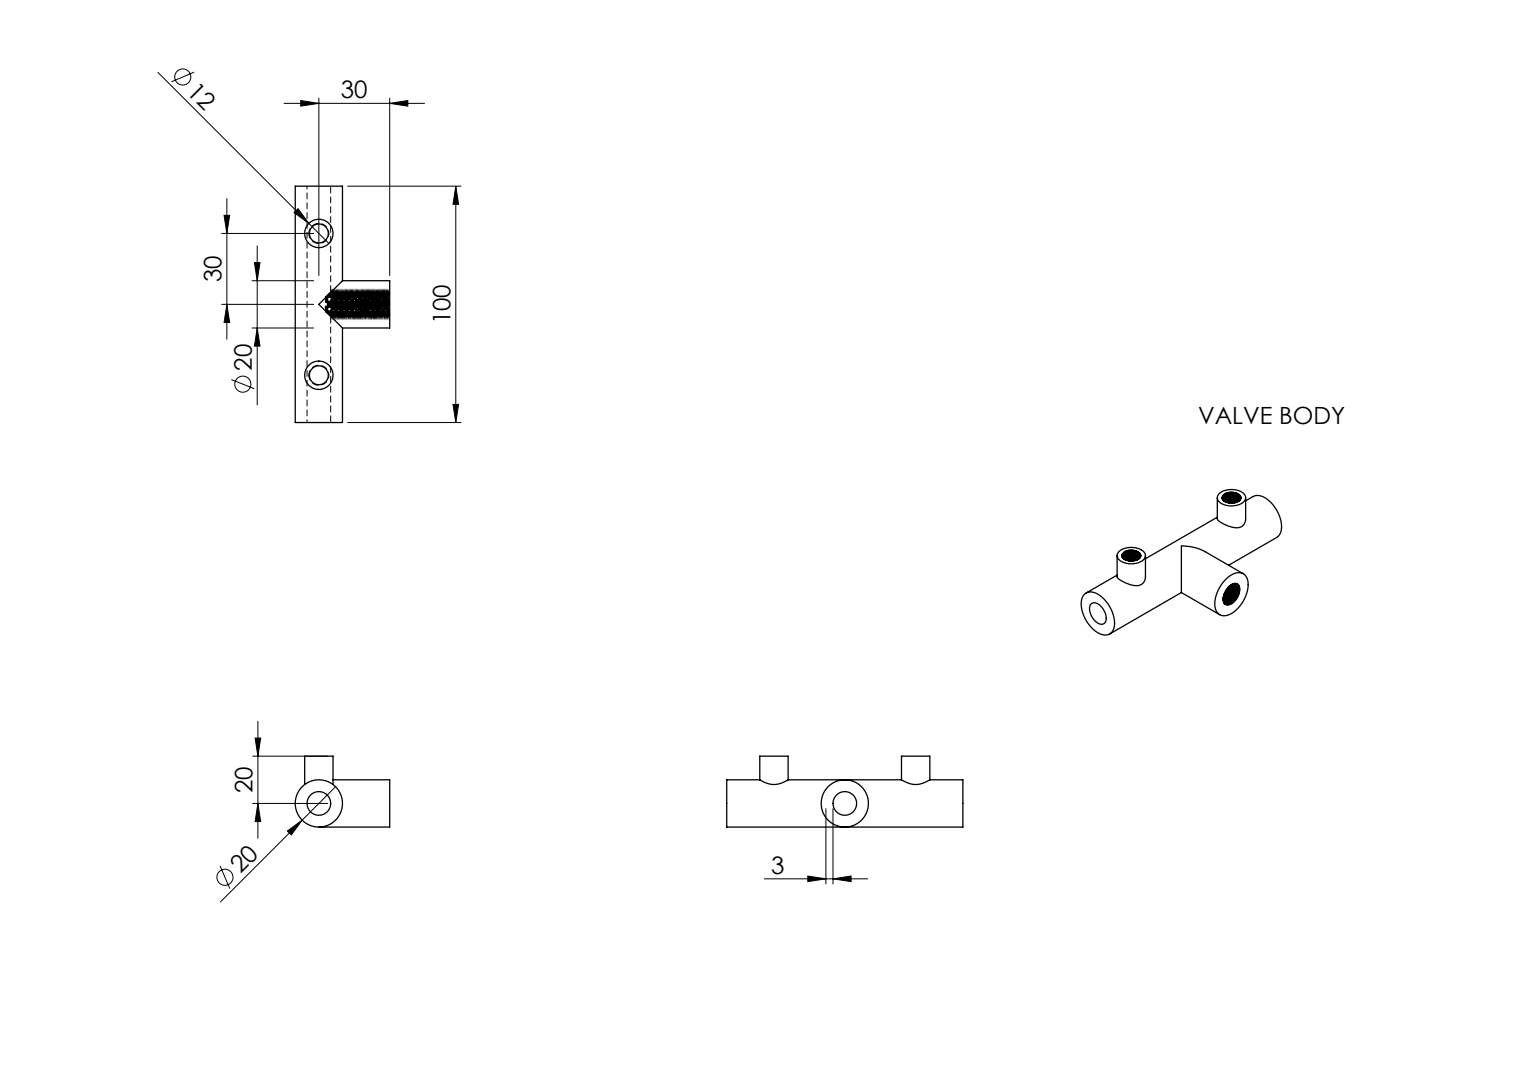
ISO-10303-21;
HEADER;
FILE_DESCRIPTION (('STEP AP214'),
    '1' );
FILE_NAME ('valve body.step',
    '2026-10-26T05:42:23',
    ( '' ),
    ( '' ),
    'SwSTEP 2.0',
    'SolidWorks 2026',
    '' );
FILE_SCHEMA (( 'AUTOMOTIVE_DESIGN' ));
ENDSEC;

DATA;
#1=CARTESIAN_POINT ( 'NONE',  ( 9.721875000614517148, -6.054752690667223547, -1.112240025338166033E-15 ) ) ;
#2=CARTESIAN_POINT ( 'NONE',  ( 3.999999999999998668, 14.07500000122903749, -32.30940107675850470 ) ) ;
#3=CARTESIAN_POINT ( 'NONE',  ( 20.46562500061451928, -6.054752690667223547, -1.112240025338166033E-15 ) ) ;
#4=CARTESIAN_POINT ( 'NONE',  ( -5.810221930991193690E-16, 14.48749999999999893, 26.00000000000000355 ) ) ;
#5=CARTESIAN_POINT ( 'NONE',  ( 2.121784821875001281, 17.25312500061459176, 33.67503911421598417 ) ) ;
#6=CARTESIAN_POINT ( 'NONE',  ( 21.83437500061451786, -4.541064518000419881, 2.621784821874995952 ) ) ;
#8=CARTESIAN_POINT ( 'NONE',  ( 27.97500000122903074, -5.773502691896255534, -1.060575238724906372E-15 ) ) ;
#10=CARTESIAN_POINT ( 'NONE',  ( 24.47812500061451502, -4.541064518000419881, 2.621784821874995952 ) ) ;
#11=CARTESIAN_POINT ( 'NONE',  ( 15.06562500061451537, -6.054752690667223547, -1.112240025338166033E-15 ) ) ;
#13=CARTESIAN_POINT ( 'NONE',  ( 10.77187500061451786, 3.027376345333613106, -5.243569643749998122 ) ) ;
#14=CARTESIAN_POINT ( 'NONE',  ( 27.89999999999999858, -4.330127018922190985, -2.500000000000001332 ) ) ;
#15=CARTESIAN_POINT ( 'NONE',  ( 25.95000000122903216, 5.773502691896255534, 3.535250795749688894E-16 ) ) ;
#16=CARTESIAN_POINT ( 'NONE',  ( 3.646875000614520079, 6.054752690667223547, 3.707466751127219781E-16 ) ) ;
#17=CARTESIAN_POINT ( 'NONE',  ( 13.58437500061451786, 4.541064518000418104, 2.621784821874999949 ) ) ;
#18=CARTESIAN_POINT ( 'NONE',  ( 28.92187500061451644, 3.027376345333611329, 5.243569643749999010 ) ) ;
#19=CARTESIAN_POINT ( 'NONE',  ( -5.810221930991193690E-16, 12.23750000000000071, -34.00000000000000000 ) ) ;
#20=ADVANCED_FACE ( 'NONE', ( #69844 ), #24040, .F. ) ;
#21=CARTESIAN_POINT ( 'NONE',  ( 18.48750000000000071, -2.886751345948126435, -5.000000000000000000 ) ) ;
#22=CARTESIAN_POINT ( 'NONE',  ( 23.74687500061451573, -3.027376345333610441, -5.243569643749999898 ) ) ;
#23=CARTESIAN_POINT ( 'NONE',  ( 13.99687500061451928, 6.054752690667223547, 3.707466751127219781E-16 ) ) ;
#25=CARTESIAN_POINT ( 'NONE',  ( 28.64999999999999858, 0.000000000000000000, 4.999999999999998224 ) ) ;
#26=CARTESIAN_POINT ( 'NONE',  ( 3.000000001229032875, 5.773502691896255534, 3.535250795749688894E-16 ) ) ;
#28=CARTESIAN_POINT ( 'NONE',  ( 18.25312500061451715, -4.541064518000417216, -2.621784821875001281 ) ) ;
#29=CARTESIAN_POINT ( 'NONE',  ( 5.962500000000002132, 2.886751345948129099, -4.999999999999998224 ) ) ;
#30=CARTESIAN_POINT ( 'NONE',  ( 13.68750000122903288, 6.123233995736764310E-16, -4.999999999999998224 ) ) ;
#31=CARTESIAN_POINT ( 'NONE',  ( 16.08749999999999503, -2.886751345948129988, 4.999999999999997335 ) ) ;
#32=CARTESIAN_POINT ( 'NONE',  ( -4.243569643749999898, 13.05312500061451786, 30.00000000000000000 ) ) ;
#33=CARTESIAN_POINT ( 'NONE',  ( -5.810221930991193690E-16, 11.78749999999999964, 26.00000000000000355 ) ) ;
#34=CARTESIAN_POINT ( 'NONE',  ( 21.63750000122903572, -4.330127018922194537, 2.499999999999995559 ) ) ;
#35=FACE_OUTER_BOUND ( 'NONE', #55826, .T. ) ;
#36=CARTESIAN_POINT ( 'NONE',  ( 26.59687500061451360, 6.054752690667223547, 3.707466751127219781E-16 ) ) ;
#37=ORIENTED_EDGE ( 'NONE', *, *, #44217, .T. ) ;
#38=CARTESIAN_POINT ( 'NONE',  ( 14.69062500061451537, -3.027376345333610441, -5.243569643749999898 ) ) ;
#39=CARTESIAN_POINT ( 'NONE',  ( 22.75312500061451360, -4.541064518000417216, -2.621784821875001281 ) ) ;
#40=CARTESIAN_POINT ( 'NONE',  ( 22.99687500061451573, 6.054752690667223547, 3.707466751127219781E-16 ) ) ;
#41=CARTESIAN_POINT ( 'NONE',  ( 6.337499999999998579, -2.886751345948125991, -5.000000000000000000 ) ) ;
#42=CARTESIAN_POINT ( 'NONE',  ( 8.990625000614516082, 6.054752690667223547, 3.707466751127219781E-16 ) ) ;
#43=CARTESIAN_POINT ( 'NONE',  ( 24.85312500061451502, 0.000000000000000000, 5.243569643749999010 ) ) ;
#44=CARTESIAN_POINT ( 'NONE',  ( 14.03437500061451715, 4.541064518000418104, 2.621784821874999949 ) ) ;
#45=CARTESIAN_POINT ( 'NONE',  ( 18.12187500061451573, 3.027376345333611329, 5.243569643749999010 ) ) ;
#47=CARTESIAN_POINT ( 'NONE',  ( -4.243569643749997233, 17.59062500061451928, 32.45002607614398471 ) ) ;
#48=CARTESIAN_POINT ( 'NONE',  ( 21.78750000122903074, 6.123233995736764310E-16, -4.999999999999998224 ) ) ;
#50=CARTESIAN_POINT ( 'NONE',  ( 11.39062500061451644, -3.027376345333614438, 5.243569643749998122 ) ) ;
#51=CARTESIAN_POINT ( 'NONE',  ( 6.684375000614518392, 6.421520780324663323E-16, -5.243569643749999010 ) ) ;
#52=CARTESIAN_POINT ( 'NONE',  ( 4.284375000614518925, -4.541064518000419881, 2.621784821874995952 ) ) ;
#53=ORIENTED_EDGE ( 'NONE', *, *, #36827, .F. ) ;
#54=CARTESIAN_POINT ( 'NONE',  ( 26.82187500061451857, -6.054752690667223547, -1.112240025338166033E-15 ) ) ;
#55=CARTESIAN_POINT ( 'NONE',  ( 16.45312500061451289, -4.541064518000417216, -2.621784821875001281 ) ) ;
#56=CARTESIAN_POINT ( 'NONE',  ( 27.82500000122903572, 2.886751345948126879, 4.999999999999999112 ) ) ;
#57=CARTESIAN_POINT ( 'NONE',  ( 28.45312500061451289, 0.000000000000000000, 5.243569643749999010 ) ) ;
#58=CARTESIAN_POINT ( 'NONE',  ( 25.02187500061451431, -6.054752690667223547, -1.112240025338166033E-15 ) ) ;
#59=CARTESIAN_POINT ( 'NONE',  ( 18.14062500061451644, -3.027376345333614438, 5.243569643749998122 ) ) ;
#60=CARTESIAN_POINT ( 'NONE',  ( 4.243569643749999010, 19.22187500061452070, 27.54997392385601174 ) ) ;
#61=CARTESIAN_POINT ( 'NONE',  ( 24.92812500061451431, -4.541064518000419881, 2.621784821874995952 ) ) ;
#62=CARTESIAN_POINT ( 'NONE',  ( 4.087500001229035007, -4.330127018922194537, 2.499999999999995559 ) ) ;
#63=ORIENTED_EDGE ( 'NONE', *, *, #30962, .F. ) ;
#64=CARTESIAN_POINT ( 'NONE',  ( 27.89999999999999858, -4.330127018922190985, -2.500000000000001332 ) ) ;
#65=CARTESIAN_POINT ( 'NONE',  ( -2.828200636599751609E-16, 15.83750000000000036, -34.61880215351700230 ) ) ;
#67=CARTESIAN_POINT ( 'NONE',  ( 5.784375000614517148, 6.421520780324663323E-16, -5.243569643749999010 ) ) ;
#68=CARTESIAN_POINT ( 'NONE',  ( 10.07812500061451644, -4.541064518000419881, 2.621784821874995952 ) ) ;
#69=CARTESIAN_POINT ( 'NONE',  ( 5.859375000614519102, 4.541064518000418104, -2.621784821874998173 ) ) ;
#70=CARTESIAN_POINT ( 'NONE',  ( 24.22500000122903430, 2.886751345948126879, 4.999999999999999112 ) ) ;
#71=CARTESIAN_POINT ( 'NONE',  ( 14.70937500061451786, -4.541064518000417216, -2.621784821875001281 ) ) ;
#72=CARTESIAN_POINT ( 'NONE',  ( 28.86562500061451786, 3.027376345333611329, 5.243569643749999010 ) ) ;
#73=CARTESIAN_POINT ( 'NONE',  ( 27.67499999999999716, 4.330127018922191873, 2.499999999999999556 ) ) ;
#75=CARTESIAN_POINT ( 'NONE',  ( 3.065625000614517592, 3.027376345333613106, -5.243569643749998122 ) ) ;
#76=CARTESIAN_POINT ( 'NONE',  ( 12.92812500061451786, 6.421520780324663323E-16, -5.243569643749999010 ) ) ;
#77=ORIENTED_EDGE ( 'NONE', *, *, #11122, .T. ) ;
#78=CARTESIAN_POINT ( 'NONE',  ( 8.953125000614518214, 4.541064518000418104, -2.621784821874998173 ) ) ;
#79=CARTESIAN_POINT ( 'NONE',  ( 5.203125000614518214, -4.541064518000417216, -2.621784821875001281 ) ) ;
#81=CARTESIAN_POINT ( 'NONE',  ( 14.10000000122903430, -2.886751345948126435, -5.000000000000000000 ) ) ;
#82=CARTESIAN_POINT ( 'NONE',  ( 14.66249999999999964, 2.886751345948126879, 4.999999999999999112 ) ) ;
#83=CARTESIAN_POINT ( 'NONE',  ( 15.90937500061451892, 0.000000000000000000, 5.243569643749999010 ) ) ;
#84=CARTESIAN_POINT ( 'NONE',  ( 11.36250000122903536, -4.330127018922190985, -2.500000000000001332 ) ) ;
#86=CARTESIAN_POINT ( 'NONE',  ( 21.72187500061451715, 3.027376345333611329, 5.243569643749999010 ) ) ;
#87=CARTESIAN_POINT ( 'NONE',  ( -3.000416591977282496E-16, 12.94062500061451537, -34.90005215228797653 ) ) ;
#90=CARTESIAN_POINT ( 'NONE',  ( 27.62812500061451360, -4.541064518000419881, 2.621784821874995952 ) ) ;
#91=CARTESIAN_POINT ( 'NONE',  ( 25.05000000000000071, 0.000000000000000000, 4.999999999999998224 ) ) ;
#92=CARTESIAN_POINT ( 'NONE',  ( 29.82187500061451502, 3.027376345333611329, 5.243569643749999010 ) ) ;
#93=CARTESIAN_POINT ( 'NONE',  ( 25.38749999999999929, 5.773502691896255534, 3.535250795749688894E-16 ) ) ;
#94=CARTESIAN_POINT ( 'NONE',  ( 8.465625000614515727, 3.027376345333613106, -5.243569643749998122 ) ) ;
#96=CARTESIAN_POINT ( 'NONE',  ( 19.09687500061451360, -3.027376345333614438, 5.243569643749998122 ) ) ;
#98=CARTESIAN_POINT ( 'NONE',  ( 4.603125000614518569, 0.000000000000000000, 5.243569643749999010 ) ) ;
#99=CARTESIAN_POINT ( 'NONE',  ( 10.69687500061451679, -3.027376345333610441, -5.243569643749999898 ) ) ;
#100=VERTEX_POINT ( 'NONE', #12957 ) ;
#101=CARTESIAN_POINT ( 'NONE',  ( 22.28437500061451715, -4.541064518000419881, 2.621784821874995952 ) ) ;
#103=CARTESIAN_POINT ( 'NONE',  ( 28.42499999999999716, 6.123233995736764310E-16, -4.999999999999998224 ) ) ;
#105=CARTESIAN_POINT ( 'NONE',  ( 5.887500000000000178, -2.886751345948125991, -5.000000000000000000 ) ) ;
#106=CARTESIAN_POINT ( 'NONE',  ( 14.36250000122903359, 0.000000000000000000, 4.999999999999998224 ) ) ;
#107=CARTESIAN_POINT ( 'NONE',  ( 1.999999999999998668, 12.31250000122903465, 26.53589838486224650 ) ) ;
#109=ORIENTED_EDGE ( 'NONE', *, *, #38380, .F. ) ;
#110=CARTESIAN_POINT ( 'NONE',  ( 12.15000000000000036, -4.330127018922190985, -2.500000000000001332 ) ) ;
#111=CARTESIAN_POINT ( 'NONE',  ( 26.84062500061451573, -3.027376345333610441, -5.243569643749999898 ) ) ;
#112=CARTESIAN_POINT ( 'NONE',  ( 16.19999999999999929, -4.330127018922190985, -2.500000000000001332 ) ) ;
#113=ADVANCED_FACE ( 'NONE', ( #65026 ), #30323, .F. ) ;
#114=CARTESIAN_POINT ( 'NONE',  ( 10.20000000122903572, 5.773502691896255534, 3.535250795749688894E-16 ) ) ;
#115=CARTESIAN_POINT ( 'NONE',  ( 8.128125000614515372, 4.541064518000418104, 2.621784821874999949 ) ) ;
#116=CARTESIAN_POINT ( 'NONE',  ( 9.225000000000001421, 4.330127018922191873, 2.499999999999999556 ) ) ;
#117=FACE_OUTER_BOUND ( 'NONE', #13285, .T. ) ;
#118=CARTESIAN_POINT ( 'NONE',  ( 4.243569643749999010, 15.17187500061451644, -32.45002607614398471 ) ) ;
#119=CARTESIAN_POINT ( 'NONE',  ( 27.00000000122903288, -2.886751345948129988, 4.999999999999997335 ) ) ;
#121=CARTESIAN_POINT ( 'NONE',  ( 7.162500000000001421, -5.773502691896255534, -1.060575238724906372E-15 ) ) ;
#124=CARTESIAN_POINT ( 'NONE',  ( 25.04062500061451502, -3.027376345333610441, -5.243569643749999898 ) ) ;
#125=CARTESIAN_POINT ( 'NONE',  ( 14.88750000122903394, -4.330127018922194537, 2.499999999999995559 ) ) ;
#126=CARTESIAN_POINT ( 'NONE',  ( 29.57812500061451644, 6.421520780324663323E-16, -5.243569643749999010 ) ) ;
#127=CARTESIAN_POINT ( 'NONE',  ( 28.62187500061451573, -6.054752690667223547, -1.112240025338166033E-15 ) ) ;
#128=CARTESIAN_POINT ( 'NONE',  ( 18.87187500061451573, 3.027376345333613106, -5.243569643749998122 ) ) ;
#129=CARTESIAN_POINT ( 'NONE',  ( 16.49062500061451786, -3.027376345333610441, -5.243569643749999898 ) ) ;
#130=CARTESIAN_POINT ( 'NONE',  ( -4.243569643749998122, 10.39062500061459460, -27.54997392385601174 ) ) ;
#131=CARTESIAN_POINT ( 'NONE',  ( 5.990625000614517859, -3.027376345333614438, 5.243569643749998122 ) ) ;
#132=CARTESIAN_POINT ( 'NONE',  ( 29.28750000122903074, -4.330127018922194537, 2.499999999999995559 ) ) ;
#134=CARTESIAN_POINT ( 'NONE',  ( 19.19062500061452070, -3.027376345333610441, -5.243569643749999898 ) ) ;
#136=CARTESIAN_POINT ( 'NONE',  ( 13.39687500061451608, -3.027376345333610441, -5.243569643749999898 ) ) ;
#137=CARTESIAN_POINT ( 'NONE',  ( 11.14687500061451608, -3.027376345333610441, -5.243569643749999898 ) ) ;
#138=CARTESIAN_POINT ( 'NONE',  ( 23.59687500061451715, -3.027376345333614438, 5.243569643749998122 ) ) ;
#140=CARTESIAN_POINT ( 'NONE',  ( 3.290625000614516793, -3.027376345333614438, 5.243569643749998122 ) ) ;
#141=CARTESIAN_POINT ( 'NONE',  ( 27.40312500061451573, 4.541064518000418104, -2.621784821874998173 ) ) ;
#142=( BOUNDED_CURVE ( )  B_SPLINE_CURVE ( 2, ( #31020, #38022, #48390, #19556, #9951, #32488, #65735 ),
 .UNSPECIFIED., .F., .F. ) 
 B_SPLINE_CURVE_WITH_KNOTS ( ( 3, 2, 2, 3 ),
 ( 0.6416666666666668295, 0.6444444444444445974, 0.6472222222222223653, 0.6500000000000001332 ),
 .UNSPECIFIED. ) 
 CURVE ( )  GEOMETRIC_REPRESENTATION_ITEM ( )  RATIONAL_B_SPLINE_CURVE ( ( 0.9999999999999946709, 0.8660254037844440367, 1.000000000000000000, 0.8660254037844387076, 1.000000000000000000, 0.8660254037844333785, 1.000000000000005329 ) ) 
 REPRESENTATION_ITEM ( '' )  );
#143=CARTESIAN_POINT ( 'NONE',  ( 27.55312500061451786, 0.000000000000000000, 5.243569643749999010 ) ) ;
#144=CARTESIAN_POINT ( 'NONE',  ( 4.000000000000000000, 12.08750000000000036, -27.69059892324149885 ) ) ;
#145=CARTESIAN_POINT ( 'NONE',  ( -2.828200636599751609E-16, 16.73750000000000071, 25.38119784648299770 ) ) ;
#146=CARTESIAN_POINT ( 'NONE',  ( 4.021875000614516082, 3.027376345333613106, -5.243569643749998122 ) ) ;
#147=CARTESIAN_POINT ( 'NONE',  ( 11.58750000122903501, 4.330127018922191873, 2.499999999999999556 ) ) ;
#148=CARTESIAN_POINT ( 'NONE',  ( 7.987500001229032698, 4.330127018922191873, 2.499999999999999556 ) ) ;
#149=CARTESIAN_POINT ( 'NONE',  ( 28.50000000122903288, -2.886751345948125991, -5.000000000000000000 ) ) ;
#152=CARTESIAN_POINT ( 'NONE',  ( 11.78437500061451892, 4.541064518000418104, 2.621784821874999949 ) ) ;
#154=CARTESIAN_POINT ( 'NONE',  ( 20.31562500061451715, 3.027376345333611329, 5.243569643749999010 ) ) ;
#155=CARTESIAN_POINT ( 'NONE',  ( 13.95937500061451786, 4.541064518000418104, -2.621784821874998173 ) ) ;
#156=CARTESIAN_POINT ( 'NONE',  ( 3.778125000614519280, -4.541064518000419881, 2.621784821874995952 ) ) ;
#157=CARTESIAN_POINT ( 'NONE',  ( 23.33437500061451786, 6.421520780324663323E-16, -5.243569643749999010 ) ) ;
#158=CARTESIAN_POINT ( 'NONE',  ( 8.746875000614515727, -3.027376345333614438, 5.243569643749998122 ) ) ;
#159=CARTESIAN_POINT ( 'NONE',  ( 4.565625000614516260, 3.027376345333611329, 5.243569643749999010 ) ) ;
#160=CARTESIAN_POINT ( 'NONE',  ( 5.812500000000001776, -5.773502691896255534, -1.060575238724906372E-15 ) ) ;
#161=CARTESIAN_POINT ( 'NONE',  ( 5.850000001229035185, -2.886751345948129988, 4.999999999999997335 ) ) ;
#162=CARTESIAN_POINT ( 'NONE',  ( 19.82812500061451644, 4.541064518000418104, 2.621784821874999949 ) ) ;
#164=CARTESIAN_POINT ( 'NONE',  ( 9.000000001229034652, -2.886751345948129988, 4.999999999999997335 ) ) ;
#165=( BOUNDED_CURVE ( )  B_SPLINE_CURVE ( 2, ( #55772, #22147, #62756, #34675, #57203, #6619, #72393 ),
 .UNSPECIFIED., .F., .F. ) 
 B_SPLINE_CURVE_WITH_KNOTS ( ( 3, 2, 2, 3 ),
 ( 0.06666666666666665186, 0.06944444444444443365, 0.07222222222222218768, 0.07499999999999996947 ),
 .UNSPECIFIED. ) 
 CURVE ( )  GEOMETRIC_REPRESENTATION_ITEM ( )  RATIONAL_B_SPLINE_CURVE ( ( 1.000000000000000666, 0.8660254037844379305, 1.000000000000000000, 0.8660254037844387076, 1.000000000000000000, 0.8660254037844400399, 0.9999999999999986677 ) ) 
 REPRESENTATION_ITEM ( '' )  );
#166=CARTESIAN_POINT ( 'NONE',  ( 18.47812500061451857, 4.541064518000418104, 2.621784821874999949 ) ) ;
#167=CARTESIAN_POINT ( 'NONE',  ( 14.35312500061451679, 4.541064518000418104, -2.621784821874998173 ) ) ;
#169=CARTESIAN_POINT ( 'NONE',  ( 12.71250000000000036, 2.886751345948129099, -4.999999999999998224 ) ) ;
#170=CARTESIAN_POINT ( 'NONE',  ( 10.16250000122903252, 4.330127018922192761, -2.499999999999997780 ) ) ;
#171=CARTESIAN_POINT ( 'NONE',  ( 4.603125000614518569, 0.000000000000000000, 5.243569643749999010 ) ) ;
#172=CARTESIAN_POINT ( 'NONE',  ( 21.45000000122903216, 5.773502691896255534, 3.535250795749688894E-16 ) ) ;
#174=CARTESIAN_POINT ( 'NONE',  ( 4.243569643749999898, 11.08437500061451786, -30.00000000000000000 ) ) ;
#175=CARTESIAN_POINT ( 'NONE',  ( 5.587500001229033231, 6.123233995736764310E-16, -4.999999999999998224 ) ) ;
#176=CARTESIAN_POINT ( 'NONE',  ( 24.07499999999999929, 4.330127018922191873, 2.499999999999999556 ) ) ;
#177=CARTESIAN_POINT ( 'NONE',  ( 6.487499999999999822, 5.773502691896255534, 3.535250795749688401E-16 ) ) ;
#178=CARTESIAN_POINT ( 'NONE',  ( 21.38437500061451502, -4.541064518000419881, 2.621784821874995952 ) ) ;
#179=CARTESIAN_POINT ( 'NONE',  ( 1.999999999999998668, 18.61250000122903359, 26.53589838486224650 ) ) ;
#180=CARTESIAN_POINT ( 'NONE',  ( 16.34062500061451573, -3.027376345333614438, 5.243569643749998122 ) ) ;
#184=CARTESIAN_POINT ( 'NONE',  ( 27.12187500061451573, 3.027376345333611329, 5.243569643749999010 ) ) ;
#186=CARTESIAN_POINT ( 'NONE',  ( 11.54062500061451857, -3.027376345333610441, -5.243569643749999898 ) ) ;
#187=CARTESIAN_POINT ( 'NONE',  ( 11.67187500061451821, 3.027376345333613106, -5.243569643749998122 ) ) ;
#189=CARTESIAN_POINT ( 'NONE',  ( -1.999999999999997113, 14.22500000000000142, -26.53589838486224295 ) ) ;
#190=CARTESIAN_POINT ( 'NONE',  ( 23.54062500061451146, -3.027376345333614438, 5.243569643749998122 ) ) ;
#191=CARTESIAN_POINT ( 'NONE',  ( 1.071796769724489895, 13.22990381179669939, -34.00000000000000000 ) ) ;
#193=CARTESIAN_POINT ( 'NONE',  ( 12.00000000000000000, 0.000000000000000000, 4.999999999999998224 ) ) ;
#194=CARTESIAN_POINT ( 'NONE',  ( 22.72500000122903430, 2.886751345948129099, -4.999999999999998224 ) ) ;
#195=CARTESIAN_POINT ( 'NONE',  ( 15.70312500061451644, 4.541064518000418104, -2.621784821874998173 ) ) ;
#198=CARTESIAN_POINT ( 'NONE',  ( 19.98749999999999716, 5.773502691896255534, 3.535250795749688894E-16 ) ) ;
#199=CARTESIAN_POINT ( 'NONE',  ( 24.78750000000000497, -2.886751345948125991, -5.000000000000000000 ) ) ;
#200=CARTESIAN_POINT ( 'NONE',  ( 21.42187500061451644, -6.054752690667223547, -1.112240025338166033E-15 ) ) ;
#201=CARTESIAN_POINT ( 'NONE',  ( 26.20312500061451644, 0.000000000000000000, 5.243569643749999010 ) ) ;
#204=CARTESIAN_POINT ( 'NONE',  ( 8.728125000614518569, -4.541064518000419881, 2.621784821874995952 ) ) ;
#205=CARTESIAN_POINT ( 'NONE',  ( 17.40000000122903145, 5.773502691896255534, 3.535250795749688401E-16 ) ) ;
#206=CARTESIAN_POINT ( 'NONE',  ( 14.40000000000000036, -4.330127018922190985, -2.500000000000001332 ) ) ;
#207=CARTESIAN_POINT ( 'NONE',  ( 2.121784821874999061, 17.85312500061451502, 26.32496088578401583 ) ) ;
#208=CARTESIAN_POINT ( 'NONE',  ( 4.171875000614517326, 3.027376345333611329, 5.243569643749999010 ) ) ;
#209=CARTESIAN_POINT ( 'NONE',  ( 27.30937500061451573, -4.541064518000417216, -2.621784821875001281 ) ) ;
#211=CARTESIAN_POINT ( 'NONE',  ( 24.70312500061451644, 4.541064518000418104, -2.621784821874998173 ) ) ;
#212=CARTESIAN_POINT ( 'NONE',  ( 25.05937500061451573, -4.541064518000417216, -2.621784821875001281 ) ) ;
#213=CARTESIAN_POINT ( 'NONE',  ( 4.243569643749999898, 19.57812500061459460, -30.00000000000000000 ) ) ;
#214=CARTESIAN_POINT ( 'NONE',  ( 10.49999999999999822, 4.330127018922192761, -2.499999999999997780 ) ) ;
#215=CARTESIAN_POINT ( 'NONE',  ( 9.478125000614515017, 4.541064518000418104, 2.621784821874999949 ) ) ;
#216=CYLINDRICAL_SURFACE ( 'NONE', #71725, 4.000000000000000000 ) ;
#218=CARTESIAN_POINT ( 'NONE',  ( 27.44062500061451715, 6.054752690667223547, 3.707466751127219781E-16 ) ) ;
#221=CARTESIAN_POINT ( 'NONE',  ( 3.665625000614517681, 3.027376345333611329, 5.243569643749999010 ) ) ;
#222=CARTESIAN_POINT ( 'NONE',  ( 19.39687500061451786, 6.054752690667223547, 3.707466751127219781E-16 ) ) ;
#223=CARTESIAN_POINT ( 'NONE',  ( 9.001249775931846008E-16, 14.57187500061451679, 34.90005215228797653 ) ) ;
#224=CARTESIAN_POINT ( 'NONE',  ( 19.65937500061451360, -4.541064518000417216, -2.621784821875001281 ) ) ;
#225=CARTESIAN_POINT ( 'NONE',  ( 29.55937500061451573, -4.541064518000417216, -2.621784821875001281 ) ) ;
#226=CARTESIAN_POINT ( 'NONE',  ( -4.243569643749999898, 18.47187500061451715, 27.54997392385601529 ) ) ;
#227=CARTESIAN_POINT ( 'NONE',  ( 10.19062500061451892, -3.027376345333610441, -5.243569643749999898 ) ) ;
#228=CARTESIAN_POINT ( 'NONE',  ( 3.112500001229034918, 0.000000000000000000, 4.999999999999998224 ) ) ;
#229=CARTESIAN_POINT ( 'NONE',  ( 7.846875000614518036, -3.027376345333614438, 5.243569643749998122 ) ) ;
#230=CARTESIAN_POINT ( 'NONE',  ( 16.16250000122903430, 0.000000000000000000, 4.999999999999998224 ) ) ;
#231=CARTESIAN_POINT ( 'NONE',  ( 8.165625000614516793, 3.027376345333611329, 5.243569643749999010 ) ) ;
#232=CARTESIAN_POINT ( 'NONE',  ( 11.22187500061451892, 3.027376345333613106, -5.243569643749998122 ) ) ;
#233=CARTESIAN_POINT ( 'NONE',  ( 18.90000000122902790, -2.886751345948129988, 4.999999999999997335 ) ) ;
#234=CARTESIAN_POINT ( 'NONE',  ( 8.446875000614518569, -3.027376345333610441, -5.243569643749999898 ) ) ;
#235=CARTESIAN_POINT ( 'NONE',  ( 9.815625000614518925, 3.027376345333613106, -5.243569643749998122 ) ) ;
#236=CARTESIAN_POINT ( 'NONE',  ( 5.803125000614517859, 4.541064518000418104, -2.621784821874998173 ) ) ;
#238=CARTESIAN_POINT ( 'NONE',  ( 20.25937500061451857, 4.541064518000418104, -2.621784821874998173 ) ) ;
#239=CARTESIAN_POINT ( 'NONE',  ( -5.810221930991193690E-16, 13.25000000122903465, 26.00000000000000355 ) ) ;
#240=CARTESIAN_POINT ( 'NONE',  ( 26.39062500061451644, -3.027376345333610441, -5.243569643749999898 ) ) ;
#241=CARTESIAN_POINT ( 'NONE',  ( 12.02812500061451573, 6.421520780324663323E-16, -5.243569643749999010 ) ) ;
#242=CARTESIAN_POINT ( 'NONE',  ( 28.99687500061451573, -3.027376345333614438, 5.243569643749998122 ) ) ;
#243=CARTESIAN_POINT ( 'NONE',  ( 2.121784821874999061, 10.25937500061451857, -33.67503911421598417 ) ) ;
#244=CARTESIAN_POINT ( 'NONE',  ( 12.78750000122903430, 6.123233995736764310E-16, -4.999999999999998224 ) ) ;
#245=CARTESIAN_POINT ( 'NONE',  ( 28.19062500061451715, -3.027376345333610441, -5.243569643749999898 ) ) ;
#246=ADVANCED_FACE ( 'NONE', ( #36587 ), #41411, .F. ) ;
#247=CARTESIAN_POINT ( 'NONE',  ( -2.121784821874999949, 15.22812500061451679, -33.67503911421598417 ) ) ;
#248=CARTESIAN_POINT ( 'NONE',  ( 15.22500000122903252, 2.886751345948126879, 4.999999999999999112 ) ) ;
#249=CARTESIAN_POINT ( 'NONE',  ( 13.68750000000000178, 5.773502691896255534, 3.535250795749688894E-16 ) ) ;
#250=CARTESIAN_POINT ( 'NONE',  ( 21.62812500061451360, 4.541064518000418104, 2.621784821874999949 ) ) ;
#251=CARTESIAN_POINT ( 'NONE',  ( 8.184375000614515727, 4.541064518000418104, 2.621784821874999949 ) ) ;
#252=CARTESIAN_POINT ( 'NONE',  ( 7.912500001229033408, 4.330127018922192761, -2.499999999999997780 ) ) ;
#253=CARTESIAN_POINT ( 'NONE',  ( 17.25000000122903288, -2.886751345948125991, -5.000000000000000000 ) ) ;
#254=CARTESIAN_POINT ( 'NONE',  ( 13.04062500061451502, 6.054752690667223547, 3.707466751127219781E-16 ) ) ;
#255=CARTESIAN_POINT ( 'NONE',  ( 16.04062500061451857, -3.027376345333610441, -5.243569643749999898 ) ) ;
#256=CARTESIAN_POINT ( 'NONE',  ( 27.56250000122902932, -4.330127018922190985, -2.500000000000001332 ) ) ;
#257=CARTESIAN_POINT ( 'NONE',  ( 21.93750000000000000, -2.886751345948129988, 4.999999999999997335 ) ) ;
#258=CARTESIAN_POINT ( 'NONE',  ( 24.15937500061451715, -4.541064518000417216, -2.621784821875001281 ) ) ;
#260=CARTESIAN_POINT ( 'NONE',  ( 10.42500000122903536, -5.773502691896255534, -1.060575238724906372E-15 ) ) ;
#261=CARTESIAN_POINT ( 'NONE',  ( 28.28437500061451715, 6.421520780324663323E-16, -5.243569643749999010 ) ) ;
#262=CARTESIAN_POINT ( 'NONE',  ( 5.146875000614517859, -3.027376345333614438, 5.243569643749998122 ) ) ;
#263=CARTESIAN_POINT ( 'NONE',  ( 24.59062500061451573, -3.027376345333610441, -5.243569643749999898 ) ) ;
#266=CARTESIAN_POINT ( 'NONE',  ( 10.69687500061451679, -3.027376345333610441, -5.243569643749999898 ) ) ;
#267=CARTESIAN_POINT ( 'NONE',  ( 3.999999999999998668, 12.61250000000000249, 27.69059892324149530 ) ) ;
#268=CARTESIAN_POINT ( 'NONE',  ( 29.09062500061451573, -3.027376345333610441, -5.243569643749999898 ) ) ;
#269=CARTESIAN_POINT ( 'NONE',  ( 7.321875000614516793, 3.027376345333611329, 5.243569643749999010 ) ) ;
#270=CARTESIAN_POINT ( 'NONE',  ( 6.825000000000001066, 6.123233995736764310E-16, -4.999999999999998224 ) ) ;
#271=CARTESIAN_POINT ( 'NONE',  ( 25.24687500061451573, 6.054752690667223547, 3.707466751127219781E-16 ) ) ;
#272=CARTESIAN_POINT ( 'NONE',  ( 2.121784821874999061, 10.65312500061459566, 26.32496088578401583 ) ) ;
#273=CARTESIAN_POINT ( 'NONE',  ( 18.56250000000000000, 2.886751345948129099, -4.999999999999998224 ) ) ;
#275=CARTESIAN_POINT ( 'NONE',  ( 26.84999999999999787, 0.000000000000000000, 4.999999999999998224 ) ) ;
#277=CARTESIAN_POINT ( 'NONE',  ( 28.99687500061451573, -3.027376345333614438, 5.243569643749998122 ) ) ;
#278=ADVANCED_FACE ( 'NONE', ( #72396 ), #26980, .F. ) ;
#279=EDGE_LOOP ( 'NONE', ( #33564, #50876, #16388, #71740 ) ) ;
#280=CARTESIAN_POINT ( 'NONE',  ( 16.45312500061451289, -4.541064518000417216, -2.621784821875001281 ) ) ;
#281=CARTESIAN_POINT ( 'NONE',  ( 7.565625000614518036, 3.027376345333613106, -5.243569643749998122 ) ) ;
#283=CARTESIAN_POINT ( 'NONE',  ( 5.821875000614519458, 3.027376345333613106, -5.243569643749998122 ) ) ;
#284=CARTESIAN_POINT ( 'NONE',  ( 18.93750000122903288, -4.330127018922194537, 2.499999999999995559 ) ) ;
#285=CARTESIAN_POINT ( 'NONE',  ( 22.64999999999999858, 4.330127018922192761, -2.499999999999997780 ) ) ;
#286=CARTESIAN_POINT ( 'NONE',  ( 3.275492200589926739, -3.777717676570560901, -3.275492200590059078 ) ) ;
#287=CARTESIAN_POINT ( 'NONE',  ( 7.734375000614517326, 4.541064518000418104, 2.621784821874999949 ) ) ;
#288=CARTESIAN_POINT ( 'NONE',  ( 12.60937500061451821, 4.541064518000418104, -2.621784821874998173 ) ) ;
#289=CARTESIAN_POINT ( 'NONE',  ( 21.60937500061451644, 4.541064518000418104, -2.621784821874998173 ) ) ;
#290=CARTESIAN_POINT ( 'NONE',  ( -5.810221930991193690E-16, 14.48749999999999893, -34.00000000000000000 ) ) ;
#291=ORIENTED_EDGE ( 'NONE', *, *, #26409, .F. ) ;
#292=CARTESIAN_POINT ( 'NONE',  ( 3.909375000614518481, -4.541064518000417216, -2.621784821875001281 ) ) ;
#293=CARTESIAN_POINT ( 'NONE',  ( 7.696875000614516793, 6.054752690667223547, 3.707466751127219781E-16 ) ) ;
#294=CARTESIAN_POINT ( 'NONE',  ( 19.46249999999999858, 2.886751345948129099, -4.999999999999998224 ) ) ;
#295=CARTESIAN_POINT ( 'NONE',  ( 15.06562500061451537, -6.054752690667223547, -1.112240025338166033E-15 ) ) ;
#299=CARTESIAN_POINT ( 'NONE',  ( 10.90312500061451928, 0.000000000000000000, 5.243569643749999010 ) ) ;
#300=CARTESIAN_POINT ( 'NONE',  ( 26.89687500061451431, -3.027376345333610441, -5.243569643749999898 ) ) ;
#301=CARTESIAN_POINT ( 'NONE',  ( 27.90937500061451715, 4.541064518000418104, -2.621784821874998173 ) ) ;
#302=CARTESIAN_POINT ( 'NONE',  ( 9.750000000000001776, 0.000000000000000000, 4.999999999999998224 ) ) ;
#303=CARTESIAN_POINT ( 'NONE',  ( -3.999999999999999112, 16.06250000122903288, 30.00000000000000000 ) ) ;
#304=CARTESIAN_POINT ( 'NONE',  ( 8.475000001229034297, 2.886751345948126879, 4.999999999999999112 ) ) ;
#305=CARTESIAN_POINT ( 'NONE',  ( 20.63437500061451857, 6.421520780324663323E-16, -5.243569643749999010 ) ) ;
#306=CARTESIAN_POINT ( 'NONE',  ( 14.70937500061451786, -4.541064518000417216, -2.621784821875001281 ) ) ;
#307=CARTESIAN_POINT ( 'NONE',  ( 9.999999999999992895, 5.857864376269048989, 9.999999999999992895 ) ) ;
#309=CARTESIAN_POINT ( 'NONE',  ( 13.97812500061451679, 4.541064518000418104, 2.621784821874999949 ) ) ;
#310=CARTESIAN_POINT ( 'NONE',  ( 27.00000000122903288, -2.886751345948129988, 4.999999999999997335 ) ) ;
#311=CARTESIAN_POINT ( 'NONE',  ( 15.38437500061451679, 4.541064518000418104, 2.621784821874999949 ) ) ;
#312=CARTESIAN_POINT ( 'NONE',  ( 3.440625000614518036, -3.027376345333610441, -5.243569643749999898 ) ) ;
#313=CARTESIAN_POINT ( 'NONE',  ( 17.42812500061451786, 6.421520780324663323E-16, -5.243569643749999010 ) ) ;
#314=ADVANCED_FACE ( 'NONE', ( #9615 ), #38044, .F. ) ;
#315=FACE_OUTER_BOUND ( 'NONE', #42185, .T. ) ;
#316=CARTESIAN_POINT ( 'NONE',  ( 25.92187500061451999, -6.054752690667223547, -1.112240025338166033E-15 ) ) ;
#317=CARTESIAN_POINT ( 'NONE',  ( 2.121784821874999061, 11.10312500061451679, 26.32496088578401583 ) ) ;
#318=CARTESIAN_POINT ( 'NONE',  ( 16.28437500061452070, 4.541064518000418104, 2.621784821874999949 ) ) ;
#319=CARTESIAN_POINT ( 'NONE',  ( 13.01250000122903394, 0.000000000000000000, 4.999999999999998224 ) ) ;
#320=CARTESIAN_POINT ( 'NONE',  ( 30.00000000000000000, 0.000000000000000000, 0.000000000000000000 ) ) ;
#321=CARTESIAN_POINT ( 'NONE',  ( -2.121784821874999949, 19.78437500061451715, -33.67503911421598417 ) ) ;
#322=CARTESIAN_POINT ( 'NONE',  ( 18.87187500061451573, 3.027376345333613106, -5.243569643749998122 ) ) ;
#323=CARTESIAN_POINT ( 'NONE',  ( 19.87500000122903288, -5.773502691896255534, -1.060575238724906372E-15 ) ) ;
#324=CARTESIAN_POINT ( 'NONE',  ( 14.89687500061451786, 6.054752690667223547, 3.707466751127219781E-16 ) ) ;
#325=CARTESIAN_POINT ( 'NONE',  ( -2.121784821874996840, 11.38437500061451679, 33.67503911421598417 ) ) ;
#326=CARTESIAN_POINT ( 'NONE',  ( 21.26250000122903572, -4.330127018922190985, -2.500000000000001332 ) ) ;
#327=CARTESIAN_POINT ( 'NONE',  ( 14.65312500061451573, -4.541064518000417216, -2.621784821875001281 ) ) ;
#328=CYLINDRICAL_SURFACE ( 'NONE', #3060, 3.999999999999996447 ) ;
#329=VERTEX_POINT ( 'NONE', #38418 ) ;
#330=ORIENTED_EDGE ( 'NONE', *, *, #52495, .F. ) ;
#331=CARTESIAN_POINT ( 'NONE',  ( 20.54999999999999716, 0.000000000000000000, 4.999999999999998224 ) ) ;
#332=CARTESIAN_POINT ( 'NONE',  ( 3.482548389542082568, 3.599757532507414481, 32.03236939885417911 ) ) ;
#333=CARTESIAN_POINT ( 'NONE',  ( 14.85000000122903252, -2.886751345948129988, 4.999999999999997335 ) ) ;
#334=CARTESIAN_POINT ( 'NONE',  ( 19.52812500061451573, -4.541064518000419881, 2.621784821874995952 ) ) ;
#335=CARTESIAN_POINT ( 'NONE',  ( 23.24062500061451786, -3.027376345333610441, -5.243569643749999898 ) ) ;
#336=EDGE_CURVE ( 'NONE', #58790, #48104, #15871, .T. ) ;
#337=CARTESIAN_POINT ( 'NONE',  ( 5.128125000614516260, -4.541064518000419881, 2.621784821874995952 ) ) ;
#338=( BOUNDED_CURVE ( )  B_SPLINE_CURVE ( 2, ( #15519, #49887, #72412, #9995, #32529, #66507, #49526 ),
 .UNSPECIFIED., .F., .F. ) 
 B_SPLINE_CURVE_WITH_KNOTS ( ( 3, 2, 2, 3 ),
 ( 0.5083333333333334147, 0.5111111111111110716, 0.5138888888888888395, 0.5166666666666666075 ),
 .UNSPECIFIED. ) 
 CURVE ( )  GEOMETRIC_REPRESENTATION_ITEM ( )  RATIONAL_B_SPLINE_CURVE ( ( 0.9999999999999946709, 0.8660254037844440367, 1.000000000000000000, 0.8660254037844387076, 1.000000000000000000, 0.8660254037844440367, 0.9999999999999946709 ) ) 
 REPRESENTATION_ITEM ( '' )  );
#340=CARTESIAN_POINT ( 'NONE',  ( 29.06250000000000000, 2.886751345948126879, 4.999999999999999112 ) ) ;
#344=CARTESIAN_POINT ( 'NONE',  ( 4.000000000000000000, 10.85000000122903430, -27.69059892324149530 ) ) ;
#345=CARTESIAN_POINT ( 'NONE',  ( 4.243569643749999010, 17.87187500061451573, -32.45002607614398471 ) ) ;
#346=CARTESIAN_POINT ( 'NONE',  ( 6.562500001229032875, 4.330127018922192761, -2.499999999999997780 ) ) ;
#347=CARTESIAN_POINT ( 'NONE',  ( 8.737500000000002487, 5.773502691896255534, 3.535250795749688894E-16 ) ) ;
#348=CARTESIAN_POINT ( 'NONE',  ( 3.787500001229033408, 6.123233995736764310E-16, -4.999999999999998224 ) ) ;
#349=CARTESIAN_POINT ( 'NONE',  ( 11.74687500061451573, 6.054752690667223547, 3.707466751127219781E-16 ) ) ;
#350=CARTESIAN_POINT ( 'NONE',  ( 4.057522967627288146, -2.921730200955767298, 4.057522967627288146 ) ) ;
#351=CARTESIAN_POINT ( 'NONE',  ( 4.396875000614516971, -3.027376345333610441, -5.243569643749999898 ) ) ;
#352=CARTESIAN_POINT ( 'NONE',  ( 12.90000000122903323, 5.773502691896255534, 3.535250795749688401E-16 ) ) ;
#353=CARTESIAN_POINT ( 'NONE',  ( 4.000000000000000000, 19.40000000122903856, 32.30940107675849760 ) ) ;
#354=CARTESIAN_POINT ( 'NONE',  ( 10.84687500061451892, 6.054752690667223547, 3.707466751127219781E-16 ) ) ;
#355=CARTESIAN_POINT ( 'NONE',  ( 14.48437500061451821, 4.541064518000418104, 2.621784821874999949 ) ) ;
#356=CARTESIAN_POINT ( 'NONE',  ( 3.609349942001692124, -3.970247583483341280, -3.123329466779292130 ) ) ;
#357=CARTESIAN_POINT ( 'NONE',  ( 2.121784821874999061, 16.50312500061459176, 26.32496088578401583 ) ) ;
#358=CARTESIAN_POINT ( 'NONE',  ( 21.15937500061451715, 4.541064518000418104, -2.621784821874998173 ) ) ;
#359=CARTESIAN_POINT ( 'NONE',  ( 26.92500000122903359, 2.886751345948126879, 4.999999999999999112 ) ) ;
#361=CARTESIAN_POINT ( 'NONE',  ( 22.52812500061451573, 4.541064518000418104, 2.621784821874999949 ) ) ;
#362=CARTESIAN_POINT ( 'NONE',  ( 15.85312500061451857, 0.000000000000000000, 5.243569643749999010 ) ) ;
#364=CARTESIAN_POINT ( 'NONE',  ( 11.55937500061451928, -4.541064518000417216, -2.621784821875001281 ) ) ;
#365=CARTESIAN_POINT ( 'NONE',  ( 29.73750000000000071, -2.886751345948125991, -5.000000000000000000 ) ) ;
#366=CARTESIAN_POINT ( 'NONE',  ( 24.75000000122902932, -2.886751345948129988, 4.999999999999997335 ) ) ;
#367=CARTESIAN_POINT ( 'NONE',  ( 4.659375000614518925, 0.000000000000000000, 5.243569643749999010 ) ) ;
#368=CARTESIAN_POINT ( 'NONE',  ( 14.93437500061451750, 4.541064518000418104, 2.621784821874999949 ) ) ;
#369=CARTESIAN_POINT ( 'NONE',  ( 29.70937500061451431, 4.541064518000418104, -2.621784821874998173 ) ) ;
#370=CARTESIAN_POINT ( 'NONE',  ( 3.070561448845197550, -4.159287105319667610, 2.795903410320249360 ) ) ;
#372=CARTESIAN_POINT ( 'NONE',  ( 22.84687500061451715, -3.027376345333610441, -5.243569643749999898 ) ) ;
#373=CARTESIAN_POINT ( 'NONE',  ( 14.82187500061451679, 3.027376345333613106, -5.243569643749998122 ) ) ;
#375=CARTESIAN_POINT ( 'NONE',  ( 25.76249999999999929, 2.886751345948129099, -4.999999999999998224 ) ) ;
#376=CARTESIAN_POINT ( 'NONE',  ( 4.350000001229033408, 5.773502691896255534, 3.535250795749688894E-16 ) ) ;
#378=CARTESIAN_POINT ( 'NONE',  ( 16.26562500061451289, 3.027376345333611329, 5.243569643749999010 ) ) ;
#379=CARTESIAN_POINT ( 'NONE',  ( 7.687500000000000000, -2.886751345948125991, -5.000000000000000000 ) ) ;
#380=EDGE_CURVE ( 'NONE', #38892, #55608, #31618, .T. ) ;
#381=CARTESIAN_POINT ( 'NONE',  ( 13.65000000122903323, -2.886751345948193048, -4.999999999999883649 ) ) ;
#382=CARTESIAN_POINT ( 'NONE',  ( 16.80000000000000071, 4.330127018922192761, -2.499999999999997780 ) ) ;
#383=CARTESIAN_POINT ( 'NONE',  ( -4.243569643749999898, 13.95312500061451821, 30.00000000000000000 ) ) ;
#385=CARTESIAN_POINT ( 'NONE',  ( 20.88750000122903572, 6.123233995736764310E-16, -4.999999999999998224 ) ) ;
#387=CARTESIAN_POINT ( 'NONE',  ( 26.18437500061451573, 4.541064518000418104, 2.621784821874999949 ) ) ;
#388=ORIENTED_EDGE ( 'NONE', *, *, #31467, .F. ) ;
#389=CARTESIAN_POINT ( 'NONE',  ( 21.36562500061451431, -6.054752690667223547, -1.112240025338166033E-15 ) ) ;
#390=CARTESIAN_POINT ( 'NONE',  ( 21.72187500061451715, 3.027376345333611329, 5.243569643749999010 ) ) ;
#391=CARTESIAN_POINT ( 'NONE',  ( 6.787500000000001421, -2.886751345948125991, -5.000000000000000000 ) ) ;
#392=CARTESIAN_POINT ( 'NONE',  ( 8.915625000614515017, 3.027376345333613106, -5.243569643749998122 ) ) ;
#393=CARTESIAN_POINT ( 'NONE',  ( 23.46562500061451573, 3.027376345333611329, 5.243569643749999010 ) ) ;
#394=CARTESIAN_POINT ( 'NONE',  ( 12.72187500061451537, 3.027376345333611329, 5.243569643749999010 ) ) ;
#395=CARTESIAN_POINT ( 'NONE',  ( 16.80937500061451573, 0.000000000000000000, 5.243569643749999010 ) ) ;
#396=CARTESIAN_POINT ( 'NONE',  ( 19.20000000000000284, 0.000000000000000000, 4.999999999999998224 ) ) ;
#397=CARTESIAN_POINT ( 'NONE',  ( 4.243569643749999898, 17.74062500061451786, 32.45002607614398471 ) ) ;
#398=CARTESIAN_POINT ( 'NONE',  ( 21.60000000122903430, -2.886751345948129988, 4.999999999999997335 ) ) ;
#400=CARTESIAN_POINT ( 'NONE',  ( 11.16562500061451679, 3.027376345333612662, -5.243569643749998122 ) ) ;
#401=CARTESIAN_POINT ( 'NONE',  ( 4.959375000614516971, 4.541064518000418104, -2.621784821874998173 ) ) ;
#402=CARTESIAN_POINT ( 'NONE',  ( 4.059375000614519280, 4.541064518000418104, -2.621784821874998173 ) ) ;
#403=VERTEX_POINT ( 'NONE', #43241 ) ;
#404=CARTESIAN_POINT ( 'NONE',  ( 24.68437500061451573, 6.421520780324663323E-16, -5.243569643749999010 ) ) ;
#405=CARTESIAN_POINT ( 'NONE',  ( 16.15312500061451573, 4.541064518000418104, -2.621784821874998173 ) ) ;
#406=CARTESIAN_POINT ( 'NONE',  ( 27.26250000122903216, 4.330127018922192761, -2.499999999999997780 ) ) ;
#407=CARTESIAN_POINT ( 'NONE',  ( 28.60312500061451502, -4.541064518000417216, -2.621784821875001281 ) ) ;
#408=CARTESIAN_POINT ( 'NONE',  ( 21.98437500061451644, 6.421520780324663323E-16, -5.243569643749999010 ) ) ;
#409=CARTESIAN_POINT ( 'NONE',  ( 16.22812500061451857, 4.541064518000418104, 2.621784821874999949 ) ) ;
#410=CARTESIAN_POINT ( 'NONE',  ( 4.243569643749999898, 19.63437500061451857, 30.00000000000000000 ) ) ;
#411=CARTESIAN_POINT ( 'NONE',  ( 22.94062500061451715, 6.054752690667223547, 3.707466751127219781E-16 ) ) ;
#412=CARTESIAN_POINT ( 'NONE',  ( 3.825000001229032609, 2.886751345948129099, -4.999999999999998224 ) ) ;
#414=CARTESIAN_POINT ( 'NONE',  ( 28.57499999999999929, 4.330127018922191873, 2.499999999999999556 ) ) ;
#415=CARTESIAN_POINT ( 'NONE',  ( -2.000000000000000000, 13.17500000000000071, -33.46410161513775705 ) ) ;
#417=CARTESIAN_POINT ( 'NONE',  ( 29.09062500061451573, -3.027376345333610441, -5.243569643749999898 ) ) ;
#418=CARTESIAN_POINT ( 'NONE',  ( 9.253125000614517148, -4.541064518000417216, -2.621784821875001281 ) ) ;
#419=CARTESIAN_POINT ( 'NONE',  ( 21.22500000122903074, -5.773502691896255534, -1.060575238724906372E-15 ) ) ;
#420=EDGE_CURVE ( 'NONE', #14890, #16300, #13688, .T. ) ;
#421=CARTESIAN_POINT ( 'NONE',  ( 12.68437500061451573, 4.541064518000418104, 2.621784821874999949 ) ) ;
#422=CARTESIAN_POINT ( 'NONE',  ( 28.07812500061451289, -4.541064518000419881, 2.621784821874995952 ) ) ;
#423=CARTESIAN_POINT ( 'NONE',  ( 27.29999999999999716, 0.000000000000000000, 4.999999999999998224 ) ) ;
#424=CARTESIAN_POINT ( 'NONE',  ( 4.000000000000000000, 17.60000000122903785, -27.69059892324149530 ) ) ;
#425=CARTESIAN_POINT ( 'NONE',  ( -1.487416814333745711E-14, 15.72500000122903430, -26.00000000000000000 ) ) ;
#426=CARTESIAN_POINT ( 'NONE',  ( 12.10312500061451857, 4.541064518000418104, -2.621784821874998173 ) ) ;
#427=VERTEX_POINT ( 'NONE', #4808 ) ;
#428=CARTESIAN_POINT ( 'NONE',  ( 11.16562500061451679, 3.027376345333613106, -5.243569643749998122 ) ) ;
#429=CARTESIAN_POINT ( 'NONE',  ( 6.253125000614517148, 4.541064518000418104, -2.621784821874998173 ) ) ;
#433=CARTESIAN_POINT ( 'NONE',  ( 15.90000000000000036, 4.330127018922192761, -2.499999999999997780 ) ) ;
#434=CARTESIAN_POINT ( 'NONE',  ( 16.54687500061451644, -3.027376345333610441, -5.243569643749999898 ) ) ;
#435=CARTESIAN_POINT ( 'NONE',  ( 10.98750000122903536, 6.123233995736764310E-16, -4.999999999999998224 ) ) ;
#436=CARTESIAN_POINT ( 'NONE',  ( 18.79687500061451644, -3.027376345333610441, -5.243569643749999898 ) ) ;
#438=CARTESIAN_POINT ( 'NONE',  ( 19.73437500061451644, 6.421520780324663323E-16, -5.243569643749999010 ) ) ;
#439=CARTESIAN_POINT ( 'NONE',  ( -2.121784821874996840, 14.92812500061451608, -26.32496088578401583 ) ) ;
#440=CARTESIAN_POINT ( 'NONE',  ( 1.071796769724497445, 16.71740381056766367, 26.00000000000000355 ) ) ;
#443=CARTESIAN_POINT ( 'NONE',  ( 27.66562500061451146, -6.054752690667223547, -1.112240025338166033E-15 ) ) ;
#445=CARTESIAN_POINT ( 'NONE',  ( 29.14687500061451075, -3.027376345333610441, -5.243569643749999898 ) ) ;
#447=CARTESIAN_POINT ( 'NONE',  ( 25.01249999999999929, 2.886751345948126879, 4.999999999999999112 ) ) ;
#448=CARTESIAN_POINT ( 'NONE',  ( 9.478125000614515017, 4.541064518000418104, 2.621784821874999949 ) ) ;
#450=CARTESIAN_POINT ( 'NONE',  ( 19.50937500061451857, 0.000000000000000000, 5.243569643749999010 ) ) ;
#452=CARTESIAN_POINT ( 'NONE',  ( 6.440625000614517148, -3.027376345333614438, 5.243569643749998122 ) ) ;
#453=CARTESIAN_POINT ( 'NONE',  ( 11.07187500061451679, -6.054752690667223547, -1.112240025338166033E-15 ) ) ;
#455=CARTESIAN_POINT ( 'NONE',  ( 22.54687500061451999, 6.054752690667223547, 3.707466751127219781E-16 ) ) ;
#459=CARTESIAN_POINT ( 'NONE',  ( 3.862500000000001155, 2.886751345948126879, 4.999999999999999112 ) ) ;
#460=CARTESIAN_POINT ( 'NONE',  ( 14.73750000122903359, 4.330127018922191873, 2.499999999999999556 ) ) ;
#462=LINE ( 'NONE', #60676, #9126 ) ;
#463=ORIENTED_EDGE ( 'NONE', *, *, #9642, .F. ) ;
#464=CARTESIAN_POINT ( 'NONE',  ( 13.23750000000000071, 5.773502691896255534, 3.535250795749688894E-16 ) ) ;
#466=CARTESIAN_POINT ( 'NONE',  ( 25.15312500061451217, 4.541064518000418104, -2.621784821874998173 ) ) ;
#467=CARTESIAN_POINT ( 'NONE',  ( 14.62500000000000000, 4.330127018922191873, 2.499999999999999556 ) ) ;
#468=CARTESIAN_POINT ( 'NONE',  ( 11.25000000122903288, -2.886751345948129988, 4.999999999999997335 ) ) ;
#469=CARTESIAN_POINT ( 'NONE',  ( 10.00312500061451715, 0.000000000000000000, 5.243569643749999010 ) ) ;
#470=CARTESIAN_POINT ( 'NONE',  ( 9.825000000000001066, -4.330127018922194537, 2.499999999999995559 ) ) ;
#471=CARTESIAN_POINT ( 'NONE',  ( 4.898734551532200499, 1.001199177798645534, 4.898734551532191617 ) ) ;
#472=CARTESIAN_POINT ( 'NONE',  ( 26.81250000122903288, 4.330127018922192761, -2.499999999999997780 ) ) ;
#474=CARTESIAN_POINT ( 'NONE',  ( 8.362500000000002487, 2.886751345948126879, 4.999999999999999112 ) ) ;
#476=ORIENTED_EDGE ( 'NONE', *, *, #37237, .F. ) ;
#477=CARTESIAN_POINT ( 'NONE',  ( 22.90312500061451573, 4.541064518000418104, -2.621784821874998173 ) ) ;
#478=CARTESIAN_POINT ( 'NONE',  ( 28.37812500061451715, 4.541064518000418104, 2.621784821874999949 ) ) ;
#479=CARTESIAN_POINT ( 'NONE',  ( 4.898587196589411843E-16, 20.00000000000000000, -26.00000000000000000 ) ) ;
#480=CARTESIAN_POINT ( 'NONE',  ( 19.05937500061451928, 0.000000000000000000, 5.243569643749999010 ) ) ;
#481=CARTESIAN_POINT ( 'NONE',  ( 17.65312500061451573, 0.000000000000000000, 5.243569643749999010 ) ) ;
#482=CARTESIAN_POINT ( 'NONE',  ( 4.243569643749999898, 11.47812500061459318, -30.00000000000000000 ) ) ;
#483=CARTESIAN_POINT ( 'NONE',  ( 6.328125000614515550, 4.541064518000418104, 2.621784821874999949 ) ) ;
#484=CARTESIAN_POINT ( 'NONE',  ( 29.21250000122903145, 0.000000000000000000, 4.999999999999998224 ) ) ;
#486=CARTESIAN_POINT ( 'NONE',  ( 18.17812500061451786, -4.541064518000419881, 2.621784821874995952 ) ) ;
#487=CARTESIAN_POINT ( 'NONE',  ( 1.999999999999998668, 11.41250000122903430, -33.46410161513775705 ) ) ;
#488=CARTESIAN_POINT ( 'NONE',  ( 3.375000001229033320, 2.886751345948129099, -4.999999999999998224 ) ) ;
#490=CARTESIAN_POINT ( 'NONE',  ( 13.13437500061451857, 4.541064518000418104, 2.621784821874999949 ) ) ;
#491=CARTESIAN_POINT ( 'NONE',  ( 12.68437500061451573, 4.541064518000418104, 2.621784821874999949 ) ) ;
#492=CARTESIAN_POINT ( 'NONE',  ( 20.67187500061451289, 3.027376345333613106, -5.243569643749998122 ) ) ;
#493=VERTEX_POINT ( 'NONE', #59846 ) ;
#494=CARTESIAN_POINT ( 'NONE',  ( -0.8062380997993553455, 9.975217491784283297, 24.04105076033751942 ) ) ;
#495=CARTESIAN_POINT ( 'NONE',  ( 23.91562500061451502, 3.027376345333611329, 5.243569643749999010 ) ) ;
#496=CARTESIAN_POINT ( 'NONE',  ( 18.00937500061451502, 4.541064518000418104, -2.621784821874998173 ) ) ;
#497=CARTESIAN_POINT ( 'NONE',  ( 25.30312500061451431, 0.000000000000000000, 5.243569643749999010 ) ) ;
#499=CARTESIAN_POINT ( 'NONE',  ( -3.999999999999999112, 15.94999999999999929, 30.00000000000000000 ) ) ;
#500=CARTESIAN_POINT ( 'NONE',  ( 3.871875000614519280, -6.054752690667223547, -1.112240025338166033E-15 ) ) ;
#502=CARTESIAN_POINT ( 'NONE',  ( 10.95000000122903394, -2.886751345948125991, -5.000000000000000000 ) ) ;
#503=CARTESIAN_POINT ( 'NONE',  ( 7.612500001229035362, 0.000000000000000000, 4.999999999999998224 ) ) ;
#504=CARTESIAN_POINT ( 'NONE',  ( 10.20000000000000107, 0.000000000000000000, 4.999999999999998224 ) ) ;
#505=CARTESIAN_POINT ( 'NONE',  ( 27.56250000122902932, -4.330127018922190985, -2.500000000000001332 ) ) ;
#508=CARTESIAN_POINT ( 'NONE',  ( 9.009375000614518569, 4.541064518000418104, -2.621784821874998173 ) ) ;
#510=CARTESIAN_POINT ( 'NONE',  ( 16.37812500061451715, -4.541064518000419881, 2.621784821874995952 ) ) ;
#511=CARTESIAN_POINT ( 'NONE',  ( 12.57187500061451857, 3.027376345333613106, -5.243569643749998122 ) ) ;
#512=CARTESIAN_POINT ( 'NONE',  ( 5.765625000614519102, 3.027376345333613106, -5.243569643749998122 ) ) ;
#513=CARTESIAN_POINT ( 'NONE',  ( 20.25937500061451857, 4.541064518000418104, -2.621784821874998173 ) ) ;
#514=CARTESIAN_POINT ( 'NONE',  ( 10.65937500061451715, -4.541064518000417216, -2.621784821875001281 ) ) ;
#515=CARTESIAN_POINT ( 'NONE',  ( 2.990625000614519191, -3.027376345333610441, -5.243569643749999898 ) ) ;
#516=CARTESIAN_POINT ( 'NONE',  ( 7.320879633048903241E-15, 17.63749999999999218, 26.00000000000000355 ) ) ;
#517=CARTESIAN_POINT ( 'NONE',  ( 6.300000001229033586, -2.886751345948129988, 4.999999999999997335 ) ) ;
#518=CARTESIAN_POINT ( 'NONE',  ( 21.14062500061451289, 6.054752690667223547, 3.707466751127219781E-16 ) ) ;
#520=CARTESIAN_POINT ( 'NONE',  ( 5.475000001229035185, -5.773502691896255534, -1.060575238724906372E-15 ) ) ;
#521=CARTESIAN_POINT ( 'NONE',  ( 18.32812500061451644, 6.421520780324663323E-16, -5.243569643749999010 ) ) ;
#522=CARTESIAN_POINT ( 'NONE',  ( 13.64062500061451644, -3.027376345333614438, 5.243569643749998122 ) ) ;
#524=CARTESIAN_POINT ( 'NONE',  ( 13.01249999999999929, -5.773502691896255534, -1.060575238724906372E-15 ) ) ;
#525=CARTESIAN_POINT ( 'NONE',  ( 9.750000001229032875, 5.773502691896255534, 3.535250795749688894E-16 ) ) ;
#526=CARTESIAN_POINT ( 'NONE',  ( 6.478125000614516793, -4.541064518000419881, 2.621784821874995952 ) ) ;
#527=CARTESIAN_POINT ( 'NONE',  ( 19.61250000122903359, 4.330127018922192761, -2.499999999999997780 ) ) ;
#529=CARTESIAN_POINT ( 'NONE',  ( -2.121784821874996840, 11.83437500061451786, -26.32496088578401583 ) ) ;
#530=CARTESIAN_POINT ( 'NONE',  ( 4.955651476953736534, 0.6855146069033769551, 5.046959488524436210 ) ) ;
#531=EDGE_CURVE ( 'NONE', #11388, #40707, #27615, .T. ) ;
#532=DIRECTION ( 'NONE',  ( 0.000000000000000000, 0.000000000000000000, 1.000000000000000000 ) ) ;
#533=( BOUNDED_CURVE ( )  B_SPLINE_CURVE ( 2, ( #30429, #71415, #70675, #37054, #15610, #8992, #71046, #4191, #26346 ),
 .UNSPECIFIED., .F., .F. ) 
 B_SPLINE_CURVE_WITH_KNOTS ( ( 3, 2, 2, 2, 3 ),
 ( 0.1630434782608695676, 0.1666666666666666574, 0.1739130434782608647, 0.1811594202898550721, 0.1847826086956521896 ),
 .UNSPECIFIED. ) 
 CURVE ( )  GEOMETRIC_REPRESENTATION_ITEM ( )  RATIONAL_B_SPLINE_CURVE ( ( 0.9330127018922194093, 0.9330127018922196314, 1.000000000000000000, 0.8660254037844387076, 1.000000000000000000, 0.8660254037844387076, 1.000000000000000000, 0.9330127018922190762, 0.9330127018922194093 ) ) 
 REPRESENTATION_ITEM ( '' )  );
#535=CARTESIAN_POINT ( 'NONE',  ( 21.19687500061451502, 6.054752690667223547, 3.707466751127219781E-16 ) ) ;
#536=CARTESIAN_POINT ( 'NONE',  ( -1.487416814333745711E-14, 16.62500000122903288, 34.00000000000000000 ) ) ;
#537=CARTESIAN_POINT ( 'NONE',  ( 15.70312500061451644, 4.541064518000418104, -2.621784821874998173 ) ) ;
#539=CARTESIAN_POINT ( 'NONE',  ( 23.02499999999999858, 6.123233995736764310E-16, -4.999999999999998224 ) ) ;
#540=CARTESIAN_POINT ( 'NONE',  ( 28.50937500061451502, 0.000000000000000000, 5.243569643749999010 ) ) ;
#541=CARTESIAN_POINT ( 'NONE',  ( 26.59687500061451360, 6.054752690667223547, 3.707466751127219781E-16 ) ) ;
#543=VECTOR ( 'NONE', #40593, 1000.000000000000000 ) ;
#544=CARTESIAN_POINT ( 'NONE',  ( 11.50312500061451892, -4.541064518000417216, -2.621784821875001281 ) ) ;
#545=CARTESIAN_POINT ( 'NONE',  ( 10.95937500061451964, 0.000000000000000000, 5.243569643749999010 ) ) ;
#546=EDGE_LOOP ( 'NONE', ( #30188, #59828, #46939, #45480 ) ) ;
#547=CARTESIAN_POINT ( 'NONE',  ( -1.071796769724488563, 14.24240381056766758, -26.00000000000000000 ) ) ;
#548=CARTESIAN_POINT ( 'NONE',  ( 20.50312500061451715, -4.541064518000417216, -2.621784821875001281 ) ) ;
#550=CARTESIAN_POINT ( 'NONE',  ( 20.96250000000000213, 2.886751345948161074, 4.999999999999941380 ) ) ;
#551=ADVANCED_FACE ( 'NONE', ( #32513 ), #31786, .F. ) ;
#552=CARTESIAN_POINT ( 'NONE',  ( 9.074999999999999289, 6.123233995736764310E-16, -4.999999999999998224 ) ) ;
#553=CARTESIAN_POINT ( 'NONE',  ( 22.20000000122903216, -2.886751345948125991, -5.000000000000000000 ) ) ;
#554=CARTESIAN_POINT ( 'NONE',  ( 16.04062500061451857, -3.027376345333610441, -5.243569643749999898 ) ) ;
#556=ORIENTED_EDGE ( 'NONE', *, *, #3876, .T. ) ;
#557=CARTESIAN_POINT ( 'NONE',  ( 19.57500000000000284, 4.330127018922191873, 2.499999999999999556 ) ) ;
#558=CARTESIAN_POINT ( 'NONE',  ( 22.19999999999999574, 4.330127018922192761, -2.499999999999997780 ) ) ;
#559=CARTESIAN_POINT ( 'NONE',  ( 21.53437500061451715, 6.421520780324663323E-16, -5.243569643749999010 ) ) ;
#560=CARTESIAN_POINT ( 'NONE',  ( 26.16562500061451502, 3.027376345333611329, 5.243569643749999010 ) ) ;
#561=EDGE_CURVE ( 'NONE', #45352, #72689, #39182, .T. ) ;
#562=( BOUNDED_CURVE ( )  B_SPLINE_CURVE ( 2, ( #23170, #34989, #67892, #57518, #62340, #11736, #40181 ),
 .UNSPECIFIED., .F., .F. ) 
 B_SPLINE_CURVE_WITH_KNOTS ( ( 3, 2, 2, 3 ),
 ( 0.1750000000000000167, 0.1777777777777778123, 0.1805555555555555525, 0.1833333333333333204 ),
 .UNSPECIFIED. ) 
 CURVE ( )  GEOMETRIC_REPRESENTATION_ITEM ( )  RATIONAL_B_SPLINE_CURVE ( ( 0.9999999999999986677, 0.8660254037844400399, 1.000000000000000000, 0.8660254037844387076, 1.000000000000000000, 0.8660254037844387076, 1.000000000000000000 ) ) 
 REPRESENTATION_ITEM ( '' )  );
#563=VECTOR ( 'NONE', #40809, 1000.000000000000000 ) ;
#564=ORIENTED_EDGE ( 'NONE', *, *, #40344, .T. ) ;
#565=CARTESIAN_POINT ( 'NONE',  ( 27.97500000122903074, -5.773502691896255534, -1.060575238724906372E-15 ) ) ;
#566=CARTESIAN_POINT ( 'NONE',  ( 7.340625000614518392, -3.027376345333614438, 5.243569643749998122 ) ) ;
#567=CARTESIAN_POINT ( 'NONE',  ( 1.071796769724489895, 12.21740381056766900, 26.00000000000000355 ) ) ;
#568=CARTESIAN_POINT ( 'NONE',  ( 14.73749999999999893, -2.886751345948129988, 4.999999999999997335 ) ) ;
#569=CARTESIAN_POINT ( 'NONE',  ( -2.121784821874999949, 18.37812500061451715, 26.32496088578401938 ) ) ;
#570=CARTESIAN_POINT ( 'NONE',  ( 28.34062500061451928, 6.054752690667223547, 3.707466751127219781E-16 ) ) ;
#571=VECTOR ( 'NONE', #21775, 1000.000000000000000 ) ;
#572=CARTESIAN_POINT ( 'NONE',  ( 27.08437500061451786, 4.541064518000418104, 2.621784821874999949 ) ) ;
#574=CARTESIAN_POINT ( 'NONE',  ( 24.77812500061451217, 4.541064518000418104, 2.621784821874999949 ) ) ;
#575=CARTESIAN_POINT ( 'NONE',  ( 25.17187500061451644, 3.027376345333613106, -5.243569643749998122 ) ) ;
#576=CARTESIAN_POINT ( 'NONE',  ( -4.243569643749999898, 19.31562500061459176, -32.45002607614398471 ) ) ;
#577=CARTESIAN_POINT ( 'NONE',  ( 11.47499999999999964, 4.330127018922191873, 2.499999999999999556 ) ) ;
#578=CARTESIAN_POINT ( 'NONE',  ( 9.740625000614516082, -3.027376345333610441, -5.243569643749999898 ) ) ;
#580=CARTESIAN_POINT ( 'NONE',  ( 29.01562500061451644, -6.054752690667223547, -1.112240025338166033E-15 ) ) ;
#581=CARTESIAN_POINT ( 'NONE',  ( 26.95312500061451644, 4.541064518000418104, -2.621784821874998173 ) ) ;
#582=CARTESIAN_POINT ( 'NONE',  ( 7.320879633048903241E-15, 18.08749999999999858, 26.00000000000000355 ) ) ;
#584=CARTESIAN_POINT ( 'NONE',  ( 18.42187500061451644, 3.027376345333613106, -5.243569643749998122 ) ) ;
#585=CARTESIAN_POINT ( 'NONE',  ( -4.243569643749999898, 13.52187500061451786, 27.54997392385601529 ) ) ;
#586=CARTESIAN_POINT ( 'NONE',  ( 20.18437500061451573, 6.421520780324663323E-16, -5.243569643749999010 ) ) ;
#587=CARTESIAN_POINT ( 'NONE',  ( 27.98437500061451289, 4.541064518000418104, 2.621784821874999949 ) ) ;
#588=CARTESIAN_POINT ( 'NONE',  ( 2.121784821874999061, 17.00937500061451857, 26.32496088578401583 ) ) ;
#589=CARTESIAN_POINT ( 'NONE',  ( 10.97812500061451679, -4.541064518000419881, 2.621784821874995952 ) ) ;
#590=FACE_OUTER_BOUND ( 'NONE', #71381, .T. ) ;
#591=CARTESIAN_POINT ( 'NONE',  ( 4.096875000614518925, 6.054752690667223547, 3.707466751127219781E-16 ) ) ;
#592=CARTESIAN_POINT ( 'NONE',  ( -1.999999999999997113, 16.13750000122903216, -26.53589838486224295 ) ) ;
#594=CARTESIAN_POINT ( 'NONE',  ( 7.828125000614517326, -4.541064518000419881, 2.621784821874995952 ) ) ;
#595=CARTESIAN_POINT ( 'NONE',  ( 11.67187500061451821, 3.027376345333613106, -5.243569643749998122 ) ) ;
#596=CARTESIAN_POINT ( 'NONE',  ( 19.35000000122903430, -2.886751345948129988, 4.999999999999997335 ) ) ;
#597=CARTESIAN_POINT ( 'NONE',  ( 4.809375000614516615, -4.541064518000417216, -2.621784821875001281 ) ) ;
#598=CARTESIAN_POINT ( 'NONE',  ( 7.903125000614515727, -4.541064518000417216, -2.621784821875001281 ) ) ;
#599=CARTESIAN_POINT ( 'NONE',  ( 5.765625000614519102, 3.027376345333612662, -5.243569643749998122 ) ) ;
#601=CARTESIAN_POINT ( 'NONE',  ( 17.93437500061451928, 6.421520780324663323E-16, -5.243569643749999010 ) ) ;
#602=ORIENTED_EDGE ( 'NONE', *, *, #7167, .F. ) ;
#603=CARTESIAN_POINT ( 'NONE',  ( 24.36562500061451786, 3.027376345333611329, 5.243569643749999010 ) ) ;
#604=CARTESIAN_POINT ( 'NONE',  ( 12.92812500061451786, 6.421520780324663323E-16, -5.243569643749999010 ) ) ;
#605=CARTESIAN_POINT ( 'NONE',  ( 26.84999999999999787, 0.000000000000000000, 4.999999999999998224 ) ) ;
#606=CARTESIAN_POINT ( 'NONE',  ( 11.76562500061451644, 3.027376345333611329, 5.243569643749999010 ) ) ;
#608=CARTESIAN_POINT ( 'NONE',  ( 11.73750000122903181, -4.330127018922194537, 2.499999999999995559 ) ) ;
#609=CARTESIAN_POINT ( 'NONE',  ( 26.80312500061451431, -4.541064518000417216, -2.621784821875001281 ) ) ;
#610=CARTESIAN_POINT ( 'NONE',  ( -3.000416591977282496E-16, 12.94062500061451537, -34.90005215228797653 ) ) ;
#611=CARTESIAN_POINT ( 'NONE',  ( 14.88750000122903394, -4.330127018922194537, 2.499999999999995559 ) ) ;
#612=CARTESIAN_POINT ( 'NONE',  ( 11.47499999999999964, 4.330127018922191873, 2.499999999999999556 ) ) ;
#613=CARTESIAN_POINT ( 'NONE',  ( 19.56562500061451715, -6.054752690667223547, -1.112240025338166033E-15 ) ) ;
#614=CARTESIAN_POINT ( 'NONE',  ( 7.921875000614517326, -6.054752690667223547, -1.112240025338166033E-15 ) ) ;
#615=CARTESIAN_POINT ( 'NONE',  ( 6.900000001229035007, -2.886751345948125991, -5.000000000000000000 ) ) ;
#616=CARTESIAN_POINT ( 'NONE',  ( 16.01250000122903216, 4.330127018922192761, -2.499999999999997780 ) ) ;
#618=CARTESIAN_POINT ( 'NONE',  ( 13.22812500061451502, -4.541064518000419881, 2.621784821874995952 ) ) ;
#619=CARTESIAN_POINT ( 'NONE',  ( 16.71562500061451573, 3.027376345333611329, 5.243569643749999010 ) ) ;
#621=CARTESIAN_POINT ( 'NONE',  ( 26.55000000122902648, -2.886751345948129988, 4.999999999999997335 ) ) ;
#622=CARTESIAN_POINT ( 'NONE',  ( 20.96250000000000213, 2.886751345948126879, 4.999999999999999112 ) ) ;
#623=AXIS2_PLACEMENT_3D ( 'NONE', #29778, #52314, #7249 ) ;
#624=CARTESIAN_POINT ( 'NONE',  ( 22.39687500061451075, -3.027376345333610441, -5.243569643749999898 ) ) ;
#626=CARTESIAN_POINT ( 'NONE',  ( 10.80000000122903536, -2.886751345948129988, 4.999999999999997335 ) ) ;
#627=CARTESIAN_POINT ( 'NONE',  ( 8.746875000614515727, -3.027376345333614438, 5.243569643749998122 ) ) ;
#628=CARTESIAN_POINT ( 'NONE',  ( 27.38437500061451857, 6.421520780324663323E-16, -5.243569643749999010 ) ) ;
#630=CARTESIAN_POINT ( 'NONE',  ( 23.54062500061451146, -3.027376345333614438, 5.243569643749998122 ) ) ;
#632=CARTESIAN_POINT ( 'NONE',  ( 4.000000000000000000, 19.73749999999999716, -27.69059892324149885 ) ) ;
#633=CARTESIAN_POINT ( 'NONE',  ( 8.334375000614516082, -4.541064518000419881, 2.621784821874995952 ) ) ;
#634=CARTESIAN_POINT ( 'NONE',  ( 1.626862140677534273E-15, 12.46250000000000213, 34.00000000000000000 ) ) ;
#635=CARTESIAN_POINT ( 'NONE',  ( 27.62812500061451360, -4.541064518000419881, 2.621784821874995952 ) ) ;
#636=CARTESIAN_POINT ( 'NONE',  ( 6.759375000614516793, 4.541064518000418104, -2.621784821874998173 ) ) ;
#637=CARTESIAN_POINT ( 'NONE',  ( 6.787500000000001421, -2.886751345948126435, -5.000000000000000000 ) ) ;
#638=CARTESIAN_POINT ( 'NONE',  ( 25.77187500061451075, 3.027376345333611329, 5.243569643749999010 ) ) ;
#639=CARTESIAN_POINT ( 'NONE',  ( 18.89999999999999858, -4.330127018922190985, -2.500000000000001332 ) ) ;
#640=EDGE_LOOP ( 'NONE', ( #68001, #59297, #35506, #56728 ) ) ;
#641=CARTESIAN_POINT ( 'NONE',  ( 27.67499999999999716, 4.330127018922191873, 2.499999999999999556 ) ) ;
#642=CARTESIAN_POINT ( 'NONE',  ( 28.54687500061451644, -3.027376345333614438, 5.243569643749998122 ) ) ;
#643=EDGE_CURVE ( 'NONE', #26767, #59300, #38760, .T. ) ;
#644=ORIENTED_EDGE ( 'NONE', *, *, #29319, .T. ) ;
#645=CARTESIAN_POINT ( 'NONE',  ( 14.46562500061451750, 3.027376345333611329, 5.243569643749999010 ) ) ;
#646=CARTESIAN_POINT ( 'NONE',  ( 8.278125000614515727, -4.541064518000419881, 2.621784821874995952 ) ) ;
#648=CARTESIAN_POINT ( 'NONE',  ( 4.246875000614519280, -3.027376345333614438, 5.243569643749998122 ) ) ;
#649=CARTESIAN_POINT ( 'NONE',  ( 18.15000000122903501, -2.886751345948125991, -5.000000000000000000 ) ) ;
#650=CARTESIAN_POINT ( 'NONE',  ( 21.75000000000000000, 4.330127018922192761, -2.499999999999997780 ) ) ;
#651=CARTESIAN_POINT ( 'NONE',  ( 29.21249999999999858, -5.773502691896255534, -1.060575238724906372E-15 ) ) ;
#652=CARTESIAN_POINT ( 'NONE',  ( 5.821875000614519458, 3.027376345333613106, -5.243569643749998122 ) ) ;
#653=CARTESIAN_POINT ( 'NONE',  ( 11.93437500061451573, -4.541064518000419881, 2.621784821874995952 ) ) ;
#654=CARTESIAN_POINT ( 'NONE',  ( 22.17187500061451644, 3.027376345333611329, 5.243569643749999010 ) ) ;
#655=CARTESIAN_POINT ( 'NONE',  ( -2.000000000000000000, 17.22500000000000142, -33.46410161513775705 ) ) ;
#656=ORIENTED_EDGE ( 'NONE', *, *, #40314, .T. ) ;
#657=CARTESIAN_POINT ( 'NONE',  ( 4.996875000614516615, 6.054752690667223547, 3.707466751127219781E-16 ) ) ;
#658=CARTESIAN_POINT ( 'NONE',  ( 7.021875000614518747, -6.054752690667223547, -1.112240025338166033E-15 ) ) ;
#659=CARTESIAN_POINT ( 'NONE',  ( 18.67500000000000071, 4.330127018922191873, 2.499999999999999556 ) ) ;
#660=CARTESIAN_POINT ( 'NONE',  ( 16.90312500061451573, -4.541064518000417216, -2.621784821875001281 ) ) ;
#664=CARTESIAN_POINT ( 'NONE',  ( 9.815625000614518925, 3.027376345333613106, -5.243569643749998122 ) ) ;
#665=CARTESIAN_POINT ( 'NONE',  ( 27.15937500061451360, 0.000000000000000000, 5.243569643749999010 ) ) ;
#666=CARTESIAN_POINT ( 'NONE',  ( 6.262500001229034829, 0.000000000000000000, 4.999999999999998224 ) ) ;
#667=CARTESIAN_POINT ( 'NONE',  ( 25.62187500061451573, 3.027376345333613106, -5.243569643749998122 ) ) ;
#668=CARTESIAN_POINT ( 'NONE',  ( 9.674999999999998934, 4.330127018922191873, 2.499999999999999556 ) ) ;
#669=CARTESIAN_POINT ( 'NONE',  ( 2.000000000000001332, 13.51250000122903394, 33.46410161513774995 ) ) ;
#670=CARTESIAN_POINT ( 'NONE',  ( 9.412500001229034297, 0.000000000000000000, 4.999999999999998224 ) ) ;
#672=CARTESIAN_POINT ( 'NONE',  ( 20.59687500061451360, -3.027376345333610441, -5.243569643749999898 ) ) ;
#673=CARTESIAN_POINT ( 'NONE',  ( 11.33437500061451608, 4.541064518000418104, 2.621784821874999949 ) ) ;
#674=CARTESIAN_POINT ( 'NONE',  ( -1.090676731616017747, 4.887066358488519668, -33.85805426562694720 ) ) ;
#676=CARTESIAN_POINT ( 'NONE',  ( 15.96562500061451573, -6.054752690667223547, -1.112240025338166033E-15 ) ) ;
#678=CARTESIAN_POINT ( 'NONE',  ( 25.80000000122903714, -2.886751345948125991, -5.000000000000000000 ) ) ;
#679=CARTESIAN_POINT ( 'NONE',  ( 12.49687500061451573, -3.027376345333610441, -5.243569643749999898 ) ) ;
#680=CARTESIAN_POINT ( 'NONE',  ( 17.16562500061451502, 3.027376345333611329, 5.243569643749999010 ) ) ;
#681=CYLINDRICAL_SURFACE ( 'NONE', #16177, 4.999999999999998224 ) ;
#682=CARTESIAN_POINT ( 'NONE',  ( 27.00937500061451857, 4.541064518000418104, -2.621784821874998173 ) ) ;
#683=CARTESIAN_POINT ( 'NONE',  ( -2.121784821874996840, 11.32812500061451644, 33.67503911421598417 ) ) ;
#684=CARTESIAN_POINT ( 'NONE',  ( 12.22500000122903430, -5.773502691896255534, -1.060575238724906372E-15 ) ) ;
#685=LINE ( 'NONE', #56105, #8000 ) ;
#686=CARTESIAN_POINT ( 'NONE',  ( -3.000416591977282496E-16, 17.49687500061451573, -34.90005215228797653 ) ) ;
#687=CARTESIAN_POINT ( 'NONE',  ( 17.33437500061451431, -4.541064518000419881, 2.621784821874995952 ) ) ;
#688=CARTESIAN_POINT ( 'NONE',  ( 20.88750000122903572, 6.123233995736764310E-16, -4.999999999999998224 ) ) ;
#689=CARTESIAN_POINT ( 'NONE',  ( 14.59687500061452070, -3.027376345333614438, 5.243569643749998122 ) ) ;
#690=CARTESIAN_POINT ( 'NONE',  ( -4.243569643749999898, 19.76562500061451644, -32.45002607614398471 ) ) ;
#691=CARTESIAN_POINT ( 'NONE',  ( 23.55000000122903359, -2.886751345948125991, -5.000000000000000000 ) ) ;
#692=CARTESIAN_POINT ( 'NONE',  ( 15.02812500061451750, -4.541064518000419881, 2.621784821874995952 ) ) ;
#693=DIRECTION ( 'NONE',  ( -0.000000000000000000, -1.000000000000000000, -0.000000000000000000 ) ) ;
#694=ORIENTED_EDGE ( 'NONE', *, *, #60253, .T. ) ;
#695=ORIENTED_EDGE ( 'NONE', *, *, #13854, .T. ) ;
#696=CARTESIAN_POINT ( 'NONE',  ( 20.62499999999999645, -4.330127018922194537, 2.499999999999995559 ) ) ;
#698=CARTESIAN_POINT ( 'NONE',  ( 2.915625000614516793, -6.054752690667223547, -1.112240025338166033E-15 ) ) ;
#699=CARTESIAN_POINT ( 'NONE',  ( 15.11250000122903359, 4.330127018922192761, -2.499999999999997780 ) ) ;
#700=CARTESIAN_POINT ( 'NONE',  ( 21.21562500061451573, 3.027376345333611329, 5.243569643749999010 ) ) ;
#701=CARTESIAN_POINT ( 'NONE',  ( 23.91562500061451502, 3.027376345333611329, 5.243569643749999010 ) ) ;
#702=CARTESIAN_POINT ( 'NONE',  ( 29.36250000122903003, -4.330127018922190985, -2.500000000000001332 ) ) ;
#703=EDGE_CURVE ( 'NONE', #27416, #27910, #5889, .T. ) ;
#704=CARTESIAN_POINT ( 'NONE',  ( 28.80000000000000071, -4.330127018922190985, -2.500000000000001332 ) ) ;
#705=CARTESIAN_POINT ( 'NONE',  ( 4.621347029917726168, 1.908772861692954237, 4.883837314020292197 ) ) ;
#708=CARTESIAN_POINT ( 'NONE',  ( 29.59687500061451715, -3.027376345333610441, -5.243569643749999898 ) ) ;
#709=B_SPLINE_CURVE_WITH_KNOTS ( 'NONE', 3,
 ( #61858, #17153, #39711, #5719, #62940, #22338, #17864, #44890, #62229, #23420 ),
 .UNSPECIFIED., .F., .F.,
 ( 4, 3, 3, 4 ),
 ( 1.810050118334583309E-16, 0.0001572268011904103229, 0.0003144534009725573147, 0.0005711762704777365160 ),
 .UNSPECIFIED. ) ;
#710=CARTESIAN_POINT ( 'NONE',  ( -1.999999999999997113, 11.18750000122903288, -26.53589838486224295 ) ) ;
#711=CARTESIAN_POINT ( 'NONE',  ( 2.121784821875001281, 19.55937500061451573, -26.32496088578401938 ) ) ;
#712=CARTESIAN_POINT ( 'NONE',  ( 5.850000001229035185, -2.886751345948129988, 4.999999999999997335 ) ) ;
#713=CARTESIAN_POINT ( 'NONE',  ( 7.537500000000002309, -2.886751345948129988, 4.999999999999997335 ) ) ;
#714=( BOUNDED_CURVE ( )  B_SPLINE_CURVE ( 2, ( #55045, #54322, #32143, #43600, #3352, #48777, #59843, #48414, #25874 ),
 .UNSPECIFIED., .F., .F. ) 
 B_SPLINE_CURVE_WITH_KNOTS ( ( 3, 2, 2, 2, 3 ),
 ( 0.1413043478260869734, 0.1449275362318840632, 0.1521739130434782705, 0.1594202898550724501, 0.1630434782608695676 ),
 .UNSPECIFIED. ) 
 CURVE ( )  GEOMETRIC_REPRESENTATION_ITEM ( )  RATIONAL_B_SPLINE_CURVE ( ( 0.9330127018922194093, 0.9330127018922196314, 1.000000000000000000, 0.8660254037844387076, 1.000000000000000000, 0.8660254037844387076, 1.000000000000000000, 0.9330127018922190762, 0.9330127018922194093 ) ) 
 REPRESENTATION_ITEM ( '' )  );
#715=CARTESIAN_POINT ( 'NONE',  ( 3.900000001229034563, 5.773502691896255534, 3.535250795749688894E-16 ) ) ;
#716=CARTESIAN_POINT ( 'NONE',  ( 12.53437500061451537, 6.421520780324663323E-16, -5.243569643749999010 ) ) ;
#717=CARTESIAN_POINT ( 'NONE',  ( 24.71250000122903145, 0.000000000000000000, 4.999999999999998224 ) ) ;
#718=CARTESIAN_POINT ( 'NONE',  ( 3.871875000614519280, -6.054752690667223547, -1.112240025338166033E-15 ) ) ;
#720=CARTESIAN_POINT ( 'NONE',  ( 29.47500000122903430, 2.886751345948139313, -4.999999999999980460 ) ) ;
#722=CARTESIAN_POINT ( 'NONE',  ( 11.14687500061451608, -3.027376345333610441, -5.243569643749999898 ) ) ;
#723=CARTESIAN_POINT ( 'NONE',  ( 14.40937500061451715, 4.541064518000418104, -2.621784821874998173 ) ) ;
#725=CARTESIAN_POINT ( 'NONE',  ( 6.899999999999999467, 4.330127018922192761, -2.499999999999997780 ) ) ;
#726=CARTESIAN_POINT ( 'NONE',  ( 4.243569643749999898, 17.29062500061459318, 32.45002607614398471 ) ) ;
#727=CARTESIAN_POINT ( 'NONE',  ( 20.63437500061451857, 6.421520780324663323E-16, -5.243569643749999010 ) ) ;
#728=CARTESIAN_POINT ( 'NONE',  ( 26.73750000122903003, 6.123233995736764310E-16, -4.999999999999998224 ) ) ;
#730=CARTESIAN_POINT ( 'NONE',  ( 22.97812500061451857, 4.541064518000418104, 2.621784821874999949 ) ) ;
#731=CARTESIAN_POINT ( 'NONE',  ( 14.87812500061451537, 4.541064518000418104, 2.621784821874999949 ) ) ;
#733=CARTESIAN_POINT ( 'NONE',  ( 12.60937500061451821, 4.541064518000418104, -2.621784821874998173 ) ) ;
#734=CARTESIAN_POINT ( 'NONE',  ( 29.39999999999999858, 4.330127018922192761, -2.499999999999997780 ) ) ;
#735=CARTESIAN_POINT ( 'NONE',  ( 25.42500000122903359, 2.886751345948129099, -4.999999999999998224 ) ) ;
#737=CARTESIAN_POINT ( 'NONE',  ( 10.84687500061451892, 6.054752690667223547, 3.707466751127219781E-16 ) ) ;
#738=CARTESIAN_POINT ( 'NONE',  ( 29.67187500061451644, 3.027376345333613106, -5.243569643749998122 ) ) ;
#739=CARTESIAN_POINT ( 'NONE',  ( 3.046875000614519990, -3.027376345333610441, -5.243569643749999898 ) ) ;
#740=DIRECTION ( 'NONE',  ( -1.000000000000000000, -0.000000000000000000, -0.000000000000000000 ) ) ;
#741=CARTESIAN_POINT ( 'NONE',  ( 21.68437500061451573, 4.541064518000418104, 2.621784821874999949 ) ) ;
#742=CARTESIAN_POINT ( 'NONE',  ( 15.38437500061451679, 4.541064518000418104, 2.621784821874999949 ) ) ;
#744=CARTESIAN_POINT ( 'NONE',  ( 25.87500000000000000, 4.330127018922191873, 2.499999999999999556 ) ) ;
#745=CARTESIAN_POINT ( 'NONE',  ( 4.575000001229033941, -5.773502691896255534, -1.060575238724906372E-15 ) ) ;
#747=CARTESIAN_POINT ( 'NONE',  ( 17.09062500061451573, 6.054752690667223547, 3.707466751127219781E-16 ) ) ;
#748=CARTESIAN_POINT ( 'NONE',  ( 5.887500000000000178, -2.886751345948125991, -5.000000000000000000 ) ) ;
#749=CARTESIAN_POINT ( 'NONE',  ( 1.999999999999998668, 13.66250000122903607, 26.53589838486224650 ) ) ;
#750=CARTESIAN_POINT ( 'NONE',  ( 16.16250000000000142, -5.773502691896255534, -1.060575238724906372E-15 ) ) ;
#751=CARTESIAN_POINT ( 'NONE',  ( 2.121784821875001281, 12.30312500061451608, 33.67503911421598417 ) ) ;
#753=CARTESIAN_POINT ( 'NONE',  ( 26.10937500061451644, 4.541064518000418104, -2.621784821874998173 ) ) ;
#755=VERTEX_POINT ( 'NONE', #11435 ) ;
#756=CARTESIAN_POINT ( 'NONE',  ( 23.09062500061451573, -3.027376345333614438, 5.243569643749998122 ) ) ;
#757=CARTESIAN_POINT ( 'NONE',  ( 21.94687500061451857, -3.027376345333610441, -5.243569643749999898 ) ) ;
#758=CARTESIAN_POINT ( 'NONE',  ( 3.525000000000000355, -4.330127018922194537, 2.499999999999995559 ) ) ;
#759=CARTESIAN_POINT ( 'NONE',  ( 6.703125000614516438, 4.541064518000418104, -2.621784821874998173 ) ) ;
#760=CARTESIAN_POINT ( 'NONE',  ( 24.77812500061451217, 4.541064518000418104, 2.621784821874999949 ) ) ;
#761=CARTESIAN_POINT ( 'NONE',  ( 13.32187500061451502, -6.054752690667223547, -1.112240025338166033E-15 ) ) ;
#762=CARTESIAN_POINT ( 'NONE',  ( 16.13437500061451502, 6.421520780324663323E-16, -5.243569643749999010 ) ) ;
#763=CARTESIAN_POINT ( 'NONE',  ( 2.121784821874999061, 18.75312500061451715, 26.32496088578401583 ) ) ;
#764=CARTESIAN_POINT ( 'NONE',  ( 18.60000000122903430, -2.886751345948125991, -5.000000000000000000 ) ) ;
#766=CARTESIAN_POINT ( 'NONE',  ( 9.440625000614517148, 6.054752690667223547, 3.707466751127219781E-16 ) ) ;
#767=CARTESIAN_POINT ( 'NONE',  ( 6.046875000614519102, -3.027376345333614438, 5.243569643749998122 ) ) ;
#768=CARTESIAN_POINT ( 'NONE',  ( 5.259375000614518569, -4.541064518000417216, -2.621784821875001281 ) ) ;
#769=ORIENTED_EDGE ( 'NONE', *, *, #18393, .F. ) ;
#770=CARTESIAN_POINT ( 'NONE',  ( 24.79687500061451999, 6.054752690667223547, 3.707466751127219781E-16 ) ) ;
#771=CARTESIAN_POINT ( 'NONE',  ( 15.85312500061451857, 0.000000000000000000, 5.243569643749999010 ) ) ;
#772=CARTESIAN_POINT ( 'NONE',  ( 26.47500000122903074, 2.886751345948126879, 4.999999999999999112 ) ) ;
#773=( BOUNDED_CURVE ( )  B_SPLINE_CURVE ( 2, ( #17330, #46145, #39889, #18045, #63124, #12520, #27707 ),
 .UNSPECIFIED., .F., .F. ) 
 B_SPLINE_CURVE_WITH_KNOTS ( ( 3, 2, 2, 3 ),
 ( 0.7500000000000000000, 0.7527777777777777679, 0.7555555555555555358, 0.7583333333333333037 ),
 .UNSPECIFIED. ) 
 CURVE ( )  GEOMETRIC_REPRESENTATION_ITEM ( )  RATIONAL_B_SPLINE_CURVE ( ( 1.000000000000000000, 0.8660254037844387076, 1.000000000000000000, 0.8660254037844387076, 1.000000000000000000, 0.8660254037844387076, 1.000000000000000000 ) ) 
 REPRESENTATION_ITEM ( '' )  );
#774=CARTESIAN_POINT ( 'NONE',  ( 27.66562500061451146, -6.054752690667223547, -1.112240025338166033E-15 ) ) ;
#775=CARTESIAN_POINT ( 'NONE',  ( 20.67187500061451289, 3.027376345333613106, -5.243569643749998122 ) ) ;
#776=CARTESIAN_POINT ( 'NONE',  ( 16.00312500061451715, -4.541064518000417216, -2.621784821875001281 ) ) ;
#777=CARTESIAN_POINT ( 'NONE',  ( 1.999999999999998668, 10.40000000000000213, 26.53589838486224650 ) ) ;
#778=CARTESIAN_POINT ( 'NONE',  ( 21.85312500061451502, -4.541064518000417216, -2.621784821875001281 ) ) ;
#779=CARTESIAN_POINT ( 'NONE',  ( 3.262500001229035718, -4.330127018922190985, -2.500000000000001332 ) ) ;
#781=CARTESIAN_POINT ( 'NONE',  ( 26.92499999999999716, -4.330127018922194537, 2.499999999999995559 ) ) ;
#782=CARTESIAN_POINT ( 'NONE',  ( -1.999999999999997113, 12.42500000000000249, -26.53589838486224295 ) ) ;
#784=CARTESIAN_POINT ( 'NONE',  ( 29.31562500061451715, 3.027376345333611329, 5.243569643749999010 ) ) ;
#785=CARTESIAN_POINT ( 'NONE',  ( 10.56562500061451715, -6.054752690667223547, -1.112240025338166033E-15 ) ) ;
#786=CARTESIAN_POINT ( 'NONE',  ( 21.63750000122903572, -4.330127018922194537, 2.499999999999995559 ) ) ;
#787=CARTESIAN_POINT ( 'NONE',  ( 27.59062500061451573, -3.027376345333614438, 5.243569643749998122 ) ) ;
#788=CARTESIAN_POINT ( 'NONE',  ( 28.38749999999999929, -2.886751345948125991, -5.000000000000000000 ) ) ;
#789=CARTESIAN_POINT ( 'NONE',  ( 2.000000000000001332, 18.46250000122903501, -26.53589838486224650 ) ) ;
#790=CARTESIAN_POINT ( 'NONE',  ( 25.27500000122903145, -5.773502691896255534, -1.060575238724906372E-15 ) ) ;
#791=CARTESIAN_POINT ( 'NONE',  ( 13.19062500061451537, -3.027376345333614438, 5.243569643749998122 ) ) ;
#792=ORIENTED_EDGE ( 'NONE', *, *, #47637, .T. ) ;
#793=EDGE_CURVE ( 'NONE', #12747, #52141, #14130, .T. ) ;
#794=CARTESIAN_POINT ( 'NONE',  ( 7.115625000614516082, 3.027376345333613106, -5.243569643749998122 ) ) ;
#795=CARTESIAN_POINT ( 'NONE',  ( 5.090625000614516615, -3.027376345333614438, 5.243569643749998122 ) ) ;
#798=EDGE_CURVE ( 'NONE', #16648, #45031, #59438, .T. ) ;
#799=CARTESIAN_POINT ( 'NONE',  ( -4.243569643749999898, 19.85937500061451644, -30.00000000000000000 ) ) ;
#800=CARTESIAN_POINT ( 'NONE',  ( 15.37500000000000000, 6.123233995736764310E-16, -4.999999999999998224 ) ) ;
#801=ADVANCED_FACE ( 'NONE', ( #17678 ), #50957, .F. ) ;
#802=CARTESIAN_POINT ( 'NONE',  ( 16.77187500061451786, 3.027376345333611329, 5.243569643749999010 ) ) ;
#803=CARTESIAN_POINT ( 'NONE',  ( 11.25000000122903288, -2.886751345948129988, 4.999999999999997335 ) ) ;
#804=CARTESIAN_POINT ( 'NONE',  ( 19.35937500061451644, 4.541064518000418104, -2.621784821874998173 ) ) ;
#806=CARTESIAN_POINT ( 'NONE',  ( 21.34687500061451715, -3.027376345333614438, 5.243569643749998122 ) ) ;
#807=CARTESIAN_POINT ( 'NONE',  ( 2.121784821875001281, 15.00312500061451715, -26.32496088578401938 ) ) ;
#810=CARTESIAN_POINT ( 'NONE',  ( 20.73750000000000071, -2.886751345948092684, -5.000000000000057732 ) ) ;
#811=CARTESIAN_POINT ( 'NONE',  ( 27.36562500061451786, 3.027376345333613106, -5.243569643749998122 ) ) ;
#812=( NAMED_UNIT ( * ) SI_UNIT ( $, .STERADIAN. ) SOLID_ANGLE_UNIT ( ) );
#813=CARTESIAN_POINT ( 'NONE',  ( 28.58437500061451786, -4.541064518000419881, 2.621784821874995952 ) ) ;
#814=CARTESIAN_POINT ( 'NONE',  ( 23.55000000000000071, 4.330127018922192761, -2.499999999999997780 ) ) ;
#815=CARTESIAN_POINT ( 'NONE',  ( 7.040625000614517681, -3.027376345333610441, -5.243569643749999898 ) ) ;
#817=CARTESIAN_POINT ( 'NONE',  ( 19.32187500061451857, 3.027376345333613106, -5.243569643749998122 ) ) ;
#819=CARTESIAN_POINT ( 'NONE',  ( 4.865625000614517859, 3.027376345333613106, -5.243569643749998122 ) ) ;
#820=CARTESIAN_POINT ( 'NONE',  ( 9.571875000614518569, 3.027376345333611329, 5.243569643749999010 ) ) ;
#822=CARTESIAN_POINT ( 'NONE',  ( 22.09687500061451715, 6.054752690667223547, 3.707466751127219781E-16 ) ) ;
#824=CARTESIAN_POINT ( 'NONE',  ( 29.62500000000000000, -4.330127018922194537, 2.499999999999995559 ) ) ;
#825=CARTESIAN_POINT ( 'NONE',  ( 29.10937500061451644, -4.541064518000417216, -2.621784821875001281 ) ) ;
#826=EDGE_CURVE ( 'NONE', #30532, #37056, #33986, .T. ) ;
#828=CARTESIAN_POINT ( 'NONE',  ( 3.319923472288579536, -4.210009680006762345, 3.195188621371491511 ) ) ;
#830=CARTESIAN_POINT ( 'NONE',  ( 9.299999999999998934, 0.000000000000000000, 4.999999999999998224 ) ) ;
#832=CARTESIAN_POINT ( 'NONE',  ( 23.95312500061451289, 0.000000000000000000, 5.243569643749999010 ) ) ;
#833=CARTESIAN_POINT ( 'NONE',  ( 13.98750000000000249, -2.886751345948125991, -5.000000000000000000 ) ) ;
#834=CARTESIAN_POINT ( 'NONE',  ( 10.83750000122903501, -4.330127018922194537, 2.499999999999995559 ) ) ;
#835=CARTESIAN_POINT ( 'NONE',  ( 8.090625000614515727, 6.054752690667223547, 3.707466751127219781E-16 ) ) ;
#836=CARTESIAN_POINT ( 'NONE',  ( 25.19999999999999929, -4.330127018922190985, -2.500000000000001332 ) ) ;
#837=CARTESIAN_POINT ( 'NONE',  ( 20.84062500061451573, -3.027376345333614438, 5.243569643749998122 ) ) ;
#838=CARTESIAN_POINT ( 'NONE',  ( 18.71250000122903145, 4.330127018922192761, -2.499999999999997780 ) ) ;
#839=CARTESIAN_POINT ( 'NONE',  ( 28.83750000122903145, -4.330127018922194537, 2.499999999999995559 ) ) ;
#841=CARTESIAN_POINT ( 'NONE',  ( 7.124999999999999112, -4.330127018922194537, 2.499999999999995559 ) ) ;
#843=CARTESIAN_POINT ( 'NONE',  ( 20.99062500061451431, -3.027376345333610441, -5.243569643749999898 ) ) ;
#844=CARTESIAN_POINT ( 'NONE',  ( 29.46562500061451573, -6.054752690667223547, -1.112240025338166033E-15 ) ) ;
#845=CARTESIAN_POINT ( 'NONE',  ( 28.43437500061451573, 4.541064518000418104, 2.621784821874999949 ) ) ;
#846=CARTESIAN_POINT ( 'NONE',  ( 18.30937500061451928, -4.541064518000417216, -2.621784821875001281 ) ) ;
#847=CARTESIAN_POINT ( 'NONE',  ( 16.04062500061451857, -3.027376345333610441, -5.243569643749999898 ) ) ;
#848=AXIS2_PLACEMENT_3D ( 'NONE', #69404, #35764, #52400 ) ;
#850=CARTESIAN_POINT ( 'NONE',  ( 4.603125000614518569, 0.000000000000000000, 5.243569643749999010 ) ) ;
#852=CARTESIAN_POINT ( 'NONE',  ( 27.48750000122903359, -4.330127018922194537, 2.499999999999995559 ) ) ;
#854=CARTESIAN_POINT ( 'NONE',  ( 19.26562500061451644, 3.027376345333612662, -5.243569643749998122 ) ) ;
#855=CARTESIAN_POINT ( 'NONE',  ( 1.071796769724489895, 11.42990381179669868, -34.00000000000000000 ) ) ;
#856=CARTESIAN_POINT ( 'NONE',  ( 4.162500001229033408, -4.330127018922190985, -2.500000000000001332 ) ) ;
#857=CARTESIAN_POINT ( 'NONE',  ( 13.80937500061451750, -4.541064518000417216, -2.621784821875001281 ) ) ;
#858=CARTESIAN_POINT ( 'NONE',  ( 12.87187500061451750, -6.054752690667223547, -1.112240025338166033E-15 ) ) ;
#859=CARTESIAN_POINT ( 'NONE',  ( 20.59687500061451360, -3.027376345333610441, -5.243569643749999898 ) ) ;
#860=VERTEX_POINT ( 'NONE', #61310 ) ;
#861=CARTESIAN_POINT ( 'NONE',  ( 29.36250000000000071, 2.886751345948160630, -4.999999999999943157 ) ) ;
#862=CARTESIAN_POINT ( 'NONE',  ( 24.25312500061451715, 4.541064518000418104, -2.621784821874998173 ) ) ;
#863=CARTESIAN_POINT ( 'NONE',  ( 18.60937500061451644, 0.000000000000000000, 5.243569643749999010 ) ) ;
#864=CARTESIAN_POINT ( 'NONE',  ( 23.24062500061451786, -3.027376345333610441, -5.243569643749999898 ) ) ;
#866=CARTESIAN_POINT ( 'NONE',  ( 3.999999999999998668, 15.76249999999999751, 27.69059892324149175 ) ) ;
#867=CARTESIAN_POINT ( 'NONE',  ( 28.97812500061451502, -4.541064518000419881, 2.621784821874995952 ) ) ;
#868=CARTESIAN_POINT ( 'NONE',  ( 9.262500001229033941, 4.330127018922192761, -2.499999999999997780 ) ) ;
#869=CARTESIAN_POINT ( 'NONE',  ( 6.487500001229034474, 6.123233995736764310E-16, -4.999999999999998224 ) ) ;
#870=CARTESIAN_POINT ( 'NONE',  ( -3.999999999999999556, 19.06249999999999645, -32.30940107675850470 ) ) ;
#871=CARTESIAN_POINT ( 'NONE',  ( 26.36250000122903003, 4.330127018922192761, -2.499999999999997780 ) ) ;
#874=CARTESIAN_POINT ( 'NONE',  ( 9.459375000614517859, 4.541064518000418104, -2.621784821874998173 ) ) ;
#875=CARTESIAN_POINT ( 'NONE',  ( 24.48749999999999716, 5.773502691896255534, 3.535250795749688401E-16 ) ) ;
#876=CARTESIAN_POINT ( 'NONE',  ( 16.86562500061451786, -6.054752690667223547, -1.112240025338166033E-15 ) ) ;
#877=CARTESIAN_POINT ( 'NONE',  ( 9.946875000614516793, 6.054752690667223547, 3.707466751127219781E-16 ) ) ;
#878=CARTESIAN_POINT ( 'NONE',  ( 29.06250000122903288, 4.330127018922192761, -2.499999999999997780 ) ) ;
#879=CARTESIAN_POINT ( 'NONE',  ( 19.77187500061451786, 3.027376345333612662, -5.243569643749998122 ) ) ;
#880=CARTESIAN_POINT ( 'NONE',  ( 6.496875000614517504, -3.027376345333614438, 5.243569643749998122 ) ) ;
#881=CARTESIAN_POINT ( 'NONE',  ( 15.00000000122903465, -2.886751345948126435, -5.000000000000000000 ) ) ;
#882=CARTESIAN_POINT ( 'NONE',  ( 1.626862140677534273E-15, 17.86250000000000071, 34.00000000000000000 ) ) ;
#883=CARTESIAN_POINT ( 'NONE',  ( 7.378125000614518036, -4.541064518000419881, 2.621784821874995952 ) ) ;
#884=CARTESIAN_POINT ( 'NONE',  ( 19.97812500061451502, -4.541064518000419881, 2.621784821874995952 ) ) ;
#885=VERTEX_POINT ( 'NONE', #33238 ) ;
#886=CARTESIAN_POINT ( 'NONE',  ( 6.187500001229032875, 4.330127018922191873, 2.499999999999999556 ) ) ;
#887=CARTESIAN_POINT ( 'NONE',  ( 14.91562500061451679, 3.027376345333611329, 5.243569643749999010 ) ) ;
#888=CARTESIAN_POINT ( 'NONE',  ( 12.89062500061451821, -3.027376345333610441, -5.243569643749999898 ) ) ;
#890=CARTESIAN_POINT ( 'NONE',  ( 12.22499999999999964, 6.123233995736764310E-16, -4.999999999999998224 ) ) ;
#891=CARTESIAN_POINT ( 'NONE',  ( 8.025000001229035007, 2.886751345948126879, 4.999999999999999112 ) ) ;
#892=CARTESIAN_POINT ( 'NONE',  ( 6.553125000614518747, -4.541064518000417216, -2.621784821875001281 ) ) ;
#894=CARTESIAN_POINT ( 'NONE',  ( 18.18750000122903288, 6.123233995736764310E-16, -4.999999999999998224 ) ) ;
#896=CARTESIAN_POINT ( 'NONE',  ( 9.001249775931846008E-16, 10.07187500061451857, -25.09994784771203058 ) ) ;
#897=CARTESIAN_POINT ( 'NONE',  ( 4.898587196589411843E-16, 20.00000000000000000, 33.99999999999999289 ) ) ;
#898=CARTESIAN_POINT ( 'NONE',  ( 3.000000001229032875, 5.773502691896255534, 3.535250795749688894E-16 ) ) ;
#899=VECTOR ( 'NONE', #33176, 1000.000000000000000 ) ;
#900=CARTESIAN_POINT ( 'NONE',  ( 3.037500001229032964, 4.330127018922191873, 2.499999999999999556 ) ) ;
#901=CARTESIAN_POINT ( 'NONE',  ( 17.97187500061451715, 3.027376345333613106, -5.243569643749998122 ) ) ;
#903=CARTESIAN_POINT ( 'NONE',  ( 13.07812500061451821, 4.541064518000418104, 2.621784821874999949 ) ) ;
#906=CARTESIAN_POINT ( 'NONE',  ( 28.95937500061451431, 0.000000000000000000, 5.243569643749999010 ) ) ;
#907=CARTESIAN_POINT ( 'NONE',  ( 26.74687500061451573, -3.027376345333614438, 5.243569643749998122 ) ) ;
#909=CARTESIAN_POINT ( 'NONE',  ( 12.89062500061451821, -3.027376345333610441, -5.243569643749999898 ) ) ;
#910=CARTESIAN_POINT ( 'NONE',  ( 10.28437500061451715, 6.421520780324663323E-16, -5.243569643749999010 ) ) ;
#913=CARTESIAN_POINT ( 'NONE',  ( 20.39062500061451644, -3.027376345333614438, 5.243569643749998122 ) ) ;
#914=CARTESIAN_POINT ( 'NONE',  ( 3.138870840040013821, 3.891985242736291539, -3.513904600516652099 ) ) ;
#915=LINE ( 'NONE', #46332, #51391 ) ;
#916=CARTESIAN_POINT ( 'NONE',  ( 10.38750000000000107, -2.886751345948125991, -5.000000000000000000 ) ) ;
#917=CARTESIAN_POINT ( 'NONE',  ( 20.66250000122903074, 0.000000000000000000, 4.999999999999998224 ) ) ;
#918=CARTESIAN_POINT ( 'NONE',  ( 15.10312500061451502, -4.541064518000417216, -2.621784821875001281 ) ) ;
#921=CARTESIAN_POINT ( 'NONE',  ( 17.96250000000000213, -5.773502691896255534, -1.060575238724906372E-15 ) ) ;
#923=CARTESIAN_POINT ( 'NONE',  ( 22.08749999999999858, -2.886751345948125991, -5.000000000000000000 ) ) ;
#924=CARTESIAN_POINT ( 'NONE',  ( 20.22187500061451715, 3.027376345333613106, -5.243569643749998122 ) ) ;
#925=CARTESIAN_POINT ( 'NONE',  ( 25.11562500061451431, 3.027376345333613106, -5.243569643749998122 ) ) ;
#927=CARTESIAN_POINT ( 'NONE',  ( -1.071796769724485010, 17.05490381179669868, 34.00000000000000000 ) ) ;
#928=CARTESIAN_POINT ( 'NONE',  ( 7.153125000614518392, 4.541064518000418104, -2.621784821874998173 ) ) ;
#930=CARTESIAN_POINT ( 'NONE',  ( 13.50000000000000178, -4.330127018922190985, -2.500000000000001332 ) ) ;
#931=CARTESIAN_POINT ( 'NONE',  ( 4.243569643749999010, 16.46562500061451573, 27.54997392385601174 ) ) ;
#932=CARTESIAN_POINT ( 'NONE',  ( 28.00312500061451715, 0.000000000000000000, 5.243569643749999010 ) ) ;
#934=CARTESIAN_POINT ( 'NONE',  ( 26.14687500061451431, 6.054752690667223547, 3.707466751127219781E-16 ) ) ;
#935=ORIENTED_EDGE ( 'NONE', *, *, #68490, .F. ) ;
#936=CARTESIAN_POINT ( 'NONE',  ( 23.87812500061451715, 4.541064518000418104, 2.621784821874999949 ) ) ;
#937=CARTESIAN_POINT ( 'NONE',  ( 24.79687500061451999, 6.054752690667223547, 3.707466751127219781E-16 ) ) ;
#939=CARTESIAN_POINT ( 'NONE',  ( 9.001249775931846008E-16, 17.66562500061459318, -25.09994784771203058 ) ) ;
#940=CARTESIAN_POINT ( 'NONE',  ( 12.00000000000000000, 0.000000000000000000, 4.999999999999998224 ) ) ;
#941=CARTESIAN_POINT ( 'NONE',  ( 8.840625000614515727, -3.027376345333610441, -5.243569643749999898 ) ) ;
#943=CARTESIAN_POINT ( 'NONE',  ( 1.626862140677534273E-15, 11.11250000000000071, 34.00000000000000000 ) ) ;
#944=CARTESIAN_POINT ( 'NONE',  ( 26.54062500061451146, 6.054752690667223547, 3.707466751127219781E-16 ) ) ;
#947=CARTESIAN_POINT ( 'NONE',  ( 20.52187500061451786, -6.054752690667223547, -1.112240025338166033E-15 ) ) ;
#948=CARTESIAN_POINT ( 'NONE',  ( -4.243569643749999898, 13.07187500061452035, 27.54997392385601529 ) ) ;
#949=CARTESIAN_POINT ( 'NONE',  ( 18.60937500061451644, 0.000000000000000000, 5.243569643749999010 ) ) ;
#950=CARTESIAN_POINT ( 'NONE',  ( 26.82187500061451857, -6.054752690667223547, -1.112240025338166033E-15 ) ) ;
#951=CARTESIAN_POINT ( 'NONE',  ( -4.243569643749999898, 17.60937500061451999, 30.00000000000000000 ) ) ;
#952=CARTESIAN_POINT ( 'NONE',  ( 8.503125000614515372, 4.541064518000418104, -2.621784821874998173 ) ) ;
#953=CARTESIAN_POINT ( 'NONE',  ( 3.999999999999999112, 16.17500000000000071, 30.00000000000000000 ) ) ;
#954=CARTESIAN_POINT ( 'NONE',  ( 3.646875000614520079, 6.054752690667223547, 3.707466751127219781E-16 ) ) ;
#955=CARTESIAN_POINT ( 'NONE',  ( 30.00000000000000000, 0.000000000000000000, 4.999999999999998224 ) ) ;
#956=CARTESIAN_POINT ( 'NONE',  ( 6.215625000614517504, 3.027376345333613106, -5.243569643749998122 ) ) ;
#957=CARTESIAN_POINT ( 'NONE',  ( 10.32187500061451679, 3.027376345333613106, -5.243569643749998122 ) ) ;
#958=CARTESIAN_POINT ( 'NONE',  ( 20.25000000122903288, -2.886751345948129988, 4.999999999999997335 ) ) ;
#959=CARTESIAN_POINT ( 'NONE',  ( 6.571875000614517681, -6.054752690667223547, -1.112240025338166033E-15 ) ) ;
#960=CARTESIAN_POINT ( 'NONE',  ( 6.853125000614516793, 0.000000000000000000, 5.243569643749999010 ) ) ;
#962=CARTESIAN_POINT ( 'NONE',  ( 17.89687500061451431, -3.027376345333610441, -5.243569643749999898 ) ) ;
#963=CARTESIAN_POINT ( 'NONE',  ( 4.457256472106807976, 2.265816029382255792, 4.511484450116618916 ) ) ;
#964=VERTEX_POINT ( 'NONE', #62041 ) ;
#965=CARTESIAN_POINT ( 'NONE',  ( 24.81562500061451715, 3.027376345333611329, 5.243569643749999010 ) ) ;
#966=CARTESIAN_POINT ( 'NONE',  ( 9.253125000614517148, -4.541064518000417216, -2.621784821875001281 ) ) ;
#967=CARTESIAN_POINT ( 'NONE',  ( 27.04687500061450933, 6.054752690667223547, 3.707466751127219781E-16 ) ) ;
#968=CARTESIAN_POINT ( 'NONE',  ( 10.75312500061451715, 4.541064518000418104, -2.621784821874998173 ) ) ;
#969=CARTESIAN_POINT ( 'NONE',  ( 4.425757632551291287, -2.326665885598202088, -4.651935364053993993 ) ) ;
#970=CARTESIAN_POINT ( 'NONE',  ( 13.35000000122903430, 5.773502691896255534, 3.535250795749688894E-16 ) ) ;
#971=CARTESIAN_POINT ( 'NONE',  ( 26.87812500061451360, 6.421520780324663323E-16, -5.243569643749999010 ) ) ;
#972=CARTESIAN_POINT ( 'NONE',  ( 4.243569643749999010, 11.96562500061451750, -32.45002607614398471 ) ) ;
#973=CARTESIAN_POINT ( 'NONE',  ( 13.50000000122903288, -2.886751345948129988, 4.999999999999997335 ) ) ;
#974=CARTESIAN_POINT ( 'NONE',  ( 10.68750000000000000, -2.886751345948129988, 4.999999999999997335 ) ) ;
#975=CARTESIAN_POINT ( 'NONE',  ( 19.37812500061451715, 4.541064518000418104, 2.621784821874999949 ) ) ;
#976=CARTESIAN_POINT ( 'NONE',  ( 6.346875000614517148, 6.054752690667223547, 3.707466751127219781E-16 ) ) ;
#977=CARTESIAN_POINT ( 'NONE',  ( 21.67500000000000071, 6.123233995736764310E-16, -4.999999999999998224 ) ) ;
#978=CARTESIAN_POINT ( 'NONE',  ( 7.800000001229035362, -2.886751345948125991, -5.000000000000000000 ) ) ;
#979=CARTESIAN_POINT ( 'NONE',  ( 17.06250000122903288, 0.000000000000000000, 4.999999999999998224 ) ) ;
#980=( BOUNDED_CURVE ( )  B_SPLINE_CURVE ( 2, ( #56330, #547, #189, #6078, #16423, #33787, #16787, #50430, #67779 ),
 .UNSPECIFIED., .F., .F. ) 
 B_SPLINE_CURVE_WITH_KNOTS ( ( 3, 2, 2, 2, 3 ),
 ( 0.5543478260869565410, 0.5579710144927536586, 0.5652173913043477826, 0.5724637681159420177, 0.5760869565217391353 ),
 .UNSPECIFIED. ) 
 CURVE ( )  GEOMETRIC_REPRESENTATION_ITEM ( )  RATIONAL_B_SPLINE_CURVE ( ( 0.9330127018922194093, 0.9330127018922194093, 1.000000000000000000, 0.8660254037844387076, 1.000000000000000000, 0.8660254037844387076, 1.000000000000000000, 0.9330127018922194093, 0.9330127018922194093 ) ) 
 REPRESENTATION_ITEM ( '' )  );
#981=CARTESIAN_POINT ( 'NONE',  ( 12.32812500061451821, -4.541064518000419881, 2.621784821874995952 ) ) ;
#982=CARTESIAN_POINT ( 'NONE',  ( 16.19062500061451715, 6.054752690667223547, 3.707466751127219781E-16 ) ) ;
#983=ADVANCED_FACE ( 'NONE', ( #48596 ), #31602, .F. ) ;
#984=CARTESIAN_POINT ( 'NONE',  ( 25.01250000122903216, 4.330127018922192761, -2.499999999999997780 ) ) ;
#985=CARTESIAN_POINT ( 'NONE',  ( 19.61249999999999716, 2.886751345948126879, 4.999999999999999112 ) ) ;
#986=CARTESIAN_POINT ( 'NONE',  ( 23.85937500061451644, 4.541064518000418104, -2.621784821874998173 ) ) ;
#988=CARTESIAN_POINT ( 'NONE',  ( 9.787500001229036073, 4.330127018922191873, 2.499999999999999556 ) ) ;
#989=CARTESIAN_POINT ( 'NONE',  ( 8.446875000614518569, -3.027376345333610441, -5.243569643749999898 ) ) ;
#990=CARTESIAN_POINT ( 'NONE',  ( 25.24687500061451573, 6.054752690667223547, 3.707466751127219781E-16 ) ) ;
#991=( BOUNDED_CURVE ( )  B_SPLINE_CURVE ( 2, ( #28868, #810, #72857, #67327, #50687, #16687, #39243 ),
 .UNSPECIFIED., .F., .F. ) 
 B_SPLINE_CURVE_WITH_KNOTS ( ( 3, 2, 2, 3 ),
 ( 0.3416666666666666186, 0.3444444444444444420, 0.3472222222222222099, 0.3500000000000000333 ),
 .UNSPECIFIED. ) 
 CURVE ( )  GEOMETRIC_REPRESENTATION_ITEM ( )  RATIONAL_B_SPLINE_CURVE ( ( 1.000000000000002665, 0.8660254037844360431, 1.000000000000000000, 0.8660254037844387076, 1.000000000000000000, 0.8660254037844360431, 1.000000000000002665 ) ) 
 REPRESENTATION_ITEM ( '' )  );
#992=CARTESIAN_POINT ( 'NONE',  ( 2.971875000614517592, -6.054752690667223547, -1.112240025338166033E-15 ) ) ;
#993=CARTESIAN_POINT ( 'NONE',  ( 24.66562500061451502, 3.027376345333613106, -5.243569643749998122 ) ) ;
#994=CARTESIAN_POINT ( 'NONE',  ( 26.48437500061451644, 6.421520780324663323E-16, -5.243569643749999010 ) ) ;
#997=CARTESIAN_POINT ( 'NONE',  ( 7.246875000614518392, 6.054752690667223547, 3.707466751127219781E-16 ) ) ;
#998=CARTESIAN_POINT ( 'NONE',  ( 1.071796769724491893, 12.48259618943233384, 33.99999999999999289 ) ) ;
#999=CARTESIAN_POINT ( 'NONE',  ( 28.37812500061451715, 4.541064518000418104, 2.621784821874999949 ) ) ;
#1000=CARTESIAN_POINT ( 'NONE',  ( 6.834375000614518747, 4.541064518000418104, 2.621784821874999949 ) ) ;
#1001=CARTESIAN_POINT ( 'NONE',  ( 25.76249999999999929, 2.886751345948095793, -5.000000000000055067 ) ) ;
#1002=CARTESIAN_POINT ( 'NONE',  ( -1.473776270879187500, 9.816672227264625405, 25.95083297442941017 ) ) ;
#1003=CARTESIAN_POINT ( 'NONE',  ( 16.31250000000000000, 2.886751345948129099, -4.999999999999998224 ) ) ;
#1004=ORIENTED_EDGE ( 'NONE', *, *, #41944, .T. ) ;
#1005=CARTESIAN_POINT ( 'NONE',  ( 27.97500000000000142, 6.123233995736764310E-16, -4.999999999999998224 ) ) ;
#1006=CARTESIAN_POINT ( 'NONE',  ( 29.44687500061451857, -3.027376345333614438, 5.243569643749998122 ) ) ;
#1008=CARTESIAN_POINT ( 'NONE',  ( 15.10312500061451502, -4.541064518000417216, -2.621784821875001281 ) ) ;
#1009=CARTESIAN_POINT ( 'NONE',  ( 5.615625000614517859, -6.054752690667223547, -1.112240025338166033E-15 ) ) ;
#1011=CARTESIAN_POINT ( 'NONE',  ( 4.809375000614516615, -4.541064518000417216, -2.621784821875001281 ) ) ;
#1013=CARTESIAN_POINT ( 'NONE',  ( 16.31250000122903288, -4.330127018922190985, -2.500000000000001332 ) ) ;
#1014=CARTESIAN_POINT ( 'NONE',  ( 21.82499999999999574, 4.330127018922191873, 2.499999999999999556 ) ) ;
#1015=CARTESIAN_POINT ( 'NONE',  ( 28.76249999999999929, -5.773502691896255534, -1.060575238724906372E-15 ) ) ;
#1016=CARTESIAN_POINT ( 'NONE',  ( 5.034375000614519813, 4.541064518000418104, 2.621784821874999949 ) ) ;
#1017=CARTESIAN_POINT ( 'NONE',  ( 8.221875000614518925, 3.027376345333611329, 5.243569643749999010 ) ) ;
#1018=CARTESIAN_POINT ( 'NONE',  ( 20.97187500061451715, -6.054752690667223547, -1.112240025338166033E-15 ) ) ;
#1019=DIRECTION ( 'NONE',  ( 0.000000000000000000, 0.000000000000000000, -1.000000000000000000 ) ) ;
#1020=ORIENTED_EDGE ( 'NONE', *, *, #66019, .T. ) ;
#1021=CARTESIAN_POINT ( 'NONE',  ( 3.009375000614516793, -4.541064518000417216, -2.621784821875001281 ) ) ;
#1022=CARTESIAN_POINT ( 'NONE',  ( 6.750000000000002665, -4.330127018922190985, -2.500000000000001332 ) ) ;
#1023=CARTESIAN_POINT ( 'NONE',  ( 6.946875000614517681, -3.027376345333614438, 5.243569643749998122 ) ) ;
#1024=CARTESIAN_POINT ( 'NONE',  ( 18.97499999999999787, 6.123233995736764310E-16, -4.999999999999998224 ) ) ;
#1025=CARTESIAN_POINT ( 'NONE',  ( 15.81562500061451537, 3.027376345333611329, 5.243569643749999010 ) ) ;
#1029=CARTESIAN_POINT ( 'NONE',  ( 11.20312500061451644, 4.541064518000418104, -2.621784821874998173 ) ) ;
#1030=CARTESIAN_POINT ( 'NONE',  ( 27.75937500061451502, -4.541064518000417216, -2.621784821875001281 ) ) ;
#1031=CARTESIAN_POINT ( 'NONE',  ( -2.121784821874996840, 19.03437500061451715, 33.67503911421598417 ) ) ;
#1032=CARTESIAN_POINT ( 'NONE',  ( 27.23437500061451644, -4.541064518000419881, 2.621784821874995952 ) ) ;
#1033=CARTESIAN_POINT ( 'NONE',  ( 8.062500000000000000, -5.773502691896255534, -1.060575238724906372E-15 ) ) ;
#1034=CARTESIAN_POINT ( 'NONE',  ( -3.999999999999997335, 13.40000000122903323, 32.30940107675850470 ) ) ;
#1035=CARTESIAN_POINT ( 'NONE',  ( 6.750000001229033764, -2.886751345948129988, 4.999999999999997335 ) ) ;
#1036=CARTESIAN_POINT ( 'NONE',  ( 18.53437500061451715, 4.541064518000418104, 2.621784821874999949 ) ) ;
#1037=CARTESIAN_POINT ( 'NONE',  ( 12.30937500061451573, 0.000000000000000000, 5.243569643749999010 ) ) ;
#1038=CARTESIAN_POINT ( 'NONE',  ( -0.1398361002794802910, 5.000000000000000000, -33.99999999999998579 ) ) ;
#1039=ORIENTED_EDGE ( 'NONE', *, *, #67203, .F. ) ;
#1040=CARTESIAN_POINT ( 'NONE',  ( 14.20312500061451644, -4.541064518000417216, -2.621784821875001281 ) ) ;
#1041=CARTESIAN_POINT ( 'NONE',  ( 26.06250000122903288, 0.000000000000000000, 4.999999999999998224 ) ) ;
#1042=CARTESIAN_POINT ( 'NONE',  ( 12.42187500061451821, -6.054752690667223547, -1.112240025338166033E-15 ) ) ;
#1044=CARTESIAN_POINT ( 'NONE',  ( 13.56562500061451892, 3.027376345333611329, 5.243569643749999010 ) ) ;
#1046=CARTESIAN_POINT ( 'NONE',  ( 23.67187500061451999, -6.054752690667223547, -1.112240025338166033E-15 ) ) ;
#1047=CARTESIAN_POINT ( 'NONE',  ( 2.874095310376903356, -4.091409605186981047, 3.279548391533174012 ) ) ;
#1048=CARTESIAN_POINT ( 'NONE',  ( 11.88750000122903216, 6.123233995736764310E-16, -4.999999999999998224 ) ) ;
#1051=CARTESIAN_POINT ( 'NONE',  ( -3.000416591977282496E-16, 16.14687500061451786, -34.90005215228797653 ) ) ;
#1052=CARTESIAN_POINT ( 'NONE',  ( 17.52187500061451431, 3.027376345333613106, -5.243569643749998122 ) ) ;
#1053=CARTESIAN_POINT ( 'NONE',  ( 19.16250000122903430, 4.330127018922192761, -2.499999999999997780 ) ) ;
#1054=CARTESIAN_POINT ( 'NONE',  ( 14.97187500061451892, 3.027376345333611329, 5.243569643749999010 ) ) ;
#1056=CARTESIAN_POINT ( 'NONE',  ( -2.121784821874999949, 10.33437500061451786, 26.32496088578401938 ) ) ;
#1057=CARTESIAN_POINT ( 'NONE',  ( 19.27500000122903145, 2.886751345948126879, 4.999999999999999112 ) ) ;
#1058=CARTESIAN_POINT ( 'NONE',  ( 15.51562500061451644, -6.054752690667223547, -1.112240025338166033E-15 ) ) ;
#1059=CARTESIAN_POINT ( 'NONE',  ( 25.46249999999999503, 2.886751345948143754, 4.999999999999969802 ) ) ;
#1060=ORIENTED_EDGE ( 'NONE', *, *, #43888, .F. ) ;
#1061=ORIENTED_EDGE ( 'NONE', *, *, #53191, .F. ) ;
#1062=CARTESIAN_POINT ( 'NONE',  ( 19.12500000000000000, 4.330127018922191873, 2.499999999999999556 ) ) ;
#1063=CARTESIAN_POINT ( 'NONE',  ( 10.00000000000000000, 1.224646799147353256E-15, -10.00000000000000888 ) ) ;
#1064=CARTESIAN_POINT ( 'NONE',  ( 3.815625000614518036, -6.054752690667223547, -1.112240025338166033E-15 ) ) ;
#1065=CARTESIAN_POINT ( 'NONE',  ( 15.67500000122903181, 2.886751345948126879, 4.999999999999999112 ) ) ;
#1066=CARTESIAN_POINT ( 'NONE',  ( 27.00937500061451857, 4.541064518000418104, -2.621784821874998173 ) ) ;
#1068=CARTESIAN_POINT ( 'NONE',  ( 21.17812500061451431, 4.541064518000418104, 2.621784821874999949 ) ) ;
#1069=CARTESIAN_POINT ( 'NONE',  ( 22.26562500061451644, -6.054752690667223547, -1.112240025338166033E-15 ) ) ;
#1070=CARTESIAN_POINT ( 'NONE',  ( 3.703125000614516882, 0.000000000000000000, 5.243569643749999010 ) ) ;
#1071=EDGE_CURVE ( 'NONE', #53683, #17652, #44373, .T. ) ;
#1072=CARTESIAN_POINT ( 'NONE',  ( 26.92499999999999716, -4.330127018922194537, 2.499999999999995559 ) ) ;
#1073=CARTESIAN_POINT ( 'NONE',  ( 4.596237264682155654, 1.968401129533140059, 4.860084320473172070 ) ) ;
#1075=DIRECTION ( 'NONE',  ( 0.000000000000000000, 0.000000000000000000, 1.000000000000000000 ) ) ;
#1076=CARTESIAN_POINT ( 'NONE',  ( -3.999999999999999556, 11.52500000122903501, -32.30940107675850470 ) ) ;
#1077=CARTESIAN_POINT ( 'NONE',  ( -4.243569643749999898, 14.90937500061451715, -30.00000000000000000 ) ) ;
#1078=CARTESIAN_POINT ( 'NONE',  ( 5.325000001229033941, 2.886751345948126879, 4.999999999999999112 ) ) ;
#1079=CARTESIAN_POINT ( 'NONE',  ( 5.475000000000000533, 6.123233995736764310E-16, -4.999999999999998224 ) ) ;
#1081=CARTESIAN_POINT ( 'NONE',  ( 3.975000001229033852, 2.886751345948126879, 4.999999999999999112 ) ) ;
#1082=CARTESIAN_POINT ( 'NONE',  ( 10.13437500061451679, -4.541064518000419881, 2.621784821874995952 ) ) ;
#1084=CARTESIAN_POINT ( 'NONE',  ( 4.898587196589411843E-16, 20.00000000000000000, -26.00000000000000000 ) ) ;
#1085=CARTESIAN_POINT ( 'NONE',  ( -4.872631645816652757, 8.733424155075976358, -33.50632029722230953 ) ) ;
#1086=CARTESIAN_POINT ( 'NONE',  ( 16.95000000122903572, 5.773502691896255534, 3.535250795749688401E-16 ) ) ;
#1087=CARTESIAN_POINT ( 'NONE',  ( 7.621875000614519280, 3.027376345333613106, -5.243569643749998122 ) ) ;
#1088=CARTESIAN_POINT ( 'NONE',  ( 12.49687500061451573, -3.027376345333610441, -5.243569643749999898 ) ) ;
#1089=CARTESIAN_POINT ( 'NONE',  ( 5.700000000000000178, 0.000000000000000000, 4.999999999999998224 ) ) ;
#1090=CARTESIAN_POINT ( 'NONE',  ( -2.121784821874999949, 16.12812500061459176, 26.32496088578401938 ) ) ;
#1091=CARTESIAN_POINT ( 'NONE',  ( 21.72187500061451715, 3.027376345333611329, 5.243569643749999010 ) ) ;
#1092=DIRECTION ( 'NONE',  ( -0.000000000000000000, -1.000000000000000000, -0.000000000000000000 ) ) ;
#1093=CARTESIAN_POINT ( 'NONE',  ( 25.76250000122903216, -4.330127018922190985, -2.500000000000001332 ) ) ;
#1095=CARTESIAN_POINT ( 'NONE',  ( 23.12812500061451360, -4.541064518000419881, 2.621784821874995952 ) ) ;
#1096=CARTESIAN_POINT ( 'NONE',  ( 13.45312500061451466, 4.541064518000418104, -2.621784821874998173 ) ) ;
#1098=CARTESIAN_POINT ( 'NONE',  ( 11.78437500061451892, 4.541064518000418104, 2.621784821874999949 ) ) ;
#1099=CARTESIAN_POINT ( 'NONE',  ( 27.93750000000000000, -2.886751345948125991, -5.000000000000000000 ) ) ;
#1100=CARTESIAN_POINT ( 'NONE',  ( 21.60000000122903430, -2.886751345948129988, 4.999999999999997335 ) ) ;
#1102=CARTESIAN_POINT ( 'NONE',  ( 12.72187500061451537, 3.027376345333611329, 5.243569643749999010 ) ) ;
#1103=CARTESIAN_POINT ( 'NONE',  ( 27.87187500061451573, 3.027376345333613106, -5.243569643749998122 ) ) ;
#1106=CARTESIAN_POINT ( 'NONE',  ( 21.72187500061451715, 3.027376345333611329, 5.243569643749999010 ) ) ;
#1107=CARTESIAN_POINT ( 'NONE',  ( 15.15937500061451715, -4.541064518000417216, -2.621784821875001281 ) ) ;
#1109=CARTESIAN_POINT ( 'NONE',  ( 26.43750000000000000, -2.886751345948129988, 4.999999999999997335 ) ) ;
#1112=CARTESIAN_POINT ( 'NONE',  ( 17.35312500061451502, -4.541064518000417216, -2.621784821875001281 ) ) ;
#1113=CARTESIAN_POINT ( 'NONE',  ( 7.162500000000001421, -5.773502691896255534, -1.060575238724906372E-15 ) ) ;
#1114=CARTESIAN_POINT ( 'NONE',  ( 1.071796769724489895, 13.67990381179670045, 26.00000000000000355 ) ) ;
#1115=CARTESIAN_POINT ( 'NONE',  ( 15.75000000000000000, -4.330127018922190985, -2.500000000000001332 ) ) ;
#1116=CARTESIAN_POINT ( 'NONE',  ( 2.121784821875001281, 10.50312500061451715, 33.67503911421598417 ) ) ;
#1117=CARTESIAN_POINT ( 'NONE',  ( 26.03437500061451715, 6.421520780324663323E-16, -5.243569643749999010 ) ) ;
#1118=ORIENTED_EDGE ( 'NONE', *, *, #30725, .F. ) ;
#1119=CARTESIAN_POINT ( 'NONE',  ( 21.74062500061451431, -3.027376345333614438, 5.243569643749998122 ) ) ;
#1120=CARTESIAN_POINT ( 'NONE',  ( 19.69687500061451857, -3.027376345333610441, -5.243569643749999898 ) ) ;
#1121=CARTESIAN_POINT ( 'NONE',  ( 5.287500000000000533, -2.886751345948129988, 4.999999999999997335 ) ) ;
#1122=CARTESIAN_POINT ( 'NONE',  ( 6.215625000614517504, 3.027376345333613106, -5.243569643749998122 ) ) ;
#1123=CARTESIAN_POINT ( 'NONE',  ( 21.17812500061451431, 4.541064518000418104, 2.621784821874999949 ) ) ;
#1124=CARTESIAN_POINT ( 'NONE',  ( 12.53437500061451537, 6.421520780324663323E-16, -5.243569643749999010 ) ) ;
#1125=CARTESIAN_POINT ( 'NONE',  ( 16.47187500061452070, -6.054752690667223547, -1.112240025338166033E-15 ) ) ;
#1126=CARTESIAN_POINT ( 'NONE',  ( 9.001249775931846008E-16, 16.76562500061451999, 34.90005215228797653 ) ) ;
#1127=CARTESIAN_POINT ( 'NONE',  ( 19.50000000122903288, -2.886751345948125991, -5.000000000000000000 ) ) ;
#1129=CARTESIAN_POINT ( 'NONE',  ( 8.803125000614517859, -4.541064518000417216, -2.621784821875001281 ) ) ;
#1130=CARTESIAN_POINT ( 'NONE',  ( 4.696875000614518569, -3.027376345333614438, 5.243569643749998122 ) ) ;
#1131=CARTESIAN_POINT ( 'NONE',  ( 5.971875000614516260, 3.027376345333611329, 5.243569643749999010 ) ) ;
#1132=CARTESIAN_POINT ( 'NONE',  ( 26.25937500061451857, 0.000000000000000000, 5.243569643749999010 ) ) ;
#1133=CARTESIAN_POINT ( 'NONE',  ( 15.77812500061451573, 4.541064518000418104, 2.621784821874999949 ) ) ;
#1134=CARTESIAN_POINT ( 'NONE',  ( 26.28750000122903430, 6.123233995736764310E-16, -4.999999999999998224 ) ) ;
#1135=CARTESIAN_POINT ( 'NONE',  ( 25.75312500061451715, 0.000000000000000000, 5.243569643749999010 ) ) ;
#1136=CARTESIAN_POINT ( 'NONE',  ( 21.83437500061451786, -4.541064518000419881, 2.621784821874995952 ) ) ;
#1137=CARTESIAN_POINT ( 'NONE',  ( 18.06562500061451715, 3.027376345333611329, 5.243569643749999010 ) ) ;
#1138=CARTESIAN_POINT ( 'NONE',  ( -4.243569643749997233, 16.29687500061451644, 32.45002607614398471 ) ) ;
#1139=CARTESIAN_POINT ( 'NONE',  ( 21.62812500061451360, 4.541064518000418104, 2.621784821874999949 ) ) ;
#1140=CARTESIAN_POINT ( 'NONE',  ( 3.112500001229034918, 0.000000000000000000, 4.999999999999998224 ) ) ;
#1141=ORIENTED_EDGE ( 'NONE', *, *, #28856, .F. ) ;
#1142=CARTESIAN_POINT ( 'NONE',  ( 25.57499999999999929, -4.330127018922194537, 2.499999999999995559 ) ) ;
#1143=CARTESIAN_POINT ( 'NONE',  ( 3.999999999999998668, 13.06250000000000355, -32.30940107675850470 ) ) ;
#1144=CARTESIAN_POINT ( 'NONE',  ( 1.999999999999998668, 18.16250000122903074, 26.53589838486224650 ) ) ;
#1146=EDGE_CURVE ( 'NONE', #35743, #36091, #69393, .T. ) ;
#1147=CARTESIAN_POINT ( 'NONE',  ( 2.971875000614517592, -6.054752690667223547, -1.112240025338166033E-15 ) ) ;
#1148=CARTESIAN_POINT ( 'NONE',  ( 9.028125000614517504, 4.541064518000418104, 2.621784821874999949 ) ) ;
#1149=CARTESIAN_POINT ( 'NONE',  ( 23.40000000122903145, -2.886751345948129988, 4.999999999999997335 ) ) ;
#1150=CARTESIAN_POINT ( 'NONE',  ( 28.11562500061451431, -6.054752690667223547, -1.112240025338166033E-15 ) ) ;
#1151=CARTESIAN_POINT ( 'NONE',  ( 27.78749999999999787, -2.886751345948129988, 4.999999999999997335 ) ) ;
#1152=CARTESIAN_POINT ( 'NONE',  ( -3.999999999999999556, 16.02500000122903501, -32.30940107675850470 ) ) ;
#1153=CARTESIAN_POINT ( 'NONE',  ( 29.76562500061451644, 3.027376345333611329, 5.243569643749999010 ) ) ;
#1154=CARTESIAN_POINT ( 'NONE',  ( 10.30312500061451431, 4.541064518000418104, -2.621784821874998173 ) ) ;
#1156=CARTESIAN_POINT ( 'NONE',  ( 25.90312500061451573, -4.541064518000417216, -2.621784821875001281 ) ) ;
#1157=CARTESIAN_POINT ( 'NONE',  ( 8.090625000614515727, 6.054752690667223547, 3.707466751127219781E-16 ) ) ;
#1158=CARTESIAN_POINT ( 'NONE',  ( 5.390625000614518214, 6.054752690667223547, 3.707466751127219781E-16 ) ) ;
#1160=DIRECTION ( 'NONE',  ( 0.000000000000000000, 0.000000000000000000, 1.000000000000000000 ) ) ;
#1161=CARTESIAN_POINT ( 'NONE',  ( 16.68750000000000000, -2.886751345948125991, -5.000000000000000000 ) ) ;
#1162=CARTESIAN_POINT ( 'NONE',  ( 15.12187500061451750, -6.054752690667223547, -1.112240025338166033E-15 ) ) ;
#1163=CARTESIAN_POINT ( 'NONE',  ( 11.06250000122903288, 4.330127018922192761, -2.499999999999997780 ) ) ;
#1164=CARTESIAN_POINT ( 'NONE',  ( 16.09687500061452070, -3.027376345333610441, -5.243569643749999898 ) ) ;
#1166=CARTESIAN_POINT ( 'NONE',  ( 20.70937500061451786, 4.541064518000418104, -2.621784821874998173 ) ) ;
#1167=CARTESIAN_POINT ( 'NONE',  ( 2.121784821875001281, 14.55312500061451786, -26.32496088578401938 ) ) ;
#1170=CARTESIAN_POINT ( 'NONE',  ( 4.121605622237005662, 2.830625451251030711, 4.413915781326256393 ) ) ;
#1171=CARTESIAN_POINT ( 'NONE',  ( 24.96562500061451573, -6.054752690667223547, -1.112240025338166033E-15 ) ) ;
#1173=CARTESIAN_POINT ( 'NONE',  ( 28.09687500061451360, -3.027376345333614438, 5.243569643749998122 ) ) ;
#1174=CARTESIAN_POINT ( 'NONE',  ( 24.82499999999999929, 6.123233995736764310E-16, -4.999999999999998224 ) ) ;
#1175=CARTESIAN_POINT ( 'NONE',  ( 5.878125000614517148, 4.541064518000418104, 2.621784821874999949 ) ) ;
#1177=CARTESIAN_POINT ( 'NONE',  ( 18.94687500061451502, 6.054752690667223547, 3.707466751127219781E-16 ) ) ;
#1179=CARTESIAN_POINT ( 'NONE',  ( 5.728125000614515905, 6.421520780324663323E-16, -5.243569643749999010 ) ) ;
#1180=CARTESIAN_POINT ( 'NONE',  ( 8.296875000614516438, -3.027376345333614438, 5.243569643749998122 ) ) ;
#1181=ORIENTED_EDGE ( 'NONE', *, *, #52747, .F. ) ;
#1182=CARTESIAN_POINT ( 'NONE',  ( 19.39687500061451786, 6.054752690667223547, 3.707466751127219781E-16 ) ) ;
#1184=CARTESIAN_POINT ( 'NONE',  ( 27.22499999999999787, 4.330127018922191873, 2.499999999999999556 ) ) ;
#1185=CARTESIAN_POINT ( 'NONE',  ( 29.74687500061451217, 6.054752690667223547, 3.707466751127219781E-16 ) ) ;
#1189=CARTESIAN_POINT ( 'NONE',  ( 10.68750000000000000, -2.886751345948129988, 4.999999999999997335 ) ) ;
#1191=CARTESIAN_POINT ( 'NONE',  ( 24.85312500061451502, 0.000000000000000000, 5.243569643749999010 ) ) ;
#1192=CARTESIAN_POINT ( 'NONE',  ( 13.38750000000000107, -2.886751345948129988, 4.999999999999997335 ) ) ;
#1193=CARTESIAN_POINT ( 'NONE',  ( 9.937500001229032875, -4.330127018922194537, 2.499999999999995559 ) ) ;
#1194=CARTESIAN_POINT ( 'NONE',  ( 8.615625000614517859, 3.027376345333611329, 5.243569643749999010 ) ) ;
#1195=( BOUNDED_CURVE ( )  B_SPLINE_CURVE ( 2, ( #11522, #40690, #45148, #17414, #39971, #63208, #11162 ),
 .UNSPECIFIED., .F., .F. ) 
 B_SPLINE_CURVE_WITH_KNOTS ( ( 3, 2, 2, 3 ),
 ( 0.4583333333333332593, 0.4611111111111111382, 0.4638888888888889062, 0.4666666666666667296 ),
 .UNSPECIFIED. ) 
 CURVE ( )  GEOMETRIC_REPRESENTATION_ITEM ( )  RATIONAL_B_SPLINE_CURVE ( ( 1.000000000000002665, 0.8660254037844360431, 1.000000000000000000, 0.8660254037844387076, 1.000000000000000000, 0.8660254037844360431, 1.000000000000002665 ) ) 
 REPRESENTATION_ITEM ( '' )  );
#1196=CARTESIAN_POINT ( 'NONE',  ( 22.53750000000000142, -2.886751345948125991, -5.000000000000000000 ) ) ;
#1198=CARTESIAN_POINT ( 'NONE',  ( 21.77812500061451928, -4.541064518000419881, 2.621784821874995952 ) ) ;
#1200=CARTESIAN_POINT ( 'NONE',  ( 26.43750000122903288, 4.330127018922191873, 2.499999999999999556 ) ) ;
#1202=CARTESIAN_POINT ( 'NONE',  ( 8.474999999999999645, -4.330127018922194537, 2.499999999999995559 ) ) ;
#1204=CARTESIAN_POINT ( 'NONE',  ( 22.52812500061451573, 4.541064518000418104, 2.621784821874999949 ) ) ;
#1205=DIRECTION ( 'NONE',  ( 0.000000000000000000, 0.000000000000000000, 1.000000000000000000 ) ) ;
#1206=CARTESIAN_POINT ( 'NONE',  ( 26.48437500061451644, 6.421520780324663323E-16, -5.243569643749999010 ) ) ;
#1207=CARTESIAN_POINT ( 'NONE',  ( 18.04687500061451999, 6.054752690667223547, 3.707466751127219781E-16 ) ) ;
#1208=CARTESIAN_POINT ( 'NONE',  ( 13.90312500061451750, 4.541064518000418104, -2.621784821874998173 ) ) ;
#1209=CARTESIAN_POINT ( 'NONE',  ( 9.001249775931846008E-16, 10.01562500061459282, -25.09994784771203058 ) ) ;
#1210=CARTESIAN_POINT ( 'NONE',  ( 25.68750000122903288, -4.330127018922194537, 2.499999999999995559 ) ) ;
#1212=CARTESIAN_POINT ( 'NONE',  ( 15.74062500061451608, 6.054752690667223547, 3.707466751127219781E-16 ) ) ;
#1213=FACE_OUTER_BOUND ( 'NONE', #2994, .T. ) ;
#1214=CARTESIAN_POINT ( 'NONE',  ( 3.975000001229033852, 2.886751345948126879, 4.999999999999999112 ) ) ;
#1215=CARTESIAN_POINT ( 'NONE',  ( 11.78437500061451892, 4.541064518000418104, 2.621784821874999949 ) ) ;
#1216=CARTESIAN_POINT ( 'NONE',  ( 11.85937500061451644, 0.000000000000000000, 5.243569643749999010 ) ) ;
#1217=CARTESIAN_POINT ( 'NONE',  ( 19.02187500061451786, 3.027376345333611329, 5.243569643749999010 ) ) ;
#1218=ORIENTED_EDGE ( 'NONE', *, *, #63369, .F. ) ;
#1219=CARTESIAN_POINT ( 'NONE',  ( 29.32499999999999929, 6.123233995736764310E-16, -4.999999999999998224 ) ) ;
#1220=CARTESIAN_POINT ( 'NONE',  ( 23.65312500061451573, -4.541064518000417216, -2.621784821875001281 ) ) ;
#1221=CARTESIAN_POINT ( 'NONE',  ( 20.10937500061451289, -4.541064518000417216, -2.621784821875001281 ) ) ;
#1222=CARTESIAN_POINT ( 'NONE',  ( 25.52812500061451573, 6.421520780324663323E-16, -5.243569643749999010 ) ) ;
#1224=CARTESIAN_POINT ( 'NONE',  ( 4.000000000000000000, 13.88750000000000107, 32.30940107675849049 ) ) ;
#1225=CARTESIAN_POINT ( 'NONE',  ( 29.05312500061451431, -4.541064518000417216, -2.621784821875001281 ) ) ;
#1226=CARTESIAN_POINT ( 'NONE',  ( 9.712500001229033231, 4.330127018922192761, -2.499999999999997780 ) ) ;
#1227=CARTESIAN_POINT ( 'NONE',  ( 8.062500001229034652, 0.000000000000000000, 4.999999999999998224 ) ) ;
#1229=CARTESIAN_POINT ( 'NONE',  ( 26.51250000122903216, 0.000000000000000000, 4.999999999999998224 ) ) ;
#1232=EDGE_CURVE ( 'NONE', #6226, #3193, #4249, .T. ) ;
#1233=CARTESIAN_POINT ( 'NONE',  ( 8.484375000614518214, 6.421520780324663323E-16, -5.243569643749999010 ) ) ;
#1234=CARTESIAN_POINT ( 'NONE',  ( 2.000000000000001332, 9.912500001229034297, 33.46410161513774995 ) ) ;
#1235=CARTESIAN_POINT ( 'NONE',  ( 18.14062500061451644, -3.027376345333614438, 5.243569643749998122 ) ) ;
#1236=CARTESIAN_POINT ( 'NONE',  ( 10.28437500061451715, 6.421520780324663323E-16, -5.243569643749999010 ) ) ;
#1237=CARTESIAN_POINT ( 'NONE',  ( 28.31250000122903288, 0.000000000000000000, 4.999999999999998224 ) ) ;
#1238=CARTESIAN_POINT ( 'NONE',  ( 19.95937500061451786, 0.000000000000000000, 5.243569643749999010 ) ) ;
#1239=CARTESIAN_POINT ( 'NONE',  ( 8.221875000614518925, 3.027376345333611329, 5.243569643749999010 ) ) ;
#1240=CARTESIAN_POINT ( 'NONE',  ( 3.103125000614517237, 4.541064518000418104, -2.621784821874998173 ) ) ;
#1242=CARTESIAN_POINT ( 'NONE',  ( 7.040625000614517681, -3.027376345333610441, -5.243569643749999898 ) ) ;
#1243=CARTESIAN_POINT ( 'NONE',  ( 18.66562500061451146, -6.054752690667223547, -1.112240025338166033E-15 ) ) ;
#1244=ORIENTED_EDGE ( 'NONE', *, *, #41134, .F. ) ;
#1245=CARTESIAN_POINT ( 'NONE',  ( 5.212500001229032343, 4.330127018922192761, -2.499999999999997780 ) ) ;
#1246=CARTESIAN_POINT ( 'NONE',  ( 14.09062500061451750, -3.027376345333614438, 5.243569643749998122 ) ) ;
#1247=CARTESIAN_POINT ( 'NONE',  ( 13.90312500061451750, 4.541064518000418104, -2.621784821874998173 ) ) ;
#1249=CARTESIAN_POINT ( 'NONE',  ( 12.44999999999999929, 0.000000000000000000, 4.999999999999998224 ) ) ;
#1250=CARTESIAN_POINT ( 'NONE',  ( 10.05000000122903181, -2.886751345948125991, -5.000000000000000000 ) ) ;
#1251=EDGE_CURVE ( 'NONE', #65794, #57266, #26423, .T. ) ;
#1252=CARTESIAN_POINT ( 'NONE',  ( 6.103125000614515905, -4.541064518000417216, -2.621784821875001281 ) ) ;
#1253=CARTESIAN_POINT ( 'NONE',  ( 19.38750000122903216, -4.330127018922194537, 2.499999999999995559 ) ) ;
#1255=CARTESIAN_POINT ( 'NONE',  ( 4.243569643749999010, 11.12187500061451928, -32.45002607614398471 ) ) ;
#1256=CARTESIAN_POINT ( 'NONE',  ( 4.087500001229035007, -4.330127018922194537, 2.499999999999995559 ) ) ;
#1257=CARTESIAN_POINT ( 'NONE',  ( 28.35000000122903430, -2.886751345948114000, 5.000000000000024869 ) ) ;
#1259=CARTESIAN_POINT ( 'NONE',  ( 18.30937500061451928, -4.541064518000417216, -2.621784821875001281 ) ) ;
#1261=CARTESIAN_POINT ( 'NONE',  ( 14.57812500061451644, -4.541064518000419881, 2.621784821874995952 ) ) ;
#1263=CARTESIAN_POINT ( 'NONE',  ( 4.898587196589411843E-16, 20.00000000000000000, -26.00000000000000000 ) ) ;
#1264=CARTESIAN_POINT ( 'NONE',  ( 26.25937500061451857, 0.000000000000000000, 5.243569643749999010 ) ) ;
#1266=CARTESIAN_POINT ( 'NONE',  ( 11.99062500061451608, -3.027376345333610441, -5.243569643749999898 ) ) ;
#1267=CARTESIAN_POINT ( 'NONE',  ( 16.47187500061452070, -6.054752690667223547, -1.112240025338166033E-15 ) ) ;
#1268=ORIENTED_EDGE ( 'NONE', *, *, #50356, .T. ) ;
#1269=CARTESIAN_POINT ( 'NONE',  ( 27.92812500061451431, 4.541064518000418104, 2.621784821874999949 ) ) ;
#1270=CARTESIAN_POINT ( 'NONE',  ( 19.82812500061451644, 4.541064518000418104, 2.621784821874999949 ) ) ;
#1271=CARTESIAN_POINT ( 'NONE',  ( 3.144856541311010556, 3.887142566792906706, -3.519253510942787599 ) ) ;
#1272=CARTESIAN_POINT ( 'NONE',  ( 9.600000000000001421, 4.330127018922192761, -2.499999999999997780 ) ) ;
#1273=CARTESIAN_POINT ( 'NONE',  ( 18.37500000122903288, 2.886751345948126879, 4.999999999999999112 ) ) ;
#1276=ORIENTED_EDGE ( 'NONE', *, *, #52094, .T. ) ;
#1277=CARTESIAN_POINT ( 'NONE',  ( 17.88749999999999929, -2.886751345948129988, 4.999999999999997335 ) ) ;
#1278=CARTESIAN_POINT ( 'NONE',  ( 20.32499999999999929, 6.123233995736764310E-16, -4.999999999999998224 ) ) ;
#1279=CARTESIAN_POINT ( 'NONE',  ( 20.07187500061451857, -6.054752690667223547, -1.112240025338166033E-15 ) ) ;
#1280=CARTESIAN_POINT ( 'NONE',  ( 24.70312500061451644, 4.541064518000418104, -2.621784821874998173 ) ) ;
#1281=ORIENTED_EDGE ( 'NONE', *, *, #64328, .F. ) ;
#1283=CARTESIAN_POINT ( 'NONE',  ( 9.103125000614515017, 0.000000000000000000, 5.243569643749999010 ) ) ;
#1284=CARTESIAN_POINT ( 'NONE',  ( 0.000000000000000000, 20.00000000000000000, 26.00000000000000000 ) ) ;
#1285=CARTESIAN_POINT ( 'NONE',  ( 15.71250000000000213, -5.773502691896255534, -1.060575238724906372E-15 ) ) ;
#1286=CARTESIAN_POINT ( 'NONE',  ( -4.243569643749997233, 16.69062500061451360, 32.45002607614398471 ) ) ;
#1287=CARTESIAN_POINT ( 'NONE',  ( 29.72812500061451502, 4.541064518000418104, 2.621784821874999949 ) ) ;
#1290=CARTESIAN_POINT ( 'NONE',  ( 26.07187500061451857, 3.027376345333613106, -5.243569643749998122 ) ) ;
#1291=ORIENTED_EDGE ( 'NONE', *, *, #3876, .F. ) ;
#1292=CARTESIAN_POINT ( 'NONE',  ( 22.34062500061451573, -3.027376345333610441, -5.243569643749999898 ) ) ;
#1293=CARTESIAN_POINT ( 'NONE',  ( 23.14687500061451786, -3.027376345333614438, 5.243569643749998122 ) ) ;
#1294=CARTESIAN_POINT ( 'NONE',  ( 4.243569643749999898, 16.87812500061459176, -30.00000000000000000 ) ) ;
#1295=CARTESIAN_POINT ( 'NONE',  ( 10.42500000000000071, 6.123233995736764310E-16, -4.999999999999998224 ) ) ;
#1296=CARTESIAN_POINT ( 'NONE',  ( 5.915625000614515905, 3.027376345333611329, 5.243569643749999010 ) ) ;
#1298=CARTESIAN_POINT ( 'NONE',  ( 23.16562500061451502, -6.054752690667223547, -1.112240025338166033E-15 ) ) ;
#1301=CARTESIAN_POINT ( 'NONE',  ( 16.65937500061452070, 4.541064518000418104, -2.621784821874998173 ) ) ;
#1302=CARTESIAN_POINT ( 'NONE',  ( 2.121784821874999061, 12.50937500061451857, 26.32496088578401583 ) ) ;
#1303=ADVANCED_FACE ( 'NONE', ( #64107 ), #16504, .T. ) ;
#1304=CARTESIAN_POINT ( 'NONE',  ( 20.14687500061451786, -3.027376345333610441, -5.243569643749999898 ) ) ;
#1305=CARTESIAN_POINT ( 'NONE',  ( 26.44687500061451502, -3.027376345333610441, -5.243569643749999898 ) ) ;
#1306=CARTESIAN_POINT ( 'NONE',  ( 2.121784821875001281, 15.95937500061451608, 33.67503911421598417 ) ) ;
#1307=CARTESIAN_POINT ( 'NONE',  ( 7.078125000614516438, 6.421520780324663323E-16, -5.243569643749999010 ) ) ;
#1309=CARTESIAN_POINT ( 'NONE',  ( 4.959375000614516971, 4.541064518000418104, -2.621784821874998173 ) ) ;
#1310=CARTESIAN_POINT ( 'NONE',  ( 25.95000000122903216, 5.773502691896255534, 3.535250795749688401E-16 ) ) ;
#1311=CARTESIAN_POINT ( 'NONE',  ( 6.140625000614516438, -3.027376345333610441, -5.243569643749999898 ) ) ;
#1312=CARTESIAN_POINT ( 'NONE',  ( 9.684375000614517504, -4.541064518000419881, 2.621784821874995952 ) ) ;
#1313=CARTESIAN_POINT ( 'NONE',  ( 15.56250000122903465, 4.330127018922192761, -2.499999999999997780 ) ) ;
#1314=CARTESIAN_POINT ( 'NONE',  ( 5.784375000614517148, 6.421520780324663323E-16, -5.243569643749999010 ) ) ;
#1315=CARTESIAN_POINT ( 'NONE',  ( 7.978125000614517681, 6.421520780324663323E-16, -5.243569643749999010 ) ) ;
#1318=CARTESIAN_POINT ( 'NONE',  ( 17.25937500061451502, 0.000000000000000000, 5.243569643749999010 ) ) ;
#1319=CARTESIAN_POINT ( 'NONE',  ( -1.071796769724488563, 10.64240381056766616, 34.00000000000000000 ) ) ;
#1320=ORIENTED_EDGE ( 'NONE', *, *, #58649, .T. ) ;
#1321=CARTESIAN_POINT ( 'NONE',  ( 25.11562500061451431, 3.027376345333613106, -5.243569643749998122 ) ) ;
#1322=CARTESIAN_POINT ( 'NONE',  ( 9.628125000614517148, -4.541064518000419881, 2.621784821874995952 ) ) ;
#1323=CARTESIAN_POINT ( 'NONE',  ( 26.74687500061451573, -3.027376345333614438, 5.243569643749998122 ) ) ;
#1324=CARTESIAN_POINT ( 'NONE',  ( 10.22812500061451679, 6.421520780324663323E-16, -5.243569643749999010 ) ) ;
#1325=CARTESIAN_POINT ( 'NONE',  ( -4.243569643749998122, 10.44687500061451679, -27.54997392385601174 ) ) ;
#1326=CARTESIAN_POINT ( 'NONE',  ( 11.25000000122903288, -2.886751345948129988, 4.999999999999997335 ) ) ;
#1327=CARTESIAN_POINT ( 'NONE',  ( 23.72812500061451502, 6.421520780324663323E-16, -5.243569643749999010 ) ) ;
#1328=CARTESIAN_POINT ( 'NONE',  ( 4.243569643749999898, 14.14062500061451644, -27.54997392385601529 ) ) ;
#1329=CARTESIAN_POINT ( 'NONE',  ( 13.65000000122903323, -2.886751345948125991, -5.000000000000000000 ) ) ;
#1330=CARTESIAN_POINT ( 'NONE',  ( 21.06562500061451715, 3.027376345333613106, -5.243569643749998122 ) ) ;
#1331=CARTESIAN_POINT ( 'NONE',  ( 12.03749999999999964, -2.886751345948129988, 4.999999999999997335 ) ) ;
#1332=CARTESIAN_POINT ( 'NONE',  ( 19.79062500061451502, 6.054752690667223547, 3.707466751127219781E-16 ) ) ;
#1333=CARTESIAN_POINT ( 'NONE',  ( 6.271875000614518747, 3.027376345333612662, -5.243569643749998122 ) ) ;
#1334=CARTESIAN_POINT ( 'NONE',  ( 20.02500000000000213, 4.330127018922191873, 2.499999999999999556 ) ) ;
#1335=CARTESIAN_POINT ( 'NONE',  ( 6.787500001229032520, -4.330127018922194537, 2.499999999999995559 ) ) ;
#1336=CARTESIAN_POINT ( 'NONE',  ( 16.83750000122903145, 6.123233995736764310E-16, -4.999999999999998224 ) ) ;
#1337=CARTESIAN_POINT ( 'NONE',  ( 13.34062500061451750, -3.027376345333610441, -5.243569643749999898 ) ) ;
#1338=CARTESIAN_POINT ( 'NONE',  ( 15.55312500061451608, -4.541064518000417216, -2.621784821875001281 ) ) ;
#1339=CARTESIAN_POINT ( 'NONE',  ( 26.40000000122902790, 5.773502691896255534, 3.535250795749688894E-16 ) ) ;
#1340=CARTESIAN_POINT ( 'NONE',  ( 20.43749999999999645, 5.773502691896255534, 3.535250795749688894E-16 ) ) ;
#1341=CARTESIAN_POINT ( 'NONE',  ( 23.25937500061451857, -4.541064518000417216, -2.621784821875001281 ) ) ;
#1344=CARTESIAN_POINT ( 'NONE',  ( 8.962500001229033231, 0.000000000000000000, 4.999999999999998224 ) ) ;
#1346=CARTESIAN_POINT ( 'NONE',  ( 9.759375000614516793, -4.541064518000417216, -2.621784821875001281 ) ) ;
#1347=CARTESIAN_POINT ( 'NONE',  ( 25.54687500061451644, -3.027376345333610441, -5.243569643749999898 ) ) ;
#1348=( BOUNDED_CURVE ( )  B_SPLINE_CURVE ( 2, ( #882, #12668, #61829, #45938, #68115, #28582, #1600, #35205, #516 ),
 .UNSPECIFIED., .F., .F. ) 
 B_SPLINE_CURVE_WITH_KNOTS ( ( 3, 2, 2, 2, 3 ),
 ( 0.2065217391304347838, 0.2101449275362318736, 0.2173913043478260809, 0.2246376811594202882, 0.2282608695652174058 ),
 .UNSPECIFIED. ) 
 CURVE ( )  GEOMETRIC_REPRESENTATION_ITEM ( )  RATIONAL_B_SPLINE_CURVE ( ( 0.9330127018922194093, 0.9330127018922194093, 1.000000000000000000, 0.8660254037844387076, 1.000000000000000000, 0.8660254037844387076, 1.000000000000000000, 0.9330127018922190762, 0.9330127018922194093 ) ) 
 REPRESENTATION_ITEM ( '' )  );
#1349=DIRECTION ( 'NONE',  ( -1.000000000000000000, -0.000000000000000000, -0.000000000000000000 ) ) ;
#1350=CARTESIAN_POINT ( 'NONE',  ( 21.81562500061451004, -6.054752690667223547, -1.112240025338166033E-15 ) ) ;
#1351=CARTESIAN_POINT ( 'NONE',  ( 25.99687500061451928, -3.027376345333610441, -5.243569643749999898 ) ) ;
#1354=CARTESIAN_POINT ( 'NONE',  ( 7.509375000614517681, -4.541064518000417216, -2.621784821875001281 ) ) ;
#1355=CARTESIAN_POINT ( 'NONE',  ( 20.35312500061451502, 0.000000000000000000, 5.243569643749999010 ) ) ;
#1356=ORIENTED_EDGE ( 'NONE', *, *, #14935, .T. ) ;
#1358=CARTESIAN_POINT ( 'NONE',  ( 27.29062500061451502, -3.027376345333610441, -5.243569643749999898 ) ) ;
#1359=CARTESIAN_POINT ( 'NONE',  ( 3.909375000614518481, -4.541064518000417216, -2.621784821875001281 ) ) ;
#1360=CARTESIAN_POINT ( 'NONE',  ( 30.00000000000000000, 6.123233995736764310E-16, -4.999999999999998224 ) ) ;
#1362=CARTESIAN_POINT ( 'NONE',  ( 16.50000000000000000, 0.000000000000000000, 4.999999999999998224 ) ) ;
#1363=CARTESIAN_POINT ( 'NONE',  ( 21.66562500061451502, 3.027376345333611329, 5.243569643749999010 ) ) ;
#1364=ORIENTED_EDGE ( 'NONE', *, *, #69679, .T. ) ;
#1365=CARTESIAN_POINT ( 'NONE',  ( 23.96249999999999858, 2.886751345948129099, -4.999999999999998224 ) ) ;
#1366=CARTESIAN_POINT ( 'NONE',  ( 26.22187500061451715, 3.027376345333611329, 5.243569643749999010 ) ) ;
#1367=ORIENTED_EDGE ( 'NONE', *, *, #63007, .F. ) ;
#1368=CARTESIAN_POINT ( 'NONE',  ( 16.26562500061451289, 3.027376345333611329, 5.243569643749999010 ) ) ;
#1369=CARTESIAN_POINT ( 'NONE',  ( 5.578125000614518214, -4.541064518000419881, 2.621784821874995952 ) ) ;
#1371=CARTESIAN_POINT ( 'NONE',  ( 28.49062500061451431, -3.027376345333614438, 5.243569643749998122 ) ) ;
#1372=CARTESIAN_POINT ( 'NONE',  ( 15.78750000122903430, -4.330127018922194537, 2.499999999999995559 ) ) ;
#1373=CARTESIAN_POINT ( 'NONE',  ( 22.19999999999999574, 4.330127018922192761, -2.499999999999997780 ) ) ;
#1374=CARTESIAN_POINT ( 'NONE',  ( 29.81250000000000000, 2.886751345948129099, -4.999999999999998224 ) ) ;
#1375=CARTESIAN_POINT ( 'NONE',  ( 4.996875000614516615, 6.054752690667223547, 3.707466751127219781E-16 ) ) ;
#1376=CARTESIAN_POINT ( 'NONE',  ( 9.834375000614517859, 6.421520780324663323E-16, -5.243569643749999010 ) ) ;
#1377=CARTESIAN_POINT ( 'NONE',  ( 19.32187500061451857, 3.027376345333613106, -5.243569643749998122 ) ) ;
#1378=CARTESIAN_POINT ( 'NONE',  ( -3.999999999999999112, 19.66250000122903430, -30.00000000000000000 ) ) ;
#1380=CARTESIAN_POINT ( 'NONE',  ( 5.259375000614518569, -4.541064518000417216, -2.621784821875001281 ) ) ;
#1381=CARTESIAN_POINT ( 'NONE',  ( 3.374999999999999556, 4.330127018922191873, 2.499999999999999556 ) ) ;
#1382=CARTESIAN_POINT ( 'NONE',  ( 4.209375000614516971, 0.000000000000000000, 5.243569643749999010 ) ) ;
#1383=CARTESIAN_POINT ( 'NONE',  ( 19.08750000000000213, 5.773502691896255534, 3.535250795749688894E-16 ) ) ;
#1384=CARTESIAN_POINT ( 'NONE',  ( 16.11562500061451786, 3.027376345333613106, -5.243569643749998122 ) ) ;
#1389=CARTESIAN_POINT ( 'NONE',  ( 9.778125000614517504, 6.421520780324663323E-16, -5.243569643749999010 ) ) ;
#1390=CARTESIAN_POINT ( 'NONE',  ( 26.48437500061451644, 6.421520780324663323E-16, -5.243569643749999010 ) ) ;
#1391=CARTESIAN_POINT ( 'NONE',  ( 9.001249775931846008E-16, 18.62187500061451928, 34.90005215228797653 ) ) ;
#1392=CARTESIAN_POINT ( 'NONE',  ( 26.78437500061451360, -4.541064518000419881, 2.621784821874995952 ) ) ;
#1393=CARTESIAN_POINT ( 'NONE',  ( 7.650000000000000355, -4.330127018922190985, -2.500000000000001332 ) ) ;
#1394=CARTESIAN_POINT ( 'NONE',  ( -3.999999999999997335, 12.05000000122903536, 32.30940107675850470 ) ) ;
#1395=CARTESIAN_POINT ( 'NONE',  ( 14.91562500061451679, 3.027376345333611329, 5.243569643749999010 ) ) ;
#1396=CARTESIAN_POINT ( 'NONE',  ( 6.225000001229036073, 2.886751345948126879, 4.999999999999999112 ) ) ;
#1397=CARTESIAN_POINT ( 'NONE',  ( 17.03437500061451715, 6.421520780324663323E-16, -5.243569643749999010 ) ) ;
#1398=CARTESIAN_POINT ( 'NONE',  ( 11.52187500061451608, -6.054752690667223547, -1.112240025338166033E-15 ) ) ;
#1399=CARTESIAN_POINT ( 'NONE',  ( -3.581514519956695342, 3.492045901024759758, -31.79929272433821552 ) ) ;
#1400=VERTEX_POINT ( 'NONE', #32601 ) ;
#1401=CARTESIAN_POINT ( 'NONE',  ( 13.49062500061451608, 6.054752690667223547, 3.707466751127219781E-16 ) ) ;
#1402=CARTESIAN_POINT ( 'NONE',  ( 23.85000000122903430, -2.886751345948129988, 4.999999999999997335 ) ) ;
#1403=CARTESIAN_POINT ( 'NONE',  ( 12.04687500061451821, -3.027376345333610441, -5.243569643749999898 ) ) ;
#1405=CARTESIAN_POINT ( 'NONE',  ( 15.70312500061451644, 4.541064518000418104, -2.621784821874998173 ) ) ;
#1406=CARTESIAN_POINT ( 'NONE',  ( 1.071796769724491893, 16.53259618943233278, -26.00000000000000355 ) ) ;
#1407=CARTESIAN_POINT ( 'NONE',  ( 23.52187500061451786, 3.027376345333611329, 5.243569643749999010 ) ) ;
#1408=DIRECTION ( 'NONE',  ( -0.000000000000000000, -1.000000000000000000, -0.000000000000000000 ) ) ;
#1409=( BOUNDED_CURVE ( )  B_SPLINE_CURVE ( 2, ( #21607, #14970, #26429, #37508, #37872, #60028, #60391 ),
 .UNSPECIFIED., .F., .F. ) 
 B_SPLINE_CURVE_WITH_KNOTS ( ( 3, 2, 2, 3 ),
 ( 0.7666666666666668295, 0.7694444444444445974, 0.7722222222222223653, 0.7750000000000001332 ),
 .UNSPECIFIED. ) 
 CURVE ( )  GEOMETRIC_REPRESENTATION_ITEM ( )  RATIONAL_B_SPLINE_CURVE ( ( 0.9999999999999946709, 0.8660254037844440367, 1.000000000000000000, 0.8660254037844387076, 1.000000000000000000, 0.8660254037844333785, 1.000000000000005329 ) ) 
 REPRESENTATION_ITEM ( '' )  );
#1410=CARTESIAN_POINT ( 'NONE',  ( 11.40000000122903501, -2.886751345948125991, -5.000000000000000000 ) ) ;
#1413=CARTESIAN_POINT ( 'NONE',  ( -4.243569643749999898, 16.70937500061451786, -30.00000000000000000 ) ) ;
#1414=CARTESIAN_POINT ( 'NONE',  ( 17.29687500061451999, -3.027376345333614438, 5.243569643749998122 ) ) ;
#1415=CARTESIAN_POINT ( 'NONE',  ( 18.26250000122903216, 4.330127018922192761, -2.499999999999997780 ) ) ;
#1416=( BOUNDED_CURVE ( )  B_SPLINE_CURVE ( 2, ( #44094, #66621, #3841, #10826, #38546, #14904, #37445 ),
 .UNSPECIFIED., .F., .F. ) 
 B_SPLINE_CURVE_WITH_KNOTS ( ( 3, 2, 2, 3 ),
 ( 0.008333333333333315870, 0.01111111111111108898, 0.01388888888888885863, 0.01666666666666663174 ),
 .UNSPECIFIED. ) 
 CURVE ( )  GEOMETRIC_REPRESENTATION_ITEM ( )  RATIONAL_B_SPLINE_CURVE ( ( 1.000000000000000888, 0.8660254037844378194, 1.000000000000000000, 0.8660254037844387076, 1.000000000000000000, 0.8660254037844403729, 0.9999999999999983347 ) ) 
 REPRESENTATION_ITEM ( '' )  );
#1417=CARTESIAN_POINT ( 'NONE',  ( 15.23437500061451644, 6.421520780324663323E-16, -5.243569643749999010 ) ) ;
#1418=CARTESIAN_POINT ( 'NONE',  ( -4.243569643749997233, 9.996875000614517504, 32.45002607614398471 ) ) ;
#1419=CARTESIAN_POINT ( 'NONE',  ( 20.88750000122903572, 6.123233995736764310E-16, -4.999999999999998224 ) ) ;
#1420=CARTESIAN_POINT ( 'NONE',  ( 14.20312500061451644, -4.541064518000417216, -2.621784821875001281 ) ) ;
#1421=ORIENTED_EDGE ( 'NONE', *, *, #69860, .F. ) ;
#1423=CARTESIAN_POINT ( 'NONE',  ( 19.34999999999999787, -4.330127018922190985, -2.500000000000001332 ) ) ;
#1425=CARTESIAN_POINT ( 'NONE',  ( 3.328125000614516438, -4.541064518000419881, 2.621784821874995952 ) ) ;
#1426=CARTESIAN_POINT ( 'NONE',  ( 14.25000000122903465, 5.773502691896255534, 3.535250795749688894E-16 ) ) ;
#1427=CARTESIAN_POINT ( 'NONE',  ( 26.07187500061451857, 3.027376345333613106, -5.243569643749998122 ) ) ;
#1428=CARTESIAN_POINT ( 'NONE',  ( 19.97812500061451502, -4.541064518000419881, 2.621784821874995952 ) ) ;
#1429=CARTESIAN_POINT ( 'NONE',  ( 24.02812500061451573, -4.541064518000419881, 2.621784821874995952 ) ) ;
#1430=CARTESIAN_POINT ( 'NONE',  ( 3.065625000614517592, 3.027376345333613106, -5.243569643749998122 ) ) ;
#1432=CARTESIAN_POINT ( 'NONE',  ( 27.56250000000000000, 2.886751345948129099, -4.999999999999998224 ) ) ;
#1433=CARTESIAN_POINT ( 'NONE',  ( -5.810221930991193690E-16, 10.10000000122903430, -34.00000000000000000 ) ) ;
#1436=CARTESIAN_POINT ( 'NONE',  ( 8.484601909799253346E-16, 9.875000001229032875, -25.38119784648299770 ) ) ;
#1437=CARTESIAN_POINT ( 'NONE',  ( -4.243569643749999898, 15.77187500061451608, -32.45002607614398471 ) ) ;
#1438=CARTESIAN_POINT ( 'NONE',  ( 7.275000001229035007, -5.773502691896255534, -1.060575238724906372E-15 ) ) ;
#1439=CARTESIAN_POINT ( 'NONE',  ( 6.975000000000002309, 4.330127018922191873, 2.499999999999999556 ) ) ;
#1441=CARTESIAN_POINT ( 'NONE',  ( 2.925000001229034918, 2.886751345948129099, -4.999999999999998224 ) ) ;
#1442=CARTESIAN_POINT ( 'NONE',  ( 9.834375000614517859, 6.421520780324663323E-16, -5.243569643749999010 ) ) ;
#1443=AXIS2_PLACEMENT_3D ( 'NONE', #5329, #54476, #14940 ) ;
#1444=CARTESIAN_POINT ( 'NONE',  ( 29.31562500061451715, 3.027376345333611329, 5.243569643749999010 ) ) ;
#1446=CARTESIAN_POINT ( 'NONE',  ( 5.437500001229035540, -4.330127018922194537, 2.499999999999995559 ) ) ;
#1447=CARTESIAN_POINT ( 'NONE',  ( 8.634375000614518569, 4.541064518000418104, 2.621784821874999949 ) ) ;
#1448=CARTESIAN_POINT ( 'NONE',  ( 11.55937500061451928, -4.541064518000417216, -2.621784821875001281 ) ) ;
#1449=CARTESIAN_POINT ( 'NONE',  ( 5.775000000000002132, -4.330127018922194537, 2.499999999999995559 ) ) ;
#1450=CARTESIAN_POINT ( 'NONE',  ( -4.243569643749998122, 14.44062500061459531, 32.45002607614398471 ) ) ;
#1451=CARTESIAN_POINT ( 'NONE',  ( 20.85937500061451644, 0.000000000000000000, 5.243569643749999010 ) ) ;
#1453=CARTESIAN_POINT ( 'NONE',  ( 6.600000000000001421, 0.000000000000000000, 4.999999999999998224 ) ) ;
#1454=CARTESIAN_POINT ( 'NONE',  ( 25.61250000122903359, 0.000000000000000000, 4.999999999999998224 ) ) ;
#1456=CARTESIAN_POINT ( 'NONE',  ( 21.55312500061451431, 4.541064518000418104, -2.621784821874998173 ) ) ;
#1457=CARTESIAN_POINT ( 'NONE',  ( 14.24062500061451608, -3.027376345333610441, -5.243569643749999898 ) ) ;
#1459=CARTESIAN_POINT ( 'NONE',  ( 10.65937500061451715, -4.541064518000417216, -2.621784821875001281 ) ) ;
#1460=CARTESIAN_POINT ( 'NONE',  ( 28.64999999999999858, 0.000000000000000000, 4.999999999999998224 ) ) ;
#1461=CARTESIAN_POINT ( 'NONE',  ( 21.97500000122903074, 2.886751345948126879, 4.999999999999999112 ) ) ;
#1462=CARTESIAN_POINT ( 'NONE',  ( -3.999999999999999112, 18.31250000122903288, -30.00000000000000000 ) ) ;
#1463=CARTESIAN_POINT ( 'NONE',  ( 12.00937500061451857, -4.541064518000417216, -2.621784821875001281 ) ) ;
#1464=CARTESIAN_POINT ( 'NONE',  ( 28.54687500061451644, -3.027376345333614438, 5.243569643749998122 ) ) ;
#1465=CARTESIAN_POINT ( 'NONE',  ( 4.171875000614517326, 3.027376345333611329, 5.243569643749999010 ) ) ;
#1466=DIRECTION ( 'NONE',  ( -1.000000000000000000, -0.000000000000000000, -0.000000000000000000 ) ) ;
#1467=CARTESIAN_POINT ( 'NONE',  ( 21.27187500061451786, 3.027376345333611329, 5.243569643749999010 ) ) ;
#1468=CARTESIAN_POINT ( 'NONE',  ( 14.33437500061451786, 6.421520780324663323E-16, -5.243569643749999010 ) ) ;
#1470=CARTESIAN_POINT ( 'NONE',  ( 26.84999999999999787, 0.000000000000000000, 4.999999999999998224 ) ) ;
#1472=CARTESIAN_POINT ( 'NONE',  ( -3.000416591977282496E-16, 14.79687500061451821, -34.90005215228797653 ) ) ;
#1474=CARTESIAN_POINT ( 'NONE',  ( 17.99062500061451786, 6.054752690667223547, 3.707466751127219781E-16 ) ) ;
#1475=CARTESIAN_POINT ( 'NONE',  ( 7.950000000000001954, 0.000000000000000000, 4.999999999999998224 ) ) ;
#1476=CARTESIAN_POINT ( 'NONE',  ( 12.22500000122903430, -5.773502691896255534, -1.060575238724906372E-15 ) ) ;
#1477=CARTESIAN_POINT ( 'NONE',  ( 14.58750000000000036, 5.773502691896255534, 3.535250795749688894E-16 ) ) ;
#1479=CARTESIAN_POINT ( 'NONE',  ( -1.473773219643375931, 9.816672173337614993, 25.95083121279759197 ) ) ;
#1480=CARTESIAN_POINT ( 'NONE',  ( 14.51250000122903394, -4.330127018922190985, -2.500000000000001332 ) ) ;
#1481=CARTESIAN_POINT ( 'NONE',  ( 25.88437500061451502, -4.541064518000419881, 2.621784821874995952 ) ) ;
#1483=CARTESIAN_POINT ( 'NONE',  ( 20.05312500061451431, -4.541064518000417216, -2.621784821875001281 ) ) ;
#1484=CARTESIAN_POINT ( 'NONE',  ( 20.63437500061451857, 6.421520780324663323E-16, -5.243569643749999010 ) ) ;
#1485=CARTESIAN_POINT ( 'NONE',  ( 3.075000000000001510, -4.330127018922194537, 2.499999999999995559 ) ) ;
#1486=CARTESIAN_POINT ( 'NONE',  ( 6.740625000614516082, 6.054752690667223547, 3.707466751127219781E-16 ) ) ;
#1487=CARTESIAN_POINT ( 'NONE',  ( 22.94062500061451715, 6.054752690667223547, 3.707466751127219781E-16 ) ) ;
#1488=CARTESIAN_POINT ( 'NONE',  ( 12.23437500061451821, 4.541064518000418104, 2.621784821874999949 ) ) ;
#1489=CARTESIAN_POINT ( 'NONE',  ( 16.24687500061451573, 6.054752690667223547, 3.707466751127219781E-16 ) ) ;
#1490=CARTESIAN_POINT ( 'NONE',  ( -4.243569643749997233, 15.34062500061451750, 32.45002607614398471 ) ) ;
#1491=CARTESIAN_POINT ( 'NONE',  ( 18.18750000122903288, 6.123233995736764310E-16, -4.999999999999998224 ) ) ;
#1493=CARTESIAN_POINT ( 'NONE',  ( 9.853125000614516793, 4.541064518000418104, -2.621784821874998173 ) ) ;
#1494=CARTESIAN_POINT ( 'NONE',  ( 3.309375000614518836, 0.000000000000000000, 5.243569643749999010 ) ) ;
#1495=CARTESIAN_POINT ( 'NONE',  ( 29.39062500061451289, -3.027376345333614438, 5.243569643749998122 ) ) ;
#1496=CARTESIAN_POINT ( 'NONE',  ( 25.17187500061451644, 3.027376345333613106, -5.243569643749998122 ) ) ;
#1497=CARTESIAN_POINT ( 'NONE',  ( 17.09062500061451573, 6.054752690667223547, 3.707466751127219781E-16 ) ) ;
#1498=CARTESIAN_POINT ( 'NONE',  ( 26.96250000122903145, 0.000000000000000000, 4.999999999999998224 ) ) ;
#1499=CARTESIAN_POINT ( 'NONE',  ( 25.67812500061451431, 4.541064518000418104, 2.621784821874999949 ) ) ;
#1500=AXIS2_PLACEMENT_3D ( 'NONE', #34507, #21976, #21609 ) ;
#1501=CARTESIAN_POINT ( 'NONE',  ( 21.08437500061451786, 6.421520780324663323E-16, -5.243569643749999010 ) ) ;
#1502=CARTESIAN_POINT ( 'NONE',  ( 17.16562500061451502, 3.027376345333611329, 5.243569643749999010 ) ) ;
#1503=CARTESIAN_POINT ( 'NONE',  ( 2.121784821875001281, 16.40937500061452070, 33.67503911421598417 ) ) ;
#1504=CARTESIAN_POINT ( 'NONE',  ( 22.75312500061451360, -4.541064518000417216, -2.621784821875001281 ) ) ;
#1505=DIRECTION ( 'NONE',  ( -1.000000000000000000, -0.000000000000000000, -0.000000000000000000 ) ) ;
#1507=CARTESIAN_POINT ( 'NONE',  ( 25.12499999999999645, -4.330127018922194537, 2.499999999999995559 ) ) ;
#1508=CARTESIAN_POINT ( 'NONE',  ( -2.828200636599751609E-16, 13.13750000000000107, -34.61880215351700230 ) ) ;
#1510=CARTESIAN_POINT ( 'NONE',  ( 29.42812500061451431, -4.541064518000419881, 2.621784821874995952 ) ) ;
#1511=CARTESIAN_POINT ( 'NONE',  ( 9.365625000614519635, 3.027376345333613106, -5.243569643749998122 ) ) ;
#1512=CARTESIAN_POINT ( 'NONE',  ( 22.98750000122903003, -4.330127018922194537, 2.499999999999995559 ) ) ;
#1513=CARTESIAN_POINT ( 'NONE',  ( 28.19062500061451715, -3.027376345333610441, -5.243569643749999898 ) ) ;
#1514=CARTESIAN_POINT ( 'NONE',  ( 26.17500000000000071, 6.123233995736764310E-16, -4.999999999999998224 ) ) ;
#1515=CARTESIAN_POINT ( 'NONE',  ( 3.999999999999998668, 15.87500000122903465, -32.30940107675850470 ) ) ;
#1516=CARTESIAN_POINT ( 'NONE',  ( -5.810221930991193690E-16, 11.45000000122903216, -34.00000000000000000 ) ) ;
#1517=CARTESIAN_POINT ( 'NONE',  ( 9.478125000614515017, 4.541064518000418104, 2.621784821874999949 ) ) ;
#1519=CARTESIAN_POINT ( 'NONE',  ( 25.52812500061451573, 6.421520780324663323E-16, -5.243569643749999010 ) ) ;
#1520=CARTESIAN_POINT ( 'NONE',  ( 8.315625000614515372, -6.054752690667223547, -1.112240025338166033E-15 ) ) ;
#1521=CARTESIAN_POINT ( 'NONE',  ( 5.015625000614518214, 3.027376345333611329, 5.243569643749999010 ) ) ;
#1523=DIRECTION ( 'NONE',  ( 0.000000000000000000, 0.000000000000000000, 1.000000000000000000 ) ) ;
#1524=CARTESIAN_POINT ( 'NONE',  ( 14.28750000000000142, -2.886751345948129988, 4.999999999999997335 ) ) ;
#1525=CARTESIAN_POINT ( 'NONE',  ( 13.50937500061451679, 4.541064518000418104, -2.621784821874998173 ) ) ;
#1526=CARTESIAN_POINT ( 'NONE',  ( 12.18750000122903465, -4.330127018922194537, 2.499999999999995559 ) ) ;
#1527=CARTESIAN_POINT ( 'NONE',  ( 16.92187500061451999, -6.054752690667223547, -1.112240025338166033E-15 ) ) ;
#1529=CARTESIAN_POINT ( 'NONE',  ( 8.034375000614518925, 6.421520780324663323E-16, -5.243569643749999010 ) ) ;
#1530=CARTESIAN_POINT ( 'NONE',  ( 2.121784821874999061, 11.10312500061451679, -33.67503911421598417 ) ) ;
#1533=CARTESIAN_POINT ( 'NONE',  ( 30.00000000000000000, 0.000000000000000000, 0.000000000000000000 ) ) ;
#1534=CARTESIAN_POINT ( 'NONE',  ( 25.30312500061451431, 0.000000000000000000, 5.243569643749999010 ) ) ;
#1536=CARTESIAN_POINT ( 'NONE',  ( 28.54687500061451644, -3.027376345333614438, 5.243569643749998122 ) ) ;
#1537=CARTESIAN_POINT ( 'NONE',  ( 24.18750000000000355, -2.886751345948129988, 4.999999999999997335 ) ) ;
#1538=CARTESIAN_POINT ( 'NONE',  ( 6.290625000614517681, 6.054752690667223547, 3.707466751127219781E-16 ) ) ;
#1540=CARTESIAN_POINT ( 'NONE',  ( 20.14687500061451786, -3.027376345333610441, -5.243569643749999898 ) ) ;
#1542=CARTESIAN_POINT ( 'NONE',  ( 3.665625000614517681, 3.027376345333611329, 5.243569643749999010 ) ) ;
#1543=CARTESIAN_POINT ( 'NONE',  ( 7.696875000614516793, 6.054752690667223547, 3.707466751127219781E-16 ) ) ;
#1545=CARTESIAN_POINT ( 'NONE',  ( 19.73437500061451644, 6.421520780324663323E-16, -5.243569643749999010 ) ) ;
#1547=CARTESIAN_POINT ( 'NONE',  ( 27.48749999999999716, -2.886751345948125991, -5.000000000000000000 ) ) ;
#1548=CARTESIAN_POINT ( 'NONE',  ( 28.69687500061451502, -3.027376345333610441, -5.243569643749999898 ) ) ;
#1551=ORIENTED_EDGE ( 'NONE', *, *, #27962, .F. ) ;
#1552=CARTESIAN_POINT ( 'NONE',  ( 9.225000000000001421, 4.330127018922191873, 2.499999999999999556 ) ) ;
#1554=CARTESIAN_POINT ( 'NONE',  ( 24.21562500061451573, 3.027376345333613106, -5.243569643749998122 ) ) ;
#1555=CARTESIAN_POINT ( 'NONE',  ( 13.27500000000000213, 4.330127018922191873, 2.499999999999999556 ) ) ;
#1556=CARTESIAN_POINT ( 'NONE',  ( 7.837500001229035007, 6.123233995736764310E-16, -4.999999999999998224 ) ) ;
#1557=CARTESIAN_POINT ( 'NONE',  ( 6.740625000614516082, 6.054752690667223547, 3.707466751127219781E-16 ) ) ;
#1558=CARTESIAN_POINT ( 'NONE',  ( 21.41250000000000497, 2.886751345948126879, 4.999999999999999112 ) ) ;
#1559=EDGE_CURVE ( 'NONE', #329, #59300, #16943, .T. ) ;
#1560=CARTESIAN_POINT ( 'NONE',  ( 21.62812500061451360, 4.541064518000418104, 2.621784821874999949 ) ) ;
#1562=CARTESIAN_POINT ( 'NONE',  ( 25.46250000122903501, 4.330127018922192761, -2.499999999999997780 ) ) ;
#1564=CARTESIAN_POINT ( 'NONE',  ( 5.700000000000000178, 0.000000000000000000, 4.999999999999998224 ) ) ;
#1566=CARTESIAN_POINT ( 'NONE',  ( 22.94062500061451715, 6.054752690667223547, 3.707466751127219781E-16 ) ) ;
#1567=CARTESIAN_POINT ( 'NONE',  ( 28.90312500061451217, 0.000000000000000000, 5.243569643749999010 ) ) ;
#1568=CARTESIAN_POINT ( 'NONE',  ( 27.94687500061451502, 6.054752690667223547, 3.707466751127219781E-16 ) ) ;
#1569=CARTESIAN_POINT ( 'NONE',  ( 17.93437500061451928, 6.421520780324663323E-16, -5.243569643749999010 ) ) ;
#1570=CARTESIAN_POINT ( 'NONE',  ( 13.94062500061451892, 6.054752690667223547, 3.707466751127219781E-16 ) ) ;
#1571=PLANE ( 'NONE',  #40404 ) ;
#1572=CARTESIAN_POINT ( 'NONE',  ( 25.05000000122903714, 5.773502691896255534, 3.535250795749688894E-16 ) ) ;
#1574=CARTESIAN_POINT ( 'NONE',  ( 15.66562500061451857, 3.027376345333612662, -5.243569643749998122 ) ) ;
#1575=CARTESIAN_POINT ( 'NONE',  ( -3.999999999999999112, 16.81250000000000000, -32.30940107675850470 ) ) ;
#1577=CARTESIAN_POINT ( 'NONE',  ( 12.34687500061452070, -3.027376345333614438, 5.243569643749998122 ) ) ;
#1578=CARTESIAN_POINT ( 'NONE',  ( 11.10937500061451644, -4.541064518000417216, -2.621784821875001281 ) ) ;
#1579=CARTESIAN_POINT ( 'NONE',  ( 19.09687500061451360, -3.027376345333614438, 5.243569643749998122 ) ) ;
#1581=CARTESIAN_POINT ( 'NONE',  ( 9.750000000000001776, 0.000000000000000000, 4.999999999999998224 ) ) ;
#1582=CARTESIAN_POINT ( 'NONE',  ( 23.61562500061451431, -6.054752690667223547, -1.112240025338166033E-15 ) ) ;
#1583=CARTESIAN_POINT ( 'NONE',  ( 18.72187500061451360, -6.054752690667223547, -1.112240025338166033E-15 ) ) ;
#1584=CARTESIAN_POINT ( 'NONE',  ( 24.96562500061451573, -6.054752690667223547, -1.112240025338166033E-15 ) ) ;
#1585=CARTESIAN_POINT ( 'NONE',  ( 9.675000001229031810, 2.886751345948129099, -4.999999999999997335 ) ) ;
#1586=CARTESIAN_POINT ( 'NONE',  ( -2.000000000000000000, 14.97499999999999964, 26.53589838486224650 ) ) ;
#1587=CARTESIAN_POINT ( 'NONE',  ( 2.934375000614518392, -4.541064518000419881, 2.621784821874995952 ) ) ;
#1588=CARTESIAN_POINT ( 'NONE',  ( 9.525000001229033231, -5.773502691896255534, -1.060575238724906372E-15 ) ) ;
#1589=CARTESIAN_POINT ( 'NONE',  ( 5.700000001229033941, 5.773502691896255534, 3.535250795749688894E-16 ) ) ;
#1591=CARTESIAN_POINT ( 'NONE',  ( 27.60000000122903430, -2.886751345948125991, -5.000000000000000000 ) ) ;
#1593=CARTESIAN_POINT ( 'NONE',  ( 8.634375000614518569, 4.541064518000418104, 2.621784821874999949 ) ) ;
#1594=CARTESIAN_POINT ( 'NONE',  ( 18.21562500061451573, -6.054752690667223547, -1.112240025338166033E-15 ) ) ;
#1595=CARTESIAN_POINT ( 'NONE',  ( 11.07187500061451679, -6.054752690667223547, -1.112240025338166033E-15 ) ) ;
#1596=CARTESIAN_POINT ( 'NONE',  ( 3.440625000614518036, -3.027376345333610441, -5.243569643749999898 ) ) ;
#1597=CARTESIAN_POINT ( 'NONE',  ( 18.64687500061451786, -3.027376345333614438, 5.243569643749998122 ) ) ;
#1598=CARTESIAN_POINT ( 'NONE',  ( 8.334375000614516082, -4.541064518000419881, 2.621784821874995952 ) ) ;
#1599=CARTESIAN_POINT ( 'NONE',  ( 3.403125000614518836, -4.541064518000417216, -2.621784821875001281 ) ) ;
#1600=CARTESIAN_POINT ( 'NONE',  ( -2.000000000000000000, 17.67500000000000071, 26.53589838486224650 ) ) ;
#1601=CARTESIAN_POINT ( 'NONE',  ( 8.953125000614518214, 4.541064518000418104, -2.621784821874998173 ) ) ;
#1602=CARTESIAN_POINT ( 'NONE',  ( 17.50312500061451715, 4.541064518000418104, -2.621784821874998173 ) ) ;
#1603=ORIENTED_EDGE ( 'NONE', *, *, #37808, .F. ) ;
#1604=CARTESIAN_POINT ( 'NONE',  ( 5.062500001229035540, -4.330127018922190985, -2.500000000000001332 ) ) ;
#1605=CARTESIAN_POINT ( 'NONE',  ( 13.79062500061451502, -3.027376345333610441, -5.243569643749999898 ) ) ;
#1606=CARTESIAN_POINT ( 'NONE',  ( 13.67812500061451786, -4.541064518000419881, 2.621784821874995952 ) ) ;
#1608=CARTESIAN_POINT ( 'NONE',  ( 13.04999999999999893, -4.330127018922190985, -2.500000000000001332 ) ) ;
#1609=CARTESIAN_POINT ( 'NONE',  ( 6.862500001229034474, -4.330127018922190985, -2.500000000000001332 ) ) ;
#1610=CARTESIAN_POINT ( 'NONE',  ( 4.265625000614517326, -6.054752690667223547, -1.112240025338166033E-15 ) ) ;
#1612=CARTESIAN_POINT ( 'NONE',  ( 15.30937500061451750, 4.541064518000418104, -2.621784821874998173 ) ) ;
#1613=CARTESIAN_POINT ( 'NONE',  ( 17.58750000122903145, -4.330127018922194537, 2.499999999999995559 ) ) ;
#1615=EDGE_CURVE ( 'NONE', #57497, #37161, #42952, .T. ) ;
#1616=CARTESIAN_POINT ( 'NONE',  ( 4.243569643749999898, 19.57812500061451644, -30.00000000000000000 ) ) ;
#1617=CARTESIAN_POINT ( 'NONE',  ( 8.587500000000002132, -2.886751345948126435, -5.000000000000000000 ) ) ;
#1619=CARTESIAN_POINT ( 'NONE',  ( 2.955228467731844333, 4.033190387708875946, -2.955228467731844333 ) ) ;
#1620=FACE_OUTER_BOUND ( 'NONE', #52178, .T. ) ;
#1621=CARTESIAN_POINT ( 'NONE',  ( 18.64687500061451786, -3.027376345333614438, 5.243569643749998122 ) ) ;
#1623=( BOUNDED_CURVE ( )  B_SPLINE_CURVE ( 2, ( #58786, #30724, #19625, #35894, #2293, #13353, #60526 ),
 .UNSPECIFIED., .F., .F. ) 
 B_SPLINE_CURVE_WITH_KNOTS ( ( 3, 2, 2, 3 ),
 ( 0.8083333333333333481, 0.8111111111111111160, 0.8138888888888888840, 0.8166666666666666519 ),
 .UNSPECIFIED. ) 
 CURVE ( )  GEOMETRIC_REPRESENTATION_ITEM ( )  RATIONAL_B_SPLINE_CURVE ( ( 1.000000000000000000, 0.8660254037844387076, 1.000000000000000000, 0.8660254037844387076, 1.000000000000000000, 0.8660254037844387076, 1.000000000000000000 ) ) 
 REPRESENTATION_ITEM ( '' )  );
#1625=CARTESIAN_POINT ( 'NONE',  ( 13.45312500061451466, 4.541064518000418104, -2.621784821874998173 ) ) ;
#1627=CARTESIAN_POINT ( 'NONE',  ( 22.68750000122903288, 6.123233995736764310E-16, -4.999999999999998224 ) ) ;
#1628=CARTESIAN_POINT ( 'NONE',  ( 25.24687500061451573, 6.054752690667223547, 3.707466751127219781E-16 ) ) ;
#1630=CARTESIAN_POINT ( 'NONE',  ( 9.478125000614515017, 4.541064518000418104, 2.621784821874999949 ) ) ;
#1631=CARTESIAN_POINT ( 'NONE',  ( 14.82187500061451679, 3.027376345333613106, -5.243569643749998122 ) ) ;
#1632=ORIENTED_EDGE ( 'NONE', *, *, #53492, .F. ) ;
#1633=CARTESIAN_POINT ( 'NONE',  ( 27.36562500061451786, 3.027376345333613106, -5.243569643749998122 ) ) ;
#1634=CARTESIAN_POINT ( 'NONE',  ( 20.05312500061451431, -4.541064518000417216, -2.621784821875001281 ) ) ;
#1635=CARTESIAN_POINT ( 'NONE',  ( -5.810221930991193690E-16, 10.88750000000000107, 26.00000000000000355 ) ) ;
#1637=CARTESIAN_POINT ( 'NONE',  ( -2.000000000000000000, 14.18750000122903288, -33.46410161513775705 ) ) ;
#1638=CARTESIAN_POINT ( 'NONE',  ( 11.06250000000000000, 2.886751345948126879, 4.999999999999999112 ) ) ;
#1639=CARTESIAN_POINT ( 'NONE',  ( 18.78750000122903430, 4.330127018922191873, 2.499999999999999556 ) ) ;
#1640=CARTESIAN_POINT ( 'NONE',  ( 23.25000000122902932, 5.773502691896255534, 3.535250795749688401E-16 ) ) ;
#1643=CARTESIAN_POINT ( 'NONE',  ( 16.94999999999999929, 0.000000000000000000, 4.999999999999998224 ) ) ;
#1644=CARTESIAN_POINT ( 'NONE',  ( 21.11249999999999716, -5.773502691896255534, -1.060575238724906372E-15 ) ) ;
#1645=CARTESIAN_POINT ( 'NONE',  ( 18.19687500061451502, -3.027376345333614438, 5.243569643749998122 ) ) ;
#1646=CARTESIAN_POINT ( 'NONE',  ( 24.02812500061451573, -4.541064518000419881, 2.621784821874995952 ) ) ;
#1647=EDGE_LOOP ( 'NONE', ( #29345, #9948, #41169, #29072 ) ) ;
#1648=CARTESIAN_POINT ( 'NONE',  ( 5.390625000614518214, 6.054752690667223547, 3.707466751127219781E-16 ) ) ;
#1650=CARTESIAN_POINT ( 'NONE',  ( 12.67499999999999893, 6.123233995736764310E-16, -4.999999999999998224 ) ) ;
#1651=CARTESIAN_POINT ( 'NONE',  ( 4.243569643749999898, 17.29062500061451502, 32.45002607614398471 ) ) ;
#1652=CARTESIAN_POINT ( 'NONE',  ( 28.45312500061451289, 0.000000000000000000, 5.243569643749999010 ) ) ;
#1655=CARTESIAN_POINT ( 'NONE',  ( 25.99687500061451928, -3.027376345333610441, -5.243569643749999898 ) ) ;
#1657=CARTESIAN_POINT ( 'NONE',  ( 21.14062500061451289, 6.054752690667223547, 3.707466751127219781E-16 ) ) ;
#1658=CARTESIAN_POINT ( 'NONE',  ( 22.69687500061451857, -3.027376345333614438, 5.243569643749998122 ) ) ;
#1659=CARTESIAN_POINT ( 'NONE',  ( -2.121784821874996840, 15.82812500061459282, -26.32496088578401583 ) ) ;
#1660=CARTESIAN_POINT ( 'NONE',  ( 6.215625000614517504, 3.027376345333613106, -5.243569643749998122 ) ) ;
#1661=CARTESIAN_POINT ( 'NONE',  ( 16.61250000122903359, 0.000000000000000000, 4.999999999999998224 ) ) ;
#1662=CARTESIAN_POINT ( 'NONE',  ( 22.82812500061451644, 6.421520780324663323E-16, -5.243569643749999010 ) ) ;
#1665=CARTESIAN_POINT ( 'NONE',  ( 17.18437500061451573, 4.541064518000418104, 2.621784821874999949 ) ) ;
#1666=CARTESIAN_POINT ( 'NONE',  ( 19.99687500061451573, -3.027376345333614438, 5.243569643749998122 ) ) ;
#1667=CARTESIAN_POINT ( 'NONE',  ( 28.17187500061451644, -6.054752690667223547, -1.112240025338166033E-15 ) ) ;
#1668=CARTESIAN_POINT ( 'NONE',  ( 2.121784821874999061, 15.65937500061451892, 26.32496088578401583 ) ) ;
#1669=CARTESIAN_POINT ( 'NONE',  ( 6.928125000614516082, -4.541064518000419881, 2.621784821874995952 ) ) ;
#1670=CARTESIAN_POINT ( 'NONE',  ( -5.810221930991193690E-16, 18.98750000000000071, 26.00000000000000355 ) ) ;
#1671=CARTESIAN_POINT ( 'NONE',  ( 5.559375000614517504, 0.000000000000000000, 5.243569643749999010 ) ) ;
#1672=CARTESIAN_POINT ( 'NONE',  ( 26.51249999999999929, -5.773502691896255534, -1.060575238724906372E-15 ) ) ;
#1673=CARTESIAN_POINT ( 'NONE',  ( 4.303125000614516971, -4.541064518000417216, -2.621784821875001281 ) ) ;
#1674=CARTESIAN_POINT ( 'NONE',  ( 10.17187500061451999, -6.054752690667223547, -1.112240025338166033E-15 ) ) ;
#1675=CARTESIAN_POINT ( 'NONE',  ( 16.12500000122903288, 2.886751345948126879, 4.999999999999999112 ) ) ;
#1676=CARTESIAN_POINT ( 'NONE',  ( 6.796875000614516438, 6.054752690667223547, 3.707466751127219781E-16 ) ) ;
#1677=CARTESIAN_POINT ( 'NONE',  ( 8.390625000614518214, -3.027376345333610441, -5.243569643749999898 ) ) ;
#1680=CARTESIAN_POINT ( 'NONE',  ( 15.94687500061451502, -3.027376345333614438, 5.243569643749998122 ) ) ;
#1682=ORIENTED_EDGE ( 'NONE', *, *, #71265, .T. ) ;
#1683=CARTESIAN_POINT ( 'NONE',  ( 25.49062500061451786, -3.027376345333610441, -5.243569643749999898 ) ) ;
#1684=CARTESIAN_POINT ( 'NONE',  ( 10.00312500061451715, 0.000000000000000000, 5.243569643749999010 ) ) ;
#1685=CARTESIAN_POINT ( 'NONE',  ( 26.25937500061451857, 0.000000000000000000, 5.243569643749999010 ) ) ;
#1686=CARTESIAN_POINT ( 'NONE',  ( 8.953125000614518214, 4.541064518000418104, -2.621784821874998173 ) ) ;
#1687=CARTESIAN_POINT ( 'NONE',  ( -4.243569643749998122, 9.996875000614517504, -27.54997392385601174 ) ) ;
#1688=CARTESIAN_POINT ( 'NONE',  ( 10.50000000122903465, -2.886751345948125991, -5.000000000000000000 ) ) ;
#1689=CARTESIAN_POINT ( 'NONE',  ( 25.26562500061451289, 3.027376345333611329, 5.243569643749999010 ) ) ;
#1690=CARTESIAN_POINT ( 'NONE',  ( -4.243569643749999898, 12.60312500061451679, -30.00000000000000000 ) ) ;
#1691=CARTESIAN_POINT ( 'NONE',  ( 13.76250000122903394, 4.330127018922192761, -2.499999999999997780 ) ) ;
#1692=CARTESIAN_POINT ( 'NONE',  ( 22.04062500061451502, 6.054752690667223547, 3.707466751127219781E-16 ) ) ;
#1693=CARTESIAN_POINT ( 'NONE',  ( 11.28749999999999787, -2.886751345948125991, -5.000000000000000000 ) ) ;
#1694=CARTESIAN_POINT ( 'NONE',  ( 20.27812500061451573, 4.541064518000418104, 2.621784821874999949 ) ) ;
#1696=CARTESIAN_POINT ( 'NONE',  ( 21.07499999999999929, -4.330127018922194537, 2.499999999999995559 ) ) ;
#1697=CARTESIAN_POINT ( 'NONE',  ( 13.16250000122903430, -4.330127018922190985, -2.500000000000001332 ) ) ;
#1698=CARTESIAN_POINT ( 'NONE',  ( 10.26562500061451644, 3.027376345333613106, -5.243569643749998122 ) ) ;
#1699=CARTESIAN_POINT ( 'NONE',  ( 16.45312500061451289, -4.541064518000417216, -2.621784821875001281 ) ) ;
#1700=CARTESIAN_POINT ( 'NONE',  ( 24.90000000122903145, -2.886751345948125991, -5.000000000000000000 ) ) ;
#1701=CARTESIAN_POINT ( 'NONE',  ( 22.54687500061451999, 6.054752690667223547, 3.707466751127219781E-16 ) ) ;
#1703=CARTESIAN_POINT ( 'NONE',  ( 8.887500001229033941, 4.330127018922191873, 2.499999999999999556 ) ) ;
#1704=CARTESIAN_POINT ( 'NONE',  ( 7.696875000614516793, 6.054752690667223547, 3.707466751127219781E-16 ) ) ;
#1705=CARTESIAN_POINT ( 'NONE',  ( 25.95937500061451431, -4.541064518000417216, -2.621784821875001281 ) ) ;
#1706=EDGE_CURVE ( 'NONE', #10824, #25563, #71026, .T. ) ;
#1707=CARTESIAN_POINT ( 'NONE',  ( 3.571875000614517237, 3.027376345333613106, -5.243569643749998122 ) ) ;
#1708=AXIS2_PLACEMENT_3D ( 'NONE', #36048, #12430, #40884 ) ;
#1709=CARTESIAN_POINT ( 'NONE',  ( 20.20312500061451644, 4.541064518000418104, -2.621784821874998173 ) ) ;
#1710=CARTESIAN_POINT ( 'NONE',  ( 25.54687500061451644, -3.027376345333610441, -5.243569643749999898 ) ) ;
#1712=CARTESIAN_POINT ( 'NONE',  ( 3.269147239230635549, -3.783209791728578519, 3.521127183980624409 ) ) ;
#1713=CARTESIAN_POINT ( 'NONE',  ( 7.471875000614519813, -6.054752690667223547, -1.112240025338166033E-15 ) ) ;
#1714=CARTESIAN_POINT ( 'NONE',  ( 20.16562500061451146, 3.027376345333613106, -5.243569643749998122 ) ) ;
#1715=CIRCLE ( 'NONE', #52442, 5.999999999999998224 ) ;
#1716=ORIENTED_EDGE ( 'NONE', *, *, #4157, .T. ) ;
#1718=CARTESIAN_POINT ( 'NONE',  ( 26.95312500061451644, 4.541064518000418104, -2.621784821874998173 ) ) ;
#1719=CARTESIAN_POINT ( 'NONE',  ( 3.871875000614519280, -6.054752690667223547, -1.112240025338166033E-15 ) ) ;
#1720=DIRECTION ( 'NONE',  ( 0.000000000000000000, 0.000000000000000000, -1.000000000000000000 ) ) ;
#1721=DIRECTION ( 'NONE',  ( -1.000000000000000000, -0.000000000000000000, -0.000000000000000000 ) ) ;
#1722=CARTESIAN_POINT ( 'NONE',  ( 17.66249999999999787, 2.886751345948129099, -4.999999999999998224 ) ) ;
#1723=CARTESIAN_POINT ( 'NONE',  ( 20.46562500061451928, -6.054752690667223547, -1.112240025338166033E-15 ) ) ;
#1725=CARTESIAN_POINT ( 'NONE',  ( 25.46249999999999858, 2.886751345948126879, 4.999999999999999112 ) ) ;
#1726=CARTESIAN_POINT ( 'NONE',  ( 27.15937500061451360, 0.000000000000000000, 5.243569643749999010 ) ) ;
#1727=ORIENTED_EDGE ( 'NONE', *, *, #16469, .F. ) ;
#1728=CARTESIAN_POINT ( 'NONE',  ( 13.37812500061451715, 6.421520780324663323E-16, -5.243569643749999010 ) ) ;
#1729=CARTESIAN_POINT ( 'NONE',  ( 5.353125000614515905, 4.541064518000418104, -2.621784821874998173 ) ) ;
#1731=CARTESIAN_POINT ( 'NONE',  ( 28.90312500061451217, 0.000000000000000000, 5.243569643749999010 ) ) ;
#1732=CARTESIAN_POINT ( 'NONE',  ( 15.75000000122902932, -2.886751345948129988, 4.999999999999997335 ) ) ;
#1733=CARTESIAN_POINT ( 'NONE',  ( 21.26249999999999574, 2.886751345948129099, -4.999999999999998224 ) ) ;
#1734=CARTESIAN_POINT ( 'NONE',  ( 28.72500000000000142, -4.330127018922194537, 2.499999999999995559 ) ) ;
#1735=CARTESIAN_POINT ( 'NONE',  ( 5.071875000614519458, 3.027376345333611329, 5.243569643749999010 ) ) ;
#1736=CARTESIAN_POINT ( 'NONE',  ( 9.796875000614519990, -3.027376345333610441, -5.243569643749999898 ) ) ;
#1737=CARTESIAN_POINT ( 'NONE',  ( 18.64687500061451786, -3.027376345333614438, 5.243569643749998122 ) ) ;
#1738=CARTESIAN_POINT ( 'NONE',  ( 15.71250000122903501, 0.000000000000000000, 4.999999999999998224 ) ) ;
#1740=CARTESIAN_POINT ( 'NONE',  ( 29.46562500061451573, -6.054752690667223547, -1.112240025338166033E-15 ) ) ;
#1741=CARTESIAN_POINT ( 'NONE',  ( 4.237500000000001599, 5.773502691896255534, 3.535250795749688894E-16 ) ) ;
#1742=CARTESIAN_POINT ( 'NONE',  ( 3.946875000614517681, -3.027376345333610441, -5.243569643749999898 ) ) ;
#1744=CARTESIAN_POINT ( 'NONE',  ( 19.76250000000000639, -5.773502691896255534, -1.060575238724906372E-15 ) ) ;
#1745=CARTESIAN_POINT ( 'NONE',  ( 14.65312500061451573, -4.541064518000417216, -2.621784821875001281 ) ) ;
#1747=FACE_OUTER_BOUND ( 'NONE', #55151, .T. ) ;
#1748=CARTESIAN_POINT ( 'NONE',  ( 20.43750000122903643, 6.123233995736764310E-16, -4.999999999999998224 ) ) ;
#1750=CARTESIAN_POINT ( 'NONE',  ( 7.078125000614516438, 6.421520780324663323E-16, -5.243569643749999010 ) ) ;
#1751=CARTESIAN_POINT ( 'NONE',  ( 25.47187500061451715, -6.054752690667223547, -1.112240025338166033E-15 ) ) ;
#1752=CARTESIAN_POINT ( 'NONE',  ( 4.243569643749999898, 19.63437500061451857, 30.00000000000000000 ) ) ;
#1753=CARTESIAN_POINT ( 'NONE',  ( 26.59687500061451360, 6.054752690667223547, 3.707466751127219781E-16 ) ) ;
#1754=CARTESIAN_POINT ( 'NONE',  ( 7.312500000000000000, 2.886751345948129099, -4.999999999999998224 ) ) ;
#1755=CARTESIAN_POINT ( 'NONE',  ( -1.999999999999997113, 13.43750000122903465, 33.46410161513775705 ) ) ;
#1756=CARTESIAN_POINT ( 'NONE',  ( 15.74062500061451608, 6.054752690667223547, 3.707466751127219781E-16 ) ) ;
#1757=CARTESIAN_POINT ( 'NONE',  ( 6.000000001229033764, -2.886751345948125991, -5.000000000000000000 ) ) ;
#1758=CARTESIAN_POINT ( 'NONE',  ( 18.04687500061451999, 6.054752690667223547, 3.707466751127219781E-16 ) ) ;
#1759=CARTESIAN_POINT ( 'NONE',  ( 12.53437500061451537, 6.421520780324663323E-16, -5.243569643749999010 ) ) ;
#1761=ORIENTED_EDGE ( 'NONE', *, *, #22002, .T. ) ;
#1762=AXIS2_PLACEMENT_3D ( 'NONE', #29323, #34855, #68483 ) ;
#1763=CARTESIAN_POINT ( 'NONE',  ( 11.95312500061451644, -4.541064518000417216, -2.621784821875001281 ) ) ;
#1764=CARTESIAN_POINT ( 'NONE',  ( 29.06250000122903288, 4.330127018922192761, -2.499999999999997780 ) ) ;
#1765=CARTESIAN_POINT ( 'NONE',  ( 24.56250000122903288, 4.330127018922192761, -2.499999999999997780 ) ) ;
#1766=CARTESIAN_POINT ( 'NONE',  ( 13.65937500061451715, 0.000000000000000000, 5.243569643749999010 ) ) ;
#1767=CARTESIAN_POINT ( 'NONE',  ( 14.31562500061451537, 3.027376345333613106, -5.243569643749998122 ) ) ;
#1768=ADVANCED_FACE ( 'NONE', ( #39607 ), #11520, .F. ) ;
#1769=CARTESIAN_POINT ( 'NONE',  ( 23.82187500061451502, 3.027376345333613106, -5.243569643749998122 ) ) ;
#1770=FACE_OUTER_BOUND ( 'NONE', #41782, .T. ) ;
#1771=AXIS2_PLACEMENT_3D ( 'NONE', #66490, #15503, #3355 ) ;
#1772=CARTESIAN_POINT ( 'NONE',  ( 11.77500000122903501, -5.773502691896255534, -1.060575238724906372E-15 ) ) ;
#1774=CARTESIAN_POINT ( 'NONE',  ( 3.089506346739232967, 3.931278485869285522, -3.469880700456108968 ) ) ;
#1775=CARTESIAN_POINT ( 'NONE',  ( 4.243569643749999010, 16.52187500061451786, -32.45002607614398471 ) ) ;
#1776=CARTESIAN_POINT ( 'NONE',  ( 16.80937500061451573, 0.000000000000000000, 5.243569643749999010 ) ) ;
#1777=CARTESIAN_POINT ( 'NONE',  ( 16.91250000122903430, 4.330127018922192761, -2.499999999999997780 ) ) ;
#1778=VECTOR ( 'NONE', #42359, 1000.000000000000000 ) ;
#1779=CARTESIAN_POINT ( 'NONE',  ( 12.83437500061451786, -4.541064518000419881, 2.621784821874995952 ) ) ;
#1780=CARTESIAN_POINT ( 'NONE',  ( -4.243569643749999898, 19.35312500061451857, -30.00000000000000000 ) ) ;
#1781=CARTESIAN_POINT ( 'NONE',  ( 19.87500000122903288, -5.773502691896255534, -1.060575238724906372E-15 ) ) ;
#1782=CARTESIAN_POINT ( 'NONE',  ( 13.82812500061451466, 6.421520780324663323E-16, -5.243569643749999010 ) ) ;
#1783=VERTEX_POINT ( 'NONE', #51771 ) ;
#1786=CARTESIAN_POINT ( 'NONE',  ( 18.30000000000000071, 0.000000000000000000, 4.999999999999998224 ) ) ;
#1787=CARTESIAN_POINT ( 'NONE',  ( -5.810221930991193690E-16, 15.50000000122903465, 26.00000000000000355 ) ) ;
#1788=CARTESIAN_POINT ( 'NONE',  ( 13.02187500061451786, 3.027376345333612662, -5.243569643749998122 ) ) ;
#1789=CARTESIAN_POINT ( 'NONE',  ( 3.075856135158071769, 3.942005890571277593, -3.420430885948836153 ) ) ;
#1790=CARTESIAN_POINT ( 'NONE',  ( 15.48750000122903359, 6.123233995736764310E-16, -4.999999999999998224 ) ) ;
#1791=CARTESIAN_POINT ( 'NONE',  ( 25.80937500061451928, 0.000000000000000000, 5.243569643749999010 ) ) ;
#1792=CARTESIAN_POINT ( 'NONE',  ( 19.11562500061451431, -6.054752690667223547, -1.112240025338166033E-15 ) ) ;
#1793=( BOUNDED_CURVE ( )  B_SPLINE_CURVE ( 2, ( #19419, #25716, #26079, #14255, #41979, #64500, #48618 ),
 .UNSPECIFIED., .F., .F. ) 
 B_SPLINE_CURVE_WITH_KNOTS ( ( 3, 2, 2, 3 ),
 ( 0.9772596827842864320, 0.9777777777777777457, 0.9805555555555555136, 0.9810043224607896128 ),
 .UNSPECIFIED. ) 
 CURVE ( )  GEOMETRIC_REPRESENTATION_ITEM ( )  RATIONAL_B_SPLINE_CURVE ( ( 0.9593449661988595611, 0.9750118356804509112, 1.000000000000000000, 0.8660254037844387076, 1.000000000000000000, 0.9783555886274875046, 0.9637047500201995076 ) ) 
 REPRESENTATION_ITEM ( '' )  );
#1794=CARTESIAN_POINT ( 'NONE',  ( 21.85312500061451502, -4.541064518000417216, -2.621784821875001281 ) ) ;
#1795=CARTESIAN_POINT ( 'NONE',  ( 3.665625000614517681, 3.027376345333611329, 5.243569643749999010 ) ) ;
#1796=CARTESIAN_POINT ( 'NONE',  ( 28.57499999999999929, 4.330127018922191873, 2.499999999999999556 ) ) ;
#1800=CARTESIAN_POINT ( 'NONE',  ( 3.977933236251851579, -3.029199096778425915, -4.197771185803018668 ) ) ;
#1801=CARTESIAN_POINT ( 'NONE',  ( 9.001249775931846008E-16, 15.02187500061451608, -25.09994784771203058 ) ) ;
#1802=CARTESIAN_POINT ( 'NONE',  ( 4.087500001229035007, -4.330127018922194537, 2.499999999999995559 ) ) ;
#1803=CARTESIAN_POINT ( 'NONE',  ( 6.712500000000000355, -5.773502691896255534, -1.060575238724906372E-15 ) ) ;
#1804=EDGE_CURVE ( 'NONE', #71417, #44451, #9952, .T. ) ;
#1805=CARTESIAN_POINT ( 'NONE',  ( 3.015379517359913386, -4.298692091864810827, -3.041586178295606846 ) ) ;
#1806=CARTESIAN_POINT ( 'NONE',  ( 9.384375000614518569, 6.421520780324663323E-16, -5.243569643749999010 ) ) ;
#1807=CARTESIAN_POINT ( 'NONE',  ( 28.82812500061451644, 4.541064518000418104, 2.621784821874999949 ) ) ;
#1811=CARTESIAN_POINT ( 'NONE',  ( 7.021875000614518747, -6.054752690667223547, -1.112240025338166033E-15 ) ) ;
#1812=CARTESIAN_POINT ( 'NONE',  ( 11.14687500061451608, -3.027376345333610441, -5.243569643749999898 ) ) ;
#1813=CARTESIAN_POINT ( 'NONE',  ( 7.275000000000000355, 6.123233995736764310E-16, -4.999999999999998224 ) ) ;
#1814=VECTOR ( 'NONE', #48157, 1000.000000000000000 ) ;
#1815=CARTESIAN_POINT ( 'NONE',  ( -2.121784821874999949, 15.67812500061459247, 26.32496088578401938 ) ) ;
#1817=CARTESIAN_POINT ( 'NONE',  ( 5.625000000000001776, 4.330127018922191873, 2.499999999999999556 ) ) ;
#1819=CARTESIAN_POINT ( 'NONE',  ( 21.85312500061451502, -4.541064518000417216, -2.621784821875001281 ) ) ;
#1820=CARTESIAN_POINT ( 'NONE',  ( 13.34062500061451750, -3.027376345333610441, -5.243569643749999898 ) ) ;
#1822=CARTESIAN_POINT ( 'NONE',  ( 10.50937500061451679, 0.000000000000000000, 5.243569643749999010 ) ) ;
#1823=CARTESIAN_POINT ( 'NONE',  ( 26.43750000000000000, -2.886751345948129988, 4.999999999999997335 ) ) ;
#1824=CARTESIAN_POINT ( 'NONE',  ( 22.31250000122903288, 4.330127018922192761, -2.499999999999997780 ) ) ;
#1825=CARTESIAN_POINT ( 'NONE',  ( 11.97187500061451892, -6.054752690667223547, -1.112240025338166033E-15 ) ) ;
#1826=CARTESIAN_POINT ( 'NONE',  ( 27.60937500061451644, 0.000000000000000000, 5.243569643749999010 ) ) ;
#1827=CARTESIAN_POINT ( 'NONE',  ( 4.209375000614516971, 0.000000000000000000, 5.243569643749999010 ) ) ;
#1828=CARTESIAN_POINT ( 'NONE',  ( -1.071796769724475906, 12.82009619066136707, -34.00000000000000711 ) ) ;
#1829=CARTESIAN_POINT ( 'NONE',  ( 19.73437500061451644, 6.421520780324663323E-16, -5.243569643749999010 ) ) ;
#1831=CARTESIAN_POINT ( 'NONE',  ( 11.59687500061451892, -3.027376345333610441, -5.243569643749999898 ) ) ;
#1833=CARTESIAN_POINT ( 'NONE',  ( 25.42500000000000071, 4.330127018922191873, 2.499999999999999556 ) ) ;
#1835=CARTESIAN_POINT ( 'NONE',  ( -3.000416591977282496E-16, 11.19687500061451679, -34.90005215228797653 ) ) ;
#1837=CARTESIAN_POINT ( 'NONE',  ( 14.69062500061451537, -3.027376345333610441, -5.243569643749999898 ) ) ;
#1838=CARTESIAN_POINT ( 'NONE',  ( 5.549999999999998934, 4.330127018922192761, -2.499999999999997780 ) ) ;
#1841=( BOUNDED_SURFACE ( )  B_SPLINE_SURFACE ( 1, 2, ( 
 ( #61791, #35169, #11915, #23710, #68800, #63240, #126, #45182, #18156, #844, #45902, #52164, #12634, #67713, #11196, #39646, #67361, #23353, #7098, #22987, #40356, #40003, #6012, #39279, #1567, #33722, #17085, #56968, #22631, #56267, #5658, #62875, #28194, #62164, #68433, #28547, #51802, #51081, #478, #45547, #68077, #17446, #62517, #6372, #17796, #12271, #34802, #57334, #6738, #8920, #7457, #29984, #35528, #18525, #52886, #47703, #19243, #70607, #36620, #30712, #24439, #69166, #41090, #18882, #41445, #52526, #2284, #63963, #36260, #59141, #63602, #3389, #25162, #47344, #30357, #53992, #12992, #31450, #1934, #58775, #42533, #46988, #8184, #25538, #53245, #14080, #3008, #8550, #48079, #24801, #64696, #65059, #69524, #19613, #14450, #58049, #13347, #69878, #31077, #35884, #58409, #53617, #19980, #2643, #41798, #36984, #7822, #59506, #64326, #13719, #42170, #70242, #46623, #48450, #26275, #20349, #38455, #66527, #70974, #55449, #55086, #27376, #32912, #15907, #60981, #66906, #71342, #72432, #37716, #10380, #31818, #4842, #20717, #9650, #43275, #4120, #15538, #44005, #72069, #48812, #15177, #49908, #49547, #32184, #65796, #21816, #65424, #44381, #54357, #21449, #42900, #14814, #59879, #60236, #37357, #54717, #26649, #71715, #16274, #38830, #61345, #3751, #9285, #49185, #55813, #60604, #10741, #21087, #33274, #43638, #66162, #38082, #25910, #10013, #32549, #4486, #27015, #68713, #67275, #756, #40634, #63153, #11103, #16634, #46174, #29184, #33631, #17711, #39, #62076, #50635, #56529, #67987, #23264, #51353, #5569, #67627, #57242, #28815, #11469, #28106, #6655, #44741, #51717, #56176, #45814, #27741, #39189, #61704, #22544, #72804, #45092, #16993, #50991, #68350, #1119, #18073, #39551, #6285, #33992, #62792, #23628, #5922, #28456, #12185, #389, #12548, #50280, #35082, #22896, #45455, #22187, #17361, #5200, #39918, #62432, #11830, #34348, #56881, #40271, #34712, #8462, #47622, #41715, #35439, #7011, #52078, #29902, #52441, #63519, #13263, #1847, #47261, #70154, #29542, #14368, #36174, #58323, #41362, #64977, #1483, #19902, #41004, #69795, #53530, #12906, #19161, #36537, #64241, #25079, #13998, #19532, #59057, #63872, #2559, #2925, #57963, #30630, #25455, #23989, #24355, #35801, #42090, #46536, #7371, #64612, #30997, #13630, #7734, #69078, #47999, #46902, #53162, #18439, #69441, #18798, #30269, #52802, #2203, #24718, #58691, #70527, #42454, #57608, #8102, #37999, #48365, #21367, #55367, #70891, #15096, #43921, #71252, #21732, #59423, #44292, #14729, #25828, #53908, #8831, #72351, #20264, #42816, #65339, #31367, #43190, #60521, #9565, #60893, #26934, #21002, #37271, #3301, #59793, #9199, #31734, #54272, #65710, #3666, #26560, #49459, #26189, #66821, #15454, #37632, #20631, #36903, #48729, #60155, #32097, #49100, #32829, #54629, #71629, #15824, #43554, #4405, #66447, #71993, #38367, #4036, #54999, #4760, #66076, #9927, #27293, #32465, #10298, #49827, #676, #55728, #22103, #34266, #28732, #5842, #39466, #34632, #61265, #17634, #27656, #61988, #11749, #28374, #50194, #38745, #16552, #10659, #51273, #56799, #33189, #45737, #45371, #40194, #23183, #6204, #68272, #57161, #44661, #5122, #6573, #62715, #67191, #12109, #11023, #73081, #61620, #67548, #50911, #29104, #62353, #39104, #5486, #51639, #39839, #22462, #33545, #1040, #45012, #23547, #72720, #46097, #56095, #309, #16194, #28025, #22819, #50553, #67906, #16911, #11389, #33908, #56452, #17277, #13545, #64527, #1401, #41638, #13921, #63072, #40928, #52359, #53081, #35003, #23910, #36092, #8019, #58246, #18720, #36459, #40554, #70073, #6933, #41284, #64157, #7651, #29464, #17995, #68996, #12474, #30555, #58612, #57533, #25001, #24637, #19447, #2476, #47544, #42007, #58974, #46458, #52000, #8381, #30911, #18355, #53452, #63441, #1763, #12827, #46825, #30189, #2842, #25371, #35361, #57885, #68633, #19083, #24276, #7294, #29824, #69362, #63795, #13185, #35724, #52719, #2126, #47183, #69715, #42372, #48281, #70805, #20542, #65995, #49380, #60806, #14284, #49014, #59336, #32375, #66364, #8747, #26106, #54915, #9116, #32747, #70444, #55285, #25744, #36821, #64894, #19820, #10214, #31280, #53822, #3215, #20180, #54187, #71546, #43100, #71910, #37918, #32014, #42735, #65254, #14644, #37185, #59709, #31654, #3584, #48645, #37551, #60436, #71170, #4679, #26474, #65626, #15013, #21284, #60073, #9485, #43471, #54549, #3951, #20919, #15376, #9846, #4322, #26847, #43837, #15739, #38278, #47915, #34184, #17196, #39756, #68188, #33105, #16109, #17552, #51190, #55644, #62274, #22020, #10939, #72636, #5402, #16832, #45289, #231, #27575, #16465, #6121, #50831, #33462, #50107, #28651, #66738, #594, #5039, #22738, #49744, #38660, #61183, #44576, #21649, #67109, #39024, #72998, #67823, #23098, #40113, #10578, #28296, #61538, #11668, #45656, #56008, #27938, #56719, #50471, #12023, #72272, #34547, #22382, #44931, #44206, #67469, #62628, #39385, #61904, #11309, #33830, #56373, #57076, #5765, #27209, #69626, #63704, #57442, #29019, #956, #51913, #1311, #12378, #35274, #23820, #69269, #18988, #51554, #36367, #58156, #7204, #63353, #13827, #23464, #41910, #62983, #18631, #2389, #34915, #41196, #58516, #13096, #47093, #35997, #41550, #7926, #12737, #24548, #24907, #6845, #52631, #47451, #46010, #46371, #57795, #64067, #68547, #29380, #13448, #30463, #35634, #29733, #69983, #7560, #68905, #52271, #18262, #52993, #19353, #40836, #1673, #17906, #64435, #40468, #24182, #46735, #6484, #30095, #2037, #21468, #16651, #67293, #31186, #20085, #4504, #42642, #8656, #53728, #25650, #3121, #47819, #61362, #65166, #58882, #8292, #19726, #48187, #44758, #38847, #10031, #27033, #66924, #53355, #15924, #15555, #10759, #70711, #60998, #30823, #25272, #36726 ),
 ( #49564, #32566, #5217, #2753, #33291, #70350, #55104, #55467, #72085, #42277, #64800, #59248, #14191, #72449, #27393, #38099, #16292, #38474, #55829, #27758, #49925, #21834, #50299, #60621, #44022, #72821, #22204, #66545, #44398, #10397, #32929, #4859, #17377, #28831, #57258, #12201, #39568, #28473, #18088, #62808, #45472, #62093, #40649, #5587, #63169, #45109, #34729, #61721, #28124, #56, #34009, #33649, #11486, #56546, #11846, #6671, #12564, #52093, #50652, #23643, #57623, #22562, #39934, #46189, #406, #24004, #11120, #46552, #17011, #67645, #56193, #5939, #1498, #51009, #22915, #68004, #62448, #34365, #40287, #56897, #35098, #29199, #23280, #6303, #51370, #772, #45830, #68366, #17728, #51733, #1134, #68728, #7026, #29557, #69093, #39207, #19174, #2219, #25842, #12921, #53921, #1862, #8117, #14382, #46917, #53176, #70540, #2574, #59072, #48012, #8476, #19915, #24732, #36552, #36917, #24369, #64626, #59437, #35454, #63886, #47276, #2939, #57978, #69455, #31010, #53543, #30645, #41729, #8845, #63534, #42469, #29916, #64256, #14013, #25093, #52456, #41019, #18813, #7386, #25468, #64992, #41376, #31381, #47636, #3315, #48379, #18455, #13277, #35815, #58337, #7748, #30284, #52817, #69809, #13644, #36188, #58706, #70170, #19546, #42104, #15837, #43934, #71268, #60168, #49840, #21380, #4048, #20646, #72364, #37286, #21745, #3681, #66460, #20278, #59809, #31750, #65723, #65354, #43203, #15109, #43568, #38383, #44307, #10672, #9214, #72005, #54287, #37645, #14744, #38759, #15467, #27306, #4773, #66836, #26205, #48744, #16207, #32479, #49473, #55741, #61279, #9578, #32110, #54644, #27669, #55013, #33202, #26574, #60906, #66089, #49113, #42831, #5135, #70906, #71642, #38012, #21015, #60534, #9941, #10310, #4418, #26947, #32842, #55379, #50567, #51286, #39479, #34280, #33558, #11763, #6946, #45026, #73094, #6219, #688, #28747, #56812, #46109, #16566, #72732, #23195, #56108, #67561, #50926, #67920, #11035, #28038, #5499, #45749, #33923, #62366, #17291, #22832, #34647, #11403, #29118, #40567, #63087, #68285, #39853, #22476, #323, #16925, #57175, #23563, #62002, #45384, #44674, #6588, #22118, #56465, #5856, #40206, #51652, #28387, #17646, #50208, #57544, #62728, #12121, #1053, #68646, #18009, #12488, #35015, #67205, #39118, #61633, #13198, #59349, #29477, #63455, #18732, #14297, #8394, #52733, #69726, #36470, #23922, #58625, #35737, #53464, #46837, #30567, #1415, #69009, #7306, #30923, #41296, #2855, #58257, #69376, #19095, #63806, #7662, #64907, #30202, #2138, #29837, #53093, #24649, #13558, #12841, #64170, #52014, #24289, #52372, #8032, #2488, #25013, #36104, #25384, #18373, #46472, #47555, #35375, #47195, #41650, #70084, #57898, #1777, #19459, #42019, #64540, #13933, #58988, #47928, #70457, #19833, #42385, #36835, #40941, #60450, #71557, #31666, #32025, #26118, #15752, #55297, #48657, #54561, #3229, #38291, #53835, #14655, #54199, #71922, #60818, #15026, #43484, #38675, #16121, #3596, #43112, #26486, #65638, #71182, #20555, #37563, #60086, #70819, #10226, #9496, #8760, #31294, #42747, #3963, #66751, #32760, #49027, #20932, #4691, #25757, #37930, #66008, #27221, #15388, #9858, #48293, #20193, #59721, #49757, #32387, #72284, #54926, #4335, #26860, #49391, #21297, #43850, #65267, #21662, #66376, #44219, #37198, #9129, #67123, #39037, #12038, #22753, #39773, #46027, #40129, #61551, #5052, #33474, #17921, #45304, #34563, #16845, #34200, #33844, #50486, #10591, #29035, #970, #10953, #28308, #44590, #51570, #50121, #56734, #23480, #61918, #5778, #22033, #56023, #16479, #62289, #44944, #244, #50845, #56388, #45670, #22396, #62643, #68563, #61196, #11685, #67838, #5414, #11323, #27954, #68206, #57091, #73011, #17211, #55656, #17567, #33119, #67482, #39399, #51208, #6500, #6137, #28667, #27589, #72652, #608, #23114, #58171, #24197, #63370, #12754, #7220, #35289, #29395, #41926, #46751, #70366, #40484, #1326, #29749, #25291, #19368, #63719, #7576, #47466, #34931, #69641, #69285, #64452, #57811, #41564, #12394, #6862, #18277, #13843, #52287, #36382, #18648, #1688, #30111, #41211, #13111, #35650, #57457, #8307, #52645, #69999, #58897, #30838, #46386, #40852, #53371, #2052, #19003, #47836, #2768, #24563, #51929, #47109, #63000, #64082, #23836, #13464, #36013, #58531, #7941, #68920, #30480, #53008, #2403, #24924, #3138, #10141, #8672, #15302, #55213, #4608, #9045, #48569, #20102, #20845, #31575, #3875, #25667, #54477, #49672, #14573, #42658, #48940, #43398, #71469, #26398, #15665, #59263, #42293, #65922, #48204, #37106, #31203, #53744, #59632, #14207, #65182, #54114, #65552, #37841, #21210, #32673, #70726, #60361, #3511, #4246, #38204, #26031, #71096, #26773, #20470, #27138, #64817, #19744, #43024, #14942, #36743, #37480, #60000, #9410, #31940, #9771, #32304, #54839, #49305, #71839, #43762, #66287, #60730, #4968, #21578, #44132, #72561, #50035, #33034, #10865, #21947, #22310, #28228, #66659, #23028, #61830, #55934, #38952, #517, #16036, #28583, #10506, #44862, #34115, #55573, #67399, #17123, #16760, #50758, #67751, #161, #39682, #61470, #5692, #56654, #27501, #56303, #6049, #38584, #44504, #33398, #22667, #61109, #67037, #45217, #62202, #39318, #5330, #51120, #16397, #11598, #27871, #50403, #72199, #72928, #11235, #33758, #65406, #59489, #4468, #32531, #36967, #21431, #21070, #66509, #72052, #55067, #26998, #32892, #70957, #53973, #55432, #15890, #20330, #49528, #59862, #48795, #37339, #43256, #54698, #9996, #38063, #14796, #54339, #43988, #15521, #71323, #9266, #38436, #31433, #60962, #42883, #60587, #14432, #4103, #10361, #8901, #21796, #43621, #65777, #20698, #72414, #3371, #27358, #48432, #26630, #4824, #31801, #49167, #49889, #71698, #65042, #25892, #3733, #26258, #15159 ) ),
 .UNSPECIFIED., .F., .F., .F. ) 
 B_SPLINE_SURFACE_WITH_KNOTS ( ( 2, 2 ),
 ( 3, 2, 2, 2, 2, 2, 2, 2, 2, 2, 2, 2, 2, 2, 2, 2, 2, 2, 2, 2, 2, 2, 2, 2, 2, 2, 2, 2, 2, 2, 2, 2, 2, 2, 2, 2, 2, 2, 2, 2, 2, 2, 2, 2, 2, 2, 2, 2, 2, 2, 2, 2, 2, 2, 2, 2, 2, 2, 2, 2, 2, 2, 2, 2, 2, 2, 2, 2, 2, 2, 2, 2, 2, 2, 2, 2, 2, 2, 2, 2, 2, 2, 2, 2, 2, 2, 2, 2, 2, 2, 2, 2, 2, 2, 2, 2, 2, 2, 2, 2, 2, 2, 2, 2, 2, 2, 2, 2, 2, 2, 2, 2, 2, 2, 2, 2, 2, 2, 2, 2, 2, 2, 2, 2, 2, 2, 2, 2, 2, 2, 2, 2, 2, 2, 2, 2, 2, 2, 2, 2, 2, 2, 2, 2, 2, 2, 2, 2, 2, 2, 2, 2, 2, 2, 2, 2, 2, 2, 2, 2, 2, 2, 2, 2, 2, 2, 2, 2, 2, 2, 2, 2, 2, 2, 2, 2, 2, 2, 2, 2, 2, 2, 2, 2, 2, 2, 2, 2, 2, 2, 2, 2, 2, 2, 2, 2, 2, 2, 2, 2, 2, 2, 2, 2, 2, 2, 2, 2, 2, 2, 2, 2, 2, 2, 2, 2, 2, 2, 2, 2, 2, 2, 2, 2, 2, 2, 2, 2, 2, 2, 2, 2, 2, 2, 2, 2, 2, 2, 2, 2, 2, 2, 2, 2, 2, 2, 2, 2, 2, 2, 2, 2, 2, 2, 2, 2, 2, 2, 2, 2, 2, 2, 2, 2, 2, 2, 2, 2, 2, 2, 2, 2, 2, 2, 2, 2, 2, 2, 2, 2, 2, 2, 2, 2, 2, 2, 2, 2, 2, 2, 2, 2, 2, 2, 2, 2, 2, 2, 2, 2, 2, 2, 2, 2, 2, 2, 2, 2, 2, 2, 2, 2, 2, 2, 2, 2, 2, 2, 2, 2, 2, 2, 2, 2, 2, 2, 2, 2, 2, 2, 2, 2, 2, 2, 2, 2, 2, 2, 2, 2, 2, 2, 2, 2, 2, 2, 2, 2, 2, 2, 2, 2, 2, 2, 2, 2, 2, 2, 2, 2, 3 ),
 ( 0.000000000000000000, 1.000000000000000000 ),
 ( 0.000000000000000000, 0.002777777777777777884, 0.005555555555555555768, 0.008333333333333333218, 0.01111111111111111154, 0.01388888888888888812, 0.01666666666666666644, 0.01944444444444444475, 0.02222222222222222307, 0.02500000000000000139, 0.02777777777777777624, 0.03055555555555555455, 0.03333333333333333287, 0.03611111111111110772, 0.03888888888888888951, 0.04166666666666666435, 0.04444444444444444614, 0.04722222222222222099, 0.05000000000000000278, 0.05277777777777777762, 0.05555555555555555247, 0.05833333333333333426, 0.06111111111111110911, 0.06388888888888888395, 0.06666666666666666574, 0.06944444444444444753, 0.07222222222222221544, 0.07499999999999999722, 0.07777777777777777901, 0.08055555555555556080, 0.08333333333333332871, 0.08611111111111111049, 0.08888888888888889228, 0.09166666666666666019, 0.09444444444444444198, 0.09722222222222222376, 0.1000000000000000056, 0.1027777777777777735, 0.1055555555555555552, 0.1083333333333333370, 0.1111111111111111049, 0.1138888888888888867, 0.1166666666666666685, 0.1194444444444444503, 0.1222222222222222182, 0.1250000000000000000, 0.1277777777777777679, 0.1305555555555555636, 0.1333333333333333315, 0.1361111111111110994, 0.1388888888888888951, 0.1416666666666666630, 0.1444444444444444309, 0.1472222222222222265, 0.1499999999999999944, 0.1527777777777777901, 0.1555555555555555580, 0.1583333333333333259, 0.1611111111111111216, 0.1638888888888888895, 0.1666666666666666574, 0.1694444444444444531, 0.1722222222222222210, 0.1749999999999999889, 0.1777777777777777846, 0.1805555555555555525, 0.1833333333333333204, 0.1861111111111111160, 0.1888888888888888840, 0.1916666666666666796, 0.1944444444444444475, 0.1972222222222222154, 0.2000000000000000111, 0.2027777777777777790, 0.2055555555555555469, 0.2083333333333333426, 0.2111111111111111105, 0.2138888888888888784, 0.2166666666666666741, 0.2194444444444444420, 0.2222222222222222099, 0.2250000000000000056, 0.2277777777777777735, 0.2305555555555555691, 0.2333333333333333370, 0.2361111111111111049, 0.2388888888888889006, 0.2416666666666666685, 0.2444444444444444364, 0.2472222222222222321, 0.2500000000000000000, 0.2527777777777777679, 0.2555555555555555358, 0.2583333333333333592, 0.2611111111111111271, 0.2638888888888888951, 0.2666666666666666630, 0.2694444444444444309, 0.2722222222222221988, 0.2750000000000000222, 0.2777777777777777901, 0.2805555555555555580, 0.2833333333333333259, 0.2861111111111110938, 0.2888888888888888618, 0.2916666666666666852, 0.2944444444444444531, 0.2972222222222222210, 0.2999999999999999889, 0.3027777777777777568, 0.3055555555555555802, 0.3083333333333333481, 0.3111111111111111160, 0.3138888888888888840, 0.3166666666666666519, 0.3194444444444444198, 0.3222222222222222432, 0.3250000000000000111, 0.3277777777777777790, 0.3305555555555555469, 0.3333333333333333148, 0.3361111111111111382, 0.3388888888888889062, 0.3416666666666666741, 0.3444444444444444420, 0.3472222222222222099, 0.3499999999999999778, 0.3527777777777778012, 0.3555555555555555691, 0.3583333333333333370, 0.3611111111111111049, 0.3638888888888888729, 0.3666666666666666408, 0.3694444444444444642, 0.3722222222222222321, 0.3750000000000000000, 0.3777777777777777679, 0.3805555555555555358, 0.3833333333333333592, 0.3861111111111111271, 0.3888888888888888951, 0.3916666666666666630, 0.3944444444444444309, 0.3972222222222221988, 0.4000000000000000222, 0.4027777777777777901, 0.4055555555555555580, 0.4083333333333333259, 0.4111111111111110938, 0.4138888888888888618, 0.4166666666666666852, 0.4194444444444444531, 0.4222222222222222210, 0.4249999999999999889, 0.4277777777777777568, 0.4305555555555555802, 0.4333333333333333481, 0.4361111111111111160, 0.4388888888888888840, 0.4416666666666666519, 0.4444444444444444198, 0.4472222222222222432, 0.4500000000000000111, 0.4527777777777777790, 0.4555555555555555469, 0.4583333333333333148, 0.4611111111111111382, 0.4638888888888889062, 0.4666666666666666741, 0.4694444444444444420, 0.4722222222222222099, 0.4749999999999999778, 0.4777777777777778012, 0.4805555555555555691, 0.4833333333333333370, 0.4861111111111111049, 0.4888888888888888729, 0.4916666666666666408, 0.4944444444444444642, 0.4972222222222222321, 0.5000000000000000000, 0.5027777777777777679, 0.5055555555555555358, 0.5083333333333333037, 0.5111111111111110716, 0.5138888888888888395, 0.5166666666666667185, 0.5194444444444444864, 0.5222222222222222543, 0.5250000000000000222, 0.5277777777777777901, 0.5305555555555555580, 0.5333333333333333259, 0.5361111111111110938, 0.5388888888888888618, 0.5416666666666666297, 0.5444444444444443976, 0.5472222222222222765, 0.5500000000000000444, 0.5527777777777778123, 0.5555555555555555802, 0.5583333333333333481, 0.5611111111111111160, 0.5638888888888888840, 0.5666666666666666519, 0.5694444444444444198, 0.5722222222222221877, 0.5749999999999999556, 0.5777777777777777235, 0.5805555555555556024, 0.5833333333333333703, 0.5861111111111111382, 0.5888888888888889062, 0.5916666666666666741, 0.5944444444444444420, 0.5972222222222222099, 0.5999999999999999778, 0.6027777777777777457, 0.6055555555555555136, 0.6083333333333332815, 0.6111111111111111605, 0.6138888888888889284, 0.6166666666666666963, 0.6194444444444444642, 0.6222222222222222321, 0.6250000000000000000, 0.6277777777777777679, 0.6305555555555555358, 0.6333333333333333037, 0.6361111111111110716, 0.6388888888888888395, 0.6416666666666667185, 0.6444444444444444864, 0.6472222222222222543, 0.6500000000000000222, 0.6527777777777777901, 0.6555555555555555580, 0.6583333333333333259, 0.6611111111111110938, 0.6638888888888888618, 0.6666666666666666297, 0.6694444444444443976, 0.6722222222222222765, 0.6750000000000000444, 0.6777777777777778123, 0.6805555555555555802, 0.6833333333333333481, 0.6861111111111111160, 0.6888888888888888840, 0.6916666666666666519, 0.6944444444444444198, 0.6972222222222221877, 0.6999999999999999556, 0.7027777777777777235, 0.7055555555555556024, 0.7083333333333333703, 0.7111111111111111382, 0.7138888888888889062, 0.7166666666666666741, 0.7194444444444444420, 0.7222222222222222099, 0.7249999999999999778, 0.7277777777777777457, 0.7305555555555555136, 0.7333333333333332815, 0.7361111111111111605, 0.7388888888888889284, 0.7416666666666666963, 0.7444444444444444642, 0.7472222222222222321, 0.7500000000000000000, 0.7527777777777777679, 0.7555555555555555358, 0.7583333333333333037, 0.7611111111111110716, 0.7638888888888888395, 0.7666666666666667185, 0.7694444444444444864, 0.7722222222222222543, 0.7750000000000000222, 0.7777777777777777901, 0.7805555555555555580, 0.7833333333333333259, 0.7861111111111110938, 0.7888888888888888618, 0.7916666666666666297, 0.7944444444444443976, 0.7972222222222222765, 0.8000000000000000444, 0.8027777777777778123, 0.8055555555555555802, 0.8083333333333333481, 0.8111111111111111160, 0.8138888888888888840, 0.8166666666666666519, 0.8194444444444444198, 0.8222222222222221877, 0.8249999999999999556, 0.8277777777777777235, 0.8305555555555556024, 0.8333333333333333703, 0.8361111111111111382, 0.8388888888888889062, 0.8416666666666666741, 0.8444444444444444420, 0.8472222222222222099, 0.8499999999999999778, 0.8527777777777777457, 0.8555555555555555136, 0.8583333333333332815, 0.8611111111111111605, 0.8638888888888889284, 0.8666666666666666963, 0.8694444444444444642, 0.8722222222222222321, 0.8750000000000000000, 0.8777777777777777679, 0.8805555555555555358, 0.8833333333333333037, 0.8861111111111110716, 0.8888888888888888395, 0.8916666666666667185, 0.8944444444444444864, 0.8972222222222222543, 0.9000000000000000222, 0.9027777777777777901, 0.9055555555555555580, 0.9083333333333333259, 0.9111111111111110938, 0.9138888888888888618, 0.9166666666666666297, 0.9194444444444443976, 0.9222222222222222765, 0.9250000000000000444, 0.9277777777777778123, 0.9305555555555555802, 0.9333333333333333481, 0.9361111111111111160, 0.9388888888888888840, 0.9416666666666666519, 0.9444444444444444198, 0.9472222222222221877, 0.9499999999999999556, 0.9527777777777777235, 0.9555555555555556024, 0.9583333333333333703, 0.9611111111111111382, 0.9638888888888889062, 0.9666666666666666741, 0.9694444444444444420, 0.9722222222222222099, 0.9749999999999999778, 0.9777777777777777457, 0.9805555555555555136, 0.9833333333333332815, 0.9861111111111111605, 0.9888888888888889284, 0.9916666666666666963, 0.9944444444444444642, 0.9972222222222222321, 1.000000000000000000 ),
 .UNSPECIFIED. ) 
 GEOMETRIC_REPRESENTATION_ITEM ( )  RATIONAL_B_SPLINE_SURFACE ( (
 ( 1.000000000000000000, 0.8660254037844387076, 1.000000000000000000, 0.8660254037844387076, 1.000000000000000000, 0.8660254037844387076, 1.000000000000000000, 0.8660254037844387076, 1.000000000000000000, 0.8660254037844387076, 1.000000000000000000, 0.8660254037844387076, 1.000000000000000000, 0.8660254037844387076, 1.000000000000000000, 0.8660254037844387076, 1.000000000000000000, 0.8660254037844387076, 1.000000000000000000, 0.8660254037844387076, 1.000000000000000000, 0.8660254037844387076, 1.000000000000000000, 0.8660254037844387076, 1.000000000000000000, 0.8660254037844387076, 1.000000000000000000, 0.8660254037844387076, 1.000000000000000000, 0.8660254037844387076, 1.000000000000000000, 0.8660254037844387076, 1.000000000000000000, 0.8660254037844387076, 1.000000000000000000, 0.8660254037844387076, 1.000000000000000000, 0.8660254037844387076, 1.000000000000000000, 0.8660254037844387076, 1.000000000000000000, 0.8660254037844387076, 1.000000000000000000, 0.8660254037844387076, 1.000000000000000000, 0.8660254037844387076, 1.000000000000000000, 0.8660254037844387076, 1.000000000000000000, 0.8660254037844387076, 1.000000000000000000, 0.8660254037844387076, 1.000000000000000000, 0.8660254037844387076, 1.000000000000000000, 0.8660254037844387076, 1.000000000000000000, 0.8660254037844387076, 1.000000000000000000, 0.8660254037844387076, 1.000000000000000000, 0.8660254037844387076, 1.000000000000000000, 0.8660254037844387076, 1.000000000000000000, 0.8660254037844387076, 1.000000000000000000, 0.8660254037844387076, 1.000000000000000000, 0.8660254037844387076, 1.000000000000000000, 0.8660254037844387076, 1.000000000000000000, 0.8660254037844387076, 1.000000000000000000, 0.8660254037844387076, 1.000000000000000000, 0.8660254037844387076, 1.000000000000000000, 0.8660254037844387076, 1.000000000000000000, 0.8660254037844387076, 1.000000000000000000, 0.8660254037844387076, 1.000000000000000000, 0.8660254037844387076, 1.000000000000000000, 0.8660254037844387076, 1.000000000000000000, 0.8660254037844387076, 1.000000000000000000, 0.8660254037844387076, 1.000000000000000000, 0.8660254037844387076, 1.000000000000000000, 0.8660254037844387076, 1.000000000000000000, 0.8660254037844387076, 1.000000000000000000, 0.8660254037844387076, 1.000000000000000000, 0.8660254037844387076, 1.000000000000000000, 0.8660254037844387076, 1.000000000000000000, 0.8660254037844387076, 1.000000000000000000, 0.8660254037844387076, 1.000000000000000000, 0.8660254037844387076, 1.000000000000000000, 0.8660254037844387076, 1.000000000000000000, 0.8660254037844387076, 1.000000000000000000, 0.8660254037844387076, 1.000000000000000000, 0.8660254037844387076, 1.000000000000000000, 0.8660254037844387076, 1.000000000000000000, 0.8660254037844387076, 1.000000000000000000, 0.8660254037844387076, 1.000000000000000000, 0.8660254037844387076, 1.000000000000000000, 0.8660254037844387076, 1.000000000000000000, 0.8660254037844387076, 1.000000000000000000, 0.8660254037844387076, 1.000000000000000000, 0.8660254037844387076, 1.000000000000000000, 0.8660254037844387076, 1.000000000000000000, 0.8660254037844387076, 1.000000000000000000, 0.8660254037844387076, 1.000000000000000000, 0.8660254037844387076, 1.000000000000000000, 0.8660254037844387076, 1.000000000000000000, 0.8660254037844387076, 1.000000000000000000, 0.8660254037844387076, 1.000000000000000000, 0.8660254037844387076, 1.000000000000000000, 0.8660254037844387076, 1.000000000000000000, 0.8660254037844387076, 1.000000000000000000, 0.8660254037844387076, 1.000000000000000000, 0.8660254037844387076, 1.000000000000000000, 0.8660254037844387076, 1.000000000000000000, 0.8660254037844387076, 1.000000000000000000, 0.8660254037844387076, 1.000000000000000000, 0.8660254037844387076, 1.000000000000000000, 0.8660254037844387076, 1.000000000000000000, 0.8660254037844387076, 1.000000000000000000, 0.8660254037844387076, 1.000000000000000000, 0.8660254037844387076, 1.000000000000000000, 0.8660254037844387076, 1.000000000000000000, 0.8660254037844387076, 1.000000000000000000, 0.8660254037844387076, 1.000000000000000000, 0.8660254037844387076, 1.000000000000000000, 0.8660254037844387076, 1.000000000000000000, 0.8660254037844387076, 1.000000000000000000, 0.8660254037844387076, 1.000000000000000000, 0.8660254037844387076, 1.000000000000000000, 0.8660254037844387076, 1.000000000000000000, 0.8660254037844387076, 1.000000000000000000, 0.8660254037844387076, 1.000000000000000000, 0.8660254037844387076, 1.000000000000000000, 0.8660254037844387076, 1.000000000000000000, 0.8660254037844387076, 1.000000000000000000, 0.8660254037844387076, 1.000000000000000000, 0.8660254037844387076, 1.000000000000000000, 0.8660254037844387076, 1.000000000000000000, 0.8660254037844387076, 1.000000000000000000, 0.8660254037844387076, 1.000000000000000000, 0.8660254037844387076, 1.000000000000000000, 0.8660254037844387076, 1.000000000000000000, 0.8660254037844387076, 1.000000000000000000, 0.8660254037844387076, 1.000000000000000000, 0.8660254037844387076, 1.000000000000000000, 0.8660254037844387076, 1.000000000000000000, 0.8660254037844387076, 1.000000000000000000, 0.8660254037844387076, 1.000000000000000000, 0.8660254037844387076, 1.000000000000000000, 0.8660254037844387076, 1.000000000000000000, 0.8660254037844387076, 1.000000000000000000, 0.8660254037844387076, 1.000000000000000000, 0.8660254037844387076, 1.000000000000000000, 0.8660254037844387076, 1.000000000000000000, 0.8660254037844387076, 1.000000000000000000, 0.8660254037844387076, 1.000000000000000000, 0.8660254037844387076, 1.000000000000000000, 0.8660254037844387076, 1.000000000000000000, 0.8660254037844387076, 1.000000000000000000, 0.8660254037844387076, 1.000000000000000000, 0.8660254037844387076, 1.000000000000000000, 0.8660254037844387076, 1.000000000000000000, 0.8660254037844387076, 1.000000000000000000, 0.8660254037844387076, 1.000000000000000000, 0.8660254037844387076, 1.000000000000000000, 0.8660254037844387076, 1.000000000000000000, 0.8660254037844387076, 1.000000000000000000, 0.8660254037844387076, 1.000000000000000000, 0.8660254037844387076, 1.000000000000000000, 0.8660254037844387076, 1.000000000000000000, 0.8660254037844387076, 1.000000000000000000, 0.8660254037844387076, 1.000000000000000000, 0.8660254037844387076, 1.000000000000000000, 0.8660254037844387076, 1.000000000000000000, 0.8660254037844387076, 1.000000000000000000, 0.8660254037844387076, 1.000000000000000000, 0.8660254037844387076, 1.000000000000000000, 0.8660254037844387076, 1.000000000000000000, 0.8660254037844387076, 1.000000000000000000, 0.8660254037844387076, 1.000000000000000000, 0.8660254037844387076, 1.000000000000000000, 0.8660254037844387076, 1.000000000000000000, 0.8660254037844387076, 1.000000000000000000, 0.8660254037844387076, 1.000000000000000000, 0.8660254037844387076, 1.000000000000000000, 0.8660254037844387076, 1.000000000000000000, 0.8660254037844387076, 1.000000000000000000, 0.8660254037844387076, 1.000000000000000000, 0.8660254037844387076, 1.000000000000000000, 0.8660254037844387076, 1.000000000000000000, 0.8660254037844387076, 1.000000000000000000, 0.8660254037844387076, 1.000000000000000000, 0.8660254037844387076, 1.000000000000000000, 0.8660254037844387076, 1.000000000000000000, 0.8660254037844387076, 1.000000000000000000, 0.8660254037844387076, 1.000000000000000000, 0.8660254037844387076, 1.000000000000000000, 0.8660254037844387076, 1.000000000000000000, 0.8660254037844387076, 1.000000000000000000, 0.8660254037844387076, 1.000000000000000000, 0.8660254037844387076, 1.000000000000000000, 0.8660254037844387076, 1.000000000000000000, 0.8660254037844387076, 1.000000000000000000, 0.8660254037844387076, 1.000000000000000000, 0.8660254037844387076, 1.000000000000000000, 0.8660254037844387076, 1.000000000000000000, 0.8660254037844387076, 1.000000000000000000, 0.8660254037844387076, 1.000000000000000000, 0.8660254037844387076, 1.000000000000000000, 0.8660254037844387076, 1.000000000000000000, 0.8660254037844387076, 1.000000000000000000, 0.8660254037844387076, 1.000000000000000000, 0.8660254037844387076, 1.000000000000000000, 0.8660254037844387076, 1.000000000000000000, 0.8660254037844387076, 1.000000000000000000, 0.8660254037844387076, 1.000000000000000000, 0.8660254037844387076, 1.000000000000000000, 0.8660254037844387076, 1.000000000000000000, 0.8660254037844387076, 1.000000000000000000, 0.8660254037844387076, 1.000000000000000000, 0.8660254037844387076, 1.000000000000000000, 0.8660254037844387076, 1.000000000000000000, 0.8660254037844387076, 1.000000000000000000, 0.8660254037844387076, 1.000000000000000000, 0.8660254037844387076, 1.000000000000000000, 0.8660254037844387076, 1.000000000000000000, 0.8660254037844387076, 1.000000000000000000, 0.8660254037844387076, 1.000000000000000000, 0.8660254037844387076, 1.000000000000000000, 0.8660254037844387076, 1.000000000000000000, 0.8660254037844387076, 1.000000000000000000, 0.8660254037844387076, 1.000000000000000000, 0.8660254037844387076, 1.000000000000000000, 0.8660254037844387076, 1.000000000000000000, 0.8660254037844387076, 1.000000000000000000, 0.8660254037844387076, 1.000000000000000000, 0.8660254037844387076, 1.000000000000000000, 0.8660254037844387076, 1.000000000000000000, 0.8660254037844387076, 1.000000000000000000, 0.8660254037844387076, 1.000000000000000000, 0.8660254037844387076, 1.000000000000000000, 0.8660254037844387076, 1.000000000000000000, 0.8660254037844387076, 1.000000000000000000, 0.8660254037844387076, 1.000000000000000000, 0.8660254037844387076, 1.000000000000000000, 0.8660254037844387076, 1.000000000000000000, 0.8660254037844387076, 1.000000000000000000, 0.8660254037844387076, 1.000000000000000000, 0.8660254037844387076, 1.000000000000000000, 0.8660254037844387076, 1.000000000000000000, 0.8660254037844387076, 1.000000000000000000, 0.8660254037844387076, 1.000000000000000000, 0.8660254037844387076, 1.000000000000000000, 0.8660254037844387076, 1.000000000000000000, 0.8660254037844387076, 1.000000000000000000, 0.8660254037844387076, 1.000000000000000000, 0.8660254037844387076, 1.000000000000000000, 0.8660254037844387076, 1.000000000000000000, 0.8660254037844387076, 1.000000000000000000, 0.8660254037844387076, 1.000000000000000000, 0.8660254037844387076, 1.000000000000000000, 0.8660254037844387076, 1.000000000000000000, 0.8660254037844387076, 1.000000000000000000, 0.8660254037844387076, 1.000000000000000000, 0.8660254037844387076, 1.000000000000000000, 0.8660254037844387076, 1.000000000000000000, 0.8660254037844387076, 1.000000000000000000, 0.8660254037844387076, 1.000000000000000000, 0.8660254037844387076, 1.000000000000000000, 0.8660254037844387076, 1.000000000000000000, 0.8660254037844387076, 1.000000000000000000, 0.8660254037844387076, 1.000000000000000000, 0.8660254037844387076, 1.000000000000000000, 0.8660254037844387076, 1.000000000000000000, 0.8660254037844387076, 1.000000000000000000, 0.8660254037844387076, 1.000000000000000000, 0.8660254037844387076, 1.000000000000000000, 0.8660254037844387076, 1.000000000000000000, 0.8660254037844387076, 1.000000000000000000, 0.8660254037844387076, 1.000000000000000000, 0.8660254037844387076, 1.000000000000000000, 0.8660254037844387076, 1.000000000000000000, 0.8660254037844387076, 1.000000000000000000, 0.8660254037844387076, 1.000000000000000000, 0.8660254037844387076, 1.000000000000000000, 0.8660254037844387076, 1.000000000000000000, 0.8660254037844387076, 1.000000000000000000, 0.8660254037844387076, 1.000000000000000000, 0.8660254037844387076, 1.000000000000000000, 0.8660254037844387076, 1.000000000000000000, 0.8660254037844387076, 1.000000000000000000, 0.8660254037844387076, 1.000000000000000000, 0.8660254037844387076, 1.000000000000000000, 0.8660254037844387076, 1.000000000000000000, 0.8660254037844387076, 1.000000000000000000, 0.8660254037844387076, 1.000000000000000000, 0.8660254037844387076, 1.000000000000000000, 0.8660254037844387076, 1.000000000000000000, 0.8660254037844387076, 1.000000000000000000, 0.8660254037844387076, 1.000000000000000000, 0.8660254037844387076, 1.000000000000000000, 0.8660254037844387076, 1.000000000000000000, 0.8660254037844387076, 1.000000000000000000, 0.8660254037844387076, 1.000000000000000000, 0.8660254037844387076, 1.000000000000000000, 0.8660254037844387076, 1.000000000000000000, 0.8660254037844387076, 1.000000000000000000, 0.8660254037844387076, 1.000000000000000000, 0.8660254037844387076, 1.000000000000000000, 0.8660254037844387076, 1.000000000000000000, 0.8660254037844387076, 1.000000000000000000, 0.8660254037844387076, 1.000000000000000000, 0.8660254037844387076, 1.000000000000000000, 0.8660254037844387076, 1.000000000000000000, 0.8660254037844387076, 1.000000000000000000, 0.8660254037844387076, 1.000000000000000000, 0.8660254037844387076, 1.000000000000000000, 0.8660254037844387076, 1.000000000000000000, 0.8660254037844387076, 1.000000000000000000, 0.8660254037844387076, 1.000000000000000000, 0.8660254037844387076, 1.000000000000000000, 0.8660254037844387076, 1.000000000000000000, 0.8660254037844387076, 1.000000000000000000, 0.8660254037844387076, 1.000000000000000000, 0.8660254037844387076, 1.000000000000000000, 0.8660254037844387076, 1.000000000000000000, 0.8660254037844387076, 1.000000000000000000, 0.8660254037844387076, 1.000000000000000000, 0.8660254037844387076, 1.000000000000000000, 0.8660254037844387076, 1.000000000000000000, 0.8660254037844387076, 1.000000000000000000, 0.8660254037844387076, 1.000000000000000000, 0.8660254037844387076, 1.000000000000000000, 0.8660254037844387076, 1.000000000000000000, 0.8660254037844387076, 1.000000000000000000, 0.8660254037844387076, 1.000000000000000000, 0.8660254037844387076, 1.000000000000000000, 0.8660254037844387076, 1.000000000000000000, 0.8660254037844387076, 1.000000000000000000, 0.8660254037844387076, 1.000000000000000000, 0.8660254037844387076, 1.000000000000000000, 0.8660254037844387076, 1.000000000000000000, 0.8660254037844387076, 1.000000000000000000, 0.8660254037844387076, 1.000000000000000000, 0.8660254037844387076, 1.000000000000000000, 0.8660254037844387076, 1.000000000000000000, 0.8660254037844387076, 1.000000000000000000, 0.8660254037844387076, 1.000000000000000000, 0.8660254037844387076, 1.000000000000000000, 0.8660254037844387076, 1.000000000000000000, 0.8660254037844387076, 1.000000000000000000, 0.8660254037844387076, 1.000000000000000000, 0.8660254037844387076, 1.000000000000000000, 0.8660254037844387076, 1.000000000000000000, 0.8660254037844387076, 1.000000000000000000, 0.8660254037844387076, 1.000000000000000000, 0.8660254037844387076, 1.000000000000000000, 0.8660254037844387076, 1.000000000000000000, 0.8660254037844387076, 1.000000000000000000, 0.8660254037844387076, 1.000000000000000000, 0.8660254037844387076, 1.000000000000000000, 0.8660254037844387076, 1.000000000000000000, 0.8660254037844387076, 1.000000000000000000, 0.8660254037844387076, 1.000000000000000000, 0.8660254037844387076, 1.000000000000000000, 0.8660254037844387076, 1.000000000000000000, 0.8660254037844387076, 1.000000000000000000, 0.8660254037844387076, 1.000000000000000000, 0.8660254037844387076, 1.000000000000000000, 0.8660254037844387076, 1.000000000000000000, 0.8660254037844387076, 1.000000000000000000, 0.8660254037844387076, 1.000000000000000000, 0.8660254037844387076, 1.000000000000000000, 0.8660254037844387076, 1.000000000000000000, 0.8660254037844387076, 1.000000000000000000, 0.8660254037844387076, 1.000000000000000000, 0.8660254037844387076, 1.000000000000000000, 0.8660254037844387076, 1.000000000000000000, 0.8660254037844387076, 1.000000000000000000, 0.8660254037844387076, 1.000000000000000000, 0.8660254037844387076, 1.000000000000000000, 0.8660254037844387076, 1.000000000000000000, 0.8660254037844387076, 1.000000000000000000, 0.8660254037844387076, 1.000000000000000000, 0.8660254037844387076, 1.000000000000000000, 0.8660254037844387076, 1.000000000000000000, 0.8660254037844387076, 1.000000000000000000, 0.8660254037844387076, 1.000000000000000000, 0.8660254037844387076, 1.000000000000000000, 0.8660254037844387076, 1.000000000000000000, 0.8660254037844387076, 1.000000000000000000, 0.8660254037844387076, 1.000000000000000000, 0.8660254037844387076, 1.000000000000000000, 0.8660254037844387076, 1.000000000000000000),
 ( 1.000000000000000000, 0.8660254037844387076, 1.000000000000000000, 0.8660254037844387076, 1.000000000000000000, 0.8660254037844387076, 1.000000000000000000, 0.8660254037844387076, 1.000000000000000000, 0.8660254037844387076, 1.000000000000000000, 0.8660254037844387076, 1.000000000000000000, 0.8660254037844387076, 1.000000000000000000, 0.8660254037844387076, 1.000000000000000000, 0.8660254037844387076, 1.000000000000000000, 0.8660254037844387076, 1.000000000000000000, 0.8660254037844387076, 1.000000000000000000, 0.8660254037844387076, 1.000000000000000000, 0.8660254037844387076, 1.000000000000000000, 0.8660254037844387076, 1.000000000000000000, 0.8660254037844387076, 1.000000000000000000, 0.8660254037844387076, 1.000000000000000000, 0.8660254037844387076, 1.000000000000000000, 0.8660254037844387076, 1.000000000000000000, 0.8660254037844387076, 1.000000000000000000, 0.8660254037844387076, 1.000000000000000000, 0.8660254037844387076, 1.000000000000000000, 0.8660254037844387076, 1.000000000000000000, 0.8660254037844387076, 1.000000000000000000, 0.8660254037844387076, 1.000000000000000000, 0.8660254037844387076, 1.000000000000000000, 0.8660254037844387076, 1.000000000000000000, 0.8660254037844387076, 1.000000000000000000, 0.8660254037844387076, 1.000000000000000000, 0.8660254037844387076, 1.000000000000000000, 0.8660254037844387076, 1.000000000000000000, 0.8660254037844387076, 1.000000000000000000, 0.8660254037844387076, 1.000000000000000000, 0.8660254037844387076, 1.000000000000000000, 0.8660254037844387076, 1.000000000000000000, 0.8660254037844387076, 1.000000000000000000, 0.8660254037844387076, 1.000000000000000000, 0.8660254037844387076, 1.000000000000000000, 0.8660254037844387076, 1.000000000000000000, 0.8660254037844387076, 1.000000000000000000, 0.8660254037844387076, 1.000000000000000000, 0.8660254037844387076, 1.000000000000000000, 0.8660254037844387076, 1.000000000000000000, 0.8660254037844387076, 1.000000000000000000, 0.8660254037844387076, 1.000000000000000000, 0.8660254037844387076, 1.000000000000000000, 0.8660254037844387076, 1.000000000000000000, 0.8660254037844387076, 1.000000000000000000, 0.8660254037844387076, 1.000000000000000000, 0.8660254037844387076, 1.000000000000000000, 0.8660254037844387076, 1.000000000000000000, 0.8660254037844387076, 1.000000000000000000, 0.8660254037844387076, 1.000000000000000000, 0.8660254037844387076, 1.000000000000000000, 0.8660254037844387076, 1.000000000000000000, 0.8660254037844387076, 1.000000000000000000, 0.8660254037844387076, 1.000000000000000000, 0.8660254037844387076, 1.000000000000000000, 0.8660254037844387076, 1.000000000000000000, 0.8660254037844387076, 1.000000000000000000, 0.8660254037844387076, 1.000000000000000000, 0.8660254037844387076, 1.000000000000000000, 0.8660254037844387076, 1.000000000000000000, 0.8660254037844387076, 1.000000000000000000, 0.8660254037844387076, 1.000000000000000000, 0.8660254037844387076, 1.000000000000000000, 0.8660254037844387076, 1.000000000000000000, 0.8660254037844387076, 1.000000000000000000, 0.8660254037844387076, 1.000000000000000000, 0.8660254037844387076, 1.000000000000000000, 0.8660254037844387076, 1.000000000000000000, 0.8660254037844387076, 1.000000000000000000, 0.8660254037844387076, 1.000000000000000000, 0.8660254037844387076, 1.000000000000000000, 0.8660254037844387076, 1.000000000000000000, 0.8660254037844387076, 1.000000000000000000, 0.8660254037844387076, 1.000000000000000000, 0.8660254037844387076, 1.000000000000000000, 0.8660254037844387076, 1.000000000000000000, 0.8660254037844387076, 1.000000000000000000, 0.8660254037844387076, 1.000000000000000000, 0.8660254037844387076, 1.000000000000000000, 0.8660254037844387076, 1.000000000000000000, 0.8660254037844387076, 1.000000000000000000, 0.8660254037844387076, 1.000000000000000000, 0.8660254037844387076, 1.000000000000000000, 0.8660254037844387076, 1.000000000000000000, 0.8660254037844387076, 1.000000000000000000, 0.8660254037844387076, 1.000000000000000000, 0.8660254037844387076, 1.000000000000000000, 0.8660254037844387076, 1.000000000000000000, 0.8660254037844387076, 1.000000000000000000, 0.8660254037844387076, 1.000000000000000000, 0.8660254037844387076, 1.000000000000000000, 0.8660254037844387076, 1.000000000000000000, 0.8660254037844387076, 1.000000000000000000, 0.8660254037844387076, 1.000000000000000000, 0.8660254037844387076, 1.000000000000000000, 0.8660254037844387076, 1.000000000000000000, 0.8660254037844387076, 1.000000000000000000, 0.8660254037844387076, 1.000000000000000000, 0.8660254037844387076, 1.000000000000000000, 0.8660254037844387076, 1.000000000000000000, 0.8660254037844387076, 1.000000000000000000, 0.8660254037844387076, 1.000000000000000000, 0.8660254037844387076, 1.000000000000000000, 0.8660254037844387076, 1.000000000000000000, 0.8660254037844387076, 1.000000000000000000, 0.8660254037844387076, 1.000000000000000000, 0.8660254037844387076, 1.000000000000000000, 0.8660254037844387076, 1.000000000000000000, 0.8660254037844387076, 1.000000000000000000, 0.8660254037844387076, 1.000000000000000000, 0.8660254037844387076, 1.000000000000000000, 0.8660254037844387076, 1.000000000000000000, 0.8660254037844387076, 1.000000000000000000, 0.8660254037844387076, 1.000000000000000000, 0.8660254037844387076, 1.000000000000000000, 0.8660254037844387076, 1.000000000000000000, 0.8660254037844387076, 1.000000000000000000, 0.8660254037844387076, 1.000000000000000000, 0.8660254037844387076, 1.000000000000000000, 0.8660254037844387076, 1.000000000000000000, 0.8660254037844387076, 1.000000000000000000, 0.8660254037844387076, 1.000000000000000000, 0.8660254037844387076, 1.000000000000000000, 0.8660254037844387076, 1.000000000000000000, 0.8660254037844387076, 1.000000000000000000, 0.8660254037844387076, 1.000000000000000000, 0.8660254037844387076, 1.000000000000000000, 0.8660254037844387076, 1.000000000000000000, 0.8660254037844387076, 1.000000000000000000, 0.8660254037844387076, 1.000000000000000000, 0.8660254037844387076, 1.000000000000000000, 0.8660254037844387076, 1.000000000000000000, 0.8660254037844387076, 1.000000000000000000, 0.8660254037844387076, 1.000000000000000000, 0.8660254037844387076, 1.000000000000000000, 0.8660254037844387076, 1.000000000000000000, 0.8660254037844387076, 1.000000000000000000, 0.8660254037844387076, 1.000000000000000000, 0.8660254037844387076, 1.000000000000000000, 0.8660254037844387076, 1.000000000000000000, 0.8660254037844387076, 1.000000000000000000, 0.8660254037844387076, 1.000000000000000000, 0.8660254037844387076, 1.000000000000000000, 0.8660254037844387076, 1.000000000000000000, 0.8660254037844387076, 1.000000000000000000, 0.8660254037844387076, 1.000000000000000000, 0.8660254037844387076, 1.000000000000000000, 0.8660254037844387076, 1.000000000000000000, 0.8660254037844387076, 1.000000000000000000, 0.8660254037844387076, 1.000000000000000000, 0.8660254037844387076, 1.000000000000000000, 0.8660254037844387076, 1.000000000000000000, 0.8660254037844387076, 1.000000000000000000, 0.8660254037844387076, 1.000000000000000000, 0.8660254037844387076, 1.000000000000000000, 0.8660254037844387076, 1.000000000000000000, 0.8660254037844387076, 1.000000000000000000, 0.8660254037844387076, 1.000000000000000000, 0.8660254037844387076, 1.000000000000000000, 0.8660254037844387076, 1.000000000000000000, 0.8660254037844387076, 1.000000000000000000, 0.8660254037844387076, 1.000000000000000000, 0.8660254037844387076, 1.000000000000000000, 0.8660254037844387076, 1.000000000000000000, 0.8660254037844387076, 1.000000000000000000, 0.8660254037844387076, 1.000000000000000000, 0.8660254037844387076, 1.000000000000000000, 0.8660254037844387076, 1.000000000000000000, 0.8660254037844387076, 1.000000000000000000, 0.8660254037844387076, 1.000000000000000000, 0.8660254037844387076, 1.000000000000000000, 0.8660254037844387076, 1.000000000000000000, 0.8660254037844387076, 1.000000000000000000, 0.8660254037844387076, 1.000000000000000000, 0.8660254037844387076, 1.000000000000000000, 0.8660254037844387076, 1.000000000000000000, 0.8660254037844387076, 1.000000000000000000, 0.8660254037844387076, 1.000000000000000000, 0.8660254037844387076, 1.000000000000000000, 0.8660254037844387076, 1.000000000000000000, 0.8660254037844387076, 1.000000000000000000, 0.8660254037844387076, 1.000000000000000000, 0.8660254037844387076, 1.000000000000000000, 0.8660254037844387076, 1.000000000000000000, 0.8660254037844387076, 1.000000000000000000, 0.8660254037844387076, 1.000000000000000000, 0.8660254037844387076, 1.000000000000000000, 0.8660254037844387076, 1.000000000000000000, 0.8660254037844387076, 1.000000000000000000, 0.8660254037844387076, 1.000000000000000000, 0.8660254037844387076, 1.000000000000000000, 0.8660254037844387076, 1.000000000000000000, 0.8660254037844387076, 1.000000000000000000, 0.8660254037844387076, 1.000000000000000000, 0.8660254037844387076, 1.000000000000000000, 0.8660254037844387076, 1.000000000000000000, 0.8660254037844387076, 1.000000000000000000, 0.8660254037844387076, 1.000000000000000000, 0.8660254037844387076, 1.000000000000000000, 0.8660254037844387076, 1.000000000000000000, 0.8660254037844387076, 1.000000000000000000, 0.8660254037844387076, 1.000000000000000000, 0.8660254037844387076, 1.000000000000000000, 0.8660254037844387076, 1.000000000000000000, 0.8660254037844387076, 1.000000000000000000, 0.8660254037844387076, 1.000000000000000000, 0.8660254037844387076, 1.000000000000000000, 0.8660254037844387076, 1.000000000000000000, 0.8660254037844387076, 1.000000000000000000, 0.8660254037844387076, 1.000000000000000000, 0.8660254037844387076, 1.000000000000000000, 0.8660254037844387076, 1.000000000000000000, 0.8660254037844387076, 1.000000000000000000, 0.8660254037844387076, 1.000000000000000000, 0.8660254037844387076, 1.000000000000000000, 0.8660254037844387076, 1.000000000000000000, 0.8660254037844387076, 1.000000000000000000, 0.8660254037844387076, 1.000000000000000000, 0.8660254037844387076, 1.000000000000000000, 0.8660254037844387076, 1.000000000000000000, 0.8660254037844387076, 1.000000000000000000, 0.8660254037844387076, 1.000000000000000000, 0.8660254037844387076, 1.000000000000000000, 0.8660254037844387076, 1.000000000000000000, 0.8660254037844387076, 1.000000000000000000, 0.8660254037844387076, 1.000000000000000000, 0.8660254037844387076, 1.000000000000000000, 0.8660254037844387076, 1.000000000000000000, 0.8660254037844387076, 1.000000000000000000, 0.8660254037844387076, 1.000000000000000000, 0.8660254037844387076, 1.000000000000000000, 0.8660254037844387076, 1.000000000000000000, 0.8660254037844387076, 1.000000000000000000, 0.8660254037844387076, 1.000000000000000000, 0.8660254037844387076, 1.000000000000000000, 0.8660254037844387076, 1.000000000000000000, 0.8660254037844387076, 1.000000000000000000, 0.8660254037844387076, 1.000000000000000000, 0.8660254037844387076, 1.000000000000000000, 0.8660254037844387076, 1.000000000000000000, 0.8660254037844387076, 1.000000000000000000, 0.8660254037844387076, 1.000000000000000000, 0.8660254037844387076, 1.000000000000000000, 0.8660254037844387076, 1.000000000000000000, 0.8660254037844387076, 1.000000000000000000, 0.8660254037844387076, 1.000000000000000000, 0.8660254037844387076, 1.000000000000000000, 0.8660254037844387076, 1.000000000000000000, 0.8660254037844387076, 1.000000000000000000, 0.8660254037844387076, 1.000000000000000000, 0.8660254037844387076, 1.000000000000000000, 0.8660254037844387076, 1.000000000000000000, 0.8660254037844387076, 1.000000000000000000, 0.8660254037844387076, 1.000000000000000000, 0.8660254037844387076, 1.000000000000000000, 0.8660254037844387076, 1.000000000000000000, 0.8660254037844387076, 1.000000000000000000, 0.8660254037844387076, 1.000000000000000000, 0.8660254037844387076, 1.000000000000000000, 0.8660254037844387076, 1.000000000000000000, 0.8660254037844387076, 1.000000000000000000, 0.8660254037844387076, 1.000000000000000000, 0.8660254037844387076, 1.000000000000000000, 0.8660254037844387076, 1.000000000000000000, 0.8660254037844387076, 1.000000000000000000, 0.8660254037844387076, 1.000000000000000000, 0.8660254037844387076, 1.000000000000000000, 0.8660254037844387076, 1.000000000000000000, 0.8660254037844387076, 1.000000000000000000, 0.8660254037844387076, 1.000000000000000000, 0.8660254037844387076, 1.000000000000000000, 0.8660254037844387076, 1.000000000000000000, 0.8660254037844387076, 1.000000000000000000, 0.8660254037844387076, 1.000000000000000000, 0.8660254037844387076, 1.000000000000000000, 0.8660254037844387076, 1.000000000000000000, 0.8660254037844387076, 1.000000000000000000, 0.8660254037844387076, 1.000000000000000000, 0.8660254037844387076, 1.000000000000000000, 0.8660254037844387076, 1.000000000000000000, 0.8660254037844387076, 1.000000000000000000, 0.8660254037844387076, 1.000000000000000000, 0.8660254037844387076, 1.000000000000000000, 0.8660254037844387076, 1.000000000000000000, 0.8660254037844387076, 1.000000000000000000, 0.8660254037844387076, 1.000000000000000000, 0.8660254037844387076, 1.000000000000000000, 0.8660254037844387076, 1.000000000000000000, 0.8660254037844387076, 1.000000000000000000, 0.8660254037844387076, 1.000000000000000000, 0.8660254037844387076, 1.000000000000000000, 0.8660254037844387076, 1.000000000000000000, 0.8660254037844387076, 1.000000000000000000, 0.8660254037844387076, 1.000000000000000000, 0.8660254037844387076, 1.000000000000000000, 0.8660254037844387076, 1.000000000000000000, 0.8660254037844387076, 1.000000000000000000, 0.8660254037844387076, 1.000000000000000000, 0.8660254037844387076, 1.000000000000000000, 0.8660254037844387076, 1.000000000000000000, 0.8660254037844387076, 1.000000000000000000, 0.8660254037844387076, 1.000000000000000000, 0.8660254037844387076, 1.000000000000000000, 0.8660254037844387076, 1.000000000000000000, 0.8660254037844387076, 1.000000000000000000, 0.8660254037844387076, 1.000000000000000000, 0.8660254037844387076, 1.000000000000000000, 0.8660254037844387076, 1.000000000000000000, 0.8660254037844387076, 1.000000000000000000, 0.8660254037844387076, 1.000000000000000000, 0.8660254037844387076, 1.000000000000000000, 0.8660254037844387076, 1.000000000000000000, 0.8660254037844387076, 1.000000000000000000, 0.8660254037844387076, 1.000000000000000000, 0.8660254037844387076, 1.000000000000000000, 0.8660254037844387076, 1.000000000000000000, 0.8660254037844387076, 1.000000000000000000, 0.8660254037844387076, 1.000000000000000000, 0.8660254037844387076, 1.000000000000000000, 0.8660254037844387076, 1.000000000000000000, 0.8660254037844387076, 1.000000000000000000, 0.8660254037844387076, 1.000000000000000000, 0.8660254037844387076, 1.000000000000000000, 0.8660254037844387076, 1.000000000000000000, 0.8660254037844387076, 1.000000000000000000, 0.8660254037844387076, 1.000000000000000000, 0.8660254037844387076, 1.000000000000000000, 0.8660254037844387076, 1.000000000000000000, 0.8660254037844387076, 1.000000000000000000, 0.8660254037844387076, 1.000000000000000000, 0.8660254037844387076, 1.000000000000000000, 0.8660254037844387076, 1.000000000000000000, 0.8660254037844387076, 1.000000000000000000, 0.8660254037844387076, 1.000000000000000000, 0.8660254037844387076, 1.000000000000000000, 0.8660254037844387076, 1.000000000000000000, 0.8660254037844387076, 1.000000000000000000, 0.8660254037844387076, 1.000000000000000000, 0.8660254037844387076, 1.000000000000000000, 0.8660254037844387076, 1.000000000000000000, 0.8660254037844387076, 1.000000000000000000, 0.8660254037844387076, 1.000000000000000000, 0.8660254037844387076, 1.000000000000000000, 0.8660254037844387076, 1.000000000000000000, 0.8660254037844387076, 1.000000000000000000, 0.8660254037844387076, 1.000000000000000000, 0.8660254037844387076, 1.000000000000000000, 0.8660254037844387076, 1.000000000000000000, 0.8660254037844387076, 1.000000000000000000, 0.8660254037844387076, 1.000000000000000000, 0.8660254037844387076, 1.000000000000000000, 0.8660254037844387076, 1.000000000000000000, 0.8660254037844387076, 1.000000000000000000, 0.8660254037844387076, 1.000000000000000000, 0.8660254037844387076, 1.000000000000000000, 0.8660254037844387076, 1.000000000000000000, 0.8660254037844387076, 1.000000000000000000, 0.8660254037844387076, 1.000000000000000000) ) ) 
 REPRESENTATION_ITEM ( '' )  SURFACE ( )  );
#1842=CARTESIAN_POINT ( 'NONE',  ( 15.03749999999999964, 5.773502691896255534, 3.535250795749688894E-16 ) ) ;
#1843=CARTESIAN_POINT ( 'NONE',  ( 4.243569643749999898, 10.12812500061451715, 30.00000000000000000 ) ) ;
#1844=CARTESIAN_POINT ( 'NONE',  ( 14.77500000122903501, 2.886751345948126879, 4.999999999999999112 ) ) ;
#1845=CARTESIAN_POINT ( 'NONE',  ( 24.49687500061451573, -3.027376345333614438, 5.243569643749998122 ) ) ;
#1847=CARTESIAN_POINT ( 'NONE',  ( 20.39062500061451644, -3.027376345333614438, 5.243569643749998122 ) ) ;
#1848=CARTESIAN_POINT ( 'NONE',  ( 19.73437500061451644, 6.421520780324663323E-16, -5.243569643749999010 ) ) ;
#1849=CARTESIAN_POINT ( 'NONE',  ( 4.949999999999999289, -4.330127018922190985, -2.500000000000001332 ) ) ;
#1850=CARTESIAN_POINT ( 'NONE',  ( 8.240625000614516082, -3.027376345333614438, 5.243569643749998122 ) ) ;
#1851=CARTESIAN_POINT ( 'NONE',  ( 21.92812500061451431, 6.421520780324663323E-16, -5.243569643749999010 ) ) ;
#1853=CARTESIAN_POINT ( 'NONE',  ( 15.75937500061451857, 4.541064518000418104, -2.621784821874998173 ) ) ;
#1854=CARTESIAN_POINT ( 'NONE',  ( 4.243569643749999898, 14.59062500061451750, 32.45002607614398471 ) ) ;
#1855=CARTESIAN_POINT ( 'NONE',  ( 18.63750000122903216, 6.123233995736764310E-16, -4.999999999999998224 ) ) ;
#1857=CARTESIAN_POINT ( 'NONE',  ( 8.353125000614518569, -4.541064518000417216, -2.621784821875001281 ) ) ;
#1858=CARTESIAN_POINT ( 'NONE',  ( 13.79999999999999893, 0.000000000000000000, 4.999999999999998224 ) ) ;
#1859=CARTESIAN_POINT ( 'NONE',  ( 3.084375000614519191, 6.421520780324663323E-16, -5.243569643749999010 ) ) ;
#1860=CARTESIAN_POINT ( 'NONE',  ( 25.47187500061451715, -6.054752690667223547, -1.112240025338166033E-15 ) ) ;
#1861=CARTESIAN_POINT ( 'NONE',  ( 15.32812500061451644, 4.541064518000418104, 2.621784821874999949 ) ) ;
#1862=CARTESIAN_POINT ( 'NONE',  ( 25.87500000122903288, 2.886751345948129099, -4.999999999999998224 ) ) ;
#1863=( BOUNDED_CURVE ( )  B_SPLINE_CURVE ( 2, ( #55253, #66705, #16078, #38627, #33075, #27911, #61151, #10546, #65962 ),
 .UNSPECIFIED., .F., .F. ) 
 B_SPLINE_CURVE_WITH_KNOTS ( ( 3, 2, 2, 2, 3 ),
 ( 0.1847826086956521896, 0.1884057971014492794, 0.1956521739130434867, 0.2028985507246376940, 0.2065217391304347838 ),
 .UNSPECIFIED. ) 
 CURVE ( )  GEOMETRIC_REPRESENTATION_ITEM ( )  RATIONAL_B_SPLINE_CURVE ( ( 0.9330127018922194093, 0.9330127018922196314, 1.000000000000000000, 0.8660254037844387076, 1.000000000000000000, 0.8660254037844387076, 1.000000000000000000, 0.9330127018922194093, 0.9330127018922194093 ) ) 
 REPRESENTATION_ITEM ( '' )  );
#1864=CARTESIAN_POINT ( 'NONE',  ( 25.97812500061451502, 6.421520780324663323E-16, -5.243569643749999010 ) ) ;
#1865=CARTESIAN_POINT ( 'NONE',  ( 20.89687500061452141, -3.027376345333614438, 5.243569643749998122 ) ) ;
#1866=CARTESIAN_POINT ( 'NONE',  ( 15.32812500061451644, 4.541064518000418104, 2.621784821874999949 ) ) ;
#1867=CARTESIAN_POINT ( 'NONE',  ( 9.001249775931846008E-16, 18.17187500061451999, 34.90005215228797653 ) ) ;
#1868=CARTESIAN_POINT ( 'NONE',  ( 21.59062500061451928, 6.054752690667223547, 3.707466751127219781E-16 ) ) ;
#1869=DIRECTION ( 'NONE',  ( -0.000000000000000000, -1.000000000000000000, -0.000000000000000000 ) ) ;
#1870=VERTEX_POINT ( 'NONE', #51407 ) ;
#1871=CARTESIAN_POINT ( 'NONE',  ( 25.72499999999999787, 6.123233995736764310E-16, -4.999999999999998224 ) ) ;
#1872=CARTESIAN_POINT ( 'NONE',  ( 8.484601909799253346E-16, 12.46250000000000213, -25.38119784648299770 ) ) ;
#1874=CARTESIAN_POINT ( 'NONE',  ( 28.75312500061451715, 4.541064518000418104, -2.621784821874998173 ) ) ;
#1875=CARTESIAN_POINT ( 'NONE',  ( 8.240625000614516082, -3.027376345333614438, 5.243569643749998122 ) ) ;
#1876=CARTESIAN_POINT ( 'NONE',  ( 21.03750000122903074, 4.330127018922191873, 2.499999999999999556 ) ) ;
#1878=CARTESIAN_POINT ( 'NONE',  ( 27.29062500061451502, -3.027376345333610441, -5.243569643749999898 ) ) ;
#1879=CARTESIAN_POINT ( 'NONE',  ( 25.53750000000000142, -2.886751345948129988, 4.999999999999997335 ) ) ;
#1880=CARTESIAN_POINT ( 'NONE',  ( 1.999999999999998668, 16.36250000122903359, -33.46410161513775705 ) ) ;
#1881=CARTESIAN_POINT ( 'NONE',  ( 11.27812500061451573, 4.541064518000418104, 2.621784821874999949 ) ) ;
#1882=ORIENTED_EDGE ( 'NONE', *, *, #22378, .F. ) ;
#1884=CARTESIAN_POINT ( 'NONE',  ( 25.60312500061451502, 4.541064518000418104, -2.621784821874998173 ) ) ;
#1885=CARTESIAN_POINT ( 'NONE',  ( 7.340625000614518392, -3.027376345333614438, 5.243569643749998122 ) ) ;
#1888=CARTESIAN_POINT ( 'NONE',  ( 3.290625000614516793, -3.027376345333614438, 5.243569643749998122 ) ) ;
#1890=CARTESIAN_POINT ( 'NONE',  ( 17.85000000122903430, 5.773502691896255534, 3.535250795749688401E-16 ) ) ;
#1891=CARTESIAN_POINT ( 'NONE',  ( 13.01249999999999929, -5.773502691896255534, -1.060575238724906372E-15 ) ) ;
#1892=EDGE_CURVE ( 'NONE', #44258, #8626, #72202, .T. ) ;
#1893=CARTESIAN_POINT ( 'NONE',  ( 14.37187500061451928, 3.027376345333613106, -5.243569643749998122 ) ) ;
#1894=CARTESIAN_POINT ( 'NONE',  ( 8.962500001229033231, 0.000000000000000000, 4.999999999999998224 ) ) ;
#1895=CARTESIAN_POINT ( 'NONE',  ( 15.98437500061451821, -4.541064518000419881, 2.621784821874995952 ) ) ;
#1897=CARTESIAN_POINT ( 'NONE',  ( 9.421875000614519990, 3.027376345333613106, -5.243569643749998122 ) ) ;
#1898=CARTESIAN_POINT ( 'NONE',  ( -4.243569643749997233, 12.19062500061451715, -27.54997392385601174 ) ) ;
#1899=CARTESIAN_POINT ( 'NONE',  ( 1.071796769724491893, 16.53259618943233278, 33.99999999999999289 ) ) ;
#1901=CARTESIAN_POINT ( 'NONE',  ( 30.00000000000000000, 0.000000000000000000, 0.000000000000000000 ) ) ;
#1902=CARTESIAN_POINT ( 'NONE',  ( 24.36562500061451786, 3.027376345333611329, 5.243569643749999010 ) ) ;
#1903=CARTESIAN_POINT ( 'NONE',  ( -1.999999999999997113, 17.48750000122903359, 33.46410161513775705 ) ) ;
#1904=CARTESIAN_POINT ( 'NONE',  ( 29.44687500061451857, -3.027376345333614438, 5.243569643749998122 ) ) ;
#1905=CARTESIAN_POINT ( 'NONE',  ( 22.05000000000000071, -4.330127018922190985, -2.500000000000001332 ) ) ;
#1906=CARTESIAN_POINT ( 'NONE',  ( 6.440625000614517148, -3.027376345333614438, 5.243569643749998122 ) ) ;
#1908=CARTESIAN_POINT ( 'NONE',  ( 16.35937500061451644, 0.000000000000000000, 5.243569643749999010 ) ) ;
#1910=AXIS2_PLACEMENT_3D ( 'NONE', #26304, #64724, #37013 ) ;
#1911=CARTESIAN_POINT ( 'NONE',  ( 3.253125000614518036, 0.000000000000000000, 5.243569643749999010 ) ) ;
#1912=CARTESIAN_POINT ( 'NONE',  ( 7.921875000614517326, -6.054752690667223547, -1.112240025338166033E-15 ) ) ;
#1913=ORIENTED_EDGE ( 'NONE', *, *, #7167, .T. ) ;
#1914=CARTESIAN_POINT ( 'NONE',  ( 18.23437500061451999, -4.541064518000419881, 2.621784821874995952 ) ) ;
#1916=CARTESIAN_POINT ( 'NONE',  ( 26.39999999999999858, 0.000000000000000000, 4.999999999999998224 ) ) ;
#1917=CARTESIAN_POINT ( 'NONE',  ( 28.43437500061451573, 4.541064518000418104, 2.621784821874999949 ) ) ;
#1920=CARTESIAN_POINT ( 'NONE',  ( 10.01250000000000107, 2.886751345948129099, -4.999999999999998224 ) ) ;
#1922=CARTESIAN_POINT ( 'NONE',  ( 23.42812500061451786, 4.541064518000418104, 2.621784821874999949 ) ) ;
#1923=CARTESIAN_POINT ( 'NONE',  ( 14.66249999999999964, 2.886751345948126879, 4.999999999999999112 ) ) ;
#1924=CARTESIAN_POINT ( 'NONE',  ( 8.512500001229033941, 0.000000000000000000, 4.999999999999998224 ) ) ;
#1925=CARTESIAN_POINT ( 'NONE',  ( 6.253125000614517148, 4.541064518000418104, -2.621784821874998173 ) ) ;
#1926=CARTESIAN_POINT ( 'NONE',  ( 20.88749999999999929, 5.773502691896255534, 3.535250795749688894E-16 ) ) ;
#1927=CARTESIAN_POINT ( 'NONE',  ( 19.82812500061451644, 4.541064518000418104, 2.621784821874999949 ) ) ;
#1928=CARTESIAN_POINT ( 'NONE',  ( 4.866723945449144217, 3.205296881438017387, 4.448262948007274176 ) ) ;
#1929=CARTESIAN_POINT ( 'NONE',  ( 24.67500000122903359, 2.886751345948126879, 4.999999999999999112 ) ) ;
#1931=CARTESIAN_POINT ( 'NONE',  ( 5.737499999999998934, -2.886751345948129988, 4.999999999999997335 ) ) ;
#1932=ORIENTED_EDGE ( 'NONE', *, *, #20120, .T. ) ;
#1933=CARTESIAN_POINT ( 'NONE',  ( 22.15312500061451573, 0.000000000000000000, 5.243569643749999010 ) ) ;
#1934=CARTESIAN_POINT ( 'NONE',  ( 26.87812500061451360, 6.421520780324663323E-16, -5.243569643749999010 ) ) ;
#1935=CARTESIAN_POINT ( 'NONE',  ( 27.64687500061452141, -3.027376345333614438, 5.243569643749998122 ) ) ;
#1936=CARTESIAN_POINT ( 'NONE',  ( 15.47812500061451679, -4.541064518000419881, 2.621784821874995952 ) ) ;
#1937=CARTESIAN_POINT ( 'NONE',  ( 4.804181228667060211, 1.395135997737601663, -4.980880193036001380 ) ) ;
#1938=CARTESIAN_POINT ( 'NONE',  ( 25.53750000122903074, 4.330127018922191873, 2.499999999999999556 ) ) ;
#1940=CARTESIAN_POINT ( 'NONE',  ( 16.37812500061451715, -4.541064518000419881, 2.621784821874995952 ) ) ;
#1941=CARTESIAN_POINT ( 'NONE',  ( 3.999999999999998668, 14.52500000122903323, -32.30940107675850470 ) ) ;
#1942=CARTESIAN_POINT ( 'NONE',  ( 5.925000001229033586, -5.773502691896255534, -1.060575238724906372E-15 ) ) ;
#1943=CARTESIAN_POINT ( 'NONE',  ( 10.43437500061451750, 4.541064518000418104, 2.621784821874999949 ) ) ;
#1944=CARTESIAN_POINT ( 'NONE',  ( 9.609375000614518214, 0.000000000000000000, 5.243569643749999010 ) ) ;
#1945=CARTESIAN_POINT ( 'NONE',  ( 19.73437500061451644, 6.421520780324663323E-16, -5.243569643749999010 ) ) ;
#1946=EDGE_LOOP ( 'NONE', ( #50933, #40270, #7996, #53284, #61619, #7313, #13137, #57510 ) ) ;
#1947=CARTESIAN_POINT ( 'NONE',  ( -3.980704297455874840, 9.178376072143944242, 25.49448230662654780 ) ) ;
#1948=CARTESIAN_POINT ( 'NONE',  ( 25.30312500061451431, 0.000000000000000000, 5.243569643749999010 ) ) ;
#1949=CARTESIAN_POINT ( 'NONE',  ( 18.75937500061451857, -4.541064518000417216, -2.621784821875001281 ) ) ;
#1950=CARTESIAN_POINT ( 'NONE',  ( 20.99062500061451431, -3.027376345333610441, -5.243569643749999898 ) ) ;
#1951=CARTESIAN_POINT ( 'NONE',  ( -2.556497649636125342E-15, 18.87500000122903288, -26.00000000000000000 ) ) ;
#1952=CARTESIAN_POINT ( 'NONE',  ( -2.000000000000000000, 14.52500000000000036, 26.53589838486224650 ) ) ;
#1953=CARTESIAN_POINT ( 'NONE',  ( 3.121875000614518836, 3.027376345333613106, -5.243569643749998122 ) ) ;
#1954=CARTESIAN_POINT ( 'NONE',  ( 8.625000001229034652, -5.773502691896255534, -1.060575238724906372E-15 ) ) ;
#1955=ORIENTED_EDGE ( 'NONE', *, *, #51760, .T. ) ;
#1956=CARTESIAN_POINT ( 'NONE',  ( 3.562500001229033764, 0.000000000000000000, 4.999999999999998224 ) ) ;
#1957=CARTESIAN_POINT ( 'NONE',  ( -2.000000000000000000, 19.47499999999999787, -33.46410161513775705 ) ) ;
#1958=CARTESIAN_POINT ( 'NONE',  ( 28.35000000122903430, -2.886751345948129988, 4.999999999999997335 ) ) ;
#1960=CARTESIAN_POINT ( 'NONE',  ( 10.65937500061451715, -4.541064518000417216, -2.621784821875001281 ) ) ;
#1961=CARTESIAN_POINT ( 'NONE',  ( 3.999999999999999112, 9.987500001229033586, 30.00000000000000000 ) ) ;
#1962=CARTESIAN_POINT ( 'NONE',  ( 17.95312500061451644, 4.541064518000418104, -2.621784821874998173 ) ) ;
#1963=CARTESIAN_POINT ( 'NONE',  ( 11.22187500061451892, 3.027376345333613106, -5.243569643749998122 ) ) ;
#1964=CARTESIAN_POINT ( 'NONE',  ( 28.80000000122903003, -2.886751345948129988, 4.999999999999997335 ) ) ;
#1965=CARTESIAN_POINT ( 'NONE',  ( 20.63437500061451857, 6.421520780324663323E-16, -5.243569643749999010 ) ) ;
#1966=CARTESIAN_POINT ( 'NONE',  ( 7.134375000614516793, 6.421520780324663323E-16, -5.243569643749999010 ) ) ;
#1967=CARTESIAN_POINT ( 'NONE',  ( 3.999999999999998668, 16.32500000122903216, 27.69059892324149530 ) ) ;
#1968=CARTESIAN_POINT ( 'NONE',  ( 7.640625000614517326, 6.054752690667223547, 3.707466751127219781E-16 ) ) ;
#1969=CARTESIAN_POINT ( 'NONE',  ( 18.81562500061452070, 3.027376345333613106, -5.243569643749998122 ) ) ;
#1970=VERTEX_POINT ( 'NONE', #68042 ) ;
#1972=CARTESIAN_POINT ( 'NONE',  ( 5.550000001229032698, -2.886751345948125991, -5.000000000000000000 ) ) ;
#1973=CARTESIAN_POINT ( 'NONE',  ( 14.80312500061451608, 4.541064518000418104, -2.621784821874998173 ) ) ;
#1974=CARTESIAN_POINT ( 'NONE',  ( 11.12812500061451715, 6.421520780324663323E-16, -5.243569643749999010 ) ) ;
#1976=CARTESIAN_POINT ( 'NONE',  ( 11.36250000000000071, 2.886751345948129099, -4.999999999999998224 ) ) ;
#1977=CARTESIAN_POINT ( 'NONE',  ( 5.400000001229032343, -2.886751345948129988, 4.999999999999997335 ) ) ;
#1978=EDGE_CURVE ( 'NONE', #11117, #72537, #991, .T. ) ;
#1979=CARTESIAN_POINT ( 'NONE',  ( 14.59687500061452070, -3.027376345333614438, 5.243569643749998122 ) ) ;
#1980=CARTESIAN_POINT ( 'NONE',  ( 18.48750000122903359, -4.330127018922194537, 2.499999999999995559 ) ) ;
#1982=CARTESIAN_POINT ( 'NONE',  ( -4.243569643749997233, 18.94062500061451715, -27.54997392385601174 ) ) ;
#1984=CARTESIAN_POINT ( 'NONE',  ( 2.000000000000001332, 10.81250000122903465, -26.53589838486224650 ) ) ;
#1985=CARTESIAN_POINT ( 'NONE',  ( 4.546875000614517326, 6.054752690667223547, 3.707466751127219781E-16 ) ) ;
#1986=CARTESIAN_POINT ( 'NONE',  ( 18.94687500061451502, 6.054752690667223547, 3.707466751127219781E-16 ) ) ;
#1987=FACE_OUTER_BOUND ( 'NONE', #53907, .T. ) ;
#1988=CARTESIAN_POINT ( 'NONE',  ( 13.64062500061451644, -3.027376345333614438, 5.243569643749998122 ) ) ;
#1990=CARTESIAN_POINT ( 'NONE',  ( 1.626862140677534273E-15, 17.52500000122903145, 34.00000000000000000 ) ) ;
#1991=CARTESIAN_POINT ( 'NONE',  ( 23.82187500061451502, 3.027376345333613106, -5.243569643749998122 ) ) ;
#1993=CARTESIAN_POINT ( 'NONE',  ( 11.09062500061451573, -3.027376345333610441, -5.243569643749999898 ) ) ;
#1994=CARTESIAN_POINT ( 'NONE',  ( 15.57187500061451679, -6.054752690667223547, -1.112240025338166033E-15 ) ) ;
#1995=ORIENTED_EDGE ( 'NONE', *, *, #58401, .T. ) ;
#1996=CARTESIAN_POINT ( 'NONE',  ( 26.33437500061451431, -4.541064518000419881, 2.621784821874995952 ) ) ;
#1998=CARTESIAN_POINT ( 'NONE',  ( 26.46562500061451573, 3.027376345333613106, -5.243569643749998122 ) ) ;
#1999=CARTESIAN_POINT ( 'NONE',  ( 19.67812500061451786, 6.421520780324663323E-16, -5.243569643749999010 ) ) ;
#2000=CARTESIAN_POINT ( 'NONE',  ( 28.94062500061452070, -3.027376345333614438, 5.243569643749998122 ) ) ;
#2001=FACE_OUTER_BOUND ( 'NONE', #10841, .T. ) ;
#2002=CARTESIAN_POINT ( 'NONE',  ( 8.849999999999999645, 0.000000000000000000, 4.999999999999998224 ) ) ;
#2003=CARTESIAN_POINT ( 'NONE',  ( 19.87500000122903288, -5.773502691896255534, -1.060575238724906372E-15 ) ) ;
#2005=ORIENTED_EDGE ( 'NONE', *, *, #60921, .F. ) ;
#2006=CARTESIAN_POINT ( 'NONE',  ( 17.21249999999999858, 2.886751345948129099, -4.999999999999998224 ) ) ;
#2007=CARTESIAN_POINT ( 'NONE',  ( 20.28750000000000142, -2.886751345948125991, -5.000000000000000000 ) ) ;
#2008=CARTESIAN_POINT ( 'NONE',  ( 18.87187500061451573, 3.027376345333613106, -5.243569643749998122 ) ) ;
#2009=CARTESIAN_POINT ( 'NONE',  ( 12.85312500061451502, -4.541064518000417216, -2.621784821875001281 ) ) ;
#2012=CARTESIAN_POINT ( 'NONE',  ( 4.828125000614518214, 6.421520780324663323E-16, -5.243569643749999010 ) ) ;
#2013=CARTESIAN_POINT ( 'NONE',  ( 3.144856541311010556, 3.887142566792906706, -3.519253510942787599 ) ) ;
#2014=CARTESIAN_POINT ( 'NONE',  ( 11.40000000000000036, 4.330127018922192761, -2.499999999999997780 ) ) ;
#2016=CARTESIAN_POINT ( 'NONE',  ( -4.243569643749997233, 15.34062500061451750, 32.45002607614398471 ) ) ;
#2017=CARTESIAN_POINT ( 'NONE',  ( 28.56562500061451715, -6.054752690667223547, -1.112240025338166033E-15 ) ) ;
#2020=CARTESIAN_POINT ( 'NONE',  ( 24.19687500061451857, -3.027376345333610441, -5.243569643749999898 ) ) ;
#2022=CARTESIAN_POINT ( 'NONE',  ( 22.22812500061451502, -4.541064518000419881, 2.621784821874995952 ) ) ;
#2023=CARTESIAN_POINT ( 'NONE',  ( 23.59687500061451715, -3.027376345333614438, 5.243569643749998122 ) ) ;
#2024=CARTESIAN_POINT ( 'NONE',  ( -3.000416591977282496E-16, 16.09062500061459744, -34.90005215228797653 ) ) ;
#2025=CARTESIAN_POINT ( 'NONE',  ( 6.890625000614516438, -3.027376345333614438, 5.243569643749998122 ) ) ;
#2027=CARTESIAN_POINT ( 'NONE',  ( 24.96562500061451217, -6.054752690667223547, -1.112240025338166033E-15 ) ) ;
#2030=CARTESIAN_POINT ( 'NONE',  ( 18.00937500061451502, 4.541064518000418104, -2.621784821874998173 ) ) ;
#2031=CARTESIAN_POINT ( 'NONE',  ( 27.79687500061451999, -3.027376345333610441, -5.243569643749999898 ) ) ;
#2032=CARTESIAN_POINT ( 'NONE',  ( -4.243569643749999898, 17.12187500061451573, 27.54997392385601529 ) ) ;
#2033=CARTESIAN_POINT ( 'NONE',  ( 7.940625000614518036, -3.027376345333610441, -5.243569643749999898 ) ) ;
#2034=CARTESIAN_POINT ( 'NONE',  ( 1.999999999999998668, 16.25000000000000000, 26.53589838486224650 ) ) ;
#2035=CARTESIAN_POINT ( 'NONE',  ( 4.359375000614517326, -4.541064518000417216, -2.621784821875001281 ) ) ;
#2036=CARTESIAN_POINT ( 'NONE',  ( 4.311958327294343363, 2.531208285321026263, 4.311958327294242999 ) ) ;
#2037=CARTESIAN_POINT ( 'NONE',  ( 4.003125000614518925, 4.541064518000418104, -2.621784821874998173 ) ) ;
#2038=CARTESIAN_POINT ( 'NONE',  ( 10.54687500061451644, -3.027376345333614438, 5.243569643749998122 ) ) ;
#2039=CARTESIAN_POINT ( 'NONE',  ( 17.13750000122903216, -4.330127018922194537, 2.499999999999995559 ) ) ;
#2040=CARTESIAN_POINT ( 'NONE',  ( 6.459375000614518747, 0.000000000000000000, 5.243569643749999010 ) ) ;
#2041=CARTESIAN_POINT ( 'NONE',  ( 7.453125000614516438, -4.541064518000417216, -2.621784821875001281 ) ) ;
#2044=CARTESIAN_POINT ( 'NONE',  ( 15.72187500061451892, 3.027376345333613106, -5.243569643749998122 ) ) ;
#2045=CYLINDRICAL_SURFACE ( 'NONE', #63174, 4.000000000000000000 ) ;
#2046=ORIENTED_EDGE ( 'NONE', *, *, #3025, .F. ) ;
#2047=CARTESIAN_POINT ( 'NONE',  ( 23.72812500061451502, 6.421520780324663323E-16, -5.243569643749999010 ) ) ;
#2048=CARTESIAN_POINT ( 'NONE',  ( 10.26562500061451644, 3.027376345333613106, -5.243569643749998122 ) ) ;
#2049=CARTESIAN_POINT ( 'NONE',  ( 27.12187500061451573, 3.027376345333611329, 5.243569643749999010 ) ) ;
#2050=CARTESIAN_POINT ( 'NONE',  ( 8.803125000614517859, -4.541064518000417216, -2.621784821875001281 ) ) ;
#2051=DIRECTION ( 'NONE',  ( -1.000000000000000000, -0.000000000000000000, -0.000000000000000000 ) ) ;
#2052=CARTESIAN_POINT ( 'NONE',  ( 9.975000001229034297, -5.773502691896255534, -1.060575238724906372E-15 ) ) ;
#2053=CARTESIAN_POINT ( 'NONE',  ( 24.06562500061451715, -6.054752690667223547, -1.112240025338166033E-15 ) ) ;
#2054=CARTESIAN_POINT ( 'NONE',  ( -4.243569643749999898, 13.05312500061451786, -30.00000000000000000 ) ) ;
#2055=CARTESIAN_POINT ( 'NONE',  ( 13.16250000122903430, -4.330127018922190985, -2.500000000000001332 ) ) ;
#2056=CARTESIAN_POINT ( 'NONE',  ( 20.95312500061451999, -4.541064518000417216, -2.621784821875001281 ) ) ;
#2057=CARTESIAN_POINT ( 'NONE',  ( 21.40312500061451573, -4.541064518000417216, -2.621784821875001281 ) ) ;
#2059=ADVANCED_FACE ( 'NONE', ( #61757 ), #11160, .F. ) ;
#2060=CARTESIAN_POINT ( 'NONE',  ( 21.41250000000000497, 2.886751345948126879, 4.999999999999999112 ) ) ;
#2061=CARTESIAN_POINT ( 'NONE',  ( 14.70000000122903394, 5.773502691896255534, 3.535250795749688894E-16 ) ) ;
#2062=AXIS2_PLACEMENT_3D ( 'NONE', #23719, #34449, #45557 ) ;
#2063=CARTESIAN_POINT ( 'NONE',  ( 10.34062500061451750, 6.054752690667223547, 3.707466751127219781E-16 ) ) ;
#2064=CARTESIAN_POINT ( 'NONE',  ( 14.50312500061451537, 0.000000000000000000, 5.243569643749999010 ) ) ;
#2065=( BOUNDED_CURVE ( )  B_SPLINE_CURVE ( 2, ( #13330, #17779, #35512, #51426, #57318, #7441, #24423 ),
 .UNSPECIFIED., .F., .F. ) 
 B_SPLINE_CURVE_WITH_KNOTS ( ( 3, 2, 2, 3 ),
 ( 0.07499999999999996947, 0.07777777777777775126, 0.08055555555555551916, 0.08333333333333328707 ),
 .UNSPECIFIED. ) 
 CURVE ( )  GEOMETRIC_REPRESENTATION_ITEM ( )  RATIONAL_B_SPLINE_CURVE ( ( 1.000000000000001332, 0.8660254037844373753, 1.000000000000000000, 0.8660254037844387076, 1.000000000000000000, 0.8660254037844407060, 0.9999999999999980016 ) ) 
 REPRESENTATION_ITEM ( '' )  );
#2066=CARTESIAN_POINT ( 'NONE',  ( 24.86250000122903359, -4.330127018922190985, -2.500000000000001332 ) ) ;
#2067=CARTESIAN_POINT ( 'NONE',  ( 20.74687500061451573, 6.054752690667223547, 3.707466751127219781E-16 ) ) ;
#2069=CARTESIAN_POINT ( 'NONE',  ( 8.137500001229033941, -4.330127018922194537, 2.499999999999995559 ) ) ;
#2070=CARTESIAN_POINT ( 'NONE',  ( 5.634375000614519458, -4.541064518000419881, 2.621784821874995952 ) ) ;
#2071=CARTESIAN_POINT ( 'NONE',  ( 26.40937500061451715, -4.541064518000417216, -2.621784821875001281 ) ) ;
#2072=CARTESIAN_POINT ( 'NONE',  ( 2.934375000614518392, -4.541064518000419881, 2.621784821874995952 ) ) ;
#2073=CARTESIAN_POINT ( 'NONE',  ( 21.44062500061452070, -3.027376345333610441, -5.243569643749999898 ) ) ;
#2074=CARTESIAN_POINT ( 'NONE',  ( 26.82187500061451857, -6.054752690667223547, -1.112240025338166033E-15 ) ) ;
#2076=DIRECTION ( 'NONE',  ( 0.000000000000000000, 0.000000000000000000, 1.000000000000000000 ) ) ;
#2078=CARTESIAN_POINT ( 'NONE',  ( 7.359375000614516438, 0.000000000000000000, 5.243569643749999010 ) ) ;
#2079=CARTESIAN_POINT ( 'NONE',  ( 17.84062500061451573, -3.027376345333610441, -5.243569643749999898 ) ) ;
#2081=CARTESIAN_POINT ( 'NONE',  ( -5.810221930991193690E-16, 12.68750000000000000, -34.00000000000000000 ) ) ;
#2082=CARTESIAN_POINT ( 'NONE',  ( 26.69062500061451715, -3.027376345333614438, 5.243569643749998122 ) ) ;
#2083=CARTESIAN_POINT ( 'NONE',  ( 4.434375000614519280, 6.421520780324663323E-16, -5.243569643749999010 ) ) ;
#2085=CARTESIAN_POINT ( 'NONE',  ( 4.093805572639152679, 3.908117946951304766, 3.718080441408566195 ) ) ;
#2086=CARTESIAN_POINT ( 'NONE',  ( 17.96250000000000213, -5.773502691896255534, -1.060575238724906372E-15 ) ) ;
#2087=CARTESIAN_POINT ( 'NONE',  ( 20.54062500061451502, -3.027376345333610441, -5.243569643749999898 ) ) ;
#2088=ORIENTED_EDGE ( 'NONE', *, *, #50142, .T. ) ;
#2089=CARTESIAN_POINT ( 'NONE',  ( 24.41250000000000142, 2.886751345948129099, -4.999999999999998224 ) ) ;
#2090=CARTESIAN_POINT ( 'NONE',  ( 25.80937500061451928, 0.000000000000000000, 5.243569643749999010 ) ) ;
#2091=VERTEX_POINT ( 'NONE', #26072 ) ;
#2092=CARTESIAN_POINT ( 'NONE',  ( 13.30312500061451786, -4.541064518000417216, -2.621784821875001281 ) ) ;
#2093=CARTESIAN_POINT ( 'NONE',  ( 4.865625000614517859, 3.027376345333613106, -5.243569643749998122 ) ) ;
#2095=CARTESIAN_POINT ( 'NONE',  ( 3.084375000614519191, 6.421520780324663323E-16, -5.243569643749999010 ) ) ;
#2096=CARTESIAN_POINT ( 'NONE',  ( 15.82500000122903216, -5.773502691896255534, -1.060575238724906372E-15 ) ) ;
#2097=CARTESIAN_POINT ( 'NONE',  ( 20.32499999999999929, 6.123233995736764310E-16, -4.999999999999998224 ) ) ;
#2098=CARTESIAN_POINT ( 'NONE',  ( 27.93750000000000000, -2.886751345948125991, -5.000000000000000000 ) ) ;
#2099=CARTESIAN_POINT ( 'NONE',  ( 4.809375000614516615, -4.541064518000417216, -2.621784821875001281 ) ) ;
#2100=CARTESIAN_POINT ( 'NONE',  ( 9.871875000614517504, 3.027376345333613106, -5.243569643749998122 ) ) ;
#2101=CARTESIAN_POINT ( 'NONE',  ( 18.23437500061451999, -4.541064518000419881, 2.621784821874995952 ) ) ;
#2104=CARTESIAN_POINT ( 'NONE',  ( 28.19062500061451715, -3.027376345333610441, -5.243569643749999898 ) ) ;
#2105=CARTESIAN_POINT ( 'NONE',  ( 3.825000000000001954, 4.330127018922191873, 2.499999999999999556 ) ) ;
#2106=CARTESIAN_POINT ( 'NONE',  ( 3.759375000614517681, 0.000000000000000000, 5.243569643749999010 ) ) ;
#2107=CARTESIAN_POINT ( 'NONE',  ( 17.28750000000000142, 5.773502691896255534, 3.535250795749688894E-16 ) ) ;
#2108=CARTESIAN_POINT ( 'NONE',  ( 14.61562500061451608, -6.054752690667223547, -1.112240025338166033E-15 ) ) ;
#2109=CARTESIAN_POINT ( 'NONE',  ( 1.626862140677534273E-15, 13.92500000122903181, 34.00000000000000000 ) ) ;
#2110=CARTESIAN_POINT ( 'NONE',  ( 26.84999999999999787, 0.000000000000000000, 4.999999999999998224 ) ) ;
#2111=CARTESIAN_POINT ( 'NONE',  ( 18.97500000122903074, -5.773502691896255534, -1.060575238724906372E-15 ) ) ;
#2112=CARTESIAN_POINT ( 'NONE',  ( 1.009598436472905814, 9.950840295117078682, 24.08220839835972527 ) ) ;
#2114=CARTESIAN_POINT ( 'NONE',  ( 7.303125000614516082, 0.000000000000000000, 5.243569643749999010 ) ) ;
#2115=CARTESIAN_POINT ( 'NONE',  ( 23.85937500061451644, 4.541064518000418104, -2.621784821874998173 ) ) ;
#2116=CARTESIAN_POINT ( 'NONE',  ( 27.18750000122903288, 6.123233995736764310E-16, -4.999999999999998224 ) ) ;
#2117=CARTESIAN_POINT ( 'NONE',  ( 27.34687500061451360, -3.027376345333610441, -5.243569643749999898 ) ) ;
#2118=CARTESIAN_POINT ( 'NONE',  ( 8.512499999999999289, -5.773502691896255534, -1.060575238724906372E-15 ) ) ;
#2119=CARTESIAN_POINT ( 'NONE',  ( 8.484601909799253346E-16, 13.02500000122903501, 34.61880215351700230 ) ) ;
#2120=CARTESIAN_POINT ( 'NONE',  ( 13.79062500061451502, -3.027376345333610441, -5.243569643749999898 ) ) ;
#2121=CARTESIAN_POINT ( 'NONE',  ( 7.800000001229035362, -2.886751345948125991, -5.000000000000000000 ) ) ;
#2123=CARTESIAN_POINT ( 'NONE',  ( 11.97187500061451892, -6.054752690667223547, -1.112240025338166033E-15 ) ) ;
#2124=CARTESIAN_POINT ( 'NONE',  ( -2.674018119152294037, 4.230323444455001969, -27.01458192567231364 ) ) ;
#2125=EDGE_LOOP ( 'NONE', ( #61952, #62682, #70320, #3688 ) ) ;
#2126=CARTESIAN_POINT ( 'NONE',  ( 11.27812500061451573, 4.541064518000418104, 2.621784821874999949 ) ) ;
#2128=CARTESIAN_POINT ( 'NONE',  ( 24.60000000122903430, 5.773502691896255534, 3.535250795749688894E-16 ) ) ;
#2129=CARTESIAN_POINT ( 'NONE',  ( 13.43437500061451750, 6.421520780324663323E-16, -5.243569643749999010 ) ) ;
#2130=CARTESIAN_POINT ( 'NONE',  ( 14.87812500061451537, 4.541064518000418104, 2.621784821874999949 ) ) ;
#2131=CARTESIAN_POINT ( 'NONE',  ( 1.626862140677534273E-15, 18.76250000000000284, -26.00000000000000355 ) ) ;
#2132=CARTESIAN_POINT ( 'NONE',  ( 23.14687500061451786, -3.027376345333614438, 5.243569643749998122 ) ) ;
#2133=DIRECTION ( 'NONE',  ( 0.000000000000000000, 0.000000000000000000, 1.000000000000000000 ) ) ;
#2134=CARTESIAN_POINT ( 'NONE',  ( 1.626862140677534273E-15, 18.42500000122903359, -26.00000000000000355 ) ) ;
#2135=CARTESIAN_POINT ( 'NONE',  ( -2.000000000000000000, 19.47499999999999787, 26.53589838486224650 ) ) ;
#2136=CARTESIAN_POINT ( 'NONE',  ( -2.121784821874996840, 15.43437500061451928, -26.32496088578401583 ) ) ;
#2137=CARTESIAN_POINT ( 'NONE',  ( 16.28437500061452070, 4.541064518000418104, 2.621784821874999949 ) ) ;
#2138=CARTESIAN_POINT ( 'NONE',  ( 17.77500000122903145, 2.886751345948129099, -4.999999999999998224 ) ) ;
#2139=CARTESIAN_POINT ( 'NONE',  ( 12.90937500061451537, -4.541064518000417216, -2.621784821875001281 ) ) ;
#2140=CARTESIAN_POINT ( 'NONE',  ( 9.001249775931846008E-16, 10.52187500061451964, 34.90005215228797653 ) ) ;
#2141=CARTESIAN_POINT ( 'NONE',  ( 19.38750000122903216, -4.330127018922194537, 2.499999999999995559 ) ) ;
#2142=CARTESIAN_POINT ( 'NONE',  ( 11.69062500061451360, 6.054752690667223547, 3.707466751127219781E-16 ) ) ;
#2143=EDGE_LOOP ( 'NONE', ( #13027, #58345, #56433, #44405 ) ) ;
#2145=CARTESIAN_POINT ( 'NONE',  ( 17.58749999999999858, -2.886751345948125991, -5.000000000000000000 ) ) ;
#2146=CARTESIAN_POINT ( 'NONE',  ( 27.48749999999999716, -2.886751345948092684, -5.000000000000057732 ) ) ;
#2147=CARTESIAN_POINT ( 'NONE',  ( 11.82187500061451857, 3.027376345333611329, 5.243569643749999010 ) ) ;
#2148=CARTESIAN_POINT ( 'NONE',  ( 22.38750000000000284, -2.886751345948096681, 5.000000000000054179 ) ) ;
#2149=CARTESIAN_POINT ( 'NONE',  ( 13.68750000122903288, 6.123233995736764310E-16, -4.999999999999998224 ) ) ;
#2150=CARTESIAN_POINT ( 'NONE',  ( 21.71250000122903501, -4.330127018922190985, -2.500000000000001332 ) ) ;
#2151=CARTESIAN_POINT ( 'NONE',  ( 18.55312500061451431, 0.000000000000000000, 5.243569643749999010 ) ) ;
#2152=CARTESIAN_POINT ( 'NONE',  ( 20.27812500061451573, 4.541064518000418104, 2.621784821874999949 ) ) ;
#2153=CARTESIAN_POINT ( 'NONE',  ( 29.06250000122903288, 4.330127018922192761, -2.499999999999997780 ) ) ;
#2154=CARTESIAN_POINT ( 'NONE',  ( 27.44999999999999929, -4.330127018922190985, -2.500000000000001332 ) ) ;
#2155=CARTESIAN_POINT ( 'NONE',  ( 27.07499999999999929, 6.123233995736764310E-16, -4.999999999999998224 ) ) ;
#2157=CARTESIAN_POINT ( 'NONE',  ( 27.49687500061451217, 6.054752690667223547, 3.707466751127219781E-16 ) ) ;
#2158=CARTESIAN_POINT ( 'NONE',  ( 4.243569643749999010, 16.07187500061451857, -32.45002607614398471 ) ) ;
#2159=ADVANCED_FACE ( 'NONE', ( #64859 ), #37519, .F. ) ;
#2160=CARTESIAN_POINT ( 'NONE',  ( 3.225000001229033408, -5.773502691896255534, -1.060575238724906372E-15 ) ) ;
#2161=CARTESIAN_POINT ( 'NONE',  ( 6.225000000000001421, -4.330127018922194537, 2.499999999999995559 ) ) ;
#2162=CARTESIAN_POINT ( 'NONE',  ( 3.598871848003822649, 4.117104574466481814, -3.356104984449806761 ) ) ;
#2163=CARTESIAN_POINT ( 'NONE',  ( 10.58437500061451964, -4.541064518000419881, 2.621784821874995952 ) ) ;
#2164=CARTESIAN_POINT ( 'NONE',  ( 29.35312500061451502, 0.000000000000000000, 5.243569643749999010 ) ) ;
#2166=CARTESIAN_POINT ( 'NONE',  ( -3.671862074746357063, 9.302863167343950579, -25.25083824868577764 ) ) ;
#2167=CARTESIAN_POINT ( 'NONE',  ( -3.999999999999997335, 19.25000000122903288, 32.30940107675850470 ) ) ;
#2168=CARTESIAN_POINT ( 'NONE',  ( 8.296875000614516438, -3.027376345333614438, 5.243569643749998122 ) ) ;
#2169=CARTESIAN_POINT ( 'NONE',  ( 10.58437500061451964, -4.541064518000419881, 2.621784821874995952 ) ) ;
#2170=CARTESIAN_POINT ( 'NONE',  ( 6.937499999999999112, 5.773502691896255534, 3.535250795749688894E-16 ) ) ;
#2171=CARTESIAN_POINT ( 'NONE',  ( 4.243569643749999010, 14.66562500061459495, 27.54997392385601174 ) ) ;
#2173=CARTESIAN_POINT ( 'NONE',  ( 6.075000000000000178, 4.330127018922191873, 2.499999999999999556 ) ) ;
#2175=CARTESIAN_POINT ( 'NONE',  ( 21.47812500061451502, 6.421520780324663323E-16, -5.243569643749999010 ) ) ;
#2176=CARTESIAN_POINT ( 'NONE',  ( 12.40312500061451573, -4.541064518000417216, -2.621784821875001281 ) ) ;
#2178=CARTESIAN_POINT ( 'NONE',  ( 9.834375000614517859, 6.421520780324663323E-16, -5.243569643749999010 ) ) ;
#2179=CARTESIAN_POINT ( 'NONE',  ( 25.76249999999999929, 2.886751345948129099, -4.999999999999998224 ) ) ;
#2180=CARTESIAN_POINT ( 'NONE',  ( 23.70000000122903216, 5.773502691896255534, 3.535250795749688894E-16 ) ) ;
#2181=CARTESIAN_POINT ( 'NONE',  ( 1.626862140677534273E-15, 18.42500000122903359, -26.00000000000000355 ) ) ;
#2182=CARTESIAN_POINT ( 'NONE',  ( 11.78437500061451892, 4.541064518000418104, 2.621784821874999949 ) ) ;
#2183=CARTESIAN_POINT ( 'NONE',  ( 26.03437500061451715, 6.421520780324663323E-16, -5.243569643749999010 ) ) ;
#2184=DIRECTION ( 'NONE',  ( -0.000000000000000000, -1.000000000000000000, -0.000000000000000000 ) ) ;
#2186=CARTESIAN_POINT ( 'NONE',  ( 19.80937500061451573, 4.541064518000418104, -2.621784821874998173 ) ) ;
#2187=CARTESIAN_POINT ( 'NONE',  ( 11.29687500061451644, 6.054752690667223547, 3.707466751127219781E-16 ) ) ;
#2189=CARTESIAN_POINT ( 'NONE',  ( 22.42500000000000071, -4.330127018922194537, 2.499999999999995559 ) ) ;
#2191=CARTESIAN_POINT ( 'NONE',  ( 4.243569643749999010, 12.92187500061451644, -32.45002607614398471 ) ) ;
#2193=CARTESIAN_POINT ( 'NONE',  ( 15.32812500061451644, 4.541064518000418104, 2.621784821874999949 ) ) ;
#2194=CARTESIAN_POINT ( 'NONE',  ( 4.912499999999999645, -5.773502691896255534, -1.060575238724906372E-15 ) ) ;
#2195=DIRECTION ( 'NONE',  ( -0.000000000000000000, -1.000000000000000000, -0.000000000000000000 ) ) ;
#2196=CARTESIAN_POINT ( 'NONE',  ( 3.242103837493086330E-14, 13.13749999999999929, -34.00000000000000000 ) ) ;
#2197=CARTESIAN_POINT ( 'NONE',  ( 14.84999999999999964, -4.330127018922190985, -2.500000000000001332 ) ) ;
#2198=CARTESIAN_POINT ( 'NONE',  ( 2.121784821874999061, 11.55312500061451786, 26.32496088578401583 ) ) ;
#2199=CARTESIAN_POINT ( 'NONE',  ( 13.38750000122903394, 4.330127018922191873, 2.499999999999999556 ) ) ;
#2200=CARTESIAN_POINT ( 'NONE',  ( 25.43437500061451573, -4.541064518000419881, 2.621784821874995952 ) ) ;
#2201=CARTESIAN_POINT ( 'NONE',  ( 4.027635003466097707, 2.962795348797195416, -4.326299380533228600 ) ) ;
#2202=EDGE_LOOP ( 'NONE', ( #21465, #47503 ) ) ;
#2203=CARTESIAN_POINT ( 'NONE',  ( 18.62812500061451715, -4.541064518000419881, 2.621784821874995952 ) ) ;
#2204=CARTESIAN_POINT ( 'NONE',  ( 3.665625000614517681, 3.027376345333611329, 5.243569643749999010 ) ) ;
#2205=CARTESIAN_POINT ( 'NONE',  ( 18.98437500061451644, 4.541064518000418104, 2.621784821874999949 ) ) ;
#2206=CARTESIAN_POINT ( 'NONE',  ( 3.937500000000000444, -2.886751345948129988, 4.999999999999997335 ) ) ;
#2207=CARTESIAN_POINT ( 'NONE',  ( 6.328125000614515550, 4.541064518000418104, 2.621784821874999949 ) ) ;
#2208=CARTESIAN_POINT ( 'NONE',  ( 21.89062500061451289, -3.027376345333610441, -5.243569643749999898 ) ) ;
#2209=CARTESIAN_POINT ( 'NONE',  ( -4.243569643749999898, 15.30312500061451608, 30.00000000000000000 ) ) ;
#2210=CARTESIAN_POINT ( 'NONE',  ( 18.15000000122903501, -2.886751345948125991, -5.000000000000000000 ) ) ;
#2212=CARTESIAN_POINT ( 'NONE',  ( 10.30312500061451431, 4.541064518000418104, -2.621784821874998173 ) ) ;
#2213=CARTESIAN_POINT ( 'NONE',  ( 3.084375000614519191, 6.421520780324663323E-16, -5.243569643749999010 ) ) ;
#2214=CARTESIAN_POINT ( 'NONE',  ( 3.496875000614518836, -3.027376345333610441, -5.243569643749999898 ) ) ;
#2217=CARTESIAN_POINT ( 'NONE',  ( 23.14687500061451786, -3.027376345333614438, 5.243569643749998122 ) ) ;
#2218=CARTESIAN_POINT ( 'NONE',  ( 13.37812500061451715, 6.421520780324663323E-16, -5.243569643749999010 ) ) ;
#2219=CARTESIAN_POINT ( 'NONE',  ( 26.02500000122903145, 2.886751345948126879, 4.999999999999999112 ) ) ;
#2220=CARTESIAN_POINT ( 'NONE',  ( 26.50312500061451360, 4.541064518000418104, -2.621784821874998173 ) ) ;
#2221=CARTESIAN_POINT ( 'NONE',  ( 19.28437500061451360, 6.421520780324663323E-16, -5.243569643749999010 ) ) ;
#2222=CARTESIAN_POINT ( 'NONE',  ( 14.20312500061451644, -4.541064518000417216, -2.621784821875001281 ) ) ;
#2223=CARTESIAN_POINT ( 'NONE',  ( 2.121784821874999061, 16.55937500061451573, 26.32496088578401583 ) ) ;
#2224=CARTESIAN_POINT ( 'NONE',  ( 20.57812500061451644, 6.421520780324663323E-16, -5.243569643749999010 ) ) ;
#2226=VERTEX_POINT ( 'NONE', #59675 ) ;
#2227=CARTESIAN_POINT ( 'NONE',  ( 24.41250000000000142, 2.886751345948129099, -4.999999999999998224 ) ) ;
#2228=CARTESIAN_POINT ( 'NONE',  ( 9.001249775931846008E-16, 19.52187500061451786, -25.09994784771203058 ) ) ;
#2230=CARTESIAN_POINT ( 'NONE',  ( 27.44062500061451715, 6.054752690667223547, 3.707466751127219781E-16 ) ) ;
#2231=CARTESIAN_POINT ( 'NONE',  ( 8.690625000614515372, -3.027376345333614438, 5.243569643749998122 ) ) ;
#2232=CARTESIAN_POINT ( 'NONE',  ( 20.73750000122903359, -4.330127018922194537, 2.499999999999995559 ) ) ;
#2233=CARTESIAN_POINT ( 'NONE',  ( 23.80312500061451786, 4.541064518000418104, -2.621784821874998173 ) ) ;
#2234=CARTESIAN_POINT ( 'NONE',  ( 26.13749999999999929, -2.886751345948125991, -5.000000000000000000 ) ) ;
#2235=CARTESIAN_POINT ( 'NONE',  ( 1.999999999999998668, 15.01250000122903394, -33.46410161513775705 ) ) ;
#2236=CARTESIAN_POINT ( 'NONE',  ( 9.553125000614517859, 0.000000000000000000, 5.243569643749999010 ) ) ;
#2237=VERTEX_POINT ( 'NONE', #13509 ) ;
#2238=CARTESIAN_POINT ( 'NONE',  ( 25.11562500061451431, 3.027376345333613106, -5.243569643749998122 ) ) ;
#2239=CARTESIAN_POINT ( 'NONE',  ( 7.828125000614517326, -4.541064518000419881, 2.621784821874995952 ) ) ;
#2241=FACE_OUTER_BOUND ( 'NONE', #15117, .T. ) ;
#2242=CARTESIAN_POINT ( 'NONE',  ( 12.37500000000000000, 4.330127018922191873, 2.499999999999999556 ) ) ;
#2243=CARTESIAN_POINT ( 'NONE',  ( 14.14687500061451786, -3.027376345333614438, 5.243569643749998122 ) ) ;
#2244=CARTESIAN_POINT ( 'NONE',  ( 8.362500001229031810, 4.330127018922192761, -2.499999999999997780 ) ) ;
#2245=CARTESIAN_POINT ( 'NONE',  ( 17.44687500061451857, -3.027376345333610441, -5.243569643749999898 ) ) ;
#2247=CARTESIAN_POINT ( 'NONE',  ( 9.121875000614517504, 3.027376345333611329, 5.243569643749999010 ) ) ;
#2248=CARTESIAN_POINT ( 'NONE',  ( -4.243569643749999898, 12.15312500061451573, -30.00000000000000000 ) ) ;
#2249=CARTESIAN_POINT ( 'NONE',  ( -0.7368881354385758975, 9.803648613939513368, 25.82089971438751519 ) ) ;
#2252=EDGE_CURVE ( 'NONE', #8622, #23877, #8520, .T. ) ;
#2253=CARTESIAN_POINT ( 'NONE',  ( 23.35312500061451857, 4.541064518000418104, -2.621784821874998173 ) ) ;
#2255=CARTESIAN_POINT ( 'NONE',  ( 25.62187500061451573, 3.027376345333613106, -5.243569643749998122 ) ) ;
#2256=CARTESIAN_POINT ( 'NONE',  ( 28.32187500061451502, 3.027376345333613106, -5.243569643749998122 ) ) ;
#2258=CARTESIAN_POINT ( 'NONE',  ( 21.48750000000000071, -2.886751345948129988, 4.999999999999997335 ) ) ;
#2259=CARTESIAN_POINT ( 'NONE',  ( 7.453125000614516438, -4.541064518000417216, -2.621784821875001281 ) ) ;
#2261=CARTESIAN_POINT ( 'NONE',  ( 15.57187500061451679, -6.054752690667223547, -1.112240025338166033E-15 ) ) ;
#2263=CARTESIAN_POINT ( 'NONE',  ( 3.553125000614516082, 4.541064518000418104, -2.621784821874998173 ) ) ;
#2264=CARTESIAN_POINT ( 'NONE',  ( 8.446875000614518569, -3.027376345333610441, -5.243569643749999898 ) ) ;
#2265=CARTESIAN_POINT ( 'NONE',  ( 19.13437500061451857, -4.541064518000419881, 2.621784821874995952 ) ) ;
#2266=CARTESIAN_POINT ( 'NONE',  ( 27.41250000000000142, -5.773502691896255534, -1.060575238724906372E-15 ) ) ;
#2267=CARTESIAN_POINT ( 'NONE',  ( 27.19687500061451857, -3.027376345333614438, 5.243569643749998122 ) ) ;
#2268=CARTESIAN_POINT ( 'NONE',  ( 1.071796769724489895, 10.41740381056766473, -34.00000000000000000 ) ) ;
#2270=CARTESIAN_POINT ( 'NONE',  ( 11.17500000000000071, -4.330127018922194537, 2.499999999999995559 ) ) ;
#2272=CARTESIAN_POINT ( 'NONE',  ( 22.11562500061451786, 3.027376345333611329, 5.243569643749999010 ) ) ;
#2273=CARTESIAN_POINT ( 'NONE',  ( 11.02500000000000036, 4.330127018922191873, 2.499999999999999556 ) ) ;
#2274=CARTESIAN_POINT ( 'NONE',  ( 9.000000001229034652, -2.886751345948129988, 4.999999999999997335 ) ) ;
#2275=CARTESIAN_POINT ( 'NONE',  ( 7.078125000614516438, 6.421520780324663323E-16, -5.243569643749999010 ) ) ;
#2276=CARTESIAN_POINT ( 'NONE',  ( 22.98749999999999716, -2.886751345948125991, -5.000000000000000000 ) ) ;
#2277=CARTESIAN_POINT ( 'NONE',  ( 21.17812500061451431, 4.541064518000418104, 2.621784821874999949 ) ) ;
#2278=CARTESIAN_POINT ( 'NONE',  ( 12.03749999999999964, -2.886751345948130876, 4.999999999999996447 ) ) ;
#2279=CARTESIAN_POINT ( 'NONE',  ( 25.95000000122903216, 5.773502691896255534, 3.535250795749688894E-16 ) ) ;
#2281=CARTESIAN_POINT ( 'NONE',  ( 4.237500000000001599, 5.773502691896255534, 3.535250795749688894E-16 ) ) ;
#2282=EDGE_LOOP ( 'NONE', ( #16211, #35541, #8208, #37007 ) ) ;
#2283=CARTESIAN_POINT ( 'NONE',  ( 20.31562500061451715, 3.027376345333611329, 5.243569643749999010 ) ) ;
#2284=CARTESIAN_POINT ( 'NONE',  ( 27.32812500061451644, 6.421520780324663323E-16, -5.243569643749999010 ) ) ;
#2285=CARTESIAN_POINT ( 'NONE',  ( 26.37187500061451217, -6.054752690667223547, -1.112240025338166033E-15 ) ) ;
#2286=CARTESIAN_POINT ( 'NONE',  ( 14.50312500061451537, 0.000000000000000000, 5.243569643749999010 ) ) ;
#2287=CARTESIAN_POINT ( 'NONE',  ( 28.64062500061451289, -3.027376345333610441, -5.243569643749999898 ) ) ;
#2288=CARTESIAN_POINT ( 'NONE',  ( 7.828125000614517326, -4.541064518000419881, 2.621784821874995952 ) ) ;
#2289=CARTESIAN_POINT ( 'NONE',  ( 4.711411573247316298, 1.674097066322985938, -4.711411573247316298 ) ) ;
#2290=CARTESIAN_POINT ( 'NONE',  ( 26.77500000122903145, 2.886751345948129099, -4.999999999999998224 ) ) ;
#2292=CARTESIAN_POINT ( 'NONE',  ( 16.56562500061451715, 3.027376345333612662, -5.243569643749998122 ) ) ;
#2293=CARTESIAN_POINT ( 'NONE',  ( 8.025000000000000355, -4.330127018922194537, 2.499999999999995559 ) ) ;
#2294=ADVANCED_FACE ( 'NONE', ( #20509 ), #58939, .F. ) ;
#2295=CARTESIAN_POINT ( 'NONE',  ( 29.67187500061451644, 3.027376345333613106, -5.243569643749998122 ) ) ;
#2296=CARTESIAN_POINT ( 'NONE',  ( 9.796875000614519990, -3.027376345333610441, -5.243569643749999898 ) ) ;
#2297=CARTESIAN_POINT ( 'NONE',  ( 9.421875000614519990, 3.027376345333613106, -5.243569643749998122 ) ) ;
#2298=CARTESIAN_POINT ( 'NONE',  ( 17.63437500061451502, 4.541064518000418104, 2.621784821874999949 ) ) ;
#2299=ORIENTED_EDGE ( 'NONE', *, *, #58543, .T. ) ;
#2300=CARTESIAN_POINT ( 'NONE',  ( 15.26249999999999929, -5.773502691896255534, -1.060575238724906372E-15 ) ) ;
#2301=CARTESIAN_POINT ( 'NONE',  ( 21.21562500061451573, 3.027376345333611329, 5.243569643749999010 ) ) ;
#2302=CARTESIAN_POINT ( 'NONE',  ( 15.57187500061451679, -6.054752690667223547, -1.112240025338166033E-15 ) ) ;
#2303=CARTESIAN_POINT ( 'NONE',  ( 22.71562500061451573, -6.054752690667223547, -1.112240025338166033E-15 ) ) ;
#2304=CARTESIAN_POINT ( 'NONE',  ( -1.999999999999997113, 13.32499999999999929, 33.46410161513775705 ) ) ;
#2305=CARTESIAN_POINT ( 'NONE',  ( 3.234375000614516438, 4.541064518000418104, 2.621784821874999949 ) ) ;
#2306=CARTESIAN_POINT ( 'NONE',  ( 8.512500001229033941, 0.000000000000000000, 4.999999999999998224 ) ) ;
#2307=ORIENTED_EDGE ( 'NONE', *, *, #42591, .T. ) ;
#2308=CARTESIAN_POINT ( 'NONE',  ( 4.837500001229035895, 4.330127018922191873, 2.499999999999999556 ) ) ;
#2309=CARTESIAN_POINT ( 'NONE',  ( 8.484601909799253346E-16, 17.86250000000000071, -25.38119784648299770 ) ) ;
#2310=CARTESIAN_POINT ( 'NONE',  ( 24.60000000122903430, 5.773502691896255534, 3.535250795749688894E-16 ) ) ;
#2312=CARTESIAN_POINT ( 'NONE',  ( 8.184375000614515727, 4.541064518000418104, 2.621784821874999949 ) ) ;
#2313=CARTESIAN_POINT ( 'NONE',  ( 24.37500000000000000, 6.123233995736764310E-16, -4.999999999999998224 ) ) ;
#2314=CARTESIAN_POINT ( 'NONE',  ( 14.54062500061451679, -3.027376345333614438, 5.243569643749998122 ) ) ;
#2315=CARTESIAN_POINT ( 'NONE',  ( 11.70937500061451608, 4.541064518000418104, -2.621784821874998173 ) ) ;
#2316=CARTESIAN_POINT ( 'NONE',  ( 25.83750000122903501, 6.123233995736764310E-16, -4.999999999999998224 ) ) ;
#2317=CARTESIAN_POINT ( 'NONE',  ( 17.97187500061451715, 3.027376345333612662, -5.243569643749998122 ) ) ;
#2318=CARTESIAN_POINT ( 'NONE',  ( 6.459375000614518747, 0.000000000000000000, 5.243569643749999010 ) ) ;
#2320=CARTESIAN_POINT ( 'NONE',  ( 7.190625000614518036, 6.054752690667223547, 3.707466751127219781E-16 ) ) ;
#2321=CARTESIAN_POINT ( 'NONE',  ( 18.36562500061451431, 3.027376345333613106, -5.243569643749998122 ) ) ;
#2323=CARTESIAN_POINT ( 'NONE',  ( 15.70312500061451644, 4.541064518000418104, -2.621784821874998173 ) ) ;
#2324=CARTESIAN_POINT ( 'NONE',  ( 10.00312500061451715, 0.000000000000000000, 5.243569643749999010 ) ) ;
#2326=CARTESIAN_POINT ( 'NONE',  ( 12.11250000000000249, -5.773502691896255534, -1.060575238724906372E-15 ) ) ;
#2327=CARTESIAN_POINT ( 'NONE',  ( 6.900000001229035007, -2.886751345948125991, -5.000000000000000000 ) ) ;
#2328=CARTESIAN_POINT ( 'NONE',  ( 14.37187500061451928, 3.027376345333613106, -5.243569643749998122 ) ) ;
#2329=CARTESIAN_POINT ( 'NONE',  ( 16.16250000122903430, 0.000000000000000000, 4.999999999999998224 ) ) ;
#2331=CARTESIAN_POINT ( 'NONE',  ( 4.243569643749999898, 19.12812500061451715, -30.00000000000000000 ) ) ;
#2333=CARTESIAN_POINT ( 'NONE',  ( 4.898587196589411843E-16, 20.00000000000000000, 33.99999999999999289 ) ) ;
#2334=CARTESIAN_POINT ( 'NONE',  ( 23.43750000122902932, -4.330127018922194537, 2.499999999999995559 ) ) ;
#2336=FACE_OUTER_BOUND ( 'NONE', #2346, .T. ) ;
#2337=CARTESIAN_POINT ( 'NONE',  ( 15.79687500061451821, 6.054752690667223547, 3.707466751127219781E-16 ) ) ;
#2339=CARTESIAN_POINT ( 'NONE',  ( 29.62500000000000000, -4.330127018922194537, 2.499999999999995559 ) ) ;
#2340=CARTESIAN_POINT ( 'NONE',  ( 13.82812500061451466, 6.421520780324663323E-16, -5.243569643749999010 ) ) ;
#2342=CARTESIAN_POINT ( 'NONE',  ( 23.29687500061451644, -3.027376345333610441, -5.243569643749999898 ) ) ;
#2344=CARTESIAN_POINT ( 'NONE',  ( 9.253125000614517148, -4.541064518000417216, -2.621784821875001281 ) ) ;
#2345=CARTESIAN_POINT ( 'NONE',  ( 15.30937500061451750, 4.541064518000418104, -2.621784821874998173 ) ) ;
#2346=EDGE_LOOP ( 'NONE', ( #15475, #56072, #64393, #27480 ) ) ;
#2347=CARTESIAN_POINT ( 'NONE',  ( 26.82187500061451857, -6.054752690667223547, -1.112240025338166033E-15 ) ) ;
#2348=VECTOR ( 'NONE', #18941, 1000.000000000000000 ) ;
#2349=CARTESIAN_POINT ( 'NONE',  ( 28.64062500061451289, -3.027376345333610441, -5.243569643749999898 ) ) ;
#2350=CARTESIAN_POINT ( 'NONE',  ( 17.72812500061451502, -4.541064518000419881, 2.621784821874995952 ) ) ;
#2351=CARTESIAN_POINT ( 'NONE',  ( 3.999999999999999112, 12.68750000122903465, -30.00000000000000000 ) ) ;
#2352=CARTESIAN_POINT ( 'NONE',  ( 7.912499999999999645, 2.886751345948126879, 4.999999999999999112 ) ) ;
#2353=CARTESIAN_POINT ( 'NONE',  ( 19.91250000122903074, -4.330127018922190985, -2.500000000000001332 ) ) ;
#2354=DIRECTION ( 'NONE',  ( 0.000000000000000000, 0.000000000000000000, -1.000000000000000000 ) ) ;
#2356=VERTEX_POINT ( 'NONE', #8346 ) ;
#2357=CARTESIAN_POINT ( 'NONE',  ( 17.28750000000000142, 5.773502691896255534, 3.535250795749688894E-16 ) ) ;
#2358=CARTESIAN_POINT ( 'NONE',  ( 20.02500000000000213, 4.330127018922191873, 2.499999999999999556 ) ) ;
#2359=CARTESIAN_POINT ( 'NONE',  ( 17.89687500061451431, -3.027376345333610441, -5.243569643749999898 ) ) ;
#2360=CARTESIAN_POINT ( 'NONE',  ( 14.87812500061451537, 4.541064518000418104, 2.621784821874999949 ) ) ;
#2361=ORIENTED_EDGE ( 'NONE', *, *, #36318, .T. ) ;
#2363=CARTESIAN_POINT ( 'NONE',  ( 6.740625000614516082, 6.054752690667223547, 3.707466751127219781E-16 ) ) ;
#2364=CARTESIAN_POINT ( 'NONE',  ( 10.27499999999999858, -4.330127018922194537, 2.499999999999995559 ) ) ;
#2365=CARTESIAN_POINT ( 'NONE',  ( 12.18750000000000000, -2.886751345948125991, -5.000000000000000000 ) ) ;
#2367=CARTESIAN_POINT ( 'NONE',  ( -4.243569643749999898, 14.81562500061451715, 27.54997392385601529 ) ) ;
#2368=CARTESIAN_POINT ( 'NONE',  ( 26.35312500061451857, -4.541064518000417216, -2.621784821875001281 ) ) ;
#2371=CARTESIAN_POINT ( 'NONE',  ( 23.78437500061451360, 6.421520780324663323E-16, -5.243569643749999010 ) ) ;
#2372=VERTEX_POINT ( 'NONE', #65221 ) ;
#2373=CARTESIAN_POINT ( 'NONE',  ( 20.99062500061451431, -3.027376345333610441, -5.243569643749999898 ) ) ;
#2374=CARTESIAN_POINT ( 'NONE',  ( 23.97187500061451360, 3.027376345333611329, 5.243569643749999010 ) ) ;
#2375=CARTESIAN_POINT ( 'NONE',  ( -4.243569643749998122, 15.34062500061459389, -27.54997392385601174 ) ) ;
#2376=CARTESIAN_POINT ( 'NONE',  ( 5.615625000614517859, -6.054752690667223547, -1.112240025338166033E-15 ) ) ;
#2378=CARTESIAN_POINT ( 'NONE',  ( 24.21562500061451573, 3.027376345333612662, -5.243569643749998122 ) ) ;
#2381=CARTESIAN_POINT ( 'NONE',  ( 17.10937500061451999, 4.541064518000418104, -2.621784821874998173 ) ) ;
#2382=CARTESIAN_POINT ( 'NONE',  ( 24.94687500061451502, -3.027376345333614438, 5.243569643749998122 ) ) ;
#2383=CARTESIAN_POINT ( 'NONE',  ( 2.121784821875001281, 14.15937500061451715, 33.67503911421598417 ) ) ;
#2384=CARTESIAN_POINT ( 'NONE',  ( 8.578125000614518214, 4.541064518000418104, 2.621784821874999949 ) ) ;
#2385=CARTESIAN_POINT ( 'NONE',  ( 16.42500000122903359, 2.886751345948129099, -4.999999999999997335 ) ) ;
#2386=EDGE_CURVE ( 'NONE', #2494, #43350, #16995, .T. ) ;
#2387=CARTESIAN_POINT ( 'NONE',  ( 29.46562500061451573, -6.054752690667223547, -1.112240025338166033E-15 ) ) ;
#2389=CARTESIAN_POINT ( 'NONE',  ( 5.540625000614515905, -3.027376345333614438, 5.243569643749998122 ) ) ;
#2390=CARTESIAN_POINT ( 'NONE',  ( 8.521875000614516082, 3.027376345333613106, -5.243569643749998122 ) ) ;
#2391=CARTESIAN_POINT ( 'NONE',  ( 16.42500000122903359, 2.886751345948129099, -4.999999999999998224 ) ) ;
#2392=CARTESIAN_POINT ( 'NONE',  ( 2.934375000614518392, -4.541064518000419881, 2.621784821874995952 ) ) ;
#2393=CARTESIAN_POINT ( 'NONE',  ( 4.790625000614518569, -3.027376345333610441, -5.243569643749999898 ) ) ;
#2395=CARTESIAN_POINT ( 'NONE',  ( 16.39687500061451786, -3.027376345333614438, 5.243569643749998122 ) ) ;
#2396=CARTESIAN_POINT ( 'NONE',  ( -2.000000000000000000, 10.47500000000000142, 26.53589838486224650 ) ) ;
#2397=ORIENTED_EDGE ( 'NONE', *, *, #3296, .F. ) ;
#2398=CARTESIAN_POINT ( 'NONE',  ( 21.74062500061451431, -3.027376345333614438, 5.243569643749998122 ) ) ;
#2399=CARTESIAN_POINT ( 'NONE',  ( 9.365625000614519635, 3.027376345333613106, -5.243569643749998122 ) ) ;
#2400=CARTESIAN_POINT ( 'NONE',  ( 26.10937500061451644, 4.541064518000418104, -2.621784821874998173 ) ) ;
#2401=CARTESIAN_POINT ( 'NONE',  ( 9.965625000614517504, 3.027376345333611329, 5.243569643749999010 ) ) ;
#2402=CARTESIAN_POINT ( 'NONE',  ( 3.397178649298551179, 3.668675132081069101, -3.397178649298551179 ) ) ;
#2403=CARTESIAN_POINT ( 'NONE',  ( 9.337500001229033231, 4.330127018922191873, 2.499999999999999556 ) ) ;
#2404=CARTESIAN_POINT ( 'NONE',  ( 24.17812500061451786, 6.421520780324663323E-16, -5.243569643749999010 ) ) ;
#2405=CARTESIAN_POINT ( 'NONE',  ( 2.121784821875001281, 10.50312500061451715, -26.32496088578401938 ) ) ;
#2406=CARTESIAN_POINT ( 'NONE',  ( 13.83750000122903323, 4.330127018922191873, 2.499999999999999556 ) ) ;
#2407=CARTESIAN_POINT ( 'NONE',  ( 21.77812500061451928, -4.541064518000419881, 2.621784821874995952 ) ) ;
#2408=CARTESIAN_POINT ( 'NONE',  ( 18.14062500061451644, -3.027376345333614438, 5.243569643749998122 ) ) ;
#2409=CARTESIAN_POINT ( 'NONE',  ( 5.521875000614517859, 3.027376345333611329, 5.243569643749999010 ) ) ;
#2410=CARTESIAN_POINT ( 'NONE',  ( 19.23749999999999716, -2.886751345948129988, 4.999999999999997335 ) ) ;
#2411=CARTESIAN_POINT ( 'NONE',  ( 12.82500000122903394, 2.886751345948129099, -4.999999999999998224 ) ) ;
#2412=CARTESIAN_POINT ( 'NONE',  ( 11.20312500061451644, 4.541064518000418104, -2.621784821874998173 ) ) ;
#2413=CARTESIAN_POINT ( 'NONE',  ( 13.07812500061451821, 4.541064518000418104, 2.621784821874999949 ) ) ;
#2414=CARTESIAN_POINT ( 'NONE',  ( 22.83750000122903501, 4.330127018922191873, 2.499999999999999556 ) ) ;
#2415=CARTESIAN_POINT ( 'NONE',  ( 20.67187500061451289, 3.027376345333613106, -5.243569643749998122 ) ) ;
#2416=CARTESIAN_POINT ( 'NONE',  ( 22.02187500061452141, 3.027376345333613106, -5.243569643749998122 ) ) ;
#2418=CARTESIAN_POINT ( 'NONE',  ( 8.437500001229034652, 4.330127018922191873, 2.499999999999999556 ) ) ;
#2419=CARTESIAN_POINT ( 'NONE',  ( 6.421875000614519102, 3.027376345333611329, 5.243569643749999010 ) ) ;
#2420=CARTESIAN_POINT ( 'NONE',  ( 24.79687500061451999, 6.054752690667223547, 3.707466751127219781E-16 ) ) ;
#2422=CARTESIAN_POINT ( 'NONE',  ( 20.91562500061451502, -6.054752690667223547, -1.112240025338166033E-15 ) ) ;
#2423=CARTESIAN_POINT ( 'NONE',  ( 25.69687500061451502, 6.054752690667223547, 3.707466751127219781E-16 ) ) ;
#2425=CARTESIAN_POINT ( 'NONE',  ( 18.63749999999999929, 5.773502691896255534, 3.535250795749688401E-16 ) ) ;
#2427=CARTESIAN_POINT ( 'NONE',  ( 6.609375000614519102, -4.541064518000417216, -2.621784821875001281 ) ) ;
#2428=CARTESIAN_POINT ( 'NONE',  ( 16.60312500061451857, 4.541064518000418104, -2.621784821874998173 ) ) ;
#2429=ORIENTED_EDGE ( 'NONE', *, *, #69330, .T. ) ;
#2430=CARTESIAN_POINT ( 'NONE',  ( 22.94999999999999929, -4.330127018922190985, -2.500000000000001332 ) ) ;
#2431=CARTESIAN_POINT ( 'NONE',  ( 25.04062500061451502, -3.027376345333610441, -5.243569643749999898 ) ) ;
#2432=CARTESIAN_POINT ( 'NONE',  ( 3.046875000614519990, -3.027376345333610441, -5.243569643749999898 ) ) ;
#2434=CYLINDRICAL_SURFACE ( 'NONE', #62037, 5.999999999999998224 ) ;
#2435=CARTESIAN_POINT ( 'NONE',  ( 16.27499999999999858, 6.123233995736764310E-16, -4.999999999999998224 ) ) ;
#2436=CARTESIAN_POINT ( 'NONE',  ( 20.05312500061451431, -4.541064518000417216, -2.621784821875001281 ) ) ;
#2438=CARTESIAN_POINT ( 'NONE',  ( 25.12499999999999645, -4.330127018922194537, 2.499999999999995559 ) ) ;
#2439=CARTESIAN_POINT ( 'NONE',  ( 25.09687500061451715, -3.027376345333610441, -5.243569643749999898 ) ) ;
#2440=ORIENTED_EDGE ( 'NONE', *, *, #36141, .F. ) ;
#2442=CARTESIAN_POINT ( 'NONE',  ( 14.01562500061451644, 3.027376345333611329, 5.243569643749999010 ) ) ;
#2443=CARTESIAN_POINT ( 'NONE',  ( 6.590625000614518392, -3.027376345333610441, -5.243569643749999898 ) ) ;
#2445=CARTESIAN_POINT ( 'NONE',  ( 28.52812500061451573, -4.541064518000419881, 2.621784821874995952 ) ) ;
#2446=CARTESIAN_POINT ( 'NONE',  ( 14.55000000122903181, -2.886751345948125991, -5.000000000000000000 ) ) ;
#2447=CARTESIAN_POINT ( 'NONE',  ( 19.08750000000000213, 5.773502691896255534, 3.535250795749688894E-16 ) ) ;
#2448=CARTESIAN_POINT ( 'NONE',  ( 26.06250000000000000, -5.773502691896255534, -1.060575238724906372E-15 ) ) ;
#2449=CARTESIAN_POINT ( 'NONE',  ( 2.896875000614518747, -3.027376345333614438, 5.243569643749998122 ) ) ;
#2450=CARTESIAN_POINT ( 'NONE',  ( 8.521875000614516082, 3.027376345333613106, -5.243569643749998122 ) ) ;
#2451=CARTESIAN_POINT ( 'NONE',  ( 19.09687500061451360, -3.027376345333614438, 5.243569643749998122 ) ) ;
#2454=CARTESIAN_POINT ( 'NONE',  ( 29.61562500061451431, 3.027376345333613106, -5.243569643749998122 ) ) ;
#2455=CARTESIAN_POINT ( 'NONE',  ( 29.85937500061451644, 0.000000000000000000, 5.243569643749999010 ) ) ;
#2456=CARTESIAN_POINT ( 'NONE',  ( 5.334375000614517859, 6.421520780324663323E-16, -5.243569643749999010 ) ) ;
#2457=CARTESIAN_POINT ( 'NONE',  ( 16.38749999999999929, 5.773502691896255534, 3.535250795749688894E-16 ) ) ;
#2458=CARTESIAN_POINT ( 'NONE',  ( 14.54062500061451679, -3.027376345333614438, 5.243569643749998122 ) ) ;
#2462=CARTESIAN_POINT ( 'NONE',  ( 18.22500000122903430, 2.886751345948129099, -4.999999999999998224 ) ) ;
#2465=CARTESIAN_POINT ( 'NONE',  ( 8.353125000614518569, -4.541064518000417216, -2.621784821875001281 ) ) ;
#2466=CARTESIAN_POINT ( 'NONE',  ( 23.82187500061451502, 3.027376345333613106, -5.243569643749998122 ) ) ;
#2467=DIRECTION ( 'NONE',  ( -1.000000000000000000, -0.000000000000000000, -0.000000000000000000 ) ) ;
#2468=CARTESIAN_POINT ( 'NONE',  ( 23.59687500061451715, -3.027376345333614438, 5.243569643749998122 ) ) ;
#2469=CARTESIAN_POINT ( 'NONE',  ( 4.800000000000002487, 0.000000000000000000, 4.999999999999998224 ) ) ;
#2470=CARTESIAN_POINT ( 'NONE',  ( 8.484601909799253346E-16, 9.875000001229032875, 34.61880215351700230 ) ) ;
#2471=CARTESIAN_POINT ( 'NONE',  ( 13.56562500061451892, 3.027376345333611329, 5.243569643749999010 ) ) ;
#2472=CARTESIAN_POINT ( 'NONE',  ( 5.700000001229033941, 5.773502691896255534, 3.535250795749688894E-16 ) ) ;
#2473=EDGE_CURVE ( 'NONE', #22068, #71409, #47880, .T. ) ;
#2474=CARTESIAN_POINT ( 'NONE',  ( 9.946875000614516793, 6.054752690667223547, 3.707466751127219781E-16 ) ) ;
#2475=EDGE_LOOP ( 'NONE', ( #65961, #44078, #25078, #64122 ) ) ;
#2476=CARTESIAN_POINT ( 'NONE',  ( 12.36562500061451608, -6.054752690667223547, -1.112240025338166033E-15 ) ) ;
#2478=CARTESIAN_POINT ( 'NONE',  ( 23.66250000122903430, 4.330127018922192761, -2.499999999999997780 ) ) ;
#2479=CARTESIAN_POINT ( 'NONE',  ( 11.10937500061451644, -4.541064518000417216, -2.621784821875001281 ) ) ;
#2480=CARTESIAN_POINT ( 'NONE',  ( 15.77812500061451573, 4.541064518000418104, 2.621784821874999949 ) ) ;
#2482=CARTESIAN_POINT ( 'NONE',  ( 23.07187500061451857, 3.027376345333611329, 5.243569643749999010 ) ) ;
#2483=DIRECTION ( 'NONE',  ( -0.000000000000000000, -1.000000000000000000, -0.000000000000000000 ) ) ;
#2484=CARTESIAN_POINT ( 'NONE',  ( 23.85000000000000142, -4.330127018922190985, -2.500000000000001332 ) ) ;
#2485=CARTESIAN_POINT ( 'NONE',  ( -3.000416591977282496E-16, 15.69687500061451857, -34.90005215228797653 ) ) ;
#2486=AXIS2_PLACEMENT_3D ( 'NONE', #65684, #36513, #25430 ) ;
#2487=CARTESIAN_POINT ( 'NONE',  ( 15.75937500061451857, 4.541064518000418104, -2.621784821874998173 ) ) ;
#2488=CARTESIAN_POINT ( 'NONE',  ( 17.36250000122903359, 4.330127018922192761, -2.499999999999997780 ) ) ;
#2489=( BOUNDED_CURVE ( )  B_SPLINE_CURVE ( 2, ( #30575, #49036, #20939, #70093, #37570, #19840, #48300, #42754, #59728 ),
 .UNSPECIFIED., .F., .F. ) 
 B_SPLINE_CURVE_WITH_KNOTS ( ( 3, 2, 2, 2, 3 ),
 ( 0.2065217391304347838, 0.2101449275362318736, 0.2173913043478260809, 0.2246376811594202882, 0.2282608695652174058 ),
 .UNSPECIFIED. ) 
 CURVE ( )  GEOMETRIC_REPRESENTATION_ITEM ( )  RATIONAL_B_SPLINE_CURVE ( ( 0.9330127018922194093, 0.9330127018922194093, 1.000000000000000000, 0.8660254037844387076, 1.000000000000000000, 0.8660254037844387076, 1.000000000000000000, 0.9330127018922190762, 0.9330127018922194093 ) ) 
 REPRESENTATION_ITEM ( '' )  );
#2490=CARTESIAN_POINT ( 'NONE',  ( 11.74687500061451573, 6.054752690667223547, 3.707466751127219781E-16 ) ) ;
#2491=CARTESIAN_POINT ( 'NONE',  ( -2.121784821874999949, 17.47812500061451502, -33.67503911421598417 ) ) ;
#2492=CARTESIAN_POINT ( 'NONE',  ( 20.70000000122903216, -2.886751345948129988, 4.999999999999997335 ) ) ;
#2493=CARTESIAN_POINT ( 'NONE',  ( 12.77812500061451750, -4.541064518000419881, 2.621784821874995952 ) ) ;
#2494=VERTEX_POINT ( 'NONE', #19046 ) ;
#2495=ORIENTED_EDGE ( 'NONE', *, *, #9420, .F. ) ;
#2496=CARTESIAN_POINT ( 'NONE',  ( 18.59999999999999787, 4.330127018922192761, -2.499999999999997780 ) ) ;
#2497=CARTESIAN_POINT ( 'NONE',  ( 19.27500000122903145, 2.886751345948093572, 5.000000000000056843 ) ) ;
#2498=CARTESIAN_POINT ( 'NONE',  ( 13.20937500061451786, 0.000000000000000000, 5.243569643749999010 ) ) ;
#2499=CARTESIAN_POINT ( 'NONE',  ( 22.53750000000000142, -2.886751345948159742, -4.999999999999942268 ) ) ;
#2501=CARTESIAN_POINT ( 'NONE',  ( 12.90000000122903145, 5.773502691896255534, 3.535250795749688894E-16 ) ) ;
#2502=CARTESIAN_POINT ( 'NONE',  ( 20.51250000122903216, 4.330127018922192761, -2.499999999999997780 ) ) ;
#2503=CARTESIAN_POINT ( 'NONE',  ( 18.51562500061451289, 3.027376345333611329, 5.243569643749999010 ) ) ;
#2504=CARTESIAN_POINT ( 'NONE',  ( 20.72812500061451502, 4.541064518000418104, 2.621784821874999949 ) ) ;
#2505=CARTESIAN_POINT ( 'NONE',  ( 28.83750000122903145, -4.330127018922194537, 2.499999999999995559 ) ) ;
#2506=CARTESIAN_POINT ( 'NONE',  ( 28.42499999999999716, 6.123233995736764310E-16, -4.999999999999998224 ) ) ;
#2507=CYLINDRICAL_SURFACE ( 'NONE', #47800, 3.999999999999996447 ) ;
#2509=CARTESIAN_POINT ( 'NONE',  ( 27.04687500061451644, 6.054752690667223547, 3.707466751127219781E-16 ) ) ;
#2510=CARTESIAN_POINT ( 'NONE',  ( 1.626862140677534273E-15, 14.26250000000000107, -26.00000000000000355 ) ) ;
#2512=CARTESIAN_POINT ( 'NONE',  ( 4.243569643749999898, 16.03437500061451715, -30.00000000000000000 ) ) ;
#2513=CARTESIAN_POINT ( 'NONE',  ( 30.00000000000000000, 0.000000000000000000, 4.999999999999998224 ) ) ;
#2514=CARTESIAN_POINT ( 'NONE',  ( 5.549999999999998934, 4.330127018922192761, -2.499999999999997780 ) ) ;
#2516=CARTESIAN_POINT ( 'NONE',  ( 16.46249999999999858, 2.886751345948126879, 4.999999999999998224 ) ) ;
#2517=CARTESIAN_POINT ( 'NONE',  ( 9.196875000614518569, -3.027376345333614438, 5.243569643749998122 ) ) ;
#2518=CARTESIAN_POINT ( 'NONE',  ( 29.42812500061451431, -4.541064518000419881, 2.621784821874995952 ) ) ;
#2520=EDGE_CURVE ( 'NONE', #7627, #10804, #55613, .T. ) ;
#2521=CARTESIAN_POINT ( 'NONE',  ( -2.699902572705014769, 9.635935948006318696, -24.62716651635609466 ) ) ;
#2522=CARTESIAN_POINT ( 'NONE',  ( 30.00000000000000000, 0.000000000000000000, 0.000000000000000000 ) ) ;
#2523=CARTESIAN_POINT ( 'NONE',  ( 6.721875000614518925, 3.027376345333613106, -5.243569643749998122 ) ) ;
#2524=CARTESIAN_POINT ( 'NONE',  ( 11.52187500061451608, -6.054752690667223547, -1.112240025338166033E-15 ) ) ;
#2525=CARTESIAN_POINT ( 'NONE',  ( 4.349999999999999645, 0.000000000000000000, 4.999999999999998224 ) ) ;
#2526=CARTESIAN_POINT ( 'NONE',  ( 9.001249775931846008E-16, 15.41562500061459495, 34.90005215228797653 ) ) ;
#2528=EDGE_CURVE ( 'NONE', #43803, #16272, #67039, .T. ) ;
#2529=CARTESIAN_POINT ( 'NONE',  ( 7.237500000000000711, -2.886751345948125991, -5.000000000000000000 ) ) ;
#2531=CARTESIAN_POINT ( 'NONE',  ( 20.24062500061451431, 6.054752690667223547, 3.707466751127219781E-16 ) ) ;
#2532=CARTESIAN_POINT ( 'NONE',  ( 13.07812500061451821, 4.541064518000418104, 2.621784821874999949 ) ) ;
#2534=CARTESIAN_POINT ( 'NONE',  ( 9.534375000614517148, 4.541064518000418104, 2.621784821874999949 ) ) ;
#2535=CARTESIAN_POINT ( 'NONE',  ( 25.94999999999999929, 0.000000000000000000, 4.999999999999998224 ) ) ;
#2536=CARTESIAN_POINT ( 'NONE',  ( 21.86250000122903003, 4.330127018922192761, -2.499999999999997780 ) ) ;
#2537=CARTESIAN_POINT ( 'NONE',  ( 1.071796769724491893, 10.79509619066136850, 33.99999999999999289 ) ) ;
#2538=CARTESIAN_POINT ( 'NONE',  ( 8.596875000614518925, 6.054752690667223547, 3.707466751127219781E-16 ) ) ;
#2539=CARTESIAN_POINT ( 'NONE',  ( 27.42187500061451644, 3.027376345333613106, -5.243569643749998122 ) ) ;
#2540=EDGE_CURVE ( 'NONE', #17100, #25696, #24047, .T. ) ;
#2543=CARTESIAN_POINT ( 'NONE',  ( 19.20937500061451786, -4.541064518000417216, -2.621784821875001281 ) ) ;
#2544=CARTESIAN_POINT ( 'NONE',  ( 10.84687500061451892, 6.054752690667223547, 3.707466751127219781E-16 ) ) ;
#2546=CARTESIAN_POINT ( 'NONE',  ( 22.27499999999999858, 4.330127018922191873, 2.499999999999999556 ) ) ;
#2548=CARTESIAN_POINT ( 'NONE',  ( -4.243569643749999898, 13.10937500061451821, -30.00000000000000000 ) ) ;
#2550=CARTESIAN_POINT ( 'NONE',  ( 15.89062500061451289, -3.027376345333614438, 5.243569643749998122 ) ) ;
#2551=CARTESIAN_POINT ( 'NONE',  ( 5.175000000000002487, 4.330127018922191873, 2.499999999999999556 ) ) ;
#2552=CARTESIAN_POINT ( 'NONE',  ( 12.30000000122903359, -2.886751345948193048, -4.999999999999883649 ) ) ;
#2554=CARTESIAN_POINT ( 'NONE',  ( 13.57500000000000107, 6.123233995736764310E-16, -4.999999999999998224 ) ) ;
#2555=CARTESIAN_POINT ( 'NONE',  ( 2.121784821874999061, 11.10312500061451679, 26.32496088578401583 ) ) ;
#2556=CARTESIAN_POINT ( 'NONE',  ( 14.06250000122903288, -4.330127018922190985, -2.500000000000001332 ) ) ;
#2557=CARTESIAN_POINT ( 'NONE',  ( 24.83437500061451431, 4.541064518000418104, 2.621784821874999949 ) ) ;
#2558=VERTEX_POINT ( 'NONE', #72607 ) ;
#2559=CARTESIAN_POINT ( 'NONE',  ( 19.52812500061451573, -4.541064518000419881, 2.621784821874995952 ) ) ;
#2560=CARTESIAN_POINT ( 'NONE',  ( 4.753125000614515372, -4.541064518000417216, -2.621784821875001281 ) ) ;
#2561=CARTESIAN_POINT ( 'NONE',  ( 20.82187500061451857, 3.027376345333611329, 5.243569643749999010 ) ) ;
#2562=CARTESIAN_POINT ( 'NONE',  ( 27.90937500061451715, 4.541064518000418104, -2.621784821874998173 ) ) ;
#2563=CARTESIAN_POINT ( 'NONE',  ( 5.240625000614516971, -3.027376345333610441, -5.243569643749999898 ) ) ;
#2564=CARTESIAN_POINT ( 'NONE',  ( 22.60312500061451857, 0.000000000000000000, 5.243569643749999010 ) ) ;
#2565=CARTESIAN_POINT ( 'NONE',  ( 2.121784821874999061, 15.60312500061451857, 26.32496088578401583 ) ) ;
#2566=CARTESIAN_POINT ( 'NONE',  ( 15.71250000122903501, 0.000000000000000000, 4.999999999999998224 ) ) ;
#2568=CARTESIAN_POINT ( 'NONE',  ( 7.603125000614517681, 4.541064518000418104, -2.621784821874998173 ) ) ;
#2569=CARTESIAN_POINT ( 'NONE',  ( 13.61250000000000071, 2.886751345948129099, -4.999999999999997335 ) ) ;
#2570=CARTESIAN_POINT ( 'NONE',  ( 29.01562500061451644, -6.054752690667223547, -1.112240025338166033E-15 ) ) ;
#2571=CARTESIAN_POINT ( 'NONE',  ( 24.00937500061451502, 0.000000000000000000, 5.243569643749999010 ) ) ;
#2572=CARTESIAN_POINT ( 'NONE',  ( 14.95312500061451644, 0.000000000000000000, 5.243569643749999010 ) ) ;
#2573=ADVANCED_FACE ( 'NONE', ( #55978 ), #38994, .F. ) ;
#2574=CARTESIAN_POINT ( 'NONE',  ( 25.65000000122903145, -2.886751345948129988, 4.999999999999997335 ) ) ;
#2575=CARTESIAN_POINT ( 'NONE',  ( 24.66562500061451502, 3.027376345333613106, -5.243569643749998122 ) ) ;
#2576=CARTESIAN_POINT ( 'NONE',  ( 20.33437500061451786, 4.541064518000418104, 2.621784821874999949 ) ) ;
#2577=CARTESIAN_POINT ( 'NONE',  ( 14.50312500061451537, 0.000000000000000000, 5.243569643749999010 ) ) ;
#2578=CARTESIAN_POINT ( 'NONE',  ( 9.001249775931846008E-16, 15.92187500061451821, 34.90005215228797653 ) ) ;
#2579=CARTESIAN_POINT ( 'NONE',  ( 19.15312500061451573, -4.541064518000417216, -2.621784821875001281 ) ) ;
#2582=CARTESIAN_POINT ( 'NONE',  ( 25.01249999999999929, 2.886751345948126879, 4.999999999999999112 ) ) ;
#2583=CARTESIAN_POINT ( 'NONE',  ( 8.484601909799253346E-16, 11.56250000000000000, -25.38119784648299770 ) ) ;
#2585=CARTESIAN_POINT ( 'NONE',  ( 26.80312500061451431, -4.541064518000417216, -2.621784821875001281 ) ) ;
#2586=CARTESIAN_POINT ( 'NONE',  ( 7.040625000614517681, -3.027376345333610441, -5.243569643749999898 ) ) ;
#2587=CARTESIAN_POINT ( 'NONE',  ( 20.51250000122903216, 4.330127018922192761, -2.499999999999997780 ) ) ;
#2588=CARTESIAN_POINT ( 'NONE',  ( 25.11562500061451431, 3.027376345333613106, -5.243569643749998122 ) ) ;
#2589=CARTESIAN_POINT ( 'NONE',  ( 25.87500000000000000, 4.330127018922191873, 2.499999999999999556 ) ) ;
#2590=CARTESIAN_POINT ( 'NONE',  ( 3.999999999999998668, 16.32500000122903216, -32.30940107675850470 ) ) ;
#2591=CARTESIAN_POINT ( 'NONE',  ( 26.80312500061451431, -4.541064518000417216, -2.621784821875001281 ) ) ;
#2592=CARTESIAN_POINT ( 'NONE',  ( 8.390625000614518214, -3.027376345333610441, -5.243569643749999898 ) ) ;
#2593=ORIENTED_EDGE ( 'NONE', *, *, #5826, .T. ) ;
#2594=CARTESIAN_POINT ( 'NONE',  ( 24.55312500061451786, -4.541064518000417216, -2.621784821875001281 ) ) ;
#2595=CARTESIAN_POINT ( 'NONE',  ( 4.565625000614516260, 3.027376345333611329, 5.243569643749999010 ) ) ;
#2597=DIRECTION ( 'NONE',  ( -1.000000000000000000, -0.000000000000000000, -0.000000000000000000 ) ) ;
#2598=CARTESIAN_POINT ( 'NONE',  ( 12.03749999999999964, -2.886751345948129988, 4.999999999999997335 ) ) ;
#2599=CARTESIAN_POINT ( 'NONE',  ( 13.05937500061451750, 4.541064518000418104, -2.621784821874998173 ) ) ;
#2600=CARTESIAN_POINT ( 'NONE',  ( 10.05000000122903181, -2.886751345948125991, -5.000000000000000000 ) ) ;
#2601=CARTESIAN_POINT ( 'NONE',  ( 17.18437500061451573, 4.541064518000418104, 2.621784821874999949 ) ) ;
#2603=CARTESIAN_POINT ( 'NONE',  ( 7.996875000614519280, -3.027376345333610441, -5.243569643749999898 ) ) ;
#2604=CARTESIAN_POINT ( 'NONE',  ( -2.121784821874996840, 12.22812500061451857, -26.32496088578401583 ) ) ;
#2605=CARTESIAN_POINT ( 'NONE',  ( -2.000000000000000000, 11.82500000000000107, -33.46410161513775705 ) ) ;
#2608=CARTESIAN_POINT ( 'NONE',  ( 23.27812500061451573, 6.421520780324663323E-16, -5.243569643749999010 ) ) ;
#2609=CARTESIAN_POINT ( 'NONE',  ( -2.121784821874999949, 10.33437500061451786, 26.32496088578401938 ) ) ;
#2610=FACE_OUTER_BOUND ( 'NONE', #2282, .T. ) ;
#2611=CARTESIAN_POINT ( 'NONE',  ( 25.02187500061451431, -6.054752690667223547, -1.112240025338166033E-15 ) ) ;
#2612=EDGE_CURVE ( 'NONE', #22784, #32666, #1863, .T. ) ;
#2613=CARTESIAN_POINT ( 'NONE',  ( 28.13437500061451502, -4.541064518000419881, 2.621784821874995952 ) ) ;
#2614=CARTESIAN_POINT ( 'NONE',  ( 4.715625000614516615, -6.054752690667223547, -1.112240025338166033E-15 ) ) ;
#2616=CARTESIAN_POINT ( 'NONE',  ( 17.78437500061451715, -4.541064518000419881, 2.621784821874995952 ) ) ;
#2618=CARTESIAN_POINT ( 'NONE',  ( 3.403125000614518836, -4.541064518000417216, -2.621784821875001281 ) ) ;
#2619=CARTESIAN_POINT ( 'NONE',  ( 7.359375000614516438, 0.000000000000000000, 5.243569643749999010 ) ) ;
#2620=CARTESIAN_POINT ( 'NONE',  ( 19.47187500061451360, 3.027376345333611329, 5.243569643749999010 ) ) ;
#2621=CARTESIAN_POINT ( 'NONE',  ( 13.68750000122903288, 6.123233995736764310E-16, -4.999999999999998224 ) ) ;
#2622=CARTESIAN_POINT ( 'NONE',  ( 25.76249999999999929, 2.886751345948129099, -4.999999999999998224 ) ) ;
#2623=CARTESIAN_POINT ( 'NONE',  ( 26.82187500061451857, -6.054752690667223547, -1.112240025338166033E-15 ) ) ;
#2627=CARTESIAN_POINT ( 'NONE',  ( 7.162500000000001421, -5.773502691896255534, -1.060575238724906372E-15 ) ) ;
#2629=CARTESIAN_POINT ( 'NONE',  ( 20.95312500061451999, -4.541064518000417216, -2.621784821875001281 ) ) ;
#2630=CARTESIAN_POINT ( 'NONE',  ( 12.15000000000000036, -4.330127018922190985, -2.500000000000001332 ) ) ;
#2632=CARTESIAN_POINT ( 'NONE',  ( 9.337500001229033231, 4.330127018922191873, 2.499999999999999556 ) ) ;
#2633=CARTESIAN_POINT ( 'NONE',  ( 5.540625000614515905, -3.027376345333614438, 5.243569643749998122 ) ) ;
#2634=CARTESIAN_POINT ( 'NONE',  ( 21.11249999999999716, -5.773502691896255534, -1.060575238724906372E-15 ) ) ;
#2635=CARTESIAN_POINT ( 'NONE',  ( 17.46562500061451217, 3.027376345333613106, -5.243569643749998122 ) ) ;
#2636=CARTESIAN_POINT ( 'NONE',  ( 12.00000000000000000, 0.000000000000000000, 4.999999999999998224 ) ) ;
#2638=CARTESIAN_POINT ( 'NONE',  ( 25.38750000122903216, 6.123233995736764310E-16, -4.999999999999998224 ) ) ;
#2640=CARTESIAN_POINT ( 'NONE',  ( 6.225000000000001421, -4.330127018922194537, 2.499999999999995559 ) ) ;
#2642=CARTESIAN_POINT ( 'NONE',  ( 19.79062500061451502, 6.054752690667223547, 3.707466751127219781E-16 ) ) ;
#2643=CARTESIAN_POINT ( 'NONE',  ( 25.94062500061451715, -3.027376345333610441, -5.243569643749999898 ) ) ;
#2644=CARTESIAN_POINT ( 'NONE',  ( 27.68437500061451573, -4.541064518000419881, 2.621784821874995952 ) ) ;
#2645=CARTESIAN_POINT ( 'NONE',  ( 8.099999999999999645, -4.330127018922190985, -2.500000000000001332 ) ) ;
#2646=CARTESIAN_POINT ( 'NONE',  ( 13.60312500061451679, 0.000000000000000000, 5.243569643749999010 ) ) ;
#2647=CARTESIAN_POINT ( 'NONE',  ( 29.65312500061451573, 4.541064518000418104, -2.621784821874998173 ) ) ;
#2648=CARTESIAN_POINT ( 'NONE',  ( 9.440625000614517148, 6.054752690667223547, 3.707466751127219781E-16 ) ) ;
#2649=CARTESIAN_POINT ( 'NONE',  ( 7.012500001229035718, 4.330127018922192761, -2.499999999999997780 ) ) ;
#2650=CARTESIAN_POINT ( 'NONE',  ( 4.243569643749999898, 11.94687500061451857, 32.45002607614398471 ) ) ;
#2652=CARTESIAN_POINT ( 'NONE',  ( 27.07500000122903216, -5.773502691896255534, -1.060575238724906372E-15 ) ) ;
#2654=CARTESIAN_POINT ( 'NONE',  ( 16.97812500061451502, 6.421520780324663323E-16, -5.243569643749999010 ) ) ;
#2656=CARTESIAN_POINT ( 'NONE',  ( 10.65937500061451715, -4.541064518000417216, -2.621784821875001281 ) ) ;
#2657=CARTESIAN_POINT ( 'NONE',  ( 10.32187500061451679, 3.027376345333613106, -5.243569643749998122 ) ) ;
#2658=CARTESIAN_POINT ( 'NONE',  ( 17.29687500061451999, -3.027376345333614438, 5.243569643749998122 ) ) ;
#2660=CARTESIAN_POINT ( 'NONE',  ( 4.000000000000000000, 13.43750000000000000, 32.30940107675849760 ) ) ;
#2661=CARTESIAN_POINT ( 'NONE',  ( 20.91562500061451502, -6.054752690667223547, -1.112240025338166033E-15 ) ) ;
#2662=CARTESIAN_POINT ( 'NONE',  ( 16.62187500061451573, 3.027376345333613106, -5.243569643749998122 ) ) ;
#2663=CARTESIAN_POINT ( 'NONE',  ( 21.32812500061451644, -4.541064518000419881, 2.621784821874995952 ) ) ;
#2664=CARTESIAN_POINT ( 'NONE',  ( 2.000000000000001332, 15.20000000000000107, 33.46410161513774995 ) ) ;
#2665=CARTESIAN_POINT ( 'NONE',  ( 27.40312500061451573, 4.541064518000418104, -2.621784821874998173 ) ) ;
#2666=CARTESIAN_POINT ( 'NONE',  ( 8.212500001229035007, -4.330127018922190985, -2.500000000000001332 ) ) ;
#2667=VERTEX_POINT ( 'NONE', #37882 ) ;
#2668=CARTESIAN_POINT ( 'NONE',  ( 3.825000001229032609, 2.886751345948129099, -4.999999999999998224 ) ) ;
#2669=CARTESIAN_POINT ( 'NONE',  ( -2.828200636599751609E-16, 18.08750000000000213, -34.61880215351700230 ) ) ;
#2670=CARTESIAN_POINT ( 'NONE',  ( 25.72500000122903074, -5.773502691896255534, -1.060575238724906372E-15 ) ) ;
#2672=CARTESIAN_POINT ( 'NONE',  ( 6.009375000614519458, 0.000000000000000000, 5.243569643749999010 ) ) ;
#2673=CARTESIAN_POINT ( 'NONE',  ( 4.337544802671691180, 2.487292970951878956, -4.464402052312094860 ) ) ;
#2675=CARTESIAN_POINT ( 'NONE',  ( 16.19062500061451715, 6.054752690667223547, 3.707466751127219781E-16 ) ) ;
#2676=CARTESIAN_POINT ( 'NONE',  ( 8.484375000614518214, 6.421520780324663323E-16, -5.243569643749999010 ) ) ;
#2677=CARTESIAN_POINT ( 'NONE',  ( 28.05000000122903359, -2.886751345948125991, -5.000000000000000000 ) ) ;
#2678=CARTESIAN_POINT ( 'NONE',  ( 16.39687500061451786, -3.027376345333614438, 5.243569643749998122 ) ) ;
#2679=CARTESIAN_POINT ( 'NONE',  ( 4.434375000614519280, 6.421520780324663323E-16, -5.243569643749999010 ) ) ;
#2680=CARTESIAN_POINT ( 'NONE',  ( 3.999999999999999112, 16.28750000122903430, 30.00000000000000000 ) ) ;
#2681=CARTESIAN_POINT ( 'NONE',  ( 6.253125000614517148, 4.541064518000418104, -2.621784821874998173 ) ) ;
#2682=CARTESIAN_POINT ( 'NONE',  ( 17.01562500061451644, 3.027376345333613106, -5.243569643749998122 ) ) ;
#2683=ORIENTED_EDGE ( 'NONE', *, *, #44097, .T. ) ;
#2684=CARTESIAN_POINT ( 'NONE',  ( 13.64062500061451644, -3.027376345333614438, 5.243569643749998122 ) ) ;
#2685=CARTESIAN_POINT ( 'NONE',  ( 6.375000001229031987, -5.773502691896255534, -1.060575238724906372E-15 ) ) ;
#2686=CARTESIAN_POINT ( 'NONE',  ( 11.65312500061451573, 4.541064518000418104, -2.621784821874998173 ) ) ;
#2688=CARTESIAN_POINT ( 'NONE',  ( 11.92500000000000071, 4.330127018922191873, 2.499999999999999556 ) ) ;
#2689=CARTESIAN_POINT ( 'NONE',  ( 7.575000001229033053, 2.886751345948126879, 4.999999999999999112 ) ) ;
#2691=CARTESIAN_POINT ( 'NONE',  ( 20.47500000000000142, 4.330127018922191873, 2.499999999999999556 ) ) ;
#2692=( BOUNDED_CURVE ( )  B_SPLINE_CURVE ( 2, ( #60582, #27352, #3727, #72408, #21790, #4095, #55062 ),
 .UNSPECIFIED., .F., .F. ) 
 B_SPLINE_CURVE_WITH_KNOTS ( ( 3, 2, 2, 3 ),
 ( 0.8250000000000000666, 0.8277777777777778345, 0.8305555555555557135, 0.8333333333333334814 ),
 .UNSPECIFIED. ) 
 CURVE ( )  GEOMETRIC_REPRESENTATION_ITEM ( )  RATIONAL_B_SPLINE_CURVE ( ( 0.9999999999999946709, 0.8660254037844440367, 1.000000000000000000, 0.8660254037844387076, 1.000000000000000000, 0.8660254037844333785, 1.000000000000005329 ) ) 
 REPRESENTATION_ITEM ( '' )  );
#2693=CARTESIAN_POINT ( 'NONE',  ( 15.49687500061451750, -3.027376345333614438, 5.243569643749998122 ) ) ;
#2694=CARTESIAN_POINT ( 'NONE',  ( 14.92500000122903181, -5.773502691896255534, -1.060575238724906372E-15 ) ) ;
#2696=CARTESIAN_POINT ( 'NONE',  ( -4.243569643749999898, 19.80312500061451786, -30.00000000000000000 ) ) ;
#2698=CARTESIAN_POINT ( 'NONE',  ( 1.071796769724497445, 15.02990381179670010, -33.99999999999998579 ) ) ;
#2699=CARTESIAN_POINT ( 'NONE',  ( 4.247151432104769420, -2.638504256727666863, 4.531370421416291983 ) ) ;
#2700=DIRECTION ( 'NONE',  ( -0.000000000000000000, -1.000000000000000000, -0.000000000000000000 ) ) ;
#2702=CARTESIAN_POINT ( 'NONE',  ( 16.84687500061451715, -3.027376345333614438, 5.243569643749998122 ) ) ;
#2703=CARTESIAN_POINT ( 'NONE',  ( 29.51249999999999929, 2.886751345948126879, 4.999999999999999112 ) ) ;
#2704=CARTESIAN_POINT ( 'NONE',  ( 12.36562500061451608, -6.054752690667223547, -1.112240025338166033E-15 ) ) ;
#2706=CARTESIAN_POINT ( 'NONE',  ( 23.07187500061451857, 3.027376345333611329, 5.243569643749999010 ) ) ;
#2708=CARTESIAN_POINT ( 'NONE',  ( 10.97812500061451679, -4.541064518000419881, 2.621784821874995952 ) ) ;
#2709=CARTESIAN_POINT ( 'NONE',  ( 15.72187500061451892, 3.027376345333613106, -5.243569643749998122 ) ) ;
#2710=ORIENTED_EDGE ( 'NONE', *, *, #35681, .F. ) ;
#2711=CARTESIAN_POINT ( 'NONE',  ( 26.89687500061451431, -3.027376345333610441, -5.243569643749999898 ) ) ;
#2712=CARTESIAN_POINT ( 'NONE',  ( 27.44062500061451715, 6.054752690667223547, 3.707466751127219781E-16 ) ) ;
#2713=CARTESIAN_POINT ( 'NONE',  ( 18.74062500061451431, -3.027376345333610441, -5.243569643749999898 ) ) ;
#2714=CARTESIAN_POINT ( 'NONE',  ( 27.66562500061451146, -6.054752690667223547, -1.112240025338166033E-15 ) ) ;
#2715=LINE ( 'NONE', #59209, #27824 ) ;
#2716=CARTESIAN_POINT ( 'NONE',  ( 7.800000000000001599, 4.330127018922192761, -2.499999999999997780 ) ) ;
#2717=CARTESIAN_POINT ( 'NONE',  ( 18.56250000122903288, -4.330127018922190985, -2.500000000000001332 ) ) ;
#2718=CARTESIAN_POINT ( 'NONE',  ( -1.999999999999997113, 18.83750000122903501, -26.53589838486224295 ) ) ;
#2720=ORIENTED_EDGE ( 'NONE', *, *, #63166, .T. ) ;
#2721=CARTESIAN_POINT ( 'NONE',  ( 15.37500000000000000, 6.123233995736764310E-16, -4.999999999999998224 ) ) ;
#2722=CARTESIAN_POINT ( 'NONE',  ( 19.94999999999999929, 4.330127018922192761, -2.499999999999997780 ) ) ;
#2723=CARTESIAN_POINT ( 'NONE',  ( 15.79687500061451821, 6.054752690667223547, 3.707466751127219781E-16 ) ) ;
#2724=CARTESIAN_POINT ( 'NONE',  ( 14.16562500061451679, -6.054752690667223547, -1.112240025338166033E-15 ) ) ;
#2725=ORIENTED_EDGE ( 'NONE', *, *, #54850, .T. ) ;
#2726=LINE ( 'NONE', #20428, #1814 ) ;
#2727=CARTESIAN_POINT ( 'NONE',  ( 4.243569643749999010, 16.07187500061451857, -32.45002607614398471 ) ) ;
#2728=CARTESIAN_POINT ( 'NONE',  ( 5.765625000614519102, 3.027376345333613106, -5.243569643749998122 ) ) ;
#2730=CARTESIAN_POINT ( 'NONE',  ( 12.15000000000000036, -4.330127018922190985, -2.500000000000001332 ) ) ;
#2732=CARTESIAN_POINT ( 'NONE',  ( 4.243569643749999010, 14.21562500061451928, 27.54997392385601174 ) ) ;
#2733=CARTESIAN_POINT ( 'NONE',  ( 26.05312500061451431, 4.541064518000418104, -2.621784821874998173 ) ) ;
#2736=CARTESIAN_POINT ( 'NONE',  ( 24.08437500061451786, -4.541064518000419881, 2.621784821874995952 ) ) ;
#2737=CARTESIAN_POINT ( 'NONE',  ( 20.57812500061451644, 6.421520780324663323E-16, -5.243569643749999010 ) ) ;
#2738=CARTESIAN_POINT ( 'NONE',  ( -2.121784821874999949, 17.47812500061459318, -33.67503911421598417 ) ) ;
#2739=CARTESIAN_POINT ( 'NONE',  ( 24.41250000122903430, -4.330127018922190985, -2.500000000000001332 ) ) ;
#2740=CARTESIAN_POINT ( 'NONE',  ( 7.640625000614517326, 6.054752690667223547, 3.707466751127219781E-16 ) ) ;
#2742=CARTESIAN_POINT ( 'NONE',  ( 23.42812500061451786, 4.541064518000418104, 2.621784821874999949 ) ) ;
#2745=CARTESIAN_POINT ( 'NONE',  ( 17.48437500061451999, 6.421520780324663323E-16, -5.243569643749999010 ) ) ;
#2746=CARTESIAN_POINT ( 'NONE',  ( 24.15937500061451715, -4.541064518000417216, -2.621784821875001281 ) ) ;
#2747=CARTESIAN_POINT ( 'NONE',  ( 2.121784821875001281, 13.70937500061451786, 33.67503911421598417 ) ) ;
#2748=CARTESIAN_POINT ( 'NONE',  ( 4.790625000614518569, -3.027376345333610441, -5.243569643749999898 ) ) ;
#2749=CARTESIAN_POINT ( 'NONE',  ( 29.72812500061451502, 4.541064518000418104, 2.621784821874999949 ) ) ;
#2750=CARTESIAN_POINT ( 'NONE',  ( 29.50312500061451360, -4.541064518000417216, -2.621784821875001281 ) ) ;
#2752=DIRECTION ( 'NONE',  ( -1.000000000000000000, -0.000000000000000000, -0.000000000000000000 ) ) ;
#2753=CARTESIAN_POINT ( 'NONE',  ( 29.55000000122903003, 5.773502691896255534, 3.535250795749688894E-16 ) ) ;
#2754=CARTESIAN_POINT ( 'NONE',  ( 7.734375000614517326, 4.541064518000418104, 2.621784821874999949 ) ) ;
#2755=CARTESIAN_POINT ( 'NONE',  ( 17.66250000122903430, -4.330127018922190985, -2.500000000000001332 ) ) ;
#2756=CARTESIAN_POINT ( 'NONE',  ( 4.284375000614518925, -4.541064518000419881, 2.621784821874995952 ) ) ;
#2757=CARTESIAN_POINT ( 'NONE',  ( 4.340625000614515727, -3.027376345333610441, -5.243569643749999898 ) ) ;
#2760=CARTESIAN_POINT ( 'NONE',  ( 15.19687500061451857, -3.027376345333610441, -5.243569643749999898 ) ) ;
#2761=CARTESIAN_POINT ( 'NONE',  ( 20.99999999999999645, 0.000000000000000000, 4.999999999999998224 ) ) ;
#2762=EDGE_LOOP ( 'NONE', ( #12032, #12705, #25248, #7136 ) ) ;
#2763=CARTESIAN_POINT ( 'NONE',  ( 22.41562500061451502, 3.027376345333613106, -5.243569643749998122 ) ) ;
#2764=CARTESIAN_POINT ( 'NONE',  ( 6.140625000614516438, -3.027376345333610441, -5.243569643749999898 ) ) ;
#2765=CARTESIAN_POINT ( 'NONE',  ( 25.73437500061451644, 4.541064518000418104, 2.621784821874999949 ) ) ;
#2766=CARTESIAN_POINT ( 'NONE',  ( 7.490625000614516082, -3.027376345333610441, -5.243569643749999898 ) ) ;
#2768=CARTESIAN_POINT ( 'NONE',  ( 9.862500001229033586, 0.000000000000000000, 4.999999999999998224 ) ) ;
#2769=CARTESIAN_POINT ( 'NONE',  ( 24.55312500061451786, -4.541064518000417216, -2.621784821875001281 ) ) ;
#2770=CARTESIAN_POINT ( 'NONE',  ( 3.999999999999999112, 19.43750000122903288, -30.00000000000000000 ) ) ;
#2771=CARTESIAN_POINT ( 'NONE',  ( 10.08750000122903323, 6.123233995736764310E-16, -4.999999999999998224 ) ) ;
#2772=CARTESIAN_POINT ( 'NONE',  ( 19.41562500061451146, 3.027376345333611329, 5.243569643749999010 ) ) ;
#2773=CARTESIAN_POINT ( 'NONE',  ( 16.94062500061451715, -3.027376345333610441, -5.243569643749999898 ) ) ;
#2775=CARTESIAN_POINT ( 'NONE',  ( 18.89999999999999858, -4.330127018922190985, -2.500000000000001332 ) ) ;
#2776=CARTESIAN_POINT ( 'NONE',  ( 14.58750000122903323, 6.123233995736764310E-16, -4.999999999999998224 ) ) ;
#2777=CARTESIAN_POINT ( 'NONE',  ( 10.15312500061451750, -4.541064518000417216, -2.621784821875001281 ) ) ;
#2778=CARTESIAN_POINT ( 'NONE',  ( 14.31562500061451537, 3.027376345333613106, -5.243569643749998122 ) ) ;
#2779=CARTESIAN_POINT ( 'NONE',  ( 22.68750000122903288, 6.123233995736764310E-16, -4.999999999999998224 ) ) ;
#2780=CARTESIAN_POINT ( 'NONE',  ( 21.90937500061451715, -4.541064518000417216, -2.621784821875001281 ) ) ;
#2781=CARTESIAN_POINT ( 'NONE',  ( 20.55937500061451573, -4.541064518000417216, -2.621784821875001281 ) ) ;
#2784=CARTESIAN_POINT ( 'NONE',  ( 8.700000001229032165, -2.886751345948125991, -5.000000000000000000 ) ) ;
#2785=CARTESIAN_POINT ( 'NONE',  ( 5.559375000614517504, 0.000000000000000000, 5.243569643749999010 ) ) ;
#2786=CARTESIAN_POINT ( 'NONE',  ( 24.12187500061451217, -6.054752690667223547, -1.112240025338166033E-15 ) ) ;
#2788=CARTESIAN_POINT ( 'NONE',  ( 21.85312500061451502, -4.541064518000417216, -2.621784821875001281 ) ) ;
#2789=CARTESIAN_POINT ( 'NONE',  ( 24.49687500061451573, -3.027376345333614438, 5.243569643749998122 ) ) ;
#2791=DIRECTION ( 'NONE',  ( 0.000000000000000000, 0.000000000000000000, 1.000000000000000000 ) ) ;
#2792=CARTESIAN_POINT ( 'NONE',  ( 5.859375000614519102, 4.541064518000418104, -2.621784821874998173 ) ) ;
#2793=CARTESIAN_POINT ( 'NONE',  ( 17.99062500061451786, 6.054752690667223547, 3.707466751127219781E-16 ) ) ;
#2794=ORIENTED_EDGE ( 'NONE', *, *, #42990, .T. ) ;
#2796=CARTESIAN_POINT ( 'NONE',  ( 24.89062500061451644, -3.027376345333614438, 5.243569643749998122 ) ) ;
#2797=CARTESIAN_POINT ( 'NONE',  ( 4.471875000614518925, 3.027376345333613106, -5.243569643749998122 ) ) ;
#2798=CARTESIAN_POINT ( 'NONE',  ( 4.779258346327469376, 1.469247991000700582, 4.779258346327429408 ) ) ;
#2799=CARTESIAN_POINT ( 'NONE',  ( 1.841668243974592611, 4.655663185590168673, -33.56086590413347892 ) ) ;
#2800=CARTESIAN_POINT ( 'NONE',  ( 13.72500000000000142, 4.330127018922191873, 2.499999999999999556 ) ) ;
#2801=CARTESIAN_POINT ( 'NONE',  ( 25.57500000122903216, 2.886751345948126879, 4.999999999999999112 ) ) ;
#2802=CARTESIAN_POINT ( 'NONE',  ( 21.96562500061451573, 3.027376345333613106, -5.243569643749998122 ) ) ;
#2804=CARTESIAN_POINT ( 'NONE',  ( 24.07499999999999929, 4.330127018922191873, 2.499999999999999556 ) ) ;
#2805=CARTESIAN_POINT ( 'NONE',  ( 27.27187500061451431, -6.054752690667223547, -1.112240025338166033E-15 ) ) ;
#2806=ORIENTED_EDGE ( 'NONE', *, *, #19846, .T. ) ;
#2807=CARTESIAN_POINT ( 'NONE',  ( 13.35000000122903430, 5.773502691896255534, 3.535250795749688401E-16 ) ) ;
#2808=CARTESIAN_POINT ( 'NONE',  ( 11.95312500061451644, -4.541064518000417216, -2.621784821875001281 ) ) ;
#2809=CARTESIAN_POINT ( 'NONE',  ( 24.93750000122903288, 6.123233995736764310E-16, -4.999999999999998224 ) ) ;
#2811=CARTESIAN_POINT ( 'NONE',  ( 29.39062500061451289, -3.027376345333614438, 5.243569643749998122 ) ) ;
#2812=CARTESIAN_POINT ( 'NONE',  ( 12.37500000122903465, 2.886751345948129099, -4.999999999999998224 ) ) ;
#2813=CARTESIAN_POINT ( 'NONE',  ( 20.21250000000000213, -5.773502691896255534, -1.060575238724906372E-15 ) ) ;
#2814=CARTESIAN_POINT ( 'NONE',  ( 25.98750000000000071, -2.886751345948129988, 4.999999999999997335 ) ) ;
#2815=CARTESIAN_POINT ( 'NONE',  ( 3.242103837493086330E-14, 12.80000000122903359, 26.00000000000000711 ) ) ;
#2816=CARTESIAN_POINT ( 'NONE',  ( 7.171875000614517326, 3.027376345333613106, -5.243569643749998122 ) ) ;
#2817=CARTESIAN_POINT ( 'NONE',  ( 19.95937500061451786, 0.000000000000000000, 5.243569643749999010 ) ) ;
#2818=CARTESIAN_POINT ( 'NONE',  ( 19.80000000122903359, -2.886751345948130876, 4.999999999999996447 ) ) ;
#2819=ORIENTED_EDGE ( 'NONE', *, *, #57401, .F. ) ;
#2820=CARTESIAN_POINT ( 'NONE',  ( 27.70312500061451289, -4.541064518000417216, -2.621784821875001281 ) ) ;
#2821=CARTESIAN_POINT ( 'NONE',  ( 4.200000000000001954, 4.330127018922192761, -2.499999999999997780 ) ) ;
#2822=CARTESIAN_POINT ( 'NONE',  ( 5.446875000614518569, 6.054752690667223547, 3.707466751127219781E-16 ) ) ;
#2823=CARTESIAN_POINT ( 'NONE',  ( 15.56250000000000000, 2.886751345948126879, 4.999999999999999112 ) ) ;
#2824=CARTESIAN_POINT ( 'NONE',  ( 14.20312500061451644, -4.541064518000417216, -2.621784821875001281 ) ) ;
#2826=CARTESIAN_POINT ( 'NONE',  ( 1.592000809091587073E-14, 15.38750000000000284, -34.00000000000000000 ) ) ;
#2827=CARTESIAN_POINT ( 'NONE',  ( 3.962290188940274405, -3.840926163143314920, 3.347320737315190531 ) ) ;
#2828=CARTESIAN_POINT ( 'NONE',  ( 17.47500000122903430, 2.886751345948126879, 4.999999999999999112 ) ) ;
#2829=CARTESIAN_POINT ( 'NONE',  ( 3.778125000614519280, -4.541064518000419881, 2.621784821874995952 ) ) ;
#2831=CARTESIAN_POINT ( 'NONE',  ( 8.428125000614517859, 6.421520780324663323E-16, -5.243569643749999010 ) ) ;
#2832=CARTESIAN_POINT ( 'NONE',  ( 24.19687500061451857, -3.027376345333610441, -5.243569643749999898 ) ) ;
#2833=CARTESIAN_POINT ( 'NONE',  ( -3.000416591977282496E-16, 17.94687500061451502, 25.09994784771203058 ) ) ;
#2834=CARTESIAN_POINT ( 'NONE',  ( 24.45937500061451786, 0.000000000000000000, 5.243569643749999010 ) ) ;
#2835=CARTESIAN_POINT ( 'NONE',  ( 6.000000000000001776, 4.330127018922192761, -2.499999999999997780 ) ) ;
#2836=CARTESIAN_POINT ( 'NONE',  ( -2.000000000000000000, 11.93750000122903465, 26.53589838486224650 ) ) ;
#2837=CARTESIAN_POINT ( 'NONE',  ( 12.44062500061451537, -3.027376345333610441, -5.243569643749999898 ) ) ;
#2838=CARTESIAN_POINT ( 'NONE',  ( 3.712500001229034563, -4.330127018922190985, -2.500000000000001332 ) ) ;
#2839=CARTESIAN_POINT ( 'NONE',  ( 8.971875000614515372, 3.027376345333613106, -5.243569643749998122 ) ) ;
#2840=CARTESIAN_POINT ( 'NONE',  ( 4.907911205059083602E-16, 5.000000000000000000, -26.00000000000000000 ) ) ;
#2841=ORIENTED_EDGE ( 'NONE', *, *, #8791, .T. ) ;
#2842=CARTESIAN_POINT ( 'NONE',  ( 11.80312500061451608, 0.000000000000000000, 5.243569643749999010 ) ) ;
#2844=CARTESIAN_POINT ( 'NONE',  ( 25.01250000122903216, 4.330127018922192761, -2.499999999999997780 ) ) ;
#2845=CARTESIAN_POINT ( 'NONE',  ( 10.05937500061451750, 0.000000000000000000, 5.243569643749999010 ) ) ;
#2846=CARTESIAN_POINT ( 'NONE',  ( 12.66562500061451502, 3.027376345333611329, 5.243569643749999010 ) ) ;
#2848=CARTESIAN_POINT ( 'NONE',  ( 21.98437500061451644, 6.421520780324663323E-16, -5.243569643749999010 ) ) ;
#2849=CARTESIAN_POINT ( 'NONE',  ( 0.000000000000000000, 20.00000000000000000, 30.00000000000000000 ) ) ;
#2850=CARTESIAN_POINT ( 'NONE',  ( 4.276577733362700862, 2.590537181842085257, -4.276577733362700862 ) ) ;
#2851=CARTESIAN_POINT ( 'NONE',  ( 30.00000000000000000, 0.000000000000000000, 4.999999999999998224 ) ) ;
#2852=CARTESIAN_POINT ( 'NONE',  ( 9.001249775931846008E-16, 15.47187500061451892, -25.09994784771203058 ) ) ;
#2853=( BOUNDED_CURVE ( )  B_SPLINE_CURVE ( 2, ( #29001, #50087, #45271, #72618, #72980, #56355, #213, #67089, #22362, #16448, #22718, #5745, #6103, #576, #22001, #44558, #67804, #27920, #61520, #23081, #5021, #17178, #38639, #55989, #61163, #28279, #44914, #23446, #5382, #34529, #27555, #39737, #34166, #45639, #50454, #62254, #55625, #11651, #28634, #51172, #67451, #40096, #45992, #68171, #61886, #16813, #68529, #39369, #51538, #11291, #33812, #50811, #17534, #62610, #12006, #57059, #6466, #939, #10558, #33086, #58140, #47804, #2738, #34896, #7546, #18617, #17890, #35259, #57425, #46720, #30807, #6829, #40450, #62966, #12723, #19340, #29718, #13814, #1294, #41895, #57781, #23804, #24893, #29364, #52256, #58503, #7190, #35984, #69970, #12362, #7913, #41536, #24535, #64422, #18975, #47438, #51896, #68889, #69255, #2024, #18246, #46355, #13434, #69614, #40819, #63335, #1659, #24168, #47079, #25256, #41182, #30080, #63691, #64054, #30450, #36354, #13082, #35620, #52979, #2375, #52618, #58867, #8277, #53340, #4212, #3104, #26741, #70333, #32639, #71437, #55180, #10109, #59969, #65522, #14176, #26000, #4575, #59232, #19710, #42262, #65150, #65891, #32273, #31910, #64785, #60696, #66253, #53712, #49274, #36710, #31544, #37810, #14540, #15271, #71807, #8640, #60330, #20812, #3845, #21177, #43367, #42991, #27105, #42626, #9739, #43729, #15631, #31169, #54806, #48905, #25633, #48171, #37076, #70695, #26366, #20070, #59600, #9377, #9013, #38172, #54084, #3482, #48539, #71066, #14908, #20441, #37450, #54446, #6376, #34081, #66625, #11919, #39650, #10830, #28551, #50727, #51086, #39283, #44830, #45185, #27470, #68082, #4936, #67717, #33001, #62169, #33366, #50371, #22635, #55540, #34444, #11200, #56273, #49638, #50002, #72164, #67365, #55902, #56972, #72527, #45552, #38918, #482, #61796, #72896, #11566, #5294, #17089, #21544, #21915, #56621, #44471, #22991, #44099, #6016, #22278, #16363, #16002, #67001, #62522, #38551, #61437, #61074, #17450, #10472, #27840, #40008, #16728, #33727, #5662, #28198, #130, #58781, #13725, #45906, #69169, #29631, #28908, #46264, #51446, #68804, #1209, #12995, #69527, #34806, #35531, #58414, #12638, #24442 ),
 .UNSPECIFIED., .F., .F. ) 
 B_SPLINE_CURVE_WITH_KNOTS ( ( 3, 2, 2, 2, 2, 2, 2, 2, 2, 2, 2, 2, 2, 2, 2, 2, 2, 2, 2, 2, 2, 2, 2, 2, 2, 2, 2, 2, 2, 2, 2, 2, 2, 2, 2, 2, 2, 2, 2, 2, 2, 2, 2, 2, 2, 2, 2, 2, 2, 2, 2, 2, 2, 2, 2, 2, 2, 2, 2, 2, 2, 2, 2, 2, 2, 2, 2, 2, 2, 2, 2, 2, 2, 2, 2, 2, 2, 2, 2, 2, 2, 2, 2, 2, 2, 2, 2, 2, 2, 2, 2, 2, 2, 2, 2, 2, 2, 2, 2, 2, 2, 2, 2, 2, 2, 2, 2, 2, 2, 2, 2, 2, 2, 2, 2, 2, 2, 2, 2, 2, 2, 2, 2, 2, 2, 2, 2, 2, 2, 2, 2, 2, 2, 2, 3 ),
 ( 0.000000000000000000, 0.007499808158871945282, 0.01499961631774389056, 0.02249942447661583411, 0.02999923263548778113, 0.03749904079435972815, 0.04499884895323166822, 0.05249865711210361524, 0.05999846527097556226, 0.06749827342984750234, 0.07499808158871945629, 0.08249788974759138249, 0.08999769790646333645, 0.09749750606533529040, 0.1049973142242072305, 0.1124971223830791706, 0.1199969305419511245, 0.1274967387008230646, 0.1349965468596950047, 0.1424963550185669448, 0.1499961631774389126, 0.1574959713363108527, 0.1649957794951827650, 0.1724955876540547328, 0.1799953958129266729, 0.1874952039717986130, 0.1949950121306705808, 0.2024948202895425209, 0.2099946284484144610, 0.2174944366072864010, 0.2249942447661583411, 0.2324940529250302812, 0.2399938610839022490, 0.2474936692427741891, 0.2549934774016461292, 0.2624932855605180970, 0.2699930937193900093, 0.2774929018782619772, 0.2849927100371338895, 0.2924925181960058573, 0.2999923263548778252, 0.3074921345137497375, 0.3149919426726217053, 0.3224917508314936176, 0.3299915589903655300, 0.3374913671492375533, 0.3449911753081094656, 0.3524909834669814335, 0.3599907916258533458, 0.3674905997847253136, 0.3749904079435972259, 0.3824902161024691938, 0.3899900242613411616, 0.3974898324202130739, 0.4049896405790850418, 0.4124894487379569541, 0.4199892568968289219, 0.4274890650557008898, 0.4349888732145728021, 0.4424886813734447699, 0.4499884895323166822, 0.4574882976911886501, 0.4649881058500605624, 0.4724879140089325302, 0.4799877221678044981, 0.4874875303266764104, 0.4949873384855483782, 0.5024871466444202905, 0.5099869548032922584, 0.5174867629621642262, 0.5249865711210361940, 0.5324863792799080509, 0.5399861874387800187, 0.5474859955976519865, 0.5549858037565239544, 0.5624856119153958112, 0.5699854200742677790, 0.5774852282331397468, 0.5849850363920117147, 0.5924848445508836825, 0.5999846527097556503, 0.6074844608686276182, 0.6149842690274994750, 0.6224840771863714428, 0.6299838853452434106, 0.6374836935041152675, 0.6449835016629872353, 0.6524833098218592031, 0.6599831179807310599, 0.6674829261396030278, 0.6749827342984751066, 0.6824825424573470745, 0.6899823506162189313, 0.6974821587750908991, 0.7049819669339628669, 0.7124817750928347238, 0.7199815832517066916, 0.7274813914105786594, 0.7349811995694506273, 0.7424810077283224841, 0.7499808158871944519, 0.7574806240460665308, 0.7649804322049383876, 0.7724802403638103554, 0.7799800485226823232, 0.7874798566815542911, 0.7949796648404261479, 0.8024794729992981157, 0.8099792811581700835, 0.8174790893170419404, 0.8249788974759139082, 0.8324787056347858760, 0.8399785137936578439, 0.8474783219525298117, 0.8549781301114017795, 0.8624779382702737474, 0.8699777464291456042, 0.8774775545880175720, 0.8849773627468895398, 0.8924771709057615077, 0.8999769790646333645, 0.9074767872235053323, 0.9149765953823773001, 0.9224764035412491570, 0.9299762117001211248, 0.9374760198589932036, 0.9449758280178650605, 0.9524756361767370283, 0.9599754443356089961, 0.9674752524944809640, 0.9749750606533528208, 0.9824748688122247886, 0.9899746769710967564, 0.9974744851299686133, 1.000000000000000000 ),
 .UNSPECIFIED. ) 
 CURVE ( )  GEOMETRIC_REPRESENTATION_ITEM ( )  RATIONAL_B_SPLINE_CURVE ( ( 1.000000000000000000, 0.8660254037844387076, 1.000000000000000000, 0.8660254037844387076, 1.000000000000000000, 0.8660254037844387076, 1.000000000000000000, 0.8660254037844387076, 1.000000000000000000, 0.8660254037844387076, 1.000000000000000000, 0.8660254037844387076, 1.000000000000000000, 0.8660254037844387076, 1.000000000000000000, 0.8660254037844387076, 1.000000000000000000, 0.8660254037844387076, 1.000000000000000000, 0.8660254037844387076, 1.000000000000000000, 0.8660254037844387076, 1.000000000000000000, 0.8660254037844387076, 1.000000000000000000, 0.8660254037844387076, 1.000000000000000000, 0.8660254037844387076, 1.000000000000000000, 0.8660254037844387076, 1.000000000000000000, 0.8660254037844387076, 1.000000000000000000, 0.8660254037844387076, 1.000000000000000000, 0.8660254037844387076, 1.000000000000000000, 0.8660254037844387076, 1.000000000000000000, 0.8660254037844387076, 1.000000000000000000, 0.8660254037844387076, 1.000000000000000000, 0.8660254037844387076, 1.000000000000000000, 0.8660254037844387076, 1.000000000000000000, 0.8660254037844387076, 1.000000000000000000, 0.8660254037844387076, 1.000000000000000000, 0.8660254037844387076, 1.000000000000000000, 0.8660254037844387076, 1.000000000000000000, 0.8660254037844387076, 1.000000000000000000, 0.8660254037844387076, 1.000000000000000000, 0.8660254037844387076, 1.000000000000000000, 0.8660254037844387076, 1.000000000000000000, 0.8660254037844387076, 1.000000000000000000, 0.8660254037844387076, 1.000000000000000000, 0.8660254037844387076, 1.000000000000000000, 0.8660254037844387076, 1.000000000000000000, 0.8660254037844387076, 1.000000000000000000, 0.8660254037844387076, 1.000000000000000000, 0.8660254037844387076, 1.000000000000000000, 0.8660254037844387076, 1.000000000000000000, 0.8660254037844387076, 1.000000000000000000, 0.8660254037844387076, 1.000000000000000000, 0.8660254037844387076, 1.000000000000000000, 0.8660254037844387076, 1.000000000000000000, 0.8660254037844387076, 1.000000000000000000, 0.8660254037844387076, 1.000000000000000000, 0.8660254037844387076, 1.000000000000000000, 0.8660254037844387076, 1.000000000000000000, 0.8660254037844387076, 1.000000000000000000, 0.8660254037844387076, 1.000000000000000000, 0.8660254037844387076, 1.000000000000000000, 0.8660254037844387076, 1.000000000000000000, 0.8660254037844387076, 1.000000000000000000, 0.8660254037844387076, 1.000000000000000000, 0.8660254037844387076, 1.000000000000000000, 0.8660254037844387076, 1.000000000000000000, 0.8660254037844387076, 1.000000000000000000, 0.8660254037844387076, 1.000000000000000000, 0.8660254037844387076, 1.000000000000000000, 0.8660254037844387076, 1.000000000000000000, 0.8660254037844387076, 1.000000000000000000, 0.8660254037844387076, 1.000000000000000000, 0.8660254037844387076, 1.000000000000000000, 0.8660254037844387076, 1.000000000000000000, 0.8660254037844387076, 1.000000000000000000, 0.8660254037844387076, 1.000000000000000000, 0.8660254037844387076, 1.000000000000000000, 0.8660254037844387076, 1.000000000000000000, 0.8660254037844387076, 1.000000000000000000, 0.8660254037844387076, 1.000000000000000000, 0.8660254037844387076, 1.000000000000000000, 0.8660254037844387076, 1.000000000000000000, 0.8660254037844387076, 1.000000000000000000, 0.8660254037844387076, 1.000000000000000000, 0.8660254037844387076, 1.000000000000000000, 0.8660254037844387076, 1.000000000000000000, 0.8660254037844387076, 1.000000000000000000, 0.8660254037844387076, 1.000000000000000000, 0.8660254037844387076, 1.000000000000000000, 0.8660254037844387076, 1.000000000000000000, 0.8660254037844387076, 1.000000000000000000, 0.8660254037844387076, 1.000000000000000000, 0.8660254037844387076, 1.000000000000000000, 0.8660254037844387076, 1.000000000000000000, 0.8660254037844387076, 1.000000000000000000, 0.8660254037844387076, 1.000000000000000000, 0.8660254037844387076, 1.000000000000000000, 0.8660254037844387076, 1.000000000000000000, 0.8660254037844387076, 1.000000000000000000, 0.8660254037844387076, 1.000000000000000000, 0.8660254037844387076, 1.000000000000000000, 0.8660254037844387076, 1.000000000000000000, 0.8660254037844387076, 1.000000000000000000, 0.8660254037844387076, 1.000000000000000000, 0.8660254037844387076, 1.000000000000000000, 0.8660254037844387076, 1.000000000000000000, 0.8660254037844387076, 1.000000000000000000, 0.8660254037844387076, 1.000000000000000000, 0.8660254037844387076, 1.000000000000000000, 0.8660254037844387076, 1.000000000000000000, 0.8660254037844387076, 1.000000000000000000, 0.8660254037844387076, 1.000000000000000000, 0.8660254037844387076, 1.000000000000000000, 0.8660254037844387076, 1.000000000000000000, 0.8660254037844387076, 1.000000000000000000, 0.8660254037844387076, 1.000000000000000000, 0.8660254037844387076, 1.000000000000000000, 0.8660254037844387076, 1.000000000000000000, 0.8660254037844387076, 1.000000000000000000, 0.8660254037844387076, 1.000000000000000000, 0.8660254037844387076, 1.000000000000000000, 0.8660254037844387076, 1.000000000000000000, 0.8660254037844387076, 1.000000000000000000, 0.8660254037844387076, 1.000000000000000000, 0.8660254037844387076, 1.000000000000000000, 0.8660254037844387076, 1.000000000000000000, 0.8660254037844387076, 1.000000000000000000, 0.8660254037844387076, 1.000000000000000000, 0.8660254037844387076, 1.000000000000000000, 0.8660254037844387076, 1.000000000000000000, 0.8660254037844387076, 1.000000000000000000, 0.8660254037844387076, 1.000000000000000000, 0.8660254037844387076, 1.000000000000000000, 0.8660254037844387076, 1.000000000000000000, 0.8660254037844387076, 1.000000000000000000, 0.8660254037844387076, 1.000000000000000000, 0.8660254037844387076, 1.000000000000000000, 0.8660254037844387076, 1.000000000000000000, 0.8660254037844387076, 1.000000000000000000, 0.8660254037844387076, 1.000000000000000000, 0.8660254037844387076, 1.000000000000000000, 0.8660254037844387076, 1.000000000000000000, 0.8660254037844387076, 1.000000000000000000, 0.8660254037844387076, 1.000000000000000000, 0.9548848677736607726, 0.9401542295229587953 ) ) 
 REPRESENTATION_ITEM ( '' )  );
#2854=CARTESIAN_POINT ( 'NONE',  ( 15.60937500061451644, -4.541064518000417216, -2.621784821875001281 ) ) ;
#2855=CARTESIAN_POINT ( 'NONE',  ( 18.07500000122903216, -5.773502691896255534, -1.060575238724906372E-15 ) ) ;
#2856=CARTESIAN_POINT ( 'NONE',  ( 12.87187500061451750, -6.054752690667223547, -1.112240025338166033E-15 ) ) ;
#2857=CARTESIAN_POINT ( 'NONE',  ( -2.121784821874996840, 18.07812500061451644, -26.32496088578401583 ) ) ;
#2858=CARTESIAN_POINT ( 'NONE',  ( 18.22500000122903430, 2.886751345948129099, -4.999999999999998224 ) ) ;
#2859=CARTESIAN_POINT ( 'NONE',  ( 13.00312500061451537, 4.541064518000418104, -2.621784821874998173 ) ) ;
#2861=VERTEX_POINT ( 'NONE', #40437 ) ;
#2862=CARTESIAN_POINT ( 'NONE',  ( 15.75000000000000000, -4.330127018922190985, -2.500000000000001332 ) ) ;
#2863=CARTESIAN_POINT ( 'NONE',  ( 19.16250000122903430, 4.330127018922192761, -2.499999999999997780 ) ) ;
#2864=CARTESIAN_POINT ( 'NONE',  ( 12.90937500061451537, -4.541064518000417216, -2.621784821875001281 ) ) ;
#2865=CARTESIAN_POINT ( 'NONE',  ( 3.027206758929961161, 3.985217399322935172, 27.37339809994529105 ) ) ;
#2866=CARTESIAN_POINT ( 'NONE',  ( 11.81250000122903465, -4.330127018922190985, -2.500000000000001332 ) ) ;
#2867=CARTESIAN_POINT ( 'NONE',  ( 20.73750000122903359, -4.330127018922194537, 2.499999999999995559 ) ) ;
#2868=CARTESIAN_POINT ( 'NONE',  ( 18.25312500061451715, -4.541064518000417216, -2.621784821875001281 ) ) ;
#2869=CARTESIAN_POINT ( 'NONE',  ( 20.54062500061451502, -3.027376345333610441, -5.243569643749999898 ) ) ;
#2870=CARTESIAN_POINT ( 'NONE',  ( 27.67500000122903359, 2.886751345948129099, -4.999999999999998224 ) ) ;
#2871=CARTESIAN_POINT ( 'NONE',  ( 25.12499999999999645, -4.330127018922194537, 2.499999999999995559 ) ) ;
#2874=CARTESIAN_POINT ( 'NONE',  ( 27.12187500061451573, 3.027376345333611329, 5.243569643749999010 ) ) ;
#2875=CARTESIAN_POINT ( 'NONE',  ( -1.389182545231912203, 9.676047173952133207, -33.81675723707382275 ) ) ;
#2876=CARTESIAN_POINT ( 'NONE',  ( -4.243569643749997233, 14.49687500061451928, -27.54997392385601174 ) ) ;
#2877=CARTESIAN_POINT ( 'NONE',  ( 4.350000001229033408, 5.773502691896255534, 3.535250795749688894E-16 ) ) ;
#2878=CARTESIAN_POINT ( 'NONE',  ( 3.900000000000000799, 0.000000000000000000, 4.999999999999998224 ) ) ;
#2879=EDGE_CURVE ( 'NONE', #12976, #35743, #16076, .T. ) ;
#2880=CARTESIAN_POINT ( 'NONE',  ( 7.096875000614517148, -3.027376345333610441, -5.243569643749999898 ) ) ;
#2881=CARTESIAN_POINT ( 'NONE',  ( 27.66562500061451146, -6.054752690667223547, -1.112240025338166033E-15 ) ) ;
#2883=CARTESIAN_POINT ( 'NONE',  ( 7.285825834671762338E-16, 10.00000000000000000, -24.00000000000000000 ) ) ;
#2884=CARTESIAN_POINT ( 'NONE',  ( 8.250000000000000000, 4.330127018922192761, -2.499999999999997780 ) ) ;
#2885=CARTESIAN_POINT ( 'NONE',  ( 5.259375000614518569, -4.541064518000417216, -2.621784821875001281 ) ) ;
#2886=CARTESIAN_POINT ( 'NONE',  ( 12.27187500061451786, 3.027376345333611329, 5.243569643749999010 ) ) ;
#2887=CARTESIAN_POINT ( 'NONE',  ( 4.800000000000002487, 0.000000000000000000, 4.999999999999998224 ) ) ;
#2889=CARTESIAN_POINT ( 'NONE',  ( -3.000416591977282496E-16, 14.29062500061459495, 25.09994784771203058 ) ) ;
#2890=CARTESIAN_POINT ( 'NONE',  ( 6.150000000000003020, 0.000000000000000000, 4.999999999999998224 ) ) ;
#2892=CARTESIAN_POINT ( 'NONE',  ( 21.06562500061451715, 3.027376345333613106, -5.243569643749998122 ) ) ;
#2893=CARTESIAN_POINT ( 'NONE',  ( 9.965625000614517504, 3.027376345333611329, 5.243569643749999010 ) ) ;
#2895=CARTESIAN_POINT ( 'NONE',  ( 8.521875000614516082, 3.027376345333613106, -5.243569643749998122 ) ) ;
#2896=CARTESIAN_POINT ( 'NONE',  ( 26.81250000000000000, 2.886751345948126879, 4.999999999999999112 ) ) ;
#2897=CARTESIAN_POINT ( 'NONE',  ( 19.23750000122903714, 4.330127018922191873, 2.499999999999999556 ) ) ;
#2898=VECTOR ( 'NONE', #20773, 1000.000000000000000 ) ;
#2899=CARTESIAN_POINT ( 'NONE',  ( 26.65312500061451573, 0.000000000000000000, 5.243569643749999010 ) ) ;
#2900=CARTESIAN_POINT ( 'NONE',  ( 3.999999999999998668, 10.92500000122903536, 27.69059892324149530 ) ) ;
#2901=CARTESIAN_POINT ( 'NONE',  ( 9.496875000614517504, 6.054752690667223547, 3.707466751127219781E-16 ) ) ;
#2902=CARTESIAN_POINT ( 'NONE',  ( 15.30937500061451750, 4.541064518000418104, -2.621784821874998173 ) ) ;
#2903=CARTESIAN_POINT ( 'NONE',  ( 26.89687500061451431, -3.027376345333610441, -5.243569643749999898 ) ) ;
#2904=CARTESIAN_POINT ( 'NONE',  ( 28.19999999999999929, 0.000000000000000000, 4.999999999999998224 ) ) ;
#2906=CARTESIAN_POINT ( 'NONE',  ( 19.77187500061451786, 3.027376345333613106, -5.243569643749998122 ) ) ;
#2907=CARTESIAN_POINT ( 'NONE',  ( 12.90937500061451537, -4.541064518000417216, -2.621784821875001281 ) ) ;
#2909=CARTESIAN_POINT ( 'NONE',  ( 23.55000000000000071, 4.330127018922192761, -2.499999999999997780 ) ) ;
#2911=CARTESIAN_POINT ( 'NONE',  ( -4.243569643749997233, 11.79687500061451999, -27.54997392385601174 ) ) ;
#2913=CARTESIAN_POINT ( 'NONE',  ( 14.46562500061451750, 3.027376345333611329, 5.243569643749999010 ) ) ;
#2914=CARTESIAN_POINT ( 'NONE',  ( 4.087500000000001243, -2.886751345948125991, -5.000000000000000000 ) ) ;
#2915=CYLINDRICAL_SURFACE ( 'NONE', #53610, 3.999999999999996447 ) ;
#2917=CARTESIAN_POINT ( 'NONE',  ( 12.00000000000000000, 0.000000000000000000, 4.999999999999998224 ) ) ;
#2918=CARTESIAN_POINT ( 'NONE',  ( 3.999999999999998668, 17.67500000122903359, 27.69059892324149175 ) ) ;
#2919=CARTESIAN_POINT ( 'NONE',  ( 12.03750000122903430, 4.330127018922191873, 2.499999999999999556 ) ) ;
#2921=CARTESIAN_POINT ( 'NONE',  ( 21.34687500061451715, -3.027376345333614438, 5.243569643749998122 ) ) ;
#2922=CARTESIAN_POINT ( 'NONE',  ( 16.73437500061451644, 4.541064518000418104, 2.621784821874999949 ) ) ;
#2923=CARTESIAN_POINT ( 'NONE',  ( 1.626862140677534273E-15, 16.51249999999999929, -26.00000000000000355 ) ) ;
#2924=ORIENTED_EDGE ( 'NONE', *, *, #37057, .T. ) ;
#2925=CARTESIAN_POINT ( 'NONE',  ( 19.49062500061451431, -3.027376345333614438, 5.243569643749998122 ) ) ;
#2927=CARTESIAN_POINT ( 'NONE',  ( 4.415625000614518569, 3.027376345333613106, -5.243569643749998122 ) ) ;
#2928=CARTESIAN_POINT ( 'NONE',  ( 17.10937500061451999, 4.541064518000418104, -2.621784821874998173 ) ) ;
#2929=CARTESIAN_POINT ( 'NONE',  ( 28.09687500061451360, -3.027376345333614438, 5.243569643749998122 ) ) ;
#2930=CARTESIAN_POINT ( 'NONE',  ( 3.928125000614516527, 6.421520780324663323E-16, -5.243569643749999010 ) ) ;
#2931=CARTESIAN_POINT ( 'NONE',  ( 18.62812500061451715, -4.541064518000419881, 2.621784821874995952 ) ) ;
#2932=CARTESIAN_POINT ( 'NONE',  ( 2.121784821875001281, 15.00312500061451715, 33.67503911421598417 ) ) ;
#2933=CARTESIAN_POINT ( 'NONE',  ( 16.57500000122903216, 2.886751345948126879, 4.999999999999999112 ) ) ;
#2935=CARTESIAN_POINT ( 'NONE',  ( 8.315625000614515372, -6.054752690667223547, -1.112240025338166033E-15 ) ) ;
#2936=CARTESIAN_POINT ( 'NONE',  ( 29.57812500061451644, 6.421520780324663323E-16, -5.243569643749999010 ) ) ;
#2937=CARTESIAN_POINT ( 'NONE',  ( 22.95937500061451431, 4.541064518000418104, -2.621784821874998173 ) ) ;
#2938=CARTESIAN_POINT ( 'NONE',  ( 13.45312500061451466, 4.541064518000418104, -2.621784821874998173 ) ) ;
#2939=CARTESIAN_POINT ( 'NONE',  ( 25.12500000122903288, 2.886751345948126879, 4.999999999999999112 ) ) ;
#2940=CARTESIAN_POINT ( 'NONE',  ( 22.56562500061451715, 3.027376345333611329, 5.243569643749999010 ) ) ;
#2941=CARTESIAN_POINT ( 'NONE',  ( 19.84687500061451360, 6.054752690667223547, 3.707466751127219781E-16 ) ) ;
#2942=CARTESIAN_POINT ( 'NONE',  ( 14.87812500061451537, 4.541064518000418104, 2.621784821874999949 ) ) ;
#2943=CARTESIAN_POINT ( 'NONE',  ( 4.243569643749999010, 15.17187500061451644, 27.54997392385601174 ) ) ;
#2945=CARTESIAN_POINT ( 'NONE',  ( 20.42812500061451431, -4.541064518000419881, 2.621784821874995952 ) ) ;
#2946=CARTESIAN_POINT ( 'NONE',  ( 28.86562500061451786, 3.027376345333611329, 5.243569643749999010 ) ) ;
#2948=ORIENTED_EDGE ( 'NONE', *, *, #66296, .T. ) ;
#2949=CARTESIAN_POINT ( 'NONE',  ( 23.13749999999999929, 5.773502691896255534, 3.535250795749688894E-16 ) ) ;
#2950=CARTESIAN_POINT ( 'NONE',  ( -3.999999999999999112, 10.55000000000000249, -30.00000000000000000 ) ) ;
#2951=CARTESIAN_POINT ( 'NONE',  ( 13.16250000122903430, -4.330127018922190985, -2.500000000000001332 ) ) ;
#2952=CARTESIAN_POINT ( 'NONE',  ( 28.04062500061451502, -3.027376345333614438, 5.243569643749998122 ) ) ;
#2953=CARTESIAN_POINT ( 'NONE',  ( 8.503125000614515372, 4.541064518000418104, -2.621784821874998173 ) ) ;
#2954=CARTESIAN_POINT ( 'NONE',  ( 19.57500000122903216, 2.886751345948129099, -4.999999999999998224 ) ) ;
#2955=CARTESIAN_POINT ( 'NONE',  ( 24.29062500061451502, 6.054752690667223547, 3.707466751127219781E-16 ) ) ;
#2956=CARTESIAN_POINT ( 'NONE',  ( 24.44999999999999929, 4.330127018922192761, -2.499999999999997780 ) ) ;
#2957=CARTESIAN_POINT ( 'NONE',  ( 27.10312500061451502, 0.000000000000000000, 5.243569643749999010 ) ) ;
#2958=CARTESIAN_POINT ( 'NONE',  ( 7.790625000614518569, -3.027376345333614438, 5.243569643749998122 ) ) ;
#2960=CARTESIAN_POINT ( 'NONE',  ( 23.09062500061451573, -3.027376345333614438, 5.243569643749998122 ) ) ;
#2961=CARTESIAN_POINT ( 'NONE',  ( 5.503125000614516260, 0.000000000000000000, 5.243569643749999010 ) ) ;
#2963=CARTESIAN_POINT ( 'NONE',  ( 3.740625000614516527, -3.027376345333614438, 5.243569643749998122 ) ) ;
#2964=EDGE_CURVE ( 'NONE', #47076, #64681, #6604, .T. ) ;
#2965=CARTESIAN_POINT ( 'NONE',  ( -3.999999999999997335, 10.25000000122903643, 32.30940107675850470 ) ) ;
#2967=CARTESIAN_POINT ( 'NONE',  ( 13.68750000000000178, 5.773502691896255534, 3.535250795749688894E-16 ) ) ;
#2969=CARTESIAN_POINT ( 'NONE',  ( 14.59687500061452070, -3.027376345333614438, 5.243569643749998122 ) ) ;
#2970=CARTESIAN_POINT ( 'NONE',  ( 9.187500001229034652, 6.123233995736764310E-16, -4.999999999999998224 ) ) ;
#2971=CARTESIAN_POINT ( 'NONE',  ( 15.53437500061451715, -4.541064518000419881, 2.621784821874995952 ) ) ;
#2973=CARTESIAN_POINT ( 'NONE',  ( 9.496875000614517504, 6.054752690667223547, 3.707466751127219781E-16 ) ) ;
#2974=CARTESIAN_POINT ( 'NONE',  ( 9.001249775931846008E-16, 11.81562500061451715, -25.09994784771203058 ) ) ;
#2976=CARTESIAN_POINT ( 'NONE',  ( 12.83437500061451786, -4.541064518000419881, 2.621784821874995952 ) ) ;
#2978=CARTESIAN_POINT ( 'NONE',  ( 21.77812500061451928, -4.541064518000419881, 2.621784821874995952 ) ) ;
#2979=CARTESIAN_POINT ( 'NONE',  ( -3.000416591977282496E-16, 10.29687500061451644, 25.09994784771203058 ) ) ;
#2980=CARTESIAN_POINT ( 'NONE',  ( 26.33437500061451431, -4.541064518000419881, 2.621784821874995952 ) ) ;
#2981=CARTESIAN_POINT ( 'NONE',  ( 29.10937500061451644, -4.541064518000417216, -2.621784821875001281 ) ) ;
#2982=CARTESIAN_POINT ( 'NONE',  ( 3.328125000614516438, -4.541064518000419881, 2.621784821874995952 ) ) ;
#2984=CARTESIAN_POINT ( 'NONE',  ( 17.29687500061451999, -3.027376345333614438, 5.243569643749998122 ) ) ;
#2986=CARTESIAN_POINT ( 'NONE',  ( 3.815625000614518036, -6.054752690667223547, -1.112240025338166033E-15 ) ) ;
#2987=CARTESIAN_POINT ( 'NONE',  ( 6.271875000614517859, 3.027376345333613106, -5.243569643749998122 ) ) ;
#2988=CARTESIAN_POINT ( 'NONE',  ( 17.59687500061451715, 6.054752690667223547, 3.707466751127219781E-16 ) ) ;
#2990=CARTESIAN_POINT ( 'NONE',  ( 24.78750000000000497, -2.886751345948125991, -5.000000000000000000 ) ) ;
#2991=CARTESIAN_POINT ( 'NONE',  ( 27.90937500061451715, 4.541064518000418104, -2.621784821874998173 ) ) ;
#2993=CARTESIAN_POINT ( 'NONE',  ( 30.00000000000000000, 0.000000000000000000, 4.999999999999998224 ) ) ;
#2994=EDGE_LOOP ( 'NONE', ( #15905, #22606, #31537, #29961 ) ) ;
#2995=CARTESIAN_POINT ( 'NONE',  ( 8.437500000000000000, -2.886751345948129988, 4.999999999999997335 ) ) ;
#2997=CARTESIAN_POINT ( 'NONE',  ( 21.81562500061451004, -6.054752690667223547, -1.112240025338166033E-15 ) ) ;
#2998=CARTESIAN_POINT ( 'NONE',  ( 11.81250000000000000, 2.886751345948129099, -4.999999999999998224 ) ) ;
#2999=CARTESIAN_POINT ( 'NONE',  ( 6.290625000614517681, 6.054752690667223547, 3.707466751127219781E-16 ) ) ;
#3000=CARTESIAN_POINT ( 'NONE',  ( 19.61249999999999716, 2.886751345948126879, 4.999999999999999112 ) ) ;
#3001=CARTESIAN_POINT ( 'NONE',  ( 19.26562500061451644, 3.027376345333613106, -5.243569643749998122 ) ) ;
#3002=LINE ( 'NONE', #42527, #72647 ) ;
#3003=CARTESIAN_POINT ( 'NONE',  ( 23.70000000122903216, 5.773502691896255534, 3.535250795749688894E-16 ) ) ;
#3005=CARTESIAN_POINT ( 'NONE',  ( 4.462500000000001243, -5.773502691896255534, -1.060575238724906372E-15 ) ) ;
#3006=ORIENTED_EDGE ( 'NONE', *, *, #11716, .F. ) ;
#3007=CARTESIAN_POINT ( 'NONE',  ( 19.75312500061451360, 4.541064518000418104, -2.621784821874998173 ) ) ;
#3008=CARTESIAN_POINT ( 'NONE',  ( 26.57812500061451644, 4.541064518000418104, 2.621784821874999949 ) ) ;
#3009=CARTESIAN_POINT ( 'NONE',  ( 25.88437500061451502, -4.541064518000419881, 2.621784821874995952 ) ) ;
#3010=CARTESIAN_POINT ( 'NONE',  ( 7.987500000000000711, -2.886751345948129988, 4.999999999999997335 ) ) ;
#3011=CARTESIAN_POINT ( 'NONE',  ( 12.59062500061451573, 6.054752690667223547, 3.707466751127219781E-16 ) ) ;
#3012=CARTESIAN_POINT ( 'NONE',  ( 29.12812500061451715, 6.421520780324663323E-16, -5.243569643749999010 ) ) ;
#3013=CARTESIAN_POINT ( 'NONE',  ( 18.08437500061451431, 4.541064518000418104, 2.621784821874999949 ) ) ;
#3014=CARTESIAN_POINT ( 'NONE',  ( 9.140625000614518214, -3.027376345333614438, 5.243569643749998122 ) ) ;
#3016=CARTESIAN_POINT ( 'NONE',  ( 4.243569643749999898, 12.84687500061451715, 32.45002607614398471 ) ) ;
#3017=CARTESIAN_POINT ( 'NONE',  ( 23.43750000122902932, -4.330127018922194537, 2.499999999999995559 ) ) ;
#3019=CARTESIAN_POINT ( 'NONE',  ( 13.30312500061451786, -4.541064518000417216, -2.621784821875001281 ) ) ;
#3020=CARTESIAN_POINT ( 'NONE',  ( 10.69687500061451679, -3.027376345333610441, -5.243569643749999898 ) ) ;
#3021=CARTESIAN_POINT ( 'NONE',  ( 9.234375000614518214, -4.541064518000419881, 2.621784821874995952 ) ) ;
#3022=CARTESIAN_POINT ( 'NONE',  ( 18.45937500061451431, 4.541064518000418104, -2.621784821874998173 ) ) ;
#3024=CARTESIAN_POINT ( 'NONE',  ( 22.75312500061451360, -4.541064518000417216, -2.621784821875001281 ) ) ;
#3025=EDGE_CURVE ( 'NONE', #38182, #55885, #22709, .T. ) ;
#3027=CARTESIAN_POINT ( 'NONE',  ( 17.44687500061451857, -3.027376345333610441, -5.243569643749999898 ) ) ;
#3028=CARTESIAN_POINT ( 'NONE',  ( 23.12812500061451360, -4.541064518000419881, 2.621784821874995952 ) ) ;
#3029=CARTESIAN_POINT ( 'NONE',  ( 4.000000000000000000, 11.18750000000000178, 32.30940107675849049 ) ) ;
#3030=CARTESIAN_POINT ( 'NONE',  ( 26.91562500061451146, 3.027376345333613106, -5.243569643749998122 ) ) ;
#3031=CARTESIAN_POINT ( 'NONE',  ( 6.787500001229032520, -4.330127018922194537, 2.499999999999995559 ) ) ;
#3032=ORIENTED_EDGE ( 'NONE', *, *, #18203, .F. ) ;
#3033=CARTESIAN_POINT ( 'NONE',  ( 3.150000001229034119, -2.886751345948129988, 4.999999999999997335 ) ) ;
#3034=CARTESIAN_POINT ( 'NONE',  ( 3.999999999999999112, 17.52499999999999858, -30.00000000000000000 ) ) ;
#3035=CARTESIAN_POINT ( 'NONE',  ( 24.26250000122903216, 0.000000000000000000, 4.999999999999998224 ) ) ;
#3038=CARTESIAN_POINT ( 'NONE',  ( 7.809375000614519280, 0.000000000000000000, 5.243569643749999010 ) ) ;
#3039=CARTESIAN_POINT ( 'NONE',  ( 12.82499999999999929, 4.330127018922191873, 2.499999999999999556 ) ) ;
#3040=CARTESIAN_POINT ( 'NONE',  ( 14.72812500061451679, 6.421520780324663323E-16, -5.243569643749999010 ) ) ;
#3041=CARTESIAN_POINT ( 'NONE',  ( 8.296875000614516438, -3.027376345333614438, 5.243569643749998122 ) ) ;
#3042=CARTESIAN_POINT ( 'NONE',  ( 26.43750000122903288, 4.330127018922191873, 2.499999999999999556 ) ) ;
#3043=CARTESIAN_POINT ( 'NONE',  ( 18.30937500061451928, -4.541064518000417216, -2.621784821875001281 ) ) ;
#3044=CARTESIAN_POINT ( 'NONE',  ( 4.884375000614518569, 6.421520780324663323E-16, -5.243569643749999010 ) ) ;
#3046=EDGE_CURVE ( 'NONE', #17794, #72719, #54288, .T. ) ;
#3047=CARTESIAN_POINT ( 'NONE',  ( 5.878125000614517148, 4.541064518000418104, 2.621784821874999949 ) ) ;
#3048=CARTESIAN_POINT ( 'NONE',  ( 16.30312500061451786, 0.000000000000000000, 5.243569643749999010 ) ) ;
#3049=ORIENTED_EDGE ( 'NONE', *, *, #50356, .F. ) ;
#3050=CARTESIAN_POINT ( 'NONE',  ( 12.47812500061451502, 6.421520780324663323E-16, -5.243569643749999010 ) ) ;
#3051=CARTESIAN_POINT ( 'NONE',  ( 4.875000001229034652, 2.886751345948126879, 4.999999999999999112 ) ) ;
#3052=CARTESIAN_POINT ( 'NONE',  ( 11.80312500061451608, 0.000000000000000000, 5.243569643749999010 ) ) ;
#3054=CARTESIAN_POINT ( 'NONE',  ( 11.96250000000000213, 2.886751345948126879, 4.999999999999999112 ) ) ;
#3055=CARTESIAN_POINT ( 'NONE',  ( 7.687500001229033764, -4.330127018922194537, 2.499999999999995559 ) ) ;
#3056=CARTESIAN_POINT ( 'NONE',  ( 20.69999999999999929, -4.330127018922190985, -2.500000000000001332 ) ) ;
#3057=CARTESIAN_POINT ( 'NONE',  ( 13.84687500061451537, -3.027376345333610441, -5.243569643749999898 ) ) ;
#3058=CARTESIAN_POINT ( 'NONE',  ( 17.10000000122903430, -2.886751345948129988, 4.999999999999997335 ) ) ;
#3060=AXIS2_PLACEMENT_3D ( 'NONE', #34285, #693, #39859 ) ;
#3061=CARTESIAN_POINT ( 'NONE',  ( 9.001249775931846008E-16, 18.11562500061451786, -25.09994784771203058 ) ) ;
#3063=CARTESIAN_POINT ( 'NONE',  ( 3.999999999999999112, 14.93750000122903288, -30.00000000000000000 ) ) ;
#3064=CARTESIAN_POINT ( 'NONE',  ( 29.20312500061451644, 4.541064518000418104, -2.621784821874998173 ) ) ;
#3066=CARTESIAN_POINT ( 'NONE',  ( 3.429892710759705476, -3.638108848382370919, 3.621991456395721620 ) ) ;
#3068=CARTESIAN_POINT ( 'NONE',  ( 15.53437500061451715, -4.541064518000419881, 2.621784821874995952 ) ) ;
#3070=CARTESIAN_POINT ( 'NONE',  ( 27.89999999999999858, -4.330127018922190985, -2.500000000000001332 ) ) ;
#3071=CARTESIAN_POINT ( 'NONE',  ( 11.87812500061451537, -4.541064518000419881, 2.621784821874995952 ) ) ;
#3074=CARTESIAN_POINT ( 'NONE',  ( 22.73437500061451644, -4.541064518000419881, 2.621784821874995952 ) ) ;
#3076=CARTESIAN_POINT ( 'NONE',  ( 9.965625000614517504, 3.027376345333611329, 5.243569643749999010 ) ) ;
#3077=CARTESIAN_POINT ( 'NONE',  ( 12.30937500061451573, 0.000000000000000000, 5.243569643749999010 ) ) ;
#3078=ORIENTED_EDGE ( 'NONE', *, *, #68758, .F. ) ;
#3079=CARTESIAN_POINT ( 'NONE',  ( 24.68437500061451573, 6.421520780324663323E-16, -5.243569643749999010 ) ) ;
#3080=CARTESIAN_POINT ( 'NONE',  ( 28.64062500061451289, -3.027376345333610441, -5.243569643749999898 ) ) ;
#3082=CARTESIAN_POINT ( 'NONE',  ( 8.324999999999999289, 4.330127018922191873, 2.499999999999999556 ) ) ;
#3083=CARTESIAN_POINT ( 'NONE',  ( 17.10000000122903430, -2.886751345948129988, 4.999999999999997335 ) ) ;
#3085=CARTESIAN_POINT ( 'NONE',  ( 3.286795329855858760, 3.767887532774327308, -3.286795329856085690 ) ) ;
#3086=ORIENTED_EDGE ( 'NONE', *, *, #28669, .T. ) ;
#3087=CARTESIAN_POINT ( 'NONE',  ( 14.69999999999999929, 0.000000000000000000, 4.999999999999998224 ) ) ;
#3088=CARTESIAN_POINT ( 'NONE',  ( 20.13749999999999929, -2.886751345948129988, 4.999999999999997335 ) ) ;
#3089=CARTESIAN_POINT ( 'NONE',  ( 12.74062500061451786, -3.027376345333614438, 5.243569643749998122 ) ) ;
#3090=VERTEX_POINT ( 'NONE', #13068 ) ;
#3092=CARTESIAN_POINT ( 'NONE',  ( 4.243569643749999898, 17.83437500061451786, -30.00000000000000000 ) ) ;
#3093=CARTESIAN_POINT ( 'NONE',  ( 6.553125000614518747, -4.541064518000417216, -2.621784821875001281 ) ) ;
#3095=CARTESIAN_POINT ( 'NONE',  ( 12.75000000000000178, 4.330127018922192761, -2.499999999999997780 ) ) ;
#3097=ORIENTED_EDGE ( 'NONE', *, *, #60084, .T. ) ;
#3098=CARTESIAN_POINT ( 'NONE',  ( -4.243569643749999898, 14.85312500061451679, 30.00000000000000000 ) ) ;
#3099=CARTESIAN_POINT ( 'NONE',  ( 26.50312500061451360, 4.541064518000418104, -2.621784821874998173 ) ) ;
#3100=CARTESIAN_POINT ( 'NONE',  ( 0.000000000000000000, 20.00000000000000000, 30.00000000000000000 ) ) ;
#3102=CARTESIAN_POINT ( 'NONE',  ( 22.99687500061451573, 6.054752690667223547, 3.707466751127219781E-16 ) ) ;
#3103=CARTESIAN_POINT ( 'NONE',  ( 18.10312500061451502, 0.000000000000000000, 5.243569643749999010 ) ) ;
#3104=CARTESIAN_POINT ( 'NONE',  ( 4.243569643749999010, 15.11562500061459424, -32.45002607614398471 ) ) ;
#3105=CARTESIAN_POINT ( 'NONE',  ( 22.91250000122903430, 0.000000000000000000, 4.999999999999998224 ) ) ;
#3106=CARTESIAN_POINT ( 'NONE',  ( 3.028125000614518392, 6.421520780324663323E-16, -5.243569643749999010 ) ) ;
#3108=CARTESIAN_POINT ( 'NONE',  ( 21.32812500061451644, -4.541064518000419881, 2.621784821874995952 ) ) ;
#3111=CARTESIAN_POINT ( 'NONE',  ( 16.58437500061451786, 6.421520780324663323E-16, -5.243569643749999010 ) ) ;
#3112=CARTESIAN_POINT ( 'NONE',  ( 16.58437500061451786, 6.421520780324663323E-16, -5.243569643749999010 ) ) ;
#3113=CARTESIAN_POINT ( 'NONE',  ( 24.23437500061451644, 6.421520780324663323E-16, -5.243569643749999010 ) ) ;
#3114=CARTESIAN_POINT ( 'NONE',  ( -4.243569643749999898, 13.07187500061452035, 27.54997392385601529 ) ) ;
#3115=CARTESIAN_POINT ( 'NONE',  ( 5.615625000614517859, -6.054752690667223547, -1.112240025338166033E-15 ) ) ;
#3116=CARTESIAN_POINT ( 'NONE',  ( 29.16562500061451502, 3.027376345333613106, -5.243569643749998122 ) ) ;
#3117=CARTESIAN_POINT ( 'NONE',  ( 28.67812500061451431, 6.421520780324663323E-16, -5.243569643749999010 ) ) ;
#3119=FACE_OUTER_BOUND ( 'NONE', #6310, .T. ) ;
#3121=CARTESIAN_POINT ( 'NONE',  ( 3.590625000614518836, 6.054752690667223547, 3.707466751127219781E-16 ) ) ;
#3122=CARTESIAN_POINT ( 'NONE',  ( 7.021875000614518747, -6.054752690667223547, -1.112240025338166033E-15 ) ) ;
#3124=CARTESIAN_POINT ( 'NONE',  ( 13.72500000122903074, 2.886751345948129099, -4.999999999999998224 ) ) ;
#3125=CARTESIAN_POINT ( 'NONE',  ( 3.609375000614516882, 4.541064518000418104, -2.621784821874998173 ) ) ;
#3126=CARTESIAN_POINT ( 'NONE',  ( 11.02500000122903501, 2.886751345948129099, -4.999999999999998224 ) ) ;
#3127=CARTESIAN_POINT ( 'NONE',  ( 4.978125000614518569, 4.541064518000418104, 2.621784821874999949 ) ) ;
#3130=CARTESIAN_POINT ( 'NONE',  ( 14.59687500061452070, -3.027376345333614438, 5.243569643749998122 ) ) ;
#3131=CARTESIAN_POINT ( 'NONE',  ( 0.000000000000000000, 20.00000000000000000, -30.00000000000000000 ) ) ;
#3132=EDGE_LOOP ( 'NONE', ( #5371, #44532, #72446, #60602 ) ) ;
#3133=CARTESIAN_POINT ( 'NONE',  ( 22.26562500061451644, -6.054752690667223547, -1.112240025338166033E-15 ) ) ;
#3134=CARTESIAN_POINT ( 'NONE',  ( 7.303125000614516082, 0.000000000000000000, 5.243569643749999010 ) ) ;
#3135=CARTESIAN_POINT ( 'NONE',  ( 24.04687500061451644, -3.027376345333614438, 5.243569643749998122 ) ) ;
#3136=CARTESIAN_POINT ( 'NONE',  ( 6.403125000614517504, 0.000000000000000000, 5.243569643749999010 ) ) ;
#3137=CARTESIAN_POINT ( 'NONE',  ( 3.495766807613835958, 4.011937492815293993, 3.051120425653408574 ) ) ;
#3138=CARTESIAN_POINT ( 'NONE',  ( 9.262500001229033941, 4.330127018922192761, -2.499999999999997780 ) ) ;
#3139=ADVANCED_FACE ( 'NONE', ( #51884 ), #35607, .F. ) ;
#3142=CARTESIAN_POINT ( 'NONE',  ( 22.60312500061451857, 0.000000000000000000, 5.243569643749999010 ) ) ;
#3143=CARTESIAN_POINT ( 'NONE',  ( -2.121784821874999949, 11.62812500061451715, -33.67503911421598417 ) ) ;
#3144=CARTESIAN_POINT ( 'NONE',  ( 9.525000001229033231, -5.773502691896255534, -1.060575238724906372E-15 ) ) ;
#3145=CARTESIAN_POINT ( 'NONE',  ( 20.01562500061451644, -6.054752690667223547, -1.112240025338166033E-15 ) ) ;
#3146=CARTESIAN_POINT ( 'NONE',  ( 18.36562500061451431, 3.027376345333613106, -5.243569643749998122 ) ) ;
#3148=CARTESIAN_POINT ( 'NONE',  ( 17.96250000000000213, -5.773502691896255534, -1.060575238724906372E-15 ) ) ;
#3149=CARTESIAN_POINT ( 'NONE',  ( 14.43750000122903288, -4.330127018922194537, 2.499999999999995559 ) ) ;
#3150=CARTESIAN_POINT ( 'NONE',  ( 9.365625000614519635, 3.027376345333613106, -5.243569643749998122 ) ) ;
#3151=CARTESIAN_POINT ( 'NONE',  ( 13.82812500061451466, 6.421520780324663323E-16, -5.243569643749999010 ) ) ;
#3152=CARTESIAN_POINT ( 'NONE',  ( 23.17500000122903359, 2.886751345948129099, -4.999999999999998224 ) ) ;
#3153=CARTESIAN_POINT ( 'NONE',  ( 22.09687500061451715, 6.054752690667223547, 3.707466751127219781E-16 ) ) ;
#3154=CARTESIAN_POINT ( 'NONE',  ( 20.59687500061451360, -3.027376345333610441, -5.243569643749999898 ) ) ;
#3155=CARTESIAN_POINT ( 'NONE',  ( 3.546502191234963242, 3.524546877579638693, -3.882356442438433586 ) ) ;
#3156=AXIS2_PLACEMENT_3D ( 'NONE', #73102, #22126, #5508 ) ;
#3157=CARTESIAN_POINT ( 'NONE',  ( 7.125000001229033764, 2.886751345948126879, 4.999999999999999112 ) ) ;
#3158=CARTESIAN_POINT ( 'NONE',  ( 6.121875000614517504, -6.054752690667223547, -1.112240025338166033E-15 ) ) ;
#3159=CARTESIAN_POINT ( 'NONE',  ( 24.04687500061451644, -3.027376345333614438, 5.243569643749998122 ) ) ;
#3160=CARTESIAN_POINT ( 'NONE',  ( 26.66250000122903430, -4.330127018922190985, -2.500000000000001332 ) ) ;
#3161=CARTESIAN_POINT ( 'NONE',  ( 18.92812500061451431, 4.541064518000418104, 2.621784821874999949 ) ) ;
#3162=CARTESIAN_POINT ( 'NONE',  ( 24.87187500061451573, 3.027376345333611329, 5.243569643749999010 ) ) ;
#3164=CARTESIAN_POINT ( 'NONE',  ( -3.999999999999999112, 11.11250000122903536, -30.00000000000000000 ) ) ;
#3167=CARTESIAN_POINT ( 'NONE',  ( 4.396875000614516971, -3.027376345333610441, -5.243569643749999898 ) ) ;
#3168=CARTESIAN_POINT ( 'NONE',  ( 18.29062500061451502, -3.027376345333610441, -5.243569643749999898 ) ) ;
#3169=ORIENTED_EDGE ( 'NONE', *, *, #67378, .T. ) ;
#3170=CARTESIAN_POINT ( 'NONE',  ( 11.51250000000000107, 2.886751345948126879, 4.999999999999998224 ) ) ;
#3171=CARTESIAN_POINT ( 'NONE',  ( 24.32812500061451289, 4.541064518000418104, 2.621784821874999949 ) ) ;
#3172=CARTESIAN_POINT ( 'NONE',  ( -1.071796769724496556, 16.04240381056766651, -26.00000000000000355 ) ) ;
#3174=CARTESIAN_POINT ( 'NONE',  ( 14.77500000000000036, -4.330127018922194537, 2.499999999999995559 ) ) ;
#3175=CARTESIAN_POINT ( 'NONE',  ( 24.22500000122903430, 2.886751345948126879, 4.999999999999999112 ) ) ;
#3176=CARTESIAN_POINT ( 'NONE',  ( 18.21562500061451573, -6.054752690667223547, -1.112240025338166033E-15 ) ) ;
#3177=ORIENTED_EDGE ( 'NONE', *, *, #46955, .T. ) ;
#3178=CARTESIAN_POINT ( 'NONE',  ( 22.98749999999999716, -2.886751345948125991, -5.000000000000000000 ) ) ;
#3179=CARTESIAN_POINT ( 'NONE',  ( 23.70937500061451786, -4.541064518000417216, -2.621784821875001281 ) ) ;
#3180=ORIENTED_EDGE ( 'NONE', *, *, #37148, .F. ) ;
#3181=DIRECTION ( 'NONE',  ( 0.000000000000000000, 0.000000000000000000, 1.000000000000000000 ) ) ;
#3182=CARTESIAN_POINT ( 'NONE',  ( 12.29062500061451857, -3.027376345333614438, 5.243569643749998122 ) ) ;
#3183=CARTESIAN_POINT ( 'NONE',  ( 4.715625000614516615, -6.054752690667223547, -1.112240025338166033E-15 ) ) ;
#3185=CARTESIAN_POINT ( 'NONE',  ( 27.17812500061451786, -4.541064518000419881, 2.621784821874995952 ) ) ;
#3186=CARTESIAN_POINT ( 'NONE',  ( 12.00000000122903465, 5.773502691896255534, 3.535250795749688894E-16 ) ) ;
#3187=CARTESIAN_POINT ( 'NONE',  ( 20.54999999999999716, 0.000000000000000000, 4.999999999999998224 ) ) ;
#3188=CARTESIAN_POINT ( 'NONE',  ( 25.72499999999999787, 6.123233995736764310E-16, -4.999999999999998224 ) ) ;
#3190=CARTESIAN_POINT ( 'NONE',  ( 7.134375000614516793, 6.421520780324663323E-16, -5.243569643749999010 ) ) ;
#3191=CARTESIAN_POINT ( 'NONE',  ( 17.67187500061451644, 3.027376345333611329, 5.243569643749999010 ) ) ;
#3193=VERTEX_POINT ( 'NONE', #39726 ) ;
#3194=CARTESIAN_POINT ( 'NONE',  ( 29.72812500061451502, 4.541064518000418104, 2.621784821874999949 ) ) ;
#3195=CARTESIAN_POINT ( 'NONE',  ( 28.24687500061451573, -3.027376345333610441, -5.243569643749999898 ) ) ;
#3196=CARTESIAN_POINT ( 'NONE',  ( 3.346875000614518036, -3.027376345333614438, 5.243569643749998122 ) ) ;
#3197=CARTESIAN_POINT ( 'NONE',  ( 15.03749999999999964, 5.773502691896255534, 3.535250795749688894E-16 ) ) ;
#3198=CARTESIAN_POINT ( 'NONE',  ( 14.31562500061451537, 3.027376345333613106, -5.243569643749998122 ) ) ;
#3199=CARTESIAN_POINT ( 'NONE',  ( 3.486133158594716510E-16, 19.55000000122903359, -34.00000000000000000 ) ) ;
#3200=CARTESIAN_POINT ( 'NONE',  ( 28.71562500061451573, 3.027376345333612662, -5.243569643749998122 ) ) ;
#3201=CARTESIAN_POINT ( 'NONE',  ( 18.78750000122903430, 4.330127018922191873, 2.499999999999999556 ) ) ;
#3202=LINE ( 'NONE', #48268, #1778 ) ;
#3204=CARTESIAN_POINT ( 'NONE',  ( 8.165625000614516793, 3.027376345333611329, 5.243569643749999010 ) ) ;
#3205=CARTESIAN_POINT ( 'NONE',  ( 23.37187500061451573, 3.027376345333613106, -5.243569643749998122 ) ) ;
#3206=CARTESIAN_POINT ( 'NONE',  ( 4.243569643749999898, 16.48437500061451644, 30.00000000000000000 ) ) ;
#3207=CARTESIAN_POINT ( 'NONE',  ( 23.70937500061451786, -4.541064518000417216, -2.621784821875001281 ) ) ;
#3208=CARTESIAN_POINT ( 'NONE',  ( 4.087500000000001243, -2.886751345948125991, -5.000000000000000000 ) ) ;
#3209=CARTESIAN_POINT ( 'NONE',  ( -2.828200636599751609E-16, 11.45000000122903394, 25.38119784648299770 ) ) ;
#3210=CARTESIAN_POINT ( 'NONE',  ( 11.50312500061451892, -4.541064518000417216, -2.621784821875001281 ) ) ;
#3211=CARTESIAN_POINT ( 'NONE',  ( 5.287500001229035185, 4.330127018922191873, 2.499999999999999556 ) ) ;
#3212=CARTESIAN_POINT ( 'NONE',  ( 10.28437500061451715, 6.421520780324663323E-16, -5.243569643749999010 ) ) ;
#3213=CARTESIAN_POINT ( 'NONE',  ( -3.026485248664591232, 3.985774251745327845, -27.37255237546152742 ) ) ;
#3215=CARTESIAN_POINT ( 'NONE',  ( 10.19062500061451892, -3.027376345333610441, -5.243569643749999898 ) ) ;
#3216=CARTESIAN_POINT ( 'NONE',  ( 14.74687500061451573, -3.027376345333610441, -5.243569643749999898 ) ) ;
#3217=CARTESIAN_POINT ( 'NONE',  ( 1.626862140677534273E-15, 12.12500000122903465, -26.00000000000000355 ) ) ;
#3218=CARTESIAN_POINT ( 'NONE',  ( 22.31250000122903288, 4.330127018922192761, -2.499999999999997780 ) ) ;
#3219=CARTESIAN_POINT ( 'NONE',  ( 9.271875000614516082, -6.054752690667223547, -1.112240025338166033E-15 ) ) ;
#3220=CARTESIAN_POINT ( 'NONE',  ( 12.21562500061451573, 3.027376345333611329, 5.243569643749999010 ) ) ;
#3222=CARTESIAN_POINT ( 'NONE',  ( 20.93437500061451573, -4.541064518000419881, 2.621784821874995952 ) ) ;
#3223=CARTESIAN_POINT ( 'NONE',  ( 14.02499999999999858, 6.123233995736764310E-16, -4.999999999999998224 ) ) ;
#3226=EDGE_CURVE ( 'NONE', #34155, #66981, #56656, .T. ) ;
#3227=CARTESIAN_POINT ( 'NONE',  ( 4.243569643749999898, 13.78437500061451715, -30.00000000000000000 ) ) ;
#3228=CARTESIAN_POINT ( 'NONE',  ( 15.72187500061451892, 3.027376345333613106, -5.243569643749998122 ) ) ;
#3229=CARTESIAN_POINT ( 'NONE',  ( 16.12500000122903288, 2.886751345948126879, 4.999999999999999112 ) ) ;
#3230=EDGE_CURVE ( 'NONE', #69635, #14969, #49540, .T. ) ;
#3231=CARTESIAN_POINT ( 'NONE',  ( 12.27187500061451786, 3.027376345333611329, 5.243569643749999010 ) ) ;
#3232=CARTESIAN_POINT ( 'NONE',  ( 9.001249775931846008E-16, 18.11562500061451786, -25.09994784771203058 ) ) ;
#3233=CARTESIAN_POINT ( 'NONE',  ( 17.47500000122903430, 2.886751345948126879, 4.999999999999999112 ) ) ;
#3234=CARTESIAN_POINT ( 'NONE',  ( 11.50312500061451892, -4.541064518000417216, -2.621784821875001281 ) ) ;
#3235=ORIENTED_EDGE ( 'NONE', *, *, #32753, .T. ) ;
#3236=CARTESIAN_POINT ( 'NONE',  ( 14.73749999999999893, -2.886751345948129988, 4.999999999999997335 ) ) ;
#3237=CARTESIAN_POINT ( 'NONE',  ( 10.95937500061451964, 0.000000000000000000, 5.243569643749999010 ) ) ;
#3238=FACE_OUTER_BOUND ( 'NONE', #30268, .T. ) ;
#3239=CARTESIAN_POINT ( 'NONE',  ( 12.48750000122903359, 4.330127018922191873, 2.499999999999999556 ) ) ;
#3240=CARTESIAN_POINT ( 'NONE',  ( 20.43750000122903643, 6.123233995736764310E-16, -4.999999999999998224 ) ) ;
#3241=CARTESIAN_POINT ( 'NONE',  ( 18.66562500061451146, -6.054752690667223547, -1.112240025338166033E-15 ) ) ;
#3242=CARTESIAN_POINT ( 'NONE',  ( 19.64062500061451644, -3.027376345333610441, -5.243569643749999898 ) ) ;
#3243=CARTESIAN_POINT ( 'NONE',  ( 28.98750000122903359, 6.123233995736764310E-16, -4.999999999999998224 ) ) ;
#3244=CARTESIAN_POINT ( 'NONE',  ( 4.228125000614517681, -4.541064518000419881, 2.621784821874995952 ) ) ;
#3245=CARTESIAN_POINT ( 'NONE',  ( 25.64999999999999858, -4.330127018922190985, -2.500000000000001332 ) ) ;
#3248=CARTESIAN_POINT ( 'NONE',  ( 27.42187500061451644, 3.027376345333613106, -5.243569643749998122 ) ) ;
#3249=CARTESIAN_POINT ( 'NONE',  ( 28.64999999999999858, 0.000000000000000000, 4.999999999999998224 ) ) ;
#3250=CARTESIAN_POINT ( 'NONE',  ( -4.243569643749997233, 13.59687500061451715, -27.54997392385601174 ) ) ;
#3251=CARTESIAN_POINT ( 'NONE',  ( 3.525000001229034119, 2.886751345948126879, 4.999999999999999112 ) ) ;
#3252=CARTESIAN_POINT ( 'NONE',  ( 3.262500000000001510, 2.886751345948129099, -4.999999999999998224 ) ) ;
#3254=CARTESIAN_POINT ( 'NONE',  ( 8.221875000614518925, 3.027376345333611329, 5.243569643749999010 ) ) ;
#3255=CARTESIAN_POINT ( 'NONE',  ( 25.97812500061451502, 6.421520780324663323E-16, -5.243569643749999010 ) ) ;
#3256=DIRECTION ( 'NONE',  ( -0.000000000000000000, -1.000000000000000000, -0.000000000000000000 ) ) ;
#3257=CARTESIAN_POINT ( 'NONE',  ( 11.66250000122903430, 0.000000000000000000, 4.999999999999998224 ) ) ;
#3259=CARTESIAN_POINT ( 'NONE',  ( 6.309375000614517504, 4.541064518000418104, -2.621784821874998173 ) ) ;
#3260=CARTESIAN_POINT ( 'NONE',  ( 9.346875000614517148, -3.027376345333610441, -5.243569643749999898 ) ) ;
#3261=CARTESIAN_POINT ( 'NONE',  ( 3.487500000000000711, -2.886751345948129988, 4.999999999999997335 ) ) ;
#3262=AXIS2_PLACEMENT_3D ( 'NONE', #70429, #46444, #7280 ) ;
#3263=CARTESIAN_POINT ( 'NONE',  ( 2.121784821874999061, 11.55312500061459424, 26.32496088578401583 ) ) ;
#3264=CARTESIAN_POINT ( 'NONE',  ( 30.00000000000000000, 0.000000000000000000, 4.999999999999998224 ) ) ;
#3265=CARTESIAN_POINT ( 'NONE',  ( 3.112500000000000711, -5.773502691896255534, -1.060575238724906372E-15 ) ) ;
#3268=CARTESIAN_POINT ( 'NONE',  ( 20.09062500061451573, -3.027376345333610441, -5.243569643749999898 ) ) ;
#3269=CARTESIAN_POINT ( 'NONE',  ( 10.00312500061451715, 0.000000000000000000, 5.243569643749999010 ) ) ;
#3271=CARTESIAN_POINT ( 'NONE',  ( 6.871875000614517504, 3.027376345333611329, 5.243569643749999010 ) ) ;
#3272=CARTESIAN_POINT ( 'NONE',  ( 26.58750000000000213, -2.886751345948125991, -5.000000000000000000 ) ) ;
#3273=CARTESIAN_POINT ( 'NONE',  ( 20.70000000122903216, -2.886751345948129988, 4.999999999999997335 ) ) ;
#3274=CARTESIAN_POINT ( 'NONE',  ( 27.55312500061451786, 0.000000000000000000, 5.243569643749999010 ) ) ;
#3276=CARTESIAN_POINT ( 'NONE',  ( 10.50937500061451679, 0.000000000000000000, 5.243569643749999010 ) ) ;
#3277=CARTESIAN_POINT ( 'NONE',  ( 14.03437500061451715, 4.541064518000418104, 2.621784821874999949 ) ) ;
#3278=CARTESIAN_POINT ( 'NONE',  ( 25.95937500061451431, -4.541064518000417216, -2.621784821875001281 ) ) ;
#3279=CARTESIAN_POINT ( 'NONE',  ( 4.898587196589411843E-16, 20.00000000000000000, -26.00000000000000000 ) ) ;
#3281=CARTESIAN_POINT ( 'NONE',  ( 19.92187500061451644, 3.027376345333611329, 5.243569643749999010 ) ) ;
#3282=CARTESIAN_POINT ( 'NONE',  ( 13.02187500061451608, 3.027376345333613106, -5.243569643749998122 ) ) ;
#3284=CARTESIAN_POINT ( 'NONE',  ( 22.94999999999999929, -4.330127018922190985, -2.500000000000001332 ) ) ;
#3286=CARTESIAN_POINT ( 'NONE',  ( 2.121784821875001281, 11.45937500061451786, -26.32496088578401938 ) ) ;
#3288=CARTESIAN_POINT ( 'NONE',  ( 13.90312500061451750, 4.541064518000418104, -2.621784821874998173 ) ) ;
#3289=CARTESIAN_POINT ( 'NONE',  ( 5.025000000000002132, 6.123233995736764310E-16, -4.999999999999998224 ) ) ;
#3291=CARTESIAN_POINT ( 'NONE',  ( -1.071796769724490117, 19.12009619066136423, -34.00000000000000000 ) ) ;
#3292=CARTESIAN_POINT ( 'NONE',  ( 1.626862140677534273E-15, 9.875000001229034652, -26.00000000000000355 ) ) ;
#3293=CARTESIAN_POINT ( 'NONE',  ( 12.11250000000000249, -5.773502691896255534, -1.060575238724906372E-15 ) ) ;
#3294=CARTESIAN_POINT ( 'NONE',  ( 3.999999999999999112, 18.98750000122903359, 30.00000000000000000 ) ) ;
#3295=CARTESIAN_POINT ( 'NONE',  ( 11.40000000122903501, -2.886751345948125991, -5.000000000000000000 ) ) ;
#3296=EDGE_CURVE ( 'NONE', #26188, #27675, #53328, .T. ) ;
#3297=CARTESIAN_POINT ( 'NONE',  ( 22.28437500061451715, -4.541064518000419881, 2.621784821874995952 ) ) ;
#3298=CARTESIAN_POINT ( 'NONE',  ( 17.44687500061451857, -3.027376345333610441, -5.243569643749999898 ) ) ;
#3299=LINE ( 'NONE', #13628, #11247 ) ;
#3301=CARTESIAN_POINT ( 'NONE',  ( 17.35312500061451502, -4.541064518000417216, -2.621784821875001281 ) ) ;
#3302=CARTESIAN_POINT ( 'NONE',  ( 3.103125000614517237, 4.541064518000418104, -2.621784821874998173 ) ) ;
#3303=CARTESIAN_POINT ( 'NONE',  ( 18.45937500061451431, 4.541064518000418104, -2.621784821874998173 ) ) ;
#3304=CARTESIAN_POINT ( 'NONE',  ( 29.22187500061451715, 3.027376345333613106, -5.243569643749998122 ) ) ;
#3305=CARTESIAN_POINT ( 'NONE',  ( 4.528125000614516615, 4.541064518000418104, 2.621784821874999949 ) ) ;
#3306=CARTESIAN_POINT ( 'NONE',  ( 19.11562500061451431, -6.054752690667223547, -1.112240025338166033E-15 ) ) ;
#3307=CARTESIAN_POINT ( 'NONE',  ( -4.243569643749997233, 12.19062500061451715, 32.45002607614398471 ) ) ;
#3308=CARTESIAN_POINT ( 'NONE',  ( 16.38750000122903216, 6.123233995736764310E-16, -4.999999999999998224 ) ) ;
#3310=CARTESIAN_POINT ( 'NONE',  ( 6.328125000614515550, 4.541064518000418104, 2.621784821874999949 ) ) ;
#3311=CARTESIAN_POINT ( 'NONE',  ( 26.24062500061451431, -3.027376345333614438, 5.243569643749998122 ) ) ;
#3312=CARTESIAN_POINT ( 'NONE',  ( 11.77500000000000036, 6.123233995736764310E-16, -4.999999999999998224 ) ) ;
#3313=CARTESIAN_POINT ( 'NONE',  ( 23.70937500061451786, -4.541064518000417216, -2.621784821875001281 ) ) ;
#3314=CARTESIAN_POINT ( 'NONE',  ( 15.47812500061451679, -4.541064518000419881, 2.621784821874995952 ) ) ;
#3315=CARTESIAN_POINT ( 'NONE',  ( 24.26250000122903216, 0.000000000000000000, 4.999999999999998224 ) ) ;
#3316=EDGE_CURVE ( 'NONE', #2861, #7111, #61832, .T. ) ;
#3317=CARTESIAN_POINT ( 'NONE',  ( 23.31562500061451715, 3.027376345333613106, -5.243569643749998122 ) ) ;
#3318=CARTESIAN_POINT ( 'NONE',  ( 20.10937500061451289, -4.541064518000417216, -2.621784821875001281 ) ) ;
#3319=CARTESIAN_POINT ( 'NONE',  ( 13.67812500061451786, -4.541064518000419881, 2.621784821874995952 ) ) ;
#3320=CARTESIAN_POINT ( 'NONE',  ( 4.243569643749999898, 15.09687500061451892, 32.45002607614398471 ) ) ;
#3321=CARTESIAN_POINT ( 'NONE',  ( 18.92812500061451431, 4.541064518000418104, 2.621784821874999949 ) ) ;
#3322=CARTESIAN_POINT ( 'NONE',  ( 29.69062500061451715, 6.054752690667223547, 3.707466751127219781E-16 ) ) ;
#3323=ORIENTED_EDGE ( 'NONE', *, *, #24627, .F. ) ;
#3325=CARTESIAN_POINT ( 'NONE',  ( 23.85000000000000142, -4.330127018922190985, -2.500000000000001332 ) ) ;
#3326=CARTESIAN_POINT ( 'NONE',  ( -3.999999999999997335, 11.03750000000000142, -27.69059892324149175 ) ) ;
#3328=CARTESIAN_POINT ( 'NONE',  ( 25.90312500061451573, -4.541064518000417216, -2.621784821875001281 ) ) ;
#3329=CARTESIAN_POINT ( 'NONE',  ( 7.190625000614518036, 6.054752690667223547, 3.707466751127219781E-16 ) ) ;
#3330=CARTESIAN_POINT ( 'NONE',  ( 19.12500000122903288, 2.886751345948129099, -4.999999999999998224 ) ) ;
#3332=CARTESIAN_POINT ( 'NONE',  ( 25.56562500061452070, 3.027376345333613106, -5.243569643749998122 ) ) ;
#3333=CARTESIAN_POINT ( 'NONE',  ( 22.68750000000000000, 5.773502691896255534, 3.535250795749688894E-16 ) ) ;
#3335=CARTESIAN_POINT ( 'NONE',  ( 27.74062500061451431, -3.027376345333610441, -5.243569643749999898 ) ) ;
#3336=CARTESIAN_POINT ( 'NONE',  ( 9.253125000614517148, -4.541064518000417216, -2.621784821875001281 ) ) ;
#3338=CARTESIAN_POINT ( 'NONE',  ( 22.79062500061451502, -3.027376345333610441, -5.243569643749999898 ) ) ;
#3339=CARTESIAN_POINT ( 'NONE',  ( 4.153125000614515727, 0.000000000000000000, 5.243569643749999010 ) ) ;
#3342=CARTESIAN_POINT ( 'NONE',  ( 3.703125000614516882, 0.000000000000000000, 5.243569643749999010 ) ) ;
#3343=CARTESIAN_POINT ( 'NONE',  ( 3.999999999999998668, 13.62500000122903288, -32.30940107675850470 ) ) ;
#3344=CARTESIAN_POINT ( 'NONE',  ( -1.071796769724488563, 10.30490381179670045, 34.00000000000000000 ) ) ;
#3345=( BOUNDED_CURVE ( )  B_SPLINE_CURVE ( 2, ( #30261, #30988, #9917, #32455, #60884, #66437, #37262 ),
 .UNSPECIFIED., .F., .F. ) 
 B_SPLINE_CURVE_WITH_KNOTS ( ( 3, 2, 2, 3 ),
 ( 0.8416666666666667851, 0.8444444444444445530, 0.8472222222222222099, 0.8499999999999999778 ),
 .UNSPECIFIED. ) 
 CURVE ( )  GEOMETRIC_REPRESENTATION_ITEM ( )  RATIONAL_B_SPLINE_CURVE ( ( 0.9999999999999946709, 0.8660254037844440367, 1.000000000000000000, 0.8660254037844387076, 1.000000000000000000, 0.8660254037844387076, 1.000000000000000000 ) ) 
 REPRESENTATION_ITEM ( '' )  );
#3346=CARTESIAN_POINT ( 'NONE',  ( 11.32500000000000107, 6.123233995736764310E-16, -4.999999999999998224 ) ) ;
#3347=CARTESIAN_POINT ( 'NONE',  ( 10.24687500061451750, -3.027376345333610441, -5.243569643749999898 ) ) ;
#3348=CARTESIAN_POINT ( 'NONE',  ( 8.437500001229034652, 4.330127018922191873, 2.499999999999999556 ) ) ;
#3349=CARTESIAN_POINT ( 'NONE',  ( 15.75937500061451857, 4.541064518000418104, -2.621784821874998173 ) ) ;
#3351=CARTESIAN_POINT ( 'NONE',  ( 6.009375000614519458, 0.000000000000000000, 5.243569643749999010 ) ) ;
#3352=CARTESIAN_POINT ( 'NONE',  ( 3.999999999999999112, 18.42500000000000071, 30.00000000000000000 ) ) ;
#3353=LINE ( 'NONE', #25875, #13495 ) ;
#3354=CARTESIAN_POINT ( 'NONE',  ( 12.30937500061451573, 0.000000000000000000, 5.243569643749999010 ) ) ;
#3355=DIRECTION ( 'NONE',  ( 0.000000000000000000, 0.000000000000000000, 1.000000000000000000 ) ) ;
#3356=CARTESIAN_POINT ( 'NONE',  ( 23.01562500061451644, 3.027376345333611329, 5.243569643749999010 ) ) ;
#3357=CARTESIAN_POINT ( 'NONE',  ( 1.071796769724476572, 11.58259618943233349, 34.00000000000000000 ) ) ;
#3359=CARTESIAN_POINT ( 'NONE',  ( 25.69687500061451502, 6.054752690667223547, 3.707466751127219781E-16 ) ) ;
#3361=( BOUNDED_CURVE ( )  B_SPLINE_CURVE ( 2, ( #72373, #21753, #38767, #10679, #5142, #50215, #27677 ),
 .UNSPECIFIED., .F., .T. ) 
 B_SPLINE_CURVE_WITH_KNOTS ( ( 3, 2, 2, 3 ),
 ( 0.05000000000000003053, 0.05277777777777779844, 0.05555555555555556635, 0.05833333333333334120 ),
 .UNSPECIFIED. ) 
 CURVE ( )  GEOMETRIC_REPRESENTATION_ITEM ( )  RATIONAL_B_SPLINE_CURVE ( ( 0.9999999999999986677, 0.8660254037844400399, 1.000000000000000000, 0.8660254037844387076, 1.000000000000000000, 0.8660254037844383745, 1.000000000000000222 ) ) 
 REPRESENTATION_ITEM ( '' )  );
#3362=CARTESIAN_POINT ( 'NONE',  ( 5.653125000614517504, -4.541064518000417216, -2.621784821875001281 ) ) ;
#3364=CARTESIAN_POINT ( 'NONE',  ( 17.03437500061451715, 6.421520780324663323E-16, -5.243569643749999010 ) ) ;
#3366=CARTESIAN_POINT ( 'NONE',  ( 26.43750000122903288, 4.330127018922191873, 2.499999999999999556 ) ) ;
#3367=CARTESIAN_POINT ( 'NONE',  ( 6.421875000614519102, 3.027376345333611329, 5.243569643749999010 ) ) ;
#3368=CARTESIAN_POINT ( 'NONE',  ( 15.90937500061451892, 0.000000000000000000, 5.243569643749999010 ) ) ;
#3370=CARTESIAN_POINT ( 'NONE',  ( 23.77499999999999858, -4.330127018922194537, 2.499999999999995559 ) ) ;
#3371=CARTESIAN_POINT ( 'NONE',  ( 3.150000001229034119, -2.886751345948129988, 4.999999999999997335 ) ) ;
#3372=CARTESIAN_POINT ( 'NONE',  ( 28.28437500061451715, 6.421520780324663323E-16, -5.243569643749999010 ) ) ;
#3374=CARTESIAN_POINT ( 'NONE',  ( 29.96250000000000213, 2.886751345948126879, 4.999999999999999112 ) ) ;
#3375=CARTESIAN_POINT ( 'NONE',  ( 7.537500000000002309, -2.886751345948129988, 4.999999999999997335 ) ) ;
#3377=CARTESIAN_POINT ( 'NONE',  ( 21.62812500061451360, 4.541064518000418104, 2.621784821874999949 ) ) ;
#3378=CARTESIAN_POINT ( 'NONE',  ( 10.65000000000000036, 0.000000000000000000, 4.999999999999998224 ) ) ;
#3379=CARTESIAN_POINT ( 'NONE',  ( 3.628125000614518036, 4.541064518000418104, 2.621784821874999949 ) ) ;
#3380=CARTESIAN_POINT ( 'NONE',  ( 20.69999999999999929, -4.330127018922190985, -2.500000000000001332 ) ) ;
#3381=CARTESIAN_POINT ( 'NONE',  ( 18.10312500061451502, 0.000000000000000000, 5.243569643749999010 ) ) ;
#3383=CARTESIAN_POINT ( 'NONE',  ( 23.21250000122903501, 4.330127018922192761, -2.499999999999997780 ) ) ;
#3386=CARTESIAN_POINT ( 'NONE',  ( 3.225000000000002309, 6.123233995736764310E-16, -4.999999999999998224 ) ) ;
#3388=CARTESIAN_POINT ( 'NONE',  ( 19.82812500061451644, 4.541064518000418104, 2.621784821874999949 ) ) ;
#3389=CARTESIAN_POINT ( 'NONE',  ( 27.14062500061451644, -3.027376345333614438, 5.243569643749998122 ) ) ;
#3390=CARTESIAN_POINT ( 'NONE',  ( 25.92187500061451999, -6.054752690667223547, -1.112240025338166033E-15 ) ) ;
#3391=CARTESIAN_POINT ( 'NONE',  ( 8.625000000000000000, 6.123233995736764310E-16, -4.999999999999998224 ) ) ;
#3392=CARTESIAN_POINT ( 'NONE',  ( 11.80312500061451608, 0.000000000000000000, 5.243569643749999010 ) ) ;
#3393=CARTESIAN_POINT ( 'NONE',  ( 26.20312500061451644, 0.000000000000000000, 5.243569643749999010 ) ) ;
#3394=CARTESIAN_POINT ( 'NONE',  ( 17.74687500061451928, -3.027376345333614438, 5.243569643749998122 ) ) ;
#3395=CARTESIAN_POINT ( 'NONE',  ( 9.215625000614515727, -6.054752690667223547, -1.112240025338166033E-15 ) ) ;
#3397=CARTESIAN_POINT ( 'NONE',  ( 9.001249775931846008E-16, 11.87187500061451750, 34.90005215228797653 ) ) ;
#3398=CARTESIAN_POINT ( 'NONE',  ( 23.21250000122903501, 4.330127018922192761, -2.499999999999997780 ) ) ;
#3400=CARTESIAN_POINT ( 'NONE',  ( 13.94062500061451537, 6.054752690667223547, 3.707466751127219781E-16 ) ) ;
#3401=CARTESIAN_POINT ( 'NONE',  ( 9.571875000614518569, 3.027376345333611329, 5.243569643749999010 ) ) ;
#3402=CARTESIAN_POINT ( 'NONE',  ( 9.084375000614517859, 4.541064518000418104, 2.621784821874999949 ) ) ;
#3403=ORIENTED_EDGE ( 'NONE', *, *, #31488, .F. ) ;
#3404=FACE_OUTER_BOUND ( 'NONE', #25177, .T. ) ;
#3405=CARTESIAN_POINT ( 'NONE',  ( 21.29062500061451502, -3.027376345333614438, 5.243569643749998122 ) ) ;
#3407=CARTESIAN_POINT ( 'NONE',  ( 16.88437500061451502, -4.541064518000419881, 2.621784821874995952 ) ) ;
#3408=CARTESIAN_POINT ( 'NONE',  ( 22.64062500061451644, -3.027376345333614438, 5.243569643749998122 ) ) ;
#3409=CARTESIAN_POINT ( 'NONE',  ( 1.999999999999998668, 10.85000000000000142, 26.53589838486224650 ) ) ;
#3410=CARTESIAN_POINT ( 'NONE',  ( 27.36562500061451786, 3.027376345333613106, -5.243569643749998122 ) ) ;
#3411=CARTESIAN_POINT ( 'NONE',  ( 8.100000001229034297, -2.886751345948129988, 4.999999999999997335 ) ) ;
#3412=ORIENTED_EDGE ( 'NONE', *, *, #48851, .T. ) ;
#3413=DIRECTION ( 'NONE',  ( -1.000000000000000000, -0.000000000000000000, -0.000000000000000000 ) ) ;
#3414=CARTESIAN_POINT ( 'NONE',  ( 8.484601909799253346E-16, 18.76250000000000284, -25.38119784648299770 ) ) ;
#3415=CARTESIAN_POINT ( 'NONE',  ( 25.42500000122903359, 2.886751345948129099, -4.999999999999998224 ) ) ;
#3417=CARTESIAN_POINT ( 'NONE',  ( 6.121875000614517504, -6.054752690667223547, -1.112240025338166033E-15 ) ) ;
#3418=DIRECTION ( 'NONE',  ( -1.000000000000000000, -0.000000000000000000, -0.000000000000000000 ) ) ;
#3419=CARTESIAN_POINT ( 'NONE',  ( 14.99062500061451786, -3.027376345333614438, 5.243569643749998122 ) ) ;
#3420=CARTESIAN_POINT ( 'NONE',  ( 8.709375000614517859, 0.000000000000000000, 5.243569643749999010 ) ) ;
#3421=CARTESIAN_POINT ( 'NONE',  ( 27.18750000122903288, 6.123233995736764310E-16, -4.999999999999998224 ) ) ;
#3422=CARTESIAN_POINT ( 'NONE',  ( 17.82187500061451502, -6.054752690667223547, -1.112240025338166033E-15 ) ) ;
#3423=CARTESIAN_POINT ( 'NONE',  ( 6.046875000614519102, -3.027376345333614438, 5.243569643749998122 ) ) ;
#3424=CARTESIAN_POINT ( 'NONE',  ( 1.071796769724495668, 17.43259618943233136, -26.00000000000000711 ) ) ;
#3425=CARTESIAN_POINT ( 'NONE',  ( 6.140625000614516438, -3.027376345333610441, -5.243569643749999898 ) ) ;
#3426=CARTESIAN_POINT ( 'NONE',  ( 15.40312500061451573, 0.000000000000000000, 5.243569643749999010 ) ) ;
#3427=VERTEX_POINT ( 'NONE', #8627 ) ;
#3428=CARTESIAN_POINT ( 'NONE',  ( 12.06562500061451537, 3.027376345333613106, -5.243569643749998122 ) ) ;
#3429=CARTESIAN_POINT ( 'NONE',  ( 5.925000001229033586, -5.773502691896255534, -1.060575238724906372E-15 ) ) ;
#3430=CARTESIAN_POINT ( 'NONE',  ( 10.41562500061451679, 3.027376345333611329, 5.243569643749999010 ) ) ;
#3432=CARTESIAN_POINT ( 'NONE',  ( 9.787499999999999645, -2.886751345948129988, 4.999999999999997335 ) ) ;
#3434=CARTESIAN_POINT ( 'NONE',  ( 3.525000001229034119, 2.886751345948126879, 4.999999999999999112 ) ) ;
#3435=CARTESIAN_POINT ( 'NONE',  ( 17.66249999999999787, 2.886751345948129099, -4.999999999999998224 ) ) ;
#3436=CARTESIAN_POINT ( 'NONE',  ( 17.78437500061451715, -4.541064518000419881, 2.621784821874995952 ) ) ;
#3437=CARTESIAN_POINT ( 'NONE',  ( 15.33750000122903323, -4.330127018922194537, 2.499999999999995559 ) ) ;
#3439=CARTESIAN_POINT ( 'NONE',  ( 2.121784821875001281, 16.80312500061451786, -26.32496088578401938 ) ) ;
#3441=CARTESIAN_POINT ( 'NONE',  ( 2.812500001229033320, -4.330127018922190985, -2.500000000000001332 ) ) ;
#3442=CARTESIAN_POINT ( 'NONE',  ( 7.347880794884118750E-16, 20.00000000000000000, -24.00000000000000000 ) ) ;
#3445=CARTESIAN_POINT ( 'NONE',  ( 15.98437500061451821, -4.541064518000419881, 2.621784821874995952 ) ) ;
#3446=CARTESIAN_POINT ( 'NONE',  ( 29.13749999999999929, -2.886751345948129988, 4.999999999999997335 ) ) ;
#3448=CARTESIAN_POINT ( 'NONE',  ( 12.40312500061451573, -4.541064518000417216, -2.621784821875001281 ) ) ;
#3450=CARTESIAN_POINT ( 'NONE',  ( 22.80937500061451573, -4.541064518000417216, -2.621784821875001281 ) ) ;
#3452=CARTESIAN_POINT ( 'NONE',  ( 6.703125000614516438, 4.541064518000418104, -2.621784821874998173 ) ) ;
#3453=CARTESIAN_POINT ( 'NONE',  ( 12.64687500061451608, 6.054752690667223547, 3.707466751127219781E-16 ) ) ;
#3455=CARTESIAN_POINT ( 'NONE',  ( 23.52187500061451786, 3.027376345333611329, 5.243569643749999010 ) ) ;
#3456=CARTESIAN_POINT ( 'NONE',  ( 27.51562500061451644, 3.027376345333611329, 5.243569643749999010 ) ) ;
#3457=CARTESIAN_POINT ( 'NONE',  ( 24.78750000000000497, -2.886751345948109559, -5.000000000000028422 ) ) ;
#3458=CARTESIAN_POINT ( 'NONE',  ( 8.062500000000000000, -5.773502691896255534, -1.060575238724906372E-15 ) ) ;
#3459=CARTESIAN_POINT ( 'NONE',  ( 15.93750000122903110, 6.123233995736764310E-16, -4.999999999999998224 ) ) ;
#3462=ORIENTED_EDGE ( 'NONE', *, *, #62341, .T. ) ;
#3463=CARTESIAN_POINT ( 'NONE',  ( 15.07499999999999929, 4.330127018922191873, 2.499999999999999556 ) ) ;
#3464=CARTESIAN_POINT ( 'NONE',  ( 18.37500000000000355, -4.330127018922194537, 2.499999999999995559 ) ) ;
#3465=CARTESIAN_POINT ( 'NONE',  ( 14.39062500061451821, 6.054752690667223547, 3.707466751127219781E-16 ) ) ;
#3467=CARTESIAN_POINT ( 'NONE',  ( 3.734827092922140768, -3.324314453528163682, -3.734827092927292203 ) ) ;
#3468=CARTESIAN_POINT ( 'NONE',  ( -2.121784821874999949, 17.53437500061451715, -33.67503911421598417 ) ) ;
#3469=CARTESIAN_POINT ( 'NONE',  ( 3.815625000614518036, -6.054752690667223547, -1.112240025338166033E-15 ) ) ;
#3470=CARTESIAN_POINT ( 'NONE',  ( 10.31250000000000178, -5.773502691896255534, -1.060575238724906372E-15 ) ) ;
#3471=CARTESIAN_POINT ( 'NONE',  ( 10.80000000000000071, -4.330127018922190985, -2.500000000000001332 ) ) ;
#3473=ORIENTED_EDGE ( 'NONE', *, *, #55966, .T. ) ;
#3474=CARTESIAN_POINT ( 'NONE',  ( -2.121784821874999949, 15.67812500061451608, 26.32496088578401938 ) ) ;
#3475=CARTESIAN_POINT ( 'NONE',  ( 27.21562500061451928, -6.054752690667223547, -1.112240025338166033E-15 ) ) ;
#3479=CARTESIAN_POINT ( 'NONE',  ( 23.44687500061451502, 6.054752690667223547, 3.707466751127219781E-16 ) ) ;
#3481=CARTESIAN_POINT ( 'NONE',  ( 18.62812500061451715, -4.541064518000419881, 2.621784821874995952 ) ) ;
#3482=CARTESIAN_POINT ( 'NONE',  ( -4.243569643749999898, 13.01562500061459460, -32.45002607614398471 ) ) ;
#3483=CARTESIAN_POINT ( 'NONE',  ( 23.40000000122903145, -2.886751345948129988, 4.999999999999997335 ) ) ;
#3484=CARTESIAN_POINT ( 'NONE',  ( 5.053125000614517859, 0.000000000000000000, 5.243569643749999010 ) ) ;
#3486=CARTESIAN_POINT ( 'NONE',  ( 21.47812500061451502, 6.421520780324663323E-16, -5.243569643749999010 ) ) ;
#3489=CARTESIAN_POINT ( 'NONE',  ( 16.43437500061451573, -4.541064518000419881, 2.621784821874995952 ) ) ;
#3490=CARTESIAN_POINT ( 'NONE',  ( 15.83437500061451608, 4.541064518000418104, 2.621784821874999949 ) ) ;
#3491=CARTESIAN_POINT ( 'NONE',  ( 25.92187500061451999, -6.054752690667223547, -1.112240025338166033E-15 ) ) ;
#3492=CARTESIAN_POINT ( 'NONE',  ( -4.243569643749999898, 13.55937500061451750, 30.00000000000000000 ) ) ;
#3493=CARTESIAN_POINT ( 'NONE',  ( 5.128125000614516260, -4.541064518000419881, 2.621784821874995952 ) ) ;
#3494=CARTESIAN_POINT ( 'NONE',  ( 27.92812500061451431, 4.541064518000418104, 2.621784821874999949 ) ) ;
#3495=CARTESIAN_POINT ( 'NONE',  ( 28.26562500061451289, 3.027376345333613106, -5.243569643749998122 ) ) ;
#3496=CARTESIAN_POINT ( 'NONE',  ( 1.071796769724491893, 16.19509619066136707, -26.00000000000000355 ) ) ;
#3497=CARTESIAN_POINT ( 'NONE',  ( -3.999999999999997335, 19.13750000000000284, 32.30940107675850470 ) ) ;
#3498=CARTESIAN_POINT ( 'NONE',  ( 6.459375000614518747, 0.000000000000000000, 5.243569643749999010 ) ) ;
#3499=CARTESIAN_POINT ( 'NONE',  ( 14.51250000122903394, -4.330127018922190985, -2.500000000000001332 ) ) ;
#3500=CARTESIAN_POINT ( 'NONE',  ( 9.787500001229036073, 4.330127018922191873, 2.499999999999999556 ) ) ;
#3501=CARTESIAN_POINT ( 'NONE',  ( 5.990625000614517859, -3.027376345333614438, 5.243569643749998122 ) ) ;
#3504=CARTESIAN_POINT ( 'NONE',  ( 13.17187500061451999, 3.027376345333611329, 5.243569643749999010 ) ) ;
#3505=CYLINDRICAL_SURFACE ( 'NONE', #30219, 3.999999999999996447 ) ;
#3506=ORIENTED_EDGE ( 'NONE', *, *, #71167, .F. ) ;
#3507=CARTESIAN_POINT ( 'NONE',  ( 22.34062500061451573, -3.027376345333610441, -5.243569643749999898 ) ) ;
#3508=CARTESIAN_POINT ( 'NONE',  ( 8.353125000614518569, -4.541064518000417216, -2.621784821875001281 ) ) ;
#3509=CARTESIAN_POINT ( 'NONE',  ( 25.02187500061451431, -6.054752690667223547, -1.112240025338166033E-15 ) ) ;
#3510=CARTESIAN_POINT ( 'NONE',  ( 7.903125000614515727, -4.541064518000417216, -2.621784821875001281 ) ) ;
#3511=CARTESIAN_POINT ( 'NONE',  ( 7.800000001229035362, -2.886751345948125991, -5.000000000000000000 ) ) ;
#3512=CARTESIAN_POINT ( 'NONE',  ( 21.47812500061451502, 6.421520780324663323E-16, -5.243569643749999010 ) ) ;
#3513=CARTESIAN_POINT ( 'NONE',  ( -4.243569643749999898, 11.70312500061451644, -30.00000000000000000 ) ) ;
#3514=CARTESIAN_POINT ( 'NONE',  ( 10.42500000122903536, -5.773502691896255534, -1.060575238724906372E-15 ) ) ;
#3515=CARTESIAN_POINT ( 'NONE',  ( 19.26562500061451644, 3.027376345333613106, -5.243569643749998122 ) ) ;
#3516=CARTESIAN_POINT ( 'NONE',  ( 17.50312500061451715, 4.541064518000418104, -2.621784821874998173 ) ) ;
#3518=CARTESIAN_POINT ( 'NONE',  ( 17.25000000000000000, 4.330127018922192761, -2.499999999999997780 ) ) ;
#3519=CARTESIAN_POINT ( 'NONE',  ( 10.83750000122903501, -4.330127018922194537, 2.499999999999995559 ) ) ;
#3520=CARTESIAN_POINT ( 'NONE',  ( 8.953125000614518214, 4.541064518000418104, -2.621784821874998173 ) ) ;
#3521=CARTESIAN_POINT ( 'NONE',  ( 12.32812500061451821, -4.541064518000419881, 2.621784821874995952 ) ) ;
#3522=( BOUNDED_CURVE ( )  B_SPLINE_CURVE ( 3, ( #7335, #47224, #41325, #57571 ),
 .UNSPECIFIED., .F., .F. ) 
 B_SPLINE_CURVE_WITH_KNOTS ( ( 4, 4 ),
 ( 5.521927013012204455, 5.555875059252146642 ),
 .UNSPECIFIED. ) 
 CURVE ( )  GEOMETRIC_REPRESENTATION_ITEM ( )  RATIONAL_B_SPLINE_CURVE ( ( 1.000000000000000000, 0.9999039631522317340, 0.9999039631522317340, 1.000000000000000000 ) ) 
 REPRESENTATION_ITEM ( '' )  );
#3523=CARTESIAN_POINT ( 'NONE',  ( 23.81250000122903288, 0.000000000000000000, 4.999999999999998224 ) ) ;
#3524=CARTESIAN_POINT ( 'NONE',  ( 22.62187500061451573, 3.027376345333611329, 5.243569643749999010 ) ) ;
#3526=CARTESIAN_POINT ( 'NONE',  ( 4.387500001229033053, 4.330127018922191873, 2.499999999999999556 ) ) ;
#3527=CARTESIAN_POINT ( 'NONE',  ( 6.159375000614517148, -4.541064518000417216, -2.621784821875001281 ) ) ;
#3528=CARTESIAN_POINT ( 'NONE',  ( 23.97187500061451360, 3.027376345333611329, 5.243569643749999010 ) ) ;
#3529=CARTESIAN_POINT ( 'NONE',  ( 4.790750098056429707, -1.432228568557152082, 4.843449711448116979 ) ) ;
#3530=CARTESIAN_POINT ( 'NONE',  ( 18.32812500061451644, 6.421520780324663323E-16, -5.243569643749999010 ) ) ;
#3531=CARTESIAN_POINT ( 'NONE',  ( 23.37187500061451573, 3.027376345333613106, -5.243569643749998122 ) ) ;
#3533=CARTESIAN_POINT ( 'NONE',  ( -3.999999999999997335, 13.40000000122903323, -27.69059892324149530 ) ) ;
#3534=CARTESIAN_POINT ( 'NONE',  ( 6.459375000614518747, 0.000000000000000000, 5.243569643749999010 ) ) ;
#3535=CARTESIAN_POINT ( 'NONE',  ( 18.10312500061451502, 0.000000000000000000, 5.243569643749999010 ) ) ;
#3536=CARTESIAN_POINT ( 'NONE',  ( 12.45937500061451786, -4.541064518000417216, -2.621784821875001281 ) ) ;
#3538=CARTESIAN_POINT ( 'NONE',  ( 22.12500000000000000, 6.123233995736764310E-16, -4.999999999999998224 ) ) ;
#3539=CARTESIAN_POINT ( 'NONE',  ( 25.30312500061451431, 0.000000000000000000, 5.243569643749999010 ) ) ;
#3540=CARTESIAN_POINT ( 'NONE',  ( 3.503166010679463760, 3.567662455396273913, -3.772175302801220376 ) ) ;
#3542=CARTESIAN_POINT ( 'NONE',  ( 14.84999999999999964, -4.330127018922190985, -2.500000000000001332 ) ) ;
#3543=CARTESIAN_POINT ( 'NONE',  ( 23.62500000122902932, 2.886751345948129099, -4.999999999999998224 ) ) ;
#3544=CARTESIAN_POINT ( 'NONE',  ( 17.42812500061451786, 6.421520780324663323E-16, -5.243569643749999010 ) ) ;
#3545=ORIENTED_EDGE ( 'NONE', *, *, #37237, .T. ) ;
#3546=CARTESIAN_POINT ( 'NONE',  ( 22.83749999999999858, -2.886751345948129988, 4.999999999999997335 ) ) ;
#3548=CARTESIAN_POINT ( 'NONE',  ( 22.69687500061451857, -3.027376345333614438, 5.243569643749998122 ) ) ;
#3549=ORIENTED_EDGE ( 'NONE', *, *, #50844, .F. ) ;
#3551=CARTESIAN_POINT ( 'NONE',  ( 10.97812500061451679, -4.541064518000419881, 2.621784821874995952 ) ) ;
#3552=CARTESIAN_POINT ( 'NONE',  ( 3.140625000614516882, 6.054752690667223547, 3.707466751127219781E-16 ) ) ;
#3554=CARTESIAN_POINT ( 'NONE',  ( 27.40312500061451573, 4.541064518000418104, -2.621784821874998173 ) ) ;
#3555=CARTESIAN_POINT ( 'NONE',  ( 18.82500000000000284, -4.330127018922194537, 2.499999999999995559 ) ) ;
#3556=CARTESIAN_POINT ( 'NONE',  ( 26.28749999999999432, 5.773502691896255534, 3.535250795749688894E-16 ) ) ;
#3557=CARTESIAN_POINT ( 'NONE',  ( 3.046875000614519990, -3.027376345333610441, -5.243569643749999898 ) ) ;
#3558=CARTESIAN_POINT ( 'NONE',  ( 7.809375000614519280, 0.000000000000000000, 5.243569643749999010 ) ) ;
#3559=CARTESIAN_POINT ( 'NONE',  ( 17.93437500061451928, 6.421520780324663323E-16, -5.243569643749999010 ) ) ;
#3562=CARTESIAN_POINT ( 'NONE',  ( 26.39062500061451644, -3.027376345333610441, -5.243569643749999898 ) ) ;
#3563=CARTESIAN_POINT ( 'NONE',  ( 27.23437500061451644, -4.541064518000419881, 2.621784821874995952 ) ) ;
#3565=CARTESIAN_POINT ( 'NONE',  ( 17.25000000000000000, 4.330127018922192761, -2.499999999999997780 ) ) ;
#3566=CARTESIAN_POINT ( 'NONE',  ( 12.17812500061451608, 4.541064518000418104, 2.621784821874999949 ) ) ;
#3568=CARTESIAN_POINT ( 'NONE',  ( 1.626862140677534273E-15, 10.66249999999999964, -26.00000000000000355 ) ) ;
#3569=CARTESIAN_POINT ( 'NONE',  ( 28.56562500061451715, -6.054752690667223547, -1.112240025338166033E-15 ) ) ;
#3570=CARTESIAN_POINT ( 'NONE',  ( 19.01250000122903216, -4.330127018922190985, -2.500000000000001332 ) ) ;
#3571=CARTESIAN_POINT ( 'NONE',  ( 1.626862140677534273E-15, 10.77500000122903323, -26.00000000000000355 ) ) ;
#3573=CARTESIAN_POINT ( 'NONE',  ( 5.953125000614519102, 0.000000000000000000, 5.243569643749999010 ) ) ;
#3574=CARTESIAN_POINT ( 'NONE',  ( 21.87187500061451573, -6.054752690667223547, -1.112240025338166033E-15 ) ) ;
#3575=CARTESIAN_POINT ( 'NONE',  ( -2.121784821874999949, 17.53437500061451715, 26.32496088578401938 ) ) ;
#3576=CARTESIAN_POINT ( 'NONE',  ( 23.89687500061451786, 6.054752690667223547, 3.707466751127219781E-16 ) ) ;
#3577=CARTESIAN_POINT ( 'NONE',  ( 5.437500000000001776, -2.886751345948125991, -5.000000000000000000 ) ) ;
#3578=CARTESIAN_POINT ( 'NONE',  ( -1.999999999999997113, 9.837500001229035007, 33.46410161513775705 ) ) ;
#3579=CARTESIAN_POINT ( 'NONE',  ( 12.77812500061451750, -4.541064518000419881, 2.621784821874995952 ) ) ;
#3580=CARTESIAN_POINT ( 'NONE',  ( 3.825000001229032609, 2.886751345948129099, -4.999999999999998224 ) ) ;
#3581=( BOUNDED_CURVE ( )  B_SPLINE_CURVE ( 2, ( #34857, #63293, #12685, #177, #57743, #7150, #46678 ),
 .UNSPECIFIED., .F., .F. ) 
 B_SPLINE_CURVE_WITH_KNOTS ( ( 3, 2, 2, 3 ),
 ( 0.8666666666666666963, 0.8694444444444444642, 0.8722222222222222321, 0.8750000000000000000 ),
 .UNSPECIFIED. ) 
 CURVE ( )  GEOMETRIC_REPRESENTATION_ITEM ( )  RATIONAL_B_SPLINE_CURVE ( ( 1.000000000000000000, 0.8660254037844387076, 1.000000000000000000, 0.8660254037844387076, 1.000000000000000000, 0.8660254037844387076, 1.000000000000000000 ) ) 
 REPRESENTATION_ITEM ( '' )  );
#3582=CARTESIAN_POINT ( 'NONE',  ( 8.859375000614518214, -4.541064518000417216, -2.621784821875001281 ) ) ;
#3584=CARTESIAN_POINT ( 'NONE',  ( 9.665625000614515017, -6.054752690667223547, -1.112240025338166033E-15 ) ) ;
#3585=CARTESIAN_POINT ( 'NONE',  ( 14.10937500061451644, 0.000000000000000000, 5.243569643749999010 ) ) ;
#3586=CARTESIAN_POINT ( 'NONE',  ( 30.00000000000000000, 0.000000000000000000, 0.000000000000000000 ) ) ;
#3587=CARTESIAN_POINT ( 'NONE',  ( 22.23750000122903003, 6.123233995736764310E-16, -4.999999999999998224 ) ) ;
#3588=CARTESIAN_POINT ( 'NONE',  ( 11.03437500061451715, -4.541064518000419881, 2.621784821874995952 ) ) ;
#3589=CARTESIAN_POINT ( 'NONE',  ( 12.36562500061451608, -6.054752690667223547, -1.112240025338166033E-15 ) ) ;
#3591=CARTESIAN_POINT ( 'NONE',  ( 22.05937500061451573, 4.541064518000418104, -2.621784821874998173 ) ) ;
#3593=CARTESIAN_POINT ( 'NONE',  ( -1.071796769724491005, 11.92009619066136850, -34.00000000000000000 ) ) ;
#3594=CARTESIAN_POINT ( 'NONE',  ( 3.144856541311010556, 3.887142566792906706, -3.519253510942787599 ) ) ;
#3595=CARTESIAN_POINT ( 'NONE',  ( 2.121784821875001281, 14.60937500061451821, -26.32496088578401938 ) ) ;
#3596=CARTESIAN_POINT ( 'NONE',  ( 15.71250000122903501, 0.000000000000000000, 4.999999999999998224 ) ) ;
#3597=CARTESIAN_POINT ( 'NONE',  ( 10.73437500061451644, 6.421520780324663323E-16, -5.243569643749999010 ) ) ;
#3598=CARTESIAN_POINT ( 'NONE',  ( -4.243569643749999898, 16.65312500061451573, -30.00000000000000000 ) ) ;
#3599=CARTESIAN_POINT ( 'NONE',  ( 17.73750000122903359, 6.123233995736764310E-16, -4.999999999999998224 ) ) ;
#3600=CARTESIAN_POINT ( 'NONE',  ( 13.71562500061451750, -6.054752690667223547, -1.112240025338166033E-15 ) ) ;
#3602=CARTESIAN_POINT ( 'NONE',  ( 15.45000000000000107, 4.330127018922192761, -2.499999999999997780 ) ) ;
#3603=CARTESIAN_POINT ( 'NONE',  ( 5.137500001229033941, 6.123233995736764310E-16, -4.999999999999998224 ) ) ;
#3604=CARTESIAN_POINT ( 'NONE',  ( 10.47187500061451715, 3.027376345333611329, 5.243569643749999010 ) ) ;
#3605=EDGE_CURVE ( 'NONE', #41592, #18509, #2726, .T. ) ;
#3606=CARTESIAN_POINT ( 'NONE',  ( 9.487500001229033586, -4.330127018922194537, 2.499999999999995559 ) ) ;
#3607=CARTESIAN_POINT ( 'NONE',  ( 18.86250000122903359, 0.000000000000000000, 4.999999999999998224 ) ) ;
#3609=CARTESIAN_POINT ( 'NONE',  ( 16.67812500061451786, 4.541064518000418104, 2.621784821874999949 ) ) ;
#3610=CARTESIAN_POINT ( 'NONE',  ( 19.82812500061451644, 4.541064518000418104, 2.621784821874999949 ) ) ;
#3611=CARTESIAN_POINT ( 'NONE',  ( 28.53750000122903074, 6.123233995736764310E-16, -4.999999999999998224 ) ) ;
#3612=CARTESIAN_POINT ( 'NONE',  ( 4.078125000614517326, 4.541064518000418104, 2.621784821874999949 ) ) ;
#3613=CARTESIAN_POINT ( 'NONE',  ( 25.72499999999999787, 6.123233995736764310E-16, -4.999999999999998224 ) ) ;
#3616=CARTESIAN_POINT ( 'NONE',  ( 27.83437500061451786, 6.421520780324663323E-16, -5.243569643749999010 ) ) ;
#3617=CARTESIAN_POINT ( 'NONE',  ( 1.626862140677534273E-15, 12.46250000000000213, -26.00000000000000355 ) ) ;
#3618=CARTESIAN_POINT ( 'NONE',  ( 12.00000000122903465, 5.773502691896255534, 3.535250795749688894E-16 ) ) ;
#3619=CARTESIAN_POINT ( 'NONE',  ( 4.687500000000000000, 5.773502691896255534, 3.535250795749688894E-16 ) ) ;
#3621=CARTESIAN_POINT ( 'NONE',  ( 6.871875000614517504, 3.027376345333611329, 5.243569643749999010 ) ) ;
#3622=CARTESIAN_POINT ( 'NONE',  ( 26.72812500061451502, -4.541064518000419881, 2.621784821874995952 ) ) ;
#3623=CARTESIAN_POINT ( 'NONE',  ( 4.710420932447848763, -3.574158126769929833, 4.296515817649278368 ) ) ;
#3624=CARTESIAN_POINT ( 'NONE',  ( -0.2030170140429786718, 10.00000000000000000, -23.99999999999999289 ) ) ;
#3625=DIRECTION ( 'NONE',  ( -1.000000000000000000, -0.000000000000000000, -0.000000000000000000 ) ) ;
#3626=CARTESIAN_POINT ( 'NONE',  ( 4.321875000614517681, -6.054752690667223547, -1.112240025338166033E-15 ) ) ;
#3627=CARTESIAN_POINT ( 'NONE',  ( 9.309375000614517504, -4.541064518000417216, -2.621784821875001281 ) ) ;
#3628=CARTESIAN_POINT ( 'NONE',  ( 3.037500000000002309, -2.886751345948129988, 4.999999999999997335 ) ) ;
#3629=CARTESIAN_POINT ( 'NONE',  ( 9.001249775931846008E-16, 12.26562500061459282, 34.90005215228797653 ) ) ;
#3630=CARTESIAN_POINT ( 'NONE',  ( 21.56250000000000000, -5.773502691896255534, -1.060575238724906372E-15 ) ) ;
#3631=CARTESIAN_POINT ( 'NONE',  ( 1.626862140677534273E-15, 17.86250000000000071, -26.00000000000000355 ) ) ;
#3632=CARTESIAN_POINT ( 'NONE',  ( 3.374999999999999556, 4.330127018922191873, 2.499999999999999556 ) ) ;
#3634=ORIENTED_EDGE ( 'NONE', *, *, #56957, .F. ) ;
#3635=CARTESIAN_POINT ( 'NONE',  ( 21.29062500061451502, -3.027376345333614438, 5.243569643749998122 ) ) ;
#3636=CARTESIAN_POINT ( 'NONE',  ( 9.703125000614514661, -4.541064518000417216, -2.621784821875001281 ) ) ;
#3638=CARTESIAN_POINT ( 'NONE',  ( 6.721875000614518925, 3.027376345333613106, -5.243569643749998122 ) ) ;
#3639=CARTESIAN_POINT ( 'NONE',  ( 24.67500000000000071, -4.330127018922194537, 2.499999999999995559 ) ) ;
#3640=CARTESIAN_POINT ( 'NONE',  ( 21.15000000122903145, -2.886751345948129988, 4.999999999999997335 ) ) ;
#3641=CARTESIAN_POINT ( 'NONE',  ( 28.04062500061451502, -3.027376345333614438, 5.243569643749998122 ) ) ;
#3642=CARTESIAN_POINT ( 'NONE',  ( 1.626862140677534273E-15, 15.61250000000000071, 34.00000000000000000 ) ) ;
#3643=CARTESIAN_POINT ( 'NONE',  ( 10.09687500061451715, -3.027376345333614438, 5.243569643749998122 ) ) ;
#3644=CARTESIAN_POINT ( 'NONE',  ( 13.65937500061451715, 0.000000000000000000, 5.243569643749999010 ) ) ;
#3645=CARTESIAN_POINT ( 'NONE',  ( 24.12187500061451217, -6.054752690667223547, -1.112240025338166033E-15 ) ) ;
#3646=CARTESIAN_POINT ( 'NONE',  ( 4.000000000000000000, 18.05000000122903359, -27.69059892324149885 ) ) ;
#3648=CARTESIAN_POINT ( 'NONE',  ( 18.75937500061451857, -4.541064518000417216, -2.621784821875001281 ) ) ;
#3649=CARTESIAN_POINT ( 'NONE',  ( 10.05937500061451750, 0.000000000000000000, 5.243569643749999010 ) ) ;
#3651=CARTESIAN_POINT ( 'NONE',  ( 24.00000000000000000, 4.330127018922192761, -2.499999999999997780 ) ) ;
#3653=CARTESIAN_POINT ( 'NONE',  ( -3.999999999999999112, 9.762500001229033941, -30.00000000000000000 ) ) ;
#3655=CARTESIAN_POINT ( 'NONE',  ( 12.85312500061451502, -4.541064518000417216, -2.621784821875001281 ) ) ;
#3656=CARTESIAN_POINT ( 'NONE',  ( 29.22187500061451715, 3.027376345333613106, -5.243569643749998122 ) ) ;
#3657=LINE ( 'NONE', #37989, #39618 ) ;
#3658=FACE_OUTER_BOUND ( 'NONE', #546, .T. ) ;
#3659=CARTESIAN_POINT ( 'NONE',  ( 11.36250000000000071, 2.886751345948129099, -4.999999999999998224 ) ) ;
#3660=CARTESIAN_POINT ( 'NONE',  ( 4.000000000000000000, 18.95000000122903216, 32.30940107675849049 ) ) ;
#3661=CARTESIAN_POINT ( 'NONE',  ( 10.38750000122903572, -4.330127018922194537, 2.499999999999995559 ) ) ;
#3662=CARTESIAN_POINT ( 'NONE',  ( 21.64687500061451786, 6.054752690667223547, 3.707466751127219781E-16 ) ) ;
#3663=CARTESIAN_POINT ( 'NONE',  ( 17.22187500061451715, 3.027376345333611329, 5.243569643749999010 ) ) ;
#3664=LINE ( 'NONE', #65337, #44264 ) ;
#3666=CARTESIAN_POINT ( 'NONE',  ( 17.12812500061451715, 4.541064518000418104, 2.621784821874999949 ) ) ;
#3667=CARTESIAN_POINT ( 'NONE',  ( 28.57500000122903572, 2.886751345948129099, -4.999999999999998224 ) ) ;
#3668=CARTESIAN_POINT ( 'NONE',  ( 18.00937500061451502, 4.541064518000418104, -2.621784821874998173 ) ) ;
#3669=CARTESIAN_POINT ( 'NONE',  ( 28.77187500061451431, 3.027376345333613106, -5.243569643749998122 ) ) ;
#3670=CARTESIAN_POINT ( 'NONE',  ( 5.015625000614518214, 3.027376345333611329, 5.243569643749999010 ) ) ;
#3671=CARTESIAN_POINT ( 'NONE',  ( 18.47812500061451857, 4.541064518000418104, 2.621784821874999949 ) ) ;
#3672=CARTESIAN_POINT ( 'NONE',  ( 28.02187500061451431, 3.027376345333611329, 5.243569643749999010 ) ) ;
#3673=CARTESIAN_POINT ( 'NONE',  ( 4.243569643749999898, 11.92812500061451608, 30.00000000000000000 ) ) ;
#3674=CARTESIAN_POINT ( 'NONE',  ( 17.25000000122903288, -2.886751345948125991, -5.000000000000000000 ) ) ;
#3676=CARTESIAN_POINT ( 'NONE',  ( 7.865625000614516082, -6.054752690667223547, -1.112240025338166033E-15 ) ) ;
#3677=CARTESIAN_POINT ( 'NONE',  ( 25.82812500061451644, -4.541064518000419881, 2.621784821874995952 ) ) ;
#3678=CARTESIAN_POINT ( 'NONE',  ( 1.999999999999998668, 19.06250000122903288, -33.46410161513775705 ) ) ;
#3679=CARTESIAN_POINT ( 'NONE',  ( 22.17187500061451644, 3.027376345333611329, 5.243569643749999010 ) ) ;
#3680=CARTESIAN_POINT ( 'NONE',  ( 13.19062500061451537, -3.027376345333614438, 5.243569643749998122 ) ) ;
#3681=CARTESIAN_POINT ( 'NONE',  ( 23.25000000122903288, 5.773502691896255534, 3.535250795749688894E-16 ) ) ;
#3682=CARTESIAN_POINT ( 'NONE',  ( 22.30312500061451431, -4.541064518000417216, -2.621784821875001281 ) ) ;
#3683=CARTESIAN_POINT ( 'NONE',  ( 17.29687500061451999, -3.027376345333614438, 5.243569643749998122 ) ) ;
#3684=CARTESIAN_POINT ( 'NONE',  ( 13.00312500061451537, 4.541064518000418104, -2.621784821874998173 ) ) ;
#3685=CARTESIAN_POINT ( 'NONE',  ( 2.121784821875001281, 14.60937500061451821, 33.67503911421598417 ) ) ;
#3686=CARTESIAN_POINT ( 'NONE',  ( 18.81562500061452070, 3.027376345333613106, -5.243569643749998122 ) ) ;
#3687=CARTESIAN_POINT ( 'NONE',  ( 10.20000000000000107, 0.000000000000000000, 4.999999999999998224 ) ) ;
#3688=ORIENTED_EDGE ( 'NONE', *, *, #34392, .T. ) ;
#3689=CARTESIAN_POINT ( 'NONE',  ( 23.36250000000000071, -5.773502691896255534, -1.060575238724906372E-15 ) ) ;
#3690=CARTESIAN_POINT ( 'NONE',  ( -4.243569643749997233, 18.54687500061451289, -27.54997392385601174 ) ) ;
#3691=CARTESIAN_POINT ( 'NONE',  ( 0.9778744620075204841, -4.999999999999998224, 0.9778744620075204841 ) ) ;
#3692=CARTESIAN_POINT ( 'NONE',  ( 26.31562500061451715, -6.054752690667223547, -1.112240025338166033E-15 ) ) ;
#3693=CARTESIAN_POINT ( 'NONE',  ( 4.565625000614516260, 3.027376345333611329, 5.243569643749999010 ) ) ;
#3694=CARTESIAN_POINT ( 'NONE',  ( 19.31250000122903288, 0.000000000000000000, 4.999999999999998224 ) ) ;
#3695=CARTESIAN_POINT ( 'NONE',  ( 24.25312500061451715, 4.541064518000418104, -2.621784821874998173 ) ) ;
#3696=CARTESIAN_POINT ( 'NONE',  ( 23.55000000000000071, 4.330127018922192761, -2.499999999999997780 ) ) ;
#3697=CARTESIAN_POINT ( 'NONE',  ( 27.55312500061451786, 0.000000000000000000, 5.243569643749999010 ) ) ;
#3698=CARTESIAN_POINT ( 'NONE',  ( 7.640625000614517326, 6.054752690667223547, 3.707466751127219781E-16 ) ) ;
#3699=ORIENTED_EDGE ( 'NONE', *, *, #55011, .T. ) ;
#3700=CARTESIAN_POINT ( 'NONE',  ( 24.14062500061451289, -3.027376345333610441, -5.243569643749999898 ) ) ;
#3701=CARTESIAN_POINT ( 'NONE',  ( 5.615625000614517859, -6.054752690667223547, -1.112240025338166033E-15 ) ) ;
#3703=CARTESIAN_POINT ( 'NONE',  ( 3.778125000614519280, -4.541064518000419881, 2.621784821874995952 ) ) ;
#3704=CARTESIAN_POINT ( 'NONE',  ( 3.999999999999998668, 13.17500000122903359, -32.30940107675850470 ) ) ;
#3705=CARTESIAN_POINT ( 'NONE',  ( -1.071796769724488563, 10.64240381056766616, -26.00000000000000000 ) ) ;
#3707=CARTESIAN_POINT ( 'NONE',  ( 9.862500000000000711, -5.773502691896255534, -1.060575238724906372E-15 ) ) ;
#3708=CARTESIAN_POINT ( 'NONE',  ( 12.45937500061451786, -4.541064518000417216, -2.621784821875001281 ) ) ;
#3709=CARTESIAN_POINT ( 'NONE',  ( 5.775000001229033231, 2.886751345948126879, 4.999999999999999112 ) ) ;
#3710=CARTESIAN_POINT ( 'NONE',  ( 13.65937500061451715, 0.000000000000000000, 5.243569643749999010 ) ) ;
#3712=CARTESIAN_POINT ( 'NONE',  ( 5.484375000614518214, 4.541064518000418104, 2.621784821874999949 ) ) ;
#3714=CARTESIAN_POINT ( 'NONE',  ( 20.96250000122903145, 4.330127018922192761, -2.499999999999997780 ) ) ;
#3715=CARTESIAN_POINT ( 'NONE',  ( 11.55937500061451928, -4.541064518000417216, -2.621784821875001281 ) ) ;
#3716=CARTESIAN_POINT ( 'NONE',  ( 0.000000000000000000, 20.00000000000000000, -30.00000000000000000 ) ) ;
#3717=CARTESIAN_POINT ( 'NONE',  ( 21.32812500061451644, -4.541064518000419881, 2.621784821874995952 ) ) ;
#3718=CARTESIAN_POINT ( 'NONE',  ( 2.121784821875001281, 10.55937500061451750, 33.67503911421598417 ) ) ;
#3719=CARTESIAN_POINT ( 'NONE',  ( 2.121784821875001281, 19.50312500061459531, 33.67503911421598417 ) ) ;
#3720=CARTESIAN_POINT ( 'NONE',  ( 26.85937500061451644, -4.541064518000417216, -2.621784821875001281 ) ) ;
#3721=( BOUNDED_CURVE ( )  B_SPLINE_CURVE ( 2, ( #30837, #3137, #48203, #47108, #69640, #70365, #2402 ),
 .UNSPECIFIED., .F., .F. ) 
 B_SPLINE_CURVE_WITH_KNOTS ( ( 3, 2, 2, 3 ),
 ( 0.9687606754894464434, 0.9694444444444444420, 0.9722222222222222099, 0.9728271748341141834 ),
 .UNSPECIFIED. ) 
 CURVE ( )  GEOMETRIC_REPRESENTATION_ITEM ( )  RATIONAL_B_SPLINE_CURVE ( ( 0.9502783720093003206, 0.9670212389257863972, 1.000000000000000000, 0.8660254037844387076, 1.000000000000000000, 0.9708226185132003971, 0.9543539088861985320 ) ) 
 REPRESENTATION_ITEM ( '' )  );
#3722=CARTESIAN_POINT ( 'NONE',  ( -2.556497649636125342E-15, 19.21250000000000213, 34.00000000000000000 ) ) ;
#3723=EDGE_CURVE ( 'NONE', #27538, #329, #64188, .T. ) ;
#3724=CARTESIAN_POINT ( 'NONE',  ( 3.740625000614516527, -3.027376345333614438, 5.243569643749998122 ) ) ;
#3726=CARTESIAN_POINT ( 'NONE',  ( 13.24687500061451750, -3.027376345333614438, 5.243569643749998122 ) ) ;
#3727=CARTESIAN_POINT ( 'NONE',  ( 7.312500001229033764, -4.330127018922190985, -2.500000000000001332 ) ) ;
#3728=CARTESIAN_POINT ( 'NONE',  ( 26.28750000122903430, 6.123233995736764310E-16, -4.999999999999998224 ) ) ;
#3729=CARTESIAN_POINT ( 'NONE',  ( 4.884375000614518569, 6.421520780324663323E-16, -5.243569643749999010 ) ) ;
#3730=CARTESIAN_POINT ( 'NONE',  ( 16.84687500061451715, -3.027376345333614438, 5.243569643749998122 ) ) ;
#3732=CARTESIAN_POINT ( 'NONE',  ( 23.92499999999999716, 6.123233995736764310E-16, -4.999999999999998224 ) ) ;
#3733=CARTESIAN_POINT ( 'NONE',  ( 2.737500001229034474, -4.330127018922194537, 2.499999999999995559 ) ) ;
#3734=CARTESIAN_POINT ( 'NONE',  ( 25.99687500061451928, -3.027376345333610441, -5.243569643749999898 ) ) ;
#3736=DIRECTION ( 'NONE',  ( -1.000000000000000000, -0.000000000000000000, -0.000000000000000000 ) ) ;
#3737=CARTESIAN_POINT ( 'NONE',  ( 9.112500000000000711, 2.886751345948129099, -4.999999999999998224 ) ) ;
#3739=CARTESIAN_POINT ( 'NONE',  ( 19.00312500061451715, 0.000000000000000000, 5.243569643749999010 ) ) ;
#3740=CARTESIAN_POINT ( 'NONE',  ( 11.06250000000000000, 2.886751345948126879, 4.999999999999999112 ) ) ;
#3741=CARTESIAN_POINT ( 'NONE',  ( 3.665625000614517681, 3.027376345333611329, 5.243569643749999010 ) ) ;
#3742=CARTESIAN_POINT ( 'NONE',  ( 18.82500000000000284, -4.330127018922194537, 2.499999999999995559 ) ) ;
#3743=CARTESIAN_POINT ( 'NONE',  ( 17.69062500061451715, -3.027376345333614438, 5.243569643749998122 ) ) ;
#3744=CARTESIAN_POINT ( 'NONE',  ( -1.071796769724491005, 18.67009619066136494, 26.00000000000000355 ) ) ;
#3745=CARTESIAN_POINT ( 'NONE',  ( 23.40000000122903145, -2.886751345948129988, 4.999999999999997335 ) ) ;
#3747=B_SPLINE_CURVE_WITH_KNOTS ( 'NONE', 3,
 ( #19091, #62189, #65635, #60446, #66005, #37560, #48655, #49024, #71179, #32384, #9855, #48290, #20928, #54923, #60082, #4332, #26856, #21294, #3960, #49388, #70814, #26483, #71554, #43481, #37927, #10223, #15385, #71919, #20189, #54196, #72280, #43109, #43846, #66373, #15749, #38288, #55294, #31662, #20552, #60815 ),
 .UNSPECIFIED., .F., .F.,
 ( 4, 2, 2, 2, 2, 2, 2, 2, 2, 2, 2, 2, 2, 2, 2, 2, 2, 2, 2, 4 ),
 ( 0.02627519828802195659, 0.02668902850172998054, 0.02710285871543800795, 0.02793051914285405585, 0.02958583999768615858, 0.03041350042510220647, 0.03124116085251825090, 0.03206882127993430226, 0.03248265149364232274, 0.03289648170735034322, 0.03331031192105837063, 0.03372414213476639111, 0.03455180256218243207, 0.03537946298959846608, 0.03620712341701450704, 0.03703478384443054106, 0.03786244427184658201, 0.03869010469926261603, 0.03910393491297063651, 0.03951776512667865005 ),
 .UNSPECIFIED. ) ;
#3748=CARTESIAN_POINT ( 'NONE',  ( 29.48437500061451644, -4.541064518000419881, 2.621784821874995952 ) ) ;
#3749=VERTEX_POINT ( 'NONE', #66613 ) ;
#3750=CARTESIAN_POINT ( 'NONE',  ( 18.62812500061451715, -4.541064518000419881, 2.621784821874995952 ) ) ;
#3751=CARTESIAN_POINT ( 'NONE',  ( 23.76562500061451644, 3.027376345333613106, -5.243569643749998122 ) ) ;
#3752=CARTESIAN_POINT ( 'NONE',  ( 24.90937500061451715, 0.000000000000000000, 5.243569643749999010 ) ) ;
#3753=CARTESIAN_POINT ( 'NONE',  ( 9.074999999999999289, 6.123233995736764310E-16, -4.999999999999998224 ) ) ;
#3754=CARTESIAN_POINT ( 'NONE',  ( 11.16562500061451679, 3.027376345333613106, -5.243569643749998122 ) ) ;
#3755=CARTESIAN_POINT ( 'NONE',  ( 26.61562500061451786, 3.027376345333611329, 5.243569643749999010 ) ) ;
#3756=CARTESIAN_POINT ( 'NONE',  ( 17.44687500061451857, -3.027376345333610441, -5.243569643749999898 ) ) ;
#3757=CARTESIAN_POINT ( 'NONE',  ( 7.940625000614518036, -3.027376345333610441, -5.243569643749999898 ) ) ;
#3758=CARTESIAN_POINT ( 'NONE',  ( 0.000000000000000000, 20.00000000000000000, -30.00000000000000000 ) ) ;
#3759=CARTESIAN_POINT ( 'NONE',  ( -4.243569643749999898, 9.959375000614517859, 30.00000000000000000 ) ) ;
#3760=CARTESIAN_POINT ( 'NONE',  ( 22.98750000122903003, -4.330127018922194537, 2.499999999999995559 ) ) ;
#3762=CARTESIAN_POINT ( 'NONE',  ( 15.10312500061451502, -4.541064518000417216, -2.621784821875001281 ) ) ;
#3763=CARTESIAN_POINT ( 'NONE',  ( 8.671875000614518214, 3.027376345333611329, 5.243569643749999010 ) ) ;
#3764=CARTESIAN_POINT ( 'NONE',  ( 6.534375000614517148, -4.541064518000419881, 2.621784821874995952 ) ) ;
#3765=ORIENTED_EDGE ( 'NONE', *, *, #66921, .T. ) ;
#3766=CARTESIAN_POINT ( 'NONE',  ( 29.18437500061451573, 6.421520780324663323E-16, -5.243569643749999010 ) ) ;
#3767=CARTESIAN_POINT ( 'NONE',  ( 21.89062500061451289, -3.027376345333610441, -5.243569643749999898 ) ) ;
#3768=CARTESIAN_POINT ( 'NONE',  ( 17.29687500061451999, -3.027376345333614438, 5.243569643749998122 ) ) ;
#3769=CARTESIAN_POINT ( 'NONE',  ( 20.50312500061451715, -4.541064518000417216, -2.621784821875001281 ) ) ;
#3770=CARTESIAN_POINT ( 'NONE',  ( -3.999999999999999556, 11.86250000000000071, 27.69059892324149530 ) ) ;
#3771=CARTESIAN_POINT ( 'NONE',  ( 27.14062500061451644, -3.027376345333614438, 5.243569643749998122 ) ) ;
#3772=CARTESIAN_POINT ( 'NONE',  ( 5.925000001229033586, -5.773502691896255534, -1.060575238724906372E-15 ) ) ;
#3774=CARTESIAN_POINT ( 'NONE',  ( 3.375000001229033320, 2.886751345948129099, -4.999999999999998224 ) ) ;
#3775=CARTESIAN_POINT ( 'NONE',  ( -2.828200636599751609E-16, 17.63749999999999929, -34.61880215351700230 ) ) ;
#3776=CARTESIAN_POINT ( 'NONE',  ( 25.46250000122903501, 4.330127018922192761, -2.499999999999997780 ) ) ;
#3778=CARTESIAN_POINT ( 'NONE',  ( 6.684375000614518392, 6.421520780324663323E-16, -5.243569643749999010 ) ) ;
#3779=LINE ( 'NONE', #14845, #55017 ) ;
#3780=CARTESIAN_POINT ( 'NONE',  ( 13.75312500061451715, -4.541064518000417216, -2.621784821875001281 ) ) ;
#3781=CARTESIAN_POINT ( 'NONE',  ( 8.859375000614518214, -4.541064518000417216, -2.621784821875001281 ) ) ;
#3782=CARTESIAN_POINT ( 'NONE',  ( 27.75000000122903288, 5.773502691896255534, 3.535250795749688894E-16 ) ) ;
#3783=( BOUNDED_CURVE ( )  B_SPLINE_CURVE ( 2, ( #58927, #30865, #36774, #42323, #13138, #7972, #18309 ),
 .UNSPECIFIED., .F., .F. ) 
 B_SPLINE_CURVE_WITH_KNOTS ( ( 3, 2, 2, 3 ),
 ( 0.1750000000000000167, 0.1777777777777778123, 0.1805555555555555525, 0.1833333333333333204 ),
 .UNSPECIFIED. ) 
 CURVE ( )  GEOMETRIC_REPRESENTATION_ITEM ( )  RATIONAL_B_SPLINE_CURVE ( ( 0.9999999999999986677, 0.8660254037844400399, 1.000000000000000000, 0.8660254037844387076, 1.000000000000000000, 0.8660254037844387076, 1.000000000000000000 ) ) 
 REPRESENTATION_ITEM ( '' )  );
#3784=CARTESIAN_POINT ( 'NONE',  ( 16.92187500061451999, -6.054752690667223547, -1.112240025338166033E-15 ) ) ;
#3785=CARTESIAN_POINT ( 'NONE',  ( 4.246875000614519280, -3.027376345333614438, 5.243569643749998122 ) ) ;
#3786=CARTESIAN_POINT ( 'NONE',  ( 29.88749999999999929, 5.773502691896255534, 3.535250795749688894E-16 ) ) ;
#3787=CARTESIAN_POINT ( 'NONE',  ( 4.715625000614516615, -6.054752690667223547, -1.112240025338166033E-15 ) ) ;
#3788=( BOUNDED_CURVE ( )  B_SPLINE_CURVE ( 2, ( #70049, #14258, #64870, #13520, #26082, #64134, #24975, #13895, #9093 ),
 .UNSPECIFIED., .F., .F. ) 
 B_SPLINE_CURVE_WITH_KNOTS ( ( 3, 2, 2, 2, 3 ),
 ( 0.7934782608695651884, 0.7971014492753623060, 0.8043478260869565410, 0.8115942028985507761, 0.8152173913043478937 ),
 .UNSPECIFIED. ) 
 CURVE ( )  GEOMETRIC_REPRESENTATION_ITEM ( )  RATIONAL_B_SPLINE_CURVE ( ( 0.9330127018922194093, 0.9330127018922194093, 1.000000000000000000, 0.8660254037844387076, 1.000000000000000000, 0.8660254037844387076, 1.000000000000000000, 0.9330127018922182991, 0.9330127018922192983 ) ) 
 REPRESENTATION_ITEM ( '' )  );
#3789=CARTESIAN_POINT ( 'NONE',  ( 14.84062500061451750, 6.054752690667223547, 3.707466751127219781E-16 ) ) ;
#3790=VERTEX_POINT ( 'NONE', #15258 ) ;
#3791=B_SPLINE_CURVE_WITH_KNOTS ( 'NONE', 3,
 ( #68225, #40147, #62665, #12060, #41950, #8326, #47488, #31958, #31597, #54496 ),
 .UNSPECIFIED., .F., .F.,
 ( 4, 3, 3, 4 ),
 ( 1.786133494513239154E-16, 0.0001572325902286019026, 0.0003144664392359658575, 0.0005105429261828870087 ),
 .UNSPECIFIED. ) ;
#3792=CARTESIAN_POINT ( 'NONE',  ( 13.41562500061451502, 3.027376345333613106, -5.243569643749998122 ) ) ;
#3793=CARTESIAN_POINT ( 'NONE',  ( 5.887500001229034829, -4.330127018922194537, 2.499999999999995559 ) ) ;
#3794=CARTESIAN_POINT ( 'NONE',  ( 9.403125000614517504, 4.541064518000418104, -2.621784821874998173 ) ) ;
#3796=CARTESIAN_POINT ( 'NONE',  ( 8.287499999999999645, 5.773502691896255534, 3.535250795749688894E-16 ) ) ;
#3797=CARTESIAN_POINT ( 'NONE',  ( 4.575000001229033941, -5.773502691896255534, -1.060575238724906372E-15 ) ) ;
#3798=CARTESIAN_POINT ( 'NONE',  ( 17.21249999999999858, 2.886751345948129099, -4.999999999999998224 ) ) ;
#3799=( BOUNDED_CURVE ( )  B_SPLINE_CURVE ( 2, ( #54792, #72152, #21902, #44458, #59957, #32989, #72885 ),
 .UNSPECIFIED., .F., .F. ) 
 B_SPLINE_CURVE_WITH_KNOTS ( ( 3, 2, 2, 3 ),
 ( 0.4083333333333333814, 0.4111111111111111494, 0.4138888888888889173, 0.4166666666666667407 ),
 .UNSPECIFIED. ) 
 CURVE ( )  GEOMETRIC_REPRESENTATION_ITEM ( )  RATIONAL_B_SPLINE_CURVE ( ( 0.9999999999999973355, 0.8660254037844413721, 1.000000000000000000, 0.8660254037844387076, 1.000000000000000000, 0.8660254037844360431, 1.000000000000002665 ) ) 
 REPRESENTATION_ITEM ( '' )  );
#3800=CARTESIAN_POINT ( 'NONE',  ( 17.52187500061451431, 3.027376345333613106, -5.243569643749998122 ) ) ;
#3801=CARTESIAN_POINT ( 'NONE',  ( 14.96250000122903323, -4.330127018922190985, -2.500000000000001332 ) ) ;
#3803=CARTESIAN_POINT ( 'NONE',  ( -4.243569643749999898, 16.65312500061451573, -30.00000000000000000 ) ) ;
#3804=CARTESIAN_POINT ( 'NONE',  ( 3.199386026630491209, 3.842393604469308777, 3.568064829105276115 ) ) ;
#3805=CARTESIAN_POINT ( 'NONE',  ( 2.817472997146174052, -4.130598735093008678, -2.817472997146206026 ) ) ;
#3807=CARTESIAN_POINT ( 'NONE',  ( 28.15312500061451573, -4.541064518000417216, -2.621784821875001281 ) ) ;
#3809=CARTESIAN_POINT ( 'NONE',  ( 3.896829055840048017, -3.132845880275759054, -4.204794798714403647 ) ) ;
#3810=CARTESIAN_POINT ( 'NONE',  ( 15.34687500061451537, 6.054752690667223547, 3.707466751127219781E-16 ) ) ;
#3811=CARTESIAN_POINT ( 'NONE',  ( 28.46249999999999858, 2.886751345948129099, -4.999999999999998224 ) ) ;
#3812=ADVANCED_FACE ( 'NONE', ( #16351 ), #38538, .F. ) ;
#3813=CARTESIAN_POINT ( 'NONE',  ( 12.47812500061451502, 6.421520780324663323E-16, -5.243569643749999010 ) ) ;
#3815=CARTESIAN_POINT ( 'NONE',  ( 20.40937500061451715, 0.000000000000000000, 5.243569643749999010 ) ) ;
#3817=CARTESIAN_POINT ( 'NONE',  ( 8.090625000614515727, 6.054752690667223547, 3.707466751127219781E-16 ) ) ;
#3818=CARTESIAN_POINT ( 'NONE',  ( 12.53437500061451537, 6.421520780324663323E-16, -5.243569643749999010 ) ) ;
#3819=ORIENTED_EDGE ( 'NONE', *, *, #23299, .T. ) ;
#3820=CARTESIAN_POINT ( 'NONE',  ( 24.83437500061451431, 4.541064518000418104, 2.621784821874999949 ) ) ;
#3821=CARTESIAN_POINT ( 'NONE',  ( 27.44062500061451715, 6.054752690667223547, 3.707466751127219781E-16 ) ) ;
#3823=CARTESIAN_POINT ( 'NONE',  ( 8.474999999999999645, -4.330127018922194537, 2.499999999999995559 ) ) ;
#3824=CARTESIAN_POINT ( 'NONE',  ( 16.16250000122903430, 0.000000000000000000, 4.999999999999998224 ) ) ;
#3828=CARTESIAN_POINT ( 'NONE',  ( 15.48749999999999893, 5.773502691896255534, 3.535250795749688894E-16 ) ) ;
#3829=CARTESIAN_POINT ( 'NONE',  ( 18.82500000000000284, -4.330127018922194537, 2.499999999999995559 ) ) ;
#3830=CARTESIAN_POINT ( 'NONE',  ( 11.46562500061451573, -6.054752690667223547, -1.112240025338166033E-15 ) ) ;
#3831=ORIENTED_EDGE ( 'NONE', *, *, #71724, .T. ) ;
#3832=CARTESIAN_POINT ( 'NONE',  ( -3.999999999999999112, 10.96250000000000213, -32.30940107675850470 ) ) ;
#3833=CARTESIAN_POINT ( 'NONE',  ( -2.121784821874999949, 17.98437500061451999, -33.67503911421598417 ) ) ;
#3834=CARTESIAN_POINT ( 'NONE',  ( 3.140625000614516882, 6.054752690667223547, 3.707466751127219781E-16 ) ) ;
#3836=CARTESIAN_POINT ( 'NONE',  ( 10.68750000000000000, -2.886751345948129988, 4.999999999999997335 ) ) ;
#3837=CARTESIAN_POINT ( 'NONE',  ( 3.837848076843224376, 3.204827942194517831, -3.837848076843224376 ) ) ;
#3838=VERTEX_POINT ( 'NONE', #26727 ) ;
#3839=CARTESIAN_POINT ( 'NONE',  ( -4.243569643749997233, 13.99062500061451786, 32.45002607614398471 ) ) ;
#3840=CARTESIAN_POINT ( 'NONE',  ( 26.69062500061451715, -3.027376345333614438, 5.243569643749998122 ) ) ;
#3841=CARTESIAN_POINT ( 'NONE',  ( 29.36250000122903003, -4.330127018922190985, -2.500000000000001332 ) ) ;
#3842=CARTESIAN_POINT ( 'NONE',  ( 20.10000000000000142, 0.000000000000000000, 4.999999999999998224 ) ) ;
#3843=CARTESIAN_POINT ( 'NONE',  ( 20.70937500061451786, 4.541064518000418104, -2.621784821874998173 ) ) ;
#3844=CARTESIAN_POINT ( 'NONE',  ( 19.94062500061451715, -3.027376345333614438, 5.243569643749998122 ) ) ;
#3845=CARTESIAN_POINT ( 'NONE',  ( -2.121784821874999949, 13.87812500061459353, -33.67503911421598417 ) ) ;
#3846=CARTESIAN_POINT ( 'NONE',  ( 23.66250000122903430, 4.330127018922192761, -2.499999999999997780 ) ) ;
#3847=CARTESIAN_POINT ( 'NONE',  ( 3.178125000614515638, 4.541064518000418104, 2.621784821874999949 ) ) ;
#3849=CARTESIAN_POINT ( 'NONE',  ( 21.59062500061451928, 6.054752690667223547, 3.707466751127219781E-16 ) ) ;
#3852=CARTESIAN_POINT ( 'NONE',  ( 15.08437500061451786, -4.541064518000419881, 2.621784821874995952 ) ) ;
#3853=CARTESIAN_POINT ( 'NONE',  ( 13.39687500061451608, -3.027376345333610441, -5.243569643749999898 ) ) ;
#3854=CARTESIAN_POINT ( 'NONE',  ( 24.04687500061451644, -3.027376345333614438, 5.243569643749998122 ) ) ;
#3855=CARTESIAN_POINT ( 'NONE',  ( 4.243569643749999898, 13.29687500061451999, 32.45002607614398471 ) ) ;
#3856=CARTESIAN_POINT ( 'NONE',  ( 4.978125000614518569, 4.541064518000418104, 2.621784821874999949 ) ) ;
#3857=CARTESIAN_POINT ( 'NONE',  ( 29.09062500061451573, -3.027376345333610441, -5.243569643749999898 ) ) ;
#3858=CARTESIAN_POINT ( 'NONE',  ( 28.07812500061451289, -4.541064518000419881, 2.621784821874995952 ) ) ;
#3859=FACE_OUTER_BOUND ( 'NONE', #40436, .T. ) ;
#3860=CARTESIAN_POINT ( 'NONE',  ( 7.284375000614518036, 4.541064518000418104, 2.621784821874999949 ) ) ;
#3862=CARTESIAN_POINT ( 'NONE',  ( 14.28750000122903430, 4.330127018922191873, 2.499999999999999556 ) ) ;
#3863=CARTESIAN_POINT ( 'NONE',  ( 8.587500001229035007, -4.330127018922194537, 2.499999999999995559 ) ) ;
#3864=CARTESIAN_POINT ( 'NONE',  ( 4.528125000614516615, 4.541064518000418104, 2.621784821874999949 ) ) ;
#3867=CARTESIAN_POINT ( 'NONE',  ( 13.62187500061451750, 3.027376345333611329, 5.243569643749999010 ) ) ;
#3868=CARTESIAN_POINT ( 'NONE',  ( 12.00000000000000000, 0.000000000000000000, 4.999999999999998224 ) ) ;
#3869=VERTEX_POINT ( 'NONE', #49989 ) ;
#3870=CARTESIAN_POINT ( 'NONE',  ( 21.96562500061451573, 3.027376345333613106, -5.243569643749998122 ) ) ;
#3871=CARTESIAN_POINT ( 'NONE',  ( 7.490625000614516082, -3.027376345333610441, -5.243569643749999898 ) ) ;
#3872=CARTESIAN_POINT ( 'NONE',  ( 24.94687500061451502, -3.027376345333614438, 5.243569643749998122 ) ) ;
#3873=CARTESIAN_POINT ( 'NONE',  ( 7.153125000614518392, 4.541064518000418104, -2.621784821874998173 ) ) ;
#3874=CARTESIAN_POINT ( 'NONE',  ( 1.626862140677534273E-15, 13.02500000122903501, 34.00000000000000000 ) ) ;
#3875=CARTESIAN_POINT ( 'NONE',  ( 8.850000001229034297, 5.773502691896255534, 3.535250795749688894E-16 ) ) ;
#3876=EDGE_CURVE ( 'NONE', #32339, #21346, #47148, .T. ) ;
#3877=CARTESIAN_POINT ( 'NONE',  ( 23.42812500061451786, 4.541064518000418104, 2.621784821874999949 ) ) ;
#3878=VECTOR ( 'NONE', #66320, 1000.000000000000000 ) ;
#3879=CARTESIAN_POINT ( 'NONE',  ( -4.243569643749999898, 11.25312500061451892, -30.00000000000000000 ) ) ;
#3880=CARTESIAN_POINT ( 'NONE',  ( 9.675000001229035362, 2.886751345948129099, -4.999999999999998224 ) ) ;
#3881=CARTESIAN_POINT ( 'NONE',  ( 20.20312500061451644, 4.541064518000418104, -2.621784821874998173 ) ) ;
#3883=CARTESIAN_POINT ( 'NONE',  ( 15.66562500061451857, 3.027376345333613106, -5.243569643749998122 ) ) ;
#3885=CARTESIAN_POINT ( 'NONE',  ( 19.01249999999999929, 2.886751345948129099, -4.999999999999998224 ) ) ;
#3886=CARTESIAN_POINT ( 'NONE',  ( 11.06250000122903288, 4.330127018922192761, -2.499999999999997780 ) ) ;
#3887=CARTESIAN_POINT ( 'NONE',  ( 7.640625000614517326, 6.054752690667223547, 3.707466751127219781E-16 ) ) ;
#3888=CARTESIAN_POINT ( 'NONE',  ( 12.10312500061451857, 4.541064518000418104, -2.621784821874998173 ) ) ;
#3889=EDGE_CURVE ( 'NONE', #52141, #43575, #36784, .T. ) ;
#3890=CARTESIAN_POINT ( 'NONE',  ( 23.88750000122903216, -4.330127018922194537, 2.499999999999995559 ) ) ;
#3891=CARTESIAN_POINT ( 'NONE',  ( 21.53437500061451715, 6.421520780324663323E-16, -5.243569643749999010 ) ) ;
#3892=CARTESIAN_POINT ( 'NONE',  ( 9.528763966825557376E-15, 17.41249999999999787, 34.00000000000000000 ) ) ;
#3893=EDGE_CURVE ( 'NONE', #19531, #54070, #3799, .T. ) ;
#3894=CARTESIAN_POINT ( 'NONE',  ( 4.800000001229032698, 5.773502691896255534, 3.535250795749688894E-16 ) ) ;
#3895=CARTESIAN_POINT ( 'NONE',  ( 4.284375000614518925, -4.541064518000419881, 2.621784821874995952 ) ) ;
#3896=CARTESIAN_POINT ( 'NONE',  ( 22.50937500061451857, 4.541064518000418104, -2.621784821874998173 ) ) ;
#3898=CARTESIAN_POINT ( 'NONE',  ( 19.82812500061451644, 4.541064518000418104, 2.621784821874999949 ) ) ;
#3899=CARTESIAN_POINT ( 'NONE',  ( 24.34687500061451715, 6.054752690667223547, 3.707466751127219781E-16 ) ) ;
#3902=CARTESIAN_POINT ( 'NONE',  ( -1.999999999999997113, 13.43750000122903465, -26.53589838486224295 ) ) ;
#3903=CARTESIAN_POINT ( 'NONE',  ( 4.959375000614516971, 4.541064518000418104, -2.621784821874998173 ) ) ;
#3904=CARTESIAN_POINT ( 'NONE',  ( 15.44062500061451537, -3.027376345333614438, 5.243569643749998122 ) ) ;
#3905=CARTESIAN_POINT ( 'NONE',  ( 13.58437500061451786, 4.541064518000418104, 2.621784821874999949 ) ) ;
#3906=EDGE_LOOP ( 'NONE', ( #30780, #16162, #10676, #50533 ) ) ;
#3907=CARTESIAN_POINT ( 'NONE',  ( 1.999999999999998668, 17.15000000000000213, -33.46410161513775705 ) ) ;
#3908=CARTESIAN_POINT ( 'NONE',  ( 25.56562500061452070, 3.027376345333613106, -5.243569643749998122 ) ) ;
#3909=CARTESIAN_POINT ( 'NONE',  ( 4.000000000000000000, 17.03750000000000142, 32.30940107675849760 ) ) ;
#3910=CARTESIAN_POINT ( 'NONE',  ( -5.810221930991193690E-16, 11.45000000122903216, -34.00000000000000000 ) ) ;
#3911=CARTESIAN_POINT ( 'NONE',  ( 14.17500000000000071, 4.330127018922191873, 2.499999999999999556 ) ) ;
#3912=CARTESIAN_POINT ( 'NONE',  ( 23.32500000122903572, 2.886751345948126879, 4.999999999999999112 ) ) ;
#3913=CARTESIAN_POINT ( 'NONE',  ( 19.64062500061451644, -3.027376345333610441, -5.243569643749999898 ) ) ;
#3915=CARTESIAN_POINT ( 'NONE',  ( 23.55000000000000071, 4.330127018922192761, -2.499999999999997780 ) ) ;
#3916=CARTESIAN_POINT ( 'NONE',  ( 24.98437500061451644, -4.541064518000419881, 2.621784821874995952 ) ) ;
#3917=VERTEX_POINT ( 'NONE', #21531 ) ;
#3919=CARTESIAN_POINT ( 'NONE',  ( 11.35312500061451679, 0.000000000000000000, 5.243569643749999010 ) ) ;
#3920=CARTESIAN_POINT ( 'NONE',  ( 4.565625000614516260, 3.027376345333611329, 5.243569643749999010 ) ) ;
#3922=CARTESIAN_POINT ( 'NONE',  ( 26.99062500061451431, 6.054752690667223547, 3.707466751127219781E-16 ) ) ;
#3923=CARTESIAN_POINT ( 'NONE',  ( 16.80000000000000071, 4.330127018922192761, -2.499999999999997780 ) ) ;
#3924=CARTESIAN_POINT ( 'NONE',  ( 27.75000000000000000, 0.000000000000000000, 4.999999999999998224 ) ) ;
#3926=CARTESIAN_POINT ( 'NONE',  ( 7.284375000614518036, 4.541064518000418104, 2.621784821874999949 ) ) ;
#3927=CARTESIAN_POINT ( 'NONE',  ( 18.12187500061451573, 3.027376345333611329, 5.243569643749999010 ) ) ;
#3928=CARTESIAN_POINT ( 'NONE',  ( 25.98750000000000782, -2.886751345948163738, 4.999999999999939604 ) ) ;
#3929=ORIENTED_EDGE ( 'NONE', *, *, #23306, .F. ) ;
#3930=CARTESIAN_POINT ( 'NONE',  ( 26.42812500061451431, 6.421520780324663323E-16, -5.243569643749999010 ) ) ;
#3931=CARTESIAN_POINT ( 'NONE',  ( 27.94687500061451502, 6.054752690667223547, 3.707466751127219781E-16 ) ) ;
#3933=CARTESIAN_POINT ( 'NONE',  ( 13.57500000000000107, 6.123233995736764310E-16, -4.999999999999998224 ) ) ;
#3934=CARTESIAN_POINT ( 'NONE',  ( 11.12812500061451715, 6.421520780324663323E-16, -5.243569643749999010 ) ) ;
#3937=CARTESIAN_POINT ( 'NONE',  ( 27.85312500061451502, 4.541064518000418104, -2.621784821874998173 ) ) ;
#3938=CARTESIAN_POINT ( 'NONE',  ( 16.76250000122903216, -4.330127018922190985, -2.500000000000001332 ) ) ;
#3939=CARTESIAN_POINT ( 'NONE',  ( 3.766124272970669651, -4.056654931390053953, 3.460806837557585336 ) ) ;
#3941=CARTESIAN_POINT ( 'NONE',  ( 4.790625000614518569, -3.027376345333610441, -5.243569643749999898 ) ) ;
#3942=CARTESIAN_POINT ( 'NONE',  ( 20.89687500061452141, -3.027376345333614438, 5.243569643749998122 ) ) ;
#3943=CARTESIAN_POINT ( 'NONE',  ( 2.121784821875001281, 17.75937500061451502, 33.67503911421598417 ) ) ;
#3944=CARTESIAN_POINT ( 'NONE',  ( 23.03437500061451715, 4.541064518000418104, 2.621784821874999949 ) ) ;
#3945=CARTESIAN_POINT ( 'NONE',  ( 4.237500000000001599, 5.773502691896255534, 3.535250795749688894E-16 ) ) ;
#3946=CARTESIAN_POINT ( 'NONE',  ( 3.999999999999999112, 11.33750000122903501, 30.00000000000000000 ) ) ;
#3947=CARTESIAN_POINT ( 'NONE',  ( 11.91562500061451857, -6.054752690667223547, -1.112240025338166033E-15 ) ) ;
#3948=CARTESIAN_POINT ( 'NONE',  ( 4.987500001229032698, -4.330127018922194537, 2.499999999999995559 ) ) ;
#3949=CARTESIAN_POINT ( 'NONE',  ( 9.646875000614516082, -3.027376345333614438, 5.243569643749998122 ) ) ;
#3951=CARTESIAN_POINT ( 'NONE',  ( 9.140625000614518214, -3.027376345333614438, 5.243569643749998122 ) ) ;
#3952=CARTESIAN_POINT ( 'NONE',  ( 14.07187500061451679, 3.027376345333611329, 5.243569643749999010 ) ) ;
#3954=CARTESIAN_POINT ( 'NONE',  ( 21.52500000122903145, 2.886751345948126879, 4.999999999999999112 ) ) ;
#3955=CARTESIAN_POINT ( 'NONE',  ( 10.17187500061451999, -6.054752690667223547, -1.112240025338166033E-15 ) ) ;
#3956=CARTESIAN_POINT ( 'NONE',  ( 11.76562500061451644, 3.027376345333611329, 5.243569643749999010 ) ) ;
#3958=CARTESIAN_POINT ( 'NONE',  ( 22.47187500061451715, 3.027376345333613106, -5.243569643749998122 ) ) ;
#3960=CARTESIAN_POINT ( 'NONE',  ( -4.000165449326166467, 2.999779401354844222, 29.86626784624999686 ) ) ;
#3961=CARTESIAN_POINT ( 'NONE',  ( 3.286795329855858760, 3.767887532774327308, -3.286795329856085690 ) ) ;
#3962=CARTESIAN_POINT ( 'NONE',  ( 4.243569643749999898, 11.49687500061451928, -27.54997392385601529 ) ) ;
#3963=CARTESIAN_POINT ( 'NONE',  ( 15.18750000122903465, 4.330127018922191873, 2.499999999999999556 ) ) ;
#3964=EDGE_CURVE ( 'NONE', #33074, #10265, #6156, .T. ) ;
#3965=CARTESIAN_POINT ( 'NONE',  ( 8.971875000614515372, 3.027376345333613106, -5.243569643749998122 ) ) ;
#3966=CARTESIAN_POINT ( 'NONE',  ( -4.243569643749999898, 16.61562500061451786, -32.45002607614398471 ) ) ;
#3967=CARTESIAN_POINT ( 'NONE',  ( 18.52500000122903145, -5.773502691896255534, -1.060575238724906372E-15 ) ) ;
#3968=CARTESIAN_POINT ( 'NONE',  ( 10.60312500061451679, -4.541064518000417216, -2.621784821875001281 ) ) ;
#3970=CARTESIAN_POINT ( 'NONE',  ( 15.15000000000000036, 0.000000000000000000, 4.999999999999998224 ) ) ;
#3971=CARTESIAN_POINT ( 'NONE',  ( 10.13437500061451679, -4.541064518000419881, 2.621784821874995952 ) ) ;
#3972=EDGE_CURVE ( 'NONE', #20508, #37144, #21249, .T. ) ;
#3974=CARTESIAN_POINT ( 'NONE',  ( 10.01250000122903394, -4.330127018922190985, -2.500000000000001332 ) ) ;
#3975=CARTESIAN_POINT ( 'NONE',  ( 18.26250000122903216, 4.330127018922192761, -2.499999999999997780 ) ) ;
#3976=CARTESIAN_POINT ( 'NONE',  ( 14.24062500061451608, -3.027376345333610441, -5.243569643749999898 ) ) ;
#3978=CARTESIAN_POINT ( 'NONE',  ( 19.22812500061451502, 6.421520780324663323E-16, -5.243569643749999010 ) ) ;
#3979=CARTESIAN_POINT ( 'NONE',  ( 27.18750000122903288, 6.123233995736764310E-16, -4.999999999999998224 ) ) ;
#3980=CARTESIAN_POINT ( 'NONE',  ( 29.55000000122903003, 5.773502691896255534, 3.535250795749688894E-16 ) ) ;
#3981=CARTESIAN_POINT ( 'NONE',  ( 24.07499999999999929, 4.330127018922191873, 2.499999999999999556 ) ) ;
#3984=CARTESIAN_POINT ( 'NONE',  ( 25.24687500061451573, 6.054752690667223547, 3.707466751127219781E-16 ) ) ;
#3985=CARTESIAN_POINT ( 'NONE',  ( -5.810221930991193690E-16, 12.68750000000000000, -34.00000000000000000 ) ) ;
#3986=CARTESIAN_POINT ( 'NONE',  ( 13.16250000122903430, -4.330127018922190985, -2.500000000000001332 ) ) ;
#3987=CARTESIAN_POINT ( 'NONE',  ( 3.825000000000001954, 4.330127018922191873, 2.499999999999999556 ) ) ;
#3988=CYLINDRICAL_SURFACE ( 'NONE', #17234, 3.999999999999996447 ) ;
#3989=CARTESIAN_POINT ( 'NONE',  ( 6.496875000614517504, -3.027376345333614438, 5.243569643749998122 ) ) ;
#3990=CARTESIAN_POINT ( 'NONE',  ( 26.54062500061451146, 6.054752690667223547, 3.707466751127219781E-16 ) ) ;
#3992=CARTESIAN_POINT ( 'NONE',  ( -0.8069677186600781038, 9.969399234781869623, -24.05111887509274737 ) ) ;
#3993=LINE ( 'NONE', #20959, #19397 ) ;
#3994=CARTESIAN_POINT ( 'NONE',  ( 6.384375000614516793, 4.541064518000418104, 2.621784821874999949 ) ) ;
#3995=CARTESIAN_POINT ( 'NONE',  ( 8.934375000614517504, 6.421520780324663323E-16, -5.243569643749999010 ) ) ;
#3996=CARTESIAN_POINT ( 'NONE',  ( 29.29687500061451644, 6.054752690667223547, 3.707466751127219781E-16 ) ) ;
#3997=EDGE_CURVE ( 'NONE', #49995, #54869, #13553, .T. ) ;
#3998=CARTESIAN_POINT ( 'NONE',  ( 2.121784821875001281, 12.75312500061459353, 33.67503911421598417 ) ) ;
#3999=CARTESIAN_POINT ( 'NONE',  ( 22.12500000000000000, 6.123233995736764310E-16, -4.999999999999998224 ) ) ;
#4001=CARTESIAN_POINT ( 'NONE',  ( 29.36250000000000071, 2.886751345948129099, -4.999999999999998224 ) ) ;
#4002=( BOUNDED_CURVE ( )  B_SPLINE_CURVE ( 2, ( #62035, #11431, #33950, #62755, #5885, #28416, #57202 ),
 .UNSPECIFIED., .F., .F. ) 
 B_SPLINE_CURVE_WITH_KNOTS ( ( 3, 2, 2, 3 ),
 ( 0.9685383496433896955, 0.9694444444444444420, 0.9722222222222222099, 0.9730456312742340463 ),
 .UNSPECIFIED. ) 
 CURVE ( )  GEOMETRIC_REPRESENTATION_ITEM ( )  RATIONAL_B_SPLINE_CURVE ( ( 0.9411070399833363354, 0.9562982733624414422, 1.000000000000000000, 0.8660254037844387076, 1.000000000000000000, 0.9602862777051311971, 0.9441170150774715886 ) ) 
 REPRESENTATION_ITEM ( '' )  );
#4003=CARTESIAN_POINT ( 'NONE',  ( 4.837500000000001243, -2.886751345948129988, 4.999999999999997335 ) ) ;
#4004=VERTEX_POINT ( 'NONE', #33714 ) ;
#4005=CARTESIAN_POINT ( 'NONE',  ( 17.35312500061451502, -4.541064518000417216, -2.621784821875001281 ) ) ;
#4006=CARTESIAN_POINT ( 'NONE',  ( 11.84062500061451750, -3.027376345333614438, 5.243569643749998122 ) ) ;
#4008=CARTESIAN_POINT ( 'NONE',  ( 8.071875000614518569, 3.027376345333613106, -5.243569643749998122 ) ) ;
#4009=CARTESIAN_POINT ( 'NONE',  ( 23.40000000000000213, -4.330127018922190985, -2.500000000000001332 ) ) ;
#4010=CARTESIAN_POINT ( 'NONE',  ( 21.18750000122903288, -4.330127018922194537, 2.499999999999995559 ) ) ;
#4012=CARTESIAN_POINT ( 'NONE',  ( 8.634375000614518569, 4.541064518000418104, 2.621784821874999949 ) ) ;
#4013=CARTESIAN_POINT ( 'NONE',  ( 15.08437500061451786, -4.541064518000419881, 2.621784821874995952 ) ) ;
#4014=CARTESIAN_POINT ( 'NONE',  ( 23.97187500061451360, 3.027376345333611329, 5.243569643749999010 ) ) ;
#4015=CARTESIAN_POINT ( 'NONE',  ( 4.342984975361706468, -2.477595912125914790, -4.621313785610477787 ) ) ;
#4017=CARTESIAN_POINT ( 'NONE',  ( 18.12187500061451573, 3.027376345333611329, 5.243569643749999010 ) ) ;
#4018=CARTESIAN_POINT ( 'NONE',  ( 8.484375000614518214, 6.421520780324663323E-16, -5.243569643749999010 ) ) ;
#4020=CARTESIAN_POINT ( 'NONE',  ( 20.85000000000000142, 4.330127018922192761, -2.499999999999997780 ) ) ;
#4022=CARTESIAN_POINT ( 'NONE',  ( -4.243569643749999898, 9.959375000614517859, -30.00000000000000000 ) ) ;
#4024=CARTESIAN_POINT ( 'NONE',  ( 13.45312500061451466, 4.541064518000418104, -2.621784821874998173 ) ) ;
#4025=CARTESIAN_POINT ( 'NONE',  ( 28.65937500061451715, -4.541064518000417216, -2.621784821875001281 ) ) ;
#4026=CARTESIAN_POINT ( 'NONE',  ( -1.071796769724490339, 19.30490381179669868, -26.00000000000000355 ) ) ;
#4028=CARTESIAN_POINT ( 'NONE',  ( 12.18750000000000000, -2.886751345948125991, -5.000000000000000000 ) ) ;
#4029=CARTESIAN_POINT ( 'NONE',  ( 3.999999999999998668, 19.02500000122903501, 27.69059892324149175 ) ) ;
#4030=CARTESIAN_POINT ( 'NONE',  ( 12.75000000122903643, -2.886751345948125991, -5.000000000000000000 ) ) ;
#4031=CARTESIAN_POINT ( 'NONE',  ( 22.73437500061451644, -4.541064518000419881, 2.621784821874995952 ) ) ;
#4032=CARTESIAN_POINT ( 'NONE',  ( 15.64687500061451608, -3.027376345333610441, -5.243569643749999898 ) ) ;
#4033=CARTESIAN_POINT ( 'NONE',  ( 3.999999999999998668, 16.77500000122903145, 27.69059892324149530 ) ) ;
#4035=AXIS2_PLACEMENT_3D ( 'NONE', #59247, #14557, #66270 ) ;
#4036=CARTESIAN_POINT ( 'NONE',  ( 16.30312500061451786, 0.000000000000000000, 5.243569643749999010 ) ) ;
#4037=CARTESIAN_POINT ( 'NONE',  ( 28.38750000122903216, -4.330127018922194537, 2.499999999999995559 ) ) ;
#4038=CARTESIAN_POINT ( 'NONE',  ( 16.73437500061451644, 4.541064518000418104, 2.621784821874999949 ) ) ;
#4039=CARTESIAN_POINT ( 'NONE',  ( 5.878125000614517148, 4.541064518000418104, 2.621784821874999949 ) ) ;
#4040=CARTESIAN_POINT ( 'NONE',  ( 20.16562500061451146, 3.027376345333613106, -5.243569643749998122 ) ) ;
#4041=CARTESIAN_POINT ( 'NONE',  ( 28.69687500061451502, -3.027376345333610441, -5.243569643749999898 ) ) ;
#4042=CARTESIAN_POINT ( 'NONE',  ( 2.121784821875001281, 11.85312500061451857, 33.67503911421598417 ) ) ;
#4043=CARTESIAN_POINT ( 'NONE',  ( 16.12500000122903288, 2.886751345948126879, 4.999999999999999112 ) ) ;
#4045=CARTESIAN_POINT ( 'NONE',  ( 27.02812500061451573, 4.541064518000418104, 2.621784821874999949 ) ) ;
#4047=CARTESIAN_POINT ( 'NONE',  ( 21.68437500061451573, 4.541064518000418104, 2.621784821874999949 ) ) ;
#4048=CARTESIAN_POINT ( 'NONE',  ( 23.43750000122902932, -4.330127018922194537, 2.499999999999995559 ) ) ;
#4049=CARTESIAN_POINT ( 'NONE',  ( 24.06562500061451715, -6.054752690667223547, -1.112240025338166033E-15 ) ) ;
#4050=CARTESIAN_POINT ( 'NONE',  ( 16.69687500061451502, 6.054752690667223547, 3.707466751127219781E-16 ) ) ;
#4051=CARTESIAN_POINT ( 'NONE',  ( 11.39062500061451644, -3.027376345333614438, 5.243569643749998122 ) ) ;
#4052=CARTESIAN_POINT ( 'NONE',  ( -2.121784821874999949, 15.73437500061451644, 26.32496088578401938 ) ) ;
#4053=CARTESIAN_POINT ( 'NONE',  ( 16.22812500061451857, 4.541064518000418104, 2.621784821874999949 ) ) ;
#4054=CARTESIAN_POINT ( 'NONE',  ( 29.31562500061451715, 3.027376345333611329, 5.243569643749999010 ) ) ;
#4055=VERTEX_POINT ( 'NONE', #69160 ) ;
#4056=CARTESIAN_POINT ( 'NONE',  ( 23.73749999999999716, -2.886751345948129988, 4.999999999999997335 ) ) ;
#4057=CARTESIAN_POINT ( 'NONE',  ( 2.121784821874999061, 18.80937500061451928, -33.67503911421598417 ) ) ;
#4059=CARTESIAN_POINT ( 'NONE',  ( 24.74062500061451786, 6.054752690667223547, 3.707466751127219781E-16 ) ) ;
#4060=CARTESIAN_POINT ( 'NONE',  ( 5.540625000614515905, -3.027376345333614438, 5.243569643749998122 ) ) ;
#4061=CARTESIAN_POINT ( 'NONE',  ( 17.88750000122903216, 4.330127018922191873, 2.499999999999999556 ) ) ;
#4062=CARTESIAN_POINT ( 'NONE',  ( 22.45312500061451644, 4.541064518000418104, -2.621784821874998173 ) ) ;
#4063=CARTESIAN_POINT ( 'NONE',  ( 23.13749999999999929, 5.773502691896255534, 3.535250795749688894E-16 ) ) ;
#4065=CARTESIAN_POINT ( 'NONE',  ( 28.41562500061451502, 3.027376345333611329, 5.243569643749999010 ) ) ;
#4066=CARTESIAN_POINT ( 'NONE',  ( 8.615625000614517859, 3.027376345333611329, 5.243569643749999010 ) ) ;
#4068=CARTESIAN_POINT ( 'NONE',  ( 23.01562500061451644, 3.027376345333611329, 5.243569643749999010 ) ) ;
#4072=CARTESIAN_POINT ( 'NONE',  ( -3.999999999999997335, 13.85000000122903607, -27.69059892324149175 ) ) ;
#4074=CARTESIAN_POINT ( 'NONE',  ( 9.637499999999999289, 5.773502691896255534, 3.535250795749688894E-16 ) ) ;
#4075=CARTESIAN_POINT ( 'NONE',  ( 10.69687500061451679, -3.027376345333610441, -5.243569643749999898 ) ) ;
#4076=CARTESIAN_POINT ( 'NONE',  ( 6.000000001229033764, -2.886751345948125991, -5.000000000000000000 ) ) ;
#4077=CARTESIAN_POINT ( 'NONE',  ( 15.38437500061451679, 4.541064518000418104, 2.621784821874999949 ) ) ;
#4078=CARTESIAN_POINT ( 'NONE',  ( 5.184375000614516615, -4.541064518000419881, 2.621784821874995952 ) ) ;
#4079=CARTESIAN_POINT ( 'NONE',  ( -4.243569643749997233, 9.940625000614515372, -27.54997392385601174 ) ) ;
#4080=CARTESIAN_POINT ( 'NONE',  ( 0.000000000000000000, 20.00000000000000000, -33.99999999999999289 ) ) ;
#4081=CARTESIAN_POINT ( 'NONE',  ( 12.23437500061451821, 4.541064518000418104, 2.621784821874999949 ) ) ;
#4082=CARTESIAN_POINT ( 'NONE',  ( 21.90000000122903856, 5.773502691896255534, 3.535250795749688401E-16 ) ) ;
#4083=CARTESIAN_POINT ( 'NONE',  ( 23.24062500061451786, -3.027376345333610441, -5.243569643749999898 ) ) ;
#4084=CARTESIAN_POINT ( 'NONE',  ( -4.243569643749998122, 9.996875000614517504, 32.45002607614398471 ) ) ;
#4085=CARTESIAN_POINT ( 'NONE',  ( -2.121784821874999949, 19.72812500061459318, 26.32496088578401938 ) ) ;
#4086=CARTESIAN_POINT ( 'NONE',  ( 23.03437500061451715, 4.541064518000418104, 2.621784821874999949 ) ) ;
#4087=CARTESIAN_POINT ( 'NONE',  ( 1.510657702057710734E-15, 19.43750000000000000, 26.00000000000000000 ) ) ;
#4088=CARTESIAN_POINT ( 'NONE',  ( 4.753125000614515372, -4.541064518000417216, -2.621784821875001281 ) ) ;
#4089=VECTOR ( 'NONE', #15173, 1000.000000000000000 ) ;
#4091=CARTESIAN_POINT ( 'NONE',  ( 25.86562500061451431, -6.054752690667223547, -1.112240025338166033E-15 ) ) ;
#4092=CARTESIAN_POINT ( 'NONE',  ( 17.65312500061451573, 0.000000000000000000, 5.243569643749999010 ) ) ;
#4094=CARTESIAN_POINT ( 'NONE',  ( 14.55937500061451573, 0.000000000000000000, 5.243569643749999010 ) ) ;
#4095=CARTESIAN_POINT ( 'NONE',  ( 7.200000001229033053, -2.886751345948063374, 5.000000000000112799 ) ) ;
#4096=CARTESIAN_POINT ( 'NONE',  ( 28.01250000122903216, -4.330127018922190985, -2.500000000000001332 ) ) ;
#4097=CARTESIAN_POINT ( 'NONE',  ( 5.521875000614517859, 3.027376345333611329, 5.243569643749999010 ) ) ;
#4099=CARTESIAN_POINT ( 'NONE',  ( 17.70937500061451431, 0.000000000000000000, 5.243569643749999010 ) ) ;
#4100=CARTESIAN_POINT ( 'NONE',  ( -3.999999999999997335, 11.93750000000000000, 32.30940107675850470 ) ) ;
#4101=CARTESIAN_POINT ( 'NONE',  ( 24.00000000000000000, 4.330127018922192761, -2.499999999999997780 ) ) ;
#4103=CARTESIAN_POINT ( 'NONE',  ( 3.450000001229036162, 5.773502691896255534, 3.535250795749688894E-16 ) ) ;
#4104=CARTESIAN_POINT ( 'NONE',  ( 24.72187500061451360, 3.027376345333613106, -5.243569643749998122 ) ) ;
#4105=CARTESIAN_POINT ( 'NONE',  ( 17.07187500061451502, 3.027376345333613106, -5.243569643749998122 ) ) ;
#4107=CARTESIAN_POINT ( 'NONE',  ( 27.11249999999999716, 2.886751345948129099, -4.999999999999998224 ) ) ;
#4108=CARTESIAN_POINT ( 'NONE',  ( 8.099999999999999645, -4.330127018922190985, -2.500000000000001332 ) ) ;
#4110=CARTESIAN_POINT ( 'NONE',  ( 18.59062500061451573, -3.027376345333614438, 5.243569643749998122 ) ) ;
#4111=CARTESIAN_POINT ( 'NONE',  ( 10.16249999999999964, 2.886751345948126879, 4.999999999999999112 ) ) ;
#4112=CARTESIAN_POINT ( 'NONE',  ( 3.815625000614518036, -6.054752690667223547, -1.112240025338166033E-15 ) ) ;
#4113=CARTESIAN_POINT ( 'NONE',  ( 20.58750000000000213, -2.886751345948129988, 4.999999999999997335 ) ) ;
#4114=CARTESIAN_POINT ( 'NONE',  ( 9.528763966825557376E-15, 17.41249999999999787, 34.00000000000000000 ) ) ;
#4115=CARTESIAN_POINT ( 'NONE',  ( 22.05000000122903714, -2.886751345948129988, 4.999999999999997335 ) ) ;
#4117=CARTESIAN_POINT ( 'NONE',  ( 29.14687500061451075, -3.027376345333610441, -5.243569643749999898 ) ) ;
#4118=ORIENTED_EDGE ( 'NONE', *, *, #36651, .T. ) ;
#4119=CARTESIAN_POINT ( 'NONE',  ( 17.31562500061451715, -6.054752690667223547, -1.112240025338166033E-15 ) ) ;
#4120=CARTESIAN_POINT ( 'NONE',  ( 24.74062500061451786, 6.054752690667223547, 3.707466751127219781E-16 ) ) ;
#4121=CARTESIAN_POINT ( 'NONE',  ( 24.30937500061451573, 4.541064518000418104, -2.621784821874998173 ) ) ;
#4122=CARTESIAN_POINT ( 'NONE',  ( 10.16249999999999964, 2.886751345948126879, 4.999999999999999112 ) ) ;
#4123=CARTESIAN_POINT ( 'NONE',  ( 11.95312500061451644, -4.541064518000417216, -2.621784821875001281 ) ) ;
#4124=CARTESIAN_POINT ( 'NONE',  ( 27.59062500061451573, -3.027376345333614438, 5.243569643749998122 ) ) ;
#4125=CARTESIAN_POINT ( 'NONE',  ( 13.62187500061451750, 3.027376345333611329, 5.243569643749999010 ) ) ;
#4126=CARTESIAN_POINT ( 'NONE',  ( 20.10937500061451289, -4.541064518000417216, -2.621784821875001281 ) ) ;
#4127=CARTESIAN_POINT ( 'NONE',  ( 3.006050052715787846, -3.995483127527877265, 3.173080537200223983 ) ) ;
#4128=CARTESIAN_POINT ( 'NONE',  ( -4.243569643749997233, 10.44687500061451857, 32.45002607614398471 ) ) ;
#4129=CARTESIAN_POINT ( 'NONE',  ( 22.76250000122903216, 4.330127018922192761, -2.499999999999997780 ) ) ;
#4131=CARTESIAN_POINT ( 'NONE',  ( 14.39062500061451821, 6.054752690667223547, 3.707466751127219781E-16 ) ) ;
#4132=CARTESIAN_POINT ( 'NONE',  ( 7.096875000614517148, -3.027376345333610441, -5.243569643749999898 ) ) ;
#4133=CARTESIAN_POINT ( 'NONE',  ( 7.396875000614519635, -3.027376345333614438, 5.243569643749998122 ) ) ;
#4134=EDGE_LOOP ( 'NONE', ( #10893, #69862, #12720, #34518 ) ) ;
#4135=CARTESIAN_POINT ( 'NONE',  ( 27.19687500061451857, -3.027376345333614438, 5.243569643749998122 ) ) ;
#4136=CARTESIAN_POINT ( 'NONE',  ( 20.12812500061451715, 6.421520780324663323E-16, -5.243569643749999010 ) ) ;
#4137=CARTESIAN_POINT ( 'NONE',  ( 23.63437500061451502, -4.541064518000419881, 2.621784821874995952 ) ) ;
#4138=CARTESIAN_POINT ( 'NONE',  ( 19.41562500061451146, 3.027376345333611329, 5.243569643749999010 ) ) ;
#4139=CARTESIAN_POINT ( 'NONE',  ( 3.999999999999999112, 12.57500000000000107, 30.00000000000000000 ) ) ;
#4140=CARTESIAN_POINT ( 'NONE',  ( 25.86562500061451431, -6.054752690667223547, -1.112240025338166033E-15 ) ) ;
#4141=CARTESIAN_POINT ( 'NONE',  ( 7.762500001229033053, -4.330127018922190985, -2.500000000000001332 ) ) ;
#4143=CARTESIAN_POINT ( 'NONE',  ( 2.962500001229034119, 4.330127018922192761, -2.499999999999997780 ) ) ;
#4144=CARTESIAN_POINT ( 'NONE',  ( 3.999999999999999112, 16.62500000000000000, -30.00000000000000000 ) ) ;
#4145=CARTESIAN_POINT ( 'NONE',  ( 23.51250000122903216, -4.330127018922190985, -2.500000000000001332 ) ) ;
#4147=CARTESIAN_POINT ( 'NONE',  ( 3.796875000614517326, -3.027376345333614438, 5.243569643749998122 ) ) ;
#4149=CARTESIAN_POINT ( 'NONE',  ( 13.26562500061451644, -6.054752690667223547, -1.112240025338166033E-15 ) ) ;
#4150=CARTESIAN_POINT ( 'NONE',  ( 9.046875000614518214, 6.054752690667223547, 3.707466751127219781E-16 ) ) ;
#4151=CARTESIAN_POINT ( 'NONE',  ( 23.96250000122903145, -4.330127018922190985, -2.500000000000001332 ) ) ;
#4152=CARTESIAN_POINT ( 'NONE',  ( 14.55937500061451573, 0.000000000000000000, 5.243569643749999010 ) ) ;
#4153=CARTESIAN_POINT ( 'NONE',  ( 5.109375000614518214, 0.000000000000000000, 5.243569643749999010 ) ) ;
#4154=CARTESIAN_POINT ( 'NONE',  ( 29.66249999999999432, -5.773502691896255534, -1.060575238724906372E-15 ) ) ;
#4155=CARTESIAN_POINT ( 'NONE',  ( 5.690625000614516260, -3.027376345333610441, -5.243569643749999898 ) ) ;
#4156=CARTESIAN_POINT ( 'NONE',  ( 15.74062500061451608, 6.054752690667223547, 3.707466751127219781E-16 ) ) ;
#4157=EDGE_CURVE ( 'NONE', #64403, #12255, #28810, .T. ) ;
#4158=VERTEX_POINT ( 'NONE', #17790 ) ;
#4160=CARTESIAN_POINT ( 'NONE',  ( 12.59062500061451573, 6.054752690667223547, 3.707466751127219781E-16 ) ) ;
#4161=CARTESIAN_POINT ( 'NONE',  ( 8.540625000614518569, 6.054752690667223547, 3.707466751127219781E-16 ) ) ;
#4163=CARTESIAN_POINT ( 'NONE',  ( 8.250000000000000000, 4.330127018922192761, -2.499999999999997780 ) ) ;
#4164=CARTESIAN_POINT ( 'NONE',  ( 4.987500001229032698, -4.330127018922194537, 2.499999999999995559 ) ) ;
#4165=CARTESIAN_POINT ( 'NONE',  ( 18.86249999999999716, -5.773502691896255534, -1.060575238724906372E-15 ) ) ;
#4166=( BOUNDED_CURVE ( )  B_SPLINE_CURVE ( 2, ( #7490, #48116, #41477, #1967, #2680, #65095, #41124, #47741, #47382 ),
 .UNSPECIFIED., .F., .F. ) 
 B_SPLINE_CURVE_WITH_KNOTS ( ( 3, 2, 2, 2, 3 ),
 ( 0.3152173913043478382, 0.3188405797101449002, 0.3260869565217391353, 0.3333333333333333148, 0.3369565217391304324 ),
 .UNSPECIFIED. ) 
 CURVE ( )  GEOMETRIC_REPRESENTATION_ITEM ( )  RATIONAL_B_SPLINE_CURVE ( ( 0.9330127018922194093, 0.9330127018922198534, 1.000000000000000000, 0.8660254037844387076, 1.000000000000000000, 0.8660254037844387076, 1.000000000000000000, 0.9330127018922194093, 0.9330127018922194093 ) ) 
 REPRESENTATION_ITEM ( '' )  );
#4167=CARTESIAN_POINT ( 'NONE',  ( 18.19687500061451502, -3.027376345333614438, 5.243569643749998122 ) ) ;
#4168=CARTESIAN_POINT ( 'NONE',  ( 14.13750000122903394, 6.123233995736764310E-16, -4.999999999999998224 ) ) ;
#4170=CARTESIAN_POINT ( 'NONE',  ( -4.243569643749999898, 17.06562500061451360, -32.45002607614398471 ) ) ;
#4173=CARTESIAN_POINT ( 'NONE',  ( 28.97812500061451502, -4.541064518000419881, 2.621784821874995952 ) ) ;
#4174=CYLINDRICAL_SURFACE ( 'NONE', #72883, 4.999999999999998224 ) ;
#4176=CARTESIAN_POINT ( 'NONE',  ( 14.52187500061451608, 3.027376345333611329, 5.243569643749999010 ) ) ;
#4177=CARTESIAN_POINT ( 'NONE',  ( 26.28749999999999432, 5.773502691896255534, 3.535250795749688894E-16 ) ) ;
#4178=CARTESIAN_POINT ( 'NONE',  ( 11.35312500061451679, 0.000000000000000000, 5.243569643749999010 ) ) ;
#4180=CARTESIAN_POINT ( 'NONE',  ( 22.02187500061452141, 3.027376345333613106, -5.243569643749998122 ) ) ;
#4182=AXIS2_PLACEMENT_3D ( 'NONE', #27291, #44290, #37997 ) ;
#4183=CARTESIAN_POINT ( 'NONE',  ( 7.903125000614515727, -4.541064518000417216, -2.621784821875001281 ) ) ;
#4184=CARTESIAN_POINT ( 'NONE',  ( 13.43437500061451750, 6.421520780324663323E-16, -5.243569643749999010 ) ) ;
#4185=ORIENTED_EDGE ( 'NONE', *, *, #42052, .F. ) ;
#4186=CARTESIAN_POINT ( 'NONE',  ( 23.48437500061451644, 4.541064518000418104, 2.621784821874999949 ) ) ;
#4187=CARTESIAN_POINT ( 'NONE',  ( 2.485350534231660191, 4.344988454211105022, -26.85539458128546286 ) ) ;
#4188=CARTESIAN_POINT ( 'NONE',  ( 7.320879633048903241E-15, 17.30000000122903003, 26.00000000000000355 ) ) ;
#4189=CARTESIAN_POINT ( 'NONE',  ( 4.837500000000001243, -2.886751345948129988, 4.999999999999997335 ) ) ;
#4190=CARTESIAN_POINT ( 'NONE',  ( 16.50000000122903288, 5.773502691896255534, 3.535250795749688894E-16 ) ) ;
#4191=CARTESIAN_POINT ( 'NONE',  ( -1.071796769724487453, 17.77009619066136636, -34.00000000000000000 ) ) ;
#4193=ORIENTED_EDGE ( 'NONE', *, *, #3893, .F. ) ;
#4194=CARTESIAN_POINT ( 'NONE',  ( 14.24999999999999822, 0.000000000000000000, 4.999999999999998224 ) ) ;
#4195=CARTESIAN_POINT ( 'NONE',  ( 16.35000000000000142, 4.330127018922192761, -2.499999999999997780 ) ) ;
#4196=CARTESIAN_POINT ( 'NONE',  ( 11.87812500061451537, -4.541064518000419881, 2.621784821874995952 ) ) ;
#4199=CARTESIAN_POINT ( 'NONE',  ( -3.999999999999999112, 15.57500000122903216, 27.69059892324149885 ) ) ;
#4200=CARTESIAN_POINT ( 'NONE',  ( -4.243569643749997233, 16.29687500061451644, -27.54997392385601174 ) ) ;
#4201=CARTESIAN_POINT ( 'NONE',  ( 29.40000000122903145, -2.886751345948125991, -5.000000000000000000 ) ) ;
#4203=CARTESIAN_POINT ( 'NONE',  ( 9.449999999999999289, -4.330127018922190985, -2.500000000000001332 ) ) ;
#4206=CARTESIAN_POINT ( 'NONE',  ( -4.243569643749999898, 12.56562500061451715, 27.54997392385601529 ) ) ;
#4207=CARTESIAN_POINT ( 'NONE',  ( 25.00312500061451715, -4.541064518000417216, -2.621784821875001281 ) ) ;
#4208=CARTESIAN_POINT ( 'NONE',  ( 3.651773823418189124, 3.415340091791402966, 3.978752903393068863 ) ) ;
#4210=CARTESIAN_POINT ( 'NONE',  ( 20.59687500061451360, -3.027376345333610441, -5.243569643749999898 ) ) ;
#4211=CARTESIAN_POINT ( 'NONE',  ( 20.24062500061451431, 6.054752690667223547, 3.707466751127219781E-16 ) ) ;
#4212=CARTESIAN_POINT ( 'NONE',  ( 2.121784821874999061, 15.15312500061459566, -33.67503911421598417 ) ) ;
#4213=CARTESIAN_POINT ( 'NONE',  ( 22.53750000122903430, -4.330127018922194537, 2.499999999999995559 ) ) ;
#4214=( BOUNDED_CURVE ( )  B_SPLINE_CURVE ( 2, ( #3805, #31505, #3441, #25960, #71025, #42951, #65479 ),
 .UNSPECIFIED., .F., .F. ) 
 B_SPLINE_CURVE_WITH_KNOTS ( ( 3, 2, 2, 3 ),
 ( 0.9942380576293760042, 0.9944444444444444642, 0.9972222222222222321, 0.9973736731814578649 ),
 .UNSPECIFIED. ) 
 CURVE ( )  GEOMETRIC_REPRESENTATION_ITEM ( )  RATIONAL_B_SPLINE_CURVE ( ( 0.9815707561575266471, 0.9900457875233154015, 1.000000000000000000, 0.8660254037844387076, 1.000000000000000000, 0.9926953908003807170, 0.9861873104512506316 ) ) 
 REPRESENTATION_ITEM ( '' )  );
#4215=CARTESIAN_POINT ( 'NONE',  ( 4.190625000614518925, -3.027376345333614438, 5.243569643749998122 ) ) ;
#4217=CARTESIAN_POINT ( 'NONE',  ( 22.67812500061451431, -4.541064518000419881, 2.621784821874995952 ) ) ;
#4220=CARTESIAN_POINT ( 'NONE',  ( 15.79687500061451821, 6.054752690667223547, 3.707466751127219781E-16 ) ) ;
#4221=CARTESIAN_POINT ( 'NONE',  ( 14.89687500061451786, 6.054752690667223547, 3.707466751127219781E-16 ) ) ;
#4222=CARTESIAN_POINT ( 'NONE',  ( 21.98437500061451644, 6.421520780324663323E-16, -5.243569643749999010 ) ) ;
#4223=CARTESIAN_POINT ( 'NONE',  ( 2.121784821875001281, 12.80937500061451928, 33.67503911421598417 ) ) ;
#4224=CARTESIAN_POINT ( 'NONE',  ( 4.303125000614516971, -4.541064518000417216, -2.621784821875001281 ) ) ;
#4225=CARTESIAN_POINT ( 'NONE',  ( 25.41562500061451146, -6.054752690667223547, -1.112240025338166033E-15 ) ) ;
#4227=ADVANCED_FACE ( 'NONE', ( #45896 ), #6365, .F. ) ;
#4228=CARTESIAN_POINT ( 'NONE',  ( 26.01562500061451289, 3.027376345333613106, -5.243569643749998122 ) ) ;
#4230=CARTESIAN_POINT ( 'NONE',  ( -3.999999999999997335, 18.23750000000000071, 32.30940107675850470 ) ) ;
#4231=CARTESIAN_POINT ( 'NONE',  ( 7.059375000614518392, -4.541064518000417216, -2.621784821875001281 ) ) ;
#4232=PRODUCT_CONTEXT ( 'NONE', #25218, 'mechanical' ) ;
#4233=CARTESIAN_POINT ( 'NONE',  ( 13.91250000122903252, 0.000000000000000000, 4.999999999999998224 ) ) ;
#4234=CARTESIAN_POINT ( 'NONE',  ( 8.362500001229031810, 4.330127018922192761, -2.499999999999997780 ) ) ;
#4235=CARTESIAN_POINT ( 'NONE',  ( 29.06250000122903288, 4.330127018922192761, -2.499999999999997780 ) ) ;
#4238=CARTESIAN_POINT ( 'NONE',  ( 14.85937500061451644, 4.541064518000418104, -2.621784821874998173 ) ) ;
#4241=CARTESIAN_POINT ( 'NONE',  ( 18.81562500061452070, 3.027376345333613106, -5.243569643749998122 ) ) ;
#4242=CARTESIAN_POINT ( 'NONE',  ( 6.515625000614516438, -6.054752690667223547, -1.112240025338166033E-15 ) ) ;
#4243=CARTESIAN_POINT ( 'NONE',  ( 21.53437500061451715, 6.421520780324663323E-16, -5.243569643749999010 ) ) ;
#4244=CARTESIAN_POINT ( 'NONE',  ( 5.840625000614516615, 6.054752690667223547, 3.707466751127219781E-16 ) ) ;
#4246=CARTESIAN_POINT ( 'NONE',  ( 7.762500001229033053, -4.330127018922190985, -2.500000000000001332 ) ) ;
#4247=CARTESIAN_POINT ( 'NONE',  ( 22.00312500061451360, 4.541064518000418104, -2.621784821874998173 ) ) ;
#4248=EDGE_CURVE ( 'NONE', #28698, #19531, #36365, .T. ) ;
#4249=( BOUNDED_CURVE ( )  B_SPLINE_CURVE ( 2, ( #54139, #36409, #3902, #3533, #26056, #58561, #37503, #58923, #60023 ),
 .UNSPECIFIED., .F., .T. ) 
 B_SPLINE_CURVE_WITH_KNOTS ( ( 3, 2, 2, 2, 3 ),
 ( 0.5978260869565217295, 0.6014492753623188470, 0.6086956521739130821, 0.6159420289855072062, 0.6195652173913043237 ),
 .UNSPECIFIED. ) 
 CURVE ( )  GEOMETRIC_REPRESENTATION_ITEM ( )  RATIONAL_B_SPLINE_CURVE ( ( 0.9330127018922194093, 0.9330127018922194093, 1.000000000000000000, 0.8660254037844387076, 1.000000000000000000, 0.8660254037844387076, 1.000000000000000000, 0.9330127018922194093, 0.9330127018922194093 ) ) 
 REPRESENTATION_ITEM ( '' )  );
#4250=CARTESIAN_POINT ( 'NONE',  ( -3.999999999999997335, 17.45000000122903216, -27.69059892324149175 ) ) ;
#4251=CARTESIAN_POINT ( 'NONE',  ( 11.25000000122903288, -2.886751345948129988, 4.999999999999997335 ) ) ;
#4252=CARTESIAN_POINT ( 'NONE',  ( 18.96562500061451573, 3.027376345333611329, 5.243569643749999010 ) ) ;
#4253=CARTESIAN_POINT ( 'NONE',  ( 16.34062500061451573, -3.027376345333614438, 5.243569643749998122 ) ) ;
#4255=CARTESIAN_POINT ( 'NONE',  ( 15.78749999999999964, -2.886751345948125991, -5.000000000000000000 ) ) ;
#4256=CARTESIAN_POINT ( 'NONE',  ( 12.33750000122903145, 6.123233995736764310E-16, -4.999999999999998224 ) ) ;
#4257=CARTESIAN_POINT ( 'NONE',  ( 7.940625000614518036, -3.027376345333610441, -5.243569643749999898 ) ) ;
#4258=CARTESIAN_POINT ( 'NONE',  ( 11.99062500061451608, -3.027376345333610441, -5.243569643749999898 ) ) ;
#4260=CARTESIAN_POINT ( 'NONE',  ( 21.30000000122903359, -2.886751345948125991, -5.000000000000000000 ) ) ;
#4261=AXIS2_PLACEMENT_3D ( 'NONE', #52143, #28882, #11894 ) ;
#4262=CARTESIAN_POINT ( 'NONE',  ( 20.59687500061451360, -3.027376345333610441, -5.243569643749999898 ) ) ;
#4264=CARTESIAN_POINT ( 'NONE',  ( 5.512500001229033941, -4.330127018922190985, -2.500000000000001332 ) ) ;
#4265=CARTESIAN_POINT ( 'NONE',  ( 5.146875000614517859, -3.027376345333614438, 5.243569643749998122 ) ) ;
#4266=CARTESIAN_POINT ( 'NONE',  ( 23.37187500061451573, 3.027376345333613106, -5.243569643749998122 ) ) ;
#4267=CARTESIAN_POINT ( 'NONE',  ( 1.071796769724491893, 18.44509619066136707, 33.99999999999999289 ) ) ;
#4268=CARTESIAN_POINT ( 'NONE',  ( 18.59062500061451573, -3.027376345333614438, 5.243569643749998122 ) ) ;
#4269=CARTESIAN_POINT ( 'NONE',  ( 23.97187500061451360, 3.027376345333611329, 5.243569643749999010 ) ) ;
#4272=CARTESIAN_POINT ( 'NONE',  ( 28.50937500061451502, 0.000000000000000000, 5.243569643749999010 ) ) ;
#4274=CARTESIAN_POINT ( 'NONE',  ( 14.24062500061451608, -3.027376345333610441, -5.243569643749999898 ) ) ;
#4275=CARTESIAN_POINT ( 'NONE',  ( 12.23437500061451821, 4.541064518000418104, 2.621784821874999949 ) ) ;
#4276=ORIENTED_EDGE ( 'NONE', *, *, #28806, .T. ) ;
#4277=CARTESIAN_POINT ( 'NONE',  ( 22.71562500061451573, -6.054752690667223547, -1.112240025338166033E-15 ) ) ;
#4278=CARTESIAN_POINT ( 'NONE',  ( 3.413604573517995622, 3.653464791278348667, -3.457471840445726752 ) ) ;
#4279=CARTESIAN_POINT ( 'NONE',  ( 13.87500000000000178, -4.330127018922194537, 2.499999999999995559 ) ) ;
#4280=CARTESIAN_POINT ( 'NONE',  ( 23.21250000122903501, 4.330127018922192761, -2.499999999999997780 ) ) ;
#4281=CARTESIAN_POINT ( 'NONE',  ( 19.67812500061451786, 6.421520780324663323E-16, -5.243569643749999010 ) ) ;
#4283=CARTESIAN_POINT ( 'NONE',  ( 22.31250000000000000, 2.886751345948126879, 4.999999999999999112 ) ) ;
#4285=CARTESIAN_POINT ( 'NONE',  ( 22.95937500061451431, 4.541064518000418104, -2.621784821874998173 ) ) ;
#4286=EDGE_LOOP ( 'NONE', ( #45626, #43800, #7187, #7569 ) ) ;
#4288=CARTESIAN_POINT ( 'NONE',  ( 9.965625000614517504, 3.027376345333611329, 5.243569643749999010 ) ) ;
#4289=LINE ( 'NONE', #47882, #49075 ) ;
#4291=CARTESIAN_POINT ( 'NONE',  ( 26.61562500061451786, 3.027376345333611329, 5.243569643749999010 ) ) ;
#4293=CARTESIAN_POINT ( 'NONE',  ( 16.19999999999999929, -4.330127018922190985, -2.500000000000001332 ) ) ;
#4294=CARTESIAN_POINT ( 'NONE',  ( 23.58749999999999858, 5.773502691896255534, 3.535250795749688894E-16 ) ) ;
#4295=DIRECTION ( 'NONE',  ( -1.000000000000000000, -0.000000000000000000, -0.000000000000000000 ) ) ;
#4296=CARTESIAN_POINT ( 'NONE',  ( 7.696875000614516793, 6.054752690667223547, 3.707466751127219781E-16 ) ) ;
#4297=CARTESIAN_POINT ( 'NONE',  ( 17.63437500061451502, 4.541064518000418104, 2.621784821874999949 ) ) ;
#4298=CARTESIAN_POINT ( 'NONE',  ( 29.48437500061451644, -4.541064518000419881, 2.621784821874995952 ) ) ;
#4300=CARTESIAN_POINT ( 'NONE',  ( 26.01562500061451289, 3.027376345333613106, -5.243569643749998122 ) ) ;
#4301=CARTESIAN_POINT ( 'NONE',  ( 28.73437500061451644, 6.421520780324663323E-16, -5.243569643749999010 ) ) ;
#4302=CARTESIAN_POINT ( 'NONE',  ( 30.00000000000000000, 6.123233995736764310E-16, -4.999999999999998224 ) ) ;
#4303=CARTESIAN_POINT ( 'NONE',  ( 12.97499999999999964, -4.330127018922194537, 2.499999999999995559 ) ) ;
#4304=CARTESIAN_POINT ( 'NONE',  ( 11.80312500061451608, 0.000000000000000000, 5.243569643749999010 ) ) ;
#4305=LINE ( 'NONE', #16094, #27556 ) ;
#4306=LINE ( 'NONE', #9831, #25391 ) ;
#4307=CARTESIAN_POINT ( 'NONE',  ( 28.19062500061451715, -3.027376345333610441, -5.243569643749999898 ) ) ;
#4308=CARTESIAN_POINT ( 'NONE',  ( 16.27500000122903501, -5.773502691896255534, -1.060575238724906372E-15 ) ) ;
#4311=CARTESIAN_POINT ( 'NONE',  ( 5.503125000614516260, 0.000000000000000000, 5.243569643749999010 ) ) ;
#4312=CARTESIAN_POINT ( 'NONE',  ( 21.75937500061451502, 0.000000000000000000, 5.243569643749999010 ) ) ;
#4313=CARTESIAN_POINT ( 'NONE',  ( -4.243569643749999898, 16.67187500061451644, 27.54997392385601529 ) ) ;
#4314=CARTESIAN_POINT ( 'NONE',  ( 20.59687500061451360, -3.027376345333610441, -5.243569643749999898 ) ) ;
#4315=CARTESIAN_POINT ( 'NONE',  ( 28.88437500061451502, 4.541064518000418104, 2.621784821874999949 ) ) ;
#4316=CARTESIAN_POINT ( 'NONE',  ( -2.121784821874996840, 18.13437500061451502, 33.67503911421598417 ) ) ;
#4317=CARTESIAN_POINT ( 'NONE',  ( 13.30312500061451786, -4.541064518000417216, -2.621784821875001281 ) ) ;
#4318=CARTESIAN_POINT ( 'NONE',  ( 5.025000001229035895, -5.773502691896255534, -1.060575238724906372E-15 ) ) ;
#4320=CARTESIAN_POINT ( 'NONE',  ( 7.584375000614516082, 6.421520780324663323E-16, -5.243569643749999010 ) ) ;
#4321=CARTESIAN_POINT ( 'NONE',  ( 3.897990869167640149, 3.131492215201401308, -4.036780346077406989 ) ) ;
#4322=CARTESIAN_POINT ( 'NONE',  ( 8.990625000614516082, 6.054752690667223547, 3.707466751127219781E-16 ) ) ;
#4323=CARTESIAN_POINT ( 'NONE',  ( 13.69687500061451679, -3.027376345333614438, 5.243569643749998122 ) ) ;
#4324=DIRECTION ( 'NONE',  ( 1.000000000000000000, 0.000000000000000000, 0.000000000000000000 ) ) ;
#4325=CARTESIAN_POINT ( 'NONE',  ( 22.05000000122903714, -2.886751345948129988, 4.999999999999997335 ) ) ;
#4326=CARTESIAN_POINT ( 'NONE',  ( 7.209375000614519635, 4.541064518000418104, -2.621784821874998173 ) ) ;
#4327=CARTESIAN_POINT ( 'NONE',  ( 12.89062500061451821, -3.027376345333610441, -5.243569643749999898 ) ) ;
#4328=ADVANCED_FACE ( 'NONE', ( #6732 ), #18150, .F. ) ;
#4330=CARTESIAN_POINT ( 'NONE',  ( 21.42187500061451644, -6.054752690667223547, -1.112240025338166033E-15 ) ) ;
#4331=CARTESIAN_POINT ( 'NONE',  ( 1.592000809091587073E-14, 16.73750000000000071, 26.00000000000000000 ) ) ;
#4332=CARTESIAN_POINT ( 'NONE',  ( -3.943440097865042571, 3.074283834720754172, 29.31637382434952954 ) ) ;
#4333=CARTESIAN_POINT ( 'NONE',  ( 3.261697542054055710, 3.789670288106804730, -3.327321037948185012 ) ) ;
#4334=CARTESIAN_POINT ( 'NONE',  ( -2.121784821874999949, 11.23437500061451821, -33.67503911421598417 ) ) ;
#4335=CARTESIAN_POINT ( 'NONE',  ( 14.47500000122903430, -5.773502691896255534, -1.060575238724906372E-15 ) ) ;
#4336=CARTESIAN_POINT ( 'NONE',  ( -2.121784821874996840, 16.27812500061451573, -26.32496088578401583 ) ) ;
#4337=CARTESIAN_POINT ( 'NONE',  ( 16.95000000122903216, 5.773502691896255534, 3.535250795749688894E-16 ) ) ;
#4338=CARTESIAN_POINT ( 'NONE',  ( 10.41562500061451679, 3.027376345333611329, 5.243569643749999010 ) ) ;
#4340=CARTESIAN_POINT ( 'NONE',  ( 14.10000000000000142, 4.330127018922192761, -2.499999999999997780 ) ) ;
#4341=AXIS2_PLACEMENT_3D ( 'NONE', #21026, #14391, #60545 ) ;
#4342=CARTESIAN_POINT ( 'NONE',  ( 23.42812500061451786, 4.541064518000418104, 2.621784821874999949 ) ) ;
#4343=CARTESIAN_POINT ( 'NONE',  ( 11.29687500061451644, 6.054752690667223547, 3.707466751127219781E-16 ) ) ;
#4345=CARTESIAN_POINT ( 'NONE',  ( 10.16250000122903252, 4.330127018922192761, -2.499999999999997780 ) ) ;
#4346=CARTESIAN_POINT ( 'NONE',  ( 19.72500000122903074, 2.886751345948126879, 4.999999999999999112 ) ) ;
#4347=CARTESIAN_POINT ( 'NONE',  ( 15.10312500061451502, -4.541064518000417216, -2.621784821875001281 ) ) ;
#4348=CARTESIAN_POINT ( 'NONE',  ( 18.32812500061451644, 6.421520780324663323E-16, -5.243569643749999010 ) ) ;
#4349=CARTESIAN_POINT ( 'NONE',  ( 25.57500000122903216, 2.886751345948126879, 4.999999999999999112 ) ) ;
#4350=CARTESIAN_POINT ( 'NONE',  ( 4.415625000614518569, 3.027376345333613106, -5.243569643749998122 ) ) ;
#4351=CARTESIAN_POINT ( 'NONE',  ( 26.17500000000000071, 6.123233995736764310E-16, -4.999999999999998224 ) ) ;
#4353=AXIS2_PLACEMENT_3D ( 'NONE', #28850, #34747, #68384 ) ;
#4354=CARTESIAN_POINT ( 'NONE',  ( 25.54687500061451644, -3.027376345333610441, -5.243569643749999898 ) ) ;
#4355=CARTESIAN_POINT ( 'NONE',  ( 9.528763966825557376E-15, 17.41249999999999787, 34.00000000000000000 ) ) ;
#4356=CARTESIAN_POINT ( 'NONE',  ( 13.31250000122903288, 4.330127018922192761, -2.499999999999997780 ) ) ;
#4357=CARTESIAN_POINT ( 'NONE',  ( 29.59687500061451715, -3.027376345333610441, -5.243569643749999898 ) ) ;
#4359=CARTESIAN_POINT ( 'NONE',  ( 6.271875000614517859, 3.027376345333613106, -5.243569643749998122 ) ) ;
#4360=CARTESIAN_POINT ( 'NONE',  ( 26.57812500061451644, 4.541064518000418104, 2.621784821874999949 ) ) ;
#4362=CARTESIAN_POINT ( 'NONE',  ( 1.626862140677534273E-15, 10.32500000122903572, 34.00000000000000000 ) ) ;
#4363=CARTESIAN_POINT ( 'NONE',  ( 4.340613942912554535, -2.482170104787147835, 4.431799429985763261 ) ) ;
#4364=CARTESIAN_POINT ( 'NONE',  ( 4.396875000614516971, -3.027376345333610441, -5.243569643749999898 ) ) ;
#4365=CARTESIAN_POINT ( 'NONE',  ( 9.009375000614518569, 4.541064518000418104, -2.621784821874998173 ) ) ;
#4366=CARTESIAN_POINT ( 'NONE',  ( 28.99687500061451573, -3.027376345333614438, 5.243569643749998122 ) ) ;
#4367=CARTESIAN_POINT ( 'NONE',  ( 4.243569643749999898, 13.24062500061459602, 32.45002607614398471 ) ) ;
#4368=CARTESIAN_POINT ( 'NONE',  ( 21.41250000000000497, 2.886751345948126879, 4.999999999999999112 ) ) ;
#4369=ORIENTED_EDGE ( 'NONE', *, *, #57401, .T. ) ;
#4371=CARTESIAN_POINT ( 'NONE',  ( 4.087500000000001243, -2.886751345948125991, -5.000000000000000000 ) ) ;
#4372=ADVANCED_FACE ( 'NONE', ( #117 ), #56259, .F. ) ;
#4374=CARTESIAN_POINT ( 'NONE',  ( 18.77812500061451573, 6.421520780324663323E-16, -5.243569643749999010 ) ) ;
#4375=CARTESIAN_POINT ( 'NONE',  ( 11.16562500061451679, 3.027376345333613106, -5.243569643749998122 ) ) ;
#4377=CARTESIAN_POINT ( 'NONE',  ( 6.984375000614516438, -4.541064518000419881, 2.621784821874995952 ) ) ;
#4378=CARTESIAN_POINT ( 'NONE',  ( 19.53750000122903430, 6.123233995736764310E-16, -4.999999999999998224 ) ) ;
#4379=CARTESIAN_POINT ( 'NONE',  ( 0.000000000000000000, 0.000000000000000000, -50.00000000000000000 ) ) ;
#4380=CARTESIAN_POINT ( 'NONE',  ( 6.046875000614519102, -3.027376345333614438, 5.243569643749998122 ) ) ;
#4381=CARTESIAN_POINT ( 'NONE',  ( 15.15937500061451715, -4.541064518000417216, -2.621784821875001281 ) ) ;
#4382=CARTESIAN_POINT ( 'NONE',  ( 23.29687500061451644, -3.027376345333610441, -5.243569643749999898 ) ) ;
#4383=CARTESIAN_POINT ( 'NONE',  ( 1.999999999999998668, 15.91250000122903430, -33.46410161513775705 ) ) ;
#4384=ORIENTED_EDGE ( 'NONE', *, *, #50466, .F. ) ;
#4386=CARTESIAN_POINT ( 'NONE',  ( 17.78437500061451715, -4.541064518000419881, 2.621784821874995952 ) ) ;
#4387=CARTESIAN_POINT ( 'NONE',  ( 10.20937500061451786, -4.541064518000417216, -2.621784821875001281 ) ) ;
#4390=CARTESIAN_POINT ( 'NONE',  ( 20.17499999999999716, -4.330127018922194537, 2.499999999999995559 ) ) ;
#4392=CARTESIAN_POINT ( 'NONE',  ( 2.121784821875001281, 10.55937500061451750, -26.32496088578401938 ) ) ;
#4394=CARTESIAN_POINT ( 'NONE',  ( 13.64062500061451644, -3.027376345333614438, 5.243569643749998122 ) ) ;
#4395=CARTESIAN_POINT ( 'NONE',  ( 29.03437500061451715, -4.541064518000419881, 2.621784821874995952 ) ) ;
#4397=CARTESIAN_POINT ( 'NONE',  ( 29.55937500061451573, -4.541064518000417216, -2.621784821875001281 ) ) ;
#4398=CARTESIAN_POINT ( 'NONE',  ( 12.56250000000000178, -5.773502691896255534, -1.060575238724906372E-15 ) ) ;
#4399=CARTESIAN_POINT ( 'NONE',  ( 4.000000000000000000, 18.05000000122903359, 32.30940107675849049 ) ) ;
#4400=CARTESIAN_POINT ( 'NONE',  ( 11.51250000122903216, 4.330127018922192761, -2.499999999999997780 ) ) ;
#4401=CARTESIAN_POINT ( 'NONE',  ( 22.84687500061451715, -3.027376345333610441, -5.243569643749999898 ) ) ;
#4402=CARTESIAN_POINT ( 'NONE',  ( 17.67187500061451644, 3.027376345333611329, 5.243569643749999010 ) ) ;
#4403=CARTESIAN_POINT ( 'NONE',  ( 1.626862140677534273E-15, 12.46250000000000213, 34.00000000000000000 ) ) ;
#4405=CARTESIAN_POINT ( 'NONE',  ( 16.45312500061451289, -4.541064518000417216, -2.621784821875001281 ) ) ;
#4406=CARTESIAN_POINT ( 'NONE',  ( 28.95000000122903572, -2.886751345948125991, -5.000000000000000000 ) ) ;
#4407=CARTESIAN_POINT ( 'NONE',  ( 15.94687500061451502, -3.027376345333614438, 5.243569643749998122 ) ) ;
#4408=CARTESIAN_POINT ( 'NONE',  ( 5.918267800642006193, 8.060802005575231632, -28.99320351616295355 ) ) ;
#4409=CARTESIAN_POINT ( 'NONE',  ( 18.70312500061451644, -4.541064518000417216, -2.621784821875001281 ) ) ;
#4411=CARTESIAN_POINT ( 'NONE',  ( 29.07187500061451502, -6.054752690667223547, -1.112240025338166033E-15 ) ) ;
#4412=CARTESIAN_POINT ( 'NONE',  ( 4.243569643749999898, 11.89062500061451644, 32.45002607614398471 ) ) ;
#4413=CARTESIAN_POINT ( 'NONE',  ( 18.19687500061451502, -3.027376345333614438, 5.243569643749998122 ) ) ;
#4414=CARTESIAN_POINT ( 'NONE',  ( 13.72500000122903074, 2.886751345948129099, -4.999999999999998224 ) ) ;
#4416=CARTESIAN_POINT ( 'NONE',  ( -4.243569643749999898, 18.95937500061451431, -30.00000000000000000 ) ) ;
#4417=CARTESIAN_POINT ( 'NONE',  ( 21.64687500061451786, 6.054752690667223547, 3.707466751127219781E-16 ) ) ;
#4418=CARTESIAN_POINT ( 'NONE',  ( 21.41250000122903074, 4.330127018922192761, -2.499999999999997780 ) ) ;
#4419=CARTESIAN_POINT ( 'NONE',  ( 17.14687500061451786, 6.054752690667223547, 3.707466751127219781E-16 ) ) ;
#4420=CARTESIAN_POINT ( 'NONE',  ( 12.89062500061451821, -3.027376345333610441, -5.243569643749999898 ) ) ;
#4421=CARTESIAN_POINT ( 'NONE',  ( 9.001249775931846008E-16, 15.47187500061451892, 34.90005215228797653 ) ) ;
#4422=CARTESIAN_POINT ( 'NONE',  ( 16.30312500061451786, 0.000000000000000000, 5.243569643749999010 ) ) ;
#4423=VERTEX_POINT ( 'NONE', #34068 ) ;
#4424=VERTEX_POINT ( 'NONE', #56608 ) ;
#4425=CARTESIAN_POINT ( 'NONE',  ( 21.97500000000000142, -4.330127018922194537, 2.499999999999995559 ) ) ;
#4426=CARTESIAN_POINT ( 'NONE',  ( 4.243569643749999010, 19.22187500061452070, -32.45002607614398471 ) ) ;
#4427=CARTESIAN_POINT ( 'NONE',  ( 24.14062500061451289, -3.027376345333610441, -5.243569643749999898 ) ) ;
#4428=CARTESIAN_POINT ( 'NONE',  ( 5.390625000614518214, 6.054752690667223547, 3.707466751127219781E-16 ) ) ;
#4429=CARTESIAN_POINT ( 'NONE',  ( 17.62500000122903288, -5.773502691896255534, -1.060575238724906372E-15 ) ) ;
#4430=EDGE_CURVE ( 'NONE', #50794, #47796, #19291, .T. ) ;
#4431=CARTESIAN_POINT ( 'NONE',  ( 22.26562500061451644, -6.054752690667223547, -1.112240025338166033E-15 ) ) ;
#4432=CARTESIAN_POINT ( 'NONE',  ( 23.81250000000000000, -5.773502691896255534, -1.060575238724906372E-15 ) ) ;
#4433=CARTESIAN_POINT ( 'NONE',  ( 26.12812500061451360, 4.541064518000418104, 2.621784821874999949 ) ) ;
#4434=CARTESIAN_POINT ( 'NONE',  ( 5.165625000614518569, -6.054752690667223547, -1.112240025338166033E-15 ) ) ;
#4436=CARTESIAN_POINT ( 'NONE',  ( 22.22812500061451502, -4.541064518000419881, 2.621784821874995952 ) ) ;
#4437=CARTESIAN_POINT ( 'NONE',  ( 3.515625000614516882, 3.027376345333613106, -5.243569643749998122 ) ) ;
#4439=FACE_OUTER_BOUND ( 'NONE', #49795, .T. ) ;
#4440=CARTESIAN_POINT ( 'NONE',  ( 1.999999999999998668, 14.11250000122903359, -33.46410161513775705 ) ) ;
#4441=CARTESIAN_POINT ( 'NONE',  ( -4.243569643749999898, 19.85937500061451644, -30.00000000000000000 ) ) ;
#4442=CARTESIAN_POINT ( 'NONE',  ( 10.80000000000000071, -4.330127018922190985, -2.500000000000001332 ) ) ;
#4443=( BOUNDED_CURVE ( )  B_SPLINE_CURVE ( 2, ( #43492, #42757, #43860, #59730, #21306, #37572, #20565, #66385, #15761 ),
 .UNSPECIFIED., .F., .F. ) 
 B_SPLINE_CURVE_WITH_KNOTS ( ( 3, 2, 2, 2, 3 ),
 ( 0.5108695652173913526, 0.5144927536231883591, 0.5217391304347825942, 0.5289855072463768293, 0.5326086956521739468 ),
 .UNSPECIFIED. ) 
 CURVE ( )  GEOMETRIC_REPRESENTATION_ITEM ( )  RATIONAL_B_SPLINE_CURVE ( ( 0.9330127018922192983, 0.9330127018922202975, 1.000000000000000000, 0.8660254037844387076, 1.000000000000000000, 0.8660254037844387076, 1.000000000000000000, 0.9330127018922194093, 0.9330127018922194093 ) ) 
 REPRESENTATION_ITEM ( '' )  );
#4444=CARTESIAN_POINT ( 'NONE',  ( 12.30937500061451573, 0.000000000000000000, 5.243569643749999010 ) ) ;
#4445=CARTESIAN_POINT ( 'NONE',  ( 7.162500001229032520, 0.000000000000000000, 4.999999999999998224 ) ) ;
#4446=CARTESIAN_POINT ( 'NONE',  ( 13.99687500061451928, 6.054752690667223547, 3.707466751127219781E-16 ) ) ;
#4447=CARTESIAN_POINT ( 'NONE',  ( 6.046875000614519102, -3.027376345333614438, 5.243569643749998122 ) ) ;
#4449=CARTESIAN_POINT ( 'NONE',  ( 3.429021053364167404, 3.639313985669003326, 3.429021053364167404 ) ) ;
#4450=CARTESIAN_POINT ( 'NONE',  ( 11.85937500061451644, 0.000000000000000000, 5.243569643749999010 ) ) ;
#4451=CARTESIAN_POINT ( 'NONE',  ( 6.112500001229034474, 4.330127018922192761, -2.499999999999997780 ) ) ;
#4452=CARTESIAN_POINT ( 'NONE',  ( 22.75312500061451360, -4.541064518000417216, -2.621784821875001281 ) ) ;
#4453=CARTESIAN_POINT ( 'NONE',  ( 16.57499999999999929, -4.330127018922194537, 2.499999999999995559 ) ) ;
#4454=DIRECTION ( 'NONE',  ( 0.000000000000000000, 0.000000000000000000, 1.000000000000000000 ) ) ;
#4455=CARTESIAN_POINT ( 'NONE',  ( 24.45937500061451786, 0.000000000000000000, 5.243569643749999010 ) ) ;
#4456=CARTESIAN_POINT ( 'NONE',  ( 4.027635003466097707, 2.962795348797195416, -4.326299380533228600 ) ) ;
#4457=CARTESIAN_POINT ( 'NONE',  ( 3.253125000614518036, 0.000000000000000000, 5.243569643749999010 ) ) ;
#4459=CARTESIAN_POINT ( 'NONE',  ( 24.74062500061451786, 6.054752690667223547, 3.707466751127219781E-16 ) ) ;
#4460=CARTESIAN_POINT ( 'NONE',  ( 18.40312500061451573, 4.541064518000418104, -2.621784821874998173 ) ) ;
#4462=CARTESIAN_POINT ( 'NONE',  ( 14.18437500061451750, -4.541064518000419881, 2.621784821874995952 ) ) ;
#4463=FACE_OUTER_BOUND ( 'NONE', #25932, .T. ) ;
#4464=CARTESIAN_POINT ( 'NONE',  ( 26.88750000122903216, 4.330127018922191873, 2.499999999999999556 ) ) ;
#4465=CARTESIAN_POINT ( 'NONE',  ( 4.771875000614516971, -6.054752690667223547, -1.112240025338166033E-15 ) ) ;
#4466=CARTESIAN_POINT ( 'NONE',  ( 15.83437500061451608, 4.541064518000418104, 2.621784821874999949 ) ) ;
#4467=CARTESIAN_POINT ( 'NONE',  ( 4.838581423605995191, -1.260210223389511386, -5.089881413325959336 ) ) ;
#4468=CARTESIAN_POINT ( 'NONE',  ( 4.762500001229033941, 4.330127018922192761, -2.499999999999997780 ) ) ;
#4469=CARTESIAN_POINT ( 'NONE',  ( 23.89687500061451786, 6.054752690667223547, 3.707466751127219781E-16 ) ) ;
#4470=CARTESIAN_POINT ( 'NONE',  ( 16.39687500061451786, -3.027376345333614438, 5.243569643749998122 ) ) ;
#4472=CARTESIAN_POINT ( 'NONE',  ( 29.17500000000000071, -4.330127018922194537, 2.499999999999995559 ) ) ;
#4473=CARTESIAN_POINT ( 'NONE',  ( 6.375000000000001776, 6.123233995736764310E-16, -4.999999999999998224 ) ) ;
#4475=CARTESIAN_POINT ( 'NONE',  ( 19.56562500061451715, -6.054752690667223547, -1.112240025338166033E-15 ) ) ;
#4476=CARTESIAN_POINT ( 'NONE',  ( 9.862500000000000711, -5.773502691896255534, -1.060575238724906372E-15 ) ) ;
#4477=EDGE_CURVE ( 'NONE', #68418, #66075, #24840, .T. ) ;
#4478=CARTESIAN_POINT ( 'NONE',  ( 5.128125000614516260, -4.541064518000419881, 2.621784821874995952 ) ) ;
#4479=CARTESIAN_POINT ( 'NONE',  ( 20.62499999999999645, -4.330127018922194537, 2.499999999999995559 ) ) ;
#4481=CARTESIAN_POINT ( 'NONE',  ( 22.68750000122903288, 6.123233995736764310E-16, -4.999999999999998224 ) ) ;
#4483=CARTESIAN_POINT ( 'NONE',  ( 28.84687500061452070, 6.054752690667223547, 3.707466751127219781E-16 ) ) ;
#4484=ORIENTED_EDGE ( 'NONE', *, *, #7700, .F. ) ;
#4485=CARTESIAN_POINT ( 'NONE',  ( 16.30312500061451786, 0.000000000000000000, 5.243569643749999010 ) ) ;
#4486=CARTESIAN_POINT ( 'NONE',  ( 23.24062500061451786, -3.027376345333610441, -5.243569643749999898 ) ) ;
#4487=CARTESIAN_POINT ( 'NONE',  ( 24.45937500061451786, 0.000000000000000000, 5.243569643749999010 ) ) ;
#4488=CARTESIAN_POINT ( 'NONE',  ( 6.299999999999999822, -4.330127018922190985, -2.500000000000001332 ) ) ;
#4489=CARTESIAN_POINT ( 'NONE',  ( 10.94062500061451537, -3.027376345333614438, 5.243569643749998122 ) ) ;
#4490=CARTESIAN_POINT ( 'NONE',  ( 25.97812500061451502, 6.421520780324663323E-16, -5.243569643749999010 ) ) ;
#4491=CARTESIAN_POINT ( 'NONE',  ( 15.42187500061451821, 3.027376345333611329, 5.243569643749999010 ) ) ;
#4492=CARTESIAN_POINT ( 'NONE',  ( 18.94687500061451502, 6.054752690667223547, 3.707466751127219781E-16 ) ) ;
#4493=CARTESIAN_POINT ( 'NONE',  ( 3.999999999999998668, 11.82500000122903394, -32.30940107675850470 ) ) ;
#4494=CARTESIAN_POINT ( 'NONE',  ( -2.121784821874999949, 10.33437500061451786, 26.32496088578401938 ) ) ;
#4495=AXIS2_PLACEMENT_3D ( 'NONE', #28384, #33555, #6215 ) ;
#4496=CARTESIAN_POINT ( 'NONE',  ( 22.61250000122903003, -4.330127018922190985, -2.500000000000001332 ) ) ;
#4498=CARTESIAN_POINT ( 'NONE',  ( 12.85312500061451502, -4.541064518000417216, -2.621784821875001281 ) ) ;
#4499=CARTESIAN_POINT ( 'NONE',  ( 6.834375000614518747, 4.541064518000418104, 2.621784821874999949 ) ) ;
#4500=CARTESIAN_POINT ( 'NONE',  ( 7.021875000614518747, -6.054752690667223547, -1.112240025338166033E-15 ) ) ;
#4502=CARTESIAN_POINT ( 'NONE',  ( 27.79687500061451999, -3.027376345333610441, -5.243569643749999898 ) ) ;
#4503=CARTESIAN_POINT ( 'NONE',  ( 18.74062500061451431, -3.027376345333610441, -5.243569643749999898 ) ) ;
#4504=CARTESIAN_POINT ( 'NONE',  ( 3.778125000614519280, -4.541064518000419881, 2.621784821874995952 ) ) ;
#4505=CARTESIAN_POINT ( 'NONE',  ( 3.984375000614517326, 6.421520780324663323E-16, -5.243569643749999010 ) ) ;
#4506=CARTESIAN_POINT ( 'NONE',  ( 23.74687500061451573, -3.027376345333610441, -5.243569643749999898 ) ) ;
#4507=CARTESIAN_POINT ( 'NONE',  ( 19.11562500061451431, -6.054752690667223547, -1.112240025338166033E-15 ) ) ;
#4508=CARTESIAN_POINT ( 'NONE',  ( 2.000000000000001332, 12.05000000000000249, 33.46410161513774995 ) ) ;
#4509=CARTESIAN_POINT ( 'NONE',  ( 25.52812500061451573, 6.421520780324663323E-16, -5.243569643749999010 ) ) ;
#4510=CARTESIAN_POINT ( 'NONE',  ( 4.762500001229033941, 4.330127018922192761, -2.499999999999997780 ) ) ;
#4511=ORIENTED_EDGE ( 'NONE', *, *, #41045, .F. ) ;
#4512=CARTESIAN_POINT ( 'NONE',  ( 29.47499999999999787, 4.330127018922191873, 2.499999999999999556 ) ) ;
#4513=CARTESIAN_POINT ( 'NONE',  ( 1.999999999999998668, 16.25000000000000000, -33.46410161513775705 ) ) ;
#4515=CARTESIAN_POINT ( 'NONE',  ( 5.446875000614518569, 6.054752690667223547, 3.707466751127219781E-16 ) ) ;
#4516=DIRECTION ( 'NONE',  ( 0.000000000000000000, 0.000000000000000000, 1.000000000000000000 ) ) ;
#4517=CARTESIAN_POINT ( 'NONE',  ( 11.42812500061451608, -4.541064518000419881, 2.621784821874995952 ) ) ;
#4518=CARTESIAN_POINT ( 'NONE',  ( 6.646875000614518747, -3.027376345333610441, -5.243569643749999898 ) ) ;
#4519=CARTESIAN_POINT ( 'NONE',  ( 24.45000000122903572, -2.886751345948125991, -5.000000000000000000 ) ) ;
#4520=CARTESIAN_POINT ( 'NONE',  ( 15.79687500061451644, 6.054752690667223547, 3.707466751127219781E-16 ) ) ;
#4521=CARTESIAN_POINT ( 'NONE',  ( 3.834375000614519635, -4.541064518000419881, 2.621784821874995952 ) ) ;
#4522=CARTESIAN_POINT ( 'NONE',  ( 9.528763966825557376E-15, 17.41249999999999787, -26.00000000000000000 ) ) ;
#4523=CARTESIAN_POINT ( 'NONE',  ( -1.999999999999997113, 15.68750000122903465, -26.53589838486224295 ) ) ;
#4524=CARTESIAN_POINT ( 'NONE',  ( 16.37812500061451715, -4.541064518000419881, 2.621784821874995952 ) ) ;
#4525=VERTEX_POINT ( 'NONE', #25531 ) ;
#4526=CARTESIAN_POINT ( 'NONE',  ( 10.52812500061451750, -4.541064518000419881, 2.621784821874995952 ) ) ;
#4527=CARTESIAN_POINT ( 'NONE',  ( 9.028125000614517504, 4.541064518000418104, 2.621784821874999949 ) ) ;
#4529=CARTESIAN_POINT ( 'NONE',  ( 9.337500000000000355, -2.886751345948129988, 4.999999999999997335 ) ) ;
#4531=CARTESIAN_POINT ( 'NONE',  ( 5.287500001229035185, 4.330127018922191873, 2.499999999999999556 ) ) ;
#4532=CARTESIAN_POINT ( 'NONE',  ( 18.26249999999999929, 2.886751345948126879, 4.999999999999999112 ) ) ;
#4533=CARTESIAN_POINT ( 'NONE',  ( 18.64687500061451786, -3.027376345333614438, 5.243569643749998122 ) ) ;
#4534=CARTESIAN_POINT ( 'NONE',  ( 14.85000000122903252, -2.886751345948129988, 4.999999999999997335 ) ) ;
#4536=CARTESIAN_POINT ( 'NONE',  ( 4.243569643749999010, 16.46562500061451573, -32.45002607614398471 ) ) ;
#4539=CARTESIAN_POINT ( 'NONE',  ( 29.42812500061451431, -4.541064518000419881, 2.621784821874995952 ) ) ;
#4541=CARTESIAN_POINT ( 'NONE',  ( 13.50937500061451679, 4.541064518000418104, -2.621784821874998173 ) ) ;
#4542=CARTESIAN_POINT ( 'NONE',  ( 27.03750000000000142, -2.886751345948125991, -5.000000000000000000 ) ) ;
#4543=CARTESIAN_POINT ( 'NONE',  ( 10.04062500061451502, -3.027376345333614438, 5.243569643749998122 ) ) ;
#4545=CARTESIAN_POINT ( 'NONE',  ( 22.54687500061451999, 6.054752690667223547, 3.707466751127219781E-16 ) ) ;
#4547=CARTESIAN_POINT ( 'NONE',  ( 7.940625000614518036, -3.027376345333610441, -5.243569643749999898 ) ) ;
#4548=CARTESIAN_POINT ( 'NONE',  ( 13.20937500061451786, 0.000000000000000000, 5.243569643749999010 ) ) ;
#4549=ORIENTED_EDGE ( 'NONE', *, *, #793, .F. ) ;
#4550=CARTESIAN_POINT ( 'NONE',  ( 22.95937500061451431, 4.541064518000418104, -2.621784821874998173 ) ) ;
#4551=CARTESIAN_POINT ( 'NONE',  ( 1.351293209486986502, 4.820886669536880831, -33.77432306116990901 ) ) ;
#4553=CARTESIAN_POINT ( 'NONE',  ( 6.000000000000001776, 4.330127018922192761, -2.499999999999997780 ) ) ;
#4554=CARTESIAN_POINT ( 'NONE',  ( 17.51250000122903216, 0.000000000000000000, 4.999999999999998224 ) ) ;
#4556=CARTESIAN_POINT ( 'NONE',  ( 17.21249999999999858, 2.886751345948095793, -5.000000000000055067 ) ) ;
#4559=CARTESIAN_POINT ( 'NONE',  ( 12.59999999999999964, -4.330127018922190985, -2.500000000000001332 ) ) ;
#4560=CARTESIAN_POINT ( 'NONE',  ( 16.38749999999999929, 5.773502691896255534, 3.535250795749688894E-16 ) ) ;
#4561=CARTESIAN_POINT ( 'NONE',  ( 13.83750000122903323, 4.330127018922191873, 2.499999999999999556 ) ) ;
#4562=CARTESIAN_POINT ( 'NONE',  ( 10.71562500061451928, 3.027376345333613106, -5.243569643749998122 ) ) ;
#4564=CARTESIAN_POINT ( 'NONE',  ( -4.243569643749997233, 13.59687500061451715, -27.54997392385601174 ) ) ;
#4565=CARTESIAN_POINT ( 'NONE',  ( 4.640625000614518214, -3.027376345333614438, 5.243569643749998122 ) ) ;
#4567=CARTESIAN_POINT ( 'NONE',  ( 9.937500000000001776, -2.886751345948125991, -5.000000000000000000 ) ) ;
#4568=CARTESIAN_POINT ( 'NONE',  ( 3.073301885803186639, 3.943998191421653310, 3.145473502252839726 ) ) ;
#4570=CARTESIAN_POINT ( 'NONE',  ( 24.81562500061451715, 3.027376345333611329, 5.243569643749999010 ) ) ;
#4573=CARTESIAN_POINT ( 'NONE',  ( 20.78437500061451715, 4.541064518000418104, 2.621784821874999949 ) ) ;
#4574=CARTESIAN_POINT ( 'NONE',  ( 18.70312500061451644, -4.541064518000417216, -2.621784821875001281 ) ) ;
#4575=CARTESIAN_POINT ( 'NONE',  ( 2.121784821874999061, 14.70312500061459282, -33.67503911421598417 ) ) ;
#4576=CARTESIAN_POINT ( 'NONE',  ( 7.190625000614518036, 6.054752690667223547, 3.707466751127219781E-16 ) ) ;
#4577=CARTESIAN_POINT ( 'NONE',  ( 4.040625000614517681, 6.054752690667223547, 3.707466751127219781E-16 ) ) ;
#4579=CARTESIAN_POINT ( 'NONE',  ( 21.10312500061451502, 4.541064518000418104, -2.621784821874998173 ) ) ;
#4582=CARTESIAN_POINT ( 'NONE',  ( 15.75937500061451857, 4.541064518000418104, -2.621784821874998173 ) ) ;
#4583=CARTESIAN_POINT ( 'NONE',  ( 15.57187500061451679, -6.054752690667223547, -1.112240025338166033E-15 ) ) ;
#4584=CARTESIAN_POINT ( 'NONE',  ( 22.09687500061451715, 6.054752690667223547, 3.707466751127219781E-16 ) ) ;
#4585=ORIENTED_EDGE ( 'NONE', *, *, #28049, .F. ) ;
#4586=CARTESIAN_POINT ( 'NONE',  ( 9.001249775931846008E-16, 11.87187500061451395, 34.90005215228797653 ) ) ;
#4588=CARTESIAN_POINT ( 'NONE',  ( 26.87812500061451360, 6.421520780324663323E-16, -5.243569643749999010 ) ) ;
#4589=CARTESIAN_POINT ( 'NONE',  ( 26.72812500061451502, -4.541064518000419881, 2.621784821874995952 ) ) ;
#4590=CARTESIAN_POINT ( 'NONE',  ( 8.325000001229033941, 2.886751345948129099, -4.999999999999997335 ) ) ;
#4591=CARTESIAN_POINT ( 'NONE',  ( 2.000000000000001332, 18.80000000000000071, 33.46410161513774995 ) ) ;
#4592=CARTESIAN_POINT ( 'NONE',  ( 4.884375000614518569, 6.421520780324663323E-16, -5.243569643749999010 ) ) ;
#4593=CARTESIAN_POINT ( 'NONE',  ( 14.02500000122903323, -5.773502691896255534, -1.060575238724906372E-15 ) ) ;
#4594=CARTESIAN_POINT ( 'NONE',  ( 10.31250000122903288, 0.000000000000000000, 4.999999999999998224 ) ) ;
#4595=CARTESIAN_POINT ( 'NONE',  ( 3.778125000614519280, -4.541064518000419881, 2.621784821874995952 ) ) ;
#4598=CARTESIAN_POINT ( 'NONE',  ( 12.75937500061451857, 0.000000000000000000, 5.243569643749999010 ) ) ;
#4600=ORIENTED_EDGE ( 'NONE', *, *, #24790, .T. ) ;
#4601=CARTESIAN_POINT ( 'NONE',  ( 19.60312500061451502, -4.541064518000417216, -2.621784821875001281 ) ) ;
#4602=CARTESIAN_POINT ( 'NONE',  ( 12.49687500061451573, -3.027376345333610441, -5.243569643749999898 ) ) ;
#4603=CARTESIAN_POINT ( 'NONE',  ( 5.203125000614518214, -4.541064518000417216, -2.621784821875001281 ) ) ;
#4604=CARTESIAN_POINT ( 'NONE',  ( 22.84687500061451715, -3.027376345333610441, -5.243569643749999898 ) ) ;
#4605=CARTESIAN_POINT ( 'NONE',  ( 5.015625000614518214, 3.027376345333611329, 5.243569643749999010 ) ) ;
#4607=( BOUNDED_CURVE ( )  B_SPLINE_CURVE ( 2, ( #21318, #70838, #32049, #20951, #60107, #43134, #42768, #66029, #4355 ),
 .UNSPECIFIED., .F., .F. ) 
 B_SPLINE_CURVE_WITH_KNOTS ( ( 3, 2, 2, 2, 3 ),
 ( 0.2282608695652174058, 0.2318840579710144956, 0.2391304347826087029, 0.2463768115942029102, 0.2500000000000000000 ),
 .UNSPECIFIED. ) 
 CURVE ( )  GEOMETRIC_REPRESENTATION_ITEM ( )  RATIONAL_B_SPLINE_CURVE ( ( 0.9330127018922194093, 0.9330127018922196314, 1.000000000000000000, 0.8660254037844387076, 1.000000000000000000, 0.8660254037844387076, 1.000000000000000000, 0.9330127018922196314, 0.9330127018922194093 ) ) 
 REPRESENTATION_ITEM ( '' )  );
#4608=CARTESIAN_POINT ( 'NONE',  ( 9.075000001229033941, -5.773502691896255534, -1.060575238724906372E-15 ) ) ;
#4609=CARTESIAN_POINT ( 'NONE',  ( 21.77812500061451928, -4.541064518000419881, 2.621784821874995952 ) ) ;
#4610=CARTESIAN_POINT ( 'NONE',  ( -2.000000000000000000, 19.13750000122903216, -33.46410161513775705 ) ) ;
#4611=CARTESIAN_POINT ( 'NONE',  ( 8.625000001229034652, -5.773502691896255534, -1.060575238724906372E-15 ) ) ;
#4612=CARTESIAN_POINT ( 'NONE',  ( 18.02812500061451573, 4.541064518000418104, 2.621784821874999949 ) ) ;
#4613=CARTESIAN_POINT ( 'NONE',  ( 15.62812500061451537, 6.421520780324663323E-16, -5.243569643749999010 ) ) ;
#4615=CARTESIAN_POINT ( 'NONE',  ( 14.96250000000000036, 2.886751345948129099, -4.999999999999998224 ) ) ;
#4616=CARTESIAN_POINT ( 'NONE',  ( 11.55000000122903181, 5.773502691896255534, 3.535250795749688894E-16 ) ) ;
#4617=CARTESIAN_POINT ( 'NONE',  ( 8.203125000614518214, 0.000000000000000000, 5.243569643749999010 ) ) ;
#4618=CARTESIAN_POINT ( 'NONE',  ( 10.67812500061451608, 6.421520780324663323E-16, -5.243569643749999010 ) ) ;
#4619=EDGE_CURVE ( 'NONE', #2237, #3790, #57073, .T. ) ;
#4620=CARTESIAN_POINT ( 'NONE',  ( 20.58750000122903145, 4.330127018922191873, 2.499999999999999556 ) ) ;
#4621=CARTESIAN_POINT ( 'NONE',  ( 2.121784821875001281, 13.25937500061451857, -26.32496088578401938 ) ) ;
#4622=CARTESIAN_POINT ( 'NONE',  ( 20.03437500061451715, -4.541064518000419881, 2.621784821874995952 ) ) ;
#4623=CYLINDRICAL_SURFACE ( 'NONE', #61922, 4.999999999999998224 ) ;
#4624=CARTESIAN_POINT ( 'NONE',  ( 4.875000001229034652, 2.886751345948126879, 4.999999999999999112 ) ) ;
#4625=CARTESIAN_POINT ( 'NONE',  ( 4.734375000614518214, -4.541064518000419881, 2.621784821874995952 ) ) ;
#4626=CARTESIAN_POINT ( 'NONE',  ( 20.52187500061451786, -6.054752690667223547, -1.112240025338166033E-15 ) ) ;
#4628=CARTESIAN_POINT ( 'NONE',  ( 18.06562500061451715, 3.027376345333611329, 5.243569643749999010 ) ) ;
#4630=CARTESIAN_POINT ( 'NONE',  ( 23.17500000000000071, 4.330127018922191873, 2.499999999999999556 ) ) ;
#4632=CARTESIAN_POINT ( 'NONE',  ( 27.57187500061451857, 3.027376345333611329, 5.243569643749999010 ) ) ;
#4634=CARTESIAN_POINT ( 'NONE',  ( 14.84062500061451750, 6.054752690667223547, 3.707466751127219781E-16 ) ) ;
#4635=CARTESIAN_POINT ( 'NONE',  ( 12.30937500061451573, 0.000000000000000000, 5.243569643749999010 ) ) ;
#4638=CARTESIAN_POINT ( 'NONE',  ( 23.27812500061451573, 6.421520780324663323E-16, -5.243569643749999010 ) ) ;
#4640=CARTESIAN_POINT ( 'NONE',  ( -1.487416814333745711E-14, 15.72500000122903430, 34.00000000000000000 ) ) ;
#4641=CARTESIAN_POINT ( 'NONE',  ( 11.77500000000000036, 6.123233995736764310E-16, -4.999999999999998224 ) ) ;
#4642=CARTESIAN_POINT ( 'NONE',  ( 23.66250000122903430, 4.330127018922192761, -2.499999999999997780 ) ) ;
#4643=CARTESIAN_POINT ( 'NONE',  ( 19.75312500061451360, 4.541064518000418104, -2.621784821874998173 ) ) ;
#4644=ORIENTED_EDGE ( 'NONE', *, *, #7878, .F. ) ;
#4645=CARTESIAN_POINT ( 'NONE',  ( 23.47499999999999787, 6.123233995736764310E-16, -4.999999999999998224 ) ) ;
#4646=( BOUNDED_CURVE ( )  B_SPLINE_CURVE ( 2, ( #24593, #3172, #69672, #36047, #19038, #70030, #41596, #13500, #52676 ),
 .UNSPECIFIED., .F., .F. ) 
 B_SPLINE_CURVE_WITH_KNOTS ( ( 3, 2, 2, 2, 3 ),
 ( 0.3804347826086956763, 0.3840579710144927383, 0.3913043478260869734, 0.3985507246376811530, 0.4021739130434782705 ),
 .UNSPECIFIED. ) 
 CURVE ( )  GEOMETRIC_REPRESENTATION_ITEM ( )  RATIONAL_B_SPLINE_CURVE ( ( 0.9330127018922194093, 0.9330127018922198534, 1.000000000000000000, 0.8660254037844387076, 1.000000000000000000, 0.8660254037844387076, 1.000000000000000000, 0.9330127018922194093, 0.9330127018922194093 ) ) 
 REPRESENTATION_ITEM ( '' )  );
#4647=CARTESIAN_POINT ( 'NONE',  ( 21.79687500061451644, -3.027376345333614438, 5.243569643749998122 ) ) ;
#4648=EDGE_CURVE ( 'NONE', #70526, #25563, #43936, .T. ) ;
#4649=ORIENTED_EDGE ( 'NONE', *, *, #20885, .F. ) ;
#4650=CARTESIAN_POINT ( 'NONE',  ( 11.16562500061451679, 3.027376345333613106, -5.243569643749998122 ) ) ;
#4651=CARTESIAN_POINT ( 'NONE',  ( 3.368666508416885197, 3.694988906523804406, 3.424053828803762745 ) ) ;
#4653=CARTESIAN_POINT ( 'NONE',  ( 17.13749999999999929, -2.886751345948125991, -5.000000000000000000 ) ) ;
#4654=CARTESIAN_POINT ( 'NONE',  ( 25.38749999999999929, 5.773502691896255534, 3.535250795749688894E-16 ) ) ;
#4655=CARTESIAN_POINT ( 'NONE',  ( -4.243569643749999898, 18.86562500061451431, 27.54997392385601529 ) ) ;
#4656=CARTESIAN_POINT ( 'NONE',  ( 5.184375000614516615, -4.541064518000419881, 2.621784821874995952 ) ) ;
#4657=CARTESIAN_POINT ( 'NONE',  ( 28.17187500061451644, -6.054752690667223547, -1.112240025338166033E-15 ) ) ;
#4658=ORIENTED_EDGE ( 'NONE', *, *, #64328, .T. ) ;
#4659=CARTESIAN_POINT ( 'NONE',  ( 26.95312500061451644, 4.541064518000418104, -2.621784821874998173 ) ) ;
#4660=CARTESIAN_POINT ( 'NONE',  ( 27.38437500061451857, 6.421520780324663323E-16, -5.243569643749999010 ) ) ;
#4661=CARTESIAN_POINT ( 'NONE',  ( 13.53749999999999964, -2.886751345948125991, -5.000000000000000000 ) ) ;
#4662=CARTESIAN_POINT ( 'NONE',  ( 10.71562500061451928, 3.027376345333613106, -5.243569643749998122 ) ) ;
#4665=CARTESIAN_POINT ( 'NONE',  ( 29.16562500061451502, 3.027376345333612662, -5.243569643749998122 ) ) ;
#4666=CARTESIAN_POINT ( 'NONE',  ( 15.56250000122903465, 4.330127018922192761, -2.499999999999997780 ) ) ;
#4669=CARTESIAN_POINT ( 'NONE',  ( 5.465625000614517504, 3.027376345333611329, 5.243569643749999010 ) ) ;
#4670=CARTESIAN_POINT ( 'NONE',  ( 22.43437500061451573, 6.421520780324663323E-16, -5.243569643749999010 ) ) ;
#4671=CARTESIAN_POINT ( 'NONE',  ( 9.001249775931846008E-16, 15.02187500061451608, 34.90005215228797653 ) ) ;
#4672=CARTESIAN_POINT ( 'NONE',  ( 21.87187500061451573, -6.054752690667223547, -1.112240025338166033E-15 ) ) ;
#4673=CARTESIAN_POINT ( 'NONE',  ( 3.787500000000002753, 5.773502691896255534, 3.535250795749688894E-16 ) ) ;
#4674=CARTESIAN_POINT ( 'NONE',  ( 4.243569643749999898, 19.63437500061451857, 30.00000000000000000 ) ) ;
#4675=CARTESIAN_POINT ( 'NONE',  ( 8.953125000614518214, 4.541064518000418104, -2.621784821874998173 ) ) ;
#4676=CARTESIAN_POINT ( 'NONE',  ( 3.075000001229035718, 2.886751345948126879, 4.999999999999999112 ) ) ;
#4677=CARTESIAN_POINT ( 'NONE',  ( 7.021875000614518747, -6.054752690667223547, -1.112240025338166033E-15 ) ) ;
#4678=DIRECTION ( 'NONE',  ( 0.000000000000000000, 0.000000000000000000, -1.000000000000000000 ) ) ;
#4679=CARTESIAN_POINT ( 'NONE',  ( 9.478125000614515017, 4.541064518000418104, 2.621784821874999949 ) ) ;
#4680=CARTESIAN_POINT ( 'NONE',  ( 15.38437500061451679, 4.541064518000418104, 2.621784821874999949 ) ) ;
#4682=CARTESIAN_POINT ( 'NONE',  ( 21.11250000122903359, 0.000000000000000000, 4.999999999999998224 ) ) ;
#4683=CARTESIAN_POINT ( 'NONE',  ( 6.909375000614518036, 0.000000000000000000, 5.243569643749999010 ) ) ;
#4684=CARTESIAN_POINT ( 'NONE',  ( 9.740625000614516082, -3.027376345333610441, -5.243569643749999898 ) ) ;
#4686=CARTESIAN_POINT ( 'NONE',  ( 18.90937500061451360, 4.541064518000418104, -2.621784821874998173 ) ) ;
#4687=CYLINDRICAL_SURFACE ( 'NONE', #26646, 5.000000000000000000 ) ;
#4689=CARTESIAN_POINT ( 'NONE',  ( 28.43437500061451573, 4.541064518000418104, 2.621784821874999949 ) ) ;
#4690=CARTESIAN_POINT ( 'NONE',  ( 9.001249775931846008E-16, 11.42187500061451644, -25.09994784771203058 ) ) ;
#4691=CARTESIAN_POINT ( 'NONE',  ( 15.00000000122903465, -2.886751345948125991, -5.000000000000000000 ) ) ;
#4692=CARTESIAN_POINT ( 'NONE',  ( -3.000416591977282496E-16, 15.64062500061451644, -34.90005215228797653 ) ) ;
#4693=CARTESIAN_POINT ( 'NONE',  ( 15.00000000122903465, -2.886751345948125991, -5.000000000000000000 ) ) ;
#4694=CARTESIAN_POINT ( 'NONE',  ( 9.740625000614516082, -3.027376345333610441, -5.243569643749999898 ) ) ;
#4695=ORIENTED_EDGE ( 'NONE', *, *, #29492, .F. ) ;
#4696=CARTESIAN_POINT ( 'NONE',  ( 14.36249999999999893, -5.773502691896255534, -1.060575238724906372E-15 ) ) ;
#4698=CARTESIAN_POINT ( 'NONE',  ( 21.92812500061451431, 6.421520780324663323E-16, -5.243569643749999010 ) ) ;
#4699=CARTESIAN_POINT ( 'NONE',  ( 10.58437500061451964, -4.541064518000419881, 2.621784821874995952 ) ) ;
#4701=CARTESIAN_POINT ( 'NONE',  ( 9.150000001229033231, -2.886751345948125991, -5.000000000000000000 ) ) ;
#4702=CARTESIAN_POINT ( 'NONE',  ( 18.07500000122903216, -5.773502691896255534, -1.060575238724906372E-15 ) ) ;
#4703=CARTESIAN_POINT ( 'NONE',  ( 15.32812500061451644, 4.541064518000418104, 2.621784821874999949 ) ) ;
#4704=CARTESIAN_POINT ( 'NONE',  ( 19.11562500061451431, -6.054752690667223547, -1.112240025338166033E-15 ) ) ;
#4705=CARTESIAN_POINT ( 'NONE',  ( 25.08750000122903145, 4.330127018922191873, 2.499999999999999556 ) ) ;
#4706=CARTESIAN_POINT ( 'NONE',  ( 28.38750000122903216, -4.330127018922194537, 2.499999999999995559 ) ) ;
#4707=CARTESIAN_POINT ( 'NONE',  ( 23.32499999999999929, -4.330127018922194537, 2.499999999999995559 ) ) ;
#4709=CARTESIAN_POINT ( 'NONE',  ( 26.33437500061451431, -4.541064518000419881, 2.621784821874995952 ) ) ;
#4710=CARTESIAN_POINT ( 'NONE',  ( 18.37500000122903288, 2.886751345948161074, 4.999999999999941380 ) ) ;
#4711=CARTESIAN_POINT ( 'NONE',  ( 11.55000000122903181, 5.773502691896255534, 3.535250795749688894E-16 ) ) ;
#4712=CARTESIAN_POINT ( 'NONE',  ( 27.19687500061451857, -3.027376345333614438, 5.243569643749998122 ) ) ;
#4714=CARTESIAN_POINT ( 'NONE',  ( 5.409375000614516260, 4.541064518000418104, -2.621784821874998173 ) ) ;
#4715=CARTESIAN_POINT ( 'NONE',  ( 26.27812500061451573, -4.541064518000419881, 2.621784821874995952 ) ) ;
#4718=CARTESIAN_POINT ( 'NONE',  ( 10.95937500061451964, 0.000000000000000000, 5.243569643749999010 ) ) ;
#4719=CARTESIAN_POINT ( 'NONE',  ( 22.08750000122903501, -4.330127018922194537, 2.499999999999995559 ) ) ;
#4720=CARTESIAN_POINT ( 'NONE',  ( 3.571875000614517237, 3.027376345333613106, -5.243569643749998122 ) ) ;
#4721=CARTESIAN_POINT ( 'NONE',  ( 8.184375000614515727, 4.541064518000418104, 2.621784821874999949 ) ) ;
#4722=CARTESIAN_POINT ( 'NONE',  ( 29.70937500061451431, 4.541064518000418104, -2.621784821874998173 ) ) ;
#4723=CARTESIAN_POINT ( 'NONE',  ( 2.121784821875001281, 12.30312500061459424, 33.67503911421598417 ) ) ;
#4724=CARTESIAN_POINT ( 'NONE',  ( 19.83750000000000213, -2.886751345948125991, -5.000000000000000000 ) ) ;
#4725=ORIENTED_EDGE ( 'NONE', *, *, #34392, .F. ) ;
#4726=CARTESIAN_POINT ( 'NONE',  ( 20.88750000122903572, 6.123233995736764310E-16, -4.999999999999998224 ) ) ;
#4727=CARTESIAN_POINT ( 'NONE',  ( 4.312500000000000000, 2.886751345948126879, 4.999999999999999112 ) ) ;
#4728=EDGE_CURVE ( 'NONE', #16013, #64135, #51484, .T. ) ;
#4730=CARTESIAN_POINT ( 'NONE',  ( 17.61562500061451786, 3.027376345333611329, 5.243569643749999010 ) ) ;
#4731=CARTESIAN_POINT ( 'NONE',  ( 8.503125000614515372, 4.541064518000418104, -2.621784821874998173 ) ) ;
#4733=CARTESIAN_POINT ( 'NONE',  ( 7.096875000614517148, -3.027376345333610441, -5.243569643749999898 ) ) ;
#4734=CARTESIAN_POINT ( 'NONE',  ( 16.68750000122903288, -4.330127018922194537, 2.499999999999995559 ) ) ;
#4735=CARTESIAN_POINT ( 'NONE',  ( 3.160880256176461511, -3.874123901750303300, -3.160880256176591185 ) ) ;
#4736=CARTESIAN_POINT ( 'NONE',  ( 7.246875000614518392, 6.054752690667223547, 3.707466751127219781E-16 ) ) ;
#4737=CARTESIAN_POINT ( 'NONE',  ( 12.83437500061451786, -4.541064518000419881, 2.621784821874995952 ) ) ;
#4738=CARTESIAN_POINT ( 'NONE',  ( 25.35937500061451644, 0.000000000000000000, 5.243569643749999010 ) ) ;
#4742=CARTESIAN_POINT ( 'NONE',  ( 18.19687500061451502, -3.027376345333614438, 5.243569643749998122 ) ) ;
#4743=CARTESIAN_POINT ( 'NONE',  ( 10.50937500061451679, 0.000000000000000000, 5.243569643749999010 ) ) ;
#4745=CARTESIAN_POINT ( 'NONE',  ( 19.83750000000000213, -2.886751345948125991, -5.000000000000000000 ) ) ;
#4749=CARTESIAN_POINT ( 'NONE',  ( 13.49062500061451608, 6.054752690667223547, 3.707466751127219781E-16 ) ) ;
#4750=CARTESIAN_POINT ( 'NONE',  ( 3.300000000000000711, 4.330127018922192761, -2.499999999999997780 ) ) ;
#4751=CARTESIAN_POINT ( 'NONE',  ( 0.000000000000000000, 20.00000000000000000, 30.00000000000000000 ) ) ;
#4752=CARTESIAN_POINT ( 'NONE',  ( 29.10937500061451644, -4.541064518000417216, -2.621784821875001281 ) ) ;
#4753=CARTESIAN_POINT ( 'NONE',  ( 10.27499999999999858, -4.330127018922194537, 2.499999999999995559 ) ) ;
#4754=CARTESIAN_POINT ( 'NONE',  ( 3.999999999999999112, 15.38750000122903394, 30.00000000000000000 ) ) ;
#4755=CARTESIAN_POINT ( 'NONE',  ( 8.025000001229035007, 2.886751345948126879, 4.999999999999999112 ) ) ;
#4756=CARTESIAN_POINT ( 'NONE',  ( 19.77187500061451786, 3.027376345333613106, -5.243569643749998122 ) ) ;
#4757=CARTESIAN_POINT ( 'NONE',  ( 14.10937500061451644, 0.000000000000000000, 5.243569643749999010 ) ) ;
#4758=CARTESIAN_POINT ( 'NONE',  ( 1.999999999999998668, 16.81250000122903643, 26.53589838486224650 ) ) ;
#4759=ORIENTED_EDGE ( 'NONE', *, *, #12791, .T. ) ;
#4760=CARTESIAN_POINT ( 'NONE',  ( 16.22812500061451857, 4.541064518000418104, 2.621784821874999949 ) ) ;
#4761=CARTESIAN_POINT ( 'NONE',  ( 29.28750000122903074, -4.330127018922194537, 2.499999999999995559 ) ) ;
#4762=CARTESIAN_POINT ( 'NONE',  ( 15.04687500061451644, -3.027376345333614438, 5.243569643749998122 ) ) ;
#4763=CARTESIAN_POINT ( 'NONE',  ( 6.000084452983059258, 7.999936660264888921, -30.40169366477969604 ) ) ;
#4764=CARTESIAN_POINT ( 'NONE',  ( 17.84062500061451573, -3.027376345333610441, -5.243569643749999898 ) ) ;
#4765=CARTESIAN_POINT ( 'NONE',  ( 3.999999999999999112, 16.62500000000000000, -30.00000000000000000 ) ) ;
#4766=CARTESIAN_POINT ( 'NONE',  ( 29.18437500061451573, 6.421520780324663323E-16, -5.243569643749999010 ) ) ;
#4767=CARTESIAN_POINT ( 'NONE',  ( -4.243569643749997233, 11.74062500061451786, 32.45002607614398471 ) ) ;
#4768=CARTESIAN_POINT ( 'NONE',  ( 14.40937500061451715, 4.541064518000418104, -2.621784821874998173 ) ) ;
#4769=CARTESIAN_POINT ( 'NONE',  ( 13.38750000122903394, 4.330127018922191873, 2.499999999999999556 ) ) ;
#4771=CARTESIAN_POINT ( 'NONE',  ( -4.243569643749999898, 18.92187500061451644, -32.45002607614398471 ) ) ;
#4772=CARTESIAN_POINT ( 'NONE',  ( 20.59687500061451360, -3.027376345333610441, -5.243569643749999898 ) ) ;
#4773=CARTESIAN_POINT ( 'NONE',  ( 22.46250000122903501, 0.000000000000000000, 4.999999999999998224 ) ) ;
#4774=CARTESIAN_POINT ( 'NONE',  ( 17.85937500061451999, -4.541064518000417216, -2.621784821875001281 ) ) ;
#4775=CARTESIAN_POINT ( 'NONE',  ( 13.22812500061451502, -4.541064518000419881, 2.621784821874995952 ) ) ;
#4776=CARTESIAN_POINT ( 'NONE',  ( -2.121784821874999949, 12.58437500061451786, 26.32496088578401938 ) ) ;
#4777=CARTESIAN_POINT ( 'NONE',  ( 18.14062500061451644, -3.027376345333614438, 5.243569643749998122 ) ) ;
#4779=ORIENTED_EDGE ( 'NONE', *, *, #48851, .F. ) ;
#4780=CARTESIAN_POINT ( 'NONE',  ( 19.65000000000000213, 0.000000000000000000, 4.999999999999998224 ) ) ;
#4781=CARTESIAN_POINT ( 'NONE',  ( 17.58749999999999858, -2.886751345948092684, -5.000000000000057732 ) ) ;
#4782=CARTESIAN_POINT ( 'NONE',  ( 24.17812500061451786, 6.421520780324663323E-16, -5.243569643749999010 ) ) ;
#4783=CARTESIAN_POINT ( 'NONE',  ( 5.465625000614517504, 3.027376345333611329, 5.243569643749999010 ) ) ;
#4784=CARTESIAN_POINT ( 'NONE',  ( 17.13750000122903216, -4.330127018922194537, 2.499999999999995559 ) ) ;
#4785=CARTESIAN_POINT ( 'NONE',  ( 22.86562500061451431, 3.027376345333613106, -5.243569643749998122 ) ) ;
#4786=CARTESIAN_POINT ( 'NONE',  ( 22.34999999999999787, 0.000000000000000000, 4.999999999999998224 ) ) ;
#4787=CARTESIAN_POINT ( 'NONE',  ( 26.42812500061451431, 6.421520780324663323E-16, -5.243569643749999010 ) ) ;
#4788=CARTESIAN_POINT ( 'NONE',  ( 6.403125000614517504, 0.000000000000000000, 5.243569643749999010 ) ) ;
#4789=ORIENTED_EDGE ( 'NONE', *, *, #35474, .T. ) ;
#4790=EDGE_CURVE ( 'NONE', #37881, #49981, #59003, .T. ) ;
#4791=CARTESIAN_POINT ( 'NONE',  ( 29.77499999999999858, 6.123233995736764310E-16, -4.999999999999998224 ) ) ;
#4792=CARTESIAN_POINT ( 'NONE',  ( 2.990625000614519191, -3.027376345333610441, -5.243569643749999898 ) ) ;
#4793=EDGE_CURVE ( 'NONE', #60642, #33795, #3002, .T. ) ;
#4795=CARTESIAN_POINT ( 'NONE',  ( 3.242103837493086330E-14, 11.00000000122903288, 26.00000000000000711 ) ) ;
#4796=CARTESIAN_POINT ( 'NONE',  ( 3.999999999999998668, 14.07500000122903572, -32.30940107675850470 ) ) ;
#4797=CARTESIAN_POINT ( 'NONE',  ( -3.000416591977282496E-16, 19.29687500061451644, -34.90005215228797653 ) ) ;
#4798=CARTESIAN_POINT ( 'NONE',  ( 9.562500000000001776, 2.886751345948129099, -4.999999999999998224 ) ) ;
#4799=ADVANCED_FACE ( 'NONE', ( #69871 ), #65053, .F. ) ;
#4800=CARTESIAN_POINT ( 'NONE',  ( 11.93437500061451573, -4.541064518000419881, 2.621784821874995952 ) ) ;
#4801=CARTESIAN_POINT ( 'NONE',  ( 6.487500001229034474, 6.123233995736764310E-16, -4.999999999999998224 ) ) ;
#4802=CARTESIAN_POINT ( 'NONE',  ( 12.72187500061451537, 3.027376345333611329, 5.243569643749999010 ) ) ;
#4803=CARTESIAN_POINT ( 'NONE',  ( 4.921875000614518214, 3.027376345333613106, -5.243569643749998122 ) ) ;
#4804=CARTESIAN_POINT ( 'NONE',  ( -4.243569643749999898, 10.31562500061451715, -32.45002607614398471 ) ) ;
#4805=CARTESIAN_POINT ( 'NONE',  ( -2.556497649636125342E-15, 19.21250000000000213, 34.00000000000000000 ) ) ;
#4806=EDGE_CURVE ( 'NONE', #28753, #71866, #32053, .T. ) ;
#4807=CARTESIAN_POINT ( 'NONE',  ( 11.25937500061451679, 4.541064518000418104, -2.621784821874998173 ) ) ;
#4808=CARTESIAN_POINT ( 'NONE',  ( 4.276577733362700862, 2.590537181842085257, -4.276577733362700862 ) ) ;
#4809=CARTESIAN_POINT ( 'NONE',  ( 19.49062500061451431, -3.027376345333614438, 5.243569643749998122 ) ) ;
#4810=CARTESIAN_POINT ( 'NONE',  ( -2.000000000000000000, 12.38750000122903394, -33.46410161513775705 ) ) ;
#4811=CARTESIAN_POINT ( 'NONE',  ( 4.243569643749999898, 19.12812500061459531, 30.00000000000000000 ) ) ;
#4812=CARTESIAN_POINT ( 'NONE',  ( 23.63437500061451502, -4.541064518000419881, 2.621784821874995952 ) ) ;
#4813=CARTESIAN_POINT ( 'NONE',  ( 28.31250000122903288, 0.000000000000000000, 4.999999999999998224 ) ) ;
#4815=CARTESIAN_POINT ( 'NONE',  ( 24.85312500061451502, 0.000000000000000000, 5.243569643749999010 ) ) ;
#4816=CARTESIAN_POINT ( 'NONE',  ( 16.86562500061451786, -6.054752690667223547, -1.112240025338166033E-15 ) ) ;
#4818=CARTESIAN_POINT ( 'NONE',  ( 15.38437500061451679, 4.541064518000418104, 2.621784821874999949 ) ) ;
#4819=CARTESIAN_POINT ( 'NONE',  ( 27.11250000122903359, -4.330127018922190985, -2.500000000000001332 ) ) ;
#4820=CARTESIAN_POINT ( 'NONE',  ( 3.609375000614516882, 4.541064518000418104, -2.621784821874998173 ) ) ;
#4821=CARTESIAN_POINT ( 'NONE',  ( 15.38437500061451679, 4.541064518000418104, 2.621784821874999949 ) ) ;
#4823=CARTESIAN_POINT ( 'NONE',  ( 14.81250000122903288, 0.000000000000000000, 4.999999999999998224 ) ) ;
#4824=CARTESIAN_POINT ( 'NONE',  ( 3.000000001229032875, 5.773502691896255534, 3.535250795749688894E-16 ) ) ;
#4825=CARTESIAN_POINT ( 'NONE',  ( 23.67187500061451999, -6.054752690667223547, -1.112240025338166033E-15 ) ) ;
#4826=CARTESIAN_POINT ( 'NONE',  ( 16.84687500061451715, -3.027376345333614438, 5.243569643749998122 ) ) ;
#4828=CARTESIAN_POINT ( 'NONE',  ( 27.63749999999999929, 5.773502691896255534, 3.535250795749688894E-16 ) ) ;
#4829=CARTESIAN_POINT ( 'NONE',  ( -5.810221930991193690E-16, 10.43750000000000000, 26.00000000000000355 ) ) ;
#4830=CARTESIAN_POINT ( 'NONE',  ( 5.549999999999998934, 4.330127018922192761, -2.499999999999997780 ) ) ;
#4832=CARTESIAN_POINT ( 'NONE',  ( 20.05312500061451431, -4.541064518000417216, -2.621784821875001281 ) ) ;
#4833=CARTESIAN_POINT ( 'NONE',  ( 9.225000000000001421, 4.330127018922191873, 2.499999999999999556 ) ) ;
#4834=CARTESIAN_POINT ( 'NONE',  ( 3.778125000614519280, -4.541064518000419881, 2.621784821874995952 ) ) ;
#4835=CARTESIAN_POINT ( 'NONE',  ( 18.18750000000000000, 5.773502691896255534, 3.535250795749688894E-16 ) ) ;
#4836=CARTESIAN_POINT ( 'NONE',  ( 15.48750000122903359, 6.123233995736764310E-16, -4.999999999999998224 ) ) ;
#4837=CARTESIAN_POINT ( 'NONE',  ( 21.03750000122903074, 4.330127018922191873, 2.499999999999999556 ) ) ;
#4838=CARTESIAN_POINT ( 'NONE',  ( 5.918267800642001752, 8.060802005575231632, 31.00679648383703935 ) ) ;
#4839=CARTESIAN_POINT ( 'NONE',  ( 3.262500000000001510, 2.886751345948129099, -4.999999999999998224 ) ) ;
#4841=CARTESIAN_POINT ( 'NONE',  ( 18.14062500061451644, -3.027376345333614438, 5.243569643749998122 ) ) ;
#4842=CARTESIAN_POINT ( 'NONE',  ( 24.89062500061451644, -3.027376345333614438, 5.243569643749998122 ) ) ;
#4843=CARTESIAN_POINT ( 'NONE',  ( 23.03437500061451715, 4.541064518000418104, 2.621784821874999949 ) ) ;
#4844=CARTESIAN_POINT ( 'NONE',  ( 6.262500000000000178, -5.773502691896255534, -1.060575238724906372E-15 ) ) ;
#4845=CARTESIAN_POINT ( 'NONE',  ( 8.465625000614515727, 3.027376345333613106, -5.243569643749998122 ) ) ;
#4846=CARTESIAN_POINT ( 'NONE',  ( 27.40312500061451573, 4.541064518000418104, -2.621784821874998173 ) ) ;
#4847=CARTESIAN_POINT ( 'NONE',  ( 15.38437500061451679, 4.541064518000418104, 2.621784821874999949 ) ) ;
#4848=CARTESIAN_POINT ( 'NONE',  ( 20.25937500061451857, 4.541064518000418104, -2.621784821874998173 ) ) ;
#4849=CYLINDRICAL_SURFACE ( 'NONE', #17960, 4.999999999999998224 ) ;
#4850=CARTESIAN_POINT ( 'NONE',  ( 9.001249775931846008E-16, 10.52187500061451964, 34.90005215228797653 ) ) ;
#4851=CARTESIAN_POINT ( 'NONE',  ( 20.92500000122903714, 2.886751345948129099, -4.999999999999998224 ) ) ;
#4853=CARTESIAN_POINT ( 'NONE',  ( 12.06562500061451537, 3.027376345333612662, -5.243569643749998122 ) ) ;
#4854=CARTESIAN_POINT ( 'NONE',  ( 8.334375000614516082, -4.541064518000419881, 2.621784821874995952 ) ) ;
#4855=CARTESIAN_POINT ( 'NONE',  ( 8.109375000614518214, 4.541064518000418104, -2.621784821874998173 ) ) ;
#4857=CARTESIAN_POINT ( 'NONE',  ( 27.75937500061451502, -4.541064518000417216, -2.621784821875001281 ) ) ;
#4858=CARTESIAN_POINT ( 'NONE',  ( 19.26562500061451644, 3.027376345333613106, -5.243569643749998122 ) ) ;
#4859=CARTESIAN_POINT ( 'NONE',  ( 28.50000000122903288, -2.886751345948125991, -5.000000000000000000 ) ) ;
#4860=CARTESIAN_POINT ( 'NONE',  ( 4.396875000614516971, -3.027376345333610441, -5.243569643749999898 ) ) ;
#4861=CARTESIAN_POINT ( 'NONE',  ( 25.35937500061451644, 0.000000000000000000, 5.243569643749999010 ) ) ;
#4862=CARTESIAN_POINT ( 'NONE',  ( 19.79062500061451502, 6.054752690667223547, 3.707466751127219781E-16 ) ) ;
#4863=CARTESIAN_POINT ( 'NONE',  ( 3.999999999999998668, 10.36250000000000071, 27.69059892324149175 ) ) ;
#4864=CARTESIAN_POINT ( 'NONE',  ( 23.42812500061451786, 4.541064518000418104, 2.621784821874999949 ) ) ;
#4865=CARTESIAN_POINT ( 'NONE',  ( 4.125000001229034652, -5.773502691896255534, -1.060575238724906372E-15 ) ) ;
#4867=CARTESIAN_POINT ( 'NONE',  ( 26.69999999999999929, 4.330127018922192761, -2.499999999999997780 ) ) ;
#4868=CARTESIAN_POINT ( 'NONE',  ( 3.999999999999999112, 15.72500000000000320, -30.00000000000000000 ) ) ;
#4870=CARTESIAN_POINT ( 'NONE',  ( 4.846875000614519813, -3.027376345333610441, -5.243569643749999898 ) ) ;
#4871=CARTESIAN_POINT ( 'NONE',  ( 12.96562500061451750, 3.027376345333613106, -5.243569643749998122 ) ) ;
#4872=CARTESIAN_POINT ( 'NONE',  ( 6.421875000614519102, 3.027376345333611329, 5.243569643749999010 ) ) ;
#4873=CARTESIAN_POINT ( 'NONE',  ( 25.80000000122903714, -2.886751345948125991, -5.000000000000000000 ) ) ;
#4874=CARTESIAN_POINT ( 'NONE',  ( 16.02187500061451786, -6.054752690667223547, -1.112240025338166033E-15 ) ) ;
#4875=CARTESIAN_POINT ( 'NONE',  ( 3.121875000614518836, 3.027376345333613106, -5.243569643749998122 ) ) ;
#4876=CARTESIAN_POINT ( 'NONE',  ( 29.06250000000000000, 2.886751345948126879, 4.999999999999999112 ) ) ;
#4877=CARTESIAN_POINT ( 'NONE',  ( 25.58437500061451431, 6.421520780324663323E-16, -5.243569643749999010 ) ) ;
#4878=CARTESIAN_POINT ( 'NONE',  ( 3.778125000614519280, -4.541064518000419881, 2.621784821874995952 ) ) ;
#4879=CARTESIAN_POINT ( 'NONE',  ( 12.51562500061451821, 3.027376345333613106, -5.243569643749998122 ) ) ;
#4880=( BOUNDED_CURVE ( )  B_SPLINE_CURVE ( 2, ( #21372, #43926, #66452, #15829, #4765, #57890, #29829, #1406, #7299 ),
 .UNSPECIFIED., .F., .F. ) 
 B_SPLINE_CURVE_WITH_KNOTS ( ( 3, 2, 2, 2, 3 ),
 ( 0.3152173913043478382, 0.3188405797101449002, 0.3260869565217391353, 0.3333333333333333148, 0.3369565217391304324 ),
 .UNSPECIFIED. ) 
 CURVE ( )  GEOMETRIC_REPRESENTATION_ITEM ( )  RATIONAL_B_SPLINE_CURVE ( ( 0.9330127018922194093, 0.9330127018922198534, 1.000000000000000000, 0.8660254037844387076, 1.000000000000000000, 0.8660254037844387076, 1.000000000000000000, 0.9330127018922194093, 0.9330127018922194093 ) ) 
 REPRESENTATION_ITEM ( '' )  );
#4882=CARTESIAN_POINT ( 'NONE',  ( 10.26562500061451644, 3.027376345333613106, -5.243569643749998122 ) ) ;
#4883=CARTESIAN_POINT ( 'NONE',  ( 9.253125000614517148, -4.541064518000417216, -2.621784821875001281 ) ) ;
#4885=CARTESIAN_POINT ( 'NONE',  ( 8.212500000000000355, 2.886751345948129099, -4.999999999999998224 ) ) ;
#4886=CARTESIAN_POINT ( 'NONE',  ( 13.98750000122903359, -4.330127018922194537, 2.499999999999995559 ) ) ;
#4887=CARTESIAN_POINT ( 'NONE',  ( 17.10000000000000142, -4.330127018922190985, -2.500000000000001332 ) ) ;
#4888=EDGE_CURVE ( 'NONE', #59956, #7528, #23624, .T. ) ;
#4889=CARTESIAN_POINT ( 'NONE',  ( 19.62187500061451573, -6.054752690667223547, -1.112240025338166033E-15 ) ) ;
#4890=CARTESIAN_POINT ( 'NONE',  ( 13.05000000122903536, -2.886751345948129988, 4.999999999999997335 ) ) ;
#4892=CARTESIAN_POINT ( 'NONE',  ( 2.121784821875001281, 15.90312500061451573, -26.32496088578401938 ) ) ;
#4896=CARTESIAN_POINT ( 'NONE',  ( 26.01562500061451289, 3.027376345333613106, -5.243569643749998122 ) ) ;
#4899=CARTESIAN_POINT ( 'NONE',  ( 12.94687500061451857, -3.027376345333610441, -5.243569643749999898 ) ) ;
#4900=CARTESIAN_POINT ( 'NONE',  ( 25.83749999999999858, 5.773502691896255534, 3.535250795749688894E-16 ) ) ;
#4901=CARTESIAN_POINT ( 'NONE',  ( 9.215625000614515727, -6.054752690667223547, -1.112240025338166033E-15 ) ) ;
#4903=CARTESIAN_POINT ( 'NONE',  ( 22.09687500061451715, 6.054752690667223547, 3.707466751127219781E-16 ) ) ;
#4905=CARTESIAN_POINT ( 'NONE',  ( 7.040625000614517681, -3.027376345333610441, -5.243569643749999898 ) ) ;
#4906=CARTESIAN_POINT ( 'NONE',  ( 10.84687500061451892, 6.054752690667223547, 3.707466751127219781E-16 ) ) ;
#4907=VERTEX_POINT ( 'NONE', #27009 ) ;
#4908=CARTESIAN_POINT ( 'NONE',  ( 22.50937500061451857, 4.541064518000418104, -2.621784821874998173 ) ) ;
#4909=CARTESIAN_POINT ( 'NONE',  ( 0.6891293861215588290, 4.954145703890282526, -26.05743059574101395 ) ) ;
#4911=CARTESIAN_POINT ( 'NONE',  ( 4.237500000000001599, 5.773502691896255534, 3.535250795749688894E-16 ) ) ;
#4913=CARTESIAN_POINT ( 'NONE',  ( 15.07500000122903394, 2.886751345948129099, -4.999999999999998224 ) ) ;
#4917=CARTESIAN_POINT ( 'NONE',  ( 11.81250000000000000, 2.886751345948129099, -4.999999999999998224 ) ) ;
#4918=CARTESIAN_POINT ( 'NONE',  ( 15.52500000000000036, 4.330127018922191873, 2.499999999999999556 ) ) ;
#4919=CARTESIAN_POINT ( 'NONE',  ( 12.45000000122903394, 5.773502691896255534, 3.535250795749688894E-16 ) ) ;
#4920=CARTESIAN_POINT ( 'NONE',  ( 12.40312500061451573, -4.541064518000417216, -2.621784821875001281 ) ) ;
#4922=CARTESIAN_POINT ( 'NONE',  ( 9.337500000000000355, -2.886751345948129988, 4.999999999999997335 ) ) ;
#4923=CARTESIAN_POINT ( 'NONE',  ( -1.999999999999997113, 15.68750000122903465, 33.46410161513775705 ) ) ;
#4924=CARTESIAN_POINT ( 'NONE',  ( 9.001249775931846008E-16, 15.02187500061451608, -25.09994784771203058 ) ) ;
#4925=CARTESIAN_POINT ( 'NONE',  ( 4.153125000614515727, 0.000000000000000000, 5.243569643749999010 ) ) ;
#4927=CARTESIAN_POINT ( 'NONE',  ( 9.074999999999999289, 6.123233995736764310E-16, -4.999999999999998224 ) ) ;
#4928=CARTESIAN_POINT ( 'NONE',  ( 3.087067283321337730, 3.933194069486794842, 3.194874766990889903 ) ) ;
#4929=EDGE_LOOP ( 'NONE', ( #11274, #18502, #65883, #67077 ) ) ;
#4930=CARTESIAN_POINT ( 'NONE',  ( 24.62812500061451715, 6.421520780324663323E-16, -5.243569643749999010 ) ) ;
#4932=CARTESIAN_POINT ( 'NONE',  ( 29.44687500061451857, -3.027376345333614438, 5.243569643749998122 ) ) ;
#4933=CARTESIAN_POINT ( 'NONE',  ( 22.58437500061451431, 4.541064518000418104, 2.621784821874999949 ) ) ;
#4934=CARTESIAN_POINT ( 'NONE',  ( 16.64062500061451289, 6.054752690667223547, 3.707466751127219781E-16 ) ) ;
#4936=CARTESIAN_POINT ( 'NONE',  ( -2.121784821874996840, 12.22812500061459495, -26.32496088578401583 ) ) ;
#4937=CARTESIAN_POINT ( 'NONE',  ( 5.953125000614519102, 0.000000000000000000, 5.243569643749999010 ) ) ;
#4938=CARTESIAN_POINT ( 'NONE',  ( 28.16250000122903074, 4.330127018922192761, -2.499999999999997780 ) ) ;
#4940=CARTESIAN_POINT ( 'NONE',  ( 20.12812500061451715, 6.421520780324663323E-16, -5.243569643749999010 ) ) ;
#4943=CARTESIAN_POINT ( 'NONE',  ( 14.10937500061451644, 0.000000000000000000, 5.243569643749999010 ) ) ;
#4944=CARTESIAN_POINT ( 'NONE',  ( 14.70937500061451786, -4.541064518000417216, -2.621784821875001281 ) ) ;
#4945=CARTESIAN_POINT ( 'NONE',  ( 23.25937500061451857, -4.541064518000417216, -2.621784821875001281 ) ) ;
#4947=CARTESIAN_POINT ( 'NONE',  ( 2.121784821874999061, 12.05937500061451750, 26.32496088578401583 ) ) ;
#4948=CARTESIAN_POINT ( 'NONE',  ( 3.065625000614517592, 3.027376345333613106, -5.243569643749998122 ) ) ;
#4949=CARTESIAN_POINT ( 'NONE',  ( 26.50312500061451360, 4.541064518000418104, -2.621784821874998173 ) ) ;
#4950=CARTESIAN_POINT ( 'NONE',  ( 27.81562500061452070, 3.027376345333613106, -5.243569643749998122 ) ) ;
#4951=DIRECTION ( 'NONE',  ( -1.000000000000000000, -0.000000000000000000, -0.000000000000000000 ) ) ;
#4952=CARTESIAN_POINT ( 'NONE',  ( 2.000000000000001332, 19.69999999999999929, 33.46410161513774995 ) ) ;
#4953=CARTESIAN_POINT ( 'NONE',  ( 5.934375000614517504, 4.541064518000418104, 2.621784821874999949 ) ) ;
#4954=CARTESIAN_POINT ( 'NONE',  ( 12.52500000122903145, 2.886751345948126879, 4.999999999999999112 ) ) ;
#4955=CARTESIAN_POINT ( 'NONE',  ( 9.187500001229034652, 6.123233995736764310E-16, -4.999999999999998224 ) ) ;
#4956=CARTESIAN_POINT ( 'NONE',  ( 28.72500000122903074, 2.886751345948126879, 4.999999999999999112 ) ) ;
#4959=CARTESIAN_POINT ( 'NONE',  ( 11.85937500061451644, 0.000000000000000000, 5.243569643749999010 ) ) ;
#4961=ORIENTED_EDGE ( 'NONE', *, *, #66576, .T. ) ;
#4962=CARTESIAN_POINT ( 'NONE',  ( 20.91562500061451502, -6.054752690667223547, -1.112240025338166033E-15 ) ) ;
#4963=CARTESIAN_POINT ( 'NONE',  ( 12.19687500061451679, 6.054752690667223547, 3.707466751127219781E-16 ) ) ;
#4964=CARTESIAN_POINT ( 'NONE',  ( 5.990625000614517859, -3.027376345333614438, 5.243569643749998122 ) ) ;
#4965=CARTESIAN_POINT ( 'NONE',  ( 21.30937500061451573, 0.000000000000000000, 5.243569643749999010 ) ) ;
#4966=CARTESIAN_POINT ( 'NONE',  ( 4.828125000614518214, 6.421520780324663323E-16, -5.243569643749999010 ) ) ;
#4968=CARTESIAN_POINT ( 'NONE',  ( 6.862500001229034474, -4.330127018922190985, -2.500000000000001332 ) ) ;
#4969=CARTESIAN_POINT ( 'NONE',  ( 20.46562500061451928, -6.054752690667223547, -1.112240025338166033E-15 ) ) ;
#4970=CARTESIAN_POINT ( 'NONE',  ( 8.062500001229034652, 0.000000000000000000, 4.999999999999998224 ) ) ;
#4971=CARTESIAN_POINT ( 'NONE',  ( 16.26562500061451289, 3.027376345333611329, 5.243569643749999010 ) ) ;
#4972=CARTESIAN_POINT ( 'NONE',  ( 16.52812500061451573, 6.421520780324663323E-16, -5.243569643749999010 ) ) ;
#4974=CARTESIAN_POINT ( 'NONE',  ( 15.52500000000000036, 4.330127018922191873, 2.499999999999999556 ) ) ;
#4975=CARTESIAN_POINT ( 'NONE',  ( 11.28750000122903252, -4.330127018922194537, 2.499999999999995559 ) ) ;
#4976=CARTESIAN_POINT ( 'NONE',  ( 6.928125000614516082, -4.541064518000419881, 2.621784821874995952 ) ) ;
#4978=CARTESIAN_POINT ( 'NONE',  ( 10.60312500061451679, -4.541064518000417216, -2.621784821875001281 ) ) ;
#4979=AXIS2_PLACEMENT_3D ( 'NONE', #66658, #72559, #10505 ) ;
#4980=CARTESIAN_POINT ( 'NONE',  ( 21.82500000122903572, 2.886751345948129099, -4.999999999999998224 ) ) ;
#4981=CARTESIAN_POINT ( 'NONE',  ( -4.243569643749999898, 12.62187500061451928, -32.45002607614398471 ) ) ;
#4982=CARTESIAN_POINT ( 'NONE',  ( 4.629056002857023344, -1.889931353889065413, 4.891133006415133266 ) ) ;
#4983=CARTESIAN_POINT ( 'NONE',  ( 4.462500001229035007, 0.000000000000000000, 4.999999999999998224 ) ) ;
#4984=CARTESIAN_POINT ( 'NONE',  ( 2.934375000614518392, -4.541064518000419881, 2.621784821874995952 ) ) ;
#4985=CARTESIAN_POINT ( 'NONE',  ( 21.98437500061451644, 6.421520780324663323E-16, -5.243569643749999010 ) ) ;
#4986=CARTESIAN_POINT ( 'NONE',  ( 12.22499999999999964, 6.123233995736764310E-16, -4.999999999999998224 ) ) ;
#4987=CARTESIAN_POINT ( 'NONE',  ( 16.52812500061451573, 6.421520780324663323E-16, -5.243569643749999010 ) ) ;
#4989=CARTESIAN_POINT ( 'NONE',  ( 10.98750000000000071, 5.773502691896255534, 3.535250795749688401E-16 ) ) ;
#4991=CARTESIAN_POINT ( 'NONE',  ( 28.80937500061451573, 4.541064518000418104, -2.621784821874998173 ) ) ;
#4993=CARTESIAN_POINT ( 'NONE',  ( 15.02812500061451750, -4.541064518000419881, 2.621784821874995952 ) ) ;
#4994=CARTESIAN_POINT ( 'NONE',  ( 13.84687500061451537, -3.027376345333610441, -5.243569643749999898 ) ) ;
#4996=CARTESIAN_POINT ( 'NONE',  ( 22.46250000122903501, 0.000000000000000000, 4.999999999999998224 ) ) ;
#4997=CARTESIAN_POINT ( 'NONE',  ( 21.66562500061451502, 3.027376345333611329, 5.243569643749999010 ) ) ;
#4999=CARTESIAN_POINT ( 'NONE',  ( 14.51250000000000107, 2.886751345948129099, -4.999999999999997335 ) ) ;
#5000=CARTESIAN_POINT ( 'NONE',  ( 12.59999999999999964, -4.330127018922190985, -2.500000000000001332 ) ) ;
#5001=CARTESIAN_POINT ( 'NONE',  ( 20.58750000122903145, 4.330127018922191873, 2.499999999999999556 ) ) ;
#5002=CARTESIAN_POINT ( 'NONE',  ( 15.92812500061451608, -4.541064518000419881, 2.621784821874995952 ) ) ;
#5004=ORIENTED_EDGE ( 'NONE', *, *, #39247, .F. ) ;
#5005=CARTESIAN_POINT ( 'NONE',  ( 18.89999999999999858, -4.330127018922190985, -2.500000000000001332 ) ) ;
#5006=CARTESIAN_POINT ( 'NONE',  ( 21.00937500061451857, -4.541064518000417216, -2.621784821875001281 ) ) ;
#5007=CARTESIAN_POINT ( 'NONE',  ( 28.67812500061451431, 6.421520780324663323E-16, -5.243569643749999010 ) ) ;
#5008=VERTEX_POINT ( 'NONE', #49902 ) ;
#5009=CARTESIAN_POINT ( 'NONE',  ( 19.91250000000000142, 2.886751345948129099, -4.999999999999997335 ) ) ;
#5010=CARTESIAN_POINT ( 'NONE',  ( 9.703125000614514661, -4.541064518000417216, -2.621784821875001281 ) ) ;
#5011=LINE ( 'NONE', #28271, #13668 ) ;
#5013=CARTESIAN_POINT ( 'NONE',  ( 16.64999999999999858, -4.330127018922190985, -2.500000000000001332 ) ) ;
#5014=CARTESIAN_POINT ( 'NONE',  ( 23.51249999999999574, 2.886751345948129099, -4.999999999999998224 ) ) ;
#5015=CARTESIAN_POINT ( 'NONE',  ( -4.243569643749999898, 19.76562500061451644, 27.54997392385601529 ) ) ;
#5016=CARTESIAN_POINT ( 'NONE',  ( 3.384375000614517237, -4.541064518000419881, 2.621784821874995952 ) ) ;
#5017=CARTESIAN_POINT ( 'NONE',  ( 29.33437500061451431, 4.541064518000418104, 2.621784821874999949 ) ) ;
#5018=ORIENTED_EDGE ( 'NONE', *, *, #56586, .F. ) ;
#5019=CARTESIAN_POINT ( 'NONE',  ( 24.21562500061451573, 3.027376345333613106, -5.243569643749998122 ) ) ;
#5020=CARTESIAN_POINT ( 'NONE',  ( 25.92187500061451999, -6.054752690667223547, -1.112240025338166033E-15 ) ) ;
#5021=CARTESIAN_POINT ( 'NONE',  ( 2.121784821875001281, 19.05312500061459247, -26.32496088578401938 ) ) ;
#5022=CARTESIAN_POINT ( 'NONE',  ( 13.95000000000000107, -4.330127018922190985, -2.500000000000001332 ) ) ;
#5023=CARTESIAN_POINT ( 'NONE',  ( 12.36562500061451608, -6.054752690667223547, -1.112240025338166033E-15 ) ) ;
#5024=CARTESIAN_POINT ( 'NONE',  ( 25.82812500061451644, -4.541064518000419881, 2.621784821874995952 ) ) ;
#5025=CARTESIAN_POINT ( 'NONE',  ( 16.80000000122903359, -2.886751345948125991, -5.000000000000000000 ) ) ;
#5027=CARTESIAN_POINT ( 'NONE',  ( 2.840625000614518392, -3.027376345333614438, 5.243569643749998122 ) ) ;
#5028=CARTESIAN_POINT ( 'NONE',  ( 21.79687500061451644, -3.027376345333614438, 5.243569643749998122 ) ) ;
#5030=CARTESIAN_POINT ( 'NONE',  ( -4.243569643749999898, 15.35937500061451644, 30.00000000000000000 ) ) ;
#5031=CARTESIAN_POINT ( 'NONE',  ( 22.05937500061451573, 4.541064518000418104, -2.621784821874998173 ) ) ;
#5032=CARTESIAN_POINT ( 'NONE',  ( 29.10937500061451644, -4.541064518000417216, -2.621784821875001281 ) ) ;
#5034=CARTESIAN_POINT ( 'NONE',  ( 9.065625000614517148, 3.027376345333611329, 5.243569643749999010 ) ) ;
#5035=CARTESIAN_POINT ( 'NONE',  ( 30.00000000000000000, 0.000000000000000000, 0.000000000000000000 ) ) ;
#5037=CARTESIAN_POINT ( 'NONE',  ( 7.284375000614518036, 4.541064518000418104, 2.621784821874999949 ) ) ;
#5038=CARTESIAN_POINT ( 'NONE',  ( 14.13750000122903394, 6.123233995736764310E-16, -4.999999999999998224 ) ) ;
#5039=CARTESIAN_POINT ( 'NONE',  ( 7.790625000614518569, -3.027376345333614438, 5.243569643749998122 ) ) ;
#5040=CARTESIAN_POINT ( 'NONE',  ( 12.98437500061451821, 6.421520780324663323E-16, -5.243569643749999010 ) ) ;
#5041=LINE ( 'NONE', #37187, #56939 ) ;
#5042=CARTESIAN_POINT ( 'NONE',  ( 19.46250000122903145, -4.330127018922190985, -2.500000000000001332 ) ) ;
#5043=CARTESIAN_POINT ( 'NONE',  ( 6.871875000614517504, 3.027376345333611329, 5.243569643749999010 ) ) ;
#5044=CARTESIAN_POINT ( 'NONE',  ( 10.41562500061451679, 3.027376345333611329, 5.243569643749999010 ) ) ;
#5045=CARTESIAN_POINT ( 'NONE',  ( 7.040625000614517681, -3.027376345333610441, -5.243569643749999898 ) ) ;
#5047=CARTESIAN_POINT ( 'NONE',  ( 18.49687500061452283, 6.054752690667223547, 3.707466751127219781E-16 ) ) ;
#5048=CARTESIAN_POINT ( 'NONE',  ( 4.575260086717170438, 2.016679235498957112, 4.840250765194281435 ) ) ;
#5049=CARTESIAN_POINT ( 'NONE',  ( 12.59062500061451573, 6.054752690667223547, 3.707466751127219781E-16 ) ) ;
#5050=CARTESIAN_POINT ( 'NONE',  ( 29.63437500061451502, 6.421520780324663323E-16, -5.243569643749999010 ) ) ;
#5051=CARTESIAN_POINT ( 'NONE',  ( 4.243569643749999010, 12.92187500061451999, -32.45002607614398471 ) ) ;
#5052=CARTESIAN_POINT ( 'NONE',  ( 13.76250000122903394, 4.330127018922192761, -2.499999999999997780 ) ) ;
#5053=CARTESIAN_POINT ( 'NONE',  ( -4.243569643749997233, 15.34062500061451750, -27.54997392385601174 ) ) ;
#5054=CARTESIAN_POINT ( 'NONE',  ( 15.48750000122903359, 6.123233995736764310E-16, -4.999999999999998224 ) ) ;
#5055=CARTESIAN_POINT ( 'NONE',  ( 11.31562500061451892, 3.027376345333611329, 5.243569643749999010 ) ) ;
#5056=ORIENTED_EDGE ( 'NONE', *, *, #30947, .F. ) ;
#5057=CARTESIAN_POINT ( 'NONE',  ( 14.13750000000000107, 5.773502691896255534, 3.535250795749688894E-16 ) ) ;
#5058=DIRECTION ( 'NONE',  ( -0.000000000000000000, -1.000000000000000000, -0.000000000000000000 ) ) ;
#5059=CARTESIAN_POINT ( 'NONE',  ( 22.86562500061451431, 3.027376345333613106, -5.243569643749998122 ) ) ;
#5060=CARTESIAN_POINT ( 'NONE',  ( 6.946875000614517681, -3.027376345333614438, 5.243569643749998122 ) ) ;
#5061=CARTESIAN_POINT ( 'NONE',  ( 11.36250000122903536, -4.330127018922190985, -2.500000000000001332 ) ) ;
#5063=CARTESIAN_POINT ( 'NONE',  ( 19.08750000122903145, 6.123233995736764310E-16, -4.999999999999998224 ) ) ;
#5064=CARTESIAN_POINT ( 'NONE',  ( 14.84062500061451750, 6.054752690667223547, 3.707466751127219781E-16 ) ) ;
#5065=CARTESIAN_POINT ( 'NONE',  ( 17.61562500061451786, 3.027376345333611329, 5.243569643749999010 ) ) ;
#5066=CARTESIAN_POINT ( 'NONE',  ( 25.42500000122903359, 2.886751345948129099, -4.999999999999998224 ) ) ;
#5068=CARTESIAN_POINT ( 'NONE',  ( 28.80000000122903003, -2.886751345948129988, 4.999999999999997335 ) ) ;
#5069=CARTESIAN_POINT ( 'NONE',  ( 23.92499999999999716, 6.123233995736764310E-16, -4.999999999999998224 ) ) ;
#5071=CARTESIAN_POINT ( 'NONE',  ( 25.47187500061451715, -6.054752690667223547, -1.112240025338166033E-15 ) ) ;
#5072=CARTESIAN_POINT ( 'NONE',  ( 18.30000000122903359, 5.773502691896255534, 3.535250795749688401E-16 ) ) ;
#5073=CARTESIAN_POINT ( 'NONE',  ( 13.57500000122903572, -5.773502691896255534, -1.060575238724906372E-15 ) ) ;
#5074=CARTESIAN_POINT ( 'NONE',  ( 28.35937500061451289, 4.541064518000418104, -2.621784821874998173 ) ) ;
#5075=( BOUNDED_CURVE ( )  B_SPLINE_CURVE ( 2, ( #52866, #42515, #65039, #24419, #18864, #35508, #14430 ),
 .UNSPECIFIED., .F., .F. ) 
 B_SPLINE_CURVE_WITH_KNOTS ( ( 3, 2, 2, 3 ),
 ( 0.3083333333333333481, 0.3111111111111111160, 0.3138888888888888840, 0.3166666666666666519 ),
 .UNSPECIFIED. ) 
 CURVE ( )  GEOMETRIC_REPRESENTATION_ITEM ( )  RATIONAL_B_SPLINE_CURVE ( ( 1.000000000000000000, 0.8660254037844387076, 1.000000000000000000, 0.8660254037844387076, 1.000000000000000000, 0.8660254037844387076, 1.000000000000000000 ) ) 
 REPRESENTATION_ITEM ( '' )  );
#5077=CARTESIAN_POINT ( 'NONE',  ( 5.109375000614518214, 0.000000000000000000, 5.243569643749999010 ) ) ;
#5078=CARTESIAN_POINT ( 'NONE',  ( 23.65312500061451573, -4.541064518000417216, -2.621784821875001281 ) ) ;
#5080=CARTESIAN_POINT ( 'NONE',  ( 10.17187500061451999, -6.054752690667223547, -1.112240025338166033E-15 ) ) ;
#5081=DIRECTION ( 'NONE',  ( -1.000000000000000000, -0.000000000000000000, -0.000000000000000000 ) ) ;
#5082=CARTESIAN_POINT ( 'NONE',  ( 29.65312500061451573, 4.541064518000418104, -2.621784821874998173 ) ) ;
#5083=CARTESIAN_POINT ( 'NONE',  ( 5.859375000614519102, 4.541064518000418104, -2.621784821874998173 ) ) ;
#5084=CARTESIAN_POINT ( 'NONE',  ( 28.84687500061452070, 6.054752690667223547, 3.707466751127219781E-16 ) ) ;
#5086=CARTESIAN_POINT ( 'NONE',  ( 18.78749999999999432, -2.886751345948129988, 4.999999999999997335 ) ) ;
#5087=ORIENTED_EDGE ( 'NONE', *, *, #33984, .T. ) ;
#5088=CARTESIAN_POINT ( 'NONE',  ( 28.08749999999999858, 5.773502691896255534, 3.535250795749688894E-16 ) ) ;
#5089=CARTESIAN_POINT ( 'NONE',  ( 28.17187500061451644, -6.054752690667223547, -1.112240025338166033E-15 ) ) ;
#5091=CARTESIAN_POINT ( 'NONE',  ( 18.44062500061451715, 6.054752690667223547, 3.707466751127219781E-16 ) ) ;
#5092=CARTESIAN_POINT ( 'NONE',  ( 8.428125000614517859, 6.421520780324663323E-16, -5.243569643749999010 ) ) ;
#5094=CARTESIAN_POINT ( 'NONE',  ( 4.096875000614518925, 6.054752690667223547, 3.707466751127219781E-16 ) ) ;
#5095=CARTESIAN_POINT ( 'NONE',  ( 17.70000000122903216, -2.886751345948125991, -5.000000000000000000 ) ) ;
#5096=CARTESIAN_POINT ( 'NONE',  ( 4.000000000000000000, 13.88750000000000107, -27.69059892324149885 ) ) ;
#5097=CARTESIAN_POINT ( 'NONE',  ( 6.384375000614516793, 4.541064518000418104, 2.621784821874999949 ) ) ;
#5098=CARTESIAN_POINT ( 'NONE',  ( 11.03437500061451715, -4.541064518000419881, 2.621784821874995952 ) ) ;
#5099=CARTESIAN_POINT ( 'NONE',  ( 20.70937500061451786, 4.541064518000418104, -2.621784821874998173 ) ) ;
#5103=CARTESIAN_POINT ( 'NONE',  ( 18.60937500061451644, 0.000000000000000000, 5.243569643749999010 ) ) ;
#5104=CARTESIAN_POINT ( 'NONE',  ( 10.32187500061451679, 3.027376345333613106, -5.243569643749998122 ) ) ;
#5106=CARTESIAN_POINT ( 'NONE',  ( 20.66250000000000142, -5.773502691896255534, -1.060575238724906372E-15 ) ) ;
#5107=CARTESIAN_POINT ( 'NONE',  ( 18.21562500061451573, -6.054752690667223547, -1.112240025338166033E-15 ) ) ;
#5109=CARTESIAN_POINT ( 'NONE',  ( -0.7368805616696193495, 9.859898480082234684, -34.17910162106521454 ) ) ;
#5111=CARTESIAN_POINT ( 'NONE',  ( 12.92812500061451786, 6.421520780324663323E-16, -5.243569643749999010 ) ) ;
#5112=CARTESIAN_POINT ( 'NONE',  ( 29.07187500061451502, -6.054752690667223547, -1.112240025338166033E-15 ) ) ;
#5113=CYLINDRICAL_SURFACE ( 'NONE', #5401, 3.999999999999996447 ) ;
#5114=CARTESIAN_POINT ( 'NONE',  ( 28.84687500061452070, 6.054752690667223547, 3.707466751127219781E-16 ) ) ;
#5115=CARTESIAN_POINT ( 'NONE',  ( 9.449999999999999289, -4.330127018922190985, -2.500000000000001332 ) ) ;
#5116=CARTESIAN_POINT ( 'NONE',  ( 3.999999999999998668, 14.97500000122903430, 27.69059892324149175 ) ) ;
#5117=CARTESIAN_POINT ( 'NONE',  ( 9.937500001229032875, -4.330127018922194537, 2.499999999999995559 ) ) ;
#5118=CARTESIAN_POINT ( 'NONE',  ( 19.58437500061451786, -4.541064518000419881, 2.621784821874995952 ) ) ;
#5119=CARTESIAN_POINT ( 'NONE',  ( 15.23437500061451644, 6.421520780324663323E-16, -5.243569643749999010 ) ) ;
#5120=FACE_OUTER_BOUND ( 'NONE', #62854, .T. ) ;
#5121=ORIENTED_EDGE ( 'NONE', *, *, #30962, .T. ) ;
#5122=CARTESIAN_POINT ( 'NONE',  ( 14.87812500061451537, 4.541064518000418104, 2.621784821874999949 ) ) ;
#5123=CARTESIAN_POINT ( 'NONE',  ( 28.91250000122903074, -4.330127018922190985, -2.500000000000001332 ) ) ;
#5124=CARTESIAN_POINT ( 'NONE',  ( 14.48437500061451821, 4.541064518000418104, 2.621784821874999949 ) ) ;
#5125=CARTESIAN_POINT ( 'NONE',  ( 3.028125000614518392, 6.421520780324663323E-16, -5.243569643749999010 ) ) ;
#5126=CARTESIAN_POINT ( 'NONE',  ( 16.26562500061451289, 3.027376345333611329, 5.243569643749999010 ) ) ;
#5127=FACE_OUTER_BOUND ( 'NONE', #9234, .T. ) ;
#5128=CARTESIAN_POINT ( 'NONE',  ( 26.97187500061451360, 3.027376345333613106, -5.243569643749998122 ) ) ;
#5129=FACE_OUTER_BOUND ( 'NONE', #7076, .T. ) ;
#5130=CARTESIAN_POINT ( 'NONE',  ( 15.34687500061451537, 6.054752690667223547, 3.707466751127219781E-16 ) ) ;
#5131=CARTESIAN_POINT ( 'NONE',  ( 13.23750000122903359, 6.123233995736764310E-16, -4.999999999999998224 ) ) ;
#5133=CARTESIAN_POINT ( 'NONE',  ( -4.243569643749999898, 19.82187500061451857, -32.45002607614398471 ) ) ;
#5134=CARTESIAN_POINT ( 'NONE',  ( 21.23437500061451644, 4.541064518000418104, 2.621784821874999949 ) ) ;
#5135=CARTESIAN_POINT ( 'NONE',  ( 21.71250000122903501, -4.330127018922190985, -2.500000000000001332 ) ) ;
#5136=CARTESIAN_POINT ( 'NONE',  ( 18.23437500061451999, -4.541064518000419881, 2.621784821874995952 ) ) ;
#5137=CARTESIAN_POINT ( 'NONE',  ( 4.243569643749999010, 11.57187500061451679, 27.54997392385601174 ) ) ;
#5138=CARTESIAN_POINT ( 'NONE',  ( 17.84062500061451573, -3.027376345333610441, -5.243569643749999898 ) ) ;
#5139=ORIENTED_EDGE ( 'NONE', *, *, #28806, .F. ) ;
#5140=VERTEX_POINT ( 'NONE', #55806 ) ;
#5141=CARTESIAN_POINT ( 'NONE',  ( 20.66250000000000142, -5.773502691896255534, -1.060575238724906372E-15 ) ) ;
#5142=CARTESIAN_POINT ( 'NONE',  ( 28.16250000122903074, 4.330127018922192761, -2.499999999999997780 ) ) ;
#5143=CARTESIAN_POINT ( 'NONE',  ( 23.72812500061451502, 6.421520780324663323E-16, -5.243569643749999010 ) ) ;
#5144=CARTESIAN_POINT ( 'NONE',  ( 4.415625000614518569, 3.027376345333613106, -5.243569643749998122 ) ) ;
#5145=CARTESIAN_POINT ( 'NONE',  ( 16.35000000122903430, -2.886751345948125991, -5.000000000000000000 ) ) ;
#5146=CARTESIAN_POINT ( 'NONE',  ( 22.30312500061451431, -4.541064518000417216, -2.621784821875001281 ) ) ;
#5147=CARTESIAN_POINT ( 'NONE',  ( 21.37499999999999645, 4.330127018922191873, 2.499999999999999556 ) ) ;
#5148=CARTESIAN_POINT ( 'NONE',  ( 26.31562500061451715, -6.054752690667223547, -1.112240025338166033E-15 ) ) ;
#5149=CARTESIAN_POINT ( 'NONE',  ( 4.903125000614516615, 4.541064518000418104, -2.621784821874998173 ) ) ;
#5150=ORIENTED_EDGE ( 'NONE', *, *, #7878, .T. ) ;
#5152=CARTESIAN_POINT ( 'NONE',  ( 29.62500000000000000, -4.330127018922194537, 2.499999999999995559 ) ) ;
#5153=CARTESIAN_POINT ( 'NONE',  ( 3.703125000614516882, 0.000000000000000000, 5.243569643749999010 ) ) ;
#5155=CARTESIAN_POINT ( 'NONE',  ( 3.999999999999998668, 18.91249999999999787, 27.69059892324149530 ) ) ;
#5156=CARTESIAN_POINT ( 'NONE',  ( 3.999999999999998668, 11.82500000122903572, -32.30940107675850470 ) ) ;
#5157=CARTESIAN_POINT ( 'NONE',  ( 9.001249775931846008E-16, 17.72187500061451715, -25.09994784771203058 ) ) ;
#5158=CARTESIAN_POINT ( 'NONE',  ( 9.337500000000000355, -2.886751345948129988, 4.999999999999997335 ) ) ;
#5159=CARTESIAN_POINT ( 'NONE',  ( 9.984375000614518214, 4.541064518000418104, 2.621784821874999949 ) ) ;
#5160=CARTESIAN_POINT ( 'NONE',  ( 7.537500001229033408, 4.330127018922191873, 2.499999999999999556 ) ) ;
#5161=CARTESIAN_POINT ( 'NONE',  ( 12.57187500061451857, 3.027376345333613106, -5.243569643749998122 ) ) ;
#5162=LINE ( 'NONE', #8236, #11193 ) ;
#5163=CARTESIAN_POINT ( 'NONE',  ( 3.196875000614516793, 6.054752690667223547, 3.707466751127219781E-16 ) ) ;
#5166=CARTESIAN_POINT ( 'NONE',  ( 9.084375000614517859, 4.541064518000418104, 2.621784821874999949 ) ) ;
#5167=CARTESIAN_POINT ( 'NONE',  ( 1.626862140677534273E-15, 13.92500000122903181, -26.00000000000000355 ) ) ;
#5168=CARTESIAN_POINT ( 'NONE',  ( 19.07812500061451644, -4.541064518000419881, 2.621784821874995952 ) ) ;
#5170=CARTESIAN_POINT ( 'NONE',  ( 9.001249775931846008E-16, 18.11562500061459602, 34.90005215228797653 ) ) ;
#5171=CARTESIAN_POINT ( 'NONE',  ( 23.82187500061451502, 3.027376345333613106, -5.243569643749998122 ) ) ;
#5173=CARTESIAN_POINT ( 'NONE',  ( 2.878125000614517592, -4.541064518000419881, 2.621784821874995952 ) ) ;
#5175=CARTESIAN_POINT ( 'NONE',  ( 24.92812500061451431, -4.541064518000419881, 2.621784821874995952 ) ) ;
#5176=CARTESIAN_POINT ( 'NONE',  ( 15.81562500061451537, 3.027376345333611329, 5.243569643749999010 ) ) ;
#5178=CARTESIAN_POINT ( 'NONE',  ( 13.28437500061451715, -4.541064518000419881, 2.621784821874995952 ) ) ;
#5179=CARTESIAN_POINT ( 'NONE',  ( 25.01250000122903216, 4.330127018922192761, -2.499999999999997780 ) ) ;
#5180=CARTESIAN_POINT ( 'NONE',  ( 3.946875000614517681, -3.027376345333610441, -5.243569643749999898 ) ) ;
#5181=CARTESIAN_POINT ( 'NONE',  ( 13.32187500061451502, -6.054752690667223547, -1.112240025338166033E-15 ) ) ;
#5182=CARTESIAN_POINT ( 'NONE',  ( -1.071796769724488563, 11.99240381056766758, 34.00000000000000000 ) ) ;
#5183=DIRECTION ( 'NONE',  ( -1.000000000000000000, -0.000000000000000000, -0.000000000000000000 ) ) ;
#5184=CARTESIAN_POINT ( 'NONE',  ( -2.000000000000000000, 11.93750000122903465, 26.53589838486224650 ) ) ;
#5185=CARTESIAN_POINT ( 'NONE',  ( 24.90937500061451715, 0.000000000000000000, 5.243569643749999010 ) ) ;
#5186=CARTESIAN_POINT ( 'NONE',  ( 16.32187500061451502, 3.027376345333611329, 5.243569643749999010 ) ) ;
#5188=CARTESIAN_POINT ( 'NONE',  ( 28.57499999999999929, 4.330127018922191873, 2.499999999999999556 ) ) ;
#5189=CARTESIAN_POINT ( 'NONE',  ( 4.462500001229035007, 0.000000000000000000, 4.999999999999998224 ) ) ;
#5190=CARTESIAN_POINT ( 'NONE',  ( 5.212500000000002132, 2.886751345948126879, 4.999999999999999112 ) ) ;
#5192=CARTESIAN_POINT ( 'NONE',  ( 18.62812500061451715, -4.541064518000419881, 2.621784821874995952 ) ) ;
#5193=CARTESIAN_POINT ( 'NONE',  ( 9.712500000000002132, 2.886751345948126879, 4.999999999999999112 ) ) ;
#5194=CARTESIAN_POINT ( 'NONE',  ( 17.62500000000000000, 6.123233995736764310E-16, -4.999999999999998224 ) ) ;
#5195=CARTESIAN_POINT ( 'NONE',  ( 19.87500000122903288, -5.773502691896255534, -1.060575238724906372E-15 ) ) ;
#5196=CARTESIAN_POINT ( 'NONE',  ( -3.999999999999997335, 10.13750000000000284, -27.69059892324149530 ) ) ;
#5197=CARTESIAN_POINT ( 'NONE',  ( 27.90937500061451715, 4.541064518000418104, -2.621784821874998173 ) ) ;
#5198=ORIENTED_EDGE ( 'NONE', *, *, #3972, .F. ) ;
#5199=CARTESIAN_POINT ( 'NONE',  ( 18.02812500061451573, 4.541064518000418104, 2.621784821874999949 ) ) ;
#5200=CARTESIAN_POINT ( 'NONE',  ( 21.06562500061451715, 3.027376345333613106, -5.243569643749998122 ) ) ;
#5201=CARTESIAN_POINT ( 'NONE',  ( 22.77187500061451786, -6.054752690667223547, -1.112240025338166033E-15 ) ) ;
#5202=CARTESIAN_POINT ( 'NONE',  ( 5.512499999999999289, 2.886751345948129099, -4.999999999999998224 ) ) ;
#5203=CARTESIAN_POINT ( 'NONE',  ( 9.253125000614517148, -4.541064518000417216, -2.621784821875001281 ) ) ;
#5204=CARTESIAN_POINT ( 'NONE',  ( 23.76562500061451644, 3.027376345333613106, -5.243569643749998122 ) ) ;
#5205=CARTESIAN_POINT ( 'NONE',  ( 14.78437500061451715, 6.421520780324663323E-16, -5.243569643749999010 ) ) ;
#5206=CARTESIAN_POINT ( 'NONE',  ( 19.80937500061451573, 4.541064518000418104, -2.621784821874998173 ) ) ;
#5208=CARTESIAN_POINT ( 'NONE',  ( 2.121784821874999061, 19.20312500061451644, 26.32496088578401583 ) ) ;
#5209=CARTESIAN_POINT ( 'NONE',  ( 21.71250000122903501, -4.330127018922190985, -2.500000000000001332 ) ) ;
#5211=CARTESIAN_POINT ( 'NONE',  ( 12.96562500061451928, 3.027376345333612662, -5.243569643749998122 ) ) ;
#5212=CARTESIAN_POINT ( 'NONE',  ( 4.396875000614516971, -3.027376345333610441, -5.243569643749999898 ) ) ;
#5213=CARTESIAN_POINT ( 'NONE',  ( 6.309375000614517504, 4.541064518000418104, -2.621784821874998173 ) ) ;
#5215=CARTESIAN_POINT ( 'NONE',  ( 27.15937500061451360, 0.000000000000000000, 5.243569643749999010 ) ) ;
#5216=CARTESIAN_POINT ( 'NONE',  ( 19.75312500061451360, 4.541064518000418104, -2.621784821874998173 ) ) ;
#5217=CARTESIAN_POINT ( 'NONE',  ( 29.58750000122903501, 4.330127018922191873, 2.499999999999999556 ) ) ;
#5218=CARTESIAN_POINT ( 'NONE',  ( 28.34062500061451928, 6.054752690667223547, 3.707466751127219781E-16 ) ) ;
#5219=CARTESIAN_POINT ( 'NONE',  ( 23.59687500061451715, -3.027376345333614438, 5.243569643749998122 ) ) ;
#5220=CARTESIAN_POINT ( 'NONE',  ( 19.71562500061451928, 3.027376345333613106, -5.243569643749998122 ) ) ;
#5221=CARTESIAN_POINT ( 'NONE',  ( -1.999999999999997113, 10.17500000000000249, 33.46410161513775705 ) ) ;
#5222=CARTESIAN_POINT ( 'NONE',  ( 25.37812500061451715, -4.541064518000419881, 2.621784821874995952 ) ) ;
#5223=CARTESIAN_POINT ( 'NONE',  ( 5.850000001229035185, -2.886751345948129988, 4.999999999999997335 ) ) ;
#5225=CARTESIAN_POINT ( 'NONE',  ( 28.04999999999999716, 4.330127018922192761, -2.499999999999997780 ) ) ;
#5226=CARTESIAN_POINT ( 'NONE',  ( -2.000000000000000000, 15.87500000000000000, -33.46410161513775705 ) ) ;
#5228=EDGE_CURVE ( 'NONE', #63939, #71801, #31182, .T. ) ;
#5229=CARTESIAN_POINT ( 'NONE',  ( 5.296875000614518214, -3.027376345333610441, -5.243569643749999898 ) ) ;
#5230=CARTESIAN_POINT ( 'NONE',  ( 13.45312500061451466, 4.541064518000418104, -2.621784821874998173 ) ) ;
#5231=CARTESIAN_POINT ( 'NONE',  ( 6.196875000614515905, -3.027376345333610441, -5.243569643749999898 ) ) ;
#5232=CARTESIAN_POINT ( 'NONE',  ( 23.58750000122903145, 6.123233995736764310E-16, -4.999999999999998224 ) ) ;
#5233=CARTESIAN_POINT ( 'NONE',  ( 14.10937500061451644, 0.000000000000000000, 5.243569643749999010 ) ) ;
#5234=CARTESIAN_POINT ( 'NONE',  ( 2.896875000614518747, -3.027376345333614438, 5.243569643749998122 ) ) ;
#5235=CARTESIAN_POINT ( 'NONE',  ( 27.15000000000000213, 4.330127018922192761, -2.499999999999997780 ) ) ;
#5236=( BOUNDED_CURVE ( )  B_SPLINE_CURVE ( 2, ( #29825, #70446, #19448, #52360, #1764, #35725, #41285 ),
 .UNSPECIFIED., .F., .F. ) 
 B_SPLINE_CURVE_WITH_KNOTS ( ( 3, 2, 2, 3 ),
 ( 0.01666666666666663174, 0.01944444444444440312, 0.02222222222222217797, 0.02499999999999994935 ),
 .UNSPECIFIED. ) 
 CURVE ( )  GEOMETRIC_REPRESENTATION_ITEM ( )  RATIONAL_B_SPLINE_CURVE ( ( 1.000000000000001554, 0.8660254037844370423, 1.000000000000000000, 0.8660254037844387076, 1.000000000000000000, 0.8660254037844412611, 0.9999999999999974465 ) ) 
 REPRESENTATION_ITEM ( '' )  );
#5237=CARTESIAN_POINT ( 'NONE',  ( 25.54687500061451644, -3.027376345333610441, -5.243569643749999898 ) ) ;
#5238=CARTESIAN_POINT ( 'NONE',  ( 2.878125000614517592, -4.541064518000419881, 2.621784821874995952 ) ) ;
#5239=CARTESIAN_POINT ( 'NONE',  ( 13.41562500061451502, 3.027376345333613106, -5.243569643749998122 ) ) ;
#5240=ORIENTED_EDGE ( 'NONE', *, *, #14959, .F. ) ;
#5241=CARTESIAN_POINT ( 'NONE',  ( 9.815625000614518925, 3.027376345333613106, -5.243569643749998122 ) ) ;
#5242=VECTOR ( 'NONE', #12140, 1000.000000000000000 ) ;
#5243=CARTESIAN_POINT ( 'NONE',  ( 7.190625000614518036, 6.054752690667223547, 3.707466751127219781E-16 ) ) ;
#5246=CARTESIAN_POINT ( 'NONE',  ( 15.18750000000000000, -2.886751345948129988, 4.999999999999997335 ) ) ;
#5247=CARTESIAN_POINT ( 'NONE',  ( 16.17187500061451644, 3.027376345333613106, -5.243569643749998122 ) ) ;
#5248=CARTESIAN_POINT ( 'NONE',  ( 13.80000000122903181, 5.773502691896255534, 3.535250795749688894E-16 ) ) ;
#5250=CARTESIAN_POINT ( 'NONE',  ( 20.44687500061451857, -3.027376345333614438, 5.243569643749998122 ) ) ;
#5251=CARTESIAN_POINT ( 'NONE',  ( -4.243569643749997233, 13.09062500061451750, -27.54997392385601174 ) ) ;
#5255=CARTESIAN_POINT ( 'NONE',  ( 26.35312500061451857, -4.541064518000417216, -2.621784821875001281 ) ) ;
#5256=CARTESIAN_POINT ( 'NONE',  ( 0.000000000000000000, 20.00000000000000000, -30.00000000000000000 ) ) ;
#5257=CARTESIAN_POINT ( 'NONE',  ( 26.13749999999999929, -2.886751345948125991, -5.000000000000000000 ) ) ;
#5258=CARTESIAN_POINT ( 'NONE',  ( 9.928125000614517859, 4.541064518000418104, 2.621784821874999949 ) ) ;
#5260=CARTESIAN_POINT ( 'NONE',  ( 20.70937500061451786, 4.541064518000418104, -2.621784821874998173 ) ) ;
#5262=CARTESIAN_POINT ( 'NONE',  ( 5.015625000614518214, 3.027376345333611329, 5.243569643749999010 ) ) ;
#5263=CARTESIAN_POINT ( 'NONE',  ( 10.88437500061451679, 4.541064518000418104, 2.621784821874999949 ) ) ;
#5264=EDGE_LOOP ( 'NONE', ( #109, #35021, #31232, #31401 ) ) ;
#5265=CARTESIAN_POINT ( 'NONE',  ( 20.67187500061451289, 3.027376345333613106, -5.243569643749998122 ) ) ;
#5266=DIRECTION ( 'NONE',  ( -1.000000000000000000, -0.000000000000000000, -0.000000000000000000 ) ) ;
#5267=FACE_OUTER_BOUND ( 'NONE', #61046, .T. ) ;
#5268=( BOUNDED_CURVE ( )  B_SPLINE_CURVE ( 2, ( #30, #381, #62067, #45808, #6278, #22888, #28807 ),
 .UNSPECIFIED., .F., .F. ) 
 B_SPLINE_CURVE_WITH_KNOTS ( ( 3, 2, 2, 3 ),
 ( 0.5916666666666667851, 0.5944444444444445530, 0.5972222222222222099, 0.5999999999999999778 ),
 .UNSPECIFIED. ) 
 CURVE ( )  GEOMETRIC_REPRESENTATION_ITEM ( )  RATIONAL_B_SPLINE_CURVE ( ( 0.9999999999999946709, 0.8660254037844440367, 1.000000000000000000, 0.8660254037844387076, 1.000000000000000000, 0.8660254037844387076, 1.000000000000000000 ) ) 
 REPRESENTATION_ITEM ( '' )  );
#5269=CARTESIAN_POINT ( 'NONE',  ( 4.200000000000001954, 4.330127018922192761, -2.499999999999997780 ) ) ;
#5270=CARTESIAN_POINT ( 'NONE',  ( 13.76250000122903394, 4.330127018922192761, -2.499999999999997780 ) ) ;
#5272=CARTESIAN_POINT ( 'NONE',  ( 3.760358691118133034, -3.295428057128597210, 4.078640785394780366 ) ) ;
#5273=ORIENTED_EDGE ( 'NONE', *, *, #29804, .T. ) ;
#5274=CARTESIAN_POINT ( 'NONE',  ( 13.16249999999999964, 2.886751345948129099, -4.999999999999998224 ) ) ;
#5275=CARTESIAN_POINT ( 'NONE',  ( 15.82499999999999929, 6.123233995736764310E-16, -4.999999999999998224 ) ) ;
#5276=CARTESIAN_POINT ( 'NONE',  ( 12.11250000122903181, 0.000000000000000000, 4.999999999999998224 ) ) ;
#5277=CARTESIAN_POINT ( 'NONE',  ( 11.16562500061451679, 3.027376345333613106, -5.243569643749998122 ) ) ;
#5279=CARTESIAN_POINT ( 'NONE',  ( 9.412499999999999645, -5.773502691896255534, -1.060575238724906372E-15 ) ) ;
#5280=CARTESIAN_POINT ( 'NONE',  ( -1.071796769724491005, 15.52009619066136814, 26.00000000000000355 ) ) ;
#5281=CARTESIAN_POINT ( 'NONE',  ( -4.243569643749999898, 14.42187500061451644, -32.45002607614398471 ) ) ;
#5282=CARTESIAN_POINT ( 'NONE',  ( 29.10000000122903074, 5.773502691896255534, 3.535250795749688894E-16 ) ) ;
#5284=CARTESIAN_POINT ( 'NONE',  ( 7.462500000000001243, 2.886751345948126879, 4.999999999999999112 ) ) ;
#5286=VECTOR ( 'NONE', #42221, 1000.000000000000000 ) ;
#5287=VERTEX_POINT ( 'NONE', #57239 ) ;
#5288=CARTESIAN_POINT ( 'NONE',  ( 25.49062500061451786, -3.027376345333610441, -5.243569643749999898 ) ) ;
#5289=CARTESIAN_POINT ( 'NONE',  ( 2.000000000000001332, 13.40000000000000213, -26.53589838486224650 ) ) ;
#5290=CARTESIAN_POINT ( 'NONE',  ( 18.97500000122903430, -5.773502691896255534, -1.060575238724906372E-15 ) ) ;
#5291=CARTESIAN_POINT ( 'NONE',  ( 21.90937500061451715, -4.541064518000417216, -2.621784821875001281 ) ) ;
#5293=CARTESIAN_POINT ( 'NONE',  ( 15.81562500061451537, 3.027376345333611329, 5.243569643749999010 ) ) ;
#5294=CARTESIAN_POINT ( 'NONE',  ( -2.121784821874996840, 11.32812500061459282, -26.32496088578401583 ) ) ;
#5295=CARTESIAN_POINT ( 'NONE',  ( 6.665625000614515905, 3.027376345333613106, -5.243569643749998122 ) ) ;
#5296=CARTESIAN_POINT ( 'NONE',  ( 28.50000000122903288, -2.886751345948125991, -5.000000000000000000 ) ) ;
#5298=CARTESIAN_POINT ( 'NONE',  ( 20.16562500061451502, 3.027376345333612662, -5.243569643749998122 ) ) ;
#5301=CARTESIAN_POINT ( 'NONE',  ( 14.93437500061451750, 4.541064518000418104, 2.621784821874999949 ) ) ;
#5303=CARTESIAN_POINT ( 'NONE',  ( 13.88437500061451679, 6.421520780324663323E-16, -5.243569643749999010 ) ) ;
#5304=CARTESIAN_POINT ( 'NONE',  ( 22.17187500061451644, 3.027376345333611329, 5.243569643749999010 ) ) ;
#5305=ORIENTED_EDGE ( 'NONE', *, *, #10249, .T. ) ;
#5306=CARTESIAN_POINT ( 'NONE',  ( -3.999999999999999112, 14.71250000122903501, -30.00000000000000000 ) ) ;
#5307=CARTESIAN_POINT ( 'NONE',  ( 27.32812500061451644, 6.421520780324663323E-16, -5.243569643749999010 ) ) ;
#5309=AXIS2_PLACEMENT_3D ( 'NONE', #15363, #60423, #9834 ) ;
#5310=CARTESIAN_POINT ( 'NONE',  ( 25.90312500061451573, -4.541064518000417216, -2.621784821875001281 ) ) ;
#5311=CARTESIAN_POINT ( 'NONE',  ( 1.071796769724491893, 12.03259618943233455, -26.00000000000000355 ) ) ;
#5312=CARTESIAN_POINT ( 'NONE',  ( -3.999999999999997335, 17.78750000000000142, 32.30940107675850470 ) ) ;
#5313=CARTESIAN_POINT ( 'NONE',  ( 5.784375000614517148, 6.421520780324663323E-16, -5.243569643749999010 ) ) ;
#5314=CARTESIAN_POINT ( 'NONE',  ( 11.06250000122903288, 4.330127018922192761, -2.499999999999997780 ) ) ;
#5315=VECTOR ( 'NONE', #27794, 1000.000000000000000 ) ;
#5316=CARTESIAN_POINT ( 'NONE',  ( 7.087500001229034119, 4.330127018922191873, 2.499999999999999556 ) ) ;
#5317=CARTESIAN_POINT ( 'NONE',  ( 3.403125000614518836, -4.541064518000417216, -2.621784821875001281 ) ) ;
#5320=CARTESIAN_POINT ( 'NONE',  ( 12.83437500061451786, -4.541064518000419881, 2.621784821874995952 ) ) ;
#5321=CARTESIAN_POINT ( 'NONE',  ( -5.810221930991193690E-16, 12.23750000000000071, 26.00000000000000355 ) ) ;
#5323=CARTESIAN_POINT ( 'NONE',  ( 19.19062500061452070, -3.027376345333610441, -5.243569643749999898 ) ) ;
#5324=CARTESIAN_POINT ( 'NONE',  ( 12.94687500061451857, -3.027376345333610441, -5.243569643749999898 ) ) ;
#5325=CARTESIAN_POINT ( 'NONE',  ( 5.803125000614517859, 4.541064518000418104, -2.621784821874998173 ) ) ;
#5326=CARTESIAN_POINT ( 'NONE',  ( 21.12187500061451573, 3.027376345333612662, -5.243569643749998122 ) ) ;
#5327=CARTESIAN_POINT ( 'NONE',  ( 9.459375000614517859, 4.541064518000418104, -2.621784821874998173 ) ) ;
#5328=CARTESIAN_POINT ( 'NONE',  ( 4.640625000614518214, -3.027376345333614438, 5.243569643749998122 ) ) ;
#5329=CARTESIAN_POINT ( 'NONE',  ( 0.000000000000000000, 20.00000000000000000, 30.00000000000000000 ) ) ;
#5330=CARTESIAN_POINT ( 'NONE',  ( 5.212500001229032343, 4.330127018922192761, -2.499999999999997780 ) ) ;
#5331=CARTESIAN_POINT ( 'NONE',  ( 19.04062500061451146, -3.027376345333614438, 5.243569643749998122 ) ) ;
#5332=CARTESIAN_POINT ( 'NONE',  ( 7.237500001229035362, -4.330127018922194537, 2.499999999999995559 ) ) ;
#5333=( BOUNDED_CURVE ( )  B_SPLINE_CURVE ( 2, ( #21141, #49600, #38136, #16329, #32604, #61037, #67330, #72127, #72859 ),
 .UNSPECIFIED., .F., .F. ) 
 B_SPLINE_CURVE_WITH_KNOTS ( ( 3, 2, 2, 2, 3 ),
 ( 0.3586956521739130821, 0.3623188405797101441, 0.3695652173913043237, 0.3768115942028985588, 0.3804347826086956763 ),
 .UNSPECIFIED. ) 
 CURVE ( )  GEOMETRIC_REPRESENTATION_ITEM ( )  RATIONAL_B_SPLINE_CURVE ( ( 0.9330127018922194093, 0.9330127018922198534, 1.000000000000000000, 0.8660254037844387076, 1.000000000000000000, 0.8660254037844387076, 1.000000000000000000, 0.9330127018922188542, 0.9330127018922194093 ) ) 
 REPRESENTATION_ITEM ( '' )  );
#5334=CARTESIAN_POINT ( 'NONE',  ( 18.36562500061451431, 3.027376345333613106, -5.243569643749998122 ) ) ;
#5335=CARTESIAN_POINT ( 'NONE',  ( 15.32812500061451644, 4.541064518000418104, 2.621784821874999949 ) ) ;
#5337=CARTESIAN_POINT ( 'NONE',  ( 15.93750000000000000, 5.773502691896255534, 3.535250795749688894E-16 ) ) ;
#5338=CARTESIAN_POINT ( 'NONE',  ( 9.487500001229033586, -4.330127018922194537, 2.499999999999995559 ) ) ;
#5339=ADVANCED_FACE ( 'NONE', ( #33987 ), #12182, .F. ) ;
#5340=CARTESIAN_POINT ( 'NONE',  ( 4.640625000614518214, -3.027376345333614438, 5.243569643749998122 ) ) ;
#5341=CARTESIAN_POINT ( 'NONE',  ( 21.97500000122903074, 2.886751345948126879, 4.999999999999999112 ) ) ;
#5343=CARTESIAN_POINT ( 'NONE',  ( -2.121784821874996840, 13.63437500061451857, -26.32496088578401583 ) ) ;
#5344=CARTESIAN_POINT ( 'NONE',  ( 21.22500000000000142, 6.123233995736764310E-16, -4.999999999999998224 ) ) ;
#5345=CARTESIAN_POINT ( 'NONE',  ( 3.525000001229034119, 2.886751345948126879, 4.999999999999999112 ) ) ;
#5346=CARTESIAN_POINT ( 'NONE',  ( 5.109375000614518214, 0.000000000000000000, 5.243569643749999010 ) ) ;
#5347=CARTESIAN_POINT ( 'NONE',  ( 20.44687500061451857, -3.027376345333614438, 5.243569643749998122 ) ) ;
#5348=CARTESIAN_POINT ( 'NONE',  ( -1.071796769724491005, 14.95759618943233527, 26.00000000000000355 ) ) ;
#5349=CARTESIAN_POINT ( 'NONE',  ( 17.39062500061451644, -3.027376345333610441, -5.243569643749999898 ) ) ;
#5351=CARTESIAN_POINT ( 'NONE',  ( -2.000000000000000000, 15.42500000000000071, -33.46410161513775705 ) ) ;
#5352=CARTESIAN_POINT ( 'NONE',  ( 1.592000809091587073E-14, 15.38750000000000284, 26.00000000000000000 ) ) ;
#5353=CARTESIAN_POINT ( 'NONE',  ( 28.24687500061451573, -3.027376345333610441, -5.243569643749999898 ) ) ;
#5355=CARTESIAN_POINT ( 'NONE',  ( 13.49062500061451608, 6.054752690667223547, 3.707466751127219781E-16 ) ) ;
#5356=CARTESIAN_POINT ( 'NONE',  ( 11.78437500061451892, 4.541064518000418104, 2.621784821874999949 ) ) ;
#5357=VERTEX_POINT ( 'NONE', #33 ) ;
#5358=CARTESIAN_POINT ( 'NONE',  ( 28.79062500061451502, 6.054752690667223547, 3.707466751127219781E-16 ) ) ;
#5359=CARTESIAN_POINT ( 'NONE',  ( 22.90312500061451573, 4.541064518000418104, -2.621784821874998173 ) ) ;
#5360=DIRECTION ( 'NONE',  ( 0.000000000000000000, 0.000000000000000000, 1.000000000000000000 ) ) ;
#5361=CARTESIAN_POINT ( 'NONE',  ( -1.999999999999997113, 12.98750000122903359, 33.46410161513775705 ) ) ;
#5362=CARTESIAN_POINT ( 'NONE',  ( 11.51250000000000107, 2.886751345948126879, 4.999999999999999112 ) ) ;
#5363=CARTESIAN_POINT ( 'NONE',  ( 21.63750000122903572, -4.330127018922194537, 2.499999999999995559 ) ) ;
#5364=CARTESIAN_POINT ( 'NONE',  ( 16.86562500061451786, -6.054752690667223547, -1.112240025338166033E-15 ) ) ;
#5366=ORIENTED_EDGE ( 'NONE', *, *, #21219, .T. ) ;
#5367=CARTESIAN_POINT ( 'NONE',  ( 19.72499999999999787, -4.330127018922194537, 2.499999999999995559 ) ) ;
#5368=CARTESIAN_POINT ( 'NONE',  ( 24.56250000000000000, 2.886751345948126879, 4.999999999999999112 ) ) ;
#5369=CARTESIAN_POINT ( 'NONE',  ( 22.02187500061452141, 3.027376345333613106, -5.243569643749998122 ) ) ;
#5370=CARTESIAN_POINT ( 'NONE',  ( 28.75312500061451715, 4.541064518000418104, -2.621784821874998173 ) ) ;
#5371=ORIENTED_EDGE ( 'NONE', *, *, #28737, .F. ) ;
#5372=CARTESIAN_POINT ( 'NONE',  ( 0.000000000000000000, 4.999999999999998224, 0.000000000000000000 ) ) ;
#5373=CARTESIAN_POINT ( 'NONE',  ( 8.015625000614518214, 3.027376345333613106, -5.243569643749998122 ) ) ;
#5375=CARTESIAN_POINT ( 'NONE',  ( 18.11250000000000071, 2.886751345948129099, -4.999999999999998224 ) ) ;
#5376=CARTESIAN_POINT ( 'NONE',  ( 24.60000000000000142, 0.000000000000000000, 4.999999999999998224 ) ) ;
#5377=CARTESIAN_POINT ( 'NONE',  ( 5.146875000614517859, -3.027376345333614438, 5.243569643749998122 ) ) ;
#5378=CARTESIAN_POINT ( 'NONE',  ( 29.10937500061451644, -4.541064518000417216, -2.621784821875001281 ) ) ;
#5379=ORIENTED_EDGE ( 'NONE', *, *, #70256, .F. ) ;
#5380=CARTESIAN_POINT ( 'NONE',  ( 24.51562500061451289, -6.054752690667223547, -1.112240025338166033E-15 ) ) ;
#5381=CARTESIAN_POINT ( 'NONE',  ( 26.07187500061451857, 3.027376345333613106, -5.243569643749998122 ) ) ;
#5382=CARTESIAN_POINT ( 'NONE',  ( 2.121784821874999061, 18.75312500061459886, -33.67503911421598417 ) ) ;
#5383=CARTESIAN_POINT ( 'NONE',  ( 11.73750000000000249, -2.886751345948125991, -5.000000000000000000 ) ) ;
#5384=CARTESIAN_POINT ( 'NONE',  ( 8.803125000614517859, -4.541064518000417216, -2.621784821875001281 ) ) ;
#5385=CARTESIAN_POINT ( 'NONE',  ( -4.243569643749999898, 19.85937500061451644, 30.00000000000000000 ) ) ;
#5387=CARTESIAN_POINT ( 'NONE',  ( 25.19062500061451715, 6.054752690667223547, 3.707466751127219781E-16 ) ) ;
#5388=CARTESIAN_POINT ( 'NONE',  ( -3.999999999999999112, 18.16250000000000142, 27.69059892324149885 ) ) ;
#5390=CARTESIAN_POINT ( 'NONE',  ( 3.403125000614518836, -4.541064518000417216, -2.621784821875001281 ) ) ;
#5391=CARTESIAN_POINT ( 'NONE',  ( 19.50937500061451857, 0.000000000000000000, 5.243569643749999010 ) ) ;
#5392=CARTESIAN_POINT ( 'NONE',  ( -2.121784821874996840, 14.98437500061451644, 33.67503911421598417 ) ) ;
#5394=CARTESIAN_POINT ( 'NONE',  ( 22.50937500061451857, 4.541064518000418104, -2.621784821874998173 ) ) ;
#5395=CARTESIAN_POINT ( 'NONE',  ( 3.675000000000001155, 6.123233995736764310E-16, -4.999999999999998224 ) ) ;
#5397=CARTESIAN_POINT ( 'NONE',  ( 11.09062500061451573, -3.027376345333610441, -5.243569643749999898 ) ) ;
#5398=CARTESIAN_POINT ( 'NONE',  ( -1.071796769724483234, 15.07009619066136885, 25.99999999999999645 ) ) ;
#5399=CARTESIAN_POINT ( 'NONE',  ( 6.121875000614517504, -6.054752690667223547, -1.112240025338166033E-15 ) ) ;
#5400=CARTESIAN_POINT ( 'NONE',  ( 7.500000001229033764, 5.773502691896255534, 3.535250795749688401E-16 ) ) ;
#5401=AXIS2_PLACEMENT_3D ( 'NONE', #29095, #73072, #56443 ) ;
#5402=CARTESIAN_POINT ( 'NONE',  ( 8.278125000614515727, -4.541064518000419881, 2.621784821874995952 ) ) ;
#5403=CARTESIAN_POINT ( 'NONE',  ( 13.05937500061451750, 4.541064518000418104, -2.621784821874998173 ) ) ;
#5404=CARTESIAN_POINT ( 'NONE',  ( 18.71250000122903145, 4.330127018922192761, -2.499999999999997780 ) ) ;
#5405=CARTESIAN_POINT ( 'NONE',  ( 9.121875000614517504, 3.027376345333611329, 5.243569643749999010 ) ) ;
#5406=CARTESIAN_POINT ( 'NONE',  ( 9.403125000614517504, 4.541064518000418104, -2.621784821874998173 ) ) ;
#5409=CARTESIAN_POINT ( 'NONE',  ( 18.23437500061451999, -4.541064518000419881, 2.621784821874995952 ) ) ;
#5410=CARTESIAN_POINT ( 'NONE',  ( 26.35312500061451857, -4.541064518000417216, -2.621784821875001281 ) ) ;
#5411=CARTESIAN_POINT ( 'NONE',  ( 11.16562500061451679, 3.027376345333613106, -5.243569643749998122 ) ) ;
#5413=CARTESIAN_POINT ( 'NONE',  ( -2.121784821874996840, 13.18437500061451750, -26.32496088578401583 ) ) ;
#5414=CARTESIAN_POINT ( 'NONE',  ( 12.41250000122903430, 4.330127018922192761, -2.499999999999997780 ) ) ;
#5415=CARTESIAN_POINT ( 'NONE',  ( 28.00312500061451715, 0.000000000000000000, 5.243569643749999010 ) ) ;
#5417=CARTESIAN_POINT ( 'NONE',  ( 2.121784821874999061, 16.50312500061451715, -33.67503911421598417 ) ) ;
#5418=CARTESIAN_POINT ( 'NONE',  ( 15.75000000122902932, -2.886751345948129988, 4.999999999999997335 ) ) ;
#5419=AXIS2_PLACEMENT_3D ( 'NONE', #61337, #56521, #68344 ) ;
#5420=CARTESIAN_POINT ( 'NONE',  ( 12.67499999999999893, 6.123233995736764310E-16, -4.999999999999998224 ) ) ;
#5422=CARTESIAN_POINT ( 'NONE',  ( 22.82812500061451644, 6.421520780324663323E-16, -5.243569643749999010 ) ) ;
#5423=CARTESIAN_POINT ( 'NONE',  ( 6.721875000614518925, 3.027376345333612662, -5.243569643749998122 ) ) ;
#5424=CARTESIAN_POINT ( 'NONE',  ( 8.812500001229034652, 4.330127018922192761, -2.499999999999997780 ) ) ;
#5425=CARTESIAN_POINT ( 'NONE',  ( 15.03750000122903252, 6.123233995736764310E-16, -4.999999999999998224 ) ) ;
#5426=CARTESIAN_POINT ( 'NONE',  ( 14.20312500061451644, -4.541064518000417216, -2.621784821875001281 ) ) ;
#5427=CARTESIAN_POINT ( 'NONE',  ( 18.77812500061451573, 6.421520780324663323E-16, -5.243569643749999010 ) ) ;
#5428=CARTESIAN_POINT ( 'NONE',  ( 26.17500000122903359, -5.773502691896255534, -1.060575238724906372E-15 ) ) ;
#5429=CARTESIAN_POINT ( 'NONE',  ( 27.41250000122903430, 0.000000000000000000, 4.999999999999998224 ) ) ;
#5430=CARTESIAN_POINT ( 'NONE',  ( 23.02499999999999858, 6.123233995736764310E-16, -4.999999999999998224 ) ) ;
#5431=CARTESIAN_POINT ( 'NONE',  ( 25.58437500061451431, 6.421520780324663323E-16, -5.243569643749999010 ) ) ;
#5434=CARTESIAN_POINT ( 'NONE',  ( 9.862500001229033586, 0.000000000000000000, 4.999999999999998224 ) ) ;
#5435=CARTESIAN_POINT ( 'NONE',  ( 26.97187500061451360, 3.027376345333613106, -5.243569643749998122 ) ) ;
#5436=CYLINDRICAL_SURFACE ( 'NONE', #58515, 4.999999999999998224 ) ;
#5437=CARTESIAN_POINT ( 'NONE',  ( 4.846875000614519813, -3.027376345333610441, -5.243569643749999898 ) ) ;
#5438=CARTESIAN_POINT ( 'NONE',  ( 24.21562500061451573, 3.027376345333613106, -5.243569643749998122 ) ) ;
#5441=CARTESIAN_POINT ( 'NONE',  ( 9.946875000614516793, 6.054752690667223547, 3.707466751127219781E-16 ) ) ;
#5442=CARTESIAN_POINT ( 'NONE',  ( 24.37500000000000000, 6.123233995736764310E-16, -4.999999999999998224 ) ) ;
#5443=CARTESIAN_POINT ( 'NONE',  ( 29.50312500061451360, -4.541064518000417216, -2.621784821875001281 ) ) ;
#5444=CARTESIAN_POINT ( 'NONE',  ( 6.609375000614519102, -4.541064518000417216, -2.621784821875001281 ) ) ;
#5445=CARTESIAN_POINT ( 'NONE',  ( 27.64687500061452141, -3.027376345333614438, 5.243569643749998122 ) ) ;
#5446=DIRECTION ( 'NONE',  ( 0.000000000000000000, 0.000000000000000000, -1.000000000000000000 ) ) ;
#5447=CARTESIAN_POINT ( 'NONE',  ( 19.50000000000000000, 4.330127018922192761, -2.499999999999997780 ) ) ;
#5448=ORIENTED_EDGE ( 'NONE', *, *, #59933, .F. ) ;
#5449=CARTESIAN_POINT ( 'NONE',  ( 28.38749999999999929, -2.886751345948125991, -5.000000000000000000 ) ) ;
#5451=CARTESIAN_POINT ( 'NONE',  ( 27.57187500061451857, 3.027376345333611329, 5.243569643749999010 ) ) ;
#5452=ORIENTED_EDGE ( 'NONE', *, *, #57133, .F. ) ;
#5453=CARTESIAN_POINT ( 'NONE',  ( 17.27812500061451217, -4.541064518000419881, 2.621784821874995952 ) ) ;
#5454=CARTESIAN_POINT ( 'NONE',  ( 8.690625000614515372, -3.027376345333614438, 5.243569643749998122 ) ) ;
#5456=CARTESIAN_POINT ( 'NONE',  ( 3.721875000614518036, 3.027376345333611329, 5.243569643749999010 ) ) ;
#5457=CARTESIAN_POINT ( 'NONE',  ( 18.22500000122903430, 2.886751345948129099, -4.999999999999998224 ) ) ;
#5458=CARTESIAN_POINT ( 'NONE',  ( 24.63749999999999574, -2.886751345948129988, 4.999999999999997335 ) ) ;
#5460=CARTESIAN_POINT ( 'NONE',  ( 6.684375000614518392, 6.421520780324663323E-16, -5.243569643749999010 ) ) ;
#5461=CARTESIAN_POINT ( 'NONE',  ( 11.52187500061451608, -6.054752690667223547, -1.112240025338166033E-15 ) ) ;
#5462=CARTESIAN_POINT ( 'NONE',  ( 22.24687500061451217, -3.027376345333614438, 5.243569643749998122 ) ) ;
#5463=CARTESIAN_POINT ( 'NONE',  ( 4.898587196589411843E-16, 20.00000000000000000, 33.99999999999999289 ) ) ;
#5464=VERTEX_POINT ( 'NONE', #18070 ) ;
#5465=CARTESIAN_POINT ( 'NONE',  ( 4.584375000614516971, 4.541064518000418104, 2.621784821874999949 ) ) ;
#5467=CARTESIAN_POINT ( 'NONE',  ( 6.121875000614517504, -6.054752690667223547, -1.112240025338166033E-15 ) ) ;
#5469=CARTESIAN_POINT ( 'NONE',  ( 21.56250000000000000, -5.773502691896255534, -1.060575238724906372E-15 ) ) ;
#5470=CARTESIAN_POINT ( 'NONE',  ( 17.27812500061451217, -4.541064518000419881, 2.621784821874995952 ) ) ;
#5472=CARTESIAN_POINT ( 'NONE',  ( 30.00000000000000000, 0.000000000000000000, 0.000000000000000000 ) ) ;
#5473=EDGE_CURVE ( 'NONE', #8533, #13160, #5917, .T. ) ;
#5475=CARTESIAN_POINT ( 'NONE',  ( 10.11562500061451608, -6.054752690667223547, -1.112240025338166033E-15 ) ) ;
#5476=CARTESIAN_POINT ( 'NONE',  ( 26.70937500061451431, 0.000000000000000000, 5.243569643749999010 ) ) ;
#5477=CARTESIAN_POINT ( 'NONE',  ( -2.000000000000000000, 19.58750000122903501, 26.53589838486224650 ) ) ;
#5478=CARTESIAN_POINT ( 'NONE',  ( 29.14687500061451075, -3.027376345333610441, -5.243569643749999898 ) ) ;
#5479=CARTESIAN_POINT ( 'NONE',  ( 9.187500000000001776, 5.773502691896255534, 3.535250795749688894E-16 ) ) ;
#5480=CARTESIAN_POINT ( 'NONE',  ( -3.999999999999999112, 16.51250000122903216, 30.00000000000000000 ) ) ;
#5481=CARTESIAN_POINT ( 'NONE',  ( 9.862500001229033586, 0.000000000000000000, 4.999999999999998224 ) ) ;
#5482=CARTESIAN_POINT ( 'NONE',  ( 20.10937500061451289, -4.541064518000417216, -2.621784821875001281 ) ) ;
#5483=CARTESIAN_POINT ( 'NONE',  ( 14.52187500061451608, 3.027376345333611329, 5.243569643749999010 ) ) ;
#5484=CARTESIAN_POINT ( 'NONE',  ( 9.225000001229034297, 2.886751345948129099, -4.999999999999997335 ) ) ;
#5486=CARTESIAN_POINT ( 'NONE',  ( 14.39062500061451821, 6.054752690667223547, 3.707466751127219781E-16 ) ) ;
#5487=CARTESIAN_POINT ( 'NONE',  ( 26.02500000122903145, 2.886751345948126879, 4.999999999999999112 ) ) ;
#5488=CARTESIAN_POINT ( 'NONE',  ( 14.07187500061451679, 3.027376345333611329, 5.243569643749999010 ) ) ;
#5489=CARTESIAN_POINT ( 'NONE',  ( 3.178125000614515638, 4.541064518000418104, 2.621784821874999949 ) ) ;
#5490=CARTESIAN_POINT ( 'NONE',  ( 16.00312500061451715, -4.541064518000417216, -2.621784821875001281 ) ) ;
#5491=LINE ( 'NONE', #28379, #48040 ) ;
#5492=CARTESIAN_POINT ( 'NONE',  ( 26.78437500061451360, -4.541064518000419881, 2.621784821874995952 ) ) ;
#5493=CARTESIAN_POINT ( 'NONE',  ( 4.243569643749999010, 10.16562500061451857, 27.54997392385601174 ) ) ;
#5494=CARTESIAN_POINT ( 'NONE',  ( 14.70937500061451786, -4.541064518000417216, -2.621784821875001281 ) ) ;
#5495=CARTESIAN_POINT ( 'NONE',  ( 14.40000000122903323, -2.886751345948129988, 4.999999999999997335 ) ) ;
#5497=DIRECTION ( 'NONE',  ( -0.000000000000000000, -1.000000000000000000, -0.000000000000000000 ) ) ;
#5498=CARTESIAN_POINT ( 'NONE',  ( 21.34687500061451715, -3.027376345333614438, 5.243569643749998122 ) ) ;
#5499=CARTESIAN_POINT ( 'NONE',  ( 20.40000000122903145, -2.886751345948125991, -5.000000000000000000 ) ) ;
#5500=CARTESIAN_POINT ( 'NONE',  ( 14.48437500061451821, 4.541064518000418104, 2.621784821874999949 ) ) ;
#5501=CARTESIAN_POINT ( 'NONE',  ( 4.243569643749999898, 12.39687500061451608, 32.45002607614398471 ) ) ;
#5502=CARTESIAN_POINT ( 'NONE',  ( 22.42500000122903359, 2.886751345948126879, 4.999999999999999112 ) ) ;
#5503=VECTOR ( 'NONE', #72848, 1000.000000000000000 ) ;
#5504=CARTESIAN_POINT ( 'NONE',  ( 17.91562500061451502, 3.027376345333613106, -5.243569643749998122 ) ) ;
#5506=VERTEX_POINT ( 'NONE', #62428 ) ;
#5507=CARTESIAN_POINT ( 'NONE',  ( 19.98749999999999716, 5.773502691896255534, 3.535250795749688894E-16 ) ) ;
#5508=DIRECTION ( 'NONE',  ( 0.000000000000000000, 0.000000000000000000, 1.000000000000000000 ) ) ;
#5509=CARTESIAN_POINT ( 'NONE',  ( 25.41562500061451146, -6.054752690667223547, -1.112240025338166033E-15 ) ) ;
#5510=CARTESIAN_POINT ( 'NONE',  ( 0.2755985575760803163, 4.994312242614637576, 33.99289732352644933 ) ) ;
#5511=CARTESIAN_POINT ( 'NONE',  ( 16.76250000122903216, -4.330127018922190985, -2.500000000000001332 ) ) ;
#5512=CARTESIAN_POINT ( 'NONE',  ( 21.59062500061451928, 6.054752690667223547, 3.707466751127219781E-16 ) ) ;
#5513=CARTESIAN_POINT ( 'NONE',  ( 24.59062500061451573, -3.027376345333610441, -5.243569643749999898 ) ) ;
#5514=CARTESIAN_POINT ( 'NONE',  ( 5.315625000614516260, 3.027376345333613106, -5.243569643749998122 ) ) ;
#5515=( BOUNDED_CURVE ( )  B_SPLINE_CURVE ( 2, ( #70208, #47312, #1903, #58744, #59476, #24407, #69846, #30683, #19212 ),
 .UNSPECIFIED., .F., .F. ) 
 B_SPLINE_CURVE_WITH_KNOTS ( ( 3, 2, 2, 2, 3 ),
 ( 0.2065217391304347838, 0.2101449275362318736, 0.2173913043478260809, 0.2246376811594202882, 0.2282608695652174058 ),
 .UNSPECIFIED. ) 
 CURVE ( )  GEOMETRIC_REPRESENTATION_ITEM ( )  RATIONAL_B_SPLINE_CURVE ( ( 0.9330127018922194093, 0.9330127018922194093, 1.000000000000000000, 0.8660254037844387076, 1.000000000000000000, 0.8660254037844387076, 1.000000000000000000, 0.9330127018922190762, 0.9330127018922194093 ) ) 
 REPRESENTATION_ITEM ( '' )  );
#5517=CARTESIAN_POINT ( 'NONE',  ( 29.66249999999999432, -5.773502691896255534, -1.060575238724906372E-15 ) ) ;
#5520=CARTESIAN_POINT ( 'NONE',  ( 0.000000000000000000, 20.00000000000000000, -30.00000000000000000 ) ) ;
#5521=CARTESIAN_POINT ( 'NONE',  ( 1.999999999999998668, 10.96250000122903501, -33.46410161513775705 ) ) ;
#5522=CARTESIAN_POINT ( 'NONE',  ( 4.243569643749999898, 18.24687500061451928, -27.54997392385601529 ) ) ;
#5523=CARTESIAN_POINT ( 'NONE',  ( 7.950000000000001954, 0.000000000000000000, 4.999999999999998224 ) ) ;
#5524=CARTESIAN_POINT ( 'NONE',  ( 3.675000001229035362, -5.773502691896255534, -1.060575238724906372E-15 ) ) ;
#5525=CARTESIAN_POINT ( 'NONE',  ( 11.82187500061451679, 3.027376345333611329, 5.243569643749999010 ) ) ;
#5526=CARTESIAN_POINT ( 'NONE',  ( 19.46250000122903145, -4.330127018922190985, -2.500000000000001332 ) ) ;
#5527=CARTESIAN_POINT ( 'NONE',  ( 3.459375000614519635, -4.541064518000417216, -2.621784821875001281 ) ) ;
#5531=CARTESIAN_POINT ( 'NONE',  ( 10.88437500061451679, 4.541064518000418104, 2.621784821874999949 ) ) ;
#5533=CARTESIAN_POINT ( 'NONE',  ( 19.00312500061451715, 0.000000000000000000, 5.243569643749999010 ) ) ;
#5535=CARTESIAN_POINT ( 'NONE',  ( 4.243569643749999898, 18.22812500061459673, 30.00000000000000000 ) ) ;
#5536=CARTESIAN_POINT ( 'NONE',  ( 24.75937500061451502, 4.541064518000418104, -2.621784821874998173 ) ) ;
#5537=DIRECTION ( 'NONE',  ( 0.000000000000000000, 0.000000000000000000, -1.000000000000000000 ) ) ;
#5538=CARTESIAN_POINT ( 'NONE',  ( 28.76250000122903216, 0.000000000000000000, 4.999999999999998224 ) ) ;
#5540=CARTESIAN_POINT ( 'NONE',  ( 25.71562500061451573, 3.027376345333611329, 5.243569643749999010 ) ) ;
#5541=CARTESIAN_POINT ( 'NONE',  ( 15.32812500061451644, 4.541064518000418104, 2.621784821874999949 ) ) ;
#5543=CARTESIAN_POINT ( 'NONE',  ( 11.48437500061451644, -4.541064518000419881, 2.621784821874995952 ) ) ;
#5544=CARTESIAN_POINT ( 'NONE',  ( 29.21249999999999858, -5.773502691896255534, -1.060575238724906372E-15 ) ) ;
#5545=CARTESIAN_POINT ( 'NONE',  ( 23.81250000122903288, 0.000000000000000000, 4.999999999999998224 ) ) ;
#5546=CARTESIAN_POINT ( 'NONE',  ( 3.121875000614518836, 3.027376345333613106, -5.243569643749998122 ) ) ;
#5547=CARTESIAN_POINT ( 'NONE',  ( 14.40937500061451715, 4.541064518000418104, -2.621784821874998173 ) ) ;
#5548=CARTESIAN_POINT ( 'NONE',  ( 29.03437500061451715, -4.541064518000419881, 2.621784821874995952 ) ) ;
#5550=CARTESIAN_POINT ( 'NONE',  ( -1.999999999999997113, 12.42500000000000249, -26.53589838486224295 ) ) ;
#5551=CARTESIAN_POINT ( 'NONE',  ( 24.53437500061451715, -4.541064518000419881, 2.621784821874995952 ) ) ;
#5552=CARTESIAN_POINT ( 'NONE',  ( 14.10937500061451644, 0.000000000000000000, 5.243569643749999010 ) ) ;
#5555=CARTESIAN_POINT ( 'NONE',  ( 28.42499999999999716, 6.123233995736764310E-16, -4.999999999999998224 ) ) ;
#5556=CARTESIAN_POINT ( 'NONE',  ( 3.075000001229035718, 2.886751345948126879, 4.999999999999999112 ) ) ;
#5558=CARTESIAN_POINT ( 'NONE',  ( 16.82812500061451644, -4.541064518000419881, 2.621784821874995952 ) ) ;
#5559=CARTESIAN_POINT ( 'NONE',  ( 8.400000000000000355, 0.000000000000000000, 4.999999999999998224 ) ) ;
#5560=CARTESIAN_POINT ( 'NONE',  ( -3.999999999999997335, 14.18750000000000000, 32.30940107675850470 ) ) ;
#5561=CARTESIAN_POINT ( 'NONE',  ( 16.27499999999999858, 6.123233995736764310E-16, -4.999999999999998224 ) ) ;
#5562=EDGE_CURVE ( 'NONE', #69508, #51457, #45449, .T. ) ;
#5563=CARTESIAN_POINT ( 'NONE',  ( -4.243569643749997233, 13.54062500061451679, 32.45002607614398471 ) ) ;
#5564=CARTESIAN_POINT ( 'NONE',  ( 21.41250000122903074, 4.330127018922192761, -2.499999999999997780 ) ) ;
#5565=CARTESIAN_POINT ( 'NONE',  ( 5.672204065618860369, 8.235970573989481736, 31.96601703155577212 ) ) ;
#5566=CARTESIAN_POINT ( 'NONE',  ( 26.82187500061451857, -6.054752690667223547, -1.112240025338166033E-15 ) ) ;
#5567=ORIENTED_EDGE ( 'NONE', *, *, #16122, .F. ) ;
#5568=CARTESIAN_POINT ( 'NONE',  ( 17.72812500061451502, -4.541064518000419881, 2.621784821874995952 ) ) ;
#5569=CARTESIAN_POINT ( 'NONE',  ( 22.49062500061451431, 6.054752690667223547, 3.707466751127219781E-16 ) ) ;
#5570=CARTESIAN_POINT ( 'NONE',  ( 22.24687500061451217, -3.027376345333614438, 5.243569643749998122 ) ) ;
#5571=CARTESIAN_POINT ( 'NONE',  ( 7.012500000000001066, 2.886751345948126879, 4.999999999999999112 ) ) ;
#5572=CARTESIAN_POINT ( 'NONE',  ( 9.440625000614517148, 6.054752690667223547, 3.707466751127219781E-16 ) ) ;
#5573=CARTESIAN_POINT ( 'NONE',  ( 24.36562500061451786, 3.027376345333611329, 5.243569643749999010 ) ) ;
#5574=CARTESIAN_POINT ( 'NONE',  ( 15.30937500061451750, 4.541064518000418104, -2.621784821874998173 ) ) ;
#5575=CARTESIAN_POINT ( 'NONE',  ( 18.30937500061451928, -4.541064518000417216, -2.621784821875001281 ) ) ;
#5576=DIRECTION ( 'NONE',  ( 0.000000000000000000, 0.000000000000000000, 1.000000000000000000 ) ) ;
#5577=CARTESIAN_POINT ( 'NONE',  ( -4.243569643749999898, 16.61562500061451786, 27.54997392385601529 ) ) ;
#5578=CARTESIAN_POINT ( 'NONE',  ( 22.27500000122903145, 2.886751345948129099, -4.999999999999998224 ) ) ;
#5580=CARTESIAN_POINT ( 'NONE',  ( 12.02812500061451573, 6.421520780324663323E-16, -5.243569643749999010 ) ) ;
#5581=CARTESIAN_POINT ( 'NONE',  ( 6.421875000614519102, 3.027376345333611329, 5.243569643749999010 ) ) ;
#5582=CARTESIAN_POINT ( 'NONE',  ( 3.871875000614519280, -6.054752690667223547, -1.112240025338166033E-15 ) ) ;
#5584=ORIENTED_EDGE ( 'NONE', *, *, #36389, .F. ) ;
#5585=CARTESIAN_POINT ( 'NONE',  ( 28.02187500061451431, 3.027376345333611329, 5.243569643749999010 ) ) ;
#5586=CARTESIAN_POINT ( 'NONE',  ( 20.46562500061451928, -6.054752690667223547, -1.112240025338166033E-15 ) ) ;
#5587=CARTESIAN_POINT ( 'NONE',  ( 28.05000000122903359, -2.886751345948125991, -5.000000000000000000 ) ) ;
#5588=CARTESIAN_POINT ( 'NONE',  ( 27.02812500061451573, 4.541064518000418104, 2.621784821874999949 ) ) ;
#5589=CARTESIAN_POINT ( 'NONE',  ( 24.42187500061451999, 3.027376345333611329, 5.243569643749999010 ) ) ;
#5590=CARTESIAN_POINT ( 'NONE',  ( 17.87812500061451715, 6.421520780324663323E-16, -5.243569643749999010 ) ) ;
#5591=CARTESIAN_POINT ( 'NONE',  ( -1.389182184750238802, 10.01354716596406824, 26.18324255480197493 ) ) ;
#5592=CARTESIAN_POINT ( 'NONE',  ( 23.91562500061451502, 3.027376345333611329, 5.243569643749999010 ) ) ;
#5593=CARTESIAN_POINT ( 'NONE',  ( 4.987500001229032698, -4.330127018922194537, 2.499999999999995559 ) ) ;
#5595=CARTESIAN_POINT ( 'NONE',  ( 27.37500000000000000, -4.330127018922194537, 2.499999999999995559 ) ) ;
#5596=CARTESIAN_POINT ( 'NONE',  ( -3.999999999999999112, 15.05000000000000071, -30.00000000000000000 ) ) ;
#5598=CARTESIAN_POINT ( 'NONE',  ( 5.746875000614517504, -3.027376345333610441, -5.243569643749999898 ) ) ;
#5599=CARTESIAN_POINT ( 'NONE',  ( 10.64062500061451644, -3.027376345333610441, -5.243569643749999898 ) ) ;
#5600=CARTESIAN_POINT ( 'NONE',  ( 6.496875000614517504, -3.027376345333614438, 5.243569643749998122 ) ) ;
#5601=CARTESIAN_POINT ( 'NONE',  ( 24.33750000122903145, -4.330127018922194537, 2.499999999999995559 ) ) ;
#5603=CARTESIAN_POINT ( 'NONE',  ( 15.08437500061451786, -4.541064518000419881, 2.621784821874995952 ) ) ;
#5604=CARTESIAN_POINT ( 'NONE',  ( 29.65312500061451573, 4.541064518000418104, -2.621784821874998173 ) ) ;
#5605=CARTESIAN_POINT ( 'NONE',  ( 27.52500000000000213, 6.123233995736764310E-16, -4.999999999999998224 ) ) ;
#5606=CARTESIAN_POINT ( 'NONE',  ( 27.75937500061451502, -4.541064518000417216, -2.621784821875001281 ) ) ;
#5607=CARTESIAN_POINT ( 'NONE',  ( 3.215625000614518836, 3.027376345333611329, 5.243569643749999010 ) ) ;
#5608=CARTESIAN_POINT ( 'NONE',  ( 13.22812500061451502, -4.541064518000419881, 2.621784821874995952 ) ) ;
#5609=ORIENTED_EDGE ( 'NONE', *, *, #2386, .T. ) ;
#5610=CARTESIAN_POINT ( 'NONE',  ( 9.065625000614517148, 3.027376345333611329, 5.243569643749999010 ) ) ;
#5611=CARTESIAN_POINT ( 'NONE',  ( 6.290625000614517681, 6.054752690667223547, 3.707466751127219781E-16 ) ) ;
#5614=CARTESIAN_POINT ( 'NONE',  ( 15.00000000000000000, 4.330127018922192761, -2.499999999999997780 ) ) ;
#5615=CARTESIAN_POINT ( 'NONE',  ( 16.32187500061451502, 3.027376345333611329, 5.243569643749999010 ) ) ;
#5616=B_SPLINE_CURVE_WITH_KNOTS ( 'NONE', 3,
 ( #19471, #41306, #19842, #12851, #35384, #8770, #42394, #63816, #42029, #14307 ),
 .UNSPECIFIED., .F., .F.,
 ( 4, 3, 3, 4 ),
 ( 0.000000000000000000, 0.0001572298629325321207, 0.0003312541060196098224, 0.0005053537190665100551 ),
 .UNSPECIFIED. ) ;
#5617=CARTESIAN_POINT ( 'NONE',  ( 12.48750000122903359, 4.330127018922191873, 2.499999999999999556 ) ) ;
#5619=CARTESIAN_POINT ( 'NONE',  ( 20.82187500061451857, 3.027376345333611329, 5.243569643749999010 ) ) ;
#5620=CARTESIAN_POINT ( 'NONE',  ( 2.121784821875001281, 14.10312500061451679, -26.32496088578401938 ) ) ;
#5623=CARTESIAN_POINT ( 'NONE',  ( 4.111889464957033447, 2.844708250062874644, 4.404844785106587501 ) ) ;
#5624=CARTESIAN_POINT ( 'NONE',  ( 26.09062500061451573, 6.054752690667223547, 3.707466751127219781E-16 ) ) ;
#5625=CARTESIAN_POINT ( 'NONE',  ( 1.510657702057710734E-15, 19.43750000000000000, -33.99999999999999289 ) ) ;
#5626=DIRECTION ( 'NONE',  ( 0.000000000000000000, 0.000000000000000000, 1.000000000000000000 ) ) ;
#5627=CARTESIAN_POINT ( 'NONE',  ( 27.29999999999999716, 0.000000000000000000, 4.999999999999998224 ) ) ;
#5628=CARTESIAN_POINT ( 'NONE',  ( 9.103125000614515017, 0.000000000000000000, 5.243569643749999010 ) ) ;
#5630=CARTESIAN_POINT ( 'NONE',  ( 19.88437500061451857, 4.541064518000418104, 2.621784821874999949 ) ) ;
#5632=CARTESIAN_POINT ( 'NONE',  ( 5.615625000614517859, -6.054752690667223547, -1.112240025338166033E-15 ) ) ;
#5633=CARTESIAN_POINT ( 'NONE',  ( 11.40937500061451892, 0.000000000000000000, 5.243569643749999010 ) ) ;
#5635=CARTESIAN_POINT ( 'NONE',  ( 21.57187500061451502, 3.027376345333613106, -5.243569643749998122 ) ) ;
#5637=CARTESIAN_POINT ( 'NONE',  ( 29.58749999999999858, -2.886751345948129988, 4.999999999999997335 ) ) ;
#5638=CARTESIAN_POINT ( 'NONE',  ( 6.150000000000003020, 0.000000000000000000, 4.999999999999998224 ) ) ;
#5640=CARTESIAN_POINT ( 'NONE',  ( 14.40000000122903323, -2.886751345948129988, 4.999999999999997335 ) ) ;
#5641=CARTESIAN_POINT ( 'NONE',  ( 1.071796769724489895, 12.32990381179670081, 26.00000000000000355 ) ) ;
#5642=ORIENTED_EDGE ( 'NONE', *, *, #27759, .T. ) ;
#5643=CARTESIAN_POINT ( 'NONE',  ( 13.46249999999999858, -5.773502691896255534, -1.060575238724906372E-15 ) ) ;
#5644=CARTESIAN_POINT ( 'NONE',  ( 26.72812500061451502, -4.541064518000419881, 2.621784821874995952 ) ) ;
#5645=CARTESIAN_POINT ( 'NONE',  ( 17.66249999999999787, 2.886751345948129099, -4.999999999999998224 ) ) ;
#5646=CARTESIAN_POINT ( 'NONE',  ( 10.68750000122903288, 4.330127018922191873, 2.499999999999999556 ) ) ;
#5647=CARTESIAN_POINT ( 'NONE',  ( 8.353125000614518569, -4.541064518000417216, -2.621784821875001281 ) ) ;
#5649=CARTESIAN_POINT ( 'NONE',  ( 9.712500000000002132, 2.886751345948126879, 4.999999999999999112 ) ) ;
#5650=CARTESIAN_POINT ( 'NONE',  ( 15.97500000122903430, 2.886751345948062486, -5.000000000000113687 ) ) ;
#5651=CARTESIAN_POINT ( 'NONE',  ( 2.121784821874999061, 15.20937500061451786, -33.67503911421598417 ) ) ;
#5652=CARTESIAN_POINT ( 'NONE',  ( 27.48750000122903359, -4.330127018922194537, 2.499999999999995559 ) ) ;
#5654=CARTESIAN_POINT ( 'NONE',  ( 7.724999999999999645, 6.123233995736764310E-16, -4.999999999999998224 ) ) ;
#5655=CARTESIAN_POINT ( 'NONE',  ( -1.487416814333745711E-14, 16.96250000000000213, -26.00000000000000000 ) ) ;
#5656=ORIENTED_EDGE ( 'NONE', *, *, #60084, .F. ) ;
#5657=CARTESIAN_POINT ( 'NONE',  ( 23.76562500061451644, 3.027376345333613106, -5.243569643749998122 ) ) ;
#5658=CARTESIAN_POINT ( 'NONE',  ( 28.67812500061451431, 6.421520780324663323E-16, -5.243569643749999010 ) ) ;
#5659=CARTESIAN_POINT ( 'NONE',  ( 28.69687500061451502, -3.027376345333610441, -5.243569643749999898 ) ) ;
#5660=CARTESIAN_POINT ( 'NONE',  ( 19.24687500061452283, -3.027376345333610441, -5.243569643749999898 ) ) ;
#5661=CARTESIAN_POINT ( 'NONE',  ( 17.84062500061451573, -3.027376345333610441, -5.243569643749999898 ) ) ;
#5662=CARTESIAN_POINT ( 'NONE',  ( 9.001249775931846008E-16, 10.46562500061459389, -25.09994784771203058 ) ) ;
#5663=CARTESIAN_POINT ( 'NONE',  ( 7.115625000614516082, 3.027376345333613106, -5.243569643749998122 ) ) ;
#5664=CARTESIAN_POINT ( 'NONE',  ( 27.67500000122903359, 2.886751345948129099, -4.999999999999998224 ) ) ;
#5666=CARTESIAN_POINT ( 'NONE',  ( 18.21562500061451573, -6.054752690667223547, -1.112240025338166033E-15 ) ) ;
#5667=DIRECTION ( 'NONE',  ( -0.000000000000000000, -1.000000000000000000, -0.000000000000000000 ) ) ;
#5669=CARTESIAN_POINT ( 'NONE',  ( 12.83437500061451786, -4.541064518000419881, 2.621784821874995952 ) ) ;
#5670=CARTESIAN_POINT ( 'NONE',  ( 12.79687500061451821, -3.027376345333614438, 5.243569643749998122 ) ) ;
#5671=CARTESIAN_POINT ( 'NONE',  ( 22.54687500061451999, 6.054752690667223547, 3.707466751127219781E-16 ) ) ;
#5672=ORIENTED_EDGE ( 'NONE', *, *, #16557, .T. ) ;
#5673=LINE ( 'NONE', #6028, #11145 ) ;
#5674=CARTESIAN_POINT ( 'NONE',  ( 26.65312500061451573, 0.000000000000000000, 5.243569643749999010 ) ) ;
#5675=CARTESIAN_POINT ( 'NONE',  ( 26.95312500061451644, 4.541064518000418104, -2.621784821874998173 ) ) ;
#5677=CARTESIAN_POINT ( 'NONE',  ( -2.000000000000000000, 16.32499999999999929, 26.53589838486224650 ) ) ;
#5678=CARTESIAN_POINT ( 'NONE',  ( 6.009375000614519458, 0.000000000000000000, 5.243569643749999010 ) ) ;
#5679=CARTESIAN_POINT ( 'NONE',  ( 12.82500000122903394, 2.886751345948129099, -4.999999999999998224 ) ) ;
#5680=CARTESIAN_POINT ( 'NONE',  ( 7.800000001229035362, -2.886751345948125991, -5.000000000000000000 ) ) ;
#5681=CARTESIAN_POINT ( 'NONE',  ( 28.57500000122903572, 2.886751345948129099, -4.999999999999998224 ) ) ;
#5684=CARTESIAN_POINT ( 'NONE',  ( 11.40937500061451892, 0.000000000000000000, 5.243569643749999010 ) ) ;
#5685=CARTESIAN_POINT ( 'NONE',  ( 18.30000000000000071, 0.000000000000000000, 4.999999999999998224 ) ) ;
#5686=CARTESIAN_POINT ( 'NONE',  ( 18.92812500061451431, 4.541064518000418104, 2.621784821874999949 ) ) ;
#5687=CARTESIAN_POINT ( 'NONE',  ( 12.64687500061451608, 6.054752690667223547, 3.707466751127219781E-16 ) ) ;
#5688=CARTESIAN_POINT ( 'NONE',  ( 3.853125000614517681, -4.541064518000417216, -2.621784821875001281 ) ) ;
#5689=CARTESIAN_POINT ( 'NONE',  ( 22.24687500061451573, -3.027376345333614438, 5.243569643749998122 ) ) ;
#5690=CARTESIAN_POINT ( 'NONE',  ( 8.821875000614518569, -6.054752690667223547, -1.112240025338166033E-15 ) ) ;
#5691=CARTESIAN_POINT ( 'NONE',  ( 5.953125000614519102, 0.000000000000000000, 5.243569643749999010 ) ) ;
#5692=CARTESIAN_POINT ( 'NONE',  ( 5.737500001229033586, 4.330127018922191873, 2.499999999999999556 ) ) ;
#5693=CARTESIAN_POINT ( 'NONE',  ( 20.27812500061451573, 4.541064518000418104, 2.621784821874999949 ) ) ;
#5694=CARTESIAN_POINT ( 'NONE',  ( 7.275000001229035007, -5.773502691896255534, -1.060575238724906372E-15 ) ) ;
#5695=CARTESIAN_POINT ( 'NONE',  ( 17.91562500061451502, 3.027376345333613106, -5.243569643749998122 ) ) ;
#5696=CARTESIAN_POINT ( 'NONE',  ( 13.60312500061451679, 0.000000000000000000, 5.243569643749999010 ) ) ;
#5698=CARTESIAN_POINT ( 'NONE',  ( 13.76250000000000107, 2.886751345948126879, 4.999999999999999112 ) ) ;
#5699=CARTESIAN_POINT ( 'NONE',  ( 8.175000001229031810, -5.773502691896255534, -1.060575238724906372E-15 ) ) ;
#5700=CARTESIAN_POINT ( 'NONE',  ( 5.653125000614517504, -4.541064518000417216, -2.621784821875001281 ) ) ;
#5702=CARTESIAN_POINT ( 'NONE',  ( 20.21250000122903145, 0.000000000000000000, 4.999999999999998224 ) ) ;
#5704=CARTESIAN_POINT ( 'NONE',  ( -4.243569643749999898, 12.20937500061451608, -30.00000000000000000 ) ) ;
#5705=CARTESIAN_POINT ( 'NONE',  ( 3.947751918878622757, -3.068428716296062841, 3.947751918878600108 ) ) ;
#5706=DIRECTION ( 'NONE',  ( -0.000000000000000000, -1.000000000000000000, -0.000000000000000000 ) ) ;
#5708=CARTESIAN_POINT ( 'NONE',  ( 28.42500000122904069, -5.773502691896255534, -1.060575238724906372E-15 ) ) ;
#5709=CARTESIAN_POINT ( 'NONE',  ( 20.78437500061451715, 4.541064518000418104, 2.621784821874999949 ) ) ;
#5710=CARTESIAN_POINT ( 'NONE',  ( 17.50312500061451715, 4.541064518000418104, -2.621784821874998173 ) ) ;
#5712=DIRECTION ( 'NONE',  ( -0.000000000000000000, -1.000000000000000000, -0.000000000000000000 ) ) ;
#5713=CARTESIAN_POINT ( 'NONE',  ( 26.69999999999999929, 4.330127018922192761, -2.499999999999997780 ) ) ;
#5714=CARTESIAN_POINT ( 'NONE',  ( 27.87187500061451573, 3.027376345333613106, -5.243569643749998122 ) ) ;
#5716=CARTESIAN_POINT ( 'NONE',  ( 12.06562500061451537, 3.027376345333613106, -5.243569643749998122 ) ) ;
#5717=CARTESIAN_POINT ( 'NONE',  ( 10.32187500061451679, 3.027376345333613106, -5.243569643749998122 ) ) ;
#5718=ORIENTED_EDGE ( 'NONE', *, *, #10486, .F. ) ;
#5719=CARTESIAN_POINT ( 'NONE',  ( 2.856422355664287593, -4.103760632159477950, -2.967416088732543145 ) ) ;
#5720=CARTESIAN_POINT ( 'NONE',  ( 22.26562500061451644, -6.054752690667223547, -1.112240025338166033E-15 ) ) ;
#5724=CARTESIAN_POINT ( 'NONE',  ( 11.40000000000000036, 4.330127018922192761, -2.499999999999997780 ) ) ;
#5725=CARTESIAN_POINT ( 'NONE',  ( 22.68750000122903288, 6.123233995736764310E-16, -4.999999999999998224 ) ) ;
#5726=CARTESIAN_POINT ( 'NONE',  ( 15.81562500061451537, 3.027376345333611329, 5.243569643749999010 ) ) ;
#5728=ORIENTED_EDGE ( 'NONE', *, *, #36745, .T. ) ;
#5729=CARTESIAN_POINT ( 'NONE',  ( 20.36249999999999716, 2.886751345948129099, -4.999999999999998224 ) ) ;
#5730=CARTESIAN_POINT ( 'NONE',  ( 23.81250000000000000, -5.773502691896255534, -1.060575238724906372E-15 ) ) ;
#5731=CARTESIAN_POINT ( 'NONE',  ( 21.30937500061451573, 0.000000000000000000, 5.243569643749999010 ) ) ;
#5732=CARTESIAN_POINT ( 'NONE',  ( 24.92812500061451431, -4.541064518000419881, 2.621784821874995952 ) ) ;
#5733=( BOUNDED_CURVE ( )  B_SPLINE_CURVE ( 2, ( #56705, #45995, #47081, #62969, #29367, #28637, #24170 ),
 .UNSPECIFIED., .F., .F. ) 
 B_SPLINE_CURVE_WITH_KNOTS ( ( 3, 2, 2, 3 ),
 ( 0.9684929749567240398, 0.9694444444444444420, 0.9722222222222222099, 0.9730758100533248856 ),
 .UNSPECIFIED. ) 
 CURVE ( )  GEOMETRIC_REPRESENTATION_ITEM ( )  RATIONAL_B_SPLINE_CURVE ( ( 0.9396570677417193096, 0.9541098134456433844, 1.000000000000000000, 0.8660254037844387076, 1.000000000000000000, 0.9588307293976606749, 0.9429634024444231155 ) ) 
 REPRESENTATION_ITEM ( '' )  );
#5736=CARTESIAN_POINT ( 'NONE',  ( 7.790625000614518569, -3.027376345333614438, 5.243569643749998122 ) ) ;
#5737=CARTESIAN_POINT ( 'NONE',  ( 29.55000000000000071, 0.000000000000000000, 4.999999999999998224 ) ) ;
#5738=CARTESIAN_POINT ( 'NONE',  ( 14.88750000000000107, -2.886751345948125991, -5.000000000000000000 ) ) ;
#5739=CARTESIAN_POINT ( 'NONE',  ( -4.243569643749997233, 19.39062500061451999, 32.45002607614398471 ) ) ;
#5740=CARTESIAN_POINT ( 'NONE',  ( 4.284375000614518925, -4.541064518000419881, 2.621784821874995952 ) ) ;
#5741=CARTESIAN_POINT ( 'NONE',  ( 28.28437500061451715, 6.421520780324663323E-16, -5.243569643749999010 ) ) ;
#5742=EDGE_LOOP ( 'NONE', ( #2005, #57763, #1995, #27992 ) ) ;
#5743=CARTESIAN_POINT ( 'NONE',  ( 24.47812500061451502, -4.541064518000419881, 2.621784821874995952 ) ) ;
#5744=CARTESIAN_POINT ( 'NONE',  ( 26.48437500061451644, 6.421520780324663323E-16, -5.243569643749999010 ) ) ;
#5745=CARTESIAN_POINT ( 'NONE',  ( -4.243569643749998122, 19.39062500061459104, -27.54997392385601174 ) ) ;
#5746=CARTESIAN_POINT ( 'NONE',  ( 10.80000000000000071, -4.330127018922190985, -2.500000000000001332 ) ) ;
#5747=CARTESIAN_POINT ( 'NONE',  ( 8.465625000614515727, 3.027376345333613106, -5.243569643749998122 ) ) ;
#5749=CARTESIAN_POINT ( 'NONE',  ( 19.61249999999999716, 2.886751345948093572, 5.000000000000056843 ) ) ;
#5750=CARTESIAN_POINT ( 'NONE',  ( 27.51562500061451644, 3.027376345333611329, 5.243569643749999010 ) ) ;
#5753=CARTESIAN_POINT ( 'NONE',  ( 2.990625000614519191, -3.027376345333610441, -5.243569643749999898 ) ) ;
#5754=CARTESIAN_POINT ( 'NONE',  ( 18.94687500061451502, 6.054752690667223547, 3.707466751127219781E-16 ) ) ;
#5755=CARTESIAN_POINT ( 'NONE',  ( -4.243569643749999898, 15.80937500061451573, 30.00000000000000000 ) ) ;
#5756=CARTESIAN_POINT ( 'NONE',  ( 22.69687500061451857, -3.027376345333614438, 5.243569643749998122 ) ) ;
#5757=CARTESIAN_POINT ( 'NONE',  ( 3.712499999999999911, 2.886751345948129099, -4.999999999999998224 ) ) ;
#5758=EDGE_CURVE ( 'NONE', #964, #27078, #20525, .T. ) ;
#5759=CARTESIAN_POINT ( 'NONE',  ( -2.121784821874999949, 18.88437500061451857, 26.32496088578401938 ) ) ;
#5760=CARTESIAN_POINT ( 'NONE',  ( 10.34062500061451750, 6.054752690667223547, 3.707466751127219781E-16 ) ) ;
#5762=CARTESIAN_POINT ( 'NONE',  ( 7.434375000614519280, -4.541064518000419881, 2.621784821874995952 ) ) ;
#5763=CARTESIAN_POINT ( 'NONE',  ( -3.999999999999997335, 16.10000000122903430, -27.69059892324149530 ) ) ;
#5765=CARTESIAN_POINT ( 'NONE',  ( 6.440625000614517148, -3.027376345333614438, 5.243569643749998122 ) ) ;
#5766=CARTESIAN_POINT ( 'NONE',  ( 12.34687500061452070, -3.027376345333614438, 5.243569643749998122 ) ) ;
#5767=CARTESIAN_POINT ( 'NONE',  ( 19.23750000122903714, 4.330127018922191873, 2.499999999999999556 ) ) ;
#5768=CARTESIAN_POINT ( 'NONE',  ( 7.246875000614518392, 6.054752690667223547, 3.707466751127219781E-16 ) ) ;
#5769=CARTESIAN_POINT ( 'NONE',  ( 8.878125000614515372, 6.421520780324663323E-16, -5.243569643749999010 ) ) ;
#5770=CARTESIAN_POINT ( 'NONE',  ( 5.503125000614516260, 0.000000000000000000, 5.243569643749999010 ) ) ;
#5772=CARTESIAN_POINT ( 'NONE',  ( 20.07187500061451857, -6.054752690667223547, -1.112240025338166033E-15 ) ) ;
#5773=CARTESIAN_POINT ( 'NONE',  ( 18.22499999999999787, 4.330127018922191873, 2.499999999999999556 ) ) ;
#5774=CARTESIAN_POINT ( 'NONE',  ( 27.32812500061451644, 6.421520780324663323E-16, -5.243569643749999010 ) ) ;
#5775=CARTESIAN_POINT ( 'NONE',  ( 12.44062500061451537, -3.027376345333610441, -5.243569643749999898 ) ) ;
#5777=CARTESIAN_POINT ( 'NONE',  ( 4.509957931155624600, -2.159147578587980121, -4.574533615465857572 ) ) ;
#5778=CARTESIAN_POINT ( 'NONE',  ( 13.01250000122903394, 0.000000000000000000, 4.999999999999998224 ) ) ;
#5779=CARTESIAN_POINT ( 'NONE',  ( 26.76562500061451644, -6.054752690667223547, -1.112240025338166033E-15 ) ) ;
#5780=CARTESIAN_POINT ( 'NONE',  ( -4.243569643749999898, 14.85312500061451679, -30.00000000000000000 ) ) ;
#5781=CARTESIAN_POINT ( 'NONE',  ( 15.71250000122903501, 0.000000000000000000, 4.999999999999998224 ) ) ;
#5782=CARTESIAN_POINT ( 'NONE',  ( 14.51250000000000107, 2.886751345948129099, -4.999999999999998224 ) ) ;
#5783=CARTESIAN_POINT ( 'NONE',  ( 23.72812500061451502, 6.421520780324663323E-16, -5.243569643749999010 ) ) ;
#5784=CARTESIAN_POINT ( 'NONE',  ( 8.296875000614518214, -3.027376345333614438, 5.243569643749998122 ) ) ;
#5785=CARTESIAN_POINT ( 'NONE',  ( 6.975000001229032520, 2.886751345948129099, -4.999999999999998224 ) ) ;
#5786=CARTESIAN_POINT ( 'NONE',  ( 15.75000000122902932, -2.886751345948129988, 4.999999999999997335 ) ) ;
#5787=CARTESIAN_POINT ( 'NONE',  ( 12.36562500061451608, -6.054752690667223547, -1.112240025338166033E-15 ) ) ;
#5788=CARTESIAN_POINT ( 'NONE',  ( 15.25312500061451715, 4.541064518000418104, -2.621784821874998173 ) ) ;
#5789=CARTESIAN_POINT ( 'NONE',  ( 27.11250000122903359, -4.330127018922190985, -2.500000000000001332 ) ) ;
#5790=CARTESIAN_POINT ( 'NONE',  ( 23.73749999999999716, -2.886751345948129988, 4.999999999999997335 ) ) ;
#5791=CARTESIAN_POINT ( 'NONE',  ( 22.35937500061451644, -4.541064518000417216, -2.621784821875001281 ) ) ;
#5793=CARTESIAN_POINT ( 'NONE',  ( 10.16250000122903252, 4.330127018922192761, -2.499999999999997780 ) ) ;
#5794=CARTESIAN_POINT ( 'NONE',  ( 27.49687500061451217, 6.054752690667223547, 3.707466751127219781E-16 ) ) ;
#5796=CARTESIAN_POINT ( 'NONE',  ( 5.896875000614518747, 6.054752690667223547, 3.707466751127219781E-16 ) ) ;
#5797=CARTESIAN_POINT ( 'NONE',  ( 24.74062500061451786, 6.054752690667223547, 3.707466751127219781E-16 ) ) ;
#5799=CARTESIAN_POINT ( 'NONE',  ( 6.975000000000002309, 4.330127018922191873, 2.499999999999999556 ) ) ;
#5800=CARTESIAN_POINT ( 'NONE',  ( 9.346875000614517148, -3.027376345333610441, -5.243569643749999898 ) ) ;
#5801=CARTESIAN_POINT ( 'NONE',  ( 1.999999999999998668, 12.65000000000000213, 26.53589838486224650 ) ) ;
#5802=CARTESIAN_POINT ( 'NONE',  ( 3.759375000614517681, 0.000000000000000000, 5.243569643749999010 ) ) ;
#5803=CARTESIAN_POINT ( 'NONE',  ( 6.196875000614515905, -3.027376345333610441, -5.243569643749999898 ) ) ;
#5804=CARTESIAN_POINT ( 'NONE',  ( -3.999999999999999112, 14.60000000000000142, 30.00000000000000000 ) ) ;
#5805=CARTESIAN_POINT ( 'NONE',  ( 26.37187500061451217, -6.054752690667223547, -1.112240025338166033E-15 ) ) ;
#5806=CARTESIAN_POINT ( 'NONE',  ( -3.000416591977282496E-16, 10.69062500061459531, 25.09994784771203058 ) ) ;
#5807=CARTESIAN_POINT ( 'NONE',  ( 18.75000000000000000, 0.000000000000000000, 4.999999999999998224 ) ) ;
#5809=CARTESIAN_POINT ( 'NONE',  ( 27.71250000000000568, 2.886751345948126879, 4.999999999999999112 ) ) ;
#5810=CARTESIAN_POINT ( 'NONE',  ( 29.52187500061451431, -6.054752690667223547, -1.112240025338166033E-15 ) ) ;
#5811=EDGE_LOOP ( 'NONE', ( #62244, #57255, #12547, #27686 ) ) ;
#5812=CARTESIAN_POINT ( 'NONE',  ( 14.91562500061451679, 3.027376345333611329, 5.243569643749999010 ) ) ;
#5813=CARTESIAN_POINT ( 'NONE',  ( 8.353125000614518569, -4.541064518000417216, -2.621784821875001281 ) ) ;
#5815=CARTESIAN_POINT ( 'NONE',  ( 4.959375000614516971, 4.541064518000418104, -2.621784821874998173 ) ) ;
#5816=CARTESIAN_POINT ( 'NONE',  ( 17.25000000122903288, -2.886751345948125991, -5.000000000000000000 ) ) ;
#5817=CARTESIAN_POINT ( 'NONE',  ( 22.38749999999999929, -2.886751345948129988, 4.999999999999997335 ) ) ;
#5819=CARTESIAN_POINT ( 'NONE',  ( 6.609375000614519102, -4.541064518000417216, -2.621784821875001281 ) ) ;
#5820=CARTESIAN_POINT ( 'NONE',  ( 11.67187500061451821, 3.027376345333613106, -5.243569643749998122 ) ) ;
#5821=CARTESIAN_POINT ( 'NONE',  ( 21.98437500061451644, 6.421520780324663323E-16, -5.243569643749999010 ) ) ;
#5823=ORIENTED_EDGE ( 'NONE', *, *, #15041, .T. ) ;
#5824=CARTESIAN_POINT ( 'NONE',  ( 3.346875000614518036, -3.027376345333614438, 5.243569643749998122 ) ) ;
#5825=CARTESIAN_POINT ( 'NONE',  ( 5.859375000614519102, 4.541064518000418104, -2.621784821874998173 ) ) ;
#5826=EDGE_CURVE ( 'NONE', #42194, #1783, #70886, .T. ) ;
#5827=CARTESIAN_POINT ( 'NONE',  ( 18.59999999999999787, 4.330127018922192761, -2.499999999999997780 ) ) ;
#5828=CARTESIAN_POINT ( 'NONE',  ( 15.66562500061451857, 3.027376345333613106, -5.243569643749998122 ) ) ;
#5831=CARTESIAN_POINT ( 'NONE',  ( 10.34062500061451750, 6.054752690667223547, 3.707466751127219781E-16 ) ) ;
#5832=CARTESIAN_POINT ( 'NONE',  ( 26.18437500061451573, 4.541064518000418104, 2.621784821874999949 ) ) ;
#5833=CARTESIAN_POINT ( 'NONE',  ( -1.071796769724490561, 19.57009619066136707, 26.00000000000000000 ) ) ;
#5834=CARTESIAN_POINT ( 'NONE',  ( 28.09687500061451360, -3.027376345333614438, 5.243569643749998122 ) ) ;
#5835=CARTESIAN_POINT ( 'NONE',  ( 9.525000000000002132, 6.123233995736764310E-16, -4.999999999999998224 ) ) ;
#5836=CARTESIAN_POINT ( 'NONE',  ( 3.999999999999998668, 14.52500000122903323, 27.69059892324149175 ) ) ;
#5837=CARTESIAN_POINT ( 'NONE',  ( 9.150000001229033231, -2.886751345948125991, -5.000000000000000000 ) ) ;
#5838=CARTESIAN_POINT ( 'NONE',  ( 18.79687500061451644, -3.027376345333610441, -5.243569643749999898 ) ) ;
#5839=CARTESIAN_POINT ( 'NONE',  ( 13.62187500061451750, 3.027376345333611329, 5.243569643749999010 ) ) ;
#5840=LINE ( 'NONE', #23545, #18282 ) ;
#5841=ORIENTED_EDGE ( 'NONE', *, *, #59933, .T. ) ;
#5842=CARTESIAN_POINT ( 'NONE',  ( 15.77812500061451573, 4.541064518000418104, 2.621784821874999949 ) ) ;
#5843=CARTESIAN_POINT ( 'NONE',  ( 27.07500000122903216, -5.773502691896255534, -1.060575238724906372E-15 ) ) ;
#5844=CARTESIAN_POINT ( 'NONE',  ( 15.49687500061451750, -3.027376345333614438, 5.243569643749998122 ) ) ;
#5845=CARTESIAN_POINT ( 'NONE',  ( 3.975671559181608306, 9.180671356215658108, -34.51033026775080970 ) ) ;
#5846=CARTESIAN_POINT ( 'NONE',  ( 17.50312500061451715, 4.541064518000418104, -2.621784821874998173 ) ) ;
#5849=CARTESIAN_POINT ( 'NONE',  ( 27.34687500061451360, -3.027376345333610441, -5.243569643749999898 ) ) ;
#5850=CARTESIAN_POINT ( 'NONE',  ( -4.243569643749997233, 11.29062500061451857, 32.45002607614398471 ) ) ;
#5851=CARTESIAN_POINT ( 'NONE',  ( 15.04687500061451644, -3.027376345333614438, 5.243569643749998122 ) ) ;
#5852=CARTESIAN_POINT ( 'NONE',  ( 13.08750000122903323, -4.330127018922194537, 2.499999999999995559 ) ) ;
#5853=FACE_OUTER_BOUND ( 'NONE', #21261, .T. ) ;
#5854=CARTESIAN_POINT ( 'NONE',  ( -2.121784821874996840, 18.58437500061451786, -26.32496088578401583 ) ) ;
#5855=CARTESIAN_POINT ( 'NONE',  ( 18.08437500061451431, 4.541064518000418104, 2.621784821874999949 ) ) ;
#5856=CARTESIAN_POINT ( 'NONE',  ( 19.50000000122903288, -2.886751345948125991, -5.000000000000000000 ) ) ;
#5857=CARTESIAN_POINT ( 'NONE',  ( 15.53437500061451715, -4.541064518000419881, 2.621784821874995952 ) ) ;
#5858=CARTESIAN_POINT ( 'NONE',  ( -2.121784821874996840, 12.28437500061451892, 33.67503911421598417 ) ) ;
#5859=CARTESIAN_POINT ( 'NONE',  ( 21.63750000122903572, -4.330127018922194537, 2.499999999999995559 ) ) ;
#5860=CARTESIAN_POINT ( 'NONE',  ( 15.32812500061451644, 4.541064518000418104, 2.621784821874999949 ) ) ;
#5861=CARTESIAN_POINT ( 'NONE',  ( 29.01562500061451644, -6.054752690667223547, -1.112240025338166033E-15 ) ) ;
#5862=EDGE_LOOP ( 'NONE', ( #33158, #41003, #23443, #42652 ) ) ;
#5863=ORIENTED_EDGE ( 'NONE', *, *, #61233, .T. ) ;
#5864=CARTESIAN_POINT ( 'NONE',  ( 20.85000000000000142, 4.330127018922192761, -2.499999999999997780 ) ) ;
#5866=CARTESIAN_POINT ( 'NONE',  ( 3.965625000614515727, 3.027376345333613106, -5.243569643749998122 ) ) ;
#5867=CARTESIAN_POINT ( 'NONE',  ( 15.18750000122903465, 4.330127018922191873, 2.499999999999999556 ) ) ;
#5868=CARTESIAN_POINT ( 'NONE',  ( 19.86562500061451786, 3.027376345333611329, 5.243569643749999010 ) ) ;
#5870=CARTESIAN_POINT ( 'NONE',  ( 25.45312500061451644, -4.541064518000417216, -2.621784821875001281 ) ) ;
#5871=CARTESIAN_POINT ( 'NONE',  ( 6.815625000614517148, 3.027376345333611329, 5.243569643749999010 ) ) ;
#5872=CARTESIAN_POINT ( 'NONE',  ( 1.626862140677534273E-15, 14.26250000000000107, 34.00000000000000000 ) ) ;
#5873=CARTESIAN_POINT ( 'NONE',  ( 30.00000000000000000, 0.000000000000000000, 4.999999999999998224 ) ) ;
#5875=CARTESIAN_POINT ( 'NONE',  ( 11.21250000122903501, 0.000000000000000000, 4.999999999999998224 ) ) ;
#5876=CARTESIAN_POINT ( 'NONE',  ( 3.999999999999998668, 12.27500000122903501, -32.30940107675850470 ) ) ;
#5877=CARTESIAN_POINT ( 'NONE',  ( -4.243569643749997233, 18.54687500061451289, -27.54997392385601174 ) ) ;
#5879=CARTESIAN_POINT ( 'NONE',  ( 6.300000001229033586, -2.886751345948129988, 4.999999999999997335 ) ) ;
#5880=CARTESIAN_POINT ( 'NONE',  ( 8.625000000000000000, 6.123233995736764310E-16, -4.999999999999998224 ) ) ;
#5882=CARTESIAN_POINT ( 'NONE',  ( 4.837500001229035895, 4.330127018922191873, 2.499999999999999556 ) ) ;
#5883=CARTESIAN_POINT ( 'NONE',  ( 12.90937500061451537, -4.541064518000417216, -2.621784821875001281 ) ) ;
#5884=B_SPLINE_CURVE_WITH_KNOTS ( 'NONE', 3,
 ( #58479, #69945, #8617, #64763, #64398, #53316, #13789, #36330, #58845, #8255 ),
 .UNSPECIFIED., .F., .F.,
 ( 4, 3, 3, 4 ),
 ( 3.346269061518779240E-14, 0.0001125120373406391218, 0.0001770538234357889697, 0.0002416132447809637063 ),
 .UNSPECIFIED. ) ;
#5885=CARTESIAN_POINT ( 'NONE',  ( 3.553125000614516082, 4.541064518000418104, -2.621784821874998173 ) ) ;
#5886=CARTESIAN_POINT ( 'NONE',  ( 12.97500000122903430, 2.886751345948126879, 4.999999999999998224 ) ) ;
#5887=CARTESIAN_POINT ( 'NONE',  ( -3.999999999999999112, 19.66250000122903430, -30.00000000000000000 ) ) ;
#5888=CARTESIAN_POINT ( 'NONE',  ( 9.534375000614517148, 4.541064518000418104, 2.621784821874999949 ) ) ;
#5889=LINE ( 'NONE', #51320, #35918 ) ;
#5891=CARTESIAN_POINT ( 'NONE',  ( 2.121784821874999061, 17.85312500061459673, 26.32496088578401583 ) ) ;
#5892=CARTESIAN_POINT ( 'NONE',  ( 21.49687500061451573, -3.027376345333610441, -5.243569643749999898 ) ) ;
#5893=CARTESIAN_POINT ( 'NONE',  ( 28.68750000122903288, 4.330127018922191873, 2.499999999999999556 ) ) ;
#5895=CARTESIAN_POINT ( 'NONE',  ( 22.00312500061451360, 4.541064518000418104, -2.621784821874998173 ) ) ;
#5896=CARTESIAN_POINT ( 'NONE',  ( 16.00312500061451715, -4.541064518000417216, -2.621784821875001281 ) ) ;
#5898=CARTESIAN_POINT ( 'NONE',  ( 11.97187500061451892, -6.054752690667223547, -1.112240025338166033E-15 ) ) ;
#5899=CARTESIAN_POINT ( 'NONE',  ( 29.69999999999999574, -4.330127018922190985, -2.500000000000001332 ) ) ;
#5900=CARTESIAN_POINT ( 'NONE',  ( 25.91250000122903074, 4.330127018922192761, -2.499999999999997780 ) ) ;
#5901=CARTESIAN_POINT ( 'NONE',  ( 3.234375000614516438, 4.541064518000418104, 2.621784821874999949 ) ) ;
#5902=CARTESIAN_POINT ( 'NONE',  ( 14.10937500061451644, 0.000000000000000000, 5.243569643749999010 ) ) ;
#5903=CARTESIAN_POINT ( 'NONE',  ( 28.50937500061451502, 0.000000000000000000, 5.243569643749999010 ) ) ;
#5904=CARTESIAN_POINT ( 'NONE',  ( 3.075000000000001510, -4.330127018922194537, 2.499999999999995559 ) ) ;
#5906=CARTESIAN_POINT ( 'NONE',  ( 22.05937500061451573, 4.541064518000418104, -2.621784821874998173 ) ) ;
#5907=CARTESIAN_POINT ( 'NONE',  ( 14.14687500061451786, -3.027376345333614438, 5.243569643749998122 ) ) ;
#5909=CARTESIAN_POINT ( 'NONE',  ( 25.98750000000000071, -2.886751345948129988, 4.999999999999997335 ) ) ;
#5910=CARTESIAN_POINT ( 'NONE',  ( 3.412500001229032964, 4.330127018922192761, -2.499999999999997780 ) ) ;
#5912=CARTESIAN_POINT ( 'NONE',  ( 18.14062500061451644, -3.027376345333614438, 5.243569643749998122 ) ) ;
#5913=CARTESIAN_POINT ( 'NONE',  ( 6.412500000000001421, 2.886751345948129099, -4.999999999999998224 ) ) ;
#5914=CARTESIAN_POINT ( 'NONE',  ( -1.071796769724488563, 14.24240381056766758, 34.00000000000000000 ) ) ;
#5915=CARTESIAN_POINT ( 'NONE',  ( 16.91250000000000142, 2.886751345948126879, 4.999999999999999112 ) ) ;
#5916=CARTESIAN_POINT ( 'NONE',  ( -4.243569643749999898, 13.01562500061451999, 27.54997392385601529 ) ) ;
#5917=LINE ( 'NONE', #11464, #17138 ) ;
#5918=CARTESIAN_POINT ( 'NONE',  ( 21.37500000122902932, 2.886751345948129099, -4.999999999999998224 ) ) ;
#5919=CARTESIAN_POINT ( 'NONE',  ( 4.520916466877475948, 8.924797207603107907, 26.03637063158135234 ) ) ;
#5920=CARTESIAN_POINT ( 'NONE',  ( 26.33437500061451431, -4.541064518000419881, 2.621784821874995952 ) ) ;
#5921=ORIENTED_EDGE ( 'NONE', *, *, #54530, .F. ) ;
#5922=CARTESIAN_POINT ( 'NONE',  ( 21.47812500061451502, 6.421520780324663323E-16, -5.243569643749999010 ) ) ;
#5923=CARTESIAN_POINT ( 'NONE',  ( 21.64687500061451786, 6.054752690667223547, 3.707466751127219781E-16 ) ) ;
#5924=CARTESIAN_POINT ( 'NONE',  ( 5.437500000000001776, -2.886751345948125991, -5.000000000000000000 ) ) ;
#5925=CARTESIAN_POINT ( 'NONE',  ( 9.965625000614517504, 3.027376345333611329, 5.243569643749999010 ) ) ;
#5926=CARTESIAN_POINT ( 'NONE',  ( 23.80312500061451786, 4.541064518000418104, -2.621784821874998173 ) ) ;
#5927=CARTESIAN_POINT ( 'NONE',  ( 12.79687500061451821, -3.027376345333614438, 5.243569643749998122 ) ) ;
#5928=CARTESIAN_POINT ( 'NONE',  ( 16.50937500061451502, -4.541064518000417216, -2.621784821875001281 ) ) ;
#5929=CARTESIAN_POINT ( 'NONE',  ( 4.458087853507603171, 2.264012079524543974, -4.729647261352303289 ) ) ;
#5930=CARTESIAN_POINT ( 'NONE',  ( -4.243569643749999898, 17.96562500061451573, 27.54997392385601529 ) ) ;
#5931=CARTESIAN_POINT ( 'NONE',  ( 22.57500000122903572, -5.773502691896255534, -1.060575238724906372E-15 ) ) ;
#5933=CARTESIAN_POINT ( 'NONE',  ( 11.87812500061451537, -4.541064518000419881, 2.621784821874995952 ) ) ;
#5934=CARTESIAN_POINT ( 'NONE',  ( 5.109375000614518214, 0.000000000000000000, 5.243569643749999010 ) ) ;
#5935=CARTESIAN_POINT ( 'NONE',  ( 4.996875000614516615, 6.054752690667223547, 3.707466751127219781E-16 ) ) ;
#5936=VERTEX_POINT ( 'NONE', #64510 ) ;
#5937=CARTESIAN_POINT ( 'NONE',  ( 25.09687500061451715, -3.027376345333610441, -5.243569643749999898 ) ) ;
#5938=CARTESIAN_POINT ( 'NONE',  ( 17.65312500061451573, 0.000000000000000000, 5.243569643749999010 ) ) ;
#5939=CARTESIAN_POINT ( 'NONE',  ( 27.00000000122903288, -2.886751345948129988, 4.999999999999997335 ) ) ;
#5941=CARTESIAN_POINT ( 'NONE',  ( 26.99062500061451431, 6.054752690667223547, 3.707466751127219781E-16 ) ) ;
#5942=CARTESIAN_POINT ( 'NONE',  ( 22.39687500061451075, -3.027376345333610441, -5.243569643749999898 ) ) ;
#5943=CARTESIAN_POINT ( 'NONE',  ( 16.45312500061451289, -4.541064518000417216, -2.621784821875001281 ) ) ;
#5944=CARTESIAN_POINT ( 'NONE',  ( -2.000000000000000000, 10.02500000000000036, 26.53589838486224650 ) ) ;
#5945=CARTESIAN_POINT ( 'NONE',  ( 23.46562500061451573, 3.027376345333611329, 5.243569643749999010 ) ) ;
#5946=CARTESIAN_POINT ( 'NONE',  ( 3.937500001229034208, 4.330127018922191873, 2.499999999999999556 ) ) ;
#5947=ORIENTED_EDGE ( 'NONE', *, *, #19674, .F. ) ;
#5948=CARTESIAN_POINT ( 'NONE',  ( 28.72500000000000142, -4.330127018922194537, 2.499999999999995559 ) ) ;
#5949=CARTESIAN_POINT ( 'NONE',  ( -2.828200636599751609E-16, 12.68750000000000000, -34.61880215351700230 ) ) ;
#5951=CARTESIAN_POINT ( 'NONE',  ( 28.56562500061451715, -6.054752690667223547, -1.112240025338166033E-15 ) ) ;
#5953=CARTESIAN_POINT ( 'NONE',  ( 10.37812500061451715, 4.541064518000418104, 2.621784821874999949 ) ) ;
#5954=CARTESIAN_POINT ( 'NONE',  ( 21.37500000122902932, 2.886751345948129099, -4.999999999999998224 ) ) ;
#5955=CARTESIAN_POINT ( 'NONE',  ( 13.24687500061451750, -3.027376345333614438, 5.243569643749998122 ) ) ;
#5956=CARTESIAN_POINT ( 'NONE',  ( 27.62812500061451360, -4.541064518000419881, 2.621784821874995952 ) ) ;
#5957=CARTESIAN_POINT ( 'NONE',  ( 28.87499999999999645, 6.123233995736764310E-16, -4.999999999999998224 ) ) ;
#5958=CARTESIAN_POINT ( 'NONE',  ( -2.828200636599751609E-16, 19.10000000122903074, -34.61880215351700230 ) ) ;
#5959=CARTESIAN_POINT ( 'NONE',  ( 14.66250000122903252, 4.330127018922192761, -2.499999999999997780 ) ) ;
#5960=CARTESIAN_POINT ( 'NONE',  ( 12.36562500061451608, -6.054752690667223547, -1.112240025338166033E-15 ) ) ;
#5962=CARTESIAN_POINT ( 'NONE',  ( 9.403125000614517504, 4.541064518000418104, -2.621784821874998173 ) ) ;
#5963=CARTESIAN_POINT ( 'NONE',  ( 6.628125000614517148, 6.421520780324663323E-16, -5.243569643749999010 ) ) ;
#5966=ADVANCED_FACE ( 'NONE', ( #53435 ), #13903, .F. ) ;
#5967=CARTESIAN_POINT ( 'NONE',  ( 15.59999999999999964, 0.000000000000000000, 4.999999999999998224 ) ) ;
#5968=EDGE_CURVE ( 'NONE', #60873, #17509, #26830, .T. ) ;
#5969=CARTESIAN_POINT ( 'NONE',  ( 17.14687500061451786, 6.054752690667223547, 3.707466751127219781E-16 ) ) ;
#5970=CARTESIAN_POINT ( 'NONE',  ( 11.43750000122903465, 6.123233995736764310E-16, -4.999999999999998224 ) ) ;
#5971=CARTESIAN_POINT ( 'NONE',  ( 18.64687500061451786, -3.027376345333614438, 5.243569643749998122 ) ) ;
#5973=EDGE_CURVE ( 'NONE', #18820, #37430, #4305, .T. ) ;
#5974=CARTESIAN_POINT ( 'NONE',  ( 20.78437500061451715, 4.541064518000418104, 2.621784821874999949 ) ) ;
#5975=CARTESIAN_POINT ( 'NONE',  ( 4.243569643749999898, 14.62812500061451715, -30.00000000000000000 ) ) ;
#5976=CARTESIAN_POINT ( 'NONE',  ( -4.243569643749999898, 19.80312500061451786, 30.00000000000000000 ) ) ;
#5978=CARTESIAN_POINT ( 'NONE',  ( 4.116754692841747776, 2.837675796283581686, 4.409386438731211832 ) ) ;
#5979=CARTESIAN_POINT ( 'NONE',  ( 27.29062500061451502, -3.027376345333610441, -5.243569643749999898 ) ) ;
#5980=CARTESIAN_POINT ( 'NONE',  ( 5.212500001229032343, 4.330127018922192761, -2.499999999999997780 ) ) ;
#5981=CARTESIAN_POINT ( 'NONE',  ( 28.65937500061451715, -4.541064518000417216, -2.621784821875001281 ) ) ;
#5982=CARTESIAN_POINT ( 'NONE',  ( 24.97499999999999787, 4.330127018922191873, 2.499999999999999556 ) ) ;
#5983=CARTESIAN_POINT ( 'NONE',  ( 8.353125000614518569, -4.541064518000417216, -2.621784821875001281 ) ) ;
#5985=CARTESIAN_POINT ( 'NONE',  ( 19.99687500061451573, -3.027376345333614438, 5.243569643749998122 ) ) ;
#5987=CARTESIAN_POINT ( 'NONE',  ( 6.140625000614516438, -3.027376345333610441, -5.243569643749999898 ) ) ;
#5988=CARTESIAN_POINT ( 'NONE',  ( 11.82187500061451679, 3.027376345333611329, 5.243569643749999010 ) ) ;
#5990=CARTESIAN_POINT ( 'NONE',  ( 21.94687500061451857, -3.027376345333610441, -5.243569643749999898 ) ) ;
#5992=CARTESIAN_POINT ( 'NONE',  ( 28.27499999999999858, -4.330127018922194537, 2.499999999999995559 ) ) ;
#5993=CARTESIAN_POINT ( 'NONE',  ( 3.412500000000002309, 2.886751345948126879, 4.999999999999999112 ) ) ;
#5994=CARTESIAN_POINT ( 'NONE',  ( 14.43750000122903288, -4.330127018922194537, 2.499999999999995559 ) ) ;
#5995=CARTESIAN_POINT ( 'NONE',  ( 4.000000000000000000, 12.20000000122903394, 32.30940107675849760 ) ) ;
#5996=CARTESIAN_POINT ( 'NONE',  ( 14.43750000122903288, -4.330127018922194537, 2.499999999999995559 ) ) ;
#5998=CARTESIAN_POINT ( 'NONE',  ( 13.61250000000000071, 2.886751345948129099, -4.999999999999998224 ) ) ;
#5999=CARTESIAN_POINT ( 'NONE',  ( 24.10312500061451502, -4.541064518000417216, -2.621784821875001281 ) ) ;
#6000=CARTESIAN_POINT ( 'NONE',  ( 14.10000000000000142, 4.330127018922192761, -2.499999999999997780 ) ) ;
#6001=CARTESIAN_POINT ( 'NONE',  ( 11.40000000122903501, -2.886751345948125991, -5.000000000000000000 ) ) ;
#6002=CARTESIAN_POINT ( 'NONE',  ( 9.590625000614517504, -3.027376345333614438, 5.243569643749998122 ) ) ;
#6003=CARTESIAN_POINT ( 'NONE',  ( 9.000000000000001776, -4.330127018922190985, -2.500000000000001332 ) ) ;
#6004=CARTESIAN_POINT ( 'NONE',  ( 9.001249775931846008E-16, 14.57187500061451679, -25.09994784771203058 ) ) ;
#6005=CARTESIAN_POINT ( 'NONE',  ( 27.75000000122903288, 5.773502691896255534, 3.535250795749688894E-16 ) ) ;
#6007=CARTESIAN_POINT ( 'NONE',  ( 8.587500000000002132, -2.886751345948125991, -5.000000000000000000 ) ) ;
#6008=CARTESIAN_POINT ( 'NONE',  ( -2.000000000000000000, 13.17500000000000071, -33.46410161513775705 ) ) ;
#6010=CARTESIAN_POINT ( 'NONE',  ( 20.76562500061451644, 3.027376345333611329, 5.243569643749999010 ) ) ;
#6011=CARTESIAN_POINT ( 'NONE',  ( 14.62500000122903288, 2.886751345948129099, -4.999999999999998224 ) ) ;
#6012=CARTESIAN_POINT ( 'NONE',  ( 28.97812500061451502, -4.541064518000419881, 2.621784821874995952 ) ) ;
#6013=CARTESIAN_POINT ( 'NONE',  ( 29.63437500061451502, 6.421520780324663323E-16, -5.243569643749999010 ) ) ;
#6014=CARTESIAN_POINT ( 'NONE',  ( 19.39687500061451786, 6.054752690667223547, 3.707466751127219781E-16 ) ) ;
#6015=CARTESIAN_POINT ( 'NONE',  ( 16.90312500061451573, -4.541064518000417216, -2.621784821875001281 ) ) ;
#6016=CARTESIAN_POINT ( 'NONE',  ( 4.243569643749999898, 11.02812500061459389, -30.00000000000000000 ) ) ;
#6017=CARTESIAN_POINT ( 'NONE',  ( 5.840625000614516615, 6.054752690667223547, 3.707466751127219781E-16 ) ) ;
#6018=CARTESIAN_POINT ( 'NONE',  ( 29.13750000122903216, 4.330127018922191873, 2.499999999999999556 ) ) ;
#6020=CARTESIAN_POINT ( 'NONE',  ( 19.45312500061451644, 0.000000000000000000, 5.243569643749999010 ) ) ;
#6021=CARTESIAN_POINT ( 'NONE',  ( 13.50000000000000178, -4.330127018922190985, -2.500000000000001332 ) ) ;
#6022=CARTESIAN_POINT ( 'NONE',  ( 4.050000001229035362, -2.886751345948129988, 4.999999999999997335 ) ) ;
#6023=CARTESIAN_POINT ( 'NONE',  ( 12.64687500061451608, 6.054752690667223547, 3.707466751127219781E-16 ) ) ;
#6024=AXIS2_PLACEMENT_3D ( 'NONE', #59768, #32074, #19878 ) ;
#6025=CARTESIAN_POINT ( 'NONE',  ( 12.34687500061452070, -3.027376345333614438, 5.243569643749998122 ) ) ;
#6026=CARTESIAN_POINT ( 'NONE',  ( 20.25937500061451857, 4.541064518000418104, -2.621784821874998173 ) ) ;
#6027=EDGE_LOOP ( 'NONE', ( #68075, #43354, #44679, #36902 ) ) ;
#6028=CARTESIAN_POINT ( 'NONE',  ( 30.00000000000000000, 6.123233995736764310E-16, -4.999999999999998224 ) ) ;
#6029=CARTESIAN_POINT ( 'NONE',  ( 23.09062500061451573, -3.027376345333614438, 5.243569643749998122 ) ) ;
#6030=CARTESIAN_POINT ( 'NONE',  ( 19.17187500061451999, -6.054752690667223547, -1.112240025338166033E-15 ) ) ;
#6031=CARTESIAN_POINT ( 'NONE',  ( 23.50312500061451360, 0.000000000000000000, 5.243569643749999010 ) ) ;
#6033=CARTESIAN_POINT ( 'NONE',  ( 2.000000000000001332, 16.55000000000000071, 33.46410161513774995 ) ) ;
#6034=CARTESIAN_POINT ( 'NONE',  ( 4.171875000614517326, 3.027376345333611329, 5.243569643749999010 ) ) ;
#6035=CARTESIAN_POINT ( 'NONE',  ( 12.60000000122903430, -2.886751345948129988, 4.999999999999997335 ) ) ;
#6036=CARTESIAN_POINT ( 'NONE',  ( 6.975000001229032520, 2.886751345948129099, -4.999999999999998224 ) ) ;
#6037=CARTESIAN_POINT ( 'NONE',  ( 27.67500000122903359, 2.886751345948129099, -4.999999999999998224 ) ) ;
#6040=CARTESIAN_POINT ( 'NONE',  ( 13.09687500061451892, 6.054752690667223547, 3.707466751127219781E-16 ) ) ;
#6041=CARTESIAN_POINT ( 'NONE',  ( -5.810221930991193690E-16, 14.93750000000000000, -34.00000000000000000 ) ) ;
#6042=CARTESIAN_POINT ( 'NONE',  ( 16.49062500061451786, -3.027376345333610441, -5.243569643749999898 ) ) ;
#6043=CARTESIAN_POINT ( 'NONE',  ( 14.55937500061451573, 0.000000000000000000, 5.243569643749999010 ) ) ;
#6044=CARTESIAN_POINT ( 'NONE',  ( 3.740625000614516527, -3.027376345333614438, 5.243569643749998122 ) ) ;
#6045=CARTESIAN_POINT ( 'NONE',  ( 20.40937500061451715, 0.000000000000000000, 5.243569643749999010 ) ) ;
#6046=CARTESIAN_POINT ( 'NONE',  ( 8.671875000614518214, 3.027376345333611329, 5.243569643749999010 ) ) ;
#6047=CARTESIAN_POINT ( 'NONE',  ( 15.03750000122903252, 6.123233995736764310E-16, -4.999999999999998224 ) ) ;
#6048=CARTESIAN_POINT ( 'NONE',  ( 5.775000000000002132, -4.330127018922194537, 2.499999999999995559 ) ) ;
#6049=CARTESIAN_POINT ( 'NONE',  ( 5.587500001229033231, 6.123233995736764310E-16, -4.999999999999998224 ) ) ;
#6050=CARTESIAN_POINT ( 'NONE',  ( 19.37812500061451715, 4.541064518000418104, 2.621784821874999949 ) ) ;
#6051=CARTESIAN_POINT ( 'NONE',  ( 8.850000001229034297, 5.773502691896255534, 3.535250795749688894E-16 ) ) ;
#6052=CARTESIAN_POINT ( 'NONE',  ( 17.09062500061451573, 6.054752690667223547, 3.707466751127219781E-16 ) ) ;
#6053=CARTESIAN_POINT ( 'NONE',  ( 12.40312500061451573, -4.541064518000417216, -2.621784821875001281 ) ) ;
#6055=CARTESIAN_POINT ( 'NONE',  ( 13.38750000000000107, -2.886751345948129988, 4.999999999999997335 ) ) ;
#6057=CARTESIAN_POINT ( 'NONE',  ( 9.937500001229032875, -4.330127018922194537, 2.499999999999995559 ) ) ;
#6058=CARTESIAN_POINT ( 'NONE',  ( 6.178125000614518747, 6.421520780324663323E-16, -5.243569643749999010 ) ) ;
#6059=EDGE_CURVE ( 'NONE', #40707, #23277, #57498, .T. ) ;
#6060=CARTESIAN_POINT ( 'NONE',  ( 19.27500000122903145, 2.886751345948126879, 4.999999999999999112 ) ) ;
#6062=CARTESIAN_POINT ( 'NONE',  ( 4.243569643749999898, 11.04687500061451999, -27.54997392385601529 ) ) ;
#6063=DIRECTION ( 'NONE',  ( -0.000000000000000000, -1.000000000000000000, -0.000000000000000000 ) ) ;
#6064=CYLINDRICAL_SURFACE ( 'NONE', #19381, 4.999999999999998224 ) ;
#6066=CARTESIAN_POINT ( 'NONE',  ( 20.29687500061451644, 6.054752690667223547, 3.707466751127219781E-16 ) ) ;
#6067=AXIS2_PLACEMENT_3D ( 'NONE', #3586, #65256, #37920 ) ;
#6069=CARTESIAN_POINT ( 'NONE',  ( 17.09062500061451573, 6.054752690667223547, 3.707466751127219781E-16 ) ) ;
#6071=CARTESIAN_POINT ( 'NONE',  ( 10.87500000000000000, 6.123233995736764310E-16, -4.999999999999998224 ) ) ;
#6073=CARTESIAN_POINT ( 'NONE',  ( 26.89687500061451431, -3.027376345333610441, -5.243569643749999898 ) ) ;
#6075=CARTESIAN_POINT ( 'NONE',  ( 11.27812500061451573, 4.541064518000418104, 2.621784821874999949 ) ) ;
#6076=CARTESIAN_POINT ( 'NONE',  ( 10.05937500061451750, 0.000000000000000000, 5.243569643749999010 ) ) ;
#6078=CARTESIAN_POINT ( 'NONE',  ( -3.999999999999997335, 14.18750000000000000, -27.69059892324149530 ) ) ;
#6079=CARTESIAN_POINT ( 'NONE',  ( 20.61562500061451431, 3.027376345333613106, -5.243569643749998122 ) ) ;
#6080=CARTESIAN_POINT ( 'NONE',  ( 17.62500000122903288, -5.773502691896255534, -1.060575238724906372E-15 ) ) ;
#6081=CARTESIAN_POINT ( 'NONE',  ( 4.000000000000000000, 15.35000000122903252, -27.69059892324149885 ) ) ;
#6082=CARTESIAN_POINT ( 'NONE',  ( 12.75000000000000178, 4.330127018922192761, -2.499999999999997780 ) ) ;
#6083=CARTESIAN_POINT ( 'NONE',  ( 22.80000000122903359, 5.773502691896255534, 3.535250795749688894E-16 ) ) ;
#6084=CARTESIAN_POINT ( 'NONE',  ( 15.44062500061451537, -3.027376345333614438, 5.243569643749998122 ) ) ;
#6087=CARTESIAN_POINT ( 'NONE',  ( 20.06250000000000000, 2.886751345948126879, 4.999999999999999112 ) ) ;
#6088=( BOUNDED_CURVE ( )  B_SPLINE_CURVE ( 2, ( #69625, #58880, #52270, #1672, #69268, #19352, #52991 ),
 .UNSPECIFIED., .F., .F. ) 
 B_SPLINE_CURVE_WITH_KNOTS ( ( 3, 2, 2, 3 ),
 ( 0.1250000000000000000, 0.1277777777777777679, 0.1305555555555555358, 0.1333333333333333037 ),
 .UNSPECIFIED. ) 
 CURVE ( )  GEOMETRIC_REPRESENTATION_ITEM ( )  RATIONAL_B_SPLINE_CURVE ( ( 1.000000000000000000, 0.8660254037844387076, 1.000000000000000000, 0.8660254037844387076, 1.000000000000000000, 0.8660254037844400399, 0.9999999999999986677 ) ) 
 REPRESENTATION_ITEM ( '' )  );
#6089=CARTESIAN_POINT ( 'NONE',  ( 23.51249999999999574, 2.886751345948129099, -4.999999999999998224 ) ) ;
#6090=CARTESIAN_POINT ( 'NONE',  ( 20.63437500061451857, 6.421520780324663323E-16, -5.243569643749999010 ) ) ;
#6091=CARTESIAN_POINT ( 'NONE',  ( 26.09062500061451573, 6.054752690667223547, 3.707466751127219781E-16 ) ) ;
#6093=CARTESIAN_POINT ( 'NONE',  ( 30.00000000000000000, 6.123233995736764310E-16, -4.999999999999998224 ) ) ;
#6094=CARTESIAN_POINT ( 'NONE',  ( 7.490625000614516082, -3.027376345333610441, -5.243569643749999898 ) ) ;
#6095=CARTESIAN_POINT ( 'NONE',  ( 3.250662400336420177, 3.799104362746421604, 3.614115195980558859 ) ) ;
#6096=CARTESIAN_POINT ( 'NONE',  ( 14.21249999999999858, 2.886751345948126879, 4.999999999999999112 ) ) ;
#6097=CARTESIAN_POINT ( 'NONE',  ( -4.243569643749999898, 18.41562500061451857, 27.54997392385601529 ) ) ;
#6098=CARTESIAN_POINT ( 'NONE',  ( 3.571875000614517237, 3.027376345333613106, -5.243569643749998122 ) ) ;
#6099=CARTESIAN_POINT ( 'NONE',  ( 26.63437500061451857, 4.541064518000418104, 2.621784821874999949 ) ) ;
#6100=EDGE_LOOP ( 'NONE', ( #46601, #21606, #13078, #18475 ) ) ;
#6101=CARTESIAN_POINT ( 'NONE',  ( 23.01562500061451644, 3.027376345333611329, 5.243569643749999010 ) ) ;
#6102=CARTESIAN_POINT ( 'NONE',  ( 24.38437500061451502, 4.541064518000418104, 2.621784821874999949 ) ) ;
#6103=CARTESIAN_POINT ( 'NONE',  ( -4.243569643749999898, 19.35312500061459318, -30.00000000000000000 ) ) ;
#6104=CARTESIAN_POINT ( 'NONE',  ( 12.33750000000000036, 5.773502691896255534, 3.535250795749688894E-16 ) ) ;
#6105=CARTESIAN_POINT ( 'NONE',  ( 10.07812500061451644, -4.541064518000419881, 2.621784821874995952 ) ) ;
#6107=CARTESIAN_POINT ( 'NONE',  ( 28.15312500061451573, -4.541064518000417216, -2.621784821875001281 ) ) ;
#6108=CARTESIAN_POINT ( 'NONE',  ( 25.56562500061451715, 3.027376345333612662, -5.243569643749998122 ) ) ;
#6109=CARTESIAN_POINT ( 'NONE',  ( -1.071796769724492338, 18.29240381056766651, 34.00000000000000000 ) ) ;
#6111=CARTESIAN_POINT ( 'NONE',  ( 18.60937500061451644, 0.000000000000000000, 5.243569643749999010 ) ) ;
#6112=CARTESIAN_POINT ( 'NONE',  ( 2.121784821875001281, 13.70937500061451786, 33.67503911421598417 ) ) ;
#6113=CARTESIAN_POINT ( 'NONE',  ( 19.17187500061451999, -6.054752690667223547, -1.112240025338166033E-15 ) ) ;
#6114=CARTESIAN_POINT ( 'NONE',  ( 28.13437500061451502, -4.541064518000419881, 2.621784821874995952 ) ) ;
#6115=CARTESIAN_POINT ( 'NONE',  ( 2.121784821874999061, 16.55937500061451573, 26.32496088578401583 ) ) ;
#6116=CARTESIAN_POINT ( 'NONE',  ( 9.553125000614517859, 0.000000000000000000, 5.243569643749999010 ) ) ;
#6117=FACE_OUTER_BOUND ( 'NONE', #42006, .T. ) ;
#6119=CARTESIAN_POINT ( 'NONE',  ( 4.509375000614518569, 4.541064518000418104, -2.621784821874998173 ) ) ;
#6121=CARTESIAN_POINT ( 'NONE',  ( 8.053125000614516082, 4.541064518000418104, -2.621784821874998173 ) ) ;
#6122=CARTESIAN_POINT ( 'NONE',  ( 12.27187500061451786, 3.027376345333611329, 5.243569643749999010 ) ) ;
#6123=CARTESIAN_POINT ( 'NONE',  ( 20.28750000122903074, -4.330127018922194537, 2.499999999999995559 ) ) ;
#6124=CARTESIAN_POINT ( 'NONE',  ( 5.821875000614519458, 3.027376345333613106, -5.243569643749998122 ) ) ;
#6125=CARTESIAN_POINT ( 'NONE',  ( 10.86562500061451431, 3.027376345333611329, 5.243569643749999010 ) ) ;
#6128=CARTESIAN_POINT ( 'NONE',  ( 18.15937500061451715, 0.000000000000000000, 5.243569643749999010 ) ) ;
#6129=CARTESIAN_POINT ( 'NONE',  ( 8.962500001229033231, 0.000000000000000000, 4.999999999999998224 ) ) ;
#6131=CARTESIAN_POINT ( 'NONE',  ( 23.80312500061451786, 4.541064518000418104, -2.621784821874998173 ) ) ;
#6132=CARTESIAN_POINT ( 'NONE',  ( 12.89062500061451821, -3.027376345333610441, -5.243569643749999898 ) ) ;
#6135=CARTESIAN_POINT ( 'NONE',  ( 11.95312500061451644, -4.541064518000417216, -2.621784821875001281 ) ) ;
#6136=CARTESIAN_POINT ( 'NONE',  ( 9.001249775931846008E-16, 10.52187500061451964, -25.09994784771203058 ) ) ;
#6137=CARTESIAN_POINT ( 'NONE',  ( 11.88750000122903216, 6.123233995736764310E-16, -4.999999999999998224 ) ) ;
#6138=CARTESIAN_POINT ( 'NONE',  ( 27.74062500061451431, -3.027376345333610441, -5.243569643749999898 ) ) ;
#6139=CARTESIAN_POINT ( 'NONE',  ( 2.121784821874999061, 13.80312500061451786, -33.67503911421598417 ) ) ;
#6140=CARTESIAN_POINT ( 'NONE',  ( 15.11250000122903359, 4.330127018922192761, -2.499999999999997780 ) ) ;
#6141=CARTESIAN_POINT ( 'NONE',  ( 10.87500000000000000, 6.123233995736764310E-16, -4.999999999999998224 ) ) ;
#6142=CARTESIAN_POINT ( 'NONE',  ( 20.01562500061451644, -6.054752690667223547, -1.112240025338166033E-15 ) ) ;
#6143=CARTESIAN_POINT ( 'NONE',  ( 7.996875000614519280, -3.027376345333610441, -5.243569643749999898 ) ) ;
#6144=EDGE_CURVE ( 'NONE', #67346, #68632, #53392, .T. ) ;
#6145=CARTESIAN_POINT ( 'NONE',  ( 7.762500001229033053, -4.330127018922190985, -2.500000000000001332 ) ) ;
#6146=CARTESIAN_POINT ( 'NONE',  ( 15.18750000122903465, 4.330127018922191873, 2.499999999999999556 ) ) ;
#6148=CARTESIAN_POINT ( 'NONE',  ( 12.62812500061451537, 4.541064518000418104, 2.621784821874999949 ) ) ;
#6149=CARTESIAN_POINT ( 'NONE',  ( 15.96562500061451573, -6.054752690667223547, -1.112240025338166033E-15 ) ) ;
#6150=CARTESIAN_POINT ( 'NONE',  ( 25.72500000122903074, -5.773502691896255534, -1.060575238724906372E-15 ) ) ;
#6151=CARTESIAN_POINT ( 'NONE',  ( 23.88749999999999929, -2.886751345948125991, -5.000000000000000000 ) ) ;
#6152=CARTESIAN_POINT ( 'NONE',  ( 24.00937500061451502, 0.000000000000000000, 5.243569643749999010 ) ) ;
#6154=CARTESIAN_POINT ( 'NONE',  ( 9.825000001229033941, 2.886751345948126879, 4.999999999999999112 ) ) ;
#6155=CARTESIAN_POINT ( 'NONE',  ( 28.84687500061452070, 6.054752690667223547, 3.707466751127219781E-16 ) ) ;
#6156=( BOUNDED_CURVE ( )  B_SPLINE_CURVE ( 2, ( #44086, #55529, #4923, #66989, #61425, #4199, #55891, #5280, #22266 ),
 .UNSPECIFIED., .F., .F. ) 
 B_SPLINE_CURVE_WITH_KNOTS ( ( 3, 2, 2, 2, 3 ),
 ( 0.3804347826086956763, 0.3840579710144927383, 0.3913043478260869734, 0.3985507246376811530, 0.4021739130434782705 ),
 .UNSPECIFIED. ) 
 CURVE ( )  GEOMETRIC_REPRESENTATION_ITEM ( )  RATIONAL_B_SPLINE_CURVE ( ( 0.9330127018922194093, 0.9330127018922198534, 1.000000000000000000, 0.8660254037844387076, 1.000000000000000000, 0.8660254037844387076, 1.000000000000000000, 0.9330127018922194093, 0.9330127018922194093 ) ) 
 REPRESENTATION_ITEM ( '' )  );
#6157=CARTESIAN_POINT ( 'NONE',  ( 4.059375000614519280, 4.541064518000418104, -2.621784821874998173 ) ) ;
#6158=CARTESIAN_POINT ( 'NONE',  ( 23.50312500061451360, 0.000000000000000000, 5.243569643749999010 ) ) ;
#6160=CARTESIAN_POINT ( 'NONE',  ( 0.000000000000000000, 20.00000000000000000, 30.00000000000000000 ) ) ;
#6161=CARTESIAN_POINT ( 'NONE',  ( 7.021875000614518747, -6.054752690667223547, -1.112240025338166033E-15 ) ) ;
#6163=CARTESIAN_POINT ( 'NONE',  ( 27.25312500061451360, -4.541064518000417216, -2.621784821875001281 ) ) ;
#6164=CARTESIAN_POINT ( 'NONE',  ( 6.421875000614519102, 3.027376345333611329, 5.243569643749999010 ) ) ;
#6166=CARTESIAN_POINT ( 'NONE',  ( 26.52187500061451431, 3.027376345333613106, -5.243569643749998122 ) ) ;
#6167=CARTESIAN_POINT ( 'NONE',  ( 4.243569643749999898, 10.12812500061459353, 30.00000000000000000 ) ) ;
#6168=CARTESIAN_POINT ( 'NONE',  ( 18.30000000000000071, 0.000000000000000000, 4.999999999999998224 ) ) ;
#6169=ORIENTED_EDGE ( 'NONE', *, *, #36318, .F. ) ;
#6170=CARTESIAN_POINT ( 'NONE',  ( 27.41250000000000142, -5.773502691896255534, -1.060575238724906372E-15 ) ) ;
#6171=CARTESIAN_POINT ( 'NONE',  ( 28.32187500061451502, 3.027376345333613106, -5.243569643749998122 ) ) ;
#6172=ORIENTED_EDGE ( 'NONE', *, *, #61587, .T. ) ;
#6173=CARTESIAN_POINT ( 'NONE',  ( 15.70312500061451644, 4.541064518000418104, -2.621784821874998173 ) ) ;
#6174=CARTESIAN_POINT ( 'NONE',  ( 8.090625000614515727, 6.054752690667223547, 3.707466751127219781E-16 ) ) ;
#6176=CARTESIAN_POINT ( 'NONE',  ( 5.634375000614519458, -4.541064518000419881, 2.621784821874995952 ) ) ;
#6178=CARTESIAN_POINT ( 'NONE',  ( 16.91250000122903430, 4.330127018922192761, -2.499999999999997780 ) ) ;
#6179=CARTESIAN_POINT ( 'NONE',  ( 21.97500000000000142, -4.330127018922194537, 2.499999999999995559 ) ) ;
#6180=CARTESIAN_POINT ( 'NONE',  ( 29.96250000000000213, 2.886751345948126879, 4.999999999999999112 ) ) ;
#6181=CARTESIAN_POINT ( 'NONE',  ( 3.496875000614518836, -3.027376345333610441, -5.243569643749999898 ) ) ;
#6182=CARTESIAN_POINT ( 'NONE',  ( 12.15937500061451892, 4.541064518000418104, -2.621784821874998173 ) ) ;
#6183=CARTESIAN_POINT ( 'NONE',  ( 22.92187500061451644, 3.027376345333613106, -5.243569643749998122 ) ) ;
#6184=CARTESIAN_POINT ( 'NONE',  ( -3.999999999999997335, 15.20000000122903572, -27.69059892324149530 ) ) ;
#6185=EDGE_LOOP ( 'NONE', ( #61084, #1603, #60824, #24890 ) ) ;
#6186=CARTESIAN_POINT ( 'NONE',  ( 3.609375000614516882, 4.541064518000418104, -2.621784821874998173 ) ) ;
#6187=CARTESIAN_POINT ( 'NONE',  ( 7.396875000614519635, -3.027376345333614438, 5.243569643749998122 ) ) ;
#6188=CARTESIAN_POINT ( 'NONE',  ( 18.71249999999999858, 2.886751345948126879, 4.999999999999999112 ) ) ;
#6189=CARTESIAN_POINT ( 'NONE',  ( 15.40312500061451573, 0.000000000000000000, 5.243569643749999010 ) ) ;
#6193=CARTESIAN_POINT ( 'NONE',  ( 9.928125000614517859, 4.541064518000418104, 2.621784821874999949 ) ) ;
#6194=CARTESIAN_POINT ( 'NONE',  ( 25.73437500061451644, 4.541064518000418104, 2.621784821874999949 ) ) ;
#6196=CARTESIAN_POINT ( 'NONE',  ( 26.07187500061451857, 3.027376345333613106, -5.243569643749998122 ) ) ;
#6197=CARTESIAN_POINT ( 'NONE',  ( 10.98750000000000071, 5.773502691896255534, 3.535250795749688894E-16 ) ) ;
#6198=CARTESIAN_POINT ( 'NONE',  ( 2.000000000000001332, 16.21250000122903501, 33.46410161513774995 ) ) ;
#6199=CARTESIAN_POINT ( 'NONE',  ( 8.212500001229035007, -4.330127018922190985, -2.500000000000001332 ) ) ;
#6200=EDGE_CURVE ( 'NONE', #70091, #8864, #45274, .T. ) ;
#6201=CARTESIAN_POINT ( 'NONE',  ( 19.54687500061451644, -3.027376345333614438, 5.243569643749998122 ) ) ;
#6202=CARTESIAN_POINT ( 'NONE',  ( 14.74687500061451573, -3.027376345333610441, -5.243569643749999898 ) ) ;
#6203=VERTEX_POINT ( 'NONE', #66721 ) ;
#6204=CARTESIAN_POINT ( 'NONE',  ( 15.02812500061451750, -4.541064518000419881, 2.621784821874995952 ) ) ;
#6205=CARTESIAN_POINT ( 'NONE',  ( 26.10000000122903430, -2.886751345948129988, 4.999999999999997335 ) ) ;
#6206=CARTESIAN_POINT ( 'NONE',  ( 13.95937500061451786, 4.541064518000418104, -2.621784821874998173 ) ) ;
#6207=CARTESIAN_POINT ( 'NONE',  ( 1.999999999999998668, 12.76250000122903394, 26.53589838486224650 ) ) ;
#6208=CARTESIAN_POINT ( 'NONE',  ( 17.57812500061451644, 4.541064518000418104, 2.621784821874999949 ) ) ;
#6211=CARTESIAN_POINT ( 'NONE',  ( 25.20937500061451431, 4.541064518000418104, -2.621784821874998173 ) ) ;
#6212=CARTESIAN_POINT ( 'NONE',  ( 2.917166856763841132, -4.060812204189049091, 3.317359856706287413 ) ) ;
#6213=CARTESIAN_POINT ( 'NONE',  ( 16.02187500061451786, -6.054752690667223547, -1.112240025338166033E-15 ) ) ;
#6214=CARTESIAN_POINT ( 'NONE',  ( 11.81250000122903465, -4.330127018922190985, -2.500000000000001332 ) ) ;
#6215=DIRECTION ( 'NONE',  ( 0.000000000000000000, 0.000000000000000000, -1.000000000000000000 ) ) ;
#6216=CARTESIAN_POINT ( 'NONE',  ( 4.243569643749999010, 17.42187500061451999, -32.45002607614398471 ) ) ;
#6217=ADVANCED_FACE ( 'NONE', ( #27559 ), #10921, .F. ) ;
#6218=CARTESIAN_POINT ( 'NONE',  ( 18.00937500061451502, 4.541064518000418104, -2.621784821874998173 ) ) ;
#6219=CARTESIAN_POINT ( 'NONE',  ( 20.92500000122903714, 2.886751345948129099, -4.999999999999998224 ) ) ;
#6220=CARTESIAN_POINT ( 'NONE',  ( 14.03437500061451715, 4.541064518000418104, 2.621784821874999949 ) ) ;
#6221=CARTESIAN_POINT ( 'NONE',  ( 4.243569643749999010, 12.92187500061451644, 27.54997392385601174 ) ) ;
#6222=CARTESIAN_POINT ( 'NONE',  ( 22.65000000122903856, -2.886751345948125991, -5.000000000000000000 ) ) ;
#6223=CARTESIAN_POINT ( 'NONE',  ( 14.39062500061451821, 6.054752690667223547, 3.707466751127219781E-16 ) ) ;
#6224=CARTESIAN_POINT ( 'NONE',  ( 29.80312500061451431, 0.000000000000000000, 5.243569643749999010 ) ) ;
#6225=ORIENTED_EDGE ( 'NONE', *, *, #37306, .T. ) ;
#6226=VERTEX_POINT ( 'NONE', #55992 ) ;
#6227=CARTESIAN_POINT ( 'NONE',  ( 20.02500000000000213, 4.330127018922191873, 2.499999999999999556 ) ) ;
#6228=CARTESIAN_POINT ( 'NONE',  ( 7.320879633048903241E-15, 17.75000000122903288, 26.00000000000000355 ) ) ;
#6229=CARTESIAN_POINT ( 'NONE',  ( 3.178125000614515638, 4.541064518000418104, 2.621784821874999949 ) ) ;
#6230=CARTESIAN_POINT ( 'NONE',  ( 14.06250000122903288, -4.330127018922190985, -2.500000000000001332 ) ) ;
#6231=CARTESIAN_POINT ( 'NONE',  ( 21.14062500061451289, 6.054752690667223547, 3.707466751127219781E-16 ) ) ;
#6232=CARTESIAN_POINT ( 'NONE',  ( 22.34062500061451573, -3.027376345333610441, -5.243569643749999898 ) ) ;
#6233=CARTESIAN_POINT ( 'NONE',  ( 29.58750000122903501, 4.330127018922191873, 2.499999999999999556 ) ) ;
#6234=VECTOR ( 'NONE', #39196, 1000.000000000000000 ) ;
#6235=CARTESIAN_POINT ( 'NONE',  ( 26.77500000122903145, 2.886751345948112668, -5.000000000000024869 ) ) ;
#6236=CARTESIAN_POINT ( 'NONE',  ( 4.582326623766785900, 2.000647313145979656, 4.846930428394146340 ) ) ;
#6239=CARTESIAN_POINT ( 'NONE',  ( 1.999999999999998668, 11.86250000122903359, -33.46410161513775705 ) ) ;
#6240=CARTESIAN_POINT ( 'NONE',  ( 4.243569643749999898, 17.79687500061451999, -27.54997392385601529 ) ) ;
#6241=EDGE_CURVE ( 'NONE', #37474, #69178, #40775, .T. ) ;
#6242=CARTESIAN_POINT ( 'NONE',  ( 5.962500001229033231, -4.330127018922190985, -2.500000000000001332 ) ) ;
#6243=CARTESIAN_POINT ( 'NONE',  ( 7.875000000000000000, 4.330127018922191873, 2.499999999999999556 ) ) ;
#6244=CARTESIAN_POINT ( 'NONE',  ( 4.350000001229033408, 5.773502691896255534, 3.535250795749688894E-16 ) ) ;
#6245=CARTESIAN_POINT ( 'NONE',  ( 11.14687500061451608, -3.027376345333610441, -5.243569643749999898 ) ) ;
#6246=CARTESIAN_POINT ( 'NONE',  ( 3.999999999999998668, 16.77500000122903145, -32.30940107675850470 ) ) ;
#6247=CARTESIAN_POINT ( 'NONE',  ( 3.046875000614519990, -3.027376345333610441, -5.243569643749999898 ) ) ;
#6248=CARTESIAN_POINT ( 'NONE',  ( 18.75000000000000000, 0.000000000000000000, 4.999999999999998224 ) ) ;
#6250=CARTESIAN_POINT ( 'NONE',  ( 11.29687500061451644, 6.054752690667223547, 3.707466751127219781E-16 ) ) ;
#6251=CARTESIAN_POINT ( 'NONE',  ( 13.77187500061451786, -6.054752690667223547, -1.112240025338166033E-15 ) ) ;
#6252=CARTESIAN_POINT ( 'NONE',  ( 1.999999999999998668, 14.11250000122903359, -33.46410161513775705 ) ) ;
#6253=CARTESIAN_POINT ( 'NONE',  ( 6.750000000000002665, -4.330127018922190985, -2.500000000000001332 ) ) ;
#6254=CARTESIAN_POINT ( 'NONE',  ( -2.121784821874999949, 17.47812500061459673, 26.32496088578401938 ) ) ;
#6255=CARTESIAN_POINT ( 'NONE',  ( 21.79687500061451644, -3.027376345333614438, 5.243569643749998122 ) ) ;
#6256=CARTESIAN_POINT ( 'NONE',  ( 2.752374072010383532, -4.174317300471400927, 2.814089559418405884 ) ) ;
#6257=CARTESIAN_POINT ( 'NONE',  ( 27.07500000122903216, -5.773502691896255534, -1.060575238724906372E-15 ) ) ;
#6259=CARTESIAN_POINT ( 'NONE',  ( 22.82812500061451644, 6.421520780324663323E-16, -5.243569643749999010 ) ) ;
#6260=CARTESIAN_POINT ( 'NONE',  ( 14.61562500061451608, -6.054752690667223547, -1.112240025338166033E-15 ) ) ;
#6262=CARTESIAN_POINT ( 'NONE',  ( 11.44687500061451857, -3.027376345333614438, 5.243569643749998122 ) ) ;
#6263=CARTESIAN_POINT ( 'NONE',  ( 28.72500000000000142, -4.330127018922194537, 2.499999999999995559 ) ) ;
#6264=CARTESIAN_POINT ( 'NONE',  ( 25.53750000122903074, 4.330127018922191873, 2.499999999999999556 ) ) ;
#6265=CARTESIAN_POINT ( 'NONE',  ( 4.209375000614516971, 0.000000000000000000, 5.243569643749999010 ) ) ;
#6266=CARTESIAN_POINT ( 'NONE',  ( 10.99687500061451750, -3.027376345333614438, 5.243569643749998122 ) ) ;
#6267=CARTESIAN_POINT ( 'NONE',  ( 28.24687500061451573, -3.027376345333610441, -5.243569643749999898 ) ) ;
#6269=CARTESIAN_POINT ( 'NONE',  ( 30.00000000000000000, 0.000000000000000000, 0.000000000000000000 ) ) ;
#6270=CARTESIAN_POINT ( 'NONE',  ( 23.33437500061451786, 6.421520780324663323E-16, -5.243569643749999010 ) ) ;
#6271=CARTESIAN_POINT ( 'NONE',  ( 13.35937500061451821, -4.541064518000417216, -2.621784821875001281 ) ) ;
#6273=CARTESIAN_POINT ( 'NONE',  ( 26.09999999999999787, -4.330127018922190985, -2.500000000000001332 ) ) ;
#6274=CARTESIAN_POINT ( 'NONE',  ( 4.162500001229033408, -4.330127018922190985, -2.500000000000001332 ) ) ;
#6276=CARTESIAN_POINT ( 'NONE',  ( 16.07812500061451289, 6.421520780324663323E-16, -5.243569643749999010 ) ) ;
#6277=CARTESIAN_POINT ( 'NONE',  ( 6.600000000000001421, 0.000000000000000000, 4.999999999999998224 ) ) ;
#6278=CARTESIAN_POINT ( 'NONE',  ( 13.53750000122903430, -4.330127018922194537, 2.499999999999995559 ) ) ;
#6279=CARTESIAN_POINT ( 'NONE',  ( 18.03749999999999787, -2.886751345948125991, -5.000000000000000000 ) ) ;
#6280=CARTESIAN_POINT ( 'NONE',  ( 2.121784821874999061, 12.45312500061451821, 26.32496088578401583 ) ) ;
#6282=CARTESIAN_POINT ( 'NONE',  ( 20.47500000122903074, 2.886751345948129099, -4.999999999999998224 ) ) ;
#6283=CARTESIAN_POINT ( 'NONE',  ( 26.70937500061451431, 0.000000000000000000, 5.243569643749999010 ) ) ;
#6284=ORIENTED_EDGE ( 'NONE', *, *, #65329, .T. ) ;
#6285=CARTESIAN_POINT ( 'NONE',  ( 21.62812500061451360, 4.541064518000418104, 2.621784821874999949 ) ) ;
#6286=B_SPLINE_CURVE_WITH_KNOTS ( 'NONE', 3,
 ( #41316, #52033, #63474, #1800, #19482, #30222, #24669, #30942, #42040, #24310 ),
 .UNSPECIFIED., .F., .F.,
 ( 4, 3, 3, 4 ),
 ( 4.080289400222272056E-17, 7.861589888542538148E-05, 0.0001572322621546033250, 0.0002879325728988927887 ),
 .UNSPECIFIED. ) ;
#6287=CARTESIAN_POINT ( 'NONE',  ( 21.53437500061451715, 6.421520780324663323E-16, -5.243569643749999010 ) ) ;
#6288=CARTESIAN_POINT ( 'NONE',  ( 4.387500000000002842, -2.886751345948129988, 4.999999999999997335 ) ) ;
#6289=CARTESIAN_POINT ( 'NONE',  ( 7.228125000614517681, 4.541064518000418104, 2.621784821874999949 ) ) ;
#6290=CARTESIAN_POINT ( 'NONE',  ( 23.20312500061451644, -4.541064518000417216, -2.621784821875001281 ) ) ;
#6291=CARTESIAN_POINT ( 'NONE',  ( 13.43437500061451750, 6.421520780324663323E-16, -5.243569643749999010 ) ) ;
#6292=CARTESIAN_POINT ( 'NONE',  ( 15.79687500061451821, 6.054752690667223547, 3.707466751127219781E-16 ) ) ;
#6293=CARTESIAN_POINT ( 'NONE',  ( -4.243569643749997233, 17.14062500061451644, 32.45002607614398471 ) ) ;
#6294=CARTESIAN_POINT ( 'NONE',  ( 22.31250000122903288, 4.330127018922192761, -2.499999999999997780 ) ) ;
#6296=CARTESIAN_POINT ( 'NONE',  ( 10.71562500061451750, 3.027376345333612662, -5.243569643749998122 ) ) ;
#6297=CARTESIAN_POINT ( 'NONE',  ( 5.559375000614517504, 0.000000000000000000, 5.243569643749999010 ) ) ;
#6298=CARTESIAN_POINT ( 'NONE',  ( 4.809375000614516615, -4.541064518000417216, -2.621784821875001281 ) ) ;
#6300=EDGE_CURVE ( 'NONE', #37421, #30066, #43821, .T. ) ;
#6301=CARTESIAN_POINT ( 'NONE',  ( 24.45937500061451786, 0.000000000000000000, 5.243569643749999010 ) ) ;
#6302=CARTESIAN_POINT ( 'NONE',  ( 15.92812500061451608, -4.541064518000419881, 2.621784821874995952 ) ) ;
#6303=CARTESIAN_POINT ( 'NONE',  ( 26.55000000122902648, -2.886751345948129988, 4.999999999999997335 ) ) ;
#6304=CARTESIAN_POINT ( 'NONE',  ( 28.79062500061451502, 6.054752690667223547, 3.707466751127219781E-16 ) ) ;
#6305=CARTESIAN_POINT ( 'NONE',  ( 20.74687500061451573, 6.054752690667223547, 3.707466751127219781E-16 ) ) ;
#6306=CARTESIAN_POINT ( 'NONE',  ( 17.76562500061451644, -6.054752690667223547, -1.112240025338166033E-15 ) ) ;
#6307=CARTESIAN_POINT ( 'NONE',  ( -4.243569643749997233, 18.99687500061451928, 32.45002607614398471 ) ) ;
#6308=CARTESIAN_POINT ( 'NONE',  ( 22.41562500061451502, 3.027376345333613106, -5.243569643749998122 ) ) ;
#6309=CARTESIAN_POINT ( 'NONE',  ( 3.187500001229033764, -4.330127018922194537, 2.499999999999995559 ) ) ;
#6310=EDGE_LOOP ( 'NONE', ( #62679, #9673, #1955, #58484 ) ) ;
#6311=CARTESIAN_POINT ( 'NONE',  ( 27.00000000000000000, -4.330127018922190985, -2.500000000000001332 ) ) ;
#6312=CARTESIAN_POINT ( 'NONE',  ( -2.828200636599751609E-16, 14.03750000000000142, -34.61880215351700230 ) ) ;
#6314=CARTESIAN_POINT ( 'NONE',  ( 29.16562500061451502, 3.027376345333613106, -5.243569643749998122 ) ) ;
#6315=CARTESIAN_POINT ( 'NONE',  ( 10.94062500061451537, -3.027376345333614438, 5.243569643749998122 ) ) ;
#6316=CARTESIAN_POINT ( 'NONE',  ( 21.71250000122903501, -4.330127018922190985, -2.500000000000001332 ) ) ;
#6317=CARTESIAN_POINT ( 'NONE',  ( 12.27187500061451608, 3.027376345333611329, 5.243569643749999010 ) ) ;
#6318=CARTESIAN_POINT ( 'NONE',  ( 27.92812500061451431, 4.541064518000418104, 2.621784821874999949 ) ) ;
#6319=CARTESIAN_POINT ( 'NONE',  ( 27.18750000000000000, 5.773502691896255534, 3.535250795749688894E-16 ) ) ;
#6320=CARTESIAN_POINT ( 'NONE',  ( -3.999999999999999556, 19.17500000122903359, -32.30940107675850470 ) ) ;
#6321=LINE ( 'NONE', #52836, #33804 ) ;
#6322=CARTESIAN_POINT ( 'NONE',  ( 11.76562500061451644, 3.027376345333611329, 5.243569643749999010 ) ) ;
#6323=ORIENTED_EDGE ( 'NONE', *, *, #39198, .T. ) ;
#6324=CARTESIAN_POINT ( 'NONE',  ( 6.553125000614518747, -4.541064518000417216, -2.621784821875001281 ) ) ;
#6325=CARTESIAN_POINT ( 'NONE',  ( 5.840625000614516615, 6.054752690667223547, 3.707466751127219781E-16 ) ) ;
#6327=CARTESIAN_POINT ( 'NONE',  ( 9.862500001229033586, 0.000000000000000000, 4.999999999999998224 ) ) ;
#6328=CARTESIAN_POINT ( 'NONE',  ( 14.77500000000000036, -4.330127018922194537, 2.499999999999995559 ) ) ;
#6329=CARTESIAN_POINT ( 'NONE',  ( 15.38437500061451679, 4.541064518000418104, 2.621784821874999949 ) ) ;
#6330=CARTESIAN_POINT ( 'NONE',  ( 10.83750000122903501, -4.330127018922194537, 2.499999999999995559 ) ) ;
#6331=CARTESIAN_POINT ( 'NONE',  ( 18.42187500061451644, 3.027376345333613106, -5.243569643749998122 ) ) ;
#6333=CARTESIAN_POINT ( 'NONE',  ( 21.30937500061451573, 0.000000000000000000, 5.243569643749999010 ) ) ;
#6334=CARTESIAN_POINT ( 'NONE',  ( -2.121784821874996840, 14.02812500061451750, -26.32496088578401583 ) ) ;
#6335=CARTESIAN_POINT ( 'NONE',  ( 7.500000000000000000, 0.000000000000000000, 4.999999999999998224 ) ) ;
#6338=ADVANCED_FACE ( 'NONE', ( #55268 ), #216, .F. ) ;
#6339=CARTESIAN_POINT ( 'NONE',  ( 26.99062500061451431, 6.054752690667223547, 3.707466751127219781E-16 ) ) ;
#6341=CARTESIAN_POINT ( 'NONE',  ( 28.17187500061451644, -6.054752690667223547, -1.112240025338166033E-15 ) ) ;
#6342=CARTESIAN_POINT ( 'NONE',  ( 24.14999999999999858, 0.000000000000000000, 4.999999999999998224 ) ) ;
#6343=CARTESIAN_POINT ( 'NONE',  ( 5.915625000614515905, 3.027376345333611329, 5.243569643749999010 ) ) ;
#6345=CARTESIAN_POINT ( 'NONE',  ( 20.03437500061451715, -4.541064518000419881, 2.621784821874995952 ) ) ;
#6347=CARTESIAN_POINT ( 'NONE',  ( 5.165625000614518569, -6.054752690667223547, -1.112240025338166033E-15 ) ) ;
#6348=CARTESIAN_POINT ( 'NONE',  ( 9.684375000614517504, -4.541064518000419881, 2.621784821874995952 ) ) ;
#6349=ORIENTED_EDGE ( 'NONE', *, *, #39819, .T. ) ;
#6350=CARTESIAN_POINT ( 'NONE',  ( 21.75937500061451502, 0.000000000000000000, 5.243569643749999010 ) ) ;
#6352=CARTESIAN_POINT ( 'NONE',  ( 29.25000000000000000, -4.330127018922190985, -2.500000000000001332 ) ) ;
#6353=CARTESIAN_POINT ( 'NONE',  ( 29.55937500061451573, -4.541064518000417216, -2.621784821875001281 ) ) ;
#6357=CARTESIAN_POINT ( 'NONE',  ( 10.49999999999999822, 4.330127018922192761, -2.499999999999997780 ) ) ;
#6359=CARTESIAN_POINT ( 'NONE',  ( 24.47812500061451502, -4.541064518000419881, 2.621784821874995952 ) ) ;
#6360=CARTESIAN_POINT ( 'NONE',  ( 14.40000000000000036, -4.330127018922190985, -2.500000000000001332 ) ) ;
#6361=CARTESIAN_POINT ( 'NONE',  ( 11.17500000122903536, 2.886751345948126879, 4.999999999999999112 ) ) ;
#6362=CARTESIAN_POINT ( 'NONE',  ( 8.578125000614518214, 4.541064518000418104, 2.621784821874999949 ) ) ;
#6363=( BOUNDED_CURVE ( )  B_SPLINE_CURVE ( 2, ( #20687, #43246, #49876, #9981, #38423, #60208, #49154, #26617, #55780 ),
 .UNSPECIFIED., .F., .F. ) 
 B_SPLINE_CURVE_WITH_KNOTS ( ( 3, 2, 2, 2, 3 ),
 ( 0.5543478260869565410, 0.5579710144927536586, 0.5652173913043477826, 0.5724637681159420177, 0.5760869565217391353 ),
 .UNSPECIFIED. ) 
 CURVE ( )  GEOMETRIC_REPRESENTATION_ITEM ( )  RATIONAL_B_SPLINE_CURVE ( ( 0.9330127018922194093, 0.9330127018922194093, 1.000000000000000000, 0.8660254037844387076, 1.000000000000000000, 0.8660254037844387076, 1.000000000000000000, 0.9330127018922194093, 0.9330127018922194093 ) ) 
 REPRESENTATION_ITEM ( '' )  );
#6364=CARTESIAN_POINT ( 'NONE',  ( 9.487500000000000711, -2.886751345948125991, -5.000000000000000000 ) ) ;
#6365=CYLINDRICAL_SURFACE ( 'NONE', #26599, 4.999999999999998224 ) ;
#6366=CARTESIAN_POINT ( 'NONE',  ( 28.46250000122903145, -4.330127018922190985, -2.500000000000001332 ) ) ;
#6368=CARTESIAN_POINT ( 'NONE',  ( 8.625000000000000000, 6.123233995736764310E-16, -4.999999999999998224 ) ) ;
#6370=ORIENTED_EDGE ( 'NONE', *, *, #41487, .T. ) ;
#6371=CARTESIAN_POINT ( 'NONE',  ( 21.70312500061451644, 0.000000000000000000, 5.243569643749999010 ) ) ;
#6372=CARTESIAN_POINT ( 'NONE',  ( 28.19062500061451715, -3.027376345333610441, -5.243569643749999898 ) ) ;
#6373=CARTESIAN_POINT ( 'NONE',  ( 29.33437500061451431, 4.541064518000418104, 2.621784821874999949 ) ) ;
#6374=CARTESIAN_POINT ( 'NONE',  ( 18.90937500061451360, 4.541064518000418104, -2.621784821874998173 ) ) ;
#6375=CARTESIAN_POINT ( 'NONE',  ( 17.31562500061451715, -6.054752690667223547, -1.112240025338166033E-15 ) ) ;
#6376=CARTESIAN_POINT ( 'NONE',  ( 2.121784821875001281, 12.75312500061459353, -26.32496088578401938 ) ) ;
#6377=CARTESIAN_POINT ( 'NONE',  ( 4.903125000614516615, 4.541064518000418104, -2.621784821874998173 ) ) ;
#6378=CARTESIAN_POINT ( 'NONE',  ( 28.12500000122902932, 2.886751345948129099, -4.999999999999998224 ) ) ;
#6380=CARTESIAN_POINT ( 'NONE',  ( 18.06562500061451715, 3.027376345333611329, 5.243569643749999010 ) ) ;
#6381=CARTESIAN_POINT ( 'NONE',  ( 3.999999999999998668, 13.96250000000000036, 27.69059892324149530 ) ) ;
#6382=CARTESIAN_POINT ( 'NONE',  ( 4.125000001229034652, -5.773502691896255534, -1.060575238724906372E-15 ) ) ;
#6383=CARTESIAN_POINT ( 'NONE',  ( 12.19687500061451679, 6.054752690667223547, 3.707466751127219781E-16 ) ) ;
#6384=CARTESIAN_POINT ( 'NONE',  ( 12.08437500061451608, 6.421520780324663323E-16, -5.243569643749999010 ) ) ;
#6385=CARTESIAN_POINT ( 'NONE',  ( 19.65937500061451360, -4.541064518000417216, -2.621784821875001281 ) ) ;
#6387=CARTESIAN_POINT ( 'NONE',  ( -5.672756003115388523, 8.235591643417166097, 31.96448613495275737 ) ) ;
#6388=CARTESIAN_POINT ( 'NONE',  ( 24.32812500061451289, 4.541064518000418104, 2.621784821874999949 ) ) ;
#6389=ADVANCED_FACE ( 'NONE', ( #39740 ), #9830, .F. ) ;
#6390=B_SPLINE_CURVE_WITH_KNOTS ( 'NONE', 3,
 ( #44450, #61053, #56250, #27450, #16344, #66980, #34059, #56600, #5272, #66232 ),
 .UNSPECIFIED., .F., .F.,
 ( 4, 3, 3, 4 ),
 ( 0.000000000000000000, 2.812507756822774961E-05, 5.625015391946155925E-05, 9.833933667866477343E-05 ),
 .UNSPECIFIED. ) ;
#6391=CARTESIAN_POINT ( 'NONE',  ( 18.45937500061451431, 4.541064518000418104, -2.621784821874998173 ) ) ;
#6392=CARTESIAN_POINT ( 'NONE',  ( 24.66562500061451502, 3.027376345333613106, -5.243569643749998122 ) ) ;
#6394=CARTESIAN_POINT ( 'NONE',  ( 1.999999999999998668, 15.80000000000000071, 26.53589838486224650 ) ) ;
#6395=AXIS2_PLACEMENT_3D ( 'NONE', #56749, #61938, #27972 ) ;
#6396=CARTESIAN_POINT ( 'NONE',  ( 3.159375000614518036, 4.541064518000418104, -2.621784821874998173 ) ) ;
#6397=CARTESIAN_POINT ( 'NONE',  ( 10.76250000122903572, 0.000000000000000000, 4.999999999999998224 ) ) ;
#6398=CARTESIAN_POINT ( 'NONE',  ( 6.637500001229035718, 4.330127018922191873, 2.499999999999999556 ) ) ;
#6399=CARTESIAN_POINT ( 'NONE',  ( -1.999999999999997113, 19.17500000000000071, -26.53589838486224295 ) ) ;
#6400=CARTESIAN_POINT ( 'NONE',  ( 26.66250000122903430, -4.330127018922190985, -2.500000000000001332 ) ) ;
#6403=CARTESIAN_POINT ( 'NONE',  ( 8.934375000614517504, 6.421520780324663323E-16, -5.243569643749999010 ) ) ;
#6404=CARTESIAN_POINT ( 'NONE',  ( 17.69999999999999929, 4.330127018922192761, -2.499999999999997780 ) ) ;
#6405=CARTESIAN_POINT ( 'NONE',  ( 17.09062500061451573, 6.054752690667223547, 3.707466751127219781E-16 ) ) ;
#6406=CARTESIAN_POINT ( 'NONE',  ( 10.65937500061451715, -4.541064518000417216, -2.621784821875001281 ) ) ;
#6407=CARTESIAN_POINT ( 'NONE',  ( 3.215625000614518836, 3.027376345333611329, 5.243569643749999010 ) ) ;
#6408=CARTESIAN_POINT ( 'NONE',  ( 19.88437500061451857, 4.541064518000418104, 2.621784821874999949 ) ) ;
#6409=CARTESIAN_POINT ( 'NONE',  ( 6.834375000614518747, 4.541064518000418104, 2.621784821874999949 ) ) ;
#6411=CARTESIAN_POINT ( 'NONE',  ( 11.77500000122903501, -5.773502691896255534, -1.060575238724906372E-15 ) ) ;
#6412=CARTESIAN_POINT ( 'NONE',  ( 10.94062500061451537, -3.027376345333614438, 5.243569643749998122 ) ) ;
#6413=CARTESIAN_POINT ( 'NONE',  ( 20.80312500061451431, 0.000000000000000000, 5.243569643749999010 ) ) ;
#6415=CARTESIAN_POINT ( 'NONE',  ( 6.487500001229034474, 6.123233995736764310E-16, -4.999999999999998224 ) ) ;
#6416=CARTESIAN_POINT ( 'NONE',  ( 15.96562500061451573, -6.054752690667223547, -1.112240025338166033E-15 ) ) ;
#6417=CARTESIAN_POINT ( 'NONE',  ( 13.86562500061451431, 3.027376345333613106, -5.243569643749998122 ) ) ;
#6419=CARTESIAN_POINT ( 'NONE',  ( 12.30000000000000249, 4.330127018922192761, -2.499999999999997780 ) ) ;
#6420=CARTESIAN_POINT ( 'NONE',  ( 9.262500001229033941, 4.330127018922192761, -2.499999999999997780 ) ) ;
#6421=CARTESIAN_POINT ( 'NONE',  ( 5.165625000614518569, -6.054752690667223547, -1.112240025338166033E-15 ) ) ;
#6422=CARTESIAN_POINT ( 'NONE',  ( 17.70000000122903216, -2.886751345948125991, -5.000000000000000000 ) ) ;
#6424=CARTESIAN_POINT ( 'NONE',  ( -3.000416591977282496E-16, 12.09687500061451715, -34.90005215228797653 ) ) ;
#6425=CARTESIAN_POINT ( 'NONE',  ( 8.474999999999999645, -4.330127018922194537, 2.499999999999995559 ) ) ;
#6426=CARTESIAN_POINT ( 'NONE',  ( 3.900000001229034563, 5.773502691896255534, 3.535250795749688894E-16 ) ) ;
#6428=CARTESIAN_POINT ( 'NONE',  ( 18.23437500061451999, -4.541064518000419881, 2.621784821874995952 ) ) ;
#6429=DIRECTION ( 'NONE',  ( -0.000000000000000000, -1.000000000000000000, -0.000000000000000000 ) ) ;
#6430=CARTESIAN_POINT ( 'NONE',  ( 16.19062500061451715, 6.054752690667223547, 3.707466751127219781E-16 ) ) ;
#6432=CARTESIAN_POINT ( 'NONE',  ( 22.65000000122903856, -2.886751345948092684, -5.000000000000057732 ) ) ;
#6433=CARTESIAN_POINT ( 'NONE',  ( 29.48437500061451644, -4.541064518000419881, 2.621784821874995952 ) ) ;
#6434=CARTESIAN_POINT ( 'NONE',  ( 27.00937500061451857, 4.541064518000418104, -2.621784821874998173 ) ) ;
#6436=AXIS2_PLACEMENT_3D ( 'NONE', #64013, #35939, #59192 ) ;
#6437=CARTESIAN_POINT ( 'NONE',  ( 13.45312500061451466, 4.541064518000418104, -2.621784821874998173 ) ) ;
#6438=CARTESIAN_POINT ( 'NONE',  ( 11.10937500061451644, -4.541064518000417216, -2.621784821875001281 ) ) ;
#6439=VERTEX_POINT ( 'NONE', #1661 ) ;
#6441=CARTESIAN_POINT ( 'NONE',  ( 21.17812500061451431, 4.541064518000418104, 2.621784821874999949 ) ) ;
#6442=CARTESIAN_POINT ( 'NONE',  ( 18.75000000000000000, 0.000000000000000000, 4.999999999999998224 ) ) ;
#6443=CARTESIAN_POINT ( 'NONE',  ( 1.071796769724489895, 14.91740381056766829, 26.00000000000000355 ) ) ;
#6444=CARTESIAN_POINT ( 'NONE',  ( 10.20000000000000107, 0.000000000000000000, 4.999999999999998224 ) ) ;
#6445=CARTESIAN_POINT ( 'NONE',  ( 20.77500000122903145, -5.773502691896255534, -1.060575238724906372E-15 ) ) ;
#6446=CARTESIAN_POINT ( 'NONE',  ( 15.14062500061451644, -3.027376345333610441, -5.243569643749999898 ) ) ;
#6448=ORIENTED_EDGE ( 'NONE', *, *, #58318, .F. ) ;
#6449=CARTESIAN_POINT ( 'NONE',  ( 16.46249999999999503, 2.886751345948126879, 4.999999999999999112 ) ) ;
#6450=CARTESIAN_POINT ( 'NONE',  ( 21.07499999999999929, -4.330127018922194537, 2.499999999999995559 ) ) ;
#6451=CARTESIAN_POINT ( 'NONE',  ( 19.88437500061451857, 4.541064518000418104, 2.621784821874999949 ) ) ;
#6452=CARTESIAN_POINT ( 'NONE',  ( 25.82812500061451644, -4.541064518000419881, 2.621784821874995952 ) ) ;
#6453=ORIENTED_EDGE ( 'NONE', *, *, #40061, .F. ) ;
#6454=EDGE_CURVE ( 'NONE', #23277, #35963, #5733, .T. ) ;
#6455=CARTESIAN_POINT ( 'NONE',  ( -3.999999999999997335, 17.00000000122903288, 32.30940107675850470 ) ) ;
#6456=CARTESIAN_POINT ( 'NONE',  ( 9.065625000614517148, 3.027376345333611329, 5.243569643749999010 ) ) ;
#6457=CARTESIAN_POINT ( 'NONE',  ( 1.626862140677534273E-15, 15.27500000122903501, 34.00000000000000000 ) ) ;
#6458=CARTESIAN_POINT ( 'NONE',  ( 13.64999999999999858, 4.330127018922192761, -2.499999999999997780 ) ) ;
#6459=CARTESIAN_POINT ( 'NONE',  ( -2.121784821874996840, 16.72812500061451857, 33.67503911421598417 ) ) ;
#6460=CARTESIAN_POINT ( 'NONE',  ( 29.61562500061451431, 3.027376345333613106, -5.243569643749998122 ) ) ;
#6461=AXIS2_PLACEMENT_3D ( 'NONE', #36951, #59471, #8882 ) ;
#6462=CARTESIAN_POINT ( 'NONE',  ( 26.10937500061451644, 4.541064518000418104, -2.621784821874998173 ) ) ;
#6464=CARTESIAN_POINT ( 'NONE',  ( 22.82812500061451644, 6.421520780324663323E-16, -5.243569643749999010 ) ) ;
#6465=CARTESIAN_POINT ( 'NONE',  ( 26.40937500061451715, -4.541064518000417216, -2.621784821875001281 ) ) ;
#6466=CARTESIAN_POINT ( 'NONE',  ( 2.121784821875001281, 17.70312500061459104, -26.32496088578401938 ) ) ;
#6467=CARTESIAN_POINT ( 'NONE',  ( 12.56250000000000178, -5.773502691896255534, -1.060575238724906372E-15 ) ) ;
#6468=CARTESIAN_POINT ( 'NONE',  ( 9.515625000614518214, 3.027376345333611329, 5.243569643749999010 ) ) ;
#6470=CARTESIAN_POINT ( 'NONE',  ( 28.71562500061451573, 3.027376345333613106, -5.243569643749998122 ) ) ;
#6471=CARTESIAN_POINT ( 'NONE',  ( 26.57812500061451644, 4.541064518000418104, 2.621784821874999949 ) ) ;
#6474=CARTESIAN_POINT ( 'NONE',  ( 19.47187500061451360, 3.027376345333611329, 5.243569643749999010 ) ) ;
#6475=CARTESIAN_POINT ( 'NONE',  ( 4.243569643749999010, 12.02187500061451786, 27.54997392385601174 ) ) ;
#6476=CARTESIAN_POINT ( 'NONE',  ( 20.10937500061451289, -4.541064518000417216, -2.621784821875001281 ) ) ;
#6477=CARTESIAN_POINT ( 'NONE',  ( 27.90937500061451715, 4.541064518000418104, -2.621784821874998173 ) ) ;
#6478=CARTESIAN_POINT ( 'NONE',  ( 2.121784821875001281, 16.85937500061451999, 33.67503911421598417 ) ) ;
#6479=CARTESIAN_POINT ( 'NONE',  ( 7.265625000614516438, 3.027376345333611329, 5.243569643749999010 ) ) ;
#6480=CARTESIAN_POINT ( 'NONE',  ( 30.00000000000000000, 0.000000000000000000, 0.000000000000000000 ) ) ;
#6482=CARTESIAN_POINT ( 'NONE',  ( 3.834375000614519635, -4.541064518000419881, 2.621784821874995952 ) ) ;
#6483=CARTESIAN_POINT ( 'NONE',  ( 3.837848076843224376, 3.204827942194517831, -3.837848076843224376 ) ) ;
#6484=CARTESIAN_POINT ( 'NONE',  ( 4.078125000614517326, 4.541064518000418104, 2.621784821874999949 ) ) ;
#6485=CARTESIAN_POINT ( 'NONE',  ( 10.20937500061451786, -4.541064518000417216, -2.621784821875001281 ) ) ;
#6486=CARTESIAN_POINT ( 'NONE',  ( 20.06250000122903643, 4.330127018922192761, -2.499999999999997780 ) ) ;
#6487=CARTESIAN_POINT ( 'NONE',  ( 5.896875000614518747, 6.054752690667223547, 3.707466751127219781E-16 ) ) ;
#6488=CARTESIAN_POINT ( 'NONE',  ( 6.590625000614518392, -3.027376345333610441, -5.243569643749999898 ) ) ;
#6491=CARTESIAN_POINT ( 'NONE',  ( 16.54687500061451644, -3.027376345333610441, -5.243569643749999898 ) ) ;
#6492=CARTESIAN_POINT ( 'NONE',  ( -1.071796769724488563, 11.65490381179670010, 34.00000000000000000 ) ) ;
#6494=CARTESIAN_POINT ( 'NONE',  ( 23.50312500061451360, 0.000000000000000000, 5.243569643749999010 ) ) ;
#6495=CARTESIAN_POINT ( 'NONE',  ( 10.45312500061451644, 0.000000000000000000, 5.243569643749999010 ) ) ;
#6496=CARTESIAN_POINT ( 'NONE',  ( 27.83437500061451786, 6.421520780324663323E-16, -5.243569643749999010 ) ) ;
#6497=CARTESIAN_POINT ( 'NONE',  ( 10.07812500061451644, -4.541064518000419881, 2.621784821874995952 ) ) ;
#6499=ADVANCED_FACE ( 'NONE', ( #5853 ), #22472, .F. ) ;
#6500=CARTESIAN_POINT ( 'NONE',  ( 11.92500000122903181, 2.886751345948129099, -4.999999999999998224 ) ) ;
#6501=CARTESIAN_POINT ( 'NONE',  ( 27.40312500061451573, 4.541064518000418104, -2.621784821874998173 ) ) ;
#6502=CARTESIAN_POINT ( 'NONE',  ( 4.243569643749999898, 12.79062500061451679, -27.54997392385601529 ) ) ;
#6503=CARTESIAN_POINT ( 'NONE',  ( 12.63750000122903394, -4.330127018922194537, 2.499999999999995559 ) ) ;
#6505=CARTESIAN_POINT ( 'NONE',  ( 10.72500000000000142, -4.330127018922194537, 2.499999999999995559 ) ) ;
#6506=CARTESIAN_POINT ( 'NONE',  ( 20.12812500061451715, 6.421520780324663323E-16, -5.243569643749999010 ) ) ;
#6508=CARTESIAN_POINT ( 'NONE',  ( 21.30000000000000071, 4.330127018922192761, -2.499999999999997780 ) ) ;
#6509=CARTESIAN_POINT ( 'NONE',  ( 6.712500001229034119, 0.000000000000000000, 4.999999999999998224 ) ) ;
#6510=CARTESIAN_POINT ( 'NONE',  ( 15.30000000122903359, -2.886751345948129988, 4.999999999999997335 ) ) ;
#6511=AXIS2_PLACEMENT_3D ( 'NONE', #53416, #31244, #64123 ) ;
#6512=CARTESIAN_POINT ( 'NONE',  ( 12.85312500061451502, -4.541064518000417216, -2.621784821875001281 ) ) ;
#6513=CARTESIAN_POINT ( 'NONE',  ( 15.85312500061451857, 0.000000000000000000, 5.243569643749999010 ) ) ;
#6515=CARTESIAN_POINT ( 'NONE',  ( 25.83750000122903501, 6.123233995736764310E-16, -4.999999999999998224 ) ) ;
#6516=CARTESIAN_POINT ( 'NONE',  ( 20.21250000000000213, -5.773502691896255534, -1.060575238724906372E-15 ) ) ;
#6517=CARTESIAN_POINT ( 'NONE',  ( 24.45937500061451786, 0.000000000000000000, 5.243569643749999010 ) ) ;
#6518=DIRECTION ( 'NONE',  ( -1.000000000000000000, -0.000000000000000000, -0.000000000000000000 ) ) ;
#6519=CARTESIAN_POINT ( 'NONE',  ( 9.037500001229034297, -4.330127018922194537, 2.499999999999995559 ) ) ;
#6520=CARTESIAN_POINT ( 'NONE',  ( 8.971875000614515372, 3.027376345333613106, -5.243569643749998122 ) ) ;
#6521=CARTESIAN_POINT ( 'NONE',  ( 24.75937500061451502, 4.541064518000418104, -2.621784821874998173 ) ) ;
#6522=( BOUNDED_CURVE ( )  B_SPLINE_CURVE ( 2, ( #42640, #60344, #21930, #31924, #66269, #61452, #16379, #48553, #71821 ),
 .UNSPECIFIED., .F., .F. ) 
 B_SPLINE_CURVE_WITH_KNOTS ( ( 3, 2, 2, 2, 3 ),
 ( 0.01086956521739130578, 0.01449275362318840597, 0.02173913043478260809, 0.02898550724637680848, 0.03260869565217391908 ),
 .UNSPECIFIED. ) 
 CURVE ( )  GEOMETRIC_REPRESENTATION_ITEM ( )  RATIONAL_B_SPLINE_CURVE ( ( 0.9330127018922194093, 0.9330127018922194093, 1.000000000000000000, 0.8660254037844387076, 1.000000000000000000, 0.8660254037844387076, 1.000000000000000000, 0.9330127018922191873, 0.9330127018922192983 ) ) 
 REPRESENTATION_ITEM ( '' )  );
#6523=CYLINDRICAL_SURFACE ( 'NONE', #23233, 4.999999999999998224 ) ;
#6524=CARTESIAN_POINT ( 'NONE',  ( 23.12812500061451360, -4.541064518000419881, 2.621784821874995952 ) ) ;
#6525=CARTESIAN_POINT ( 'NONE',  ( 27.34687500061451360, -3.027376345333610441, -5.243569643749999898 ) ) ;
#6528=CARTESIAN_POINT ( 'NONE',  ( 8.371875000614515727, -6.054752690667223547, -1.112240025338166033E-15 ) ) ;
#6529=CARTESIAN_POINT ( 'NONE',  ( 5.000000000000945022, -0.1513208456332415797, 5.148249888508871663 ) ) ;
#6530=CARTESIAN_POINT ( 'NONE',  ( 26.72812500061451502, -4.541064518000419881, 2.621784821874995952 ) ) ;
#6531=CARTESIAN_POINT ( 'NONE',  ( 5.446875000614518569, 6.054752690667223547, 3.707466751127219781E-16 ) ) ;
#6532=CARTESIAN_POINT ( 'NONE',  ( 3.160880256176461511, -3.874123901750303300, -3.160880256176591185 ) ) ;
#6533=CARTESIAN_POINT ( 'NONE',  ( -4.243569643749999898, 10.35312500061459673, 30.00000000000000000 ) ) ;
#6534=CARTESIAN_POINT ( 'NONE',  ( 15.97499999999999964, 4.330127018922191873, 2.499999999999999556 ) ) ;
#6536=CARTESIAN_POINT ( 'NONE',  ( 28.12499999999999645, 4.330127018922191873, 2.499999999999999556 ) ) ;
#6537=CARTESIAN_POINT ( 'NONE',  ( 29.55937500061451573, -4.541064518000417216, -2.621784821875001281 ) ) ;
#6539=CARTESIAN_POINT ( 'NONE',  ( 15.02812500061451750, -4.541064518000419881, 2.621784821874995952 ) ) ;
#6540=CARTESIAN_POINT ( 'NONE',  ( 5.765625000614519102, 3.027376345333613106, -5.243569643749998122 ) ) ;
#6542=CARTESIAN_POINT ( 'NONE',  ( 4.434375000614519280, 6.421520780324663323E-16, -5.243569643749999010 ) ) ;
#6543=CARTESIAN_POINT ( 'NONE',  ( 14.85000000122903252, -2.886751345948129988, 4.999999999999997335 ) ) ;
#6544=CARTESIAN_POINT ( 'NONE',  ( 21.44999999999999929, 0.000000000000000000, 4.999999999999998224 ) ) ;
#6545=CARTESIAN_POINT ( 'NONE',  ( 29.62500000000000000, -4.330127018922194537, 2.499999999999995559 ) ) ;
#6546=CARTESIAN_POINT ( 'NONE',  ( 4.959375000614516971, 4.541064518000418104, -2.621784821874998173 ) ) ;
#6547=CARTESIAN_POINT ( 'NONE',  ( 8.709375000614517859, 0.000000000000000000, 5.243569643749999010 ) ) ;
#6548=CARTESIAN_POINT ( 'NONE',  ( 22.62187500061451573, 3.027376345333611329, 5.243569643749999010 ) ) ;
#6549=ADVANCED_FACE ( 'NONE', ( #11032 ), #28743, .F. ) ;
#6550=CARTESIAN_POINT ( 'NONE',  ( 17.17500000000000071, 6.123233995736764310E-16, -4.999999999999998224 ) ) ;
#6552=CARTESIAN_POINT ( 'NONE',  ( 4.021875000614516082, 3.027376345333613106, -5.243569643749998122 ) ) ;
#6553=CARTESIAN_POINT ( 'NONE',  ( 6.337499999999998579, -2.886751345948125991, -5.000000000000000000 ) ) ;
#6555=CARTESIAN_POINT ( 'NONE',  ( 6.684375000614518392, 6.421520780324663323E-16, -5.243569643749999010 ) ) ;
#6556=CARTESIAN_POINT ( 'NONE',  ( 17.62500000000000000, 6.123233995736764310E-16, -4.999999999999998224 ) ) ;
#6557=CARTESIAN_POINT ( 'NONE',  ( 15.89062500061451289, -3.027376345333614438, 5.243569643749998122 ) ) ;
#6559=CARTESIAN_POINT ( 'NONE',  ( 4.194367172679521083, 2.721727781396576784, 4.432111563841672819 ) ) ;
#6561=CARTESIAN_POINT ( 'NONE',  ( 9.553125000614517859, 0.000000000000000000, 5.243569643749999010 ) ) ;
#6562=CARTESIAN_POINT ( 'NONE',  ( 25.99687500061451928, -3.027376345333610441, -5.243569643749999898 ) ) ;
#6564=CARTESIAN_POINT ( 'NONE',  ( 26.55937500061451573, 4.541064518000418104, -2.621784821874998173 ) ) ;
#6565=CARTESIAN_POINT ( 'NONE',  ( 8.699999999999999289, 4.330127018922192761, -2.499999999999997780 ) ) ;
#6566=CARTESIAN_POINT ( 'NONE',  ( -1.999999999999997113, 13.88750000122903394, 33.46410161513775705 ) ) ;
#6567=CARTESIAN_POINT ( 'NONE',  ( 7.837500001229035007, 6.123233995736764310E-16, -4.999999999999998224 ) ) ;
#6569=CARTESIAN_POINT ( 'NONE',  ( 17.37187500061451573, -6.054752690667223547, -1.112240025338166033E-15 ) ) ;
#6570=CARTESIAN_POINT ( 'NONE',  ( 12.08437500061451608, 6.421520780324663323E-16, -5.243569643749999010 ) ) ;
#6571=CARTESIAN_POINT ( 'NONE',  ( -3.992949912593975359, 3.009468837316803924, -30.27463465970910406 ) ) ;
#6573=CARTESIAN_POINT ( 'NONE',  ( 14.84062500061451750, 6.054752690667223547, 3.707466751127219781E-16 ) ) ;
#6574=AXIS2_PLACEMENT_3D ( 'NONE', #30059, #53319, #2354 ) ;
#6575=CARTESIAN_POINT ( 'NONE',  ( 25.61250000122903359, 0.000000000000000000, 4.999999999999998224 ) ) ;
#6576=CARTESIAN_POINT ( 'NONE',  ( 12.57187500061451857, 3.027376345333613106, -5.243569643749998122 ) ) ;
#6577=CARTESIAN_POINT ( 'NONE',  ( 3.999999999999998668, 12.72500000122903430, 27.69059892324149530 ) ) ;
#6578=CARTESIAN_POINT ( 'NONE',  ( 13.71562500061451750, -6.054752690667223547, -1.112240025338166033E-15 ) ) ;
#6579=CARTESIAN_POINT ( 'NONE',  ( 26.36250000122903003, 4.330127018922192761, -2.499999999999997780 ) ) ;
#6580=CARTESIAN_POINT ( 'NONE',  ( 26.14687500061451431, 6.054752690667223547, 3.707466751127219781E-16 ) ) ;
#6581=CARTESIAN_POINT ( 'NONE',  ( 5.190092854996874117, 9.698896338944486217, 24.77581305162949832 ) ) ;
#6583=CARTESIAN_POINT ( 'NONE',  ( 12.15000000122903501, -2.886751345948129988, 4.999999999999997335 ) ) ;
#6586=CARTESIAN_POINT ( 'NONE',  ( 4.243569643749999898, 17.34687500061451715, -27.54997392385601529 ) ) ;
#6587=CARTESIAN_POINT ( 'NONE',  ( 18.30937500061451928, -4.541064518000417216, -2.621784821875001281 ) ) ;
#6588=CARTESIAN_POINT ( 'NONE',  ( 19.61250000122903359, 4.330127018922192761, -2.499999999999997780 ) ) ;
#6589=( BOUNDED_CURVE ( )  B_SPLINE_CURVE ( 2, ( #22167, #45073, #61684, #55431, #21430, #49888, #43987, #62057, #16975 ),
 .UNSPECIFIED., .F., .F. ) 
 B_SPLINE_CURVE_WITH_KNOTS ( ( 3, 2, 2, 2, 3 ),
 ( 0.8152173913043478937, 0.8188405797101449002, 0.8260869565217391353, 0.8333333333333333703, 0.8369565217391304879 ),
 .UNSPECIFIED. ) 
 CURVE ( )  GEOMETRIC_REPRESENTATION_ITEM ( )  RATIONAL_B_SPLINE_CURVE ( ( 0.9330127018922192983, 0.9330127018922202975, 1.000000000000000000, 0.8660254037844387076, 1.000000000000000000, 0.8660254037844387076, 1.000000000000000000, 0.9330127018922182991, 0.9330127018922192983 ) ) 
 REPRESENTATION_ITEM ( '' )  );
#6590=CARTESIAN_POINT ( 'NONE',  ( 14.63437500061451679, -4.541064518000419881, 2.621784821874995952 ) ) ;
#6591=FACE_OUTER_BOUND ( 'NONE', #59994, .T. ) ;
#6592=CARTESIAN_POINT ( 'NONE',  ( 22.31250000122903288, 4.330127018922192761, -2.499999999999997780 ) ) ;
#6593=CARTESIAN_POINT ( 'NONE',  ( 15.85312500061451857, 0.000000000000000000, 5.243569643749999010 ) ) ;
#6594=CARTESIAN_POINT ( 'NONE',  ( 29.72812500061451502, 4.541064518000418104, 2.621784821874999949 ) ) ;
#6595=ORIENTED_EDGE ( 'NONE', *, *, #39975, .F. ) ;
#6596=ORIENTED_EDGE ( 'NONE', *, *, #38656, .F. ) ;
#6597=CARTESIAN_POINT ( 'NONE',  ( 17.39999999999999858, 0.000000000000000000, 4.999999999999998224 ) ) ;
#6599=CARTESIAN_POINT ( 'NONE',  ( 3.103125000614517237, 4.541064518000418104, -2.621784821874998173 ) ) ;
#6600=CARTESIAN_POINT ( 'NONE',  ( 14.62500000122903288, 2.886751345948129099, -4.999999999999998224 ) ) ;
#6601=CARTESIAN_POINT ( 'NONE',  ( 20.72812500061451502, 4.541064518000418104, 2.621784821874999949 ) ) ;
#6602=CARTESIAN_POINT ( 'NONE',  ( 23.99062500061451786, -3.027376345333614438, 5.243569643749998122 ) ) ;
#6603=CARTESIAN_POINT ( 'NONE',  ( 2.803125000614518747, 0.000000000000000000, 5.243569643749999010 ) ) ;
#6604=( BOUNDED_CURVE ( )  B_SPLINE_CURVE ( 2, ( #56693, #57049, #52244, #68161, #68517, #12712, #18234 ),
 .UNSPECIFIED., .F., .F. ) 
 B_SPLINE_CURVE_WITH_KNOTS ( ( 3, 2, 2, 3 ),
 ( 0.7666666666666668295, 0.7694444444444445974, 0.7722222222222223653, 0.7750000000000001332 ),
 .UNSPECIFIED. ) 
 CURVE ( )  GEOMETRIC_REPRESENTATION_ITEM ( )  RATIONAL_B_SPLINE_CURVE ( ( 0.9999999999999946709, 0.8660254037844440367, 1.000000000000000000, 0.8660254037844387076, 1.000000000000000000, 0.8660254037844333785, 1.000000000000005329 ) ) 
 REPRESENTATION_ITEM ( '' )  );
#6605=CARTESIAN_POINT ( 'NONE',  ( 27.37500000000000000, -4.330127018922194537, 2.499999999999995559 ) ) ;
#6606=CARTESIAN_POINT ( 'NONE',  ( 4.575260086717170438, 2.016679235498957112, 4.840250765194281435 ) ) ;
#6607=AXIS2_PLACEMENT_3D ( 'NONE', #16146, #42772, #72305 ) ;
#6609=LINE ( 'NONE', #29137, #5242 ) ;
#6610=CARTESIAN_POINT ( 'NONE',  ( 3.999999999999999112, 11.33750000122903501, -30.00000000000000000 ) ) ;
#6611=CARTESIAN_POINT ( 'NONE',  ( -4.243569643749997233, 15.84687500061451715, -27.54997392385601174 ) ) ;
#6612=CARTESIAN_POINT ( 'NONE',  ( 6.487500001229034474, 6.123233995736764310E-16, -4.999999999999998224 ) ) ;
#6613=CARTESIAN_POINT ( 'NONE',  ( 9.187500000000001776, 5.773502691896255534, 3.535250795749688894E-16 ) ) ;
#6614=EDGE_CURVE ( 'NONE', #65643, #53042, #685, .T. ) ;
#6615=CARTESIAN_POINT ( 'NONE',  ( 4.987500001229032698, -4.330127018922194537, 2.499999999999995559 ) ) ;
#6616=CARTESIAN_POINT ( 'NONE',  ( 9.609375000614518214, 0.000000000000000000, 5.243569643749999010 ) ) ;
#6618=CARTESIAN_POINT ( 'NONE',  ( 3.121875000614518836, 3.027376345333613106, -5.243569643749998122 ) ) ;
#6619=CARTESIAN_POINT ( 'NONE',  ( 28.01249999999999929, 2.886751345948146419, -4.999999999999968914 ) ) ;
#6620=CARTESIAN_POINT ( 'NONE',  ( 7.320879633048903241E-15, 18.53750000000000142, -34.00000000000000000 ) ) ;
#6621=CARTESIAN_POINT ( 'NONE',  ( 7.471875000614519813, -6.054752690667223547, -1.112240025338166033E-15 ) ) ;
#6622=CARTESIAN_POINT ( 'NONE',  ( 12.60937500061451821, 4.541064518000418104, -2.621784821874998173 ) ) ;
#6623=CARTESIAN_POINT ( 'NONE',  ( 6.075000001229034829, 2.886751345948129099, -4.999999999999997335 ) ) ;
#6624=CARTESIAN_POINT ( 'NONE',  ( 6.450000000000001066, 4.330127018922192761, -2.499999999999997780 ) ) ;
#6625=CARTESIAN_POINT ( 'NONE',  ( -4.243569643749999898, 16.20312500061459815, 30.00000000000000000 ) ) ;
#6626=CARTESIAN_POINT ( 'NONE',  ( 22.35937500061451644, -4.541064518000417216, -2.621784821875001281 ) ) ;
#6628=CARTESIAN_POINT ( 'NONE',  ( 25.83750000122903501, 6.123233995736764310E-16, -4.999999999999998224 ) ) ;
#6630=CARTESIAN_POINT ( 'NONE',  ( 21.81562500061451004, -6.054752690667223547, -1.112240025338166033E-15 ) ) ;
#6631=CARTESIAN_POINT ( 'NONE',  ( 15.74062500061451608, 6.054752690667223547, 3.707466751127219781E-16 ) ) ;
#6633=CARTESIAN_POINT ( 'NONE',  ( 11.89687500061451608, -3.027376345333614438, 5.243569643749998122 ) ) ;
#6634=CARTESIAN_POINT ( 'NONE',  ( 29.02499999999999858, 4.330127018922191873, 2.499999999999999556 ) ) ;
#6635=CARTESIAN_POINT ( 'NONE',  ( 22.68750000122903288, 6.123233995736764310E-16, -4.999999999999998224 ) ) ;
#6637=CARTESIAN_POINT ( 'NONE',  ( 11.44687500061451857, -3.027376345333614438, 5.243569643749998122 ) ) ;
#6638=CARTESIAN_POINT ( 'NONE',  ( 29.18437500061451573, 6.421520780324663323E-16, -5.243569643749999010 ) ) ;
#6639=ADVANCED_FACE ( 'NONE', ( #61630 ), #22829, .F. ) ;
#6642=CARTESIAN_POINT ( 'NONE',  ( 21.98437500061451644, 6.421520780324663323E-16, -5.243569643749999010 ) ) ;
#6643=CARTESIAN_POINT ( 'NONE',  ( 13.20937500061451786, 0.000000000000000000, 5.243569643749999010 ) ) ;
#6645=CARTESIAN_POINT ( 'NONE',  ( 25.38749999999999929, 5.773502691896255534, 3.535250795749688894E-16 ) ) ;
#6648=CARTESIAN_POINT ( 'NONE',  ( 17.24062500061451786, -3.027376345333614438, 5.243569643749998122 ) ) ;
#6649=CARTESIAN_POINT ( 'NONE',  ( 7.724999999999999645, 6.123233995736764310E-16, -4.999999999999998224 ) ) ;
#6650=CARTESIAN_POINT ( 'NONE',  ( 15.67500000000000071, -4.330127018922194537, 2.499999999999995559 ) ) ;
#6651=CARTESIAN_POINT ( 'NONE',  ( -3.999999999999999556, 19.62500000122903643, 27.69059892324149530 ) ) ;
#6653=CARTESIAN_POINT ( 'NONE',  ( 26.29687500061451644, -3.027376345333614438, 5.243569643749998122 ) ) ;
#6655=CARTESIAN_POINT ( 'NONE',  ( 22.26562500061451644, -6.054752690667223547, -1.112240025338166033E-15 ) ) ;
#6656=CARTESIAN_POINT ( 'NONE',  ( 20.25937500061451857, 4.541064518000418104, -2.621784821874998173 ) ) ;
#6657=CARTESIAN_POINT ( 'NONE',  ( 3.600000000000002309, -4.330127018922190985, -2.500000000000001332 ) ) ;
#6658=CARTESIAN_POINT ( 'NONE',  ( 7.190625000614518036, 6.054752690667223547, 3.707466751127219781E-16 ) ) ;
#6659=CARTESIAN_POINT ( 'NONE',  ( 21.51562500061451644, 3.027376345333613106, -5.243569643749998122 ) ) ;
#6660=CARTESIAN_POINT ( 'NONE',  ( 11.70937500061451608, 4.541064518000418104, -2.621784821874998173 ) ) ;
#6661=CARTESIAN_POINT ( 'NONE',  ( 17.33437500061451431, -4.541064518000419881, 2.621784821874995952 ) ) ;
#6662=CARTESIAN_POINT ( 'NONE',  ( 4.243569643749999898, 17.32812500061451644, 30.00000000000000000 ) ) ;
#6663=EDGE_CURVE ( 'NONE', #10265, #9450, #39476, .T. ) ;
#6664=CARTESIAN_POINT ( 'NONE',  ( 20.02500000122903145, 2.886751345948129099, -4.999999999999998224 ) ) ;
#6666=CARTESIAN_POINT ( 'NONE',  ( 10.15312500061451750, -4.541064518000417216, -2.621784821875001281 ) ) ;
#6667=CARTESIAN_POINT ( 'NONE',  ( 6.196875000614515905, -3.027376345333610441, -5.243569643749999898 ) ) ;
#6668=CARTESIAN_POINT ( 'NONE',  ( 4.884375000614518569, 6.421520780324663323E-16, -5.243569643749999010 ) ) ;
#6669=CARTESIAN_POINT ( 'NONE',  ( 26.18437500061451573, 4.541064518000418104, 2.621784821874999949 ) ) ;
#6670=CARTESIAN_POINT ( 'NONE',  ( 16.22812500061451857, 4.541064518000418104, 2.621784821874999949 ) ) ;
#6671=CARTESIAN_POINT ( 'NONE',  ( 27.60000000122903430, -2.886751345948125991, -5.000000000000000000 ) ) ;
#6672=CARTESIAN_POINT ( 'NONE',  ( 25.22812500061451502, 4.541064518000418104, 2.621784821874999949 ) ) ;
#6673=CARTESIAN_POINT ( 'NONE',  ( 21.53437500061451715, 6.421520780324663323E-16, -5.243569643749999010 ) ) ;
#6674=CARTESIAN_POINT ( 'NONE',  ( 18.36562500061451431, 3.027376345333613106, -5.243569643749998122 ) ) ;
#6675=CARTESIAN_POINT ( 'NONE',  ( -3.000416591977282496E-16, 16.59687500061452070, 25.09994784771203058 ) ) ;
#6676=CARTESIAN_POINT ( 'NONE',  ( 22.82812500061451644, 6.421520780324663323E-16, -5.243569643749999010 ) ) ;
#6677=CARTESIAN_POINT ( 'NONE',  ( 0.000000000000000000, 20.00000000000000000, -33.99999999999999289 ) ) ;
#6679=CARTESIAN_POINT ( 'NONE',  ( 25.42500000000000071, 4.330127018922191873, 2.499999999999999556 ) ) ;
#6680=CARTESIAN_POINT ( 'NONE',  ( -2.828200636599751609E-16, 13.58750000000000213, -34.61880215351700230 ) ) ;
#6682=CARTESIAN_POINT ( 'NONE',  ( 28.94062500061452070, -3.027376345333614438, 5.243569643749998122 ) ) ;
#6683=CARTESIAN_POINT ( 'NONE',  ( 9.215625000614515727, -6.054752690667223547, -1.112240025338166033E-15 ) ) ;
#6684=CARTESIAN_POINT ( 'NONE',  ( 21.48750000122903003, 4.330127018922191873, 2.499999999999999556 ) ) ;
#6685=CARTESIAN_POINT ( 'NONE',  ( 27.89062500061451289, 6.054752690667223547, 3.707466751127219781E-16 ) ) ;
#6686=CARTESIAN_POINT ( 'NONE',  ( 26.81250000000000000, 2.886751345948126879, 4.999999999999999112 ) ) ;
#6687=CARTESIAN_POINT ( 'NONE',  ( -3.999999999999999556, 17.82500000122903572, -32.30940107675850470 ) ) ;
#6688=CARTESIAN_POINT ( 'NONE',  ( 29.80312500061451431, 0.000000000000000000, 5.243569643749999010 ) ) ;
#6689=CARTESIAN_POINT ( 'NONE',  ( 10.22812500061451679, 6.421520780324663323E-16, -5.243569643749999010 ) ) ;
#6690=ORIENTED_EDGE ( 'NONE', *, *, #68921, .T. ) ;
#6691=CARTESIAN_POINT ( 'NONE',  ( 7.490625000614516082, -3.027376345333610441, -5.243569643749999898 ) ) ;
#6692=CARTESIAN_POINT ( 'NONE',  ( 6.965625000614518392, -6.054752690667223547, -1.112240025338166033E-15 ) ) ;
#6695=CARTESIAN_POINT ( 'NONE',  ( 4.676989713315623298, -1.768073502771440486, 4.936522198724768273 ) ) ;
#6696=CARTESIAN_POINT ( 'NONE',  ( 14.40000000000000036, -4.330127018922190985, -2.500000000000001332 ) ) ;
#6697=CARTESIAN_POINT ( 'NONE',  ( 16.65937500061452070, 4.541064518000418104, -2.621784821874998173 ) ) ;
#6698=CARTESIAN_POINT ( 'NONE',  ( 11.96250000122903501, 4.330127018922192761, -2.499999999999997780 ) ) ;
#6699=CARTESIAN_POINT ( 'NONE',  ( 16.65937500061452070, 4.541064518000418104, -2.621784821874998173 ) ) ;
#6701=CARTESIAN_POINT ( 'NONE',  ( 20.33437500061451786, 4.541064518000418104, 2.621784821874999949 ) ) ;
#6702=CARTESIAN_POINT ( 'NONE',  ( 4.243569643749999898, 13.69062500061451537, -27.54997392385601529 ) ) ;
#6703=CARTESIAN_POINT ( 'NONE',  ( 1.592000809091587073E-14, 16.73750000000000071, 26.00000000000000000 ) ) ;
#6706=CARTESIAN_POINT ( 'NONE',  ( 24.17812500061451786, 6.421520780324663323E-16, -5.243569643749999010 ) ) ;
#6707=CARTESIAN_POINT ( 'NONE',  ( 28.43437500061451573, 4.541064518000418104, 2.621784821874999949 ) ) ;
#6709=CARTESIAN_POINT ( 'NONE',  ( 23.09999999999999787, 4.330127018922192761, -2.499999999999997780 ) ) ;
#6710=CARTESIAN_POINT ( 'NONE',  ( 7.303125000614516082, 0.000000000000000000, 5.243569643749999010 ) ) ;
#6712=CARTESIAN_POINT ( 'NONE',  ( 19.17187500061451999, -6.054752690667223547, -1.112240025338166033E-15 ) ) ;
#6714=CARTESIAN_POINT ( 'NONE',  ( 4.528125000614516615, 4.541064518000418104, 2.621784821874999949 ) ) ;
#6715=CARTESIAN_POINT ( 'NONE',  ( 8.821875000614518569, -6.054752690667223547, -1.112240025338166033E-15 ) ) ;
#6716=VERTEX_POINT ( 'NONE', #12484 ) ;
#6717=CARTESIAN_POINT ( 'NONE',  ( 19.43437500061451928, 4.541064518000418104, 2.621784821874999949 ) ) ;
#6719=CARTESIAN_POINT ( 'NONE',  ( 30.00000000000000000, 0.000000000000000000, 4.999999999999998224 ) ) ;
#6720=CARTESIAN_POINT ( 'NONE',  ( 3.075000000000001510, -4.330127018922194537, 2.499999999999995559 ) ) ;
#6721=CARTESIAN_POINT ( 'NONE',  ( 1.626862140677534273E-15, 10.21250000000000036, -26.00000000000000355 ) ) ;
#6723=ORIENTED_EDGE ( 'NONE', *, *, #26985, .F. ) ;
#6724=CARTESIAN_POINT ( 'NONE',  ( 10.53750000000000320, 5.773502691896255534, 3.535250795749688894E-16 ) ) ;
#6726=CARTESIAN_POINT ( 'NONE',  ( 23.27812500061451573, 6.421520780324663323E-16, -5.243569643749999010 ) ) ;
#6727=CARTESIAN_POINT ( 'NONE',  ( 13.50000000000000178, -4.330127018922190985, -2.500000000000001332 ) ) ;
#6728=CARTESIAN_POINT ( 'NONE',  ( 10.80000000122903536, -2.886751345948129988, 4.999999999999997335 ) ) ;
#6729=CARTESIAN_POINT ( 'NONE',  ( 9.628125000614517148, -4.541064518000419881, 2.621784821874995952 ) ) ;
#6730=CARTESIAN_POINT ( 'NONE',  ( 23.13749999999999929, 5.773502691896255534, 3.535250795749688894E-16 ) ) ;
#6731=CARTESIAN_POINT ( 'NONE',  ( 20.87812500061451715, -4.541064518000419881, 2.621784821874995952 ) ) ;
#6732=FACE_OUTER_BOUND ( 'NONE', #279, .T. ) ;
#6733=CARTESIAN_POINT ( 'NONE',  ( 28.53750000122903074, 6.123233995736764310E-16, -4.999999999999998224 ) ) ;
#6735=CARTESIAN_POINT ( 'NONE',  ( 6.450000000000001066, 4.330127018922192761, -2.499999999999997780 ) ) ;
#6736=ORIENTED_EDGE ( 'NONE', *, *, #58814, .F. ) ;
#6737=CARTESIAN_POINT ( 'NONE',  ( 22.30312500061451431, -4.541064518000417216, -2.621784821875001281 ) ) ;
#6738=CARTESIAN_POINT ( 'NONE',  ( 28.00312500061451715, 0.000000000000000000, 5.243569643749999010 ) ) ;
#6739=CARTESIAN_POINT ( 'NONE',  ( 26.07187500061451857, 3.027376345333613106, -5.243569643749998122 ) ) ;
#6740=CARTESIAN_POINT ( 'NONE',  ( 18.12187500061451573, 3.027376345333611329, 5.243569643749999010 ) ) ;
#6741=CARTESIAN_POINT ( 'NONE',  ( 14.01562500061451644, 3.027376345333611329, 5.243569643749999010 ) ) ;
#6743=AXIS2_PLACEMENT_3D ( 'NONE', #56627, #17804, #17455 ) ;
#6744=CARTESIAN_POINT ( 'NONE',  ( 25.95000000122903216, 5.773502691896255534, 3.535250795749688894E-16 ) ) ;
#6746=CARTESIAN_POINT ( 'NONE',  ( 15.85312500061451857, 0.000000000000000000, 5.243569643749999010 ) ) ;
#6747=CARTESIAN_POINT ( 'NONE',  ( -5.810221930991193690E-16, 11.45000000122903216, -34.00000000000000000 ) ) ;
#6748=CARTESIAN_POINT ( 'NONE',  ( 3.000000001229032875, 5.773502691896255534, 3.535250795749688894E-16 ) ) ;
#6749=CARTESIAN_POINT ( 'NONE',  ( 12.57187500061451857, 3.027376345333613106, -5.243569643749998122 ) ) ;
#6750=CARTESIAN_POINT ( 'NONE',  ( 12.38437500061451857, -4.541064518000419881, 2.621784821874995952 ) ) ;
#6751=CARTESIAN_POINT ( 'NONE',  ( 19.17187500061451999, -6.054752690667223547, -1.112240025338166033E-15 ) ) ;
#6753=CARTESIAN_POINT ( 'NONE',  ( 29.47499999999999787, 4.330127018922191873, 2.499999999999999556 ) ) ;
#6754=CARTESIAN_POINT ( 'NONE',  ( 24.44062500061451715, -3.027376345333614438, 5.243569643749998122 ) ) ;
#6755=CARTESIAN_POINT ( 'NONE',  ( 19.39687500061451786, 6.054752690667223547, 3.707466751127219781E-16 ) ) ;
#6756=CARTESIAN_POINT ( 'NONE',  ( 23.76562500061451644, 3.027376345333613106, -5.243569643749998122 ) ) ;
#6757=CARTESIAN_POINT ( 'NONE',  ( -1.999999999999997113, 16.92500000000000426, 33.46410161513775705 ) ) ;
#6758=CARTESIAN_POINT ( 'NONE',  ( 28.79062500061451502, 6.054752690667223547, 3.707466751127219781E-16 ) ) ;
#6759=CARTESIAN_POINT ( 'NONE',  ( 10.27500000122903323, 2.886751345948126879, 4.999999999999999112 ) ) ;
#6760=CARTESIAN_POINT ( 'NONE',  ( 6.750000001229033764, -2.886751345948129988, 4.999999999999997335 ) ) ;
#6761=LINE ( 'NONE', #62899, #31585 ) ;
#6762=CARTESIAN_POINT ( 'NONE',  ( 26.25000000122903288, -2.886751345948125991, -5.000000000000000000 ) ) ;
#6765=CARTESIAN_POINT ( 'NONE',  ( 8.521875000614516082, 3.027376345333613106, -5.243569643749998122 ) ) ;
#6768=CARTESIAN_POINT ( 'NONE',  ( 17.35312500061451502, -4.541064518000417216, -2.621784821875001281 ) ) ;
#6769=CARTESIAN_POINT ( 'NONE',  ( 10.43437500061451750, 4.541064518000418104, 2.621784821874999949 ) ) ;
#6770=CARTESIAN_POINT ( 'NONE',  ( 28.35000000122903430, -2.886751345948129988, 4.999999999999997335 ) ) ;
#6772=CARTESIAN_POINT ( 'NONE',  ( 19.39687500061451786, 6.054752690667223547, 3.707466751127219781E-16 ) ) ;
#6773=CARTESIAN_POINT ( 'NONE',  ( 7.359375000614516438, 0.000000000000000000, 5.243569643749999010 ) ) ;
#6774=CARTESIAN_POINT ( 'NONE',  ( 3.740625000614516527, -3.027376345333614438, 5.243569643749998122 ) ) ;
#6776=CARTESIAN_POINT ( 'NONE',  ( 7.565625000614518036, 3.027376345333613106, -5.243569643749998122 ) ) ;
#6777=CARTESIAN_POINT ( 'NONE',  ( 17.12812500061451715, 4.541064518000418104, 2.621784821874999949 ) ) ;
#6778=VERTEX_POINT ( 'NONE', #42015 ) ;
#6779=CARTESIAN_POINT ( 'NONE',  ( 5.962500001229033231, -4.330127018922190985, -2.500000000000001332 ) ) ;
#6780=CARTESIAN_POINT ( 'NONE',  ( 15.36562500061451608, 3.027376345333611329, 5.243569643749999010 ) ) ;
#6781=CARTESIAN_POINT ( 'NONE',  ( 12.44062500061451537, -3.027376345333610441, -5.243569643749999898 ) ) ;
#6783=CARTESIAN_POINT ( 'NONE',  ( 12.59999999999999964, -4.330127018922190985, -2.500000000000001332 ) ) ;
#6784=CARTESIAN_POINT ( 'NONE',  ( 8.475000001229034297, 2.886751345948126879, 4.999999999999999112 ) ) ;
#6785=CARTESIAN_POINT ( 'NONE',  ( 4.715625000614516615, -6.054752690667223547, -1.112240025338166033E-15 ) ) ;
#6786=CARTESIAN_POINT ( 'NONE',  ( 18.22500000122903430, 2.886751345948129099, -4.999999999999998224 ) ) ;
#6788=CARTESIAN_POINT ( 'NONE',  ( 4.243569643749999010, 12.02187500061451786, -32.45002607614398471 ) ) ;
#6792=CARTESIAN_POINT ( 'NONE',  ( 19.05937500061451928, 0.000000000000000000, 5.243569643749999010 ) ) ;
#6793=( BOUNDED_CURVE ( )  B_SPLINE_CURVE ( 2, ( #10664, #39844, #16199, #55733, #33194, #50200, #67196 ),
 .UNSPECIFIED., .F., .F. ) 
 B_SPLINE_CURVE_WITH_KNOTS ( ( 3, 2, 2, 3 ),
 ( 0.4249999999999999889, 0.4277777777777777568, 0.4305555555555555802, 0.4333333333333333481 ),
 .UNSPECIFIED. ) 
 CURVE ( )  GEOMETRIC_REPRESENTATION_ITEM ( )  RATIONAL_B_SPLINE_CURVE ( ( 1.000000000000000000, 0.8660254037844387076, 1.000000000000000000, 0.8660254037844387076, 1.000000000000000000, 0.8660254037844387076, 1.000000000000000000 ) ) 
 REPRESENTATION_ITEM ( '' )  );
#6794=CARTESIAN_POINT ( 'NONE',  ( -3.999999999999999112, 16.51250000122903216, 30.00000000000000000 ) ) ;
#6795=CARTESIAN_POINT ( 'NONE',  ( 13.22812500061451502, -4.541064518000419881, 2.621784821874995952 ) ) ;
#6797=CARTESIAN_POINT ( 'NONE',  ( 4.898587196589411843E-16, 20.00000000000000000, -26.00000000000000000 ) ) ;
#6798=CARTESIAN_POINT ( 'NONE',  ( 25.95937500061451431, -4.541064518000417216, -2.621784821875001281 ) ) ;
#6800=CARTESIAN_POINT ( 'NONE',  ( 12.92812500061451786, 6.421520780324663323E-16, -5.243569643749999010 ) ) ;
#6801=CARTESIAN_POINT ( 'NONE',  ( 10.99687500061451750, -3.027376345333614438, 5.243569643749998122 ) ) ;
#6802=VERTEX_POINT ( 'NONE', #8027 ) ;
#6803=CARTESIAN_POINT ( 'NONE',  ( 26.84062500061451573, -3.027376345333610441, -5.243569643749999898 ) ) ;
#6804=CARTESIAN_POINT ( 'NONE',  ( 21.47812500061451502, 6.421520780324663323E-16, -5.243569643749999010 ) ) ;
#6805=CARTESIAN_POINT ( 'NONE',  ( 29.27812500061451573, 4.541064518000418104, 2.621784821874999949 ) ) ;
#6806=CARTESIAN_POINT ( 'NONE',  ( -1.071796769724487453, 18.22009619066136565, 26.00000000000000000 ) ) ;
#6807=CARTESIAN_POINT ( 'NONE',  ( 10.98750000000000071, 5.773502691896255534, 3.535250795749688894E-16 ) ) ;
#6808=CARTESIAN_POINT ( 'NONE',  ( 18.45000000122903216, -2.886751345948129988, 4.999999999999997335 ) ) ;
#6809=CARTESIAN_POINT ( 'NONE',  ( 23.36250000122903359, 0.000000000000000000, 4.999999999999998224 ) ) ;
#6811=VERTEX_POINT ( 'NONE', #53090 ) ;
#6812=CARTESIAN_POINT ( 'NONE',  ( 18.03749999999999787, -2.886751345948125991, -5.000000000000000000 ) ) ;
#6813=CARTESIAN_POINT ( 'NONE',  ( 20.47500000000000142, 4.330127018922191873, 2.499999999999999556 ) ) ;
#6814=CARTESIAN_POINT ( 'NONE',  ( 18.53437500061451715, 4.541064518000418104, 2.621784821874999949 ) ) ;
#6815=CARTESIAN_POINT ( 'NONE',  ( 26.05312500061451431, 4.541064518000418104, -2.621784821874998173 ) ) ;
#6818=CARTESIAN_POINT ( 'NONE',  ( 8.240625000614516082, -3.027376345333614438, 5.243569643749998122 ) ) ;
#6819=CARTESIAN_POINT ( 'NONE',  ( 1.999999999999998668, 15.46250000122903501, 26.53589838486224650 ) ) ;
#6820=CARTESIAN_POINT ( 'NONE',  ( 14.84999999999999964, -4.330127018922190985, -2.500000000000001332 ) ) ;
#6821=CARTESIAN_POINT ( 'NONE',  ( 4.243569643749999898, 17.74062500061451786, 32.45002607614398471 ) ) ;
#6822=CARTESIAN_POINT ( 'NONE',  ( 29.35312500061451502, 0.000000000000000000, 5.243569643749999010 ) ) ;
#6825=CARTESIAN_POINT ( 'NONE',  ( 25.32187500061451857, 3.027376345333611329, 5.243569643749999010 ) ) ;
#6827=CARTESIAN_POINT ( 'NONE',  ( 22.41562500061451502, 3.027376345333613106, -5.243569643749998122 ) ) ;
#6828=CARTESIAN_POINT ( 'NONE',  ( 23.40937500061451715, 4.541064518000418104, -2.621784821874998173 ) ) ;
#6829=CARTESIAN_POINT ( 'NONE',  ( -4.243569643749998122, 17.14062500061459460, -27.54997392385601174 ) ) ;
#6830=CARTESIAN_POINT ( 'NONE',  ( 11.81250000000000000, 2.886751345948129099, -4.999999999999998224 ) ) ;
#6831=CARTESIAN_POINT ( 'NONE',  ( 9.590625000614517504, -3.027376345333614438, 5.243569643749998122 ) ) ;
#6833=CARTESIAN_POINT ( 'NONE',  ( 23.24062500061451786, -3.027376345333610441, -5.243569643749999898 ) ) ;
#6836=CARTESIAN_POINT ( 'NONE',  ( 19.24687500061452283, -3.027376345333610441, -5.243569643749999898 ) ) ;
#6837=CARTESIAN_POINT ( 'NONE',  ( 4.243569643749999898, 12.39687500061451608, 32.45002607614398471 ) ) ;
#6838=CARTESIAN_POINT ( 'NONE',  ( 18.08437500061451431, 4.541064518000418104, 2.621784821874999949 ) ) ;
#6839=CARTESIAN_POINT ( 'NONE',  ( 26.59687500061451360, 6.054752690667223547, 3.707466751127219781E-16 ) ) ;
#6840=CARTESIAN_POINT ( 'NONE',  ( 9.001249775931846008E-16, 17.72187500061451715, 34.90005215228797653 ) ) ;
#6841=CARTESIAN_POINT ( 'NONE',  ( 7.415625000614516793, -6.054752690667223547, -1.112240025338166033E-15 ) ) ;
#6843=CARTESIAN_POINT ( 'NONE',  ( 3.684375000614518836, 4.541064518000418104, 2.621784821874999949 ) ) ;
#6845=CARTESIAN_POINT ( 'NONE',  ( 5.090625000614516615, -3.027376345333614438, 5.243569643749998122 ) ) ;
#6846=CARTESIAN_POINT ( 'NONE',  ( 8.821875000614518569, -6.054752690667223547, -1.112240025338166033E-15 ) ) ;
#6847=( NAMED_UNIT ( * ) SI_UNIT ( $, .STERADIAN. ) SOLID_ANGLE_UNIT ( ) );
#6848=CARTESIAN_POINT ( 'NONE',  ( 15.75000000122902932, -2.886751345948129988, 4.999999999999997335 ) ) ;
#6849=CARTESIAN_POINT ( 'NONE',  ( 5.259375000614518569, -4.541064518000417216, -2.621784821875001281 ) ) ;
#6850=CARTESIAN_POINT ( 'NONE',  ( 7.565625000614518036, 3.027376345333613106, -5.243569643749998122 ) ) ;
#6853=CARTESIAN_POINT ( 'NONE',  ( 16.09687500061452070, -3.027376345333610441, -5.243569643749999898 ) ) ;
#6856=CARTESIAN_POINT ( 'NONE',  ( 25.22812500061451502, 4.541064518000418104, 2.621784821874999949 ) ) ;
#6857=CARTESIAN_POINT ( 'NONE',  ( 9.478125000614515017, 4.541064518000418104, 2.621784821874999949 ) ) ;
#6859=CARTESIAN_POINT ( 'NONE',  ( 26.44687500061451502, -3.027376345333610441, -5.243569643749999898 ) ) ;
#6860=CARTESIAN_POINT ( 'NONE',  ( 9.403125000614517504, 4.541064518000418104, -2.621784821874998173 ) ) ;
#6861=CARTESIAN_POINT ( 'NONE',  ( 4.437985916418120347, -2.303102473984535603, -4.640431841391475132 ) ) ;
#6862=CARTESIAN_POINT ( 'NONE',  ( 10.72500000122903252, 2.886751345948126879, 4.999999999999999112 ) ) ;
#6863=ADVANCED_FACE ( 'NONE', ( #46468 ), #36100, .F. ) ;
#6864=CARTESIAN_POINT ( 'NONE',  ( 26.35312500061451857, -4.541064518000417216, -2.621784821875001281 ) ) ;
#6865=CARTESIAN_POINT ( 'NONE',  ( 9.001249775931846008E-16, 11.81562500061451715, -25.09994784771203058 ) ) ;
#6866=CARTESIAN_POINT ( 'NONE',  ( 12.03750000122903430, 4.330127018922191873, 2.499999999999999556 ) ) ;
#6867=CARTESIAN_POINT ( 'NONE',  ( 21.40312500061451573, -4.541064518000417216, -2.621784821875001281 ) ) ;
#6868=CARTESIAN_POINT ( 'NONE',  ( 11.06250000000000000, 2.886751345948126879, 4.999999999999999112 ) ) ;
#6869=CARTESIAN_POINT ( 'NONE',  ( 20.95312500061451999, -4.541064518000417216, -2.621784821875001281 ) ) ;
#6870=CARTESIAN_POINT ( 'NONE',  ( 5.634375000614519458, -4.541064518000419881, 2.621784821874995952 ) ) ;
#6871=CARTESIAN_POINT ( 'NONE',  ( 21.22500000000000142, 6.123233995736764310E-16, -4.999999999999998224 ) ) ;
#6872=CARTESIAN_POINT ( 'NONE',  ( 8.287500001229034297, 6.123233995736764310E-16, -4.999999999999998224 ) ) ;
#6873=CARTESIAN_POINT ( 'NONE',  ( 16.35000000122903430, -2.886751345948125991, -5.000000000000000000 ) ) ;
#6874=CARTESIAN_POINT ( 'NONE',  ( 13.45312500061451466, 4.541064518000418104, -2.621784821874998173 ) ) ;
#6875=CARTESIAN_POINT ( 'NONE',  ( 15.62812500061451537, 6.421520780324663323E-16, -5.243569643749999010 ) ) ;
#6876=CARTESIAN_POINT ( 'NONE',  ( 26.36250000122903003, 4.330127018922192761, -2.499999999999997780 ) ) ;
#6877=CARTESIAN_POINT ( 'NONE',  ( 20.28750000000000142, -2.886751345948125991, -5.000000000000000000 ) ) ;
#6878=CARTESIAN_POINT ( 'NONE',  ( 24.49687500061451573, -3.027376345333614438, 5.243569643749998122 ) ) ;
#6879=LINE ( 'NONE', #30495, #35949 ) ;
#6880=CARTESIAN_POINT ( 'NONE',  ( 10.23750000122903359, 4.330127018922191873, 2.499999999999999556 ) ) ;
#6881=CARTESIAN_POINT ( 'NONE',  ( 8.934375000614517504, 6.421520780324663323E-16, -5.243569643749999010 ) ) ;
#6882=CARTESIAN_POINT ( 'NONE',  ( 26.37187500061451217, -6.054752690667223547, -1.112240025338166033E-15 ) ) ;
#6883=ADVANCED_FACE ( 'NONE', ( #70080 ), #18367, .F. ) ;
#6884=CARTESIAN_POINT ( 'NONE',  ( 21.74062500061451431, -3.027376345333614438, 5.243569643749998122 ) ) ;
#6885=CARTESIAN_POINT ( 'NONE',  ( 27.79687500061451999, -3.027376345333610441, -5.243569643749999898 ) ) ;
#6888=CARTESIAN_POINT ( 'NONE',  ( 6.796875000614516438, 6.054752690667223547, 3.707466751127219781E-16 ) ) ;
#6889=CARTESIAN_POINT ( 'NONE',  ( 19.22812500061451502, 6.421520780324663323E-16, -5.243569643749999010 ) ) ;
#6890=ORIENTED_EDGE ( 'NONE', *, *, #55011, .F. ) ;
#6891=DIRECTION ( 'NONE',  ( 0.000000000000000000, 0.000000000000000000, 1.000000000000000000 ) ) ;
#6892=CARTESIAN_POINT ( 'NONE',  ( 27.55312500061451786, 0.000000000000000000, 5.243569643749999010 ) ) ;
#6893=CARTESIAN_POINT ( 'NONE',  ( 4.059375000614519280, 4.541064518000418104, -2.621784821874998173 ) ) ;
#6894=CARTESIAN_POINT ( 'NONE',  ( 26.39999999999999858, 0.000000000000000000, 4.999999999999998224 ) ) ;
#6895=CARTESIAN_POINT ( 'NONE',  ( 3.972658874145789110, 3.036112888163414514, -4.275165627105516286 ) ) ;
#6896=CARTESIAN_POINT ( 'NONE',  ( 16.72500000000000142, 6.123233995736764310E-16, -4.999999999999998224 ) ) ;
#6898=CARTESIAN_POINT ( 'NONE',  ( 24.48749999999999716, 5.773502691896255534, 3.535250795749688894E-16 ) ) ;
#6899=CARTESIAN_POINT ( 'NONE',  ( 26.40937500061451715, -4.541064518000417216, -2.621784821875001281 ) ) ;
#6901=CARTESIAN_POINT ( 'NONE',  ( 14.39062500061451821, 6.054752690667223547, 3.707466751127219781E-16 ) ) ;
#6902=CARTESIAN_POINT ( 'NONE',  ( 5.953125000614519102, 0.000000000000000000, 5.243569643749999010 ) ) ;
#6904=CARTESIAN_POINT ( 'NONE',  ( 3.009375000614516793, -4.541064518000417216, -2.621784821875001281 ) ) ;
#6905=CARTESIAN_POINT ( 'NONE',  ( 15.71250000122903501, 0.000000000000000000, 4.999999999999998224 ) ) ;
#6906=CARTESIAN_POINT ( 'NONE',  ( 20.81250000000000000, 2.886751345948129099, -4.999999999999998224 ) ) ;
#6907=CARTESIAN_POINT ( 'NONE',  ( 28.38749999999999929, -2.886751345948125991, -5.000000000000000000 ) ) ;
#6908=CARTESIAN_POINT ( 'NONE',  ( 5.446875000614518569, 6.054752690667223547, 3.707466751127219781E-16 ) ) ;
#6909=CARTESIAN_POINT ( 'NONE',  ( 9.759375000614516793, -4.541064518000417216, -2.621784821875001281 ) ) ;
#6910=CARTESIAN_POINT ( 'NONE',  ( 20.48437500061451289, -4.541064518000419881, 2.621784821874995952 ) ) ;
#6913=CARTESIAN_POINT ( 'NONE',  ( 4.659375000614518925, 0.000000000000000000, 5.243569643749999010 ) ) ;
#6914=CARTESIAN_POINT ( 'NONE',  ( 6.225000000000001421, -4.330127018922194537, 2.499999999999995559 ) ) ;
#6915=CARTESIAN_POINT ( 'NONE',  ( 5.709375000614517859, -4.541064518000417216, -2.621784821875001281 ) ) ;
#6916=CARTESIAN_POINT ( 'NONE',  ( 19.12500000000000000, 4.330127018922191873, 2.499999999999999556 ) ) ;
#6917=CARTESIAN_POINT ( 'NONE',  ( 16.79062500061451857, -3.027376345333614438, 5.243569643749998122 ) ) ;
#6921=CARTESIAN_POINT ( 'NONE',  ( 9.665625000614515017, -6.054752690667223547, -1.112240025338166033E-15 ) ) ;
#6922=CARTESIAN_POINT ( 'NONE',  ( 26.55937500061451573, 4.541064518000418104, -2.621784821874998173 ) ) ;
#6923=DIRECTION ( 'NONE',  ( 0.000000000000000000, 0.000000000000000000, 1.000000000000000000 ) ) ;
#6924=CARTESIAN_POINT ( 'NONE',  ( 26.97187500061451360, 3.027376345333613106, -5.243569643749998122 ) ) ;
#6925=CARTESIAN_POINT ( 'NONE',  ( 8.474999999999999645, -4.330127018922194537, 2.499999999999995559 ) ) ;
#6926=CARTESIAN_POINT ( 'NONE',  ( 2.000000000000001332, 12.16250000122903430, 33.46410161513774995 ) ) ;
#6927=CARTESIAN_POINT ( 'NONE',  ( 15.51562500061451644, -6.054752690667223547, -1.112240025338166033E-15 ) ) ;
#6928=CARTESIAN_POINT ( 'NONE',  ( 7.425000001229034474, 2.886751345948129099, -4.999999999999998224 ) ) ;
#6929=CARTESIAN_POINT ( 'NONE',  ( 17.70937500061451431, 0.000000000000000000, 5.243569643749999010 ) ) ;
#6930=CARTESIAN_POINT ( 'NONE',  ( 11.74687500061451573, 6.054752690667223547, 3.707466751127219781E-16 ) ) ;
#6931=LINE ( 'NONE', #52357, #28901 ) ;
#6933=CARTESIAN_POINT ( 'NONE',  ( 12.89062500061451821, -3.027376345333610441, -5.243569643749999898 ) ) ;
#6934=CARTESIAN_POINT ( 'NONE',  ( 26.92500000122903359, 2.886751345948126879, 4.999999999999999112 ) ) ;
#6935=CARTESIAN_POINT ( 'NONE',  ( 12.15937500061451892, 4.541064518000418104, -2.621784821874998173 ) ) ;
#6937=CARTESIAN_POINT ( 'NONE',  ( 14.35312500061451679, 4.541064518000418104, -2.621784821874998173 ) ) ;
#6939=CARTESIAN_POINT ( 'NONE',  ( 23.78437500061451360, 6.421520780324663323E-16, -5.243569643749999010 ) ) ;
#6940=CARTESIAN_POINT ( 'NONE',  ( 1.626862140677534273E-15, 10.21250000000000036, -26.00000000000000355 ) ) ;
#6941=CARTESIAN_POINT ( 'NONE',  ( 12.67500000122903536, -5.773502691896255534, -1.060575238724906372E-15 ) ) ;
#6943=CARTESIAN_POINT ( 'NONE',  ( 5.475000000000000533, 6.123233995736764310E-16, -4.999999999999998224 ) ) ;
#6944=CARTESIAN_POINT ( 'NONE',  ( 2.121784821875001281, 16.85937500061451999, -26.32496088578401938 ) ) ;
#6945=CARTESIAN_POINT ( 'NONE',  ( 18.64687500061451786, -3.027376345333614438, 5.243569643749998122 ) ) ;
#6946=CARTESIAN_POINT ( 'NONE',  ( 21.03750000122903074, 4.330127018922191873, 2.499999999999999556 ) ) ;
#6947=CARTESIAN_POINT ( 'NONE',  ( 13.50937500061451679, 4.541064518000418104, -2.621784821874998173 ) ) ;
#6948=CARTESIAN_POINT ( 'NONE',  ( 4.243569643749999898, 11.08437500061451786, 30.00000000000000000 ) ) ;
#6949=CARTESIAN_POINT ( 'NONE',  ( 19.35000000122903430, -2.886751345948129988, 4.999999999999997335 ) ) ;
#6950=CARTESIAN_POINT ( 'NONE',  ( 16.00312500061451715, -4.541064518000417216, -2.621784821875001281 ) ) ;
#6951=ORIENTED_EDGE ( 'NONE', *, *, #55418, .F. ) ;
#6952=ORIENTED_EDGE ( 'NONE', *, *, #30275, .F. ) ;
#6953=CARTESIAN_POINT ( 'NONE',  ( 18.86249999999999716, -5.773502691896255534, -1.060575238724906372E-15 ) ) ;
#6955=CARTESIAN_POINT ( 'NONE',  ( 3.853125000614517681, -4.541064518000417216, -2.621784821875001281 ) ) ;
#6956=CARTESIAN_POINT ( 'NONE',  ( 14.36250000122903359, 0.000000000000000000, 4.999999999999998224 ) ) ;
#6957=CARTESIAN_POINT ( 'NONE',  ( 26.14687500061451431, 6.054752690667223547, 3.707466751127219781E-16 ) ) ;
#6958=CARTESIAN_POINT ( 'NONE',  ( 19.60312500061451502, -4.541064518000417216, -2.621784821875001281 ) ) ;
#6959=( BOUNDED_CURVE ( )  B_SPLINE_CURVE ( 2, ( #69793, #36171, #48363, #47997, #19159, #58689, #9197 ),
 .UNSPECIFIED., .F., .F. ) 
 B_SPLINE_CURVE_WITH_KNOTS ( ( 3, 2, 2, 3 ),
 ( 0.3416666666666666186, 0.3444444444444444420, 0.3472222222222222099, 0.3500000000000000333 ),
 .UNSPECIFIED. ) 
 CURVE ( )  GEOMETRIC_REPRESENTATION_ITEM ( )  RATIONAL_B_SPLINE_CURVE ( ( 1.000000000000002665, 0.8660254037844360431, 1.000000000000000000, 0.8660254037844387076, 1.000000000000000000, 0.8660254037844360431, 1.000000000000002665 ) ) 
 REPRESENTATION_ITEM ( '' )  );
#6960=CARTESIAN_POINT ( 'NONE',  ( 22.67812500061451431, -4.541064518000419881, 2.621784821874995952 ) ) ;
#6961=CARTESIAN_POINT ( 'NONE',  ( 3.628125000614518036, 4.541064518000418104, 2.621784821874999949 ) ) ;
#6962=CARTESIAN_POINT ( 'NONE',  ( 26.62500000000000000, 6.123233995736764310E-16, -4.999999999999998224 ) ) ;
#6966=CARTESIAN_POINT ( 'NONE',  ( 3.999999999999998668, 10.02500000122903501, -32.30940107675850470 ) ) ;
#6967=CARTESIAN_POINT ( 'NONE',  ( 4.243569643749999898, 15.99687500061451573, -27.54997392385601529 ) ) ;
#6968=CARTESIAN_POINT ( 'NONE',  ( 5.512500001229033941, -4.330127018922190985, -2.500000000000001332 ) ) ;
#6969=CARTESIAN_POINT ( 'NONE',  ( 5.400000000000002132, -4.330127018922190985, -2.500000000000001332 ) ) ;
#6970=EDGE_CURVE ( 'NONE', #29785, #60995, #19829, .T. ) ;
#6971=CARTESIAN_POINT ( 'NONE',  ( 4.462500001229035007, 0.000000000000000000, 4.999999999999998224 ) ) ;
#6972=CARTESIAN_POINT ( 'NONE',  ( 8.821875000614518569, -6.054752690667223547, -1.112240025338166033E-15 ) ) ;
#6973=CARTESIAN_POINT ( 'NONE',  ( 28.86562500061451786, 3.027376345333611329, 5.243569643749999010 ) ) ;
#6975=CARTESIAN_POINT ( 'NONE',  ( 18.41250000122903430, 0.000000000000000000, 4.999999999999998224 ) ) ;
#6976=CARTESIAN_POINT ( 'NONE',  ( 3.486133158594716510E-16, 19.55000000122903359, -34.00000000000000000 ) ) ;
#6977=CARTESIAN_POINT ( 'NONE',  ( 7.696875000614516793, 6.054752690667223547, 3.707466751127219781E-16 ) ) ;
#6978=CARTESIAN_POINT ( 'NONE',  ( 10.28437500061451715, 6.421520780324663323E-16, -5.243569643749999010 ) ) ;
#6979=CARTESIAN_POINT ( 'NONE',  ( 6.225000000000001421, -4.330127018922194537, 2.499999999999995559 ) ) ;
#6980=CARTESIAN_POINT ( 'NONE',  ( 4.243569643749999898, 15.94062500061459176, 32.45002607614398471 ) ) ;
#6981=CARTESIAN_POINT ( 'NONE',  ( 22.32187500061451502, -6.054752690667223547, -1.112240025338166033E-15 ) ) ;
#6982=CARTESIAN_POINT ( 'NONE',  ( 1.071796769724493892, 18.06740381056766864, 26.00000000000000711 ) ) ;
#6983=CARTESIAN_POINT ( 'NONE',  ( 5.737499999999998934, -2.886751345948129988, 4.999999999999997335 ) ) ;
#6984=CARTESIAN_POINT ( 'NONE',  ( 27.22500000122903430, 2.886751345948129099, -4.999999999999998224 ) ) ;
#6986=CARTESIAN_POINT ( 'NONE',  ( 21.59062500061451928, 6.054752690667223547, 3.707466751127219781E-16 ) ) ;
#6987=CARTESIAN_POINT ( 'NONE',  ( 12.74062500061451786, -3.027376345333614438, 5.243569643749998122 ) ) ;
#6989=CARTESIAN_POINT ( 'NONE',  ( 10.92187500061451644, 3.027376345333611329, 5.243569643749999010 ) ) ;
#6990=CARTESIAN_POINT ( 'NONE',  ( 28.83749999999999858, -2.886751345948125991, -5.000000000000000000 ) ) ;
#6991=CARTESIAN_POINT ( 'NONE',  ( 22.20000000122903216, -2.886751345948125991, -5.000000000000000000 ) ) ;
#6992=CARTESIAN_POINT ( 'NONE',  ( -3.999999999999999112, 18.27500000122903501, -32.30940107675850470 ) ) ;
#6993=CARTESIAN_POINT ( 'NONE',  ( 12.57187500061451857, 3.027376345333613106, -5.243569643749998122 ) ) ;
#6994=CARTESIAN_POINT ( 'NONE',  ( 27.94687500061451502, 6.054752690667223547, 3.707466751127219781E-16 ) ) ;
#6996=CARTESIAN_POINT ( 'NONE',  ( -1.071796769724504328, 14.69240381056766687, 33.99999999999999289 ) ) ;
#6997=CARTESIAN_POINT ( 'NONE',  ( 23.25937500061451857, -4.541064518000417216, -2.621784821875001281 ) ) ;
#6998=CARTESIAN_POINT ( 'NONE',  ( 15.12187500061451750, -6.054752690667223547, -1.112240025338166033E-15 ) ) ;
#7000=CARTESIAN_POINT ( 'NONE',  ( 25.19999999999999929, -4.330127018922190985, -2.500000000000001332 ) ) ;
#7003=CARTESIAN_POINT ( 'NONE',  ( 17.54062500061451502, 6.054752690667223547, 3.707466751127219781E-16 ) ) ;
#7004=CARTESIAN_POINT ( 'NONE',  ( 7.387500000000001066, 5.773502691896255534, 3.535250795749688894E-16 ) ) ;
#7007=CARTESIAN_POINT ( 'NONE',  ( 15.33750000000000036, -2.886751345948125991, -5.000000000000000000 ) ) ;
#7008=CARTESIAN_POINT ( 'NONE',  ( 2.121784821874999061, 10.65312500061451750, 26.32496088578401583 ) ) ;
#7009=CARTESIAN_POINT ( 'NONE',  ( 25.20937500061451431, 4.541064518000418104, -2.621784821874998173 ) ) ;
#7011=CARTESIAN_POINT ( 'NONE',  ( 20.61562500061451431, 3.027376345333613106, -5.243569643749998122 ) ) ;
#7012=CARTESIAN_POINT ( 'NONE',  ( 21.04687500061451644, -3.027376345333610441, -5.243569643749999898 ) ) ;
#7013=CARTESIAN_POINT ( 'NONE',  ( 3.675000000000001155, 6.123233995736764310E-16, -4.999999999999998224 ) ) ;
#7014=CARTESIAN_POINT ( 'NONE',  ( 6.853125000614516793, 0.000000000000000000, 5.243569643749999010 ) ) ;
#7015=CARTESIAN_POINT ( 'NONE',  ( 20.84062500061451573, -3.027376345333614438, 5.243569643749998122 ) ) ;
#7016=CARTESIAN_POINT ( 'NONE',  ( 12.42187500061451821, -6.054752690667223547, -1.112240025338166033E-15 ) ) ;
#7017=CARTESIAN_POINT ( 'NONE',  ( 16.73437500061451644, 4.541064518000418104, 2.621784821874999949 ) ) ;
#7018=CARTESIAN_POINT ( 'NONE',  ( 4.243569643749999010, 18.26562500061451644, 27.54997392385601174 ) ) ;
#7019=CARTESIAN_POINT ( 'NONE',  ( 18.22500000122903430, 2.886751345948129099, -4.999999999999998224 ) ) ;
#7021=CARTESIAN_POINT ( 'NONE',  ( 10.22812500061451679, 6.421520780324663323E-16, -5.243569643749999010 ) ) ;
#7022=CARTESIAN_POINT ( 'NONE',  ( 4.209375000614516971, 0.000000000000000000, 5.243569643749999010 ) ) ;
#7023=CARTESIAN_POINT ( 'NONE',  ( 4.846875000614519813, -3.027376345333610441, -5.243569643749999898 ) ) ;
#7024=CARTESIAN_POINT ( 'NONE',  ( 25.32187500061451857, 3.027376345333611329, 5.243569643749999010 ) ) ;
#7025=CARTESIAN_POINT ( 'NONE',  ( 17.42812500061451786, 6.421520780324663323E-16, -5.243569643749999010 ) ) ;
#7026=CARTESIAN_POINT ( 'NONE',  ( 26.21250000122903501, -4.330127018922190985, -2.500000000000001332 ) ) ;
#7027=EDGE_CURVE ( 'NONE', #25241, #16013, #25579, .T. ) ;
#7028=CARTESIAN_POINT ( 'NONE',  ( 25.64062500061451644, 6.054752690667223547, 3.707466751127219781E-16 ) ) ;
#7029=CARTESIAN_POINT ( 'NONE',  ( 21.57187500061451502, 3.027376345333613106, -5.243569643749998122 ) ) ;
#7030=CARTESIAN_POINT ( 'NONE',  ( 17.24062500061451786, -3.027376345333614438, 5.243569643749998122 ) ) ;
#7031=CARTESIAN_POINT ( 'NONE',  ( -4.243569643749997233, 16.74687500061451928, 32.45002607614398471 ) ) ;
#7032=EDGE_CURVE ( 'NONE', #41820, #427, #28388, .T. ) ;
#7033=CARTESIAN_POINT ( 'NONE',  ( 21.89062500061451289, -3.027376345333610441, -5.243569643749999898 ) ) ;
#7034=CARTESIAN_POINT ( 'NONE',  ( 2.962500001229034119, 4.330127018922192761, -2.499999999999997780 ) ) ;
#7035=ORIENTED_EDGE ( 'NONE', *, *, #58291, .F. ) ;
#7036=CARTESIAN_POINT ( 'NONE',  ( 24.82499999999999929, 6.123233995736764310E-16, -4.999999999999998224 ) ) ;
#7037=CARTESIAN_POINT ( 'NONE',  ( 2.000000000000001332, 13.40000000000000213, -26.53589838486224650 ) ) ;
#7039=CARTESIAN_POINT ( 'NONE',  ( 29.39062500061451289, -3.027376345333614438, 5.243569643749998122 ) ) ;
#7040=CARTESIAN_POINT ( 'NONE',  ( 9.890625000614516438, 6.054752690667223547, 3.707466751127219781E-16 ) ) ;
#7041=CARTESIAN_POINT ( 'NONE',  ( 22.65000000122903856, -2.886751345948125991, -5.000000000000000000 ) ) ;
#7042=CARTESIAN_POINT ( 'NONE',  ( 26.61562500061451786, 3.027376345333611329, 5.243569643749999010 ) ) ;
#7043=CARTESIAN_POINT ( 'NONE',  ( 24.93750000000000355, 5.773502691896255534, 3.535250795749688894E-16 ) ) ;
#7044=CARTESIAN_POINT ( 'NONE',  ( 2.000000000000001332, 16.21250000122903501, -26.53589838486224650 ) ) ;
#7046=CARTESIAN_POINT ( 'NONE',  ( 29.50312500061451360, -4.541064518000417216, -2.621784821875001281 ) ) ;
#7047=CARTESIAN_POINT ( 'NONE',  ( 10.15312500061451750, -4.541064518000417216, -2.621784821875001281 ) ) ;
#7048=ORIENTED_EDGE ( 'NONE', *, *, #38793, .T. ) ;
#7049=CARTESIAN_POINT ( 'NONE',  ( 26.16562500061451502, 3.027376345333611329, 5.243569643749999010 ) ) ;
#7050=CARTESIAN_POINT ( 'NONE',  ( 7.640625000614517326, 6.054752690667223547, 3.707466751127219781E-16 ) ) ;
#7051=UNCERTAINTY_MEASURE_WITH_UNIT (LENGTH_MEASURE( 1.000000000000000082E-05 ), #33832, 'distance_accuracy_value', 'NONE');
#7052=CARTESIAN_POINT ( 'NONE',  ( 5.353125000614515905, 4.541064518000418104, -2.621784821874998173 ) ) ;
#7054=EDGE_CURVE ( 'NONE', #29691, #41395, #51037, .T. ) ;
#7055=CARTESIAN_POINT ( 'NONE',  ( 4.664282881542661130, -1.801239906550150316, 4.924485496770981463 ) ) ;
#7056=CARTESIAN_POINT ( 'NONE',  ( 13.50000000000000178, -4.330127018922190985, -2.500000000000001332 ) ) ;
#7057=CARTESIAN_POINT ( 'NONE',  ( 13.92187500061451644, 3.027376345333613106, -5.243569643749998122 ) ) ;
#7058=CARTESIAN_POINT ( 'NONE',  ( 12.26250000122903394, -4.330127018922190985, -2.500000000000001332 ) ) ;
#7059=CARTESIAN_POINT ( 'NONE',  ( 16.73437500061451644, 4.541064518000418104, 2.621784821874999949 ) ) ;
#7061=CARTESIAN_POINT ( 'NONE',  ( 8.221875000614518925, 3.027376345333611329, 5.243569643749999010 ) ) ;
#7062=CARTESIAN_POINT ( 'NONE',  ( 2.121784821875001281, 10.95312500061451821, -26.32496088578401938 ) ) ;
#7065=CARTESIAN_POINT ( 'NONE',  ( 1.071796769724476572, 11.58259618943233349, -25.99999999999999289 ) ) ;
#7066=CARTESIAN_POINT ( 'NONE',  ( 23.87812500061451715, 4.541064518000418104, 2.621784821874999949 ) ) ;
#7067=( NAMED_UNIT ( * ) PLANE_ANGLE_UNIT ( ) SI_UNIT ( $, .RADIAN. ) );
#7068=CARTESIAN_POINT ( 'NONE',  ( 29.48437500061451644, -4.541064518000419881, 2.621784821874995952 ) ) ;
#7069=CARTESIAN_POINT ( 'NONE',  ( 24.93750000000000355, 5.773502691896255534, 3.535250795749688894E-16 ) ) ;
#7070=CARTESIAN_POINT ( 'NONE',  ( 7.115625000614516082, 3.027376345333613106, -5.243569643749998122 ) ) ;
#7072=CARTESIAN_POINT ( 'NONE',  ( 18.90937500061451360, 4.541064518000418104, -2.621784821874998173 ) ) ;
#7074=CARTESIAN_POINT ( 'NONE',  ( 2.840625000614518392, -3.027376345333614438, 5.243569643749998122 ) ) ;
#7075=CARTESIAN_POINT ( 'NONE',  ( 8.146875000614516082, 6.054752690667223547, 3.707466751127219781E-16 ) ) ;
#7076=EDGE_LOOP ( 'NONE', ( #16722, #40633, #37631, #31100 ) ) ;
#7077=CARTESIAN_POINT ( 'NONE',  ( 19.35937500061451644, 4.541064518000418104, -2.621784821874998173 ) ) ;
#7078=DIRECTION ( 'NONE',  ( -1.000000000000000000, -0.000000000000000000, -0.000000000000000000 ) ) ;
#7079=CARTESIAN_POINT ( 'NONE',  ( 26.92499999999999716, -4.330127018922194537, 2.499999999999995559 ) ) ;
#7080=CARTESIAN_POINT ( 'NONE',  ( 28.62187500061451573, -6.054752690667223547, -1.112240025338166033E-15 ) ) ;
#7084=CARTESIAN_POINT ( 'NONE',  ( 10.65000000000000036, 0.000000000000000000, 4.999999999999998224 ) ) ;
#7086=CARTESIAN_POINT ( 'NONE',  ( 25.34062500061451217, -3.027376345333614438, 5.243569643749998122 ) ) ;
#7087=CARTESIAN_POINT ( 'NONE',  ( 14.73749999999999893, -2.886751345948129988, 4.999999999999997335 ) ) ;
#7088=CARTESIAN_POINT ( 'NONE',  ( 9.862500001229033586, 0.000000000000000000, 4.999999999999998224 ) ) ;
#7089=CARTESIAN_POINT ( 'NONE',  ( 8.053125000614516082, 4.541064518000418104, -2.621784821874998173 ) ) ;
#7090=CARTESIAN_POINT ( 'NONE',  ( 22.94999999999999929, -4.330127018922190985, -2.500000000000001332 ) ) ;
#7091=CARTESIAN_POINT ( 'NONE',  ( 19.86562500061451786, 3.027376345333611329, 5.243569643749999010 ) ) ;
#7093=CARTESIAN_POINT ( 'NONE',  ( 26.13750000122903216, -4.330127018922194537, 2.499999999999995559 ) ) ;
#7095=CARTESIAN_POINT ( 'NONE',  ( 5.250000000000000888, 0.000000000000000000, 4.999999999999998224 ) ) ;
#7097=CARTESIAN_POINT ( 'NONE',  ( 22.97812500061451857, 4.541064518000418104, 2.621784821874999949 ) ) ;
#7098=CARTESIAN_POINT ( 'NONE',  ( 29.12812500061451715, 6.421520780324663323E-16, -5.243569643749999010 ) ) ;
#7099=CARTESIAN_POINT ( 'NONE',  ( 28.28437500061451715, 6.421520780324663323E-16, -5.243569643749999010 ) ) ;
#7100=CARTESIAN_POINT ( 'NONE',  ( 18.19687500061451502, -3.027376345333614438, 5.243569643749998122 ) ) ;
#7101=CARTESIAN_POINT ( 'NONE',  ( 14.87812500061451537, 4.541064518000418104, 2.621784821874999949 ) ) ;
#7103=CARTESIAN_POINT ( 'NONE',  ( 27.22500000122903430, 2.886751345948129099, -4.999999999999998224 ) ) ;
#7105=CARTESIAN_POINT ( 'NONE',  ( 17.69062500061451715, -3.027376345333614438, 5.243569643749998122 ) ) ;
#7106=LINE ( 'NONE', #22997, #42126 ) ;
#7107=CARTESIAN_POINT ( 'NONE',  ( 3.075000001229035718, 2.886751345948126879, 4.999999999999999112 ) ) ;
#7108=CARTESIAN_POINT ( 'NONE',  ( 11.63437500061451857, 6.421520780324663323E-16, -5.243569643749999010 ) ) ;
#7109=CARTESIAN_POINT ( 'NONE',  ( 11.33437500061451608, 4.541064518000418104, 2.621784821874999949 ) ) ;
#7110=CARTESIAN_POINT ( 'NONE',  ( 19.24687500061452283, -3.027376345333610441, -5.243569643749999898 ) ) ;
#7111=VERTEX_POINT ( 'NONE', #2134 ) ;
#7112=CARTESIAN_POINT ( 'NONE',  ( 9.825000000000001066, -4.330127018922194537, 2.499999999999995559 ) ) ;
#7113=CARTESIAN_POINT ( 'NONE',  ( 25.07812500061451644, 6.421520780324663323E-16, -5.243569643749999010 ) ) ;
#7114=CARTESIAN_POINT ( 'NONE',  ( 18.53437500061451715, 4.541064518000418104, 2.621784821874999949 ) ) ;
#7115=CARTESIAN_POINT ( 'NONE',  ( 24.25312500061451715, 4.541064518000418104, -2.621784821874998173 ) ) ;
#7116=CARTESIAN_POINT ( 'NONE',  ( 9.000000000000001776, -4.330127018922190985, -2.500000000000001332 ) ) ;
#7117=CARTESIAN_POINT ( 'NONE',  ( -3.999999999999999112, 15.50000000000000000, 30.00000000000000000 ) ) ;
#7118=CARTESIAN_POINT ( 'NONE',  ( 29.69062500061451715, 6.054752690667223547, 3.707466751127219781E-16 ) ) ;
#7119=CARTESIAN_POINT ( 'NONE',  ( 10.42500000122903536, -5.773502691896255534, -1.060575238724906372E-15 ) ) ;
#7120=CARTESIAN_POINT ( 'NONE',  ( 3.487500001229035362, 4.330127018922191873, 2.499999999999999556 ) ) ;
#7122=CARTESIAN_POINT ( 'NONE',  ( 26.43750000122903288, 4.330127018922191873, 2.499999999999999556 ) ) ;
#7124=CARTESIAN_POINT ( 'NONE',  ( 9.196875000614518569, -3.027376345333614438, 5.243569643749998122 ) ) ;
#7125=CARTESIAN_POINT ( 'NONE',  ( 4.000000000000000000, 9.950000001229033941, 32.30940107675849760 ) ) ;
#7126=CARTESIAN_POINT ( 'NONE',  ( 17.54062500061451502, 6.054752690667223547, 3.707466751127219781E-16 ) ) ;
#7127=CARTESIAN_POINT ( 'NONE',  ( 11.03437500061451715, -4.541064518000419881, 2.621784821874995952 ) ) ;
#7128=CARTESIAN_POINT ( 'NONE',  ( 2.803125000614518747, 0.000000000000000000, 5.243569643749999010 ) ) ;
#7129=CARTESIAN_POINT ( 'NONE',  ( 18.90937500061451360, 4.541064518000418104, -2.621784821874998173 ) ) ;
#7130=CARTESIAN_POINT ( 'NONE',  ( 7.209375000614519635, 4.541064518000418104, -2.621784821874998173 ) ) ;
#7131=CARTESIAN_POINT ( 'NONE',  ( 3.028125000614518392, 6.421520780324663323E-16, -5.243569643749999010 ) ) ;
#7132=CARTESIAN_POINT ( 'NONE',  ( 11.85000000122903430, -2.886751345948193048, -4.999999999999883649 ) ) ;
#7134=CARTESIAN_POINT ( 'NONE',  ( 6.740625000614516082, 6.054752690667223547, 3.707466751127219781E-16 ) ) ;
#7135=CARTESIAN_POINT ( 'NONE',  ( 17.99062500061451786, 6.054752690667223547, 3.707466751127219781E-16 ) ) ;
#7136=ORIENTED_EDGE ( 'NONE', *, *, #1559, .F. ) ;
#7137=CARTESIAN_POINT ( 'NONE',  ( 5.587500001229033231, 6.123233995736764310E-16, -4.999999999999998224 ) ) ;
#7138=CARTESIAN_POINT ( 'NONE',  ( 14.76562500061451821, 3.027376345333613106, -5.243569643749998122 ) ) ;
#7139=CARTESIAN_POINT ( 'NONE',  ( 12.74062500061451786, -3.027376345333614438, 5.243569643749998122 ) ) ;
#7141=CARTESIAN_POINT ( 'NONE',  ( 14.55000000000000071, 4.330127018922192761, -2.499999999999997780 ) ) ;
#7142=CARTESIAN_POINT ( 'NONE',  ( 5.587500001229033231, 6.123233995736764310E-16, -4.999999999999998224 ) ) ;
#7144=CARTESIAN_POINT ( 'NONE',  ( 19.01250000122903216, -4.330127018922190985, -2.500000000000001332 ) ) ;
#7146=CARTESIAN_POINT ( 'NONE',  ( -4.243569643749999898, 9.959375000614517859, -30.00000000000000000 ) ) ;
#7147=CARTESIAN_POINT ( 'NONE',  ( 4.158798725700454391, -2.776528725802326125, -4.158798725700454391 ) ) ;
#7148=CARTESIAN_POINT ( 'NONE',  ( 23.58750000122903145, 6.123233995736764310E-16, -4.999999999999998224 ) ) ;
#7149=EDGE_CURVE ( 'NONE', #20263, #39861, #3747, .T. ) ;
#7150=CARTESIAN_POINT ( 'NONE',  ( 6.412500000000001421, 2.886751345948129099, -4.999999999999997335 ) ) ;
#7151=CARTESIAN_POINT ( 'NONE',  ( 4.509375000614518569, 4.541064518000418104, -2.621784821874998173 ) ) ;
#7152=CARTESIAN_POINT ( 'NONE',  ( 19.62187500061451573, -6.054752690667223547, -1.112240025338166033E-15 ) ) ;
#7153=CARTESIAN_POINT ( 'NONE',  ( -1.071796769724496556, 16.60490381179669939, 33.99999999999998579 ) ) ;
#7154=CARTESIAN_POINT ( 'NONE',  ( 14.76562500061451821, 3.027376345333613106, -5.243569643749998122 ) ) ;
#7157=CARTESIAN_POINT ( 'NONE',  ( 15.82500000122903216, -5.773502691896255534, -1.060575238724906372E-15 ) ) ;
#7158=CARTESIAN_POINT ( 'NONE',  ( 25.50937500061451502, -4.541064518000417216, -2.621784821875001281 ) ) ;
#7160=CARTESIAN_POINT ( 'NONE',  ( 10.71562500061451928, 3.027376345333613106, -5.243569643749998122 ) ) ;
#7161=CARTESIAN_POINT ( 'NONE',  ( 16.09687500061452070, -3.027376345333610441, -5.243569643749999898 ) ) ;
#7162=ORIENTED_EDGE ( 'NONE', *, *, #29219, .T. ) ;
#7163=CARTESIAN_POINT ( 'NONE',  ( 27.55312500061451786, 0.000000000000000000, 5.243569643749999010 ) ) ;
#7164=CARTESIAN_POINT ( 'NONE',  ( 19.64062500061451644, -3.027376345333610441, -5.243569643749999898 ) ) ;
#7165=CARTESIAN_POINT ( 'NONE',  ( 4.000000000000000000, 13.10000000122903430, -27.69059892324149885 ) ) ;
#7166=CARTESIAN_POINT ( 'NONE',  ( -1.999999999999997113, 14.33750000122903323, -26.53589838486224295 ) ) ;
#7167=EDGE_CURVE ( 'NONE', #52378, #23627, #60959, .T. ) ;
#7168=CARTESIAN_POINT ( 'NONE',  ( 10.95000000000000107, 4.330127018922192761, -2.499999999999997780 ) ) ;
#7169=CARTESIAN_POINT ( 'NONE',  ( 19.46250000122903145, -4.330127018922190985, -2.500000000000001332 ) ) ;
#7170=DIRECTION ( 'NONE',  ( -0.000000000000000000, -1.000000000000000000, -0.000000000000000000 ) ) ;
#7172=EDGE_LOOP ( 'NONE', ( #5379, #56471, #55522, #12450 ) ) ;
#7173=CARTESIAN_POINT ( 'NONE',  ( 17.55000000000000071, -4.330127018922190985, -2.500000000000001332 ) ) ;
#7174=CARTESIAN_POINT ( 'NONE',  ( 21.37499999999999645, 4.330127018922191873, 2.499999999999999556 ) ) ;
#7175=CARTESIAN_POINT ( 'NONE',  ( 19.35937500061451644, 4.541064518000418104, -2.621784821874998173 ) ) ;
#7176=CARTESIAN_POINT ( 'NONE',  ( 24.21562500061451573, 3.027376345333613106, -5.243569643749998122 ) ) ;
#7177=EDGE_LOOP ( 'NONE', ( #11101, #3235, #72498, #29360 ) ) ;
#7179=CARTESIAN_POINT ( 'NONE',  ( 5.878125000614517148, 4.541064518000418104, 2.621784821874999949 ) ) ;
#7181=CARTESIAN_POINT ( 'NONE',  ( 14.62500000000000000, 4.330127018922191873, 2.499999999999999556 ) ) ;
#7182=CARTESIAN_POINT ( 'NONE',  ( -4.243569643749997233, 18.04062500061451857, 32.45002607614398471 ) ) ;
#7183=CARTESIAN_POINT ( 'NONE',  ( 3.159375000614518036, 4.541064518000418104, -2.621784821874998173 ) ) ;
#7186=CARTESIAN_POINT ( 'NONE',  ( 25.35937500061451644, 0.000000000000000000, 5.243569643749999010 ) ) ;
#7187=ORIENTED_EDGE ( 'NONE', *, *, #38408, .T. ) ;
#7188=CARTESIAN_POINT ( 'NONE',  ( 20.35312500061451502, 0.000000000000000000, 5.243569643749999010 ) ) ;
#7189=CARTESIAN_POINT ( 'NONE',  ( 23.37187500061451573, 3.027376345333613106, -5.243569643749998122 ) ) ;
#7190=CARTESIAN_POINT ( 'NONE',  ( -2.121784821874999949, 16.57812500061459460, -33.67503911421598417 ) ) ;
#7191=CARTESIAN_POINT ( 'NONE',  ( 6.590625000614518392, -3.027376345333610441, -5.243569643749999898 ) ) ;
#7193=CARTESIAN_POINT ( 'NONE',  ( 23.87812500061451715, 4.541064518000418104, 2.621784821874999949 ) ) ;
#7196=CARTESIAN_POINT ( 'NONE',  ( 17.70937500061451431, 0.000000000000000000, 5.243569643749999010 ) ) ;
#7197=CARTESIAN_POINT ( 'NONE',  ( 19.62187500061451573, -6.054752690667223547, -1.112240025338166033E-15 ) ) ;
#7198=CARTESIAN_POINT ( 'NONE',  ( 26.48437500061451644, 6.421520780324663323E-16, -5.243569643749999010 ) ) ;
#7199=CARTESIAN_POINT ( 'NONE',  ( 2.121784821874999061, 17.45937500061451786, 26.32496088578401583 ) ) ;
#7200=CARTESIAN_POINT ( 'NONE',  ( 7.603125000614517681, 4.541064518000418104, -2.621784821874998173 ) ) ;
#7202=CARTESIAN_POINT ( 'NONE',  ( 5.259375000614518569, -4.541064518000417216, -2.621784821875001281 ) ) ;
#7204=CARTESIAN_POINT ( 'NONE',  ( 5.803125000614517859, 4.541064518000418104, -2.621784821874998173 ) ) ;
#7205=CARTESIAN_POINT ( 'NONE',  ( 9.009375000614518569, 4.541064518000418104, -2.621784821874998173 ) ) ;
#7207=CARTESIAN_POINT ( 'NONE',  ( 17.55000000122903359, -2.886751345948129988, 4.999999999999997335 ) ) ;
#7208=CARTESIAN_POINT ( 'NONE',  ( 4.734375000614518214, -4.541064518000419881, 2.621784821874995952 ) ) ;
#7209=CARTESIAN_POINT ( 'NONE',  ( 6.328125000614515550, 4.541064518000418104, 2.621784821874999949 ) ) ;
#7212=CARTESIAN_POINT ( 'NONE',  ( 16.02187500061451786, -6.054752690667223547, -1.112240025338166033E-15 ) ) ;
#7213=DIRECTION ( 'NONE',  ( 0.000000000000000000, 0.000000000000000000, 1.000000000000000000 ) ) ;
#7215=CARTESIAN_POINT ( 'NONE',  ( 23.91562500061451502, 3.027376345333611329, 5.243569643749999010 ) ) ;
#7216=CARTESIAN_POINT ( 'NONE',  ( 8.690625000614515372, -3.027376345333614438, 5.243569643749998122 ) ) ;
#7217=CARTESIAN_POINT ( 'NONE',  ( 26.85937500061451644, -4.541064518000417216, -2.621784821875001281 ) ) ;
#7218=CARTESIAN_POINT ( 'NONE',  ( 9.328125000614518214, 6.421520780324663323E-16, -5.243569643749999010 ) ) ;
#7220=CARTESIAN_POINT ( 'NONE',  ( 11.51250000122903216, 4.330127018922192761, -2.499999999999997780 ) ) ;
#7222=CARTESIAN_POINT ( 'NONE',  ( 25.45312500061451644, -4.541064518000417216, -2.621784821875001281 ) ) ;
#7223=CARTESIAN_POINT ( 'NONE',  ( 4.243569643749999898, 13.24062500061451786, -27.54997392385601529 ) ) ;
#7224=CARTESIAN_POINT ( 'NONE',  ( 11.77500000122903501, -5.773502691896255534, -1.060575238724906372E-15 ) ) ;
#7225=CARTESIAN_POINT ( 'NONE',  ( 23.12812500061451360, -4.541064518000419881, 2.621784821874995952 ) ) ;
#7226=CARTESIAN_POINT ( 'NONE',  ( 10.27499999999999858, -4.330127018922194537, 2.499999999999995559 ) ) ;
#7227=CARTESIAN_POINT ( 'NONE',  ( 19.97812500061451502, -4.541064518000419881, 2.621784821874995952 ) ) ;
#7228=CARTESIAN_POINT ( 'NONE',  ( 5.934375000614517504, 4.541064518000418104, 2.621784821874999949 ) ) ;
#7229=CARTESIAN_POINT ( 'NONE',  ( 20.54999999999999716, 0.000000000000000000, 4.999999999999998224 ) ) ;
#7230=CARTESIAN_POINT ( 'NONE',  ( 14.55000000122903181, -2.886751345948125991, -5.000000000000000000 ) ) ;
#7231=CARTESIAN_POINT ( 'NONE',  ( 10.07812500061451644, -4.541064518000419881, 2.621784821874995952 ) ) ;
#7232=CARTESIAN_POINT ( 'NONE',  ( 14.65312500061451573, -4.541064518000417216, -2.621784821875001281 ) ) ;
#7233=( BOUNDED_CURVE ( )  B_SPLINE_CURVE ( 2, ( #26791, #9789, #55952, #43781, #22328, #44880, #50052, #5348, #60752 ),
 .UNSPECIFIED., .F., .F. ) 
 B_SPLINE_CURVE_WITH_KNOTS ( ( 3, 2, 2, 2, 3 ),
 ( 0.4673913043478261087, 0.4710144927536231707, 0.4782608695652174058, 0.4855072463768115854, 0.4891304347826087029 ),
 .UNSPECIFIED. ) 
 CURVE ( )  GEOMETRIC_REPRESENTATION_ITEM ( )  RATIONAL_B_SPLINE_CURVE ( ( 0.9330127018922194093, 0.9330127018922198534, 1.000000000000000000, 0.8660254037844387076, 1.000000000000000000, 0.8660254037844387076, 1.000000000000000000, 0.9330127018922194093, 0.9330127018922194093 ) ) 
 REPRESENTATION_ITEM ( '' )  );
#7234=CARTESIAN_POINT ( 'NONE',  ( 25.27500000122903145, -5.773502691896255534, -1.060575238724906372E-15 ) ) ;
#7235=CARTESIAN_POINT ( 'NONE',  ( 21.07499999999999929, -4.330127018922194537, 2.499999999999995559 ) ) ;
#7236=CARTESIAN_POINT ( 'NONE',  ( 23.14687500061451786, -3.027376345333614438, 5.243569643749998122 ) ) ;
#7238=CARTESIAN_POINT ( 'NONE',  ( 6.637500001229035718, 4.330127018922191873, 2.499999999999999556 ) ) ;
#7239=CARTESIAN_POINT ( 'NONE',  ( 7.921875000614517326, -6.054752690667223547, -1.112240025338166033E-15 ) ) ;
#7240=CARTESIAN_POINT ( 'NONE',  ( 25.92187500061451999, -6.054752690667223547, -1.112240025338166033E-15 ) ) ;
#7241=CARTESIAN_POINT ( 'NONE',  ( 23.81250000122903288, 0.000000000000000000, 4.999999999999998224 ) ) ;
#7242=CARTESIAN_POINT ( 'NONE',  ( 21.70312500061451644, 0.000000000000000000, 5.243569643749999010 ) ) ;
#7243=CARTESIAN_POINT ( 'NONE',  ( 25.62187500061451573, 3.027376345333613106, -5.243569643749998122 ) ) ;
#7245=CARTESIAN_POINT ( 'NONE',  ( 30.00000000000000000, 0.000000000000000000, 0.000000000000000000 ) ) ;
#7246=CARTESIAN_POINT ( 'NONE',  ( 7.846875000614518036, -3.027376345333614438, 5.243569643749998122 ) ) ;
#7247=CARTESIAN_POINT ( 'NONE',  ( 19.56562500061451715, -6.054752690667223547, -1.112240025338166033E-15 ) ) ;
#7249=DIRECTION ( 'NONE',  ( 0.000000000000000000, 0.000000000000000000, -1.000000000000000000 ) ) ;
#7250=CARTESIAN_POINT ( 'NONE',  ( 27.59062500061451573, -3.027376345333614438, 5.243569643749998122 ) ) ;
#7251=CARTESIAN_POINT ( 'NONE',  ( 4.771875000614516971, -6.054752690667223547, -1.112240025338166033E-15 ) ) ;
#7252=DIRECTION ( 'NONE',  ( -1.000000000000000000, -0.000000000000000000, -0.000000000000000000 ) ) ;
#7253=EDGE_CURVE ( 'NONE', #16300, #9370, #66130, .T. ) ;
#7255=CARTESIAN_POINT ( 'NONE',  ( 17.88749999999999929, -2.886751345948129988, 4.999999999999997335 ) ) ;
#7256=CARTESIAN_POINT ( 'NONE',  ( 21.17812500061451431, 4.541064518000418104, 2.621784821874999949 ) ) ;
#7258=CARTESIAN_POINT ( 'NONE',  ( 23.92499999999999716, 6.123233995736764310E-16, -4.999999999999998224 ) ) ;
#7259=CARTESIAN_POINT ( 'NONE',  ( 25.88437500061451502, -4.541064518000419881, 2.621784821874995952 ) ) ;
#7260=ORIENTED_EDGE ( 'NONE', *, *, #51252, .T. ) ;
#7261=CARTESIAN_POINT ( 'NONE',  ( 15.81562500061451537, 3.027376345333611329, 5.243569643749999010 ) ) ;
#7262=CARTESIAN_POINT ( 'NONE',  ( 5.990625000614517859, -3.027376345333614438, 5.243569643749998122 ) ) ;
#7264=CARTESIAN_POINT ( 'NONE',  ( 28.86562500061451786, 3.027376345333611329, 5.243569643749999010 ) ) ;
#7265=CARTESIAN_POINT ( 'NONE',  ( 15.30000000122903359, -2.886751345948129988, 4.999999999999997335 ) ) ;
#7266=CARTESIAN_POINT ( 'NONE',  ( 21.37499999999999645, 4.330127018922191873, 2.499999999999999556 ) ) ;
#7267=CARTESIAN_POINT ( 'NONE',  ( 16.50000000000000000, 0.000000000000000000, 4.999999999999998224 ) ) ;
#7268=CARTESIAN_POINT ( 'NONE',  ( 5.221875000614519813, -6.054752690667223547, -1.112240025338166033E-15 ) ) ;
#7269=CARTESIAN_POINT ( 'NONE',  ( 9.346875000614517148, -3.027376345333610441, -5.243569643749999898 ) ) ;
#7270=CARTESIAN_POINT ( 'NONE',  ( 20.37187500061451573, 3.027376345333611329, 5.243569643749999010 ) ) ;
#7271=FACE_OUTER_BOUND ( 'NONE', #7177, .T. ) ;
#7272=VERTEX_POINT ( 'NONE', #53832 ) ;
#7273=CARTESIAN_POINT ( 'NONE',  ( 27.85312500061451502, 4.541064518000418104, -2.621784821874998173 ) ) ;
#7274=CARTESIAN_POINT ( 'NONE',  ( 29.74687500061451217, 6.054752690667223547, 3.707466751127219781E-16 ) ) ;
#7275=CARTESIAN_POINT ( 'NONE',  ( 4.284375000614518925, -4.541064518000419881, 2.621784821874995952 ) ) ;
#7276=CARTESIAN_POINT ( 'NONE',  ( 17.77499999999999858, 4.330127018922191873, 2.499999999999999556 ) ) ;
#7277=CARTESIAN_POINT ( 'NONE',  ( 13.22812500061451502, -4.541064518000419881, 2.621784821874995952 ) ) ;
#7278=CARTESIAN_POINT ( 'NONE',  ( 1.071796769724489895, 14.12990381179669797, 26.00000000000000355 ) ) ;
#7280=DIRECTION ( 'NONE',  ( 0.000000000000000000, 0.000000000000000000, -1.000000000000000000 ) ) ;
#7283=CARTESIAN_POINT ( 'NONE',  ( 7.190625000614518036, 6.054752690667223547, 3.707466751127219781E-16 ) ) ;
#7284=CARTESIAN_POINT ( 'NONE',  ( 25.02187500061451431, -6.054752690667223547, -1.112240025338166033E-15 ) ) ;
#7285=CARTESIAN_POINT ( 'NONE',  ( 4.243569643749999010, 18.32187500061451502, 27.54997392385601174 ) ) ;
#7286=CARTESIAN_POINT ( 'NONE',  ( 26.48437500061451644, 6.421520780324663323E-16, -5.243569643749999010 ) ) ;
#7287=CARTESIAN_POINT ( 'NONE',  ( 6.450000000000001066, 4.330127018922192761, -2.499999999999997780 ) ) ;
#7288=CARTESIAN_POINT ( 'NONE',  ( 3.999999999999999112, 14.03750000122903430, 30.00000000000000000 ) ) ;
#7289=CARTESIAN_POINT ( 'NONE',  ( 15.59062500061451573, -3.027376345333610441, -5.243569643749999898 ) ) ;
#7290=CARTESIAN_POINT ( 'NONE',  ( 7.912500001229033408, 4.330127018922192761, -2.499999999999997780 ) ) ;
#7291=CARTESIAN_POINT ( 'NONE',  ( 18.00937500061451502, 4.541064518000418104, -2.621784821874998173 ) ) ;
#7292=CARTESIAN_POINT ( 'NONE',  ( 11.22187500061451892, 3.027376345333613106, -5.243569643749998122 ) ) ;
#7293=ORIENTED_EDGE ( 'NONE', *, *, #41790, .F. ) ;
#7294=CARTESIAN_POINT ( 'NONE',  ( 11.54062500061451857, -3.027376345333610441, -5.243569643749999898 ) ) ;
#7296=CARTESIAN_POINT ( 'NONE',  ( 23.43750000122902932, -4.330127018922194537, 2.499999999999995559 ) ) ;
#7297=CARTESIAN_POINT ( 'NONE',  ( 12.75937500061451857, 0.000000000000000000, 5.243569643749999010 ) ) ;
#7298=CARTESIAN_POINT ( 'NONE',  ( 15.59062500061451573, -3.027376345333610441, -5.243569643749999898 ) ) ;
#7299=CARTESIAN_POINT ( 'NONE',  ( 1.626862140677534273E-15, 16.51249999999999929, -26.00000000000000355 ) ) ;
#7300=CARTESIAN_POINT ( 'NONE',  ( 24.19687500061451857, -3.027376345333610441, -5.243569643749999898 ) ) ;
#7301=CARTESIAN_POINT ( 'NONE',  ( 12.45000000122903394, 5.773502691896255534, 3.535250795749688894E-16 ) ) ;
#7302=DIRECTION ( 'NONE',  ( 0.000000000000000000, 0.000000000000000000, 1.000000000000000000 ) ) ;
#7304=CARTESIAN_POINT ( 'NONE',  ( -4.243569643749998122, 16.29687500061451644, -27.54997392385601174 ) ) ;
#7305=CARTESIAN_POINT ( 'NONE',  ( 19.20937500061451786, -4.541064518000417216, -2.621784821875001281 ) ) ;
#7306=CARTESIAN_POINT ( 'NONE',  ( 18.18750000122903288, 6.123233995736764310E-16, -4.999999999999998224 ) ) ;
#7307=EDGE_CURVE ( 'NONE', #13801, #14992, #60516, .T. ) ;
#7308=CARTESIAN_POINT ( 'NONE',  ( 12.12187500061451573, 3.027376345333613106, -5.243569643749998122 ) ) ;
#7309=CARTESIAN_POINT ( 'NONE',  ( 4.243569643749999010, 19.61562500061451431, -32.45002607614398471 ) ) ;
#7310=CARTESIAN_POINT ( 'NONE',  ( 20.13750000122903216, 4.330127018922191873, 2.499999999999999556 ) ) ;
#7311=CARTESIAN_POINT ( 'NONE',  ( 13.90312500061451750, 4.541064518000418104, -2.621784821874998173 ) ) ;
#7312=ORIENTED_EDGE ( 'NONE', *, *, #16702, .F. ) ;
#7313=ORIENTED_EDGE ( 'NONE', *, *, #34980, .T. ) ;
#7314=CARTESIAN_POINT ( 'NONE',  ( 17.17500000000000071, 6.123233995736764310E-16, -4.999999999999998224 ) ) ;
#7317=CARTESIAN_POINT ( 'NONE',  ( 15.86250000122903181, -4.330127018922190985, -2.500000000000001332 ) ) ;
#7318=CARTESIAN_POINT ( 'NONE',  ( 25.99687500061451928, -3.027376345333610441, -5.243569643749999898 ) ) ;
#7319=CARTESIAN_POINT ( 'NONE',  ( 20.39062500061451644, -3.027376345333614438, 5.243569643749998122 ) ) ;
#7320=CARTESIAN_POINT ( 'NONE',  ( 23.05312500061451431, 0.000000000000000000, 5.243569643749999010 ) ) ;
#7321=CARTESIAN_POINT ( 'NONE',  ( 29.40000000122903145, -2.886751345948125991, -5.000000000000000000 ) ) ;
#7322=CARTESIAN_POINT ( 'NONE',  ( 27.41250000000000142, -5.773502691896255534, -1.060575238724906372E-15 ) ) ;
#7325=CYLINDRICAL_SURFACE ( 'NONE', #45318, 3.999999999999996447 ) ;
#7326=CARTESIAN_POINT ( 'NONE',  ( 3.999999999999999112, 9.987500001229033586, -30.00000000000000000 ) ) ;
#7327=CARTESIAN_POINT ( 'NONE',  ( -4.243569643749999898, 15.35937500061451644, -30.00000000000000000 ) ) ;
#7328=CARTESIAN_POINT ( 'NONE',  ( 6.900000001229035007, -2.886751345948125991, -5.000000000000000000 ) ) ;
#7329=CARTESIAN_POINT ( 'NONE',  ( 5.025000000000002132, 6.123233995736764310E-16, -4.999999999999998224 ) ) ;
#7330=CARTESIAN_POINT ( 'NONE',  ( 2.934375000614518392, -4.541064518000419881, 2.621784821874995952 ) ) ;
#7331=CARTESIAN_POINT ( 'NONE',  ( 10.62187500061451928, -6.054752690667223547, -1.112240025338166033E-15 ) ) ;
#7333=CARTESIAN_POINT ( 'NONE',  ( 28.79062500061451502, 6.054752690667223547, 3.707466751127219781E-16 ) ) ;
#7334=DIRECTION ( 'NONE',  ( -0.000000000000000000, -1.000000000000000000, -0.000000000000000000 ) ) ;
#7335=CARTESIAN_POINT ( 'NONE',  ( 3.619842856578028734, -3.449164782042274169, -3.619842856578066481 ) ) ;
#7336=CARTESIAN_POINT ( 'NONE',  ( -3.999999999999999112, 19.17500000122903359, 27.69059892324149885 ) ) ;
#7337=CARTESIAN_POINT ( 'NONE',  ( 7.734375000614517326, 4.541064518000418104, 2.621784821874999949 ) ) ;
#7338=CARTESIAN_POINT ( 'NONE',  ( 11.70937500061451608, 4.541064518000418104, -2.621784821874998173 ) ) ;
#7339=CARTESIAN_POINT ( 'NONE',  ( 6.075000000000000178, 4.330127018922191873, 2.499999999999999556 ) ) ;
#7340=CARTESIAN_POINT ( 'NONE',  ( -4.243569643749999898, 13.95312500061459282, 30.00000000000000000 ) ) ;
#7342=CARTESIAN_POINT ( 'NONE',  ( 5.812500000000001776, -5.773502691896255534, -1.060575238724906372E-15 ) ) ;
#7343=CARTESIAN_POINT ( 'NONE',  ( 27.52500000122903145, -5.773502691896255534, -1.060575238724906372E-15 ) ) ;
#7345=CARTESIAN_POINT ( 'NONE',  ( 22.07812500061451644, 4.541064518000418104, 2.621784821874999949 ) ) ;
#7346=CARTESIAN_POINT ( 'NONE',  ( 13.60312500061451679, 0.000000000000000000, 5.243569643749999010 ) ) ;
#7348=CARTESIAN_POINT ( 'NONE',  ( 10.17187500061451999, -6.054752690667223547, -1.112240025338166033E-15 ) ) ;
#7349=CARTESIAN_POINT ( 'NONE',  ( 26.92499999999999716, -4.330127018922194537, 2.499999999999995559 ) ) ;
#7350=CARTESIAN_POINT ( 'NONE',  ( 21.37500000122902932, 2.886751345948129099, -4.999999999999998224 ) ) ;
#7351=CARTESIAN_POINT ( 'NONE',  ( 0.000000000000000000, -10.00000000000000000, 0.000000000000000000 ) ) ;
#7352=CARTESIAN_POINT ( 'NONE',  ( 12.83437500061451786, -4.541064518000419881, 2.621784821874995952 ) ) ;
#7353=CARTESIAN_POINT ( 'NONE',  ( 26.37187500061451217, -6.054752690667223547, -1.112240025338166033E-15 ) ) ;
#7354=CARTESIAN_POINT ( 'NONE',  ( 3.196875000614516793, 6.054752690667223547, 3.707466751127219781E-16 ) ) ;
#7355=CARTESIAN_POINT ( 'NONE',  ( 3.999999999999998668, 13.62500000122903465, -32.30940107675850470 ) ) ;
#7356=CARTESIAN_POINT ( 'NONE',  ( 22.02187500061452141, 3.027376345333613106, -5.243569643749998122 ) ) ;
#7357=CARTESIAN_POINT ( 'NONE',  ( 11.82187500061451679, 3.027376345333611329, 5.243569643749999010 ) ) ;
#7359=CARTESIAN_POINT ( 'NONE',  ( 25.64999999999999858, -4.330127018922190985, -2.500000000000001332 ) ) ;
#7361=CARTESIAN_POINT ( 'NONE',  ( -2.121784821874999949, 13.03437500061451715, -33.67503911421598417 ) ) ;
#7363=CARTESIAN_POINT ( 'NONE',  ( 13.71562500061451750, -6.054752690667223547, -1.112240025338166033E-15 ) ) ;
#7364=CARTESIAN_POINT ( 'NONE',  ( 6.037500000000001421, 5.773502691896255534, 3.535250795749688894E-16 ) ) ;
#7365=CARTESIAN_POINT ( 'NONE',  ( 0.000000000000000000, 20.00000000000000000, -30.00000000000000000 ) ) ;
#7366=CARTESIAN_POINT ( 'NONE',  ( 15.37500000000000000, 6.123233995736764310E-16, -4.999999999999998224 ) ) ;
#7367=CARTESIAN_POINT ( 'NONE',  ( -2.121784821874999949, 11.17812500061451786, 26.32496088578401938 ) ) ;
#7368=CARTESIAN_POINT ( 'NONE',  ( 14.40000000122903323, -2.886751345948129988, 4.999999999999997335 ) ) ;
#7369=CARTESIAN_POINT ( 'NONE',  ( 25.35937500061451644, 0.000000000000000000, 5.243569643749999010 ) ) ;
#7371=CARTESIAN_POINT ( 'NONE',  ( 19.15312500061451573, -4.541064518000417216, -2.621784821875001281 ) ) ;
#7372=CARTESIAN_POINT ( 'NONE',  ( 20.85937500061451644, 0.000000000000000000, 5.243569643749999010 ) ) ;
#7373=CARTESIAN_POINT ( 'NONE',  ( 5.362500000000003375, -5.773502691896255534, -1.060575238724906372E-15 ) ) ;
#7374=CARTESIAN_POINT ( 'NONE',  ( 7.490625000614516082, -3.027376345333610441, -5.243569643749999898 ) ) ;
#7375=CARTESIAN_POINT ( 'NONE',  ( 21.70312500061451644, 0.000000000000000000, 5.243569643749999010 ) ) ;
#7376=CARTESIAN_POINT ( 'NONE',  ( 15.98437500061451821, -4.541064518000419881, 2.621784821874995952 ) ) ;
#7377=CARTESIAN_POINT ( 'NONE',  ( 2.121784821874999061, 14.70312500061451644, 26.32496088578401583 ) ) ;
#7378=CARTESIAN_POINT ( 'NONE',  ( 19.08750000122903145, 6.123233995736764310E-16, -4.999999999999998224 ) ) ;
#7380=CARTESIAN_POINT ( 'NONE',  ( 8.540625000614518569, 6.054752690667223547, 3.707466751127219781E-16 ) ) ;
#7381=CARTESIAN_POINT ( 'NONE',  ( 3.234375000614516438, 4.541064518000418104, 2.621784821874999949 ) ) ;
#7382=CARTESIAN_POINT ( 'NONE',  ( 29.61562500061451431, 3.027376345333613106, -5.243569643749998122 ) ) ;
#7383=( BOUNDED_CURVE ( )  B_SPLINE_CURVE ( 2, ( #57536, #25649, #36725, #62718, #35365, #12112, #30822 ),
 .UNSPECIFIED., .F., .F. ) 
 B_SPLINE_CURVE_WITH_KNOTS ( ( 3, 2, 2, 3 ),
 ( 0.9599923174713632656, 0.9611111111111111382, 0.9638888888888889062, 0.9649074199495660809 ),
 .UNSPECIFIED. ) 
 CURVE ( )  GEOMETRIC_REPRESENTATION_ITEM ( )  RATIONAL_B_SPLINE_CURVE ( ( 0.9355460294322659465, 0.9460396265918464831, 1.000000000000000000, 0.8660254037844387076, 1.000000000000000000, 0.9508753764685963228, 0.9377759204729740894 ) ) 
 REPRESENTATION_ITEM ( '' )  );
#7384=CARTESIAN_POINT ( 'NONE',  ( 25.43437500061451573, -4.541064518000419881, 2.621784821874995952 ) ) ;
#7385=CARTESIAN_POINT ( 'NONE',  ( 16.79062500061451857, -3.027376345333614438, 5.243569643749998122 ) ) ;
#7386=CARTESIAN_POINT ( 'NONE',  ( 24.48750000122903359, 6.123233995736764310E-16, -4.999999999999998224 ) ) ;
#7387=EDGE_CURVE ( 'NONE', #43953, #14078, #10905, .T. ) ;
#7388=CARTESIAN_POINT ( 'NONE',  ( 25.15312500061451217, 4.541064518000418104, -2.621784821874998173 ) ) ;
#7389=VECTOR ( 'NONE', #67578, 1000.000000000000000 ) ;
#7390=CARTESIAN_POINT ( 'NONE',  ( 20.93437500061451573, -4.541064518000419881, 2.621784821874995952 ) ) ;
#7391=CARTESIAN_POINT ( 'NONE',  ( 14.76562500061451821, 3.027376345333613106, -5.243569643749998122 ) ) ;
#7392=CARTESIAN_POINT ( 'NONE',  ( -4.243569643749999898, 18.02187500061452141, 27.54997392385601529 ) ) ;
#7393=CARTESIAN_POINT ( 'NONE',  ( 21.51562500061451644, 3.027376345333613106, -5.243569643749998122 ) ) ;
#7395=ORIENTED_EDGE ( 'NONE', *, *, #33218, .T. ) ;
#7396=CARTESIAN_POINT ( 'NONE',  ( 24.75000000000000000, -4.330127018922190985, -2.500000000000001332 ) ) ;
#7397=CARTESIAN_POINT ( 'NONE',  ( -3.999999999999999112, 12.80000000000000071, -30.00000000000000000 ) ) ;
#7399=CARTESIAN_POINT ( 'NONE',  ( 3.421875000614516882, -6.054752690667223547, -1.112240025338166033E-15 ) ) ;
#7400=CARTESIAN_POINT ( 'NONE',  ( 6.853125000614516793, 0.000000000000000000, 5.243569643749999010 ) ) ;
#7401=CARTESIAN_POINT ( 'NONE',  ( 21.18750000122903288, -4.330127018922194537, 2.499999999999995559 ) ) ;
#7402=CARTESIAN_POINT ( 'NONE',  ( 26.20312500061451644, 0.000000000000000000, 5.243569643749999010 ) ) ;
#7403=CARTESIAN_POINT ( 'NONE',  ( 24.63749999999999574, -2.886751345948129988, 4.999999999999997335 ) ) ;
#7404=CARTESIAN_POINT ( 'NONE',  ( -1.999999999999997113, 15.23750000122903536, -26.53589838486224295 ) ) ;
#7406=CARTESIAN_POINT ( 'NONE',  ( 10.60312500061451679, -4.541064518000417216, -2.621784821875001281 ) ) ;
#7408=CARTESIAN_POINT ( 'NONE',  ( 25.82812500061451644, -4.541064518000419881, 2.621784821874995952 ) ) ;
#7409=CARTESIAN_POINT ( 'NONE',  ( 7.190625000614518036, 6.054752690667223547, 3.707466751127219781E-16 ) ) ;
#7410=CARTESIAN_POINT ( 'NONE',  ( 3.815625000614518036, -6.054752690667223547, -1.112240025338166033E-15 ) ) ;
#7412=CYLINDRICAL_SURFACE ( 'NONE', #32657, 4.999999999999998224 ) ;
#7413=CARTESIAN_POINT ( 'NONE',  ( 13.35000000000000142, 0.000000000000000000, 4.999999999999998224 ) ) ;
#7414=CARTESIAN_POINT ( 'NONE',  ( 12.87187500061451750, -6.054752690667223547, -1.112240025338166033E-15 ) ) ;
#7415=CARTESIAN_POINT ( 'NONE',  ( 9.750000001229032875, 5.773502691896255534, 3.535250795749688894E-16 ) ) ;
#7416=CARTESIAN_POINT ( 'NONE',  ( 16.13437500061451502, 6.421520780324663323E-16, -5.243569643749999010 ) ) ;
#7418=CARTESIAN_POINT ( 'NONE',  ( 8.409375000614518925, -4.541064518000417216, -2.621784821875001281 ) ) ;
#7419=CARTESIAN_POINT ( 'NONE',  ( -4.243569643749999898, 12.11562500061451608, -32.45002607614398471 ) ) ;
#7420=CARTESIAN_POINT ( 'NONE',  ( -3.999999999999997335, 16.88749999999999929, 32.30940107675850470 ) ) ;
#7422=EDGE_LOOP ( 'NONE', ( #35380, #4511, #41457, #34982 ) ) ;
#7423=CARTESIAN_POINT ( 'NONE',  ( 23.65312500061451573, -4.541064518000417216, -2.621784821875001281 ) ) ;
#7424=CARTESIAN_POINT ( 'NONE',  ( 0.000000000000000000, 20.00000000000000000, 30.00000000000000000 ) ) ;
#7425=CARTESIAN_POINT ( 'NONE',  ( 29.25937500061451502, 4.541064518000418104, -2.621784821874998173 ) ) ;
#7426=( BOUNDED_CURVE ( )  B_SPLINE_CURVE ( 2, ( #40616, #52061, #13978, #54249, #26169, #3646, #14708, #36516, #65689 ),
 .UNSPECIFIED., .F., .F. ) 
 B_SPLINE_CURVE_WITH_KNOTS ( ( 3, 2, 2, 2, 3 ),
 ( 0.1413043478260869734, 0.1449275362318840632, 0.1521739130434782705, 0.1594202898550724501, 0.1630434782608695676 ),
 .UNSPECIFIED. ) 
 CURVE ( )  GEOMETRIC_REPRESENTATION_ITEM ( )  RATIONAL_B_SPLINE_CURVE ( ( 0.9330127018922194093, 0.9330127018922196314, 1.000000000000000000, 0.8660254037844387076, 1.000000000000000000, 0.8660254037844387076, 1.000000000000000000, 0.9330127018922190762, 0.9330127018922194093 ) ) 
 REPRESENTATION_ITEM ( '' )  );
#7427=CARTESIAN_POINT ( 'NONE',  ( 24.67500000000000071, -4.330127018922194537, 2.499999999999995559 ) ) ;
#7428=CARTESIAN_POINT ( 'NONE',  ( 7.153125000614518392, 4.541064518000418104, -2.621784821874998173 ) ) ;
#7429=B_SPLINE_CURVE_WITH_KNOTS ( 'NONE', 3,
 ( #59358, #1789, #24659, #53844, #24299, #46847, #69387, #13208, #26496, #71567 ),
 .UNSPECIFIED., .F., .F.,
 ( 4, 3, 3, 4 ),
 ( 0.000000000000000000, 0.0001572266096559048090, 0.0003144533513551280631, 0.0005416000942056856159 ),
 .UNSPECIFIED. ) ;
#7431=CARTESIAN_POINT ( 'NONE',  ( 16.54687500061451644, -3.027376345333610441, -5.243569643749999898 ) ) ;
#7433=CARTESIAN_POINT ( 'NONE',  ( 29.62500000122903288, 2.886751345948126879, 4.999999999999999112 ) ) ;
#7434=CARTESIAN_POINT ( 'NONE',  ( 9.159375000614515372, 0.000000000000000000, 5.243569643749999010 ) ) ;
#7436=CARTESIAN_POINT ( 'NONE',  ( 19.28437500061451360, 6.421520780324663323E-16, -5.243569643749999010 ) ) ;
#7438=CARTESIAN_POINT ( 'NONE',  ( 27.82499999999999929, -4.330127018922194537, 2.499999999999995559 ) ) ;
#7439=CARTESIAN_POINT ( 'NONE',  ( 28.77187500061451431, 3.027376345333613106, -5.243569643749998122 ) ) ;
#7441=CARTESIAN_POINT ( 'NONE',  ( 27.78750000000000142, -2.886751345948155301, 4.999999999999952927 ) ) ;
#7443=CARTESIAN_POINT ( 'NONE',  ( 11.02500000000000036, 4.330127018922191873, 2.499999999999999556 ) ) ;
#7445=CARTESIAN_POINT ( 'NONE',  ( 25.64062500061451644, 6.054752690667223547, 3.707466751127219781E-16 ) ) ;
#7446=CARTESIAN_POINT ( 'NONE',  ( 14.47499999999999964, 6.123233995736764310E-16, -4.999999999999998224 ) ) ;
#7447=CARTESIAN_POINT ( 'NONE',  ( 9.112500001229033586, -4.330127018922190985, -2.500000000000001332 ) ) ;
#7448=CARTESIAN_POINT ( 'NONE',  ( 7.415625000614516793, -6.054752690667223547, -1.112240025338166033E-15 ) ) ;
#7449=CARTESIAN_POINT ( 'NONE',  ( 21.75000000000000000, 4.330127018922192761, -2.499999999999997780 ) ) ;
#7450=CARTESIAN_POINT ( 'NONE',  ( 21.25312500061451715, 0.000000000000000000, 5.243569643749999010 ) ) ;
#7452=CARTESIAN_POINT ( 'NONE',  ( 24.75000000122902932, -2.886751345948129988, 4.999999999999997335 ) ) ;
#7454=CARTESIAN_POINT ( 'NONE',  ( 6.000000000000001776, 4.330127018922192761, -2.499999999999997780 ) ) ;
#7455=ORIENTED_EDGE ( 'NONE', *, *, #40125, .T. ) ;
#7456=CARTESIAN_POINT ( 'NONE',  ( 21.17812500061451431, 4.541064518000418104, 2.621784821874999949 ) ) ;
#7457=CARTESIAN_POINT ( 'NONE',  ( 27.92812500061451431, 4.541064518000418104, 2.621784821874999949 ) ) ;
#7458=CARTESIAN_POINT ( 'NONE',  ( 27.23437500061451644, -4.541064518000419881, 2.621784821874995952 ) ) ;
#7460=CARTESIAN_POINT ( 'NONE',  ( 14.16562500061451679, -6.054752690667223547, -1.112240025338166033E-15 ) ) ;
#7462=CARTESIAN_POINT ( 'NONE',  ( 26.36250000122903003, 4.330127018922192761, -2.499999999999997780 ) ) ;
#7464=CARTESIAN_POINT ( 'NONE',  ( 17.24062500061451786, -3.027376345333614438, 5.243569643749998122 ) ) ;
#7466=CARTESIAN_POINT ( 'NONE',  ( 5.850000001229035185, -2.886751345948130876, 4.999999999999996447 ) ) ;
#7467=CARTESIAN_POINT ( 'NONE',  ( 10.95937500061451964, 0.000000000000000000, 5.243569643749999010 ) ) ;
#7468=CARTESIAN_POINT ( 'NONE',  ( 9.496875000614517504, 6.054752690667223547, 3.707466751127219781E-16 ) ) ;
#7469=CARTESIAN_POINT ( 'NONE',  ( 21.19687500061451502, 6.054752690667223547, 3.707466751127219781E-16 ) ) ;
#7471=CARTESIAN_POINT ( 'NONE',  ( -1.974232797588184596, 9.810253314282338266, 24.32048149236734247 ) ) ;
#7472=CARTESIAN_POINT ( 'NONE',  ( 23.01562500061451644, 3.027376345333611329, 5.243569643749999010 ) ) ;
#7473=CARTESIAN_POINT ( 'NONE',  ( 19.73437500061451644, 6.421520780324663323E-16, -5.243569643749999010 ) ) ;
#7474=CARTESIAN_POINT ( 'NONE',  ( 23.39062500061451289, 6.054752690667223547, 3.707466751127219781E-16 ) ) ;
#7475=CARTESIAN_POINT ( 'NONE',  ( 4.057522967627288146, -2.921730200955767298, 4.057522967627288146 ) ) ;
#7476=CARTESIAN_POINT ( 'NONE',  ( 1.999999999999998668, 14.00000000000000178, 26.53589838486224650 ) ) ;
#7477=CARTESIAN_POINT ( 'NONE',  ( 3.009375000614516793, -4.541064518000417216, -2.621784821875001281 ) ) ;
#7478=CARTESIAN_POINT ( 'NONE',  ( 9.037500001229034297, -4.330127018922194537, 2.499999999999995559 ) ) ;
#7479=CARTESIAN_POINT ( 'NONE',  ( 5.475000001229035185, -5.773502691896255534, -1.060575238724906372E-15 ) ) ;
#7480=CARTESIAN_POINT ( 'NONE',  ( -3.999999999999997335, 19.58749999999999858, -27.69059892324149175 ) ) ;
#7481=CARTESIAN_POINT ( 'NONE',  ( 26.02500000122903145, 2.886751345948126879, 4.999999999999999112 ) ) ;
#7483=CARTESIAN_POINT ( 'NONE',  ( 10.09687500061451715, -3.027376345333614438, 5.243569643749998122 ) ) ;
#7484=CARTESIAN_POINT ( 'NONE',  ( 18.55312500061451431, 0.000000000000000000, 5.243569643749999010 ) ) ;
#7485=CARTESIAN_POINT ( 'NONE',  ( 9.871875000614517504, 3.027376345333613106, -5.243569643749998122 ) ) ;
#7486=CARTESIAN_POINT ( 'NONE',  ( 28.98750000122903359, 6.123233995736764310E-16, -4.999999999999998224 ) ) ;
#7487=CARTESIAN_POINT ( 'NONE',  ( 19.43437500061451928, 4.541064518000418104, 2.621784821874999949 ) ) ;
#7488=CARTESIAN_POINT ( 'NONE',  ( 7.059375000614518392, -4.541064518000417216, -2.621784821875001281 ) ) ;
#7489=CARTESIAN_POINT ( 'NONE',  ( 3.138359732036306138, -3.892498296044141437, -3.200804231420348422 ) ) ;
#7490=CARTESIAN_POINT ( 'NONE',  ( 1.592000809091587073E-14, 16.40000000122903501, 26.00000000000000000 ) ) ;
#7491=CARTESIAN_POINT ( 'NONE',  ( 8.128125000614515372, 4.541064518000418104, 2.621784821874999949 ) ) ;
#7492=CARTESIAN_POINT ( 'NONE',  ( 16.75312500061451715, 0.000000000000000000, 5.243569643749999010 ) ) ;
#7493=EDGE_LOOP ( 'NONE', ( #44255, #52202, #2683, #33376 ) ) ;
#7494=CARTESIAN_POINT ( 'NONE',  ( 5.700000001229033941, 5.773502691896255534, 3.535250795749688894E-16 ) ) ;
#7495=CARTESIAN_POINT ( 'NONE',  ( 15.21562500061451750, 3.027376345333613106, -5.243569643749998122 ) ) ;
#7496=CARTESIAN_POINT ( 'NONE',  ( 10.07812500061451644, -4.541064518000419881, 2.621784821874995952 ) ) ;
#7498=CARTESIAN_POINT ( 'NONE',  ( 11.13750000000000284, -2.886751345948129988, 4.999999999999997335 ) ) ;
#7499=CARTESIAN_POINT ( 'NONE',  ( 5.475000001229035185, -5.773502691896255534, -1.060575238724906372E-15 ) ) ;
#7500=CARTESIAN_POINT ( 'NONE',  ( 14.70937500061451786, -4.541064518000417216, -2.621784821875001281 ) ) ;
#7501=CARTESIAN_POINT ( 'NONE',  ( 18.97500000122903074, -5.773502691896255534, -1.060575238724906372E-15 ) ) ;
#7503=CARTESIAN_POINT ( 'NONE',  ( 4.243569643749999898, 17.74062500061451786, -27.54997392385601529 ) ) ;
#7504=CARTESIAN_POINT ( 'NONE',  ( 4.120265700342371495, -2.833395342107308590, -4.120265700342371495 ) ) ;
#7506=CARTESIAN_POINT ( 'NONE',  ( 9.450000001229033941, -2.886751345948130876, 4.999999999999996447 ) ) ;
#7507=DIRECTION ( 'NONE',  ( -1.000000000000000000, -0.000000000000000000, -0.000000000000000000 ) ) ;
#7508=CARTESIAN_POINT ( 'NONE',  ( 19.39687500061451786, 6.054752690667223547, 3.707466751127219781E-16 ) ) ;
#7509=CARTESIAN_POINT ( 'NONE',  ( 21.37500000122903288, 2.886751345948129099, -4.999999999999997335 ) ) ;
#7511=CARTESIAN_POINT ( 'NONE',  ( 14.61562500061451608, -6.054752690667223547, -1.112240025338166033E-15 ) ) ;
#7514=CARTESIAN_POINT ( 'NONE',  ( 25.32187500061451857, 3.027376345333611329, 5.243569643749999010 ) ) ;
#7516=CARTESIAN_POINT ( 'NONE',  ( 10.11562500061451608, -6.054752690667223547, -1.112240025338166033E-15 ) ) ;
#7517=CARTESIAN_POINT ( 'NONE',  ( 16.02187500061451786, -6.054752690667223547, -1.112240025338166033E-15 ) ) ;
#7519=CARTESIAN_POINT ( 'NONE',  ( 25.09687500061451715, -3.027376345333610441, -5.243569643749999898 ) ) ;
#7520=CARTESIAN_POINT ( 'NONE',  ( 26.50312500061451360, 4.541064518000418104, -2.621784821874998173 ) ) ;
#7521=CARTESIAN_POINT ( 'NONE',  ( 19.94062500061451715, -3.027376345333614438, 5.243569643749998122 ) ) ;
#7522=CARTESIAN_POINT ( 'NONE',  ( 29.65312500061451573, 4.541064518000418104, -2.621784821874998173 ) ) ;
#7524=CARTESIAN_POINT ( 'NONE',  ( 10.57500000000000107, 4.330127018922191873, 2.499999999999999556 ) ) ;
#7525=CARTESIAN_POINT ( 'NONE',  ( 19.50000000122903288, -2.886751345948125991, -5.000000000000000000 ) ) ;
#7526=CARTESIAN_POINT ( 'NONE',  ( 1.999999999999998668, 10.40000000000000213, 26.53589838486224650 ) ) ;
#7528=VERTEX_POINT ( 'NONE', #40380 ) ;
#7529=CARTESIAN_POINT ( 'NONE',  ( 18.71249999999999858, 2.886751345948126879, 4.999999999999999112 ) ) ;
#7530=CARTESIAN_POINT ( 'NONE',  ( 22.38749999999999929, -2.886751345948129988, 4.999999999999997335 ) ) ;
#7531=CARTESIAN_POINT ( 'NONE',  ( 19.02187500061451786, 3.027376345333611329, 5.243569643749999010 ) ) ;
#7532=CARTESIAN_POINT ( 'NONE',  ( 13.67812500061451786, -4.541064518000419881, 2.621784821874995952 ) ) ;
#7534=CARTESIAN_POINT ( 'NONE',  ( 1.999999999999998668, 18.61250000122903359, -33.46410161513775705 ) ) ;
#7535=CARTESIAN_POINT ( 'NONE',  ( 6.515625000614516438, -6.054752690667223547, -1.112240025338166033E-15 ) ) ;
#7536=CARTESIAN_POINT ( 'NONE',  ( 13.38750000000000107, -2.886751345948129988, 4.999999999999997335 ) ) ;
#7538=CARTESIAN_POINT ( 'NONE',  ( -4.243569643749999898, 15.75312500061451537, 30.00000000000000000 ) ) ;
#7539=CARTESIAN_POINT ( 'NONE',  ( 29.31562500061451715, 3.027376345333611329, 5.243569643749999010 ) ) ;
#7542=CARTESIAN_POINT ( 'NONE',  ( 25.05937500061451573, -4.541064518000417216, -2.621784821875001281 ) ) ;
#7544=CARTESIAN_POINT ( 'NONE',  ( 21.06562500061451715, 3.027376345333613106, -5.243569643749998122 ) ) ;
#7545=CARTESIAN_POINT ( 'NONE',  ( 23.85937500061451644, 4.541064518000418104, -2.621784821874998173 ) ) ;
#7546=CARTESIAN_POINT ( 'NONE',  ( 2.121784821874999061, 17.40312500061459389, -33.67503911421598417 ) ) ;
#7547=CARTESIAN_POINT ( 'NONE',  ( 6.815625000614517148, 3.027376345333611329, 5.243569643749999010 ) ) ;
#7549=CARTESIAN_POINT ( 'NONE',  ( 25.04062500061451502, -3.027376345333610441, -5.243569643749999898 ) ) ;
#7552=CARTESIAN_POINT ( 'NONE',  ( 17.48437500061451999, 6.421520780324663323E-16, -5.243569643749999010 ) ) ;
#7553=CARTESIAN_POINT ( 'NONE',  ( 18.38437500061451857, 6.421520780324663323E-16, -5.243569643749999010 ) ) ;
#7554=CARTESIAN_POINT ( 'NONE',  ( 27.23437500061451644, -4.541064518000419881, 2.621784821874995952 ) ) ;
#7555=CARTESIAN_POINT ( 'NONE',  ( 4.243569643749999010, 15.62187500061451928, 27.54997392385601174 ) ) ;
#7556=CARTESIAN_POINT ( 'NONE',  ( 7.978125000614517681, 6.421520780324663323E-16, -5.243569643749999010 ) ) ;
#7557=CARTESIAN_POINT ( 'NONE',  ( 1.626862140677534273E-15, 10.32500000122903572, -26.00000000000000355 ) ) ;
#7558=CARTESIAN_POINT ( 'NONE',  ( 5.409375000614516260, 4.541064518000418104, -2.621784821874998173 ) ) ;
#7560=CARTESIAN_POINT ( 'NONE',  ( 4.565625000614516260, 3.027376345333611329, 5.243569643749999010 ) ) ;
#7561=CARTESIAN_POINT ( 'NONE',  ( 9.384375000614518569, 6.421520780324663323E-16, -5.243569643749999010 ) ) ;
#7562=CARTESIAN_POINT ( 'NONE',  ( 15.86250000122903181, -4.330127018922190985, -2.500000000000001332 ) ) ;
#7563=CARTESIAN_POINT ( 'NONE',  ( 4.884375000614518569, 6.421520780324663323E-16, -5.243569643749999010 ) ) ;
#7564=CARTESIAN_POINT ( 'NONE',  ( 8.578125000614518214, 4.541064518000418104, 2.621784821874999949 ) ) ;
#7567=CARTESIAN_POINT ( 'NONE',  ( 17.59687500061451715, 6.054752690667223547, 3.707466751127219781E-16 ) ) ;
#7568=CYLINDRICAL_SURFACE ( 'NONE', #29018, 3.999999999999996447 ) ;
#7569=ORIENTED_EDGE ( 'NONE', *, *, #68436, .F. ) ;
#7570=CARTESIAN_POINT ( 'NONE',  ( 23.99062500061451786, -3.027376345333614438, 5.243569643749998122 ) ) ;
#7571=CARTESIAN_POINT ( 'NONE',  ( 10.75312500061451715, 4.541064518000418104, -2.621784821874998173 ) ) ;
#7572=EDGE_CURVE ( 'NONE', #48607, #43803, #6761, .T. ) ;
#7573=CARTESIAN_POINT ( 'NONE',  ( 26.18437500061451573, 4.541064518000418104, 2.621784821874999949 ) ) ;
#7574=CARTESIAN_POINT ( 'NONE',  ( 8.878125000614515372, 6.421520780324663323E-16, -5.243569643749999010 ) ) ;
#7575=CARTESIAN_POINT ( 'NONE',  ( 20.47500000000000142, 4.330127018922191873, 2.499999999999999556 ) ) ;
#7576=CARTESIAN_POINT ( 'NONE',  ( 11.06250000122903288, 4.330127018922192761, -2.499999999999997780 ) ) ;
#7577=CARTESIAN_POINT ( 'NONE',  ( 24.81562500061451715, 3.027376345333611329, 5.243569643749999010 ) ) ;
#7578=CARTESIAN_POINT ( 'NONE',  ( 2.121784821875001281, 12.30312500061451608, -26.32496088578401938 ) ) ;
#7579=CARTESIAN_POINT ( 'NONE',  ( 13.91250000122903252, 0.000000000000000000, 4.999999999999998224 ) ) ;
#7580=CARTESIAN_POINT ( 'NONE',  ( 21.02812500061451573, 6.421520780324663323E-16, -5.243569643749999010 ) ) ;
#7581=CARTESIAN_POINT ( 'NONE',  ( 11.81250000000000000, 2.886751345948129099, -4.999999999999998224 ) ) ;
#7582=CARTESIAN_POINT ( 'NONE',  ( 19.45312500061451644, 0.000000000000000000, 5.243569643749999010 ) ) ;
#7583=CARTESIAN_POINT ( 'NONE',  ( 5.746875000614517504, -3.027376345333610441, -5.243569643749999898 ) ) ;
#7584=CARTESIAN_POINT ( 'NONE',  ( 20.85000000000000142, 4.330127018922192761, -2.499999999999997780 ) ) ;
#7585=CARTESIAN_POINT ( 'NONE',  ( 13.46250000122903323, 0.000000000000000000, 4.999999999999998224 ) ) ;
#7586=CARTESIAN_POINT ( 'NONE',  ( 11.27812500061451573, 4.541064518000418104, 2.621784821874999949 ) ) ;
#7587=CARTESIAN_POINT ( 'NONE',  ( 13.86562500061451431, 3.027376345333613106, -5.243569643749998122 ) ) ;
#7588=CARTESIAN_POINT ( 'NONE',  ( 26.32500000122903216, 2.886751345948129099, -4.999999999999998224 ) ) ;
#7589=AXIS2_PLACEMENT_3D ( 'NONE', #71577, #49410, #37220 ) ;
#7590=CARTESIAN_POINT ( 'NONE',  ( 21.08437500061451786, 6.421520780324663323E-16, -5.243569643749999010 ) ) ;
#7592=CARTESIAN_POINT ( 'NONE',  ( 6.900000001229035007, -2.886751345948125991, -5.000000000000000000 ) ) ;
#7593=CARTESIAN_POINT ( 'NONE',  ( 7.809375000614519280, 0.000000000000000000, 5.243569643749999010 ) ) ;
#7594=CARTESIAN_POINT ( 'NONE',  ( 25.88437500061451502, -4.541064518000419881, 2.621784821874995952 ) ) ;
#7595=CARTESIAN_POINT ( 'NONE',  ( 3.009375000614516793, -4.541064518000417216, -2.621784821875001281 ) ) ;
#7596=CARTESIAN_POINT ( 'NONE',  ( 22.45312500061451644, 4.541064518000418104, -2.621784821874998173 ) ) ;
#7597=CARTESIAN_POINT ( 'NONE',  ( 27.19687500061451857, -3.027376345333614438, 5.243569643749998122 ) ) ;
#7599=DIRECTION ( 'NONE',  ( -1.000000000000000000, -0.000000000000000000, -0.000000000000000000 ) ) ;
#7600=CARTESIAN_POINT ( 'NONE',  ( 8.634375000614518569, 4.541064518000418104, 2.621784821874999949 ) ) ;
#7601=CARTESIAN_POINT ( 'NONE',  ( 17.09062500061451573, 6.054752690667223547, 3.707466751127219781E-16 ) ) ;
#7602=AXIS2_PLACEMENT_3D ( 'NONE', #26977, #38416, #9613 ) ;
#7604=CARTESIAN_POINT ( 'NONE',  ( 30.00000000000000000, 0.000000000000000000, 0.000000000000000000 ) ) ;
#7605=CARTESIAN_POINT ( 'NONE',  ( 28.04062500061451502, -3.027376345333614438, 5.243569643749998122 ) ) ;
#7606=CARTESIAN_POINT ( 'NONE',  ( 4.996875000614516615, 6.054752690667223547, 3.707466751127219781E-16 ) ) ;
#7607=CARTESIAN_POINT ( 'NONE',  ( 10.20000000122903572, 5.773502691896255534, 3.535250795749688401E-16 ) ) ;
#7608=LINE ( 'NONE', #60671, #34756 ) ;
#7609=CARTESIAN_POINT ( 'NONE',  ( 16.94999999999999929, 0.000000000000000000, 4.999999999999998224 ) ) ;
#7610=CARTESIAN_POINT ( 'NONE',  ( 20.69062500061451715, 6.054752690667223547, 3.707466751127219781E-16 ) ) ;
#7611=ORIENTED_EDGE ( 'NONE', *, *, #61652, .T. ) ;
#7612=CARTESIAN_POINT ( 'NONE',  ( 25.16249999999999432, -5.773502691896255534, -1.060575238724906372E-15 ) ) ;
#7614=CARTESIAN_POINT ( 'NONE',  ( 26.63437500061451857, 4.541064518000418104, 2.621784821874999949 ) ) ;
#7615=EDGE_LOOP ( 'NONE', ( #13757, #34736 ) ) ;
#7616=CARTESIAN_POINT ( 'NONE',  ( 14.24062500061451608, -3.027376345333610441, -5.243569643749999898 ) ) ;
#7617=CARTESIAN_POINT ( 'NONE',  ( 6.290625000614517681, 6.054752690667223547, 3.707466751127219781E-16 ) ) ;
#7619=CARTESIAN_POINT ( 'NONE',  ( 29.65312500061451573, 4.541064518000418104, -2.621784821874998173 ) ) ;
#7620=CARTESIAN_POINT ( 'NONE',  ( 15.97500000122903430, 2.886751345948129099, -4.999999999999998224 ) ) ;
#7621=CARTESIAN_POINT ( 'NONE',  ( 19.94999999999999929, 4.330127018922192761, -2.499999999999997780 ) ) ;
#7622=CARTESIAN_POINT ( 'NONE',  ( 28.04999999999999716, 4.330127018922192761, -2.499999999999997780 ) ) ;
#7623=CARTESIAN_POINT ( 'NONE',  ( 3.759375000614517681, 0.000000000000000000, 5.243569643749999010 ) ) ;
#7624=CARTESIAN_POINT ( 'NONE',  ( 9.309375000614517504, -4.541064518000417216, -2.621784821875001281 ) ) ;
#7625=CARTESIAN_POINT ( 'NONE',  ( 18.60937500061451644, 0.000000000000000000, 5.243569643749999010 ) ) ;
#7626=CARTESIAN_POINT ( 'NONE',  ( 18.86250000122903359, 0.000000000000000000, 4.999999999999998224 ) ) ;
#7627=VERTEX_POINT ( 'NONE', #13013 ) ;
#7628=CARTESIAN_POINT ( 'NONE',  ( 28.26562500061451289, 3.027376345333613106, -5.243569643749998122 ) ) ;
#7629=CARTESIAN_POINT ( 'NONE',  ( 29.44687500061451857, -3.027376345333614438, 5.243569643749998122 ) ) ;
#7630=( BOUNDED_CURVE ( )  B_SPLINE_CURVE ( 2, ( #72622, #5749, #60420, #28283, #26831, #22006, #27924 ),
 .UNSPECIFIED., .F., .F. ) 
 B_SPLINE_CURVE_WITH_KNOTS ( ( 3, 2, 2, 3 ),
 ( 0.3833333333333333037, 0.3861111111111111271, 0.3888888888888889506, 0.3916666666666667740 ),
 .UNSPECIFIED. ) 
 CURVE ( )  GEOMETRIC_REPRESENTATION_ITEM ( )  RATIONAL_B_SPLINE_CURVE ( ( 1.000000000000002665, 0.8660254037844360431, 1.000000000000000000, 0.8660254037844387076, 1.000000000000000000, 0.8660254037844333785, 1.000000000000005329 ) ) 
 REPRESENTATION_ITEM ( '' )  );
#7631=CARTESIAN_POINT ( 'NONE',  ( 4.059375000614519280, 4.541064518000418104, -2.621784821874998173 ) ) ;
#7632=CARTESIAN_POINT ( 'NONE',  ( 16.08749999999999503, -2.886751345948129988, 4.999999999999997335 ) ) ;
#7633=CARTESIAN_POINT ( 'NONE',  ( 12.89062500061451821, -3.027376345333610441, -5.243569643749999898 ) ) ;
#7636=CARTESIAN_POINT ( 'NONE',  ( 18.45000000122903216, -2.886751345948129988, 4.999999999999997335 ) ) ;
#7639=CARTESIAN_POINT ( 'NONE',  ( 6.478125000614516793, -4.541064518000419881, 2.621784821874995952 ) ) ;
#7640=CARTESIAN_POINT ( 'NONE',  ( 25.32187500061451857, 3.027376345333611329, 5.243569643749999010 ) ) ;
#7641=CARTESIAN_POINT ( 'NONE',  ( 2.121784821875001281, 18.65937500061451715, 33.67503911421598417 ) ) ;
#7642=CARTESIAN_POINT ( 'NONE',  ( 25.54687500061451644, -3.027376345333610441, -5.243569643749999898 ) ) ;
#7643=CARTESIAN_POINT ( 'NONE',  ( 8.137500000000002842, -2.886751345948125991, -5.000000000000000000 ) ) ;
#7644=CARTESIAN_POINT ( 'NONE',  ( -1.999999999999997113, 14.33750000122903323, 33.46410161513775705 ) ) ;
#7645=CARTESIAN_POINT ( 'NONE',  ( 14.87812500061451537, 4.541064518000418104, 2.621784821874999949 ) ) ;
#7646=CARTESIAN_POINT ( 'NONE',  ( 5.775000001229033231, 2.886751345948126879, 4.999999999999999112 ) ) ;
#7647=CARTESIAN_POINT ( 'NONE',  ( 12.15937500061451892, 4.541064518000418104, -2.621784821874998173 ) ) ;
#7649=VERTEX_POINT ( 'NONE', #504 ) ;
#7650=AXIS2_PLACEMENT_3D ( 'NONE', #65481, #59561, #60656 ) ;
#7651=CARTESIAN_POINT ( 'NONE',  ( 12.77812500061451750, -4.541064518000419881, 2.621784821874995952 ) ) ;
#7653=CARTESIAN_POINT ( 'NONE',  ( 24.37500000122903288, -5.773502691896255534, -1.060575238724906372E-15 ) ) ;
#7654=CARTESIAN_POINT ( 'NONE',  ( 12.68437500061451573, 4.541064518000418104, 2.621784821874999949 ) ) ;
#7655=CARTESIAN_POINT ( 'NONE',  ( 15.25312500061451715, 4.541064518000418104, -2.621784821874998173 ) ) ;
#7656=CARTESIAN_POINT ( 'NONE',  ( 26.28750000122903430, 6.123233995736764310E-16, -4.999999999999998224 ) ) ;
#7657=CARTESIAN_POINT ( 'NONE',  ( 24.87187500061451573, 3.027376345333611329, 5.243569643749999010 ) ) ;
#7659=CARTESIAN_POINT ( 'NONE',  ( -1.394453263437886604E-15, 19.66249999999999787, 33.99999999999999289 ) ) ;
#7660=CARTESIAN_POINT ( 'NONE',  ( -2.121784821874999949, 17.98437500061451999, -33.67503911421598417 ) ) ;
#7661=CARTESIAN_POINT ( 'NONE',  ( 16.62187500061451573, 3.027376345333613106, -5.243569643749998122 ) ) ;
#7662=CARTESIAN_POINT ( 'NONE',  ( 17.88750000122903216, 4.330127018922191873, 2.499999999999999556 ) ) ;
#7663=( BOUNDED_CURVE ( )  B_SPLINE_CURVE ( 2, ( #56473, #4781, #62375, #15845, #33209, #33568, #44314 ),
 .UNSPECIFIED., .F., .F. ) 
 B_SPLINE_CURVE_WITH_KNOTS ( ( 3, 2, 2, 3 ),
 ( 0.4583333333333332593, 0.4611111111111111382, 0.4638888888888889062, 0.4666666666666667296 ),
 .UNSPECIFIED. ) 
 CURVE ( )  GEOMETRIC_REPRESENTATION_ITEM ( )  RATIONAL_B_SPLINE_CURVE ( ( 1.000000000000002665, 0.8660254037844360431, 1.000000000000000000, 0.8660254037844387076, 1.000000000000000000, 0.8660254037844360431, 1.000000000000002665 ) ) 
 REPRESENTATION_ITEM ( '' )  );
#7664=CARTESIAN_POINT ( 'NONE',  ( 12.75937500061451857, 0.000000000000000000, 5.243569643749999010 ) ) ;
#7665=CARTESIAN_POINT ( 'NONE',  ( 4.243569643749999898, 19.09062500061451573, -27.54997392385601529 ) ) ;
#7666=CARTESIAN_POINT ( 'NONE',  ( 19.46250000122903145, -4.330127018922190985, -2.500000000000001332 ) ) ;
#7667=CARTESIAN_POINT ( 'NONE',  ( 12.51562500061451821, 3.027376345333613106, -5.243569643749998122 ) ) ;
#7668=ORIENTED_EDGE ( 'NONE', *, *, #35039, .T. ) ;
#7669=ORIENTED_EDGE ( 'NONE', *, *, #37449, .F. ) ;
#7671=CARTESIAN_POINT ( 'NONE',  ( 17.66249999999999787, 2.886751345948129099, -4.999999999999998224 ) ) ;
#7672=CARTESIAN_POINT ( 'NONE',  ( 27.41250000000000142, -5.773502691896255534, -1.060575238724906372E-15 ) ) ;
#7673=CARTESIAN_POINT ( 'NONE',  ( 13.58437500061451786, 4.541064518000418104, 2.621784821874999949 ) ) ;
#7674=CARTESIAN_POINT ( 'NONE',  ( 30.00000000000000000, 0.000000000000000000, 0.000000000000000000 ) ) ;
#7675=ADVANCED_FACE ( 'NONE', ( #34464 ), #48223, .T. ) ;
#7676=CARTESIAN_POINT ( 'NONE',  ( 13.46250000122903323, 0.000000000000000000, 4.999999999999998224 ) ) ;
#7677=CARTESIAN_POINT ( 'NONE',  ( 21.48750000122903003, 4.330127018922191873, 2.499999999999999556 ) ) ;
#7678=CARTESIAN_POINT ( 'NONE',  ( 18.10312500061451502, 0.000000000000000000, 5.243569643749999010 ) ) ;
#7679=CARTESIAN_POINT ( 'NONE',  ( 23.01562500061451644, 3.027376345333611329, 5.243569643749999010 ) ) ;
#7680=CARTESIAN_POINT ( 'NONE',  ( 29.66250000122903074, 0.000000000000000000, 4.999999999999998224 ) ) ;
#7681=CARTESIAN_POINT ( 'NONE',  ( 28.68749999999999645, -2.886751345948129988, 4.999999999999997335 ) ) ;
#7682=CYLINDRICAL_SURFACE ( 'NONE', #45433, 4.999999999999998224 ) ;
#7683=( BOUNDED_CURVE ( )  B_SPLINE_CURVE ( 2, ( #66036, #15414, #42415, #19862, #9524, #70848, #64935 ),
 .UNSPECIFIED., .F., .F. ) 
 B_SPLINE_CURVE_WITH_KNOTS ( ( 3, 2, 2, 3 ),
 ( 0.9000000000000001332, 0.9027777777777779011, 0.9055555555555556690, 0.9083333333333334370 ),
 .UNSPECIFIED. ) 
 CURVE ( )  GEOMETRIC_REPRESENTATION_ITEM ( )  RATIONAL_B_SPLINE_CURVE ( ( 0.9999999999999946709, 0.8660254037844440367, 1.000000000000000000, 0.8660254037844387076, 1.000000000000000000, 0.8660254037844333785, 1.000000000000005329 ) ) 
 REPRESENTATION_ITEM ( '' )  );
#7685=CARTESIAN_POINT ( 'NONE',  ( 2.000000000000001332, 9.912500001229034297, -26.53589838486224650 ) ) ;
#7686=CARTESIAN_POINT ( 'NONE',  ( -4.243569643749999898, 16.22187500061452070, -32.45002607614398471 ) ) ;
#7687=CARTESIAN_POINT ( 'NONE',  ( 3.975000001229033852, 2.886751345948126879, 4.999999999999999112 ) ) ;
#7688=CARTESIAN_POINT ( 'NONE',  ( 7.012500000000001066, 2.886751345948126879, 4.999999999999999112 ) ) ;
#7690=CARTESIAN_POINT ( 'NONE',  ( 10.32187500061451679, 3.027376345333613106, -5.243569643749998122 ) ) ;
#7691=CARTESIAN_POINT ( 'NONE',  ( 27.29062500061451502, -3.027376345333610441, -5.243569643749999898 ) ) ;
#7693=CARTESIAN_POINT ( 'NONE',  ( -3.980704297455869511, 9.178376072143947795, -34.50551769337345576 ) ) ;
#7694=AXIS2_PLACEMENT_3D ( 'NONE', #19530, #8460, #48727 ) ;
#7696=CARTESIAN_POINT ( 'NONE',  ( 8.559375000614515727, 4.541064518000418104, -2.621784821874998173 ) ) ;
#7697=CARTESIAN_POINT ( 'NONE',  ( 11.78437500061451892, 4.541064518000418104, 2.621784821874999949 ) ) ;
#7698=CARTESIAN_POINT ( 'NONE',  ( 7.425000000000000711, 4.330127018922191873, 2.499999999999999556 ) ) ;
#7699=CARTESIAN_POINT ( 'NONE',  ( -3.000416591977282496E-16, 14.74062500061459424, 25.09994784771203058 ) ) ;
#7700=EDGE_CURVE ( 'NONE', #30519, #66542, #33133, .T. ) ;
#7702=CARTESIAN_POINT ( 'NONE',  ( 7.612500000000000711, -5.773502691896255534, -1.060575238724906372E-15 ) ) ;
#7705=B_SPLINE_CURVE_WITH_KNOTS ( 'NONE', 3,
 ( #54802, #15997, #59965, #54442, #65886, #16359, #26736, #61433, #15626, #4208 ),
 .UNSPECIFIED., .F., .F.,
 ( 4, 3, 3, 4 ),
 ( 1.799357552115988686E-16, 0.0001572276214405268226, 0.0003144552949517756741, 0.0005183884262692322036 ),
 .UNSPECIFIED. ) ;
#7706=CARTESIAN_POINT ( 'NONE',  ( 21.40312500061451573, -4.541064518000417216, -2.621784821875001281 ) ) ;
#7707=CARTESIAN_POINT ( 'NONE',  ( 12.51562500061451821, 3.027376345333613106, -5.243569643749998122 ) ) ;
#7709=CARTESIAN_POINT ( 'NONE',  ( 10.32187500061451679, 3.027376345333613106, -5.243569643749998122 ) ) ;
#7710=CARTESIAN_POINT ( 'NONE',  ( 25.87500000000000000, 4.330127018922191873, 2.499999999999999556 ) ) ;
#7711=CARTESIAN_POINT ( 'NONE',  ( 22.91250000122903430, 0.000000000000000000, 4.999999999999998224 ) ) ;
#7712=CARTESIAN_POINT ( 'NONE',  ( 17.17500000000000071, 6.123233995736764310E-16, -4.999999999999998224 ) ) ;
#7714=CARTESIAN_POINT ( 'NONE',  ( 12.08437500061451608, 6.421520780324663323E-16, -5.243569643749999010 ) ) ;
#7715=CARTESIAN_POINT ( 'NONE',  ( 25.58437500061451431, 6.421520780324663323E-16, -5.243569643749999010 ) ) ;
#7717=CARTESIAN_POINT ( 'NONE',  ( 24.45000000122903572, -2.886751345948109559, -5.000000000000028422 ) ) ;
#7718=CARTESIAN_POINT ( 'NONE',  ( 20.89687500061452141, -3.027376345333614438, 5.243569643749998122 ) ) ;
#7719=CARTESIAN_POINT ( 'NONE',  ( 11.44687500061451857, -3.027376345333614438, 5.243569643749998122 ) ) ;
#7721=CARTESIAN_POINT ( 'NONE',  ( 23.28750000000000142, -2.886751345948129988, 4.999999999999997335 ) ) ;
#7723=CARTESIAN_POINT ( 'NONE',  ( -2.121784821874999949, 12.58437500061451786, -33.67503911421598417 ) ) ;
#7725=CARTESIAN_POINT ( 'NONE',  ( 14.27812500061451573, 6.421520780324663323E-16, -5.243569643749999010 ) ) ;
#7726=CARTESIAN_POINT ( 'NONE',  ( 5.662500000000000533, 2.886751345948126879, 4.999999999999999112 ) ) ;
#7728=CARTESIAN_POINT ( 'NONE',  ( -3.999999999999999112, 13.21250000000000213, -32.30940107675850470 ) ) ;
#7729=CARTESIAN_POINT ( 'NONE',  ( 13.95000000000000107, -4.330127018922190985, -2.500000000000001332 ) ) ;
#7730=CARTESIAN_POINT ( 'NONE',  ( -2.121784821874999949, 10.72812500061451679, 26.32496088578401938 ) ) ;
#7731=CARTESIAN_POINT ( 'NONE',  ( 14.17500000122903536, 2.886751345948129099, -4.999999999999998224 ) ) ;
#7732=CARTESIAN_POINT ( 'NONE',  ( 25.92187500061451999, -6.054752690667223547, -1.112240025338166033E-15 ) ) ;
#7734=CARTESIAN_POINT ( 'NONE',  ( 19.00312500061451715, 0.000000000000000000, 5.243569643749999010 ) ) ;
#7735=CARTESIAN_POINT ( 'NONE',  ( 4.490625000614516971, 6.054752690667223547, 3.707466751127219781E-16 ) ) ;
#7736=CARTESIAN_POINT ( 'NONE',  ( 19.09687500061451360, -3.027376345333614438, 5.243569643749998122 ) ) ;
#7737=CARTESIAN_POINT ( 'NONE',  ( 3.562500000000000444, -5.773502691896255534, -1.060575238724906372E-15 ) ) ;
#7738=CARTESIAN_POINT ( 'NONE',  ( 8.278125000614515727, -4.541064518000419881, 2.621784821874995952 ) ) ;
#7739=CARTESIAN_POINT ( 'NONE',  ( 20.72812500061451502, 4.541064518000418104, 2.621784821874999949 ) ) ;
#7740=CARTESIAN_POINT ( 'NONE',  ( 4.243569643749999898, 14.17812500061451608, 30.00000000000000000 ) ) ;
#7741=CARTESIAN_POINT ( 'NONE',  ( 19.80000000122903359, -2.886751345948129988, 4.999999999999997335 ) ) ;
#7743=CARTESIAN_POINT ( 'NONE',  ( 9.215625000614515727, -6.054752690667223547, -1.112240025338166033E-15 ) ) ;
#7744=CARTESIAN_POINT ( 'NONE',  ( 4.284375000614518925, -4.541064518000419881, 2.621784821874995952 ) ) ;
#7745=CARTESIAN_POINT ( 'NONE',  ( 3.421875000614516882, -6.054752690667223547, -1.112240025338166033E-15 ) ) ;
#7746=CARTESIAN_POINT ( 'NONE',  ( 23.74687500061451573, -3.027376345333610441, -5.243569643749999898 ) ) ;
#7747=CARTESIAN_POINT ( 'NONE',  ( 14.16562500061451679, -6.054752690667223547, -1.112240025338166033E-15 ) ) ;
#7748=CARTESIAN_POINT ( 'NONE',  ( 24.03750000122903430, 6.123233995736764310E-16, -4.999999999999998224 ) ) ;
#7749=CARTESIAN_POINT ( 'NONE',  ( 26.01562500061451289, 3.027376345333613106, -5.243569643749998122 ) ) ;
#7750=CARTESIAN_POINT ( 'NONE',  ( 19.09687500061451360, -3.027376345333614438, 5.243569643749998122 ) ) ;
#7751=CARTESIAN_POINT ( 'NONE',  ( 14.65312500061451573, -4.541064518000417216, -2.621784821875001281 ) ) ;
#7752=CARTESIAN_POINT ( 'NONE',  ( 2.121784821875001281, 17.30937500061451573, 33.67503911421598417 ) ) ;
#7754=CARTESIAN_POINT ( 'NONE',  ( 20.12812500061451715, 6.421520780324663323E-16, -5.243569643749999010 ) ) ;
#7755=CARTESIAN_POINT ( 'NONE',  ( 3.337500001229034563, 6.123233995736764310E-16, -4.999999999999998224 ) ) ;
#7756=ORIENTED_EDGE ( 'NONE', *, *, #41935, .T. ) ;
#7757=CARTESIAN_POINT ( 'NONE',  ( 24.48749999999999716, 5.773502691896255534, 3.535250795749688894E-16 ) ) ;
#7758=CARTESIAN_POINT ( 'NONE',  ( -3.999999999999997335, 11.48750000000000071, -27.69059892324149175 ) ) ;
#7760=CARTESIAN_POINT ( 'NONE',  ( 26.09062500061451573, 6.054752690667223547, 3.707466751127219781E-16 ) ) ;
#7761=CARTESIAN_POINT ( 'NONE',  ( 6.665625000614515905, 3.027376345333613106, -5.243569643749998122 ) ) ;
#7762=CARTESIAN_POINT ( 'NONE',  ( 18.90000000122902790, -2.886751345948129988, 4.999999999999997335 ) ) ;
#7763=CARTESIAN_POINT ( 'NONE',  ( 24.74062500061451786, 6.054752690667223547, 3.707466751127219781E-16 ) ) ;
#7764=CARTESIAN_POINT ( 'NONE',  ( 24.18750000000000355, -2.886751345948129988, 4.999999999999997335 ) ) ;
#7765=CARTESIAN_POINT ( 'NONE',  ( -2.000000000000000000, 16.43750000122903643, -33.46410161513775705 ) ) ;
#7766=EDGE_CURVE ( 'NONE', #62319, #29541, #14716, .T. ) ;
#7767=CARTESIAN_POINT ( 'NONE',  ( 25.38750000122903216, 6.123233995736764310E-16, -4.999999999999998224 ) ) ;
#7768=CARTESIAN_POINT ( 'NONE',  ( 10.79062500061451679, 6.054752690667223547, 3.707466751127219781E-16 ) ) ;
#7769=ORIENTED_EDGE ( 'NONE', *, *, #36745, .F. ) ;
#7771=CARTESIAN_POINT ( 'NONE',  ( 25.30312500061451431, 0.000000000000000000, 5.243569643749999010 ) ) ;
#7772=CARTESIAN_POINT ( 'NONE',  ( 8.503125000614515372, 4.541064518000418104, -2.621784821874998173 ) ) ;
#7774=AXIS2_PLACEMENT_3D ( 'NONE', #45881, #34419, #57672 ) ;
#7775=CARTESIAN_POINT ( 'NONE',  ( 4.640625000614518214, -3.027376345333614438, 5.243569643749998122 ) ) ;
#7777=CARTESIAN_POINT ( 'NONE',  ( 14.13750000000000107, 5.773502691896255534, 3.535250795749688894E-16 ) ) ;
#7778=CARTESIAN_POINT ( 'NONE',  ( 14.78437500061451715, 6.421520780324663323E-16, -5.243569643749999010 ) ) ;
#7779=CARTESIAN_POINT ( 'NONE',  ( 8.512500001229033941, 0.000000000000000000, 4.999999999999998224 ) ) ;
#7780=CARTESIAN_POINT ( 'NONE',  ( 18.19687500061451502, -3.027376345333614438, 5.243569643749998122 ) ) ;
#7782=CARTESIAN_POINT ( 'NONE',  ( 8.521875000614516082, 3.027376345333613106, -5.243569643749998122 ) ) ;
#7783=CARTESIAN_POINT ( 'NONE',  ( 4.243569643749999898, 11.44062500061451715, -27.54997392385601529 ) ) ;
#7784=CARTESIAN_POINT ( 'NONE',  ( 30.00000000000000000, 0.000000000000000000, 0.000000000000000000 ) ) ;
#7786=DIRECTION ( 'NONE',  ( 0.000000000000000000, 0.000000000000000000, 1.000000000000000000 ) ) ;
#7787=CARTESIAN_POINT ( 'NONE',  ( 23.42812500061451786, 4.541064518000418104, 2.621784821874999949 ) ) ;
#7788=CARTESIAN_POINT ( 'NONE',  ( 26.63437500061451857, 4.541064518000418104, 2.621784821874999949 ) ) ;
#7789=CARTESIAN_POINT ( 'NONE',  ( 29.59687500061451715, -3.027376345333610441, -5.243569643749999898 ) ) ;
#7790=CARTESIAN_POINT ( 'NONE',  ( 21.78750000000000142, 5.773502691896255534, 3.535250795749688894E-16 ) ) ;
#7792=CARTESIAN_POINT ( 'NONE',  ( 6.253125000614517148, 4.541064518000418104, -2.621784821874998173 ) ) ;
#7794=CARTESIAN_POINT ( 'NONE',  ( 15.64687500061451608, -3.027376345333610441, -5.243569643749999898 ) ) ;
#7796=AXIS2_PLACEMENT_3D ( 'NONE', #48682, #60844, #54223 ) ;
#7797=CARTESIAN_POINT ( 'NONE',  ( 4.040625000614517681, 6.054752690667223547, 3.707466751127219781E-16 ) ) ;
#7798=CARTESIAN_POINT ( 'NONE',  ( 7.584375000614516082, 6.421520780324663323E-16, -5.243569643749999010 ) ) ;
#7799=ORIENTED_EDGE ( 'NONE', *, *, #16945, .F. ) ;
#7800=CARTESIAN_POINT ( 'NONE',  ( 18.30937500061451928, -4.541064518000417216, -2.621784821875001281 ) ) ;
#7802=CARTESIAN_POINT ( 'NONE',  ( 27.44999999999999929, -4.330127018922190985, -2.500000000000001332 ) ) ;
#7803=CARTESIAN_POINT ( 'NONE',  ( 27.53437500061451360, 4.541064518000418104, 2.621784821874999949 ) ) ;
#7804=CYLINDRICAL_SURFACE ( 'NONE', #28972, 4.999999999999998224 ) ;
#7807=CARTESIAN_POINT ( 'NONE',  ( 11.51250000000000107, 2.886751345948126879, 4.999999999999999112 ) ) ;
#7809=CARTESIAN_POINT ( 'NONE',  ( 22.30312500061451431, -4.541064518000417216, -2.621784821875001281 ) ) ;
#7810=CARTESIAN_POINT ( 'NONE',  ( 12.56250000000000178, -5.773502691896255534, -1.060575238724906372E-15 ) ) ;
#7811=( BOUNDED_CURVE ( )  B_SPLINE_CURVE ( 2, ( #20303, #20672, #48407, #36577, #49498, #53569, #9241, #8871, #65750 ),
 .UNSPECIFIED., .F., .T. ) 
 B_SPLINE_CURVE_WITH_KNOTS ( ( 3, 2, 2, 2, 3 ),
 ( 0.5978260869565217295, 0.6014492753623188470, 0.6086956521739130821, 0.6159420289855072062, 0.6195652173913043237 ),
 .UNSPECIFIED. ) 
 CURVE ( )  GEOMETRIC_REPRESENTATION_ITEM ( )  RATIONAL_B_SPLINE_CURVE ( ( 0.9330127018922194093, 0.9330127018922194093, 1.000000000000000000, 0.8660254037844387076, 1.000000000000000000, 0.8660254037844387076, 1.000000000000000000, 0.9330127018922194093, 0.9330127018922194093 ) ) 
 REPRESENTATION_ITEM ( '' )  );
#7812=CARTESIAN_POINT ( 'NONE',  ( 8.325000001229033941, 2.886751345948129099, -4.999999999999998224 ) ) ;
#7813=CARTESIAN_POINT ( 'NONE',  ( 6.403125000614517504, 0.000000000000000000, 5.243569643749999010 ) ) ;
#7814=CARTESIAN_POINT ( 'NONE',  ( 21.86250000000000071, 2.886751345948126879, 4.999999999999999112 ) ) ;
#7815=CARTESIAN_POINT ( 'NONE',  ( 20.16562500061451146, 3.027376345333613106, -5.243569643749998122 ) ) ;
#7817=CARTESIAN_POINT ( 'NONE',  ( 25.80000000122903714, -2.886751345948125991, -5.000000000000000000 ) ) ;
#7819=CARTESIAN_POINT ( 'NONE',  ( 4.275000000000001243, 4.330127018922191873, 2.499999999999999556 ) ) ;
#7821=CARTESIAN_POINT ( 'NONE',  ( 18.66562500061451146, -6.054752690667223547, -1.112240025338166033E-15 ) ) ;
#7822=CARTESIAN_POINT ( 'NONE',  ( 25.82812500061451644, -4.541064518000419881, 2.621784821874995952 ) ) ;
#7823=CARTESIAN_POINT ( 'NONE',  ( 26.52187500061451431, 3.027376345333613106, -5.243569643749998122 ) ) ;
#7824=CARTESIAN_POINT ( 'NONE',  ( 14.57812500061451644, -4.541064518000419881, 2.621784821874995952 ) ) ;
#7825=CARTESIAN_POINT ( 'NONE',  ( 29.76562500061451644, 3.027376345333611329, 5.243569643749999010 ) ) ;
#7826=CARTESIAN_POINT ( 'NONE',  ( 8.465625000614515727, 3.027376345333613106, -5.243569643749998122 ) ) ;
#7828=CARTESIAN_POINT ( 'NONE',  ( 27.18750000122903288, 6.123233995736764310E-16, -4.999999999999998224 ) ) ;
#7830=CARTESIAN_POINT ( 'NONE',  ( 17.05312500061451786, 4.541064518000418104, -2.621784821874998173 ) ) ;
#7831=CARTESIAN_POINT ( 'NONE',  ( 29.29687500061451644, 6.054752690667223547, 3.707466751127219781E-16 ) ) ;
#7832=CARTESIAN_POINT ( 'NONE',  ( 9.534375000614517148, 4.541064518000418104, 2.621784821874999949 ) ) ;
#7833=CARTESIAN_POINT ( 'NONE',  ( 8.934375000614517504, 6.421520780324663323E-16, -5.243569643749999010 ) ) ;
#7834=CARTESIAN_POINT ( 'NONE',  ( 18.23437500061451999, -4.541064518000419881, 2.621784821874995952 ) ) ;
#7835=ORIENTED_EDGE ( 'NONE', *, *, #561, .T. ) ;
#7836=CARTESIAN_POINT ( 'NONE',  ( 29.43750000000000000, 5.773502691896255534, 3.535250795749688401E-16 ) ) ;
#7837=CARTESIAN_POINT ( 'NONE',  ( 20.54062500061451502, -3.027376345333610441, -5.243569643749999898 ) ) ;
#7838=CARTESIAN_POINT ( 'NONE',  ( 16.92187500061451999, -6.054752690667223547, -1.112240025338166033E-15 ) ) ;
#7839=CARTESIAN_POINT ( 'NONE',  ( 22.37812500061451360, 6.421520780324663323E-16, -5.243569643749999010 ) ) ;
#7840=CARTESIAN_POINT ( 'NONE',  ( -2.828200636599751609E-16, 15.38750000000000284, 25.38119784648299770 ) ) ;
#7841=CARTESIAN_POINT ( 'NONE',  ( 28.60312500061451502, -4.541064518000417216, -2.621784821875001281 ) ) ;
#7842=CARTESIAN_POINT ( 'NONE',  ( 9.375000001229036428, 2.886751345948126879, 4.999999999999999112 ) ) ;
#7844=CARTESIAN_POINT ( 'NONE',  ( 3.712500001229034563, -4.330127018922190985, -2.500000000000001332 ) ) ;
#7845=CARTESIAN_POINT ( 'NONE',  ( -3.999999999999999556, 18.61250000000000426, -32.30940107675850470 ) ) ;
#7846=CIRCLE ( 'NONE', #49146, 4.000000000000000000 ) ;
#7847=CARTESIAN_POINT ( 'NONE',  ( 23.92500000122903359, -5.773502691896255534, -1.060575238724906372E-15 ) ) ;
#7849=CARTESIAN_POINT ( 'NONE',  ( 10.35937500061451644, 4.541064518000418104, -2.621784821874998173 ) ) ;
#7850=CARTESIAN_POINT ( 'NONE',  ( 24.56250000000000355, 2.886751345948093572, 5.000000000000056843 ) ) ;
#7851=CARTESIAN_POINT ( 'NONE',  ( 13.97812500061451679, 4.541064518000418104, 2.621784821874999949 ) ) ;
#7852=CARTESIAN_POINT ( 'NONE',  ( 10.62187500061451928, -6.054752690667223547, -1.112240025338166033E-15 ) ) ;
#7853=CARTESIAN_POINT ( 'NONE',  ( 3.028125000614518392, 6.421520780324663323E-16, -5.243569643749999010 ) ) ;
#7854=CARTESIAN_POINT ( 'NONE',  ( 18.00937500061451502, 4.541064518000418104, -2.621784821874998173 ) ) ;
#7855=CARTESIAN_POINT ( 'NONE',  ( 8.071875000614518569, 3.027376345333613106, -5.243569643749998122 ) ) ;
#7857=CARTESIAN_POINT ( 'NONE',  ( 6.890625000614516438, -3.027376345333614438, 5.243569643749998122 ) ) ;
#7858=CARTESIAN_POINT ( 'NONE',  ( 18.70312500061451644, -4.541064518000417216, -2.621784821875001281 ) ) ;
#7860=CARTESIAN_POINT ( 'NONE',  ( 15.66562500061451857, 3.027376345333613106, -5.243569643749998122 ) ) ;
#7861=AXIS2_PLACEMENT_3D ( 'NONE', #13302, #57290, #8142 ) ;
#7862=CARTESIAN_POINT ( 'NONE',  ( 11.09062500061451573, -3.027376345333610441, -5.243569643749999898 ) ) ;
#7864=CARTESIAN_POINT ( 'NONE',  ( 10.49999999999999822, 4.330127018922192761, -2.499999999999997780 ) ) ;
#7865=CARTESIAN_POINT ( 'NONE',  ( 6.337500001229033231, -4.330127018922194537, 2.499999999999995559 ) ) ;
#7866=( BOUNDED_CURVE ( )  B_SPLINE_CURVE ( 2, ( #44920, #72986, #27926, #17184, #16453, #11657, #23087 ),
 .UNSPECIFIED., .F., .F. ) 
 B_SPLINE_CURVE_WITH_KNOTS ( ( 3, 2, 2, 3 ),
 ( 0.6250000000000000000, 0.6277777777777777679, 0.6305555555555555358, 0.6333333333333333037 ),
 .UNSPECIFIED. ) 
 CURVE ( )  GEOMETRIC_REPRESENTATION_ITEM ( )  RATIONAL_B_SPLINE_CURVE ( ( 1.000000000000000000, 0.8660254037844387076, 1.000000000000000000, 0.8660254037844387076, 1.000000000000000000, 0.8660254037844387076, 1.000000000000000000 ) ) 
 REPRESENTATION_ITEM ( '' )  );
#7867=CARTESIAN_POINT ( 'NONE',  ( 13.99687500061451928, 6.054752690667223547, 3.707466751127219781E-16 ) ) ;
#7868=CARTESIAN_POINT ( 'NONE',  ( 17.17500000122903359, -5.773502691896255534, -1.060575238724906372E-15 ) ) ;
#7870=CARTESIAN_POINT ( 'NONE',  ( 4.243569643749999898, 18.22812500061451502, -30.00000000000000000 ) ) ;
#7871=CARTESIAN_POINT ( 'NONE',  ( 16.20000000122903216, -2.886751345948130876, 4.999999999999996447 ) ) ;
#7875=CARTESIAN_POINT ( 'NONE',  ( 13.79999999999999893, 0.000000000000000000, 4.999999999999998224 ) ) ;
#7876=CARTESIAN_POINT ( 'NONE',  ( 18.57187500061451857, 3.027376345333611329, 5.243569643749999010 ) ) ;
#7877=CARTESIAN_POINT ( 'NONE',  ( 28.04999999999999716, 4.330127018922192761, -2.499999999999997780 ) ) ;
#7878=EDGE_CURVE ( 'NONE', #36605, #18379, #58554, .T. ) ;
#7879=CARTESIAN_POINT ( 'NONE',  ( 15.14062500061451644, -3.027376345333610441, -5.243569643749999898 ) ) ;
#7881=CARTESIAN_POINT ( 'NONE',  ( 22.95937500061451431, 4.541064518000418104, -2.621784821874998173 ) ) ;
#7883=CARTESIAN_POINT ( 'NONE',  ( 10.41562500061451679, 3.027376345333611329, 5.243569643749999010 ) ) ;
#7884=CARTESIAN_POINT ( 'NONE',  ( 14.63437500061451679, -4.541064518000419881, 2.621784821874995952 ) ) ;
#7885=EDGE_LOOP ( 'NONE', ( #27374, #49428, #51883 ) ) ;
#7886=CARTESIAN_POINT ( 'NONE',  ( 25.47187500061451715, -6.054752690667223547, -1.112240025338166033E-15 ) ) ;
#7887=CARTESIAN_POINT ( 'NONE',  ( 26.31562500061451715, -6.054752690667223547, -1.112240025338166033E-15 ) ) ;
#7888=CARTESIAN_POINT ( 'NONE',  ( 17.57812500061451644, 4.541064518000418104, 2.621784821874999949 ) ) ;
#7889=CARTESIAN_POINT ( 'NONE',  ( 29.76562500061451644, 3.027376345333611329, 5.243569643749999010 ) ) ;
#7891=CARTESIAN_POINT ( 'NONE',  ( 10.49999999999999822, 4.330127018922192761, -2.499999999999997780 ) ) ;
#7892=CARTESIAN_POINT ( 'NONE',  ( 20.55000000122903359, 5.773502691896255534, 3.535250795749688894E-16 ) ) ;
#7895=CARTESIAN_POINT ( 'NONE',  ( 16.98750000000000426, -2.886751345948129988, 4.999999999999997335 ) ) ;
#7896=CARTESIAN_POINT ( 'NONE',  ( 22.46250000000000213, -5.773502691896255534, -1.060575238724906372E-15 ) ) ;
#7897=CARTESIAN_POINT ( 'NONE',  ( 19.62187500061451573, -6.054752690667223547, -1.112240025338166033E-15 ) ) ;
#7898=CARTESIAN_POINT ( 'NONE',  ( 13.71562500061451750, -6.054752690667223547, -1.112240025338166033E-15 ) ) ;
#7900=CARTESIAN_POINT ( 'NONE',  ( 2.000000000000001332, 18.46250000122903501, -26.53589838486224650 ) ) ;
#7901=CARTESIAN_POINT ( 'NONE',  ( 6.628125000614517148, 6.421520780324663323E-16, -5.243569643749999010 ) ) ;
#7902=CARTESIAN_POINT ( 'NONE',  ( 13.23750000000000071, 5.773502691896255534, 3.535250795749688894E-16 ) ) ;
#7904=CARTESIAN_POINT ( 'NONE',  ( -2.121784821874996840, 15.82812500061451644, 33.67503911421598417 ) ) ;
#7905=CARTESIAN_POINT ( 'NONE',  ( 27.77812500061451573, 6.421520780324663323E-16, -5.243569643749999010 ) ) ;
#7908=CARTESIAN_POINT ( 'NONE',  ( 23.48437500061451644, 4.541064518000418104, 2.621784821874999949 ) ) ;
#7909=ORIENTED_EDGE ( 'NONE', *, *, #36869, .T. ) ;
#7910=CARTESIAN_POINT ( 'NONE',  ( 21.02812500061451573, 6.421520780324663323E-16, -5.243569643749999010 ) ) ;
#7911=CARTESIAN_POINT ( 'NONE',  ( 23.93437500061451573, 4.541064518000418104, 2.621784821874999949 ) ) ;
#7913=CARTESIAN_POINT ( 'NONE',  ( 4.243569643749999898, 16.42812500061459247, -30.00000000000000000 ) ) ;
#7914=CARTESIAN_POINT ( 'NONE',  ( 5.503125000614516260, 0.000000000000000000, 5.243569643749999010 ) ) ;
#7916=CARTESIAN_POINT ( 'NONE',  ( 24.40312500061451573, 0.000000000000000000, 5.243569643749999010 ) ) ;
#7919=CARTESIAN_POINT ( 'NONE',  ( 17.78437500061451715, -4.541064518000419881, 2.621784821874995952 ) ) ;
#7920=CARTESIAN_POINT ( 'NONE',  ( 24.87187500061451573, 3.027376345333611329, 5.243569643749999010 ) ) ;
#7921=CARTESIAN_POINT ( 'NONE',  ( 9.001249775931846008E-16, 15.02187500061451608, 34.90005215228797653 ) ) ;
#7922=CARTESIAN_POINT ( 'NONE',  ( 6.740625000614516082, 6.054752690667223547, 3.707466751127219781E-16 ) ) ;
#7923=DIRECTION ( 'NONE',  ( 0.000000000000000000, 0.000000000000000000, 1.000000000000000000 ) ) ;
#7924=CARTESIAN_POINT ( 'NONE',  ( 28.82812500061451644, 4.541064518000418104, 2.621784821874999949 ) ) ;
#7925=DIRECTION ( 'NONE',  ( -0.000000000000000000, -1.000000000000000000, -0.000000000000000000 ) ) ;
#7926=CARTESIAN_POINT ( 'NONE',  ( 5.240625000614516971, -3.027376345333610441, -5.243569643749999898 ) ) ;
#7927=CARTESIAN_POINT ( 'NONE',  ( 10.69687500061451679, -3.027376345333610441, -5.243569643749999898 ) ) ;
#7928=CARTESIAN_POINT ( 'NONE',  ( 17.43750000122903288, 4.330127018922191873, 2.499999999999999556 ) ) ;
#7929=CARTESIAN_POINT ( 'NONE',  ( 29.09062500061451573, -3.027376345333610441, -5.243569643749999898 ) ) ;
#7930=CARTESIAN_POINT ( 'NONE',  ( 4.115625000614516082, 3.027376345333611329, 5.243569643749999010 ) ) ;
#7933=CARTESIAN_POINT ( 'NONE',  ( 16.88437500061451502, -4.541064518000419881, 2.621784821874995952 ) ) ;
#7936=CARTESIAN_POINT ( 'NONE',  ( 23.09062500061451573, -3.027376345333614438, 5.243569643749998122 ) ) ;
#7937=CARTESIAN_POINT ( 'NONE',  ( 9.590625000614517504, -3.027376345333614438, 5.243569643749998122 ) ) ;
#7938=CARTESIAN_POINT ( 'NONE',  ( 25.88437500061451502, -4.541064518000419881, 2.621784821874995952 ) ) ;
#7939=CARTESIAN_POINT ( 'NONE',  ( 10.41562500061451679, 3.027376345333611329, 5.243569643749999010 ) ) ;
#7940=CARTESIAN_POINT ( 'NONE',  ( 20.43749999999999645, 5.773502691896255534, 3.535250795749688401E-16 ) ) ;
#7941=CARTESIAN_POINT ( 'NONE',  ( 9.487500001229033586, -4.330127018922194537, 2.499999999999995559 ) ) ;
#7942=EDGE_CURVE ( 'NONE', #65447, #18641, #562, .T. ) ;
#7943=CARTESIAN_POINT ( 'NONE',  ( 25.75312500061451715, 0.000000000000000000, 5.243569643749999010 ) ) ;
#7944=B_SPLINE_CURVE_WITH_KNOTS ( 'NONE', 3,
 ( #71028, #14138, #8603, #42588, #59562, #63651, #3066, #69573, #35940, #25596 ),
 .UNSPECIFIED., .F., .F.,
 ( 4, 3, 3, 4 ),
 ( 3.881383207071731149E-17, 7.861371910493904853E-05, 0.0001572271722546394167, 0.0002869866954567743423 ),
 .UNSPECIFIED. ) ;
#7945=CARTESIAN_POINT ( 'NONE',  ( -1.473773219643375931, 9.816672173337614993, -34.04916878720240447 ) ) ;
#7946=CARTESIAN_POINT ( 'NONE',  ( 12.15000000122903501, -2.886751345948129988, 4.999999999999997335 ) ) ;
#7947=CARTESIAN_POINT ( 'NONE',  ( 22.11562500061451786, 3.027376345333611329, 5.243569643749999010 ) ) ;
#7948=CARTESIAN_POINT ( 'NONE',  ( 18.44062500061451715, 6.054752690667223547, 3.707466751127219781E-16 ) ) ;
#7949=CARTESIAN_POINT ( 'NONE',  ( 5.596875000614516260, -3.027376345333614438, 5.243569643749998122 ) ) ;
#7950=CARTESIAN_POINT ( 'NONE',  ( 17.73750000000000071, 5.773502691896255534, 3.535250795749688894E-16 ) ) ;
#7951=CARTESIAN_POINT ( 'NONE',  ( 12.90000000122903145, 5.773502691896255534, 3.535250795749688894E-16 ) ) ;
#7952=VECTOR ( 'NONE', #48065, 1000.000000000000000 ) ;
#7953=CARTESIAN_POINT ( 'NONE',  ( 10.75312500061451715, 4.541064518000418104, -2.621784821874998173 ) ) ;
#7954=CARTESIAN_POINT ( 'NONE',  ( 13.30312500061451786, -4.541064518000417216, -2.621784821875001281 ) ) ;
#7955=CARTESIAN_POINT ( 'NONE',  ( 23.02500000122903145, -5.773502691896255534, -1.060575238724906372E-15 ) ) ;
#7956=CARTESIAN_POINT ( 'NONE',  ( 20.89687500061452141, -3.027376345333614438, 5.243569643749998122 ) ) ;
#7957=CARTESIAN_POINT ( 'NONE',  ( 21.57187500061451502, 3.027376345333613106, -5.243569643749998122 ) ) ;
#7960=CARTESIAN_POINT ( 'NONE',  ( 7.087500001229034119, 4.330127018922191873, 2.499999999999999556 ) ) ;
#7961=CARTESIAN_POINT ( 'NONE',  ( 7.584375000614516082, 6.421520780324663323E-16, -5.243569643749999010 ) ) ;
#7962=CARTESIAN_POINT ( 'NONE',  ( 25.69687500061451502, 6.054752690667223547, 3.707466751127219781E-16 ) ) ;
#7963=LINE ( 'NONE', #53027, #43346 ) ;
#7964=CARTESIAN_POINT ( 'NONE',  ( 20.80312500061451431, 0.000000000000000000, 5.243569643749999010 ) ) ;
#7965=CARTESIAN_POINT ( 'NONE',  ( 25.80937500061451928, 0.000000000000000000, 5.243569643749999010 ) ) ;
#7969=CARTESIAN_POINT ( 'NONE',  ( 6.084375000614518747, -4.541064518000419881, 2.621784821874995952 ) ) ;
#7970=CARTESIAN_POINT ( 'NONE',  ( 17.16562500061451502, 3.027376345333611329, 5.243569643749999010 ) ) ;
#7971=EDGE_LOOP ( 'NONE', ( #22359, #27390, #564, #39187 ) ) ;
#7972=CARTESIAN_POINT ( 'NONE',  ( 25.08749999999999858, -2.886751345948130876, 4.999999999999996447 ) ) ;
#7973=CARTESIAN_POINT ( 'NONE',  ( 26.09062500061451573, 6.054752690667223547, 3.707466751127219781E-16 ) ) ;
#7974=CARTESIAN_POINT ( 'NONE',  ( 3.609375000614516882, 4.541064518000418104, -2.621784821874998173 ) ) ;
#7975=CARTESIAN_POINT ( 'NONE',  ( 10.08750000122903323, 6.123233995736764310E-16, -4.999999999999998224 ) ) ;
#7976=CARTESIAN_POINT ( 'NONE',  ( 3.701615863222355252, 3.361311753005875591, -3.762615002631680916 ) ) ;
#7977=CARTESIAN_POINT ( 'NONE',  ( 17.02499999999999858, -4.330127018922194537, 2.499999999999995559 ) ) ;
#7978=CARTESIAN_POINT ( 'NONE',  ( 20.84062500061451573, -3.027376345333614438, 5.243569643749998122 ) ) ;
#7979=ORIENTED_EDGE ( 'NONE', *, *, #1706, .F. ) ;
#7980=CARTESIAN_POINT ( 'NONE',  ( 25.38749999999999929, 5.773502691896255534, 3.535250795749688894E-16 ) ) ;
#7981=ADVANCED_FACE ( 'NONE', ( #34253 ), #39826, .F. ) ;
#7982=CARTESIAN_POINT ( 'NONE',  ( 26.78437500061451360, -4.541064518000419881, 2.621784821874995952 ) ) ;
#7984=DIRECTION ( 'NONE',  ( -1.000000000000000000, -0.000000000000000000, -0.000000000000000000 ) ) ;
#7985=CARTESIAN_POINT ( 'NONE',  ( 12.92812500061451786, 6.421520780324663323E-16, -5.243569643749999010 ) ) ;
#7986=CARTESIAN_POINT ( 'NONE',  ( 6.103125000614515905, -4.541064518000417216, -2.621784821875001281 ) ) ;
#7988=CARTESIAN_POINT ( 'NONE',  ( 28.71562500061451573, 3.027376345333613106, -5.243569643749998122 ) ) ;
#7989=CARTESIAN_POINT ( 'NONE',  ( 16.38750000122903216, 6.123233995736764310E-16, -4.999999999999998224 ) ) ;
#7990=CARTESIAN_POINT ( 'NONE',  ( 19.23749999999999716, -2.886751345948129988, 4.999999999999997335 ) ) ;
#7991=CARTESIAN_POINT ( 'NONE',  ( 26.92499999999999716, -4.330127018922194537, 2.499999999999995559 ) ) ;
#7992=CARTESIAN_POINT ( 'NONE',  ( 3.309375000614518836, 0.000000000000000000, 5.243569643749999010 ) ) ;
#7993=CARTESIAN_POINT ( 'NONE',  ( 9.009375000614518569, 4.541064518000418104, -2.621784821874998173 ) ) ;
#7994=CARTESIAN_POINT ( 'NONE',  ( 19.39687500061451786, 6.054752690667223547, 3.707466751127219781E-16 ) ) ;
#7995=CARTESIAN_POINT ( 'NONE',  ( 19.87500000122903288, -5.773502691896255534, -1.060575238724906372E-15 ) ) ;
#7996=ORIENTED_EDGE ( 'NONE', *, *, #42304, .T. ) ;
#7997=CARTESIAN_POINT ( 'NONE',  ( 28.97812500061451502, -4.541064518000419881, 2.621784821874995952 ) ) ;
#7998=CARTESIAN_POINT ( 'NONE',  ( 3.225000000000002309, 6.123233995736764310E-16, -4.999999999999998224 ) ) ;
#7999=CARTESIAN_POINT ( 'NONE',  ( 5.109375000614518214, 0.000000000000000000, 5.243569643749999010 ) ) ;
#8000=VECTOR ( 'NONE', #51648, 1000.000000000000000 ) ;
#8001=CARTESIAN_POINT ( 'NONE',  ( 16.46249999999999503, 2.886751345948126879, 4.999999999999999112 ) ) ;
#8002=CARTESIAN_POINT ( 'NONE',  ( 13.90312500061451750, 4.541064518000418104, -2.621784821874998173 ) ) ;
#8005=CARTESIAN_POINT ( 'NONE',  ( 18.33750000122903501, 4.330127018922191873, 2.499999999999999556 ) ) ;
#8008=CARTESIAN_POINT ( 'NONE',  ( 8.015625000614518214, 3.027376345333613106, -5.243569643749998122 ) ) ;
#8009=CARTESIAN_POINT ( 'NONE',  ( 23.63437500061451502, -4.541064518000419881, 2.621784821874995952 ) ) ;
#8010=CARTESIAN_POINT ( 'NONE',  ( -4.243569643749999898, 18.92187500061451644, 27.54997392385601529 ) ) ;
#8011=CARTESIAN_POINT ( 'NONE',  ( 23.67187500061451999, -6.054752690667223547, -1.112240025338166033E-15 ) ) ;
#8012=CARTESIAN_POINT ( 'NONE',  ( 7.124999999999999112, -4.330127018922194537, 2.499999999999995559 ) ) ;
#8013=CARTESIAN_POINT ( 'NONE',  ( -2.828200636599751609E-16, 14.15000000122903501, 25.38119784648299770 ) ) ;
#8014=CARTESIAN_POINT ( 'NONE',  ( 13.67812500061451786, -4.541064518000419881, 2.621784821874995952 ) ) ;
#8015=CARTESIAN_POINT ( 'NONE',  ( 7.125000001229033764, 2.886751345948126879, 4.999999999999999112 ) ) ;
#8016=CARTESIAN_POINT ( 'NONE',  ( 10.77187500061451786, 3.027376345333613106, -5.243569643749998122 ) ) ;
#8019=CARTESIAN_POINT ( 'NONE',  ( 13.11562500061451786, 3.027376345333611329, 5.243569643749999010 ) ) ;
#8021=CARTESIAN_POINT ( 'NONE',  ( 24.78750000122903074, -4.330127018922194537, 2.499999999999995559 ) ) ;
#8022=CARTESIAN_POINT ( 'NONE',  ( 10.84687500061451892, 6.054752690667223547, 3.707466751127219781E-16 ) ) ;
#8023=CARTESIAN_POINT ( 'NONE',  ( 15.40312500061451573, 0.000000000000000000, 5.243569643749999010 ) ) ;
#8025=CARTESIAN_POINT ( 'NONE',  ( 22.88437500061451857, 6.421520780324663323E-16, -5.243569643749999010 ) ) ;
#8026=CARTESIAN_POINT ( 'NONE',  ( 24.26250000122903216, 0.000000000000000000, 4.999999999999998224 ) ) ;
#8027=CARTESIAN_POINT ( 'NONE',  ( 9.975000000000001421, 6.123233995736764310E-16, -4.999999999999998224 ) ) ;
#8029=CARTESIAN_POINT ( 'NONE',  ( -3.000416591977282496E-16, 15.24687500061451928, -34.90005215228797653 ) ) ;
#8031=CARTESIAN_POINT ( 'NONE',  ( 16.58437500061451786, 6.421520780324663323E-16, -5.243569643749999010 ) ) ;
#8032=CARTESIAN_POINT ( 'NONE',  ( 17.40000000122903145, 5.773502691896255534, 3.535250795749688894E-16 ) ) ;
#8033=CARTESIAN_POINT ( 'NONE',  ( 13.02187500061451608, 3.027376345333613106, -5.243569643749998122 ) ) ;
#8034=CARTESIAN_POINT ( 'NONE',  ( -2.121784821874996840, 10.93437500061451928, 33.67503911421598417 ) ) ;
#8035=CARTESIAN_POINT ( 'NONE',  ( 19.83750000122903145, -4.330127018922194537, 2.499999999999995559 ) ) ;
#8036=CARTESIAN_POINT ( 'NONE',  ( 12.96562500061451750, 3.027376345333613106, -5.243569643749998122 ) ) ;
#8037=ORIENTED_EDGE ( 'NONE', *, *, #53290, .F. ) ;
#8039=CARTESIAN_POINT ( 'NONE',  ( 16.98750000000000426, -2.886751345948129988, 4.999999999999997335 ) ) ;
#8040=CARTESIAN_POINT ( 'NONE',  ( 17.88749999999999574, -2.886751345948063374, 5.000000000000112799 ) ) ;
#8041=CARTESIAN_POINT ( 'NONE',  ( 11.44687500061451679, -3.027376345333614438, 5.243569643749998122 ) ) ;
#8043=CARTESIAN_POINT ( 'NONE',  ( 12.56250000122903465, 0.000000000000000000, 4.999999999999998224 ) ) ;
#8044=CARTESIAN_POINT ( 'NONE',  ( 22.08750000122903501, -4.330127018922194537, 2.499999999999995559 ) ) ;
#8045=CARTESIAN_POINT ( 'NONE',  ( 16.60312500061451857, 4.541064518000418104, -2.621784821874998173 ) ) ;
#8047=CARTESIAN_POINT ( 'NONE',  ( 21.29062500061451502, -3.027376345333614438, 5.243569643749998122 ) ) ;
#8048=CARTESIAN_POINT ( 'NONE',  ( 27.30000000122903359, 5.773502691896255534, 3.535250795749688894E-16 ) ) ;
#8049=CARTESIAN_POINT ( 'NONE',  ( 26.43750000000000000, -2.886751345948129988, 4.999999999999997335 ) ) ;
#8052=CARTESIAN_POINT ( 'NONE',  ( 28.32187500061451502, 3.027376345333613106, -5.243569643749998122 ) ) ;
#8053=CARTESIAN_POINT ( 'NONE',  ( 2.000000000000001332, 14.30000000000000071, -26.53589838486224650 ) ) ;
#8054=CARTESIAN_POINT ( 'NONE',  ( 2.121784821875001281, 16.85937500061451999, -26.32496088578401938 ) ) ;
#8055=CARTESIAN_POINT ( 'NONE',  ( 2.662500001229036073, 0.000000000000000000, 4.999999999999998224 ) ) ;
#8056=CARTESIAN_POINT ( 'NONE',  ( 5.887500000000000178, -2.886751345948125991, -5.000000000000000000 ) ) ;
#8058=CARTESIAN_POINT ( 'NONE',  ( 10.77187500061451786, 3.027376345333613106, -5.243569643749998122 ) ) ;
#8059=CARTESIAN_POINT ( 'NONE',  ( 28.67812500061451431, 6.421520780324663323E-16, -5.243569643749999010 ) ) ;
#8061=CARTESIAN_POINT ( 'NONE',  ( -0.8062380997993551235, 9.975217491784283297, -35.95894923966248058 ) ) ;
#8063=CARTESIAN_POINT ( 'NONE',  ( 6.796875000614516438, 6.054752690667223547, 3.707466751127219781E-16 ) ) ;
#8064=CARTESIAN_POINT ( 'NONE',  ( 11.29687500061451644, 6.054752690667223547, 3.707466751127219781E-16 ) ) ;
#8065=CARTESIAN_POINT ( 'NONE',  ( 4.462500000000001243, -5.773502691896255534, -1.060575238724906372E-15 ) ) ;
#8066=( BOUNDED_CURVE ( )  B_SPLINE_CURVE ( 2, ( #55159, #48519, #37428, #54064, #42969, #48885, #25613 ),
 .UNSPECIFIED., .F., .F. ) 
 B_SPLINE_CURVE_WITH_KNOTS ( ( 3, 2, 2, 3 ),
 ( 0.08333333333333328707, 0.08611111111111106886, 0.08888888888888883677, 0.09166666666666660468 ),
 .UNSPECIFIED. ) 
 CURVE ( )  GEOMETRIC_REPRESENTATION_ITEM ( )  RATIONAL_B_SPLINE_CURVE ( ( 1.000000000000001998, 0.8660254037844365982, 1.000000000000000000, 0.8660254037844387076, 1.000000000000000000, 0.8660254037844413721, 0.9999999999999973355 ) ) 
 REPRESENTATION_ITEM ( '' )  );
#8068=CARTESIAN_POINT ( 'NONE',  ( 4.243569643749999898, 15.49062500061459779, 32.45002607614398471 ) ) ;
#8070=CARTESIAN_POINT ( 'NONE',  ( 5.362500000000003375, -5.773502691896255534, -1.060575238724906372E-15 ) ) ;
#8072=CARTESIAN_POINT ( 'NONE',  ( 19.67812500061451786, 6.421520780324663323E-16, -5.243569643749999010 ) ) ;
#8073=CARTESIAN_POINT ( 'NONE',  ( 13.82812500061451466, 6.421520780324663323E-16, -5.243569643749999010 ) ) ;
#8075=CARTESIAN_POINT ( 'NONE',  ( 9.946875000614516793, 6.054752690667223547, 3.707466751127219781E-16 ) ) ;
#8076=CARTESIAN_POINT ( 'NONE',  ( 25.61250000000000071, -5.773502691896255534, -1.060575238724906372E-15 ) ) ;
#8077=CARTESIAN_POINT ( 'NONE',  ( 23.73750000122903359, 4.330127018922191873, 2.499999999999999556 ) ) ;
#8078=CARTESIAN_POINT ( 'NONE',  ( 16.94999999999999929, 0.000000000000000000, 4.999999999999998224 ) ) ;
#8079=CARTESIAN_POINT ( 'NONE',  ( 9.271875000614516082, -6.054752690667223547, -1.112240025338166033E-15 ) ) ;
#8080=CARTESIAN_POINT ( 'NONE',  ( 25.43437500061451573, -4.541064518000419881, 2.621784821874995952 ) ) ;
#8083=CARTESIAN_POINT ( 'NONE',  ( -3.999999999999999112, 12.91250000122903430, -30.00000000000000000 ) ) ;
#8084=CARTESIAN_POINT ( 'NONE',  ( 20.44687500061451857, -3.027376345333614438, 5.243569643749998122 ) ) ;
#8085=CARTESIAN_POINT ( 'NONE',  ( 10.95937500061451964, 0.000000000000000000, 5.243569643749999010 ) ) ;
#8087=CARTESIAN_POINT ( 'NONE',  ( 22.64999999999999858, 4.330127018922192761, -2.499999999999997780 ) ) ;
#8089=CARTESIAN_POINT ( 'NONE',  ( 9.001249775931846008E-16, 12.32187500061451857, -25.09994784771203058 ) ) ;
#8091=CARTESIAN_POINT ( 'NONE',  ( 15.96562500061451573, -6.054752690667223547, -1.112240025338166033E-15 ) ) ;
#8092=CARTESIAN_POINT ( 'NONE',  ( 5.137500000000000178, 5.773502691896255534, 3.535250795749688894E-16 ) ) ;
#8094=DIRECTION ( 'NONE',  ( -0.000000000000000000, -1.000000000000000000, -0.000000000000000000 ) ) ;
#8095=CARTESIAN_POINT ( 'NONE',  ( 13.68750000000000178, 5.773502691896255534, 3.535250795749688894E-16 ) ) ;
#8096=CARTESIAN_POINT ( 'NONE',  ( 3.999999999999998668, 19.47500000122903430, 27.69059892324149175 ) ) ;
#8097=CARTESIAN_POINT ( 'NONE',  ( 13.57500000122903572, -5.773502691896255534, -1.060575238724906372E-15 ) ) ;
#8099=CARTESIAN_POINT ( 'NONE',  ( 24.45937500061451786, 0.000000000000000000, 5.243569643749999010 ) ) ;
#8101=ORIENTED_EDGE ( 'NONE', *, *, #39400, .T. ) ;
#8102=CARTESIAN_POINT ( 'NONE',  ( 18.40312500061451573, 4.541064518000418104, -2.621784821874998173 ) ) ;
#8103=CARTESIAN_POINT ( 'NONE',  ( 3.515625000614516882, 3.027376345333613106, -5.243569643749998122 ) ) ;
#8104=CARTESIAN_POINT ( 'NONE',  ( 18.83437500061451431, 6.421520780324663323E-16, -5.243569643749999010 ) ) ;
#8105=CARTESIAN_POINT ( 'NONE',  ( 29.67187500061451644, 3.027376345333613106, -5.243569643749998122 ) ) ;
#8106=CARTESIAN_POINT ( 'NONE',  ( 4.453125000614517326, 4.541064518000418104, -2.621784821874998173 ) ) ;
#8107=CARTESIAN_POINT ( 'NONE',  ( 22.00312500061451360, 4.541064518000418104, -2.621784821874998173 ) ) ;
#8108=CARTESIAN_POINT ( 'NONE',  ( -2.121784821874999949, 15.67812500061451608, 26.32496088578401938 ) ) ;
#8109=CARTESIAN_POINT ( 'NONE',  ( 19.91250000122903074, -4.330127018922190985, -2.500000000000001332 ) ) ;
#8111=CARTESIAN_POINT ( 'NONE',  ( 5.953125000614519102, 0.000000000000000000, 5.243569643749999010 ) ) ;
#8112=EDGE_CURVE ( 'NONE', #37474, #43716, #20388, .T. ) ;
#8113=CARTESIAN_POINT ( 'NONE',  ( 13.72500000000000142, 4.330127018922191873, 2.499999999999999556 ) ) ;
#8114=CARTESIAN_POINT ( 'NONE',  ( 2.934375000614518392, -4.541064518000419881, 2.621784821874995952 ) ) ;
#8115=CARTESIAN_POINT ( 'NONE',  ( 21.79687500061451644, -3.027376345333614438, 5.243569643749998122 ) ) ;
#8116=CARTESIAN_POINT ( 'NONE',  ( 15.14062500061451644, -3.027376345333610441, -5.243569643749999898 ) ) ;
#8117=CARTESIAN_POINT ( 'NONE',  ( 25.83750000122903501, 6.123233995736764310E-16, -4.999999999999998224 ) ) ;
#8118=CARTESIAN_POINT ( 'NONE',  ( 26.57812500061451644, 4.541064518000418104, 2.621784821874999949 ) ) ;
#8119=CARTESIAN_POINT ( 'NONE',  ( 19.77187500061451786, 3.027376345333613106, -5.243569643749998122 ) ) ;
#8120=CARTESIAN_POINT ( 'NONE',  ( 14.95312500061451644, 0.000000000000000000, 5.243569643749999010 ) ) ;
#8121=CARTESIAN_POINT ( 'NONE',  ( 4.243569643749999898, 16.03437500061451715, 30.00000000000000000 ) ) ;
#8122=( BOUNDED_CURVE ( )  B_SPLINE_CURVE ( 2, ( #40385, #40754, #24828, #30012, #1961, #7125, #1234, #19273, #47016 ),
 .UNSPECIFIED., .F., .F. ) 
 B_SPLINE_CURVE_WITH_KNOTS ( ( 3, 2, 2, 2, 3 ),
 ( 0.9239130434782608647, 0.9275362318840579823, 0.9347826086956522174, 0.9420289855072463414, 0.9456521739130434590 ),
 .UNSPECIFIED. ) 
 CURVE ( )  GEOMETRIC_REPRESENTATION_ITEM ( )  RATIONAL_B_SPLINE_CURVE ( ( 0.9330127018922194093, 0.9330127018922194093, 1.000000000000000000, 0.8660254037844387076, 1.000000000000000000, 0.8660254037844387076, 1.000000000000000000, 0.9330127018922194093, 0.9330127018922194093 ) ) 
 REPRESENTATION_ITEM ( '' )  );
#8123=CARTESIAN_POINT ( 'NONE',  ( 19.86562500061451786, 3.027376345333611329, 5.243569643749999010 ) ) ;
#8124=CARTESIAN_POINT ( 'NONE',  ( 28.60312500061451502, -4.541064518000417216, -2.621784821875001281 ) ) ;
#8126=CARTESIAN_POINT ( 'NONE',  ( 25.16249999999999432, -5.773502691896255534, -1.060575238724906372E-15 ) ) ;
#8127=CARTESIAN_POINT ( 'NONE',  ( -2.000000000000000000, 10.47500000000000142, -33.46410161513775705 ) ) ;
#8129=CARTESIAN_POINT ( 'NONE',  ( 26.39062500061451644, -3.027376345333610441, -5.243569643749999898 ) ) ;
#8130=CARTESIAN_POINT ( 'NONE',  ( 7.078125000614516438, 6.421520780324663323E-16, -5.243569643749999010 ) ) ;
#8131=CARTESIAN_POINT ( 'NONE',  ( 20.77500000122903145, -5.773502691896255534, -1.060575238724906372E-15 ) ) ;
#8132=EDGE_CURVE ( 'NONE', #44451, #10990, #41847, .T. ) ;
#8133=CARTESIAN_POINT ( 'NONE',  ( 25.30312500061451431, 0.000000000000000000, 5.243569643749999010 ) ) ;
#8134=CARTESIAN_POINT ( 'NONE',  ( 24.60000000000000142, 0.000000000000000000, 4.999999999999998224 ) ) ;
#8135=CARTESIAN_POINT ( 'NONE',  ( 1.999999999999998668, 16.81250000122903643, -33.46410161513775705 ) ) ;
#8136=CARTESIAN_POINT ( 'NONE',  ( 28.90312500061451217, 0.000000000000000000, 5.243569643749999010 ) ) ;
#8137=CARTESIAN_POINT ( 'NONE',  ( 10.90312500061451928, 0.000000000000000000, 5.243569643749999010 ) ) ;
#8139=CARTESIAN_POINT ( 'NONE',  ( 24.59062500061451573, -3.027376345333610441, -5.243569643749999898 ) ) ;
#8140=CARTESIAN_POINT ( 'NONE',  ( 4.903125000614516615, 4.541064518000418104, -2.621784821874998173 ) ) ;
#8142=DIRECTION ( 'NONE',  ( 0.000000000000000000, 0.000000000000000000, -1.000000000000000000 ) ) ;
#8143=CARTESIAN_POINT ( 'NONE',  ( 12.22499999999999964, 6.123233995736764310E-16, -4.999999999999998224 ) ) ;
#8144=CARTESIAN_POINT ( 'NONE',  ( 13.43437500061451750, 6.421520780324663323E-16, -5.243569643749999010 ) ) ;
#8145=CARTESIAN_POINT ( 'NONE',  ( 10.01250000122903394, -4.330127018922190985, -2.500000000000001332 ) ) ;
#8146=CARTESIAN_POINT ( 'NONE',  ( 16.84687500061451715, -3.027376345333614438, 5.243569643749998122 ) ) ;
#8148=CARTESIAN_POINT ( 'NONE',  ( 7.809375000614519280, 0.000000000000000000, 5.243569643749999010 ) ) ;
#8149=CARTESIAN_POINT ( 'NONE',  ( 4.243569643749999898, 12.37812500061451715, -30.00000000000000000 ) ) ;
#8153=CARTESIAN_POINT ( 'NONE',  ( 25.45312500061451644, -4.541064518000417216, -2.621784821875001281 ) ) ;
#8155=CARTESIAN_POINT ( 'NONE',  ( 27.12187500061451573, 3.027376345333611329, 5.243569643749999010 ) ) ;
#8156=CARTESIAN_POINT ( 'NONE',  ( 28.09687500061451360, -3.027376345333614438, 5.243569643749998122 ) ) ;
#8157=CARTESIAN_POINT ( 'NONE',  ( 4.153125000614515727, 0.000000000000000000, 5.243569643749999010 ) ) ;
#8159=CARTESIAN_POINT ( 'NONE',  ( 16.95937500061451786, -4.541064518000417216, -2.621784821875001281 ) ) ;
#8161=CARTESIAN_POINT ( 'NONE',  ( 29.28750000122903074, -4.330127018922194537, 2.499999999999995559 ) ) ;
#8162=CARTESIAN_POINT ( 'NONE',  ( 7.809375000614519280, 0.000000000000000000, 5.243569643749999010 ) ) ;
#8163=CARTESIAN_POINT ( 'NONE',  ( 18.68437500061451928, -4.541064518000419881, 2.621784821874995952 ) ) ;
#8165=CARTESIAN_POINT ( 'NONE',  ( 26.13749999999999929, -2.886751345948125991, -5.000000000000000000 ) ) ;
#8166=CARTESIAN_POINT ( 'NONE',  ( 27.04687500061451644, 6.054752690667223547, 3.707466751127219781E-16 ) ) ;
#8167=CARTESIAN_POINT ( 'NONE',  ( 4.000000000000000000, 10.28750000000000142, -27.69059892324149885 ) ) ;
#8168=CARTESIAN_POINT ( 'NONE',  ( 29.92500000000000071, 4.330127018922191873, 2.499999999999999556 ) ) ;
#8169=ORIENTED_EDGE ( 'NONE', *, *, #30275, .T. ) ;
#8170=CARTESIAN_POINT ( 'NONE',  ( 7.425000000000000711, 4.330127018922191873, 2.499999999999999556 ) ) ;
#8172=CARTESIAN_POINT ( 'NONE',  ( 21.14062500061451289, 6.054752690667223547, 3.707466751127219781E-16 ) ) ;
#8173=CARTESIAN_POINT ( 'NONE',  ( 12.33750000000000036, 5.773502691896255534, 3.535250795749688894E-16 ) ) ;
#8174=CARTESIAN_POINT ( 'NONE',  ( 9.150000001229033231, -2.886751345948125991, -5.000000000000000000 ) ) ;
#8175=CARTESIAN_POINT ( 'NONE',  ( 5.840625000614516615, 6.054752690667223547, 3.707466751127219781E-16 ) ) ;
#8176=CARTESIAN_POINT ( 'NONE',  ( 21.33749999999999858, 5.773502691896255534, 3.535250795749688894E-16 ) ) ;
#8177=CARTESIAN_POINT ( 'NONE',  ( 18.36562500061451431, 3.027376345333613106, -5.243569643749998122 ) ) ;
#8178=CARTESIAN_POINT ( 'NONE',  ( 4.762500001229033941, 4.330127018922192761, -2.499999999999997780 ) ) ;
#8179=CARTESIAN_POINT ( 'NONE',  ( 25.83750000122903501, 6.123233995736764310E-16, -4.999999999999998224 ) ) ;
#8181=CARTESIAN_POINT ( 'NONE',  ( 3.900000000000000799, 0.000000000000000000, 4.999999999999998224 ) ) ;
#8183=CARTESIAN_POINT ( 'NONE',  ( 19.71562500061451928, 3.027376345333613106, -5.243569643749998122 ) ) ;
#8184=CARTESIAN_POINT ( 'NONE',  ( 26.72812500061451502, -4.541064518000419881, 2.621784821874995952 ) ) ;
#8185=CARTESIAN_POINT ( 'NONE',  ( 27.30937500061451573, -4.541064518000417216, -2.621784821875001281 ) ) ;
#8186=CARTESIAN_POINT ( 'NONE',  ( 9.862500000000000711, -5.773502691896255534, -1.060575238724906372E-15 ) ) ;
#8187=CARTESIAN_POINT ( 'NONE',  ( 13.56562500061451892, 3.027376345333611329, 5.243569643749999010 ) ) ;
#8188=CARTESIAN_POINT ( 'NONE',  ( 28.04062500061451502, -3.027376345333614438, 5.243569643749998122 ) ) ;
#8190=CARTESIAN_POINT ( 'NONE',  ( 10.15312500061451750, -4.541064518000417216, -2.621784821875001281 ) ) ;
#8192=CARTESIAN_POINT ( 'NONE',  ( 2.121784821874999061, 13.40937500061451892, 26.32496088578401583 ) ) ;
#8193=CARTESIAN_POINT ( 'NONE',  ( 26.92500000122903359, 2.886751345948126879, 4.999999999999999112 ) ) ;
#8195=CARTESIAN_POINT ( 'NONE',  ( 16.67812500061451786, 4.541064518000418104, 2.621784821874999949 ) ) ;
#8196=DIRECTION ( 'NONE',  ( -0.000000000000000000, -1.000000000000000000, -0.000000000000000000 ) ) ;
#8197=CARTESIAN_POINT ( 'NONE',  ( 10.05937500061451750, 0.000000000000000000, 5.243569643749999010 ) ) ;
#8198=CARTESIAN_POINT ( 'NONE',  ( 9.796875000614519990, -3.027376345333610441, -5.243569643749999898 ) ) ;
#8199=CARTESIAN_POINT ( 'NONE',  ( 18.38437500061451857, 6.421520780324663323E-16, -5.243569643749999010 ) ) ;
#8201=CARTESIAN_POINT ( 'NONE',  ( -0.8069677186600735519, 9.969399234781874952, 35.94888112490725263 ) ) ;
#8202=CARTESIAN_POINT ( 'NONE',  ( 21.06562500061451715, 3.027376345333613106, -5.243569643749998122 ) ) ;
#8203=CARTESIAN_POINT ( 'NONE',  ( 16.28437500061452070, 4.541064518000418104, 2.621784821874999949 ) ) ;
#8204=CARTESIAN_POINT ( 'NONE',  ( 22.56562500061451715, 3.027376345333611329, 5.243569643749999010 ) ) ;
#8205=CARTESIAN_POINT ( 'NONE',  ( 3.999999999999998668, 15.31250000000000000, 27.69059892324149175 ) ) ;
#8206=CARTESIAN_POINT ( 'NONE',  ( 27.85312500061451502, 4.541064518000418104, -2.621784821874998173 ) ) ;
#8207=CARTESIAN_POINT ( 'NONE',  ( 8.325000001229033941, 2.886751345948129099, -4.999999999999998224 ) ) ;
#8208=ORIENTED_EDGE ( 'NONE', *, *, #26740, .T. ) ;
#8209=CARTESIAN_POINT ( 'NONE',  ( 4.050000001229035362, -2.886751345948129988, 4.999999999999997335 ) ) ;
#8210=CARTESIAN_POINT ( 'NONE',  ( -2.828200636599751609E-16, 16.73750000000000071, -34.61880215351700230 ) ) ;
#8211=CARTESIAN_POINT ( 'NONE',  ( 24.30000000122903359, -2.886751345948129988, 4.999999999999997335 ) ) ;
#8213=CARTESIAN_POINT ( 'NONE',  ( 7.021875000614518747, -6.054752690667223547, -1.112240025338166033E-15 ) ) ;
#8214=CARTESIAN_POINT ( 'NONE',  ( 2.000000000000001332, 15.20000000000000107, 33.46410161513774995 ) ) ;
#8215=CARTESIAN_POINT ( 'NONE',  ( 15.89062500061451289, -3.027376345333614438, 5.243569643749998122 ) ) ;
#8216=CARTESIAN_POINT ( 'NONE',  ( 8.259375000614518569, 0.000000000000000000, 5.243569643749999010 ) ) ;
#8218=CARTESIAN_POINT ( 'NONE',  ( 27.71250000122903145, 4.330127018922192761, -2.499999999999997780 ) ) ;
#8219=CARTESIAN_POINT ( 'NONE',  ( 17.40937500061451715, -4.541064518000417216, -2.621784821875001281 ) ) ;
#8220=CARTESIAN_POINT ( 'NONE',  ( 5.371875000614516615, 3.027376345333613106, -5.243569643749998122 ) ) ;
#8222=CARTESIAN_POINT ( 'NONE',  ( 7.528125000614515727, 6.421520780324663323E-16, -5.243569643749999010 ) ) ;
#8223=CARTESIAN_POINT ( 'NONE',  ( 16.71562500061451573, 3.027376345333611329, 5.243569643749999010 ) ) ;
#8226=CARTESIAN_POINT ( 'NONE',  ( 13.26562500061451644, -6.054752690667223547, -1.112240025338166033E-15 ) ) ;
#8227=CARTESIAN_POINT ( 'NONE',  ( 6.450000001229034829, -2.886751345948125991, -5.000000000000000000 ) ) ;
#8228=CARTESIAN_POINT ( 'NONE',  ( 10.82812500061451644, 4.541064518000418104, 2.621784821874999949 ) ) ;
#8230=CARTESIAN_POINT ( 'NONE',  ( 10.27499999999999858, -4.330127018922194537, 2.499999999999995559 ) ) ;
#8231=CARTESIAN_POINT ( 'NONE',  ( 6.150000001229033231, 5.773502691896255534, 3.535250795749688894E-16 ) ) ;
#8232=CARTESIAN_POINT ( 'NONE',  ( 15.00937500061451679, 0.000000000000000000, 5.243569643749999010 ) ) ;
#8233=CARTESIAN_POINT ( 'NONE',  ( 15.11250000122903359, 4.330127018922192761, -2.499999999999997780 ) ) ;
#8235=CARTESIAN_POINT ( 'NONE',  ( -4.243569643749999898, 18.41562500061451857, -32.45002607614398471 ) ) ;
#8236=CARTESIAN_POINT ( 'NONE',  ( 30.00000000000000000, 0.000000000000000000, 4.999999999999998224 ) ) ;
#8239=CARTESIAN_POINT ( 'NONE',  ( 4.000000000000000000, 10.85000000122903430, -27.69059892324149885 ) ) ;
#8241=CARTESIAN_POINT ( 'NONE',  ( 16.73437500061451644, 4.541064518000418104, 2.621784821874999949 ) ) ;
#8242=( BOUNDED_CURVE ( )  B_SPLINE_CURVE ( 2, ( #30310, #52480, #68754, #70192, #46944, #69481, #18838 ),
 .UNSPECIFIED., .F., .F. ) 
 B_SPLINE_CURVE_WITH_KNOTS ( ( 3, 2, 2, 3 ),
 ( 0.6250000000000000000, 0.6277777777777777679, 0.6305555555555555358, 0.6333333333333333037 ),
 .UNSPECIFIED. ) 
 CURVE ( )  GEOMETRIC_REPRESENTATION_ITEM ( )  RATIONAL_B_SPLINE_CURVE ( ( 1.000000000000000000, 0.8660254037844387076, 1.000000000000000000, 0.8660254037844387076, 1.000000000000000000, 0.8660254037844387076, 1.000000000000000000 ) ) 
 REPRESENTATION_ITEM ( '' )  );
#8243=CARTESIAN_POINT ( 'NONE',  ( 29.84999999999999787, 4.330127018922192761, -2.499999999999997780 ) ) ;
#8244=CARTESIAN_POINT ( 'NONE',  ( 11.91562500061451857, -6.054752690667223547, -1.112240025338166033E-15 ) ) ;
#8246=CARTESIAN_POINT ( 'NONE',  ( 23.70937500061451786, -4.541064518000417216, -2.621784821875001281 ) ) ;
#8248=CARTESIAN_POINT ( 'NONE',  ( 9.590625000614517504, -3.027376345333614438, 5.243569643749998122 ) ) ;
#8249=CARTESIAN_POINT ( 'NONE',  ( 14.40937500061451715, 4.541064518000418104, -2.621784821874998173 ) ) ;
#8250=ORIENTED_EDGE ( 'NONE', *, *, #7387, .T. ) ;
#8251=CARTESIAN_POINT ( 'NONE',  ( 25.80937500061451928, 0.000000000000000000, 5.243569643749999010 ) ) ;
#8252=CARTESIAN_POINT ( 'NONE',  ( 28.22812500061451502, 6.421520780324663323E-16, -5.243569643749999010 ) ) ;
#8253=CARTESIAN_POINT ( 'NONE',  ( 17.87812500061451715, 6.421520780324663323E-16, -5.243569643749999010 ) ) ;
#8254=CARTESIAN_POINT ( 'NONE',  ( 28.37812500061451715, 4.541064518000418104, 2.621784821874999949 ) ) ;
#8255=CARTESIAN_POINT ( 'NONE',  ( 4.844509297411972781, 1.237226603047926421, -5.095516945469514170 ) ) ;
#8256=CARTESIAN_POINT ( 'NONE',  ( 7.050000000000000711, 0.000000000000000000, 4.999999999999998224 ) ) ;
#8257=CARTESIAN_POINT ( 'NONE',  ( 19.80000000122903359, -2.886751345948129988, 4.999999999999997335 ) ) ;
#8260=ORIENTED_EDGE ( 'NONE', *, *, #52094, .F. ) ;
#8261=CARTESIAN_POINT ( 'NONE',  ( 14.02499999999999858, 6.123233995736764310E-16, -4.999999999999998224 ) ) ;
#8262=CARTESIAN_POINT ( 'NONE',  ( 19.76250000000000639, -5.773502691896255534, -1.060575238724906372E-15 ) ) ;
#8263=CARTESIAN_POINT ( 'NONE',  ( 16.35937500061451644, 0.000000000000000000, 5.243569643749999010 ) ) ;
#8264=CARTESIAN_POINT ( 'NONE',  ( 12.81562500061451537, -6.054752690667223547, -1.112240025338166033E-15 ) ) ;
#8267=CARTESIAN_POINT ( 'NONE',  ( 5.803125000614517859, 4.541064518000418104, -2.621784821874998173 ) ) ;
#8268=CARTESIAN_POINT ( 'NONE',  ( 10.23750000000000071, -2.886751345948130876, 4.999999999999996447 ) ) ;
#8269=CARTESIAN_POINT ( 'NONE',  ( 11.77500000000000036, 6.123233995736764310E-16, -4.999999999999998224 ) ) ;
#8271=CARTESIAN_POINT ( 'NONE',  ( 4.243569643749999010, 14.66562500061451857, 27.54997392385601174 ) ) ;
#8272=CARTESIAN_POINT ( 'NONE',  ( 26.99062500061451431, 6.054752690667223547, 3.707466751127219781E-16 ) ) ;
#8275=CARTESIAN_POINT ( 'NONE',  ( 23.82187500061451502, 3.027376345333613106, -5.243569643749998122 ) ) ;
#8276=CARTESIAN_POINT ( 'NONE',  ( 21.59062500061451928, 6.054752690667223547, 3.707466751127219781E-16 ) ) ;
#8277=CARTESIAN_POINT ( 'NONE',  ( -2.121784821874999949, 15.22812500061459318, -33.67503911421598417 ) ) ;
#8278=CARTESIAN_POINT ( 'NONE',  ( 23.47500000122903430, -5.773502691896255534, -1.060575238724906372E-15 ) ) ;
#8279=CARTESIAN_POINT ( 'NONE',  ( 6.853125000614516793, 0.000000000000000000, 5.243569643749999010 ) ) ;
#8281=CARTESIAN_POINT ( 'NONE',  ( 23.54062500061451502, -3.027376345333614438, 5.243569643749998122 ) ) ;
#8284=CARTESIAN_POINT ( 'NONE',  ( 16.09687500061452070, -3.027376345333610441, -5.243569643749999898 ) ) ;
#8285=CARTESIAN_POINT ( 'NONE',  ( 24.90937500061451715, 0.000000000000000000, 5.243569643749999010 ) ) ;
#8286=CARTESIAN_POINT ( 'NONE',  ( -4.243569643749998122, 14.04687500061451999, 32.45002607614398471 ) ) ;
#8287=CARTESIAN_POINT ( 'NONE',  ( 5.503125000614516260, 0.000000000000000000, 5.243569643749999010 ) ) ;
#8288=CARTESIAN_POINT ( 'NONE',  ( 28.26562500061451289, 3.027376345333613106, -5.243569643749998122 ) ) ;
#8289=CARTESIAN_POINT ( 'NONE',  ( 29.61562500061451431, 3.027376345333613106, -5.243569643749998122 ) ) ;
#8291=CARTESIAN_POINT ( 'NONE',  ( 1.009598436472904703, 9.950840295117078682, -35.91779160164027473 ) ) ;
#8292=CARTESIAN_POINT ( 'NONE',  ( 3.403125000614518836, -4.541064518000417216, -2.621784821875001281 ) ) ;
#8293=CARTESIAN_POINT ( 'NONE',  ( 6.984375000614516438, -4.541064518000419881, 2.621784821874995952 ) ) ;
#8295=CARTESIAN_POINT ( 'NONE',  ( 16.35000000122903430, -2.886751345948125991, -5.000000000000000000 ) ) ;
#8296=CARTESIAN_POINT ( 'NONE',  ( 4.096875000614518925, 6.054752690667223547, 3.707466751127219781E-16 ) ) ;
#8297=CARTESIAN_POINT ( 'NONE',  ( 5.165625000614518569, -6.054752690667223547, -1.112240025338166033E-15 ) ) ;
#8300=CARTESIAN_POINT ( 'NONE',  ( 13.99687500061451928, 6.054752690667223547, 3.707466751127219781E-16 ) ) ;
#8301=CARTESIAN_POINT ( 'NONE',  ( -3.999999999999999112, 10.51250000000000107, 27.69059892324149885 ) ) ;
#8303=CARTESIAN_POINT ( 'NONE',  ( 23.20312500061451644, -4.541064518000417216, -2.621784821875001281 ) ) ;
#8304=CARTESIAN_POINT ( 'NONE',  ( 7.753125000614518036, 0.000000000000000000, 5.243569643749999010 ) ) ;
#8305=CARTESIAN_POINT ( 'NONE',  ( 23.48437500061451644, 4.541064518000418104, 2.621784821874999949 ) ) ;
#8306=CARTESIAN_POINT ( 'NONE',  ( 8.615625000614517859, 3.027376345333611329, 5.243569643749999010 ) ) ;
#8307=CARTESIAN_POINT ( 'NONE',  ( 10.27500000122903323, 2.886751345948126879, 4.999999999999999112 ) ) ;
#8309=CARTESIAN_POINT ( 'NONE',  ( 25.52812500061451573, 6.421520780324663323E-16, -5.243569643749999010 ) ) ;
#8311=CARTESIAN_POINT ( 'NONE',  ( -4.243569643749999898, 10.80312500061451786, -30.00000000000000000 ) ) ;
#8312=CARTESIAN_POINT ( 'NONE',  ( 10.57500000122903572, 2.886751345948129099, -4.999999999999998224 ) ) ;
#8313=CARTESIAN_POINT ( 'NONE',  ( 22.67812500061451431, -4.541064518000419881, 2.621784821874995952 ) ) ;
#8314=CARTESIAN_POINT ( 'NONE',  ( 17.87812500061451715, 6.421520780324663323E-16, -5.243569643749999010 ) ) ;
#8316=CARTESIAN_POINT ( 'NONE',  ( 19.34999999999999787, -4.330127018922190985, -2.500000000000001332 ) ) ;
#8317=CARTESIAN_POINT ( 'NONE',  ( 14.47500000122903430, -5.773502691896255534, -1.060575238724906372E-15 ) ) ;
#8318=CARTESIAN_POINT ( 'NONE',  ( 10.41562500061451679, 3.027376345333611329, 5.243569643749999010 ) ) ;
#8319=CARTESIAN_POINT ( 'NONE',  ( 12.89062500061451821, -3.027376345333610441, -5.243569643749999898 ) ) ;
#8320=CARTESIAN_POINT ( 'NONE',  ( 22.57500000122903572, -5.773502691896255534, -1.060575238724906372E-15 ) ) ;
#8321=CARTESIAN_POINT ( 'NONE',  ( 20.70937500061451786, 4.541064518000418104, -2.621784821874998173 ) ) ;
#8322=CARTESIAN_POINT ( 'NONE',  ( 20.70937500061451786, 4.541064518000418104, -2.621784821874998173 ) ) ;
#8323=CARTESIAN_POINT ( 'NONE',  ( 7.537500001229033408, 4.330127018922191873, 2.499999999999999556 ) ) ;
#8324=CARTESIAN_POINT ( 'NONE',  ( 7.171875000614517326, 3.027376345333613106, -5.243569643749998122 ) ) ;
#8325=CARTESIAN_POINT ( 'NONE',  ( 22.84687500061451715, -3.027376345333610441, -5.243569643749999898 ) ) ;
#8326=CARTESIAN_POINT ( 'NONE',  ( 4.271383450090062261, -2.599258264455263312, -4.416836559537284046 ) ) ;
#8327=CARTESIAN_POINT ( 'NONE',  ( 20.57812500061451644, 6.421520780324663323E-16, -5.243569643749999010 ) ) ;
#8328=CARTESIAN_POINT ( 'NONE',  ( 25.39687500061451431, -3.027376345333614438, 5.243569643749998122 ) ) ;
#8330=CARTESIAN_POINT ( 'NONE',  ( 3.421875000614516882, -6.054752690667223547, -1.112240025338166033E-15 ) ) ;
#8331=CARTESIAN_POINT ( 'NONE',  ( 2.000000000000001332, 15.65000000000000036, 33.46410161513774995 ) ) ;
#8332=CARTESIAN_POINT ( 'NONE',  ( 5.259375000614518569, -4.541064518000417216, -2.621784821875001281 ) ) ;
#8333=CARTESIAN_POINT ( 'NONE',  ( 17.35312500061451502, -4.541064518000417216, -2.621784821875001281 ) ) ;
#8334=ORIENTED_EDGE ( 'NONE', *, *, #63321, .T. ) ;
#8335=DIRECTION ( 'NONE',  ( -0.000000000000000000, -1.000000000000000000, -0.000000000000000000 ) ) ;
#8336=CARTESIAN_POINT ( 'NONE',  ( 25.97812500061451502, 6.421520780324663323E-16, -5.243569643749999010 ) ) ;
#8337=CARTESIAN_POINT ( 'NONE',  ( 3.721875000614518036, 3.027376345333611329, 5.243569643749999010 ) ) ;
#8338=CARTESIAN_POINT ( 'NONE',  ( 10.12500000122903288, 2.886751345948129099, -4.999999999999997335 ) ) ;
#8340=CARTESIAN_POINT ( 'NONE',  ( 15.59999999999999964, 0.000000000000000000, 4.999999999999998224 ) ) ;
#8341=CARTESIAN_POINT ( 'NONE',  ( 19.79062500061451502, 6.054752690667223547, 3.707466751127219781E-16 ) ) ;
#8342=VERTEX_POINT ( 'NONE', #58958 ) ;
#8343=CARTESIAN_POINT ( 'NONE',  ( 23.66250000000000142, 2.886751345948126879, 4.999999999999999112 ) ) ;
#8344=CARTESIAN_POINT ( 'NONE',  ( 26.89687500061451431, -3.027376345333610441, -5.243569643749999898 ) ) ;
#8345=ORIENTED_EDGE ( 'NONE', *, *, #32039, .F. ) ;
#8346=CARTESIAN_POINT ( 'NONE',  ( 9.525000000000002132, 6.123233995736764310E-16, -4.999999999999998224 ) ) ;
#8347=CARTESIAN_POINT ( 'NONE',  ( 14.16562500061451679, -6.054752690667223547, -1.112240025338166033E-15 ) ) ;
#8348=CARTESIAN_POINT ( 'NONE',  ( 3.328125000614516438, -4.541064518000419881, 2.621784821874995952 ) ) ;
#8350=CARTESIAN_POINT ( 'NONE',  ( 28.34062500061451928, 6.054752690667223547, 3.707466751127219781E-16 ) ) ;
#8351=CARTESIAN_POINT ( 'NONE',  ( 12.60000000122903430, -2.886751345948129988, 4.999999999999997335 ) ) ;
#8352=CARTESIAN_POINT ( 'NONE',  ( 18.67500000000000071, 4.330127018922191873, 2.499999999999999556 ) ) ;
#8353=CARTESIAN_POINT ( 'NONE',  ( 27.48749999999999716, -2.886751345948125991, -5.000000000000000000 ) ) ;
#8355=CARTESIAN_POINT ( 'NONE',  ( 8.109375000614518214, 4.541064518000418104, -2.621784821874998173 ) ) ;
#8356=CARTESIAN_POINT ( 'NONE',  ( 18.42187500061451644, 3.027376345333613106, -5.243569643749998122 ) ) ;
#8357=CARTESIAN_POINT ( 'NONE',  ( 26.09999999999999787, -4.330127018922190985, -2.500000000000001332 ) ) ;
#8359=CARTESIAN_POINT ( 'NONE',  ( 28.41562500061451502, 3.027376345333611329, 5.243569643749999010 ) ) ;
#8360=CARTESIAN_POINT ( 'NONE',  ( 4.275000000000001243, 4.330127018922191873, 2.499999999999999556 ) ) ;
#8361=CARTESIAN_POINT ( 'NONE',  ( 4.434375000614519280, 6.421520780324663323E-16, -5.243569643749999010 ) ) ;
#8362=CARTESIAN_POINT ( 'NONE',  ( 16.53750000000000142, -2.886751345948129988, 4.999999999999997335 ) ) ;
#8363=CARTESIAN_POINT ( 'NONE',  ( 13.52812500061451750, 4.541064518000418104, 2.621784821874999949 ) ) ;
#8366=CYLINDRICAL_SURFACE ( 'NONE', #15060, 4.000000000000000000 ) ;
#8367=CARTESIAN_POINT ( 'NONE',  ( 17.70000000122903216, -2.886751345948125991, -5.000000000000000000 ) ) ;
#8368=CARTESIAN_POINT ( 'NONE',  ( 0.000000000000000000, 20.00000000000000000, -30.00000000000000000 ) ) ;
#8370=CARTESIAN_POINT ( 'NONE',  ( 7.040625000614517681, -3.027376345333610441, -5.243569643749999898 ) ) ;
#8371=CARTESIAN_POINT ( 'NONE',  ( 24.87187500061451573, 3.027376345333611329, 5.243569643749999010 ) ) ;
#8372=CARTESIAN_POINT ( 'NONE',  ( 19.65000000122902790, 5.773502691896255534, 3.535250795749688401E-16 ) ) ;
#8373=CARTESIAN_POINT ( 'NONE',  ( 24.04687500061451644, -3.027376345333614438, 5.243569643749998122 ) ) ;
#8374=CARTESIAN_POINT ( 'NONE',  ( 5.812500000000001776, -5.773502691896255534, -1.060575238724906372E-15 ) ) ;
#8375=CARTESIAN_POINT ( 'NONE',  ( 4.000000000000000000, 10.85000000122903430, 32.30940107675849049 ) ) ;
#8376=CARTESIAN_POINT ( 'NONE',  ( 15.66562500061451857, 3.027376345333613106, -5.243569643749998122 ) ) ;
#8377=CARTESIAN_POINT ( 'NONE',  ( 3.787500001229033408, 6.123233995736764310E-16, -4.999999999999998224 ) ) ;
#8378=CARTESIAN_POINT ( 'NONE',  ( 10.43437500061451750, 4.541064518000418104, 2.621784821874999949 ) ) ;
#8379=CARTESIAN_POINT ( 'NONE',  ( 3.046343057529203424, 3.964819538874875704, 3.046343057529141696 ) ) ;
#8381=CARTESIAN_POINT ( 'NONE',  ( 12.14062500061451821, 6.054752690667223547, 3.707466751127219781E-16 ) ) ;
#8383=CARTESIAN_POINT ( 'NONE',  ( 25.08750000122903145, 4.330127018922191873, 2.499999999999999556 ) ) ;
#8384=CARTESIAN_POINT ( 'NONE',  ( 9.796875000614519990, -3.027376345333610441, -5.243569643749999898 ) ) ;
#8385=CARTESIAN_POINT ( 'NONE',  ( 11.20312500061451644, 4.541064518000418104, -2.621784821874998173 ) ) ;
#8386=ADVANCED_FACE ( 'NONE', ( #19066 ), #8366, .F. ) ;
#8388=CARTESIAN_POINT ( 'NONE',  ( 24.98437500061451644, -4.541064518000419881, 2.621784821874995952 ) ) ;
#8389=CARTESIAN_POINT ( 'NONE',  ( 4.312500001229034652, 4.330127018922192761, -2.499999999999997780 ) ) ;
#8390=DIRECTION ( 'NONE',  ( -1.000000000000000000, -0.000000000000000000, -0.000000000000000000 ) ) ;
#8391=CARTESIAN_POINT ( 'NONE',  ( -2.121784821874999949, 14.38437500061451679, -33.67503911421598417 ) ) ;
#8392=AXIS2_PLACEMENT_3D ( 'NONE', #32888, #72781, #50257 ) ;
#8393=CARTESIAN_POINT ( 'NONE',  ( 16.32187500061451502, 3.027376345333611329, 5.243569643749999010 ) ) ;
#8394=CARTESIAN_POINT ( 'NONE',  ( 18.63750000122903216, 6.123233995736764310E-16, -4.999999999999998224 ) ) ;
#8395=CARTESIAN_POINT ( 'NONE',  ( 11.63437500061451857, 6.421520780324663323E-16, -5.243569643749999010 ) ) ;
#8396=CARTESIAN_POINT ( 'NONE',  ( -4.243569643749999898, 18.86562500061451431, -32.45002607614398471 ) ) ;
#8397=CARTESIAN_POINT ( 'NONE',  ( 20.25000000122903288, -2.886751345948129988, 4.999999999999997335 ) ) ;
#8398=CARTESIAN_POINT ( 'NONE',  ( 12.44062500061451537, -3.027376345333610441, -5.243569643749999898 ) ) ;
#8399=VERTEX_POINT ( 'NONE', #40912 ) ;
#8400=CARTESIAN_POINT ( 'NONE',  ( 16.12500000000000000, -4.330127018922194537, 2.499999999999995559 ) ) ;
#8401=CARTESIAN_POINT ( 'NONE',  ( 29.09999999999999787, 0.000000000000000000, 4.999999999999998224 ) ) ;
#8402=CARTESIAN_POINT ( 'NONE',  ( 11.37187500061451928, 3.027376345333611329, 5.243569643749999010 ) ) ;
#8403=CARTESIAN_POINT ( 'NONE',  ( -3.305248395036964552E-15, 5.000000000000034639, 25.99999999999995737 ) ) ;
#8404=CARTESIAN_POINT ( 'NONE',  ( 13.53750000122903430, -4.330127018922194537, 2.499999999999995559 ) ) ;
#8405=CARTESIAN_POINT ( 'NONE',  ( 21.67500000122903359, -5.773502691896255534, -1.060575238724906372E-15 ) ) ;
#8406=CARTESIAN_POINT ( 'NONE',  ( 18.81562500061452070, 3.027376345333613106, -5.243569643749998122 ) ) ;
#8407=CARTESIAN_POINT ( 'NONE',  ( 21.44062500061452070, -3.027376345333610441, -5.243569643749999898 ) ) ;
#8408=CARTESIAN_POINT ( 'NONE',  ( 28.16250000122903074, 4.330127018922192761, -2.499999999999997780 ) ) ;
#8409=CARTESIAN_POINT ( 'NONE',  ( 25.83749999999999858, 5.773502691896255534, 3.535250795749688894E-16 ) ) ;
#8411=CARTESIAN_POINT ( 'NONE',  ( 28.39687500061452141, 6.054752690667223547, 3.707466751127219781E-16 ) ) ;
#8412=CARTESIAN_POINT ( 'NONE',  ( -2.000000000000000000, 9.687500001229034652, -33.46410161513775705 ) ) ;
#8413=CARTESIAN_POINT ( 'NONE',  ( 4.243569643749999010, 13.37187500061451750, -32.45002607614398471 ) ) ;
#8414=CARTESIAN_POINT ( 'NONE',  ( 4.687500001229034652, 6.123233995736764310E-16, -4.999999999999998224 ) ) ;
#8415=CARTESIAN_POINT ( 'NONE',  ( 5.325000000000000178, -4.330127018922194537, 2.499999999999995559 ) ) ;
#8417=CARTESIAN_POINT ( 'NONE',  ( 7.359375000614516438, 0.000000000000000000, 5.243569643749999010 ) ) ;
#8418=CARTESIAN_POINT ( 'NONE',  ( 28.34062500061451928, 6.054752690667223547, 3.707466751127219781E-16 ) ) ;
#8419=DIRECTION ( 'NONE',  ( -1.000000000000000000, -0.000000000000000000, -0.000000000000000000 ) ) ;
#8420=CARTESIAN_POINT ( 'NONE',  ( 1.071796769724489895, 10.52990381179670010, 26.00000000000000355 ) ) ;
#8421=CARTESIAN_POINT ( 'NONE',  ( 6.159375000614517148, -4.541064518000417216, -2.621784821875001281 ) ) ;
#8422=CARTESIAN_POINT ( 'NONE',  ( 10.20937500061451786, -4.541064518000417216, -2.621784821875001281 ) ) ;
#8423=CARTESIAN_POINT ( 'NONE',  ( 4.125000000000000000, 6.123233995736764310E-16, -4.999999999999998224 ) ) ;
#8424=CARTESIAN_POINT ( 'NONE',  ( 4.243569643749999898, 13.72812500061459495, 30.00000000000000000 ) ) ;
#8426=CARTESIAN_POINT ( 'NONE',  ( 7.500000000000000000, 0.000000000000000000, 4.999999999999998224 ) ) ;
#8429=CARTESIAN_POINT ( 'NONE',  ( 20.42812500061451431, -4.541064518000419881, 2.621784821874995952 ) ) ;
#8430=CARTESIAN_POINT ( 'NONE',  ( 10.34062500061451750, 6.054752690667223547, 3.707466751127219781E-16 ) ) ;
#8432=CARTESIAN_POINT ( 'NONE',  ( 10.62187500061451928, -6.054752690667223547, -1.112240025338166033E-15 ) ) ;
#8433=CARTESIAN_POINT ( 'NONE',  ( 25.98750000000000071, -2.886751345948129988, 4.999999999999997335 ) ) ;
#8434=CARTESIAN_POINT ( 'NONE',  ( 19.50000000122903288, -2.886751345948125991, -5.000000000000000000 ) ) ;
#8435=CARTESIAN_POINT ( 'NONE',  ( 27.70312500061451289, -4.541064518000417216, -2.621784821875001281 ) ) ;
#8437=CARTESIAN_POINT ( 'NONE',  ( 10.35937500061451644, 4.541064518000418104, -2.621784821874998173 ) ) ;
#8438=CARTESIAN_POINT ( 'NONE',  ( 14.18437500061451750, -4.541064518000419881, 2.621784821874995952 ) ) ;
#8439=CARTESIAN_POINT ( 'NONE',  ( 26.70937500061451431, 0.000000000000000000, 5.243569643749999010 ) ) ;
#8441=CARTESIAN_POINT ( 'NONE',  ( 4.265625000614517326, -6.054752690667223547, -1.112240025338166033E-15 ) ) ;
#8443=CARTESIAN_POINT ( 'NONE',  ( 19.02187500061451786, 3.027376345333611329, 5.243569643749999010 ) ) ;
#8444=CARTESIAN_POINT ( 'NONE',  ( 10.73437500061451644, 6.421520780324663323E-16, -5.243569643749999010 ) ) ;
#8446=CARTESIAN_POINT ( 'NONE',  ( 22.34999999999999787, 0.000000000000000000, 4.999999999999998224 ) ) ;
#8448=CARTESIAN_POINT ( 'NONE',  ( -4.243569643749999898, 12.62187500061451928, -32.45002607614398471 ) ) ;
#8450=CARTESIAN_POINT ( 'NONE',  ( 14.76562500061451821, 3.027376345333613106, -5.243569643749998122 ) ) ;
#8451=CARTESIAN_POINT ( 'NONE',  ( 3.450000000000001510, 0.000000000000000000, 4.999999999999998224 ) ) ;
#8453=EDGE_CURVE ( 'NONE', #31017, #60322, #45423, .T. ) ;
#8454=CARTESIAN_POINT ( 'NONE',  ( 25.57499999999999929, -4.330127018922194537, 2.499999999999995559 ) ) ;
#8455=CARTESIAN_POINT ( 'NONE',  ( 13.12500000000000178, 6.123233995736764310E-16, -4.999999999999998224 ) ) ;
#8456=CARTESIAN_POINT ( 'NONE',  ( -2.000000000000000000, 16.88750000122903572, 26.53589838486224650 ) ) ;
#8457=CARTESIAN_POINT ( 'NONE',  ( 10.80000000122903536, -2.886751345948129988, 4.999999999999997335 ) ) ;
#8458=CARTESIAN_POINT ( 'NONE',  ( 23.67187500061451999, -6.054752690667223547, -1.112240025338166033E-15 ) ) ;
#8459=CARTESIAN_POINT ( 'NONE',  ( 16.99687500061451573, -3.027376345333610441, -5.243569643749999898 ) ) ;
#8460=DIRECTION ( 'NONE',  ( -1.000000000000000000, -0.000000000000000000, -0.000000000000000000 ) ) ;
#8462=CARTESIAN_POINT ( 'NONE',  ( 20.76562500061451644, 3.027376345333611329, 5.243569643749999010 ) ) ;
#8463=CARTESIAN_POINT ( 'NONE',  ( 4.678125000614516971, -4.541064518000419881, 2.621784821874995952 ) ) ;
#8464=CARTESIAN_POINT ( 'NONE',  ( 17.25937500061451502, 0.000000000000000000, 5.243569643749999010 ) ) ;
#8465=CARTESIAN_POINT ( 'NONE',  ( 29.29687500061451644, 6.054752690667223547, 3.707466751127219781E-16 ) ) ;
#8466=CARTESIAN_POINT ( 'NONE',  ( 5.653125000614517504, -4.541064518000417216, -2.621784821875001281 ) ) ;
#8467=CARTESIAN_POINT ( 'NONE',  ( 19.60312500061451502, -4.541064518000417216, -2.621784821875001281 ) ) ;
#8468=CARTESIAN_POINT ( 'NONE',  ( 4.243569643749999898, 16.39062500061451999, 32.45002607614398471 ) ) ;
#8469=CARTESIAN_POINT ( 'NONE',  ( 17.36250000122903359, 4.330127018922192761, -2.499999999999997780 ) ) ;
#8471=CARTESIAN_POINT ( 'NONE',  ( 6.028125000614517504, -4.541064518000419881, 2.621784821874995952 ) ) ;
#8472=CARTESIAN_POINT ( 'NONE',  ( 4.171875000614517326, 3.027376345333611329, 5.243569643749999010 ) ) ;
#8473=CARTESIAN_POINT ( 'NONE',  ( 3.571875000614517237, 3.027376345333613106, -5.243569643749998122 ) ) ;
#8474=CARTESIAN_POINT ( 'NONE',  ( 23.48437500061451644, 4.541064518000418104, 2.621784821874999949 ) ) ;
#8475=CARTESIAN_POINT ( 'NONE',  ( 13.71562500061451750, -6.054752690667223547, -1.112240025338166033E-15 ) ) ;
#8476=CARTESIAN_POINT ( 'NONE',  ( 25.53750000122903074, 4.330127018922191873, 2.499999999999999556 ) ) ;
#8477=CARTESIAN_POINT ( 'NONE',  ( 23.84062500061451928, 6.054752690667223547, 3.707466751127219781E-16 ) ) ;
#8478=CARTESIAN_POINT ( 'NONE',  ( 20.03437500061451715, -4.541064518000419881, 2.621784821874995952 ) ) ;
#8479=CARTESIAN_POINT ( 'NONE',  ( 13.60312500061451679, 0.000000000000000000, 5.243569643749999010 ) ) ;
#8480=CARTESIAN_POINT ( 'NONE',  ( 9.001249775931846008E-16, 14.57187500061451679, 34.90005215228797653 ) ) ;
#8481=CARTESIAN_POINT ( 'NONE',  ( 20.39062500061451644, -3.027376345333614438, 5.243569643749998122 ) ) ;
#8484=ORIENTED_EDGE ( 'NONE', *, *, #70743, .F. ) ;
#8485=CARTESIAN_POINT ( 'NONE',  ( 23.77499999999999858, -4.330127018922194537, 2.499999999999995559 ) ) ;
#8486=CARTESIAN_POINT ( 'NONE',  ( -3.999999999999999112, 11.45000000000000107, -30.00000000000000000 ) ) ;
#8488=CARTESIAN_POINT ( 'NONE',  ( 26.12812500061451360, 4.541064518000418104, 2.621784821874999949 ) ) ;
#8489=CARTESIAN_POINT ( 'NONE',  ( 7.715625000614515727, 3.027376345333611329, 5.243569643749999010 ) ) ;
#8490=CARTESIAN_POINT ( 'NONE',  ( 19.65000000122902790, 5.773502691896255534, 3.535250795749688894E-16 ) ) ;
#8492=CARTESIAN_POINT ( 'NONE',  ( 25.52812500061451573, 6.421520780324663323E-16, -5.243569643749999010 ) ) ;
#8493=CARTESIAN_POINT ( 'NONE',  ( 25.12499999999999645, -4.330127018922194537, 2.499999999999995559 ) ) ;
#8494=CARTESIAN_POINT ( 'NONE',  ( 28.11562500061451431, -6.054752690667223547, -1.112240025338166033E-15 ) ) ;
#8495=CARTESIAN_POINT ( 'NONE',  ( 8.728125000614518569, -4.541064518000419881, 2.621784821874995952 ) ) ;
#8497=AXIS2_PLACEMENT_3D ( 'NONE', #42292, #41925, #14572 ) ;
#8498=CARTESIAN_POINT ( 'NONE',  ( 23.61562500061451431, -6.054752690667223547, -1.112240025338166033E-15 ) ) ;
#8499=CARTESIAN_POINT ( 'NONE',  ( 4.378125000614518925, 6.421520780324663323E-16, -5.243569643749999010 ) ) ;
#8502=CARTESIAN_POINT ( 'NONE',  ( 3.665625000614517681, 3.027376345333611329, 5.243569643749999010 ) ) ;
#8503=CARTESIAN_POINT ( 'NONE',  ( 4.243569643749999898, 19.59687500061452070, -27.54997392385601529 ) ) ;
#8504=( BOUNDED_CURVE ( )  B_SPLINE_CURVE ( 2, ( #12020, #62980, #58512, #62625, #57792, #34543, #12376, #23817, #41193 ),
 .UNSPECIFIED., .F., .F. ) 
 B_SPLINE_CURVE_WITH_KNOTS ( ( 3, 2, 2, 2, 3 ),
 ( 0.1630434782608695676, 0.1666666666666666574, 0.1739130434782608647, 0.1811594202898550721, 0.1847826086956521896 ),
 .UNSPECIFIED. ) 
 CURVE ( )  GEOMETRIC_REPRESENTATION_ITEM ( )  RATIONAL_B_SPLINE_CURVE ( ( 0.9330127018922194093, 0.9330127018922196314, 1.000000000000000000, 0.8660254037844387076, 1.000000000000000000, 0.8660254037844387076, 1.000000000000000000, 0.9330127018922190762, 0.9330127018922194093 ) ) 
 REPRESENTATION_ITEM ( '' )  );
#8505=CARTESIAN_POINT ( 'NONE',  ( 11.96250000000000213, 2.886751345948126879, 4.999999999999999112 ) ) ;
#8506=CARTESIAN_POINT ( 'NONE',  ( 13.84687500061451537, -3.027376345333610441, -5.243569643749999898 ) ) ;
#8507=CARTESIAN_POINT ( 'NONE',  ( 8.550000001229031810, -2.886751345948129988, 4.999999999999997335 ) ) ;
#8508=CARTESIAN_POINT ( 'NONE',  ( 15.19687500061451857, -3.027376345333610441, -5.243569643749999898 ) ) ;
#8510=CARTESIAN_POINT ( 'NONE',  ( 9.459375000614517859, 4.541064518000418104, -2.621784821874998173 ) ) ;
#8511=CARTESIAN_POINT ( 'NONE',  ( 4.243569643749999898, 11.92812500061451608, -30.00000000000000000 ) ) ;
#8513=CARTESIAN_POINT ( 'NONE',  ( 13.62187500061451750, 3.027376345333611329, 5.243569643749999010 ) ) ;
#8515=CARTESIAN_POINT ( 'NONE',  ( 22.56562500061451715, 3.027376345333611329, 5.243569643749999010 ) ) ;
#8516=CARTESIAN_POINT ( 'NONE',  ( -0.7368805616696195715, 9.859898480082234684, 25.82089837893477480 ) ) ;
#8517=CARTESIAN_POINT ( 'NONE',  ( 11.32500000000000107, 6.123233995736764310E-16, -4.999999999999998224 ) ) ;
#8518=CARTESIAN_POINT ( 'NONE',  ( 25.92187500061451999, -6.054752690667223547, -1.112240025338166033E-15 ) ) ;
#8519=CARTESIAN_POINT ( 'NONE',  ( 28.28437500061451715, 6.421520780324663323E-16, -5.243569643749999010 ) ) ;
#8520=( BOUNDED_CURVE ( )  B_SPLINE_CURVE ( 2, ( #58576, #59301, #25708, #2807, #70769, #20145, #71136 ),
 .UNSPECIFIED., .F., .F. ) 
 B_SPLINE_CURVE_WITH_KNOTS ( ( 3, 2, 2, 3 ),
 ( 0.5999999999999999778, 0.6027777777777777457, 0.6055555555555555136, 0.6083333333333332815 ),
 .UNSPECIFIED. ) 
 CURVE ( )  GEOMETRIC_REPRESENTATION_ITEM ( )  RATIONAL_B_SPLINE_CURVE ( ( 1.000000000000000000, 0.8660254037844387076, 1.000000000000000000, 0.8660254037844387076, 1.000000000000000000, 0.8660254037844387076, 1.000000000000000000 ) ) 
 REPRESENTATION_ITEM ( '' )  );
#8521=CARTESIAN_POINT ( 'NONE',  ( 4.303125000614516971, -4.541064518000417216, -2.621784821875001281 ) ) ;
#8523=CARTESIAN_POINT ( 'NONE',  ( 17.48437500061451999, 6.421520780324663323E-16, -5.243569643749999010 ) ) ;
#8525=CARTESIAN_POINT ( 'NONE',  ( 2.953125000614516438, -4.541064518000417216, -2.621784821875001281 ) ) ;
#8526=CARTESIAN_POINT ( 'NONE',  ( 5.484375000614518214, 4.541064518000418104, 2.621784821874999949 ) ) ;
#8527=CARTESIAN_POINT ( 'NONE',  ( 16.24687500061451573, 6.054752690667223547, 3.707466751127219781E-16 ) ) ;
#8529=CARTESIAN_POINT ( 'NONE',  ( 27.56250000000000000, 2.886751345948129099, -4.999999999999998224 ) ) ;
#8530=CARTESIAN_POINT ( 'NONE',  ( 26.52187500061451431, 3.027376345333613106, -5.243569643749998122 ) ) ;
#8532=CARTESIAN_POINT ( 'NONE',  ( 21.82499999999999574, 4.330127018922191873, 2.499999999999999556 ) ) ;
#8533=VERTEX_POINT ( 'NONE', #58597 ) ;
#8534=CARTESIAN_POINT ( 'NONE',  ( 7.050000000000000711, 0.000000000000000000, 4.999999999999998224 ) ) ;
#8536=CARTESIAN_POINT ( 'NONE',  ( 22.60312500061451857, 0.000000000000000000, 5.243569643749999010 ) ) ;
#8537=CARTESIAN_POINT ( 'NONE',  ( 12.90000000000000213, 0.000000000000000000, 4.999999999999998224 ) ) ;
#8538=EDGE_CURVE ( 'NONE', #40887, #30395, #30752, .T. ) ;
#8539=CARTESIAN_POINT ( 'NONE',  ( 9.075000001229033941, -5.773502691896255534, -1.060575238724906372E-15 ) ) ;
#8540=CARTESIAN_POINT ( 'NONE',  ( 6.140625000614516438, -3.027376345333610441, -5.243569643749999898 ) ) ;
#8541=CARTESIAN_POINT ( 'NONE',  ( 21.71249999999999858, 2.886751345948129099, -4.999999999999998224 ) ) ;
#8542=CARTESIAN_POINT ( 'NONE',  ( 19.49062500061451431, -3.027376345333614438, 5.243569643749998122 ) ) ;
#8543=CARTESIAN_POINT ( 'NONE',  ( 23.47499999999999787, 6.123233995736764310E-16, -4.999999999999998224 ) ) ;
#8544=CARTESIAN_POINT ( 'NONE',  ( 25.98750000122903003, 4.330127018922191873, 2.499999999999999556 ) ) ;
#8547=CARTESIAN_POINT ( 'NONE',  ( 4.724999999999999645, 4.330127018922191873, 2.499999999999999556 ) ) ;
#8549=CARTESIAN_POINT ( 'NONE',  ( 20.54062500061451502, -3.027376345333610441, -5.243569643749999898 ) ) ;
#8550=CARTESIAN_POINT ( 'NONE',  ( 26.54062500061451146, 6.054752690667223547, 3.707466751127219781E-16 ) ) ;
#8551=CARTESIAN_POINT ( 'NONE',  ( 25.05937500061451573, -4.541064518000417216, -2.621784821875001281 ) ) ;
#8552=CARTESIAN_POINT ( 'NONE',  ( 9.750000000000001776, 0.000000000000000000, 4.999999999999998224 ) ) ;
#8553=CARTESIAN_POINT ( 'NONE',  ( 12.55312500061451786, 4.541064518000418104, -2.621784821874998173 ) ) ;
#8554=CARTESIAN_POINT ( 'NONE',  ( 27.96562500061451928, 3.027376345333611329, 5.243569643749999010 ) ) ;
#8555=CARTESIAN_POINT ( 'NONE',  ( 9.553125000614517859, 0.000000000000000000, 5.243569643749999010 ) ) ;
#8556=FACE_OUTER_BOUND ( 'NONE', #20970, .T. ) ;
#8557=CARTESIAN_POINT ( 'NONE',  ( -3.000416591977282496E-16, 11.64687500061451786, 25.09994784771203058 ) ) ;
#8558=CARTESIAN_POINT ( 'NONE',  ( 24.71250000122903145, 0.000000000000000000, 4.999999999999998224 ) ) ;
#8560=CARTESIAN_POINT ( 'NONE',  ( 13.37812500061451715, 6.421520780324663323E-16, -5.243569643749999010 ) ) ;
#8561=CARTESIAN_POINT ( 'NONE',  ( 10.80937500061451928, 4.541064518000418104, -2.621784821874998173 ) ) ;
#8562=CARTESIAN_POINT ( 'NONE',  ( 8.671875000614518214, 3.027376345333611329, 5.243569643749999010 ) ) ;
#8563=CARTESIAN_POINT ( 'NONE',  ( 16.84687500061451715, -3.027376345333614438, 5.243569643749998122 ) ) ;
#8564=EDGE_LOOP ( 'NONE', ( #5921, #66714, #29257, #61200 ) ) ;
#8565=CARTESIAN_POINT ( 'NONE',  ( -1.585543809737898213, 9.875380255848558164, 35.79011327352668559 ) ) ;
#8566=CARTESIAN_POINT ( 'NONE',  ( 22.07812500061451644, 4.541064518000418104, 2.621784821874999949 ) ) ;
#8567=CARTESIAN_POINT ( 'NONE',  ( 16.47187500061452070, -6.054752690667223547, -1.112240025338166033E-15 ) ) ;
#8568=CARTESIAN_POINT ( 'NONE',  ( 23.09062500061451573, -3.027376345333614438, 5.243569643749998122 ) ) ;
#8569=CARTESIAN_POINT ( 'NONE',  ( -1.999999999999997113, 12.87500000000000178, 33.46410161513775705 ) ) ;
#8570=CARTESIAN_POINT ( 'NONE',  ( 27.70312500061451289, -4.541064518000417216, -2.621784821875001281 ) ) ;
#8571=CARTESIAN_POINT ( 'NONE',  ( 6.825000001229034829, -5.773502691896255534, -1.060575238724906372E-15 ) ) ;
#8573=CARTESIAN_POINT ( 'NONE',  ( 4.612500001229032698, -4.330127018922190985, -2.500000000000001332 ) ) ;
#8574=CARTESIAN_POINT ( 'NONE',  ( 3.999999999999998668, 16.66249999999999787, -32.30940107675850470 ) ) ;
#8575=CARTESIAN_POINT ( 'NONE',  ( 25.87500000122903288, 2.886751345948129099, -4.999999999999998224 ) ) ;
#8577=CARTESIAN_POINT ( 'NONE',  ( 7.996875000614519280, -3.027376345333610441, -5.243569643749999898 ) ) ;
#8578=CARTESIAN_POINT ( 'NONE',  ( 4.322286709174337105, 2.513530903668243610, -4.417718143658825980 ) ) ;
#8579=CARTESIAN_POINT ( 'NONE',  ( 15.85312500061451857, 0.000000000000000000, 5.243569643749999010 ) ) ;
#8580=CARTESIAN_POINT ( 'NONE',  ( 9.459375000614517859, 4.541064518000418104, -2.621784821874998173 ) ) ;
#8581=CARTESIAN_POINT ( 'NONE',  ( 27.90000000122903145, -2.886751345948129988, 4.999999999999997335 ) ) ;
#8582=CARTESIAN_POINT ( 'NONE',  ( 17.10937500061451999, 4.541064518000418104, -2.621784821874998173 ) ) ;
#8583=CARTESIAN_POINT ( 'NONE',  ( 5.334375000614517859, 6.421520780324663323E-16, -5.243569643749999010 ) ) ;
#8585=CARTESIAN_POINT ( 'NONE',  ( 5.765625000614519102, 3.027376345333613106, -5.243569643749998122 ) ) ;
#8586=CARTESIAN_POINT ( 'NONE',  ( 15.96562500061451573, -6.054752690667223547, -1.112240025338166033E-15 ) ) ;
#8588=CARTESIAN_POINT ( 'NONE',  ( 13.19062500061451537, -3.027376345333614438, 5.243569643749998122 ) ) ;
#8589=CARTESIAN_POINT ( 'NONE',  ( 5.100000001229034297, -2.886751345948125991, -5.000000000000000000 ) ) ;
#8590=CARTESIAN_POINT ( 'NONE',  ( 9.778125000614517504, 6.421520780324663323E-16, -5.243569643749999010 ) ) ;
#8592=CARTESIAN_POINT ( 'NONE',  ( 11.58750000000000036, -2.886751345948129988, 4.999999999999997335 ) ) ;
#8593=ADVANCED_FACE ( 'NONE', ( #1747 ), #36076, .F. ) ;
#8594=CARTESIAN_POINT ( 'NONE',  ( 6.675000001229034474, 2.886751345948126879, 4.999999999999999112 ) ) ;
#8595=CARTESIAN_POINT ( 'NONE',  ( 19.87500000000000000, 6.123233995736764310E-16, -4.999999999999998224 ) ) ;
#8596=CARTESIAN_POINT ( 'NONE',  ( 14.25937500061451679, -4.541064518000417216, -2.621784821875001281 ) ) ;
#8597=CARTESIAN_POINT ( 'NONE',  ( 15.37500000122903465, -5.773502691896255534, -1.060575238724906372E-15 ) ) ;
#8599=CARTESIAN_POINT ( 'NONE',  ( 4.243569643749999898, 18.67812500061451431, -30.00000000000000000 ) ) ;
#8600=CARTESIAN_POINT ( 'NONE',  ( 3.236215399915419511, 3.811430163627435252, 3.601125184156294345 ) ) ;
#8603=CARTESIAN_POINT ( 'NONE',  ( 3.481582908954544919, -3.588718827790031263, 3.545339672739869830 ) ) ;
#8604=CARTESIAN_POINT ( 'NONE',  ( 3.921087004242067131, -3.102464839086551240, -4.227284519891857606 ) ) ;
#8605=CARTESIAN_POINT ( 'NONE',  ( 15.57187500061451679, -6.054752690667223547, -1.112240025338166033E-15 ) ) ;
#8606=CARTESIAN_POINT ( 'NONE',  ( 29.66249999999999432, -5.773502691896255534, -1.060575238724906372E-15 ) ) ;
#8607=CARTESIAN_POINT ( 'NONE',  ( 12.70312500061451821, 0.000000000000000000, 5.243569643749999010 ) ) ;
#8609=CARTESIAN_POINT ( 'NONE',  ( 23.97187500061451360, 3.027376345333611329, 5.243569643749999010 ) ) ;
#8611=CARTESIAN_POINT ( 'NONE',  ( 9.703125000614514661, -4.541064518000417216, -2.621784821875001281 ) ) ;
#8612=CARTESIAN_POINT ( 'NONE',  ( 12.12187500061451573, 3.027376345333613106, -5.243569643749998122 ) ) ;
#8613=ORIENTED_EDGE ( 'NONE', *, *, #11628, .T. ) ;
#8614=CARTESIAN_POINT ( 'NONE',  ( 23.97187500061451360, 3.027376345333611329, 5.243569643749999010 ) ) ;
#8615=CARTESIAN_POINT ( 'NONE',  ( 24.81562500061451715, 3.027376345333611329, 5.243569643749999010 ) ) ;
#8616=CARTESIAN_POINT ( 'NONE',  ( 28.26562500061451289, 3.027376345333613106, -5.243569643749998122 ) ) ;
#8617=CARTESIAN_POINT ( 'NONE',  ( 4.882324679417408220, 1.079004970772768246, -5.131482293177458409 ) ) ;
#8618=CARTESIAN_POINT ( 'NONE',  ( 8.287499999999999645, 5.773502691896255534, 3.535250795749688894E-16 ) ) ;
#8619=CARTESIAN_POINT ( 'NONE',  ( 16.61250000122903359, 0.000000000000000000, 4.999999999999998224 ) ) ;
#8622=VERTEX_POINT ( 'NONE', #47529 ) ;
#8623=CARTESIAN_POINT ( 'NONE',  ( 16.08749999999999503, -2.886751345948129988, 4.999999999999997335 ) ) ;
#8624=CARTESIAN_POINT ( 'NONE',  ( 18.86249999999999716, -5.773502691896255534, -1.060575238724906372E-15 ) ) ;
#8625=CARTESIAN_POINT ( 'NONE',  ( 13.07812500061451821, 4.541064518000418104, 2.621784821874999949 ) ) ;
#8626=VERTEX_POINT ( 'NONE', #31264 ) ;
#8627=CARTESIAN_POINT ( 'NONE',  ( 1.626862140677534273E-15, 16.17500000122903359, -26.00000000000000355 ) ) ;
#8628=CARTESIAN_POINT ( 'NONE',  ( 4.243569643749999898, 16.48437500061451644, -30.00000000000000000 ) ) ;
#8629=CARTESIAN_POINT ( 'NONE',  ( 5.203125000614518214, -4.541064518000417216, -2.621784821875001281 ) ) ;
#8631=CARTESIAN_POINT ( 'NONE',  ( 13.46249999999999858, -5.773502691896255534, -1.060575238724906372E-15 ) ) ;
#8634=CARTESIAN_POINT ( 'NONE',  ( 9.001249775931846008E-16, 14.96562500061451750, 34.90005215228797653 ) ) ;
#8635=CARTESIAN_POINT ( 'NONE',  ( 26.46562500061451573, 3.027376345333613106, -5.243569643749998122 ) ) ;
#8638=CARTESIAN_POINT ( 'NONE',  ( 23.37187500061451573, 3.027376345333613106, -5.243569643749998122 ) ) ;
#8639=CARTESIAN_POINT ( 'NONE',  ( 18.17812500061451786, -4.541064518000419881, 2.621784821874995952 ) ) ;
#8640=CARTESIAN_POINT ( 'NONE',  ( -4.243569643749998122, 13.99062500061459602, -27.54997392385601174 ) ) ;
#8641=CARTESIAN_POINT ( 'NONE',  ( 23.58750000122903145, 6.123233995736764310E-16, -4.999999999999998224 ) ) ;
#8642=CARTESIAN_POINT ( 'NONE',  ( 6.253125000614517148, 4.541064518000418104, -2.621784821874998173 ) ) ;
#8644=CARTESIAN_POINT ( 'NONE',  ( 22.04062500061451502, 6.054752690667223547, 3.707466751127219781E-16 ) ) ;
#8647=CARTESIAN_POINT ( 'NONE',  ( 16.65937500061452070, 4.541064518000418104, -2.621784821874998173 ) ) ;
#8648=CARTESIAN_POINT ( 'NONE',  ( 16.24687500061451573, 6.054752690667223547, 3.707466751127219781E-16 ) ) ;
#8649=CARTESIAN_POINT ( 'NONE',  ( 24.57187500061451502, -6.054752690667223547, -1.112240025338166033E-15 ) ) ;
#8650=CARTESIAN_POINT ( 'NONE',  ( -4.243569643749999898, 14.42187500061451999, 27.54997392385601529 ) ) ;
#8651=CARTESIAN_POINT ( 'NONE',  ( 5.578125000614518214, -4.541064518000419881, 2.621784821874995952 ) ) ;
#8652=CARTESIAN_POINT ( 'NONE',  ( 28.71562500061451573, 3.027376345333613106, -5.243569643749998122 ) ) ;
#8653=CARTESIAN_POINT ( 'NONE',  ( 29.69062500061451715, 6.054752690667223547, 3.707466751127219781E-16 ) ) ;
#8655=CARTESIAN_POINT ( 'NONE',  ( 1.970565482296603443, 9.811066920826823079, -35.68093638750369223 ) ) ;
#8656=CARTESIAN_POINT ( 'NONE',  ( 3.703125000614516882, 0.000000000000000000, 5.243569643749999010 ) ) ;
#8657=CARTESIAN_POINT ( 'NONE',  ( 6.721875000614518925, 3.027376345333613106, -5.243569643749998122 ) ) ;
#8658=CARTESIAN_POINT ( 'NONE',  ( 13.95000000122903572, -2.886751345948129988, 4.999999999999997335 ) ) ;
#8659=CARTESIAN_POINT ( 'NONE',  ( 4.359375000614517326, -4.541064518000417216, -2.621784821875001281 ) ) ;
#8660=CARTESIAN_POINT ( 'NONE',  ( 10.65000000122903323, 5.773502691896255534, 3.535250795749688894E-16 ) ) ;
#8661=CARTESIAN_POINT ( 'NONE',  ( 3.965625000614515727, 3.027376345333613106, -5.243569643749998122 ) ) ;
#8664=CARTESIAN_POINT ( 'NONE',  ( 13.69687500061451679, -3.027376345333614438, 5.243569643749998122 ) ) ;
#8665=CARTESIAN_POINT ( 'NONE',  ( 7.650000000000000355, -4.330127018922190985, -2.500000000000001332 ) ) ;
#8666=ORIENTED_EDGE ( 'NONE', *, *, #61233, .F. ) ;
#8667=CARTESIAN_POINT ( 'NONE',  ( 23.24062500061451786, -3.027376345333610441, -5.243569643749999898 ) ) ;
#8668=CARTESIAN_POINT ( 'NONE',  ( 7.565625000614518036, 3.027376345333613106, -5.243569643749998122 ) ) ;
#8669=CARTESIAN_POINT ( 'NONE',  ( 25.43437500061451573, -4.541064518000419881, 2.621784821874995952 ) ) ;
#8670=CARTESIAN_POINT ( 'NONE',  ( 7.378125000614518036, -4.541064518000419881, 2.621784821874995952 ) ) ;
#8671=DIRECTION ( 'NONE',  ( -1.000000000000000000, -0.000000000000000000, -0.000000000000000000 ) ) ;
#8672=CARTESIAN_POINT ( 'NONE',  ( 9.187500001229034652, 6.123233995736764310E-16, -4.999999999999998224 ) ) ;
#8673=CARTESIAN_POINT ( 'NONE',  ( 23.95312500061451289, 0.000000000000000000, 5.243569643749999010 ) ) ;
#8674=CARTESIAN_POINT ( 'NONE',  ( -2.121784821874996840, 11.32812500061451644, -26.32496088578401583 ) ) ;
#8675=CARTESIAN_POINT ( 'NONE',  ( 9.937500001229032875, -4.330127018922194537, 2.499999999999995559 ) ) ;
#8676=CARTESIAN_POINT ( 'NONE',  ( 20.35312500061451502, 0.000000000000000000, 5.243569643749999010 ) ) ;
#8677=CARTESIAN_POINT ( 'NONE',  ( 18.02812500061451573, 4.541064518000418104, 2.621784821874999949 ) ) ;
#8679=CARTESIAN_POINT ( 'NONE',  ( 19.27500000000000213, -4.330127018922194537, 2.499999999999995559 ) ) ;
#8680=CARTESIAN_POINT ( 'NONE',  ( 13.12500000122903288, -5.773502691896255534, -1.060575238724906372E-15 ) ) ;
#8681=CARTESIAN_POINT ( 'NONE',  ( 9.515625000614518214, 3.027376345333611329, 5.243569643749999010 ) ) ;
#8682=CARTESIAN_POINT ( 'NONE',  ( 13.41562500061451502, 3.027376345333613106, -5.243569643749998122 ) ) ;
#8683=CARTESIAN_POINT ( 'NONE',  ( 22.53750000122903430, -4.330127018922194537, 2.499999999999995559 ) ) ;
#8684=CARTESIAN_POINT ( 'NONE',  ( 21.23437500061451644, 4.541064518000418104, 2.621784821874999949 ) ) ;
#8685=CARTESIAN_POINT ( 'NONE',  ( 21.27187500061451786, 3.027376345333611329, 5.243569643749999010 ) ) ;
#8687=CARTESIAN_POINT ( 'NONE',  ( 8.662500001229034297, -4.330127018922190985, -2.500000000000001332 ) ) ;
#8688=CARTESIAN_POINT ( 'NONE',  ( 6.684375000614518392, 6.421520780324663323E-16, -5.243569643749999010 ) ) ;
#8689=CARTESIAN_POINT ( 'NONE',  ( 23.10937500061451644, 0.000000000000000000, 5.243569643749999010 ) ) ;
#8690=CARTESIAN_POINT ( 'NONE',  ( 4.715814460642238970, -1.662339852463772916, 4.911777014959029408 ) ) ;
#8692=CARTESIAN_POINT ( 'NONE',  ( 19.22812500061451502, 6.421520780324663323E-16, -5.243569643749999010 ) ) ;
#8693=CARTESIAN_POINT ( 'NONE',  ( 24.00937500061451502, 0.000000000000000000, 5.243569643749999010 ) ) ;
#8697=CARTESIAN_POINT ( 'NONE',  ( 6.384375000614516793, 4.541064518000418104, 2.621784821874999949 ) ) ;
#8698=CARTESIAN_POINT ( 'NONE',  ( 17.20312500061451644, 0.000000000000000000, 5.243569643749999010 ) ) ;
#8699=ORIENTED_EDGE ( 'NONE', *, *, #16481, .T. ) ;
#8700=CARTESIAN_POINT ( 'NONE',  ( 22.80000000000000071, 0.000000000000000000, 4.999999999999998224 ) ) ;
#8701=CARTESIAN_POINT ( 'NONE',  ( 24.44062500061451715, -3.027376345333614438, 5.243569643749998122 ) ) ;
#8702=CARTESIAN_POINT ( 'NONE',  ( 2.000000000000001332, 17.00000000000000000, 33.46410161513774995 ) ) ;
#8703=CARTESIAN_POINT ( 'NONE',  ( 30.00000000000000000, 1.224646799147353059E-15, -9.999999999999998224 ) ) ;
#8704=CARTESIAN_POINT ( 'NONE',  ( 15.37500000000000000, 6.123233995736764310E-16, -4.999999999999998224 ) ) ;
#8705=CARTESIAN_POINT ( 'NONE',  ( 27.33750000122903145, 4.330127018922191873, 2.499999999999999556 ) ) ;
#8706=CARTESIAN_POINT ( 'NONE',  ( 21.44062500061452070, -3.027376345333610441, -5.243569643749999898 ) ) ;
#8708=CARTESIAN_POINT ( 'NONE',  ( 22.23750000000000071, 5.773502691896255534, 3.535250795749688894E-16 ) ) ;
#8709=CARTESIAN_POINT ( 'NONE',  ( 23.63437500061451502, -4.541064518000419881, 2.621784821874995952 ) ) ;
#8711=ORIENTED_EDGE ( 'NONE', *, *, #64551, .T. ) ;
#8713=CARTESIAN_POINT ( 'NONE',  ( 13.90312500061451750, 4.541064518000418104, -2.621784821874998173 ) ) ;
#8714=CARTESIAN_POINT ( 'NONE',  ( 3.440625000614518036, -3.027376345333610441, -5.243569643749999898 ) ) ;
#8716=CARTESIAN_POINT ( 'NONE',  ( 26.27812500061451573, -4.541064518000419881, 2.621784821874995952 ) ) ;
#8717=CARTESIAN_POINT ( 'NONE',  ( 13.01250000122903394, 0.000000000000000000, 4.999999999999998224 ) ) ;
#8718=CARTESIAN_POINT ( 'NONE',  ( 20.58750000000000213, -2.886751345948129988, 4.999999999999997335 ) ) ;
#8719=CARTESIAN_POINT ( 'NONE',  ( 25.91250000000000142, 2.886751345948126879, 4.999999999999999112 ) ) ;
#8720=CARTESIAN_POINT ( 'NONE',  ( 6.121875000614517504, -6.054752690667223547, -1.112240025338166033E-15 ) ) ;
#8721=CARTESIAN_POINT ( 'NONE',  ( 16.24687500061451573, 6.054752690667223547, 3.707466751127219781E-16 ) ) ;
#8722=VERTEX_POINT ( 'NONE', #26460 ) ;
#8723=CARTESIAN_POINT ( 'NONE',  ( 29.20312500061451644, 4.541064518000418104, -2.621784821874998173 ) ) ;
#8724=CARTESIAN_POINT ( 'NONE',  ( 26.74687500061451573, -3.027376345333614438, 5.243569643749998122 ) ) ;
#8726=CARTESIAN_POINT ( 'NONE',  ( 15.11249999999999893, 2.886751345948126879, 4.999999999999999112 ) ) ;
#8727=CARTESIAN_POINT ( 'NONE',  ( 12.51562500061451821, 3.027376345333613106, -5.243569643749998122 ) ) ;
#8730=CARTESIAN_POINT ( 'NONE',  ( 26.92499999999999716, -4.330127018922194537, 2.499999999999995559 ) ) ;
#8731=CARTESIAN_POINT ( 'NONE',  ( 19.16250000122903430, 4.330127018922192761, -2.499999999999997780 ) ) ;
#8732=CARTESIAN_POINT ( 'NONE',  ( 15.18750000122903465, 4.330127018922191873, 2.499999999999999556 ) ) ;
#8734=CARTESIAN_POINT ( 'NONE',  ( 8.765625000614518214, -6.054752690667223547, -1.112240025338166033E-15 ) ) ;
#8735=CARTESIAN_POINT ( 'NONE',  ( 25.39687500061451431, -3.027376345333614438, 5.243569643749998122 ) ) ;
#8736=EDGE_CURVE ( 'NONE', #44903, #53469, #38308, .T. ) ;
#8737=CARTESIAN_POINT ( 'NONE',  ( -2.121784821874996840, 17.23437500061451999, 33.67503911421598417 ) ) ;
#8738=CARTESIAN_POINT ( 'NONE',  ( 24.87187500061451573, 3.027376345333611329, 5.243569643749999010 ) ) ;
#8739=CARTESIAN_POINT ( 'NONE',  ( 5.362500000000003375, -5.773502691896255534, -1.060575238724906372E-15 ) ) ;
#8740=CARTESIAN_POINT ( 'NONE',  ( -2.828200636599751609E-16, 11.90000000122903501, 25.38119784648299770 ) ) ;
#8741=CARTESIAN_POINT ( 'NONE',  ( 12.89062500061451821, -3.027376345333610441, -5.243569643749999898 ) ) ;
#8742=CARTESIAN_POINT ( 'NONE',  ( 3.412500001229032964, 4.330127018922192761, -2.499999999999997780 ) ) ;
#8744=CARTESIAN_POINT ( 'NONE',  ( 9.121875000614517504, 3.027376345333611329, 5.243569643749999010 ) ) ;
#8745=CARTESIAN_POINT ( 'NONE',  ( -3.182292052831503071, 3.860956188314065507, -27.56400650891052351 ) ) ;
#8746=ORIENTED_EDGE ( 'NONE', *, *, #30487, .F. ) ;
#8747=CARTESIAN_POINT ( 'NONE',  ( 10.71562500061451928, 3.027376345333613106, -5.243569643749998122 ) ) ;
#8748=CARTESIAN_POINT ( 'NONE',  ( 13.62187500061451750, 3.027376345333611329, 5.243569643749999010 ) ) ;
#8750=CARTESIAN_POINT ( 'NONE',  ( 20.92500000122903714, 2.886751345948129099, -4.999999999999998224 ) ) ;
#8751=CARTESIAN_POINT ( 'NONE',  ( 11.18437500061451928, 6.421520780324663323E-16, -5.243569643749999010 ) ) ;
#8752=CARTESIAN_POINT ( 'NONE',  ( 13.22812500061451502, -4.541064518000419881, 2.621784821874995952 ) ) ;
#8754=CARTESIAN_POINT ( 'NONE',  ( 20.78437500061451715, 4.541064518000418104, 2.621784821874999949 ) ) ;
#8755=CARTESIAN_POINT ( 'NONE',  ( 0.000000000000000000, 0.000000000000000000, 50.00000000000000000 ) ) ;
#8758=CARTESIAN_POINT ( 'NONE',  ( 2.121784821874999061, 15.20937500061451786, -33.67503911421598417 ) ) ;
#8759=CARTESIAN_POINT ( 'NONE',  ( 16.73437500061451644, 4.541064518000418104, 2.621784821874999949 ) ) ;
#8760=CARTESIAN_POINT ( 'NONE',  ( 15.30000000122903359, -2.886751345948129988, 4.999999999999997335 ) ) ;
#8761=CARTESIAN_POINT ( 'NONE',  ( 11.07187500061451679, -6.054752690667223547, -1.112240025338166033E-15 ) ) ;
#8762=CARTESIAN_POINT ( 'NONE',  ( 4.243569643749999898, 17.32812500061451644, -30.00000000000000000 ) ) ;
#8763=CARTESIAN_POINT ( 'NONE',  ( 17.58750000122903145, -4.330127018922194537, 2.499999999999995559 ) ) ;
#8764=CARTESIAN_POINT ( 'NONE',  ( 11.57812500061451644, 6.421520780324663323E-16, -5.243569643749999010 ) ) ;
#8766=ORIENTED_EDGE ( 'NONE', *, *, #19281, .T. ) ;
#8767=CARTESIAN_POINT ( 'NONE',  ( 16.83749999999999858, 5.773502691896255534, 3.535250795749688894E-16 ) ) ;
#8768=CARTESIAN_POINT ( 'NONE',  ( 29.25000000000000000, -4.330127018922190985, -2.500000000000001332 ) ) ;
#8769=CARTESIAN_POINT ( 'NONE',  ( 9.346875000614517148, -3.027376345333610441, -5.243569643749999898 ) ) ;
#8770=CARTESIAN_POINT ( 'NONE',  ( 4.043974773626141328, 2.940596785297640459, 4.204683744944501811 ) ) ;
#8771=CARTESIAN_POINT ( 'NONE',  ( 12.11250000122903181, 0.000000000000000000, 4.999999999999998224 ) ) ;
#8772=CARTESIAN_POINT ( 'NONE',  ( 21.33750000122903145, 6.123233995736764310E-16, -4.999999999999998224 ) ) ;
#8773=CARTESIAN_POINT ( 'NONE',  ( 17.20312500061451644, 0.000000000000000000, 5.243569643749999010 ) ) ;
#8774=CARTESIAN_POINT ( 'NONE',  ( 19.71562500061451928, 3.027376345333613106, -5.243569643749998122 ) ) ;
#8775=CARTESIAN_POINT ( 'NONE',  ( 26.85000000122903430, 5.773502691896255534, 3.535250795749688894E-16 ) ) ;
#8776=CARTESIAN_POINT ( 'NONE',  ( 24.82499999999999929, 6.123233995736764310E-16, -4.999999999999998224 ) ) ;
#8777=CARTESIAN_POINT ( 'NONE',  ( 9.999999999999992895, -5.857864376269048101, 9.999999999999992895 ) ) ;
#8779=CARTESIAN_POINT ( 'NONE',  ( 28.88437500061451502, 4.541064518000418104, 2.621784821874999949 ) ) ;
#8780=CARTESIAN_POINT ( 'NONE',  ( -2.000000000000000000, 15.87500000000000000, 26.53589838486224650 ) ) ;
#8781=CARTESIAN_POINT ( 'NONE',  ( 4.243569643749999898, 14.19687500061451857, -27.54997392385601529 ) ) ;
#8782=CARTESIAN_POINT ( 'NONE',  ( 3.337500001229034563, 6.123233995736764310E-16, -4.999999999999998224 ) ) ;
#8783=CARTESIAN_POINT ( 'NONE',  ( 3.937500000000000444, -2.886751345948129988, 4.999999999999997335 ) ) ;
#8785=CARTESIAN_POINT ( 'NONE',  ( 7.434375000614519280, -4.541064518000419881, 2.621784821874995952 ) ) ;
#8786=CARTESIAN_POINT ( 'NONE',  ( 25.19062500061451715, 6.054752690667223547, 3.707466751127219781E-16 ) ) ;
#8788=CARTESIAN_POINT ( 'NONE',  ( 14.47499999999999964, 6.123233995736764310E-16, -4.999999999999998224 ) ) ;
#8791=EDGE_CURVE ( 'NONE', #28731, #66075, #26013, .T. ) ;
#8792=CARTESIAN_POINT ( 'NONE',  ( 5.559375000614517504, 0.000000000000000000, 5.243569643749999010 ) ) ;
#8793=CARTESIAN_POINT ( 'NONE',  ( 8.746875000614515727, -3.027376345333614438, 5.243569643749998122 ) ) ;
#8794=CARTESIAN_POINT ( 'NONE',  ( 3.225000000000002309, 6.123233995736764310E-16, -4.999999999999998224 ) ) ;
#8795=CARTESIAN_POINT ( 'NONE',  ( -4.243569643749998122, 12.19062500061459531, 32.45002607614398471 ) ) ;
#8796=CARTESIAN_POINT ( 'NONE',  ( 7.320879633048903241E-15, 17.63749999999999218, -34.00000000000000000 ) ) ;
#8797=CARTESIAN_POINT ( 'NONE',  ( 3.149999999999999911, -4.330127018922190985, -2.500000000000001332 ) ) ;
#8799=CARTESIAN_POINT ( 'NONE',  ( 19.90312500061451573, 0.000000000000000000, 5.243569643749999010 ) ) ;
#8800=CARTESIAN_POINT ( 'NONE',  ( 10.52812500061451750, -4.541064518000419881, 2.621784821874995952 ) ) ;
#8802=CARTESIAN_POINT ( 'NONE',  ( 9.196875000614518569, -3.027376345333614438, 5.243569643749998122 ) ) ;
#8803=CARTESIAN_POINT ( 'NONE',  ( 25.01249999999999929, 2.886751345948126879, 4.999999999999999112 ) ) ;
#8804=CARTESIAN_POINT ( 'NONE',  ( 19.38750000122903216, -4.330127018922194537, 2.499999999999995559 ) ) ;
#8805=CARTESIAN_POINT ( 'NONE',  ( 27.21562500061451928, -6.054752690667223547, -1.112240025338166033E-15 ) ) ;
#8807=CARTESIAN_POINT ( 'NONE',  ( 9.909375000614517148, 4.541064518000418104, -2.621784821874998173 ) ) ;
#8808=CARTESIAN_POINT ( 'NONE',  ( 14.48437500061451821, 4.541064518000418104, 2.621784821874999949 ) ) ;
#8809=CARTESIAN_POINT ( 'NONE',  ( 26.14687500061451431, 6.054752690667223547, 3.707466751127219781E-16 ) ) ;
#8812=CARTESIAN_POINT ( 'NONE',  ( 20.67187500061451289, 3.027376345333613106, -5.243569643749998122 ) ) ;
#8813=CARTESIAN_POINT ( 'NONE',  ( 11.67187500061451821, 3.027376345333613106, -5.243569643749998122 ) ) ;
#8815=CARTESIAN_POINT ( 'NONE',  ( 23.32499999999999929, -4.330127018922194537, 2.499999999999995559 ) ) ;
#8817=CARTESIAN_POINT ( 'NONE',  ( 4.243569643749999898, 11.53437500061451892, -30.00000000000000000 ) ) ;
#8819=CARTESIAN_POINT ( 'NONE',  ( 15.47812500061451679, -4.541064518000419881, 2.621784821874995952 ) ) ;
#8820=CARTESIAN_POINT ( 'NONE',  ( 3.937500000000000444, -2.886751345948129988, 4.999999999999997335 ) ) ;
#8821=CARTESIAN_POINT ( 'NONE',  ( -1.394453263437886604E-15, 19.32500000122903216, -26.00000000000000000 ) ) ;
#8822=CARTESIAN_POINT ( 'NONE',  ( 30.00000000000000000, 0.000000000000000000, 0.000000000000000000 ) ) ;
#8823=CARTESIAN_POINT ( 'NONE',  ( 11.92500000000000071, 4.330127018922191873, 2.499999999999999556 ) ) ;
#8824=CARTESIAN_POINT ( 'NONE',  ( 2.000000000000001332, 18.91250000122903430, 33.46410161513774995 ) ) ;
#8825=CARTESIAN_POINT ( 'NONE',  ( 10.65000000122903323, 5.773502691896255534, 3.535250795749688894E-16 ) ) ;
#8826=VECTOR ( 'NONE', #45717, 1000.000000000000000 ) ;
#8827=CARTESIAN_POINT ( 'NONE',  ( 23.40937500061451715, 4.541064518000418104, -2.621784821874998173 ) ) ;
#8828=CARTESIAN_POINT ( 'NONE',  ( 15.68437500061451573, 6.421520780324663323E-16, -5.243569643749999010 ) ) ;
#8830=ORIENTED_EDGE ( 'NONE', *, *, #53492, .T. ) ;
#8831=CARTESIAN_POINT ( 'NONE',  ( 17.84062500061451573, -3.027376345333610441, -5.243569643749999898 ) ) ;
#8832=CARTESIAN_POINT ( 'NONE',  ( 3.853125000614517681, -4.541064518000417216, -2.621784821875001281 ) ) ;
#8833=CARTESIAN_POINT ( 'NONE',  ( 17.40937500061451715, -4.541064518000417216, -2.621784821875001281 ) ) ;
#8834=CARTESIAN_POINT ( 'NONE',  ( 28.95937500061451431, 0.000000000000000000, 5.243569643749999010 ) ) ;
#8835=CARTESIAN_POINT ( 'NONE',  ( 4.003125000614518925, 4.541064518000418104, -2.621784821874998173 ) ) ;
#8836=CARTESIAN_POINT ( 'NONE',  ( 19.30312500061451786, 4.541064518000418104, -2.621784821874998173 ) ) ;
#8837=CARTESIAN_POINT ( 'NONE',  ( -4.243569643749999898, 14.40312500061451750, 30.00000000000000000 ) ) ;
#8838=CARTESIAN_POINT ( 'NONE',  ( 17.43750000122903288, 4.330127018922191873, 2.499999999999999556 ) ) ;
#8840=CARTESIAN_POINT ( 'NONE',  ( 7.078125000614516438, 6.421520780324663323E-16, -5.243569643749999010 ) ) ;
#8841=CARTESIAN_POINT ( 'NONE',  ( 28.82812500061451644, 4.541064518000418104, 2.621784821874999949 ) ) ;
#8842=CARTESIAN_POINT ( 'NONE',  ( 9.825000001229032165, 2.886751345948126879, 4.999999999999998224 ) ) ;
#8843=CARTESIAN_POINT ( 'NONE',  ( 22.32187500061451502, -6.054752690667223547, -1.112240025338166033E-15 ) ) ;
#8844=CARTESIAN_POINT ( 'NONE',  ( 14.39062500061451821, 6.054752690667223547, 3.707466751127219781E-16 ) ) ;
#8845=CARTESIAN_POINT ( 'NONE',  ( 24.86250000122903359, -4.330127018922190985, -2.500000000000001332 ) ) ;
#8846=CARTESIAN_POINT ( 'NONE',  ( 23.69062500061451004, -3.027376345333610441, -5.243569643749999898 ) ) ;
#8847=CARTESIAN_POINT ( 'NONE',  ( 19.54687500061451644, -3.027376345333614438, 5.243569643749998122 ) ) ;
#8848=CARTESIAN_POINT ( 'NONE',  ( 14.05312500061451431, 0.000000000000000000, 5.243569643749999010 ) ) ;
#8849=CARTESIAN_POINT ( 'NONE',  ( 4.243569643749999010, 14.27187500061451964, 27.54997392385601174 ) ) ;
#8850=CARTESIAN_POINT ( 'NONE',  ( 19.30312500061451786, 4.541064518000418104, -2.621784821874998173 ) ) ;
#8851=CARTESIAN_POINT ( 'NONE',  ( 29.35312500061451502, 0.000000000000000000, 5.243569643749999010 ) ) ;
#8852=EDGE_LOOP ( 'NONE', ( #41260, #26213, #43941, #556 ) ) ;
#8854=CARTESIAN_POINT ( 'NONE',  ( 24.11249999999999716, 2.886751345948126879, 4.999999999999999112 ) ) ;
#8855=CARTESIAN_POINT ( 'NONE',  ( 3.999999999999999112, 10.32500000000000107, -30.00000000000000000 ) ) ;
#8856=CARTESIAN_POINT ( 'NONE',  ( 13.08750000122903323, -4.330127018922194537, 2.499999999999995559 ) ) ;
#8857=CARTESIAN_POINT ( 'NONE',  ( 27.14062500061451644, -3.027376345333614438, 5.243569643749998122 ) ) ;
#8858=CARTESIAN_POINT ( 'NONE',  ( 7.528125000614515727, 6.421520780324663323E-16, -5.243569643749999010 ) ) ;
#8859=CARTESIAN_POINT ( 'NONE',  ( 19.16250000122903430, 4.330127018922192761, -2.499999999999997780 ) ) ;
#8860=CARTESIAN_POINT ( 'NONE',  ( 24.32812500061451289, 4.541064518000418104, 2.621784821874999949 ) ) ;
#8861=CARTESIAN_POINT ( 'NONE',  ( 23.85000000000000142, -4.330127018922190985, -2.500000000000001332 ) ) ;
#8862=CARTESIAN_POINT ( 'NONE',  ( 28.26562500061451289, 3.027376345333613106, -5.243569643749998122 ) ) ;
#8863=CARTESIAN_POINT ( 'NONE',  ( 8.765625000614518214, -6.054752690667223547, -1.112240025338166033E-15 ) ) ;
#8864=VERTEX_POINT ( 'NONE', #40474 ) ;
#8866=CARTESIAN_POINT ( 'NONE',  ( 24.36562500061451786, 3.027376345333611329, 5.243569643749999010 ) ) ;
#8867=CARTESIAN_POINT ( 'NONE',  ( 5.465625000614517504, 3.027376345333611329, 5.243569643749999010 ) ) ;
#8869=CARTESIAN_POINT ( 'NONE',  ( 3.253125000614518036, 0.000000000000000000, 5.243569643749999010 ) ) ;
#8870=CARTESIAN_POINT ( 'NONE',  ( 8.484601909799253346E-16, 12.57500000122903216, -25.38119784648299770 ) ) ;
#8871=CARTESIAN_POINT ( 'NONE',  ( -1.071796769724491005, 13.60759618943233384, -34.00000000000000000 ) ) ;
#8873=CARTESIAN_POINT ( 'NONE',  ( 10.83750000000000036, -2.886751345948125991, -5.000000000000000000 ) ) ;
#8875=CARTESIAN_POINT ( 'NONE',  ( 11.07187500061451679, -6.054752690667223547, -1.112240025338166033E-15 ) ) ;
#8876=CARTESIAN_POINT ( 'NONE',  ( 9.975000001229034297, -5.773502691896255534, -1.060575238724906372E-15 ) ) ;
#8877=CARTESIAN_POINT ( 'NONE',  ( 14.82187500061451679, 3.027376345333613106, -5.243569643749998122 ) ) ;
#8879=CARTESIAN_POINT ( 'NONE',  ( 6.871875000614517504, 3.027376345333611329, 5.243569643749999010 ) ) ;
#8880=CARTESIAN_POINT ( 'NONE',  ( 2.121784821875001281, 10.05312500061451608, -26.32496088578401938 ) ) ;
#8881=CIRCLE ( 'NONE', #60761, 5.999999999999998224 ) ;
#8882=DIRECTION ( 'NONE',  ( 0.000000000000000000, 0.000000000000000000, 1.000000000000000000 ) ) ;
#8884=CARTESIAN_POINT ( 'NONE',  ( 13.05937500061451750, 4.541064518000418104, -2.621784821874998173 ) ) ;
#8885=CARTESIAN_POINT ( 'NONE',  ( 13.23750000000000071, 5.773502691896255534, 3.535250795749688401E-16 ) ) ;
#8886=CARTESIAN_POINT ( 'NONE',  ( 23.09062500061451573, -3.027376345333614438, 5.243569643749998122 ) ) ;
#8887=CARTESIAN_POINT ( 'NONE',  ( 2.121784821875001281, 11.00937500061451857, 33.67503911421598417 ) ) ;
#8888=CARTESIAN_POINT ( 'NONE',  ( 11.28749999999999964, -2.886751345948126435, -5.000000000000000000 ) ) ;
#8889=CARTESIAN_POINT ( 'NONE',  ( 27.04687500061451644, 6.054752690667223547, 3.707466751127219781E-16 ) ) ;
#8890=( BOUNDED_CURVE ( )  B_SPLINE_CURVE ( 2, ( #71518, #39363, #44908, #54888, #27914, #15349, #10187 ),
 .UNSPECIFIED., .F., .F. ) 
 B_SPLINE_CURVE_WITH_KNOTS ( ( 3, 2, 2, 3 ),
 ( 0.8083333333333333481, 0.8111111111111111160, 0.8138888888888888840, 0.8166666666666666519 ),
 .UNSPECIFIED. ) 
 CURVE ( )  GEOMETRIC_REPRESENTATION_ITEM ( )  RATIONAL_B_SPLINE_CURVE ( ( 1.000000000000000000, 0.8660254037844387076, 1.000000000000000000, 0.8660254037844387076, 1.000000000000000000, 0.8660254037844387076, 1.000000000000000000 ) ) 
 REPRESENTATION_ITEM ( '' )  );
#8891=CARTESIAN_POINT ( 'NONE',  ( 15.78750000122903430, -4.330127018922194537, 2.499999999999995559 ) ) ;
#8892=CARTESIAN_POINT ( 'NONE',  ( 5.353125000614515905, 4.541064518000418104, -2.621784821874998173 ) ) ;
#8894=CARTESIAN_POINT ( 'NONE',  ( 17.37187500061451573, -6.054752690667223547, -1.112240025338166033E-15 ) ) ;
#8896=CARTESIAN_POINT ( 'NONE',  ( 27.52500000122903145, -5.773502691896255534, -1.060575238724906372E-15 ) ) ;
#8897=CARTESIAN_POINT ( 'NONE',  ( 5.559375000614517504, 0.000000000000000000, 5.243569643749999010 ) ) ;
#8898=CARTESIAN_POINT ( 'NONE',  ( 17.29687500061451999, -3.027376345333614438, 5.243569643749998122 ) ) ;
#8900=CARTESIAN_POINT ( 'NONE',  ( 23.47499999999999787, 6.123233995736764310E-16, -4.999999999999998224 ) ) ;
#8901=CARTESIAN_POINT ( 'NONE',  ( 3.375000001229033320, 2.886751345948129099, -4.999999999999998224 ) ) ;
#8902=CARTESIAN_POINT ( 'NONE',  ( 27.38437500061451857, 6.421520780324663323E-16, -5.243569643749999010 ) ) ;
#8905=CARTESIAN_POINT ( 'NONE',  ( 5.775000001229033231, 2.886751345948126879, 4.999999999999998224 ) ) ;
#8906=CARTESIAN_POINT ( 'NONE',  ( 8.662499999999999645, 2.886751345948129099, -4.999999999999998224 ) ) ;
#8908=CARTESIAN_POINT ( 'NONE',  ( 22.34062500061451573, -3.027376345333610441, -5.243569643749999898 ) ) ;
#8909=CARTESIAN_POINT ( 'NONE',  ( 11.43750000000000000, 5.773502691896255534, 3.535250795749688894E-16 ) ) ;
#8910=CARTESIAN_POINT ( 'NONE',  ( 3.065625000614517592, 3.027376345333613106, -5.243569643749998122 ) ) ;
#8911=CARTESIAN_POINT ( 'NONE',  ( 18.78749999999999432, -2.886751345948129988, 4.999999999999997335 ) ) ;
#8912=CARTESIAN_POINT ( 'NONE',  ( 19.22812500061451502, 6.421520780324663323E-16, -5.243569643749999010 ) ) ;
#8913=CARTESIAN_POINT ( 'NONE',  ( 4.102673862605173305, -2.857983061023190441, 4.201819747086521062 ) ) ;
#8914=CARTESIAN_POINT ( 'NONE',  ( 23.81250000122903288, 0.000000000000000000, 4.999999999999998224 ) ) ;
#8916=CARTESIAN_POINT ( 'NONE',  ( 29.78437500061451715, 4.541064518000418104, 2.621784821874999949 ) ) ;
#8917=AXIS2_PLACEMENT_3D ( 'NONE', #46832, #57892, #63802 ) ;
#8918=ORIENTED_EDGE ( 'NONE', *, *, #25401, .T. ) ;
#8919=CARTESIAN_POINT ( 'NONE',  ( 19.97812500061451502, -4.541064518000419881, 2.621784821874995952 ) ) ;
#8920=CARTESIAN_POINT ( 'NONE',  ( 27.96562500061451928, 3.027376345333611329, 5.243569643749999010 ) ) ;
#8921=CARTESIAN_POINT ( 'NONE',  ( 25.39687500061451431, -3.027376345333614438, 5.243569643749998122 ) ) ;
#8922=CARTESIAN_POINT ( 'NONE',  ( 7.800000000000001599, 4.330127018922192761, -2.499999999999997780 ) ) ;
#8923=CARTESIAN_POINT ( 'NONE',  ( 11.42812500061451608, -4.541064518000419881, 2.621784821874995952 ) ) ;
#8924=CARTESIAN_POINT ( 'NONE',  ( 27.10312500061451502, 0.000000000000000000, 5.243569643749999010 ) ) ;
#8925=CARTESIAN_POINT ( 'NONE',  ( 17.22187500061451715, 3.027376345333611329, 5.243569643749999010 ) ) ;
#8926=CARTESIAN_POINT ( 'NONE',  ( 8.653125000614515727, 0.000000000000000000, 5.243569643749999010 ) ) ;
#8927=CARTESIAN_POINT ( 'NONE',  ( 3.017996468573438396, -3.986467487895139605, 3.151570663109291459 ) ) ;
#8928=CARTESIAN_POINT ( 'NONE',  ( -4.243569643749999898, 11.27187500061451608, 27.54997392385601529 ) ) ;
#8929=CARTESIAN_POINT ( 'NONE',  ( 24.26250000122903216, 0.000000000000000000, 4.999999999999998224 ) ) ;
#8931=CARTESIAN_POINT ( 'NONE',  ( 14.16562500061451679, -6.054752690667223547, -1.112240025338166033E-15 ) ) ;
#8932=CARTESIAN_POINT ( 'NONE',  ( 9.871875000614517504, 3.027376345333613106, -5.243569643749998122 ) ) ;
#8933=CARTESIAN_POINT ( 'NONE',  ( 10.28437500061451715, 6.421520780324663323E-16, -5.243569643749999010 ) ) ;
#8934=ORIENTED_EDGE ( 'NONE', *, *, #26985, .T. ) ;
#8935=CARTESIAN_POINT ( 'NONE',  ( 15.15000000000000036, 0.000000000000000000, 4.999999999999998224 ) ) ;
#8936=CARTESIAN_POINT ( 'NONE',  ( 21.66562500061451502, 3.027376345333611329, 5.243569643749999010 ) ) ;
#8937=CARTESIAN_POINT ( 'NONE',  ( 17.14687500061451786, 6.054752690667223547, 3.707466751127219781E-16 ) ) ;
#8938=CARTESIAN_POINT ( 'NONE',  ( 20.95312500061451999, -4.541064518000417216, -2.621784821875001281 ) ) ;
#8939=CARTESIAN_POINT ( 'NONE',  ( 4.000000000000000000, 11.63750000000000284, 32.30940107675849049 ) ) ;
#8940=CARTESIAN_POINT ( 'NONE',  ( 27.21562500061451928, -6.054752690667223547, -1.112240025338166033E-15 ) ) ;
#8941=CARTESIAN_POINT ( 'NONE',  ( 6.112500001229034474, 4.330127018922192761, -2.499999999999997780 ) ) ;
#8943=CARTESIAN_POINT ( 'NONE',  ( 3.112500001229034918, 0.000000000000000000, 4.999999999999998224 ) ) ;
#8944=CARTESIAN_POINT ( 'NONE',  ( 2.000000000000001332, 17.44999999999999929, -26.53589838486224650 ) ) ;
#8945=CARTESIAN_POINT ( 'NONE',  ( 25.80000000122903714, -2.886751345948125991, -5.000000000000000000 ) ) ;
#8947=CARTESIAN_POINT ( 'NONE',  ( 6.309375000614517504, 4.541064518000418104, -2.621784821874998173 ) ) ;
#8948=CARTESIAN_POINT ( 'NONE',  ( 15.62812500061451537, 6.421520780324663323E-16, -5.243569643749999010 ) ) ;
#8949=CARTESIAN_POINT ( 'NONE',  ( 8.409375000614518925, -4.541064518000417216, -2.621784821875001281 ) ) ;
#8950=CARTESIAN_POINT ( 'NONE',  ( 26.25000000122903288, -2.886751345948125991, -5.000000000000000000 ) ) ;
#8952=CARTESIAN_POINT ( 'NONE',  ( 17.52187500061451431, 3.027376345333612662, -5.243569643749998122 ) ) ;
#8953=CARTESIAN_POINT ( 'NONE',  ( 6.159375000614517148, -4.541064518000417216, -2.621784821875001281 ) ) ;
#8954=DIRECTION ( 'NONE',  ( 0.000000000000000000, 0.000000000000000000, 1.000000000000000000 ) ) ;
#8955=CARTESIAN_POINT ( 'NONE',  ( 5.728125000614515905, 6.421520780324663323E-16, -5.243569643749999010 ) ) ;
#8956=( BOUNDED_CURVE ( )  B_SPLINE_CURVE ( 2, ( #270, #637, #67867, #57490, #46417, #39799, #23144 ),
 .UNSPECIFIED., .F., .F. ) 
 B_SPLINE_CURVE_WITH_KNOTS ( ( 3, 2, 2, 3 ),
 ( 0.8583333333333332815, 0.8611111111111111605, 0.8638888888888889284, 0.8666666666666666963 ),
 .UNSPECIFIED. ) 
 CURVE ( )  GEOMETRIC_REPRESENTATION_ITEM ( )  RATIONAL_B_SPLINE_CURVE ( ( 1.000000000000000000, 0.8660254037844387076, 1.000000000000000000, 0.8660254037844387076, 1.000000000000000000, 0.8660254037844387076, 1.000000000000000000 ) ) 
 REPRESENTATION_ITEM ( '' )  );
#8957=CARTESIAN_POINT ( 'NONE',  ( 15.02812500061451750, -4.541064518000419881, 2.621784821874995952 ) ) ;
#8958=VERTEX_POINT ( 'NONE', #46376 ) ;
#8959=CARTESIAN_POINT ( 'NONE',  ( 12.51562500061451821, 3.027376345333613106, -5.243569643749998122 ) ) ;
#8960=CARTESIAN_POINT ( 'NONE',  ( 6.262500001229034829, 0.000000000000000000, 4.999999999999998224 ) ) ;
#8961=CARTESIAN_POINT ( 'NONE',  ( 10.60312500061451679, -4.541064518000417216, -2.621784821875001281 ) ) ;
#8963=CARTESIAN_POINT ( 'NONE',  ( 11.28749999999999787, -2.886751345948125991, -5.000000000000000000 ) ) ;
#8964=CARTESIAN_POINT ( 'NONE',  ( 4.012500001229033053, 0.000000000000000000, 4.999999999999998224 ) ) ;
#8965=CARTESIAN_POINT ( 'NONE',  ( 20.36249999999999716, 2.886751345948129099, -4.999999999999998224 ) ) ;
#8968=CARTESIAN_POINT ( 'NONE',  ( 17.97187500061451715, 3.027376345333613106, -5.243569643749998122 ) ) ;
#8969=CARTESIAN_POINT ( 'NONE',  ( 16.12500000122903288, 2.886751345948126879, 4.999999999999999112 ) ) ;
#8971=AXIS2_PLACEMENT_3D ( 'NONE', #62194, #68108, #45209 ) ;
#8972=CARTESIAN_POINT ( 'NONE',  ( 4.243569643749999898, 16.87812500061451715, -30.00000000000000000 ) ) ;
#8973=DIRECTION ( 'NONE',  ( 0.000000000000000000, 0.000000000000000000, -1.000000000000000000 ) ) ;
#8974=CARTESIAN_POINT ( 'NONE',  ( 29.05312500061451431, -4.541064518000417216, -2.621784821875001281 ) ) ;
#8977=CARTESIAN_POINT ( 'NONE',  ( 16.43437500061451573, -4.541064518000419881, 2.621784821874995952 ) ) ;
#8979=CARTESIAN_POINT ( 'NONE',  ( 11.05312500061451608, -4.541064518000417216, -2.621784821875001281 ) ) ;
#8981=PRODUCT_DEFINITION_SHAPE ( 'NONE', 'NONE',  #45867 ) ;
#8982=CARTESIAN_POINT ( 'NONE',  ( 23.18437500061451573, -4.541064518000419881, 2.621784821874995952 ) ) ;
#8984=CARTESIAN_POINT ( 'NONE',  ( 6.815625000614517148, 3.027376345333611329, 5.243569643749999010 ) ) ;
#8985=CARTESIAN_POINT ( 'NONE',  ( 14.25937500061451679, -4.541064518000417216, -2.621784821875001281 ) ) ;
#8986=ORIENTED_EDGE ( 'NONE', *, *, #32530, .T. ) ;
#8987=CARTESIAN_POINT ( 'NONE',  ( 24.42187500061451999, 3.027376345333611329, 5.243569643749999010 ) ) ;
#8988=CARTESIAN_POINT ( 'NONE',  ( 28.11562500061451431, -6.054752690667223547, -1.112240025338166033E-15 ) ) ;
#8990=CARTESIAN_POINT ( 'NONE',  ( 6.450000000000001066, 4.330127018922192761, -2.499999999999997780 ) ) ;
#8991=CARTESIAN_POINT ( 'NONE',  ( 15.97500000122903430, 2.886751345948129099, -4.999999999999998224 ) ) ;
#8992=CARTESIAN_POINT ( 'NONE',  ( -3.999999999999999112, 17.82500000122903572, -32.30940107675850470 ) ) ;
#8995=CARTESIAN_POINT ( 'NONE',  ( 15.15000000000000036, 0.000000000000000000, 4.999999999999998224 ) ) ;
#8996=CARTESIAN_POINT ( 'NONE',  ( 19.72499999999999787, -4.330127018922194537, 2.499999999999995559 ) ) ;
#8997=CARTESIAN_POINT ( 'NONE',  ( 12.59062500061451573, 6.054752690667223547, 3.707466751127219781E-16 ) ) ;
#9000=CARTESIAN_POINT ( 'NONE',  ( -3.000416591977282496E-16, 16.59687500061452070, -34.90005215228797653 ) ) ;
#9001=CARTESIAN_POINT ( 'NONE',  ( 3.928125000614516527, 6.421520780324663323E-16, -5.243569643749999010 ) ) ;
#9003=CARTESIAN_POINT ( 'NONE',  ( 13.12500000000000178, 6.123233995736764310E-16, -4.999999999999998224 ) ) ;
#9006=CARTESIAN_POINT ( 'NONE',  ( 2.121784821875001281, 16.35312500061451857, 33.67503911421598417 ) ) ;
#9007=CARTESIAN_POINT ( 'NONE',  ( 26.31562500061451715, -6.054752690667223547, -1.112240025338166033E-15 ) ) ;
#9008=DIRECTION ( 'NONE',  ( 0.000000000000000000, 0.000000000000000000, -1.000000000000000000 ) ) ;
#9010=CARTESIAN_POINT ( 'NONE',  ( 24.57187500061451502, -6.054752690667223547, -1.112240025338166033E-15 ) ) ;
#9011=CARTESIAN_POINT ( 'NONE',  ( 18.32812500061451644, 6.421520780324663323E-16, -5.243569643749999010 ) ) ;
#9013=CARTESIAN_POINT ( 'NONE',  ( -2.121784821874996840, 13.12812500061459176, -26.32496088578401583 ) ) ;
#9014=CARTESIAN_POINT ( 'NONE',  ( 24.56250000122903288, 4.330127018922192761, -2.499999999999997780 ) ) ;
#9016=CARTESIAN_POINT ( 'NONE',  ( 5.090625000614516615, -3.027376345333614438, 5.243569643749998122 ) ) ;
#9018=CARTESIAN_POINT ( 'NONE',  ( 20.35312500061451502, 0.000000000000000000, 5.243569643749999010 ) ) ;
#9021=CARTESIAN_POINT ( 'NONE',  ( 17.89687500061451431, -3.027376345333610441, -5.243569643749999898 ) ) ;
#9022=CARTESIAN_POINT ( 'NONE',  ( 16.32187500061451502, 3.027376345333611329, 5.243569643749999010 ) ) ;
#9023=CARTESIAN_POINT ( 'NONE',  ( 25.35937500061451644, 0.000000000000000000, 5.243569643749999010 ) ) ;
#9024=CARTESIAN_POINT ( 'NONE',  ( -2.121784821874999949, 13.93437500061451750, 26.32496088578401938 ) ) ;
#9025=CARTESIAN_POINT ( 'NONE',  ( 5.428125000614517859, 4.541064518000418104, 2.621784821874999949 ) ) ;
#9026=CARTESIAN_POINT ( 'NONE',  ( 28.15312500061451573, -4.541064518000417216, -2.621784821875001281 ) ) ;
#9027=CARTESIAN_POINT ( 'NONE',  ( 2.896875000614518747, -3.027376345333614438, 5.243569643749998122 ) ) ;
#9029=CARTESIAN_POINT ( 'NONE',  ( -3.999999999999999112, 18.64999999999999858, 30.00000000000000000 ) ) ;
#9030=AXIS2_PLACEMENT_3D ( 'NONE', #62036, #12148, #49869 ) ;
#9031=CARTESIAN_POINT ( 'NONE',  ( 7.246875000614518392, 6.054752690667223547, 3.707466751127219781E-16 ) ) ;
#9032=CARTESIAN_POINT ( 'NONE',  ( 13.76250000122903394, 4.330127018922192761, -2.499999999999997780 ) ) ;
#9033=CARTESIAN_POINT ( 'NONE',  ( 10.05000000122903181, -2.886751345948125991, -5.000000000000000000 ) ) ;
#9034=CARTESIAN_POINT ( 'NONE',  ( 5.015625000614518214, 3.027376345333611329, 5.243569643749999010 ) ) ;
#9037=CARTESIAN_POINT ( 'NONE',  ( 14.63437500061451679, -4.541064518000419881, 2.621784821874995952 ) ) ;
#9038=CARTESIAN_POINT ( 'NONE',  ( 10.00000000000000000, 1.224646799147353256E-15, 50.00000000000000000 ) ) ;
#9039=EDGE_LOOP ( 'NONE', ( #49478, #2361, #5672, #54652 ) ) ;
#9040=CARTESIAN_POINT ( 'NONE',  ( 22.37812500061451360, 6.421520780324663323E-16, -5.243569643749999010 ) ) ;
#9041=CARTESIAN_POINT ( 'NONE',  ( 6.553125000614518747, -4.541064518000417216, -2.621784821875001281 ) ) ;
#9042=CARTESIAN_POINT ( 'NONE',  ( 24.75937500061451502, 4.541064518000418104, -2.621784821874998173 ) ) ;
#9043=CARTESIAN_POINT ( 'NONE',  ( 7.303125000614516082, 0.000000000000000000, 5.243569643749999010 ) ) ;
#9045=CARTESIAN_POINT ( 'NONE',  ( 9.037500001229034297, -4.330127018922194537, 2.499999999999995559 ) ) ;
#9046=CARTESIAN_POINT ( 'NONE',  ( 21.74062500061451431, -3.027376345333614438, 5.243569643749998122 ) ) ;
#9047=CARTESIAN_POINT ( 'NONE',  ( -4.243569643749999898, 10.31562500061451715, -32.45002607614398471 ) ) ;
#9048=CARTESIAN_POINT ( 'NONE',  ( 11.32500000122903394, -5.773502691896255534, -1.060575238724906372E-15 ) ) ;
#9049=CARTESIAN_POINT ( 'NONE',  ( 20.24062500061451431, 6.054752690667223547, 3.707466751127219781E-16 ) ) ;
#9050=CARTESIAN_POINT ( 'NONE',  ( 19.00312500061451715, 0.000000000000000000, 5.243569643749999010 ) ) ;
#9052=CARTESIAN_POINT ( 'NONE',  ( 18.93750000000000000, -2.886751345948125991, -5.000000000000000000 ) ) ;
#9053=CARTESIAN_POINT ( 'NONE',  ( 11.36250000122903536, -4.330127018922190985, -2.500000000000001332 ) ) ;
#9055=CARTESIAN_POINT ( 'NONE',  ( 7.715625000614515727, 3.027376345333611329, 5.243569643749999010 ) ) ;
#9056=CARTESIAN_POINT ( 'NONE',  ( 13.94062500061451892, 6.054752690667223547, 3.707466751127219781E-16 ) ) ;
#9057=CARTESIAN_POINT ( 'NONE',  ( 22.61250000122903003, -4.330127018922190985, -2.500000000000001332 ) ) ;
#9058=CARTESIAN_POINT ( 'NONE',  ( 20.78437500061451715, 4.541064518000418104, 2.621784821874999949 ) ) ;
#9060=CARTESIAN_POINT ( 'NONE',  ( 4.350000001229033408, 5.773502691896255534, 3.535250795749688894E-16 ) ) ;
#9061=CARTESIAN_POINT ( 'NONE',  ( 7.396875000614519635, -3.027376345333614438, 5.243569643749998122 ) ) ;
#9062=CARTESIAN_POINT ( 'NONE',  ( 22.20937500061451431, 0.000000000000000000, 5.243569643749999010 ) ) ;
#9064=CARTESIAN_POINT ( 'NONE',  ( 19.64062500061451644, -3.027376345333610441, -5.243569643749999898 ) ) ;
#9065=CARTESIAN_POINT ( 'NONE',  ( 23.48437500061451644, 4.541064518000418104, 2.621784821874999949 ) ) ;
#9067=CARTESIAN_POINT ( 'NONE',  ( 27.67500000122903359, 2.886751345948146419, -4.999999999999968914 ) ) ;
#9068=CARTESIAN_POINT ( 'NONE',  ( 5.296875000614518214, -3.027376345333610441, -5.243569643749999898 ) ) ;
#9069=CARTESIAN_POINT ( 'NONE',  ( 16.07812500061451289, 6.421520780324663323E-16, -5.243569643749999010 ) ) ;
#9070=CARTESIAN_POINT ( 'NONE',  ( 13.35937500061451821, -4.541064518000417216, -2.621784821875001281 ) ) ;
#9071=VERTEX_POINT ( 'NONE', #13655 ) ;
#9072=CARTESIAN_POINT ( 'NONE',  ( 22.19999999999999574, 4.330127018922192761, -2.499999999999997780 ) ) ;
#9073=CARTESIAN_POINT ( 'NONE',  ( 24.36562500061451786, 3.027376345333611329, 5.243569643749999010 ) ) ;
#9074=CARTESIAN_POINT ( 'NONE',  ( 1.071796769724484344, 16.98259618943233562, 34.00000000000000000 ) ) ;
#9075=CARTESIAN_POINT ( 'NONE',  ( -3.999999999999999112, 18.27500000122903501, 27.69059892324149885 ) ) ;
#9076=CARTESIAN_POINT ( 'NONE',  ( 15.33750000000000036, -2.886751345948125991, -5.000000000000000000 ) ) ;
#9077=CARTESIAN_POINT ( 'NONE',  ( 23.85000000122903430, -2.886751345948129988, 4.999999999999997335 ) ) ;
#9078=CARTESIAN_POINT ( 'NONE',  ( 17.50312500061451715, 4.541064518000418104, -2.621784821874998173 ) ) ;
#9080=CARTESIAN_POINT ( 'NONE',  ( 23.36250000000000071, -5.773502691896255534, -1.060575238724906372E-15 ) ) ;
#9081=CARTESIAN_POINT ( 'NONE',  ( 24.34687500061451715, 6.054752690667223547, 3.707466751127219781E-16 ) ) ;
#9082=ORIENTED_EDGE ( 'NONE', *, *, #50559, .T. ) ;
#9084=CARTESIAN_POINT ( 'NONE',  ( 9.553125000614517859, 0.000000000000000000, 5.243569643749999010 ) ) ;
#9085=CARTESIAN_POINT ( 'NONE',  ( 4.340625000614515727, -3.027376345333610441, -5.243569643749999898 ) ) ;
#9087=CARTESIAN_POINT ( 'NONE',  ( 26.57812500061451644, 4.541064518000418104, 2.621784821874999949 ) ) ;
#9088=CARTESIAN_POINT ( 'NONE',  ( 20.43749999999999645, 5.773502691896255534, 3.535250795749688894E-16 ) ) ;
#9089=CARTESIAN_POINT ( 'NONE',  ( 27.11249999999999716, 2.886751345948129099, -4.999999999999998224 ) ) ;
#9091=CARTESIAN_POINT ( 'NONE',  ( 7.921875000614517326, -6.054752690667223547, -1.112240025338166033E-15 ) ) ;
#9092=CARTESIAN_POINT ( 'NONE',  ( 17.74687500061451928, -3.027376345333614438, 5.243569643749998122 ) ) ;
#9093=CARTESIAN_POINT ( 'NONE',  ( -3.137519842735245283E-14, 11.22500000122903430, 34.00000000000000000 ) ) ;
#9095=CARTESIAN_POINT ( 'NONE',  ( 25.90312500061451573, -4.541064518000417216, -2.621784821875001281 ) ) ;
#9096=CARTESIAN_POINT ( 'NONE',  ( 28.28437500061451715, 6.421520780324663323E-16, -5.243569643749999010 ) ) ;
#9098=CARTESIAN_POINT ( 'NONE',  ( 15.78749999999999964, -2.886751345948125991, -5.000000000000000000 ) ) ;
#9099=CARTESIAN_POINT ( 'NONE',  ( 12.10312500061451857, 4.541064518000418104, -2.621784821874998173 ) ) ;
#9100=DIRECTION ( 'NONE',  ( -1.000000000000000000, -0.000000000000000000, -0.000000000000000000 ) ) ;
#9102=CARTESIAN_POINT ( 'NONE',  ( 28.30312500061451431, 4.541064518000418104, -2.621784821874998173 ) ) ;
#9103=CARTESIAN_POINT ( 'NONE',  ( 18.82500000122903216, 2.886751345948126879, 4.999999999999999112 ) ) ;
#9106=CARTESIAN_POINT ( 'NONE',  ( 6.140625000614516438, -3.027376345333610441, -5.243569643749999898 ) ) ;
#9107=CARTESIAN_POINT ( 'NONE',  ( 23.07187500061451857, 3.027376345333611329, 5.243569643749999010 ) ) ;
#9108=CARTESIAN_POINT ( 'NONE',  ( 4.243569643749999898, 17.83437500061451786, 30.00000000000000000 ) ) ;
#9109=CARTESIAN_POINT ( 'NONE',  ( 24.68437500061451573, 6.421520780324663323E-16, -5.243569643749999010 ) ) ;
#9110=CARTESIAN_POINT ( 'NONE',  ( 5.325000000000000178, -4.330127018922194537, 2.499999999999995559 ) ) ;
#9111=CARTESIAN_POINT ( 'NONE',  ( -3.999999999999999556, 10.17500000122903359, 27.69059892324149530 ) ) ;
#9112=CARTESIAN_POINT ( 'NONE',  ( 13.15312500061451750, 0.000000000000000000, 5.243569643749999010 ) ) ;
#9113=CARTESIAN_POINT ( 'NONE',  ( 5.437500001229035540, -4.330127018922194537, 2.499999999999995559 ) ) ;
#9114=CARTESIAN_POINT ( 'NONE',  ( 9.684375000614517504, -4.541064518000419881, 2.621784821874995952 ) ) ;
#9115=CARTESIAN_POINT ( 'NONE',  ( 7.050000000000000711, 0.000000000000000000, 4.999999999999998224 ) ) ;
#9116=CARTESIAN_POINT ( 'NONE',  ( 10.60312500061451679, -4.541064518000417216, -2.621784821875001281 ) ) ;
#9117=CARTESIAN_POINT ( 'NONE',  ( 14.44687500061451679, 6.054752690667223547, 3.707466751127219781E-16 ) ) ;
#9119=CARTESIAN_POINT ( 'NONE',  ( 21.67500000122903359, -5.773502691896255534, -1.060575238724906372E-15 ) ) ;
#9120=CARTESIAN_POINT ( 'NONE',  ( 11.33437500061451608, 4.541064518000418104, 2.621784821874999949 ) ) ;
#9121=CARTESIAN_POINT ( 'NONE',  ( 11.80312500061451608, 0.000000000000000000, 5.243569643749999010 ) ) ;
#9123=CARTESIAN_POINT ( 'NONE',  ( 20.89687500061452141, -3.027376345333614438, 5.243569643749998122 ) ) ;
#9125=CARTESIAN_POINT ( 'NONE',  ( -2.000000000000000000, 11.93750000122903465, -33.46410161513775705 ) ) ;
#9126=VECTOR ( 'NONE', #50705, 1000.000000000000000 ) ;
#9127=CARTESIAN_POINT ( 'NONE',  ( -2.556497649636125342E-15, 18.87500000122903288, -26.00000000000000355 ) ) ;
#9128=CARTESIAN_POINT ( 'NONE',  ( -2.121784821874999949, 14.83437500061451786, -33.67503911421598417 ) ) ;
#9129=CARTESIAN_POINT ( 'NONE',  ( 14.10000000122903252, -2.886751345948125991, -5.000000000000000000 ) ) ;
#9130=CARTESIAN_POINT ( 'NONE',  ( 10.80937500061451928, 4.541064518000418104, -2.621784821874998173 ) ) ;
#9131=CARTESIAN_POINT ( 'NONE',  ( -2.121784821874996840, 18.97812500061451857, -26.32496088578401583 ) ) ;
#9132=CARTESIAN_POINT ( 'NONE',  ( 17.36250000122903359, 4.330127018922192761, -2.499999999999997780 ) ) ;
#9133=CARTESIAN_POINT ( 'NONE',  ( 12.70312500061451821, 0.000000000000000000, 5.243569643749999010 ) ) ;
#9135=CARTESIAN_POINT ( 'NONE',  ( 15.86250000000000249, 2.886751345948129099, -4.999999999999998224 ) ) ;
#9136=CARTESIAN_POINT ( 'NONE',  ( 4.603329117574985752, 1.951758446961684434, -4.603329117574985752 ) ) ;
#9137=CARTESIAN_POINT ( 'NONE',  ( 9.159375000614515372, 0.000000000000000000, 5.243569643749999010 ) ) ;
#9138=CARTESIAN_POINT ( 'NONE',  ( 30.00000000000000000, 6.123233995736764310E-16, -4.999999999999998224 ) ) ;
#9139=CARTESIAN_POINT ( 'NONE',  ( 13.80000000122903181, 5.773502691896255534, 3.535250795749688894E-16 ) ) ;
#9140=CARTESIAN_POINT ( 'NONE',  ( 19.83750000122903145, -4.330127018922194537, 2.499999999999995559 ) ) ;
#9141=CARTESIAN_POINT ( 'NONE',  ( 16.75312500061451715, 0.000000000000000000, 5.243569643749999010 ) ) ;
#9142=CARTESIAN_POINT ( 'NONE',  ( 21.17812500061451431, 4.541064518000418104, 2.621784821874999949 ) ) ;
#9143=CARTESIAN_POINT ( 'NONE',  ( 28.87500000122902932, -5.773502691896255534, -1.060575238724906372E-15 ) ) ;
#9144=EDGE_CURVE ( 'NONE', #59952, #57422, #60946, .T. ) ;
#9145=CARTESIAN_POINT ( 'NONE',  ( 4.753125000614515372, -4.541064518000417216, -2.621784821875001281 ) ) ;
#9146=CARTESIAN_POINT ( 'NONE',  ( 25.08749999999999858, -2.886751345948129988, 4.999999999999997335 ) ) ;
#9147=DIRECTION ( 'NONE',  ( -1.000000000000000000, -0.000000000000000000, -0.000000000000000000 ) ) ;
#9149=CARTESIAN_POINT ( 'NONE',  ( 29.14687500061451075, -3.027376345333610441, -5.243569643749999898 ) ) ;
#9150=CARTESIAN_POINT ( 'NONE',  ( -5.810221930991193690E-16, 15.83749999999999680, 26.00000000000000355 ) ) ;
#9151=CARTESIAN_POINT ( 'NONE',  ( 2.812500001229033320, -4.330127018922190985, -2.500000000000001332 ) ) ;
#9152=CARTESIAN_POINT ( 'NONE',  ( 29.70937500061451431, 4.541064518000418104, -2.621784821874998173 ) ) ;
#9154=CARTESIAN_POINT ( 'NONE',  ( 7.471875000614519813, -6.054752690667223547, -1.112240025338166033E-15 ) ) ;
#9155=CARTESIAN_POINT ( 'NONE',  ( 25.26562500061451289, 3.027376345333611329, 5.243569643749999010 ) ) ;
#9158=CARTESIAN_POINT ( 'NONE',  ( 3.708868255654138135, -3.353251595422250375, 3.928382055777434267 ) ) ;
#9159=CARTESIAN_POINT ( 'NONE',  ( 4.471875000614518925, 3.027376345333613106, -5.243569643749998122 ) ) ;
#9160=CARTESIAN_POINT ( 'NONE',  ( 8.596875000614518925, 6.054752690667223547, 3.707466751127219781E-16 ) ) ;
#9161=CARTESIAN_POINT ( 'NONE',  ( 3.112500000000000711, -5.773502691896255534, -1.060575238724906372E-15 ) ) ;
#9162=CARTESIAN_POINT ( 'NONE',  ( -4.243569643749998122, 11.29062500061459495, 32.45002607614398471 ) ) ;
#9163=CARTESIAN_POINT ( 'NONE',  ( 21.30000000000000071, 4.330127018922192761, -2.499999999999997780 ) ) ;
#9165=CARTESIAN_POINT ( 'NONE',  ( 3.900000000000000799, 0.000000000000000000, 4.999999999999998224 ) ) ;
#9167=ORIENTED_EDGE ( 'NONE', *, *, #68280, .T. ) ;
#9168=CARTESIAN_POINT ( 'NONE',  ( 21.44062500061452070, -3.027376345333610441, -5.243569643749999898 ) ) ;
#9169=CARTESIAN_POINT ( 'NONE',  ( 10.26562500061451644, 3.027376345333613106, -5.243569643749998122 ) ) ;
#9171=CARTESIAN_POINT ( 'NONE',  ( 6.646875000614518747, -3.027376345333610441, -5.243569643749999898 ) ) ;
#9172=CARTESIAN_POINT ( 'NONE',  ( 24.11249999999999716, 2.886751345948126879, 4.999999999999999112 ) ) ;
#9173=CARTESIAN_POINT ( 'NONE',  ( 19.05000000122903359, -2.886751345948125991, -5.000000000000000000 ) ) ;
#9174=CARTESIAN_POINT ( 'NONE',  ( 27.40312500061451573, 4.541064518000418104, -2.621784821874998173 ) ) ;
#9176=CARTESIAN_POINT ( 'NONE',  ( 9.046875000614518214, 6.054752690667223547, 3.707466751127219781E-16 ) ) ;
#9177=CARTESIAN_POINT ( 'NONE',  ( 13.35937500061451821, -4.541064518000417216, -2.621784821875001281 ) ) ;
#9178=CARTESIAN_POINT ( 'NONE',  ( 24.27187500061452141, 3.027376345333613106, -5.243569643749998122 ) ) ;
#9179=CARTESIAN_POINT ( 'NONE',  ( -1.487416814333745711E-14, 16.06250000000000000, 34.00000000000000000 ) ) ;
#9181=CARTESIAN_POINT ( 'NONE',  ( 19.17187500061451999, -6.054752690667223547, -1.112240025338166033E-15 ) ) ;
#9182=CARTESIAN_POINT ( 'NONE',  ( 8.409375000614518925, -4.541064518000417216, -2.621784821875001281 ) ) ;
#9184=CARTESIAN_POINT ( 'NONE',  ( 23.88749999999999929, -2.886751345948125991, -5.000000000000000000 ) ) ;
#9188=CARTESIAN_POINT ( 'NONE',  ( 12.66562500061451502, 3.027376345333611329, 5.243569643749999010 ) ) ;
#9189=CARTESIAN_POINT ( 'NONE',  ( 4.500000000000000888, -4.330127018922190985, -2.500000000000001332 ) ) ;
#9191=DIRECTION ( 'NONE',  ( 0.000000000000000000, 1.000000000000000000, -0.000000000000000000 ) ) ;
#9192=CARTESIAN_POINT ( 'NONE',  ( 11.70000000000000284, -4.330127018922190985, -2.500000000000001332 ) ) ;
#9193=CARTESIAN_POINT ( 'NONE',  ( 1.999999999999998668, 18.16250000122903074, 26.53589838486224650 ) ) ;
#9194=CARTESIAN_POINT ( 'NONE',  ( 10.50000000122903465, -2.886751345948125991, -5.000000000000000000 ) ) ;
#9195=CARTESIAN_POINT ( 'NONE',  ( 21.98437500061451644, 6.421520780324663323E-16, -5.243569643749999010 ) ) ;
#9196=CARTESIAN_POINT ( 'NONE',  ( 16.50937500061451502, -4.541064518000417216, -2.621784821875001281 ) ) ;
#9197=CARTESIAN_POINT ( 'NONE',  ( 20.21250000122903145, 0.000000000000000000, 4.999999999999998224 ) ) ;
#9198=ORIENTED_EDGE ( 'NONE', *, *, #37402, .F. ) ;
#9199=CARTESIAN_POINT ( 'NONE',  ( 17.27812500061451217, -4.541064518000419881, 2.621784821874995952 ) ) ;
#9200=CARTESIAN_POINT ( 'NONE',  ( 2.915625000614516793, -6.054752690667223547, -1.112240025338166033E-15 ) ) ;
#9201=CARTESIAN_POINT ( 'NONE',  ( 17.85937500061451999, -4.541064518000417216, -2.621784821875001281 ) ) ;
#9202=CARTESIAN_POINT ( 'NONE',  ( 29.78437500061451715, 4.541064518000418104, 2.621784821874999949 ) ) ;
#9203=CARTESIAN_POINT ( 'NONE',  ( 3.703125000614516882, 0.000000000000000000, 5.243569643749999010 ) ) ;
#9204=CARTESIAN_POINT ( 'NONE',  ( 18.55312500061451431, 0.000000000000000000, 5.243569643749999010 ) ) ;
#9205=CARTESIAN_POINT ( 'NONE',  ( 28.17187500061451644, -6.054752690667223547, -1.112240025338166033E-15 ) ) ;
#9206=CARTESIAN_POINT ( 'NONE',  ( 4.243569643749999898, 13.72812500061451679, 30.00000000000000000 ) ) ;
#9207=CARTESIAN_POINT ( 'NONE',  ( 17.62500000122903288, -5.773502691896255534, -1.060575238724906372E-15 ) ) ;
#9209=CARTESIAN_POINT ( 'NONE',  ( 8.240625000614516082, -3.027376345333614438, 5.243569643749998122 ) ) ;
#9210=CARTESIAN_POINT ( 'NONE',  ( 26.01562500061451289, 3.027376345333613106, -5.243569643749998122 ) ) ;
#9211=CARTESIAN_POINT ( 'NONE',  ( 1.510657702057710734E-15, 19.10000000122903430, -33.99999999999999289 ) ) ;
#9212=CARTESIAN_POINT ( 'NONE',  ( 22.39687500061451075, -3.027376345333610441, -5.243569643749999898 ) ) ;
#9213=CARTESIAN_POINT ( 'NONE',  ( 13.34062500061451750, -3.027376345333610441, -5.243569643749999898 ) ) ;
#9214=CARTESIAN_POINT ( 'NONE',  ( 22.76250000122903216, 4.330127018922192761, -2.499999999999997780 ) ) ;
#9215=CARTESIAN_POINT ( 'NONE',  ( 23.91562500061451502, 3.027376345333611329, 5.243569643749999010 ) ) ;
#9216=CARTESIAN_POINT ( 'NONE',  ( 18.49687500061452283, 6.054752690667223547, 3.707466751127219781E-16 ) ) ;
#9217=CARTESIAN_POINT ( 'NONE',  ( 12.62812500061451537, 4.541064518000418104, 2.621784821874999949 ) ) ;
#9218=CARTESIAN_POINT ( 'NONE',  ( 2.121784821874999061, 15.65937500061451892, 26.32496088578401583 ) ) ;
#9219=CARTESIAN_POINT ( 'NONE',  ( 20.35312500061451502, 0.000000000000000000, 5.243569643749999010 ) ) ;
#9223=CARTESIAN_POINT ( 'NONE',  ( 21.89999999999999858, 0.000000000000000000, 4.999999999999998224 ) ) ;
#9224=CARTESIAN_POINT ( 'NONE',  ( 3.999999999999998668, 10.36250000000000071, -32.30940107675850470 ) ) ;
#9226=CARTESIAN_POINT ( 'NONE',  ( 26.46562500061451573, 3.027376345333613106, -5.243569643749998122 ) ) ;
#9227=CARTESIAN_POINT ( 'NONE',  ( 6.215625000614517504, 3.027376345333613106, -5.243569643749998122 ) ) ;
#9228=CARTESIAN_POINT ( 'NONE',  ( 19.91250000122903074, -4.330127018922190985, -2.500000000000001332 ) ) ;
#9230=CARTESIAN_POINT ( 'NONE',  ( 23.99062500061451786, -3.027376345333614438, 5.243569643749998122 ) ) ;
#9231=CARTESIAN_POINT ( 'NONE',  ( 23.21250000000000213, 2.886751345948126879, 4.999999999999999112 ) ) ;
#9232=CARTESIAN_POINT ( 'NONE',  ( 27.89062500061451289, 6.054752690667223547, 3.707466751127219781E-16 ) ) ;
#9233=CARTESIAN_POINT ( 'NONE',  ( 9.065625000614517148, 3.027376345333611329, 5.243569643749999010 ) ) ;
#9234=EDGE_LOOP ( 'NONE', ( #62532, #61431, #41521, #35208 ) ) ;
#9235=EDGE_CURVE ( 'NONE', #23877, #58137, #68515, .T. ) ;
#9236=CARTESIAN_POINT ( 'NONE',  ( 23.84062500061451928, 6.054752690667223547, 3.707466751127219781E-16 ) ) ;
#9237=CARTESIAN_POINT ( 'NONE',  ( 6.178125000614518747, 6.421520780324663323E-16, -5.243569643749999010 ) ) ;
#9239=CARTESIAN_POINT ( 'NONE',  ( 3.928125000614516527, 6.421520780324663323E-16, -5.243569643749999010 ) ) ;
#9240=CARTESIAN_POINT ( 'NONE',  ( -2.828200636599751609E-16, 14.60000000122903430, -34.61880215351700230 ) ) ;
#9241=CARTESIAN_POINT ( 'NONE',  ( -2.000000000000000000, 13.62500000000000178, -33.46410161513775705 ) ) ;
#9242=CARTESIAN_POINT ( 'NONE',  ( 10.12500000000000178, 4.330127018922191873, 2.499999999999999556 ) ) ;
#9243=CARTESIAN_POINT ( 'NONE',  ( 11.10937500061451644, -4.541064518000417216, -2.621784821875001281 ) ) ;
#9244=CARTESIAN_POINT ( 'NONE',  ( 6.825000001229034829, -5.773502691896255534, -1.060575238724906372E-15 ) ) ;
#9245=CARTESIAN_POINT ( 'NONE',  ( 15.30937500061451750, 4.541064518000418104, -2.621784821874998173 ) ) ;
#9247=CARTESIAN_POINT ( 'NONE',  ( 7.021875000614518747, -6.054752690667223547, -1.112240025338166033E-15 ) ) ;
#9248=CARTESIAN_POINT ( 'NONE',  ( -3.000416591977282496E-16, 10.24062500061451608, -34.90005215228797653 ) ) ;
#9250=CARTESIAN_POINT ( 'NONE',  ( 13.32187500061451502, -6.054752690667223547, -1.112240025338166033E-15 ) ) ;
#9251=CARTESIAN_POINT ( 'NONE',  ( 3.668019400630285531, 3.397886648580393132, 3.993668605712777264 ) ) ;
#9252=CARTESIAN_POINT ( 'NONE',  ( 22.60312500061451857, 0.000000000000000000, 5.243569643749999010 ) ) ;
#9254=DIRECTION ( 'NONE',  ( -0.000000000000000000, -1.000000000000000000, -0.000000000000000000 ) ) ;
#9255=CARTESIAN_POINT ( 'NONE',  ( 25.88437500061451502, -4.541064518000419881, 2.621784821874995952 ) ) ;
#9257=CARTESIAN_POINT ( 'NONE',  ( 4.378125000614518925, 6.421520780324663323E-16, -5.243569643749999010 ) ) ;
#9259=CARTESIAN_POINT ( 'NONE',  ( 13.35937500061451821, -4.541064518000417216, -2.621784821875001281 ) ) ;
#9260=CARTESIAN_POINT ( 'NONE',  ( 26.13750000122903216, -4.330127018922194537, 2.499999999999995559 ) ) ;
#9261=CARTESIAN_POINT ( 'NONE',  ( 26.36250000122903003, 4.330127018922192761, -2.499999999999997780 ) ) ;
#9262=CARTESIAN_POINT ( 'NONE',  ( 6.234375000614519102, 6.421520780324663323E-16, -5.243569643749999010 ) ) ;
#9263=CARTESIAN_POINT ( 'NONE',  ( 15.45937500061451608, 0.000000000000000000, 5.243569643749999010 ) ) ;
#9265=CARTESIAN_POINT ( 'NONE',  ( 24.41250000000000142, 2.886751345948129099, -4.999999999999998224 ) ) ;
#9266=CARTESIAN_POINT ( 'NONE',  ( 3.712500001229034563, -4.330127018922190985, -2.500000000000001332 ) ) ;
#9267=CARTESIAN_POINT ( 'NONE',  ( 26.29687500061451644, -3.027376345333614438, 5.243569643749998122 ) ) ;
#9270=CARTESIAN_POINT ( 'NONE',  ( 9.037499999999999645, -2.886751345948125991, -5.000000000000000000 ) ) ;
#9272=CARTESIAN_POINT ( 'NONE',  ( 21.29062500061451502, -3.027376345333614438, 5.243569643749998122 ) ) ;
#9273=CARTESIAN_POINT ( 'NONE',  ( 11.25000000000000000, -4.330127018922190985, -2.500000000000001332 ) ) ;
#9274=CARTESIAN_POINT ( 'NONE',  ( 4.040625000614517681, 6.054752690667223547, 3.707466751127219781E-16 ) ) ;
#9275=CARTESIAN_POINT ( 'NONE',  ( 19.42499999999999716, 6.123233995736764310E-16, -4.999999999999998224 ) ) ;
#9276=EDGE_CURVE ( 'NONE', #20937, #2237, #27968, .T. ) ;
#9277=CARTESIAN_POINT ( 'NONE',  ( 19.07812500061451644, -4.541064518000419881, 2.621784821874995952 ) ) ;
#9278=CARTESIAN_POINT ( 'NONE',  ( -3.999999999999999112, 18.72500000122903074, 27.69059892324149885 ) ) ;
#9279=CARTESIAN_POINT ( 'NONE',  ( 22.61250000122903003, -4.330127018922190985, -2.500000000000001332 ) ) ;
#9281=CARTESIAN_POINT ( 'NONE',  ( 29.74687500061451217, 6.054752690667223547, 3.707466751127219781E-16 ) ) ;
#9283=ORIENTED_EDGE ( 'NONE', *, *, #54421, .F. ) ;
#9284=CARTESIAN_POINT ( 'NONE',  ( 20.39062500061451644, -3.027376345333614438, 5.243569643749998122 ) ) ;
#9285=CARTESIAN_POINT ( 'NONE',  ( 23.72812500061451502, 6.421520780324663323E-16, -5.243569643749999010 ) ) ;
#9286=CARTESIAN_POINT ( 'NONE',  ( 25.02187500061451431, -6.054752690667223547, -1.112240025338166033E-15 ) ) ;
#9287=CARTESIAN_POINT ( 'NONE',  ( 10.01250000000000107, 2.886751345948129099, -4.999999999999998224 ) ) ;
#9288=CARTESIAN_POINT ( 'NONE',  ( 11.31562500061451892, 3.027376345333611329, 5.243569643749999010 ) ) ;
#9289=CARTESIAN_POINT ( 'NONE',  ( 26.50312500061451360, 4.541064518000418104, -2.621784821874998173 ) ) ;
#9290=CARTESIAN_POINT ( 'NONE',  ( 16.99687500061451573, -3.027376345333610441, -5.243569643749999898 ) ) ;
#9291=CARTESIAN_POINT ( 'NONE',  ( 9.890625000614516438, 6.054752690667223547, 3.707466751127219781E-16 ) ) ;
#9293=CARTESIAN_POINT ( 'NONE',  ( -4.243569643749999898, 18.86562500061451431, 27.54997392385601529 ) ) ;
#9294=CARTESIAN_POINT ( 'NONE',  ( 24.86250000122903359, -4.330127018922190985, -2.500000000000001332 ) ) ;
#9296=CARTESIAN_POINT ( 'NONE',  ( 15.29062500061451502, 6.054752690667223547, 3.707466751127219781E-16 ) ) ;
#9297=CARTESIAN_POINT ( 'NONE',  ( 8.821875000614518569, -6.054752690667223547, -1.112240025338166033E-15 ) ) ;
#9298=CARTESIAN_POINT ( 'NONE',  ( 6.609375000614519102, -4.541064518000417216, -2.621784821875001281 ) ) ;
#9299=EDGE_CURVE ( 'NONE', #27538, #53550, #65663, .T. ) ;
#9300=ORIENTED_EDGE ( 'NONE', *, *, #55763, .T. ) ;
#9301=CARTESIAN_POINT ( 'NONE',  ( 29.25937500061451502, 4.541064518000418104, -2.621784821874998173 ) ) ;
#9302=CARTESIAN_POINT ( 'NONE',  ( 20.65312500061451573, 4.541064518000418104, -2.621784821874998173 ) ) ;
#9303=CARTESIAN_POINT ( 'NONE',  ( 17.25937500061451502, 0.000000000000000000, 5.243569643749999010 ) ) ;
#9304=CARTESIAN_POINT ( 'NONE',  ( 21.47812500061451502, 6.421520780324663323E-16, -5.243569643749999010 ) ) ;
#9305=CARTESIAN_POINT ( 'NONE',  ( -2.000000000000000000, 11.82500000000000107, 26.53589838486224650 ) ) ;
#9306=CARTESIAN_POINT ( 'NONE',  ( 26.72812500061451502, -4.541064518000419881, 2.621784821874995952 ) ) ;
#9307=CARTESIAN_POINT ( 'NONE',  ( 7.537500001229033408, 4.330127018922191873, 2.499999999999999556 ) ) ;
#9308=ORIENTED_EDGE ( 'NONE', *, *, #63007, .T. ) ;
#9309=CARTESIAN_POINT ( 'NONE',  ( 28.98750000000000071, 5.773502691896255534, 3.535250795749688894E-16 ) ) ;
#9310=CARTESIAN_POINT ( 'NONE',  ( -1.999999999999997113, 16.92500000000000426, -26.53589838486224295 ) ) ;
#9311=CARTESIAN_POINT ( 'NONE',  ( 25.95000000122903216, 5.773502691896255534, 3.535250795749688894E-16 ) ) ;
#9313=ADVANCED_FACE ( 'NONE', ( #42480 ), #65003, .T. ) ;
#9314=CARTESIAN_POINT ( 'NONE',  ( 7.246875000614518392, 6.054752690667223547, 3.707466751127219781E-16 ) ) ;
#9315=CARTESIAN_POINT ( 'NONE',  ( 3.999999999999999112, 15.27500000000000036, 30.00000000000000000 ) ) ;
#9316=CARTESIAN_POINT ( 'NONE',  ( 14.09062500061451750, -3.027376345333614438, 5.243569643749998122 ) ) ;
#9317=CARTESIAN_POINT ( 'NONE',  ( 9.609375000614518214, 0.000000000000000000, 5.243569643749999010 ) ) ;
#9318=CARTESIAN_POINT ( 'NONE',  ( 27.03750000122903430, -4.330127018922194537, 2.499999999999995559 ) ) ;
#9319=CARTESIAN_POINT ( 'NONE',  ( 17.70937500061451431, 0.000000000000000000, 5.243569643749999010 ) ) ;
#9320=CARTESIAN_POINT ( 'NONE',  ( 6.234375000614519102, 6.421520780324663323E-16, -5.243569643749999010 ) ) ;
#9321=CARTESIAN_POINT ( 'NONE',  ( 4.575260086717170438, 2.016679235498957112, 4.840250765194281435 ) ) ;
#9322=CARTESIAN_POINT ( 'NONE',  ( 5.953125000614519102, 0.000000000000000000, 5.243569643749999010 ) ) ;
#9323=CARTESIAN_POINT ( 'NONE',  ( 15.17812500061451608, 6.421520780324663323E-16, -5.243569643749999010 ) ) ;
#9324=ORIENTED_EDGE ( 'NONE', *, *, #68758, .T. ) ;
#9325=CARTESIAN_POINT ( 'NONE',  ( 12.17812500061451608, 4.541064518000418104, 2.621784821874999949 ) ) ;
#9326=CARTESIAN_POINT ( 'NONE',  ( 5.850000001229035185, -2.886751345948129988, 4.999999999999997335 ) ) ;
#9327=CARTESIAN_POINT ( 'NONE',  ( 9.178125000614517859, -4.541064518000419881, 2.621784821874995952 ) ) ;
#9329=CARTESIAN_POINT ( 'NONE',  ( 9.074999999999999289, 6.123233995736764310E-16, -4.999999999999998224 ) ) ;
#9330=CARTESIAN_POINT ( 'NONE',  ( 4.950000001229033941, -2.886751345948129988, 4.999999999999997335 ) ) ;
#9331=CARTESIAN_POINT ( 'NONE',  ( 18.03749999999999787, -2.886751345948125991, -5.000000000000000000 ) ) ;
#9333=CARTESIAN_POINT ( 'NONE',  ( 18.42187500061451644, 3.027376345333613106, -5.243569643749998122 ) ) ;
#9334=CARTESIAN_POINT ( 'NONE',  ( 16.23750000122903359, -4.330127018922194537, 2.499999999999995559 ) ) ;
#9336=CARTESIAN_POINT ( 'NONE',  ( -4.243569643749999898, 15.30312500061451608, -30.00000000000000000 ) ) ;
#9337=CARTESIAN_POINT ( 'NONE',  ( 3.193447721043152665, 3.847322660365763536, 3.562742055761627835 ) ) ;
#9338=CARTESIAN_POINT ( 'NONE',  ( 1.592000809091587073E-14, 15.05000000122903714, -34.00000000000000000 ) ) ;
#9340=CARTESIAN_POINT ( 'NONE',  ( 28.22812500061451502, 6.421520780324663323E-16, -5.243569643749999010 ) ) ;
#9342=CARTESIAN_POINT ( 'NONE',  ( 3.999999999999998668, 14.52500000122903323, 27.69059892324149530 ) ) ;
#9343=CARTESIAN_POINT ( 'NONE',  ( 17.14687500061451786, 6.054752690667223547, 3.707466751127219781E-16 ) ) ;
#9344=CARTESIAN_POINT ( 'NONE',  ( 29.58749999999999858, -2.886751345948129988, 4.999999999999997335 ) ) ;
#9345=CARTESIAN_POINT ( 'NONE',  ( 10.71562500061451928, 3.027376345333613106, -5.243569643749998122 ) ) ;
#9347=CARTESIAN_POINT ( 'NONE',  ( 24.64687500061451431, -3.027376345333610441, -5.243569643749999898 ) ) ;
#9349=CARTESIAN_POINT ( 'NONE',  ( 8.165625000614516793, 3.027376345333611329, 5.243569643749999010 ) ) ;
#9350=CARTESIAN_POINT ( 'NONE',  ( 12.60937500061451821, 4.541064518000418104, -2.621784821874998173 ) ) ;
#9351=VERTEX_POINT ( 'NONE', #43215 ) ;
#9352=CARTESIAN_POINT ( 'NONE',  ( 24.45937500061451786, 0.000000000000000000, 5.243569643749999010 ) ) ;
#9353=CARTESIAN_POINT ( 'NONE',  ( 27.77812500061451573, 6.421520780324663323E-16, -5.243569643749999010 ) ) ;
#9355=CARTESIAN_POINT ( 'NONE',  ( 6.750000000000002665, -4.330127018922190985, -2.500000000000001332 ) ) ;
#9356=CARTESIAN_POINT ( 'NONE',  ( 17.02500000122903145, 2.886751345948126879, 4.999999999999999112 ) ) ;
#9357=DIRECTION ( 'NONE',  ( -0.000000000000000000, -1.000000000000000000, -0.000000000000000000 ) ) ;
#9359=ORIENTED_EDGE ( 'NONE', *, *, #42162, .T. ) ;
#9360=CARTESIAN_POINT ( 'NONE',  ( 14.66249999999999964, 2.886751345948126879, 4.999999999999999112 ) ) ;
#9361=CARTESIAN_POINT ( 'NONE',  ( 19.08750000000000213, 5.773502691896255534, 3.535250795749688894E-16 ) ) ;
#9362=CARTESIAN_POINT ( 'NONE',  ( 10.22812500061451679, 6.421520780324663323E-16, -5.243569643749999010 ) ) ;
#9363=ORIENTED_EDGE ( 'NONE', *, *, #18203, .T. ) ;
#9364=CARTESIAN_POINT ( 'NONE',  ( -1.999999999999997113, 11.07500000000000107, -26.53589838486224295 ) ) ;
#9365=CARTESIAN_POINT ( 'NONE',  ( 4.243569643749999898, 16.89687500061451786, -27.54997392385601529 ) ) ;
#9366=CARTESIAN_POINT ( 'NONE',  ( 4.340625000614515727, -3.027376345333610441, -5.243569643749999898 ) ) ;
#9368=CARTESIAN_POINT ( 'NONE',  ( 9.150000000000002132, 4.330127018922192761, -2.499999999999997780 ) ) ;
#9369=CARTESIAN_POINT ( 'NONE',  ( 1.626862140677534273E-15, 13.36250000000000071, -26.00000000000000355 ) ) ;
#9370=VERTEX_POINT ( 'NONE', #25853 ) ;
#9371=CARTESIAN_POINT ( 'NONE',  ( 4.243569643749999010, 11.96562500061451750, 27.54997392385601174 ) ) ;
#9372=CARTESIAN_POINT ( 'NONE',  ( 26.42812500061451431, 6.421520780324663323E-16, -5.243569643749999010 ) ) ;
#9373=CARTESIAN_POINT ( 'NONE',  ( 13.57500000000000107, 6.123233995736764310E-16, -4.999999999999998224 ) ) ;
#9375=CARTESIAN_POINT ( 'NONE',  ( 20.67187500061451289, 3.027376345333613106, -5.243569643749998122 ) ) ;
#9376=CARTESIAN_POINT ( 'NONE',  ( 18.66562500061451146, -6.054752690667223547, -1.112240025338166033E-15 ) ) ;
#9377=CARTESIAN_POINT ( 'NONE',  ( 9.001249775931846008E-16, 13.16562500061459140, -25.09994784771203058 ) ) ;
#9378=CARTESIAN_POINT ( 'NONE',  ( 22.50000000122903288, -2.886751345948129988, 4.999999999999997335 ) ) ;
#9379=( BOUNDED_CURVE ( )  B_SPLINE_CURVE ( 2, ( #24765, #69489, #41409, #19208, #64292, #52851, #2605, #13679, #36585 ),
 .UNSPECIFIED., .F., .F. ) 
 B_SPLINE_CURVE_WITH_KNOTS ( ( 3, 2, 2, 2, 3 ),
 ( 0.7717391304347825942, 0.7753623188405797118, 0.7826086956521739468, 0.7898550724637680709, 0.7934782608695651884 ),
 .UNSPECIFIED. ) 
 CURVE ( )  GEOMETRIC_REPRESENTATION_ITEM ( )  RATIONAL_B_SPLINE_CURVE ( ( 0.9330127018922194093, 0.9330127018922194093, 1.000000000000000000, 0.8660254037844387076, 1.000000000000000000, 0.8660254037844387076, 1.000000000000000000, 0.9330127018922194093, 0.9330127018922194093 ) ) 
 REPRESENTATION_ITEM ( '' )  );
#9380=CARTESIAN_POINT ( 'NONE',  ( 3.928125000614516527, 6.421520780324663323E-16, -5.243569643749999010 ) ) ;
#9382=CARTESIAN_POINT ( 'NONE',  ( 22.41562500061451502, 3.027376345333612662, -5.243569643749998122 ) ) ;
#9385=CARTESIAN_POINT ( 'NONE',  ( 16.28437500061452070, 4.541064518000418104, 2.621784821874999949 ) ) ;
#9387=CARTESIAN_POINT ( 'NONE',  ( 17.40937500061451715, -4.541064518000417216, -2.621784821875001281 ) ) ;
#9388=CARTESIAN_POINT ( 'NONE',  ( 24.38437500061451502, 4.541064518000418104, 2.621784821874999949 ) ) ;
#9389=CARTESIAN_POINT ( 'NONE',  ( -3.000416591977282496E-16, 13.44687500061451679, 25.09994784771203058 ) ) ;
#9390=CARTESIAN_POINT ( 'NONE',  ( 4.490625000614516971, 6.054752690667223547, 3.707466751127219781E-16 ) ) ;
#9391=CARTESIAN_POINT ( 'NONE',  ( 28.04062500061451502, -3.027376345333614438, 5.243569643749998122 ) ) ;
#9392=( BOUNDED_CURVE ( )  B_SPLINE_CURVE ( 2, ( #36518, #63138, #24699, #35067, #8083, #42069, #57593, #1828, #30613 ),
 .UNSPECIFIED., .F., .F. ) 
 B_SPLINE_CURVE_WITH_KNOTS ( ( 3, 2, 2, 2, 3 ),
 ( 0.6413043478260869179, 0.6449275362318840354, 0.6521739130434782705, 0.6594202898550725056, 0.6630434782608696231 ),
 .UNSPECIFIED. ) 
 CURVE ( )  GEOMETRIC_REPRESENTATION_ITEM ( )  RATIONAL_B_SPLINE_CURVE ( ( 0.9330127018922194093, 0.9330127018922194093, 1.000000000000000000, 0.8660254037844387076, 1.000000000000000000, 0.8660254037844387076, 1.000000000000000000, 0.9330127018922182991, 0.9330127018922192983 ) ) 
 REPRESENTATION_ITEM ( '' )  );
#9393=CARTESIAN_POINT ( 'NONE',  ( 28.97812500061451502, -4.541064518000419881, 2.621784821874995952 ) ) ;
#9395=CARTESIAN_POINT ( 'NONE',  ( 4.000000000000000000, 18.38749999999999929, 32.30940107675849049 ) ) ;
#9396=CARTESIAN_POINT ( 'NONE',  ( 6.346875000614517148, 6.054752690667223547, 3.707466751127219781E-16 ) ) ;
#9397=CARTESIAN_POINT ( 'NONE',  ( 15.33750000122903323, -4.330127018922194537, 2.499999999999995559 ) ) ;
#9398=CARTESIAN_POINT ( 'NONE',  ( 9.900000001229033231, -2.886751345948129988, 4.999999999999997335 ) ) ;
#9399=CARTESIAN_POINT ( 'NONE',  ( 5.915625000614515905, 3.027376345333611329, 5.243569643749999010 ) ) ;
#9402=CARTESIAN_POINT ( 'NONE',  ( 13.88437500061451679, 6.421520780324663323E-16, -5.243569643749999010 ) ) ;
#9403=FACE_OUTER_BOUND ( 'NONE', #72136, .T. ) ;
#9404=ORIENTED_EDGE ( 'NONE', *, *, #43004, .F. ) ;
#9405=CARTESIAN_POINT ( 'NONE',  ( 21.40312500061451573, -4.541064518000417216, -2.621784821875001281 ) ) ;
#9406=CARTESIAN_POINT ( 'NONE',  ( 7.453125000614516438, -4.541064518000417216, -2.621784821875001281 ) ) ;
#9407=CARTESIAN_POINT ( 'NONE',  ( 24.00937500061451502, 0.000000000000000000, 5.243569643749999010 ) ) ;
#9408=CARTESIAN_POINT ( 'NONE',  ( 8.128125000614515372, 4.541064518000418104, 2.621784821874999949 ) ) ;
#9410=CARTESIAN_POINT ( 'NONE',  ( 7.237500001229035362, -4.330127018922194537, 2.499999999999995559 ) ) ;
#9411=CARTESIAN_POINT ( 'NONE',  ( 21.32812500061451644, -4.541064518000419881, 2.621784821874995952 ) ) ;
#9413=CARTESIAN_POINT ( 'NONE',  ( -3.999999999999999556, 19.62500000122903643, -32.30940107675850470 ) ) ;
#9414=CARTESIAN_POINT ( 'NONE',  ( 10.50000000122903465, -2.886751345948125991, -5.000000000000000000 ) ) ;
#9415=CARTESIAN_POINT ( 'NONE',  ( 20.05312500061451431, -4.541064518000417216, -2.621784821875001281 ) ) ;
#9416=CARTESIAN_POINT ( 'NONE',  ( 16.79062500061451857, -3.027376345333614438, 5.243569643749998122 ) ) ;
#9418=CARTESIAN_POINT ( 'NONE',  ( 19.04999999999999716, 4.330127018922192761, -2.499999999999997780 ) ) ;
#9419=CARTESIAN_POINT ( 'NONE',  ( 10.23750000122903359, 4.330127018922191873, 2.499999999999999556 ) ) ;
#9420=EDGE_CURVE ( 'NONE', #40801, #61496, #142, .T. ) ;
#9421=CARTESIAN_POINT ( 'NONE',  ( 8.278125000614515727, -4.541064518000419881, 2.621784821874995952 ) ) ;
#9422=CARTESIAN_POINT ( 'NONE',  ( 10.22812500061451679, 6.421520780324663323E-16, -5.243569643749999010 ) ) ;
#9423=CARTESIAN_POINT ( 'NONE',  ( 22.27500000122903145, 2.886751345948129099, -4.999999999999998224 ) ) ;
#9424=CARTESIAN_POINT ( 'NONE',  ( 22.50937500061451857, 4.541064518000418104, -2.621784821874998173 ) ) ;
#9425=CARTESIAN_POINT ( 'NONE',  ( 4.753125000614515372, -4.541064518000417216, -2.621784821875001281 ) ) ;
#9427=CARTESIAN_POINT ( 'NONE',  ( 5.475000001229035185, -5.773502691896255534, -1.060575238724906372E-15 ) ) ;
#9428=CARTESIAN_POINT ( 'NONE',  ( 5.821875000614519458, 3.027376345333613106, -5.243569643749998122 ) ) ;
#9429=CARTESIAN_POINT ( 'NONE',  ( 23.70937500061451786, -4.541064518000417216, -2.621784821875001281 ) ) ;
#9431=CARTESIAN_POINT ( 'NONE',  ( 18.96562500061451573, 3.027376345333611329, 5.243569643749999010 ) ) ;
#9432=CARTESIAN_POINT ( 'NONE',  ( 24.94687500061451502, -3.027376345333614438, 5.243569643749998122 ) ) ;
#9434=CARTESIAN_POINT ( 'NONE',  ( 12.45000000122903394, 5.773502691896255534, 3.535250795749688401E-16 ) ) ;
#9436=CARTESIAN_POINT ( 'NONE',  ( 6.234375000614519102, 6.421520780324663323E-16, -5.243569643749999010 ) ) ;
#9437=CARTESIAN_POINT ( 'NONE',  ( 15.10312500061451502, -4.541064518000417216, -2.621784821875001281 ) ) ;
#9438=CARTESIAN_POINT ( 'NONE',  ( 12.64687500061451608, 6.054752690667223547, 3.707466751127219781E-16 ) ) ;
#9440=CARTESIAN_POINT ( 'NONE',  ( 22.23750000122903003, 6.123233995736764310E-16, -4.999999999999998224 ) ) ;
#9441=CARTESIAN_POINT ( 'NONE',  ( 24.85312500061451502, 0.000000000000000000, 5.243569643749999010 ) ) ;
#9444=CARTESIAN_POINT ( 'NONE',  ( 14.24999999999999822, 0.000000000000000000, 4.999999999999998224 ) ) ;
#9445=CARTESIAN_POINT ( 'NONE',  ( 24.03750000122903430, 6.123233995736764310E-16, -4.999999999999998224 ) ) ;
#9446=CARTESIAN_POINT ( 'NONE',  ( 19.56562500061451715, -6.054752690667223547, -1.112240025338166033E-15 ) ) ;
#9448=CARTESIAN_POINT ( 'NONE',  ( 21.22500000000000142, 6.123233995736764310E-16, -4.999999999999998224 ) ) ;
#9449=CARTESIAN_POINT ( 'NONE',  ( 23.85937500061451644, 4.541064518000418104, -2.621784821874998173 ) ) ;
#9450=VERTEX_POINT ( 'NONE', #53554 ) ;
#9451=CARTESIAN_POINT ( 'NONE',  ( 2.977075986255253159, -4.017098088058328464, -3.370162576270459454 ) ) ;
#9452=CARTESIAN_POINT ( 'NONE',  ( 11.54062500061451857, -3.027376345333610441, -5.243569643749999898 ) ) ;
#9453=CARTESIAN_POINT ( 'NONE',  ( 3.853125000614517681, -4.541064518000417216, -2.621784821875001281 ) ) ;
#9455=CARTESIAN_POINT ( 'NONE',  ( 27.44062500061451715, 6.054752690667223547, 3.707466751127219781E-16 ) ) ;
#9456=CARTESIAN_POINT ( 'NONE',  ( 17.28750000000000142, 5.773502691896255534, 3.535250795749688894E-16 ) ) ;
#9457=CARTESIAN_POINT ( 'NONE',  ( 25.76249999999999929, 2.886751345948129099, -4.999999999999998224 ) ) ;
#9458=CARTESIAN_POINT ( 'NONE',  ( 1.999999999999998668, 10.85000000000000142, -33.46410161513775705 ) ) ;
#9459=CARTESIAN_POINT ( 'NONE',  ( 6.159375000614517148, -4.541064518000417216, -2.621784821875001281 ) ) ;
#9460=CARTESIAN_POINT ( 'NONE',  ( 16.92187500061451999, -6.054752690667223547, -1.112240025338166033E-15 ) ) ;
#9461=CARTESIAN_POINT ( 'NONE',  ( 26.02499999999999858, -4.330127018922194537, 2.499999999999995559 ) ) ;
#9462=ORIENTED_EDGE ( 'NONE', *, *, #18001, .F. ) ;
#9463=CARTESIAN_POINT ( 'NONE',  ( 27.06562500061451004, 3.027376345333611329, 5.243569643749999010 ) ) ;
#9464=CARTESIAN_POINT ( 'NONE',  ( 28.54687500061451644, -3.027376345333614438, 5.243569643749998122 ) ) ;
#9465=CARTESIAN_POINT ( 'NONE',  ( 3.271875000614519635, 3.027376345333611329, 5.243569643749999010 ) ) ;
#9466=CARTESIAN_POINT ( 'NONE',  ( 12.63749999999999929, -2.886751345948125991, -5.000000000000000000 ) ) ;
#9467=CARTESIAN_POINT ( 'NONE',  ( 12.06562500061451537, 3.027376345333613106, -5.243569643749998122 ) ) ;
#9469=CARTESIAN_POINT ( 'NONE',  ( 4.897546610576117843, 1.006994139586731674, -5.145967878999484491 ) ) ;
#9470=CARTESIAN_POINT ( 'NONE',  ( 28.22812500061451502, 6.421520780324663323E-16, -5.243569643749999010 ) ) ;
#9471=CARTESIAN_POINT ( 'NONE',  ( 15.26250000122903216, 0.000000000000000000, 4.999999999999998224 ) ) ;
#9472=CARTESIAN_POINT ( 'NONE',  ( 3.881554241669678884, -3.151751365348489653, -4.190642664303462439 ) ) ;
#9474=CARTESIAN_POINT ( 'NONE',  ( 4.978125000614518569, 4.541064518000418104, 2.621784821874999949 ) ) ;
#9475=CARTESIAN_POINT ( 'NONE',  ( 22.65937500061451715, 0.000000000000000000, 5.243569643749999010 ) ) ;
#9476=CARTESIAN_POINT ( 'NONE',  ( -2.121784821874999949, 16.63437500061451857, 26.32496088578401938 ) ) ;
#9478=CARTESIAN_POINT ( 'NONE',  ( 23.55937500061451573, 0.000000000000000000, 5.243569643749999010 ) ) ;
#9479=CARTESIAN_POINT ( 'NONE',  ( 5.662500000000000533, 2.886751345948126879, 4.999999999999999112 ) ) ;
#9480=CARTESIAN_POINT ( 'NONE',  ( 8.484601909799253346E-16, 11.67500000122903359, 34.61880215351700230 ) ) ;
#9481=CARTESIAN_POINT ( 'NONE',  ( 13.37812500061451715, 6.421520780324663323E-16, -5.243569643749999010 ) ) ;
#9482=CARTESIAN_POINT ( 'NONE',  ( 5.362500001229033586, 0.000000000000000000, 4.999999999999998224 ) ) ;
#9483=CARTESIAN_POINT ( 'NONE',  ( 9.721875000614517148, -6.054752690667223547, -1.112240025338166033E-15 ) ) ;
#9484=CARTESIAN_POINT ( 'NONE',  ( 1.999999999999998668, 15.80000000000000071, -33.46410161513775705 ) ) ;
#9485=CARTESIAN_POINT ( 'NONE',  ( 9.253125000614517148, -4.541064518000417216, -2.621784821875001281 ) ) ;
#9486=CARTESIAN_POINT ( 'NONE',  ( 14.85937500061451644, 4.541064518000418104, -2.621784821874998173 ) ) ;
#9487=CARTESIAN_POINT ( 'NONE',  ( 20.36250000122903359, -4.330127018922190985, -2.500000000000001332 ) ) ;
#9488=CARTESIAN_POINT ( 'NONE',  ( 10.39687500061451786, 6.054752690667223547, 3.707466751127219781E-16 ) ) ;
#9489=CARTESIAN_POINT ( 'NONE',  ( 11.69062500061451360, 6.054752690667223547, 3.707466751127219781E-16 ) ) ;
#9491=CARTESIAN_POINT ( 'NONE',  ( 20.37187500061451573, 3.027376345333611329, 5.243569643749999010 ) ) ;
#9494=CARTESIAN_POINT ( 'NONE',  ( 3.189326098586207081, 3.850849880488091515, -3.445552266572465605 ) ) ;
#9495=CARTESIAN_POINT ( 'NONE',  ( -3.000416591977282496E-16, 14.34687500061451715, -34.90005215228797653 ) ) ;
#9496=CARTESIAN_POINT ( 'NONE',  ( 15.33750000122903323, -4.330127018922194537, 2.499999999999995559 ) ) ;
#9497=CARTESIAN_POINT ( 'NONE',  ( 10.88437500061451679, 4.541064518000418104, 2.621784821874999949 ) ) ;
#9498=CARTESIAN_POINT ( 'NONE',  ( -4.243569643749999898, 18.90312500061451573, -30.00000000000000000 ) ) ;
#9499=CARTESIAN_POINT ( 'NONE',  ( 16.68750000122903288, -4.330127018922194537, 2.499999999999995559 ) ) ;
#9500=CARTESIAN_POINT ( 'NONE',  ( 9.853125000614516793, 4.541064518000418104, -2.621784821874998173 ) ) ;
#9501=ORIENTED_EDGE ( 'NONE', *, *, #16801, .F. ) ;
#9502=CARTESIAN_POINT ( 'NONE',  ( 16.68750000000000000, -2.886751345948125991, -5.000000000000000000 ) ) ;
#9503=CARTESIAN_POINT ( 'NONE',  ( 19.12500000122902932, 2.886751345948062486, -5.000000000000113687 ) ) ;
#9504=CARTESIAN_POINT ( 'NONE',  ( 10.84687500061451715, 6.054752690667223547, 3.707466751127219781E-16 ) ) ;
#9506=CARTESIAN_POINT ( 'NONE',  ( 9.675000001229035362, 2.886751345948129099, -4.999999999999998224 ) ) ;
#9507=CARTESIAN_POINT ( 'NONE',  ( 19.20000000122903572, 5.773502691896255534, 3.535250795749688894E-16 ) ) ;
#9508=CARTESIAN_POINT ( 'NONE',  ( 15.44062500061451537, -3.027376345333614438, 5.243569643749998122 ) ) ;
#9509=CARTESIAN_POINT ( 'NONE',  ( 19.45312500061451644, 0.000000000000000000, 5.243569643749999010 ) ) ;
#9510=CARTESIAN_POINT ( 'NONE',  ( 26.73750000122903003, 6.123233995736764310E-16, -4.999999999999998224 ) ) ;
#9511=CARTESIAN_POINT ( 'NONE',  ( 2.990625000614519191, -3.027376345333610441, -5.243569643749999898 ) ) ;
#9512=CARTESIAN_POINT ( 'NONE',  ( 24.14999999999999858, 0.000000000000000000, 4.999999999999998224 ) ) ;
#9515=CARTESIAN_POINT ( 'NONE',  ( 26.03437500061451715, 6.421520780324663323E-16, -5.243569643749999010 ) ) ;
#9518=CARTESIAN_POINT ( 'NONE',  ( 12.82500000122903394, 2.886751345948129099, -4.999999999999998224 ) ) ;
#9519=CARTESIAN_POINT ( 'NONE',  ( 3.600000000000002309, -4.330127018922190985, -2.500000000000001332 ) ) ;
#9520=CARTESIAN_POINT ( 'NONE',  ( 14.69999999999999929, 0.000000000000000000, 4.999999999999998224 ) ) ;
#9521=CARTESIAN_POINT ( 'NONE',  ( 8.296875000614516438, -3.027376345333614438, 5.243569643749998122 ) ) ;
#9522=CARTESIAN_POINT ( 'NONE',  ( 25.00312500061451715, -4.541064518000417216, -2.621784821875001281 ) ) ;
#9524=CARTESIAN_POINT ( 'NONE',  ( 5.549999999999998934, 4.330127018922192761, -2.499999999999997780 ) ) ;
#9526=CARTESIAN_POINT ( 'NONE',  ( 4.209375000614516971, 0.000000000000000000, 5.243569643749999010 ) ) ;
#9527=CARTESIAN_POINT ( 'NONE',  ( 7.696875000614516793, 6.054752690667223547, 3.707466751127219781E-16 ) ) ;
#9528=CARTESIAN_POINT ( 'NONE',  ( 5.062500000000000888, 2.886751345948129099, -4.999999999999998224 ) ) ;
#9529=CARTESIAN_POINT ( 'NONE',  ( 9.001249775931846008E-16, 13.61562500061459602, 34.90005215228797653 ) ) ;
#9530=CARTESIAN_POINT ( 'NONE',  ( 22.57499999999999929, 6.123233995736764310E-16, -4.999999999999998224 ) ) ;
#9531=FACE_OUTER_BOUND ( 'NONE', #69545, .T. ) ;
#9532=CARTESIAN_POINT ( 'NONE',  ( 3.412500000000002309, 2.886751345948126879, 4.999999999999999112 ) ) ;
#9533=EDGE_LOOP ( 'NONE', ( #13204, #49395, #6349, #33646 ) ) ;
#9534=CARTESIAN_POINT ( 'NONE',  ( 17.54062500061451502, 6.054752690667223547, 3.707466751127219781E-16 ) ) ;
#9535=CARTESIAN_POINT ( 'NONE',  ( 11.27812500061451573, 4.541064518000418104, 2.621784821874999949 ) ) ;
#9537=CARTESIAN_POINT ( 'NONE',  ( 6.196875000614515905, -3.027376345333610441, -5.243569643749999898 ) ) ;
#9538=CARTESIAN_POINT ( 'NONE',  ( 22.76249999999999574, 2.886751345948126879, 4.999999999999999112 ) ) ;
#9539=CARTESIAN_POINT ( 'NONE',  ( 20.51250000122903216, 4.330127018922192761, -2.499999999999997780 ) ) ;
#9541=CARTESIAN_POINT ( 'NONE',  ( 9.196875000614518569, -3.027376345333614438, 5.243569643749998122 ) ) ;
#9542=CARTESIAN_POINT ( 'NONE',  ( 13.20937500061451786, 0.000000000000000000, 5.243569643749999010 ) ) ;
#9543=CARTESIAN_POINT ( 'NONE',  ( 23.55937500061451573, 0.000000000000000000, 5.243569643749999010 ) ) ;
#9546=CARTESIAN_POINT ( 'NONE',  ( 17.18437500061451573, 4.541064518000418104, 2.621784821874999949 ) ) ;
#9547=CARTESIAN_POINT ( 'NONE',  ( 8.559375000614515727, 4.541064518000418104, -2.621784821874998173 ) ) ;
#9549=CARTESIAN_POINT ( 'NONE',  ( 20.24999999999999645, -4.330127018922190985, -2.500000000000001332 ) ) ;
#9551=CARTESIAN_POINT ( 'NONE',  ( -1.999999999999997113, 9.837500001229035007, -26.53589838486224295 ) ) ;
#9553=CARTESIAN_POINT ( 'NONE',  ( 12.77812500061451750, -4.541064518000419881, 2.621784821874995952 ) ) ;
#9554=CARTESIAN_POINT ( 'NONE',  ( 29.33437500061451431, 4.541064518000418104, 2.621784821874999949 ) ) ;
#9556=CARTESIAN_POINT ( 'NONE',  ( 0.000000000000000000, 20.00000000000000000, -33.99999999999999289 ) ) ;
#9557=CARTESIAN_POINT ( 'NONE',  ( 12.78749999999999964, 5.773502691896255534, 3.535250795749688894E-16 ) ) ;
#9559=CARTESIAN_POINT ( 'NONE',  ( 3.999999999999999112, 18.53750000122903430, 30.00000000000000000 ) ) ;
#9560=CARTESIAN_POINT ( 'NONE',  ( 11.32500000122903394, -5.773502691896255534, -1.060575238724906372E-15 ) ) ;
#9561=CARTESIAN_POINT ( 'NONE',  ( 21.38437500061451502, -4.541064518000419881, 2.621784821874995952 ) ) ;
#9562=CARTESIAN_POINT ( 'NONE',  ( 16.24687500061451573, 6.054752690667223547, 3.707466751127219781E-16 ) ) ;
#9563=DIRECTION ( 'NONE',  ( -0.000000000000000000, -1.000000000000000000, -0.000000000000000000 ) ) ;
#9564=ORIENTED_EDGE ( 'NONE', *, *, #43169, .T. ) ;
#9565=CARTESIAN_POINT ( 'NONE',  ( 17.54062500061451502, 6.054752690667223547, 3.707466751127219781E-16 ) ) ;
#9566=CARTESIAN_POINT ( 'NONE',  ( 27.71250000122903145, 4.330127018922192761, -2.499999999999997780 ) ) ;
#9567=CARTESIAN_POINT ( 'NONE',  ( 17.33437500061451431, -4.541064518000419881, 2.621784821874995952 ) ) ;
#9568=CARTESIAN_POINT ( 'NONE',  ( 3.590625000614518836, 6.054752690667223547, 3.707466751127219781E-16 ) ) ;
#9569=CARTESIAN_POINT ( 'NONE',  ( 20.20312500061451644, 4.541064518000418104, -2.621784821874998173 ) ) ;
#9570=CARTESIAN_POINT ( 'NONE',  ( 3.999999999999999112, 18.42500000000000071, -30.00000000000000000 ) ) ;
#9571=CARTESIAN_POINT ( 'NONE',  ( 27.79687500061451999, -3.027376345333610441, -5.243569643749999898 ) ) ;
#9572=CARTESIAN_POINT ( 'NONE',  ( 2.121784821875001281, 12.30312500061451608, 33.67503911421598417 ) ) ;
#9573=CARTESIAN_POINT ( 'NONE',  ( 17.06250000122903288, 0.000000000000000000, 4.999999999999998224 ) ) ;
#9575=CARTESIAN_POINT ( 'NONE',  ( 26.16562500061451502, 3.027376345333611329, 5.243569643749999010 ) ) ;
#9577=CARTESIAN_POINT ( 'NONE',  ( 19.73437500061451644, 6.421520780324663323E-16, -5.243569643749999010 ) ) ;
#9578=CARTESIAN_POINT ( 'NONE',  ( 22.12500000122903288, -5.773502691896255534, -1.060575238724906372E-15 ) ) ;
#9579=CARTESIAN_POINT ( 'NONE',  ( 22.94062500061451715, 6.054752690667223547, 3.707466751127219781E-16 ) ) ;
#9580=CARTESIAN_POINT ( 'NONE',  ( 18.12187500061451573, 3.027376345333611329, 5.243569643749999010 ) ) ;
#9581=CARTESIAN_POINT ( 'NONE',  ( 11.46562500061451573, -6.054752690667223547, -1.112240025338166033E-15 ) ) ;
#9582=CARTESIAN_POINT ( 'NONE',  ( 4.243569643749999898, 15.13437500061451679, 30.00000000000000000 ) ) ;
#9583=CARTESIAN_POINT ( 'NONE',  ( 17.31562500061451715, -6.054752690667223547, -1.112240025338166033E-15 ) ) ;
#9584=CARTESIAN_POINT ( 'NONE',  ( 10.05000000000000071, 4.330127018922192761, -2.499999999999997780 ) ) ;
#9587=CARTESIAN_POINT ( 'NONE',  ( 22.46250000000000213, -5.773502691896255534, -1.060575238724906372E-15 ) ) ;
#9588=CARTESIAN_POINT ( 'NONE',  ( 4.243569643749999898, 18.24687500061451928, -27.54997392385601529 ) ) ;
#9589=CARTESIAN_POINT ( 'NONE',  ( 13.23750000122903359, 6.123233995736764310E-16, -4.999999999999998224 ) ) ;
#9590=CARTESIAN_POINT ( 'NONE',  ( 23.99062500061451786, -3.027376345333614438, 5.243569643749998122 ) ) ;
#9591=CARTESIAN_POINT ( 'NONE',  ( 6.328125000614515550, 4.541064518000418104, 2.621784821874999949 ) ) ;
#9592=CARTESIAN_POINT ( 'NONE',  ( 16.53750000122903430, 4.330127018922191873, 2.499999999999999556 ) ) ;
#9593=CARTESIAN_POINT ( 'NONE',  ( 21.32812500061451644, -4.541064518000419881, 2.621784821874995952 ) ) ;
#9594=CARTESIAN_POINT ( 'NONE',  ( 22.19999999999999574, 4.330127018922192761, -2.499999999999997780 ) ) ;
#9595=CARTESIAN_POINT ( 'NONE',  ( 26.91562500061451146, 3.027376345333613106, -5.243569643749998122 ) ) ;
#9596=CARTESIAN_POINT ( 'NONE',  ( 7.115625000614516082, 3.027376345333613106, -5.243569643749998122 ) ) ;
#9597=VERTEX_POINT ( 'NONE', #39863 ) ;
#9599=CARTESIAN_POINT ( 'NONE',  ( 24.29062500061451502, 6.054752690667223547, 3.707466751127219781E-16 ) ) ;
#9600=CARTESIAN_POINT ( 'NONE',  ( 5.128125000614516260, -4.541064518000419881, 2.621784821874995952 ) ) ;
#9602=CARTESIAN_POINT ( 'NONE',  ( 4.340625000614515727, -3.027376345333610441, -5.243569643749999898 ) ) ;
#9603=CARTESIAN_POINT ( 'NONE',  ( 4.000000000000000000, 13.55000000122903359, -27.69059892324149530 ) ) ;
#9604=CARTESIAN_POINT ( 'NONE',  ( -1.999999999999997113, 10.62500000000000000, -26.53589838486224295 ) ) ;
#9605=AXIS2_PLACEMENT_3D ( 'NONE', #21651, #55287, #49016 ) ;
#9606=CARTESIAN_POINT ( 'NONE',  ( 10.01250000000000107, 2.886751345948129099, -4.999999999999998224 ) ) ;
#9608=CARTESIAN_POINT ( 'NONE',  ( 11.22187500061451892, 3.027376345333613106, -5.243569643749998122 ) ) ;
#9609=CARTESIAN_POINT ( 'NONE',  ( 5.625000001229036428, 2.886751345948129099, -4.999999999999998224 ) ) ;
#9610=CARTESIAN_POINT ( 'NONE',  ( 15.27187500061451786, 3.027376345333613106, -5.243569643749998122 ) ) ;
#9611=CARTESIAN_POINT ( 'NONE',  ( 5.296875000614518214, -3.027376345333610441, -5.243569643749999898 ) ) ;
#9612=DIRECTION ( 'NONE',  ( 0.000000000000000000, 0.000000000000000000, 1.000000000000000000 ) ) ;
#9613=DIRECTION ( 'NONE',  ( 0.000000000000000000, 0.000000000000000000, -1.000000000000000000 ) ) ;
#9614=CARTESIAN_POINT ( 'NONE',  ( 12.19687500061451679, 6.054752690667223547, 3.707466751127219781E-16 ) ) ;
#9615=FACE_OUTER_BOUND ( 'NONE', #70642, .T. ) ;
#9616=CARTESIAN_POINT ( 'NONE',  ( 23.20312500061451644, -4.541064518000417216, -2.621784821875001281 ) ) ;
#9617=CARTESIAN_POINT ( 'NONE',  ( 3.999999999999999112, 11.67500000000000071, 30.00000000000000000 ) ) ;
#9618=CARTESIAN_POINT ( 'NONE',  ( -4.243569643749999898, 18.86562500061459247, 27.54997392385601529 ) ) ;
#9619=CARTESIAN_POINT ( 'NONE',  ( 23.78437500061451360, 6.421520780324663323E-16, -5.243569643749999010 ) ) ;
#9620=CARTESIAN_POINT ( 'NONE',  ( 4.142324674002726859, 2.800292288406700969, -4.194544246395793152 ) ) ;
#9621=CARTESIAN_POINT ( 'NONE',  ( 3.628125000614518036, 4.541064518000418104, 2.621784821874999949 ) ) ;
#9622=EDGE_CURVE ( 'NONE', #29484, #44903, #11414, .T. ) ;
#9624=CARTESIAN_POINT ( 'NONE',  ( 17.84062500061451573, -3.027376345333610441, -5.243569643749999898 ) ) ;
#9625=CARTESIAN_POINT ( 'NONE',  ( 15.27187500061451786, 3.027376345333613106, -5.243569643749998122 ) ) ;
#9627=CARTESIAN_POINT ( 'NONE',  ( 26.77500000122903145, 2.886751345948129099, -4.999999999999998224 ) ) ;
#9628=CARTESIAN_POINT ( 'NONE',  ( 5.934375000614517504, 4.541064518000418104, 2.621784821874999949 ) ) ;
#9629=CARTESIAN_POINT ( 'NONE',  ( 16.35937500061451644, 0.000000000000000000, 5.243569643749999010 ) ) ;
#9630=CARTESIAN_POINT ( 'NONE',  ( 23.32499999999999929, -4.330127018922194537, 2.499999999999995559 ) ) ;
#9631=CARTESIAN_POINT ( 'NONE',  ( 16.83750000122903145, 6.123233995736764310E-16, -4.999999999999998224 ) ) ;
#9632=CARTESIAN_POINT ( 'NONE',  ( 25.58437500061451431, 6.421520780324663323E-16, -5.243569643749999010 ) ) ;
#9633=CARTESIAN_POINT ( 'NONE',  ( 16.62187500061451573, 3.027376345333613106, -5.243569643749998122 ) ) ;
#9635=CARTESIAN_POINT ( 'NONE',  ( 29.81250000000000000, 2.886751345948129099, -4.999999999999998224 ) ) ;
#9636=CARTESIAN_POINT ( 'NONE',  ( 7.687500000000000000, -2.886751345948125991, -5.000000000000000000 ) ) ;
#9638=CARTESIAN_POINT ( 'NONE',  ( 20.69062500061451715, 6.054752690667223547, 3.707466751127219781E-16 ) ) ;
#9639=CARTESIAN_POINT ( 'NONE',  ( 8.474999999999999645, -4.330127018922194537, 2.499999999999995559 ) ) ;
#9640=CARTESIAN_POINT ( 'NONE',  ( 3.215625000614518836, 3.027376345333611329, 5.243569643749999010 ) ) ;
#9641=CARTESIAN_POINT ( 'NONE',  ( 19.94999999999999929, 4.330127018922192761, -2.499999999999997780 ) ) ;
#9642=EDGE_CURVE ( 'NONE', #30208, #47001, #7663, .T. ) ;
#9643=CARTESIAN_POINT ( 'NONE',  ( 18.29062500061451502, -3.027376345333610441, -5.243569643749999898 ) ) ;
#9645=CARTESIAN_POINT ( 'NONE',  ( 22.80000000122903359, 5.773502691896255534, 3.535250795749688894E-16 ) ) ;
#9646=CARTESIAN_POINT ( 'NONE',  ( 2.923357432354301455, -4.056350739605543154, 3.322806236625610588 ) ) ;
#9647=CARTESIAN_POINT ( 'NONE',  ( 28.77187500061451431, 3.027376345333613106, -5.243569643749998122 ) ) ;
#9648=ORIENTED_EDGE ( 'NONE', *, *, #15704, .F. ) ;
#9649=CARTESIAN_POINT ( 'NONE',  ( 17.84062500061451573, -3.027376345333610441, -5.243569643749999898 ) ) ;
#9650=CARTESIAN_POINT ( 'NONE',  ( 24.81562500061451715, 3.027376345333611329, 5.243569643749999010 ) ) ;
#9651=CARTESIAN_POINT ( 'NONE',  ( 25.84687500061451360, -3.027376345333614438, 5.243569643749998122 ) ) ;
#9652=CARTESIAN_POINT ( 'NONE',  ( 10.05000000000000071, 4.330127018922192761, -2.499999999999997780 ) ) ;
#9653=CARTESIAN_POINT ( 'NONE',  ( 11.12812500061451715, 6.421520780324663323E-16, -5.243569643749999010 ) ) ;
#9654=CARTESIAN_POINT ( 'NONE',  ( 25.71562500061451573, 3.027376345333611329, 5.243569643749999010 ) ) ;
#9655=CARTESIAN_POINT ( 'NONE',  ( 18.00937500061451502, 4.541064518000418104, -2.621784821874998173 ) ) ;
#9656=CARTESIAN_POINT ( 'NONE',  ( 18.57187500061451857, 3.027376345333611329, 5.243569643749999010 ) ) ;
#9657=CARTESIAN_POINT ( 'NONE',  ( 3.065815551951259543, -3.949781639713015657, 3.065815551951216467 ) ) ;
#9658=CARTESIAN_POINT ( 'NONE',  ( -4.243569643749997233, 9.996875000614517504, 32.45002607614398471 ) ) ;
#9659=CARTESIAN_POINT ( 'NONE',  ( 23.40000000122903145, -2.886751345948129988, 4.999999999999997335 ) ) ;
#9661=CARTESIAN_POINT ( 'NONE',  ( 13.86562500061451431, 3.027376345333612662, -5.243569643749998122 ) ) ;
#9663=CARTESIAN_POINT ( 'NONE',  ( 8.296875000614516438, -3.027376345333614438, 5.243569643749998122 ) ) ;
#9664=CARTESIAN_POINT ( 'NONE',  ( 6.984375000614516438, -4.541064518000419881, 2.621784821874995952 ) ) ;
#9665=ORIENTED_EDGE ( 'NONE', *, *, #12071, .T. ) ;
#9666=CARTESIAN_POINT ( 'NONE',  ( 29.78437500061451715, 4.541064518000418104, 2.621784821874999949 ) ) ;
#9667=CARTESIAN_POINT ( 'NONE',  ( 20.24062500061451431, 6.054752690667223547, 3.707466751127219781E-16 ) ) ;
#9668=CARTESIAN_POINT ( 'NONE',  ( 23.37187500061451573, 3.027376345333613106, -5.243569643749998122 ) ) ;
#9669=CARTESIAN_POINT ( 'NONE',  ( 20.09062500061451573, -3.027376345333610441, -5.243569643749999898 ) ) ;
#9670=CARTESIAN_POINT ( 'NONE',  ( 3.999999999999999112, 11.67500000000000071, 30.00000000000000000 ) ) ;
#9671=CARTESIAN_POINT ( 'NONE',  ( 25.90312500061451573, -4.541064518000417216, -2.621784821875001281 ) ) ;
#9672=CARTESIAN_POINT ( 'NONE',  ( 7.837500001229035007, 6.123233995736764310E-16, -4.999999999999998224 ) ) ;
#9673=ORIENTED_EDGE ( 'NONE', *, *, #70375, .F. ) ;
#9674=CARTESIAN_POINT ( 'NONE',  ( 3.187500001229033764, -4.330127018922194537, 2.499999999999995559 ) ) ;
#9675=CARTESIAN_POINT ( 'NONE',  ( -1.999999999999997113, 15.12500000000000000, -26.53589838486224295 ) ) ;
#9676=CARTESIAN_POINT ( 'NONE',  ( 21.97500000122903074, 2.886751345948126879, 4.999999999999999112 ) ) ;
#9678=CARTESIAN_POINT ( 'NONE',  ( 6.159375000614517148, -4.541064518000417216, -2.621784821875001281 ) ) ;
#9679=CARTESIAN_POINT ( 'NONE',  ( 12.86250000000000071, 2.886751345948126879, 4.999999999999998224 ) ) ;
#9680=CARTESIAN_POINT ( 'NONE',  ( 11.50312500061451892, -4.541064518000417216, -2.621784821875001281 ) ) ;
#9681=CARTESIAN_POINT ( 'NONE',  ( 9.159375000614515372, 0.000000000000000000, 5.243569643749999010 ) ) ;
#9682=CARTESIAN_POINT ( 'NONE',  ( 26.88750000122903216, 4.330127018922191873, 2.499999999999999556 ) ) ;
#9683=CARTESIAN_POINT ( 'NONE',  ( 14.29687500061451821, -3.027376345333610441, -5.243569643749999898 ) ) ;
#9684=CARTESIAN_POINT ( 'NONE',  ( 5.784375000614517148, 6.421520780324663323E-16, -5.243569643749999010 ) ) ;
#9685=CARTESIAN_POINT ( 'NONE',  ( 29.39999999999999858, 4.330127018922192761, -2.499999999999997780 ) ) ;
#9686=CARTESIAN_POINT ( 'NONE',  ( 4.903125000614516615, 4.541064518000418104, -2.621784821874998173 ) ) ;
#9687=CARTESIAN_POINT ( 'NONE',  ( 15.77812500061451573, 4.541064518000418104, 2.621784821874999949 ) ) ;
#9688=ORIENTED_EDGE ( 'NONE', *, *, #61648, .F. ) ;
#9689=CARTESIAN_POINT ( 'NONE',  ( 12.66562500061451502, 3.027376345333611329, 5.243569643749999010 ) ) ;
#9690=CARTESIAN_POINT ( 'NONE',  ( 8.278125000614515727, -4.541064518000419881, 2.621784821874995952 ) ) ;
#9692=CARTESIAN_POINT ( 'NONE',  ( 9.000000000000001776, -4.330127018922190985, -2.500000000000001332 ) ) ;
#9693=CARTESIAN_POINT ( 'NONE',  ( 3.487500001229035362, 4.330127018922191873, 2.499999999999999556 ) ) ;
#9694=CARTESIAN_POINT ( 'NONE',  ( 17.02499999999999858, -4.330127018922194537, 2.499999999999995559 ) ) ;
#9695=CARTESIAN_POINT ( 'NONE',  ( 17.82187500061451502, -6.054752690667223547, -1.112240025338166033E-15 ) ) ;
#9696=CARTESIAN_POINT ( 'NONE',  ( 14.73750000122903359, 4.330127018922191873, 2.499999999999999556 ) ) ;
#9698=CARTESIAN_POINT ( 'NONE',  ( 2.121784821875001281, 17.25312500061451715, -26.32496088578401938 ) ) ;
#9701=CARTESIAN_POINT ( 'NONE',  ( 29.65312500061451573, 4.541064518000418104, -2.621784821874998173 ) ) ;
#9702=DIRECTION ( 'NONE',  ( -1.000000000000000000, -0.000000000000000000, -0.000000000000000000 ) ) ;
#9703=CARTESIAN_POINT ( 'NONE',  ( 15.94687500061451502, -3.027376345333614438, 5.243569643749998122 ) ) ;
#9704=CARTESIAN_POINT ( 'NONE',  ( 26.62500000000000000, 6.123233995736764310E-16, -4.999999999999998224 ) ) ;
#9705=CARTESIAN_POINT ( 'NONE',  ( 11.20312500061451644, 4.541064518000418104, -2.621784821874998173 ) ) ;
#9706=VECTOR ( 'NONE', #2051, 1000.000000000000000 ) ;
#9708=CARTESIAN_POINT ( 'NONE',  ( 21.12187500061451573, 3.027376345333613106, -5.243569643749998122 ) ) ;
#9710=CARTESIAN_POINT ( 'NONE',  ( 6.515625000614516438, -6.054752690667223547, -1.112240025338166033E-15 ) ) ;
#9711=CARTESIAN_POINT ( 'NONE',  ( 14.18437500061451750, -4.541064518000419881, 2.621784821874995952 ) ) ;
#9712=ORIENTED_EDGE ( 'NONE', *, *, #8453, .F. ) ;
#9713=CARTESIAN_POINT ( 'NONE',  ( 23.07187500061451857, 3.027376345333611329, 5.243569643749999010 ) ) ;
#9714=CARTESIAN_POINT ( 'NONE',  ( 3.861486210907941086, 3.177525289277527420, -28.92245512961235576 ) ) ;
#9716=CARTESIAN_POINT ( 'NONE',  ( 24.71250000000000213, -5.773502691896255534, -1.060575238724906372E-15 ) ) ;
#9717=CARTESIAN_POINT ( 'NONE',  ( 6.524999999999999467, 4.330127018922191873, 2.499999999999999556 ) ) ;
#9718=CARTESIAN_POINT ( 'NONE',  ( 16.46250000122903501, 4.330127018922192761, -2.499999999999997780 ) ) ;
#9719=CARTESIAN_POINT ( 'NONE',  ( -1.487416814333745711E-14, 16.62500000122903288, 34.00000000000000000 ) ) ;
#9721=ORIENTED_EDGE ( 'NONE', *, *, #25362, .T. ) ;
#9722=CARTESIAN_POINT ( 'NONE',  ( 14.88750000000000107, -2.886751345948125991, -5.000000000000000000 ) ) ;
#9723=CARTESIAN_POINT ( 'NONE',  ( 16.01249999999999929, 2.886751345948126879, 4.999999999999999112 ) ) ;
#9724=CARTESIAN_POINT ( 'NONE',  ( 12.51562500061451821, 3.027376345333613106, -5.243569643749998122 ) ) ;
#9725=ORIENTED_EDGE ( 'NONE', *, *, #38684, .F. ) ;
#9726=CARTESIAN_POINT ( 'NONE',  ( -3.999999999999997335, 17.00000000122903288, -27.69059892324149530 ) ) ;
#9727=CARTESIAN_POINT ( 'NONE',  ( 2.121784821875001281, 17.75937500061451502, -26.32496088578401938 ) ) ;
#9728=CARTESIAN_POINT ( 'NONE',  ( 4.490625000614516971, 6.054752690667223547, 3.707466751127219781E-16 ) ) ;
#9730=CARTESIAN_POINT ( 'NONE',  ( 10.95000000000000107, 4.330127018922192761, -2.499999999999997780 ) ) ;
#9731=CARTESIAN_POINT ( 'NONE',  ( 3.046343057529203424, 3.964819538874875704, 3.046343057529141696 ) ) ;
#9732=ORIENTED_EDGE ( 'NONE', *, *, #28241, .F. ) ;
#9733=CARTESIAN_POINT ( 'NONE',  ( 2.121784821875001281, 11.85312500061451857, 33.67503911421598417 ) ) ;
#9734=CARTESIAN_POINT ( 'NONE',  ( 23.39062500061451289, 6.054752690667223547, 3.707466751127219781E-16 ) ) ;
#9737=CARTESIAN_POINT ( 'NONE',  ( 20.89687500061452141, -3.027376345333614438, 5.243569643749998122 ) ) ;
#9738=CARTESIAN_POINT ( 'NONE',  ( 19.11562500061451431, -6.054752690667223547, -1.112240025338166033E-15 ) ) ;
#9739=CARTESIAN_POINT ( 'NONE',  ( 2.121784821875001281, 13.65312500061459566, -26.32496088578401938 ) ) ;
#9740=CARTESIAN_POINT ( 'NONE',  ( 24.07500000122903216, 2.886751345948129099, -4.999999999999998224 ) ) ;
#9741=CARTESIAN_POINT ( 'NONE',  ( 3.890625000614517326, -3.027376345333610441, -5.243569643749999898 ) ) ;
#9743=CARTESIAN_POINT ( 'NONE',  ( 20.95312500061451999, -4.541064518000417216, -2.621784821875001281 ) ) ;
#9746=CARTESIAN_POINT ( 'NONE',  ( 15.94687500061451502, -3.027376345333614438, 5.243569643749998122 ) ) ;
#9747=CARTESIAN_POINT ( 'NONE',  ( 13.84687500061451537, -3.027376345333610441, -5.243569643749999898 ) ) ;
#9748=CARTESIAN_POINT ( 'NONE',  ( 21.64687500061451786, 6.054752690667223547, 3.707466751127219781E-16 ) ) ;
#9749=CARTESIAN_POINT ( 'NONE',  ( 4.243569643749999898, 11.49687500061451928, 32.45002607614398471 ) ) ;
#9750=CARTESIAN_POINT ( 'NONE',  ( 4.528125000614516615, 4.541064518000418104, 2.621784821874999949 ) ) ;
#9751=CARTESIAN_POINT ( 'NONE',  ( 25.94062500061451715, -3.027376345333610441, -5.243569643749999898 ) ) ;
#9752=CARTESIAN_POINT ( 'NONE',  ( 26.27812500061451573, -4.541064518000419881, 2.621784821874995952 ) ) ;
#9754=CARTESIAN_POINT ( 'NONE',  ( 7.275000000000000355, 6.123233995736764310E-16, -4.999999999999998224 ) ) ;
#9755=CARTESIAN_POINT ( 'NONE',  ( 7.771875000614516971, 3.027376345333611329, 5.243569643749999010 ) ) ;
#9757=CARTESIAN_POINT ( 'NONE',  ( 14.06250000122903288, -4.330127018922190985, -2.500000000000001332 ) ) ;
#9758=CARTESIAN_POINT ( 'NONE',  ( 10.46250000122903323, -4.330127018922190985, -2.500000000000001332 ) ) ;
#9759=CARTESIAN_POINT ( 'NONE',  ( 3.703125000614516882, 0.000000000000000000, 5.243569643749999010 ) ) ;
#9762=CARTESIAN_POINT ( 'NONE',  ( 13.73437500061451821, -4.541064518000419881, 2.621784821874995952 ) ) ;
#9763=CARTESIAN_POINT ( 'NONE',  ( 1.510657702057710734E-15, 19.10000000122903430, -33.99999999999999289 ) ) ;
#9765=CARTESIAN_POINT ( 'NONE',  ( 20.39062500061451644, -3.027376345333614438, 5.243569643749998122 ) ) ;
#9766=CARTESIAN_POINT ( 'NONE',  ( 6.215625000614517504, 3.027376345333613106, -5.243569643749998122 ) ) ;
#9767=CARTESIAN_POINT ( 'NONE',  ( 24.98437500061451644, -4.541064518000419881, 2.621784821874995952 ) ) ;
#9768=CARTESIAN_POINT ( 'NONE',  ( 8.428125000614517859, 6.421520780324663323E-16, -5.243569643749999010 ) ) ;
#9769=CYLINDRICAL_SURFACE ( 'NONE', #68674, 4.999999999999998224 ) ;
#9770=( BOUNDED_CURVE ( )  B_SPLINE_CURVE ( 2, ( #41492, #64012, #13392, #35937, #58460, #7871, #30407 ),
 .UNSPECIFIED., .F., .F. ) 
 B_SPLINE_CURVE_WITH_KNOTS ( ( 3, 2, 2, 3 ),
 ( 0.4916666666666666408, 0.4944444444444444642, 0.4972222222222222321, 0.5000000000000000000 ),
 .UNSPECIFIED. ) 
 CURVE ( )  GEOMETRIC_REPRESENTATION_ITEM ( )  RATIONAL_B_SPLINE_CURVE ( ( 1.000000000000000000, 0.8660254037844387076, 1.000000000000000000, 0.8660254037844387076, 1.000000000000000000, 0.8660254037844387076, 1.000000000000000000 ) ) 
 REPRESENTATION_ITEM ( '' )  );
#9771=CARTESIAN_POINT ( 'NONE',  ( 7.162500001229032520, 0.000000000000000000, 4.999999999999998224 ) ) ;
#9772=CARTESIAN_POINT ( 'NONE',  ( 22.34062500061451573, -3.027376345333610441, -5.243569643749999898 ) ) ;
#9773=CARTESIAN_POINT ( 'NONE',  ( -2.828200636599751609E-16, 18.20000000122903216, -34.61880215351700230 ) ) ;
#9774=CARTESIAN_POINT ( 'NONE',  ( 9.862500001229033586, 0.000000000000000000, 4.999999999999998224 ) ) ;
#9775=CARTESIAN_POINT ( 'NONE',  ( 19.00312500061451715, 0.000000000000000000, 5.243569643749999010 ) ) ;
#9776=CARTESIAN_POINT ( 'NONE',  ( 15.44062500061451537, -3.027376345333614438, 5.243569643749998122 ) ) ;
#9778=CARTESIAN_POINT ( 'NONE',  ( 15.56250000000000000, 2.886751345948126879, 4.999999999999999112 ) ) ;
#9779=CARTESIAN_POINT ( 'NONE',  ( 12.03750000122903430, 4.330127018922191873, 2.499999999999999556 ) ) ;
#9780=CARTESIAN_POINT ( 'NONE',  ( 9.103125000614515017, 0.000000000000000000, 5.243569643749999010 ) ) ;
#9781=CARTESIAN_POINT ( 'NONE',  ( 10.56562500061451715, -6.054752690667223547, -1.112240025338166033E-15 ) ) ;
#9782=EDGE_CURVE ( 'NONE', #40370, #8399, #66844, .T. ) ;
#9783=CARTESIAN_POINT ( 'NONE',  ( 20.43750000122903643, 6.123233995736764310E-16, -4.999999999999998224 ) ) ;
#9784=CARTESIAN_POINT ( 'NONE',  ( 18.98437500061451644, 4.541064518000418104, 2.621784821874999949 ) ) ;
#9785=CARTESIAN_POINT ( 'NONE',  ( 4.655204990825274614, -3.615897911723494840, 4.224220389412703724 ) ) ;
#9786=CARTESIAN_POINT ( 'NONE',  ( 5.925000001229033586, -5.773502691896255534, -1.060575238724906372E-15 ) ) ;
#9787=CARTESIAN_POINT ( 'NONE',  ( 3.834375000614519635, -4.541064518000419881, 2.621784821874995952 ) ) ;
#9788=CARTESIAN_POINT ( 'NONE',  ( 22.09687500061451715, 6.054752690667223547, 3.707466751127219781E-16 ) ) ;
#9789=CARTESIAN_POINT ( 'NONE',  ( -1.071796769724496556, 15.14240381056766616, 33.99999999999998579 ) ) ;
#9790=CARTESIAN_POINT ( 'NONE',  ( 18.51562500061451289, 3.027376345333611329, 5.243569643749999010 ) ) ;
#9791=CARTESIAN_POINT ( 'NONE',  ( 23.22187500061451715, -6.054752690667223547, -1.112240025338166033E-15 ) ) ;
#9793=CARTESIAN_POINT ( 'NONE',  ( -2.000000000000000000, 11.03750000122903430, -33.46410161513775705 ) ) ;
#9794=CARTESIAN_POINT ( 'NONE',  ( 27.72187500061451715, -6.054752690667223547, -1.112240025338166033E-15 ) ) ;
#9796=CARTESIAN_POINT ( 'NONE',  ( 14.35312500061451679, 4.541064518000418104, -2.621784821874998173 ) ) ;
#9797=CARTESIAN_POINT ( 'NONE',  ( 12.53437500061451537, 6.421520780324663323E-16, -5.243569643749999010 ) ) ;
#9798=ORIENTED_EDGE ( 'NONE', *, *, #56271, .F. ) ;
#9799=CARTESIAN_POINT ( 'NONE',  ( 13.35000000000000142, 0.000000000000000000, 4.999999999999998224 ) ) ;
#9800=CARTESIAN_POINT ( 'NONE',  ( 22.00312500061451360, 4.541064518000418104, -2.621784821874998173 ) ) ;
#9801=CARTESIAN_POINT ( 'NONE',  ( 1.999999999999998668, 17.15000000000000213, 26.53589838486224650 ) ) ;
#9802=CARTESIAN_POINT ( 'NONE',  ( 14.47499999999999964, 6.123233995736764310E-16, -4.999999999999998224 ) ) ;
#9803=CARTESIAN_POINT ( 'NONE',  ( 14.62500000000000000, 4.330127018922191873, 2.499999999999999556 ) ) ;
#9804=CARTESIAN_POINT ( 'NONE',  ( 23.77500000122903145, 2.886751345948126879, 4.999999999999999112 ) ) ;
#9805=CARTESIAN_POINT ( 'NONE',  ( 19.11562500061451431, -6.054752690667223547, -1.112240025338166033E-15 ) ) ;
#9806=ORIENTED_EDGE ( 'NONE', *, *, #49507, .F. ) ;
#9807=CARTESIAN_POINT ( 'NONE',  ( 21.67500000000000071, 6.123233995736764310E-16, -4.999999999999998224 ) ) ;
#9808=( BOUNDED_CURVE ( )  B_SPLINE_CURVE ( 2, ( #8517, #8888, #63571, #12959, #35496, #69493, #58016 ),
 .UNSPECIFIED., .F., .F. ) 
 B_SPLINE_CURVE_WITH_KNOTS ( ( 3, 2, 2, 3 ),
 ( 0.6916666666666666519, 0.6944444444444444198, 0.6972222222222221877, 0.6999999999999999556 ),
 .UNSPECIFIED. ) 
 CURVE ( )  GEOMETRIC_REPRESENTATION_ITEM ( )  RATIONAL_B_SPLINE_CURVE ( ( 1.000000000000000000, 0.8660254037844387076, 1.000000000000000000, 0.8660254037844387076, 1.000000000000000000, 0.8660254037844387076, 1.000000000000000000 ) ) 
 REPRESENTATION_ITEM ( '' )  );
#9809=CARTESIAN_POINT ( 'NONE',  ( 24.19687500061451857, -3.027376345333610441, -5.243569643749999898 ) ) ;
#9810=EDGE_LOOP ( 'NONE', ( #28610, #60092, #63638, #63542, #4644, #38636, #26963, #63152 ) ) ;
#9812=CARTESIAN_POINT ( 'NONE',  ( 10.11562500061451608, -6.054752690667223547, -1.112240025338166033E-15 ) ) ;
#9813=CARTESIAN_POINT ( 'NONE',  ( 4.453125000614517326, 4.541064518000418104, -2.621784821874998173 ) ) ;
#9815=CARTESIAN_POINT ( 'NONE',  ( 27.74062500061451431, -3.027376345333610441, -5.243569643749999898 ) ) ;
#9816=CARTESIAN_POINT ( 'NONE',  ( 16.31250000000000000, 2.886751345948129099, -4.999999999999998224 ) ) ;
#9817=CARTESIAN_POINT ( 'NONE',  ( 23.85000000000000142, -4.330127018922190985, -2.500000000000001332 ) ) ;
#9818=CARTESIAN_POINT ( 'NONE',  ( 2.121784821875001281, 19.05312500061451431, 33.67503911421598417 ) ) ;
#9819=CARTESIAN_POINT ( 'NONE',  ( 5.859375000614519102, 4.541064518000418104, -2.621784821874998173 ) ) ;
#9820=CARTESIAN_POINT ( 'NONE',  ( 17.25937500061451502, 0.000000000000000000, 5.243569643749999010 ) ) ;
#9821=CARTESIAN_POINT ( 'NONE',  ( 28.88437500061451502, 4.541064518000418104, 2.621784821874999949 ) ) ;
#9823=CARTESIAN_POINT ( 'NONE',  ( 27.44062500061451715, 6.054752690667223547, 3.707466751127219781E-16 ) ) ;
#9824=CARTESIAN_POINT ( 'NONE',  ( 27.12187500061451573, 3.027376345333611329, 5.243569643749999010 ) ) ;
#9825=CARTESIAN_POINT ( 'NONE',  ( 2.934375000614518392, -4.541064518000419881, 2.621784821874995952 ) ) ;
#9826=ADVANCED_FACE ( 'NONE', ( #67212 ), #50935, .F. ) ;
#9827=AXIS2_PLACEMENT_3D ( 'NONE', #36442, #47899, #72255 ) ;
#9828=CARTESIAN_POINT ( 'NONE',  ( 14.21249999999999858, 2.886751345948126879, 4.999999999999999112 ) ) ;
#9829=CARTESIAN_POINT ( 'NONE',  ( 11.46562500061451573, -6.054752690667223547, -1.112240025338166033E-15 ) ) ;
#9830=CYLINDRICAL_SURFACE ( 'NONE', #59888, 4.999999999999998224 ) ;
#9831=CARTESIAN_POINT ( 'NONE',  ( 0.000000000000000000, 20.00000000000000000, -33.99999999999999289 ) ) ;
#9832=CARTESIAN_POINT ( 'NONE',  ( 29.72812500061451502, 4.541064518000418104, 2.621784821874999949 ) ) ;
#9833=CARTESIAN_POINT ( 'NONE',  ( 16.87500000122903288, 2.886751345948129099, -4.999999999999998224 ) ) ;
#9834=DIRECTION ( 'NONE',  ( 0.000000000000000000, 0.000000000000000000, -1.000000000000000000 ) ) ;
#9836=CARTESIAN_POINT ( 'NONE',  ( 6.440625000614517148, -3.027376345333614438, 5.243569643749998122 ) ) ;
#9837=CARTESIAN_POINT ( 'NONE',  ( 20.74687500061451573, 6.054752690667223547, 3.707466751127219781E-16 ) ) ;
#9838=CARTESIAN_POINT ( 'NONE',  ( 4.243569643749999010, 16.52187500061451786, 27.54997392385601174 ) ) ;
#9839=CARTESIAN_POINT ( 'NONE',  ( 21.08437500061451786, 6.421520780324663323E-16, -5.243569643749999010 ) ) ;
#9840=CARTESIAN_POINT ( 'NONE',  ( 6.225000000000001421, -4.330127018922194537, 2.499999999999995559 ) ) ;
#9841=CARTESIAN_POINT ( 'NONE',  ( 2.121784821874999061, 19.70937500061451786, 26.32496088578401583 ) ) ;
#9842=CARTESIAN_POINT ( 'NONE',  ( 12.06562500061451537, 3.027376345333613106, -5.243569643749998122 ) ) ;
#9843=CARTESIAN_POINT ( 'NONE',  ( 5.512500001229033941, -4.330127018922190985, -2.500000000000001332 ) ) ;
#9844=CARTESIAN_POINT ( 'NONE',  ( 8.259375000614518569, 0.000000000000000000, 5.243569643749999010 ) ) ;
#9846=CARTESIAN_POINT ( 'NONE',  ( 9.028125000614517504, 4.541064518000418104, 2.621784821874999949 ) ) ;
#9847=CARTESIAN_POINT ( 'NONE',  ( 13.88437500061451679, 6.421520780324663323E-16, -5.243569643749999010 ) ) ;
#9848=CARTESIAN_POINT ( 'NONE',  ( 3.456510739548324551, -3.612829017181165892, -3.800327499238720819 ) ) ;
#9849=CARTESIAN_POINT ( 'NONE',  ( 20.77500000122903145, -5.773502691896255534, -1.060575238724906372E-15 ) ) ;
#9850=CARTESIAN_POINT ( 'NONE',  ( 7.846875000614518036, -3.027376345333614438, 5.243569643749998122 ) ) ;
#9851=CARTESIAN_POINT ( 'NONE',  ( 11.61562500061451608, 3.027376345333613106, -5.243569643749998122 ) ) ;
#9853=CARTESIAN_POINT ( 'NONE',  ( 21.57187500061451502, 3.027376345333613106, -5.243569643749998122 ) ) ;
#9855=CARTESIAN_POINT ( 'NONE',  ( -3.183805653906653266, 3.859810113929996067, 27.56566125170668258 ) ) ;
#9856=CARTESIAN_POINT ( 'NONE',  ( -3.999999999999999112, 20.00000000000000000, -30.00000000000000000 ) ) ;
#9857=CARTESIAN_POINT ( 'NONE',  ( -4.243569643749999898, 11.27187500061451786, -32.45002607614398471 ) ) ;
#9858=CARTESIAN_POINT ( 'NONE',  ( 14.77500000122903501, 2.886751345948126879, 4.999999999999999112 ) ) ;
#9859=CARTESIAN_POINT ( 'NONE',  ( 4.243569643749999898, 15.94062500061451537, -27.54997392385601529 ) ) ;
#9860=CARTESIAN_POINT ( 'NONE',  ( 18.33750000122903501, 4.330127018922191873, 2.499999999999999556 ) ) ;
#9861=CARTESIAN_POINT ( 'NONE',  ( 9.028125000614517504, 4.541064518000418104, 2.621784821874999949 ) ) ;
#9862=ORIENTED_EDGE ( 'NONE', *, *, #2528, .F. ) ;
#9863=CARTESIAN_POINT ( 'NONE',  ( 16.42500000000000071, 4.330127018922191873, 2.499999999999999556 ) ) ;
#9865=CARTESIAN_POINT ( 'NONE',  ( 23.95312500061451289, 0.000000000000000000, 5.243569643749999010 ) ) ;
#9866=CARTESIAN_POINT ( 'NONE',  ( 10.02187500061451964, 3.027376345333611329, 5.243569643749999010 ) ) ;
#9868=CARTESIAN_POINT ( 'NONE',  ( 9.862500001229033586, 0.000000000000000000, 4.999999999999998224 ) ) ;
#9869=CARTESIAN_POINT ( 'NONE',  ( 19.23750000122903714, 4.330127018922191873, 2.499999999999999556 ) ) ;
#9870=CARTESIAN_POINT ( 'NONE',  ( 15.17812500061451608, 6.421520780324663323E-16, -5.243569643749999010 ) ) ;
#9871=CARTESIAN_POINT ( 'NONE',  ( 17.65312500061451573, 0.000000000000000000, 5.243569643749999010 ) ) ;
#9872=CARTESIAN_POINT ( 'NONE',  ( 24.67500000122903359, 2.886751345948126879, 4.999999999999999112 ) ) ;
#9873=CARTESIAN_POINT ( 'NONE',  ( 29.32500000122903216, -5.773502691896255534, -1.060575238724906372E-15 ) ) ;
#9874=CARTESIAN_POINT ( 'NONE',  ( 26.32499999999999929, 4.330127018922191873, 2.499999999999999556 ) ) ;
#9876=CARTESIAN_POINT ( 'NONE',  ( 26.82187500061451857, -6.054752690667223547, -1.112240025338166033E-15 ) ) ;
#9878=CARTESIAN_POINT ( 'NONE',  ( 12.45000000122903394, 5.773502691896255534, 3.535250795749688894E-16 ) ) ;
#9879=CARTESIAN_POINT ( 'NONE',  ( 3.562500000000000444, -5.773502691896255534, -1.060575238724906372E-15 ) ) ;
#9880=EDGE_CURVE ( 'NONE', #49995, #52378, #66590, .T. ) ;
#9881=FACE_OUTER_BOUND ( 'NONE', #12309, .T. ) ;
#9882=CARTESIAN_POINT ( 'NONE',  ( 6.421875000614519102, 3.027376345333611329, 5.243569643749999010 ) ) ;
#9883=CARTESIAN_POINT ( 'NONE',  ( 27.25312500061451360, -4.541064518000417216, -2.621784821875001281 ) ) ;
#9885=CARTESIAN_POINT ( 'NONE',  ( 3.999999999999998668, 10.47500000122903430, 27.69059892324149530 ) ) ;
#9886=CARTESIAN_POINT ( 'NONE',  ( 3.662819313031858925, -3.403491542531015046, 3.773569494236241439 ) ) ;
#9887=CARTESIAN_POINT ( 'NONE',  ( 5.409375000614516260, 4.541064518000418104, -2.621784821874998173 ) ) ;
#9888=CARTESIAN_POINT ( 'NONE',  ( 9.834375000614517859, 6.421520780324663323E-16, -5.243569643749999010 ) ) ;
#9889=CARTESIAN_POINT ( 'NONE',  ( 29.63437500061451502, 6.421520780324663323E-16, -5.243569643749999010 ) ) ;
#9890=CARTESIAN_POINT ( 'NONE',  ( -2.121784821874999949, 12.52812500061459211, 26.32496088578401938 ) ) ;
#9891=CARTESIAN_POINT ( 'NONE',  ( 21.37499999999999645, 4.330127018922191873, 2.499999999999999556 ) ) ;
#9892=CARTESIAN_POINT ( 'NONE',  ( 28.61249999999999716, 2.886751345948126879, 4.999999999999999112 ) ) ;
#9893=CARTESIAN_POINT ( 'NONE',  ( 4.462500000000001243, -5.773502691896255534, -1.060575238724906372E-15 ) ) ;
#9895=CARTESIAN_POINT ( 'NONE',  ( 17.99062500061451786, 6.054752690667223547, 3.707466751127219781E-16 ) ) ;
#9896=CARTESIAN_POINT ( 'NONE',  ( 11.39062500061451644, -3.027376345333614438, 5.243569643749998122 ) ) ;
#9898=CARTESIAN_POINT ( 'NONE',  ( 7.321875000614516793, 3.027376345333611329, 5.243569643749999010 ) ) ;
#9899=CARTESIAN_POINT ( 'NONE',  ( 23.21250000000000213, 2.886751345948126879, 4.999999999999999112 ) ) ;
#9900=CARTESIAN_POINT ( 'NONE',  ( 20.43750000122903643, 6.123233995736764310E-16, -4.999999999999998224 ) ) ;
#9902=CARTESIAN_POINT ( 'NONE',  ( 5.971875000614516260, 3.027376345333611329, 5.243569643749999010 ) ) ;
#9903=CARTESIAN_POINT ( 'NONE',  ( 12.98437500061451821, 6.421520780324663323E-16, -5.243569643749999010 ) ) ;
#9904=CARTESIAN_POINT ( 'NONE',  ( 23.78437500061451360, 6.421520780324663323E-16, -5.243569643749999010 ) ) ;
#9905=CARTESIAN_POINT ( 'NONE',  ( -1.071796769724488563, 16.49240381056766580, 34.00000000000000000 ) ) ;
#9906=VERTEX_POINT ( 'NONE', #55748 ) ;
#9908=CARTESIAN_POINT ( 'NONE',  ( 18.15937500061451715, 0.000000000000000000, 5.243569643749999010 ) ) ;
#9909=CARTESIAN_POINT ( 'NONE',  ( 9.571875000614518569, 3.027376345333611329, 5.243569643749999010 ) ) ;
#9911=CARTESIAN_POINT ( 'NONE',  ( 21.11249999999999716, -5.773502691896255534, -1.060575238724906372E-15 ) ) ;
#9915=CARTESIAN_POINT ( 'NONE',  ( 12.81562500061451537, -6.054752690667223547, -1.112240025338166033E-15 ) ) ;
#9916=CARTESIAN_POINT ( 'NONE',  ( 28.99687500061451573, -3.027376345333614438, 5.243569643749998122 ) ) ;
#9917=CARTESIAN_POINT ( 'NONE',  ( 6.862500001229034474, -4.330127018922190985, -2.500000000000001332 ) ) ;
#9918=CARTESIAN_POINT ( 'NONE',  ( 28.43437500061451573, 4.541064518000418104, 2.621784821874999949 ) ) ;
#9919=CARTESIAN_POINT ( 'NONE',  ( 11.43750000000000000, 5.773502691896255534, 3.535250795749688894E-16 ) ) ;
#9920=CARTESIAN_POINT ( 'NONE',  ( -2.828200636599751609E-16, 16.85000000122903430, 25.38119784648299770 ) ) ;
#9921=CARTESIAN_POINT ( 'NONE',  ( 12.33750000122903145, 6.123233995736764310E-16, -4.999999999999998224 ) ) ;
#9922=CARTESIAN_POINT ( 'NONE',  ( 23.55937500061451573, 0.000000000000000000, 5.243569643749999010 ) ) ;
#9923=CARTESIAN_POINT ( 'NONE',  ( 17.29687500061451999, -3.027376345333614438, 5.243569643749998122 ) ) ;
#9924=CARTESIAN_POINT ( 'NONE',  ( 4.003212292754231072, 2.995723341028087017, -4.303571541022567892 ) ) ;
#9925=ORIENTED_EDGE ( 'NONE', *, *, #54220, .F. ) ;
#9926=VECTOR ( 'NONE', #65748, 1000.000000000000000 ) ;
#9927=CARTESIAN_POINT ( 'NONE',  ( 16.15312500061451573, 4.541064518000418104, -2.621784821874998173 ) ) ;
#9928=CARTESIAN_POINT ( 'NONE',  ( 29.02500000122903145, 2.886751345948129099, -4.999999999999998224 ) ) ;
#9929=CARTESIAN_POINT ( 'NONE',  ( 18.08437500061451431, 4.541064518000418104, 2.621784821874999949 ) ) ;
#9930=CARTESIAN_POINT ( 'NONE',  ( 5.672204065618859481, 8.235970573989483512, -28.03398296844422433 ) ) ;
#9931=CARTESIAN_POINT ( 'NONE',  ( 20.05312500061451431, -4.541064518000417216, -2.621784821875001281 ) ) ;
#9933=EDGE_CURVE ( 'NONE', #57422, #50074, #15216, .T. ) ;
#9934=CARTESIAN_POINT ( 'NONE',  ( 29.63437500061451502, 6.421520780324663323E-16, -5.243569643749999010 ) ) ;
#9935=CARTESIAN_POINT ( 'NONE',  ( 4.243569643749999010, 11.96562500061451750, 27.54997392385601174 ) ) ;
#9936=CARTESIAN_POINT ( 'NONE',  ( 17.59687500061451715, 6.054752690667223547, 3.707466751127219781E-16 ) ) ;
#9937=CARTESIAN_POINT ( 'NONE',  ( 16.83750000122903145, 6.123233995736764310E-16, -4.999999999999998224 ) ) ;
#9939=CARTESIAN_POINT ( 'NONE',  ( 9.001249775931846008E-16, 19.52187500061451786, -25.09994784771203058 ) ) ;
#9940=CARTESIAN_POINT ( 'NONE',  ( 19.88437500061451857, 4.541064518000418104, 2.621784821874999949 ) ) ;
#9941=CARTESIAN_POINT ( 'NONE',  ( 21.48750000122903003, 4.330127018922191873, 2.499999999999999556 ) ) ;
#9942=CARTESIAN_POINT ( 'NONE',  ( 22.71562500061451573, -6.054752690667223547, -1.112240025338166033E-15 ) ) ;
#9943=CARTESIAN_POINT ( 'NONE',  ( 18.08437500061451431, 4.541064518000418104, 2.621784821874999949 ) ) ;
#9944=CARTESIAN_POINT ( 'NONE',  ( 11.24062500061451608, 6.054752690667223547, 3.707466751127219781E-16 ) ) ;
#9945=CARTESIAN_POINT ( 'NONE',  ( 9.001249775931846008E-16, 13.67187500061451999, 34.90005215228797653 ) ) ;
#9946=CARTESIAN_POINT ( 'NONE',  ( 16.60312500061451857, 4.541064518000418104, -2.621784821874998173 ) ) ;
#9947=ORIENTED_EDGE ( 'NONE', *, *, #64920, .F. ) ;
#9948=ORIENTED_EDGE ( 'NONE', *, *, #1146, .F. ) ;
#9949=CARTESIAN_POINT ( 'NONE',  ( 22.05000000000000071, -4.330127018922190985, -2.500000000000001332 ) ) ;
#9950=CARTESIAN_POINT ( 'NONE',  ( -3.000416591977282496E-16, 19.29687500061451644, -34.90005215228797653 ) ) ;
#9951=CARTESIAN_POINT ( 'NONE',  ( 12.52500000000000213, -4.330127018922194537, 2.499999999999995559 ) ) ;
#9952=B_SPLINE_CURVE_WITH_KNOTS ( 'NONE', 3,
 ( #5623, #5978, #1170, #17050, #17412, #62843, #40321, #51046, #33685, #23317 ),
 .UNSPECIFIED., .F., .F.,
 ( 4, 3, 3, 4 ),
 ( 1.952816364424374816E-16, 2.904775715151696798E-05, 7.262233730042978481E-05, 0.0001161998171129827076 ),
 .UNSPECIFIED. ) ;
#9953=CARTESIAN_POINT ( 'NONE',  ( 23.57812500061451289, -4.541064518000419881, 2.621784821874995952 ) ) ;
#9954=CARTESIAN_POINT ( 'NONE',  ( 6.365625000614518747, 3.027376345333611329, 5.243569643749999010 ) ) ;
#9955=CARTESIAN_POINT ( 'NONE',  ( 18.22500000122903430, 2.886751345948129099, -4.999999999999998224 ) ) ;
#9956=CARTESIAN_POINT ( 'NONE',  ( 23.31562500061451715, 3.027376345333613106, -5.243569643749998122 ) ) ;
#9957=CARTESIAN_POINT ( 'NONE',  ( 22.31250000000000000, 2.886751345948126879, 4.999999999999999112 ) ) ;
#9958=CARTESIAN_POINT ( 'NONE',  ( 26.50312500061451360, 4.541064518000418104, -2.621784821874998173 ) ) ;
#9959=CARTESIAN_POINT ( 'NONE',  ( 8.653125000614515727, 0.000000000000000000, 5.243569643749999010 ) ) ;
#9961=CARTESIAN_POINT ( 'NONE',  ( 22.49062500061451431, 6.054752690667223547, 3.707466751127219781E-16 ) ) ;
#9962=CARTESIAN_POINT ( 'NONE',  ( 3.140625000614516882, 6.054752690667223547, 3.707466751127219781E-16 ) ) ;
#9964=CARTESIAN_POINT ( 'NONE',  ( -3.999999999999999112, 11.07500000122903394, 27.69059892324149885 ) ) ;
#9965=CARTESIAN_POINT ( 'NONE',  ( 4.000000000000000000, 14.90000000122903323, -27.69059892324149530 ) ) ;
#9968=CARTESIAN_POINT ( 'NONE',  ( 10.68750000000000000, -2.886751345948129988, 4.999999999999997335 ) ) ;
#9969=CARTESIAN_POINT ( 'NONE',  ( 11.59687500061451892, -3.027376345333610441, -5.243569643749999898 ) ) ;
#9970=CARTESIAN_POINT ( 'NONE',  ( 7.012500001229035718, 4.330127018922192761, -2.499999999999997780 ) ) ;
#9971=CARTESIAN_POINT ( 'NONE',  ( 15.79687500061451821, 6.054752690667223547, 3.707466751127219781E-16 ) ) ;
#9972=CARTESIAN_POINT ( 'NONE',  ( 6.421875000614519102, 3.027376345333611329, 5.243569643749999010 ) ) ;
#9973=CARTESIAN_POINT ( 'NONE',  ( -2.121784821874999949, 9.828125000614516438, -33.67503911421598417 ) ) ;
#9974=CARTESIAN_POINT ( 'NONE',  ( -1.071796769724491005, 10.57009619066136707, 26.00000000000000355 ) ) ;
#9975=CARTESIAN_POINT ( 'NONE',  ( 13.47187500061451537, 3.027376345333613106, -5.243569643749998122 ) ) ;
#9977=CARTESIAN_POINT ( 'NONE',  ( 21.55312500061451431, 4.541064518000418104, -2.621784821874998173 ) ) ;
#9978=DIRECTION ( 'NONE',  ( -1.000000000000000000, -0.000000000000000000, -0.000000000000000000 ) ) ;
#9979=CARTESIAN_POINT ( 'NONE',  ( 2.121784821874999061, 19.20312500061459460, 26.32496088578401583 ) ) ;
#9980=CARTESIAN_POINT ( 'NONE',  ( 23.22187500061451715, -6.054752690667223547, -1.112240025338166033E-15 ) ) ;
#9981=CARTESIAN_POINT ( 'NONE',  ( -3.999999999999997335, 13.85000000122903607, -27.69059892324149530 ) ) ;
#9982=CARTESIAN_POINT ( 'NONE',  ( 28.98750000122903359, 6.123233995736764310E-16, -4.999999999999998224 ) ) ;
#9986=CARTESIAN_POINT ( 'NONE',  ( 25.41562500061451146, -6.054752690667223547, -1.112240025338166033E-15 ) ) ;
#9987=CARTESIAN_POINT ( 'NONE',  ( 18.66562500061451146, -6.054752690667223547, -1.112240025338166033E-15 ) ) ;
#9989=CARTESIAN_POINT ( 'NONE',  ( 14.82187500061451679, 3.027376345333613106, -5.243569643749998122 ) ) ;
#9991=CARTESIAN_POINT ( 'NONE',  ( 26.92500000122903359, 2.886751345948126879, 4.999999999999999112 ) ) ;
#9992=CARTESIAN_POINT ( 'NONE',  ( 4.846875000614519813, -3.027376345333610441, -5.243569643749999898 ) ) ;
#9993=VECTOR ( 'NONE', #3625, 1000.000000000000000 ) ;
#9994=CARTESIAN_POINT ( 'NONE',  ( 16.65937500061452070, 4.541064518000418104, -2.621784821874998173 ) ) ;
#9995=CARTESIAN_POINT ( 'NONE',  ( 16.16250000000000142, -5.773502691896255534, -1.060575238724906372E-15 ) ) ;
#9996=CARTESIAN_POINT ( 'NONE',  ( 3.975000001229033852, 2.886751345948126879, 4.999999999999999112 ) ) ;
#9997=CARTESIAN_POINT ( 'NONE',  ( 24.57187500061451502, -6.054752690667223547, -1.112240025338166033E-15 ) ) ;
#9998=CARTESIAN_POINT ( 'NONE',  ( 17.78437500061451715, -4.541064518000419881, 2.621784821874995952 ) ) ;
#10000=CARTESIAN_POINT ( 'NONE',  ( 29.21249999999999858, -5.773502691896255534, -1.060575238724906372E-15 ) ) ;
#10001=CARTESIAN_POINT ( 'NONE',  ( 4.724999999999999645, 4.330127018922191873, 2.499999999999999556 ) ) ;
#10003=CARTESIAN_POINT ( 'NONE',  ( 19.64062500061451644, -3.027376345333610441, -5.243569643749999898 ) ) ;
#10004=CARTESIAN_POINT ( 'NONE',  ( 8.775000000000002132, 4.330127018922191873, 2.499999999999999556 ) ) ;
#10005=CARTESIAN_POINT ( 'NONE',  ( 5.315625000614516260, 3.027376345333613106, -5.243569643749998122 ) ) ;
#10006=CARTESIAN_POINT ( 'NONE',  ( 20.47500000000000142, 4.330127018922191873, 2.499999999999999556 ) ) ;
#10007=CARTESIAN_POINT ( 'NONE',  ( -1.071796769724483234, 17.20759618943233704, 25.99999999999999645 ) ) ;
#10008=CARTESIAN_POINT ( 'NONE',  ( 22.20000000122903216, -2.886751345948125991, -5.000000000000000000 ) ) ;
#10009=CARTESIAN_POINT ( 'NONE',  ( 4.765820465973550135, 8.794739343793304798, 33.66511406871330081 ) ) ;
#10010=CARTESIAN_POINT ( 'NONE',  ( 3.337499999999999911, 5.773502691896255534, 3.535250795749688894E-16 ) ) ;
#10011=VERTEX_POINT ( 'NONE', #32850 ) ;
#10012=CARTESIAN_POINT ( 'NONE',  ( 17.69062500061451715, -3.027376345333614438, 5.243569643749998122 ) ) ;
#10013=CARTESIAN_POINT ( 'NONE',  ( 23.31562500061451715, 3.027376345333613106, -5.243569643749998122 ) ) ;
#10014=CARTESIAN_POINT ( 'NONE',  ( 25.17187500061451644, 3.027376345333613106, -5.243569643749998122 ) ) ;
#10015=CARTESIAN_POINT ( 'NONE',  ( 6.825000000000001066, 6.123233995736764310E-16, -4.999999999999998224 ) ) ;
#10016=CARTESIAN_POINT ( 'NONE',  ( 11.50312500061451892, -4.541064518000417216, -2.621784821875001281 ) ) ;
#10017=CARTESIAN_POINT ( 'NONE',  ( 26.09062500061451573, 6.054752690667223547, 3.707466751127219781E-16 ) ) ;
#10018=CARTESIAN_POINT ( 'NONE',  ( 13.50937500061451679, 4.541064518000418104, -2.621784821874998173 ) ) ;
#10019=CARTESIAN_POINT ( 'NONE',  ( 19.43437500061451928, 4.541064518000418104, 2.621784821874999949 ) ) ;
#10020=CARTESIAN_POINT ( 'NONE',  ( 19.23749999999999716, -2.886751345948197045, 4.999999999999880096 ) ) ;
#10021=CARTESIAN_POINT ( 'NONE',  ( -4.243569643749999898, 19.80312500061451786, 30.00000000000000000 ) ) ;
#10022=CARTESIAN_POINT ( 'NONE',  ( 24.15000000122903145, 5.773502691896255534, 3.535250795749688894E-16 ) ) ;
#10024=CARTESIAN_POINT ( 'NONE',  ( 13.67812500061451786, -4.541064518000419881, 2.621784821874995952 ) ) ;
#10025=CARTESIAN_POINT ( 'NONE',  ( 6.909375000614518036, 0.000000000000000000, 5.243569643749999010 ) ) ;
#10026=CARTESIAN_POINT ( 'NONE',  ( 7.809375000614519280, 0.000000000000000000, 5.243569643749999010 ) ) ;
#10027=ORIENTED_EDGE ( 'NONE', *, *, #10344, .T. ) ;
#10028=EDGE_CURVE ( 'NONE', #26188, #12976, #3361, .T. ) ;
#10029=CARTESIAN_POINT ( 'NONE',  ( 28.32187500061451502, 3.027376345333613106, -5.243569643749998122 ) ) ;
#10030=CARTESIAN_POINT ( 'NONE',  ( 19.15312500061451573, -4.541064518000417216, -2.621784821875001281 ) ) ;
#10031=CARTESIAN_POINT ( 'NONE',  ( 3.215625000614518836, 3.027376345333611329, 5.243569643749999010 ) ) ;
#10032=CARTESIAN_POINT ( 'NONE',  ( 29.50312500061451360, -4.541064518000417216, -2.621784821875001281 ) ) ;
#10033=CARTESIAN_POINT ( 'NONE',  ( 24.00937500061451502, 0.000000000000000000, 5.243569643749999010 ) ) ;
#10034=CARTESIAN_POINT ( 'NONE',  ( 20.65312500061451573, 4.541064518000418104, -2.621784821874998173 ) ) ;
#10035=CARTESIAN_POINT ( 'NONE',  ( -2.828200636599751609E-16, 11.78749999999999964, 25.38119784648299770 ) ) ;
#10036=VECTOR ( 'NONE', #39102, 1000.000000000000000 ) ;
#10037=CARTESIAN_POINT ( 'NONE',  ( 24.47812500061451502, -4.541064518000419881, 2.621784821874995952 ) ) ;
#10038=CARTESIAN_POINT ( 'NONE',  ( 5.550000001229032698, -2.886751345948125991, -5.000000000000000000 ) ) ;
#10040=CARTESIAN_POINT ( 'NONE',  ( 29.09999999999999787, 0.000000000000000000, 4.999999999999998224 ) ) ;
#10041=CARTESIAN_POINT ( 'NONE',  ( -2.000000000000000000, 16.32499999999999929, -33.46410161513775705 ) ) ;
#10042=CARTESIAN_POINT ( 'NONE',  ( 22.87500000122903288, 2.886751345948126879, 4.999999999999999112 ) ) ;
#10044=CARTESIAN_POINT ( 'NONE',  ( 3.571875000614517237, 3.027376345333613106, -5.243569643749998122 ) ) ;
#10045=CARTESIAN_POINT ( 'NONE',  ( 28.82812500061451644, 4.541064518000418104, 2.621784821874999949 ) ) ;
#10046=CARTESIAN_POINT ( 'NONE',  ( 11.87812500061451537, -4.541064518000419881, 2.621784821874995952 ) ) ;
#10047=CARTESIAN_POINT ( 'NONE',  ( 6.121875000614517504, -6.054752690667223547, -1.112240025338166033E-15 ) ) ;
#10048=CARTESIAN_POINT ( 'NONE',  ( 24.71250000122903145, 0.000000000000000000, 4.999999999999998224 ) ) ;
#10050=CARTESIAN_POINT ( 'NONE',  ( 16.09687500061451715, -3.027376345333610441, -5.243569643749999898 ) ) ;
#10051=CARTESIAN_POINT ( 'NONE',  ( 3.234375000614516438, 4.541064518000418104, 2.621784821874999949 ) ) ;
#10052=CARTESIAN_POINT ( 'NONE',  ( 29.17500000000000071, -4.330127018922194537, 2.499999999999995559 ) ) ;
#10053=CARTESIAN_POINT ( 'NONE',  ( 3.928125000614516527, 6.421520780324663323E-16, -5.243569643749999010 ) ) ;
#10054=CARTESIAN_POINT ( 'NONE',  ( 14.65312500061451573, -4.541064518000417216, -2.621784821875001281 ) ) ;
#10055=( BOUNDED_CURVE ( )  B_SPLINE_CURVE ( 3, ( #53842, #26493, #59356, #9136 ),
 .UNSPECIFIED., .F., .F. ) 
 B_SPLINE_CURVE_WITH_KNOTS ( ( 4, 4 ),
 ( 0.3414135753472636314, 0.4010135564025098520 ),
 .UNSPECIFIED. ) 
 CURVE ( )  GEOMETRIC_REPRESENTATION_ITEM ( )  RATIONAL_B_SPLINE_CURVE ( ( 1.000000000000000000, 0.9997040087601481995, 0.9997040087601481995, 1.000000000000000000 ) ) 
 REPRESENTATION_ITEM ( '' )  );
#10058=CARTESIAN_POINT ( 'NONE',  ( 9.178125000614517859, -4.541064518000419881, 2.621784821874995952 ) ) ;
#10059=CARTESIAN_POINT ( 'NONE',  ( 8.990625000614516082, 6.054752690667223547, 3.707466751127219781E-16 ) ) ;
#10061=CARTESIAN_POINT ( 'NONE',  ( 9.225000000000001421, 4.330127018922191873, 2.499999999999999556 ) ) ;
#10062=CARTESIAN_POINT ( 'NONE',  ( 3.562500001229033764, 0.000000000000000000, 4.999999999999998224 ) ) ;
#10063=CARTESIAN_POINT ( 'NONE',  ( 17.69999999999999929, 4.330127018922192761, -2.499999999999997780 ) ) ;
#10064=EDGE_CURVE ( 'NONE', #71866, #51638, #12496, .T. ) ;
#10065=CARTESIAN_POINT ( 'NONE',  ( 18.34687500061451715, -3.027376345333610441, -5.243569643749999898 ) ) ;
#10066=CARTESIAN_POINT ( 'NONE',  ( 12.63750000122903394, -4.330127018922194537, 2.499999999999995559 ) ) ;
#10068=CARTESIAN_POINT ( 'NONE',  ( -4.243569643749997233, 16.69062500061451360, -27.54997392385601174 ) ) ;
#10071=CARTESIAN_POINT ( 'NONE',  ( -5.810221930991193690E-16, 12.35000000122903430, -34.00000000000000000 ) ) ;
#10074=CARTESIAN_POINT ( 'NONE',  ( 13.58437500061451786, 4.541064518000418104, 2.621784821874999949 ) ) ;
#10075=CARTESIAN_POINT ( 'NONE',  ( 26.43750000000000000, -2.886751345948129988, 4.999999999999997335 ) ) ;
#10076=CARTESIAN_POINT ( 'NONE',  ( 10.11562500061451608, -6.054752690667223547, -1.112240025338166033E-15 ) ) ;
#10078=CARTESIAN_POINT ( 'NONE',  ( 22.05937500061451573, 4.541064518000418104, -2.621784821874998173 ) ) ;
#10080=VECTOR ( 'NONE', #1408, 1000.000000000000000 ) ;
#10081=CARTESIAN_POINT ( 'NONE',  ( 7.678125000614516082, 4.541064518000418104, 2.621784821874999949 ) ) ;
#10082=CARTESIAN_POINT ( 'NONE',  ( 13.24687500061451750, -3.027376345333614438, 5.243569643749998122 ) ) ;
#10083=ORIENTED_EDGE ( 'NONE', *, *, #2879, .F. ) ;
#10084=CARTESIAN_POINT ( 'NONE',  ( 22.73437500061451644, -4.541064518000419881, 2.621784821874995952 ) ) ;
#10085=CARTESIAN_POINT ( 'NONE',  ( 0.5511252142286452438, 4.971455555459576736, -26.03572899521184425 ) ) ;
#10087=CARTESIAN_POINT ( 'NONE',  ( 5.475000000000000533, 6.123233995736764310E-16, -4.999999999999998224 ) ) ;
#10088=CARTESIAN_POINT ( 'NONE',  ( 16.53750000122903430, 4.330127018922191873, 2.499999999999999556 ) ) ;
#10090=CARTESIAN_POINT ( 'NONE',  ( 14.55000000122903359, -2.886751345948126435, -5.000000000000000000 ) ) ;
#10091=ORIENTED_EDGE ( 'NONE', *, *, #58291, .T. ) ;
#10092=CARTESIAN_POINT ( 'NONE',  ( 12.90000000000000213, 0.000000000000000000, 4.999999999999998224 ) ) ;
#10093=CARTESIAN_POINT ( 'NONE',  ( 17.02499999999999858, -4.330127018922194537, 2.499999999999995559 ) ) ;
#10094=CARTESIAN_POINT ( 'NONE',  ( 12.78750000122903430, 6.123233995736764310E-16, -4.999999999999998224 ) ) ;
#10095=CARTESIAN_POINT ( 'NONE',  ( 10.90312500061451928, 0.000000000000000000, 5.243569643749999010 ) ) ;
#10096=VECTOR ( 'NONE', #22341, 1000.000000000000000 ) ;
#10097=ORIENTED_EDGE ( 'NONE', *, *, #16399, .F. ) ;
#10098=DIRECTION ( 'NONE',  ( -0.000000000000000000, -1.000000000000000000, -0.000000000000000000 ) ) ;
#10099=CARTESIAN_POINT ( 'NONE',  ( -4.243569643749997233, 18.09687500061452070, -27.54997392385601174 ) ) ;
#10100=CARTESIAN_POINT ( 'NONE',  ( 3.740625000614516527, -3.027376345333614438, 5.243569643749998122 ) ) ;
#10102=CARTESIAN_POINT ( 'NONE',  ( 9.975000000000001421, 6.123233995736764310E-16, -4.999999999999998224 ) ) ;
#10103=EDGE_LOOP ( 'NONE', ( #48887, #2429, #41244, #1421, #3545 ) ) ;
#10104=CARTESIAN_POINT ( 'NONE',  ( 23.16562500061451502, -6.054752690667223547, -1.112240025338166033E-15 ) ) ;
#10107=CARTESIAN_POINT ( 'NONE',  ( 21.68437500061451573, 4.541064518000418104, 2.621784821874999949 ) ) ;
#10108=CARTESIAN_POINT ( 'NONE',  ( 18.89062500061451644, 6.054752690667223547, 3.707466751127219781E-16 ) ) ;
#10109=CARTESIAN_POINT ( 'NONE',  ( -4.243569643749998122, 14.89062500061459282, -27.54997392385601174 ) ) ;
#10110=CARTESIAN_POINT ( 'NONE',  ( 6.928125000614516082, -4.541064518000419881, 2.621784821874995952 ) ) ;
#10111=CARTESIAN_POINT ( 'NONE',  ( 4.303125000614516971, -4.541064518000417216, -2.621784821875001281 ) ) ;
#10113=CARTESIAN_POINT ( 'NONE',  ( 20.65312500061451573, 4.541064518000418104, -2.621784821874998173 ) ) ;
#10114=DIRECTION ( 'NONE',  ( -0.000000000000000000, -1.000000000000000000, -0.000000000000000000 ) ) ;
#10116=CARTESIAN_POINT ( 'NONE',  ( 14.29687500061451821, -3.027376345333610441, -5.243569643749999898 ) ) ;
#10117=CARTESIAN_POINT ( 'NONE',  ( 15.49687500061451750, -3.027376345333614438, 5.243569643749998122 ) ) ;
#10118=CARTESIAN_POINT ( 'NONE',  ( 23.07187500061451857, 3.027376345333611329, 5.243569643749999010 ) ) ;
#10120=CARTESIAN_POINT ( 'NONE',  ( 4.243569643749999898, 12.43437500061451750, 30.00000000000000000 ) ) ;
#10121=CARTESIAN_POINT ( 'NONE',  ( -3.999999999999999112, 14.67500000122903536, -32.30940107675850470 ) ) ;
#10122=CARTESIAN_POINT ( 'NONE',  ( 26.84062500061451573, -3.027376345333610441, -5.243569643749999898 ) ) ;
#10123=CARTESIAN_POINT ( 'NONE',  ( 25.97812500061451502, 6.421520780324663323E-16, -5.243569643749999010 ) ) ;
#10124=CARTESIAN_POINT ( 'NONE',  ( 1.071796769724497445, 16.37990381179669797, -33.99999999999998579 ) ) ;
#10126=CARTESIAN_POINT ( 'NONE',  ( 3.834375000614519635, -4.541064518000419881, 2.621784821874995952 ) ) ;
#10127=CARTESIAN_POINT ( 'NONE',  ( 13.38750000122903394, 4.330127018922191873, 2.499999999999999556 ) ) ;
#10128=CARTESIAN_POINT ( 'NONE',  ( 10.38750000122903572, -4.330127018922194537, 2.499999999999995559 ) ) ;
#10129=CARTESIAN_POINT ( 'NONE',  ( 28.95000000122903572, -2.886751345948125991, -5.000000000000000000 ) ) ;
#10132=CARTESIAN_POINT ( 'NONE',  ( 12.72187500061451537, 3.027376345333611329, 5.243569643749999010 ) ) ;
#10133=CARTESIAN_POINT ( 'NONE',  ( 4.683223236373093457, -1.751405183929441556, 4.942428804804532838 ) ) ;
#10135=CARTESIAN_POINT ( 'NONE',  ( 19.56562500061451715, -6.054752690667223547, -1.112240025338166033E-15 ) ) ;
#10136=CARTESIAN_POINT ( 'NONE',  ( 14.85937500061451644, 4.541064518000418104, -2.621784821874998173 ) ) ;
#10137=CARTESIAN_POINT ( 'NONE',  ( 5.878125000614517148, 4.541064518000418104, 2.621784821874999949 ) ) ;
#10138=CARTESIAN_POINT ( 'NONE',  ( 23.29687500061451644, -3.027376345333610441, -5.243569643749999898 ) ) ;
#10139=CARTESIAN_POINT ( 'NONE',  ( 4.415625000614518569, 3.027376345333613106, -5.243569643749998122 ) ) ;
#10140=CARTESIAN_POINT ( 'NONE',  ( 6.675000001229034474, 2.886751345948126879, 4.999999999999998224 ) ) ;
#10141=CARTESIAN_POINT ( 'NONE',  ( 9.225000001229034297, 2.886751345948129099, -4.999999999999998224 ) ) ;
#10142=CARTESIAN_POINT ( 'NONE',  ( 22.04062500061451502, 6.054752690667223547, 3.707466751127219781E-16 ) ) ;
#10143=CARTESIAN_POINT ( 'NONE',  ( 1.999999999999998668, 19.06250000122903288, -33.46410161513775705 ) ) ;
#10144=CARTESIAN_POINT ( 'NONE',  ( 8.362500001229031810, 4.330127018922192761, -2.499999999999997780 ) ) ;
#10145=CARTESIAN_POINT ( 'NONE',  ( 20.61562500061451431, 3.027376345333613106, -5.243569643749998122 ) ) ;
#10146=AXIS2_PLACEMENT_3D ( 'NONE', #52939, #71400, #20774 ) ;
#10147=CARTESIAN_POINT ( 'NONE',  ( 14.50312500061451537, 0.000000000000000000, 5.243569643749999010 ) ) ;
#10149=CARTESIAN_POINT ( 'NONE',  ( 15.03749999999999964, 5.773502691896255534, 3.535250795749688894E-16 ) ) ;
#10150=CARTESIAN_POINT ( 'NONE',  ( 11.17500000122903536, 2.886751345948126879, 4.999999999999999112 ) ) ;
#10151=CARTESIAN_POINT ( 'NONE',  ( 7.040625000614517681, -3.027376345333610441, -5.243569643749999898 ) ) ;
#10152=CARTESIAN_POINT ( 'NONE',  ( 11.01562500061451821, -6.054752690667223547, -1.112240025338166033E-15 ) ) ;
#10153=EDGE_CURVE ( 'NONE', #22971, #25850, #22764, .T. ) ;
#10154=CARTESIAN_POINT ( 'NONE',  ( 21.15000000122903145, -2.886751345948129988, 4.999999999999997335 ) ) ;
#10155=CARTESIAN_POINT ( 'NONE',  ( 2.121784821875001281, 13.70937500061451786, -26.32496088578401938 ) ) ;
#10156=CARTESIAN_POINT ( 'NONE',  ( 19.20937500061451786, -4.541064518000417216, -2.621784821875001281 ) ) ;
#10158=CARTESIAN_POINT ( 'NONE',  ( 5.962500001229033231, -4.330127018922190985, -2.500000000000001332 ) ) ;
#10159=CARTESIAN_POINT ( 'NONE',  ( 3.496875000614518836, -3.027376345333610441, -5.243569643749999898 ) ) ;
#10160=CARTESIAN_POINT ( 'NONE',  ( 22.02187500061452141, 3.027376345333613106, -5.243569643749998122 ) ) ;
#10162=CARTESIAN_POINT ( 'NONE',  ( 18.10312500061451502, 0.000000000000000000, 5.243569643749999010 ) ) ;
#10165=CARTESIAN_POINT ( 'NONE',  ( -1.071796769724483234, 15.40759618943233811, 25.99999999999999645 ) ) ;
#10166=CARTESIAN_POINT ( 'NONE',  ( 29.44687500061451857, -3.027376345333614438, 5.243569643749998122 ) ) ;
#10168=CARTESIAN_POINT ( 'NONE',  ( 15.81562500061451537, 3.027376345333611329, 5.243569643749999010 ) ) ;
#10169=CARTESIAN_POINT ( 'NONE',  ( 12.90937500061451537, -4.541064518000417216, -2.621784821875001281 ) ) ;
#10170=VERTEX_POINT ( 'NONE', #46480 ) ;
#10171=CARTESIAN_POINT ( 'NONE',  ( 22.67812500061451431, -4.541064518000419881, 2.621784821874995952 ) ) ;
#10172=CARTESIAN_POINT ( 'NONE',  ( -1.071796769724488563, 10.75490381179670152, -26.00000000000000000 ) ) ;
#10173=CARTESIAN_POINT ( 'NONE',  ( -3.999999999999999112, 11.56250000122903465, -30.00000000000000000 ) ) ;
#10174=CARTESIAN_POINT ( 'NONE',  ( 13.19999999999999929, 4.330127018922192761, -2.499999999999997780 ) ) ;
#10175=CARTESIAN_POINT ( 'NONE',  ( 24.56250000122903288, 4.330127018922192761, -2.499999999999997780 ) ) ;
#10176=CARTESIAN_POINT ( 'NONE',  ( 17.91562500061451502, 3.027376345333613106, -5.243569643749998122 ) ) ;
#10178=CARTESIAN_POINT ( 'NONE',  ( 23.02499999999999858, 6.123233995736764310E-16, -4.999999999999998224 ) ) ;
#10179=CARTESIAN_POINT ( 'NONE',  ( 24.75937500061451502, 4.541064518000418104, -2.621784821874998173 ) ) ;
#10180=ORIENTED_EDGE ( 'NONE', *, *, #61111, .F. ) ;
#10181=CARTESIAN_POINT ( 'NONE',  ( 30.00000000000000000, 0.000000000000000000, 0.000000000000000000 ) ) ;
#10182=CARTESIAN_POINT ( 'NONE',  ( 9.778125000614517504, 6.421520780324663323E-16, -5.243569643749999010 ) ) ;
#10185=CARTESIAN_POINT ( 'NONE',  ( 16.05000000000000071, 0.000000000000000000, 4.999999999999998224 ) ) ;
#10186=CARTESIAN_POINT ( 'NONE',  ( 23.69999999999999929, 0.000000000000000000, 4.999999999999998224 ) ) ;
#10187=CARTESIAN_POINT ( 'NONE',  ( 7.612500001229035362, 0.000000000000000000, 4.999999999999998224 ) ) ;
#10188=CARTESIAN_POINT ( 'NONE',  ( 3.534375000614518036, 6.421520780324663323E-16, -5.243569643749999010 ) ) ;
#10189=CARTESIAN_POINT ( 'NONE',  ( 27.64687500061452141, -3.027376345333614438, 5.243569643749998122 ) ) ;
#10190=VERTEX_POINT ( 'NONE', #23206 ) ;
#10191=CARTESIAN_POINT ( 'NONE',  ( 26.09062500061451573, 6.054752690667223547, 3.707466751127219781E-16 ) ) ;
#10192=CARTESIAN_POINT ( 'NONE',  ( 27.42187500061451644, 3.027376345333613106, -5.243569643749998122 ) ) ;
#10194=CARTESIAN_POINT ( 'NONE',  ( 14.13750000000000107, 5.773502691896255534, 3.535250795749688894E-16 ) ) ;
#10195=CARTESIAN_POINT ( 'NONE',  ( 11.76562500061451644, 3.027376345333611329, 5.243569643749999010 ) ) ;
#10196=CARTESIAN_POINT ( 'NONE',  ( 6.000000000000001776, 4.330127018922192761, -2.499999999999997780 ) ) ;
#10197=CARTESIAN_POINT ( 'NONE',  ( 3.999999999999998668, 19.36249999999999716, -32.30940107675850470 ) ) ;
#10198=CARTESIAN_POINT ( 'NONE',  ( 28.67812500061451431, 6.421520780324663323E-16, -5.243569643749999010 ) ) ;
#10199=CARTESIAN_POINT ( 'NONE',  ( 16.46250000122903501, 4.330127018922192761, -2.499999999999997780 ) ) ;
#10201=CARTESIAN_POINT ( 'NONE',  ( 5.128125000614516260, -4.541064518000419881, 2.621784821874995952 ) ) ;
#10202=CARTESIAN_POINT ( 'NONE',  ( 22.39687500061451075, -3.027376345333610441, -5.243569643749999898 ) ) ;
#10203=( BOUNDED_CURVE ( )  B_SPLINE_CURVE ( 2, ( #717, #67947, #12513, #72759, #63114, #56490, #22145 ),
 .UNSPECIFIED., .F., .F. ) 
 B_SPLINE_CURVE_WITH_KNOTS ( ( 3, 2, 2, 3 ),
 ( 0.1833333333333333204, 0.1861111111111111160, 0.1888888888888888562, 0.1916666666666666519 ),
 .UNSPECIFIED. ) 
 CURVE ( )  GEOMETRIC_REPRESENTATION_ITEM ( )  RATIONAL_B_SPLINE_CURVE ( ( 1.000000000000000000, 0.8660254037844387076, 1.000000000000000000, 0.8660254037844387076, 1.000000000000000000, 0.8660254037844400399, 0.9999999999999986677 ) ) 
 REPRESENTATION_ITEM ( '' )  );
#10204=CARTESIAN_POINT ( 'NONE',  ( 2.121784821875001281, 15.05937500061451928, 33.67503911421598417 ) ) ;
#10205=CARTESIAN_POINT ( 'NONE',  ( 22.20937500061451431, 0.000000000000000000, 5.243569643749999010 ) ) ;
#10206=CARTESIAN_POINT ( 'NONE',  ( 29.52187500061451431, -6.054752690667223547, -1.112240025338166033E-15 ) ) ;
#10207=CARTESIAN_POINT ( 'NONE',  ( -4.243569643749999898, 19.40937500061451715, 30.00000000000000000 ) ) ;
#10208=CARTESIAN_POINT ( 'NONE',  ( 9.590625000614517504, -3.027376345333614438, 5.243569643749998122 ) ) ;
#10209=CARTESIAN_POINT ( 'NONE',  ( 21.67500000000000071, 6.123233995736764310E-16, -4.999999999999998224 ) ) ;
#10210=EDGE_CURVE ( 'NONE', #69178, #66787, #61219, .T. ) ;
#10211=CARTESIAN_POINT ( 'NONE',  ( 7.696875000614516793, 6.054752690667223547, 3.707466751127219781E-16 ) ) ;
#10212=CARTESIAN_POINT ( 'NONE',  ( 3.852725565712457723, 3.187011840027719423, -3.887821400885792311 ) ) ;
#10214=CARTESIAN_POINT ( 'NONE',  ( 10.30312500061451431, 4.541064518000418104, -2.621784821874998173 ) ) ;
#10215=CARTESIAN_POINT ( 'NONE',  ( 15.60937500061451644, -4.541064518000417216, -2.621784821875001281 ) ) ;
#10216=CARTESIAN_POINT ( 'NONE',  ( 3.472008138778309494, -3.597954294344049675, -3.814426947577870930 ) ) ;
#10217=CARTESIAN_POINT ( 'NONE',  ( 21.41250000122903074, 4.330127018922192761, -2.499999999999997780 ) ) ;
#10218=CARTESIAN_POINT ( 'NONE',  ( 8.184375000614515727, 4.541064518000418104, 2.621784821874999949 ) ) ;
#10219=CARTESIAN_POINT ( 'NONE',  ( 10.30312500061451431, 4.541064518000418104, -2.621784821874998173 ) ) ;
#10221=CARTESIAN_POINT ( 'NONE',  ( 18.53437500061451715, 4.541064518000418104, 2.621784821874999949 ) ) ;
#10222=CARTESIAN_POINT ( 'NONE',  ( 14.13750000000000107, 5.773502691896255534, 3.535250795749688401E-16 ) ) ;
#10223=CARTESIAN_POINT ( 'NONE',  ( -3.578127771932954726, 3.495591672637166525, 31.80636524853745684 ) ) ;
#10224=CARTESIAN_POINT ( 'NONE',  ( 2.121784821875001281, 11.00937500061451857, -26.32496088578401938 ) ) ;
#10226=CARTESIAN_POINT ( 'NONE',  ( 15.37500000122903465, -5.773502691896255534, -1.060575238724906372E-15 ) ) ;
#10227=CARTESIAN_POINT ( 'NONE',  ( -4.243569643749999898, 14.40312500061451750, -30.00000000000000000 ) ) ;
#10228=CARTESIAN_POINT ( 'NONE',  ( 15.33750000122903323, -4.330127018922194537, 2.499999999999995559 ) ) ;
#10229=CARTESIAN_POINT ( 'NONE',  ( 10.04062500061451502, -3.027376345333614438, 5.243569643749998122 ) ) ;
#10230=ORIENTED_EDGE ( 'NONE', *, *, #44518, .T. ) ;
#10231=CARTESIAN_POINT ( 'NONE',  ( 13.42499999999999893, -4.330127018922194537, 2.499999999999995559 ) ) ;
#10233=CARTESIAN_POINT ( 'NONE',  ( 22.11562500061451786, 3.027376345333611329, 5.243569643749999010 ) ) ;
#10234=CARTESIAN_POINT ( 'NONE',  ( 9.946875000614516793, 6.054752690667223547, 3.707466751127219781E-16 ) ) ;
#10235=ADVANCED_FACE ( 'NONE', ( #18381 ), #52741, .F. ) ;
#10236=CARTESIAN_POINT ( 'NONE',  ( 4.400918202330496243, -2.373166445152071535, -4.675799785326651303 ) ) ;
#10237=CARTESIAN_POINT ( 'NONE',  ( 10.12500000122903465, 2.886751345948129099, -4.999999999999998224 ) ) ;
#10238=CARTESIAN_POINT ( 'NONE',  ( 19.53750000122903430, 6.123233995736764310E-16, -4.999999999999998224 ) ) ;
#10239=CARTESIAN_POINT ( 'NONE',  ( 15.77812500061451573, 4.541064518000418104, 2.621784821874999949 ) ) ;
#10240=CARTESIAN_POINT ( 'NONE',  ( 18.14062500061451644, -3.027376345333614438, 5.243569643749998122 ) ) ;
#10241=CARTESIAN_POINT ( 'NONE',  ( 24.78750000122903074, -4.330127018922194537, 2.499999999999995559 ) ) ;
#10242=CARTESIAN_POINT ( 'NONE',  ( 28.61250000122903359, 4.330127018922192761, -2.499999999999997780 ) ) ;
#10243=CARTESIAN_POINT ( 'NONE',  ( 22.83749999999999858, -2.886751345948129988, 4.999999999999997335 ) ) ;
#10245=VECTOR ( 'NONE', #43048, 1000.000000000000000 ) ;
#10246=CARTESIAN_POINT ( 'NONE',  ( 26.29687500061451644, -3.027376345333614438, 5.243569643749998122 ) ) ;
#10247=CARTESIAN_POINT ( 'NONE',  ( 11.66250000122903430, 0.000000000000000000, 4.999999999999998224 ) ) ;
#10248=CARTESIAN_POINT ( 'NONE',  ( 4.012500000000001954, -5.773502691896255534, -1.060575238724906372E-15 ) ) ;
#10249=EDGE_CURVE ( 'NONE', #16314, #4423, #52964, .T. ) ;
#10251=CARTESIAN_POINT ( 'NONE',  ( 14.24999999999999822, 0.000000000000000000, 4.999999999999998224 ) ) ;
#10252=CARTESIAN_POINT ( 'NONE',  ( 4.471875000614518925, 3.027376345333613106, -5.243569643749998122 ) ) ;
#10253=CARTESIAN_POINT ( 'NONE',  ( 27.17812500061451786, -4.541064518000419881, 2.621784821874995952 ) ) ;
#10255=CARTESIAN_POINT ( 'NONE',  ( 2.000000000000001332, 19.69999999999999929, -26.53589838486224650 ) ) ;
#10256=CARTESIAN_POINT ( 'NONE',  ( 10.02187500061451964, 3.027376345333611329, 5.243569643749999010 ) ) ;
#10257=CARTESIAN_POINT ( 'NONE',  ( 4.134375000614517681, 4.541064518000418104, 2.621784821874999949 ) ) ;
#10258=CARTESIAN_POINT ( 'NONE',  ( 8.146875000614516082, 6.054752690667223547, 3.707466751127219781E-16 ) ) ;
#10259=CARTESIAN_POINT ( 'NONE',  ( 28.77187500061451431, 3.027376345333613106, -5.243569643749998122 ) ) ;
#10260=CARTESIAN_POINT ( 'NONE',  ( -2.121784821874996840, 13.12812500061459353, 33.67503911421598417 ) ) ;
#10261=CARTESIAN_POINT ( 'NONE',  ( 20.58750000000000213, -2.886751345948129988, 4.999999999999997335 ) ) ;
#10262=ORIENTED_EDGE ( 'NONE', *, *, #27962, .T. ) ;
#10263=CARTESIAN_POINT ( 'NONE',  ( 29.28749999999999787, -2.886751345948125991, -5.000000000000000000 ) ) ;
#10264=CARTESIAN_POINT ( 'NONE',  ( 4.275000000000001243, 4.330127018922191873, 2.499999999999999556 ) ) ;
#10265=VERTEX_POINT ( 'NONE', #1787 ) ;
#10266=CARTESIAN_POINT ( 'NONE',  ( 17.46562500061451217, 3.027376345333613106, -5.243569643749998122 ) ) ;
#10267=CARTESIAN_POINT ( 'NONE',  ( 8.653125000614515727, 0.000000000000000000, 5.243569643749999010 ) ) ;
#10269=CARTESIAN_POINT ( 'NONE',  ( 7.959375000614516971, -4.541064518000417216, -2.621784821875001281 ) ) ;
#10270=CARTESIAN_POINT ( 'NONE',  ( 16.95000000122903216, 5.773502691896255534, 3.535250795749688894E-16 ) ) ;
#10272=CARTESIAN_POINT ( 'NONE',  ( 7.659375000614518036, 4.541064518000418104, -2.621784821874998173 ) ) ;
#10273=CARTESIAN_POINT ( 'NONE',  ( 11.63437500061451857, 6.421520780324663323E-16, -5.243569643749999010 ) ) ;
#10274=CARTESIAN_POINT ( 'NONE',  ( 24.64687500061451431, -3.027376345333610441, -5.243569643749999898 ) ) ;
#10276=ORIENTED_EDGE ( 'NONE', *, *, #60328, .F. ) ;
#10278=CIRCLE ( 'NONE', #49214, 5.000000000000000000 ) ;
#10279=CARTESIAN_POINT ( 'NONE',  ( 18.23437500061451999, -4.541064518000419881, 2.621784821874995952 ) ) ;
#10280=CARTESIAN_POINT ( 'NONE',  ( 9.009375000614518569, 4.541064518000418104, -2.621784821874998173 ) ) ;
#10283=CARTESIAN_POINT ( 'NONE',  ( 21.48750000000000071, -2.886751345948129988, 4.999999999999997335 ) ) ;
#10285=CARTESIAN_POINT ( 'NONE',  ( 29.92500000000000071, 4.330127018922191873, 2.499999999999999556 ) ) ;
#10287=CARTESIAN_POINT ( 'NONE',  ( 13.34062500061451750, -3.027376345333610441, -5.243569643749999898 ) ) ;
#10288=CARTESIAN_POINT ( 'NONE',  ( 28.32187500061451502, 3.027376345333613106, -5.243569643749998122 ) ) ;
#10289=DIRECTION ( 'NONE',  ( -0.000000000000000000, -1.000000000000000000, -0.000000000000000000 ) ) ;
#10290=CARTESIAN_POINT ( 'NONE',  ( 29.52187500061451431, -6.054752690667223547, -1.112240025338166033E-15 ) ) ;
#10291=CARTESIAN_POINT ( 'NONE',  ( 10.31250000000000355, -5.773502691896255534, -1.060575238724906372E-15 ) ) ;
#10292=CARTESIAN_POINT ( 'NONE',  ( -3.999999999999997335, 16.55000000122903003, 32.30940107675850470 ) ) ;
#10293=CARTESIAN_POINT ( 'NONE',  ( 8.137500001229033941, -4.330127018922194537, 2.499999999999995559 ) ) ;
#10294=CARTESIAN_POINT ( 'NONE',  ( 22.35937500061451644, -4.541064518000417216, -2.621784821875001281 ) ) ;
#10295=CARTESIAN_POINT ( 'NONE',  ( 14.03437500061451715, 4.541064518000418104, 2.621784821874999949 ) ) ;
#10296=CARTESIAN_POINT ( 'NONE',  ( -1.487416814333745711E-14, 15.16250000000000142, 34.00000000000000000 ) ) ;
#10297=ORIENTED_EDGE ( 'NONE', *, *, #46318, .T. ) ;
#10298=CARTESIAN_POINT ( 'NONE',  ( 16.04062500061451857, -3.027376345333610441, -5.243569643749999898 ) ) ;
#10299=CARTESIAN_POINT ( 'NONE',  ( 28.72500000122903074, 2.886751345948126879, 4.999999999999999112 ) ) ;
#10300=CARTESIAN_POINT ( 'NONE',  ( 16.35937500061451644, 0.000000000000000000, 5.243569643749999010 ) ) ;
#10301=CARTESIAN_POINT ( 'NONE',  ( 16.52812500061451573, 6.421520780324663323E-16, -5.243569643749999010 ) ) ;
#10302=CARTESIAN_POINT ( 'NONE',  ( 27.53437500061451360, 4.541064518000418104, 2.621784821874999949 ) ) ;
#10303=CARTESIAN_POINT ( 'NONE',  ( -4.243569643749997233, 12.64062500061451999, 32.45002607614398471 ) ) ;
#10304=CARTESIAN_POINT ( 'NONE',  ( 16.99687500061451573, -3.027376345333610441, -5.243569643749999898 ) ) ;
#10305=CARTESIAN_POINT ( 'NONE',  ( 13.46250000122903323, 0.000000000000000000, 4.999999999999998224 ) ) ;
#10307=CARTESIAN_POINT ( 'NONE',  ( -3.000416591977282496E-16, 19.29687500061451644, -34.90005215228797653 ) ) ;
#10309=CARTESIAN_POINT ( 'NONE',  ( 20.93437500061451573, -4.541064518000419881, 2.621784821874995952 ) ) ;
#10310=CARTESIAN_POINT ( 'NONE',  ( 21.45000000122903216, 5.773502691896255534, 3.535250795749688894E-16 ) ) ;
#10311=CARTESIAN_POINT ( 'NONE',  ( 17.97187500061451715, 3.027376345333613106, -5.243569643749998122 ) ) ;
#10312=CARTESIAN_POINT ( 'NONE',  ( 13.52812500061451750, 4.541064518000418104, 2.621784821874999949 ) ) ;
#10313=CARTESIAN_POINT ( 'NONE',  ( 4.243569643749999010, 13.37187500061451750, 27.54997392385601174 ) ) ;
#10314=CARTESIAN_POINT ( 'NONE',  ( 16.90312500061451573, -4.541064518000417216, -2.621784821875001281 ) ) ;
#10317=CARTESIAN_POINT ( 'NONE',  ( 20.24999999999999645, -4.330127018922190985, -2.500000000000001332 ) ) ;
#10318=CARTESIAN_POINT ( 'NONE',  ( -3.999999999999997335, 17.90000000122903501, 32.30940107675850470 ) ) ;
#10319=CARTESIAN_POINT ( 'NONE',  ( 25.60312500061451502, 4.541064518000418104, -2.621784821874998173 ) ) ;
#10320=CARTESIAN_POINT ( 'NONE',  ( 5.503125000614516260, 0.000000000000000000, 5.243569643749999010 ) ) ;
#10321=CARTESIAN_POINT ( 'NONE',  ( 18.41250000122903430, 0.000000000000000000, 4.999999999999998224 ) ) ;
#10322=CARTESIAN_POINT ( 'NONE',  ( 23.35312500061451857, 4.541064518000418104, -2.621784821874998173 ) ) ;
#10323=CARTESIAN_POINT ( 'NONE',  ( 22.53750000000000142, -2.886751345948125991, -5.000000000000000000 ) ) ;
#10324=CARTESIAN_POINT ( 'NONE',  ( 25.90312500061451573, -4.541064518000417216, -2.621784821875001281 ) ) ;
#10325=CARTESIAN_POINT ( 'NONE',  ( 6.140625000614516438, -3.027376345333610441, -5.243569643749999898 ) ) ;
#10326=ORIENTED_EDGE ( 'NONE', *, *, #55566, .T. ) ;
#10327=CARTESIAN_POINT ( 'NONE',  ( 30.00000000000000000, 0.000000000000000000, 4.999999999999998224 ) ) ;
#10328=CARTESIAN_POINT ( 'NONE',  ( 3.740625000614516527, -3.027376345333614438, 5.243569643749998122 ) ) ;
#10330=CARTESIAN_POINT ( 'NONE',  ( 3.999999999999999112, 13.02500000000000213, 30.00000000000000000 ) ) ;
#10331=CARTESIAN_POINT ( 'NONE',  ( -3.999999999999997335, 14.30000000122903359, -27.69059892324149175 ) ) ;
#10332=CARTESIAN_POINT ( 'NONE',  ( -2.121784821874999949, 17.98437500061451999, -33.67503911421598417 ) ) ;
#10334=VECTOR ( 'NONE', #62725, 1000.000000000000000 ) ;
#10335=CARTESIAN_POINT ( 'NONE',  ( 10.31250000000000355, -5.773502691896255534, -1.060575238724906372E-15 ) ) ;
#10336=CARTESIAN_POINT ( 'NONE',  ( 12.19687500061451679, 6.054752690667223547, 3.707466751127219781E-16 ) ) ;
#10337=CARTESIAN_POINT ( 'NONE',  ( 6.187500001229032875, 4.330127018922191873, 2.499999999999999556 ) ) ;
#10338=CARTESIAN_POINT ( 'NONE',  ( 12.87187500061451750, -6.054752690667223547, -1.112240025338166033E-15 ) ) ;
#10339=CARTESIAN_POINT ( 'NONE',  ( 4.959375000614516971, 4.541064518000418104, -2.621784821874998173 ) ) ;
#10341=CARTESIAN_POINT ( 'NONE',  ( 3.390184931900214860, 3.675138926287994767, 3.390184931900133147 ) ) ;
#10342=CARTESIAN_POINT ( 'NONE',  ( 9.796875000614519990, -3.027376345333610441, -5.243569643749999898 ) ) ;
#10343=CARTESIAN_POINT ( 'NONE',  ( 21.93750000122903288, 4.330127018922191873, 2.499999999999999556 ) ) ;
#10344=EDGE_CURVE ( 'NONE', #4424, #33565, #68096, .T. ) ;
#10345=CARTESIAN_POINT ( 'NONE',  ( 19.71562500061451928, 3.027376345333613106, -5.243569643749998122 ) ) ;
#10346=CARTESIAN_POINT ( 'NONE',  ( -1.999999999999997113, 12.53750000122903430, -26.53589838486224295 ) ) ;
#10347=CARTESIAN_POINT ( 'NONE',  ( -3.000416591977282496E-16, 19.24062500061459247, 25.09994784771203058 ) ) ;
#10348=CARTESIAN_POINT ( 'NONE',  ( 24.49687500061451573, -3.027376345333614438, 5.243569643749998122 ) ) ;
#10349=DIRECTION ( 'NONE',  ( -1.000000000000000000, -0.000000000000000000, -0.000000000000000000 ) ) ;
#10350=CARTESIAN_POINT ( 'NONE',  ( 28.72500000122903074, 2.886751345948126879, 4.999999999999999112 ) ) ;
#10352=CARTESIAN_POINT ( 'NONE',  ( 24.10312500061451502, -4.541064518000417216, -2.621784821875001281 ) ) ;
#10353=CARTESIAN_POINT ( 'NONE',  ( 16.97812500061451502, 6.421520780324663323E-16, -5.243569643749999010 ) ) ;
#10355=CARTESIAN_POINT ( 'NONE',  ( 13.65937500061451715, 0.000000000000000000, 5.243569643749999010 ) ) ;
#10356=CARTESIAN_POINT ( 'NONE',  ( 26.10000000122903785, -2.886751345948146863, 4.999999999999968026 ) ) ;
#10357=CARTESIAN_POINT ( 'NONE',  ( 27.93750000122903288, -4.330127018922194537, 2.499999999999995559 ) ) ;
#10358=CARTESIAN_POINT ( 'NONE',  ( 3.009375000614516793, -4.541064518000417216, -2.621784821875001281 ) ) ;
#10359=CARTESIAN_POINT ( 'NONE',  ( 15.04687500061451644, -3.027376345333614438, 5.243569643749998122 ) ) ;
#10361=CARTESIAN_POINT ( 'NONE',  ( 3.412500001229032964, 4.330127018922192761, -2.499999999999997780 ) ) ;
#10362=CARTESIAN_POINT ( 'NONE',  ( 23.93437500061451573, 4.541064518000418104, 2.621784821874999949 ) ) ;
#10363=CARTESIAN_POINT ( 'NONE',  ( 16.95937500061451786, -4.541064518000417216, -2.621784821875001281 ) ) ;
#10365=CARTESIAN_POINT ( 'NONE',  ( 28.31250000000000000, -5.773502691896255534, -1.060575238724906372E-15 ) ) ;
#10367=CARTESIAN_POINT ( 'NONE',  ( 3.712500001229034563, -4.330127018922190985, -2.500000000000001332 ) ) ;
#10368=CARTESIAN_POINT ( 'NONE',  ( 4.612500000000002487, 2.886751345948129099, -4.999999999999998224 ) ) ;
#10370=CARTESIAN_POINT ( 'NONE',  ( 19.75312500061451360, 4.541064518000418104, -2.621784821874998173 ) ) ;
#10371=CARTESIAN_POINT ( 'NONE',  ( 9.487500000000000711, -2.886751345948125991, -5.000000000000000000 ) ) ;
#10372=CARTESIAN_POINT ( 'NONE',  ( 5.203125000614518214, -4.541064518000417216, -2.621784821875001281 ) ) ;
#10373=CARTESIAN_POINT ( 'NONE',  ( 19.38749999999999929, -2.886751345948125991, -5.000000000000000000 ) ) ;
#10375=CARTESIAN_POINT ( 'NONE',  ( 20.28750000122903074, -4.330127018922194537, 2.499999999999995559 ) ) ;
#10376=CARTESIAN_POINT ( 'NONE',  ( -1.999999999999997113, 10.17500000000000249, -26.53589838486224295 ) ) ;
#10377=CARTESIAN_POINT ( 'NONE',  ( 3.075000000000001510, -4.330127018922194537, 2.499999999999995559 ) ) ;
#10379=CARTESIAN_POINT ( 'NONE',  ( 16.41562500061451857, -6.054752690667223547, -1.112240025338166033E-15 ) ) ;
#10380=CARTESIAN_POINT ( 'NONE',  ( 24.96562500061451573, -6.054752690667223547, -1.112240025338166033E-15 ) ) ;
#10381=CARTESIAN_POINT ( 'NONE',  ( 21.90937500061451715, -4.541064518000417216, -2.621784821875001281 ) ) ;
#10382=CARTESIAN_POINT ( 'NONE',  ( 7.612500000000000711, -5.773502691896255534, -1.060575238724906372E-15 ) ) ;
#10383=CARTESIAN_POINT ( 'NONE',  ( 10.22812500061451679, 6.421520780324663323E-16, -5.243569643749999010 ) ) ;
#10384=CARTESIAN_POINT ( 'NONE',  ( 27.77812500061451573, 6.421520780324663323E-16, -5.243569643749999010 ) ) ;
#10385=CARTESIAN_POINT ( 'NONE',  ( 14.63437500061451679, -4.541064518000419881, 2.621784821874995952 ) ) ;
#10386=CARTESIAN_POINT ( 'NONE',  ( 18.53437500061451715, 4.541064518000418104, 2.621784821874999949 ) ) ;
#10387=CARTESIAN_POINT ( 'NONE',  ( -5.810221930991193690E-16, 11.90000000122903501, -34.00000000000000000 ) ) ;
#10388=CARTESIAN_POINT ( 'NONE',  ( 4.243569643749999010, 10.22187500061451892, 27.54997392385601174 ) ) ;
#10389=CARTESIAN_POINT ( 'NONE',  ( 21.00000000122903288, 5.773502691896255534, 3.535250795749688894E-16 ) ) ;
#10391=CARTESIAN_POINT ( 'NONE',  ( 10.90312500061451928, 0.000000000000000000, 5.243569643749999010 ) ) ;
#10392=CARTESIAN_POINT ( 'NONE',  ( 9.009375000614518569, 4.541064518000418104, -2.621784821874998173 ) ) ;
#10393=CARTESIAN_POINT ( 'NONE',  ( 7.621875000614519280, 3.027376345333613106, -5.243569643749998122 ) ) ;
#10394=ORIENTED_EDGE ( 'NONE', *, *, #18647, .F. ) ;
#10395=CARTESIAN_POINT ( 'NONE',  ( 28.50937500061451502, 0.000000000000000000, 5.243569643749999010 ) ) ;
#10396=CARTESIAN_POINT ( 'NONE',  ( 18.55312500061451431, 0.000000000000000000, 5.243569643749999010 ) ) ;
#10397=CARTESIAN_POINT ( 'NONE',  ( 28.57500000122903572, 2.886751345948129099, -4.999999999999998224 ) ) ;
#10398=CARTESIAN_POINT ( 'NONE',  ( 3.796875000614517326, -3.027376345333614438, 5.243569643749998122 ) ) ;
#10399=CARTESIAN_POINT ( 'NONE',  ( 24.57187500061451502, -6.054752690667223547, -1.112240025338166033E-15 ) ) ;
#10400=CARTESIAN_POINT ( 'NONE',  ( 18.70312500061451644, -4.541064518000417216, -2.621784821875001281 ) ) ;
#10401=CARTESIAN_POINT ( 'NONE',  ( 4.243569643749999898, 19.14687500061451431, 32.45002607614398471 ) ) ;
#10402=CARTESIAN_POINT ( 'NONE',  ( 23.57812500061451289, -4.541064518000419881, 2.621784821874995952 ) ) ;
#10403=CARTESIAN_POINT ( 'NONE',  ( 3.900000001229034563, 5.773502691896255534, 3.535250795749688894E-16 ) ) ;
#10405=CARTESIAN_POINT ( 'NONE',  ( 29.96250000000000213, 2.886751345948126879, 4.999999999999999112 ) ) ;
#10406=CARTESIAN_POINT ( 'NONE',  ( 8.484601909799253346E-16, 15.61250000000000249, -25.38119784648299770 ) ) ;
#10408=CARTESIAN_POINT ( 'NONE',  ( 5.409375000614516260, 4.541064518000418104, -2.621784821874998173 ) ) ;
#10409=CARTESIAN_POINT ( 'NONE',  ( 11.80312500061451608, 0.000000000000000000, 5.243569643749999010 ) ) ;
#10410=CARTESIAN_POINT ( 'NONE',  ( 5.709375000614517859, -4.541064518000417216, -2.621784821875001281 ) ) ;
#10411=CARTESIAN_POINT ( 'NONE',  ( 24.90000000122903145, -2.886751345948125991, -5.000000000000000000 ) ) ;
#10412=CARTESIAN_POINT ( 'NONE',  ( 14.89687500061451786, 6.054752690667223547, 3.707466751127219781E-16 ) ) ;
#10413=CARTESIAN_POINT ( 'NONE',  ( 3.759375000614517681, 0.000000000000000000, 5.243569643749999010 ) ) ;
#10414=CARTESIAN_POINT ( 'NONE',  ( 2.000000000000001332, 17.44999999999999929, -26.53589838486224650 ) ) ;
#10415=( BOUNDED_CURVE ( )  B_SPLINE_CURVE ( 2, ( #56332, #191, #50432, #40073, #58114, #7165, #40795, #13787, #47414 ),
 .UNSPECIFIED., .F., .F. ) 
 B_SPLINE_CURVE_WITH_KNOTS ( ( 3, 2, 2, 2, 3 ),
 ( 0.6195652173913043237, 0.6231884057971014412, 0.6304347826086956763, 0.6376811594202898004, 0.6413043478260869179 ),
 .UNSPECIFIED. ) 
 CURVE ( )  GEOMETRIC_REPRESENTATION_ITEM ( )  RATIONAL_B_SPLINE_CURVE ( ( 0.9330127018922194093, 0.9330127018922194093, 1.000000000000000000, 0.8660254037844387076, 1.000000000000000000, 0.8660254037844387076, 1.000000000000000000, 0.9330127018922194093, 0.9330127018922194093 ) ) 
 REPRESENTATION_ITEM ( '' )  );
#10416=CARTESIAN_POINT ( 'NONE',  ( 26.85937500061451644, -4.541064518000417216, -2.621784821875001281 ) ) ;
#10418=CARTESIAN_POINT ( 'NONE',  ( 13.30312500061451786, -4.541064518000417216, -2.621784821875001281 ) ) ;
#10419=ORIENTED_EDGE ( 'NONE', *, *, #10486, .T. ) ;
#10420=CARTESIAN_POINT ( 'NONE',  ( 10.86562500061451431, 3.027376345333611329, 5.243569643749999010 ) ) ;
#10421=CARTESIAN_POINT ( 'NONE',  ( 8.015625000614518214, 3.027376345333613106, -5.243569643749998122 ) ) ;
#10423=CARTESIAN_POINT ( 'NONE',  ( 9.674999999999998934, 4.330127018922191873, 2.499999999999999556 ) ) ;
#10424=CARTESIAN_POINT ( 'NONE',  ( 4.462500001229035007, 0.000000000000000000, 4.999999999999998224 ) ) ;
#10425=VECTOR ( 'NONE', #31873, 1000.000000000000000 ) ;
#10426=CARTESIAN_POINT ( 'NONE',  ( 17.36249999999999716, 2.886751345948126879, 4.999999999999999112 ) ) ;
#10427=CARTESIAN_POINT ( 'NONE',  ( 18.15937500061451715, 0.000000000000000000, 5.243569643749999010 ) ) ;
#10428=CARTESIAN_POINT ( 'NONE',  ( 13.12500000122903288, -5.773502691896255534, -1.060575238724906372E-15 ) ) ;
#10430=CARTESIAN_POINT ( 'NONE',  ( -4.243569643749999898, 17.10312500061451502, -30.00000000000000000 ) ) ;
#10431=CARTESIAN_POINT ( 'NONE',  ( 21.93750000000000000, -2.886751345948130876, 4.999999999999996447 ) ) ;
#10433=CARTESIAN_POINT ( 'NONE',  ( 29.50312500061451360, -4.541064518000417216, -2.621784821875001281 ) ) ;
#10434=CARTESIAN_POINT ( 'NONE',  ( 1.071796769724490783, 19.68259618943233491, 34.00000000000000000 ) ) ;
#10436=CARTESIAN_POINT ( 'NONE',  ( 13.24687500061451750, -3.027376345333614438, 5.243569643749998122 ) ) ;
#10437=CARTESIAN_POINT ( 'NONE',  ( 26.36249999999999716, 2.886751345948126879, 4.999999999999999112 ) ) ;
#10438=CARTESIAN_POINT ( 'NONE',  ( 9.290625000614515017, -3.027376345333610441, -5.243569643749999898 ) ) ;
#10440=CARTESIAN_POINT ( 'NONE',  ( 21.00937500061451857, -4.541064518000417216, -2.621784821875001281 ) ) ;
#10442=CARTESIAN_POINT ( 'NONE',  ( 7.453125000614516438, -4.541064518000417216, -2.621784821875001281 ) ) ;
#10443=CARTESIAN_POINT ( 'NONE',  ( 10.99687500061451750, -3.027376345333614438, 5.243569643749998122 ) ) ;
#10445=CARTESIAN_POINT ( 'NONE',  ( 21.00937500061451857, -4.541064518000417216, -2.621784821875001281 ) ) ;
#10446=CARTESIAN_POINT ( 'NONE',  ( 28.98750000000000071, 5.773502691896255534, 3.535250795749688401E-16 ) ) ;
#10447=FACE_OUTER_BOUND ( 'NONE', #63927, .T. ) ;
#10448=( BOUNDED_CURVE ( )  B_SPLINE_CURVE ( 2, ( #29610, #2268, #69507, #52146, #68782, #8167, #40337, #24783, #6721 ),
 .UNSPECIFIED., .F., .T. ) 
 B_SPLINE_CURVE_WITH_KNOTS ( ( 3, 2, 2, 2, 3 ),
 ( 0.9239130434782608647, 0.9275362318840579823, 0.9347826086956522174, 0.9420289855072463414, 0.9456521739130434590 ),
 .UNSPECIFIED. ) 
 CURVE ( )  GEOMETRIC_REPRESENTATION_ITEM ( )  RATIONAL_B_SPLINE_CURVE ( ( 0.9330127018922194093, 0.9330127018922194093, 1.000000000000000000, 0.8660254037844387076, 1.000000000000000000, 0.8660254037844387076, 1.000000000000000000, 0.9330127018922194093, 0.9330127018922194093 ) ) 
 REPRESENTATION_ITEM ( '' )  );
#10449=CARTESIAN_POINT ( 'NONE',  ( 4.875000000000000888, -4.330127018922194537, 2.499999999999995559 ) ) ;
#10450=CARTESIAN_POINT ( 'NONE',  ( 14.70000000122903394, 5.773502691896255534, 3.535250795749688894E-16 ) ) ;
#10454=CARTESIAN_POINT ( 'NONE',  ( 12.18750000000000000, -2.886751345948125991, -5.000000000000000000 ) ) ;
#10455=CARTESIAN_POINT ( 'NONE',  ( 15.48749999999999893, 5.773502691896255534, 3.535250795749688894E-16 ) ) ;
#10456=CARTESIAN_POINT ( 'NONE',  ( 12.63750000122903394, -4.330127018922194537, 2.499999999999995559 ) ) ;
#10457=CARTESIAN_POINT ( 'NONE',  ( 11.31562500061451892, 3.027376345333611329, 5.243569643749999010 ) ) ;
#10458=VERTEX_POINT ( 'NONE', #53101 ) ;
#10459=CARTESIAN_POINT ( 'NONE',  ( 8.250000000000000000, 4.330127018922192761, -2.499999999999997780 ) ) ;
#10460=CARTESIAN_POINT ( 'NONE',  ( -3.000416591977282496E-16, 13.44687500061451857, -34.90005215228797653 ) ) ;
#10461=CARTESIAN_POINT ( 'NONE',  ( 29.62500000122903288, 2.886751345948126879, 4.999999999999999112 ) ) ;
#10463=CARTESIAN_POINT ( 'NONE',  ( 9.262499999999999289, 2.886751345948126879, 4.999999999999999112 ) ) ;
#10464=CARTESIAN_POINT ( 'NONE',  ( 3.965171583692859603, 3.045884815923804556, 3.965171583692790325 ) ) ;
#10465=ORIENTED_EDGE ( 'NONE', *, *, #10153, .T. ) ;
#10466=CARTESIAN_POINT ( 'NONE',  ( 24.14062500061451289, -3.027376345333610441, -5.243569643749999898 ) ) ;
#10467=DIRECTION ( 'NONE',  ( -1.000000000000000000, -0.000000000000000000, -0.000000000000000000 ) ) ;
#10469=CARTESIAN_POINT ( 'NONE',  ( 22.02187500061452141, 3.027376345333613106, -5.243569643749998122 ) ) ;
#10470=CARTESIAN_POINT ( 'NONE',  ( 16.94062500061451715, -3.027376345333610441, -5.243569643749999898 ) ) ;
#10471=EDGE_CURVE ( 'NONE', #2226, #12747, #2489, .T. ) ;
#10472=CARTESIAN_POINT ( 'NONE',  ( 2.121784821874999061, 10.65312500061459389, -33.67503911421598417 ) ) ;
#10473=CARTESIAN_POINT ( 'NONE',  ( 6.028125000614517504, -4.541064518000419881, 2.621784821874995952 ) ) ;
#10474=CARTESIAN_POINT ( 'NONE',  ( 29.62500000122903288, 2.886751345948126879, 4.999999999999999112 ) ) ;
#10476=CARTESIAN_POINT ( 'NONE',  ( 18.81562500061451715, 3.027376345333612662, -5.243569643749998122 ) ) ;
#10479=CARTESIAN_POINT ( 'NONE',  ( 14.44687500061451679, 6.054752690667223547, 3.707466751127219781E-16 ) ) ;
#10480=CARTESIAN_POINT ( 'NONE',  ( 14.03437500061451715, 4.541064518000418104, 2.621784821874999949 ) ) ;
#10481=CARTESIAN_POINT ( 'NONE',  ( 21.87187500061451573, -6.054752690667223547, -1.112240025338166033E-15 ) ) ;
#10483=CARTESIAN_POINT ( 'NONE',  ( 4.243569643749999010, 12.47187500061451715, 27.54997392385601174 ) ) ;
#10484=CARTESIAN_POINT ( 'NONE',  ( 3.890625000614517326, -3.027376345333610441, -5.243569643749999898 ) ) ;
#10485=CARTESIAN_POINT ( 'NONE',  ( 26.42812500061451431, 6.421520780324663323E-16, -5.243569643749999010 ) ) ;
#10486=EDGE_CURVE ( 'NONE', #47796, #55334, #10055, .T. ) ;
#10488=CARTESIAN_POINT ( 'NONE',  ( 27.14062500061451644, -3.027376345333614438, 5.243569643749998122 ) ) ;
#10490=CARTESIAN_POINT ( 'NONE',  ( 8.484601909799253346E-16, 18.76250000000000284, 34.61880215351700230 ) ) ;
#10491=CARTESIAN_POINT ( 'NONE',  ( 4.846875000614519813, -3.027376345333610441, -5.243569643749999898 ) ) ;
#10492=CARTESIAN_POINT ( 'NONE',  ( 12.86250000122903359, 4.330127018922192761, -2.499999999999997780 ) ) ;
#10493=CARTESIAN_POINT ( 'NONE',  ( 8.212500001229035007, -4.330127018922190985, -2.500000000000001332 ) ) ;
#10494=CARTESIAN_POINT ( 'NONE',  ( 28.91250000122903074, -4.330127018922190985, -2.500000000000001332 ) ) ;
#10497=CARTESIAN_POINT ( 'NONE',  ( 11.59687500061451892, -3.027376345333610441, -5.243569643749999898 ) ) ;
#10499=ORIENTED_EDGE ( 'NONE', *, *, #68490, .T. ) ;
#10500=CARTESIAN_POINT ( 'NONE',  ( 19.94062500061451715, -3.027376345333614438, 5.243569643749998122 ) ) ;
#10501=CARTESIAN_POINT ( 'NONE',  ( 12.34687500061452070, -3.027376345333614438, 5.243569643749998122 ) ) ;
#10502=CARTESIAN_POINT ( 'NONE',  ( 5.953125000614519102, 0.000000000000000000, 5.243569643749999010 ) ) ;
#10503=CARTESIAN_POINT ( 'NONE',  ( 21.79687500061451644, -3.027376345333614438, 5.243569643749998122 ) ) ;
#10504=CARTESIAN_POINT ( 'NONE',  ( 5.915625000614515905, 3.027376345333611329, 5.243569643749999010 ) ) ;
#10505=DIRECTION ( 'NONE',  ( 0.000000000000000000, 0.000000000000000000, -1.000000000000000000 ) ) ;
#10506=CARTESIAN_POINT ( 'NONE',  ( 6.187500001229032875, 4.330127018922191873, 2.499999999999999556 ) ) ;
#10507=CARTESIAN_POINT ( 'NONE',  ( 21.81562500061451004, -6.054752690667223547, -1.112240025338166033E-15 ) ) ;
#10508=CARTESIAN_POINT ( 'NONE',  ( -2.828200636599751609E-16, 18.65000000122903501, -34.61880215351700230 ) ) ;
#10509=CARTESIAN_POINT ( 'NONE',  ( 9.037500001229034297, -4.330127018922194537, 2.499999999999995559 ) ) ;
#10511=CARTESIAN_POINT ( 'NONE',  ( 16.64062500061451289, 6.054752690667223547, 3.707466751127219781E-16 ) ) ;
#10512=CARTESIAN_POINT ( 'NONE',  ( 16.00312500061451715, -4.541064518000417216, -2.621784821875001281 ) ) ;
#10514=CARTESIAN_POINT ( 'NONE',  ( 15.90000000000000036, 4.330127018922192761, -2.499999999999997780 ) ) ;
#10515=CARTESIAN_POINT ( 'NONE',  ( 10.91250000122903252, -4.330127018922190985, -2.500000000000001332 ) ) ;
#10516=CARTESIAN_POINT ( 'NONE',  ( 8.615625000614517859, 3.027376345333611329, 5.243569643749999010 ) ) ;
#10517=CARTESIAN_POINT ( 'NONE',  ( 11.35312500061451679, 0.000000000000000000, 5.243569643749999010 ) ) ;
#10518=CARTESIAN_POINT ( 'NONE',  ( 20.96250000122903145, 4.330127018922192761, -2.499999999999997780 ) ) ;
#10519=CARTESIAN_POINT ( 'NONE',  ( 9.001249775931846008E-16, 12.77187500061451786, -25.09994784771203058 ) ) ;
#10520=FACE_OUTER_BOUND ( 'NONE', #48532, .T. ) ;
#10521=CARTESIAN_POINT ( 'NONE',  ( 4.575000001229033941, -5.773502691896255534, -1.060575238724906372E-15 ) ) ;
#10522=CARTESIAN_POINT ( 'NONE',  ( 3.909375000614518481, -4.541064518000417216, -2.621784821875001281 ) ) ;
#10523=CARTESIAN_POINT ( 'NONE',  ( 20.33437500061451786, 4.541064518000418104, 2.621784821874999949 ) ) ;
#10524=CARTESIAN_POINT ( 'NONE',  ( 5.025000000000002132, 6.123233995736764310E-16, -4.999999999999998224 ) ) ;
#10525=CARTESIAN_POINT ( 'NONE',  ( 16.49062500061451786, -3.027376345333610441, -5.243569643749999898 ) ) ;
#10527=CARTESIAN_POINT ( 'NONE',  ( -2.000000000000000000, 14.63750000122903394, 26.53589838486224650 ) ) ;
#10528=CARTESIAN_POINT ( 'NONE',  ( 1.626862140677534273E-15, 15.61250000000000071, 34.00000000000000000 ) ) ;
#10529=CARTESIAN_POINT ( 'NONE',  ( 29.63437500061451502, 6.421520780324663323E-16, -5.243569643749999010 ) ) ;
#10531=CARTESIAN_POINT ( 'NONE',  ( 15.29062500061451679, 6.054752690667223547, 3.707466751127219781E-16 ) ) ;
#10532=CARTESIAN_POINT ( 'NONE',  ( 12.00937500061451857, -4.541064518000417216, -2.621784821875001281 ) ) ;
#10533=ORIENTED_EDGE ( 'NONE', *, *, #14215, .F. ) ;
#10534=CARTESIAN_POINT ( 'NONE',  ( 22.34062500061451573, -3.027376345333610441, -5.243569643749999898 ) ) ;
#10536=CARTESIAN_POINT ( 'NONE',  ( -3.999999999999997335, 18.35000000122903074, 32.30940107675850470 ) ) ;
#10537=CARTESIAN_POINT ( 'NONE',  ( 12.41249999999999964, 2.886751345948126879, 4.999999999999999112 ) ) ;
#10538=CARTESIAN_POINT ( 'NONE',  ( 21.45000000122903216, 5.773502691896255534, 3.535250795749688894E-16 ) ) ;
#10539=CARTESIAN_POINT ( 'NONE',  ( 16.56562500061451715, 3.027376345333613106, -5.243569643749998122 ) ) ;
#10541=ORIENTED_EDGE ( 'NONE', *, *, #64554, .F. ) ;
#10542=CARTESIAN_POINT ( 'NONE',  ( 19.31250000000000000, -5.773502691896255534, -1.060575238724906372E-15 ) ) ;
#10543=CARTESIAN_POINT ( 'NONE',  ( 21.75937500061451502, 0.000000000000000000, 5.243569643749999010 ) ) ;
#10544=CARTESIAN_POINT ( 'NONE',  ( 27.47812500061451502, 4.541064518000418104, 2.621784821874999949 ) ) ;
#10546=CARTESIAN_POINT ( 'NONE',  ( 1.071796769724491893, 17.88259618943233065, -26.00000000000000355 ) ) ;
#10547=CARTESIAN_POINT ( 'NONE',  ( 11.24062500061451608, 6.054752690667223547, 3.707466751127219781E-16 ) ) ;
#10548=CARTESIAN_POINT ( 'NONE',  ( 17.28750000122903430, 6.123233995736764310E-16, -4.999999999999998224 ) ) ;
#10550=CARTESIAN_POINT ( 'NONE',  ( 17.21249999999999858, 2.886751345948129099, -4.999999999999998224 ) ) ;
#10551=CARTESIAN_POINT ( 'NONE',  ( 23.92499999999999716, 6.123233995736764310E-16, -4.999999999999998224 ) ) ;
#10552=CARTESIAN_POINT ( 'NONE',  ( 3.492642502296683382, -3.577956359659812513, -3.802396965202827772 ) ) ;
#10553=CARTESIAN_POINT ( 'NONE',  ( 3.721875000614518036, 3.027376345333611329, 5.243569643749999010 ) ) ;
#10554=CARTESIAN_POINT ( 'NONE',  ( 28.77187500061451431, 3.027376345333613106, -5.243569643749998122 ) ) ;
#10556=CARTESIAN_POINT ( 'NONE',  ( 26.57812500061451644, 4.541064518000418104, 2.621784821874999949 ) ) ;
#10557=CARTESIAN_POINT ( 'NONE',  ( 24.68437500061451573, 6.421520780324663323E-16, -5.243569643749999010 ) ) ;
#10558=CARTESIAN_POINT ( 'NONE',  ( -2.121784821874996840, 17.62812500061459176, -26.32496088578401583 ) ) ;
#10559=CARTESIAN_POINT ( 'NONE',  ( 14.81250000000000000, -5.773502691896255534, -1.060575238724906372E-15 ) ) ;
#10560=CARTESIAN_POINT ( 'NONE',  ( 10.94062500061451537, -3.027376345333614438, 5.243569643749998122 ) ) ;
#10561=CARTESIAN_POINT ( 'NONE',  ( 3.774699069111469019, 3.279031861275984561, 3.945388500768145956 ) ) ;
#10563=CARTESIAN_POINT ( 'NONE',  ( 29.69062500061451715, 6.054752690667223547, 3.707466751127219781E-16 ) ) ;
#10564=CARTESIAN_POINT ( 'NONE',  ( 15.82500000122903216, -5.773502691896255534, -1.060575238724906372E-15 ) ) ;
#10565=CARTESIAN_POINT ( 'NONE',  ( -6.275039685470489619E-15, 18.31250000000000000, 33.99999999999999289 ) ) ;
#10567=CARTESIAN_POINT ( 'NONE',  ( 4.190625000614518925, -3.027376345333614438, 5.243569643749998122 ) ) ;
#10568=CARTESIAN_POINT ( 'NONE',  ( 22.62187500061451573, 3.027376345333611329, 5.243569643749999010 ) ) ;
#10569=CARTESIAN_POINT ( 'NONE',  ( -4.243569643749999898, 15.32187500061451679, 27.54997392385601529 ) ) ;
#10570=CARTESIAN_POINT ( 'NONE',  ( 22.28437500061451715, -4.541064518000419881, 2.621784821874995952 ) ) ;
#10571=CARTESIAN_POINT ( 'NONE',  ( 29.22187500061451715, 3.027376345333613106, -5.243569643749998122 ) ) ;
#10572=CARTESIAN_POINT ( 'NONE',  ( 4.243569643749999010, 18.32187500061451502, 27.54997392385601174 ) ) ;
#10573=CARTESIAN_POINT ( 'NONE',  ( 8.878125000614515372, 6.421520780324663323E-16, -5.243569643749999010 ) ) ;
#10575=EDGE_CURVE ( 'NONE', #39103, #13160, #46297, .T. ) ;
#10576=CARTESIAN_POINT ( 'NONE',  ( 6.909375000614518036, 0.000000000000000000, 5.243569643749999010 ) ) ;
#10578=CARTESIAN_POINT ( 'NONE',  ( 7.303125000614516082, 0.000000000000000000, 5.243569643749999010 ) ) ;
#10579=CARTESIAN_POINT ( 'NONE',  ( 10.84687500061451892, 6.054752690667223547, 3.707466751127219781E-16 ) ) ;
#10580=CARTESIAN_POINT ( 'NONE',  ( 1.592000809091587073E-14, 16.85000000122903785, 26.00000000000000000 ) ) ;
#10581=CARTESIAN_POINT ( 'NONE',  ( 17.92500000122903359, 2.886751345948126879, 4.999999999999999112 ) ) ;
#10582=CARTESIAN_POINT ( 'NONE',  ( 7.809375000614519280, 0.000000000000000000, 5.243569643749999010 ) ) ;
#10583=CARTESIAN_POINT ( 'NONE',  ( 10.75312500061451715, 4.541064518000418104, -2.621784821874998173 ) ) ;
#10584=CARTESIAN_POINT ( 'NONE',  ( 7.228125000614517681, 4.541064518000418104, 2.621784821874999949 ) ) ;
#10586=CARTESIAN_POINT ( 'NONE',  ( 19.24687500061452283, -3.027376345333610441, -5.243569643749999898 ) ) ;
#10587=CARTESIAN_POINT ( 'NONE',  ( 18.30000000000000071, 0.000000000000000000, 4.999999999999998224 ) ) ;
#10588=CARTESIAN_POINT ( 'NONE',  ( 11.42812500061451608, -4.541064518000419881, 2.621784821874995952 ) ) ;
#10589=CARTESIAN_POINT ( 'NONE',  ( 29.18437500061451573, 6.421520780324663323E-16, -5.243569643749999010 ) ) ;
#10590=CARTESIAN_POINT ( 'NONE',  ( -4.243569643749999898, 12.20937500061451608, -30.00000000000000000 ) ) ;
#10591=CARTESIAN_POINT ( 'NONE',  ( 13.42500000122903536, 2.886751345948126879, 4.999999999999999112 ) ) ;
#10592=CARTESIAN_POINT ( 'NONE',  ( 2.121784821874999061, 14.25312500061451715, -33.67503911421598417 ) ) ;
#10593=CARTESIAN_POINT ( 'NONE',  ( 14.62500000122903288, 2.886751345948129099, -4.999999999999998224 ) ) ;
#10594=CARTESIAN_POINT ( 'NONE',  ( 10.75312500061451715, 4.541064518000418104, -2.621784821874998173 ) ) ;
#10595=EDGE_LOOP ( 'NONE', ( #6169, #26713, #24601, #3412 ) ) ;
#10596=CARTESIAN_POINT ( 'NONE',  ( 12.63749999999999929, -2.886751345948125991, -5.000000000000000000 ) ) ;
#10598=CARTESIAN_POINT ( 'NONE',  ( 22.71562500061451573, -6.054752690667223547, -1.112240025338166033E-15 ) ) ;
#10599=CARTESIAN_POINT ( 'NONE',  ( 8.484375000614518214, 6.421520780324663323E-16, -5.243569643749999010 ) ) ;
#10600=CARTESIAN_POINT ( 'NONE',  ( 10.80000000122903536, -2.886751345948129988, 4.999999999999997335 ) ) ;
#10601=CARTESIAN_POINT ( 'NONE',  ( 17.58750000122903145, -4.330127018922194537, 2.499999999999995559 ) ) ;
#10602=CARTESIAN_POINT ( 'NONE',  ( 15.29062500061451679, 6.054752690667223547, 3.707466751127219781E-16 ) ) ;
#10603=CARTESIAN_POINT ( 'NONE',  ( 18.55312500061451431, 0.000000000000000000, 5.243569643749999010 ) ) ;
#10604=CARTESIAN_POINT ( 'NONE',  ( 25.80000000122903714, -2.886751345948125991, -5.000000000000000000 ) ) ;
#10605=CARTESIAN_POINT ( 'NONE',  ( 27.00000000122903288, -2.886751345948129988, 4.999999999999997335 ) ) ;
#10606=CARTESIAN_POINT ( 'NONE',  ( 21.86250000000000071, 2.886751345948126879, 4.999999999999999112 ) ) ;
#10608=CARTESIAN_POINT ( 'NONE',  ( 25.50937500061451502, -4.541064518000417216, -2.621784821875001281 ) ) ;
#10610=CARTESIAN_POINT ( 'NONE',  ( 12.15000000122903501, -2.886751345948129988, 4.999999999999997335 ) ) ;
#10611=CARTESIAN_POINT ( 'NONE',  ( 28.39687500061452141, 6.054752690667223547, 3.707466751127219781E-16 ) ) ;
#10613=CARTESIAN_POINT ( 'NONE',  ( 4.209375000614516971, 0.000000000000000000, 5.243569643749999010 ) ) ;
#10614=CARTESIAN_POINT ( 'NONE',  ( 22.64062500061451644, -3.027376345333614438, 5.243569643749998122 ) ) ;
#10616=CARTESIAN_POINT ( 'NONE',  ( -1.394453263437886604E-15, 19.66249999999999787, -26.00000000000000000 ) ) ;
#10617=CARTESIAN_POINT ( 'NONE',  ( 9.871875000614517504, 3.027376345333613106, -5.243569643749998122 ) ) ;
#10618=CARTESIAN_POINT ( 'NONE',  ( 4.282566015150520933, -2.580625568709436379, 4.493093119413346770 ) ) ;
#10619=CARTESIAN_POINT ( 'NONE',  ( 3.721875000614518036, 3.027376345333611329, 5.243569643749999010 ) ) ;
#10620=CARTESIAN_POINT ( 'NONE',  ( 6.459375000614518747, 0.000000000000000000, 5.243569643749999010 ) ) ;
#10621=CARTESIAN_POINT ( 'NONE',  ( 27.60937500061451644, 0.000000000000000000, 5.243569643749999010 ) ) ;
#10622=CARTESIAN_POINT ( 'NONE',  ( 9.001249775931846008E-16, 10.46562500061459389, 34.90005215228797653 ) ) ;
#10623=CARTESIAN_POINT ( 'NONE',  ( 20.51249999999999929, 2.886751345948126879, 4.999999999999999112 ) ) ;
#10625=CARTESIAN_POINT ( 'NONE',  ( 27.29999999999999716, 0.000000000000000000, 4.999999999999998224 ) ) ;
#10626=( BOUNDED_CURVE ( )  B_SPLINE_CURVE ( 2, ( #27613, #28329, #27251, #61222, #33146, #632, #10255, #55683, #10616 ),
 .UNSPECIFIED., .F., .F. ) 
 B_SPLINE_CURVE_WITH_KNOTS ( ( 3, 2, 2, 2, 3 ),
 ( 0.01086956521739130578, 0.01449275362318840597, 0.02173913043478260809, 0.02898550724637680848, 0.03260869565217391908 ),
 .UNSPECIFIED. ) 
 CURVE ( )  GEOMETRIC_REPRESENTATION_ITEM ( )  RATIONAL_B_SPLINE_CURVE ( ( 0.9330127018922194093, 0.9330127018922194093, 1.000000000000000000, 0.8660254037844387076, 1.000000000000000000, 0.8660254037844387076, 1.000000000000000000, 0.9330127018922191873, 0.9330127018922192983 ) ) 
 REPRESENTATION_ITEM ( '' )  );
#10627=CARTESIAN_POINT ( 'NONE',  ( 28.43437500061451573, 4.541064518000418104, 2.621784821874999949 ) ) ;
#10628=EDGE_LOOP ( 'NONE', ( #57607, #53697, #42839, #35952 ) ) ;
#10629=CARTESIAN_POINT ( 'NONE',  ( 16.71562500061451573, 3.027376345333611329, 5.243569643749999010 ) ) ;
#10630=CARTESIAN_POINT ( 'NONE',  ( 8.878125000614515372, 6.421520780324663323E-16, -5.243569643749999010 ) ) ;
#10632=CARTESIAN_POINT ( 'NONE',  ( 8.184375000614515727, 4.541064518000418104, 2.621784821874999949 ) ) ;
#10633=CARTESIAN_POINT ( 'NONE',  ( 17.40000000122903145, 5.773502691896255534, 3.535250795749688894E-16 ) ) ;
#10634=CARTESIAN_POINT ( 'NONE',  ( 7.059375000614518392, -4.541064518000417216, -2.621784821875001281 ) ) ;
#10635=CARTESIAN_POINT ( 'NONE',  ( 11.25937500061451679, 4.541064518000418104, -2.621784821874998173 ) ) ;
#10636=CARTESIAN_POINT ( 'NONE',  ( 23.10937500061451644, 0.000000000000000000, 5.243569643749999010 ) ) ;
#10637=EDGE_CURVE ( 'NONE', #42547, #39133, #61392, .T. ) ;
#10641=CARTESIAN_POINT ( 'NONE',  ( 17.59687500061451715, 6.054752690667223547, 3.707466751127219781E-16 ) ) ;
#10642=CARTESIAN_POINT ( 'NONE',  ( 9.421875000614519990, 3.027376345333613106, -5.243569643749998122 ) ) ;
#10644=CARTESIAN_POINT ( 'NONE',  ( 19.91250000000000142, 2.886751345948129099, -4.999999999999998224 ) ) ;
#10646=CARTESIAN_POINT ( 'NONE',  ( 9.001249775931846008E-16, 10.52187500061451964, -25.09994784771203058 ) ) ;
#10648=CARTESIAN_POINT ( 'NONE',  ( 11.61562500061451608, 3.027376345333613106, -5.243569643749998122 ) ) ;
#10649=CARTESIAN_POINT ( 'NONE',  ( 3.075000000000001510, -4.330127018922194537, 2.499999999999995559 ) ) ;
#10650=CARTESIAN_POINT ( 'NONE',  ( 3.486133158594716510E-16, 19.55000000122903359, 26.00000000000000355 ) ) ;
#10651=CARTESIAN_POINT ( 'NONE',  ( 4.204793154262189248, 2.706354874286773349, -4.204793154262189248 ) ) ;
#10652=CARTESIAN_POINT ( 'NONE',  ( 10.95000000000000107, 4.330127018922192761, -2.499999999999997780 ) ) ;
#10653=CARTESIAN_POINT ( 'NONE',  ( -3.999999999999999556, 15.12500000122903288, 27.69059892324149530 ) ) ;
#10654=CARTESIAN_POINT ( 'NONE',  ( 9.262500001229033941, 4.330127018922192761, -2.499999999999997780 ) ) ;
#10655=CARTESIAN_POINT ( 'NONE',  ( 20.97187500061451715, -6.054752690667223547, -1.112240025338166033E-15 ) ) ;
#10656=CARTESIAN_POINT ( 'NONE',  ( 15.27187500061451786, 3.027376345333613106, -5.243569643749998122 ) ) ;
#10657=DIRECTION ( 'NONE',  ( 0.000000000000000000, 0.000000000000000000, -1.000000000000000000 ) ) ;
#10658=ORIENTED_EDGE ( 'NONE', *, *, #40061, .T. ) ;
#10659=CARTESIAN_POINT ( 'NONE',  ( 15.32812500061451644, 4.541064518000418104, 2.621784821874999949 ) ) ;
#10660=CARTESIAN_POINT ( 'NONE',  ( 29.25000000122903288, -2.886751345948129988, 4.999999999999997335 ) ) ;
#10661=CARTESIAN_POINT ( 'NONE',  ( 15.87187500061451573, 3.027376345333611329, 5.243569643749999010 ) ) ;
#10663=CARTESIAN_POINT ( 'NONE',  ( 17.91562500061451502, 3.027376345333613106, -5.243569643749998122 ) ) ;
#10664=CARTESIAN_POINT ( 'NONE',  ( 18.18750000122903288, 6.123233995736764310E-16, -4.999999999999998224 ) ) ;
#10665=CARTESIAN_POINT ( 'NONE',  ( 27.38437500061451857, 6.421520780324663323E-16, -5.243569643749999010 ) ) ;
#10666=CARTESIAN_POINT ( 'NONE',  ( -3.000416591977282496E-16, 13.39062500061451644, 25.09994784771203058 ) ) ;
#10667=CARTESIAN_POINT ( 'NONE',  ( 16.35937500061451644, 0.000000000000000000, 5.243569643749999010 ) ) ;
#10668=CARTESIAN_POINT ( 'NONE',  ( 13.42500000122903536, 2.886751345948126879, 4.999999999999999112 ) ) ;
#10670=CARTESIAN_POINT ( 'NONE',  ( 4.243569643749999010, 19.67187500061451644, -32.45002607614398471 ) ) ;
#10671=CARTESIAN_POINT ( 'NONE',  ( 21.08437500061451786, 6.421520780324663323E-16, -5.243569643749999010 ) ) ;
#10672=CARTESIAN_POINT ( 'NONE',  ( 22.80000000122903359, 5.773502691896255534, 3.535250795749688894E-16 ) ) ;
#10673=CARTESIAN_POINT ( 'NONE',  ( 15.90937500061451892, 0.000000000000000000, 5.243569643749999010 ) ) ;
#10674=CARTESIAN_POINT ( 'NONE',  ( 4.243569643749999898, 11.94687500061451857, 32.45002607614398471 ) ) ;
#10675=CARTESIAN_POINT ( 'NONE',  ( 18.10312500061451502, 0.000000000000000000, 5.243569643749999010 ) ) ;
#10676=ORIENTED_EDGE ( 'NONE', *, *, #35455, .T. ) ;
#10678=CARTESIAN_POINT ( 'NONE',  ( 21.71249999999999858, 2.886751345948129099, -4.999999999999998224 ) ) ;
#10679=CARTESIAN_POINT ( 'NONE',  ( 28.20000000122903216, 5.773502691896255534, 3.535250795749688401E-16 ) ) ;
#10680=CARTESIAN_POINT ( 'NONE',  ( 25.19062500061451715, 6.054752690667223547, 3.707466751127219781E-16 ) ) ;
#10681=CARTESIAN_POINT ( 'NONE',  ( 4.603125000614518569, 0.000000000000000000, 5.243569643749999010 ) ) ;
#10682=CARTESIAN_POINT ( 'NONE',  ( 17.58750000122903145, -4.330127018922194537, 2.499999999999995559 ) ) ;
#10683=CARTESIAN_POINT ( 'NONE',  ( 21.77812500061451928, -4.541064518000419881, 2.621784821874995952 ) ) ;
#10684=CARTESIAN_POINT ( 'NONE',  ( 19.72499999999999787, -4.330127018922194537, 2.499999999999995559 ) ) ;
#10685=CARTESIAN_POINT ( 'NONE',  ( 25.37812500061451715, -4.541064518000419881, 2.621784821874995952 ) ) ;
#10686=CARTESIAN_POINT ( 'NONE',  ( 4.753125000614515372, -4.541064518000417216, -2.621784821875001281 ) ) ;
#10687=( BOUNDED_CURVE ( )  B_SPLINE_CURVE ( 2, ( #27432, #49963, #15593, #38135, #21506, #26330, #60657 ),
 .UNSPECIFIED., .F., .F. ) 
 B_SPLINE_CURVE_WITH_KNOTS ( ( 3, 2, 2, 3 ),
 ( 0.3500000000000000333, 0.3527777777777778567, 0.3555555555555556246, 0.3583333333333333925 ),
 .UNSPECIFIED. ) 
 CURVE ( )  GEOMETRIC_REPRESENTATION_ITEM ( )  RATIONAL_B_SPLINE_CURVE ( ( 0.9999999999999973355, 0.8660254037844413721, 1.000000000000000000, 0.8660254037844387076, 1.000000000000000000, 0.8660254037844360431, 1.000000000000002665 ) ) 
 REPRESENTATION_ITEM ( '' )  );
#10689=CARTESIAN_POINT ( 'NONE',  ( 29.84999999999999787, 4.330127018922192761, -2.499999999999997780 ) ) ;
#10690=CARTESIAN_POINT ( 'NONE',  ( 3.553125000614516082, 4.541064518000418104, -2.621784821874998173 ) ) ;
#10692=CARTESIAN_POINT ( 'NONE',  ( -5.810221930991193690E-16, 18.98750000000000071, 26.00000000000000355 ) ) ;
#10693=CARTESIAN_POINT ( 'NONE',  ( -2.000000000000000000, 11.48750000122903359, -33.46410161513775705 ) ) ;
#10694=CARTESIAN_POINT ( 'NONE',  ( 2.121784821874999061, 19.25937500061451857, -33.67503911421598417 ) ) ;
#10695=CARTESIAN_POINT ( 'NONE',  ( 8.925000000000002487, -4.330127018922194537, 2.499999999999995559 ) ) ;
#10696=ADVANCED_FACE ( 'NONE', ( #54206 ), #60094, .F. ) ;
#10697=CARTESIAN_POINT ( 'NONE',  ( 8.034375000614518925, 6.421520780324663323E-16, -5.243569643749999010 ) ) ;
#10698=CARTESIAN_POINT ( 'NONE',  ( 7.500000001229034652, 5.773502691896255534, 3.535250795749688894E-16 ) ) ;
#10699=CARTESIAN_POINT ( 'NONE',  ( 13.24687500061451750, -3.027376345333614438, 5.243569643749998122 ) ) ;
#10700=CARTESIAN_POINT ( 'NONE',  ( 4.621875000614516615, 3.027376345333611329, 5.243569643749999010 ) ) ;
#10701=CARTESIAN_POINT ( 'NONE',  ( -2.556497649636125342E-15, 18.87500000122903288, 34.00000000000000000 ) ) ;
#10702=CARTESIAN_POINT ( 'NONE',  ( 19.83750000000000213, -2.886751345948126435, -5.000000000000000000 ) ) ;
#10703=CARTESIAN_POINT ( 'NONE',  ( 9.309375000614517504, -4.541064518000417216, -2.621784821875001281 ) ) ;
#10704=EDGE_CURVE ( 'NONE', #13105, #6716, #53851, .T. ) ;
#10705=CARTESIAN_POINT ( 'NONE',  ( 3.999999999999999112, 17.18750000122903288, -30.00000000000000000 ) ) ;
#10706=CARTESIAN_POINT ( 'NONE',  ( 19.15312500061451573, -4.541064518000417216, -2.621784821875001281 ) ) ;
#10707=CARTESIAN_POINT ( 'NONE',  ( 16.72500000000000142, 6.123233995736764310E-16, -4.999999999999998224 ) ) ;
#10708=CARTESIAN_POINT ( 'NONE',  ( -2.121784821874996840, 18.97812500061459673, 33.67503911421598417 ) ) ;
#10709=CARTESIAN_POINT ( 'NONE',  ( 23.18437500061451573, -4.541064518000419881, 2.621784821874995952 ) ) ;
#10710=EDGE_CURVE ( 'NONE', #38182, #50028, #68943, .T. ) ;
#10711=CARTESIAN_POINT ( 'NONE',  ( 2.000000000000001332, 19.25000000000000000, 33.46410161513774995 ) ) ;
#10712=CARTESIAN_POINT ( 'NONE',  ( 29.43750000122903288, 6.123233995736764310E-16, -4.999999999999998224 ) ) ;
#10714=CARTESIAN_POINT ( 'NONE',  ( 25.07812500061451644, 6.421520780324663323E-16, -5.243569643749999010 ) ) ;
#10715=CARTESIAN_POINT ( 'NONE',  ( 14.35312500061451679, 4.541064518000418104, -2.621784821874998173 ) ) ;
#10717=CARTESIAN_POINT ( 'NONE',  ( 13.32187500061451502, -6.054752690667223547, -1.112240025338166033E-15 ) ) ;
#10718=CARTESIAN_POINT ( 'NONE',  ( 16.83749999999999858, 5.773502691896255534, 3.535250795749688401E-16 ) ) ;
#10719=CARTESIAN_POINT ( 'NONE',  ( 25.20000000122903216, -2.886751345948129988, 4.999999999999997335 ) ) ;
#10720=CARTESIAN_POINT ( 'NONE',  ( 2.859375000614519546, 0.000000000000000000, 5.243569643749999010 ) ) ;
#10721=CARTESIAN_POINT ( 'NONE',  ( 13.43437500061451750, 6.421520780324663323E-16, -5.243569643749999010 ) ) ;
#10723=CARTESIAN_POINT ( 'NONE',  ( 30.00000000000000000, 0.000000000000000000, 0.000000000000000000 ) ) ;
#10724=CARTESIAN_POINT ( 'NONE',  ( 30.00000000000000000, 6.123233995736764310E-16, -4.999999999999998224 ) ) ;
#10725=CARTESIAN_POINT ( 'NONE',  ( 25.50937500061451502, -4.541064518000417216, -2.621784821875001281 ) ) ;
#10726=CARTESIAN_POINT ( 'NONE',  ( 17.10937500061451999, 4.541064518000418104, -2.621784821874998173 ) ) ;
#10728=CARTESIAN_POINT ( 'NONE',  ( 28.04999999999999716, 4.330127018922192761, -2.499999999999997780 ) ) ;
#10729=CARTESIAN_POINT ( 'NONE',  ( 4.725000001229034297, 2.886751345948129099, -4.999999999999998224 ) ) ;
#10730=CARTESIAN_POINT ( 'NONE',  ( 4.687500000000000000, 5.773502691896255534, 3.535250795749688894E-16 ) ) ;
#10732=CARTESIAN_POINT ( 'NONE',  ( 18.85312500061451502, 4.541064518000418104, -2.621784821874998173 ) ) ;
#10733=CARTESIAN_POINT ( 'NONE',  ( 9.000000000000001776, -4.330127018922190985, -2.500000000000001332 ) ) ;
#10734=CARTESIAN_POINT ( 'NONE',  ( 17.47499999999999787, -4.330127018922194537, 2.499999999999995559 ) ) ;
#10735=DIRECTION ( 'NONE',  ( -0.000000000000000000, -1.000000000000000000, -0.000000000000000000 ) ) ;
#10736=CARTESIAN_POINT ( 'NONE',  ( 20.10000000122903074, 5.773502691896255534, 3.535250795749688894E-16 ) ) ;
#10737=CARTESIAN_POINT ( 'NONE',  ( 0.4052273161492640496, 10.00000000000000000, 36.00000000000000711 ) ) ;
#10738=CARTESIAN_POINT ( 'NONE',  ( 27.45937500061451786, 4.541064518000418104, -2.621784821874998173 ) ) ;
#10739=ORIENTED_EDGE ( 'NONE', *, *, #58225, .F. ) ;
#10740=CARTESIAN_POINT ( 'NONE',  ( 16.07812500061451289, 6.421520780324663323E-16, -5.243569643749999010 ) ) ;
#10741=CARTESIAN_POINT ( 'NONE',  ( 23.57812500061451289, -4.541064518000419881, 2.621784821874995952 ) ) ;
#10742=CARTESIAN_POINT ( 'NONE',  ( 22.50937500061451857, 4.541064518000418104, -2.621784821874998173 ) ) ;
#10743=CARTESIAN_POINT ( 'NONE',  ( 5.737499999999998934, -2.886751345948129988, 4.999999999999997335 ) ) ;
#10744=CARTESIAN_POINT ( 'NONE',  ( 9.703125000614514661, -4.541064518000417216, -2.621784821875001281 ) ) ;
#10745=CARTESIAN_POINT ( 'NONE',  ( 24.92812500061451431, -4.541064518000419881, 2.621784821874995952 ) ) ;
#10746=CARTESIAN_POINT ( 'NONE',  ( 14.89687500061451786, 6.054752690667223547, 3.707466751127219781E-16 ) ) ;
#10747=CARTESIAN_POINT ( 'NONE',  ( 20.14687500061451786, -3.027376345333610441, -5.243569643749999898 ) ) ;
#10749=CARTESIAN_POINT ( 'NONE',  ( -4.243569643749999898, 19.35312500061451857, 30.00000000000000000 ) ) ;
#10751=CARTESIAN_POINT ( 'NONE',  ( 20.77500000122903145, -5.773502691896255534, -1.060575238724906372E-15 ) ) ;
#10753=CARTESIAN_POINT ( 'NONE',  ( 12.59062500061451573, 6.054752690667223547, 3.707466751127219781E-16 ) ) ;
#10754=CARTESIAN_POINT ( 'NONE',  ( 8.784375000614518925, -4.541064518000419881, 2.621784821874995952 ) ) ;
#10755=CARTESIAN_POINT ( 'NONE',  ( 6.496875000614517504, -3.027376345333614438, 5.243569643749998122 ) ) ;
#10756=ORIENTED_EDGE ( 'NONE', *, *, #27024, .T. ) ;
#10757=CARTESIAN_POINT ( 'NONE',  ( 28.20937500061451786, -4.541064518000417216, -2.621784821875001281 ) ) ;
#10758=CARTESIAN_POINT ( 'NONE',  ( 19.97812500061451502, -4.541064518000419881, 2.621784821874995952 ) ) ;
#10759=CARTESIAN_POINT ( 'NONE',  ( 2.990625000614519191, -3.027376345333610441, -5.243569643749999898 ) ) ;
#10760=CARTESIAN_POINT ( 'NONE',  ( 27.62812500061451360, -4.541064518000419881, 2.621784821874995952 ) ) ;
#10761=CARTESIAN_POINT ( 'NONE',  ( 24.94687500061451502, -3.027376345333614438, 5.243569643749998122 ) ) ;
#10762=CARTESIAN_POINT ( 'NONE',  ( 19.90312500061451573, 0.000000000000000000, 5.243569643749999010 ) ) ;
#10763=CARTESIAN_POINT ( 'NONE',  ( -2.121784821874999949, 18.43437500061451928, 26.32496088578401938 ) ) ;
#10764=CARTESIAN_POINT ( 'NONE',  ( 25.07812500061451644, 6.421520780324663323E-16, -5.243569643749999010 ) ) ;
#10765=CARTESIAN_POINT ( 'NONE',  ( 5.812500001229035540, 0.000000000000000000, 4.999999999999998224 ) ) ;
#10766=ORIENTED_EDGE ( 'NONE', *, *, #10575, .T. ) ;
#10767=CARTESIAN_POINT ( 'NONE',  ( 28.83749999999999858, -2.886751345948125991, -5.000000000000000000 ) ) ;
#10768=CARTESIAN_POINT ( 'NONE',  ( 2.000000000000001332, 16.10000000000000142, -26.53589838486224650 ) ) ;
#10770=CARTESIAN_POINT ( 'NONE',  ( 3.759375000614517681, 0.000000000000000000, 5.243569643749999010 ) ) ;
#10771=CARTESIAN_POINT ( 'NONE',  ( 13.04062500061451502, 6.054752690667223547, 3.707466751127219781E-16 ) ) ;
#10772=CARTESIAN_POINT ( 'NONE',  ( 6.834375000614518747, 4.541064518000418104, 2.621784821874999949 ) ) ;
#10773=CARTESIAN_POINT ( 'NONE',  ( 24.07500000122903216, 2.886751345948129099, -4.999999999999998224 ) ) ;
#10774=CARTESIAN_POINT ( 'NONE',  ( 14.22187500061451892, -6.054752690667223547, -1.112240025338166033E-15 ) ) ;
#10775=CARTESIAN_POINT ( 'NONE',  ( 3.534375000614518036, 6.421520780324663323E-16, -5.243569643749999010 ) ) ;
#10776=CARTESIAN_POINT ( 'NONE',  ( 7.987500001229032698, 4.330127018922191873, 2.499999999999999556 ) ) ;
#10777=CARTESIAN_POINT ( 'NONE',  ( 26.29687500061451644, -3.027376345333614438, 5.243569643749998122 ) ) ;
#10778=CARTESIAN_POINT ( 'NONE',  ( 3.890625000614517326, -3.027376345333610441, -5.243569643749999898 ) ) ;
#10779=CARTESIAN_POINT ( 'NONE',  ( 13.37812500061451715, 6.421520780324663323E-16, -5.243569643749999010 ) ) ;
#10781=CARTESIAN_POINT ( 'NONE',  ( 11.05312500061451608, -4.541064518000417216, -2.621784821875001281 ) ) ;
#10782=CARTESIAN_POINT ( 'NONE',  ( 7.265625000614516438, 3.027376345333611329, 5.243569643749999010 ) ) ;
#10784=CARTESIAN_POINT ( 'NONE',  ( 30.00000000000000000, 0.000000000000000000, 0.000000000000000000 ) ) ;
#10785=CARTESIAN_POINT ( 'NONE',  ( 16.38749999999999929, 5.773502691896255534, 3.535250795749688894E-16 ) ) ;
#10786=CARTESIAN_POINT ( 'NONE',  ( 17.03437500061451715, 6.421520780324663323E-16, -5.243569643749999010 ) ) ;
#10787=CARTESIAN_POINT ( 'NONE',  ( 14.81250000122903288, 0.000000000000000000, 4.999999999999998224 ) ) ;
#10789=CARTESIAN_POINT ( 'NONE',  ( 4.243569643749999010, 14.66562500061451857, -32.45002607614398471 ) ) ;
#10793=CARTESIAN_POINT ( 'NONE',  ( 26.46562500061451573, 3.027376345333613106, -5.243569643749998122 ) ) ;
#10794=CARTESIAN_POINT ( 'NONE',  ( 3.999999999999998668, 19.81250000000000000, 27.69059892324149530 ) ) ;
#10797=CARTESIAN_POINT ( 'NONE',  ( 26.73749999999999716, 5.773502691896255534, 3.535250795749688894E-16 ) ) ;
#10798=CARTESIAN_POINT ( 'NONE',  ( 8.390625000614518214, -3.027376345333610441, -5.243569643749999898 ) ) ;
#10800=CARTESIAN_POINT ( 'NONE',  ( 22.50937500061451857, 4.541064518000418104, -2.621784821874998173 ) ) ;
#10802=CARTESIAN_POINT ( 'NONE',  ( 4.415625000614518569, 3.027376345333613106, -5.243569643749998122 ) ) ;
#10803=CARTESIAN_POINT ( 'NONE',  ( 10.80937500061451928, 4.541064518000418104, -2.621784821874998173 ) ) ;
#10804=VERTEX_POINT ( 'NONE', #67128 ) ;
#10805=CARTESIAN_POINT ( 'NONE',  ( 20.74687500061451573, 6.054752690667223547, 3.707466751127219781E-16 ) ) ;
#10806=CARTESIAN_POINT ( 'NONE',  ( 3.963750086740945200, 3.047826611959361109, -30.55459297196504309 ) ) ;
#10807=CARTESIAN_POINT ( 'NONE',  ( 28.61249999999999716, 2.886751345948126879, 4.999999999999999112 ) ) ;
#10808=CARTESIAN_POINT ( 'NONE',  ( 5.437500000000001776, -2.886751345948125991, -5.000000000000000000 ) ) ;
#10809=CARTESIAN_POINT ( 'NONE',  ( 13.83750000122903323, 4.330127018922191873, 2.499999999999999556 ) ) ;
#10810=CARTESIAN_POINT ( 'NONE',  ( 3.999999999999998668, 15.31250000000000000, -32.30940107675850470 ) ) ;
#10813=ORIENTED_EDGE ( 'NONE', *, *, #69202, .F. ) ;
#10814=CARTESIAN_POINT ( 'NONE',  ( 11.77500000000000036, 6.123233995736764310E-16, -4.999999999999998224 ) ) ;
#10815=CARTESIAN_POINT ( 'NONE',  ( 17.58749999999999858, -2.886751345948125991, -5.000000000000000000 ) ) ;
#10816=CARTESIAN_POINT ( 'NONE',  ( 12.18750000122903465, -4.330127018922194537, 2.499999999999995559 ) ) ;
#10817=CARTESIAN_POINT ( 'NONE',  ( 12.21562500061451573, 3.027376345333611329, 5.243569643749999010 ) ) ;
#10818=CARTESIAN_POINT ( 'NONE',  ( 8.099999999999999645, -4.330127018922190985, -2.500000000000001332 ) ) ;
#10819=CARTESIAN_POINT ( 'NONE',  ( -4.243569643749999898, 14.87187500061451928, -32.45002607614398471 ) ) ;
#10820=CARTESIAN_POINT ( 'NONE',  ( 28.80000000122903003, -2.886751345948129988, 4.999999999999997335 ) ) ;
#10822=CARTESIAN_POINT ( 'NONE',  ( 11.06250000000000000, 2.886751345948126879, 4.999999999999999112 ) ) ;
#10823=CARTESIAN_POINT ( 'NONE',  ( 0.000000000000000000, 20.00000000000000000, -30.00000000000000000 ) ) ;
#10824=VERTEX_POINT ( 'NONE', #39042 ) ;
#10825=CARTESIAN_POINT ( 'NONE',  ( 25.34062500061451217, -3.027376345333614438, 5.243569643749998122 ) ) ;
#10826=CARTESIAN_POINT ( 'NONE',  ( 29.32500000122903216, -5.773502691896255534, -1.060575238724906372E-15 ) ) ;
#10827=CARTESIAN_POINT ( 'NONE',  ( 29.14687500061451075, -3.027376345333610441, -5.243569643749999898 ) ) ;
#10828=CARTESIAN_POINT ( 'NONE',  ( 22.13437500061451502, 4.541064518000418104, 2.621784821874999949 ) ) ;
#10829=CARTESIAN_POINT ( 'NONE',  ( 15.85312500061451857, 0.000000000000000000, 5.243569643749999010 ) ) ;
#10830=CARTESIAN_POINT ( 'NONE',  ( -4.243569643749999898, 12.56562500061459176, -32.45002607614398471 ) ) ;
#10831=CARTESIAN_POINT ( 'NONE',  ( 7.265625000614516438, 3.027376345333611329, 5.243569643749999010 ) ) ;
#10832=CARTESIAN_POINT ( 'NONE',  ( 28.57500000122903572, 2.886751345948129099, -4.999999999999998224 ) ) ;
#10834=CARTESIAN_POINT ( 'NONE',  ( 17.95312500061451644, 4.541064518000418104, -2.621784821874998173 ) ) ;
#10837=( BOUNDED_CURVE ( )  B_SPLINE_CURVE ( 2, ( #67427, #11984, #49703, #6080, #27530, #72594, #16789 ),
 .UNSPECIFIED., .F., .F. ) 
 B_SPLINE_CURVE_WITH_KNOTS ( ( 3, 2, 2, 3 ),
 ( 0.4416666666666666519, 0.4444444444444444753, 0.4472222222222222987, 0.4500000000000001221 ),
 .UNSPECIFIED. ) 
 CURVE ( )  GEOMETRIC_REPRESENTATION_ITEM ( )  RATIONAL_B_SPLINE_CURVE ( ( 1.000000000000000000, 0.8660254037844387076, 1.000000000000000000, 0.8660254037844387076, 1.000000000000000000, 0.8660254037844333785, 1.000000000000005329 ) ) 
 REPRESENTATION_ITEM ( '' )  );
#10838=CARTESIAN_POINT ( 'NONE',  ( 15.42187500061451821, 3.027376345333611329, 5.243569643749999010 ) ) ;
#10839=CARTESIAN_POINT ( 'NONE',  ( 14.29687500061451821, -3.027376345333610441, -5.243569643749999898 ) ) ;
#10840=CARTESIAN_POINT ( 'NONE',  ( 22.77187500061451786, -6.054752690667223547, -1.112240025338166033E-15 ) ) ;
#10841=EDGE_LOOP ( 'NONE', ( #65731, #3473, #38399, #20427 ) ) ;
#10842=CARTESIAN_POINT ( 'NONE',  ( 4.243569643749999898, 12.88437500061451857, 30.00000000000000000 ) ) ;
#10843=CARTESIAN_POINT ( 'NONE',  ( 3.478125000614517237, 6.421520780324663323E-16, -5.243569643749999010 ) ) ;
#10844=CARTESIAN_POINT ( 'NONE',  ( 27.17812500061451786, -4.541064518000419881, 2.621784821874995952 ) ) ;
#10845=CARTESIAN_POINT ( 'NONE',  ( 26.39062500061451644, -3.027376345333610441, -5.243569643749999898 ) ) ;
#10847=CARTESIAN_POINT ( 'NONE',  ( 4.000000000000000000, 16.58750000000000213, 32.30940107675849049 ) ) ;
#10848=CARTESIAN_POINT ( 'NONE',  ( 5.971875000614516260, 3.027376345333611329, 5.243569643749999010 ) ) ;
#10849=CARTESIAN_POINT ( 'NONE',  ( 11.51250000122903216, 4.330127018922192761, -2.499999999999997780 ) ) ;
#10850=CARTESIAN_POINT ( 'NONE',  ( 6.375000001229031987, -5.773502691896255534, -1.060575238724906372E-15 ) ) ;
#10851=CARTESIAN_POINT ( 'NONE',  ( 3.215625000614518836, 3.027376345333611329, 5.243569643749999010 ) ) ;
#10854=CARTESIAN_POINT ( 'NONE',  ( 12.12187500061451573, 3.027376345333613106, -5.243569643749998122 ) ) ;
#10855=CARTESIAN_POINT ( 'NONE',  ( 1.071796769724489895, 14.91740381056766829, -34.00000000000000000 ) ) ;
#10856=EDGE_LOOP ( 'NONE', ( #28024, #19160, #53321, #31491 ) ) ;
#10858=CARTESIAN_POINT ( 'NONE',  ( 19.64062500061451644, -3.027376345333610441, -5.243569643749999898 ) ) ;
#10859=CARTESIAN_POINT ( 'NONE',  ( 13.50937500061451679, 4.541064518000418104, -2.621784821874998173 ) ) ;
#10860=CARTESIAN_POINT ( 'NONE',  ( 4.528125000614516615, 4.541064518000418104, 2.621784821874999949 ) ) ;
#10861=CARTESIAN_POINT ( 'NONE',  ( 21.57187500061451502, 3.027376345333612662, -5.243569643749998122 ) ) ;
#10862=CARTESIAN_POINT ( 'NONE',  ( 9.421875000614519990, 3.027376345333613106, -5.243569643749998122 ) ) ;
#10863=CARTESIAN_POINT ( 'NONE',  ( 4.340625000614515727, -3.027376345333610441, -5.243569643749999898 ) ) ;
#10864=CARTESIAN_POINT ( 'NONE',  ( 10.80000000122903536, -2.886751345948130876, 4.999999999999996447 ) ) ;
#10865=CARTESIAN_POINT ( 'NONE',  ( 6.637500001229035718, 4.330127018922191873, 2.499999999999999556 ) ) ;
#10866=CARTESIAN_POINT ( 'NONE',  ( 20.39062500061451644, -3.027376345333614438, 5.243569643749998122 ) ) ;
#10867=CARTESIAN_POINT ( 'NONE',  ( 7.425000001229034474, 2.886751345948129099, -4.999999999999998224 ) ) ;
#10868=CARTESIAN_POINT ( 'NONE',  ( 16.82812500061451644, -4.541064518000419881, 2.621784821874995952 ) ) ;
#10869=CARTESIAN_POINT ( 'NONE',  ( 16.71562500061451573, 3.027376345333611329, 5.243569643749999010 ) ) ;
#10871=CARTESIAN_POINT ( 'NONE',  ( 16.35000000000000142, 4.330127018922192761, -2.499999999999997780 ) ) ;
#10872=CARTESIAN_POINT ( 'NONE',  ( 8.700000001229032165, -2.886751345948125991, -5.000000000000000000 ) ) ;
#10873=CARTESIAN_POINT ( 'NONE',  ( 6.215625000614517504, 3.027376345333613106, -5.243569643749998122 ) ) ;
#10874=CARTESIAN_POINT ( 'NONE',  ( 20.25000000122903288, -2.886751345948129988, 4.999999999999997335 ) ) ;
#10876=CARTESIAN_POINT ( 'NONE',  ( 4.243569643749999898, 12.88437500061451857, -30.00000000000000000 ) ) ;
#10877=CARTESIAN_POINT ( 'NONE',  ( 30.00000000000000000, 6.123233995736764310E-16, -4.999999999999998224 ) ) ;
#10879=CARTESIAN_POINT ( 'NONE',  ( 3.037500001229032964, 4.330127018922191873, 2.499999999999999556 ) ) ;
#10881=CARTESIAN_POINT ( 'NONE',  ( 5.184375000614516615, -4.541064518000419881, 2.621784821874995952 ) ) ;
#10882=CARTESIAN_POINT ( 'NONE',  ( 19.73437500061451644, 6.421520780324663323E-16, -5.243569643749999010 ) ) ;
#10884=CARTESIAN_POINT ( 'NONE',  ( 12.41249999999999609, 2.886751345948193936, 4.999999999999883649 ) ) ;
#10885=CARTESIAN_POINT ( 'NONE',  ( 15.40312500061451573, 0.000000000000000000, 5.243569643749999010 ) ) ;
#10889=CARTESIAN_POINT ( 'NONE',  ( 29.48437500061451644, -4.541064518000419881, 2.621784821874995952 ) ) ;
#10891=CARTESIAN_POINT ( 'NONE',  ( 16.04062500061451857, -3.027376345333610441, -5.243569643749999898 ) ) ;
#10892=CARTESIAN_POINT ( 'NONE',  ( 10.80937500061451928, 4.541064518000418104, -2.621784821874998173 ) ) ;
#10893=ORIENTED_EDGE ( 'NONE', *, *, #38374, .F. ) ;
#10894=CARTESIAN_POINT ( 'NONE',  ( 28.82812500061451644, 4.541064518000418104, 2.621784821874999949 ) ) ;
#10895=CARTESIAN_POINT ( 'NONE',  ( 22.86562500061451431, 3.027376345333613106, -5.243569643749998122 ) ) ;
#10896=CARTESIAN_POINT ( 'NONE',  ( -1.071796769724488563, 13.00490381179669974, 34.00000000000000000 ) ) ;
#10897=CARTESIAN_POINT ( 'NONE',  ( 12.48750000000000249, -2.886751345948129988, 4.999999999999997335 ) ) ;
#10898=CARTESIAN_POINT ( 'NONE',  ( 22.65000000122903856, -2.886751345948125991, -5.000000000000000000 ) ) ;
#10899=CARTESIAN_POINT ( 'NONE',  ( 16.52812500061451573, 6.421520780324663323E-16, -5.243569643749999010 ) ) ;
#10902=CARTESIAN_POINT ( 'NONE',  ( 20.96250000000000213, 2.886751345948126879, 4.999999999999999112 ) ) ;
#10903=CARTESIAN_POINT ( 'NONE',  ( 22.05937500061451573, 4.541064518000418104, -2.621784821874998173 ) ) ;
#10904=CARTESIAN_POINT ( 'NONE',  ( 26.69062500061451715, -3.027376345333614438, 5.243569643749998122 ) ) ;
#10905=( BOUNDED_CURVE ( )  B_SPLINE_CURVE ( 2, ( #11939, #45925, #45572, #68823, #62542, #63623, #68457 ),
 .UNSPECIFIED., .F., .F. ) 
 B_SPLINE_CURVE_WITH_KNOTS ( ( 3, 2, 2, 3 ),
 ( 0.02499999999999994935, 0.02777777777777776236, 0.03055555555555557884, 0.03333333333333339532 ),
 .UNSPECIFIED. ) 
 CURVE ( )  GEOMETRIC_REPRESENTATION_ITEM ( )  RATIONAL_B_SPLINE_CURVE ( ( 1.000000000000002442, 0.8660254037844360431, 1.000000000000000000, 0.8660254037844387076, 1.000000000000000000, 0.8660254037844357100, 1.000000000000003109 ) ) 
 REPRESENTATION_ITEM ( '' )  );
#10906=ORIENTED_EDGE ( 'NONE', *, *, #24383, .F. ) ;
#10907=CARTESIAN_POINT ( 'NONE',  ( 19.87500000000000000, 6.123233995736764310E-16, -4.999999999999998224 ) ) ;
#10908=CARTESIAN_POINT ( 'NONE',  ( 9.140625000614518214, -3.027376345333614438, 5.243569643749998122 ) ) ;
#10909=DIRECTION ( 'NONE',  ( 0.000000000000000000, 0.000000000000000000, 1.000000000000000000 ) ) ;
#10910=CARTESIAN_POINT ( 'NONE',  ( 17.47499999999999787, -4.330127018922194537, 2.499999999999995559 ) ) ;
#10911=CARTESIAN_POINT ( 'NONE',  ( 24.22500000000000142, -4.330127018922194537, 2.499999999999995559 ) ) ;
#10912=CARTESIAN_POINT ( 'NONE',  ( 7.912499999999999645, 2.886751345948126879, 4.999999999999998224 ) ) ;
#10913=CARTESIAN_POINT ( 'NONE',  ( 5.446875000614518569, 6.054752690667223547, 3.707466751127219781E-16 ) ) ;
#10914=CARTESIAN_POINT ( 'NONE',  ( 29.40937500061451715, 0.000000000000000000, 5.243569643749999010 ) ) ;
#10916=CARTESIAN_POINT ( 'NONE',  ( 24.02812500061451573, -4.541064518000419881, 2.621784821874995952 ) ) ;
#10917=CARTESIAN_POINT ( 'NONE',  ( 24.57187500061451502, -6.054752690667223547, -1.112240025338166033E-15 ) ) ;
#10918=DIRECTION ( 'NONE',  ( 0.000000000000000000, 0.000000000000000000, -1.000000000000000000 ) ) ;
#10919=CARTESIAN_POINT ( 'NONE',  ( 14.06250000000000000, 2.886751345948129099, -4.999999999999998224 ) ) ;
#10920=CARTESIAN_POINT ( 'NONE',  ( 7.715625000614515727, 3.027376345333611329, 5.243569643749999010 ) ) ;
#10921=CYLINDRICAL_SURFACE ( 'NONE', #24494, 4.999999999999998224 ) ;
#10923=CARTESIAN_POINT ( 'NONE',  ( 25.30312500061451431, 0.000000000000000000, 5.243569643749999010 ) ) ;
#10926=CARTESIAN_POINT ( 'NONE',  ( 3.853125000614517681, -4.541064518000417216, -2.621784821875001281 ) ) ;
#10927=CARTESIAN_POINT ( 'NONE',  ( 19.95937500061451786, 0.000000000000000000, 5.243569643749999010 ) ) ;
#10928=CARTESIAN_POINT ( 'NONE',  ( -2.121784821874996840, 13.63437500061451857, 33.67503911421598417 ) ) ;
#10929=CARTESIAN_POINT ( 'NONE',  ( 22.39687500061451075, -3.027376345333610441, -5.243569643749999898 ) ) ;
#10930=CARTESIAN_POINT ( 'NONE',  ( 3.037500000000002309, -2.886751345948129988, 4.999999999999997335 ) ) ;
#10931=CARTESIAN_POINT ( 'NONE',  ( 2.121784821874999061, 19.25937500061451857, 26.32496088578401583 ) ) ;
#10932=CARTESIAN_POINT ( 'NONE',  ( 9.853125000614516793, 4.541064518000418104, -2.621784821874998173 ) ) ;
#10936=CARTESIAN_POINT ( 'NONE',  ( 6.684375000614518392, 6.421520780324663323E-16, -5.243569643749999010 ) ) ;
#10938=( BOUNDED_CURVE ( )  B_SPLINE_CURVE ( 2, ( #53830, #60444, #71553, #10222, #66004, #54195, #3223 ),
 .UNSPECIFIED., .F., .F. ) 
 B_SPLINE_CURVE_WITH_KNOTS ( ( 3, 2, 2, 3 ),
 ( 0.5833333333333334814, 0.5861111111111112493, 0.5888888888888890172, 0.5916666666666667851 ),
 .UNSPECIFIED. ) 
 CURVE ( )  GEOMETRIC_REPRESENTATION_ITEM ( )  RATIONAL_B_SPLINE_CURVE ( ( 0.9999999999999946709, 0.8660254037844440367, 1.000000000000000000, 0.8660254037844387076, 1.000000000000000000, 0.8660254037844333785, 1.000000000000005329 ) ) 
 REPRESENTATION_ITEM ( '' )  );
#10939=CARTESIAN_POINT ( 'NONE',  ( 8.353125000614518569, -4.541064518000417216, -2.621784821875001281 ) ) ;
#10940=CARTESIAN_POINT ( 'NONE',  ( 11.85937500061451644, 0.000000000000000000, 5.243569643749999010 ) ) ;
#10942=CARTESIAN_POINT ( 'NONE',  ( 18.97500000122903074, -5.773502691896255534, -1.060575238724906372E-15 ) ) ;
#10943=CARTESIAN_POINT ( 'NONE',  ( 8.934375000614517504, 6.421520780324663323E-16, -5.243569643749999010 ) ) ;
#10944=CARTESIAN_POINT ( 'NONE',  ( 10.90312500061451928, 0.000000000000000000, 5.243569643749999010 ) ) ;
#10945=CARTESIAN_POINT ( 'NONE',  ( 5.615625000614517859, -6.054752690667223547, -1.112240025338166033E-15 ) ) ;
#10947=CARTESIAN_POINT ( 'NONE',  ( 18.38437500061451857, 6.421520780324663323E-16, -5.243569643749999010 ) ) ;
#10949=CARTESIAN_POINT ( 'NONE',  ( 26.69062500061451715, -3.027376345333614438, 5.243569643749998122 ) ) ;
#10950=CARTESIAN_POINT ( 'NONE',  ( 12.55312500061451786, 4.541064518000418104, -2.621784821874998173 ) ) ;
#10951=CARTESIAN_POINT ( 'NONE',  ( 28.28437500061451715, 6.421520780324663323E-16, -5.243569643749999010 ) ) ;
#10952=CARTESIAN_POINT ( 'NONE',  ( -4.243569643749999898, 12.62187500061451750, -32.45002607614398471 ) ) ;
#10953=CARTESIAN_POINT ( 'NONE',  ( 13.31250000122903288, 4.330127018922192761, -2.499999999999997780 ) ) ;
#10954=CARTESIAN_POINT ( 'NONE',  ( 27.89062500061451289, 6.054752690667223547, 3.707466751127219781E-16 ) ) ;
#10955=CARTESIAN_POINT ( 'NONE',  ( 2.121784821875001281, 15.45312500061451644, -26.32496088578401938 ) ) ;
#10956=CARTESIAN_POINT ( 'NONE',  ( 14.77500000122903501, 2.886751345948126879, 4.999999999999999112 ) ) ;
#10957=CARTESIAN_POINT ( 'NONE',  ( 13.12500000000000178, 6.123233995736764310E-16, -4.999999999999998224 ) ) ;
#10959=CARTESIAN_POINT ( 'NONE',  ( 23.76562500061451644, 3.027376345333613106, -5.243569643749998122 ) ) ;
#10960=CARTESIAN_POINT ( 'NONE',  ( 6.909375000614518036, 0.000000000000000000, 5.243569643749999010 ) ) ;
#10961=CARTESIAN_POINT ( 'NONE',  ( 11.06250000122903288, 4.330127018922192761, -2.499999999999997780 ) ) ;
#10962=CARTESIAN_POINT ( 'NONE',  ( 19.12500000122903288, 2.886751345948129099, -4.999999999999998224 ) ) ;
#10963=CARTESIAN_POINT ( 'NONE',  ( 14.42812500061451786, 4.541064518000418104, 2.621784821874999949 ) ) ;
#10964=CARTESIAN_POINT ( 'NONE',  ( 18.85312500061451502, 4.541064518000418104, -2.621784821874998173 ) ) ;
#10965=CARTESIAN_POINT ( 'NONE',  ( 25.61250000122903359, 0.000000000000000000, 4.999999999999998224 ) ) ;
#10966=CARTESIAN_POINT ( 'NONE',  ( 28.35000000122903430, -2.886751345948129988, 4.999999999999997335 ) ) ;
#10967=CARTESIAN_POINT ( 'NONE',  ( 23.28750000000000142, -2.886751345948129988, 4.999999999999997335 ) ) ;
#10968=CARTESIAN_POINT ( 'NONE',  ( 26.25937500061451857, 0.000000000000000000, 5.243569643749999010 ) ) ;
#10970=CARTESIAN_POINT ( 'NONE',  ( 13.23750000122903359, 6.123233995736764310E-16, -4.999999999999998224 ) ) ;
#10971=EDGE_CURVE ( 'NONE', #55851, #46843, #48673, .T. ) ;
#10972=CARTESIAN_POINT ( 'NONE',  ( 27.23437500061451644, -4.541064518000419881, 2.621784821874995952 ) ) ;
#10974=CARTESIAN_POINT ( 'NONE',  ( 4.584375000614516971, 4.541064518000418104, 2.621784821874999949 ) ) ;
#10975=CARTESIAN_POINT ( 'NONE',  ( 3.909375000614518481, -4.541064518000417216, -2.621784821875001281 ) ) ;
#10976=CARTESIAN_POINT ( 'NONE',  ( 23.09062500061451573, -3.027376345333614438, 5.243569643749998122 ) ) ;
#10979=CARTESIAN_POINT ( 'NONE',  ( 10.43437500061451750, 4.541064518000418104, 2.621784821874999949 ) ) ;
#10980=CARTESIAN_POINT ( 'NONE',  ( 4.000000000000000000, 12.53749999999999964, 32.30940107675849760 ) ) ;
#10981=CARTESIAN_POINT ( 'NONE',  ( 29.27812500061451573, 4.541064518000418104, 2.621784821874999949 ) ) ;
#10982=CARTESIAN_POINT ( 'NONE',  ( 7.209375000614519635, 4.541064518000418104, -2.621784821874998173 ) ) ;
#10983=CARTESIAN_POINT ( 'NONE',  ( 28.28437500061451715, 6.421520780324663323E-16, -5.243569643749999010 ) ) ;
#10984=DIRECTION ( 'NONE',  ( 1.000000000000000000, 0.000000000000000000, 0.000000000000000000 ) ) ;
#10985=CARTESIAN_POINT ( 'NONE',  ( 19.76250000000000639, -5.773502691896255534, -1.060575238724906372E-15 ) ) ;
#10987=CARTESIAN_POINT ( 'NONE',  ( 26.39999999999999858, 0.000000000000000000, 4.999999999999998224 ) ) ;
#10988=EDGE_CURVE ( 'NONE', #72145, #52358, #39406, .T. ) ;
#10989=CARTESIAN_POINT ( 'NONE',  ( 28.28437500061451715, 6.421520780324663323E-16, -5.243569643749999010 ) ) ;
#10990=VERTEX_POINT ( 'NONE', #61924 ) ;
#10991=CARTESIAN_POINT ( 'NONE',  ( 18.29062500061451502, -3.027376345333610441, -5.243569643749999898 ) ) ;
#10992=CARTESIAN_POINT ( 'NONE',  ( 9.140625000614518214, -3.027376345333614438, 5.243569643749998122 ) ) ;
#10994=CARTESIAN_POINT ( 'NONE',  ( 3.834375000614519635, -4.541064518000419881, 2.621784821874995952 ) ) ;
#10995=CARTESIAN_POINT ( 'NONE',  ( 18.37500000122903288, 2.886751345948126879, 4.999999999999999112 ) ) ;
#10996=CARTESIAN_POINT ( 'NONE',  ( 25.16249999999999432, -5.773502691896255534, -1.060575238724906372E-15 ) ) ;
#10997=CARTESIAN_POINT ( 'NONE',  ( -0.6945881563830144101, 20.00000000000000000, -33.93923181508938569 ) ) ;
#10998=CARTESIAN_POINT ( 'NONE',  ( 6.646875000614518747, -3.027376345333610441, -5.243569643749999898 ) ) ;
#10999=CARTESIAN_POINT ( 'NONE',  ( 11.48437500061451644, -4.541064518000419881, 2.621784821874995952 ) ) ;
#11000=CARTESIAN_POINT ( 'NONE',  ( 22.50937500061451857, 4.541064518000418104, -2.621784821874998173 ) ) ;
#11001=FACE_OUTER_BOUND ( 'NONE', #52718, .T. ) ;
#11002=ORIENTED_EDGE ( 'NONE', *, *, #54124, .F. ) ;
#11003=CARTESIAN_POINT ( 'NONE',  ( 4.809375000614516615, -4.541064518000417216, -2.621784821875001281 ) ) ;
#11005=CARTESIAN_POINT ( 'NONE',  ( 6.646875000614518747, -3.027376345333610441, -5.243569643749999898 ) ) ;
#11007=CARTESIAN_POINT ( 'NONE',  ( 21.71249999999999858, 2.886751345948129099, -4.999999999999998224 ) ) ;
#11008=CARTESIAN_POINT ( 'NONE',  ( 15.62812500061451537, 6.421520780324663323E-16, -5.243569643749999010 ) ) ;
#11010=CARTESIAN_POINT ( 'NONE',  ( 4.218973316782503424, 2.683427332786226582, 4.406139393528273551 ) ) ;
#11012=CARTESIAN_POINT ( 'NONE',  ( 9.215625000614515727, -6.054752690667223547, -1.112240025338166033E-15 ) ) ;
#11013=CARTESIAN_POINT ( 'NONE',  ( 26.07187500061451857, 3.027376345333613106, -5.243569643749998122 ) ) ;
#11014=CARTESIAN_POINT ( 'NONE',  ( 19.76250000122903216, 0.000000000000000000, 4.999999999999998224 ) ) ;
#11015=CARTESIAN_POINT ( 'NONE',  ( 29.03437500061451715, -4.541064518000419881, 2.621784821874995952 ) ) ;
#11016=CARTESIAN_POINT ( 'NONE',  ( 9.299999999999998934, 0.000000000000000000, 4.999999999999998224 ) ) ;
#11017=CARTESIAN_POINT ( 'NONE',  ( -3.999999999999997335, 14.75000000122903288, 32.30940107675850470 ) ) ;
#11018=CARTESIAN_POINT ( 'NONE',  ( 9.225000001229034297, 2.886751345948129099, -4.999999999999998224 ) ) ;
#11019=CARTESIAN_POINT ( 'NONE',  ( 19.13437500061451857, -4.541064518000419881, 2.621784821874995952 ) ) ;
#11020=CARTESIAN_POINT ( 'NONE',  ( 14.14687500061451786, -3.027376345333614438, 5.243569643749998122 ) ) ;
#11021=CARTESIAN_POINT ( 'NONE',  ( 9.412500001229034297, 0.000000000000000000, 4.999999999999998224 ) ) ;
#11022=EDGE_LOOP ( 'NONE', ( #58759, #8169, #40927, #61295 ) ) ;
#11023=CARTESIAN_POINT ( 'NONE',  ( 14.69062500061451537, -3.027376345333610441, -5.243569643749999898 ) ) ;
#11024=CARTESIAN_POINT ( 'NONE',  ( 25.38750000122903216, 6.123233995736764310E-16, -4.999999999999998224 ) ) ;
#11025=CARTESIAN_POINT ( 'NONE',  ( 14.40937500061451715, 4.541064518000418104, -2.621784821874998173 ) ) ;
#11026=CARTESIAN_POINT ( 'NONE',  ( 5.999957575222543582, 8.000031818581998522, -29.79726394907932274 ) ) ;
#11027=CARTESIAN_POINT ( 'NONE',  ( 17.69062500061451715, -3.027376345333614438, 5.243569643749998122 ) ) ;
#11028=CARTESIAN_POINT ( 'NONE',  ( 26.82187500061451857, -6.054752690667223547, -1.112240025338166033E-15 ) ) ;
#11029=CARTESIAN_POINT ( 'NONE',  ( 4.243569643749999898, 10.99062500061451786, 32.45002607614398471 ) ) ;
#11030=CARTESIAN_POINT ( 'NONE',  ( 14.82187500061451679, 3.027376345333613106, -5.243569643749998122 ) ) ;
#11031=CARTESIAN_POINT ( 'NONE',  ( 14.73750000122903359, 4.330127018922191873, 2.499999999999999556 ) ) ;
#11032=FACE_OUTER_BOUND ( 'NONE', #32808, .T. ) ;
#11033=DIRECTION ( 'NONE',  ( 0.000000000000000000, 0.000000000000000000, -1.000000000000000000 ) ) ;
#11034=CARTESIAN_POINT ( 'NONE',  ( 21.57187500061451502, 3.027376345333613106, -5.243569643749998122 ) ) ;
#11035=CARTESIAN_POINT ( 'NONE',  ( 20.47500000122903074, 2.886751345948129099, -4.999999999999998224 ) ) ;
#11036=CARTESIAN_POINT ( 'NONE',  ( 17.67187500061451644, 3.027376345333611329, 5.243569643749999010 ) ) ;
#11037=CARTESIAN_POINT ( 'NONE',  ( -3.000416591977282496E-16, 12.99687500061451750, 25.09994784771203058 ) ) ;
#11038=CARTESIAN_POINT ( 'NONE',  ( 16.52812500061451573, 6.421520780324663323E-16, -5.243569643749999010 ) ) ;
#11040=ORIENTED_EDGE ( 'NONE', *, *, #47637, .F. ) ;
#11041=CARTESIAN_POINT ( 'NONE',  ( 20.81250000000000000, 2.886751345948129099, -4.999999999999998224 ) ) ;
#11043=CARTESIAN_POINT ( 'NONE',  ( 23.31562500061451715, 3.027376345333613106, -5.243569643749998122 ) ) ;
#11044=CARTESIAN_POINT ( 'NONE',  ( 3.028125000614518392, 6.421520780324663323E-16, -5.243569643749999010 ) ) ;
#11045=CARTESIAN_POINT ( 'NONE',  ( 16.91250000122903430, 4.330127018922192761, -2.499999999999997780 ) ) ;
#11046=CARTESIAN_POINT ( 'NONE',  ( 21.70312500061451644, 0.000000000000000000, 5.243569643749999010 ) ) ;
#11047=CARTESIAN_POINT ( 'NONE',  ( 25.52812500061451573, 6.421520780324663323E-16, -5.243569643749999010 ) ) ;
#11048=CARTESIAN_POINT ( 'NONE',  ( 6.178125000614518747, 6.421520780324663323E-16, -5.243569643749999010 ) ) ;
#11049=ORIENTED_EDGE ( 'NONE', *, *, #7387, .F. ) ;
#11050=CARTESIAN_POINT ( 'NONE',  ( -1.487416814333745711E-14, 16.96250000000000213, 34.00000000000000000 ) ) ;
#11053=CARTESIAN_POINT ( 'NONE',  ( 12.56250000122903465, 0.000000000000000000, 4.999999999999998224 ) ) ;
#11054=CARTESIAN_POINT ( 'NONE',  ( -3.999999999999997335, 12.05000000122903536, -27.69059892324149175 ) ) ;
#11055=CARTESIAN_POINT ( 'NONE',  ( 2.121784821874999061, 18.35937500061451644, -33.67503911421598417 ) ) ;
#11056=CARTESIAN_POINT ( 'NONE',  ( 8.887499999999999289, -2.886751345948129988, 4.999999999999997335 ) ) ;
#11059=CARTESIAN_POINT ( 'NONE',  ( 4.687500001229034652, 6.123233995736764310E-16, -4.999999999999998224 ) ) ;
#11060=CARTESIAN_POINT ( 'NONE',  ( 13.20937500061451786, 0.000000000000000000, 5.243569643749999010 ) ) ;
#11061=CARTESIAN_POINT ( 'NONE',  ( 1.071796769724497445, 16.82990381179670081, -33.99999999999998579 ) ) ;
#11062=CARTESIAN_POINT ( 'NONE',  ( 4.209375000614516971, 0.000000000000000000, 5.243569643749999010 ) ) ;
#11064=CARTESIAN_POINT ( 'NONE',  ( 19.87500000000000000, 6.123233995736764310E-16, -4.999999999999998224 ) ) ;
#11065=CARTESIAN_POINT ( 'NONE',  ( 9.009375000614518569, 4.541064518000418104, -2.621784821874998173 ) ) ;
#11066=CARTESIAN_POINT ( 'NONE',  ( 4.000000000000000000, 17.15000000122903145, -27.69059892324149885 ) ) ;
#11067=CARTESIAN_POINT ( 'NONE',  ( 19.04062500061451146, -3.027376345333614438, 5.243569643749998122 ) ) ;
#11068=CARTESIAN_POINT ( 'NONE',  ( 4.635370124282374604, -3.449855572172436879, -4.024674870222735734 ) ) ;
#11069=CARTESIAN_POINT ( 'NONE',  ( 2.121784821875001281, 17.70312500061459104, 33.67503911421598417 ) ) ;
#11070=CARTESIAN_POINT ( 'NONE',  ( 22.69687500061451857, -3.027376345333614438, 5.243569643749998122 ) ) ;
#11072=CARTESIAN_POINT ( 'NONE',  ( 3.178125000614515638, 4.541064518000418104, 2.621784821874999949 ) ) ;
#11074=CARTESIAN_POINT ( 'NONE',  ( 26.24062500061451431, -3.027376345333614438, 5.243569643749998122 ) ) ;
#11075=CARTESIAN_POINT ( 'NONE',  ( 16.26562500061451289, 3.027376345333611329, 5.243569643749999010 ) ) ;
#11077=CARTESIAN_POINT ( 'NONE',  ( 12.27187500061451786, 3.027376345333611329, 5.243569643749999010 ) ) ;
#11078=CARTESIAN_POINT ( 'NONE',  ( 28.42499999999999716, 6.123233995736764310E-16, -4.999999999999998224 ) ) ;
#11079=CARTESIAN_POINT ( 'NONE',  ( 24.33750000122903145, -4.330127018922194537, 2.499999999999995559 ) ) ;
#11080=CARTESIAN_POINT ( 'NONE',  ( 3.759375000614517681, 0.000000000000000000, 5.243569643749999010 ) ) ;
#11081=CARTESIAN_POINT ( 'NONE',  ( 15.34687500061451537, 6.054752690667223547, 3.707466751127219781E-16 ) ) ;
#11082=CARTESIAN_POINT ( 'NONE',  ( 29.59687500061451715, -3.027376345333610441, -5.243569643749999898 ) ) ;
#11083=LINE ( 'NONE', #67610, #28922 ) ;
#11085=CARTESIAN_POINT ( 'NONE',  ( 24.15937500061451715, -4.541064518000417216, -2.621784821875001281 ) ) ;
#11086=CARTESIAN_POINT ( 'NONE',  ( 13.95937500061451786, 4.541064518000418104, -2.621784821874998173 ) ) ;
#11088=CARTESIAN_POINT ( 'NONE',  ( 28.16249999999999787, 2.886751345948126879, 4.999999999999999112 ) ) ;
#11089=CARTESIAN_POINT ( 'NONE',  ( 4.650000001229035895, -2.886751345948125991, -5.000000000000000000 ) ) ;
#11090=CARTESIAN_POINT ( 'NONE',  ( 5.362500000000003375, -5.773502691896255534, -1.060575238724906372E-15 ) ) ;
#11092=CARTESIAN_POINT ( 'NONE',  ( 19.07812500061451644, -4.541064518000419881, 2.621784821874995952 ) ) ;
#11093=CARTESIAN_POINT ( 'NONE',  ( 9.600000000000001421, 4.330127018922192761, -2.499999999999997780 ) ) ;
#11094=FACE_OUTER_BOUND ( 'NONE', #25580, .T. ) ;
#11095=CARTESIAN_POINT ( 'NONE',  ( 16.53750000000000142, -2.886751345948129988, 4.999999999999997335 ) ) ;
#11096=CARTESIAN_POINT ( 'NONE',  ( 9.001249775931846008E-16, 13.16562500061451857, 34.90005215228797653 ) ) ;
#11098=CARTESIAN_POINT ( 'NONE',  ( 19.61250000122903359, 4.330127018922192761, -2.499999999999997780 ) ) ;
#11099=CARTESIAN_POINT ( 'NONE',  ( 1.587219675395664886, 9.875134926496691889, 35.78969804657884168 ) ) ;
#11100=CARTESIAN_POINT ( 'NONE',  ( 27.08437500061451786, 4.541064518000418104, 2.621784821874999949 ) ) ;
#11101=ORIENTED_EDGE ( 'NONE', *, *, #42409, .F. ) ;
#11102=CARTESIAN_POINT ( 'NONE',  ( 16.45312500061451289, -4.541064518000417216, -2.621784821875001281 ) ) ;
#11103=CARTESIAN_POINT ( 'NONE',  ( 22.97812500061451857, 4.541064518000418104, 2.621784821874999949 ) ) ;
#11104=CARTESIAN_POINT ( 'NONE',  ( 23.55937500061451573, 0.000000000000000000, 5.243569643749999010 ) ) ;
#11105=CARTESIAN_POINT ( 'NONE',  ( 6.412500000000001421, 2.886751345948129099, -4.999999999999998224 ) ) ;
#11106=CARTESIAN_POINT ( 'NONE',  ( 9.665625000614515017, -6.054752690667223547, -1.112240025338166033E-15 ) ) ;
#11107=CARTESIAN_POINT ( 'NONE',  ( 25.22812500061451502, 4.541064518000418104, 2.621784821874999949 ) ) ;
#11108=CARTESIAN_POINT ( 'NONE',  ( 15.34687500061451537, 6.054752690667223547, 3.707466751127219781E-16 ) ) ;
#11109=CARTESIAN_POINT ( 'NONE',  ( 18.19687500061451502, -3.027376345333614438, 5.243569643749998122 ) ) ;
#11111=CARTESIAN_POINT ( 'NONE',  ( 4.243569643749999898, 17.29062500061451502, 32.45002607614398471 ) ) ;
#11112=CARTESIAN_POINT ( 'NONE',  ( 22.50000000122903288, -2.886751345948129988, 4.999999999999997335 ) ) ;
#11114=CARTESIAN_POINT ( 'NONE',  ( 11.42812500061451608, -4.541064518000419881, 2.621784821874995952 ) ) ;
#11115=CARTESIAN_POINT ( 'NONE',  ( 6.759375000614516793, 4.541064518000418104, -2.621784821874998173 ) ) ;
#11116=CARTESIAN_POINT ( 'NONE',  ( 5.446875000614518569, 6.054752690667223547, 3.707466751127219781E-16 ) ) ;
#11117=VERTEX_POINT ( 'NONE', #26358 ) ;
#11118=CARTESIAN_POINT ( 'NONE',  ( 28.13437500061451502, -4.541064518000419881, 2.621784821874995952 ) ) ;
#11119=CARTESIAN_POINT ( 'NONE',  ( 18.17812500061451786, -4.541064518000419881, 2.621784821874995952 ) ) ;
#11120=CARTESIAN_POINT ( 'NONE',  ( 27.18750000122903288, 6.123233995736764310E-16, -4.999999999999998224 ) ) ;
#11121=( BOUNDED_CURVE ( )  B_SPLINE_CURVE ( 2, ( #18577, #41143, #45233, #30410, #59193, #7506, #53673 ),
 .UNSPECIFIED., .F., .F. ) 
 B_SPLINE_CURVE_WITH_KNOTS ( ( 3, 2, 2, 3 ),
 ( 0.7416666666666666963, 0.7444444444444444642, 0.7472222222222222321, 0.7500000000000000000 ),
 .UNSPECIFIED. ) 
 CURVE ( )  GEOMETRIC_REPRESENTATION_ITEM ( )  RATIONAL_B_SPLINE_CURVE ( ( 1.000000000000000000, 0.8660254037844387076, 1.000000000000000000, 0.8660254037844387076, 1.000000000000000000, 0.8660254037844387076, 1.000000000000000000 ) ) 
 REPRESENTATION_ITEM ( '' )  );
#11122=EDGE_CURVE ( 'NONE', #32974, #64445, #71310, .T. ) ;
#11123=CARTESIAN_POINT ( 'NONE',  ( 28.75312500061451715, 4.541064518000418104, -2.621784821874998173 ) ) ;
#11124=CARTESIAN_POINT ( 'NONE',  ( 25.20937500061451431, 4.541064518000418104, -2.621784821874998173 ) ) ;
#11125=CARTESIAN_POINT ( 'NONE',  ( 20.46562500061451928, -6.054752690667223547, -1.112240025338166033E-15 ) ) ;
#11126=CARTESIAN_POINT ( 'NONE',  ( 4.243569643749999010, 18.77187500061451786, 27.54997392385601174 ) ) ;
#11127=CARTESIAN_POINT ( 'NONE',  ( 24.70312500061451644, 4.541064518000418104, -2.621784821874998173 ) ) ;
#11128=CARTESIAN_POINT ( 'NONE',  ( 4.312500001229034652, 4.330127018922192761, -2.499999999999997780 ) ) ;
#11130=CARTESIAN_POINT ( 'NONE',  ( 28.91250000000000497, 2.886751345948129099, -4.999999999999998224 ) ) ;
#11131=CARTESIAN_POINT ( 'NONE',  ( -3.999999999999997335, 14.63750000000000107, -27.69059892324149175 ) ) ;
#11133=CARTESIAN_POINT ( 'NONE',  ( 5.184375000614516615, -4.541064518000419881, 2.621784821874995952 ) ) ;
#11134=CARTESIAN_POINT ( 'NONE',  ( 12.77812500061451750, -4.541064518000419881, 2.621784821874995952 ) ) ;
#11135=CARTESIAN_POINT ( 'NONE',  ( 6.946875000614517681, -3.027376345333614438, 5.243569643749998122 ) ) ;
#11136=CARTESIAN_POINT ( 'NONE',  ( 25.23750000122903359, -4.330127018922194537, 2.499999999999995559 ) ) ;
#11137=CARTESIAN_POINT ( 'NONE',  ( 14.14687500061451786, -3.027376345333614438, 5.243569643749998122 ) ) ;
#11138=CARTESIAN_POINT ( 'NONE',  ( 3.196875000614516793, 6.054752690667223547, 3.707466751127219781E-16 ) ) ;
#11139=CARTESIAN_POINT ( 'NONE',  ( 28.64999999999999858, 0.000000000000000000, 4.999999999999998224 ) ) ;
#11140=CARTESIAN_POINT ( 'NONE',  ( 25.73437500061451644, 4.541064518000418104, 2.621784821874999949 ) ) ;
#11142=CARTESIAN_POINT ( 'NONE',  ( 13.82812500061451466, 6.421520780324663323E-16, -5.243569643749999010 ) ) ;
#11143=VERTEX_POINT ( 'NONE', #38911 ) ;
#11144=CARTESIAN_POINT ( 'NONE',  ( 10.22812500061451679, 6.421520780324663323E-16, -5.243569643749999010 ) ) ;
#11145=VECTOR ( 'NONE', #44483, 1000.000000000000000 ) ;
#11146=CARTESIAN_POINT ( 'NONE',  ( 5.765625000614519102, 3.027376345333613106, -5.243569643749998122 ) ) ;
#11149=LINE ( 'NONE', #40310, #5503 ) ;
#11150=VECTOR ( 'NONE', #66869, 1000.000000000000000 ) ;
#11151=CARTESIAN_POINT ( 'NONE',  ( 16.64999999999999858, -4.330127018922190985, -2.500000000000001332 ) ) ;
#11152=CARTESIAN_POINT ( 'NONE',  ( 14.93437500061451750, 4.541064518000418104, 2.621784821874999949 ) ) ;
#11153=CARTESIAN_POINT ( 'NONE',  ( 13.65000000122903323, -2.886751345948125991, -5.000000000000000000 ) ) ;
#11155=CARTESIAN_POINT ( 'NONE',  ( 21.38437500061451502, -4.541064518000419881, 2.621784821874995952 ) ) ;
#11156=CARTESIAN_POINT ( 'NONE',  ( -4.243569643749999898, 13.05312500061451786, -30.00000000000000000 ) ) ;
#11160=CYLINDRICAL_SURFACE ( 'NONE', #65496, 4.999999999999998224 ) ;
#11161=CARTESIAN_POINT ( 'NONE',  ( 26.24062500061451431, -3.027376345333614438, 5.243569643749998122 ) ) ;
#11162=CARTESIAN_POINT ( 'NONE',  ( 17.06250000122903288, 0.000000000000000000, 4.999999999999998224 ) ) ;
#11163=CYLINDRICAL_SURFACE ( 'NONE', #66839, 4.999999999999998224 ) ;
#11164=EDGE_CURVE ( 'NONE', #64445, #35963, #40243, .T. ) ;
#11165=CARTESIAN_POINT ( 'NONE',  ( 25.50000000000000000, 0.000000000000000000, 4.999999999999998224 ) ) ;
#11166=CARTESIAN_POINT ( 'NONE',  ( 8.728125000614518569, -4.541064518000419881, 2.621784821874995952 ) ) ;
#11168=CARTESIAN_POINT ( 'NONE',  ( 18.19687500061451502, -3.027376345333614438, 5.243569643749998122 ) ) ;
#11170=CARTESIAN_POINT ( 'NONE',  ( 5.540625000614515905, -3.027376345333614438, 5.243569643749998122 ) ) ;
#11171=CARTESIAN_POINT ( 'NONE',  ( 10.32187500061451679, 3.027376345333613106, -5.243569643749998122 ) ) ;
#11173=CARTESIAN_POINT ( 'NONE',  ( 22.20937500061451431, 0.000000000000000000, 5.243569643749999010 ) ) ;
#11174=DIRECTION ( 'NONE',  ( 0.000000000000000000, 0.000000000000000000, -1.000000000000000000 ) ) ;
#11175=CARTESIAN_POINT ( 'NONE',  ( 29.06250000000000000, 2.886751345948126879, 4.999999999999999112 ) ) ;
#11176=CARTESIAN_POINT ( 'NONE',  ( 5.850000000000001421, -4.330127018922190985, -2.500000000000001332 ) ) ;
#11177=CARTESIAN_POINT ( 'NONE',  ( 15.48750000122903359, 6.123233995736764310E-16, -4.999999999999998224 ) ) ;
#11179=CARTESIAN_POINT ( 'NONE',  ( 19.01249999999999929, 2.886751345948095793, -5.000000000000055067 ) ) ;
#11180=ORIENTED_EDGE ( 'NONE', *, *, #29228, .T. ) ;
#11181=CARTESIAN_POINT ( 'NONE',  ( 12.22499999999999964, 6.123233995736764310E-16, -4.999999999999998224 ) ) ;
#11182=CARTESIAN_POINT ( 'NONE',  ( 25.90312500061451573, -4.541064518000417216, -2.621784821875001281 ) ) ;
#11183=CARTESIAN_POINT ( 'NONE',  ( 17.28750000000000142, 5.773502691896255534, 3.535250795749688894E-16 ) ) ;
#11184=CARTESIAN_POINT ( 'NONE',  ( 11.66250000122903430, 0.000000000000000000, 4.999999999999998224 ) ) ;
#11185=CARTESIAN_POINT ( 'NONE',  ( 9.703125000614514661, -4.541064518000417216, -2.621784821875001281 ) ) ;
#11186=CARTESIAN_POINT ( 'NONE',  ( 7.875000000000000000, 4.330127018922191873, 2.499999999999999556 ) ) ;
#11188=CARTESIAN_POINT ( 'NONE',  ( 9.001249775931846008E-16, 15.47187500061451892, -25.09994784771203058 ) ) ;
#11189=CARTESIAN_POINT ( 'NONE',  ( 27.11250000122903359, -4.330127018922190985, -2.500000000000001332 ) ) ;
#11191=CARTESIAN_POINT ( 'NONE',  ( 7.200000000000001954, -4.330127018922190985, -2.500000000000001332 ) ) ;
#11192=FACE_OUTER_BOUND ( 'NONE', #2125, .T. ) ;
#11193=VECTOR ( 'NONE', #13770, 1000.000000000000000 ) ;
#11194=ORIENTED_EDGE ( 'NONE', *, *, #66354, .T. ) ;
#11195=CARTESIAN_POINT ( 'NONE',  ( 25.26562500061451289, 3.027376345333611329, 5.243569643749999010 ) ) ;
#11196=CARTESIAN_POINT ( 'NONE',  ( 29.27812500061451573, 4.541064518000418104, 2.621784821874999949 ) ) ;
#11197=CARTESIAN_POINT ( 'NONE',  ( 28.88437500061451502, 4.541064518000418104, 2.621784821874999949 ) ) ;
#11198=CARTESIAN_POINT ( 'NONE',  ( 19.17187500061451999, -6.054752690667223547, -1.112240025338166033E-15 ) ) ;
#11199=CARTESIAN_POINT ( 'NONE',  ( 16.71562500061451573, 3.027376345333611329, 5.243569643749999010 ) ) ;
#11200=CARTESIAN_POINT ( 'NONE',  ( 4.243569643749999898, 11.89062500061459282, -27.54997392385601529 ) ) ;
#11201=CARTESIAN_POINT ( 'NONE',  ( 6.065625000614516260, -6.054752690667223547, -1.112240025338166033E-15 ) ) ;
#11202=CARTESIAN_POINT ( 'NONE',  ( 27.78750000122903074, 4.330127018922191873, 2.499999999999999556 ) ) ;
#11204=CARTESIAN_POINT ( 'NONE',  ( 18.89062500061451644, 6.054752690667223547, 3.707466751127219781E-16 ) ) ;
#11205=CARTESIAN_POINT ( 'NONE',  ( -1.487416814333745711E-14, 16.06250000000000000, -26.00000000000000000 ) ) ;
#11207=CARTESIAN_POINT ( 'NONE',  ( 12.87187500061451750, -6.054752690667223547, -1.112240025338166033E-15 ) ) ;
#11208=CARTESIAN_POINT ( 'NONE',  ( 11.67187500061451821, 3.027376345333613106, -5.243569643749998122 ) ) ;
#11209=CARTESIAN_POINT ( 'NONE',  ( 21.49687500061451573, -3.027376345333610441, -5.243569643749999898 ) ) ;
#11211=CARTESIAN_POINT ( 'NONE',  ( -1.071796769724496556, 14.80490381179669690, -26.00000000000000355 ) ) ;
#11212=CARTESIAN_POINT ( 'NONE',  ( 25.64062500061451644, 6.054752690667223547, 3.707466751127219781E-16 ) ) ;
#11213=VECTOR ( 'NONE', #5183, 1000.000000000000000 ) ;
#11214=CARTESIAN_POINT ( 'NONE',  ( 27.25312500061451360, -4.541064518000417216, -2.621784821875001281 ) ) ;
#11215=CARTESIAN_POINT ( 'NONE',  ( 1.999999999999998668, 12.20000000000000107, -33.46410161513775705 ) ) ;
#11216=CARTESIAN_POINT ( 'NONE',  ( 4.000000000000000000, 17.48750000000000071, 32.30940107675849049 ) ) ;
#11217=CARTESIAN_POINT ( 'NONE',  ( 4.059375000614519280, 4.541064518000418104, -2.621784821874998173 ) ) ;
#11219=CARTESIAN_POINT ( 'NONE',  ( 12.67500000122903536, -5.773502691896255534, -1.060575238724906372E-15 ) ) ;
#11221=CARTESIAN_POINT ( 'NONE',  ( 7.500000001229034652, 5.773502691896255534, 3.535250795749688894E-16 ) ) ;
#11222=CARTESIAN_POINT ( 'NONE',  ( 29.25000000122903288, -2.886751345948129988, 4.999999999999997335 ) ) ;
#11225=CARTESIAN_POINT ( 'NONE',  ( 12.49687500061451573, -3.027376345333610441, -5.243569643749999898 ) ) ;
#11226=CARTESIAN_POINT ( 'NONE',  ( -3.137519842735245283E-14, 14.71250000000000213, -26.00000000000000711 ) ) ;
#11227=EDGE_LOOP ( 'NONE', ( #24614, #39277, #9167, #58690 ) ) ;
#11228=CARTESIAN_POINT ( 'NONE',  ( 20.80312500061451431, 0.000000000000000000, 5.243569643749999010 ) ) ;
#11229=CARTESIAN_POINT ( 'NONE',  ( 12.79687500061451821, -3.027376345333614438, 5.243569643749998122 ) ) ;
#11230=CARTESIAN_POINT ( 'NONE',  ( 4.903125000614516615, 4.541064518000418104, -2.621784821874998173 ) ) ;
#11231=CARTESIAN_POINT ( 'NONE',  ( 22.20937500061451431, 0.000000000000000000, 5.243569643749999010 ) ) ;
#11232=CARTESIAN_POINT ( 'NONE',  ( 9.084375000614517859, 4.541064518000418104, 2.621784821874999949 ) ) ;
#11233=CARTESIAN_POINT ( 'NONE',  ( 5.578125000614518214, -4.541064518000419881, 2.621784821874995952 ) ) ;
#11234=CARTESIAN_POINT ( 'NONE',  ( 11.66250000122903430, 0.000000000000000000, 4.999999999999998224 ) ) ;
#11235=CARTESIAN_POINT ( 'NONE',  ( 4.912500001229034297, 0.000000000000000000, 4.999999999999998224 ) ) ;
#11236=EDGE_CURVE ( 'NONE', #63910, #24148, #30330, .T. ) ;
#11237=CARTESIAN_POINT ( 'NONE',  ( 20.65312500061451573, 4.541064518000418104, -2.621784821874998173 ) ) ;
#11238=CARTESIAN_POINT ( 'NONE',  ( 8.587500001229035007, -4.330127018922194537, 2.499999999999995559 ) ) ;
#11239=CARTESIAN_POINT ( 'NONE',  ( 16.52812500061451573, 6.421520780324663323E-16, -5.243569643749999010 ) ) ;
#11240=CARTESIAN_POINT ( 'NONE',  ( 14.69062500061451537, -3.027376345333610441, -5.243569643749999898 ) ) ;
#11242=CARTESIAN_POINT ( 'NONE',  ( 16.91250000000000142, 2.886751345948126879, 4.999999999999999112 ) ) ;
#11243=CARTESIAN_POINT ( 'NONE',  ( 9.000000001229034652, -2.886751345948129988, 4.999999999999997335 ) ) ;
#11244=CARTESIAN_POINT ( 'NONE',  ( 5.503125000614516260, 0.000000000000000000, 5.243569643749999010 ) ) ;
#11245=CARTESIAN_POINT ( 'NONE',  ( 21.11250000122903359, 0.000000000000000000, 4.999999999999998224 ) ) ;
#11247=VECTOR ( 'NONE', #64610, 1000.000000000000000 ) ;
#11248=CARTESIAN_POINT ( 'NONE',  ( 4.243569643749999898, 10.59687500061451715, -27.54997392385601529 ) ) ;
#11249=CARTESIAN_POINT ( 'NONE',  ( 0.000000000000000000, 20.00000000000000000, 26.00000000000000000 ) ) ;
#11250=FACE_OUTER_BOUND ( 'NONE', #62816, .T. ) ;
#11252=CARTESIAN_POINT ( 'NONE',  ( 3.000000001229033320, 5.773502691896255534, 3.535250795749688401E-16 ) ) ;
#11253=CARTESIAN_POINT ( 'NONE',  ( 21.94687500061451857, -3.027376345333610441, -5.243569643749999898 ) ) ;
#11254=CARTESIAN_POINT ( 'NONE',  ( 5.175000000000002487, 4.330127018922191873, 2.499999999999999556 ) ) ;
#11255=AXIS2_PLACEMENT_3D ( 'NONE', #6269, #740, #29527 ) ;
#11256=CARTESIAN_POINT ( 'NONE',  ( 17.61562500061451786, 3.027376345333611329, 5.243569643749999010 ) ) ;
#11259=CARTESIAN_POINT ( 'NONE',  ( 4.520699896614321034, -3.533387626757130029, -3.879993107621428905 ) ) ;
#11260=CARTESIAN_POINT ( 'NONE',  ( 29.14687500061451075, -3.027376345333610441, -5.243569643749999898 ) ) ;
#11262=CARTESIAN_POINT ( 'NONE',  ( 12.62812500061451537, 4.541064518000418104, 2.621784821874999949 ) ) ;
#11263=CARTESIAN_POINT ( 'NONE',  ( 10.02187500061451964, 3.027376345333611329, 5.243569643749999010 ) ) ;
#11265=CARTESIAN_POINT ( 'NONE',  ( 21.96562500061451573, 3.027376345333613106, -5.243569643749998122 ) ) ;
#11266=CARTESIAN_POINT ( 'NONE',  ( 1.999999999999998668, 11.30000000000000071, -33.46410161513775705 ) ) ;
#11267=CARTESIAN_POINT ( 'NONE',  ( 1.999999999999998668, 15.46250000122903501, -33.46410161513775705 ) ) ;
#11268=ADVANCED_FACE ( 'NONE', ( #20433 ), #21169, .F. ) ;
#11269=CARTESIAN_POINT ( 'NONE',  ( 12.30000000000000249, 4.330127018922192761, -2.499999999999997780 ) ) ;
#11270=EDGE_CURVE ( 'NONE', #30207, #30864, #49994, .T. ) ;
#11271=CARTESIAN_POINT ( 'NONE',  ( 22.12500000122903288, -5.773502691896255534, -1.060575238724906372E-15 ) ) ;
#11272=CARTESIAN_POINT ( 'NONE',  ( 16.19062500061451715, 6.054752690667223547, 3.707466751127219781E-16 ) ) ;
#11274=ORIENTED_EDGE ( 'NONE', *, *, #9235, .F. ) ;
#11275=CARTESIAN_POINT ( 'NONE',  ( 19.01249999999999929, 2.886751345948129099, -4.999999999999998224 ) ) ;
#11276=( BOUNDED_CURVE ( )  B_SPLINE_CURVE ( 2, ( #71169, #24999, #47542, #64892, #26105, #64525, #14282, #13919, #36457 ),
 .UNSPECIFIED., .F., .F. ) 
 B_SPLINE_CURVE_WITH_KNOTS ( ( 3, 2, 2, 2, 3 ),
 ( 0.4456521739130435145, 0.4492753623188405765, 0.4565217391304347561, 0.4637681159420289911, 0.4673913043478261087 ),
 .UNSPECIFIED. ) 
 CURVE ( )  GEOMETRIC_REPRESENTATION_ITEM ( )  RATIONAL_B_SPLINE_CURVE ( ( 0.9330127018922194093, 0.9330127018922198534, 1.000000000000000000, 0.8660254037844387076, 1.000000000000000000, 0.8660254037844387076, 1.000000000000000000, 0.9330127018922188542, 0.9330127018922194093 ) ) 
 REPRESENTATION_ITEM ( '' )  );
#11277=CARTESIAN_POINT ( 'NONE',  ( 24.37500000000000000, 6.123233995736764310E-16, -4.999999999999998224 ) ) ;
#11278=CARTESIAN_POINT ( 'NONE',  ( 22.47187500061451715, 3.027376345333613106, -5.243569643749998122 ) ) ;
#11279=CARTESIAN_POINT ( 'NONE',  ( 23.99062500061451786, -3.027376345333614438, 5.243569643749998122 ) ) ;
#11282=CARTESIAN_POINT ( 'NONE',  ( 8.578125000614518214, 4.541064518000418104, 2.621784821874999949 ) ) ;
#11284=CARTESIAN_POINT ( 'NONE',  ( 15.33750000000000036, -2.886751345948125991, -5.000000000000000000 ) ) ;
#11285=CARTESIAN_POINT ( 'NONE',  ( 3.544399568801740674, -3.526694215397601528, -3.727027268090089329 ) ) ;
#11286=CARTESIAN_POINT ( 'NONE',  ( 4.546875000614517326, 6.054752690667223547, 3.707466751127219781E-16 ) ) ;
#11287=CARTESIAN_POINT ( 'NONE',  ( 28.39687500061452141, 6.054752690667223547, 3.707466751127219781E-16 ) ) ;
#11289=CARTESIAN_POINT ( 'NONE',  ( 24.62812500061451715, 6.421520780324663323E-16, -5.243569643749999010 ) ) ;
#11290=CARTESIAN_POINT ( 'NONE',  ( 26.33437500061451431, -4.541064518000419881, 2.621784821874995952 ) ) ;
#11291=CARTESIAN_POINT ( 'NONE',  ( -4.243569643749999898, 17.96562500061459389, -32.45002607614398471 ) ) ;
#11292=CARTESIAN_POINT ( 'NONE',  ( 11.13750000000000284, -2.886751345948129988, 4.999999999999997335 ) ) ;
#11293=CARTESIAN_POINT ( 'NONE',  ( 9.365625000614519635, 3.027376345333613106, -5.243569643749998122 ) ) ;
#11294=DIRECTION ( 'NONE',  ( -1.000000000000000000, -0.000000000000000000, -0.000000000000000000 ) ) ;
#11295=CARTESIAN_POINT ( 'NONE',  ( 3.999999999999999112, 19.32500000000000284, -30.00000000000000000 ) ) ;
#11296=CARTESIAN_POINT ( 'NONE',  ( 25.94062500061451715, -3.027376345333610441, -5.243569643749999898 ) ) ;
#11299=CARTESIAN_POINT ( 'NONE',  ( 3.515625000614516882, 3.027376345333613106, -5.243569643749998122 ) ) ;
#11300=CARTESIAN_POINT ( 'NONE',  ( 20.37187500061451573, 3.027376345333611329, 5.243569643749999010 ) ) ;
#11301=CARTESIAN_POINT ( 'NONE',  ( -2.121784821874999949, 15.28437500061451892, 26.32496088578401938 ) ) ;
#11302=CARTESIAN_POINT ( 'NONE',  ( 20.89687500061452141, -3.027376345333614438, 5.243569643749998122 ) ) ;
#11303=CARTESIAN_POINT ( 'NONE',  ( 3.562500000000000444, -5.773502691896255534, -1.060575238724906372E-15 ) ) ;
#11304=CARTESIAN_POINT ( 'NONE',  ( 4.243569643749999898, 18.73437500061451644, 30.00000000000000000 ) ) ;
#11305=CARTESIAN_POINT ( 'NONE',  ( 9.740625000614516082, -3.027376345333610441, -5.243569643749999898 ) ) ;
#11307=CARTESIAN_POINT ( 'NONE',  ( 5.934375000614517504, 4.541064518000418104, 2.621784821874999949 ) ) ;
#11309=CARTESIAN_POINT ( 'NONE',  ( 6.590625000614518392, -3.027376345333610441, -5.243569643749999898 ) ) ;
#11310=CARTESIAN_POINT ( 'NONE',  ( 12.08437500061451608, 6.421520780324663323E-16, -5.243569643749999010 ) ) ;
#11311=FILL_AREA_STYLE_COLOUR ( '', #17852 ) ;
#11312=CARTESIAN_POINT ( 'NONE',  ( 18.26250000122903216, 4.330127018922192761, -2.499999999999997780 ) ) ;
#11313=CARTESIAN_POINT ( 'NONE',  ( 7.959375000614516971, -4.541064518000417216, -2.621784821875001281 ) ) ;
#11314=CARTESIAN_POINT ( 'NONE',  ( 9.065625000614517148, 3.027376345333611329, 5.243569643749999010 ) ) ;
#11315=CARTESIAN_POINT ( 'NONE',  ( 5.165625000614517681, -6.054752690667223547, -1.112240025338166033E-15 ) ) ;
#11317=CARTESIAN_POINT ( 'NONE',  ( 19.09687500061451360, -3.027376345333614438, 5.243569643749998122 ) ) ;
#11318=CARTESIAN_POINT ( 'NONE',  ( 9.187500001229034652, 6.123233995736764310E-16, -4.999999999999998224 ) ) ;
#11319=CARTESIAN_POINT ( 'NONE',  ( 27.77812500061451573, 6.421520780324663323E-16, -5.243569643749999010 ) ) ;
#11320=CARTESIAN_POINT ( 'NONE',  ( 10.94062500061451537, -3.027376345333614438, 5.243569643749998122 ) ) ;
#11322=CARTESIAN_POINT ( 'NONE',  ( 4.243569643749999898, 11.53437500061451892, -30.00000000000000000 ) ) ;
#11323=CARTESIAN_POINT ( 'NONE',  ( 12.37500000122903465, 2.886751345948129099, -4.999999999999998224 ) ) ;
#11324=CARTESIAN_POINT ( 'NONE',  ( 27.47812500061451502, 4.541064518000418104, 2.621784821874999949 ) ) ;
#11326=CARTESIAN_POINT ( 'NONE',  ( -2.121784821874996840, 15.37812500061451892, -26.32496088578401583 ) ) ;
#11327=CARTESIAN_POINT ( 'NONE',  ( 13.98750000122903359, -4.330127018922194537, 2.499999999999995559 ) ) ;
#11328=AXIS2_PLACEMENT_3D ( 'NONE', #40628, #19522, #46895 ) ;
#11329=CARTESIAN_POINT ( 'NONE',  ( 12.30000000000000249, 4.330127018922192761, -2.499999999999997780 ) ) ;
#11331=CARTESIAN_POINT ( 'NONE',  ( 23.54062500061451146, -3.027376345333614438, 5.243569643749998122 ) ) ;
#11332=CARTESIAN_POINT ( 'NONE',  ( 8.521875000614517859, 3.027376345333612662, -5.243569643749998122 ) ) ;
#11333=CARTESIAN_POINT ( 'NONE',  ( 7.987500001229032698, 4.330127018922191873, 2.499999999999999556 ) ) ;
#11334=CARTESIAN_POINT ( 'NONE',  ( 15.90000000122903501, -2.886751345948125991, -5.000000000000000000 ) ) ;
#11335=( BOUNDED_CURVE ( )  B_SPLINE_CURVE ( 2, ( #6703, #440, #58012, #56579, #24038, #29948, #52488, #1899, #46588 ),
 .UNSPECIFIED., .F., .F. ) 
 B_SPLINE_CURVE_WITH_KNOTS ( ( 3, 2, 2, 2, 3 ),
 ( 0.3152173913043478382, 0.3188405797101449002, 0.3260869565217391353, 0.3333333333333333148, 0.3369565217391304324 ),
 .UNSPECIFIED. ) 
 CURVE ( )  GEOMETRIC_REPRESENTATION_ITEM ( )  RATIONAL_B_SPLINE_CURVE ( ( 0.9330127018922194093, 0.9330127018922198534, 1.000000000000000000, 0.8660254037844387076, 1.000000000000000000, 0.8660254037844387076, 1.000000000000000000, 0.9330127018922194093, 0.9330127018922194093 ) ) 
 REPRESENTATION_ITEM ( '' )  );
#11336=CARTESIAN_POINT ( 'NONE',  ( 12.92812500061451786, 6.421520780324663323E-16, -5.243569643749999010 ) ) ;
#11337=CARTESIAN_POINT ( 'NONE',  ( 16.49062500061451786, -3.027376345333610441, -5.243569643749999898 ) ) ;
#11338=( BOUNDED_CURVE ( )  B_SPLINE_CURVE ( 2, ( #7659, #46469, #64167, #24646, #13555, #18368, #2135, #30564, #63083 ),
 .UNSPECIFIED., .F., .F. ) 
 B_SPLINE_CURVE_WITH_KNOTS ( ( 3, 2, 2, 2, 3 ),
 ( 0.03260869565217391908, 0.03623188405797101580, 0.04347826086956521618, 0.05072463768115942351, 0.05434782608695652717 ),
 .UNSPECIFIED. ) 
 CURVE ( )  GEOMETRIC_REPRESENTATION_ITEM ( )  RATIONAL_B_SPLINE_CURVE ( ( 0.9330127018922192983, 0.9330127018922194093, 1.000000000000000000, 0.8660254037844387076, 1.000000000000000000, 0.8660254037844387076, 1.000000000000000000, 0.9330127018922192983, 0.9330127018922194093 ) ) 
 REPRESENTATION_ITEM ( '' )  );
#11339=CARTESIAN_POINT ( 'NONE',  ( 28.53750000122903074, 6.123233995736764310E-16, -4.999999999999998224 ) ) ;
#11340=CARTESIAN_POINT ( 'NONE',  ( 22.27499999999999858, 4.330127018922191873, 2.499999999999999556 ) ) ;
#11341=CARTESIAN_POINT ( 'NONE',  ( 23.63437500061451502, -4.541064518000419881, 2.621784821874995952 ) ) ;
#11342=CARTESIAN_POINT ( 'NONE',  ( 10.53750000122903252, 6.123233995736764310E-16, -4.999999999999998224 ) ) ;
#11343=CARTESIAN_POINT ( 'NONE',  ( 28.92187500061451644, 3.027376345333611329, 5.243569643749999010 ) ) ;
#11345=CARTESIAN_POINT ( 'NONE',  ( 4.659375000614518925, 0.000000000000000000, 5.243569643749999010 ) ) ;
#11346=CARTESIAN_POINT ( 'NONE',  ( 22.67812500061451431, -4.541064518000419881, 2.621784821874995952 ) ) ;
#11348=CARTESIAN_POINT ( 'NONE',  ( 7.050000000000000711, 0.000000000000000000, 4.999999999999998224 ) ) ;
#11349=CARTESIAN_POINT ( 'NONE',  ( 11.29687500061451644, 6.054752690667223547, 3.707466751127219781E-16 ) ) ;
#11350=CARTESIAN_POINT ( 'NONE',  ( 3.384375000614517237, -4.541064518000419881, 2.621784821874995952 ) ) ;
#11351=CARTESIAN_POINT ( 'NONE',  ( 7.021875000614518747, -6.054752690667223547, -1.112240025338166033E-15 ) ) ;
#11352=CARTESIAN_POINT ( 'NONE',  ( 25.94999999999999929, 0.000000000000000000, 4.999999999999998224 ) ) ;
#11353=CARTESIAN_POINT ( 'NONE',  ( 28.43437500061451573, 4.541064518000418104, 2.621784821874999949 ) ) ;
#11355=CARTESIAN_POINT ( 'NONE',  ( 19.94999999999999929, 4.330127018922192761, -2.499999999999997780 ) ) ;
#11357=CARTESIAN_POINT ( 'NONE',  ( 26.02499999999999858, -4.330127018922194537, 2.499999999999995559 ) ) ;
#11358=CARTESIAN_POINT ( 'NONE',  ( 28.84687500061452070, 6.054752690667223547, 3.707466751127219781E-16 ) ) ;
#11359=VERTEX_POINT ( 'NONE', #15263 ) ;
#11360=CARTESIAN_POINT ( 'NONE',  ( 14.54062500061451679, -3.027376345333614438, 5.243569643749998122 ) ) ;
#11361=CARTESIAN_POINT ( 'NONE',  ( 8.953125000614518214, 4.541064518000418104, -2.621784821874998173 ) ) ;
#11363=CARTESIAN_POINT ( 'NONE',  ( 4.321875000614517681, -6.054752690667223547, -1.112240025338166033E-15 ) ) ;
#11364=CARTESIAN_POINT ( 'NONE',  ( 17.36250000122903359, 4.330127018922192761, -2.499999999999997780 ) ) ;
#11365=CARTESIAN_POINT ( 'NONE',  ( 21.56250000000000000, -5.773502691896255534, -1.060575238724906372E-15 ) ) ;
#11367=CARTESIAN_POINT ( 'NONE',  ( 6.946875000614517681, -3.027376345333614438, 5.243569643749998122 ) ) ;
#11368=CARTESIAN_POINT ( 'NONE',  ( 10.69687500061451679, -3.027376345333610441, -5.243569643749999898 ) ) ;
#11369=CARTESIAN_POINT ( 'NONE',  ( 22.09687500061451715, 6.054752690667223547, 3.707466751127219781E-16 ) ) ;
#11371=CARTESIAN_POINT ( 'NONE',  ( 3.984375000614517326, 6.421520780324663323E-16, -5.243569643749999010 ) ) ;
#11372=CARTESIAN_POINT ( 'NONE',  ( 6.759375000614516793, 4.541064518000418104, -2.621784821874998173 ) ) ;
#11373=CARTESIAN_POINT ( 'NONE',  ( 18.26249999999999929, 2.886751345948126879, 4.999999999999999112 ) ) ;
#11374=CARTESIAN_POINT ( 'NONE',  ( 16.52812500061451573, 6.421520780324663323E-16, -5.243569643749999010 ) ) ;
#11378=CARTESIAN_POINT ( 'NONE',  ( 9.515625000614518214, 3.027376345333611329, 5.243569643749999010 ) ) ;
#11379=CARTESIAN_POINT ( 'NONE',  ( 26.74687500061451573, -3.027376345333614438, 5.243569643749998122 ) ) ;
#11381=CARTESIAN_POINT ( 'NONE',  ( 29.25937500061451502, 4.541064518000418104, -2.621784821874998173 ) ) ;
#11382=CARTESIAN_POINT ( 'NONE',  ( 10.83750000000000036, -2.886751345948125991, -5.000000000000000000 ) ) ;
#11383=CARTESIAN_POINT ( 'NONE',  ( 1.999999999999998668, 14.56250000122903288, 26.53589838486224650 ) ) ;
#11384=CARTESIAN_POINT ( 'NONE',  ( 9.712500001229033231, 4.330127018922192761, -2.499999999999997780 ) ) ;
#11385=CARTESIAN_POINT ( 'NONE',  ( 19.50937500061451857, 0.000000000000000000, 5.243569643749999010 ) ) ;
#11386=CARTESIAN_POINT ( 'NONE',  ( 15.00937500061451679, 0.000000000000000000, 5.243569643749999010 ) ) ;
#11387=CARTESIAN_POINT ( 'NONE',  ( -3.183805653906651933, 3.859810113929996067, -32.43433874829330676 ) ) ;
#11388=VERTEX_POINT ( 'NONE', #65513 ) ;
#11389=CARTESIAN_POINT ( 'NONE',  ( 13.71562500061451750, -6.054752690667223547, -1.112240025338166033E-15 ) ) ;
#11390=CARTESIAN_POINT ( 'NONE',  ( 25.16250000122903074, 0.000000000000000000, 4.999999999999998224 ) ) ;
#11391=CARTESIAN_POINT ( 'NONE',  ( 14.97187500061451892, 3.027376345333611329, 5.243569643749999010 ) ) ;
#11392=CARTESIAN_POINT ( 'NONE',  ( 5.191822204397932516, 8.550203871005534140, -33.03186005587161134 ) ) ;
#11393=CARTESIAN_POINT ( 'NONE',  ( 18.14062500061451644, -3.027376345333614438, 5.243569643749998122 ) ) ;
#11395=CARTESIAN_POINT ( 'NONE',  ( 25.54687500061451644, -3.027376345333610441, -5.243569643749999898 ) ) ;
#11396=CARTESIAN_POINT ( 'NONE',  ( 4.243569643749999010, 11.06562500061451715, 27.54997392385601174 ) ) ;
#11397=ADVANCED_FACE ( 'NONE', ( #60688 ), #66245, .F. ) ;
#11398=CARTESIAN_POINT ( 'NONE',  ( 15.64687500061451608, -3.027376345333610441, -5.243569643749999898 ) ) ;
#11399=CARTESIAN_POINT ( 'NONE',  ( 14.06250000122903288, -4.330127018922190985, -2.500000000000001332 ) ) ;
#11401=CARTESIAN_POINT ( 'NONE',  ( 9.001249775931846008E-16, 19.07187500061451857, -25.09994784771203058 ) ) ;
#11402=CARTESIAN_POINT ( 'NONE',  ( 17.03437500061451715, 6.421520780324663323E-16, -5.243569643749999010 ) ) ;
#11403=CARTESIAN_POINT ( 'NONE',  ( 20.13750000122903216, 4.330127018922191873, 2.499999999999999556 ) ) ;
#11405=CARTESIAN_POINT ( 'NONE',  ( 15.34687500061451537, 6.054752690667223547, 3.707466751127219781E-16 ) ) ;
#11406=CARTESIAN_POINT ( 'NONE',  ( -4.243569643749997233, 13.14687500061451786, 32.45002607614398471 ) ) ;
#11407=CARTESIAN_POINT ( 'NONE',  ( 22.98750000122903003, -4.330127018922194537, 2.499999999999995559 ) ) ;
#11408=VECTOR ( 'NONE', #49139, 1000.000000000000000 ) ;
#11409=CARTESIAN_POINT ( 'NONE',  ( 15.10312500061451502, -4.541064518000417216, -2.621784821875001281 ) ) ;
#11410=CARTESIAN_POINT ( 'NONE',  ( 29.27812500061451573, 4.541064518000418104, 2.621784821874999949 ) ) ;
#11413=CARTESIAN_POINT ( 'NONE',  ( 21.67500000000000071, 6.123233995736764310E-16, -4.999999999999998224 ) ) ;
#11414=LINE ( 'NONE', #39125, #38547 ) ;
#11415=CARTESIAN_POINT ( 'NONE',  ( 3.065625000614517592, 3.027376345333613106, -5.243569643749998122 ) ) ;
#11416=CARTESIAN_POINT ( 'NONE',  ( 14.13750000122903394, 6.123233995736764310E-16, -4.999999999999998224 ) ) ;
#11417=CARTESIAN_POINT ( 'NONE',  ( 18.92812500061451431, 4.541064518000418104, 2.621784821874999949 ) ) ;
#11418=CARTESIAN_POINT ( 'NONE',  ( 24.44062500061451715, -3.027376345333614438, 5.243569643749998122 ) ) ;
#11419=CARTESIAN_POINT ( 'NONE',  ( 6.853125000614516793, 0.000000000000000000, 5.243569643749999010 ) ) ;
#11421=CARTESIAN_POINT ( 'NONE',  ( 3.365625000614516082, -6.054752690667223547, -1.112240025338166033E-15 ) ) ;
#11424=CARTESIAN_POINT ( 'NONE',  ( 8.484601909799253346E-16, 10.77500000122903501, -25.38119784648299770 ) ) ;
#11425=CARTESIAN_POINT ( 'NONE',  ( 4.243569643749999898, 17.38437500061451502, -30.00000000000000000 ) ) ;
#11426=CARTESIAN_POINT ( 'NONE',  ( 5.400000001229032343, -2.886751345948129988, 4.999999999999997335 ) ) ;
#11427=CARTESIAN_POINT ( 'NONE',  ( 8.287499999999999645, 5.773502691896255534, 3.535250795749688894E-16 ) ) ;
#11428=CARTESIAN_POINT ( 'NONE',  ( 5.250000001229035540, 5.773502691896255534, 3.535250795749688894E-16 ) ) ;
#11429=CARTESIAN_POINT ( 'NONE',  ( 12.42187500061451821, -6.054752690667223547, -1.112240025338166033E-15 ) ) ;
#11430=CARTESIAN_POINT ( 'NONE',  ( 19.42500000122903714, -5.773502691896255534, -1.060575238724906372E-15 ) ) ;
#11431=CARTESIAN_POINT ( 'NONE',  ( 3.639202574798650947, 4.093918037350785966, 3.396265244785773074 ) ) ;
#11432=CARTESIAN_POINT ( 'NONE',  ( 12.86250000122903359, 4.330127018922192761, -2.499999999999997780 ) ) ;
#11434=CARTESIAN_POINT ( 'NONE',  ( 11.22187500061451892, 3.027376345333613106, -5.243569643749998122 ) ) ;
#11435=CARTESIAN_POINT ( 'NONE',  ( 17.51250000122903216, 0.000000000000000000, 4.999999999999998224 ) ) ;
#11437=DIRECTION ( 'NONE',  ( -1.000000000000000000, -0.000000000000000000, -0.000000000000000000 ) ) ;
#11438=CARTESIAN_POINT ( 'NONE',  ( -2.121784821874996840, 16.72812500061459673, 33.67503911421598417 ) ) ;
#11439=CARTESIAN_POINT ( 'NONE',  ( 21.87187500061451573, -6.054752690667223547, -1.112240025338166033E-15 ) ) ;
#11440=DIRECTION ( 'NONE',  ( -0.000000000000000000, -1.000000000000000000, -0.000000000000000000 ) ) ;
#11441=CARTESIAN_POINT ( 'NONE',  ( 28.50000000122903288, -2.886751345948125991, -5.000000000000000000 ) ) ;
#11443=CARTESIAN_POINT ( 'NONE',  ( 23.35312500061451857, 4.541064518000418104, -2.621784821874998173 ) ) ;
#11444=CARTESIAN_POINT ( 'NONE',  ( 16.04062500061451857, -3.027376345333610441, -5.243569643749999898 ) ) ;
#11446=CARTESIAN_POINT ( 'NONE',  ( 12.87187500061451750, -6.054752690667223547, -1.112240025338166033E-15 ) ) ;
#11447=CARTESIAN_POINT ( 'NONE',  ( 29.17500000000000071, -4.330127018922194537, 2.499999999999995559 ) ) ;
#11448=CARTESIAN_POINT ( 'NONE',  ( 26.13750000122903216, -4.330127018922194537, 2.499999999999995559 ) ) ;
#11449=CARTESIAN_POINT ( 'NONE',  ( 3.459375000614519635, -4.541064518000417216, -2.621784821875001281 ) ) ;
#11450=CARTESIAN_POINT ( 'NONE',  ( 15.00937500061451679, 0.000000000000000000, 5.243569643749999010 ) ) ;
#11451=CARTESIAN_POINT ( 'NONE',  ( 28.88437500061451502, 4.541064518000418104, 2.621784821874999949 ) ) ;
#11453=CARTESIAN_POINT ( 'NONE',  ( 21.23437500061451644, 4.541064518000418104, 2.621784821874999949 ) ) ;
#11454=CARTESIAN_POINT ( 'NONE',  ( 13.88437500061451679, 6.421520780324663323E-16, -5.243569643749999010 ) ) ;
#11456=CARTESIAN_POINT ( 'NONE',  ( 28.83749999999999858, -2.886751345948125991, -5.000000000000000000 ) ) ;
#11457=CARTESIAN_POINT ( 'NONE',  ( 3.937500001229034208, 4.330127018922191873, 2.499999999999999556 ) ) ;
#11459=CARTESIAN_POINT ( 'NONE',  ( 16.56562500061451715, 3.027376345333613106, -5.243569643749998122 ) ) ;
#11460=CARTESIAN_POINT ( 'NONE',  ( 7.912499999999999645, 2.886751345948126879, 4.999999999999999112 ) ) ;
#11462=CARTESIAN_POINT ( 'NONE',  ( 17.77499999999999858, 4.330127018922191873, 2.499999999999999556 ) ) ;
#11463=CARTESIAN_POINT ( 'NONE',  ( -3.000416591977282496E-16, 12.94062500061451537, 25.09994784771203058 ) ) ;
#11464=CARTESIAN_POINT ( 'NONE',  ( 30.00000000000000000, 0.000000000000000000, 4.999999999999998224 ) ) ;
#11465=CARTESIAN_POINT ( 'NONE',  ( 19.91250000122903074, -4.330127018922190985, -2.500000000000001332 ) ) ;
#11467=CARTESIAN_POINT ( 'NONE',  ( 26.37187500061451217, -6.054752690667223547, -1.112240025338166033E-15 ) ) ;
#11468=VERTEX_POINT ( 'NONE', #55172 ) ;
#11469=CARTESIAN_POINT ( 'NONE',  ( 22.34062500061451573, -3.027376345333610441, -5.243569643749999898 ) ) ;
#11470=CARTESIAN_POINT ( 'NONE',  ( 21.75937500061451502, 0.000000000000000000, 5.243569643749999010 ) ) ;
#11471=CARTESIAN_POINT ( 'NONE',  ( 6.675000000000000711, -4.330127018922194537, 2.499999999999995559 ) ) ;
#11472=CARTESIAN_POINT ( 'NONE',  ( 10.64062500061451644, -3.027376345333610441, -5.243569643749999898 ) ) ;
#11473=CARTESIAN_POINT ( 'NONE',  ( 24.66562500061451502, 3.027376345333613106, -5.243569643749998122 ) ) ;
#11474=CARTESIAN_POINT ( 'NONE',  ( 14.33437500061451786, 6.421520780324663323E-16, -5.243569643749999010 ) ) ;
#11475=CARTESIAN_POINT ( 'NONE',  ( 16.58437500061451786, 6.421520780324663323E-16, -5.243569643749999010 ) ) ;
#11476=CARTESIAN_POINT ( 'NONE',  ( 4.416509438036825941, 2.344049510472278719, -4.690477066236870662 ) ) ;
#11477=CARTESIAN_POINT ( 'NONE',  ( -2.121784821874996840, 16.72812500061451857, 33.67503911421598417 ) ) ;
#11478=CARTESIAN_POINT ( 'NONE',  ( 20.32500000122903572, -5.773502691896255534, -1.060575238724906372E-15 ) ) ;
#11480=CARTESIAN_POINT ( 'NONE',  ( 12.74062500061451786, -3.027376345333614438, 5.243569643749998122 ) ) ;
#11481=CARTESIAN_POINT ( 'NONE',  ( 6.271875000614517859, 3.027376345333613106, -5.243569643749998122 ) ) ;
#11482=CARTESIAN_POINT ( 'NONE',  ( 5.821875000614519458, 3.027376345333613106, -5.243569643749998122 ) ) ;
#11484=CARTESIAN_POINT ( 'NONE',  ( 25.88437500061451502, -4.541064518000419881, 2.621784821874995952 ) ) ;
#11485=CARTESIAN_POINT ( 'NONE',  ( 17.05312500061451786, 4.541064518000418104, -2.621784821874998173 ) ) ;
#11486=CARTESIAN_POINT ( 'NONE',  ( 27.71250000122903145, 4.330127018922192761, -2.499999999999997780 ) ) ;
#11488=CARTESIAN_POINT ( 'NONE',  ( 27.29062500061451502, -3.027376345333610441, -5.243569643749999898 ) ) ;
#11489=CARTESIAN_POINT ( 'NONE',  ( 21.68437500061451573, 4.541064518000418104, 2.621784821874999949 ) ) ;
#11490=CARTESIAN_POINT ( 'NONE',  ( 16.37812500061451715, -4.541064518000419881, 2.621784821874995952 ) ) ;
#11491=CARTESIAN_POINT ( 'NONE',  ( 2.000000000000001332, 10.70000000000000107, 33.46410161513774995 ) ) ;
#11492=CARTESIAN_POINT ( 'NONE',  ( 23.95312500061451289, 0.000000000000000000, 5.243569643749999010 ) ) ;
#11493=CARTESIAN_POINT ( 'NONE',  ( 5.775000001229033231, 2.886751345948126879, 4.999999999999999112 ) ) ;
#11494=VERTEX_POINT ( 'NONE', #37441 ) ;
#11495=CARTESIAN_POINT ( 'NONE',  ( 28.19999999999999929, 0.000000000000000000, 4.999999999999998224 ) ) ;
#11496=CARTESIAN_POINT ( 'NONE',  ( -1.999999999999997113, 14.22500000000000142, -26.53589838486224295 ) ) ;
#11498=CARTESIAN_POINT ( 'NONE',  ( 28.60312500061451502, -4.541064518000417216, -2.621784821875001281 ) ) ;
#11499=CARTESIAN_POINT ( 'NONE',  ( 9.553125000614517859, 0.000000000000000000, 5.243569643749999010 ) ) ;
#11500=CARTESIAN_POINT ( 'NONE',  ( 24.00000000122902932, -2.886751345948125991, -5.000000000000000000 ) ) ;
#11501=CARTESIAN_POINT ( 'NONE',  ( 12.79687500061451821, -3.027376345333614438, 5.243569643749998122 ) ) ;
#11502=CARTESIAN_POINT ( 'NONE',  ( 29.27812500061451573, 4.541064518000418104, 2.621784821874999949 ) ) ;
#11503=CARTESIAN_POINT ( 'NONE',  ( 28.72500000000000142, -4.330127018922194537, 2.499999999999995559 ) ) ;
#11504=CARTESIAN_POINT ( 'NONE',  ( 4.003125000614518925, 4.541064518000418104, -2.621784821874998173 ) ) ;
#11505=CARTESIAN_POINT ( 'NONE',  ( 14.05312500061451431, 0.000000000000000000, 5.243569643749999010 ) ) ;
#11507=CARTESIAN_POINT ( 'NONE',  ( 9.553125000614517859, 0.000000000000000000, 5.243569643749999010 ) ) ;
#11508=CARTESIAN_POINT ( 'NONE',  ( 4.940625000614515372, 6.054752690667223547, 3.707466751127219781E-16 ) ) ;
#11511=CARTESIAN_POINT ( 'NONE',  ( 16.42500000000000071, 4.330127018922191873, 2.499999999999999556 ) ) ;
#11512=CARTESIAN_POINT ( 'NONE',  ( 16.58437500061451786, 6.421520780324663323E-16, -5.243569643749999010 ) ) ;
#11513=CARTESIAN_POINT ( 'NONE',  ( 11.81250000122903465, -4.330127018922190985, -2.500000000000001332 ) ) ;
#11514=CARTESIAN_POINT ( 'NONE',  ( 18.90937500061451360, 4.541064518000418104, -2.621784821874998173 ) ) ;
#11516=CARTESIAN_POINT ( 'NONE',  ( 20.03437500061451715, -4.541064518000419881, 2.621784821874995952 ) ) ;
#11517=CARTESIAN_POINT ( 'NONE',  ( 4.243569643749999898, 14.14062500061451644, -27.54997392385601529 ) ) ;
#11518=CARTESIAN_POINT ( 'NONE',  ( 21.03750000122903074, 4.330127018922191873, 2.499999999999999556 ) ) ;
#11520=CYLINDRICAL_SURFACE ( 'NONE', #57210, 4.999999999999998224 ) ;
#11521=CARTESIAN_POINT ( 'NONE',  ( 26.65312500061451573, 0.000000000000000000, 5.243569643749999010 ) ) ;
#11522=CARTESIAN_POINT ( 'NONE',  ( 17.28750000122903430, 6.123233995736764310E-16, -4.999999999999998224 ) ) ;
#11523=CARTESIAN_POINT ( 'NONE',  ( 27.27187500061451431, -6.054752690667223547, -1.112240025338166033E-15 ) ) ;
#11524=CARTESIAN_POINT ( 'NONE',  ( 23.85000000000000142, -4.330127018922190985, -2.500000000000001332 ) ) ;
#11525=EDGE_CURVE ( 'NONE', #65099, #18895, #50189, .T. ) ;
#11526=CARTESIAN_POINT ( 'NONE',  ( 8.165625000614516793, 3.027376345333611329, 5.243569643749999010 ) ) ;
#11528=CARTESIAN_POINT ( 'NONE',  ( 18.00937500061451502, 4.541064518000418104, -2.621784821874998173 ) ) ;
#11531=CARTESIAN_POINT ( 'NONE',  ( 4.078125000614517326, 4.541064518000418104, 2.621784821874999949 ) ) ;
#11532=CARTESIAN_POINT ( 'NONE',  ( 11.29687500061451644, 6.054752690667223547, 3.707466751127219781E-16 ) ) ;
#11533=VERTEX_POINT ( 'NONE', #13256 ) ;
#11534=CARTESIAN_POINT ( 'NONE',  ( 20.40937500061451715, 0.000000000000000000, 5.243569643749999010 ) ) ;
#11536=CARTESIAN_POINT ( 'NONE',  ( 29.28749999999999787, -2.886751345948125991, -5.000000000000000000 ) ) ;
#11537=CARTESIAN_POINT ( 'NONE',  ( 3.037500000000002309, -2.886751345948129988, 4.999999999999997335 ) ) ;
#11539=CARTESIAN_POINT ( 'NONE',  ( 14.06250000122903288, -4.330127018922190985, -2.500000000000001332 ) ) ;
#11541=CARTESIAN_POINT ( 'NONE',  ( 14.47500000122903430, -5.773502691896255534, -1.060575238724906372E-15 ) ) ;
#11542=ORIENTED_EDGE ( 'NONE', *, *, #43393, .T. ) ;
#11544=CARTESIAN_POINT ( 'NONE',  ( 11.84999999999999964, 4.330127018922192761, -2.499999999999997780 ) ) ;
#11545=CARTESIAN_POINT ( 'NONE',  ( 25.11562500061451431, 3.027376345333613106, -5.243569643749998122 ) ) ;
#11546=CARTESIAN_POINT ( 'NONE',  ( 15.03749999999999964, 5.773502691896255534, 3.535250795749688894E-16 ) ) ;
#11548=CARTESIAN_POINT ( 'NONE',  ( 9.637500001229033941, 6.123233995736764310E-16, -4.999999999999998224 ) ) ;
#11549=CARTESIAN_POINT ( 'NONE',  ( 8.915625000614515017, 3.027376345333613106, -5.243569643749998122 ) ) ;
#11550=( BOUNDED_CURVE ( )  B_SPLINE_CURVE ( 2, ( #46506, #6982, #14333, #30601, #58294, #41332, #64942, #69044, #42421 ),
 .UNSPECIFIED., .F., .F. ) 
 B_SPLINE_CURVE_WITH_KNOTS ( ( 3, 2, 2, 2, 3 ),
 ( 0.1847826086956521896, 0.1884057971014492794, 0.1956521739130434867, 0.2028985507246376940, 0.2065217391304347838 ),
 .UNSPECIFIED. ) 
 CURVE ( )  GEOMETRIC_REPRESENTATION_ITEM ( )  RATIONAL_B_SPLINE_CURVE ( ( 0.9330127018922194093, 0.9330127018922196314, 1.000000000000000000, 0.8660254037844387076, 1.000000000000000000, 0.8660254037844387076, 1.000000000000000000, 0.9330127018922194093, 0.9330127018922194093 ) ) 
 REPRESENTATION_ITEM ( '' )  );
#11551=CARTESIAN_POINT ( 'NONE',  ( 8.212500000000000355, 2.886751345948129099, -4.999999999999998224 ) ) ;
#11553=CARTESIAN_POINT ( 'NONE',  ( 4.243569643749999898, 13.74687500061451750, -27.54997392385601529 ) ) ;
#11554=CARTESIAN_POINT ( 'NONE',  ( 28.68750000122903288, 4.330127018922191873, 2.499999999999999556 ) ) ;
#11556=CARTESIAN_POINT ( 'NONE',  ( 8.062500000000000000, -5.773502691896255534, -1.060575238724906372E-15 ) ) ;
#11557=CARTESIAN_POINT ( 'NONE',  ( -1.071796769724491005, 12.70759618943233349, 26.00000000000000355 ) ) ;
#11558=EDGE_LOOP ( 'NONE', ( #14162, #22645, #29640, #11714 ) ) ;
#11559=CARTESIAN_POINT ( 'NONE',  ( 22.26562500061451644, -6.054752690667223547, -1.112240025338166033E-15 ) ) ;
#11560=CARTESIAN_POINT ( 'NONE',  ( 14.96250000122903323, -4.330127018922190985, -2.500000000000001332 ) ) ;
#11561=CARTESIAN_POINT ( 'NONE',  ( 3.289418471268391819, -3.765642822148987712, -3.324553038165963148 ) ) ;
#11562=LINE ( 'NONE', #479, #21911 ) ;
#11563=CARTESIAN_POINT ( 'NONE',  ( 20.14687500061451786, -3.027376345333610441, -5.243569643749999898 ) ) ;
#11565=CARTESIAN_POINT ( 'NONE',  ( 17.16562500061451502, 3.027376345333611329, 5.243569643749999010 ) ) ;
#11566=CARTESIAN_POINT ( 'NONE',  ( 9.001249775931846008E-16, 11.36562500061459424, -25.09994784771203058 ) ) ;
#11567=CARTESIAN_POINT ( 'NONE',  ( 7.790625000614518569, -3.027376345333614438, 5.243569643749998122 ) ) ;
#11568=CARTESIAN_POINT ( 'NONE',  ( 28.46250000122903145, -4.330127018922190985, -2.500000000000001332 ) ) ;
#11570=CARTESIAN_POINT ( 'NONE',  ( 18.59062500061451573, -3.027376345333614438, 5.243569643749998122 ) ) ;
#11572=CARTESIAN_POINT ( 'NONE',  ( 4.200000001229033053, -2.886751345948125991, -5.000000000000000000 ) ) ;
#11573=CARTESIAN_POINT ( 'NONE',  ( 13.58437500061451786, 4.541064518000418104, 2.621784821874999949 ) ) ;
#11574=CARTESIAN_POINT ( 'NONE',  ( 12.75937500061451857, 0.000000000000000000, 5.243569643749999010 ) ) ;
#11575=CARTESIAN_POINT ( 'NONE',  ( 20.29687500061451644, 6.054752690667223547, 3.707466751127219781E-16 ) ) ;
#11577=CARTESIAN_POINT ( 'NONE',  ( 3.140625000614516882, 6.054752690667223547, 3.707466751127219781E-16 ) ) ;
#11578=CARTESIAN_POINT ( 'NONE',  ( 24.06562500061451715, -6.054752690667223547, -1.112240025338166033E-15 ) ) ;
#11579=CARTESIAN_POINT ( 'NONE',  ( 23.61562500061451431, -6.054752690667223547, -1.112240025338166033E-15 ) ) ;
#11580=DIRECTION ( 'NONE',  ( 0.000000000000000000, 0.000000000000000000, 1.000000000000000000 ) ) ;
#11581=CARTESIAN_POINT ( 'NONE',  ( -3.999999999999997335, 16.43750000000000000, 32.30940107675850470 ) ) ;
#11582=CARTESIAN_POINT ( 'NONE',  ( 4.359375000614517326, -4.541064518000417216, -2.621784821875001281 ) ) ;
#11583=CARTESIAN_POINT ( 'NONE',  ( 11.70000000122903216, -2.886751345948129988, 4.999999999999997335 ) ) ;
#11584=CARTESIAN_POINT ( 'NONE',  ( 7.012500001229035718, 4.330127018922192761, -2.499999999999997780 ) ) ;
#11585=CARTESIAN_POINT ( 'NONE',  ( 21.56250000122903288, 0.000000000000000000, 4.999999999999998224 ) ) ;
#11586=CARTESIAN_POINT ( 'NONE',  ( 27.07500000122903216, -5.773502691896255534, -1.060575238724906372E-15 ) ) ;
#11589=CARTESIAN_POINT ( 'NONE',  ( 11.55937500061451928, -4.541064518000417216, -2.621784821875001281 ) ) ;
#11591=CARTESIAN_POINT ( 'NONE',  ( 18.25312500061451715, -4.541064518000417216, -2.621784821875001281 ) ) ;
#11592=CARTESIAN_POINT ( 'NONE',  ( 13.24687500061451750, -3.027376345333614438, 5.243569643749998122 ) ) ;
#11593=CARTESIAN_POINT ( 'NONE',  ( 4.228125000614517681, -4.541064518000419881, 2.621784821874995952 ) ) ;
#11594=CARTESIAN_POINT ( 'NONE',  ( 21.68437500061451573, 4.541064518000418104, 2.621784821874999949 ) ) ;
#11595=CARTESIAN_POINT ( 'NONE',  ( 9.009375000614518569, 4.541064518000418104, -2.621784821874998173 ) ) ;
#11596=CARTESIAN_POINT ( 'NONE',  ( 5.128125000614516260, -4.541064518000419881, 2.621784821874995952 ) ) ;
#11598=CARTESIAN_POINT ( 'NONE',  ( 5.100000001229034297, -2.886751345948125991, -5.000000000000000000 ) ) ;
#11599=CARTESIAN_POINT ( 'NONE',  ( 19.79062500061451502, 6.054752690667223547, 3.707466751127219781E-16 ) ) ;
#11600=CARTESIAN_POINT ( 'NONE',  ( 6.937500001229033764, 6.123233995736764310E-16, -4.999999999999998224 ) ) ;
#11601=CARTESIAN_POINT ( 'NONE',  ( 17.16562500061451502, 3.027376345333611329, 5.243569643749999010 ) ) ;
#11602=CARTESIAN_POINT ( 'NONE',  ( 14.05312500061451431, 0.000000000000000000, 5.243569643749999010 ) ) ;
#11604=CARTESIAN_POINT ( 'NONE',  ( 14.13750000000000107, 5.773502691896255534, 3.535250795749688894E-16 ) ) ;
#11605=CARTESIAN_POINT ( 'NONE',  ( 9.825000001229033941, 2.886751345948126879, 4.999999999999999112 ) ) ;
#11606=CARTESIAN_POINT ( 'NONE',  ( 5.690625000614516260, -3.027376345333610441, -5.243569643749999898 ) ) ;
#11607=CARTESIAN_POINT ( 'NONE',  ( 18.90000000122902790, -2.886751345948129988, 4.999999999999997335 ) ) ;
#11609=CARTESIAN_POINT ( 'NONE',  ( 2.121784821874999061, 11.60937500061451821, -33.67503911421598417 ) ) ;
#11610=CARTESIAN_POINT ( 'NONE',  ( 4.588602605000858148, -1.986133463133878285, 4.773510639627289720 ) ) ;
#11611=CARTESIAN_POINT ( 'NONE',  ( 3.600000001229033408, -2.886751345948129988, 4.999999999999997335 ) ) ;
#11612=CARTESIAN_POINT ( 'NONE',  ( 28.46250000122903145, -4.330127018922190985, -2.500000000000001332 ) ) ;
#11613=CARTESIAN_POINT ( 'NONE',  ( 20.14687500061451786, -3.027376345333610441, -5.243569643749999898 ) ) ;
#11615=ADVANCED_FACE ( 'NONE', ( #11192 ), #34437, .F. ) ;
#11616=CARTESIAN_POINT ( 'NONE',  ( 15.92812500061451608, -4.541064518000419881, 2.621784821874995952 ) ) ;
#11618=CARTESIAN_POINT ( 'NONE',  ( -1.071796769724496556, 14.80490381179669690, 33.99999999999998579 ) ) ;
#11620=CARTESIAN_POINT ( 'NONE',  ( 25.47187500061451715, -6.054752690667223547, -1.112240025338166033E-15 ) ) ;
#11622=CARTESIAN_POINT ( 'NONE',  ( 11.65312500061451573, 4.541064518000418104, -2.621784821874998173 ) ) ;
#11623=CARTESIAN_POINT ( 'NONE',  ( 9.646875000614516082, -3.027376345333614438, 5.243569643749998122 ) ) ;
#11625=CARTESIAN_POINT ( 'NONE',  ( 29.80312500061451431, 0.000000000000000000, 5.243569643749999010 ) ) ;
#11626=CARTESIAN_POINT ( 'NONE',  ( 21.51562500061451644, 3.027376345333613106, -5.243569643749998122 ) ) ;
#11627=CARTESIAN_POINT ( 'NONE',  ( 22.91250000122903430, 0.000000000000000000, 4.999999999999998224 ) ) ;
#11628=EDGE_CURVE ( 'NONE', #57370, #53683, #56965, .T. ) ;
#11630=CARTESIAN_POINT ( 'NONE',  ( 11.13750000000000284, -2.886751345948129988, 4.999999999999997335 ) ) ;
#11631=CARTESIAN_POINT ( 'NONE',  ( 21.60000000122903430, -2.886751345948129988, 4.999999999999997335 ) ) ;
#11632=CARTESIAN_POINT ( 'NONE',  ( 16.15312500061451573, 4.541064518000418104, -2.621784821874998173 ) ) ;
#11634=VERTEX_POINT ( 'NONE', #35794 ) ;
#11635=CARTESIAN_POINT ( 'NONE',  ( 21.18749999999999645, -2.886751345948125991, -5.000000000000000000 ) ) ;
#11637=CARTESIAN_POINT ( 'NONE',  ( 24.75000000000000000, -4.330127018922190985, -2.500000000000001332 ) ) ;
#11638=CARTESIAN_POINT ( 'NONE',  ( 21.38437500061451502, -4.541064518000419881, 2.621784821874995952 ) ) ;
#11639=CARTESIAN_POINT ( 'NONE',  ( 24.89062500061451644, -3.027376345333614438, 5.243569643749998122 ) ) ;
#11642=CARTESIAN_POINT ( 'NONE',  ( 9.328125000614518214, 6.421520780324663323E-16, -5.243569643749999010 ) ) ;
#11644=CARTESIAN_POINT ( 'NONE',  ( 15.75000000000000000, -4.330127018922190985, -2.500000000000001332 ) ) ;
#11645=CARTESIAN_POINT ( 'NONE',  ( 4.243569643749999898, 17.77812500061451928, 30.00000000000000000 ) ) ;
#11646=CARTESIAN_POINT ( 'NONE',  ( 4.659375000614518925, 0.000000000000000000, 5.243569643749999010 ) ) ;
#11647=CARTESIAN_POINT ( 'NONE',  ( 27.23437500061451644, -4.541064518000419881, 2.621784821874995952 ) ) ;
#11649=CARTESIAN_POINT ( 'NONE',  ( 23.05312500061451431, 0.000000000000000000, 5.243569643749999010 ) ) ;
#11650=CARTESIAN_POINT ( 'NONE',  ( 25.35937500061451644, 0.000000000000000000, 5.243569643749999010 ) ) ;
#11651=CARTESIAN_POINT ( 'NONE',  ( -4.243569643749999898, 18.41562500061459318, -32.45002607614398471 ) ) ;
#11652=CARTESIAN_POINT ( 'NONE',  ( 12.30000000000000249, 4.330127018922192761, -2.499999999999997780 ) ) ;
#11653=CARTESIAN_POINT ( 'NONE',  ( 8.353125000614518569, -4.541064518000417216, -2.621784821875001281 ) ) ;
#11655=CARTESIAN_POINT ( 'NONE',  ( 28.45312500061451289, 0.000000000000000000, 5.243569643749999010 ) ) ;
#11656=CARTESIAN_POINT ( 'NONE',  ( 25.71562500061451573, 3.027376345333611329, 5.243569643749999010 ) ) ;
#11657=CARTESIAN_POINT ( 'NONE',  ( 12.60000000122903430, -2.886751345948130876, 4.999999999999996447 ) ) ;
#11659=CARTESIAN_POINT ( 'NONE',  ( 20.67187500061451289, 3.027376345333613106, -5.243569643749998122 ) ) ;
#11660=CARTESIAN_POINT ( 'NONE',  ( -4.243569643749999898, 14.00937500061451857, 30.00000000000000000 ) ) ;
#11661=CARTESIAN_POINT ( 'NONE',  ( 18.79687500061451644, -3.027376345333610441, -5.243569643749999898 ) ) ;
#11662=CARTESIAN_POINT ( 'NONE',  ( 29.18437500061451573, 6.421520780324663323E-16, -5.243569643749999010 ) ) ;
#11663=CARTESIAN_POINT ( 'NONE',  ( -2.121784821874999949, 16.63437500061451857, 26.32496088578401938 ) ) ;
#11664=CARTESIAN_POINT ( 'NONE',  ( 10.37812500061451715, 4.541064518000418104, 2.621784821874999949 ) ) ;
#11665=CARTESIAN_POINT ( 'NONE',  ( 0.000000000000000000, 20.00000000000000000, 24.00000000000000000 ) ) ;
#11666=CARTESIAN_POINT ( 'NONE',  ( 3.946875000614517681, -3.027376345333610441, -5.243569643749999898 ) ) ;
#11667=CARTESIAN_POINT ( 'NONE',  ( -3.999999999999999112, 16.06250000122903288, -30.00000000000000000 ) ) ;
#11668=CARTESIAN_POINT ( 'NONE',  ( 7.190625000614518036, 6.054752690667223547, 3.707466751127219781E-16 ) ) ;
#11669=CARTESIAN_POINT ( 'NONE',  ( 11.07187500061451679, -6.054752690667223547, -1.112240025338166033E-15 ) ) ;
#11670=CARTESIAN_POINT ( 'NONE',  ( 18.33750000122903501, 4.330127018922191873, 2.499999999999999556 ) ) ;
#11671=CARTESIAN_POINT ( 'NONE',  ( 4.996875000614516615, 6.054752690667223547, 3.707466751127219781E-16 ) ) ;
#11672=B_SPLINE_CURVE_WITH_KNOTS ( 'NONE', 3,
 ( #46051, #17947, #64106, #1712, #18671, #24948, #19030, #40509, #23503, #13491 ),
 .UNSPECIFIED., .F., .F.,
 ( 4, 3, 3, 4 ),
 ( 0.000000000000000000, 0.0001572268757737857144, 0.0003144538226509923230, 0.0005227749235523226640 ),
 .UNSPECIFIED. ) ;
#11673=CARTESIAN_POINT ( 'NONE',  ( 8.840625000614515727, -3.027376345333610441, -5.243569643749999898 ) ) ;
#11674=CARTESIAN_POINT ( 'NONE',  ( 5.878125000614517148, 4.541064518000418104, 2.621784821874999949 ) ) ;
#11676=CARTESIAN_POINT ( 'NONE',  ( 19.99687500061451573, -3.027376345333614438, 5.243569643749998122 ) ) ;
#11677=CARTESIAN_POINT ( 'NONE',  ( 9.150000001229033231, -2.886751345948126435, -5.000000000000000000 ) ) ;
#11678=ORIENTED_EDGE ( 'NONE', *, *, #56574, .F. ) ;
#11679=CARTESIAN_POINT ( 'NONE',  ( 26.65312500061451573, 0.000000000000000000, 5.243569643749999010 ) ) ;
#11680=CARTESIAN_POINT ( 'NONE',  ( 12.66562500061451502, 3.027376345333611329, 5.243569643749999010 ) ) ;
#11682=CARTESIAN_POINT ( 'NONE',  ( 28.39687500061451431, 6.054752690667223547, 3.707466751127219781E-16 ) ) ;
#11683=CARTESIAN_POINT ( 'NONE',  ( 13.11562500061451786, 3.027376345333611329, 5.243569643749999010 ) ) ;
#11684=CARTESIAN_POINT ( 'NONE',  ( 2.121784821875001281, 10.55937500061451750, -26.32496088578401938 ) ) ;
#11685=CARTESIAN_POINT ( 'NONE',  ( 12.48750000122903359, 4.330127018922191873, 2.499999999999999556 ) ) ;
#11686=CARTESIAN_POINT ( 'NONE',  ( 26.42812500061451431, 6.421520780324663323E-16, -5.243569643749999010 ) ) ;
#11687=CARTESIAN_POINT ( 'NONE',  ( -2.121784821874999949, 12.52812500061451573, -33.67503911421598417 ) ) ;
#11688=CARTESIAN_POINT ( 'NONE',  ( 15.82500000122903216, -5.773502691896255534, -1.060575238724906372E-15 ) ) ;
#11689=CARTESIAN_POINT ( 'NONE',  ( 14.55000000000000071, 4.330127018922192761, -2.499999999999997780 ) ) ;
#11690=CARTESIAN_POINT ( 'NONE',  ( 20.76562500061451644, 3.027376345333611329, 5.243569643749999010 ) ) ;
#11691=CARTESIAN_POINT ( 'NONE',  ( 6.759375000614516793, 4.541064518000418104, -2.621784821874998173 ) ) ;
#11692=CARTESIAN_POINT ( 'NONE',  ( 8.662500001229034297, -4.330127018922190985, -2.500000000000001332 ) ) ;
#11693=CARTESIAN_POINT ( 'NONE',  ( 15.63750000122903216, 4.330127018922191873, 2.499999999999999556 ) ) ;
#11694=CARTESIAN_POINT ( 'NONE',  ( 11.84062500061451750, -3.027376345333614438, 5.243569643749998122 ) ) ;
#11695=CARTESIAN_POINT ( 'NONE',  ( 16.60312500061451857, 4.541064518000418104, -2.621784821874998173 ) ) ;
#11696=CARTESIAN_POINT ( 'NONE',  ( 26.96250000122903145, 0.000000000000000000, 4.999999999999998224 ) ) ;
#11697=CARTESIAN_POINT ( 'NONE',  ( 22.50000000000000000, -4.330127018922190985, -2.500000000000001332 ) ) ;
#11698=CARTESIAN_POINT ( 'NONE',  ( 24.19687500061451857, -3.027376345333610441, -5.243569643749999898 ) ) ;
#11700=CARTESIAN_POINT ( 'NONE',  ( 10.72500000122903252, 2.886751345948126879, 4.999999999999999112 ) ) ;
#11701=CARTESIAN_POINT ( 'NONE',  ( 27.60937500061451644, 0.000000000000000000, 5.243569643749999010 ) ) ;
#11702=( BOUNDED_CURVE ( )  B_SPLINE_CURVE ( 2, ( #48376, #8842, #31747, #26202, #46642, #1585, #70903 ),
 .UNSPECIFIED., .F., .F. ) 
 B_SPLINE_CURVE_WITH_KNOTS ( ( 3, 2, 2, 3 ),
 ( 0.7333333333333332815, 0.7361111111111111605, 0.7388888888888889284, 0.7416666666666666963 ),
 .UNSPECIFIED. ) 
 CURVE ( )  GEOMETRIC_REPRESENTATION_ITEM ( )  RATIONAL_B_SPLINE_CURVE ( ( 1.000000000000000000, 0.8660254037844387076, 1.000000000000000000, 0.8660254037844387076, 1.000000000000000000, 0.8660254037844387076, 1.000000000000000000 ) ) 
 REPRESENTATION_ITEM ( '' )  );
#11703=CARTESIAN_POINT ( 'NONE',  ( 5.559375000614517504, 0.000000000000000000, 5.243569643749999010 ) ) ;
#11704=CARTESIAN_POINT ( 'NONE',  ( 22.71562500061451573, -6.054752690667223547, -1.112240025338166033E-15 ) ) ;
#11706=CARTESIAN_POINT ( 'NONE',  ( 1.626862140677534273E-15, 10.77500000122903323, 34.00000000000000000 ) ) ;
#11707=CARTESIAN_POINT ( 'NONE',  ( 11.07187500061451679, -6.054752690667223547, -1.112240025338166033E-15 ) ) ;
#11708=CARTESIAN_POINT ( 'NONE',  ( 15.86249999999999893, 2.886751345948129099, -4.999999999999997335 ) ) ;
#11709=CARTESIAN_POINT ( 'NONE',  ( 29.01562500061451644, -6.054752690667223547, -1.112240025338166033E-15 ) ) ;
#11710=CARTESIAN_POINT ( 'NONE',  ( 7.059375000614518392, -4.541064518000417216, -2.621784821875001281 ) ) ;
#11711=CARTESIAN_POINT ( 'NONE',  ( 26.85937500061451644, -4.541064518000417216, -2.621784821875001281 ) ) ;
#11712=CARTESIAN_POINT ( 'NONE',  ( -2.121784821874999949, 10.27812500061459566, 26.32496088578401938 ) ) ;
#11713=CARTESIAN_POINT ( 'NONE',  ( 20.24999999999999645, -4.330127018922190985, -2.500000000000001332 ) ) ;
#11714=ORIENTED_EDGE ( 'NONE', *, *, #2386, .F. ) ;
#11715=CARTESIAN_POINT ( 'NONE',  ( 28.04999999999999716, 4.330127018922192761, -2.499999999999997780 ) ) ;
#11716=EDGE_CURVE ( 'NONE', #38366, #36659, #52795, .T. ) ;
#11717=CARTESIAN_POINT ( 'NONE',  ( 29.33437500061451431, 4.541064518000418104, 2.621784821874999949 ) ) ;
#11718=VERTEX_POINT ( 'NONE', #24711 ) ;
#11719=CARTESIAN_POINT ( 'NONE',  ( 15.47812500061451679, -4.541064518000419881, 2.621784821874995952 ) ) ;
#11720=CARTESIAN_POINT ( 'NONE',  ( 8.840625000614515727, -3.027376345333610441, -5.243569643749999898 ) ) ;
#11722=CARTESIAN_POINT ( 'NONE',  ( 4.696875000614518569, -3.027376345333614438, 5.243569643749998122 ) ) ;
#11723=CARTESIAN_POINT ( 'NONE',  ( 17.85000000122903430, 5.773502691896255534, 3.535250795749688894E-16 ) ) ;
#11724=CARTESIAN_POINT ( 'NONE',  ( 22.12500000000000000, 6.123233995736764310E-16, -4.999999999999998224 ) ) ;
#11726=CARTESIAN_POINT ( 'NONE',  ( 5.259375000614518569, -4.541064518000417216, -2.621784821875001281 ) ) ;
#11727=CARTESIAN_POINT ( 'NONE',  ( 11.07187500061451679, -6.054752690667223547, -1.112240025338166033E-15 ) ) ;
#11728=CARTESIAN_POINT ( 'NONE',  ( 22.39687500061451075, -3.027376345333610441, -5.243569643749999898 ) ) ;
#11729=CARTESIAN_POINT ( 'NONE',  ( -3.999999999999997335, 17.33749999999999858, -27.69059892324149530 ) ) ;
#11730=ORIENTED_EDGE ( 'NONE', *, *, #39611, .F. ) ;
#11731=CARTESIAN_POINT ( 'NONE',  ( 3.796875000614517326, -3.027376345333614438, 5.243569643749998122 ) ) ;
#11732=CARTESIAN_POINT ( 'NONE',  ( 8.221875000614518925, 3.027376345333611329, 5.243569643749999010 ) ) ;
#11733=CARTESIAN_POINT ( 'NONE',  ( 18.30000000000000071, 0.000000000000000000, 4.999999999999998224 ) ) ;
#11734=CARTESIAN_POINT ( 'NONE',  ( 16.67812500061451786, 4.541064518000418104, 2.621784821874999949 ) ) ;
#11736=CARTESIAN_POINT ( 'NONE',  ( 24.75000000122903288, -2.886751345948130876, 4.999999999999996447 ) ) ;
#11738=CARTESIAN_POINT ( 'NONE',  ( 10.37812500061451715, 4.541064518000418104, 2.621784821874999949 ) ) ;
#11739=CARTESIAN_POINT ( 'NONE',  ( 25.77187500061451075, 3.027376345333611329, 5.243569643749999010 ) ) ;
#11740=CARTESIAN_POINT ( 'NONE',  ( 4.898587196589411843E-16, 20.00000000000000000, -26.00000000000000000 ) ) ;
#11741=CARTESIAN_POINT ( 'NONE',  ( 27.42187500061451644, 3.027376345333613106, -5.243569643749998122 ) ) ;
#11742=CARTESIAN_POINT ( 'NONE',  ( 9.787499999999999645, -2.886751345948129988, 4.999999999999997335 ) ) ;
#11743=CARTESIAN_POINT ( 'NONE',  ( -2.828200636599751609E-16, 15.95000000122903216, 25.38119784648299770 ) ) ;
#11744=CARTESIAN_POINT ( 'NONE',  ( 8.325000001229033941, 2.886751345948129099, -4.999999999999998224 ) ) ;
#11745=CARTESIAN_POINT ( 'NONE',  ( 20.78437500061451715, 4.541064518000418104, 2.621784821874999949 ) ) ;
#11746=CARTESIAN_POINT ( 'NONE',  ( 14.25937500061451679, -4.541064518000417216, -2.621784821875001281 ) ) ;
#11749=CARTESIAN_POINT ( 'NONE',  ( 15.51562500061451644, -6.054752690667223547, -1.112240025338166033E-15 ) ) ;
#11750=CARTESIAN_POINT ( 'NONE',  ( 26.13750000122903216, -4.330127018922194537, 2.499999999999995559 ) ) ;
#11751=CARTESIAN_POINT ( 'NONE',  ( 14.18437500061451750, -4.541064518000419881, 2.621784821874995952 ) ) ;
#11752=DIRECTION ( 'NONE',  ( -1.000000000000000000, -0.000000000000000000, -0.000000000000000000 ) ) ;
#11753=CARTESIAN_POINT ( 'NONE',  ( 17.20312500061451644, 0.000000000000000000, 5.243569643749999010 ) ) ;
#11755=CARTESIAN_POINT ( 'NONE',  ( 25.39687500061451431, -3.027376345333614438, 5.243569643749998122 ) ) ;
#11756=CARTESIAN_POINT ( 'NONE',  ( -4.243569643749999898, 10.35312500061451857, 30.00000000000000000 ) ) ;
#11757=CARTESIAN_POINT ( 'NONE',  ( 14.44687500061451679, 6.054752690667223547, 3.707466751127219781E-16 ) ) ;
#11758=( BOUNDED_CURVE ( )  B_SPLINE_CURVE ( 2, ( #5887, #28418, #51317, #23593, #6976 ),
 .UNSPECIFIED., .F., .F. ) 
 B_SPLINE_CURVE_WITH_KNOTS ( ( 3, 2, 3 ),
 ( 0.000000000000000000, 0.007246376811594202987, 0.01086956521739130578 ),
 .UNSPECIFIED. ) 
 CURVE ( )  GEOMETRIC_REPRESENTATION_ITEM ( )  RATIONAL_B_SPLINE_CURVE ( ( 1.000000000000000000, 0.8660254037844387076, 1.000000000000000000, 0.9330127018922192983, 0.9330127018922194093 ) ) 
 REPRESENTATION_ITEM ( '' )  );
#11759=CARTESIAN_POINT ( 'NONE',  ( 12.18750000122903465, -4.330127018922194537, 2.499999999999995559 ) ) ;
#11761=CARTESIAN_POINT ( 'NONE',  ( -2.121784821874996840, 15.88437500061451857, -26.32496088578401583 ) ) ;
#11762=CARTESIAN_POINT ( 'NONE',  ( 17.89687500061451431, -3.027376345333610441, -5.243569643749999898 ) ) ;
#11763=CARTESIAN_POINT ( 'NONE',  ( 21.07500000122903572, 2.886751345948126879, 4.999999999999999112 ) ) ;
#11764=( BOUNDED_CURVE ( )  B_SPLINE_CURVE ( 2, ( #38237, #15333, #33064, #26432, #10173, #54147, #48603, #37511, #3910 ),
 .UNSPECIFIED., .F., .F. ) 
 B_SPLINE_CURVE_WITH_KNOTS ( ( 3, 2, 2, 2, 3 ),
 ( 0.7717391304347825942, 0.7753623188405797118, 0.7826086956521739468, 0.7898550724637680709, 0.7934782608695651884 ),
 .UNSPECIFIED. ) 
 CURVE ( )  GEOMETRIC_REPRESENTATION_ITEM ( )  RATIONAL_B_SPLINE_CURVE ( ( 0.9330127018922194093, 0.9330127018922194093, 1.000000000000000000, 0.8660254037844387076, 1.000000000000000000, 0.8660254037844387076, 1.000000000000000000, 0.9330127018922194093, 0.9330127018922194093 ) ) 
 REPRESENTATION_ITEM ( '' )  );
#11765=CARTESIAN_POINT ( 'NONE',  ( 15.00937500061451679, 0.000000000000000000, 5.243569643749999010 ) ) ;
#11766=CARTESIAN_POINT ( 'NONE',  ( 4.243569643749999010, 11.12187500061451928, 27.54997392385601174 ) ) ;
#11767=CARTESIAN_POINT ( 'NONE',  ( 23.13750000122903216, 6.123233995736764310E-16, -4.999999999999998224 ) ) ;
#11768=CARTESIAN_POINT ( 'NONE',  ( 15.29062500061451679, 6.054752690667223547, 3.707466751127219781E-16 ) ) ;
#11769=DIRECTION ( 'NONE',  ( -1.000000000000000000, -0.000000000000000000, -0.000000000000000000 ) ) ;
#11772=CARTESIAN_POINT ( 'NONE',  ( 20.17499999999999716, -4.330127018922194537, 2.499999999999995559 ) ) ;
#11774=CARTESIAN_POINT ( 'NONE',  ( 3.478125000614517237, 6.421520780324663323E-16, -5.243569643749999010 ) ) ;
#11776=CARTESIAN_POINT ( 'NONE',  ( 14.70000000122903394, 5.773502691896255534, 3.535250795749688894E-16 ) ) ;
#11777=CARTESIAN_POINT ( 'NONE',  ( 20.80312500061451431, 0.000000000000000000, 5.243569643749999010 ) ) ;
#11778=CARTESIAN_POINT ( 'NONE',  ( 22.75312500061451360, -4.541064518000417216, -2.621784821875001281 ) ) ;
#11779=CARTESIAN_POINT ( 'NONE',  ( 6.290625000614517681, 6.054752690667223547, 3.707466751127219781E-16 ) ) ;
#11781=CARTESIAN_POINT ( 'NONE',  ( 28.91250000000000497, 2.886751345948129099, -4.999999999999998224 ) ) ;
#11783=CARTESIAN_POINT ( 'NONE',  ( 29.70937500061451431, 4.541064518000418104, -2.621784821874998173 ) ) ;
#11784=CARTESIAN_POINT ( 'NONE',  ( 2.000000000000001332, 11.26250000122903394, -26.53589838486224650 ) ) ;
#11785=CARTESIAN_POINT ( 'NONE',  ( -3.000416591977282496E-16, 17.94687500061451502, -34.90005215228797653 ) ) ;
#11786=CARTESIAN_POINT ( 'NONE',  ( 6.225000001229036073, 2.886751345948126879, 4.999999999999999112 ) ) ;
#11787=CARTESIAN_POINT ( 'NONE',  ( 8.587500000000002132, -2.886751345948125991, -5.000000000000000000 ) ) ;
#11788=CARTESIAN_POINT ( 'NONE',  ( 3.112500001229034918, 0.000000000000000000, 4.999999999999998224 ) ) ;
#11789=CARTESIAN_POINT ( 'NONE',  ( 11.78437500061451892, 4.541064518000418104, 2.621784821874999949 ) ) ;
#11790=CARTESIAN_POINT ( 'NONE',  ( 23.62500000122902932, 2.886751345948095793, -5.000000000000055067 ) ) ;
#11791=CARTESIAN_POINT ( 'NONE',  ( 3.946875000614517681, -3.027376345333610441, -5.243569643749999898 ) ) ;
#11793=FACE_OUTER_BOUND ( 'NONE', #53184, .T. ) ;
#11794=CARTESIAN_POINT ( 'NONE',  ( 10.54687500061451644, -3.027376345333614438, 5.243569643749998122 ) ) ;
#11795=CARTESIAN_POINT ( 'NONE',  ( 14.10937500061451644, 0.000000000000000000, 5.243569643749999010 ) ) ;
#11796=CARTESIAN_POINT ( 'NONE',  ( -1.999999999999997113, 18.72500000000000142, -26.53589838486224295 ) ) ;
#11797=CARTESIAN_POINT ( 'NONE',  ( 6.262500000000000178, -5.773502691896255534, -1.060575238724906372E-15 ) ) ;
#11798=CARTESIAN_POINT ( 'NONE',  ( -3.000416591977282496E-16, 16.99062500061459602, 25.09994784771203058 ) ) ;
#11799=CARTESIAN_POINT ( 'NONE',  ( 20.82187500061451857, 3.027376345333611329, 5.243569643749999010 ) ) ;
#11801=EDGE_CURVE ( 'NONE', #18961, #7272, #32258, .T. ) ;
#11802=CARTESIAN_POINT ( 'NONE',  ( 26.66250000122903430, -4.330127018922190985, -2.500000000000001332 ) ) ;
#11804=CARTESIAN_POINT ( 'NONE',  ( 23.27812500061451573, 6.421520780324663323E-16, -5.243569643749999010 ) ) ;
#11805=CARTESIAN_POINT ( 'NONE',  ( 14.65312500061451573, -4.541064518000417216, -2.621784821875001281 ) ) ;
#11807=CARTESIAN_POINT ( 'NONE',  ( 13.05937500061451750, 4.541064518000418104, -2.621784821874998173 ) ) ;
#11808=CARTESIAN_POINT ( 'NONE',  ( 27.48749999999999716, -2.886751345948125991, -5.000000000000000000 ) ) ;
#11809=CARTESIAN_POINT ( 'NONE',  ( 24.30000000122903359, -2.886751345948129988, 4.999999999999997335 ) ) ;
#11810=CARTESIAN_POINT ( 'NONE',  ( 2.934375000614518392, -4.541064518000419881, 2.621784821874995952 ) ) ;
#11811=CARTESIAN_POINT ( 'NONE',  ( 14.74687500061451573, -3.027376345333610441, -5.243569643749999898 ) ) ;
#11813=CARTESIAN_POINT ( 'NONE',  ( 8.175000001229031810, -5.773502691896255534, -1.060575238724906372E-15 ) ) ;
#11814=FACE_OUTER_BOUND ( 'NONE', #21555, .T. ) ;
#11815=CARTESIAN_POINT ( 'NONE',  ( 22.28437500061451715, -4.541064518000419881, 2.621784821874995952 ) ) ;
#11816=CARTESIAN_POINT ( 'NONE',  ( 13.39687500061451608, -3.027376345333610441, -5.243569643749999898 ) ) ;
#11818=CARTESIAN_POINT ( 'NONE',  ( 26.36249999999999716, 2.886751345948126879, 4.999999999999999112 ) ) ;
#11819=CARTESIAN_POINT ( 'NONE',  ( 2.737500001229034474, -4.330127018922194537, 2.499999999999995559 ) ) ;
#11821=CARTESIAN_POINT ( 'NONE',  ( 16.71562500061451573, 3.027376345333611329, 5.243569643749999010 ) ) ;
#11822=CARTESIAN_POINT ( 'NONE',  ( 6.150000000000003020, 0.000000000000000000, 4.999999999999998224 ) ) ;
#11824=CARTESIAN_POINT ( 'NONE',  ( 16.76249999999999929, 2.886751345948129099, -4.999999999999998224 ) ) ;
#11825=CARTESIAN_POINT ( 'NONE',  ( -4.243569643749999898, 13.91562500061451679, 27.54997392385601529 ) ) ;
#11827=CARTESIAN_POINT ( 'NONE',  ( 21.48750000122903003, 4.330127018922191873, 2.499999999999999556 ) ) ;
#11828=CARTESIAN_POINT ( 'NONE',  ( 27.34687500061451360, -3.027376345333610441, -5.243569643749999898 ) ) ;
#11829=ORIENTED_EDGE ( 'NONE', *, *, #38793, .F. ) ;
#11830=CARTESIAN_POINT ( 'NONE',  ( 20.95312500061451999, -4.541064518000417216, -2.621784821875001281 ) ) ;
#11831=CARTESIAN_POINT ( 'NONE',  ( 21.27187500061451786, 3.027376345333611329, 5.243569643749999010 ) ) ;
#11832=CARTESIAN_POINT ( 'NONE',  ( 4.312500000000000000, 2.886751345948126879, 4.999999999999999112 ) ) ;
#11833=CARTESIAN_POINT ( 'NONE',  ( 8.690625000614515372, -3.027376345333614438, 5.243569643749998122 ) ) ;
#11834=CARTESIAN_POINT ( 'NONE',  ( 24.10312500061451502, -4.541064518000417216, -2.621784821875001281 ) ) ;
#11835=CARTESIAN_POINT ( 'NONE',  ( 12.57187500061451857, 3.027376345333613106, -5.243569643749998122 ) ) ;
#11836=CARTESIAN_POINT ( 'NONE',  ( 17.67187500061451644, 3.027376345333611329, 5.243569643749999010 ) ) ;
#11837=CARTESIAN_POINT ( 'NONE',  ( -4.243569643749999898, 18.00312500061451715, 30.00000000000000000 ) ) ;
#11838=CARTESIAN_POINT ( 'NONE',  ( 22.01250000122903216, 0.000000000000000000, 4.999999999999998224 ) ) ;
#11840=CARTESIAN_POINT ( 'NONE',  ( 11.76562500061451644, 3.027376345333611329, 5.243569643749999010 ) ) ;
#11841=CARTESIAN_POINT ( 'NONE',  ( 4.621875000614516615, 3.027376345333611329, 5.243569643749999010 ) ) ;
#11842=CARTESIAN_POINT ( 'NONE',  ( 5.071875000614519458, 3.027376345333611329, 5.243569643749999010 ) ) ;
#11843=ORIENTED_EDGE ( 'NONE', *, *, #72200, .T. ) ;
#11844=CARTESIAN_POINT ( 'NONE',  ( 25.39687500061451431, -3.027376345333614438, 5.243569643749998122 ) ) ;
#11845=CARTESIAN_POINT ( 'NONE',  ( 16.00312500061451715, -4.541064518000417216, -2.621784821875001281 ) ) ;
#11846=CARTESIAN_POINT ( 'NONE',  ( 27.63750000122903216, 6.123233995736764310E-16, -4.999999999999998224 ) ) ;
#11847=CARTESIAN_POINT ( 'NONE',  ( 28.41562500061451502, 3.027376345333611329, 5.243569643749999010 ) ) ;
#11848=CARTESIAN_POINT ( 'NONE',  ( 22.69687500061451857, -3.027376345333614438, 5.243569643749998122 ) ) ;
#11849=CARTESIAN_POINT ( 'NONE',  ( 16.11562500061451786, 3.027376345333613106, -5.243569643749998122 ) ) ;
#11850=CARTESIAN_POINT ( 'NONE',  ( -1.999999999999997113, 10.62500000000000000, 33.46410161513775705 ) ) ;
#11851=CARTESIAN_POINT ( 'NONE',  ( 22.64062500061451644, -3.027376345333614438, 5.243569643749998122 ) ) ;
#11854=CARTESIAN_POINT ( 'NONE',  ( 28.49999999999999645, 4.330127018922192761, -2.499999999999997780 ) ) ;
#11855=CARTESIAN_POINT ( 'NONE',  ( 8.484601909799253346E-16, 13.81250000000000000, -25.38119784648299770 ) ) ;
#11857=CARTESIAN_POINT ( 'NONE',  ( 29.35312500061451502, 0.000000000000000000, 5.243569643749999010 ) ) ;
#11858=CARTESIAN_POINT ( 'NONE',  ( 9.778125000614517504, 6.421520780324663323E-16, -5.243569643749999010 ) ) ;
#11859=CARTESIAN_POINT ( 'NONE',  ( 22.23750000122903003, 6.123233995736764310E-16, -4.999999999999998224 ) ) ;
#11860=CARTESIAN_POINT ( 'NONE',  ( 12.38437500061451857, -4.541064518000419881, 2.621784821874995952 ) ) ;
#11861=CARTESIAN_POINT ( 'NONE',  ( 27.44062500061451715, 6.054752690667223547, 3.707466751127219781E-16 ) ) ;
#11862=CARTESIAN_POINT ( 'NONE',  ( 28.01249999999999574, 2.886751345948129099, -4.999999999999998224 ) ) ;
#11863=CARTESIAN_POINT ( 'NONE',  ( 8.484601909799253346E-16, 19.32500000122902861, -25.38119784648299770 ) ) ;
#11864=CARTESIAN_POINT ( 'NONE',  ( 25.23750000122903359, -4.330127018922194537, 2.499999999999995559 ) ) ;
#11865=CARTESIAN_POINT ( 'NONE',  ( 11.87812500061451537, -4.541064518000419881, 2.621784821874995952 ) ) ;
#11866=VERTEX_POINT ( 'NONE', #5655 ) ;
#11867=CARTESIAN_POINT ( 'NONE',  ( 6.853125000614516793, 0.000000000000000000, 5.243569643749999010 ) ) ;
#11868=CARTESIAN_POINT ( 'NONE',  ( 6.328125000614515550, 4.541064518000418104, 2.621784821874999949 ) ) ;
#11871=CARTESIAN_POINT ( 'NONE',  ( 15.75000000000000000, -4.330127018922190985, -2.500000000000001332 ) ) ;
#11872=CARTESIAN_POINT ( 'NONE',  ( 15.60937500061451644, -4.541064518000417216, -2.621784821875001281 ) ) ;
#11873=CARTESIAN_POINT ( 'NONE',  ( 11.92500000122903181, 2.886751345948129099, -4.999999999999998224 ) ) ;
#11874=EDGE_CURVE ( 'NONE', #56056, #5140, #50719, .T. ) ;
#11875=CARTESIAN_POINT ( 'NONE',  ( 18.53437500061451715, 4.541064518000418104, 2.621784821874999949 ) ) ;
#11877=CARTESIAN_POINT ( 'NONE',  ( 20.63437500061451857, 6.421520780324663323E-16, -5.243569643749999010 ) ) ;
#11878=CARTESIAN_POINT ( 'NONE',  ( 4.243569643749999010, 13.76562500061451644, -32.45002607614398471 ) ) ;
#11879=CARTESIAN_POINT ( 'NONE',  ( 30.00000000000000000, 0.000000000000000000, 0.000000000000000000 ) ) ;
#11882=CARTESIAN_POINT ( 'NONE',  ( 26.31562500061451715, -6.054752690667223547, -1.112240025338166033E-15 ) ) ;
#11883=CARTESIAN_POINT ( 'NONE',  ( 28.28437500061451715, 6.421520780324663323E-16, -5.243569643749999010 ) ) ;
#11884=CARTESIAN_POINT ( 'NONE',  ( 23.73749999999999716, -2.886751345948129988, 4.999999999999997335 ) ) ;
#11885=EDGE_CURVE ( 'NONE', #54799, #11143, #51078, .T. ) ;
#11886=CARTESIAN_POINT ( 'NONE',  ( 6.028125000614517504, -4.541064518000419881, 2.621784821874995952 ) ) ;
#11888=CARTESIAN_POINT ( 'NONE',  ( 17.89687500061451431, -3.027376345333610441, -5.243569643749999898 ) ) ;
#11890=CARTESIAN_POINT ( 'NONE',  ( 5.353125000614515905, 4.541064518000418104, -2.621784821874998173 ) ) ;
#11891=CARTESIAN_POINT ( 'NONE',  ( 10.28437500061451715, 6.421520780324663323E-16, -5.243569643749999010 ) ) ;
#11892=VERTEX_POINT ( 'NONE', #32090 ) ;
#11893=CARTESIAN_POINT ( 'NONE',  ( 20.33437500061451786, 4.541064518000418104, 2.621784821874999949 ) ) ;
#11894=DIRECTION ( 'NONE',  ( 0.000000000000000000, 0.000000000000000000, 1.000000000000000000 ) ) ;
#11895=CARTESIAN_POINT ( 'NONE',  ( 28.08749999999999858, 5.773502691896255534, 3.535250795749688894E-16 ) ) ;
#11896=CARTESIAN_POINT ( 'NONE',  ( 29.63437500061451502, 6.421520780324663323E-16, -5.243569643749999010 ) ) ;
#11899=ORIENTED_EDGE ( 'NONE', *, *, #26844, .F. ) ;
#11900=CARTESIAN_POINT ( 'NONE',  ( 9.449999999999999289, -4.330127018922190985, -2.500000000000001332 ) ) ;
#11902=CARTESIAN_POINT ( 'NONE',  ( 24.14062500061451289, -3.027376345333610441, -5.243569643749999898 ) ) ;
#11903=CARTESIAN_POINT ( 'NONE',  ( 14.84999999999999964, -4.330127018922190985, -2.500000000000001332 ) ) ;
#11904=ADVANCED_FACE ( 'NONE', ( #3658 ), #49092, .F. ) ;
#11905=CARTESIAN_POINT ( 'NONE',  ( 11.28750000122903252, -4.330127018922194537, 2.499999999999995559 ) ) ;
#11906=CARTESIAN_POINT ( 'NONE',  ( 9.103125000614515017, 0.000000000000000000, 5.243569643749999010 ) ) ;
#11907=CARTESIAN_POINT ( 'NONE',  ( 7.762500000000001954, 2.886751345948129099, -4.999999999999998224 ) ) ;
#11908=DIRECTION ( 'NONE',  ( -1.000000000000000000, -0.000000000000000000, -0.000000000000000000 ) ) ;
#11909=CARTESIAN_POINT ( 'NONE',  ( 29.02500000122903145, 2.886751345948129099, -4.999999999999998224 ) ) ;
#11911=CARTESIAN_POINT ( 'NONE',  ( 7.612500000000000711, -5.773502691896255534, -1.060575238724906372E-15 ) ) ;
#11913=ORIENTED_EDGE ( 'NONE', *, *, #29578, .T. ) ;
#11914=CARTESIAN_POINT ( 'NONE',  ( 21.55312500061451431, 4.541064518000418104, -2.621784821874998173 ) ) ;
#11915=CARTESIAN_POINT ( 'NONE',  ( 29.72812500061451502, 4.541064518000418104, 2.621784821874999949 ) ) ;
#11916=CARTESIAN_POINT ( 'NONE',  ( 28.84687500061452070, 6.054752690667223547, 3.707466751127219781E-16 ) ) ;
#11917=CARTESIAN_POINT ( 'NONE',  ( 19.65937500061451360, -4.541064518000417216, -2.621784821875001281 ) ) ;
#11918=CARTESIAN_POINT ( 'NONE',  ( 17.27812500061451217, -4.541064518000419881, 2.621784821874995952 ) ) ;
#11919=CARTESIAN_POINT ( 'NONE',  ( -4.243569643749998122, 12.64062500061459460, -27.54997392385601174 ) ) ;
#11920=CARTESIAN_POINT ( 'NONE',  ( 4.115625000614516082, 3.027376345333611329, 5.243569643749999010 ) ) ;
#11921=CARTESIAN_POINT ( 'NONE',  ( 28.95000000122903572, -2.886751345948125991, -5.000000000000000000 ) ) ;
#11923=CARTESIAN_POINT ( 'NONE',  ( 19.90312500061451573, 0.000000000000000000, 5.243569643749999010 ) ) ;
#11925=CARTESIAN_POINT ( 'NONE',  ( 3.862500001229035362, 4.330127018922192761, -2.499999999999997780 ) ) ;
#11926=CARTESIAN_POINT ( 'NONE',  ( 13.50937500061451679, 4.541064518000418104, -2.621784821874998173 ) ) ;
#11927=CARTESIAN_POINT ( 'NONE',  ( 13.17187500061451999, 3.027376345333611329, 5.243569643749999010 ) ) ;
#11928=CARTESIAN_POINT ( 'NONE',  ( 20.93437500061451573, -4.541064518000419881, 2.621784821874995952 ) ) ;
#11930=CARTESIAN_POINT ( 'NONE',  ( -5.810221930991193690E-16, 15.83749999999999680, -34.00000000000000000 ) ) ;
#11931=CARTESIAN_POINT ( 'NONE',  ( 25.19062500061451715, 6.054752690667223547, 3.707466751127219781E-16 ) ) ;
#11932=CARTESIAN_POINT ( 'NONE',  ( 17.93437500061451928, 6.421520780324663323E-16, -5.243569643749999010 ) ) ;
#11933=CARTESIAN_POINT ( 'NONE',  ( 24.29062500061451502, 6.054752690667223547, 3.707466751127219781E-16 ) ) ;
#11934=CARTESIAN_POINT ( 'NONE',  ( 27.26249999999999929, 2.886751345948161074, 4.999999999999941380 ) ) ;
#11935=CARTESIAN_POINT ( 'NONE',  ( -3.999999999999999112, 16.85000000000000142, 30.00000000000000000 ) ) ;
#11936=CARTESIAN_POINT ( 'NONE',  ( 3.459375000614519635, -4.541064518000417216, -2.621784821875001281 ) ) ;
#11937=CARTESIAN_POINT ( 'NONE',  ( 11.81250000122903465, -4.330127018922190985, -2.500000000000001332 ) ) ;
#11938=CARTESIAN_POINT ( 'NONE',  ( 7.575000001229033053, 2.886751345948126879, 4.999999999999999112 ) ) ;
#11939=CARTESIAN_POINT ( 'NONE',  ( 28.98750000122903359, 6.123233995736764310E-16, -4.999999999999998224 ) ) ;
#11940=CARTESIAN_POINT ( 'NONE',  ( 26.70000000122903572, -2.886751345948125991, -5.000000000000000000 ) ) ;
#11943=CARTESIAN_POINT ( 'NONE',  ( 10.62187500061451928, -6.054752690667223547, -1.112240025338166033E-15 ) ) ;
#11944=CARTESIAN_POINT ( 'NONE',  ( 1.999999999999998668, 14.90000000000000036, -33.46410161513775705 ) ) ;
#11945=CARTESIAN_POINT ( 'NONE',  ( 16.22812500061451857, 4.541064518000418104, 2.621784821874999949 ) ) ;
#11946=CARTESIAN_POINT ( 'NONE',  ( 13.43437500061451750, 6.421520780324663323E-16, -5.243569643749999010 ) ) ;
#11947=CARTESIAN_POINT ( 'NONE',  ( 3.403125000614518836, -4.541064518000417216, -2.621784821875001281 ) ) ;
#11948=CARTESIAN_POINT ( 'NONE',  ( 19.73437500061451644, 6.421520780324663323E-16, -5.243569643749999010 ) ) ;
#11949=CARTESIAN_POINT ( 'NONE',  ( 8.034375000614518925, 6.421520780324663323E-16, -5.243569643749999010 ) ) ;
#11950=CARTESIAN_POINT ( 'NONE',  ( 3.065625000614517592, 3.027376345333613106, -5.243569643749998122 ) ) ;
#11952=CARTESIAN_POINT ( 'NONE',  ( 11.27812500061451573, 4.541064518000418104, 2.621784821874999949 ) ) ;
#11953=CARTESIAN_POINT ( 'NONE',  ( 19.56562500061451715, -6.054752690667223547, -1.112240025338166033E-15 ) ) ;
#11955=CARTESIAN_POINT ( 'NONE',  ( 4.950000001229033941, -2.886751345948129988, 4.999999999999997335 ) ) ;
#11956=CARTESIAN_POINT ( 'NONE',  ( 16.79062500061451857, -3.027376345333614438, 5.243569643749998122 ) ) ;
#11957=CARTESIAN_POINT ( 'NONE',  ( 12.96562500061451750, 3.027376345333613106, -5.243569643749998122 ) ) ;
#11959=CARTESIAN_POINT ( 'NONE',  ( 12.48750000000000249, -2.886751345948129988, 4.999999999999997335 ) ) ;
#11960=CARTESIAN_POINT ( 'NONE',  ( 8.100000001229034297, -2.886751345948129988, 4.999999999999997335 ) ) ;
#11962=CARTESIAN_POINT ( 'NONE',  ( 5.203125000614518214, -4.541064518000417216, -2.621784821875001281 ) ) ;
#11963=CARTESIAN_POINT ( 'NONE',  ( 18.82500000122903216, 2.886751345948126879, 4.999999999999999112 ) ) ;
#11965=CARTESIAN_POINT ( 'NONE',  ( -4.243569643749999898, 10.40937500061451892, -30.00000000000000000 ) ) ;
#11968=CARTESIAN_POINT ( 'NONE',  ( 3.862500001229035362, 4.330127018922192761, -2.499999999999997780 ) ) ;
#11970=CARTESIAN_POINT ( 'NONE',  ( 18.34687500061451715, -3.027376345333610441, -5.243569643749999898 ) ) ;
#11971=( BOUNDED_CURVE ( )  B_SPLINE_CURVE ( 2, ( #12833, #63078, #17639, #18363, #51278, #24282, #40199, #46830, #2131 ),
 .UNSPECIFIED., .F., .F. ) 
 B_SPLINE_CURVE_WITH_KNOTS ( ( 3, 2, 2, 2, 3 ),
 ( 0.09782608695652174335, 0.1014492753623188470, 0.1086956521739130405, 0.1159420289855072478, 0.1195652173913043514 ),
 .UNSPECIFIED. ) 
 CURVE ( )  GEOMETRIC_REPRESENTATION_ITEM ( )  RATIONAL_B_SPLINE_CURVE ( ( 0.9330127018922194093, 0.9330127018922194093, 1.000000000000000000, 0.8660254037844387076, 1.000000000000000000, 0.8660254037844387076, 1.000000000000000000, 0.9330127018922194093, 0.9330127018922194093 ) ) 
 REPRESENTATION_ITEM ( '' )  );
#11972=CYLINDRICAL_SURFACE ( 'NONE', #30363, 4.999999999999998224 ) ;
#11973=CARTESIAN_POINT ( 'NONE',  ( 17.24062500061451786, -3.027376345333614438, 5.243569643749998122 ) ) ;
#11975=DIRECTION ( 'NONE',  ( 0.000000000000000000, 0.000000000000000000, 1.000000000000000000 ) ) ;
#11976=CARTESIAN_POINT ( 'NONE',  ( 28.99687500061451573, -3.027376345333614438, 5.243569643749998122 ) ) ;
#11977=CARTESIAN_POINT ( 'NONE',  ( 27.04687500061451644, 6.054752690667223547, 3.707466751127219781E-16 ) ) ;
#11979=CARTESIAN_POINT ( 'NONE',  ( 12.59062500061451573, 6.054752690667223547, 3.707466751127219781E-16 ) ) ;
#11980=CARTESIAN_POINT ( 'NONE',  ( 10.13437500061451679, -4.541064518000419881, 2.621784821874995952 ) ) ;
#11982=CARTESIAN_POINT ( 'NONE',  ( 9.487499999999997158, -2.886751345948126435, -5.000000000000000000 ) ) ;
#11983=CARTESIAN_POINT ( 'NONE',  ( 19.41562500061451146, 3.027376345333611329, 5.243569643749999010 ) ) ;
#11984=CARTESIAN_POINT ( 'NONE',  ( 17.70000000122903216, -2.886751345948126435, -5.000000000000000000 ) ) ;
#11986=CARTESIAN_POINT ( 'NONE',  ( 10.01250000000000107, 2.886751345948129099, -4.999999999999998224 ) ) ;
#11987=CARTESIAN_POINT ( 'NONE',  ( 21.30000000122903359, -2.886751345948125991, -5.000000000000000000 ) ) ;
#11988=CARTESIAN_POINT ( 'NONE',  ( 15.21562500061451750, 3.027376345333613106, -5.243569643749998122 ) ) ;
#11991=CARTESIAN_POINT ( 'NONE',  ( 19.87500000000000000, 6.123233995736764310E-16, -4.999999999999998224 ) ) ;
#11992=CARTESIAN_POINT ( 'NONE',  ( 21.15000000000000213, -4.330127018922190985, -2.500000000000001332 ) ) ;
#11993=CARTESIAN_POINT ( 'NONE',  ( 22.17187500061451644, 3.027376345333611329, 5.243569643749999010 ) ) ;
#11994=CARTESIAN_POINT ( 'NONE',  ( 26.01562500061451289, 3.027376345333613106, -5.243569643749998122 ) ) ;
#11995=ORIENTED_EDGE ( 'NONE', *, *, #17977, .F. ) ;
#11997=CARTESIAN_POINT ( 'NONE',  ( 7.303125000614516082, 0.000000000000000000, 5.243569643749999010 ) ) ;
#11998=CARTESIAN_POINT ( 'NONE',  ( 4.000000000000000000, 12.08750000000000036, 32.30940107675849760 ) ) ;
#11999=CARTESIAN_POINT ( 'NONE',  ( 13.98750000000000249, -2.886751345948125991, -5.000000000000000000 ) ) ;
#12000=CARTESIAN_POINT ( 'NONE',  ( 2.121784821875001281, 16.80312500061451786, 33.67503911421598417 ) ) ;
#12001=CARTESIAN_POINT ( 'NONE',  ( 29.05312500061451431, -4.541064518000417216, -2.621784821875001281 ) ) ;
#12002=CARTESIAN_POINT ( 'NONE',  ( 25.80937500061451928, 0.000000000000000000, 5.243569643749999010 ) ) ;
#12004=CARTESIAN_POINT ( 'NONE',  ( 23.31562500061451715, 3.027376345333613106, -5.243569643749998122 ) ) ;
#12005=CARTESIAN_POINT ( 'NONE',  ( 26.10937500061451644, 4.541064518000418104, -2.621784821874998173 ) ) ;
#12006=CARTESIAN_POINT ( 'NONE',  ( 4.243569643749999898, 17.77812500061459389, -30.00000000000000000 ) ) ;
#12007=CARTESIAN_POINT ( 'NONE',  ( 10.95000000000000107, 4.330127018922192761, -2.499999999999997780 ) ) ;
#12008=CARTESIAN_POINT ( 'NONE',  ( 9.178125000614517859, -4.541064518000419881, 2.621784821874995952 ) ) ;
#12010=CARTESIAN_POINT ( 'NONE',  ( 29.80312500061451431, 0.000000000000000000, 5.243569643749999010 ) ) ;
#12011=CARTESIAN_POINT ( 'NONE',  ( 26.20312500061451644, 0.000000000000000000, 5.243569643749999010 ) ) ;
#12014=CARTESIAN_POINT ( 'NONE',  ( 18.75937500061451857, -4.541064518000417216, -2.621784821875001281 ) ) ;
#12015=CARTESIAN_POINT ( 'NONE',  ( -3.000416591977282496E-16, 12.09687500061451715, 25.09994784771203058 ) ) ;
#12016=CARTESIAN_POINT ( 'NONE',  ( 20.29687500061451644, 6.054752690667223547, 3.707466751127219781E-16 ) ) ;
#12017=CARTESIAN_POINT ( 'NONE',  ( 26.85937500061451644, -4.541064518000417216, -2.621784821875001281 ) ) ;
#12018=CARTESIAN_POINT ( 'NONE',  ( -4.243569643749999898, 16.22187500061452070, 27.54997392385601529 ) ) ;
#12019=CARTESIAN_POINT ( 'NONE',  ( 6.965625000614518392, -6.054752690667223547, -1.112240025338166033E-15 ) ) ;
#12020=CARTESIAN_POINT ( 'NONE',  ( -6.275039685470489619E-15, 18.31250000000000000, -26.00000000000000355 ) ) ;
#12021=CARTESIAN_POINT ( 'NONE',  ( 5.071875000614519458, 3.027376345333611329, 5.243569643749999010 ) ) ;
#12022=CARTESIAN_POINT ( 'NONE',  ( -1.071796769724483234, 15.97009619066136565, -34.00000000000000711 ) ) ;
#12023=CARTESIAN_POINT ( 'NONE',  ( 6.965625000614518392, -6.054752690667223547, -1.112240025338166033E-15 ) ) ;
#12024=CARTESIAN_POINT ( 'NONE',  ( 12.79687500061451821, -3.027376345333614438, 5.243569643749998122 ) ) ;
#12025=CARTESIAN_POINT ( 'NONE',  ( 19.57500000122903216, 2.886751345948129099, -4.999999999999998224 ) ) ;
#12026=CARTESIAN_POINT ( 'NONE',  ( 6.159375000614517148, -4.541064518000417216, -2.621784821875001281 ) ) ;
#12027=CARTESIAN_POINT ( 'NONE',  ( 7.415625000614516793, -6.054752690667223547, -1.112240025338166033E-15 ) ) ;
#12028=CARTESIAN_POINT ( 'NONE',  ( 5.203125000614518214, -4.541064518000417216, -2.621784821875001281 ) ) ;
#12030=CARTESIAN_POINT ( 'NONE',  ( 15.79687500061451821, 6.054752690667223547, 3.707466751127219781E-16 ) ) ;
#12031=CARTESIAN_POINT ( 'NONE',  ( 19.53750000122903430, 6.123233995736764310E-16, -4.999999999999998224 ) ) ;
#12032=ORIENTED_EDGE ( 'NONE', *, *, #3723, .F. ) ;
#12033=CARTESIAN_POINT ( 'NONE',  ( 24.32812500061451289, 4.541064518000418104, 2.621784821874999949 ) ) ;
#12034=CARTESIAN_POINT ( 'NONE',  ( 8.990625000614516082, 6.054752690667223547, 3.707466751127219781E-16 ) ) ;
#12035=CARTESIAN_POINT ( 'NONE',  ( 28.05937500061451573, 0.000000000000000000, 5.243569643749999010 ) ) ;
#12036=CARTESIAN_POINT ( 'NONE',  ( 11.01562500061451821, -6.054752690667223547, -1.112240025338166033E-15 ) ) ;
#12038=CARTESIAN_POINT ( 'NONE',  ( 13.98750000122903359, -4.330127018922194537, 2.499999999999995559 ) ) ;
#12040=CARTESIAN_POINT ( 'NONE',  ( 27.66562500061451146, -6.054752690667223547, -1.112240025338166033E-15 ) ) ;
#12041=VECTOR ( 'NONE', #69183, 1000.000000000000000 ) ;
#12042=CARTESIAN_POINT ( 'NONE',  ( -4.243569643749999898, 12.11562500061451608, -32.45002607614398471 ) ) ;
#12043=CARTESIAN_POINT ( 'NONE',  ( 13.42500000122903536, 2.886751345948126879, 4.999999999999999112 ) ) ;
#12044=CARTESIAN_POINT ( 'NONE',  ( 11.13750000000000284, -2.886751345948129988, 4.999999999999997335 ) ) ;
#12045=CARTESIAN_POINT ( 'NONE',  ( 19.64062500061451644, -3.027376345333610441, -5.243569643749999898 ) ) ;
#12046=CARTESIAN_POINT ( 'NONE',  ( 8.746875000614515727, -3.027376345333614438, 5.243569643749998122 ) ) ;
#12047=CARTESIAN_POINT ( 'NONE',  ( 20.32499999999999929, 6.123233995736764310E-16, -4.999999999999998224 ) ) ;
#12048=CARTESIAN_POINT ( 'NONE',  ( 7.237500001229035362, -4.330127018922194537, 2.499999999999995559 ) ) ;
#12049=CARTESIAN_POINT ( 'NONE',  ( 15.82500000122903216, -5.773502691896255534, -1.060575238724906372E-15 ) ) ;
#12050=CARTESIAN_POINT ( 'NONE',  ( 12.74062500061451786, -3.027376345333614438, 5.243569643749998122 ) ) ;
#12051=CARTESIAN_POINT ( 'NONE',  ( 15.77812500061451573, 4.541064518000418104, 2.621784821874999949 ) ) ;
#12052=CARTESIAN_POINT ( 'NONE',  ( 24.48750000122903359, 6.123233995736764310E-16, -4.999999999999998224 ) ) ;
#12053=CARTESIAN_POINT ( 'NONE',  ( 21.03750000000000142, -2.886751345948129988, 4.999999999999997335 ) ) ;
#12054=CARTESIAN_POINT ( 'NONE',  ( 23.18437500061451573, -4.541064518000419881, 2.621784821874995952 ) ) ;
#12055=CARTESIAN_POINT ( 'NONE',  ( 25.61250000122903359, 0.000000000000000000, 4.999999999999998224 ) ) ;
#12056=EDGE_CURVE ( 'NONE', #6778, #36605, #29871, .T. ) ;
#12057=CARTESIAN_POINT ( 'NONE',  ( 9.300000001229035362, 5.773502691896255534, 3.535250795749688894E-16 ) ) ;
#12058=CARTESIAN_POINT ( 'NONE',  ( 9.121875000614517504, 3.027376345333611329, 5.243569643749999010 ) ) ;
#12059=CARTESIAN_POINT ( 'NONE',  ( 25.28437500061451715, 4.541064518000418104, 2.621784821874999949 ) ) ;
#12060=CARTESIAN_POINT ( 'NONE',  ( 4.241234947910677455, -2.648004176096003803, -4.329066063250716745 ) ) ;
#12061=CARTESIAN_POINT ( 'NONE',  ( 24.36562500061451786, 3.027376345333611329, 5.243569643749999010 ) ) ;
#12062=CARTESIAN_POINT ( 'NONE',  ( 27.00937500061451857, 4.541064518000418104, -2.621784821874998173 ) ) ;
#12065=CARTESIAN_POINT ( 'NONE',  ( 9.009375000614518569, 4.541064518000418104, -2.621784821874998173 ) ) ;
#12066=CARTESIAN_POINT ( 'NONE',  ( 4.411272977760241965, 2.353862934769528792, -4.685547128476531320 ) ) ;
#12067=CARTESIAN_POINT ( 'NONE',  ( 28.67812500061451431, 6.421520780324663323E-16, -5.243569643749999010 ) ) ;
#12068=CARTESIAN_POINT ( 'NONE',  ( 5.934375000614517504, 4.541064518000418104, 2.621784821874999949 ) ) ;
#12069=CARTESIAN_POINT ( 'NONE',  ( -1.071796769724483234, 16.42009619066137205, -34.00000000000000711 ) ) ;
#12070=CARTESIAN_POINT ( 'NONE',  ( 25.39687500061451431, -3.027376345333614438, 5.243569643749998122 ) ) ;
#12071=EDGE_CURVE ( 'NONE', #60642, #58564, #7846, .T. ) ;
#12072=CARTESIAN_POINT ( 'NONE',  ( 4.243569643749999010, 11.06562500061459531, 27.54997392385601174 ) ) ;
#12073=CARTESIAN_POINT ( 'NONE',  ( 18.07499999999999929, 6.123233995736764310E-16, -4.999999999999998224 ) ) ;
#12075=CARTESIAN_POINT ( 'NONE',  ( 26.28749999999999432, 5.773502691896255534, 3.535250795749688894E-16 ) ) ;
#12076=CARTESIAN_POINT ( 'NONE',  ( 29.40937500061451715, 0.000000000000000000, 5.243569643749999010 ) ) ;
#12078=VECTOR ( 'NONE', #71891, 1000.000000000000000 ) ;
#12079=CARTESIAN_POINT ( 'NONE',  ( 16.07812500061451289, 6.421520780324663323E-16, -5.243569643749999010 ) ) ;
#12080=CARTESIAN_POINT ( 'NONE',  ( 6.140625000614516438, -3.027376345333610441, -5.243569643749999898 ) ) ;
#12082=CARTESIAN_POINT ( 'NONE',  ( 5.146875000614517859, -3.027376345333614438, 5.243569643749998122 ) ) ;
#12083=CARTESIAN_POINT ( 'NONE',  ( 16.01250000122903216, 4.330127018922192761, -2.499999999999997780 ) ) ;
#12084=CARTESIAN_POINT ( 'NONE',  ( 21.63749999999999929, -2.886751345948125991, -5.000000000000000000 ) ) ;
#12085=CARTESIAN_POINT ( 'NONE',  ( 29.92500000000000071, 4.330127018922191873, 2.499999999999999556 ) ) ;
#12086=CARTESIAN_POINT ( 'NONE',  ( 4.621875000614516615, 3.027376345333611329, 5.243569643749999010 ) ) ;
#12087=CARTESIAN_POINT ( 'NONE',  ( 10.39687500061451786, 6.054752690667223547, 3.707466751127219781E-16 ) ) ;
#12088=CARTESIAN_POINT ( 'NONE',  ( 21.19687500061451502, 6.054752690667223547, 3.707466751127219781E-16 ) ) ;
#12089=LINE ( 'NONE', #23525, #8826 ) ;
#12090=ORIENTED_EDGE ( 'NONE', *, *, #56574, .T. ) ;
#12091=CARTESIAN_POINT ( 'NONE',  ( 4.059375000614519280, 4.541064518000418104, -2.621784821874998173 ) ) ;
#12092=CARTESIAN_POINT ( 'NONE',  ( 7.996875000614519280, -3.027376345333610441, -5.243569643749999898 ) ) ;
#12093=CARTESIAN_POINT ( 'NONE',  ( 17.55000000000000071, -4.330127018922190985, -2.500000000000001332 ) ) ;
#12094=CARTESIAN_POINT ( 'NONE',  ( 16.60312500061451857, 4.541064518000418104, -2.621784821874998173 ) ) ;
#12096=CARTESIAN_POINT ( 'NONE',  ( -2.000000000000000000, 19.92500000000000071, 26.53589838486224650 ) ) ;
#12098=CARTESIAN_POINT ( 'NONE',  ( 10.67812500061451608, 6.421520780324663323E-16, -5.243569643749999010 ) ) ;
#12099=CARTESIAN_POINT ( 'NONE',  ( 25.50937500061451502, -4.541064518000417216, -2.621784821875001281 ) ) ;
#12101=CARTESIAN_POINT ( 'NONE',  ( 25.32187500061451857, 3.027376345333611329, 5.243569643749999010 ) ) ;
#12102=CARTESIAN_POINT ( 'NONE',  ( 7.575000000000001954, -4.330127018922194537, 2.499999999999995559 ) ) ;
#12103=CARTESIAN_POINT ( 'NONE',  ( 8.484601909799253346E-16, 12.12500000122903465, 34.61880215351700230 ) ) ;
#12104=CARTESIAN_POINT ( 'NONE',  ( 6.637500001229035718, 4.330127018922191873, 2.499999999999999556 ) ) ;
#12105=CARTESIAN_POINT ( 'NONE',  ( 19.35937500061451644, 4.541064518000418104, -2.621784821874998173 ) ) ;
#12106=CARTESIAN_POINT ( 'NONE',  ( 10.62187500061451928, -6.054752690667223547, -1.112240025338166033E-15 ) ) ;
#12107=CARTESIAN_POINT ( 'NONE',  ( -3.992479141629562633, 3.010095094815111505, -29.71890115206955585 ) ) ;
#12109=CARTESIAN_POINT ( 'NONE',  ( 14.72812500061451679, 6.421520780324663323E-16, -5.243569643749999010 ) ) ;
#12110=CARTESIAN_POINT ( 'NONE',  ( 27.11250000122903359, -4.330127018922190985, -2.500000000000001332 ) ) ;
#12111=CARTESIAN_POINT ( 'NONE',  ( 12.94687500061451857, -3.027376345333610441, -5.243569643749999898 ) ) ;
#12112=CARTESIAN_POINT ( 'NONE',  ( 3.821851807532226530, -4.035565604595362288, 3.497334623063416803 ) ) ;
#12113=CARTESIAN_POINT ( 'NONE',  ( 14.16562500061451679, -6.054752690667223547, -1.112240025338166033E-15 ) ) ;
#12114=DIRECTION ( 'NONE',  ( -1.000000000000000000, -0.000000000000000000, -0.000000000000000000 ) ) ;
#12115=CARTESIAN_POINT ( 'NONE',  ( 25.88437500061451502, -4.541064518000419881, 2.621784821874995952 ) ) ;
#12116=CARTESIAN_POINT ( 'NONE',  ( -2.121784821874999949, 10.27812500061451750, 26.32496088578401938 ) ) ;
#12117=CARTESIAN_POINT ( 'NONE',  ( 12.11250000122903181, 0.000000000000000000, 4.999999999999998224 ) ) ;
#12119=CARTESIAN_POINT ( 'NONE',  ( 4.243569643749999898, 17.83437500061451786, -30.00000000000000000 ) ) ;
#12120=CARTESIAN_POINT ( 'NONE',  ( 18.57187500061451857, 3.027376345333611329, 5.243569643749999010 ) ) ;
#12121=CARTESIAN_POINT ( 'NONE',  ( 19.20000000122903572, 5.773502691896255534, 3.535250795749688894E-16 ) ) ;
#12122=CARTESIAN_POINT ( 'NONE',  ( 15.49687500061451750, -3.027376345333614438, 5.243569643749998122 ) ) ;
#12123=CARTESIAN_POINT ( 'NONE',  ( 23.06250000122903288, -4.330127018922190985, -2.500000000000001332 ) ) ;
#12124=CARTESIAN_POINT ( 'NONE',  ( 15.77812500061451573, 4.541064518000418104, 2.621784821874999949 ) ) ;
#12125=CARTESIAN_POINT ( 'NONE',  ( 29.16562500061451502, 3.027376345333613106, -5.243569643749998122 ) ) ;
#12126=ORIENTED_EDGE ( 'NONE', *, *, #63735, .T. ) ;
#12127=ORIENTED_EDGE ( 'NONE', *, *, #32319, .T. ) ;
#12128=CARTESIAN_POINT ( 'NONE',  ( 17.55000000000000071, -4.330127018922190985, -2.500000000000001332 ) ) ;
#12130=CARTESIAN_POINT ( 'NONE',  ( 2.990625000614519191, -3.027376345333610441, -5.243569643749999898 ) ) ;
#12131=CARTESIAN_POINT ( 'NONE',  ( 16.05000000122903359, 5.773502691896255534, 3.535250795749688894E-16 ) ) ;
#12132=CARTESIAN_POINT ( 'NONE',  ( 20.84062500061451573, -3.027376345333614438, 5.243569643749998122 ) ) ;
#12134=ADVANCED_FACE ( 'NONE', ( #54262 ), #31726, .F. ) ;
#12135=CARTESIAN_POINT ( 'NONE',  ( 24.21562500061451573, 3.027376345333613106, -5.243569643749998122 ) ) ;
#12136=CARTESIAN_POINT ( 'NONE',  ( 3.515625000614516882, 3.027376345333613106, -5.243569643749998122 ) ) ;
#12137=CARTESIAN_POINT ( 'NONE',  ( 27.29999999999999716, 0.000000000000000000, 4.999999999999998224 ) ) ;
#12138=CARTESIAN_POINT ( 'NONE',  ( 4.603329117574985752, 1.951758446961684434, -4.603329117574985752 ) ) ;
#12140=DIRECTION ( 'NONE',  ( -0.000000000000000000, -1.000000000000000000, -0.000000000000000000 ) ) ;
#12141=CARTESIAN_POINT ( 'NONE',  ( 8.484601909799253346E-16, 12.12500000122903465, -25.38119784648299770 ) ) ;
#12142=CARTESIAN_POINT ( 'NONE',  ( -2.121784821874999949, 15.28437500061451892, -33.67503911421598417 ) ) ;
#12143=CARTESIAN_POINT ( 'NONE',  ( 5.550000001229032698, -2.886751345948125991, -5.000000000000000000 ) ) ;
#12144=CARTESIAN_POINT ( 'NONE',  ( 7.762500000000001954, 2.886751345948129099, -4.999999999999998224 ) ) ;
#12145=CARTESIAN_POINT ( 'NONE',  ( 4.500000001229034652, -2.886751345948129988, 4.999999999999997335 ) ) ;
#12146=CARTESIAN_POINT ( 'NONE',  ( 8.971875000614515372, 3.027376345333613106, -5.243569643749998122 ) ) ;
#12147=CARTESIAN_POINT ( 'NONE',  ( 4.171875000614517326, 3.027376345333611329, 5.243569643749999010 ) ) ;
#12148=DIRECTION ( 'NONE',  ( -0.000000000000000000, -1.000000000000000000, -0.000000000000000000 ) ) ;
#12149=DIRECTION ( 'NONE',  ( -1.000000000000000000, -0.000000000000000000, -0.000000000000000000 ) ) ;
#12150=CARTESIAN_POINT ( 'NONE',  ( 7.959375000614516971, -4.541064518000417216, -2.621784821875001281 ) ) ;
#12151=CARTESIAN_POINT ( 'NONE',  ( 12.64687500061451608, 6.054752690667223547, 3.707466751127219781E-16 ) ) ;
#12153=CARTESIAN_POINT ( 'NONE',  ( 6.975000000000002309, 4.330127018922191873, 2.499999999999999556 ) ) ;
#12154=CARTESIAN_POINT ( 'NONE',  ( 2.121784821874999061, 17.40312500061459744, 26.32496088578401583 ) ) ;
#12155=CARTESIAN_POINT ( 'NONE',  ( 22.09687500061451715, 6.054752690667223547, 3.707466751127219781E-16 ) ) ;
#12156=CARTESIAN_POINT ( 'NONE',  ( 26.06250000122903288, 0.000000000000000000, 4.999999999999998224 ) ) ;
#12158=CARTESIAN_POINT ( 'NONE',  ( 23.46562500061451573, 3.027376345333611329, 5.243569643749999010 ) ) ;
#12159=CARTESIAN_POINT ( 'NONE',  ( 16.49062500061451786, -3.027376345333610441, -5.243569643749999898 ) ) ;
#12161=CARTESIAN_POINT ( 'NONE',  ( 12.90937500061451537, -4.541064518000417216, -2.621784821875001281 ) ) ;
#12162=CARTESIAN_POINT ( 'NONE',  ( 28.46249999999999858, 2.886751345948129099, -4.999999999999998224 ) ) ;
#12163=CARTESIAN_POINT ( 'NONE',  ( 25.23750000122903359, -4.330127018922194537, 2.499999999999995559 ) ) ;
#12165=CARTESIAN_POINT ( 'NONE',  ( 11.74687500061451573, 6.054752690667223547, 3.707466751127219781E-16 ) ) ;
#12167=CARTESIAN_POINT ( 'NONE',  ( 3.909375000614518481, -4.541064518000417216, -2.621784821875001281 ) ) ;
#12169=CARTESIAN_POINT ( 'NONE',  ( 16.65000000122903501, -2.886751345948096681, 5.000000000000054179 ) ) ;
#12170=CARTESIAN_POINT ( 'NONE',  ( 22.50937500061451857, 4.541064518000418104, -2.621784821874998173 ) ) ;
#12171=CARTESIAN_POINT ( 'NONE',  ( 13.28437500061451715, -4.541064518000419881, 2.621784821874995952 ) ) ;
#12173=CARTESIAN_POINT ( 'NONE',  ( 25.94999999999999929, 0.000000000000000000, 4.999999999999998224 ) ) ;
#12176=CARTESIAN_POINT ( 'NONE',  ( 17.76562500061451644, -6.054752690667223547, -1.112240025338166033E-15 ) ) ;
#12177=CARTESIAN_POINT ( 'NONE',  ( 7.012500000000001066, 2.886751345948126879, 4.999999999999999112 ) ) ;
#12178=CARTESIAN_POINT ( 'NONE',  ( 1.071796769724491893, 13.49509619066136779, 33.99999999999999289 ) ) ;
#12179=( BOUNDED_CURVE ( )  B_SPLINE_CURVE ( 2, ( #11352, #33870, #61948, #57120, #29065, #1001, #23508 ),
 .UNSPECIFIED., .F., .F. ) 
 B_SPLINE_CURVE_WITH_KNOTS ( ( 3, 2, 2, 3 ),
 ( 0.1499999999999999389, 0.1527777777777777624, 0.1555555555555555858, 0.1583333333333333814 ),
 .UNSPECIFIED. ) 
 CURVE ( )  GEOMETRIC_REPRESENTATION_ITEM ( )  RATIONAL_B_SPLINE_CURVE ( ( 1.000000000000002665, 0.8660254037844360431, 1.000000000000000000, 0.8660254037844387076, 1.000000000000000000, 0.8660254037844360431, 1.000000000000002665 ) ) 
 REPRESENTATION_ITEM ( '' )  );
#12180=CARTESIAN_POINT ( 'NONE',  ( 14.81250000000000000, -5.773502691896255534, -1.060575238724906372E-15 ) ) ;
#12181=CARTESIAN_POINT ( 'NONE',  ( 2.121784821875001281, 10.05312500061451608, 33.67503911421598417 ) ) ;
#12182=CYLINDRICAL_SURFACE ( 'NONE', #64334, 4.999999999999998224 ) ;
#12183=CARTESIAN_POINT ( 'NONE',  ( 26.74687500061451573, -3.027376345333614438, 5.243569643749998122 ) ) ;
#12185=CARTESIAN_POINT ( 'NONE',  ( 21.40312500061451573, -4.541064518000417216, -2.621784821875001281 ) ) ;
#12186=CARTESIAN_POINT ( 'NONE',  ( 20.93437500061451573, -4.541064518000419881, 2.621784821874995952 ) ) ;
#12187=CARTESIAN_POINT ( 'NONE',  ( 4.349999999999999645, 0.000000000000000000, 4.999999999999998224 ) ) ;
#12188=CARTESIAN_POINT ( 'NONE',  ( 6.065625000614516260, -6.054752690667223547, -1.112240025338166033E-15 ) ) ;
#12189=CARTESIAN_POINT ( 'NONE',  ( 25.04062500061451502, -3.027376345333610441, -5.243569643749999898 ) ) ;
#12190=CARTESIAN_POINT ( 'NONE',  ( 11.63437500061451857, 6.421520780324663323E-16, -5.243569643749999010 ) ) ;
#12191=CARTESIAN_POINT ( 'NONE',  ( 16.92187500061451999, -6.054752690667223547, -1.112240025338166033E-15 ) ) ;
#12192=CARTESIAN_POINT ( 'NONE',  ( 4.243569643749999898, 18.22812500061451502, 30.00000000000000000 ) ) ;
#12193=CARTESIAN_POINT ( 'NONE',  ( 18.90000000122902790, -2.886751345948129988, 4.999999999999997335 ) ) ;
#12195=CARTESIAN_POINT ( 'NONE',  ( 8.915625000614515017, 3.027376345333612662, -5.243569643749998122 ) ) ;
#12196=CARTESIAN_POINT ( 'NONE',  ( 4.771875000614516971, -6.054752690667223547, -1.112240025338166033E-15 ) ) ;
#12197=CARTESIAN_POINT ( 'NONE',  ( 4.509375000614518569, 4.541064518000418104, -2.621784821874998173 ) ) ;
#12199=CARTESIAN_POINT ( 'NONE',  ( 26.14687500061451431, 6.054752690667223547, 3.707466751127219781E-16 ) ) ;
#12200=CARTESIAN_POINT ( 'NONE',  ( 17.24062500061451786, -3.027376345333614438, 5.243569643749998122 ) ) ;
#12201=CARTESIAN_POINT ( 'NONE',  ( 28.35000000122903430, -2.886751345948129988, 4.999999999999997335 ) ) ;
#12202=CARTESIAN_POINT ( 'NONE',  ( 27.17812500061451786, -4.541064518000419881, 2.621784821874995952 ) ) ;
#12203=CARTESIAN_POINT ( 'NONE',  ( 21.15937500061451715, 4.541064518000418104, -2.621784821874998173 ) ) ;
#12204=CARTESIAN_POINT ( 'NONE',  ( 17.01562500061451644, 3.027376345333613106, -5.243569643749998122 ) ) ;
#12205=CARTESIAN_POINT ( 'NONE',  ( 4.243569643749999898, 16.44687500061451857, 32.45002607614398471 ) ) ;
#12206=CARTESIAN_POINT ( 'NONE',  ( 21.40312500061451573, -4.541064518000417216, -2.621784821875001281 ) ) ;
#12207=CARTESIAN_POINT ( 'NONE',  ( 30.00000000000000000, 0.000000000000000000, 4.999999999999998224 ) ) ;
#12209=CARTESIAN_POINT ( 'NONE',  ( 28.31250000000000000, -5.773502691896255534, -1.060575238724906372E-15 ) ) ;
#12210=CARTESIAN_POINT ( 'NONE',  ( -3.999999999999999556, 14.11249999999999893, -32.30940107675850470 ) ) ;
#12212=CARTESIAN_POINT ( 'NONE',  ( 28.30312500061451431, 4.541064518000418104, -2.621784821874998173 ) ) ;
#12213=CARTESIAN_POINT ( 'NONE',  ( 11.05312500061451608, -4.541064518000417216, -2.621784821875001281 ) ) ;
#12214=CARTESIAN_POINT ( 'NONE',  ( 21.33750000122903145, 6.123233995736764310E-16, -4.999999999999998224 ) ) ;
#12215=CARTESIAN_POINT ( 'NONE',  ( 28.04062500061451502, -3.027376345333614438, 5.243569643749998122 ) ) ;
#12216=CARTESIAN_POINT ( 'NONE',  ( 28.31250000000000000, -5.773502691896255534, -1.060575238724906372E-15 ) ) ;
#12218=CARTESIAN_POINT ( 'NONE',  ( -3.999999999999999112, 18.31250000122903288, -30.00000000000000000 ) ) ;
#12219=PLANE ( 'NONE',  #4353 ) ;
#12220=CARTESIAN_POINT ( 'NONE',  ( 10.82812500061451644, 4.541064518000418104, 2.621784821874999949 ) ) ;
#12222=CARTESIAN_POINT ( 'NONE',  ( 7.865625000614516971, -6.054752690667223547, -1.112240025338166033E-15 ) ) ;
#12224=CARTESIAN_POINT ( 'NONE',  ( 7.003125000614518036, -4.541064518000417216, -2.621784821875001281 ) ) ;
#12227=CARTESIAN_POINT ( 'NONE',  ( 14.51250000000000107, 2.886751345948129099, -4.999999999999998224 ) ) ;
#12228=CARTESIAN_POINT ( 'NONE',  ( 16.35937500061451644, 0.000000000000000000, 5.243569643749999010 ) ) ;
#12229=CARTESIAN_POINT ( 'NONE',  ( 11.62500000122903465, 2.886751345948126879, 4.999999999999999112 ) ) ;
#12230=CARTESIAN_POINT ( 'NONE',  ( 18.68437500061451928, -4.541064518000419881, 2.621784821874995952 ) ) ;
#12232=CARTESIAN_POINT ( 'NONE',  ( 21.57187500061451502, 3.027376345333613106, -5.243569643749998122 ) ) ;
#12233=CARTESIAN_POINT ( 'NONE',  ( -4.243569643749999898, 14.36562500061451786, -32.45002607614398471 ) ) ;
#12234=CARTESIAN_POINT ( 'NONE',  ( 21.11250000122903359, 0.000000000000000000, 4.999999999999998224 ) ) ;
#12236=CARTESIAN_POINT ( 'NONE',  ( 4.000000000000000000, 11.63750000000000284, -27.69059892324149885 ) ) ;
#12237=CARTESIAN_POINT ( 'NONE',  ( 27.14062500061451644, -3.027376345333614438, 5.243569643749998122 ) ) ;
#12238=CARTESIAN_POINT ( 'NONE',  ( 24.93750000000000000, 5.773502691896255534, 3.535250795749688401E-16 ) ) ;
#12239=CARTESIAN_POINT ( 'NONE',  ( 28.88437500061451502, 4.541064518000418104, 2.621784821874999949 ) ) ;
#12240=CARTESIAN_POINT ( 'NONE',  ( 23.62500000000000000, 4.330127018922191873, 2.499999999999999556 ) ) ;
#12241=B_SPLINE_CURVE_WITH_KNOTS ( 'NONE', 3,
 ( #6095, #66331, #34158, #55255, #61511, #67795, #49714, #72972, #4651, #38629 ),
 .UNSPECIFIED., .F., .F.,
 ( 4, 3, 3, 4 ),
 ( 6.133173666733496745E-19, 7.861287778095982833E-05, 0.0001572259190930990044, 0.0002915343808913384120 ),
 .UNSPECIFIED. ) ;
#12242=CARTESIAN_POINT ( 'NONE',  ( 7.378125000614518036, -4.541064518000419881, 2.621784821874995952 ) ) ;
#12244=CARTESIAN_POINT ( 'NONE',  ( 19.73437500061451644, 6.421520780324663323E-16, -5.243569643749999010 ) ) ;
#12246=CARTESIAN_POINT ( 'NONE',  ( 4.678125000614516971, -4.541064518000419881, 2.621784821874995952 ) ) ;
#12247=CARTESIAN_POINT ( 'NONE',  ( 8.859375000614518214, -4.541064518000417216, -2.621784821875001281 ) ) ;
#12249=CARTESIAN_POINT ( 'NONE',  ( 20.14687500061451786, -3.027376345333610441, -5.243569643749999898 ) ) ;
#12250=CARTESIAN_POINT ( 'NONE',  ( 13.91250000122903252, 0.000000000000000000, 4.999999999999998224 ) ) ;
#12251=CARTESIAN_POINT ( 'NONE',  ( 28.19999999999999929, 0.000000000000000000, 4.999999999999998224 ) ) ;
#12252=CARTESIAN_POINT ( 'NONE',  ( 3.000000000000002665, 0.000000000000000000, 4.999999999999998224 ) ) ;
#12255=VERTEX_POINT ( 'NONE', #42808 ) ;
#12256=CARTESIAN_POINT ( 'NONE',  ( 10.80000000000000071, -4.330127018922190985, -2.500000000000001332 ) ) ;
#12258=CARTESIAN_POINT ( 'NONE',  ( 24.89062500061451644, -3.027376345333614438, 5.243569643749998122 ) ) ;
#12259=CARTESIAN_POINT ( 'NONE',  ( 13.87500000000000178, -4.330127018922194537, 2.499999999999995559 ) ) ;
#12261=CARTESIAN_POINT ( 'NONE',  ( 11.70000000122903216, -2.886751345948129988, 4.999999999999997335 ) ) ;
#12262=CARTESIAN_POINT ( 'NONE',  ( 9.253125000614517148, -4.541064518000417216, -2.621784821875001281 ) ) ;
#12263=CARTESIAN_POINT ( 'NONE',  ( 23.25000000000000000, 0.000000000000000000, 4.999999999999998224 ) ) ;
#12264=CARTESIAN_POINT ( 'NONE',  ( 21.85312500061451502, -4.541064518000417216, -2.621784821875001281 ) ) ;
#12266=CARTESIAN_POINT ( 'NONE',  ( 27.71250000122903145, 4.330127018922192761, -2.499999999999997780 ) ) ;
#12268=CARTESIAN_POINT ( 'NONE',  ( 6.862500000000002487, 2.886751345948129099, -4.999999999999998224 ) ) ;
#12269=VERTEX_POINT ( 'NONE', #13990 ) ;
#12270=CARTESIAN_POINT ( 'NONE',  ( 21.74062500061451431, -3.027376345333614438, 5.243569643749998122 ) ) ;
#12271=CARTESIAN_POINT ( 'NONE',  ( 28.11562500061451431, -6.054752690667223547, -1.112240025338166033E-15 ) ) ;
#12273=CARTESIAN_POINT ( 'NONE',  ( 18.68437500061451928, -4.541064518000419881, 2.621784821874995952 ) ) ;
#12274=CARTESIAN_POINT ( 'NONE',  ( 14.61562500061451608, -6.054752690667223547, -1.112240025338166033E-15 ) ) ;
#12275=DIRECTION ( 'NONE',  ( 1.000000000000000000, 0.000000000000000000, 0.000000000000000000 ) ) ;
#12276=CARTESIAN_POINT ( 'NONE',  ( 26.40000000122902790, 5.773502691896255534, 3.535250795749688894E-16 ) ) ;
#12278=CARTESIAN_POINT ( 'NONE',  ( 16.04062500061451857, -3.027376345333610441, -5.243569643749999898 ) ) ;
#12279=CARTESIAN_POINT ( 'NONE',  ( 4.312500001229034652, 4.330127018922192761, -2.499999999999997780 ) ) ;
#12280=CARTESIAN_POINT ( 'NONE',  ( 12.00937500061451857, -4.541064518000417216, -2.621784821875001281 ) ) ;
#12281=CARTESIAN_POINT ( 'NONE',  ( 12.27187500061451786, 3.027376345333611329, 5.243569643749999010 ) ) ;
#12282=CARTESIAN_POINT ( 'NONE',  ( 19.28437500061451360, 6.421520780324663323E-16, -5.243569643749999010 ) ) ;
#12283=ORIENTED_EDGE ( 'NONE', *, *, #24627, .T. ) ;
#12284=CARTESIAN_POINT ( 'NONE',  ( -5.378075516623670893, 8.432637420806665673, 32.68862326928266526 ) ) ;
#12285=CARTESIAN_POINT ( 'NONE',  ( 25.15312500061451217, 4.541064518000418104, -2.621784821874998173 ) ) ;
#12286=CARTESIAN_POINT ( 'NONE',  ( 18.79687500061451644, -3.027376345333610441, -5.243569643749999898 ) ) ;
#12287=CARTESIAN_POINT ( 'NONE',  ( 25.49062500061451786, -3.027376345333610441, -5.243569643749999898 ) ) ;
#12288=CARTESIAN_POINT ( 'NONE',  ( 30.00000000000000000, 0.000000000000000000, 4.999999999999998224 ) ) ;
#12289=CARTESIAN_POINT ( 'NONE',  ( 3.999999999999999112, 16.17500000000000071, 30.00000000000000000 ) ) ;
#12291=CARTESIAN_POINT ( 'NONE',  ( 28.71562500061451573, 3.027376345333613106, -5.243569643749998122 ) ) ;
#12292=CARTESIAN_POINT ( 'NONE',  ( 10.68750000122903288, 4.330127018922191873, 2.499999999999999556 ) ) ;
#12293=CARTESIAN_POINT ( 'NONE',  ( 5.812500001229035540, 0.000000000000000000, 4.999999999999998224 ) ) ;
#12294=CARTESIAN_POINT ( 'NONE',  ( 3.999999999999998668, 19.81250000000000000, -32.30940107675850470 ) ) ;
#12295=CARTESIAN_POINT ( 'NONE',  ( 26.96250000122903145, 0.000000000000000000, 4.999999999999998224 ) ) ;
#12298=CARTESIAN_POINT ( 'NONE',  ( 9.084375000614517859, 4.541064518000418104, 2.621784821874999949 ) ) ;
#12299=CARTESIAN_POINT ( 'NONE',  ( 17.12812500061451715, 4.541064518000418104, 2.621784821874999949 ) ) ;
#12300=CARTESIAN_POINT ( 'NONE',  ( 10.80937500061451928, 4.541064518000418104, -2.621784821874998173 ) ) ;
#12301=CARTESIAN_POINT ( 'NONE',  ( 3.328125000614516438, -4.541064518000419881, 2.621784821874995952 ) ) ;
#12302=CARTESIAN_POINT ( 'NONE',  ( 19.92187500061451644, 3.027376345333611329, 5.243569643749999010 ) ) ;
#12303=CARTESIAN_POINT ( 'NONE',  ( 7.884375000614517681, -4.541064518000419881, 2.621784821874995952 ) ) ;
#12304=CARTESIAN_POINT ( 'NONE',  ( 3.021917804904423743, -3.983467431823952687, -3.409840147052992432 ) ) ;
#12306=CARTESIAN_POINT ( 'NONE',  ( 8.578125000614518214, 4.541064518000418104, 2.621784821874999949 ) ) ;
#12307=CARTESIAN_POINT ( 'NONE',  ( 18.25312500061451715, -4.541064518000417216, -2.621784821875001281 ) ) ;
#12308=EDGE_CURVE ( 'NONE', #49458, #72969, #42188, .T. ) ;
#12309=EDGE_LOOP ( 'NONE', ( #59894, #58264, #4369, #22558 ) ) ;
#12310=CARTESIAN_POINT ( 'NONE',  ( 6.037500001229035185, 6.123233995736764310E-16, -4.999999999999998224 ) ) ;
#12311=CARTESIAN_POINT ( 'NONE',  ( 14.16562500061451679, -6.054752690667223547, -1.112240025338166033E-15 ) ) ;
#12312=CARTESIAN_POINT ( 'NONE',  ( 12.62812500061451537, 4.541064518000418104, 2.621784821874999949 ) ) ;
#12314=CARTESIAN_POINT ( 'NONE',  ( 13.46249999999999858, -5.773502691896255534, -1.060575238724906372E-15 ) ) ;
#12315=CARTESIAN_POINT ( 'NONE',  ( 7.875000001229034652, 2.886751345948129099, -4.999999999999998224 ) ) ;
#12316=CARTESIAN_POINT ( 'NONE',  ( 5.803125000614517859, 4.541064518000418104, -2.621784821874998173 ) ) ;
#12317=CARTESIAN_POINT ( 'NONE',  ( 18.15000000122903501, -2.886751345948125991, -5.000000000000000000 ) ) ;
#12319=CARTESIAN_POINT ( 'NONE',  ( -2.121784821874999949, 10.78437500061451715, -33.67503911421598417 ) ) ;
#12321=CARTESIAN_POINT ( 'NONE',  ( 2.962500001229034119, 4.330127018922192761, -2.499999999999997780 ) ) ;
#12322=CARTESIAN_POINT ( 'NONE',  ( 26.17500000000000071, 6.123233995736764310E-16, -4.999999999999998224 ) ) ;
#12323=CARTESIAN_POINT ( 'NONE',  ( 17.89687500061451431, -3.027376345333610441, -5.243569643749999898 ) ) ;
#12324=CARTESIAN_POINT ( 'NONE',  ( 21.48750000122903003, 4.330127018922191873, 2.499999999999999556 ) ) ;
#12325=CARTESIAN_POINT ( 'NONE',  ( 12.96562500061451750, 3.027376345333613106, -5.243569643749998122 ) ) ;
#12327=LINE ( 'NONE', #40786, #14107 ) ;
#12328=CARTESIAN_POINT ( 'NONE',  ( 26.37187500061451217, -6.054752690667223547, -1.112240025338166033E-15 ) ) ;
#12331=CARTESIAN_POINT ( 'NONE',  ( 12.70312500061451821, 0.000000000000000000, 5.243569643749999010 ) ) ;
#12332=CARTESIAN_POINT ( 'NONE',  ( 11.82187500061451679, 3.027376345333611329, 5.243569643749999010 ) ) ;
#12333=VERTEX_POINT ( 'NONE', #19894 ) ;
#12334=CARTESIAN_POINT ( 'NONE',  ( 29.72812500061451502, 4.541064518000418104, 2.621784821874999949 ) ) ;
#12335=CARTESIAN_POINT ( 'NONE',  ( 20.09062500061451573, -3.027376345333610441, -5.243569643749999898 ) ) ;
#12336=CARTESIAN_POINT ( 'NONE',  ( 29.35312500061451502, 0.000000000000000000, 5.243569643749999010 ) ) ;
#12337=CARTESIAN_POINT ( 'NONE',  ( 1.626862140677534273E-15, 10.66249999999999964, 34.00000000000000000 ) ) ;
#12338=CARTESIAN_POINT ( 'NONE',  ( 9.150000000000002132, 4.330127018922192761, -2.499999999999997780 ) ) ;
#12339=CARTESIAN_POINT ( 'NONE',  ( 20.28750000122903074, -4.330127018922194537, 2.499999999999995559 ) ) ;
#12340=CARTESIAN_POINT ( 'NONE',  ( -2.000000000000000000, 10.02500000000000036, 26.53589838486224650 ) ) ;
#12343=CARTESIAN_POINT ( 'NONE',  ( 17.84999999999999787, 0.000000000000000000, 4.999999999999998224 ) ) ;
#12344=CARTESIAN_POINT ( 'NONE',  ( 21.63749999999999929, -2.886751345948125991, -5.000000000000000000 ) ) ;
#12345=CARTESIAN_POINT ( 'NONE',  ( 19.13437500061451857, -4.541064518000419881, 2.621784821874995952 ) ) ;
#12346=CARTESIAN_POINT ( 'NONE',  ( 24.32812500061451289, 4.541064518000418104, 2.621784821874999949 ) ) ;
#12347=VECTOR ( 'NONE', #41962, 1000.000000000000000 ) ;
#12348=EDGE_LOOP ( 'NONE', ( #63772, #22123, #30355, #24597 ) ) ;
#12349=CARTESIAN_POINT ( 'NONE',  ( -2.000000000000000000, 16.88750000122903572, 26.53589838486224650 ) ) ;
#12350=CARTESIAN_POINT ( 'NONE',  ( 8.390625000614518214, -3.027376345333610441, -5.243569643749999898 ) ) ;
#12352=CARTESIAN_POINT ( 'NONE',  ( 14.28750000000000142, -2.886751345948129988, 4.999999999999997335 ) ) ;
#12353=CARTESIAN_POINT ( 'NONE',  ( -3.000416591977282496E-16, 18.34062500061451928, 25.09994784771203058 ) ) ;
#12354=CARTESIAN_POINT ( 'NONE',  ( 3.084375000614519191, 6.421520780324663323E-16, -5.243569643749999010 ) ) ;
#12358=CARTESIAN_POINT ( 'NONE',  ( 25.47187500061451715, -6.054752690667223547, -1.112240025338166033E-15 ) ) ;
#12359=ORIENTED_EDGE ( 'NONE', *, *, #63501, .T. ) ;
#12360=CARTESIAN_POINT ( 'NONE',  ( 24.59062500061451573, -3.027376345333610441, -5.243569643749999898 ) ) ;
#12361=CARTESIAN_POINT ( 'NONE',  ( 23.33437500061451786, 6.421520780324663323E-16, -5.243569643749999010 ) ) ;
#12362=CARTESIAN_POINT ( 'NONE',  ( 4.243569643749999010, 16.46562500061459389, -32.45002607614398471 ) ) ;
#12363=CARTESIAN_POINT ( 'NONE',  ( 10.65000000000000036, 0.000000000000000000, 4.999999999999998224 ) ) ;
#12364=CARTESIAN_POINT ( 'NONE',  ( 7.978125000614517681, 6.421520780324663323E-16, -5.243569643749999010 ) ) ;
#12366=CARTESIAN_POINT ( 'NONE',  ( 28.19062500061451715, -3.027376345333610441, -5.243569643749999898 ) ) ;
#12367=CARTESIAN_POINT ( 'NONE',  ( 26.61562500061451786, 3.027376345333611329, 5.243569643749999010 ) ) ;
#12370=CARTESIAN_POINT ( 'NONE',  ( 18.87187500061451573, 3.027376345333613106, -5.243569643749998122 ) ) ;
#12371=CARTESIAN_POINT ( 'NONE',  ( -4.243569643749999898, 11.75937500061451857, 30.00000000000000000 ) ) ;
#12372=CARTESIAN_POINT ( 'NONE',  ( 18.27187500061451431, -6.054752690667223547, -1.112240025338166033E-15 ) ) ;
#12373=CARTESIAN_POINT ( 'NONE',  ( 27.00937500061451857, 4.541064518000418104, -2.621784821874998173 ) ) ;
#12374=CARTESIAN_POINT ( 'NONE',  ( 9.001249775931846008E-16, 17.27187500061451786, 34.90005215228797653 ) ) ;
#12375=CARTESIAN_POINT ( 'NONE',  ( 8.053125000614516082, 4.541064518000418104, -2.621784821874998173 ) ) ;
#12376=CARTESIAN_POINT ( 'NONE',  ( -2.000000000000000000, 18.12500000000000355, -33.46410161513775705 ) ) ;
#12377=CARTESIAN_POINT ( 'NONE',  ( 3.496875000614518836, -3.027376345333610441, -5.243569643749999898 ) ) ;
#12378=CARTESIAN_POINT ( 'NONE',  ( 6.103125000614515905, -4.541064518000417216, -2.621784821875001281 ) ) ;
#12379=CARTESIAN_POINT ( 'NONE',  ( 9.459375000614517859, 4.541064518000418104, -2.621784821874998173 ) ) ;
#12381=CARTESIAN_POINT ( 'NONE',  ( 17.17500000122903359, -5.773502691896255534, -1.060575238724906372E-15 ) ) ;
#12382=CARTESIAN_POINT ( 'NONE',  ( 6.346875000614517148, 6.054752690667223547, 3.707466751127219781E-16 ) ) ;
#12383=CARTESIAN_POINT ( 'NONE',  ( 8.540625000614518569, 6.054752690667223547, 3.707466751127219781E-16 ) ) ;
#12386=CARTESIAN_POINT ( 'NONE',  ( 17.10937500061451999, 4.541064518000418104, -2.621784821874998173 ) ) ;
#12388=EDGE_LOOP ( 'NONE', ( #68168, #31151, #10326, #71463 ) ) ;
#12389=CARTESIAN_POINT ( 'NONE',  ( 23.42812500061451786, 4.541064518000418104, 2.621784821874999949 ) ) ;
#12390=CARTESIAN_POINT ( 'NONE',  ( 9.665625000614515017, -6.054752690667223547, -1.112240025338166033E-15 ) ) ;
#12391=CARTESIAN_POINT ( 'NONE',  ( 27.23437500061451644, -4.541064518000419881, 2.621784821874995952 ) ) ;
#12392=CARTESIAN_POINT ( 'NONE',  ( 10.19062500061451892, -3.027376345333610441, -5.243569643749999898 ) ) ;
#12393=CARTESIAN_POINT ( 'NONE',  ( 0.000000000000000000, 20.00000000000000000, 30.00000000000000000 ) ) ;
#12394=CARTESIAN_POINT ( 'NONE',  ( 10.76250000122903572, 0.000000000000000000, 4.999999999999998224 ) ) ;
#12395=CARTESIAN_POINT ( 'NONE',  ( 26.84062500061451573, -3.027376345333610441, -5.243569643749999898 ) ) ;
#12396=EDGE_CURVE ( 'NONE', #427, #11359, #46938, .T. ) ;
#12397=CARTESIAN_POINT ( 'NONE',  ( -4.243569643749999898, 13.95312500061451821, -30.00000000000000000 ) ) ;
#12398=CARTESIAN_POINT ( 'NONE',  ( 12.37500000122903465, 2.886751345948129099, -4.999999999999998224 ) ) ;
#12399=CARTESIAN_POINT ( 'NONE',  ( 22.94062500061451715, 6.054752690667223547, 3.707466751127219781E-16 ) ) ;
#12401=CARTESIAN_POINT ( 'NONE',  ( 10.31250000000000355, -5.773502691896255534, -1.060575238724906372E-15 ) ) ;
#12402=CARTESIAN_POINT ( 'NONE',  ( 21.29062500061451502, -3.027376345333614438, 5.243569643749998122 ) ) ;
#12403=CARTESIAN_POINT ( 'NONE',  ( 6.234375000614519102, 6.421520780324663323E-16, -5.243569643749999010 ) ) ;
#12404=CARTESIAN_POINT ( 'NONE',  ( 20.17499999999999716, -4.330127018922194537, 2.499999999999995559 ) ) ;
#12405=CARTESIAN_POINT ( 'NONE',  ( 7.200000001229035718, -2.886751345948129988, 4.999999999999997335 ) ) ;
#12406=CARTESIAN_POINT ( 'NONE',  ( 15.71250000122903501, 0.000000000000000000, 4.999999999999998224 ) ) ;
#12407=VECTOR ( 'NONE', #15591, 1000.000000000000000 ) ;
#12408=CARTESIAN_POINT ( 'NONE',  ( 12.21562500061451573, 3.027376345333611329, 5.243569643749999010 ) ) ;
#12409=CARTESIAN_POINT ( 'NONE',  ( 15.44062500061451537, -3.027376345333614438, 5.243569643749998122 ) ) ;
#12411=CARTESIAN_POINT ( 'NONE',  ( 25.76250000122903216, -4.330127018922190985, -2.500000000000001332 ) ) ;
#12412=CARTESIAN_POINT ( 'NONE',  ( 20.99999999999999645, 0.000000000000000000, 4.999999999999998224 ) ) ;
#12413=VECTOR ( 'NONE', #53805, 1000.000000000000000 ) ;
#12414=CARTESIAN_POINT ( 'NONE',  ( 23.22187500061451715, -6.054752690667223547, -1.112240025338166033E-15 ) ) ;
#12415=CARTESIAN_POINT ( 'NONE',  ( 30.00000000000000000, 0.000000000000000000, 0.000000000000000000 ) ) ;
#12416=CARTESIAN_POINT ( 'NONE',  ( 11.25000000122903288, -2.886751345948129988, 4.999999999999997335 ) ) ;
#12417=CARTESIAN_POINT ( 'NONE',  ( 7.884375000614517681, -4.541064518000419881, 2.621784821874995952 ) ) ;
#12418=CARTESIAN_POINT ( 'NONE',  ( 25.20937500061451431, 4.541064518000418104, -2.621784821874998173 ) ) ;
#12419=CARTESIAN_POINT ( 'NONE',  ( 3.609375000614516882, 4.541064518000418104, -2.621784821874998173 ) ) ;
#12420=CARTESIAN_POINT ( 'NONE',  ( 20.61562500061451431, 3.027376345333613106, -5.243569643749998122 ) ) ;
#12421=CARTESIAN_POINT ( 'NONE',  ( 26.63437500061451857, 4.541064518000418104, 2.621784821874999949 ) ) ;
#12423=CARTESIAN_POINT ( 'NONE',  ( 18.52499999999999858, 6.123233995736764310E-16, -4.999999999999998224 ) ) ;
#12424=CARTESIAN_POINT ( 'NONE',  ( 7.284375000614518036, 4.541064518000418104, 2.621784821874999949 ) ) ;
#12425=CARTESIAN_POINT ( 'NONE',  ( 18.96562500061451573, 3.027376345333611329, 5.243569643749999010 ) ) ;
#12426=CARTESIAN_POINT ( 'NONE',  ( 15.97499999999999964, 4.330127018922191873, 2.499999999999999556 ) ) ;
#12427=CARTESIAN_POINT ( 'NONE',  ( 28.26562500061451289, 3.027376345333613106, -5.243569643749998122 ) ) ;
#12428=CARTESIAN_POINT ( 'NONE',  ( 4.584375000614516971, 4.541064518000418104, 2.621784821874999949 ) ) ;
#12429=CARTESIAN_POINT ( 'NONE',  ( 22.83750000122903501, 4.330127018922191873, 2.499999999999999556 ) ) ;
#12430=DIRECTION ( 'NONE',  ( -0.000000000000000000, -1.000000000000000000, -0.000000000000000000 ) ) ;
#12431=CARTESIAN_POINT ( 'NONE',  ( 17.51249999999999929, -5.773502691896255534, -1.060575238724906372E-15 ) ) ;
#12432=ORIENTED_EDGE ( 'NONE', *, *, #5228, .F. ) ;
#12433=CARTESIAN_POINT ( 'NONE',  ( 24.78750000000000497, -2.886751345948125991, -5.000000000000000000 ) ) ;
#12434=CARTESIAN_POINT ( 'NONE',  ( 27.19687500061451857, -3.027376345333614438, 5.243569643749998122 ) ) ;
#12435=ADVANCED_FACE ( 'NONE', ( #59414 ), #31835, .T. ) ;
#12436=ORIENTED_EDGE ( 'NONE', *, *, #45135, .T. ) ;
#12437=CARTESIAN_POINT ( 'NONE',  ( 14.65312500061451573, -4.541064518000417216, -2.621784821875001281 ) ) ;
#12438=CARTESIAN_POINT ( 'NONE',  ( 7.115625000614516082, 3.027376345333613106, -5.243569643749998122 ) ) ;
#12440=CARTESIAN_POINT ( 'NONE',  ( 29.20312500061451644, 4.541064518000418104, -2.621784821874998173 ) ) ;
#12441=EDGE_CURVE ( 'NONE', #39861, #20263, #50628, .T. ) ;
#12442=CARTESIAN_POINT ( 'NONE',  ( 15.37500000122903465, -5.773502691896255534, -1.060575238724906372E-15 ) ) ;
#12444=CARTESIAN_POINT ( 'NONE',  ( 22.31250000000000000, 2.886751345948126879, 4.999999999999999112 ) ) ;
#12445=CARTESIAN_POINT ( 'NONE',  ( 28.64999999999999858, 0.000000000000000000, 4.999999999999998224 ) ) ;
#12446=CARTESIAN_POINT ( 'NONE',  ( 3.609375000614516882, 4.541064518000418104, -2.621784821874998173 ) ) ;
#12447=CARTESIAN_POINT ( 'NONE',  ( 9.421875000614519990, 3.027376345333613106, -5.243569643749998122 ) ) ;
#12448=CARTESIAN_POINT ( 'NONE',  ( 20.74687500061451573, 6.054752690667223547, 3.707466751127219781E-16 ) ) ;
#12449=DIRECTION ( 'NONE',  ( -1.000000000000000000, -0.000000000000000000, -0.000000000000000000 ) ) ;
#12450=ORIENTED_EDGE ( 'NONE', *, *, #45017, .F. ) ;
#12451=CARTESIAN_POINT ( 'NONE',  ( 3.271875000614519635, 3.027376345333611329, 5.243569643749999010 ) ) ;
#12452=CARTESIAN_POINT ( 'NONE',  ( 6.000000000000001776, 4.330127018922192761, -2.499999999999997780 ) ) ;
#12454=CARTESIAN_POINT ( 'NONE',  ( 7.171875000614517326, 3.027376345333613106, -5.243569643749998122 ) ) ;
#12455=CARTESIAN_POINT ( 'NONE',  ( 19.38749999999999929, -2.886751345948125991, -5.000000000000000000 ) ) ;
#12456=CARTESIAN_POINT ( 'NONE',  ( 15.17812500061451608, 6.421520780324663323E-16, -5.243569643749999010 ) ) ;
#12458=DIRECTION ( 'NONE',  ( -1.000000000000000000, -0.000000000000000000, -0.000000000000000000 ) ) ;
#12460=CARTESIAN_POINT ( 'NONE',  ( 9.178125000614517859, -4.541064518000419881, 2.621784821874995952 ) ) ;
#12461=CARTESIAN_POINT ( 'NONE',  ( 27.64687500061452141, -3.027376345333614438, 5.243569643749998122 ) ) ;
#12462=ADVANCED_FACE ( 'NONE', ( #3238 ), #25395, .F. ) ;
#12463=CARTESIAN_POINT ( 'NONE',  ( -2.121784821874996840, 19.48437500061451644, 33.67503911421598417 ) ) ;
#12464=CARTESIAN_POINT ( 'NONE',  ( 27.04687500061451644, 6.054752690667223547, 3.707466751127219781E-16 ) ) ;
#12465=CARTESIAN_POINT ( 'NONE',  ( 7.087499999999999467, -2.886751345948129988, 4.999999999999997335 ) ) ;
#12466=CARTESIAN_POINT ( 'NONE',  ( 1.999999999999998668, 12.76250000122903394, 26.53589838486224650 ) ) ;
#12467=CARTESIAN_POINT ( 'NONE',  ( 13.86562500061451431, 3.027376345333613106, -5.243569643749998122 ) ) ;
#12468=CARTESIAN_POINT ( 'NONE',  ( 6.375000001229031987, -5.773502691896255534, -1.060575238724906372E-15 ) ) ;
#12469=AXIS2_PLACEMENT_3D ( 'NONE', #34077, #1205, #40724 ) ;
#12470=CARTESIAN_POINT ( 'NONE',  ( 17.33437500061451431, -4.541064518000419881, 2.621784821874995952 ) ) ;
#12471=CARTESIAN_POINT ( 'NONE',  ( 11.59687500061451892, -3.027376345333610441, -5.243569643749999898 ) ) ;
#12472=LINE ( 'NONE', #39837, #31279 ) ;
#12473=ORIENTED_EDGE ( 'NONE', *, *, #58187, .T. ) ;
#12474=CARTESIAN_POINT ( 'NONE',  ( 12.62812500061451537, 4.541064518000418104, 2.621784821874999949 ) ) ;
#12475=CARTESIAN_POINT ( 'NONE',  ( 26.47500000122903074, 2.886751345948126879, 4.999999999999999112 ) ) ;
#12476=CARTESIAN_POINT ( 'NONE',  ( 12.34687500061452070, -3.027376345333614438, 5.243569643749998122 ) ) ;
#12477=CARTESIAN_POINT ( 'NONE',  ( 3.038088735723365019, 9.529008066655462628, -35.17764897947208169 ) ) ;
#12478=CARTESIAN_POINT ( 'NONE',  ( 15.44062500061451537, -3.027376345333614438, 5.243569643749998122 ) ) ;
#12479=EDGE_CURVE ( 'NONE', #51420, #32936, #67229, .T. ) ;
#12481=CARTESIAN_POINT ( 'NONE',  ( 24.68437500061451573, 6.421520780324663323E-16, -5.243569643749999010 ) ) ;
#12483=CARTESIAN_POINT ( 'NONE',  ( 10.80000000122903536, -2.886751345948129988, 4.999999999999997335 ) ) ;
#12484=CARTESIAN_POINT ( 'NONE',  ( 4.924325218087134637, -0.8666147624583920850, 4.924325218087160394 ) ) ;
#12485=CYLINDRICAL_SURFACE ( 'NONE', #44287, 4.000000000000000000 ) ;
#12486=CARTESIAN_POINT ( 'NONE',  ( -2.121784821874996840, 17.68437500061451928, -26.32496088578401583 ) ) ;
#12487=CARTESIAN_POINT ( 'NONE',  ( 18.04687500061451999, 6.054752690667223547, 3.707466751127219781E-16 ) ) ;
#12488=CARTESIAN_POINT ( 'NONE',  ( 19.05000000122903359, -2.886751345948125991, -5.000000000000000000 ) ) ;
#12489=CARTESIAN_POINT ( 'NONE',  ( 13.77187500061451786, -6.054752690667223547, -1.112240025338166033E-15 ) ) ;
#12490=CARTESIAN_POINT ( 'NONE',  ( -4.243569643749997233, 19.39062500061451999, -27.54997392385601174 ) ) ;
#12491=CARTESIAN_POINT ( 'NONE',  ( 18.97500000122903074, -5.773502691896255534, -1.060575238724906372E-15 ) ) ;
#12492=CARTESIAN_POINT ( 'NONE',  ( 14.57812500061451644, -4.541064518000419881, 2.621784821874995952 ) ) ;
#12494=ORIENTED_EDGE ( 'NONE', *, *, #69679, .F. ) ;
#12495=CARTESIAN_POINT ( 'NONE',  ( 18.48750000000000071, -2.886751345948125991, -5.000000000000000000 ) ) ;
#12496=LINE ( 'NONE', #13568, #44467 ) ;
#12497=CARTESIAN_POINT ( 'NONE',  ( 4.000175247584509819, 2.999766337098574098, 30.13334590365527177 ) ) ;
#12498=CARTESIAN_POINT ( 'NONE',  ( 15.63750000122903216, 4.330127018922191873, 2.499999999999999556 ) ) ;
#12499=CARTESIAN_POINT ( 'NONE',  ( 26.78437500061451360, -4.541064518000419881, 2.621784821874995952 ) ) ;
#12500=CARTESIAN_POINT ( 'NONE',  ( 19.75312500061451360, 4.541064518000418104, -2.621784821874998173 ) ) ;
#12501=CARTESIAN_POINT ( 'NONE',  ( 23.50312500061451360, 0.000000000000000000, 5.243569643749999010 ) ) ;
#12502=CARTESIAN_POINT ( 'NONE',  ( 2.990625000614519191, -3.027376345333610441, -5.243569643749999898 ) ) ;
#12503=CARTESIAN_POINT ( 'NONE',  ( 26.84999999999999787, 0.000000000000000000, 4.999999999999998224 ) ) ;
#12506=CARTESIAN_POINT ( 'NONE',  ( 6.375000001229033764, -5.773502691896255534, -1.060575238724906372E-15 ) ) ;
#12507=CARTESIAN_POINT ( 'NONE',  ( 3.999999999999999112, 14.37500000000000000, -30.00000000000000000 ) ) ;
#12508=CARTESIAN_POINT ( 'NONE',  ( -4.243569643749997233, 16.74687500061451928, -27.54997392385601174 ) ) ;
#12509=CARTESIAN_POINT ( 'NONE',  ( 6.375000001229031987, -5.773502691896255534, -1.060575238724906372E-15 ) ) ;
#12510=CARTESIAN_POINT ( 'NONE',  ( 5.812500000000001776, -5.773502691896255534, -1.060575238724906372E-15 ) ) ;
#12511=CARTESIAN_POINT ( 'NONE',  ( 3.000000001229032875, 5.773502691896255534, 3.535250795749688894E-16 ) ) ;
#12512=CARTESIAN_POINT ( 'NONE',  ( 11.03437500061451715, -4.541064518000419881, 2.621784821874995952 ) ) ;
#12513=CARTESIAN_POINT ( 'NONE',  ( 24.63750000122903216, 4.330127018922191873, 2.499999999999999556 ) ) ;
#12515=CARTESIAN_POINT ( 'NONE',  ( 8.109375000614518214, 4.541064518000418104, -2.621784821874998173 ) ) ;
#12516=CARTESIAN_POINT ( 'NONE',  ( 14.14687500061451786, -3.027376345333614438, 5.243569643749998122 ) ) ;
#12517=CARTESIAN_POINT ( 'NONE',  ( 7.500000000000000000, 0.000000000000000000, 4.999999999999998224 ) ) ;
#12518=CARTESIAN_POINT ( 'NONE',  ( 2.121784821875001281, 13.65312500061459566, 33.67503911421598417 ) ) ;
#12519=CARTESIAN_POINT ( 'NONE',  ( 20.48437500061451289, -4.541064518000419881, 2.621784821874995952 ) ) ;
#12520=CARTESIAN_POINT ( 'NONE',  ( 9.562500000000001776, 2.886751345948129099, -4.999999999999997335 ) ) ;
#12521=CARTESIAN_POINT ( 'NONE',  ( 26.58750000122903145, -4.330127018922194537, 2.499999999999995559 ) ) ;
#12523=CARTESIAN_POINT ( 'NONE',  ( 21.77812500061451928, -4.541064518000419881, 2.621784821874995952 ) ) ;
#12524=CARTESIAN_POINT ( 'NONE',  ( 11.99062500061451608, -3.027376345333610441, -5.243569643749999898 ) ) ;
#12526=CARTESIAN_POINT ( 'NONE',  ( 12.34687500061452070, -3.027376345333614438, 5.243569643749998122 ) ) ;
#12527=CARTESIAN_POINT ( 'NONE',  ( 27.52500000000000213, 6.123233995736764310E-16, -4.999999999999998224 ) ) ;
#12528=CARTESIAN_POINT ( 'NONE',  ( 22.87500000122903288, 2.886751345948126879, 4.999999999999999112 ) ) ;
#12529=CARTESIAN_POINT ( 'NONE',  ( -3.999999999999997335, 18.35000000122903074, -27.69059892324149530 ) ) ;
#12530=CARTESIAN_POINT ( 'NONE',  ( 11.48437500061451644, -4.541064518000419881, 2.621784821874995952 ) ) ;
#12531=CARTESIAN_POINT ( 'NONE',  ( 28.05937500061451573, 0.000000000000000000, 5.243569643749999010 ) ) ;
#12532=CARTESIAN_POINT ( 'NONE',  ( -3.137519842735245283E-14, 11.22500000122903430, 34.00000000000000000 ) ) ;
#12533=CARTESIAN_POINT ( 'NONE',  ( -1.999999999999997113, 14.67500000000000071, 33.46410161513775705 ) ) ;
#12534=CARTESIAN_POINT ( 'NONE',  ( 22.95937500061451431, 4.541064518000418104, -2.621784821874998173 ) ) ;
#12535=CARTESIAN_POINT ( 'NONE',  ( 13.77187500061451786, -6.054752690667223547, -1.112240025338166033E-15 ) ) ;
#12537=CARTESIAN_POINT ( 'NONE',  ( 26.13749999999999929, -2.886751345948125991, -5.000000000000000000 ) ) ;
#12540=CARTESIAN_POINT ( 'NONE',  ( 17.84062500061451573, -3.027376345333610441, -5.243569643749999898 ) ) ;
#12541=CARTESIAN_POINT ( 'NONE',  ( 8.137500000000002842, -2.886751345948125991, -5.000000000000000000 ) ) ;
#12543=CARTESIAN_POINT ( 'NONE',  ( 15.78749999999999964, -2.886751345948125991, -5.000000000000000000 ) ) ;
#12544=CARTESIAN_POINT ( 'NONE',  ( -4.243569643749997233, 10.84062500061451395, 32.45002607614398471 ) ) ;
#12546=CARTESIAN_POINT ( 'NONE',  ( 24.42187500061451999, 3.027376345333611329, 5.243569643749999010 ) ) ;
#12547=ORIENTED_EDGE ( 'NONE', *, *, #8453, .T. ) ;
#12548=CARTESIAN_POINT ( 'NONE',  ( 21.32812500061451644, -4.541064518000419881, 2.621784821874995952 ) ) ;
#12549=CARTESIAN_POINT ( 'NONE',  ( 21.00937500061451857, -4.541064518000417216, -2.621784821875001281 ) ) ;
#12550=CARTESIAN_POINT ( 'NONE',  ( 4.012500000000001954, -5.773502691896255534, -1.060575238724906372E-15 ) ) ;
#12551=CARTESIAN_POINT ( 'NONE',  ( 6.665625000614515905, 3.027376345333613106, -5.243569643749998122 ) ) ;
#12552=CARTESIAN_POINT ( 'NONE',  ( 22.56562500061451715, 3.027376345333611329, 5.243569643749999010 ) ) ;
#12553=CARTESIAN_POINT ( 'NONE',  ( 12.38437500061451857, -4.541064518000419881, 2.621784821874995952 ) ) ;
#12554=CARTESIAN_POINT ( 'NONE',  ( 17.93437500061451928, 6.421520780324663323E-16, -5.243569643749999010 ) ) ;
#12555=CARTESIAN_POINT ( 'NONE',  ( -3.000416591977282496E-16, 18.79062500061451857, 25.09994784771203058 ) ) ;
#12556=CARTESIAN_POINT ( 'NONE',  ( 18.37500000122903288, 2.886751345948126879, 4.999999999999999112 ) ) ;
#12558=CARTESIAN_POINT ( 'NONE',  ( 8.840625000614517504, -3.027376345333610441, -5.243569643749999898 ) ) ;
#12559=CARTESIAN_POINT ( 'NONE',  ( 5.184375000614516615, -4.541064518000419881, 2.621784821874995952 ) ) ;
#12560=CARTESIAN_POINT ( 'NONE',  ( 5.221875000614519813, -6.054752690667223547, -1.112240025338166033E-15 ) ) ;
#12561=( BOUNDED_CURVE ( )  B_SPLINE_CURVE ( 3, ( #35577, #7504, #7147, #18207 ),
 .UNSPECIFIED., .F., .F. ) 
 B_SPLINE_CURVE_WITH_KNOTS ( ( 4, 4 ),
 ( 5.667042959702281557, 5.708255309384981047 ),
 .UNSPECIFIED. ) 
 CURVE ( )  GEOMETRIC_REPRESENTATION_ITEM ( )  RATIONAL_B_SPLINE_CURVE ( ( 1.000000000000000000, 0.9998584668609933335, 0.9998584668609933335, 1.000000000000000000 ) ) 
 REPRESENTATION_ITEM ( '' )  );
#12562=CARTESIAN_POINT ( 'NONE',  ( 25.28437500061451715, 4.541064518000418104, 2.621784821874999949 ) ) ;
#12563=CARTESIAN_POINT ( 'NONE',  ( 17.27812500061451217, -4.541064518000419881, 2.621784821874995952 ) ) ;
#12564=CARTESIAN_POINT ( 'NONE',  ( 27.56250000122902932, -4.330127018922190985, -2.500000000000001332 ) ) ;
#12565=CARTESIAN_POINT ( 'NONE',  ( 26.54062500061451146, 6.054752690667223547, 3.707466751127219781E-16 ) ) ;
#12566=CARTESIAN_POINT ( 'NONE',  ( 22.77187500061451786, -6.054752690667223547, -1.112240025338166033E-15 ) ) ;
#12567=CARTESIAN_POINT ( 'NONE',  ( 17.27812500061451217, -4.541064518000419881, 2.621784821874995952 ) ) ;
#12568=CARTESIAN_POINT ( 'NONE',  ( 4.243569643749999898, 17.38437500061451502, 30.00000000000000000 ) ) ;
#12569=CARTESIAN_POINT ( 'NONE',  ( 22.37812500061451360, 6.421520780324663323E-16, -5.243569643749999010 ) ) ;
#12572=CARTESIAN_POINT ( 'NONE',  ( 25.08749999999999858, -2.886751345948129988, 4.999999999999997335 ) ) ;
#12573=CARTESIAN_POINT ( 'NONE',  ( -2.000000000000000000, 13.62500000000000178, -33.46410161513775705 ) ) ;
#12575=CARTESIAN_POINT ( 'NONE',  ( 28.11562500061451431, -6.054752690667223547, -1.112240025338166033E-15 ) ) ;
#12576=CARTESIAN_POINT ( 'NONE',  ( 9.815625000614518925, 3.027376345333613106, -5.243569643749998122 ) ) ;
#12577=CARTESIAN_POINT ( 'NONE',  ( 23.10000000122903074, -2.886751345948125991, -5.000000000000000000 ) ) ;
#12578=ADVANCED_FACE ( 'NONE', ( #64550 ), #58635, .F. ) ;
#12579=CARTESIAN_POINT ( 'NONE',  ( 26.72812500061451502, -4.541064518000419881, 2.621784821874995952 ) ) ;
#12580=CARTESIAN_POINT ( 'NONE',  ( 28.80000000000000071, -4.330127018922190985, -2.500000000000001332 ) ) ;
#12581=CARTESIAN_POINT ( 'NONE',  ( -2.828200636599751609E-16, 16.85000000122903430, -34.61880215351700230 ) ) ;
#12582=CARTESIAN_POINT ( 'NONE',  ( -3.999999999999999112, 15.57500000122903216, -32.30940107675850470 ) ) ;
#12583=CARTESIAN_POINT ( 'NONE',  ( 9.965625000614517504, 3.027376345333611329, 5.243569643749999010 ) ) ;
#12584=VERTEX_POINT ( 'NONE', #63464 ) ;
#12585=CARTESIAN_POINT ( 'NONE',  ( 26.27812500061451573, -4.541064518000419881, 2.621784821874995952 ) ) ;
#12586=CARTESIAN_POINT ( 'NONE',  ( 8.690625000614515372, -3.027376345333614438, 5.243569643749998122 ) ) ;
#12587=CARTESIAN_POINT ( 'NONE',  ( 5.878125000614517148, 4.541064518000418104, 2.621784821874999949 ) ) ;
#12588=VECTOR ( 'NONE', #61286, 1000.000000000000000 ) ;
#12591=DIRECTION ( 'NONE',  ( -1.000000000000000000, -0.000000000000000000, -0.000000000000000000 ) ) ;
#12592=CARTESIAN_POINT ( 'NONE',  ( 13.38750000000000107, -2.886751345948129988, 4.999999999999997335 ) ) ;
#12593=CARTESIAN_POINT ( 'NONE',  ( 13.88437500061451679, 6.421520780324663323E-16, -5.243569643749999010 ) ) ;
#12594=CARTESIAN_POINT ( 'NONE',  ( 10.57500000122903572, 2.886751345948129099, -4.999999999999998224 ) ) ;
#12595=CARTESIAN_POINT ( 'NONE',  ( 17.82187500061451502, -6.054752690667223547, -1.112240025338166033E-15 ) ) ;
#12598=CARTESIAN_POINT ( 'NONE',  ( 8.371875000614515727, -6.054752690667223547, -1.112240025338166033E-15 ) ) ;
#12599=CARTESIAN_POINT ( 'NONE',  ( 4.243569643749999010, 12.41562500061451857, -32.45002607614398471 ) ) ;
#12602=CARTESIAN_POINT ( 'NONE',  ( 24.44062500061451715, -3.027376345333614438, 5.243569643749998122 ) ) ;
#12604=CARTESIAN_POINT ( 'NONE',  ( 27.75937500061451502, -4.541064518000417216, -2.621784821875001281 ) ) ;
#12605=( BOUNDED_SURFACE ( )  B_SPLINE_SURFACE ( 1, 2, ( 
 ( #28436, #16612, #68333, #34695, #369, #738, #56154, #11082, #39168, #29525, #22525, #57224, #40615, #17341, #22877, #17693, #62413, #18056, #6638, #51336, #45072, #33610, #5548, #39531, #62056, #18, #11451, #56510, #46156, #28086, #50614, #23970, #45798, #67968, #50973, #1464, #5903, #52060, #45435, #56861, #63136, #34329, #40254, #6267, #28795, #29167, #68696, #51699, #12531, #23247, #35064, #6994, #62775, #1103, #57591, #67254, #53140, #52420, #30975, #12888, #1826, #64589, #42066, #58305, #30248, #2539, #57946, #47240, #18777, #19141, #13244, #14347, #69422, #25059, #46883, #40985, #59037, #13977, #18419, #2903, #47602, #47976, #53510, #36515, #8439, #36881, #63500, #52781, #70132, #41343, #35421, #25434, #70504, #7353, #19881, #19510, #42434, #64955, #59399, #8809, #31346, #29882, #2183, #53886, #3278, #46518, #24334, #36153, #69058, #58672, #24696, #63853, #69773, #35781, #7715, #41695, #64219, #13608, #8080, #30611, #4738, #55343, #26538, #54609, #43533, #48344, #65316, #59771, #20610, #20243, #26168, #48708, #71605, #43900, #27272, #38722, #14706, #26911, #37250, #10274, #44268, #33167, #42795, #60134, #70869, #49437, #66424, #32077, #32441, #9178, #31713, #54248, #61243, #3645, #15802, #72330, #49078, #4014, #71971, #20980, #49805, #38343, #9904, #71231, #43168, #65687, #15075, #37612, #9543, #66054, #15432, #21710, #37977, #60498, #55705, #4382, #54977, #21345, #25806, #60871, #10636, #32806, #66800, #16171, #33520, #6183, #61599, #44989, #23162, #34609, #68250, #57139, #61966, #6548, #17970, #33887, #11000, #45716, #51251, #11728, #56070, #62692, #44639, #5462, #17613, #654, #16891, #11369, #34244, #16529, #5821, #50531, #50889, #67526, #46074, #28002, #67168, #50169, #28352, #34979, #289, #56431, #39445, #45350, #22797, #51617, #73059, #67884, #17256, #40173, #22080, #12088, #28712, #22440, #39816, #29082, #62332, #1018, #56777, #23524, #68609, #40531, #63047, #12448, #5099, #27635, #72698, #39081, #53427, #46799, #6910, #25345, #70419, #7270, #24612, #40903, #47890, #46434, #53057, #19795, #42346, #30530, #64869, #63416, #2817, #18694, #14257, #47159, #41981, #57508, #58948, #19056, #13519, #58587, #36067, #64133, #29441, #23887, #51978, #7994, #12802, #1377, #68973, #41258, #35338, #57861, #29799, #2451, #63770, #69691, #41614, #30162, #64502, #13158, #36434, #18330, #52335, #24974, #47519, #1737, #7625, #35700, #24251, #70048, #19421, #8356, #69336, #58220, #13894, #52695, #2101, #30885, #32352, #3927, #14620, #42709, #26450, #37159, #3559, #14990, #26081, #59685, #65230, #9092, #31629, #3191, #4297, #48620, #60782, #37892, #37528, #71145, #71886, #54890, #20518, #60049, #9820, #31254, #48990, #43076, #26822, #54163, #71520, #59311, #65602, #9460, #31990, #49356, #70779, #54524, #20895, #43449, #53796, #15351, #65971, #20155, #60411, #21259, #43812, #66337, #15715, #38253, #36796, #8721, #25718, #48256, #29674, #59186, #70291, #20025, #25588, #18928, #52210, #70651, #42581, #52571, #69922, #13036, #65107, #18570, #25208, #14497, #37031, #2693, #59555, #35573, #48127, #64007, #1612, #19292, #14131, #24122, #31125, #64374, #58822, #30761, #8232, #36307, #46672, #69212, #41136, #53293, #58093, #63645, #7500, #13388, #30030, #1979, #24488, #47755, #35932, #41846, #13766, #2328, #36667, #58455, #8596, #47032, #69567, #19663, #42217, #41488, #52931, #7867, #30403, #64741, #53666, #3057, #24846, #47392, #32145, #25504, #53580, #8513, #72036, #65025, #54678, #9975, #59845, #42866, #37680, #9250, #60568, #26610, #20681, #14415, #59106, #31042, #8884, #31417, #42502, #36952, #59472, #66123, #2976, #48049, #66489, #15142, #37322, #20313, #43969, #70574, #21412, #19950, #26242, #32512, #53957, #60202, #3354, #25876, #4081, #9614, #48415, #70942, #55048, #71303, #49148, #65389, #31785, #14780, #4450, #26978, #48779, #36586, #15502, #71676, #49508, #54324, #3715, #43239, #65760, #21051, #43602, #38043, #72395, #6250, #4807, #11434, #51318, #722, #62040, #28777, #21776, #34311, #50242, #23228, #5531, #354, #56844, #17324, #50597, #45056, #16959, #67593, #22507, #11794, #55411, #38417, #39512, #44340, #60939, #45781, #72764, #66868, #16238, #38791, #33953, #22149, #28068, #56137, #61666, #22861, #44702, #67952, #15870, #10342, #56494, #1, #61309, #39148, #67236, #32874, #5888, #28419, #39883, #50956, #27339, #16595, #10703, #33237, #45416, #62396, #49870, #55774, #5166, #27701, #11065, #33592, #12872, #52043, #18040, #40597, #35046, #63119, #57206, #69758, #1447, #25044, #7696, #35404, #23952, #13590, #47226, #18402, #57930, #2168, #62758, #24319, #46502, #19126, #12515, #69407, #40235, #34677, #12150, #40969, #68316, #69040, #63484, #57574, #7337, #6977, #41680, #1087, #29508, #29866, #63837, #6621, #58289, #24679, #46867, #64203, #36137, #30233, #52765, #58656, #29149, #52403, #18762, #1811, #41328, #51683, #13228, #30597, #35767, #8063, #53124, #2523, #17676, #68679, #23594, #46140, #71212, #53868, #47959, #26521, #3994, #48325, #3259, #65297, #70116, #13962, #8421, #42417, #42050, #70487, #19864, #20223, #65668, #49059, #60479, #36499, #48688, #59020, #32058, #66038, #54959, #64573, #8792, #19493, #71587, #37959, #9887, #43146, #30957, #53493, #2885, #32422, #25415, #15057, #20960, #70850, #25788, #20589, #42777, #43515, #37595, #31694, #64937, #14328, #36863, #59381, #31325, #14687, #37229, #59752, #15416, #9159, #54229, #4364, #26148, #3626, #60116, #47587, #9526, #54592, #10257, #16511, #22778, #55326, #27983, #32789, #66781, #44969, #56411, #16872, #5802, #10619, #28332, #39797, #55686, #4720, #67507, #73039, #33502, #27254, #11350, #66407, #49787, #39426, #22422, #38705, #33149, #56051, #38325, #27617, #72312, #72681, #16153, #67865, #21693 ),
 ( #50513, #44250, #49419, #56758, #5082, #61225, #50151, #22063, #5443, #44621, #39064, #67151, #61578, #33868, #10981, #50870, #17237, #62313, #61946, #268, #45329, #11709, #34225, #26893, #71952, #21328, #43881, #15783, #60853, #40513, #12067, #51599, #69315, #35678, #35319, #29063, #57118, #57841, #999, #63028, #23867, #12427, #23506, #46055, #68589, #17951, #68230, #7605, #34961, #36045, #18676, #46415, #57488, #24591, #58201, #29423, #68952, #13139, #635, #7250, #6892, #30143, #51958, #29779, #51231, #45697, #23142, #1358, #6163, #18310, #40881, #63397, #12782, #52315, #52674, #34590, #1718, #24230, #46780, #17594, #41238, #63750, #6530, #2082, #47139, #69670, #19036, #41594, #64112, #13498, #28692, #40153, #62672, #58566, #14971, #26062, #48971, #54506, #47868, #7973, #26430, #71500, #8336, #25698, #41959, #20877, #47497, #54145, #43430, #65952, #31608, #15331, #64481, #3908, #19400, #53404, #53036, #58928, #30866, #31234, #3539, #60029, #30509, #24954, #59665, #70028, #43056, #2431, #13874, #36413, #19773, #2796, #9441, #25323, #70397, #48601, #42324, #64849, #14237, #36775, #59291, #71126, #31969, #8701, #53775, #9073, #3171, #48234, #20499, #42689, #70759, #20134, #65211, #14601, #37137, #65581, #37509, #43792, #67426, #32333, #60392, #67780, #16424, #38615, #21608, #45246, #54871, #190, #21240, #27529, #33788, #66319, #38982, #15696, #4638, #55964, #16788, #27897, #39346, #44163, #61859, #50787, #66692, #38235, #5359, #10895, #44535, #60765, #22339, #4277, #10171, #50431, #33423, #49702, #16066, #67067, #49336, #61138, #32706, #10534, #27168, #5720, #55243, #61498, #72229, #26802, #72957, #44891, #9800, #11265, #56331, #28256, #22695, #37873, #71868, #33063, #55601, #4997, #50063, #72593, #21975, #11626, #6804, #52592, #29338, #45968, #69230, #40424, #63307, #17511, #6441, #18591, #40794, #23421, #40072, #41156, #46693, #17865, #68501, #34870, #39712, #56681, #46329, #23777, #13055, #6079, #62230, #12698, #548, #34142, #47053, #913, #23059, #68147, #45614, #68864, #62941, #51868, #57398, #12335, #1634, #51514, #63665, #7521, #30052, #18220, #1270, #62586, #35235, #57756, #1999, #7164, #29693, #35594, #52230, #58113, #24141, #11983, #34506, #24509, #17154, #28611, #57034, #28976, #51148, #41866, #30783, #15151, #53314, #19313, #64396, #36328, #13786, #58476, #72044, #2713, #27349, #9987, #37688, #25229, #15882, #49519, #20690, #60211, #4460, #64028, #26621, #47775, #21422, #58843, #71689, #41508, #35955, #13407, #43249, #69587, #71314, #65769, #8253, #9624, #32157, #43979, #2350, #54690, #4092, #66134, #7888, #60579, #21061, #24866, #47413, #66500, #49158, #32522, #43612, #15512, #38054, #38427, #60950, #55059, #18949, #26990, #10353, #32883, #55423, #4816, #30424, #52952, #69943, #72775, #16967, #33247, #40247, #38802, #45427, #12159, #34687, #22869, #62768, #55785, #68326, #11075, #57218, #39523, #34322, #17686, #51329, #11444, #5896, #50966, #16246, #72405, #362, #5176, #21787, #6631, #33603, #27712, #50252, #22159, #28429, #56147, #62049, #33964, #22518, #56854, #5541, #28788, #49880, #44353, #67961, #56503, #44711, #11, #28079, #66878, #17334, #39893, #731, #62406, #45791, #50607, #67247, #16605, #11805, #6260, #23240, #39161, #61676, #61318, #45065, #67602, #10715, #12881, #52053, #1457, #69050, #23963, #18049, #30605, #35414, #59028, #41688, #46876, #57939, #47595, #8073, #52412, #69415, #36146, #23604, #58298, #7346, #53133, #46511, #30241, #1096, #68689, #46149, #1820, #29160, #29876, #24327, #18412, #18770, #40978, #2532, #35057, #63493, #41336, #24689, #40607, #19134, #52774, #57584, #6987, #25052, #63846, #64211, #13237, #35775, #7707, #70124, #19502, #2176, #51692, #58665, #69766, #42059, #64582, #47233, #63128, #13970, #36508, #13600, #12524, #29518, #71964, #70495, #4006, #43893, #66417, #54601, #21338, #14338, #26904, #42786, #15795, #71222, #66047, #49430, #9896, #43159, #37604, #9535, #60126, #15067, #4375, #48335, #26529, #37969, #71597, #60490, #65307, #32432, #38335, #37241, #36872, #49069, #20972, #32069, #59390, #15425, #47967, #8800, #43525, #54969, #20234, #14697, #8430, #19872, #9169, #53877, #54239, #70860, #30966, #31336, #53501, #3269, #2893, #25424, #42425, #64946, #25797, #59762, #31704, #3636, #26160, #48699, #20600, #65679, #44632, #61957, #67518, #33879, #55336, #50523, #23154, #73051, #16522, #39808, #10992, #56424, #61236, #50161, #62324, #11361, #67161, #10630, #11720, #17248, #61591, #39074, #5454, #10267, #27265, #21703, #55698, #4731, #33160, #5092, #33512, #5813, #34236, #646, #49798, #28344, #72323, #45342, #6174, #68242, #44260, #22073, #32800, #56770, #51243, #45708, #50881, #66793, #16164, #38716, #17605, #27628, #281, #28704, #56061, #27994, #22789, #22433, #60864, #67876, #44981, #72691, #16883, #39437, #12438, #34971, #46066, #40523, #68601, #69683, #34601, #62684, #70040, #18686, #40894, #23879, #47511, #57130, #2443, #23516, #29791, #36058, #17962, #41250, #63039, #19048, #7617, #30522, #58578, #29433, #12080, #7986, #53049, #57500, #7262, #6902, #24966, #29074, #35692, #40165, #6540, #13150, #51609, #51970, #1009, #1369, #46426, #52327, #24603, #68964, #41606, #1729, #69327, #63761, #58212, #46791, #18321, #63408, #12794, #30153, #35330, #57853, #24242, #52687, #2093, #47151, #64125, #13511, #3183, #31622, #59677, #65223, #3920, #53787, #71512, #9813, #32345, #71138, #9085, #42338, #42701, #70771, #54883, #43068, #14983, #20888, #37521, #15344, #25710, #25337, #64861, #9453, #48983, #48613, #14249, #70411, #20511, #36788, #48247, #37152, #20147, #59303, #8714, #31246, #14613, #8348, #43442, #54156, #49349, #31983, #3552, #26074, #37884, #65964, #65594, #60042, #26443, #13886, #54517, #60404 ) ),
 .UNSPECIFIED., .F., .F., .F. ) 
 B_SPLINE_SURFACE_WITH_KNOTS ( ( 2, 2 ),
 ( 3, 2, 2, 2, 2, 2, 2, 2, 2, 2, 2, 2, 2, 2, 2, 2, 2, 2, 2, 2, 2, 2, 2, 2, 2, 2, 2, 2, 2, 2, 2, 2, 2, 2, 2, 2, 2, 2, 2, 2, 2, 2, 2, 2, 2, 2, 2, 2, 2, 2, 2, 2, 2, 2, 2, 2, 2, 2, 2, 2, 2, 2, 2, 2, 2, 2, 2, 2, 2, 2, 2, 2, 2, 2, 2, 2, 2, 2, 2, 2, 2, 2, 2, 2, 2, 2, 2, 2, 2, 2, 2, 2, 2, 2, 2, 2, 2, 2, 2, 2, 2, 2, 2, 2, 2, 2, 2, 2, 2, 2, 2, 2, 2, 2, 2, 2, 2, 2, 2, 2, 2, 2, 2, 2, 2, 2, 2, 2, 2, 2, 2, 2, 2, 2, 2, 2, 2, 2, 2, 2, 2, 2, 2, 2, 2, 2, 2, 2, 2, 2, 2, 2, 2, 2, 2, 2, 2, 2, 2, 2, 2, 2, 2, 2, 2, 2, 2, 2, 2, 2, 2, 2, 2, 2, 2, 2, 2, 2, 2, 2, 2, 2, 2, 2, 2, 2, 2, 2, 2, 2, 2, 2, 2, 2, 2, 2, 2, 2, 2, 2, 2, 2, 2, 2, 2, 2, 2, 2, 2, 2, 2, 2, 2, 2, 2, 2, 2, 2, 2, 2, 2, 2, 2, 2, 2, 2, 2, 2, 2, 2, 2, 2, 2, 2, 2, 2, 2, 2, 2, 2, 2, 2, 2, 2, 2, 2, 2, 2, 2, 2, 2, 2, 2, 2, 2, 2, 2, 2, 2, 2, 2, 2, 2, 2, 2, 2, 2, 2, 2, 2, 2, 2, 2, 2, 2, 2, 2, 2, 2, 2, 2, 2, 2, 2, 2, 2, 2, 2, 2, 2, 2, 2, 2, 2, 2, 2, 2, 2, 2, 2, 2, 2, 2, 2, 2, 2, 2, 2, 2, 2, 2, 2, 2, 2, 2, 2, 2, 2, 2, 2, 2, 2, 2, 2, 2, 2, 2, 2, 2, 2, 2, 2, 2, 2, 2, 2, 2, 2, 2, 2, 2, 2, 2, 2, 2, 2, 2, 2, 2, 2, 2, 2, 2, 2, 2, 2, 2, 2, 2, 2, 3 ),
 ( 0.000000000000000000, 1.000000000000000000 ),
 ( 0.000000000000000000, 0.002777777777777777884, 0.005555555555555555768, 0.008333333333333333218, 0.01111111111111111154, 0.01388888888888888812, 0.01666666666666666644, 0.01944444444444444475, 0.02222222222222222307, 0.02500000000000000139, 0.02777777777777777624, 0.03055555555555555455, 0.03333333333333333287, 0.03611111111111110772, 0.03888888888888888951, 0.04166666666666666435, 0.04444444444444444614, 0.04722222222222222099, 0.05000000000000000278, 0.05277777777777777762, 0.05555555555555555247, 0.05833333333333333426, 0.06111111111111110911, 0.06388888888888888395, 0.06666666666666666574, 0.06944444444444444753, 0.07222222222222221544, 0.07499999999999999722, 0.07777777777777777901, 0.08055555555555556080, 0.08333333333333332871, 0.08611111111111111049, 0.08888888888888889228, 0.09166666666666666019, 0.09444444444444444198, 0.09722222222222222376, 0.1000000000000000056, 0.1027777777777777735, 0.1055555555555555552, 0.1083333333333333370, 0.1111111111111111049, 0.1138888888888888867, 0.1166666666666666685, 0.1194444444444444503, 0.1222222222222222182, 0.1250000000000000000, 0.1277777777777777679, 0.1305555555555555636, 0.1333333333333333315, 0.1361111111111110994, 0.1388888888888888951, 0.1416666666666666630, 0.1444444444444444309, 0.1472222222222222265, 0.1499999999999999944, 0.1527777777777777901, 0.1555555555555555580, 0.1583333333333333259, 0.1611111111111111216, 0.1638888888888888895, 0.1666666666666666574, 0.1694444444444444531, 0.1722222222222222210, 0.1749999999999999889, 0.1777777777777777846, 0.1805555555555555525, 0.1833333333333333204, 0.1861111111111111160, 0.1888888888888888840, 0.1916666666666666796, 0.1944444444444444475, 0.1972222222222222154, 0.2000000000000000111, 0.2027777777777777790, 0.2055555555555555469, 0.2083333333333333426, 0.2111111111111111105, 0.2138888888888888784, 0.2166666666666666741, 0.2194444444444444420, 0.2222222222222222099, 0.2250000000000000056, 0.2277777777777777735, 0.2305555555555555691, 0.2333333333333333370, 0.2361111111111111049, 0.2388888888888889006, 0.2416666666666666685, 0.2444444444444444364, 0.2472222222222222321, 0.2500000000000000000, 0.2527777777777777679, 0.2555555555555555358, 0.2583333333333333592, 0.2611111111111111271, 0.2638888888888888951, 0.2666666666666666630, 0.2694444444444444309, 0.2722222222222221988, 0.2750000000000000222, 0.2777777777777777901, 0.2805555555555555580, 0.2833333333333333259, 0.2861111111111110938, 0.2888888888888888618, 0.2916666666666666852, 0.2944444444444444531, 0.2972222222222222210, 0.2999999999999999889, 0.3027777777777777568, 0.3055555555555555802, 0.3083333333333333481, 0.3111111111111111160, 0.3138888888888888840, 0.3166666666666666519, 0.3194444444444444198, 0.3222222222222222432, 0.3250000000000000111, 0.3277777777777777790, 0.3305555555555555469, 0.3333333333333333148, 0.3361111111111111382, 0.3388888888888889062, 0.3416666666666666741, 0.3444444444444444420, 0.3472222222222222099, 0.3499999999999999778, 0.3527777777777778012, 0.3555555555555555691, 0.3583333333333333370, 0.3611111111111111049, 0.3638888888888888729, 0.3666666666666666408, 0.3694444444444444642, 0.3722222222222222321, 0.3750000000000000000, 0.3777777777777777679, 0.3805555555555555358, 0.3833333333333333592, 0.3861111111111111271, 0.3888888888888888951, 0.3916666666666666630, 0.3944444444444444309, 0.3972222222222221988, 0.4000000000000000222, 0.4027777777777777901, 0.4055555555555555580, 0.4083333333333333259, 0.4111111111111110938, 0.4138888888888888618, 0.4166666666666666852, 0.4194444444444444531, 0.4222222222222222210, 0.4249999999999999889, 0.4277777777777777568, 0.4305555555555555802, 0.4333333333333333481, 0.4361111111111111160, 0.4388888888888888840, 0.4416666666666666519, 0.4444444444444444198, 0.4472222222222222432, 0.4500000000000000111, 0.4527777777777777790, 0.4555555555555555469, 0.4583333333333333148, 0.4611111111111111382, 0.4638888888888889062, 0.4666666666666666741, 0.4694444444444444420, 0.4722222222222222099, 0.4749999999999999778, 0.4777777777777778012, 0.4805555555555555691, 0.4833333333333333370, 0.4861111111111111049, 0.4888888888888888729, 0.4916666666666666408, 0.4944444444444444642, 0.4972222222222222321, 0.5000000000000000000, 0.5027777777777777679, 0.5055555555555555358, 0.5083333333333333037, 0.5111111111111110716, 0.5138888888888888395, 0.5166666666666667185, 0.5194444444444444864, 0.5222222222222222543, 0.5250000000000000222, 0.5277777777777777901, 0.5305555555555555580, 0.5333333333333333259, 0.5361111111111110938, 0.5388888888888888618, 0.5416666666666666297, 0.5444444444444443976, 0.5472222222222222765, 0.5500000000000000444, 0.5527777777777778123, 0.5555555555555555802, 0.5583333333333333481, 0.5611111111111111160, 0.5638888888888888840, 0.5666666666666666519, 0.5694444444444444198, 0.5722222222222221877, 0.5749999999999999556, 0.5777777777777777235, 0.5805555555555556024, 0.5833333333333333703, 0.5861111111111111382, 0.5888888888888889062, 0.5916666666666666741, 0.5944444444444444420, 0.5972222222222222099, 0.5999999999999999778, 0.6027777777777777457, 0.6055555555555555136, 0.6083333333333332815, 0.6111111111111111605, 0.6138888888888889284, 0.6166666666666666963, 0.6194444444444444642, 0.6222222222222222321, 0.6250000000000000000, 0.6277777777777777679, 0.6305555555555555358, 0.6333333333333333037, 0.6361111111111110716, 0.6388888888888888395, 0.6416666666666667185, 0.6444444444444444864, 0.6472222222222222543, 0.6500000000000000222, 0.6527777777777777901, 0.6555555555555555580, 0.6583333333333333259, 0.6611111111111110938, 0.6638888888888888618, 0.6666666666666666297, 0.6694444444444443976, 0.6722222222222222765, 0.6750000000000000444, 0.6777777777777778123, 0.6805555555555555802, 0.6833333333333333481, 0.6861111111111111160, 0.6888888888888888840, 0.6916666666666666519, 0.6944444444444444198, 0.6972222222222221877, 0.6999999999999999556, 0.7027777777777777235, 0.7055555555555556024, 0.7083333333333333703, 0.7111111111111111382, 0.7138888888888889062, 0.7166666666666666741, 0.7194444444444444420, 0.7222222222222222099, 0.7249999999999999778, 0.7277777777777777457, 0.7305555555555555136, 0.7333333333333332815, 0.7361111111111111605, 0.7388888888888889284, 0.7416666666666666963, 0.7444444444444444642, 0.7472222222222222321, 0.7500000000000000000, 0.7527777777777777679, 0.7555555555555555358, 0.7583333333333333037, 0.7611111111111110716, 0.7638888888888888395, 0.7666666666666667185, 0.7694444444444444864, 0.7722222222222222543, 0.7750000000000000222, 0.7777777777777777901, 0.7805555555555555580, 0.7833333333333333259, 0.7861111111111110938, 0.7888888888888888618, 0.7916666666666666297, 0.7944444444444443976, 0.7972222222222222765, 0.8000000000000000444, 0.8027777777777778123, 0.8055555555555555802, 0.8083333333333333481, 0.8111111111111111160, 0.8138888888888888840, 0.8166666666666666519, 0.8194444444444444198, 0.8222222222222221877, 0.8249999999999999556, 0.8277777777777777235, 0.8305555555555556024, 0.8333333333333333703, 0.8361111111111111382, 0.8388888888888889062, 0.8416666666666666741, 0.8444444444444444420, 0.8472222222222222099, 0.8499999999999999778, 0.8527777777777777457, 0.8555555555555555136, 0.8583333333333332815, 0.8611111111111111605, 0.8638888888888889284, 0.8666666666666666963, 0.8694444444444444642, 0.8722222222222222321, 0.8750000000000000000, 0.8777777777777777679, 0.8805555555555555358, 0.8833333333333333037, 0.8861111111111110716, 0.8888888888888888395, 0.8916666666666667185, 0.8944444444444444864, 0.8972222222222222543, 0.9000000000000000222, 0.9027777777777777901, 0.9055555555555555580, 0.9083333333333333259, 0.9111111111111110938, 0.9138888888888888618, 0.9166666666666666297, 0.9194444444444443976, 0.9222222222222222765, 0.9250000000000000444, 0.9277777777777778123, 0.9305555555555555802, 0.9333333333333333481, 0.9361111111111111160, 0.9388888888888888840, 0.9416666666666666519, 0.9444444444444444198, 0.9472222222222221877, 0.9499999999999999556, 0.9527777777777777235, 0.9555555555555556024, 0.9583333333333333703, 0.9611111111111111382, 0.9638888888888889062, 0.9666666666666666741, 0.9694444444444444420, 0.9722222222222222099, 0.9749999999999999778, 0.9777777777777777457, 0.9805555555555555136, 0.9833333333333332815, 0.9861111111111111605, 0.9888888888888889284, 0.9916666666666666963, 0.9944444444444444642, 0.9972222222222222321, 1.000000000000000000 ),
 .UNSPECIFIED. ) 
 GEOMETRIC_REPRESENTATION_ITEM ( )  RATIONAL_B_SPLINE_SURFACE ( (
 ( 1.000000000000000000, 0.8660254037844387076, 1.000000000000000000, 0.8660254037844387076, 1.000000000000000000, 0.8660254037844387076, 1.000000000000000000, 0.8660254037844387076, 1.000000000000000000, 0.8660254037844387076, 1.000000000000000000, 0.8660254037844387076, 1.000000000000000000, 0.8660254037844387076, 1.000000000000000000, 0.8660254037844387076, 1.000000000000000000, 0.8660254037844387076, 1.000000000000000000, 0.8660254037844387076, 1.000000000000000000, 0.8660254037844387076, 1.000000000000000000, 0.8660254037844387076, 1.000000000000000000, 0.8660254037844387076, 1.000000000000000000, 0.8660254037844387076, 1.000000000000000000, 0.8660254037844387076, 1.000000000000000000, 0.8660254037844387076, 1.000000000000000000, 0.8660254037844387076, 1.000000000000000000, 0.8660254037844387076, 1.000000000000000000, 0.8660254037844387076, 1.000000000000000000, 0.8660254037844387076, 1.000000000000000000, 0.8660254037844387076, 1.000000000000000000, 0.8660254037844387076, 1.000000000000000000, 0.8660254037844387076, 1.000000000000000000, 0.8660254037844387076, 1.000000000000000000, 0.8660254037844387076, 1.000000000000000000, 0.8660254037844387076, 1.000000000000000000, 0.8660254037844387076, 1.000000000000000000, 0.8660254037844387076, 1.000000000000000000, 0.8660254037844387076, 1.000000000000000000, 0.8660254037844387076, 1.000000000000000000, 0.8660254037844387076, 1.000000000000000000, 0.8660254037844387076, 1.000000000000000000, 0.8660254037844387076, 1.000000000000000000, 0.8660254037844387076, 1.000000000000000000, 0.8660254037844387076, 1.000000000000000000, 0.8660254037844387076, 1.000000000000000000, 0.8660254037844387076, 1.000000000000000000, 0.8660254037844387076, 1.000000000000000000, 0.8660254037844387076, 1.000000000000000000, 0.8660254037844387076, 1.000000000000000000, 0.8660254037844387076, 1.000000000000000000, 0.8660254037844387076, 1.000000000000000000, 0.8660254037844387076, 1.000000000000000000, 0.8660254037844387076, 1.000000000000000000, 0.8660254037844387076, 1.000000000000000000, 0.8660254037844387076, 1.000000000000000000, 0.8660254037844387076, 1.000000000000000000, 0.8660254037844387076, 1.000000000000000000, 0.8660254037844387076, 1.000000000000000000, 0.8660254037844387076, 1.000000000000000000, 0.8660254037844387076, 1.000000000000000000, 0.8660254037844387076, 1.000000000000000000, 0.8660254037844387076, 1.000000000000000000, 0.8660254037844387076, 1.000000000000000000, 0.8660254037844387076, 1.000000000000000000, 0.8660254037844387076, 1.000000000000000000, 0.8660254037844387076, 1.000000000000000000, 0.8660254037844387076, 1.000000000000000000, 0.8660254037844387076, 1.000000000000000000, 0.8660254037844387076, 1.000000000000000000, 0.8660254037844387076, 1.000000000000000000, 0.8660254037844387076, 1.000000000000000000, 0.8660254037844387076, 1.000000000000000000, 0.8660254037844387076, 1.000000000000000000, 0.8660254037844387076, 1.000000000000000000, 0.8660254037844387076, 1.000000000000000000, 0.8660254037844387076, 1.000000000000000000, 0.8660254037844387076, 1.000000000000000000, 0.8660254037844387076, 1.000000000000000000, 0.8660254037844387076, 1.000000000000000000, 0.8660254037844387076, 1.000000000000000000, 0.8660254037844387076, 1.000000000000000000, 0.8660254037844387076, 1.000000000000000000, 0.8660254037844387076, 1.000000000000000000, 0.8660254037844387076, 1.000000000000000000, 0.8660254037844387076, 1.000000000000000000, 0.8660254037844387076, 1.000000000000000000, 0.8660254037844387076, 1.000000000000000000, 0.8660254037844387076, 1.000000000000000000, 0.8660254037844387076, 1.000000000000000000, 0.8660254037844387076, 1.000000000000000000, 0.8660254037844387076, 1.000000000000000000, 0.8660254037844387076, 1.000000000000000000, 0.8660254037844387076, 1.000000000000000000, 0.8660254037844387076, 1.000000000000000000, 0.8660254037844387076, 1.000000000000000000, 0.8660254037844387076, 1.000000000000000000, 0.8660254037844387076, 1.000000000000000000, 0.8660254037844387076, 1.000000000000000000, 0.8660254037844387076, 1.000000000000000000, 0.8660254037844387076, 1.000000000000000000, 0.8660254037844387076, 1.000000000000000000, 0.8660254037844387076, 1.000000000000000000, 0.8660254037844387076, 1.000000000000000000, 0.8660254037844387076, 1.000000000000000000, 0.8660254037844387076, 1.000000000000000000, 0.8660254037844387076, 1.000000000000000000, 0.8660254037844387076, 1.000000000000000000, 0.8660254037844387076, 1.000000000000000000, 0.8660254037844387076, 1.000000000000000000, 0.8660254037844387076, 1.000000000000000000, 0.8660254037844387076, 1.000000000000000000, 0.8660254037844387076, 1.000000000000000000, 0.8660254037844387076, 1.000000000000000000, 0.8660254037844387076, 1.000000000000000000, 0.8660254037844387076, 1.000000000000000000, 0.8660254037844387076, 1.000000000000000000, 0.8660254037844387076, 1.000000000000000000, 0.8660254037844387076, 1.000000000000000000, 0.8660254037844387076, 1.000000000000000000, 0.8660254037844387076, 1.000000000000000000, 0.8660254037844387076, 1.000000000000000000, 0.8660254037844387076, 1.000000000000000000, 0.8660254037844387076, 1.000000000000000000, 0.8660254037844387076, 1.000000000000000000, 0.8660254037844387076, 1.000000000000000000, 0.8660254037844387076, 1.000000000000000000, 0.8660254037844387076, 1.000000000000000000, 0.8660254037844387076, 1.000000000000000000, 0.8660254037844387076, 1.000000000000000000, 0.8660254037844387076, 1.000000000000000000, 0.8660254037844387076, 1.000000000000000000, 0.8660254037844387076, 1.000000000000000000, 0.8660254037844387076, 1.000000000000000000, 0.8660254037844387076, 1.000000000000000000, 0.8660254037844387076, 1.000000000000000000, 0.8660254037844387076, 1.000000000000000000, 0.8660254037844387076, 1.000000000000000000, 0.8660254037844387076, 1.000000000000000000, 0.8660254037844387076, 1.000000000000000000, 0.8660254037844387076, 1.000000000000000000, 0.8660254037844387076, 1.000000000000000000, 0.8660254037844387076, 1.000000000000000000, 0.8660254037844387076, 1.000000000000000000, 0.8660254037844387076, 1.000000000000000000, 0.8660254037844387076, 1.000000000000000000, 0.8660254037844387076, 1.000000000000000000, 0.8660254037844387076, 1.000000000000000000, 0.8660254037844387076, 1.000000000000000000, 0.8660254037844387076, 1.000000000000000000, 0.8660254037844387076, 1.000000000000000000, 0.8660254037844387076, 1.000000000000000000, 0.8660254037844387076, 1.000000000000000000, 0.8660254037844387076, 1.000000000000000000, 0.8660254037844387076, 1.000000000000000000, 0.8660254037844387076, 1.000000000000000000, 0.8660254037844387076, 1.000000000000000000, 0.8660254037844387076, 1.000000000000000000, 0.8660254037844387076, 1.000000000000000000, 0.8660254037844387076, 1.000000000000000000, 0.8660254037844387076, 1.000000000000000000, 0.8660254037844387076, 1.000000000000000000, 0.8660254037844387076, 1.000000000000000000, 0.8660254037844387076, 1.000000000000000000, 0.8660254037844387076, 1.000000000000000000, 0.8660254037844387076, 1.000000000000000000, 0.8660254037844387076, 1.000000000000000000, 0.8660254037844387076, 1.000000000000000000, 0.8660254037844387076, 1.000000000000000000, 0.8660254037844387076, 1.000000000000000000, 0.8660254037844387076, 1.000000000000000000, 0.8660254037844387076, 1.000000000000000000, 0.8660254037844387076, 1.000000000000000000, 0.8660254037844387076, 1.000000000000000000, 0.8660254037844387076, 1.000000000000000000, 0.8660254037844387076, 1.000000000000000000, 0.8660254037844387076, 1.000000000000000000, 0.8660254037844387076, 1.000000000000000000, 0.8660254037844387076, 1.000000000000000000, 0.8660254037844387076, 1.000000000000000000, 0.8660254037844387076, 1.000000000000000000, 0.8660254037844387076, 1.000000000000000000, 0.8660254037844387076, 1.000000000000000000, 0.8660254037844387076, 1.000000000000000000, 0.8660254037844387076, 1.000000000000000000, 0.8660254037844387076, 1.000000000000000000, 0.8660254037844387076, 1.000000000000000000, 0.8660254037844387076, 1.000000000000000000, 0.8660254037844387076, 1.000000000000000000, 0.8660254037844387076, 1.000000000000000000, 0.8660254037844387076, 1.000000000000000000, 0.8660254037844387076, 1.000000000000000000, 0.8660254037844387076, 1.000000000000000000, 0.8660254037844387076, 1.000000000000000000, 0.8660254037844387076, 1.000000000000000000, 0.8660254037844387076, 1.000000000000000000, 0.8660254037844387076, 1.000000000000000000, 0.8660254037844387076, 1.000000000000000000, 0.8660254037844387076, 1.000000000000000000, 0.8660254037844387076, 1.000000000000000000, 0.8660254037844387076, 1.000000000000000000, 0.8660254037844387076, 1.000000000000000000, 0.8660254037844387076, 1.000000000000000000, 0.8660254037844387076, 1.000000000000000000, 0.8660254037844387076, 1.000000000000000000, 0.8660254037844387076, 1.000000000000000000, 0.8660254037844387076, 1.000000000000000000, 0.8660254037844387076, 1.000000000000000000, 0.8660254037844387076, 1.000000000000000000, 0.8660254037844387076, 1.000000000000000000, 0.8660254037844387076, 1.000000000000000000, 0.8660254037844387076, 1.000000000000000000, 0.8660254037844387076, 1.000000000000000000, 0.8660254037844387076, 1.000000000000000000, 0.8660254037844387076, 1.000000000000000000, 0.8660254037844387076, 1.000000000000000000, 0.8660254037844387076, 1.000000000000000000, 0.8660254037844387076, 1.000000000000000000, 0.8660254037844387076, 1.000000000000000000, 0.8660254037844387076, 1.000000000000000000, 0.8660254037844387076, 1.000000000000000000, 0.8660254037844387076, 1.000000000000000000, 0.8660254037844387076, 1.000000000000000000, 0.8660254037844387076, 1.000000000000000000, 0.8660254037844387076, 1.000000000000000000, 0.8660254037844387076, 1.000000000000000000, 0.8660254037844387076, 1.000000000000000000, 0.8660254037844387076, 1.000000000000000000, 0.8660254037844387076, 1.000000000000000000, 0.8660254037844387076, 1.000000000000000000, 0.8660254037844387076, 1.000000000000000000, 0.8660254037844387076, 1.000000000000000000, 0.8660254037844387076, 1.000000000000000000, 0.8660254037844387076, 1.000000000000000000, 0.8660254037844387076, 1.000000000000000000, 0.8660254037844387076, 1.000000000000000000, 0.8660254037844387076, 1.000000000000000000, 0.8660254037844387076, 1.000000000000000000, 0.8660254037844387076, 1.000000000000000000, 0.8660254037844387076, 1.000000000000000000, 0.8660254037844387076, 1.000000000000000000, 0.8660254037844387076, 1.000000000000000000, 0.8660254037844387076, 1.000000000000000000, 0.8660254037844387076, 1.000000000000000000, 0.8660254037844387076, 1.000000000000000000, 0.8660254037844387076, 1.000000000000000000, 0.8660254037844387076, 1.000000000000000000, 0.8660254037844387076, 1.000000000000000000, 0.8660254037844387076, 1.000000000000000000, 0.8660254037844387076, 1.000000000000000000, 0.8660254037844387076, 1.000000000000000000, 0.8660254037844387076, 1.000000000000000000, 0.8660254037844387076, 1.000000000000000000, 0.8660254037844387076, 1.000000000000000000, 0.8660254037844387076, 1.000000000000000000, 0.8660254037844387076, 1.000000000000000000, 0.8660254037844387076, 1.000000000000000000, 0.8660254037844387076, 1.000000000000000000, 0.8660254037844387076, 1.000000000000000000, 0.8660254037844387076, 1.000000000000000000, 0.8660254037844387076, 1.000000000000000000, 0.8660254037844387076, 1.000000000000000000, 0.8660254037844387076, 1.000000000000000000, 0.8660254037844387076, 1.000000000000000000, 0.8660254037844387076, 1.000000000000000000, 0.8660254037844387076, 1.000000000000000000, 0.8660254037844387076, 1.000000000000000000, 0.8660254037844387076, 1.000000000000000000, 0.8660254037844387076, 1.000000000000000000, 0.8660254037844387076, 1.000000000000000000, 0.8660254037844387076, 1.000000000000000000, 0.8660254037844387076, 1.000000000000000000, 0.8660254037844387076, 1.000000000000000000, 0.8660254037844387076, 1.000000000000000000, 0.8660254037844387076, 1.000000000000000000, 0.8660254037844387076, 1.000000000000000000, 0.8660254037844387076, 1.000000000000000000, 0.8660254037844387076, 1.000000000000000000, 0.8660254037844387076, 1.000000000000000000, 0.8660254037844387076, 1.000000000000000000, 0.8660254037844387076, 1.000000000000000000, 0.8660254037844387076, 1.000000000000000000, 0.8660254037844387076, 1.000000000000000000, 0.8660254037844387076, 1.000000000000000000, 0.8660254037844387076, 1.000000000000000000, 0.8660254037844387076, 1.000000000000000000, 0.8660254037844387076, 1.000000000000000000, 0.8660254037844387076, 1.000000000000000000, 0.8660254037844387076, 1.000000000000000000, 0.8660254037844387076, 1.000000000000000000, 0.8660254037844387076, 1.000000000000000000, 0.8660254037844387076, 1.000000000000000000, 0.8660254037844387076, 1.000000000000000000, 0.8660254037844387076, 1.000000000000000000, 0.8660254037844387076, 1.000000000000000000, 0.8660254037844387076, 1.000000000000000000, 0.8660254037844387076, 1.000000000000000000, 0.8660254037844387076, 1.000000000000000000, 0.8660254037844387076, 1.000000000000000000, 0.8660254037844387076, 1.000000000000000000, 0.8660254037844387076, 1.000000000000000000, 0.8660254037844387076, 1.000000000000000000, 0.8660254037844387076, 1.000000000000000000, 0.8660254037844387076, 1.000000000000000000, 0.8660254037844387076, 1.000000000000000000, 0.8660254037844387076, 1.000000000000000000, 0.8660254037844387076, 1.000000000000000000, 0.8660254037844387076, 1.000000000000000000, 0.8660254037844387076, 1.000000000000000000, 0.8660254037844387076, 1.000000000000000000, 0.8660254037844387076, 1.000000000000000000, 0.8660254037844387076, 1.000000000000000000, 0.8660254037844387076, 1.000000000000000000, 0.8660254037844387076, 1.000000000000000000, 0.8660254037844387076, 1.000000000000000000, 0.8660254037844387076, 1.000000000000000000, 0.8660254037844387076, 1.000000000000000000, 0.8660254037844387076, 1.000000000000000000, 0.8660254037844387076, 1.000000000000000000, 0.8660254037844387076, 1.000000000000000000, 0.8660254037844387076, 1.000000000000000000, 0.8660254037844387076, 1.000000000000000000, 0.8660254037844387076, 1.000000000000000000, 0.8660254037844387076, 1.000000000000000000, 0.8660254037844387076, 1.000000000000000000, 0.8660254037844387076, 1.000000000000000000, 0.8660254037844387076, 1.000000000000000000, 0.8660254037844387076, 1.000000000000000000, 0.8660254037844387076, 1.000000000000000000, 0.8660254037844387076, 1.000000000000000000, 0.8660254037844387076, 1.000000000000000000, 0.8660254037844387076, 1.000000000000000000, 0.8660254037844387076, 1.000000000000000000, 0.8660254037844387076, 1.000000000000000000, 0.8660254037844387076, 1.000000000000000000, 0.8660254037844387076, 1.000000000000000000, 0.8660254037844387076, 1.000000000000000000, 0.8660254037844387076, 1.000000000000000000, 0.8660254037844387076, 1.000000000000000000, 0.8660254037844387076, 1.000000000000000000, 0.8660254037844387076, 1.000000000000000000, 0.8660254037844387076, 1.000000000000000000, 0.8660254037844387076, 1.000000000000000000, 0.8660254037844387076, 1.000000000000000000, 0.8660254037844387076, 1.000000000000000000, 0.8660254037844387076, 1.000000000000000000, 0.8660254037844387076, 1.000000000000000000, 0.8660254037844387076, 1.000000000000000000, 0.8660254037844387076, 1.000000000000000000, 0.8660254037844387076, 1.000000000000000000, 0.8660254037844387076, 1.000000000000000000, 0.8660254037844387076, 1.000000000000000000, 0.8660254037844387076, 1.000000000000000000, 0.8660254037844387076, 1.000000000000000000, 0.8660254037844387076, 1.000000000000000000, 0.8660254037844387076, 1.000000000000000000, 0.8660254037844387076, 1.000000000000000000, 0.8660254037844387076, 1.000000000000000000, 0.8660254037844387076, 1.000000000000000000, 0.8660254037844387076, 1.000000000000000000, 0.8660254037844387076, 1.000000000000000000, 0.8660254037844387076, 1.000000000000000000, 0.8660254037844387076, 1.000000000000000000, 0.8660254037844387076, 1.000000000000000000, 0.8660254037844387076, 1.000000000000000000, 0.8660254037844387076, 1.000000000000000000, 0.8660254037844387076, 1.000000000000000000, 0.8660254037844387076, 1.000000000000000000, 0.8660254037844387076, 1.000000000000000000, 0.8660254037844387076, 1.000000000000000000),
 ( 1.000000000000000000, 0.8660254037844387076, 1.000000000000000000, 0.8660254037844387076, 1.000000000000000000, 0.8660254037844387076, 1.000000000000000000, 0.8660254037844387076, 1.000000000000000000, 0.8660254037844387076, 1.000000000000000000, 0.8660254037844387076, 1.000000000000000000, 0.8660254037844387076, 1.000000000000000000, 0.8660254037844387076, 1.000000000000000000, 0.8660254037844387076, 1.000000000000000000, 0.8660254037844387076, 1.000000000000000000, 0.8660254037844387076, 1.000000000000000000, 0.8660254037844387076, 1.000000000000000000, 0.8660254037844387076, 1.000000000000000000, 0.8660254037844387076, 1.000000000000000000, 0.8660254037844387076, 1.000000000000000000, 0.8660254037844387076, 1.000000000000000000, 0.8660254037844387076, 1.000000000000000000, 0.8660254037844387076, 1.000000000000000000, 0.8660254037844387076, 1.000000000000000000, 0.8660254037844387076, 1.000000000000000000, 0.8660254037844387076, 1.000000000000000000, 0.8660254037844387076, 1.000000000000000000, 0.8660254037844387076, 1.000000000000000000, 0.8660254037844387076, 1.000000000000000000, 0.8660254037844387076, 1.000000000000000000, 0.8660254037844387076, 1.000000000000000000, 0.8660254037844387076, 1.000000000000000000, 0.8660254037844387076, 1.000000000000000000, 0.8660254037844387076, 1.000000000000000000, 0.8660254037844387076, 1.000000000000000000, 0.8660254037844387076, 1.000000000000000000, 0.8660254037844387076, 1.000000000000000000, 0.8660254037844387076, 1.000000000000000000, 0.8660254037844387076, 1.000000000000000000, 0.8660254037844387076, 1.000000000000000000, 0.8660254037844387076, 1.000000000000000000, 0.8660254037844387076, 1.000000000000000000, 0.8660254037844387076, 1.000000000000000000, 0.8660254037844387076, 1.000000000000000000, 0.8660254037844387076, 1.000000000000000000, 0.8660254037844387076, 1.000000000000000000, 0.8660254037844387076, 1.000000000000000000, 0.8660254037844387076, 1.000000000000000000, 0.8660254037844387076, 1.000000000000000000, 0.8660254037844387076, 1.000000000000000000, 0.8660254037844387076, 1.000000000000000000, 0.8660254037844387076, 1.000000000000000000, 0.8660254037844387076, 1.000000000000000000, 0.8660254037844387076, 1.000000000000000000, 0.8660254037844387076, 1.000000000000000000, 0.8660254037844387076, 1.000000000000000000, 0.8660254037844387076, 1.000000000000000000, 0.8660254037844387076, 1.000000000000000000, 0.8660254037844387076, 1.000000000000000000, 0.8660254037844387076, 1.000000000000000000, 0.8660254037844387076, 1.000000000000000000, 0.8660254037844387076, 1.000000000000000000, 0.8660254037844387076, 1.000000000000000000, 0.8660254037844387076, 1.000000000000000000, 0.8660254037844387076, 1.000000000000000000, 0.8660254037844387076, 1.000000000000000000, 0.8660254037844387076, 1.000000000000000000, 0.8660254037844387076, 1.000000000000000000, 0.8660254037844387076, 1.000000000000000000, 0.8660254037844387076, 1.000000000000000000, 0.8660254037844387076, 1.000000000000000000, 0.8660254037844387076, 1.000000000000000000, 0.8660254037844387076, 1.000000000000000000, 0.8660254037844387076, 1.000000000000000000, 0.8660254037844387076, 1.000000000000000000, 0.8660254037844387076, 1.000000000000000000, 0.8660254037844387076, 1.000000000000000000, 0.8660254037844387076, 1.000000000000000000, 0.8660254037844387076, 1.000000000000000000, 0.8660254037844387076, 1.000000000000000000, 0.8660254037844387076, 1.000000000000000000, 0.8660254037844387076, 1.000000000000000000, 0.8660254037844387076, 1.000000000000000000, 0.8660254037844387076, 1.000000000000000000, 0.8660254037844387076, 1.000000000000000000, 0.8660254037844387076, 1.000000000000000000, 0.8660254037844387076, 1.000000000000000000, 0.8660254037844387076, 1.000000000000000000, 0.8660254037844387076, 1.000000000000000000, 0.8660254037844387076, 1.000000000000000000, 0.8660254037844387076, 1.000000000000000000, 0.8660254037844387076, 1.000000000000000000, 0.8660254037844387076, 1.000000000000000000, 0.8660254037844387076, 1.000000000000000000, 0.8660254037844387076, 1.000000000000000000, 0.8660254037844387076, 1.000000000000000000, 0.8660254037844387076, 1.000000000000000000, 0.8660254037844387076, 1.000000000000000000, 0.8660254037844387076, 1.000000000000000000, 0.8660254037844387076, 1.000000000000000000, 0.8660254037844387076, 1.000000000000000000, 0.8660254037844387076, 1.000000000000000000, 0.8660254037844387076, 1.000000000000000000, 0.8660254037844387076, 1.000000000000000000, 0.8660254037844387076, 1.000000000000000000, 0.8660254037844387076, 1.000000000000000000, 0.8660254037844387076, 1.000000000000000000, 0.8660254037844387076, 1.000000000000000000, 0.8660254037844387076, 1.000000000000000000, 0.8660254037844387076, 1.000000000000000000, 0.8660254037844387076, 1.000000000000000000, 0.8660254037844387076, 1.000000000000000000, 0.8660254037844387076, 1.000000000000000000, 0.8660254037844387076, 1.000000000000000000, 0.8660254037844387076, 1.000000000000000000, 0.8660254037844387076, 1.000000000000000000, 0.8660254037844387076, 1.000000000000000000, 0.8660254037844387076, 1.000000000000000000, 0.8660254037844387076, 1.000000000000000000, 0.8660254037844387076, 1.000000000000000000, 0.8660254037844387076, 1.000000000000000000, 0.8660254037844387076, 1.000000000000000000, 0.8660254037844387076, 1.000000000000000000, 0.8660254037844387076, 1.000000000000000000, 0.8660254037844387076, 1.000000000000000000, 0.8660254037844387076, 1.000000000000000000, 0.8660254037844387076, 1.000000000000000000, 0.8660254037844387076, 1.000000000000000000, 0.8660254037844387076, 1.000000000000000000, 0.8660254037844387076, 1.000000000000000000, 0.8660254037844387076, 1.000000000000000000, 0.8660254037844387076, 1.000000000000000000, 0.8660254037844387076, 1.000000000000000000, 0.8660254037844387076, 1.000000000000000000, 0.8660254037844387076, 1.000000000000000000, 0.8660254037844387076, 1.000000000000000000, 0.8660254037844387076, 1.000000000000000000, 0.8660254037844387076, 1.000000000000000000, 0.8660254037844387076, 1.000000000000000000, 0.8660254037844387076, 1.000000000000000000, 0.8660254037844387076, 1.000000000000000000, 0.8660254037844387076, 1.000000000000000000, 0.8660254037844387076, 1.000000000000000000, 0.8660254037844387076, 1.000000000000000000, 0.8660254037844387076, 1.000000000000000000, 0.8660254037844387076, 1.000000000000000000, 0.8660254037844387076, 1.000000000000000000, 0.8660254037844387076, 1.000000000000000000, 0.8660254037844387076, 1.000000000000000000, 0.8660254037844387076, 1.000000000000000000, 0.8660254037844387076, 1.000000000000000000, 0.8660254037844387076, 1.000000000000000000, 0.8660254037844387076, 1.000000000000000000, 0.8660254037844387076, 1.000000000000000000, 0.8660254037844387076, 1.000000000000000000, 0.8660254037844387076, 1.000000000000000000, 0.8660254037844387076, 1.000000000000000000, 0.8660254037844387076, 1.000000000000000000, 0.8660254037844387076, 1.000000000000000000, 0.8660254037844387076, 1.000000000000000000, 0.8660254037844387076, 1.000000000000000000, 0.8660254037844387076, 1.000000000000000000, 0.8660254037844387076, 1.000000000000000000, 0.8660254037844387076, 1.000000000000000000, 0.8660254037844387076, 1.000000000000000000, 0.8660254037844387076, 1.000000000000000000, 0.8660254037844387076, 1.000000000000000000, 0.8660254037844387076, 1.000000000000000000, 0.8660254037844387076, 1.000000000000000000, 0.8660254037844387076, 1.000000000000000000, 0.8660254037844387076, 1.000000000000000000, 0.8660254037844387076, 1.000000000000000000, 0.8660254037844387076, 1.000000000000000000, 0.8660254037844387076, 1.000000000000000000, 0.8660254037844387076, 1.000000000000000000, 0.8660254037844387076, 1.000000000000000000, 0.8660254037844387076, 1.000000000000000000, 0.8660254037844387076, 1.000000000000000000, 0.8660254037844387076, 1.000000000000000000, 0.8660254037844387076, 1.000000000000000000, 0.8660254037844387076, 1.000000000000000000, 0.8660254037844387076, 1.000000000000000000, 0.8660254037844387076, 1.000000000000000000, 0.8660254037844387076, 1.000000000000000000, 0.8660254037844387076, 1.000000000000000000, 0.8660254037844387076, 1.000000000000000000, 0.8660254037844387076, 1.000000000000000000, 0.8660254037844387076, 1.000000000000000000, 0.8660254037844387076, 1.000000000000000000, 0.8660254037844387076, 1.000000000000000000, 0.8660254037844387076, 1.000000000000000000, 0.8660254037844387076, 1.000000000000000000, 0.8660254037844387076, 1.000000000000000000, 0.8660254037844387076, 1.000000000000000000, 0.8660254037844387076, 1.000000000000000000, 0.8660254037844387076, 1.000000000000000000, 0.8660254037844387076, 1.000000000000000000, 0.8660254037844387076, 1.000000000000000000, 0.8660254037844387076, 1.000000000000000000, 0.8660254037844387076, 1.000000000000000000, 0.8660254037844387076, 1.000000000000000000, 0.8660254037844387076, 1.000000000000000000, 0.8660254037844387076, 1.000000000000000000, 0.8660254037844387076, 1.000000000000000000, 0.8660254037844387076, 1.000000000000000000, 0.8660254037844387076, 1.000000000000000000, 0.8660254037844387076, 1.000000000000000000, 0.8660254037844387076, 1.000000000000000000, 0.8660254037844387076, 1.000000000000000000, 0.8660254037844387076, 1.000000000000000000, 0.8660254037844387076, 1.000000000000000000, 0.8660254037844387076, 1.000000000000000000, 0.8660254037844387076, 1.000000000000000000, 0.8660254037844387076, 1.000000000000000000, 0.8660254037844387076, 1.000000000000000000, 0.8660254037844387076, 1.000000000000000000, 0.8660254037844387076, 1.000000000000000000, 0.8660254037844387076, 1.000000000000000000, 0.8660254037844387076, 1.000000000000000000, 0.8660254037844387076, 1.000000000000000000, 0.8660254037844387076, 1.000000000000000000, 0.8660254037844387076, 1.000000000000000000, 0.8660254037844387076, 1.000000000000000000, 0.8660254037844387076, 1.000000000000000000, 0.8660254037844387076, 1.000000000000000000, 0.8660254037844387076, 1.000000000000000000, 0.8660254037844387076, 1.000000000000000000, 0.8660254037844387076, 1.000000000000000000, 0.8660254037844387076, 1.000000000000000000, 0.8660254037844387076, 1.000000000000000000, 0.8660254037844387076, 1.000000000000000000, 0.8660254037844387076, 1.000000000000000000, 0.8660254037844387076, 1.000000000000000000, 0.8660254037844387076, 1.000000000000000000, 0.8660254037844387076, 1.000000000000000000, 0.8660254037844387076, 1.000000000000000000, 0.8660254037844387076, 1.000000000000000000, 0.8660254037844387076, 1.000000000000000000, 0.8660254037844387076, 1.000000000000000000, 0.8660254037844387076, 1.000000000000000000, 0.8660254037844387076, 1.000000000000000000, 0.8660254037844387076, 1.000000000000000000, 0.8660254037844387076, 1.000000000000000000, 0.8660254037844387076, 1.000000000000000000, 0.8660254037844387076, 1.000000000000000000, 0.8660254037844387076, 1.000000000000000000, 0.8660254037844387076, 1.000000000000000000, 0.8660254037844387076, 1.000000000000000000, 0.8660254037844387076, 1.000000000000000000, 0.8660254037844387076, 1.000000000000000000, 0.8660254037844387076, 1.000000000000000000, 0.8660254037844387076, 1.000000000000000000, 0.8660254037844387076, 1.000000000000000000, 0.8660254037844387076, 1.000000000000000000, 0.8660254037844387076, 1.000000000000000000, 0.8660254037844387076, 1.000000000000000000, 0.8660254037844387076, 1.000000000000000000, 0.8660254037844387076, 1.000000000000000000, 0.8660254037844387076, 1.000000000000000000, 0.8660254037844387076, 1.000000000000000000, 0.8660254037844387076, 1.000000000000000000, 0.8660254037844387076, 1.000000000000000000, 0.8660254037844387076, 1.000000000000000000, 0.8660254037844387076, 1.000000000000000000, 0.8660254037844387076, 1.000000000000000000, 0.8660254037844387076, 1.000000000000000000, 0.8660254037844387076, 1.000000000000000000, 0.8660254037844387076, 1.000000000000000000, 0.8660254037844387076, 1.000000000000000000, 0.8660254037844387076, 1.000000000000000000, 0.8660254037844387076, 1.000000000000000000, 0.8660254037844387076, 1.000000000000000000, 0.8660254037844387076, 1.000000000000000000, 0.8660254037844387076, 1.000000000000000000, 0.8660254037844387076, 1.000000000000000000, 0.8660254037844387076, 1.000000000000000000, 0.8660254037844387076, 1.000000000000000000, 0.8660254037844387076, 1.000000000000000000, 0.8660254037844387076, 1.000000000000000000, 0.8660254037844387076, 1.000000000000000000, 0.8660254037844387076, 1.000000000000000000, 0.8660254037844387076, 1.000000000000000000, 0.8660254037844387076, 1.000000000000000000, 0.8660254037844387076, 1.000000000000000000, 0.8660254037844387076, 1.000000000000000000, 0.8660254037844387076, 1.000000000000000000, 0.8660254037844387076, 1.000000000000000000, 0.8660254037844387076, 1.000000000000000000, 0.8660254037844387076, 1.000000000000000000, 0.8660254037844387076, 1.000000000000000000, 0.8660254037844387076, 1.000000000000000000, 0.8660254037844387076, 1.000000000000000000, 0.8660254037844387076, 1.000000000000000000, 0.8660254037844387076, 1.000000000000000000, 0.8660254037844387076, 1.000000000000000000, 0.8660254037844387076, 1.000000000000000000, 0.8660254037844387076, 1.000000000000000000, 0.8660254037844387076, 1.000000000000000000, 0.8660254037844387076, 1.000000000000000000, 0.8660254037844387076, 1.000000000000000000, 0.8660254037844387076, 1.000000000000000000, 0.8660254037844387076, 1.000000000000000000, 0.8660254037844387076, 1.000000000000000000, 0.8660254037844387076, 1.000000000000000000, 0.8660254037844387076, 1.000000000000000000, 0.8660254037844387076, 1.000000000000000000, 0.8660254037844387076, 1.000000000000000000, 0.8660254037844387076, 1.000000000000000000, 0.8660254037844387076, 1.000000000000000000, 0.8660254037844387076, 1.000000000000000000, 0.8660254037844387076, 1.000000000000000000, 0.8660254037844387076, 1.000000000000000000, 0.8660254037844387076, 1.000000000000000000, 0.8660254037844387076, 1.000000000000000000, 0.8660254037844387076, 1.000000000000000000, 0.8660254037844387076, 1.000000000000000000, 0.8660254037844387076, 1.000000000000000000, 0.8660254037844387076, 1.000000000000000000, 0.8660254037844387076, 1.000000000000000000, 0.8660254037844387076, 1.000000000000000000, 0.8660254037844387076, 1.000000000000000000, 0.8660254037844387076, 1.000000000000000000, 0.8660254037844387076, 1.000000000000000000, 0.8660254037844387076, 1.000000000000000000, 0.8660254037844387076, 1.000000000000000000, 0.8660254037844387076, 1.000000000000000000, 0.8660254037844387076, 1.000000000000000000, 0.8660254037844387076, 1.000000000000000000, 0.8660254037844387076, 1.000000000000000000, 0.8660254037844387076, 1.000000000000000000, 0.8660254037844387076, 1.000000000000000000, 0.8660254037844387076, 1.000000000000000000, 0.8660254037844387076, 1.000000000000000000, 0.8660254037844387076, 1.000000000000000000, 0.8660254037844387076, 1.000000000000000000, 0.8660254037844387076, 1.000000000000000000, 0.8660254037844387076, 1.000000000000000000, 0.8660254037844387076, 1.000000000000000000, 0.8660254037844387076, 1.000000000000000000, 0.8660254037844387076, 1.000000000000000000, 0.8660254037844387076, 1.000000000000000000, 0.8660254037844387076, 1.000000000000000000, 0.8660254037844387076, 1.000000000000000000, 0.8660254037844387076, 1.000000000000000000, 0.8660254037844387076, 1.000000000000000000, 0.8660254037844387076, 1.000000000000000000, 0.8660254037844387076, 1.000000000000000000, 0.8660254037844387076, 1.000000000000000000, 0.8660254037844387076, 1.000000000000000000, 0.8660254037844387076, 1.000000000000000000, 0.8660254037844387076, 1.000000000000000000, 0.8660254037844387076, 1.000000000000000000, 0.8660254037844387076, 1.000000000000000000, 0.8660254037844387076, 1.000000000000000000, 0.8660254037844387076, 1.000000000000000000, 0.8660254037844387076, 1.000000000000000000, 0.8660254037844387076, 1.000000000000000000, 0.8660254037844387076, 1.000000000000000000, 0.8660254037844387076, 1.000000000000000000, 0.8660254037844387076, 1.000000000000000000, 0.8660254037844387076, 1.000000000000000000, 0.8660254037844387076, 1.000000000000000000, 0.8660254037844387076, 1.000000000000000000, 0.8660254037844387076, 1.000000000000000000, 0.8660254037844387076, 1.000000000000000000) ) ) 
 REPRESENTATION_ITEM ( '' )  SURFACE ( )  );
#12606=CARTESIAN_POINT ( 'NONE',  ( 23.88749999999999929, -2.886751345948125991, -5.000000000000000000 ) ) ;
#12607=CARTESIAN_POINT ( 'NONE',  ( 5.728125000614515905, 6.421520780324663323E-16, -5.243569643749999010 ) ) ;
#12609=CARTESIAN_POINT ( 'NONE',  ( 18.23437500061451999, -4.541064518000419881, 2.621784821874995952 ) ) ;
#12611=CARTESIAN_POINT ( 'NONE',  ( 28.65000000122903145, 5.773502691896255534, 3.535250795749688894E-16 ) ) ;
#12612=CARTESIAN_POINT ( 'NONE',  ( 8.521875000614516082, 3.027376345333613106, -5.243569643749998122 ) ) ;
#12613=EDGE_LOOP ( 'NONE', ( #39256, #69680, #8711, #65709 ) ) ;
#12614=CARTESIAN_POINT ( 'NONE',  ( 18.49687500061452283, 6.054752690667223547, 3.707466751127219781E-16 ) ) ;
#12615=FACE_OUTER_BOUND ( 'NONE', #37835, .T. ) ;
#12616=CARTESIAN_POINT ( 'NONE',  ( 27.00000000000000000, -4.330127018922190985, -2.500000000000001332 ) ) ;
#12617=CARTESIAN_POINT ( 'NONE',  ( 3.525000000000000355, -4.330127018922194537, 2.499999999999995559 ) ) ;
#12620=CARTESIAN_POINT ( 'NONE',  ( 9.487500000000000711, -2.886751345948125991, -5.000000000000000000 ) ) ;
#12622=CARTESIAN_POINT ( 'NONE',  ( 25.52812500061451573, 6.421520780324663323E-16, -5.243569643749999010 ) ) ;
#12623=CARTESIAN_POINT ( 'NONE',  ( 15.33750000000000036, -2.886751345948125991, -5.000000000000000000 ) ) ;
#12624=CARTESIAN_POINT ( 'NONE',  ( 10.91250000122903252, -4.330127018922190985, -2.500000000000001332 ) ) ;
#12625=CARTESIAN_POINT ( 'NONE',  ( 8.315625000614515372, -6.054752690667223547, -1.112240025338166033E-15 ) ) ;
#12626=CARTESIAN_POINT ( 'NONE',  ( 22.38749999999999929, -2.886751345948129988, 4.999999999999997335 ) ) ;
#12627=CARTESIAN_POINT ( 'NONE',  ( 20.46562500061451928, -6.054752690667223547, -1.112240025338166033E-15 ) ) ;
#12629=CARTESIAN_POINT ( 'NONE',  ( 26.55000000122902648, -2.886751345948129988, 4.999999999999997335 ) ) ;
#12631=CARTESIAN_POINT ( 'NONE',  ( 5.587500000000003020, 5.773502691896255534, 3.535250795749688894E-16 ) ) ;
#12633=CARTESIAN_POINT ( 'NONE',  ( 21.62812500061451360, 4.541064518000418104, 2.621784821874999949 ) ) ;
#12634=CARTESIAN_POINT ( 'NONE',  ( 29.35312500061451502, 0.000000000000000000, 5.243569643749999010 ) ) ;
#12635=CARTESIAN_POINT ( 'NONE',  ( 28.39687500061452141, 6.054752690667223547, 3.707466751127219781E-16 ) ) ;
#12636=CARTESIAN_POINT ( 'NONE',  ( 19.43437500061451928, 4.541064518000418104, 2.621784821874999949 ) ) ;
#12637=CARTESIAN_POINT ( 'NONE',  ( 15.36562500061451608, 3.027376345333611329, 5.243569643749999010 ) ) ;
#12638=CARTESIAN_POINT ( 'NONE',  ( -1.473776270879187500, 9.816672227264625405, -34.04916702557058983 ) ) ;
#12639=CARTESIAN_POINT ( 'NONE',  ( 25.38750000122903216, 6.123233995736764310E-16, -4.999999999999998224 ) ) ;
#12641=CARTESIAN_POINT ( 'NONE',  ( 17.46562500061451217, 3.027376345333612662, -5.243569643749998122 ) ) ;
#12642=CARTESIAN_POINT ( 'NONE',  ( 4.537500001229034297, -4.330127018922194537, 2.499999999999995559 ) ) ;
#12643=CARTESIAN_POINT ( 'NONE',  ( 12.15937500061451892, 4.541064518000418104, -2.621784821874998173 ) ) ;
#12644=CARTESIAN_POINT ( 'NONE',  ( 12.49687500061451573, -3.027376345333610441, -5.243569643749999898 ) ) ;
#12645=CARTESIAN_POINT ( 'NONE',  ( 20.82187500061451857, 3.027376345333611329, 5.243569643749999010 ) ) ;
#12646=ORIENTED_EDGE ( 'NONE', *, *, #54952, .F. ) ;
#12647=CARTESIAN_POINT ( 'NONE',  ( 24.03750000122903430, 6.123233995736764310E-16, -4.999999999999998224 ) ) ;
#12648=CARTESIAN_POINT ( 'NONE',  ( 23.35312500061451857, 4.541064518000418104, -2.621784821874998173 ) ) ;
#12649=CARTESIAN_POINT ( 'NONE',  ( 19.13437500061451857, -4.541064518000419881, 2.621784821874995952 ) ) ;
#12650=CARTESIAN_POINT ( 'NONE',  ( 25.00312500061451715, -4.541064518000417216, -2.621784821875001281 ) ) ;
#12651=LINE ( 'NONE', #24458, #26226 ) ;
#12652=CARTESIAN_POINT ( 'NONE',  ( 4.000000000000000000, 15.23750000000000071, 32.30940107675849049 ) ) ;
#12653=CARTESIAN_POINT ( 'NONE',  ( 3.421875000614516882, -6.054752690667223547, -1.112240025338166033E-15 ) ) ;
#12654=CARTESIAN_POINT ( 'NONE',  ( 8.775000001229033231, 2.886751345948129099, -4.999999999999998224 ) ) ;
#12655=CARTESIAN_POINT ( 'NONE',  ( 4.800000001229032698, 5.773502691896255534, 3.535250795749688894E-16 ) ) ;
#12656=CARTESIAN_POINT ( 'NONE',  ( -5.810221930991193690E-16, 11.90000000122903501, -34.00000000000000000 ) ) ;
#12657=CARTESIAN_POINT ( 'NONE',  ( 27.90000000122903145, -2.886751345948129988, 4.999999999999997335 ) ) ;
#12660=CARTESIAN_POINT ( 'NONE',  ( 10.50937500061451679, 0.000000000000000000, 5.243569643749999010 ) ) ;
#12662=CARTESIAN_POINT ( 'NONE',  ( 16.82812500061451644, -4.541064518000419881, 2.621784821874995952 ) ) ;
#12663=CARTESIAN_POINT ( 'NONE',  ( 10.99687500061451750, -3.027376345333614438, 5.243569643749998122 ) ) ;
#12664=CARTESIAN_POINT ( 'NONE',  ( 2.915625000614516793, -6.054752690667223547, -1.112240025338166033E-15 ) ) ;
#12665=CARTESIAN_POINT ( 'NONE',  ( 19.02187500061451786, 3.027376345333611329, 5.243569643749999010 ) ) ;
#12666=CARTESIAN_POINT ( 'NONE',  ( 7.659375000614518036, 4.541064518000418104, -2.621784821874998173 ) ) ;
#12667=CARTESIAN_POINT ( 'NONE',  ( 3.440625000614518036, -3.027376345333610441, -5.243569643749999898 ) ) ;
#12668=CARTESIAN_POINT ( 'NONE',  ( -1.071796769724488563, 17.84240381056766367, 34.00000000000000000 ) ) ;
#12669=CARTESIAN_POINT ( 'NONE',  ( 7.003125000614518036, -4.541064518000417216, -2.621784821875001281 ) ) ;
#12670=CARTESIAN_POINT ( 'NONE',  ( 17.57812500061451644, 4.541064518000418104, 2.621784821874999949 ) ) ;
#12671=ORIENTED_EDGE ( 'NONE', *, *, #24843, .F. ) ;
#12672=CARTESIAN_POINT ( 'NONE',  ( 5.437500001229035540, -4.330127018922194537, 2.499999999999995559 ) ) ;
#12673=CARTESIAN_POINT ( 'NONE',  ( 15.32812500061451644, 4.541064518000418104, 2.621784821874999949 ) ) ;
#12674=CARTESIAN_POINT ( 'NONE',  ( 13.71562500061451750, -6.054752690667223547, -1.112240025338166033E-15 ) ) ;
#12676=CARTESIAN_POINT ( 'NONE',  ( 12.97499999999999964, -4.330127018922194537, 2.499999999999995559 ) ) ;
#12677=EDGE_CURVE ( 'NONE', #32974, #71417, #5616, .T. ) ;
#12678=CARTESIAN_POINT ( 'NONE',  ( 7.462500001229035007, 4.330127018922192761, -2.499999999999997780 ) ) ;
#12679=CARTESIAN_POINT ( 'NONE',  ( 3.965625000614515727, 3.027376345333613106, -5.243569643749998122 ) ) ;
#12680=CARTESIAN_POINT ( 'NONE',  ( 18.63750000122903216, 6.123233995736764310E-16, -4.999999999999998224 ) ) ;
#12682=CARTESIAN_POINT ( 'NONE',  ( 2.121784821874999061, 12.05937500061451750, -33.67503911421598417 ) ) ;
#12685=CARTESIAN_POINT ( 'NONE',  ( 6.524999999999999467, 4.330127018922191873, 2.499999999999999556 ) ) ;
#12686=CARTESIAN_POINT ( 'NONE',  ( -3.999999999999997335, 13.28749999999999964, 32.30940107675850470 ) ) ;
#12687=CARTESIAN_POINT ( 'NONE',  ( 17.55937500061451573, 4.541064518000418104, -2.621784821874998173 ) ) ;
#12688=AXIS2_PLACEMENT_3D ( 'NONE', #49599, #54408, #43693 ) ;
#12689=CARTESIAN_POINT ( 'NONE',  ( 14.87812500061451537, 4.541064518000418104, 2.621784821874999949 ) ) ;
#12691=CARTESIAN_POINT ( 'NONE',  ( -1.071796769724491005, 14.62009619066136779, 26.00000000000000355 ) ) ;
#12692=CARTESIAN_POINT ( 'NONE',  ( 26.55937500061451573, 4.541064518000418104, -2.621784821874998173 ) ) ;
#12694=CARTESIAN_POINT ( 'NONE',  ( 12.21562500061451573, 3.027376345333611329, 5.243569643749999010 ) ) ;
#12695=CARTESIAN_POINT ( 'NONE',  ( 15.23437500061451644, 6.421520780324663323E-16, -5.243569643749999010 ) ) ;
#12696=ORIENTED_EDGE ( 'NONE', *, *, #31768, .T. ) ;
#12697=CARTESIAN_POINT ( 'NONE',  ( 27.21562500061451928, -6.054752690667223547, -1.112240025338166033E-15 ) ) ;
#12698=CARTESIAN_POINT ( 'NONE',  ( 20.54062500061451502, -3.027376345333610441, -5.243569643749999898 ) ) ;
#12699=CARTESIAN_POINT ( 'NONE',  ( 3.132876461932173395, 3.896812063161361195, -3.508551012645405365 ) ) ;
#12700=CARTESIAN_POINT ( 'NONE',  ( -3.137519842735245283E-14, 14.37500000122903288, -26.00000000000000711 ) ) ;
#12701=CARTESIAN_POINT ( 'NONE',  ( 9.037499999999999645, -2.886751345948125991, -5.000000000000000000 ) ) ;
#12702=CARTESIAN_POINT ( 'NONE',  ( 18.33750000122903501, 4.330127018922191873, 2.499999999999999556 ) ) ;
#12703=CYLINDRICAL_SURFACE ( 'NONE', #54933, 10.00000000000000000 ) ;
#12705=ORIENTED_EDGE ( 'NONE', *, *, #54021, .F. ) ;
#12706=CARTESIAN_POINT ( 'NONE',  ( 18.63749999999999929, 5.773502691896255534, 3.535250795749688894E-16 ) ) ;
#12707=CARTESIAN_POINT ( 'NONE',  ( 22.42500000000000071, -4.330127018922194537, 2.499999999999995559 ) ) ;
#12708=CARTESIAN_POINT ( 'NONE',  ( 19.99687500061451573, -3.027376345333614438, 5.243569643749998122 ) ) ;
#12709=CARTESIAN_POINT ( 'NONE',  ( 24.40312500061451573, 0.000000000000000000, 5.243569643749999010 ) ) ;
#12710=EDGE_CURVE ( 'NONE', #32129, #48891, #57907, .T. ) ;
#12711=EDGE_LOOP ( 'NONE', ( #15487, #48728, #57141, #62009 ) ) ;
#12712=CARTESIAN_POINT ( 'NONE',  ( 8.775000001229031454, 2.886751345948062486, -5.000000000000113687 ) ) ;
#12713=CARTESIAN_POINT ( 'NONE',  ( 5.615625000614517859, -6.054752690667223547, -1.112240025338166033E-15 ) ) ;
#12714=CARTESIAN_POINT ( 'NONE',  ( 13.91249999999999964, -5.773502691896255534, -1.060575238724906372E-15 ) ) ;
#12715=CARTESIAN_POINT ( 'NONE',  ( -3.000416591977282496E-16, 16.54062500061451857, 25.09994784771203058 ) ) ;
#12716=CARTESIAN_POINT ( 'NONE',  ( 29.16562500061451502, 3.027376345333613106, -5.243569643749998122 ) ) ;
#12719=CARTESIAN_POINT ( 'NONE',  ( 25.20937500061451431, 4.541064518000418104, -2.621784821874998173 ) ) ;
#12720=ORIENTED_EDGE ( 'NONE', *, *, #12941, .T. ) ;
#12721=CARTESIAN_POINT ( 'NONE',  ( 20.87812500061451715, -4.541064518000419881, 2.621784821874995952 ) ) ;
#12722=CARTESIAN_POINT ( 'NONE',  ( 22.47187500061451715, 3.027376345333613106, -5.243569643749998122 ) ) ;
#12723=CARTESIAN_POINT ( 'NONE',  ( -2.121784821874999949, 17.02812500061459744, -33.67503911421598417 ) ) ;
#12724=CARTESIAN_POINT ( 'NONE',  ( 7.153125000614518392, 4.541064518000418104, -2.621784821874998173 ) ) ;
#12726=CARTESIAN_POINT ( 'NONE',  ( 22.86562500061451431, 3.027376345333612662, -5.243569643749998122 ) ) ;
#12729=CARTESIAN_POINT ( 'NONE',  ( 16.28437500061452070, 4.541064518000418104, 2.621784821874999949 ) ) ;
#12730=CARTESIAN_POINT ( 'NONE',  ( 20.07187500061451857, -6.054752690667223547, -1.112240025338166033E-15 ) ) ;
#12731=CARTESIAN_POINT ( 'NONE',  ( 26.97187500061451360, 3.027376345333613106, -5.243569643749998122 ) ) ;
#12732=CARTESIAN_POINT ( 'NONE',  ( 4.243569643749999898, 15.58437500061451786, 30.00000000000000000 ) ) ;
#12733=CARTESIAN_POINT ( 'NONE',  ( 7.865625000614516971, -6.054752690667223547, -1.112240025338166033E-15 ) ) ;
#12734=CARTESIAN_POINT ( 'NONE',  ( -1.999999999999997113, 19.17500000000000071, 33.46410161513775705 ) ) ;
#12735=CARTESIAN_POINT ( 'NONE',  ( 5.746875000614517504, -3.027376345333610441, -5.243569643749999898 ) ) ;
#12736=DIRECTION ( 'NONE',  ( -1.000000000000000000, -0.000000000000000000, -0.000000000000000000 ) ) ;
#12737=CARTESIAN_POINT ( 'NONE',  ( 5.203125000614518214, -4.541064518000417216, -2.621784821875001281 ) ) ;
#12738=CARTESIAN_POINT ( 'NONE',  ( 8.671875000614518214, 3.027376345333611329, 5.243569643749999010 ) ) ;
#12740=CARTESIAN_POINT ( 'NONE',  ( 16.83750000122903145, 6.123233995736764310E-16, -4.999999999999998224 ) ) ;
#12741=CARTESIAN_POINT ( 'NONE',  ( 4.921875000614518214, 3.027376345333613106, -5.243569643749998122 ) ) ;
#12742=CARTESIAN_POINT ( 'NONE',  ( 7.003125000614518036, -4.541064518000417216, -2.621784821875001281 ) ) ;
#12745=CARTESIAN_POINT ( 'NONE',  ( 16.13437500061451502, 6.421520780324663323E-16, -5.243569643749999010 ) ) ;
#12747=VERTEX_POINT ( 'NONE', #52382 ) ;
#12748=CARTESIAN_POINT ( 'NONE',  ( 25.30312500061451431, 0.000000000000000000, 5.243569643749999010 ) ) ;
#12749=CARTESIAN_POINT ( 'NONE',  ( 8.765625000614518214, -6.054752690667223547, -1.112240025338166033E-15 ) ) ;
#12751=CARTESIAN_POINT ( 'NONE',  ( 28.13437500061451502, -4.541064518000419881, 2.621784821874995952 ) ) ;
#12752=CARTESIAN_POINT ( 'NONE',  ( 9.815625000614518925, 3.027376345333613106, -5.243569643749998122 ) ) ;
#12753=CARTESIAN_POINT ( 'NONE',  ( 4.243569643749999898, 10.18437500061451750, -30.00000000000000000 ) ) ;
#12754=CARTESIAN_POINT ( 'NONE',  ( 11.55000000122903181, 5.773502691896255534, 3.535250795749688894E-16 ) ) ;
#12755=CARTESIAN_POINT ( 'NONE',  ( 25.79062500061451502, -3.027376345333614438, 5.243569643749998122 ) ) ;
#12756=CARTESIAN_POINT ( 'NONE',  ( 4.243569643749999898, 12.82812500061451821, -30.00000000000000000 ) ) ;
#12757=CARTESIAN_POINT ( 'NONE',  ( 11.85000000122903430, -2.886751345948125991, -5.000000000000000000 ) ) ;
#12758=CARTESIAN_POINT ( 'NONE',  ( 22.71562500061451573, -6.054752690667223547, -1.112240025338166033E-15 ) ) ;
#12759=CARTESIAN_POINT ( 'NONE',  ( 11.36250000000000071, 2.886751345948129099, -4.999999999999998224 ) ) ;
#12760=CARTESIAN_POINT ( 'NONE',  ( 21.44062500061452070, -3.027376345333610441, -5.243569643749999898 ) ) ;
#12761=CARTESIAN_POINT ( 'NONE',  ( 5.484375000614518214, 4.541064518000418104, 2.621784821874999949 ) ) ;
#12762=CARTESIAN_POINT ( 'NONE',  ( 20.96250000000000213, 2.886751345948126879, 4.999999999999999112 ) ) ;
#12763=CARTESIAN_POINT ( 'NONE',  ( 16.68750000122903288, -4.330127018922194537, 2.499999999999995559 ) ) ;
#12764=CARTESIAN_POINT ( 'NONE',  ( 13.15312500061451750, 0.000000000000000000, 5.243569643749999010 ) ) ;
#12766=CARTESIAN_POINT ( 'NONE',  ( 14.69062500061451537, -3.027376345333610441, -5.243569643749999898 ) ) ;
#12767=CARTESIAN_POINT ( 'NONE',  ( 25.16250000122903074, 0.000000000000000000, 4.999999999999998224 ) ) ;
#12768=CARTESIAN_POINT ( 'NONE',  ( 19.31250000000000000, -5.773502691896255534, -1.060575238724906372E-15 ) ) ;
#12769=CARTESIAN_POINT ( 'NONE',  ( 22.62187500061451573, 3.027376345333611329, 5.243569643749999010 ) ) ;
#12771=CARTESIAN_POINT ( 'NONE',  ( 7.462500001229035007, 4.330127018922192761, -2.499999999999997780 ) ) ;
#12772=CARTESIAN_POINT ( 'NONE',  ( 9.571875000614518569, 3.027376345333611329, 5.243569643749999010 ) ) ;
#12773=CARTESIAN_POINT ( 'NONE',  ( 26.48437500061451644, 6.421520780324663323E-16, -5.243569643749999010 ) ) ;
#12774=CARTESIAN_POINT ( 'NONE',  ( 15.41250000122903252, -4.330127018922190985, -2.500000000000001332 ) ) ;
#12775=CARTESIAN_POINT ( 'NONE',  ( 20.27812500061451573, 4.541064518000418104, 2.621784821874999949 ) ) ;
#12776=CARTESIAN_POINT ( 'NONE',  ( 27.12187500061451573, 3.027376345333611329, 5.243569643749999010 ) ) ;
#12778=CARTESIAN_POINT ( 'NONE',  ( 9.046875000614518214, 6.054752690667223547, 3.707466751127219781E-16 ) ) ;
#12779=CARTESIAN_POINT ( 'NONE',  ( 18.59062500061451573, -3.027376345333614438, 5.243569643749998122 ) ) ;
#12780=ORIENTED_EDGE ( 'NONE', *, *, #26740, .F. ) ;
#12781=CYLINDRICAL_SURFACE ( 'NONE', #18295, 4.000000000000000000 ) ;
#12782=CARTESIAN_POINT ( 'NONE',  ( 27.10312500061451502, 0.000000000000000000, 5.243569643749999010 ) ) ;
#12783=CARTESIAN_POINT ( 'NONE',  ( 3.196875000614516793, 6.054752690667223547, 3.707466751127219781E-16 ) ) ;
#12785=CYLINDRICAL_SURFACE ( 'NONE', #25312, 4.999999999999998224 ) ;
#12786=CARTESIAN_POINT ( 'NONE',  ( 16.01249999999999929, 2.886751345948126879, 4.999999999999999112 ) ) ;
#12787=CARTESIAN_POINT ( 'NONE',  ( 21.77812500061451928, -4.541064518000419881, 2.621784821874995952 ) ) ;
#12788=EDGE_LOOP ( 'NONE', ( #14894, #48364 ) ) ;
#12789=CARTESIAN_POINT ( 'NONE',  ( 24.93750000000000355, 5.773502691896255534, 3.535250795749688894E-16 ) ) ;
#12790=CARTESIAN_POINT ( 'NONE',  ( 26.37187500061451217, -6.054752690667223547, -1.112240025338166033E-15 ) ) ;
#12791=EDGE_CURVE ( 'NONE', #68292, #17100, #7429, .T. ) ;
#12792=VERTEX_POINT ( 'NONE', #20941 ) ;
#12793=CARTESIAN_POINT ( 'NONE',  ( 15.21562500061451750, 3.027376345333613106, -5.243569643749998122 ) ) ;
#12794=CARTESIAN_POINT ( 'NONE',  ( 5.090625000614516615, -3.027376345333614438, 5.243569643749998122 ) ) ;
#12796=CARTESIAN_POINT ( 'NONE',  ( 2.971875000614517592, -6.054752690667223547, -1.112240025338166033E-15 ) ) ;
#12797=CARTESIAN_POINT ( 'NONE',  ( 14.17500000122903536, 2.886751345948129099, -4.999999999999998224 ) ) ;
#12798=CARTESIAN_POINT ( 'NONE',  ( 20.73750000000000071, -2.886751345948125991, -5.000000000000000000 ) ) ;
#12799=CARTESIAN_POINT ( 'NONE',  ( 28.61249999999999716, 2.886751345948126879, 4.999999999999999112 ) ) ;
#12800=CARTESIAN_POINT ( 'NONE',  ( 3.721875000614518036, 3.027376345333611329, 5.243569643749999010 ) ) ;
#12801=CARTESIAN_POINT ( 'NONE',  ( 10.43437500061451750, 4.541064518000418104, 2.621784821874999949 ) ) ;
#12802=CARTESIAN_POINT ( 'NONE',  ( 19.35937500061451644, 4.541064518000418104, -2.621784821874998173 ) ) ;
#12804=ORIENTED_EDGE ( 'NONE', *, *, #68955, .T. ) ;
#12805=CARTESIAN_POINT ( 'NONE',  ( 28.71562500061451573, 3.027376345333613106, -5.243569643749998122 ) ) ;
#12806=CARTESIAN_POINT ( 'NONE',  ( 3.149999999999999911, -4.330127018922190985, -2.500000000000001332 ) ) ;
#12807=( BOUNDED_CURVE ( )  B_SPLINE_CURVE ( 2, ( #61417, #39262, #21521, #10810, #50704, #49979, #16343, #68060, #55883 ),
 .UNSPECIFIED., .F., .F. ) 
 B_SPLINE_CURVE_WITH_KNOTS ( ( 3, 2, 2, 2, 3 ),
 ( 0.4456521739130435145, 0.4492753623188405765, 0.4565217391304347561, 0.4637681159420289911, 0.4673913043478261087 ),
 .UNSPECIFIED. ) 
 CURVE ( )  GEOMETRIC_REPRESENTATION_ITEM ( )  RATIONAL_B_SPLINE_CURVE ( ( 0.9330127018922194093, 0.9330127018922198534, 1.000000000000000000, 0.8660254037844387076, 1.000000000000000000, 0.8660254037844387076, 1.000000000000000000, 0.9330127018922188542, 0.9330127018922194093 ) ) 
 REPRESENTATION_ITEM ( '' )  );
#12808=CARTESIAN_POINT ( 'NONE',  ( 5.484375000614518214, 4.541064518000418104, 2.621784821874999949 ) ) ;
#12809=CARTESIAN_POINT ( 'NONE',  ( 19.16250000000000142, 2.886751345948126879, 4.999999999999999112 ) ) ;
#12810=CARTESIAN_POINT ( 'NONE',  ( 12.92812500061451786, 6.421520780324663323E-16, -5.243569643749999010 ) ) ;
#12812=CARTESIAN_POINT ( 'NONE',  ( 4.080569135018654592, -2.889455923578380769, -4.080569135022440896 ) ) ;
#12815=CARTESIAN_POINT ( 'NONE',  ( 8.465625000614515727, 3.027376345333613106, -5.243569643749998122 ) ) ;
#12816=CARTESIAN_POINT ( 'NONE',  ( 25.17187500061451644, 3.027376345333613106, -5.243569643749998122 ) ) ;
#12817=CARTESIAN_POINT ( 'NONE',  ( -4.243569643749997233, 18.54687500061451289, 32.45002607614398471 ) ) ;
#12818=CARTESIAN_POINT ( 'NONE',  ( 25.99687500061451928, -3.027376345333610441, -5.243569643749999898 ) ) ;
#12819=CARTESIAN_POINT ( 'NONE',  ( 6.862500000000002487, 2.886751345948129099, -4.999999999999998224 ) ) ;
#12820=CARTESIAN_POINT ( 'NONE',  ( -2.000000000000000000, 13.73750000122903359, 26.53589838486224650 ) ) ;
#12821=CARTESIAN_POINT ( 'NONE',  ( 14.12812500061451715, -4.541064518000419881, 2.621784821874995952 ) ) ;
#12822=CARTESIAN_POINT ( 'NONE',  ( 6.525000001229033231, 2.886751345948129099, -4.999999999999998224 ) ) ;
#12823=CARTESIAN_POINT ( 'NONE',  ( 16.99687500061451573, -3.027376345333610441, -5.243569643749999898 ) ) ;
#12824=CARTESIAN_POINT ( 'NONE',  ( 12.83437500061451786, -4.541064518000419881, 2.621784821874995952 ) ) ;
#12827=CARTESIAN_POINT ( 'NONE',  ( 11.91562500061451857, -6.054752690667223547, -1.112240025338166033E-15 ) ) ;
#12829=CARTESIAN_POINT ( 'NONE',  ( 23.81250000122903288, 0.000000000000000000, 4.999999999999998224 ) ) ;
#12830=CARTESIAN_POINT ( 'NONE',  ( 12.60937500061451821, 4.541064518000418104, -2.621784821874998173 ) ) ;
#12831=CARTESIAN_POINT ( 'NONE',  ( 3.300000000000000711, 4.330127018922192761, -2.499999999999997780 ) ) ;
#12832=CARTESIAN_POINT ( 'NONE',  ( 14.61562500061451608, -6.054752690667223547, -1.112240025338166033E-15 ) ) ;
#12833=CARTESIAN_POINT ( 'NONE',  ( -5.810221930991193690E-16, 18.98750000000000071, -34.00000000000000000 ) ) ;
#12834=CARTESIAN_POINT ( 'NONE',  ( 24.08437500061451786, -4.541064518000419881, 2.621784821874995952 ) ) ;
#12836=CARTESIAN_POINT ( 'NONE',  ( 12.82500000122903394, 2.886751345948129099, -4.999999999999998224 ) ) ;
#12837=CARTESIAN_POINT ( 'NONE',  ( 4.428044609675158227, 2.322158679919935409, 4.428044609675073850 ) ) ;
#12839=CARTESIAN_POINT ( 'NONE',  ( 9.001249775931846008E-16, 17.72187500061451715, -25.09994784771203058 ) ) ;
#12840=CARTESIAN_POINT ( 'NONE',  ( 18.90937500061451360, 4.541064518000418104, -2.621784821874998173 ) ) ;
#12841=CARTESIAN_POINT ( 'NONE',  ( 17.58750000122903145, -4.330127018922194537, 2.499999999999995559 ) ) ;
#12843=CARTESIAN_POINT ( 'NONE',  ( 15.60937500061451644, -4.541064518000417216, -2.621784821875001281 ) ) ;
#12844=CARTESIAN_POINT ( 'NONE',  ( 9.001249775931846008E-16, 10.97187500061451715, 34.90005215228797653 ) ) ;
#12845=CARTESIAN_POINT ( 'NONE',  ( 19.95000000122903572, -2.886751345948125991, -5.000000000000000000 ) ) ;
#12846=CARTESIAN_POINT ( 'NONE',  ( 14.01562500061451644, 3.027376345333611329, 5.243569643749999010 ) ) ;
#12849=CARTESIAN_POINT ( 'NONE',  ( 17.77499999999999858, 4.330127018922191873, 2.499999999999999556 ) ) ;
#12850=CARTESIAN_POINT ( 'NONE',  ( 27.37500000000000000, -4.330127018922194537, 2.499999999999995559 ) ) ;
#12851=CARTESIAN_POINT ( 'NONE',  ( 4.010363759615468204, 2.986131697625305836, 4.103404943945538896 ) ) ;
#12852=CARTESIAN_POINT ( 'NONE',  ( 14.43750000122903288, -4.330127018922194537, 2.499999999999995559 ) ) ;
#12853=CARTESIAN_POINT ( 'NONE',  ( 26.22187500061451715, 3.027376345333611329, 5.243569643749999010 ) ) ;
#12854=CARTESIAN_POINT ( 'NONE',  ( 19.26562500061451644, 3.027376345333613106, -5.243569643749998122 ) ) ;
#12855=CARTESIAN_POINT ( 'NONE',  ( 22.79062500061451502, -3.027376345333610441, -5.243569643749999898 ) ) ;
#12856=CARTESIAN_POINT ( 'NONE',  ( 3.290625000614516793, -3.027376345333614438, 5.243569643749998122 ) ) ;
#12857=CARTESIAN_POINT ( 'NONE',  ( 28.49999999999999645, 4.330127018922192761, -2.499999999999997780 ) ) ;
#12861=CARTESIAN_POINT ( 'NONE',  ( -0.6945863667395647534, 9.663023495605401081, -33.93923213064925193 ) ) ;
#12863=CARTESIAN_POINT ( 'NONE',  ( 2.121784821874999061, 16.10937500061451644, -33.67503911421598417 ) ) ;
#12864=CARTESIAN_POINT ( 'NONE',  ( 7.050000001229036251, 5.773502691896255534, 3.535250795749688894E-16 ) ) ;
#12865=CARTESIAN_POINT ( 'NONE',  ( 6.825000000000001066, 6.123233995736764310E-16, -4.999999999999998224 ) ) ;
#12867=CARTESIAN_POINT ( 'NONE',  ( 8.671875000614518214, 3.027376345333611329, 5.243569643749999010 ) ) ;
#12868=CARTESIAN_POINT ( 'NONE',  ( 27.96562500061451928, 3.027376345333611329, 5.243569643749999010 ) ) ;
#12869=CARTESIAN_POINT ( 'NONE',  ( 27.45000000122903216, -2.886751345948155301, 4.999999999999952927 ) ) ;
#12870=CARTESIAN_POINT ( 'NONE',  ( -5.840105773466370387, 8.117609419225257028, -28.60964832515872658 ) ) ;
#12872=CARTESIAN_POINT ( 'NONE',  ( 8.934375000614517504, 6.421520780324663323E-16, -5.243569643749999010 ) ) ;
#12873=CARTESIAN_POINT ( 'NONE',  ( 12.34687500061452070, -3.027376345333614438, 5.243569643749998122 ) ) ;
#12874=CARTESIAN_POINT ( 'NONE',  ( 7.050000000000000711, 0.000000000000000000, 4.999999999999998224 ) ) ;
#12875=CARTESIAN_POINT ( 'NONE',  ( -4.243569643749999898, 14.85312500061459495, 30.00000000000000000 ) ) ;
#12877=CARTESIAN_POINT ( 'NONE',  ( 7.012500000000001066, 2.886751345948126879, 4.999999999999999112 ) ) ;
#12878=CARTESIAN_POINT ( 'NONE',  ( 26.43750000122903288, 4.330127018922191873, 2.499999999999999556 ) ) ;
#12880=CARTESIAN_POINT ( 'NONE',  ( 22.37812500061451360, 6.421520780324663323E-16, -5.243569643749999010 ) ) ;
#12881=CARTESIAN_POINT ( 'NONE',  ( 14.31562500061451537, 3.027376345333613106, -5.243569643749998122 ) ) ;
#12883=CARTESIAN_POINT ( 'NONE',  ( 9.459375000614517859, 4.541064518000418104, -2.621784821874998173 ) ) ;
#12884=CARTESIAN_POINT ( 'NONE',  ( 27.18750000000000000, 5.773502691896255534, 3.535250795749688894E-16 ) ) ;
#12885=CARTESIAN_POINT ( 'NONE',  ( 22.46250000122903501, 0.000000000000000000, 4.999999999999998224 ) ) ;
#12886=CARTESIAN_POINT ( 'NONE',  ( -1.071796769724488563, 18.40490381179670365, -26.00000000000000000 ) ) ;
#12887=CARTESIAN_POINT ( 'NONE',  ( 11.67187500061451821, 3.027376345333613106, -5.243569643749998122 ) ) ;
#12888=CARTESIAN_POINT ( 'NONE',  ( 27.64687500061452141, -3.027376345333614438, 5.243569643749998122 ) ) ;
#12891=CARTESIAN_POINT ( 'NONE',  ( 22.54687500061451999, 6.054752690667223547, 3.707466751127219781E-16 ) ) ;
#12892=CARTESIAN_POINT ( 'NONE',  ( 12.83437500061451786, -4.541064518000419881, 2.621784821874995952 ) ) ;
#12894=CARTESIAN_POINT ( 'NONE',  ( 26.17500000000000071, 6.123233995736764310E-16, -4.999999999999998224 ) ) ;
#12896=CARTESIAN_POINT ( 'NONE',  ( 2.121784821875001281, 11.90937500061451892, -26.32496088578401938 ) ) ;
#12898=CARTESIAN_POINT ( 'NONE',  ( 17.57812500061451644, 4.541064518000418104, 2.621784821874999949 ) ) ;
#12899=CARTESIAN_POINT ( 'NONE',  ( 6.450000000000001066, 4.330127018922192761, -2.499999999999997780 ) ) ;
#12900=CARTESIAN_POINT ( 'NONE',  ( 0.000000000000000000, 20.00000000000000000, -33.99999999999999289 ) ) ;
#12901=CARTESIAN_POINT ( 'NONE',  ( 14.32500000000000107, -4.330127018922194537, 2.499999999999995559 ) ) ;
#12902=CARTESIAN_POINT ( 'NONE',  ( -3.000416591977282496E-16, 10.69062500061451715, 25.09994784771203058 ) ) ;
#12903=CARTESIAN_POINT ( 'NONE',  ( 13.53750000122903430, -4.330127018922194537, 2.499999999999995559 ) ) ;
#12904=CARTESIAN_POINT ( 'NONE',  ( 24.98437500061451644, -4.541064518000419881, 2.621784821874995952 ) ) ;
#12905=EDGE_LOOP ( 'NONE', ( #10276, #4789, #19737 ) ) ;
#12906=CARTESIAN_POINT ( 'NONE',  ( 19.86562500061451786, 3.027376345333611329, 5.243569643749999010 ) ) ;
#12907=CARTESIAN_POINT ( 'NONE',  ( 19.84687500061451360, 6.054752690667223547, 3.707466751127219781E-16 ) ) ;
#12908=CARTESIAN_POINT ( 'NONE',  ( 4.800000000000002487, 0.000000000000000000, 4.999999999999998224 ) ) ;
#12909=CARTESIAN_POINT ( 'NONE',  ( 7.940625000614518036, -3.027376345333610441, -5.243569643749999898 ) ) ;
#12910=CARTESIAN_POINT ( 'NONE',  ( 20.76562500061451644, 3.027376345333611329, 5.243569643749999010 ) ) ;
#12911=CARTESIAN_POINT ( 'NONE',  ( 12.08437500061451608, 6.421520780324663323E-16, -5.243569643749999010 ) ) ;
#12912=CARTESIAN_POINT ( 'NONE',  ( 17.70937500061451431, 0.000000000000000000, 5.243569643749999010 ) ) ;
#12913=CARTESIAN_POINT ( 'NONE',  ( 4.243569643749999898, 15.52812500061451750, 30.00000000000000000 ) ) ;
#12914=CARTESIAN_POINT ( 'NONE',  ( 19.35000000122903430, -2.886751345948129988, 4.999999999999997335 ) ) ;
#12916=CARTESIAN_POINT ( 'NONE',  ( 8.503125000614515372, 4.541064518000418104, -2.621784821874998173 ) ) ;
#12917=CARTESIAN_POINT ( 'NONE',  ( 3.271875000614519635, 3.027376345333611329, 5.243569643749999010 ) ) ;
#12918=CARTESIAN_POINT ( 'NONE',  ( 28.52812500061451573, -4.541064518000419881, 2.621784821874995952 ) ) ;
#12919=CARTESIAN_POINT ( 'NONE',  ( 26.10937500061451644, 4.541064518000418104, -2.621784821874998173 ) ) ;
#12920=CARTESIAN_POINT ( 'NONE',  ( 16.52812500061451573, 6.421520780324663323E-16, -5.243569643749999010 ) ) ;
#12921=CARTESIAN_POINT ( 'NONE',  ( 25.95000000122903216, 5.773502691896255534, 3.535250795749688894E-16 ) ) ;
#12922=CARTESIAN_POINT ( 'NONE',  ( 26.05312500061451431, 4.541064518000418104, -2.621784821874998173 ) ) ;
#12923=CARTESIAN_POINT ( 'NONE',  ( 22.99687500061451573, 6.054752690667223547, 3.707466751127219781E-16 ) ) ;
#12924=CARTESIAN_POINT ( 'NONE',  ( 14.24062500061451608, -3.027376345333610441, -5.243569643749999898 ) ) ;
#12925=CARTESIAN_POINT ( 'NONE',  ( -2.121784821874996840, 16.78437500061452070, 33.67503911421598417 ) ) ;
#12926=CARTESIAN_POINT ( 'NONE',  ( 22.26562500061451644, -6.054752690667223547, -1.112240025338166033E-15 ) ) ;
#12928=ORIENTED_EDGE ( 'NONE', *, *, #64752, .F. ) ;
#12929=CARTESIAN_POINT ( 'NONE',  ( 25.53750000000000142, -2.886751345948129988, 4.999999999999997335 ) ) ;
#12930=CARTESIAN_POINT ( 'NONE',  ( 3.999999999999998668, 12.16250000000000142, -32.30940107675850470 ) ) ;
#12931=CARTESIAN_POINT ( 'NONE',  ( 3.999999999999998668, 18.12500000122903288, 27.69059892324149530 ) ) ;
#12932=CARTESIAN_POINT ( 'NONE',  ( 29.05312500061451431, -4.541064518000417216, -2.621784821875001281 ) ) ;
#12933=CARTESIAN_POINT ( 'NONE',  ( 9.628125000614517148, -4.541064518000419881, 2.621784821874995952 ) ) ;
#12934=CARTESIAN_POINT ( 'NONE',  ( 21.90000000122903145, 5.773502691896255534, 3.535250795749688894E-16 ) ) ;
#12935=CARTESIAN_POINT ( 'NONE',  ( 26.35312500061451857, -4.541064518000417216, -2.621784821875001281 ) ) ;
#12936=CARTESIAN_POINT ( 'NONE',  ( 25.23749999999999716, -2.886751345948125991, -5.000000000000000000 ) ) ;
#12937=CARTESIAN_POINT ( 'NONE',  ( -3.999999999999997335, 15.20000000122903572, -27.69059892324149175 ) ) ;
#12938=CARTESIAN_POINT ( 'NONE',  ( 29.12812500061451715, 6.421520780324663323E-16, -5.243569643749999010 ) ) ;
#12939=CARTESIAN_POINT ( 'NONE',  ( 10.49062500061451431, -3.027376345333614438, 5.243569643749998122 ) ) ;
#12940=ORIENTED_EDGE ( 'NONE', *, *, #15134, .F. ) ;
#12941=EDGE_CURVE ( 'NONE', #58137, #15201, #49400, .T. ) ;
#12942=CARTESIAN_POINT ( 'NONE',  ( 25.94062500061451715, -3.027376345333610441, -5.243569643749999898 ) ) ;
#12943=CARTESIAN_POINT ( 'NONE',  ( 8.278125000614515727, -4.541064518000419881, 2.621784821874995952 ) ) ;
#12944=CARTESIAN_POINT ( 'NONE',  ( 4.528125000614516615, 4.541064518000418104, 2.621784821874999949 ) ) ;
#12946=LINE ( 'NONE', #46215, #46775 ) ;
#12947=CARTESIAN_POINT ( 'NONE',  ( 13.98750000000000249, -2.886751345948125991, -5.000000000000000000 ) ) ;
#12948=EDGE_CURVE ( 'NONE', #10190, #55745, #4443, .T. ) ;
#12949=CARTESIAN_POINT ( 'NONE',  ( 13.77187500061451786, -6.054752690667223547, -1.112240025338166033E-15 ) ) ;
#12950=CARTESIAN_POINT ( 'NONE',  ( 10.61250000122903536, 4.330127018922192761, -2.499999999999997780 ) ) ;
#12951=CARTESIAN_POINT ( 'NONE',  ( 17.37187500061451573, -6.054752690667223547, -1.112240025338166033E-15 ) ) ;
#12953=CARTESIAN_POINT ( 'NONE',  ( 8.484375000614518214, 6.421520780324663323E-16, -5.243569643749999010 ) ) ;
#12954=CARTESIAN_POINT ( 'NONE',  ( 4.243569643749999010, 10.61562500061451786, -32.45002607614398471 ) ) ;
#12955=CARTESIAN_POINT ( 'NONE',  ( 27.86250000122903359, 0.000000000000000000, 4.999999999999998224 ) ) ;
#12957=CARTESIAN_POINT ( 'NONE',  ( 30.00000000000000000, 0.000000000000000000, 9.999999999999998224 ) ) ;
#12958=CARTESIAN_POINT ( 'NONE',  ( 23.72812500061451502, 6.421520780324663323E-16, -5.243569643749999010 ) ) ;
#12959=CARTESIAN_POINT ( 'NONE',  ( 11.21250000000000036, -5.773502691896255534, -1.060575238724906372E-15 ) ) ;
#12960=CARTESIAN_POINT ( 'NONE',  ( 28.77187500061451431, 3.027376345333613106, -5.243569643749998122 ) ) ;
#12961=CARTESIAN_POINT ( 'NONE',  ( 24.60000000000000142, 0.000000000000000000, 4.999999999999998224 ) ) ;
#12962=CARTESIAN_POINT ( 'NONE',  ( 6.890625000614516438, -3.027376345333614438, 5.243569643749998122 ) ) ;
#12964=CARTESIAN_POINT ( 'NONE',  ( 16.88437500061451502, -4.541064518000419881, 2.621784821874995952 ) ) ;
#12966=CARTESIAN_POINT ( 'NONE',  ( 29.40000000122903145, -2.886751345948125991, -5.000000000000000000 ) ) ;
#12967=CARTESIAN_POINT ( 'NONE',  ( 8.746875000614515727, -3.027376345333614438, 5.243569643749998122 ) ) ;
#12969=CARTESIAN_POINT ( 'NONE',  ( 17.93437500061451928, 6.421520780324663323E-16, -5.243569643749999010 ) ) ;
#12971=CARTESIAN_POINT ( 'NONE',  ( 26.66250000000000142, 2.886751345948129099, -4.999999999999998224 ) ) ;
#12972=CARTESIAN_POINT ( 'NONE',  ( 3.825000000000001954, 4.330127018922191873, 2.499999999999999556 ) ) ;
#12974=DIRECTION ( 'NONE',  ( -1.000000000000000000, -0.000000000000000000, -0.000000000000000000 ) ) ;
#12976=VERTEX_POINT ( 'NONE', #32034 ) ;
#12977=CARTESIAN_POINT ( 'NONE',  ( 11.28749999999999787, -2.886751345948125991, -5.000000000000000000 ) ) ;
#12979=CARTESIAN_POINT ( 'NONE',  ( 25.22812500061451502, 4.541064518000418104, 2.621784821874999949 ) ) ;
#12980=CARTESIAN_POINT ( 'NONE',  ( 15.15000000000000036, 0.000000000000000000, 4.999999999999998224 ) ) ;
#12982=CARTESIAN_POINT ( 'NONE',  ( 8.850000001229034297, 5.773502691896255534, 3.535250795749688894E-16 ) ) ;
#12983=CARTESIAN_POINT ( 'NONE',  ( 7.228125000614517681, 4.541064518000418104, 2.621784821874999949 ) ) ;
#12984=CARTESIAN_POINT ( 'NONE',  ( 20.81250000000000000, 2.886751345948129099, -4.999999999999998224 ) ) ;
#12985=CARTESIAN_POINT ( 'NONE',  ( 21.14062500061451289, 6.054752690667223547, 3.707466751127219781E-16 ) ) ;
#12986=CARTESIAN_POINT ( 'NONE',  ( 4.800000001229032698, 5.773502691896255534, 3.535250795749688401E-16 ) ) ;
#12987=CARTESIAN_POINT ( 'NONE',  ( 25.31250000122903288, -4.330127018922190985, -2.500000000000001332 ) ) ;
#12989=CARTESIAN_POINT ( 'NONE',  ( 4.050000000000001599, -4.330127018922190985, -2.500000000000001332 ) ) ;
#12990=ORIENTED_EDGE ( 'NONE', *, *, #72086, .T. ) ;
#12991=CARTESIAN_POINT ( 'NONE',  ( 21.85312500061451502, -4.541064518000417216, -2.621784821875001281 ) ) ;
#12992=CARTESIAN_POINT ( 'NONE',  ( 26.95312500061451644, 4.541064518000418104, -2.621784821874998173 ) ) ;
#12993=CARTESIAN_POINT ( 'NONE',  ( 27.34687500061451360, -3.027376345333610441, -5.243569643749999898 ) ) ;
#12994=CARTESIAN_POINT ( 'NONE',  ( 15.17812500061451608, 6.421520780324663323E-16, -5.243569643749999010 ) ) ;
#12995=CARTESIAN_POINT ( 'NONE',  ( -2.121784821874996840, 9.978125000614594953, -26.32496088578401583 ) ) ;
#12996=CARTESIAN_POINT ( 'NONE',  ( 25.12500000122903288, 2.886751345948126879, 4.999999999999999112 ) ) ;
#12998=CARTESIAN_POINT ( 'NONE',  ( 17.84062500061451573, -3.027376345333610441, -5.243569643749999898 ) ) ;
#12999=CARTESIAN_POINT ( 'NONE',  ( -5.810221930991193690E-16, 14.60000000122903252, -34.00000000000000000 ) ) ;
#13000=CARTESIAN_POINT ( 'NONE',  ( 3.037500001229032964, 4.330127018922191873, 2.499999999999999556 ) ) ;
#13001=CARTESIAN_POINT ( 'NONE',  ( 11.44687500061451857, -3.027376345333614438, 5.243569643749998122 ) ) ;
#13002=CARTESIAN_POINT ( 'NONE',  ( 8.559375000614515727, 4.541064518000418104, -2.621784821874998173 ) ) ;
#13003=CARTESIAN_POINT ( 'NONE',  ( 19.77187500061451786, 3.027376345333613106, -5.243569643749998122 ) ) ;
#13004=ORIENTED_EDGE ( 'NONE', *, *, #31222, .F. ) ;
#13005=CARTESIAN_POINT ( 'NONE',  ( 23.54062500061451146, -3.027376345333614438, 5.243569643749998122 ) ) ;
#13006=CARTESIAN_POINT ( 'NONE',  ( 19.84687500061451360, 6.054752690667223547, 3.707466751127219781E-16 ) ) ;
#13007=CARTESIAN_POINT ( 'NONE',  ( 23.54062500061451146, -3.027376345333614438, 5.243569643749998122 ) ) ;
#13008=CARTESIAN_POINT ( 'NONE',  ( -1.071796769724488563, 9.854903811796701163, 34.00000000000000000 ) ) ;
#13009=CARTESIAN_POINT ( 'NONE',  ( 1.999999999999998668, 14.90000000000000036, 26.53589838486224650 ) ) ;
#13010=CARTESIAN_POINT ( 'NONE',  ( 3.384375000614517237, -4.541064518000419881, 2.621784821874995952 ) ) ;
#13011=CARTESIAN_POINT ( 'NONE',  ( 8.962500001229033231, 0.000000000000000000, 4.999999999999998224 ) ) ;
#13012=CARTESIAN_POINT ( 'NONE',  ( 4.462500001229035007, 0.000000000000000000, 4.999999999999998224 ) ) ;
#13013=CARTESIAN_POINT ( 'NONE',  ( -5.810221930991193690E-16, 13.70000000122903394, -34.00000000000000000 ) ) ;
#13014=CARTESIAN_POINT ( 'NONE',  ( 26.47500000122903074, 2.886751345948126879, 4.999999999999999112 ) ) ;
#13016=CARTESIAN_POINT ( 'NONE',  ( 10.02187500061451964, 3.027376345333611329, 5.243569643749999010 ) ) ;
#13018=CARTESIAN_POINT ( 'NONE',  ( 17.65312500061451573, 0.000000000000000000, 5.243569643749999010 ) ) ;
#13019=CARTESIAN_POINT ( 'NONE',  ( 10.69687500061451679, -3.027376345333610441, -5.243569643749999898 ) ) ;
#13020=CARTESIAN_POINT ( 'NONE',  ( 29.47500000122903430, 2.886751345948129099, -4.999999999999998224 ) ) ;
#13021=CARTESIAN_POINT ( 'NONE',  ( 20.52187500061451786, -6.054752690667223547, -1.112240025338166033E-15 ) ) ;
#13022=CARTESIAN_POINT ( 'NONE',  ( 7.696875000614516793, 6.054752690667223547, 3.707466751127219781E-16 ) ) ;
#13023=CARTESIAN_POINT ( 'NONE',  ( 3.815625000614518036, -6.054752690667223547, -1.112240025338166033E-15 ) ) ;
#13024=CARTESIAN_POINT ( 'NONE',  ( 30.00000000000000000, 0.000000000000000000, 4.999999999999998224 ) ) ;
#13025=CARTESIAN_POINT ( 'NONE',  ( 8.840625000614515727, -3.027376345333610441, -5.243569643749999898 ) ) ;
#13026=CARTESIAN_POINT ( 'NONE',  ( 18.21562500061451573, -6.054752690667223547, -1.112240025338166033E-15 ) ) ;
#13027=ORIENTED_EDGE ( 'NONE', *, *, #63628, .F. ) ;
#13028=CARTESIAN_POINT ( 'NONE',  ( 6.450000001229034829, -2.886751345948125991, -5.000000000000000000 ) ) ;
#13029=CARTESIAN_POINT ( 'NONE',  ( 13.75312500061451715, -4.541064518000417216, -2.621784821875001281 ) ) ;
#13030=CARTESIAN_POINT ( 'NONE',  ( 12.85312500061451502, -4.541064518000417216, -2.621784821875001281 ) ) ;
#13032=CARTESIAN_POINT ( 'NONE',  ( 14.36249999999999893, -5.773502691896255534, -1.060575238724906372E-15 ) ) ;
#13033=CARTESIAN_POINT ( 'NONE',  ( 7.237500001229035362, -4.330127018922194537, 2.499999999999995559 ) ) ;
#13034=EDGE_CURVE ( 'NONE', #69794, #14534, #40046, .T. ) ;
#13035=( BOUNDED_CURVE ( )  B_SPLINE_CURVE ( 2, ( #66872, #32877, #4085, #54683, #48783, #26615, #43243, #16241, #3719, #60572, #71308, #70946, #38421, #60943, #25880, #10347, #9979, #55416, #4811, #27343, #61312, #26983, #10708, #59849, #53961, #9618, #20317, #15506, #65393, #14784, #37326, #32516, #49512, #31789, #65764, #49152, #21055, #72768, #55778, #56848, #16599, #44706, #5535, #22153, #67241, #5170, #39153, #61670, #28072, #27705, #33596, #56141, #5891, #51322, #34681, #46143, #11069, #34315, #50600, #17680, #51686, #23598, #6254, #28782, #12154, #29154, #68682, #726, #5, #22512, #23234, #62762, #62400, #45059, #67596, #11798, #16962, #39516, #50959, #62043, #22864, #45785, #11438, #68320, #50246, #33957, #56496, #28422, #357, #45420, #57211, #67956, #17328, #63122, #40239, #39887, #6625, #40600, #1090, #18043, #33241, #57577, #52046, #6980, #35770, #42420, #13232, #18765, #52406, #52769, #1815, #59023, #18406, #46871, #24322, #8068, #29511, #2526, #13595, #40972, #63487, #47229, #25047, #69410, #58293, #41331, #30960, #53496, #64576, #23955, #63840, #69043, #12875, #35407, #64206, #7699, #24682, #2171, #30236, #70119, #69761, #13965, #25419, #1450, #36140, #46505, #19496, #2889, #19867, #57933, #19129, #35049, #58660, #53127, #41683, #30600, #7340, #29869, #47590, #47962, #42054, #36503, #8424, #70490, #12518, #9529, #48692, #54595, #14331, #49790, #54232, #53871, #66410, #71215, #21696, #4367, #32062, #20592, #10260, #43884, #15061, #43518, #65672, #43149, #72315, #59384, #27257, #48329, #3998, #60857, #20227, #66041, #70854, #31697, #9890, #21331, #54962, #15787, #37598, #38328, #4723, #3629, #60484, #8795, #26897, #15419, #42780, #65300, #32792, #26524, #49422, #26151, #60119, #49062, #55329, #64941, #71590, #36866, #31329, #32426, #3263, #20964, #14690, #25791, #71955, #37233, #59755, #9162, #37962, #45701, #51235, #34229, #56763, #12072, #61228, #27986, #45334, #50874, #17241, #38708, #33872, #62677, #68234, #5806, #272, #67869, #22782, #39801, #40157, #10622, #66784, #62317, #6533, #72684, #11712, #17598, #67511, #50516, #6167, #16875, #34594, #16157, #29066, #33505, #33152, #57122, #73044, #1002, #28696 ),
 .UNSPECIFIED., .F., .F. ) 
 B_SPLINE_CURVE_WITH_KNOTS ( ( 3, 2, 2, 2, 2, 2, 2, 2, 2, 2, 2, 2, 2, 2, 2, 2, 2, 2, 2, 2, 2, 2, 2, 2, 2, 2, 2, 2, 2, 2, 2, 2, 2, 2, 2, 2, 2, 2, 2, 2, 2, 2, 2, 2, 2, 2, 2, 2, 2, 2, 2, 2, 2, 2, 2, 2, 2, 2, 2, 2, 2, 2, 2, 2, 2, 2, 2, 2, 2, 2, 2, 2, 2, 2, 2, 2, 2, 2, 2, 2, 2, 2, 2, 2, 2, 2, 2, 2, 2, 2, 2, 2, 2, 2, 2, 2, 2, 2, 2, 2, 2, 2, 2, 2, 2, 2, 2, 2, 2, 2, 2, 2, 2, 2, 2, 2, 2, 2, 2, 2, 2, 2, 2, 2, 2, 2, 2, 2, 2, 2, 2, 2, 2, 2, 3 ),
 ( 0.000000000000000000, 0.007499808158871946150, 0.01499961631774389230, 0.02249942447661583758, 0.02999923263548778460, 0.03749904079435972815, 0.04499884895323167516, 0.05249865711210362218, 0.05999846527097556920, 0.06749827342984751621, 0.07499808158871945629, 0.08249788974759139637, 0.08999769790646335033, 0.09749750606533530428, 0.1049973142242072444, 0.1124971223830791844, 0.1199969305419511384, 0.1274967387008230923, 0.1349965468596950324, 0.1424963550185669725, 0.1499961631774389126, 0.1574959713363108804, 0.1649957794951827927, 0.1724955876540547328, 0.1799953958129267007, 0.1874952039717986407, 0.1949950121306706086, 0.2024948202895425486, 0.2099946284484144887, 0.2174944366072864288, 0.2249942447661583689, 0.2324940529250303090, 0.2399938610839022768, 0.2474936692427742169, 0.2549934774016461847, 0.2624932855605180970, 0.2699930937193900649, 0.2774929018782620327, 0.2849927100371339450, 0.2924925181960058573, 0.2999923263548778252, 0.3074921345137497930, 0.3149919426726217608, 0.3224917508314936732, 0.3299915589903655855, 0.3374913671492375533, 0.3449911753081094656, 0.3524909834669814890, 0.3599907916258534013, 0.3674905997847253691, 0.3749904079435972815, 0.3824902161024691938, 0.3899900242613412171, 0.3974898324202131294, 0.4049896405790850973, 0.4124894487379570096, 0.4199892568968289774, 0.4274890650557008898, 0.4349888732145728576, 0.4424886813734448254, 0.4499884895323167378, 0.4574882976911887056, 0.4649881058500606179, 0.4724879140089325857, 0.4799877221678045536, 0.4874875303266764659, 0.4949873384855484337, 0.5024871466444204016, 0.5099869548032923694, 0.5174867629621642262, 0.5249865711210361940, 0.5324863792799081619, 0.5399861874387801297, 0.5474859955976520975, 0.5549858037565240654, 0.5624856119153959222, 0.5699854200742678900, 0.5774852282331398579, 0.5849850363920117147, 0.5924848445508836825, 0.5999846527097556503, 0.6074844608686276182, 0.6149842690274995860, 0.6224840771863715538, 0.6299838853452435217, 0.6374836935041153785, 0.6449835016629873463, 0.6524833098218593141, 0.6599831179807311710, 0.6674829261396031388, 0.6749827342984751066, 0.6824825424573470745, 0.6899823506162189313, 0.6974821587750910101, 0.7049819669339629780, 0.7124817750928348348, 0.7199815832517068026, 0.7274813914105787704, 0.7349811995694507383, 0.7424810077283225951, 0.7499808158871945629, 0.7574806240460665308, 0.7649804322049383876, 0.7724802403638103554, 0.7799800485226824343, 0.7874798566815544021, 0.7949796648404262589, 0.8024794729992982267, 0.8099792811581701946, 0.8174790893170420514, 0.8249788974759140192, 0.8324787056347859870, 0.8399785137936579549, 0.8474783219525298117, 0.8549781301114017795, 0.8624779382702738584, 0.8699777464291457152, 0.8774775545880176830, 0.8849773627468896509, 0.8924771709057616187, 0.8999769790646334755, 0.9074767872235054433, 0.9149765953823774112, 0.9224764035412492680, 0.9299762117001212358, 0.9374760198589933147, 0.9449758280178651715, 0.9524756361767371393, 0.9599754443356091071, 0.9674752524944810750, 0.9749750606533529318, 0.9824748688122248996, 0.9899746769710968675, 0.9974744851299687243, 1.000000000000000000 ),
 .UNSPECIFIED. ) 
 CURVE ( )  GEOMETRIC_REPRESENTATION_ITEM ( )  RATIONAL_B_SPLINE_CURVE ( ( 1.000000000000000000, 0.8660254037844387076, 1.000000000000000000, 0.8660254037844387076, 1.000000000000000000, 0.8660254037844387076, 1.000000000000000000, 0.8660254037844387076, 1.000000000000000000, 0.8660254037844387076, 1.000000000000000000, 0.8660254037844387076, 1.000000000000000000, 0.8660254037844387076, 1.000000000000000000, 0.8660254037844387076, 1.000000000000000000, 0.8660254037844387076, 1.000000000000000000, 0.8660254037844387076, 1.000000000000000000, 0.8660254037844387076, 1.000000000000000000, 0.8660254037844387076, 1.000000000000000000, 0.8660254037844387076, 1.000000000000000000, 0.8660254037844387076, 1.000000000000000000, 0.8660254037844387076, 1.000000000000000000, 0.8660254037844387076, 1.000000000000000000, 0.8660254037844387076, 1.000000000000000000, 0.8660254037844387076, 1.000000000000000000, 0.8660254037844387076, 1.000000000000000000, 0.8660254037844387076, 1.000000000000000000, 0.8660254037844387076, 1.000000000000000000, 0.8660254037844387076, 1.000000000000000000, 0.8660254037844387076, 1.000000000000000000, 0.8660254037844387076, 1.000000000000000000, 0.8660254037844387076, 1.000000000000000000, 0.8660254037844387076, 1.000000000000000000, 0.8660254037844387076, 1.000000000000000000, 0.8660254037844387076, 1.000000000000000000, 0.8660254037844387076, 1.000000000000000000, 0.8660254037844387076, 1.000000000000000000, 0.8660254037844387076, 1.000000000000000000, 0.8660254037844387076, 1.000000000000000000, 0.8660254037844387076, 1.000000000000000000, 0.8660254037844387076, 1.000000000000000000, 0.8660254037844387076, 1.000000000000000000, 0.8660254037844387076, 1.000000000000000000, 0.8660254037844387076, 1.000000000000000000, 0.8660254037844387076, 1.000000000000000000, 0.8660254037844387076, 1.000000000000000000, 0.8660254037844387076, 1.000000000000000000, 0.8660254037844387076, 1.000000000000000000, 0.8660254037844387076, 1.000000000000000000, 0.8660254037844387076, 1.000000000000000000, 0.8660254037844387076, 1.000000000000000000, 0.8660254037844387076, 1.000000000000000000, 0.8660254037844387076, 1.000000000000000000, 0.8660254037844387076, 1.000000000000000000, 0.8660254037844387076, 1.000000000000000000, 0.8660254037844387076, 1.000000000000000000, 0.8660254037844387076, 1.000000000000000000, 0.8660254037844387076, 1.000000000000000000, 0.8660254037844387076, 1.000000000000000000, 0.8660254037844387076, 1.000000000000000000, 0.8660254037844387076, 1.000000000000000000, 0.8660254037844387076, 1.000000000000000000, 0.8660254037844387076, 1.000000000000000000, 0.8660254037844387076, 1.000000000000000000, 0.8660254037844387076, 1.000000000000000000, 0.8660254037844387076, 1.000000000000000000, 0.8660254037844387076, 1.000000000000000000, 0.8660254037844387076, 1.000000000000000000, 0.8660254037844387076, 1.000000000000000000, 0.8660254037844387076, 1.000000000000000000, 0.8660254037844387076, 1.000000000000000000, 0.8660254037844387076, 1.000000000000000000, 0.8660254037844387076, 1.000000000000000000, 0.8660254037844387076, 1.000000000000000000, 0.8660254037844387076, 1.000000000000000000, 0.8660254037844387076, 1.000000000000000000, 0.8660254037844387076, 1.000000000000000000, 0.8660254037844387076, 1.000000000000000000, 0.8660254037844387076, 1.000000000000000000, 0.8660254037844387076, 1.000000000000000000, 0.8660254037844387076, 1.000000000000000000, 0.8660254037844387076, 1.000000000000000000, 0.8660254037844387076, 1.000000000000000000, 0.8660254037844387076, 1.000000000000000000, 0.8660254037844387076, 1.000000000000000000, 0.8660254037844387076, 1.000000000000000000, 0.8660254037844387076, 1.000000000000000000, 0.8660254037844387076, 1.000000000000000000, 0.8660254037844387076, 1.000000000000000000, 0.8660254037844387076, 1.000000000000000000, 0.8660254037844387076, 1.000000000000000000, 0.8660254037844387076, 1.000000000000000000, 0.8660254037844387076, 1.000000000000000000, 0.8660254037844387076, 1.000000000000000000, 0.8660254037844387076, 1.000000000000000000, 0.8660254037844387076, 1.000000000000000000, 0.8660254037844387076, 1.000000000000000000, 0.8660254037844387076, 1.000000000000000000, 0.8660254037844387076, 1.000000000000000000, 0.8660254037844387076, 1.000000000000000000, 0.8660254037844387076, 1.000000000000000000, 0.8660254037844387076, 1.000000000000000000, 0.8660254037844387076, 1.000000000000000000, 0.8660254037844387076, 1.000000000000000000, 0.8660254037844387076, 1.000000000000000000, 0.8660254037844387076, 1.000000000000000000, 0.8660254037844387076, 1.000000000000000000, 0.8660254037844387076, 1.000000000000000000, 0.8660254037844387076, 1.000000000000000000, 0.8660254037844387076, 1.000000000000000000, 0.8660254037844387076, 1.000000000000000000, 0.8660254037844387076, 1.000000000000000000, 0.8660254037844387076, 1.000000000000000000, 0.8660254037844387076, 1.000000000000000000, 0.8660254037844387076, 1.000000000000000000, 0.8660254037844387076, 1.000000000000000000, 0.8660254037844387076, 1.000000000000000000, 0.8660254037844387076, 1.000000000000000000, 0.8660254037844387076, 1.000000000000000000, 0.8660254037844387076, 1.000000000000000000, 0.8660254037844387076, 1.000000000000000000, 0.8660254037844387076, 1.000000000000000000, 0.8660254037844387076, 1.000000000000000000, 0.8660254037844387076, 1.000000000000000000, 0.8660254037844387076, 1.000000000000000000, 0.8660254037844387076, 1.000000000000000000, 0.8660254037844387076, 1.000000000000000000, 0.8660254037844387076, 1.000000000000000000, 0.8660254037844387076, 1.000000000000000000, 0.8660254037844387076, 1.000000000000000000, 0.8660254037844387076, 1.000000000000000000, 0.8660254037844387076, 1.000000000000000000, 0.8660254037844387076, 1.000000000000000000, 0.8660254037844387076, 1.000000000000000000, 0.8660254037844387076, 1.000000000000000000, 0.8660254037844387076, 1.000000000000000000, 0.8660254037844387076, 1.000000000000000000, 0.8660254037844387076, 1.000000000000000000, 0.8660254037844387076, 1.000000000000000000, 0.8660254037844387076, 1.000000000000000000, 0.9548848677736607726, 0.9401542295229587953 ) ) 
 REPRESENTATION_ITEM ( '' )  );
#13036=CARTESIAN_POINT ( 'NONE',  ( 15.72187500061451892, 3.027376345333613106, -5.243569643749998122 ) ) ;
#13037=CARTESIAN_POINT ( 'NONE',  ( 17.40000000122903145, 5.773502691896255534, 3.535250795749688894E-16 ) ) ;
#13039=CARTESIAN_POINT ( 'NONE',  ( -0.7368881354385758975, 9.859898613939513723, -34.17910028561248481 ) ) ;
#13042=CARTESIAN_POINT ( 'NONE',  ( 4.779258346327469376, 1.469247991000700582, 4.779258346327429408 ) ) ;
#13043=CARTESIAN_POINT ( 'NONE',  ( 13.95000000000000107, -4.330127018922190985, -2.500000000000001332 ) ) ;
#13044=CARTESIAN_POINT ( 'NONE',  ( 17.40937500061451715, -4.541064518000417216, -2.621784821875001281 ) ) ;
#13046=CARTESIAN_POINT ( 'NONE',  ( 14.84062500061451750, 6.054752690667223547, 3.707466751127219781E-16 ) ) ;
#13049=CARTESIAN_POINT ( 'NONE',  ( 25.62187500061451573, 3.027376345333613106, -5.243569643749998122 ) ) ;
#13051=CARTESIAN_POINT ( 'NONE',  ( 10.75312500061451715, 4.541064518000418104, -2.621784821874998173 ) ) ;
#13052=CARTESIAN_POINT ( 'NONE',  ( 14.85937500061451644, 4.541064518000418104, -2.621784821874998173 ) ) ;
#13053=ORIENTED_EDGE ( 'NONE', *, *, #19020, .T. ) ;
#13054=CARTESIAN_POINT ( 'NONE',  ( 27.40312500061451573, 4.541064518000418104, -2.621784821874998173 ) ) ;
#13055=CARTESIAN_POINT ( 'NONE',  ( 20.65312500061451573, 4.541064518000418104, -2.621784821874998173 ) ) ;
#13056=CARTESIAN_POINT ( 'NONE',  ( 29.01562500061451644, -6.054752690667223547, -1.112240025338166033E-15 ) ) ;
#13057=CARTESIAN_POINT ( 'NONE',  ( 3.242103837493086330E-14, 12.80000000122903536, -34.00000000000000000 ) ) ;
#13058=CARTESIAN_POINT ( 'NONE',  ( 10.35000000000000142, -4.330127018922190985, -2.500000000000001332 ) ) ;
#13059=CARTESIAN_POINT ( 'NONE',  ( 19.83750000122903145, -4.330127018922194537, 2.499999999999995559 ) ) ;
#13060=DIRECTION ( 'NONE',  ( -0.000000000000000000, -0.000000000000000000, -1.000000000000000000 ) ) ;
#13062=ORIENTED_EDGE ( 'NONE', *, *, #9622, .F. ) ;
#13063=CARTESIAN_POINT ( 'NONE',  ( 18.59999999999999787, 4.330127018922192761, -2.499999999999997780 ) ) ;
#13064=CARTESIAN_POINT ( 'NONE',  ( 20.40000000000000213, 4.330127018922192761, -2.499999999999997780 ) ) ;
#13065=CARTESIAN_POINT ( 'NONE',  ( 19.50937500061451857, 0.000000000000000000, 5.243569643749999010 ) ) ;
#13066=CARTESIAN_POINT ( 'NONE',  ( 14.80312500061451608, 4.541064518000418104, -2.621784821874998173 ) ) ;
#13068=CARTESIAN_POINT ( 'NONE',  ( 9.750000000000001776, 0.000000000000000000, 4.999999999999998224 ) ) ;
#13069=CARTESIAN_POINT ( 'NONE',  ( 4.790625000614518569, -3.027376345333610441, -5.243569643749999898 ) ) ;
#13071=CARTESIAN_POINT ( 'NONE',  ( 11.66249999999999964, -5.773502691896255534, -1.060575238724906372E-15 ) ) ;
#13073=CARTESIAN_POINT ( 'NONE',  ( 4.243569643749999898, 18.67812500061451431, 30.00000000000000000 ) ) ;
#13074=CARTESIAN_POINT ( 'NONE',  ( 2.859375000614519546, 0.000000000000000000, 5.243569643749999010 ) ) ;
#13077=CARTESIAN_POINT ( 'NONE',  ( 26.29687500061451644, -3.027376345333614438, 5.243569643749998122 ) ) ;
#13078=ORIENTED_EDGE ( 'NONE', *, *, #9420, .T. ) ;
#13079=CARTESIAN_POINT ( 'NONE',  ( 21.17812500061451431, 4.541064518000418104, 2.621784821874999949 ) ) ;
#13080=CARTESIAN_POINT ( 'NONE',  ( 23.89687500061451786, 6.054752690667223547, 3.707466751127219781E-16 ) ) ;
#13082=CARTESIAN_POINT ( 'NONE',  ( 2.121784821875001281, 15.45312500061459282, -26.32496088578401938 ) ) ;
#13083=CARTESIAN_POINT ( 'NONE',  ( 6.328125000614515550, 4.541064518000418104, 2.621784821874999949 ) ) ;
#13085=CARTESIAN_POINT ( 'NONE',  ( 23.01562500061451644, 3.027376345333611329, 5.243569643749999010 ) ) ;
#13088=CARTESIAN_POINT ( 'NONE',  ( 16.09687500061452070, -3.027376345333610441, -5.243569643749999898 ) ) ;
#13089=CARTESIAN_POINT ( 'NONE',  ( 18.72187500061451360, -6.054752690667223547, -1.112240025338166033E-15 ) ) ;
#13090=CARTESIAN_POINT ( 'NONE',  ( 26.63437500061451857, 4.541064518000418104, 2.621784821874999949 ) ) ;
#13091=CARTESIAN_POINT ( 'NONE',  ( 4.243569643749999898, 16.03437500061451715, 30.00000000000000000 ) ) ;
#13092=CARTESIAN_POINT ( 'NONE',  ( 6.628125000614517148, 6.421520780324663323E-16, -5.243569643749999010 ) ) ;
#13093=CARTESIAN_POINT ( 'NONE',  ( 1.071796769724484344, 16.08259618943233704, 34.00000000000000000 ) ) ;
#13094=CARTESIAN_POINT ( 'NONE',  ( 4.809375000614516615, -4.541064518000417216, -2.621784821875001281 ) ) ;
#13096=CARTESIAN_POINT ( 'NONE',  ( 5.390625000614518214, 6.054752690667223547, 3.707466751127219781E-16 ) ) ;
#13097=CARTESIAN_POINT ( 'NONE',  ( 10.58437500061451964, -4.541064518000419881, 2.621784821874995952 ) ) ;
#13098=CARTESIAN_POINT ( 'NONE',  ( 15.93750000122903110, 6.123233995736764310E-16, -4.999999999999998224 ) ) ;
#13099=CARTESIAN_POINT ( 'NONE',  ( 4.509375000614518569, 4.541064518000418104, -2.621784821874998173 ) ) ;
#13100=CARTESIAN_POINT ( 'NONE',  ( 8.240625000614516082, -3.027376345333614438, 5.243569643749998122 ) ) ;
#13103=CARTESIAN_POINT ( 'NONE',  ( 16.24687500061451573, 6.054752690667223547, 3.707466751127219781E-16 ) ) ;
#13104=CYLINDRICAL_SURFACE ( 'NONE', #36062, 4.999999999999998224 ) ;
#13105=VERTEX_POINT ( 'NONE', #71192 ) ;
#13106=CARTESIAN_POINT ( 'NONE',  ( 24.40312500061451573, 0.000000000000000000, 5.243569643749999010 ) ) ;
#13107=CARTESIAN_POINT ( 'NONE',  ( 8.803125000614517859, -4.541064518000417216, -2.621784821875001281 ) ) ;
#13108=CARTESIAN_POINT ( 'NONE',  ( 26.03437500061451715, 6.421520780324663323E-16, -5.243569643749999010 ) ) ;
#13109=CARTESIAN_POINT ( 'NONE',  ( 10.34062500061451750, 6.054752690667223547, 3.707466751127219781E-16 ) ) ;
#13111=CARTESIAN_POINT ( 'NONE',  ( 10.38750000122903572, -4.330127018922194537, 2.499999999999995559 ) ) ;
#13112=CARTESIAN_POINT ( 'NONE',  ( 26.09062500061451573, 6.054752690667223547, 3.707466751127219781E-16 ) ) ;
#13113=CARTESIAN_POINT ( 'NONE',  ( 4.243569643749999898, 12.37812500061451715, -30.00000000000000000 ) ) ;
#13114=CARTESIAN_POINT ( 'NONE',  ( 11.62500000122903465, 2.886751345948126879, 4.999999999999999112 ) ) ;
#13115=CARTESIAN_POINT ( 'NONE',  ( 22.19062500061451715, -3.027376345333614438, 5.243569643749998122 ) ) ;
#13116=CARTESIAN_POINT ( 'NONE',  ( 10.38750000000000107, -2.886751345948125991, -5.000000000000000000 ) ) ;
#13117=CARTESIAN_POINT ( 'NONE',  ( 20.05312500061451431, -4.541064518000417216, -2.621784821875001281 ) ) ;
#13118=CARTESIAN_POINT ( 'NONE',  ( 20.69999999999999929, -4.330127018922190985, -2.500000000000001332 ) ) ;
#13119=CARTESIAN_POINT ( 'NONE',  ( 14.02500000122903323, -5.773502691896255534, -1.060575238724906372E-15 ) ) ;
#13120=CARTESIAN_POINT ( 'NONE',  ( 10.67812500061451608, 6.421520780324663323E-16, -5.243569643749999010 ) ) ;
#13122=EDGE_CURVE ( 'NONE', #860, #33359, #37208, .T. ) ;
#13123=CARTESIAN_POINT ( 'NONE',  ( 12.66562500061451502, 3.027376345333611329, 5.243569643749999010 ) ) ;
#13124=CARTESIAN_POINT ( 'NONE',  ( 24.56250000122903288, 4.330127018922192761, -2.499999999999997780 ) ) ;
#13125=CARTESIAN_POINT ( 'NONE',  ( 20.22187500061451715, 3.027376345333613106, -5.243569643749998122 ) ) ;
#13127=CARTESIAN_POINT ( 'NONE',  ( 6.975000001229032520, 2.886751345948129099, -4.999999999999998224 ) ) ;
#13128=CARTESIAN_POINT ( 'NONE',  ( 8.671875000614518214, 3.027376345333611329, 5.243569643749999010 ) ) ;
#13129=CARTESIAN_POINT ( 'NONE',  ( 26.74687500061451573, -3.027376345333614438, 5.243569643749998122 ) ) ;
#13131=CARTESIAN_POINT ( 'NONE',  ( 20.69062500061451715, 6.054752690667223547, 3.707466751127219781E-16 ) ) ;
#13132=CARTESIAN_POINT ( 'NONE',  ( 27.08437500061451786, 4.541064518000418104, 2.621784821874999949 ) ) ;
#13135=CARTESIAN_POINT ( 'NONE',  ( 8.071875000614518569, 3.027376345333613106, -5.243569643749998122 ) ) ;
#13136=CARTESIAN_POINT ( 'NONE',  ( 18.14062500061451644, -3.027376345333614438, 5.243569643749998122 ) ) ;
#13137=ORIENTED_EDGE ( 'NONE', *, *, #7149, .F. ) ;
#13138=CARTESIAN_POINT ( 'NONE',  ( 25.12499999999999645, -4.330127018922194537, 2.499999999999995559 ) ) ;
#13139=CARTESIAN_POINT ( 'NONE',  ( 27.66562500061451146, -6.054752690667223547, -1.112240025338166033E-15 ) ) ;
#13140=CARTESIAN_POINT ( 'NONE',  ( 4.546875000614517326, 6.054752690667223547, 3.707466751127219781E-16 ) ) ;
#13141=CARTESIAN_POINT ( 'NONE',  ( 10.16250000122903252, 4.330127018922192761, -2.499999999999997780 ) ) ;
#13142=CARTESIAN_POINT ( 'NONE',  ( 3.607718959681897264, 3.461971838192151818, -3.890427558041640754 ) ) ;
#13143=CARTESIAN_POINT ( 'NONE',  ( 18.03749999999999787, -2.886751345948125991, -5.000000000000000000 ) ) ;
#13144=CARTESIAN_POINT ( 'NONE',  ( 21.14062500061451289, 6.054752690667223547, 3.707466751127219781E-16 ) ) ;
#13145=ORIENTED_EDGE ( 'NONE', *, *, #60921, .T. ) ;
#13146=CARTESIAN_POINT ( 'NONE',  ( 25.76249999999999929, 2.886751345948129099, -4.999999999999998224 ) ) ;
#13147=CARTESIAN_POINT ( 'NONE',  ( 27.34687500061451360, -3.027376345333610441, -5.243569643749999898 ) ) ;
#13148=ORIENTED_EDGE ( 'NONE', *, *, #56915, .T. ) ;
#13149=CARTESIAN_POINT ( 'NONE',  ( 14.20312500061451644, -4.541064518000417216, -2.621784821875001281 ) ) ;
#13150=CARTESIAN_POINT ( 'NONE',  ( 5.728125000614515905, 6.421520780324663323E-16, -5.243569643749999010 ) ) ;
#13152=CARTESIAN_POINT ( 'NONE',  ( 3.384375000614517237, -4.541064518000419881, 2.621784821874995952 ) ) ;
#13153=CARTESIAN_POINT ( 'NONE',  ( 16.23750000122903359, -4.330127018922194537, 2.499999999999995559 ) ) ;
#13154=CARTESIAN_POINT ( 'NONE',  ( 20.13749999999999929, -2.886751345948129988, 4.999999999999997335 ) ) ;
#13155=CARTESIAN_POINT ( 'NONE',  ( 28.08749999999999858, 5.773502691896255534, 3.535250795749688894E-16 ) ) ;
#13156=CARTESIAN_POINT ( 'NONE',  ( 3.946875000614517681, -3.027376345333610441, -5.243569643749999898 ) ) ;
#13157=CARTESIAN_POINT ( 'NONE',  ( 10.50937500061451679, 0.000000000000000000, 5.243569643749999010 ) ) ;
#13158=CARTESIAN_POINT ( 'NONE',  ( 18.87187500061451573, 3.027376345333613106, -5.243569643749998122 ) ) ;
#13159=CARTESIAN_POINT ( 'NONE',  ( -4.243569643749999898, 19.80312500061451786, -30.00000000000000000 ) ) ;
#13160=VERTEX_POINT ( 'NONE', #31675 ) ;
#13161=CARTESIAN_POINT ( 'NONE',  ( 28.79062500061451502, 6.054752690667223547, 3.707466751127219781E-16 ) ) ;
#13162=CARTESIAN_POINT ( 'NONE',  ( 29.78437500061451715, 4.541064518000418104, 2.621784821874999949 ) ) ;
#13163=CARTESIAN_POINT ( 'NONE',  ( 4.659375000614518925, 0.000000000000000000, 5.243569643749999010 ) ) ;
#13164=CARTESIAN_POINT ( 'NONE',  ( 15.41250000000000142, 2.886751345948129099, -4.999999999999998224 ) ) ;
#13165=CARTESIAN_POINT ( 'NONE',  ( 13.30312500061451786, -4.541064518000417216, -2.621784821875001281 ) ) ;
#13167=CARTESIAN_POINT ( 'NONE',  ( 4.844509297411972781, 1.237226603047926421, -5.095516945469514170 ) ) ;
#13169=CARTESIAN_POINT ( 'NONE',  ( 19.38750000122903216, -4.330127018922194537, 2.499999999999995559 ) ) ;
#13172=CARTESIAN_POINT ( 'NONE',  ( 6.553125000614518747, -4.541064518000417216, -2.621784821875001281 ) ) ;
#13173=CARTESIAN_POINT ( 'NONE',  ( 24.53437500061451715, -4.541064518000419881, 2.621784821874995952 ) ) ;
#13174=CARTESIAN_POINT ( 'NONE',  ( -2.121784821874999949, 19.33437500061451786, 26.32496088578401938 ) ) ;
#13176=CARTESIAN_POINT ( 'NONE',  ( 25.80937500061451928, 0.000000000000000000, 5.243569643749999010 ) ) ;
#13177=CARTESIAN_POINT ( 'NONE',  ( 8.550000000000002487, -4.330127018922190985, -2.500000000000001332 ) ) ;
#13178=CARTESIAN_POINT ( 'NONE',  ( -1.999999999999997113, 12.53750000122903430, 33.46410161513775705 ) ) ;
#13179=CARTESIAN_POINT ( 'NONE',  ( 14.31562500061451537, 3.027376345333613106, -5.243569643749998122 ) ) ;
#13180=CARTESIAN_POINT ( 'NONE',  ( 5.887500001229034829, -4.330127018922194537, 2.499999999999995559 ) ) ;
#13181=CARTESIAN_POINT ( 'NONE',  ( 18.15937500061451715, 0.000000000000000000, 5.243569643749999010 ) ) ;
#13182=CARTESIAN_POINT ( 'NONE',  ( 10.99687500061451750, -3.027376345333614438, 5.243569643749998122 ) ) ;
#13183=CARTESIAN_POINT ( 'NONE',  ( 13.91250000122903252, 0.000000000000000000, 4.999999999999998224 ) ) ;
#13185=CARTESIAN_POINT ( 'NONE',  ( 11.39062500061451644, -3.027376345333614438, 5.243569643749998122 ) ) ;
#13186=CARTESIAN_POINT ( 'NONE',  ( 1.071796769724491893, 12.14509619066136814, -26.00000000000000355 ) ) ;
#13187=CARTESIAN_POINT ( 'NONE',  ( 24.75000000122902932, -2.886751345948129988, 4.999999999999997335 ) ) ;
#13188=CARTESIAN_POINT ( 'NONE',  ( 11.89687500061451608, -3.027376345333614438, 5.243569643749998122 ) ) ;
#13189=CARTESIAN_POINT ( 'NONE',  ( 14.39062500061451821, 6.054752690667223547, 3.707466751127219781E-16 ) ) ;
#13191=CARTESIAN_POINT ( 'NONE',  ( 23.18437500061451573, -4.541064518000419881, 2.621784821874995952 ) ) ;
#13192=FACE_OUTER_BOUND ( 'NONE', #56114, .T. ) ;
#13194=CARTESIAN_POINT ( 'NONE',  ( 3.140625000614516882, 6.054752690667223547, 3.707466751127219781E-16 ) ) ;
#13195=CARTESIAN_POINT ( 'NONE',  ( -4.243569643749999898, 15.80937500061451573, -30.00000000000000000 ) ) ;
#13196=SHAPE_REPRESENTATION ( 'valve body', ( #23765 ), #56785 ) ;
#13197=CARTESIAN_POINT ( 'NONE',  ( 16.17187500061451644, 3.027376345333613106, -5.243569643749998122 ) ) ;
#13198=CARTESIAN_POINT ( 'NONE',  ( 18.86250000122903359, 0.000000000000000000, 4.999999999999998224 ) ) ;
#13199=CARTESIAN_POINT ( 'NONE',  ( 12.19687500061451679, 6.054752690667223547, 3.707466751127219781E-16 ) ) ;
#13200=CARTESIAN_POINT ( 'NONE',  ( 2.121784821874999061, 19.65312500061451573, -33.67503911421598417 ) ) ;
#13201=CARTESIAN_POINT ( 'NONE',  ( 20.51250000122903216, 4.330127018922192761, -2.499999999999997780 ) ) ;
#13202=CARTESIAN_POINT ( 'NONE',  ( 11.72812500061451857, 4.541064518000418104, 2.621784821874999949 ) ) ;
#13204=ORIENTED_EDGE ( 'NONE', *, *, #17223, .F. ) ;
#13205=CARTESIAN_POINT ( 'NONE',  ( 18.56250000000000000, 2.886751345948129099, -4.999999999999998224 ) ) ;
#13207=CARTESIAN_POINT ( 'NONE',  ( 12.49687500061451573, -3.027376345333610441, -5.243569643749999898 ) ) ;
#13208=CARTESIAN_POINT ( 'NONE',  ( 2.991194101639602199, 4.006657223659620293, -3.099915294692820122 ) ) ;
#13209=CARTESIAN_POINT ( 'NONE',  ( 13.42500000122903536, 2.886751345948126879, 4.999999999999999112 ) ) ;
#13210=CARTESIAN_POINT ( 'NONE',  ( 21.82500000122903572, 2.886751345948129099, -4.999999999999998224 ) ) ;
#13211=CARTESIAN_POINT ( 'NONE',  ( 16.71562500061451573, 3.027376345333611329, 5.243569643749999010 ) ) ;
#13212=CARTESIAN_POINT ( 'NONE',  ( 23.84062500061451928, 6.054752690667223547, 3.707466751127219781E-16 ) ) ;
#13213=CARTESIAN_POINT ( 'NONE',  ( 29.17500000122903714, 2.886751345948126879, 4.999999999999999112 ) ) ;
#13215=CARTESIAN_POINT ( 'NONE',  ( 27.89999999999999858, -4.330127018922190985, -2.500000000000001332 ) ) ;
#13216=CARTESIAN_POINT ( 'NONE',  ( 4.608887683030311599, 1.938663576234528341, 4.872049282877938481 ) ) ;
#13218=CARTESIAN_POINT ( 'NONE',  ( 29.92968750030725644, 0.000000000000000000, 5.121784821874998173 ) ) ;
#13219=CARTESIAN_POINT ( 'NONE',  ( -2.121784821874996840, 14.98437500061451644, -26.32496088578401583 ) ) ;
#13220=CARTESIAN_POINT ( 'NONE',  ( 4.200000001229033053, -2.886751345948125991, -5.000000000000000000 ) ) ;
#13221=CARTESIAN_POINT ( 'NONE',  ( 6.150000000000003020, 0.000000000000000000, 4.999999999999998224 ) ) ;
#13222=CARTESIAN_POINT ( 'NONE',  ( 3.009375000614516793, -4.541064518000417216, -2.621784821875001281 ) ) ;
#13223=CARTESIAN_POINT ( 'NONE',  ( 10.17187500061451999, -6.054752690667223547, -1.112240025338166033E-15 ) ) ;
#13225=CARTESIAN_POINT ( 'NONE',  ( 29.27812500061451573, 4.541064518000418104, 2.621784821874999949 ) ) ;
#13226=CARTESIAN_POINT ( 'NONE',  ( 3.999999999999999112, 10.77500000000000213, 30.00000000000000000 ) ) ;
#13227=CARTESIAN_POINT ( 'NONE',  ( -5.378075516623670893, 8.432637420806662121, -27.31137673071734184 ) ) ;
#13228=CARTESIAN_POINT ( 'NONE',  ( 6.909375000614518036, 0.000000000000000000, 5.243569643749999010 ) ) ;
#13229=CARTESIAN_POINT ( 'NONE',  ( 10.13437500061451679, -4.541064518000419881, 2.621784821874995952 ) ) ;
#13230=CARTESIAN_POINT ( 'NONE',  ( 5.362500000000003375, -5.773502691896255534, -1.060575238724906372E-15 ) ) ;
#13231=( BOUNDED_CURVE ( )  B_SPLINE_CURVE ( 2, ( #17662, #40223, #56481, #35391, #46126, #23581, #34663, #18749, #51303 ),
 .UNSPECIFIED., .F., .F. ) 
 B_SPLINE_CURVE_WITH_KNOTS ( ( 3, 2, 2, 2, 3 ),
 ( 0.7500000000000000000, 0.7536231884057971175, 0.7608695652173913526, 0.7681159420289854767, 0.7717391304347825942 ),
 .UNSPECIFIED. ) 
 CURVE ( )  GEOMETRIC_REPRESENTATION_ITEM ( )  RATIONAL_B_SPLINE_CURVE ( ( 0.9330127018922194093, 0.9330127018922194093, 1.000000000000000000, 0.8660254037844387076, 1.000000000000000000, 0.8660254037844387076, 1.000000000000000000, 0.9330127018922194093, 0.9330127018922194093 ) ) 
 REPRESENTATION_ITEM ( '' )  );
#13232=CARTESIAN_POINT ( 'NONE',  ( -2.121784821874996840, 15.82812500061459637, 33.67503911421598417 ) ) ;
#13234=CARTESIAN_POINT ( 'NONE',  ( 5.475000000000000533, 6.123233995736764310E-16, -4.999999999999998224 ) ) ;
#13236=CARTESIAN_POINT ( 'NONE',  ( 19.56562500061451715, -6.054752690667223547, -1.112240025338166033E-15 ) ) ;
#13237=CARTESIAN_POINT ( 'NONE',  ( 12.59062500061451573, 6.054752690667223547, 3.707466751127219781E-16 ) ) ;
#13239=CARTESIAN_POINT ( 'NONE',  ( 8.296875000614516438, -3.027376345333614438, 5.243569643749998122 ) ) ;
#13240=CARTESIAN_POINT ( 'NONE',  ( 27.22499999999999787, 4.330127018922191873, 2.499999999999999556 ) ) ;
#13241=CARTESIAN_POINT ( 'NONE',  ( 23.40000000122903145, -2.886751345948129988, 4.999999999999997335 ) ) ;
#13242=LINE ( 'NONE', #24332, #69724 ) ;
#13243=CARTESIAN_POINT ( 'NONE',  ( 12.60937500061451821, 4.541064518000418104, -2.621784821874998173 ) ) ;
#13244=CARTESIAN_POINT ( 'NONE',  ( 27.23437500061451644, -4.541064518000419881, 2.621784821874995952 ) ) ;
#13245=CARTESIAN_POINT ( 'NONE',  ( 3.421875000614516882, -6.054752690667223547, -1.112240025338166033E-15 ) ) ;
#13246=CARTESIAN_POINT ( 'NONE',  ( 18.87187500061451573, 3.027376345333613106, -5.243569643749998122 ) ) ;
#13247=CARTESIAN_POINT ( 'NONE',  ( 12.08437500061451608, 6.421520780324663323E-16, -5.243569643749999010 ) ) ;
#13249=CARTESIAN_POINT ( 'NONE',  ( 26.32499999999999929, 4.330127018922191873, 2.499999999999999556 ) ) ;
#13251=CARTESIAN_POINT ( 'NONE',  ( -3.000416591977282496E-16, 12.99687500061451750, -34.90005215228797653 ) ) ;
#13253=CARTESIAN_POINT ( 'NONE',  ( 15.36562500061451608, 3.027376345333611329, 5.243569643749999010 ) ) ;
#13254=CARTESIAN_POINT ( 'NONE',  ( 4.312500000000000000, 2.886751345948126879, 4.999999999999999112 ) ) ;
#13256=CARTESIAN_POINT ( 'NONE',  ( 9.299999999999998934, 0.000000000000000000, 4.999999999999998224 ) ) ;
#13257=CARTESIAN_POINT ( 'NONE',  ( 14.40000000000000036, -4.330127018922190985, -2.500000000000001332 ) ) ;
#13258=CARTESIAN_POINT ( 'NONE',  ( -3.999999999999999112, 19.21250000122903501, 30.00000000000000000 ) ) ;
#13259=CARTESIAN_POINT ( 'NONE',  ( 15.03750000122903252, 6.123233995736764310E-16, -4.999999999999998224 ) ) ;
#13261=CARTESIAN_POINT ( 'NONE',  ( 25.58437500061451431, 6.421520780324663323E-16, -5.243569643749999010 ) ) ;
#13263=CARTESIAN_POINT ( 'NONE',  ( 20.42812500061451431, -4.541064518000419881, 2.621784821874995952 ) ) ;
#13264=CARTESIAN_POINT ( 'NONE',  ( 4.978125000614518569, 4.541064518000418104, 2.621784821874999949 ) ) ;
#13265=CARTESIAN_POINT ( 'NONE',  ( 19.95937500061451786, 0.000000000000000000, 5.243569643749999010 ) ) ;
#13266=CARTESIAN_POINT ( 'NONE',  ( 5.212500000000002132, 2.886751345948126879, 4.999999999999999112 ) ) ;
#13267=CARTESIAN_POINT ( 'NONE',  ( 7.715625000614515727, 3.027376345333611329, 5.243569643749999010 ) ) ;
#13268=CARTESIAN_POINT ( 'NONE',  ( 21.14062500061451289, 6.054752690667223547, 3.707466751127219781E-16 ) ) ;
#13269=CARTESIAN_POINT ( 'NONE',  ( 9.001249775931846008E-16, 14.06562500061451715, 34.90005215228797653 ) ) ;
#13270=CARTESIAN_POINT ( 'NONE',  ( 18.93750000122903288, -4.330127018922194537, 2.499999999999995559 ) ) ;
#13272=CARTESIAN_POINT ( 'NONE',  ( 10.56562500061451715, -6.054752690667223547, -1.112240025338166033E-15 ) ) ;
#13273=CARTESIAN_POINT ( 'NONE',  ( 3.421875000614516882, -6.054752690667223547, -1.112240025338166033E-15 ) ) ;
#13274=CARTESIAN_POINT ( 'NONE',  ( 29.50312500061451360, -4.541064518000417216, -2.621784821875001281 ) ) ;
#13275=CARTESIAN_POINT ( 'NONE',  ( 22.35937500061451644, -4.541064518000417216, -2.621784821875001281 ) ) ;
#13276=CARTESIAN_POINT ( 'NONE',  ( 13.41562500061451502, 3.027376345333613106, -5.243569643749998122 ) ) ;
#13277=CARTESIAN_POINT ( 'NONE',  ( 24.15000000122903145, 5.773502691896255534, 3.535250795749688894E-16 ) ) ;
#13278=CARTESIAN_POINT ( 'NONE',  ( 25.86562500061451431, -6.054752690667223547, -1.112240025338166033E-15 ) ) ;
#13279=CARTESIAN_POINT ( 'NONE',  ( 19.43437500061451928, 4.541064518000418104, 2.621784821874999949 ) ) ;
#13280=CARTESIAN_POINT ( 'NONE',  ( 15.17812500061451608, 6.421520780324663323E-16, -5.243569643749999010 ) ) ;
#13281=CARTESIAN_POINT ( 'NONE',  ( -4.243569643749999898, 16.22187500061452070, 27.54997392385601529 ) ) ;
#13282=( BOUNDED_CURVE ( )  B_SPLINE_CURVE ( 2, ( #30918, #64164, #13552, #41291, #36099, #58619, #53459, #42743, #31288 ),
 .UNSPECIFIED., .F., .F. ) 
 B_SPLINE_CURVE_WITH_KNOTS ( ( 3, 2, 2, 2, 3 ),
 ( 0.3586956521739130821, 0.3623188405797101441, 0.3695652173913043237, 0.3768115942028985588, 0.3804347826086956763 ),
 .UNSPECIFIED. ) 
 CURVE ( )  GEOMETRIC_REPRESENTATION_ITEM ( )  RATIONAL_B_SPLINE_CURVE ( ( 0.9330127018922194093, 0.9330127018922198534, 1.000000000000000000, 0.8660254037844387076, 1.000000000000000000, 0.8660254037844387076, 1.000000000000000000, 0.9330127018922188542, 0.9330127018922194093 ) ) 
 REPRESENTATION_ITEM ( '' )  );
#13283=CARTESIAN_POINT ( 'NONE',  ( 21.10312500061451502, 4.541064518000418104, -2.621784821874998173 ) ) ;
#13284=CARTESIAN_POINT ( 'NONE',  ( 3.300000001229034918, -2.886751345948125991, -5.000000000000000000 ) ) ;
#13285=EDGE_LOOP ( 'NONE', ( #1039, #54108, #25522, #10541 ) ) ;
#13286=CARTESIAN_POINT ( 'NONE',  ( 24.52499999999999858, 4.330127018922191873, 2.499999999999999556 ) ) ;
#13287=CARTESIAN_POINT ( 'NONE',  ( 1.999999999999998668, 10.40000000000000213, -33.46410161513775705 ) ) ;
#13289=CARTESIAN_POINT ( 'NONE',  ( 27.47812500061451502, 4.541064518000418104, 2.621784821874999949 ) ) ;
#13290=CARTESIAN_POINT ( 'NONE',  ( 8.203125000614518214, 0.000000000000000000, 5.243569643749999010 ) ) ;
#13291=CARTESIAN_POINT ( 'NONE',  ( 20.58750000122903145, 4.330127018922191873, 2.499999999999999556 ) ) ;
#13292=CARTESIAN_POINT ( 'NONE',  ( 28.00312500061451715, 0.000000000000000000, 5.243569643749999010 ) ) ;
#13293=CARTESIAN_POINT ( 'NONE',  ( 24.26249999999999929, -5.773502691896255534, -1.060575238724906372E-15 ) ) ;
#13294=CARTESIAN_POINT ( 'NONE',  ( 2.000000000000001332, 15.76250000122903216, -26.53589838486224650 ) ) ;
#13295=CARTESIAN_POINT ( 'NONE',  ( 10.67812500061451608, 6.421520780324663323E-16, -5.243569643749999010 ) ) ;
#13297=ADVANCED_FACE ( 'NONE', ( #66630 ), #38177, .F. ) ;
#13298=CARTESIAN_POINT ( 'NONE',  ( 24.77812500061451217, 4.541064518000418104, 2.621784821874999949 ) ) ;
#13299=CARTESIAN_POINT ( 'NONE',  ( 6.628125000614517148, 6.421520780324663323E-16, -5.243569643749999010 ) ) ;
#13300=CARTESIAN_POINT ( 'NONE',  ( 4.603125000614518569, 0.000000000000000000, 5.243569643749999010 ) ) ;
#13302=CARTESIAN_POINT ( 'NONE',  ( 0.000000000000000000, 20.00000000000000000, -30.00000000000000000 ) ) ;
#13303=CARTESIAN_POINT ( 'NONE',  ( 12.63749999999999929, -2.886751345948125991, -5.000000000000000000 ) ) ;
#13304=CARTESIAN_POINT ( 'NONE',  ( 12.53437500061451537, 6.421520780324663323E-16, -5.243569643749999010 ) ) ;
#13305=CARTESIAN_POINT ( 'NONE',  ( 9.600000001229034297, -2.886751345948125991, -5.000000000000000000 ) ) ;
#13306=CARTESIAN_POINT ( 'NONE',  ( 15.94687500061451502, -3.027376345333614438, 5.243569643749998122 ) ) ;
#13308=CARTESIAN_POINT ( 'NONE',  ( 7.771875000614516971, 3.027376345333611329, 5.243569643749999010 ) ) ;
#13309=CARTESIAN_POINT ( 'NONE',  ( -4.243569643749999898, 11.70312500061451644, -30.00000000000000000 ) ) ;
#13310=CARTESIAN_POINT ( 'NONE',  ( 27.63750000122903216, 6.123233995736764310E-16, -4.999999999999998224 ) ) ;
#13313=CARTESIAN_POINT ( 'NONE',  ( 23.54062500061451146, -3.027376345333614438, 5.243569643749998122 ) ) ;
#13315=CARTESIAN_POINT ( 'NONE',  ( 26.37187500061451217, -6.054752690667223547, -1.112240025338166033E-15 ) ) ;
#13316=CARTESIAN_POINT ( 'NONE',  ( 28.43437500061451573, 4.541064518000418104, 2.621784821874999949 ) ) ;
#13317=CARTESIAN_POINT ( 'NONE',  ( 22.91249999999999432, -5.773502691896255534, -1.060575238724906372E-15 ) ) ;
#13318=CARTESIAN_POINT ( 'NONE',  ( 6.665625000614515905, 3.027376345333613106, -5.243569643749998122 ) ) ;
#13320=CARTESIAN_POINT ( 'NONE',  ( 15.68437500061451573, 6.421520780324663323E-16, -5.243569643749999010 ) ) ;
#13322=CARTESIAN_POINT ( 'NONE',  ( 29.17500000122903714, 2.886751345948126879, 4.999999999999999112 ) ) ;
#13323=CARTESIAN_POINT ( 'NONE',  ( 7.434375000614519280, -4.541064518000419881, 2.621784821874995952 ) ) ;
#13325=CARTESIAN_POINT ( 'NONE',  ( 19.02187500061451786, 3.027376345333611329, 5.243569643749999010 ) ) ;
#13327=CARTESIAN_POINT ( 'NONE',  ( 27.59999999999999787, 4.330127018922192761, -2.499999999999997780 ) ) ;
#13328=CARTESIAN_POINT ( 'NONE',  ( 28.20937500061451786, -4.541064518000417216, -2.621784821875001281 ) ) ;
#13330=CARTESIAN_POINT ( 'NONE',  ( 27.97500000000000142, 6.123233995736764310E-16, -4.999999999999998224 ) ) ;
#13331=ORIENTED_EDGE ( 'NONE', *, *, #43332, .T. ) ;
#13332=CARTESIAN_POINT ( 'NONE',  ( 11.21250000000000036, -5.773502691896255534, -1.060575238724906372E-15 ) ) ;
#13334=CARTESIAN_POINT ( 'NONE',  ( 21.10312500061451502, 4.541064518000418104, -2.621784821874998173 ) ) ;
#13335=CARTESIAN_POINT ( 'NONE',  ( 12.59999999999999964, -4.330127018922190985, -2.500000000000001332 ) ) ;
#13336=CARTESIAN_POINT ( 'NONE',  ( 7.650000001229034119, -2.886751345948129988, 4.999999999999997335 ) ) ;
#13337=CARTESIAN_POINT ( 'NONE',  ( 5.503125000614516260, 0.000000000000000000, 5.243569643749999010 ) ) ;
#13338=CARTESIAN_POINT ( 'NONE',  ( 22.05000000000000071, -4.330127018922190985, -2.500000000000001332 ) ) ;
#13340=CARTESIAN_POINT ( 'NONE',  ( 20.42812500061451431, -4.541064518000419881, 2.621784821874995952 ) ) ;
#13341=CARTESIAN_POINT ( 'NONE',  ( 23.58749999999999858, 5.773502691896255534, 3.535250795749688401E-16 ) ) ;
#13342=CARTESIAN_POINT ( 'NONE',  ( 25.20000000122903216, -2.886751345948129988, 4.999999999999997335 ) ) ;
#13344=CARTESIAN_POINT ( 'NONE',  ( 5.100000000000000533, 4.330127018922192761, -2.499999999999997780 ) ) ;
#13345=ORIENTED_EDGE ( 'NONE', *, *, #10988, .F. ) ;
#13346=CARTESIAN_POINT ( 'NONE',  ( 20.01562500061451644, -6.054752690667223547, -1.112240025338166033E-15 ) ) ;
#13347=CARTESIAN_POINT ( 'NONE',  ( 26.20312500061451644, 0.000000000000000000, 5.243569643749999010 ) ) ;
#13348=CARTESIAN_POINT ( 'NONE',  ( 26.74687500061451573, -3.027376345333614438, 5.243569643749998122 ) ) ;
#13349=CARTESIAN_POINT ( 'NONE',  ( 15.21562500061451750, 3.027376345333613106, -5.243569643749998122 ) ) ;
#13350=CARTESIAN_POINT ( 'NONE',  ( 25.87500000122903288, 2.886751345948129099, -4.999999999999998224 ) ) ;
#13352=CARTESIAN_POINT ( 'NONE',  ( 17.27812500061451217, -4.541064518000419881, 2.621784821874995952 ) ) ;
#13353=CARTESIAN_POINT ( 'NONE',  ( 7.987500000000000711, -2.886751345948130876, 4.999999999999996447 ) ) ;
#13354=CARTESIAN_POINT ( 'NONE',  ( 28.39687500061452141, 6.054752690667223547, 3.707466751127219781E-16 ) ) ;
#13355=CARTESIAN_POINT ( 'NONE',  ( 9.759375000614516793, -4.541064518000417216, -2.621784821875001281 ) ) ;
#13356=CARTESIAN_POINT ( 'NONE',  ( 10.43437500061451750, 4.541064518000418104, 2.621784821874999949 ) ) ;
#13357=CARTESIAN_POINT ( 'NONE',  ( 17.85937500061451999, -4.541064518000417216, -2.621784821875001281 ) ) ;
#13358=ORIENTED_EDGE ( 'NONE', *, *, #18629, .F. ) ;
#13359=CARTESIAN_POINT ( 'NONE',  ( -5.989433049342594906, 8.007954590042436038, 29.59128506087665400 ) ) ;
#13360=CARTESIAN_POINT ( 'NONE',  ( 20.61562500061451431, 3.027376345333613106, -5.243569643749998122 ) ) ;
#13361=CARTESIAN_POINT ( 'NONE',  ( 17.70937500061451431, 0.000000000000000000, 5.243569643749999010 ) ) ;
#13362=CARTESIAN_POINT ( 'NONE',  ( 21.89062500061451289, -3.027376345333610441, -5.243569643749999898 ) ) ;
#13363=CARTESIAN_POINT ( 'NONE',  ( -2.828200636599751609E-16, 13.58750000000000213, 25.38119784648299770 ) ) ;
#13364=CARTESIAN_POINT ( 'NONE',  ( 29.31562500061451715, 3.027376345333611329, 5.243569643749999010 ) ) ;
#13365=CARTESIAN_POINT ( 'NONE',  ( 10.38750000122903572, -4.330127018922194537, 2.499999999999995559 ) ) ;
#13366=ORIENTED_EDGE ( 'NONE', *, *, #41986, .T. ) ;
#13367=CARTESIAN_POINT ( 'NONE',  ( 3.975000001229033852, 2.886751345948126879, 4.999999999999999112 ) ) ;
#13368=CARTESIAN_POINT ( 'NONE',  ( 4.000000000000000000, 18.83749999999999858, -27.69059892324149530 ) ) ;
#13369=CARTESIAN_POINT ( 'NONE',  ( 24.22500000122903430, 2.886751345948126879, 4.999999999999999112 ) ) ;
#13372=CARTESIAN_POINT ( 'NONE',  ( 9.271875000614516082, -6.054752690667223547, -1.112240025338166033E-15 ) ) ;
#13373=CARTESIAN_POINT ( 'NONE',  ( 14.87812500061451537, 4.541064518000418104, 2.621784821874999949 ) ) ;
#13374=CARTESIAN_POINT ( 'NONE',  ( 11.52187500061451608, -6.054752690667223547, -1.112240025338166033E-15 ) ) ;
#13375=CARTESIAN_POINT ( 'NONE',  ( 3.178125000614515638, 4.541064518000418104, 2.621784821874999949 ) ) ;
#13376=CARTESIAN_POINT ( 'NONE',  ( 20.07187500061451857, -6.054752690667223547, -1.112240025338166033E-15 ) ) ;
#13377=CARTESIAN_POINT ( 'NONE',  ( 6.646875000614518747, -3.027376345333610441, -5.243569643749999898 ) ) ;
#13379=CARTESIAN_POINT ( 'NONE',  ( 7.490625000614516082, -3.027376345333610441, -5.243569643749999898 ) ) ;
#13380=CARTESIAN_POINT ( 'NONE',  ( 18.51562500061451289, 3.027376345333611329, 5.243569643749999010 ) ) ;
#13382=CARTESIAN_POINT ( 'NONE',  ( 15.44062500061451537, -3.027376345333614438, 5.243569643749998122 ) ) ;
#13383=CARTESIAN_POINT ( 'NONE',  ( 11.91562500061451857, -6.054752690667223547, -1.112240025338166033E-15 ) ) ;
#13385=CARTESIAN_POINT ( 'NONE',  ( 10.76250000000000107, -5.773502691896255534, -1.060575238724906372E-15 ) ) ;
#13386=CARTESIAN_POINT ( 'NONE',  ( 6.375000001229031987, -5.773502691896255534, -1.060575238724906372E-15 ) ) ;
#13387=EDGE_CURVE ( 'NONE', #51427, #3917, #54488, .T. ) ;
#13388=CARTESIAN_POINT ( 'NONE',  ( 14.67187500061451821, -6.054752690667223547, -1.112240025338166033E-15 ) ) ;
#13389=CARTESIAN_POINT ( 'NONE',  ( 16.46250000122903501, 4.330127018922192761, -2.499999999999997780 ) ) ;
#13391=CARTESIAN_POINT ( 'NONE',  ( -4.243569643749999898, 18.45312500061451644, -30.00000000000000000 ) ) ;
#13392=CARTESIAN_POINT ( 'NONE',  ( 16.31250000122903288, -4.330127018922190985, -2.500000000000001332 ) ) ;
#13393=CYLINDRICAL_SURFACE ( 'NONE', #6436, 4.999999999999998224 ) ;
#13394=CARTESIAN_POINT ( 'NONE',  ( 19.35937500061451644, 4.541064518000418104, -2.621784821874998173 ) ) ;
#13395=( BOUNDED_CURVE ( )  B_SPLINE_CURVE ( 2, ( #52310, #35314, #18305, #2425, #35673, #63024, #12423 ),
 .UNSPECIFIED., .F., .F. ) 
 B_SPLINE_CURVE_WITH_KNOTS ( ( 3, 2, 2, 3 ),
 ( 0.4166666666666667407, 0.4194444444444445086, 0.4222222222222222210, 0.4249999999999999889 ),
 .UNSPECIFIED. ) 
 CURVE ( )  GEOMETRIC_REPRESENTATION_ITEM ( )  RATIONAL_B_SPLINE_CURVE ( ( 0.9999999999999973355, 0.8660254037844413721, 1.000000000000000000, 0.8660254037844387076, 1.000000000000000000, 0.8660254037844387076, 1.000000000000000000 ) ) 
 REPRESENTATION_ITEM ( '' )  );
#13396=CARTESIAN_POINT ( 'NONE',  ( 29.92500000000000071, 4.330127018922191873, 2.499999999999999556 ) ) ;
#13397=CARTESIAN_POINT ( 'NONE',  ( 14.91562500061451679, 3.027376345333611329, 5.243569643749999010 ) ) ;
#13399=LINE ( 'NONE', #6797, #2348 ) ;
#13400=CARTESIAN_POINT ( 'NONE',  ( 23.85937500061451644, 4.541064518000418104, -2.621784821874998173 ) ) ;
#13402=CARTESIAN_POINT ( 'NONE',  ( 9.215625000614515727, -6.054752690667223547, -1.112240025338166033E-15 ) ) ;
#13403=CARTESIAN_POINT ( 'NONE',  ( 14.89687500061451786, 6.054752690667223547, 3.707466751127219781E-16 ) ) ;
#13404=ORIENTED_EDGE ( 'NONE', *, *, #49345, .F. ) ;
#13405=CARTESIAN_POINT ( 'NONE',  ( 25.62187500061451573, 3.027376345333613106, -5.243569643749998122 ) ) ;
#13406=CARTESIAN_POINT ( 'NONE',  ( 26.87812500061451360, 6.421520780324663323E-16, -5.243569643749999010 ) ) ;
#13407=CARTESIAN_POINT ( 'NONE',  ( 18.06562500061451715, 3.027376345333611329, 5.243569643749999010 ) ) ;
#13408=CARTESIAN_POINT ( 'NONE',  ( 29.72812500061451502, 4.541064518000418104, 2.621784821874999949 ) ) ;
#13409=DIRECTION ( 'NONE',  ( 0.000000000000000000, 0.000000000000000000, 1.000000000000000000 ) ) ;
#13410=CARTESIAN_POINT ( 'NONE',  ( 8.699999999999999289, 4.330127018922192761, -2.499999999999997780 ) ) ;
#13411=CARTESIAN_POINT ( 'NONE',  ( 19.27500000122903145, 2.886751345948126879, 4.999999999999999112 ) ) ;
#13412=CYLINDRICAL_SURFACE ( 'NONE', #6574, 4.000000000000000000 ) ;
#13415=CARTESIAN_POINT ( 'NONE',  ( 16.72500000000000142, 6.123233995736764310E-16, -4.999999999999998224 ) ) ;
#13416=CARTESIAN_POINT ( 'NONE',  ( 21.97500000000000142, -4.330127018922194537, 2.499999999999995559 ) ) ;
#13417=CARTESIAN_POINT ( 'NONE',  ( 18.79687500061451644, -3.027376345333610441, -5.243569643749999898 ) ) ;
#13418=CARTESIAN_POINT ( 'NONE',  ( 13.19062500061451537, -3.027376345333614438, 5.243569643749998122 ) ) ;
#13420=CARTESIAN_POINT ( 'NONE',  ( -0.6945831915928805111, 10.00052343484236950, -33.93923269050669944 ) ) ;
#13421=CARTESIAN_POINT ( 'NONE',  ( 5.690625000614516260, -3.027376345333610441, -5.243569643749999898 ) ) ;
#13422=CARTESIAN_POINT ( 'NONE',  ( 12.00000000000000000, 0.000000000000000000, 4.999999999999998224 ) ) ;
#13423=CARTESIAN_POINT ( 'NONE',  ( 12.56250000000000178, -5.773502691896255534, -1.060575238724906372E-15 ) ) ;
#13425=VECTOR ( 'NONE', #18752, 1000.000000000000000 ) ;
#13426=CARTESIAN_POINT ( 'NONE',  ( 4.243569643749999010, 16.01562500061451644, 27.54997392385601174 ) ) ;
#13427=CARTESIAN_POINT ( 'NONE',  ( 29.42812500061451431, -4.541064518000419881, 2.621784821874995952 ) ) ;
#13430=CARTESIAN_POINT ( 'NONE',  ( 23.63437500061451502, -4.541064518000419881, 2.621784821874995952 ) ) ;
#13431=EDGE_LOOP ( 'NONE', ( #29593, #62251 ) ) ;
#13432=CARTESIAN_POINT ( 'NONE',  ( 21.77812500061451928, -4.541064518000419881, 2.621784821874995952 ) ) ;
#13433=CARTESIAN_POINT ( 'NONE',  ( 23.48437500061451644, 4.541064518000418104, 2.621784821874999949 ) ) ;
#13434=CARTESIAN_POINT ( 'NONE',  ( 4.243569643749999898, 15.97812500061459495, -30.00000000000000000 ) ) ;
#13435=CARTESIAN_POINT ( 'NONE',  ( 5.578125000614518214, -4.541064518000419881, 2.621784821874995952 ) ) ;
#13437=CARTESIAN_POINT ( 'NONE',  ( 24.62812500061451715, 6.421520780324663323E-16, -5.243569643749999010 ) ) ;
#13441=CARTESIAN_POINT ( 'NONE',  ( 15.90937500061451892, 0.000000000000000000, 5.243569643749999010 ) ) ;
#13442=CARTESIAN_POINT ( 'NONE',  ( 24.00937500061451502, 0.000000000000000000, 5.243569643749999010 ) ) ;
#13443=CARTESIAN_POINT ( 'NONE',  ( 9.001249775931846008E-16, 14.12187500061451750, 34.90005215228797653 ) ) ;
#13444=CARTESIAN_POINT ( 'NONE',  ( 8.390625000614518214, -3.027376345333610441, -5.243569643749999898 ) ) ;
#13445=CARTESIAN_POINT ( 'NONE',  ( 3.999999999999998668, 10.47500000122903430, -32.30940107675850470 ) ) ;
#13446=CARTESIAN_POINT ( 'NONE',  ( 3.196875000614516793, 6.054752690667223547, 3.707466751127219781E-16 ) ) ;
#13447=CYLINDRICAL_SURFACE ( 'NONE', #64280, 4.000000000000000000 ) ;
#13448=CARTESIAN_POINT ( 'NONE',  ( 4.753125000614515372, -4.541064518000417216, -2.621784821875001281 ) ) ;
#13449=CARTESIAN_POINT ( 'NONE',  ( 10.09687500061451715, -3.027376345333614438, 5.243569643749998122 ) ) ;
#13451=CARTESIAN_POINT ( 'NONE',  ( 15.71250000122903501, 0.000000000000000000, 4.999999999999998224 ) ) ;
#13452=CARTESIAN_POINT ( 'NONE',  ( 29.35312500061451502, 0.000000000000000000, 5.243569643749999010 ) ) ;
#13453=CARTESIAN_POINT ( 'NONE',  ( 8.278125000614515727, -4.541064518000419881, 2.621784821874995952 ) ) ;
#13456=CARTESIAN_POINT ( 'NONE',  ( 16.92187500061451999, -6.054752690667223547, -1.112240025338166033E-15 ) ) ;
#13458=ORIENTED_EDGE ( 'NONE', *, *, #53850, .F. ) ;
#13459=CARTESIAN_POINT ( 'NONE',  ( 21.44062500061452070, -3.027376345333610441, -5.243569643749999898 ) ) ;
#13460=CARTESIAN_POINT ( 'NONE',  ( 10.86562500061451431, 3.027376345333611329, 5.243569643749999010 ) ) ;
#13461=CARTESIAN_POINT ( 'NONE',  ( 25.92187500061451644, -6.054752690667223547, -1.112240025338166033E-15 ) ) ;
#13462=CARTESIAN_POINT ( 'NONE',  ( 10.71562500061451928, 3.027376345333613106, -5.243569643749998122 ) ) ;
#13463=CARTESIAN_POINT ( 'NONE',  ( 30.00000000000000000, 0.000000000000000000, 4.999999999999998224 ) ) ;
#13464=CARTESIAN_POINT ( 'NONE',  ( 9.600000001229034297, -2.886751345948125991, -5.000000000000000000 ) ) ;
#13466=CARTESIAN_POINT ( 'NONE',  ( 25.60312500061451502, 4.541064518000418104, -2.621784821874998173 ) ) ;
#13467=CARTESIAN_POINT ( 'NONE',  ( 2.121784821875001281, 10.05312500061451608, -26.32496088578401938 ) ) ;
#13468=CARTESIAN_POINT ( 'NONE',  ( 13.72500000122903074, 2.886751345948129099, -4.999999999999998224 ) ) ;
#13469=CARTESIAN_POINT ( 'NONE',  ( 22.45312500061451644, 4.541064518000418104, -2.621784821874998173 ) ) ;
#13470=CARTESIAN_POINT ( 'NONE',  ( 19.04062500061451146, -3.027376345333614438, 5.243569643749998122 ) ) ;
#13471=CARTESIAN_POINT ( 'NONE',  ( 5.109375000614518214, 0.000000000000000000, 5.243569643749999010 ) ) ;
#13472=CARTESIAN_POINT ( 'NONE',  ( 18.48750000000000071, -2.886751345948125991, -5.000000000000000000 ) ) ;
#13473=CARTESIAN_POINT ( 'NONE',  ( 13.01250000122903394, 0.000000000000000000, 4.999999999999998224 ) ) ;
#13475=CARTESIAN_POINT ( 'NONE',  ( 9.665625000614515017, -6.054752690667223547, -1.112240025338166033E-15 ) ) ;
#13476=CARTESIAN_POINT ( 'NONE',  ( 13.56562500061451892, 3.027376345333611329, 5.243569643749999010 ) ) ;
#13477=CARTESIAN_POINT ( 'NONE',  ( 24.71250000122903145, 0.000000000000000000, 4.999999999999998224 ) ) ;
#13478=AXIS2_PLACEMENT_3D ( 'NONE', #12415, #6518, #69301 ) ;
#13479=CARTESIAN_POINT ( 'NONE',  ( 22.80937500061451573, -4.541064518000417216, -2.621784821875001281 ) ) ;
#13480=CARTESIAN_POINT ( 'NONE',  ( 21.15937500061451715, 4.541064518000418104, -2.621784821874998173 ) ) ;
#13482=EDGE_CURVE ( 'NONE', #2226, #46707, #7106, .T. ) ;
#13483=CARTESIAN_POINT ( 'NONE',  ( 6.750000001229033764, -2.886751345948129988, 4.999999999999997335 ) ) ;
#13484=CARTESIAN_POINT ( 'NONE',  ( 5.446875000614518569, 6.054752690667223547, 3.707466751127219781E-16 ) ) ;
#13485=CARTESIAN_POINT ( 'NONE',  ( 25.99687500061451928, -3.027376345333610441, -5.243569643749999898 ) ) ;
#13486=CARTESIAN_POINT ( 'NONE',  ( 3.759375000614517681, 0.000000000000000000, 5.243569643749999010 ) ) ;
#13487=VECTOR ( 'NONE', #63583, 1000.000000000000000 ) ;
#13488=CARTESIAN_POINT ( 'NONE',  ( 22.00312500061451360, 4.541064518000418104, -2.621784821874998173 ) ) ;
#13489=CARTESIAN_POINT ( 'NONE',  ( 25.88437500061451502, -4.541064518000419881, 2.621784821874995952 ) ) ;
#13491=CARTESIAN_POINT ( 'NONE',  ( 3.176339285701963888, -3.861459405730729433, 3.176339285701963888 ) ) ;
#13492=CARTESIAN_POINT ( 'NONE',  ( 27.75000000122903288, 5.773502691896255534, 3.535250795749688401E-16 ) ) ;
#13493=CARTESIAN_POINT ( 'NONE',  ( 7.171875000614517326, 3.027376345333613106, -5.243569643749998122 ) ) ;
#13494=CARTESIAN_POINT ( 'NONE',  ( 17.72812500061451502, -4.541064518000419881, 2.621784821874995952 ) ) ;
#13495=VECTOR ( 'NONE', #20312, 1000.000000000000000 ) ;
#13496=ORIENTED_EDGE ( 'NONE', *, *, #48843, .F. ) ;
#13497=CARTESIAN_POINT ( 'NONE',  ( -3.137519842735245283E-14, 12.91250000000000142, -26.00000000000000711 ) ) ;
#13498=CARTESIAN_POINT ( 'NONE',  ( 26.46562500061451573, 3.027376345333613106, -5.243569643749998122 ) ) ;
#13499=CARTESIAN_POINT ( 'NONE',  ( 4.284375000614518925, -4.541064518000419881, 2.621784821874995952 ) ) ;
#13500=CARTESIAN_POINT ( 'NONE',  ( -1.071796769724491005, 15.85759618943233207, -34.00000000000000000 ) ) ;
#13501=DIRECTION ( 'NONE',  ( -1.000000000000000000, -0.000000000000000000, -0.000000000000000000 ) ) ;
#13502=CARTESIAN_POINT ( 'NONE',  ( 17.43750000000000355, -2.886751345948129988, 4.999999999999997335 ) ) ;
#13503=CARTESIAN_POINT ( 'NONE',  ( 20.27812500061451573, 4.541064518000418104, 2.621784821874999949 ) ) ;
#13504=ADVANCED_FACE ( 'NONE', ( #22640 ), #45190, .F. ) ;
#13505=ORIENTED_EDGE ( 'NONE', *, *, #71944, .T. ) ;
#13506=CARTESIAN_POINT ( 'NONE',  ( 23.88749999999999929, -2.886751345948125991, -5.000000000000000000 ) ) ;
#13507=CARTESIAN_POINT ( 'NONE',  ( 25.28437500061451715, 4.541064518000418104, 2.621784821874999949 ) ) ;
#13508=ORIENTED_EDGE ( 'NONE', *, *, #72232, .T. ) ;
#13509=CARTESIAN_POINT ( 'NONE',  ( 0.000000000000000000, -4.999999999999998224, 0.000000000000000000 ) ) ;
#13510=CARTESIAN_POINT ( 'NONE',  ( 14.12812500061451715, -4.541064518000419881, 2.621784821874995952 ) ) ;
#13511=CARTESIAN_POINT ( 'NONE',  ( 4.753125000614515372, -4.541064518000417216, -2.621784821875001281 ) ) ;
#13513=CARTESIAN_POINT ( 'NONE',  ( 29.01562500061451644, -6.054752690667223547, -1.112240025338166033E-15 ) ) ;
#13514=CARTESIAN_POINT ( 'NONE',  ( 16.35000000122903430, -2.886751345948125991, -5.000000000000000000 ) ) ;
#13515=CARTESIAN_POINT ( 'NONE',  ( 19.31250000000000000, -5.773502691896255534, -1.060575238724906372E-15 ) ) ;
#13516=CARTESIAN_POINT ( 'NONE',  ( 26.21249999999999858, 2.886751345948129099, -4.999999999999998224 ) ) ;
#13517=CARTESIAN_POINT ( 'NONE',  ( 1.626862140677534273E-15, 10.66249999999999964, -26.00000000000000355 ) ) ;
#13518=CARTESIAN_POINT ( 'NONE',  ( 8.596875000614518925, 6.054752690667223547, 3.707466751127219781E-16 ) ) ;
#13519=CARTESIAN_POINT ( 'NONE',  ( 19.65937500061451360, -4.541064518000417216, -2.621784821875001281 ) ) ;
#13520=CARTESIAN_POINT ( 'NONE',  ( 3.999999999999998668, 11.37500000122903643, 27.69059892324149530 ) ) ;
#13522=CARTESIAN_POINT ( 'NONE',  ( 28.04062500061451502, -3.027376345333614438, 5.243569643749998122 ) ) ;
#13523=CARTESIAN_POINT ( 'NONE',  ( 3.637500000000001954, -2.886751345948125991, -5.000000000000000000 ) ) ;
#13524=ADVANCED_FACE ( 'NONE', ( #1213 ), #28914, .F. ) ;
#13525=CARTESIAN_POINT ( 'NONE',  ( 5.746875000614517504, -3.027376345333610441, -5.243569643749999898 ) ) ;
#13526=CARTESIAN_POINT ( 'NONE',  ( 15.90000000000000036, 4.330127018922192761, -2.499999999999997780 ) ) ;
#13527=CARTESIAN_POINT ( 'NONE',  ( 12.70312500061451821, 0.000000000000000000, 5.243569643749999010 ) ) ;
#13530=CARTESIAN_POINT ( 'NONE',  ( 18.52500000122903145, -5.773502691896255534, -1.060575238724906372E-15 ) ) ;
#13531=CARTESIAN_POINT ( 'NONE',  ( 0.2033016277077261402, 10.00000000000000533, 24.00000000000001066 ) ) ;
#13533=CARTESIAN_POINT ( 'NONE',  ( 6.703125000614516438, 4.541064518000418104, -2.621784821874998173 ) ) ;
#13534=CARTESIAN_POINT ( 'NONE',  ( 24.79687500061451999, 6.054752690667223547, 3.707466751127219781E-16 ) ) ;
#13535=CARTESIAN_POINT ( 'NONE',  ( 4.243569643749999010, 19.22187500061452070, 27.54997392385601174 ) ) ;
#13536=CARTESIAN_POINT ( 'NONE',  ( 24.34687500061451715, 6.054752690667223547, 3.707466751127219781E-16 ) ) ;
#13537=CARTESIAN_POINT ( 'NONE',  ( 6.675000000000000711, -4.330127018922194537, 2.499999999999995559 ) ) ;
#13538=CARTESIAN_POINT ( 'NONE',  ( 4.000000000000000000, 12.20000000122903394, 32.30940107675849049 ) ) ;
#13539=CARTESIAN_POINT ( 'NONE',  ( 14.35312500061451679, 4.541064518000418104, -2.621784821874998173 ) ) ;
#13540=CARTESIAN_POINT ( 'NONE',  ( 7.462500001229035007, 4.330127018922192761, -2.499999999999997780 ) ) ;
#13541=CARTESIAN_POINT ( 'NONE',  ( 12.57187500061451857, 3.027376345333613106, -5.243569643749998122 ) ) ;
#13542=CARTESIAN_POINT ( 'NONE',  ( 3.908869731033371764, -3.117809716100492512, 3.994975926305053271 ) ) ;
#13543=ORIENTED_EDGE ( 'NONE', *, *, #4806, .F. ) ;
#13544=AXIS2_PLACEMENT_3D ( 'NONE', #37917, #67107, #4678 ) ;
#13545=CARTESIAN_POINT ( 'NONE',  ( 13.56562500061451892, 3.027376345333611329, 5.243569643749999010 ) ) ;
#13547=CARTESIAN_POINT ( 'NONE',  ( 23.28750000122903430, 4.330127018922191873, 2.499999999999999556 ) ) ;
#13548=CARTESIAN_POINT ( 'NONE',  ( 11.67187500061451821, 3.027376345333613106, -5.243569643749998122 ) ) ;
#13549=CARTESIAN_POINT ( 'NONE',  ( 15.10312500061451502, -4.541064518000417216, -2.621784821875001281 ) ) ;
#13551=CARTESIAN_POINT ( 'NONE',  ( 22.99687500061451573, 6.054752690667223547, 3.707466751127219781E-16 ) ) ;
#13552=CARTESIAN_POINT ( 'NONE',  ( 1.999999999999998668, 15.91250000122903430, 26.53589838486224650 ) ) ;
#13553=CIRCLE ( 'NONE', #17091, 4.000000000000000000 ) ;
#13554=DIRECTION ( 'NONE',  ( -0.000000000000000000, -1.000000000000000000, -0.000000000000000000 ) ) ;
#13555=CARTESIAN_POINT ( 'NONE',  ( -3.999999999999999112, 19.55000000000000071, 30.00000000000000000 ) ) ;
#13556=CARTESIAN_POINT ( 'NONE',  ( -3.000416591977282496E-16, 14.79687500061451821, -34.90005215228797653 ) ) ;
#13557=CARTESIAN_POINT ( 'NONE',  ( 14.82187500061451679, 3.027376345333613106, -5.243569643749998122 ) ) ;
#13558=CARTESIAN_POINT ( 'NONE',  ( 17.62500000122903288, -5.773502691896255534, -1.060575238724906372E-15 ) ) ;
#13560=CARTESIAN_POINT ( 'NONE',  ( 11.33437500061451608, 4.541064518000418104, 2.621784821874999949 ) ) ;
#13561=CARTESIAN_POINT ( 'NONE',  ( -2.121784821874999949, 9.884375000614518569, 26.32496088578401938 ) ) ;
#13562=CARTESIAN_POINT ( 'NONE',  ( 19.05000000122903359, -2.886751345948125991, -5.000000000000000000 ) ) ;
#13563=CARTESIAN_POINT ( 'NONE',  ( 12.36562500061451608, -6.054752690667223547, -1.112240025338166033E-15 ) ) ;
#13564=ORIENTED_EDGE ( 'NONE', *, *, #22499, .T. ) ;
#13565=ORIENTED_EDGE ( 'NONE', *, *, #37148, .T. ) ;
#13567=CARTESIAN_POINT ( 'NONE',  ( 18.26249999999999929, 2.886751345948126879, 4.999999999999999112 ) ) ;
#13568=CARTESIAN_POINT ( 'NONE',  ( 30.00000000000000000, 6.123233995736764310E-16, -4.999999999999998224 ) ) ;
#13569=CARTESIAN_POINT ( 'NONE',  ( 11.63437500061451857, 6.421520780324663323E-16, -5.243569643749999010 ) ) ;
#13571=CARTESIAN_POINT ( 'NONE',  ( 12.30000000122903181, -2.886751345948125991, -5.000000000000000000 ) ) ;
#13572=CARTESIAN_POINT ( 'NONE',  ( 21.41250000122903074, 4.330127018922192761, -2.499999999999997780 ) ) ;
#13573=CARTESIAN_POINT ( 'NONE',  ( 17.95312500061451644, 4.541064518000418104, -2.621784821874998173 ) ) ;
#13574=CARTESIAN_POINT ( 'NONE',  ( 21.70312500061451644, 0.000000000000000000, 5.243569643749999010 ) ) ;
#13575=CARTESIAN_POINT ( 'NONE',  ( 28.42500000122904069, -5.773502691896255534, -1.060575238724906372E-15 ) ) ;
#13576=CARTESIAN_POINT ( 'NONE',  ( 26.73749999999999716, 5.773502691896255534, 3.535250795749688894E-16 ) ) ;
#13577=CARTESIAN_POINT ( 'NONE',  ( 3.397178649298551179, 3.668675132081069545, -3.397178649298551179 ) ) ;
#13579=CARTESIAN_POINT ( 'NONE',  ( 28.13437500061451502, -4.541064518000419881, 2.621784821874995952 ) ) ;
#13580=DIRECTION ( 'NONE',  ( -0.4999999999999975575, 0.000000000000000000, 0.8660254037844400399 ) ) ;
#13581=CARTESIAN_POINT ( 'NONE',  ( -2.121784821874996840, 15.43437500061451928, -26.32496088578401583 ) ) ;
#13582=CARTESIAN_POINT ( 'NONE',  ( 4.575000001229033941, -5.773502691896255534, -1.060575238724906372E-15 ) ) ;
#13583=CARTESIAN_POINT ( 'NONE',  ( 6.375000000000001776, 6.123233995736764310E-16, -4.999999999999998224 ) ) ;
#13585=CARTESIAN_POINT ( 'NONE',  ( 9.496875000614517504, 6.054752690667223547, 3.707466751127219781E-16 ) ) ;
#13586=CARTESIAN_POINT ( 'NONE',  ( 27.81562500061452070, 3.027376345333613106, -5.243569643749998122 ) ) ;
#13587=DIRECTION ( 'NONE',  ( -1.000000000000000000, -0.000000000000000000, -0.000000000000000000 ) ) ;
#13588=CARTESIAN_POINT ( 'NONE',  ( -3.039972894299037609, 9.532883912050412079, -35.18750932600423909 ) ) ;
#13589=CARTESIAN_POINT ( 'NONE',  ( 3.999999999999999112, 17.63750000122903572, -30.00000000000000000 ) ) ;
#13590=CARTESIAN_POINT ( 'NONE',  ( 8.446875000614518569, -3.027376345333610441, -5.243569643749999898 ) ) ;
#13591=CARTESIAN_POINT ( 'NONE',  ( 11.48437500061451644, -4.541064518000419881, 2.621784821874995952 ) ) ;
#13592=EDGE_CURVE ( 'NONE', #30864, #38892, #62891, .T. ) ;
#13593=CARTESIAN_POINT ( 'NONE',  ( 4.724999999999999645, 4.330127018922191873, 2.499999999999999556 ) ) ;
#13594=VECTOR ( 'NONE', #9100, 1000.000000000000000 ) ;
#13595=CARTESIAN_POINT ( 'NONE',  ( -2.121784821874996840, 15.37812500061459531, 33.67503911421598417 ) ) ;
#13597=CARTESIAN_POINT ( 'NONE',  ( 6.337499999999998579, -2.886751345948125991, -5.000000000000000000 ) ) ;
#13599=CARTESIAN_POINT ( 'NONE',  ( 20.91562500061451502, -6.054752690667223547, -1.112240025338166033E-15 ) ) ;
#13600=CARTESIAN_POINT ( 'NONE',  ( 12.02812500061451573, 6.421520780324663323E-16, -5.243569643749999010 ) ) ;
#13602=CARTESIAN_POINT ( 'NONE',  ( 9.571875000614518569, 3.027376345333611329, 5.243569643749999010 ) ) ;
#13603=CARTESIAN_POINT ( 'NONE',  ( 26.06250000000000000, -5.773502691896255534, -1.060575238724906372E-15 ) ) ;
#13604=CARTESIAN_POINT ( 'NONE',  ( 23.17500000122903359, 2.886751345948129099, -4.999999999999998224 ) ) ;
#13606=AXIS2_PLACEMENT_3D ( 'NONE', #67615, #16981, #28444 ) ;
#13607=CARTESIAN_POINT ( 'NONE',  ( 12.68437500061451573, 4.541064518000418104, 2.621784821874999949 ) ) ;
#13608=CARTESIAN_POINT ( 'NONE',  ( 25.47187500061451715, -6.054752690667223547, -1.112240025338166033E-15 ) ) ;
#13609=CARTESIAN_POINT ( 'NONE',  ( 3.721875000614518036, 3.027376345333611329, 5.243569643749999010 ) ) ;
#13610=CARTESIAN_POINT ( 'NONE',  ( 24.26250000122903216, 0.000000000000000000, 4.999999999999998224 ) ) ;
#13611=CARTESIAN_POINT ( 'NONE',  ( 19.47187500061451360, 3.027376345333611329, 5.243569643749999010 ) ) ;
#13612=CARTESIAN_POINT ( 'NONE',  ( 11.03437500061451715, -4.541064518000419881, 2.621784821874995952 ) ) ;
#13614=CARTESIAN_POINT ( 'NONE',  ( 24.29999999999999716, -4.330127018922190985, -2.500000000000001332 ) ) ;
#13616=CARTESIAN_POINT ( 'NONE',  ( -4.243569643749997233, 11.34687500061451892, -27.54997392385601174 ) ) ;
#13618=CARTESIAN_POINT ( 'NONE',  ( 14.20312500061451644, -4.541064518000417216, -2.621784821875001281 ) ) ;
#13619=CARTESIAN_POINT ( 'NONE',  ( 4.050000000000001599, -4.330127018922190985, -2.500000000000001332 ) ) ;
#13620=( BOUNDED_CURVE ( )  B_SPLINE_CURVE ( 2, ( #43932, #5133, #321, #28385, #60532, #10670, #44304, #43565, #60904, #9939, #72362, #56463, #32477, #15465, #55010, #10307, #38381, #50565, #39115, #26945, #62000, #11401, #49470, #73092, #4416, #4771, #22473, #55377, #61631, #45024, #72003, #33920, #16564, #22116, #5854, #50923, #49838, #44672, #66834, #16205, #21378, #66458, #15835, #38756, #61277, #33200, #55739, #17644, #23193, #52012, #7660, #28744, #35013, #51284, #12119, #41294, #17289, #12839, #12486, #18007, #18369, #30200, #63804, #686, #40939, #6216, #35373, #6586, #23560, #69007, #45747, #57173, #62726, #68283, #62364, #29475, #63084, #68644, #29835, #63453, #6944, #40204, #34644, #57542, #1413, #58255, #22830, #23920, #52370, #1775, #24287, #57896, #29116, #46835, #52731, #7304, #46107, #51650, #45382, #1051, #35735, #40565, #46470, #67918, #69374, #39851, #11761, #18730, #13195, #34278, #56810, #2485, #36833, #32024, #60085, #19093, #42383, #2852, #2136, #19457, #41648, #59347, #42746, #8029, #8758, #31665, #19831, #64168, #30565, #54198, #24647, #65637, #71181, #58623, #9128, #13556, #36468, #65266, #42017, #20191, #3595, #30921, #70816, #53091, #70455, #69723, #8391, #9495, #47926, #47553, #14654, #26117, #48656, #36102, #37197, #53833, #25011, #47193, #70082, #64538, #31292, #64905, #3227, #13931, #20554, #58986, #53462, #25382, #43111, #14295, #25755, #48291, #59720, #15025, #37562, #39036, #71556, #67121, #5413, #16478, #22032, #55655, #27953, #61550, #44589, #5051, #33473, #44218, #49756, #50120, #32386, #38673, #72283, #10952, #56022, #15387, #66007, #61195, #43849, #37929, #50485, #21296, #54925, #20931, #10590, #21661, #27220, #73010, #72651, #33118, #22394, #66750, #43483, #16120, #39398, #61917, #66375, #44943, #67481, #54560, #16844, #26859, #11322, #3962, #26485, #4690, #15751, #49026, #60448, #9857, #4334, #38290, #49390, #71921, #60817, #27588, #10224, #32759, #55296, #51928, #68562, #18646, #41210, #35288, #62288, #56386, #23479, #57456, #11684, #6136, #17920, #1325, #39772, #40483, #63368, #51569, #243, #34199, #12753, #33843, #24196, #56733, #62999, #1687, #50843, #34929, #57090, #17566, #63718 ),
 .UNSPECIFIED., .F., .F. ) 
 B_SPLINE_CURVE_WITH_KNOTS ( ( 3, 2, 2, 2, 2, 2, 2, 2, 2, 2, 2, 2, 2, 2, 2, 2, 2, 2, 2, 2, 2, 2, 2, 2, 2, 2, 2, 2, 2, 2, 2, 2, 2, 2, 2, 2, 2, 2, 2, 2, 2, 2, 2, 2, 2, 2, 2, 2, 2, 2, 2, 2, 2, 2, 2, 2, 2, 2, 2, 2, 2, 2, 2, 2, 2, 2, 2, 2, 2, 2, 2, 2, 2, 2, 2, 2, 2, 2, 2, 2, 2, 2, 2, 2, 2, 2, 2, 2, 2, 2, 2, 2, 2, 2, 2, 2, 2, 2, 2, 2, 2, 2, 2, 2, 2, 2, 2, 2, 2, 2, 2, 2, 2, 2, 2, 2, 2, 2, 2, 2, 2, 2, 2, 2, 2, 2, 2, 2, 2, 2, 2, 2, 2, 2, 3 ),
 ( 0.000000000000000000, 0.007499808062934601276, 0.01499961612586920255, 0.02249942418880380296, 0.02999923225173840510, 0.03749904031467300725, 0.04499884837760760592, 0.05249865644054221153, 0.05999846450347681021, 0.06749827256641140194, 0.07499808062934601449, 0.08249788869228059929, 0.08999769675521521184, 0.09749750481814981051, 0.1049973128810844231, 0.1124971209440190079, 0.1199969290069536204, 0.1274967370698882330, 0.1349965451328228039, 0.1424963531957574303, 0.1499961612586920290, 0.1574959693216266277, 0.1649957773845611986, 0.1724955854474958250, 0.1799953935104304237, 0.1874952015733650224, 0.1949950096362996210, 0.2024948176992342197, 0.2099946257621688461, 0.2174944338251034170, 0.2249942418880380157, 0.2324940499509726144, 0.2399938580139072408, 0.2474936660768418395, 0.2549934741397764659, 0.2624932822027110646, 0.2699930902656456078, 0.2774928983285802619, 0.2849927063915148606, 0.2924925144544494038, 0.2999923225173840580, 0.3074921305803186011, 0.3149919386432532553, 0.3224917467061878540, 0.3299915547691223972, 0.3374913628320570513, 0.3449911708949916500, 0.3524909789579262487, 0.3599907870208608474, 0.3674905950837954460, 0.3749904031467300447, 0.3824902112096646434, 0.3899900192725992421, 0.3974898273355338407, 0.4049896353984684394, 0.4124894434614030381, 0.4199892515243376923, 0.4274890595872722354, 0.4349888676502068341, 0.4424886757131414883, 0.4499884837760760314, 0.4574882918390106856, 0.4649880999019452288, 0.4724879079648798275, 0.4799877160278144816, 0.4874875240907490248, 0.4949873321536836790, 0.5024871402166182222, 0.5099869482795529319, 0.5174867563424874195, 0.5249865644054221292, 0.5324863724683566168, 0.5399861805312912155, 0.5474859885942259252, 0.5549857966571605239, 0.5624856047200950115, 0.5699854127830297212, 0.5774852208459643199, 0.5849850289088988076, 0.5924848369718334062, 0.5999846450347681159, 0.6074844530977027146, 0.6149842611606372023, 0.6224840692235719120, 0.6299838772865065106, 0.6374836853494409983, 0.6449834934123757080, 0.6524833014753103066, 0.6599831095382447943, 0.6674829176011795040, 0.6749827256641141027, 0.6824825337270487013, 0.6899823417899833000, 0.6974821498529178987, 0.7049819579158524974, 0.7124817659787869850, 0.7199815740417216947, 0.7274813821046562934, 0.7349811901675908921, 0.7424809982305254907, 0.7499808062934600894, 0.7574806143563946881, 0.7649804224193292868, 0.7724802304822638854, 0.7799800385451984841, 0.7874798466081331938, 0.7949796546710676814, 0.8024794627340022801, 0.8099792707969368788, 0.8174790788598714775, 0.8249788869228060761, 0.8324786949857406748, 0.8399785030486753845, 0.8474783111116098722, 0.8549781191745444708, 0.8624779272374791805, 0.8699777353004136682, 0.8774775433633482669, 0.8849773514262829766, 0.8924771594892175752, 0.8999769675521520629, 0.9074767756150867726, 0.9149765836780213712, 0.9224763917409558589, 0.9299761998038904576, 0.9374760078668251673, 0.9449758159297596549, 0.9524756239926942536, 0.9599754320556289633, 0.9674752401185635620, 0.9749750481814980496, 0.9824748562444327593, 0.9899746643073673580, 0.9974744723703018456, 1.000000000000000000 ),
 .UNSPECIFIED. ) 
 CURVE ( )  GEOMETRIC_REPRESENTATION_ITEM ( )  RATIONAL_B_SPLINE_CURVE ( ( 1.000000000000000000, 0.8660254037844387076, 1.000000000000000000, 0.8660254037844387076, 1.000000000000000000, 0.8660254037844387076, 1.000000000000000000, 0.8660254037844387076, 1.000000000000000000, 0.8660254037844387076, 1.000000000000000000, 0.8660254037844387076, 1.000000000000000000, 0.8660254037844387076, 1.000000000000000000, 0.8660254037844387076, 1.000000000000000000, 0.8660254037844387076, 1.000000000000000000, 0.8660254037844387076, 1.000000000000000000, 0.8660254037844387076, 1.000000000000000000, 0.8660254037844387076, 1.000000000000000000, 0.8660254037844387076, 1.000000000000000000, 0.8660254037844387076, 1.000000000000000000, 0.8660254037844387076, 1.000000000000000000, 0.8660254037844387076, 1.000000000000000000, 0.8660254037844387076, 1.000000000000000000, 0.8660254037844387076, 1.000000000000000000, 0.8660254037844387076, 1.000000000000000000, 0.8660254037844387076, 1.000000000000000000, 0.8660254037844387076, 1.000000000000000000, 0.8660254037844387076, 1.000000000000000000, 0.8660254037844387076, 1.000000000000000000, 0.8660254037844387076, 1.000000000000000000, 0.8660254037844387076, 1.000000000000000000, 0.8660254037844387076, 1.000000000000000000, 0.8660254037844387076, 1.000000000000000000, 0.8660254037844387076, 1.000000000000000000, 0.8660254037844387076, 1.000000000000000000, 0.8660254037844387076, 1.000000000000000000, 0.8660254037844387076, 1.000000000000000000, 0.8660254037844387076, 1.000000000000000000, 0.8660254037844387076, 1.000000000000000000, 0.8660254037844387076, 1.000000000000000000, 0.8660254037844387076, 1.000000000000000000, 0.8660254037844387076, 1.000000000000000000, 0.8660254037844387076, 1.000000000000000000, 0.8660254037844387076, 1.000000000000000000, 0.8660254037844387076, 1.000000000000000000, 0.8660254037844387076, 1.000000000000000000, 0.8660254037844387076, 1.000000000000000000, 0.8660254037844387076, 1.000000000000000000, 0.8660254037844387076, 1.000000000000000000, 0.8660254037844387076, 1.000000000000000000, 0.8660254037844387076, 1.000000000000000000, 0.8660254037844387076, 1.000000000000000000, 0.8660254037844387076, 1.000000000000000000, 0.8660254037844387076, 1.000000000000000000, 0.8660254037844387076, 1.000000000000000000, 0.8660254037844387076, 1.000000000000000000, 0.8660254037844387076, 1.000000000000000000, 0.8660254037844387076, 1.000000000000000000, 0.8660254037844387076, 1.000000000000000000, 0.8660254037844387076, 1.000000000000000000, 0.8660254037844387076, 1.000000000000000000, 0.8660254037844387076, 1.000000000000000000, 0.8660254037844387076, 1.000000000000000000, 0.8660254037844387076, 1.000000000000000000, 0.8660254037844387076, 1.000000000000000000, 0.8660254037844387076, 1.000000000000000000, 0.8660254037844387076, 1.000000000000000000, 0.8660254037844387076, 1.000000000000000000, 0.8660254037844387076, 1.000000000000000000, 0.8660254037844387076, 1.000000000000000000, 0.8660254037844387076, 1.000000000000000000, 0.8660254037844387076, 1.000000000000000000, 0.8660254037844387076, 1.000000000000000000, 0.8660254037844387076, 1.000000000000000000, 0.8660254037844387076, 1.000000000000000000, 0.8660254037844387076, 1.000000000000000000, 0.8660254037844387076, 1.000000000000000000, 0.8660254037844387076, 1.000000000000000000, 0.8660254037844387076, 1.000000000000000000, 0.8660254037844387076, 1.000000000000000000, 0.8660254037844387076, 1.000000000000000000, 0.8660254037844387076, 1.000000000000000000, 0.8660254037844387076, 1.000000000000000000, 0.8660254037844387076, 1.000000000000000000, 0.8660254037844387076, 1.000000000000000000, 0.8660254037844387076, 1.000000000000000000, 0.8660254037844387076, 1.000000000000000000, 0.8660254037844387076, 1.000000000000000000, 0.8660254037844387076, 1.000000000000000000, 0.8660254037844387076, 1.000000000000000000, 0.8660254037844387076, 1.000000000000000000, 0.8660254037844387076, 1.000000000000000000, 0.8660254037844387076, 1.000000000000000000, 0.8660254037844387076, 1.000000000000000000, 0.8660254037844387076, 1.000000000000000000, 0.8660254037844387076, 1.000000000000000000, 0.8660254037844387076, 1.000000000000000000, 0.8660254037844387076, 1.000000000000000000, 0.8660254037844387076, 1.000000000000000000, 0.8660254037844387076, 1.000000000000000000, 0.8660254037844387076, 1.000000000000000000, 0.8660254037844387076, 1.000000000000000000, 0.8660254037844387076, 1.000000000000000000, 0.8660254037844387076, 1.000000000000000000, 0.8660254037844387076, 1.000000000000000000, 0.8660254037844387076, 1.000000000000000000, 0.8660254037844387076, 1.000000000000000000, 0.8660254037844387076, 1.000000000000000000, 0.8660254037844387076, 1.000000000000000000, 0.8660254037844387076, 1.000000000000000000, 0.8660254037844387076, 1.000000000000000000, 0.8660254037844387076, 1.000000000000000000, 0.8660254037844387076, 1.000000000000000000, 0.8660254037844387076, 1.000000000000000000, 0.8660254037844387076, 1.000000000000000000, 0.8660254037844387076, 1.000000000000000000, 0.8660254037844387076, 1.000000000000000000, 0.8660254037844387076, 1.000000000000000000, 0.8660254037844387076, 1.000000000000000000, 0.8660254037844387076, 1.000000000000000000, 0.8660254037844387076, 1.000000000000000000, 0.8660254037844387076, 1.000000000000000000, 0.8660254037844387076, 1.000000000000000000, 0.8660254037844387076, 1.000000000000000000, 0.8660254037844387076, 1.000000000000000000, 0.8660254037844387076, 1.000000000000000000, 0.8660254037844387076, 1.000000000000000000, 0.8660254037844387076, 1.000000000000000000, 0.8660254037844387076, 1.000000000000000000, 0.8660254037844387076, 1.000000000000000000, 0.8660254037844387076, 1.000000000000000000, 0.8660254037844387076, 1.000000000000000000, 0.8660254037844387076, 1.000000000000000000, 0.8660254037844387076, 1.000000000000000000, 0.8660254037844387076, 1.000000000000000000, 0.8660254037844387076, 1.000000000000000000, 0.8660254037844387076, 1.000000000000000000, 0.8660254037844387076, 1.000000000000000000, 0.8660254037844387076, 1.000000000000000000, 0.9548846395026737710, 0.9401540804572410259 ) ) 
 REPRESENTATION_ITEM ( '' )  );
#13622=DIRECTION ( 'NONE',  ( -1.000000000000000000, -0.000000000000000000, -0.000000000000000000 ) ) ;
#13623=CARTESIAN_POINT ( 'NONE',  ( 15.45000000000000107, 4.330127018922192761, -2.499999999999997780 ) ) ;
#13624=ADVANCED_FACE ( 'NONE', ( #63248 ), #68441, .F. ) ;
#13625=CARTESIAN_POINT ( 'NONE',  ( -3.000416591977282496E-16, 10.24062500061451608, 25.09994784771203058 ) ) ;
#13626=CARTESIAN_POINT ( 'NONE',  ( 13.61250000122903359, -4.330127018922190985, -2.500000000000001332 ) ) ;
#13627=CARTESIAN_POINT ( 'NONE',  ( 25.95937500061451431, -4.541064518000417216, -2.621784821875001281 ) ) ;
#13628=CARTESIAN_POINT ( 'NONE',  ( 30.00000000000000000, 6.123233995736764310E-16, -4.999999999999998224 ) ) ;
#13629=VERTEX_POINT ( 'NONE', #17095 ) ;
#13630=CARTESIAN_POINT ( 'NONE',  ( 19.04062500061451146, -3.027376345333614438, 5.243569643749998122 ) ) ;
#13631=CARTESIAN_POINT ( 'NONE',  ( 3.328125000614516438, -4.541064518000419881, 2.621784821874995952 ) ) ;
#13632=CARTESIAN_POINT ( 'NONE',  ( 19.28437500061451360, 6.421520780324663323E-16, -5.243569643749999010 ) ) ;
#13633=CARTESIAN_POINT ( 'NONE',  ( 29.70937500061451431, 4.541064518000418104, -2.621784821874998173 ) ) ;
#13634=CARTESIAN_POINT ( 'NONE',  ( 7.565625000614518036, 3.027376345333613106, -5.243569643749998122 ) ) ;
#13635=CARTESIAN_POINT ( 'NONE',  ( 22.34062500061451573, -3.027376345333610441, -5.243569643749999898 ) ) ;
#13636=CARTESIAN_POINT ( 'NONE',  ( -4.243569643749999898, 16.20312500061451644, 30.00000000000000000 ) ) ;
#13637=CARTESIAN_POINT ( 'NONE',  ( 18.56250000122903288, -4.330127018922190985, -2.500000000000001332 ) ) ;
#13639=CARTESIAN_POINT ( 'NONE',  ( 8.953125000614518214, 4.541064518000418104, -2.621784821874998173 ) ) ;
#13640=CARTESIAN_POINT ( 'NONE',  ( 4.246875000614519280, -3.027376345333614438, 5.243569643749998122 ) ) ;
#13641=CARTESIAN_POINT ( 'NONE',  ( 3.159375000614518036, 4.541064518000418104, -2.621784821874998173 ) ) ;
#13642=CARTESIAN_POINT ( 'NONE',  ( 21.90937500061451715, -4.541064518000417216, -2.621784821875001281 ) ) ;
#13643=CARTESIAN_POINT ( 'NONE',  ( 14.46562500061451750, 3.027376345333611329, 5.243569643749999010 ) ) ;
#13644=CARTESIAN_POINT ( 'NONE',  ( 23.88750000122903216, -4.330127018922194537, 2.499999999999995559 ) ) ;
#13645=CARTESIAN_POINT ( 'NONE',  ( 24.81562500061451715, 3.027376345333611329, 5.243569643749999010 ) ) ;
#13646=CARTESIAN_POINT ( 'NONE',  ( 18.98437500061451644, 4.541064518000418104, 2.621784821874999949 ) ) ;
#13647=CARTESIAN_POINT ( 'NONE',  ( 14.31562500061451537, 3.027376345333613106, -5.243569643749998122 ) ) ;
#13648=CARTESIAN_POINT ( 'NONE',  ( 2.121784821874999061, 17.45937500061451786, 26.32496088578401583 ) ) ;
#13650=CARTESIAN_POINT ( 'NONE',  ( 18.62812500061451715, -4.541064518000419881, 2.621784821874995952 ) ) ;
#13651=CARTESIAN_POINT ( 'NONE',  ( 10.01250000000000107, 2.886751345948129099, -4.999999999999997335 ) ) ;
#13652=ORIENTED_EDGE ( 'NONE', *, *, #19932, .T. ) ;
#13653=CARTESIAN_POINT ( 'NONE',  ( 26.17500000000000071, 6.123233995736764310E-16, -4.999999999999998224 ) ) ;
#13654=CARTESIAN_POINT ( 'NONE',  ( -3.999999999999999556, 11.41250000000000142, -32.30940107675850470 ) ) ;
#13655=CARTESIAN_POINT ( 'NONE',  ( 4.818692141996693046, -1.334243621178544226, 4.818692141997074074 ) ) ;
#13656=STYLED_ITEM('',(#73130),#22240);
#13657=CARTESIAN_POINT ( 'NONE',  ( 26.99062500061451431, 6.054752690667223547, 3.707466751127219781E-16 ) ) ;
#13658=CARTESIAN_POINT ( 'NONE',  ( 7.228125000614517681, 4.541064518000418104, 2.621784821874999949 ) ) ;
#13659=CARTESIAN_POINT ( 'NONE',  ( 19.68750000122903288, 4.330127018922191873, 2.499999999999999556 ) ) ;
#13660=CARTESIAN_POINT ( 'NONE',  ( 24.77812500061451217, 4.541064518000418104, 2.621784821874999949 ) ) ;
#13661=CARTESIAN_POINT ( 'NONE',  ( 25.19999999999999929, -4.330127018922190985, -2.500000000000001332 ) ) ;
#13662=CARTESIAN_POINT ( 'NONE',  ( -3.999999999999999112, 16.51250000122903216, -30.00000000000000000 ) ) ;
#13663=CARTESIAN_POINT ( 'NONE',  ( 26.87812500061451360, 6.421520780324663323E-16, -5.243569643749999010 ) ) ;
#13664=CARTESIAN_POINT ( 'NONE',  ( 9.328125000614518214, 6.421520780324663323E-16, -5.243569643749999010 ) ) ;
#13665=VERTEX_POINT ( 'NONE', #51452 ) ;
#13666=CARTESIAN_POINT ( 'NONE',  ( 24.62812500061451715, 6.421520780324663323E-16, -5.243569643749999010 ) ) ;
#13667=CARTESIAN_POINT ( 'NONE',  ( 4.640625000614518214, -3.027376345333614438, 5.243569643749998122 ) ) ;
#13668=VECTOR ( 'NONE', #50802, 1000.000000000000000 ) ;
#13670=FACE_OUTER_BOUND ( 'NONE', #2202, .T. ) ;
#13671=( BOUNDED_CURVE ( )  B_SPLINE_CURVE ( 2, ( #49234, #21503, #54767, #15959, #61033, #10431, #55863 ),
 .UNSPECIFIED., .F., .F. ) 
 B_SPLINE_CURVE_WITH_KNOTS ( ( 3, 2, 2, 3 ),
 ( 0.2916666666666667407, 0.2944444444444445086, 0.2972222222222222210, 0.2999999999999999889 ),
 .UNSPECIFIED. ) 
 CURVE ( )  GEOMETRIC_REPRESENTATION_ITEM ( )  RATIONAL_B_SPLINE_CURVE ( ( 0.9999999999999973355, 0.8660254037844413721, 1.000000000000000000, 0.8660254037844387076, 1.000000000000000000, 0.8660254037844387076, 1.000000000000000000 ) ) 
 REPRESENTATION_ITEM ( '' )  );
#13672=CARTESIAN_POINT ( 'NONE',  ( 12.30000000000000249, 4.330127018922192761, -2.499999999999997780 ) ) ;
#13673=CARTESIAN_POINT ( 'NONE',  ( 13.99687500061451928, 6.054752690667223547, 3.707466751127219781E-16 ) ) ;
#13674=CARTESIAN_POINT ( 'NONE',  ( 7.762500001229033053, -4.330127018922190985, -2.500000000000001332 ) ) ;
#13675=CARTESIAN_POINT ( 'NONE',  ( 17.59687500061451715, 6.054752690667223547, 3.707466751127219781E-16 ) ) ;
#13677=CARTESIAN_POINT ( 'NONE',  ( 7.321875000614516793, 3.027376345333611329, 5.243569643749999010 ) ) ;
#13678=CARTESIAN_POINT ( 'NONE',  ( -4.243569643749997233, 12.64062500061451999, -27.54997392385601174 ) ) ;
#13679=CARTESIAN_POINT ( 'NONE',  ( -1.071796769724491005, 11.80759618943233669, -34.00000000000000000 ) ) ;
#13681=ORIENTED_EDGE ( 'NONE', *, *, #27532, .T. ) ;
#13682=CARTESIAN_POINT ( 'NONE',  ( 25.56562500061452070, 3.027376345333613106, -5.243569643749998122 ) ) ;
#13683=CARTESIAN_POINT ( 'NONE',  ( -4.243569643749998122, 10.44687500061451679, 32.45002607614398471 ) ) ;
#13685=CARTESIAN_POINT ( 'NONE',  ( 25.17187500061451644, 3.027376345333613106, -5.243569643749998122 ) ) ;
#13686=CARTESIAN_POINT ( 'NONE',  ( 28.20937500061451786, -4.541064518000417216, -2.621784821875001281 ) ) ;
#13687=CARTESIAN_POINT ( 'NONE',  ( 22.80000000000000071, 0.000000000000000000, 4.999999999999998224 ) ) ;
#13688=( BOUNDED_CURVE ( )  B_SPLINE_CURVE ( 2, ( #71304, #71678, #10343, #4082, #65761, #31418, #21052 ),
 .UNSPECIFIED., .F., .T. ) 
 B_SPLINE_CURVE_WITH_KNOTS ( ( 3, 2, 2, 3 ),
 ( 0.2833333333333333814, 0.2861111111111111494, 0.2888888888888889173, 0.2916666666666667407 ),
 .UNSPECIFIED. ) 
 CURVE ( )  GEOMETRIC_REPRESENTATION_ITEM ( )  RATIONAL_B_SPLINE_CURVE ( ( 0.9999999999999973355, 0.8660254037844413721, 1.000000000000000000, 0.8660254037844387076, 1.000000000000000000, 0.8660254037844360431, 1.000000000000002665 ) ) 
 REPRESENTATION_ITEM ( '' )  );
#13689=CARTESIAN_POINT ( 'NONE',  ( 3.553125000614516082, 4.541064518000418104, -2.621784821874998173 ) ) ;
#13691=CARTESIAN_POINT ( 'NONE',  ( 16.92187500061451999, -6.054752690667223547, -1.112240025338166033E-15 ) ) ;
#13693=AXIS2_PLACEMENT_3D ( 'NONE', #58463, #44614, #16503 ) ;
#13694=CARTESIAN_POINT ( 'NONE',  ( 3.140625000614516882, 6.054752690667223547, 3.707466751127219781E-16 ) ) ;
#13695=CARTESIAN_POINT ( 'NONE',  ( 8.559375000614515727, 4.541064518000418104, -2.621784821874998173 ) ) ;
#13696=CARTESIAN_POINT ( 'NONE',  ( 17.85937500061451999, -4.541064518000417216, -2.621784821875001281 ) ) ;
#13698=CARTESIAN_POINT ( 'NONE',  ( 25.87500000000000000, 4.330127018922191873, 2.499999999999999556 ) ) ;
#13699=CARTESIAN_POINT ( 'NONE',  ( 27.98437500061451289, 4.541064518000418104, 2.621784821874999949 ) ) ;
#13700=DIRECTION ( 'NONE',  ( 0.000000000000000000, 0.000000000000000000, 1.000000000000000000 ) ) ;
#13701=CARTESIAN_POINT ( 'NONE',  ( 5.625000001229036428, 2.886751345948129099, -4.999999999999997335 ) ) ;
#13703=CARTESIAN_POINT ( 'NONE',  ( 7.912499999999999645, 2.886751345948126879, 4.999999999999999112 ) ) ;
#13705=CARTESIAN_POINT ( 'NONE',  ( 21.17812500061451431, 4.541064518000418104, 2.621784821874999949 ) ) ;
#13706=CARTESIAN_POINT ( 'NONE',  ( 11.58750000000000036, -2.886751345948129988, 4.999999999999997335 ) ) ;
#13707=CARTESIAN_POINT ( 'NONE',  ( 8.625000001229034652, -5.773502691896255534, -1.060575238724906372E-15 ) ) ;
#13708=CARTESIAN_POINT ( 'NONE',  ( 7.265625000614516438, 3.027376345333611329, 5.243569643749999010 ) ) ;
#13709=CARTESIAN_POINT ( 'NONE',  ( 22.80000000000000071, 0.000000000000000000, 4.999999999999998224 ) ) ;
#13710=EDGE_CURVE ( 'NONE', #67926, #55851, #17578, .T. ) ;
#13711=CARTESIAN_POINT ( 'NONE',  ( 21.70312500061451644, 0.000000000000000000, 5.243569643749999010 ) ) ;
#13713=CARTESIAN_POINT ( 'NONE',  ( 26.58750000122903145, -4.330127018922194537, 2.499999999999995559 ) ) ;
#13715=( BOUNDED_CURVE ( )  B_SPLINE_CURVE ( 2, ( #42411, #1805, #13222, #35398, #7330, #30227, #13956 ),
 .UNSPECIFIED., .F., .F. ) 
 B_SPLINE_CURVE_WITH_KNOTS ( ( 3, 2, 2, 3 ),
 ( 0.9939432722679919507, 0.9944444444444444642, 0.9972222222222222321, 0.9976655291192481068 ),
 .UNSPECIFIED. ) 
 CURVE ( )  GEOMETRIC_REPRESENTATION_ITEM ( )  RATIONAL_B_SPLINE_CURVE ( ( 0.9603783820186277964, 0.9758280376091080788, 1.000000000000000000, 0.8660254037844387076, 1.000000000000000000, 0.9786189294896985302, 0.9640622897159665250 ) ) 
 REPRESENTATION_ITEM ( '' )  );
#13716=CARTESIAN_POINT ( 'NONE',  ( 5.062500000000000888, 2.886751345948129099, -4.999999999999998224 ) ) ;
#13717=VERTEX_POINT ( 'NONE', #11205 ) ;
#13718=CARTESIAN_POINT ( 'NONE',  ( 19.37812500061451715, 4.541064518000418104, 2.621784821874999949 ) ) ;
#13719=CARTESIAN_POINT ( 'NONE',  ( 25.71562500061451573, 3.027376345333611329, 5.243569643749999010 ) ) ;
#13720=CARTESIAN_POINT ( 'NONE',  ( 27.75937500061451502, -4.541064518000417216, -2.621784821875001281 ) ) ;
#13721=CARTESIAN_POINT ( 'NONE',  ( 10.20000000000000107, 0.000000000000000000, 4.999999999999998224 ) ) ;
#13722=CARTESIAN_POINT ( 'NONE',  ( 13.75312500061451715, -4.541064518000417216, -2.621784821875001281 ) ) ;
#13723=CARTESIAN_POINT ( 'NONE',  ( 29.42812500061451431, -4.541064518000419881, 2.621784821874995952 ) ) ;
#13724=CARTESIAN_POINT ( 'NONE',  ( 8.878125000614515372, 6.421520780324663323E-16, -5.243569643749999010 ) ) ;
#13725=CARTESIAN_POINT ( 'NONE',  ( -4.243569643749999898, 10.31562500061459353, -32.45002607614398471 ) ) ;
#13726=CARTESIAN_POINT ( 'NONE',  ( 9.001249775931846008E-16, 12.32187500061451857, 34.90005215228797653 ) ) ;
#13727=CARTESIAN_POINT ( 'NONE',  ( 25.76250000122903216, -4.330127018922190985, -2.500000000000001332 ) ) ;
#13729=CARTESIAN_POINT ( 'NONE',  ( 16.86562500061451786, -6.054752690667223547, -1.112240025338166033E-15 ) ) ;
#13730=CARTESIAN_POINT ( 'NONE',  ( 4.000000000000000000, 18.38750000000000284, -27.69059892324149885 ) ) ;
#13731=CARTESIAN_POINT ( 'NONE',  ( 9.384375000614518569, 6.421520780324663323E-16, -5.243569643749999010 ) ) ;
#13732=CARTESIAN_POINT ( 'NONE',  ( 10.80937500061451928, 4.541064518000418104, -2.621784821874998173 ) ) ;
#13733=CARTESIAN_POINT ( 'NONE',  ( 17.78437500061451715, -4.541064518000419881, 2.621784821874995952 ) ) ;
#13734=ORIENTED_EDGE ( 'NONE', *, *, #15386, .T. ) ;
#13735=CARTESIAN_POINT ( 'NONE',  ( -4.518949595698570576, 8.925733855591197141, 33.96564934234342559 ) ) ;
#13736=CARTESIAN_POINT ( 'NONE',  ( 22.52812500061451573, 4.541064518000418104, 2.621784821874999949 ) ) ;
#13737=CARTESIAN_POINT ( 'NONE',  ( 15.38437500061451679, 4.541064518000418104, 2.621784821874999949 ) ) ;
#13738=CARTESIAN_POINT ( 'NONE',  ( 21.40312500061451573, -4.541064518000417216, -2.621784821875001281 ) ) ;
#13739=CARTESIAN_POINT ( 'NONE',  ( -3.999999999999999112, 13.70000000000000107, 30.00000000000000000 ) ) ;
#13740=CARTESIAN_POINT ( 'NONE',  ( 27.77812500061451573, 6.421520780324663323E-16, -5.243569643749999010 ) ) ;
#13741=CARTESIAN_POINT ( 'NONE',  ( 9.225000001229034297, 2.886751345948129099, -4.999999999999998224 ) ) ;
#13743=CARTESIAN_POINT ( 'NONE',  ( 4.350000001229033408, 5.773502691896255534, 3.535250795749688894E-16 ) ) ;
#13744=CARTESIAN_POINT ( 'NONE',  ( -3.999999999999997335, 18.68750000000000000, -27.69059892324149175 ) ) ;
#13745=VECTOR ( 'NONE', #71427, 1000.000000000000000 ) ;
#13746=CARTESIAN_POINT ( 'NONE',  ( 25.91250000122903074, 4.330127018922192761, -2.499999999999997780 ) ) ;
#13748=CARTESIAN_POINT ( 'NONE',  ( 6.271875000614517859, 3.027376345333613106, -5.243569643749998122 ) ) ;
#13749=CARTESIAN_POINT ( 'NONE',  ( 14.76562500061451821, 3.027376345333613106, -5.243569643749998122 ) ) ;
#13750=CARTESIAN_POINT ( 'NONE',  ( 9.196875000614518569, -3.027376345333614438, 5.243569643749998122 ) ) ;
#13751=CARTESIAN_POINT ( 'NONE',  ( 27.22500000122903430, 2.886751345948129099, -4.999999999999998224 ) ) ;
#13752=CARTESIAN_POINT ( 'NONE',  ( 17.93437500061451928, 6.421520780324663323E-16, -5.243569643749999010 ) ) ;
#13753=CARTESIAN_POINT ( 'NONE',  ( 4.734375000614518214, -4.541064518000419881, 2.621784821874995952 ) ) ;
#13755=CARTESIAN_POINT ( 'NONE',  ( 8.465625000614515727, 3.027376345333613106, -5.243569643749998122 ) ) ;
#13756=CARTESIAN_POINT ( 'NONE',  ( 16.97812500061451502, 6.421520780324663323E-16, -5.243569643749999010 ) ) ;
#13757=ORIENTED_EDGE ( 'NONE', *, *, #54130, .F. ) ;
#13758=CARTESIAN_POINT ( 'NONE',  ( 11.91562500061451857, -6.054752690667223547, -1.112240025338166033E-15 ) ) ;
#13759=VECTOR ( 'NONE', #44424, 1000.000000000000000 ) ;
#13760=CARTESIAN_POINT ( 'NONE',  ( 7.687500001229033764, -4.330127018922194537, 2.499999999999995559 ) ) ;
#13761=CARTESIAN_POINT ( 'NONE',  ( 11.57812500061451644, 6.421520780324663323E-16, -5.243569643749999010 ) ) ;
#13763=CARTESIAN_POINT ( 'NONE',  ( 10.83750000000000036, -2.886751345948125991, -5.000000000000000000 ) ) ;
#13764=CARTESIAN_POINT ( 'NONE',  ( 7.200000001229035718, -2.886751345948129988, 4.999999999999997335 ) ) ;
#13765=ADVANCED_FACE ( 'NONE', ( #33732 ), #50732, .F. ) ;
#13766=CARTESIAN_POINT ( 'NONE',  ( 14.40937500061451715, 4.541064518000418104, -2.621784821874998173 ) ) ;
#13767=CARTESIAN_POINT ( 'NONE',  ( 16.95000000122903216, 5.773502691896255534, 3.535250795749688894E-16 ) ) ;
#13769=CARTESIAN_POINT ( 'NONE',  ( 9.001249775931846008E-16, 19.46562500061451573, -25.09994784771203058 ) ) ;
#13770=DIRECTION ( 'NONE',  ( -1.000000000000000000, -0.000000000000000000, -0.000000000000000000 ) ) ;
#13771=CARTESIAN_POINT ( 'NONE',  ( -2.000000000000000000, 18.57500000000000284, 26.53589838486224650 ) ) ;
#13775=CARTESIAN_POINT ( 'NONE',  ( 16.24687500061451573, 6.054752690667223547, 3.707466751127219781E-16 ) ) ;
#13776=CARTESIAN_POINT ( 'NONE',  ( 28.31250000000000000, -5.773502691896255534, -1.060575238724906372E-15 ) ) ;
#13777=CARTESIAN_POINT ( 'NONE',  ( 13.90312500061451750, 4.541064518000418104, -2.621784821874998173 ) ) ;
#13779=CARTESIAN_POINT ( 'NONE',  ( 24.23437500061451644, 6.421520780324663323E-16, -5.243569643749999010 ) ) ;
#13781=CARTESIAN_POINT ( 'NONE',  ( 9.853125000614516793, 4.541064518000418104, -2.621784821874998173 ) ) ;
#13782=CARTESIAN_POINT ( 'NONE',  ( 14.48437500061451821, 4.541064518000418104, 2.621784821874999949 ) ) ;
#13784=CARTESIAN_POINT ( 'NONE',  ( 26.18437500061451573, 4.541064518000418104, 2.621784821874999949 ) ) ;
#13785=CARTESIAN_POINT ( 'NONE',  ( 28.19062500061451715, -3.027376345333610441, -5.243569643749999898 ) ) ;
#13786=CARTESIAN_POINT ( 'NONE',  ( 18.85312500061451502, 4.541064518000418104, -2.621784821874998173 ) ) ;
#13787=CARTESIAN_POINT ( 'NONE',  ( 1.071796769724491893, 13.04509619066137027, -26.00000000000000355 ) ) ;
#13788=EDGE_CURVE ( 'NONE', #57550, #18233, #1623, .T. ) ;
#13789=CARTESIAN_POINT ( 'NONE',  ( 4.859696611844813496, 1.176158510076063646, -5.109958294157806336 ) ) ;
#13790=VECTOR ( 'NONE', #39078, 1000.000000000000000 ) ;
#13791=CARTESIAN_POINT ( 'NONE',  ( 7.575000000000001954, -4.330127018922194537, 2.499999999999995559 ) ) ;
#13792=VECTOR ( 'NONE', #55884, 1000.000000000000000 ) ;
#13793=CARTESIAN_POINT ( 'NONE',  ( 19.20000000122903572, 5.773502691896255534, 3.535250795749688894E-16 ) ) ;
#13794=CARTESIAN_POINT ( 'NONE',  ( 23.13750000122903216, 6.123233995736764310E-16, -4.999999999999998224 ) ) ;
#13796=ORIENTED_EDGE ( 'NONE', *, *, #69469, .F. ) ;
#13797=CARTESIAN_POINT ( 'NONE',  ( 17.47499999999999787, -4.330127018922194537, 2.499999999999995559 ) ) ;
#13798=CARTESIAN_POINT ( 'NONE',  ( 18.63749999999999929, 5.773502691896255534, 3.535250795749688894E-16 ) ) ;
#13799=CARTESIAN_POINT ( 'NONE',  ( 20.10937500061451289, -4.541064518000417216, -2.621784821875001281 ) ) ;
#13800=CARTESIAN_POINT ( 'NONE',  ( 14.65312500061451573, -4.541064518000417216, -2.621784821875001281 ) ) ;
#13801=VERTEX_POINT ( 'NONE', #41807 ) ;
#13803=CARTESIAN_POINT ( 'NONE',  ( 6.103125000614515905, -4.541064518000417216, -2.621784821875001281 ) ) ;
#13805=CARTESIAN_POINT ( 'NONE',  ( 11.84999999999999964, 4.330127018922192761, -2.499999999999997780 ) ) ;
#13807=CARTESIAN_POINT ( 'NONE',  ( 2.121784821874999061, 14.70312500061451644, 26.32496088578401583 ) ) ;
#13808=CARTESIAN_POINT ( 'NONE',  ( 27.32812500061451644, 6.421520780324663323E-16, -5.243569643749999010 ) ) ;
#13811=CARTESIAN_POINT ( 'NONE',  ( 24.79687500061451999, 6.054752690667223547, 3.707466751127219781E-16 ) ) ;
#13812=ORIENTED_EDGE ( 'NONE', *, *, #12071, .F. ) ;
#13813=CARTESIAN_POINT ( 'NONE',  ( 20.76562500061451644, 3.027376345333611329, 5.243569643749999010 ) ) ;
#13814=CARTESIAN_POINT ( 'NONE',  ( 4.243569643749999010, 16.91562500061459318, -32.45002607614398471 ) ) ;
#13815=CARTESIAN_POINT ( 'NONE',  ( 7.603125000614517681, 4.541064518000418104, -2.621784821874998173 ) ) ;
#13817=CARTESIAN_POINT ( 'NONE',  ( 23.65312500061451573, -4.541064518000417216, -2.621784821875001281 ) ) ;
#13820=CARTESIAN_POINT ( 'NONE',  ( 16.39687500061451786, -3.027376345333614438, 5.243569643749998122 ) ) ;
#13821=CARTESIAN_POINT ( 'NONE',  ( 24.98437500061451644, -4.541064518000419881, 2.621784821874995952 ) ) ;
#13822=CARTESIAN_POINT ( 'NONE',  ( -2.121784821874999949, 15.28437500061451892, 26.32496088578401938 ) ) ;
#13823=CARTESIAN_POINT ( 'NONE',  ( 4.903125000614516615, 4.541064518000418104, -2.621784821874998173 ) ) ;
#13824=CARTESIAN_POINT ( 'NONE',  ( 29.24062500061451431, 6.054752690667223547, 3.707466751127219781E-16 ) ) ;
#13825=CARTESIAN_POINT ( 'NONE',  ( 2.971875000614517592, -6.054752690667223547, -1.112240025338166033E-15 ) ) ;
#13826=CARTESIAN_POINT ( 'NONE',  ( 4.275000000000001243, 4.330127018922191873, 2.499999999999999556 ) ) ;
#13827=CARTESIAN_POINT ( 'NONE',  ( 5.728125000614515905, 6.421520780324663323E-16, -5.243569643749999010 ) ) ;
#13828=CARTESIAN_POINT ( 'NONE',  ( 8.446875000614518569, -3.027376345333610441, -5.243569643749999898 ) ) ;
#13830=CARTESIAN_POINT ( 'NONE',  ( 17.51250000122903216, 0.000000000000000000, 4.999999999999998224 ) ) ;
#13831=CARTESIAN_POINT ( 'NONE',  ( 29.39062500061451289, -3.027376345333614438, 5.243569643749998122 ) ) ;
#13832=CARTESIAN_POINT ( 'NONE',  ( 5.578125000614518214, -4.541064518000419881, 2.621784821874995952 ) ) ;
#13835=CARTESIAN_POINT ( 'NONE',  ( 14.44687500061451679, 6.054752690667223547, 3.707466751127219781E-16 ) ) ;
#13836=CARTESIAN_POINT ( 'NONE',  ( 3.999999999999999112, 17.63750000122903572, 30.00000000000000000 ) ) ;
#13838=CARTESIAN_POINT ( 'NONE',  ( 22.19062500061451715, -3.027376345333614438, 5.243569643749998122 ) ) ;
#13839=CARTESIAN_POINT ( 'NONE',  ( 8.465625000614515727, 3.027376345333613106, -5.243569643749998122 ) ) ;
#13840=CARTESIAN_POINT ( 'NONE',  ( 23.59687500061451715, -3.027376345333614438, 5.243569643749998122 ) ) ;
#13841=CARTESIAN_POINT ( 'NONE',  ( 8.540625000614518569, 6.054752690667223547, 3.707466751127219781E-16 ) ) ;
#13843=CARTESIAN_POINT ( 'NONE',  ( 10.65000000122903323, 5.773502691896255534, 3.535250795749688894E-16 ) ) ;
#13844=CARTESIAN_POINT ( 'NONE',  ( 25.11562500061451431, 3.027376345333613106, -5.243569643749998122 ) ) ;
#13845=CARTESIAN_POINT ( 'NONE',  ( -3.999999999999999112, 19.66250000122903430, -30.00000000000000000 ) ) ;
#13846=CARTESIAN_POINT ( 'NONE',  ( 10.31250000122903288, 0.000000000000000000, 4.999999999999998224 ) ) ;
#13847=CARTESIAN_POINT ( 'NONE',  ( 21.32812500061451644, -4.541064518000419881, 2.621784821874995952 ) ) ;
#13848=CARTESIAN_POINT ( 'NONE',  ( 18.17812500061451786, -4.541064518000419881, 2.621784821874995952 ) ) ;
#13849=CARTESIAN_POINT ( 'NONE',  ( 5.859375000614519102, 4.541064518000418104, -2.621784821874998173 ) ) ;
#13850=CARTESIAN_POINT ( 'NONE',  ( 18.26249999999999929, 2.886751345948126879, 4.999999999999999112 ) ) ;
#13851=CARTESIAN_POINT ( 'NONE',  ( 13.50000000122903288, -2.886751345948129988, 4.999999999999997335 ) ) ;
#13852=CARTESIAN_POINT ( 'NONE',  ( 11.09062500061451573, -3.027376345333610441, -5.243569643749999898 ) ) ;
#13853=CARTESIAN_POINT ( 'NONE',  ( 13.37812500061451715, 6.421520780324663323E-16, -5.243569643749999010 ) ) ;
#13854=EDGE_CURVE ( 'NONE', #4424, #6811, #19252, .T. ) ;
#13855=CARTESIAN_POINT ( 'NONE',  ( 23.85000000122903430, -2.886751345948129988, 4.999999999999997335 ) ) ;
#13856=CARTESIAN_POINT ( 'NONE',  ( 21.83437500061451786, -4.541064518000419881, 2.621784821874995952 ) ) ;
#13857=CARTESIAN_POINT ( 'NONE',  ( 20.67187500061451289, 3.027376345333613106, -5.243569643749998122 ) ) ;
#13860=CARTESIAN_POINT ( 'NONE',  ( 7.762500001229033053, -4.330127018922190985, -2.500000000000001332 ) ) ;
#13861=CARTESIAN_POINT ( 'NONE',  ( 5.409375000614516260, 4.541064518000418104, -2.621784821874998173 ) ) ;
#13862=CARTESIAN_POINT ( 'NONE',  ( 23.89687500061451786, 6.054752690667223547, 3.707466751127219781E-16 ) ) ;
#13864=CARTESIAN_POINT ( 'NONE',  ( 4.818692141996693046, -1.334243621178544226, 4.818692141997074074 ) ) ;
#13865=CARTESIAN_POINT ( 'NONE',  ( 21.47812500061451502, 6.421520780324663323E-16, -5.243569643749999010 ) ) ;
#13866=CARTESIAN_POINT ( 'NONE',  ( 24.30937500061451573, 4.541064518000418104, -2.621784821874998173 ) ) ;
#13868=CARTESIAN_POINT ( 'NONE',  ( 12.37500000122903110, 2.886751345948062486, -5.000000000000113687 ) ) ;
#13870=CARTESIAN_POINT ( 'NONE',  ( 6.496875000614517504, -3.027376345333614438, 5.243569643749998122 ) ) ;
#13871=CARTESIAN_POINT ( 'NONE',  ( 16.49062500061451786, -3.027376345333610441, -5.243569643749999898 ) ) ;
#13872=ORIENTED_EDGE ( 'NONE', *, *, #45678, .T. ) ;
#13873=CARTESIAN_POINT ( 'NONE',  ( 11.55000000000000071, 0.000000000000000000, 4.999999999999998224 ) ) ;
#13874=CARTESIAN_POINT ( 'NONE',  ( 25.00312500061451715, -4.541064518000417216, -2.621784821875001281 ) ) ;
#13875=CARTESIAN_POINT ( 'NONE',  ( 2.859375000614519546, 0.000000000000000000, 5.243569643749999010 ) ) ;
#13877=CARTESIAN_POINT ( 'NONE',  ( 3.662307474140069186, 3.404096216171143219, -3.815575040102499482 ) ) ;
#13878=CARTESIAN_POINT ( 'NONE',  ( 15.63749999999999751, -2.886751345948129988, 4.999999999999997335 ) ) ;
#13879=CARTESIAN_POINT ( 'NONE',  ( 21.81562500061451004, -6.054752690667223547, -1.112240025338166033E-15 ) ) ;
#13881=CARTESIAN_POINT ( 'NONE',  ( 25.27499999999999858, 6.123233995736764310E-16, -4.999999999999998224 ) ) ;
#13882=CARTESIAN_POINT ( 'NONE',  ( 25.77187500061451075, 3.027376345333611329, 5.243569643749999010 ) ) ;
#13883=VERTEX_POINT ( 'NONE', #60160 ) ;
#13885=CARTESIAN_POINT ( 'NONE',  ( 12.66562500061451502, 3.027376345333611329, 5.243569643749999010 ) ) ;
#13886=CARTESIAN_POINT ( 'NONE',  ( 2.878125000614517592, -4.541064518000419881, 2.621784821874995952 ) ) ;
#13888=CARTESIAN_POINT ( 'NONE',  ( 29.69062500061451715, 6.054752690667223547, 3.707466751127219781E-16 ) ) ;
#13889=CARTESIAN_POINT ( 'NONE',  ( 12.22500000122903430, -5.773502691896255534, -1.060575238724906372E-15 ) ) ;
#13890=CARTESIAN_POINT ( 'NONE',  ( 20.47500000000000142, 4.330127018922191873, 2.499999999999999556 ) ) ;
#13891=CARTESIAN_POINT ( 'NONE',  ( 26.58750000000000213, -2.886751345948125991, -5.000000000000000000 ) ) ;
#13893=CARTESIAN_POINT ( 'NONE',  ( 6.046875000614519102, -3.027376345333614438, 5.243569643749998122 ) ) ;
#13894=CARTESIAN_POINT ( 'NONE',  ( 18.30937500061451928, -4.541064518000417216, -2.621784821875001281 ) ) ;
#13895=CARTESIAN_POINT ( 'NONE',  ( 1.071796769724476572, 11.24509619066136779, 34.00000000000000000 ) ) ;
#13896=ORIENTED_EDGE ( 'NONE', *, *, #25145, .T. ) ;
#13897=CARTESIAN_POINT ( 'NONE',  ( 29.09062500061451573, -3.027376345333610441, -5.243569643749999898 ) ) ;
#13898=CARTESIAN_POINT ( 'NONE',  ( 29.29687500061451644, 6.054752690667223547, 3.707466751127219781E-16 ) ) ;
#13899=CARTESIAN_POINT ( 'NONE',  ( 5.296875000614518214, -3.027376345333610441, -5.243569643749999898 ) ) ;
#13900=EDGE_CURVE ( 'NONE', #37056, #29389, #52540, .T. ) ;
#13901=CARTESIAN_POINT ( 'NONE',  ( 16.91250000000000142, 2.886751345948126879, 4.999999999999999112 ) ) ;
#13902=CARTESIAN_POINT ( 'NONE',  ( 12.74062500061451786, -3.027376345333614438, 5.243569643749998122 ) ) ;
#13903=CYLINDRICAL_SURFACE ( 'NONE', #9827, 4.000000000000000000 ) ;
#13904=CARTESIAN_POINT ( 'NONE',  ( 4.898587196589411843E-16, 20.00000000000000000, 33.99999999999999289 ) ) ;
#13906=CARTESIAN_POINT ( 'NONE',  ( 17.77500000122903145, 2.886751345948129099, -4.999999999999998224 ) ) ;
#13909=CARTESIAN_POINT ( 'NONE',  ( 7.265625000614516438, 3.027376345333611329, 5.243569643749999010 ) ) ;
#13910=CARTESIAN_POINT ( 'NONE',  ( 23.70937500061451786, -4.541064518000417216, -2.621784821875001281 ) ) ;
#13911=CARTESIAN_POINT ( 'NONE',  ( -2.121784821874999949, 18.88437500061451857, 26.32496088578401938 ) ) ;
#13912=CARTESIAN_POINT ( 'NONE',  ( 25.13437500061451502, 6.421520780324663323E-16, -5.243569643749999010 ) ) ;
#13913=CARTESIAN_POINT ( 'NONE',  ( 5.250000000000000888, 0.000000000000000000, 4.999999999999998224 ) ) ;
#13914=CARTESIAN_POINT ( 'NONE',  ( -3.999999999999999112, 11.56250000122903465, 30.00000000000000000 ) ) ;
#13915=CARTESIAN_POINT ( 'NONE',  ( 14.46562500061451750, 3.027376345333611329, 5.243569643749999010 ) ) ;
#13916=CARTESIAN_POINT ( 'NONE',  ( 4.200000001229033053, -2.886751345948125991, -5.000000000000000000 ) ) ;
#13917=( BOUNDED_CURVE ( )  B_SPLINE_CURVE ( 2, ( #29680, #52216, #900, #11252, #40779, #51855, #1619 ),
 .UNSPECIFIED., .F., .F. ) 
 B_SPLINE_CURVE_WITH_KNOTS ( ( 3, 2, 2, 3 ),
 ( 0.9857515426466298969, 0.9861111111111111605, 0.9888888888888889284, 0.9891869394448051800 ),
 .UNSPECIFIED. ) 
 CURVE ( )  GEOMETRIC_REPRESENTATION_ITEM ( )  RATIONAL_B_SPLINE_CURVE ( ( 0.9698051456607861276, 0.9826577056573390090, 1.000000000000000000, 0.8660254037844387076, 1.000000000000000000, 0.9856247669629467634, 0.9743344071885395863 ) ) 
 REPRESENTATION_ITEM ( '' )  );
#13918=CARTESIAN_POINT ( 'NONE',  ( 9.984375000614518214, 4.541064518000418104, 2.621784821874999949 ) ) ;
#13919=CARTESIAN_POINT ( 'NONE',  ( 1.071796769724484344, 14.84509619066137098, 34.00000000000000000 ) ) ;
#13921=CARTESIAN_POINT ( 'NONE',  ( 13.41562500061451502, 3.027376345333613106, -5.243569643749998122 ) ) ;
#13922=CARTESIAN_POINT ( 'NONE',  ( 3.445179128855461848, -3.623644852411430417, -3.790023247856260102 ) ) ;
#13923=CARTESIAN_POINT ( 'NONE',  ( 23.17500000122903359, 2.886751345948129099, -4.999999999999998224 ) ) ;
#13924=CARTESIAN_POINT ( 'NONE',  ( 11.07187500061451679, -6.054752690667223547, -1.112240025338166033E-15 ) ) ;
#13925=CARTESIAN_POINT ( 'NONE',  ( 13.34062500061451750, -3.027376345333610441, -5.243569643749999898 ) ) ;
#13927=CARTESIAN_POINT ( 'NONE',  ( 24.34687500061451715, 6.054752690667223547, 3.707466751127219781E-16 ) ) ;
#13929=CARTESIAN_POINT ( 'NONE',  ( 30.00000000000000000, 0.000000000000000000, 0.000000000000000000 ) ) ;
#13931=CARTESIAN_POINT ( 'NONE',  ( 4.243569643749999898, 13.74687500061451750, -27.54997392385601529 ) ) ;
#13932=CARTESIAN_POINT ( 'NONE',  ( 16.88437500061451502, -4.541064518000419881, 2.621784821874995952 ) ) ;
#13933=CARTESIAN_POINT ( 'NONE',  ( 16.76250000122903216, -4.330127018922190985, -2.500000000000001332 ) ) ;
#13934=CARTESIAN_POINT ( 'NONE',  ( 11.78437500061451892, 4.541064518000418104, 2.621784821874999949 ) ) ;
#13935=CARTESIAN_POINT ( 'NONE',  ( -2.121784821874999949, 18.82812500061451644, -33.67503911421598417 ) ) ;
#13936=CARTESIAN_POINT ( 'NONE',  ( 19.65000000122902790, 5.773502691896255534, 3.535250795749688894E-16 ) ) ;
#13937=CARTESIAN_POINT ( 'NONE',  ( 13.49062500061451608, 6.054752690667223547, 3.707466751127219781E-16 ) ) ;
#13938=VERTEX_POINT ( 'NONE', #53256 ) ;
#13940=CARTESIAN_POINT ( 'NONE',  ( 14.58750000000000036, 5.773502691896255534, 3.535250795749688894E-16 ) ) ;
#13941=CARTESIAN_POINT ( 'NONE',  ( 18.00000000000000355, -4.330127018922190985, -2.500000000000001332 ) ) ;
#13942=CARTESIAN_POINT ( 'NONE',  ( 13.17187500061451821, 3.027376345333611329, 5.243569643749999010 ) ) ;
#13943=CARTESIAN_POINT ( 'NONE',  ( 12.82500000122903394, 2.886751345948129099, -4.999999999999998224 ) ) ;
#13944=CARTESIAN_POINT ( 'NONE',  ( 19.98750000122903359, 6.123233995736764310E-16, -4.999999999999998224 ) ) ;
#13945=CARTESIAN_POINT ( 'NONE',  ( 17.12812500061451715, 4.541064518000418104, 2.621784821874999949 ) ) ;
#13946=CARTESIAN_POINT ( 'NONE',  ( 19.79062500061451502, 6.054752690667223547, 3.707466751127219781E-16 ) ) ;
#13947=CARTESIAN_POINT ( 'NONE',  ( 27.75000000122903288, 5.773502691896255534, 3.535250795749688894E-16 ) ) ;
#13948=CARTESIAN_POINT ( 'NONE',  ( 25.31250000000000000, 2.886751345948129099, -4.999999999999998224 ) ) ;
#13951=CARTESIAN_POINT ( 'NONE',  ( 28.80937500061451573, 4.541064518000418104, -2.621784821874998173 ) ) ;
#13952=CARTESIAN_POINT ( 'NONE',  ( -2.121784821874996840, 14.08437500061451786, -26.32496088578401583 ) ) ;
#13953=CARTESIAN_POINT ( 'NONE',  ( 3.562500001229033764, 0.000000000000000000, 4.999999999999998224 ) ) ;
#13954=CARTESIAN_POINT ( 'NONE',  ( 4.800000000000002487, 0.000000000000000000, 4.999999999999998224 ) ) ;
#13955=EDGE_CURVE ( 'NONE', #11866, #20886, #32695, .T. ) ;
#13956=CARTESIAN_POINT ( 'NONE',  ( 2.923357432354301455, -4.056350739605543154, 3.322806236625610588 ) ) ;
#13957=CARTESIAN_POINT ( 'NONE',  ( 7.696875000614516793, 6.054752690667223547, 3.707466751127219781E-16 ) ) ;
#13958=CARTESIAN_POINT ( 'NONE',  ( 29.09062500061451573, -3.027376345333610441, -5.243569643749999898 ) ) ;
#13959=CARTESIAN_POINT ( 'NONE',  ( 3.242103837493086330E-14, 13.13749999999999929, -34.00000000000000000 ) ) ;
#13960=CARTESIAN_POINT ( 'NONE',  ( -5.810221930991193690E-16, 18.98750000000000071, -34.00000000000000000 ) ) ;
#13961=CARTESIAN_POINT ( 'NONE',  ( 16.87500000122902932, 2.886751345948095793, -5.000000000000055067 ) ) ;
#13962=CARTESIAN_POINT ( 'NONE',  ( 6.196875000614515905, -3.027376345333610441, -5.243569643749999898 ) ) ;
#13963=CARTESIAN_POINT ( 'NONE',  ( 10.47187500061451715, 3.027376345333611329, 5.243569643749999010 ) ) ;
#13964=CARTESIAN_POINT ( 'NONE',  ( 4.387500000000002842, -2.886751345948129988, 4.999999999999997335 ) ) ;
#13965=CARTESIAN_POINT ( 'NONE',  ( 9.001249775931846008E-16, 14.51562500061459460, 34.90005215228797653 ) ) ;
#13967=CARTESIAN_POINT ( 'NONE',  ( 7.162500000000001421, -5.773502691896255534, -1.060575238724906372E-15 ) ) ;
#13969=CARTESIAN_POINT ( 'NONE',  ( 20.54062500061451502, -3.027376345333610441, -5.243569643749999898 ) ) ;
#13970=CARTESIAN_POINT ( 'NONE',  ( 12.10312500061451857, 4.541064518000418104, -2.621784821874998173 ) ) ;
#13972=CARTESIAN_POINT ( 'NONE',  ( 9.871875000614517504, 3.027376345333613106, -5.243569643749998122 ) ) ;
#13973=CARTESIAN_POINT ( 'NONE',  ( 27.37500000000000000, -4.330127018922194537, 2.499999999999995559 ) ) ;
#13974=CARTESIAN_POINT ( 'NONE',  ( 23.02500000122903145, -5.773502691896255534, -1.060575238724906372E-15 ) ) ;
#13976=CARTESIAN_POINT ( 'NONE',  ( 10.43437500061451750, 4.541064518000418104, 2.621784821874999949 ) ) ;
#13977=CARTESIAN_POINT ( 'NONE',  ( 26.97187500061451360, 3.027376345333613106, -5.243569643749998122 ) ) ;
#13978=CARTESIAN_POINT ( 'NONE',  ( 1.999999999999998668, 18.16250000122903074, -33.46410161513775705 ) ) ;
#13980=CARTESIAN_POINT ( 'NONE',  ( 20.78437500061451715, 4.541064518000418104, 2.621784821874999949 ) ) ;
#13981=CARTESIAN_POINT ( 'NONE',  ( 12.79687500061451821, -3.027376345333614438, 5.243569643749998122 ) ) ;
#13983=CARTESIAN_POINT ( 'NONE',  ( 23.13749999999999929, 5.773502691896255534, 3.535250795749688894E-16 ) ) ;
#13985=CARTESIAN_POINT ( 'NONE',  ( 2.121784821874999061, 12.50937500061451857, -33.67503911421598417 ) ) ;
#13987=CARTESIAN_POINT ( 'NONE',  ( 15.06562500061451537, -6.054752690667223547, -1.112240025338166033E-15 ) ) ;
#13988=CARTESIAN_POINT ( 'NONE',  ( 3.675000000000001155, 6.123233995736764310E-16, -4.999999999999998224 ) ) ;
#13990=CARTESIAN_POINT ( 'NONE',  ( 22.12500000000000000, 6.123233995736764310E-16, -4.999999999999998224 ) ) ;
#13991=CARTESIAN_POINT ( 'NONE',  ( 13.35000000000000142, 0.000000000000000000, 4.999999999999998224 ) ) ;
#13992=CARTESIAN_POINT ( 'NONE',  ( 3.999999999999998668, 18.57500000122903216, 27.69059892324149175 ) ) ;
#13993=CARTESIAN_POINT ( 'NONE',  ( 13.27500000122903323, 2.886751345948129099, -4.999999999999998224 ) ) ;
#13994=CARTESIAN_POINT ( 'NONE',  ( 25.02187500061451431, -6.054752690667223547, -1.112240025338166033E-15 ) ) ;
#13995=CARTESIAN_POINT ( 'NONE',  ( 16.02187500061451786, -6.054752690667223547, -1.112240025338166033E-15 ) ) ;
#13997=EDGE_LOOP ( 'NONE', ( #18737, #39216, #63461, #1004 ) ) ;
#13998=CARTESIAN_POINT ( 'NONE',  ( 19.67812500061451786, 6.421520780324663323E-16, -5.243569643749999010 ) ) ;
#13999=CARTESIAN_POINT ( 'NONE',  ( 4.828125000614518214, 6.421520780324663323E-16, -5.243569643749999010 ) ) ;
#14000=CARTESIAN_POINT ( 'NONE',  ( 18.19687500061451502, -3.027376345333614438, 5.243569643749998122 ) ) ;
#14001=CARTESIAN_POINT ( 'NONE',  ( 29.63437500061451502, 6.421520780324663323E-16, -5.243569643749999010 ) ) ;
#14002=CARTESIAN_POINT ( 'NONE',  ( 5.053125000614517859, 0.000000000000000000, 5.243569643749999010 ) ) ;
#14003=CARTESIAN_POINT ( 'NONE',  ( 21.32812500061451644, -4.541064518000419881, 2.621784821874995952 ) ) ;
#14004=EDGE_CURVE ( 'NONE', #6203, #20497, #24684, .T. ) ;
#14005=CARTESIAN_POINT ( 'NONE',  ( -2.121784821874996840, 14.92812500061451608, 33.67503911421598417 ) ) ;
#14006=CARTESIAN_POINT ( 'NONE',  ( 15.52500000122903323, 2.886751345948129099, -4.999999999999998224 ) ) ;
#14008=CARTESIAN_POINT ( 'NONE',  ( 7.565625000614518036, 3.027376345333612662, -5.243569643749998122 ) ) ;
#14009=CARTESIAN_POINT ( 'NONE',  ( 3.946875000614517681, -3.027376345333610441, -5.243569643749999898 ) ) ;
#14010=CARTESIAN_POINT ( 'NONE',  ( 28.60312500061451502, -4.541064518000417216, -2.621784821875001281 ) ) ;
#14011=CARTESIAN_POINT ( 'NONE',  ( 22.77187500061451786, -6.054752690667223547, -1.112240025338166033E-15 ) ) ;
#14012=CARTESIAN_POINT ( 'NONE',  ( 14.42812500061451786, 4.541064518000418104, 2.621784821874999949 ) ) ;
#14013=CARTESIAN_POINT ( 'NONE',  ( 24.67500000122903359, 2.886751345948126879, 4.999999999999999112 ) ) ;
#14014=CARTESIAN_POINT ( 'NONE',  ( 24.29062500061451502, 6.054752690667223547, 3.707466751127219781E-16 ) ) ;
#14015=CARTESIAN_POINT ( 'NONE',  ( 20.29687500061451644, 6.054752690667223547, 3.707466751127219781E-16 ) ) ;
#14016=CARTESIAN_POINT ( 'NONE',  ( 15.77812500061451573, 4.541064518000418104, 2.621784821874999949 ) ) ;
#14017=CARTESIAN_POINT ( 'NONE',  ( 4.243569643749999898, 13.74687500061451750, 32.45002607614398471 ) ) ;
#14018=CARTESIAN_POINT ( 'NONE',  ( 19.79062500061451502, 6.054752690667223547, 3.707466751127219781E-16 ) ) ;
#14019=CARTESIAN_POINT ( 'NONE',  ( 29.01562500061451644, -6.054752690667223547, -1.112240025338166033E-15 ) ) ;
#14020=ORIENTED_EDGE ( 'NONE', *, *, #68767, .F. ) ;
#14021=CARTESIAN_POINT ( 'NONE',  ( 22.64999999999999858, 4.330127018922192761, -2.499999999999997780 ) ) ;
#14022=CARTESIAN_POINT ( 'NONE',  ( -3.999999999999999556, 10.06250000000000178, -32.30940107675850470 ) ) ;
#14024=CARTESIAN_POINT ( 'NONE',  ( 26.35312500061451857, -4.541064518000417216, -2.621784821875001281 ) ) ;
#14025=CARTESIAN_POINT ( 'NONE',  ( 7.940625000614518036, -3.027376345333610441, -5.243569643749999898 ) ) ;
#14026=CARTESIAN_POINT ( 'NONE',  ( 19.83750000122903145, -4.330127018922194537, 2.499999999999995559 ) ) ;
#14027=CARTESIAN_POINT ( 'NONE',  ( 23.65312500061451573, -4.541064518000417216, -2.621784821875001281 ) ) ;
#14028=CARTESIAN_POINT ( 'NONE',  ( 25.80000000000000071, 4.330127018922192761, -2.499999999999997780 ) ) ;
#14029=CARTESIAN_POINT ( 'NONE',  ( 28.82812500061451644, 4.541064518000418104, 2.621784821874999949 ) ) ;
#14030=CARTESIAN_POINT ( 'NONE',  ( 9.103125000614515017, 0.000000000000000000, 5.243569643749999010 ) ) ;
#14032=CARTESIAN_POINT ( 'NONE',  ( 26.87812500061451360, 6.421520780324663323E-16, -5.243569643749999010 ) ) ;
#14033=CARTESIAN_POINT ( 'NONE',  ( 5.315625000614516260, 3.027376345333613106, -5.243569643749998122 ) ) ;
#14035=CARTESIAN_POINT ( 'NONE',  ( 3.328125000614516438, -4.541064518000419881, 2.621784821874995952 ) ) ;
#14036=DIRECTION ( 'NONE',  ( 1.000000000000000000, 0.000000000000000000, -0.000000000000000000 ) ) ;
#14037=CARTESIAN_POINT ( 'NONE',  ( 13.04999999999999893, -4.330127018922190985, -2.500000000000001332 ) ) ;
#14039=CARTESIAN_POINT ( 'NONE',  ( 12.94687500061451857, -3.027376345333610441, -5.243569643749999898 ) ) ;
#14040=CARTESIAN_POINT ( 'NONE',  ( 9.225000001229034297, 2.886751345948129099, -4.999999999999998224 ) ) ;
#14041=CARTESIAN_POINT ( 'NONE',  ( 16.20937500061451786, 4.541064518000418104, -2.621784821874998173 ) ) ;
#14043=CARTESIAN_POINT ( 'NONE',  ( 8.596875000614518925, 6.054752690667223547, 3.707466751127219781E-16 ) ) ;
#14044=CARTESIAN_POINT ( 'NONE',  ( -3.000416591977282496E-16, 11.14062500061451644, -34.90005215228797653 ) ) ;
#14048=CARTESIAN_POINT ( 'NONE',  ( 22.11562500061451786, 3.027376345333611329, 5.243569643749999010 ) ) ;
#14049=CARTESIAN_POINT ( 'NONE',  ( -4.243569643749999898, 9.959375000614517859, 30.00000000000000000 ) ) ;
#14050=CARTESIAN_POINT ( 'NONE',  ( 26.74687500061451573, -3.027376345333614438, 5.243569643749998122 ) ) ;
#14051=( BOUNDED_CURVE ( )  B_SPLINE_CURVE ( 2, ( #31574, #54113, #7575, #7940, #19367, #30478, #47465 ),
 .UNSPECIFIED., .F., .F. ) 
 B_SPLINE_CURVE_WITH_KNOTS ( ( 3, 2, 2, 3 ),
 ( 0.3500000000000000333, 0.3527777777777778567, 0.3555555555555556246, 0.3583333333333333925 ),
 .UNSPECIFIED. ) 
 CURVE ( )  GEOMETRIC_REPRESENTATION_ITEM ( )  RATIONAL_B_SPLINE_CURVE ( ( 0.9999999999999973355, 0.8660254037844413721, 1.000000000000000000, 0.8660254037844387076, 1.000000000000000000, 0.8660254037844360431, 1.000000000000002665 ) ) 
 REPRESENTATION_ITEM ( '' )  );
#14052=CARTESIAN_POINT ( 'NONE',  ( 28.35937500061451289, 4.541064518000418104, -2.621784821874998173 ) ) ;
#14053=CARTESIAN_POINT ( 'NONE',  ( 3.440625000614518036, -3.027376345333610441, -5.243569643749999898 ) ) ;
#14054=B_SPLINE_CURVE_WITH_KNOTS ( 'NONE', 3,
 ( #46025, #68919, #969, #6861, #67837, #57810, #51205, #5777, #17210, #40850 ),
 .UNSPECIFIED., .F., .F.,
 ( 4, 3, 3, 4 ),
 ( 4.336808689942017736E-19, 8.679785101976316634E-05, 0.0002172003593263750992, 0.0003478061572614656602 ),
 .UNSPECIFIED. ) ;
#14056=CARTESIAN_POINT ( 'NONE',  ( 15.94687500061451502, -3.027376345333614438, 5.243569643749998122 ) ) ;
#14058=CARTESIAN_POINT ( 'NONE',  ( 28.76250000122903216, 0.000000000000000000, 4.999999999999998224 ) ) ;
#14059=CARTESIAN_POINT ( 'NONE',  ( 6.871875000614517504, 3.027376345333611329, 5.243569643749999010 ) ) ;
#14060=CARTESIAN_POINT ( 'NONE',  ( 17.63437500061451502, 4.541064518000418104, 2.621784821874999949 ) ) ;
#14062=CARTESIAN_POINT ( 'NONE',  ( 25.64999999999999858, -4.330127018922190985, -2.500000000000001332 ) ) ;
#14063=CARTESIAN_POINT ( 'NONE',  ( 27.30937500061451573, -4.541064518000417216, -2.621784821875001281 ) ) ;
#14065=CARTESIAN_POINT ( 'NONE',  ( 29.55000000000000071, 0.000000000000000000, 4.999999999999998224 ) ) ;
#14067=CARTESIAN_POINT ( 'NONE',  ( 7.950000000000001954, 0.000000000000000000, 4.999999999999998224 ) ) ;
#14069=CARTESIAN_POINT ( 'NONE',  ( 22.52812500061451573, 4.541064518000418104, 2.621784821874999949 ) ) ;
#14070=CARTESIAN_POINT ( 'NONE',  ( 12.48750000000000249, -2.886751345948129988, 4.999999999999997335 ) ) ;
#14071=CARTESIAN_POINT ( 'NONE',  ( 7.612500001229035362, 0.000000000000000000, 4.999999999999998224 ) ) ;
#14072=CARTESIAN_POINT ( 'NONE',  ( 7.303125000614516082, 0.000000000000000000, 5.243569643749999010 ) ) ;
#14073=CARTESIAN_POINT ( 'NONE',  ( 22.23750000000000071, 5.773502691896255534, 3.535250795749688894E-16 ) ) ;
#14074=CARTESIAN_POINT ( 'NONE',  ( 18.89062500061451644, 6.054752690667223547, 3.707466751127219781E-16 ) ) ;
#14075=CARTESIAN_POINT ( 'NONE',  ( 4.133006999854208274, -2.814071958334764201, 4.297262197382941906 ) ) ;
#14076=CARTESIAN_POINT ( 'NONE',  ( 26.21250000122903501, -4.330127018922190985, -2.500000000000001332 ) ) ;
#14077=CARTESIAN_POINT ( 'NONE',  ( 5.662500000000000533, 2.886751345948126879, 4.999999999999999112 ) ) ;
#14078=VERTEX_POINT ( 'NONE', #44666 ) ;
#14079=CARTESIAN_POINT ( 'NONE',  ( 19.07812500061451644, -4.541064518000419881, 2.621784821874995952 ) ) ;
#14080=CARTESIAN_POINT ( 'NONE',  ( 26.61562500061451786, 3.027376345333611329, 5.243569643749999010 ) ) ;
#14081=CARTESIAN_POINT ( 'NONE',  ( 25.09687500061451715, -3.027376345333610441, -5.243569643749999898 ) ) ;
#14082=CARTESIAN_POINT ( 'NONE',  ( 8.737500000000002487, 5.773502691896255534, 3.535250795749688894E-16 ) ) ;
#14083=CARTESIAN_POINT ( 'NONE',  ( 10.75312500061451715, 4.541064518000418104, -2.621784821874998173 ) ) ;
#14084=CARTESIAN_POINT ( 'NONE',  ( 28.30312500061451431, 4.541064518000418104, -2.621784821874998173 ) ) ;
#14085=CARTESIAN_POINT ( 'NONE',  ( 8.090625000614515727, 6.054752690667223547, 3.707466751127219781E-16 ) ) ;
#14086=CARTESIAN_POINT ( 'NONE',  ( 3.053854506608032704, -3.959065788097787753, 3.087202309779018883 ) ) ;
#14087=CARTESIAN_POINT ( 'NONE',  ( 2.121784821875001281, 11.90937500061451892, 33.67503911421598417 ) ) ;
#14088=CARTESIAN_POINT ( 'NONE',  ( 24.52500000122903145, 2.886751345948129099, -4.999999999999998224 ) ) ;
#14090=CARTESIAN_POINT ( 'NONE',  ( 13.49062500061451786, 6.054752690667223547, 3.707466751127219781E-16 ) ) ;
#14091=CARTESIAN_POINT ( 'NONE',  ( 10.77187500061451786, 3.027376345333613106, -5.243569643749998122 ) ) ;
#14092=CARTESIAN_POINT ( 'NONE',  ( 8.971875000614515372, 3.027376345333613106, -5.243569643749998122 ) ) ;
#14093=CARTESIAN_POINT ( 'NONE',  ( 17.03437500061451715, 6.421520780324663323E-16, -5.243569643749999010 ) ) ;
#14094=ORIENTED_EDGE ( 'NONE', *, *, #23957, .T. ) ;
#14095=CARTESIAN_POINT ( 'NONE',  ( -2.152738742430648777, 9.767338418468105132, 35.60400921600815138 ) ) ;
#14096=CARTESIAN_POINT ( 'NONE',  ( 22.30312500061451431, -4.541064518000417216, -2.621784821875001281 ) ) ;
#14097=CARTESIAN_POINT ( 'NONE',  ( 15.68437500061451573, 6.421520780324663323E-16, -5.243569643749999010 ) ) ;
#14098=CARTESIAN_POINT ( 'NONE',  ( 22.90312500061451573, 4.541064518000418104, -2.621784821874998173 ) ) ;
#14099=CARTESIAN_POINT ( 'NONE',  ( 1.999999999999998668, 15.35000000000000142, 26.53589838486224650 ) ) ;
#14100=CARTESIAN_POINT ( 'NONE',  ( 26.61562500061451786, 3.027376345333611329, 5.243569643749999010 ) ) ;
#14101=CARTESIAN_POINT ( 'NONE',  ( 7.275000001229035007, -5.773502691896255534, -1.060575238724906372E-15 ) ) ;
#14103=CARTESIAN_POINT ( 'NONE',  ( 5.400000001229032343, -2.886751345948129988, 4.999999999999997335 ) ) ;
#14104=CARTESIAN_POINT ( 'NONE',  ( 1.999999999999998668, 16.69999999999999929, -33.46410161513775705 ) ) ;
#14105=CARTESIAN_POINT ( 'NONE',  ( 24.97500000122903430, 2.886751345948129099, -4.999999999999998224 ) ) ;
#14107=VECTOR ( 'NONE', #63299, 1000.000000000000000 ) ;
#14108=CARTESIAN_POINT ( 'NONE',  ( 7.321875000614516793, 3.027376345333611329, 5.243569643749999010 ) ) ;
#14110=CARTESIAN_POINT ( 'NONE',  ( 14.95312500061451644, 0.000000000000000000, 5.243569643749999010 ) ) ;
#14111=CARTESIAN_POINT ( 'NONE',  ( 9.421875000614519990, 3.027376345333613106, -5.243569643749998122 ) ) ;
#14112=CARTESIAN_POINT ( 'NONE',  ( 26.55000000122902648, -2.886751345948129988, 4.999999999999997335 ) ) ;
#14113=( BOUNDED_CURVE ( )  B_SPLINE_CURVE ( 2, ( #26716, #44073, #38149, #49250, #71785, #66602, #59576 ),
 .UNSPECIFIED., .F., .F. ) 
 B_SPLINE_CURVE_WITH_KNOTS ( ( 3, 2, 2, 3 ),
 ( 0.7833333333333334370, 0.7861111111111112049, 0.7888888888888888618, 0.7916666666666666297 ),
 .UNSPECIFIED. ) 
 CURVE ( )  GEOMETRIC_REPRESENTATION_ITEM ( )  RATIONAL_B_SPLINE_CURVE ( ( 0.9999999999999946709, 0.8660254037844440367, 1.000000000000000000, 0.8660254037844387076, 1.000000000000000000, 0.8660254037844387076, 1.000000000000000000 ) ) 
 REPRESENTATION_ITEM ( '' )  );
#14114=CARTESIAN_POINT ( 'NONE',  ( 16.88437500061451502, -4.541064518000419881, 2.621784821874995952 ) ) ;
#14115=CARTESIAN_POINT ( 'NONE',  ( 4.096875000614518925, 6.054752690667223547, 3.707466751127219781E-16 ) ) ;
#14117=CARTESIAN_POINT ( 'NONE',  ( 6.590625000614518392, -3.027376345333610441, -5.243569643749999898 ) ) ;
#14118=( BOUNDED_CURVE ( )  B_SPLINE_CURVE ( 2, ( #68643, #52011, #18006, #13194, #40938, #18729, #1774 ),
 .UNSPECIFIED., .F., .F. ) 
 B_SPLINE_CURVE_WITH_KNOTS ( ( 3, 2, 2, 3 ),
 ( 0.9855061078632572080, 0.9861111111111111605, 0.9888888888888889284, 0.9894304826859887658 ),
 .UNSPECIFIED. ) 
 CURVE ( )  GEOMETRIC_REPRESENTATION_ITEM ( )  RATIONAL_B_SPLINE_CURVE ( ( 0.9543511520354772681, 0.9708201762974799642, 1.000000000000000000, 0.8660254037844387076, 1.000000000000000000, 0.9738784682994507946, 0.9579429634675318272 ) ) 
 REPRESENTATION_ITEM ( '' )  );
#14119=CARTESIAN_POINT ( 'NONE',  ( 14.91562500061451679, 3.027376345333611329, 5.243569643749999010 ) ) ;
#14121=ADVANCED_FACE ( 'NONE', ( #33914, #38373, #315 ), #60898, .T. ) ;
#14122=CARTESIAN_POINT ( 'NONE',  ( 12.85312500061451502, -4.541064518000417216, -2.621784821875001281 ) ) ;
#14123=CARTESIAN_POINT ( 'NONE',  ( 4.800000001229032698, 5.773502691896255534, 3.535250795749688894E-16 ) ) ;
#14124=CARTESIAN_POINT ( 'NONE',  ( 11.27812500061451573, 4.541064518000418104, 2.621784821874999949 ) ) ;
#14126=CARTESIAN_POINT ( 'NONE',  ( 10.35000000000000142, -4.330127018922190985, -2.500000000000001332 ) ) ;
#14127=CARTESIAN_POINT ( 'NONE',  ( 7.350000001229033408, -2.886751345948125991, -5.000000000000000000 ) ) ;
#14128=CARTESIAN_POINT ( 'NONE',  ( 19.27500000000000213, -4.330127018922194537, 2.499999999999995559 ) ) ;
#14129=ADVANCED_FACE ( 'NONE', ( #5127 ), #22824, .F. ) ;
#14130=( BOUNDED_CURVE ( )  B_SPLINE_CURVE ( 2, ( #17326, #45057, #28069, #22150, #10705, #11066, #62398, #67594, #45783 ),
 .UNSPECIFIED., .F., .T. ) 
 B_SPLINE_CURVE_WITH_KNOTS ( ( 3, 2, 2, 2, 3 ),
 ( 0.2282608695652174058, 0.2318840579710144956, 0.2391304347826087029, 0.2463768115942029102, 0.2500000000000000000 ),
 .UNSPECIFIED. ) 
 CURVE ( )  GEOMETRIC_REPRESENTATION_ITEM ( )  RATIONAL_B_SPLINE_CURVE ( ( 0.9330127018922194093, 0.9330127018922196314, 1.000000000000000000, 0.8660254037844387076, 1.000000000000000000, 0.8660254037844387076, 1.000000000000000000, 0.9330127018922196314, 0.9330127018922194093 ) ) 
 REPRESENTATION_ITEM ( '' )  );
#14131=CARTESIAN_POINT ( 'NONE',  ( 15.23437500061451644, 6.421520780324663323E-16, -5.243569643749999010 ) ) ;
#14132=CARTESIAN_POINT ( 'NONE',  ( 16.98750000122903359, 4.330127018922191873, 2.499999999999999556 ) ) ;
#14134=CARTESIAN_POINT ( 'NONE',  ( -4.243569643749997233, 19.39062500061451999, -27.54997392385601174 ) ) ;
#14136=CARTESIAN_POINT ( 'NONE',  ( -3.999999999999997335, 18.68750000000000000, 32.30940107675850470 ) ) ;
#14137=CARTESIAN_POINT ( 'NONE',  ( 23.10000000122903074, -2.886751345948142422, -4.999999999999970690 ) ) ;
#14138=CARTESIAN_POINT ( 'NONE',  ( 3.494527216699953698, -3.576116613012044976, 3.526356099291672042 ) ) ;
#14140=CARTESIAN_POINT ( 'NONE',  ( 15.27187500061451786, 3.027376345333613106, -5.243569643749998122 ) ) ;
#14141=EDGE_CURVE ( 'NONE', #2091, #8533, #6793, .T. ) ;
#14142=CARTESIAN_POINT ( 'NONE',  ( 28.01249999999999574, 2.886751345948129099, -4.999999999999998224 ) ) ;
#14143=CARTESIAN_POINT ( 'NONE',  ( 11.72812500061451857, 4.541064518000418104, 2.621784821874999949 ) ) ;
#14145=CARTESIAN_POINT ( 'NONE',  ( 22.88437500061451857, 6.421520780324663323E-16, -5.243569643749999010 ) ) ;
#14147=CARTESIAN_POINT ( 'NONE',  ( 8.915625000614515017, 3.027376345333613106, -5.243569643749998122 ) ) ;
#14148=CARTESIAN_POINT ( 'NONE',  ( 14.67187500061451821, -6.054752690667223547, -1.112240025338166033E-15 ) ) ;
#14150=CARTESIAN_POINT ( 'NONE',  ( 26.03437500061451715, 6.421520780324663323E-16, -5.243569643749999010 ) ) ;
#14151=CARTESIAN_POINT ( 'NONE',  ( 28.45312500061451289, 0.000000000000000000, 5.243569643749999010 ) ) ;
#14152=CARTESIAN_POINT ( 'NONE',  ( 27.89062500061451289, 6.054752690667223547, 3.707466751127219781E-16 ) ) ;
#14153=CARTESIAN_POINT ( 'NONE',  ( 3.939080010846523372, -3.079553322829319928, -4.243980907203444453 ) ) ;
#14154=CARTESIAN_POINT ( 'NONE',  ( 8.362500000000002487, 2.886751345948126879, 4.999999999999999112 ) ) ;
#14155=CARTESIAN_POINT ( 'NONE',  ( 16.08750000122903501, 4.330127018922191873, 2.499999999999999556 ) ) ;
#14159=CARTESIAN_POINT ( 'NONE',  ( 15.00000000000000000, 4.330127018922192761, -2.499999999999997780 ) ) ;
#14160=CARTESIAN_POINT ( 'NONE',  ( 19.57500000000000284, 4.330127018922191873, 2.499999999999999556 ) ) ;
#14161=CARTESIAN_POINT ( 'NONE',  ( 13.64062500061451644, -3.027376345333614438, 5.243569643749998122 ) ) ;
#14162=ORIENTED_EDGE ( 'NONE', *, *, #30313, .T. ) ;
#14164=CARTESIAN_POINT ( 'NONE',  ( 4.243569643749999898, 15.99687500061451573, -27.54997392385601529 ) ) ;
#14165=CARTESIAN_POINT ( 'NONE',  ( 6.778125000614518392, 4.541064518000418104, 2.621784821874999949 ) ) ;
#14167=CARTESIAN_POINT ( 'NONE',  ( 11.17500000000000071, -4.330127018922194537, 2.499999999999995559 ) ) ;
#14170=CARTESIAN_POINT ( 'NONE',  ( 4.243569643749999898, 15.97812500061451857, 30.00000000000000000 ) ) ;
#14171=CARTESIAN_POINT ( 'NONE',  ( 27.29062500061451502, -3.027376345333610441, -5.243569643749999898 ) ) ;
#14174=CARTESIAN_POINT ( 'NONE',  ( 23.10937500061451644, 0.000000000000000000, 5.243569643749999010 ) ) ;
#14175=CARTESIAN_POINT ( 'NONE',  ( 20.46562500061451928, -6.054752690667223547, -1.112240025338166033E-15 ) ) ;
#14176=CARTESIAN_POINT ( 'NONE',  ( -2.121784821874999949, 14.77812500061459389, -33.67503911421598417 ) ) ;
#14177=CARTESIAN_POINT ( 'NONE',  ( 22.65000000122903856, -2.886751345948125991, -5.000000000000000000 ) ) ;
#14178=CARTESIAN_POINT ( 'NONE',  ( 5.465625000614517504, 3.027376345333611329, 5.243569643749999010 ) ) ;
#14180=CARTESIAN_POINT ( 'NONE',  ( 21.92812500061451431, 6.421520780324663323E-16, -5.243569643749999010 ) ) ;
#14183=CARTESIAN_POINT ( 'NONE',  ( 16.43437500061451573, -4.541064518000419881, 2.621784821874995952 ) ) ;
#14184=CARTESIAN_POINT ( 'NONE',  ( 25.17187500061451644, 3.027376345333613106, -5.243569643749998122 ) ) ;
#14185=CARTESIAN_POINT ( 'NONE',  ( -4.243569643749999898, 15.32187500061451502, 27.54997392385601529 ) ) ;
#14186=CARTESIAN_POINT ( 'NONE',  ( 4.715625000614516615, -6.054752690667223547, -1.112240025338166033E-15 ) ) ;
#14187=CARTESIAN_POINT ( 'NONE',  ( 29.80312500061451431, 0.000000000000000000, 5.243569643749999010 ) ) ;
#14188=CARTESIAN_POINT ( 'NONE',  ( 29.05312500061451431, -4.541064518000417216, -2.621784821875001281 ) ) ;
#14190=CARTESIAN_POINT ( 'NONE',  ( 0.8114860633430618364, 9.969066991719973458, -35.94832491657660256 ) ) ;
#14191=CARTESIAN_POINT ( 'NONE',  ( 29.21250000122903145, 0.000000000000000000, 4.999999999999998224 ) ) ;
#14192=CARTESIAN_POINT ( 'NONE',  ( 7.996875000614519280, -3.027376345333610441, -5.243569643749999898 ) ) ;
#14193=CARTESIAN_POINT ( 'NONE',  ( 14.81250000122903288, 0.000000000000000000, 4.999999999999998224 ) ) ;
#14194=CARTESIAN_POINT ( 'NONE',  ( 3.646875000614520079, 6.054752690667223547, 3.707466751127219781E-16 ) ) ;
#14195=CARTESIAN_POINT ( 'NONE',  ( 10.95000000122903394, -2.886751345948125991, -5.000000000000000000 ) ) ;
#14196=CARTESIAN_POINT ( 'NONE',  ( 5.053125000614517859, 0.000000000000000000, 5.243569643749999010 ) ) ;
#14199=CARTESIAN_POINT ( 'NONE',  ( 14.07187500061451679, 3.027376345333611329, 5.243569643749999010 ) ) ;
#14200=CARTESIAN_POINT ( 'NONE',  ( 7.687499999999998224, -2.886751345948193048, -4.999999999999883649 ) ) ;
#14202=CARTESIAN_POINT ( 'NONE',  ( 21.89062500061451289, -3.027376345333610441, -5.243569643749999898 ) ) ;
#14203=CARTESIAN_POINT ( 'NONE',  ( 6.365625000614518747, 3.027376345333611329, 5.243569643749999010 ) ) ;
#14204=CARTESIAN_POINT ( 'NONE',  ( 25.47187500061451715, -6.054752690667223547, -1.112240025338166033E-15 ) ) ;
#14205=CARTESIAN_POINT ( 'NONE',  ( 6.553125000614518747, -4.541064518000417216, -2.621784821875001281 ) ) ;
#14207=CARTESIAN_POINT ( 'NONE',  ( 8.137500001229033941, -4.330127018922194537, 2.499999999999995559 ) ) ;
#14208=CARTESIAN_POINT ( 'NONE',  ( 24.14062500061451289, -3.027376345333610441, -5.243569643749999898 ) ) ;
#14209=CARTESIAN_POINT ( 'NONE',  ( -4.243569643749997233, 10.84062500061451395, -27.54997392385601174 ) ) ;
#14210=CARTESIAN_POINT ( 'NONE',  ( 9.262500001229033941, 4.330127018922192761, -2.499999999999997780 ) ) ;
#14211=CARTESIAN_POINT ( 'NONE',  ( 20.72812500061451502, 4.541064518000418104, 2.621784821874999949 ) ) ;
#14212=CARTESIAN_POINT ( 'NONE',  ( 18.66562500061451146, -6.054752690667223547, -1.112240025338166033E-15 ) ) ;
#14215=EDGE_CURVE ( 'NONE', #50028, #7649, #5491, .T. ) ;
#14216=CARTESIAN_POINT ( 'NONE',  ( 18.63749999999999929, 5.773502691896255534, 3.535250795749688894E-16 ) ) ;
#14217=CARTESIAN_POINT ( 'NONE',  ( 13.31250000122903288, 4.330127018922192761, -2.499999999999997780 ) ) ;
#14218=CARTESIAN_POINT ( 'NONE',  ( 10.37812500061451715, 4.541064518000418104, 2.621784821874999949 ) ) ;
#14219=CARTESIAN_POINT ( 'NONE',  ( 12.81562500061451537, -6.054752690667223547, -1.112240025338166033E-15 ) ) ;
#14220=CARTESIAN_POINT ( 'NONE',  ( 23.13750000122903216, 6.123233995736764310E-16, -4.999999999999998224 ) ) ;
#14221=CARTESIAN_POINT ( 'NONE',  ( 22.95937500061451431, 4.541064518000418104, -2.621784821874998173 ) ) ;
#14222=CARTESIAN_POINT ( 'NONE',  ( 21.38437500061451502, -4.541064518000419881, 2.621784821874995952 ) ) ;
#14224=CARTESIAN_POINT ( 'NONE',  ( 7.387500001229032165, 6.123233995736764310E-16, -4.999999999999998224 ) ) ;
#14225=CARTESIAN_POINT ( 'NONE',  ( 5.596875000614516260, -3.027376345333614438, 5.243569643749998122 ) ) ;
#14226=CARTESIAN_POINT ( 'NONE',  ( 23.22187500061451715, -6.054752690667223547, -1.112240025338166033E-15 ) ) ;
#14227=CARTESIAN_POINT ( 'NONE',  ( 4.761519200037192867, -1.526514057201037611, 4.869786965056912997 ) ) ;
#14228=CARTESIAN_POINT ( 'NONE',  ( 18.55312500061451431, 0.000000000000000000, 5.243569643749999010 ) ) ;
#14229=CARTESIAN_POINT ( 'NONE',  ( 24.68437500061451573, 6.421520780324663323E-16, -5.243569643749999010 ) ) ;
#14231=CARTESIAN_POINT ( 'NONE',  ( 3.384375000614517237, -4.541064518000419881, 2.621784821874995952 ) ) ;
#14232=CARTESIAN_POINT ( 'NONE',  ( 1.071796769724489895, 15.81740381056766509, 26.00000000000000355 ) ) ;
#14233=CARTESIAN_POINT ( 'NONE',  ( 5.896875000614518747, 6.054752690667223547, 3.707466751127219781E-16 ) ) ;
#14234=CARTESIAN_POINT ( 'NONE',  ( 17.61562500061451786, 3.027376345333611329, 5.243569643749999010 ) ) ;
#14236=CARTESIAN_POINT ( 'NONE',  ( 22.83749999999999858, -2.886751345948163738, 4.999999999999939604 ) ) ;
#14237=CARTESIAN_POINT ( 'NONE',  ( 24.62812500061451715, 6.421520780324663323E-16, -5.243569643749999010 ) ) ;
#14238=CARTESIAN_POINT ( 'NONE',  ( -3.999999999999999112, 10.66250000122903430, -30.00000000000000000 ) ) ;
#14240=CARTESIAN_POINT ( 'NONE',  ( 13.79999999999999893, 0.000000000000000000, 4.999999999999998224 ) ) ;
#14241=CARTESIAN_POINT ( 'NONE',  ( 25.38750000122903216, 6.123233995736764310E-16, -4.999999999999998224 ) ) ;
#14242=CARTESIAN_POINT ( 'NONE',  ( 21.92812500061451431, 6.421520780324663323E-16, -5.243569643749999010 ) ) ;
#14244=CARTESIAN_POINT ( 'NONE',  ( 23.09999999999999787, 4.330127018922192761, -2.499999999999997780 ) ) ;
#14245=CARTESIAN_POINT ( 'NONE',  ( 22.99687500061451573, 6.054752690667223547, 3.707466751127219781E-16 ) ) ;
#14246=ORIENTED_EDGE ( 'NONE', *, *, #34911, .T. ) ;
#14248=CARTESIAN_POINT ( 'NONE',  ( 13.97812500061451679, 4.541064518000418104, 2.621784821874999949 ) ) ;
#14249=CARTESIAN_POINT ( 'NONE',  ( 3.740625000614516527, -3.027376345333614438, 5.243569643749998122 ) ) ;
#14251=CARTESIAN_POINT ( 'NONE',  ( 25.71562500061451573, 3.027376345333611329, 5.243569643749999010 ) ) ;
#14252=CARTESIAN_POINT ( 'NONE',  ( 13.68750000122903288, 6.123233995736764310E-16, -4.999999999999998224 ) ) ;
#14253=CARTESIAN_POINT ( 'NONE',  ( 18.48750000000000071, -2.886751345948125991, -5.000000000000000000 ) ) ;
#14254=CARTESIAN_POINT ( 'NONE',  ( 26.55000000000000071, -4.330127018922190985, -2.500000000000001332 ) ) ;
#14255=CARTESIAN_POINT ( 'NONE',  ( 3.225000001229032964, -5.773502691896255534, -1.060575238724906372E-15 ) ) ;
#14256=CARTESIAN_POINT ( 'NONE',  ( 6.571875000614517681, -6.054752690667223547, -1.112240025338166033E-15 ) ) ;
#14257=CARTESIAN_POINT ( 'NONE',  ( 19.88437500061451857, 4.541064518000418104, 2.621784821874999949 ) ) ;
#14258=CARTESIAN_POINT ( 'NONE',  ( 1.071796769724489895, 11.42990381179669868, 26.00000000000000355 ) ) ;
#14259=VERTEX_POINT ( 'NONE', #67912 ) ;
#14260=CARTESIAN_POINT ( 'NONE',  ( 29.31562500061451715, 3.027376345333611329, 5.243569643749999010 ) ) ;
#14261=CARTESIAN_POINT ( 'NONE',  ( 29.67187500061451644, 3.027376345333613106, -5.243569643749998122 ) ) ;
#14262=CARTESIAN_POINT ( 'NONE',  ( 5.521875000614517859, 3.027376345333611329, 5.243569643749999010 ) ) ;
#14263=CARTESIAN_POINT ( 'NONE',  ( 15.22500000000000142, -4.330127018922194537, 2.499999999999995559 ) ) ;
#14264=CARTESIAN_POINT ( 'NONE',  ( 13.15312500061451750, 0.000000000000000000, 5.243569643749999010 ) ) ;
#14265=CARTESIAN_POINT ( 'NONE',  ( -1.999999999999997113, 15.12500000000000000, -26.53589838486224295 ) ) ;
#14267=DIRECTION ( 'NONE',  ( -0.000000000000000000, -1.000000000000000000, -0.000000000000000000 ) ) ;
#14268=CARTESIAN_POINT ( 'NONE',  ( 19.20000000122903572, 5.773502691896255534, 3.535250795749688894E-16 ) ) ;
#14271=CARTESIAN_POINT ( 'NONE',  ( 8.090625000614515727, 6.054752690667223547, 3.707466751127219781E-16 ) ) ;
#14272=CARTESIAN_POINT ( 'NONE',  ( 24.64687500061451431, -3.027376345333610441, -5.243569643749999898 ) ) ;
#14273=CARTESIAN_POINT ( 'NONE',  ( -4.243569643749997233, 17.64687500061452141, 32.45002607614398471 ) ) ;
#14274=CARTESIAN_POINT ( 'NONE',  ( 24.64687500061451431, -3.027376345333610441, -5.243569643749999898 ) ) ;
#14275=CARTESIAN_POINT ( 'NONE',  ( 4.275000000000001243, 4.330127018922191873, 2.499999999999999556 ) ) ;
#14276=CARTESIAN_POINT ( 'NONE',  ( -0.6945863667395647534, 9.663023495605401081, 26.06076786935073741 ) ) ;
#14277=CARTESIAN_POINT ( 'NONE',  ( 13.45312500061451466, 4.541064518000418104, -2.621784821874998173 ) ) ;
#14278=CARTESIAN_POINT ( 'NONE',  ( 5.550000001229032698, -2.886751345948125991, -5.000000000000000000 ) ) ;
#14281=CARTESIAN_POINT ( 'NONE',  ( 8.446875000614518569, -3.027376345333610441, -5.243569643749999898 ) ) ;
#14282=CARTESIAN_POINT ( 'NONE',  ( 2.000000000000001332, 14.86250000122903536, 33.46410161513774995 ) ) ;
#14283=EDGE_LOOP ( 'NONE', ( #14020, #50633, #18140, #65950 ) ) ;
#14284=CARTESIAN_POINT ( 'NONE',  ( 10.90312500061451928, 0.000000000000000000, 5.243569643749999010 ) ) ;
#14285=CARTESIAN_POINT ( 'NONE',  ( 14.33437500061451786, 6.421520780324663323E-16, -5.243569643749999010 ) ) ;
#14287=CARTESIAN_POINT ( 'NONE',  ( 24.26250000122903216, 0.000000000000000000, 4.999999999999998224 ) ) ;
#14288=CARTESIAN_POINT ( 'NONE',  ( 9.759375000614516793, -4.541064518000417216, -2.621784821875001281 ) ) ;
#14289=CARTESIAN_POINT ( 'NONE',  ( 12.14062500061451821, 6.054752690667223547, 3.707466751127219781E-16 ) ) ;
#14291=CARTESIAN_POINT ( 'NONE',  ( 20.82187500061451857, 3.027376345333611329, 5.243569643749999010 ) ) ;
#14293=CARTESIAN_POINT ( 'NONE',  ( 5.250000000000000888, 0.000000000000000000, 4.999999999999998224 ) ) ;
#14295=CARTESIAN_POINT ( 'NONE',  ( -4.243569643749999898, 13.52187500061451786, -32.45002607614398471 ) ) ;
#14296=CARTESIAN_POINT ( 'NONE',  ( 15.27187500061451786, 3.027376345333613106, -5.243569643749998122 ) ) ;
#14297=CARTESIAN_POINT ( 'NONE',  ( 18.67500000122903714, 2.886751345948129099, -4.999999999999998224 ) ) ;
#14298=CARTESIAN_POINT ( 'NONE',  ( 13.43437500061451750, 6.421520780324663323E-16, -5.243569643749999010 ) ) ;
#14299=CARTESIAN_POINT ( 'NONE',  ( -4.243569643749997233, 18.49062500061451431, -27.54997392385601174 ) ) ;
#14300=CARTESIAN_POINT ( 'NONE',  ( 17.96250000122903501, 0.000000000000000000, 4.999999999999998224 ) ) ;
#14301=CARTESIAN_POINT ( 'NONE',  ( 11.61562500061451608, 3.027376345333613106, -5.243569643749998122 ) ) ;
#14302=ORIENTED_EDGE ( 'NONE', *, *, #16136, .T. ) ;
#14303=CARTESIAN_POINT ( 'NONE',  ( 14.77500000000000036, -4.330127018922194537, 2.499999999999995559 ) ) ;
#14304=CARTESIAN_POINT ( 'NONE',  ( 4.924325218087134637, -0.8666147624583920850, 4.924325218087160394 ) ) ;
#14305=CARTESIAN_POINT ( 'NONE',  ( 9.459375000614517859, 4.541064518000418104, -2.621784821874998173 ) ) ;
#14307=CARTESIAN_POINT ( 'NONE',  ( 4.111889464957033447, 2.844708250062874644, 4.404844785106587501 ) ) ;
#14308=CARTESIAN_POINT ( 'NONE',  ( 13.20000000122903394, -2.886751345948125991, -5.000000000000000000 ) ) ;
#14309=CARTESIAN_POINT ( 'NONE',  ( 20.88750000122903572, 6.123233995736764310E-16, -4.999999999999998224 ) ) ;
#14310=CARTESIAN_POINT ( 'NONE',  ( 18.40312500061451573, 4.541064518000418104, -2.621784821874998173 ) ) ;
#14311=CARTESIAN_POINT ( 'NONE',  ( 19.97812500061451502, -4.541064518000419881, 2.621784821874995952 ) ) ;
#14312=CARTESIAN_POINT ( 'NONE',  ( 28.35000000122903430, -2.886751345948129988, 4.999999999999997335 ) ) ;
#14313=CARTESIAN_POINT ( 'NONE',  ( 24.86250000000000071, 2.886751345948129099, -4.999999999999998224 ) ) ;
#14314=CARTESIAN_POINT ( 'NONE',  ( 28.42499999999999716, 6.123233995736764310E-16, -4.999999999999998224 ) ) ;
#14316=CARTESIAN_POINT ( 'NONE',  ( 28.28437500061451715, 6.421520780324663323E-16, -5.243569643749999010 ) ) ;
#14317=CARTESIAN_POINT ( 'NONE',  ( 11.58750000000000036, -2.886751345948130876, 4.999999999999996447 ) ) ;
#14318=CARTESIAN_POINT ( 'NONE',  ( 2.121784821875001281, 14.15937500061451715, -26.32496088578401938 ) ) ;
#14320=CARTESIAN_POINT ( 'NONE',  ( 3.787500001229033408, 6.123233995736764310E-16, -4.999999999999998224 ) ) ;
#14321=CARTESIAN_POINT ( 'NONE',  ( 4.349999999999999645, 0.000000000000000000, 4.999999999999998224 ) ) ;
#14323=CARTESIAN_POINT ( 'NONE',  ( 7.846875000614518036, -3.027376345333614438, 5.243569643749998122 ) ) ;
#14324=CARTESIAN_POINT ( 'NONE',  ( 29.24062500061451431, 6.054752690667223547, 3.707466751127219781E-16 ) ) ;
#14326=CARTESIAN_POINT ( 'NONE',  ( 2.000000000000001332, 10.36250000122903359, 33.46410161513774995 ) ) ;
#14327=CARTESIAN_POINT ( 'NONE',  ( 1.510657702057710734E-15, 19.10000000122903430, 26.00000000000000000 ) ) ;
#14328=CARTESIAN_POINT ( 'NONE',  ( 4.771875000614516971, -6.054752690667223547, -1.112240025338166033E-15 ) ) ;
#14329=CARTESIAN_POINT ( 'NONE',  ( 9.909375000614517148, 4.541064518000418104, -2.621784821874998173 ) ) ;
#14330=CARTESIAN_POINT ( 'NONE',  ( 3.337499999999999911, 5.773502691896255534, 3.535250795749688894E-16 ) ) ;
#14331=CARTESIAN_POINT ( 'NONE',  ( -4.243569643749999898, 13.50312500061459531, 30.00000000000000000 ) ) ;
#14333=CARTESIAN_POINT ( 'NONE',  ( 1.999999999999998668, 18.05000000000000071, 26.53589838486224650 ) ) ;
#14334=( BOUNDED_CURVE ( )  B_SPLINE_CURVE ( 2, ( #38899, #10090, #15611, #11541, #5996, #72504, #21893 ),
 .UNSPECIFIED., .F., .F. ) 
 B_SPLINE_CURVE_WITH_KNOTS ( ( 3, 2, 2, 3 ),
 ( 0.5583333333333333481, 0.5611111111111111160, 0.5638888888888889950, 0.5666666666666667629 ),
 .UNSPECIFIED. ) 
 CURVE ( )  GEOMETRIC_REPRESENTATION_ITEM ( )  RATIONAL_B_SPLINE_CURVE ( ( 1.000000000000000000, 0.8660254037844387076, 1.000000000000000000, 0.8660254037844387076, 1.000000000000000000, 0.8660254037844333785, 1.000000000000005329 ) ) 
 REPRESENTATION_ITEM ( '' )  );
#14335=CARTESIAN_POINT ( 'NONE',  ( 4.349999999999999645, 0.000000000000000000, 4.999999999999998224 ) ) ;
#14337=CARTESIAN_POINT ( 'NONE',  ( 21.36562500061451431, -6.054752690667223547, -1.112240025338166033E-15 ) ) ;
#14338=CARTESIAN_POINT ( 'NONE',  ( 11.65312500061451573, 4.541064518000418104, -2.621784821874998173 ) ) ;
#14340=CARTESIAN_POINT ( 'NONE',  ( 9.609375000614518214, 0.000000000000000000, 5.243569643749999010 ) ) ;
#14341=CARTESIAN_POINT ( 'NONE',  ( 25.16249999999999432, -5.773502691896255534, -1.060575238724906372E-15 ) ) ;
#14342=CARTESIAN_POINT ( 'NONE',  ( 21.07500000122903572, 2.886751345948126879, 4.999999999999999112 ) ) ;
#14343=CARTESIAN_POINT ( 'NONE',  ( 28.71562500061451573, 3.027376345333613106, -5.243569643749998122 ) ) ;
#14345=CARTESIAN_POINT ( 'NONE',  ( 8.671875000614518214, 3.027376345333611329, 5.243569643749999010 ) ) ;
#14346=CARTESIAN_POINT ( 'NONE',  ( 15.12187500061451750, -6.054752690667223547, -1.112240025338166033E-15 ) ) ;
#14347=CARTESIAN_POINT ( 'NONE',  ( 27.19687500061451857, -3.027376345333614438, 5.243569643749998122 ) ) ;
#14348=CARTESIAN_POINT ( 'NONE',  ( 4.303125000614516971, -4.541064518000417216, -2.621784821875001281 ) ) ;
#14350=CARTESIAN_POINT ( 'NONE',  ( 21.08437500061451786, 6.421520780324663323E-16, -5.243569643749999010 ) ) ;
#14351=CARTESIAN_POINT ( 'NONE',  ( 10.65937500061451715, -4.541064518000417216, -2.621784821875001281 ) ) ;
#14353=CARTESIAN_POINT ( 'NONE',  ( 23.17500000000000071, 4.330127018922191873, 2.499999999999999556 ) ) ;
#14355=CARTESIAN_POINT ( 'NONE',  ( -2.121784821874996840, 12.73437500061451821, -26.32496088578401583 ) ) ;
#14357=CARTESIAN_POINT ( 'NONE',  ( 14.87812500061451537, 4.541064518000418104, 2.621784821874999949 ) ) ;
#14358=CARTESIAN_POINT ( 'NONE',  ( 3.900000000000000799, 0.000000000000000000, 4.999999999999998224 ) ) ;
#14360=CARTESIAN_POINT ( 'NONE',  ( 2.000000000000001332, 9.912500001229034297, -26.53589838486224650 ) ) ;
#14361=CARTESIAN_POINT ( 'NONE',  ( 12.48750000000000249, -2.886751345948129988, 4.999999999999997335 ) ) ;
#14362=CARTESIAN_POINT ( 'NONE',  ( 3.999999999999999112, 18.08750000122903501, 30.00000000000000000 ) ) ;
#14363=CARTESIAN_POINT ( 'NONE',  ( 10.72500000122903252, 2.886751345948126879, 4.999999999999999112 ) ) ;
#14364=CARTESIAN_POINT ( 'NONE',  ( 22.69687500061451857, -3.027376345333614438, 5.243569643749998122 ) ) ;
#14365=CARTESIAN_POINT ( 'NONE',  ( 15.53437500061451715, -4.541064518000419881, 2.621784821874995952 ) ) ;
#14367=ORIENTED_EDGE ( 'NONE', *, *, #1615, .T. ) ;
#14368=CARTESIAN_POINT ( 'NONE',  ( 20.24062500061451431, 6.054752690667223547, 3.707466751127219781E-16 ) ) ;
#14369=CARTESIAN_POINT ( 'NONE',  ( 3.365625000614516082, -6.054752690667223547, -1.112240025338166033E-15 ) ) ;
#14370=CARTESIAN_POINT ( 'NONE',  ( 18.23437500061451999, -4.541064518000419881, 2.621784821874995952 ) ) ;
#14371=CARTESIAN_POINT ( 'NONE',  ( 28.05937500061451573, 0.000000000000000000, 5.243569643749999010 ) ) ;
#14372=CARTESIAN_POINT ( 'NONE',  ( 3.778125000614519280, -4.541064518000419881, 2.621784821874995952 ) ) ;
#14373=CARTESIAN_POINT ( 'NONE',  ( 19.71562500061451928, 3.027376345333613106, -5.243569643749998122 ) ) ;
#14374=CARTESIAN_POINT ( 'NONE',  ( -2.121784821874996840, 15.82812500061451644, 33.67503911421598417 ) ) ;
#14375=CARTESIAN_POINT ( 'NONE',  ( 15.63750000122903216, 4.330127018922191873, 2.499999999999999556 ) ) ;
#14377=CARTESIAN_POINT ( 'NONE',  ( 7.003125000614518036, -4.541064518000417216, -2.621784821875001281 ) ) ;
#14378=CARTESIAN_POINT ( 'NONE',  ( 29.16562500061451502, 3.027376345333613106, -5.243569643749998122 ) ) ;
#14379=EDGE_CURVE ( 'NONE', #56216, #61496, #32471, .T. ) ;
#14380=CARTESIAN_POINT ( 'NONE',  ( 22.69687500061451857, -3.027376345333614438, 5.243569643749998122 ) ) ;
#14381=CARTESIAN_POINT ( 'NONE',  ( 14.35312500061451679, 4.541064518000418104, -2.621784821874998173 ) ) ;
#14382=CARTESIAN_POINT ( 'NONE',  ( 25.80000000122903714, -2.886751345948125991, -5.000000000000000000 ) ) ;
#14383=CARTESIAN_POINT ( 'NONE',  ( 22.34062500061451573, -3.027376345333610441, -5.243569643749999898 ) ) ;
#14384=CARTESIAN_POINT ( 'NONE',  ( 19.17187500061451999, -6.054752690667223547, -1.112240025338166033E-15 ) ) ;
#14385=CARTESIAN_POINT ( 'NONE',  ( 15.89062500061451289, -3.027376345333614438, 5.243569643749998122 ) ) ;
#14386=CARTESIAN_POINT ( 'NONE',  ( -3.000416591977282496E-16, 14.34687500061451715, 25.09994784771203058 ) ) ;
#14387=CARTESIAN_POINT ( 'NONE',  ( 19.34062500061451573, 6.054752690667223547, 3.707466751127219781E-16 ) ) ;
#14388=ORIENTED_EDGE ( 'NONE', *, *, #38075, .T. ) ;
#14389=CARTESIAN_POINT ( 'NONE',  ( 24.07499999999999929, 4.330127018922191873, 2.499999999999999556 ) ) ;
#14390=CARTESIAN_POINT ( 'NONE',  ( -2.828200636599751609E-16, 11.33750000000000036, -34.61880215351700230 ) ) ;
#14391=DIRECTION ( 'NONE',  ( -1.000000000000000000, -0.000000000000000000, -0.000000000000000000 ) ) ;
#14392=CARTESIAN_POINT ( 'NONE',  ( 26.50312500061451360, 4.541064518000418104, -2.621784821874998173 ) ) ;
#14393=CARTESIAN_POINT ( 'NONE',  ( 7.865625000614516971, -6.054752690667223547, -1.112240025338166033E-15 ) ) ;
#14394=CARTESIAN_POINT ( 'NONE',  ( 19.23750000122903714, 4.330127018922191873, 2.499999999999999556 ) ) ;
#14395=CARTESIAN_POINT ( 'NONE',  ( 24.70312500061451644, 4.541064518000418104, -2.621784821874998173 ) ) ;
#14396=CARTESIAN_POINT ( 'NONE',  ( 22.76249999999999574, 2.886751345948126879, 4.999999999999999112 ) ) ;
#14397=CARTESIAN_POINT ( 'NONE',  ( 28.22812500061451502, 6.421520780324663323E-16, -5.243569643749999010 ) ) ;
#14398=CARTESIAN_POINT ( 'NONE',  ( 7.603125000614517681, 4.541064518000418104, -2.621784821874998173 ) ) ;
#14400=CARTESIAN_POINT ( 'NONE',  ( 23.76562500061451644, 3.027376345333613106, -5.243569643749998122 ) ) ;
#14401=CARTESIAN_POINT ( 'NONE',  ( 5.690625000614516260, -3.027376345333610441, -5.243569643749999898 ) ) ;
#14402=PRODUCT_DEFINITION_CONTEXT ( 'detailed design', #29032, 'design' ) ;
#14404=CARTESIAN_POINT ( 'NONE',  ( 3.365625000614516082, -6.054752690667223547, -1.112240025338166033E-15 ) ) ;
#14405=CARTESIAN_POINT ( 'NONE',  ( -1.999999999999997113, 14.33750000122903323, -26.53589838486224295 ) ) ;
#14406=CARTESIAN_POINT ( 'NONE',  ( -3.999999999999997335, 10.58750000000000213, -27.69059892324149530 ) ) ;
#14407=CARTESIAN_POINT ( 'NONE',  ( 9.750000000000001776, 0.000000000000000000, 4.999999999999998224 ) ) ;
#14408=CARTESIAN_POINT ( 'NONE',  ( 10.62187500061451928, -6.054752690667223547, -1.112240025338166033E-15 ) ) ;
#14409=CARTESIAN_POINT ( 'NONE',  ( 8.737500001229033586, 6.123233995736764310E-16, -4.999999999999998224 ) ) ;
#14410=CARTESIAN_POINT ( 'NONE',  ( 15.42187500061451821, 3.027376345333611329, 5.243569643749999010 ) ) ;
#14412=CARTESIAN_POINT ( 'NONE',  ( 6.796875000614516438, 6.054752690667223547, 3.707466751127219781E-16 ) ) ;
#14414=CARTESIAN_POINT ( 'NONE',  ( 20.13750000000000639, -2.886751345948130876, 4.999999999999996447 ) ) ;
#14415=CARTESIAN_POINT ( 'NONE',  ( 13.17187500061451999, 3.027376345333611329, 5.243569643749999010 ) ) ;
#14416=EDGE_LOOP ( 'NONE', ( #41616, #28618, #5305, #58500 ) ) ;
#14417=EDGE_CURVE ( 'NONE', #20886, #16658, #4880, .T. ) ;
#14418=CARTESIAN_POINT ( 'NONE',  ( 22.90312500061451573, 4.541064518000418104, -2.621784821874998173 ) ) ;
#14422=CARTESIAN_POINT ( 'NONE',  ( 26.70937500061451431, 0.000000000000000000, 5.243569643749999010 ) ) ;
#14423=CARTESIAN_POINT ( 'NONE',  ( 4.340625000614515727, -3.027376345333610441, -5.243569643749999898 ) ) ;
#14425=CARTESIAN_POINT ( 'NONE',  ( 15.83437500061451608, 4.541064518000418104, 2.621784821874999949 ) ) ;
#14427=CARTESIAN_POINT ( 'NONE',  ( 26.40000000122902790, 5.773502691896255534, 3.535250795749688894E-16 ) ) ;
#14428=CARTESIAN_POINT ( 'NONE',  ( 6.796875000614516438, 6.054752690667223547, 3.707466751127219781E-16 ) ) ;
#14429=CARTESIAN_POINT ( 'NONE',  ( 16.50937500061451502, -4.541064518000417216, -2.621784821875001281 ) ) ;
#14430=CARTESIAN_POINT ( 'NONE',  ( 21.44999999999999929, 0.000000000000000000, 4.999999999999998224 ) ) ;
#14431=CARTESIAN_POINT ( 'NONE',  ( 23.51249999999999574, 2.886751345948129099, -4.999999999999998224 ) ) ;
#14432=CARTESIAN_POINT ( 'NONE',  ( 3.487500001229035362, 4.330127018922191873, 2.499999999999999556 ) ) ;
#14433=CARTESIAN_POINT ( 'NONE',  ( 27.27187500061451431, -6.054752690667223547, -1.112240025338166033E-15 ) ) ;
#14436=CARTESIAN_POINT ( 'NONE',  ( 8.474999999999999645, -4.330127018922194537, 2.499999999999995559 ) ) ;
#14438=CARTESIAN_POINT ( 'NONE',  ( 21.55312500061451431, 4.541064518000418104, -2.621784821874998173 ) ) ;
#14439=CARTESIAN_POINT ( 'NONE',  ( 10.87500000000000000, 6.123233995736764310E-16, -4.999999999999998224 ) ) ;
#14440=CARTESIAN_POINT ( 'NONE',  ( 7.528125000614515727, 6.421520780324663323E-16, -5.243569643749999010 ) ) ;
#14441=CARTESIAN_POINT ( 'NONE',  ( 19.08750000000000213, 5.773502691896255534, 3.535250795749688894E-16 ) ) ;
#14442=CARTESIAN_POINT ( 'NONE',  ( 18.25312500061451715, -4.541064518000417216, -2.621784821875001281 ) ) ;
#14443=CARTESIAN_POINT ( 'NONE',  ( 0.000000000000000000, 20.00000000000000000, -30.00000000000000000 ) ) ;
#14444=VECTOR ( 'NONE', #16641, 1000.000000000000000 ) ;
#14445=CARTESIAN_POINT ( 'NONE',  ( 23.96250000122903145, -4.330127018922190985, -2.500000000000001332 ) ) ;
#14447=CARTESIAN_POINT ( 'NONE',  ( 3.637500000000001954, -2.886751345948125991, -5.000000000000000000 ) ) ;
#14449=CARTESIAN_POINT ( 'NONE',  ( 20.24062500061451431, 6.054752690667223547, 3.707466751127219781E-16 ) ) ;
#14450=CARTESIAN_POINT ( 'NONE',  ( 26.27812500061451573, -4.541064518000419881, 2.621784821874995952 ) ) ;
#14451=CARTESIAN_POINT ( 'NONE',  ( 25.35937500061451644, 0.000000000000000000, 5.243569643749999010 ) ) ;
#14452=CARTESIAN_POINT ( 'NONE',  ( 9.150000000000002132, 4.330127018922192761, -2.499999999999997780 ) ) ;
#14453=CARTESIAN_POINT ( 'NONE',  ( 12.85312500061451502, -4.541064518000417216, -2.621784821875001281 ) ) ;
#14454=CARTESIAN_POINT ( 'NONE',  ( 26.01562500061451289, 3.027376345333613106, -5.243569643749998122 ) ) ;
#14455=CARTESIAN_POINT ( 'NONE',  ( 17.85937500061451999, -4.541064518000417216, -2.621784821875001281 ) ) ;
#14456=CARTESIAN_POINT ( 'NONE',  ( 9.853125000614516793, 4.541064518000418104, -2.621784821874998173 ) ) ;
#14458=CARTESIAN_POINT ( 'NONE',  ( -2.121784821874999949, 11.68437500061451750, 26.32496088578401938 ) ) ;
#14459=ADVANCED_FACE ( 'NONE', ( #63447 ), #681, .F. ) ;
#14460=CARTESIAN_POINT ( 'NONE',  ( 23.58750000122903145, 6.123233995736764310E-16, -4.999999999999998224 ) ) ;
#14462=CARTESIAN_POINT ( 'NONE',  ( 14.46562500061451573, 3.027376345333611329, 5.243569643749999010 ) ) ;
#14463=CARTESIAN_POINT ( 'NONE',  ( 10.47187500061451715, 3.027376345333611329, 5.243569643749999010 ) ) ;
#14464=CARTESIAN_POINT ( 'NONE',  ( 8.746875000614515727, -3.027376345333614438, 5.243569643749998122 ) ) ;
#14465=ORIENTED_EDGE ( 'NONE', *, *, #31222, .T. ) ;
#14466=CARTESIAN_POINT ( 'NONE',  ( -3.671862074746357063, 9.302863167343950579, 34.74916175131421170 ) ) ;
#14467=CARTESIAN_POINT ( 'NONE',  ( 22.34062500061451573, -3.027376345333610441, -5.243569643749999898 ) ) ;
#14468=CARTESIAN_POINT ( 'NONE',  ( 16.09687500061452070, -3.027376345333610441, -5.243569643749999898 ) ) ;
#14469=CARTESIAN_POINT ( 'NONE',  ( 21.21562500061451573, 3.027376345333611329, 5.243569643749999010 ) ) ;
#14470=CARTESIAN_POINT ( 'NONE',  ( -2.828200636599751609E-16, 12.68750000000000000, 25.38119784648299770 ) ) ;
#14471=CARTESIAN_POINT ( 'NONE',  ( 27.55312500061451786, 0.000000000000000000, 5.243569643749999010 ) ) ;
#14472=CARTESIAN_POINT ( 'NONE',  ( 7.500000001229034652, 5.773502691896255534, 3.535250795749688894E-16 ) ) ;
#14473=ORIENTED_EDGE ( 'NONE', *, *, #69351, .T. ) ;
#14474=CARTESIAN_POINT ( 'NONE',  ( 29.55000000000000071, 0.000000000000000000, 4.999999999999998224 ) ) ;
#14475=CARTESIAN_POINT ( 'NONE',  ( -3.999999999999997335, 17.33749999999999858, -27.69059892324149175 ) ) ;
#14476=CARTESIAN_POINT ( 'NONE',  ( 24.93750000122903288, 6.123233995736764310E-16, -4.999999999999998224 ) ) ;
#14478=CARTESIAN_POINT ( 'NONE',  ( 7.284375000614518036, 4.541064518000418104, 2.621784821874999949 ) ) ;
#14479=CARTESIAN_POINT ( 'NONE',  ( 4.368115381025522659, 2.433016238755435268, -4.556724453905077965 ) ) ;
#14480=CARTESIAN_POINT ( 'NONE',  ( 14.24062500061451608, -3.027376345333610441, -5.243569643749999898 ) ) ;
#14481=CARTESIAN_POINT ( 'NONE',  ( 9.759375000614516793, -4.541064518000417216, -2.621784821875001281 ) ) ;
#14482=CARTESIAN_POINT ( 'NONE',  ( 26.73750000122903003, 6.123233995736764310E-16, -4.999999999999998224 ) ) ;
#14483=CARTESIAN_POINT ( 'NONE',  ( 16.20937500061451786, 4.541064518000418104, -2.621784821874998173 ) ) ;
#14484=CARTESIAN_POINT ( 'NONE',  ( 5.859375000614519102, 4.541064518000418104, -2.621784821874998173 ) ) ;
#14485=CARTESIAN_POINT ( 'NONE',  ( 0.000000000000000000, 20.00000000000000000, -33.99999999999999289 ) ) ;
#14486=CARTESIAN_POINT ( 'NONE',  ( 4.790625000614518569, -3.027376345333610441, -5.243569643749999898 ) ) ;
#14487=CARTESIAN_POINT ( 'NONE',  ( 15.70312500061451644, 4.541064518000418104, -2.621784821874998173 ) ) ;
#14488=ORIENTED_EDGE ( 'NONE', *, *, #35039, .F. ) ;
#14489=CARTESIAN_POINT ( 'NONE',  ( 12.44062500061451537, -3.027376345333610441, -5.243569643749999898 ) ) ;
#14490=CARTESIAN_POINT ( 'NONE',  ( 5.287500001229035185, 4.330127018922191873, 2.499999999999999556 ) ) ;
#14491=CARTESIAN_POINT ( 'NONE',  ( 11.20312500061451644, 4.541064518000418104, -2.621784821874998173 ) ) ;
#14493=CARTESIAN_POINT ( 'NONE',  ( 9.862500000000000711, -5.773502691896255534, -1.060575238724906372E-15 ) ) ;
#14494=CARTESIAN_POINT ( 'NONE',  ( 4.387500001229033053, 4.330127018922191873, 2.499999999999999556 ) ) ;
#14495=CARTESIAN_POINT ( 'NONE',  ( 19.16250000000000142, 2.886751345948126879, 4.999999999999999112 ) ) ;
#14497=CARTESIAN_POINT ( 'NONE',  ( 15.57187500061451679, -6.054752690667223547, -1.112240025338166033E-15 ) ) ;
#14498=CARTESIAN_POINT ( 'NONE',  ( 16.91250000122903430, 4.330127018922192761, -2.499999999999997780 ) ) ;
#14500=CARTESIAN_POINT ( 'NONE',  ( 4.243569643749999010, 17.81562500061451715, -32.45002607614398471 ) ) ;
#14501=LINE ( 'NONE', #42585, #35905 ) ;
#14502=CARTESIAN_POINT ( 'NONE',  ( 4.898587196589411843E-16, 20.00000000000000000, 33.99999999999999289 ) ) ;
#14503=CARTESIAN_POINT ( 'NONE',  ( 29.80312500061451431, 0.000000000000000000, 5.243569643749999010 ) ) ;
#14505=CARTESIAN_POINT ( 'NONE',  ( 3.881554241669678884, -3.151751365348489653, -4.190642664303462439 ) ) ;
#14506=CARTESIAN_POINT ( 'NONE',  ( 16.69687500061451502, 6.054752690667223547, 3.707466751127219781E-16 ) ) ;
#14508=CARTESIAN_POINT ( 'NONE',  ( 28.72500000000000142, -4.330127018922194537, 2.499999999999995559 ) ) ;
#14509=CARTESIAN_POINT ( 'NONE',  ( 12.32812500061451821, -4.541064518000419881, 2.621784821874995952 ) ) ;
#14511=CARTESIAN_POINT ( 'NONE',  ( 24.49687500061451573, -3.027376345333614438, 5.243569643749998122 ) ) ;
#14513=CARTESIAN_POINT ( 'NONE',  ( 10.34062500061451750, 6.054752690667223547, 3.707466751127219781E-16 ) ) ;
#14514=CARTESIAN_POINT ( 'NONE',  ( 13.80937500061451750, -4.541064518000417216, -2.621784821875001281 ) ) ;
#14516=CARTESIAN_POINT ( 'NONE',  ( 23.14687500061451786, -3.027376345333614438, 5.243569643749998122 ) ) ;
#14517=CARTESIAN_POINT ( 'NONE',  ( 27.14062500061451644, -3.027376345333614438, 5.243569643749998122 ) ) ;
#14519=CARTESIAN_POINT ( 'NONE',  ( 8.437500000000000000, -2.886751345948129988, 4.999999999999997335 ) ) ;
#14520=CARTESIAN_POINT ( 'NONE',  ( 17.43750000122903288, 4.330127018922191873, 2.499999999999999556 ) ) ;
#14523=ORIENTED_EDGE ( 'NONE', *, *, #70232, .T. ) ;
#14524=CARTESIAN_POINT ( 'NONE',  ( 15.22500000000000142, -4.330127018922194537, 2.499999999999995559 ) ) ;
#14525=CARTESIAN_POINT ( 'NONE',  ( 18.45000000000000284, -4.330127018922190985, -2.500000000000001332 ) ) ;
#14526=CARTESIAN_POINT ( 'NONE',  ( 13.75312500061451715, -4.541064518000417216, -2.621784821875001281 ) ) ;
#14527=VERTEX_POINT ( 'NONE', #24643 ) ;
#14528=CARTESIAN_POINT ( 'NONE',  ( 3.999999999999998668, 18.57500000122903216, -32.30940107675850470 ) ) ;
#14529=CARTESIAN_POINT ( 'NONE',  ( 4.243569643749999010, 17.87187500061451573, -32.45002607614398471 ) ) ;
#14530=CARTESIAN_POINT ( 'NONE',  ( 29.36250000122903003, -4.330127018922190985, -2.500000000000001332 ) ) ;
#14532=CARTESIAN_POINT ( 'NONE',  ( 11.47499999999999964, 4.330127018922191873, 2.499999999999999556 ) ) ;
#14534=VERTEX_POINT ( 'NONE', #40933 ) ;
#14535=CARTESIAN_POINT ( 'NONE',  ( 2.121784821874999061, 15.60312500061451857, 26.32496088578401583 ) ) ;
#14536=CARTESIAN_POINT ( 'NONE',  ( 27.02812500061451573, 4.541064518000418104, 2.621784821874999949 ) ) ;
#14538=CARTESIAN_POINT ( 'NONE',  ( 22.69687500061451857, -3.027376345333614438, 5.243569643749998122 ) ) ;
#14539=CARTESIAN_POINT ( 'NONE',  ( 20.01562500061451644, -6.054752690667223547, -1.112240025338166033E-15 ) ) ;
#14540=CARTESIAN_POINT ( 'NONE',  ( 2.121784821875001281, 14.10312500061459318, -26.32496088578401938 ) ) ;
#14541=CARTESIAN_POINT ( 'NONE',  ( 22.76250000122903216, 4.330127018922192761, -2.499999999999997780 ) ) ;
#14542=CARTESIAN_POINT ( 'NONE',  ( 4.565625000614516260, 3.027376345333611329, 5.243569643749999010 ) ) ;
#14544=CARTESIAN_POINT ( 'NONE',  ( 20.39062500061451644, -3.027376345333614438, 5.243569643749998122 ) ) ;
#14547=CARTESIAN_POINT ( 'NONE',  ( 18.72187500061451360, -6.054752690667223547, -1.112240025338166033E-15 ) ) ;
#14548=CARTESIAN_POINT ( 'NONE',  ( 17.82187500061451502, -6.054752690667223547, -1.112240025338166033E-15 ) ) ;
#14549=CARTESIAN_POINT ( 'NONE',  ( 23.63437500061451502, -4.541064518000419881, 2.621784821874995952 ) ) ;
#14550=CARTESIAN_POINT ( 'NONE',  ( -2.121784821874999949, 13.03437500061451715, 26.32496088578401938 ) ) ;
#14551=CARTESIAN_POINT ( 'NONE',  ( 6.290625000614517681, 6.054752690667223547, 3.707466751127219781E-16 ) ) ;
#14552=CARTESIAN_POINT ( 'NONE',  ( 28.97812500061451502, -4.541064518000419881, 2.621784821874995952 ) ) ;
#14553=( BOUNDED_CURVE ( )  B_SPLINE_CURVE ( 2, ( #43432, #32708, #72231, #21610, #15698, #4999, #9802 ),
 .UNSPECIFIED., .F., .F. ) 
 B_SPLINE_CURVE_WITH_KNOTS ( ( 3, 2, 2, 3 ),
 ( 0.5666666666666667629, 0.5694444444444445308, 0.5722222222222221877, 0.5749999999999999556 ),
 .UNSPECIFIED. ) 
 CURVE ( )  GEOMETRIC_REPRESENTATION_ITEM ( )  RATIONAL_B_SPLINE_CURVE ( ( 0.9999999999999946709, 0.8660254037844440367, 1.000000000000000000, 0.8660254037844387076, 1.000000000000000000, 0.8660254037844387076, 1.000000000000000000 ) ) 
 REPRESENTATION_ITEM ( '' )  );
#14555=CARTESIAN_POINT ( 'NONE',  ( 28.41562500061451502, 3.027376345333611329, 5.243569643749999010 ) ) ;
#14556=CARTESIAN_POINT ( 'NONE',  ( 4.167140676845648706, 2.763139261668956514, -4.167140676845877856 ) ) ;
#14557=DIRECTION ( 'NONE',  ( -0.000000000000000000, -1.000000000000000000, -0.000000000000000000 ) ) ;
#14558=CARTESIAN_POINT ( 'NONE',  ( 8.146875000614516082, 6.054752690667223547, 3.707466751127219781E-16 ) ) ;
#14560=CARTESIAN_POINT ( 'NONE',  ( 14.17500000122903536, 2.886751345948129099, -4.999999999999998224 ) ) ;
#14561=CARTESIAN_POINT ( 'NONE',  ( 10.50000000122903465, -2.886751345948125991, -5.000000000000000000 ) ) ;
#14562=CARTESIAN_POINT ( 'NONE',  ( 4.865625000614517859, 3.027376345333613106, -5.243569643749998122 ) ) ;
#14565=CARTESIAN_POINT ( 'NONE',  ( 14.14687500061451786, -3.027376345333614438, 5.243569643749998122 ) ) ;
#14566=CYLINDRICAL_SURFACE ( 'NONE', #31386, 3.999999999999996447 ) ;
#14568=CARTESIAN_POINT ( 'NONE',  ( 22.94062500061451715, 6.054752690667223547, 3.707466751127219781E-16 ) ) ;
#14569=CARTESIAN_POINT ( 'NONE',  ( 7.415625000614516793, -6.054752690667223547, -1.112240025338166033E-15 ) ) ;
#14570=CARTESIAN_POINT ( 'NONE',  ( 23.40937500061451715, 4.541064518000418104, -2.621784821874998173 ) ) ;
#14571=CARTESIAN_POINT ( 'NONE',  ( 8.165625000614516793, 3.027376345333611329, 5.243569643749999010 ) ) ;
#14572=DIRECTION ( 'NONE',  ( 0.000000000000000000, 0.000000000000000000, 1.000000000000000000 ) ) ;
#14573=CARTESIAN_POINT ( 'NONE',  ( 8.700000001229032165, -2.886751345948125991, -5.000000000000000000 ) ) ;
#14574=CARTESIAN_POINT ( 'NONE',  ( 22.86562500061451431, 3.027376345333613106, -5.243569643749998122 ) ) ;
#14575=CARTESIAN_POINT ( 'NONE',  ( -4.243569643749999898, 10.35312500061451857, -30.00000000000000000 ) ) ;
#14576=CARTESIAN_POINT ( 'NONE',  ( 10.38750000122903572, -4.330127018922194537, 2.499999999999995559 ) ) ;
#14577=CARTESIAN_POINT ( 'NONE',  ( 20.87812500061451715, -4.541064518000419881, 2.621784821874995952 ) ) ;
#14578=CARTESIAN_POINT ( 'NONE',  ( 18.89062500061451644, 6.054752690667223547, 3.707466751127219781E-16 ) ) ;
#14580=CARTESIAN_POINT ( 'NONE',  ( 17.32499999999999929, 4.330127018922191873, 2.499999999999999556 ) ) ;
#14581=CARTESIAN_POINT ( 'NONE',  ( 11.73750000122903181, -4.330127018922194537, 2.499999999999995559 ) ) ;
#14582=CARTESIAN_POINT ( 'NONE',  ( 11.01562500061451821, -6.054752690667223547, -1.112240025338166033E-15 ) ) ;
#14583=CARTESIAN_POINT ( 'NONE',  ( 12.44062500061451537, -3.027376345333610441, -5.243569643749999898 ) ) ;
#14584=CARTESIAN_POINT ( 'NONE',  ( 22.98750000122903003, -4.330127018922194537, 2.499999999999995559 ) ) ;
#14585=CARTESIAN_POINT ( 'NONE',  ( 20.85937500061451644, 0.000000000000000000, 5.243569643749999010 ) ) ;
#14586=CARTESIAN_POINT ( 'NONE',  ( 3.575968405063141731, 3.494640511729611099, -3.909292473339659235 ) ) ;
#14587=CARTESIAN_POINT ( 'NONE',  ( 6.300000001229033586, -2.886751345948129988, 4.999999999999997335 ) ) ;
#14588=CARTESIAN_POINT ( 'NONE',  ( 6.271875000614517859, 3.027376345333613106, -5.243569643749998122 ) ) ;
#14589=CARTESIAN_POINT ( 'NONE',  ( 24.42187500061451999, 3.027376345333611329, 5.243569643749999010 ) ) ;
#14590=CARTESIAN_POINT ( 'NONE',  ( 4.746675283896760078, -1.572051564878419683, 4.883304218962898346 ) ) ;
#14591=CARTESIAN_POINT ( 'NONE',  ( 19.60312500061451502, -4.541064518000417216, -2.621784821875001281 ) ) ;
#14592=CARTESIAN_POINT ( 'NONE',  ( 24.64687500061451431, -3.027376345333610441, -5.243569643749999898 ) ) ;
#14595=CARTESIAN_POINT ( 'NONE',  ( 27.86250000122903359, 0.000000000000000000, 4.999999999999998224 ) ) ;
#14596=CARTESIAN_POINT ( 'NONE',  ( 4.284375000614518925, -4.541064518000419881, 2.621784821874995952 ) ) ;
#14597=CARTESIAN_POINT ( 'NONE',  ( 16.22812500061451857, 4.541064518000418104, 2.621784821874999949 ) ) ;
#14598=CARTESIAN_POINT ( 'NONE',  ( 12.68437500061451573, 4.541064518000418104, 2.621784821874999949 ) ) ;
#14599=ORIENTED_EDGE ( 'NONE', *, *, #36502, .T. ) ;
#14600=CARTESIAN_POINT ( 'NONE',  ( 2.000000000000001332, 17.00000000000000000, -26.53589838486224650 ) ) ;
#14601=CARTESIAN_POINT ( 'NONE',  ( 24.06562500061451715, -6.054752690667223547, -1.112240025338166033E-15 ) ) ;
#14602=CARTESIAN_POINT ( 'NONE',  ( 1.071796769724497445, 17.16740381056766651, 26.00000000000000355 ) ) ;
#14604=CARTESIAN_POINT ( 'NONE',  ( 14.73749999999999893, -2.886751345948129988, 4.999999999999997335 ) ) ;
#14605=CARTESIAN_POINT ( 'NONE',  ( 23.92500000122903359, -5.773502691896255534, -1.060575238724906372E-15 ) ) ;
#14606=CARTESIAN_POINT ( 'NONE',  ( 17.57812500061451644, 4.541064518000418104, 2.621784821874999949 ) ) ;
#14607=ORIENTED_EDGE ( 'NONE', *, *, #61749, .F. ) ;
#14608=CARTESIAN_POINT ( 'NONE',  ( 21.93750000000000000, -2.886751345948129988, 4.999999999999997335 ) ) ;
#14609=CARTESIAN_POINT ( 'NONE',  ( 23.25937500061451857, -4.541064518000417216, -2.621784821875001281 ) ) ;
#14611=CARTESIAN_POINT ( 'NONE',  ( 2.964777361493091679, -4.026176250088806086, -3.359304602455296607 ) ) ;
#14612=CARTESIAN_POINT ( 'NONE',  ( 12.02812500061451573, 6.421520780324663323E-16, -5.243569643749999010 ) ) ;
#14613=CARTESIAN_POINT ( 'NONE',  ( 3.365625000614516082, -6.054752690667223547, -1.112240025338166033E-15 ) ) ;
#14615=CARTESIAN_POINT ( 'NONE',  ( 27.36562500061451786, 3.027376345333613106, -5.243569643749998122 ) ) ;
#14616=CARTESIAN_POINT ( 'NONE',  ( 19.83750000000000213, -2.886751345948125991, -5.000000000000000000 ) ) ;
#14617=CARTESIAN_POINT ( 'NONE',  ( 27.07499999999999929, 6.123233995736764310E-16, -4.999999999999998224 ) ) ;
#14619=CARTESIAN_POINT ( 'NONE',  ( 7.546875000614517326, -3.027376345333610441, -5.243569643749999898 ) ) ;
#14620=CARTESIAN_POINT ( 'NONE',  ( 18.08437500061451431, 4.541064518000418104, 2.621784821874999949 ) ) ;
#14621=CARTESIAN_POINT ( 'NONE',  ( -1.999999999999997113, 13.88750000122903394, 33.46410161513775705 ) ) ;
#14622=ORIENTED_EDGE ( 'NONE', *, *, #1071, .T. ) ;
#14623=CARTESIAN_POINT ( 'NONE',  ( 27.40312500061451573, 4.541064518000418104, -2.621784821874998173 ) ) ;
#14624=CARTESIAN_POINT ( 'NONE',  ( 28.80937500061451573, 4.541064518000418104, -2.621784821874998173 ) ) ;
#14625=CARTESIAN_POINT ( 'NONE',  ( 3.046875000614519990, -3.027376345333610441, -5.243569643749999898 ) ) ;
#14626=CARTESIAN_POINT ( 'NONE',  ( 16.31250000000000000, 2.886751345948129099, -4.999999999999998224 ) ) ;
#14627=CARTESIAN_POINT ( 'NONE',  ( 10.56562500061451715, -6.054752690667223547, -1.112240025338166033E-15 ) ) ;
#14629=CARTESIAN_POINT ( 'NONE',  ( 28.45312500061451289, 0.000000000000000000, 5.243569643749999010 ) ) ;
#14630=CARTESIAN_POINT ( 'NONE',  ( 19.05000000122903359, -2.886751345948125991, -5.000000000000000000 ) ) ;
#14631=CARTESIAN_POINT ( 'NONE',  ( 3.139915822865742445, -3.891420429212240073, 3.139915822865742445 ) ) ;
#14633=CARTESIAN_POINT ( 'NONE',  ( 4.153125000614515727, 0.000000000000000000, 5.243569643749999010 ) ) ;
#14634=CARTESIAN_POINT ( 'NONE',  ( 22.80937500061451573, -4.541064518000417216, -2.621784821875001281 ) ) ;
#14635=CARTESIAN_POINT ( 'NONE',  ( 2.121784821874999061, 16.10937500061451644, 26.32496088578401583 ) ) ;
#14636=CARTESIAN_POINT ( 'NONE',  ( 24.60937500061451644, -4.541064518000417216, -2.621784821875001281 ) ) ;
#14637=CARTESIAN_POINT ( 'NONE',  ( 5.887500000000000178, -2.886751345948125991, -5.000000000000000000 ) ) ;
#14638=CARTESIAN_POINT ( 'NONE',  ( 2.000000000000001332, 10.81250000122903465, 33.46410161513774995 ) ) ;
#14639=CARTESIAN_POINT ( 'NONE',  ( 11.80312500061451608, 0.000000000000000000, 5.243569643749999010 ) ) ;
#14640=CARTESIAN_POINT ( 'NONE',  ( 4.537500001229034297, -4.330127018922194537, 2.499999999999995559 ) ) ;
#14642=CARTESIAN_POINT ( 'NONE',  ( 9.234375000614518214, -4.541064518000419881, 2.621784821874995952 ) ) ;
#14644=CARTESIAN_POINT ( 'NONE',  ( 9.815625000614518925, 3.027376345333613106, -5.243569643749998122 ) ) ;
#14645=CARTESIAN_POINT ( 'NONE',  ( 15.30937500061451750, 4.541064518000418104, -2.621784821874998173 ) ) ;
#14647=CARTESIAN_POINT ( 'NONE',  ( 22.20000000122903216, -2.886751345948125991, -5.000000000000000000 ) ) ;
#14648=CARTESIAN_POINT ( 'NONE',  ( 9.496875000614517504, 6.054752690667223547, 3.707466751127219781E-16 ) ) ;
#14649=CARTESIAN_POINT ( 'NONE',  ( 12.62812500061451537, 4.541064518000418104, 2.621784821874999949 ) ) ;
#14651=CARTESIAN_POINT ( 'NONE',  ( 22.62187500061451573, 3.027376345333611329, 5.243569643749999010 ) ) ;
#14652=CARTESIAN_POINT ( 'NONE',  ( -3.999999999999997335, 12.05000000122903359, -27.69059892324149530 ) ) ;
#14654=CARTESIAN_POINT ( 'NONE',  ( 4.243569643749999898, 14.23437500061451821, -30.00000000000000000 ) ) ;
#14655=CARTESIAN_POINT ( 'NONE',  ( 16.01250000122903216, 4.330127018922192761, -2.499999999999997780 ) ) ;
#14656=CARTESIAN_POINT ( 'NONE',  ( 9.946875000614516793, 6.054752690667223547, 3.707466751127219781E-16 ) ) ;
#14657=CARTESIAN_POINT ( 'NONE',  ( 4.243569643749999010, 16.91562500061451502, -32.45002607614398471 ) ) ;
#14658=CARTESIAN_POINT ( 'NONE',  ( 17.06250000122903288, 0.000000000000000000, 4.999999999999998224 ) ) ;
#14659=CARTESIAN_POINT ( 'NONE',  ( 11.87812500061451537, -4.541064518000419881, 2.621784821874995952 ) ) ;
#14660=VECTOR ( 'NONE', #68814, 1000.000000000000000 ) ;
#14662=CARTESIAN_POINT ( 'NONE',  ( 16.61250000000000426, -5.773502691896255534, -1.060575238724906372E-15 ) ) ;
#14664=CARTESIAN_POINT ( 'NONE',  ( 9.196875000614518569, -3.027376345333614438, 5.243569643749998122 ) ) ;
#14666=CARTESIAN_POINT ( 'NONE',  ( 12.26250000122903394, -4.330127018922190985, -2.500000000000001332 ) ) ;
#14667=CARTESIAN_POINT ( 'NONE',  ( 20.92500000122903714, 2.886751345948129099, -4.999999999999998224 ) ) ;
#14668=CARTESIAN_POINT ( 'NONE',  ( 17.09062500061451573, 6.054752690667223547, 3.707466751127219781E-16 ) ) ;
#14669=CARTESIAN_POINT ( 'NONE',  ( 21.74062500061451431, -3.027376345333614438, 5.243569643749998122 ) ) ;
#14670=CARTESIAN_POINT ( 'NONE',  ( 28.68750000122903288, 4.330127018922191873, 2.499999999999999556 ) ) ;
#14671=CARTESIAN_POINT ( 'NONE',  ( 4.153125000614515727, 0.000000000000000000, 5.243569643749999010 ) ) ;
#14672=CARTESIAN_POINT ( 'NONE',  ( 24.63749999999999574, -2.886751345948129988, 4.999999999999997335 ) ) ;
#14673=FACE_OUTER_BOUND ( 'NONE', #10103, .T. ) ;
#14675=CARTESIAN_POINT ( 'NONE',  ( 28.58437500061451786, -4.541064518000419881, 2.621784821874995952 ) ) ;
#14676=CARTESIAN_POINT ( 'NONE',  ( 2.000000000000001332, 12.50000000000000000, -26.53589838486224650 ) ) ;
#14677=CARTESIAN_POINT ( 'NONE',  ( 2.887500001229035274, 6.123233995736764310E-16, -4.999999999999998224 ) ) ;
#14678=CARTESIAN_POINT ( 'NONE',  ( 3.149999999999999911, -4.330127018922190985, -2.500000000000001332 ) ) ;
#14681=CARTESIAN_POINT ( 'NONE',  ( 8.259375000614518569, 0.000000000000000000, 5.243569643749999010 ) ) ;
#14682=CARTESIAN_POINT ( 'NONE',  ( 25.37812500061451715, -4.541064518000419881, 2.621784821874995952 ) ) ;
#14685=CARTESIAN_POINT ( 'NONE',  ( 1.071796769724491893, 10.34509619066136921, 33.99999999999999289 ) ) ;
#14687=CARTESIAN_POINT ( 'NONE',  ( 4.621875000614516615, 3.027376345333611329, 5.243569643749999010 ) ) ;
#14688=CARTESIAN_POINT ( 'NONE',  ( 8.634375000614518569, 4.541064518000418104, 2.621784821874999949 ) ) ;
#14689=CARTESIAN_POINT ( 'NONE',  ( 4.537500000000000533, -2.886751345948125991, -5.000000000000000000 ) ) ;
#14690=CARTESIAN_POINT ( 'NONE',  ( 4.243569643749999898, 11.47812500061459495, 30.00000000000000000 ) ) ;
#14691=CARTESIAN_POINT ( 'NONE',  ( 29.84999999999999787, 4.330127018922192761, -2.499999999999997780 ) ) ;
#14692=EDGE_CURVE ( 'NONE', #54008, #30532, #11971, .T. ) ;
#14693=CARTESIAN_POINT ( 'NONE',  ( 3.975000000000002753, -4.330127018922194537, 2.499999999999995559 ) ) ;
#14696=CARTESIAN_POINT ( 'NONE',  ( 20.69062500061451715, 6.054752690667223547, 3.707466751127219781E-16 ) ) ;
#14697=CARTESIAN_POINT ( 'NONE',  ( 10.37812500061451715, 4.541064518000418104, 2.621784821874999949 ) ) ;
#14699=CARTESIAN_POINT ( 'NONE',  ( 7.171875000614517326, 3.027376345333613106, -5.243569643749998122 ) ) ;
#14700=CARTESIAN_POINT ( 'NONE',  ( 23.73749999999999716, -2.886751345948129988, 4.999999999999997335 ) ) ;
#14701=CARTESIAN_POINT ( 'NONE',  ( 19.08750000122903145, 6.123233995736764310E-16, -4.999999999999998224 ) ) ;
#14702=CARTESIAN_POINT ( 'NONE',  ( 28.00312500061451715, 0.000000000000000000, 5.243569643749999010 ) ) ;
#14704=CARTESIAN_POINT ( 'NONE',  ( 9.346875000614517148, -3.027376345333610441, -5.243569643749999898 ) ) ;
#14705=CARTESIAN_POINT ( 'NONE',  ( 14.14687500061451786, -3.027376345333614438, 5.243569643749998122 ) ) ;
#14706=CARTESIAN_POINT ( 'NONE',  ( 24.75937500061451502, 4.541064518000418104, -2.621784821874998173 ) ) ;
#14708=CARTESIAN_POINT ( 'NONE',  ( 2.000000000000001332, 18.01250000122903572, -26.53589838486224650 ) ) ;
#14710=CARTESIAN_POINT ( 'NONE',  ( 19.39687500061451786, 6.054752690667223547, 3.707466751127219781E-16 ) ) ;
#14711=AXIS2_PLACEMENT_3D ( 'NONE', #46590, #25505, #43603 ) ;
#14712=CARTESIAN_POINT ( 'NONE',  ( 10.35937500061451644, 4.541064518000418104, -2.621784821874998173 ) ) ;
#14714=CARTESIAN_POINT ( 'NONE',  ( 22.53750000000000142, -2.886751345948125991, -5.000000000000000000 ) ) ;
#14716=LINE ( 'NONE', #66063, #899 ) ;
#14718=CARTESIAN_POINT ( 'NONE',  ( 11.39062500061451644, -3.027376345333614438, 5.243569643749998122 ) ) ;
#14719=CARTESIAN_POINT ( 'NONE',  ( 5.325000000000000178, -4.330127018922194537, 2.499999999999995559 ) ) ;
#14720=FACE_OUTER_BOUND ( 'NONE', #15031, .T. ) ;
#14721=CARTESIAN_POINT ( 'NONE',  ( 11.96250000000000213, 2.886751345948126879, 4.999999999999999112 ) ) ;
#14722=CARTESIAN_POINT ( 'NONE',  ( -3.999999999999999112, 17.86250000122903359, 30.00000000000000000 ) ) ;
#14723=CARTESIAN_POINT ( 'NONE',  ( 11.06250000122903288, 4.330127018922192761, -2.499999999999997780 ) ) ;
#14724=AXIS2_PLACEMENT_3D ( 'NONE', #27563, #21636, #34172 ) ;
#14725=CARTESIAN_POINT ( 'NONE',  ( 21.75937500061451502, 0.000000000000000000, 5.243569643749999010 ) ) ;
#14726=CARTESIAN_POINT ( 'NONE',  ( 16.47187500061452070, -6.054752690667223547, -1.112240025338166033E-15 ) ) ;
#14728=VERTEX_POINT ( 'NONE', #35729 ) ;
#14729=CARTESIAN_POINT ( 'NONE',  ( 17.95312500061451644, 4.541064518000418104, -2.621784821874998173 ) ) ;
#14730=CARTESIAN_POINT ( 'NONE',  ( 29.66250000122903074, 0.000000000000000000, 4.999999999999998224 ) ) ;
#14731=CARTESIAN_POINT ( 'NONE',  ( 16.43437500061451573, -4.541064518000419881, 2.621784821874995952 ) ) ;
#14732=CARTESIAN_POINT ( 'NONE',  ( 28.65937500061451715, -4.541064518000417216, -2.621784821875001281 ) ) ;
#14733=CARTESIAN_POINT ( 'NONE',  ( 4.265625000614517326, -6.054752690667223547, -1.112240025338166033E-15 ) ) ;
#14734=CARTESIAN_POINT ( 'NONE',  ( 19.45312500061451644, 0.000000000000000000, 5.243569643749999010 ) ) ;
#14735=CARTESIAN_POINT ( 'NONE',  ( 28.50937500061451502, 0.000000000000000000, 5.243569643749999010 ) ) ;
#14736=CARTESIAN_POINT ( 'NONE',  ( 4.243569643749999898, 12.34062500061451750, 32.45002607614398471 ) ) ;
#14737=CARTESIAN_POINT ( 'NONE',  ( 16.08750000122903501, 4.330127018922191873, 2.499999999999999556 ) ) ;
#14739=CARTESIAN_POINT ( 'NONE',  ( 6.665625000614517681, 3.027376345333612662, -5.243569643749998122 ) ) ;
#14740=CARTESIAN_POINT ( 'NONE',  ( 26.54062500061451146, 6.054752690667223547, 3.707466751127219781E-16 ) ) ;
#14741=DIRECTION ( 'NONE',  ( 0.000000000000000000, 0.000000000000000000, 1.000000000000000000 ) ) ;
#14742=CARTESIAN_POINT ( 'NONE',  ( 23.67187500061451999, -6.054752690667223547, -1.112240025338166033E-15 ) ) ;
#14743=CARTESIAN_POINT ( 'NONE',  ( 14.57812500061451644, -4.541064518000419881, 2.621784821874995952 ) ) ;
#14744=CARTESIAN_POINT ( 'NONE',  ( 22.61250000122903003, -4.330127018922190985, -2.500000000000001332 ) ) ;
#14745=CARTESIAN_POINT ( 'NONE',  ( 23.99062500061451786, -3.027376345333614438, 5.243569643749998122 ) ) ;
#14746=CARTESIAN_POINT ( 'NONE',  ( 19.95937500061451786, 0.000000000000000000, 5.243569643749999010 ) ) ;
#14747=CARTESIAN_POINT ( 'NONE',  ( 12.81562500061451537, -6.054752690667223547, -1.112240025338166033E-15 ) ) ;
#14748=CARTESIAN_POINT ( 'NONE',  ( -4.243569643749999898, 15.35937500061451644, 30.00000000000000000 ) ) ;
#14749=CARTESIAN_POINT ( 'NONE',  ( 18.66562500061451146, -6.054752690667223547, -1.112240025338166033E-15 ) ) ;
#14750=CARTESIAN_POINT ( 'NONE',  ( 28.79062500061451502, 6.054752690667223547, 3.707466751127219781E-16 ) ) ;
#14752=CARTESIAN_POINT ( 'NONE',  ( 22.16250000000000142, 2.886751345948129099, -4.999999999999998224 ) ) ;
#14753=CARTESIAN_POINT ( 'NONE',  ( 2.121784821874999061, 19.70937500061451786, -33.67503911421598417 ) ) ;
#14754=CARTESIAN_POINT ( 'NONE',  ( 27.62812500061451360, -4.541064518000419881, 2.621784821874995952 ) ) ;
#14755=CARTESIAN_POINT ( 'NONE',  ( 4.790625000614518569, -3.027376345333610441, -5.243569643749999898 ) ) ;
#14756=CARTESIAN_POINT ( 'NONE',  ( 20.70000000122903216, -2.886751345948129988, 4.999999999999997335 ) ) ;
#14757=CARTESIAN_POINT ( 'NONE',  ( 25.79062500061451502, -3.027376345333614438, 5.243569643749998122 ) ) ;
#14758=CARTESIAN_POINT ( 'NONE',  ( 23.43750000000000000, -2.886751345948125991, -5.000000000000000000 ) ) ;
#14759=CARTESIAN_POINT ( 'NONE',  ( 27.66562500061451146, -6.054752690667223547, -1.112240025338166033E-15 ) ) ;
#14760=CARTESIAN_POINT ( 'NONE',  ( 7.303125000614516082, 0.000000000000000000, 5.243569643749999010 ) ) ;
#14762=CARTESIAN_POINT ( 'NONE',  ( 22.71562500061451573, -6.054752690667223547, -1.112240025338166033E-15 ) ) ;
#14763=CARTESIAN_POINT ( 'NONE',  ( 5.953125000614519102, 0.000000000000000000, 5.243569643749999010 ) ) ;
#14764=VECTOR ( 'NONE', #22737, 1000.000000000000000 ) ;
#14766=CARTESIAN_POINT ( 'NONE',  ( 4.190625000614518925, -3.027376345333614438, 5.243569643749998122 ) ) ;
#14767=CARTESIAN_POINT ( 'NONE',  ( 1.999999999999998668, 14.56250000122903288, -33.46410161513775705 ) ) ;
#14769=CARTESIAN_POINT ( 'NONE',  ( 11.25000000000000000, -4.330127018922190985, -2.500000000000001332 ) ) ;
#14772=CARTESIAN_POINT ( 'NONE',  ( 11.37187500061451750, 3.027376345333611329, 5.243569643749999010 ) ) ;
#14773=CARTESIAN_POINT ( 'NONE',  ( 7.687500001229033764, -4.330127018922194537, 2.499999999999995559 ) ) ;
#14774=CARTESIAN_POINT ( 'NONE',  ( 15.12187500061451750, -6.054752690667223547, -1.112240025338166033E-15 ) ) ;
#14776=CARTESIAN_POINT ( 'NONE',  ( 5.859375000614519102, 4.541064518000418104, -2.621784821874998173 ) ) ;
#14778=VECTOR ( 'NONE', #47212, 1000.000000000000000 ) ;
#14779=CARTESIAN_POINT ( 'NONE',  ( 0.000000000000000000, 20.00000000000000000, -30.00000000000000000 ) ) ;
#14780=CARTESIAN_POINT ( 'NONE',  ( 11.89687500061451608, -3.027376345333614438, 5.243569643749998122 ) ) ;
#14781=CARTESIAN_POINT ( 'NONE',  ( 3.709174336338540989, 3.352913023424228811, 4.031500572517469294 ) ) ;
#14782=CARTESIAN_POINT ( 'NONE',  ( 21.51562500061451644, 3.027376345333613106, -5.243569643749998122 ) ) ;
#14783=CARTESIAN_POINT ( 'NONE',  ( 4.000000000000000000, 11.63750000000000284, 32.30940107675849760 ) ) ;
#14784=CARTESIAN_POINT ( 'NONE',  ( 4.243569643749999010, 18.71562500061459389, 27.54997392385601174 ) ) ;
#14785=CARTESIAN_POINT ( 'NONE',  ( 25.20937500061451431, 4.541064518000418104, -2.621784821874998173 ) ) ;
#14786=EDGE_CURVE ( 'NONE', #48144, #66704, #72388, .T. ) ;
#14787=CARTESIAN_POINT ( 'NONE',  ( 29.69999999999999574, -4.330127018922190985, -2.500000000000001332 ) ) ;
#14788=CARTESIAN_POINT ( 'NONE',  ( 4.903125000614516615, 4.541064518000418104, -2.621784821874998173 ) ) ;
#14790=CARTESIAN_POINT ( 'NONE',  ( 13.13437500061451857, 4.541064518000418104, 2.621784821874999949 ) ) ;
#14792=CARTESIAN_POINT ( 'NONE',  ( 27.78750000122903074, 4.330127018922191873, 2.499999999999999556 ) ) ;
#14793=CARTESIAN_POINT ( 'NONE',  ( 5.109375000614518214, 0.000000000000000000, 5.243569643749999010 ) ) ;
#14794=CARTESIAN_POINT ( 'NONE',  ( 16.32187500061451502, 3.027376345333611329, 5.243569643749999010 ) ) ;
#14795=CARTESIAN_POINT ( 'NONE',  ( 25.38749999999999929, 5.773502691896255534, 3.535250795749688894E-16 ) ) ;
#14796=CARTESIAN_POINT ( 'NONE',  ( 3.900000001229034563, 5.773502691896255534, 3.535250795749688894E-16 ) ) ;
#14797=CARTESIAN_POINT ( 'NONE',  ( 26.10937500061451644, 4.541064518000418104, -2.621784821874998173 ) ) ;
#14799=CARTESIAN_POINT ( 'NONE',  ( 29.66249999999999432, -5.773502691896255534, -1.060575238724906372E-15 ) ) ;
#14800=CARTESIAN_POINT ( 'NONE',  ( 8.887499999999999289, -2.886751345948129988, 4.999999999999997335 ) ) ;
#14802=CARTESIAN_POINT ( 'NONE',  ( 22.94062500061451715, 6.054752690667223547, 3.707466751127219781E-16 ) ) ;
#14803=CARTESIAN_POINT ( 'NONE',  ( 12.22499999999999964, 6.123233995736764310E-16, -4.999999999999998224 ) ) ;
#14804=CARTESIAN_POINT ( 'NONE',  ( 5.165625000614518569, -6.054752690667223547, -1.112240025338166033E-15 ) ) ;
#14805=CARTESIAN_POINT ( 'NONE',  ( 18.97499999999999787, 6.123233995736764310E-16, -4.999999999999998224 ) ) ;
#14806=CARTESIAN_POINT ( 'NONE',  ( 19.41562500061451146, 3.027376345333611329, 5.243569643749999010 ) ) ;
#14808=CARTESIAN_POINT ( 'NONE',  ( 22.72500000122903430, 2.886751345948129099, -4.999999999999998224 ) ) ;
#14810=CARTESIAN_POINT ( 'NONE',  ( 3.450000000000001510, 0.000000000000000000, 4.999999999999998224 ) ) ;
#14811=AXIS2_PLACEMENT_3D ( 'NONE', #64534, #63449, #29471 ) ;
#14812=EDGE_LOOP ( 'NONE', ( #18218, #23002, #62515, #69440 ) ) ;
#14813=CARTESIAN_POINT ( 'NONE',  ( 20.35312500061451502, 0.000000000000000000, 5.243569643749999010 ) ) ;
#14814=CARTESIAN_POINT ( 'NONE',  ( 24.14062500061451289, -3.027376345333610441, -5.243569643749999898 ) ) ;
#14815=CARTESIAN_POINT ( 'NONE',  ( 24.94687500061451502, -3.027376345333614438, 5.243569643749998122 ) ) ;
#14816=CARTESIAN_POINT ( 'NONE',  ( 8.400000000000000355, 0.000000000000000000, 4.999999999999998224 ) ) ;
#14817=CARTESIAN_POINT ( 'NONE',  ( 11.99062500061451608, -3.027376345333610441, -5.243569643749999898 ) ) ;
#14818=CARTESIAN_POINT ( 'NONE',  ( 25.86562500061451431, -6.054752690667223547, -1.112240025338166033E-15 ) ) ;
#14819=CARTESIAN_POINT ( 'NONE',  ( 17.55937500061451573, 4.541064518000418104, -2.621784821874998173 ) ) ;
#14820=CARTESIAN_POINT ( 'NONE',  ( 8.053125000614516082, 4.541064518000418104, -2.621784821874998173 ) ) ;
#14821=CARTESIAN_POINT ( 'NONE',  ( 2.923357432354301455, -4.056350739605543154, 3.322806236625610588 ) ) ;
#14822=CARTESIAN_POINT ( 'NONE',  ( -1.473776270879187500, 9.872922227264545825, 25.95083297442941017 ) ) ;
#14824=CARTESIAN_POINT ( 'NONE',  ( 23.66250000122903430, 4.330127018922192761, -2.499999999999997780 ) ) ;
#14826=CARTESIAN_POINT ( 'NONE',  ( 15.21562500061451750, 3.027376345333612662, -5.243569643749998122 ) ) ;
#14827=CARTESIAN_POINT ( 'NONE',  ( 8.634375000614518569, 4.541064518000418104, 2.621784821874999949 ) ) ;
#14828=CARTESIAN_POINT ( 'NONE',  ( 7.284375000614518036, 4.541064518000418104, 2.621784821874999949 ) ) ;
#14829=VERTEX_POINT ( 'NONE', #53691 ) ;
#14830=CARTESIAN_POINT ( 'NONE',  ( -3.517994946560660807, 9.362281625417800512, 34.86422368405397521 ) ) ;
#14831=CARTESIAN_POINT ( 'NONE',  ( 22.90312500061451573, 4.541064518000418104, -2.621784821874998173 ) ) ;
#14832=AXIS2_PLACEMENT_3D ( 'NONE', #42602, #37051, #71412 ) ;
#14833=CARTESIAN_POINT ( 'NONE',  ( 16.02187500061451786, -6.054752690667223547, -1.112240025338166033E-15 ) ) ;
#14834=CARTESIAN_POINT ( 'NONE',  ( 21.92812500061451431, 6.421520780324663323E-16, -5.243569643749999010 ) ) ;
#14835=CARTESIAN_POINT ( 'NONE',  ( 1.999999999999998668, 12.65000000000000213, 26.53589838486224650 ) ) ;
#14836=CARTESIAN_POINT ( 'NONE',  ( 26.35312500061451857, -4.541064518000417216, -2.621784821875001281 ) ) ;
#14837=CARTESIAN_POINT ( 'NONE',  ( 7.312500001229033764, -4.330127018922190985, -2.500000000000001332 ) ) ;
#14839=VERTEX_POINT ( 'NONE', #3085 ) ;
#14840=CARTESIAN_POINT ( 'NONE',  ( 29.43750000000000000, 5.773502691896255534, 3.535250795749688894E-16 ) ) ;
#14841=CARTESIAN_POINT ( 'NONE',  ( -1.999999999999997113, 17.82499999999999929, -26.53589838486224295 ) ) ;
#14842=CARTESIAN_POINT ( 'NONE',  ( 25.65000000122903145, -2.886751345948129988, 4.999999999999997335 ) ) ;
#14844=CARTESIAN_POINT ( 'NONE',  ( 7.209375000614519635, 4.541064518000418104, -2.621784821874998173 ) ) ;
#14845=CARTESIAN_POINT ( 'NONE',  ( 30.00000000000000000, 0.000000000000000000, 4.999999999999998224 ) ) ;
#14846=ADVANCED_FACE ( 'NONE', ( #70676 ), #65131, .F. ) ;
#14847=CARTESIAN_POINT ( 'NONE',  ( 15.96562500061451573, -6.054752690667223547, -1.112240025338166033E-15 ) ) ;
#14848=CARTESIAN_POINT ( 'NONE',  ( 7.884375000614517681, -4.541064518000419881, 2.621784821874995952 ) ) ;
#14849=CARTESIAN_POINT ( 'NONE',  ( 27.37500000122903288, 2.886751345948126879, 4.999999999999999112 ) ) ;
#14850=CARTESIAN_POINT ( 'NONE',  ( 18.38437500061451857, 6.421520780324663323E-16, -5.243569643749999010 ) ) ;
#14851=CARTESIAN_POINT ( 'NONE',  ( 4.771875000614516971, -6.054752690667223547, -1.112240025338166033E-15 ) ) ;
#14852=CARTESIAN_POINT ( 'NONE',  ( 7.875000001229034652, 2.886751345948129099, -4.999999999999997335 ) ) ;
#14853=CARTESIAN_POINT ( 'NONE',  ( 6.403125000614517504, 0.000000000000000000, 5.243569643749999010 ) ) ;
#14854=CARTESIAN_POINT ( 'NONE',  ( 15.66562500061451857, 3.027376345333613106, -5.243569643749998122 ) ) ;
#14856=CARTESIAN_POINT ( 'NONE',  ( 13.52812500061451750, 4.541064518000418104, 2.621784821874999949 ) ) ;
#14857=CARTESIAN_POINT ( 'NONE',  ( 5.812500001229035540, 0.000000000000000000, 4.999999999999998224 ) ) ;
#14858=CARTESIAN_POINT ( 'NONE',  ( 8.353125000614518569, -4.541064518000417216, -2.621784821875001281 ) ) ;
#14860=CARTESIAN_POINT ( 'NONE',  ( 11.43750000000000000, 5.773502691896255534, 3.535250795749688894E-16 ) ) ;
#14861=CARTESIAN_POINT ( 'NONE',  ( 4.200000001229033053, -2.886751345948125991, -5.000000000000000000 ) ) ;
#14862=CARTESIAN_POINT ( 'NONE',  ( 18.41250000000000142, -5.773502691896255534, -1.060575238724906372E-15 ) ) ;
#14863=CARTESIAN_POINT ( 'NONE',  ( 19.24687500061452283, -3.027376345333610441, -5.243569643749999898 ) ) ;
#14864=CARTESIAN_POINT ( 'NONE',  ( 16.05000000122903359, 5.773502691896255534, 3.535250795749688894E-16 ) ) ;
#14867=CARTESIAN_POINT ( 'NONE',  ( -4.243569643749999898, 15.71562500061451573, -32.45002607614398471 ) ) ;
#14868=CARTESIAN_POINT ( 'NONE',  ( -1.487416814333745711E-14, 16.62500000122903288, -26.00000000000000000 ) ) ;
#14870=CARTESIAN_POINT ( 'NONE',  ( 30.00000000000000000, 0.000000000000000000, 4.999999999999998224 ) ) ;
#14871=CARTESIAN_POINT ( 'NONE',  ( 28.52812500061451573, -4.541064518000419881, 2.621784821874995952 ) ) ;
#14873=CARTESIAN_POINT ( 'NONE',  ( 15.68437500061451573, 6.421520780324663323E-16, -5.243569643749999010 ) ) ;
#14874=EDGE_CURVE ( 'NONE', #55745, #67926, #14889, .T. ) ;
#14875=CARTESIAN_POINT ( 'NONE',  ( 28.87499999999999645, 6.123233995736764310E-16, -4.999999999999998224 ) ) ;
#14876=CARTESIAN_POINT ( 'NONE',  ( 10.82812500061451644, 4.541064518000418104, 2.621784821874999949 ) ) ;
#14878=CARTESIAN_POINT ( 'NONE',  ( 25.02187500061451431, -6.054752690667223547, -1.112240025338166033E-15 ) ) ;
#14880=CARTESIAN_POINT ( 'NONE',  ( 6.965625000614518392, -6.054752690667223547, -1.112240025338166033E-15 ) ) ;
#14881=CARTESIAN_POINT ( 'NONE',  ( 13.28437500061451715, -4.541064518000419881, 2.621784821874995952 ) ) ;
#14882=ORIENTED_EDGE ( 'NONE', *, *, #58832, .F. ) ;
#14883=CARTESIAN_POINT ( 'NONE',  ( 22.99687500061451573, 6.054752690667223547, 3.707466751127219781E-16 ) ) ;
#14884=CARTESIAN_POINT ( 'NONE',  ( 27.81562500061452070, 3.027376345333613106, -5.243569643749998122 ) ) ;
#14886=CARTESIAN_POINT ( 'NONE',  ( 6.975000000000002309, 4.330127018922191873, 2.499999999999999556 ) ) ;
#14887=CARTESIAN_POINT ( 'NONE',  ( 15.82500000122903216, -5.773502691896255534, -1.060575238724906372E-15 ) ) ;
#14889=LINE ( 'NONE', #37429, #13792 ) ;
#14890=VERTEX_POINT ( 'NONE', #28526 ) ;
#14891=CARTESIAN_POINT ( 'NONE',  ( 16.05000000000000071, 0.000000000000000000, 4.999999999999998224 ) ) ;
#14892=CARTESIAN_POINT ( 'NONE',  ( 18.03749999999999787, -2.886751345948125991, -5.000000000000000000 ) ) ;
#14893=CARTESIAN_POINT ( 'NONE',  ( 11.57812500061451644, 6.421520780324663323E-16, -5.243569643749999010 ) ) ;
#14894=ORIENTED_EDGE ( 'NONE', *, *, #57289, .F. ) ;
#14896=CARTESIAN_POINT ( 'NONE',  ( -4.243569643749997233, 17.64687500061452141, -27.54997392385601174 ) ) ;
#14897=CARTESIAN_POINT ( 'NONE',  ( 4.190625000614518925, -3.027376345333614438, 5.243569643749998122 ) ) ;
#14899=CARTESIAN_POINT ( 'NONE',  ( 8.849999999999999645, 0.000000000000000000, 4.999999999999998224 ) ) ;
#14901=ORIENTED_EDGE ( 'NONE', *, *, #31908, .F. ) ;
#14902=CARTESIAN_POINT ( 'NONE',  ( -4.243569643749999898, 14.36562500061451786, 27.54997392385601529 ) ) ;
#14903=CARTESIAN_POINT ( 'NONE',  ( 27.44062500061451715, 6.054752690667223547, 3.707466751127219781E-16 ) ) ;
#14904=CARTESIAN_POINT ( 'NONE',  ( 29.25000000122903288, -2.886751345948150860, 4.999999999999960920 ) ) ;
#14906=CARTESIAN_POINT ( 'NONE',  ( 24.60937500061451644, -4.541064518000417216, -2.621784821875001281 ) ) ;
#14907=CARTESIAN_POINT ( 'NONE',  ( 19.22812500061451502, 6.421520780324663323E-16, -5.243569643749999010 ) ) ;
#14908=CARTESIAN_POINT ( 'NONE',  ( 2.121784821874999061, 12.90312500061459389, -33.67503911421598417 ) ) ;
#14909=CARTESIAN_POINT ( 'NONE',  ( 22.68750000122903288, 6.123233995736764310E-16, -4.999999999999998224 ) ) ;
#14910=CARTESIAN_POINT ( 'NONE',  ( 4.828125000614518214, 6.421520780324663323E-16, -5.243569643749999010 ) ) ;
#14912=CARTESIAN_POINT ( 'NONE',  ( 20.69062500061451715, 6.054752690667223547, 3.707466751127219781E-16 ) ) ;
#14915=CARTESIAN_POINT ( 'NONE',  ( 14.40937500061451715, 4.541064518000418104, -2.621784821874998173 ) ) ;
#14916=CARTESIAN_POINT ( 'NONE',  ( 16.65937500061452070, 4.541064518000418104, -2.621784821874998173 ) ) ;
#14917=CARTESIAN_POINT ( 'NONE',  ( 25.80937500061451928, 0.000000000000000000, 5.243569643749999010 ) ) ;
#14918=CARTESIAN_POINT ( 'NONE',  ( -4.243569643749999898, 13.52187500061451786, 27.54997392385601529 ) ) ;
#14919=CARTESIAN_POINT ( 'NONE',  ( 5.690625000614516260, -3.027376345333610441, -5.243569643749999898 ) ) ;
#14920=CARTESIAN_POINT ( 'NONE',  ( 28.41562500061451502, 3.027376345333611329, 5.243569643749999010 ) ) ;
#14921=CARTESIAN_POINT ( 'NONE',  ( 2.859375000614519546, 0.000000000000000000, 5.243569643749999010 ) ) ;
#14922=LINE ( 'NONE', #55555, #33293 ) ;
#14923=CARTESIAN_POINT ( 'NONE',  ( 3.999999999999999112, 18.87500000000000000, 30.00000000000000000 ) ) ;
#14925=CARTESIAN_POINT ( 'NONE',  ( 6.571875000614517681, -6.054752690667223547, -1.112240025338166033E-15 ) ) ;
#14927=CARTESIAN_POINT ( 'NONE',  ( 14.66250000122903252, 4.330127018922192761, -2.499999999999997780 ) ) ;
#14928=CARTESIAN_POINT ( 'NONE',  ( 9.487500001229033586, -4.330127018922194537, 2.499999999999995559 ) ) ;
#14929=CARTESIAN_POINT ( 'NONE',  ( 4.903125000614516615, 4.541064518000418104, -2.621784821874998173 ) ) ;
#14932=CARTESIAN_POINT ( 'NONE',  ( 14.74687500061451573, -3.027376345333610441, -5.243569643749999898 ) ) ;
#14933=CARTESIAN_POINT ( 'NONE',  ( 11.92500000000000071, 4.330127018922191873, 2.499999999999999556 ) ) ;
#14934=EDGE_LOOP ( 'NONE', ( #31733, #59918, #13812 ) ) ;
#14935=EDGE_CURVE ( 'NONE', #44045, #2558, #14334, .T. ) ;
#14936=CARTESIAN_POINT ( 'NONE',  ( 21.77812500061451928, -4.541064518000419881, 2.621784821874995952 ) ) ;
#14937=CARTESIAN_POINT ( 'NONE',  ( 6.403125000614517504, 0.000000000000000000, 5.243569643749999010 ) ) ;
#14938=CARTESIAN_POINT ( 'NONE',  ( 24.23437500061451644, 6.421520780324663323E-16, -5.243569643749999010 ) ) ;
#14939=CARTESIAN_POINT ( 'NONE',  ( 7.003125000614518036, -4.541064518000417216, -2.621784821875001281 ) ) ;
#14940=DIRECTION ( 'NONE',  ( 0.000000000000000000, 0.000000000000000000, -1.000000000000000000 ) ) ;
#14941=( BOUNDED_CURVE ( )  B_SPLINE_CURVE ( 2, ( #61661, #11061, #33587, #6246, #67589, #68675, #34307, #45777, #56840 ),
 .UNSPECIFIED., .F., .F. ) 
 B_SPLINE_CURVE_WITH_KNOTS ( ( 3, 2, 2, 2, 3 ),
 ( 0.2717391304347826497, 0.2753623188405797118, 0.2826086956521738913, 0.2898550724637681264, 0.2934782608695652439 ),
 .UNSPECIFIED. ) 
 CURVE ( )  GEOMETRIC_REPRESENTATION_ITEM ( )  RATIONAL_B_SPLINE_CURVE ( ( 0.9330127018922194093, 0.9330127018922198534, 1.000000000000000000, 0.8660254037844387076, 1.000000000000000000, 0.8660254037844387076, 1.000000000000000000, 0.9330127018922188542, 0.9330127018922194093 ) ) 
 REPRESENTATION_ITEM ( '' )  );
#14942=CARTESIAN_POINT ( 'NONE',  ( 7.387500001229032165, 6.123233995736764310E-16, -4.999999999999998224 ) ) ;
#14943=CARTESIAN_POINT ( 'NONE',  ( 21.44062500061452070, -3.027376345333610441, -5.243569643749999898 ) ) ;
#14944=CARTESIAN_POINT ( 'NONE',  ( 2.121784821875001281, 10.95312500061451821, -26.32496088578401938 ) ) ;
#14945=CARTESIAN_POINT ( 'NONE',  ( 10.80000000122903536, -2.886751345948129988, 4.999999999999997335 ) ) ;
#14946=CARTESIAN_POINT ( 'NONE',  ( 20.54062500061451502, -3.027376345333610441, -5.243569643749999898 ) ) ;
#14947=CARTESIAN_POINT ( 'NONE',  ( 16.82812500061451644, -4.541064518000419881, 2.621784821874995952 ) ) ;
#14949=CARTESIAN_POINT ( 'NONE',  ( 17.92500000000000071, -4.330127018922194537, 2.499999999999995559 ) ) ;
#14950=CARTESIAN_POINT ( 'NONE',  ( 11.25000000122903288, -2.886751345948129988, 4.999999999999997335 ) ) ;
#14951=CARTESIAN_POINT ( 'NONE',  ( 7.865625000614516971, -6.054752690667223547, -1.112240025338166033E-15 ) ) ;
#14952=CARTESIAN_POINT ( 'NONE',  ( 10.41562500061451679, 3.027376345333611329, 5.243569643749999010 ) ) ;
#14953=CARTESIAN_POINT ( 'NONE',  ( 22.42500000122903359, 2.886751345948126879, 4.999999999999999112 ) ) ;
#14954=CARTESIAN_POINT ( 'NONE',  ( 22.43437500061451573, 6.421520780324663323E-16, -5.243569643749999010 ) ) ;
#14955=CARTESIAN_POINT ( 'NONE',  ( 4.809916128174254624, -1.365542690628744449, -5.062639209831853115 ) ) ;
#14956=CARTESIAN_POINT ( 'NONE',  ( 4.950000001229033941, -2.886751345948129988, 4.999999999999997335 ) ) ;
#14957=CARTESIAN_POINT ( 'NONE',  ( 5.971875000614516260, 3.027376345333611329, 5.243569643749999010 ) ) ;
#14958=CARTESIAN_POINT ( 'NONE',  ( 22.65937500061451715, 0.000000000000000000, 5.243569643749999010 ) ) ;
#14959=EDGE_CURVE ( 'NONE', #65447, #12584, #462, .T. ) ;
#14960=CARTESIAN_POINT ( 'NONE',  ( 4.518533959972518943, 2.140970262095818200, -4.684411254032723626 ) ) ;
#14961=CARTESIAN_POINT ( 'NONE',  ( 19.41562500061451146, 3.027376345333611329, 5.243569643749999010 ) ) ;
#14962=CARTESIAN_POINT ( 'NONE',  ( 23.85937500061451644, 4.541064518000418104, -2.621784821874998173 ) ) ;
#14964=CARTESIAN_POINT ( 'NONE',  ( 3.242103837493086330E-14, 11.00000000122903288, -34.00000000000000000 ) ) ;
#14966=CARTESIAN_POINT ( 'NONE',  ( 5.146875000614517859, -3.027376345333614438, 5.243569643749998122 ) ) ;
#14967=CARTESIAN_POINT ( 'NONE',  ( 15.77812500061451573, 4.541064518000418104, 2.621784821874999949 ) ) ;
#14968=CARTESIAN_POINT ( 'NONE',  ( 12.98437500061451821, 6.421520780324663323E-16, -5.243569643749999010 ) ) ;
#14969=VERTEX_POINT ( 'NONE', #55160 ) ;
#14970=CARTESIAN_POINT ( 'NONE',  ( 9.262499999999997513, 2.886751345948193936, 4.999999999999883649 ) ) ;
#14971=CARTESIAN_POINT ( 'NONE',  ( 26.27812500061451573, -4.541064518000419881, 2.621784821874995952 ) ) ;
#14972=CARTESIAN_POINT ( 'NONE',  ( 3.489066138150112018, 3.581398816609729252, -3.723603497192741862 ) ) ;
#14974=CARTESIAN_POINT ( 'NONE',  ( 14.36249999999999893, -5.773502691896255534, -1.060575238724906372E-15 ) ) ;
#14975=CARTESIAN_POINT ( 'NONE',  ( 24.67500000122903359, 2.886751345948126879, 4.999999999999999112 ) ) ;
#14976=CARTESIAN_POINT ( 'NONE',  ( 18.14062500061451644, -3.027376345333614438, 5.243569643749998122 ) ) ;
#14977=ORIENTED_EDGE ( 'NONE', *, *, #54670, .T. ) ;
#14978=CARTESIAN_POINT ( 'NONE',  ( 21.41250000000000497, 2.886751345948126879, 4.999999999999999112 ) ) ;
#14979=( BOUNDED_CURVE ( )  B_SPLINE_CURVE ( 2, ( #42068, #70505, #66055, #60135, #31347, #48345, #15076 ),
 .UNSPECIFIED., .F., .F. ) 
 B_SPLINE_CURVE_WITH_KNOTS ( ( 3, 2, 2, 3 ),
 ( 0.7750000000000001332, 0.7777777777777779011, 0.7805555555555556690, 0.7833333333333334370 ),
 .UNSPECIFIED. ) 
 CURVE ( )  GEOMETRIC_REPRESENTATION_ITEM ( )  RATIONAL_B_SPLINE_CURVE ( ( 0.9999999999999946709, 0.8660254037844440367, 1.000000000000000000, 0.8660254037844387076, 1.000000000000000000, 0.8660254037844333785, 1.000000000000005329 ) ) 
 REPRESENTATION_ITEM ( '' )  );
#14980=CARTESIAN_POINT ( 'NONE',  ( 24.12187500061451217, -6.054752690667223547, -1.112240025338166033E-15 ) ) ;
#14981=ORIENTED_EDGE ( 'NONE', *, *, #42052, .T. ) ;
#14982=CARTESIAN_POINT ( 'NONE',  ( 11.20312500061451644, 4.541064518000418104, -2.621784821874998173 ) ) ;
#14983=CARTESIAN_POINT ( 'NONE',  ( 4.115625000614516082, 3.027376345333611329, 5.243569643749999010 ) ) ;
#14985=CARTESIAN_POINT ( 'NONE',  ( 26.87812500061451360, 6.421520780324663323E-16, -5.243569643749999010 ) ) ;
#14986=CARTESIAN_POINT ( 'NONE',  ( 17.02499999999999858, -4.330127018922194537, 2.499999999999995559 ) ) ;
#14987=CARTESIAN_POINT ( 'NONE',  ( 26.09999999999999787, -4.330127018922190985, -2.500000000000001332 ) ) ;
#14989=CARTESIAN_POINT ( 'NONE',  ( 7.021875000614518747, -6.054752690667223547, -1.112240025338166033E-15 ) ) ;
#14990=CARTESIAN_POINT ( 'NONE',  ( 17.89687500061451431, -3.027376345333610441, -5.243569643749999898 ) ) ;
#14991=CARTESIAN_POINT ( 'NONE',  ( 29.85937500061451644, 0.000000000000000000, 5.243569643749999010 ) ) ;
#14992=VERTEX_POINT ( 'NONE', #49980 ) ;
#14993=CARTESIAN_POINT ( 'NONE',  ( 25.52812500061451573, 6.421520780324663323E-16, -5.243569643749999010 ) ) ;
#14994=CARTESIAN_POINT ( 'NONE',  ( 28.05937500061451573, 0.000000000000000000, 5.243569643749999010 ) ) ;
#14995=CARTESIAN_POINT ( 'NONE',  ( 3.121875000614518836, 3.027376345333613106, -5.243569643749998122 ) ) ;
#14996=CARTESIAN_POINT ( 'NONE',  ( 14.62500000000000000, 4.330127018922191873, 2.499999999999999556 ) ) ;
#14997=CARTESIAN_POINT ( 'NONE',  ( 11.35312500061451679, 0.000000000000000000, 5.243569643749999010 ) ) ;
#15000=CARTESIAN_POINT ( 'NONE',  ( 29.09062500061451217, -3.027376345333610441, -5.243569643749999898 ) ) ;
#15001=CARTESIAN_POINT ( 'NONE',  ( 15.30000000122903359, -2.886751345948129988, 4.999999999999997335 ) ) ;
#15004=CARTESIAN_POINT ( 'NONE',  ( 5.015625000614518214, 3.027376345333611329, 5.243569643749999010 ) ) ;
#15005=CARTESIAN_POINT ( 'NONE',  ( 21.42187500061451644, -6.054752690667223547, -1.112240025338166033E-15 ) ) ;
#15006=CARTESIAN_POINT ( 'NONE',  ( 9.001249775931846008E-16, 16.82187500061451857, 34.90005215228797653 ) ) ;
#15007=CARTESIAN_POINT ( 'NONE',  ( 23.37187500061451573, 3.027376345333613106, -5.243569643749998122 ) ) ;
#15008=CARTESIAN_POINT ( 'NONE',  ( 6.262500000000000178, -5.773502691896255534, -1.060575238724906372E-15 ) ) ;
#15009=CARTESIAN_POINT ( 'NONE',  ( 2.000000000000001332, 11.26250000122903394, 33.46410161513774995 ) ) ;
#15010=CARTESIAN_POINT ( 'NONE',  ( 13.26562500061451644, -6.054752690667223547, -1.112240025338166033E-15 ) ) ;
#15011=CARTESIAN_POINT ( 'NONE',  ( 4.500000001229034652, -2.886751345948129988, 4.999999999999997335 ) ) ;
#15012=CARTESIAN_POINT ( 'NONE',  ( 9.834375000614517859, 6.421520780324663323E-16, -5.243569643749999010 ) ) ;
#15013=CARTESIAN_POINT ( 'NONE',  ( 9.365625000614519635, 3.027376345333613106, -5.243569643749998122 ) ) ;
#15014=CARTESIAN_POINT ( 'NONE',  ( 15.00937500061451679, 0.000000000000000000, 5.243569643749999010 ) ) ;
#15015=DIRECTION ( 'NONE',  ( 0.000000000000000000, 0.000000000000000000, 1.000000000000000000 ) ) ;
#15016=CARTESIAN_POINT ( 'NONE',  ( 22.12500000122903288, -5.773502691896255534, -1.060575238724906372E-15 ) ) ;
#15017=CARTESIAN_POINT ( 'NONE',  ( 11.52187500061451608, -6.054752690667223547, -1.112240025338166033E-15 ) ) ;
#15018=CARTESIAN_POINT ( 'NONE',  ( 12.40312500061451573, -4.541064518000417216, -2.621784821875001281 ) ) ;
#15020=CARTESIAN_POINT ( 'NONE',  ( 21.08437500061451786, 6.421520780324663323E-16, -5.243569643749999010 ) ) ;
#15021=CARTESIAN_POINT ( 'NONE',  ( 25.61250000122903359, 0.000000000000000000, 4.999999999999998224 ) ) ;
#15022=CARTESIAN_POINT ( 'NONE',  ( -4.243569643749999898, 19.85937500061451644, -30.00000000000000000 ) ) ;
#15023=AXIS2_PLACEMENT_3D ( 'NONE', #21549, #10114, #16007 ) ;
#15024=CARTESIAN_POINT ( 'NONE',  ( 3.224120815779399241, 3.821689571648150707, -3.388499519612508060 ) ) ;
#15025=CARTESIAN_POINT ( 'NONE',  ( 4.243569643749999010, 13.37187500061451750, -32.45002607614398471 ) ) ;
#15026=CARTESIAN_POINT ( 'NONE',  ( 15.86250000122903181, -4.330127018922190985, -2.500000000000001332 ) ) ;
#15027=CARTESIAN_POINT ( 'NONE',  ( 9.234375000614518214, -4.541064518000419881, 2.621784821874995952 ) ) ;
#15028=CARTESIAN_POINT ( 'NONE',  ( 2.121784821875001281, 17.25312500061451715, -26.32496088578401938 ) ) ;
#15029=CARTESIAN_POINT ( 'NONE',  ( 18.00000000122903288, -2.886751345948129988, 4.999999999999997335 ) ) ;
#15030=CARTESIAN_POINT ( 'NONE',  ( 9.103125000614515017, 0.000000000000000000, 5.243569643749999010 ) ) ;
#15031=EDGE_LOOP ( 'NONE', ( #62888, #6370, #64178, #31256 ) ) ;
#15032=CARTESIAN_POINT ( 'NONE',  ( 16.08749999999999503, -2.886751345948129988, 4.999999999999997335 ) ) ;
#15033=CARTESIAN_POINT ( 'NONE',  ( 17.84999999999999787, 0.000000000000000000, 4.999999999999998224 ) ) ;
#15034=CARTESIAN_POINT ( 'NONE',  ( 8.971875000614515372, 3.027376345333612662, -5.243569643749998122 ) ) ;
#15035=CARTESIAN_POINT ( 'NONE',  ( 4.384576699563885960, -2.403224326949449097, -4.660422238726323663 ) ) ;
#15036=CARTESIAN_POINT ( 'NONE',  ( 11.32500000122903394, -5.773502691896255534, -1.060575238724906372E-15 ) ) ;
#15037=CARTESIAN_POINT ( 'NONE',  ( 19.57500000122903216, 2.886751345948129099, -4.999999999999998224 ) ) ;
#15038=CARTESIAN_POINT ( 'NONE',  ( 14.95312500061451644, 0.000000000000000000, 5.243569643749999010 ) ) ;
#15039=CARTESIAN_POINT ( 'NONE',  ( 20.24062500061451431, 6.054752690667223547, 3.707466751127219781E-16 ) ) ;
#15040=CARTESIAN_POINT ( 'NONE',  ( 27.15000000122902790, -2.886751345948125991, -5.000000000000000000 ) ) ;
#15041=EDGE_CURVE ( 'NONE', #4907, #42330, #6390, .T. ) ;
#15042=CARTESIAN_POINT ( 'NONE',  ( 3.515625000614516882, 3.027376345333613106, -5.243569643749998122 ) ) ;
#15043=CARTESIAN_POINT ( 'NONE',  ( 24.26249999999999929, -5.773502691896255534, -1.060575238724906372E-15 ) ) ;
#15046=CARTESIAN_POINT ( 'NONE',  ( 27.38437500061451857, 6.421520780324663323E-16, -5.243569643749999010 ) ) ;
#15047=CARTESIAN_POINT ( 'NONE',  ( -1.487416814333745711E-14, 16.06250000000000000, 34.00000000000000000 ) ) ;
#15048=CARTESIAN_POINT ( 'NONE',  ( 11.70000000122903216, -2.886751345948129988, 4.999999999999997335 ) ) ;
#15049=CARTESIAN_POINT ( 'NONE',  ( 4.125000000000000000, 6.123233995736764310E-16, -4.999999999999998224 ) ) ;
#15052=CARTESIAN_POINT ( 'NONE',  ( 7.284375000614518036, 4.541064518000418104, 2.621784821874999949 ) ) ;
#15053=CARTESIAN_POINT ( 'NONE',  ( 25.15312500061451217, 4.541064518000418104, -2.621784821874998173 ) ) ;
#15056=CARTESIAN_POINT ( 'NONE',  ( -3.999999999999999112, 19.66250000122903430, 30.00000000000000000 ) ) ;
#15057=CARTESIAN_POINT ( 'NONE',  ( 5.146875000614517859, -3.027376345333614438, 5.243569643749998122 ) ) ;
#15058=CARTESIAN_POINT ( 'NONE',  ( 7.771875000614516971, 3.027376345333611329, 5.243569643749999010 ) ) ;
#15059=CARTESIAN_POINT ( 'NONE',  ( 5.212500000000002132, 2.886751345948126879, 4.999999999999999112 ) ) ;
#15060=AXIS2_PLACEMENT_3D ( 'NONE', #29809, #14267, #18339 ) ;
#15061=CARTESIAN_POINT ( 'NONE',  ( -4.243569643749999898, 13.05312500061459602, 30.00000000000000000 ) ) ;
#15062=CARTESIAN_POINT ( 'NONE',  ( 21.60000000000000142, -4.330127018922190985, -2.500000000000001332 ) ) ;
#15063=CARTESIAN_POINT ( 'NONE',  ( 28.94999999999999929, 4.330127018922192761, -2.499999999999997780 ) ) ;
#15064=CARTESIAN_POINT ( 'NONE',  ( 3.037500000000002309, -2.886751345948129988, 4.999999999999997335 ) ) ;
#15066=CARTESIAN_POINT ( 'NONE',  ( 17.39062500061451644, -3.027376345333610441, -5.243569643749999898 ) ) ;
#15067=CARTESIAN_POINT ( 'NONE',  ( 11.20312500061451644, 4.541064518000418104, -2.621784821874998173 ) ) ;
#15069=CARTESIAN_POINT ( 'NONE',  ( 6.009375000614519458, 0.000000000000000000, 5.243569643749999010 ) ) ;
#15070=CARTESIAN_POINT ( 'NONE',  ( 22.83749999999999858, -2.886751345948129988, 4.999999999999997335 ) ) ;
#15071=CARTESIAN_POINT ( 'NONE',  ( 20.47500000122903074, 2.886751345948129099, -4.999999999999998224 ) ) ;
#15073=CARTESIAN_POINT ( 'NONE',  ( 10.13437500061451679, -4.541064518000419881, 2.621784821874995952 ) ) ;
#15074=CARTESIAN_POINT ( 'NONE',  ( 14.63437500061451679, -4.541064518000419881, 2.621784821874995952 ) ) ;
#15075=CARTESIAN_POINT ( 'NONE',  ( 23.63437500061451502, -4.541064518000419881, 2.621784821874995952 ) ) ;
#15076=CARTESIAN_POINT ( 'NONE',  ( 8.512500001229033941, 0.000000000000000000, 4.999999999999998224 ) ) ;
#15078=CARTESIAN_POINT ( 'NONE',  ( 17.33437500061451431, -4.541064518000419881, 2.621784821874995952 ) ) ;
#15079=CARTESIAN_POINT ( 'NONE',  ( 9.909375000614517148, 4.541064518000418104, -2.621784821874998173 ) ) ;
#15081=CARTESIAN_POINT ( 'NONE',  ( 20.43749999999999645, 5.773502691896255534, 3.535250795749688894E-16 ) ) ;
#15083=CARTESIAN_POINT ( 'NONE',  ( 4.243569643749999010, 10.67187500061451644, -32.45002607614398471 ) ) ;
#15085=CARTESIAN_POINT ( 'NONE',  ( 11.76562500061451644, 3.027376345333611329, 5.243569643749999010 ) ) ;
#15086=CARTESIAN_POINT ( 'NONE',  ( 28.69687500061451502, -3.027376345333610441, -5.243569643749999898 ) ) ;
#15088=CARTESIAN_POINT ( 'NONE',  ( 1.071796769724491893, 9.895096190661368141, -26.00000000000000355 ) ) ;
#15089=CARTESIAN_POINT ( 'NONE',  ( 11.47499999999999964, 4.330127018922191873, 2.499999999999999556 ) ) ;
#15090=CARTESIAN_POINT ( 'NONE',  ( 2.000000000000001332, 18.01250000122903572, 33.46410161513774995 ) ) ;
#15091=CARTESIAN_POINT ( 'NONE',  ( 11.62500000122903465, 2.886751345948126879, 4.999999999999999112 ) ) ;
#15092=CARTESIAN_POINT ( 'NONE',  ( 21.49687500061451573, -3.027376345333610441, -5.243569643749999898 ) ) ;
#15093=CARTESIAN_POINT ( 'NONE',  ( 17.59687500061451715, 6.054752690667223547, 3.707466751127219781E-16 ) ) ;
#15096=CARTESIAN_POINT ( 'NONE',  ( 18.17812500061451786, -4.541064518000419881, 2.621784821874995952 ) ) ;
#15097=CARTESIAN_POINT ( 'NONE',  ( 27.82500000122903572, 2.886751345948126879, 4.999999999999999112 ) ) ;
#15098=CARTESIAN_POINT ( 'NONE',  ( 17.70937500061451431, 0.000000000000000000, 5.243569643749999010 ) ) ;
#15099=CARTESIAN_POINT ( 'NONE',  ( 4.078125000614517326, 4.541064518000418104, 2.621784821874999949 ) ) ;
#15100=CARTESIAN_POINT ( 'NONE',  ( 18.51562500061451289, 3.027376345333611329, 5.243569643749999010 ) ) ;
#15102=CARTESIAN_POINT ( 'NONE',  ( 28.43437500061451573, 4.541064518000418104, 2.621784821874999949 ) ) ;
#15103=CARTESIAN_POINT ( 'NONE',  ( 2.121784821874999061, 12.45312500061451821, 26.32496088578401583 ) ) ;
#15104=CARTESIAN_POINT ( 'NONE',  ( 16.95000000122903216, 5.773502691896255534, 3.535250795749688894E-16 ) ) ;
#15106=CARTESIAN_POINT ( 'NONE',  ( 27.74062500061451431, -3.027376345333610441, -5.243569643749999898 ) ) ;
#15107=FACE_OUTER_BOUND ( 'NONE', #7422, .T. ) ;
#15108=CARTESIAN_POINT ( 'NONE',  ( 20.03437500061451715, -4.541064518000419881, 2.621784821874995952 ) ) ;
#15109=CARTESIAN_POINT ( 'NONE',  ( 22.95000000122903216, -2.886751345948129988, 4.999999999999997335 ) ) ;
#15110=CARTESIAN_POINT ( 'NONE',  ( 22.67812500061451431, -4.541064518000419881, 2.621784821874995952 ) ) ;
#15111=CARTESIAN_POINT ( 'NONE',  ( 16.99687500061451573, -3.027376345333610441, -5.243569643749999898 ) ) ;
#15112=CARTESIAN_POINT ( 'NONE',  ( 11.84062500061451750, -3.027376345333614438, 5.243569643749998122 ) ) ;
#15113=CARTESIAN_POINT ( 'NONE',  ( -2.121784821874996840, 14.53437500061451715, 33.67503911421598417 ) ) ;
#15114=CARTESIAN_POINT ( 'NONE',  ( 18.74062500061451431, -3.027376345333610441, -5.243569643749999898 ) ) ;
#15115=CARTESIAN_POINT ( 'NONE',  ( 29.46562500061451573, -6.054752690667223547, -1.112240025338166033E-15 ) ) ;
#15116=ORIENTED_EDGE ( 'NONE', *, *, #17491, .T. ) ;
#15117=EDGE_LOOP ( 'NONE', ( #49906, #65000, #40093, #20798 ) ) ;
#15118=CARTESIAN_POINT ( 'NONE',  ( 22.76249999999999574, 2.886751345948126879, 4.999999999999999112 ) ) ;
#15119=CARTESIAN_POINT ( 'NONE',  ( 4.243569643749999898, 18.28437500061451715, -30.00000000000000000 ) ) ;
#15121=CARTESIAN_POINT ( 'NONE',  ( 24.36562500061451786, 3.027376345333611329, 5.243569643749999010 ) ) ;
#15122=CARTESIAN_POINT ( 'NONE',  ( 5.315625000614516260, 3.027376345333613106, -5.243569643749998122 ) ) ;
#15123=CARTESIAN_POINT ( 'NONE',  ( 18.03750000122903430, -4.330127018922194537, 2.499999999999995559 ) ) ;
#15124=CARTESIAN_POINT ( 'NONE',  ( 23.84062500061451928, 6.054752690667223547, 3.707466751127219781E-16 ) ) ;
#15125=CARTESIAN_POINT ( 'NONE',  ( 23.17500000000000071, 4.330127018922191873, 2.499999999999999556 ) ) ;
#15126=CARTESIAN_POINT ( 'NONE',  ( 28.56562500061451715, -6.054752690667223547, -1.112240025338166033E-15 ) ) ;
#15127=CARTESIAN_POINT ( 'NONE',  ( 8.953125000614518214, 4.541064518000418104, -2.621784821874998173 ) ) ;
#15128=VERTEX_POINT ( 'NONE', #55521 ) ;
#15129=CARTESIAN_POINT ( 'NONE',  ( 23.65312500061451573, -4.541064518000417216, -2.621784821875001281 ) ) ;
#15130=CARTESIAN_POINT ( 'NONE',  ( 4.978125000614518569, 4.541064518000418104, 2.621784821874999949 ) ) ;
#15132=CARTESIAN_POINT ( 'NONE',  ( 4.303125000614516971, -4.541064518000417216, -2.621784821875001281 ) ) ;
#15133=CARTESIAN_POINT ( 'NONE',  ( -2.828200636599751609E-16, 13.25000000122903288, -34.61880215351700230 ) ) ;
#15134=EDGE_CURVE ( 'NONE', #6811, #66841, #37434, .T. ) ;
#15135=CARTESIAN_POINT ( 'NONE',  ( 11.06250000000000000, 2.886751345948126879, 4.999999999999999112 ) ) ;
#15136=CARTESIAN_POINT ( 'NONE',  ( 10.73437500061451644, 6.421520780324663323E-16, -5.243569643749999010 ) ) ;
#15137=CARTESIAN_POINT ( 'NONE',  ( 6.862500001229034474, -4.330127018922190985, -2.500000000000001332 ) ) ;
#15138=CARTESIAN_POINT ( 'NONE',  ( 13.47187500061451537, 3.027376345333613106, -5.243569643749998122 ) ) ;
#15139=CARTESIAN_POINT ( 'NONE',  ( 6.346875000614517148, 6.054752690667223547, 3.707466751127219781E-16 ) ) ;
#15140=CARTESIAN_POINT ( 'NONE',  ( -4.243569643749997233, 10.39062500061451644, -27.54997392385601174 ) ) ;
#15141=CARTESIAN_POINT ( 'NONE',  ( 3.467284487300496654, 3.602878009983967900, 3.467284487300496654 ) ) ;
#15142=CARTESIAN_POINT ( 'NONE',  ( 12.72187500061451537, 3.027376345333611329, 5.243569643749999010 ) ) ;
#15143=CARTESIAN_POINT ( 'NONE',  ( 3.700875911142169628, 3.362093191700385564, 4.023865622399847020 ) ) ;
#15144=CARTESIAN_POINT ( 'NONE',  ( 21.02812500061451573, 6.421520780324663323E-16, -5.243569643749999010 ) ) ;
#15145=CARTESIAN_POINT ( 'NONE',  ( 4.243569643749999898, 10.63437500061451857, 30.00000000000000000 ) ) ;
#15147=CARTESIAN_POINT ( 'NONE',  ( 24.34687500061451715, 6.054752690667223547, 3.707466751127219781E-16 ) ) ;
#15148=CYLINDRICAL_SURFACE ( 'NONE', #72122, 4.999999999999998224 ) ;
#15149=CARTESIAN_POINT ( 'NONE',  ( 4.565625000614516260, 3.027376345333611329, 5.243569643749999010 ) ) ;
#15151=CARTESIAN_POINT ( 'NONE',  ( 19.04062500061451146, -3.027376345333614438, 5.243569643749998122 ) ) ;
#15152=CARTESIAN_POINT ( 'NONE',  ( 14.52187500061451608, 3.027376345333611329, 5.243569643749999010 ) ) ;
#15154=CARTESIAN_POINT ( 'NONE',  ( 27.60000000122903430, -2.886751345948125991, -5.000000000000000000 ) ) ;
#15155=CARTESIAN_POINT ( 'NONE',  ( 5.371875000614516615, 3.027376345333613106, -5.243569643749998122 ) ) ;
#15156=CARTESIAN_POINT ( 'NONE',  ( 17.82187500061451502, -6.054752690667223547, -1.112240025338166033E-15 ) ) ;
#15157=CARTESIAN_POINT ( 'NONE',  ( 15.15000000000000036, 0.000000000000000000, 4.999999999999998224 ) ) ;
#15158=CARTESIAN_POINT ( 'NONE',  ( 23.40000000000000213, -4.330127018922190985, -2.500000000000001332 ) ) ;
#15159=CARTESIAN_POINT ( 'NONE',  ( 2.662500001229036073, 0.000000000000000000, 4.999999999999998224 ) ) ;
#15160=CARTESIAN_POINT ( 'NONE',  ( 24.87187500061451573, 3.027376345333611329, 5.243569643749999010 ) ) ;
#15161=CARTESIAN_POINT ( 'NONE',  ( 17.22187500061451715, 3.027376345333611329, 5.243569643749999010 ) ) ;
#15163=CARTESIAN_POINT ( 'NONE',  ( 21.89999999999999858, 0.000000000000000000, 4.999999999999998224 ) ) ;
#15164=CARTESIAN_POINT ( 'NONE',  ( 6.937499999999999112, 5.773502691896255534, 3.535250795749688894E-16 ) ) ;
#15166=CARTESIAN_POINT ( 'NONE',  ( 19.26562500061451644, 3.027376345333613106, -5.243569643749998122 ) ) ;
#15167=CARTESIAN_POINT ( 'NONE',  ( 9.187500000000001776, 5.773502691896255534, 3.535250795749688894E-16 ) ) ;
#15168=CARTESIAN_POINT ( 'NONE',  ( 3.890625000614517326, -3.027376345333610441, -5.243569643749999898 ) ) ;
#15169=CARTESIAN_POINT ( 'NONE',  ( 18.48750000000000071, -2.886751345948125991, -5.000000000000000000 ) ) ;
#15170=CARTESIAN_POINT ( 'NONE',  ( 18.85312500061451502, 4.541064518000418104, -2.621784821874998173 ) ) ;
#15172=CARTESIAN_POINT ( 'NONE',  ( 23.28750000122903430, 4.330127018922191873, 2.499999999999999556 ) ) ;
#15173=DIRECTION ( 'NONE',  ( -1.000000000000000000, -0.000000000000000000, -0.000000000000000000 ) ) ;
#15174=CARTESIAN_POINT ( 'NONE',  ( 29.03437500061451715, -4.541064518000419881, 2.621784821874995952 ) ) ;
#15175=ORIENTED_EDGE ( 'NONE', *, *, #28049, .T. ) ;
#15176=CARTESIAN_POINT ( 'NONE',  ( 16.64062500061451289, 6.054752690667223547, 3.707466751127219781E-16 ) ) ;
#15177=CARTESIAN_POINT ( 'NONE',  ( 24.55312500061451786, -4.541064518000417216, -2.621784821875001281 ) ) ;
#15178=CARTESIAN_POINT ( 'NONE',  ( 25.32187500061451857, 3.027376345333611329, 5.243569643749999010 ) ) ;
#15179=CARTESIAN_POINT ( 'NONE',  ( 8.287499999999999645, 5.773502691896255534, 3.535250795749688894E-16 ) ) ;
#15180=CARTESIAN_POINT ( 'NONE',  ( 12.36562500061451608, -6.054752690667223547, -1.112240025338166033E-15 ) ) ;
#15181=CARTESIAN_POINT ( 'NONE',  ( 27.62812500061451360, -4.541064518000419881, 2.621784821874995952 ) ) ;
#15182=CARTESIAN_POINT ( 'NONE',  ( 17.40937500061451715, -4.541064518000417216, -2.621784821875001281 ) ) ;
#15183=CARTESIAN_POINT ( 'NONE',  ( 19.69687500061451857, -3.027376345333610441, -5.243569643749999898 ) ) ;
#15184=DIRECTION ( 'NONE',  ( 0.000000000000000000, 0.000000000000000000, -1.000000000000000000 ) ) ;
#15185=CARTESIAN_POINT ( 'NONE',  ( -4.243569643749999898, 10.40937500061451892, 30.00000000000000000 ) ) ;
#15186=( BOUNDED_CURVE ( )  B_SPLINE_CURVE ( 2, ( #35178, #24085, #69174, #1942, #18535, #7466, #29992 ),
 .UNSPECIFIED., .F., .F. ) 
 B_SPLINE_CURVE_WITH_KNOTS ( ( 3, 2, 2, 3 ),
 ( 0.8750000000000000000, 0.8777777777777777679, 0.8805555555555555358, 0.8833333333333333037 ),
 .UNSPECIFIED. ) 
 CURVE ( )  GEOMETRIC_REPRESENTATION_ITEM ( )  RATIONAL_B_SPLINE_CURVE ( ( 1.000000000000000000, 0.8660254037844387076, 1.000000000000000000, 0.8660254037844387076, 1.000000000000000000, 0.8660254037844387076, 1.000000000000000000 ) ) 
 REPRESENTATION_ITEM ( '' )  );
#15187=CARTESIAN_POINT ( 'NONE',  ( 23.17500000122903359, 2.886751345948129099, -4.999999999999998224 ) ) ;
#15189=CARTESIAN_POINT ( 'NONE',  ( 14.27812500061451573, 6.421520780324663323E-16, -5.243569643749999010 ) ) ;
#15190=CARTESIAN_POINT ( 'NONE',  ( 7.396875000614519635, -3.027376345333614438, 5.243569643749998122 ) ) ;
#15191=CARTESIAN_POINT ( 'NONE',  ( 8.071875000614518569, 3.027376345333613106, -5.243569643749998122 ) ) ;
#15192=ORIENTED_EDGE ( 'NONE', *, *, #4728, .F. ) ;
#15193=CARTESIAN_POINT ( 'NONE',  ( 2.000000000000001332, 13.40000000000000213, 33.46410161513774995 ) ) ;
#15194=CARTESIAN_POINT ( 'NONE',  ( 19.11562500061451431, -6.054752690667223547, -1.112240025338166033E-15 ) ) ;
#15195=EDGE_CURVE ( 'NONE', #47001, #28339, #19942, .T. ) ;
#15196=CARTESIAN_POINT ( 'NONE',  ( 23.55937500061451573, 0.000000000000000000, 5.243569643749999010 ) ) ;
#15197=CARTESIAN_POINT ( 'NONE',  ( 18.40312500061451573, 4.541064518000418104, -2.621784821874998173 ) ) ;
#15198=CARTESIAN_POINT ( 'NONE',  ( 8.484601909799253346E-16, 12.01250000000000107, 34.61880215351700230 ) ) ;
#15199=CARTESIAN_POINT ( 'NONE',  ( 27.92812500061451431, 4.541064518000418104, 2.621784821874999949 ) ) ;
#15200=CARTESIAN_POINT ( 'NONE',  ( 7.125000001229033764, 2.886751345948126879, 4.999999999999999112 ) ) ;
#15201=VERTEX_POINT ( 'NONE', #22258 ) ;
#15203=CARTESIAN_POINT ( 'NONE',  ( 3.999999999999999112, 14.37500000000000000, -30.00000000000000000 ) ) ;
#15204=CARTESIAN_POINT ( 'NONE',  ( 21.18750000122903288, -4.330127018922194537, 2.499999999999995559 ) ) ;
#15206=CARTESIAN_POINT ( 'NONE',  ( 7.434375000614519280, -4.541064518000419881, 2.621784821874995952 ) ) ;
#15207=CARTESIAN_POINT ( 'NONE',  ( 4.411272977760241965, 2.353862934769528348, -4.685547128476531320 ) ) ;
#15208=CARTESIAN_POINT ( 'NONE',  ( 11.76562500061451644, 3.027376345333611329, 5.243569643749999010 ) ) ;
#15209=CARTESIAN_POINT ( 'NONE',  ( 7.471875000614519813, -6.054752690667223547, -1.112240025338166033E-15 ) ) ;
#15210=CARTESIAN_POINT ( 'NONE',  ( 27.26250000122903216, 4.330127018922192761, -2.499999999999997780 ) ) ;
#15211=CARTESIAN_POINT ( 'NONE',  ( 13.77187500061451786, -6.054752690667223547, -1.112240025338166033E-15 ) ) ;
#15212=CARTESIAN_POINT ( 'NONE',  ( 5.259375000614518569, -4.541064518000417216, -2.621784821875001281 ) ) ;
#15213=CARTESIAN_POINT ( 'NONE',  ( 29.55000000000000071, 0.000000000000000000, 4.999999999999998224 ) ) ;
#15214=CARTESIAN_POINT ( 'NONE',  ( 6.553125000614518747, -4.541064518000417216, -2.621784821875001281 ) ) ;
#15215=CARTESIAN_POINT ( 'NONE',  ( 14.50312500061451537, 0.000000000000000000, 5.243569643749999010 ) ) ;
#15216=( BOUNDED_CURVE ( )  B_SPLINE_CURVE ( 2, ( #56821, #39489, #22841, #10318, #45393, #67929, #17302, #34289, #6228 ),
 .UNSPECIFIED., .F., .F. ) 
 B_SPLINE_CURVE_WITH_KNOTS ( ( 3, 2, 2, 2, 3 ),
 ( 0.1630434782608695676, 0.1666666666666666574, 0.1739130434782608647, 0.1811594202898550721, 0.1847826086956521896 ),
 .UNSPECIFIED. ) 
 CURVE ( )  GEOMETRIC_REPRESENTATION_ITEM ( )  RATIONAL_B_SPLINE_CURVE ( ( 0.9330127018922194093, 0.9330127018922196314, 1.000000000000000000, 0.8660254037844387076, 1.000000000000000000, 0.8660254037844387076, 1.000000000000000000, 0.9330127018922190762, 0.9330127018922194093 ) ) 
 REPRESENTATION_ITEM ( '' )  );
#15218=CARTESIAN_POINT ( 'NONE',  ( 11.84062500061451750, -3.027376345333614438, 5.243569643749998122 ) ) ;
#15219=CARTESIAN_POINT ( 'NONE',  ( 5.362500001229033586, 0.000000000000000000, 4.999999999999998224 ) ) ;
#15220=CARTESIAN_POINT ( 'NONE',  ( 7.978125000614517681, 6.421520780324663323E-16, -5.243569643749999010 ) ) ;
#15222=CARTESIAN_POINT ( 'NONE',  ( 9.750000000000001776, 0.000000000000000000, 4.999999999999998224 ) ) ;
#15223=CARTESIAN_POINT ( 'NONE',  ( 4.537500001229034297, -4.330127018922194537, 2.499999999999995559 ) ) ;
#15224=CARTESIAN_POINT ( 'NONE',  ( 19.12500000000000000, 4.330127018922191873, 2.499999999999999556 ) ) ;
#15225=CARTESIAN_POINT ( 'NONE',  ( 18.30937500061451928, -4.541064518000417216, -2.621784821875001281 ) ) ;
#15226=CARTESIAN_POINT ( 'NONE',  ( 13.46250000122903323, 0.000000000000000000, 4.999999999999998224 ) ) ;
#15228=( BOUNDED_CURVE ( )  B_SPLINE_CURVE ( 2, ( #19393, #20127, #26055, #8330, #14231, #53398, #48595 ),
 .UNSPECIFIED., .F., .F. ) 
 B_SPLINE_CURVE_WITH_KNOTS ( ( 3, 2, 2, 3 ),
 ( 0.9769893167920098431, 0.9777777777777777457, 0.9805555555555555136, 0.9812695158790134542 ),
 .UNSPECIFIED. ) 
 CURVE ( )  GEOMETRIC_REPRESENTATION_ITEM ( )  RATIONAL_B_SPLINE_CURVE ( ( 0.9455319771198016365, 0.9619718528080076769, 1.000000000000000000, 0.8660254037844387076, 1.000000000000000000, 0.9655650834222846424, 0.9488314850527816979 ) ) 
 REPRESENTATION_ITEM ( '' )  );
#15229=CARTESIAN_POINT ( 'NONE',  ( 2.121784821874999061, 17.40312500061451573, -33.67503911421598417 ) ) ;
#15233=CARTESIAN_POINT ( 'NONE',  ( 29.31562500061451715, 3.027376345333611329, 5.243569643749999010 ) ) ;
#15234=EDGE_CURVE ( 'NONE', #15804, #54008, #45007, .T. ) ;
#15235=DIRECTION ( 'NONE',  ( -1.000000000000000000, -0.000000000000000000, -0.000000000000000000 ) ) ;
#15236=CARTESIAN_POINT ( 'NONE',  ( 15.90937500061451892, 0.000000000000000000, 5.243569643749999010 ) ) ;
#15237=CARTESIAN_POINT ( 'NONE',  ( 26.51249999999999929, -5.773502691896255534, -1.060575238724906372E-15 ) ) ;
#15238=CARTESIAN_POINT ( 'NONE',  ( 12.14062500061451821, 6.054752690667223547, 3.707466751127219781E-16 ) ) ;
#15240=CARTESIAN_POINT ( 'NONE',  ( 20.74687500061451573, 6.054752690667223547, 3.707466751127219781E-16 ) ) ;
#15242=CARTESIAN_POINT ( 'NONE',  ( 8.353125000614518569, -4.541064518000417216, -2.621784821875001281 ) ) ;
#15243=CARTESIAN_POINT ( 'NONE',  ( 13.02187500061451608, 3.027376345333613106, -5.243569643749998122 ) ) ;
#15244=ORIENTED_EDGE ( 'NONE', *, *, #57647, .F. ) ;
#15245=CARTESIAN_POINT ( 'NONE',  ( 24.19687500061451857, -3.027376345333610441, -5.243569643749999898 ) ) ;
#15246=CARTESIAN_POINT ( 'NONE',  ( 2.675063744352809358, 4.229653939133389606, -32.98446850650686457 ) ) ;
#15247=CARTESIAN_POINT ( 'NONE',  ( 28.52812500061451573, -4.541064518000419881, 2.621784821874995952 ) ) ;
#15249=CARTESIAN_POINT ( 'NONE',  ( 7.687500000000000000, -2.886751345948125991, -5.000000000000000000 ) ) ;
#15250=CARTESIAN_POINT ( 'NONE',  ( 16.95000000122903216, 5.773502691896255534, 3.535250795749688894E-16 ) ) ;
#15253=ORIENTED_EDGE ( 'NONE', *, *, #34980, .F. ) ;
#15254=CARTESIAN_POINT ( 'NONE',  ( 15.82499999999999929, 6.123233995736764310E-16, -4.999999999999998224 ) ) ;
#15255=CARTESIAN_POINT ( 'NONE',  ( 19.12500000000000000, 4.330127018922191873, 2.499999999999999556 ) ) ;
#15256=CARTESIAN_POINT ( 'NONE',  ( 11.39062500061451644, -3.027376345333614438, 5.243569643749998122 ) ) ;
#15258=CARTESIAN_POINT ( 'NONE',  ( 2.817472997146174052, -4.130598735093008678, -2.817472997146206026 ) ) ;
#15259=CARTESIAN_POINT ( 'NONE',  ( -4.243569643749999898, 16.70937500061451786, -30.00000000000000000 ) ) ;
#15260=CARTESIAN_POINT ( 'NONE',  ( 2.878125000614517592, -4.541064518000419881, 2.621784821874995952 ) ) ;
#15262=CARTESIAN_POINT ( 'NONE',  ( 10.23750000000000071, -2.886751345948129988, 4.999999999999997335 ) ) ;
#15263=CARTESIAN_POINT ( 'NONE',  ( 4.167140676845648706, 2.763139261668956514, -4.167140676845877856 ) ) ;
#15264=VERTEX_POINT ( 'NONE', #38530 ) ;
#15265=CARTESIAN_POINT ( 'NONE',  ( 2.121784821875001281, 12.75312500061451715, 33.67503911421598417 ) ) ;
#15266=CARTESIAN_POINT ( 'NONE',  ( 27.85312500061451502, 4.541064518000418104, -2.621784821874998173 ) ) ;
#15267=CARTESIAN_POINT ( 'NONE',  ( 18.52499999999999858, 6.123233995736764310E-16, -4.999999999999998224 ) ) ;
#15269=CARTESIAN_POINT ( 'NONE',  ( 22.39687500061451075, -3.027376345333610441, -5.243569643749999898 ) ) ;
#15270=CARTESIAN_POINT ( 'NONE',  ( 19.34062500061451573, 6.054752690667223547, 3.707466751127219781E-16 ) ) ;
#15271=CARTESIAN_POINT ( 'NONE',  ( 9.001249775931846008E-16, 14.06562500061459353, -25.09994784771203058 ) ) ;
#15272=CARTESIAN_POINT ( 'NONE',  ( 23.36250000122903359, 0.000000000000000000, 4.999999999999998224 ) ) ;
#15273=CARTESIAN_POINT ( 'NONE',  ( 5.015625000614518214, 3.027376345333611329, 5.243569643749999010 ) ) ;
#15275=CARTESIAN_POINT ( 'NONE',  ( 21.14062500061451644, 6.054752690667223547, 3.707466751127219781E-16 ) ) ;
#15278=CARTESIAN_POINT ( 'NONE',  ( 15.12187500061451750, -6.054752690667223547, -1.112240025338166033E-15 ) ) ;
#15279=CARTESIAN_POINT ( 'NONE',  ( 13.32187500061451502, -6.054752690667223547, -1.112240025338166033E-15 ) ) ;
#15280=CARTESIAN_POINT ( 'NONE',  ( 23.55937500061451573, 0.000000000000000000, 5.243569643749999010 ) ) ;
#15281=CARTESIAN_POINT ( 'NONE',  ( 4.243569643749999010, 12.92187500061451999, 27.54997392385601174 ) ) ;
#15282=CARTESIAN_POINT ( 'NONE',  ( 4.115625000614516082, 3.027376345333611329, 5.243569643749999010 ) ) ;
#15283=CARTESIAN_POINT ( 'NONE',  ( 29.35312500061451502, 0.000000000000000000, 5.243569643749999010 ) ) ;
#15284=CARTESIAN_POINT ( 'NONE',  ( 26.69062500061451715, -3.027376345333614438, 5.243569643749998122 ) ) ;
#15285=CARTESIAN_POINT ( 'NONE',  ( 24.93750000122903288, 6.123233995736764310E-16, -4.999999999999998224 ) ) ;
#15286=CARTESIAN_POINT ( 'NONE',  ( 3.999999999999998668, 19.81250000000000000, 27.69059892324149175 ) ) ;
#15287=CARTESIAN_POINT ( 'NONE',  ( 7.096875000614517148, -3.027376345333610441, -5.243569643749999898 ) ) ;
#15289=CARTESIAN_POINT ( 'NONE',  ( 15.03750000122903252, 6.123233995736764310E-16, -4.999999999999998224 ) ) ;
#15290=CARTESIAN_POINT ( 'NONE',  ( 8.512500001229033941, 0.000000000000000000, 4.999999999999998224 ) ) ;
#15291=CARTESIAN_POINT ( 'NONE',  ( 5.428125000614517859, 4.541064518000418104, 2.621784821874999949 ) ) ;
#15294=CARTESIAN_POINT ( 'NONE',  ( 13.50937500061451679, 4.541064518000418104, -2.621784821874998173 ) ) ;
#15296=ORIENTED_EDGE ( 'NONE', *, *, #16945, .T. ) ;
#15297=CARTESIAN_POINT ( 'NONE',  ( 19.90312500061451573, 0.000000000000000000, 5.243569643749999010 ) ) ;
#15298=CARTESIAN_POINT ( 'NONE',  ( 7.940625000614518036, -3.027376345333610441, -5.243569643749999898 ) ) ;
#15299=CARTESIAN_POINT ( 'NONE',  ( 24.30937500061451573, 4.541064518000418104, -2.621784821874998173 ) ) ;
#15300=CARTESIAN_POINT ( 'NONE',  ( 8.578125000614518214, 4.541064518000418104, 2.621784821874999949 ) ) ;
#15302=CARTESIAN_POINT ( 'NONE',  ( 9.150000001229033231, -2.886751345948125991, -5.000000000000000000 ) ) ;
#15304=CARTESIAN_POINT ( 'NONE',  ( 23.12812500061451360, -4.541064518000419881, 2.621784821874995952 ) ) ;
#15305=CARTESIAN_POINT ( 'NONE',  ( -2.828200636599751609E-16, 17.30000000122903359, -34.61880215351700230 ) ) ;
#15306=CARTESIAN_POINT ( 'NONE',  ( 10.01250000122903394, -4.330127018922190985, -2.500000000000001332 ) ) ;
#15307=CARTESIAN_POINT ( 'NONE',  ( 19.67812500061451786, 6.421520780324663323E-16, -5.243569643749999010 ) ) ;
#15308=CARTESIAN_POINT ( 'NONE',  ( 16.07812500061451289, 6.421520780324663323E-16, -5.243569643749999010 ) ) ;
#15310=CARTESIAN_POINT ( 'NONE',  ( 14.66249999999999964, 2.886751345948126879, 4.999999999999999112 ) ) ;
#15311=CARTESIAN_POINT ( 'NONE',  ( 12.00000000122903465, 5.773502691896255534, 3.535250795749688894E-16 ) ) ;
#15312=CARTESIAN_POINT ( 'NONE',  ( 9.178125000614517859, -4.541064518000419881, 2.621784821874995952 ) ) ;
#15314=CARTESIAN_POINT ( 'NONE',  ( 12.17812500061451608, 4.541064518000418104, 2.621784821874999949 ) ) ;
#15315=CARTESIAN_POINT ( 'NONE',  ( 23.32500000122903572, 2.886751345948126879, 4.999999999999999112 ) ) ;
#15316=CARTESIAN_POINT ( 'NONE',  ( 20.07187500061451857, -6.054752690667223547, -1.112240025338166033E-15 ) ) ;
#15318=CARTESIAN_POINT ( 'NONE',  ( 4.200000001229033053, -2.886751345948125991, -5.000000000000000000 ) ) ;
#15319=CARTESIAN_POINT ( 'NONE',  ( 3.459375000614519635, -4.541064518000417216, -2.621784821875001281 ) ) ;
#15320=CARTESIAN_POINT ( 'NONE',  ( 22.80937500061451573, -4.541064518000417216, -2.621784821875001281 ) ) ;
#15322=CARTESIAN_POINT ( 'NONE',  ( 19.45312500061451644, 0.000000000000000000, 5.243569643749999010 ) ) ;
#15323=CARTESIAN_POINT ( 'NONE',  ( 23.59687500061451715, -3.027376345333614438, 5.243569643749998122 ) ) ;
#15325=CARTESIAN_POINT ( 'NONE',  ( 28.65937500061451715, -4.541064518000417216, -2.621784821875001281 ) ) ;
#15326=CARTESIAN_POINT ( 'NONE',  ( 5.709375000614517859, -4.541064518000417216, -2.621784821875001281 ) ) ;
#15327=CARTESIAN_POINT ( 'NONE',  ( 14.27812500061451573, 6.421520780324663323E-16, -5.243569643749999010 ) ) ;
#15328=CARTESIAN_POINT ( 'NONE',  ( 13.62187500061451750, 3.027376345333611329, 5.243569643749999010 ) ) ;
#15329=ORIENTED_EDGE ( 'NONE', *, *, #57151, .T. ) ;
#15331=CARTESIAN_POINT ( 'NONE',  ( 25.64062500061451644, 6.054752690667223547, 3.707466751127219781E-16 ) ) ;
#15332=CARTESIAN_POINT ( 'NONE',  ( 3.999999999999998668, 13.06250000000000000, -32.30940107675850470 ) ) ;
#15333=CARTESIAN_POINT ( 'NONE',  ( -1.071796769724488563, 11.65490381179670010, -26.00000000000000000 ) ) ;
#15335=CARTESIAN_POINT ( 'NONE',  ( 14.88750000000000107, -2.886751345948125991, -5.000000000000000000 ) ) ;
#15336=CARTESIAN_POINT ( 'NONE',  ( 25.05000000122903714, 5.773502691896255534, 3.535250795749688894E-16 ) ) ;
#15337=CARTESIAN_POINT ( 'NONE',  ( 18.96562500061451573, 3.027376345333611329, 5.243569643749999010 ) ) ;
#15339=CARTESIAN_POINT ( 'NONE',  ( 23.25000000000000000, 0.000000000000000000, 4.999999999999998224 ) ) ;
#15340=CARTESIAN_POINT ( 'NONE',  ( 23.67187500061451999, -6.054752690667223547, -1.112240025338166033E-15 ) ) ;
#15341=ORIENTED_EDGE ( 'NONE', *, *, #42238, .T. ) ;
#15342=CARTESIAN_POINT ( 'NONE',  ( 1.071873214313479261, 4.999999999999998224, -1.071873214313479261 ) ) ;
#15343=CARTESIAN_POINT ( 'NONE',  ( 11.39062500061451644, -3.027376345333614438, 5.243569643749998122 ) ) ;
#15344=CARTESIAN_POINT ( 'NONE',  ( 4.003125000614518925, 4.541064518000418104, -2.621784821874998173 ) ) ;
#15346=CARTESIAN_POINT ( 'NONE',  ( 26.05312500061451431, 4.541064518000418104, -2.621784821874998173 ) ) ;
#15347=CARTESIAN_POINT ( 'NONE',  ( 17.39999999999999858, 0.000000000000000000, 4.999999999999998224 ) ) ;
#15348=CARTESIAN_POINT ( 'NONE',  ( 24.86250000000000071, 2.886751345948129099, -4.999999999999998224 ) ) ;
#15349=CARTESIAN_POINT ( 'NONE',  ( 7.650000001229034119, -2.886751345948130876, 4.999999999999996447 ) ) ;
#15350=CARTESIAN_POINT ( 'NONE',  ( 6.084375000614518747, -4.541064518000419881, 2.621784821874995952 ) ) ;
#15351=CARTESIAN_POINT ( 'NONE',  ( 16.62187500061451573, 3.027376345333613106, -5.243569643749998122 ) ) ;
#15352=CARTESIAN_POINT ( 'NONE',  ( 28.50937500061451502, 0.000000000000000000, 5.243569643749999010 ) ) ;
#15353=ORIENTED_EDGE ( 'NONE', *, *, #14141, .F. ) ;
#15354=CARTESIAN_POINT ( 'NONE',  ( 25.97812500061451502, 6.421520780324663323E-16, -5.243569643749999010 ) ) ;
#15355=CARTESIAN_POINT ( 'NONE',  ( 28.62187500061451573, -6.054752690667223547, -1.112240025338166033E-15 ) ) ;
#15356=CARTESIAN_POINT ( 'NONE',  ( 3.421875000614516882, -6.054752690667223547, -1.112240025338166033E-15 ) ) ;
#15357=CARTESIAN_POINT ( 'NONE',  ( 13.38750000000000107, -2.886751345948129988, 4.999999999999997335 ) ) ;
#15358=CARTESIAN_POINT ( 'NONE',  ( 10.19062500061451892, -3.027376345333610441, -5.243569643749999898 ) ) ;
#15360=DIRECTION ( 'NONE',  ( 0.000000000000000000, 0.000000000000000000, -1.000000000000000000 ) ) ;
#15361=CARTESIAN_POINT ( 'NONE',  ( 28.86562500061451786, 3.027376345333611329, 5.243569643749999010 ) ) ;
#15362=CARTESIAN_POINT ( 'NONE',  ( 16.20000000122903216, -2.886751345948129988, 4.999999999999997335 ) ) ;
#15363=CARTESIAN_POINT ( 'NONE',  ( 30.00000000000000000, 0.000000000000000000, 0.000000000000000000 ) ) ;
#15365=CARTESIAN_POINT ( 'NONE',  ( 5.690625000614516260, -3.027376345333610441, -5.243569643749999898 ) ) ;
#15366=CARTESIAN_POINT ( 'NONE',  ( 22.69687500061451857, -3.027376345333614438, 5.243569643749998122 ) ) ;
#15367=( BOUNDED_CURVE ( )  B_SPLINE_CURVE ( 2, ( #23590, #50594, #40232, #39144, #57201, #11790, #17320 ),
 .UNSPECIFIED., .F., .F. ) 
 B_SPLINE_CURVE_WITH_KNOTS ( ( 3, 2, 2, 3 ),
 ( 0.2166666666666667296, 0.2194444444444444975, 0.2222222222222222654, 0.2250000000000000611 ),
 .UNSPECIFIED. ) 
 CURVE ( )  GEOMETRIC_REPRESENTATION_ITEM ( )  RATIONAL_B_SPLINE_CURVE ( ( 0.9999999999999973355, 0.8660254037844413721, 1.000000000000000000, 0.8660254037844387076, 1.000000000000000000, 0.8660254037844360431, 1.000000000000002665 ) ) 
 REPRESENTATION_ITEM ( '' )  );
#15368=CARTESIAN_POINT ( 'NONE',  ( -4.243569643749999898, 16.25937500061451857, 30.00000000000000000 ) ) ;
#15369=CARTESIAN_POINT ( 'NONE',  ( 22.43437500061451573, 6.421520780324663323E-16, -5.243569643749999010 ) ) ;
#15370=CARTESIAN_POINT ( 'NONE',  ( 4.125000000000000000, 6.123233995736764310E-16, -4.999999999999998224 ) ) ;
#15371=CARTESIAN_POINT ( 'NONE',  ( -3.999999999999999556, 9.725000001229034297, 27.69059892324149530 ) ) ;
#15372=CARTESIAN_POINT ( 'NONE',  ( 12.74062500061451786, -3.027376345333614438, 5.243569643749998122 ) ) ;
#15373=CARTESIAN_POINT ( 'NONE',  ( 5.212500001229032343, 4.330127018922192761, -2.499999999999997780 ) ) ;
#15374=CARTESIAN_POINT ( 'NONE',  ( 9.196875000614518569, -3.027376345333614438, 5.243569643749998122 ) ) ;
#15376=CARTESIAN_POINT ( 'NONE',  ( 9.065625000614517148, 3.027376345333611329, 5.243569643749999010 ) ) ;
#15377=CARTESIAN_POINT ( 'NONE',  ( 15.08437500061451786, -4.541064518000419881, 2.621784821874995952 ) ) ;
#15379=CARTESIAN_POINT ( 'NONE',  ( 21.30000000122903359, -2.886751345948125991, -5.000000000000000000 ) ) ;
#15380=CARTESIAN_POINT ( 'NONE',  ( 7.621875000614519280, 3.027376345333613106, -5.243569643749998122 ) ) ;
#15381=CARTESIAN_POINT ( 'NONE',  ( 11.27812500061451573, 4.541064518000418104, 2.621784821874999949 ) ) ;
#15383=CARTESIAN_POINT ( 'NONE',  ( 22.32187500061451502, -6.054752690667223547, -1.112240025338166033E-15 ) ) ;
#15385=CARTESIAN_POINT ( 'NONE',  ( -3.457895701286862966, 3.616202803579614322, 32.02583422746450026 ) ) ;
#15386=EDGE_CURVE ( 'NONE', #62948, #29428, #67665, .T. ) ;
#15387=CARTESIAN_POINT ( 'NONE',  ( -3.000416591977282496E-16, 12.54687500061451999, -34.90005215228797653 ) ) ;
#15388=CARTESIAN_POINT ( 'NONE',  ( 14.81250000122903288, 0.000000000000000000, 4.999999999999998224 ) ) ;
#15389=CARTESIAN_POINT ( 'NONE',  ( -4.243569643749997233, 18.94062500061451715, -27.54997392385601174 ) ) ;
#15390=CARTESIAN_POINT ( 'NONE',  ( 16.50000000122903288, 5.773502691896255534, 3.535250795749688894E-16 ) ) ;
#15391=CARTESIAN_POINT ( 'NONE',  ( 10.15312500061451750, -4.541064518000417216, -2.621784821875001281 ) ) ;
#15393=CARTESIAN_POINT ( 'NONE',  ( 15.03749999999999964, 5.773502691896255534, 3.535250795749688894E-16 ) ) ;
#15394=CARTESIAN_POINT ( 'NONE',  ( 10.42500000122903181, -5.773502691896255534, -1.060575238724906372E-15 ) ) ;
#15395=CARTESIAN_POINT ( 'NONE',  ( 22.49062500061451431, 6.054752690667223547, 3.707466751127219781E-16 ) ) ;
#15396=CARTESIAN_POINT ( 'NONE',  ( 10.24687500061451573, -3.027376345333610441, -5.243569643749999898 ) ) ;
#15397=CARTESIAN_POINT ( 'NONE',  ( 4.351407642015760580, -2.462831795607901775, -4.629229178597866756 ) ) ;
#15398=CARTESIAN_POINT ( 'NONE',  ( 9.300000001229035362, 5.773502691896255534, 3.535250795749688894E-16 ) ) ;
#15399=CARTESIAN_POINT ( 'NONE',  ( 17.92500000122903359, 2.886751345948126879, 4.999999999999999112 ) ) ;
#15400=CARTESIAN_POINT ( 'NONE',  ( 15.74062500061451608, 6.054752690667223547, 3.707466751127219781E-16 ) ) ;
#15401=CARTESIAN_POINT ( 'NONE',  ( 18.44062500061451715, 6.054752690667223547, 3.707466751127219781E-16 ) ) ;
#15402=CARTESIAN_POINT ( 'NONE',  ( 26.36250000122903003, 4.330127018922192761, -2.499999999999997780 ) ) ;
#15403=CARTESIAN_POINT ( 'NONE',  ( 29.43750000122903288, 6.123233995736764310E-16, -4.999999999999998224 ) ) ;
#15404=CARTESIAN_POINT ( 'NONE',  ( 24.60000000000000142, 0.000000000000000000, 4.999999999999998224 ) ) ;
#15406=CARTESIAN_POINT ( 'NONE',  ( 25.88437500061451502, -4.541064518000419881, 2.621784821874995952 ) ) ;
#15407=CARTESIAN_POINT ( 'NONE',  ( -1.071796769724491005, 15.85759618943233207, 26.00000000000000355 ) ) ;
#15408=CARTESIAN_POINT ( 'NONE',  ( 12.52500000122903145, 2.886751345948126879, 4.999999999999999112 ) ) ;
#15409=CARTESIAN_POINT ( 'NONE',  ( 3.450000000000001510, 0.000000000000000000, 4.999999999999998224 ) ) ;
#15412=CARTESIAN_POINT ( 'NONE',  ( 8.184375000614515727, 4.541064518000418104, 2.621784821874999949 ) ) ;
#15413=CARTESIAN_POINT ( 'NONE',  ( 26.95312500061451644, 4.541064518000418104, -2.621784821874998173 ) ) ;
#15414=CARTESIAN_POINT ( 'NONE',  ( 5.662499999999998757, 2.886751345948193936, 4.999999999999883649 ) ) ;
#15416=CARTESIAN_POINT ( 'NONE',  ( 4.509375000614518569, 4.541064518000418104, -2.621784821874998173 ) ) ;
#15417=CARTESIAN_POINT ( 'NONE',  ( 8.446875000614518569, -3.027376345333610441, -5.243569643749999898 ) ) ;
#15418=CARTESIAN_POINT ( 'NONE',  ( 29.37187500061451928, 3.027376345333611329, 5.243569643749999010 ) ) ;
#15419=CARTESIAN_POINT ( 'NONE',  ( -4.243569643749999898, 12.11562500061459424, 27.54997392385601529 ) ) ;
#15420=CARTESIAN_POINT ( 'NONE',  ( 22.42500000000000071, -4.330127018922194537, 2.499999999999995559 ) ) ;
#15421=EDGE_CURVE ( 'NONE', #21571, #72350, #57281, .T. ) ;
#15422=CARTESIAN_POINT ( 'NONE',  ( 4.387500000000002842, -2.886751345948129988, 4.999999999999997335 ) ) ;
#15423=ORIENTED_EDGE ( 'NONE', *, *, #37449, .T. ) ;
#15424=CARTESIAN_POINT ( 'NONE',  ( 18.06562500061451715, 3.027376345333611329, 5.243569643749999010 ) ) ;
#15425=CARTESIAN_POINT ( 'NONE',  ( 10.60312500061451679, -4.541064518000417216, -2.621784821875001281 ) ) ;
#15427=CARTESIAN_POINT ( 'NONE',  ( 7.246875000614518392, 6.054752690667223547, 3.707466751127219781E-16 ) ) ;
#15428=CARTESIAN_POINT ( 'NONE',  ( 22.64999999999999858, 4.330127018922192761, -2.499999999999997780 ) ) ;
#15429=CARTESIAN_POINT ( 'NONE',  ( 19.57500000122903216, 2.886751345948129099, -4.999999999999998224 ) ) ;
#15430=CARTESIAN_POINT ( 'NONE',  ( 10.20937500061451786, -4.541064518000417216, -2.621784821875001281 ) ) ;
#15431=CARTESIAN_POINT ( 'NONE',  ( 13.09687500061451892, 6.054752690667223547, 3.707466751127219781E-16 ) ) ;
#15432=CARTESIAN_POINT ( 'NONE',  ( 23.48437500061451644, 4.541064518000418104, 2.621784821874999949 ) ) ;
#15433=CARTESIAN_POINT ( 'NONE',  ( 4.192336996406676342, -2.724758798235080715, 4.480034832487019614 ) ) ;
#15436=CARTESIAN_POINT ( 'NONE',  ( 18.00937500061451502, 4.541064518000418104, -2.621784821874998173 ) ) ;
#15437=CARTESIAN_POINT ( 'NONE',  ( 8.259375000614518569, 0.000000000000000000, 5.243569643749999010 ) ) ;
#15439=CARTESIAN_POINT ( 'NONE',  ( 20.32499999999999929, 6.123233995736764310E-16, -4.999999999999998224 ) ) ;
#15441=CARTESIAN_POINT ( 'NONE',  ( 1.626862140677534273E-15, 9.875000001229034652, -26.00000000000000355 ) ) ;
#15443=CARTESIAN_POINT ( 'NONE',  ( 13.60312500061451679, 0.000000000000000000, 5.243569643749999010 ) ) ;
#15444=CARTESIAN_POINT ( 'NONE',  ( 28.24687500061451573, -3.027376345333610441, -5.243569643749999898 ) ) ;
#15447=CARTESIAN_POINT ( 'NONE',  ( 12.59999999999999964, -4.330127018922190985, -2.500000000000001332 ) ) ;
#15448=CARTESIAN_POINT ( 'NONE',  ( 8.484601909799253346E-16, 17.07500000122903572, 34.61880215351700230 ) ) ;
#15449=CARTESIAN_POINT ( 'NONE',  ( 12.30000000122903181, -2.886751345948125991, -5.000000000000000000 ) ) ;
#15450=CARTESIAN_POINT ( 'NONE',  ( 23.48437500061451644, 4.541064518000418104, 2.621784821874999949 ) ) ;
#15451=CARTESIAN_POINT ( 'NONE',  ( 15.87187500061451573, 3.027376345333611329, 5.243569643749999010 ) ) ;
#15452=CARTESIAN_POINT ( 'NONE',  ( -3.999999999999999112, 12.34999999999999964, 30.00000000000000000 ) ) ;
#15454=CARTESIAN_POINT ( 'NONE',  ( 16.94062500061451715, -3.027376345333610441, -5.243569643749999898 ) ) ;
#15455=CARTESIAN_POINT ( 'NONE',  ( 29.62500000122903288, 2.886751345948126879, 4.999999999999999112 ) ) ;
#15456=CARTESIAN_POINT ( 'NONE',  ( 16.58437500061451786, 6.421520780324663323E-16, -5.243569643749999010 ) ) ;
#15457=CARTESIAN_POINT ( 'NONE',  ( 5.128125000614516260, -4.541064518000419881, 2.621784821874995952 ) ) ;
#15458=CARTESIAN_POINT ( 'NONE',  ( 19.04062500061451146, -3.027376345333614438, 5.243569643749998122 ) ) ;
#15459=CARTESIAN_POINT ( 'NONE',  ( -2.000000000000000000, 16.77500000000000213, -33.46410161513775705 ) ) ;
#15460=CARTESIAN_POINT ( 'NONE',  ( 29.74687500061451217, 6.054752690667223547, 3.707466751127219781E-16 ) ) ;
#15461=CARTESIAN_POINT ( 'NONE',  ( -4.243569643749999898, 12.56562500061451715, 27.54997392385601529 ) ) ;
#15462=CARTESIAN_POINT ( 'NONE',  ( 16.62187500061451573, 3.027376345333613106, -5.243569643749998122 ) ) ;
#15463=CARTESIAN_POINT ( 'NONE',  ( 15.93750000122903110, 6.123233995736764310E-16, -4.999999999999998224 ) ) ;
#15465=CARTESIAN_POINT ( 'NONE',  ( -4.243569643749999898, 19.37187500061451928, -32.45002607614398471 ) ) ;
#15466=CARTESIAN_POINT ( 'NONE',  ( 20.29687500061451644, 6.054752690667223547, 3.707466751127219781E-16 ) ) ;
#15467=CARTESIAN_POINT ( 'NONE',  ( 22.53750000122903430, -4.330127018922194537, 2.499999999999995559 ) ) ;
#15469=CARTESIAN_POINT ( 'NONE',  ( 23.12812500061451360, -4.541064518000419881, 2.621784821874995952 ) ) ;
#15470=CARTESIAN_POINT ( 'NONE',  ( 15.98437500061451821, -4.541064518000419881, 2.621784821874995952 ) ) ;
#15471=CARTESIAN_POINT ( 'NONE',  ( 13.15312500061451750, 0.000000000000000000, 5.243569643749999010 ) ) ;
#15472=CARTESIAN_POINT ( 'NONE',  ( -2.121784821874996840, 15.88437500061451857, 33.67503911421598417 ) ) ;
#15473=CARTESIAN_POINT ( 'NONE',  ( 17.87812500061451715, 6.421520780324663323E-16, -5.243569643749999010 ) ) ;
#15474=ORIENTED_EDGE ( 'NONE', *, *, #57411, .F. ) ;
#15475=ORIENTED_EDGE ( 'NONE', *, *, #53989, .F. ) ;
#15476=CARTESIAN_POINT ( 'NONE',  ( 22.61250000000000071, 2.886751345948129099, -4.999999999999998224 ) ) ;
#15477=CARTESIAN_POINT ( 'NONE',  ( 2.121784821874999061, 19.25937500061451857, -33.67503911421598417 ) ) ;
#15479=CARTESIAN_POINT ( 'NONE',  ( 23.76562500061451644, 3.027376345333613106, -5.243569643749998122 ) ) ;
#15481=CARTESIAN_POINT ( 'NONE',  ( 4.640625000614518214, -3.027376345333614438, 5.243569643749998122 ) ) ;
#15482=CARTESIAN_POINT ( 'NONE',  ( 18.33750000122903501, 4.330127018922191873, 2.499999999999999556 ) ) ;
#15483=CARTESIAN_POINT ( 'NONE',  ( 22.07812500061451644, 4.541064518000418104, 2.621784821874999949 ) ) ;
#15484=CARTESIAN_POINT ( 'NONE',  ( 23.02499999999999858, 6.123233995736764310E-16, -4.999999999999998224 ) ) ;
#15485=CARTESIAN_POINT ( 'NONE',  ( 24.47812500061451502, -4.541064518000419881, 2.621784821874995952 ) ) ;
#15486=CARTESIAN_POINT ( 'NONE',  ( 8.165625000614516793, 3.027376345333611329, 5.243569643749999010 ) ) ;
#15487=ORIENTED_EDGE ( 'NONE', *, *, #51411, .F. ) ;
#15489=CARTESIAN_POINT ( 'NONE',  ( 22.75312500061451360, -4.541064518000417216, -2.621784821875001281 ) ) ;
#15490=CARTESIAN_POINT ( 'NONE',  ( 3.065625000614517592, 3.027376345333613106, -5.243569643749998122 ) ) ;
#15492=CARTESIAN_POINT ( 'NONE',  ( 11.02500000122903501, 2.886751345948129099, -4.999999999999997335 ) ) ;
#15493=CARTESIAN_POINT ( 'NONE',  ( -2.828200636599751609E-16, 12.80000000122903181, -34.61880215351700230 ) ) ;
#15494=CARTESIAN_POINT ( 'NONE',  ( -5.810221930991193690E-16, 10.43750000000000000, -34.00000000000000000 ) ) ;
#15495=CARTESIAN_POINT ( 'NONE',  ( 9.787499999999999645, -2.886751345948129988, 4.999999999999997335 ) ) ;
#15496=CARTESIAN_POINT ( 'NONE',  ( 11.85937500061451644, 0.000000000000000000, 5.243569643749999010 ) ) ;
#15497=CARTESIAN_POINT ( 'NONE',  ( 5.287500001229035185, 4.330127018922191873, 2.499999999999999556 ) ) ;
#15498=CARTESIAN_POINT ( 'NONE',  ( 14.74687500061451573, -3.027376345333610441, -5.243569643749999898 ) ) ;
#15499=CARTESIAN_POINT ( 'NONE',  ( 6.309375000614517504, 4.541064518000418104, -2.621784821874998173 ) ) ;
#15501=DIRECTION ( 'NONE',  ( 0.000000000000000000, 0.000000000000000000, -1.000000000000000000 ) ) ;
#15502=CARTESIAN_POINT ( 'NONE',  ( 11.70937500061451608, 4.541064518000418104, -2.621784821874998173 ) ) ;
#15503=DIRECTION ( 'NONE',  ( -1.000000000000000000, -0.000000000000000000, -0.000000000000000000 ) ) ;
#15504=CARTESIAN_POINT ( 'NONE',  ( 21.59062500061451928, 6.054752690667223547, 3.707466751127219781E-16 ) ) ;
#15505=LINE ( 'NONE', #16598, #43954 ) ;
#15506=CARTESIAN_POINT ( 'NONE',  ( -3.000416591977282496E-16, 18.79062500061460028, 25.09994784771203058 ) ) ;
#15507=CARTESIAN_POINT ( 'NONE',  ( 22.65937500061451715, 0.000000000000000000, 5.243569643749999010 ) ) ;
#15509=CARTESIAN_POINT ( 'NONE',  ( 28.65000000122903145, 5.773502691896255534, 3.535250795749688894E-16 ) ) ;
#15511=CARTESIAN_POINT ( 'NONE',  ( 24.89062500061451644, -3.027376345333614438, 5.243569643749998122 ) ) ;
#15512=CARTESIAN_POINT ( 'NONE',  ( 17.24062500061451786, -3.027376345333614438, 5.243569643749998122 ) ) ;
#15514=CARTESIAN_POINT ( 'NONE',  ( 15.08437500061451786, -4.541064518000419881, 2.621784821874995952 ) ) ;
#15516=CARTESIAN_POINT ( 'NONE',  ( 27.63750000122903216, 6.123233995736764310E-16, -4.999999999999998224 ) ) ;
#15517=CARTESIAN_POINT ( 'NONE',  ( 6.196875000614515905, -3.027376345333610441, -5.243569643749999898 ) ) ;
#15518=CARTESIAN_POINT ( 'NONE',  ( 15.94687500061451502, -3.027376345333614438, 5.243569643749998122 ) ) ;
#15519=CARTESIAN_POINT ( 'NONE',  ( 16.27499999999999858, 6.123233995736764310E-16, -4.999999999999998224 ) ) ;
#15520=CARTESIAN_POINT ( 'NONE',  ( 23.09999999999999787, 4.330127018922192761, -2.499999999999997780 ) ) ;
#15521=CARTESIAN_POINT ( 'NONE',  ( 3.787500001229033408, 6.123233995736764310E-16, -4.999999999999998224 ) ) ;
#15522=CARTESIAN_POINT ( 'NONE',  ( 25.24687500061451573, 6.054752690667223547, 3.707466751127219781E-16 ) ) ;
#15523=CARTESIAN_POINT ( 'NONE',  ( 15.45937500061451608, 0.000000000000000000, 5.243569643749999010 ) ) ;
#15525=CARTESIAN_POINT ( 'NONE',  ( 27.93750000000000000, -2.886751345948125991, -5.000000000000000000 ) ) ;
#15526=CARTESIAN_POINT ( 'NONE',  ( 6.037500000000001421, 5.773502691896255534, 3.535250795749688894E-16 ) ) ;
#15528=CARTESIAN_POINT ( 'NONE',  ( 20.84062500061451573, -3.027376345333614438, 5.243569643749998122 ) ) ;
#15529=CARTESIAN_POINT ( 'NONE',  ( 8.887499999999999289, -2.886751345948129988, 4.999999999999997335 ) ) ;
#15530=CARTESIAN_POINT ( 'NONE',  ( 3.703125000614516882, 0.000000000000000000, 5.243569643749999010 ) ) ;
#15531=CARTESIAN_POINT ( 'NONE',  ( 18.33749999999999858, -2.886751345948129988, 4.999999999999997335 ) ) ;
#15532=CARTESIAN_POINT ( 'NONE',  ( -1.071796769724485010, 17.39240381056766083, 34.00000000000000000 ) ) ;
#15533=CARTESIAN_POINT ( 'NONE',  ( 24.15000000122903145, 5.773502691896255534, 3.535250795749688894E-16 ) ) ;
#15534=CARTESIAN_POINT ( 'NONE',  ( 3.685019977366418509, 9.302529035819389946, 34.75091536352346111 ) ) ;
#15535=CARTESIAN_POINT ( 'NONE',  ( 28.39687500061452141, 6.054752690667223547, 3.707466751127219781E-16 ) ) ;
#15537=CARTESIAN_POINT ( 'NONE',  ( 17.42812500061451786, 6.421520780324663323E-16, -5.243569643749999010 ) ) ;
#15538=CARTESIAN_POINT ( 'NONE',  ( 24.70312500061451644, 4.541064518000418104, -2.621784821874998173 ) ) ;
#15539=CARTESIAN_POINT ( 'NONE',  ( 24.34687500061451715, 6.054752690667223547, 3.707466751127219781E-16 ) ) ;
#15540=CARTESIAN_POINT ( 'NONE',  ( 8.550000000000002487, -4.330127018922190985, -2.500000000000001332 ) ) ;
#15541=CARTESIAN_POINT ( 'NONE',  ( 11.20312500061451644, 4.541064518000418104, -2.621784821874998173 ) ) ;
#15542=CARTESIAN_POINT ( 'NONE',  ( 27.55312500061451786, 0.000000000000000000, 5.243569643749999010 ) ) ;
#15543=CARTESIAN_POINT ( 'NONE',  ( 14.25937500061451679, -4.541064518000417216, -2.621784821875001281 ) ) ;
#15544=CARTESIAN_POINT ( 'NONE',  ( 19.02187500061451786, 3.027376345333611329, 5.243569643749999010 ) ) ;
#15545=CYLINDRICAL_SURFACE ( 'NONE', #49857, 3.999999999999996447 ) ;
#15546=CARTESIAN_POINT ( 'NONE',  ( -4.243569643749997233, 18.94062500061451715, 32.45002607614398471 ) ) ;
#15547=CARTESIAN_POINT ( 'NONE',  ( 22.65000000122903856, -2.886751345948125991, -5.000000000000000000 ) ) ;
#15549=CARTESIAN_POINT ( 'NONE',  ( 15.06562500061451892, -6.054752690667223547, -1.112240025338166033E-15 ) ) ;
#15550=CARTESIAN_POINT ( 'NONE',  ( 8.446875000614518569, -3.027376345333610441, -5.243569643749999898 ) ) ;
#15551=CARTESIAN_POINT ( 'NONE',  ( 8.296875000614516438, -3.027376345333614438, 5.243569643749998122 ) ) ;
#15552=ORIENTED_EDGE ( 'NONE', *, *, #65470, .T. ) ;
#15553=CARTESIAN_POINT ( 'NONE',  ( 28.05937500061451573, 0.000000000000000000, 5.243569643749999010 ) ) ;
#15554=CARTESIAN_POINT ( 'NONE',  ( 20.16562500061451146, 3.027376345333613106, -5.243569643749998122 ) ) ;
#15555=CARTESIAN_POINT ( 'NONE',  ( 3.028125000614518392, 6.421520780324663323E-16, -5.243569643749999010 ) ) ;
#15557=CARTESIAN_POINT ( 'NONE',  ( 3.571875000614517237, 3.027376345333613106, -5.243569643749998122 ) ) ;
#15558=CARTESIAN_POINT ( 'NONE',  ( 24.72187500061451360, 3.027376345333613106, -5.243569643749998122 ) ) ;
#15559=CARTESIAN_POINT ( 'NONE',  ( 19.34062500061451573, 6.054752690667223547, 3.707466751127219781E-16 ) ) ;
#15560=CARTESIAN_POINT ( 'NONE',  ( -3.999999999999999112, 12.80000000000000071, 30.00000000000000000 ) ) ;
#15561=CARTESIAN_POINT ( 'NONE',  ( 25.75312500061451715, 0.000000000000000000, 5.243569643749999010 ) ) ;
#15562=CARTESIAN_POINT ( 'NONE',  ( 6.412500001229036073, -4.330127018922190985, -2.500000000000001332 ) ) ;
#15563=VERTEX_POINT ( 'NONE', #41073 ) ;
#15564=CARTESIAN_POINT ( 'NONE',  ( 3.037500001229032964, 4.330127018922191873, 2.499999999999999556 ) ) ;
#15565=CARTESIAN_POINT ( 'NONE',  ( -3.999999999999999556, 14.56250000000000000, -32.30940107675850470 ) ) ;
#15566=CARTESIAN_POINT ( 'NONE',  ( 22.01250000122903216, 0.000000000000000000, 4.999999999999998224 ) ) ;
#15568=( GEOMETRIC_REPRESENTATION_CONTEXT ( 3 ) GLOBAL_UNCERTAINTY_ASSIGNED_CONTEXT ( ( #18835 ) ) GLOBAL_UNIT_ASSIGNED_CONTEXT ( ( #51409, #7067, #812 ) ) REPRESENTATION_CONTEXT ( 'NONE', 'WORKASPACE' ) );
#15569=CARTESIAN_POINT ( 'NONE',  ( 4.809375000614516615, -4.541064518000417216, -2.621784821875001281 ) ) ;
#15570=CARTESIAN_POINT ( 'NONE',  ( 29.12812500061451715, 6.421520780324663323E-16, -5.243569643749999010 ) ) ;
#15571=CARTESIAN_POINT ( 'NONE',  ( 12.10312500061451857, 4.541064518000418104, -2.621784821874998173 ) ) ;
#15572=CARTESIAN_POINT ( 'NONE',  ( 5.821875000614519458, 3.027376345333613106, -5.243569643749998122 ) ) ;
#15573=CARTESIAN_POINT ( 'NONE',  ( 23.47500000122903430, -5.773502691896255534, -1.060575238724906372E-15 ) ) ;
#15574=CARTESIAN_POINT ( 'NONE',  ( 15.83437500061451608, 4.541064518000418104, 2.621784821874999949 ) ) ;
#15575=CARTESIAN_POINT ( 'NONE',  ( 28.49062500061451431, -3.027376345333614438, 5.243569643749998122 ) ) ;
#15576=CARTESIAN_POINT ( 'NONE',  ( 29.28749999999999787, -2.886751345948125991, -5.000000000000000000 ) ) ;
#15577=CARTESIAN_POINT ( 'NONE',  ( 4.228125000614517681, -4.541064518000419881, 2.621784821874995952 ) ) ;
#15578=CARTESIAN_POINT ( 'NONE',  ( 16.19062500061451715, 6.054752690667223547, 3.707466751127219781E-16 ) ) ;
#15579=ORIENTED_EDGE ( 'NONE', *, *, #6144, .F. ) ;
#15580=CARTESIAN_POINT ( 'NONE',  ( 10.67812500061451608, 6.421520780324663323E-16, -5.243569643749999010 ) ) ;
#15581=CARTESIAN_POINT ( 'NONE',  ( 7.678125000614516082, 4.541064518000418104, 2.621784821874999949 ) ) ;
#15583=CARTESIAN_POINT ( 'NONE',  ( 8.362500000000002487, 2.886751345948126879, 4.999999999999999112 ) ) ;
#15584=CARTESIAN_POINT ( 'NONE',  ( 4.350000001229033408, 5.773502691896255534, 3.535250795749688894E-16 ) ) ;
#15585=CARTESIAN_POINT ( 'NONE',  ( 18.14999999999999858, 4.330127018922192761, -2.499999999999997780 ) ) ;
#15586=CARTESIAN_POINT ( 'NONE',  ( 19.65937500061451360, -4.541064518000417216, -2.621784821875001281 ) ) ;
#15587=CARTESIAN_POINT ( 'NONE',  ( 13.91250000122903252, 0.000000000000000000, 4.999999999999998224 ) ) ;
#15589=CARTESIAN_POINT ( 'NONE',  ( -2.121784821874996840, 17.17812500061451786, -26.32496088578401583 ) ) ;
#15591=DIRECTION ( 'NONE',  ( -1.000000000000000000, -0.000000000000000000, -0.000000000000000000 ) ) ;
#15592=LINE ( 'NONE', #3442, #58360 ) ;
#15593=CARTESIAN_POINT ( 'NONE',  ( 20.13750000122903216, 4.330127018922191873, 2.499999999999999556 ) ) ;
#15594=CARTESIAN_POINT ( 'NONE',  ( 13.73437500061451821, -4.541064518000419881, 2.621784821874995952 ) ) ;
#15595=CARTESIAN_POINT ( 'NONE',  ( 26.55000000000000071, -4.330127018922190985, -2.500000000000001332 ) ) ;
#15596=EDGE_CURVE ( 'NONE', #32725, #34653, #2065, .T. ) ;
#15597=CARTESIAN_POINT ( 'NONE',  ( 12.29062500061451857, -3.027376345333614438, 5.243569643749998122 ) ) ;
#15599=CARTESIAN_POINT ( 'NONE',  ( 21.98437500061451644, 6.421520780324663323E-16, -5.243569643749999010 ) ) ;
#15602=CARTESIAN_POINT ( 'NONE',  ( 8.203125000614518214, 0.000000000000000000, 5.243569643749999010 ) ) ;
#15603=CARTESIAN_POINT ( 'NONE',  ( 13.58437500061451786, 4.541064518000418104, 2.621784821874999949 ) ) ;
#15604=ORIENTED_EDGE ( 'NONE', *, *, #65676, .F. ) ;
#15605=CARTESIAN_POINT ( 'NONE',  ( 22.84687500061451715, -3.027376345333610441, -5.243569643749999898 ) ) ;
#15606=DIRECTION ( 'NONE',  ( -1.000000000000000000, -0.000000000000000000, -0.000000000000000000 ) ) ;
#15608=CARTESIAN_POINT ( 'NONE',  ( 4.575000000000002842, 6.123233995736764310E-16, -4.999999999999998224 ) ) ;
#15609=CARTESIAN_POINT ( 'NONE',  ( 18.11250000122903359, -4.330127018922190985, -2.500000000000001332 ) ) ;
#15610=CARTESIAN_POINT ( 'NONE',  ( -3.999999999999999112, 17.86250000122903359, -30.00000000000000000 ) ) ;
#15611=CARTESIAN_POINT ( 'NONE',  ( 14.51250000122903394, -4.330127018922190985, -2.500000000000001332 ) ) ;
#15612=ORIENTED_EDGE ( 'NONE', *, *, #22319, .F. ) ;
#15613=CARTESIAN_POINT ( 'NONE',  ( 14.47499999999999964, 6.123233995736764310E-16, -4.999999999999998224 ) ) ;
#15614=CARTESIAN_POINT ( 'NONE',  ( 17.55000000000000071, -4.330127018922190985, -2.500000000000001332 ) ) ;
#15615=CARTESIAN_POINT ( 'NONE',  ( 14.13750000122903394, 6.123233995736764310E-16, -4.999999999999998224 ) ) ;
#15616=CARTESIAN_POINT ( 'NONE',  ( 10.97812500061451679, -4.541064518000419881, 2.621784821874995952 ) ) ;
#15617=ORIENTED_EDGE ( 'NONE', *, *, #69599, .F. ) ;
#15618=CARTESIAN_POINT ( 'NONE',  ( 9.528763966825557376E-15, 17.07500000122903572, -26.00000000000000000 ) ) ;
#15619=CARTESIAN_POINT ( 'NONE',  ( -4.243569643749997233, 17.19687500061451502, -27.54997392385601174 ) ) ;
#15620=CARTESIAN_POINT ( 'NONE',  ( 4.003125000614518925, 4.541064518000418104, -2.621784821874998173 ) ) ;
#15622=CARTESIAN_POINT ( 'NONE',  ( 11.02500000000000036, 4.330127018922191873, 2.499999999999999556 ) ) ;
#15623=DIRECTION ( 'NONE',  ( -0.000000000000000000, -1.000000000000000000, -0.000000000000000000 ) ) ;
#15625=CARTESIAN_POINT ( 'NONE',  ( 23.24062500061451786, -3.027376345333610441, -5.243569643749999898 ) ) ;
#15626=CARTESIAN_POINT ( 'NONE',  ( 3.631995133754550853, 3.436488000706471535, 3.917251957431123088 ) ) ;
#15628=CARTESIAN_POINT ( 'NONE',  ( 21.27187500061451786, 3.027376345333611329, 5.243569643749999010 ) ) ;
#15630=CARTESIAN_POINT ( 'NONE',  ( 18.92812500061451431, 4.541064518000418104, 2.621784821874999949 ) ) ;
#15631=CARTESIAN_POINT ( 'NONE',  ( -2.121784821874996840, 13.57812500061459460, -26.32496088578401583 ) ) ;
#15632=CARTESIAN_POINT ( 'NONE',  ( 24.48750000122903359, 6.123233995736764310E-16, -4.999999999999998224 ) ) ;
#15633=CARTESIAN_POINT ( 'NONE',  ( 3.778125000614519280, -4.541064518000419881, 2.621784821874995952 ) ) ;
#15635=CARTESIAN_POINT ( 'NONE',  ( 22.60312500061451857, 0.000000000000000000, 5.243569643749999010 ) ) ;
#15638=CARTESIAN_POINT ( 'NONE',  ( 14.63437500061451679, -4.541064518000419881, 2.621784821874995952 ) ) ;
#15639=CARTESIAN_POINT ( 'NONE',  ( 15.19687500061451857, -3.027376345333610441, -5.243569643749999898 ) ) ;
#15640=CARTESIAN_POINT ( 'NONE',  ( 23.33437500061451786, 6.421520780324663323E-16, -5.243569643749999010 ) ) ;
#15642=CARTESIAN_POINT ( 'NONE',  ( -2.121784821874996840, 11.38437500061451679, 33.67503911421598417 ) ) ;
#15643=DIRECTION ( 'NONE',  ( -1.000000000000000000, -0.000000000000000000, -0.000000000000000000 ) ) ;
#15644=CARTESIAN_POINT ( 'NONE',  ( 26.99062500061451431, 6.054752690667223547, 3.707466751127219781E-16 ) ) ;
#15646=CARTESIAN_POINT ( 'NONE',  ( 27.59062500061451573, -3.027376345333614438, 5.243569643749998122 ) ) ;
#15648=CARTESIAN_POINT ( 'NONE',  ( -2.828200636599751609E-16, 19.88749999999999929, 25.38119784648299770 ) ) ;
#15649=CARTESIAN_POINT ( 'NONE',  ( 6.609375000614519102, -4.541064518000417216, -2.621784821875001281 ) ) ;
#15651=CARTESIAN_POINT ( 'NONE',  ( 13.35000000122903430, 5.773502691896255534, 3.535250795749688894E-16 ) ) ;
#15652=CARTESIAN_POINT ( 'NONE',  ( 9.750000001229032875, 5.773502691896255534, 3.535250795749688894E-16 ) ) ;
#15653=CARTESIAN_POINT ( 'NONE',  ( 29.47500000122903430, 2.886751345948129099, -4.999999999999998224 ) ) ;
#15656=CARTESIAN_POINT ( 'NONE',  ( 12.38437500061451857, -4.541064518000419881, 2.621784821874995952 ) ) ;
#15657=CARTESIAN_POINT ( 'NONE',  ( 2.000000000000001332, 17.56250000122903288, 33.46410161513774995 ) ) ;
#15658=EDGE_LOOP ( 'NONE', ( #39621, #31530, #30148, #694 ) ) ;
#15659=CARTESIAN_POINT ( 'NONE',  ( 19.34062500061451573, 6.054752690667223547, 3.707466751127219781E-16 ) ) ;
#15660=CARTESIAN_POINT ( 'NONE',  ( 14.89687500061451786, 6.054752690667223547, 3.707466751127219781E-16 ) ) ;
#15661=CARTESIAN_POINT ( 'NONE',  ( 6.028125000614517504, -4.541064518000419881, 2.621784821874995952 ) ) ;
#15662=CARTESIAN_POINT ( 'NONE',  ( 20.97187500061451715, -6.054752690667223547, -1.112240025338166033E-15 ) ) ;
#15663=CARTESIAN_POINT ( 'NONE',  ( 5.390625000614518214, 6.054752690667223547, 3.707466751127219781E-16 ) ) ;
#15665=CARTESIAN_POINT ( 'NONE',  ( 8.475000001229034297, 2.886751345948126879, 4.999999999999999112 ) ) ;
#15667=CARTESIAN_POINT ( 'NONE',  ( 22.11562500061451786, 3.027376345333611329, 5.243569643749999010 ) ) ;
#15668=CARTESIAN_POINT ( 'NONE',  ( -3.999999999999999556, 18.72500000122903074, -32.30940107675850470 ) ) ;
#15669=CARTESIAN_POINT ( 'NONE',  ( 6.825000001229034829, -5.773502691896255534, -1.060575238724906372E-15 ) ) ;
#15670=( BOUNDED_CURVE ( )  B_SPLINE_CURVE ( 2, ( #11318, #11677, #22028, #22747, #33839, #34193, #6129 ),
 .UNSPECIFIED., .F., .F. ) 
 B_SPLINE_CURVE_WITH_KNOTS ( ( 3, 2, 2, 3 ),
 ( 0.7583333333333333037, 0.7611111111111110716, 0.7638888888888889506, 0.7666666666666668295 ),
 .UNSPECIFIED. ) 
 CURVE ( )  GEOMETRIC_REPRESENTATION_ITEM ( )  RATIONAL_B_SPLINE_CURVE ( ( 1.000000000000000000, 0.8660254037844387076, 1.000000000000000000, 0.8660254037844387076, 1.000000000000000000, 0.8660254037844333785, 1.000000000000005329 ) ) 
 REPRESENTATION_ITEM ( '' )  );
#15671=CARTESIAN_POINT ( 'NONE',  ( 18.51562500061451289, 3.027376345333611329, 5.243569643749999010 ) ) ;
#15672=CARTESIAN_POINT ( 'NONE',  ( 14.61562500061451608, -6.054752690667223547, -1.112240025338166033E-15 ) ) ;
#15674=CARTESIAN_POINT ( 'NONE',  ( 16.76249999999999929, 2.886751345948129099, -4.999999999999998224 ) ) ;
#15675=CARTESIAN_POINT ( 'NONE',  ( 11.21250000122903501, 0.000000000000000000, 4.999999999999998224 ) ) ;
#15676=CARTESIAN_POINT ( 'NONE',  ( 7.228125000614517681, 4.541064518000418104, 2.621784821874999949 ) ) ;
#15677=CARTESIAN_POINT ( 'NONE',  ( 11.50312500061451892, -4.541064518000417216, -2.621784821875001281 ) ) ;
#15678=CARTESIAN_POINT ( 'NONE',  ( 21.56250000122903288, 0.000000000000000000, 4.999999999999998224 ) ) ;
#15679=CARTESIAN_POINT ( 'NONE',  ( 2.121784821875001281, 14.60937500061451821, -26.32496088578401938 ) ) ;
#15680=CARTESIAN_POINT ( 'NONE',  ( 20.22187500061451715, 3.027376345333613106, -5.243569643749998122 ) ) ;
#15682=CARTESIAN_POINT ( 'NONE',  ( 5.287500001229035185, 4.330127018922191873, 2.499999999999999556 ) ) ;
#15683=CARTESIAN_POINT ( 'NONE',  ( 3.721875000614518036, 3.027376345333611329, 5.243569643749999010 ) ) ;
#15684=CARTESIAN_POINT ( 'NONE',  ( 19.88437500061451857, 4.541064518000418104, 2.621784821874999949 ) ) ;
#15686=CARTESIAN_POINT ( 'NONE',  ( 19.15312500061451573, -4.541064518000417216, -2.621784821875001281 ) ) ;
#15688=CARTESIAN_POINT ( 'NONE',  ( 10.95000000000000107, 4.330127018922192761, -2.499999999999997780 ) ) ;
#15690=CARTESIAN_POINT ( 'NONE',  ( 28.20937500061451786, -4.541064518000417216, -2.621784821875001281 ) ) ;
#15692=CARTESIAN_POINT ( 'NONE',  ( 14.72812500061451679, 6.421520780324663323E-16, -5.243569643749999010 ) ) ;
#15693=CARTESIAN_POINT ( 'NONE',  ( 14.03437500061451715, 4.541064518000418104, 2.621784821874999949 ) ) ;
#15695=CARTESIAN_POINT ( 'NONE',  ( 22.27500000122903145, 2.886751345948095793, -5.000000000000055067 ) ) ;
#15696=CARTESIAN_POINT ( 'NONE',  ( 23.31562500061451715, 3.027376345333613106, -5.243569643749998122 ) ) ;
#15697=CARTESIAN_POINT ( 'NONE',  ( 3.999999999999998668, 17.11250000000000071, 27.69059892324149530 ) ) ;
#15698=CARTESIAN_POINT ( 'NONE',  ( 14.55000000000000071, 4.330127018922192761, -2.499999999999997780 ) ) ;
#15699=CARTESIAN_POINT ( 'NONE',  ( 13.12500000000000178, 6.123233995736764310E-16, -4.999999999999998224 ) ) ;
#15700=CARTESIAN_POINT ( 'NONE',  ( 24.41250000122903430, -4.330127018922190985, -2.500000000000001332 ) ) ;
#15701=CARTESIAN_POINT ( 'NONE',  ( 17.69062500061451715, -3.027376345333614438, 5.243569643749998122 ) ) ;
#15702=EDGE_LOOP ( 'NONE', ( #21492, #69876, #2088, #60520 ) ) ;
#15703=CARTESIAN_POINT ( 'NONE',  ( 21.30000000000000071, 4.330127018922192761, -2.499999999999997780 ) ) ;
#15704=EDGE_CURVE ( 'NONE', #6439, #18523, #71327, .T. ) ;
#15705=CARTESIAN_POINT ( 'NONE',  ( 22.73437500061451644, -4.541064518000419881, 2.621784821874995952 ) ) ;
#15707=DIRECTION ( 'NONE',  ( 0.000000000000000000, 0.000000000000000000, 1.000000000000000000 ) ) ;
#15708=CARTESIAN_POINT ( 'NONE',  ( 9.853125000614516793, 4.541064518000418104, -2.621784821874998173 ) ) ;
#15711=CARTESIAN_POINT ( 'NONE',  ( 16.91250000000000142, 2.886751345948126879, 4.999999999999999112 ) ) ;
#15712=CARTESIAN_POINT ( 'NONE',  ( 24.89999999999999858, 4.330127018922192761, -2.499999999999997780 ) ) ;
#15713=CARTESIAN_POINT ( 'NONE',  ( -2.121784821874999949, 19.27812500061451573, 26.32496088578401938 ) ) ;
#15714=CARTESIAN_POINT ( 'NONE',  ( 4.996875000614516615, 6.054752690667223547, 3.707466751127219781E-16 ) ) ;
#15715=CARTESIAN_POINT ( 'NONE',  ( 16.35937500061451644, 0.000000000000000000, 5.243569643749999010 ) ) ;
#15716=CARTESIAN_POINT ( 'NONE',  ( 27.72187500061451715, -6.054752690667223547, -1.112240025338166033E-15 ) ) ;
#15718=CARTESIAN_POINT ( 'NONE',  ( 25.94062500061451715, -3.027376345333610441, -5.243569643749999898 ) ) ;
#15719=CARTESIAN_POINT ( 'NONE',  ( 27.90937500061451715, 4.541064518000418104, -2.621784821874998173 ) ) ;
#15720=CYLINDRICAL_SURFACE ( 'NONE', #54587, 3.999999999999996447 ) ;
#15721=CARTESIAN_POINT ( 'NONE',  ( 13.35000000000000142, 0.000000000000000000, 4.999999999999998224 ) ) ;
#15722=CARTESIAN_POINT ( 'NONE',  ( 11.09062500061451573, -3.027376345333610441, -5.243569643749999898 ) ) ;
#15724=CARTESIAN_POINT ( 'NONE',  ( 7.237499999999998934, -2.886751345948193048, -4.999999999999883649 ) ) ;
#15725=CARTESIAN_POINT ( 'NONE',  ( 28.37812500061451715, 4.541064518000418104, 2.621784821874999949 ) ) ;
#15726=CARTESIAN_POINT ( 'NONE',  ( 15.78750000122903430, -4.330127018922194537, 2.499999999999995559 ) ) ;
#15727=CARTESIAN_POINT ( 'NONE',  ( 3.176339285701963888, -3.861459405730729433, 3.176339285701963888 ) ) ;
#15729=CARTESIAN_POINT ( 'NONE',  ( 4.490625000614516971, 6.054752690667223547, 3.707466751127219781E-16 ) ) ;
#15730=CARTESIAN_POINT ( 'NONE',  ( 21.90937500061451715, -4.541064518000417216, -2.621784821875001281 ) ) ;
#15731=CARTESIAN_POINT ( 'NONE',  ( -3.000416591977282496E-16, 17.04687500061451644, 25.09994784771203058 ) ) ;
#15732=CARTESIAN_POINT ( 'NONE',  ( 21.19687500061451502, 6.054752690667223547, 3.707466751127219781E-16 ) ) ;
#15733=CARTESIAN_POINT ( 'NONE',  ( 28.58437500061451786, -4.541064518000419881, 2.621784821874995952 ) ) ;
#15734=CARTESIAN_POINT ( 'NONE',  ( 4.243569643749999898, 18.24687500061451928, 32.45002607614398471 ) ) ;
#15735=CARTESIAN_POINT ( 'NONE',  ( 11.31562500061451892, 3.027376345333611329, 5.243569643749999010 ) ) ;
#15736=CARTESIAN_POINT ( 'NONE',  ( -3.999999999999999112, 15.16250000122903252, 30.00000000000000000 ) ) ;
#15737=CARTESIAN_POINT ( 'NONE',  ( 6.759375000614516793, 4.541064518000418104, -2.621784821874998173 ) ) ;
#15738=CARTESIAN_POINT ( 'NONE',  ( 3.999999999999999112, 15.72500000000000320, -30.00000000000000000 ) ) ;
#15739=CARTESIAN_POINT ( 'NONE',  ( 8.878125000614515372, 6.421520780324663323E-16, -5.243569643749999010 ) ) ;
#15740=CARTESIAN_POINT ( 'NONE',  ( 13.32187500061451502, -6.054752690667223547, -1.112240025338166033E-15 ) ) ;
#15742=CARTESIAN_POINT ( 'NONE',  ( 21.75000000122903288, -2.886751345948125991, -5.000000000000000000 ) ) ;
#15743=CARTESIAN_POINT ( 'NONE',  ( 8.146875000614516082, 6.054752690667223547, 3.707466751127219781E-16 ) ) ;
#15744=CARTESIAN_POINT ( 'NONE',  ( 10.97812500061451679, -4.541064518000419881, 2.621784821874995952 ) ) ;
#15746=CARTESIAN_POINT ( 'NONE',  ( 22.35937500061451644, -4.541064518000417216, -2.621784821875001281 ) ) ;
#15748=EDGE_CURVE ( 'NONE', #23263, #39486, #22327, .T. ) ;
#15749=CARTESIAN_POINT ( 'NONE',  ( -1.092898315830470590, 4.886665047895962566, 33.85754803517728817 ) ) ;
#15750=CARTESIAN_POINT ( 'NONE',  ( 29.59687500061451715, -3.027376345333610441, -5.243569643749999898 ) ) ;
#15751=CARTESIAN_POINT ( 'NONE',  ( -2.121784821874996840, 11.38437500061451679, -26.32496088578401583 ) ) ;
#15752=CARTESIAN_POINT ( 'NONE',  ( 16.27500000122903501, -5.773502691896255534, -1.060575238724906372E-15 ) ) ;
#15753=CARTESIAN_POINT ( 'NONE',  ( -2.121784821874996840, 14.47812500061451679, -26.32496088578401583 ) ) ;
#15754=CARTESIAN_POINT ( 'NONE',  ( 18.60000000122903430, -2.886751345948125991, -5.000000000000000000 ) ) ;
#15755=CARTESIAN_POINT ( 'NONE',  ( 11.05312500061451608, -4.541064518000417216, -2.621784821875001281 ) ) ;
#15757=CARTESIAN_POINT ( 'NONE',  ( 13.46249999999999858, -5.773502691896255534, -1.060575238724906372E-15 ) ) ;
#15758=CARTESIAN_POINT ( 'NONE',  ( 1.626862140677534273E-15, 13.81250000000000000, 34.00000000000000000 ) ) ;
#15759=CARTESIAN_POINT ( 'NONE',  ( 22.19062500061451715, -3.027376345333614438, 5.243569643749998122 ) ) ;
#15760=CARTESIAN_POINT ( 'NONE',  ( 10.17187500061451999, -6.054752690667223547, -1.112240025338166033E-15 ) ) ;
#15761=CARTESIAN_POINT ( 'NONE',  ( -5.810221930991193690E-16, 14.15000000122903145, 26.00000000000000355 ) ) ;
#15762=EDGE_CURVE ( 'NONE', #2558, #64110, #39401, .T. ) ;
#15763=CARTESIAN_POINT ( 'NONE',  ( 11.21250000122903501, 0.000000000000000000, 4.999999999999998224 ) ) ;
#15764=CARTESIAN_POINT ( 'NONE',  ( 17.66250000122903430, -4.330127018922190985, -2.500000000000001332 ) ) ;
#15765=CARTESIAN_POINT ( 'NONE',  ( 15.36562500061451608, 3.027376345333611329, 5.243569643749999010 ) ) ;
#15766=CARTESIAN_POINT ( 'NONE',  ( 18.51562500061451289, 3.027376345333611329, 5.243569643749999010 ) ) ;
#15767=CARTESIAN_POINT ( 'NONE',  ( 26.40000000122902790, 5.773502691896255534, 3.535250795749688894E-16 ) ) ;
#15768=CARTESIAN_POINT ( 'NONE',  ( 29.25000000122903288, -2.886751345948129988, 4.999999999999997335 ) ) ;
#15769=CARTESIAN_POINT ( 'NONE',  ( 23.66250000000000142, 2.886751345948126879, 4.999999999999999112 ) ) ;
#15771=CARTESIAN_POINT ( 'NONE',  ( 24.68437500061451573, 6.421520780324663323E-16, -5.243569643749999010 ) ) ;
#15772=CARTESIAN_POINT ( 'NONE',  ( 11.77500000000000036, 6.123233995736764310E-16, -4.999999999999998224 ) ) ;
#15773=CARTESIAN_POINT ( 'NONE',  ( 11.77500000122903501, -5.773502691896255534, -1.060575238724906372E-15 ) ) ;
#15775=CARTESIAN_POINT ( 'NONE',  ( 29.40937500061451715, 0.000000000000000000, 5.243569643749999010 ) ) ;
#15777=CARTESIAN_POINT ( 'NONE',  ( 5.596875000614516260, -3.027376345333614438, 5.243569643749998122 ) ) ;
#15778=CARTESIAN_POINT ( 'NONE',  ( 25.56562500061452070, 3.027376345333613106, -5.243569643749998122 ) ) ;
#15781=CARTESIAN_POINT ( 'NONE',  ( 10.92187500061451644, 3.027376345333611329, 5.243569643749999010 ) ) ;
#15782=CARTESIAN_POINT ( 'NONE',  ( 4.247151432104769420, -2.638504256727666863, 4.531370421416291983 ) ) ;
#15783=CARTESIAN_POINT ( 'NONE',  ( 28.79062500061451502, 6.054752690667223547, 3.707466751127219781E-16 ) ) ;
#15784=CARTESIAN_POINT ( 'NONE',  ( 9.646875000614516082, -3.027376345333614438, 5.243569643749998122 ) ) ;
#15785=CARTESIAN_POINT ( 'NONE',  ( 28.05937500061451573, 0.000000000000000000, 5.243569643749999010 ) ) ;
#15786=EDGE_CURVE ( 'NONE', #40370, #60188, #39834, .T. ) ;
#15787=CARTESIAN_POINT ( 'NONE',  ( 4.243569643749999010, 12.41562500061459673, 27.54997392385601174 ) ) ;
#15788=CARTESIAN_POINT ( 'NONE',  ( 21.15000000000000213, -4.330127018922190985, -2.500000000000001332 ) ) ;
#15790=CARTESIAN_POINT ( 'NONE',  ( 29.43750000000000000, 5.773502691896255534, 3.535250795749688894E-16 ) ) ;
#15791=( BOUNDED_SURFACE ( )  B_SPLINE_SURFACE ( 1, 2, ( 
 ( #4441, #26969, #21404, #31033, #70565, #43961, #59097, #8503, #711, #44694, #27692, #67941, #45771, #16587, #73116, #4797, #10694, #27331, #22498, #49863, #50230, #28410, #55764, #56485, #61656, #38782, #23218, #17314, #51307, #15861, #39874, #50946, #67226, #45048, #39138, #5877, #38406, #60929, #32866, #56129, #11055, #33583, #28768, #5522, #72386, #21767, #66858, #62386, #50588, #67583, #10332, #11785, #16229, #345, #55402, #6240, #28060, #5157, #33942, #22851, #61300, #16949, #72755, #44329, #33225, #39502, #11425, #22140, #62026, #45405, #34301, #56833, #40960, #68668, #69031, #35036, #35758, #34667, #18032, #40588, #8054, #25034, #63108, #12508, #24311, #23585, #41671, #46858, #19116, #57196, #57564, #41317, #62749, #36127, #46130, #30588, #53114, #7686, #46492, #63475, #12863, #2158, #2512, #6967, #18392, #29498, #58279, #6611, #52034, #1437, #68307, #17666, #23943, #35394, #69398, #57920, #64194, #18753, #13581, #29139, #7327, #63827, #12142, #58646, #29858, #40227, #51672, #30223, #52394, #1801, #13219, #24670, #1077, #52756, #47216, #69748, #43775, #72213, #66302, #38217, #15679, #55947, #67051, #2876, #66673, #30943, #38597, #31315, #48316, #21591, #53484, #8781, #14318, #25407, #13952, #55226, #60744, #21223, #55586, #42406, #47950, #42041, #36490, #59009, #10155, #33409, #5343, #3250, #59370, #27513, #47577, #70839, #32687, #8413, #64928, #70478, #4621, #19855, #53859, #61124, #36854, #16048, #27150, #25777, #70107, #50047, #10876, #19483, #72574, #10519, #49684, #44145, #33047, #4981, #64564, #21960, #44516, #16410, #38965, #61482, #40776, #23041, #39329, #33772, #5704, #51851, #62570, #6424, #12682, #6788, #28239, #62925, #57740, #18206, #529, #17136, #45952, #40407, #50771, #51132, #11609, #27882, #63289, #56666, #23403, #56314, #45598, #22322, #34127, #35219, #68129, #29322, #57019, #1255, #174, #6062, #23759, #68482, #17846, #17495, #67762, #50416, #12319, #57381, #46312, #45229, #61843, #11248, #22679, #28957, #39695, #68847, #11965, #34854, #40056, #28596, #34490, #51496, #72940, #62214, #44875, #896, #67410, #16772, #7146, #52934, #64744, #46675, #13039, #25211, #19666 ),
 ( #2696, #41850, #24849, #24491, #47758, #59189, #1616, #70295, #30765, #13769, #31128, #14134, #64011, #64378, #69570, #29677, #20028, #24125, #2331, #52574, #36310, #47035, #47395, #1982, #58459, #69926, #42220, #42584, #36670, #69215, #8599, #18931, #37034, #30406, #58825, #41491, #13391, #8235, #35936, #18573, #53296, #25592, #7870, #53669, #48130, #3061, #41140, #19295, #63648, #35576, #70654, #65110, #58097, #14500, #52213, #7503, #30035, #20401, #71023, #43688, #48863, #42949, #44055, #71766, #15229, #21502, #66211, #21136, #9698, #66958, #15589, #59558, #10430, #4170, #31503, #26700, #38131, #21868, #8972, #60653, #3439, #32231, #31868, #10068, #3803, #54766, #54403, #37767, #49233, #4536, #72482, #55138, #48498, #27064, #71395, #16324, #32599, #49595, #20769, #43325, #72120, #60286, #65477, #66581, #4892, #65846, #15958, #27427, #32961, #14867, #26326, #25958, #37406, #38508, #61032, #59929, #55497, #49958, #44430, #54043, #9336, #50330, #22948, #28156, #22236, #23314, #51043, #67676, #807, #45509, #439, #62125, #46223, #68040, #38877, #62841, #56578, #10789, #5975, #17409, #1167, #61396, #39966, #40318, #62480, #12233, #44792, #45143, #34762, #34402, #56930, #11517, #5620, #23676, #6334, #68397, #57297, #56227, #72854, #67324, #16684, #11878, #50684, #6702, #28865, #51404, #28505, #17046, #34039, #39604, #29235, #39240, #33324, #45863, #61754, #17758, #55862, #51768, #68762, #5251, #11156, #27793, #33683, #87, #22592, #36584, #18120, #24764, #59104, #69129, #47307, #13678, #52850, #35847, #35491, #36222, #70201, #12599, #8149, #41761, #69842, #42133, #2604, #1898, #2248, #7419, #40684, #31040, #64290, #35131, #8511, #18487, #53576, #2974, #30676, #69488, #13309, #58372, #25125, #25502, #53208, #58738, #19207, #7783, #47667, #30320, #19577, #64659, #48047, #63202, #46587, #14044, #1530, #57656, #24402, #18847, #7062, #24037, #52487, #58011, #41053, #29590, #52128, #63566, #63924, #12954, #29947, #46951, #41408, #36950, #59470, #15140, #55409, #4804, #26240, #9248, #49505, #27337, #71301, #54676, #8880, #65386, #31415, #4079, #53955, #31783, #9973, #37319, #38042, #43237, #20311 ) ),
 .UNSPECIFIED., .F., .F., .F. ) 
 B_SPLINE_SURFACE_WITH_KNOTS ( ( 2, 2 ),
 ( 3, 2, 2, 2, 2, 2, 2, 2, 2, 2, 2, 2, 2, 2, 2, 2, 2, 2, 2, 2, 2, 2, 2, 2, 2, 2, 2, 2, 2, 2, 2, 2, 2, 2, 2, 2, 2, 2, 2, 2, 2, 2, 2, 2, 2, 2, 2, 2, 2, 2, 2, 2, 2, 2, 2, 2, 2, 2, 2, 2, 2, 2, 2, 2, 2, 2, 2, 2, 2, 2, 2, 2, 2, 2, 2, 2, 2, 2, 2, 2, 2, 2, 2, 2, 2, 2, 2, 2, 2, 2, 2, 2, 2, 2, 2, 2, 2, 2, 2, 2, 2, 2, 2, 2, 2, 2, 2, 2, 2, 2, 2, 2, 2, 2, 2, 2, 2, 2, 2, 2, 2, 2, 2, 2, 2, 2, 2, 2, 2, 2, 2, 2, 2, 2, 2, 3 ),
 ( 0.000000000000000000, 1.000000000000000000 ),
 ( 0.000000000000000000, 0.007246376811594202987, 0.01449275362318840597, 0.02173913043478260809, 0.02898550724637681195, 0.03623188405797101580, 0.04347826086956521618, 0.05072463768115942351, 0.05797101449275362389, 0.06521739130434782428, 0.07246376811594203160, 0.07971014492753622505, 0.08695652173913043237, 0.09420289855072463969, 0.1014492753623188470, 0.1086956521739130405, 0.1159420289855072478, 0.1231884057971014551, 0.1304347826086956486, 0.1376811594202898559, 0.1449275362318840632, 0.1521739130434782705, 0.1594202898550724501, 0.1666666666666666574, 0.1739130434782608647, 0.1811594202898550721, 0.1884057971014492794, 0.1956521739130434867, 0.2028985507246376940, 0.2101449275362318736, 0.2173913043478260809, 0.2246376811594202882, 0.2318840579710144956, 0.2391304347826087029, 0.2463768115942029102, 0.2536231884057971175, 0.2608695652173912971, 0.2681159420289855322, 0.2753623188405797118, 0.2826086956521738913, 0.2898550724637681264, 0.2971014492753623060, 0.3043478260869565410, 0.3115942028985507206, 0.3188405797101449002, 0.3260869565217391353, 0.3333333333333333148, 0.3405797101449275499, 0.3478260869565217295, 0.3550724637681159646, 0.3623188405797101441, 0.3695652173913043237, 0.3768115942028985588, 0.3840579710144927383, 0.3913043478260869734, 0.3985507246376811530, 0.4057971014492753881, 0.4130434782608695676, 0.4202898550724637472, 0.4275362318840579823, 0.4347826086956521618, 0.4420289855072463969, 0.4492753623188405765, 0.4565217391304347561, 0.4637681159420289911, 0.4710144927536231707, 0.4782608695652174058, 0.4855072463768115854, 0.4927536231884058204, 0.5000000000000000000, 0.5072463768115942351, 0.5144927536231883591, 0.5217391304347825942, 0.5289855072463768293, 0.5362318840579710644, 0.5434782608695651884, 0.5507246376811594235, 0.5579710144927536586, 0.5652173913043477826, 0.5724637681159420177, 0.5797101449275362528, 0.5869565217391304879, 0.5942028985507246119, 0.6014492753623188470, 0.6086956521739130821, 0.6159420289855072062, 0.6231884057971014412, 0.6304347826086956763, 0.6376811594202898004, 0.6449275362318840354, 0.6521739130434782705, 0.6594202898550725056, 0.6666666666666666297, 0.6739130434782608647, 0.6811594202898550998, 0.6884057971014492239, 0.6956521739130434590, 0.7028985507246376940, 0.7101449275362319291, 0.7173913043478260532, 0.7246376811594202882, 0.7318840579710145233, 0.7391304347826086474, 0.7463768115942028825, 0.7536231884057971175, 0.7608695652173913526, 0.7681159420289854767, 0.7753623188405797118, 0.7826086956521739468, 0.7898550724637680709, 0.7971014492753623060, 0.8043478260869565410, 0.8115942028985507761, 0.8188405797101449002, 0.8260869565217391353, 0.8333333333333333703, 0.8405797101449274944, 0.8478260869565217295, 0.8550724637681159646, 0.8623188405797101996, 0.8695652173913043237, 0.8768115942028985588, 0.8840579710144927938, 0.8913043478260869179, 0.8985507246376811530, 0.9057971014492753881, 0.9130434782608695121, 0.9202898550724637472, 0.9275362318840579823, 0.9347826086956522174, 0.9420289855072463414, 0.9492753623188405765, 0.9565217391304348116, 0.9637681159420289356, 0.9662082893573751274, 0.9758703722509488587 ),
 .UNSPECIFIED. ) 
 GEOMETRIC_REPRESENTATION_ITEM ( )  RATIONAL_B_SPLINE_SURFACE ( (
 ( 1.000000000000000000, 0.8660254037844387076, 1.000000000000000000, 0.8660254037844387076, 1.000000000000000000, 0.8660254037844387076, 1.000000000000000000, 0.8660254037844387076, 1.000000000000000000, 0.8660254037844387076, 1.000000000000000000, 0.8660254037844387076, 1.000000000000000000, 0.8660254037844387076, 1.000000000000000000, 0.8660254037844387076, 1.000000000000000000, 0.8660254037844387076, 1.000000000000000000, 0.8660254037844387076, 1.000000000000000000, 0.8660254037844387076, 1.000000000000000000, 0.8660254037844387076, 1.000000000000000000, 0.8660254037844387076, 1.000000000000000000, 0.8660254037844387076, 1.000000000000000000, 0.8660254037844387076, 1.000000000000000000, 0.8660254037844387076, 1.000000000000000000, 0.8660254037844387076, 1.000000000000000000, 0.8660254037844387076, 1.000000000000000000, 0.8660254037844387076, 1.000000000000000000, 0.8660254037844387076, 1.000000000000000000, 0.8660254037844387076, 1.000000000000000000, 0.8660254037844387076, 1.000000000000000000, 0.8660254037844387076, 1.000000000000000000, 0.8660254037844387076, 1.000000000000000000, 0.8660254037844387076, 1.000000000000000000, 0.8660254037844387076, 1.000000000000000000, 0.8660254037844387076, 1.000000000000000000, 0.8660254037844387076, 1.000000000000000000, 0.8660254037844387076, 1.000000000000000000, 0.8660254037844387076, 1.000000000000000000, 0.8660254037844387076, 1.000000000000000000, 0.8660254037844387076, 1.000000000000000000, 0.8660254037844387076, 1.000000000000000000, 0.8660254037844387076, 1.000000000000000000, 0.8660254037844387076, 1.000000000000000000, 0.8660254037844387076, 1.000000000000000000, 0.8660254037844387076, 1.000000000000000000, 0.8660254037844387076, 1.000000000000000000, 0.8660254037844387076, 1.000000000000000000, 0.8660254037844387076, 1.000000000000000000, 0.8660254037844387076, 1.000000000000000000, 0.8660254037844387076, 1.000000000000000000, 0.8660254037844387076, 1.000000000000000000, 0.8660254037844387076, 1.000000000000000000, 0.8660254037844387076, 1.000000000000000000, 0.8660254037844387076, 1.000000000000000000, 0.8660254037844387076, 1.000000000000000000, 0.8660254037844387076, 1.000000000000000000, 0.8660254037844387076, 1.000000000000000000, 0.8660254037844387076, 1.000000000000000000, 0.8660254037844387076, 1.000000000000000000, 0.8660254037844387076, 1.000000000000000000, 0.8660254037844387076, 1.000000000000000000, 0.8660254037844387076, 1.000000000000000000, 0.8660254037844387076, 1.000000000000000000, 0.8660254037844387076, 1.000000000000000000, 0.8660254037844387076, 1.000000000000000000, 0.8660254037844387076, 1.000000000000000000, 0.8660254037844387076, 1.000000000000000000, 0.8660254037844387076, 1.000000000000000000, 0.8660254037844387076, 1.000000000000000000, 0.8660254037844387076, 1.000000000000000000, 0.8660254037844387076, 1.000000000000000000, 0.8660254037844387076, 1.000000000000000000, 0.8660254037844387076, 1.000000000000000000, 0.8660254037844387076, 1.000000000000000000, 0.8660254037844387076, 1.000000000000000000, 0.8660254037844387076, 1.000000000000000000, 0.8660254037844387076, 1.000000000000000000, 0.8660254037844387076, 1.000000000000000000, 0.8660254037844387076, 1.000000000000000000, 0.8660254037844387076, 1.000000000000000000, 0.8660254037844387076, 1.000000000000000000, 0.8660254037844387076, 1.000000000000000000, 0.8660254037844387076, 1.000000000000000000, 0.8660254037844387076, 1.000000000000000000, 0.8660254037844387076, 1.000000000000000000, 0.8660254037844387076, 1.000000000000000000, 0.8660254037844387076, 1.000000000000000000, 0.8660254037844387076, 1.000000000000000000, 0.8660254037844387076, 1.000000000000000000, 0.8660254037844387076, 1.000000000000000000, 0.8660254037844387076, 1.000000000000000000, 0.8660254037844387076, 1.000000000000000000, 0.8660254037844387076, 1.000000000000000000, 0.8660254037844387076, 1.000000000000000000, 0.8660254037844387076, 1.000000000000000000, 0.8660254037844387076, 1.000000000000000000, 0.8660254037844387076, 1.000000000000000000, 0.8660254037844387076, 1.000000000000000000, 0.8660254037844387076, 1.000000000000000000, 0.8660254037844387076, 1.000000000000000000, 0.8660254037844387076, 1.000000000000000000, 0.8660254037844387076, 1.000000000000000000, 0.8660254037844387076, 1.000000000000000000, 0.8660254037844387076, 1.000000000000000000, 0.8660254037844387076, 1.000000000000000000, 0.8660254037844387076, 1.000000000000000000, 0.8660254037844387076, 1.000000000000000000, 0.8660254037844387076, 1.000000000000000000, 0.8660254037844387076, 1.000000000000000000, 0.8660254037844387076, 1.000000000000000000, 0.8660254037844387076, 1.000000000000000000, 0.8660254037844387076, 1.000000000000000000, 0.8660254037844387076, 1.000000000000000000, 0.8660254037844387076, 1.000000000000000000, 0.8660254037844387076, 1.000000000000000000, 0.8660254037844387076, 1.000000000000000000, 0.8660254037844387076, 1.000000000000000000, 0.8660254037844387076, 1.000000000000000000, 0.8660254037844387076, 1.000000000000000000, 0.8660254037844387076, 1.000000000000000000, 0.8660254037844387076, 1.000000000000000000, 0.8660254037844387076, 1.000000000000000000, 0.8660254037844387076, 1.000000000000000000, 0.8660254037844387076, 1.000000000000000000, 0.8660254037844387076, 1.000000000000000000, 0.8660254037844387076, 1.000000000000000000, 0.8660254037844387076, 1.000000000000000000, 0.8660254037844387076, 1.000000000000000000, 0.8660254037844387076, 1.000000000000000000, 0.8660254037844387076, 1.000000000000000000, 0.8660254037844387076, 1.000000000000000000, 0.8660254037844387076, 1.000000000000000000, 0.8660254037844387076, 1.000000000000000000, 0.8660254037844387076, 1.000000000000000000, 0.8660254037844387076, 1.000000000000000000, 0.8660254037844387076, 1.000000000000000000, 0.8660254037844387076, 1.000000000000000000, 0.8660254037844387076, 1.000000000000000000, 0.8660254037844387076, 1.000000000000000000, 0.8660254037844387076, 1.000000000000000000, 0.8660254037844387076, 1.000000000000000000, 0.9548848677736607726, 0.9401542295229587953, 0.9401542295229587953, 0.9401542295229587953),
 ( 1.000000000000000000, 0.8660254037844387076, 1.000000000000000000, 0.8660254037844387076, 1.000000000000000000, 0.8660254037844387076, 1.000000000000000000, 0.8660254037844387076, 1.000000000000000000, 0.8660254037844387076, 1.000000000000000000, 0.8660254037844387076, 1.000000000000000000, 0.8660254037844387076, 1.000000000000000000, 0.8660254037844387076, 1.000000000000000000, 0.8660254037844387076, 1.000000000000000000, 0.8660254037844387076, 1.000000000000000000, 0.8660254037844387076, 1.000000000000000000, 0.8660254037844387076, 1.000000000000000000, 0.8660254037844387076, 1.000000000000000000, 0.8660254037844387076, 1.000000000000000000, 0.8660254037844387076, 1.000000000000000000, 0.8660254037844387076, 1.000000000000000000, 0.8660254037844387076, 1.000000000000000000, 0.8660254037844387076, 1.000000000000000000, 0.8660254037844387076, 1.000000000000000000, 0.8660254037844387076, 1.000000000000000000, 0.8660254037844387076, 1.000000000000000000, 0.8660254037844387076, 1.000000000000000000, 0.8660254037844387076, 1.000000000000000000, 0.8660254037844387076, 1.000000000000000000, 0.8660254037844387076, 1.000000000000000000, 0.8660254037844387076, 1.000000000000000000, 0.8660254037844387076, 1.000000000000000000, 0.8660254037844387076, 1.000000000000000000, 0.8660254037844387076, 1.000000000000000000, 0.8660254037844387076, 1.000000000000000000, 0.8660254037844387076, 1.000000000000000000, 0.8660254037844387076, 1.000000000000000000, 0.8660254037844387076, 1.000000000000000000, 0.8660254037844387076, 1.000000000000000000, 0.8660254037844387076, 1.000000000000000000, 0.8660254037844387076, 1.000000000000000000, 0.8660254037844387076, 1.000000000000000000, 0.8660254037844387076, 1.000000000000000000, 0.8660254037844387076, 1.000000000000000000, 0.8660254037844387076, 1.000000000000000000, 0.8660254037844387076, 1.000000000000000000, 0.8660254037844387076, 1.000000000000000000, 0.8660254037844387076, 1.000000000000000000, 0.8660254037844387076, 1.000000000000000000, 0.8660254037844387076, 1.000000000000000000, 0.8660254037844387076, 1.000000000000000000, 0.8660254037844387076, 1.000000000000000000, 0.8660254037844387076, 1.000000000000000000, 0.8660254037844387076, 1.000000000000000000, 0.8660254037844387076, 1.000000000000000000, 0.8660254037844387076, 1.000000000000000000, 0.8660254037844387076, 1.000000000000000000, 0.8660254037844387076, 1.000000000000000000, 0.8660254037844387076, 1.000000000000000000, 0.8660254037844387076, 1.000000000000000000, 0.8660254037844387076, 1.000000000000000000, 0.8660254037844387076, 1.000000000000000000, 0.8660254037844387076, 1.000000000000000000, 0.8660254037844387076, 1.000000000000000000, 0.8660254037844387076, 1.000000000000000000, 0.8660254037844387076, 1.000000000000000000, 0.8660254037844387076, 1.000000000000000000, 0.8660254037844387076, 1.000000000000000000, 0.8660254037844387076, 1.000000000000000000, 0.8660254037844387076, 1.000000000000000000, 0.8660254037844387076, 1.000000000000000000, 0.8660254037844387076, 1.000000000000000000, 0.8660254037844387076, 1.000000000000000000, 0.8660254037844387076, 1.000000000000000000, 0.8660254037844387076, 1.000000000000000000, 0.8660254037844387076, 1.000000000000000000, 0.8660254037844387076, 1.000000000000000000, 0.8660254037844387076, 1.000000000000000000, 0.8660254037844387076, 1.000000000000000000, 0.8660254037844387076, 1.000000000000000000, 0.8660254037844387076, 1.000000000000000000, 0.8660254037844387076, 1.000000000000000000, 0.8660254037844387076, 1.000000000000000000, 0.8660254037844387076, 1.000000000000000000, 0.8660254037844387076, 1.000000000000000000, 0.8660254037844387076, 1.000000000000000000, 0.8660254037844387076, 1.000000000000000000, 0.8660254037844387076, 1.000000000000000000, 0.8660254037844387076, 1.000000000000000000, 0.8660254037844387076, 1.000000000000000000, 0.8660254037844387076, 1.000000000000000000, 0.8660254037844387076, 1.000000000000000000, 0.8660254037844387076, 1.000000000000000000, 0.8660254037844387076, 1.000000000000000000, 0.8660254037844387076, 1.000000000000000000, 0.8660254037844387076, 1.000000000000000000, 0.8660254037844387076, 1.000000000000000000, 0.8660254037844387076, 1.000000000000000000, 0.8660254037844387076, 1.000000000000000000, 0.8660254037844387076, 1.000000000000000000, 0.8660254037844387076, 1.000000000000000000, 0.8660254037844387076, 1.000000000000000000, 0.8660254037844387076, 1.000000000000000000, 0.8660254037844387076, 1.000000000000000000, 0.8660254037844387076, 1.000000000000000000, 0.8660254037844387076, 1.000000000000000000, 0.8660254037844387076, 1.000000000000000000, 0.8660254037844387076, 1.000000000000000000, 0.8660254037844387076, 1.000000000000000000, 0.8660254037844387076, 1.000000000000000000, 0.8660254037844387076, 1.000000000000000000, 0.8660254037844387076, 1.000000000000000000, 0.8660254037844387076, 1.000000000000000000, 0.8660254037844387076, 1.000000000000000000, 0.8660254037844387076, 1.000000000000000000, 0.8660254037844387076, 1.000000000000000000, 0.8660254037844387076, 1.000000000000000000, 0.8660254037844387076, 1.000000000000000000, 0.8660254037844387076, 1.000000000000000000, 0.8660254037844387076, 1.000000000000000000, 0.8660254037844387076, 1.000000000000000000, 0.8660254037844387076, 1.000000000000000000, 0.8660254037844387076, 1.000000000000000000, 0.8660254037844387076, 1.000000000000000000, 0.8660254037844387076, 1.000000000000000000, 0.8660254037844387076, 1.000000000000000000, 0.8660254037844387076, 1.000000000000000000, 0.8660254037844387076, 1.000000000000000000, 0.8660254037844387076, 1.000000000000000000, 0.8660254037844387076, 1.000000000000000000, 0.8660254037844387076, 1.000000000000000000, 0.8660254037844387076, 1.000000000000000000, 0.8660254037844387076, 1.000000000000000000, 0.8660254037844387076, 1.000000000000000000, 0.8660254037844387076, 1.000000000000000000, 0.8660254037844387076, 1.000000000000000000, 0.8660254037844387076, 1.000000000000000000, 0.8660254037844387076, 1.000000000000000000, 0.9548848677736607726, 0.9401542295229587953, 0.9401542295229587953, 0.9401542295229587953) ) ) 
 REPRESENTATION_ITEM ( '' )  SURFACE ( )  );
#15792=CARTESIAN_POINT ( 'NONE',  ( 4.949999999999999289, -4.330127018922190985, -2.500000000000001332 ) ) ;
#15793=ORIENTED_EDGE ( 'NONE', *, *, #13955, .F. ) ;
#15794=CARTESIAN_POINT ( 'NONE',  ( 19.07812500061451644, -4.541064518000419881, 2.621784821874995952 ) ) ;
#15795=CARTESIAN_POINT ( 'NONE',  ( 11.54062500061451857, -3.027376345333610441, -5.243569643749999898 ) ) ;
#15797=CARTESIAN_POINT ( 'NONE',  ( 7.734375000614517326, 4.541064518000418104, 2.621784821874999949 ) ) ;
#15798=CARTESIAN_POINT ( 'NONE',  ( 19.31250000122903288, 0.000000000000000000, 4.999999999999998224 ) ) ;
#15799=CARTESIAN_POINT ( 'NONE',  ( 23.96250000122903145, -4.330127018922190985, -2.500000000000001332 ) ) ;
#15800=CARTESIAN_POINT ( 'NONE',  ( 6.459375000614518747, 0.000000000000000000, 5.243569643749999010 ) ) ;
#15801=CARTESIAN_POINT ( 'NONE',  ( 14.74687500061451573, -3.027376345333610441, -5.243569643749999898 ) ) ;
#15802=CARTESIAN_POINT ( 'NONE',  ( 24.08437500061451786, -4.541064518000419881, 2.621784821874995952 ) ) ;
#15803=CARTESIAN_POINT ( 'NONE',  ( 1.071796769724484344, 15.74509619066136956, -25.99999999999999645 ) ) ;
#15804=VERTEX_POINT ( 'NONE', #70223 ) ;
#15806=CARTESIAN_POINT ( 'NONE',  ( 17.22187500061451715, 3.027376345333611329, 5.243569643749999010 ) ) ;
#15807=CARTESIAN_POINT ( 'NONE',  ( 9.984375000614518214, 4.541064518000418104, 2.621784821874999949 ) ) ;
#15809=CARTESIAN_POINT ( 'NONE',  ( 21.15000000000000213, -4.330127018922190985, -2.500000000000001332 ) ) ;
#15813=CARTESIAN_POINT ( 'NONE',  ( 12.74062500061451786, -3.027376345333614438, 5.243569643749998122 ) ) ;
#15814=CARTESIAN_POINT ( 'NONE',  ( 28.80937500061451573, 4.541064518000418104, -2.621784821874998173 ) ) ;
#15815=LINE ( 'NONE', #71620, #50226 ) ;
#15816=CARTESIAN_POINT ( 'NONE',  ( 9.712500000000002132, 2.886751345948126879, 4.999999999999999112 ) ) ;
#15817=CARTESIAN_POINT ( 'NONE',  ( 2.000000000000001332, 15.76250000122903216, 33.46410161513774995 ) ) ;
#15818=CARTESIAN_POINT ( 'NONE',  ( 12.56250000122903465, 0.000000000000000000, 4.999999999999998224 ) ) ;
#15819=CARTESIAN_POINT ( 'NONE',  ( 22.80937500061451573, -4.541064518000417216, -2.621784821875001281 ) ) ;
#15820=CARTESIAN_POINT ( 'NONE',  ( 15.15937500061451715, -4.541064518000417216, -2.621784821875001281 ) ) ;
#15821=CARTESIAN_POINT ( 'NONE',  ( 3.999999999999999112, 16.73750000122903359, 30.00000000000000000 ) ) ;
#15822=ORIENTED_EDGE ( 'NONE', *, *, #67839, .F. ) ;
#15824=CARTESIAN_POINT ( 'NONE',  ( 16.52812500061451573, 6.421520780324663323E-16, -5.243569643749999010 ) ) ;
#15825=CARTESIAN_POINT ( 'NONE',  ( 28.80000000122903003, -2.886751345948129988, 4.999999999999997335 ) ) ;
#15826=CARTESIAN_POINT ( 'NONE',  ( 14.74687500061451573, -3.027376345333610441, -5.243569643749999898 ) ) ;
#15827=CARTESIAN_POINT ( 'NONE',  ( 1.391695283777659053, 9.904653401742692154, -24.16020628980599483 ) ) ;
#15828=CARTESIAN_POINT ( 'NONE',  ( 19.56562500061451715, -6.054752690667223547, -1.112240025338166033E-15 ) ) ;
#15829=CARTESIAN_POINT ( 'NONE',  ( 3.999999999999998668, 16.66250000000000142, -32.30940107675850470 ) ) ;
#15830=CARTESIAN_POINT ( 'NONE',  ( 27.64687500061452141, -3.027376345333614438, 5.243569643749998122 ) ) ;
#15831=CARTESIAN_POINT ( 'NONE',  ( 9.001249775931846008E-16, 12.71562500061451750, 34.90005215228797653 ) ) ;
#15832=CARTESIAN_POINT ( 'NONE',  ( 16.47187500061452070, -6.054752690667223547, -1.112240025338166033E-15 ) ) ;
#15833=CARTESIAN_POINT ( 'NONE',  ( 15.37500000122903465, -5.773502691896255534, -1.060575238724906372E-15 ) ) ;
#15835=CARTESIAN_POINT ( 'NONE',  ( 4.243569643749999898, 18.28437500061451715, -30.00000000000000000 ) ) ;
#15836=CARTESIAN_POINT ( 'NONE',  ( 20.10937500061451289, -4.541064518000417216, -2.621784821875001281 ) ) ;
#15837=CARTESIAN_POINT ( 'NONE',  ( 23.66250000122903430, 4.330127018922192761, -2.499999999999997780 ) ) ;
#15838=CARTESIAN_POINT ( 'NONE',  ( 16.02187500061451786, -6.054752690667223547, -1.112240025338166033E-15 ) ) ;
#15839=CARTESIAN_POINT ( 'NONE',  ( 11.72812500061451857, 4.541064518000418104, 2.621784821874999949 ) ) ;
#15840=CARTESIAN_POINT ( 'NONE',  ( -2.121784821874999949, 13.03437500061451715, 26.32496088578401938 ) ) ;
#15841=CARTESIAN_POINT ( 'NONE',  ( 17.24062500061451786, -3.027376345333614438, 5.243569643749998122 ) ) ;
#15843=VERTEX_POINT ( 'NONE', #19597 ) ;
#15844=CARTESIAN_POINT ( 'NONE',  ( 19.72499999999999787, -4.330127018922194537, 2.499999999999995559 ) ) ;
#15845=CARTESIAN_POINT ( 'NONE',  ( 17.51249999999999929, -5.773502691896255534, -1.060575238724906372E-15 ) ) ;
#15846=CARTESIAN_POINT ( 'NONE',  ( 23.69062500061451004, -3.027376345333610441, -5.243569643749999898 ) ) ;
#15847=CARTESIAN_POINT ( 'NONE',  ( 6.065625000614516260, -6.054752690667223547, -1.112240025338166033E-15 ) ) ;
#15848=CARTESIAN_POINT ( 'NONE',  ( 17.28750000122903430, 6.123233995736764310E-16, -4.999999999999998224 ) ) ;
#15849=CARTESIAN_POINT ( 'NONE',  ( 23.12812500061451360, -4.541064518000419881, 2.621784821874995952 ) ) ;
#15850=CARTESIAN_POINT ( 'NONE',  ( 22.94999999999999929, -4.330127018922190985, -2.500000000000001332 ) ) ;
#15851=CARTESIAN_POINT ( 'NONE',  ( 26.24062500061451431, -3.027376345333614438, 5.243569643749998122 ) ) ;
#15852=CARTESIAN_POINT ( 'NONE',  ( 4.678125000614516971, -4.541064518000419881, 2.621784821874995952 ) ) ;
#15853=( BOUNDED_SURFACE ( )  B_SPLINE_SURFACE ( 1, 2, ( 
 ( #3264, #43887, #37965, #42781, #14691, #60860, #71592, #66413, #71217, #60121, #65674, #55332, #49793, #49064, #36867, #15790, #38331, #4001, #26154, #10263, #65301, #20594, #48694, #32428, #25792, #32795, #60486, #43152, #15063, #72318, #20966, #21699, #37600, #32065, #54597, #44256, #66788, #9892, #59385, #48330, #70855, #20229, #54965, #5449, #38712, #57125, #29069, #39070, #56418, #72687, #6536, #5088, #11715, #51605, #1005, #61231, #22785, #23512, #67872, #50519, #46061, #5809, #641, #34597, #17601, #50877, #45337, #50157, #16517, #6170, #17244, #55692, #10625, #39804, #22069, #28699, #23150, #33875, #62320, #67157, #44628, #34232, #73047, #28340, #275, #61953, #45704, #22429, #68237, #16160, #33155, #27623, #61584, #56766, #40160, #67514, #10987, #51238, #62680, #12075, #33508, #56057, #27989, #44976, #16878, #39432, #11357, #24598, #18317, #46422, #47146, #40888, #29786, #13146, #52322, #58208, #17957, #53412, #57848, #57494, #70035, #1725, #25331, #7980, #35686, #24237, #13881, #47504, #18682, #7612, #2438, #63034, #69677, #46787, #19408, #12789, #19043, #40519, #34967, #12433, #41245, #68595, #69322, #63757, #35326, #41967, #30149, #6898, #52681, #2089, #23874, #41601, #64120, #68960, #64488, #63404, #36420, #30516, #2804, #29429, #51966, #1365, #7258, #13506, #36052, #58573, #53043, #24960, #58936, #8343, #30872, #31976, #3915, #54512, #4645, #55250, #64856, #9080, #70406, #48978, #15339, #54152, #26437, #36782, #14244, #19781, #10178, #3178, #65959, #21247, #71133, #3546, #71507, #20506, #71875, #26069, #20883, #48241, #60399, #42331, #20141, #42696, #53782, #70766, #25705, #4283, #59298, #8708, #47877, #43437, #48608, #31616, #31241, #65218, #32713, #14608, #37516, #43801, #37145, #37879, #59672, #43063, #9807, #26809, #32340, #49343, #65588, #66326, #60771, #14978, #60037, #54878, #15703, #38242, #9448, #11635, #66701, #33070, #45255, #22703, #38990, #10902, #33796, #38623, #27905, #72601, #72965, #67074, #68156, #50071, #56339, #27539, #21615, #39721, #67788, #72237, #56688, #5729, #28619, #34151, #17162, #62239, #17519, #21984, #62595, #6087, #33430, #198, #44170, #16797, #11991, #39354, #55973, #50795, #5367, #44543, #51156, #16432, #557, #23067, #34514, #49709, #16073, #61147, #61505, #10542, #50440, #22347, #44899, #45622, #40080, #57043, #55609, #11275, #28264, #27175, #5005, #67435, #61868, #40802, #28984, #7529, #47061, #12706, #13063, #68510, #23430, #51522, #41875, #34878, #24517, #52960, #29701, #35243, #30062, #52238, #30432, #57764, #58121, #6812, #18957, #921, #51878, #1277, #12343, #29346, #57407, #35964, #45976, #17873, #36337, #52600, #7173, #63315, #13797, #40432, #64404, #62949, #69238, #2357, #23786, #2006, #46338, #68872, #69595, #58485, #41517, #7895, #1643, #24874, #19321, #24149, #18228, #64036, #13415, #35602, #46702, #47421, #18600, #41164, #69951, #6449, #63673, #42608, #65503, #70317, #59582, #31152, #31527, #25616, #26723, #8623, #14891, #59215, #53322, #71418, #26349, #30791, #15254, #37431, #60312, #65873, #48888, #20795, #49258, #53693, #21160, #3828, #65133, #31893, #2721, #48522, #43713, #71049, #14524, #37791, #8995, #58851, #3463, #37058, #14159, #54067, #25983, #9722, #25237, #59953, #20424, #32255, #3087, #9360, #47783, #19692, #42245, #42972, #15613, #54429, #43351, #48152, #54788, #70678, #4194, #64769, #20053, #71791, #66235, #36693, #8261, #39265, #44079, #15982, #62148, #72878, #28179, #72506, #61420, #66982, #56602, #5998, #27819, #38155, #67698, #5643, #28529, #34061, #27452, #60678, #51067, #464, #61055, #5274, #21524, #22972, #27087, #33705, #45534, #68063, #10092, #44813, #32622, #16709, #21895, #55162, #50352, #22616, #4559, #39630, #22260, #67347, #72146, #38532, #50707, #61777, #49619, #66607, #11181, #10454, #110, #45167, #55886, #56252, #32983, #55523, #17070, #44452, #11544, #4917, #10814, #49982, #16346, #38901, #33348, #30344, #47330, #7807, #58033, #41431, #68785, #52872, #41075, #12977, #69509, #13332, #2270, #35514, #23338, #62861, #7443, #46974, #46608, #40340, #68419, #69151, #12256, #51788, #35155, #1189, #7084, #39989, #24786, #6724, #6357, #18869, #23697, #17431, #29969, #57679, #46245, #35870, #63947, #52510, #63589, #24062, #45887, #1920, #56953, #17781, #24425, #58394, #29258, #18141, #18510, #28889, #40708, #34787, #63226, #57320, #62502, #12620, #11900, #29613, #34425, #51428, #830, #52149, #1552, #25896, #71328, #3737, #59866, #9270, #37701, #64682, #32170, #14800, #53601, #42887, #64313, #59493, #54703, #8906, #25523, #48799, #19967, #69863, #14436, #2995, #25149, #20334, #48066, #70225, #20703, #42155, #43261, #31805, #4108, #19229, #36246, #30698, #14067, #13703, #19599, #36606, #42520, #37343, #65782, #9636, #58760, #53977, #48436, #3375, #26636, #41783, #8170, #31063, #53230, #70961, #54343, #70592, #65410, #2627, #47689, #59127, #8534, #65046, #26262, #15164, #36970, #31437, #60222, #21803, #1022, #55438, #27728, #49533, #61691, #43626, #21436, #43993, #55073, #72057, #4473, #6553, #66148, #71703, #6914, #50266, #49895, #32898, #57512, #15526, #12452, #32536, #38817, #46078, #27003, #72791, #66515, #15895, #67262, #29086, #39175, #51621, #4830, #23528, #63051, #27364, #38442, #11090, #16620, #21075, #68613, #5190, #17974, #56162, #33618, #40535, #34984, #60968, #49172, #38068, #72420, #22174, #60592, #61332, #10001, #10730, #44367, #10368, #66894, #16262, #33262, #55800, #44727, #53061, #35703, #29803, #8360, #1741, #2821, #41985, #36800, #51982, #68977, #63420, #24255, #23891, #52339, #46803, #2105, #47523, #30889, #42350, #18334, #13523, #58591, #36071, #59315, #29444, #46438, #63774, #1381, #30534, #70052, #58224, #7998, #40907, #12806, #35342, #64873, #57865, #19425 ),
 ( #2455, #30166, #13162, #7274, #69339, #14261, #18698, #19060, #25349, #41262, #24978, #7629, #52699, #64506, #58952, #13898, #53431, #24616, #47895, #47163, #69695, #41618, #36438, #70423, #19798, #64137, #66341, #48260, #14624, #26826, #4301, #20522, #65606, #15355, #20159, #9464, #54166, #54528, #48624, #49724, #31633, #37897, #9096, #3195, #54894, #59689, #65234, #60415, #14994, #20899, #48994, #3931, #15719, #43080, #60786, #72251, #21628, #38638, #44186, #49360, #32727, #60053, #66716, #32356, #71890, #10192, #4660, #16090, #21263, #37163, #3563, #43817, #38257, #9824, #26085, #71149, #55264, #37531, #31994, #26454, #71524, #43453, #31258, #8724, #65975, #70783, #27189, #53800, #25722, #42713, #5744, #44913, #6465, #40095, #11290, #28278, #68170, #55624, #17176, #67450, #12005, #5381, #62253, #33085, #27554, #5020, #33811, #17889, #61884, #16812, #27919, #50810, #50453, #34528, #67088, #22361, #72979, #56702, #50086, #51171, #11650, #16447, #39004, #57058, #22717, #575, #39368, #56354, #212, #29000, #51537, #45270, #61162, #17533, #28633, #937, #23445, #67803, #10557, #45991, #68528, #10917, #39736, #44557, #72617, #22000, #6102, #61519, #33443, #55988, #34165, #23080, #45637, #62609, #41894, #63690, #64053, #2374, #7911, #13080, #7545, #29362, #68888, #18974, #52617, #57424, #62965, #2023, #51895, #41534, #13433, #18616, #6828, #7189, #12361, #24534, #69613, #29717, #30079, #1293, #34895, #23803, #69968, #46354, #47078, #30449, #24167, #52255, #35983, #69254, #52978, #1658, #58502, #18245, #24892, #40818, #63334, #12722, #35258, #57779, #46719, #47437, #41181, #35619, #64421, #19339, #58139, #40449, #40683, #27792, #68761, #16683, #22947, #29234, #61753, #34401, #39239, #86, #51403, #62840, #23313, #12232, #17045, #34761, #46222, #62124, #11155, #806, #6333, #39965, #33682, #17757, #72853, #56226, #45862, #28864, #45142, #39603, #62479, #44791, #34038, #5619, #5974, #22591, #1166, #28155, #11877, #50683, #50329, #68396, #40317, #5250, #57296, #56929, #6701, #51767, #23675, #18119, #63201, #67675, #33323, #55861, #11516, #22235, #67323, #45508, #56577, #68039, #28504, #51042, #438, #17408, #15586, #4889, #48495, #31500, #32596, #65474, #21499, #66578, #26696, #55135, #59926, #14863, #60650, #65843, #21133, #49230, #54763, #15955, #43322, #61029, #72479, #21865, #38874, #44426, #49592, #32958, #60283, #4533, #37403, #44052, #38504, #71763, #27061, #9333, #31865, #10065, #15225, #43685, #66208, #4167, #10427, #37764, #55494, #66955, #16321, #8968, #54040, #72117, #27424, #9695, #3436, #49955, #25955, #71020, #20397, #42946, #54400, #3800, #26323, #48860, #71391, #38128, #20765, #32228, #39961, #33679, #22588, #5969, #45139, #51038, #10786, #46218, #50680, #50326, #62836, #67672, #18115, #802, #28500, #17041, #6697, #40312, #11512, #434, #68392, #55858, #17404, #39599, #12228, #5615, #62475, #33320, #27789, #5247, #34034, #61393, #62120, #56572, #28151, #22943, #83, #34757, #67320, #45504, #68034, #56925, #72850, #51399, #11872, #16680, #39236, #57292, #34397, #23309, #6329, #28860, #45858, #29230, #51763, #17753, #22232, #1162, #23671, #68756, #44788, #61750, #11152, #56223, #53571, #63561, #7778, #24032, #31035, #29585, #36217, #2969, #25497, #63197, #47302, #48042, #19202, #1893, #70567, #30315, #25120, #59099, #42128, #2243, #69837, #41756, #64285, #13673, #36579, #7057, #12593, #8506, #40679, #12949, #52845, #46581, #35126, #52123, #58733, #57651, #1525, #69124, #8144, #18482, #30671, #24397, #41048, #24759, #47662, #35486, #64654, #53203, #2599, #70196, #19572, #14039, #58006, #7414, #29942, #52482, #46946, #69483, #18842, #58367, #41403, #63919, #13304, #35842, #3708, #32139, #60196, #65752, #4444, #54317, #72030, #10336, #32868, #49865, #55405, #60562, #43963, #71296, #4800, #43596, #15496, #21406, #15863, #27333, #38038, #25869, #65381, #9969, #49501, #49141, #42859, #70935, #71670, #14772, #26235, #37674, #48772, #9608, #42496, #19943, #9243, #8875, #66484, #20675, #65019, #32506, #54672, #43232, #38411, #60932, #15136, #4075, #26972, #14408, #21044, #26603, #36945, #37314, #66117, #59465, #31410, #53950, #55041, #3347, #48409, #20306, #59838, #31778, #40145, #46768, #5159, #34581, #62661, #68941, #16232, #63387, #1346, #27694, #50234, #24219, #34949, #12772, #57109, #23497, #29053, #18665, #41226, #63018, #72389, #29768, #40870, #63737, #69303, #12058, #21769, #23856, #35307, #6520, #6881, #61302, #38785, #44333, #35667, #627, #18299, #13128, #46045, #51589, #46403, #68580, #58190, #989, #51947, #23133, #57830, #66861, #45689, #68223, #17586, #17940, #40503, #52303, #10697, #33229, #30131, #7239, #12417, #57476, #7593, #55767, #29414, #1704, #42311, #48588, #7961, #53763, #36033, #19386, #70745, #9061, #42676, #31594, #36403, #54132, #65568, #8324, #58551, #20122, #25687, #59280, #30497, #37122, #19022, #53025, #65199, #48221, #64468, #58915, #8688, #64099, #53389, #24941, #25309, #41947, #20486, #2419, #31220, #47485, #47126, #14588, #59651, #24579, #3527, #3158, #26048, #71114, #43041, #14957, #37496, #70016, #60016, #9428, #30854, #52663, #69657, #64838, #2070, #14225, #2785, #41582, #47856, #13484, #13861, #70385, #19761, #36762, #38221, #32321, #10881, #4265, #5346, #44521, #39332, #54494, #71487, #65939, #26789, #26415, #54856, #49323, #4625, #50050, #33412, #44878, #20864, #16053, #61127, #38601, #61846, #31956, #48957, #66306, #3895, #27516, #55950, #27884, #22325, #72578, #37858, #71854, #21963, #61485, #10522, #21227, #9787, #33050, #43779, #15683, #49688, #60750, #21595, #43415, #16775, #10159, #15319, #50418, #32693, #60379, #67054, #72217, #55230, #72944, #67413, #27154, #44149, #38969, #66678, #55589, #4984, #16413, #28599 ) ),
 .UNSPECIFIED., .F., .F., .F. ) 
 B_SPLINE_SURFACE_WITH_KNOTS ( ( 2, 2 ),
 ( 3, 2, 2, 2, 2, 2, 2, 2, 2, 2, 2, 2, 2, 2, 2, 2, 2, 2, 2, 2, 2, 2, 2, 2, 2, 2, 2, 2, 2, 2, 2, 2, 2, 2, 2, 2, 2, 2, 2, 2, 2, 2, 2, 2, 2, 2, 2, 2, 2, 2, 2, 2, 2, 2, 2, 2, 2, 2, 2, 2, 2, 2, 2, 2, 2, 2, 2, 2, 2, 2, 2, 2, 2, 2, 2, 2, 2, 2, 2, 2, 2, 2, 2, 2, 2, 2, 2, 2, 2, 2, 2, 2, 2, 2, 2, 2, 2, 2, 2, 2, 2, 2, 2, 2, 2, 2, 2, 2, 2, 2, 2, 2, 2, 2, 2, 2, 2, 2, 2, 2, 2, 2, 2, 2, 2, 2, 2, 2, 2, 2, 2, 2, 2, 2, 2, 2, 2, 2, 2, 2, 2, 2, 2, 2, 2, 2, 2, 2, 2, 2, 2, 2, 2, 2, 2, 2, 2, 2, 2, 2, 2, 2, 2, 2, 2, 2, 2, 2, 2, 2, 2, 2, 2, 2, 2, 2, 2, 2, 2, 2, 2, 2, 2, 2, 2, 2, 2, 2, 2, 2, 2, 2, 2, 2, 2, 2, 2, 2, 2, 2, 2, 2, 2, 2, 2, 2, 2, 2, 2, 2, 2, 2, 2, 2, 2, 2, 2, 2, 2, 2, 2, 2, 2, 2, 2, 2, 2, 2, 2, 2, 2, 2, 2, 2, 2, 2, 2, 2, 2, 2, 2, 2, 2, 2, 2, 2, 2, 2, 2, 2, 2, 2, 2, 2, 2, 2, 2, 2, 2, 2, 2, 2, 2, 2, 2, 2, 2, 2, 2, 2, 2, 2, 2, 2, 2, 2, 2, 2, 2, 2, 2, 2, 2, 2, 2, 2, 2, 2, 2, 2, 2, 2, 2, 2, 2, 2, 2, 2, 2, 2, 2, 2, 2, 2, 2, 2, 2, 2, 2, 2, 2, 2, 2, 2, 2, 2, 2, 2, 2, 2, 2, 2, 2, 2, 2, 2, 2, 2, 2, 2, 2, 2, 2, 2, 2, 2, 2, 2, 2, 2, 2, 2, 2, 2, 2, 2, 2, 2, 2, 2, 2, 2, 2, 2, 2, 2, 2, 2, 2, 2, 3 ),
 ( 0.000000000000000000, 1.000000000000000000 ),
 ( 0.000000000000000000, 0.002777777777777777884, 0.005555555555555555768, 0.008333333333333333218, 0.01111111111111111154, 0.01388888888888888812, 0.01666666666666666644, 0.01944444444444444475, 0.02222222222222222307, 0.02500000000000000139, 0.02777777777777777624, 0.03055555555555555455, 0.03333333333333333287, 0.03611111111111110772, 0.03888888888888888951, 0.04166666666666666435, 0.04444444444444444614, 0.04722222222222222099, 0.05000000000000000278, 0.05277777777777777762, 0.05555555555555555247, 0.05833333333333333426, 0.06111111111111110911, 0.06388888888888888395, 0.06666666666666666574, 0.06944444444444444753, 0.07222222222222221544, 0.07499999999999999722, 0.07777777777777777901, 0.08055555555555556080, 0.08333333333333332871, 0.08611111111111111049, 0.08888888888888889228, 0.09166666666666666019, 0.09444444444444444198, 0.09722222222222222376, 0.1000000000000000056, 0.1027777777777777735, 0.1055555555555555552, 0.1083333333333333370, 0.1111111111111111049, 0.1138888888888888867, 0.1166666666666666685, 0.1194444444444444503, 0.1222222222222222182, 0.1250000000000000000, 0.1277777777777777679, 0.1305555555555555636, 0.1333333333333333315, 0.1361111111111110994, 0.1388888888888888951, 0.1416666666666666630, 0.1444444444444444309, 0.1472222222222222265, 0.1499999999999999944, 0.1527777777777777901, 0.1555555555555555580, 0.1583333333333333259, 0.1611111111111111216, 0.1638888888888888895, 0.1666666666666666574, 0.1694444444444444531, 0.1722222222222222210, 0.1749999999999999889, 0.1777777777777777846, 0.1805555555555555525, 0.1833333333333333204, 0.1861111111111111160, 0.1888888888888888840, 0.1916666666666666796, 0.1944444444444444475, 0.1972222222222222154, 0.2000000000000000111, 0.2027777777777777790, 0.2055555555555555469, 0.2083333333333333426, 0.2111111111111111105, 0.2138888888888888784, 0.2166666666666666741, 0.2194444444444444420, 0.2222222222222222099, 0.2250000000000000056, 0.2277777777777777735, 0.2305555555555555691, 0.2333333333333333370, 0.2361111111111111049, 0.2388888888888889006, 0.2416666666666666685, 0.2444444444444444364, 0.2472222222222222321, 0.2500000000000000000, 0.2527777777777777679, 0.2555555555555555358, 0.2583333333333333592, 0.2611111111111111271, 0.2638888888888888951, 0.2666666666666666630, 0.2694444444444444309, 0.2722222222222221988, 0.2750000000000000222, 0.2777777777777777901, 0.2805555555555555580, 0.2833333333333333259, 0.2861111111111110938, 0.2888888888888888618, 0.2916666666666666852, 0.2944444444444444531, 0.2972222222222222210, 0.2999999999999999889, 0.3027777777777777568, 0.3055555555555555802, 0.3083333333333333481, 0.3111111111111111160, 0.3138888888888888840, 0.3166666666666666519, 0.3194444444444444198, 0.3222222222222222432, 0.3250000000000000111, 0.3277777777777777790, 0.3305555555555555469, 0.3333333333333333148, 0.3361111111111111382, 0.3388888888888889062, 0.3416666666666666741, 0.3444444444444444420, 0.3472222222222222099, 0.3499999999999999778, 0.3527777777777778012, 0.3555555555555555691, 0.3583333333333333370, 0.3611111111111111049, 0.3638888888888888729, 0.3666666666666666408, 0.3694444444444444642, 0.3722222222222222321, 0.3750000000000000000, 0.3777777777777777679, 0.3805555555555555358, 0.3833333333333333592, 0.3861111111111111271, 0.3888888888888888951, 0.3916666666666666630, 0.3944444444444444309, 0.3972222222222221988, 0.4000000000000000222, 0.4027777777777777901, 0.4055555555555555580, 0.4083333333333333259, 0.4111111111111110938, 0.4138888888888888618, 0.4166666666666666852, 0.4194444444444444531, 0.4222222222222222210, 0.4249999999999999889, 0.4277777777777777568, 0.4305555555555555802, 0.4333333333333333481, 0.4361111111111111160, 0.4388888888888888840, 0.4416666666666666519, 0.4444444444444444198, 0.4472222222222222432, 0.4500000000000000111, 0.4527777777777777790, 0.4555555555555555469, 0.4583333333333333148, 0.4611111111111111382, 0.4638888888888889062, 0.4666666666666666741, 0.4694444444444444420, 0.4722222222222222099, 0.4749999999999999778, 0.4777777777777778012, 0.4805555555555555691, 0.4833333333333333370, 0.4861111111111111049, 0.4888888888888888729, 0.4916666666666666408, 0.4944444444444444642, 0.4972222222222222321, 0.5000000000000000000, 0.5027777777777777679, 0.5055555555555555358, 0.5083333333333333037, 0.5111111111111110716, 0.5138888888888888395, 0.5166666666666667185, 0.5194444444444444864, 0.5222222222222222543, 0.5250000000000000222, 0.5277777777777777901, 0.5305555555555555580, 0.5333333333333333259, 0.5361111111111110938, 0.5388888888888888618, 0.5416666666666666297, 0.5444444444444443976, 0.5472222222222222765, 0.5500000000000000444, 0.5527777777777778123, 0.5555555555555555802, 0.5583333333333333481, 0.5611111111111111160, 0.5638888888888888840, 0.5666666666666666519, 0.5694444444444444198, 0.5722222222222221877, 0.5749999999999999556, 0.5777777777777777235, 0.5805555555555556024, 0.5833333333333333703, 0.5861111111111111382, 0.5888888888888889062, 0.5916666666666666741, 0.5944444444444444420, 0.5972222222222222099, 0.5999999999999999778, 0.6027777777777777457, 0.6055555555555555136, 0.6083333333333332815, 0.6111111111111111605, 0.6138888888888889284, 0.6166666666666666963, 0.6194444444444444642, 0.6222222222222222321, 0.6250000000000000000, 0.6277777777777777679, 0.6305555555555555358, 0.6333333333333333037, 0.6361111111111110716, 0.6388888888888888395, 0.6416666666666667185, 0.6444444444444444864, 0.6472222222222222543, 0.6500000000000000222, 0.6527777777777777901, 0.6555555555555555580, 0.6583333333333333259, 0.6611111111111110938, 0.6638888888888888618, 0.6666666666666666297, 0.6694444444444443976, 0.6722222222222222765, 0.6750000000000000444, 0.6777777777777778123, 0.6805555555555555802, 0.6833333333333333481, 0.6861111111111111160, 0.6888888888888888840, 0.6916666666666666519, 0.6944444444444444198, 0.6972222222222221877, 0.6999999999999999556, 0.7027777777777777235, 0.7055555555555556024, 0.7083333333333333703, 0.7111111111111111382, 0.7138888888888889062, 0.7166666666666666741, 0.7194444444444444420, 0.7222222222222222099, 0.7249999999999999778, 0.7277777777777777457, 0.7305555555555555136, 0.7333333333333332815, 0.7361111111111111605, 0.7388888888888889284, 0.7416666666666666963, 0.7444444444444444642, 0.7472222222222222321, 0.7500000000000000000, 0.7527777777777777679, 0.7555555555555555358, 0.7583333333333333037, 0.7611111111111110716, 0.7638888888888888395, 0.7666666666666667185, 0.7694444444444444864, 0.7722222222222222543, 0.7750000000000000222, 0.7777777777777777901, 0.7805555555555555580, 0.7833333333333333259, 0.7861111111111110938, 0.7888888888888888618, 0.7916666666666666297, 0.7944444444444443976, 0.7972222222222222765, 0.8000000000000000444, 0.8027777777777778123, 0.8055555555555555802, 0.8083333333333333481, 0.8111111111111111160, 0.8138888888888888840, 0.8166666666666666519, 0.8194444444444444198, 0.8222222222222221877, 0.8249999999999999556, 0.8277777777777777235, 0.8305555555555556024, 0.8333333333333333703, 0.8361111111111111382, 0.8388888888888889062, 0.8416666666666666741, 0.8444444444444444420, 0.8472222222222222099, 0.8499999999999999778, 0.8527777777777777457, 0.8555555555555555136, 0.8583333333333332815, 0.8611111111111111605, 0.8638888888888889284, 0.8666666666666666963, 0.8694444444444444642, 0.8722222222222222321, 0.8750000000000000000, 0.8777777777777777679, 0.8805555555555555358, 0.8833333333333333037, 0.8861111111111110716, 0.8888888888888888395, 0.8916666666666667185, 0.8944444444444444864, 0.8972222222222222543, 0.9000000000000000222, 0.9027777777777777901, 0.9055555555555555580, 0.9083333333333333259, 0.9111111111111110938, 0.9138888888888888618, 0.9166666666666666297, 0.9194444444444443976, 0.9222222222222222765, 0.9250000000000000444, 0.9277777777777778123, 0.9305555555555555802, 0.9333333333333333481, 0.9361111111111111160, 0.9388888888888888840, 0.9416666666666666519, 0.9444444444444444198, 0.9472222222222221877, 0.9499999999999999556, 0.9527777777777777235, 0.9555555555555556024, 0.9583333333333333703, 0.9611111111111111382, 0.9638888888888889062, 0.9666666666666666741, 0.9694444444444444420, 0.9722222222222222099, 0.9749999999999999778, 0.9777777777777777457, 0.9805555555555555136, 0.9833333333333332815, 0.9861111111111111605, 0.9888888888888889284, 0.9916666666666666963, 0.9944444444444444642, 0.9972222222222222321, 1.000000000000000000 ),
 .UNSPECIFIED. ) 
 GEOMETRIC_REPRESENTATION_ITEM ( )  RATIONAL_B_SPLINE_SURFACE ( (
 ( 1.000000000000000000, 0.8660254037844387076, 1.000000000000000000, 0.8660254037844387076, 1.000000000000000000, 0.8660254037844387076, 1.000000000000000000, 0.8660254037844387076, 1.000000000000000000, 0.8660254037844387076, 1.000000000000000000, 0.8660254037844387076, 1.000000000000000000, 0.8660254037844387076, 1.000000000000000000, 0.8660254037844387076, 1.000000000000000000, 0.8660254037844387076, 1.000000000000000000, 0.8660254037844387076, 1.000000000000000000, 0.8660254037844387076, 1.000000000000000000, 0.8660254037844387076, 1.000000000000000000, 0.8660254037844387076, 1.000000000000000000, 0.8660254037844387076, 1.000000000000000000, 0.8660254037844387076, 1.000000000000000000, 0.8660254037844387076, 1.000000000000000000, 0.8660254037844387076, 1.000000000000000000, 0.8660254037844387076, 1.000000000000000000, 0.8660254037844387076, 1.000000000000000000, 0.8660254037844387076, 1.000000000000000000, 0.8660254037844387076, 1.000000000000000000, 0.8660254037844387076, 1.000000000000000000, 0.8660254037844387076, 1.000000000000000000, 0.8660254037844387076, 1.000000000000000000, 0.8660254037844387076, 1.000000000000000000, 0.8660254037844387076, 1.000000000000000000, 0.8660254037844387076, 1.000000000000000000, 0.8660254037844387076, 1.000000000000000000, 0.8660254037844387076, 1.000000000000000000, 0.8660254037844387076, 1.000000000000000000, 0.8660254037844387076, 1.000000000000000000, 0.8660254037844387076, 1.000000000000000000, 0.8660254037844387076, 1.000000000000000000, 0.8660254037844387076, 1.000000000000000000, 0.8660254037844387076, 1.000000000000000000, 0.8660254037844387076, 1.000000000000000000, 0.8660254037844387076, 1.000000000000000000, 0.8660254037844387076, 1.000000000000000000, 0.8660254037844387076, 1.000000000000000000, 0.8660254037844387076, 1.000000000000000000, 0.8660254037844387076, 1.000000000000000000, 0.8660254037844387076, 1.000000000000000000, 0.8660254037844387076, 1.000000000000000000, 0.8660254037844387076, 1.000000000000000000, 0.8660254037844387076, 1.000000000000000000, 0.8660254037844387076, 1.000000000000000000, 0.8660254037844387076, 1.000000000000000000, 0.8660254037844387076, 1.000000000000000000, 0.8660254037844387076, 1.000000000000000000, 0.8660254037844387076, 1.000000000000000000, 0.8660254037844387076, 1.000000000000000000, 0.8660254037844387076, 1.000000000000000000, 0.8660254037844387076, 1.000000000000000000, 0.8660254037844387076, 1.000000000000000000, 0.8660254037844387076, 1.000000000000000000, 0.8660254037844387076, 1.000000000000000000, 0.8660254037844387076, 1.000000000000000000, 0.8660254037844387076, 1.000000000000000000, 0.8660254037844387076, 1.000000000000000000, 0.8660254037844387076, 1.000000000000000000, 0.8660254037844387076, 1.000000000000000000, 0.8660254037844387076, 1.000000000000000000, 0.8660254037844387076, 1.000000000000000000, 0.8660254037844387076, 1.000000000000000000, 0.8660254037844387076, 1.000000000000000000, 0.8660254037844387076, 1.000000000000000000, 0.8660254037844387076, 1.000000000000000000, 0.8660254037844387076, 1.000000000000000000, 0.8660254037844387076, 1.000000000000000000, 0.8660254037844387076, 1.000000000000000000, 0.8660254037844387076, 1.000000000000000000, 0.8660254037844387076, 1.000000000000000000, 0.8660254037844387076, 1.000000000000000000, 0.8660254037844387076, 1.000000000000000000, 0.8660254037844387076, 1.000000000000000000, 0.8660254037844387076, 1.000000000000000000, 0.8660254037844387076, 1.000000000000000000, 0.8660254037844387076, 1.000000000000000000, 0.8660254037844387076, 1.000000000000000000, 0.8660254037844387076, 1.000000000000000000, 0.8660254037844387076, 1.000000000000000000, 0.8660254037844387076, 1.000000000000000000, 0.8660254037844387076, 1.000000000000000000, 0.8660254037844387076, 1.000000000000000000, 0.8660254037844387076, 1.000000000000000000, 0.8660254037844387076, 1.000000000000000000, 0.8660254037844387076, 1.000000000000000000, 0.8660254037844387076, 1.000000000000000000, 0.8660254037844387076, 1.000000000000000000, 0.8660254037844387076, 1.000000000000000000, 0.8660254037844387076, 1.000000000000000000, 0.8660254037844387076, 1.000000000000000000, 0.8660254037844387076, 1.000000000000000000, 0.8660254037844387076, 1.000000000000000000, 0.8660254037844387076, 1.000000000000000000, 0.8660254037844387076, 1.000000000000000000, 0.8660254037844387076, 1.000000000000000000, 0.8660254037844387076, 1.000000000000000000, 0.8660254037844387076, 1.000000000000000000, 0.8660254037844387076, 1.000000000000000000, 0.8660254037844387076, 1.000000000000000000, 0.8660254037844387076, 1.000000000000000000, 0.8660254037844387076, 1.000000000000000000, 0.8660254037844387076, 1.000000000000000000, 0.8660254037844387076, 1.000000000000000000, 0.8660254037844387076, 1.000000000000000000, 0.8660254037844387076, 1.000000000000000000, 0.8660254037844387076, 1.000000000000000000, 0.8660254037844387076, 1.000000000000000000, 0.8660254037844387076, 1.000000000000000000, 0.8660254037844387076, 1.000000000000000000, 0.8660254037844387076, 1.000000000000000000, 0.8660254037844387076, 1.000000000000000000, 0.8660254037844387076, 1.000000000000000000, 0.8660254037844387076, 1.000000000000000000, 0.8660254037844387076, 1.000000000000000000, 0.8660254037844387076, 1.000000000000000000, 0.8660254037844387076, 1.000000000000000000, 0.8660254037844387076, 1.000000000000000000, 0.8660254037844387076, 1.000000000000000000, 0.8660254037844387076, 1.000000000000000000, 0.8660254037844387076, 1.000000000000000000, 0.8660254037844387076, 1.000000000000000000, 0.8660254037844387076, 1.000000000000000000, 0.8660254037844387076, 1.000000000000000000, 0.8660254037844387076, 1.000000000000000000, 0.8660254037844387076, 1.000000000000000000, 0.8660254037844387076, 1.000000000000000000, 0.8660254037844387076, 1.000000000000000000, 0.8660254037844387076, 1.000000000000000000, 0.8660254037844387076, 1.000000000000000000, 0.8660254037844387076, 1.000000000000000000, 0.8660254037844387076, 1.000000000000000000, 0.8660254037844387076, 1.000000000000000000, 0.8660254037844387076, 1.000000000000000000, 0.8660254037844387076, 1.000000000000000000, 0.8660254037844387076, 1.000000000000000000, 0.8660254037844387076, 1.000000000000000000, 0.8660254037844387076, 1.000000000000000000, 0.8660254037844387076, 1.000000000000000000, 0.8660254037844387076, 1.000000000000000000, 0.8660254037844387076, 1.000000000000000000, 0.8660254037844387076, 1.000000000000000000, 0.8660254037844387076, 1.000000000000000000, 0.8660254037844387076, 1.000000000000000000, 0.8660254037844387076, 1.000000000000000000, 0.8660254037844387076, 1.000000000000000000, 0.8660254037844387076, 1.000000000000000000, 0.8660254037844387076, 1.000000000000000000, 0.8660254037844387076, 1.000000000000000000, 0.8660254037844387076, 1.000000000000000000, 0.8660254037844387076, 1.000000000000000000, 0.8660254037844387076, 1.000000000000000000, 0.8660254037844387076, 1.000000000000000000, 0.8660254037844387076, 1.000000000000000000, 0.8660254037844387076, 1.000000000000000000, 0.8660254037844387076, 1.000000000000000000, 0.8660254037844387076, 1.000000000000000000, 0.8660254037844387076, 1.000000000000000000, 0.8660254037844387076, 1.000000000000000000, 0.8660254037844387076, 1.000000000000000000, 0.8660254037844387076, 1.000000000000000000, 0.8660254037844387076, 1.000000000000000000, 0.8660254037844387076, 1.000000000000000000, 0.8660254037844387076, 1.000000000000000000, 0.8660254037844387076, 1.000000000000000000, 0.8660254037844387076, 1.000000000000000000, 0.8660254037844387076, 1.000000000000000000, 0.8660254037844387076, 1.000000000000000000, 0.8660254037844387076, 1.000000000000000000, 0.8660254037844387076, 1.000000000000000000, 0.8660254037844387076, 1.000000000000000000, 0.8660254037844387076, 1.000000000000000000, 0.8660254037844387076, 1.000000000000000000, 0.8660254037844387076, 1.000000000000000000, 0.8660254037844387076, 1.000000000000000000, 0.8660254037844387076, 1.000000000000000000, 0.8660254037844387076, 1.000000000000000000, 0.8660254037844387076, 1.000000000000000000, 0.8660254037844387076, 1.000000000000000000, 0.8660254037844387076, 1.000000000000000000, 0.8660254037844387076, 1.000000000000000000, 0.8660254037844387076, 1.000000000000000000, 0.8660254037844387076, 1.000000000000000000, 0.8660254037844387076, 1.000000000000000000, 0.8660254037844387076, 1.000000000000000000, 0.8660254037844387076, 1.000000000000000000, 0.8660254037844387076, 1.000000000000000000, 0.8660254037844387076, 1.000000000000000000, 0.8660254037844387076, 1.000000000000000000, 0.8660254037844387076, 1.000000000000000000, 0.8660254037844387076, 1.000000000000000000, 0.8660254037844387076, 1.000000000000000000, 0.8660254037844387076, 1.000000000000000000, 0.8660254037844387076, 1.000000000000000000, 0.8660254037844387076, 1.000000000000000000, 0.8660254037844387076, 1.000000000000000000, 0.8660254037844387076, 1.000000000000000000, 0.8660254037844387076, 1.000000000000000000, 0.8660254037844387076, 1.000000000000000000, 0.8660254037844387076, 1.000000000000000000, 0.8660254037844387076, 1.000000000000000000, 0.8660254037844387076, 1.000000000000000000, 0.8660254037844387076, 1.000000000000000000, 0.8660254037844387076, 1.000000000000000000, 0.8660254037844387076, 1.000000000000000000, 0.8660254037844387076, 1.000000000000000000, 0.8660254037844387076, 1.000000000000000000, 0.8660254037844387076, 1.000000000000000000, 0.8660254037844387076, 1.000000000000000000, 0.8660254037844387076, 1.000000000000000000, 0.8660254037844387076, 1.000000000000000000, 0.8660254037844387076, 1.000000000000000000, 0.8660254037844387076, 1.000000000000000000, 0.8660254037844387076, 1.000000000000000000, 0.8660254037844387076, 1.000000000000000000, 0.8660254037844387076, 1.000000000000000000, 0.8660254037844387076, 1.000000000000000000, 0.8660254037844387076, 1.000000000000000000, 0.8660254037844387076, 1.000000000000000000, 0.8660254037844387076, 1.000000000000000000, 0.8660254037844387076, 1.000000000000000000, 0.8660254037844387076, 1.000000000000000000, 0.8660254037844387076, 1.000000000000000000, 0.8660254037844387076, 1.000000000000000000, 0.8660254037844387076, 1.000000000000000000, 0.8660254037844387076, 1.000000000000000000, 0.8660254037844387076, 1.000000000000000000, 0.8660254037844387076, 1.000000000000000000, 0.8660254037844387076, 1.000000000000000000, 0.8660254037844387076, 1.000000000000000000, 0.8660254037844387076, 1.000000000000000000, 0.8660254037844387076, 1.000000000000000000, 0.8660254037844387076, 1.000000000000000000, 0.8660254037844387076, 1.000000000000000000, 0.8660254037844387076, 1.000000000000000000, 0.8660254037844387076, 1.000000000000000000, 0.8660254037844387076, 1.000000000000000000, 0.8660254037844387076, 1.000000000000000000, 0.8660254037844387076, 1.000000000000000000, 0.8660254037844387076, 1.000000000000000000, 0.8660254037844387076, 1.000000000000000000, 0.8660254037844387076, 1.000000000000000000, 0.8660254037844387076, 1.000000000000000000, 0.8660254037844387076, 1.000000000000000000, 0.8660254037844387076, 1.000000000000000000, 0.8660254037844387076, 1.000000000000000000, 0.8660254037844387076, 1.000000000000000000, 0.8660254037844387076, 1.000000000000000000, 0.8660254037844387076, 1.000000000000000000, 0.8660254037844387076, 1.000000000000000000, 0.8660254037844387076, 1.000000000000000000, 0.8660254037844387076, 1.000000000000000000, 0.8660254037844387076, 1.000000000000000000, 0.8660254037844387076, 1.000000000000000000, 0.8660254037844387076, 1.000000000000000000, 0.8660254037844387076, 1.000000000000000000, 0.8660254037844387076, 1.000000000000000000, 0.8660254037844387076, 1.000000000000000000, 0.8660254037844387076, 1.000000000000000000, 0.8660254037844387076, 1.000000000000000000, 0.8660254037844387076, 1.000000000000000000, 0.8660254037844387076, 1.000000000000000000, 0.8660254037844387076, 1.000000000000000000, 0.8660254037844387076, 1.000000000000000000, 0.8660254037844387076, 1.000000000000000000, 0.8660254037844387076, 1.000000000000000000, 0.8660254037844387076, 1.000000000000000000, 0.8660254037844387076, 1.000000000000000000, 0.8660254037844387076, 1.000000000000000000, 0.8660254037844387076, 1.000000000000000000, 0.8660254037844387076, 1.000000000000000000, 0.8660254037844387076, 1.000000000000000000, 0.8660254037844387076, 1.000000000000000000, 0.8660254037844387076, 1.000000000000000000, 0.8660254037844387076, 1.000000000000000000, 0.8660254037844387076, 1.000000000000000000, 0.8660254037844387076, 1.000000000000000000, 0.8660254037844387076, 1.000000000000000000, 0.8660254037844387076, 1.000000000000000000, 0.8660254037844387076, 1.000000000000000000, 0.8660254037844387076, 1.000000000000000000, 0.8660254037844387076, 1.000000000000000000, 0.8660254037844387076, 1.000000000000000000, 0.8660254037844387076, 1.000000000000000000, 0.8660254037844387076, 1.000000000000000000, 0.8660254037844387076, 1.000000000000000000, 0.8660254037844387076, 1.000000000000000000, 0.8660254037844387076, 1.000000000000000000, 0.8660254037844387076, 1.000000000000000000, 0.8660254037844387076, 1.000000000000000000, 0.8660254037844387076, 1.000000000000000000, 0.8660254037844387076, 1.000000000000000000, 0.8660254037844387076, 1.000000000000000000, 0.8660254037844387076, 1.000000000000000000, 0.8660254037844387076, 1.000000000000000000, 0.8660254037844387076, 1.000000000000000000, 0.8660254037844387076, 1.000000000000000000, 0.8660254037844387076, 1.000000000000000000, 0.8660254037844387076, 1.000000000000000000, 0.8660254037844387076, 1.000000000000000000, 0.8660254037844387076, 1.000000000000000000, 0.8660254037844387076, 1.000000000000000000, 0.8660254037844387076, 1.000000000000000000, 0.8660254037844387076, 1.000000000000000000, 0.8660254037844387076, 1.000000000000000000, 0.8660254037844387076, 1.000000000000000000, 0.8660254037844387076, 1.000000000000000000, 0.8660254037844387076, 1.000000000000000000, 0.8660254037844387076, 1.000000000000000000, 0.8660254037844387076, 1.000000000000000000, 0.8660254037844387076, 1.000000000000000000, 0.8660254037844387076, 1.000000000000000000, 0.8660254037844387076, 1.000000000000000000, 0.8660254037844387076, 1.000000000000000000, 0.8660254037844387076, 1.000000000000000000, 0.8660254037844387076, 1.000000000000000000, 0.8660254037844387076, 1.000000000000000000, 0.8660254037844387076, 1.000000000000000000, 0.8660254037844387076, 1.000000000000000000, 0.8660254037844387076, 1.000000000000000000, 0.8660254037844387076, 1.000000000000000000, 0.8660254037844387076, 1.000000000000000000, 0.8660254037844387076, 1.000000000000000000, 0.8660254037844387076, 1.000000000000000000, 0.8660254037844387076, 1.000000000000000000, 0.8660254037844387076, 1.000000000000000000, 0.8660254037844387076, 1.000000000000000000, 0.8660254037844387076, 1.000000000000000000, 0.8660254037844387076, 1.000000000000000000, 0.8660254037844387076, 1.000000000000000000, 0.8660254037844387076, 1.000000000000000000, 0.8660254037844387076, 1.000000000000000000, 0.8660254037844387076, 1.000000000000000000, 0.8660254037844387076, 1.000000000000000000, 0.8660254037844387076, 1.000000000000000000, 0.8660254037844387076, 1.000000000000000000, 0.8660254037844387076, 1.000000000000000000, 0.8660254037844387076, 1.000000000000000000, 0.8660254037844387076, 1.000000000000000000, 0.8660254037844387076, 1.000000000000000000, 0.8660254037844387076, 1.000000000000000000, 0.8660254037844387076, 1.000000000000000000, 0.8660254037844387076, 1.000000000000000000, 0.8660254037844387076, 1.000000000000000000, 0.8660254037844387076, 1.000000000000000000, 0.8660254037844387076, 1.000000000000000000, 0.8660254037844387076, 1.000000000000000000, 0.8660254037844387076, 1.000000000000000000, 0.8660254037844387076, 1.000000000000000000, 0.8660254037844387076, 1.000000000000000000, 0.8660254037844387076, 1.000000000000000000, 0.8660254037844387076, 1.000000000000000000, 0.8660254037844387076, 1.000000000000000000, 0.8660254037844387076, 1.000000000000000000, 0.8660254037844387076, 1.000000000000000000, 0.8660254037844387076, 1.000000000000000000, 0.8660254037844387076, 1.000000000000000000, 0.8660254037844387076, 1.000000000000000000, 0.8660254037844387076, 1.000000000000000000),
 ( 1.000000000000000000, 0.8660254037844387076, 1.000000000000000000, 0.8660254037844387076, 1.000000000000000000, 0.8660254037844387076, 1.000000000000000000, 0.8660254037844387076, 1.000000000000000000, 0.8660254037844387076, 1.000000000000000000, 0.8660254037844387076, 1.000000000000000000, 0.8660254037844387076, 1.000000000000000000, 0.8660254037844387076, 1.000000000000000000, 0.8660254037844387076, 1.000000000000000000, 0.8660254037844387076, 1.000000000000000000, 0.8660254037844387076, 1.000000000000000000, 0.8660254037844387076, 1.000000000000000000, 0.8660254037844387076, 1.000000000000000000, 0.8660254037844387076, 1.000000000000000000, 0.8660254037844387076, 1.000000000000000000, 0.8660254037844387076, 1.000000000000000000, 0.8660254037844387076, 1.000000000000000000, 0.8660254037844387076, 1.000000000000000000, 0.8660254037844387076, 1.000000000000000000, 0.8660254037844387076, 1.000000000000000000, 0.8660254037844387076, 1.000000000000000000, 0.8660254037844387076, 1.000000000000000000, 0.8660254037844387076, 1.000000000000000000, 0.8660254037844387076, 1.000000000000000000, 0.8660254037844387076, 1.000000000000000000, 0.8660254037844387076, 1.000000000000000000, 0.8660254037844387076, 1.000000000000000000, 0.8660254037844387076, 1.000000000000000000, 0.8660254037844387076, 1.000000000000000000, 0.8660254037844387076, 1.000000000000000000, 0.8660254037844387076, 1.000000000000000000, 0.8660254037844387076, 1.000000000000000000, 0.8660254037844387076, 1.000000000000000000, 0.8660254037844387076, 1.000000000000000000, 0.8660254037844387076, 1.000000000000000000, 0.8660254037844387076, 1.000000000000000000, 0.8660254037844387076, 1.000000000000000000, 0.8660254037844387076, 1.000000000000000000, 0.8660254037844387076, 1.000000000000000000, 0.8660254037844387076, 1.000000000000000000, 0.8660254037844387076, 1.000000000000000000, 0.8660254037844387076, 1.000000000000000000, 0.8660254037844387076, 1.000000000000000000, 0.8660254037844387076, 1.000000000000000000, 0.8660254037844387076, 1.000000000000000000, 0.8660254037844387076, 1.000000000000000000, 0.8660254037844387076, 1.000000000000000000, 0.8660254037844387076, 1.000000000000000000, 0.8660254037844387076, 1.000000000000000000, 0.8660254037844387076, 1.000000000000000000, 0.8660254037844387076, 1.000000000000000000, 0.8660254037844387076, 1.000000000000000000, 0.8660254037844387076, 1.000000000000000000, 0.8660254037844387076, 1.000000000000000000, 0.8660254037844387076, 1.000000000000000000, 0.8660254037844387076, 1.000000000000000000, 0.8660254037844387076, 1.000000000000000000, 0.8660254037844387076, 1.000000000000000000, 0.8660254037844387076, 1.000000000000000000, 0.8660254037844387076, 1.000000000000000000, 0.8660254037844387076, 1.000000000000000000, 0.8660254037844387076, 1.000000000000000000, 0.8660254037844387076, 1.000000000000000000, 0.8660254037844387076, 1.000000000000000000, 0.8660254037844387076, 1.000000000000000000, 0.8660254037844387076, 1.000000000000000000, 0.8660254037844387076, 1.000000000000000000, 0.8660254037844387076, 1.000000000000000000, 0.8660254037844387076, 1.000000000000000000, 0.8660254037844387076, 1.000000000000000000, 0.8660254037844387076, 1.000000000000000000, 0.8660254037844387076, 1.000000000000000000, 0.8660254037844387076, 1.000000000000000000, 0.8660254037844387076, 1.000000000000000000, 0.8660254037844387076, 1.000000000000000000, 0.8660254037844387076, 1.000000000000000000, 0.8660254037844387076, 1.000000000000000000, 0.8660254037844387076, 1.000000000000000000, 0.8660254037844387076, 1.000000000000000000, 0.8660254037844387076, 1.000000000000000000, 0.8660254037844387076, 1.000000000000000000, 0.8660254037844387076, 1.000000000000000000, 0.8660254037844387076, 1.000000000000000000, 0.8660254037844387076, 1.000000000000000000, 0.8660254037844387076, 1.000000000000000000, 0.8660254037844387076, 1.000000000000000000, 0.8660254037844387076, 1.000000000000000000, 0.8660254037844387076, 1.000000000000000000, 0.8660254037844387076, 1.000000000000000000, 0.8660254037844387076, 1.000000000000000000, 0.8660254037844387076, 1.000000000000000000, 0.8660254037844387076, 1.000000000000000000, 0.8660254037844387076, 1.000000000000000000, 0.8660254037844387076, 1.000000000000000000, 0.8660254037844387076, 1.000000000000000000, 0.8660254037844387076, 1.000000000000000000, 0.8660254037844387076, 1.000000000000000000, 0.8660254037844387076, 1.000000000000000000, 0.8660254037844387076, 1.000000000000000000, 0.8660254037844387076, 1.000000000000000000, 0.8660254037844387076, 1.000000000000000000, 0.8660254037844387076, 1.000000000000000000, 0.8660254037844387076, 1.000000000000000000, 0.8660254037844387076, 1.000000000000000000, 0.8660254037844387076, 1.000000000000000000, 0.8660254037844387076, 1.000000000000000000, 0.8660254037844387076, 1.000000000000000000, 0.8660254037844387076, 1.000000000000000000, 0.8660254037844387076, 1.000000000000000000, 0.8660254037844387076, 1.000000000000000000, 0.8660254037844387076, 1.000000000000000000, 0.8660254037844387076, 1.000000000000000000, 0.8660254037844387076, 1.000000000000000000, 0.8660254037844387076, 1.000000000000000000, 0.8660254037844387076, 1.000000000000000000, 0.8660254037844387076, 1.000000000000000000, 0.8660254037844387076, 1.000000000000000000, 0.8660254037844387076, 1.000000000000000000, 0.8660254037844387076, 1.000000000000000000, 0.8660254037844387076, 1.000000000000000000, 0.8660254037844387076, 1.000000000000000000, 0.8660254037844387076, 1.000000000000000000, 0.8660254037844387076, 1.000000000000000000, 0.8660254037844387076, 1.000000000000000000, 0.8660254037844387076, 1.000000000000000000, 0.8660254037844387076, 1.000000000000000000, 0.8660254037844387076, 1.000000000000000000, 0.8660254037844387076, 1.000000000000000000, 0.8660254037844387076, 1.000000000000000000, 0.8660254037844387076, 1.000000000000000000, 0.8660254037844387076, 1.000000000000000000, 0.8660254037844387076, 1.000000000000000000, 0.8660254037844387076, 1.000000000000000000, 0.8660254037844387076, 1.000000000000000000, 0.8660254037844387076, 1.000000000000000000, 0.8660254037844387076, 1.000000000000000000, 0.8660254037844387076, 1.000000000000000000, 0.8660254037844387076, 1.000000000000000000, 0.8660254037844387076, 1.000000000000000000, 0.8660254037844387076, 1.000000000000000000, 0.8660254037844387076, 1.000000000000000000, 0.8660254037844387076, 1.000000000000000000, 0.8660254037844387076, 1.000000000000000000, 0.8660254037844387076, 1.000000000000000000, 0.8660254037844387076, 1.000000000000000000, 0.8660254037844387076, 1.000000000000000000, 0.8660254037844387076, 1.000000000000000000, 0.8660254037844387076, 1.000000000000000000, 0.8660254037844387076, 1.000000000000000000, 0.8660254037844387076, 1.000000000000000000, 0.8660254037844387076, 1.000000000000000000, 0.8660254037844387076, 1.000000000000000000, 0.8660254037844387076, 1.000000000000000000, 0.8660254037844387076, 1.000000000000000000, 0.8660254037844387076, 1.000000000000000000, 0.8660254037844387076, 1.000000000000000000, 0.8660254037844387076, 1.000000000000000000, 0.8660254037844387076, 1.000000000000000000, 0.8660254037844387076, 1.000000000000000000, 0.8660254037844387076, 1.000000000000000000, 0.8660254037844387076, 1.000000000000000000, 0.8660254037844387076, 1.000000000000000000, 0.8660254037844387076, 1.000000000000000000, 0.8660254037844387076, 1.000000000000000000, 0.8660254037844387076, 1.000000000000000000, 0.8660254037844387076, 1.000000000000000000, 0.8660254037844387076, 1.000000000000000000, 0.8660254037844387076, 1.000000000000000000, 0.8660254037844387076, 1.000000000000000000, 0.8660254037844387076, 1.000000000000000000, 0.8660254037844387076, 1.000000000000000000, 0.8660254037844387076, 1.000000000000000000, 0.8660254037844387076, 1.000000000000000000, 0.8660254037844387076, 1.000000000000000000, 0.8660254037844387076, 1.000000000000000000, 0.8660254037844387076, 1.000000000000000000, 0.8660254037844387076, 1.000000000000000000, 0.8660254037844387076, 1.000000000000000000, 0.8660254037844387076, 1.000000000000000000, 0.8660254037844387076, 1.000000000000000000, 0.8660254037844387076, 1.000000000000000000, 0.8660254037844387076, 1.000000000000000000, 0.8660254037844387076, 1.000000000000000000, 0.8660254037844387076, 1.000000000000000000, 0.8660254037844387076, 1.000000000000000000, 0.8660254037844387076, 1.000000000000000000, 0.8660254037844387076, 1.000000000000000000, 0.8660254037844387076, 1.000000000000000000, 0.8660254037844387076, 1.000000000000000000, 0.8660254037844387076, 1.000000000000000000, 0.8660254037844387076, 1.000000000000000000, 0.8660254037844387076, 1.000000000000000000, 0.8660254037844387076, 1.000000000000000000, 0.8660254037844387076, 1.000000000000000000, 0.8660254037844387076, 1.000000000000000000, 0.8660254037844387076, 1.000000000000000000, 0.8660254037844387076, 1.000000000000000000, 0.8660254037844387076, 1.000000000000000000, 0.8660254037844387076, 1.000000000000000000, 0.8660254037844387076, 1.000000000000000000, 0.8660254037844387076, 1.000000000000000000, 0.8660254037844387076, 1.000000000000000000, 0.8660254037844387076, 1.000000000000000000, 0.8660254037844387076, 1.000000000000000000, 0.8660254037844387076, 1.000000000000000000, 0.8660254037844387076, 1.000000000000000000, 0.8660254037844387076, 1.000000000000000000, 0.8660254037844387076, 1.000000000000000000, 0.8660254037844387076, 1.000000000000000000, 0.8660254037844387076, 1.000000000000000000, 0.8660254037844387076, 1.000000000000000000, 0.8660254037844387076, 1.000000000000000000, 0.8660254037844387076, 1.000000000000000000, 0.8660254037844387076, 1.000000000000000000, 0.8660254037844387076, 1.000000000000000000, 0.8660254037844387076, 1.000000000000000000, 0.8660254037844387076, 1.000000000000000000, 0.8660254037844387076, 1.000000000000000000, 0.8660254037844387076, 1.000000000000000000, 0.8660254037844387076, 1.000000000000000000, 0.8660254037844387076, 1.000000000000000000, 0.8660254037844387076, 1.000000000000000000, 0.8660254037844387076, 1.000000000000000000, 0.8660254037844387076, 1.000000000000000000, 0.8660254037844387076, 1.000000000000000000, 0.8660254037844387076, 1.000000000000000000, 0.8660254037844387076, 1.000000000000000000, 0.8660254037844387076, 1.000000000000000000, 0.8660254037844387076, 1.000000000000000000, 0.8660254037844387076, 1.000000000000000000, 0.8660254037844387076, 1.000000000000000000, 0.8660254037844387076, 1.000000000000000000, 0.8660254037844387076, 1.000000000000000000, 0.8660254037844387076, 1.000000000000000000, 0.8660254037844387076, 1.000000000000000000, 0.8660254037844387076, 1.000000000000000000, 0.8660254037844387076, 1.000000000000000000, 0.8660254037844387076, 1.000000000000000000, 0.8660254037844387076, 1.000000000000000000, 0.8660254037844387076, 1.000000000000000000, 0.8660254037844387076, 1.000000000000000000, 0.8660254037844387076, 1.000000000000000000, 0.8660254037844387076, 1.000000000000000000, 0.8660254037844387076, 1.000000000000000000, 0.8660254037844387076, 1.000000000000000000, 0.8660254037844387076, 1.000000000000000000, 0.8660254037844387076, 1.000000000000000000, 0.8660254037844387076, 1.000000000000000000, 0.8660254037844387076, 1.000000000000000000, 0.8660254037844387076, 1.000000000000000000, 0.8660254037844387076, 1.000000000000000000, 0.8660254037844387076, 1.000000000000000000, 0.8660254037844387076, 1.000000000000000000, 0.8660254037844387076, 1.000000000000000000, 0.8660254037844387076, 1.000000000000000000, 0.8660254037844387076, 1.000000000000000000, 0.8660254037844387076, 1.000000000000000000, 0.8660254037844387076, 1.000000000000000000, 0.8660254037844387076, 1.000000000000000000, 0.8660254037844387076, 1.000000000000000000, 0.8660254037844387076, 1.000000000000000000, 0.8660254037844387076, 1.000000000000000000, 0.8660254037844387076, 1.000000000000000000, 0.8660254037844387076, 1.000000000000000000, 0.8660254037844387076, 1.000000000000000000, 0.8660254037844387076, 1.000000000000000000, 0.8660254037844387076, 1.000000000000000000, 0.8660254037844387076, 1.000000000000000000, 0.8660254037844387076, 1.000000000000000000, 0.8660254037844387076, 1.000000000000000000, 0.8660254037844387076, 1.000000000000000000, 0.8660254037844387076, 1.000000000000000000, 0.8660254037844387076, 1.000000000000000000, 0.8660254037844387076, 1.000000000000000000, 0.8660254037844387076, 1.000000000000000000, 0.8660254037844387076, 1.000000000000000000, 0.8660254037844387076, 1.000000000000000000, 0.8660254037844387076, 1.000000000000000000, 0.8660254037844387076, 1.000000000000000000, 0.8660254037844387076, 1.000000000000000000, 0.8660254037844387076, 1.000000000000000000, 0.8660254037844387076, 1.000000000000000000, 0.8660254037844387076, 1.000000000000000000, 0.8660254037844387076, 1.000000000000000000, 0.8660254037844387076, 1.000000000000000000, 0.8660254037844387076, 1.000000000000000000, 0.8660254037844387076, 1.000000000000000000, 0.8660254037844387076, 1.000000000000000000, 0.8660254037844387076, 1.000000000000000000, 0.8660254037844387076, 1.000000000000000000, 0.8660254037844387076, 1.000000000000000000, 0.8660254037844387076, 1.000000000000000000, 0.8660254037844387076, 1.000000000000000000, 0.8660254037844387076, 1.000000000000000000, 0.8660254037844387076, 1.000000000000000000, 0.8660254037844387076, 1.000000000000000000, 0.8660254037844387076, 1.000000000000000000, 0.8660254037844387076, 1.000000000000000000, 0.8660254037844387076, 1.000000000000000000, 0.8660254037844387076, 1.000000000000000000, 0.8660254037844387076, 1.000000000000000000, 0.8660254037844387076, 1.000000000000000000, 0.8660254037844387076, 1.000000000000000000, 0.8660254037844387076, 1.000000000000000000, 0.8660254037844387076, 1.000000000000000000, 0.8660254037844387076, 1.000000000000000000, 0.8660254037844387076, 1.000000000000000000, 0.8660254037844387076, 1.000000000000000000, 0.8660254037844387076, 1.000000000000000000, 0.8660254037844387076, 1.000000000000000000, 0.8660254037844387076, 1.000000000000000000, 0.8660254037844387076, 1.000000000000000000, 0.8660254037844387076, 1.000000000000000000, 0.8660254037844387076, 1.000000000000000000, 0.8660254037844387076, 1.000000000000000000, 0.8660254037844387076, 1.000000000000000000, 0.8660254037844387076, 1.000000000000000000, 0.8660254037844387076, 1.000000000000000000, 0.8660254037844387076, 1.000000000000000000, 0.8660254037844387076, 1.000000000000000000, 0.8660254037844387076, 1.000000000000000000, 0.8660254037844387076, 1.000000000000000000, 0.8660254037844387076, 1.000000000000000000, 0.8660254037844387076, 1.000000000000000000, 0.8660254037844387076, 1.000000000000000000, 0.8660254037844387076, 1.000000000000000000, 0.8660254037844387076, 1.000000000000000000, 0.8660254037844387076, 1.000000000000000000, 0.8660254037844387076, 1.000000000000000000, 0.8660254037844387076, 1.000000000000000000, 0.8660254037844387076, 1.000000000000000000, 0.8660254037844387076, 1.000000000000000000, 0.8660254037844387076, 1.000000000000000000, 0.8660254037844387076, 1.000000000000000000, 0.8660254037844387076, 1.000000000000000000, 0.8660254037844387076, 1.000000000000000000, 0.8660254037844387076, 1.000000000000000000, 0.8660254037844387076, 1.000000000000000000, 0.8660254037844387076, 1.000000000000000000, 0.8660254037844387076, 1.000000000000000000, 0.8660254037844387076, 1.000000000000000000, 0.8660254037844387076, 1.000000000000000000, 0.8660254037844387076, 1.000000000000000000, 0.8660254037844387076, 1.000000000000000000, 0.8660254037844387076, 1.000000000000000000, 0.8660254037844387076, 1.000000000000000000, 0.8660254037844387076, 1.000000000000000000, 0.8660254037844387076, 1.000000000000000000, 0.8660254037844387076, 1.000000000000000000, 0.8660254037844387076, 1.000000000000000000, 0.8660254037844387076, 1.000000000000000000, 0.8660254037844387076, 1.000000000000000000, 0.8660254037844387076, 1.000000000000000000, 0.8660254037844387076, 1.000000000000000000, 0.8660254037844387076, 1.000000000000000000, 0.8660254037844387076, 1.000000000000000000, 0.8660254037844387076, 1.000000000000000000, 0.8660254037844387076, 1.000000000000000000, 0.8660254037844387076, 1.000000000000000000, 0.8660254037844387076, 1.000000000000000000) ) ) 
 REPRESENTATION_ITEM ( '' )  SURFACE ( )  );
#15855=CARTESIAN_POINT ( 'NONE',  ( 24.10312500061451502, -4.541064518000417216, -2.621784821875001281 ) ) ;
#15858=CARTESIAN_POINT ( 'NONE',  ( -3.999999999999999112, 11.11250000122903536, 30.00000000000000000 ) ) ;
#15859=CARTESIAN_POINT ( 'NONE',  ( -3.999999999999999556, 13.32500000122903572, -32.30940107675850470 ) ) ;
#15860=EDGE_CURVE ( 'NONE', #14728, #69731, #25895, .T. ) ;
#15861=CARTESIAN_POINT ( 'NONE',  ( 4.243569643749999010, 18.77187500061451786, -32.45002607614398471 ) ) ;
#15862=CARTESIAN_POINT ( 'NONE',  ( 10.95000000000000107, 4.330127018922192761, -2.499999999999997780 ) ) ;
#15863=CARTESIAN_POINT ( 'NONE',  ( 11.78437500061451892, 4.541064518000418104, 2.621784821874999949 ) ) ;
#15864=CARTESIAN_POINT ( 'NONE',  ( 6.712500001229034119, 0.000000000000000000, 4.999999999999998224 ) ) ;
#15865=CARTESIAN_POINT ( 'NONE',  ( 14.48437500061451821, 4.541064518000418104, 2.621784821874999949 ) ) ;
#15866=CARTESIAN_POINT ( 'NONE',  ( 5.034375000614519813, 4.541064518000418104, 2.621784821874999949 ) ) ;
#15869=DIRECTION ( 'NONE',  ( -0.000000000000000000, -0.000000000000000000, -1.000000000000000000 ) ) ;
#15870=CARTESIAN_POINT ( 'NONE',  ( 9.834375000614517859, 6.421520780324663323E-16, -5.243569643749999010 ) ) ;
#15871=LINE ( 'NONE', #55413, #11150 ) ;
#15872=CARTESIAN_POINT ( 'NONE',  ( 18.77812500061451573, 6.421520780324663323E-16, -5.243569643749999010 ) ) ;
#15873=ADVANCED_FACE ( 'NONE', ( #26261 ), #47363, .T. ) ;
#15875=CARTESIAN_POINT ( 'NONE',  ( 10.00000000000000000, 1.224646799147353256E-15, -10.00000000000000888 ) ) ;
#15876=CARTESIAN_POINT ( 'NONE',  ( 24.19687500061451857, -3.027376345333610441, -5.243569643749999898 ) ) ;
#15877=CARTESIAN_POINT ( 'NONE',  ( 4.391019444462268773, 2.392760695475801835, 4.391019444462268773 ) ) ;
#15879=CARTESIAN_POINT ( 'NONE',  ( 29.21250000122903145, 0.000000000000000000, 4.999999999999998224 ) ) ;
#15881=CARTESIAN_POINT ( 'NONE',  ( 25.67812500061451431, 4.541064518000418104, 2.621784821874999949 ) ) ;
#15882=CARTESIAN_POINT ( 'NONE',  ( 18.55312500061451431, 0.000000000000000000, 5.243569643749999010 ) ) ;
#15884=CARTESIAN_POINT ( 'NONE',  ( 14.29687500061451821, -3.027376345333610441, -5.243569643749999898 ) ) ;
#15885=CARTESIAN_POINT ( 'NONE',  ( 26.28750000122903430, 6.123233995736764310E-16, -4.999999999999998224 ) ) ;
#15886=CARTESIAN_POINT ( 'NONE',  ( 26.73750000122903003, 6.123233995736764310E-16, -4.999999999999998224 ) ) ;
#15887=CARTESIAN_POINT ( 'NONE',  ( 13.88437500061451679, 6.421520780324663323E-16, -5.243569643749999010 ) ) ;
#15889=CARTESIAN_POINT ( 'NONE',  ( 30.00000000000000000, 6.123233995736764310E-16, -4.999999999999998224 ) ) ;
#15890=CARTESIAN_POINT ( 'NONE',  ( 4.275000001229035895, 2.886751345948129099, -4.999999999999998224 ) ) ;
#15891=CARTESIAN_POINT ( 'NONE',  ( 25.20937500061451431, 4.541064518000418104, -2.621784821874998173 ) ) ;
#15892=CARTESIAN_POINT ( 'NONE',  ( 16.43437500061451573, -4.541064518000419881, 2.621784821874995952 ) ) ;
#15894=CARTESIAN_POINT ( 'NONE',  ( 27.78749999999999787, -2.886751345948129988, 4.999999999999997335 ) ) ;
#15895=CARTESIAN_POINT ( 'NONE',  ( 5.737499999999998934, -2.886751345948129988, 4.999999999999997335 ) ) ;
#15897=CARTESIAN_POINT ( 'NONE',  ( 20.16562500061451146, 3.027376345333613106, -5.243569643749998122 ) ) ;
#15898=CARTESIAN_POINT ( 'NONE',  ( 9.262499999999999289, 2.886751345948126879, 4.999999999999999112 ) ) ;
#15899=CARTESIAN_POINT ( 'NONE',  ( 4.115625000614516082, 3.027376345333611329, 5.243569643749999010 ) ) ;
#15900=CARTESIAN_POINT ( 'NONE',  ( 19.27500000000000213, -4.330127018922194537, 2.499999999999995559 ) ) ;
#15902=CARTESIAN_POINT ( 'NONE',  ( 23.92500000122903359, -5.773502691896255534, -1.060575238724906372E-15 ) ) ;
#15903=CARTESIAN_POINT ( 'NONE',  ( 5.375648687660714131, 8.434199909737650103, 32.69359484207353717 ) ) ;
#15904=CARTESIAN_POINT ( 'NONE',  ( 3.300000000000000711, 4.330127018922192761, -2.499999999999997780 ) ) ;
#15905=ORIENTED_EDGE ( 'NONE', *, *, #23424, .F. ) ;
#15906=CARTESIAN_POINT ( 'NONE',  ( 17.80312500061451786, -4.541064518000417216, -2.621784821875001281 ) ) ;
#15907=CARTESIAN_POINT ( 'NONE',  ( 25.19062500061451715, 6.054752690667223547, 3.707466751127219781E-16 ) ) ;
#15908=CARTESIAN_POINT ( 'NONE',  ( 22.69687500061451857, -3.027376345333614438, 5.243569643749998122 ) ) ;
#15909=CARTESIAN_POINT ( 'NONE',  ( 7.425000000000000711, 4.330127018922191873, 2.499999999999999556 ) ) ;
#15910=CARTESIAN_POINT ( 'NONE',  ( 8.578125000614518214, 4.541064518000418104, 2.621784821874999949 ) ) ;
#15911=CARTESIAN_POINT ( 'NONE',  ( 25.49062500061451786, -3.027376345333610441, -5.243569643749999898 ) ) ;
#15912=CARTESIAN_POINT ( 'NONE',  ( 15.64687500061451608, -3.027376345333610441, -5.243569643749999898 ) ) ;
#15913=CARTESIAN_POINT ( 'NONE',  ( 19.65937500061451360, -4.541064518000417216, -2.621784821875001281 ) ) ;
#15914=CARTESIAN_POINT ( 'NONE',  ( 1.999999999999998668, 11.86250000122903359, -33.46410161513775705 ) ) ;
#15915=CARTESIAN_POINT ( 'NONE',  ( -4.243569643749999898, 19.31562500061451715, 27.54997392385601529 ) ) ;
#15916=CARTESIAN_POINT ( 'NONE',  ( 21.07500000122903572, 2.886751345948126879, 4.999999999999999112 ) ) ;
#15918=CARTESIAN_POINT ( 'NONE',  ( 10.94062500061451537, -3.027376345333614438, 5.243569643749998122 ) ) ;
#15919=CARTESIAN_POINT ( 'NONE',  ( 8.371875000614515727, -6.054752690667223547, -1.112240025338166033E-15 ) ) ;
#15920=CARTESIAN_POINT ( 'NONE',  ( 7.546875000614517326, -3.027376345333610441, -5.243569643749999898 ) ) ;
#15921=ORIENTED_EDGE ( 'NONE', *, *, #32136, .T. ) ;
#15922=CARTESIAN_POINT ( 'NONE',  ( 27.72187500061451715, -6.054752690667223547, -1.112240025338166033E-15 ) ) ;
#15923=CARTESIAN_POINT ( 'NONE',  ( 18.59062500061451573, -3.027376345333614438, 5.243569643749998122 ) ) ;
#15924=CARTESIAN_POINT ( 'NONE',  ( 3.065625000614517592, 3.027376345333613106, -5.243569643749998122 ) ) ;
#15925=CARTESIAN_POINT ( 'NONE',  ( 29.12812500061451715, 6.421520780324663323E-16, -5.243569643749999010 ) ) ;
#15926=CARTESIAN_POINT ( 'NONE',  ( 23.33437500061451786, 6.421520780324663323E-16, -5.243569643749999010 ) ) ;
#15927=CARTESIAN_POINT ( 'NONE',  ( 19.30312500061451786, 4.541064518000418104, -2.621784821874998173 ) ) ;
#15928=CARTESIAN_POINT ( 'NONE',  ( -3.999999999999999556, 10.96250000000000213, 27.69059892324149530 ) ) ;
#15930=CARTESIAN_POINT ( 'NONE',  ( 23.76562500061451644, 3.027376345333613106, -5.243569643749998122 ) ) ;
#15931=CARTESIAN_POINT ( 'NONE',  ( 5.400000001229032343, -2.886751345948129988, 4.999999999999997335 ) ) ;
#15932=ORIENTED_EDGE ( 'NONE', *, *, #18629, .T. ) ;
#15933=CARTESIAN_POINT ( 'NONE',  ( 10.00000000000000000, 1.224646799147353256E-15, 50.00000000000000000 ) ) ;
#15934=CARTESIAN_POINT ( 'NONE',  ( 2.000000000000001332, 15.20000000000000107, -26.53589838486224650 ) ) ;
#15936=CARTESIAN_POINT ( 'NONE',  ( 4.321875000614517681, -6.054752690667223547, -1.112240025338166033E-15 ) ) ;
#15938=CARTESIAN_POINT ( 'NONE',  ( 12.06562500061451537, 3.027376345333613106, -5.243569643749998122 ) ) ;
#15939=CARTESIAN_POINT ( 'NONE',  ( 5.521875000614517859, 3.027376345333611329, 5.243569643749999010 ) ) ;
#15940=CARTESIAN_POINT ( 'NONE',  ( 23.85000000122903430, -2.886751345948129988, 4.999999999999997335 ) ) ;
#15941=AXIS2_PLACEMENT_3D ( 'NONE', #10181, #72240, #15707 ) ;
#15942=CARTESIAN_POINT ( 'NONE',  ( 15.57187500061451857, -6.054752690667223547, -1.112240025338166033E-15 ) ) ;
#15943=CARTESIAN_POINT ( 'NONE',  ( 3.271875000614519635, 3.027376345333611329, 5.243569643749999010 ) ) ;
#15944=CARTESIAN_POINT ( 'NONE',  ( -2.000000000000000000, 10.92500000000000071, 26.53589838486224650 ) ) ;
#15945=CARTESIAN_POINT ( 'NONE',  ( 26.59687500061451360, 6.054752690667223547, 3.707466751127219781E-16 ) ) ;
#15946=CARTESIAN_POINT ( 'NONE',  ( 3.365625000614516082, -6.054752690667223547, -1.112240025338166033E-15 ) ) ;
#15947=CARTESIAN_POINT ( 'NONE',  ( 12.70312500061451821, 0.000000000000000000, 5.243569643749999010 ) ) ;
#15948=ORIENTED_EDGE ( 'NONE', *, *, #48843, .T. ) ;
#15949=CARTESIAN_POINT ( 'NONE',  ( 10.97812500061451679, -4.541064518000419881, 2.621784821874995952 ) ) ;
#15950=CARTESIAN_POINT ( 'NONE',  ( 7.565625000614518036, 3.027376345333613106, -5.243569643749998122 ) ) ;
#15952=CARTESIAN_POINT ( 'NONE',  ( 9.037499999999999645, -2.886751345948125991, -5.000000000000000000 ) ) ;
#15953=CARTESIAN_POINT ( 'NONE',  ( 3.825000001229032609, 2.886751345948129099, -4.999999999999998224 ) ) ;
#15954=CARTESIAN_POINT ( 'NONE',  ( 18.97499999999999787, 6.123233995736764310E-16, -4.999999999999998224 ) ) ;
#15955=CARTESIAN_POINT ( 'NONE',  ( 19.02187500061451786, 3.027376345333611329, 5.243569643749999010 ) ) ;
#15956=CARTESIAN_POINT ( 'NONE',  ( 13.27500000122903323, 2.886751345948129099, -4.999999999999998224 ) ) ;
#15958=CARTESIAN_POINT ( 'NONE',  ( -2.121784821874996840, 15.82812500061451644, -26.32496088578401583 ) ) ;
#15959=CARTESIAN_POINT ( 'NONE',  ( 22.01249999999999574, -5.773502691896255534, -1.060575238724906372E-15 ) ) ;
#15961=CARTESIAN_POINT ( 'NONE',  ( 28.45312500061451289, 0.000000000000000000, 5.243569643749999010 ) ) ;
#15963=CARTESIAN_POINT ( 'NONE',  ( 24.14999999999999858, 0.000000000000000000, 4.999999999999998224 ) ) ;
#15964=CARTESIAN_POINT ( 'NONE',  ( 14.44687500061451679, 6.054752690667223547, 3.707466751127219781E-16 ) ) ;
#15965=CARTESIAN_POINT ( 'NONE',  ( 27.07499999999999929, 6.123233995736764310E-16, -4.999999999999998224 ) ) ;
#15967=CARTESIAN_POINT ( 'NONE',  ( 9.365625000614519635, 3.027376345333613106, -5.243569643749998122 ) ) ;
#15969=CARTESIAN_POINT ( 'NONE',  ( 21.64687500061451786, 6.054752690667223547, 3.707466751127219781E-16 ) ) ;
#15971=CARTESIAN_POINT ( 'NONE',  ( 8.728125000614518569, -4.541064518000419881, 2.621784821874995952 ) ) ;
#15972=CARTESIAN_POINT ( 'NONE',  ( 12.23437500061451821, 4.541064518000418104, 2.621784821874999949 ) ) ;
#15974=CARTESIAN_POINT ( 'NONE',  ( 21.90937500061451715, -4.541064518000417216, -2.621784821875001281 ) ) ;
#15975=CARTESIAN_POINT ( 'NONE',  ( 29.09999999999999787, 0.000000000000000000, 4.999999999999998224 ) ) ;
#15977=CARTESIAN_POINT ( 'NONE',  ( 6.112499999999999822, 2.886751345948126879, 4.999999999999999112 ) ) ;
#15978=CARTESIAN_POINT ( 'NONE',  ( 13.95000000122903572, -2.886751345948129988, 4.999999999999997335 ) ) ;
#15979=CARTESIAN_POINT ( 'NONE',  ( -5.810221930991193690E-16, 12.35000000122903430, 26.00000000000000355 ) ) ;
#15980=CARTESIAN_POINT ( 'NONE',  ( -1.071796769724491005, 19.00759618943233775, -34.00000000000000000 ) ) ;
#15981=VERTEX_POINT ( 'NONE', #7241 ) ;
#15982=CARTESIAN_POINT ( 'NONE',  ( 13.91249999999999964, -5.773502691896255534, -1.060575238724906372E-15 ) ) ;
#15983=CARTESIAN_POINT ( 'NONE',  ( 15.90000000000000036, 4.330127018922192761, -2.499999999999997780 ) ) ;
#15984=CARTESIAN_POINT ( 'NONE',  ( 13.65000000122903323, -2.886751345948125991, -5.000000000000000000 ) ) ;
#15985=CARTESIAN_POINT ( 'NONE',  ( 11.99062500061451608, -3.027376345333610441, -5.243569643749999898 ) ) ;
#15988=CARTESIAN_POINT ( 'NONE',  ( 8.962500000000002132, -5.773502691896255534, -1.060575238724906372E-15 ) ) ;
#15989=DIRECTION ( 'NONE',  ( 0.000000000000000000, 0.000000000000000000, -1.000000000000000000 ) ) ;
#15990=CARTESIAN_POINT ( 'NONE',  ( -4.243569643749999898, 13.55937500061451750, -30.00000000000000000 ) ) ;
#15991=CARTESIAN_POINT ( 'NONE',  ( 3.328125000614516438, -4.541064518000419881, 2.621784821874995952 ) ) ;
#15993=CARTESIAN_POINT ( 'NONE',  ( 8.775000000000002132, 4.330127018922191873, 2.499999999999999556 ) ) ;
#15995=ORIENTED_EDGE ( 'NONE', *, *, #10637, .T. ) ;
#15996=CARTESIAN_POINT ( 'NONE',  ( 24.21562500061451573, 3.027376345333613106, -5.243569643749998122 ) ) ;
#15997=CARTESIAN_POINT ( 'NONE',  ( 3.519358070056033849, 3.551693405655444113, 3.553333502389941945 ) ) ;
#16000=CARTESIAN_POINT ( 'NONE',  ( 21.94687500061451857, -3.027376345333610441, -5.243569643749999898 ) ) ;
#16001=CARTESIAN_POINT ( 'NONE',  ( 17.72812500061451502, -4.541064518000419881, 2.621784821874995952 ) ) ;
#16002=CARTESIAN_POINT ( 'NONE',  ( 9.001249775931846008E-16, 10.91562500061459140, -25.09994784771203058 ) ) ;
#16003=CARTESIAN_POINT ( 'NONE',  ( 7.378125000614518036, -4.541064518000419881, 2.621784821874995952 ) ) ;
#16004=CARTESIAN_POINT ( 'NONE',  ( 3.215625000614518836, 3.027376345333611329, 5.243569643749999010 ) ) ;
#16006=CARTESIAN_POINT ( 'NONE',  ( 19.34062500061451573, 6.054752690667223547, 3.707466751127219781E-16 ) ) ;
#16007=DIRECTION ( 'NONE',  ( 0.000000000000000000, 0.000000000000000000, -1.000000000000000000 ) ) ;
#16009=( BOUNDED_CURVE ( )  B_SPLINE_CURVE ( 2, ( #27119, #10124, #71080, #54099, #26381, #71453, #32655, #3496, #37464 ),
 .UNSPECIFIED., .F., .F. ) 
 B_SPLINE_CURVE_WITH_KNOTS ( ( 3, 2, 2, 2, 3 ),
 ( 0.3152173913043478382, 0.3188405797101449002, 0.3260869565217391353, 0.3333333333333333148, 0.3369565217391304324 ),
 .UNSPECIFIED. ) 
 CURVE ( )  GEOMETRIC_REPRESENTATION_ITEM ( )  RATIONAL_B_SPLINE_CURVE ( ( 0.9330127018922194093, 0.9330127018922198534, 1.000000000000000000, 0.8660254037844387076, 1.000000000000000000, 0.8660254037844387076, 1.000000000000000000, 0.9330127018922194093, 0.9330127018922194093 ) ) 
 REPRESENTATION_ITEM ( '' )  );
#16010=CARTESIAN_POINT ( 'NONE',  ( 16.09687500061452070, -3.027376345333610441, -5.243569643749999898 ) ) ;
#16011=CARTESIAN_POINT ( 'NONE',  ( 15.15937500061451715, -4.541064518000417216, -2.621784821875001281 ) ) ;
#16012=CARTESIAN_POINT ( 'NONE',  ( 21.83437500061451786, -4.541064518000419881, 2.621784821874995952 ) ) ;
#16013=VERTEX_POINT ( 'NONE', #51949 ) ;
#16014=CARTESIAN_POINT ( 'NONE',  ( 2.121784821875001281, 12.35937500061451821, 33.67503911421598417 ) ) ;
#16015=CARTESIAN_POINT ( 'NONE',  ( 3.553125000614516082, 4.541064518000418104, -2.621784821874998173 ) ) ;
#16016=CARTESIAN_POINT ( 'NONE',  ( 27.59062500061451573, -3.027376345333614438, 5.243569643749998122 ) ) ;
#16017=CARTESIAN_POINT ( 'NONE',  ( 27.36562500061451786, 3.027376345333613106, -5.243569643749998122 ) ) ;
#16019=CARTESIAN_POINT ( 'NONE',  ( 1.999999999999998668, 18.95000000000000284, 26.53589838486224650 ) ) ;
#16020=CARTESIAN_POINT ( 'NONE',  ( 5.671875000614519102, -6.054752690667223547, -1.112240025338166033E-15 ) ) ;
#16022=CARTESIAN_POINT ( 'NONE',  ( 12.22500000122903430, -5.773502691896255534, -1.060575238724906372E-15 ) ) ;
#16023=CARTESIAN_POINT ( 'NONE',  ( 8.550000001229031810, -2.886751345948129988, 4.999999999999997335 ) ) ;
#16024=CARTESIAN_POINT ( 'NONE',  ( 29.62500000122903288, 2.886751345948126879, 4.999999999999999112 ) ) ;
#16027=CARTESIAN_POINT ( 'NONE',  ( 12.27187500061451786, 3.027376345333611329, 5.243569643749999010 ) ) ;
#16028=CARTESIAN_POINT ( 'NONE',  ( 1.071796769724476572, 14.73259618943233562, -25.99999999999999289 ) ) ;
#16030=CARTESIAN_POINT ( 'NONE',  ( 20.16562500061451146, 3.027376345333613106, -5.243569643749998122 ) ) ;
#16031=CARTESIAN_POINT ( 'NONE',  ( 13.84687500061451537, -3.027376345333610441, -5.243569643749999898 ) ) ;
#16032=CARTESIAN_POINT ( 'NONE',  ( 5.690625000614516260, -3.027376345333610441, -5.243569643749999898 ) ) ;
#16033=CARTESIAN_POINT ( 'NONE',  ( 21.98437500061451644, 6.421520780324663323E-16, -5.243569643749999010 ) ) ;
#16034=CARTESIAN_POINT ( 'NONE',  ( 5.240625000614516971, -3.027376345333610441, -5.243569643749999898 ) ) ;
#16035=CARTESIAN_POINT ( 'NONE',  ( 28.42499999999999716, 6.123233995736764310E-16, -4.999999999999998224 ) ) ;
#16036=CARTESIAN_POINT ( 'NONE',  ( 6.262500001229034829, 0.000000000000000000, 4.999999999999998224 ) ) ;
#16037=CARTESIAN_POINT ( 'NONE',  ( 22.75312500061451360, -4.541064518000417216, -2.621784821875001281 ) ) ;
#16038=CARTESIAN_POINT ( 'NONE',  ( 8.484601909799253346E-16, 18.42500000122903714, -25.38119784648299770 ) ) ;
#16039=CARTESIAN_POINT ( 'NONE',  ( 8.175000001229031810, -5.773502691896255534, -1.060575238724906372E-15 ) ) ;
#16040=CARTESIAN_POINT ( 'NONE',  ( 18.06562500061451715, 3.027376345333611329, 5.243569643749999010 ) ) ;
#16041=CARTESIAN_POINT ( 'NONE',  ( 15.29062500061451679, 6.054752690667223547, 3.707466751127219781E-16 ) ) ;
#16043=CARTESIAN_POINT ( 'NONE',  ( 16.27499999999999858, 6.123233995736764310E-16, -4.999999999999998224 ) ) ;
#16044=CARTESIAN_POINT ( 'NONE',  ( 11.96250000122903501, 4.330127018922192761, -2.499999999999997780 ) ) ;
#16045=CARTESIAN_POINT ( 'NONE',  ( 7.078125000614516438, 6.421520780324663323E-16, -5.243569643749999010 ) ) ;
#16046=CARTESIAN_POINT ( 'NONE',  ( 10.37812500061451715, 4.541064518000418104, 2.621784821874999949 ) ) ;
#16047=CARTESIAN_POINT ( 'NONE',  ( 21.75000000122903288, -2.886751345948125991, -5.000000000000000000 ) ) ;
#16048=CARTESIAN_POINT ( 'NONE',  ( -4.243569643749999898, 13.07187500061452035, -32.45002607614398471 ) ) ;
#16049=FACE_OUTER_BOUND ( 'NONE', #26733, .T. ) ;
#16050=ADVANCED_FACE ( 'NONE', ( #17943 ), #6523, .F. ) ;
#16051=CARTESIAN_POINT ( 'NONE',  ( 5.400000001229032343, -2.886751345948129988, 4.999999999999997335 ) ) ;
#16052=( BOUNDED_CURVE ( )  B_SPLINE_CURVE ( 2, ( #32511, #60938, #56136, #33591, #21049, #60567, #43968, #9974, #49147 ),
 .UNSPECIFIED., .F., .F. ) 
 B_SPLINE_CURVE_WITH_KNOTS ( ( 3, 2, 2, 2, 3 ),
 ( 0.8586956521739130821, 0.8623188405797101996, 0.8695652173913043237, 0.8768115942028985588, 0.8804347826086956763 ),
 .UNSPECIFIED. ) 
 CURVE ( )  GEOMETRIC_REPRESENTATION_ITEM ( )  RATIONAL_B_SPLINE_CURVE ( ( 0.9330127018922194093, 0.9330127018922194093, 1.000000000000000000, 0.8660254037844387076, 1.000000000000000000, 0.8660254037844387076, 1.000000000000000000, 0.9330127018922194093, 0.9330127018922194093 ) ) 
 REPRESENTATION_ITEM ( '' )  );
#16053=CARTESIAN_POINT ( 'NONE',  ( 4.546875000614517326, 6.054752690667223547, 3.707466751127219781E-16 ) ) ;
#16054=CARTESIAN_POINT ( 'NONE',  ( 21.49687500061451573, -3.027376345333610441, -5.243569643749999898 ) ) ;
#16056=CARTESIAN_POINT ( 'NONE',  ( 15.77812500061451573, 4.541064518000418104, 2.621784821874999949 ) ) ;
#16058=CARTESIAN_POINT ( 'NONE',  ( -3.999999999999999112, 14.67500000122903536, 27.69059892324149885 ) ) ;
#16059=CARTESIAN_POINT ( 'NONE',  ( 4.425000000000001599, -4.330127018922194537, 2.499999999999995559 ) ) ;
#16060=CARTESIAN_POINT ( 'NONE',  ( 28.88437500061451502, 4.541064518000418104, 2.621784821874999949 ) ) ;
#16062=CARTESIAN_POINT ( 'NONE',  ( 15.92812500061451608, -4.541064518000419881, 2.621784821874995952 ) ) ;
#16063=CARTESIAN_POINT ( 'NONE',  ( 12.08437500061451608, 6.421520780324663323E-16, -5.243569643749999010 ) ) ;
#16064=EDGE_LOOP ( 'NONE', ( #22492, #6172, #52959, #40738 ) ) ;
#16065=CARTESIAN_POINT ( 'NONE',  ( 22.31249999999999645, 2.886751345948161074, 4.999999999999941380 ) ) ;
#16066=CARTESIAN_POINT ( 'NONE',  ( 22.52812500061451573, 4.541064518000418104, 2.621784821874999949 ) ) ;
#16067=CARTESIAN_POINT ( 'NONE',  ( 1.071796769724505438, 11.31740381056766864, -33.99999999999999289 ) ) ;
#16068=CARTESIAN_POINT ( 'NONE',  ( 13.16249999999999964, 2.886751345948129099, -4.999999999999998224 ) ) ;
#16069=CARTESIAN_POINT ( 'NONE',  ( 25.31250000122903288, -4.330127018922190985, -2.500000000000001332 ) ) ;
#16070=CARTESIAN_POINT ( 'NONE',  ( 19.19062500061452070, -3.027376345333610441, -5.243569643749999898 ) ) ;
#16073=CARTESIAN_POINT ( 'NONE',  ( 19.42499999999999716, 6.123233995736764310E-16, -4.999999999999998224 ) ) ;
#16074=CARTESIAN_POINT ( 'NONE',  ( 22.50937500061451857, 4.541064518000418104, -2.621784821874998173 ) ) ;
#16075=CARTESIAN_POINT ( 'NONE',  ( 27.85312500061451502, 4.541064518000418104, -2.621784821874998173 ) ) ;
#16076=( BOUNDED_CURVE ( )  B_SPLINE_CURVE ( 2, ( #46708, #63678, #40807, #565, #28990, #63322, #68877 ),
 .UNSPECIFIED., .F., .F. ) 
 B_SPLINE_CURVE_WITH_KNOTS ( ( 3, 2, 2, 3 ),
 ( 0.05833333333333334120, 0.06111111111111110911, 0.06388888888888888395, 0.06666666666666665186 ),
 .UNSPECIFIED. ) 
 CURVE ( )  GEOMETRIC_REPRESENTATION_ITEM ( )  RATIONAL_B_SPLINE_CURVE ( ( 0.9999999999999995559, 0.8660254037844390407, 1.000000000000000000, 0.8660254037844387076, 1.000000000000000000, 0.8660254037844393737, 0.9999999999999993339 ) ) 
 REPRESENTATION_ITEM ( '' )  );
#16078=CARTESIAN_POINT ( 'NONE',  ( 1.999999999999998668, 18.05000000000000071, -33.46410161513775705 ) ) ;
#16079=CARTESIAN_POINT ( 'NONE',  ( 10.34062500061451750, 6.054752690667223547, 3.707466751127219781E-16 ) ) ;
#16080=CARTESIAN_POINT ( 'NONE',  ( 17.32500000122903216, 2.886751345948162850, -4.999999999999940492 ) ) ;
#16082=AXIS2_PLACEMENT_3D ( 'NONE', #49238, #55869, #27799 ) ;
#16083=CARTESIAN_POINT ( 'NONE',  ( 17.51249999999999929, -5.773502691896255534, -1.060575238724906372E-15 ) ) ;
#16084=CARTESIAN_POINT ( 'NONE',  ( 24.56250000000000000, 2.886751345948126879, 4.999999999999999112 ) ) ;
#16085=CARTESIAN_POINT ( 'NONE',  ( -4.243569643749999898, 19.80312500061451786, 30.00000000000000000 ) ) ;
#16086=CARTESIAN_POINT ( 'NONE',  ( 4.434375000614519280, 6.421520780324663323E-16, -5.243569643749999010 ) ) ;
#16087=CARTESIAN_POINT ( 'NONE',  ( 27.45937500061451786, 4.541064518000418104, -2.621784821874998173 ) ) ;
#16088=VERTEX_POINT ( 'NONE', #58192 ) ;
#16089=CARTESIAN_POINT ( 'NONE',  ( 25.15312500061451217, 4.541064518000418104, -2.621784821874998173 ) ) ;
#16090=CARTESIAN_POINT ( 'NONE',  ( 27.34687500061451360, -3.027376345333610441, -5.243569643749999898 ) ) ;
#16091=CARTESIAN_POINT ( 'NONE',  ( 3.196875000614516793, 6.054752690667223547, 3.707466751127219781E-16 ) ) ;
#16092=CARTESIAN_POINT ( 'NONE',  ( 13.72500000000000142, 4.330127018922191873, 2.499999999999999556 ) ) ;
#16093=CARTESIAN_POINT ( 'NONE',  ( 10.90312500061451928, 0.000000000000000000, 5.243569643749999010 ) ) ;
#16094=CARTESIAN_POINT ( 'NONE',  ( 4.898587196589411843E-16, 20.00000000000000000, 33.99999999999999289 ) ) ;
#16095=CARTESIAN_POINT ( 'NONE',  ( 27.59062500061451573, -3.027376345333614438, 5.243569643749998122 ) ) ;
#16096=CARTESIAN_POINT ( 'NONE',  ( 16.53750000122903430, 4.330127018922191873, 2.499999999999999556 ) ) ;
#16098=CARTESIAN_POINT ( 'NONE',  ( 4.940625000614515372, 6.054752690667223547, 3.707466751127219781E-16 ) ) ;
#16099=CARTESIAN_POINT ( 'NONE',  ( 21.27187500061451786, 3.027376345333611329, 5.243569643749999010 ) ) ;
#16100=CARTESIAN_POINT ( 'NONE',  ( 9.001249775931846008E-16, 15.47187500061451892, 34.90005215228797653 ) ) ;
#16101=CARTESIAN_POINT ( 'NONE',  ( 21.90937500061451715, -4.541064518000417216, -2.621784821875001281 ) ) ;
#16102=CARTESIAN_POINT ( 'NONE',  ( 28.50937500061451502, 0.000000000000000000, 5.243569643749999010 ) ) ;
#16103=CARTESIAN_POINT ( 'NONE',  ( 2.121784821874999061, 17.90937500061451715, 26.32496088578401583 ) ) ;
#16104=CARTESIAN_POINT ( 'NONE',  ( 9.103125000614515017, 0.000000000000000000, 5.243569643749999010 ) ) ;
#16105=CARTESIAN_POINT ( 'NONE',  ( 0.000000000000000000, 0.000000000000000000, 50.00000000000000000 ) ) ;
#16106=CARTESIAN_POINT ( 'NONE',  ( 6.609375000614519102, -4.541064518000417216, -2.621784821875001281 ) ) ;
#16107=FACE_OUTER_BOUND ( 'NONE', #21333, .T. ) ;
#16109=CARTESIAN_POINT ( 'NONE',  ( 8.578125000614518214, 4.541064518000418104, 2.621784821874999949 ) ) ;
#16110=CARTESIAN_POINT ( 'NONE',  ( 11.59687500061451892, -3.027376345333610441, -5.243569643749999898 ) ) ;
#16111=CARTESIAN_POINT ( 'NONE',  ( 20.85000000122903430, -2.886751345948125991, -5.000000000000000000 ) ) ;
#16112=CARTESIAN_POINT ( 'NONE',  ( 7.734375000614517326, 4.541064518000418104, 2.621784821874999949 ) ) ;
#16113=CARTESIAN_POINT ( 'NONE',  ( 11.05312500061451608, -4.541064518000417216, -2.621784821875001281 ) ) ;
#16114=CARTESIAN_POINT ( 'NONE',  ( 6.853125000614516793, 0.000000000000000000, 5.243569643749999010 ) ) ;
#16116=CARTESIAN_POINT ( 'NONE',  ( 19.65937500061451360, -4.541064518000417216, -2.621784821875001281 ) ) ;
#16117=CARTESIAN_POINT ( 'NONE',  ( 1.626862140677534273E-15, 13.02500000122903323, 34.00000000000000000 ) ) ;
#16118=CARTESIAN_POINT ( 'NONE',  ( 11.84062500061451750, -3.027376345333614438, 5.243569643749998122 ) ) ;
#16119=CARTESIAN_POINT ( 'NONE',  ( 29.48437500061451644, -4.541064518000419881, 2.621784821874995952 ) ) ;
#16120=CARTESIAN_POINT ( 'NONE',  ( 9.001249775931846008E-16, 11.87187500061451395, -25.09994784771203058 ) ) ;
#16121=CARTESIAN_POINT ( 'NONE',  ( 15.75000000122902932, -2.886751345948129988, 4.999999999999997335 ) ) ;
#16122=EDGE_CURVE ( 'NONE', #45352, #67346, #52665, .T. ) ;
#16123=CARTESIAN_POINT ( 'NONE',  ( 2.121784821874999061, 14.70312500061451644, -33.67503911421598417 ) ) ;
#16124=CARTESIAN_POINT ( 'NONE',  ( 16.08750000122903501, 4.330127018922191873, 2.499999999999999556 ) ) ;
#16125=CARTESIAN_POINT ( 'NONE',  ( 10.82812500061451644, 4.541064518000418104, 2.621784821874999949 ) ) ;
#16127=CARTESIAN_POINT ( 'NONE',  ( 13.72500000000000142, 4.330127018922191873, 2.499999999999999556 ) ) ;
#16128=CARTESIAN_POINT ( 'NONE',  ( -2.000000000000000000, 13.62500000000000178, 26.53589838486224650 ) ) ;
#16129=AXIS2_PLACEMENT_3D ( 'NONE', #52434, #13622, #62514 ) ;
#16130=CARTESIAN_POINT ( 'NONE',  ( 23.16562500061451502, -6.054752690667223547, -1.112240025338166033E-15 ) ) ;
#16131=CARTESIAN_POINT ( 'NONE',  ( 7.959375000614516971, -4.541064518000417216, -2.621784821875001281 ) ) ;
#16132=EDGE_CURVE ( 'NONE', #71866, #37421, #57709, .T. ) ;
#16133=CARTESIAN_POINT ( 'NONE',  ( 10.72500000122903252, 2.886751345948126879, 4.999999999999999112 ) ) ;
#16134=CARTESIAN_POINT ( 'NONE',  ( 19.42500000122903714, -5.773502691896255534, -1.060575238724906372E-15 ) ) ;
#16135=CARTESIAN_POINT ( 'NONE',  ( 15.55312500061451608, -4.541064518000417216, -2.621784821875001281 ) ) ;
#16136=EDGE_CURVE ( 'NONE', #28731, #69794, #3791, .T. ) ;
#16137=CARTESIAN_POINT ( 'NONE',  ( 18.40312500061451573, 4.541064518000418104, -2.621784821874998173 ) ) ;
#16138=CARTESIAN_POINT ( 'NONE',  ( 26.28750000122903430, 6.123233995736764310E-16, -4.999999999999998224 ) ) ;
#16139=CARTESIAN_POINT ( 'NONE',  ( 27.30000000122903359, 5.773502691896255534, 3.535250795749688894E-16 ) ) ;
#16140=CARTESIAN_POINT ( 'NONE',  ( 22.64999999999999858, 4.330127018922192761, -2.499999999999997780 ) ) ;
#16142=AXIS2_PLACEMENT_3D ( 'NONE', #6160, #24225, #57836 ) ;
#16143=CARTESIAN_POINT ( 'NONE',  ( 26.85937500061451644, -4.541064518000417216, -2.621784821875001281 ) ) ;
#16144=CARTESIAN_POINT ( 'NONE',  ( 13.12500000122903288, -5.773502691896255534, -1.060575238724906372E-15 ) ) ;
#16145=CARTESIAN_POINT ( 'NONE',  ( 29.18437500061451573, 6.421520780324663323E-16, -5.243569643749999010 ) ) ;
#16146=CARTESIAN_POINT ( 'NONE',  ( 0.000000000000000000, 20.00000000000000000, 30.00000000000000000 ) ) ;
#16147=CARTESIAN_POINT ( 'NONE',  ( 5.296875000614518214, -3.027376345333610441, -5.243569643749999898 ) ) ;
#16148=CARTESIAN_POINT ( 'NONE',  ( 26.05312500061451431, 4.541064518000418104, -2.621784821874998173 ) ) ;
#16151=CARTESIAN_POINT ( 'NONE',  ( 9.796875000614519990, -3.027376345333610441, -5.243569643749999898 ) ) ;
#16152=CARTESIAN_POINT ( 'NONE',  ( 22.16250000122903074, -4.330127018922190985, -2.500000000000001332 ) ) ;
#16153=CARTESIAN_POINT ( 'NONE',  ( 2.934375000614518392, -4.541064518000419881, 2.621784821874995952 ) ) ;
#16154=CARTESIAN_POINT ( 'NONE',  ( 5.409375000614516260, 4.541064518000418104, -2.621784821874998173 ) ) ;
#16155=CARTESIAN_POINT ( 'NONE',  ( 27.83437500061451786, 6.421520780324663323E-16, -5.243569643749999010 ) ) ;
#16157=CARTESIAN_POINT ( 'NONE',  ( 9.001249775931846008E-16, 10.01562500061459637, 34.90005215228797653 ) ) ;
#16158=CARTESIAN_POINT ( 'NONE',  ( 19.12500000000000000, 4.330127018922191873, 2.499999999999999556 ) ) ;
#16160=CARTESIAN_POINT ( 'NONE',  ( 26.66250000000000142, 2.886751345948129099, -4.999999999999998224 ) ) ;
#16161=CARTESIAN_POINT ( 'NONE',  ( 28.88437500061451502, 4.541064518000418104, 2.621784821874999949 ) ) ;
#16162=ORIENTED_EDGE ( 'NONE', *, *, #28153, .T. ) ;
#16163=CARTESIAN_POINT ( 'NONE',  ( 18.25312500061451715, -4.541064518000417216, -2.621784821875001281 ) ) ;
#16164=CARTESIAN_POINT ( 'NONE',  ( 7.715625000614515727, 3.027376345333611329, 5.243569643749999010 ) ) ;
#16166=CARTESIAN_POINT ( 'NONE',  ( 6.046875000614519102, -3.027376345333614438, 5.243569643749998122 ) ) ;
#16167=CARTESIAN_POINT ( 'NONE',  ( 17.62500000122903288, -5.773502691896255534, -1.060575238724906372E-15 ) ) ;
#16169=CARTESIAN_POINT ( 'NONE',  ( 7.846875000614518036, -3.027376345333614438, 5.243569643749998122 ) ) ;
#16170=CARTESIAN_POINT ( 'NONE',  ( 12.90937500061451537, -4.541064518000417216, -2.621784821875001281 ) ) ;
#16171=CARTESIAN_POINT ( 'NONE',  ( 22.99687500061451573, 6.054752690667223547, 3.707466751127219781E-16 ) ) ;
#16172=CARTESIAN_POINT ( 'NONE',  ( -1.999999999999997113, 14.67500000000000071, -26.53589838486224295 ) ) ;
#16173=ORIENTED_EDGE ( 'NONE', *, *, #33228, .T. ) ;
#16175=CARTESIAN_POINT ( 'NONE',  ( 16.88437500061451502, -4.541064518000419881, 2.621784821874995952 ) ) ;
#16176=CARTESIAN_POINT ( 'NONE',  ( 8.371875000614515727, -6.054752690667223547, -1.112240025338166033E-15 ) ) ;
#16177=AXIS2_PLACEMENT_3D ( 'NONE', #52364, #12114, #23188 ) ;
#16179=CARTESIAN_POINT ( 'NONE',  ( 20.99999999999999645, 0.000000000000000000, 4.999999999999998224 ) ) ;
#16181=CARTESIAN_POINT ( 'NONE',  ( 9.001249775931846008E-16, 10.07187500061451857, -25.09994784771203058 ) ) ;
#16183=CARTESIAN_POINT ( 'NONE',  ( 11.95312500061451644, -4.541064518000417216, -2.621784821875001281 ) ) ;
#16184=CARTESIAN_POINT ( 'NONE',  ( 29.67187500061451644, 3.027376345333613106, -5.243569643749998122 ) ) ;
#16186=CARTESIAN_POINT ( 'NONE',  ( 29.85937500061451644, 0.000000000000000000, 5.243569643749999010 ) ) ;
#16187=CARTESIAN_POINT ( 'NONE',  ( 10.49999999999999822, 4.330127018922192761, -2.499999999999997780 ) ) ;
#16188=CARTESIAN_POINT ( 'NONE',  ( 2.000000000000001332, 16.66250000122903430, 33.46410161513774995 ) ) ;
#16189=CARTESIAN_POINT ( 'NONE',  ( 9.187500001229034652, 6.123233995736764310E-16, -4.999999999999998224 ) ) ;
#16190=CARTESIAN_POINT ( 'NONE',  ( 19.80937500061451573, 4.541064518000418104, -2.621784821874998173 ) ) ;
#16191=CARTESIAN_POINT ( 'NONE',  ( 14.18437500061451750, -4.541064518000419881, 2.621784821874995952 ) ) ;
#16192=CARTESIAN_POINT ( 'NONE',  ( 3.989788714780147405, 3.013600307987785776, -4.291086904670110336 ) ) ;
#16194=CARTESIAN_POINT ( 'NONE',  ( 13.94062500061451892, 6.054752690667223547, 3.707466751127219781E-16 ) ) ;
#16195=CARTESIAN_POINT ( 'NONE',  ( 28.87500000122902932, -5.773502691896255534, -1.060575238724906372E-15 ) ) ;
#16196=CARTESIAN_POINT ( 'NONE',  ( 16.02187500061451786, -6.054752690667223547, -1.112240025338166033E-15 ) ) ;
#16197=CARTESIAN_POINT ( 'NONE',  ( 2.953125000614516438, -4.541064518000417216, -2.621784821875001281 ) ) ;
#16198=CARTESIAN_POINT ( 'NONE',  ( 16.82812500061451644, -4.541064518000419881, 2.621784821874995952 ) ) ;
#16199=CARTESIAN_POINT ( 'NONE',  ( 18.11250000122903359, -4.330127018922190985, -2.500000000000001332 ) ) ;
#16200=CARTESIAN_POINT ( 'NONE',  ( 26.03437500061451715, 6.421520780324663323E-16, -5.243569643749999010 ) ) ;
#16201=CARTESIAN_POINT ( 'NONE',  ( 2.121784821874999061, 13.35312500061451679, 26.32496088578401583 ) ) ;
#16202=CARTESIAN_POINT ( 'NONE',  ( 15.90937500061451892, 0.000000000000000000, 5.243569643749999010 ) ) ;
#16203=CARTESIAN_POINT ( 'NONE',  ( 14.32500000122903394, 2.886751345948126879, 4.999999999999999112 ) ) ;
#16205=CARTESIAN_POINT ( 'NONE',  ( -3.000416591977282496E-16, 18.39687500061451786, -34.90005215228797653 ) ) ;
#16206=CARTESIAN_POINT ( 'NONE',  ( 19.58437500061451786, -4.541064518000419881, 2.621784821874995952 ) ) ;
#16207=CARTESIAN_POINT ( 'NONE',  ( 22.31250000122903288, 4.330127018922192761, -2.499999999999997780 ) ) ;
#16208=CARTESIAN_POINT ( 'NONE',  ( 16.43437500061451573, -4.541064518000419881, 2.621784821874995952 ) ) ;
#16209=CARTESIAN_POINT ( 'NONE',  ( -2.121784821874999949, 11.68437500061451750, 26.32496088578401938 ) ) ;
#16210=CARTESIAN_POINT ( 'NONE',  ( 17.12812500061451715, 4.541064518000418104, 2.621784821874999949 ) ) ;
#16211=ORIENTED_EDGE ( 'NONE', *, *, #41487, .F. ) ;
#16212=ORIENTED_EDGE ( 'NONE', *, *, #31507, .F. ) ;
#16213=CARTESIAN_POINT ( 'NONE',  ( 19.87500000000000000, 6.123233995736764310E-16, -4.999999999999998224 ) ) ;
#16215=CARTESIAN_POINT ( 'NONE',  ( 24.85312500061451502, 0.000000000000000000, 5.243569643749999010 ) ) ;
#16216=CARTESIAN_POINT ( 'NONE',  ( 5.128125000614516260, -4.541064518000419881, 2.621784821874995952 ) ) ;
#16217=CARTESIAN_POINT ( 'NONE',  ( 16.68750000122903288, -4.330127018922194537, 2.499999999999995559 ) ) ;
#16218=CARTESIAN_POINT ( 'NONE',  ( 22.64062500061451644, -3.027376345333614438, 5.243569643749998122 ) ) ;
#16219=CARTESIAN_POINT ( 'NONE',  ( 21.44999999999999929, 0.000000000000000000, 4.999999999999998224 ) ) ;
#16221=EDGE_CURVE ( 'NONE', #9071, #47727, #32824, .T. ) ;
#16222=CARTESIAN_POINT ( 'NONE',  ( 25.34062500061451217, -3.027376345333614438, 5.243569643749998122 ) ) ;
#16223=CARTESIAN_POINT ( 'NONE',  ( 5.653125000614517504, -4.541064518000417216, -2.621784821875001281 ) ) ;
#16224=EDGE_LOOP ( 'NONE', ( #17246, #9564, #52685, #16581 ) ) ;
#16225=CARTESIAN_POINT ( 'NONE',  ( 26.92500000122903003, 2.886751345948161074, 4.999999999999941380 ) ) ;
#16226=CARTESIAN_POINT ( 'NONE',  ( 4.040625000614517681, 6.054752690667223547, 3.707466751127219781E-16 ) ) ;
#16228=CARTESIAN_POINT ( 'NONE',  ( 3.999999999999998668, 11.37500000122903288, -32.30940107675850470 ) ) ;
#16229=CARTESIAN_POINT ( 'NONE',  ( 2.121784821874999061, 17.90937500061451715, -33.67503911421598417 ) ) ;
#16231=CARTESIAN_POINT ( 'NONE',  ( 8.324999999999999289, 4.330127018922191873, 2.499999999999999556 ) ) ;
#16232=CARTESIAN_POINT ( 'NONE',  ( 9.834375000614517859, 6.421520780324663323E-16, -5.243569643749999010 ) ) ;
#16233=CARTESIAN_POINT ( 'NONE',  ( 6.112500001229034474, 4.330127018922192761, -2.499999999999997780 ) ) ;
#16234=CARTESIAN_POINT ( 'NONE',  ( 11.52187500061451608, -6.054752690667223547, -1.112240025338166033E-15 ) ) ;
#16235=CARTESIAN_POINT ( 'NONE',  ( 3.909375000614518481, -4.541064518000417216, -2.621784821875001281 ) ) ;
#16237=LINE ( 'NONE', #60201, #31231 ) ;
#16238=CARTESIAN_POINT ( 'NONE',  ( 10.20937500061451786, -4.541064518000417216, -2.621784821875001281 ) ) ;
#16239=CARTESIAN_POINT ( 'NONE',  ( 20.20312500061451644, 4.541064518000418104, -2.621784821874998173 ) ) ;
#16240=CARTESIAN_POINT ( 'NONE',  ( -3.137519842735245283E-14, 11.56250000000000178, 34.00000000000000000 ) ) ;
#16241=CARTESIAN_POINT ( 'NONE',  ( 4.243569643749999898, 19.54062500061459673, 32.45002607614398471 ) ) ;
#16242=CARTESIAN_POINT ( 'NONE',  ( 23.33437500061451786, 6.421520780324663323E-16, -5.243569643749999010 ) ) ;
#16243=CARTESIAN_POINT ( 'NONE',  ( 28.12500000122902932, 2.886751345948129099, -4.999999999999998224 ) ) ;
#16245=CARTESIAN_POINT ( 'NONE',  ( 25.00312500061451715, -4.541064518000417216, -2.621784821875001281 ) ) ;
#16246=CARTESIAN_POINT ( 'NONE',  ( 15.92812500061451608, -4.541064518000419881, 2.621784821874995952 ) ) ;
#16248=CARTESIAN_POINT ( 'NONE',  ( 13.50937500061451679, 4.541064518000418104, -2.621784821874998173 ) ) ;
#16250=CARTESIAN_POINT ( 'NONE',  ( 25.12500000122903288, 2.886751345948126879, 4.999999999999999112 ) ) ;
#16251=CARTESIAN_POINT ( 'NONE',  ( 2.955228467731844333, 4.033190387708875946, -2.955228467731844333 ) ) ;
#16252=CARTESIAN_POINT ( 'NONE',  ( 15.08437500061451786, -4.541064518000419881, 2.621784821874995952 ) ) ;
#16254=CARTESIAN_POINT ( 'NONE',  ( 24.14999999999999858, 0.000000000000000000, 4.999999999999998224 ) ) ;
#16255=EDGE_CURVE ( 'NONE', #55334, #70765, #62765, .T. ) ;
#16256=CARTESIAN_POINT ( 'NONE',  ( -3.999999999999999112, 12.34999999999999964, -30.00000000000000000 ) ) ;
#16257=CARTESIAN_POINT ( 'NONE',  ( 25.73437500061451644, 4.541064518000418104, 2.621784821874999949 ) ) ;
#16258=CARTESIAN_POINT ( 'NONE',  ( 15.90937500061451892, 0.000000000000000000, 5.243569643749999010 ) ) ;
#16260=CARTESIAN_POINT ( 'NONE',  ( 27.33750000000000213, -2.886751345948129988, 4.999999999999997335 ) ) ;
#16261=CARTESIAN_POINT ( 'NONE',  ( 2.925000001229034918, 2.886751345948129099, -4.999999999999998224 ) ) ;
#16262=CARTESIAN_POINT ( 'NONE',  ( 4.537500000000000533, -2.886751345948125991, -5.000000000000000000 ) ) ;
#16264=CARTESIAN_POINT ( 'NONE',  ( 20.35312500061451502, 0.000000000000000000, 5.243569643749999010 ) ) ;
#16265=CARTESIAN_POINT ( 'NONE',  ( 9.525000000000002132, 6.123233995736764310E-16, -4.999999999999998224 ) ) ;
#16266=CARTESIAN_POINT ( 'NONE',  ( 4.265625000614517326, -6.054752690667223547, -1.112240025338166033E-15 ) ) ;
#16267=CARTESIAN_POINT ( 'NONE',  ( 17.06250000000000000, -5.773502691896255534, -1.060575238724906372E-15 ) ) ;
#16268=CARTESIAN_POINT ( 'NONE',  ( -3.999999999999999112, 17.26249999999999929, 27.69059892324149885 ) ) ;
#16269=CARTESIAN_POINT ( 'NONE',  ( 21.75000000122903288, -2.886751345948125991, -5.000000000000000000 ) ) ;
#16271=CARTESIAN_POINT ( 'NONE',  ( 28.13437500061451502, -4.541064518000419881, 2.621784821874995952 ) ) ;
#16272=VERTEX_POINT ( 'NONE', #43419 ) ;
#16273=CARTESIAN_POINT ( 'NONE',  ( 17.16562500061451502, 3.027376345333611329, 5.243569643749999010 ) ) ;
#16274=CARTESIAN_POINT ( 'NONE',  ( 23.87812500061451715, 4.541064518000418104, 2.621784821874999949 ) ) ;
#16275=CARTESIAN_POINT ( 'NONE',  ( 23.48437500061451644, 4.541064518000418104, 2.621784821874999949 ) ) ;
#16276=CARTESIAN_POINT ( 'NONE',  ( 6.450000000000001066, 4.330127018922192761, -2.499999999999997780 ) ) ;
#16277=CARTESIAN_POINT ( 'NONE',  ( 9.628125000614517148, -4.541064518000419881, 2.621784821874995952 ) ) ;
#16278=CARTESIAN_POINT ( 'NONE',  ( 25.30312500061451431, 0.000000000000000000, 5.243569643749999010 ) ) ;
#16279=CARTESIAN_POINT ( 'NONE',  ( 14.67187500061451821, -6.054752690667223547, -1.112240025338166033E-15 ) ) ;
#16280=CARTESIAN_POINT ( 'NONE',  ( 19.95937500061451786, 0.000000000000000000, 5.243569643749999010 ) ) ;
#16281=CARTESIAN_POINT ( 'NONE',  ( 1.071796769724491893, 11.69509619066136885, -26.00000000000000355 ) ) ;
#16282=CARTESIAN_POINT ( 'NONE',  ( 2.121784821874999061, 10.70937500061451964, 26.32496088578401583 ) ) ;
#16284=CARTESIAN_POINT ( 'NONE',  ( 20.81250000122903643, -4.330127018922190985, -2.500000000000001332 ) ) ;
#16286=CARTESIAN_POINT ( 'NONE',  ( 12.17812500061451608, 4.541064518000418104, 2.621784821874999949 ) ) ;
#16287=CARTESIAN_POINT ( 'NONE',  ( 8.521875000614516082, 3.027376345333613106, -5.243569643749998122 ) ) ;
#16288=CARTESIAN_POINT ( 'NONE',  ( 6.646875000614518747, -3.027376345333610441, -5.243569643749999898 ) ) ;
#16290=CARTESIAN_POINT ( 'NONE',  ( 27.45937500061451786, 4.541064518000418104, -2.621784821874998173 ) ) ;
#16291=CARTESIAN_POINT ( 'NONE',  ( 20.31562500061451715, 3.027376345333611329, 5.243569643749999010 ) ) ;
#16292=CARTESIAN_POINT ( 'NONE',  ( 29.06250000122903288, 4.330127018922192761, -2.499999999999997780 ) ) ;
#16294=CARTESIAN_POINT ( 'NONE',  ( 26.91562500061451146, 3.027376345333613106, -5.243569643749998122 ) ) ;
#16295=CARTESIAN_POINT ( 'NONE',  ( 24.60937500061451644, -4.541064518000417216, -2.621784821875001281 ) ) ;
#16296=CARTESIAN_POINT ( 'NONE',  ( 19.67812500061451786, 6.421520780324663323E-16, -5.243569643749999010 ) ) ;
#16297=CARTESIAN_POINT ( 'NONE',  ( -4.243569643749999898, 18.50937500061451857, 30.00000000000000000 ) ) ;
#16298=CARTESIAN_POINT ( 'NONE',  ( 24.62812500061451715, 6.421520780324663323E-16, -5.243569643749999010 ) ) ;
#16299=CARTESIAN_POINT ( 'NONE',  ( 3.562500001229033764, 0.000000000000000000, 4.999999999999998224 ) ) ;
#16300=VERTEX_POINT ( 'NONE', #37498 ) ;
#16301=CARTESIAN_POINT ( 'NONE',  ( 27.63749999999999929, 5.773502691896255534, 3.535250795749688894E-16 ) ) ;
#16302=CARTESIAN_POINT ( 'NONE',  ( 3.999999999999998668, 15.31250000000000000, -32.30940107675850470 ) ) ;
#16304=CARTESIAN_POINT ( 'NONE',  ( 4.284375000614518925, -4.541064518000419881, 2.621784821874995952 ) ) ;
#16305=CARTESIAN_POINT ( 'NONE',  ( 13.19062500061451537, -3.027376345333614438, 5.243569643749998122 ) ) ;
#16306=CARTESIAN_POINT ( 'NONE',  ( 6.046875000614519102, -3.027376345333614438, 5.243569643749998122 ) ) ;
#16307=CARTESIAN_POINT ( 'NONE',  ( 24.60000000122903430, 5.773502691896255534, 3.535250795749688894E-16 ) ) ;
#16308=CARTESIAN_POINT ( 'NONE',  ( 15.00937500061451679, 0.000000000000000000, 5.243569643749999010 ) ) ;
#16309=CARTESIAN_POINT ( 'NONE',  ( 29.16562500061451502, 3.027376345333613106, -5.243569643749998122 ) ) ;
#16310=CARTESIAN_POINT ( 'NONE',  ( 29.47499999999999787, 4.330127018922191873, 2.499999999999999556 ) ) ;
#16311=CARTESIAN_POINT ( 'NONE',  ( 26.48437500061451644, 6.421520780324663323E-16, -5.243569643749999010 ) ) ;
#16312=CARTESIAN_POINT ( 'NONE',  ( 3.403125000614518836, -4.541064518000417216, -2.621784821875001281 ) ) ;
#16313=CARTESIAN_POINT ( 'NONE',  ( 12.44062500061451537, -3.027376345333610441, -5.243569643749999898 ) ) ;
#16314=VERTEX_POINT ( 'NONE', #60018 ) ;
#16315=CARTESIAN_POINT ( 'NONE',  ( 9.965625000614517504, 3.027376345333611329, 5.243569643749999010 ) ) ;
#16316=CARTESIAN_POINT ( 'NONE',  ( 7.340625000614518392, -3.027376345333614438, 5.243569643749998122 ) ) ;
#16318=CARTESIAN_POINT ( 'NONE',  ( 9.299999999999998934, 0.000000000000000000, 4.999999999999998224 ) ) ;
#16320=CARTESIAN_POINT ( 'NONE',  ( 18.71249999999999858, 2.886751345948126879, 4.999999999999999112 ) ) ;
#16321=CARTESIAN_POINT ( 'NONE',  ( 18.00937500061451502, 4.541064518000418104, -2.621784821874998173 ) ) ;
#16322=CARTESIAN_POINT ( 'NONE',  ( 13.83750000122903323, 4.330127018922191873, 2.499999999999999556 ) ) ;
#16324=CARTESIAN_POINT ( 'NONE',  ( -4.243569643749997233, 16.24062500061451431, -27.54997392385601174 ) ) ;
#16328=CARTESIAN_POINT ( 'NONE',  ( 27.55312500061451786, 0.000000000000000000, 5.243569643749999010 ) ) ;
#16329=CARTESIAN_POINT ( 'NONE',  ( 3.999999999999998668, 16.21250000000000213, -32.30940107675850470 ) ) ;
#16330=CARTESIAN_POINT ( 'NONE',  ( 27.48749999999999716, -2.886751345948125991, -5.000000000000000000 ) ) ;
#16331=CARTESIAN_POINT ( 'NONE',  ( 8.578125000614518214, 4.541064518000418104, 2.621784821874999949 ) ) ;
#16333=CARTESIAN_POINT ( 'NONE',  ( 21.72187500061451715, 3.027376345333611329, 5.243569643749999010 ) ) ;
#16335=CARTESIAN_POINT ( 'NONE',  ( 5.990625000614517859, -3.027376345333614438, 5.243569643749998122 ) ) ;
#16336=CARTESIAN_POINT ( 'NONE',  ( 11.33437500061451608, 4.541064518000418104, 2.621784821874999949 ) ) ;
#16337=ORIENTED_EDGE ( 'NONE', *, *, #24471, .F. ) ;
#16338=CARTESIAN_POINT ( 'NONE',  ( 21.08437500061451786, 6.421520780324663323E-16, -5.243569643749999010 ) ) ;
#16339=CARTESIAN_POINT ( 'NONE',  ( 2.679675080847534030, 4.226630133448150417, -27.01986178876142830 ) ) ;
#16340=CARTESIAN_POINT ( 'NONE',  ( 29.21249999999999858, -5.773502691896255534, -1.060575238724906372E-15 ) ) ;
#16341=CARTESIAN_POINT ( 'NONE',  ( 6.037500000000001421, 5.773502691896255534, 3.535250795749688894E-16 ) ) ;
#16342=CARTESIAN_POINT ( 'NONE',  ( 14.85000000122903252, -2.886751345948129988, 4.999999999999997335 ) ) ;
#16343=CARTESIAN_POINT ( 'NONE',  ( 2.000000000000001332, 15.20000000000000107, -26.53589838486224650 ) ) ;
#16344=CARTESIAN_POINT ( 'NONE',  ( 3.786627597484739649, -3.265197691826910553, 4.102873032019218158 ) ) ;
#16346=CARTESIAN_POINT ( 'NONE',  ( 11.70000000000000284, -4.330127018922190985, -2.500000000000001332 ) ) ;
#16347=CARTESIAN_POINT ( 'NONE',  ( 17.06250000000000000, -5.773502691896255534, -1.060575238724906372E-15 ) ) ;
#16348=CARTESIAN_POINT ( 'NONE',  ( 12.52500000122903145, 2.886751345948126879, 4.999999999999999112 ) ) ;
#16349=CARTESIAN_POINT ( 'NONE',  ( 10.49062500061451431, -3.027376345333614438, 5.243569643749998122 ) ) ;
#16350=CARTESIAN_POINT ( 'NONE',  ( 8.400000000000000355, 0.000000000000000000, 4.999999999999998224 ) ) ;
#16351=FACE_OUTER_BOUND ( 'NONE', #7971, .T. ) ;
#16352=CARTESIAN_POINT ( 'NONE',  ( 4.243569643749999010, 15.62187500061451928, -32.45002607614398471 ) ) ;
#16353=CARTESIAN_POINT ( 'NONE',  ( 28.01250000122903216, -4.330127018922190985, -2.500000000000001332 ) ) ;
#16355=CARTESIAN_POINT ( 'NONE',  ( 10.46249999999999858, 2.886751345948129099, -4.999999999999998224 ) ) ;
#16357=ORIENTED_EDGE ( 'NONE', *, *, #35944, .F. ) ;
#16358=CARTESIAN_POINT ( 'NONE',  ( 24.92812500061451431, -4.541064518000419881, 2.621784821874995952 ) ) ;
#16359=CARTESIAN_POINT ( 'NONE',  ( 3.578077538329305973, 3.492538166020475732, 3.745691089025586784 ) ) ;
#16360=DIRECTION ( 'NONE',  ( 0.000000000000000000, 0.000000000000000000, 1.000000000000000000 ) ) ;
#16361=CARTESIAN_POINT ( 'NONE',  ( 21.30937500061451573, 0.000000000000000000, 5.243569643749999010 ) ) ;
#16362=CARTESIAN_POINT ( 'NONE',  ( 16.60312500061451857, 4.541064518000418104, -2.621784821874998173 ) ) ;
#16363=CARTESIAN_POINT ( 'NONE',  ( 2.121784821875001281, 10.95312500061459460, -26.32496088578401938 ) ) ;
#16364=CARTESIAN_POINT ( 'NONE',  ( 7.640625000614517326, 6.054752690667223547, 3.707466751127219781E-16 ) ) ;
#16365=CARTESIAN_POINT ( 'NONE',  ( 29.40000000122903145, -2.886751345948125991, -5.000000000000000000 ) ) ;
#16367=CARTESIAN_POINT ( 'NONE',  ( 18.62812500061451715, -4.541064518000419881, 2.621784821874995952 ) ) ;
#16370=CARTESIAN_POINT ( 'NONE',  ( 15.15937500061451715, -4.541064518000417216, -2.621784821875001281 ) ) ;
#16371=CARTESIAN_POINT ( 'NONE',  ( 14.93437500061451750, 4.541064518000418104, 2.621784821874999949 ) ) ;
#16372=CARTESIAN_POINT ( 'NONE',  ( 21.45937500061451786, -4.541064518000417216, -2.621784821875001281 ) ) ;
#16374=CARTESIAN_POINT ( 'NONE',  ( -4.243569643749999898, 11.75937500061451857, 30.00000000000000000 ) ) ;
#16375=CARTESIAN_POINT ( 'NONE',  ( 3.253125000614518036, 0.000000000000000000, 5.243569643749999010 ) ) ;
#16376=CARTESIAN_POINT ( 'NONE',  ( 26.69062500061451715, -3.027376345333614438, 5.243569643749998122 ) ) ;
#16378=CARTESIAN_POINT ( 'NONE',  ( 27.40312500061451573, 4.541064518000418104, -2.621784821874998173 ) ) ;
#16379=CARTESIAN_POINT ( 'NONE',  ( 2.000000000000001332, 19.36250000122903359, -26.53589838486224650 ) ) ;
#16380=CARTESIAN_POINT ( 'NONE',  ( -1.999999999999997113, 17.37500000000000000, 33.46410161513775705 ) ) ;
#16381=CARTESIAN_POINT ( 'NONE',  ( 5.746875000614517504, -3.027376345333610441, -5.243569643749999898 ) ) ;
#16382=CARTESIAN_POINT ( 'NONE',  ( 12.03750000122903430, 4.330127018922191873, 2.499999999999999556 ) ) ;
#16383=CARTESIAN_POINT ( 'NONE',  ( 6.450000001229034829, -2.886751345948125991, -5.000000000000000000 ) ) ;
#16384=CARTESIAN_POINT ( 'NONE',  ( 29.17500000122903714, 2.886751345948126879, 4.999999999999999112 ) ) ;
#16387=CARTESIAN_POINT ( 'NONE',  ( 11.33437500061451608, 4.541064518000418104, 2.621784821874999949 ) ) ;
#16388=ORIENTED_EDGE ( 'NONE', *, *, #50186, .T. ) ;
#16389=CARTESIAN_POINT ( 'NONE',  ( 20.09062500061451573, -3.027376345333610441, -5.243569643749999898 ) ) ;
#16390=CARTESIAN_POINT ( 'NONE',  ( 13.62187500061451750, 3.027376345333611329, 5.243569643749999010 ) ) ;
#16391=CARTESIAN_POINT ( 'NONE',  ( 4.940625000614515372, 6.054752690667223547, 3.707466751127219781E-16 ) ) ;
#16392=EDGE_CURVE ( 'NONE', #72350, #55885, #65268, .T. ) ;
#16393=CARTESIAN_POINT ( 'NONE',  ( 21.08437500061451786, 6.421520780324663323E-16, -5.243569643749999010 ) ) ;
#16394=CARTESIAN_POINT ( 'NONE',  ( 10.43437500061451750, 4.541064518000418104, 2.621784821874999949 ) ) ;
#16395=CARTESIAN_POINT ( 'NONE',  ( 4.453125000614517326, 4.541064518000418104, -2.621784821874998173 ) ) ;
#16396=CARTESIAN_POINT ( 'NONE',  ( 10.91250000122903252, -4.330127018922190985, -2.500000000000001332 ) ) ;
#16397=CARTESIAN_POINT ( 'NONE',  ( 5.137500001229033941, 6.123233995736764310E-16, -4.999999999999998224 ) ) ;
#16398=CARTESIAN_POINT ( 'NONE',  ( 19.19062500061452070, -3.027376345333610441, -5.243569643749999898 ) ) ;
#16399=EDGE_CURVE ( 'NONE', #860, #48144, #21899, .T. ) ;
#16400=CARTESIAN_POINT ( 'NONE',  ( 7.500000001229034652, 5.773502691896255534, 3.535250795749688894E-16 ) ) ;
#16401=CARTESIAN_POINT ( 'NONE',  ( 16.15312500061451573, 4.541064518000418104, -2.621784821874998173 ) ) ;
#16402=CARTESIAN_POINT ( 'NONE',  ( 15.77812500061451573, 4.541064518000418104, 2.621784821874999949 ) ) ;
#16404=CARTESIAN_POINT ( 'NONE',  ( 16.64999999999999858, -4.330127018922190985, -2.500000000000001332 ) ) ;
#16405=CARTESIAN_POINT ( 'NONE',  ( 9.600000001229034297, -2.886751345948125991, -5.000000000000000000 ) ) ;
#16406=CARTESIAN_POINT ( 'NONE',  ( 9.028125000614517504, 4.541064518000418104, 2.621784821874999949 ) ) ;
#16407=EDGE_CURVE ( 'NONE', #403, #31197, #7963, .T. ) ;
#16408=CARTESIAN_POINT ( 'NONE',  ( 21.37500000122902932, 2.886751345948129099, -4.999999999999998224 ) ) ;
#16410=CARTESIAN_POINT ( 'NONE',  ( 4.243569643749999010, 12.47187500061451715, -32.45002607614398471 ) ) ;
#16411=CARTESIAN_POINT ( 'NONE',  ( 4.615679581435968792, -1.922694556504207286, 4.852467576076502809 ) ) ;
#16413=CARTESIAN_POINT ( 'NONE',  ( 2.896875000614518747, -3.027376345333614438, 5.243569643749998122 ) ) ;
#16414=CARTESIAN_POINT ( 'NONE',  ( 20.37187500061451573, 3.027376345333611329, 5.243569643749999010 ) ) ;
#16415=CARTESIAN_POINT ( 'NONE',  ( 1.626862140677534273E-15, 16.51249999999999929, -26.00000000000000355 ) ) ;
#16416=CARTESIAN_POINT ( 'NONE',  ( 16.79062500061451857, -3.027376345333614438, 5.243569643749998122 ) ) ;
#16418=CARTESIAN_POINT ( 'NONE',  ( 29.33437500061451431, 4.541064518000418104, 2.621784821874999949 ) ) ;
#16420=CARTESIAN_POINT ( 'NONE',  ( 14.95312500061451644, 0.000000000000000000, 5.243569643749999010 ) ) ;
#16421=CARTESIAN_POINT ( 'NONE',  ( 11.07187500061451679, -6.054752690667223547, -1.112240025338166033E-15 ) ) ;
#16423=CARTESIAN_POINT ( 'NONE',  ( -3.999999999999999112, 14.15000000000000036, -30.00000000000000000 ) ) ;
#16424=CARTESIAN_POINT ( 'NONE',  ( 23.72812500061451502, 6.421520780324663323E-16, -5.243569643749999010 ) ) ;
#16427=CARTESIAN_POINT ( 'NONE',  ( 12.82499999999999929, 4.330127018922191873, 2.499999999999999556 ) ) ;
#16428=CARTESIAN_POINT ( 'NONE',  ( 22.05000000122903714, -2.886751345948129988, 4.999999999999997335 ) ) ;
#16429=CARTESIAN_POINT ( 'NONE',  ( 16.30312500061451786, 0.000000000000000000, 5.243569643749999010 ) ) ;
#16431=VERTEX_POINT ( 'NONE', #55232 ) ;
#16432=CARTESIAN_POINT ( 'NONE',  ( 19.61249999999999716, 2.886751345948126879, 4.999999999999999112 ) ) ;
#16434=CARTESIAN_POINT ( 'NONE',  ( 20.70937500061451786, 4.541064518000418104, -2.621784821874998173 ) ) ;
#16435=CARTESIAN_POINT ( 'NONE',  ( 26.76562500061451644, -6.054752690667223547, -1.112240025338166033E-15 ) ) ;
#16438=CARTESIAN_POINT ( 'NONE',  ( 10.00312500061451715, 0.000000000000000000, 5.243569643749999010 ) ) ;
#16439=CARTESIAN_POINT ( 'NONE',  ( 6.187500000000001776, -2.886751345948130876, 4.999999999999996447 ) ) ;
#16440=CARTESIAN_POINT ( 'NONE',  ( 16.46249999999999503, 2.886751345948126879, 4.999999999999999112 ) ) ;
#16441=CARTESIAN_POINT ( 'NONE',  ( 23.36250000000000071, -5.773502691896255534, -1.060575238724906372E-15 ) ) ;
#16442=CARTESIAN_POINT ( 'NONE',  ( 2.121784821875001281, 19.50312500061451360, 33.67503911421598417 ) ) ;
#16443=CARTESIAN_POINT ( 'NONE',  ( 4.471875000614518925, 3.027376345333613106, -5.243569643749998122 ) ) ;
#16444=CARTESIAN_POINT ( 'NONE',  ( 29.74687500061451217, 6.054752690667223547, 3.707466751127219781E-16 ) ) ;
#16445=ORIENTED_EDGE ( 'NONE', *, *, #36482, .T. ) ;
#16446=CARTESIAN_POINT ( 'NONE',  ( 23.54062500061451146, -3.027376345333614438, 5.243569643749998122 ) ) ;
#16447=CARTESIAN_POINT ( 'NONE',  ( 25.32187500061451857, 3.027376345333611329, 5.243569643749999010 ) ) ;
#16448=CARTESIAN_POINT ( 'NONE',  ( 9.001249775931846008E-16, 19.46562500061459033, -25.09994784771203058 ) ) ;
#16449=CARTESIAN_POINT ( 'NONE',  ( 13.87500000000000178, -4.330127018922194537, 2.499999999999995559 ) ) ;
#16450=CARTESIAN_POINT ( 'NONE',  ( 9.215625000614515727, -6.054752690667223547, -1.112240025338166033E-15 ) ) ;
#16452=CARTESIAN_POINT ( 'NONE',  ( 25.41562500061451146, -6.054752690667223547, -1.112240025338166033E-15 ) ) ;
#16453=CARTESIAN_POINT ( 'NONE',  ( 12.63750000122903394, -4.330127018922194537, 2.499999999999995559 ) ) ;
#16455=CARTESIAN_POINT ( 'NONE',  ( 3.740625000614516527, -3.027376345333614438, 5.243569643749998122 ) ) ;
#16456=CARTESIAN_POINT ( 'NONE',  ( 19.84687500061451360, 6.054752690667223547, 3.707466751127219781E-16 ) ) ;
#16457=CARTESIAN_POINT ( 'NONE',  ( 4.243569643749999898, 13.78437500061451715, 30.00000000000000000 ) ) ;
#16458=CARTESIAN_POINT ( 'NONE',  ( 22.65937500061451715, 0.000000000000000000, 5.243569643749999010 ) ) ;
#16459=CARTESIAN_POINT ( 'NONE',  ( 28.43437500061451573, 4.541064518000418104, 2.621784821874999949 ) ) ;
#16460=CARTESIAN_POINT ( 'NONE',  ( 4.243569643749999898, 19.18437500061451928, 30.00000000000000000 ) ) ;
#16461=CARTESIAN_POINT ( 'NONE',  ( 10.75312500061451715, 4.541064518000418104, -2.621784821874998173 ) ) ;
#16462=CARTESIAN_POINT ( 'NONE',  ( -3.999999999999999112, 15.12500000122903465, 27.69059892324149885 ) ) ;
#16463=CARTESIAN_POINT ( 'NONE',  ( 7.171875000614517326, 3.027376345333613106, -5.243569643749998122 ) ) ;
#16465=CARTESIAN_POINT ( 'NONE',  ( 8.090625000614515727, 6.054752690667223547, 3.707466751127219781E-16 ) ) ;
#16466=CARTESIAN_POINT ( 'NONE',  ( 12.04687500061451821, -3.027376345333610441, -5.243569643749999898 ) ) ;
#16467=CARTESIAN_POINT ( 'NONE',  ( 19.12500000122903288, 2.886751345948129099, -4.999999999999998224 ) ) ;
#16468=CARTESIAN_POINT ( 'NONE',  ( 8.071875000614518569, 3.027376345333613106, -5.243569643749998122 ) ) ;
#16469=EDGE_CURVE ( 'NONE', #41395, #4055, #72843, .T. ) ;
#16470=CARTESIAN_POINT ( 'NONE',  ( 9.590625000614517504, -3.027376345333614438, 5.243569643749998122 ) ) ;
#16471=CARTESIAN_POINT ( 'NONE',  ( 4.875318576323432573, 3.418657702705165669, -4.565850452727954867 ) ) ;
#16473=CARTESIAN_POINT ( 'NONE',  ( 19.13437500061451857, -4.541064518000419881, 2.621784821874995952 ) ) ;
#16474=CARTESIAN_POINT ( 'NONE',  ( 18.11250000000000071, 2.886751345948129099, -4.999999999999997335 ) ) ;
#16475=CARTESIAN_POINT ( 'NONE',  ( 27.70312500061451289, -4.541064518000417216, -2.621784821875001281 ) ) ;
#16476=CARTESIAN_POINT ( 'NONE',  ( 11.27812500061451573, 4.541064518000418104, 2.621784821874999949 ) ) ;
#16478=CARTESIAN_POINT ( 'NONE',  ( -4.243569643749998122, 13.14687500061451786, -27.54997392385601174 ) ) ;
#16479=CARTESIAN_POINT ( 'NONE',  ( 12.90000000122903145, 5.773502691896255534, 3.535250795749688894E-16 ) ) ;
#16480=CARTESIAN_POINT ( 'NONE',  ( 27.10312500061451502, 0.000000000000000000, 5.243569643749999010 ) ) ;
#16481=EDGE_CURVE ( 'NONE', #61496, #70526, #19498, .T. ) ;
#16482=CARTESIAN_POINT ( 'NONE',  ( -3.000416591977282496E-16, 16.54062500061451857, -34.90005215228797653 ) ) ;
#16483=CARTESIAN_POINT ( 'NONE',  ( 14.47500000122903430, -5.773502691896255534, -1.060575238724906372E-15 ) ) ;
#16484=CARTESIAN_POINT ( 'NONE',  ( 13.38750000000000107, -2.886751345948129988, 4.999999999999997335 ) ) ;
#16486=CARTESIAN_POINT ( 'NONE',  ( 22.22812500061451502, -4.541064518000419881, 2.621784821874995952 ) ) ;
#16487=CARTESIAN_POINT ( 'NONE',  ( 8.559375000614515727, 4.541064518000418104, -2.621784821874998173 ) ) ;
#16488=CARTESIAN_POINT ( 'NONE',  ( 9.712500001229033231, 4.330127018922192761, -2.499999999999997780 ) ) ;
#16489=CARTESIAN_POINT ( 'NONE',  ( 18.63750000122903216, 6.123233995736764310E-16, -4.999999999999998224 ) ) ;
#16490=( BOUNDED_CURVE ( )  B_SPLINE_CURVE ( 2, ( #66691, #16065, #38614, #61137, #9072, #31607, #3538 ),
 .UNSPECIFIED., .F., .F. ) 
 B_SPLINE_CURVE_WITH_KNOTS ( ( 3, 2, 2, 3 ),
 ( 0.2833333333333333814, 0.2861111111111111494, 0.2888888888888889173, 0.2916666666666667407 ),
 .UNSPECIFIED. ) 
 CURVE ( )  GEOMETRIC_REPRESENTATION_ITEM ( )  RATIONAL_B_SPLINE_CURVE ( ( 0.9999999999999973355, 0.8660254037844413721, 1.000000000000000000, 0.8660254037844387076, 1.000000000000000000, 0.8660254037844360431, 1.000000000000002665 ) ) 
 REPRESENTATION_ITEM ( '' )  );
#16491=CARTESIAN_POINT ( 'NONE',  ( 14.46562500061451750, 3.027376345333611329, 5.243569643749999010 ) ) ;
#16492=CARTESIAN_POINT ( 'NONE',  ( 17.69062500061451715, -3.027376345333614438, 5.243569643749998122 ) ) ;
#16493=CARTESIAN_POINT ( 'NONE',  ( 24.97500000122903430, 2.886751345948129099, -4.999999999999998224 ) ) ;
#16494=( BOUNDED_CURVE ( )  B_SPLINE_CURVE ( 2, ( #46075, #40174, #18695, #6184, #41259, #68251, #35339, #62333, #28713 ),
 .UNSPECIFIED., .F., .F. ) 
 B_SPLINE_CURVE_WITH_KNOTS ( ( 3, 2, 2, 2, 3 ),
 ( 0.4239130434782608647, 0.4275362318840579823, 0.4347826086956521618, 0.4420289855072463969, 0.4456521739130435145 ),
 .UNSPECIFIED. ) 
 CURVE ( )  GEOMETRIC_REPRESENTATION_ITEM ( )  RATIONAL_B_SPLINE_CURVE ( ( 0.9330127018922194093, 0.9330127018922194093, 1.000000000000000000, 0.8660254037844387076, 1.000000000000000000, 0.8660254037844387076, 1.000000000000000000, 0.9330127018922188542, 0.9330127018922194093 ) ) 
 REPRESENTATION_ITEM ( '' )  );
#16495=CARTESIAN_POINT ( 'NONE',  ( 28.46250000122903145, -4.330127018922190985, -2.500000000000001332 ) ) ;
#16496=CARTESIAN_POINT ( 'NONE',  ( 22.42500000000000071, -4.330127018922194537, 2.499999999999995559 ) ) ;
#16498=CARTESIAN_POINT ( 'NONE',  ( 25.13437500061451502, 6.421520780324663323E-16, -5.243569643749999010 ) ) ;
#16501=CARTESIAN_POINT ( 'NONE',  ( 11.36250000122903536, -4.330127018922190985, -2.500000000000001332 ) ) ;
#16502=CARTESIAN_POINT ( 'NONE',  ( 28.13437500061451502, -4.541064518000419881, 2.621784821874995952 ) ) ;
#16503=DIRECTION ( 'NONE',  ( 0.000000000000000000, 0.000000000000000000, 1.000000000000000000 ) ) ;
#16504=( BOUNDED_SURFACE ( )  B_SPLINE_SURFACE ( 1, 2, ( 
 ( #32700, #32327, #55596, #49330, #50425, #55237, #10529, #21602, #61132, #60386, #10889, #10166, #67061, #56325, #16418, #38976, #61492, #33417, #72586, #11260, #27891, #38609, #44156, #50781, #27162, #66685, #16060, #33057, #4991, #72951, #27523, #50056, #15325, #21234, #39340, #55957, #4272, #54864, #67420, #21969, #22333, #71862, #60758, #5353, #15690, #37867, #44528, #28250, #44885, #16782, #26796, #61852, #33782, #5714, #20871, #43424, #65946, #9794, #43786, #66313, #38228, #4632, #49696, #72223, #28606, #18214, #40066, #57028, #63658, #57391, #23052, #45962, #51507, #184, #56675, #11977, #6434, #28969, #40418, #6073, #68495, #62580, #51142, #907, #24135, #34500, #62935, #541, #12692, #67773, #68858, #46323, #17148, #12328, #35588, #45607, #1264, #69224, #34864, #18585, #17859, #23415, #39706, #29687, #6798, #29332, #63300, #51862, #23771, #40787, #30045, #46686, #41150, #13049, #35229, #57750, #7158, #11620, #58107, #52224, #62224, #7514, #22689, #1628, #45240, #34136, #68141, #17505, #25602, #14878, #25968, #42959, #47046, #36321, #36680, #70664, #59940, #37417, #71036, #9347, #65121, #24859, #53307, #14511, #20040, #52585, #48140, #69580, #47406, #65488, #13779, #47768, #30776, #24502, #35947, #59201, #41859, #8609, #58836, #19306, #13400, #1991, #52945, #53679, #8246, #42595, #31514, #54055, #18942, #37044, #70304, #41501, #19677, #58468, #20411, #2342, #64021, #59568, #8982, #31138, #69936, #2706, #25222, #30417, #7881, #42230, #14145, #64389, #3450, #64755, #3074, #48509, #60665, #72132, #22247, #4545, #10800, #60297, #21146, #49605, #43700, #54775, #20780, #61406, #66221, #21512, #43336, #4903, #10078, #4180, #15599, #44065, #33335, #27074, #38141, #39252, #66593, #16333, #44801, #15969, #71778, #44439, #49243, #16694, #27439, #72493, #38519, #49969, #38888, #61042, #26336, #21878, #71405, #9708, #32609, #65858, #10440, #32242, #55873, #55147, #32970, #55510, #66968, #15240, #5260, #27804, #50340, #67334, #72864, #61764, #31880, #54414, #3815, #48875, #37777, #26709, #18498, #22959, #52137, #1540, #39616, #50694, #6345, #5985, #62850, #17769, #5630, #51415, #40329, #68050, #12244, #34775, #51777, #34413, #57307, #56941, #450, #62135, #39978, #35143, #51055, #817, #17057, #23685, #28167, #6712, #29245, #96, #23325, #46597, #34049, #1177, #7072, #45875, #29601, #28876, #45519, #22602, #40696, #46233, #68773, #18129, #17419, #68407, #62490, #41063, #57666, #24050, #69139, #63213, #12609, #11168, #45154, #33692, #56238, #67686, #11528, #56589, #28515, #11888, #41773, #25137, #2616, #36595, #25885, #36960, #53966, #58021, #47319, #47678, #8523, #70951, #48425, #8894, #20322, #2984, #35859, #64302, #25512, #31052, #63577, #59116, #3364, #70582, #8159, #13691, #12964, #69852, #36235, #58749, #30688, #70214, #19958, #53219, #19588, #7431, #63935, #31426, #48057, #46962, #1908, #59482, #42144, #65034, #41419, #30333, #53589, #58382, #29957, #64671, #35502, #14056, #42510, #24413, #14425, #52498, #69498, #18858, #13320, #7794, #52861, #2261, #24775, #19219, #66136, #20691, #4818, #71315, #60952, #9625, #26623, #33249, #26992, #65770, #15514, #21063, #42876, #26251, #54691, #49160, #71691, #9989, #48788, #38056, #21789, #43250, #32158, #60581, #4094, #15152, #31794, #72407, #43614, #32524, #54333, #15884, #55061, #37689, #4462, #49521, #44355, #72046, #21424, #50254, #43981, #27351, #55787, #66502, #38429, #55425, #60212, #27714, #10355, #32885, #49882, #66880, #16248, #38804, #37331, #61320, #9259, #10717, #5178, #3726, #72777, #65399, #14790, #59855, #11807, #22871, #62408, #61678, #12161, #11446, #68328, #57586, #17688, #40249, #62770, #34689, #733, #29162, #67963, #57220, #29520, #33966, #63130, #12526, #50609, #11077, #17336, #16969, #23242, #28790, #16607, #34324, #51331, #5898, #45793, #6633, #51694, #45429, #1098, #39163, #67604, #35059, #56505, #39895, #364, #67249, #5543, #6262, #28431, #23606, #50968, #62051, #56149, #44713, #22520, #46151, #56856, #68691, #18051, #40609, #33605, #6989, #52055, #28081, #22161, #13, #45067, #39525, #1459, #8432, #64584, #30607, #1822, #35777, #58300, #52414, #42427, #7709, #36148, #69052, #53503, #7348, #30243, #19504, #52776, #41690, #64948, #8075, #53135, #13972, #2178, #47235, #24691, #31338, #25426, #19874, #14340, #13602, #2534, #47597, #12883, #36874, #25054, #18414, #59392, #47969, #69768, #8802, #19136, #58667, #70126, #42061, #23965, #70497, #46513, #40980, #64213, #36510, #59030, #63495, #35416, #57941, #29878, #30968, #46878, #2895, #24329, #69417, #18772, #41338, #63848, #13239, #71599, #54603, #10632, #60128, #26531, #4008, #20974, #37971, #10269, #43527, #66049, #48337, #54241, #72325, #15797, #37243, #65309, #27267, #60492, #55338, #31706, #20602, #49432, #48701, #70862, #9898, #61238, #15427, #32434, #14699, #49071, #4733, #54971, #32802, #4377, #26906, #71966, #3271, #20236, #49800, #21340, #3638, #38337, #9171, #43895, #43161, #37606, #44262, #66419, #26162, #60866, #32071, #53879, #59764, #65681, #9537, #21705, #66795, #71224, #16166, #15069, #38718, #25799, #42788, #73053, #283, #39076, #45710, #27630, #28706, #6176, #50163, #22791, #68603, #56063, #34238, #29076, #45344, #51611, #28346, #22435, #72693, #62686, #12082, #39810, #62326, #23156, #39439, #5815, #16885, #63041, #57132, #1011, #23518, #67878, #11722, #51245, #44634, #46068, #56772, #22075, #17964, #6542, #50883, #40525, #11363, #17250, #648, #68244, #33162, #55700, #5094, #67163, #61959, #17607, #40167, #16524, #61593, #10994, #33514, #34603, #5456, #33881, #27996, #50525, #44983, #67520, #56426, #19415, #30155, #13152, #42340, #18688, #58214, #35694, #52689, #69685, #41975, #2095, #24605, #6904, #12796, #30879, #47513, #68966 ),
 ( #47153, #34973, #29435, #13888, #7619, #63410, #70042, #40896, #30524, #52329, #69329, #2811, #19050, #35332, #41608, #63763, #12440, #18323, #24244, #41252, #64127, #13513, #57855, #36060, #1731, #7264, #58580, #36428, #46793, #7988, #29793, #24968, #51972, #53051, #2445, #1371, #64496, #47884, #58942, #8350, #53420, #25339, #70413, #19789, #57502, #23881, #46428, #42703, #33706, #26076, #26445, #59305, #44814, #70773, #71140, #9815, #20513, #31985, #56253, #37523, #67348, #20149, #54158, #9455, #3554, #14615, #53789, #22261, #48615, #54519, #3185, #37886, #43070, #37154, #65596, #3922, #16710, #60044, #14985, #111, #48985, #49351, #5644, #71514, #31624, #4291, #9087, #50708, #60406, #32347, #20890, #54885, #72879, #43444, #8716, #26817, #31248, #65225, #65966, #25712, #15346, #59679, #39266, #61778, #11182, #28180, #22617, #48249, #64863, #14251, #36790, #7445, #18143, #40710, #12622, #57681, #23699, #52151, #17783, #7086, #52512, #56955, #12979, #35516, #466, #11545, #40342, #39991, #46247, #51790, #39631, #12258, #1191, #28891, #68787, #63228, #35157, #68421, #29615, #62149, #17433, #58035, #6359, #62863, #23340, #17071, #28530, #29260, #34427, #1554, #51430, #11902, #5999, #67699, #45536, #24064, #832, #46610, #69153, #18512, #34062, #41077, #34789, #56603, #57322, #51068, #29971, #68065, #45168, #63591, #1922, #22974, #62504, #45889, #6726, #59868, #36972, #69865, #25151, #59495, #65048, #24427, #70594, #14802, #31439, #42157, #47691, #54345, #30700, #70227, #19601, #64684, #8536, #53979, #14069, #36608, #18871, #24788, #42889, #8908, #7809, #35872, #70963, #31065, #25898, #2272, #64315, #19969, #19231, #41433, #53603, #31807, #59129, #2997, #58396, #25525, #48438, #48068, #3377, #42522, #14438, #20336, #46976, #63949, #65412, #37345, #47332, #9272, #52874, #69511, #13705, #8172, #13334, #30346, #41785, #36248, #2629, #58762, #53232, #15528, #60594, #32538, #43995, #9638, #49535, #66150, #32172, #55075, #27730, #43628, #66517, #54705, #16264, #71330, #72422, #49897, #20705, #15897, #39177, #26638, #4832, #72793, #38444, #22176, #72059, #38070, #43263, #33264, #10370, #32900, #66896, #10003, #21438, #4475, #33620, #50268, #44729, #67264, #60970, #55440, #21805, #15166, #16622, #27366, #65784, #61693, #11092, #44369, #3739, #27005, #38819, #61334, #10732, #26264, #48801, #37703, #60224, #55802, #5192, #4110, #49174, #71705, #21077, #62065, #68705, #50623, #51709, #29175, #28, #45806, #18429, #5912, #57233, #52069, #68342, #1474, #51345, #45444, #22534, #12540, #62784, #12176, #46165, #62422, #28804, #39909, #12898, #7003, #23980, #46528, #17702, #34704, #1112, #67617, #69070, #6648, #45081, #40995, #29534, #747, #63511, #34338, #40263, #23619, #18065, #56164, #5558, #28095, #16983, #11821, #40626, #63145, #39540, #11459, #33980, #56519, #35074, #28446, #56872, #57600, #50981, #378, #22886, #67977, #17350, #23256, #6276, #65327, #41705, #8091, #58681, #2550, #19520, #64966, #25069, #47612, #29892, #35791, #53897, #70515, #18788, #46893, #8819, #42078, #36892, #13253, #2193, #30986, #30259, #52431, #64600, #42805, #70142, #13987, #69431, #30621, #59411, #36526, #14357, #59046, #53151, #8450, #57955, #1837, #31356, #53519, #58314, #19891, #63863, #2913, #24707, #19151, #25816, #25444, #7725, #47987, #13618, #35431, #41353, #47251, #64229, #36163, #42444, #52792, #3288, #69784, #48354, #70879, #20253, #7363, #24345, #4394, #15443, #54988, #54259, #4749, #4024, #60882, #50181, #10287, #32817, #55355, #27283, #66435, #21721, #60509, #49816, #22092, #26549, #55716, #5111, #43179, #3655, #9915, #9553, #15813, #21355, #9188, #26923, #43911, #71618, #38355, #72340, #44280, #37987, #66811, #31723, #60144, #27645, #49090, #32453, #66065, #59782, #71241, #71982, #20991, #16183, #43544, #54618, #48719, #37260, #15085, #38734, #49448, #61254, #10648, #33178, #26178, #72709, #44650, #20621, #14718, #65698, #37622, #32087, #67180, #1029, #57149, #23172, #67537, #28363, #50899, #45000, #34991, #299, #28721, #61611, #46085, #73070, #22808, #12098, #45360, #34255, #57520, #39828, #68621, #22451, #56441, #11738, #5831, #16900, #56083, #23535, #67894, #56788, #5475, #40183, #17266, #39455, #62343, #6193, #17983, #51262, #664, #1389, #45726, #51629, #6921, #68261, #33897, #6561, #11378, #51988, #62704, #34619, #17624, #29093, #40542, #63058, #11012, #12460, #33533, #61976, #29451, #28014, #23898, #16541, #39094, #50542, #40915, #36080, #8734, #69349, #47533, #42361, #58601, #64883, #41626, #35712, #12815, #2831, #53070, #2465, #36448, #52708, #19070, #30177, #3204, #70433, #14271, #36809, #8008, #24988, #19435, #57873, #59324, #70061, #63428, #31268, #19808, #64146, #53810, #24625, #30543, #41996, #64516, #46446, #68984, #18341, #35349, #2114, #13909, #58962, #7283, #29812, #52347, #1750, #8370, #18707, #47172, #30898, #53440, #24263, #25359, #46812, #47904, #13533, #69704, #41271, #63783, #13172, #58234, #7639, #9836, #55274, #65985, #37907, #20169, #26096, #44196, #60796, #9106, #37173, #72261, #32365, #27199, #3573, #65615, #21273, #20531, #42723, #54903, #33095, #15365, #60425, #59699, #49003, #49734, #4311, #4669, #49370, #71534, #43461, #48270, #65244, #21638, #20909, #48634, #10201, #54176, #43827, #15004, #9474, #16098, #26836, #71159, #71900, #3941, #25732, #31644, #37541, #32004, #54539, #66351, #43088, #15729, #60063, #26464, #38268, #66727, #32737, #38648, #61172, #10567, #14633, #55634, #70794, #22370, #67812, #50461, #50818, #67097, #10926, #44922, #33453, #16455, #72627, #221, #55997, #67458, #22011, #11299, #27928, #39013, #5390, #16821, #22726, #72988, #39375, #39746, #61894, #28287, #17186, #33819, #56363, #5753, #61528, #62262, #45279, #5027, #27565 ) ),
 .UNSPECIFIED., .F., .F., .T. ) 
 B_SPLINE_SURFACE_WITH_KNOTS ( ( 2, 2 ),
 ( 3, 2, 2, 2, 2, 2, 2, 2, 2, 2, 2, 2, 2, 2, 2, 2, 2, 2, 2, 2, 2, 2, 2, 2, 2, 2, 2, 2, 2, 2, 2, 2, 2, 2, 2, 2, 2, 2, 2, 2, 2, 2, 2, 2, 2, 2, 2, 2, 2, 2, 2, 2, 2, 2, 2, 2, 2, 2, 2, 2, 2, 2, 2, 2, 2, 2, 2, 2, 2, 2, 2, 2, 2, 2, 2, 2, 2, 2, 2, 2, 2, 2, 2, 2, 2, 2, 2, 2, 2, 2, 2, 2, 2, 2, 2, 2, 2, 2, 2, 2, 2, 2, 2, 2, 2, 2, 2, 2, 2, 2, 2, 2, 2, 2, 2, 2, 2, 2, 2, 2, 2, 2, 2, 2, 2, 2, 2, 2, 2, 2, 2, 2, 2, 2, 2, 2, 2, 2, 2, 2, 2, 2, 2, 2, 2, 2, 2, 2, 2, 2, 2, 2, 2, 2, 2, 2, 2, 2, 2, 2, 2, 2, 2, 2, 2, 2, 2, 2, 2, 2, 2, 2, 2, 2, 2, 2, 2, 2, 2, 2, 2, 2, 2, 2, 2, 2, 2, 2, 2, 2, 2, 2, 2, 2, 2, 2, 2, 2, 2, 2, 2, 2, 2, 2, 2, 2, 2, 2, 2, 2, 2, 2, 2, 2, 2, 2, 2, 2, 2, 2, 2, 2, 2, 2, 2, 2, 2, 2, 2, 2, 2, 2, 2, 2, 2, 2, 2, 2, 2, 2, 2, 2, 2, 2, 2, 2, 2, 2, 2, 2, 2, 2, 2, 2, 2, 2, 2, 2, 2, 2, 2, 2, 2, 2, 2, 2, 2, 2, 2, 2, 2, 2, 2, 2, 2, 2, 2, 2, 2, 2, 2, 2, 2, 2, 2, 2, 2, 2, 2, 2, 2, 2, 2, 2, 2, 2, 2, 2, 2, 2, 2, 2, 2, 2, 2, 2, 2, 2, 2, 2, 2, 2, 2, 2, 2, 2, 2, 2, 2, 2, 2, 2, 2, 2, 2, 2, 2, 2, 2, 2, 2, 2, 2, 2, 2, 2, 2, 2, 2, 2, 2, 2, 2, 2, 2, 2, 2, 2, 2, 2, 2, 2, 2, 2, 2, 2, 2, 2, 2, 2, 3 ),
 ( 0.000000000000000000, 1.000000000000000000 ),
 ( 0.000000000000000000, 0.002777777777777777884, 0.005555555555555555768, 0.008333333333333333218, 0.01111111111111111154, 0.01388888888888888812, 0.01666666666666666644, 0.01944444444444444475, 0.02222222222222222307, 0.02500000000000000139, 0.02777777777777777624, 0.03055555555555555455, 0.03333333333333333287, 0.03611111111111110772, 0.03888888888888888951, 0.04166666666666666435, 0.04444444444444444614, 0.04722222222222222099, 0.05000000000000000278, 0.05277777777777777762, 0.05555555555555555247, 0.05833333333333333426, 0.06111111111111110911, 0.06388888888888888395, 0.06666666666666666574, 0.06944444444444444753, 0.07222222222222221544, 0.07499999999999999722, 0.07777777777777777901, 0.08055555555555556080, 0.08333333333333332871, 0.08611111111111111049, 0.08888888888888889228, 0.09166666666666666019, 0.09444444444444444198, 0.09722222222222222376, 0.1000000000000000056, 0.1027777777777777735, 0.1055555555555555552, 0.1083333333333333370, 0.1111111111111111049, 0.1138888888888888867, 0.1166666666666666685, 0.1194444444444444503, 0.1222222222222222182, 0.1250000000000000000, 0.1277777777777777679, 0.1305555555555555636, 0.1333333333333333315, 0.1361111111111110994, 0.1388888888888888951, 0.1416666666666666630, 0.1444444444444444309, 0.1472222222222222265, 0.1499999999999999944, 0.1527777777777777901, 0.1555555555555555580, 0.1583333333333333259, 0.1611111111111111216, 0.1638888888888888895, 0.1666666666666666574, 0.1694444444444444531, 0.1722222222222222210, 0.1749999999999999889, 0.1777777777777777846, 0.1805555555555555525, 0.1833333333333333204, 0.1861111111111111160, 0.1888888888888888840, 0.1916666666666666796, 0.1944444444444444475, 0.1972222222222222154, 0.2000000000000000111, 0.2027777777777777790, 0.2055555555555555469, 0.2083333333333333426, 0.2111111111111111105, 0.2138888888888888784, 0.2166666666666666741, 0.2194444444444444420, 0.2222222222222222099, 0.2250000000000000056, 0.2277777777777777735, 0.2305555555555555691, 0.2333333333333333370, 0.2361111111111111049, 0.2388888888888889006, 0.2416666666666666685, 0.2444444444444444364, 0.2472222222222222321, 0.2500000000000000000, 0.2527777777777777679, 0.2555555555555555358, 0.2583333333333333592, 0.2611111111111111271, 0.2638888888888888951, 0.2666666666666666630, 0.2694444444444444309, 0.2722222222222221988, 0.2750000000000000222, 0.2777777777777777901, 0.2805555555555555580, 0.2833333333333333259, 0.2861111111111110938, 0.2888888888888888618, 0.2916666666666666852, 0.2944444444444444531, 0.2972222222222222210, 0.2999999999999999889, 0.3027777777777777568, 0.3055555555555555802, 0.3083333333333333481, 0.3111111111111111160, 0.3138888888888888840, 0.3166666666666666519, 0.3194444444444444198, 0.3222222222222222432, 0.3250000000000000111, 0.3277777777777777790, 0.3305555555555555469, 0.3333333333333333148, 0.3361111111111111382, 0.3388888888888889062, 0.3416666666666666741, 0.3444444444444444420, 0.3472222222222222099, 0.3499999999999999778, 0.3527777777777778012, 0.3555555555555555691, 0.3583333333333333370, 0.3611111111111111049, 0.3638888888888888729, 0.3666666666666666408, 0.3694444444444444642, 0.3722222222222222321, 0.3750000000000000000, 0.3777777777777777679, 0.3805555555555555358, 0.3833333333333333592, 0.3861111111111111271, 0.3888888888888888951, 0.3916666666666666630, 0.3944444444444444309, 0.3972222222222221988, 0.4000000000000000222, 0.4027777777777777901, 0.4055555555555555580, 0.4083333333333333259, 0.4111111111111110938, 0.4138888888888888618, 0.4166666666666666852, 0.4194444444444444531, 0.4222222222222222210, 0.4249999999999999889, 0.4277777777777777568, 0.4305555555555555802, 0.4333333333333333481, 0.4361111111111111160, 0.4388888888888888840, 0.4416666666666666519, 0.4444444444444444198, 0.4472222222222222432, 0.4500000000000000111, 0.4527777777777777790, 0.4555555555555555469, 0.4583333333333333148, 0.4611111111111111382, 0.4638888888888889062, 0.4666666666666666741, 0.4694444444444444420, 0.4722222222222222099, 0.4749999999999999778, 0.4777777777777778012, 0.4805555555555555691, 0.4833333333333333370, 0.4861111111111111049, 0.4888888888888888729, 0.4916666666666666408, 0.4944444444444444642, 0.4972222222222222321, 0.5000000000000000000, 0.5027777777777777679, 0.5055555555555555358, 0.5083333333333333037, 0.5111111111111110716, 0.5138888888888888395, 0.5166666666666667185, 0.5194444444444444864, 0.5222222222222222543, 0.5250000000000000222, 0.5277777777777777901, 0.5305555555555555580, 0.5333333333333333259, 0.5361111111111110938, 0.5388888888888888618, 0.5416666666666666297, 0.5444444444444443976, 0.5472222222222222765, 0.5500000000000000444, 0.5527777777777778123, 0.5555555555555555802, 0.5583333333333333481, 0.5611111111111111160, 0.5638888888888888840, 0.5666666666666666519, 0.5694444444444444198, 0.5722222222222221877, 0.5749999999999999556, 0.5777777777777777235, 0.5805555555555556024, 0.5833333333333333703, 0.5861111111111111382, 0.5888888888888889062, 0.5916666666666666741, 0.5944444444444444420, 0.5972222222222222099, 0.5999999999999999778, 0.6027777777777777457, 0.6055555555555555136, 0.6083333333333332815, 0.6111111111111111605, 0.6138888888888889284, 0.6166666666666666963, 0.6194444444444444642, 0.6222222222222222321, 0.6250000000000000000, 0.6277777777777777679, 0.6305555555555555358, 0.6333333333333333037, 0.6361111111111110716, 0.6388888888888888395, 0.6416666666666667185, 0.6444444444444444864, 0.6472222222222222543, 0.6500000000000000222, 0.6527777777777777901, 0.6555555555555555580, 0.6583333333333333259, 0.6611111111111110938, 0.6638888888888888618, 0.6666666666666666297, 0.6694444444444443976, 0.6722222222222222765, 0.6750000000000000444, 0.6777777777777778123, 0.6805555555555555802, 0.6833333333333333481, 0.6861111111111111160, 0.6888888888888888840, 0.6916666666666666519, 0.6944444444444444198, 0.6972222222222221877, 0.6999999999999999556, 0.7027777777777777235, 0.7055555555555556024, 0.7083333333333333703, 0.7111111111111111382, 0.7138888888888889062, 0.7166666666666666741, 0.7194444444444444420, 0.7222222222222222099, 0.7249999999999999778, 0.7277777777777777457, 0.7305555555555555136, 0.7333333333333332815, 0.7361111111111111605, 0.7388888888888889284, 0.7416666666666666963, 0.7444444444444444642, 0.7472222222222222321, 0.7500000000000000000, 0.7527777777777777679, 0.7555555555555555358, 0.7583333333333333037, 0.7611111111111110716, 0.7638888888888888395, 0.7666666666666667185, 0.7694444444444444864, 0.7722222222222222543, 0.7750000000000000222, 0.7777777777777777901, 0.7805555555555555580, 0.7833333333333333259, 0.7861111111111110938, 0.7888888888888888618, 0.7916666666666666297, 0.7944444444444443976, 0.7972222222222222765, 0.8000000000000000444, 0.8027777777777778123, 0.8055555555555555802, 0.8083333333333333481, 0.8111111111111111160, 0.8138888888888888840, 0.8166666666666666519, 0.8194444444444444198, 0.8222222222222221877, 0.8249999999999999556, 0.8277777777777777235, 0.8305555555555556024, 0.8333333333333333703, 0.8361111111111111382, 0.8388888888888889062, 0.8416666666666666741, 0.8444444444444444420, 0.8472222222222222099, 0.8499999999999999778, 0.8527777777777777457, 0.8555555555555555136, 0.8583333333333332815, 0.8611111111111111605, 0.8638888888888889284, 0.8666666666666666963, 0.8694444444444444642, 0.8722222222222222321, 0.8750000000000000000, 0.8777777777777777679, 0.8805555555555555358, 0.8833333333333333037, 0.8861111111111110716, 0.8888888888888888395, 0.8916666666666667185, 0.8944444444444444864, 0.8972222222222222543, 0.9000000000000000222, 0.9027777777777777901, 0.9055555555555555580, 0.9083333333333333259, 0.9111111111111110938, 0.9138888888888888618, 0.9166666666666666297, 0.9194444444444443976, 0.9222222222222222765, 0.9250000000000000444, 0.9277777777777778123, 0.9305555555555555802, 0.9333333333333333481, 0.9361111111111111160, 0.9388888888888888840, 0.9416666666666666519, 0.9444444444444444198, 0.9472222222222221877, 0.9499999999999999556, 0.9527777777777777235, 0.9555555555555556024, 0.9583333333333333703, 0.9611111111111111382, 0.9638888888888889062, 0.9666666666666666741, 0.9694444444444444420, 0.9722222222222222099, 0.9749999999999999778, 0.9777777777777777457, 0.9805555555555555136, 0.9833333333333332815, 0.9861111111111111605, 0.9888888888888889284, 0.9916666666666666963, 0.9944444444444444642, 0.9972222222222222321, 1.000000000000000000 ),
 .UNSPECIFIED. ) 
 GEOMETRIC_REPRESENTATION_ITEM ( )  RATIONAL_B_SPLINE_SURFACE ( (
 ( 1.000000000000000000, 0.8660254037844387076, 1.000000000000000000, 0.8660254037844387076, 1.000000000000000000, 0.8660254037844387076, 1.000000000000000000, 0.8660254037844387076, 1.000000000000000000, 0.8660254037844387076, 1.000000000000000000, 0.8660254037844387076, 1.000000000000000000, 0.8660254037844387076, 1.000000000000000000, 0.8660254037844387076, 1.000000000000000000, 0.8660254037844387076, 1.000000000000000000, 0.8660254037844387076, 1.000000000000000000, 0.8660254037844387076, 1.000000000000000000, 0.8660254037844387076, 1.000000000000000000, 0.8660254037844387076, 1.000000000000000000, 0.8660254037844387076, 1.000000000000000000, 0.8660254037844387076, 1.000000000000000000, 0.8660254037844387076, 1.000000000000000000, 0.8660254037844387076, 1.000000000000000000, 0.8660254037844387076, 1.000000000000000000, 0.8660254037844387076, 1.000000000000000000, 0.8660254037844387076, 1.000000000000000000, 0.8660254037844387076, 1.000000000000000000, 0.8660254037844387076, 1.000000000000000000, 0.8660254037844387076, 1.000000000000000000, 0.8660254037844387076, 1.000000000000000000, 0.8660254037844387076, 1.000000000000000000, 0.8660254037844387076, 1.000000000000000000, 0.8660254037844387076, 1.000000000000000000, 0.8660254037844387076, 1.000000000000000000, 0.8660254037844387076, 1.000000000000000000, 0.8660254037844387076, 1.000000000000000000, 0.8660254037844387076, 1.000000000000000000, 0.8660254037844387076, 1.000000000000000000, 0.8660254037844387076, 1.000000000000000000, 0.8660254037844387076, 1.000000000000000000, 0.8660254037844387076, 1.000000000000000000, 0.8660254037844387076, 1.000000000000000000, 0.8660254037844387076, 1.000000000000000000, 0.8660254037844387076, 1.000000000000000000, 0.8660254037844387076, 1.000000000000000000, 0.8660254037844387076, 1.000000000000000000, 0.8660254037844387076, 1.000000000000000000, 0.8660254037844387076, 1.000000000000000000, 0.8660254037844387076, 1.000000000000000000, 0.8660254037844387076, 1.000000000000000000, 0.8660254037844387076, 1.000000000000000000, 0.8660254037844387076, 1.000000000000000000, 0.8660254037844387076, 1.000000000000000000, 0.8660254037844387076, 1.000000000000000000, 0.8660254037844387076, 1.000000000000000000, 0.8660254037844387076, 1.000000000000000000, 0.8660254037844387076, 1.000000000000000000, 0.8660254037844387076, 1.000000000000000000, 0.8660254037844387076, 1.000000000000000000, 0.8660254037844387076, 1.000000000000000000, 0.8660254037844387076, 1.000000000000000000, 0.8660254037844387076, 1.000000000000000000, 0.8660254037844387076, 1.000000000000000000, 0.8660254037844387076, 1.000000000000000000, 0.8660254037844387076, 1.000000000000000000, 0.8660254037844387076, 1.000000000000000000, 0.8660254037844387076, 1.000000000000000000, 0.8660254037844387076, 1.000000000000000000, 0.8660254037844387076, 1.000000000000000000, 0.8660254037844387076, 1.000000000000000000, 0.8660254037844387076, 1.000000000000000000, 0.8660254037844387076, 1.000000000000000000, 0.8660254037844387076, 1.000000000000000000, 0.8660254037844387076, 1.000000000000000000, 0.8660254037844387076, 1.000000000000000000, 0.8660254037844387076, 1.000000000000000000, 0.8660254037844387076, 1.000000000000000000, 0.8660254037844387076, 1.000000000000000000, 0.8660254037844387076, 1.000000000000000000, 0.8660254037844387076, 1.000000000000000000, 0.8660254037844387076, 1.000000000000000000, 0.8660254037844387076, 1.000000000000000000, 0.8660254037844387076, 1.000000000000000000, 0.8660254037844387076, 1.000000000000000000, 0.8660254037844387076, 1.000000000000000000, 0.8660254037844387076, 1.000000000000000000, 0.8660254037844387076, 1.000000000000000000, 0.8660254037844387076, 1.000000000000000000, 0.8660254037844387076, 1.000000000000000000, 0.8660254037844387076, 1.000000000000000000, 0.8660254037844387076, 1.000000000000000000, 0.8660254037844387076, 1.000000000000000000, 0.8660254037844387076, 1.000000000000000000, 0.8660254037844387076, 1.000000000000000000, 0.8660254037844387076, 1.000000000000000000, 0.8660254037844387076, 1.000000000000000000, 0.8660254037844387076, 1.000000000000000000, 0.8660254037844387076, 1.000000000000000000, 0.8660254037844387076, 1.000000000000000000, 0.8660254037844387076, 1.000000000000000000, 0.8660254037844387076, 1.000000000000000000, 0.8660254037844387076, 1.000000000000000000, 0.8660254037844387076, 1.000000000000000000, 0.8660254037844387076, 1.000000000000000000, 0.8660254037844387076, 1.000000000000000000, 0.8660254037844387076, 1.000000000000000000, 0.8660254037844387076, 1.000000000000000000, 0.8660254037844387076, 1.000000000000000000, 0.8660254037844387076, 1.000000000000000000, 0.8660254037844387076, 1.000000000000000000, 0.8660254037844387076, 1.000000000000000000, 0.8660254037844387076, 1.000000000000000000, 0.8660254037844387076, 1.000000000000000000, 0.8660254037844387076, 1.000000000000000000, 0.8660254037844387076, 1.000000000000000000, 0.8660254037844387076, 1.000000000000000000, 0.8660254037844387076, 1.000000000000000000, 0.8660254037844387076, 1.000000000000000000, 0.8660254037844387076, 1.000000000000000000, 0.8660254037844387076, 1.000000000000000000, 0.8660254037844387076, 1.000000000000000000, 0.8660254037844387076, 1.000000000000000000, 0.8660254037844387076, 1.000000000000000000, 0.8660254037844387076, 1.000000000000000000, 0.8660254037844387076, 1.000000000000000000, 0.8660254037844387076, 1.000000000000000000, 0.8660254037844387076, 1.000000000000000000, 0.8660254037844387076, 1.000000000000000000, 0.8660254037844387076, 1.000000000000000000, 0.8660254037844387076, 1.000000000000000000, 0.8660254037844387076, 1.000000000000000000, 0.8660254037844387076, 1.000000000000000000, 0.8660254037844387076, 1.000000000000000000, 0.8660254037844387076, 1.000000000000000000, 0.8660254037844387076, 1.000000000000000000, 0.8660254037844387076, 1.000000000000000000, 0.8660254037844387076, 1.000000000000000000, 0.8660254037844387076, 1.000000000000000000, 0.8660254037844387076, 1.000000000000000000, 0.8660254037844387076, 1.000000000000000000, 0.8660254037844387076, 1.000000000000000000, 0.8660254037844387076, 1.000000000000000000, 0.8660254037844387076, 1.000000000000000000, 0.8660254037844387076, 1.000000000000000000, 0.8660254037844387076, 1.000000000000000000, 0.8660254037844387076, 1.000000000000000000, 0.8660254037844387076, 1.000000000000000000, 0.8660254037844387076, 1.000000000000000000, 0.8660254037844387076, 1.000000000000000000, 0.8660254037844387076, 1.000000000000000000, 0.8660254037844387076, 1.000000000000000000, 0.8660254037844387076, 1.000000000000000000, 0.8660254037844387076, 1.000000000000000000, 0.8660254037844387076, 1.000000000000000000, 0.8660254037844387076, 1.000000000000000000, 0.8660254037844387076, 1.000000000000000000, 0.8660254037844387076, 1.000000000000000000, 0.8660254037844387076, 1.000000000000000000, 0.8660254037844387076, 1.000000000000000000, 0.8660254037844387076, 1.000000000000000000, 0.8660254037844387076, 1.000000000000000000, 0.8660254037844387076, 1.000000000000000000, 0.8660254037844387076, 1.000000000000000000, 0.8660254037844387076, 1.000000000000000000, 0.8660254037844387076, 1.000000000000000000, 0.8660254037844387076, 1.000000000000000000, 0.8660254037844387076, 1.000000000000000000, 0.8660254037844387076, 1.000000000000000000, 0.8660254037844387076, 1.000000000000000000, 0.8660254037844387076, 1.000000000000000000, 0.8660254037844387076, 1.000000000000000000, 0.8660254037844387076, 1.000000000000000000, 0.8660254037844387076, 1.000000000000000000, 0.8660254037844387076, 1.000000000000000000, 0.8660254037844387076, 1.000000000000000000, 0.8660254037844387076, 1.000000000000000000, 0.8660254037844387076, 1.000000000000000000, 0.8660254037844387076, 1.000000000000000000, 0.8660254037844387076, 1.000000000000000000, 0.8660254037844387076, 1.000000000000000000, 0.8660254037844387076, 1.000000000000000000, 0.8660254037844387076, 1.000000000000000000, 0.8660254037844387076, 1.000000000000000000, 0.8660254037844387076, 1.000000000000000000, 0.8660254037844387076, 1.000000000000000000, 0.8660254037844387076, 1.000000000000000000, 0.8660254037844387076, 1.000000000000000000, 0.8660254037844387076, 1.000000000000000000, 0.8660254037844387076, 1.000000000000000000, 0.8660254037844387076, 1.000000000000000000, 0.8660254037844387076, 1.000000000000000000, 0.8660254037844387076, 1.000000000000000000, 0.8660254037844387076, 1.000000000000000000, 0.8660254037844387076, 1.000000000000000000, 0.8660254037844387076, 1.000000000000000000, 0.8660254037844387076, 1.000000000000000000, 0.8660254037844387076, 1.000000000000000000, 0.8660254037844387076, 1.000000000000000000, 0.8660254037844387076, 1.000000000000000000, 0.8660254037844387076, 1.000000000000000000, 0.8660254037844387076, 1.000000000000000000, 0.8660254037844387076, 1.000000000000000000, 0.8660254037844387076, 1.000000000000000000, 0.8660254037844387076, 1.000000000000000000, 0.8660254037844387076, 1.000000000000000000, 0.8660254037844387076, 1.000000000000000000, 0.8660254037844387076, 1.000000000000000000, 0.8660254037844387076, 1.000000000000000000, 0.8660254037844387076, 1.000000000000000000, 0.8660254037844387076, 1.000000000000000000, 0.8660254037844387076, 1.000000000000000000, 0.8660254037844387076, 1.000000000000000000, 0.8660254037844387076, 1.000000000000000000, 0.8660254037844387076, 1.000000000000000000, 0.8660254037844387076, 1.000000000000000000, 0.8660254037844387076, 1.000000000000000000, 0.8660254037844387076, 1.000000000000000000, 0.8660254037844387076, 1.000000000000000000, 0.8660254037844387076, 1.000000000000000000, 0.8660254037844387076, 1.000000000000000000, 0.8660254037844387076, 1.000000000000000000, 0.8660254037844387076, 1.000000000000000000, 0.8660254037844387076, 1.000000000000000000, 0.8660254037844387076, 1.000000000000000000, 0.8660254037844387076, 1.000000000000000000, 0.8660254037844387076, 1.000000000000000000, 0.8660254037844387076, 1.000000000000000000, 0.8660254037844387076, 1.000000000000000000, 0.8660254037844387076, 1.000000000000000000, 0.8660254037844387076, 1.000000000000000000, 0.8660254037844387076, 1.000000000000000000, 0.8660254037844387076, 1.000000000000000000, 0.8660254037844387076, 1.000000000000000000, 0.8660254037844387076, 1.000000000000000000, 0.8660254037844387076, 1.000000000000000000, 0.8660254037844387076, 1.000000000000000000, 0.8660254037844387076, 1.000000000000000000, 0.8660254037844387076, 1.000000000000000000, 0.8660254037844387076, 1.000000000000000000, 0.8660254037844387076, 1.000000000000000000, 0.8660254037844387076, 1.000000000000000000, 0.8660254037844387076, 1.000000000000000000, 0.8660254037844387076, 1.000000000000000000, 0.8660254037844387076, 1.000000000000000000, 0.8660254037844387076, 1.000000000000000000, 0.8660254037844387076, 1.000000000000000000, 0.8660254037844387076, 1.000000000000000000, 0.8660254037844387076, 1.000000000000000000, 0.8660254037844387076, 1.000000000000000000, 0.8660254037844387076, 1.000000000000000000, 0.8660254037844387076, 1.000000000000000000, 0.8660254037844387076, 1.000000000000000000, 0.8660254037844387076, 1.000000000000000000, 0.8660254037844387076, 1.000000000000000000, 0.8660254037844387076, 1.000000000000000000, 0.8660254037844387076, 1.000000000000000000, 0.8660254037844387076, 1.000000000000000000, 0.8660254037844387076, 1.000000000000000000, 0.8660254037844387076, 1.000000000000000000, 0.8660254037844387076, 1.000000000000000000, 0.8660254037844387076, 1.000000000000000000, 0.8660254037844387076, 1.000000000000000000, 0.8660254037844387076, 1.000000000000000000, 0.8660254037844387076, 1.000000000000000000, 0.8660254037844387076, 1.000000000000000000, 0.8660254037844387076, 1.000000000000000000, 0.8660254037844387076, 1.000000000000000000, 0.8660254037844387076, 1.000000000000000000, 0.8660254037844387076, 1.000000000000000000, 0.8660254037844387076, 1.000000000000000000, 0.8660254037844387076, 1.000000000000000000, 0.8660254037844387076, 1.000000000000000000, 0.8660254037844387076, 1.000000000000000000, 0.8660254037844387076, 1.000000000000000000, 0.8660254037844387076, 1.000000000000000000, 0.8660254037844387076, 1.000000000000000000, 0.8660254037844387076, 1.000000000000000000, 0.8660254037844387076, 1.000000000000000000, 0.8660254037844387076, 1.000000000000000000, 0.8660254037844387076, 1.000000000000000000, 0.8660254037844387076, 1.000000000000000000, 0.8660254037844387076, 1.000000000000000000, 0.8660254037844387076, 1.000000000000000000, 0.8660254037844387076, 1.000000000000000000, 0.8660254037844387076, 1.000000000000000000, 0.8660254037844387076, 1.000000000000000000, 0.8660254037844387076, 1.000000000000000000, 0.8660254037844387076, 1.000000000000000000, 0.8660254037844387076, 1.000000000000000000, 0.8660254037844387076, 1.000000000000000000, 0.8660254037844387076, 1.000000000000000000, 0.8660254037844387076, 1.000000000000000000, 0.8660254037844387076, 1.000000000000000000, 0.8660254037844387076, 1.000000000000000000, 0.8660254037844387076, 1.000000000000000000, 0.8660254037844387076, 1.000000000000000000, 0.8660254037844387076, 1.000000000000000000, 0.8660254037844387076, 1.000000000000000000, 0.8660254037844387076, 1.000000000000000000, 0.8660254037844387076, 1.000000000000000000, 0.8660254037844387076, 1.000000000000000000, 0.8660254037844387076, 1.000000000000000000, 0.8660254037844387076, 1.000000000000000000, 0.8660254037844387076, 1.000000000000000000, 0.8660254037844387076, 1.000000000000000000, 0.8660254037844387076, 1.000000000000000000, 0.8660254037844387076, 1.000000000000000000, 0.8660254037844387076, 1.000000000000000000, 0.8660254037844387076, 1.000000000000000000, 0.8660254037844387076, 1.000000000000000000, 0.8660254037844387076, 1.000000000000000000, 0.8660254037844387076, 1.000000000000000000, 0.8660254037844387076, 1.000000000000000000, 0.8660254037844387076, 1.000000000000000000, 0.8660254037844387076, 1.000000000000000000, 0.8660254037844387076, 1.000000000000000000, 0.8660254037844387076, 1.000000000000000000, 0.8660254037844387076, 1.000000000000000000, 0.8660254037844387076, 1.000000000000000000, 0.8660254037844387076, 1.000000000000000000, 0.8660254037844387076, 1.000000000000000000, 0.8660254037844387076, 1.000000000000000000, 0.8660254037844387076, 1.000000000000000000, 0.8660254037844387076, 1.000000000000000000, 0.8660254037844387076, 1.000000000000000000, 0.8660254037844387076, 1.000000000000000000, 0.8660254037844387076, 1.000000000000000000, 0.8660254037844387076, 1.000000000000000000, 0.8660254037844387076, 1.000000000000000000, 0.8660254037844387076, 1.000000000000000000, 0.8660254037844387076, 1.000000000000000000, 0.8660254037844387076, 1.000000000000000000, 0.8660254037844387076, 1.000000000000000000, 0.8660254037844387076, 1.000000000000000000, 0.8660254037844387076, 1.000000000000000000, 0.8660254037844387076, 1.000000000000000000, 0.8660254037844387076, 1.000000000000000000, 0.8660254037844387076, 1.000000000000000000, 0.8660254037844387076, 1.000000000000000000, 0.8660254037844387076, 1.000000000000000000, 0.8660254037844387076, 1.000000000000000000, 0.8660254037844387076, 1.000000000000000000, 0.8660254037844387076, 1.000000000000000000, 0.8660254037844387076, 1.000000000000000000, 0.8660254037844387076, 1.000000000000000000, 0.8660254037844387076, 1.000000000000000000, 0.8660254037844387076, 1.000000000000000000, 0.8660254037844387076, 1.000000000000000000, 0.8660254037844387076, 1.000000000000000000, 0.8660254037844387076, 1.000000000000000000, 0.8660254037844387076, 1.000000000000000000, 0.8660254037844387076, 1.000000000000000000, 0.8660254037844387076, 1.000000000000000000, 0.8660254037844387076, 1.000000000000000000, 0.8660254037844387076, 1.000000000000000000, 0.8660254037844387076, 1.000000000000000000, 0.8660254037844387076, 1.000000000000000000, 0.8660254037844387076, 1.000000000000000000, 0.8660254037844387076, 1.000000000000000000, 0.8660254037844387076, 1.000000000000000000, 0.8660254037844387076, 1.000000000000000000, 0.8660254037844387076, 1.000000000000000000, 0.8660254037844387076, 1.000000000000000000, 0.8660254037844387076, 1.000000000000000000, 0.8660254037844387076, 1.000000000000000000, 0.8660254037844387076, 1.000000000000000000),
 ( 1.000000000000000000, 0.8660254037844387076, 1.000000000000000000, 0.8660254037844387076, 1.000000000000000000, 0.8660254037844387076, 1.000000000000000000, 0.8660254037844387076, 1.000000000000000000, 0.8660254037844387076, 1.000000000000000000, 0.8660254037844387076, 1.000000000000000000, 0.8660254037844387076, 1.000000000000000000, 0.8660254037844387076, 1.000000000000000000, 0.8660254037844387076, 1.000000000000000000, 0.8660254037844387076, 1.000000000000000000, 0.8660254037844387076, 1.000000000000000000, 0.8660254037844387076, 1.000000000000000000, 0.8660254037844387076, 1.000000000000000000, 0.8660254037844387076, 1.000000000000000000, 0.8660254037844387076, 1.000000000000000000, 0.8660254037844387076, 1.000000000000000000, 0.8660254037844387076, 1.000000000000000000, 0.8660254037844387076, 1.000000000000000000, 0.8660254037844387076, 1.000000000000000000, 0.8660254037844387076, 1.000000000000000000, 0.8660254037844387076, 1.000000000000000000, 0.8660254037844387076, 1.000000000000000000, 0.8660254037844387076, 1.000000000000000000, 0.8660254037844387076, 1.000000000000000000, 0.8660254037844387076, 1.000000000000000000, 0.8660254037844387076, 1.000000000000000000, 0.8660254037844387076, 1.000000000000000000, 0.8660254037844387076, 1.000000000000000000, 0.8660254037844387076, 1.000000000000000000, 0.8660254037844387076, 1.000000000000000000, 0.8660254037844387076, 1.000000000000000000, 0.8660254037844387076, 1.000000000000000000, 0.8660254037844387076, 1.000000000000000000, 0.8660254037844387076, 1.000000000000000000, 0.8660254037844387076, 1.000000000000000000, 0.8660254037844387076, 1.000000000000000000, 0.8660254037844387076, 1.000000000000000000, 0.8660254037844387076, 1.000000000000000000, 0.8660254037844387076, 1.000000000000000000, 0.8660254037844387076, 1.000000000000000000, 0.8660254037844387076, 1.000000000000000000, 0.8660254037844387076, 1.000000000000000000, 0.8660254037844387076, 1.000000000000000000, 0.8660254037844387076, 1.000000000000000000, 0.8660254037844387076, 1.000000000000000000, 0.8660254037844387076, 1.000000000000000000, 0.8660254037844387076, 1.000000000000000000, 0.8660254037844387076, 1.000000000000000000, 0.8660254037844387076, 1.000000000000000000, 0.8660254037844387076, 1.000000000000000000, 0.8660254037844387076, 1.000000000000000000, 0.8660254037844387076, 1.000000000000000000, 0.8660254037844387076, 1.000000000000000000, 0.8660254037844387076, 1.000000000000000000, 0.8660254037844387076, 1.000000000000000000, 0.8660254037844387076, 1.000000000000000000, 0.8660254037844387076, 1.000000000000000000, 0.8660254037844387076, 1.000000000000000000, 0.8660254037844387076, 1.000000000000000000, 0.8660254037844387076, 1.000000000000000000, 0.8660254037844387076, 1.000000000000000000, 0.8660254037844387076, 1.000000000000000000, 0.8660254037844387076, 1.000000000000000000, 0.8660254037844387076, 1.000000000000000000, 0.8660254037844387076, 1.000000000000000000, 0.8660254037844387076, 1.000000000000000000, 0.8660254037844387076, 1.000000000000000000, 0.8660254037844387076, 1.000000000000000000, 0.8660254037844387076, 1.000000000000000000, 0.8660254037844387076, 1.000000000000000000, 0.8660254037844387076, 1.000000000000000000, 0.8660254037844387076, 1.000000000000000000, 0.8660254037844387076, 1.000000000000000000, 0.8660254037844387076, 1.000000000000000000, 0.8660254037844387076, 1.000000000000000000, 0.8660254037844387076, 1.000000000000000000, 0.8660254037844387076, 1.000000000000000000, 0.8660254037844387076, 1.000000000000000000, 0.8660254037844387076, 1.000000000000000000, 0.8660254037844387076, 1.000000000000000000, 0.8660254037844387076, 1.000000000000000000, 0.8660254037844387076, 1.000000000000000000, 0.8660254037844387076, 1.000000000000000000, 0.8660254037844387076, 1.000000000000000000, 0.8660254037844387076, 1.000000000000000000, 0.8660254037844387076, 1.000000000000000000, 0.8660254037844387076, 1.000000000000000000, 0.8660254037844387076, 1.000000000000000000, 0.8660254037844387076, 1.000000000000000000, 0.8660254037844387076, 1.000000000000000000, 0.8660254037844387076, 1.000000000000000000, 0.8660254037844387076, 1.000000000000000000, 0.8660254037844387076, 1.000000000000000000, 0.8660254037844387076, 1.000000000000000000, 0.8660254037844387076, 1.000000000000000000, 0.8660254037844387076, 1.000000000000000000, 0.8660254037844387076, 1.000000000000000000, 0.8660254037844387076, 1.000000000000000000, 0.8660254037844387076, 1.000000000000000000, 0.8660254037844387076, 1.000000000000000000, 0.8660254037844387076, 1.000000000000000000, 0.8660254037844387076, 1.000000000000000000, 0.8660254037844387076, 1.000000000000000000, 0.8660254037844387076, 1.000000000000000000, 0.8660254037844387076, 1.000000000000000000, 0.8660254037844387076, 1.000000000000000000, 0.8660254037844387076, 1.000000000000000000, 0.8660254037844387076, 1.000000000000000000, 0.8660254037844387076, 1.000000000000000000, 0.8660254037844387076, 1.000000000000000000, 0.8660254037844387076, 1.000000000000000000, 0.8660254037844387076, 1.000000000000000000, 0.8660254037844387076, 1.000000000000000000, 0.8660254037844387076, 1.000000000000000000, 0.8660254037844387076, 1.000000000000000000, 0.8660254037844387076, 1.000000000000000000, 0.8660254037844387076, 1.000000000000000000, 0.8660254037844387076, 1.000000000000000000, 0.8660254037844387076, 1.000000000000000000, 0.8660254037844387076, 1.000000000000000000, 0.8660254037844387076, 1.000000000000000000, 0.8660254037844387076, 1.000000000000000000, 0.8660254037844387076, 1.000000000000000000, 0.8660254037844387076, 1.000000000000000000, 0.8660254037844387076, 1.000000000000000000, 0.8660254037844387076, 1.000000000000000000, 0.8660254037844387076, 1.000000000000000000, 0.8660254037844387076, 1.000000000000000000, 0.8660254037844387076, 1.000000000000000000, 0.8660254037844387076, 1.000000000000000000, 0.8660254037844387076, 1.000000000000000000, 0.8660254037844387076, 1.000000000000000000, 0.8660254037844387076, 1.000000000000000000, 0.8660254037844387076, 1.000000000000000000, 0.8660254037844387076, 1.000000000000000000, 0.8660254037844387076, 1.000000000000000000, 0.8660254037844387076, 1.000000000000000000, 0.8660254037844387076, 1.000000000000000000, 0.8660254037844387076, 1.000000000000000000, 0.8660254037844387076, 1.000000000000000000, 0.8660254037844387076, 1.000000000000000000, 0.8660254037844387076, 1.000000000000000000, 0.8660254037844387076, 1.000000000000000000, 0.8660254037844387076, 1.000000000000000000, 0.8660254037844387076, 1.000000000000000000, 0.8660254037844387076, 1.000000000000000000, 0.8660254037844387076, 1.000000000000000000, 0.8660254037844387076, 1.000000000000000000, 0.8660254037844387076, 1.000000000000000000, 0.8660254037844387076, 1.000000000000000000, 0.8660254037844387076, 1.000000000000000000, 0.8660254037844387076, 1.000000000000000000, 0.8660254037844387076, 1.000000000000000000, 0.8660254037844387076, 1.000000000000000000, 0.8660254037844387076, 1.000000000000000000, 0.8660254037844387076, 1.000000000000000000, 0.8660254037844387076, 1.000000000000000000, 0.8660254037844387076, 1.000000000000000000, 0.8660254037844387076, 1.000000000000000000, 0.8660254037844387076, 1.000000000000000000, 0.8660254037844387076, 1.000000000000000000, 0.8660254037844387076, 1.000000000000000000, 0.8660254037844387076, 1.000000000000000000, 0.8660254037844387076, 1.000000000000000000, 0.8660254037844387076, 1.000000000000000000, 0.8660254037844387076, 1.000000000000000000, 0.8660254037844387076, 1.000000000000000000, 0.8660254037844387076, 1.000000000000000000, 0.8660254037844387076, 1.000000000000000000, 0.8660254037844387076, 1.000000000000000000, 0.8660254037844387076, 1.000000000000000000, 0.8660254037844387076, 1.000000000000000000, 0.8660254037844387076, 1.000000000000000000, 0.8660254037844387076, 1.000000000000000000, 0.8660254037844387076, 1.000000000000000000, 0.8660254037844387076, 1.000000000000000000, 0.8660254037844387076, 1.000000000000000000, 0.8660254037844387076, 1.000000000000000000, 0.8660254037844387076, 1.000000000000000000, 0.8660254037844387076, 1.000000000000000000, 0.8660254037844387076, 1.000000000000000000, 0.8660254037844387076, 1.000000000000000000, 0.8660254037844387076, 1.000000000000000000, 0.8660254037844387076, 1.000000000000000000, 0.8660254037844387076, 1.000000000000000000, 0.8660254037844387076, 1.000000000000000000, 0.8660254037844387076, 1.000000000000000000, 0.8660254037844387076, 1.000000000000000000, 0.8660254037844387076, 1.000000000000000000, 0.8660254037844387076, 1.000000000000000000, 0.8660254037844387076, 1.000000000000000000, 0.8660254037844387076, 1.000000000000000000, 0.8660254037844387076, 1.000000000000000000, 0.8660254037844387076, 1.000000000000000000, 0.8660254037844387076, 1.000000000000000000, 0.8660254037844387076, 1.000000000000000000, 0.8660254037844387076, 1.000000000000000000, 0.8660254037844387076, 1.000000000000000000, 0.8660254037844387076, 1.000000000000000000, 0.8660254037844387076, 1.000000000000000000, 0.8660254037844387076, 1.000000000000000000, 0.8660254037844387076, 1.000000000000000000, 0.8660254037844387076, 1.000000000000000000, 0.8660254037844387076, 1.000000000000000000, 0.8660254037844387076, 1.000000000000000000, 0.8660254037844387076, 1.000000000000000000, 0.8660254037844387076, 1.000000000000000000, 0.8660254037844387076, 1.000000000000000000, 0.8660254037844387076, 1.000000000000000000, 0.8660254037844387076, 1.000000000000000000, 0.8660254037844387076, 1.000000000000000000, 0.8660254037844387076, 1.000000000000000000, 0.8660254037844387076, 1.000000000000000000, 0.8660254037844387076, 1.000000000000000000, 0.8660254037844387076, 1.000000000000000000, 0.8660254037844387076, 1.000000000000000000, 0.8660254037844387076, 1.000000000000000000, 0.8660254037844387076, 1.000000000000000000, 0.8660254037844387076, 1.000000000000000000, 0.8660254037844387076, 1.000000000000000000, 0.8660254037844387076, 1.000000000000000000, 0.8660254037844387076, 1.000000000000000000, 0.8660254037844387076, 1.000000000000000000, 0.8660254037844387076, 1.000000000000000000, 0.8660254037844387076, 1.000000000000000000, 0.8660254037844387076, 1.000000000000000000, 0.8660254037844387076, 1.000000000000000000, 0.8660254037844387076, 1.000000000000000000, 0.8660254037844387076, 1.000000000000000000, 0.8660254037844387076, 1.000000000000000000, 0.8660254037844387076, 1.000000000000000000, 0.8660254037844387076, 1.000000000000000000, 0.8660254037844387076, 1.000000000000000000, 0.8660254037844387076, 1.000000000000000000, 0.8660254037844387076, 1.000000000000000000, 0.8660254037844387076, 1.000000000000000000, 0.8660254037844387076, 1.000000000000000000, 0.8660254037844387076, 1.000000000000000000, 0.8660254037844387076, 1.000000000000000000, 0.8660254037844387076, 1.000000000000000000, 0.8660254037844387076, 1.000000000000000000, 0.8660254037844387076, 1.000000000000000000, 0.8660254037844387076, 1.000000000000000000, 0.8660254037844387076, 1.000000000000000000, 0.8660254037844387076, 1.000000000000000000, 0.8660254037844387076, 1.000000000000000000, 0.8660254037844387076, 1.000000000000000000, 0.8660254037844387076, 1.000000000000000000, 0.8660254037844387076, 1.000000000000000000, 0.8660254037844387076, 1.000000000000000000, 0.8660254037844387076, 1.000000000000000000, 0.8660254037844387076, 1.000000000000000000, 0.8660254037844387076, 1.000000000000000000, 0.8660254037844387076, 1.000000000000000000, 0.8660254037844387076, 1.000000000000000000, 0.8660254037844387076, 1.000000000000000000, 0.8660254037844387076, 1.000000000000000000, 0.8660254037844387076, 1.000000000000000000, 0.8660254037844387076, 1.000000000000000000, 0.8660254037844387076, 1.000000000000000000, 0.8660254037844387076, 1.000000000000000000, 0.8660254037844387076, 1.000000000000000000, 0.8660254037844387076, 1.000000000000000000, 0.8660254037844387076, 1.000000000000000000, 0.8660254037844387076, 1.000000000000000000, 0.8660254037844387076, 1.000000000000000000, 0.8660254037844387076, 1.000000000000000000, 0.8660254037844387076, 1.000000000000000000, 0.8660254037844387076, 1.000000000000000000, 0.8660254037844387076, 1.000000000000000000, 0.8660254037844387076, 1.000000000000000000, 0.8660254037844387076, 1.000000000000000000, 0.8660254037844387076, 1.000000000000000000, 0.8660254037844387076, 1.000000000000000000, 0.8660254037844387076, 1.000000000000000000, 0.8660254037844387076, 1.000000000000000000, 0.8660254037844387076, 1.000000000000000000, 0.8660254037844387076, 1.000000000000000000, 0.8660254037844387076, 1.000000000000000000, 0.8660254037844387076, 1.000000000000000000, 0.8660254037844387076, 1.000000000000000000, 0.8660254037844387076, 1.000000000000000000, 0.8660254037844387076, 1.000000000000000000, 0.8660254037844387076, 1.000000000000000000, 0.8660254037844387076, 1.000000000000000000, 0.8660254037844387076, 1.000000000000000000, 0.8660254037844387076, 1.000000000000000000, 0.8660254037844387076, 1.000000000000000000, 0.8660254037844387076, 1.000000000000000000, 0.8660254037844387076, 1.000000000000000000, 0.8660254037844387076, 1.000000000000000000, 0.8660254037844387076, 1.000000000000000000, 0.8660254037844387076, 1.000000000000000000, 0.8660254037844387076, 1.000000000000000000, 0.8660254037844387076, 1.000000000000000000, 0.8660254037844387076, 1.000000000000000000, 0.8660254037844387076, 1.000000000000000000, 0.8660254037844387076, 1.000000000000000000, 0.8660254037844387076, 1.000000000000000000, 0.8660254037844387076, 1.000000000000000000, 0.8660254037844387076, 1.000000000000000000, 0.8660254037844387076, 1.000000000000000000, 0.8660254037844387076, 1.000000000000000000, 0.8660254037844387076, 1.000000000000000000, 0.8660254037844387076, 1.000000000000000000, 0.8660254037844387076, 1.000000000000000000, 0.8660254037844387076, 1.000000000000000000, 0.8660254037844387076, 1.000000000000000000, 0.8660254037844387076, 1.000000000000000000, 0.8660254037844387076, 1.000000000000000000, 0.8660254037844387076, 1.000000000000000000, 0.8660254037844387076, 1.000000000000000000, 0.8660254037844387076, 1.000000000000000000, 0.8660254037844387076, 1.000000000000000000, 0.8660254037844387076, 1.000000000000000000, 0.8660254037844387076, 1.000000000000000000, 0.8660254037844387076, 1.000000000000000000, 0.8660254037844387076, 1.000000000000000000, 0.8660254037844387076, 1.000000000000000000, 0.8660254037844387076, 1.000000000000000000, 0.8660254037844387076, 1.000000000000000000, 0.8660254037844387076, 1.000000000000000000, 0.8660254037844387076, 1.000000000000000000, 0.8660254037844387076, 1.000000000000000000, 0.8660254037844387076, 1.000000000000000000, 0.8660254037844387076, 1.000000000000000000, 0.8660254037844387076, 1.000000000000000000, 0.8660254037844387076, 1.000000000000000000, 0.8660254037844387076, 1.000000000000000000, 0.8660254037844387076, 1.000000000000000000, 0.8660254037844387076, 1.000000000000000000, 0.8660254037844387076, 1.000000000000000000, 0.8660254037844387076, 1.000000000000000000, 0.8660254037844387076, 1.000000000000000000, 0.8660254037844387076, 1.000000000000000000, 0.8660254037844387076, 1.000000000000000000, 0.8660254037844387076, 1.000000000000000000, 0.8660254037844387076, 1.000000000000000000, 0.8660254037844387076, 1.000000000000000000, 0.8660254037844387076, 1.000000000000000000, 0.8660254037844387076, 1.000000000000000000, 0.8660254037844387076, 1.000000000000000000, 0.8660254037844387076, 1.000000000000000000, 0.8660254037844387076, 1.000000000000000000, 0.8660254037844387076, 1.000000000000000000, 0.8660254037844387076, 1.000000000000000000, 0.8660254037844387076, 1.000000000000000000, 0.8660254037844387076, 1.000000000000000000, 0.8660254037844387076, 1.000000000000000000, 0.8660254037844387076, 1.000000000000000000, 0.8660254037844387076, 1.000000000000000000, 0.8660254037844387076, 1.000000000000000000, 0.8660254037844387076, 1.000000000000000000, 0.8660254037844387076, 1.000000000000000000, 0.8660254037844387076, 1.000000000000000000, 0.8660254037844387076, 1.000000000000000000, 0.8660254037844387076, 1.000000000000000000, 0.8660254037844387076, 1.000000000000000000, 0.8660254037844387076, 1.000000000000000000, 0.8660254037844387076, 1.000000000000000000) ) ) 
 REPRESENTATION_ITEM ( '' )  SURFACE ( )  );
#16505=CARTESIAN_POINT ( 'NONE',  ( 6.196875000614515905, -3.027376345333610441, -5.243569643749999898 ) ) ;
#16506=CARTESIAN_POINT ( 'NONE',  ( 23.84062500061451928, 6.054752690667223547, 3.707466751127219781E-16 ) ) ;
#16509=CARTESIAN_POINT ( 'NONE',  ( 10.09687500061451715, -3.027376345333614438, 5.243569643749998122 ) ) ;
#16511=CARTESIAN_POINT ( 'NONE',  ( 4.096875000614518925, 6.054752690667223547, 3.707466751127219781E-16 ) ) ;
#16512=CARTESIAN_POINT ( 'NONE',  ( 6.084375000614518747, -4.541064518000419881, 2.621784821874995952 ) ) ;
#16513=CARTESIAN_POINT ( 'NONE',  ( 29.18437500061451573, 6.421520780324663323E-16, -5.243569643749999010 ) ) ;
#16515=CARTESIAN_POINT ( 'NONE',  ( 20.54999999999999716, 0.000000000000000000, 4.999999999999998224 ) ) ;
#16516=ORIENTED_EDGE ( 'NONE', *, *, #21398, .F. ) ;
#16517=CARTESIAN_POINT ( 'NONE',  ( 27.44999999999999929, -4.330127018922190985, -2.500000000000001332 ) ) ;
#16518=CARTESIAN_POINT ( 'NONE',  ( 28.73437500061451644, 6.421520780324663323E-16, -5.243569643749999010 ) ) ;
#16520=ORIENTED_EDGE ( 'NONE', *, *, #36401, .T. ) ;
#16521=CARTESIAN_POINT ( 'NONE',  ( 17.24062500061451786, -3.027376345333614438, 5.243569643749998122 ) ) ;
#16522=CARTESIAN_POINT ( 'NONE',  ( 9.215625000614515727, -6.054752690667223547, -1.112240025338166033E-15 ) ) ;
#16524=CARTESIAN_POINT ( 'NONE',  ( 3.909375000614518481, -4.541064518000417216, -2.621784821875001281 ) ) ;
#16525=CARTESIAN_POINT ( 'NONE',  ( 16.65000000122903501, -2.886751345948129988, 4.999999999999997335 ) ) ;
#16526=LINE ( 'NONE', #10997, #47301 ) ;
#16527=CARTESIAN_POINT ( 'NONE',  ( 7.696875000614516793, 6.054752690667223547, 3.707466751127219781E-16 ) ) ;
#16528=CARTESIAN_POINT ( 'NONE',  ( 11.44687500061451857, -3.027376345333614438, 5.243569643749998122 ) ) ;
#16529=CARTESIAN_POINT ( 'NONE',  ( 22.02187500061452141, 3.027376345333613106, -5.243569643749998122 ) ) ;
#16530=CARTESIAN_POINT ( 'NONE',  ( 4.385796401931335353, -2.400997692794667682, 4.385796401931427724 ) ) ;
#16532=CARTESIAN_POINT ( 'NONE',  ( 4.359375000614517326, -4.541064518000417216, -2.621784821875001281 ) ) ;
#16534=CARTESIAN_POINT ( 'NONE',  ( 7.359375000614516438, 0.000000000000000000, 5.243569643749999010 ) ) ;
#16536=CARTESIAN_POINT ( 'NONE',  ( 21.22500000000000142, 6.123233995736764310E-16, -4.999999999999998224 ) ) ;
#16537=CARTESIAN_POINT ( 'NONE',  ( 18.92812500061451431, 4.541064518000418104, 2.621784821874999949 ) ) ;
#16539=CARTESIAN_POINT ( 'NONE',  ( 4.266506403143407233, 2.607457314201153231, 4.357040118942011375 ) ) ;
#16541=CARTESIAN_POINT ( 'NONE',  ( 8.953125000614518214, 4.541064518000418104, -2.621784821874998173 ) ) ;
#16542=CARTESIAN_POINT ( 'NONE',  ( 29.44687500061451857, -3.027376345333614438, 5.243569643749998122 ) ) ;
#16544=CARTESIAN_POINT ( 'NONE',  ( 29.37187500061451928, 3.027376345333611329, 5.243569643749999010 ) ) ;
#16545=CARTESIAN_POINT ( 'NONE',  ( 10.08749999999999858, 5.773502691896255534, 3.535250795749688894E-16 ) ) ;
#16546=CARTESIAN_POINT ( 'NONE',  ( -2.828200636599751609E-16, 16.40000000122903501, 25.38119784648299770 ) ) ;
#16547=CARTESIAN_POINT ( 'NONE',  ( 9.600000001229034297, -2.886751345948125991, -5.000000000000000000 ) ) ;
#16548=CARTESIAN_POINT ( 'NONE',  ( 19.17187500061451999, -6.054752690667223547, -1.112240025338166033E-15 ) ) ;
#16549=CARTESIAN_POINT ( 'NONE',  ( 13.09687500061451892, 6.054752690667223547, 3.707466751127219781E-16 ) ) ;
#16551=ORIENTED_EDGE ( 'NONE', *, *, #41902, .T. ) ;
#16552=CARTESIAN_POINT ( 'NONE',  ( 15.36562500061451608, 3.027376345333611329, 5.243569643749999010 ) ) ;
#16553=CARTESIAN_POINT ( 'NONE',  ( 25.72500000122903074, -5.773502691896255534, -1.060575238724906372E-15 ) ) ;
#16554=CARTESIAN_POINT ( 'NONE',  ( 15.60937500061451644, -4.541064518000417216, -2.621784821875001281 ) ) ;
#16555=CARTESIAN_POINT ( 'NONE',  ( 5.789369777004289119, 8.154036291478783838, -28.41181880268660009 ) ) ;
#16556=CARTESIAN_POINT ( 'NONE',  ( 18.25312500061451715, -4.541064518000417216, -2.621784821875001281 ) ) ;
#16557=EDGE_CURVE ( 'NONE', #63279, #60995, #7233, .T. ) ;
#16559=CARTESIAN_POINT ( 'NONE',  ( 25.99687500061451928, -3.027376345333610441, -5.243569643749999898 ) ) ;
#16560=CARTESIAN_POINT ( 'NONE',  ( 4.243569643749999898, 10.54062500061451679, 32.45002607614398471 ) ) ;
#16561=CARTESIAN_POINT ( 'NONE',  ( 15.38437500061451679, 4.541064518000418104, 2.621784821874999949 ) ) ;
#16562=CARTESIAN_POINT ( 'NONE',  ( 15.00000000122903465, -2.886751345948125991, -5.000000000000000000 ) ) ;
#16564=CARTESIAN_POINT ( 'NONE',  ( 2.121784821875001281, 18.65937500061451715, -26.32496088578401938 ) ) ;
#16565=CARTESIAN_POINT ( 'NONE',  ( 20.48437500061451289, -4.541064518000419881, 2.621784821874995952 ) ) ;
#16566=CARTESIAN_POINT ( 'NONE',  ( 20.73750000122903359, -4.330127018922194537, 2.499999999999995559 ) ) ;
#16567=CARTESIAN_POINT ( 'NONE',  ( 17.07187500061451502, 3.027376345333613106, -5.243569643749998122 ) ) ;
#16568=CARTESIAN_POINT ( 'NONE',  ( 9.001249775931846008E-16, 12.32187500061451857, 34.90005215228797653 ) ) ;
#16569=CARTESIAN_POINT ( 'NONE',  ( 16.64062500061451289, 6.054752690667223547, 3.707466751127219781E-16 ) ) ;
#16570=ORIENTED_EDGE ( 'NONE', *, *, #8132, .F. ) ;
#16571=ORIENTED_EDGE ( 'NONE', *, *, #13710, .F. ) ;
#16572=CARTESIAN_POINT ( 'NONE',  ( 20.51249999999999929, 2.886751345948126879, 4.999999999999999112 ) ) ;
#16574=CARTESIAN_POINT ( 'NONE',  ( 23.39062500061451289, 6.054752690667223547, 3.707466751127219781E-16 ) ) ;
#16575=CARTESIAN_POINT ( 'NONE',  ( 3.928125000614516527, 6.421520780324663323E-16, -5.243569643749999010 ) ) ;
#16576=CARTESIAN_POINT ( 'NONE',  ( 17.51250000122903216, 0.000000000000000000, 4.999999999999998224 ) ) ;
#16577=CARTESIAN_POINT ( 'NONE',  ( 22.90312500061451573, 4.541064518000418104, -2.621784821874998173 ) ) ;
#16578=CARTESIAN_POINT ( 'NONE',  ( 21.52499999999999858, -4.330127018922194537, 2.499999999999995559 ) ) ;
#16579=CARTESIAN_POINT ( 'NONE',  ( 25.67812500061451431, 4.541064518000418104, 2.621784821874999949 ) ) ;
#16580=CARTESIAN_POINT ( 'NONE',  ( 5.278125000614516615, 6.421520780324663323E-16, -5.243569643749999010 ) ) ;
#16581=ORIENTED_EDGE ( 'NONE', *, *, #58905, .F. ) ;
#16582=CARTESIAN_POINT ( 'NONE',  ( 29.92500000000000071, 4.330127018922191873, 2.499999999999999556 ) ) ;
#16583=CARTESIAN_POINT ( 'NONE',  ( 2.840625000614518392, -3.027376345333614438, 5.243569643749998122 ) ) ;
#16585=CARTESIAN_POINT ( 'NONE',  ( -2.000000000000000000, 11.03750000122903430, 26.53589838486224650 ) ) ;
#16586=CARTESIAN_POINT ( 'NONE',  ( -2.828200636599751609E-16, 11.90000000122903501, -34.61880215351700230 ) ) ;
#16587=CARTESIAN_POINT ( 'NONE',  ( -4.243569643749999898, 19.37187500061451928, -32.45002607614398471 ) ) ;
#16588=CARTESIAN_POINT ( 'NONE',  ( 8.175000000000002487, 6.123233995736764310E-16, -4.999999999999998224 ) ) ;
#16589=CARTESIAN_POINT ( 'NONE',  ( 5.700000001229033941, 5.773502691896255534, 3.535250795749688894E-16 ) ) ;
#16590=CARTESIAN_POINT ( 'NONE',  ( 12.04687500061451821, -3.027376345333610441, -5.243569643749999898 ) ) ;
#16591=CARTESIAN_POINT ( 'NONE',  ( 29.69062500061451715, 6.054752690667223547, 3.707466751127219781E-16 ) ) ;
#16592=CARTESIAN_POINT ( 'NONE',  ( 4.284375000614518925, -4.541064518000419881, 2.621784821874995952 ) ) ;
#16593=CARTESIAN_POINT ( 'NONE',  ( 2.000000000000001332, 18.91250000122903430, 33.46410161513774995 ) ) ;
#16595=CARTESIAN_POINT ( 'NONE',  ( 9.346875000614517148, -3.027376345333610441, -5.243569643749999898 ) ) ;
#16596=CARTESIAN_POINT ( 'NONE',  ( 1.071796769724489895, 14.12990381179669797, -34.00000000000000000 ) ) ;
#16597=CARTESIAN_POINT ( 'NONE',  ( 19.64062500061451644, -3.027376345333610441, -5.243569643749999898 ) ) ;
#16598=CARTESIAN_POINT ( 'NONE',  ( 30.00000000000000000, 6.123233995736764310E-16, -4.999999999999998224 ) ) ;
#16599=CARTESIAN_POINT ( 'NONE',  ( 2.121784821874999061, 18.30312500061459602, 26.32496088578401583 ) ) ;
#16600=CARTESIAN_POINT ( 'NONE',  ( 22.84687500061451715, -3.027376345333610441, -5.243569643749999898 ) ) ;
#16602=CARTESIAN_POINT ( 'NONE',  ( 3.215625000614518836, 3.027376345333611329, 5.243569643749999010 ) ) ;
#16604=CARTESIAN_POINT ( 'NONE',  ( 24.06562500061451715, -6.054752690667223547, -1.112240025338166033E-15 ) ) ;
#16605=CARTESIAN_POINT ( 'NONE',  ( 14.69062500061451537, -3.027376345333610441, -5.243569643749999898 ) ) ;
#16607=CARTESIAN_POINT ( 'NONE',  ( 12.08437500061451608, 6.421520780324663323E-16, -5.243569643749999010 ) ) ;
#16609=CARTESIAN_POINT ( 'NONE',  ( 25.08750000122903145, 4.330127018922191873, 2.499999999999999556 ) ) ;
#16610=CARTESIAN_POINT ( 'NONE',  ( 3.984375000614517326, 6.421520780324663323E-16, -5.243569643749999010 ) ) ;
#16611=CARTESIAN_POINT ( 'NONE',  ( 14.55937500061451573, 0.000000000000000000, 5.243569643749999010 ) ) ;
#16612=CARTESIAN_POINT ( 'NONE',  ( 29.82187500061451502, 3.027376345333611329, 5.243569643749999010 ) ) ;
#16615=CARTESIAN_POINT ( 'NONE',  ( 24.42187500061451999, 3.027376345333611329, 5.243569643749999010 ) ) ;
#16616=CARTESIAN_POINT ( 'NONE',  ( 14.37187500061451928, 3.027376345333613106, -5.243569643749998122 ) ) ;
#16618=CARTESIAN_POINT ( 'NONE',  ( 29.36250000000000071, 2.886751345948129099, -4.999999999999998224 ) ) ;
#16619=CARTESIAN_POINT ( 'NONE',  ( 4.012500001229033053, 0.000000000000000000, 4.999999999999998224 ) ) ;
#16620=CARTESIAN_POINT ( 'NONE',  ( 5.325000000000000178, -4.330127018922194537, 2.499999999999995559 ) ) ;
#16622=CARTESIAN_POINT ( 'NONE',  ( 19.22812500061451502, 6.421520780324663323E-16, -5.243569643749999010 ) ) ;
#16623=CARTESIAN_POINT ( 'NONE',  ( 10.31250000000000355, -5.773502691896255534, -1.060575238724906372E-15 ) ) ;
#16625=CARTESIAN_POINT ( 'NONE',  ( 15.52500000000000036, 4.330127018922191873, 2.499999999999999556 ) ) ;
#16626=CARTESIAN_POINT ( 'NONE',  ( 17.21249999999999858, 2.886751345948129099, -4.999999999999998224 ) ) ;
#16627=CARTESIAN_POINT ( 'NONE',  ( -2.121784821874999949, 11.62812500061451715, 26.32496088578401938 ) ) ;
#16629=CARTESIAN_POINT ( 'NONE',  ( 19.65000000122902790, 5.773502691896255534, 3.535250795749688894E-16 ) ) ;
#16630=CARTESIAN_POINT ( 'NONE',  ( 30.00000000000000000, 6.123233995736764310E-16, -4.999999999999998224 ) ) ;
#16631=CARTESIAN_POINT ( 'NONE',  ( 27.53437500061451360, 4.541064518000418104, 2.621784821874999949 ) ) ;
#16633=CARTESIAN_POINT ( 'NONE',  ( 15.96562500061451573, -6.054752690667223547, -1.112240025338166033E-15 ) ) ;
#16634=CARTESIAN_POINT ( 'NONE',  ( 22.94062500061451715, 6.054752690667223547, 3.707466751127219781E-16 ) ) ;
#16635=CARTESIAN_POINT ( 'NONE',  ( 22.05937500061451573, 4.541064518000418104, -2.621784821874998173 ) ) ;
#16636=CARTESIAN_POINT ( 'NONE',  ( 7.387500000000001066, 5.773502691896255534, 3.535250795749688894E-16 ) ) ;
#16637=CARTESIAN_POINT ( 'NONE',  ( 10.45312500061451644, 0.000000000000000000, 5.243569643749999010 ) ) ;
#16638=CARTESIAN_POINT ( 'NONE',  ( 25.07812500061451644, 6.421520780324663323E-16, -5.243569643749999010 ) ) ;
#16639=CARTESIAN_POINT ( 'NONE',  ( 13.65937500061451715, 0.000000000000000000, 5.243569643749999010 ) ) ;
#16640=CARTESIAN_POINT ( 'NONE',  ( 18.27187500061451431, -6.054752690667223547, -1.112240025338166033E-15 ) ) ;
#16641=DIRECTION ( 'NONE',  ( -1.000000000000000000, -0.000000000000000000, -0.000000000000000000 ) ) ;
#16642=CARTESIAN_POINT ( 'NONE',  ( 4.243569643749999010, 18.71562500061451217, 27.54997392385601174 ) ) ;
#16643=CARTESIAN_POINT ( 'NONE',  ( 20.51250000122903216, 4.330127018922192761, -2.499999999999997780 ) ) ;
#16645=CARTESIAN_POINT ( 'NONE',  ( 11.61562500061451608, 3.027376345333612662, -5.243569643749998122 ) ) ;
#16646=CARTESIAN_POINT ( 'NONE',  ( 5.596875000614516260, -3.027376345333614438, 5.243569643749998122 ) ) ;
#16647=CARTESIAN_POINT ( 'NONE',  ( 6.009375000614519458, 0.000000000000000000, 5.243569643749999010 ) ) ;
#16648=VERTEX_POINT ( 'NONE', #50776 ) ;
#16649=CARTESIAN_POINT ( 'NONE',  ( 26.85937500061451644, -4.541064518000417216, -2.621784821875001281 ) ) ;
#16650=CARTESIAN_POINT ( 'NONE',  ( 18.47812500061451857, 4.541064518000418104, 2.621784821874999949 ) ) ;
#16651=CARTESIAN_POINT ( 'NONE',  ( 3.928125000614516527, 6.421520780324663323E-16, -5.243569643749999010 ) ) ;
#16652=CARTESIAN_POINT ( 'NONE',  ( 27.32812500061451644, 6.421520780324663323E-16, -5.243569643749999010 ) ) ;
#16653=CARTESIAN_POINT ( 'NONE',  ( 23.10937500061451644, 0.000000000000000000, 5.243569643749999010 ) ) ;
#16654=CARTESIAN_POINT ( 'NONE',  ( 20.24062500061451431, 6.054752690667223547, 3.707466751127219781E-16 ) ) ;
#16655=CARTESIAN_POINT ( 'NONE',  ( -4.243569643749999898, 18.92187500061451644, 27.54997392385601529 ) ) ;
#16656=CARTESIAN_POINT ( 'NONE',  ( 24.74062500061451786, 6.054752690667223547, 3.707466751127219781E-16 ) ) ;
#16657=CARTESIAN_POINT ( 'NONE',  ( 5.025000001229035895, -5.773502691896255534, -1.060575238724906372E-15 ) ) ;
#16658=VERTEX_POINT ( 'NONE', #16415 ) ;
#16659=CARTESIAN_POINT ( 'NONE',  ( 27.11249999999999716, 2.886751345948129099, -4.999999999999998224 ) ) ;
#16660=CARTESIAN_POINT ( 'NONE',  ( 2.000000000000001332, 14.75000000000000178, -26.53589838486224650 ) ) ;
#16662=CARTESIAN_POINT ( 'NONE',  ( 5.521875000614517859, 3.027376345333611329, 5.243569643749999010 ) ) ;
#16663=CARTESIAN_POINT ( 'NONE',  ( 12.92812500061451786, 6.421520780324663323E-16, -5.243569643749999010 ) ) ;
#16664=CARTESIAN_POINT ( 'NONE',  ( 6.759375000614516793, 4.541064518000418104, -2.621784821874998173 ) ) ;
#16665=CARTESIAN_POINT ( 'NONE',  ( 23.51250000122903216, -4.330127018922190985, -2.500000000000001332 ) ) ;
#16666=CARTESIAN_POINT ( 'NONE',  ( 15.75937500061451857, 4.541064518000418104, -2.621784821874998173 ) ) ;
#16667=CARTESIAN_POINT ( 'NONE',  ( 29.35312500061451502, 0.000000000000000000, 5.243569643749999010 ) ) ;
#16668=CARTESIAN_POINT ( 'NONE',  ( 27.44999999999999929, -4.330127018922190985, -2.500000000000001332 ) ) ;
#16669=CARTESIAN_POINT ( 'NONE',  ( 26.93437500061451573, 6.421520780324663323E-16, -5.243569643749999010 ) ) ;
#16670=CARTESIAN_POINT ( 'NONE',  ( 3.853125000614517681, -4.541064518000417216, -2.621784821875001281 ) ) ;
#16671=CARTESIAN_POINT ( 'NONE',  ( 12.25312500061451537, 0.000000000000000000, 5.243569643749999010 ) ) ;
#16673=CARTESIAN_POINT ( 'NONE',  ( 9.365625000614519635, 3.027376345333613106, -5.243569643749998122 ) ) ;
#16674=CARTESIAN_POINT ( 'NONE',  ( 6.140625000614516438, -3.027376345333610441, -5.243569643749999898 ) ) ;
#16676=EDGE_CURVE ( 'NONE', #26352, #47876, #49691, .T. ) ;
#16677=DIRECTION ( 'NONE',  ( 0.000000000000000000, 0.000000000000000000, -1.000000000000000000 ) ) ;
#16679=CARTESIAN_POINT ( 'NONE',  ( 15.22500000000000142, -4.330127018922194537, 2.499999999999995559 ) ) ;
#16680=CARTESIAN_POINT ( 'NONE',  ( 15.57187500061451679, -6.054752690667223547, -1.112240025338166033E-15 ) ) ;
#16681=CARTESIAN_POINT ( 'NONE',  ( 12.67500000122903536, -5.773502691896255534, -1.060575238724906372E-15 ) ) ;
#16683=CARTESIAN_POINT ( 'NONE',  ( 21.94687500061451857, -3.027376345333610441, -5.243569643749999898 ) ) ;
#16684=CARTESIAN_POINT ( 'NONE',  ( 2.121784821874999061, 13.80312500061451786, -33.67503911421598417 ) ) ;
#16687=CARTESIAN_POINT ( 'NONE',  ( 20.58749999999999858, -2.886751345948096681, 5.000000000000054179 ) ) ;
#16688=CARTESIAN_POINT ( 'NONE',  ( 25.79062500061451502, -3.027376345333614438, 5.243569643749998122 ) ) ;
#16689=CARTESIAN_POINT ( 'NONE',  ( -3.999999999999999112, 19.51250000000000284, -32.30940107675850470 ) ) ;
#16690=DIRECTION ( 'NONE',  ( 0.000000000000000000, 1.000000000000000000, 0.000000000000000000 ) ) ;
#16691=CARTESIAN_POINT ( 'NONE',  ( 25.57499999999999929, -4.330127018922194537, 2.499999999999995559 ) ) ;
#16692=CARTESIAN_POINT ( 'NONE',  ( 9.140625000614518214, -3.027376345333614438, 5.243569643749998122 ) ) ;
#16694=CARTESIAN_POINT ( 'NONE',  ( 21.49687500061451573, -3.027376345333610441, -5.243569643749999898 ) ) ;
#16696=CARTESIAN_POINT ( 'NONE',  ( 5.765625000614519102, 3.027376345333613106, -5.243569643749998122 ) ) ;
#16697=CARTESIAN_POINT ( 'NONE',  ( 11.25937500061451679, 4.541064518000418104, -2.621784821874998173 ) ) ;
#16698=ORIENTED_EDGE ( 'NONE', *, *, #25145, .F. ) ;
#16699=CARTESIAN_POINT ( 'NONE',  ( 20.85937500061451644, 0.000000000000000000, 5.243569643749999010 ) ) ;
#16700=FACE_OUTER_BOUND ( 'NONE', #45989, .T. ) ;
#16701=CARTESIAN_POINT ( 'NONE',  ( 29.69999999999999574, -4.330127018922190985, -2.500000000000001332 ) ) ;
#16702=EDGE_CURVE ( 'NONE', #71801, #46607, #27091, .T. ) ;
#16703=CARTESIAN_POINT ( 'NONE',  ( 3.937500000000000444, -2.886751345948129988, 4.999999999999997335 ) ) ;
#16704=CARTESIAN_POINT ( 'NONE',  ( 15.71250000122903501, 0.000000000000000000, 4.999999999999998224 ) ) ;
#16706=CARTESIAN_POINT ( 'NONE',  ( -3.999999999999999112, 19.06250000000000000, -32.30940107675850470 ) ) ;
#16709=CARTESIAN_POINT ( 'NONE',  ( 12.78749999999999964, 5.773502691896255534, 3.535250795749688894E-16 ) ) ;
#16710=CARTESIAN_POINT ( 'NONE',  ( 26.95312500061451644, 4.541064518000418104, -2.621784821874998173 ) ) ;
#16711=CARTESIAN_POINT ( 'NONE',  ( 16.31250000000000000, 2.886751345948129099, -4.999999999999998224 ) ) ;
#16712=CARTESIAN_POINT ( 'NONE',  ( 9.525000001229033231, -5.773502691896255534, -1.060575238724906372E-15 ) ) ;
#16713=CARTESIAN_POINT ( 'NONE',  ( 8.428125000614517859, 6.421520780324663323E-16, -5.243569643749999010 ) ) ;
#16715=CARTESIAN_POINT ( 'NONE',  ( 8.474999999999999645, -4.330127018922194537, 2.499999999999995559 ) ) ;
#16716=CARTESIAN_POINT ( 'NONE',  ( -1.071796769724488563, 11.09240381056766545, -26.00000000000000000 ) ) ;
#16717=CARTESIAN_POINT ( 'NONE',  ( 2.121784821874999061, 14.30937500061451750, -33.67503911421598417 ) ) ;
#16718=CARTESIAN_POINT ( 'NONE',  ( 28.08750000122903145, 6.123233995736764310E-16, -4.999999999999998224 ) ) ;
#16720=CARTESIAN_POINT ( 'NONE',  ( 8.324999999999999289, 4.330127018922191873, 2.499999999999999556 ) ) ;
#16721=CARTESIAN_POINT ( 'NONE',  ( 0.000000000000000000, 20.00000000000000000, 26.00000000000000000 ) ) ;
#16722=ORIENTED_EDGE ( 'NONE', *, *, #19527, .F. ) ;
#16723=CARTESIAN_POINT ( 'NONE',  ( 23.95312500061451289, 0.000000000000000000, 5.243569643749999010 ) ) ;
#16724=FACE_OUTER_BOUND ( 'NONE', #45975, .T. ) ;
#16725=CARTESIAN_POINT ( 'NONE',  ( 14.58750000122903323, 6.123233995736764310E-16, -4.999999999999998224 ) ) ;
#16726=CARTESIAN_POINT ( 'NONE',  ( 22.28437500061451715, -4.541064518000419881, 2.621784821874995952 ) ) ;
#16727=CARTESIAN_POINT ( 'NONE',  ( 15.55312500061451608, -4.541064518000417216, -2.621784821875001281 ) ) ;
#16728=CARTESIAN_POINT ( 'NONE',  ( 4.243569643749999898, 10.54062500061459318, -27.54997392385601529 ) ) ;
#16729=CARTESIAN_POINT ( 'NONE',  ( 6.703125000614516438, 4.541064518000418104, -2.621784821874998173 ) ) ;
#16730=CARTESIAN_POINT ( 'NONE',  ( 27.93750000122903288, -4.330127018922194537, 2.499999999999995559 ) ) ;
#16732=CARTESIAN_POINT ( 'NONE',  ( 19.64062500061451644, -3.027376345333610441, -5.243569643749999898 ) ) ;
#16735=CARTESIAN_POINT ( 'NONE',  ( 13.69687500061451679, -3.027376345333614438, 5.243569643749998122 ) ) ;
#16736=CARTESIAN_POINT ( 'NONE',  ( 13.47187500061451537, 3.027376345333613106, -5.243569643749998122 ) ) ;
#16737=CARTESIAN_POINT ( 'NONE',  ( 22.28437500061451715, -4.541064518000419881, 2.621784821874995952 ) ) ;
#16738=VERTEX_POINT ( 'NONE', #21229 ) ;
#16740=CARTESIAN_POINT ( 'NONE',  ( 26.09062500061451573, 6.054752690667223547, 3.707466751127219781E-16 ) ) ;
#16741=CARTESIAN_POINT ( 'NONE',  ( 27.47812500061451502, 4.541064518000418104, 2.621784821874999949 ) ) ;
#16743=CARTESIAN_POINT ( 'NONE',  ( 2.000000000000001332, 17.44999999999999929, 33.46410161513774995 ) ) ;
#16744=CARTESIAN_POINT ( 'NONE',  ( 5.034375000614519813, 4.541064518000418104, 2.621784821874999949 ) ) ;
#16745=CARTESIAN_POINT ( 'NONE',  ( 13.01250000122903394, 0.000000000000000000, 4.999999999999998224 ) ) ;
#16746=CARTESIAN_POINT ( 'NONE',  ( 6.075000001229034829, 2.886751345948129099, -4.999999999999998224 ) ) ;
#16747=CARTESIAN_POINT ( 'NONE',  ( 28.80000000122903003, -2.886751345948129988, 4.999999999999997335 ) ) ;
#16750=CARTESIAN_POINT ( 'NONE',  ( 10.77187500061451786, 3.027376345333613106, -5.243569643749998122 ) ) ;
#16752=ORIENTED_EDGE ( 'NONE', *, *, #68046, .T. ) ;
#16753=CARTESIAN_POINT ( 'NONE',  ( 20.12812500061451715, 6.421520780324663323E-16, -5.243569643749999010 ) ) ;
#16754=CARTESIAN_POINT ( 'NONE',  ( 13.73437500061451821, -4.541064518000419881, 2.621784821874995952 ) ) ;
#16755=CARTESIAN_POINT ( 'NONE',  ( 4.153125000614515727, 0.000000000000000000, 5.243569643749999010 ) ) ;
#16756=CARTESIAN_POINT ( 'NONE',  ( 22.13437500061451502, 4.541064518000418104, 2.621784821874999949 ) ) ;
#16757=CARTESIAN_POINT ( 'NONE',  ( 10.13437500061451679, -4.541064518000419881, 2.621784821874995952 ) ) ;
#16758=CARTESIAN_POINT ( 'NONE',  ( 4.153125000614515727, 0.000000000000000000, 5.243569643749999010 ) ) ;
#16760=CARTESIAN_POINT ( 'NONE',  ( 5.962500001229033231, -4.330127018922190985, -2.500000000000001332 ) ) ;
#16761=CARTESIAN_POINT ( 'NONE',  ( 20.87812500061451715, -4.541064518000419881, 2.621784821874995952 ) ) ;
#16762=CARTESIAN_POINT ( 'NONE',  ( 8.700000001229032165, -2.886751345948125991, -5.000000000000000000 ) ) ;
#16763=CARTESIAN_POINT ( 'NONE',  ( 17.84062500061451573, -3.027376345333610441, -5.243569643749999898 ) ) ;
#16764=CARTESIAN_POINT ( 'NONE',  ( 16.15312500061451573, 4.541064518000418104, -2.621784821874998173 ) ) ;
#16766=CARTESIAN_POINT ( 'NONE',  ( 15.15000000000000036, 0.000000000000000000, 4.999999999999998224 ) ) ;
#16767=CARTESIAN_POINT ( 'NONE',  ( 8.362500001229031810, 4.330127018922192761, -2.499999999999997780 ) ) ;
#16768=CARTESIAN_POINT ( 'NONE',  ( 5.353125000614515905, 4.541064518000418104, -2.621784821874998173 ) ) ;
#16770=CARTESIAN_POINT ( 'NONE',  ( 19.87500000122903288, -5.773502691896255534, -1.060575238724906372E-15 ) ) ;
#16772=CARTESIAN_POINT ( 'NONE',  ( -4.243569643749997233, 9.996875000614517504, -27.54997392385601174 ) ) ;
#16773=CARTESIAN_POINT ( 'NONE',  ( 5.000000000000000888, 2.882564675336284927E-11, 5.151554443534156036 ) ) ;
#16775=CARTESIAN_POINT ( 'NONE',  ( 3.534375000614518036, 6.421520780324663323E-16, -5.243569643749999010 ) ) ;
#16776=CARTESIAN_POINT ( 'NONE',  ( 20.67187500061451289, 3.027376345333613106, -5.243569643749998122 ) ) ;
#16778=CARTESIAN_POINT ( 'NONE',  ( 17.31562500061451715, -6.054752690667223547, -1.112240025338166033E-15 ) ) ;
#16781=CARTESIAN_POINT ( 'NONE',  ( 26.81250000000000355, 2.886751345948135317, 4.999999999999984013 ) ) ;
#16782=CARTESIAN_POINT ( 'NONE',  ( 28.02187500061451431, 3.027376345333611329, 5.243569643749999010 ) ) ;
#16784=CARTESIAN_POINT ( 'NONE',  ( 13.60312500061451679, 0.000000000000000000, 5.243569643749999010 ) ) ;
#16785=CARTESIAN_POINT ( 'NONE',  ( 10.54687500061451644, -3.027376345333614438, 5.243569643749998122 ) ) ;
#16787=CARTESIAN_POINT ( 'NONE',  ( -2.000000000000000000, 14.07500000000000107, -33.46410161513775705 ) ) ;
#16788=CARTESIAN_POINT ( 'NONE',  ( 23.20312500061451644, -4.541064518000417216, -2.621784821875001281 ) ) ;
#16789=CARTESIAN_POINT ( 'NONE',  ( 17.51250000122903216, 0.000000000000000000, 4.999999999999998224 ) ) ;
#16790=CARTESIAN_POINT ( 'NONE',  ( 20.92500000000000071, 4.330127018922191873, 2.499999999999999556 ) ) ;
#16791=EDGE_CURVE ( 'NONE', #16738, #48333, #18211, .T. ) ;
#16792=CARTESIAN_POINT ( 'NONE',  ( 11.32500000000000107, 6.123233995736764310E-16, -4.999999999999998224 ) ) ;
#16793=CARTESIAN_POINT ( 'NONE',  ( 22.95000000122903216, -2.886751345948129988, 4.999999999999997335 ) ) ;
#16794=CARTESIAN_POINT ( 'NONE',  ( 17.20312500061451644, 0.000000000000000000, 5.243569643749999010 ) ) ;
#16797=CARTESIAN_POINT ( 'NONE',  ( 19.91250000000000142, 2.886751345948129099, -4.999999999999998224 ) ) ;
#16798=CARTESIAN_POINT ( 'NONE',  ( 24.97499999999999787, 4.330127018922191873, 2.499999999999999556 ) ) ;
#16799=CARTESIAN_POINT ( 'NONE',  ( 20.29687500061451644, 6.054752690667223547, 3.707466751127219781E-16 ) ) ;
#16800=CARTESIAN_POINT ( 'NONE',  ( 28.19062500061451715, -3.027376345333610441, -5.243569643749999898 ) ) ;
#16801=EDGE_CURVE ( 'NONE', #36412, #38182, #59644, .T. ) ;
#16802=EDGE_LOOP ( 'NONE', ( #62939, #37394, #44312, #42136 ) ) ;
#16804=CARTESIAN_POINT ( 'NONE',  ( 8.915625000614515017, 3.027376345333613106, -5.243569643749998122 ) ) ;
#16806=CARTESIAN_POINT ( 'NONE',  ( 15.22500000000000142, -4.330127018922194537, 2.499999999999995559 ) ) ;
#16807=CARTESIAN_POINT ( 'NONE',  ( -2.121784821874996840, 19.42812500061451786, 33.67503911421598417 ) ) ;
#16808=CARTESIAN_POINT ( 'NONE',  ( 4.921875000614518214, 3.027376345333613106, -5.243569643749998122 ) ) ;
#16809=CARTESIAN_POINT ( 'NONE',  ( 28.99687500061451573, -3.027376345333614438, 5.243569643749998122 ) ) ;
#16811=CARTESIAN_POINT ( 'NONE',  ( 23.61562500061451431, -6.054752690667223547, -1.112240025338166033E-15 ) ) ;
#16812=CARTESIAN_POINT ( 'NONE',  ( 25.77187500061451075, 3.027376345333611329, 5.243569643749999010 ) ) ;
#16813=CARTESIAN_POINT ( 'NONE',  ( 9.001249775931846008E-16, 18.11562500061459602, -25.09994784771203058 ) ) ;
#16814=CARTESIAN_POINT ( 'NONE',  ( 11.84999999999999964, 4.330127018922192761, -2.499999999999997780 ) ) ;
#16815=CARTESIAN_POINT ( 'NONE',  ( 9.965625000614517504, 3.027376345333611329, 5.243569643749999010 ) ) ;
#16816=CARTESIAN_POINT ( 'NONE',  ( 6.037500000000001421, 5.773502691896255534, 3.535250795749688401E-16 ) ) ;
#16817=CYLINDRICAL_SURFACE ( 'NONE', #45497, 5.999999999999998224 ) ;
#16818=CARTESIAN_POINT ( 'NONE',  ( 27.32812500061451644, 6.421520780324663323E-16, -5.243569643749999010 ) ) ;
#16819=FACE_OUTER_BOUND ( 'NONE', #11227, .T. ) ;
#16821=CARTESIAN_POINT ( 'NONE',  ( 3.365625000614516082, -6.054752690667223547, -1.112240025338166033E-15 ) ) ;
#16822=CARTESIAN_POINT ( 'NONE',  ( 19.88437500061451857, 4.541064518000418104, 2.621784821874999949 ) ) ;
#16823=CARTESIAN_POINT ( 'NONE',  ( 2.121784821874999061, 14.30937500061451750, 26.32496088578401583 ) ) ;
#16824=CARTESIAN_POINT ( 'NONE',  ( 21.49687500061451573, -3.027376345333610441, -5.243569643749999898 ) ) ;
#16825=CARTESIAN_POINT ( 'NONE',  ( 29.03437500061451715, -4.541064518000419881, 2.621784821874995952 ) ) ;
#16826=CARTESIAN_POINT ( 'NONE',  ( -3.000416591977282496E-16, 18.84687500061451360, 25.09994784771203058 ) ) ;
#16827=CARTESIAN_POINT ( 'NONE',  ( 10.04062500061451502, -3.027376345333614438, 5.243569643749998122 ) ) ;
#16828=CARTESIAN_POINT ( 'NONE',  ( 2.775000001229033675, -5.773502691896255534, -1.060575238724906372E-15 ) ) ;
#16829=VECTOR ( 'NONE', #49151, 1000.000000000000000 ) ;
#16830=CARTESIAN_POINT ( 'NONE',  ( 8.034375000614518925, 6.421520780324663323E-16, -5.243569643749999010 ) ) ;
#16831=CARTESIAN_POINT ( 'NONE',  ( 1.626862140677534273E-15, 16.17500000122903359, -26.00000000000000355 ) ) ;
#16832=CARTESIAN_POINT ( 'NONE',  ( 8.240625000614516082, -3.027376345333614438, 5.243569643749998122 ) ) ;
#16833=CARTESIAN_POINT ( 'NONE',  ( 12.72187500061451537, 3.027376345333611329, 5.243569643749999010 ) ) ;
#16834=CARTESIAN_POINT ( 'NONE',  ( 18.86250000122903359, 0.000000000000000000, 4.999999999999998224 ) ) ;
#16835=CARTESIAN_POINT ( 'NONE',  ( 8.859375000614518214, -4.541064518000417216, -2.621784821875001281 ) ) ;
#16836=CARTESIAN_POINT ( 'NONE',  ( 10.00312500061451715, 0.000000000000000000, 5.243569643749999010 ) ) ;
#16837=CARTESIAN_POINT ( 'NONE',  ( 5.578125000614518214, -4.541064518000419881, 2.621784821874995952 ) ) ;
#16839=CARTESIAN_POINT ( 'NONE',  ( 18.94687500061451502, 6.054752690667223547, 3.707466751127219781E-16 ) ) ;
#16840=CARTESIAN_POINT ( 'NONE',  ( 17.39999999999999858, 0.000000000000000000, 4.999999999999998224 ) ) ;
#16841=CARTESIAN_POINT ( 'NONE',  ( 27.21562500061451928, -6.054752690667223547, -1.112240025338166033E-15 ) ) ;
#16842=CARTESIAN_POINT ( 'NONE',  ( 11.01562500061451821, -6.054752690667223547, -1.112240025338166033E-15 ) ) ;
#16843=CARTESIAN_POINT ( 'NONE',  ( 28.58437500061451786, -4.541064518000419881, 2.621784821874995952 ) ) ;
#16844=CARTESIAN_POINT ( 'NONE',  ( 2.121784821874999061, 11.60937500061451821, -33.67503911421598417 ) ) ;
#16845=CARTESIAN_POINT ( 'NONE',  ( 13.57500000122903572, -5.773502691896255534, -1.060575238724906372E-15 ) ) ;
#16846=CARTESIAN_POINT ( 'NONE',  ( 27.96562500061451928, 3.027376345333611329, 5.243569643749999010 ) ) ;
#16847=CARTESIAN_POINT ( 'NONE',  ( 9.001249775931846008E-16, 14.96562500061451750, -25.09994784771203058 ) ) ;
#16848=CARTESIAN_POINT ( 'NONE',  ( 14.73750000122903359, 4.330127018922191873, 2.499999999999999556 ) ) ;
#16849=CARTESIAN_POINT ( 'NONE',  ( 12.33750000000000036, 5.773502691896255534, 3.535250795749688894E-16 ) ) ;
#16850=CARTESIAN_POINT ( 'NONE',  ( -5.810221930991193690E-16, 13.58750000000000036, 26.00000000000000355 ) ) ;
#16851=CARTESIAN_POINT ( 'NONE',  ( 23.05312500061451431, 0.000000000000000000, 5.243569643749999010 ) ) ;
#16852=CARTESIAN_POINT ( 'NONE',  ( 6.609375000614519102, -4.541064518000417216, -2.621784821875001281 ) ) ;
#16853=CARTESIAN_POINT ( 'NONE',  ( 8.925000001229033586, 2.886751345948126879, 4.999999999999999112 ) ) ;
#16854=CARTESIAN_POINT ( 'NONE',  ( 16.57500000122903216, 2.886751345948126879, 4.999999999999999112 ) ) ;
#16855=CARTESIAN_POINT ( 'NONE',  ( 11.99062500061451608, -3.027376345333610441, -5.243569643749999898 ) ) ;
#16856=CARTESIAN_POINT ( 'NONE',  ( 17.46562500061451217, 3.027376345333613106, -5.243569643749998122 ) ) ;
#16857=CARTESIAN_POINT ( 'NONE',  ( 24.71250000122903145, 0.000000000000000000, 4.999999999999998224 ) ) ;
#16858=CARTESIAN_POINT ( 'NONE',  ( 28.27500000122903145, 2.886751345948126879, 4.999999999999999112 ) ) ;
#16859=CARTESIAN_POINT ( 'NONE',  ( 23.62500000000000000, 4.330127018922191873, 2.499999999999999556 ) ) ;
#16860=CARTESIAN_POINT ( 'NONE',  ( 24.60937500061451644, -4.541064518000417216, -2.621784821875001281 ) ) ;
#16861=DIRECTION ( 'NONE',  ( -1.000000000000000000, -0.000000000000000000, -0.000000000000000000 ) ) ;
#16862=CARTESIAN_POINT ( 'NONE',  ( 10.27500000122903323, 2.886751345948126879, 4.999999999999999112 ) ) ;
#16863=CARTESIAN_POINT ( 'NONE',  ( 28.80937500061451573, 4.541064518000418104, -2.621784821874998173 ) ) ;
#16865=CARTESIAN_POINT ( 'NONE',  ( 4.921875000614518214, 3.027376345333613106, -5.243569643749998122 ) ) ;
#16866=CARTESIAN_POINT ( 'NONE',  ( 22.82812500061451644, 6.421520780324663323E-16, -5.243569643749999010 ) ) ;
#16869=CARTESIAN_POINT ( 'NONE',  ( 10.47187500061451715, 3.027376345333611329, 5.243569643749999010 ) ) ;
#16870=B_SPLINE_CURVE_WITH_KNOTS ( 'NONE', 3,
 ( #21370, #61992, #55370, #15827, #27296, #28028, #50556, #38371, #50198, #21735, #60524, #28377, #72723, #33548, #66450, #22106, #32469, #44296, #9930, #16555, #60896, #4408, #26937, #61623, #11026, #4763, #49830, #72354, #45015, #67551, #11392, #33912, #56455, #5845, #51276, #70348, #12477, #52003, #53354, #8655, #17281, #8291, #14190, #40197, #58881, #28735 ),
 .UNSPECIFIED., .F., .F.,
 ( 4, 2, 2, 2, 2, 2, 2, 2, 2, 2, 2, 2, 2, 2, 2, 2, 2, 2, 2, 2, 2, 2, 4 ),
 ( 0.01924954336552996484, 0.02045024950336954417, 0.02105060257228933210, 0.02165095564120912003, 0.02225130871012891143, 0.02285166177904869936, 0.02405236791688827175, 0.02525307405472784761, 0.02645378019256742000, 0.02705413326148721140, 0.02765448633040700280, 0.02825483939932679073, 0.02885519246824658213, 0.03005589860608615452, 0.03125660474392572691, 0.03245731088176529583, 0.03365801701960486475, 0.03485872315744444061, 0.03545907622636421813, 0.03605942929528400259, 0.03726013543312356457, 0.03786048850204334210, 0.03846084157096311962 ),
 .UNSPECIFIED. ) ;
#16871=CARTESIAN_POINT ( 'NONE',  ( 4.898587196589411843E-16, 20.00000000000000000, -26.00000000000000000 ) ) ;
#16872=CARTESIAN_POINT ( 'NONE',  ( 3.796875000614517326, -3.027376345333614438, 5.243569643749998122 ) ) ;
#16873=CARTESIAN_POINT ( 'NONE',  ( 6.721875000614518925, 3.027376345333613106, -5.243569643749998122 ) ) ;
#16874=CARTESIAN_POINT ( 'NONE',  ( 27.49687500061451217, 6.054752690667223547, 3.707466751127219781E-16 ) ) ;
#16875=CARTESIAN_POINT ( 'NONE',  ( 4.243569643749999898, 10.09062500061459566, 32.45002607614398471 ) ) ;
#16876=CARTESIAN_POINT ( 'NONE',  ( 18.82500000000000284, -4.330127018922194537, 2.499999999999995559 ) ) ;
#16878=CARTESIAN_POINT ( 'NONE',  ( 26.09999999999999787, -4.330127018922190985, -2.500000000000001332 ) ) ;
#16879=CARTESIAN_POINT ( 'NONE',  ( 27.53437500061451360, 4.541064518000418104, 2.621784821874999949 ) ) ;
#16880=EDGE_CURVE ( 'NONE', #9370, #26592, #34626, .T. ) ;
#16881=VERTEX_POINT ( 'NONE', #68489 ) ;
#16882=CARTESIAN_POINT ( 'NONE',  ( 14.31562500061451537, 3.027376345333613106, -5.243569643749998122 ) ) ;
#16883=CARTESIAN_POINT ( 'NONE',  ( 7.190625000614518036, 6.054752690667223547, 3.707466751127219781E-16 ) ) ;
#16885=CARTESIAN_POINT ( 'NONE',  ( 4.921875000614518214, 3.027376345333613106, -5.243569643749998122 ) ) ;
#16886=CARTESIAN_POINT ( 'NONE',  ( 18.33750000122903501, 4.330127018922191873, 2.499999999999999556 ) ) ;
#16887=CARTESIAN_POINT ( 'NONE',  ( 25.19999999999999929, -4.330127018922190985, -2.500000000000001332 ) ) ;
#16888=CARTESIAN_POINT ( 'NONE',  ( 15.82499999999999929, 6.123233995736764310E-16, -4.999999999999998224 ) ) ;
#16889=CARTESIAN_POINT ( 'NONE',  ( 8.221875000614518925, 3.027376345333611329, 5.243569643749999010 ) ) ;
#16890=CARTESIAN_POINT ( 'NONE',  ( 11.14687500061451608, -3.027376345333610441, -5.243569643749999898 ) ) ;
#16891=CARTESIAN_POINT ( 'NONE',  ( 22.13437500061451502, 4.541064518000418104, 2.621784821874999949 ) ) ;
#16892=VERTEX_POINT ( 'NONE', #68136 ) ;
#16893=CARTESIAN_POINT ( 'NONE',  ( 5.296875000614518214, -3.027376345333610441, -5.243569643749999898 ) ) ;
#16894=CARTESIAN_POINT ( 'NONE',  ( 6.459375000614518747, 0.000000000000000000, 5.243569643749999010 ) ) ;
#16895=CARTESIAN_POINT ( 'NONE',  ( 17.58749999999999858, -2.886751345948125991, -5.000000000000000000 ) ) ;
#16896=CARTESIAN_POINT ( 'NONE',  ( 16.86562500061451786, -6.054752690667223547, -1.112240025338166033E-15 ) ) ;
#16900=CARTESIAN_POINT ( 'NONE',  ( 10.30312500061451431, 4.541064518000418104, -2.621784821874998173 ) ) ;
#16901=CARTESIAN_POINT ( 'NONE',  ( 27.53437500061451360, 4.541064518000418104, 2.621784821874999949 ) ) ;
#16903=CARTESIAN_POINT ( 'NONE',  ( 28.39687500061452141, 6.054752690667223547, 3.707466751127219781E-16 ) ) ;
#16904=CARTESIAN_POINT ( 'NONE',  ( 11.10000000000000142, 0.000000000000000000, 4.999999999999998224 ) ) ;
#16905=CARTESIAN_POINT ( 'NONE',  ( 4.000000000000000000, 16.70000000122903572, 32.30940107675849049 ) ) ;
#16906=CARTESIAN_POINT ( 'NONE',  ( 10.27500000122903323, 2.886751345948126879, 4.999999999999999112 ) ) ;
#16907=CARTESIAN_POINT ( 'NONE',  ( 20.14687500061451786, -3.027376345333610441, -5.243569643749999898 ) ) ;
#16908=CARTESIAN_POINT ( 'NONE',  ( 15.08437500061451786, -4.541064518000419881, 2.621784821874995952 ) ) ;
#16910=ORIENTED_EDGE ( 'NONE', *, *, #380, .F. ) ;
#16911=CARTESIAN_POINT ( 'NONE',  ( 13.75312500061451715, -4.541064518000417216, -2.621784821875001281 ) ) ;
#16912=CARTESIAN_POINT ( 'NONE',  ( 27.45000000122903572, -2.886751345948129988, 4.999999999999997335 ) ) ;
#16913=CARTESIAN_POINT ( 'NONE',  ( 15.53437500061451715, -4.541064518000419881, 2.621784821874995952 ) ) ;
#16914=CARTESIAN_POINT ( 'NONE',  ( 3.478125000614517237, 6.421520780324663323E-16, -5.243569643749999010 ) ) ;
#16915=CARTESIAN_POINT ( 'NONE',  ( 15.89062500061451289, -3.027376345333614438, 5.243569643749998122 ) ) ;
#16917=CARTESIAN_POINT ( 'NONE',  ( 25.62187500061451573, 3.027376345333613106, -5.243569643749998122 ) ) ;
#16918=CARTESIAN_POINT ( 'NONE',  ( -4.243569643749997233, 9.940625000614515372, 32.45002607614398471 ) ) ;
#16919=CARTESIAN_POINT ( 'NONE',  ( 15.75937500061451857, 4.541064518000418104, -2.621784821874998173 ) ) ;
#16920=( BOUNDED_CURVE ( )  B_SPLINE_CURVE ( 2, ( #9338, #2698, #42222, #25213, #3063, #47760, #19668, #58827, #30408 ),
 .UNSPECIFIED., .F., .F. ) 
 B_SPLINE_CURVE_WITH_KNOTS ( ( 3, 2, 2, 2, 3 ),
 ( 0.4456521739130435145, 0.4492753623188405765, 0.4565217391304347561, 0.4637681159420289911, 0.4673913043478261087 ),
 .UNSPECIFIED. ) 
 CURVE ( )  GEOMETRIC_REPRESENTATION_ITEM ( )  RATIONAL_B_SPLINE_CURVE ( ( 0.9330127018922194093, 0.9330127018922198534, 1.000000000000000000, 0.8660254037844387076, 1.000000000000000000, 0.8660254037844387076, 1.000000000000000000, 0.9330127018922188542, 0.9330127018922194093 ) ) 
 REPRESENTATION_ITEM ( '' )  );
#16921=CARTESIAN_POINT ( 'NONE',  ( 14.51250000122903394, -4.330127018922190985, -2.500000000000001332 ) ) ;
#16922=DIRECTION ( 'NONE',  ( -1.000000000000000000, -0.000000000000000000, -0.000000000000000000 ) ) ;
#16923=CARTESIAN_POINT ( 'NONE',  ( 0.000000000000000000, 20.00000000000000000, 30.00000000000000000 ) ) ;
#16924=CARTESIAN_POINT ( 'NONE',  ( 17.14687500061451786, 6.054752690667223547, 3.707466751127219781E-16 ) ) ;
#16925=CARTESIAN_POINT ( 'NONE',  ( 19.83750000122903145, -4.330127018922194537, 2.499999999999995559 ) ) ;
#16926=( BOUNDED_CURVE ( )  B_SPLINE_CURVE ( 2, ( #44165, #50065, #49338, #21242, #72595, #27531, #43794 ),
 .UNSPECIFIED., .F., .F. ) 
 B_SPLINE_CURVE_WITH_KNOTS ( ( 3, 2, 2, 3 ),
 ( 0.03333333333333339532, 0.03611111111111116323, 0.03888888888888894502, 0.04166666666666671293 ),
 .UNSPECIFIED. ) 
 CURVE ( )  GEOMETRIC_REPRESENTATION_ITEM ( )  RATIONAL_B_SPLINE_CURVE ( ( 0.9999999999999968914, 0.8660254037844417052, 1.000000000000000000, 0.8660254037844387076, 1.000000000000000000, 0.8660254037844363761, 1.000000000000002442 ) ) 
 REPRESENTATION_ITEM ( '' )  );
#16927=CARTESIAN_POINT ( 'NONE',  ( 13.65937500061451715, 0.000000000000000000, 5.243569643749999010 ) ) ;
#16928=CARTESIAN_POINT ( 'NONE',  ( 2.121784821875001281, 12.80937500061451928, 33.67503911421598417 ) ) ;
#16929=CARTESIAN_POINT ( 'NONE',  ( 22.20000000122903216, -2.886751345948125991, -5.000000000000000000 ) ) ;
#16930=CARTESIAN_POINT ( 'NONE',  ( 18.51562500061451289, 3.027376345333611329, 5.243569643749999010 ) ) ;
#16931=ORIENTED_EDGE ( 'NONE', *, *, #67466, .F. ) ;
#16932=ORIENTED_EDGE ( 'NONE', *, *, #21809, .T. ) ;
#16933=CARTESIAN_POINT ( 'NONE',  ( 21.52499999999999858, -4.330127018922194537, 2.499999999999995559 ) ) ;
#16935=CARTESIAN_POINT ( 'NONE',  ( 21.62812500061451360, 4.541064518000418104, 2.621784821874999949 ) ) ;
#16936=CARTESIAN_POINT ( 'NONE',  ( 3.963750086740946088, 3.047826611959361554, 29.44540702803496401 ) ) ;
#16937=CARTESIAN_POINT ( 'NONE',  ( 13.98750000122903359, -4.330127018922194537, 2.499999999999995559 ) ) ;
#16938=CARTESIAN_POINT ( 'NONE',  ( 21.10312500061451502, 4.541064518000418104, -2.621784821874998173 ) ) ;
#16939=CARTESIAN_POINT ( 'NONE',  ( 24.36562500061451786, 3.027376345333611329, 5.243569643749999010 ) ) ;
#16940=CARTESIAN_POINT ( 'NONE',  ( 4.978125000614518569, 4.541064518000418104, 2.621784821874999949 ) ) ;
#16941=EDGE_LOOP ( 'NONE', ( #36634, #63049, #21750, #41465 ) ) ;
#16942=ADVANCED_FACE ( 'NONE', ( #1987 ), #11972, .F. ) ;
#16943=( BOUNDED_CURVE ( )  B_SPLINE_CURVE ( 3, ( #31871, #20404, #71397, #66583 ),
 .UNSPECIFIED., .F., .F. ) 
 B_SPLINE_CURVE_WITH_KNOTS ( ( 4, 4 ),
 ( 3.903471329280879143, 3.934893574429339846 ),
 .UNSPECIFIED. ) 
 CURVE ( )  GEOMETRIC_REPRESENTATION_ITEM ( )  RATIONAL_B_SPLINE_CURVE ( ( 1.000000000000000000, 0.9999177219016296414, 0.9999177219016296414, 1.000000000000000000 ) ) 
 REPRESENTATION_ITEM ( '' )  );
#16944=CARTESIAN_POINT ( 'NONE',  ( -3.999999999999999112, 10.21250000122903501, -30.00000000000000000 ) ) ;
#16945=EDGE_CURVE ( 'NONE', #70308, #37144, #29328, .T. ) ;
#16948=CARTESIAN_POINT ( 'NONE',  ( -1.999999999999997113, 10.28750000122903430, -26.53589838486224295 ) ) ;
#16949=CARTESIAN_POINT ( 'NONE',  ( -4.243569643749999898, 17.57187500061451502, -32.45002607614398471 ) ) ;
#16950=CARTESIAN_POINT ( 'NONE',  ( 6.712500001229034119, 0.000000000000000000, 4.999999999999998224 ) ) ;
#16951=CARTESIAN_POINT ( 'NONE',  ( 7.237500000000000711, -2.886751345948125991, -5.000000000000000000 ) ) ;
#16952=EDGE_CURVE ( 'NONE', #42898, #69508, #44591, .T. ) ;
#16953=CARTESIAN_POINT ( 'NONE',  ( 3.825000001229032609, 2.886751345948129099, -4.999999999999998224 ) ) ;
#16954=CARTESIAN_POINT ( 'NONE',  ( 11.40937500061451892, 0.000000000000000000, 5.243569643749999010 ) ) ;
#16956=CARTESIAN_POINT ( 'NONE',  ( 4.246875000614519280, -3.027376345333614438, 5.243569643749998122 ) ) ;
#16957=CARTESIAN_POINT ( 'NONE',  ( 3.881554241669678884, -3.151751365348489653, -4.190642664303462439 ) ) ;
#16958=EDGE_CURVE ( 'NONE', #66380, #15804, #51502, .T. ) ;
#16959=CARTESIAN_POINT ( 'NONE',  ( 10.65937500061451715, -4.541064518000417216, -2.621784821875001281 ) ) ;
#16960=CARTESIAN_POINT ( 'NONE',  ( 3.999999999999999112, 14.03750000122903430, -30.00000000000000000 ) ) ;
#16961=CARTESIAN_POINT ( 'NONE',  ( 1.999999999999998668, 14.45000000000000107, 26.53589838486224650 ) ) ;
#16962=CARTESIAN_POINT ( 'NONE',  ( 2.121784821874999061, 16.95312500061459815, 26.32496088578401583 ) ) ;
#16963=CARTESIAN_POINT ( 'NONE',  ( 20.44687500061451857, -3.027376345333614438, 5.243569643749998122 ) ) ;
#16964=CARTESIAN_POINT ( 'NONE',  ( 3.065625000614517592, 3.027376345333613106, -5.243569643749998122 ) ) ;
#16966=CARTESIAN_POINT ( 'NONE',  ( 25.79062500061451502, -3.027376345333614438, 5.243569643749998122 ) ) ;
#16967=CARTESIAN_POINT ( 'NONE',  ( 16.67812500061451786, 4.541064518000418104, 2.621784821874999949 ) ) ;
#16969=CARTESIAN_POINT ( 'NONE',  ( 12.19687500061451679, 6.054752690667223547, 3.707466751127219781E-16 ) ) ;
#16970=CARTESIAN_POINT ( 'NONE',  ( 29.47499999999999787, 4.330127018922191873, 2.499999999999999556 ) ) ;
#16971=CARTESIAN_POINT ( 'NONE',  ( 25.83750000122903501, 6.123233995736764310E-16, -4.999999999999998224 ) ) ;
#16972=CARTESIAN_POINT ( 'NONE',  ( 4.396875000614516971, -3.027376345333610441, -5.243569643749999898 ) ) ;
#16973=CARTESIAN_POINT ( 'NONE',  ( 14.37187500061451928, 3.027376345333613106, -5.243569643749998122 ) ) ;
#16975=CARTESIAN_POINT ( 'NONE',  ( 3.242103837493086330E-14, 11.33750000000000213, 26.00000000000000711 ) ) ;
#16977=CARTESIAN_POINT ( 'NONE',  ( 23.52187500061451786, 3.027376345333611329, 5.243569643749999010 ) ) ;
#16978=CARTESIAN_POINT ( 'NONE',  ( 14.44687500061451679, 6.054752690667223547, 3.707466751127219781E-16 ) ) ;
#16980=CARTESIAN_POINT ( 'NONE',  ( 27.29999999999999716, 0.000000000000000000, 4.999999999999998224 ) ) ;
#16981=DIRECTION ( 'NONE',  ( -0.000000000000000000, -1.000000000000000000, -0.000000000000000000 ) ) ;
#16983=CARTESIAN_POINT ( 'NONE',  ( 16.75312500061451715, 0.000000000000000000, 5.243569643749999010 ) ) ;
#16984=CARTESIAN_POINT ( 'NONE',  ( 7.537500000000002309, -2.886751345948129988, 4.999999999999997335 ) ) ;
#16986=CARTESIAN_POINT ( 'NONE',  ( 15.93750000000000000, 5.773502691896255534, 3.535250795749688894E-16 ) ) ;
#16987=CARTESIAN_POINT ( 'NONE',  ( -4.243569643749999898, 12.11562500061451608, 27.54997392385601529 ) ) ;
#16989=CARTESIAN_POINT ( 'NONE',  ( 20.21250000122903145, 0.000000000000000000, 4.999999999999998224 ) ) ;
#16991=CARTESIAN_POINT ( 'NONE',  ( 28.02187500061451431, 3.027376345333611329, 5.243569643749999010 ) ) ;
#16993=CARTESIAN_POINT ( 'NONE',  ( 21.85312500061451502, -4.541064518000417216, -2.621784821875001281 ) ) ;
#16994=CARTESIAN_POINT ( 'NONE',  ( 22.35937500061451644, -4.541064518000417216, -2.621784821875001281 ) ) ;
#16995=B_SPLINE_CURVE_WITH_KNOTS ( 'NONE', 3,
 ( #14611, #60040, #9451, #31981, #47509, #36424, #26441, #64492, #30520, #69681 ),
 .UNSPECIFIED., .F., .F.,
 ( 4, 3, 3, 4 ),
 ( 1.664927911480095392E-16, 2.812505234851141628E-05, 5.777440207181503025E-05, 8.742424744633160846E-05 ),
 .UNSPECIFIED. ) ;
#16996=CARTESIAN_POINT ( 'NONE',  ( 6.075000000000000178, 4.330127018922191873, 2.499999999999999556 ) ) ;
#16997=CARTESIAN_POINT ( 'NONE',  ( 9.890625000614516438, 6.054752690667223547, 3.707466751127219781E-16 ) ) ;
#16998=CARTESIAN_POINT ( 'NONE',  ( 23.65312500061451573, -4.541064518000417216, -2.621784821875001281 ) ) ;
#16999=CARTESIAN_POINT ( 'NONE',  ( 13.58437500061451786, 4.541064518000418104, 2.621784821874999949 ) ) ;
#17000=CARTESIAN_POINT ( 'NONE',  ( 17.63437500061451502, 4.541064518000418104, 2.621784821874999949 ) ) ;
#17001=CARTESIAN_POINT ( 'NONE',  ( 19.42499999999999716, 6.123233995736764310E-16, -4.999999999999998224 ) ) ;
#17002=CARTESIAN_POINT ( 'NONE',  ( 4.243569643749999898, 18.64062500061451644, 32.45002607614398471 ) ) ;
#17003=CARTESIAN_POINT ( 'NONE',  ( 20.47500000122903074, 2.886751345948129099, -4.999999999999998224 ) ) ;
#17005=CARTESIAN_POINT ( 'NONE',  ( 13.04062500061451502, 6.054752690667223547, 3.707466751127219781E-16 ) ) ;
#17006=CARTESIAN_POINT ( 'NONE',  ( 5.784375000614517148, 6.421520780324663323E-16, -5.243569643749999010 ) ) ;
#17007=CARTESIAN_POINT ( 'NONE',  ( 3.684375000614518836, 4.541064518000418104, 2.621784821874999949 ) ) ;
#17008=ORIENTED_EDGE ( 'NONE', *, *, #19932, .F. ) ;
#17009=CARTESIAN_POINT ( 'NONE',  ( 28.65937500061451715, -4.541064518000417216, -2.621784821875001281 ) ) ;
#17010=CARTESIAN_POINT ( 'NONE',  ( 16.41562500061451857, -6.054752690667223547, -1.112240025338166033E-15 ) ) ;
#17011=CARTESIAN_POINT ( 'NONE',  ( 27.11250000122903359, -4.330127018922190985, -2.500000000000001332 ) ) ;
#17012=CARTESIAN_POINT ( 'NONE',  ( 28.90312500061451217, 0.000000000000000000, 5.243569643749999010 ) ) ;
#17013=CARTESIAN_POINT ( 'NONE',  ( 21.42187500061451644, -6.054752690667223547, -1.112240025338166033E-15 ) ) ;
#17014=CARTESIAN_POINT ( 'NONE',  ( 16.94062500061451715, -3.027376345333610441, -5.243569643749999898 ) ) ;
#17015=CARTESIAN_POINT ( 'NONE',  ( 4.000000000000000000, 10.28750000000000142, 32.30940107675849049 ) ) ;
#17016=CARTESIAN_POINT ( 'NONE',  ( 24.59062500061451573, -3.027376345333610441, -5.243569643749999898 ) ) ;
#17017=CARTESIAN_POINT ( 'NONE',  ( 4.537500001229034297, -4.330127018922194537, 2.499999999999995559 ) ) ;
#17019=CARTESIAN_POINT ( 'NONE',  ( 26.66250000000000142, 2.886751345948129099, -4.999999999999998224 ) ) ;
#17020=CARTESIAN_POINT ( 'NONE',  ( -1.999999999999997113, 11.97500000000000142, -26.53589838486224295 ) ) ;
#17022=CARTESIAN_POINT ( 'NONE',  ( 5.034375000614519813, 4.541064518000418104, 2.621784821874999949 ) ) ;
#17023=CARTESIAN_POINT ( 'NONE',  ( 10.45312500061451644, 0.000000000000000000, 5.243569643749999010 ) ) ;
#17024=CARTESIAN_POINT ( 'NONE',  ( 7.321875000614516793, 3.027376345333611329, 5.243569643749999010 ) ) ;
#17025=CARTESIAN_POINT ( 'NONE',  ( 25.42500000122903359, 2.886751345948129099, -4.999999999999998224 ) ) ;
#17026=CARTESIAN_POINT ( 'NONE',  ( 12.94687500061451857, -3.027376345333610441, -5.243569643749999898 ) ) ;
#17027=CARTESIAN_POINT ( 'NONE',  ( 3.684375000614518836, 4.541064518000418104, 2.621784821874999949 ) ) ;
#17028=CARTESIAN_POINT ( 'NONE',  ( 26.66250000000000142, 2.886751345948129099, -4.999999999999998224 ) ) ;
#17029=CARTESIAN_POINT ( 'NONE',  ( 14.81250000122903288, 0.000000000000000000, 4.999999999999998224 ) ) ;
#17030=CARTESIAN_POINT ( 'NONE',  ( 13.49062500061451608, 6.054752690667223547, 3.707466751127219781E-16 ) ) ;
#17033=CARTESIAN_POINT ( 'NONE',  ( 10.15312500061451750, -4.541064518000417216, -2.621784821875001281 ) ) ;
#17035=CARTESIAN_POINT ( 'NONE',  ( 4.978125000614518569, 4.541064518000418104, 2.621784821874999949 ) ) ;
#17038=CYLINDRICAL_SURFACE ( 'NONE', #45630, 4.999999999999998224 ) ;
#17039=CARTESIAN_POINT ( 'NONE',  ( 15.33750000000000036, -2.886751345948125991, -5.000000000000000000 ) ) ;
#17041=CARTESIAN_POINT ( 'NONE',  ( 16.69687500061451502, 6.054752690667223547, 3.707466751127219781E-16 ) ) ;
#17042=CARTESIAN_POINT ( 'NONE',  ( 11.40000000122903501, -2.886751345948125991, -5.000000000000000000 ) ) ;
#17043=CARTESIAN_POINT ( 'NONE',  ( 19.43437500061451928, 4.541064518000418104, 2.621784821874999949 ) ) ;
#17045=CARTESIAN_POINT ( 'NONE',  ( 21.53437500061451715, 6.421520780324663323E-16, -5.243569643749999010 ) ) ;
#17046=CARTESIAN_POINT ( 'NONE',  ( -4.243569643749997233, 13.54062500061451679, -27.54997392385601174 ) ) ;
#17047=VECTOR ( 'NONE', #24318, 1000.000000000000000 ) ;
#17048=CARTESIAN_POINT ( 'NONE',  ( 7.387500000000001954, 5.773502691896255534, 3.535250795749688401E-16 ) ) ;
#17050=CARTESIAN_POINT ( 'NONE',  ( 4.126442089077904107, 2.823557275049659143, 4.418432631982811110 ) ) ;
#17051=CARTESIAN_POINT ( 'NONE',  ( 26.61562500061451786, 3.027376345333611329, 5.243569643749999010 ) ) ;
#17053=CARTESIAN_POINT ( 'NONE',  ( 29.70937500061451431, 4.541064518000418104, -2.621784821874998173 ) ) ;
#17054=CARTESIAN_POINT ( 'NONE',  ( 24.86250000000000071, 2.886751345948129099, -4.999999999999998224 ) ) ;
#17055=CARTESIAN_POINT ( 'NONE',  ( 8.315625000614515372, -6.054752690667223547, -1.112240025338166033E-15 ) ) ;
#17057=CARTESIAN_POINT ( 'NONE',  ( 19.28437500061451360, 6.421520780324663323E-16, -5.243569643749999010 ) ) ;
#17059=CARTESIAN_POINT ( 'NONE',  ( 5.503125000614516260, 0.000000000000000000, 5.243569643749999010 ) ) ;
#17060=CARTESIAN_POINT ( 'NONE',  ( 9.984375000614518214, 4.541064518000418104, 2.621784821874999949 ) ) ;
#17061=ORIENTED_EDGE ( 'NONE', *, *, #17352, .F. ) ;
#17062=CARTESIAN_POINT ( 'NONE',  ( 20.52187500061451786, -6.054752690667223547, -1.112240025338166033E-15 ) ) ;
#17065=CARTESIAN_POINT ( 'NONE',  ( 5.175000000000002487, 4.330127018922191873, 2.499999999999999556 ) ) ;
#17066=ADVANCED_FACE ( 'NONE', ( #64018 ), #26667, .T. ) ;
#17067=CARTESIAN_POINT ( 'NONE',  ( 15.18750000122903465, 4.330127018922191873, 2.499999999999999556 ) ) ;
#17070=CARTESIAN_POINT ( 'NONE',  ( 11.92500000000000071, 4.330127018922191873, 2.499999999999999556 ) ) ;
#17071=CARTESIAN_POINT ( 'NONE',  ( 24.36562500061451786, 3.027376345333611329, 5.243569643749999010 ) ) ;
#17072=CARTESIAN_POINT ( 'NONE',  ( 16.08749999999999503, -2.886751345948129988, 4.999999999999997335 ) ) ;
#17073=CARTESIAN_POINT ( 'NONE',  ( 10.46250000122903323, -4.330127018922190985, -2.500000000000001332 ) ) ;
#17074=CARTESIAN_POINT ( 'NONE',  ( 9.140625000614518214, -3.027376345333614438, 5.243569643749998122 ) ) ;
#17075=CARTESIAN_POINT ( 'NONE',  ( 8.925000000000002487, -4.330127018922194537, 2.499999999999995559 ) ) ;
#17076=DIRECTION ( 'NONE',  ( -1.000000000000000000, -0.000000000000000000, -0.000000000000000000 ) ) ;
#17077=CARTESIAN_POINT ( 'NONE',  ( -4.243569643749999898, 13.97187500061451715, -32.45002607614398471 ) ) ;
#17078=CARTESIAN_POINT ( 'NONE',  ( 26.92500000122903359, 2.886751345948126879, 4.999999999999999112 ) ) ;
#17080=CARTESIAN_POINT ( 'NONE',  ( 7.087499999999999467, -2.886751345948129988, 4.999999999999997335 ) ) ;
#17082=ORIENTED_EDGE ( 'NONE', *, *, #16407, .T. ) ;
#17083=CARTESIAN_POINT ( 'NONE',  ( 23.42812500061451786, 4.541064518000418104, 2.621784821874999949 ) ) ;
#17084=CARTESIAN_POINT ( 'NONE',  ( 14.92500000122903181, -5.773502691896255534, -1.060575238724906372E-15 ) ) ;
#17085=CARTESIAN_POINT ( 'NONE',  ( 28.82812500061451644, 4.541064518000418104, 2.621784821874999949 ) ) ;
#17086=CARTESIAN_POINT ( 'NONE',  ( 28.92187500061451644, 3.027376345333611329, 5.243569643749999010 ) ) ;
#17087=CARTESIAN_POINT ( 'NONE',  ( 18.34687500061451715, -3.027376345333610441, -5.243569643749999898 ) ) ;
#17088=CARTESIAN_POINT ( 'NONE',  ( 16.79062500061451857, -3.027376345333614438, 5.243569643749998122 ) ) ;
#17089=CARTESIAN_POINT ( 'NONE',  ( -4.243569643749998122, 11.29062500061459495, -27.54997392385601174 ) ) ;
#17090=CARTESIAN_POINT ( 'NONE',  ( 6.553125000614518747, -4.541064518000417216, -2.621784821875001281 ) ) ;
#17091=AXIS2_PLACEMENT_3D ( 'NONE', #40349, #45541, #29266 ) ;
#17092=CARTESIAN_POINT ( 'NONE',  ( 27.86250000122903359, 0.000000000000000000, 4.999999999999998224 ) ) ;
#17094=CARTESIAN_POINT ( 'NONE',  ( 19.04062500061451146, -3.027376345333614438, 5.243569643749998122 ) ) ;
#17095=CARTESIAN_POINT ( 'NONE',  ( -5.810221930991193690E-16, 10.10000000122903430, 26.00000000000000355 ) ) ;
#17097=CARTESIAN_POINT ( 'NONE',  ( 13.24687500061451750, -3.027376345333614438, 5.243569643749998122 ) ) ;
#17098=CARTESIAN_POINT ( 'NONE',  ( 11.03437500061451715, -4.541064518000419881, 2.621784821874995952 ) ) ;
#17099=CARTESIAN_POINT ( 'NONE',  ( 19.62187500061451573, -6.054752690667223547, -1.112240025338166033E-15 ) ) ;
#17100=VERTEX_POINT ( 'NONE', #16251 ) ;
#17102=CARTESIAN_POINT ( 'NONE',  ( 27.21562500061451928, -6.054752690667223547, -1.112240025338166033E-15 ) ) ;
#17103=CARTESIAN_POINT ( 'NONE',  ( 25.19062500061451715, 6.054752690667223547, 3.707466751127219781E-16 ) ) ;
#17104=DIRECTION ( 'NONE',  ( -1.000000000000000000, -0.000000000000000000, -0.000000000000000000 ) ) ;
#17105=CARTESIAN_POINT ( 'NONE',  ( -3.999999999999999112, 17.30000000000000071, 30.00000000000000000 ) ) ;
#17106=CARTESIAN_POINT ( 'NONE',  ( 4.959375000614516971, 4.541064518000418104, -2.621784821874998173 ) ) ;
#17107=CARTESIAN_POINT ( 'NONE',  ( 11.85000000122903430, -2.886751345948125991, -5.000000000000000000 ) ) ;
#17109=CARTESIAN_POINT ( 'NONE',  ( 6.300000001229033586, -2.886751345948129988, 4.999999999999997335 ) ) ;
#17111=CARTESIAN_POINT ( 'NONE',  ( 28.42500000122904069, -5.773502691896255534, -1.060575238724906372E-15 ) ) ;
#17114=CARTESIAN_POINT ( 'NONE',  ( 11.25937500061451679, 4.541064518000418104, -2.621784821874998173 ) ) ;
#17115=CARTESIAN_POINT ( 'NONE',  ( 30.00000000000000000, 6.123233995736764310E-16, -4.999999999999998224 ) ) ;
#17116=CARTESIAN_POINT ( 'NONE',  ( 17.80312500061451786, -4.541064518000417216, -2.621784821875001281 ) ) ;
#17117=CARTESIAN_POINT ( 'NONE',  ( 13.69687500061451679, -3.027376345333614438, 5.243569643749998122 ) ) ;
#17118=CARTESIAN_POINT ( 'NONE',  ( 4.865625000614517859, 3.027376345333613106, -5.243569643749998122 ) ) ;
#17119=CARTESIAN_POINT ( 'NONE',  ( 22.39687500061451075, -3.027376345333610441, -5.243569643749999898 ) ) ;
#17120=CARTESIAN_POINT ( 'NONE',  ( 9.909375000614517148, 4.541064518000418104, -2.621784821874998173 ) ) ;
#17121=CARTESIAN_POINT ( 'NONE',  ( 4.003125000614518925, 4.541064518000418104, -2.621784821874998173 ) ) ;
#17123=CARTESIAN_POINT ( 'NONE',  ( 6.000000001229033764, -2.886751345948125991, -5.000000000000000000 ) ) ;
#17124=CARTESIAN_POINT ( 'NONE',  ( 20.76562500061451644, 3.027376345333611329, 5.243569643749999010 ) ) ;
#17125=CARTESIAN_POINT ( 'NONE',  ( 7.200000001229035718, -2.886751345948129988, 4.999999999999997335 ) ) ;
#17126=CARTESIAN_POINT ( 'NONE',  ( 17.76562500061451644, -6.054752690667223547, -1.112240025338166033E-15 ) ) ;
#17127=CARTESIAN_POINT ( 'NONE',  ( 12.55312500061451786, 4.541064518000418104, -2.621784821874998173 ) ) ;
#17129=CARTESIAN_POINT ( 'NONE',  ( 14.17500000000000071, 4.330127018922191873, 2.499999999999999556 ) ) ;
#17130=CARTESIAN_POINT ( 'NONE',  ( 8.775000001229033231, 2.886751345948129099, -4.999999999999998224 ) ) ;
#17131=CARTESIAN_POINT ( 'NONE',  ( 5.090625000614516615, -3.027376345333614438, 5.243569643749998122 ) ) ;
#17132=ADVANCED_FACE ( 'NONE', ( #33252 ), #50612, .F. ) ;
#17133=CARTESIAN_POINT ( 'NONE',  ( 17.62500000122903288, -5.773502691896255534, -1.060575238724906372E-15 ) ) ;
#17136=CARTESIAN_POINT ( 'NONE',  ( -4.243569643749997233, 11.79687500061451999, -27.54997392385601174 ) ) ;
#17137=CARTESIAN_POINT ( 'NONE',  ( 24.00000000000000000, 4.330127018922192761, -2.499999999999997780 ) ) ;
#17138=VECTOR ( 'NONE', #68347, 1000.000000000000000 ) ;
#17140=CARTESIAN_POINT ( 'NONE',  ( 20.48437500061451289, -4.541064518000419881, 2.621784821874995952 ) ) ;
#17142=CARTESIAN_POINT ( 'NONE',  ( 12.30000000000000249, 4.330127018922192761, -2.499999999999997780 ) ) ;
#17143=VECTOR ( 'NONE', #65213, 1000.000000000000000 ) ;
#17144=CARTESIAN_POINT ( 'NONE',  ( 16.30312500061451786, 0.000000000000000000, 5.243569643749999010 ) ) ;
#17147=CARTESIAN_POINT ( 'NONE',  ( 14.81250000122903288, 0.000000000000000000, 4.999999999999998224 ) ) ;
#17148=CARTESIAN_POINT ( 'NONE',  ( 26.40937500061451715, -4.541064518000417216, -2.621784821875001281 ) ) ;
#17150=CARTESIAN_POINT ( 'NONE',  ( 11.39062500061451644, -3.027376345333614438, 5.243569643749998122 ) ) ;
#17151=CARTESIAN_POINT ( 'NONE',  ( 9.759375000614516793, -4.541064518000417216, -2.621784821875001281 ) ) ;
#17153=CARTESIAN_POINT ( 'NONE',  ( 2.830238065994760355, -4.121891707590733311, -2.867552304490421200 ) ) ;
#17154=CARTESIAN_POINT ( 'NONE',  ( 19.30312500061451786, 4.541064518000418104, -2.621784821874998173 ) ) ;
#17156=CARTESIAN_POINT ( 'NONE',  ( -3.999999999999999112, 12.91250000122903430, 30.00000000000000000 ) ) ;
#17157=CARTESIAN_POINT ( 'NONE',  ( 11.21250000000000036, -5.773502691896255534, -1.060575238724906372E-15 ) ) ;
#17158=CARTESIAN_POINT ( 'NONE',  ( 21.86250000122903003, 4.330127018922192761, -2.499999999999997780 ) ) ;
#17159=CARTESIAN_POINT ( 'NONE',  ( 16.00312500061451715, -4.541064518000417216, -2.621784821875001281 ) ) ;
#17161=ORIENTED_EDGE ( 'NONE', *, *, #40617, .T. ) ;
#17162=CARTESIAN_POINT ( 'NONE',  ( 20.24999999999999645, -4.330127018922190985, -2.500000000000001332 ) ) ;
#17163=CARTESIAN_POINT ( 'NONE',  ( 24.22500000000000142, -4.330127018922194537, 2.499999999999995559 ) ) ;
#17164=CARTESIAN_POINT ( 'NONE',  ( 20.97187500061451715, -6.054752690667223547, -1.112240025338166033E-15 ) ) ;
#17165=CARTESIAN_POINT ( 'NONE',  ( 25.71562500061451573, 3.027376345333611329, 5.243569643749999010 ) ) ;
#17166=VERTEX_POINT ( 'NONE', #43984 ) ;
#17168=CARTESIAN_POINT ( 'NONE',  ( 7.715625000614515727, 3.027376345333611329, 5.243569643749999010 ) ) ;
#17169=LINE ( 'NONE', #72609, #54974 ) ;
#17170=CARTESIAN_POINT ( 'NONE',  ( 15.26249999999999929, -5.773502691896255534, -1.060575238724906372E-15 ) ) ;
#17171=CARTESIAN_POINT ( 'NONE',  ( 4.243569643749999010, 17.81562500061451715, 27.54997392385601174 ) ) ;
#17172=CARTESIAN_POINT ( 'NONE',  ( 4.771875000614516971, -6.054752690667223547, -1.112240025338166033E-15 ) ) ;
#17173=CARTESIAN_POINT ( 'NONE',  ( 27.27187500061451431, -6.054752690667223547, -1.112240025338166033E-15 ) ) ;
#17175=CARTESIAN_POINT ( 'NONE',  ( 23.99062500061451786, -3.027376345333614438, 5.243569643749998122 ) ) ;
#17176=CARTESIAN_POINT ( 'NONE',  ( 26.18437500061451573, 4.541064518000418104, 2.621784821874999949 ) ) ;
#17178=CARTESIAN_POINT ( 'NONE',  ( 9.001249775931846008E-16, 19.01562500061459104, -25.09994784771203058 ) ) ;
#17179=CARTESIAN_POINT ( 'NONE',  ( 11.88749999999999751, 5.773502691896255534, 3.535250795749688894E-16 ) ) ;
#17180=CARTESIAN_POINT ( 'NONE',  ( 9.778125000614517504, 6.421520780324663323E-16, -5.243569643749999010 ) ) ;
#17181=DIRECTION ( 'NONE',  ( 0.000000000000000000, 0.000000000000000000, -1.000000000000000000 ) ) ;
#17182=CARTESIAN_POINT ( 'NONE',  ( 29.72812500061451502, 4.541064518000418104, 2.621784821874999949 ) ) ;
#17183=CARTESIAN_POINT ( 'NONE',  ( 26.87812500061451360, 6.421520780324663323E-16, -5.243569643749999010 ) ) ;
#17184=CARTESIAN_POINT ( 'NONE',  ( 12.67500000122903536, -5.773502691896255534, -1.060575238724906372E-15 ) ) ;
#17186=CARTESIAN_POINT ( 'NONE',  ( 3.103125000614517237, 4.541064518000418104, -2.621784821874998173 ) ) ;
#17187=CARTESIAN_POINT ( 'NONE',  ( 18.83437500061451431, 6.421520780324663323E-16, -5.243569643749999010 ) ) ;
#17188=CARTESIAN_POINT ( 'NONE',  ( 4.243569643749999898, 14.64687500061451964, 32.45002607614398471 ) ) ;
#17189=CARTESIAN_POINT ( 'NONE',  ( 19.24687500061452283, -3.027376345333610441, -5.243569643749999898 ) ) ;
#17190=CARTESIAN_POINT ( 'NONE',  ( 29.67187500061451644, 3.027376345333613106, -5.243569643749998122 ) ) ;
#17191=CARTESIAN_POINT ( 'NONE',  ( 2.121784821875001281, 18.20937500061451786, 33.67503911421598417 ) ) ;
#17192=CARTESIAN_POINT ( 'NONE',  ( 10.71562500061451928, 3.027376345333613106, -5.243569643749998122 ) ) ;
#17193=CARTESIAN_POINT ( 'NONE',  ( 7.809375000614519280, 0.000000000000000000, 5.243569643749999010 ) ) ;
#17194=DIRECTION ( 'NONE',  ( -1.000000000000000000, -0.000000000000000000, -0.000000000000000000 ) ) ;
#17195=AXIS2_PLACEMENT_3D ( 'NONE', #58964, #2467, #6923 ) ;
#17196=CARTESIAN_POINT ( 'NONE',  ( 8.728125000614518569, -4.541064518000419881, 2.621784821874995952 ) ) ;
#17197=CARTESIAN_POINT ( 'NONE',  ( 11.18437500061451928, 6.421520780324663323E-16, -5.243569643749999010 ) ) ;
#17198=CARTESIAN_POINT ( 'NONE',  ( 19.05000000122903359, -2.886751345948125991, -5.000000000000000000 ) ) ;
#17199=CARTESIAN_POINT ( 'NONE',  ( 5.971875000614516260, 3.027376345333611329, 5.243569643749999010 ) ) ;
#17200=CARTESIAN_POINT ( 'NONE',  ( 8.728125000614518569, -4.541064518000419881, 2.621784821874995952 ) ) ;
#17203=CARTESIAN_POINT ( 'NONE',  ( 18.98437500061451644, 4.541064518000418104, 2.621784821874999949 ) ) ;
#17204=CARTESIAN_POINT ( 'NONE',  ( -3.999999999999999112, 11.56250000122903465, 30.00000000000000000 ) ) ;
#17206=CARTESIAN_POINT ( 'NONE',  ( 27.44062500061451715, 6.054752690667223547, 3.707466751127219781E-16 ) ) ;
#17207=CARTESIAN_POINT ( 'NONE',  ( 13.22812500061451502, -4.541064518000419881, 2.621784821874995952 ) ) ;
#17208=CARTESIAN_POINT ( 'NONE',  ( 28.47187500061451715, 3.027376345333611329, 5.243569643749999010 ) ) ;
#17209=CARTESIAN_POINT ( 'NONE',  ( 12.51562500061451821, 3.027376345333613106, -5.243569643749998122 ) ) ;
#17210=CARTESIAN_POINT ( 'NONE',  ( 4.527409397281981995, -2.122320272585544565, -4.559184932251166167 ) ) ;
#17211=CARTESIAN_POINT ( 'NONE',  ( 12.18750000122903465, -4.330127018922194537, 2.499999999999995559 ) ) ;
#17212=CARTESIAN_POINT ( 'NONE',  ( 26.61562500061451786, 3.027376345333611329, 5.243569643749999010 ) ) ;
#17213=CARTESIAN_POINT ( 'NONE',  ( 4.243569643749999898, 14.59062500061451750, -27.54997392385601529 ) ) ;
#17214=CARTESIAN_POINT ( 'NONE',  ( 16.16250000122903430, 0.000000000000000000, 4.999999999999998224 ) ) ;
#17216=CARTESIAN_POINT ( 'NONE',  ( 13.95000000000000107, -4.330127018922190985, -2.500000000000001332 ) ) ;
#17217=CARTESIAN_POINT ( 'NONE',  ( 19.71562500061451928, 3.027376345333613106, -5.243569643749998122 ) ) ;
#17218=CARTESIAN_POINT ( 'NONE',  ( 7.359375000614516438, 0.000000000000000000, 5.243569643749999010 ) ) ;
#17219=CARTESIAN_POINT ( 'NONE',  ( 7.275000001229035007, -5.773502691896255534, -1.060575238724906372E-15 ) ) ;
#17220=CARTESIAN_POINT ( 'NONE',  ( 15.78750000122903430, -4.330127018922194537, 2.499999999999995559 ) ) ;
#17221=CARTESIAN_POINT ( 'NONE',  ( 12.06562500061451537, 3.027376345333613106, -5.243569643749998122 ) ) ;
#17222=CARTESIAN_POINT ( 'NONE',  ( 15.17812500061451608, 6.421520780324663323E-16, -5.243569643749999010 ) ) ;
#17223=EDGE_CURVE ( 'NONE', #7111, #27030, #21034, .T. ) ;
#17224=CARTESIAN_POINT ( 'NONE',  ( 28.01250000122903216, -4.330127018922190985, -2.500000000000001332 ) ) ;
#17225=CARTESIAN_POINT ( 'NONE',  ( 23.17500000000000071, 4.330127018922191873, 2.499999999999999556 ) ) ;
#17226=CARTESIAN_POINT ( 'NONE',  ( 23.67187500061451999, -6.054752690667223547, -1.112240025338166033E-15 ) ) ;
#17228=CARTESIAN_POINT ( 'NONE',  ( 9.937500001229032875, -4.330127018922194537, 2.499999999999995559 ) ) ;
#17229=CARTESIAN_POINT ( 'NONE',  ( 27.53437500061451360, 4.541064518000418104, 2.621784821874999949 ) ) ;
#17230=CARTESIAN_POINT ( 'NONE',  ( 4.621875000614516615, 3.027376345333611329, 5.243569643749999010 ) ) ;
#17231=CARTESIAN_POINT ( 'NONE',  ( 22.86562500061451431, 3.027376345333613106, -5.243569643749998122 ) ) ;
#17233=CARTESIAN_POINT ( 'NONE',  ( 6.825000000000001066, 6.123233995736764310E-16, -4.999999999999998224 ) ) ;
#17234=AXIS2_PLACEMENT_3D ( 'NONE', #54953, #60472, #70844 ) ;
#17235=CARTESIAN_POINT ( 'NONE',  ( 9.234375000614518214, -4.541064518000419881, 2.621784821874995952 ) ) ;
#17236=CARTESIAN_POINT ( 'NONE',  ( 15.93750000000000000, 5.773502691896255534, 3.535250795749688401E-16 ) ) ;
#17237=CARTESIAN_POINT ( 'NONE',  ( 29.20312500061451644, 4.541064518000418104, -2.621784821874998173 ) ) ;
#17238=CARTESIAN_POINT ( 'NONE',  ( 6.984375000614516438, -4.541064518000419881, 2.621784821874995952 ) ) ;
#17239=CARTESIAN_POINT ( 'NONE',  ( -1.071796769724491005, 14.50759618943233420, 26.00000000000000355 ) ) ;
#17240=CARTESIAN_POINT ( 'NONE',  ( 25.65937500061451715, 4.541064518000418104, -2.621784821874998173 ) ) ;
#17241=CARTESIAN_POINT ( 'NONE',  ( -2.121784821874996840, 10.87812500061459531, 33.67503911421598417 ) ) ;
#17242=CARTESIAN_POINT ( 'NONE',  ( 18.41250000000000142, -5.773502691896255534, -1.060575238724906372E-15 ) ) ;
#17244=CARTESIAN_POINT ( 'NONE',  ( 27.37500000000000000, -4.330127018922194537, 2.499999999999995559 ) ) ;
#17245=CARTESIAN_POINT ( 'NONE',  ( 28.39687500061452141, 6.054752690667223547, 3.707466751127219781E-16 ) ) ;
#17246=ORIENTED_EDGE ( 'NONE', *, *, #27246, .F. ) ;
#17247=CARTESIAN_POINT ( 'NONE',  ( 16.67812500061451786, 4.541064518000418104, 2.621784821874999949 ) ) ;
#17248=CARTESIAN_POINT ( 'NONE',  ( 8.803125000614517859, -4.541064518000417216, -2.621784821875001281 ) ) ;
#17250=CARTESIAN_POINT ( 'NONE',  ( 4.284375000614518925, -4.541064518000419881, 2.621784821874995952 ) ) ;
#17251=CARTESIAN_POINT ( 'NONE',  ( 18.00000000122903288, -2.886751345948129988, 4.999999999999997335 ) ) ;
#17252=CARTESIAN_POINT ( 'NONE',  ( 22.46250000000000213, -5.773502691896255534, -1.060575238724906372E-15 ) ) ;
#17253=CARTESIAN_POINT ( 'NONE',  ( 15.75000000000000000, -4.330127018922190985, -2.500000000000001332 ) ) ;
#17254=CARTESIAN_POINT ( 'NONE',  ( 5.484375000614518214, 4.541064518000418104, 2.621784821874999949 ) ) ;
#17255=CARTESIAN_POINT ( 'NONE',  ( 11.97187500061451892, -6.054752690667223547, -1.112240025338166033E-15 ) ) ;
#17256=CARTESIAN_POINT ( 'NONE',  ( 21.30937500061451573, 0.000000000000000000, 5.243569643749999010 ) ) ;
#17257=CARTESIAN_POINT ( 'NONE',  ( -1.999999999999997113, 16.47500000000000142, 33.46410161513775705 ) ) ;
#17258=ORIENTED_EDGE ( 'NONE', *, *, #32653, .F. ) ;
#17259=CARTESIAN_POINT ( 'NONE',  ( 4.959375000614516971, 4.541064518000418104, -2.621784821874998173 ) ) ;
#17260=CARTESIAN_POINT ( 'NONE',  ( 6.534375000614517148, -4.541064518000419881, 2.621784821874995952 ) ) ;
#17261=CARTESIAN_POINT ( 'NONE',  ( 18.45000000000000284, -4.330127018922190985, -2.500000000000001332 ) ) ;
#17262=CARTESIAN_POINT ( 'NONE',  ( 14.95312500061451644, 0.000000000000000000, 5.243569643749999010 ) ) ;
#17266=CARTESIAN_POINT ( 'NONE',  ( 10.04062500061451502, -3.027376345333614438, 5.243569643749998122 ) ) ;
#17267=CARTESIAN_POINT ( 'NONE',  ( 26.22187500061451715, 3.027376345333611329, 5.243569643749999010 ) ) ;
#17269=CARTESIAN_POINT ( 'NONE',  ( 28.99687500061451573, -3.027376345333614438, 5.243569643749998122 ) ) ;
#17270=CARTESIAN_POINT ( 'NONE',  ( 10.46249999999999858, 2.886751345948129099, -4.999999999999998224 ) ) ;
#17271=CARTESIAN_POINT ( 'NONE',  ( 8.484601909799253346E-16, 14.37500000122903288, 34.61880215351700230 ) ) ;
#17272=CARTESIAN_POINT ( 'NONE',  ( 8.962500001229033231, 0.000000000000000000, 4.999999999999998224 ) ) ;
#17273=CARTESIAN_POINT ( 'NONE',  ( 19.65937500061451360, -4.541064518000417216, -2.621784821875001281 ) ) ;
#17274=CARTESIAN_POINT ( 'NONE',  ( 13.32187500061451502, -6.054752690667223547, -1.112240025338166033E-15 ) ) ;
#17277=CARTESIAN_POINT ( 'NONE',  ( 13.60312500061451679, 0.000000000000000000, 5.243569643749999010 ) ) ;
#17278=CARTESIAN_POINT ( 'NONE',  ( 26.81250000122903288, 4.330127018922192761, -2.499999999999997780 ) ) ;
#17279=CARTESIAN_POINT ( 'NONE',  ( 14.37187500061451928, 3.027376345333613106, -5.243569643749998122 ) ) ;
#17280=AXIS2_PLACEMENT_3D ( 'NONE', #20994, #70882, #43546 ) ;
#17281=CARTESIAN_POINT ( 'NONE',  ( 1.594043775273461083, 9.879932731042712746, -35.79803503059465442 ) ) ;
#17282=CARTESIAN_POINT ( 'NONE',  ( 18.02812500061451573, 4.541064518000418104, 2.621784821874999949 ) ) ;
#17284=CARTESIAN_POINT ( 'NONE',  ( 27.08437500061451786, 4.541064518000418104, 2.621784821874999949 ) ) ;
#17285=CARTESIAN_POINT ( 'NONE',  ( 4.243569643749999898, 10.09062500061451928, 32.45002607614398471 ) ) ;
#17286=CARTESIAN_POINT ( 'NONE',  ( 14.52187500061451608, 3.027376345333611329, 5.243569643749999010 ) ) ;
#17287=CARTESIAN_POINT ( 'NONE',  ( 15.33750000122903323, -4.330127018922194537, 2.499999999999995559 ) ) ;
#17289=CARTESIAN_POINT ( 'NONE',  ( 2.121784821875001281, 17.75937500061451502, -26.32496088578401938 ) ) ;
#17290=CARTESIAN_POINT ( 'NONE',  ( 19.32187500061451857, 3.027376345333613106, -5.243569643749998122 ) ) ;
#17291=CARTESIAN_POINT ( 'NONE',  ( 20.25000000122903288, -2.886751345948129988, 4.999999999999997335 ) ) ;
#17292=CARTESIAN_POINT ( 'NONE',  ( 14.14687500061451786, -3.027376345333614438, 5.243569643749998122 ) ) ;
#17294=CARTESIAN_POINT ( 'NONE',  ( 4.243569643749999898, 12.88437500061451857, 30.00000000000000000 ) ) ;
#17295=CARTESIAN_POINT ( 'NONE',  ( 23.21250000122903501, 4.330127018922192761, -2.499999999999997780 ) ) ;
#17296=AXIS2_PLACEMENT_3D ( 'NONE', #35839, #51761, #30668 ) ;
#17297=CARTESIAN_POINT ( 'NONE',  ( 16.11562500061451786, 3.027376345333613106, -5.243569643749998122 ) ) ;
#17299=VERTEX_POINT ( 'NONE', #7351 ) ;
#17300=ORIENTED_EDGE ( 'NONE', *, *, #1804, .F. ) ;
#17301=CARTESIAN_POINT ( 'NONE',  ( 21.44999999999999929, 0.000000000000000000, 4.999999999999998224 ) ) ;
#17302=CARTESIAN_POINT ( 'NONE',  ( -2.000000000000000000, 17.78750000122903430, 26.53589838486224650 ) ) ;
#17303=CARTESIAN_POINT ( 'NONE',  ( 3.553125000614516082, 4.541064518000418104, -2.621784821874998173 ) ) ;
#17304=CARTESIAN_POINT ( 'NONE',  ( 14.51250000122903394, -4.330127018922190985, -2.500000000000001332 ) ) ;
#17305=CARTESIAN_POINT ( 'NONE',  ( 18.89062500061451644, 6.054752690667223547, 3.707466751127219781E-16 ) ) ;
#17307=CARTESIAN_POINT ( 'NONE',  ( 22.41562500061451502, 3.027376345333613106, -5.243569643749998122 ) ) ;
#17308=CARTESIAN_POINT ( 'NONE',  ( 5.953125000614519102, 0.000000000000000000, 5.243569643749999010 ) ) ;
#17309=ADVANCED_FACE ( 'NONE', ( #51334 ), #18054, .F. ) ;
#17310=CARTESIAN_POINT ( 'NONE',  ( 29.55000000000000071, 0.000000000000000000, 4.999999999999998224 ) ) ;
#17312=DIRECTION ( 'NONE',  ( 0.000000000000000000, 0.000000000000000000, -1.000000000000000000 ) ) ;
#17313=CARTESIAN_POINT ( 'NONE',  ( -3.999999999999997335, 10.25000000122903288, -27.69059892324149175 ) ) ;
#17314=CARTESIAN_POINT ( 'NONE',  ( -3.000416591977282496E-16, 18.84687500061452070, -34.90005215228797653 ) ) ;
#17315=CARTESIAN_POINT ( 'NONE',  ( 6.412500001229036073, -4.330127018922190985, -2.500000000000001332 ) ) ;
#17316=CARTESIAN_POINT ( 'NONE',  ( 9.412499999999999645, -5.773502691896255534, -1.060575238724906372E-15 ) ) ;
#17318=CARTESIAN_POINT ( 'NONE',  ( 5.212500001229032343, 4.330127018922192761, -2.499999999999997780 ) ) ;
#17319=CARTESIAN_POINT ( 'NONE',  ( 11.85937500061451644, 0.000000000000000000, 5.243569643749999010 ) ) ;
#17320=CARTESIAN_POINT ( 'NONE',  ( 23.58750000122903145, 6.123233995736764310E-16, -4.999999999999998224 ) ) ;
#17321=CARTESIAN_POINT ( 'NONE',  ( 4.771875000614516971, -6.054752690667223547, -1.112240025338166033E-15 ) ) ;
#17323=CARTESIAN_POINT ( 'NONE',  ( 29.51250000122903216, 4.330127018922192761, -2.499999999999997780 ) ) ;
#17324=CARTESIAN_POINT ( 'NONE',  ( 10.77187500061451786, 3.027376345333613106, -5.243569643749998122 ) ) ;
#17325=CARTESIAN_POINT ( 'NONE',  ( 14.67187500061451821, -6.054752690667223547, -1.112240025338166033E-15 ) ) ;
#17326=CARTESIAN_POINT ( 'NONE',  ( 7.320879633048903241E-15, 17.30000000122903003, -34.00000000000000000 ) ) ;
#17327=CARTESIAN_POINT ( 'NONE',  ( 6.150000000000003020, 0.000000000000000000, 4.999999999999998224 ) ) ;
#17328=CARTESIAN_POINT ( 'NONE',  ( 2.121784821875001281, 16.35312500061459318, 33.67503911421598417 ) ) ;
#17329=CARTESIAN_POINT ( 'NONE',  ( 20.78437500061451715, 4.541064518000418104, 2.621784821874999949 ) ) ;
#17330=CARTESIAN_POINT ( 'NONE',  ( 9.750000000000001776, 0.000000000000000000, 4.999999999999998224 ) ) ;
#17331=CARTESIAN_POINT ( 'NONE',  ( 27.71250000122903145, 4.330127018922192761, -2.499999999999997780 ) ) ;
#17333=CARTESIAN_POINT ( 'NONE',  ( 22.30312500061451431, -4.541064518000417216, -2.621784821875001281 ) ) ;
#17334=CARTESIAN_POINT ( 'NONE',  ( 14.95312500061451644, 0.000000000000000000, 5.243569643749999010 ) ) ;
#17336=CARTESIAN_POINT ( 'NONE',  ( 12.23437500061451821, 4.541064518000418104, 2.621784821874999949 ) ) ;
#17337=CARTESIAN_POINT ( 'NONE',  ( 27.59999999999999787, 4.330127018922192761, -2.499999999999997780 ) ) ;
#17338=CARTESIAN_POINT ( 'NONE',  ( 24.71250000122903145, 0.000000000000000000, 4.999999999999998224 ) ) ;
#17339=CARTESIAN_POINT ( 'NONE',  ( 3.346875000614518036, -3.027376345333614438, 5.243569643749998122 ) ) ;
#17340=CARTESIAN_POINT ( 'NONE',  ( 14.03437500061451715, 4.541064518000418104, 2.621784821874999949 ) ) ;
#17341=CARTESIAN_POINT ( 'NONE',  ( 29.37187500061451928, 3.027376345333611329, 5.243569643749999010 ) ) ;
#17343=CARTESIAN_POINT ( 'NONE',  ( 18.45000000000000284, -4.330127018922190985, -2.500000000000001332 ) ) ;
#17344=CARTESIAN_POINT ( 'NONE',  ( 23.55937500061451573, 0.000000000000000000, 5.243569643749999010 ) ) ;
#17345=CARTESIAN_POINT ( 'NONE',  ( 14.22187500061451537, -6.054752690667223547, -1.112240025338166033E-15 ) ) ;
#17347=CARTESIAN_POINT ( 'NONE',  ( 25.23749999999999716, -2.886751345948125991, -5.000000000000000000 ) ) ;
#17348=CARTESIAN_POINT ( 'NONE',  ( 3.337500001229034563, 6.123233995736764310E-16, -4.999999999999998224 ) ) ;
#17350=CARTESIAN_POINT ( 'NONE',  ( 16.15312500061451573, 4.541064518000418104, -2.621784821874998173 ) ) ;
#17351=CARTESIAN_POINT ( 'NONE',  ( 6.225000000000001421, -4.330127018922194537, 2.499999999999995559 ) ) ;
#17352=EDGE_CURVE ( 'NONE', #20497, #11634, #13242, .T. ) ;
#17353=CARTESIAN_POINT ( 'NONE',  ( -3.999999999999999112, 14.11250000000000071, 27.69059892324149885 ) ) ;
#17354=( BOUNDED_CURVE ( )  B_SPLINE_CURVE ( 3, ( #19593, #58027, #20327, #42881 ),
 .UNSPECIFIED., .F., .F. ) 
 B_SPLINE_CURVE_WITH_KNOTS ( ( 4, 4 ),
 ( 0.8238030042635362538, 0.8534874751081462652 ),
 .UNSPECIFIED. ) 
 CURVE ( )  GEOMETRIC_REPRESENTATION_ITEM ( )  RATIONAL_B_SPLINE_CURVE ( ( 1.000000000000000000, 0.9999265706972281231, 0.9999265706972281231, 1.000000000000000000 ) ) 
 REPRESENTATION_ITEM ( '' )  );
#17355=CARTESIAN_POINT ( 'NONE',  ( 16.31250000000000000, 2.886751345948129099, -4.999999999999998224 ) ) ;
#17356=CARTESIAN_POINT ( 'NONE',  ( 9.001249775931846008E-16, 12.71562500061451750, 34.90005215228797653 ) ) ;
#17358=CARTESIAN_POINT ( 'NONE',  ( 21.82500000122903572, 2.886751345948129099, -4.999999999999998224 ) ) ;
#17359=CARTESIAN_POINT ( 'NONE',  ( 27.75937500061451502, -4.541064518000417216, -2.621784821875001281 ) ) ;
#17360=EDGE_LOOP ( 'NONE', ( #935, #29743, #66525, #11899 ) ) ;
#17361=CARTESIAN_POINT ( 'NONE',  ( 21.10312500061451502, 4.541064518000418104, -2.621784821874998173 ) ) ;
#17362=CARTESIAN_POINT ( 'NONE',  ( 21.45937500061451786, -4.541064518000417216, -2.621784821875001281 ) ) ;
#17363=CARTESIAN_POINT ( 'NONE',  ( 3.450000000000001510, 0.000000000000000000, 4.999999999999998224 ) ) ;
#17364=CARTESIAN_POINT ( 'NONE',  ( 10.30312500061451431, 4.541064518000418104, -2.621784821874998173 ) ) ;
#17365=CARTESIAN_POINT ( 'NONE',  ( 23.84062500061451928, 6.054752690667223547, 3.707466751127219781E-16 ) ) ;
#17366=CARTESIAN_POINT ( 'NONE',  ( 13.13437500061451857, 4.541064518000418104, 2.621784821874999949 ) ) ;
#17367=CARTESIAN_POINT ( 'NONE',  ( 15.87187500061451573, 3.027376345333611329, 5.243569643749999010 ) ) ;
#17368=CARTESIAN_POINT ( 'NONE',  ( 2.121784821875001281, 17.70312500061451644, 33.67503911421598417 ) ) ;
#17369=CARTESIAN_POINT ( 'NONE',  ( 20.66250000122903074, 0.000000000000000000, 4.999999999999998224 ) ) ;
#17371=CARTESIAN_POINT ( 'NONE',  ( 10.97812500061451679, -4.541064518000419881, 2.621784821874995952 ) ) ;
#17372=CARTESIAN_POINT ( 'NONE',  ( 4.846875000614519813, -3.027376345333610441, -5.243569643749999898 ) ) ;
#17373=CARTESIAN_POINT ( 'NONE',  ( 3.646875000614520079, 6.054752690667223547, 3.707466751127219781E-16 ) ) ;
#17375=CARTESIAN_POINT ( 'NONE',  ( 25.73437500061451644, 4.541064518000418104, 2.621784821874999949 ) ) ;
#17376=CARTESIAN_POINT ( 'NONE',  ( 17.95312500061451644, 4.541064518000418104, -2.621784821874998173 ) ) ;
#17377=CARTESIAN_POINT ( 'NONE',  ( 28.46250000122903145, -4.330127018922190985, -2.500000000000001332 ) ) ;
#17378=CARTESIAN_POINT ( 'NONE',  ( 28.82812500061451644, 4.541064518000418104, 2.621784821874999949 ) ) ;
#17379=CARTESIAN_POINT ( 'NONE',  ( 22.54687500061451999, 6.054752690667223547, 3.707466751127219781E-16 ) ) ;
#17380=CARTESIAN_POINT ( 'NONE',  ( 17.09062500061451573, 6.054752690667223547, 3.707466751127219781E-16 ) ) ;
#17381=CARTESIAN_POINT ( 'NONE',  ( 9.001249775931846008E-16, 19.07187500061451502, 34.90005215228797653 ) ) ;
#17382=CARTESIAN_POINT ( 'NONE',  ( 23.27812500061451573, 6.421520780324663323E-16, -5.243569643749999010 ) ) ;
#17383=CARTESIAN_POINT ( 'NONE',  ( 3.787500001229033408, 6.123233995736764310E-16, -4.999999999999998224 ) ) ;
#17384=ORIENTED_EDGE ( 'NONE', *, *, #26884, .F. ) ;
#17385=CARTESIAN_POINT ( 'NONE',  ( 27.67499999999999716, 4.330127018922191873, 2.499999999999999556 ) ) ;
#17386=CARTESIAN_POINT ( 'NONE',  ( -3.999999999999999556, 11.86250000000000071, -32.30940107675850470 ) ) ;
#17388=ADVANCED_FACE ( 'NONE', ( #63133 ), #68331, .F. ) ;
#17389=CARTESIAN_POINT ( 'NONE',  ( 3.384375000614517237, -4.541064518000419881, 2.621784821874995952 ) ) ;
#17390=CARTESIAN_POINT ( 'NONE',  ( 11.31562500061451892, 3.027376345333611329, 5.243569643749999010 ) ) ;
#17391=CARTESIAN_POINT ( 'NONE',  ( 23.36250000122903359, 0.000000000000000000, 4.999999999999998224 ) ) ;
#17392=CARTESIAN_POINT ( 'NONE',  ( 12.60937500061451821, 4.541064518000418104, -2.621784821874998173 ) ) ;
#17393=CARTESIAN_POINT ( 'NONE',  ( 26.16562500061451502, 3.027376345333611329, 5.243569643749999010 ) ) ;
#17394=CARTESIAN_POINT ( 'NONE',  ( 27.37500000000000000, -4.330127018922194537, 2.499999999999995559 ) ) ;
#17395=CARTESIAN_POINT ( 'NONE',  ( 3.999999999999998668, 17.67500000122903359, -32.30940107675850470 ) ) ;
#17396=CARTESIAN_POINT ( 'NONE',  ( -1.071796769724496556, 15.70490381179669903, -26.00000000000000355 ) ) ;
#17397=CARTESIAN_POINT ( 'NONE',  ( 11.95312500061451644, -4.541064518000417216, -2.621784821875001281 ) ) ;
#17398=ORIENTED_EDGE ( 'NONE', *, *, #19782, .F. ) ;
#17399=CARTESIAN_POINT ( 'NONE',  ( 6.965625000614518392, -6.054752690667223547, -1.112240025338166033E-15 ) ) ;
#17400=CARTESIAN_POINT ( 'NONE',  ( 6.890625000614516438, -3.027376345333614438, 5.243569643749998122 ) ) ;
#17402=CARTESIAN_POINT ( 'NONE',  ( 14.02500000122903323, -5.773502691896255534, -1.060575238724906372E-15 ) ) ;
#17403=CARTESIAN_POINT ( 'NONE',  ( 15.15000000000000036, 0.000000000000000000, 4.999999999999998224 ) ) ;
#17404=CARTESIAN_POINT ( 'NONE',  ( 16.43437500061451573, -4.541064518000419881, 2.621784821874995952 ) ) ;
#17405=CARTESIAN_POINT ( 'NONE',  ( 10.65000000122903323, 5.773502691896255534, 3.535250795749688894E-16 ) ) ;
#17406=CARTESIAN_POINT ( 'NONE',  ( 19.95937500061451786, 0.000000000000000000, 5.243569643749999010 ) ) ;
#17408=CARTESIAN_POINT ( 'NONE',  ( 19.69687500061451857, -3.027376345333610441, -5.243569643749999898 ) ) ;
#17409=CARTESIAN_POINT ( 'NONE',  ( 4.243569643749999898, 14.59062500061451750, -27.54997392385601529 ) ) ;
#17410=CARTESIAN_POINT ( 'NONE',  ( -2.000000000000000000, 16.77500000000000213, 26.53589838486224650 ) ) ;
#17412=CARTESIAN_POINT ( 'NONE',  ( 4.133697246135442427, 2.812954343170202431, 4.425208334576621105 ) ) ;
#17413=CARTESIAN_POINT ( 'NONE',  ( 26.95312500061451644, 4.541064518000418104, -2.621784821874998173 ) ) ;
#17414=CARTESIAN_POINT ( 'NONE',  ( 17.17500000122903359, -5.773502691896255534, -1.060575238724906372E-15 ) ) ;
#17415=CARTESIAN_POINT ( 'NONE',  ( 28.32187500061451502, 3.027376345333613106, -5.243569643749998122 ) ) ;
#17416=CARTESIAN_POINT ( 'NONE',  ( 24.33749999999999858, -2.886751345948125991, -5.000000000000000000 ) ) ;
#17417=CARTESIAN_POINT ( 'NONE',  ( 8.990625000614516082, 6.054752690667223547, 3.707466751127219781E-16 ) ) ;
#17419=CARTESIAN_POINT ( 'NONE',  ( 18.53437500061451715, 4.541064518000418104, 2.621784821874999949 ) ) ;
#17421=CARTESIAN_POINT ( 'NONE',  ( 5.803125000614517859, 4.541064518000418104, -2.621784821874998173 ) ) ;
#17422=CARTESIAN_POINT ( 'NONE',  ( 10.02187500061451964, 3.027376345333611329, 5.243569643749999010 ) ) ;
#17423=VERTEX_POINT ( 'NONE', #57944 ) ;
#17424=CARTESIAN_POINT ( 'NONE',  ( 21.23437500061451644, 4.541064518000418104, 2.621784821874999949 ) ) ;
#17426=CARTESIAN_POINT ( 'NONE',  ( 29.40937500061451715, 0.000000000000000000, 5.243569643749999010 ) ) ;
#17429=CARTESIAN_POINT ( 'NONE',  ( 3.365625000614516082, -6.054752690667223547, -1.112240025338166033E-15 ) ) ;
#17431=CARTESIAN_POINT ( 'NONE',  ( 10.38750000000000107, -2.886751345948125991, -5.000000000000000000 ) ) ;
#17433=CARTESIAN_POINT ( 'NONE',  ( 24.55312500061451786, -4.541064518000417216, -2.621784821875001281 ) ) ;
#17434=CARTESIAN_POINT ( 'NONE',  ( 14.36249999999999893, -5.773502691896255534, -1.060575238724906372E-15 ) ) ;
#17435=CARTESIAN_POINT ( 'NONE',  ( 10.98750000122903536, 6.123233995736764310E-16, -4.999999999999998224 ) ) ;
#17436=CARTESIAN_POINT ( 'NONE',  ( 7.790625000614518569, -3.027376345333614438, 5.243569643749998122 ) ) ;
#17438=CARTESIAN_POINT ( 'NONE',  ( 9.674999999999998934, 4.330127018922191873, 2.499999999999999556 ) ) ;
#17440=CARTESIAN_POINT ( 'NONE',  ( 29.06250000122903288, 4.330127018922192761, -2.499999999999997780 ) ) ;
#17442=CARTESIAN_POINT ( 'NONE',  ( 7.912499999999999645, 2.886751345948126879, 4.999999999999999112 ) ) ;
#17444=ORIENTED_EDGE ( 'NONE', *, *, #33444, .T. ) ;
#17445=CARTESIAN_POINT ( 'NONE',  ( 23.09062500061451573, -3.027376345333614438, 5.243569643749998122 ) ) ;
#17446=CARTESIAN_POINT ( 'NONE',  ( 28.26562500061451289, 3.027376345333613106, -5.243569643749998122 ) ) ;
#17447=CARTESIAN_POINT ( 'NONE',  ( 29.52187500061451431, -6.054752690667223547, -1.112240025338166033E-15 ) ) ;
#17448=CARTESIAN_POINT ( 'NONE',  ( 19.47187500061451360, 3.027376345333611329, 5.243569643749999010 ) ) ;
#17449=CARTESIAN_POINT ( 'NONE',  ( 16.19062500061451715, 6.054752690667223547, 3.707466751127219781E-16 ) ) ;
#17450=CARTESIAN_POINT ( 'NONE',  ( -3.000416591977282496E-16, 10.69062500061459531, -34.90005215228797653 ) ) ;
#17451=CARTESIAN_POINT ( 'NONE',  ( 5.240625000614516971, -3.027376345333610441, -5.243569643749999898 ) ) ;
#17452=CARTESIAN_POINT ( 'NONE',  ( 27.82500000122903572, 2.886751345948126879, 4.999999999999999112 ) ) ;
#17454=CARTESIAN_POINT ( 'NONE',  ( 19.07812500061451644, -4.541064518000419881, 2.621784821874995952 ) ) ;
#17455=DIRECTION ( 'NONE',  ( 0.000000000000000000, 0.000000000000000000, 1.000000000000000000 ) ) ;
#17456=CARTESIAN_POINT ( 'NONE',  ( 4.087500001229035007, -4.330127018922194537, 2.499999999999995559 ) ) ;
#17457=CARTESIAN_POINT ( 'NONE',  ( 12.42187500061451821, -6.054752690667223547, -1.112240025338166033E-15 ) ) ;
#17458=CARTESIAN_POINT ( 'NONE',  ( 13.09687500061451892, 6.054752690667223547, 3.707466751127219781E-16 ) ) ;
#17459=CARTESIAN_POINT ( 'NONE',  ( 20.48437500061451289, -4.541064518000419881, 2.621784821874995952 ) ) ;
#17461=CARTESIAN_POINT ( 'NONE',  ( 25.11562500061451431, 3.027376345333613106, -5.243569643749998122 ) ) ;
#17462=CARTESIAN_POINT ( 'NONE',  ( 18.34687500061451715, -3.027376345333610441, -5.243569643749999898 ) ) ;
#17463=CARTESIAN_POINT ( 'NONE',  ( 24.89062500061451644, -3.027376345333614438, 5.243569643749998122 ) ) ;
#17465=CARTESIAN_POINT ( 'NONE',  ( -3.999999999999999556, 15.91249999999999964, 27.69059892324149530 ) ) ;
#17466=CARTESIAN_POINT ( 'NONE',  ( 29.24062500061451431, 6.054752690667223547, 3.707466751127219781E-16 ) ) ;
#17467=CARTESIAN_POINT ( 'NONE',  ( 12.30000000122903181, -2.886751345948125991, -5.000000000000000000 ) ) ;
#17468=CARTESIAN_POINT ( 'NONE',  ( 7.125000001229033764, 2.886751345948126879, 4.999999999999999112 ) ) ;
#17469=CARTESIAN_POINT ( 'NONE',  ( -2.000000000000000000, 19.92500000000000071, -33.46410161513775705 ) ) ;
#17470=CARTESIAN_POINT ( 'NONE',  ( 27.37500000122903288, 2.886751345948126879, 4.999999999999999112 ) ) ;
#17473=CARTESIAN_POINT ( 'NONE',  ( 9.834375000614517859, 6.421520780324663323E-16, -5.243569643749999010 ) ) ;
#17475=CARTESIAN_POINT ( 'NONE',  ( 16.64062500061451289, 6.054752690667223547, 3.707466751127219781E-16 ) ) ;
#17476=CARTESIAN_POINT ( 'NONE',  ( 12.45937500061451786, -4.541064518000417216, -2.621784821875001281 ) ) ;
#17477=CARTESIAN_POINT ( 'NONE',  ( 28.83750000122903145, -4.330127018922194537, 2.499999999999995559 ) ) ;
#17478=CARTESIAN_POINT ( 'NONE',  ( 20.59687500061451715, -3.027376345333610441, -5.243569643749999898 ) ) ;
#17479=CARTESIAN_POINT ( 'NONE',  ( 6.421875000614519102, 3.027376345333611329, 5.243569643749999010 ) ) ;
#17480=CARTESIAN_POINT ( 'NONE',  ( 3.590625000614518836, 6.054752690667223547, 3.707466751127219781E-16 ) ) ;
#17482=CARTESIAN_POINT ( 'NONE',  ( 10.90312500061451928, 0.000000000000000000, 5.243569643749999010 ) ) ;
#17483=CARTESIAN_POINT ( 'NONE',  ( 20.24062500061451431, 6.054752690667223547, 3.707466751127219781E-16 ) ) ;
#17485=CARTESIAN_POINT ( 'NONE',  ( 5.925000001229033586, -5.773502691896255534, -1.060575238724906372E-15 ) ) ;
#17486=CARTESIAN_POINT ( 'NONE',  ( 17.35312500061451502, -4.541064518000417216, -2.621784821875001281 ) ) ;
#17487=CARTESIAN_POINT ( 'NONE',  ( 12.36562500061451608, -6.054752690667223547, -1.112240025338166033E-15 ) ) ;
#17489=CARTESIAN_POINT ( 'NONE',  ( 12.93750000000000178, -2.886751345948129988, 4.999999999999997335 ) ) ;
#17490=CARTESIAN_POINT ( 'NONE',  ( 8.437500001229034652, 4.330127018922191873, 2.499999999999999556 ) ) ;
#17491=EDGE_CURVE ( 'NONE', #40395, #64264, #53607, .T. ) ;
#17492=CARTESIAN_POINT ( 'NONE',  ( 6.140625000614516438, -3.027376345333610441, -5.243569643749999898 ) ) ;
#17493=CARTESIAN_POINT ( 'NONE',  ( 17.81250000122903288, 4.330127018922192761, -2.499999999999997780 ) ) ;
#17495=CARTESIAN_POINT ( 'NONE',  ( -4.243569643749997233, 10.89687500061451786, -27.54997392385601174 ) ) ;
#17497=CARTESIAN_POINT ( 'NONE',  ( 3.375000001229033320, 2.886751345948129099, -4.999999999999998224 ) ) ;
#17499=CARTESIAN_POINT ( 'NONE',  ( 18.19687500061451502, -3.027376345333614438, 5.243569643749998122 ) ) ;
#17500=CARTESIAN_POINT ( 'NONE',  ( -3.999999999999999112, 16.47500000122903430, 27.69059892324149885 ) ) ;
#17501=CARTESIAN_POINT ( 'NONE',  ( 15.62812500061451537, 6.421520780324663323E-16, -5.243569643749999010 ) ) ;
#17504=CARTESIAN_POINT ( 'NONE',  ( 29.40937500061451715, 0.000000000000000000, 5.243569643749999010 ) ) ;
#17505=CARTESIAN_POINT ( 'NONE',  ( 25.09687500061451715, -3.027376345333610441, -5.243569643749999898 ) ) ;
#17507=CARTESIAN_POINT ( 'NONE',  ( 12.44062500061451537, -3.027376345333610441, -5.243569643749999898 ) ) ;
#17508=CARTESIAN_POINT ( 'NONE',  ( 10.47187500061451715, 3.027376345333611329, 5.243569643749999010 ) ) ;
#17509=VERTEX_POINT ( 'NONE', #63498 ) ;
#17510=CARTESIAN_POINT ( 'NONE',  ( 29.50312500061451360, -4.541064518000417216, -2.621784821875001281 ) ) ;
#17511=CARTESIAN_POINT ( 'NONE',  ( 21.21562500061451573, 3.027376345333611329, 5.243569643749999010 ) ) ;
#17513=CARTESIAN_POINT ( 'NONE',  ( 4.907911205059083602E-16, 5.000000000000000000, -26.00000000000000000 ) ) ;
#17514=CARTESIAN_POINT ( 'NONE',  ( 10.87500000000000000, 6.123233995736764310E-16, -4.999999999999998224 ) ) ;
#17515=CARTESIAN_POINT ( 'NONE',  ( 21.75000000122903288, -2.886751345948125991, -5.000000000000000000 ) ) ;
#17516=CARTESIAN_POINT ( 'NONE',  ( 15.36562500061451608, 3.027376345333611329, 5.243569643749999010 ) ) ;
#17518=VERTEX_POINT ( 'NONE', #35419 ) ;
#17519=CARTESIAN_POINT ( 'NONE',  ( 20.17499999999999716, -4.330127018922194537, 2.499999999999995559 ) ) ;
#17520=CARTESIAN_POINT ( 'NONE',  ( 21.22500000000000142, 6.123233995736764310E-16, -4.999999999999998224 ) ) ;
#17521=CARTESIAN_POINT ( 'NONE',  ( 21.04687500061451644, -3.027376345333610441, -5.243569643749999898 ) ) ;
#17522=CARTESIAN_POINT ( 'NONE',  ( 25.79062500061451502, -3.027376345333614438, 5.243569643749998122 ) ) ;
#17525=CARTESIAN_POINT ( 'NONE',  ( 7.378125000614518036, -4.541064518000419881, 2.621784821874995952 ) ) ;
#17527=CARTESIAN_POINT ( 'NONE',  ( 14.10000000000000142, 4.330127018922192761, -2.499999999999997780 ) ) ;
#17528=CARTESIAN_POINT ( 'NONE',  ( 4.243569643749999898, 16.87812500061451715, 30.00000000000000000 ) ) ;
#17529=CARTESIAN_POINT ( 'NONE',  ( 29.54062500061451502, -3.027376345333610441, -5.243569643749999898 ) ) ;
#17530=CARTESIAN_POINT ( 'NONE',  ( 26.25937500061451857, 0.000000000000000000, 5.243569643749999010 ) ) ;
#17532=CARTESIAN_POINT ( 'NONE',  ( 25.04062500061451502, -3.027376345333610441, -5.243569643749999898 ) ) ;
#17533=CARTESIAN_POINT ( 'NONE',  ( 24.87187500061451573, 3.027376345333611329, 5.243569643749999010 ) ) ;
#17534=CARTESIAN_POINT ( 'NONE',  ( 2.121784821874999061, 17.85312500061459318, -33.67503911421598417 ) ) ;
#17535=CARTESIAN_POINT ( 'NONE',  ( 11.32500000000000107, 6.123233995736764310E-16, -4.999999999999998224 ) ) ;
#17536=CARTESIAN_POINT ( 'NONE',  ( 9.815625000614518925, 3.027376345333613106, -5.243569643749998122 ) ) ;
#17538=CARTESIAN_POINT ( 'NONE',  ( 28.79062500061451502, 6.054752690667223547, 3.707466751127219781E-16 ) ) ;
#17539=CARTESIAN_POINT ( 'NONE',  ( 26.76562500061451644, -6.054752690667223547, -1.112240025338166033E-15 ) ) ;
#17542=CARTESIAN_POINT ( 'NONE',  ( 20.03437500061451715, -4.541064518000419881, 2.621784821874995952 ) ) ;
#17543=CARTESIAN_POINT ( 'NONE',  ( -3.000416591977282496E-16, 15.69687500061451857, 25.09994784771203058 ) ) ;
#17544=EDGE_CURVE ( 'NONE', #28339, #45340, #23400, .T. ) ;
#17545=CARTESIAN_POINT ( 'NONE',  ( 18.15937500061451715, 0.000000000000000000, 5.243569643749999010 ) ) ;
#17546=CARTESIAN_POINT ( 'NONE',  ( 27.38437500061451857, 6.421520780324663323E-16, -5.243569643749999010 ) ) ;
#17547=CARTESIAN_POINT ( 'NONE',  ( 9.001249775931846008E-16, 16.37187500061451573, 34.90005215228797653 ) ) ;
#17548=CARTESIAN_POINT ( 'NONE',  ( 9.665625000614515017, -6.054752690667223547, -1.112240025338166033E-15 ) ) ;
#17549=CARTESIAN_POINT ( 'NONE',  ( 4.907911205059083602E-16, 5.000000000000000000, 33.99999999999999289 ) ) ;
#17550=CARTESIAN_POINT ( 'NONE',  ( 5.371875000614516615, 3.027376345333613106, -5.243569643749998122 ) ) ;
#17552=CARTESIAN_POINT ( 'NONE',  ( 8.540625000614518569, 6.054752690667223547, 3.707466751127219781E-16 ) ) ;
#17553=CARTESIAN_POINT ( 'NONE',  ( 11.78437500061451892, 4.541064518000418104, 2.621784821874999949 ) ) ;
#17554=CARTESIAN_POINT ( 'NONE',  ( 18.82500000122903216, 2.886751345948126879, 4.999999999999999112 ) ) ;
#17555=CARTESIAN_POINT ( 'NONE',  ( 6.271875000614517859, 3.027376345333613106, -5.243569643749998122 ) ) ;
#17556=CARTESIAN_POINT ( 'NONE',  ( 6.703125000614516438, 4.541064518000418104, -2.621784821874998173 ) ) ;
#17557=CARTESIAN_POINT ( 'NONE',  ( 5.090625000614516615, -3.027376345333614438, 5.243569643749998122 ) ) ;
#17559=CARTESIAN_POINT ( 'NONE',  ( 19.50937500061451857, 0.000000000000000000, 5.243569643749999010 ) ) ;
#17560=CARTESIAN_POINT ( 'NONE',  ( 2.000000000000001332, 13.06250000122903465, 33.46410161513774995 ) ) ;
#17562=CARTESIAN_POINT ( 'NONE',  ( 23.57812500061451289, -4.541064518000419881, 2.621784821874995952 ) ) ;
#17563=CARTESIAN_POINT ( 'NONE',  ( 12.17812500061451608, 4.541064518000418104, 2.621784821874999949 ) ) ;
#17564=CARTESIAN_POINT ( 'NONE',  ( 27.08437500061451786, 4.541064518000418104, 2.621784821874999949 ) ) ;
#17565=CARTESIAN_POINT ( 'NONE',  ( 10.45312500061451644, 0.000000000000000000, 5.243569643749999010 ) ) ;
#17566=CARTESIAN_POINT ( 'NONE',  ( -1.473772837211104303, 9.872922166578582903, -34.04916900799978663 ) ) ;
#17567=CARTESIAN_POINT ( 'NONE',  ( 12.11250000122903181, 0.000000000000000000, 4.999999999999998224 ) ) ;
#17568=CARTESIAN_POINT ( 'NONE',  ( 27.81562500061452070, 3.027376345333613106, -5.243569643749998122 ) ) ;
#17569=CARTESIAN_POINT ( 'NONE',  ( 2.121784821874999061, 12.90312500061451750, -33.67503911421598417 ) ) ;
#17570=CARTESIAN_POINT ( 'NONE',  ( 14.40000000122903323, -2.886751345948129988, 4.999999999999997335 ) ) ;
#17571=CARTESIAN_POINT ( 'NONE',  ( 11.21250000000000036, -5.773502691896255534, -1.060575238724906372E-15 ) ) ;
#17572=CARTESIAN_POINT ( 'NONE',  ( 20.72812500061451502, 4.541064518000418104, 2.621784821874999949 ) ) ;
#17573=CARTESIAN_POINT ( 'NONE',  ( 8.634375000614518569, 4.541064518000418104, 2.621784821874999949 ) ) ;
#17574=CARTESIAN_POINT ( 'NONE',  ( 7.500000001229034652, 5.773502691896255534, 3.535250795749688894E-16 ) ) ;
#17575=CARTESIAN_POINT ( 'NONE',  ( 17.28750000122903430, 6.123233995736764310E-16, -4.999999999999998224 ) ) ;
#17576=CARTESIAN_POINT ( 'NONE',  ( 13.56562500061451892, 3.027376345333611329, 5.243569643749999010 ) ) ;
#17577=CARTESIAN_POINT ( 'NONE',  ( 15.40312500061451573, 0.000000000000000000, 5.243569643749999010 ) ) ;
#17578=( BOUNDED_CURVE ( )  B_SPLINE_CURVE ( 2, ( #39288, #56977, #28556, #6381, #23362, #57701, #40364, #34811, #61802 ),
 .UNSPECIFIED., .F., .F. ) 
 B_SPLINE_CURVE_WITH_KNOTS ( ( 3, 2, 2, 2, 3 ),
 ( 0.5760869565217391353, 0.5797101449275362528, 0.5869565217391304879, 0.5942028985507246119, 0.5978260869565217295 ),
 .UNSPECIFIED. ) 
 CURVE ( )  GEOMETRIC_REPRESENTATION_ITEM ( )  RATIONAL_B_SPLINE_CURVE ( ( 0.9330127018922194093, 0.9330127018922194093, 1.000000000000000000, 0.8660254037844387076, 1.000000000000000000, 0.8660254037844387076, 1.000000000000000000, 0.9330127018922194093, 0.9330127018922194093 ) ) 
 REPRESENTATION_ITEM ( '' )  );
#17579=CARTESIAN_POINT ( 'NONE',  ( 25.20000000122903216, -2.886751345948129988, 4.999999999999997335 ) ) ;
#17580=CARTESIAN_POINT ( 'NONE',  ( 20.51249999999999929, 2.886751345948126879, 4.999999999999999112 ) ) ;
#17581=CARTESIAN_POINT ( 'NONE',  ( 22.17187500061451644, 3.027376345333611329, 5.243569643749999010 ) ) ;
#17583=EDGE_CURVE ( 'NONE', #47866, #54008, #25057, .T. ) ;
#17584=CARTESIAN_POINT ( 'NONE',  ( 10.46250000122903323, -4.330127018922190985, -2.500000000000001332 ) ) ;
#17586=CARTESIAN_POINT ( 'NONE',  ( 8.184375000614515727, 4.541064518000418104, 2.621784821874999949 ) ) ;
#17587=CARTESIAN_POINT ( 'NONE',  ( 29.22187500061451715, 3.027376345333613106, -5.243569643749998122 ) ) ;
#17588=CARTESIAN_POINT ( 'NONE',  ( 3.346875000614518036, -3.027376345333614438, 5.243569643749998122 ) ) ;
#17589=CARTESIAN_POINT ( 'NONE',  ( 24.47812500061451502, -4.541064518000419881, 2.621784821874995952 ) ) ;
#17592=CARTESIAN_POINT ( 'NONE',  ( 8.596875000614518925, 6.054752690667223547, 3.707466751127219781E-16 ) ) ;
#17593=CARTESIAN_POINT ( 'NONE',  ( 15.82499999999999929, 6.123233995736764310E-16, -4.999999999999998224 ) ) ;
#17594=CARTESIAN_POINT ( 'NONE',  ( 26.84062500061451573, -3.027376345333610441, -5.243569643749999898 ) ) ;
#17595=CARTESIAN_POINT ( 'NONE',  ( 6.384375000614516793, 4.541064518000418104, 2.621784821874999949 ) ) ;
#17596=CARTESIAN_POINT ( 'NONE',  ( -3.999999999999999112, 16.51250000122903216, -30.00000000000000000 ) ) ;
#17597=CARTESIAN_POINT ( 'NONE',  ( 26.29687500061451644, -3.027376345333614438, 5.243569643749998122 ) ) ;
#17598=CARTESIAN_POINT ( 'NONE',  ( -3.000416591977282496E-16, 10.24062500061459424, 25.09994784771203058 ) ) ;
#17599=CARTESIAN_POINT ( 'NONE',  ( 18.52499999999999858, 6.123233995736764310E-16, -4.999999999999998224 ) ) ;
#17601=CARTESIAN_POINT ( 'NONE',  ( 27.59999999999999787, 4.330127018922192761, -2.499999999999997780 ) ) ;
#17602=CARTESIAN_POINT ( 'NONE',  ( 27.64687500061452141, -3.027376345333614438, 5.243569643749998122 ) ) ;
#17603=ORIENTED_EDGE ( 'NONE', *, *, #63887, .F. ) ;
#17604=CARTESIAN_POINT ( 'NONE',  ( 16.56562500061451715, 3.027376345333613106, -5.243569643749998122 ) ) ;
#17605=CARTESIAN_POINT ( 'NONE',  ( 7.640625000614517326, 6.054752690667223547, 3.707466751127219781E-16 ) ) ;
#17607=CARTESIAN_POINT ( 'NONE',  ( 3.984375000614517326, 6.421520780324663323E-16, -5.243569643749999010 ) ) ;
#17608=CARTESIAN_POINT ( 'NONE',  ( 16.42500000122903359, 2.886751345948129099, -4.999999999999998224 ) ) ;
#17609=CARTESIAN_POINT ( 'NONE',  ( 22.34999999999999787, 0.000000000000000000, 4.999999999999998224 ) ) ;
#17610=CARTESIAN_POINT ( 'NONE',  ( 29.06250000000000000, 2.886751345948126879, 4.999999999999999112 ) ) ;
#17611=CARTESIAN_POINT ( 'NONE',  ( 4.846875000614519813, -3.027376345333610441, -5.243569643749999898 ) ) ;
#17612=CARTESIAN_POINT ( 'NONE',  ( 9.721875000614517148, -6.054752690667223547, -1.112240025338166033E-15 ) ) ;
#17613=CARTESIAN_POINT ( 'NONE',  ( 22.20937500061451431, 0.000000000000000000, 5.243569643749999010 ) ) ;
#17614=CARTESIAN_POINT ( 'NONE',  ( 9.528763966825557376E-15, 17.41249999999999787, -26.00000000000000000 ) ) ;
#17615=ORIENTED_EDGE ( 'NONE', *, *, #21641, .F. ) ;
#17616=CARTESIAN_POINT ( 'NONE',  ( 3.196875000614516793, 6.054752690667223547, 3.707466751127219781E-16 ) ) ;
#17617=CARTESIAN_POINT ( 'NONE',  ( 6.984375000614516438, -4.541064518000419881, 2.621784821874995952 ) ) ;
#17618=CARTESIAN_POINT ( 'NONE',  ( 17.66249999999999787, 2.886751345948129099, -4.999999999999998224 ) ) ;
#17619=CARTESIAN_POINT ( 'NONE',  ( 17.01562500061451644, 3.027376345333613106, -5.243569643749998122 ) ) ;
#17622=EDGE_CURVE ( 'NONE', #18316, #54892, #56420, .T. ) ;
#17624=CARTESIAN_POINT ( 'NONE',  ( 9.365625000614519635, 3.027376345333613106, -5.243569643749998122 ) ) ;
#17625=CARTESIAN_POINT ( 'NONE',  ( 27.42187500061451644, 3.027376345333613106, -5.243569643749998122 ) ) ;
#17626=CARTESIAN_POINT ( 'NONE',  ( 27.49687500061451217, 6.054752690667223547, 3.707466751127219781E-16 ) ) ;
#17627=CARTESIAN_POINT ( 'NONE',  ( 7.500000000000000000, 0.000000000000000000, 4.999999999999998224 ) ) ;
#17628=CARTESIAN_POINT ( 'NONE',  ( -2.000000000000000000, 14.18750000122903288, 26.53589838486224650 ) ) ;
#17629=CARTESIAN_POINT ( 'NONE',  ( 8.662500001229034297, -4.330127018922190985, -2.500000000000001332 ) ) ;
#17630=CARTESIAN_POINT ( 'NONE',  ( 21.12187500061451573, 3.027376345333613106, -5.243569643749998122 ) ) ;
#17631=CARTESIAN_POINT ( 'NONE',  ( 10.69687500061451679, -3.027376345333610441, -5.243569643749999898 ) ) ;
#17634=CARTESIAN_POINT ( 'NONE',  ( 15.62812500061451537, 6.421520780324663323E-16, -5.243569643749999010 ) ) ;
#17635=CARTESIAN_POINT ( 'NONE',  ( 27.41250000122903430, 0.000000000000000000, 4.999999999999998224 ) ) ;
#17636=CARTESIAN_POINT ( 'NONE',  ( 13.02187500061451608, 3.027376345333613106, -5.243569643749998122 ) ) ;
#17637=CARTESIAN_POINT ( 'NONE',  ( 2.000000000000001332, 12.61250000122903536, 33.46410161513774995 ) ) ;
#17638=CARTESIAN_POINT ( 'NONE',  ( 15.66562500061451857, 3.027376345333613106, -5.243569643749998122 ) ) ;
#17639=CARTESIAN_POINT ( 'NONE',  ( 1.999999999999998668, 18.95000000000000284, -33.46410161513775705 ) ) ;
#17640=CARTESIAN_POINT ( 'NONE',  ( 26.37187500061451217, -6.054752690667223547, -1.112240025338166033E-15 ) ) ;
#17641=CARTESIAN_POINT ( 'NONE',  ( 2.904760919847030110, -4.069688439982819261, 3.306457108496466901 ) ) ;
#17642=CARTESIAN_POINT ( 'NONE',  ( 12.63750000122903394, -4.330127018922194537, 2.499999999999995559 ) ) ;
#17644=CARTESIAN_POINT ( 'NONE',  ( -4.243569643749998122, 18.09687500061451715, -27.54997392385601174 ) ) ;
#17645=CARTESIAN_POINT ( 'NONE',  ( 18.27187500061451431, -6.054752690667223547, -1.112240025338166033E-15 ) ) ;
#17646=CARTESIAN_POINT ( 'NONE',  ( 19.35000000122903430, -2.886751345948129988, 4.999999999999997335 ) ) ;
#17647=CARTESIAN_POINT ( 'NONE',  ( 14.93437500061451750, 4.541064518000418104, 2.621784821874999949 ) ) ;
#17648=CARTESIAN_POINT ( 'NONE',  ( 9.001249775931846008E-16, 19.46562500061451573, -25.09994784771203058 ) ) ;
#17649=CARTESIAN_POINT ( 'NONE',  ( 21.45000000122903216, 5.773502691896255534, 3.535250795749688894E-16 ) ) ;
#17650=CARTESIAN_POINT ( 'NONE',  ( 16.19062500061451715, 6.054752690667223547, 3.707466751127219781E-16 ) ) ;
#17651=CARTESIAN_POINT ( 'NONE',  ( 28.86562500061451786, 3.027376345333611329, 5.243569643749999010 ) ) ;
#17652=VERTEX_POINT ( 'NONE', #3642 ) ;
#17654=CARTESIAN_POINT ( 'NONE',  ( 18.07499999999999929, 6.123233995736764310E-16, -4.999999999999998224 ) ) ;
#17655=CARTESIAN_POINT ( 'NONE',  ( 27.44999999999999929, -4.330127018922190985, -2.500000000000001332 ) ) ;
#17656=CARTESIAN_POINT ( 'NONE',  ( 2.064291216241245230, 4.560108959200714907, 33.43572587555581066 ) ) ;
#17657=CARTESIAN_POINT ( 'NONE',  ( 14.55000000122903181, -2.886751345948125991, -5.000000000000000000 ) ) ;
#17658=CARTESIAN_POINT ( 'NONE',  ( 20.16562500061451146, 3.027376345333613106, -5.243569643749998122 ) ) ;
#17659=CARTESIAN_POINT ( 'NONE',  ( 23.72812500061451502, 6.421520780324663323E-16, -5.243569643749999010 ) ) ;
#17660=CARTESIAN_POINT ( 'NONE',  ( 4.378125000614518925, 6.421520780324663323E-16, -5.243569643749999010 ) ) ;
#17662=CARTESIAN_POINT ( 'NONE',  ( -5.810221930991193690E-16, 11.90000000122903501, 26.00000000000000355 ) ) ;
#17664=CARTESIAN_POINT ( 'NONE',  ( 29.48437500061451644, -4.541064518000419881, 2.621784821874995952 ) ) ;
#17665=CARTESIAN_POINT ( 'NONE',  ( -3.999999999999999112, 10.21250000122903501, -30.00000000000000000 ) ) ;
#17666=CARTESIAN_POINT ( 'NONE',  ( -3.000416591977282496E-16, 15.69687500061451857, -34.90005215228797653 ) ) ;
#17667=CARTESIAN_POINT ( 'NONE',  ( 5.737500001229033586, 4.330127018922191873, 2.499999999999999556 ) ) ;
#17668=CARTESIAN_POINT ( 'NONE',  ( 7.724999999999999645, 6.123233995736764310E-16, -4.999999999999998224 ) ) ;
#17669=ADVANCED_FACE ( 'NONE', ( #71228 ), #43530, .F. ) ;
#17670=CARTESIAN_POINT ( 'NONE',  ( 3.937500001229034208, 4.330127018922191873, 2.499999999999999556 ) ) ;
#17671=CARTESIAN_POINT ( 'NONE',  ( 9.121875000614517504, 3.027376345333611329, 5.243569643749999010 ) ) ;
#17672=DIRECTION ( 'NONE',  ( 0.000000000000000000, 0.000000000000000000, 1.000000000000000000 ) ) ;
#17673=CARTESIAN_POINT ( 'NONE',  ( 3.009375000614516793, -4.541064518000417216, -2.621784821875001281 ) ) ;
#17675=CARTESIAN_POINT ( 'NONE',  ( -1.394453263437886604E-15, 19.32500000122903216, 33.99999999999999289 ) ) ;
#17676=CARTESIAN_POINT ( 'NONE',  ( 6.684375000614518392, 6.421520780324663323E-16, -5.243569643749999010 ) ) ;
#17677=CARTESIAN_POINT ( 'NONE',  ( 13.28437500061451715, -4.541064518000419881, 2.621784821874995952 ) ) ;
#17678=FACE_OUTER_BOUND ( 'NONE', #44379, .T. ) ;
#17679=CARTESIAN_POINT ( 'NONE',  ( 7.162500000000001421, -5.773502691896255534, -1.060575238724906372E-15 ) ) ;
#17680=CARTESIAN_POINT ( 'NONE',  ( -4.243569643749998122, 17.59062500061459744, 32.45002607614398471 ) ) ;
#17681=CARTESIAN_POINT ( 'NONE',  ( 22.17187500061451644, 3.027376345333611329, 5.243569643749999010 ) ) ;
#17683=CARTESIAN_POINT ( 'NONE',  ( 26.96250000122903145, 0.000000000000000000, 4.999999999999998224 ) ) ;
#17685=CARTESIAN_POINT ( 'NONE',  ( 22.49062500061451431, 6.054752690667223547, 3.707466751127219781E-16 ) ) ;
#17686=CARTESIAN_POINT ( 'NONE',  ( 16.11562500061451786, 3.027376345333613106, -5.243569643749998122 ) ) ;
#17688=CARTESIAN_POINT ( 'NONE',  ( 12.75937500061451857, 0.000000000000000000, 5.243569643749999010 ) ) ;
#17689=CARTESIAN_POINT ( 'NONE',  ( 29.36250000000000071, 2.886751345948129099, -4.999999999999998224 ) ) ;
#17690=CARTESIAN_POINT ( 'NONE',  ( 23.96250000122903145, -4.330127018922190985, -2.500000000000001332 ) ) ;
#17692=CARTESIAN_POINT ( 'NONE',  ( 11.70937500061451608, 4.541064518000418104, -2.621784821874998173 ) ) ;
#17693=CARTESIAN_POINT ( 'NONE',  ( 29.29687500061451644, 6.054752690667223547, 3.707466751127219781E-16 ) ) ;
#17694=CARTESIAN_POINT ( 'NONE',  ( 3.834375000614519635, -4.541064518000419881, 2.621784821874995952 ) ) ;
#17695=CARTESIAN_POINT ( 'NONE',  ( 18.52499999999999858, 6.123233995736764310E-16, -4.999999999999998224 ) ) ;
#17696=CARTESIAN_POINT ( 'NONE',  ( 23.22187500061451715, -6.054752690667223547, -1.112240025338166033E-15 ) ) ;
#17697=CARTESIAN_POINT ( 'NONE',  ( 15.27187500061451786, 3.027376345333613106, -5.243569643749998122 ) ) ;
#17699=CARTESIAN_POINT ( 'NONE',  ( 24.97499999999999787, 4.330127018922191873, 2.499999999999999556 ) ) ;
#17702=CARTESIAN_POINT ( 'NONE',  ( 17.42812500061451786, 6.421520780324663323E-16, -5.243569643749999010 ) ) ;
#17703=CARTESIAN_POINT ( 'NONE',  ( 6.075000000000000178, 4.330127018922191873, 2.499999999999999556 ) ) ;
#17704=CARTESIAN_POINT ( 'NONE',  ( 3.999999999999999112, 13.58750000122903323, 30.00000000000000000 ) ) ;
#17705=CARTESIAN_POINT ( 'NONE',  ( 17.10000000000000142, -4.330127018922190985, -2.500000000000001332 ) ) ;
#17707=CARTESIAN_POINT ( 'NONE',  ( -3.000416591977282496E-16, 12.49062500061451608, 25.09994784771203058 ) ) ;
#17709=CARTESIAN_POINT ( 'NONE',  ( 27.42187500061451644, 3.027376345333613106, -5.243569643749998122 ) ) ;
#17710=ORIENTED_EDGE ( 'NONE', *, *, #47762, .T. ) ;
#17711=CARTESIAN_POINT ( 'NONE',  ( 22.79062500061451502, -3.027376345333610441, -5.243569643749999898 ) ) ;
#17712=CARTESIAN_POINT ( 'NONE',  ( 21.08437500061451786, 6.421520780324663323E-16, -5.243569643749999010 ) ) ;
#17713=CARTESIAN_POINT ( 'NONE',  ( 4.425000000000001599, -4.330127018922194537, 2.499999999999995559 ) ) ;
#17714=CARTESIAN_POINT ( 'NONE',  ( 7.978125000614517681, 6.421520780324663323E-16, -5.243569643749999010 ) ) ;
#17715=CARTESIAN_POINT ( 'NONE',  ( 23.99062500061451786, -3.027376345333614438, 5.243569643749998122 ) ) ;
#17716=CARTESIAN_POINT ( 'NONE',  ( 11.52187500061451608, -6.054752690667223547, -1.112240025338166033E-15 ) ) ;
#17717=CARTESIAN_POINT ( 'NONE',  ( 17.89687500061451431, -3.027376345333610441, -5.243569643749999898 ) ) ;
#17718=CARTESIAN_POINT ( 'NONE',  ( -4.243569643749999898, 18.45312500061451644, 30.00000000000000000 ) ) ;
#17719=CARTESIAN_POINT ( 'NONE',  ( 19.72500000122903074, 2.886751345948126879, 4.999999999999999112 ) ) ;
#17721=CARTESIAN_POINT ( 'NONE',  ( 9.740625000614519635, -3.027376345333610441, -5.243569643749999898 ) ) ;
#17722=CARTESIAN_POINT ( 'NONE',  ( 6.721875000614518925, 3.027376345333613106, -5.243569643749998122 ) ) ;
#17723=CARTESIAN_POINT ( 'NONE',  ( 5.034375000614519813, 4.541064518000418104, 2.621784821874999949 ) ) ;
#17724=( BOUNDED_CURVE ( )  B_SPLINE_CURVE ( 2, ( #41458, #51458, #35900, #58424, #29286, #18540, #12647 ),
 .UNSPECIFIED., .F., .F. ) 
 B_SPLINE_CURVE_WITH_KNOTS ( ( 3, 2, 2, 3 ),
 ( 0.1999999999999999556, 0.2027777777777777235, 0.2055555555555554914, 0.2083333333333332871 ),
 .UNSPECIFIED. ) 
 CURVE ( )  GEOMETRIC_REPRESENTATION_ITEM ( )  RATIONAL_B_SPLINE_CURVE ( ( 1.000000000000002665, 0.8660254037844360431, 1.000000000000000000, 0.8660254037844387076, 1.000000000000000000, 0.8660254037844413721, 0.9999999999999973355 ) ) 
 REPRESENTATION_ITEM ( '' )  );
#17726=CARTESIAN_POINT ( 'NONE',  ( 24.23437500061451644, 6.421520780324663323E-16, -5.243569643749999010 ) ) ;
#17727=CARTESIAN_POINT ( 'NONE',  ( 15.81562500061451537, 3.027376345333611329, 5.243569643749999010 ) ) ;
#17728=CARTESIAN_POINT ( 'NONE',  ( 26.36250000122903003, 4.330127018922192761, -2.499999999999997780 ) ) ;
#17729=CARTESIAN_POINT ( 'NONE',  ( 28.97812500061451502, -4.541064518000419881, 2.621784821874995952 ) ) ;
#17730=CARTESIAN_POINT ( 'NONE',  ( 21.75937500061451502, 0.000000000000000000, 5.243569643749999010 ) ) ;
#17731=CARTESIAN_POINT ( 'NONE',  ( 16.82812500061451644, -4.541064518000419881, 2.621784821874995952 ) ) ;
#17732=CARTESIAN_POINT ( 'NONE',  ( -3.000416591977282496E-16, 19.74687500061451928, 25.09994784771203058 ) ) ;
#17733=CARTESIAN_POINT ( 'NONE',  ( 22.11562500061451786, 3.027376345333611329, 5.243569643749999010 ) ) ;
#17736=CARTESIAN_POINT ( 'NONE',  ( 26.73749999999999716, 5.773502691896255534, 3.535250795749688894E-16 ) ) ;
#17737=CARTESIAN_POINT ( 'NONE',  ( 4.000000000000000000, 12.53749999999999964, -27.69059892324149530 ) ) ;
#17739=CARTESIAN_POINT ( 'NONE',  ( 29.20312500061451644, 4.541064518000418104, -2.621784821874998173 ) ) ;
#17740=CARTESIAN_POINT ( 'NONE',  ( 9.965625000614517504, 3.027376345333611329, 5.243569643749999010 ) ) ;
#17741=CARTESIAN_POINT ( 'NONE',  ( 22.12500000122903288, -5.773502691896255534, -1.060575238724906372E-15 ) ) ;
#17742=CARTESIAN_POINT ( 'NONE',  ( 27.14062500061451644, -3.027376345333614438, 5.243569643749998122 ) ) ;
#17743=CARTESIAN_POINT ( 'NONE',  ( 27.59999999999999787, 4.330127018922192761, -2.499999999999997780 ) ) ;
#17744=CARTESIAN_POINT ( 'NONE',  ( -1.999999999999997113, 17.93750000122903288, -26.53589838486224295 ) ) ;
#17745=CARTESIAN_POINT ( 'NONE',  ( -3.999999999999997335, 12.50000000122903465, 32.30940107675850470 ) ) ;
#17746=CARTESIAN_POINT ( 'NONE',  ( 11.12812500061451715, 6.421520780324663323E-16, -5.243569643749999010 ) ) ;
#17748=CARTESIAN_POINT ( 'NONE',  ( 8.203125000614518214, 0.000000000000000000, 5.243569643749999010 ) ) ;
#17749=CARTESIAN_POINT ( 'NONE',  ( 4.790625000614518569, -3.027376345333610441, -5.243569643749999898 ) ) ;
#17752=CARTESIAN_POINT ( 'NONE',  ( 14.69999999999999929, 0.000000000000000000, 4.999999999999998224 ) ) ;
#17753=CARTESIAN_POINT ( 'NONE',  ( 15.19687500061451857, -3.027376345333610441, -5.243569643749999898 ) ) ;
#17754=CARTESIAN_POINT ( 'NONE',  ( 10.35000000122903074, -2.886751345948129988, 4.999999999999997335 ) ) ;
#17755=CARTESIAN_POINT ( 'NONE',  ( 19.13437500061451857, -4.541064518000419881, 2.621784821874995952 ) ) ;
#17757=CARTESIAN_POINT ( 'NONE',  ( 21.19687500061451502, 6.054752690667223547, 3.707466751127219781E-16 ) ) ;
#17758=CARTESIAN_POINT ( 'NONE',  ( 4.243569643749999898, 13.24062500061451786, -27.54997392385601529 ) ) ;
#17759=CARTESIAN_POINT ( 'NONE',  ( -1.071796769724483234, 16.75759618943233420, 25.99999999999999645 ) ) ;
#17762=CARTESIAN_POINT ( 'NONE',  ( 27.96562500061451928, 3.027376345333611329, 5.243569643749999010 ) ) ;
#17763=CARTESIAN_POINT ( 'NONE',  ( 5.287500001229035185, 4.330127018922191873, 2.499999999999999556 ) ) ;
#17764=CARTESIAN_POINT ( 'NONE',  ( 28.05937500061451573, 0.000000000000000000, 5.243569643749999010 ) ) ;
#17765=( BOUNDED_CURVE ( )  B_SPLINE_CURVE ( 2, ( #55430, #5182, #33254, #4100, #37337, #55792, #44718, #54696, #55066 ),
 .UNSPECIFIED., .F., .F. ) 
 B_SPLINE_CURVE_WITH_KNOTS ( ( 3, 2, 2, 2, 3 ),
 ( 0.7717391304347825942, 0.7753623188405797118, 0.7826086956521739468, 0.7898550724637680709, 0.7934782608695651884 ),
 .UNSPECIFIED. ) 
 CURVE ( )  GEOMETRIC_REPRESENTATION_ITEM ( )  RATIONAL_B_SPLINE_CURVE ( ( 0.9330127018922194093, 0.9330127018922194093, 1.000000000000000000, 0.8660254037844387076, 1.000000000000000000, 0.8660254037844387076, 1.000000000000000000, 0.9330127018922194093, 0.9330127018922194093 ) ) 
 REPRESENTATION_ITEM ( '' )  );
#17766=CARTESIAN_POINT ( 'NONE',  ( 24.11249999999999716, 2.886751345948126879, 4.999999999999999112 ) ) ;
#17767=CARTESIAN_POINT ( 'NONE',  ( 6.178125000614518747, 6.421520780324663323E-16, -5.243569643749999010 ) ) ;
#17769=CARTESIAN_POINT ( 'NONE',  ( 19.92187500061451644, 3.027376345333611329, 5.243569643749999010 ) ) ;
#17771=CARTESIAN_POINT ( 'NONE',  ( 4.715625000614516615, -6.054752690667223547, -1.112240025338166033E-15 ) ) ;
#17772=CARTESIAN_POINT ( 'NONE',  ( 11.03437500061451715, -4.541064518000419881, 2.621784821874995952 ) ) ;
#17773=ORIENTED_EDGE ( 'NONE', *, *, #11270, .F. ) ;
#17774=CARTESIAN_POINT ( 'NONE',  ( 19.20937500061451786, -4.541064518000417216, -2.621784821875001281 ) ) ;
#17775=LINE ( 'NONE', #28521, #48919 ) ;
#17776=CARTESIAN_POINT ( 'NONE',  ( 28.46249999999999858, 2.886751345948129099, -4.999999999999998224 ) ) ;
#17777=CARTESIAN_POINT ( 'NONE',  ( 3.637500000000001954, -2.886751345948125991, -5.000000000000000000 ) ) ;
#17779=CARTESIAN_POINT ( 'NONE',  ( 27.93750000000000355, -2.886751345948109559, -5.000000000000028422 ) ) ;
#17780=EDGE_LOOP ( 'NONE', ( #11002, #46327, #45545, #71962 ) ) ;
#17781=CARTESIAN_POINT ( 'NONE',  ( 9.937500000000001776, -2.886751345948125991, -5.000000000000000000 ) ) ;
#17783=CARTESIAN_POINT ( 'NONE',  ( 25.37812500061451715, -4.541064518000419881, 2.621784821874995952 ) ) ;
#17784=CARTESIAN_POINT ( 'NONE',  ( 14.43750000000000000, -2.886751345948125991, -5.000000000000000000 ) ) ;
#17785=CARTESIAN_POINT ( 'NONE',  ( 11.73750000122903181, -4.330127018922194537, 2.499999999999995559 ) ) ;
#17786=CARTESIAN_POINT ( 'NONE',  ( 8.765625000614518214, -6.054752690667223547, -1.112240025338166033E-15 ) ) ;
#17787=CARTESIAN_POINT ( 'NONE',  ( 23.28750000000000142, -2.886751345948129988, 4.999999999999997335 ) ) ;
#17789=CARTESIAN_POINT ( 'NONE',  ( 21.44062500061452070, -3.027376345333610441, -5.243569643749999898 ) ) ;
#17790=CARTESIAN_POINT ( 'NONE',  ( 5.362500001229033586, 0.000000000000000000, 4.999999999999998224 ) ) ;
#17791=CARTESIAN_POINT ( 'NONE',  ( 28.91250000122903074, -4.330127018922190985, -2.500000000000001332 ) ) ;
#17793=CARTESIAN_POINT ( 'NONE',  ( 6.937499999999999112, 5.773502691896255534, 3.535250795749688894E-16 ) ) ;
#17794=VERTEX_POINT ( 'NONE', #59034 ) ;
#17795=CARTESIAN_POINT ( 'NONE',  ( 21.14062500061451289, 6.054752690667223547, 3.707466751127219781E-16 ) ) ;
#17796=CARTESIAN_POINT ( 'NONE',  ( 28.15312500061451573, -4.541064518000417216, -2.621784821875001281 ) ) ;
#17797=CARTESIAN_POINT ( 'NONE',  ( 28.98750000122903359, 6.123233995736764310E-16, -4.999999999999998224 ) ) ;
#17798=CARTESIAN_POINT ( 'NONE',  ( 19.50937500061451857, 0.000000000000000000, 5.243569643749999010 ) ) ;
#17799=CARTESIAN_POINT ( 'NONE',  ( 13.41562500061451502, 3.027376345333613106, -5.243569643749998122 ) ) ;
#17801=CARTESIAN_POINT ( 'NONE',  ( 29.47500000122903430, 2.886751345948129099, -4.999999999999998224 ) ) ;
#17803=CARTESIAN_POINT ( 'NONE',  ( 16.15312500061451573, 4.541064518000418104, -2.621784821874998173 ) ) ;
#17804=DIRECTION ( 'NONE',  ( -1.000000000000000000, -0.000000000000000000, -0.000000000000000000 ) ) ;
#17805=CARTESIAN_POINT ( 'NONE',  ( 3.487500001229035362, 4.330127018922191873, 2.499999999999999556 ) ) ;
#17806=CARTESIAN_POINT ( 'NONE',  ( 13.65937500061451715, 0.000000000000000000, 5.243569643749999010 ) ) ;
#17807=CARTESIAN_POINT ( 'NONE',  ( 12.60937500061451821, 4.541064518000418104, -2.621784821874998173 ) ) ;
#17808=CARTESIAN_POINT ( 'NONE',  ( 20.07187500061451857, -6.054752690667223547, -1.112240025338166033E-15 ) ) ;
#17810=CARTESIAN_POINT ( 'NONE',  ( -5.840105773466367722, 8.117609419225253475, 31.39035167484127697 ) ) ;
#17811=CARTESIAN_POINT ( 'NONE',  ( 24.40312500061451573, 0.000000000000000000, 5.243569643749999010 ) ) ;
#17812=CARTESIAN_POINT ( 'NONE',  ( 17.74687500061451928, -3.027376345333614438, 5.243569643749998122 ) ) ;
#17813=CARTESIAN_POINT ( 'NONE',  ( 25.26562500061451289, 3.027376345333611329, 5.243569643749999010 ) ) ;
#17814=LINE ( 'NONE', #45920, #19079 ) ;
#17815=CARTESIAN_POINT ( 'NONE',  ( 8.484601909799253346E-16, 15.61250000000000249, 34.61880215351700230 ) ) ;
#17816=CARTESIAN_POINT ( 'NONE',  ( 28.45312500061451289, 0.000000000000000000, 5.243569643749999010 ) ) ;
#17817=CARTESIAN_POINT ( 'NONE',  ( 8.737500001229033586, 6.123233995736764310E-16, -4.999999999999998224 ) ) ;
#17818=CARTESIAN_POINT ( 'NONE',  ( 5.925000001229033586, -5.773502691896255534, -1.060575238724906372E-15 ) ) ;
#17820=CARTESIAN_POINT ( 'NONE',  ( 27.30000000122903359, 5.773502691896255534, 3.535250795749688894E-16 ) ) ;
#17823=CARTESIAN_POINT ( 'NONE',  ( 9.909375000614517148, 4.541064518000418104, -2.621784821874998173 ) ) ;
#17825=CARTESIAN_POINT ( 'NONE',  ( 18.02812500061451573, 4.541064518000418104, 2.621784821874999949 ) ) ;
#17826=CARTESIAN_POINT ( 'NONE',  ( 10.88437500061451679, 4.541064518000418104, 2.621784821874999949 ) ) ;
#17827=CARTESIAN_POINT ( 'NONE',  ( 29.62500000122903288, 2.886751345948126879, 4.999999999999999112 ) ) ;
#17828=CARTESIAN_POINT ( 'NONE',  ( 20.89687500061451786, -3.027376345333614438, 5.243569643749998122 ) ) ;
#17829=CARTESIAN_POINT ( 'NONE',  ( 6.271875000614517859, 3.027376345333613106, -5.243569643749998122 ) ) ;
#17830=CARTESIAN_POINT ( 'NONE',  ( 3.160880256176461511, -3.874123901750303300, -3.160880256176591185 ) ) ;
#17832=CARTESIAN_POINT ( 'NONE',  ( 8.315625000614515372, -6.054752690667223547, -1.112240025338166033E-15 ) ) ;
#17833=CARTESIAN_POINT ( 'NONE',  ( 21.17812500061451431, 4.541064518000418104, 2.621784821874999949 ) ) ;
#17835=CARTESIAN_POINT ( 'NONE',  ( 5.850000001229035185, -2.886751345948129988, 4.999999999999997335 ) ) ;
#17836=CARTESIAN_POINT ( 'NONE',  ( 14.72812500061451679, 6.421520780324663323E-16, -5.243569643749999010 ) ) ;
#17837=CARTESIAN_POINT ( 'NONE',  ( 13.04062500061451502, 6.054752690667223547, 3.707466751127219781E-16 ) ) ;
#17839=CARTESIAN_POINT ( 'NONE',  ( 12.18750000000000000, -2.886751345948125991, -5.000000000000000000 ) ) ;
#17840=CARTESIAN_POINT ( 'NONE',  ( 8.925000001229033586, 2.886751345948126879, 4.999999999999999112 ) ) ;
#17841=CARTESIAN_POINT ( 'NONE',  ( 5.915625000614515905, 3.027376345333611329, 5.243569643749999010 ) ) ;
#17842=ADVANCED_FACE ( 'NONE', ( #47973 ), #60131, .F. ) ;
#17843=CARTESIAN_POINT ( 'NONE',  ( 17.96250000122903501, 0.000000000000000000, 4.999999999999998224 ) ) ;
#17846=CARTESIAN_POINT ( 'NONE',  ( -2.121784821874996840, 10.93437500061451928, -26.32496088578401583 ) ) ;
#17847=FACE_OUTER_BOUND ( 'NONE', #39264, .T. ) ;
#17848=CARTESIAN_POINT ( 'NONE',  ( 4.125000001229034652, -5.773502691896255534, -1.060575238724906372E-15 ) ) ;
#17849=CARTESIAN_POINT ( 'NONE',  ( 28.50000000122903643, -2.886751345948155745, -4.999999999999948486 ) ) ;
#17851=CARTESIAN_POINT ( 'NONE',  ( 18.12187500061451573, 3.027376345333611329, 5.243569643749999010 ) ) ;
#17852=COLOUR_RGB ( '',0.8941176470588234615, 0.8941176470588234615, 0.8941176470588234615 ) ;
#17854=CARTESIAN_POINT ( 'NONE',  ( 30.00000000000000000, 0.000000000000000000, 0.000000000000000000 ) ) ;
#17855=CARTESIAN_POINT ( 'NONE',  ( 12.89062500061451821, -3.027376345333610441, -5.243569643749999898 ) ) ;
#17857=CARTESIAN_POINT ( 'NONE',  ( 0.000000000000000000, 20.00000000000000000, 30.00000000000000000 ) ) ;
#17858=CARTESIAN_POINT ( 'NONE',  ( 28.80937500061451573, 4.541064518000418104, -2.621784821874998173 ) ) ;
#17859=CARTESIAN_POINT ( 'NONE',  ( 26.10937500061451644, 4.541064518000418104, -2.621784821874998173 ) ) ;
#17861=CARTESIAN_POINT ( 'NONE',  ( 13.19062500061451537, -3.027376345333614438, 5.243569643749998122 ) ) ;
#17862=CARTESIAN_POINT ( 'NONE',  ( 9.834375000614517859, 6.421520780324663323E-16, -5.243569643749999010 ) ) ;
#17863=ORIENTED_EDGE ( 'NONE', *, *, #50844, .T. ) ;
#17864=CARTESIAN_POINT ( 'NONE',  ( 2.896627646276317858, -4.075481355475408130, -3.116761479535832713 ) ) ;
#17865=CARTESIAN_POINT ( 'NONE',  ( 20.91562500061451502, -6.054752690667223547, -1.112240025338166033E-15 ) ) ;
#17866=DIRECTION ( 'NONE',  ( -1.000000000000000000, -0.000000000000000000, -0.000000000000000000 ) ) ;
#17868=CARTESIAN_POINT ( 'NONE',  ( 9.299999999999998934, 0.000000000000000000, 4.999999999999998224 ) ) ;
#17869=CARTESIAN_POINT ( 'NONE',  ( 22.91250000122903430, 0.000000000000000000, 4.999999999999998224 ) ) ;
#17870=CARTESIAN_POINT ( 'NONE',  ( 17.09062500061451573, 6.054752690667223547, 3.707466751127219781E-16 ) ) ;
#17872=ORIENTED_EDGE ( 'NONE', *, *, #68046, .F. ) ;
#17873=CARTESIAN_POINT ( 'NONE',  ( 17.66249999999999787, 2.886751345948129099, -4.999999999999998224 ) ) ;
#17874=CARTESIAN_POINT ( 'NONE',  ( 20.85000000000000142, 4.330127018922192761, -2.499999999999997780 ) ) ;
#17875=CARTESIAN_POINT ( 'NONE',  ( 18.75937500061451857, -4.541064518000417216, -2.621784821875001281 ) ) ;
#17876=CARTESIAN_POINT ( 'NONE',  ( 25.07812500061451644, 6.421520780324663323E-16, -5.243569643749999010 ) ) ;
#17877=ORIENTED_EDGE ( 'NONE', *, *, #72232, .F. ) ;
#17878=CARTESIAN_POINT ( 'NONE',  ( 9.528763966825557376E-15, 17.07500000122903572, 34.00000000000000000 ) ) ;
#17879=CARTESIAN_POINT ( 'NONE',  ( 7.115625000614516082, 3.027376345333613106, -5.243569643749998122 ) ) ;
#17880=CARTESIAN_POINT ( 'NONE',  ( 3.999999999999998668, 15.42500000122903359, 27.69059892324149530 ) ) ;
#17881=CARTESIAN_POINT ( 'NONE',  ( 15.41250000000000142, 2.886751345948129099, -4.999999999999998224 ) ) ;
#17882=CARTESIAN_POINT ( 'NONE',  ( -4.243569643749997233, 18.49062500061451431, 32.45002607614398471 ) ) ;
#17883=CARTESIAN_POINT ( 'NONE',  ( 27.92812500061451431, 4.541064518000418104, 2.621784821874999949 ) ) ;
#17886=CARTESIAN_POINT ( 'NONE',  ( 25.62187500061451573, 3.027376345333613106, -5.243569643749998122 ) ) ;
#17887=EDGE_LOOP ( 'NONE', ( #62637, #44690, #48899, #5718 ) ) ;
#17888=CARTESIAN_POINT ( 'NONE',  ( 23.76562500061451644, 3.027376345333613106, -5.243569643749998122 ) ) ;
#17889=CARTESIAN_POINT ( 'NONE',  ( 25.84687500061451360, -3.027376345333614438, 5.243569643749998122 ) ) ;
#17890=CARTESIAN_POINT ( 'NONE',  ( 4.243569643749999898, 17.32812500061459460, -30.00000000000000000 ) ) ;
#17891=CARTESIAN_POINT ( 'NONE',  ( 11.70000000000000284, -4.330127018922190985, -2.500000000000001332 ) ) ;
#17892=CARTESIAN_POINT ( 'NONE',  ( 8.315625000614515372, -6.054752690667223547, -1.112240025338166033E-15 ) ) ;
#17894=CARTESIAN_POINT ( 'NONE',  ( 28.26562500061451289, 3.027376345333613106, -5.243569643749998122 ) ) ;
#17895=CARTESIAN_POINT ( 'NONE',  ( 26.31562500061451715, -6.054752690667223547, -1.112240025338166033E-15 ) ) ;
#17898=CARTESIAN_POINT ( 'NONE',  ( 19.65937500061451360, -4.541064518000417216, -2.621784821875001281 ) ) ;
#17899=CARTESIAN_POINT ( 'NONE',  ( 4.243569643749999898, 12.43437500061451750, 30.00000000000000000 ) ) ;
#17900=CARTESIAN_POINT ( 'NONE',  ( 19.88437500061451857, 4.541064518000418104, 2.621784821874999949 ) ) ;
#17901=CARTESIAN_POINT ( 'NONE',  ( 26.70937500061451431, 0.000000000000000000, 5.243569643749999010 ) ) ;
#17902=CARTESIAN_POINT ( 'NONE',  ( -2.121784821874996840, 16.78437500061452070, 33.67503911421598417 ) ) ;
#17903=CARTESIAN_POINT ( 'NONE',  ( 7.640625000614517326, 6.054752690667223547, 3.707466751127219781E-16 ) ) ;
#17904=CARTESIAN_POINT ( 'NONE',  ( 4.059375000614519280, 4.541064518000418104, -2.621784821874998173 ) ) ;
#17906=CARTESIAN_POINT ( 'NONE',  ( 4.265625000614517326, -6.054752690667223547, -1.112240025338166033E-15 ) ) ;
#17907=CARTESIAN_POINT ( 'NONE',  ( 10.65937500061451715, -4.541064518000417216, -2.621784821875001281 ) ) ;
#17908=CARTESIAN_POINT ( 'NONE',  ( 19.91250000122903074, -4.330127018922190985, -2.500000000000001332 ) ) ;
#17909=CARTESIAN_POINT ( 'NONE',  ( 5.559375000614517504, 0.000000000000000000, 5.243569643749999010 ) ) ;
#17910=CARTESIAN_POINT ( 'NONE',  ( 6.628125000614517148, 6.421520780324663323E-16, -5.243569643749999010 ) ) ;
#17911=CARTESIAN_POINT ( 'NONE',  ( 5.315625000614516260, 3.027376345333612662, -5.243569643749998122 ) ) ;
#17913=CARTESIAN_POINT ( 'NONE',  ( 17.44687500061451857, -3.027376345333610441, -5.243569643749999898 ) ) ;
#17916=CARTESIAN_POINT ( 'NONE',  ( 24.10312500061451502, -4.541064518000417216, -2.621784821875001281 ) ) ;
#17917=CARTESIAN_POINT ( 'NONE',  ( 9.328125000614518214, 6.421520780324663323E-16, -5.243569643749999010 ) ) ;
#17918=CARTESIAN_POINT ( 'NONE',  ( 27.42187500061451644, 3.027376345333612662, -5.243569643749998122 ) ) ;
#17919=CARTESIAN_POINT ( 'NONE',  ( 9.553125000614517859, 0.000000000000000000, 5.243569643749999010 ) ) ;
#17920=CARTESIAN_POINT ( 'NONE',  ( -2.121784821874996840, 10.48437500061451821, -26.32496088578401583 ) ) ;
#17921=CARTESIAN_POINT ( 'NONE',  ( 13.68750000122903288, 6.123233995736764310E-16, -4.999999999999998224 ) ) ;
#17922=CARTESIAN_POINT ( 'NONE',  ( 26.27812500061451573, -4.541064518000419881, 2.621784821874995952 ) ) ;
#17923=VECTOR ( 'NONE', #47022, 1000.000000000000000 ) ;
#17924=CARTESIAN_POINT ( 'NONE',  ( 2.121784821875001281, 14.10312500061451679, -26.32496088578401938 ) ) ;
#17925=CARTESIAN_POINT ( 'NONE',  ( 12.41250000122903430, 4.330127018922192761, -2.499999999999997780 ) ) ;
#17926=CARTESIAN_POINT ( 'NONE',  ( 10.61250000000000071, 2.886751345948126879, 4.999999999999999112 ) ) ;
#17927=CARTESIAN_POINT ( 'NONE',  ( 20.46562500061451928, -6.054752690667223547, -1.112240025338166033E-15 ) ) ;
#17928=CARTESIAN_POINT ( 'NONE',  ( 4.996875000614516615, 6.054752690667223547, 3.707466751127219781E-16 ) ) ;
#17929=CARTESIAN_POINT ( 'NONE',  ( 19.50000000000000000, 4.330127018922192761, -2.499999999999997780 ) ) ;
#17930=CARTESIAN_POINT ( 'NONE',  ( 8.962500001229033231, 0.000000000000000000, 4.999999999999998224 ) ) ;
#17931=CARTESIAN_POINT ( 'NONE',  ( 16.12500000122903288, 2.886751345948126879, 4.999999999999999112 ) ) ;
#17932=CARTESIAN_POINT ( 'NONE',  ( 12.25312500061451537, 0.000000000000000000, 5.243569643749999010 ) ) ;
#17934=CARTESIAN_POINT ( 'NONE',  ( 15.51562500061451644, -6.054752690667223547, -1.112240025338166033E-15 ) ) ;
#17935=CARTESIAN_POINT ( 'NONE',  ( 25.53750000122903074, 4.330127018922191873, 2.499999999999999556 ) ) ;
#17936=CARTESIAN_POINT ( 'NONE',  ( 20.66250000000000142, -5.773502691896255534, -1.060575238724906372E-15 ) ) ;
#17937=CARTESIAN_POINT ( 'NONE',  ( 23.52187500061451786, 3.027376345333611329, 5.243569643749999010 ) ) ;
#17938=CARTESIAN_POINT ( 'NONE',  ( 4.898587196589411843E-16, 20.00000000000000000, -26.00000000000000000 ) ) ;
#17939=CARTESIAN_POINT ( 'NONE',  ( 9.487500001229033586, -4.330127018922194537, 2.499999999999995559 ) ) ;
#17940=CARTESIAN_POINT ( 'NONE',  ( 8.146875000614516082, 6.054752690667223547, 3.707466751127219781E-16 ) ) ;
#17941=CARTESIAN_POINT ( 'NONE',  ( 25.65937500061451715, 4.541064518000418104, -2.621784821874998173 ) ) ;
#17943=FACE_OUTER_BOUND ( 'NONE', #17360, .T. ) ;
#17944=CARTESIAN_POINT ( 'NONE',  ( 22.30312500061451431, -4.541064518000417216, -2.621784821875001281 ) ) ;
#17945=CARTESIAN_POINT ( 'NONE',  ( 27.23437500061451644, -4.541064518000419881, 2.621784821874995952 ) ) ;
#17947=CARTESIAN_POINT ( 'NONE',  ( 3.296756130434198351, -3.759222042027491995, 3.619358968842379287 ) ) ;
#17948=CARTESIAN_POINT ( 'NONE',  ( 6.871875000614517504, 3.027376345333611329, 5.243569643749999010 ) ) ;
#17949=CARTESIAN_POINT ( 'NONE',  ( 18.70312500061451644, -4.541064518000417216, -2.621784821875001281 ) ) ;
#17950=CARTESIAN_POINT ( 'NONE',  ( 4.490625000614516971, 6.054752690667223547, 3.707466751127219781E-16 ) ) ;
#17951=CARTESIAN_POINT ( 'NONE',  ( 28.11562500061451431, -6.054752690667223547, -1.112240025338166033E-15 ) ) ;
#17952=CARTESIAN_POINT ( 'NONE',  ( 3.796875000614517326, -3.027376345333614438, 5.243569643749998122 ) ) ;
#17953=CARTESIAN_POINT ( 'NONE',  ( 22.91250000122903430, 0.000000000000000000, 4.999999999999998224 ) ) ;
#17955=CARTESIAN_POINT ( 'NONE',  ( 16.91250000000000142, 2.886751345948126879, 4.999999999999999112 ) ) ;
#17957=CARTESIAN_POINT ( 'NONE',  ( 25.64999999999999858, -4.330127018922190985, -2.500000000000001332 ) ) ;
#17958=CARTESIAN_POINT ( 'NONE',  ( 26.59687500061451360, 6.054752690667223547, 3.707466751127219781E-16 ) ) ;
#17959=ORIENTED_EDGE ( 'NONE', *, *, #24471, .T. ) ;
#17960=AXIS2_PLACEMENT_3D ( 'NONE', #33999, #44748, #5576 ) ;
#17961=CARTESIAN_POINT ( 'NONE',  ( 14.99062500061451786, -3.027376345333614438, 5.243569643749998122 ) ) ;
#17962=CARTESIAN_POINT ( 'NONE',  ( 6.440625000614517148, -3.027376345333614438, 5.243569643749998122 ) ) ;
#17964=CARTESIAN_POINT ( 'NONE',  ( 4.471875000614518925, 3.027376345333613106, -5.243569643749998122 ) ) ;
#17965=CARTESIAN_POINT ( 'NONE',  ( 15.60000000122903607, 5.773502691896255534, 3.535250795749688894E-16 ) ) ;
#17966=CARTESIAN_POINT ( 'NONE',  ( 21.18749999999999645, -2.886751345948125991, -5.000000000000000000 ) ) ;
#17967=CARTESIAN_POINT ( 'NONE',  ( 28.53749999999999787, 5.773502691896255534, 3.535250795749688894E-16 ) ) ;
#17968=CARTESIAN_POINT ( 'NONE',  ( 4.584375000614516971, 4.541064518000418104, 2.621784821874999949 ) ) ;
#17969=CARTESIAN_POINT ( 'NONE',  ( 10.24687500061451750, -3.027376345333610441, -5.243569643749999898 ) ) ;
#17970=CARTESIAN_POINT ( 'NONE',  ( 22.58437500061451431, 4.541064518000418104, 2.621784821874999949 ) ) ;
#17972=ORIENTED_EDGE ( 'NONE', *, *, #12479, .T. ) ;
#17973=CARTESIAN_POINT ( 'NONE',  ( 4.471875000614518925, 3.027376345333613106, -5.243569643749998122 ) ) ;
#17974=CARTESIAN_POINT ( 'NONE',  ( 5.175000000000002487, 4.330127018922191873, 2.499999999999999556 ) ) ;
#17976=CARTESIAN_POINT ( 'NONE',  ( 7.959375000614516971, -4.541064518000417216, -2.621784821875001281 ) ) ;
#17977=EDGE_CURVE ( 'NONE', #14969, #18379, #16526, .T. ) ;
#17978=CARTESIAN_POINT ( 'NONE',  ( 17.39999999999999858, 0.000000000000000000, 4.999999999999998224 ) ) ;
#17979=CARTESIAN_POINT ( 'NONE',  ( 15.32812500061451644, 4.541064518000418104, 2.621784821874999949 ) ) ;
#17983=CARTESIAN_POINT ( 'NONE',  ( 9.890625000614516438, 6.054752690667223547, 3.707466751127219781E-16 ) ) ;
#17984=CARTESIAN_POINT ( 'NONE',  ( 26.67187500061451644, 3.027376345333611329, 5.243569643749999010 ) ) ;
#17985=CARTESIAN_POINT ( 'NONE',  ( 27.07500000122903216, -5.773502691896255534, -1.060575238724906372E-15 ) ) ;
#17986=CARTESIAN_POINT ( 'NONE',  ( 25.77187500061451075, 3.027376345333611329, 5.243569643749999010 ) ) ;
#17987=CARTESIAN_POINT ( 'NONE',  ( 7.537500000000002309, -2.886751345948129988, 4.999999999999997335 ) ) ;
#17988=CARTESIAN_POINT ( 'NONE',  ( 2.000000000000001332, 13.06250000122903465, 33.46410161513774995 ) ) ;
#17989=CARTESIAN_POINT ( 'NONE',  ( 15.02812500061451750, -4.541064518000419881, 2.621784821874995952 ) ) ;
#17990=CARTESIAN_POINT ( 'NONE',  ( 6.900000001229035007, -2.886751345948125991, -5.000000000000000000 ) ) ;
#17991=CARTESIAN_POINT ( 'NONE',  ( 17.55937500061451573, 4.541064518000418104, -2.621784821874998173 ) ) ;
#17992=CARTESIAN_POINT ( 'NONE',  ( 11.85937500061451644, 0.000000000000000000, 5.243569643749999010 ) ) ;
#17994=ORIENTED_EDGE ( 'NONE', *, *, #7027, .F. ) ;
#17995=CARTESIAN_POINT ( 'NONE',  ( 12.70312500061451821, 0.000000000000000000, 5.243569643749999010 ) ) ;
#17996=CARTESIAN_POINT ( 'NONE',  ( 25.50000000122903288, 5.773502691896255534, 3.535250795749688894E-16 ) ) ;
#17997=CARTESIAN_POINT ( 'NONE',  ( 13.80937500061451750, -4.541064518000417216, -2.621784821875001281 ) ) ;
#17999=CARTESIAN_POINT ( 'NONE',  ( 13.90312500061451750, 4.541064518000418104, -2.621784821874998173 ) ) ;
#18000=CARTESIAN_POINT ( 'NONE',  ( 26.47500000122903430, 2.886751345948135317, 4.999999999999984013 ) ) ;
#18001=EDGE_CURVE ( 'NONE', #18095, #46571, #58766, .T. ) ;
#18002=CARTESIAN_POINT ( 'NONE',  ( 23.10937500061451644, 0.000000000000000000, 5.243569643749999010 ) ) ;
#18003=CARTESIAN_POINT ( 'NONE',  ( -4.243569643749999898, 10.80312500061451786, 30.00000000000000000 ) ) ;
#18004=CARTESIAN_POINT ( 'NONE',  ( 11.62500000122903465, 2.886751345948126879, 4.999999999999999112 ) ) ;
#18006=CARTESIAN_POINT ( 'NONE',  ( 3.178125000614515638, 4.541064518000418104, 2.621784821874999949 ) ) ;
#18007=CARTESIAN_POINT ( 'NONE',  ( -4.243569643749998122, 17.64687500061451786, -27.54997392385601174 ) ) ;
#18008=CARTESIAN_POINT ( 'NONE',  ( 17.82187500061451502, -6.054752690667223547, -1.112240025338166033E-15 ) ) ;
#18009=CARTESIAN_POINT ( 'NONE',  ( 19.08750000122903145, 6.123233995736764310E-16, -4.999999999999998224 ) ) ;
#18011=CARTESIAN_POINT ( 'NONE',  ( 13.88437500061451679, 6.421520780324663323E-16, -5.243569643749999010 ) ) ;
#18013=CARTESIAN_POINT ( 'NONE',  ( 20.02500000122903145, 2.886751345948129099, -4.999999999999998224 ) ) ;
#18014=CARTESIAN_POINT ( 'NONE',  ( 15.47812500061451679, -4.541064518000419881, 2.621784821874995952 ) ) ;
#18015=CARTESIAN_POINT ( 'NONE',  ( 29.35312500061451502, 0.000000000000000000, 5.243569643749999010 ) ) ;
#18016=ORIENTED_EDGE ( 'NONE', *, *, #48583, .F. ) ;
#18017=ORIENTED_EDGE ( 'NONE', *, *, #60732, .F. ) ;
#18018=CARTESIAN_POINT ( 'NONE',  ( 18.67500000000000071, 4.330127018922191873, 2.499999999999999556 ) ) ;
#18019=CARTESIAN_POINT ( 'NONE',  ( 19.31250000122903288, 0.000000000000000000, 4.999999999999998224 ) ) ;
#18020=CARTESIAN_POINT ( 'NONE',  ( 4.153125000614515727, 0.000000000000000000, 5.243569643749999010 ) ) ;
#18021=CARTESIAN_POINT ( 'NONE',  ( 15.30000000122903359, -2.886751345948129988, 4.999999999999997335 ) ) ;
#18022=CARTESIAN_POINT ( 'NONE',  ( 26.37187500061451217, -6.054752690667223547, -1.112240025338166033E-15 ) ) ;
#18023=CARTESIAN_POINT ( 'NONE',  ( 20.61562500061451431, 3.027376345333613106, -5.243569643749998122 ) ) ;
#18024=CARTESIAN_POINT ( 'NONE',  ( 24.06562500061451715, -6.054752690667223547, -1.112240025338166033E-15 ) ) ;
#18025=CARTESIAN_POINT ( 'NONE',  ( 4.115625000614516082, 3.027376345333611329, 5.243569643749999010 ) ) ;
#18026=CARTESIAN_POINT ( 'NONE',  ( 27.67499999999999716, 4.330127018922191873, 2.499999999999999556 ) ) ;
#18027=CARTESIAN_POINT ( 'NONE',  ( 4.602594079845841790, 1.953557899511747964, 4.866096033195304926 ) ) ;
#18028=( BOUNDED_CURVE ( )  B_SPLINE_CURVE ( 2, ( #18936, #57385, #22056, #12686, #35223, #33495, #68487, #23408, #29681 ),
 .UNSPECIFIED., .F., .F. ) 
 B_SPLINE_CURVE_WITH_KNOTS ( ( 3, 2, 2, 2, 3 ),
 ( 0.6413043478260869179, 0.6449275362318840354, 0.6521739130434782705, 0.6594202898550725056, 0.6630434782608696231 ),
 .UNSPECIFIED. ) 
 CURVE ( )  GEOMETRIC_REPRESENTATION_ITEM ( )  RATIONAL_B_SPLINE_CURVE ( ( 0.9330127018922194093, 0.9330127018922194093, 1.000000000000000000, 0.8660254037844387076, 1.000000000000000000, 0.8660254037844387076, 1.000000000000000000, 0.9330127018922182991, 0.9330127018922192983 ) ) 
 REPRESENTATION_ITEM ( '' )  );
#18031=CARTESIAN_POINT ( 'NONE',  ( 28.76250000000000284, -5.773502691896255534, -1.060575238724906372E-15 ) ) ;
#18032=CARTESIAN_POINT ( 'NONE',  ( 4.243569643749999898, 16.93437500061451573, -30.00000000000000000 ) ) ;
#18033=CARTESIAN_POINT ( 'NONE',  ( 6.337500001229033231, -4.330127018922194537, 2.499999999999995559 ) ) ;
#18034=CARTESIAN_POINT ( 'NONE',  ( 6.412500000000001421, 2.886751345948129099, -4.999999999999998224 ) ) ;
#18035=CARTESIAN_POINT ( 'NONE',  ( 3.037500001229032964, 4.330127018922191873, 2.499999999999999556 ) ) ;
#18036=CARTESIAN_POINT ( 'NONE',  ( 10.35937500061451644, 4.541064518000418104, -2.621784821874998173 ) ) ;
#18038=DIRECTION ( 'NONE',  ( 0.000000000000000000, 0.000000000000000000, 1.000000000000000000 ) ) ;
#18039=CARTESIAN_POINT ( 'NONE',  ( -5.918438294331348715, 8.060677219855273634, -31.00586393815197894 ) ) ;
#18040=CARTESIAN_POINT ( 'NONE',  ( 8.859375000614518214, -4.541064518000417216, -2.621784821875001281 ) ) ;
#18041=CARTESIAN_POINT ( 'NONE',  ( 13.39687500061451608, -3.027376345333610441, -5.243569643749999898 ) ) ;
#18042=CARTESIAN_POINT ( 'NONE',  ( 5.512499999999999289, 2.886751345948129099, -4.999999999999998224 ) ) ;
#18043=CARTESIAN_POINT ( 'NONE',  ( -3.000416591977282496E-16, 16.09062500061459744, 25.09994784771203058 ) ) ;
#18044=CARTESIAN_POINT ( 'NONE',  ( 20.55937500061451573, -4.541064518000417216, -2.621784821875001281 ) ) ;
#18045=CARTESIAN_POINT ( 'NONE',  ( 9.637499999999999289, 5.773502691896255534, 3.535250795749688401E-16 ) ) ;
#18046=CARTESIAN_POINT ( 'NONE',  ( 25.72500000122903074, -5.773502691896255534, -1.060575238724906372E-15 ) ) ;
#18048=CARTESIAN_POINT ( 'NONE',  ( 23.76562500061451644, 3.027376345333613106, -5.243569643749998122 ) ) ;
#18049=CARTESIAN_POINT ( 'NONE',  ( 14.12812500061451715, -4.541064518000419881, 2.621784821874995952 ) ) ;
#18051=CARTESIAN_POINT ( 'NONE',  ( 11.03437500061451715, -4.541064518000419881, 2.621784821874995952 ) ) ;
#18052=CARTESIAN_POINT ( 'NONE',  ( 29.28749999999999787, -2.886751345948125991, -5.000000000000000000 ) ) ;
#18053=CARTESIAN_POINT ( 'NONE',  ( 23.43750000122902932, -4.330127018922194537, 2.499999999999995559 ) ) ;
#18054=CYLINDRICAL_SURFACE ( 'NONE', #21357, 4.000000000000000000 ) ;
#18055=CARTESIAN_POINT ( 'NONE',  ( 10.95937500061451964, 0.000000000000000000, 5.243569643749999010 ) ) ;
#18056=CARTESIAN_POINT ( 'NONE',  ( 29.22187500061451715, 3.027376345333613106, -5.243569643749998122 ) ) ;
#18057=CARTESIAN_POINT ( 'NONE',  ( 4.134375000614517681, 4.541064518000418104, 2.621784821874999949 ) ) ;
#18059=CARTESIAN_POINT ( 'NONE',  ( 21.49687500061451573, -3.027376345333610441, -5.243569643749999898 ) ) ;
#18060=CARTESIAN_POINT ( 'NONE',  ( 14.59687500061452070, -3.027376345333614438, 5.243569643749998122 ) ) ;
#18062=CARTESIAN_POINT ( 'NONE',  ( 25.16249999999999432, -5.773502691896255534, -1.060575238724906372E-15 ) ) ;
#18065=CARTESIAN_POINT ( 'NONE',  ( 16.90312500061451573, -4.541064518000417216, -2.621784821875001281 ) ) ;
#18066=CARTESIAN_POINT ( 'NONE',  ( 8.175000000000002487, 6.123233995736764310E-16, -4.999999999999998224 ) ) ;
#18067=CARTESIAN_POINT ( 'NONE',  ( -1.999999999999997113, 14.22500000000000142, 33.46410161513775705 ) ) ;
#18068=CARTESIAN_POINT ( 'NONE',  ( 14.21249999999999858, 2.886751345948126879, 4.999999999999999112 ) ) ;
#18069=CARTESIAN_POINT ( 'NONE',  ( -2.121784821874996840, 10.42812500061451786, 33.67503911421598417 ) ) ;
#18070=CARTESIAN_POINT ( 'NONE',  ( 17.06250000122903288, 0.000000000000000000, 4.999999999999998224 ) ) ;
#18071=CARTESIAN_POINT ( 'NONE',  ( 25.80937500061451928, 0.000000000000000000, 5.243569643749999010 ) ) ;
#18072=ORIENTED_EDGE ( 'NONE', *, *, #40917, .T. ) ;
#18073=CARTESIAN_POINT ( 'NONE',  ( 21.70312500061451644, 0.000000000000000000, 5.243569643749999010 ) ) ;
#18074=CARTESIAN_POINT ( 'NONE',  ( 20.74687500061451573, 6.054752690667223547, 3.707466751127219781E-16 ) ) ;
#18075=CARTESIAN_POINT ( 'NONE',  ( 4.612500000000002487, 2.886751345948129099, -4.999999999999998224 ) ) ;
#18076=CARTESIAN_POINT ( 'NONE',  ( 7.153125000614518392, 4.541064518000418104, -2.621784821874998173 ) ) ;
#18077=CARTESIAN_POINT ( 'NONE',  ( 21.96562500061451573, 3.027376345333613106, -5.243569643749998122 ) ) ;
#18078=CARTESIAN_POINT ( 'NONE',  ( 13.28437500061451715, -4.541064518000419881, 2.621784821874995952 ) ) ;
#18079=CARTESIAN_POINT ( 'NONE',  ( 16.32187500061451502, 3.027376345333611329, 5.243569643749999010 ) ) ;
#18080=CARTESIAN_POINT ( 'NONE',  ( -4.243569643749997233, 16.69062500061451360, 32.45002607614398471 ) ) ;
#18081=CARTESIAN_POINT ( 'NONE',  ( 18.97500000122903074, -5.773502691896255534, -1.060575238724906372E-15 ) ) ;
#18083=CARTESIAN_POINT ( 'NONE',  ( 9.478125000614515017, 4.541064518000418104, 2.621784821874999949 ) ) ;
#18084=CARTESIAN_POINT ( 'NONE',  ( 5.634375000614519458, -4.541064518000419881, 2.621784821874995952 ) ) ;
#18085=CARTESIAN_POINT ( 'NONE',  ( 4.096875000614518925, 6.054752690667223547, 3.707466751127219781E-16 ) ) ;
#18086=CARTESIAN_POINT ( 'NONE',  ( 25.35937500061451644, 0.000000000000000000, 5.243569643749999010 ) ) ;
#18087=CARTESIAN_POINT ( 'NONE',  ( 17.72812500061451502, -4.541064518000419881, 2.621784821874995952 ) ) ;
#18088=CARTESIAN_POINT ( 'NONE',  ( 28.23750000122903359, 4.330127018922191873, 2.499999999999999556 ) ) ;
#18089=CARTESIAN_POINT ( 'NONE',  ( 24.21562500061451573, 3.027376345333613106, -5.243569643749998122 ) ) ;
#18090=CARTESIAN_POINT ( 'NONE',  ( 21.27187500061451786, 3.027376345333611329, 5.243569643749999010 ) ) ;
#18091=CARTESIAN_POINT ( 'NONE',  ( 18.17812500061451786, -4.541064518000419881, 2.621784821874995952 ) ) ;
#18092=CARTESIAN_POINT ( 'NONE',  ( 2.121784821875001281, 17.75937500061451502, 33.67503911421598417 ) ) ;
#18093=CARTESIAN_POINT ( 'NONE',  ( 21.25312500061451715, 0.000000000000000000, 5.243569643749999010 ) ) ;
#18095=VERTEX_POINT ( 'NONE', #56067 ) ;
#18096=CARTESIAN_POINT ( 'NONE',  ( 25.19999999999999929, -4.330127018922190985, -2.500000000000001332 ) ) ;
#18097=CARTESIAN_POINT ( 'NONE',  ( -3.999999999999997335, 12.83750000000000213, -27.69059892324149175 ) ) ;
#18099=CARTESIAN_POINT ( 'NONE',  ( 28.49062500061451431, -3.027376345333614438, 5.243569643749998122 ) ) ;
#18100=CARTESIAN_POINT ( 'NONE',  ( 10.26562500061451644, 3.027376345333613106, -5.243569643749998122 ) ) ;
#18101=CARTESIAN_POINT ( 'NONE',  ( 22.95000000122903216, -2.886751345948129988, 4.999999999999997335 ) ) ;
#18102=CARTESIAN_POINT ( 'NONE',  ( 27.40312500061451573, 4.541064518000418104, -2.621784821874998173 ) ) ;
#18103=CARTESIAN_POINT ( 'NONE',  ( 27.22499999999999787, 4.330127018922191873, 2.499999999999999556 ) ) ;
#18104=CARTESIAN_POINT ( 'NONE',  ( -3.999999999999999556, 15.57500000122903216, -32.30940107675850470 ) ) ;
#18105=CARTESIAN_POINT ( 'NONE',  ( 29.54062500061451502, -3.027376345333610441, -5.243569643749999898 ) ) ;
#18106=CARTESIAN_POINT ( 'NONE',  ( 11.46562500061451573, -6.054752690667223547, -1.112240025338166033E-15 ) ) ;
#18107=ORIENTED_EDGE ( 'NONE', *, *, #63501, .F. ) ;
#18108=CARTESIAN_POINT ( 'NONE',  ( 26.54062500061451146, 6.054752690667223547, 3.707466751127219781E-16 ) ) ;
#18109=CARTESIAN_POINT ( 'NONE',  ( 7.228125000614517681, 4.541064518000418104, 2.621784821874999949 ) ) ;
#18110=CARTESIAN_POINT ( 'NONE',  ( 6.665625000614515905, 3.027376345333613106, -5.243569643749998122 ) ) ;
#18112=CARTESIAN_POINT ( 'NONE',  ( 17.73750000122903359, 6.123233995736764310E-16, -4.999999999999998224 ) ) ;
#18113=CARTESIAN_POINT ( 'NONE',  ( 15.71250000000000213, -5.773502691896255534, -1.060575238724906372E-15 ) ) ;
#18115=CARTESIAN_POINT ( 'NONE',  ( 16.80937500061451573, 0.000000000000000000, 5.243569643749999010 ) ) ;
#18116=CARTESIAN_POINT ( 'NONE',  ( 11.13750000122903216, 4.330127018922191873, 2.499999999999999556 ) ) ;
#18117=CARTESIAN_POINT ( 'NONE',  ( 16.35937500061451644, 0.000000000000000000, 5.243569643749999010 ) ) ;
#18119=CARTESIAN_POINT ( 'NONE',  ( 20.22187500061451715, 3.027376345333613106, -5.243569643749998122 ) ) ;
#18120=CARTESIAN_POINT ( 'NONE',  ( 4.243569643749999898, 12.82812500061451821, -30.00000000000000000 ) ) ;
#18121=DIRECTION ( 'NONE',  ( 0.000000000000000000, 1.000000000000000000, -0.000000000000000000 ) ) ;
#18124=CARTESIAN_POINT ( 'NONE',  ( 25.22812500061451502, 4.541064518000418104, 2.621784821874999949 ) ) ;
#18125=CARTESIAN_POINT ( 'NONE',  ( 28.24687500061451573, -3.027376345333610441, -5.243569643749999898 ) ) ;
#18126=CARTESIAN_POINT ( 'NONE',  ( 23.92499999999999716, 6.123233995736764310E-16, -4.999999999999998224 ) ) ;
#18127=CARTESIAN_POINT ( 'NONE',  ( 7.565625000614518036, 3.027376345333613106, -5.243569643749998122 ) ) ;
#18129=CARTESIAN_POINT ( 'NONE',  ( 18.57187500061451857, 3.027376345333611329, 5.243569643749999010 ) ) ;
#18131=CARTESIAN_POINT ( 'NONE',  ( 28.80000000122903003, -2.886751345948129988, 4.999999999999997335 ) ) ;
#18132=CARTESIAN_POINT ( 'NONE',  ( 7.734375000614517326, 4.541064518000418104, 2.621784821874999949 ) ) ;
#18133=ORIENTED_EDGE ( 'NONE', *, *, #26472, .T. ) ;
#18134=CARTESIAN_POINT ( 'NONE',  ( 18.57187500061451857, 3.027376345333611329, 5.243569643749999010 ) ) ;
#18136=CARTESIAN_POINT ( 'NONE',  ( 27.26249999999999929, 2.886751345948126879, 4.999999999999999112 ) ) ;
#18137=CARTESIAN_POINT ( 'NONE',  ( 28.88437500061451502, 4.541064518000418104, 2.621784821874999949 ) ) ;
#18140=ORIENTED_EDGE ( 'NONE', *, *, #47732, .T. ) ;
#18141=CARTESIAN_POINT ( 'NONE',  ( 9.787499999999999645, -2.886751345948129988, 4.999999999999997335 ) ) ;
#18143=CARTESIAN_POINT ( 'NONE',  ( 25.60312500061451502, 4.541064518000418104, -2.621784821874998173 ) ) ;
#18144=CARTESIAN_POINT ( 'NONE',  ( 13.23750000000000071, 5.773502691896255534, 3.535250795749688894E-16 ) ) ;
#18145=( BOUNDED_CURVE ( )  B_SPLINE_CURVE ( 2, ( #11348, #56408, #5799, #22775, #45326, #67862, #17233 ),
 .UNSPECIFIED., .F., .F. ) 
 B_SPLINE_CURVE_WITH_KNOTS ( ( 3, 2, 2, 3 ),
 ( 0.8499999999999999778, 0.8527777777777777457, 0.8555555555555555136, 0.8583333333333332815 ),
 .UNSPECIFIED. ) 
 CURVE ( )  GEOMETRIC_REPRESENTATION_ITEM ( )  RATIONAL_B_SPLINE_CURVE ( ( 1.000000000000000000, 0.8660254037844387076, 1.000000000000000000, 0.8660254037844387076, 1.000000000000000000, 0.8660254037844387076, 1.000000000000000000 ) ) 
 REPRESENTATION_ITEM ( '' )  );
#18146=CARTESIAN_POINT ( 'NONE',  ( 9.787500001229036073, 4.330127018922191873, 2.499999999999999556 ) ) ;
#18147=CARTESIAN_POINT ( 'NONE',  ( 9.215625000614515727, -6.054752690667223547, -1.112240025338166033E-15 ) ) ;
#18148=CARTESIAN_POINT ( 'NONE',  ( 23.06250000000000355, 2.886751345948129099, -4.999999999999998224 ) ) ;
#18149=CARTESIAN_POINT ( 'NONE',  ( 21.40312500061451573, -4.541064518000417216, -2.621784821875001281 ) ) ;
#18150=CYLINDRICAL_SURFACE ( 'NONE', #50231, 4.999999999999998224 ) ;
#18151=CARTESIAN_POINT ( 'NONE',  ( 25.87500000122903288, 2.886751345948129099, -4.999999999999998224 ) ) ;
#18153=CARTESIAN_POINT ( 'NONE',  ( 8.137500000000002842, -2.886751345948125991, -5.000000000000000000 ) ) ;
#18154=EDGE_LOOP ( 'NONE', ( #28839, #27904, #2593, #67778 ) ) ;
#18155=CARTESIAN_POINT ( 'NONE',  ( 22.41562500061451502, 3.027376345333613106, -5.243569643749998122 ) ) ;
#18156=CARTESIAN_POINT ( 'NONE',  ( 29.50312500061451360, -4.541064518000417216, -2.621784821875001281 ) ) ;
#18157=CARTESIAN_POINT ( 'NONE',  ( 26.03437500061451715, 6.421520780324663323E-16, -5.243569643749999010 ) ) ;
#18158=CARTESIAN_POINT ( 'NONE',  ( 17.85937500061451999, -4.541064518000417216, -2.621784821875001281 ) ) ;
#18159=CARTESIAN_POINT ( 'NONE',  ( 13.19062500061451537, -3.027376345333614438, 5.243569643749998122 ) ) ;
#18161=CARTESIAN_POINT ( 'NONE',  ( 26.88750000122903216, 4.330127018922191873, 2.499999999999999556 ) ) ;
#18163=CARTESIAN_POINT ( 'NONE',  ( 16.00312500061451715, -4.541064518000417216, -2.621784821875001281 ) ) ;
#18164=CARTESIAN_POINT ( 'NONE',  ( 13.38750000000000107, -2.886751345948130876, 4.999999999999996447 ) ) ;
#18165=CARTESIAN_POINT ( 'NONE',  ( 2.662500001229036073, 0.000000000000000000, 4.999999999999998224 ) ) ;
#18166=CARTESIAN_POINT ( 'NONE',  ( 13.02187500061451608, 3.027376345333613106, -5.243569643749998122 ) ) ;
#18167=CARTESIAN_POINT ( 'NONE',  ( 11.44687500061451857, -3.027376345333614438, 5.243569643749998122 ) ) ;
#18168=CARTESIAN_POINT ( 'NONE',  ( 21.08437500061451786, 6.421520780324663323E-16, -5.243569643749999010 ) ) ;
#18170=CARTESIAN_POINT ( 'NONE',  ( 29.55000000000000071, 0.000000000000000000, 4.999999999999998224 ) ) ;
#18171=CARTESIAN_POINT ( 'NONE',  ( 23.46562500061451573, 3.027376345333611329, 5.243569643749999010 ) ) ;
#18172=CARTESIAN_POINT ( 'NONE',  ( 19.47187500061451360, 3.027376345333611329, 5.243569643749999010 ) ) ;
#18173=CARTESIAN_POINT ( 'NONE',  ( 24.36562500061451786, 3.027376345333611329, 5.243569643749999010 ) ) ;
#18174=CARTESIAN_POINT ( 'NONE',  ( 27.11250000000000071, 2.886751345948112668, -5.000000000000024869 ) ) ;
#18175=CARTESIAN_POINT ( 'NONE',  ( -3.999999999999999556, 13.21250000000000213, 27.69059892324149530 ) ) ;
#18176=AXIS2_PLACEMENT_3D ( 'NONE', #18390, #29496, #17312 ) ;
#18177=CARTESIAN_POINT ( 'NONE',  ( 28.26562500061451289, 3.027376345333613106, -5.243569643749998122 ) ) ;
#18178=CARTESIAN_POINT ( 'NONE',  ( 9.487500001229033586, -4.330127018922194537, 2.499999999999995559 ) ) ;
#18179=CARTESIAN_POINT ( 'NONE',  ( 4.387500001229033053, 4.330127018922191873, 2.499999999999999556 ) ) ;
#18181=CARTESIAN_POINT ( 'NONE',  ( 26.13750000122903216, -4.330127018922194537, 2.499999999999995559 ) ) ;
#18184=CARTESIAN_POINT ( 'NONE',  ( 8.371875000614515727, -6.054752690667223547, -1.112240025338166033E-15 ) ) ;
#18185=CARTESIAN_POINT ( 'NONE',  ( 17.72812500061451502, -4.541064518000419881, 2.621784821874995952 ) ) ;
#18186=CARTESIAN_POINT ( 'NONE',  ( 10.20937500061451786, -4.541064518000417216, -2.621784821875001281 ) ) ;
#18187=CARTESIAN_POINT ( 'NONE',  ( 29.17500000122903714, 2.886751345948126879, 4.999999999999999112 ) ) ;
#18188=CARTESIAN_POINT ( 'NONE',  ( 19.17187500061451644, -6.054752690667223547, -1.112240025338166033E-15 ) ) ;
#18189=CARTESIAN_POINT ( 'NONE',  ( 8.634375000614518569, 4.541064518000418104, 2.621784821874999949 ) ) ;
#18190=CARTESIAN_POINT ( 'NONE',  ( 3.140625000614516882, 6.054752690667223547, 3.707466751127219781E-16 ) ) ;
#18192=CARTESIAN_POINT ( 'NONE',  ( 8.090625000614515727, 6.054752690667223547, 3.707466751127219781E-16 ) ) ;
#18193=CARTESIAN_POINT ( 'NONE',  ( 17.91562500061451502, 3.027376345333613106, -5.243569643749998122 ) ) ;
#18194=VERTEX_POINT ( 'NONE', #27999 ) ;
#18195=CARTESIAN_POINT ( 'NONE',  ( 6.412500001229036073, -4.330127018922190985, -2.500000000000001332 ) ) ;
#18196=CARTESIAN_POINT ( 'NONE',  ( 14.05312500061451431, 0.000000000000000000, 5.243569643749999010 ) ) ;
#18197=CARTESIAN_POINT ( 'NONE',  ( 12.25312500061451537, 0.000000000000000000, 5.243569643749999010 ) ) ;
#18199=CARTESIAN_POINT ( 'NONE',  ( 12.86250000000000071, 2.886751345948126879, 4.999999999999999112 ) ) ;
#18200=CARTESIAN_POINT ( 'NONE',  ( 5.662500001229035185, 4.330127018922192761, -2.499999999999997780 ) ) ;
#18201=CARTESIAN_POINT ( 'NONE',  ( 4.378125000614518925, 6.421520780324663323E-16, -5.243569643749999010 ) ) ;
#18203=EDGE_CURVE ( 'NONE', #31631, #15981, #34201, .T. ) ;
#18204=CARTESIAN_POINT ( 'NONE',  ( 19.57500000122903216, 2.886751345948129099, -4.999999999999998224 ) ) ;
#18206=CARTESIAN_POINT ( 'NONE',  ( 9.001249775931846008E-16, 11.87187500061451750, -25.09994784771203058 ) ) ;
#18207=CARTESIAN_POINT ( 'NONE',  ( 4.196151849995945149, -2.718880220196457476, -4.196151849995952254 ) ) ;
#18208=CARTESIAN_POINT ( 'NONE',  ( 22.91250000122903430, 0.000000000000000000, 4.999999999999998224 ) ) ;
#18209=DIRECTION ( 'NONE',  ( -1.000000000000000000, -0.000000000000000000, -0.000000000000000000 ) ) ;
#18210=CARTESIAN_POINT ( 'NONE',  ( 17.59687500061451715, 6.054752690667223547, 3.707466751127219781E-16 ) ) ;
#18211=LINE ( 'NONE', #23410, #46870 ) ;
#18212=CARTESIAN_POINT ( 'NONE',  ( 14.80312500061451608, 4.541064518000418104, -2.621784821874998173 ) ) ;
#18214=CARTESIAN_POINT ( 'NONE',  ( 27.42187500061451644, 3.027376345333613106, -5.243569643749998122 ) ) ;
#18216=CARTESIAN_POINT ( 'NONE',  ( 11.80312500061451608, 0.000000000000000000, 5.243569643749999010 ) ) ;
#18217=CARTESIAN_POINT ( 'NONE',  ( 16.05937500061451573, -4.541064518000417216, -2.621784821875001281 ) ) ;
#18218=ORIENTED_EDGE ( 'NONE', *, *, #32403, .F. ) ;
#18219=CARTESIAN_POINT ( 'NONE',  ( 26.69062500061451715, -3.027376345333614438, 5.243569643749998122 ) ) ;
#18220=CARTESIAN_POINT ( 'NONE',  ( 19.86562500061451786, 3.027376345333611329, 5.243569643749999010 ) ) ;
#18221=CARTESIAN_POINT ( 'NONE',  ( 29.16562500061451502, 3.027376345333613106, -5.243569643749998122 ) ) ;
#18223=CARTESIAN_POINT ( 'NONE',  ( 9.712500000000002132, 2.886751345948126879, 4.999999999999999112 ) ) ;
#18224=CARTESIAN_POINT ( 'NONE',  ( 20.32500000122903572, -5.773502691896255534, -1.060575238724906372E-15 ) ) ;
#18225=CARTESIAN_POINT ( 'NONE',  ( 2.000000000000001332, 10.25000000000000000, 33.46410161513774995 ) ) ;
#18227=ORIENTED_EDGE ( 'NONE', *, *, #38783, .T. ) ;
#18228=CARTESIAN_POINT ( 'NONE',  ( 16.80000000000000071, 4.330127018922192761, -2.499999999999997780 ) ) ;
#18229=CARTESIAN_POINT ( 'NONE',  ( 22.05000000000000071, -4.330127018922190985, -2.500000000000001332 ) ) ;
#18230=CARTESIAN_POINT ( 'NONE',  ( 18.42187500061451644, 3.027376345333613106, -5.243569643749998122 ) ) ;
#18231=CARTESIAN_POINT ( 'NONE',  ( 25.00312500061451715, -4.541064518000417216, -2.621784821875001281 ) ) ;
#18233=VERTEX_POINT ( 'NONE', #43897 ) ;
#18234=CARTESIAN_POINT ( 'NONE',  ( 8.737500001229033586, 6.123233995736764310E-16, -4.999999999999998224 ) ) ;
#18235=CARTESIAN_POINT ( 'NONE',  ( 7.940625000614518036, -3.027376345333610441, -5.243569643749999898 ) ) ;
#18237=CARTESIAN_POINT ( 'NONE',  ( 14.43750000000000000, -2.886751345948125991, -5.000000000000000000 ) ) ;
#18238=CARTESIAN_POINT ( 'NONE',  ( 2.121784821875001281, 17.25312500061451715, 33.67503911421598417 ) ) ;
#18239=CARTESIAN_POINT ( 'NONE',  ( 28.41562500061451502, 3.027376345333611329, 5.243569643749999010 ) ) ;
#18242=CARTESIAN_POINT ( 'NONE',  ( 26.22187500061451715, 3.027376345333611329, 5.243569643749999010 ) ) ;
#18243=ORIENTED_EDGE ( 'NONE', *, *, #17583, .F. ) ;
#18244=CARTESIAN_POINT ( 'NONE',  ( 21.81562500061451004, -6.054752690667223547, -1.112240025338166033E-15 ) ) ;
#18245=CARTESIAN_POINT ( 'NONE',  ( 22.62187500061451573, 3.027376345333611329, 5.243569643749999010 ) ) ;
#18246=CARTESIAN_POINT ( 'NONE',  ( 2.121784821874999061, 16.05312500061459247, -33.67503911421598417 ) ) ;
#18247=CARTESIAN_POINT ( 'NONE',  ( 10.31250000000000355, -5.773502691896255534, -1.060575238724906372E-15 ) ) ;
#18248=CARTESIAN_POINT ( 'NONE',  ( 6.928125000614516082, -4.541064518000419881, 2.621784821874995952 ) ) ;
#18250=CARTESIAN_POINT ( 'NONE',  ( 22.97812500061451857, 4.541064518000418104, 2.621784821874999949 ) ) ;
#18253=CARTESIAN_POINT ( 'NONE',  ( 16.35937500061451644, 0.000000000000000000, 5.243569643749999010 ) ) ;
#18254=CARTESIAN_POINT ( 'NONE',  ( -4.243569643749997233, 12.69687500061451857, 32.45002607614398471 ) ) ;
#18255=CARTESIAN_POINT ( 'NONE',  ( 18.04687500061451999, 6.054752690667223547, 3.707466751127219781E-16 ) ) ;
#18256=CARTESIAN_POINT ( 'NONE',  ( 26.29687500061451644, -3.027376345333614438, 5.243569643749998122 ) ) ;
#18257=CARTESIAN_POINT ( 'NONE',  ( -4.243569643749999898, 15.77187500061451608, 27.54997392385601529 ) ) ;
#18258=CARTESIAN_POINT ( 'NONE',  ( 7.715625000614515727, 3.027376345333611329, 5.243569643749999010 ) ) ;
#18259=CARTESIAN_POINT ( 'NONE',  ( 1.071796769724489895, 10.52990381179670010, -34.00000000000000000 ) ) ;
#18260=CARTESIAN_POINT ( 'NONE',  ( 5.221875000614519813, -6.054752690667223547, -1.112240025338166033E-15 ) ) ;
#18261=FACE_OUTER_BOUND ( 'NONE', #34074, .T. ) ;
#18262=CARTESIAN_POINT ( 'NONE',  ( 4.453125000614517326, 4.541064518000418104, -2.621784821874998173 ) ) ;
#18263=CARTESIAN_POINT ( 'NONE',  ( 8.784375000614518925, -4.541064518000419881, 2.621784821874995952 ) ) ;
#18265=CARTESIAN_POINT ( 'NONE',  ( 17.10000000122903430, -2.886751345948129988, 4.999999999999997335 ) ) ;
#18266=CARTESIAN_POINT ( 'NONE',  ( 5.109375000614518214, 0.000000000000000000, 5.243569643749999010 ) ) ;
#18267=CARTESIAN_POINT ( 'NONE',  ( 8.015625000614518214, 3.027376345333613106, -5.243569643749998122 ) ) ;
#18270=CARTESIAN_POINT ( 'NONE',  ( 17.14687500061451786, 6.054752690667223547, 3.707466751127219781E-16 ) ) ;
#18272=CARTESIAN_POINT ( 'NONE',  ( 24.59062500061451573, -3.027376345333610441, -5.243569643749999898 ) ) ;
#18273=CARTESIAN_POINT ( 'NONE',  ( 9.515625000614518214, 3.027376345333611329, 5.243569643749999010 ) ) ;
#18274=CARTESIAN_POINT ( 'NONE',  ( 28.09687500061451715, -3.027376345333614438, 5.243569643749998122 ) ) ;
#18275=CARTESIAN_POINT ( 'NONE',  ( 11.16562500061451679, 3.027376345333613106, -5.243569643749998122 ) ) ;
#18277=CARTESIAN_POINT ( 'NONE',  ( 10.68750000122903288, 4.330127018922191873, 2.499999999999999556 ) ) ;
#18278=CARTESIAN_POINT ( 'NONE',  ( 25.15312500061451217, 4.541064518000418104, -2.621784821874998173 ) ) ;
#18279=CARTESIAN_POINT ( 'NONE',  ( -2.121784821874999949, 13.87812500061451715, -33.67503911421598417 ) ) ;
#18280=CARTESIAN_POINT ( 'NONE',  ( 13.27500000122903323, 2.886751345948129099, -4.999999999999998224 ) ) ;
#18281=CARTESIAN_POINT ( 'NONE',  ( 23.05312500061451431, 0.000000000000000000, 5.243569643749999010 ) ) ;
#18282=VECTOR ( 'NONE', #35359, 1000.000000000000000 ) ;
#18283=CARTESIAN_POINT ( 'NONE',  ( 11.40000000000000036, 4.330127018922192761, -2.499999999999997780 ) ) ;
#18284=CARTESIAN_POINT ( 'NONE',  ( 19.41562500061451146, 3.027376345333611329, 5.243569643749999010 ) ) ;
#18285=CARTESIAN_POINT ( 'NONE',  ( 5.559375000614517504, 0.000000000000000000, 5.243569643749999010 ) ) ;
#18287=CARTESIAN_POINT ( 'NONE',  ( 21.71249999999999858, 2.886751345948129099, -4.999999999999998224 ) ) ;
#18288=CARTESIAN_POINT ( 'NONE',  ( 7.387500001229032165, 6.123233995736764310E-16, -4.999999999999998224 ) ) ;
#18289=CARTESIAN_POINT ( 'NONE',  ( 15.56250000122903465, 4.330127018922192761, -2.499999999999997780 ) ) ;
#18290=CARTESIAN_POINT ( 'NONE',  ( 11.72812500061451857, 4.541064518000418104, 2.621784821874999949 ) ) ;
#18291=CARTESIAN_POINT ( 'NONE',  ( 14.72812500061451679, 6.421520780324663323E-16, -5.243569643749999010 ) ) ;
#18293=CARTESIAN_POINT ( 'NONE',  ( 26.47500000122903074, 2.886751345948126879, 4.999999999999999112 ) ) ;
#18294=CARTESIAN_POINT ( 'NONE',  ( 19.42499999999999716, 6.123233995736764310E-16, -4.999999999999998224 ) ) ;
#18295=AXIS2_PLACEMENT_3D ( 'NONE', #25697, #46779, #69314 ) ;
#18296=CARTESIAN_POINT ( 'NONE',  ( 22.65937500061451715, 0.000000000000000000, 5.243569643749999010 ) ) ;
#18298=CARTESIAN_POINT ( 'NONE',  ( 10.87500000122903288, -5.773502691896255534, -1.060575238724906372E-15 ) ) ;
#18299=CARTESIAN_POINT ( 'NONE',  ( 8.709375000614517859, 0.000000000000000000, 5.243569643749999010 ) ) ;
#18300=CARTESIAN_POINT ( 'NONE',  ( 24.57187500061451502, -6.054752690667223547, -1.112240025338166033E-15 ) ) ;
#18301=CARTESIAN_POINT ( 'NONE',  ( 3.496875000614518836, -3.027376345333610441, -5.243569643749999898 ) ) ;
#18302=CARTESIAN_POINT ( 'NONE',  ( 21.06562500061451715, 3.027376345333613106, -5.243569643749998122 ) ) ;
#18303=CARTESIAN_POINT ( 'NONE',  ( 26.93437500061451573, 6.421520780324663323E-16, -5.243569643749999010 ) ) ;
#18305=CARTESIAN_POINT ( 'NONE',  ( 18.67500000000000071, 4.330127018922191873, 2.499999999999999556 ) ) ;
#18306=CARTESIAN_POINT ( 'NONE',  ( 7.696875000614516793, 6.054752690667223547, 3.707466751127219781E-16 ) ) ;
#18307=CARTESIAN_POINT ( 'NONE',  ( 20.31562500061451715, 3.027376345333611329, 5.243569643749999010 ) ) ;
#18308=ORIENTED_EDGE ( 'NONE', *, *, #28846, .F. ) ;
#18309=CARTESIAN_POINT ( 'NONE',  ( 25.05000000000000071, 0.000000000000000000, 4.999999999999998224 ) ) ;
#18310=CARTESIAN_POINT ( 'NONE',  ( 27.21562500061451928, -6.054752690667223547, -1.112240025338166033E-15 ) ) ;
#18311=CARTESIAN_POINT ( 'NONE',  ( 3.346875000614518036, -3.027376345333614438, 5.243569643749998122 ) ) ;
#18313=CYLINDRICAL_SURFACE ( 'NONE', #1708, 3.999999999999996447 ) ;
#18314=CARTESIAN_POINT ( 'NONE',  ( 16.57499999999999929, -4.330127018922194537, 2.499999999999995559 ) ) ;
#18315=CARTESIAN_POINT ( 'NONE',  ( 22.04062500061451502, 6.054752690667223547, 3.707466751127219781E-16 ) ) ;
#18316=VERTEX_POINT ( 'NONE', #61596 ) ;
#18317=CARTESIAN_POINT ( 'NONE',  ( 25.94999999999999929, 0.000000000000000000, 4.999999999999998224 ) ) ;
#18318=CARTESIAN_POINT ( 'NONE',  ( 25.95937500061451431, -4.541064518000417216, -2.621784821875001281 ) ) ;
#18319=ORIENTED_EDGE ( 'NONE', *, *, #14004, .F. ) ;
#18320=CARTESIAN_POINT ( 'NONE',  ( 16.37812500061451715, -4.541064518000419881, 2.621784821874995952 ) ) ;
#18321=CARTESIAN_POINT ( 'NONE',  ( 5.165625000614518569, -6.054752690667223547, -1.112240025338166033E-15 ) ) ;
#18323=CARTESIAN_POINT ( 'NONE',  ( 29.16562500061451502, 3.027376345333613106, -5.243569643749998122 ) ) ;
#18324=CARTESIAN_POINT ( 'NONE',  ( 15.33750000122903323, -4.330127018922194537, 2.499999999999995559 ) ) ;
#18325=VECTOR ( 'NONE', #51264, 1000.000000000000000 ) ;
#18326=CARTESIAN_POINT ( 'NONE',  ( 22.87500000000000000, -4.330127018922194537, 2.499999999999995559 ) ) ;
#18327=CARTESIAN_POINT ( 'NONE',  ( 28.94999999999999929, 4.330127018922192761, -2.499999999999997780 ) ) ;
#18328=CARTESIAN_POINT ( 'NONE',  ( 4.771875000614516971, -6.054752690667223547, -1.112240025338166033E-15 ) ) ;
#18329=CARTESIAN_POINT ( 'NONE',  ( 10.20937500061451786, -4.541064518000417216, -2.621784821875001281 ) ) ;
#18330=CARTESIAN_POINT ( 'NONE',  ( 18.79687500061451644, -3.027376345333610441, -5.243569643749999898 ) ) ;
#18331=CARTESIAN_POINT ( 'NONE',  ( 9.937500001229032875, -4.330127018922194537, 2.499999999999995559 ) ) ;
#18333=CARTESIAN_POINT ( 'NONE',  ( 28.60312500061451502, -4.541064518000417216, -2.621784821875001281 ) ) ;
#18334=CARTESIAN_POINT ( 'NONE',  ( 3.675000000000001155, 6.123233995736764310E-16, -4.999999999999998224 ) ) ;
#18335=CARTESIAN_POINT ( 'NONE',  ( 4.921875000614518214, 3.027376345333613106, -5.243569643749998122 ) ) ;
#18336=CARTESIAN_POINT ( 'NONE',  ( 18.22499999999999787, 4.330127018922191873, 2.499999999999999556 ) ) ;
#18337=CARTESIAN_POINT ( 'NONE',  ( 17.12812500061451715, 4.541064518000418104, 2.621784821874999949 ) ) ;
#18339=DIRECTION ( 'NONE',  ( 0.000000000000000000, 0.000000000000000000, -1.000000000000000000 ) ) ;
#18341=CARTESIAN_POINT ( 'NONE',  ( 7.378125000614518036, -4.541064518000419881, 2.621784821874995952 ) ) ;
#18342=CARTESIAN_POINT ( 'NONE',  ( 26.29687500061451644, -3.027376345333614438, 5.243569643749998122 ) ) ;
#18343=CARTESIAN_POINT ( 'NONE',  ( 4.243569643749999010, 18.77187500061451786, 27.54997392385601174 ) ) ;
#18344=CARTESIAN_POINT ( 'NONE',  ( 26.29687500061451644, -3.027376345333614438, 5.243569643749998122 ) ) ;
#18345=CARTESIAN_POINT ( 'NONE',  ( 7.200000000000001954, -4.330127018922190985, -2.500000000000001332 ) ) ;
#18346=CARTESIAN_POINT ( 'NONE',  ( -2.828200636599751609E-16, 13.70000000122903572, 25.38119784648299770 ) ) ;
#18347=CARTESIAN_POINT ( 'NONE',  ( 15.21562500061451750, 3.027376345333613106, -5.243569643749998122 ) ) ;
#18348=CARTESIAN_POINT ( 'NONE',  ( 6.600000001229032520, 5.773502691896255534, 3.535250795749688894E-16 ) ) ;
#18349=EDGE_CURVE ( 'NONE', #47876, #19994, #10278, .T. ) ;
#18350=VECTOR ( 'NONE', #65848, 1000.000000000000000 ) ;
#18351=CARTESIAN_POINT ( 'NONE',  ( 18.12187500061451573, 3.027376345333611329, 5.243569643749999010 ) ) ;
#18352=CARTESIAN_POINT ( 'NONE',  ( 12.23437500061451821, 4.541064518000418104, 2.621784821874999949 ) ) ;
#18353=CARTESIAN_POINT ( 'NONE',  ( -3.999828644916963327, 3.000228472979579841, -29.85654714282670952 ) ) ;
#18355=CARTESIAN_POINT ( 'NONE',  ( 12.06562500061451537, 3.027376345333613106, -5.243569643749998122 ) ) ;
#18358=CARTESIAN_POINT ( 'NONE',  ( 24.18750000122903288, 4.330127018922191873, 2.499999999999999556 ) ) ;
#18359=CARTESIAN_POINT ( 'NONE',  ( 13.69687500061451679, -3.027376345333614438, 5.243569643749998122 ) ) ;
#18360=CARTESIAN_POINT ( 'NONE',  ( 28.87499999999999645, 6.123233995736764310E-16, -4.999999999999998224 ) ) ;
#18361=CARTESIAN_POINT ( 'NONE',  ( 14.24062500061451608, -3.027376345333610441, -5.243569643749999898 ) ) ;
#18362=EDGE_CURVE ( 'NONE', #32246, #5287, #46062, .T. ) ;
#18363=CARTESIAN_POINT ( 'NONE',  ( 3.999999999999998668, 18.91249999999999787, -32.30940107675850470 ) ) ;
#18364=CARTESIAN_POINT ( 'NONE',  ( 23.55937500061451573, 0.000000000000000000, 5.243569643749999010 ) ) ;
#18366=CARTESIAN_POINT ( 'NONE',  ( 11.70000000122903216, -2.886751345948129988, 4.999999999999997335 ) ) ;
#18367=CYLINDRICAL_SURFACE ( 'NONE', #35112, 4.999999999999998224 ) ;
#18368=CARTESIAN_POINT ( 'NONE',  ( -3.999999999999999112, 19.51250000000000284, 27.69059892324149885 ) ) ;
#18369=CARTESIAN_POINT ( 'NONE',  ( -4.243569643749999898, 17.60937500061451999, -30.00000000000000000 ) ) ;
#18372=CARTESIAN_POINT ( 'NONE',  ( 19.02187500061451786, 3.027376345333611329, 5.243569643749999010 ) ) ;
#18373=CARTESIAN_POINT ( 'NONE',  ( 17.21250000122903145, -4.330127018922190985, -2.500000000000001332 ) ) ;
#18374=CARTESIAN_POINT ( 'NONE',  ( 15.08437500061451786, -4.541064518000419881, 2.621784821874995952 ) ) ;
#18375=CARTESIAN_POINT ( 'NONE',  ( -4.243569643749999898, 10.82187500061451857, 27.54997392385601529 ) ) ;
#18376=CARTESIAN_POINT ( 'NONE',  ( 21.11250000122903359, 0.000000000000000000, 4.999999999999998224 ) ) ;
#18377=CARTESIAN_POINT ( 'NONE',  ( 15.40312500061451573, 0.000000000000000000, 5.243569643749999010 ) ) ;
#18379=VERTEX_POINT ( 'NONE', #49802 ) ;
#18380=CARTESIAN_POINT ( 'NONE',  ( 18.52499999999999858, 6.123233995736764310E-16, -4.999999999999998224 ) ) ;
#18381=FACE_OUTER_BOUND ( 'NONE', #52604, .T. ) ;
#18382=CARTESIAN_POINT ( 'NONE',  ( 22.34999999999999787, 0.000000000000000000, 4.999999999999998224 ) ) ;
#18383=CARTESIAN_POINT ( 'NONE',  ( 13.95000000122903572, -2.886751345948129988, 4.999999999999997335 ) ) ;
#18384=CARTESIAN_POINT ( 'NONE',  ( 27.45937500061451786, 4.541064518000418104, -2.621784821874998173 ) ) ;
#18385=CARTESIAN_POINT ( 'NONE',  ( 19.34062500061451573, 6.054752690667223547, 3.707466751127219781E-16 ) ) ;
#18386=CARTESIAN_POINT ( 'NONE',  ( 22.86562500061451431, 3.027376345333613106, -5.243569643749998122 ) ) ;
#18387=CARTESIAN_POINT ( 'NONE',  ( 4.340625000614515727, -3.027376345333610441, -5.243569643749999898 ) ) ;
#18388=CARTESIAN_POINT ( 'NONE',  ( 26.39999999999999858, 0.000000000000000000, 4.999999999999998224 ) ) ;
#18390=CARTESIAN_POINT ( 'NONE',  ( 0.000000000000000000, 20.00000000000000000, 30.00000000000000000 ) ) ;
#18392=CARTESIAN_POINT ( 'NONE',  ( 2.121784821875001281, 15.95937500061451608, -26.32496088578401938 ) ) ;
#18393=EDGE_CURVE ( 'NONE', #36225, #19466, #19078, .T. ) ;
#18394=CARTESIAN_POINT ( 'NONE',  ( 5.362500001229033586, 0.000000000000000000, 4.999999999999998224 ) ) ;
#18395=CARTESIAN_POINT ( 'NONE',  ( 6.787500000000001421, -2.886751345948125991, -5.000000000000000000 ) ) ;
#18396=CARTESIAN_POINT ( 'NONE',  ( 16.31249999999999645, 2.886751345948062486, -5.000000000000113687 ) ) ;
#18397=CARTESIAN_POINT ( 'NONE',  ( 9.459375000614517859, 4.541064518000418104, -2.621784821874998173 ) ) ;
#18398=CARTESIAN_POINT ( 'NONE',  ( 28.11562500061451431, -6.054752690667223547, -1.112240025338166033E-15 ) ) ;
#18399=CARTESIAN_POINT ( 'NONE',  ( 27.56250000122902932, -4.330127018922190985, -2.500000000000001332 ) ) ;
#18401=CARTESIAN_POINT ( 'NONE',  ( 10.00000000000000000, 1.224646799147353256E-15, -50.00000000000000000 ) ) ;
#18402=CARTESIAN_POINT ( 'NONE',  ( 8.371875000614515727, -6.054752690667223547, -1.112240025338166033E-15 ) ) ;
#18403=CARTESIAN_POINT ( 'NONE',  ( 10.24687500061451750, -3.027376345333610441, -5.243569643749999898 ) ) ;
#18404=CARTESIAN_POINT ( 'NONE',  ( 5.625000000000001776, 4.330127018922191873, 2.499999999999999556 ) ) ;
#18405=( BOUNDED_CURVE ( )  B_SPLINE_CURVE ( 2, ( #23258, #34341, #16625, #39179, #50270, #55804, #67619 ),
 .UNSPECIFIED., .F., .F. ) 
 B_SPLINE_CURVE_WITH_KNOTS ( ( 3, 2, 2, 3 ),
 ( 0.5333333333333334370, 0.5361111111111112049, 0.5388888888888888618, 0.5416666666666666297 ),
 .UNSPECIFIED. ) 
 CURVE ( )  GEOMETRIC_REPRESENTATION_ITEM ( )  RATIONAL_B_SPLINE_CURVE ( ( 0.9999999999999946709, 0.8660254037844440367, 1.000000000000000000, 0.8660254037844387076, 1.000000000000000000, 0.8660254037844387076, 1.000000000000000000 ) ) 
 REPRESENTATION_ITEM ( '' )  );
#18406=CARTESIAN_POINT ( 'NONE',  ( 2.121784821874999061, 15.60312500061459495, 26.32496088578401583 ) ) ;
#18407=CARTESIAN_POINT ( 'NONE',  ( 4.949999999999999289, -4.330127018922190985, -2.500000000000001332 ) ) ;
#18408=CARTESIAN_POINT ( 'NONE',  ( 6.675000000000000711, -4.330127018922194537, 2.499999999999995559 ) ) ;
#18409=CARTESIAN_POINT ( 'NONE',  ( 26.85000000122903430, 5.773502691896255534, 3.535250795749688894E-16 ) ) ;
#18411=CARTESIAN_POINT ( 'NONE',  ( 23.87812500061451715, 4.541064518000418104, 2.621784821874999949 ) ) ;
#18412=CARTESIAN_POINT ( 'NONE',  ( 13.19062500061451537, -3.027376345333614438, 5.243569643749998122 ) ) ;
#18414=CARTESIAN_POINT ( 'NONE',  ( 9.346875000614517148, -3.027376345333610441, -5.243569643749999898 ) ) ;
#18415=CARTESIAN_POINT ( 'NONE',  ( 25.34999999999999787, 4.330127018922192761, -2.499999999999997780 ) ) ;
#18416=CARTESIAN_POINT ( 'NONE',  ( 22.08750000122903501, -4.330127018922194537, 2.499999999999995559 ) ) ;
#18417=CARTESIAN_POINT ( 'NONE',  ( 0.000000000000000000, 20.00000000000000000, 30.00000000000000000 ) ) ;
#18418=CARTESIAN_POINT ( 'NONE',  ( 12.04687500061451821, -3.027376345333610441, -5.243569643749999898 ) ) ;
#18419=CARTESIAN_POINT ( 'NONE',  ( 26.93437500061451573, 6.421520780324663323E-16, -5.243569643749999010 ) ) ;
#18420=CARTESIAN_POINT ( 'NONE',  ( 3.459375000614519635, -4.541064518000417216, -2.621784821875001281 ) ) ;
#18421=CARTESIAN_POINT ( 'NONE',  ( 2.000000000000001332, 13.51250000122903394, -26.53589838486224650 ) ) ;
#18422=CARTESIAN_POINT ( 'NONE',  ( 21.42187500061451644, -6.054752690667223547, -1.112240025338166033E-15 ) ) ;
#18423=CARTESIAN_POINT ( 'NONE',  ( 12.27187500061451786, 3.027376345333611329, 5.243569643749999010 ) ) ;
#18425=CARTESIAN_POINT ( 'NONE',  ( 24.86250000000000071, 2.886751345948129099, -4.999999999999998224 ) ) ;
#18427=CARTESIAN_POINT ( 'NONE',  ( 4.243569643749999898, 14.19687500061451857, -27.54997392385601529 ) ) ;
#18429=CARTESIAN_POINT ( 'NONE',  ( 18.17812500061451786, -4.541064518000419881, 2.621784821874995952 ) ) ;
#18430=CARTESIAN_POINT ( 'NONE',  ( 8.025000000000000355, -4.330127018922194537, 2.499999999999995559 ) ) ;
#18432=CARTESIAN_POINT ( 'NONE',  ( 14.73749999999999893, -2.886751345948129988, 4.999999999999997335 ) ) ;
#18433=CARTESIAN_POINT ( 'NONE',  ( 3.999999999999999112, 19.43750000122903288, 30.00000000000000000 ) ) ;
#18434=CARTESIAN_POINT ( 'NONE',  ( 14.10000000122903252, -2.886751345948125991, -5.000000000000000000 ) ) ;
#18436=CARTESIAN_POINT ( 'NONE',  ( 25.73437500061451644, 4.541064518000418104, 2.621784821874999949 ) ) ;
#18437=AXIS2_PLACEMENT_3D ( 'NONE', #21854, #67663, #62111 ) ;
#18438=EDGE_LOOP ( 'NONE', ( #56265, #35247, #17959, #18604 ) ) ;
#18439=CARTESIAN_POINT ( 'NONE',  ( 18.81562500061452070, 3.027376345333613106, -5.243569643749998122 ) ) ;
#18440=CARTESIAN_POINT ( 'NONE',  ( 21.19687500061451502, 6.054752690667223547, 3.707466751127219781E-16 ) ) ;
#18441=CARTESIAN_POINT ( 'NONE',  ( 3.037500000000002309, -2.886751345948129988, 4.999999999999997335 ) ) ;
#18442=CARTESIAN_POINT ( 'NONE',  ( 7.790625000614518569, -3.027376345333614438, 5.243569643749998122 ) ) ;
#18443=CARTESIAN_POINT ( 'NONE',  ( 21.25312500061451715, 0.000000000000000000, 5.243569643749999010 ) ) ;
#18444=CARTESIAN_POINT ( 'NONE',  ( 12.60937500061451821, 4.541064518000418104, -2.621784821874998173 ) ) ;
#18445=CARTESIAN_POINT ( 'NONE',  ( 16.54687500061451644, -3.027376345333610441, -5.243569643749999898 ) ) ;
#18446=CARTESIAN_POINT ( 'NONE',  ( 4.243569643749999010, 14.21562500061451928, 27.54997392385601174 ) ) ;
#18447=CARTESIAN_POINT ( 'NONE',  ( 18.75000000122903288, 5.773502691896255534, 3.535250795749688894E-16 ) ) ;
#18449=CARTESIAN_POINT ( 'NONE',  ( 9.290625000614515017, -3.027376345333610441, -5.243569643749999898 ) ) ;
#18450=CARTESIAN_POINT ( 'NONE',  ( 3.496875000614518836, -3.027376345333610441, -5.243569643749999898 ) ) ;
#18451=CARTESIAN_POINT ( 'NONE',  ( 29.69062500061451715, 6.054752690667223547, 3.707466751127219781E-16 ) ) ;
#18452=EDGE_CURVE ( 'NONE', #16648, #36225, #44636, .T. ) ;
#18453=CARTESIAN_POINT ( 'NONE',  ( 24.90937500061451715, 0.000000000000000000, 5.243569643749999010 ) ) ;
#18454=CARTESIAN_POINT ( 'NONE',  ( 17.16562500061451502, 3.027376345333611329, 5.243569643749999010 ) ) ;
#18455=CARTESIAN_POINT ( 'NONE',  ( 24.18750000122903288, 4.330127018922191873, 2.499999999999999556 ) ) ;
#18456=CARTESIAN_POINT ( 'NONE',  ( 25.30312500061451431, 0.000000000000000000, 5.243569643749999010 ) ) ;
#18457=CARTESIAN_POINT ( 'NONE',  ( 22.28437500061451715, -4.541064518000419881, 2.621784821874995952 ) ) ;
#18458=CARTESIAN_POINT ( 'NONE',  ( 16.67812500061451786, 4.541064518000418104, 2.621784821874999949 ) ) ;
#18459=CARTESIAN_POINT ( 'NONE',  ( -3.000416591977282496E-16, 17.94687500061451502, 25.09994784771203058 ) ) ;
#18460=( BOUNDED_SURFACE ( )  B_SPLINE_SURFACE ( 1, 2, ( 
 ( #36083, #63060, #57522, #69706, #64148, #41274, #1752, #70063, #23537, #19437, #12463, #46814, #58236, #19072, #13174, #69352, #68986, #13535, #30545, #46087, #64518, #34993, #1031, #18709, #58603, #8010, #13911, #36450, #29453, #18343, #63785, #51990, #7641, #1391, #23900, #12817, #46448, #29814, #40918, #63430, #57875, #7285, #19810, #26466, #37543, #49372, #32006, #70796, #42363, #60798, #71536, #2833, #64885, #30901, #9108, #31646, #3943, #71902, #54905, #14273, #71161, #20911, #3575, #20171, #37176, #36811, #25735, #20534, #54178, #49005, #8737, #60065, #26098, #43463, #53443, #15731, #47906, #43090, #48636, #65618, #43829, #15006, #59326, #31270, #53812, #4313, #9476, #54541, #38270, #9838, #3206, #70435, #48272, #25361, #65987, #42725, #15368, #37909, #65246, #60427, #14635, #59701, #21275, #32367, #26838, #66353, #72629, #72263, #5755, #45647, #68181, #17543, #61896, #50463, #39377, #50820, #67460, #16100, #27930, #40105, #5030, #10569, #11301, #38650, #56711, #33821, #34175, #22372, #10204, #4671, #5392, #28289, #72991, #55999, #32739, #55276, #50098, #21640, #67815, #17188, #23090, #223, #22728, #27201, #49736, #22013, #56365, #44924, #16823, #44198, #28643, #61174, #45281, #66729, #39748, #62264, #11660, #55636, #33097, #44569, #67099, #27567, #16457, #39015, #6112, #61530, #10928, #33455, #51181, #585, #46363, #47710, #8192, #20357, #25169, #51547, #65067, #68897, #62619, #64333, #70249, #948, #57434, #23456, #19621, #46001, #23812, #3016, #29372, #42177, #68538, #18254, #25546, #51904, #31084, #36267, #1302, #40827, #17899, #6837, #30719, #13726, #59148, #40459, #64703, #58782, #53624, #12015, #48458, #6475, #53252, #2650, #14087, #3397, #36627, #62975, #12371, #34906, #14458, #8557, #48089, #70982, #42541, #70614, #29010, #19988, #34538, #36992, #59514, #8928, #31458, #54000, #25918, #57068, #72812, #33281, #21095, #72440, #66914, #32192, #31826, #38463, #21458, #26657, #16282, #60244, #55094, #65432, #32557, #4850, #27384, #4128, #15185, #43646, #4494, #60989, #55820, #10388, #54364, #32920, #49555, #61353, #44013, #9658, #3759, #42908, #55457, #14822, #26283, #37365, #66170 ),
 ( #10021, #49916, #20725, #27023, #60612, #21824, #44389, #48820, #71350, #72076, #43283, #66535, #10749, #15915, #71723, #38838, #5208, #65804, #37724, #54725, #59887, #49192, #27749, #15546, #50288, #9293, #38089, #12555, #763, #16642, #67635, #17002, #28114, #50643, #28464, #68720, #17718, #40278, #62799, #45463, #62084, #7018, #12192, #51725, #40641, #39559, #44749, #57615, #11837, #5930, #67995, #68357, #39197, #61712, #34356, #397, #17368, #22904, #23635, #47, #67283, #56888, #22552, #51360, #22195, #39925, #6662, #11111, #45100, #34719, #57249, #6293, #62439, #63160, #33640, #46181, #56184, #28822, #23271, #29191, #45821, #1126, #11477, #18080, #35089, #5577, #29549, #34000, #56537, #52085, #50999, #8468, #53168, #58329, #48005, #18804, #13636, #23996, #64248, #36543, #59063, #35807, #46908, #52808, #36180, #19538, #14374, #70161, #63526, #42096, #8108, #19908, #2565, #41368, #12913, #31373, #64618, #46544, #35446, #1490, #2209, #24724, #47628, #42461, #25461, #57970, #41721, #31003, #2932, #58698, #14005, #52448, #30636, #19167, #53536, #70533, #7377, #29908, #25085, #1854, #64983, #36909, #59429, #30276, #8837, #69085, #24361, #69447, #63878, #18446, #7740, #41011, #47267, #13269, #69801, #43928, #44300, #32473, #48371, #26197, #48736, #59800, #9206, #60162, #27300, #49466, #70898, #49107, #71999, #71636, #26567, #10666, #16201, #20639, #42822, #38376, #60900, #66829, #66454, #21374, #20270, #25834, #65717, #26941, #43561, #21009, #61273, #72358, #31741, #15831, #37278, #10303, #55006, #15461, #71259, #65346, #15103, #43197, #54279, #14736, #9572, #38006, #53914, #3307, #37639, #32104, #66083, #54637, #60528, #9935, #3673, #4412, #4042, #55373, #32836, #4767, #49834, #21739, #38752, #28032, #44668, #39846, #67198, #67555, #45744, #73088, #683, #5850, #22469, #39473, #39111, #50561, #317, #11396, #28740, #11029, #62360, #56459, #23190, #63080, #18003, #50202, #22826, #33916, #28381, #46103, #50919, #16560, #61627, #33552, #57169, #67914, #11756, #40561, #12116, #56102, #72727, #5493, #33196, #17285, #45020, #51280, #68279, #16918, #45378, #61996, #55735, #23555, #34274, #62723, #6581 ) ),
 .UNSPECIFIED., .F., .F., .F. ) 
 B_SPLINE_SURFACE_WITH_KNOTS ( ( 2, 2 ),
 ( 3, 2, 2, 2, 2, 2, 2, 2, 2, 2, 2, 2, 2, 2, 2, 2, 2, 2, 2, 2, 2, 2, 2, 2, 2, 2, 2, 2, 2, 2, 2, 2, 2, 2, 2, 2, 2, 2, 2, 2, 2, 2, 2, 2, 2, 2, 2, 2, 2, 2, 2, 2, 2, 2, 2, 2, 2, 2, 2, 2, 2, 2, 2, 2, 2, 2, 2, 2, 2, 2, 2, 2, 2, 2, 2, 2, 2, 2, 2, 2, 2, 2, 2, 2, 2, 2, 2, 2, 2, 2, 2, 2, 2, 2, 2, 2, 2, 2, 2, 2, 2, 2, 2, 2, 2, 2, 2, 2, 2, 2, 2, 2, 2, 2, 2, 2, 2, 2, 2, 2, 2, 2, 2, 2, 2, 2, 2, 2, 2, 2, 2, 2, 2, 2, 2, 3 ),
 ( 0.000000000000000000, 1.000000000000000000 ),
 ( 0.000000000000000000, 0.007246376811594202987, 0.01449275362318840597, 0.02173913043478260809, 0.02898550724637681195, 0.03623188405797101580, 0.04347826086956521618, 0.05072463768115942351, 0.05797101449275362389, 0.06521739130434782428, 0.07246376811594203160, 0.07971014492753622505, 0.08695652173913043237, 0.09420289855072463969, 0.1014492753623188470, 0.1086956521739130405, 0.1159420289855072478, 0.1231884057971014551, 0.1304347826086956486, 0.1376811594202898559, 0.1449275362318840632, 0.1521739130434782705, 0.1594202898550724501, 0.1666666666666666574, 0.1739130434782608647, 0.1811594202898550721, 0.1884057971014492794, 0.1956521739130434867, 0.2028985507246376940, 0.2101449275362318736, 0.2173913043478260809, 0.2246376811594202882, 0.2318840579710144956, 0.2391304347826087029, 0.2463768115942029102, 0.2536231884057971175, 0.2608695652173912971, 0.2681159420289855322, 0.2753623188405797118, 0.2826086956521738913, 0.2898550724637681264, 0.2971014492753623060, 0.3043478260869565410, 0.3115942028985507206, 0.3188405797101449002, 0.3260869565217391353, 0.3333333333333333148, 0.3405797101449275499, 0.3478260869565217295, 0.3550724637681159646, 0.3623188405797101441, 0.3695652173913043237, 0.3768115942028985588, 0.3840579710144927383, 0.3913043478260869734, 0.3985507246376811530, 0.4057971014492753881, 0.4130434782608695676, 0.4202898550724637472, 0.4275362318840579823, 0.4347826086956521618, 0.4420289855072463969, 0.4492753623188405765, 0.4565217391304347561, 0.4637681159420289911, 0.4710144927536231707, 0.4782608695652174058, 0.4855072463768115854, 0.4927536231884058204, 0.5000000000000000000, 0.5072463768115942351, 0.5144927536231883591, 0.5217391304347825942, 0.5289855072463768293, 0.5362318840579710644, 0.5434782608695651884, 0.5507246376811594235, 0.5579710144927536586, 0.5652173913043477826, 0.5724637681159420177, 0.5797101449275362528, 0.5869565217391304879, 0.5942028985507246119, 0.6014492753623188470, 0.6086956521739130821, 0.6159420289855072062, 0.6231884057971014412, 0.6304347826086956763, 0.6376811594202898004, 0.6449275362318840354, 0.6521739130434782705, 0.6594202898550725056, 0.6666666666666666297, 0.6739130434782608647, 0.6811594202898550998, 0.6884057971014492239, 0.6956521739130434590, 0.7028985507246376940, 0.7101449275362319291, 0.7173913043478260532, 0.7246376811594202882, 0.7318840579710145233, 0.7391304347826086474, 0.7463768115942028825, 0.7536231884057971175, 0.7608695652173913526, 0.7681159420289854767, 0.7753623188405797118, 0.7826086956521739468, 0.7898550724637680709, 0.7971014492753623060, 0.8043478260869565410, 0.8115942028985507761, 0.8188405797101449002, 0.8260869565217391353, 0.8333333333333333703, 0.8405797101449274944, 0.8478260869565217295, 0.8550724637681159646, 0.8623188405797101996, 0.8695652173913043237, 0.8768115942028985588, 0.8840579710144927938, 0.8913043478260869179, 0.8985507246376811530, 0.9057971014492753881, 0.9130434782608695121, 0.9202898550724637472, 0.9275362318840579823, 0.9347826086956522174, 0.9420289855072463414, 0.9492753623188405765, 0.9565217391304348116, 0.9637681159420289356, 0.9662082893573751274, 0.9758703722509488587 ),
 .UNSPECIFIED. ) 
 GEOMETRIC_REPRESENTATION_ITEM ( )  RATIONAL_B_SPLINE_SURFACE ( (
 ( 1.000000000000000000, 0.8660254037844387076, 1.000000000000000000, 0.8660254037844387076, 1.000000000000000000, 0.8660254037844387076, 1.000000000000000000, 0.8660254037844387076, 1.000000000000000000, 0.8660254037844387076, 1.000000000000000000, 0.8660254037844387076, 1.000000000000000000, 0.8660254037844387076, 1.000000000000000000, 0.8660254037844387076, 1.000000000000000000, 0.8660254037844387076, 1.000000000000000000, 0.8660254037844387076, 1.000000000000000000, 0.8660254037844387076, 1.000000000000000000, 0.8660254037844387076, 1.000000000000000000, 0.8660254037844387076, 1.000000000000000000, 0.8660254037844387076, 1.000000000000000000, 0.8660254037844387076, 1.000000000000000000, 0.8660254037844387076, 1.000000000000000000, 0.8660254037844387076, 1.000000000000000000, 0.8660254037844387076, 1.000000000000000000, 0.8660254037844387076, 1.000000000000000000, 0.8660254037844387076, 1.000000000000000000, 0.8660254037844387076, 1.000000000000000000, 0.8660254037844387076, 1.000000000000000000, 0.8660254037844387076, 1.000000000000000000, 0.8660254037844387076, 1.000000000000000000, 0.8660254037844387076, 1.000000000000000000, 0.8660254037844387076, 1.000000000000000000, 0.8660254037844387076, 1.000000000000000000, 0.8660254037844387076, 1.000000000000000000, 0.8660254037844387076, 1.000000000000000000, 0.8660254037844387076, 1.000000000000000000, 0.8660254037844387076, 1.000000000000000000, 0.8660254037844387076, 1.000000000000000000, 0.8660254037844387076, 1.000000000000000000, 0.8660254037844387076, 1.000000000000000000, 0.8660254037844387076, 1.000000000000000000, 0.8660254037844387076, 1.000000000000000000, 0.8660254037844387076, 1.000000000000000000, 0.8660254037844387076, 1.000000000000000000, 0.8660254037844387076, 1.000000000000000000, 0.8660254037844387076, 1.000000000000000000, 0.8660254037844387076, 1.000000000000000000, 0.8660254037844387076, 1.000000000000000000, 0.8660254037844387076, 1.000000000000000000, 0.8660254037844387076, 1.000000000000000000, 0.8660254037844387076, 1.000000000000000000, 0.8660254037844387076, 1.000000000000000000, 0.8660254037844387076, 1.000000000000000000, 0.8660254037844387076, 1.000000000000000000, 0.8660254037844387076, 1.000000000000000000, 0.8660254037844387076, 1.000000000000000000, 0.8660254037844387076, 1.000000000000000000, 0.8660254037844387076, 1.000000000000000000, 0.8660254037844387076, 1.000000000000000000, 0.8660254037844387076, 1.000000000000000000, 0.8660254037844387076, 1.000000000000000000, 0.8660254037844387076, 1.000000000000000000, 0.8660254037844387076, 1.000000000000000000, 0.8660254037844387076, 1.000000000000000000, 0.8660254037844387076, 1.000000000000000000, 0.8660254037844387076, 1.000000000000000000, 0.8660254037844387076, 1.000000000000000000, 0.8660254037844387076, 1.000000000000000000, 0.8660254037844387076, 1.000000000000000000, 0.8660254037844387076, 1.000000000000000000, 0.8660254037844387076, 1.000000000000000000, 0.8660254037844387076, 1.000000000000000000, 0.8660254037844387076, 1.000000000000000000, 0.8660254037844387076, 1.000000000000000000, 0.8660254037844387076, 1.000000000000000000, 0.8660254037844387076, 1.000000000000000000, 0.8660254037844387076, 1.000000000000000000, 0.8660254037844387076, 1.000000000000000000, 0.8660254037844387076, 1.000000000000000000, 0.8660254037844387076, 1.000000000000000000, 0.8660254037844387076, 1.000000000000000000, 0.8660254037844387076, 1.000000000000000000, 0.8660254037844387076, 1.000000000000000000, 0.8660254037844387076, 1.000000000000000000, 0.8660254037844387076, 1.000000000000000000, 0.8660254037844387076, 1.000000000000000000, 0.8660254037844387076, 1.000000000000000000, 0.8660254037844387076, 1.000000000000000000, 0.8660254037844387076, 1.000000000000000000, 0.8660254037844387076, 1.000000000000000000, 0.8660254037844387076, 1.000000000000000000, 0.8660254037844387076, 1.000000000000000000, 0.8660254037844387076, 1.000000000000000000, 0.8660254037844387076, 1.000000000000000000, 0.8660254037844387076, 1.000000000000000000, 0.8660254037844387076, 1.000000000000000000, 0.8660254037844387076, 1.000000000000000000, 0.8660254037844387076, 1.000000000000000000, 0.8660254037844387076, 1.000000000000000000, 0.8660254037844387076, 1.000000000000000000, 0.8660254037844387076, 1.000000000000000000, 0.8660254037844387076, 1.000000000000000000, 0.8660254037844387076, 1.000000000000000000, 0.8660254037844387076, 1.000000000000000000, 0.8660254037844387076, 1.000000000000000000, 0.8660254037844387076, 1.000000000000000000, 0.8660254037844387076, 1.000000000000000000, 0.8660254037844387076, 1.000000000000000000, 0.8660254037844387076, 1.000000000000000000, 0.8660254037844387076, 1.000000000000000000, 0.8660254037844387076, 1.000000000000000000, 0.8660254037844387076, 1.000000000000000000, 0.8660254037844387076, 1.000000000000000000, 0.8660254037844387076, 1.000000000000000000, 0.8660254037844387076, 1.000000000000000000, 0.8660254037844387076, 1.000000000000000000, 0.8660254037844387076, 1.000000000000000000, 0.8660254037844387076, 1.000000000000000000, 0.8660254037844387076, 1.000000000000000000, 0.8660254037844387076, 1.000000000000000000, 0.8660254037844387076, 1.000000000000000000, 0.8660254037844387076, 1.000000000000000000, 0.8660254037844387076, 1.000000000000000000, 0.8660254037844387076, 1.000000000000000000, 0.8660254037844387076, 1.000000000000000000, 0.8660254037844387076, 1.000000000000000000, 0.8660254037844387076, 1.000000000000000000, 0.8660254037844387076, 1.000000000000000000, 0.8660254037844387076, 1.000000000000000000, 0.8660254037844387076, 1.000000000000000000, 0.8660254037844387076, 1.000000000000000000, 0.8660254037844387076, 1.000000000000000000, 0.8660254037844387076, 1.000000000000000000, 0.8660254037844387076, 1.000000000000000000, 0.8660254037844387076, 1.000000000000000000, 0.8660254037844387076, 1.000000000000000000, 0.8660254037844387076, 1.000000000000000000, 0.8660254037844387076, 1.000000000000000000, 0.8660254037844387076, 1.000000000000000000, 0.9548848677736607726, 0.9401542295229587953, 0.9401542295229587953, 0.9401542295229587953),
 ( 1.000000000000000000, 0.8660254037844387076, 1.000000000000000000, 0.8660254037844387076, 1.000000000000000000, 0.8660254037844387076, 1.000000000000000000, 0.8660254037844387076, 1.000000000000000000, 0.8660254037844387076, 1.000000000000000000, 0.8660254037844387076, 1.000000000000000000, 0.8660254037844387076, 1.000000000000000000, 0.8660254037844387076, 1.000000000000000000, 0.8660254037844387076, 1.000000000000000000, 0.8660254037844387076, 1.000000000000000000, 0.8660254037844387076, 1.000000000000000000, 0.8660254037844387076, 1.000000000000000000, 0.8660254037844387076, 1.000000000000000000, 0.8660254037844387076, 1.000000000000000000, 0.8660254037844387076, 1.000000000000000000, 0.8660254037844387076, 1.000000000000000000, 0.8660254037844387076, 1.000000000000000000, 0.8660254037844387076, 1.000000000000000000, 0.8660254037844387076, 1.000000000000000000, 0.8660254037844387076, 1.000000000000000000, 0.8660254037844387076, 1.000000000000000000, 0.8660254037844387076, 1.000000000000000000, 0.8660254037844387076, 1.000000000000000000, 0.8660254037844387076, 1.000000000000000000, 0.8660254037844387076, 1.000000000000000000, 0.8660254037844387076, 1.000000000000000000, 0.8660254037844387076, 1.000000000000000000, 0.8660254037844387076, 1.000000000000000000, 0.8660254037844387076, 1.000000000000000000, 0.8660254037844387076, 1.000000000000000000, 0.8660254037844387076, 1.000000000000000000, 0.8660254037844387076, 1.000000000000000000, 0.8660254037844387076, 1.000000000000000000, 0.8660254037844387076, 1.000000000000000000, 0.8660254037844387076, 1.000000000000000000, 0.8660254037844387076, 1.000000000000000000, 0.8660254037844387076, 1.000000000000000000, 0.8660254037844387076, 1.000000000000000000, 0.8660254037844387076, 1.000000000000000000, 0.8660254037844387076, 1.000000000000000000, 0.8660254037844387076, 1.000000000000000000, 0.8660254037844387076, 1.000000000000000000, 0.8660254037844387076, 1.000000000000000000, 0.8660254037844387076, 1.000000000000000000, 0.8660254037844387076, 1.000000000000000000, 0.8660254037844387076, 1.000000000000000000, 0.8660254037844387076, 1.000000000000000000, 0.8660254037844387076, 1.000000000000000000, 0.8660254037844387076, 1.000000000000000000, 0.8660254037844387076, 1.000000000000000000, 0.8660254037844387076, 1.000000000000000000, 0.8660254037844387076, 1.000000000000000000, 0.8660254037844387076, 1.000000000000000000, 0.8660254037844387076, 1.000000000000000000, 0.8660254037844387076, 1.000000000000000000, 0.8660254037844387076, 1.000000000000000000, 0.8660254037844387076, 1.000000000000000000, 0.8660254037844387076, 1.000000000000000000, 0.8660254037844387076, 1.000000000000000000, 0.8660254037844387076, 1.000000000000000000, 0.8660254037844387076, 1.000000000000000000, 0.8660254037844387076, 1.000000000000000000, 0.8660254037844387076, 1.000000000000000000, 0.8660254037844387076, 1.000000000000000000, 0.8660254037844387076, 1.000000000000000000, 0.8660254037844387076, 1.000000000000000000, 0.8660254037844387076, 1.000000000000000000, 0.8660254037844387076, 1.000000000000000000, 0.8660254037844387076, 1.000000000000000000, 0.8660254037844387076, 1.000000000000000000, 0.8660254037844387076, 1.000000000000000000, 0.8660254037844387076, 1.000000000000000000, 0.8660254037844387076, 1.000000000000000000, 0.8660254037844387076, 1.000000000000000000, 0.8660254037844387076, 1.000000000000000000, 0.8660254037844387076, 1.000000000000000000, 0.8660254037844387076, 1.000000000000000000, 0.8660254037844387076, 1.000000000000000000, 0.8660254037844387076, 1.000000000000000000, 0.8660254037844387076, 1.000000000000000000, 0.8660254037844387076, 1.000000000000000000, 0.8660254037844387076, 1.000000000000000000, 0.8660254037844387076, 1.000000000000000000, 0.8660254037844387076, 1.000000000000000000, 0.8660254037844387076, 1.000000000000000000, 0.8660254037844387076, 1.000000000000000000, 0.8660254037844387076, 1.000000000000000000, 0.8660254037844387076, 1.000000000000000000, 0.8660254037844387076, 1.000000000000000000, 0.8660254037844387076, 1.000000000000000000, 0.8660254037844387076, 1.000000000000000000, 0.8660254037844387076, 1.000000000000000000, 0.8660254037844387076, 1.000000000000000000, 0.8660254037844387076, 1.000000000000000000, 0.8660254037844387076, 1.000000000000000000, 0.8660254037844387076, 1.000000000000000000, 0.8660254037844387076, 1.000000000000000000, 0.8660254037844387076, 1.000000000000000000, 0.8660254037844387076, 1.000000000000000000, 0.8660254037844387076, 1.000000000000000000, 0.8660254037844387076, 1.000000000000000000, 0.8660254037844387076, 1.000000000000000000, 0.8660254037844387076, 1.000000000000000000, 0.8660254037844387076, 1.000000000000000000, 0.8660254037844387076, 1.000000000000000000, 0.8660254037844387076, 1.000000000000000000, 0.8660254037844387076, 1.000000000000000000, 0.8660254037844387076, 1.000000000000000000, 0.8660254037844387076, 1.000000000000000000, 0.8660254037844387076, 1.000000000000000000, 0.8660254037844387076, 1.000000000000000000, 0.8660254037844387076, 1.000000000000000000, 0.8660254037844387076, 1.000000000000000000, 0.8660254037844387076, 1.000000000000000000, 0.8660254037844387076, 1.000000000000000000, 0.8660254037844387076, 1.000000000000000000, 0.8660254037844387076, 1.000000000000000000, 0.8660254037844387076, 1.000000000000000000, 0.8660254037844387076, 1.000000000000000000, 0.8660254037844387076, 1.000000000000000000, 0.8660254037844387076, 1.000000000000000000, 0.8660254037844387076, 1.000000000000000000, 0.8660254037844387076, 1.000000000000000000, 0.8660254037844387076, 1.000000000000000000, 0.8660254037844387076, 1.000000000000000000, 0.8660254037844387076, 1.000000000000000000, 0.8660254037844387076, 1.000000000000000000, 0.8660254037844387076, 1.000000000000000000, 0.8660254037844387076, 1.000000000000000000, 0.8660254037844387076, 1.000000000000000000, 0.8660254037844387076, 1.000000000000000000, 0.8660254037844387076, 1.000000000000000000, 0.8660254037844387076, 1.000000000000000000, 0.9548848677736607726, 0.9401542295229587953, 0.9401542295229587953, 0.9401542295229587953) ) ) 
 REPRESENTATION_ITEM ( '' )  SURFACE ( )  );
#18461=CARTESIAN_POINT ( 'NONE',  ( 22.97812500061451857, 4.541064518000418104, 2.621784821874999949 ) ) ;
#18462=FACE_OUTER_BOUND ( 'NONE', #5811, .T. ) ;
#18464=CARTESIAN_POINT ( 'NONE',  ( 26.28749999999999432, 5.773502691896255534, 3.535250795749688894E-16 ) ) ;
#18465=CARTESIAN_POINT ( 'NONE',  ( 1.999999999999998668, 12.65000000000000213, -33.46410161513775705 ) ) ;
#18467=CARTESIAN_POINT ( 'NONE',  ( 3.159375000614518036, 4.541064518000418104, -2.621784821874998173 ) ) ;
#18468=CARTESIAN_POINT ( 'NONE',  ( 9.403125000614517504, 4.541064518000418104, -2.621784821874998173 ) ) ;
#18469=CARTESIAN_POINT ( 'NONE',  ( 21.60000000122903430, -2.886751345948129988, 4.999999999999997335 ) ) ;
#18470=CARTESIAN_POINT ( 'NONE',  ( 26.42812500061451431, 6.421520780324663323E-16, -5.243569643749999010 ) ) ;
#18471=CARTESIAN_POINT ( 'NONE',  ( 25.46249999999999858, 2.886751345948126879, 4.999999999999999112 ) ) ;
#18472=CARTESIAN_POINT ( 'NONE',  ( 1.999999999999998668, 15.46250000122903501, -33.46410161513775705 ) ) ;
#18473=CARTESIAN_POINT ( 'NONE',  ( 29.20312500061451644, 4.541064518000418104, -2.621784821874998173 ) ) ;
#18474=CARTESIAN_POINT ( 'NONE',  ( 11.09062500061451573, -3.027376345333610441, -5.243569643749999898 ) ) ;
#18475=ORIENTED_EDGE ( 'NONE', *, *, #14379, .F. ) ;
#18476=CARTESIAN_POINT ( 'NONE',  ( 25.19062500061451715, 6.054752690667223547, 3.707466751127219781E-16 ) ) ;
#18477=CARTESIAN_POINT ( 'NONE',  ( 7.078125000614516438, 6.421520780324663323E-16, -5.243569643749999010 ) ) ;
#18478=CARTESIAN_POINT ( 'NONE',  ( 3.365625000614516082, -6.054752690667223547, -1.112240025338166033E-15 ) ) ;
#18480=FACE_OUTER_BOUND ( 'NONE', #52325, .T. ) ;
#18481=CARTESIAN_POINT ( 'NONE',  ( 14.06250000000000000, 2.886751345948129099, -4.999999999999998224 ) ) ;
#18482=CARTESIAN_POINT ( 'NONE',  ( 13.39687500061451608, -3.027376345333610441, -5.243569643749999898 ) ) ;
#18483=CARTESIAN_POINT ( 'NONE',  ( 11.10000000122903252, 5.773502691896255534, 3.535250795749688894E-16 ) ) ;
#18484=CARTESIAN_POINT ( 'NONE',  ( 16.39687500061451786, -3.027376345333614438, 5.243569643749998122 ) ) ;
#18486=CARTESIAN_POINT ( 'NONE',  ( 7.546875000614517326, -3.027376345333610441, -5.243569643749999898 ) ) ;
#18487=CARTESIAN_POINT ( 'NONE',  ( 4.243569643749999898, 11.89062500061451644, -27.54997392385601529 ) ) ;
#18488=DIRECTION ( 'NONE',  ( -1.000000000000000000, -0.000000000000000000, -0.000000000000000000 ) ) ;
#18492=CARTESIAN_POINT ( 'NONE',  ( 24.25312500061451715, 4.541064518000418104, -2.621784821874998173 ) ) ;
#18494=CARTESIAN_POINT ( 'NONE',  ( 28.02187500061451431, 3.027376345333611329, 5.243569643749999010 ) ) ;
#18495=CARTESIAN_POINT ( 'NONE',  ( 23.58749999999999858, 5.773502691896255534, 3.535250795749688894E-16 ) ) ;
#18496=CARTESIAN_POINT ( 'NONE',  ( 7.415625000614516793, -6.054752690667223547, -1.112240025338166033E-15 ) ) ;
#18498=CARTESIAN_POINT ( 'NONE',  ( 20.25937500061451857, 4.541064518000418104, -2.621784821874998173 ) ) ;
#18500=CARTESIAN_POINT ( 'NONE',  ( 29.36250000122903003, -4.330127018922190985, -2.500000000000001332 ) ) ;
#18501=CARTESIAN_POINT ( 'NONE',  ( 8.634375000614518569, 4.541064518000418104, 2.621784821874999949 ) ) ;
#18502=ORIENTED_EDGE ( 'NONE', *, *, #54530, .T. ) ;
#18503=CARTESIAN_POINT ( 'NONE',  ( 20.07187500061451857, -6.054752690667223547, -1.112240025338166033E-15 ) ) ;
#18505=CARTESIAN_POINT ( 'NONE',  ( 26.36249999999999716, 2.886751345948126879, 4.999999999999999112 ) ) ;
#18506=CARTESIAN_POINT ( 'NONE',  ( 28.54687500061451644, -3.027376345333614438, 5.243569643749998122 ) ) ;
#18508=CARTESIAN_POINT ( 'NONE',  ( 10.65000000000000036, 0.000000000000000000, 4.999999999999998224 ) ) ;
#18509=VERTEX_POINT ( 'NONE', #34241 ) ;
#18510=CARTESIAN_POINT ( 'NONE',  ( 9.750000000000001776, 0.000000000000000000, 4.999999999999998224 ) ) ;
#18512=CARTESIAN_POINT ( 'NONE',  ( 23.84062500061451928, 6.054752690667223547, 3.707466751127219781E-16 ) ) ;
#18513=CARTESIAN_POINT ( 'NONE',  ( 13.01249999999999929, -5.773502691896255534, -1.060575238724906372E-15 ) ) ;
#18514=CARTESIAN_POINT ( 'NONE',  ( 8.100000001229034297, -2.886751345948129988, 4.999999999999997335 ) ) ;
#18515=CARTESIAN_POINT ( 'NONE',  ( 5.878125000614517148, 4.541064518000418104, 2.621784821874999949 ) ) ;
#18516=CARTESIAN_POINT ( 'NONE',  ( 20.96250000000000213, 2.886751345948126879, 4.999999999999999112 ) ) ;
#18517=B_SPLINE_CURVE_WITH_KNOTS ( 'NONE', 3,
 ( #21885, #50346, #27080, #10085, #4909, #49611, #72870, #32615, #55516, #4187, #16339, #19776, #49249, #71784, #9714, #26715, #32248, #55879, #43342, #25326, #33698, #10806, #65864, #32976, #55153, #44807, #21152, #27445, #47872, #15246, #37783, #72138, #2799, #4551, #21518, #43706, #44072, #66227 ),
 .UNSPECIFIED., .F., .F.,
 ( 4, 2, 2, 2, 2, 2, 2, 2, 2, 2, 2, 2, 2, 2, 2, 2, 2, 2, 4 ),
 ( 0.01305910913008847749, 0.01347211191627390239, 0.01388511470245932730, 0.01471112027483017712, 0.01553712584720102867, 0.01636313141957188022, 0.01801514256431357638, 0.01884114813668442273, 0.01925415092286984764, 0.01966715370905527255, 0.02008015649524069746, 0.02049315928142611890, 0.02131916485379695830, 0.02214517042616779424, 0.02297117599853863018, 0.02379718157090946959, 0.02462318714328030553, 0.02544919271565114494, 0.02627519828802198087 ),
 .UNSPECIFIED. ) ;
#18518=CARTESIAN_POINT ( 'NONE',  ( 22.07812500061451644, 4.541064518000418104, 2.621784821874999949 ) ) ;
#18520=CARTESIAN_POINT ( 'NONE',  ( 24.90000000122903145, -2.886751345948125991, -5.000000000000000000 ) ) ;
#18522=CARTESIAN_POINT ( 'NONE',  ( 4.537500000000000533, -2.886751345948125991, -5.000000000000000000 ) ) ;
#18523=VERTEX_POINT ( 'NONE', #7267 ) ;
#18524=CARTESIAN_POINT ( 'NONE',  ( 22.00312500061451360, 4.541064518000418104, -2.621784821874998173 ) ) ;
#18525=CARTESIAN_POINT ( 'NONE',  ( 27.81562500061452070, 3.027376345333613106, -5.243569643749998122 ) ) ;
#18526=CARTESIAN_POINT ( 'NONE',  ( 27.83437500061451786, 6.421520780324663323E-16, -5.243569643749999010 ) ) ;
#18527=CARTESIAN_POINT ( 'NONE',  ( 13.64062500061451644, -3.027376345333614438, 5.243569643749998122 ) ) ;
#18529=VECTOR ( 'NONE', #49464, 1000.000000000000000 ) ;
#18530=CARTESIAN_POINT ( 'NONE',  ( 25.57500000122903216, 2.886751345948126879, 4.999999999999999112 ) ) ;
#18532=CARTESIAN_POINT ( 'NONE',  ( 16.49062500061451786, -3.027376345333610441, -5.243569643749999898 ) ) ;
#18533=CARTESIAN_POINT ( 'NONE',  ( -1.071796769724483234, 16.75759618943233420, -34.00000000000000711 ) ) ;
#18534=ADVANCED_FACE ( 'NONE', ( #18691 ), #71542, .T. ) ;
#18535=CARTESIAN_POINT ( 'NONE',  ( 5.887500001229034829, -4.330127018922194537, 2.499999999999995559 ) ) ;
#18536=CARTESIAN_POINT ( 'NONE',  ( 11.18437500061451928, 6.421520780324663323E-16, -5.243569643749999010 ) ) ;
#18537=CARTESIAN_POINT ( 'NONE',  ( 12.23437500061451821, 4.541064518000418104, 2.621784821874999949 ) ) ;
#18538=CARTESIAN_POINT ( 'NONE',  ( 20.44687500061451857, -3.027376345333614438, 5.243569643749998122 ) ) ;
#18539=ORIENTED_EDGE ( 'NONE', *, *, #31941, .F. ) ;
#18540=CARTESIAN_POINT ( 'NONE',  ( 24.07500000122903572, 2.886751345948162850, -4.999999999999940492 ) ) ;
#18541=CARTESIAN_POINT ( 'NONE',  ( 23.16562500061451502, -6.054752690667223547, -1.112240025338166033E-15 ) ) ;
#18542=CARTESIAN_POINT ( 'NONE',  ( 18.15937500061451715, 0.000000000000000000, 5.243569643749999010 ) ) ;
#18543=CARTESIAN_POINT ( 'NONE',  ( 24.51562500061451289, -6.054752690667223547, -1.112240025338166033E-15 ) ) ;
#18544=CARTESIAN_POINT ( 'NONE',  ( -3.999999999999997335, 15.08750000000000036, 32.30940107675850470 ) ) ;
#18545=CARTESIAN_POINT ( 'NONE',  ( 29.72812500061451502, 4.541064518000418104, 2.621784821874999949 ) ) ;
#18546=CARTESIAN_POINT ( 'NONE',  ( 8.475000001229034297, 2.886751345948126879, 4.999999999999999112 ) ) ;
#18547=CARTESIAN_POINT ( 'NONE',  ( 5.737500001229033586, 4.330127018922191873, 2.499999999999999556 ) ) ;
#18549=CARTESIAN_POINT ( 'NONE',  ( 28.08750000122903145, 6.123233995736764310E-16, -4.999999999999998224 ) ) ;
#18551=CARTESIAN_POINT ( 'NONE',  ( 10.39687500061451786, 6.054752690667223547, 3.707466751127219781E-16 ) ) ;
#18553=CARTESIAN_POINT ( 'NONE',  ( 17.61562500061451786, 3.027376345333611329, 5.243569643749999010 ) ) ;
#18554=CARTESIAN_POINT ( 'NONE',  ( 12.00937500061451857, -4.541064518000417216, -2.621784821875001281 ) ) ;
#18555=CARTESIAN_POINT ( 'NONE',  ( 3.103125000614517237, 4.541064518000418104, -2.621784821874998173 ) ) ;
#18556=CARTESIAN_POINT ( 'NONE',  ( 18.57187500061451857, 3.027376345333611329, 5.243569643749999010 ) ) ;
#18557=CARTESIAN_POINT ( 'NONE',  ( 8.371875000614515727, -6.054752690667223547, -1.112240025338166033E-15 ) ) ;
#18558=CARTESIAN_POINT ( 'NONE',  ( 3.703125000614516882, 0.000000000000000000, 5.243569643749999010 ) ) ;
#18559=DIRECTION ( 'NONE',  ( -1.000000000000000000, -0.000000000000000000, -0.000000000000000000 ) ) ;
#18560=CARTESIAN_POINT ( 'NONE',  ( 7.303125000614516082, 0.000000000000000000, 5.243569643749999010 ) ) ;
#18561=CARTESIAN_POINT ( 'NONE',  ( 17.05312500061451786, 4.541064518000418104, -2.621784821874998173 ) ) ;
#18563=CARTESIAN_POINT ( 'NONE',  ( 6.300000001229033586, -2.886751345948129988, 4.999999999999997335 ) ) ;
#18564=CARTESIAN_POINT ( 'NONE',  ( 14.31562500061451537, 3.027376345333613106, -5.243569643749998122 ) ) ;
#18565=CARTESIAN_POINT ( 'NONE',  ( 13.56562500061451892, 3.027376345333611329, 5.243569643749999010 ) ) ;
#18567=CARTESIAN_POINT ( 'NONE',  ( 14.28750000000000142, -2.886751345948129988, 4.999999999999997335 ) ) ;
#18568=CARTESIAN_POINT ( 'NONE',  ( 7.087500001229034119, 4.330127018922191873, 2.499999999999999556 ) ) ;
#18570=CARTESIAN_POINT ( 'NONE',  ( 15.64687500061451608, -3.027376345333610441, -5.243569643749999898 ) ) ;
#18571=CARTESIAN_POINT ( 'NONE',  ( 17.85000000122903430, 5.773502691896255534, 3.535250795749688894E-16 ) ) ;
#18573=CARTESIAN_POINT ( 'NONE',  ( -3.000416591977282496E-16, 18.34062500061451928, -34.90005215228797653 ) ) ;
#18575=CARTESIAN_POINT ( 'NONE',  ( 6.825000000000001066, 6.123233995736764310E-16, -4.999999999999998224 ) ) ;
#18577=CARTESIAN_POINT ( 'NONE',  ( 9.637500001229033941, 6.123233995736764310E-16, -4.999999999999998224 ) ) ;
#18579=CARTESIAN_POINT ( 'NONE',  ( 17.48437500061451999, 6.421520780324663323E-16, -5.243569643749999010 ) ) ;
#18582=CARTESIAN_POINT ( 'NONE',  ( 14.39062500061451821, 6.054752690667223547, 3.707466751127219781E-16 ) ) ;
#18585=CARTESIAN_POINT ( 'NONE',  ( 26.14687500061451431, 6.054752690667223547, 3.707466751127219781E-16 ) ) ;
#18587=CARTESIAN_POINT ( 'NONE',  ( 11.16562500061451679, 3.027376345333613106, -5.243569643749998122 ) ) ;
#18588=CARTESIAN_POINT ( 'NONE',  ( 16.13437500061451502, 6.421520780324663323E-16, -5.243569643749999010 ) ) ;
#18590=CARTESIAN_POINT ( 'NONE',  ( 26.65312500061451573, 0.000000000000000000, 5.243569643749999010 ) ) ;
#18591=CARTESIAN_POINT ( 'NONE',  ( 21.14062500061451289, 6.054752690667223547, 3.707466751127219781E-16 ) ) ;
#18592=CARTESIAN_POINT ( 'NONE',  ( 29.05312500061451431, -4.541064518000417216, -2.621784821875001281 ) ) ;
#18594=CARTESIAN_POINT ( 'NONE',  ( -3.999999999999997335, 14.30000000122903359, -27.69059892324149530 ) ) ;
#18595=CARTESIAN_POINT ( 'NONE',  ( 10.72500000000000142, -4.330127018922194537, 2.499999999999995559 ) ) ;
#18596=CARTESIAN_POINT ( 'NONE',  ( 18.22500000122903430, 2.886751345948129099, -4.999999999999998224 ) ) ;
#18597=CARTESIAN_POINT ( 'NONE',  ( 0.000000000000000000, 0.000000000000000000, 50.00000000000000000 ) ) ;
#18599=ORIENTED_EDGE ( 'NONE', *, *, #72525, .T. ) ;
#18600=CARTESIAN_POINT ( 'NONE',  ( 16.57499999999999929, -4.330127018922194537, 2.499999999999995559 ) ) ;
#18601=CARTESIAN_POINT ( 'NONE',  ( 22.34999999999999787, 0.000000000000000000, 4.999999999999998224 ) ) ;
#18602=CARTESIAN_POINT ( 'NONE',  ( 18.04687500061451999, 6.054752690667223547, 3.707466751127219781E-16 ) ) ;
#18603=CARTESIAN_POINT ( 'NONE',  ( 13.52812500061451750, 4.541064518000418104, 2.621784821874999949 ) ) ;
#18604=ORIENTED_EDGE ( 'NONE', *, *, #53983, .F. ) ;
#18605=CARTESIAN_POINT ( 'NONE',  ( 4.940625000614515372, 6.054752690667223547, 3.707466751127219781E-16 ) ) ;
#18607=CARTESIAN_POINT ( 'NONE',  ( 12.11250000000000249, -5.773502691896255534, -1.060575238724906372E-15 ) ) ;
#18609=CARTESIAN_POINT ( 'NONE',  ( -4.243569643749999898, 17.96562500061451573, 27.54997392385601529 ) ) ;
#18610=CARTESIAN_POINT ( 'NONE',  ( 29.27812500061451573, 4.541064518000418104, 2.621784821874999949 ) ) ;
#18613=CARTESIAN_POINT ( 'NONE',  ( 26.59687500061451360, 6.054752690667223547, 3.707466751127219781E-16 ) ) ;
#18614=ORIENTED_EDGE ( 'NONE', *, *, #53086, .T. ) ;
#18615=CARTESIAN_POINT ( 'NONE',  ( 22.71562500061451573, -6.054752690667223547, -1.112240025338166033E-15 ) ) ;
#18616=CARTESIAN_POINT ( 'NONE',  ( 23.44687500061451502, 6.054752690667223547, 3.707466751127219781E-16 ) ) ;
#18617=CARTESIAN_POINT ( 'NONE',  ( 4.243569643749999010, 17.36562500061459602, -32.45002607614398471 ) ) ;
#18618=CARTESIAN_POINT ( 'NONE',  ( 5.953125000614519102, 0.000000000000000000, 5.243569643749999010 ) ) ;
#18620=CARTESIAN_POINT ( 'NONE',  ( 24.17812500061451786, 6.421520780324663323E-16, -5.243569643749999010 ) ) ;
#18623=CARTESIAN_POINT ( 'NONE',  ( 16.17187500061451644, 3.027376345333613106, -5.243569643749998122 ) ) ;
#18624=CARTESIAN_POINT ( 'NONE',  ( 18.64687500061451786, -3.027376345333614438, 5.243569643749998122 ) ) ;
#18625=CARTESIAN_POINT ( 'NONE',  ( 26.22187500061451715, 3.027376345333611329, 5.243569643749999010 ) ) ;
#18626=CARTESIAN_POINT ( 'NONE',  ( -2.121784821874999949, 17.53437500061451715, 26.32496088578401938 ) ) ;
#18627=CARTESIAN_POINT ( 'NONE',  ( 7.003125000614518036, -4.541064518000417216, -2.621784821875001281 ) ) ;
#18628=CARTESIAN_POINT ( 'NONE',  ( -3.999999999999997335, 19.13750000000000284, 32.30940107675850470 ) ) ;
#18629=EDGE_CURVE ( 'NONE', #11388, #57032, #4002, .T. ) ;
#18630=CARTESIAN_POINT ( 'NONE',  ( 4.996875000614516615, 6.054752690667223547, 3.707466751127219781E-16 ) ) ;
#18631=CARTESIAN_POINT ( 'NONE',  ( 5.578125000614518214, -4.541064518000419881, 2.621784821874995952 ) ) ;
#18632=CARTESIAN_POINT ( 'NONE',  ( 8.971875000614515372, 3.027376345333613106, -5.243569643749998122 ) ) ;
#18634=CARTESIAN_POINT ( 'NONE',  ( 17.36250000122903359, 4.330127018922192761, -2.499999999999997780 ) ) ;
#18635=CARTESIAN_POINT ( 'NONE',  ( 4.696875000614518569, -3.027376345333614438, 5.243569643749998122 ) ) ;
#18636=CARTESIAN_POINT ( 'NONE',  ( 8.615625000614517859, 3.027376345333611329, 5.243569643749999010 ) ) ;
#18639=CARTESIAN_POINT ( 'NONE',  ( 16.95937500061451786, -4.541064518000417216, -2.621784821875001281 ) ) ;
#18640=CARTESIAN_POINT ( 'NONE',  ( 27.71250000000000568, 2.886751345948102454, 5.000000000000042633 ) ) ;
#18641=VERTEX_POINT ( 'NONE', #29145 ) ;
#18642=CARTESIAN_POINT ( 'NONE',  ( 24.92812500061451431, -4.541064518000419881, 2.621784821874995952 ) ) ;
#18643=CARTESIAN_POINT ( 'NONE',  ( 8.578125000614518214, 4.541064518000418104, 2.621784821874999949 ) ) ;
#18644=CARTESIAN_POINT ( 'NONE',  ( 26.14687500061451431, 6.054752690667223547, 3.707466751127219781E-16 ) ) ;
#18645=CARTESIAN_POINT ( 'NONE',  ( 9.478125000614515017, 4.541064518000418104, 2.621784821874999949 ) ) ;
#18646=CARTESIAN_POINT ( 'NONE',  ( -4.243569643749999898, 10.82187500061451857, -32.45002607614398471 ) ) ;
#18647=EDGE_CURVE ( 'NONE', #61789, #8626, #44336, .T. ) ;
#18648=CARTESIAN_POINT ( 'NONE',  ( 10.53750000122903252, 6.123233995736764310E-16, -4.999999999999998224 ) ) ;
#18649=( BOUNDED_CURVE ( )  B_SPLINE_CURVE ( 3, ( #13042, #31508, #35580, #58462 ),
 .UNSPECIFIED., .F., .F. ) 
 B_SPLINE_CURVE_WITH_KNOTS ( ( 4, 4 ),
 ( 2.843340893843762540, 2.939989945538246996 ),
 .UNSPECIFIED. ) 
 CURVE ( )  GEOMETRIC_REPRESENTATION_ITEM ( )  RATIONAL_B_SPLINE_CURVE ( ( 1.000000000000000000, 0.9992217315398195243, 0.9992217315398195243, 1.000000000000000000 ) ) 
 REPRESENTATION_ITEM ( '' )  );
#18650=CARTESIAN_POINT ( 'NONE',  ( 24.85312500061451502, 0.000000000000000000, 5.243569643749999010 ) ) ;
#18651=CARTESIAN_POINT ( 'NONE',  ( -4.243569643749999898, 13.46562500061451928, -32.45002607614398471 ) ) ;
#18652=CARTESIAN_POINT ( 'NONE',  ( 12.45000000122903394, 5.773502691896255534, 3.535250795749688894E-16 ) ) ;
#18653=CARTESIAN_POINT ( 'NONE',  ( 21.66562500061451502, 3.027376345333611329, 5.243569643749999010 ) ) ;
#18654=CARTESIAN_POINT ( 'NONE',  ( 10.20000000000000107, 0.000000000000000000, 4.999999999999998224 ) ) ;
#18655=CARTESIAN_POINT ( 'NONE',  ( 20.24062500061451431, 6.054752690667223547, 3.707466751127219781E-16 ) ) ;
#18657=CARTESIAN_POINT ( 'NONE',  ( 20.28750000000000142, -2.886751345948125991, -5.000000000000000000 ) ) ;
#18658=CARTESIAN_POINT ( 'NONE',  ( 14.25000000122903465, 5.773502691896255534, 3.535250795749688894E-16 ) ) ;
#18659=CARTESIAN_POINT ( 'NONE',  ( 10.19062500061451892, -3.027376345333610441, -5.243569643749999898 ) ) ;
#18660=CARTESIAN_POINT ( 'NONE',  ( 15.02812500061451750, -4.541064518000419881, 2.621784821874995952 ) ) ;
#18661=CARTESIAN_POINT ( 'NONE',  ( 25.87500000122903288, 2.886751345948129099, -4.999999999999998224 ) ) ;
#18662=CARTESIAN_POINT ( 'NONE',  ( 22.32187500061451502, -6.054752690667223547, -1.112240025338166033E-15 ) ) ;
#18664=CARTESIAN_POINT ( 'NONE',  ( 8.100000001229034297, -2.886751345948129988, 4.999999999999997335 ) ) ;
#18665=CARTESIAN_POINT ( 'NONE',  ( 9.421875000614519990, 3.027376345333613106, -5.243569643749998122 ) ) ;
#18666=CARTESIAN_POINT ( 'NONE',  ( 25.58437500061451431, 6.421520780324663323E-16, -5.243569643749999010 ) ) ;
#18668=CARTESIAN_POINT ( 'NONE',  ( 20.09062500061451573, -3.027376345333610441, -5.243569643749999898 ) ) ;
#18669=CARTESIAN_POINT ( 'NONE',  ( 25.50937500061451502, -4.541064518000417216, -2.621784821875001281 ) ) ;
#18671=CARTESIAN_POINT ( 'NONE',  ( 3.255427375287384351, -3.795065400537469102, 3.471954933061189852 ) ) ;
#18672=CARTESIAN_POINT ( 'NONE',  ( 8.821875000614518569, -6.054752690667223547, -1.112240025338166033E-15 ) ) ;
#18673=CARTESIAN_POINT ( 'NONE',  ( 16.19062500061451715, 6.054752690667223547, 3.707466751127219781E-16 ) ) ;
#18674=ORIENTED_EDGE ( 'NONE', *, *, #48506, .F. ) ;
#18675=CARTESIAN_POINT ( 'NONE',  ( -1.999999999999997113, 12.87500000000000178, -26.53589838486224295 ) ) ;
#18676=CARTESIAN_POINT ( 'NONE',  ( 27.92812500061451431, 4.541064518000418104, 2.621784821874999949 ) ) ;
#18677=CARTESIAN_POINT ( 'NONE',  ( 3.121875000614518836, 3.027376345333613106, -5.243569643749998122 ) ) ;
#18679=CARTESIAN_POINT ( 'NONE',  ( 16.76249999999999929, 2.886751345948129099, -4.999999999999998224 ) ) ;
#18680=CARTESIAN_POINT ( 'NONE',  ( 20.99062500061451431, -3.027376345333610441, -5.243569643749999898 ) ) ;
#18682=CARTESIAN_POINT ( 'NONE',  ( 25.19999999999999929, -4.330127018922190985, -2.500000000000001332 ) ) ;
#18683=CARTESIAN_POINT ( 'NONE',  ( 26.29687500061451644, -3.027376345333614438, 5.243569643749998122 ) ) ;
#18684=ORIENTED_EDGE ( 'NONE', *, *, #66354, .F. ) ;
#18685=CARTESIAN_POINT ( 'NONE',  ( 11.91562500061451857, -6.054752690667223547, -1.112240025338166033E-15 ) ) ;
#18686=CARTESIAN_POINT ( 'NONE',  ( 6.778125000614518392, 4.541064518000418104, 2.621784821874999949 ) ) ;
#18688=CARTESIAN_POINT ( 'NONE',  ( 3.309375000614518836, 0.000000000000000000, 5.243569643749999010 ) ) ;
#18689=CARTESIAN_POINT ( 'NONE',  ( 15.52500000122903323, 2.886751345948129099, -4.999999999999998224 ) ) ;
#18690=CARTESIAN_POINT ( 'NONE',  ( 22.72499999999999787, 4.330127018922191873, 2.499999999999999556 ) ) ;
#18691=FACE_OUTER_BOUND ( 'NONE', #6185, .T. ) ;
#18692=CARTESIAN_POINT ( 'NONE',  ( 4.359375000614517326, -4.541064518000417216, -2.621784821875001281 ) ) ;
#18693=CARTESIAN_POINT ( 'NONE',  ( 9.234375000614518214, -4.541064518000419881, 2.621784821874995952 ) ) ;
#18694=CARTESIAN_POINT ( 'NONE',  ( 19.92187500061451644, 3.027376345333611329, 5.243569643749999010 ) ) ;
#18695=CARTESIAN_POINT ( 'NONE',  ( -1.999999999999997113, 15.23750000122903536, -26.53589838486224295 ) ) ;
#18697=CARTESIAN_POINT ( 'NONE',  ( 29.12812500061451715, 6.421520780324663323E-16, -5.243569643749999010 ) ) ;
#18698=CARTESIAN_POINT ( 'NONE',  ( 29.63437500061451502, 6.421520780324663323E-16, -5.243569643749999010 ) ) ;
#18699=CARTESIAN_POINT ( 'NONE',  ( 3.871875000614519280, -6.054752690667223547, -1.112240025338166033E-15 ) ) ;
#18700=CARTESIAN_POINT ( 'NONE',  ( 15.59999999999999964, 0.000000000000000000, 4.999999999999998224 ) ) ;
#18701=CARTESIAN_POINT ( 'NONE',  ( 13.64062500061451644, -3.027376345333614438, 5.243569643749998122 ) ) ;
#18702=CARTESIAN_POINT ( 'NONE',  ( 4.000000000000000000, 14.00000000122903465, 32.30940107675849760 ) ) ;
#18704=CARTESIAN_POINT ( 'NONE',  ( 20.70000000122903216, -2.886751345948129988, 4.999999999999997335 ) ) ;
#18705=CARTESIAN_POINT ( 'NONE',  ( 16.72500000000000142, 6.123233995736764310E-16, -4.999999999999998224 ) ) ;
#18707=CARTESIAN_POINT ( 'NONE',  ( 7.003125000614518036, -4.541064518000417216, -2.621784821875001281 ) ) ;
#18708=CARTESIAN_POINT ( 'NONE',  ( 25.28437500061451715, 4.541064518000418104, 2.621784821874999949 ) ) ;
#18709=CARTESIAN_POINT ( 'NONE',  ( -4.243569643749997233, 18.99687500061451928, 32.45002607614398471 ) ) ;
#18710=CARTESIAN_POINT ( 'NONE',  ( 27.27187500061451431, -6.054752690667223547, -1.112240025338166033E-15 ) ) ;
#18711=CARTESIAN_POINT ( 'NONE',  ( 7.987500000000000711, -2.886751345948129988, 4.999999999999997335 ) ) ;
#18712=CARTESIAN_POINT ( 'NONE',  ( -2.000000000000000000, 13.28750000122903430, 26.53589838486224650 ) ) ;
#18713=CARTESIAN_POINT ( 'NONE',  ( 14.05312500061451431, 0.000000000000000000, 5.243569643749999010 ) ) ;
#18714=CARTESIAN_POINT ( 'NONE',  ( 6.412500001229036073, -4.330127018922190985, -2.500000000000001332 ) ) ;
#18716=CARTESIAN_POINT ( 'NONE',  ( 16.84687500061451715, -3.027376345333614438, 5.243569643749998122 ) ) ;
#18717=CARTESIAN_POINT ( 'NONE',  ( 11.07187500061451679, -6.054752690667223547, -1.112240025338166033E-15 ) ) ;
#18720=CARTESIAN_POINT ( 'NONE',  ( 13.04062500061451502, 6.054752690667223547, 3.707466751127219781E-16 ) ) ;
#18722=CARTESIAN_POINT ( 'NONE',  ( 23.51250000122903216, -4.330127018922190985, -2.500000000000001332 ) ) ;
#18723=CARTESIAN_POINT ( 'NONE',  ( 13.88437500061451679, 6.421520780324663323E-16, -5.243569643749999010 ) ) ;
#18724=CARTESIAN_POINT ( 'NONE',  ( 13.60312500061451679, 0.000000000000000000, 5.243569643749999010 ) ) ;
#18726=CARTESIAN_POINT ( 'NONE',  ( 24.45937500061451786, 0.000000000000000000, 5.243569643749999010 ) ) ;
#18729=CARTESIAN_POINT ( 'NONE',  ( 3.096623204930365691, 4.278619418581859790, -3.076353068265403667 ) ) ;
#18730=CARTESIAN_POINT ( 'NONE',  ( -4.243569643749998122, 15.84687500061451892, -27.54997392385601174 ) ) ;
#18731=CARTESIAN_POINT ( 'NONE',  ( 14.74687500061451573, -3.027376345333610441, -5.243569643749999898 ) ) ;
#18732=CARTESIAN_POINT ( 'NONE',  ( 18.71250000122903145, 4.330127018922192761, -2.499999999999997780 ) ) ;
#18733=CARTESIAN_POINT ( 'NONE',  ( 11.40937500061451892, 0.000000000000000000, 5.243569643749999010 ) ) ;
#18734=CARTESIAN_POINT ( 'NONE',  ( -2.121784821874999949, 19.27812500061451573, -33.67503911421598417 ) ) ;
#18735=CARTESIAN_POINT ( 'NONE',  ( 21.00000000122903288, 5.773502691896255534, 3.535250795749688894E-16 ) ) ;
#18736=CARTESIAN_POINT ( 'NONE',  ( 13.04062500061451502, 6.054752690667223547, 3.707466751127219781E-16 ) ) ;
#18737=ORIENTED_EDGE ( 'NONE', *, *, #23644, .F. ) ;
#18739=CARTESIAN_POINT ( 'NONE',  ( 17.47499999999999787, -4.330127018922194537, 2.499999999999995559 ) ) ;
#18741=CARTESIAN_POINT ( 'NONE',  ( 12.19687500061451857, 6.054752690667223547, 3.707466751127219781E-16 ) ) ;
#18743=CARTESIAN_POINT ( 'NONE',  ( 13.08750000122903323, -4.330127018922194537, 2.499999999999995559 ) ) ;
#18744=CARTESIAN_POINT ( 'NONE',  ( 20.70000000122903216, -2.886751345948129988, 4.999999999999997335 ) ) ;
#18745=CARTESIAN_POINT ( 'NONE',  ( 17.57812500061451644, 4.541064518000418104, 2.621784821874999949 ) ) ;
#18746=CARTESIAN_POINT ( 'NONE',  ( 22.64062500061451644, -3.027376345333614438, 5.243569643749998122 ) ) ;
#18747=CARTESIAN_POINT ( 'NONE',  ( 29.25000000122903288, -2.886751345948129988, 4.999999999999997335 ) ) ;
#18748=CARTESIAN_POINT ( 'NONE',  ( 27.33750000000000213, -2.886751345948129988, 4.999999999999997335 ) ) ;
#18749=CARTESIAN_POINT ( 'NONE',  ( 1.071796769724491893, 11.69509619066136885, 33.99999999999999289 ) ) ;
#18752=DIRECTION ( 'NONE',  ( -1.000000000000000000, -0.000000000000000000, -0.000000000000000000 ) ) ;
#18753=CARTESIAN_POINT ( 'NONE',  ( 9.001249775931846008E-16, 15.47187500061451892, -25.09994784771203058 ) ) ;
#18754=CARTESIAN_POINT ( 'NONE',  ( 3.825000001229032609, 2.886751345948129099, -4.999999999999998224 ) ) ;
#18755=CARTESIAN_POINT ( 'NONE',  ( 6.600000000000001421, 0.000000000000000000, 4.999999999999998224 ) ) ;
#18756=ADVANCED_FACE ( 'NONE', ( #46865 ), #46499, .F. ) ;
#18757=CARTESIAN_POINT ( 'NONE',  ( 3.684375000614518836, 4.541064518000418104, 2.621784821874999949 ) ) ;
#18758=CARTESIAN_POINT ( 'NONE',  ( 10.92187500061451644, 3.027376345333611329, 5.243569643749999010 ) ) ;
#18759=CARTESIAN_POINT ( 'NONE',  ( 27.44062500061451715, 6.054752690667223547, 3.707466751127219781E-16 ) ) ;
#18760=CARTESIAN_POINT ( 'NONE',  ( -5.798826918071315895, 8.147596131390992369, -31.59132108569609443 ) ) ;
#18761=CARTESIAN_POINT ( 'NONE',  ( 8.400000000000000355, 0.000000000000000000, 4.999999999999998224 ) ) ;
#18762=CARTESIAN_POINT ( 'NONE',  ( 7.059375000614518392, -4.541064518000417216, -2.621784821875001281 ) ) ;
#18763=CARTESIAN_POINT ( 'NONE',  ( 12.12187500061451573, 3.027376345333613106, -5.243569643749998122 ) ) ;
#18764=CARTESIAN_POINT ( 'NONE',  ( 6.562500000000001776, 2.886751345948126879, 4.999999999999999112 ) ) ;
#18765=CARTESIAN_POINT ( 'NONE',  ( -4.243569643749998122, 15.79062500061459495, 32.45002607614398471 ) ) ;
#18766=CARTESIAN_POINT ( 'NONE',  ( 4.848412143738765501, -3.306759954282229685, 4.272523750749039451 ) ) ;
#18767=CARTESIAN_POINT ( 'NONE',  ( 7.724999999999999645, 6.123233995736764310E-16, -4.999999999999998224 ) ) ;
#18769=CARTESIAN_POINT ( 'NONE',  ( 19.97812500061451502, -4.541064518000419881, 2.621784821874995952 ) ) ;
#18770=CARTESIAN_POINT ( 'NONE',  ( 13.15312500061451750, 0.000000000000000000, 5.243569643749999010 ) ) ;
#18772=CARTESIAN_POINT ( 'NONE',  ( 8.409375000614518925, -4.541064518000417216, -2.621784821875001281 ) ) ;
#18773=CARTESIAN_POINT ( 'NONE',  ( 27.15000000000000213, 4.330127018922192761, -2.499999999999997780 ) ) ;
#18774=CARTESIAN_POINT ( 'NONE',  ( 23.25000000122903288, 5.773502691896255534, 3.535250795749688894E-16 ) ) ;
#18775=CARTESIAN_POINT ( 'NONE',  ( 11.21250000122903501, 0.000000000000000000, 4.999999999999998224 ) ) ;
#18776=CARTESIAN_POINT ( 'NONE',  ( 12.27187500061451786, 3.027376345333611329, 5.243569643749999010 ) ) ;
#18777=CARTESIAN_POINT ( 'NONE',  ( 27.30937500061451573, -4.541064518000417216, -2.621784821875001281 ) ) ;
#18780=DIRECTION ( 'NONE',  ( -0.000000000000000000, -1.000000000000000000, -0.000000000000000000 ) ) ;
#18781=CARTESIAN_POINT ( 'NONE',  ( 18.90937500061451360, 4.541064518000418104, -2.621784821874998173 ) ) ;
#18782=CARTESIAN_POINT ( 'NONE',  ( 12.42187500061451821, -6.054752690667223547, -1.112240025338166033E-15 ) ) ;
#18784=CARTESIAN_POINT ( 'NONE',  ( 26.88749999999999574, -2.886751345948129988, 4.999999999999997335 ) ) ;
#18786=CARTESIAN_POINT ( 'NONE',  ( -4.243569643749999898, 11.27187500061451608, -32.45002607614398471 ) ) ;
#18788=CARTESIAN_POINT ( 'NONE',  ( 15.55312500061451608, -4.541064518000417216, -2.621784821875001281 ) ) ;
#18789=CARTESIAN_POINT ( 'NONE',  ( 4.837500000000001243, -2.886751345948129988, 4.999999999999997335 ) ) ;
#18790=( BOUNDED_SURFACE ( )  B_SPLINE_SURFACE ( 1, 2, ( 
 ( #38492, #54752, #66942, #3786, #60639, #48484, #61380, #48848, #43675, #4154, #71378, #43311, #15213, #49219, #16310, #60271, #9685, #21122, #66198, #15576, #61017, #21489, #10052, #27412, #32946, #4876, #49943, #44415, #72839, #56914, #5957, #39586, #12580, #46205, #11503, #51386, #11139, #51027, #50316, #62110, #63184, #28490, #28141, #788, #62824, #12216, #22221, #23297, #34383, #44775, #55847, #50669, #56212, #11862, #40665, #61738, #68021, #33668, #45128, #1151, #67310, #45847, #73, #68382, #17743, #51750, #5605, #40302, #16668, #34745, #17394, #45490, #423, #22579, #18103, #6319, #5235, #68745, #39951, #22931, #27777, #23660, #67662, #57277, #39226, #6686, #34025, #56562, #28848, #17028, #29214, #62464, #19562, #24018, #70184, #30301, #47291, #64643, #53193, #19191, #47652, #52834, #1514, #2234, #19931, #42485, #46933, #42118, #25108, #35114, #2589, #52471, #14028, #25484, #46567, #41744, #65008, #36568, #58353, #1879, #57637, #18471, #48030, #69111, #24385, #41035, #63550, #12936, #13661, #69471, #8493, #64272, #59088, #69826, #24748, #7043, #29573, #31025, #35472, #52110, #36203, #58721, #57994, #7403, #8134, #53559, #29931, #30660, #2956, #70556, #18828, #41391, #63904, #13293, #35830, #7764, #70923, #21394, #53937, #48760, #55028, #31767, #32493, #66473, #8861, #4432, #38027, #21031, #38396, #72018, #71284, #71658, #3696, #65740, #43584, #14758, #49852, #66105, #59825, #26221, #54304, #9231, #15125, #4063, #26960, #32126, #15484, #48395, #15850, #20663, #21758, #20293, #43950, #14396, #60550, #3333, #25858, #60920, #44319, #10323, #31397, #49487, #32856, #55392, #4786, #9957, #27320, #26589, #9594, #72378, #65370, #36934, #54660, #59454, #42848, #37302, #43220, #37662, #60185, #49130, #52295, #18287, #977, #67217, #35298, #72746, #16578, #41219, #16219, #2060, #5147, #50220, #6508, #34939, #6871, #30119, #66849, #57465, #1696, #24207, #46760, #12762, #39130, #69294, #7584, #29403, #63008, #24571, #13118, #22131, #57819, #44686, #7229, #51578, #68570, #40861, #62650, #29758, #12047, #18657, #55753, #63727, #12404, #51937, #35659, #58179, #1334, #52653, #23846, #33214, #46394, #38772, #61292, #29043, #10684, #27682, #34571, #57099, #23487, #46034, #17929, #40492, #68929, #63378, #8316, #64826, #8679, #2410, #30845, #70006, #54484, #26039, #9418, #3885, #48578, #9052, #2775, #37487, #47474, #31211, #47116, #31948, #64090, #14216, #47845, #69648, #64459, #13472, #25298, #60008, #36021, #19010, #41572, #13850, #41933, #37113, #42666, #30488, #71105, #36392, #24931, #3148, #14949, #58538, #48211, #70373, #53379, #7950, #53016, #19751, #65190, #19376, #42300, #58906, #36751, #59271, #53751, #25674, #14580, #54122, #3518, #70733, #59640, #20111, #31583, #20478, #43031, #65560, #55581, #11242, #32312, #38591, #54846, #15674, #44869, #20853, #16404, #43770, #67044, #38958, #22316, #49312, #61476, #37848, #10871, #61117, #16043, #72208, #26780, #61837, #27508, #33765, #33404, #55941, #50041, #5337, #10514, #21585, #21953, #4255, #33041, #44139, #27877, #50410, #60369, #9778, #4974, #38211, #71846, #72934, #72567, #32681, #21217, #67405, #66294, #60739, #16766, #48948, #56309, #10149, #55220, #4615, #66666, #44510, #26405, #71477, #39324, #43405, #65930, #15310, #27145, #49679, #7141, #63643, #23754, #28951, #45590, #13032, #62208, #18567, #67757, #68124, #17129, #11604, #39690, #57376, #23035, #52207, #62919, #46303, #40400, #45946, #35571, #5698, #29671, #34121, #28234, #68477, #29315, #56661, #51127, #12314, #68842, #6055, #34849, #35213, #23397, #45224, #28590, #57735, #50764, #69209, #1608, #524, #12676, #17489, #40051, #18199, #62563, #40770, #24119, #169, #63284, #51846, #6783, #46668, #41133, #11959, #1249, #34484, #57014, #22673, #6419, #51490, #890, #17839, #47389, #2326, #30400, #36305, #47752, #3054, #2688, #59183, #18925, #37027, #52929, #65469, #41485, #65104, #58090, #8592, #47029, #69564, #31497, #14860, #42576, #1976, #70647, #8963, #48492, #58452, #19659, #7498, #42943, #24485, #25204, #58819, #30026, #24842, #64005, #13763, #71016, #13385, #52569, #35930, #69919, #19289, #48124, #53662, #7864, #54037, #41843, #64372, #14126, #25952, #8230, #31122, #30758, #53289, #70287, #20394, #42214, #25585, #64738, #36664, #20022, #14493, #59552, #3432, #15222, #21496, #10423, #32954, #31862, #44049, #27058, #54397, #61388, #60279, #65839, #4529, #16318, #20761, #10061, #71388, #32225, #72476, #9329, #15952, #9692, #66573, #38500, #49951, #37761, #61026, #26318, #55491, #32593, #60646, #43682, #54759, #38871, #49588, #66950, #37399, #55131, #15583, #59923, #3796, #4163, #4885, #26693, #27420, #38125, #72112, #21862, #49226, #44423, #71760, #48857, #21129, #43319, #66205, #28780, #23954, #52767, #56847, #51321, #57209, #12517, #57576, #7698, #45419, #35048, #52405, #1813, #24321, #63486, #17679, #46869, #30235, #12874, #68681, #12153, #2170, #725, #58292, #34314, #34680, #6253, #23232, #45784, #46504, #62761, #18764, #29510, #63121, #6624, #35406, #52045, #57932, #40599, #11797, #6979, #67955, #17327, #29152, #7339, #29868, #39886, #69409, #51685, #41330, #35769, #68319, #1449, #40238, #1089, #69042, #18404, #23596, #46142, #18042, #62399, #63839, #40971, #13230, #26150, #59754, #53495, #15059, #25046, #59383, #54594, #9528, #41682, #64939, #25417, #24681, #42053, #64205, #2887, #37597, #13593, #47228, #69760, #64575, #19495, #14689, #20225, #8065, #48690, #13964, #2525, #53870, #65670, #36139, #25790, #47961, #8423, #19128, #60118, #70489, #42779, #53126, #19866, #58658, #30959, #32060, #42419, #70118, #65299, #31696, #54231, #30599, #37231, #3261, #47589, #36501, #59022, #14330, #48327, #36865, #8794, #31327, #70852, #9161, #43148, #3628, #71214 ),
 ( #20591, #60481, #67153, #60855, #4722, #50153, #9889, #22065, #26895, #61580, #66040, #32424, #26523, #15418, #49061, #3996, #43883, #71954, #16513, #72683, #54961, #27985, #21330, #4366, #33151, #44972, #20962, #5084, #27256, #10259, #33871, #67510, #32791, #44623, #49421, #72314, #71589, #55328, #11353, #49789, #66409, #39066, #10983, #33504, #43517, #56053, #55688, #37961, #15785, #38327, #21695, #27619, #61949, #44252, #16155, #66783, #38707, #22425, #61227, #5445, #10621, #50515, #73042, #16874, #39429, #24864, #67868, #41864, #18947, #47051, #30050, #56761, #19682, #58474, #42235, #70309, #69585, #52590, #64760, #2711, #11711, #2347, #39800, #47411, #40156, #57121, #30422, #62316, #69941, #6166, #64394, #45333, #34228, #5805, #1996, #17597, #19311, #41506, #13784, #24507, #22781, #64026, #14150, #56414, #68233, #36326, #58841, #28335, #8251, #638, #30781, #47773, #17240, #13405, #28695, #62676, #35953, #7886, #51234, #12070, #23146, #50873, #53312, #271, #45700, #25227, #34593, #7519, #52950, #37049, #71410, #66598, #21517, #53684, #3820, #37422, #36685, #54060, #3079, #65493, #49610, #31143, #42964, #44071, #9352, #8987, #32247, #43705, #66226, #25607, #54780, #15245, #48145, #59206, #31519, #59574, #65863, #8614, #42600, #48880, #65126, #25973, #55152, #70669, #26714, #59945, #43341, #60302, #20416, #3455, #4186, #20045, #21151, #20785, #26341, #31885, #48514, #72137, #37782, #14516, #71041, #9713, #54419, #14883, #4550, #49248, #71783, #15605, #38146, #60670, #10084, #32614, #27079, #34054, #38893, #455, #4908, #72499, #38524, #33697, #50345, #56594, #101, #28520, #11173, #55515, #56244, #822, #23330, #27811, #51060, #5990, #15974, #22964, #33340, #45525, #6350, #27444, #22607, #49974, #72869, #5635, #50699, #44444, #22252, #61411, #45880, #68055, #51421, #61047, #17424, #39983, #44806, #28881, #16338, #45159, #10445, #32975, #21884, #28172, #16699, #66973, #55878, #10805, #67339, #5265, #39257, #61769, #67691, #17062, #39622, #62495, #11534, #62140, #11893, #34418, #56946, #24418, #36239, #12249, #69503, #18503, #52142, #25141, #58753, #24055, #63940, #23690, #63582, #18863, #1545, #68778, #35864, #68412, #57313, #51782, #46967, #2620, #6717, #1182, #7077, #35507, #7436, #30692, #17774, #58026, #2265, #24779, #47323, #13325, #40701, #69856, #53223, #58387, #41068, #35148, #40334, #46238, #8163, #29250, #57671, #18134, #63219, #12614, #41424, #29606, #41777, #52503, #7800, #29962, #1914, #62855, #34780, #19223, #46602, #69144, #30337, #52865, #12969, #64306, #13696, #15156, #53593, #31798, #4099, #65403, #14060, #2988, #26627, #47682, #38060, #43618, #31056, #54695, #36599, #8898, #37693, #65038, #65774, #49164, #42148, #60216, #71320, #54336, #71695, #32162, #31430, #3730, #36964, #25889, #26255, #48061, #9994, #48792, #19962, #59486, #14429, #42514, #48429, #37336, #9629, #14794, #20695, #8527, #21067, #53970, #55065, #25516, #66140, #70955, #20326, #15518, #3368, #60585, #4466, #32528, #64675, #70218, #19592, #59120, #70586, #43254, #42880, #59859, #9263, #22524, #4821, #11081, #44717, #67608, #62055, #60957, #38433, #33609, #16252, #10359, #11450, #44359, #368, #56153, #45071, #61682, #67253, #11811, #34328, #28435, #55429, #49525, #16611, #50613, #27355, #72411, #5547, #16973, #32889, #28085, #56509, #39167, #66506, #49886, #5902, #26996, #17340, #22876, #21793, #33970, #15887, #61323, #39530, #66885, #50972, #45434, #21428, #67967, #17, #39899, #62412, #56860, #10721, #72050, #38808, #5181, #43985, #33253, #55791, #27719, #50258, #72782, #22165, #51698, #57590, #69057, #24333, #23969, #7352, #40253, #58304, #1102, #13607, #62774, #13243, #6993, #52059, #69421, #23610, #52780, #36152, #63852, #23246, #18776, #30247, #41342, #46882, #29881, #7714, #18418, #1463, #1825, #57223, #63499, #46517, #35780, #2182, #12165, #17692, #12887, #68695, #34694, #24695, #52419, #12530, #6637, #29166, #28794, #40984, #40614, #47239, #35420, #69772, #57945, #45797, #19140, #64218, #6266, #18055, #41694, #51335, #737, #68332, #46155, #63135, #35063, #29524, #65314, #19509, #19879, #3276, #20241, #13976, #42432, #8437, #66052, #37610, #20978, #15430, #65685, #15073, #3643, #30973, #60132, #43531, #26166, #8807, #25432, #58671, #42065, #71603, #47601, #47974, #70131, #64588, #36514, #37248, #2901, #32075, #42793, #48706, #14704, #25804, #8079, #30610, #9541, #59035, #53139, #48342, #9176, #53508, #70502, #59769, #71229, #64953, #31711, #54607, #70867, #25058, #14345, #4012, #2538, #49076, #26536, #36879, #59397, #31344, #53884, #20608, #54246, #43166, #16889, #32439, #28000, #61597, #44637, #61964, #22438, #21708, #22078, #27270, #16169, #67166, #38341, #287, #16527, #10272, #49803, #55341, #32804, #38720, #27633, #56068, #55703, #39079, #71969, #39443, #4736, #45348, #21343, #44987, #61241, #10634, #50529, #72328, #11367, #67882, #67524, #54975, #73057, #33885, #56429, #5460, #10998, #5819, #50167, #33165, #33518, #15800, #28350, #5097, #50887, #22795, #43898, #49435, #37975, #44266, #66422, #60496, #4380, #72696, #9902, #66798, #26909, #60869, #652, #68971, #24610, #28710, #23160, #29080, #57506, #29439, #52693, #17254, #6908, #24249, #34607, #35336, #69334, #11726, #7268, #40901, #23885, #41256, #1735, #1016, #1375, #6546, #68607, #46432, #17611, #2099, #18328, #62690, #51615, #57137, #12086, #17968, #51976, #57859, #34977, #63414, #51249, #18692, #23522, #47157, #45714, #46797, #40529, #63045, #29797, #46072, #63768, #39814, #13156, #34242, #52333, #35698, #58218, #7623, #12800, #30160, #62330, #12446, #56775, #68248, #6181, #40171, #37157, #31627, #30528, #7992, #53794, #58946, #53055, #54161, #36065, #19793, #3557, #25343, #69689, #58585, #2449, #48254 ) ),
 .UNSPECIFIED., .F., .F., .F. ) 
 B_SPLINE_SURFACE_WITH_KNOTS ( ( 2, 2 ),
 ( 3, 2, 2, 2, 2, 2, 2, 2, 2, 2, 2, 2, 2, 2, 2, 2, 2, 2, 2, 2, 2, 2, 2, 2, 2, 2, 2, 2, 2, 2, 2, 2, 2, 2, 2, 2, 2, 2, 2, 2, 2, 2, 2, 2, 2, 2, 2, 2, 2, 2, 2, 2, 2, 2, 2, 2, 2, 2, 2, 2, 2, 2, 2, 2, 2, 2, 2, 2, 2, 2, 2, 2, 2, 2, 2, 2, 2, 2, 2, 2, 2, 2, 2, 2, 2, 2, 2, 2, 2, 2, 2, 2, 2, 2, 2, 2, 2, 2, 2, 2, 2, 2, 2, 2, 2, 2, 2, 2, 2, 2, 2, 2, 2, 2, 2, 2, 2, 2, 2, 2, 2, 2, 2, 2, 2, 2, 2, 2, 2, 2, 2, 2, 2, 2, 2, 2, 2, 2, 2, 2, 2, 2, 2, 2, 2, 2, 2, 2, 2, 2, 2, 2, 2, 2, 2, 2, 2, 2, 2, 2, 2, 2, 2, 2, 2, 2, 2, 2, 2, 2, 2, 2, 2, 2, 2, 2, 2, 2, 2, 2, 2, 2, 2, 2, 2, 2, 2, 2, 2, 2, 2, 2, 2, 2, 2, 2, 2, 2, 2, 2, 2, 2, 2, 2, 2, 2, 2, 2, 2, 2, 2, 2, 2, 2, 2, 2, 2, 2, 2, 2, 2, 2, 2, 2, 2, 2, 2, 2, 2, 2, 2, 2, 2, 2, 2, 2, 2, 2, 2, 2, 2, 2, 2, 2, 2, 2, 2, 2, 2, 2, 2, 2, 2, 2, 2, 2, 2, 2, 2, 2, 2, 2, 2, 2, 2, 2, 2, 2, 2, 2, 2, 2, 2, 2, 2, 2, 2, 2, 2, 2, 2, 2, 2, 2, 2, 2, 2, 2, 2, 2, 2, 2, 2, 2, 2, 2, 2, 2, 2, 2, 2, 2, 2, 2, 2, 2, 2, 2, 2, 2, 2, 2, 2, 2, 2, 2, 2, 2, 2, 2, 2, 2, 2, 2, 2, 2, 2, 2, 2, 2, 2, 2, 2, 2, 2, 2, 2, 2, 2, 2, 2, 2, 2, 2, 2, 2, 2, 2, 2, 2, 2, 2, 2, 2, 2, 2, 2, 2, 2, 2, 3 ),
 ( 0.000000000000000000, 1.000000000000000000 ),
 ( 0.000000000000000000, 0.002777777777777777884, 0.005555555555555555768, 0.008333333333333333218, 0.01111111111111111154, 0.01388888888888888812, 0.01666666666666666644, 0.01944444444444444475, 0.02222222222222222307, 0.02500000000000000139, 0.02777777777777777624, 0.03055555555555555455, 0.03333333333333333287, 0.03611111111111110772, 0.03888888888888888951, 0.04166666666666666435, 0.04444444444444444614, 0.04722222222222222099, 0.05000000000000000278, 0.05277777777777777762, 0.05555555555555555247, 0.05833333333333333426, 0.06111111111111110911, 0.06388888888888888395, 0.06666666666666666574, 0.06944444444444444753, 0.07222222222222221544, 0.07499999999999999722, 0.07777777777777777901, 0.08055555555555556080, 0.08333333333333332871, 0.08611111111111111049, 0.08888888888888889228, 0.09166666666666666019, 0.09444444444444444198, 0.09722222222222222376, 0.1000000000000000056, 0.1027777777777777735, 0.1055555555555555552, 0.1083333333333333370, 0.1111111111111111049, 0.1138888888888888867, 0.1166666666666666685, 0.1194444444444444503, 0.1222222222222222182, 0.1250000000000000000, 0.1277777777777777679, 0.1305555555555555636, 0.1333333333333333315, 0.1361111111111110994, 0.1388888888888888951, 0.1416666666666666630, 0.1444444444444444309, 0.1472222222222222265, 0.1499999999999999944, 0.1527777777777777901, 0.1555555555555555580, 0.1583333333333333259, 0.1611111111111111216, 0.1638888888888888895, 0.1666666666666666574, 0.1694444444444444531, 0.1722222222222222210, 0.1749999999999999889, 0.1777777777777777846, 0.1805555555555555525, 0.1833333333333333204, 0.1861111111111111160, 0.1888888888888888840, 0.1916666666666666796, 0.1944444444444444475, 0.1972222222222222154, 0.2000000000000000111, 0.2027777777777777790, 0.2055555555555555469, 0.2083333333333333426, 0.2111111111111111105, 0.2138888888888888784, 0.2166666666666666741, 0.2194444444444444420, 0.2222222222222222099, 0.2250000000000000056, 0.2277777777777777735, 0.2305555555555555691, 0.2333333333333333370, 0.2361111111111111049, 0.2388888888888889006, 0.2416666666666666685, 0.2444444444444444364, 0.2472222222222222321, 0.2500000000000000000, 0.2527777777777777679, 0.2555555555555555358, 0.2583333333333333592, 0.2611111111111111271, 0.2638888888888888951, 0.2666666666666666630, 0.2694444444444444309, 0.2722222222222221988, 0.2750000000000000222, 0.2777777777777777901, 0.2805555555555555580, 0.2833333333333333259, 0.2861111111111110938, 0.2888888888888888618, 0.2916666666666666852, 0.2944444444444444531, 0.2972222222222222210, 0.2999999999999999889, 0.3027777777777777568, 0.3055555555555555802, 0.3083333333333333481, 0.3111111111111111160, 0.3138888888888888840, 0.3166666666666666519, 0.3194444444444444198, 0.3222222222222222432, 0.3250000000000000111, 0.3277777777777777790, 0.3305555555555555469, 0.3333333333333333148, 0.3361111111111111382, 0.3388888888888889062, 0.3416666666666666741, 0.3444444444444444420, 0.3472222222222222099, 0.3499999999999999778, 0.3527777777777778012, 0.3555555555555555691, 0.3583333333333333370, 0.3611111111111111049, 0.3638888888888888729, 0.3666666666666666408, 0.3694444444444444642, 0.3722222222222222321, 0.3750000000000000000, 0.3777777777777777679, 0.3805555555555555358, 0.3833333333333333592, 0.3861111111111111271, 0.3888888888888888951, 0.3916666666666666630, 0.3944444444444444309, 0.3972222222222221988, 0.4000000000000000222, 0.4027777777777777901, 0.4055555555555555580, 0.4083333333333333259, 0.4111111111111110938, 0.4138888888888888618, 0.4166666666666666852, 0.4194444444444444531, 0.4222222222222222210, 0.4249999999999999889, 0.4277777777777777568, 0.4305555555555555802, 0.4333333333333333481, 0.4361111111111111160, 0.4388888888888888840, 0.4416666666666666519, 0.4444444444444444198, 0.4472222222222222432, 0.4500000000000000111, 0.4527777777777777790, 0.4555555555555555469, 0.4583333333333333148, 0.4611111111111111382, 0.4638888888888889062, 0.4666666666666666741, 0.4694444444444444420, 0.4722222222222222099, 0.4749999999999999778, 0.4777777777777778012, 0.4805555555555555691, 0.4833333333333333370, 0.4861111111111111049, 0.4888888888888888729, 0.4916666666666666408, 0.4944444444444444642, 0.4972222222222222321, 0.5000000000000000000, 0.5027777777777777679, 0.5055555555555555358, 0.5083333333333333037, 0.5111111111111110716, 0.5138888888888888395, 0.5166666666666667185, 0.5194444444444444864, 0.5222222222222222543, 0.5250000000000000222, 0.5277777777777777901, 0.5305555555555555580, 0.5333333333333333259, 0.5361111111111110938, 0.5388888888888888618, 0.5416666666666666297, 0.5444444444444443976, 0.5472222222222222765, 0.5500000000000000444, 0.5527777777777778123, 0.5555555555555555802, 0.5583333333333333481, 0.5611111111111111160, 0.5638888888888888840, 0.5666666666666666519, 0.5694444444444444198, 0.5722222222222221877, 0.5749999999999999556, 0.5777777777777777235, 0.5805555555555556024, 0.5833333333333333703, 0.5861111111111111382, 0.5888888888888889062, 0.5916666666666666741, 0.5944444444444444420, 0.5972222222222222099, 0.5999999999999999778, 0.6027777777777777457, 0.6055555555555555136, 0.6083333333333332815, 0.6111111111111111605, 0.6138888888888889284, 0.6166666666666666963, 0.6194444444444444642, 0.6222222222222222321, 0.6250000000000000000, 0.6277777777777777679, 0.6305555555555555358, 0.6333333333333333037, 0.6361111111111110716, 0.6388888888888888395, 0.6416666666666667185, 0.6444444444444444864, 0.6472222222222222543, 0.6500000000000000222, 0.6527777777777777901, 0.6555555555555555580, 0.6583333333333333259, 0.6611111111111110938, 0.6638888888888888618, 0.6666666666666666297, 0.6694444444444443976, 0.6722222222222222765, 0.6750000000000000444, 0.6777777777777778123, 0.6805555555555555802, 0.6833333333333333481, 0.6861111111111111160, 0.6888888888888888840, 0.6916666666666666519, 0.6944444444444444198, 0.6972222222222221877, 0.6999999999999999556, 0.7027777777777777235, 0.7055555555555556024, 0.7083333333333333703, 0.7111111111111111382, 0.7138888888888889062, 0.7166666666666666741, 0.7194444444444444420, 0.7222222222222222099, 0.7249999999999999778, 0.7277777777777777457, 0.7305555555555555136, 0.7333333333333332815, 0.7361111111111111605, 0.7388888888888889284, 0.7416666666666666963, 0.7444444444444444642, 0.7472222222222222321, 0.7500000000000000000, 0.7527777777777777679, 0.7555555555555555358, 0.7583333333333333037, 0.7611111111111110716, 0.7638888888888888395, 0.7666666666666667185, 0.7694444444444444864, 0.7722222222222222543, 0.7750000000000000222, 0.7777777777777777901, 0.7805555555555555580, 0.7833333333333333259, 0.7861111111111110938, 0.7888888888888888618, 0.7916666666666666297, 0.7944444444444443976, 0.7972222222222222765, 0.8000000000000000444, 0.8027777777777778123, 0.8055555555555555802, 0.8083333333333333481, 0.8111111111111111160, 0.8138888888888888840, 0.8166666666666666519, 0.8194444444444444198, 0.8222222222222221877, 0.8249999999999999556, 0.8277777777777777235, 0.8305555555555556024, 0.8333333333333333703, 0.8361111111111111382, 0.8388888888888889062, 0.8416666666666666741, 0.8444444444444444420, 0.8472222222222222099, 0.8499999999999999778, 0.8527777777777777457, 0.8555555555555555136, 0.8583333333333332815, 0.8611111111111111605, 0.8638888888888889284, 0.8666666666666666963, 0.8694444444444444642, 0.8722222222222222321, 0.8750000000000000000, 0.8777777777777777679, 0.8805555555555555358, 0.8833333333333333037, 0.8861111111111110716, 0.8888888888888888395, 0.8916666666666667185, 0.8944444444444444864, 0.8972222222222222543, 0.9000000000000000222, 0.9027777777777777901, 0.9055555555555555580, 0.9083333333333333259, 0.9111111111111110938, 0.9138888888888888618, 0.9166666666666666297, 0.9194444444444443976, 0.9222222222222222765, 0.9250000000000000444, 0.9277777777777778123, 0.9305555555555555802, 0.9333333333333333481, 0.9361111111111111160, 0.9388888888888888840, 0.9416666666666666519, 0.9444444444444444198, 0.9472222222222221877, 0.9499999999999999556, 0.9527777777777777235, 0.9555555555555556024, 0.9583333333333333703, 0.9611111111111111382, 0.9638888888888889062, 0.9666666666666666741, 0.9694444444444444420, 0.9722222222222222099, 0.9749999999999999778, 0.9777777777777777457, 0.9805555555555555136, 0.9833333333333332815, 0.9861111111111111605, 0.9888888888888889284, 0.9916666666666666963, 0.9944444444444444642, 0.9972222222222222321, 1.000000000000000000 ),
 .UNSPECIFIED. ) 
 GEOMETRIC_REPRESENTATION_ITEM ( )  RATIONAL_B_SPLINE_SURFACE ( (
 ( 1.000000000000000000, 0.8660254037844387076, 1.000000000000000000, 0.8660254037844387076, 1.000000000000000000, 0.8660254037844387076, 1.000000000000000000, 0.8660254037844387076, 1.000000000000000000, 0.8660254037844387076, 1.000000000000000000, 0.8660254037844387076, 1.000000000000000000, 0.8660254037844387076, 1.000000000000000000, 0.8660254037844387076, 1.000000000000000000, 0.8660254037844387076, 1.000000000000000000, 0.8660254037844387076, 1.000000000000000000, 0.8660254037844387076, 1.000000000000000000, 0.8660254037844387076, 1.000000000000000000, 0.8660254037844387076, 1.000000000000000000, 0.8660254037844387076, 1.000000000000000000, 0.8660254037844387076, 1.000000000000000000, 0.8660254037844387076, 1.000000000000000000, 0.8660254037844387076, 1.000000000000000000, 0.8660254037844387076, 1.000000000000000000, 0.8660254037844387076, 1.000000000000000000, 0.8660254037844387076, 1.000000000000000000, 0.8660254037844387076, 1.000000000000000000, 0.8660254037844387076, 1.000000000000000000, 0.8660254037844387076, 1.000000000000000000, 0.8660254037844387076, 1.000000000000000000, 0.8660254037844387076, 1.000000000000000000, 0.8660254037844387076, 1.000000000000000000, 0.8660254037844387076, 1.000000000000000000, 0.8660254037844387076, 1.000000000000000000, 0.8660254037844387076, 1.000000000000000000, 0.8660254037844387076, 1.000000000000000000, 0.8660254037844387076, 1.000000000000000000, 0.8660254037844387076, 1.000000000000000000, 0.8660254037844387076, 1.000000000000000000, 0.8660254037844387076, 1.000000000000000000, 0.8660254037844387076, 1.000000000000000000, 0.8660254037844387076, 1.000000000000000000, 0.8660254037844387076, 1.000000000000000000, 0.8660254037844387076, 1.000000000000000000, 0.8660254037844387076, 1.000000000000000000, 0.8660254037844387076, 1.000000000000000000, 0.8660254037844387076, 1.000000000000000000, 0.8660254037844387076, 1.000000000000000000, 0.8660254037844387076, 1.000000000000000000, 0.8660254037844387076, 1.000000000000000000, 0.8660254037844387076, 1.000000000000000000, 0.8660254037844387076, 1.000000000000000000, 0.8660254037844387076, 1.000000000000000000, 0.8660254037844387076, 1.000000000000000000, 0.8660254037844387076, 1.000000000000000000, 0.8660254037844387076, 1.000000000000000000, 0.8660254037844387076, 1.000000000000000000, 0.8660254037844387076, 1.000000000000000000, 0.8660254037844387076, 1.000000000000000000, 0.8660254037844387076, 1.000000000000000000, 0.8660254037844387076, 1.000000000000000000, 0.8660254037844387076, 1.000000000000000000, 0.8660254037844387076, 1.000000000000000000, 0.8660254037844387076, 1.000000000000000000, 0.8660254037844387076, 1.000000000000000000, 0.8660254037844387076, 1.000000000000000000, 0.8660254037844387076, 1.000000000000000000, 0.8660254037844387076, 1.000000000000000000, 0.8660254037844387076, 1.000000000000000000, 0.8660254037844387076, 1.000000000000000000, 0.8660254037844387076, 1.000000000000000000, 0.8660254037844387076, 1.000000000000000000, 0.8660254037844387076, 1.000000000000000000, 0.8660254037844387076, 1.000000000000000000, 0.8660254037844387076, 1.000000000000000000, 0.8660254037844387076, 1.000000000000000000, 0.8660254037844387076, 1.000000000000000000, 0.8660254037844387076, 1.000000000000000000, 0.8660254037844387076, 1.000000000000000000, 0.8660254037844387076, 1.000000000000000000, 0.8660254037844387076, 1.000000000000000000, 0.8660254037844387076, 1.000000000000000000, 0.8660254037844387076, 1.000000000000000000, 0.8660254037844387076, 1.000000000000000000, 0.8660254037844387076, 1.000000000000000000, 0.8660254037844387076, 1.000000000000000000, 0.8660254037844387076, 1.000000000000000000, 0.8660254037844387076, 1.000000000000000000, 0.8660254037844387076, 1.000000000000000000, 0.8660254037844387076, 1.000000000000000000, 0.8660254037844387076, 1.000000000000000000, 0.8660254037844387076, 1.000000000000000000, 0.8660254037844387076, 1.000000000000000000, 0.8660254037844387076, 1.000000000000000000, 0.8660254037844387076, 1.000000000000000000, 0.8660254037844387076, 1.000000000000000000, 0.8660254037844387076, 1.000000000000000000, 0.8660254037844387076, 1.000000000000000000, 0.8660254037844387076, 1.000000000000000000, 0.8660254037844387076, 1.000000000000000000, 0.8660254037844387076, 1.000000000000000000, 0.8660254037844387076, 1.000000000000000000, 0.8660254037844387076, 1.000000000000000000, 0.8660254037844387076, 1.000000000000000000, 0.8660254037844387076, 1.000000000000000000, 0.8660254037844387076, 1.000000000000000000, 0.8660254037844387076, 1.000000000000000000, 0.8660254037844387076, 1.000000000000000000, 0.8660254037844387076, 1.000000000000000000, 0.8660254037844387076, 1.000000000000000000, 0.8660254037844387076, 1.000000000000000000, 0.8660254037844387076, 1.000000000000000000, 0.8660254037844387076, 1.000000000000000000, 0.8660254037844387076, 1.000000000000000000, 0.8660254037844387076, 1.000000000000000000, 0.8660254037844387076, 1.000000000000000000, 0.8660254037844387076, 1.000000000000000000, 0.8660254037844387076, 1.000000000000000000, 0.8660254037844387076, 1.000000000000000000, 0.8660254037844387076, 1.000000000000000000, 0.8660254037844387076, 1.000000000000000000, 0.8660254037844387076, 1.000000000000000000, 0.8660254037844387076, 1.000000000000000000, 0.8660254037844387076, 1.000000000000000000, 0.8660254037844387076, 1.000000000000000000, 0.8660254037844387076, 1.000000000000000000, 0.8660254037844387076, 1.000000000000000000, 0.8660254037844387076, 1.000000000000000000, 0.8660254037844387076, 1.000000000000000000, 0.8660254037844387076, 1.000000000000000000, 0.8660254037844387076, 1.000000000000000000, 0.8660254037844387076, 1.000000000000000000, 0.8660254037844387076, 1.000000000000000000, 0.8660254037844387076, 1.000000000000000000, 0.8660254037844387076, 1.000000000000000000, 0.8660254037844387076, 1.000000000000000000, 0.8660254037844387076, 1.000000000000000000, 0.8660254037844387076, 1.000000000000000000, 0.8660254037844387076, 1.000000000000000000, 0.8660254037844387076, 1.000000000000000000, 0.8660254037844387076, 1.000000000000000000, 0.8660254037844387076, 1.000000000000000000, 0.8660254037844387076, 1.000000000000000000, 0.8660254037844387076, 1.000000000000000000, 0.8660254037844387076, 1.000000000000000000, 0.8660254037844387076, 1.000000000000000000, 0.8660254037844387076, 1.000000000000000000, 0.8660254037844387076, 1.000000000000000000, 0.8660254037844387076, 1.000000000000000000, 0.8660254037844387076, 1.000000000000000000, 0.8660254037844387076, 1.000000000000000000, 0.8660254037844387076, 1.000000000000000000, 0.8660254037844387076, 1.000000000000000000, 0.8660254037844387076, 1.000000000000000000, 0.8660254037844387076, 1.000000000000000000, 0.8660254037844387076, 1.000000000000000000, 0.8660254037844387076, 1.000000000000000000, 0.8660254037844387076, 1.000000000000000000, 0.8660254037844387076, 1.000000000000000000, 0.8660254037844387076, 1.000000000000000000, 0.8660254037844387076, 1.000000000000000000, 0.8660254037844387076, 1.000000000000000000, 0.8660254037844387076, 1.000000000000000000, 0.8660254037844387076, 1.000000000000000000, 0.8660254037844387076, 1.000000000000000000, 0.8660254037844387076, 1.000000000000000000, 0.8660254037844387076, 1.000000000000000000, 0.8660254037844387076, 1.000000000000000000, 0.8660254037844387076, 1.000000000000000000, 0.8660254037844387076, 1.000000000000000000, 0.8660254037844387076, 1.000000000000000000, 0.8660254037844387076, 1.000000000000000000, 0.8660254037844387076, 1.000000000000000000, 0.8660254037844387076, 1.000000000000000000, 0.8660254037844387076, 1.000000000000000000, 0.8660254037844387076, 1.000000000000000000, 0.8660254037844387076, 1.000000000000000000, 0.8660254037844387076, 1.000000000000000000, 0.8660254037844387076, 1.000000000000000000, 0.8660254037844387076, 1.000000000000000000, 0.8660254037844387076, 1.000000000000000000, 0.8660254037844387076, 1.000000000000000000, 0.8660254037844387076, 1.000000000000000000, 0.8660254037844387076, 1.000000000000000000, 0.8660254037844387076, 1.000000000000000000, 0.8660254037844387076, 1.000000000000000000, 0.8660254037844387076, 1.000000000000000000, 0.8660254037844387076, 1.000000000000000000, 0.8660254037844387076, 1.000000000000000000, 0.8660254037844387076, 1.000000000000000000, 0.8660254037844387076, 1.000000000000000000, 0.8660254037844387076, 1.000000000000000000, 0.8660254037844387076, 1.000000000000000000, 0.8660254037844387076, 1.000000000000000000, 0.8660254037844387076, 1.000000000000000000, 0.8660254037844387076, 1.000000000000000000, 0.8660254037844387076, 1.000000000000000000, 0.8660254037844387076, 1.000000000000000000, 0.8660254037844387076, 1.000000000000000000, 0.8660254037844387076, 1.000000000000000000, 0.8660254037844387076, 1.000000000000000000, 0.8660254037844387076, 1.000000000000000000, 0.8660254037844387076, 1.000000000000000000, 0.8660254037844387076, 1.000000000000000000, 0.8660254037844387076, 1.000000000000000000, 0.8660254037844387076, 1.000000000000000000, 0.8660254037844387076, 1.000000000000000000, 0.8660254037844387076, 1.000000000000000000, 0.8660254037844387076, 1.000000000000000000, 0.8660254037844387076, 1.000000000000000000, 0.8660254037844387076, 1.000000000000000000, 0.8660254037844387076, 1.000000000000000000, 0.8660254037844387076, 1.000000000000000000, 0.8660254037844387076, 1.000000000000000000, 0.8660254037844387076, 1.000000000000000000, 0.8660254037844387076, 1.000000000000000000, 0.8660254037844387076, 1.000000000000000000, 0.8660254037844387076, 1.000000000000000000, 0.8660254037844387076, 1.000000000000000000, 0.8660254037844387076, 1.000000000000000000, 0.8660254037844387076, 1.000000000000000000, 0.8660254037844387076, 1.000000000000000000, 0.8660254037844387076, 1.000000000000000000, 0.8660254037844387076, 1.000000000000000000, 0.8660254037844387076, 1.000000000000000000, 0.8660254037844387076, 1.000000000000000000, 0.8660254037844387076, 1.000000000000000000, 0.8660254037844387076, 1.000000000000000000, 0.8660254037844387076, 1.000000000000000000, 0.8660254037844387076, 1.000000000000000000, 0.8660254037844387076, 1.000000000000000000, 0.8660254037844387076, 1.000000000000000000, 0.8660254037844387076, 1.000000000000000000, 0.8660254037844387076, 1.000000000000000000, 0.8660254037844387076, 1.000000000000000000, 0.8660254037844387076, 1.000000000000000000, 0.8660254037844387076, 1.000000000000000000, 0.8660254037844387076, 1.000000000000000000, 0.8660254037844387076, 1.000000000000000000, 0.8660254037844387076, 1.000000000000000000, 0.8660254037844387076, 1.000000000000000000, 0.8660254037844387076, 1.000000000000000000, 0.8660254037844387076, 1.000000000000000000, 0.8660254037844387076, 1.000000000000000000, 0.8660254037844387076, 1.000000000000000000, 0.8660254037844387076, 1.000000000000000000, 0.8660254037844387076, 1.000000000000000000, 0.8660254037844387076, 1.000000000000000000, 0.8660254037844387076, 1.000000000000000000, 0.8660254037844387076, 1.000000000000000000, 0.8660254037844387076, 1.000000000000000000, 0.8660254037844387076, 1.000000000000000000, 0.8660254037844387076, 1.000000000000000000, 0.8660254037844387076, 1.000000000000000000, 0.8660254037844387076, 1.000000000000000000, 0.8660254037844387076, 1.000000000000000000, 0.8660254037844387076, 1.000000000000000000, 0.8660254037844387076, 1.000000000000000000, 0.8660254037844387076, 1.000000000000000000, 0.8660254037844387076, 1.000000000000000000, 0.8660254037844387076, 1.000000000000000000, 0.8660254037844387076, 1.000000000000000000, 0.8660254037844387076, 1.000000000000000000, 0.8660254037844387076, 1.000000000000000000, 0.8660254037844387076, 1.000000000000000000, 0.8660254037844387076, 1.000000000000000000, 0.8660254037844387076, 1.000000000000000000, 0.8660254037844387076, 1.000000000000000000, 0.8660254037844387076, 1.000000000000000000, 0.8660254037844387076, 1.000000000000000000, 0.8660254037844387076, 1.000000000000000000, 0.8660254037844387076, 1.000000000000000000, 0.8660254037844387076, 1.000000000000000000, 0.8660254037844387076, 1.000000000000000000, 0.8660254037844387076, 1.000000000000000000, 0.8660254037844387076, 1.000000000000000000, 0.8660254037844387076, 1.000000000000000000, 0.8660254037844387076, 1.000000000000000000, 0.8660254037844387076, 1.000000000000000000, 0.8660254037844387076, 1.000000000000000000, 0.8660254037844387076, 1.000000000000000000, 0.8660254037844387076, 1.000000000000000000, 0.8660254037844387076, 1.000000000000000000, 0.8660254037844387076, 1.000000000000000000, 0.8660254037844387076, 1.000000000000000000, 0.8660254037844387076, 1.000000000000000000, 0.8660254037844387076, 1.000000000000000000, 0.8660254037844387076, 1.000000000000000000, 0.8660254037844387076, 1.000000000000000000, 0.8660254037844387076, 1.000000000000000000, 0.8660254037844387076, 1.000000000000000000, 0.8660254037844387076, 1.000000000000000000, 0.8660254037844387076, 1.000000000000000000, 0.8660254037844387076, 1.000000000000000000, 0.8660254037844387076, 1.000000000000000000, 0.8660254037844387076, 1.000000000000000000, 0.8660254037844387076, 1.000000000000000000, 0.8660254037844387076, 1.000000000000000000, 0.8660254037844387076, 1.000000000000000000, 0.8660254037844387076, 1.000000000000000000, 0.8660254037844387076, 1.000000000000000000, 0.8660254037844387076, 1.000000000000000000, 0.8660254037844387076, 1.000000000000000000, 0.8660254037844387076, 1.000000000000000000, 0.8660254037844387076, 1.000000000000000000, 0.8660254037844387076, 1.000000000000000000, 0.8660254037844387076, 1.000000000000000000, 0.8660254037844387076, 1.000000000000000000, 0.8660254037844387076, 1.000000000000000000, 0.8660254037844387076, 1.000000000000000000, 0.8660254037844387076, 1.000000000000000000, 0.8660254037844387076, 1.000000000000000000, 0.8660254037844387076, 1.000000000000000000, 0.8660254037844387076, 1.000000000000000000, 0.8660254037844387076, 1.000000000000000000, 0.8660254037844387076, 1.000000000000000000, 0.8660254037844387076, 1.000000000000000000, 0.8660254037844387076, 1.000000000000000000, 0.8660254037844387076, 1.000000000000000000, 0.8660254037844387076, 1.000000000000000000, 0.8660254037844387076, 1.000000000000000000, 0.8660254037844387076, 1.000000000000000000, 0.8660254037844387076, 1.000000000000000000, 0.8660254037844387076, 1.000000000000000000, 0.8660254037844387076, 1.000000000000000000, 0.8660254037844387076, 1.000000000000000000, 0.8660254037844387076, 1.000000000000000000, 0.8660254037844387076, 1.000000000000000000, 0.8660254037844387076, 1.000000000000000000, 0.8660254037844387076, 1.000000000000000000, 0.8660254037844387076, 1.000000000000000000, 0.8660254037844387076, 1.000000000000000000, 0.8660254037844387076, 1.000000000000000000, 0.8660254037844387076, 1.000000000000000000, 0.8660254037844387076, 1.000000000000000000, 0.8660254037844387076, 1.000000000000000000, 0.8660254037844387076, 1.000000000000000000, 0.8660254037844387076, 1.000000000000000000, 0.8660254037844387076, 1.000000000000000000, 0.8660254037844387076, 1.000000000000000000, 0.8660254037844387076, 1.000000000000000000, 0.8660254037844387076, 1.000000000000000000, 0.8660254037844387076, 1.000000000000000000, 0.8660254037844387076, 1.000000000000000000, 0.8660254037844387076, 1.000000000000000000, 0.8660254037844387076, 1.000000000000000000, 0.8660254037844387076, 1.000000000000000000, 0.8660254037844387076, 1.000000000000000000, 0.8660254037844387076, 1.000000000000000000, 0.8660254037844387076, 1.000000000000000000, 0.8660254037844387076, 1.000000000000000000, 0.8660254037844387076, 1.000000000000000000, 0.8660254037844387076, 1.000000000000000000, 0.8660254037844387076, 1.000000000000000000, 0.8660254037844387076, 1.000000000000000000, 0.8660254037844387076, 1.000000000000000000, 0.8660254037844387076, 1.000000000000000000, 0.8660254037844387076, 1.000000000000000000, 0.8660254037844387076, 1.000000000000000000, 0.8660254037844387076, 1.000000000000000000, 0.8660254037844387076, 1.000000000000000000, 0.8660254037844387076, 1.000000000000000000, 0.8660254037844387076, 1.000000000000000000, 0.8660254037844387076, 1.000000000000000000, 0.8660254037844387076, 1.000000000000000000, 0.8660254037844387076, 1.000000000000000000),
 ( 1.000000000000000000, 0.8660254037844387076, 1.000000000000000000, 0.8660254037844387076, 1.000000000000000000, 0.8660254037844387076, 1.000000000000000000, 0.8660254037844387076, 1.000000000000000000, 0.8660254037844387076, 1.000000000000000000, 0.8660254037844387076, 1.000000000000000000, 0.8660254037844387076, 1.000000000000000000, 0.8660254037844387076, 1.000000000000000000, 0.8660254037844387076, 1.000000000000000000, 0.8660254037844387076, 1.000000000000000000, 0.8660254037844387076, 1.000000000000000000, 0.8660254037844387076, 1.000000000000000000, 0.8660254037844387076, 1.000000000000000000, 0.8660254037844387076, 1.000000000000000000, 0.8660254037844387076, 1.000000000000000000, 0.8660254037844387076, 1.000000000000000000, 0.8660254037844387076, 1.000000000000000000, 0.8660254037844387076, 1.000000000000000000, 0.8660254037844387076, 1.000000000000000000, 0.8660254037844387076, 1.000000000000000000, 0.8660254037844387076, 1.000000000000000000, 0.8660254037844387076, 1.000000000000000000, 0.8660254037844387076, 1.000000000000000000, 0.8660254037844387076, 1.000000000000000000, 0.8660254037844387076, 1.000000000000000000, 0.8660254037844387076, 1.000000000000000000, 0.8660254037844387076, 1.000000000000000000, 0.8660254037844387076, 1.000000000000000000, 0.8660254037844387076, 1.000000000000000000, 0.8660254037844387076, 1.000000000000000000, 0.8660254037844387076, 1.000000000000000000, 0.8660254037844387076, 1.000000000000000000, 0.8660254037844387076, 1.000000000000000000, 0.8660254037844387076, 1.000000000000000000, 0.8660254037844387076, 1.000000000000000000, 0.8660254037844387076, 1.000000000000000000, 0.8660254037844387076, 1.000000000000000000, 0.8660254037844387076, 1.000000000000000000, 0.8660254037844387076, 1.000000000000000000, 0.8660254037844387076, 1.000000000000000000, 0.8660254037844387076, 1.000000000000000000, 0.8660254037844387076, 1.000000000000000000, 0.8660254037844387076, 1.000000000000000000, 0.8660254037844387076, 1.000000000000000000, 0.8660254037844387076, 1.000000000000000000, 0.8660254037844387076, 1.000000000000000000, 0.8660254037844387076, 1.000000000000000000, 0.8660254037844387076, 1.000000000000000000, 0.8660254037844387076, 1.000000000000000000, 0.8660254037844387076, 1.000000000000000000, 0.8660254037844387076, 1.000000000000000000, 0.8660254037844387076, 1.000000000000000000, 0.8660254037844387076, 1.000000000000000000, 0.8660254037844387076, 1.000000000000000000, 0.8660254037844387076, 1.000000000000000000, 0.8660254037844387076, 1.000000000000000000, 0.8660254037844387076, 1.000000000000000000, 0.8660254037844387076, 1.000000000000000000, 0.8660254037844387076, 1.000000000000000000, 0.8660254037844387076, 1.000000000000000000, 0.8660254037844387076, 1.000000000000000000, 0.8660254037844387076, 1.000000000000000000, 0.8660254037844387076, 1.000000000000000000, 0.8660254037844387076, 1.000000000000000000, 0.8660254037844387076, 1.000000000000000000, 0.8660254037844387076, 1.000000000000000000, 0.8660254037844387076, 1.000000000000000000, 0.8660254037844387076, 1.000000000000000000, 0.8660254037844387076, 1.000000000000000000, 0.8660254037844387076, 1.000000000000000000, 0.8660254037844387076, 1.000000000000000000, 0.8660254037844387076, 1.000000000000000000, 0.8660254037844387076, 1.000000000000000000, 0.8660254037844387076, 1.000000000000000000, 0.8660254037844387076, 1.000000000000000000, 0.8660254037844387076, 1.000000000000000000, 0.8660254037844387076, 1.000000000000000000, 0.8660254037844387076, 1.000000000000000000, 0.8660254037844387076, 1.000000000000000000, 0.8660254037844387076, 1.000000000000000000, 0.8660254037844387076, 1.000000000000000000, 0.8660254037844387076, 1.000000000000000000, 0.8660254037844387076, 1.000000000000000000, 0.8660254037844387076, 1.000000000000000000, 0.8660254037844387076, 1.000000000000000000, 0.8660254037844387076, 1.000000000000000000, 0.8660254037844387076, 1.000000000000000000, 0.8660254037844387076, 1.000000000000000000, 0.8660254037844387076, 1.000000000000000000, 0.8660254037844387076, 1.000000000000000000, 0.8660254037844387076, 1.000000000000000000, 0.8660254037844387076, 1.000000000000000000, 0.8660254037844387076, 1.000000000000000000, 0.8660254037844387076, 1.000000000000000000, 0.8660254037844387076, 1.000000000000000000, 0.8660254037844387076, 1.000000000000000000, 0.8660254037844387076, 1.000000000000000000, 0.8660254037844387076, 1.000000000000000000, 0.8660254037844387076, 1.000000000000000000, 0.8660254037844387076, 1.000000000000000000, 0.8660254037844387076, 1.000000000000000000, 0.8660254037844387076, 1.000000000000000000, 0.8660254037844387076, 1.000000000000000000, 0.8660254037844387076, 1.000000000000000000, 0.8660254037844387076, 1.000000000000000000, 0.8660254037844387076, 1.000000000000000000, 0.8660254037844387076, 1.000000000000000000, 0.8660254037844387076, 1.000000000000000000, 0.8660254037844387076, 1.000000000000000000, 0.8660254037844387076, 1.000000000000000000, 0.8660254037844387076, 1.000000000000000000, 0.8660254037844387076, 1.000000000000000000, 0.8660254037844387076, 1.000000000000000000, 0.8660254037844387076, 1.000000000000000000, 0.8660254037844387076, 1.000000000000000000, 0.8660254037844387076, 1.000000000000000000, 0.8660254037844387076, 1.000000000000000000, 0.8660254037844387076, 1.000000000000000000, 0.8660254037844387076, 1.000000000000000000, 0.8660254037844387076, 1.000000000000000000, 0.8660254037844387076, 1.000000000000000000, 0.8660254037844387076, 1.000000000000000000, 0.8660254037844387076, 1.000000000000000000, 0.8660254037844387076, 1.000000000000000000, 0.8660254037844387076, 1.000000000000000000, 0.8660254037844387076, 1.000000000000000000, 0.8660254037844387076, 1.000000000000000000, 0.8660254037844387076, 1.000000000000000000, 0.8660254037844387076, 1.000000000000000000, 0.8660254037844387076, 1.000000000000000000, 0.8660254037844387076, 1.000000000000000000, 0.8660254037844387076, 1.000000000000000000, 0.8660254037844387076, 1.000000000000000000, 0.8660254037844387076, 1.000000000000000000, 0.8660254037844387076, 1.000000000000000000, 0.8660254037844387076, 1.000000000000000000, 0.8660254037844387076, 1.000000000000000000, 0.8660254037844387076, 1.000000000000000000, 0.8660254037844387076, 1.000000000000000000, 0.8660254037844387076, 1.000000000000000000, 0.8660254037844387076, 1.000000000000000000, 0.8660254037844387076, 1.000000000000000000, 0.8660254037844387076, 1.000000000000000000, 0.8660254037844387076, 1.000000000000000000, 0.8660254037844387076, 1.000000000000000000, 0.8660254037844387076, 1.000000000000000000, 0.8660254037844387076, 1.000000000000000000, 0.8660254037844387076, 1.000000000000000000, 0.8660254037844387076, 1.000000000000000000, 0.8660254037844387076, 1.000000000000000000, 0.8660254037844387076, 1.000000000000000000, 0.8660254037844387076, 1.000000000000000000, 0.8660254037844387076, 1.000000000000000000, 0.8660254037844387076, 1.000000000000000000, 0.8660254037844387076, 1.000000000000000000, 0.8660254037844387076, 1.000000000000000000, 0.8660254037844387076, 1.000000000000000000, 0.8660254037844387076, 1.000000000000000000, 0.8660254037844387076, 1.000000000000000000, 0.8660254037844387076, 1.000000000000000000, 0.8660254037844387076, 1.000000000000000000, 0.8660254037844387076, 1.000000000000000000, 0.8660254037844387076, 1.000000000000000000, 0.8660254037844387076, 1.000000000000000000, 0.8660254037844387076, 1.000000000000000000, 0.8660254037844387076, 1.000000000000000000, 0.8660254037844387076, 1.000000000000000000, 0.8660254037844387076, 1.000000000000000000, 0.8660254037844387076, 1.000000000000000000, 0.8660254037844387076, 1.000000000000000000, 0.8660254037844387076, 1.000000000000000000, 0.8660254037844387076, 1.000000000000000000, 0.8660254037844387076, 1.000000000000000000, 0.8660254037844387076, 1.000000000000000000, 0.8660254037844387076, 1.000000000000000000, 0.8660254037844387076, 1.000000000000000000, 0.8660254037844387076, 1.000000000000000000, 0.8660254037844387076, 1.000000000000000000, 0.8660254037844387076, 1.000000000000000000, 0.8660254037844387076, 1.000000000000000000, 0.8660254037844387076, 1.000000000000000000, 0.8660254037844387076, 1.000000000000000000, 0.8660254037844387076, 1.000000000000000000, 0.8660254037844387076, 1.000000000000000000, 0.8660254037844387076, 1.000000000000000000, 0.8660254037844387076, 1.000000000000000000, 0.8660254037844387076, 1.000000000000000000, 0.8660254037844387076, 1.000000000000000000, 0.8660254037844387076, 1.000000000000000000, 0.8660254037844387076, 1.000000000000000000, 0.8660254037844387076, 1.000000000000000000, 0.8660254037844387076, 1.000000000000000000, 0.8660254037844387076, 1.000000000000000000, 0.8660254037844387076, 1.000000000000000000, 0.8660254037844387076, 1.000000000000000000, 0.8660254037844387076, 1.000000000000000000, 0.8660254037844387076, 1.000000000000000000, 0.8660254037844387076, 1.000000000000000000, 0.8660254037844387076, 1.000000000000000000, 0.8660254037844387076, 1.000000000000000000, 0.8660254037844387076, 1.000000000000000000, 0.8660254037844387076, 1.000000000000000000, 0.8660254037844387076, 1.000000000000000000, 0.8660254037844387076, 1.000000000000000000, 0.8660254037844387076, 1.000000000000000000, 0.8660254037844387076, 1.000000000000000000, 0.8660254037844387076, 1.000000000000000000, 0.8660254037844387076, 1.000000000000000000, 0.8660254037844387076, 1.000000000000000000, 0.8660254037844387076, 1.000000000000000000, 0.8660254037844387076, 1.000000000000000000, 0.8660254037844387076, 1.000000000000000000, 0.8660254037844387076, 1.000000000000000000, 0.8660254037844387076, 1.000000000000000000, 0.8660254037844387076, 1.000000000000000000, 0.8660254037844387076, 1.000000000000000000, 0.8660254037844387076, 1.000000000000000000, 0.8660254037844387076, 1.000000000000000000, 0.8660254037844387076, 1.000000000000000000, 0.8660254037844387076, 1.000000000000000000, 0.8660254037844387076, 1.000000000000000000, 0.8660254037844387076, 1.000000000000000000, 0.8660254037844387076, 1.000000000000000000, 0.8660254037844387076, 1.000000000000000000, 0.8660254037844387076, 1.000000000000000000, 0.8660254037844387076, 1.000000000000000000, 0.8660254037844387076, 1.000000000000000000, 0.8660254037844387076, 1.000000000000000000, 0.8660254037844387076, 1.000000000000000000, 0.8660254037844387076, 1.000000000000000000, 0.8660254037844387076, 1.000000000000000000, 0.8660254037844387076, 1.000000000000000000, 0.8660254037844387076, 1.000000000000000000, 0.8660254037844387076, 1.000000000000000000, 0.8660254037844387076, 1.000000000000000000, 0.8660254037844387076, 1.000000000000000000, 0.8660254037844387076, 1.000000000000000000, 0.8660254037844387076, 1.000000000000000000, 0.8660254037844387076, 1.000000000000000000, 0.8660254037844387076, 1.000000000000000000, 0.8660254037844387076, 1.000000000000000000, 0.8660254037844387076, 1.000000000000000000, 0.8660254037844387076, 1.000000000000000000, 0.8660254037844387076, 1.000000000000000000, 0.8660254037844387076, 1.000000000000000000, 0.8660254037844387076, 1.000000000000000000, 0.8660254037844387076, 1.000000000000000000, 0.8660254037844387076, 1.000000000000000000, 0.8660254037844387076, 1.000000000000000000, 0.8660254037844387076, 1.000000000000000000, 0.8660254037844387076, 1.000000000000000000, 0.8660254037844387076, 1.000000000000000000, 0.8660254037844387076, 1.000000000000000000, 0.8660254037844387076, 1.000000000000000000, 0.8660254037844387076, 1.000000000000000000, 0.8660254037844387076, 1.000000000000000000, 0.8660254037844387076, 1.000000000000000000, 0.8660254037844387076, 1.000000000000000000, 0.8660254037844387076, 1.000000000000000000, 0.8660254037844387076, 1.000000000000000000, 0.8660254037844387076, 1.000000000000000000, 0.8660254037844387076, 1.000000000000000000, 0.8660254037844387076, 1.000000000000000000, 0.8660254037844387076, 1.000000000000000000, 0.8660254037844387076, 1.000000000000000000, 0.8660254037844387076, 1.000000000000000000, 0.8660254037844387076, 1.000000000000000000, 0.8660254037844387076, 1.000000000000000000, 0.8660254037844387076, 1.000000000000000000, 0.8660254037844387076, 1.000000000000000000, 0.8660254037844387076, 1.000000000000000000, 0.8660254037844387076, 1.000000000000000000, 0.8660254037844387076, 1.000000000000000000, 0.8660254037844387076, 1.000000000000000000, 0.8660254037844387076, 1.000000000000000000, 0.8660254037844387076, 1.000000000000000000, 0.8660254037844387076, 1.000000000000000000, 0.8660254037844387076, 1.000000000000000000, 0.8660254037844387076, 1.000000000000000000, 0.8660254037844387076, 1.000000000000000000, 0.8660254037844387076, 1.000000000000000000, 0.8660254037844387076, 1.000000000000000000, 0.8660254037844387076, 1.000000000000000000, 0.8660254037844387076, 1.000000000000000000, 0.8660254037844387076, 1.000000000000000000, 0.8660254037844387076, 1.000000000000000000, 0.8660254037844387076, 1.000000000000000000, 0.8660254037844387076, 1.000000000000000000, 0.8660254037844387076, 1.000000000000000000, 0.8660254037844387076, 1.000000000000000000, 0.8660254037844387076, 1.000000000000000000, 0.8660254037844387076, 1.000000000000000000, 0.8660254037844387076, 1.000000000000000000, 0.8660254037844387076, 1.000000000000000000, 0.8660254037844387076, 1.000000000000000000, 0.8660254037844387076, 1.000000000000000000, 0.8660254037844387076, 1.000000000000000000, 0.8660254037844387076, 1.000000000000000000, 0.8660254037844387076, 1.000000000000000000, 0.8660254037844387076, 1.000000000000000000, 0.8660254037844387076, 1.000000000000000000, 0.8660254037844387076, 1.000000000000000000, 0.8660254037844387076, 1.000000000000000000, 0.8660254037844387076, 1.000000000000000000, 0.8660254037844387076, 1.000000000000000000, 0.8660254037844387076, 1.000000000000000000, 0.8660254037844387076, 1.000000000000000000, 0.8660254037844387076, 1.000000000000000000, 0.8660254037844387076, 1.000000000000000000, 0.8660254037844387076, 1.000000000000000000, 0.8660254037844387076, 1.000000000000000000, 0.8660254037844387076, 1.000000000000000000, 0.8660254037844387076, 1.000000000000000000, 0.8660254037844387076, 1.000000000000000000, 0.8660254037844387076, 1.000000000000000000, 0.8660254037844387076, 1.000000000000000000, 0.8660254037844387076, 1.000000000000000000, 0.8660254037844387076, 1.000000000000000000, 0.8660254037844387076, 1.000000000000000000, 0.8660254037844387076, 1.000000000000000000, 0.8660254037844387076, 1.000000000000000000, 0.8660254037844387076, 1.000000000000000000, 0.8660254037844387076, 1.000000000000000000, 0.8660254037844387076, 1.000000000000000000, 0.8660254037844387076, 1.000000000000000000, 0.8660254037844387076, 1.000000000000000000, 0.8660254037844387076, 1.000000000000000000, 0.8660254037844387076, 1.000000000000000000, 0.8660254037844387076, 1.000000000000000000, 0.8660254037844387076, 1.000000000000000000, 0.8660254037844387076, 1.000000000000000000, 0.8660254037844387076, 1.000000000000000000, 0.8660254037844387076, 1.000000000000000000, 0.8660254037844387076, 1.000000000000000000, 0.8660254037844387076, 1.000000000000000000, 0.8660254037844387076, 1.000000000000000000, 0.8660254037844387076, 1.000000000000000000, 0.8660254037844387076, 1.000000000000000000, 0.8660254037844387076, 1.000000000000000000, 0.8660254037844387076, 1.000000000000000000, 0.8660254037844387076, 1.000000000000000000, 0.8660254037844387076, 1.000000000000000000, 0.8660254037844387076, 1.000000000000000000, 0.8660254037844387076, 1.000000000000000000, 0.8660254037844387076, 1.000000000000000000, 0.8660254037844387076, 1.000000000000000000, 0.8660254037844387076, 1.000000000000000000, 0.8660254037844387076, 1.000000000000000000, 0.8660254037844387076, 1.000000000000000000, 0.8660254037844387076, 1.000000000000000000, 0.8660254037844387076, 1.000000000000000000, 0.8660254037844387076, 1.000000000000000000, 0.8660254037844387076, 1.000000000000000000, 0.8660254037844387076, 1.000000000000000000, 0.8660254037844387076, 1.000000000000000000, 0.8660254037844387076, 1.000000000000000000, 0.8660254037844387076, 1.000000000000000000, 0.8660254037844387076, 1.000000000000000000, 0.8660254037844387076, 1.000000000000000000, 0.8660254037844387076, 1.000000000000000000) ) ) 
 REPRESENTATION_ITEM ( '' )  SURFACE ( )  );
#18792=DIRECTION ( 'NONE',  ( -0.000000000000000000, -1.000000000000000000, -0.000000000000000000 ) ) ;
#18793=CARTESIAN_POINT ( 'NONE',  ( 14.28750000000000142, -2.886751345948129988, 4.999999999999997335 ) ) ;
#18794=CARTESIAN_POINT ( 'NONE',  ( 9.001249775931846008E-16, 11.36562500061451786, 34.90005215228797653 ) ) ;
#18795=CARTESIAN_POINT ( 'NONE',  ( 14.32500000122903394, 2.886751345948126879, 4.999999999999999112 ) ) ;
#18796=CARTESIAN_POINT ( 'NONE',  ( 23.89687500061451786, 6.054752690667223547, 3.707466751127219781E-16 ) ) ;
#18797=ORIENTED_EDGE ( 'NONE', *, *, #15596, .F. ) ;
#18798=CARTESIAN_POINT ( 'NONE',  ( 18.74062500061451431, -3.027376345333610441, -5.243569643749999898 ) ) ;
#18799=CARTESIAN_POINT ( 'NONE',  ( 4.228125000614517681, -4.541064518000419881, 2.621784821874995952 ) ) ;
#18800=CARTESIAN_POINT ( 'NONE',  ( 19.43437500061451928, 4.541064518000418104, 2.621784821874999949 ) ) ;
#18801=CARTESIAN_POINT ( 'NONE',  ( 5.250000000000000888, 0.000000000000000000, 4.999999999999998224 ) ) ;
#18802=CARTESIAN_POINT ( 'NONE',  ( 7.078125000614516438, 6.421520780324663323E-16, -5.243569643749999010 ) ) ;
#18803=CARTESIAN_POINT ( 'NONE',  ( 22.15312500061451573, 0.000000000000000000, 5.243569643749999010 ) ) ;
#18804=CARTESIAN_POINT ( 'NONE',  ( -4.243569643749997233, 16.24062500061451431, 32.45002607614398471 ) ) ;
#18805=CARTESIAN_POINT ( 'NONE',  ( 19.83750000122903145, -4.330127018922194537, 2.499999999999995559 ) ) ;
#18807=CARTESIAN_POINT ( 'NONE',  ( 9.328125000614518214, 6.421520780324663323E-16, -5.243569643749999010 ) ) ;
#18808=CARTESIAN_POINT ( 'NONE',  ( 2.971875000614517592, -6.054752690667223547, -1.112240025338166033E-15 ) ) ;
#18809=CARTESIAN_POINT ( 'NONE',  ( 28.37812500061451715, 4.541064518000418104, 2.621784821874999949 ) ) ;
#18810=CARTESIAN_POINT ( 'NONE',  ( 24.34687500061451715, 6.054752690667223547, 3.707466751127219781E-16 ) ) ;
#18811=CARTESIAN_POINT ( 'NONE',  ( 13.90312500061451750, 4.541064518000418104, -2.621784821874998173 ) ) ;
#18813=CARTESIAN_POINT ( 'NONE',  ( 24.52500000122903145, 2.886751345948129099, -4.999999999999998224 ) ) ;
#18814=CARTESIAN_POINT ( 'NONE',  ( 26.35312500061451857, -4.541064518000417216, -2.621784821875001281 ) ) ;
#18815=CARTESIAN_POINT ( 'NONE',  ( 18.34687500061451715, -3.027376345333610441, -5.243569643749999898 ) ) ;
#18816=CARTESIAN_POINT ( 'NONE',  ( 14.61562500061451608, -6.054752690667223547, -1.112240025338166033E-15 ) ) ;
#18817=CARTESIAN_POINT ( 'NONE',  ( -4.243569643749997233, 17.64687500061452141, 32.45002607614398471 ) ) ;
#18818=CARTESIAN_POINT ( 'NONE',  ( 21.47812500061451502, 6.421520780324663323E-16, -5.243569643749999010 ) ) ;
#18819=DIRECTION ( 'NONE',  ( -1.000000000000000000, -0.000000000000000000, -0.000000000000000000 ) ) ;
#18820=VERTEX_POINT ( 'NONE', #30594 ) ;
#18821=CARTESIAN_POINT ( 'NONE',  ( 25.87500000000000000, 4.330127018922191873, 2.499999999999999556 ) ) ;
#18822=CARTESIAN_POINT ( 'NONE',  ( 1.999999999999998668, 11.75000000000000178, -33.46410161513775705 ) ) ;
#18824=CARTESIAN_POINT ( 'NONE',  ( 29.12812500061451715, 6.421520780324663323E-16, -5.243569643749999010 ) ) ;
#18825=CARTESIAN_POINT ( 'NONE',  ( 6.815625000614517148, 3.027376345333611329, 5.243569643749999010 ) ) ;
#18826=CARTESIAN_POINT ( 'NONE',  ( 23.17500000122903359, 2.886751345948129099, -4.999999999999998224 ) ) ;
#18827=CARTESIAN_POINT ( 'NONE',  ( 27.66562500061451146, -6.054752690667223547, -1.112240025338166033E-15 ) ) ;
#18828=CARTESIAN_POINT ( 'NONE',  ( 24.37500000000000000, 6.123233995736764310E-16, -4.999999999999998224 ) ) ;
#18829=CARTESIAN_POINT ( 'NONE',  ( -2.000000000000000000, 15.98750000122903181, -33.46410161513775705 ) ) ;
#18830=CARTESIAN_POINT ( 'NONE',  ( 29.57812500061451644, 6.421520780324663323E-16, -5.243569643749999010 ) ) ;
#18831=CARTESIAN_POINT ( 'NONE',  ( 11.05312500061451608, -4.541064518000417216, -2.621784821875001281 ) ) ;
#18832=ORIENTED_EDGE ( 'NONE', *, *, #69351, .F. ) ;
#18833=CARTESIAN_POINT ( 'NONE',  ( 24.92812500061451431, -4.541064518000419881, 2.621784821874995952 ) ) ;
#18834=CARTESIAN_POINT ( 'NONE',  ( 6.740625000614516082, 6.054752690667223547, 3.707466751127219781E-16 ) ) ;
#18835=UNCERTAINTY_MEASURE_WITH_UNIT (LENGTH_MEASURE( 1.000000000000000082E-05 ), #51409, 'distance_accuracy_value', 'NONE');
#18836=CARTESIAN_POINT ( 'NONE',  ( 4.715625000614516615, -6.054752690667223547, -1.112240025338166033E-15 ) ) ;
#18838=CARTESIAN_POINT ( 'NONE',  ( 12.90000000000000213, 0.000000000000000000, 4.999999999999998224 ) ) ;
#18839=( BOUNDED_CURVE ( )  B_SPLINE_CURVE ( 2, ( #12234, #51769, #11518, #34040, #3714, #41763, #47308 ),
 .UNSPECIFIED., .F., .F. ) 
 B_SPLINE_CURVE_WITH_KNOTS ( ( 3, 2, 2, 3 ),
 ( 0.3166666666666666519, 0.3194444444444444198, 0.3222222222222222432, 0.3250000000000000111 ),
 .UNSPECIFIED. ) 
 CURVE ( )  GEOMETRIC_REPRESENTATION_ITEM ( )  RATIONAL_B_SPLINE_CURVE ( ( 1.000000000000000000, 0.8660254037844387076, 1.000000000000000000, 0.8660254037844387076, 1.000000000000000000, 0.8660254037844387076, 1.000000000000000000 ) ) 
 REPRESENTATION_ITEM ( '' )  );
#18840=CARTESIAN_POINT ( 'NONE',  ( 13.72500000000000142, 4.330127018922191873, 2.499999999999999556 ) ) ;
#18841=( BOUNDED_CURVE ( )  B_SPLINE_CURVE ( 2, ( #22527, #51338, #5550, #29168, #16256, #51701, #22168, #33256, #61326 ),
 .UNSPECIFIED., .F., .F. ) 
 B_SPLINE_CURVE_WITH_KNOTS ( ( 3, 2, 2, 2, 3 ),
 ( 0.7282608695652174058, 0.7318840579710145233, 0.7391304347826086474, 0.7463768115942028825, 0.7500000000000000000 ),
 .UNSPECIFIED. ) 
 CURVE ( )  GEOMETRIC_REPRESENTATION_ITEM ( )  RATIONAL_B_SPLINE_CURVE ( ( 0.9330127018922194093, 0.9330127018922194093, 1.000000000000000000, 0.8660254037844387076, 1.000000000000000000, 0.8660254037844387076, 1.000000000000000000, 0.9330127018922194093, 0.9330127018922194093 ) ) 
 REPRESENTATION_ITEM ( '' )  );
#18842=CARTESIAN_POINT ( 'NONE',  ( 12.68437500061451573, 4.541064518000418104, 2.621784821874999949 ) ) ;
#18843=CARTESIAN_POINT ( 'NONE',  ( 9.300000001229035362, 5.773502691896255534, 3.535250795749688894E-16 ) ) ;
#18844=CARTESIAN_POINT ( 'NONE',  ( 17.70937500061451431, 0.000000000000000000, 5.243569643749999010 ) ) ;
#18846=CARTESIAN_POINT ( 'NONE',  ( 8.296875000614516438, -3.027376345333614438, 5.243569643749998122 ) ) ;
#18847=CARTESIAN_POINT ( 'NONE',  ( 4.243569643749999898, 10.99062500061451786, -27.54997392385601529 ) ) ;
#18848=DIRECTION ( 'NONE',  ( 0.000000000000000000, 0.000000000000000000, 1.000000000000000000 ) ) ;
#18851=CARTESIAN_POINT ( 'NONE',  ( 24.62812500061451715, 6.421520780324663323E-16, -5.243569643749999010 ) ) ;
#18852=CARTESIAN_POINT ( 'NONE',  ( 29.10937500061451644, -4.541064518000417216, -2.621784821875001281 ) ) ;
#18853=EDGE_CURVE ( 'NONE', #70559, #33433, #41748, .T. ) ;
#18854=CARTESIAN_POINT ( 'NONE',  ( 21.44999999999999929, 0.000000000000000000, 4.999999999999998224 ) ) ;
#18856=CARTESIAN_POINT ( 'NONE',  ( 7.940625000614518036, -3.027376345333610441, -5.243569643749999898 ) ) ;
#18858=CARTESIAN_POINT ( 'NONE',  ( 15.72187500061451892, 3.027376345333613106, -5.243569643749998122 ) ) ;
#18860=CARTESIAN_POINT ( 'NONE',  ( 3.853125000614517681, -4.541064518000417216, -2.621784821875001281 ) ) ;
#18861=CARTESIAN_POINT ( 'NONE',  ( 7.471875000614519813, -6.054752690667223547, -1.112240025338166033E-15 ) ) ;
#18862=ORIENTED_EDGE ( 'NONE', *, *, #68921, .F. ) ;
#18863=CARTESIAN_POINT ( 'NONE',  ( 19.77187500061451786, 3.027376345333613106, -5.243569643749998122 ) ) ;
#18864=CARTESIAN_POINT ( 'NONE',  ( 21.52499999999999858, -4.330127018922194537, 2.499999999999995559 ) ) ;
#18865=CARTESIAN_POINT ( 'NONE',  ( 26.77499999999999858, 4.330127018922191873, 2.499999999999999556 ) ) ;
#18866=CARTESIAN_POINT ( 'NONE',  ( 28.84687500061452070, 6.054752690667223547, 3.707466751127219781E-16 ) ) ;
#18868=ORIENTED_EDGE ( 'NONE', *, *, #13955, .T. ) ;
#18869=CARTESIAN_POINT ( 'NONE',  ( 10.46249999999999858, 2.886751345948129099, -4.999999999999998224 ) ) ;
#18871=CARTESIAN_POINT ( 'NONE',  ( 22.45312500061451644, 4.541064518000418104, -2.621784821874998173 ) ) ;
#18872=CARTESIAN_POINT ( 'NONE',  ( 13.19999999999999929, 4.330127018922192761, -2.499999999999997780 ) ) ;
#18873=CARTESIAN_POINT ( 'NONE',  ( 7.950000001229033053, 5.773502691896255534, 3.535250795749688894E-16 ) ) ;
#18874=CARTESIAN_POINT ( 'NONE',  ( 5.690625000614516260, -3.027376345333610441, -5.243569643749999898 ) ) ;
#18875=CARTESIAN_POINT ( 'NONE',  ( 21.07499999999999929, -4.330127018922194537, 2.499999999999995559 ) ) ;
#18876=CARTESIAN_POINT ( 'NONE',  ( 22.00312500061451360, 4.541064518000418104, -2.621784821874998173 ) ) ;
#18877=CARTESIAN_POINT ( 'NONE',  ( 24.52500000122903145, 2.886751345948129099, -4.999999999999998224 ) ) ;
#18879=CARTESIAN_POINT ( 'NONE',  ( 6.150000000000003020, 0.000000000000000000, 4.999999999999998224 ) ) ;
#18880=ORIENTED_EDGE ( 'NONE', *, *, #23767, .F. ) ;
#18881=CARTESIAN_POINT ( 'NONE',  ( 20.42812500061451431, -4.541064518000419881, 2.621784821874995952 ) ) ;
#18882=CARTESIAN_POINT ( 'NONE',  ( 27.44062500061451715, 6.054752690667223547, 3.707466751127219781E-16 ) ) ;
#18883=CARTESIAN_POINT ( 'NONE',  ( 27.08437500061451786, 4.541064518000418104, 2.621784821874999949 ) ) ;
#18884=CARTESIAN_POINT ( 'NONE',  ( 13.82812500061451466, 6.421520780324663323E-16, -5.243569643749999010 ) ) ;
#18887=CARTESIAN_POINT ( 'NONE',  ( 26.13750000122903216, -4.330127018922194537, 2.499999999999995559 ) ) ;
#18889=CARTESIAN_POINT ( 'NONE',  ( 16.75312500061451715, 0.000000000000000000, 5.243569643749999010 ) ) ;
#18890=CARTESIAN_POINT ( 'NONE',  ( 0.000000000000000000, 20.00000000000000000, 30.00000000000000000 ) ) ;
#18891=CARTESIAN_POINT ( 'NONE',  ( 28.05937500061451573, 0.000000000000000000, 5.243569643749999010 ) ) ;
#18892=CARTESIAN_POINT ( 'NONE',  ( 11.55937500061451928, -4.541064518000417216, -2.621784821875001281 ) ) ;
#18893=CARTESIAN_POINT ( 'NONE',  ( 8.521875000614516082, 3.027376345333613106, -5.243569643749998122 ) ) ;
#18894=CARTESIAN_POINT ( 'NONE',  ( 18.57187500061451857, 3.027376345333611329, 5.243569643749999010 ) ) ;
#18895=VERTEX_POINT ( 'NONE', #13959 ) ;
#18896=CARTESIAN_POINT ( 'NONE',  ( -5.678847837524353181, 8.233079231341500659, 28.02470760206609057 ) ) ;
#18897=CARTESIAN_POINT ( 'NONE',  ( 24.59062500061451573, -3.027376345333610441, -5.243569643749999898 ) ) ;
#18898=CARTESIAN_POINT ( 'NONE',  ( 19.05937500061451928, 0.000000000000000000, 5.243569643749999010 ) ) ;
#18899=CARTESIAN_POINT ( 'NONE',  ( 22.15312500061451573, 0.000000000000000000, 5.243569643749999010 ) ) ;
#18900=CARTESIAN_POINT ( 'NONE',  ( -0.6945863667395647534, 9.663023495605401081, 26.06076786935074097 ) ) ;
#18901=CARTESIAN_POINT ( 'NONE',  ( 3.999999999999998668, 13.51250000000000107, 27.69059892324149175 ) ) ;
#18902=CARTESIAN_POINT ( 'NONE',  ( 28.82812500061451644, 4.541064518000418104, 2.621784821874999949 ) ) ;
#18903=CARTESIAN_POINT ( 'NONE',  ( 10.05000000122903181, -2.886751345948125991, -5.000000000000000000 ) ) ;
#18904=ORIENTED_EDGE ( 'NONE', *, *, #16392, .F. ) ;
#18905=CARTESIAN_POINT ( 'NONE',  ( 5.250000001229035540, 5.773502691896255534, 3.535250795749688894E-16 ) ) ;
#18906=CARTESIAN_POINT ( 'NONE',  ( 3.999999999999998668, 19.36250000000000426, -32.30940107675850470 ) ) ;
#18907=CARTESIAN_POINT ( 'NONE',  ( 24.56250000122903288, 4.330127018922192761, -2.499999999999997780 ) ) ;
#18909=CARTESIAN_POINT ( 'NONE',  ( 9.346875000614517148, -3.027376345333610441, -5.243569643749999898 ) ) ;
#18912=CARTESIAN_POINT ( 'NONE',  ( 15.92812500061451608, -4.541064518000419881, 2.621784821874995952 ) ) ;
#18913=CARTESIAN_POINT ( 'NONE',  ( 11.37187500061451750, 3.027376345333611329, 5.243569643749999010 ) ) ;
#18914=CARTESIAN_POINT ( 'NONE',  ( 28.76250000122903216, 0.000000000000000000, 4.999999999999998224 ) ) ;
#18915=ADVANCED_FACE ( 'NONE', ( #53490 ), #23591, .F. ) ;
#18916=CARTESIAN_POINT ( 'NONE',  ( 20.18437500061451573, 6.421520780324663323E-16, -5.243569643749999010 ) ) ;
#18917=CARTESIAN_POINT ( 'NONE',  ( 8.296875000614516438, -3.027376345333614438, 5.243569643749998122 ) ) ;
#18918=LINE ( 'NONE', #20014, #21471 ) ;
#18919=CARTESIAN_POINT ( 'NONE',  ( 7.903125000614515727, -4.541064518000417216, -2.621784821875001281 ) ) ;
#18920=CARTESIAN_POINT ( 'NONE',  ( 18.59062500061451573, -3.027376345333614438, 5.243569643749998122 ) ) ;
#18921=ORIENTED_EDGE ( 'NONE', *, *, #3889, .F. ) ;
#18922=CARTESIAN_POINT ( 'NONE',  ( 16.00312500061451715, -4.541064518000417216, -2.621784821875001281 ) ) ;
#18923=CARTESIAN_POINT ( 'NONE',  ( 10.22812500061451679, 6.421520780324663323E-16, -5.243569643749999010 ) ) ;
#18925=CARTESIAN_POINT ( 'NONE',  ( 11.84999999999999964, 4.330127018922192761, -2.499999999999997780 ) ) ;
#18926=CARTESIAN_POINT ( 'NONE',  ( 6.487500001229034474, 6.123233995736764310E-16, -4.999999999999998224 ) ) ;
#18927=ADVANCED_FACE ( 'NONE', ( #64570 ), #68676, .F. ) ;
#18928=CARTESIAN_POINT ( 'NONE',  ( 15.94687500061451502, -3.027376345333614438, 5.243569643749998122 ) ) ;
#18929=CARTESIAN_POINT ( 'NONE',  ( 15.75000000122902932, -2.886751345948129988, 4.999999999999997335 ) ) ;
#18931=CARTESIAN_POINT ( 'NONE',  ( 4.243569643749999898, 18.64062500061451644, -27.54997392385601529 ) ) ;
#18933=CARTESIAN_POINT ( 'NONE',  ( 22.95000000122903216, -2.886751345948130876, 4.999999999999996447 ) ) ;
#18934=EDGE_CURVE ( 'NONE', #36091, #3869, #48871, .T. ) ;
#18936=CARTESIAN_POINT ( 'NONE',  ( 1.626862140677534273E-15, 13.36250000000000071, 34.00000000000000000 ) ) ;
#18937=CARTESIAN_POINT ( 'NONE',  ( 18.00937500061451502, 4.541064518000418104, -2.621784821874998173 ) ) ;
#18938=CARTESIAN_POINT ( 'NONE',  ( 27.93750000000000000, -2.886751345948125991, -5.000000000000000000 ) ) ;
#18939=CARTESIAN_POINT ( 'NONE',  ( 15.06562500061451537, -6.054752690667223547, -1.112240025338166033E-15 ) ) ;
#18941=DIRECTION ( 'NONE',  ( -0.000000000000000000, -1.000000000000000000, -0.000000000000000000 ) ) ;
#18942=CARTESIAN_POINT ( 'NONE',  ( 23.55937500061451573, 0.000000000000000000, 5.243569643749999010 ) ) ;
#18944=CARTESIAN_POINT ( 'NONE',  ( 9.553125000614517859, 0.000000000000000000, 5.243569643749999010 ) ) ;
#18945=CARTESIAN_POINT ( 'NONE',  ( 15.42187500061451821, 3.027376345333611329, 5.243569643749999010 ) ) ;
#18947=CARTESIAN_POINT ( 'NONE',  ( 27.30937500061451573, -4.541064518000417216, -2.621784821875001281 ) ) ;
#18948=CARTESIAN_POINT ( 'NONE',  ( 28.60312500061451502, -4.541064518000417216, -2.621784821875001281 ) ) ;
#18949=CARTESIAN_POINT ( 'NONE',  ( 17.05312500061451786, 4.541064518000418104, -2.621784821874998173 ) ) ;
#18950=CARTESIAN_POINT ( 'NONE',  ( 29.80312500061451431, 0.000000000000000000, 5.243569643749999010 ) ) ;
#18951=CARTESIAN_POINT ( 'NONE',  ( 3.999999999999998668, 12.72500000122903430, -32.30940107675850470 ) ) ;
#18952=CARTESIAN_POINT ( 'NONE',  ( 9.637499999999999289, 5.773502691896255534, 3.535250795749688894E-16 ) ) ;
#18953=CARTESIAN_POINT ( 'NONE',  ( 20.17500000122903359, 2.886751345948126879, 4.999999999999999112 ) ) ;
#18954=CARTESIAN_POINT ( 'NONE',  ( 4.000000000000000000, 10.28750000000000142, 32.30940107675849760 ) ) ;
#18957=CARTESIAN_POINT ( 'NONE',  ( 18.00000000000000355, -4.330127018922190985, -2.500000000000001332 ) ) ;
#18958=CARTESIAN_POINT ( 'NONE',  ( 22.16250000000000142, 2.886751345948129099, -4.999999999999998224 ) ) ;
#18959=CARTESIAN_POINT ( 'NONE',  ( 18.08437500061451431, 4.541064518000418104, 2.621784821874999949 ) ) ;
#18960=CARTESIAN_POINT ( 'NONE',  ( 14.31562500061451537, 3.027376345333613106, -5.243569643749998122 ) ) ;
#18961=VERTEX_POINT ( 'NONE', #57927 ) ;
#18963=CARTESIAN_POINT ( 'NONE',  ( 6.590625000614518392, -3.027376345333610441, -5.243569643749999898 ) ) ;
#18965=CARTESIAN_POINT ( 'NONE',  ( 12.90000000000000213, 0.000000000000000000, 4.999999999999998224 ) ) ;
#18967=CARTESIAN_POINT ( 'NONE',  ( -2.121784821874996840, 14.02812500061451750, 33.67503911421598417 ) ) ;
#18968=CARTESIAN_POINT ( 'NONE',  ( 3.271875000614519635, 3.027376345333611329, 5.243569643749999010 ) ) ;
#18971=CARTESIAN_POINT ( 'NONE',  ( 24.87187500061451573, 3.027376345333611329, 5.243569643749999010 ) ) ;
#18972=ORIENTED_EDGE ( 'NONE', *, *, #39310, .T. ) ;
#18973=CARTESIAN_POINT ( 'NONE',  ( 21.62812500061451360, 4.541064518000418104, 2.621784821874999949 ) ) ;
#18974=CARTESIAN_POINT ( 'NONE',  ( 23.74687500061451573, -3.027376345333610441, -5.243569643749999898 ) ) ;
#18975=CARTESIAN_POINT ( 'NONE',  ( -2.121784821874996840, 16.27812500061459389, -26.32496088578401583 ) ) ;
#18976=CARTESIAN_POINT ( 'NONE',  ( 5.990625000614517859, -3.027376345333614438, 5.243569643749998122 ) ) ;
#18978=CARTESIAN_POINT ( 'NONE',  ( 24.92812500061451431, -4.541064518000419881, 2.621784821874995952 ) ) ;
#18981=CARTESIAN_POINT ( 'NONE',  ( 16.73437500061451644, 4.541064518000418104, 2.621784821874999949 ) ) ;
#18982=CARTESIAN_POINT ( 'NONE',  ( 27.87187500061451573, 3.027376345333613106, -5.243569643749998122 ) ) ;
#18983=CARTESIAN_POINT ( 'NONE',  ( 4.243569643749999898, 17.34687500061451715, 32.45002607614398471 ) ) ;
#18984=CARTESIAN_POINT ( 'NONE',  ( 6.365625000614518747, 3.027376345333611329, 5.243569643749999010 ) ) ;
#18985=CARTESIAN_POINT ( 'NONE',  ( 30.00000000000000000, 0.000000000000000000, 0.000000000000000000 ) ) ;
#18986=CARTESIAN_POINT ( 'NONE',  ( 4.171875000614517326, 3.027376345333611329, 5.243569643749999010 ) ) ;
#18988=CARTESIAN_POINT ( 'NONE',  ( 5.953125000614519102, 0.000000000000000000, 5.243569643749999010 ) ) ;
#18989=CARTESIAN_POINT ( 'NONE',  ( 9.421875000614519990, 3.027376345333613106, -5.243569643749998122 ) ) ;
#18990=CARTESIAN_POINT ( 'NONE',  ( 16.91250000122903430, 4.330127018922192761, -2.499999999999997780 ) ) ;
#18991=CARTESIAN_POINT ( 'NONE',  ( 3.084375000614519191, 6.421520780324663323E-16, -5.243569643749999010 ) ) ;
#18992=CARTESIAN_POINT ( 'NONE',  ( 7.228125000614517681, 4.541064518000418104, 2.621784821874999949 ) ) ;
#18995=CARTESIAN_POINT ( 'NONE',  ( 15.60937500061451644, -4.541064518000417216, -2.621784821875001281 ) ) ;
#18997=VERTEX_POINT ( 'NONE', #26518 ) ;
#18998=CARTESIAN_POINT ( 'NONE',  ( 24.89062500061451644, -3.027376345333614438, 5.243569643749998122 ) ) ;
#18999=CARTESIAN_POINT ( 'NONE',  ( 10.30312500061451431, 4.541064518000418104, -2.621784821874998173 ) ) ;
#19000=CARTESIAN_POINT ( 'NONE',  ( 27.27187500061451431, -6.054752690667223547, -1.112240025338166033E-15 ) ) ;
#19001=CARTESIAN_POINT ( 'NONE',  ( 10.30312500061451431, 4.541064518000418104, -2.621784821874998173 ) ) ;
#19002=FACE_OUTER_BOUND ( 'NONE', #12905, .T. ) ;
#19003=CARTESIAN_POINT ( 'NONE',  ( 9.937500001229032875, -4.330127018922194537, 2.499999999999995559 ) ) ;
#19004=CARTESIAN_POINT ( 'NONE',  ( 25.94062500061451715, -3.027376345333610441, -5.243569643749999898 ) ) ;
#19005=CARTESIAN_POINT ( 'NONE',  ( -4.243569643749999898, 12.56562500061451715, -32.45002607614398471 ) ) ;
#19006=CARTESIAN_POINT ( 'NONE',  ( 12.82500000122903394, 2.886751345948129099, -4.999999999999998224 ) ) ;
#19007=CARTESIAN_POINT ( 'NONE',  ( 21.47812500061451502, 6.421520780324663323E-16, -5.243569643749999010 ) ) ;
#19008=CARTESIAN_POINT ( 'NONE',  ( 18.81562500061452070, 3.027376345333613106, -5.243569643749998122 ) ) ;
#19009=CARTESIAN_POINT ( 'NONE',  ( 6.084375000614518747, -4.541064518000419881, 2.621784821874995952 ) ) ;
#19010=CARTESIAN_POINT ( 'NONE',  ( 18.33749999999999858, -2.886751345948129988, 4.999999999999997335 ) ) ;
#19011=EDGE_CURVE ( 'NONE', #58630, #41088, #26889, .T. ) ;
#19012=CARTESIAN_POINT ( 'NONE',  ( 14.40000000122903323, -2.886751345948129988, 4.999999999999997335 ) ) ;
#19013=CARTESIAN_POINT ( 'NONE',  ( 10.04062500061451502, -3.027376345333614438, 5.243569643749998122 ) ) ;
#19015=CARTESIAN_POINT ( 'NONE',  ( 14.12812500061451715, -4.541064518000419881, 2.621784821874995952 ) ) ;
#19016=CARTESIAN_POINT ( 'NONE',  ( 24.78750000122903074, -4.330127018922194537, 2.499999999999995559 ) ) ;
#19017=CARTESIAN_POINT ( 'NONE',  ( 21.08437500061451786, 6.421520780324663323E-16, -5.243569643749999010 ) ) ;
#19018=CARTESIAN_POINT ( 'NONE',  ( 20.14687500061451786, -3.027376345333610441, -5.243569643749999898 ) ) ;
#19019=LINE ( 'NONE', #17938, #50125 ) ;
#19020=EDGE_CURVE ( 'NONE', #48662, #47727, #43696, .T. ) ;
#19021=CARTESIAN_POINT ( 'NONE',  ( 7.237500001229035362, -4.330127018922194537, 2.499999999999995559 ) ) ;
#19022=CARTESIAN_POINT ( 'NONE',  ( 6.909375000614518036, 0.000000000000000000, 5.243569643749999010 ) ) ;
#19023=CARTESIAN_POINT ( 'NONE',  ( 26.52187500061451431, 3.027376345333613106, -5.243569643749998122 ) ) ;
#19025=CARTESIAN_POINT ( 'NONE',  ( 15.30000000122903181, -2.886751345948063374, 5.000000000000112799 ) ) ;
#19026=CARTESIAN_POINT ( 'NONE',  ( 21.10312500061451502, 4.541064518000418104, -2.621784821874998173 ) ) ;
#19027=CARTESIAN_POINT ( 'NONE',  ( 27.04687500061451644, 6.054752690667223547, 3.707466751127219781E-16 ) ) ;
#19028=ADVANCED_FACE ( 'NONE', ( #59377 ), #25785, .F. ) ;
#19030=CARTESIAN_POINT ( 'NONE',  ( 3.228505727505837974, -3.817951121670090320, 3.373270459396892296 ) ) ;
#19031=DIRECTION ( 'NONE',  ( 0.000000000000000000, -1.000000000000000000, 0.000000000000000000 ) ) ;
#19032=CARTESIAN_POINT ( 'NONE',  ( 7.321875000614516793, 3.027376345333611329, 5.243569643749999010 ) ) ;
#19033=CARTESIAN_POINT ( 'NONE',  ( 18.40312500061451573, 4.541064518000418104, -2.621784821874998173 ) ) ;
#19034=VERTEX_POINT ( 'NONE', #64934 ) ;
#19035=LINE ( 'NONE', #68951, #34827 ) ;
#19036=CARTESIAN_POINT ( 'NONE',  ( 26.57812500061451644, 4.541064518000418104, 2.621784821874999949 ) ) ;
#19037=CARTESIAN_POINT ( 'NONE',  ( 5.109375000614518214, 0.000000000000000000, 5.243569643749999010 ) ) ;
#19038=CARTESIAN_POINT ( 'NONE',  ( -3.999999999999999112, 15.94999999999999929, -30.00000000000000000 ) ) ;
#19040=CARTESIAN_POINT ( 'NONE',  ( 17.28750000000000142, 5.773502691896255534, 3.535250795749688894E-16 ) ) ;
#19041=CARTESIAN_POINT ( 'NONE',  ( 20.57812500061451644, 6.421520780324663323E-16, -5.243569643749999010 ) ) ;
#19043=CARTESIAN_POINT ( 'NONE',  ( 24.89999999999999858, 4.330127018922192761, -2.499999999999997780 ) ) ;
#19044=CARTESIAN_POINT ( 'NONE',  ( 25.35937500061451644, 0.000000000000000000, 5.243569643749999010 ) ) ;
#19046=CARTESIAN_POINT ( 'NONE',  ( 2.964777361493091679, -4.026176250088806086, -3.359304602455296607 ) ) ;
#19047=CARTESIAN_POINT ( 'NONE',  ( 12.81562500061451537, -6.054752690667223547, -1.112240025338166033E-15 ) ) ;
#19048=CARTESIAN_POINT ( 'NONE',  ( 6.328125000614515550, 4.541064518000418104, 2.621784821874999949 ) ) ;
#19050=CARTESIAN_POINT ( 'NONE',  ( 29.35312500061451502, 0.000000000000000000, 5.243569643749999010 ) ) ;
#19051=CARTESIAN_POINT ( 'NONE',  ( 16.05000000122903359, 5.773502691896255534, 3.535250795749688894E-16 ) ) ;
#19052=CARTESIAN_POINT ( 'NONE',  ( 19.65000000000000213, 0.000000000000000000, 4.999999999999998224 ) ) ;
#19053=CARTESIAN_POINT ( 'NONE',  ( 28.49999999999999645, 4.330127018922192761, -2.499999999999997780 ) ) ;
#19054=CARTESIAN_POINT ( 'NONE',  ( 2.000000000000001332, 10.70000000000000107, -26.53589838486224650 ) ) ;
#19055=CARTESIAN_POINT ( 'NONE',  ( 8.671875000614518214, 3.027376345333611329, 5.243569643749999010 ) ) ;
#19056=CARTESIAN_POINT ( 'NONE',  ( 19.69687500061451857, -3.027376345333610441, -5.243569643749999898 ) ) ;
#19057=DIRECTION ( 'NONE',  ( -1.000000000000000000, -0.000000000000000000, -0.000000000000000000 ) ) ;
#19059=CARTESIAN_POINT ( 'NONE',  ( 28.90312500061451217, 0.000000000000000000, 5.243569643749999010 ) ) ;
#19060=CARTESIAN_POINT ( 'NONE',  ( 29.59687500061451715, -3.027376345333610441, -5.243569643749999898 ) ) ;
#19061=CARTESIAN_POINT ( 'NONE',  ( 3.721875000614518036, 3.027376345333611329, 5.243569643749999010 ) ) ;
#19062=CARTESIAN_POINT ( 'NONE',  ( 17.10000000000000142, -4.330127018922190985, -2.500000000000001332 ) ) ;
#19063=CARTESIAN_POINT ( 'NONE',  ( 13.11562500061451786, 3.027376345333611329, 5.243569643749999010 ) ) ;
#19065=PRODUCT_DEFINITION_FORMATION_WITH_SPECIFIED_SOURCE ( 'ANY', '', #65012, .NOT_KNOWN. ) ;
#19066=FACE_OUTER_BOUND ( 'NONE', #63225, .T. ) ;
#19067=CARTESIAN_POINT ( 'NONE',  ( 18.90000000122902790, -2.886751345948129988, 4.999999999999997335 ) ) ;
#19068=DIRECTION ( 'NONE',  ( -0.000000000000000000, -1.000000000000000000, -0.000000000000000000 ) ) ;
#19070=CARTESIAN_POINT ( 'NONE',  ( 8.240625000614516082, -3.027376345333614438, 5.243569643749998122 ) ) ;
#19071=CARTESIAN_POINT ( 'NONE',  ( 24.75937500061451502, 4.541064518000418104, -2.621784821874998173 ) ) ;
#19072=CARTESIAN_POINT ( 'NONE',  ( -4.243569643749999898, 19.37187500061451928, 27.54997392385601529 ) ) ;
#19073=CARTESIAN_POINT ( 'NONE',  ( 27.57187500061451857, 3.027376345333611329, 5.243569643749999010 ) ) ;
#19074=CARTESIAN_POINT ( 'NONE',  ( 7.012500000000001066, 2.886751345948126879, 4.999999999999999112 ) ) ;
#19075=CARTESIAN_POINT ( 'NONE',  ( -3.999999999999999556, 12.42500000122903359, 27.69059892324149530 ) ) ;
#19076=CARTESIAN_POINT ( 'NONE',  ( 15.17812500061451608, 6.421520780324663323E-16, -5.243569643749999010 ) ) ;
#19077=CARTESIAN_POINT ( 'NONE',  ( 5.737500001229033586, 4.330127018922191873, 2.499999999999999556 ) ) ;
#19078=( BOUNDED_CURVE ( )  B_SPLINE_CURVE ( 2, ( #22794, #67881, #33164, #39813, #55702, #5096, #50166, #72695, #22077 ),
 .UNSPECIFIED., .F., .F. ) 
 B_SPLINE_CURVE_WITH_KNOTS ( ( 3, 2, 2, 2, 3 ),
 ( 0.5760869565217391353, 0.5797101449275362528, 0.5869565217391304879, 0.5942028985507246119, 0.5978260869565217295 ),
 .UNSPECIFIED. ) 
 CURVE ( )  GEOMETRIC_REPRESENTATION_ITEM ( )  RATIONAL_B_SPLINE_CURVE ( ( 0.9330127018922194093, 0.9330127018922194093, 1.000000000000000000, 0.8660254037844387076, 1.000000000000000000, 0.8660254037844387076, 1.000000000000000000, 0.9330127018922194093, 0.9330127018922194093 ) ) 
 REPRESENTATION_ITEM ( '' )  );
#19079=VECTOR ( 'NONE', #40375, 1000.000000000000000 ) ;
#19080=CARTESIAN_POINT ( 'NONE',  ( 10.95937500061451964, 0.000000000000000000, 5.243569643749999010 ) ) ;
#19083=CARTESIAN_POINT ( 'NONE',  ( 11.61562500061451608, 3.027376345333613106, -5.243569643749998122 ) ) ;
#19085=CARTESIAN_POINT ( 'NONE',  ( 24.33750000122903145, -4.330127018922194537, 2.499999999999995559 ) ) ;
#19086=CARTESIAN_POINT ( 'NONE',  ( 11.74687500061451573, 6.054752690667223547, 3.707466751127219781E-16 ) ) ;
#19087=CARTESIAN_POINT ( 'NONE',  ( 15.21562500061451750, 3.027376345333613106, -5.243569643749998122 ) ) ;
#19089=CARTESIAN_POINT ( 'NONE',  ( 23.33437500061451786, 6.421520780324663323E-16, -5.243569643749999010 ) ) ;
#19090=FACE_OUTER_BOUND ( 'NONE', #20198, .T. ) ;
#19091=CARTESIAN_POINT ( 'NONE',  ( -3.305248395036964552E-15, 5.000000000000034639, 25.99999999999995737 ) ) ;
#19092=DIRECTION ( 'NONE',  ( 0.000000000000000000, 0.000000000000000000, -1.000000000000000000 ) ) ;
#19093=CARTESIAN_POINT ( 'NONE',  ( 4.243569643749999898, 15.54687500061451644, -27.54997392385601529 ) ) ;
#19094=CARTESIAN_POINT ( 'NONE',  ( 16.02187500061451786, -6.054752690667223547, -1.112240025338166033E-15 ) ) ;
#19095=CARTESIAN_POINT ( 'NONE',  ( 17.96250000122903501, 0.000000000000000000, 4.999999999999998224 ) ) ;
#19096=CARTESIAN_POINT ( 'NONE',  ( 11.48437500061451644, -4.541064518000419881, 2.621784821874995952 ) ) ;
#19097=CARTESIAN_POINT ( 'NONE',  ( 9.001249775931846008E-16, 19.01562500061451644, -25.09994784771203058 ) ) ;
#19098=CARTESIAN_POINT ( 'NONE',  ( 19.42500000122903714, -5.773502691896255534, -1.060575238724906372E-15 ) ) ;
#19099=CARTESIAN_POINT ( 'NONE',  ( 13.15312500061451750, 0.000000000000000000, 5.243569643749999010 ) ) ;
#19102=CARTESIAN_POINT ( 'NONE',  ( 17.28750000000000142, 5.773502691896255534, 3.535250795749688894E-16 ) ) ;
#19103=CARTESIAN_POINT ( 'NONE',  ( 27.29999999999999716, 0.000000000000000000, 4.999999999999998224 ) ) ;
#19104=CARTESIAN_POINT ( 'NONE',  ( 11.74687500061451573, 6.054752690667223547, 3.707466751127219781E-16 ) ) ;
#19105=CARTESIAN_POINT ( 'NONE',  ( 22.42500000000000071, -4.330127018922194537, 2.499999999999995559 ) ) ;
#19106=CARTESIAN_POINT ( 'NONE',  ( 12.97500000122903252, 2.886751345948126879, 4.999999999999999112 ) ) ;
#19107=CARTESIAN_POINT ( 'NONE',  ( 21.90000000122903145, 5.773502691896255534, 3.535250795749688894E-16 ) ) ;
#19108=CARTESIAN_POINT ( 'NONE',  ( 18.14062500061451644, -3.027376345333614438, 5.243569643749998122 ) ) ;
#19109=CARTESIAN_POINT ( 'NONE',  ( 20.05312500061451431, -4.541064518000417216, -2.621784821875001281 ) ) ;
#19110=CARTESIAN_POINT ( 'NONE',  ( 3.140625000614516882, 6.054752690667223547, 3.707466751127219781E-16 ) ) ;
#19111=CARTESIAN_POINT ( 'NONE',  ( 27.00000000000000000, -4.330127018922190985, -2.500000000000001332 ) ) ;
#19114=CARTESIAN_POINT ( 'NONE',  ( 28.43437500061451573, 4.541064518000418104, 2.621784821874999949 ) ) ;
#19115=CARTESIAN_POINT ( 'NONE',  ( 3.999999999999998668, 14.41250000000000142, -32.30940107675850470 ) ) ;
#19116=CARTESIAN_POINT ( 'NONE',  ( 2.121784821874999061, 16.55937500061451573, -33.67503911421598417 ) ) ;
#19117=CARTESIAN_POINT ( 'NONE',  ( 4.800000001229032698, 5.773502691896255534, 3.535250795749688894E-16 ) ) ;
#19118=CARTESIAN_POINT ( 'NONE',  ( 6.637500000000001066, -2.886751345948129988, 4.999999999999997335 ) ) ;
#19121=CARTESIAN_POINT ( 'NONE',  ( 9.534375000614517148, 4.541064518000418104, 2.621784821874999949 ) ) ;
#19122=CARTESIAN_POINT ( 'NONE',  ( 27.85312500061451502, 4.541064518000418104, -2.621784821874998173 ) ) ;
#19123=CARTESIAN_POINT ( 'NONE',  ( 1.071796769724491893, 10.68259618943233313, 33.99999999999999289 ) ) ;
#19124=CARTESIAN_POINT ( 'NONE',  ( -4.513148444473915610, 8.924709038934331318, -33.95832947008857872 ) ) ;
#19125=CARTESIAN_POINT ( 'NONE',  ( 1.071796769724493892, 17.72990381179669583, -34.00000000000000000 ) ) ;
#19126=CARTESIAN_POINT ( 'NONE',  ( 8.146875000614516082, 6.054752690667223547, 3.707466751127219781E-16 ) ) ;
#19127=CARTESIAN_POINT ( 'NONE',  ( 10.35937500061451644, 4.541064518000418104, -2.621784821874998173 ) ) ;
#19128=CARTESIAN_POINT ( 'NONE',  ( 4.087500000000001243, -2.886751345948125991, -5.000000000000000000 ) ) ;
#19129=CARTESIAN_POINT ( 'NONE',  ( 4.243569643749999898, 14.17812500061459247, 30.00000000000000000 ) ) ;
#19131=CARTESIAN_POINT ( 'NONE',  ( 6.975000000000002309, 4.330127018922191873, 2.499999999999999556 ) ) ;
#19133=CARTESIAN_POINT ( 'NONE',  ( 20.87812500061451715, -4.541064518000419881, 2.621784821874995952 ) ) ;
#19134=CARTESIAN_POINT ( 'NONE',  ( 12.85312500061451502, -4.541064518000417216, -2.621784821875001281 ) ) ;
#19136=CARTESIAN_POINT ( 'NONE',  ( 9.159375000614515372, 0.000000000000000000, 5.243569643749999010 ) ) ;
#19137=CARTESIAN_POINT ( 'NONE',  ( 25.68750000000000000, -2.886751345948125991, -5.000000000000000000 ) ) ;
#19138=CARTESIAN_POINT ( 'NONE',  ( 21.93750000122903288, 4.330127018922191873, 2.499999999999999556 ) ) ;
#19139=CARTESIAN_POINT ( 'NONE',  ( -1.071796769724487453, 18.22009619066136565, -34.00000000000000000 ) ) ;
#19140=CARTESIAN_POINT ( 'NONE',  ( 11.07187500061451679, -6.054752690667223547, -1.112240025338166033E-15 ) ) ;
#19141=CARTESIAN_POINT ( 'NONE',  ( 27.27187500061451431, -6.054752690667223547, -1.112240025338166033E-15 ) ) ;
#19142=CARTESIAN_POINT ( 'NONE',  ( 3.871875000614519280, -6.054752690667223547, -1.112240025338166033E-15 ) ) ;
#19144=CARTESIAN_POINT ( 'NONE',  ( 19.84687500061451360, 6.054752690667223547, 3.707466751127219781E-16 ) ) ;
#19145=CARTESIAN_POINT ( 'NONE',  ( 11.25937500061451679, 4.541064518000418104, -2.621784821874998173 ) ) ;
#19147=CARTESIAN_POINT ( 'NONE',  ( 23.51249999999999574, 2.886751345948129099, -4.999999999999998224 ) ) ;
#19149=CARTESIAN_POINT ( 'NONE',  ( 4.243569643749999898, 13.33437500061451786, -30.00000000000000000 ) ) ;
#19151=CARTESIAN_POINT ( 'NONE',  ( 14.39062500061451821, 6.054752690667223547, 3.707466751127219781E-16 ) ) ;
#19152=CARTESIAN_POINT ( 'NONE',  ( 4.650000000000001243, 4.330127018922192761, -2.499999999999997780 ) ) ;
#19154=CARTESIAN_POINT ( 'NONE',  ( -1.999999999999997113, 12.87500000000000178, 33.46410161513775705 ) ) ;
#19155=CARTESIAN_POINT ( 'NONE',  ( 13.91249999999999964, -5.773502691896255534, -1.060575238724906372E-15 ) ) ;
#19156=CARTESIAN_POINT ( 'NONE',  ( 9.001249775931846008E-16, 10.91562500061451857, 34.90005215228797653 ) ) ;
#19157=CARTESIAN_POINT ( 'NONE',  ( 14.70000000122903394, 5.773502691896255534, 3.535250795749688894E-16 ) ) ;
#19158=CARTESIAN_POINT ( 'NONE',  ( 24.00937500061451502, 0.000000000000000000, 5.243569643749999010 ) ) ;
#19159=CARTESIAN_POINT ( 'NONE',  ( 20.28750000122903074, -4.330127018922194537, 2.499999999999995559 ) ) ;
#19160=ORIENTED_EDGE ( 'NONE', *, *, #21528, .F. ) ;
#19161=CARTESIAN_POINT ( 'NONE',  ( 19.82812500061451644, 4.541064518000418104, 2.621784821874999949 ) ) ;
#19162=CARTESIAN_POINT ( 'NONE',  ( 5.165625000614518569, -6.054752690667223547, -1.112240025338166033E-15 ) ) ;
#19163=CARTESIAN_POINT ( 'NONE',  ( 19.92187500061451644, 3.027376345333611329, 5.243569643749999010 ) ) ;
#19164=CARTESIAN_POINT ( 'NONE',  ( 29.59687500061451715, -3.027376345333610441, -5.243569643749999898 ) ) ;
#19165=CARTESIAN_POINT ( 'NONE',  ( 5.953125000614519102, 0.000000000000000000, 5.243569643749999010 ) ) ;
#19166=CARTESIAN_POINT ( 'NONE',  ( 22.19062500061451715, -3.027376345333614438, 5.243569643749998122 ) ) ;
#19167=CARTESIAN_POINT ( 'NONE',  ( -4.243569643749999898, 14.81562500061451715, 27.54997392385601529 ) ) ;
#19168=CARTESIAN_POINT ( 'NONE',  ( 19.23750000122903714, 4.330127018922191873, 2.499999999999999556 ) ) ;
#19170=CARTESIAN_POINT ( 'NONE',  ( 8.765625000614518214, -6.054752690667223547, -1.112240025338166033E-15 ) ) ;
#19171=CARTESIAN_POINT ( 'NONE',  ( 3.534375000614518036, 6.421520780324663323E-16, -5.243569643749999010 ) ) ;
#19172=CARTESIAN_POINT ( 'NONE',  ( 21.94687500061451857, -3.027376345333610441, -5.243569643749999898 ) ) ;
#19173=CARTESIAN_POINT ( 'NONE',  ( 14.91562500061451679, 3.027376345333611329, 5.243569643749999010 ) ) ;
#19174=CARTESIAN_POINT ( 'NONE',  ( 26.06250000122903288, 0.000000000000000000, 4.999999999999998224 ) ) ;
#19176=CARTESIAN_POINT ( 'NONE',  ( 25.90312500061451573, -4.541064518000417216, -2.621784821875001281 ) ) ;
#19178=CARTESIAN_POINT ( 'NONE',  ( 20.37187500061451573, 3.027376345333611329, 5.243569643749999010 ) ) ;
#19179=CARTESIAN_POINT ( 'NONE',  ( 15.62812500061451537, 6.421520780324663323E-16, -5.243569643749999010 ) ) ;
#19180=CARTESIAN_POINT ( 'NONE',  ( -4.243569643749999898, 17.57187500061451502, 27.54997392385601529 ) ) ;
#19181=CARTESIAN_POINT ( 'NONE',  ( 19.52812500061451573, -4.541064518000419881, 2.621784821874995952 ) ) ;
#19184=CARTESIAN_POINT ( 'NONE',  ( 24.22500000000000142, -4.330127018922194537, 2.499999999999995559 ) ) ;
#19185=CARTESIAN_POINT ( 'NONE',  ( -3.999999999999999556, 10.51250000000000107, -32.30940107675850470 ) ) ;
#19187=CARTESIAN_POINT ( 'NONE',  ( 27.02812500061451573, 4.541064518000418104, 2.621784821874999949 ) ) ;
#19188=CARTESIAN_POINT ( 'NONE',  ( 7.978125000614517681, 6.421520780324663323E-16, -5.243569643749999010 ) ) ;
#19189=CARTESIAN_POINT ( 'NONE',  ( 20.02500000122903145, 2.886751345948129099, -4.999999999999998224 ) ) ;
#19190=CARTESIAN_POINT ( 'NONE',  ( 25.19062500061451715, 6.054752690667223547, 3.707466751127219781E-16 ) ) ;
#19191=CARTESIAN_POINT ( 'NONE',  ( 26.28749999999999432, 5.773502691896255534, 3.535250795749688894E-16 ) ) ;
#19192=CARTESIAN_POINT ( 'NONE',  ( 3.999999999999999112, 15.38750000122903394, -30.00000000000000000 ) ) ;
#19193=CARTESIAN_POINT ( 'NONE',  ( -1.071796769724491005, 15.52009619066136814, -34.00000000000000000 ) ) ;
#19194=CARTESIAN_POINT ( 'NONE',  ( 9.440625000614517148, 6.054752690667223547, 3.707466751127219781E-16 ) ) ;
#19196=CARTESIAN_POINT ( 'NONE',  ( 24.81562500061451715, 3.027376345333611329, 5.243569643749999010 ) ) ;
#19197=CARTESIAN_POINT ( 'NONE',  ( 5.728125000614515905, 6.421520780324663323E-16, -5.243569643749999010 ) ) ;
#19200=CARTESIAN_POINT ( 'NONE',  ( 17.77500000122903501, 2.886751345948129099, -4.999999999999997335 ) ) ;
#19201=CARTESIAN_POINT ( 'NONE',  ( 12.78749999999999964, 5.773502691896255534, 3.535250795749688894E-16 ) ) ;
#19202=CARTESIAN_POINT ( 'NONE',  ( 14.40937500061451715, 4.541064518000418104, -2.621784821874998173 ) ) ;
#19203=CARTESIAN_POINT ( 'NONE',  ( 7.912500001229033408, 4.330127018922192761, -2.499999999999997780 ) ) ;
#19204=CARTESIAN_POINT ( 'NONE',  ( 18.00937500061451502, 4.541064518000418104, -2.621784821874998173 ) ) ;
#19206=CARTESIAN_POINT ( 'NONE',  ( 8.934375000614517504, 6.421520780324663323E-16, -5.243569643749999010 ) ) ;
#19207=CARTESIAN_POINT ( 'NONE',  ( 4.243569643749999898, 11.47812500061451679, -30.00000000000000000 ) ) ;
#19208=CARTESIAN_POINT ( 'NONE',  ( -3.999999999999997335, 11.93750000000000000, -27.69059892324149530 ) ) ;
#19211=CARTESIAN_POINT ( 'NONE',  ( 25.04062500061451502, -3.027376345333610441, -5.243569643749999898 ) ) ;
#19212=CARTESIAN_POINT ( 'NONE',  ( 7.320879633048903241E-15, 17.30000000122903003, 26.00000000000000355 ) ) ;
#19213=CARTESIAN_POINT ( 'NONE',  ( 26.29687500061451644, -3.027376345333614438, 5.243569643749998122 ) ) ;
#19214=( BOUNDED_CURVE ( )  B_SPLINE_CURVE ( 2, ( #23027, #7132, #45216, #6411, #44861, #29662, #11234 ),
 .UNSPECIFIED., .F., .F. ) 
 B_SPLINE_CURVE_WITH_KNOTS ( ( 3, 2, 2, 3 ),
 ( 0.6583333333333334370, 0.6611111111111112049, 0.6638888888888888618, 0.6666666666666666297 ),
 .UNSPECIFIED. ) 
 CURVE ( )  GEOMETRIC_REPRESENTATION_ITEM ( )  RATIONAL_B_SPLINE_CURVE ( ( 0.9999999999999946709, 0.8660254037844440367, 1.000000000000000000, 0.8660254037844387076, 1.000000000000000000, 0.8660254037844387076, 1.000000000000000000 ) ) 
 REPRESENTATION_ITEM ( '' )  );
#19215=CARTESIAN_POINT ( 'NONE',  ( 29.67187500061451644, 3.027376345333613106, -5.243569643749998122 ) ) ;
#19216=CARTESIAN_POINT ( 'NONE',  ( 20.85000000000000142, 4.330127018922192761, -2.499999999999997780 ) ) ;
#19217=CARTESIAN_POINT ( 'NONE',  ( 5.203125000614518214, -4.541064518000417216, -2.621784821875001281 ) ) ;
#19219=CARTESIAN_POINT ( 'NONE',  ( 15.49687500061451750, -3.027376345333614438, 5.243569643749998122 ) ) ;
#19221=CARTESIAN_POINT ( 'NONE',  ( 29.66250000122903074, 0.000000000000000000, 4.999999999999998224 ) ) ;
#19222=CARTESIAN_POINT ( 'NONE',  ( 9.234375000614518214, -4.541064518000419881, 2.621784821874995952 ) ) ;
#19223=CARTESIAN_POINT ( 'NONE',  ( 18.12187500061451573, 3.027376345333611329, 5.243569643749999010 ) ) ;
#19225=CARTESIAN_POINT ( 'NONE',  ( 26.02499999999999858, -4.330127018922194537, 2.499999999999995559 ) ) ;
#19226=CARTESIAN_POINT ( 'NONE',  ( 27.42187500061451644, 3.027376345333613106, -5.243569643749998122 ) ) ;
#19227=FACE_OUTER_BOUND ( 'NONE', #55962, .T. ) ;
#19229=CARTESIAN_POINT ( 'NONE',  ( 8.062500000000000000, -5.773502691896255534, -1.060575238724906372E-15 ) ) ;
#19231=CARTESIAN_POINT ( 'NONE',  ( 22.00312500061451360, 4.541064518000418104, -2.621784821874998173 ) ) ;
#19232=CARTESIAN_POINT ( 'NONE',  ( 11.88749999999999751, 5.773502691896255534, 3.535250795749688894E-16 ) ) ;
#19233=CARTESIAN_POINT ( 'NONE',  ( 7.687500001229033764, -4.330127018922194537, 2.499999999999995559 ) ) ;
#19234=CARTESIAN_POINT ( 'NONE',  ( 6.853125000614516793, 0.000000000000000000, 5.243569643749999010 ) ) ;
#19235=CARTESIAN_POINT ( 'NONE',  ( 21.56250000000000000, -5.773502691896255534, -1.060575238724906372E-15 ) ) ;
#19236=CARTESIAN_POINT ( 'NONE',  ( 20.27812500061451573, 4.541064518000418104, 2.621784821874999949 ) ) ;
#19237=DIRECTION ( 'NONE',  ( -0.000000000000000000, -1.000000000000000000, -0.000000000000000000 ) ) ;
#19238=CARTESIAN_POINT ( 'NONE',  ( 26.62500000122903288, -5.773502691896255534, -1.060575238724906372E-15 ) ) ;
#19240=CARTESIAN_POINT ( 'NONE',  ( 4.012500000000001954, -5.773502691896255534, -1.060575238724906372E-15 ) ) ;
#19241=EDGE_LOOP ( 'NONE', ( #16212, #48050, #12283, #8666 ) ) ;
#19242=CARTESIAN_POINT ( 'NONE',  ( 18.36562500061451431, 3.027376345333613106, -5.243569643749998122 ) ) ;
#19243=CARTESIAN_POINT ( 'NONE',  ( 27.70312500061451289, -4.541064518000417216, -2.621784821875001281 ) ) ;
#19244=CARTESIAN_POINT ( 'NONE',  ( 26.22187500061451715, 3.027376345333611329, 5.243569643749999010 ) ) ;
#19245=CARTESIAN_POINT ( 'NONE',  ( 14.54062500061451679, -3.027376345333614438, 5.243569643749998122 ) ) ;
#19246=CARTESIAN_POINT ( 'NONE',  ( 29.24062500061451431, 6.054752690667223547, 3.707466751127219781E-16 ) ) ;
#19247=CARTESIAN_POINT ( 'NONE',  ( 8.803125000614517859, -4.541064518000417216, -2.621784821875001281 ) ) ;
#19248=DIRECTION ( 'NONE',  ( 0.000000000000000000, 0.000000000000000000, -1.000000000000000000 ) ) ;
#19249=CARTESIAN_POINT ( 'NONE',  ( 26.06250000122903288, 0.000000000000000000, 4.999999999999998224 ) ) ;
#19251=CARTESIAN_POINT ( 'NONE',  ( 16.64062500061451289, 6.054752690667223547, 3.707466751127219781E-16 ) ) ;
#19252=LINE ( 'NONE', #37637, #44520 ) ;
#19253=CARTESIAN_POINT ( 'NONE',  ( 28.65937500061451715, -4.541064518000417216, -2.621784821875001281 ) ) ;
#19254=CARTESIAN_POINT ( 'NONE',  ( 11.07187500061451679, -6.054752690667223547, -1.112240025338166033E-15 ) ) ;
#19255=CARTESIAN_POINT ( 'NONE',  ( 9.009375000614518569, 4.541064518000418104, -2.621784821874998173 ) ) ;
#19256=CARTESIAN_POINT ( 'NONE',  ( 18.75937500061451857, -4.541064518000417216, -2.621784821875001281 ) ) ;
#19257=VERTEX_POINT ( 'NONE', #22331 ) ;
#19258=CARTESIAN_POINT ( 'NONE',  ( 1.592000809091587073E-14, 15.95000000122903394, 26.00000000000000000 ) ) ;
#19259=CARTESIAN_POINT ( 'NONE',  ( 22.82812500061451644, 6.421520780324663323E-16, -5.243569643749999010 ) ) ;
#19260=EDGE_CURVE ( 'NONE', #46535, #41088, #64384, .T. ) ;
#19261=CARTESIAN_POINT ( 'NONE',  ( 17.55937500061451573, 4.541064518000418104, -2.621784821874998173 ) ) ;
#19262=CARTESIAN_POINT ( 'NONE',  ( 22.07812500061451644, 4.541064518000418104, 2.621784821874999949 ) ) ;
#19263=CARTESIAN_POINT ( 'NONE',  ( 2.000000000000001332, 14.30000000000000071, 33.46410161513774995 ) ) ;
#19264=CARTESIAN_POINT ( 'NONE',  ( 26.01562500061451289, 3.027376345333613106, -5.243569643749998122 ) ) ;
#19265=CARTESIAN_POINT ( 'NONE',  ( 9.337500001229033231, 4.330127018922191873, 2.499999999999999556 ) ) ;
#19266=ORIENTED_EDGE ( 'NONE', *, *, #48691, .T. ) ;
#19267=CARTESIAN_POINT ( 'NONE',  ( 5.325000001229033941, 2.886751345948126879, 4.999999999999999112 ) ) ;
#19268=CARTESIAN_POINT ( 'NONE',  ( 2.000000000000001332, 18.35000000000000142, -26.53589838486224650 ) ) ;
#19269=CARTESIAN_POINT ( 'NONE',  ( 23.85000000122903430, -2.886751345948129988, 4.999999999999997335 ) ) ;
#19272=CARTESIAN_POINT ( 'NONE',  ( 6.759375000614516793, 4.541064518000418104, -2.621784821874998173 ) ) ;
#19273=CARTESIAN_POINT ( 'NONE',  ( 1.071796769724491893, 9.895096190661368141, 33.99999999999999289 ) ) ;
#19274=CARTESIAN_POINT ( 'NONE',  ( 16.07812500061451289, 6.421520780324663323E-16, -5.243569643749999010 ) ) ;
#19275=CARTESIAN_POINT ( 'NONE',  ( 11.14687500061451608, -3.027376345333610441, -5.243569643749999898 ) ) ;
#19276=CARTESIAN_POINT ( 'NONE',  ( 26.17500000122903359, -5.773502691896255534, -1.060575238724906372E-15 ) ) ;
#19277=( BOUNDED_CURVE ( )  B_SPLINE_CURVE ( 2, ( #28776, #40234, #50596, #73118, #17323, #720, #23227 ),
 .UNSPECIFIED., .F., .F. ) 
 B_SPLINE_CURVE_WITH_KNOTS ( ( 3, 2, 2, 3 ),
 ( 0.000000000000000000, 0.002777777777777771812, 0.005555555555555543625, 0.008333333333333315870 ),
 .UNSPECIFIED. ) 
 CURVE ( )  GEOMETRIC_REPRESENTATION_ITEM ( )  RATIONAL_B_SPLINE_CURVE ( ( 1.000000000000000000, 0.8660254037844387076, 1.000000000000000000, 0.8660254037844387076, 1.000000000000000000, 0.8660254037844395958, 0.9999999999999991118 ) ) 
 REPRESENTATION_ITEM ( '' )  );
#19278=CARTESIAN_POINT ( 'NONE',  ( 16.54687500061451644, -3.027376345333610441, -5.243569643749999898 ) ) ;
#19279=CARTESIAN_POINT ( 'NONE',  ( 5.896875000614518747, 6.054752690667223547, 3.707466751127219781E-16 ) ) ;
#19280=CYLINDRICAL_SURFACE ( 'NONE', #42732, 4.999999999999998224 ) ;
#19281=EDGE_CURVE ( 'NONE', #47295, #21571, #46495, .T. ) ;
#19282=CARTESIAN_POINT ( 'NONE',  ( 7.228125000614517681, 4.541064518000418104, 2.621784821874999949 ) ) ;
#19283=( BOUNDED_CURVE ( )  B_SPLINE_CURVE ( 2, ( #28087, #39169, #21795, #72784, #5904, #370, #27357 ),
 .UNSPECIFIED., .F., .F. ) 
 B_SPLINE_CURVE_WITH_KNOTS ( ( 3, 2, 2, 3 ),
 ( 0.9940063808490070540, 0.9944444444444444642, 0.9972222222222222321, 0.9975950399704071048 ),
 .UNSPECIFIED. ) 
 CURVE ( )  GEOMETRIC_REPRESENTATION_ITEM ( )  RATIONAL_B_SPLINE_CURVE ( ( 0.9644075875924971175, 0.9788718184064328920, 1.000000000000000000, 0.8660254037844387076, 1.000000000000000000, 0.9820186813809772541, 0.9688640661581504610 ) ) 
 REPRESENTATION_ITEM ( '' )  );
#19284=CARTESIAN_POINT ( 'NONE',  ( 17.42812500061451786, 6.421520780324663323E-16, -5.243569643749999010 ) ) ;
#19286=CARTESIAN_POINT ( 'NONE',  ( 14.95312500061451644, 0.000000000000000000, 5.243569643749999010 ) ) ;
#19287=CARTESIAN_POINT ( 'NONE',  ( 10.79062500061451679, 6.054752690667223547, 3.707466751127219781E-16 ) ) ;
#19289=CARTESIAN_POINT ( 'NONE',  ( 10.61250000000000071, 2.886751345948126879, 4.999999999999999112 ) ) ;
#19290=CARTESIAN_POINT ( 'NONE',  ( 6.000000001229033764, -2.886751345948125991, -5.000000000000000000 ) ) ;
#19291=( BOUNDED_CURVE ( )  B_SPLINE_CURVE ( 2, ( #471, #1928, #64690, #12986, #8178, #53985, #41439 ),
 .UNSPECIFIED., .F., .F. ) 
 B_SPLINE_CURVE_WITH_KNOTS ( ( 3, 2, 2, 3 ),
 ( 0.9172137518328628003, 0.9194444444444443976, 0.9222222222222222765, 0.9240845911989643557 ),
 .UNSPECIFIED. ) 
 CURVE ( )  GEOMETRIC_REPRESENTATION_ITEM ( )  RATIONAL_B_SPLINE_CURVE ( ( 0.9576208616715126132, 0.8924117889096346845, 1.000000000000000000, 0.8660254037844387076, 1.000000000000000000, 0.9101763526011728000, 0.9407977426935905108 ) ) 
 REPRESENTATION_ITEM ( '' )  );
#19292=CARTESIAN_POINT ( 'NONE',  ( 15.27187500061451786, 3.027376345333613106, -5.243569643749998122 ) ) ;
#19293=CARTESIAN_POINT ( 'NONE',  ( 15.52500000122903323, 2.886751345948129099, -4.999999999999998224 ) ) ;
#19295=CARTESIAN_POINT ( 'NONE',  ( -4.243569643749997233, 18.04062500061451857, -27.54997392385601174 ) ) ;
#19296=CARTESIAN_POINT ( 'NONE',  ( 11.88750000122903216, 6.123233995736764310E-16, -4.999999999999998224 ) ) ;
#19297=CARTESIAN_POINT ( 'NONE',  ( -3.999999999999999112, 18.61250000000000426, 27.69059892324149885 ) ) ;
#19298=CARTESIAN_POINT ( 'NONE',  ( 23.02500000122903856, -5.773502691896255534, -1.060575238724906372E-15 ) ) ;
#19299=EDGE_CURVE ( 'NONE', #68293, #7272, #27160, .T. ) ;
#19301=CARTESIAN_POINT ( 'NONE',  ( 3.886657622141069357, -3.145466273087292208, -4.195369635725843871 ) ) ;
#19302=CARTESIAN_POINT ( 'NONE',  ( 17.07187500061451502, 3.027376345333613106, -5.243569643749998122 ) ) ;
#19303=CARTESIAN_POINT ( 'NONE',  ( 28.53749999999999787, 5.773502691896255534, 3.535250795749688894E-16 ) ) ;
#19304=CARTESIAN_POINT ( 'NONE',  ( 13.71562500061451750, -6.054752690667223547, -1.112240025338166033E-15 ) ) ;
#19306=CARTESIAN_POINT ( 'NONE',  ( 23.89687500061451786, 6.054752690667223547, 3.707466751127219781E-16 ) ) ;
#19308=CARTESIAN_POINT ( 'NONE',  ( 10.94062500061451537, -3.027376345333614438, 5.243569643749998122 ) ) ;
#19309=CARTESIAN_POINT ( 'NONE',  ( 15.87187500061451573, 3.027376345333611329, 5.243569643749999010 ) ) ;
#19310=EDGE_LOOP ( 'NONE', ( #31857, #61807, #29336, #36069 ) ) ;
#19311=CARTESIAN_POINT ( 'NONE',  ( 26.25937500061451857, 0.000000000000000000, 5.243569643749999010 ) ) ;
#19312=CARTESIAN_POINT ( 'NONE',  ( 28.11562500061451431, -6.054752690667223547, -1.112240025338166033E-15 ) ) ;
#19313=CARTESIAN_POINT ( 'NONE',  ( 18.96562500061451573, 3.027376345333611329, 5.243569643749999010 ) ) ;
#19314=CARTESIAN_POINT ( 'NONE',  ( 12.22499999999999964, 6.123233995736764310E-16, -4.999999999999998224 ) ) ;
#19315=FACE_OUTER_BOUND ( 'NONE', #54066, .T. ) ;
#19316=CARTESIAN_POINT ( 'NONE',  ( 6.899999999999999467, 4.330127018922192761, -2.499999999999997780 ) ) ;
#19317=CARTESIAN_POINT ( 'NONE',  ( 18.86250000122903359, 0.000000000000000000, 4.999999999999998224 ) ) ;
#19318=CARTESIAN_POINT ( 'NONE',  ( -1.487416814333745711E-14, 15.16250000000000142, -26.00000000000000000 ) ) ;
#19320=ORIENTED_EDGE ( 'NONE', *, *, #3723, .T. ) ;
#19321=CARTESIAN_POINT ( 'NONE',  ( 16.87500000000000000, 4.330127018922191873, 2.499999999999999556 ) ) ;
#19322=CARTESIAN_POINT ( 'NONE',  ( 19.38749999999999929, -2.886751345948125991, -5.000000000000000000 ) ) ;
#19323=CARTESIAN_POINT ( 'NONE',  ( 17.85937500061451999, -4.541064518000417216, -2.621784821875001281 ) ) ;
#19324=CARTESIAN_POINT ( 'NONE',  ( 13.94062500061451892, 6.054752690667223547, 3.707466751127219781E-16 ) ) ;
#19327=CARTESIAN_POINT ( 'NONE',  ( 6.890625000614516438, -3.027376345333614438, 5.243569643749998122 ) ) ;
#19329=CARTESIAN_POINT ( 'NONE',  ( 13.01249999999999929, -5.773502691896255534, -1.060575238724906372E-15 ) ) ;
#19332=CARTESIAN_POINT ( 'NONE',  ( -2.121784821874999949, 14.77812500061451750, 26.32496088578401938 ) ) ;
#19333=CARTESIAN_POINT ( 'NONE',  ( 26.87812500061451360, 6.421520780324663323E-16, -5.243569643749999010 ) ) ;
#19336=CARTESIAN_POINT ( 'NONE',  ( 24.64687500061451431, -3.027376345333610441, -5.243569643749999898 ) ) ;
#19337=EDGE_LOOP ( 'NONE', ( #17398, #8334, #42234, #15604 ) ) ;
#19338=CARTESIAN_POINT ( 'NONE',  ( 22.07812500061451644, 4.541064518000418104, 2.621784821874999949 ) ) ;
#19339=CARTESIAN_POINT ( 'NONE',  ( 22.17187500061451644, 3.027376345333611329, 5.243569643749999010 ) ) ;
#19340=CARTESIAN_POINT ( 'NONE',  ( -3.000416591977282496E-16, 16.99062500061459247, -34.90005215228797653 ) ) ;
#19341=CARTESIAN_POINT ( 'NONE',  ( 7.565625000614518036, 3.027376345333613106, -5.243569643749998122 ) ) ;
#19343=CARTESIAN_POINT ( 'NONE',  ( 23.91562500061451502, 3.027376345333611329, 5.243569643749999010 ) ) ;
#19346=CARTESIAN_POINT ( 'NONE',  ( 17.70937500061451431, 0.000000000000000000, 5.243569643749999010 ) ) ;
#19347=CARTESIAN_POINT ( 'NONE',  ( 25.69687500061451502, 6.054752690667223547, 3.707466751127219781E-16 ) ) ;
#19348=CARTESIAN_POINT ( 'NONE',  ( -3.000416591977282496E-16, 13.89687500061451608, 25.09994784771203058 ) ) ;
#19349=CARTESIAN_POINT ( 'NONE',  ( 7.790625000614518569, -3.027376345333614438, 5.243569643749998122 ) ) ;
#19350=CARTESIAN_POINT ( 'NONE',  ( 29.61562500061451431, 3.027376345333613106, -5.243569643749998122 ) ) ;
#19351=CARTESIAN_POINT ( 'NONE',  ( 29.09062500061451573, -3.027376345333610441, -5.243569643749999898 ) ) ;
#19352=CARTESIAN_POINT ( 'NONE',  ( 26.43749999999999645, -2.886751345948146863, 4.999999999999968026 ) ) ;
#19353=CARTESIAN_POINT ( 'NONE',  ( 4.378125000614518925, 6.421520780324663323E-16, -5.243569643749999010 ) ) ;
#19354=CARTESIAN_POINT ( 'NONE',  ( 9.534375000614517148, 4.541064518000418104, 2.621784821874999949 ) ) ;
#19356=CARTESIAN_POINT ( 'NONE',  ( 16.38750000122903216, 6.123233995736764310E-16, -4.999999999999998224 ) ) ;
#19357=CARTESIAN_POINT ( 'NONE',  ( 29.72812500061451502, 4.541064518000418104, 2.621784821874999949 ) ) ;
#19358=CARTESIAN_POINT ( 'NONE',  ( 5.540625000614515905, -3.027376345333614438, 5.243569643749998122 ) ) ;
#19361=CARTESIAN_POINT ( 'NONE',  ( 16.47187500061452070, -6.054752690667223547, -1.112240025338166033E-15 ) ) ;
#19362=EDGE_LOOP ( 'NONE', ( #1060, #36798, #38764, #39577 ) ) ;
#19363=CARTESIAN_POINT ( 'NONE',  ( 22.00312500061451360, 4.541064518000418104, -2.621784821874998173 ) ) ;
#19364=CARTESIAN_POINT ( 'NONE',  ( 10.56562500061451715, -6.054752690667223547, -1.112240025338166033E-15 ) ) ;
#19365=CARTESIAN_POINT ( 'NONE',  ( 25.35937500061451644, 0.000000000000000000, 5.243569643749999010 ) ) ;
#19366=CARTESIAN_POINT ( 'NONE',  ( 7.078125000614516438, 6.421520780324663323E-16, -5.243569643749999010 ) ) ;
#19367=CARTESIAN_POINT ( 'NONE',  ( 20.40000000000000213, 4.330127018922192761, -2.499999999999997780 ) ) ;
#19368=CARTESIAN_POINT ( 'NONE',  ( 11.13750000122903216, 4.330127018922191873, 2.499999999999999556 ) ) ;
#19370=CARTESIAN_POINT ( 'NONE',  ( 24.74062500061451786, 6.054752690667223547, 3.707466751127219781E-16 ) ) ;
#19371=CARTESIAN_POINT ( 'NONE',  ( 4.243569643749999898, 10.09062500061451928, -27.54997392385601529 ) ) ;
#19372=CARTESIAN_POINT ( 'NONE',  ( 13.08750000122903323, -4.330127018922194537, 2.499999999999995559 ) ) ;
#19373=CARTESIAN_POINT ( 'NONE',  ( 21.55312500061451431, 4.541064518000418104, -2.621784821874998173 ) ) ;
#19374=CARTESIAN_POINT ( 'NONE',  ( 17.91562500061451502, 3.027376345333613106, -5.243569643749998122 ) ) ;
#19376=CARTESIAN_POINT ( 'NONE',  ( 17.58749999999999858, -2.886751345948125991, -5.000000000000000000 ) ) ;
#19377=CARTESIAN_POINT ( 'NONE',  ( 13.98750000122903359, -4.330127018922194537, 2.499999999999995559 ) ) ;
#19378=CARTESIAN_POINT ( 'NONE',  ( 11.46562500061451573, -6.054752690667223547, -1.112240025338166033E-15 ) ) ;
#19379=CARTESIAN_POINT ( 'NONE',  ( 14.27812500061451573, 6.421520780324663323E-16, -5.243569643749999010 ) ) ;
#19380=CARTESIAN_POINT ( 'NONE',  ( 22.95000000122903216, -2.886751345948129988, 4.999999999999997335 ) ) ;
#19381=AXIS2_PLACEMENT_3D ( 'NONE', #28598, #51134, #532 ) ;
#19382=CARTESIAN_POINT ( 'NONE',  ( 22.54687500061451999, 6.054752690667223547, 3.707466751127219781E-16 ) ) ;
#19383=CARTESIAN_POINT ( 'NONE',  ( 21.90937500061451715, -4.541064518000417216, -2.621784821875001281 ) ) ;
#19385=CARTESIAN_POINT ( 'NONE',  ( 8.175000001229031810, -5.773502691896255534, -1.060575238724906372E-15 ) ) ;
#19386=CARTESIAN_POINT ( 'NONE',  ( 7.471875000614519813, -6.054752690667223547, -1.112240025338166033E-15 ) ) ;
#19387=CARTESIAN_POINT ( 'NONE',  ( 26.59687500061451360, 6.054752690667223547, 3.707466751127219781E-16 ) ) ;
#19388=CARTESIAN_POINT ( 'NONE',  ( 4.731257479987296399, -1.617158822770780269, 4.897528984835215482 ) ) ;
#19389=AXIS2_PLACEMENT_3D ( 'NONE', #61770, #49975, #11174 ) ;
#19390=CARTESIAN_POINT ( 'NONE',  ( 21.21562500061451573, 3.027376345333611329, 5.243569643749999010 ) ) ;
#19391=CARTESIAN_POINT ( 'NONE',  ( 26.29687500061451644, -3.027376345333614438, 5.243569643749998122 ) ) ;
#19393=CARTESIAN_POINT ( 'NONE',  ( 3.479729569495786379, -3.590471016896914946, -3.821457900550485398 ) ) ;
#19395=CARTESIAN_POINT ( 'NONE',  ( 4.659375000614518925, 0.000000000000000000, 5.243569643749999010 ) ) ;
#19396=CARTESIAN_POINT ( 'NONE',  ( 18.44062500061451715, 6.054752690667223547, 3.707466751127219781E-16 ) ) ;
#19397=VECTOR ( 'NONE', #60115, 1000.000000000000000 ) ;
#19398=ORIENTED_EDGE ( 'NONE', *, *, #6200, .T. ) ;
#19399=CARTESIAN_POINT ( 'NONE',  ( 11.47499999999999964, 4.330127018922191873, 2.499999999999999556 ) ) ;
#19400=CARTESIAN_POINT ( 'NONE',  ( 25.52812500061451573, 6.421520780324663323E-16, -5.243569643749999010 ) ) ;
#19401=CARTESIAN_POINT ( 'NONE',  ( 2.971875000614517592, -6.054752690667223547, -1.112240025338166033E-15 ) ) ;
#19402=CARTESIAN_POINT ( 'NONE',  ( 4.688072943975824636, 1.738382027048589684, 4.849960349263820802 ) ) ;
#19404=CARTESIAN_POINT ( 'NONE',  ( 4.078125000614517326, 4.541064518000418104, 2.621784821874999949 ) ) ;
#19405=CARTESIAN_POINT ( 'NONE',  ( 16.19999999999999929, -4.330127018922190985, -2.500000000000001332 ) ) ;
#19406=CARTESIAN_POINT ( 'NONE',  ( 21.85312500061451502, -4.541064518000417216, -2.621784821875001281 ) ) ;
#19408=CARTESIAN_POINT ( 'NONE',  ( 24.97499999999999787, 4.330127018922191873, 2.499999999999999556 ) ) ;
#19409=CARTESIAN_POINT ( 'NONE',  ( 26.07187500061451857, 3.027376345333613106, -5.243569643749998122 ) ) ;
#19410=ORIENTED_EDGE ( 'NONE', *, *, #37713, .F. ) ;
#19411=CARTESIAN_POINT ( 'NONE',  ( 30.00000000000000000, 0.000000000000000000, 0.000000000000000000 ) ) ;
#19412=CARTESIAN_POINT ( 'NONE',  ( 13.75312500061451715, -4.541064518000417216, -2.621784821875001281 ) ) ;
#19413=CARTESIAN_POINT ( 'NONE',  ( 25.16250000122903074, 0.000000000000000000, 4.999999999999998224 ) ) ;
#19415=CARTESIAN_POINT ( 'NONE',  ( 3.459375000614519635, -4.541064518000417216, -2.621784821875001281 ) ) ;
#19416=CARTESIAN_POINT ( 'NONE',  ( 12.48750000122903359, 4.330127018922191873, 2.499999999999999556 ) ) ;
#19417=CARTESIAN_POINT ( 'NONE',  ( 18.97499999999999787, 6.123233995736764310E-16, -4.999999999999998224 ) ) ;
#19418=CARTESIAN_POINT ( 'NONE',  ( 27.15000000000000213, 4.330127018922192761, -2.499999999999997780 ) ) ;
#19419=CARTESIAN_POINT ( 'NONE',  ( 3.275492200589926739, -3.777717676570560901, -3.275492200590059522 ) ) ;
#19420=CARTESIAN_POINT ( 'NONE',  ( 7.359375000614516438, 0.000000000000000000, 5.243569643749999010 ) ) ;
#19421=CARTESIAN_POINT ( 'NONE',  ( 18.45937500061451431, 4.541064518000418104, -2.621784821874998173 ) ) ;
#19423=ORIENTED_EDGE ( 'NONE', *, *, #2520, .T. ) ;
#19424=CARTESIAN_POINT ( 'NONE',  ( 28.30312500061451431, 4.541064518000418104, -2.621784821874998173 ) ) ;
#19425=CARTESIAN_POINT ( 'NONE',  ( 3.000000000000002665, 0.000000000000000000, 4.999999999999998224 ) ) ;
#19426=CARTESIAN_POINT ( 'NONE',  ( 3.571875000614517237, 3.027376345333613106, -5.243569643749998122 ) ) ;
#19427=CARTESIAN_POINT ( 'NONE',  ( 15.29999999999999893, -4.330127018922190985, -2.500000000000001332 ) ) ;
#19428=CARTESIAN_POINT ( 'NONE',  ( 13.37812500061451715, 6.421520780324663323E-16, -5.243569643749999010 ) ) ;
#19429=CARTESIAN_POINT ( 'NONE',  ( -2.000000000000000000, 14.97499999999999964, -33.46410161513775705 ) ) ;
#19432=CARTESIAN_POINT ( 'NONE',  ( 17.88750000122903216, 4.330127018922191873, 2.499999999999999556 ) ) ;
#19435=CARTESIAN_POINT ( 'NONE',  ( 7.940625000614518036, -3.027376345333610441, -5.243569643749999898 ) ) ;
#19436=CARTESIAN_POINT ( 'NONE',  ( 23.18437500061451573, -4.541064518000419881, 2.621784821874995952 ) ) ;
#19437=CARTESIAN_POINT ( 'NONE',  ( 9.001249775931846008E-16, 19.52187500061451786, 34.90005215228797653 ) ) ;
#19438=CARTESIAN_POINT ( 'NONE',  ( 22.84687500061451715, -3.027376345333610441, -5.243569643749999898 ) ) ;
#19439=CARTESIAN_POINT ( 'NONE',  ( 5.549999999999998934, 4.330127018922192761, -2.499999999999997780 ) ) ;
#19440=CARTESIAN_POINT ( 'NONE',  ( -3.999999999999997335, 10.25000000122903288, 32.30940107675850470 ) ) ;
#19441=CARTESIAN_POINT ( 'NONE',  ( 14.57812500061451644, -4.541064518000419881, 2.621784821874995952 ) ) ;
#19442=CARTESIAN_POINT ( 'NONE',  ( 3.937500001229034208, 4.330127018922191873, 2.499999999999999556 ) ) ;
#19443=CARTESIAN_POINT ( 'NONE',  ( 10.47187500061451715, 3.027376345333611329, 5.243569643749999010 ) ) ;
#19445=ORIENTED_EDGE ( 'NONE', *, *, #20206, .F. ) ;
#19447=CARTESIAN_POINT ( 'NONE',  ( 12.40312500061451573, -4.541064518000417216, -2.621784821875001281 ) ) ;
#19448=CARTESIAN_POINT ( 'NONE',  ( 29.13750000122903216, 4.330127018922191873, 2.499999999999999556 ) ) ;
#19449=CARTESIAN_POINT ( 'NONE',  ( 23.88750000122903216, -4.330127018922194537, 2.499999999999995559 ) ) ;
#19450=CARTESIAN_POINT ( 'NONE',  ( 10.35937500061451644, 4.541064518000418104, -2.621784821874998173 ) ) ;
#19451=CARTESIAN_POINT ( 'NONE',  ( 11.95312500061451644, -4.541064518000417216, -2.621784821875001281 ) ) ;
#19453=CARTESIAN_POINT ( 'NONE',  ( 22.73437500061451644, -4.541064518000419881, 2.621784821874995952 ) ) ;
#19454=CYLINDRICAL_SURFACE ( 'NONE', #24246, 4.000000000000000000 ) ;
#19455=CARTESIAN_POINT ( 'NONE',  ( 23.73749999999999716, -2.886751345948114000, 5.000000000000024869 ) ) ;
#19456=CARTESIAN_POINT ( 'NONE',  ( 20.58750000122903145, 4.330127018922191873, 2.499999999999999556 ) ) ;
#19457=CARTESIAN_POINT ( 'NONE',  ( -4.243569643749998122, 15.39687500061451786, -27.54997392385601174 ) ) ;
#19458=CARTESIAN_POINT ( 'NONE',  ( 15.19687500061451857, -3.027376345333610441, -5.243569643749999898 ) ) ;
#19459=CARTESIAN_POINT ( 'NONE',  ( 16.87500000122903288, 2.886751345948129099, -4.999999999999998224 ) ) ;
#19460=EDGE_CURVE ( 'NONE', #56329, #40333, #29036, .T. ) ;
#19461=AXIS2_PLACEMENT_3D ( 'NONE', #8368, #56526, #36807 ) ;
#19462=CARTESIAN_POINT ( 'NONE',  ( 13.32187500061451502, -6.054752690667223547, -1.112240025338166033E-15 ) ) ;
#19463=CARTESIAN_POINT ( 'NONE',  ( 2.121784821875001281, 16.80312500061451786, -26.32496088578401938 ) ) ;
#19464=CARTESIAN_POINT ( 'NONE',  ( 20.81250000122903643, -4.330127018922190985, -2.500000000000001332 ) ) ;
#19465=CARTESIAN_POINT ( 'NONE',  ( 13.60312500061451679, 0.000000000000000000, 5.243569643749999010 ) ) ;
#19466=VERTEX_POINT ( 'NONE', #27521 ) ;
#19468=VECTOR ( 'NONE', #54534, 1000.000000000000000 ) ;
#19469=CARTESIAN_POINT ( 'NONE',  ( 14.66249999999999964, 2.886751345948126879, 4.999999999999999112 ) ) ;
#19470=CARTESIAN_POINT ( 'NONE',  ( 11.97187500061451892, -6.054752690667223547, -1.112240025338166033E-15 ) ) ;
#19471=CARTESIAN_POINT ( 'NONE',  ( 3.965171583692859603, 3.045884815923804556, 3.965171583692790325 ) ) ;
#19472=CARTESIAN_POINT ( 'NONE',  ( 12.03750000122903430, 4.330127018922191873, 2.499999999999999556 ) ) ;
#19473=CARTESIAN_POINT ( 'NONE',  ( 20.13750000122903216, 4.330127018922191873, 2.499999999999999556 ) ) ;
#19474=CARTESIAN_POINT ( 'NONE',  ( 18.36562500061451431, 3.027376345333613106, -5.243569643749998122 ) ) ;
#19475=CARTESIAN_POINT ( 'NONE',  ( 20.50312500061451715, -4.541064518000417216, -2.621784821875001281 ) ) ;
#19476=CARTESIAN_POINT ( 'NONE',  ( 28.08750000122903145, 6.123233995736764310E-16, -4.999999999999998224 ) ) ;
#19477=CARTESIAN_POINT ( 'NONE',  ( 26.02499999999999858, -4.330127018922194537, 2.499999999999995559 ) ) ;
#19478=CARTESIAN_POINT ( 'NONE',  ( 4.869423765992945796, -1.135214599616954256, -5.119209941160161037 ) ) ;
#19479=B_SPLINE_CURVE_WITH_KNOTS ( 'NONE', 3,
 ( #20484, #70741, #14586, #43039, #53761, #58913, #65566, #3155, #42674, #65197 ),
 .UNSPECIFIED., .F., .F.,
 ( 4, 3, 3, 4 ),
 ( 1.780036773976668796E-16, 2.812506838582382114E-05, 5.625013576972328906E-05, 9.339561289900664856E-05 ),
 .UNSPECIFIED. ) ;
#19481=CARTESIAN_POINT ( 'NONE',  ( 28.02187500061451431, 3.027376345333611329, 5.243569643749999010 ) ) ;
#19482=CARTESIAN_POINT ( 'NONE',  ( 3.990860739963187687, -3.012222745923910594, -4.182559159433559159 ) ) ;
#19483=CARTESIAN_POINT ( 'NONE',  ( 4.243569643749999898, 12.84687500061451715, -27.54997392385601529 ) ) ;
#19484=CARTESIAN_POINT ( 'NONE',  ( 4.387500001229033053, 4.330127018922191873, 2.499999999999999556 ) ) ;
#19485=CARTESIAN_POINT ( 'NONE',  ( 4.987500000000002487, -2.886751345948125991, -5.000000000000000000 ) ) ;
#19487=CARTESIAN_POINT ( 'NONE',  ( 8.559375000614515727, 4.541064518000418104, -2.621784821874998173 ) ) ;
#19488=CARTESIAN_POINT ( 'NONE',  ( 27.92812500061451431, 4.541064518000418104, 2.621784821874999949 ) ) ;
#19489=CARTESIAN_POINT ( 'NONE',  ( 1.999999999999998668, 10.85000000000000142, 26.53589838486224650 ) ) ;
#19490=CARTESIAN_POINT ( 'NONE',  ( -4.112406224592633386, 9.116497278081073574, -25.62679350102753872 ) ) ;
#19493=CARTESIAN_POINT ( 'NONE',  ( 5.521875000614517859, 3.027376345333611329, 5.243569643749999010 ) ) ;
#19494=CARTESIAN_POINT ( 'NONE',  ( 10.69687500061451679, -3.027376345333610441, -5.243569643749999898 ) ) ;
#19495=CARTESIAN_POINT ( 'NONE',  ( 4.575000000000002842, 6.123233995736764310E-16, -4.999999999999998224 ) ) ;
#19496=CARTESIAN_POINT ( 'NONE',  ( -2.121784821874999949, 14.32812500061459460, 26.32496088578401938 ) ) ;
#19498=( BOUNDED_CURVE ( )  B_SPLINE_CURVE ( 2, ( #33777, #10884, #56320, #44151, #17142, #72946, #4986 ),
 .UNSPECIFIED., .F., .F. ) 
 B_SPLINE_CURVE_WITH_KNOTS ( ( 3, 2, 2, 3 ),
 ( 0.6500000000000001332, 0.6527777777777779011, 0.6555555555555556690, 0.6583333333333334370 ),
 .UNSPECIFIED. ) 
 CURVE ( )  GEOMETRIC_REPRESENTATION_ITEM ( )  RATIONAL_B_SPLINE_CURVE ( ( 0.9999999999999946709, 0.8660254037844440367, 1.000000000000000000, 0.8660254037844387076, 1.000000000000000000, 0.8660254037844333785, 1.000000000000005329 ) ) 
 REPRESENTATION_ITEM ( '' )  );
#19499=CARTESIAN_POINT ( 'NONE',  ( 7.425000000000000711, 4.330127018922191873, 2.499999999999999556 ) ) ;
#19501=CARTESIAN_POINT ( 'NONE',  ( 20.46562500061451928, -6.054752690667223547, -1.112240025338166033E-15 ) ) ;
#19502=CARTESIAN_POINT ( 'NONE',  ( 12.44062500061451537, -3.027376345333610441, -5.243569643749999898 ) ) ;
#19504=CARTESIAN_POINT ( 'NONE',  ( 10.09687500061451715, -3.027376345333614438, 5.243569643749998122 ) ) ;
#19505=CARTESIAN_POINT ( 'NONE',  ( 26.88749999999999574, -2.886751345948129988, 4.999999999999997335 ) ) ;
#19506=CARTESIAN_POINT ( 'NONE',  ( 22.16250000122903074, -4.330127018922190985, -2.500000000000001332 ) ) ;
#19509=CARTESIAN_POINT ( 'NONE',  ( 10.58437500061451964, -4.541064518000419881, 2.621784821874995952 ) ) ;
#19510=CARTESIAN_POINT ( 'NONE',  ( 26.29687500061451644, -3.027376345333614438, 5.243569643749998122 ) ) ;
#19513=CARTESIAN_POINT ( 'NONE',  ( 21.00937500061451857, -4.541064518000417216, -2.621784821875001281 ) ) ;
#19514=CARTESIAN_POINT ( 'NONE',  ( 11.10937500061451644, -4.541064518000417216, -2.621784821875001281 ) ) ;
#19516=CARTESIAN_POINT ( 'NONE',  ( 23.40000000000000213, -4.330127018922190985, -2.500000000000001332 ) ) ;
#19518=CARTESIAN_POINT ( 'NONE',  ( 4.243569643749999898, 12.84687500061451715, -27.54997392385601529 ) ) ;
#19520=CARTESIAN_POINT ( 'NONE',  ( 15.85312500061451857, 0.000000000000000000, 5.243569643749999010 ) ) ;
#19521=CARTESIAN_POINT ( 'NONE',  ( 3.712499999999999911, 2.886751345948129099, -4.999999999999998224 ) ) ;
#19522=DIRECTION ( 'NONE',  ( -0.000000000000000000, -1.000000000000000000, -0.000000000000000000 ) ) ;
#19523=DIRECTION ( 'NONE',  ( 0.000000000000000000, 0.000000000000000000, -1.000000000000000000 ) ) ;
#19524=CARTESIAN_POINT ( 'NONE',  ( 15.00000000000000000, 4.330127018922192761, -2.499999999999997780 ) ) ;
#19525=CARTESIAN_POINT ( 'NONE',  ( -3.999999999999997335, 17.45000000122903216, 32.30940107675850470 ) ) ;
#19526=CARTESIAN_POINT ( 'NONE',  ( 13.76250000122903394, 4.330127018922192761, -2.499999999999997780 ) ) ;
#19527=EDGE_CURVE ( 'NONE', #18820, #40294, #23837, .T. ) ;
#19528=CARTESIAN_POINT ( 'NONE',  ( 25.13437500061451502, 6.421520780324663323E-16, -5.243569643749999010 ) ) ;
#19529=CARTESIAN_POINT ( 'NONE',  ( 19.88437500061451857, 4.541064518000418104, 2.621784821874999949 ) ) ;
#19530=CARTESIAN_POINT ( 'NONE',  ( 30.00000000000000000, 0.000000000000000000, 0.000000000000000000 ) ) ;
#19531=VERTEX_POINT ( 'NONE', #51861 ) ;
#19532=CARTESIAN_POINT ( 'NONE',  ( 19.64062500061451644, -3.027376345333610441, -5.243569643749999898 ) ) ;
#19533=CARTESIAN_POINT ( 'NONE',  ( 3.253125000614518036, 0.000000000000000000, 5.243569643749999010 ) ) ;
#19534=CARTESIAN_POINT ( 'NONE',  ( 17.14687500061451786, 6.054752690667223547, 3.707466751127219781E-16 ) ) ;
#19535=CARTESIAN_POINT ( 'NONE',  ( 29.48437500061451644, -4.541064518000419881, 2.621784821874995952 ) ) ;
#19536=CARTESIAN_POINT ( 'NONE',  ( 4.303125000614516971, -4.541064518000417216, -2.621784821875001281 ) ) ;
#19537=CARTESIAN_POINT ( 'NONE',  ( 21.36562500061451431, -6.054752690667223547, -1.112240025338166033E-15 ) ) ;
#19538=CARTESIAN_POINT ( 'NONE',  ( 9.001249775931846008E-16, 15.86562500061451608, 34.90005215228797653 ) ) ;
#19539=CARTESIAN_POINT ( 'NONE',  ( 16.87500000122903288, 2.886751345948129099, -4.999999999999998224 ) ) ;
#19541=CARTESIAN_POINT ( 'NONE',  ( 6.553125000614518747, -4.541064518000417216, -2.621784821875001281 ) ) ;
#19542=CARTESIAN_POINT ( 'NONE',  ( 3.834375000614519635, -4.541064518000419881, 2.621784821874995952 ) ) ;
#19543=CARTESIAN_POINT ( 'NONE',  ( 28.75312500061451715, 4.541064518000418104, -2.621784821874998173 ) ) ;
#19544=CARTESIAN_POINT ( 'NONE',  ( 23.89687500061451786, 6.054752690667223547, 3.707466751127219781E-16 ) ) ;
#19545=CARTESIAN_POINT ( 'NONE',  ( 14.65312500061451573, -4.541064518000417216, -2.621784821875001281 ) ) ;
#19546=CARTESIAN_POINT ( 'NONE',  ( 23.73750000122903359, 4.330127018922191873, 2.499999999999999556 ) ) ;
#19547=ADVANCED_FACE ( 'NONE', ( #45960 ), #52223, .F. ) ;
#19548=CARTESIAN_POINT ( 'NONE',  ( 24.40312500061451573, 0.000000000000000000, 5.243569643749999010 ) ) ;
#19549=CARTESIAN_POINT ( 'NONE',  ( 20.40937500061451715, 0.000000000000000000, 5.243569643749999010 ) ) ;
#19550=CARTESIAN_POINT ( 'NONE',  ( 13.71562500061451750, -6.054752690667223547, -1.112240025338166033E-15 ) ) ;
#19551=CARTESIAN_POINT ( 'NONE',  ( -4.243569643749997233, 14.04687500061451999, 32.45002607614398471 ) ) ;
#19552=CARTESIAN_POINT ( 'NONE',  ( 19.56562500061451715, -6.054752690667223547, -1.112240025338166033E-15 ) ) ;
#19554=CARTESIAN_POINT ( 'NONE',  ( 25.80000000000000071, 4.330127018922192761, -2.499999999999997780 ) ) ;
#19555=CARTESIAN_POINT ( 'NONE',  ( 2.000000000000001332, 11.60000000000000142, -26.53589838486224650 ) ) ;
#19556=CARTESIAN_POINT ( 'NONE',  ( 12.56250000000000000, -5.773502691896255534, -1.060575238724906372E-15 ) ) ;
#19557=AXIS2_PLACEMENT_3D ( 'NONE', #28510, #23319, #68044 ) ;
#19558=CARTESIAN_POINT ( 'NONE',  ( 28.00312500061451715, 0.000000000000000000, 5.243569643749999010 ) ) ;
#19559=CARTESIAN_POINT ( 'NONE',  ( 8.165625000614516793, 3.027376345333611329, 5.243569643749999010 ) ) ;
#19560=CARTESIAN_POINT ( 'NONE',  ( 20.66250000122903074, 0.000000000000000000, 4.999999999999998224 ) ) ;
#19561=CARTESIAN_POINT ( 'NONE',  ( 23.72812500061451502, 6.421520780324663323E-16, -5.243569643749999010 ) ) ;
#19562=CARTESIAN_POINT ( 'NONE',  ( 26.55000000000000071, -4.330127018922190985, -2.500000000000001332 ) ) ;
#19563=EDGE_CURVE ( 'NONE', #62090, #24437, #47045, .T. ) ;
#19564=CARTESIAN_POINT ( 'NONE',  ( 27.40312500061451573, 4.541064518000418104, -2.621784821874998173 ) ) ;
#19565=CARTESIAN_POINT ( 'NONE',  ( 8.315625000614515372, -6.054752690667223547, -1.112240025338166033E-15 ) ) ;
#19566=EDGE_LOOP ( 'NONE', ( #29823, #23392, #23928, #33429 ) ) ;
#19567=CARTESIAN_POINT ( 'NONE',  ( 25.86562500061451431, -6.054752690667223547, -1.112240025338166033E-15 ) ) ;
#19568=CARTESIAN_POINT ( 'NONE',  ( 5.165625000614518569, -6.054752690667223547, -1.112240025338166033E-15 ) ) ;
#19570=CYLINDRICAL_SURFACE ( 'NONE', #21991, 4.000000000000000000 ) ;
#19571=CARTESIAN_POINT ( 'NONE',  ( 12.07499999999999929, -4.330127018922194537, 2.499999999999995559 ) ) ;
#19572=CARTESIAN_POINT ( 'NONE',  ( 12.98437500061451821, 6.421520780324663323E-16, -5.243569643749999010 ) ) ;
#19573=CARTESIAN_POINT ( 'NONE',  ( 9.487500001229033586, -4.330127018922194537, 2.499999999999995559 ) ) ;
#19574=CARTESIAN_POINT ( 'NONE',  ( 16.32187500061451502, 3.027376345333611329, 5.243569643749999010 ) ) ;
#19576=CARTESIAN_POINT ( 'NONE',  ( 7.246875000614518392, 6.054752690667223547, 3.707466751127219781E-16 ) ) ;
#19577=CARTESIAN_POINT ( 'NONE',  ( -2.121784821874996840, 11.32812500061451644, -26.32496088578401583 ) ) ;
#19578=CARTESIAN_POINT ( 'NONE',  ( 20.21250000000000213, -5.773502691896255534, -1.060575238724906372E-15 ) ) ;
#19581=CARTESIAN_POINT ( 'NONE',  ( 25.26562500061451289, 3.027376345333611329, 5.243569643749999010 ) ) ;
#19582=CARTESIAN_POINT ( 'NONE',  ( -4.243569643749999898, 10.40937500061451892, 30.00000000000000000 ) ) ;
#19584=CARTESIAN_POINT ( 'NONE',  ( 26.55937500061451573, 4.541064518000418104, -2.621784821874998173 ) ) ;
#19585=CARTESIAN_POINT ( 'NONE',  ( 28.54687500061451644, -3.027376345333614438, 5.243569643749998122 ) ) ;
#19586=CARTESIAN_POINT ( 'NONE',  ( 4.040625000614517681, 6.054752690667223547, 3.707466751127219781E-16 ) ) ;
#19588=CARTESIAN_POINT ( 'NONE',  ( 16.58437500061451786, 6.421520780324663323E-16, -5.243569643749999010 ) ) ;
#19590=CARTESIAN_POINT ( 'NONE',  ( 29.43750000122903288, 6.123233995736764310E-16, -4.999999999999998224 ) ) ;
#19591=CARTESIAN_POINT ( 'NONE',  ( 6.384375000614516793, 4.541064518000418104, 2.621784821874999949 ) ) ;
#19592=CARTESIAN_POINT ( 'NONE',  ( 15.68437500061451573, 6.421520780324663323E-16, -5.243569643749999010 ) ) ;
#19593=CARTESIAN_POINT ( 'NONE',  ( 3.397178649298551179, 3.668675132081069545, -3.397178649298551179 ) ) ;
#19594=CARTESIAN_POINT ( 'NONE',  ( 25.68750000000000000, -2.886751345948125991, -5.000000000000000000 ) ) ;
#19595=CARTESIAN_POINT ( 'NONE',  ( 27.12187500061451573, 3.027376345333611329, 5.243569643749999010 ) ) ;
#19597=CARTESIAN_POINT ( 'NONE',  ( 4.247151432104769420, -2.638504256727666863, 4.531370421416291983 ) ) ;
#19598=ORIENTED_EDGE ( 'NONE', *, *, #19260, .T. ) ;
#19599=CARTESIAN_POINT ( 'NONE',  ( 7.875000000000000000, 4.330127018922191873, 2.499999999999999556 ) ) ;
#19601=CARTESIAN_POINT ( 'NONE',  ( 22.67812500061451431, -4.541064518000419881, 2.621784821874995952 ) ) ;
#19602=CARTESIAN_POINT ( 'NONE',  ( 10.83750000000000036, -2.886751345948125991, -5.000000000000000000 ) ) ;
#19603=CARTESIAN_POINT ( 'NONE',  ( 8.250000001229034652, -2.886751345948125991, -5.000000000000000000 ) ) ;
#19604=CARTESIAN_POINT ( 'NONE',  ( 6.103125000614515905, -4.541064518000417216, -2.621784821875001281 ) ) ;
#19605=CARTESIAN_POINT ( 'NONE',  ( 22.64999999999999858, 4.330127018922192761, -2.499999999999997780 ) ) ;
#19606=CARTESIAN_POINT ( 'NONE',  ( 17.31562500061451715, -6.054752690667223547, -1.112240025338166033E-15 ) ) ;
#19607=CARTESIAN_POINT ( 'NONE',  ( 14.92500000000000071, 6.123233995736764310E-16, -4.999999999999998224 ) ) ;
#19608=CARTESIAN_POINT ( 'NONE',  ( 25.61250000122903359, 0.000000000000000000, 4.999999999999998224 ) ) ;
#19610=CARTESIAN_POINT ( 'NONE',  ( 5.287500000000000533, -2.886751345948129988, 4.999999999999997335 ) ) ;
#19612=CARTESIAN_POINT ( 'NONE',  ( 18.77812500061451573, 6.421520780324663323E-16, -5.243569643749999010 ) ) ;
#19613=CARTESIAN_POINT ( 'NONE',  ( 26.31562500061451715, -6.054752690667223547, -1.112240025338166033E-15 ) ) ;
#19614=CARTESIAN_POINT ( 'NONE',  ( 27.90937500061451715, 4.541064518000418104, -2.621784821874998173 ) ) ;
#19615=CARTESIAN_POINT ( 'NONE',  ( 9.525000000000002132, 6.123233995736764310E-16, -4.999999999999998224 ) ) ;
#19616=EDGE_CURVE ( 'NONE', #17423, #70720, #31400, .T. ) ;
#19617=CARTESIAN_POINT ( 'NONE',  ( 10.86562500061451431, 3.027376345333611329, 5.243569643749999010 ) ) ;
#19618=CARTESIAN_POINT ( 'NONE',  ( 28.67812500061451431, 6.421520780324663323E-16, -5.243569643749999010 ) ) ;
#19619=CARTESIAN_POINT ( 'NONE',  ( 8.728125000614518569, -4.541064518000419881, 2.621784821874995952 ) ) ;
#19620=CARTESIAN_POINT ( 'NONE',  ( 30.00000000000000000, 0.000000000000000000, 0.000000000000000000 ) ) ;
#19621=CARTESIAN_POINT ( 'NONE',  ( 2.121784821874999061, 12.95937500061451786, 26.32496088578401583 ) ) ;
#19622=CARTESIAN_POINT ( 'NONE',  ( 25.35000000122903074, -2.886751345948125991, -5.000000000000000000 ) ) ;
#19624=CARTESIAN_POINT ( 'NONE',  ( 13.56562500061451537, 3.027376345333611329, 5.243569643749999010 ) ) ;
#19625=CARTESIAN_POINT ( 'NONE',  ( 8.099999999999999645, -4.330127018922190985, -2.500000000000001332 ) ) ;
#19626=CARTESIAN_POINT ( 'NONE',  ( 9.984375000614518214, 4.541064518000418104, 2.621784821874999949 ) ) ;
#19627=CARTESIAN_POINT ( 'NONE',  ( 10.05937500061451750, 0.000000000000000000, 5.243569643749999010 ) ) ;
#19628=CARTESIAN_POINT ( 'NONE',  ( 17.55937500061451573, 4.541064518000418104, -2.621784821874998173 ) ) ;
#19630=CARTESIAN_POINT ( 'NONE',  ( 29.10937500061451644, -4.541064518000417216, -2.621784821875001281 ) ) ;
#19631=CARTESIAN_POINT ( 'NONE',  ( 21.14062500061451289, 6.054752690667223547, 3.707466751127219781E-16 ) ) ;
#19632=CARTESIAN_POINT ( 'NONE',  ( 15.79687500061451821, 6.054752690667223547, 3.707466751127219781E-16 ) ) ;
#19633=CARTESIAN_POINT ( 'NONE',  ( 21.14062500061451289, 6.054752690667223547, 3.707466751127219781E-16 ) ) ;
#19634=CARTESIAN_POINT ( 'NONE',  ( 3.999999999999999112, 14.82500000000000107, 30.00000000000000000 ) ) ;
#19635=CARTESIAN_POINT ( 'NONE',  ( 27.02812500061451573, 4.541064518000418104, 2.621784821874999949 ) ) ;
#19636=CARTESIAN_POINT ( 'NONE',  ( 7.200000001229035718, -2.886751345948129988, 4.999999999999997335 ) ) ;
#19637=ORIENTED_EDGE ( 'NONE', *, *, #32035, .F. ) ;
#19638=CARTESIAN_POINT ( 'NONE',  ( 3.450000001229036162, 5.773502691896255534, 3.535250795749688894E-16 ) ) ;
#19639=CARTESIAN_POINT ( 'NONE',  ( -3.999999999999997335, 17.78750000000000142, -27.69059892324149175 ) ) ;
#19641=CARTESIAN_POINT ( 'NONE',  ( 24.00000000122902932, -2.886751345948125991, -5.000000000000000000 ) ) ;
#19643=CARTESIAN_POINT ( 'NONE',  ( 7.771875000614516971, 3.027376345333611329, 5.243569643749999010 ) ) ;
#19644=CARTESIAN_POINT ( 'NONE',  ( 4.898587196589411843E-16, 20.00000000000000000, -26.00000000000000000 ) ) ;
#19645=CARTESIAN_POINT ( 'NONE',  ( 15.10312500061451502, -4.541064518000417216, -2.621784821875001281 ) ) ;
#19646=CARTESIAN_POINT ( 'NONE',  ( 9.309375000614517504, -4.541064518000417216, -2.621784821875001281 ) ) ;
#19647=CARTESIAN_POINT ( 'NONE',  ( 26.77500000122903145, 2.886751345948129099, -4.999999999999998224 ) ) ;
#19648=CARTESIAN_POINT ( 'NONE',  ( 17.67187500061451999, 3.027376345333611329, 5.243569643749999010 ) ) ;
#19649=CARTESIAN_POINT ( 'NONE',  ( 4.209375000614516971, 0.000000000000000000, 5.243569643749999010 ) ) ;
#19651=CARTESIAN_POINT ( 'NONE',  ( 6.290625000614517681, 6.054752690667223547, 3.707466751127219781E-16 ) ) ;
#19652=CARTESIAN_POINT ( 'NONE',  ( 16.56562500061451715, 3.027376345333613106, -5.243569643749998122 ) ) ;
#19653=ORIENTED_EDGE ( 'NONE', *, *, #47041, .F. ) ;
#19654=CARTESIAN_POINT ( 'NONE',  ( 13.15312500061451750, 0.000000000000000000, 5.243569643749999010 ) ) ;
#19656=CARTESIAN_POINT ( 'NONE',  ( 4.912500001229034297, 0.000000000000000000, 4.999999999999998224 ) ) ;
#19657=CARTESIAN_POINT ( 'NONE',  ( 11.01562500061451821, -6.054752690667223547, -1.112240025338166033E-15 ) ) ;
#19659=CARTESIAN_POINT ( 'NONE',  ( 11.17500000000000071, -4.330127018922194537, 2.499999999999995559 ) ) ;
#19660=CARTESIAN_POINT ( 'NONE',  ( 6.825000001229034829, -5.773502691896255534, -1.060575238724906372E-15 ) ) ;
#19661=CARTESIAN_POINT ( 'NONE',  ( 19.94999999999999929, 4.330127018922192761, -2.499999999999997780 ) ) ;
#19662=( BOUNDED_SURFACE ( )  B_SPLINE_SURFACE ( 1, 2, ( 
 ( #52735, #690, #23198, #47197, #13200, #7309, #45752, #63089, #52374, #17648, #40208, #12490, #1780, #24291, #18734, #57546, #41298, #35740, #58259, #7665, #69728, #19097, #9131, #15389, #9498, #8396, #13935, #54563, #25387, #30925, #19835, #48659, #43115, #53466, #53837, #14299, #60451, #20934, #59351, #26120, #58990, #25759, #25015, #36837, #37931, #3232, #2857, #31296, #70460, #71184, #47557, #20557, #31668, #70086, #30569, #47931, #42387, #59723, #53095, #36472, #42749, #64909, #2491, #26488, #49030, #71559, #8762, #65640, #15028, #43485, #48295, #37565, #42021, #60089, #65270, #20195, #70821, #14657, #32027, #37200, #19463, #54201, #66009, #64542, #3598, #3966, #66377, #16482, #5417, #44593, #27590, #27222, #27956, #61920, #4336, #73014, #33476, #39039, #33846, #67484, #66753, #67124, #72285, #9859, #22755, #26861, #55657, #61553, #55298, #21663, #49759, #4692, #61197, #72653, #50488, #50122, #10955, #43852, #11326, #5053, #56025, #44947, #247, #32389, #22398, #71923, #21298, #56390, #39775, #16847, #49392, #39403, #5780, #28311, #50847, #67841, #16123, #22034, #45306, #17213, #60821, #54929, #15753, #38292, #10227, #32761, #44220, #38676, #10592, #33120, #46753, #1328, #17924, #24200, #46388, #23840, #12397, #69643, #18279, #68923, #6139, #40487, #51931, #29397, #40855, #24566, #62291, #63372, #69288, #18651, #41213, #68208, #68565, #35653, #57813, #7223, #34933, #29038, #47111, #45672, #2054, #51210, #51573, #610, #17569, #23117, #12756, #6502, #58173, #35292, #29752, #52289, #1690, #19005, #11687, #63721, #40131, #34203, #13113, #62645, #7578, #56737, #57459, #30113, #28670, #12042, #52648, #34565, #57094, #972, #23482, #46029, #63002, #6865, #53746, #70368, #3513, #25669, #3143, #64820, #48943, #70728, #48206, #58533, #19746, #31205, #8674, #20105, #3879, #41567, #42660, #48572, #71100, #20473, #47469, #47839, #14944, #37108, #59634, #14209, #8311, #26400, #24926, #54479, #30482, #30840, #53011, #70001, #2405, #65185, #58899, #37482, #14575, #9047, #31578, #54117, #71471, #64085, #43026, #19371, #13467, #26033, #41928, #65554, #36015, #36746, #60003, #7945, #64454 ),
 ( #13845, #9413, #31943, #36385, #59266, #53374, #2770, #25293, #42295, #11863, #45491, #28492, #45848, #6320, #4610, #5958, #10143, #20847, #34746, #37843, #66661, #51028, #66289, #32676, #38206, #15668, #72203, #10508, #39952, #38586, #22932, #54841, #789, #16038, #55576, #56916, #12218, #43400, #68022, #9773, #32307, #68383, #51751, #28849, #60364, #34384, #17744, #51387, #62465, #6687, #27140, #61112, #23298, #17395, #71841, #424, #33036, #40303, #62825, #4250, #57278, #29215, #65925, #15305, #26775, #49307, #21212, #43765, #49674, #60734, #55215, #21580, #44134, #46568, #53194, #12581, #8135, #40666, #69112, #63185, #35115, #57638, #63905, #24019, #13662, #69472, #7765, #46935, #1880, #2590, #25109, #41745, #7044, #23661, #24386, #29574, #41392, #1152, #18829, #69827, #52111, #1515, #52835, #47292, #13294, #52472, #30661, #46206, #68746, #18104, #35831, #58722, #18472, #36204, #19192, #58354, #41036, #63551, #7404, #12937, #35473, #57995, #29932, #30302, #2235, #24749, #64273, #9965, #21403, #43960, #31406, #32503, #66114, #53946, #44328, #9240, #14767, #43592, #72385, #20302, #26598, #42856, #14405, #10331, #32865, #55401, #31776, #55037, #4440, #4796, #37311, #26968, #25866, #72026, #49138, #4072, #60193, #59833, #49497, #54314, #21766, #3343, #71666, #9603, #36942, #27329, #65378, #66481, #70931, #15859, #71292, #15133, #60558, #3704, #48769, #26231, #20671, #48406, #21041, #54668, #32135, #38405, #59462, #15493, #43229, #60928, #65749, #38036, #49862, #8870, #37671, #23584, #61655, #67225, #22850, #51671, #72754, #5876, #22139, #66857, #62748, #12141, #34666, #11054, #34300, #56832, #57195, #16586, #6239, #5156, #51306, #28409, #56484, #39501, #39137, #28767, #33582, #1076, #10693, #50945, #62025, #16228, #6610, #44693, #11784, #50229, #710, #50587, #67582, #39873, #56128, #28059, #5521, #73115, #33224, #344, #33941, #11424, #23217, #38781, #45404, #55762, #62385, #27691, #67940, #61299, #22497, #45047, #45770, #68306, #16948, #17313, #17665, #40226, #29138, #57563, #52755, #6966, #7326, #63826, #7685, #1436, #29857, #69030, #53483, #25033, #8412, #2875, #47576 ) ),
 .UNSPECIFIED., .F., .F., .F. ) 
 B_SPLINE_SURFACE_WITH_KNOTS ( ( 2, 2 ),
 ( 3, 2, 2, 2, 2, 2, 2, 2, 2, 2, 2, 2, 2, 2, 2, 2, 2, 2, 2, 2, 2, 2, 2, 2, 2, 2, 2, 2, 2, 2, 2, 2, 2, 2, 2, 2, 2, 2, 2, 2, 2, 2, 2, 2, 2, 2, 2, 2, 2, 2, 2, 2, 2, 2, 2, 2, 2, 2, 2, 2, 2, 2, 2, 2, 2, 2, 2, 2, 2, 2, 2, 2, 2, 2, 2, 2, 2, 2, 2, 2, 2, 2, 2, 2, 2, 2, 2, 2, 2, 2, 2, 2, 2, 2, 2, 2, 2, 2, 2, 2, 2, 2, 2, 2, 2, 2, 2, 2, 2, 2, 2, 2, 2, 2, 2, 2, 2, 2, 2, 2, 2, 2, 2, 2, 2, 2, 2, 2, 2, 2, 2, 2, 2, 2, 3 ),
 ( 0.000000000000000000, 1.000000000000000000 ),
 ( 0.000000000000000000, 0.007246376811594202987, 0.01449275362318840597, 0.02173913043478260809, 0.02898550724637681195, 0.03623188405797101580, 0.04347826086956521618, 0.05072463768115942351, 0.05797101449275362389, 0.06521739130434782428, 0.07246376811594203160, 0.07971014492753622505, 0.08695652173913043237, 0.09420289855072463969, 0.1014492753623188470, 0.1086956521739130405, 0.1159420289855072478, 0.1231884057971014551, 0.1304347826086956486, 0.1376811594202898559, 0.1449275362318840632, 0.1521739130434782705, 0.1594202898550724501, 0.1666666666666666574, 0.1739130434782608647, 0.1811594202898550721, 0.1884057971014492794, 0.1956521739130434867, 0.2028985507246376940, 0.2101449275362318736, 0.2173913043478260809, 0.2246376811594202882, 0.2318840579710144956, 0.2391304347826087029, 0.2463768115942029102, 0.2536231884057971175, 0.2608695652173912971, 0.2681159420289855322, 0.2753623188405797118, 0.2826086956521738913, 0.2898550724637681264, 0.2971014492753623060, 0.3043478260869565410, 0.3115942028985507206, 0.3188405797101449002, 0.3260869565217391353, 0.3333333333333333148, 0.3405797101449275499, 0.3478260869565217295, 0.3550724637681159646, 0.3623188405797101441, 0.3695652173913043237, 0.3768115942028985588, 0.3840579710144927383, 0.3913043478260869734, 0.3985507246376811530, 0.4057971014492753881, 0.4130434782608695676, 0.4202898550724637472, 0.4275362318840579823, 0.4347826086956521618, 0.4420289855072463969, 0.4492753623188405765, 0.4565217391304347561, 0.4637681159420289911, 0.4710144927536231707, 0.4782608695652174058, 0.4855072463768115854, 0.4927536231884058204, 0.5000000000000000000, 0.5072463768115942351, 0.5144927536231883591, 0.5217391304347825942, 0.5289855072463768293, 0.5362318840579710644, 0.5434782608695651884, 0.5507246376811594235, 0.5579710144927536586, 0.5652173913043477826, 0.5724637681159420177, 0.5797101449275362528, 0.5869565217391304879, 0.5942028985507246119, 0.6014492753623188470, 0.6086956521739130821, 0.6159420289855072062, 0.6231884057971014412, 0.6304347826086956763, 0.6376811594202898004, 0.6449275362318840354, 0.6521739130434782705, 0.6594202898550725056, 0.6666666666666666297, 0.6739130434782608647, 0.6811594202898550998, 0.6884057971014492239, 0.6956521739130434590, 0.7028985507246376940, 0.7101449275362319291, 0.7173913043478260532, 0.7246376811594202882, 0.7318840579710145233, 0.7391304347826086474, 0.7463768115942028825, 0.7536231884057971175, 0.7608695652173913526, 0.7681159420289854767, 0.7753623188405797118, 0.7826086956521739468, 0.7898550724637680709, 0.7971014492753623060, 0.8043478260869565410, 0.8115942028985507761, 0.8188405797101449002, 0.8260869565217391353, 0.8333333333333333703, 0.8405797101449274944, 0.8478260869565217295, 0.8550724637681159646, 0.8623188405797101996, 0.8695652173913043237, 0.8768115942028985588, 0.8840579710144927938, 0.8913043478260869179, 0.8985507246376811530, 0.9057971014492753881, 0.9130434782608695121, 0.9202898550724637472, 0.9275362318840579823, 0.9347826086956522174, 0.9420289855072463414, 0.9492753623188405765, 0.9565217391304348116, 0.9637681159420289356, 0.9662083003288912675 ),
 .UNSPECIFIED. ) 
 GEOMETRIC_REPRESENTATION_ITEM ( )  RATIONAL_B_SPLINE_SURFACE ( (
 ( 1.000000000000000000, 0.8660254037844387076, 1.000000000000000000, 0.8660254037844387076, 1.000000000000000000, 0.8660254037844387076, 1.000000000000000000, 0.8660254037844387076, 1.000000000000000000, 0.8660254037844387076, 1.000000000000000000, 0.8660254037844387076, 1.000000000000000000, 0.8660254037844387076, 1.000000000000000000, 0.8660254037844387076, 1.000000000000000000, 0.8660254037844387076, 1.000000000000000000, 0.8660254037844387076, 1.000000000000000000, 0.8660254037844387076, 1.000000000000000000, 0.8660254037844387076, 1.000000000000000000, 0.8660254037844387076, 1.000000000000000000, 0.8660254037844387076, 1.000000000000000000, 0.8660254037844387076, 1.000000000000000000, 0.8660254037844387076, 1.000000000000000000, 0.8660254037844387076, 1.000000000000000000, 0.8660254037844387076, 1.000000000000000000, 0.8660254037844387076, 1.000000000000000000, 0.8660254037844387076, 1.000000000000000000, 0.8660254037844387076, 1.000000000000000000, 0.8660254037844387076, 1.000000000000000000, 0.8660254037844387076, 1.000000000000000000, 0.8660254037844387076, 1.000000000000000000, 0.8660254037844387076, 1.000000000000000000, 0.8660254037844387076, 1.000000000000000000, 0.8660254037844387076, 1.000000000000000000, 0.8660254037844387076, 1.000000000000000000, 0.8660254037844387076, 1.000000000000000000, 0.8660254037844387076, 1.000000000000000000, 0.8660254037844387076, 1.000000000000000000, 0.8660254037844387076, 1.000000000000000000, 0.8660254037844387076, 1.000000000000000000, 0.8660254037844387076, 1.000000000000000000, 0.8660254037844387076, 1.000000000000000000, 0.8660254037844387076, 1.000000000000000000, 0.8660254037844387076, 1.000000000000000000, 0.8660254037844387076, 1.000000000000000000, 0.8660254037844387076, 1.000000000000000000, 0.8660254037844387076, 1.000000000000000000, 0.8660254037844387076, 1.000000000000000000, 0.8660254037844387076, 1.000000000000000000, 0.8660254037844387076, 1.000000000000000000, 0.8660254037844387076, 1.000000000000000000, 0.8660254037844387076, 1.000000000000000000, 0.8660254037844387076, 1.000000000000000000, 0.8660254037844387076, 1.000000000000000000, 0.8660254037844387076, 1.000000000000000000, 0.8660254037844387076, 1.000000000000000000, 0.8660254037844387076, 1.000000000000000000, 0.8660254037844387076, 1.000000000000000000, 0.8660254037844387076, 1.000000000000000000, 0.8660254037844387076, 1.000000000000000000, 0.8660254037844387076, 1.000000000000000000, 0.8660254037844387076, 1.000000000000000000, 0.8660254037844387076, 1.000000000000000000, 0.8660254037844387076, 1.000000000000000000, 0.8660254037844387076, 1.000000000000000000, 0.8660254037844387076, 1.000000000000000000, 0.8660254037844387076, 1.000000000000000000, 0.8660254037844387076, 1.000000000000000000, 0.8660254037844387076, 1.000000000000000000, 0.8660254037844387076, 1.000000000000000000, 0.8660254037844387076, 1.000000000000000000, 0.8660254037844387076, 1.000000000000000000, 0.8660254037844387076, 1.000000000000000000, 0.8660254037844387076, 1.000000000000000000, 0.8660254037844387076, 1.000000000000000000, 0.8660254037844387076, 1.000000000000000000, 0.8660254037844387076, 1.000000000000000000, 0.8660254037844387076, 1.000000000000000000, 0.8660254037844387076, 1.000000000000000000, 0.8660254037844387076, 1.000000000000000000, 0.8660254037844387076, 1.000000000000000000, 0.8660254037844387076, 1.000000000000000000, 0.8660254037844387076, 1.000000000000000000, 0.8660254037844387076, 1.000000000000000000, 0.8660254037844387076, 1.000000000000000000, 0.8660254037844387076, 1.000000000000000000, 0.8660254037844387076, 1.000000000000000000, 0.8660254037844387076, 1.000000000000000000, 0.8660254037844387076, 1.000000000000000000, 0.8660254037844387076, 1.000000000000000000, 0.8660254037844387076, 1.000000000000000000, 0.8660254037844387076, 1.000000000000000000, 0.8660254037844387076, 1.000000000000000000, 0.8660254037844387076, 1.000000000000000000, 0.8660254037844387076, 1.000000000000000000, 0.8660254037844387076, 1.000000000000000000, 0.8660254037844387076, 1.000000000000000000, 0.8660254037844387076, 1.000000000000000000, 0.8660254037844387076, 1.000000000000000000, 0.8660254037844387076, 1.000000000000000000, 0.8660254037844387076, 1.000000000000000000, 0.8660254037844387076, 1.000000000000000000, 0.8660254037844387076, 1.000000000000000000, 0.8660254037844387076, 1.000000000000000000, 0.8660254037844387076, 1.000000000000000000, 0.8660254037844387076, 1.000000000000000000, 0.8660254037844387076, 1.000000000000000000, 0.8660254037844387076, 1.000000000000000000, 0.8660254037844387076, 1.000000000000000000, 0.8660254037844387076, 1.000000000000000000, 0.8660254037844387076, 1.000000000000000000, 0.8660254037844387076, 1.000000000000000000, 0.8660254037844387076, 1.000000000000000000, 0.8660254037844387076, 1.000000000000000000, 0.8660254037844387076, 1.000000000000000000, 0.8660254037844387076, 1.000000000000000000, 0.8660254037844387076, 1.000000000000000000, 0.8660254037844387076, 1.000000000000000000, 0.8660254037844387076, 1.000000000000000000, 0.8660254037844387076, 1.000000000000000000, 0.8660254037844387076, 1.000000000000000000, 0.8660254037844387076, 1.000000000000000000, 0.8660254037844387076, 1.000000000000000000, 0.8660254037844387076, 1.000000000000000000, 0.8660254037844387076, 1.000000000000000000, 0.8660254037844387076, 1.000000000000000000, 0.8660254037844387076, 1.000000000000000000, 0.8660254037844387076, 1.000000000000000000, 0.8660254037844387076, 1.000000000000000000, 0.8660254037844387076, 1.000000000000000000, 0.8660254037844387076, 1.000000000000000000, 0.8660254037844387076, 1.000000000000000000, 0.8660254037844387076, 1.000000000000000000, 0.8660254037844387076, 1.000000000000000000, 0.8660254037844387076, 1.000000000000000000, 0.8660254037844387076, 1.000000000000000000, 0.8660254037844387076, 1.000000000000000000, 0.8660254037844387076, 1.000000000000000000, 0.8660254037844387076, 1.000000000000000000, 0.8660254037844387076, 1.000000000000000000, 0.9548846649268474263, 0.9401540970596797830),
 ( 1.000000000000000000, 0.8660254037844387076, 1.000000000000000000, 0.8660254037844387076, 1.000000000000000000, 0.8660254037844387076, 1.000000000000000000, 0.8660254037844387076, 1.000000000000000000, 0.8660254037844387076, 1.000000000000000000, 0.8660254037844387076, 1.000000000000000000, 0.8660254037844387076, 1.000000000000000000, 0.8660254037844387076, 1.000000000000000000, 0.8660254037844387076, 1.000000000000000000, 0.8660254037844387076, 1.000000000000000000, 0.8660254037844387076, 1.000000000000000000, 0.8660254037844387076, 1.000000000000000000, 0.8660254037844387076, 1.000000000000000000, 0.8660254037844387076, 1.000000000000000000, 0.8660254037844387076, 1.000000000000000000, 0.8660254037844387076, 1.000000000000000000, 0.8660254037844387076, 1.000000000000000000, 0.8660254037844387076, 1.000000000000000000, 0.8660254037844387076, 1.000000000000000000, 0.8660254037844387076, 1.000000000000000000, 0.8660254037844387076, 1.000000000000000000, 0.8660254037844387076, 1.000000000000000000, 0.8660254037844387076, 1.000000000000000000, 0.8660254037844387076, 1.000000000000000000, 0.8660254037844387076, 1.000000000000000000, 0.8660254037844387076, 1.000000000000000000, 0.8660254037844387076, 1.000000000000000000, 0.8660254037844387076, 1.000000000000000000, 0.8660254037844387076, 1.000000000000000000, 0.8660254037844387076, 1.000000000000000000, 0.8660254037844387076, 1.000000000000000000, 0.8660254037844387076, 1.000000000000000000, 0.8660254037844387076, 1.000000000000000000, 0.8660254037844387076, 1.000000000000000000, 0.8660254037844387076, 1.000000000000000000, 0.8660254037844387076, 1.000000000000000000, 0.8660254037844387076, 1.000000000000000000, 0.8660254037844387076, 1.000000000000000000, 0.8660254037844387076, 1.000000000000000000, 0.8660254037844387076, 1.000000000000000000, 0.8660254037844387076, 1.000000000000000000, 0.8660254037844387076, 1.000000000000000000, 0.8660254037844387076, 1.000000000000000000, 0.8660254037844387076, 1.000000000000000000, 0.8660254037844387076, 1.000000000000000000, 0.8660254037844387076, 1.000000000000000000, 0.8660254037844387076, 1.000000000000000000, 0.8660254037844387076, 1.000000000000000000, 0.8660254037844387076, 1.000000000000000000, 0.8660254037844387076, 1.000000000000000000, 0.8660254037844387076, 1.000000000000000000, 0.8660254037844387076, 1.000000000000000000, 0.8660254037844387076, 1.000000000000000000, 0.8660254037844387076, 1.000000000000000000, 0.8660254037844387076, 1.000000000000000000, 0.8660254037844387076, 1.000000000000000000, 0.8660254037844387076, 1.000000000000000000, 0.8660254037844387076, 1.000000000000000000, 0.8660254037844387076, 1.000000000000000000, 0.8660254037844387076, 1.000000000000000000, 0.8660254037844387076, 1.000000000000000000, 0.8660254037844387076, 1.000000000000000000, 0.8660254037844387076, 1.000000000000000000, 0.8660254037844387076, 1.000000000000000000, 0.8660254037844387076, 1.000000000000000000, 0.8660254037844387076, 1.000000000000000000, 0.8660254037844387076, 1.000000000000000000, 0.8660254037844387076, 1.000000000000000000, 0.8660254037844387076, 1.000000000000000000, 0.8660254037844387076, 1.000000000000000000, 0.8660254037844387076, 1.000000000000000000, 0.8660254037844387076, 1.000000000000000000, 0.8660254037844387076, 1.000000000000000000, 0.8660254037844387076, 1.000000000000000000, 0.8660254037844387076, 1.000000000000000000, 0.8660254037844387076, 1.000000000000000000, 0.8660254037844387076, 1.000000000000000000, 0.8660254037844387076, 1.000000000000000000, 0.8660254037844387076, 1.000000000000000000, 0.8660254037844387076, 1.000000000000000000, 0.8660254037844387076, 1.000000000000000000, 0.8660254037844387076, 1.000000000000000000, 0.8660254037844387076, 1.000000000000000000, 0.8660254037844387076, 1.000000000000000000, 0.8660254037844387076, 1.000000000000000000, 0.8660254037844387076, 1.000000000000000000, 0.8660254037844387076, 1.000000000000000000, 0.8660254037844387076, 1.000000000000000000, 0.8660254037844387076, 1.000000000000000000, 0.8660254037844387076, 1.000000000000000000, 0.8660254037844387076, 1.000000000000000000, 0.8660254037844387076, 1.000000000000000000, 0.8660254037844387076, 1.000000000000000000, 0.8660254037844387076, 1.000000000000000000, 0.8660254037844387076, 1.000000000000000000, 0.8660254037844387076, 1.000000000000000000, 0.8660254037844387076, 1.000000000000000000, 0.8660254037844387076, 1.000000000000000000, 0.8660254037844387076, 1.000000000000000000, 0.8660254037844387076, 1.000000000000000000, 0.8660254037844387076, 1.000000000000000000, 0.8660254037844387076, 1.000000000000000000, 0.8660254037844387076, 1.000000000000000000, 0.8660254037844387076, 1.000000000000000000, 0.8660254037844387076, 1.000000000000000000, 0.8660254037844387076, 1.000000000000000000, 0.8660254037844387076, 1.000000000000000000, 0.8660254037844387076, 1.000000000000000000, 0.8660254037844387076, 1.000000000000000000, 0.8660254037844387076, 1.000000000000000000, 0.8660254037844387076, 1.000000000000000000, 0.8660254037844387076, 1.000000000000000000, 0.8660254037844387076, 1.000000000000000000, 0.8660254037844387076, 1.000000000000000000, 0.8660254037844387076, 1.000000000000000000, 0.8660254037844387076, 1.000000000000000000, 0.8660254037844387076, 1.000000000000000000, 0.8660254037844387076, 1.000000000000000000, 0.8660254037844387076, 1.000000000000000000, 0.8660254037844387076, 1.000000000000000000, 0.8660254037844387076, 1.000000000000000000, 0.8660254037844387076, 1.000000000000000000, 0.8660254037844387076, 1.000000000000000000, 0.8660254037844387076, 1.000000000000000000, 0.8660254037844387076, 1.000000000000000000, 0.8660254037844387076, 1.000000000000000000, 0.8660254037844387076, 1.000000000000000000, 0.8660254037844387076, 1.000000000000000000, 0.8660254037844387076, 1.000000000000000000, 0.8660254037844387076, 1.000000000000000000, 0.8660254037844387076, 1.000000000000000000, 0.8660254037844387076, 1.000000000000000000, 0.8660254037844387076, 1.000000000000000000, 0.9548846649268474263, 0.9401540970596797830) ) ) 
 REPRESENTATION_ITEM ( '' )  SURFACE ( )  );
#19663=CARTESIAN_POINT ( 'NONE',  ( 14.14687500061451786, -3.027376345333614438, 5.243569643749998122 ) ) ;
#19664=CARTESIAN_POINT ( 'NONE',  ( 17.13750000122903216, -4.330127018922194537, 2.499999999999995559 ) ) ;
#19666=CARTESIAN_POINT ( 'NONE',  ( 5.190092854996874117, 9.755146338944483020, -35.22418694837048037 ) ) ;
#19668=CARTESIAN_POINT ( 'NONE',  ( 2.000000000000001332, 14.86250000122903536, -26.53589838486224650 ) ) ;
#19669=CARTESIAN_POINT ( 'NONE',  ( 4.284375000614518925, -4.541064518000419881, 2.621784821874995952 ) ) ;
#19671=CARTESIAN_POINT ( 'NONE',  ( 4.714058847239782857, -1.672958453767266818, -4.806836186950011580 ) ) ;
#19672=CARTESIAN_POINT ( 'NONE',  ( 16.05937500061451573, -4.541064518000417216, -2.621784821875001281 ) ) ;
#19673=CARTESIAN_POINT ( 'NONE',  ( 28.27499999999999858, -4.330127018922194537, 2.499999999999995559 ) ) ;
#19674=EDGE_CURVE ( 'NONE', #3427, #13717, #35228, .T. ) ;
#19675=CARTESIAN_POINT ( 'NONE',  ( 11.24062500061451608, 6.054752690667223547, 3.707466751127219781E-16 ) ) ;
#19677=CARTESIAN_POINT ( 'NONE',  ( 23.40937500061451715, 4.541064518000418104, -2.621784821874998173 ) ) ;
#19679=CARTESIAN_POINT ( 'NONE',  ( 8.953125000614518214, 4.541064518000418104, -2.621784821874998173 ) ) ;
#19680=CARTESIAN_POINT ( 'NONE',  ( 15.12187500061451750, -6.054752690667223547, -1.112240025338166033E-15 ) ) ;
#19682=CARTESIAN_POINT ( 'NONE',  ( 27.15937500061451360, 0.000000000000000000, 5.243569643749999010 ) ) ;
#19683=CARTESIAN_POINT ( 'NONE',  ( 27.02812500061451573, 4.541064518000418104, 2.621784821874999949 ) ) ;
#19684=CARTESIAN_POINT ( 'NONE',  ( 28.67812500061451431, 6.421520780324663323E-16, -5.243569643749999010 ) ) ;
#19685=DIRECTION ( 'NONE',  ( -1.000000000000000000, -0.000000000000000000, -0.000000000000000000 ) ) ;
#19686=CARTESIAN_POINT ( 'NONE',  ( 6.412500000000001421, 2.886751345948129099, -4.999999999999998224 ) ) ;
#19688=CARTESIAN_POINT ( 'NONE',  ( 18.52500000122903145, -5.773502691896255534, -1.060575238724906372E-15 ) ) ;
#19689=CARTESIAN_POINT ( 'NONE',  ( 4.898587196589411843E-16, 20.00000000000000000, -26.00000000000000000 ) ) ;
#19692=CARTESIAN_POINT ( 'NONE',  ( 14.58750000000000036, 5.773502691896255534, 3.535250795749688894E-16 ) ) ;
#19693=CARTESIAN_POINT ( 'NONE',  ( 19.46249999999999858, 2.886751345948129099, -4.999999999999998224 ) ) ;
#19694=CARTESIAN_POINT ( 'NONE',  ( 14.91562500061451679, 3.027376345333611329, 5.243569643749999010 ) ) ;
#19697=CARTESIAN_POINT ( 'NONE',  ( -4.243569643749999898, 16.67187500061451644, -32.45002607614398471 ) ) ;
#19698=CARTESIAN_POINT ( 'NONE',  ( 6.290625000614517681, 6.054752690667223547, 3.707466751127219781E-16 ) ) ;
#19700=CARTESIAN_POINT ( 'NONE',  ( 11.28749999999999787, -2.886751345948125991, -5.000000000000000000 ) ) ;
#19702=ORIENTED_EDGE ( 'NONE', *, *, #65676, .T. ) ;
#19703=CARTESIAN_POINT ( 'NONE',  ( 4.243569643749999898, 14.62812500061451715, 30.00000000000000000 ) ) ;
#19704=CARTESIAN_POINT ( 'NONE',  ( 25.64062500061451644, 6.054752690667223547, 3.707466751127219781E-16 ) ) ;
#19707=CARTESIAN_POINT ( 'NONE',  ( 23.89687500061451786, 6.054752690667223547, 3.707466751127219781E-16 ) ) ;
#19708=ADVANCED_FACE ( 'NONE', ( #53963 ), #23770, .T. ) ;
#19709=CARTESIAN_POINT ( 'NONE',  ( 20.50312500061451715, -4.541064518000417216, -2.621784821875001281 ) ) ;
#19710=CARTESIAN_POINT ( 'NONE',  ( 4.243569643749999898, 14.62812500061459353, -30.00000000000000000 ) ) ;
#19711=CARTESIAN_POINT ( 'NONE',  ( 22.95000000122903216, -2.886751345948129988, 4.999999999999997335 ) ) ;
#19712=CARTESIAN_POINT ( 'NONE',  ( 6.028125000614517504, -4.541064518000419881, 2.621784821874995952 ) ) ;
#19714=CARTESIAN_POINT ( 'NONE',  ( 23.27812500061451573, 6.421520780324663323E-16, -5.243569643749999010 ) ) ;
#19717=CARTESIAN_POINT ( 'NONE',  ( 16.95937500061451786, -4.541064518000417216, -2.621784821875001281 ) ) ;
#19718=CARTESIAN_POINT ( 'NONE',  ( 25.28437500061451715, 4.541064518000418104, 2.621784821874999949 ) ) ;
#19719=CARTESIAN_POINT ( 'NONE',  ( -4.243569643749998122, 13.59687500061451892, 32.45002607614398471 ) ) ;
#19720=CARTESIAN_POINT ( 'NONE',  ( 5.540625000614515905, -3.027376345333614438, 5.243569643749998122 ) ) ;
#19721=CARTESIAN_POINT ( 'NONE',  ( 29.39062500061451289, -3.027376345333614438, 5.243569643749998122 ) ) ;
#19723=CARTESIAN_POINT ( 'NONE',  ( 29.35312500061451502, 0.000000000000000000, 5.243569643749999010 ) ) ;
#19725=CARTESIAN_POINT ( 'NONE',  ( 3.293689335155384867, 4.087229415801913568, -2.920710989641019495 ) ) ;
#19726=CARTESIAN_POINT ( 'NONE',  ( 3.365625000614516082, -6.054752690667223547, -1.112240025338166033E-15 ) ) ;
#19727=CARTESIAN_POINT ( 'NONE',  ( 8.409375000614518925, -4.541064518000417216, -2.621784821875001281 ) ) ;
#19729=CARTESIAN_POINT ( 'NONE',  ( 14.70000000122903394, 5.773502691896255534, 3.535250795749688894E-16 ) ) ;
#19730=CARTESIAN_POINT ( 'NONE',  ( 4.209375000614516971, 0.000000000000000000, 5.243569643749999010 ) ) ;
#19731=CARTESIAN_POINT ( 'NONE',  ( 12.41250000122903430, 4.330127018922192761, -2.499999999999997780 ) ) ;
#19732=CARTESIAN_POINT ( 'NONE',  ( 5.690625000614516260, -3.027376345333610441, -5.243569643749999898 ) ) ;
#19735=CARTESIAN_POINT ( 'NONE',  ( 13.92187500061451644, 3.027376345333613106, -5.243569643749998122 ) ) ;
#19737=ORIENTED_EDGE ( 'NONE', *, *, #8112, .T. ) ;
#19738=CARTESIAN_POINT ( 'NONE',  ( 22.11562500061451786, 3.027376345333611329, 5.243569643749999010 ) ) ;
#19739=CARTESIAN_POINT ( 'NONE',  ( 6.628125000614517148, 6.421520780324663323E-16, -5.243569643749999010 ) ) ;
#19741=CARTESIAN_POINT ( 'NONE',  ( 24.83437500061451431, 4.541064518000418104, 2.621784821874999949 ) ) ;
#19742=CARTESIAN_POINT ( 'NONE',  ( 6.815625000614517148, 3.027376345333611329, 5.243569643749999010 ) ) ;
#19743=FACE_OUTER_BOUND ( 'NONE', #58575, .T. ) ;
#19744=CARTESIAN_POINT ( 'NONE',  ( 7.462500001229035007, 4.330127018922192761, -2.499999999999997780 ) ) ;
#19745=CARTESIAN_POINT ( 'NONE',  ( 25.22812500061451502, 4.541064518000418104, 2.621784821874999949 ) ) ;
#19746=CARTESIAN_POINT ( 'NONE',  ( 2.121784821875001281, 11.40312500061451750, -26.32496088578401938 ) ) ;
#19747=CARTESIAN_POINT ( 'NONE',  ( 9.450000001229033941, -2.886751345948129988, 4.999999999999997335 ) ) ;
#19748=CARTESIAN_POINT ( 'NONE',  ( 19.94062500061451715, -3.027376345333614438, 5.243569643749998122 ) ) ;
#19749=CARTESIAN_POINT ( 'NONE',  ( 18.62812500061451715, -4.541064518000419881, 2.621784821874995952 ) ) ;
#19751=CARTESIAN_POINT ( 'NONE',  ( 17.66249999999999787, 2.886751345948129099, -4.999999999999998224 ) ) ;
#19752=CARTESIAN_POINT ( 'NONE',  ( 13.87500000122903465, 2.886751345948126879, 4.999999999999999112 ) ) ;
#19754=CARTESIAN_POINT ( 'NONE',  ( 9.965625000614517504, 3.027376345333611329, 5.243569643749999010 ) ) ;
#19755=CARTESIAN_POINT ( 'NONE',  ( 13.00312500061451537, 4.541064518000418104, -2.621784821874998173 ) ) ;
#19756=CARTESIAN_POINT ( 'NONE',  ( 23.55000000122903359, -2.886751345948125991, -5.000000000000000000 ) ) ;
#19757=CARTESIAN_POINT ( 'NONE',  ( 22.92187500061451644, 3.027376345333613106, -5.243569643749998122 ) ) ;
#19758=CARTESIAN_POINT ( 'NONE',  ( 21.30937500061451573, 0.000000000000000000, 5.243569643749999010 ) ) ;
#19760=CARTESIAN_POINT ( 'NONE',  ( 8.287500001229034297, 6.123233995736764310E-16, -4.999999999999998224 ) ) ;
#19761=CARTESIAN_POINT ( 'NONE',  ( 5.334375000614517859, 6.421520780324663323E-16, -5.243569643749999010 ) ) ;
#19762=CARTESIAN_POINT ( 'NONE',  ( 23.74687500061451573, -3.027376345333610441, -5.243569643749999898 ) ) ;
#19763=CARTESIAN_POINT ( 'NONE',  ( 4.775752298065365054, -1.480604602020447969, 4.856962839292451761 ) ) ;
#19764=CARTESIAN_POINT ( 'NONE',  ( 18.81562500061452070, 3.027376345333613106, -5.243569643749998122 ) ) ;
#19765=CARTESIAN_POINT ( 'NONE',  ( 24.98437500061451644, -4.541064518000419881, 2.621784821874995952 ) ) ;
#19768=CARTESIAN_POINT ( 'NONE',  ( 3.999999999999999112, 15.72500000000000320, 30.00000000000000000 ) ) ;
#19769=CARTESIAN_POINT ( 'NONE',  ( 4.621875000614516615, 3.027376345333611329, 5.243569643749999010 ) ) ;
#19770=CARTESIAN_POINT ( 'NONE',  ( 16.67812500061451786, 4.541064518000418104, 2.621784821874999949 ) ) ;
#19772=DIRECTION ( 'NONE',  ( -1.000000000000000000, -0.000000000000000000, -0.000000000000000000 ) ) ;
#19773=CARTESIAN_POINT ( 'NONE',  ( 24.92812500061451431, -4.541064518000419881, 2.621784821874995952 ) ) ;
#19774=CARTESIAN_POINT ( 'NONE',  ( 4.000000000000000000, 12.98749999999999893, -27.69059892324149885 ) ) ;
#19776=CARTESIAN_POINT ( 'NONE',  ( 3.202568429182105270, 3.863133281671067731, -27.55233077308146505 ) ) ;
#19777=CARTESIAN_POINT ( 'NONE',  ( 15.26249999999999929, -5.773502691896255534, -1.060575238724906372E-15 ) ) ;
#19778=CARTESIAN_POINT ( 'NONE',  ( 25.50000000122903288, 5.773502691896255534, 3.535250795749688894E-16 ) ) ;
#19779=CARTESIAN_POINT ( 'NONE',  ( 20.39062500061451644, -3.027376345333614438, 5.243569643749998122 ) ) ;
#19781=CARTESIAN_POINT ( 'NONE',  ( 23.06250000000000355, 2.886751345948129099, -4.999999999999998224 ) ) ;
#19782=EDGE_CURVE ( 'NONE', #12255, #28753, #66360, .T. ) ;
#19783=CARTESIAN_POINT ( 'NONE',  ( 23.22187500061451715, -6.054752690667223547, -1.112240025338166033E-15 ) ) ;
#19786=CARTESIAN_POINT ( 'NONE',  ( 13.52812500061451750, 4.541064518000418104, 2.621784821874999949 ) ) ;
#19787=CARTESIAN_POINT ( 'NONE',  ( 25.08750000122903145, 4.330127018922191873, 2.499999999999999556 ) ) ;
#19789=CARTESIAN_POINT ( 'NONE',  ( 28.19062500061451715, -3.027376345333610441, -5.243569643749999898 ) ) ;
#19790=CARTESIAN_POINT ( 'NONE',  ( 11.96250000122903501, 4.330127018922192761, -2.499999999999997780 ) ) ;
#19791=CARTESIAN_POINT ( 'NONE',  ( 19.87500000000000000, 6.123233995736764310E-16, -4.999999999999998224 ) ) ;
#19792=CARTESIAN_POINT ( 'NONE',  ( 26.73749999999999716, 5.773502691896255534, 3.535250795749688894E-16 ) ) ;
#19793=CARTESIAN_POINT ( 'NONE',  ( 3.084375000614519191, 6.421520780324663323E-16, -5.243569643749999010 ) ) ;
#19794=CARTESIAN_POINT ( 'NONE',  ( 6.759375000614516793, 4.541064518000418104, -2.621784821874998173 ) ) ;
#19795=CARTESIAN_POINT ( 'NONE',  ( 20.14687500061451786, -3.027376345333610441, -5.243569643749999898 ) ) ;
#19796=VERTEX_POINT ( 'NONE', #1990 ) ;
#19797=CARTESIAN_POINT ( 'NONE',  ( 27.55312500061451786, 0.000000000000000000, 5.243569643749999010 ) ) ;
#19798=CARTESIAN_POINT ( 'NONE',  ( 28.95937500061451431, 0.000000000000000000, 5.243569643749999010 ) ) ;
#19799=CARTESIAN_POINT ( 'NONE',  ( 4.321875000614517681, -6.054752690667223547, -1.112240025338166033E-15 ) ) ;
#19800=CARTESIAN_POINT ( 'NONE',  ( 15.63749999999999751, -2.886751345948129988, 4.999999999999997335 ) ) ;
#19801=CARTESIAN_POINT ( 'NONE',  ( 14.35312500061451679, 4.541064518000418104, -2.621784821874998173 ) ) ;
#19802=CARTESIAN_POINT ( 'NONE',  ( -5.810221930991193690E-16, 14.93750000000000000, -34.00000000000000000 ) ) ;
#19803=CARTESIAN_POINT ( 'NONE',  ( 30.00000000000000000, 6.123233995736764310E-16, -4.999999999999998224 ) ) ;
#19805=CARTESIAN_POINT ( 'NONE',  ( 17.32500000122903216, 2.886751345948129099, -4.999999999999998224 ) ) ;
#19806=CARTESIAN_POINT ( 'NONE',  ( 3.815625000614518481, -6.054752690667223547, -1.112240025338166033E-15 ) ) ;
#19808=CARTESIAN_POINT ( 'NONE',  ( 7.715625000614515727, 3.027376345333611329, 5.243569643749999010 ) ) ;
#19809=CARTESIAN_POINT ( 'NONE',  ( 23.55937500061451573, 0.000000000000000000, 5.243569643749999010 ) ) ;
#19810=CARTESIAN_POINT ( 'NONE',  ( 4.243569643749999898, 18.28437500061451715, 30.00000000000000000 ) ) ;
#19811=CARTESIAN_POINT ( 'NONE',  ( 24.38437500061451502, 4.541064518000418104, 2.621784821874999949 ) ) ;
#19812=CARTESIAN_POINT ( 'NONE',  ( 5.700000000000000178, 0.000000000000000000, 4.999999999999998224 ) ) ;
#19813=CARTESIAN_POINT ( 'NONE',  ( -2.828200636599751609E-16, 10.55000000122903359, 25.38119784648299770 ) ) ;
#19814=CARTESIAN_POINT ( 'NONE',  ( 11.61562500061451608, 3.027376345333613106, -5.243569643749998122 ) ) ;
#19815=CARTESIAN_POINT ( 'NONE',  ( 3.487500001229035362, 4.330127018922191873, 2.499999999999999556 ) ) ;
#19816=B_SPLINE_CURVE_WITH_KNOTS ( 'NONE', 3,
 ( #63605, #1937, #52892, #2289 ),
 .UNSPECIFIED., .F., .F.,
 ( 4, 4 ),
 ( 2.168404344971008868E-19, 0.0005975612829869297133 ),
 .UNSPECIFIED. ) ;
#19817=CARTESIAN_POINT ( 'NONE',  ( 8.521875000614516082, 3.027376345333613106, -5.243569643749998122 ) ) ;
#19818=CARTESIAN_POINT ( 'NONE',  ( 3.828346580387561371, -3.216332247866912741, 4.095469943695211335 ) ) ;
#19820=CARTESIAN_POINT ( 'NONE',  ( 10.34062500061451750, 6.054752690667223547, 3.707466751127219781E-16 ) ) ;
#19821=CARTESIAN_POINT ( 'NONE',  ( 13.92187500061451644, 3.027376345333613106, -5.243569643749998122 ) ) ;
#19822=CARTESIAN_POINT ( 'NONE',  ( 20.54999999999999716, 0.000000000000000000, 4.999999999999998224 ) ) ;
#19823=CARTESIAN_POINT ( 'NONE',  ( 22.76250000122903216, 4.330127018922192761, -2.499999999999997780 ) ) ;
#19824=CARTESIAN_POINT ( 'NONE',  ( 11.48437500061451644, -4.541064518000419881, 2.621784821874995952 ) ) ;
#19825=CARTESIAN_POINT ( 'NONE',  ( 11.16562500061451679, 3.027376345333613106, -5.243569643749998122 ) ) ;
#19827=CARTESIAN_POINT ( 'NONE',  ( 21.00937500061451857, -4.541064518000417216, -2.621784821875001281 ) ) ;
#19829=LINE ( 'NONE', #58621, #51623 ) ;
#19830=CARTESIAN_POINT ( 'NONE',  ( -3.999999999999999112, 19.96250000000000213, -32.30940107675850470 ) ) ;
#19831=CARTESIAN_POINT ( 'NONE',  ( 4.243569643749999898, 15.13437500061451679, -30.00000000000000000 ) ) ;
#19832=CARTESIAN_POINT ( 'NONE',  ( 16.47187500061452070, -6.054752690667223547, -1.112240025338166033E-15 ) ) ;
#19833=CARTESIAN_POINT ( 'NONE',  ( 16.61250000122903359, 0.000000000000000000, 4.999999999999998224 ) ) ;
#19834=CARTESIAN_POINT ( 'NONE',  ( 11.25937500061451679, 4.541064518000418104, -2.621784821874998173 ) ) ;
#19835=CARTESIAN_POINT ( 'NONE',  ( 4.243569643749999898, 18.67812500061451431, -30.00000000000000000 ) ) ;
#19836=CARTESIAN_POINT ( 'NONE',  ( 17.88750000122903216, 4.330127018922191873, 2.499999999999999556 ) ) ;
#19837=CARTESIAN_POINT ( 'NONE',  ( 12.29062500061451857, -3.027376345333614438, 5.243569643749998122 ) ) ;
#19839=CARTESIAN_POINT ( 'NONE',  ( 14.92500000000000071, 6.123233995736764310E-16, -4.999999999999998224 ) ) ;
#19840=CARTESIAN_POINT ( 'NONE',  ( -3.999999999999999112, 17.37500000122903288, -32.30940107675850470 ) ) ;
#19841=CARTESIAN_POINT ( 'NONE',  ( 10.20937500061451786, -4.541064518000417216, -2.621784821875001281 ) ) ;
#19842=CARTESIAN_POINT ( 'NONE',  ( 3.995221338070210848, 3.006467913421217553, 4.057536123296732633 ) ) ;
#19844=CARTESIAN_POINT ( 'NONE',  ( 11.47500000122903252, 2.886751345948129099, -4.999999999999998224 ) ) ;
#19845=CARTESIAN_POINT ( 'NONE',  ( 22.05000000122903714, -2.886751345948129988, 4.999999999999997335 ) ) ;
#19846=EDGE_CURVE ( 'NONE', #6778, #47420, #12327, .T. ) ;
#19847=CARTESIAN_POINT ( 'NONE',  ( 16.82812500061451644, -4.541064518000419881, 2.621784821874995952 ) ) ;
#19848=CARTESIAN_POINT ( 'NONE',  ( 19.75312500061451360, 4.541064518000418104, -2.621784821874998173 ) ) ;
#19849=CARTESIAN_POINT ( 'NONE',  ( 26.96250000122903145, 0.000000000000000000, 4.999999999999998224 ) ) ;
#19850=CARTESIAN_POINT ( 'NONE',  ( 26.28749999999999432, 5.773502691896255534, 3.535250795749688894E-16 ) ) ;
#19853=CARTESIAN_POINT ( 'NONE',  ( 27.45937500061451786, 4.541064518000418104, -2.621784821874998173 ) ) ;
#19854=CARTESIAN_POINT ( 'NONE',  ( 11.70000000000000284, -4.330127018922190985, -2.500000000000001332 ) ) ;
#19855=CARTESIAN_POINT ( 'NONE',  ( 9.001249775931846008E-16, 13.22187500061451715, -25.09994784771203058 ) ) ;
#19856=CARTESIAN_POINT ( 'NONE',  ( 4.425000001229032698, 2.886751345948126879, 4.999999999999999112 ) ) ;
#19857=CARTESIAN_POINT ( 'NONE',  ( 3.187500000000002220, -2.886751345948125991, -5.000000000000000000 ) ) ;
#19859=CARTESIAN_POINT ( 'NONE',  ( 7.059375000614518392, -4.541064518000417216, -2.621784821875001281 ) ) ;
#19860=CARTESIAN_POINT ( 'NONE',  ( 27.70312500061451289, -4.541064518000417216, -2.621784821875001281 ) ) ;
#19861=DIRECTION ( 'NONE',  ( 0.000000000000000000, 0.000000000000000000, -1.000000000000000000 ) ) ;
#19862=CARTESIAN_POINT ( 'NONE',  ( 5.587500000000003020, 5.773502691896255534, 3.535250795749688401E-16 ) ) ;
#19864=CARTESIAN_POINT ( 'NONE',  ( 6.009375000614519458, 0.000000000000000000, 5.243569643749999010 ) ) ;
#19865=CARTESIAN_POINT ( 'NONE',  ( 11.25937500061451679, 4.541064518000418104, -2.621784821874998173 ) ) ;
#19866=CARTESIAN_POINT ( 'NONE',  ( 3.900000000000000799, 0.000000000000000000, 4.999999999999998224 ) ) ;
#19867=CARTESIAN_POINT ( 'NONE',  ( 2.121784821874999061, 14.25312500061459531, 26.32496088578401583 ) ) ;
#19869=CARTESIAN_POINT ( 'NONE',  ( 6.225000000000001421, -4.330127018922194537, 2.499999999999995559 ) ) ;
#19871=CARTESIAN_POINT ( 'NONE',  ( 20.84062500061451573, -3.027376345333614438, 5.243569643749998122 ) ) ;
#19872=CARTESIAN_POINT ( 'NONE',  ( 10.30312500061451431, 4.541064518000418104, -2.621784821874998173 ) ) ;
#19874=CARTESIAN_POINT ( 'NONE',  ( 9.646875000614516082, -3.027376345333614438, 5.243569643749998122 ) ) ;
#19875=CARTESIAN_POINT ( 'NONE',  ( 27.00000000000000000, -4.330127018922190985, -2.500000000000001332 ) ) ;
#19876=CARTESIAN_POINT ( 'NONE',  ( 19.72500000122903074, 2.886751345948126879, 4.999999999999999112 ) ) ;
#19877=CARTESIAN_POINT ( 'NONE',  ( 27.59062500061451573, -3.027376345333614438, 5.243569643749998122 ) ) ;
#19878=DIRECTION ( 'NONE',  ( 0.000000000000000000, 0.000000000000000000, 1.000000000000000000 ) ) ;
#19879=CARTESIAN_POINT ( 'NONE',  ( 10.54687500061451644, -3.027376345333614438, 5.243569643749998122 ) ) ;
#19880=CARTESIAN_POINT ( 'NONE',  ( 13.13437500061451857, 4.541064518000418104, 2.621784821874999949 ) ) ;
#19881=CARTESIAN_POINT ( 'NONE',  ( 26.33437500061451431, -4.541064518000419881, 2.621784821874995952 ) ) ;
#19884=CARTESIAN_POINT ( 'NONE',  ( 20.07187500061451857, -6.054752690667223547, -1.112240025338166033E-15 ) ) ;
#19885=CARTESIAN_POINT ( 'NONE',  ( 11.48437500061451644, -4.541064518000419881, 2.621784821874995952 ) ) ;
#19887=CARTESIAN_POINT ( 'NONE',  ( 23.06250000000000355, 2.886751345948129099, -4.999999999999998224 ) ) ;
#19889=CARTESIAN_POINT ( 'NONE',  ( 4.243569643749999010, 11.57187500061451679, -32.45002607614398471 ) ) ;
#19891=CARTESIAN_POINT ( 'NONE',  ( 14.54062500061451679, -3.027376345333614438, 5.243569643749998122 ) ) ;
#19892=CARTESIAN_POINT ( 'NONE',  ( 3.975000000000002753, -4.330127018922194537, 2.499999999999995559 ) ) ;
#19894=CARTESIAN_POINT ( 'NONE',  ( 1.626862140677534273E-15, 10.21250000000000036, 34.00000000000000000 ) ) ;
#19895=CARTESIAN_POINT ( 'NONE',  ( 12.93750000000000178, -2.886751345948129988, 4.999999999999997335 ) ) ;
#19896=CARTESIAN_POINT ( 'NONE',  ( -3.999999999999997335, 18.80000000122903359, 32.30940107675850470 ) ) ;
#19897=CARTESIAN_POINT ( 'NONE',  ( 10.83750000122903501, -4.330127018922194537, 2.499999999999995559 ) ) ;
#19898=CARTESIAN_POINT ( 'NONE',  ( 22.24687500061451217, -3.027376345333614438, 5.243569643749998122 ) ) ;
#19899=CARTESIAN_POINT ( 'NONE',  ( 16.69687500061451502, 6.054752690667223547, 3.707466751127219781E-16 ) ) ;
#19901=ORIENTED_EDGE ( 'NONE', *, *, #10704, .T. ) ;
#19902=CARTESIAN_POINT ( 'NONE',  ( 20.01562500061451644, -6.054752690667223547, -1.112240025338166033E-15 ) ) ;
#19903=CARTESIAN_POINT ( 'NONE',  ( 3.703125000614516882, 0.000000000000000000, 5.243569643749999010 ) ) ;
#19904=CARTESIAN_POINT ( 'NONE',  ( 16.80937500061451573, 0.000000000000000000, 5.243569643749999010 ) ) ;
#19905=CARTESIAN_POINT ( 'NONE',  ( 29.85937500061451644, 0.000000000000000000, 5.243569643749999010 ) ) ;
#19906=CARTESIAN_POINT ( 'NONE',  ( 4.753125000614515372, -4.541064518000417216, -2.621784821875001281 ) ) ;
#19907=CARTESIAN_POINT ( 'NONE',  ( 20.24062500061451431, 6.054752690667223547, 3.707466751127219781E-16 ) ) ;
#19908=CARTESIAN_POINT ( 'NONE',  ( -3.000416591977282496E-16, 15.64062500061451644, 25.09994784771203058 ) ) ;
#19909=CARTESIAN_POINT ( 'NONE',  ( 17.51250000122903216, 0.000000000000000000, 4.999999999999998224 ) ) ;
#19911=CARTESIAN_POINT ( 'NONE',  ( 7.115625000614516971, 3.027376345333612662, -5.243569643749998122 ) ) ;
#19912=CARTESIAN_POINT ( 'NONE',  ( 3.046875000614519990, -3.027376345333610441, -5.243569643749999898 ) ) ;
#19913=CARTESIAN_POINT ( 'NONE',  ( 22.84687500061451715, -3.027376345333610441, -5.243569643749999898 ) ) ;
#19914=CARTESIAN_POINT ( 'NONE',  ( 14.24062500061451608, -3.027376345333610441, -5.243569643749999898 ) ) ;
#19915=CARTESIAN_POINT ( 'NONE',  ( 25.50000000122903288, 5.773502691896255534, 3.535250795749688894E-16 ) ) ;
#19916=CARTESIAN_POINT ( 'NONE',  ( 22.60312500061451857, 0.000000000000000000, 5.243569643749999010 ) ) ;
#19917=CARTESIAN_POINT ( 'NONE',  ( 19.32187500061451857, 3.027376345333613106, -5.243569643749998122 ) ) ;
#19918=CARTESIAN_POINT ( 'NONE',  ( 13.79062500061451502, -3.027376345333610441, -5.243569643749999898 ) ) ;
#19919=CARTESIAN_POINT ( 'NONE',  ( 4.243569643749999898, 15.58437500061451786, 30.00000000000000000 ) ) ;
#19920=CARTESIAN_POINT ( 'NONE',  ( 20.50312500061451715, -4.541064518000417216, -2.621784821875001281 ) ) ;
#19921=FACE_OUTER_BOUND ( 'NONE', #28263, .T. ) ;
#19924=CARTESIAN_POINT ( 'NONE',  ( 23.96249999999999858, 2.886751345948129099, -4.999999999999998224 ) ) ;
#19925=CARTESIAN_POINT ( 'NONE',  ( 4.243569643749999010, 19.67187500061451644, -32.45002607614398471 ) ) ;
#19926=CARTESIAN_POINT ( 'NONE',  ( 3.881554241669678884, -3.151751365348489653, -4.190642664303462439 ) ) ;
#19927=CARTESIAN_POINT ( 'NONE',  ( 27.40312500061451573, 4.541064518000418104, -2.621784821874998173 ) ) ;
#19928=CARTESIAN_POINT ( 'NONE',  ( 8.803125000614517859, -4.541064518000417216, -2.621784821875001281 ) ) ;
#19929=CARTESIAN_POINT ( 'NONE',  ( 20.40000000122903145, -2.886751345948125991, -5.000000000000000000 ) ) ;
#19930=CARTESIAN_POINT ( 'NONE',  ( 24.96562500061451573, -6.054752690667223547, -1.112240025338166033E-15 ) ) ;
#19931=CARTESIAN_POINT ( 'NONE',  ( 26.09999999999999787, -4.330127018922190985, -2.500000000000001332 ) ) ;
#19932=EDGE_CURVE ( 'NONE', #3917, #20508, #13399, .T. ) ;
#19933=CARTESIAN_POINT ( 'NONE',  ( 26.69062500061451715, -3.027376345333614438, 5.243569643749998122 ) ) ;
#19934=CARTESIAN_POINT ( 'NONE',  ( 8.690625000614515372, -3.027376345333614438, 5.243569643749998122 ) ) ;
#19935=EDGE_LOOP ( 'NONE', ( #56094, #5139, #2307, #13366 ) ) ;
#19936=CARTESIAN_POINT ( 'NONE',  ( 23.39062500061451289, 6.054752690667223547, 3.707466751127219781E-16 ) ) ;
#19937=CARTESIAN_POINT ( 'NONE',  ( 4.265625000614517326, -6.054752690667223547, -1.112240025338166033E-15 ) ) ;
#19939=CARTESIAN_POINT ( 'NONE',  ( 1.071796769724505438, 13.11740381056766580, 26.00000000000001421 ) ) ;
#19941=CARTESIAN_POINT ( 'NONE',  ( 13.83749999999999858, -2.886751345948129988, 4.999999999999997335 ) ) ;
#19942=( BOUNDED_CURVE ( )  B_SPLINE_CURVE ( 2, ( #38153, #27817, #66605, #44077, #50350, #4556, #22970 ),
 .UNSPECIFIED., .F., .F. ) 
 B_SPLINE_CURVE_WITH_KNOTS ( ( 3, 2, 2, 3 ),
 ( 0.4666666666666667296, 0.4694444444444444975, 0.4722222222222222654, 0.4750000000000000333 ),
 .UNSPECIFIED. ) 
 CURVE ( )  GEOMETRIC_REPRESENTATION_ITEM ( )  RATIONAL_B_SPLINE_CURVE ( ( 0.9999999999999973355, 0.8660254037844413721, 1.000000000000000000, 0.8660254037844387076, 1.000000000000000000, 0.8660254037844360431, 1.000000000000002665 ) ) 
 REPRESENTATION_ITEM ( '' )  );
#19943=CARTESIAN_POINT ( 'NONE',  ( 11.14687500061451608, -3.027376345333610441, -5.243569643749999898 ) ) ;
#19944=CARTESIAN_POINT ( 'NONE',  ( 9.525000001229033231, -5.773502691896255534, -1.060575238724906372E-15 ) ) ;
#19945=CARTESIAN_POINT ( 'NONE',  ( 14.97187500061451892, 3.027376345333611329, 5.243569643749999010 ) ) ;
#19947=CARTESIAN_POINT ( 'NONE',  ( 8.784375000614518925, -4.541064518000419881, 2.621784821874995952 ) ) ;
#19949=CARTESIAN_POINT ( 'NONE',  ( 20.32499999999999929, 6.123233995736764310E-16, -4.999999999999998224 ) ) ;
#19950=CARTESIAN_POINT ( 'NONE',  ( 12.49687500061451573, -3.027376345333610441, -5.243569643749999898 ) ) ;
#19951=CARTESIAN_POINT ( 'NONE',  ( 21.92812500061451431, 6.421520780324663323E-16, -5.243569643749999010 ) ) ;
#19954=CARTESIAN_POINT ( 'NONE',  ( 25.65937500061451715, 4.541064518000418104, -2.621784821874998173 ) ) ;
#19956=CARTESIAN_POINT ( 'NONE',  ( 3.290625000614516793, -3.027376345333614438, 5.243569643749998122 ) ) ;
#19958=CARTESIAN_POINT ( 'NONE',  ( 16.65937500061452070, 4.541064518000418104, -2.621784821874998173 ) ) ;
#19960=CARTESIAN_POINT ( 'NONE',  ( 26.51250000122903216, 0.000000000000000000, 4.999999999999998224 ) ) ;
#19961=CARTESIAN_POINT ( 'NONE',  ( 6.946875000614517681, -3.027376345333614438, 5.243569643749998122 ) ) ;
#19962=CARTESIAN_POINT ( 'NONE',  ( 16.58437500061451786, 6.421520780324663323E-16, -5.243569643749999010 ) ) ;
#19963=CARTESIAN_POINT ( 'NONE',  ( 25.46249999999999858, 2.886751345948126879, 4.999999999999999112 ) ) ;
#19964=CARTESIAN_POINT ( 'NONE',  ( 26.25937500061451857, 0.000000000000000000, 5.243569643749999010 ) ) ;
#19967=CARTESIAN_POINT ( 'NONE',  ( 8.550000000000002487, -4.330127018922190985, -2.500000000000001332 ) ) ;
#19969=CARTESIAN_POINT ( 'NONE',  ( 22.04062500061451502, 6.054752690667223547, 3.707466751127219781E-16 ) ) ;
#19970=CARTESIAN_POINT ( 'NONE',  ( 11.77500000000000036, 6.123233995736764310E-16, -4.999999999999998224 ) ) ;
#19971=CARTESIAN_POINT ( 'NONE',  ( 5.803125000614517859, 4.541064518000418104, -2.621784821874998173 ) ) ;
#19972=CARTESIAN_POINT ( 'NONE',  ( 20.66250000000000142, -5.773502691896255534, -1.060575238724906372E-15 ) ) ;
#19973=CARTESIAN_POINT ( 'NONE',  ( 18.70312500061451644, -4.541064518000417216, -2.621784821875001281 ) ) ;
#19974=CARTESIAN_POINT ( 'NONE',  ( 23.66249999999999787, 2.886751345948143754, 4.999999999999969802 ) ) ;
#19975=CARTESIAN_POINT ( 'NONE',  ( 23.77500000122903145, 2.886751345948126879, 4.999999999999999112 ) ) ;
#19977=CARTESIAN_POINT ( 'NONE',  ( 6.037500000000001421, 5.773502691896255534, 3.535250795749688894E-16 ) ) ;
#19979=CARTESIAN_POINT ( 'NONE',  ( 19.19062500061452070, -3.027376345333610441, -5.243569643749999898 ) ) ;
#19980=CARTESIAN_POINT ( 'NONE',  ( 25.97812500061451502, 6.421520780324663323E-16, -5.243569643749999010 ) ) ;
#19981=CARTESIAN_POINT ( 'NONE',  ( 25.50937500061451502, -4.541064518000417216, -2.621784821875001281 ) ) ;
#19982=CARTESIAN_POINT ( 'NONE',  ( 9.299999999999998934, 0.000000000000000000, 4.999999999999998224 ) ) ;
#19983=CARTESIAN_POINT ( 'NONE',  ( 11.54062500061451857, -3.027376345333610441, -5.243569643749999898 ) ) ;
#19984=CARTESIAN_POINT ( 'NONE',  ( 26.72812500061451502, -4.541064518000419881, 2.621784821874995952 ) ) ;
#19985=CARTESIAN_POINT ( 'NONE',  ( 16.02187500061451786, -6.054752690667223547, -1.112240025338166033E-15 ) ) ;
#19986=CARTESIAN_POINT ( 'NONE',  ( 9.178125000614517859, -4.541064518000419881, 2.621784821874995952 ) ) ;
#19988=CARTESIAN_POINT ( 'NONE',  ( 9.001249775931846008E-16, 11.42187500061451999, 34.90005215228797653 ) ) ;
#19989=CARTESIAN_POINT ( 'NONE',  ( 24.22500000122903430, 2.886751345948126879, 4.999999999999999112 ) ) ;
#19991=CARTESIAN_POINT ( 'NONE',  ( 13.22812500061451502, -4.541064518000419881, 2.621784821874995952 ) ) ;
#19992=CARTESIAN_POINT ( 'NONE',  ( 10.32187500061451679, 3.027376345333613106, -5.243569643749998122 ) ) ;
#19993=CARTESIAN_POINT ( 'NONE',  ( 10.13437500061451679, -4.541064518000419881, 2.621784821874995952 ) ) ;
#19994=VERTEX_POINT ( 'NONE', #26248 ) ;
#19995=CARTESIAN_POINT ( 'NONE',  ( 1.626862140677534273E-15, 13.36250000000000071, 34.00000000000000000 ) ) ;
#19996=CARTESIAN_POINT ( 'NONE',  ( 22.71562500061451573, -6.054752690667223547, -1.112240025338166033E-15 ) ) ;
#19997=CARTESIAN_POINT ( 'NONE',  ( 17.18437500061451573, 4.541064518000418104, 2.621784821874999949 ) ) ;
#19998=CARTESIAN_POINT ( 'NONE',  ( 22.34062500061451573, -3.027376345333610441, -5.243569643749999898 ) ) ;
#19999=CARTESIAN_POINT ( 'NONE',  ( -2.828200636599751609E-16, 12.23750000000000249, 25.38119784648299770 ) ) ;
#20000=CARTESIAN_POINT ( 'NONE',  ( 26.46562500061451573, 3.027376345333613106, -5.243569643749998122 ) ) ;
#20001=CARTESIAN_POINT ( 'NONE',  ( 6.262500001229034829, 0.000000000000000000, 4.999999999999998224 ) ) ;
#20002=ORIENTED_EDGE ( 'NONE', *, *, #12677, .F. ) ;
#20003=CARTESIAN_POINT ( 'NONE',  ( 29.92500000000000071, 4.330127018922191873, 2.499999999999999556 ) ) ;
#20004=CARTESIAN_POINT ( 'NONE',  ( 4.000000000000000000, 17.48750000000000071, -27.69059892324149530 ) ) ;
#20005=CARTESIAN_POINT ( 'NONE',  ( 23.58750000122903145, 6.123233995736764310E-16, -4.999999999999998224 ) ) ;
#20007=CARTESIAN_POINT ( 'NONE',  ( 7.509375000614517681, -4.541064518000417216, -2.621784821875001281 ) ) ;
#20008=CARTESIAN_POINT ( 'NONE',  ( -1.487416814333745711E-14, 15.16250000000000142, 34.00000000000000000 ) ) ;
#20009=CARTESIAN_POINT ( 'NONE',  ( 14.46562500061451750, 3.027376345333611329, 5.243569643749999010 ) ) ;
#20010=CARTESIAN_POINT ( 'NONE',  ( 7.959375000614516971, -4.541064518000417216, -2.621784821875001281 ) ) ;
#20011=CARTESIAN_POINT ( 'NONE',  ( 26.06250000122903288, 0.000000000000000000, 4.999999999999998224 ) ) ;
#20012=CARTESIAN_POINT ( 'NONE',  ( 16.28437500061452070, 4.541064518000418104, 2.621784821874999949 ) ) ;
#20013=CARTESIAN_POINT ( 'NONE',  ( 4.809375000614516615, -4.541064518000417216, -2.621784821875001281 ) ) ;
#20014=CARTESIAN_POINT ( 'NONE',  ( 30.00000000000000000, 6.123233995736764310E-16, -4.999999999999998224 ) ) ;
#20015=CARTESIAN_POINT ( 'NONE',  ( 4.603125000614518569, 0.000000000000000000, 5.243569643749999010 ) ) ;
#20016=CARTESIAN_POINT ( 'NONE',  ( 14.76562500061451821, 3.027376345333613106, -5.243569643749998122 ) ) ;
#20017=ORIENTED_EDGE ( 'NONE', *, *, #42731, .T. ) ;
#20018=CARTESIAN_POINT ( 'NONE',  ( 13.56562500061451892, 3.027376345333611329, 5.243569643749999010 ) ) ;
#20019=CARTESIAN_POINT ( 'NONE',  ( 5.437500001229035540, -4.330127018922194537, 2.499999999999995559 ) ) ;
#20020=CARTESIAN_POINT ( 'NONE',  ( 9.665625000614515017, -6.054752690667223547, -1.112240025338166033E-15 ) ) ;
#20022=CARTESIAN_POINT ( 'NONE',  ( 9.899999999999998579, -4.330127018922190985, -2.500000000000001332 ) ) ;
#20023=CARTESIAN_POINT ( 'NONE',  ( 5.250000001229035540, 5.773502691896255534, 3.535250795749688894E-16 ) ) ;
#20024=CARTESIAN_POINT ( 'NONE',  ( 20.54999999999999716, 0.000000000000000000, 4.999999999999998224 ) ) ;
#20025=CARTESIAN_POINT ( 'NONE',  ( 16.02187500061451786, -6.054752690667223547, -1.112240025338166033E-15 ) ) ;
#20026=CARTESIAN_POINT ( 'NONE',  ( 15.22500000122903252, 2.886751345948126879, 4.999999999999999112 ) ) ;
#20028=CARTESIAN_POINT ( 'NONE',  ( 2.121784821874999061, 19.20312500061451644, -33.67503911421598417 ) ) ;
#20031=CARTESIAN_POINT ( 'NONE',  ( 28.34062500061451928, 6.054752690667223547, 3.707466751127219781E-16 ) ) ;
#20033=CARTESIAN_POINT ( 'NONE',  ( 3.930102994493983370, -3.091035892528488649, -4.235648827855108323 ) ) ;
#20034=CARTESIAN_POINT ( 'NONE',  ( 15.19687500061451857, -3.027376345333610441, -5.243569643749999898 ) ) ;
#20036=CARTESIAN_POINT ( 'NONE',  ( 29.06250000000000000, 2.886751345948126879, 4.999999999999999112 ) ) ;
#20037=EDGE_CURVE ( 'NONE', #66542, #24963, #25781, .T. ) ;
#20038=CARTESIAN_POINT ( 'NONE',  ( 11.54062500061451857, -3.027376345333610441, -5.243569643749999898 ) ) ;
#20040=CARTESIAN_POINT ( 'NONE',  ( 24.45937500061451786, 0.000000000000000000, 5.243569643749999010 ) ) ;
#20042=CARTESIAN_POINT ( 'NONE',  ( 8.878125000614515372, 6.421520780324663323E-16, -5.243569643749999010 ) ) ;
#20043=CARTESIAN_POINT ( 'NONE',  ( 12.90937500061451537, -4.541064518000417216, -2.621784821875001281 ) ) ;
#20045=CARTESIAN_POINT ( 'NONE',  ( 23.44687500061451502, 6.054752690667223547, 3.707466751127219781E-16 ) ) ;
#20046=CARTESIAN_POINT ( 'NONE',  ( 27.55312500061451786, 0.000000000000000000, 5.243569643749999010 ) ) ;
#20048=CARTESIAN_POINT ( 'NONE',  ( 7.762500000000001954, 2.886751345948129099, -4.999999999999998224 ) ) ;
#20049=CARTESIAN_POINT ( 'NONE',  ( 16.23750000122903359, -4.330127018922194537, 2.499999999999995559 ) ) ;
#20053=CARTESIAN_POINT ( 'NONE',  ( 14.17500000000000071, 4.330127018922191873, 2.499999999999999556 ) ) ;
#20054=CARTESIAN_POINT ( 'NONE',  ( 18.59999999999999787, 4.330127018922192761, -2.499999999999997780 ) ) ;
#20055=CARTESIAN_POINT ( 'NONE',  ( 12.62812500061451537, 4.541064518000418104, 2.621784821874999949 ) ) ;
#20058=CARTESIAN_POINT ( 'NONE',  ( -4.243569643749999898, 17.12187500061451573, -32.45002607614398471 ) ) ;
#20059=CARTESIAN_POINT ( 'NONE',  ( 29.47500000122903430, 2.886751345948129099, -4.999999999999998224 ) ) ;
#20061=CARTESIAN_POINT ( 'NONE',  ( 11.55000000000000071, 0.000000000000000000, 4.999999999999998224 ) ) ;
#20063=ORIENTED_EDGE ( 'NONE', *, *, #55458, .F. ) ;
#20064=CARTESIAN_POINT ( 'NONE',  ( -4.243569643749999898, 15.30312500061451608, 30.00000000000000000 ) ) ;
#20065=CARTESIAN_POINT ( 'NONE',  ( 27.59062500061451573, -3.027376345333614438, 5.243569643749998122 ) ) ;
#20066=CARTESIAN_POINT ( 'NONE',  ( 0.000000000000000000, 0.000000000000000000, 50.00000000000000000 ) ) ;
#20068=CARTESIAN_POINT ( 'NONE',  ( 23.59687500061451715, -3.027376345333614438, 5.243569643749998122 ) ) ;
#20069=CARTESIAN_POINT ( 'NONE',  ( 19.67812500061451786, 6.421520780324663323E-16, -5.243569643749999010 ) ) ;
#20070=CARTESIAN_POINT ( 'NONE',  ( 4.243569643749999898, 13.24062500061459424, -27.54997392385601529 ) ) ;
#20071=CARTESIAN_POINT ( 'NONE',  ( 23.21250000122903501, 4.330127018922192761, -2.499999999999997780 ) ) ;
#20072=CARTESIAN_POINT ( 'NONE',  ( 2.953125000614516438, -4.541064518000417216, -2.621784821875001281 ) ) ;
#20074=CARTESIAN_POINT ( 'NONE',  ( 20.42812500061451431, -4.541064518000419881, 2.621784821874995952 ) ) ;
#20077=CARTESIAN_POINT ( 'NONE',  ( 17.97187500061451715, 3.027376345333613106, -5.243569643749998122 ) ) ;
#20078=CARTESIAN_POINT ( 'NONE',  ( 17.25937500061451502, 0.000000000000000000, 5.243569643749999010 ) ) ;
#20079=CARTESIAN_POINT ( 'NONE',  ( 25.58437500061451431, 6.421520780324663323E-16, -5.243569643749999010 ) ) ;
#20080=CARTESIAN_POINT ( 'NONE',  ( 2.121784821875001281, 15.05937500061451928, 33.67503911421598417 ) ) ;
#20081=CARTESIAN_POINT ( 'NONE',  ( 3.965625000614515727, 3.027376345333613106, -5.243569643749998122 ) ) ;
#20082=CARTESIAN_POINT ( 'NONE',  ( 16.53750000122903430, 4.330127018922191873, 2.499999999999999556 ) ) ;
#20083=CARTESIAN_POINT ( 'NONE',  ( 28.79062500061451502, 6.054752690667223547, 3.707466751127219781E-16 ) ) ;
#20084=CARTESIAN_POINT ( 'NONE',  ( -2.000000000000000000, 19.02499999999999858, 26.53589838486224650 ) ) ;
#20085=CARTESIAN_POINT ( 'NONE',  ( 3.815625000614518036, -6.054752690667223547, -1.112240025338166033E-15 ) ) ;
#20086=CARTESIAN_POINT ( 'NONE',  ( 6.309375000614517504, 4.541064518000418104, -2.621784821874998173 ) ) ;
#20088=CARTESIAN_POINT ( 'NONE',  ( 13.53750000122903430, -4.330127018922194537, 2.499999999999995559 ) ) ;
#20089=CARTESIAN_POINT ( 'NONE',  ( 12.52500000122903145, 2.886751345948126879, 4.999999999999999112 ) ) ;
#20090=CARTESIAN_POINT ( 'NONE',  ( 5.803125000614517859, 4.541064518000418104, -2.621784821874998173 ) ) ;
#20093=CARTESIAN_POINT ( 'NONE',  ( 14.10937500061451644, 0.000000000000000000, 5.243569643749999010 ) ) ;
#20094=DIRECTION ( 'NONE',  ( -0.000000000000000000, -0.000000000000000000, -1.000000000000000000 ) ) ;
#20095=ORIENTED_EDGE ( 'NONE', *, *, #51501, .F. ) ;
#20096=CARTESIAN_POINT ( 'NONE',  ( 23.12812500061451360, -4.541064518000419881, 2.621784821874995952 ) ) ;
#20097=CARTESIAN_POINT ( 'NONE',  ( 8.315625000614515372, -6.054752690667223547, -1.112240025338166033E-15 ) ) ;
#20098=CARTESIAN_POINT ( 'NONE',  ( 23.44687500061451502, 6.054752690667223547, 3.707466751127219781E-16 ) ) ;
#20099=CARTESIAN_POINT ( 'NONE',  ( 6.778125000614518392, 4.541064518000418104, 2.621784821874999949 ) ) ;
#20100=LINE ( 'NONE', #13463, #9706 ) ;
#20102=CARTESIAN_POINT ( 'NONE',  ( 8.962500001229033231, 0.000000000000000000, 4.999999999999998224 ) ) ;
#20104=CARTESIAN_POINT ( 'NONE',  ( 23.61562500061451431, -6.054752690667223547, -1.112240025338166033E-15 ) ) ;
#20105=CARTESIAN_POINT ( 'NONE',  ( -4.243569643749997233, 11.29062500061451857, -27.54997392385601174 ) ) ;
#20106=CARTESIAN_POINT ( 'NONE',  ( 11.28750000122903252, -4.330127018922194537, 2.499999999999995559 ) ) ;
#20107=CARTESIAN_POINT ( 'NONE',  ( 19.75312500061451360, 4.541064518000418104, -2.621784821874998173 ) ) ;
#20108=EDGE_CURVE ( 'NONE', #52020, #36659, #36130, .T. ) ;
#20109=CARTESIAN_POINT ( 'NONE',  ( 17.16562500061451502, 3.027376345333611329, 5.243569643749999010 ) ) ;
#20111=CARTESIAN_POINT ( 'NONE',  ( 17.13749999999999929, -2.886751345948125991, -5.000000000000000000 ) ) ;
#20112=CARTESIAN_POINT ( 'NONE',  ( 13.08750000122903323, -4.330127018922194537, 2.499999999999995559 ) ) ;
#20113=CARTESIAN_POINT ( 'NONE',  ( 9.253125000614517148, -4.541064518000417216, -2.621784821875001281 ) ) ;
#20114=CARTESIAN_POINT ( 'NONE',  ( 14.01562500061451644, 3.027376345333611329, 5.243569643749999010 ) ) ;
#20116=CARTESIAN_POINT ( 'NONE',  ( 23.66250000122903430, 4.330127018922192761, -2.499999999999997780 ) ) ;
#20117=CARTESIAN_POINT ( 'NONE',  ( 21.15937500061451715, 4.541064518000418104, -2.621784821874998173 ) ) ;
#20118=CARTESIAN_POINT ( 'NONE',  ( 20.40937500061451715, 0.000000000000000000, 5.243569643749999010 ) ) ;
#20120=EDGE_CURVE ( 'NONE', #10990, #41820, #51239, .T. ) ;
#20121=CARTESIAN_POINT ( 'NONE',  ( 7.800000001229035362, -2.886751345948125991, -5.000000000000000000 ) ) ;
#20122=CARTESIAN_POINT ( 'NONE',  ( 7.096875000614517148, -3.027376345333610441, -5.243569643749999898 ) ) ;
#20123=CARTESIAN_POINT ( 'NONE',  ( 24.34687500061451715, 6.054752690667223547, 3.707466751127219781E-16 ) ) ;
#20124=CARTESIAN_POINT ( 'NONE',  ( 17.99062500061451786, 6.054752690667223547, 3.707466751127219781E-16 ) ) ;
#20125=CARTESIAN_POINT ( 'NONE',  ( 23.89687500061451786, 6.054752690667223547, 3.707466751127219781E-16 ) ) ;
#20127=CARTESIAN_POINT ( 'NONE',  ( 3.468957575989525477, -4.154263691098152300, -3.291743506479378301 ) ) ;
#20129=CARTESIAN_POINT ( 'NONE',  ( 4.509375000614518569, 4.541064518000418104, -2.621784821874998173 ) ) ;
#20130=CARTESIAN_POINT ( 'NONE',  ( 16.30312500061451786, 0.000000000000000000, 5.243569643749999010 ) ) ;
#20131=CARTESIAN_POINT ( 'NONE',  ( 13.28437500061451715, -4.541064518000419881, 2.621784821874995952 ) ) ;
#20132=ORIENTED_EDGE ( 'NONE', *, *, #68150, .F. ) ;
#20134=CARTESIAN_POINT ( 'NONE',  ( 24.14062500061451289, -3.027376345333610441, -5.243569643749999898 ) ) ;
#20135=CARTESIAN_POINT ( 'NONE',  ( 3.397178649298551179, 3.668675132081069545, -3.397178649298551179 ) ) ;
#20137=CARTESIAN_POINT ( 'NONE',  ( 15.18750000000000000, -2.886751345948129988, 4.999999999999997335 ) ) ;
#20138=CARTESIAN_POINT ( 'NONE',  ( 25.01250000122903216, 4.330127018922192761, -2.499999999999997780 ) ) ;
#20139=CARTESIAN_POINT ( 'NONE',  ( 19.30312500061451786, 4.541064518000418104, -2.621784821874998173 ) ) ;
#20141=CARTESIAN_POINT ( 'NONE',  ( 22.50000000000000000, -4.330127018922190985, -2.500000000000001332 ) ) ;
#20143=CARTESIAN_POINT ( 'NONE',  ( 24.87187500061451573, 3.027376345333611329, 5.243569643749999010 ) ) ;
#20144=ORIENTED_EDGE ( 'NONE', *, *, #61389, .T. ) ;
#20145=CARTESIAN_POINT ( 'NONE',  ( 13.27500000122903323, 2.886751345948129099, -4.999999999999997335 ) ) ;
#20146=CARTESIAN_POINT ( 'NONE',  ( 13.86562500061451431, 3.027376345333613106, -5.243569643749998122 ) ) ;
#20147=CARTESIAN_POINT ( 'NONE',  ( 3.515625000614516882, 3.027376345333613106, -5.243569643749998122 ) ) ;
#20149=CARTESIAN_POINT ( 'NONE',  ( 27.51562500061451644, 3.027376345333611329, 5.243569643749999010 ) ) ;
#20150=CARTESIAN_POINT ( 'NONE',  ( 11.85000000122903430, -2.886751345948125991, -5.000000000000000000 ) ) ;
#20151=CARTESIAN_POINT ( 'NONE',  ( 19.91250000000000142, 2.886751345948129099, -4.999999999999998224 ) ) ;
#20152=CARTESIAN_POINT ( 'NONE',  ( 26.13749999999999929, -2.886751345948125991, -5.000000000000000000 ) ) ;
#20154=CARTESIAN_POINT ( 'NONE',  ( 7.734375000614517326, 4.541064518000418104, 2.621784821874999949 ) ) ;
#20155=CARTESIAN_POINT ( 'NONE',  ( 16.54687500061451644, -3.027376345333610441, -5.243569643749999898 ) ) ;
#20156=CARTESIAN_POINT ( 'NONE',  ( -3.999999999999999112, 13.77500000122903678, 27.69059892324149885 ) ) ;
#20158=CARTESIAN_POINT ( 'NONE',  ( 26.20312500061451644, 0.000000000000000000, 5.243569643749999010 ) ) ;
#20159=CARTESIAN_POINT ( 'NONE',  ( 28.58437500061451786, -4.541064518000419881, 2.621784821874995952 ) ) ;
#20161=CARTESIAN_POINT ( 'NONE',  ( 17.06250000000000000, -5.773502691896255534, -1.060575238724906372E-15 ) ) ;
#20162=CARTESIAN_POINT ( 'NONE',  ( 11.61562500061451608, 3.027376345333613106, -5.243569643749998122 ) ) ;
#20165=CARTESIAN_POINT ( 'NONE',  ( 29.76562500061451644, 3.027376345333611329, 5.243569643749999010 ) ) ;
#20166=CARTESIAN_POINT ( 'NONE',  ( 17.62500000122903288, -5.773502691896255534, -1.060575238724906372E-15 ) ) ;
#20167=CARTESIAN_POINT ( 'NONE',  ( 15.07500000122903394, 2.886751345948129099, -4.999999999999997335 ) ) ;
#20169=CARTESIAN_POINT ( 'NONE',  ( 6.290625000614517681, 6.054752690667223547, 3.707466751127219781E-16 ) ) ;
#20170=CARTESIAN_POINT ( 'NONE',  ( 24.12187500061451217, -6.054752690667223547, -1.112240025338166033E-15 ) ) ;
#20171=CARTESIAN_POINT ( 'NONE',  ( -3.000416591977282496E-16, 17.49687500061451573, 25.09994784771203058 ) ) ;
#20172=CARTESIAN_POINT ( 'NONE',  ( 24.98437500061451644, -4.541064518000419881, 2.621784821874995952 ) ) ;
#20173=CARTESIAN_POINT ( 'NONE',  ( 4.162499999999999645, 2.886751345948129099, -4.999999999999998224 ) ) ;
#20174=CARTESIAN_POINT ( 'NONE',  ( 1.999999999999998668, 11.86250000122903359, 26.53589838486224650 ) ) ;
#20175=CARTESIAN_POINT ( 'NONE',  ( 11.72812500061451857, 4.541064518000418104, 2.621784821874999949 ) ) ;
#20176=CARTESIAN_POINT ( 'NONE',  ( 3.300000001229034918, -2.886751345948125991, -5.000000000000000000 ) ) ;
#20178=CARTESIAN_POINT ( 'NONE',  ( 8.296875000614516438, -3.027376345333614438, 5.243569643749998122 ) ) ;
#20179=CARTESIAN_POINT ( 'NONE',  ( 3.934813120841985423, -3.085075400804674572, 3.963314313556091761 ) ) ;
#20180=CARTESIAN_POINT ( 'NONE',  ( 10.15312500061451750, -4.541064518000417216, -2.621784821875001281 ) ) ;
#20181=CARTESIAN_POINT ( 'NONE',  ( 14.14687500061451786, -3.027376345333614438, 5.243569643749998122 ) ) ;
#20182=FACE_OUTER_BOUND ( 'NONE', #53739, .T. ) ;
#20183=CARTESIAN_POINT ( 'NONE',  ( 21.45000000122903216, 5.773502691896255534, 3.535250795749688894E-16 ) ) ;
#20184=CARTESIAN_POINT ( 'NONE',  ( 9.946875000614516793, 6.054752690667223547, 3.707466751127219781E-16 ) ) ;
#20185=CARTESIAN_POINT ( 'NONE',  ( 12.10312500061451857, 4.541064518000418104, -2.621784821874998173 ) ) ;
#20187=CARTESIAN_POINT ( 'NONE',  ( 20.70937500061451786, 4.541064518000418104, -2.621784821874998173 ) ) ;
#20189=CARTESIAN_POINT ( 'NONE',  ( -3.026485248664595673, 3.985774251745325181, 32.62744762453846903 ) ) ;
#20190=CYLINDRICAL_SURFACE ( 'NONE', #60820, 4.999999999999998224 ) ;
#20191=CARTESIAN_POINT ( 'NONE',  ( 4.243569643749999898, 14.64687500061451964, -27.54997392385601529 ) ) ;
#20192=CARTESIAN_POINT ( 'NONE',  ( 15.15937500061451715, -4.541064518000417216, -2.621784821875001281 ) ) ;
#20193=CARTESIAN_POINT ( 'NONE',  ( 14.70000000122903394, 5.773502691896255534, 3.535250795749688894E-16 ) ) ;
#20194=CARTESIAN_POINT ( 'NONE',  ( 12.53437500061451537, 6.421520780324663323E-16, -5.243569643749999010 ) ) ;
#20195=CARTESIAN_POINT ( 'NONE',  ( -3.000416591977282496E-16, 16.99062500061451786, -34.90005215228797653 ) ) ;
#20196=CARTESIAN_POINT ( 'NONE',  ( 16.76250000122903216, -4.330127018922190985, -2.500000000000001332 ) ) ;
#20197=CARTESIAN_POINT ( 'NONE',  ( 11.42812500061451608, -4.541064518000419881, 2.621784821874995952 ) ) ;
#20198=EDGE_LOOP ( 'NONE', ( #13004, #52313, #69522, #9648 ) ) ;
#20199=CARTESIAN_POINT ( 'NONE',  ( 16.31250000000000000, 2.886751345948129099, -4.999999999999998224 ) ) ;
#20200=DIRECTION ( 'NONE',  ( -1.000000000000000000, -0.000000000000000000, -0.000000000000000000 ) ) ;
#20201=CARTESIAN_POINT ( 'NONE',  ( 10.62187500061451750, -6.054752690667223547, -1.112240025338166033E-15 ) ) ;
#20203=CARTESIAN_POINT ( 'NONE',  ( 11.96250000122903501, 4.330127018922192761, -2.499999999999997780 ) ) ;
#20204=CARTESIAN_POINT ( 'NONE',  ( 19.91250000122903074, -4.330127018922190985, -2.500000000000001332 ) ) ;
#20205=CARTESIAN_POINT ( 'NONE',  ( 16.86562500061451786, -6.054752690667223547, -1.112240025338166033E-15 ) ) ;
#20206=EDGE_CURVE ( 'NONE', #45031, #7627, #6363, .T. ) ;
#20207=CARTESIAN_POINT ( 'NONE',  ( 21.77812500061451928, -4.541064518000419881, 2.621784821874995952 ) ) ;
#20208=CARTESIAN_POINT ( 'NONE',  ( 28.76250000122903216, 0.000000000000000000, 4.999999999999998224 ) ) ;
#20209=CARTESIAN_POINT ( 'NONE',  ( 3.478125000614517237, 6.421520780324663323E-16, -5.243569643749999010 ) ) ;
#20210=CARTESIAN_POINT ( 'NONE',  ( 26.06250000000000000, -5.773502691896255534, -1.060575238724906372E-15 ) ) ;
#20213=CARTESIAN_POINT ( 'NONE',  ( 28.20937500061451786, -4.541064518000417216, -2.621784821875001281 ) ) ;
#20215=CARTESIAN_POINT ( 'NONE',  ( 4.125000001229034652, -5.773502691896255534, -1.060575238724906372E-15 ) ) ;
#20216=CARTESIAN_POINT ( 'NONE',  ( 4.650000000000001243, 4.330127018922192761, -2.499999999999997780 ) ) ;
#20218=CARTESIAN_POINT ( 'NONE',  ( 8.071875000614518569, 3.027376345333613106, -5.243569643749998122 ) ) ;
#20219=CARTESIAN_POINT ( 'NONE',  ( 26.46562500061451573, 3.027376345333613106, -5.243569643749998122 ) ) ;
#20221=CARTESIAN_POINT ( 'NONE',  ( 14.24999999999999822, 0.000000000000000000, 4.999999999999998224 ) ) ;
#20222=CARTESIAN_POINT ( 'NONE',  ( 1.626862140677534273E-15, 17.52500000122903145, -26.00000000000000355 ) ) ;
#20223=CARTESIAN_POINT ( 'NONE',  ( 5.971875000614516260, 3.027376345333611329, 5.243569643749999010 ) ) ;
#20224=CARTESIAN_POINT ( 'NONE',  ( 9.421875000614519990, 3.027376345333613106, -5.243569643749998122 ) ) ;
#20225=CARTESIAN_POINT ( 'NONE',  ( 4.500000000000000888, -4.330127018922190985, -2.500000000000001332 ) ) ;
#20226=EDGE_CURVE ( 'NONE', #11359, #72067, #52942, .T. ) ;
#20227=CARTESIAN_POINT ( 'NONE',  ( -2.121784821874996840, 12.67812500061459602, 33.67503911421598417 ) ) ;
#20229=CARTESIAN_POINT ( 'NONE',  ( 28.46249999999999858, 2.886751345948129099, -4.999999999999998224 ) ) ;
#20230=CARTESIAN_POINT ( 'NONE',  ( 4.612500000000002487, 2.886751345948129099, -4.999999999999998224 ) ) ;
#20233=CARTESIAN_POINT ( 'NONE',  ( 19.52812500061451573, -4.541064518000419881, 2.621784821874995952 ) ) ;
#20234=CARTESIAN_POINT ( 'NONE',  ( 10.41562500061451679, 3.027376345333611329, 5.243569643749999010 ) ) ;
#20236=CARTESIAN_POINT ( 'NONE',  ( 6.834375000614518747, 4.541064518000418104, 2.621784821874999949 ) ) ;
#20237=CARTESIAN_POINT ( 'NONE',  ( 23.06250000000000355, 2.886751345948129099, -4.999999999999998224 ) ) ;
#20238=CARTESIAN_POINT ( 'NONE',  ( 19.12500000122903288, 2.886751345948129099, -4.999999999999998224 ) ) ;
#20239=CARTESIAN_POINT ( 'NONE',  ( 28.41562500061451502, 3.027376345333611329, 5.243569643749999010 ) ) ;
#20241=CARTESIAN_POINT ( 'NONE',  ( 10.47187500061451715, 3.027376345333611329, 5.243569643749999010 ) ) ;
#20242=CARTESIAN_POINT ( 'NONE',  ( 14.82187500061451679, 3.027376345333613106, -5.243569643749998122 ) ) ;
#20243=CARTESIAN_POINT ( 'NONE',  ( 25.02187500061451431, -6.054752690667223547, -1.112240025338166033E-15 ) ) ;
#20244=ADVANCED_FACE ( 'NONE', ( #65766 ), #15148, .F. ) ;
#20246=CARTESIAN_POINT ( 'NONE',  ( 20.14687500061451786, -3.027376345333610441, -5.243569643749999898 ) ) ;
#20247=CARTESIAN_POINT ( 'NONE',  ( 8.709375000614517859, 0.000000000000000000, 5.243569643749999010 ) ) ;
#20249=CARTESIAN_POINT ( 'NONE',  ( 23.02499999999999858, 6.123233995736764310E-16, -4.999999999999998224 ) ) ;
#20251=CARTESIAN_POINT ( 'NONE',  ( 4.243569643749999010, 12.47187500061451715, -32.45002607614398471 ) ) ;
#20253=CARTESIAN_POINT ( 'NONE',  ( 13.75312500061451715, -4.541064518000417216, -2.621784821875001281 ) ) ;
#20254=CARTESIAN_POINT ( 'NONE',  ( 5.625000000000001776, 4.330127018922191873, 2.499999999999999556 ) ) ;
#20255=CYLINDRICAL_SURFACE ( 'NONE', #27807, 4.000000000000000000 ) ;
#20257=CARTESIAN_POINT ( 'NONE',  ( 12.52500000000000213, -4.330127018922194537, 2.499999999999995559 ) ) ;
#20258=CARTESIAN_POINT ( 'NONE',  ( 2.000000000000001332, 17.56250000122903288, 33.46410161513774995 ) ) ;
#20259=CARTESIAN_POINT ( 'NONE',  ( 10.57500000122903572, 2.886751345948129099, -4.999999999999998224 ) ) ;
#20260=CARTESIAN_POINT ( 'NONE',  ( 22.13437500061451502, 4.541064518000418104, 2.621784821874999949 ) ) ;
#20261=CARTESIAN_POINT ( 'NONE',  ( 15.42187500061451821, 3.027376345333611329, 5.243569643749999010 ) ) ;
#20263=VERTEX_POINT ( 'NONE', #59851 ) ;
#20264=CARTESIAN_POINT ( 'NONE',  ( 17.76562500061451644, -6.054752690667223547, -1.112240025338166033E-15 ) ) ;
#20265=CARTESIAN_POINT ( 'NONE',  ( 28.31250000122903288, 0.000000000000000000, 4.999999999999998224 ) ) ;
#20266=CARTESIAN_POINT ( 'NONE',  ( 16.69687500061451502, 6.054752690667223547, 3.707466751127219781E-16 ) ) ;
#20267=CARTESIAN_POINT ( 'NONE',  ( 28.58437500061451786, -4.541064518000419881, 2.621784821874995952 ) ) ;
#20268=CARTESIAN_POINT ( 'NONE',  ( 5.503125000614516260, 0.000000000000000000, 5.243569643749999010 ) ) ;
#20269=CARTESIAN_POINT ( 'NONE',  ( 18.85312500061451502, 4.541064518000418104, -2.621784821874998173 ) ) ;
#20270=CARTESIAN_POINT ( 'NONE',  ( -4.243569643749999898, 13.05312500061451786, 30.00000000000000000 ) ) ;
#20271=CARTESIAN_POINT ( 'NONE',  ( 16.01250000122903216, 4.330127018922192761, -2.499999999999997780 ) ) ;
#20273=CARTESIAN_POINT ( 'NONE',  ( 7.303125000614516082, 0.000000000000000000, 5.243569643749999010 ) ) ;
#20274=CARTESIAN_POINT ( 'NONE',  ( 28.00312500061451715, 0.000000000000000000, 5.243569643749999010 ) ) ;
#20275=DIRECTION ( 'NONE',  ( 1.000000000000000000, 0.000000000000000000, 0.000000000000000000 ) ) ;
#20276=CARTESIAN_POINT ( 'NONE',  ( 23.22187500061451715, -6.054752690667223547, -1.112240025338166033E-15 ) ) ;
#20277=CARTESIAN_POINT ( 'NONE',  ( 13.67812500061451786, -4.541064518000419881, 2.621784821874995952 ) ) ;
#20278=CARTESIAN_POINT ( 'NONE',  ( 23.17500000122903359, 2.886751345948129099, -4.999999999999998224 ) ) ;
#20279=CARTESIAN_POINT ( 'NONE',  ( 22.82812500061451644, 6.421520780324663323E-16, -5.243569643749999010 ) ) ;
#20280=CARTESIAN_POINT ( 'NONE',  ( 18.72187500061451360, -6.054752690667223547, -1.112240025338166033E-15 ) ) ;
#20281=CARTESIAN_POINT ( 'NONE',  ( 15.40312500061451573, 0.000000000000000000, 5.243569643749999010 ) ) ;
#20282=CARTESIAN_POINT ( 'NONE',  ( 2.121784821875001281, 15.05937500061451928, 33.67503911421598417 ) ) ;
#20283=CARTESIAN_POINT ( 'NONE',  ( 19.90312500061451573, 0.000000000000000000, 5.243569643749999010 ) ) ;
#20284=CARTESIAN_POINT ( 'NONE',  ( 29.24062500061451431, 6.054752690667223547, 3.707466751127219781E-16 ) ) ;
#20286=ORIENTED_EDGE ( 'NONE', *, *, #70743, .T. ) ;
#20287=CARTESIAN_POINT ( 'NONE',  ( 22.42500000000000071, -4.330127018922194537, 2.499999999999995559 ) ) ;
#20288=CARTESIAN_POINT ( 'NONE',  ( 2.121784821875001281, 19.55937500061451573, -26.32496088578401938 ) ) ;
#20289=CARTESIAN_POINT ( 'NONE',  ( 25.82812500061451644, -4.541064518000419881, 2.621784821874995952 ) ) ;
#20290=CARTESIAN_POINT ( 'NONE',  ( 8.578125000614518214, 4.541064518000418104, 2.621784821874999949 ) ) ;
#20291=CARTESIAN_POINT ( 'NONE',  ( 19.46250000122903145, -4.330127018922190985, -2.500000000000001332 ) ) ;
#20292=CARTESIAN_POINT ( 'NONE',  ( 24.02812500061451573, -4.541064518000419881, 2.621784821874995952 ) ) ;
#20293=CARTESIAN_POINT ( 'NONE',  ( 22.83749999999999858, -2.886751345948129988, 4.999999999999997335 ) ) ;
#20294=CARTESIAN_POINT ( 'NONE',  ( 28.52812500061451573, -4.541064518000419881, 2.621784821874995952 ) ) ;
#20295=CARTESIAN_POINT ( 'NONE',  ( 8.128125000614515372, 4.541064518000418104, 2.621784821874999949 ) ) ;
#20297=AXIS2_PLACEMENT_3D ( 'NONE', #72104, #55124, #65460 ) ;
#20298=CARTESIAN_POINT ( 'NONE',  ( 22.15312500061451573, 0.000000000000000000, 5.243569643749999010 ) ) ;
#20299=CARTESIAN_POINT ( 'NONE',  ( 6.440625000614517148, -3.027376345333614438, 5.243569643749998122 ) ) ;
#20301=CARTESIAN_POINT ( 'NONE',  ( 3.140625000614516882, 6.054752690667223547, 3.707466751127219781E-16 ) ) ;
#20302=CARTESIAN_POINT ( 'NONE',  ( 4.000000000000000000, 14.45000000122903572, -27.69059892324149530 ) ) ;
#20303=CARTESIAN_POINT ( 'NONE',  ( 1.626862140677534273E-15, 13.81250000000000000, -26.00000000000000355 ) ) ;
#20304=CARTESIAN_POINT ( 'NONE',  ( 10.46249999999999858, 2.886751345948129099, -4.999999999999998224 ) ) ;
#20305=( BOUNDED_CURVE ( )  B_SPLINE_CURVE ( 2, ( #60393, #14602, #9801, #15697, #36776, #3909, #8702, #9074, #37510 ),
 .UNSPECIFIED., .F., .F. ) 
 B_SPLINE_CURVE_WITH_KNOTS ( ( 3, 2, 2, 2, 3 ),
 ( 0.2717391304347826497, 0.2753623188405797118, 0.2826086956521738913, 0.2898550724637681264, 0.2934782608695652439 ),
 .UNSPECIFIED. ) 
 CURVE ( )  GEOMETRIC_REPRESENTATION_ITEM ( )  RATIONAL_B_SPLINE_CURVE ( ( 0.9330127018922194093, 0.9330127018922198534, 1.000000000000000000, 0.8660254037844387076, 1.000000000000000000, 0.8660254037844387076, 1.000000000000000000, 0.9330127018922188542, 0.9330127018922194093 ) ) 
 REPRESENTATION_ITEM ( '' )  );
#20306=CARTESIAN_POINT ( 'NONE',  ( 10.17187500061451999, -6.054752690667223547, -1.112240025338166033E-15 ) ) ;
#20307=CARTESIAN_POINT ( 'NONE',  ( 8.175000001229031810, -5.773502691896255534, -1.060575238724906372E-15 ) ) ;
#20308=CARTESIAN_POINT ( 'NONE',  ( 14.25937500061451679, -4.541064518000417216, -2.621784821875001281 ) ) ;
#20310=CARTESIAN_POINT ( 'NONE',  ( 6.459375000614518747, 0.000000000000000000, 5.243569643749999010 ) ) ;
#20311=CARTESIAN_POINT ( 'NONE',  ( 5.190092854996874117, 9.698896338944486217, -35.22418694837048037 ) ) ;
#20312=DIRECTION ( 'NONE',  ( -0.000000000000000000, -1.000000000000000000, -0.000000000000000000 ) ) ;
#20313=CARTESIAN_POINT ( 'NONE',  ( 12.64687500061451608, 6.054752690667223547, 3.707466751127219781E-16 ) ) ;
#20314=CARTESIAN_POINT ( 'NONE',  ( 3.657199499170772139, 3.409538812810354536, 3.983732690067115723 ) ) ;
#20315=CARTESIAN_POINT ( 'NONE',  ( 22.52812500061451573, 4.541064518000418104, 2.621784821874999949 ) ) ;
#20316=CARTESIAN_POINT ( 'NONE',  ( -4.243569643749999898, 10.82187500061451857, 27.54997392385601529 ) ) ;
#20317=CARTESIAN_POINT ( 'NONE',  ( -2.121784821874999949, 18.82812500061459104, 26.32496088578401938 ) ) ;
#20318=CARTESIAN_POINT ( 'NONE',  ( 25.28437500061451715, 4.541064518000418104, 2.621784821874999949 ) ) ;
#20319=CARTESIAN_POINT ( 'NONE',  ( 4.117352459450578372, 2.836881972790640916, -4.222552775064624342 ) ) ;
#20320=CARTESIAN_POINT ( 'NONE',  ( 4.678125000614516971, -4.541064518000419881, 2.621784821874995952 ) ) ;
#20322=CARTESIAN_POINT ( 'NONE',  ( 17.33437500061451431, -4.541064518000419881, 2.621784821874995952 ) ) ;
#20324=CARTESIAN_POINT ( 'NONE',  ( 27.86250000122903359, 0.000000000000000000, 4.999999999999998224 ) ) ;
#20325=CARTESIAN_POINT ( 'NONE',  ( 6.459375000614518747, 0.000000000000000000, 5.243569643749999010 ) ) ;
#20326=CARTESIAN_POINT ( 'NONE',  ( 15.98437500061451821, -4.541064518000419881, 2.621784821874995952 ) ) ;
#20327=CARTESIAN_POINT ( 'NONE',  ( 3.324079281300976962, 3.735364078604925364, -3.324079281300976962 ) ) ;
#20328=CARTESIAN_POINT ( 'NONE',  ( 25.23749999999999716, -2.886751345948125991, -5.000000000000000000 ) ) ;
#20330=CARTESIAN_POINT ( 'NONE',  ( 4.237500001229036251, 6.123233995736764310E-16, -4.999999999999998224 ) ) ;
#20331=CARTESIAN_POINT ( 'NONE',  ( 26.74687500061451573, -3.027376345333614438, 5.243569643749998122 ) ) ;
#20333=CARTESIAN_POINT ( 'NONE',  ( 14.17500000122903536, 2.886751345948129099, -4.999999999999997335 ) ) ;
#20334=CARTESIAN_POINT ( 'NONE',  ( 8.362500000000002487, 2.886751345948126879, 4.999999999999999112 ) ) ;
#20336=CARTESIAN_POINT ( 'NONE',  ( 21.51562500061451644, 3.027376345333613106, -5.243569643749998122 ) ) ;
#20337=CARTESIAN_POINT ( 'NONE',  ( 12.97499999999999964, -4.330127018922194537, 2.499999999999995559 ) ) ;
#20338=CARTESIAN_POINT ( 'NONE',  ( 4.378125000614518925, 6.421520780324663323E-16, -5.243569643749999010 ) ) ;
#20339=CARTESIAN_POINT ( 'NONE',  ( 19.31250000000000000, -5.773502691896255534, -1.060575238724906372E-15 ) ) ;
#20340=CARTESIAN_POINT ( 'NONE',  ( 17.84062500061451573, -3.027376345333610441, -5.243569643749999898 ) ) ;
#20341=CARTESIAN_POINT ( 'NONE',  ( -1.999999999999997113, 18.83750000122903501, 33.46410161513775705 ) ) ;
#20342=VECTOR ( 'NONE', #48602, 1000.000000000000000 ) ;
#20343=B_SPLINE_CURVE_WITH_KNOTS ( 'NONE', 3,
 ( #31277, #20179, #64155, #13542, #70442, #53079, #36090, #42734, #19818, #42005 ),
 .UNSPECIFIED., .F., .F.,
 ( 4, 3, 3, 4 ),
 ( 2.616501308845268417E-17, 7.861561263978005779E-05, 0.0001572308220202767550, 0.0002825258805215967667 ),
 .UNSPECIFIED. ) ;
#20344=CARTESIAN_POINT ( 'NONE',  ( 23.06250000122903288, -4.330127018922190985, -2.500000000000001332 ) ) ;
#20346=CARTESIAN_POINT ( 'NONE',  ( 29.67187500061451644, 3.027376345333613106, -5.243569643749998122 ) ) ;
#20348=CARTESIAN_POINT ( 'NONE',  ( 19.11562500061451431, -6.054752690667223547, -1.112240025338166033E-15 ) ) ;
#20349=CARTESIAN_POINT ( 'NONE',  ( 25.49062500061451786, -3.027376345333610441, -5.243569643749999898 ) ) ;
#20350=CARTESIAN_POINT ( 'NONE',  ( 23.78437500061451360, 6.421520780324663323E-16, -5.243569643749999010 ) ) ;
#20351=CARTESIAN_POINT ( 'NONE',  ( 9.225000000000001421, 4.330127018922191873, 2.499999999999999556 ) ) ;
#20352=CARTESIAN_POINT ( 'NONE',  ( 11.65312500061451573, 4.541064518000418104, -2.621784821874998173 ) ) ;
#20353=CARTESIAN_POINT ( 'NONE',  ( 25.79062500061451502, -3.027376345333614438, 5.243569643749998122 ) ) ;
#20354=CARTESIAN_POINT ( 'NONE',  ( 17.63437500061451502, 4.541064518000418104, 2.621784821874999949 ) ) ;
#20355=CARTESIAN_POINT ( 'NONE',  ( 9.365625000614519635, 3.027376345333613106, -5.243569643749998122 ) ) ;
#20357=CARTESIAN_POINT ( 'NONE',  ( 4.243569643749999010, 13.37187500061451750, 27.54997392385601174 ) ) ;
#20359=CARTESIAN_POINT ( 'NONE',  ( 23.88750000122903216, -4.330127018922194537, 2.499999999999995559 ) ) ;
#20361=CARTESIAN_POINT ( 'NONE',  ( 15.02812500061451750, -4.541064518000419881, 2.621784821874995952 ) ) ;
#20362=CARTESIAN_POINT ( 'NONE',  ( 8.071875000614518569, 3.027376345333613106, -5.243569643749998122 ) ) ;
#20363=CARTESIAN_POINT ( 'NONE',  ( 9.871875000614517504, 3.027376345333613106, -5.243569643749998122 ) ) ;
#20365=CARTESIAN_POINT ( 'NONE',  ( 29.37187500061451928, 3.027376345333611329, 5.243569643749999010 ) ) ;
#20366=CARTESIAN_POINT ( 'NONE',  ( 22.64062500061451644, -3.027376345333614438, 5.243569643749998122 ) ) ;
#20367=CARTESIAN_POINT ( 'NONE',  ( 16.73437500061451644, 4.541064518000418104, 2.621784821874999949 ) ) ;
#20368=CARTESIAN_POINT ( 'NONE',  ( 21.74062500061451431, -3.027376345333614438, 5.243569643749998122 ) ) ;
#20369=CARTESIAN_POINT ( 'NONE',  ( -2.828200636599751609E-16, 10.88750000000000107, 25.38119784648299770 ) ) ;
#20370=CARTESIAN_POINT ( 'NONE',  ( 25.94062500061451715, -3.027376345333610441, -5.243569643749999898 ) ) ;
#20371=CARTESIAN_POINT ( 'NONE',  ( 6.150000001229033231, 5.773502691896255534, 3.535250795749688894E-16 ) ) ;
#20372=ORIENTED_EDGE ( 'NONE', *, *, #4888, .T. ) ;
#20373=CARTESIAN_POINT ( 'NONE',  ( 29.77499999999999858, 6.123233995736764310E-16, -4.999999999999998224 ) ) ;
#20374=CARTESIAN_POINT ( 'NONE',  ( 2.000000000000001332, 18.80000000000000071, -26.53589838486224650 ) ) ;
#20375=CARTESIAN_POINT ( 'NONE',  ( 25.05000000122903714, 5.773502691896255534, 3.535250795749688894E-16 ) ) ;
#20377=CARTESIAN_POINT ( 'NONE',  ( 7.096875000614517148, -3.027376345333610441, -5.243569643749999898 ) ) ;
#20378=CARTESIAN_POINT ( 'NONE',  ( 4.291775470143723403, 2.565448060106937600, -4.323948581960670445 ) ) ;
#20379=CARTESIAN_POINT ( 'NONE',  ( 14.16562500061451679, -6.054752690667223547, -1.112240025338166033E-15 ) ) ;
#20380=CARTESIAN_POINT ( 'NONE',  ( 8.109375000614518214, 4.541064518000418104, -2.621784821874998173 ) ) ;
#20381=CARTESIAN_POINT ( 'NONE',  ( 28.12500000122902932, 2.886751345948129099, -4.999999999999998224 ) ) ;
#20382=CARTESIAN_POINT ( 'NONE',  ( 17.33437500061451431, -4.541064518000419881, 2.621784821874995952 ) ) ;
#20383=CARTESIAN_POINT ( 'NONE',  ( 4.846875000614519813, -3.027376345333610441, -5.243569643749999898 ) ) ;
#20385=CARTESIAN_POINT ( 'NONE',  ( 5.090625000614516615, -3.027376345333614438, 5.243569643749998122 ) ) ;
#20386=CARTESIAN_POINT ( 'NONE',  ( 14.87812500061451537, 4.541064518000418104, 2.621784821874999949 ) ) ;
#20387=ADVANCED_FACE ( 'NONE', ( #26986 ), #33598, .F. ) ;
#20388=( BOUNDED_CURVE ( )  B_SPLINE_CURVE ( 2, ( #62702, #50540, #12096, #68619, #57147 ),
 .UNSPECIFIED., .F., .F. ) 
 B_SPLINE_CURVE_WITH_KNOTS ( ( 3, 2, 3 ),
 ( 0.000000000000000000, 0.007246376811594202987, 0.01086956521739130578 ),
 .UNSPECIFIED. ) 
 CURVE ( )  GEOMETRIC_REPRESENTATION_ITEM ( )  RATIONAL_B_SPLINE_CURVE ( ( 1.000000000000000000, 0.8660254037844387076, 1.000000000000000000, 0.9330127018922192983, 0.9330127018922194093 ) ) 
 REPRESENTATION_ITEM ( '' )  );
#20390=CARTESIAN_POINT ( 'NONE',  ( 13.04062500061451502, 6.054752690667223547, 3.707466751127219781E-16 ) ) ;
#20391=CARTESIAN_POINT ( 'NONE',  ( 6.300000001229033586, -2.886751345948129988, 4.999999999999997335 ) ) ;
#20392=CARTESIAN_POINT ( 'NONE',  ( 11.72812500061451857, 4.541064518000418104, 2.621784821874999949 ) ) ;
#20394=CARTESIAN_POINT ( 'NONE',  ( 10.08749999999999858, 5.773502691896255534, 3.535250795749688894E-16 ) ) ;
#20395=CARTESIAN_POINT ( 'NONE',  ( 4.612500001229032698, -4.330127018922190985, -2.500000000000001332 ) ) ;
#20396=CARTESIAN_POINT ( 'NONE',  ( 16.94999999999999929, 0.000000000000000000, 4.999999999999998224 ) ) ;
#20397=CARTESIAN_POINT ( 'NONE',  ( 17.63437500061451502, 4.541064518000418104, 2.621784821874999949 ) ) ;
#20398=CARTESIAN_POINT ( 'NONE',  ( 15.56250000122903465, 4.330127018922192761, -2.499999999999997780 ) ) ;
#20400=( BOUNDED_CURVE ( )  B_SPLINE_CURVE ( 2, ( #40412, #41144, #13043, #50506, #46316, #34858, #7875 ),
 .UNSPECIFIED., .F., .F. ) 
 B_SPLINE_CURVE_WITH_KNOTS ( ( 3, 2, 2, 3 ),
 ( 0.5916666666666667851, 0.5944444444444445530, 0.5972222222222222099, 0.5999999999999999778 ),
 .UNSPECIFIED. ) 
 CURVE ( )  GEOMETRIC_REPRESENTATION_ITEM ( )  RATIONAL_B_SPLINE_CURVE ( ( 0.9999999999999946709, 0.8660254037844440367, 1.000000000000000000, 0.8660254037844387076, 1.000000000000000000, 0.8660254037844387076, 1.000000000000000000 ) ) 
 REPRESENTATION_ITEM ( '' )  );
#20401=CARTESIAN_POINT ( 'NONE',  ( 9.001249775931846008E-16, 17.66562500061451502, -25.09994784771203058 ) ) ;
#20402=CARTESIAN_POINT ( 'NONE',  ( 3.243445638651676344, 3.805279306527807659, 3.607624186539012623 ) ) ;
#20403=CARTESIAN_POINT ( 'NONE',  ( -3.999999999999999112, 18.64999999999999858, 30.00000000000000000 ) ) ;
#20404=CARTESIAN_POINT ( 'NONE',  ( 3.581550526421168001, -3.489303470904949744, 3.581550526421168001 ) ) ;
#20405=CARTESIAN_POINT ( 'NONE',  ( 29.72812500061451502, 4.541064518000418104, 2.621784821874999949 ) ) ;
#20407=CARTESIAN_POINT ( 'NONE',  ( 17.03437500061451715, 6.421520780324663323E-16, -5.243569643749999010 ) ) ;
#20408=CARTESIAN_POINT ( 'NONE',  ( 28.91250000000000497, 2.886751345948129099, -4.999999999999998224 ) ) ;
#20409=CARTESIAN_POINT ( 'NONE',  ( 11.69062500061451360, 6.054752690667223547, 3.707466751127219781E-16 ) ) ;
#20411=CARTESIAN_POINT ( 'NONE',  ( 23.33437500061451786, 6.421520780324663323E-16, -5.243569643749999010 ) ) ;
#20413=CARTESIAN_POINT ( 'NONE',  ( 7.490625000614516082, -3.027376345333610441, -5.243569643749999898 ) ) ;
#20414=CARTESIAN_POINT ( 'NONE',  ( 12.75937500061451857, 0.000000000000000000, 5.243569643749999010 ) ) ;
#20415=ORIENTED_EDGE ( 'NONE', *, *, #42313, .F. ) ;
#20416=CARTESIAN_POINT ( 'NONE',  ( 23.55937500061451573, 0.000000000000000000, 5.243569643749999010 ) ) ;
#20417=CARTESIAN_POINT ( 'NONE',  ( 27.92812500061451431, 4.541064518000418104, 2.621784821874999949 ) ) ;
#20419=CARTESIAN_POINT ( 'NONE',  ( 6.937499999999999112, 5.773502691896255534, 3.535250795749688894E-16 ) ) ;
#20420=CARTESIAN_POINT ( 'NONE',  ( 17.62500000122903288, -5.773502691896255534, -1.060575238724906372E-15 ) ) ;
#20421=LINE ( 'NONE', #65870, #31343 ) ;
#20424=CARTESIAN_POINT ( 'NONE',  ( 14.77500000000000036, -4.330127018922194537, 2.499999999999995559 ) ) ;
#20425=CARTESIAN_POINT ( 'NONE',  ( 19.91250000000000142, 2.886751345948129099, -4.999999999999998224 ) ) ;
#20426=CARTESIAN_POINT ( 'NONE',  ( 11.61562500061451608, 3.027376345333613106, -5.243569643749998122 ) ) ;
#20427=ORIENTED_EDGE ( 'NONE', *, *, #19299, .F. ) ;
#20428=CARTESIAN_POINT ( 'NONE',  ( 0.000000000000000000, 20.00000000000000000, -33.99999999999999289 ) ) ;
#20429=CARTESIAN_POINT ( 'NONE',  ( -2.121784821874996840, 17.68437500061451928, -26.32496088578401583 ) ) ;
#20430=CARTESIAN_POINT ( 'NONE',  ( 4.378125000614518925, 6.421520780324663323E-16, -5.243569643749999010 ) ) ;
#20432=CARTESIAN_POINT ( 'NONE',  ( 9.787499999999999645, -2.886751345948129988, 4.999999999999997335 ) ) ;
#20433=FACE_OUTER_BOUND ( 'NONE', #5264, .T. ) ;
#20434=ORIENTED_EDGE ( 'NONE', *, *, #53141, .F. ) ;
#20435=CARTESIAN_POINT ( 'NONE',  ( -3.000416591977282496E-16, 14.29062500061451679, 25.09994784771203058 ) ) ;
#20436=CARTESIAN_POINT ( 'NONE',  ( 25.97812500061451502, 6.421520780324663323E-16, -5.243569643749999010 ) ) ;
#20439=CARTESIAN_POINT ( 'NONE',  ( 22.84687500061451715, -3.027376345333610441, -5.243569643749999898 ) ) ;
#20440=CARTESIAN_POINT ( 'NONE',  ( 20.16562500061451146, 3.027376345333613106, -5.243569643749998122 ) ) ;
#20441=CARTESIAN_POINT ( 'NONE',  ( 4.243569643749999010, 12.86562500061459424, -32.45002607614398471 ) ) ;
#20442=CARTESIAN_POINT ( 'NONE',  ( 24.03750000122903430, 6.123233995736764310E-16, -4.999999999999998224 ) ) ;
#20443=CARTESIAN_POINT ( 'NONE',  ( 3.703125000614516882, 0.000000000000000000, 5.243569643749999010 ) ) ;
#20445=CARTESIAN_POINT ( 'NONE',  ( 22.71562500061451573, -6.054752690667223547, -1.112240025338166033E-15 ) ) ;
#20448=CARTESIAN_POINT ( 'NONE',  ( 16.47187500061452070, -6.054752690667223547, -1.112240025338166033E-15 ) ) ;
#20449=CARTESIAN_POINT ( 'NONE',  ( 15.75937500061451857, 4.541064518000418104, -2.621784821874998173 ) ) ;
#20450=CARTESIAN_POINT ( 'NONE',  ( 24.79687500061451999, 6.054752690667223547, 3.707466751127219781E-16 ) ) ;
#20451=CARTESIAN_POINT ( 'NONE',  ( 9.001249775931846008E-16, 14.57187500061451679, 34.90005215228797653 ) ) ;
#20452=CARTESIAN_POINT ( 'NONE',  ( 4.078125000614517326, 4.541064518000418104, 2.621784821874999949 ) ) ;
#20453=CARTESIAN_POINT ( 'NONE',  ( 28.15312500061451573, -4.541064518000417216, -2.621784821875001281 ) ) ;
#20455=CARTESIAN_POINT ( 'NONE',  ( 2.000000000000001332, 19.25000000000000000, 33.46410161513774995 ) ) ;
#20456=CARTESIAN_POINT ( 'NONE',  ( 6.684375000614518392, 6.421520780324663323E-16, -5.243569643749999010 ) ) ;
#20457=CARTESIAN_POINT ( 'NONE',  ( 13.50000000122903288, -2.886751345948129988, 4.999999999999997335 ) ) ;
#20458=CARTESIAN_POINT ( 'NONE',  ( 9.562500001229032875, -4.330127018922190985, -2.500000000000001332 ) ) ;
#20459=CARTESIAN_POINT ( 'NONE',  ( 5.653125000614517504, -4.541064518000417216, -2.621784821875001281 ) ) ;
#20462=CARTESIAN_POINT ( 'NONE',  ( 15.30937500061451750, 4.541064518000418104, -2.621784821874998173 ) ) ;
#20463=CARTESIAN_POINT ( 'NONE',  ( 11.81250000000000000, 2.886751345948129099, -4.999999999999997335 ) ) ;
#20465=CARTESIAN_POINT ( 'NONE',  ( 21.62812500061451360, 4.541064518000418104, 2.621784821874999949 ) ) ;
#20466=CARTESIAN_POINT ( 'NONE',  ( 6.890625000614516438, -3.027376345333614438, 5.243569643749998122 ) ) ;
#20467=CARTESIAN_POINT ( 'NONE',  ( 23.67187500061451644, -6.054752690667223547, -1.112240025338166033E-15 ) ) ;
#20468=CARTESIAN_POINT ( 'NONE',  ( 8.503125000614515372, 4.541064518000418104, -2.621784821874998173 ) ) ;
#20469=DIRECTION ( 'NONE',  ( 0.000000000000000000, 0.000000000000000000, -1.000000000000000000 ) ) ;
#20470=CARTESIAN_POINT ( 'NONE',  ( 7.575000001229033053, 2.886751345948126879, 4.999999999999999112 ) ) ;
#20471=CARTESIAN_POINT ( 'NONE',  ( 22.37812500061451360, 6.421520780324663323E-16, -5.243569643749999010 ) ) ;
#20472=EDGE_CURVE ( 'NONE', #38561, #20937, #36209, .T. ) ;
#20473=CARTESIAN_POINT ( 'NONE',  ( 4.243569643749999010, 11.06562500061451715, -32.45002607614398471 ) ) ;
#20474=CARTESIAN_POINT ( 'NONE',  ( 9.300000001229035362, 5.773502691896255534, 3.535250795749688894E-16 ) ) ;
#20475=CARTESIAN_POINT ( 'NONE',  ( 18.92812500061451431, 4.541064518000418104, 2.621784821874999949 ) ) ;
#20476=CARTESIAN_POINT ( 'NONE',  ( 16.90312500061451573, -4.541064518000417216, -2.621784821875001281 ) ) ;
#20478=CARTESIAN_POINT ( 'NONE',  ( 17.06250000000000000, -5.773502691896255534, -1.060575238724906372E-15 ) ) ;
#20479=CARTESIAN_POINT ( 'NONE',  ( 11.58750000122903501, 4.330127018922191873, 2.499999999999999556 ) ) ;
#20480=CARTESIAN_POINT ( 'NONE',  ( 7.153125000614518392, 4.541064518000418104, -2.621784821874998173 ) ) ;
#20481=CARTESIAN_POINT ( 'NONE',  ( 13.15312500061451750, 0.000000000000000000, 5.243569643749999010 ) ) ;
#20482=CARTESIAN_POINT ( 'NONE',  ( 22.50000000122903288, -2.886751345948129988, 4.999999999999997335 ) ) ;
#20483=CARTESIAN_POINT ( 'NONE',  ( 22.69687500061451857, -3.027376345333614438, 5.243569643749998122 ) ) ;
#20484=CARTESIAN_POINT ( 'NONE',  ( 3.586992791275801729, 3.483314903268937446, -3.919380039434936513 ) ) ;
#20485=CARTESIAN_POINT ( 'NONE',  ( 6.337500001229033231, -4.330127018922194537, 2.499999999999995559 ) ) ;
#20486=CARTESIAN_POINT ( 'NONE',  ( 6.459375000614518747, 0.000000000000000000, 5.243569643749999010 ) ) ;
#20487=CARTESIAN_POINT ( 'NONE',  ( 22.54687500061451999, 6.054752690667223547, 3.707466751127219781E-16 ) ) ;
#20489=CARTESIAN_POINT ( 'NONE',  ( 17.76562500061451644, -6.054752690667223547, -1.112240025338166033E-15 ) ) ;
#20490=CARTESIAN_POINT ( 'NONE',  ( 24.79687500061451999, 6.054752690667223547, 3.707466751127219781E-16 ) ) ;
#20494=CARTESIAN_POINT ( 'NONE',  ( 5.109375000614518214, 0.000000000000000000, 5.243569643749999010 ) ) ;
#20495=CARTESIAN_POINT ( 'NONE',  ( 14.57812500061451644, -4.541064518000419881, 2.621784821874995952 ) ) ;
#20496=CARTESIAN_POINT ( 'NONE',  ( 13.43437500061451750, 6.421520780324663323E-16, -5.243569643749999010 ) ) ;
#20497=VERTEX_POINT ( 'NONE', #56850 ) ;
#20499=CARTESIAN_POINT ( 'NONE',  ( 24.25312500061451715, 4.541064518000418104, -2.621784821874998173 ) ) ;
#20500=CARTESIAN_POINT ( 'NONE',  ( 26.96250000122903145, 0.000000000000000000, 4.999999999999998224 ) ) ;
#20502=CARTESIAN_POINT ( 'NONE',  ( 13.50000000000000178, -4.330127018922190985, -2.500000000000001332 ) ) ;
#20503=CARTESIAN_POINT ( 'NONE',  ( 23.47500000122903430, -5.773502691896255534, -1.060575238724906372E-15 ) ) ;
#20504=CARTESIAN_POINT ( 'NONE',  ( 19.34062500061451573, 6.054752690667223547, 3.707466751127219781E-16 ) ) ;
#20505=ORIENTED_EDGE ( 'NONE', *, *, #30054, .T. ) ;
#20506=CARTESIAN_POINT ( 'NONE',  ( 22.76249999999999574, 2.886751345948126879, 4.999999999999999112 ) ) ;
#20507=CARTESIAN_POINT ( 'NONE',  ( 23.82187500061451502, 3.027376345333613106, -5.243569643749998122 ) ) ;
#20508=VERTEX_POINT ( 'NONE', #29156 ) ;
#20509=FACE_OUTER_BOUND ( 'NONE', #46973, .T. ) ;
#20510=CARTESIAN_POINT ( 'NONE',  ( 9.665625000614515017, -6.054752690667223547, -1.112240025338166033E-15 ) ) ;
#20511=CARTESIAN_POINT ( 'NONE',  ( 3.665625000614517681, 3.027376345333611329, 5.243569643749999010 ) ) ;
#20513=CARTESIAN_POINT ( 'NONE',  ( 27.70312500061451289, -4.541064518000417216, -2.621784821875001281 ) ) ;
#20514=CARTESIAN_POINT ( 'NONE',  ( 18.33749999999999858, -2.886751345948129988, 4.999999999999997335 ) ) ;
#20515=CARTESIAN_POINT ( 'NONE',  ( 27.33750000000000213, -2.886751345948129988, 4.999999999999997335 ) ) ;
#20516=CARTESIAN_POINT ( 'NONE',  ( 3.089506346739232967, 3.931278485869285522, -3.469880700456108968 ) ) ;
#20517=CARTESIAN_POINT ( 'NONE',  ( 6.609375000614519102, -4.541064518000417216, -2.621784821875001281 ) ) ;
#20518=CARTESIAN_POINT ( 'NONE',  ( 17.33437500061451431, -4.541064518000419881, 2.621784821874995952 ) ) ;
#20519=CARTESIAN_POINT ( 'NONE',  ( 19.83750000122903145, -4.330127018922194537, 2.499999999999995559 ) ) ;
#20521=CARTESIAN_POINT ( 'NONE',  ( 27.36562500061451786, 3.027376345333613106, -5.243569643749998122 ) ) ;
#20522=CARTESIAN_POINT ( 'NONE',  ( 28.69687500061451502, -3.027376345333610441, -5.243569643749999898 ) ) ;
#20523=CARTESIAN_POINT ( 'NONE',  ( 12.75000000000000178, 4.330127018922192761, -2.499999999999997780 ) ) ;
#20524=CARTESIAN_POINT ( 'NONE',  ( 11.24062500061451608, 6.054752690667223547, 3.707466751127219781E-16 ) ) ;
#20525=LINE ( 'NONE', #42717, #13594 ) ;
#20527=CARTESIAN_POINT ( 'NONE',  ( 27.74062500061451431, -3.027376345333610441, -5.243569643749999898 ) ) ;
#20528=CARTESIAN_POINT ( 'NONE',  ( 18.56250000122903288, -4.330127018922190985, -2.500000000000001332 ) ) ;
#20531=CARTESIAN_POINT ( 'NONE',  ( 5.840625000614516615, 6.054752690667223547, 3.707466751127219781E-16 ) ) ;
#20532=CARTESIAN_POINT ( 'NONE',  ( 21.19687500061451502, 6.054752690667223547, 3.707466751127219781E-16 ) ) ;
#20534=CARTESIAN_POINT ( 'NONE',  ( 4.243569643749999898, 17.34687500061451715, 32.45002607614398471 ) ) ;
#20535=CARTESIAN_POINT ( 'NONE',  ( 23.85937500061451644, 4.541064518000418104, -2.621784821874998173 ) ) ;
#20536=CARTESIAN_POINT ( 'NONE',  ( 5.100000000000000533, 4.330127018922192761, -2.499999999999997780 ) ) ;
#20537=CARTESIAN_POINT ( 'NONE',  ( 1.999999999999998668, 11.41250000122903430, 26.53589838486224650 ) ) ;
#20538=CARTESIAN_POINT ( 'NONE',  ( 13.19062500061451537, -3.027376345333614438, 5.243569643749998122 ) ) ;
#20539=CARTESIAN_POINT ( 'NONE',  ( 3.187500001229033764, -4.330127018922194537, 2.499999999999995559 ) ) ;
#20540=CARTESIAN_POINT ( 'NONE',  ( 9.796875000614519990, -3.027376345333610441, -5.243569643749999898 ) ) ;
#20542=CARTESIAN_POINT ( 'NONE',  ( 11.05312500061451608, -4.541064518000417216, -2.621784821875001281 ) ) ;
#20543=CARTESIAN_POINT ( 'NONE',  ( 15.42187500061451821, 3.027376345333611329, 5.243569643749999010 ) ) ;
#20544=DIRECTION ( 'NONE',  ( -0.000000000000000000, -1.000000000000000000, -0.000000000000000000 ) ) ;
#20545=CARTESIAN_POINT ( 'NONE',  ( 20.62500000122903288, 2.886751345948126879, 4.999999999999999112 ) ) ;
#20546=CARTESIAN_POINT ( 'NONE',  ( 11.14687500061451608, -3.027376345333610441, -5.243569643749999898 ) ) ;
#20547=CARTESIAN_POINT ( 'NONE',  ( 12.44062500061451537, -3.027376345333610441, -5.243569643749999898 ) ) ;
#20548=ADVANCED_FACE ( 'NONE', ( #22514 ), #45787, .F. ) ;
#20550=CARTESIAN_POINT ( 'NONE',  ( 22.09687500061451715, 6.054752690667223547, 3.707466751127219781E-16 ) ) ;
#20552=CARTESIAN_POINT ( 'NONE',  ( -0.1380872570243143471, 5.000000000000001776, 34.00000000000000000 ) ) ;
#20553=CARTESIAN_POINT ( 'NONE',  ( 3.211615563433569243, 3.832169812614073745, -3.409004327678504698 ) ) ;
#20554=CARTESIAN_POINT ( 'NONE',  ( 2.121784821875001281, 13.70937500061451786, -26.32496088578401938 ) ) ;
#20555=CARTESIAN_POINT ( 'NONE',  ( 15.52500000122903323, 2.886751345948129099, -4.999999999999998224 ) ) ;
#20556=CARTESIAN_POINT ( 'NONE',  ( 9.496875000614517504, 6.054752690667223547, 3.707466751127219781E-16 ) ) ;
#20557=CARTESIAN_POINT ( 'NONE',  ( -3.000416591977282496E-16, 17.89062500061451644, -34.90005215228797653 ) ) ;
#20558=CARTESIAN_POINT ( 'NONE',  ( 17.28750000122903430, 6.123233995736764310E-16, -4.999999999999998224 ) ) ;
#20559=CARTESIAN_POINT ( 'NONE',  ( 10.11562500061451608, -6.054752690667223547, -1.112240025338166033E-15 ) ) ;
#20560=VECTOR ( 'NONE', #2752, 1000.000000000000000 ) ;
#20562=CARTESIAN_POINT ( 'NONE',  ( 15.41250000000000142, 2.886751345948129099, -4.999999999999998224 ) ) ;
#20563=CARTESIAN_POINT ( 'NONE',  ( 10.53750000122903252, 6.123233995736764310E-16, -4.999999999999998224 ) ) ;
#20564=CARTESIAN_POINT ( 'NONE',  ( 10.39687500061451786, 6.054752690667223547, 3.707466751127219781E-16 ) ) ;
#20565=CARTESIAN_POINT ( 'NONE',  ( -2.000000000000000000, 14.18750000122903288, 26.53589838486224650 ) ) ;
#20566=CARTESIAN_POINT ( 'NONE',  ( 10.53750000122903252, 6.123233995736764310E-16, -4.999999999999998224 ) ) ;
#20567=CARTESIAN_POINT ( 'NONE',  ( 18.78750000122903430, 4.330127018922191873, 2.499999999999999556 ) ) ;
#20569=CARTESIAN_POINT ( 'NONE',  ( 14.12812500061451715, -4.541064518000419881, 2.621784821874995952 ) ) ;
#20570=CARTESIAN_POINT ( 'NONE',  ( 20.35312500061451502, 0.000000000000000000, 5.243569643749999010 ) ) ;
#20571=CARTESIAN_POINT ( 'NONE',  ( 27.60000000122903430, -2.886751345948125991, -5.000000000000000000 ) ) ;
#20572=AXIS2_PLACEMENT_3D ( 'NONE', #63324, #58129, #69603 ) ;
#20573=CARTESIAN_POINT ( 'NONE',  ( 2.953125000614516438, -4.541064518000417216, -2.621784821875001281 ) ) ;
#20574=CARTESIAN_POINT ( 'NONE',  ( 24.41250000000000142, 2.886751345948129099, -4.999999999999998224 ) ) ;
#20575=CARTESIAN_POINT ( 'NONE',  ( 28.38749999999999929, -2.886751345948130432, -4.999999999999991118 ) ) ;
#20576=VECTOR ( 'NONE', #71302, 1000.000000000000000 ) ;
#20578=CARTESIAN_POINT ( 'NONE',  ( 29.22187500061451715, 3.027376345333613106, -5.243569643749998122 ) ) ;
#20579=CARTESIAN_POINT ( 'NONE',  ( -1.071796769724496556, 16.04240381056766651, 33.99999999999998579 ) ) ;
#20580=CARTESIAN_POINT ( 'NONE',  ( 12.41250000122903430, 4.330127018922192761, -2.499999999999997780 ) ) ;
#20581=CARTESIAN_POINT ( 'NONE',  ( 4.087500000000001243, -2.886751345948125991, -5.000000000000000000 ) ) ;
#20584=CARTESIAN_POINT ( 'NONE',  ( 7.809375000614519280, 0.000000000000000000, 5.243569643749999010 ) ) ;
#20585=CARTESIAN_POINT ( 'NONE',  ( 25.30312500061451431, 0.000000000000000000, 5.243569643749999010 ) ) ;
#20588=CARTESIAN_POINT ( 'NONE',  ( 3.737800990869664552, -3.321044174263025006, 4.023844142270481150 ) ) ;
#20589=CARTESIAN_POINT ( 'NONE',  ( 4.996875000614516615, 6.054752690667223547, 3.707466751127219781E-16 ) ) ;
#20590=CARTESIAN_POINT ( 'NONE',  ( 7.996875000614519280, -3.027376345333610441, -5.243569643749999898 ) ) ;
#20591=CARTESIAN_POINT ( 'NONE',  ( 29.85937500061451644, 0.000000000000000000, 5.243569643749999010 ) ) ;
#20592=CARTESIAN_POINT ( 'NONE',  ( 9.001249775931846008E-16, 13.16562500061459673, 34.90005215228797653 ) ) ;
#20593=CARTESIAN_POINT ( 'NONE',  ( 22.83749999999999858, -2.886751345948129988, 4.999999999999997335 ) ) ;
#20594=CARTESIAN_POINT ( 'NONE',  ( 29.21249999999999858, -5.773502691896255534, -1.060575238724906372E-15 ) ) ;
#20595=CARTESIAN_POINT ( 'NONE',  ( 3.637500000000001954, -2.886751345948125991, -5.000000000000000000 ) ) ;
#20598=ORIENTED_EDGE ( 'NONE', *, *, #25778, .T. ) ;
#20599=CARTESIAN_POINT ( 'NONE',  ( 18.32812500061451644, 6.421520780324663323E-16, -5.243569643749999010 ) ) ;
#20600=CARTESIAN_POINT ( 'NONE',  ( 9.590625000614517504, -3.027376345333614438, 5.243569643749998122 ) ) ;
#20602=CARTESIAN_POINT ( 'NONE',  ( 7.471875000614519813, -6.054752690667223547, -1.112240025338166033E-15 ) ) ;
#20603=CARTESIAN_POINT ( 'NONE',  ( 23.96249999999999858, 2.886751345948129099, -4.999999999999998224 ) ) ;
#20604=CARTESIAN_POINT ( 'NONE',  ( 20.77500000122903145, -5.773502691896255534, -1.060575238724906372E-15 ) ) ;
#20606=CARTESIAN_POINT ( 'NONE',  ( 28.52812500061451573, -4.541064518000419881, 2.621784821874995952 ) ) ;
#20607=CARTESIAN_POINT ( 'NONE',  ( 3.999999999999999112, 10.88750000122903394, 30.00000000000000000 ) ) ;
#20608=CARTESIAN_POINT ( 'NONE',  ( 8.334375000614516082, -4.541064518000419881, 2.621784821874995952 ) ) ;
#20609=CARTESIAN_POINT ( 'NONE',  ( 14.07187500061451679, 3.027376345333611329, 5.243569643749999010 ) ) ;
#20610=CARTESIAN_POINT ( 'NONE',  ( 25.05937500061451573, -4.541064518000417216, -2.621784821875001281 ) ) ;
#20613=CARTESIAN_POINT ( 'NONE',  ( 18.34687500061451715, -3.027376345333610441, -5.243569643749999898 ) ) ;
#20615=CARTESIAN_POINT ( 'NONE',  ( 10.62187500061451928, -6.054752690667223547, -1.112240025338166033E-15 ) ) ;
#20617=CARTESIAN_POINT ( 'NONE',  ( 23.21250000000000213, 2.886751345948126879, 4.999999999999999112 ) ) ;
#20619=CARTESIAN_POINT ( 'NONE',  ( 29.96249999999999858, 2.886751345948126879, 4.999999999999998224 ) ) ;
#20621=CARTESIAN_POINT ( 'NONE',  ( 11.42812500061451608, -4.541064518000419881, 2.621784821874995952 ) ) ;
#20622=CARTESIAN_POINT ( 'NONE',  ( 29.29687500061451644, 6.054752690667223547, 3.707466751127219781E-16 ) ) ;
#20623=CARTESIAN_POINT ( 'NONE',  ( 3.999999999999998668, 10.02500000122903323, -32.30940107675850470 ) ) ;
#20624=CARTESIAN_POINT ( 'NONE',  ( 12.03749999999999964, -2.886751345948129988, 4.999999999999997335 ) ) ;
#20625=CARTESIAN_POINT ( 'NONE',  ( 2.000000000000001332, 18.46250000122903501, 33.46410161513774995 ) ) ;
#20626=CARTESIAN_POINT ( 'NONE',  ( 12.71250000122903145, -4.330127018922190985, -2.500000000000001332 ) ) ;
#20627=CARTESIAN_POINT ( 'NONE',  ( 21.57187500061451502, 3.027376345333613106, -5.243569643749998122 ) ) ;
#20628=CARTESIAN_POINT ( 'NONE',  ( 17.10937500061451999, 4.541064518000418104, -2.621784821874998173 ) ) ;
#20630=VERTEX_POINT ( 'NONE', #72770 ) ;
#20631=CARTESIAN_POINT ( 'NONE',  ( 16.86562500061451786, -6.054752690667223547, -1.112240025338166033E-15 ) ) ;
#20633=CARTESIAN_POINT ( 'NONE',  ( 28.12500000122902932, 2.886751345948129099, -4.999999999999998224 ) ) ;
#20634=CARTESIAN_POINT ( 'NONE',  ( 18.15937500061451715, 0.000000000000000000, 5.243569643749999010 ) ) ;
#20635=CARTESIAN_POINT ( 'NONE',  ( 29.10937500061451644, -4.541064518000417216, -2.621784821875001281 ) ) ;
#20636=CARTESIAN_POINT ( 'NONE',  ( 4.115625000614516082, 3.027376345333611329, 5.243569643749999010 ) ) ;
#20637=CARTESIAN_POINT ( 'NONE',  ( 19.49062500061451431, -3.027376345333614438, 5.243569643749998122 ) ) ;
#20638=CARTESIAN_POINT ( 'NONE',  ( 27.94687500061451502, 6.054752690667223547, 3.707466751127219781E-16 ) ) ;
#20639=CARTESIAN_POINT ( 'NONE',  ( 4.243569643749999010, 13.31562500061451537, 27.54997392385601174 ) ) ;
#20640=CARTESIAN_POINT ( 'NONE',  ( 17.40000000122903145, 5.773502691896255534, 3.535250795749688894E-16 ) ) ;
#20642=CARTESIAN_POINT ( 'NONE',  ( 7.753125000614518036, 0.000000000000000000, 5.243569643749999010 ) ) ;
#20643=CARTESIAN_POINT ( 'NONE',  ( 26.84062500061451573, -3.027376345333610441, -5.243569643749999898 ) ) ;
#20645=CARTESIAN_POINT ( 'NONE',  ( 23.82187500061451502, 3.027376345333613106, -5.243569643749998122 ) ) ;
#20646=CARTESIAN_POINT ( 'NONE',  ( 23.40000000122903145, -2.886751345948129988, 4.999999999999997335 ) ) ;
#20647=CARTESIAN_POINT ( 'NONE',  ( 22.75312500061451360, -4.541064518000417216, -2.621784821875001281 ) ) ;
#20648=CARTESIAN_POINT ( 'NONE',  ( 17.22187500061451715, 3.027376345333611329, 5.243569643749999010 ) ) ;
#20649=CARTESIAN_POINT ( 'NONE',  ( 13.30312500061451786, -4.541064518000417216, -2.621784821875001281 ) ) ;
#20650=CARTESIAN_POINT ( 'NONE',  ( 9.001249775931846008E-16, 14.12187500061451750, 34.90005215228797653 ) ) ;
#20651=CARTESIAN_POINT ( 'NONE',  ( 19.11562500061451431, -6.054752690667223547, -1.112240025338166033E-15 ) ) ;
#20652=CARTESIAN_POINT ( 'NONE',  ( 29.54062500061451502, -3.027376345333610441, -5.243569643749999898 ) ) ;
#20653=VERTEX_POINT ( 'NONE', #61672 ) ;
#20654=CARTESIAN_POINT ( 'NONE',  ( 23.66250000000000142, 2.886751345948126879, 4.999999999999999112 ) ) ;
#20655=CARTESIAN_POINT ( 'NONE',  ( -3.000416591977282496E-16, 18.84687500061452070, -34.90005215228797653 ) ) ;
#20656=CARTESIAN_POINT ( 'NONE',  ( 1.915124944151129771, -4.721073491456853510, 1.915124944151129771 ) ) ;
#20657=CARTESIAN_POINT ( 'NONE',  ( 26.01562500061451289, 3.027376345333613106, -5.243569643749998122 ) ) ;
#20658=CARTESIAN_POINT ( 'NONE',  ( 4.378125000614518925, 6.421520780324663323E-16, -5.243569643749999010 ) ) ;
#20660=CARTESIAN_POINT ( 'NONE',  ( 18.75000000122903288, 5.773502691896255534, 3.535250795749688894E-16 ) ) ;
#20662=CARTESIAN_POINT ( 'NONE',  ( 25.94062500061451715, -3.027376345333610441, -5.243569643749999898 ) ) ;
#20663=CARTESIAN_POINT ( 'NONE',  ( 22.91249999999999432, -5.773502691896255534, -1.060575238724906372E-15 ) ) ;
#20664=CARTESIAN_POINT ( 'NONE',  ( 27.36562500061451786, 3.027376345333613106, -5.243569643749998122 ) ) ;
#20665=CARTESIAN_POINT ( 'NONE',  ( 7.565625000614518036, 3.027376345333613106, -5.243569643749998122 ) ) ;
#20667=CARTESIAN_POINT ( 'NONE',  ( 24.17812500061451786, 6.421520780324663323E-16, -5.243569643749999010 ) ) ;
#20668=CARTESIAN_POINT ( 'NONE',  ( 5.240625000614516971, -3.027376345333610441, -5.243569643749999898 ) ) ;
#20670=CARTESIAN_POINT ( 'NONE',  ( 3.065625000614517592, 3.027376345333613106, -5.243569643749998122 ) ) ;
#20671=CARTESIAN_POINT ( 'NONE',  ( 2.000000000000001332, 13.06250000122903465, -26.53589838486224650 ) ) ;
#20672=CARTESIAN_POINT ( 'NONE',  ( -1.071796769724488563, 13.79240381056766829, -26.00000000000000000 ) ) ;
#20673=AXIS2_PLACEMENT_3D ( 'NONE', #27458, #10098, #15989 ) ;
#20674=CARTESIAN_POINT ( 'NONE',  ( 9.674999999999998934, 4.330127018922191873, 2.499999999999999556 ) ) ;
#20675=CARTESIAN_POINT ( 'NONE',  ( 10.99687500061451750, -3.027376345333614438, 5.243569643749998122 ) ) ;
#20676=CARTESIAN_POINT ( 'NONE',  ( 6.225000001229036073, 2.886751345948126879, 4.999999999999999112 ) ) ;
#20677=CARTESIAN_POINT ( 'NONE',  ( 13.54687500061451999, 6.054752690667223547, 3.707466751127219781E-16 ) ) ;
#20679=CARTESIAN_POINT ( 'NONE',  ( 6.159375000614517148, -4.541064518000417216, -2.621784821875001281 ) ) ;
#20680=FACE_OUTER_BOUND ( 'NONE', #59290, .T. ) ;
#20681=CARTESIAN_POINT ( 'NONE',  ( 13.20937500061451786, 0.000000000000000000, 5.243569643749999010 ) ) ;
#20682=DIRECTION ( 'NONE',  ( 0.000000000000000000, 0.000000000000000000, -1.000000000000000000 ) ) ;
#20683=CARTESIAN_POINT ( 'NONE',  ( 21.06562500061451715, 3.027376345333613106, -5.243569643749998122 ) ) ;
#20684=CARTESIAN_POINT ( 'NONE',  ( 30.00000000000000000, 6.123233995736764310E-16, -4.999999999999998224 ) ) ;
#20685=CARTESIAN_POINT ( 'NONE',  ( 1.626862140677534273E-15, 16.51249999999999929, 34.00000000000000000 ) ) ;
#20686=CARTESIAN_POINT ( 'NONE',  ( 23.89687500061451786, 6.054752690667223547, 3.707466751127219781E-16 ) ) ;
#20687=CARTESIAN_POINT ( 'NONE',  ( 1.626862140677534273E-15, 13.92500000122903181, -26.00000000000000355 ) ) ;
#20688=CARTESIAN_POINT ( 'NONE',  ( 4.640625000614518214, -3.027376345333614438, 5.243569643749998122 ) ) ;
#20690=CARTESIAN_POINT ( 'NONE',  ( 18.47812500061451857, 4.541064518000418104, 2.621784821874999949 ) ) ;
#20691=CARTESIAN_POINT ( 'NONE',  ( 15.42187500061451821, 3.027376345333611329, 5.243569643749999010 ) ) ;
#20692=CARTESIAN_POINT ( 'NONE',  ( 29.81250000000000000, 2.886751345948129099, -4.999999999999998224 ) ) ;
#20693=CARTESIAN_POINT ( 'NONE',  ( 26.21250000122903501, -4.330127018922190985, -2.500000000000001332 ) ) ;
#20694=CARTESIAN_POINT ( 'NONE',  ( 6.496875000614517504, -3.027376345333614438, 5.243569643749998122 ) ) ;
#20695=CARTESIAN_POINT ( 'NONE',  ( 16.28437500061452070, 4.541064518000418104, 2.621784821874999949 ) ) ;
#20697=CARTESIAN_POINT ( 'NONE',  ( 24.48749999999999716, 5.773502691896255534, 3.535250795749688894E-16 ) ) ;
#20698=CARTESIAN_POINT ( 'NONE',  ( 3.225000001229033408, -5.773502691896255534, -1.060575238724906372E-15 ) ) ;
#20699=CARTESIAN_POINT ( 'NONE',  ( 27.15937500061451360, 0.000000000000000000, 5.243569643749999010 ) ) ;
#20700=CARTESIAN_POINT ( 'NONE',  ( 17.33437500061451431, -4.541064518000419881, 2.621784821874995952 ) ) ;
#20702=CARTESIAN_POINT ( 'NONE',  ( 30.00000000000000000, 0.000000000000000000, 4.999999999999998224 ) ) ;
#20703=CARTESIAN_POINT ( 'NONE',  ( 8.250000000000000000, 4.330127018922192761, -2.499999999999997780 ) ) ;
#20705=CARTESIAN_POINT ( 'NONE',  ( 20.20312500061451644, 4.541064518000418104, -2.621784821874998173 ) ) ;
#20706=CARTESIAN_POINT ( 'NONE',  ( 8.287499999999999645, 5.773502691896255534, 3.535250795749688894E-16 ) ) ;
#20707=EDGE_CURVE ( 'NONE', #3090, #2356, #773, .T. ) ;
#20708=CARTESIAN_POINT ( 'NONE',  ( 4.528125000614516615, 4.541064518000418104, 2.621784821874999949 ) ) ;
#20709=CARTESIAN_POINT ( 'NONE',  ( 18.52499999999999858, 6.123233995736764310E-16, -4.999999999999998224 ) ) ;
#20710=CARTESIAN_POINT ( 'NONE',  ( 17.54062500061451502, 6.054752690667223547, 3.707466751127219781E-16 ) ) ;
#20711=CARTESIAN_POINT ( 'NONE',  ( 22.95000000122903216, -2.886751345948129988, 4.999999999999997335 ) ) ;
#20712=CARTESIAN_POINT ( 'NONE',  ( 6.000084452983056593, 7.999936660264885369, 29.59830633522030396 ) ) ;
#20713=CARTESIAN_POINT ( 'NONE',  ( 29.63437500061451502, 6.421520780324663323E-16, -5.243569643749999010 ) ) ;
#20715=VERTEX_POINT ( 'NONE', #62402 ) ;
#20716=CARTESIAN_POINT ( 'NONE',  ( 16.94062500061451715, -3.027376345333610441, -5.243569643749999898 ) ) ;
#20717=CARTESIAN_POINT ( 'NONE',  ( 24.85312500061451502, 0.000000000000000000, 5.243569643749999010 ) ) ;
#20718=CARTESIAN_POINT ( 'NONE',  ( 25.20937500061451431, 4.541064518000418104, -2.621784821874998173 ) ) ;
#20719=CARTESIAN_POINT ( 'NONE',  ( 8.362500000000002487, 2.886751345948126879, 4.999999999999999112 ) ) ;
#20720=CARTESIAN_POINT ( 'NONE',  ( 11.05312500061451608, -4.541064518000417216, -2.621784821875001281 ) ) ;
#20721=CARTESIAN_POINT ( 'NONE',  ( 26.05312500061451431, 4.541064518000418104, -2.621784821874998173 ) ) ;
#20722=CARTESIAN_POINT ( 'NONE',  ( 16.88437500061451502, -4.541064518000419881, 2.621784821874995952 ) ) ;
#20723=CARTESIAN_POINT ( 'NONE',  ( 9.478125000614515017, 4.541064518000418104, 2.621784821874999949 ) ) ;
#20724=CARTESIAN_POINT ( 'NONE',  ( 7.087500001229034119, 4.330127018922191873, 2.499999999999999556 ) ) ;
#20725=CARTESIAN_POINT ( 'NONE',  ( -2.121784821874999949, 19.72812500061451857, 26.32496088578401938 ) ) ;
#20726=CARTESIAN_POINT ( 'NONE',  ( 23.36250000122903359, 0.000000000000000000, 4.999999999999998224 ) ) ;
#20728=CARTESIAN_POINT ( 'NONE',  ( 14.87812500061451537, 4.541064518000418104, 2.621784821874999949 ) ) ;
#20729=CARTESIAN_POINT ( 'NONE',  ( 8.559375000614515727, 4.541064518000418104, -2.621784821874998173 ) ) ;
#20730=CARTESIAN_POINT ( 'NONE',  ( 6.046875000614519102, -3.027376345333614438, 5.243569643749998122 ) ) ;
#20731=ORIENTED_EDGE ( 'NONE', *, *, #41134, .T. ) ;
#20732=CARTESIAN_POINT ( 'NONE',  ( 3.999999999999999112, 13.47500000000000142, 30.00000000000000000 ) ) ;
#20733=CARTESIAN_POINT ( 'NONE',  ( 18.36562500061451431, 3.027376345333613106, -5.243569643749998122 ) ) ;
#20735=CARTESIAN_POINT ( 'NONE',  ( 15.60937500061451644, -4.541064518000417216, -2.621784821875001281 ) ) ;
#20736=CARTESIAN_POINT ( 'NONE',  ( 19.22812500061451502, 6.421520780324663323E-16, -5.243569643749999010 ) ) ;
#20737=CARTESIAN_POINT ( 'NONE',  ( 2.000000000000001332, 12.95000000000000107, 33.46410161513774995 ) ) ;
#20738=CARTESIAN_POINT ( 'NONE',  ( 27.89062500061451289, 6.054752690667223547, 3.707466751127219781E-16 ) ) ;
#20739=CARTESIAN_POINT ( 'NONE',  ( 6.937500001229033764, 6.123233995736764310E-16, -4.999999999999998224 ) ) ;
#20740=AXIS2_PLACEMENT_3D ( 'NONE', #22253, #5266, #38525 ) ;
#20741=ORIENTED_EDGE ( 'NONE', *, *, #24238, .T. ) ;
#20742=CARTESIAN_POINT ( 'NONE',  ( 2.700000001229035718, -2.886751345948129988, 4.999999999999997335 ) ) ;
#20743=CARTESIAN_POINT ( 'NONE',  ( -1.999999999999997113, 17.37500000000000000, -26.53589838486224295 ) ) ;
#20744=CARTESIAN_POINT ( 'NONE',  ( 21.82500000122903572, 2.886751345948129099, -4.999999999999998224 ) ) ;
#20746=CARTESIAN_POINT ( 'NONE',  ( 6.459375000614518747, 0.000000000000000000, 5.243569643749999010 ) ) ;
#20747=CARTESIAN_POINT ( 'NONE',  ( 1.071796769724484344, 15.18259618943233669, 34.00000000000000000 ) ) ;
#20748=CARTESIAN_POINT ( 'NONE',  ( 12.62812500061451537, 4.541064518000418104, 2.621784821874999949 ) ) ;
#20749=CARTESIAN_POINT ( 'NONE',  ( 7.584375000614516082, 6.421520780324663323E-16, -5.243569643749999010 ) ) ;
#20750=CARTESIAN_POINT ( 'NONE',  ( 27.07500000122903216, -5.773502691896255534, -1.060575238724906372E-15 ) ) ;
#20751=CARTESIAN_POINT ( 'NONE',  ( 18.42187500061451999, 3.027376345333612662, -5.243569643749998122 ) ) ;
#20752=CARTESIAN_POINT ( 'NONE',  ( 4.321875000614517681, -6.054752690667223547, -1.112240025338166033E-15 ) ) ;
#20753=CARTESIAN_POINT ( 'NONE',  ( -3.999999999999999112, 11.00000000000000178, 30.00000000000000000 ) ) ;
#20754=CARTESIAN_POINT ( 'NONE',  ( 6.028125000614517504, -4.541064518000419881, 2.621784821874995952 ) ) ;
#20755=CARTESIAN_POINT ( 'NONE',  ( 14.80312500061451608, 4.541064518000418104, -2.621784821874998173 ) ) ;
#20757=CARTESIAN_POINT ( 'NONE',  ( 12.10312500061451857, 4.541064518000418104, -2.621784821874998173 ) ) ;
#20758=CARTESIAN_POINT ( 'NONE',  ( 5.737500001229033586, 4.330127018922191873, 2.499999999999999556 ) ) ;
#20759=CARTESIAN_POINT ( 'NONE',  ( 8.165625000614516793, 3.027376345333611329, 5.243569643749999010 ) ) ;
#20761=CARTESIAN_POINT ( 'NONE',  ( 9.262499999999999289, 2.886751345948126879, 4.999999999999999112 ) ) ;
#20763=CARTESIAN_POINT ( 'NONE',  ( 5.100000001229034297, -2.886751345948125991, -5.000000000000000000 ) ) ;
#20764=CARTESIAN_POINT ( 'NONE',  ( 16.87500000000000000, 4.330127018922191873, 2.499999999999999556 ) ) ;
#20765=CARTESIAN_POINT ( 'NONE',  ( 17.33437500061451431, -4.541064518000419881, 2.621784821874995952 ) ) ;
#20766=CARTESIAN_POINT ( 'NONE',  ( 14.62500000122903288, 2.886751345948129099, -4.999999999999998224 ) ) ;
#20768=CIRCLE ( 'NONE', #24308, 4.000000000000000000 ) ;
#20769=CARTESIAN_POINT ( 'NONE',  ( -2.121784821874999949, 16.12812500061451715, -33.67503911421598417 ) ) ;
#20773=DIRECTION ( 'NONE',  ( -1.000000000000000000, -0.000000000000000000, -0.000000000000000000 ) ) ;
#20774=DIRECTION ( 'NONE',  ( 0.000000000000000000, 0.000000000000000000, 1.000000000000000000 ) ) ;
#20775=CARTESIAN_POINT ( 'NONE',  ( 16.58437500061451786, 6.421520780324663323E-16, -5.243569643749999010 ) ) ;
#20776=CARTESIAN_POINT ( 'NONE',  ( 26.66250000000000142, 2.886751345948129099, -4.999999999999998224 ) ) ;
#20777=CARTESIAN_POINT ( 'NONE',  ( 12.74062500061451786, -3.027376345333614438, 5.243569643749998122 ) ) ;
#20780=CARTESIAN_POINT ( 'NONE',  ( 22.28437500061451715, -4.541064518000419881, 2.621784821874995952 ) ) ;
#20782=CARTESIAN_POINT ( 'NONE',  ( 8.465625000614515727, 3.027376345333613106, -5.243569643749998122 ) ) ;
#20783=CARTESIAN_POINT ( 'NONE',  ( 13.69687500061451679, -3.027376345333614438, 5.243569643749998122 ) ) ;
#20784=ORIENTED_EDGE ( 'NONE', *, *, #420, .T. ) ;
#20785=CARTESIAN_POINT ( 'NONE',  ( 23.37187500061451573, 3.027376345333613106, -5.243569643749998122 ) ) ;
#20786=CARTESIAN_POINT ( 'NONE',  ( 27.02812500061451573, 4.541064518000418104, 2.621784821874999949 ) ) ;
#20788=( BOUNDED_CURVE ( )  B_SPLINE_CURVE ( 3, ( #47573, #8777, #64560, #31312 ),
 .UNSPECIFIED., .F., .F. ) 
 B_SPLINE_CURVE_WITH_KNOTS ( ( 4, 4 ),
 ( 3.141592653589793116, 4.712388980384689674 ),
 .UNSPECIFIED. ) 
 CURVE ( )  GEOMETRIC_REPRESENTATION_ITEM ( )  RATIONAL_B_SPLINE_CURVE ( ( 1.000000000000000000, 0.8047378541243649375, 0.8047378541243649375, 1.000000000000000000 ) ) 
 REPRESENTATION_ITEM ( '' )  );
#20789=CARTESIAN_POINT ( 'NONE',  ( 8.212500000000000355, 2.886751345948129099, -4.999999999999998224 ) ) ;
#20790=CARTESIAN_POINT ( 'NONE',  ( 17.47500000122903430, 2.886751345948126879, 4.999999999999999112 ) ) ;
#20793=ORIENTED_EDGE ( 'NONE', *, *, #28153, .F. ) ;
#20795=CARTESIAN_POINT ( 'NONE',  ( 15.63749999999999751, -2.886751345948129988, 4.999999999999997335 ) ) ;
#20796=CARTESIAN_POINT ( 'NONE',  ( 17.92500000000000071, -4.330127018922194537, 2.499999999999995559 ) ) ;
#20797=CARTESIAN_POINT ( 'NONE',  ( 10.45312500061451644, 0.000000000000000000, 5.243569643749999010 ) ) ;
#20798=ORIENTED_EDGE ( 'NONE', *, *, #21398, .T. ) ;
#20800=CARTESIAN_POINT ( 'NONE',  ( 4.243569643749999898, 16.93437500061451573, -30.00000000000000000 ) ) ;
#20801=CARTESIAN_POINT ( 'NONE',  ( 2.990625000614519191, -3.027376345333610441, -5.243569643749999898 ) ) ;
#20803=CARTESIAN_POINT ( 'NONE',  ( 9.637499999999999289, 5.773502691896255534, 3.535250795749688894E-16 ) ) ;
#20806=CARTESIAN_POINT ( 'NONE',  ( -2.121784821874999949, 13.42812500061451786, 26.32496088578401938 ) ) ;
#20807=CARTESIAN_POINT ( 'NONE',  ( 25.75312500061451715, 0.000000000000000000, 5.243569643749999010 ) ) ;
#20809=CARTESIAN_POINT ( 'NONE',  ( 30.00000000000000000, 0.000000000000000000, 0.000000000000000000 ) ) ;
#20810=CARTESIAN_POINT ( 'NONE',  ( 20.22187500061451715, 3.027376345333613106, -5.243569643749998122 ) ) ;
#20811=CARTESIAN_POINT ( 'NONE',  ( 19.97812500061451502, -4.541064518000419881, 2.621784821874995952 ) ) ;
#20812=CARTESIAN_POINT ( 'NONE',  ( -4.243569643749999898, 13.91562500061459495, -32.45002607614398471 ) ) ;
#20813=CARTESIAN_POINT ( 'NONE',  ( 22.31250000122903288, 4.330127018922192761, -2.499999999999997780 ) ) ;
#20814=CARTESIAN_POINT ( 'NONE',  ( 5.165625000614518569, -6.054752690667223547, -1.112240025338166033E-15 ) ) ;
#20816=CARTESIAN_POINT ( 'NONE',  ( 21.17812500061451431, 4.541064518000418104, 2.621784821874999949 ) ) ;
#20819=CARTESIAN_POINT ( 'NONE',  ( 15.38437500061451679, 4.541064518000418104, 2.621784821874999949 ) ) ;
#20820=CARTESIAN_POINT ( 'NONE',  ( 14.18437500061451750, -4.541064518000419881, 2.621784821874995952 ) ) ;
#20821=CARTESIAN_POINT ( 'NONE',  ( 24.19687500061451857, -3.027376345333610441, -5.243569643749999898 ) ) ;
#20822=CARTESIAN_POINT ( 'NONE',  ( -4.243569643749998122, 12.24687500061451750, 32.45002607614398471 ) ) ;
#20823=CARTESIAN_POINT ( 'NONE',  ( 4.340625000614515727, -3.027376345333610441, -5.243569643749999898 ) ) ;
#20824=CARTESIAN_POINT ( 'NONE',  ( 28.45312500061451289, 0.000000000000000000, 5.243569643749999010 ) ) ;
#20826=CARTESIAN_POINT ( 'NONE',  ( 29.16562500061451502, 3.027376345333613106, -5.243569643749998122 ) ) ;
#20828=CARTESIAN_POINT ( 'NONE',  ( -2.828200636599751609E-16, 18.08750000000000213, 25.38119784648299770 ) ) ;
#20830=CARTESIAN_POINT ( 'NONE',  ( 8.109375000614518214, 4.541064518000418104, -2.621784821874998173 ) ) ;
#20832=CARTESIAN_POINT ( 'NONE',  ( 13.87500000122903465, 2.886751345948126879, 4.999999999999999112 ) ) ;
#20833=CARTESIAN_POINT ( 'NONE',  ( 9.225000001229034297, 2.886751345948129099, -4.999999999999998224 ) ) ;
#20834=CARTESIAN_POINT ( 'NONE',  ( 5.878125000614517148, 4.541064518000418104, 2.621784821874999949 ) ) ;
#20837=CARTESIAN_POINT ( 'NONE',  ( 14.55937500061451573, 0.000000000000000000, 5.243569643749999010 ) ) ;
#20838=CARTESIAN_POINT ( 'NONE',  ( 4.000000000000000000, 17.60000000122903430, 32.30940107675849760 ) ) ;
#20840=CARTESIAN_POINT ( 'NONE',  ( 21.25312500061451715, 0.000000000000000000, 5.243569643749999010 ) ) ;
#20841=CARTESIAN_POINT ( 'NONE',  ( 6.853125000614516793, 0.000000000000000000, 5.243569643749999010 ) ) ;
#20842=CARTESIAN_POINT ( 'NONE',  ( 25.20937500061451431, 4.541064518000418104, -2.621784821874998173 ) ) ;
#20843=CARTESIAN_POINT ( 'NONE',  ( 7.828125000614517326, -4.541064518000419881, 2.621784821874995952 ) ) ;
#20845=CARTESIAN_POINT ( 'NONE',  ( 8.925000001229033586, 2.886751345948126879, 4.999999999999999112 ) ) ;
#20846=CARTESIAN_POINT ( 'NONE',  ( 22.79062500061451502, -3.027376345333610441, -5.243569643749999898 ) ) ;
#20847=CARTESIAN_POINT ( 'NONE',  ( 3.999999999999998668, 19.02500000122903501, -32.30940107675850470 ) ) ;
#20848=CARTESIAN_POINT ( 'NONE',  ( 11.40000000122903501, -2.886751345948125991, -5.000000000000000000 ) ) ;
#20850=CARTESIAN_POINT ( 'NONE',  ( 19.64062500061451644, -3.027376345333610441, -5.243569643749999898 ) ) ;
#20851=CARTESIAN_POINT ( 'NONE',  ( 16.37812500061451715, -4.541064518000419881, 2.621784821874995952 ) ) ;
#20853=CARTESIAN_POINT ( 'NONE',  ( 16.68750000000000000, -2.886751345948125991, -5.000000000000000000 ) ) ;
#20854=CARTESIAN_POINT ( 'NONE',  ( 10.46250000122903323, -4.330127018922190985, -2.500000000000001332 ) ) ;
#20855=CARTESIAN_POINT ( 'NONE',  ( 7.415625000614516793, -6.054752690667223547, -1.112240025338166033E-15 ) ) ;
#20856=CARTESIAN_POINT ( 'NONE',  ( 11.16562500061451679, 3.027376345333613106, -5.243569643749998122 ) ) ;
#20858=CARTESIAN_POINT ( 'NONE',  ( 24.45000000122903572, -2.886751345948125991, -5.000000000000000000 ) ) ;
#20859=CARTESIAN_POINT ( 'NONE',  ( 19.28437500061451360, 6.421520780324663323E-16, -5.243569643749999010 ) ) ;
#20861=AXIS2_PLACEMENT_3D ( 'NONE', #7674, #36114, #47205 ) ;
#20863=CARTESIAN_POINT ( 'NONE',  ( 4.237500001229036251, 6.123233995736764310E-16, -4.999999999999998224 ) ) ;
#20864=CARTESIAN_POINT ( 'NONE',  ( 4.584375000614516971, 4.541064518000418104, 2.621784821874999949 ) ) ;
#20865=CARTESIAN_POINT ( 'NONE',  ( 22.39687500061451075, -3.027376345333610441, -5.243569643749999898 ) ) ;
#20866=CARTESIAN_POINT ( 'NONE',  ( 10.53750000000000320, 5.773502691896255534, 3.535250795749688401E-16 ) ) ;
#20867=CARTESIAN_POINT ( 'NONE',  ( 19.07812500061451644, -4.541064518000419881, 2.621784821874995952 ) ) ;
#20868=CARTESIAN_POINT ( 'NONE',  ( 23.93437500061451573, 4.541064518000418104, 2.621784821874999949 ) ) ;
#20871=CARTESIAN_POINT ( 'NONE',  ( 27.83437500061451786, 6.421520780324663323E-16, -5.243569643749999010 ) ) ;
#20872=CARTESIAN_POINT ( 'NONE',  ( 6.534375000614517148, -4.541064518000419881, 2.621784821874995952 ) ) ;
#20873=CARTESIAN_POINT ( 'NONE',  ( 15.74062500061451608, 6.054752690667223547, 3.707466751127219781E-16 ) ) ;
#20874=CARTESIAN_POINT ( 'NONE',  ( 12.49687500061451573, -3.027376345333610441, -5.243569643749999898 ) ) ;
#20875=ORIENTED_EDGE ( 'NONE', *, *, #15762, .F. ) ;
#20876=DIRECTION ( 'NONE',  ( -1.000000000000000000, -0.000000000000000000, -0.000000000000000000 ) ) ;
#20877=CARTESIAN_POINT ( 'NONE',  ( 25.86562500061451431, -6.054752690667223547, -1.112240025338166033E-15 ) ) ;
#20879=CARTESIAN_POINT ( 'NONE',  ( 14.13750000000000107, 5.773502691896255534, 3.535250795749688894E-16 ) ) ;
#20880=CARTESIAN_POINT ( 'NONE',  ( 24.11250000122903359, 4.330127018922192761, -2.499999999999997780 ) ) ;
#20881=CARTESIAN_POINT ( 'NONE',  ( 18.32812500061451644, 6.421520780324663323E-16, -5.243569643749999010 ) ) ;
#20883=CARTESIAN_POINT ( 'NONE',  ( 22.64999999999999858, 4.330127018922192761, -2.499999999999997780 ) ) ;
#20884=CARTESIAN_POINT ( 'NONE',  ( 25.02187500061451431, -6.054752690667223547, -1.112240025338166033E-15 ) ) ;
#20885=EDGE_CURVE ( 'NONE', #62607, #60454, #11550, .T. ) ;
#20886=VERTEX_POINT ( 'NONE', #53128 ) ;
#20887=CARTESIAN_POINT ( 'NONE',  ( 10.64062500061451644, -3.027376345333610441, -5.243569643749999898 ) ) ;
#20888=CARTESIAN_POINT ( 'NONE',  ( 4.078125000614517326, 4.541064518000418104, 2.621784821874999949 ) ) ;
#20890=CARTESIAN_POINT ( 'NONE',  ( 26.42812500061451431, 6.421520780324663323E-16, -5.243569643749999010 ) ) ;
#20891=CARTESIAN_POINT ( 'NONE',  ( 17.25000000000000000, 4.330127018922192761, -2.499999999999997780 ) ) ;
#20892=CARTESIAN_POINT ( 'NONE',  ( 25.46249999999999858, 2.886751345948126879, 4.999999999999999112 ) ) ;
#20893=CARTESIAN_POINT ( 'NONE',  ( -3.000416591977282496E-16, 19.69062500061451360, 25.09994784771203058 ) ) ;
#20894=CARTESIAN_POINT ( 'NONE',  ( 7.584375000614516082, 6.421520780324663323E-16, -5.243569643749999010 ) ) ;
#20895=CARTESIAN_POINT ( 'NONE',  ( 16.73437500061451644, 4.541064518000418104, 2.621784821874999949 ) ) ;
#20896=CARTESIAN_POINT ( 'NONE',  ( 28.69687500061451502, -3.027376345333610441, -5.243569643749999898 ) ) ;
#20898=CARTESIAN_POINT ( 'NONE',  ( 26.05312500061451431, 4.541064518000418104, -2.621784821874998173 ) ) ;
#20899=CARTESIAN_POINT ( 'NONE',  ( 28.02187500061451431, 3.027376345333611329, 5.243569643749999010 ) ) ;
#20900=CARTESIAN_POINT ( 'NONE',  ( 0.000000000000000000, 20.00000000000000000, -30.00000000000000000 ) ) ;
#20901=CARTESIAN_POINT ( 'NONE',  ( 14.10000000000000142, 4.330127018922192761, -2.499999999999997780 ) ) ;
#20902=CARTESIAN_POINT ( 'NONE',  ( 10.26562500061451644, 3.027376345333613106, -5.243569643749998122 ) ) ;
#20904=LINE ( 'NONE', #19803, #19468 ) ;
#20905=CARTESIAN_POINT ( 'NONE',  ( 29.31562500061451715, 3.027376345333611329, 5.243569643749999010 ) ) ;
#20906=CARTESIAN_POINT ( 'NONE',  ( 15.52500000122903323, 2.886751345948129099, -4.999999999999998224 ) ) ;
#20907=DIRECTION ( 'NONE',  ( -0.000000000000000000, -1.000000000000000000, -0.000000000000000000 ) ) ;
#20909=CARTESIAN_POINT ( 'NONE',  ( 5.203125000614518214, -4.541064518000417216, -2.621784821875001281 ) ) ;
#20910=CARTESIAN_POINT ( 'NONE',  ( 20.82187500061451857, 3.027376345333611329, 5.243569643749999010 ) ) ;
#20911=CARTESIAN_POINT ( 'NONE',  ( -4.243569643749999898, 17.57187500061451502, 27.54997392385601529 ) ) ;
#20912=CARTESIAN_POINT ( 'NONE',  ( 20.78437500061451715, 4.541064518000418104, 2.621784821874999949 ) ) ;
#20913=CARTESIAN_POINT ( 'NONE',  ( 4.200000000000001954, 4.330127018922192761, -2.499999999999997780 ) ) ;
#20914=CARTESIAN_POINT ( 'NONE',  ( -3.999999999999997335, 9.800000001229033586, 32.30940107675850470 ) ) ;
#20915=CARTESIAN_POINT ( 'NONE',  ( 12.10312500061451857, 4.541064518000418104, -2.621784821874998173 ) ) ;
#20916=CARTESIAN_POINT ( 'NONE',  ( 4.612500001229032698, -4.330127018922190985, -2.500000000000001332 ) ) ;
#20917=CARTESIAN_POINT ( 'NONE',  ( 9.496875000614517504, 6.054752690667223547, 3.707466751127219781E-16 ) ) ;
#20919=CARTESIAN_POINT ( 'NONE',  ( 9.103125000614515017, 0.000000000000000000, 5.243569643749999010 ) ) ;
#20920=CARTESIAN_POINT ( 'NONE',  ( 14.52187500061451608, 3.027376345333611329, 5.243569643749999010 ) ) ;
#20922=CARTESIAN_POINT ( 'NONE',  ( 20.88750000122903572, 6.123233995736764310E-16, -4.999999999999998224 ) ) ;
#20923=CARTESIAN_POINT ( 'NONE',  ( 9.871875000614517504, 3.027376345333613106, -5.243569643749998122 ) ) ;
#20924=CARTESIAN_POINT ( 'NONE',  ( 13.11562500061451786, 3.027376345333611329, 5.243569643749999010 ) ) ;
#20926=CARTESIAN_POINT ( 'NONE',  ( 22.69687500061451857, -3.027376345333614438, 5.243569643749998122 ) ) ;
#20928=CARTESIAN_POINT ( 'NONE',  ( -3.581514519956692677, 3.492045901024761534, 28.20070727566179869 ) ) ;
#20929=VECTOR ( 'NONE', #6429, 1000.000000000000000 ) ;
#20931=CARTESIAN_POINT ( 'NONE',  ( -4.243569643749998122, 12.24687500061451750, -27.54997392385601174 ) ) ;
#20932=CARTESIAN_POINT ( 'NONE',  ( 15.03750000122903252, 6.123233995736764310E-16, -4.999999999999998224 ) ) ;
#20933=CARTESIAN_POINT ( 'NONE',  ( 8.859375000614518214, -4.541064518000417216, -2.621784821875001281 ) ) ;
#20934=CARTESIAN_POINT ( 'NONE',  ( -4.243569643749999898, 18.41562500061451857, -32.45002607614398471 ) ) ;
#20935=CARTESIAN_POINT ( 'NONE',  ( 17.66250000122903430, -4.330127018922190985, -2.500000000000001332 ) ) ;
#20936=CARTESIAN_POINT ( 'NONE',  ( 9.515625000614518214, 3.027376345333611329, 5.243569643749999010 ) ) ;
#20937=VERTEX_POINT ( 'NONE', #69762 ) ;
#20938=CARTESIAN_POINT ( 'NONE',  ( 15.52500000000000036, 4.330127018922191873, 2.499999999999999556 ) ) ;
#20939=CARTESIAN_POINT ( 'NONE',  ( -1.999999999999997113, 17.48750000122903359, -26.53589838486224295 ) ) ;
#20940=CARTESIAN_POINT ( 'NONE',  ( 11.10937500061451644, -4.541064518000417216, -2.621784821875001281 ) ) ;
#20941=CARTESIAN_POINT ( 'NONE',  ( 1.626862140677534273E-15, 13.47500000122903252, 34.00000000000000000 ) ) ;
#20942=CARTESIAN_POINT ( 'NONE',  ( 10.61250000122903536, 4.330127018922192761, -2.499999999999997780 ) ) ;
#20943=CARTESIAN_POINT ( 'NONE',  ( 19.16250000122903430, 4.330127018922192761, -2.499999999999997780 ) ) ;
#20944=CARTESIAN_POINT ( 'NONE',  ( 15.81562500061451537, 3.027376345333611329, 5.243569643749999010 ) ) ;
#20945=CARTESIAN_POINT ( 'NONE',  ( 18.36562500061451431, 3.027376345333613106, -5.243569643749998122 ) ) ;
#20946=CARTESIAN_POINT ( 'NONE',  ( 26.66250000122903430, -4.330127018922190985, -2.500000000000001332 ) ) ;
#20947=CARTESIAN_POINT ( 'NONE',  ( 29.58750000122903501, 4.330127018922191873, 2.499999999999999556 ) ) ;
#20948=CARTESIAN_POINT ( 'NONE',  ( 25.42500000000000071, 4.330127018922191873, 2.499999999999999556 ) ) ;
#20950=CARTESIAN_POINT ( 'NONE',  ( 26.70937500061451431, 0.000000000000000000, 5.243569643749999010 ) ) ;
#20951=CARTESIAN_POINT ( 'NONE',  ( 3.999999999999998668, 17.56250000000000000, 27.69059892324149530 ) ) ;
#20952=CARTESIAN_POINT ( 'NONE',  ( 12.56250000122903465, 0.000000000000000000, 4.999999999999998224 ) ) ;
#20953=CARTESIAN_POINT ( 'NONE',  ( 4.162499999999999645, 2.886751345948129099, -4.999999999999998224 ) ) ;
#20955=CARTESIAN_POINT ( 'NONE',  ( 7.884375000614517681, -4.541064518000419881, 2.621784821874995952 ) ) ;
#20956=CARTESIAN_POINT ( 'NONE',  ( 25.52812500061451573, 6.421520780324663323E-16, -5.243569643749999010 ) ) ;
#20959=CARTESIAN_POINT ( 'NONE',  ( 30.00000000000000000, 6.123233995736764310E-16, -4.999999999999998224 ) ) ;
#20960=CARTESIAN_POINT ( 'NONE',  ( 5.109375000614518214, 0.000000000000000000, 5.243569643749999010 ) ) ;
#20961=CARTESIAN_POINT ( 'NONE',  ( 8.709375000614517859, 0.000000000000000000, 5.243569643749999010 ) ) ;
#20962=CARTESIAN_POINT ( 'NONE',  ( 28.88437500061451502, 4.541064518000418104, 2.621784821874999949 ) ) ;
#20963=AXIS2_PLACEMENT_3D ( 'NONE', #40203, #16922, #67558 ) ;
#20964=CARTESIAN_POINT ( 'NONE',  ( 4.243569643749999010, 11.51562500061459460, 27.54997392385601174 ) ) ;
#20965=CARTESIAN_POINT ( 'NONE',  ( 22.16250000000000142, 2.886751345948129099, -4.999999999999998224 ) ) ;
#20966=CARTESIAN_POINT ( 'NONE',  ( 28.87499999999999645, 6.123233995736764310E-16, -4.999999999999998224 ) ) ;
#20968=CARTESIAN_POINT ( 'NONE',  ( 4.687500000000000000, 5.773502691896255534, 3.535250795749688894E-16 ) ) ;
#20969=EDGE_CURVE ( 'NONE', #4055, #9071, #21469, .T. ) ;
#20970=EDGE_LOOP ( 'NONE', ( #40765, #21203, #14367, #32067 ) ) ;
#20971=CARTESIAN_POINT ( 'NONE',  ( 19.00312500061451715, 0.000000000000000000, 5.243569643749999010 ) ) ;
#20972=CARTESIAN_POINT ( 'NONE',  ( 10.71562500061451928, 3.027376345333613106, -5.243569643749998122 ) ) ;
#20974=CARTESIAN_POINT ( 'NONE',  ( 8.034375000614518925, 6.421520780324663323E-16, -5.243569643749999010 ) ) ;
#20975=CARTESIAN_POINT ( 'NONE',  ( 24.26249999999999929, -5.773502691896255534, -1.060575238724906372E-15 ) ) ;
#20976=CARTESIAN_POINT ( 'NONE',  ( 19.65000000122902790, 5.773502691896255534, 3.535250795749688894E-16 ) ) ;
#20978=CARTESIAN_POINT ( 'NONE',  ( 10.24687500061451750, -3.027376345333610441, -5.243569643749999898 ) ) ;
#20979=CARTESIAN_POINT ( 'NONE',  ( 13.50937500061451679, 4.541064518000418104, -2.621784821874998173 ) ) ;
#20980=CARTESIAN_POINT ( 'NONE',  ( 23.89687500061451786, 6.054752690667223547, 3.707466751127219781E-16 ) ) ;
#20984=CARTESIAN_POINT ( 'NONE',  ( 17.03437500061451715, 6.421520780324663323E-16, -5.243569643749999010 ) ) ;
#20985=CARTESIAN_POINT ( 'NONE',  ( 9.496875000614517504, 6.054752690667223547, 3.707466751127219781E-16 ) ) ;
#20987=CARTESIAN_POINT ( 'NONE',  ( 21.37499999999999645, 4.330127018922191873, 2.499999999999999556 ) ) ;
#20989=CARTESIAN_POINT ( 'NONE',  ( 29.77499999999999858, 6.123233995736764310E-16, -4.999999999999998224 ) ) ;
#20991=CARTESIAN_POINT ( 'NONE',  ( 11.99062500061451608, -3.027376345333610441, -5.243569643749999898 ) ) ;
#20992=CARTESIAN_POINT ( 'NONE',  ( 28.39687500061452141, 6.054752690667223547, 3.707466751127219781E-16 ) ) ;
#20994=CARTESIAN_POINT ( 'NONE',  ( -4.243569643749999898, 19.83125000061451715, -30.00000000000000000 ) ) ;
#20995=CARTESIAN_POINT ( 'NONE',  ( 13.42499999999999893, -4.330127018922194537, 2.499999999999995559 ) ) ;
#20996=CARTESIAN_POINT ( 'NONE',  ( 4.000000000000000000, 17.15000000122903145, 32.30940107675849049 ) ) ;
#20997=CARTESIAN_POINT ( 'NONE',  ( 12.22500000122903430, -5.773502691896255534, -1.060575238724906372E-15 ) ) ;
#20998=CARTESIAN_POINT ( 'NONE',  ( 22.99687500061451573, 6.054752690667223547, 3.707466751127219781E-16 ) ) ;
#20999=CARTESIAN_POINT ( 'NONE',  ( 16.35937500061451644, 0.000000000000000000, 5.243569643749999010 ) ) ;
#21000=CARTESIAN_POINT ( 'NONE',  ( -1.071796769724491005, 12.25759618943233775, 26.00000000000000355 ) ) ;
#21001=ORIENTED_EDGE ( 'NONE', *, *, #10344, .F. ) ;
#21002=CARTESIAN_POINT ( 'NONE',  ( 17.42812500061451786, 6.421520780324663323E-16, -5.243569643749999010 ) ) ;
#21003=CARTESIAN_POINT ( 'NONE',  ( 27.78750000122903074, 4.330127018922191873, 2.499999999999999556 ) ) ;
#21004=CARTESIAN_POINT ( 'NONE',  ( 17.48437500061451999, 6.421520780324663323E-16, -5.243569643749999010 ) ) ;
#21005=CARTESIAN_POINT ( 'NONE',  ( 5.728125000614515905, 6.421520780324663323E-16, -5.243569643749999010 ) ) ;
#21006=CARTESIAN_POINT ( 'NONE',  ( 19.79062500061451502, 6.054752690667223547, 3.707466751127219781E-16 ) ) ;
#21007=CARTESIAN_POINT ( 'NONE',  ( 2.000000000000001332, 18.35000000000000142, -26.53589838486224650 ) ) ;
#21008=CARTESIAN_POINT ( 'NONE',  ( 27.68437500061451573, -4.541064518000419881, 2.621784821874995952 ) ) ;
#21009=CARTESIAN_POINT ( 'NONE',  ( 4.243569643749999010, 12.86562500061451608, 27.54997392385601174 ) ) ;
#21010=CARTESIAN_POINT ( 'NONE',  ( 16.65937500061452070, 4.541064518000418104, -2.621784821874998173 ) ) ;
#21011=CARTESIAN_POINT ( 'NONE',  ( 15.75000000122902932, -2.886751345948129988, 4.999999999999997335 ) ) ;
#21013=CARTESIAN_POINT ( 'NONE',  ( -1.999999999999997113, 9.837500001229035007, 33.46410161513775705 ) ) ;
#21014=CARTESIAN_POINT ( 'NONE',  ( 20.67187500061451289, 3.027376345333613106, -5.243569643749998122 ) ) ;
#21015=CARTESIAN_POINT ( 'NONE',  ( 21.56250000122903288, 0.000000000000000000, 4.999999999999998224 ) ) ;
#21016=CARTESIAN_POINT ( 'NONE',  ( 24.14062500061451289, -3.027376345333610441, -5.243569643749999898 ) ) ;
#21017=CARTESIAN_POINT ( 'NONE',  ( 16.39687500061451786, -3.027376345333614438, 5.243569643749998122 ) ) ;
#21018=CARTESIAN_POINT ( 'NONE',  ( 11.99062500061451608, -3.027376345333610441, -5.243569643749999898 ) ) ;
#21019=CARTESIAN_POINT ( 'NONE',  ( 4.243569643749999898, 13.78437500061451715, 30.00000000000000000 ) ) ;
#21020=CARTESIAN_POINT ( 'NONE',  ( 16.75312500061451715, 0.000000000000000000, 5.243569643749999010 ) ) ;
#21021=CARTESIAN_POINT ( 'NONE',  ( 28.22812500061451502, 6.421520780324663323E-16, -5.243569643749999010 ) ) ;
#21023=ORIENTED_EDGE ( 'NONE', *, *, #42304, .F. ) ;
#21024=CARTESIAN_POINT ( 'NONE',  ( 22.23750000000000071, 5.773502691896255534, 3.535250795749688894E-16 ) ) ;
#21025=CARTESIAN_POINT ( 'NONE',  ( -2.121784821874999949, 18.88437500061451857, -33.67503911421598417 ) ) ;
#21026=CARTESIAN_POINT ( 'NONE',  ( 30.00000000000000000, 0.000000000000000000, 0.000000000000000000 ) ) ;
#21027=CARTESIAN_POINT ( 'NONE',  ( 23.84062500061451928, 6.054752690667223547, 3.707466751127219781E-16 ) ) ;
#21028=CARTESIAN_POINT ( 'NONE',  ( 5.428125000614517859, 4.541064518000418104, 2.621784821874999949 ) ) ;
#21029=CARTESIAN_POINT ( 'NONE',  ( 17.43750000122903288, 4.330127018922191873, 2.499999999999999556 ) ) ;
#21030=CARTESIAN_POINT ( 'NONE',  ( 21.89062500061451289, -3.027376345333610441, -5.243569643749999898 ) ) ;
#21031=CARTESIAN_POINT ( 'NONE',  ( 23.73749999999999716, -2.886751345948129988, 4.999999999999997335 ) ) ;
#21032=CARTESIAN_POINT ( 'NONE',  ( 26.39062500061451644, -3.027376345333610441, -5.243569643749999898 ) ) ;
#21033=CARTESIAN_POINT ( 'NONE',  ( 7.003125000614518036, -4.541064518000417216, -2.621784821875001281 ) ) ;
#21034=( BOUNDED_CURVE ( )  B_SPLINE_CURVE ( 2, ( #2181, #12886, #41341, #12529, #1462, #6992, #69771, #19139, #40983 ),
 .UNSPECIFIED., .F., .F. ) 
 B_SPLINE_CURVE_WITH_KNOTS ( ( 3, 2, 2, 2, 3 ),
 ( 0.1195652173913043514, 0.1231884057971014551, 0.1304347826086956486, 0.1376811594202898559, 0.1413043478260869734 ),
 .UNSPECIFIED. ) 
 CURVE ( )  GEOMETRIC_REPRESENTATION_ITEM ( )  RATIONAL_B_SPLINE_CURVE ( ( 0.9330127018922194093, 0.9330127018922194093, 1.000000000000000000, 0.8660254037844387076, 1.000000000000000000, 0.8660254037844387076, 1.000000000000000000, 0.9330127018922190762, 0.9330127018922194093 ) ) 
 REPRESENTATION_ITEM ( '' )  );
#21035=ORIENTED_EDGE ( 'NONE', *, *, #14417, .F. ) ;
#21037=CARTESIAN_POINT ( 'NONE',  ( 22.97812500061451857, 4.541064518000418104, 2.621784821874999949 ) ) ;
#21038=CARTESIAN_POINT ( 'NONE',  ( 3.028125000614518392, 6.421520780324663323E-16, -5.243569643749999010 ) ) ;
#21040=CARTESIAN_POINT ( 'NONE',  ( -3.137519842735245283E-14, 11.22500000122903430, 34.00000000000000000 ) ) ;
#21041=CARTESIAN_POINT ( 'NONE',  ( -1.999999999999997113, 12.98750000122903359, -26.53589838486224295 ) ) ;
#21043=CARTESIAN_POINT ( 'NONE',  ( 10.20000000000000107, 0.000000000000000000, 4.999999999999998224 ) ) ;
#21044=CARTESIAN_POINT ( 'NONE',  ( 10.58437500061451964, -4.541064518000419881, 2.621784821874995952 ) ) ;
#21045=CARTESIAN_POINT ( 'NONE',  ( 5.362500001229033586, 0.000000000000000000, 4.999999999999998224 ) ) ;
#21046=CARTESIAN_POINT ( 'NONE',  ( 14.03437500061451715, 4.541064518000418104, 2.621784821874999949 ) ) ;
#21047=CARTESIAN_POINT ( 'NONE',  ( 4.846875000614519813, -3.027376345333610441, -5.243569643749999898 ) ) ;
#21048=CYLINDRICAL_SURFACE ( 'NONE', #60910, 4.999999999999998224 ) ;
#21049=CARTESIAN_POINT ( 'NONE',  ( -3.999999999999999112, 10.66250000122903430, 30.00000000000000000 ) ) ;
#21050=EDGE_CURVE ( 'NONE', #14259, #72082, #54051, .T. ) ;
#21051=CARTESIAN_POINT ( 'NONE',  ( 11.44687500061451857, -3.027376345333614438, 5.243569643749998122 ) ) ;
#21052=CARTESIAN_POINT ( 'NONE',  ( 21.78750000122903074, 6.123233995736764310E-16, -4.999999999999998224 ) ) ;
#21053=CARTESIAN_POINT ( 'NONE',  ( 22.34062500061451573, -3.027376345333610441, -5.243569643749999898 ) ) ;
#21054=CARTESIAN_POINT ( 'NONE',  ( -4.243569643749999898, 10.85937500061451821, 30.00000000000000000 ) ) ;
#21055=CARTESIAN_POINT ( 'NONE',  ( -4.243569643749999898, 18.45312500061459104, 30.00000000000000000 ) ) ;
#21056=CARTESIAN_POINT ( 'NONE',  ( 22.99687500061451573, 6.054752690667223547, 3.707466751127219781E-16 ) ) ;
#21057=DIRECTION ( 'NONE',  ( 0.000000000000000000, 0.000000000000000000, 1.000000000000000000 ) ) ;
#21058=CARTESIAN_POINT ( 'NONE',  ( 29.25000000122903288, -2.886751345948129988, 4.999999999999997335 ) ) ;
#21060=CARTESIAN_POINT ( 'NONE',  ( 24.51562500061451289, -6.054752690667223547, -1.112240025338166033E-15 ) ) ;
#21061=CARTESIAN_POINT ( 'NONE',  ( 17.50312500061451715, 4.541064518000418104, -2.621784821874998173 ) ) ;
#21063=CARTESIAN_POINT ( 'NONE',  ( 15.04687500061451644, -3.027376345333614438, 5.243569643749998122 ) ) ;
#21065=CARTESIAN_POINT ( 'NONE',  ( 27.37500000122903288, 2.886751345948126879, 4.999999999999999112 ) ) ;
#21066=CARTESIAN_POINT ( 'NONE',  ( 5.896875000614518747, 6.054752690667223547, 3.707466751127219781E-16 ) ) ;
#21067=CARTESIAN_POINT ( 'NONE',  ( 16.20937500061451786, 4.541064518000418104, -2.621784821874998173 ) ) ;
#21069=CARTESIAN_POINT ( 'NONE',  ( 23.25000000000000000, 0.000000000000000000, 4.999999999999998224 ) ) ;
#21070=CARTESIAN_POINT ( 'NONE',  ( 4.612500001229032698, -4.330127018922190985, -2.500000000000001332 ) ) ;
#21071=CARTESIAN_POINT ( 'NONE',  ( 24.00937500061451502, 0.000000000000000000, 5.243569643749999010 ) ) ;
#21072=CARTESIAN_POINT ( 'NONE',  ( 16.92187500061451999, -6.054752690667223547, -1.112240025338166033E-15 ) ) ;
#21074=CARTESIAN_POINT ( 'NONE',  ( 29.06250000000000000, 2.886751345948126879, 4.999999999999999112 ) ) ;
#21075=CARTESIAN_POINT ( 'NONE',  ( 5.287500000000000533, -2.886751345948129988, 4.999999999999997335 ) ) ;
#21077=CARTESIAN_POINT ( 'NONE',  ( 18.47812500061451857, 4.541064518000418104, 2.621784821874999949 ) ) ;
#21078=CARTESIAN_POINT ( 'NONE',  ( 9.299999999999998934, 0.000000000000000000, 4.999999999999998224 ) ) ;
#21079=EDGE_CURVE ( 'NONE', #32666, #32497, #66789, .T. ) ;
#21080=CARTESIAN_POINT ( 'NONE',  ( 4.640625000614518214, -3.027376345333614438, 5.243569643749998122 ) ) ;
#21081=CARTESIAN_POINT ( 'NONE',  ( 18.37500000000000355, -4.330127018922194537, 2.499999999999995559 ) ) ;
#21082=CARTESIAN_POINT ( 'NONE',  ( 23.32500000122903572, 2.886751345948126879, 4.999999999999999112 ) ) ;
#21083=CARTESIAN_POINT ( 'NONE',  ( 1.391695283777658831, 9.904653401742692154, 35.83979371019399451 ) ) ;
#21084=CARTESIAN_POINT ( 'NONE',  ( 28.47187500061451715, 3.027376345333611329, 5.243569643749999010 ) ) ;
#21086=CARTESIAN_POINT ( 'NONE',  ( 17.09062500061451573, 6.054752690667223547, 3.707466751127219781E-16 ) ) ;
#21087=CARTESIAN_POINT ( 'NONE',  ( 23.54062500061451146, -3.027376345333614438, 5.243569643749998122 ) ) ;
#21088=CARTESIAN_POINT ( 'NONE',  ( 24.60937500061451644, -4.541064518000417216, -2.621784821875001281 ) ) ;
#21089=CARTESIAN_POINT ( 'NONE',  ( 9.375000000000001776, -4.330127018922194537, 2.499999999999995559 ) ) ;
#21090=CARTESIAN_POINT ( 'NONE',  ( 13.00312500061451537, 4.541064518000418104, -2.621784821874998173 ) ) ;
#21091=CARTESIAN_POINT ( 'NONE',  ( 27.21562500061451928, -6.054752690667223547, -1.112240025338166033E-15 ) ) ;
#21092=CARTESIAN_POINT ( 'NONE',  ( 13.77187500061451786, -6.054752690667223547, -1.112240025338166033E-15 ) ) ;
#21093=CARTESIAN_POINT ( 'NONE',  ( 19.35937500061451644, 4.541064518000418104, -2.621784821874998173 ) ) ;
#21094=CYLINDRICAL_SURFACE ( 'NONE', #56899, 4.999999999999998224 ) ;
#21095=CARTESIAN_POINT ( 'NONE',  ( 2.121784821875001281, 11.00937500061451857, 33.67503911421598417 ) ) ;
#21096=CARTESIAN_POINT ( 'NONE',  ( 22.68750000122903288, 6.123233995736764310E-16, -4.999999999999998224 ) ) ;
#21098=CARTESIAN_POINT ( 'NONE',  ( 14.61562500061451786, -6.054752690667223547, -1.112240025338166033E-15 ) ) ;
#21099=CARTESIAN_POINT ( 'NONE',  ( 7.021875000614518747, -6.054752690667223547, -1.112240025338166033E-15 ) ) ;
#21100=CARTESIAN_POINT ( 'NONE',  ( 7.321875000614516793, 3.027376345333611329, 5.243569643749999010 ) ) ;
#21101=ORIENTED_EDGE ( 'NONE', *, *, #11164, .T. ) ;
#21102=CARTESIAN_POINT ( 'NONE',  ( 26.70937500061451431, 0.000000000000000000, 5.243569643749999010 ) ) ;
#21103=CARTESIAN_POINT ( 'NONE',  ( 19.56562500061451715, -6.054752690667223547, -1.112240025338166033E-15 ) ) ;
#21104=CARTESIAN_POINT ( 'NONE',  ( 4.246875000614519280, -3.027376345333614438, 5.243569643749998122 ) ) ;
#21105=CARTESIAN_POINT ( 'NONE',  ( 25.32187500061451857, 3.027376345333611329, 5.243569643749999010 ) ) ;
#21106=CARTESIAN_POINT ( 'NONE',  ( 19.97812500061451502, -4.541064518000419881, 2.621784821874995952 ) ) ;
#21107=CARTESIAN_POINT ( 'NONE',  ( -2.828200636599751609E-16, 11.33750000000000036, 25.38119784648299770 ) ) ;
#21108=CARTESIAN_POINT ( 'NONE',  ( 24.96562500061451573, -6.054752690667223547, -1.112240025338166033E-15 ) ) ;
#21109=CARTESIAN_POINT ( 'NONE',  ( 6.900000001229035007, -2.886751345948125991, -5.000000000000000000 ) ) ;
#21110=ORIENTED_EDGE ( 'NONE', *, *, #4806, .T. ) ;
#21112=CARTESIAN_POINT ( 'NONE',  ( 2.000000000000001332, 16.55000000000000071, -26.53589838486224650 ) ) ;
#21113=CARTESIAN_POINT ( 'NONE',  ( 22.12500000122903288, -5.773502691896255534, -1.060575238724906372E-15 ) ) ;
#21115=CARTESIAN_POINT ( 'NONE',  ( 3.646875000614520079, 6.054752690667223547, 3.707466751127219781E-16 ) ) ;
#21116=CARTESIAN_POINT ( 'NONE',  ( 1.071796769724497445, 15.36740381056766758, 26.00000000000000355 ) ) ;
#21117=CARTESIAN_POINT ( 'NONE',  ( 13.49062500061451608, 6.054752690667223547, 3.707466751127219781E-16 ) ) ;
#21118=CARTESIAN_POINT ( 'NONE',  ( 8.934375000614517504, 6.421520780324663323E-16, -5.243569643749999010 ) ) ;
#21119=CARTESIAN_POINT ( 'NONE',  ( 24.75000000122902932, -2.886751345948129988, 4.999999999999997335 ) ) ;
#21120=CARTESIAN_POINT ( 'NONE',  ( 14.40937500061451715, 4.541064518000418104, -2.621784821874998173 ) ) ;
#21121=CARTESIAN_POINT ( 'NONE',  ( 29.31562500061451715, 3.027376345333611329, 5.243569643749999010 ) ) ;
#21122=CARTESIAN_POINT ( 'NONE',  ( 29.36250000000000071, 2.886751345948129099, -4.999999999999998224 ) ) ;
#21123=CARTESIAN_POINT ( 'NONE',  ( 5.990625000614517859, -3.027376345333614438, 5.243569643749998122 ) ) ;
#21124=CARTESIAN_POINT ( 'NONE',  ( 15.47812500061451679, -4.541064518000419881, 2.621784821874995952 ) ) ;
#21125=ORIENTED_EDGE ( 'NONE', *, *, #3997, .T. ) ;
#21126=CARTESIAN_POINT ( 'NONE',  ( 12.32812500061451821, -4.541064518000419881, 2.621784821874995952 ) ) ;
#21127=CARTESIAN_POINT ( 'NONE',  ( 8.428125000614517859, 6.421520780324663323E-16, -5.243569643749999010 ) ) ;
#21129=CARTESIAN_POINT ( 'NONE',  ( 7.837499999999999467, 5.773502691896255534, 3.535250795749688894E-16 ) ) ;
#21130=CARTESIAN_POINT ( 'NONE',  ( 4.425000001229032698, 2.886751345948126879, 4.999999999999999112 ) ) ;
#21131=CARTESIAN_POINT ( 'NONE',  ( 18.89999999999999858, -4.330127018922190985, -2.500000000000001332 ) ) ;
#21132=ADVANCED_FACE ( 'NONE', ( #9531 ), #15853, .T. ) ;
#21133=CARTESIAN_POINT ( 'NONE',  ( 19.13437500061451857, -4.541064518000419881, 2.621784821874995952 ) ) ;
#21134=CARTESIAN_POINT ( 'NONE',  ( 14.25000000122903465, 5.773502691896255534, 3.535250795749688894E-16 ) ) ;
#21136=CARTESIAN_POINT ( 'NONE',  ( 4.243569643749999898, 17.29062500061451502, -27.54997392385601529 ) ) ;
#21140=CARTESIAN_POINT ( 'NONE',  ( 0.000000000000000000, 0.000000000000000000, -50.00000000000000000 ) ) ;
#21141=CARTESIAN_POINT ( 'NONE',  ( 1.592000809091587073E-14, 16.28750000000000142, -34.00000000000000000 ) ) ;
#21142=CARTESIAN_POINT ( 'NONE',  ( 14.25937500061451679, -4.541064518000417216, -2.621784821875001281 ) ) ;
#21143=CARTESIAN_POINT ( 'NONE',  ( 26.88749999999999574, -2.886751345948129988, 4.999999999999997335 ) ) ;
#21144=CARTESIAN_POINT ( 'NONE',  ( 10.52812500061451750, -4.541064518000419881, 2.621784821874995952 ) ) ;
#21146=CARTESIAN_POINT ( 'NONE',  ( 22.43437500061451573, 6.421520780324663323E-16, -5.243569643749999010 ) ) ;
#21148=CARTESIAN_POINT ( 'NONE',  ( 8.428125000614517859, 6.421520780324663323E-16, -5.243569643749999010 ) ) ;
#21149=CARTESIAN_POINT ( 'NONE',  ( 13.99687500061451928, 6.054752690667223547, 3.707466751127219781E-16 ) ) ;
#21150=ORIENTED_EDGE ( 'NONE', *, *, #14141, .T. ) ;
#21151=CARTESIAN_POINT ( 'NONE',  ( 23.40937500061451715, 4.541064518000418104, -2.621784821874998173 ) ) ;
#21152=CARTESIAN_POINT ( 'NONE',  ( 3.458282317606260037, 3.615826433065251422, -32.02515933644849611 ) ) ;
#21154=CARTESIAN_POINT ( 'NONE',  ( 5.100000000000000533, 4.330127018922192761, -2.499999999999997780 ) ) ;
#21156=CARTESIAN_POINT ( 'NONE',  ( 17.06250000122903288, 0.000000000000000000, 4.999999999999998224 ) ) ;
#21160=CARTESIAN_POINT ( 'NONE',  ( 15.52500000000000036, 4.330127018922191873, 2.499999999999999556 ) ) ;
#21161=CARTESIAN_POINT ( 'NONE',  ( 16.61250000000000426, -5.773502691896255534, -1.060575238724906372E-15 ) ) ;
#21162=CARTESIAN_POINT ( 'NONE',  ( 12.06562500061451537, 3.027376345333613106, -5.243569643749998122 ) ) ;
#21164=CARTESIAN_POINT ( 'NONE',  ( 26.28750000000000142, 5.773502691896255534, 3.535250795749688401E-16 ) ) ;
#21165=CARTESIAN_POINT ( 'NONE',  ( -3.000416591977282496E-16, 16.14687500061451431, -34.90005215228797653 ) ) ;
#21166=CARTESIAN_POINT ( 'NONE',  ( 3.515625000614516882, 3.027376345333613106, -5.243569643749998122 ) ) ;
#21168=CARTESIAN_POINT ( 'NONE',  ( 10.65000000000000036, 0.000000000000000000, 4.999999999999998224 ) ) ;
#21169=CYLINDRICAL_SURFACE ( 'NONE', #70382, 3.999999999999996447 ) ;
#21171=CARTESIAN_POINT ( 'NONE',  ( 24.55312500061451786, -4.541064518000417216, -2.621784821875001281 ) ) ;
#21174=CARTESIAN_POINT ( 'NONE',  ( 20.37187500061451573, 3.027376345333611329, 5.243569643749999010 ) ) ;
#21175=CARTESIAN_POINT ( 'NONE',  ( 19.64062500061451644, -3.027376345333610441, -5.243569643749999898 ) ) ;
#21176=EDGE_CURVE ( 'NONE', #63910, #17100, #13917, .T. ) ;
#21177=CARTESIAN_POINT ( 'NONE',  ( -3.000416591977282496E-16, 13.84062500061459744, -34.90005215228797653 ) ) ;
#21178=CARTESIAN_POINT ( 'NONE',  ( 22.83750000122903501, 4.330127018922191873, 2.499999999999999556 ) ) ;
#21179=CARTESIAN_POINT ( 'NONE',  ( 4.415625000614518569, 3.027376345333613106, -5.243569643749998122 ) ) ;
#21181=CARTESIAN_POINT ( 'NONE',  ( 20.72812500061451502, 4.541064518000418104, 2.621784821874999949 ) ) ;
#21185=CARTESIAN_POINT ( 'NONE',  ( 16.20937500061451786, 4.541064518000418104, -2.621784821874998173 ) ) ;
#21186=CARTESIAN_POINT ( 'NONE',  ( 14.07187500061451679, 3.027376345333611329, 5.243569643749999010 ) ) ;
#21187=CARTESIAN_POINT ( 'NONE',  ( 22.92187500061451644, 3.027376345333613106, -5.243569643749998122 ) ) ;
#21188=ORIENTED_EDGE ( 'NONE', *, *, #58553, .T. ) ;
#21189=CARTESIAN_POINT ( 'NONE',  ( -2.121784821874999949, 12.58437500061451786, 26.32496088578401938 ) ) ;
#21190=CARTESIAN_POINT ( 'NONE',  ( 3.853125000614517681, -4.541064518000417216, -2.621784821875001281 ) ) ;
#21191=CARTESIAN_POINT ( 'NONE',  ( 27.36562500061451786, 3.027376345333613106, -5.243569643749998122 ) ) ;
#21192=CARTESIAN_POINT ( 'NONE',  ( 27.89062500061451289, 6.054752690667223547, 3.707466751127219781E-16 ) ) ;
#21194=CARTESIAN_POINT ( 'NONE',  ( 3.999999999999998668, 18.01249999999999929, 27.69059892324149175 ) ) ;
#21195=CARTESIAN_POINT ( 'NONE',  ( 6.946875000614517681, -3.027376345333614438, 5.243569643749998122 ) ) ;
#21196=CARTESIAN_POINT ( 'NONE',  ( 15.18750000122903465, 4.330127018922191873, 2.499999999999999556 ) ) ;
#21197=CARTESIAN_POINT ( 'NONE',  ( 10.23750000122903359, 4.330127018922191873, 2.499999999999999556 ) ) ;
#21198=CARTESIAN_POINT ( 'NONE',  ( 29.51250000122903216, 4.330127018922192761, -2.499999999999997780 ) ) ;
#21201=CARTESIAN_POINT ( 'NONE',  ( 11.82187500061451679, 3.027376345333611329, 5.243569643749999010 ) ) ;
#21202=DIRECTION ( 'NONE',  ( 0.000000000000000000, 0.000000000000000000, -1.000000000000000000 ) ) ;
#21203=ORIENTED_EDGE ( 'NONE', *, *, #64083, .F. ) ;
#21204=CARTESIAN_POINT ( 'NONE',  ( 19.67812500061451786, 6.421520780324663323E-16, -5.243569643749999010 ) ) ;
#21205=CARTESIAN_POINT ( 'NONE',  ( 7.340625000614518392, -3.027376345333614438, 5.243569643749998122 ) ) ;
#21206=CARTESIAN_POINT ( 'NONE',  ( 22.80937500061451573, -4.541064518000417216, -2.621784821875001281 ) ) ;
#21207=EDGE_CURVE ( 'NONE', #4525, #26188, #61585, .T. ) ;
#21208=CARTESIAN_POINT ( 'NONE',  ( 4.940625000614515372, 6.054752690667223547, 3.707466751127219781E-16 ) ) ;
#21209=CARTESIAN_POINT ( 'NONE',  ( 30.00000000000000000, 0.000000000000000000, 0.000000000000000000 ) ) ;
#21210=CARTESIAN_POINT ( 'NONE',  ( 7.950000001229033053, 5.773502691896255534, 3.535250795749688894E-16 ) ) ;
#21211=CARTESIAN_POINT ( 'NONE',  ( 23.01562500061451644, 3.027376345333611329, 5.243569643749999010 ) ) ;
#21212=CARTESIAN_POINT ( 'NONE',  ( 3.999999999999999112, 17.18750000122903288, -30.00000000000000000 ) ) ;
#21213=CARTESIAN_POINT ( 'NONE',  ( 7.762500001229033053, -4.330127018922190985, -2.500000000000001332 ) ) ;
#21214=CARTESIAN_POINT ( 'NONE',  ( 18.62812500061451715, -4.541064518000419881, 2.621784821874995952 ) ) ;
#21215=CARTESIAN_POINT ( 'NONE',  ( 14.91562500061451679, 3.027376345333611329, 5.243569643749999010 ) ) ;
#21217=CARTESIAN_POINT ( 'NONE',  ( 15.29999999999999893, -4.330127018922190985, -2.500000000000001332 ) ) ;
#21218=CARTESIAN_POINT ( 'NONE',  ( 11.47500000122903252, 2.886751345948129099, -4.999999999999998224 ) ) ;
#21219=EDGE_CURVE ( 'NONE', #8626, #5506, #51675, .T. ) ;
#21220=CARTESIAN_POINT ( 'NONE',  ( 8.578125000614518214, 4.541064518000418104, 2.621784821874999949 ) ) ;
#21221=CARTESIAN_POINT ( 'NONE',  ( 11.57812500061451644, 6.421520780324663323E-16, -5.243569643749999010 ) ) ;
#21222=CARTESIAN_POINT ( 'NONE',  ( 21.07500000122903572, 2.886751345948126879, 4.999999999999999112 ) ) ;
#21223=CARTESIAN_POINT ( 'NONE',  ( -4.243569643749999898, 13.97187500061451715, -32.45002607614398471 ) ) ;
#21224=CARTESIAN_POINT ( 'NONE',  ( 18.30937500061451928, -4.541064518000417216, -2.621784821875001281 ) ) ;
#21225=CARTESIAN_POINT ( 'NONE',  ( 6.187500001229032875, 4.330127018922191873, 2.499999999999999556 ) ) ;
#21226=( BOUNDED_CURVE ( )  B_SPLINE_CURVE ( 2, ( #19949, #53578, #30677, #19578, #53209, #14414, #25126 ),
 .UNSPECIFIED., .F., .F. ) 
 B_SPLINE_CURVE_WITH_KNOTS ( ( 3, 2, 2, 3 ),
 ( 0.3583333333333333925, 0.3611111111111111605, 0.3638888888888888729, 0.3666666666666666408 ),
 .UNSPECIFIED. ) 
 CURVE ( )  GEOMETRIC_REPRESENTATION_ITEM ( )  RATIONAL_B_SPLINE_CURVE ( ( 0.9999999999999973355, 0.8660254037844413721, 1.000000000000000000, 0.8660254037844387076, 1.000000000000000000, 0.8660254037844387076, 1.000000000000000000 ) ) 
 REPRESENTATION_ITEM ( '' )  );
#21227=CARTESIAN_POINT ( 'NONE',  ( 3.871875000614519280, -6.054752690667223547, -1.112240025338166033E-15 ) ) ;
#21228=CARTESIAN_POINT ( 'NONE',  ( 23.78437500061451360, 6.421520780324663323E-16, -5.243569643749999010 ) ) ;
#21229=CARTESIAN_POINT ( 'NONE',  ( 7.837500001229035007, 6.123233995736764310E-16, -4.999999999999998224 ) ) ;
#21230=CARTESIAN_POINT ( 'NONE',  ( 20.05312500061451431, -4.541064518000417216, -2.621784821875001281 ) ) ;
#21233=LINE ( 'NONE', #44884, #53577 ) ;
#21234=CARTESIAN_POINT ( 'NONE',  ( 28.62187500061451573, -6.054752690667223547, -1.112240025338166033E-15 ) ) ;
#21236=CARTESIAN_POINT ( 'NONE',  ( 13.90312500061451750, 4.541064518000418104, -2.621784821874998173 ) ) ;
#21237=CARTESIAN_POINT ( 'NONE',  ( 13.50937500061451679, 4.541064518000418104, -2.621784821874998173 ) ) ;
#21238=ORIENTED_EDGE ( 'NONE', *, *, #11885, .F. ) ;
#21239=CARTESIAN_POINT ( 'NONE',  ( 1.592000809091587073E-14, 17.18750000000000355, -34.00000000000000000 ) ) ;
#21240=CARTESIAN_POINT ( 'NONE',  ( 23.50312500061451360, 0.000000000000000000, 5.243569643749999010 ) ) ;
#21241=FACE_OUTER_BOUND ( 'NONE', #56338, .T. ) ;
#21242=CARTESIAN_POINT ( 'NONE',  ( 28.65000000122903145, 5.773502691896255534, 3.535250795749688401E-16 ) ) ;
#21243=CARTESIAN_POINT ( 'NONE',  ( 12.26249999999999929, 2.886751345948129099, -4.999999999999998224 ) ) ;
#21244=CARTESIAN_POINT ( 'NONE',  ( 25.16250000122903074, 0.000000000000000000, 4.999999999999998224 ) ) ;
#21245=CARTESIAN_POINT ( 'NONE',  ( 18.10312500061451502, 0.000000000000000000, 5.243569643749999010 ) ) ;
#21247=CARTESIAN_POINT ( 'NONE',  ( 22.91249999999999432, -5.773502691896255534, -1.060575238724906372E-15 ) ) ;
#21248=CARTESIAN_POINT ( 'NONE',  ( 23.03437500061451715, 4.541064518000418104, 2.621784821874999949 ) ) ;
#21249=( BOUNDED_CURVE ( )  B_SPLINE_CURVE ( 2, ( #67353, #16716, #9364, #31897, #54433, #3832, #26353, #48892, #71422 ),
 .UNSPECIFIED., .F., .F. ) 
 B_SPLINE_CURVE_WITH_KNOTS ( ( 3, 2, 2, 2, 3 ),
 ( 0.8586956521739130821, 0.8623188405797101996, 0.8695652173913043237, 0.8768115942028985588, 0.8804347826086956763 ),
 .UNSPECIFIED. ) 
 CURVE ( )  GEOMETRIC_REPRESENTATION_ITEM ( )  RATIONAL_B_SPLINE_CURVE ( ( 0.9330127018922194093, 0.9330127018922194093, 1.000000000000000000, 0.8660254037844387076, 1.000000000000000000, 0.8660254037844387076, 1.000000000000000000, 0.9330127018922194093, 0.9330127018922194093 ) ) 
 REPRESENTATION_ITEM ( '' )  );
#21250=ORIENTED_EDGE ( 'NONE', *, *, #35651, .F. ) ;
#21252=CARTESIAN_POINT ( 'NONE',  ( 11.65312500061451573, 4.541064518000418104, -2.621784821874998173 ) ) ;
#21255=CARTESIAN_POINT ( 'NONE',  ( 16.16250000000000142, -5.773502691896255534, -1.060575238724906372E-15 ) ) ;
#21256=CARTESIAN_POINT ( 'NONE',  ( 25.23749999999999716, -2.886751345948125991, -5.000000000000000000 ) ) ;
#21257=CARTESIAN_POINT ( 'NONE',  ( 9.001249775931846008E-16, 19.46562500061451573, 34.90005215228797653 ) ) ;
#21258=CARTESIAN_POINT ( 'NONE',  ( 4.734375000614518214, -4.541064518000419881, 2.621784821874995952 ) ) ;
#21259=CARTESIAN_POINT ( 'NONE',  ( 16.47187500061452070, -6.054752690667223547, -1.112240025338166033E-15 ) ) ;
#21260=CARTESIAN_POINT ( 'NONE',  ( 27.94687500061451502, 6.054752690667223547, 3.707466751127219781E-16 ) ) ;
#21261=EDGE_LOOP ( 'NONE', ( #17008, #59671, #12436, #14523 ) ) ;
#21262=CARTESIAN_POINT ( 'NONE',  ( 25.45312500061451644, -4.541064518000417216, -2.621784821875001281 ) ) ;
#21263=CARTESIAN_POINT ( 'NONE',  ( 27.30937500061451573, -4.541064518000417216, -2.621784821875001281 ) ) ;
#21265=CARTESIAN_POINT ( 'NONE',  ( 14.47499999999999964, 6.123233995736764310E-16, -4.999999999999998224 ) ) ;
#21266=CARTESIAN_POINT ( 'NONE',  ( 11.01562500061451821, -6.054752690667223547, -1.112240025338166033E-15 ) ) ;
#21267=CARTESIAN_POINT ( 'NONE',  ( -3.999999999999999112, 20.00000000000000000, 30.00000000000000000 ) ) ;
#21269=CARTESIAN_POINT ( 'NONE',  ( 28.26562500061450933, 3.027376345333612662, -5.243569643749998122 ) ) ;
#21270=CARTESIAN_POINT ( 'NONE',  ( 16.12500000122903288, 2.886751345948126879, 4.999999999999999112 ) ) ;
#21273=CARTESIAN_POINT ( 'NONE',  ( 5.878125000614517148, 4.541064518000418104, 2.621784821874999949 ) ) ;
#21274=CARTESIAN_POINT ( 'NONE',  ( 21.94687500061451857, -3.027376345333610441, -5.243569643749999898 ) ) ;
#21275=CARTESIAN_POINT ( 'NONE',  ( 4.243569643749999898, 16.03437500061451715, 30.00000000000000000 ) ) ;
#21276=CARTESIAN_POINT ( 'NONE',  ( 20.48437500061451289, -4.541064518000419881, 2.621784821874995952 ) ) ;
#21277=CARTESIAN_POINT ( 'NONE',  ( 3.750000000000000000, 4.330127018922192761, -2.499999999999997780 ) ) ;
#21278=CARTESIAN_POINT ( 'NONE',  ( 2.121784821874999061, 18.35937500061451644, 26.32496088578401583 ) ) ;
#21279=CARTESIAN_POINT ( 'NONE',  ( 12.40312500061451573, -4.541064518000417216, -2.621784821875001281 ) ) ;
#21280=CARTESIAN_POINT ( 'NONE',  ( 3.000000001229032875, 5.773502691896255534, 3.535250795749688894E-16 ) ) ;
#21281=CARTESIAN_POINT ( 'NONE',  ( 7.659375000614518036, 4.541064518000418104, -2.621784821874998173 ) ) ;
#21283=( BOUNDED_CURVE ( )  B_SPLINE_CURVE ( 2, ( #54023, #31481, #65088, #26680, #42929, #70273, #42200 ),
 .UNSPECIFIED., .F., .F. ) 
 B_SPLINE_CURVE_WITH_KNOTS ( ( 3, 2, 2, 3 ),
 ( 0.2416666666666666963, 0.2444444444444444642, 0.2472222222222222321, 0.2500000000000000000 ),
 .UNSPECIFIED. ) 
 CURVE ( )  GEOMETRIC_REPRESENTATION_ITEM ( )  RATIONAL_B_SPLINE_CURVE ( ( 0.9999999999999986677, 0.8660254037844400399, 1.000000000000000000, 0.8660254037844387076, 1.000000000000000000, 0.8660254037844387076, 1.000000000000000000 ) ) 
 REPRESENTATION_ITEM ( '' )  );
#21284=CARTESIAN_POINT ( 'NONE',  ( 9.328125000614518214, 6.421520780324663323E-16, -5.243569643749999010 ) ) ;
#21285=CARTESIAN_POINT ( 'NONE',  ( 13.43437500061451750, 6.421520780324663323E-16, -5.243569643749999010 ) ) ;
#21287=CARTESIAN_POINT ( 'NONE',  ( 21.86250000122903003, 4.330127018922192761, -2.499999999999997780 ) ) ;
#21288=CARTESIAN_POINT ( 'NONE',  ( 8.521875000614516082, 3.027376345333613106, -5.243569643749998122 ) ) ;
#21289=CARTESIAN_POINT ( 'NONE',  ( 9.140625000614518214, -3.027376345333614438, 5.243569643749998122 ) ) ;
#21292=CARTESIAN_POINT ( 'NONE',  ( 21.34687500061451715, -3.027376345333614438, 5.243569643749998122 ) ) ;
#21294=CARTESIAN_POINT ( 'NONE',  ( -3.992949912593974471, 3.009468837316803480, 29.72536534029088884 ) ) ;
#21296=CARTESIAN_POINT ( 'NONE',  ( 9.001249775931846008E-16, 12.32187500061451857, -25.09994784771203058 ) ) ;
#21297=CARTESIAN_POINT ( 'NONE',  ( 14.36250000122903359, 0.000000000000000000, 4.999999999999998224 ) ) ;
#21298=CARTESIAN_POINT ( 'NONE',  ( 4.243569643749999898, 15.07812500061451644, -30.00000000000000000 ) ) ;
#21299=CARTESIAN_POINT ( 'NONE',  ( 18.30000000122903359, 5.773502691896255534, 3.535250795749688894E-16 ) ) ;
#21300=CARTESIAN_POINT ( 'NONE',  ( 10.37812500061451715, 4.541064518000418104, 2.621784821874999949 ) ) ;
#21302=CARTESIAN_POINT ( 'NONE',  ( 14.21249999999999858, 2.886751345948126879, 4.999999999999999112 ) ) ;
#21304=CARTESIAN_POINT ( 'NONE',  ( 22.41562500061451502, 3.027376345333613106, -5.243569643749998122 ) ) ;
#21305=CARTESIAN_POINT ( 'NONE',  ( 10.99687500061451928, -3.027376345333614438, 5.243569643749998122 ) ) ;
#21306=CARTESIAN_POINT ( 'NONE',  ( -3.999999999999999112, 14.26250000122903572, 30.00000000000000000 ) ) ;
#21307=CARTESIAN_POINT ( 'NONE',  ( 9.112500001229033586, -4.330127018922190985, -2.500000000000001332 ) ) ;
#21309=CARTESIAN_POINT ( 'NONE',  ( 18.60000000122903430, -2.886751345948125991, -5.000000000000000000 ) ) ;
#21310=CARTESIAN_POINT ( 'NONE',  ( 15.85312500061451857, 0.000000000000000000, 5.243569643749999010 ) ) ;
#21311=CARTESIAN_POINT ( 'NONE',  ( 18.02812500061451573, 4.541064518000418104, 2.621784821874999949 ) ) ;
#21312=CARTESIAN_POINT ( 'NONE',  ( 25.12500000122903288, 2.886751345948126879, 4.999999999999999112 ) ) ;
#21314=CARTESIAN_POINT ( 'NONE',  ( 27.71250000122903145, 4.330127018922192761, -2.499999999999997780 ) ) ;
#21315=CARTESIAN_POINT ( 'NONE',  ( 22.38749999999999929, -2.886751345948129988, 4.999999999999997335 ) ) ;
#21317=CARTESIAN_POINT ( 'NONE',  ( 24.94687500061451502, -3.027376345333614438, 5.243569643749998122 ) ) ;
#21318=CARTESIAN_POINT ( 'NONE',  ( 7.320879633048903241E-15, 17.63749999999999218, 26.00000000000000355 ) ) ;
#21319=CARTESIAN_POINT ( 'NONE',  ( 12.33750000122903145, 6.123233995736764310E-16, -4.999999999999998224 ) ) ;
#21320=CARTESIAN_POINT ( 'NONE',  ( 29.48437500061451644, -4.541064518000419881, 2.621784821874995952 ) ) ;
#21322=CARTESIAN_POINT ( 'NONE',  ( 4.021875000614516082, 3.027376345333613106, -5.243569643749998122 ) ) ;
#21323=CARTESIAN_POINT ( 'NONE',  ( 25.86562500061451431, -6.054752690667223547, -1.112240025338166033E-15 ) ) ;
#21325=CARTESIAN_POINT ( 'NONE',  ( 11.51250000122903216, 4.330127018922192761, -2.499999999999997780 ) ) ;
#21326=CARTESIAN_POINT ( 'NONE',  ( 10.35937500061451644, 4.541064518000418104, -2.621784821874998173 ) ) ;
#21327=CARTESIAN_POINT ( 'NONE',  ( 3.617702362022032325, -3.451409801779584452, 3.617702362022032325 ) ) ;
#21328=CARTESIAN_POINT ( 'NONE',  ( 28.86562500061451786, 3.027376345333611329, 5.243569643749999010 ) ) ;
#21329=CARTESIAN_POINT ( 'NONE',  ( 8.071875000614518569, 3.027376345333613106, -5.243569643749998122 ) ) ;
#21330=CARTESIAN_POINT ( 'NONE',  ( 29.03437500061451715, -4.541064518000419881, 2.621784821874995952 ) ) ;
#21331=CARTESIAN_POINT ( 'NONE',  ( -3.000416591977282496E-16, 12.49062500061459602, 25.09994784771203058 ) ) ;
#21332=CARTESIAN_POINT ( 'NONE',  ( 22.87500000000000000, -4.330127018922194537, 2.499999999999995559 ) ) ;
#21333=EDGE_LOOP ( 'NONE', ( #69115, #21730, #19398, #58061 ) ) ;
#21334=CARTESIAN_POINT ( 'NONE',  ( -1.071796769724487453, 17.65759618943233633, -34.00000000000000000 ) ) ;
#21335=CARTESIAN_POINT ( 'NONE',  ( 4.200000000000001954, 4.330127018922192761, -2.499999999999997780 ) ) ;
#21336=ORIENTED_EDGE ( 'NONE', *, *, #25207, .T. ) ;
#21337=CARTESIAN_POINT ( 'NONE',  ( 18.51562500061451289, 3.027376345333611329, 5.243569643749999010 ) ) ;
#21338=CARTESIAN_POINT ( 'NONE',  ( 11.69062500061451360, 6.054752690667223547, 3.707466751127219781E-16 ) ) ;
#21340=CARTESIAN_POINT ( 'NONE',  ( 6.759375000614516793, 4.541064518000418104, -2.621784821874998173 ) ) ;
#21341=CARTESIAN_POINT ( 'NONE',  ( 20.13750000122903216, 4.330127018922191873, 2.499999999999999556 ) ) ;
#21343=CARTESIAN_POINT ( 'NONE',  ( 7.171875000614517326, 3.027376345333613106, -5.243569643749998122 ) ) ;
#21344=CARTESIAN_POINT ( 'NONE',  ( 14.22187500061451537, -6.054752690667223547, -1.112240025338166033E-15 ) ) ;
#21345=CARTESIAN_POINT ( 'NONE',  ( 23.22187500061451715, -6.054752690667223547, -1.112240025338166033E-15 ) ) ;
#21346=VERTEX_POINT ( 'NONE', #12322 ) ;
#21348=CARTESIAN_POINT ( 'NONE',  ( 17.74687500061451928, -3.027376345333614438, 5.243569643749998122 ) ) ;
#21349=CARTESIAN_POINT ( 'NONE',  ( 9.796875000614519990, -3.027376345333610441, -5.243569643749999898 ) ) ;
#21351=CARTESIAN_POINT ( 'NONE',  ( 21.41250000000000497, 2.886751345948126879, 4.999999999999999112 ) ) ;
#21353=CARTESIAN_POINT ( 'NONE',  ( -3.000416591977282496E-16, 10.29687500061451644, -34.90005215228797653 ) ) ;
#21355=CARTESIAN_POINT ( 'NONE',  ( 12.70312500061451821, 0.000000000000000000, 5.243569643749999010 ) ) ;
#21356=CARTESIAN_POINT ( 'NONE',  ( 3.225000000000002309, 6.123233995736764310E-16, -4.999999999999998224 ) ) ;
#21357=AXIS2_PLACEMENT_3D ( 'NONE', #18417, #40613, #29165 ) ;
#21359=CARTESIAN_POINT ( 'NONE',  ( 27.68437500061451573, -4.541064518000419881, 2.621784821874995952 ) ) ;
#21360=CARTESIAN_POINT ( 'NONE',  ( 13.31250000000000178, 2.886751345948126879, 4.999999999999999112 ) ) ;
#21361=CARTESIAN_POINT ( 'NONE',  ( 3.999999999999999112, 15.83750000122903501, 30.00000000000000000 ) ) ;
#21362=CARTESIAN_POINT ( 'NONE',  ( 11.13750000122903216, 4.330127018922191873, 2.499999999999999556 ) ) ;
#21363=CARTESIAN_POINT ( 'NONE',  ( 22.62187500061451573, 3.027376345333611329, 5.243569643749999010 ) ) ;
#21364=CARTESIAN_POINT ( 'NONE',  ( 13.92187500061451644, 3.027376345333613106, -5.243569643749998122 ) ) ;
#21365=CARTESIAN_POINT ( 'NONE',  ( 3.972658874145789110, 3.036112888163414514, -4.275165627105516286 ) ) ;
#21366=ORIENTED_EDGE ( 'NONE', *, *, #38881, .T. ) ;
#21367=CARTESIAN_POINT ( 'NONE',  ( 18.29062500061451502, -3.027376345333610441, -5.243569643749999898 ) ) ;
#21368=CARTESIAN_POINT ( 'NONE',  ( 29.06250000122903288, 4.330127018922192761, -2.499999999999997780 ) ) ;
#21369=CARTESIAN_POINT ( 'NONE',  ( 14.29687500061451821, -3.027376345333610441, -5.243569643749999898 ) ) ;
#21370=CARTESIAN_POINT ( 'NONE',  ( 7.285825834671762338E-16, 10.00000000000000000, -24.00000000000000000 ) ) ;
#21371=CARTESIAN_POINT ( 'NONE',  ( 19.86562500061451786, 3.027376345333611329, 5.243569643749999010 ) ) ;
#21372=CARTESIAN_POINT ( 'NONE',  ( 1.592000809091587073E-14, 16.73750000000000071, -34.00000000000000000 ) ) ;
#21373=CARTESIAN_POINT ( 'NONE',  ( 29.82187500061451502, 3.027376345333611329, 5.243569643749999010 ) ) ;
#21374=CARTESIAN_POINT ( 'NONE',  ( -4.243569643749997233, 13.09062500061451750, 32.45002607614398471 ) ) ;
#21375=CARTESIAN_POINT ( 'NONE',  ( 16.88437500061451502, -4.541064518000419881, 2.621784821874995952 ) ) ;
#21376=CARTESIAN_POINT ( 'NONE',  ( 13.53750000122903430, -4.330127018922194537, 2.499999999999995559 ) ) ;
#21378=CARTESIAN_POINT ( 'NONE',  ( 2.121784821874999061, 18.35937500061451644, -33.67503911421598417 ) ) ;
#21379=CARTESIAN_POINT ( 'NONE',  ( 20.85937500061451644, 0.000000000000000000, 5.243569643749999010 ) ) ;
#21380=CARTESIAN_POINT ( 'NONE',  ( 23.47500000122903430, -5.773502691896255534, -1.060575238724906372E-15 ) ) ;
#21381=CARTESIAN_POINT ( 'NONE',  ( 16.20937500061451786, 4.541064518000418104, -2.621784821874998173 ) ) ;
#21382=CARTESIAN_POINT ( 'NONE',  ( 12.55312500061451786, 4.541064518000418104, -2.621784821874998173 ) ) ;
#21383=CARTESIAN_POINT ( 'NONE',  ( -4.243569643749997233, 12.24687500061451928, 32.45002607614398471 ) ) ;
#21384=CARTESIAN_POINT ( 'NONE',  ( 17.57812500061451644, 4.541064518000418104, 2.621784821874999949 ) ) ;
#21385=ORIENTED_EDGE ( 'NONE', *, *, #31048, .F. ) ;
#21387=CARTESIAN_POINT ( 'NONE',  ( 22.68750000000000000, 5.773502691896255534, 3.535250795749688894E-16 ) ) ;
#21388=CARTESIAN_POINT ( 'NONE',  ( 2.121784821874999061, 18.35937500061451644, -33.67503911421598417 ) ) ;
#21390=CARTESIAN_POINT ( 'NONE',  ( 23.50312500061451360, 0.000000000000000000, 5.243569643749999010 ) ) ;
#21391=CARTESIAN_POINT ( 'NONE',  ( 6.253125000614517148, 4.541064518000418104, -2.621784821874998173 ) ) ;
#21392=CARTESIAN_POINT ( 'NONE',  ( 17.77500000122903145, 2.886751345948129099, -4.999999999999998224 ) ) ;
#21393=CARTESIAN_POINT ( 'NONE',  ( 23.57812500061451289, -4.541064518000419881, 2.621784821874995952 ) ) ;
#21394=CARTESIAN_POINT ( 'NONE',  ( 24.11249999999999716, 2.886751345948126879, 4.999999999999999112 ) ) ;
#21395=CARTESIAN_POINT ( 'NONE',  ( 25.15312500061451217, 4.541064518000418104, -2.621784821874998173 ) ) ;
#21396=CARTESIAN_POINT ( 'NONE',  ( 6.740625000614516082, 6.054752690667223547, 3.707466751127219781E-16 ) ) ;
#21397=ORIENTED_EDGE ( 'NONE', *, *, #15860, .F. ) ;
#21398=EDGE_CURVE ( 'NONE', #24437, #10170, #3581, .T. ) ;
#21399=CARTESIAN_POINT ( 'NONE',  ( 24.21562500061451573, 3.027376345333613106, -5.243569643749998122 ) ) ;
#21402=CYLINDRICAL_SURFACE ( 'NONE', #40612, 4.999999999999998224 ) ;
#21403=CARTESIAN_POINT ( 'NONE',  ( 2.000000000000001332, 14.86250000122903536, -26.53589838486224650 ) ) ;
#21404=CARTESIAN_POINT ( 'NONE',  ( -2.121784821874999949, 19.78437500061451715, -33.67503911421598417 ) ) ;
#21405=CARTESIAN_POINT ( 'NONE',  ( 11.28749999999999787, -2.886751345948125991, -5.000000000000000000 ) ) ;
#21406=CARTESIAN_POINT ( 'NONE',  ( 11.82187500061451679, 3.027376345333611329, 5.243569643749999010 ) ) ;
#21407=CARTESIAN_POINT ( 'NONE',  ( 6.787500001229032520, -4.330127018922194537, 2.499999999999995559 ) ) ;
#21408=CARTESIAN_POINT ( 'NONE',  ( 15.45937500061451608, 0.000000000000000000, 5.243569643749999010 ) ) ;
#21409=CARTESIAN_POINT ( 'NONE',  ( 6.271875000614517859, 3.027376345333613106, -5.243569643749998122 ) ) ;
#21411=FACE_OUTER_BOUND ( 'NONE', #65876, .T. ) ;
#21412=CARTESIAN_POINT ( 'NONE',  ( 12.53437500061451537, 6.421520780324663323E-16, -5.243569643749999010 ) ) ;
#21413=CARTESIAN_POINT ( 'NONE',  ( 13.12500000000000178, 6.123233995736764310E-16, -4.999999999999998224 ) ) ;
#21414=CARTESIAN_POINT ( 'NONE',  ( 22.49062500061451431, 6.054752690667223547, 3.707466751127219781E-16 ) ) ;
#21416=CARTESIAN_POINT ( 'NONE',  ( -5.810221930991193690E-16, 10.43750000000000000, -34.00000000000000000 ) ) ;
#21417=CARTESIAN_POINT ( 'NONE',  ( 24.15937500061451715, -4.541064518000417216, -2.621784821875001281 ) ) ;
#21419=CARTESIAN_POINT ( 'NONE',  ( 29.06250000122903288, 4.330127018922192761, -2.499999999999997780 ) ) ;
#21421=CARTESIAN_POINT ( 'NONE',  ( 24.21562500061451573, 3.027376345333613106, -5.243569643749998122 ) ) ;
#21422=CARTESIAN_POINT ( 'NONE',  ( 18.25312500061451715, -4.541064518000417216, -2.621784821875001281 ) ) ;
#21424=CARTESIAN_POINT ( 'NONE',  ( 14.03437500061451715, 4.541064518000418104, 2.621784821874999949 ) ) ;
#21426=CARTESIAN_POINT ( 'NONE',  ( 27.15000000122902790, -2.886751345948125991, -5.000000000000000000 ) ) ;
#21427=CARTESIAN_POINT ( 'NONE',  ( 2.896875000614518747, -3.027376345333614438, 5.243569643749998122 ) ) ;
#21428=CARTESIAN_POINT ( 'NONE',  ( 13.65937500061451715, 0.000000000000000000, 5.243569643749999010 ) ) ;
#21430=CARTESIAN_POINT ( 'NONE',  ( -3.999999999999999112, 11.45000000000000107, 30.00000000000000000 ) ) ;
#21431=CARTESIAN_POINT ( 'NONE',  ( 4.650000001229035895, -2.886751345948125991, -5.000000000000000000 ) ) ;
#21432=CARTESIAN_POINT ( 'NONE',  ( 24.45937500061451786, 0.000000000000000000, 5.243569643749999010 ) ) ;
#21433=CARTESIAN_POINT ( 'NONE',  ( 16.73437500061451644, 4.541064518000418104, 2.621784821874999949 ) ) ;
#21435=CARTESIAN_POINT ( 'NONE',  ( 28.01249999999999574, 2.886751345948129099, -4.999999999999998224 ) ) ;
#21436=CARTESIAN_POINT ( 'NONE',  ( 6.524999999999999467, 4.330127018922191873, 2.499999999999999556 ) ) ;
#21438=CARTESIAN_POINT ( 'NONE',  ( 19.60312500061451502, -4.541064518000417216, -2.621784821875001281 ) ) ;
#21439=CARTESIAN_POINT ( 'NONE',  ( 10.08749999999999858, 5.773502691896255534, 3.535250795749688894E-16 ) ) ;
#21440=CARTESIAN_POINT ( 'NONE',  ( 4.790625000614518569, -3.027376345333610441, -5.243569643749999898 ) ) ;
#21441=CARTESIAN_POINT ( 'NONE',  ( 19.34999999999999787, -4.330127018922190985, -2.500000000000001332 ) ) ;
#21442=EDGE_CURVE ( 'NONE', #59726, #55474, #11121, .T. ) ;
#21444=CARTESIAN_POINT ( 'NONE',  ( 22.38750000122903216, 4.330127018922191873, 2.499999999999999556 ) ) ;
#21445=CARTESIAN_POINT ( 'NONE',  ( 5.681944431425976383, 8.230953001180113304, 28.03323168659990117 ) ) ;
#21446=CARTESIAN_POINT ( 'NONE',  ( 28.88437500061451502, 4.541064518000418104, 2.621784821874999949 ) ) ;
#21448=CARTESIAN_POINT ( 'NONE',  ( 16.75312500061451715, 0.000000000000000000, 5.243569643749999010 ) ) ;
#21449=CARTESIAN_POINT ( 'NONE',  ( 24.21562500061451573, 3.027376345333613106, -5.243569643749998122 ) ) ;
#21450=CARTESIAN_POINT ( 'NONE',  ( 25.73437500061451644, 4.541064518000418104, 2.621784821874999949 ) ) ;
#21452=CARTESIAN_POINT ( 'NONE',  ( 5.775000000000002132, -4.330127018922194537, 2.499999999999995559 ) ) ;
#21453=CARTESIAN_POINT ( 'NONE',  ( 9.928125000614517859, 4.541064518000418104, 2.621784821874999949 ) ) ;
#21454=CARTESIAN_POINT ( 'NONE',  ( 25.56562500061452070, 3.027376345333613106, -5.243569643749998122 ) ) ;
#21455=CARTESIAN_POINT ( 'NONE',  ( 14.59687500061452070, -3.027376345333614438, 5.243569643749998122 ) ) ;
#21456=CARTESIAN_POINT ( 'NONE',  ( 18.60937500061451644, 0.000000000000000000, 5.243569643749999010 ) ) ;
#21457=CARTESIAN_POINT ( 'NONE',  ( 4.437233173123817487, 2.304579454652033732, -4.709995530123128660 ) ) ;
#21458=CARTESIAN_POINT ( 'NONE',  ( -2.121784821874999949, 10.78437500061451715, 26.32496088578401938 ) ) ;
#21459=CARTESIAN_POINT ( 'NONE',  ( 21.52500000122903145, 2.886751345948126879, 4.999999999999999112 ) ) ;
#21461=CARTESIAN_POINT ( 'NONE',  ( 13.11562500061451786, 3.027376345333611329, 5.243569643749999010 ) ) ;
#21463=CARTESIAN_POINT ( 'NONE',  ( 7.509375000614517681, -4.541064518000417216, -2.621784821875001281 ) ) ;
#21464=CARTESIAN_POINT ( 'NONE',  ( 7.921875000614517326, -6.054752690667223547, -1.112240025338166033E-15 ) ) ;
#21465=ORIENTED_EDGE ( 'NONE', *, *, #30679, .T. ) ;
#21466=CARTESIAN_POINT ( 'NONE',  ( 27.90937500061451715, 4.541064518000418104, -2.621784821874998173 ) ) ;
#21467=CARTESIAN_POINT ( 'NONE',  ( 18.66562500061451146, -6.054752690667223547, -1.112240025338166033E-15 ) ) ;
#21468=CARTESIAN_POINT ( 'NONE',  ( 3.965625000614515727, 3.027376345333613106, -5.243569643749998122 ) ) ;
#21469=( BOUNDED_CURVE ( )  B_SPLINE_CURVE ( 2, ( #47591, #41684, #18407, #40973, #24323, #18766, #46872 ),
 .UNSPECIFIED., .F., .F. ) 
 B_SPLINE_CURVE_WITH_KNOTS ( ( 3, 2, 2, 3 ),
 ( 0.9249999999999999334, 0.9277777777777777013, 0.9305555555555555802, 0.9326049216113281304 ),
 .UNSPECIFIED. ) 
 CURVE ( )  GEOMETRIC_REPRESENTATION_ITEM ( )  RATIONAL_B_SPLINE_CURVE ( ( 1.000000000000005329, 0.8660254037844333785, 1.000000000000000000, 0.8660254037844387076, 1.000000000000000000, 0.9011573236647978380, 0.9481613218646109953 ) ) 
 REPRESENTATION_ITEM ( '' )  );
#21470=CARTESIAN_POINT ( 'NONE',  ( 4.321875000614517681, -6.054752690667223547, -1.112240025338166033E-15 ) ) ;
#21471=VECTOR ( 'NONE', #53281, 1000.000000000000000 ) ;
#21472=CARTESIAN_POINT ( 'NONE',  ( 24.98437500061451644, -4.541064518000419881, 2.621784821874995952 ) ) ;
#21473=CARTESIAN_POINT ( 'NONE',  ( 18.74062500061451431, -3.027376345333610441, -5.243569643749999898 ) ) ;
#21474=CARTESIAN_POINT ( 'NONE',  ( -3.999999999999999112, 12.34999999999999964, 30.00000000000000000 ) ) ;
#21475=CARTESIAN_POINT ( 'NONE',  ( 24.02812500061451573, -4.541064518000419881, 2.621784821874995952 ) ) ;
#21476=CARTESIAN_POINT ( 'NONE',  ( 5.100000001229034297, -2.886751345948125991, -5.000000000000000000 ) ) ;
#21477=VERTEX_POINT ( 'NONE', #54048 ) ;
#21478=CARTESIAN_POINT ( 'NONE',  ( 29.32499999999999929, 6.123233995736764310E-16, -4.999999999999998224 ) ) ;
#21479=CARTESIAN_POINT ( 'NONE',  ( 1.999999999999998668, 15.35000000000000142, -33.46410161513775705 ) ) ;
#21482=CARTESIAN_POINT ( 'NONE',  ( 5.221875000614519813, -6.054752690667223547, -1.112240025338166033E-15 ) ) ;
#21483=CARTESIAN_POINT ( 'NONE',  ( 29.76562500061451644, 3.027376345333611329, 5.243569643749999010 ) ) ;
#21484=CARTESIAN_POINT ( 'NONE',  ( 12.21562500061451573, 3.027376345333611329, 5.243569643749999010 ) ) ;
#21485=CARTESIAN_POINT ( 'NONE',  ( 5.634375000614519458, -4.541064518000419881, 2.621784821874995952 ) ) ;
#21486=CARTESIAN_POINT ( 'NONE',  ( 25.76250000122903216, -4.330127018922190985, -2.500000000000001332 ) ) ;
#21487=CARTESIAN_POINT ( 'NONE',  ( 15.68437500061451573, 6.421520780324663323E-16, -5.243569643749999010 ) ) ;
#21488=CARTESIAN_POINT ( 'NONE',  ( 28.71562500061451573, 3.027376345333613106, -5.243569643749998122 ) ) ;
#21489=CARTESIAN_POINT ( 'NONE',  ( 29.21249999999999858, -5.773502691896255534, -1.060575238724906372E-15 ) ) ;
#21490=CARTESIAN_POINT ( 'NONE',  ( 3.815625000614518036, -6.054752690667223547, -1.112240025338166033E-15 ) ) ;
#21491=CARTESIAN_POINT ( 'NONE',  ( 15.89062500061451289, -3.027376345333614438, 5.243569643749998122 ) ) ;
#21492=ORIENTED_EDGE ( 'NONE', *, *, #52383, .F. ) ;
#21493=CARTESIAN_POINT ( 'NONE',  ( 10.07812500061451644, -4.541064518000419881, 2.621784821874995952 ) ) ;
#21494=CARTESIAN_POINT ( 'NONE',  ( 7.940625000614518036, -3.027376345333610441, -5.243569643749999898 ) ) ;
#21496=CARTESIAN_POINT ( 'NONE',  ( 9.712500000000002132, 2.886751345948126879, 4.999999999999999112 ) ) ;
#21497=CARTESIAN_POINT ( 'NONE',  ( 3.150000001229034119, -2.886751345948129988, 4.999999999999997335 ) ) ;
#21498=CARTESIAN_POINT ( 'NONE',  ( 18.37500000000000355, -4.330127018922194537, 2.499999999999995559 ) ) ;
#21499=CARTESIAN_POINT ( 'NONE',  ( 19.43437500061451928, 4.541064518000418104, 2.621784821874999949 ) ) ;
#21500=CARTESIAN_POINT ( 'NONE',  ( 14.51250000122903394, -4.330127018922190985, -2.500000000000001332 ) ) ;
#21502=CARTESIAN_POINT ( 'NONE',  ( 4.243569643749999010, 17.36562500061451786, -32.45002607614398471 ) ) ;
#21503=CARTESIAN_POINT ( 'NONE',  ( 22.08749999999999858, -2.886751345948159742, -4.999999999999942268 ) ) ;
#21505=CARTESIAN_POINT ( 'NONE',  ( 28.56562500061451715, -6.054752690667223547, -1.112240025338166033E-15 ) ) ;
#21506=CARTESIAN_POINT ( 'NONE',  ( 20.06250000122903643, 4.330127018922192761, -2.499999999999997780 ) ) ;
#21507=CARTESIAN_POINT ( 'NONE',  ( 12.87187500061451750, -6.054752690667223547, -1.112240025338166033E-15 ) ) ;
#21508=CARTESIAN_POINT ( 'NONE',  ( 26.02499999999999858, -4.330127018922194537, 2.499999999999995559 ) ) ;
#21509=CARTESIAN_POINT ( 'NONE',  ( 9.515625000614518214, 3.027376345333611329, 5.243569643749999010 ) ) ;
#21510=VECTOR ( 'NONE', #60611, 1000.000000000000000 ) ;
#21512=CARTESIAN_POINT ( 'NONE',  ( 22.17187500061451644, 3.027376345333611329, 5.243569643749999010 ) ) ;
#21514=CARTESIAN_POINT ( 'NONE',  ( 8.503125000614515372, 4.541064518000418104, -2.621784821874998173 ) ) ;
#21515=CARTESIAN_POINT ( 'NONE',  ( 12.83437500061451786, -4.541064518000419881, 2.621784821874995952 ) ) ;
#21516=ORIENTED_EDGE ( 'NONE', *, *, #3316, .F. ) ;
#21517=CARTESIAN_POINT ( 'NONE',  ( 24.90937500061451715, 0.000000000000000000, 5.243569643749999010 ) ) ;
#21518=CARTESIAN_POINT ( 'NONE',  ( 1.095284332908923686, 4.886121113889972278, -33.85685977295008087 ) ) ;
#21519=CARTESIAN_POINT ( 'NONE',  ( 5.137500000000000178, 5.773502691896255534, 3.535250795749688894E-16 ) ) ;
#21520=CARTESIAN_POINT ( 'NONE',  ( 15.26250000122903216, 0.000000000000000000, 4.999999999999998224 ) ) ;
#21521=CARTESIAN_POINT ( 'NONE',  ( 1.999999999999998668, 15.35000000000000142, -33.46410161513775705 ) ) ;
#21522=CARTESIAN_POINT ( 'NONE',  ( 19.04999999999999716, 4.330127018922192761, -2.499999999999997780 ) ) ;
#21524=CARTESIAN_POINT ( 'NONE',  ( 13.12500000000000178, 6.123233995736764310E-16, -4.999999999999998224 ) ) ;
#21525=CARTESIAN_POINT ( 'NONE',  ( 15.67500000000000071, -4.330127018922194537, 2.499999999999995559 ) ) ;
#21526=CARTESIAN_POINT ( 'NONE',  ( 13.50000000122903288, -2.886751345948129988, 4.999999999999997335 ) ) ;
#21527=CARTESIAN_POINT ( 'NONE',  ( 10.37812500061451715, 4.541064518000418104, 2.621784821874999949 ) ) ;
#21528=EDGE_CURVE ( 'NONE', #59300, #11494, #7944, .T. ) ;
#21529=ORIENTED_EDGE ( 'NONE', *, *, #56383, .T. ) ;
#21530=CARTESIAN_POINT ( 'NONE',  ( 8.775000000000002132, 4.330127018922191873, 2.499999999999999556 ) ) ;
#21531=CARTESIAN_POINT ( 'NONE',  ( -3.137519842735245283E-14, 11.22500000122903430, -26.00000000000000711 ) ) ;
#21532=CARTESIAN_POINT ( 'NONE',  ( 4.243569643749999898, 14.23437500061451821, -30.00000000000000000 ) ) ;
#21533=CARTESIAN_POINT ( 'NONE',  ( 4.078125000614517326, 4.541064518000418104, 2.621784821874999949 ) ) ;
#21535=CARTESIAN_POINT ( 'NONE',  ( 9.037499999999999645, -2.886751345948125991, -5.000000000000000000 ) ) ;
#21538=CARTESIAN_POINT ( 'NONE',  ( 24.32812500061451289, 4.541064518000418104, 2.621784821874999949 ) ) ;
#21541=CARTESIAN_POINT ( 'NONE',  ( 21.42187500061451644, -6.054752690667223547, -1.112240025338166033E-15 ) ) ;
#21542=EDGE_CURVE ( 'NONE', #14527, #50794, #18649, .T. ) ;
#21543=CARTESIAN_POINT ( 'NONE',  ( 20.20312500061451644, 4.541064518000418104, -2.621784821874998173 ) ) ;
#21544=CARTESIAN_POINT ( 'NONE',  ( -4.243569643749999898, 11.25312500061459531, -30.00000000000000000 ) ) ;
#21545=CARTESIAN_POINT ( 'NONE',  ( 6.103125000614515905, -4.541064518000417216, -2.621784821875001281 ) ) ;
#21546=CARTESIAN_POINT ( 'NONE',  ( 4.640625000614518214, -3.027376345333614438, 5.243569643749998122 ) ) ;
#21548=CARTESIAN_POINT ( 'NONE',  ( 20.84062500061451217, -3.027376345333614438, 5.243569643749998122 ) ) ;
#21549=CARTESIAN_POINT ( 'NONE',  ( 0.000000000000000000, 20.00000000000000000, -30.00000000000000000 ) ) ;
#21551=CARTESIAN_POINT ( 'NONE',  ( 14.25937500061451679, -4.541064518000417216, -2.621784821875001281 ) ) ;
#21553=CARTESIAN_POINT ( 'NONE',  ( 14.37187500061451928, 3.027376345333613106, -5.243569643749998122 ) ) ;
#21554=CARTESIAN_POINT ( 'NONE',  ( 22.50937500061451857, 4.541064518000418104, -2.621784821874998173 ) ) ;
#21555=EDGE_LOOP ( 'NONE', ( #30871, #30996, #55384, #30790 ) ) ;
#21556=CARTESIAN_POINT ( 'NONE',  ( 2.121784821875001281, 11.90937500061451892, 33.67503911421598417 ) ) ;
#21558=CARTESIAN_POINT ( 'NONE',  ( 25.71562500061451573, 3.027376345333611329, 5.243569643749999010 ) ) ;
#21559=CARTESIAN_POINT ( 'NONE',  ( 25.64062500061451644, 6.054752690667223547, 3.707466751127219781E-16 ) ) ;
#21561=CARTESIAN_POINT ( 'NONE',  ( 3.999999999999998668, 18.46249999999999858, 27.69059892324149175 ) ) ;
#21562=CARTESIAN_POINT ( 'NONE',  ( 3.646875000614520079, 6.054752690667223547, 3.707466751127219781E-16 ) ) ;
#21564=CARTESIAN_POINT ( 'NONE',  ( 10.72500000122903252, 2.886751345948126879, 4.999999999999999112 ) ) ;
#21565=CARTESIAN_POINT ( 'NONE',  ( 8.287500001229034297, 6.123233995736764310E-16, -4.999999999999998224 ) ) ;
#21566=CARTESIAN_POINT ( 'NONE',  ( 3.553125000614516082, 4.541064518000418104, -2.621784821874998173 ) ) ;
#21569=CARTESIAN_POINT ( 'NONE',  ( 12.42187500061451821, -6.054752690667223547, -1.112240025338166033E-15 ) ) ;
#21571=VERTEX_POINT ( 'NONE', #37038 ) ;
#21572=CARTESIAN_POINT ( 'NONE',  ( 18.74062500061451431, -3.027376345333610441, -5.243569643749999898 ) ) ;
#21573=CARTESIAN_POINT ( 'NONE',  ( 13.35937500061451821, -4.541064518000417216, -2.621784821875001281 ) ) ;
#21574=CARTESIAN_POINT ( 'NONE',  ( 5.915625000614515905, 3.027376345333611329, 5.243569643749999010 ) ) ;
#21575=CARTESIAN_POINT ( 'NONE',  ( 22.05937500061451573, 4.541064518000418104, -2.621784821874998173 ) ) ;
#21576=CARTESIAN_POINT ( 'NONE',  ( 6.028125000614517504, -4.541064518000419881, 2.621784821874995952 ) ) ;
#21578=CARTESIAN_POINT ( 'NONE',  ( 6.825000001229034829, -5.773502691896255534, -1.060575238724906372E-15 ) ) ;
#21579=CARTESIAN_POINT ( 'NONE',  ( 21.96562500061451573, 3.027376345333613106, -5.243569643749998122 ) ) ;
#21580=CARTESIAN_POINT ( 'NONE',  ( -3.999999999999997335, 17.00000000122903288, -27.69059892324149175 ) ) ;
#21581=CARTESIAN_POINT ( 'NONE',  ( 9.075000001229033941, -5.773502691896255534, -1.060575238724906372E-15 ) ) ;
#21582=CARTESIAN_POINT ( 'NONE',  ( 16.67812500061451786, 4.541064518000418104, 2.621784821874999949 ) ) ;
#21583=CARTESIAN_POINT ( 'NONE',  ( 15.14062500061451644, -3.027376345333610441, -5.243569643749999898 ) ) ;
#21585=CARTESIAN_POINT ( 'NONE',  ( 15.86250000000000249, 2.886751345948129099, -4.999999999999998224 ) ) ;
#21586=CARTESIAN_POINT ( 'NONE',  ( 10.72500000122903252, 2.886751345948126879, 4.999999999999999112 ) ) ;
#21588=CARTESIAN_POINT ( 'NONE',  ( 9.215625000614515727, -6.054752690667223547, -1.112240025338166033E-15 ) ) ;
#21589=CARTESIAN_POINT ( 'NONE',  ( 10.94062500061451537, -3.027376345333614438, 5.243569643749998122 ) ) ;
#21590=CARTESIAN_POINT ( 'NONE',  ( 21.33750000122903145, 6.123233995736764310E-16, -4.999999999999998224 ) ) ;
#21591=CARTESIAN_POINT ( 'NONE',  ( 4.243569643749999010, 14.27187500061451964, -32.45002607614398471 ) ) ;
#21592=CARTESIAN_POINT ( 'NONE',  ( 19.54687500061451644, -3.027376345333614438, 5.243569643749998122 ) ) ;
#21593=CARTESIAN_POINT ( 'NONE',  ( 30.00000000000000000, 0.000000000000000000, 0.000000000000000000 ) ) ;
#21594=CARTESIAN_POINT ( 'NONE',  ( 4.612500001229032698, -4.330127018922190985, -2.500000000000001332 ) ) ;
#21595=CARTESIAN_POINT ( 'NONE',  ( 3.609375000614516882, 4.541064518000418104, -2.621784821874998173 ) ) ;
#21596=CARTESIAN_POINT ( 'NONE',  ( 19.99687500061451573, -3.027376345333614438, 5.243569643749998122 ) ) ;
#21597=CARTESIAN_POINT ( 'NONE',  ( 5.062500000000002665, 2.886751345948196157, -4.999999999999881872 ) ) ;
#21598=CARTESIAN_POINT ( 'NONE',  ( 16.04062500061451857, -3.027376345333610441, -5.243569643749999898 ) ) ;
#21600=CARTESIAN_POINT ( 'NONE',  ( -1.487416814333745711E-14, 14.82500000122903572, 34.00000000000000000 ) ) ;
#21601=CARTESIAN_POINT ( 'NONE',  ( 1.626862140677534273E-15, 13.81250000000000000, 34.00000000000000000 ) ) ;
#21602=CARTESIAN_POINT ( 'NONE',  ( 29.59687500061451715, -3.027376345333610441, -5.243569643749999898 ) ) ;
#21604=CARTESIAN_POINT ( 'NONE',  ( 14.80312500061451608, 4.541064518000418104, -2.621784821874998173 ) ) ;
#21605=CARTESIAN_POINT ( 'NONE',  ( 13.77187500061451786, -6.054752690667223547, -1.112240025338166033E-15 ) ) ;
#21606=ORIENTED_EDGE ( 'NONE', *, *, #38374, .T. ) ;
#21607=CARTESIAN_POINT ( 'NONE',  ( 9.299999999999998934, 0.000000000000000000, 4.999999999999998224 ) ) ;
#21608=CARTESIAN_POINT ( 'NONE',  ( 23.65312500061451573, -4.541064518000417216, -2.621784821875001281 ) ) ;
#21609=DIRECTION ( 'NONE',  ( 0.000000000000000000, 0.000000000000000000, -1.000000000000000000 ) ) ;
#21610=CARTESIAN_POINT ( 'NONE',  ( 14.58750000000000036, 5.773502691896255534, 3.535250795749688401E-16 ) ) ;
#21611=CARTESIAN_POINT ( 'NONE',  ( 13.23750000000000071, 5.773502691896255534, 3.535250795749688894E-16 ) ) ;
#21612=CARTESIAN_POINT ( 'NONE',  ( 24.33750000122903145, -4.330127018922194537, 2.499999999999995559 ) ) ;
#21613=CARTESIAN_POINT ( 'NONE',  ( 17.87812500061451715, 6.421520780324663323E-16, -5.243569643749999010 ) ) ;
#21614=EDGE_LOOP ( 'NONE', ( #43157, #21666 ) ) ;
#21615=CARTESIAN_POINT ( 'NONE',  ( 20.54999999999999716, 0.000000000000000000, 4.999999999999998224 ) ) ;
#21617=CARTESIAN_POINT ( 'NONE',  ( 21.27187500061451786, 3.027376345333611329, 5.243569643749999010 ) ) ;
#21618=ORIENTED_EDGE ( 'NONE', *, *, #16392, .T. ) ;
#21619=CARTESIAN_POINT ( 'NONE',  ( 10.19062500061451892, -3.027376345333610441, -5.243569643749999898 ) ) ;
#21621=CARTESIAN_POINT ( 'NONE',  ( 15.97499999999999964, 4.330127018922191873, 2.499999999999999556 ) ) ;
#21622=CARTESIAN_POINT ( 'NONE',  ( 24.07499999999999929, 4.330127018922191873, 2.499999999999999556 ) ) ;
#21623=CARTESIAN_POINT ( 'NONE',  ( 3.518507979705963518, -3.552478233113482542, -3.764599296078968926 ) ) ;
#21624=CARTESIAN_POINT ( 'NONE',  ( 3.796875000614517326, -3.027376345333614438, 5.243569643749998122 ) ) ;
#21625=CARTESIAN_POINT ( 'NONE',  ( 29.03437500061451715, -4.541064518000419881, 2.621784821874995952 ) ) ;
#21626=ORIENTED_EDGE ( 'NONE', *, *, #72282, .F. ) ;
#21627=CARTESIAN_POINT ( 'NONE',  ( 25.49062500061451786, -3.027376345333610441, -5.243569643749999898 ) ) ;
#21628=CARTESIAN_POINT ( 'NONE',  ( 27.75937500061451502, -4.541064518000417216, -2.621784821875001281 ) ) ;
#21630=CARTESIAN_POINT ( 'NONE',  ( 12.78749999999999964, 5.773502691896255534, 3.535250795749688894E-16 ) ) ;
#21631=CARTESIAN_POINT ( 'NONE',  ( 12.40312500061451573, -4.541064518000417216, -2.621784821875001281 ) ) ;
#21632=CARTESIAN_POINT ( 'NONE',  ( 3.849931240356728512, 3.190302406438068505, 3.849931240356827544 ) ) ;
#21633=CARTESIAN_POINT ( 'NONE',  ( 2.000000000000001332, 19.25000000000000000, -26.53589838486224650 ) ) ;
#21634=CARTESIAN_POINT ( 'NONE',  ( 27.66562500061451502, -6.054752690667223547, -1.112240025338166033E-15 ) ) ;
#21635=CARTESIAN_POINT ( 'NONE',  ( 15.90000000122903501, -2.886751345948125991, -5.000000000000000000 ) ) ;
#21636=DIRECTION ( 'NONE',  ( -0.000000000000000000, -1.000000000000000000, -0.000000000000000000 ) ) ;
#21638=CARTESIAN_POINT ( 'NONE',  ( 5.240625000614516971, -3.027376345333610441, -5.243569643749999898 ) ) ;
#21639=CARTESIAN_POINT ( 'NONE',  ( 21.68437500061451573, 4.541064518000418104, 2.621784821874999949 ) ) ;
#21640=CARTESIAN_POINT ( 'NONE',  ( 4.243569643749999010, 14.72187500061451715, 27.54997392385601174 ) ) ;
#21641=EDGE_CURVE ( 'NONE', #70308, #26824, #41320, .T. ) ;
#21642=CARTESIAN_POINT ( 'NONE',  ( 22.02187500061452141, 3.027376345333613106, -5.243569643749998122 ) ) ;
#21643=CARTESIAN_POINT ( 'NONE',  ( 29.40937500061451715, 0.000000000000000000, 5.243569643749999010 ) ) ;
#21644=CARTESIAN_POINT ( 'NONE',  ( -2.121784821874999949, 17.98437500061451999, 26.32496088578401938 ) ) ;
#21645=CARTESIAN_POINT ( 'NONE',  ( 10.07812500061451644, -4.541064518000419881, 2.621784821874995952 ) ) ;
#21646=DIRECTION ( 'NONE',  ( 0.000000000000000000, 0.000000000000000000, 1.000000000000000000 ) ) ;
#21647=CARTESIAN_POINT ( 'NONE',  ( 6.534375000614517148, -4.541064518000419881, 2.621784821874995952 ) ) ;
#21648=CARTESIAN_POINT ( 'NONE',  ( 23.47499999999999787, 6.123233995736764310E-16, -4.999999999999998224 ) ) ;
#21649=CARTESIAN_POINT ( 'NONE',  ( 7.565625000614518036, 3.027376345333613106, -5.243569643749998122 ) ) ;
#21650=CARTESIAN_POINT ( 'NONE',  ( 11.10937500061451644, -4.541064518000417216, -2.621784821875001281 ) ) ;
#21651=CARTESIAN_POINT ( 'NONE',  ( 30.00000000000000000, 0.000000000000000000, 0.000000000000000000 ) ) ;
#21652=CARTESIAN_POINT ( 'NONE',  ( 21.07500000122903572, 2.886751345948126879, 4.999999999999999112 ) ) ;
#21653=CARTESIAN_POINT ( 'NONE',  ( 6.834375000614518747, 4.541064518000418104, 2.621784821874999949 ) ) ;
#21654=CARTESIAN_POINT ( 'NONE',  ( 10.79062500061451679, 6.054752690667223547, 3.707466751127219781E-16 ) ) ;
#21656=CARTESIAN_POINT ( 'NONE',  ( 19.62187500061451573, -6.054752690667223547, -1.112240025338166033E-15 ) ) ;
#21657=CARTESIAN_POINT ( 'NONE',  ( 1.626862140677534273E-15, 15.61250000000000071, -26.00000000000000355 ) ) ;
#21658=CARTESIAN_POINT ( 'NONE',  ( 11.95312500061451644, -4.541064518000417216, -2.621784821875001281 ) ) ;
#21659=CARTESIAN_POINT ( 'NONE',  ( 21.63750000122903572, -4.330127018922194537, 2.499999999999995559 ) ) ;
#21660=CARTESIAN_POINT ( 'NONE',  ( 28.35937500061451289, 4.541064518000418104, -2.621784821874998173 ) ) ;
#21661=CARTESIAN_POINT ( 'NONE',  ( -4.243569643749999898, 12.17187500061451999, -32.45002607614398471 ) ) ;
#21662=CARTESIAN_POINT ( 'NONE',  ( 14.25000000122903465, 5.773502691896255534, 3.535250795749688894E-16 ) ) ;
#21663=CARTESIAN_POINT ( 'NONE',  ( -4.243569643749999898, 15.71562500061451573, -32.45002607614398471 ) ) ;
#21664=CARTESIAN_POINT ( 'NONE',  ( 15.78750000122903430, -4.330127018922194537, 2.499999999999995559 ) ) ;
#21665=CARTESIAN_POINT ( 'NONE',  ( 11.09062500061451573, -3.027376345333610441, -5.243569643749999898 ) ) ;
#21666=ORIENTED_EDGE ( 'NONE', *, *, #18349, .T. ) ;
#21667=CARTESIAN_POINT ( 'NONE',  ( 14.06250000000000000, 2.886751345948129099, -4.999999999999998224 ) ) ;
#21669=CARTESIAN_POINT ( 'NONE',  ( 21.77812500061451928, -4.541064518000419881, 2.621784821874995952 ) ) ;
#21670=CARTESIAN_POINT ( 'NONE',  ( 7.659375000614518036, 4.541064518000418104, -2.621784821874998173 ) ) ;
#21671=CARTESIAN_POINT ( 'NONE',  ( 11.10000000122903252, 5.773502691896255534, 3.535250795749688894E-16 ) ) ;
#21672=CARTESIAN_POINT ( 'NONE',  ( 17.88750000122903216, 4.330127018922191873, 2.499999999999999556 ) ) ;
#21673=( BOUNDED_CURVE ( )  B_SPLINE_CURVE ( 2, ( #11064, #10702, #33235, #65758, #32144, #44339, #38790 ),
 .UNSPECIFIED., .F., .F. ) 
 B_SPLINE_CURVE_WITH_KNOTS ( ( 3, 2, 2, 3 ),
 ( 0.3750000000000000000, 0.3777777777777777679, 0.3805555555555554803, 0.3833333333333333037 ),
 .UNSPECIFIED. ) 
 CURVE ( )  GEOMETRIC_REPRESENTATION_ITEM ( )  RATIONAL_B_SPLINE_CURVE ( ( 1.000000000000000000, 0.8660254037844387076, 1.000000000000000000, 0.8660254037844387076, 1.000000000000000000, 0.8660254037844413721, 0.9999999999999973355 ) ) 
 REPRESENTATION_ITEM ( '' )  );
#21674=CARTESIAN_POINT ( 'NONE',  ( 14.54062500061451679, -3.027376345333614438, 5.243569643749998122 ) ) ;
#21675=CARTESIAN_POINT ( 'NONE',  ( 19.34062500061451573, 6.054752690667223547, 3.707466751127219781E-16 ) ) ;
#21676=CARTESIAN_POINT ( 'NONE',  ( 24.86250000122903359, -4.330127018922190985, -2.500000000000001332 ) ) ;
#21678=CARTESIAN_POINT ( 'NONE',  ( 27.75000000122903288, 5.773502691896255534, 3.535250795749688894E-16 ) ) ;
#21679=CARTESIAN_POINT ( 'NONE',  ( 22.91249999999999432, -5.773502691896255534, -1.060575238724906372E-15 ) ) ;
#21681=CARTESIAN_POINT ( 'NONE',  ( 26.14687500061451431, 6.054752690667223547, 3.707466751127219781E-16 ) ) ;
#21684=CARTESIAN_POINT ( 'NONE',  ( 12.78750000122903430, 6.123233995736764310E-16, -4.999999999999998224 ) ) ;
#21685=CARTESIAN_POINT ( 'NONE',  ( 29.10937500061451644, -4.541064518000417216, -2.621784821875001281 ) ) ;
#21688=CARTESIAN_POINT ( 'NONE',  ( 4.696875000614518569, -3.027376345333614438, 5.243569643749998122 ) ) ;
#21689=CARTESIAN_POINT ( 'NONE',  ( 26.87812500061451360, 6.421520780324663323E-16, -5.243569643749999010 ) ) ;
#21691=CARTESIAN_POINT ( 'NONE',  ( 10.24687500061451750, -3.027376345333610441, -5.243569643749999898 ) ) ;
#21692=LINE ( 'NONE', #43145, #9993 ) ;
#21693=CARTESIAN_POINT ( 'NONE',  ( 2.859375000614519546, 0.000000000000000000, 5.243569643749999010 ) ) ;
#21694=CARTESIAN_POINT ( 'NONE',  ( 9.796875000614519990, -3.027376345333610441, -5.243569643749999898 ) ) ;
#21695=CARTESIAN_POINT ( 'NONE',  ( 27.98437500061451289, 4.541064518000418104, 2.621784821874999949 ) ) ;
#21696=CARTESIAN_POINT ( 'NONE',  ( 4.243569643749999898, 13.27812500061459566, 30.00000000000000000 ) ) ;
#21697=CARTESIAN_POINT ( 'NONE',  ( 19.46249999999999858, 2.886751345948129099, -4.999999999999998224 ) ) ;
#21699=CARTESIAN_POINT ( 'NONE',  ( 28.83749999999999858, -2.886751345948125991, -5.000000000000000000 ) ) ;
#21700=CARTESIAN_POINT ( 'NONE',  ( 4.987500000000002487, -2.886751345948125991, -5.000000000000000000 ) ) ;
#21701=EDGE_LOOP ( 'NONE', ( #70688, #52589, #31389, #43018 ) ) ;
#21702=CARTESIAN_POINT ( 'NONE',  ( 16.86562500061451786, -6.054752690667223547, -1.112240025338166033E-15 ) ) ;
#21703=CARTESIAN_POINT ( 'NONE',  ( 8.578125000614518214, 4.541064518000418104, 2.621784821874999949 ) ) ;
#21705=CARTESIAN_POINT ( 'NONE',  ( 6.159375000614517148, -4.541064518000417216, -2.621784821875001281 ) ) ;
#21706=CARTESIAN_POINT ( 'NONE',  ( 18.75000000122903288, 5.773502691896255534, 3.535250795749688894E-16 ) ) ;
#21707=CARTESIAN_POINT ( 'NONE',  ( 23.85000000122903430, -2.886751345948096681, 5.000000000000054179 ) ) ;
#21708=CARTESIAN_POINT ( 'NONE',  ( 7.959375000614516971, -4.541064518000417216, -2.621784821875001281 ) ) ;
#21709=CARTESIAN_POINT ( 'NONE',  ( 12.27187500061451786, 3.027376345333611329, 5.243569643749999010 ) ) ;
#21710=CARTESIAN_POINT ( 'NONE',  ( 23.44687500061451502, 6.054752690667223547, 3.707466751127219781E-16 ) ) ;
#21711=DIRECTION ( 'NONE',  ( -0.000000000000000000, -1.000000000000000000, -0.000000000000000000 ) ) ;
#21712=EDGE_LOOP ( 'NONE', ( #5240, #12671, #27622, #61588 ) ) ;
#21714=CARTESIAN_POINT ( 'NONE',  ( 16.95937500061451786, -4.541064518000417216, -2.621784821875001281 ) ) ;
#21715=CARTESIAN_POINT ( 'NONE',  ( 9.946875000614516793, 6.054752690667223547, 3.707466751127219781E-16 ) ) ;
#21717=CARTESIAN_POINT ( 'NONE',  ( 20.88749999999999929, 5.773502691896255534, 3.535250795749688894E-16 ) ) ;
#21719=CARTESIAN_POINT ( 'NONE',  ( -4.243569643749999898, 10.37187500061451750, -32.45002607614398471 ) ) ;
#21721=CARTESIAN_POINT ( 'NONE',  ( 13.15312500061451750, 0.000000000000000000, 5.243569643749999010 ) ) ;
#21722=CARTESIAN_POINT ( 'NONE',  ( 28.84687500061452070, 6.054752690667223547, 3.707466751127219781E-16 ) ) ;
#21724=CARTESIAN_POINT ( 'NONE',  ( 28.28437500061451715, 6.421520780324663323E-16, -5.243569643749999010 ) ) ;
#21725=CARTESIAN_POINT ( 'NONE',  ( 9.375000000000001776, -4.330127018922194537, 2.499999999999995559 ) ) ;
#21726=CARTESIAN_POINT ( 'NONE',  ( 4.000000000000000000, 16.25000000122903643, 32.30940107675849049 ) ) ;
#21727=CARTESIAN_POINT ( 'NONE',  ( 10.08750000122903323, 6.123233995736764310E-16, -4.999999999999998224 ) ) ;
#21728=CARTESIAN_POINT ( 'NONE',  ( 20.29687500061451644, 6.054752690667223547, 3.707466751127219781E-16 ) ) ;
#21729=CARTESIAN_POINT ( 'NONE',  ( 14.67187500061451821, -6.054752690667223547, -1.112240025338166033E-15 ) ) ;
#21730=ORIENTED_EDGE ( 'NONE', *, *, #32398, .F. ) ;
#21732=CARTESIAN_POINT ( 'NONE',  ( 18.06562500061451715, 3.027376345333611329, 5.243569643749999010 ) ) ;
#21733=CARTESIAN_POINT ( 'NONE',  ( 27.63750000122903216, 6.123233995736764310E-16, -4.999999999999998224 ) ) ;
#21734=CARTESIAN_POINT ( 'NONE',  ( 15.72187500061451892, 3.027376345333613106, -5.243569643749998122 ) ) ;
#21735=CARTESIAN_POINT ( 'NONE',  ( 3.035296952380283297, 9.529902216964481809, -24.82070563642345462 ) ) ;
#21736=CARTESIAN_POINT ( 'NONE',  ( 17.65312500061451573, 0.000000000000000000, 5.243569643749999010 ) ) ;
#21737=DIRECTION ( 'NONE',  ( -1.000000000000000000, 0.000000000000000000, 0.000000000000000000 ) ) ;
#21738=CARTESIAN_POINT ( 'NONE',  ( 25.32187500061451857, 3.027376345333611329, 5.243569643749999010 ) ) ;
#21739=CARTESIAN_POINT ( 'NONE',  ( -4.243569643749999898, 11.66562500061451679, 27.54997392385601529 ) ) ;
#21740=CARTESIAN_POINT ( 'NONE',  ( 15.12187500061451750, -6.054752690667223547, -1.112240025338166033E-15 ) ) ;
#21741=CARTESIAN_POINT ( 'NONE',  ( 13.50000000122903288, -2.886751345948129988, 4.999999999999997335 ) ) ;
#21743=CARTESIAN_POINT ( 'NONE',  ( 3.310802318797580579, -3.746810377620464205, 3.668301323911666412 ) ) ;
#21744=CARTESIAN_POINT ( 'NONE',  ( 20.55937500061451573, -4.541064518000417216, -2.621784821875001281 ) ) ;
#21745=CARTESIAN_POINT ( 'NONE',  ( 23.28750000122903430, 4.330127018922191873, 2.499999999999999556 ) ) ;
#21746=CARTESIAN_POINT ( 'NONE',  ( 17.78437500061451715, -4.541064518000419881, 2.621784821874995952 ) ) ;
#21747=CARTESIAN_POINT ( 'NONE',  ( 12.59062500061451573, 6.054752690667223547, 3.707466751127219781E-16 ) ) ;
#21748=CARTESIAN_POINT ( 'NONE',  ( -3.000416591977282496E-16, 13.44687500061451857, 25.09994784771203058 ) ) ;
#21749=CARTESIAN_POINT ( 'NONE',  ( 17.39062500061451644, -3.027376345333610441, -5.243569643749999898 ) ) ;
#21750=ORIENTED_EDGE ( 'NONE', *, *, #25488, .F. ) ;
#21752=CARTESIAN_POINT ( 'NONE',  ( 19.68750000000000355, -2.886751345948129988, 4.999999999999997335 ) ) ;
#21753=CARTESIAN_POINT ( 'NONE',  ( 28.27500000122902435, 2.886751345948143754, 4.999999999999969802 ) ) ;
#21754=CARTESIAN_POINT ( 'NONE',  ( 25.30312500061451431, 0.000000000000000000, 5.243569643749999010 ) ) ;
#21755=CARTESIAN_POINT ( 'NONE',  ( 4.940625000614515372, 6.054752690667223547, 3.707466751127219781E-16 ) ) ;
#21756=CARTESIAN_POINT ( 'NONE',  ( 17.10000000122903430, -2.886751345948129988, 4.999999999999997335 ) ) ;
#21757=CARTESIAN_POINT ( 'NONE',  ( 23.54062500061451146, -3.027376345333614438, 5.243569643749998122 ) ) ;
#21758=CARTESIAN_POINT ( 'NONE',  ( 22.87500000000000000, -4.330127018922194537, 2.499999999999995559 ) ) ;
#21759=CARTESIAN_POINT ( 'NONE',  ( 26.35312500061451857, -4.541064518000417216, -2.621784821875001281 ) ) ;
#21760=CARTESIAN_POINT ( 'NONE',  ( 6.515625000614516438, -6.054752690667223547, -1.112240025338166033E-15 ) ) ;
#21765=CARTESIAN_POINT ( 'NONE',  ( -1.071796769724504328, 11.20490381179670081, 33.99999999999999289 ) ) ;
#21766=CARTESIAN_POINT ( 'NONE',  ( 1.999999999999998668, 13.66250000122903607, -33.46410161513775705 ) ) ;
#21767=CARTESIAN_POINT ( 'NONE',  ( 9.001249775931846008E-16, 18.17187500061451999, -25.09994784771203058 ) ) ;
#21768=CARTESIAN_POINT ( 'NONE',  ( 9.487500000000000711, -2.886751345948125991, -5.000000000000000000 ) ) ;
#21769=CARTESIAN_POINT ( 'NONE',  ( 9.084375000614517859, 4.541064518000418104, 2.621784821874999949 ) ) ;
#21770=CARTESIAN_POINT ( 'NONE',  ( 7.087500001229034119, 4.330127018922191873, 2.499999999999999556 ) ) ;
#21771=CARTESIAN_POINT ( 'NONE',  ( 11.63437500061451857, 6.421520780324663323E-16, -5.243569643749999010 ) ) ;
#21772=CARTESIAN_POINT ( 'NONE',  ( 6.196875000614515905, -3.027376345333610441, -5.243569643749999898 ) ) ;
#21773=LINE ( 'NONE', #67234, #57415 ) ;
#21775=DIRECTION ( 'NONE',  ( -1.000000000000000000, -0.000000000000000000, -0.000000000000000000 ) ) ;
#21776=CARTESIAN_POINT ( 'NONE',  ( 11.03437500061451715, -4.541064518000419881, 2.621784821874995952 ) ) ;
#21777=DIRECTION ( 'NONE',  ( 0.000000000000000000, 0.000000000000000000, 1.000000000000000000 ) ) ;
#21778=CARTESIAN_POINT ( 'NONE',  ( 19.45312500061451644, 0.000000000000000000, 5.243569643749999010 ) ) ;
#21779=CARTESIAN_POINT ( 'NONE',  ( -5.810221930991193690E-16, 12.35000000122903430, -34.00000000000000000 ) ) ;
#21781=CARTESIAN_POINT ( 'NONE',  ( 23.29687500061451644, -3.027376345333610441, -5.243569643749999898 ) ) ;
#21782=CARTESIAN_POINT ( 'NONE',  ( 4.000000000000000000, 19.28749999999999787, 32.30940107675849760 ) ) ;
#21783=CARTESIAN_POINT ( 'NONE',  ( 3.103125000614517237, 4.541064518000418104, -2.621784821874998173 ) ) ;
#21786=CARTESIAN_POINT ( 'NONE',  ( 26.05312500061451431, 4.541064518000418104, -2.621784821874998173 ) ) ;
#21787=CARTESIAN_POINT ( 'NONE',  ( 15.77812500061451573, 4.541064518000418104, 2.621784821874999949 ) ) ;
#21789=CARTESIAN_POINT ( 'NONE',  ( 14.70937500061451786, -4.541064518000417216, -2.621784821875001281 ) ) ;
#21790=CARTESIAN_POINT ( 'NONE',  ( 7.237500001229035362, -4.330127018922194537, 2.499999999999995559 ) ) ;
#21791=CARTESIAN_POINT ( 'NONE',  ( 24.41250000122903430, -4.330127018922190985, -2.500000000000001332 ) ) ;
#21792=CARTESIAN_POINT ( 'NONE',  ( 3.084375000614519191, 6.421520780324663323E-16, -5.243569643749999010 ) ) ;
#21793=CARTESIAN_POINT ( 'NONE',  ( 13.95937500061451786, 4.541064518000418104, -2.621784821874998173 ) ) ;
#21795=CARTESIAN_POINT ( 'NONE',  ( 3.149999999999999911, -4.330127018922190985, -2.500000000000001332 ) ) ;
#21796=CARTESIAN_POINT ( 'NONE',  ( 3.337500001229034563, 6.123233995736764310E-16, -4.999999999999998224 ) ) ;
#21797=CARTESIAN_POINT ( 'NONE',  ( 24.79687500061451999, 6.054752690667223547, 3.707466751127219781E-16 ) ) ;
#21798=CARTESIAN_POINT ( 'NONE',  ( 16.77187500061451786, 3.027376345333611329, 5.243569643749999010 ) ) ;
#21800=ADVANCED_FACE ( 'NONE', ( #30769 ), #53300, .F. ) ;
#21801=CARTESIAN_POINT ( 'NONE',  ( 27.41250000000000142, -5.773502691896255534, -1.060575238724906372E-15 ) ) ;
#21802=CARTESIAN_POINT ( 'NONE',  ( 3.975000001229033852, 2.886751345948126879, 4.999999999999999112 ) ) ;
#21803=CARTESIAN_POINT ( 'NONE',  ( 6.787500000000001421, -2.886751345948125991, -5.000000000000000000 ) ) ;
#21805=CARTESIAN_POINT ( 'NONE',  ( 19.30312500061451786, 4.541064518000418104, -2.621784821874998173 ) ) ;
#21806=CARTESIAN_POINT ( 'NONE',  ( 10.42500000000000071, 6.123233995736764310E-16, -4.999999999999998224 ) ) ;
#21807=CARTESIAN_POINT ( 'NONE',  ( 4.715625000614516615, -6.054752690667223547, -1.112240025338166033E-15 ) ) ;
#21808=CARTESIAN_POINT ( 'NONE',  ( 18.26249999999999929, 2.886751345948126879, 4.999999999999999112 ) ) ;
#21809=EDGE_CURVE ( 'NONE', #43716, #33795, #38515, .T. ) ;
#21810=CARTESIAN_POINT ( 'NONE',  ( -3.999999999999999112, 17.30000000000000071, 30.00000000000000000 ) ) ;
#21811=CARTESIAN_POINT ( 'NONE',  ( 21.45000000122903216, 5.773502691896255534, 3.535250795749688894E-16 ) ) ;
#21812=CARTESIAN_POINT ( 'NONE',  ( -0.6945831915928805111, 10.00052343484236772, -33.93923269050669944 ) ) ;
#21813=CARTESIAN_POINT ( 'NONE',  ( 29.44687500061451857, -3.027376345333614438, 5.243569643749998122 ) ) ;
#21814=ORIENTED_EDGE ( 'NONE', *, *, #54584, .F. ) ;
#21815=CARTESIAN_POINT ( 'NONE',  ( 17.12812500061451715, 4.541064518000418104, 2.621784821874999949 ) ) ;
#21816=CARTESIAN_POINT ( 'NONE',  ( 24.36562500061451786, 3.027376345333611329, 5.243569643749999010 ) ) ;
#21817=CARTESIAN_POINT ( 'NONE',  ( 21.49687500061451573, -3.027376345333610441, -5.243569643749999898 ) ) ;
#21818=CARTESIAN_POINT ( 'NONE',  ( 6.112499999999999822, 2.886751345948126879, 4.999999999999999112 ) ) ;
#21819=CARTESIAN_POINT ( 'NONE',  ( 9.290625000614515017, -3.027376345333610441, -5.243569643749999898 ) ) ;
#21820=CARTESIAN_POINT ( 'NONE',  ( 24.17812500061451786, 6.421520780324663323E-16, -5.243569643749999010 ) ) ;
#21821=CARTESIAN_POINT ( 'NONE',  ( 15.75937500061451857, 4.541064518000418104, -2.621784821874998173 ) ) ;
#21822=CARTESIAN_POINT ( 'NONE',  ( 20.03437500061451715, -4.541064518000419881, 2.621784821874995952 ) ) ;
#21824=CARTESIAN_POINT ( 'NONE',  ( 4.243569643749999010, 19.61562500061451431, 27.54997392385601174 ) ) ;
#21825=CARTESIAN_POINT ( 'NONE',  ( 22.42500000122903359, 2.886751345948126879, 4.999999999999999112 ) ) ;
#21827=CARTESIAN_POINT ( 'NONE',  ( 10.75312500061451715, 4.541064518000418104, -2.621784821874998173 ) ) ;
#21828=CARTESIAN_POINT ( 'NONE',  ( 8.221875000614518925, 3.027376345333611329, 5.243569643749999010 ) ) ;
#21829=CARTESIAN_POINT ( 'NONE',  ( 6.796875000614516438, 6.054752690667223547, 3.707466751127219781E-16 ) ) ;
#21830=EDGE_CURVE ( 'NONE', #48891, #37048, #66986, .T. ) ;
#21832=CARTESIAN_POINT ( 'NONE',  ( 27.49687500061451217, 6.054752690667223547, 3.707466751127219781E-16 ) ) ;
#21833=CARTESIAN_POINT ( 'NONE',  ( 19.82812500061451644, 4.541064518000418104, 2.621784821874999949 ) ) ;
#21834=CARTESIAN_POINT ( 'NONE',  ( 28.87500000122902932, -5.773502691896255534, -1.060575238724906372E-15 ) ) ;
#21835=CARTESIAN_POINT ( 'NONE',  ( 27.59062500061451573, -3.027376345333614438, 5.243569643749998122 ) ) ;
#21836=CARTESIAN_POINT ( 'NONE',  ( 24.53437500061451715, -4.541064518000419881, 2.621784821874995952 ) ) ;
#21837=CARTESIAN_POINT ( 'NONE',  ( 18.66562500061451146, -6.054752690667223547, -1.112240025338166033E-15 ) ) ;
#21838=CARTESIAN_POINT ( 'NONE',  ( -2.121784821874996840, 18.58437500061451786, 33.67503911421598417 ) ) ;
#21840=CARTESIAN_POINT ( 'NONE',  ( 25.30312500061451431, 0.000000000000000000, 5.243569643749999010 ) ) ;
#21841=CARTESIAN_POINT ( 'NONE',  ( 3.637500001229036162, -4.330127018922194537, 2.499999999999995559 ) ) ;
#21842=ORIENTED_EDGE ( 'NONE', *, *, #35681, .T. ) ;
#21843=CARTESIAN_POINT ( 'NONE',  ( 28.35000000000000142, -4.330127018922190985, -2.500000000000001332 ) ) ;
#21844=CARTESIAN_POINT ( 'NONE',  ( -3.999999999999999112, 15.50000000000000000, -30.00000000000000000 ) ) ;
#21846=CARTESIAN_POINT ( 'NONE',  ( 5.596875000614516260, -3.027376345333614438, 5.243569643749998122 ) ) ;
#21847=CARTESIAN_POINT ( 'NONE',  ( 13.64062500061451644, -3.027376345333614438, 5.243569643749998122 ) ) ;
#21848=CARTESIAN_POINT ( 'NONE',  ( 5.371875000614516615, 3.027376345333613106, -5.243569643749998122 ) ) ;
#21849=CARTESIAN_POINT ( 'NONE',  ( 25.50000000122903288, 5.773502691896255534, 3.535250795749688894E-16 ) ) ;
#21850=CARTESIAN_POINT ( 'NONE',  ( 14.74687500061451750, -3.027376345333610441, -5.243569643749999898 ) ) ;
#21851=CARTESIAN_POINT ( 'NONE',  ( 29.39062500061451289, -3.027376345333614438, 5.243569643749998122 ) ) ;
#21852=CARTESIAN_POINT ( 'NONE',  ( -1.071796769724488563, 11.09240381056766545, 34.00000000000000000 ) ) ;
#21853=CARTESIAN_POINT ( 'NONE',  ( 27.83437500061451786, 6.421520780324663323E-16, -5.243569643749999010 ) ) ;
#21854=CARTESIAN_POINT ( 'NONE',  ( 30.00000000000000000, 0.000000000000000000, 0.000000000000000000 ) ) ;
#21855=CARTESIAN_POINT ( 'NONE',  ( 13.34062500061451750, -3.027376345333610441, -5.243569643749999898 ) ) ;
#21856=ORIENTED_EDGE ( 'NONE', *, *, #70520, .F. ) ;
#21858=CARTESIAN_POINT ( 'NONE',  ( 10.75312500061451715, 4.541064518000418104, -2.621784821874998173 ) ) ;
#21860=CARTESIAN_POINT ( 'NONE',  ( 9.328125000614518214, 6.421520780324663323E-16, -5.243569643749999010 ) ) ;
#21862=CARTESIAN_POINT ( 'NONE',  ( 8.025000000000000355, -4.330127018922194537, 2.499999999999995559 ) ) ;
#21863=CARTESIAN_POINT ( 'NONE',  ( 2.662500001229036073, 0.000000000000000000, 4.999999999999998224 ) ) ;
#21864=CARTESIAN_POINT ( 'NONE',  ( 17.32499999999999929, 4.330127018922191873, 2.499999999999999556 ) ) ;
#21865=CARTESIAN_POINT ( 'NONE',  ( 18.87187500061451573, 3.027376345333613106, -5.243569643749998122 ) ) ;
#21866=CARTESIAN_POINT ( 'NONE',  ( 13.50000000122903288, -2.886751345948129988, 4.999999999999997335 ) ) ;
#21868=CARTESIAN_POINT ( 'NONE',  ( 4.243569643749999010, 16.91562500061451502, -32.45002607614398471 ) ) ;
#21872=CARTESIAN_POINT ( 'NONE',  ( 25.82812500061451644, -4.541064518000419881, 2.621784821874995952 ) ) ;
#21875=CARTESIAN_POINT ( 'NONE',  ( 26.96249999999999858, -5.773502691896255534, -1.060575238724906372E-15 ) ) ;
#21876=CARTESIAN_POINT ( 'NONE',  ( 10.41562500061451679, 3.027376345333611329, 5.243569643749999010 ) ) ;
#21878=CARTESIAN_POINT ( 'NONE',  ( 21.19687500061451502, 6.054752690667223547, 3.707466751127219781E-16 ) ) ;
#21881=CARTESIAN_POINT ( 'NONE',  ( 7.153125000614518392, 4.541064518000418104, -2.621784821874998173 ) ) ;
#21882=CARTESIAN_POINT ( 'NONE',  ( 10.92187500061451644, 3.027376345333611329, 5.243569643749999010 ) ) ;
#21884=CARTESIAN_POINT ( 'NONE',  ( 20.93437500061451573, -4.541064518000419881, 2.621784821874995952 ) ) ;
#21885=CARTESIAN_POINT ( 'NONE',  ( 4.907911205059083602E-16, 5.000000000000000000, -26.00000000000000000 ) ) ;
#21886=ADVANCED_FACE ( 'NONE', ( #71770 ), #4174, .F. ) ;
#21887=ADVANCED_FACE ( 'NONE', ( #61036, #26704 ), #55868, .F. ) ;
#21888=CARTESIAN_POINT ( 'NONE',  ( 28.72500000000000142, -4.330127018922194537, 2.499999999999995559 ) ) ;
#21890=CARTESIAN_POINT ( 'NONE',  ( 5.250000000000000888, 0.000000000000000000, 4.999999999999998224 ) ) ;
#21891=CARTESIAN_POINT ( 'NONE',  ( 14.13750000122903394, 6.123233995736764310E-16, -4.999999999999998224 ) ) ;
#21893=CARTESIAN_POINT ( 'NONE',  ( 14.36250000122903359, 0.000000000000000000, 4.999999999999998224 ) ) ;
#21894=ORIENTED_EDGE ( 'NONE', *, *, #7572, .T. ) ;
#21895=CARTESIAN_POINT ( 'NONE',  ( 12.75000000000000178, 4.330127018922192761, -2.499999999999997780 ) ) ;
#21896=CARTESIAN_POINT ( 'NONE',  ( 16.80000000000000071, 4.330127018922192761, -2.499999999999997780 ) ) ;
#21897=CARTESIAN_POINT ( 'NONE',  ( 13.42500000122903536, 2.886751345948126879, 4.999999999999999112 ) ) ;
#21898=CARTESIAN_POINT ( 'NONE',  ( 11.76562500061451644, 3.027376345333611329, 5.243569643749999010 ) ) ;
#21899=( BOUNDED_CURVE ( )  B_SPLINE_CURVE ( 2, ( #37124, #30856, #3160, #47858, #42678, #70387, #37862 ),
 .UNSPECIFIED., .F., .F. ) 
 B_SPLINE_CURVE_WITH_KNOTS ( ( 3, 2, 2, 3 ),
 ( 0.1083333333333333648, 0.1111111111111111327, 0.1138888888888889006, 0.1166666666666666824 ),
 .UNSPECIFIED. ) 
 CURVE ( )  GEOMETRIC_REPRESENTATION_ITEM ( )  RATIONAL_B_SPLINE_CURVE ( ( 0.9999999999999986677, 0.8660254037844400399, 1.000000000000000000, 0.8660254037844387076, 1.000000000000000000, 0.8660254037844380415, 1.000000000000000666 ) ) 
 REPRESENTATION_ITEM ( '' )  );
#21900=ORIENTED_EDGE ( 'NONE', *, *, #41575, .F. ) ;
#21901=CARTESIAN_POINT ( 'NONE',  ( 9.112500000000000711, 2.886751345948129099, -4.999999999999998224 ) ) ;
#21902=CARTESIAN_POINT ( 'NONE',  ( 18.56250000122903288, -4.330127018922190985, -2.500000000000001332 ) ) ;
#21903=CARTESIAN_POINT ( 'NONE',  ( 2.121784821874999061, 13.85937500061451821, -33.67503911421598417 ) ) ;
#21904=CARTESIAN_POINT ( 'NONE',  ( 28.61250000122903359, 4.330127018922192761, -2.499999999999997780 ) ) ;
#21906=CARTESIAN_POINT ( 'NONE',  ( 10.76250000000000107, -5.773502691896255534, -1.060575238724906372E-15 ) ) ;
#21908=ORIENTED_EDGE ( 'NONE', *, *, #20969, .T. ) ;
#21909=CARTESIAN_POINT ( 'NONE',  ( 24.44062500061451715, -3.027376345333614438, 5.243569643749998122 ) ) ;
#21910=CARTESIAN_POINT ( 'NONE',  ( 4.000000000000000000, 13.43750000000000000, -27.69059892324149885 ) ) ;
#21911=VECTOR ( 'NONE', #34078, 1000.000000000000000 ) ;
#21912=CARTESIAN_POINT ( 'NONE',  ( 29.40937500061451715, 0.000000000000000000, 5.243569643749999010 ) ) ;
#21913=CARTESIAN_POINT ( 'NONE',  ( 20.52187500061451786, -6.054752690667223547, -1.112240025338166033E-15 ) ) ;
#21914=CARTESIAN_POINT ( 'NONE',  ( 17.57812500061451644, 4.541064518000418104, 2.621784821874999949 ) ) ;
#21915=CARTESIAN_POINT ( 'NONE',  ( -4.243569643749999898, 11.21562500061459389, -32.45002607614398471 ) ) ;
#21916=CARTESIAN_POINT ( 'NONE',  ( 6.215625000614517504, 3.027376345333613106, -5.243569643749998122 ) ) ;
#21917=CARTESIAN_POINT ( 'NONE',  ( 29.43750000122903288, 6.123233995736764310E-16, -4.999999999999998224 ) ) ;
#21919=CARTESIAN_POINT ( 'NONE',  ( 20.05312500061451431, -4.541064518000417216, -2.621784821875001281 ) ) ;
#21922=CARTESIAN_POINT ( 'NONE',  ( 16.32187500061451502, 3.027376345333611329, 5.243569643749999010 ) ) ;
#21923=CARTESIAN_POINT ( 'NONE',  ( 13.58437500061451786, 4.541064518000418104, 2.621784821874999949 ) ) ;
#21924=CARTESIAN_POINT ( 'NONE',  ( 22.02187500061452141, 3.027376345333613106, -5.243569643749998122 ) ) ;
#21925=ORIENTED_EDGE ( 'NONE', *, *, #48397, .T. ) ;
#21926=CARTESIAN_POINT ( 'NONE',  ( -3.000416591977282496E-16, 12.09687500061451892, 25.09994784771203058 ) ) ;
#21927=CARTESIAN_POINT ( 'NONE',  ( 2.915625000614516793, -6.054752690667223547, -1.112240025338166033E-15 ) ) ;
#21928=CARTESIAN_POINT ( 'NONE',  ( 26.39062500061451644, -3.027376345333610441, -5.243569643749999898 ) ) ;
#21929=CARTESIAN_POINT ( 'NONE',  ( 27.77812500061451573, 6.421520780324663323E-16, -5.243569643749999010 ) ) ;
#21930=CARTESIAN_POINT ( 'NONE',  ( 1.999999999999998668, 19.51250000122903216, -33.46410161513775705 ) ) ;
#21931=CARTESIAN_POINT ( 'NONE',  ( 1.999999999999998668, 16.25000000000000000, 26.53589838486224650 ) ) ;
#21932=CARTESIAN_POINT ( 'NONE',  ( 4.546875000614517326, 6.054752690667223547, 3.707466751127219781E-16 ) ) ;
#21933=CARTESIAN_POINT ( 'NONE',  ( 11.73750000122903181, -4.330127018922194537, 2.499999999999995559 ) ) ;
#21934=CARTESIAN_POINT ( 'NONE',  ( 9.337500001229033231, 4.330127018922191873, 2.499999999999999556 ) ) ;
#21935=CARTESIAN_POINT ( 'NONE',  ( 3.440625000614518036, -3.027376345333610441, -5.243569643749999898 ) ) ;
#21938=CARTESIAN_POINT ( 'NONE',  ( 11.67187500061451821, 3.027376345333613106, -5.243569643749998122 ) ) ;
#21942=CARTESIAN_POINT ( 'NONE',  ( 20.61562500061451431, 3.027376345333613106, -5.243569643749998122 ) ) ;
#21943=CARTESIAN_POINT ( 'NONE',  ( 12.75937500061451857, 0.000000000000000000, 5.243569643749999010 ) ) ;
#21944=CARTESIAN_POINT ( 'NONE',  ( 5.315625000614516260, 3.027376345333613106, -5.243569643749998122 ) ) ;
#21945=CARTESIAN_POINT ( 'NONE',  ( 21.27187500061451786, 3.027376345333611329, 5.243569643749999010 ) ) ;
#21946=CARTESIAN_POINT ( 'NONE',  ( 6.215625000614517504, 3.027376345333613106, -5.243569643749998122 ) ) ;
#21947=CARTESIAN_POINT ( 'NONE',  ( 6.600000001229032520, 5.773502691896255534, 3.535250795749688894E-16 ) ) ;
#21948=CARTESIAN_POINT ( 'NONE',  ( 19.41562500061451146, 3.027376345333611329, 5.243569643749999010 ) ) ;
#21949=CARTESIAN_POINT ( 'NONE',  ( 7.650000001229034119, -2.886751345948129988, 4.999999999999997335 ) ) ;
#21950=CARTESIAN_POINT ( 'NONE',  ( 17.69062500061451715, -3.027376345333614438, 5.243569643749998122 ) ) ;
#21951=CARTESIAN_POINT ( 'NONE',  ( 16.60312500061451857, 4.541064518000418104, -2.621784821874998173 ) ) ;
#21953=CARTESIAN_POINT ( 'NONE',  ( 15.82499999999999929, 6.123233995736764310E-16, -4.999999999999998224 ) ) ;
#21954=CARTESIAN_POINT ( 'NONE',  ( 10.68750000122903288, 4.330127018922191873, 2.499999999999999556 ) ) ;
#21955=CARTESIAN_POINT ( 'NONE',  ( 7.378125000614518036, -4.541064518000419881, 2.621784821874995952 ) ) ;
#21956=CARTESIAN_POINT ( 'NONE',  ( 11.72812500061451857, 4.541064518000418104, 2.621784821874999949 ) ) ;
#21958=CARTESIAN_POINT ( 'NONE',  ( 21.22500000122903074, -5.773502691896255534, -1.060575238724906372E-15 ) ) ;
#21960=CARTESIAN_POINT ( 'NONE',  ( -3.000416591977282496E-16, 12.54687500061451999, -34.90005215228797653 ) ) ;
#21962=CARTESIAN_POINT ( 'NONE',  ( 4.425000001229032698, 2.886751345948126879, 4.999999999999999112 ) ) ;
#21963=CARTESIAN_POINT ( 'NONE',  ( 3.984375000614517326, 6.421520780324663323E-16, -5.243569643749999010 ) ) ;
#21964=CARTESIAN_POINT ( 'NONE',  ( 19.69687500061451857, -3.027376345333610441, -5.243569643749999898 ) ) ;
#21965=CARTESIAN_POINT ( 'NONE',  ( 5.137499999999999289, 5.773502691896255534, 3.535250795749688401E-16 ) ) ;
#21966=CARTESIAN_POINT ( 'NONE',  ( 15.51562500061451644, -6.054752690667223547, -1.112240025338166033E-15 ) ) ;
#21968=CARTESIAN_POINT ( 'NONE',  ( 1.626862140677534273E-15, 9.875000001229034652, 34.00000000000000000 ) ) ;
#21969=CARTESIAN_POINT ( 'NONE',  ( 28.39687500061452141, 6.054752690667223547, 3.707466751127219781E-16 ) ) ;
#21971=CARTESIAN_POINT ( 'NONE',  ( 14.91562500061451679, 3.027376345333611329, 5.243569643749999010 ) ) ;
#21972=CARTESIAN_POINT ( 'NONE',  ( 11.85937500061451644, 0.000000000000000000, 5.243569643749999010 ) ) ;
#21975=CARTESIAN_POINT ( 'NONE',  ( 21.55312500061451431, 4.541064518000418104, -2.621784821874998173 ) ) ;
#21976=DIRECTION ( 'NONE',  ( -0.000000000000000000, -1.000000000000000000, -0.000000000000000000 ) ) ;
#21977=EDGE_CURVE ( 'NONE', #48607, #2372, #10687, .T. ) ;
#21978=CARTESIAN_POINT ( 'NONE',  ( -3.999999999999999112, 18.31250000122903288, 30.00000000000000000 ) ) ;
#21979=CARTESIAN_POINT ( 'NONE',  ( 13.42499999999999893, -4.330127018922194537, 2.499999999999995559 ) ) ;
#21980=CARTESIAN_POINT ( 'NONE',  ( 20.81250000122903643, -4.330127018922190985, -2.500000000000001332 ) ) ;
#21981=CARTESIAN_POINT ( 'NONE',  ( 16.67812500061451786, 4.541064518000418104, 2.621784821874999949 ) ) ;
#21983=ORIENTED_EDGE ( 'NONE', *, *, #15704, .T. ) ;
#21984=CARTESIAN_POINT ( 'NONE',  ( 20.13749999999999929, -2.886751345948129988, 4.999999999999997335 ) ) ;
#21985=CARTESIAN_POINT ( 'NONE',  ( 22.62187500061451573, 3.027376345333611329, 5.243569643749999010 ) ) ;
#21986=CARTESIAN_POINT ( 'NONE',  ( 26.87812500061451360, 6.421520780324663323E-16, -5.243569643749999010 ) ) ;
#21987=ORIENTED_EDGE ( 'NONE', *, *, #39247, .T. ) ;
#21989=CARTESIAN_POINT ( 'NONE',  ( 10.75312500061451715, 4.541064518000418104, -2.621784821874998173 ) ) ;
#21990=CARTESIAN_POINT ( 'NONE',  ( 6.337500000000000355, -2.886751345948126435, -5.000000000000000000 ) ) ;
#21991=AXIS2_PLACEMENT_3D ( 'NONE', #42125, #32137, #71293 ) ;
#21992=CARTESIAN_POINT ( 'NONE',  ( 17.69999999999999929, 4.330127018922192761, -2.499999999999997780 ) ) ;
#21993=CARTESIAN_POINT ( 'NONE',  ( 24.26249999999999929, -5.773502691896255534, -1.060575238724906372E-15 ) ) ;
#21995=CARTESIAN_POINT ( 'NONE',  ( 5.071875000614519458, 3.027376345333611329, 5.243569643749999010 ) ) ;
#21996=CARTESIAN_POINT ( 'NONE',  ( 27.60937500061451644, 0.000000000000000000, 5.243569643749999010 ) ) ;
#21997=ORIENTED_EDGE ( 'NONE', *, *, #5228, .T. ) ;
#21998=CARTESIAN_POINT ( 'NONE',  ( 24.36562500061451786, 3.027376345333611329, 5.243569643749999010 ) ) ;
#22000=CARTESIAN_POINT ( 'NONE',  ( 24.42187500061451999, 3.027376345333611329, 5.243569643749999010 ) ) ;
#22001=CARTESIAN_POINT ( 'NONE',  ( -2.121784821874999949, 19.27812500061459033, -33.67503911421598417 ) ) ;
#22002=EDGE_CURVE ( 'NONE', #23329, #60892, #66963, .T. ) ;
#22003=CARTESIAN_POINT ( 'NONE',  ( 14.02499999999999858, 6.123233995736764310E-16, -4.999999999999998224 ) ) ;
#22004=CARTESIAN_POINT ( 'NONE',  ( 7.903125000614515727, -4.541064518000417216, -2.621784821875001281 ) ) ;
#22005=CARTESIAN_POINT ( 'NONE',  ( 5.924999999999999822, 6.123233995736764310E-16, -4.999999999999998224 ) ) ;
#22006=CARTESIAN_POINT ( 'NONE',  ( 19.46249999999999503, 2.886751345948062486, -5.000000000000113687 ) ) ;
#22007=CARTESIAN_POINT ( 'NONE',  ( 25.49062500061451431, -3.027376345333610441, -5.243569643749999898 ) ) ;
#22008=CARTESIAN_POINT ( 'NONE',  ( 16.61250000122903359, 0.000000000000000000, 4.999999999999998224 ) ) ;
#22011=CARTESIAN_POINT ( 'NONE',  ( 3.553125000614516082, 4.541064518000418104, -2.621784821874998173 ) ) ;
#22012=CARTESIAN_POINT ( 'NONE',  ( 18.68437500061451928, -4.541064518000419881, 2.621784821874995952 ) ) ;
#22013=CARTESIAN_POINT ( 'NONE',  ( -4.243569643749999898, 14.42187500061451644, 27.54997392385601529 ) ) ;
#22014=CARTESIAN_POINT ( 'NONE',  ( 21.12187500061451573, 3.027376345333613106, -5.243569643749998122 ) ) ;
#22015=CARTESIAN_POINT ( 'NONE',  ( 3.900000000000000799, 0.000000000000000000, 4.999999999999998224 ) ) ;
#22016=CARTESIAN_POINT ( 'NONE',  ( 4.243569643749999898, 18.69687500061451857, 32.45002607614398471 ) ) ;
#22017=CARTESIAN_POINT ( 'NONE',  ( 10.94062500061451537, -3.027376345333614438, 5.243569643749998122 ) ) ;
#22018=CARTESIAN_POINT ( 'NONE',  ( 9.528763966825557376E-15, 17.07500000122903572, 34.00000000000000000 ) ) ;
#22019=CARTESIAN_POINT ( 'NONE',  ( 6.834375000614518747, 4.541064518000418104, 2.621784821874999949 ) ) ;
#22020=CARTESIAN_POINT ( 'NONE',  ( 8.390625000614518214, -3.027376345333610441, -5.243569643749999898 ) ) ;
#22021=CARTESIAN_POINT ( 'NONE',  ( 13.13437500061451857, 4.541064518000418104, 2.621784821874999949 ) ) ;
#22022=CARTESIAN_POINT ( 'NONE',  ( 19.80000000122903359, -2.886751345948129988, 4.999999999999997335 ) ) ;
#22023=CARTESIAN_POINT ( 'NONE',  ( 7.996875000614519280, -3.027376345333610441, -5.243569643749999898 ) ) ;
#22024=CARTESIAN_POINT ( 'NONE',  ( 10.04062500061451502, -3.027376345333614438, 5.243569643749998122 ) ) ;
#22025=CARTESIAN_POINT ( 'NONE',  ( 7.940625000614518036, -3.027376345333610441, -5.243569643749999898 ) ) ;
#22027=CARTESIAN_POINT ( 'NONE',  ( 19.77187500061451786, 3.027376345333613106, -5.243569643749998122 ) ) ;
#22028=CARTESIAN_POINT ( 'NONE',  ( 9.112500001229033586, -4.330127018922190985, -2.500000000000001332 ) ) ;
#22029=CARTESIAN_POINT ( 'NONE',  ( 26.61562500061451786, 3.027376345333611329, 5.243569643749999010 ) ) ;
#22030=CARTESIAN_POINT ( 'NONE',  ( 12.36562500061451608, -6.054752690667223547, -1.112240025338166033E-15 ) ) ;
#22031=CARTESIAN_POINT ( 'NONE',  ( 2.873218894584086858, -4.343029460077421078, 2.964791603877473314 ) ) ;
#22032=CARTESIAN_POINT ( 'NONE',  ( -4.243569643749999898, 13.10937500061451821, -30.00000000000000000 ) ) ;
#22033=CARTESIAN_POINT ( 'NONE',  ( 12.97500000122903252, 2.886751345948126879, 4.999999999999999112 ) ) ;
#22034=CARTESIAN_POINT ( 'NONE',  ( 4.243569643749999010, 14.66562500061451857, -32.45002607614398471 ) ) ;
#22035=CARTESIAN_POINT ( 'NONE',  ( 14.43750000122903288, -4.330127018922194537, 2.499999999999995559 ) ) ;
#22036=CARTESIAN_POINT ( 'NONE',  ( 9.365625000614519635, 3.027376345333613106, -5.243569643749998122 ) ) ;
#22037=CARTESIAN_POINT ( 'NONE',  ( 12.52500000000000213, -4.330127018922194537, 2.499999999999995559 ) ) ;
#22038=CARTESIAN_POINT ( 'NONE',  ( 10.38750000122903572, -4.330127018922194537, 2.499999999999995559 ) ) ;
#22039=CARTESIAN_POINT ( 'NONE',  ( 22.56562500061451715, 3.027376345333611329, 5.243569643749999010 ) ) ;
#22040=CARTESIAN_POINT ( 'NONE',  ( 7.696875000614516793, 6.054752690667223547, 3.707466751127219781E-16 ) ) ;
#22041=CARTESIAN_POINT ( 'NONE',  ( 9.937500001229032875, -4.330127018922194537, 2.499999999999995559 ) ) ;
#22042=CARTESIAN_POINT ( 'NONE',  ( 18.15000000122903501, -2.886751345948125991, -5.000000000000000000 ) ) ;
#22043=CARTESIAN_POINT ( 'NONE',  ( 14.87812500061451537, 4.541064518000418104, 2.621784821874999949 ) ) ;
#22044=CARTESIAN_POINT ( 'NONE',  ( 17.99062500061451786, 6.054752690667223547, 3.707466751127219781E-16 ) ) ;
#22045=CARTESIAN_POINT ( 'NONE',  ( 26.10000000122903430, -2.886751345948129988, 4.999999999999997335 ) ) ;
#22046=CARTESIAN_POINT ( 'NONE',  ( 27.03750000122903430, -4.330127018922194537, 2.499999999999995559 ) ) ;
#22047=CARTESIAN_POINT ( 'NONE',  ( 23.06250000000000355, 2.886751345948129099, -4.999999999999998224 ) ) ;
#22050=CARTESIAN_POINT ( 'NONE',  ( 25.80937500061451928, 0.000000000000000000, 5.243569643749999010 ) ) ;
#22051=LINE ( 'NONE', #44611, #48898 ) ;
#22052=CARTESIAN_POINT ( 'NONE',  ( 11.47500000122903252, 2.886751345948129099, -4.999999999999998224 ) ) ;
#22053=CARTESIAN_POINT ( 'NONE',  ( 29.07187500061451502, -6.054752690667223547, -1.112240025338166033E-15 ) ) ;
#22055=EDGE_CURVE ( 'NONE', #64264, #47295, #66585, .T. ) ;
#22056=CARTESIAN_POINT ( 'NONE',  ( -1.999999999999997113, 13.32499999999999929, 33.46410161513775705 ) ) ;
#22057=CARTESIAN_POINT ( 'NONE',  ( 4.359375000614517326, -4.541064518000417216, -2.621784821875001281 ) ) ;
#22058=CARTESIAN_POINT ( 'NONE',  ( 24.14062500061451289, -3.027376345333610441, -5.243569643749999898 ) ) ;
#22060=CARTESIAN_POINT ( 'NONE',  ( 4.544497808834801589, -2.085075457992688897, -4.544497808831748920 ) ) ;
#22061=CARTESIAN_POINT ( 'NONE',  ( 9.609375000614518214, 0.000000000000000000, 5.243569643749999010 ) ) ;
#22062=CARTESIAN_POINT ( 'NONE',  ( 22.20000000122903216, -2.886751345948159742, -4.999999999999942268 ) ) ;
#22063=CARTESIAN_POINT ( 'NONE',  ( 29.54062500061451502, -3.027376345333610441, -5.243569643749999898 ) ) ;
#22064=CARTESIAN_POINT ( 'NONE',  ( 5.896875000614518747, 6.054752690667223547, 3.707466751127219781E-16 ) ) ;
#22065=CARTESIAN_POINT ( 'NONE',  ( 29.59687500061451715, -3.027376345333610441, -5.243569643749999898 ) ) ;
#22067=CARTESIAN_POINT ( 'NONE',  ( 19.16250000000000142, 2.886751345948126879, 4.999999999999999112 ) ) ;
#22068=VERTEX_POINT ( 'NONE', #71399 ) ;
#22069=CARTESIAN_POINT ( 'NONE',  ( 27.22499999999999787, 4.330127018922191873, 2.499999999999999556 ) ) ;
#22070=CARTESIAN_POINT ( 'NONE',  ( 29.37187500061451928, 3.027376345333611329, 5.243569643749999010 ) ) ;
#22072=CARTESIAN_POINT ( 'NONE',  ( 18.17812500061451786, -4.541064518000419881, 2.621784821874995952 ) ) ;
#22073=CARTESIAN_POINT ( 'NONE',  ( 7.978125000614517681, 6.421520780324663323E-16, -5.243569643749999010 ) ) ;
#22075=CARTESIAN_POINT ( 'NONE',  ( 4.509375000614518569, 4.541064518000418104, -2.621784821874998173 ) ) ;
#22076=CARTESIAN_POINT ( 'NONE',  ( 16.76250000122903216, -4.330127018922190985, -2.500000000000001332 ) ) ;
#22077=CARTESIAN_POINT ( 'NONE',  ( 1.626862140677534273E-15, 13.81250000000000000, -26.00000000000000355 ) ) ;
#22078=CARTESIAN_POINT ( 'NONE',  ( 7.921875000614517326, -6.054752690667223547, -1.112240025338166033E-15 ) ) ;
#22079=CARTESIAN_POINT ( 'NONE',  ( 10.92187500061451644, 3.027376345333611329, 5.243569643749999010 ) ) ;
#22080=CARTESIAN_POINT ( 'NONE',  ( 21.23437500061451644, 4.541064518000418104, 2.621784821874999949 ) ) ;
#22081=CARTESIAN_POINT ( 'NONE',  ( -3.137519842735245283E-14, 14.71250000000000213, -26.00000000000000711 ) ) ;
#22082=ORIENTED_EDGE ( 'NONE', *, *, #32388, .T. ) ;
#22084=CARTESIAN_POINT ( 'NONE',  ( 6.009375000614519458, 0.000000000000000000, 5.243569643749999010 ) ) ;
#22085=AXIS2_PLACEMENT_3D ( 'NONE', #44298, #27661, #61271 ) ;
#22087=CARTESIAN_POINT ( 'NONE',  ( 21.33749999999999858, 5.773502691896255534, 3.535250795749688894E-16 ) ) ;
#22088=CARTESIAN_POINT ( 'NONE',  ( 18.47812500061451857, 4.541064518000418104, 2.621784821874999949 ) ) ;
#22090=CARTESIAN_POINT ( 'NONE',  ( 2.121784821875001281, 10.10937500061451821, -26.32496088578401938 ) ) ;
#22092=CARTESIAN_POINT ( 'NONE',  ( 13.04062500061451502, 6.054752690667223547, 3.707466751127219781E-16 ) ) ;
#22093=CARTESIAN_POINT ( 'NONE',  ( 27.90937500061451715, 4.541064518000418104, -2.621784821874998173 ) ) ;
#22095=CARTESIAN_POINT ( 'NONE',  ( 29.59687500061451715, -3.027376345333610441, -5.243569643749999898 ) ) ;
#22096=CARTESIAN_POINT ( 'NONE',  ( 9.637499999999999289, 5.773502691896255534, 3.535250795749688894E-16 ) ) ;
#22097=CARTESIAN_POINT ( 'NONE',  ( 4.000000000000000000, 14.90000000122903323, 32.30940107675849049 ) ) ;
#22098=CARTESIAN_POINT ( 'NONE',  ( 9.487500001229033586, -4.330127018922194537, 2.499999999999995559 ) ) ;
#22099=CARTESIAN_POINT ( 'NONE',  ( 19.28437500061451360, 6.421520780324663323E-16, -5.243569643749999010 ) ) ;
#22100=CARTESIAN_POINT ( 'NONE',  ( 13.17187500061451999, 3.027376345333611329, 5.243569643749999010 ) ) ;
#22101=CARTESIAN_POINT ( 'NONE',  ( -1.487416814333745711E-14, 16.62500000122903288, 34.00000000000000000 ) ) ;
#22102=ORIENTED_EDGE ( 'NONE', *, *, #21050, .T. ) ;
#22103=CARTESIAN_POINT ( 'NONE',  ( 15.89062500061451289, -3.027376345333614438, 5.243569643749998122 ) ) ;
#22104=CARTESIAN_POINT ( 'NONE',  ( 25.98750000122903003, 4.330127018922191873, 2.499999999999999556 ) ) ;
#22105=CARTESIAN_POINT ( 'NONE',  ( 14.70937500061451786, -4.541064518000417216, -2.621784821875001281 ) ) ;
#22106=CARTESIAN_POINT ( 'NONE',  ( 5.192387018522393483, 8.549830518147029323, -26.96928673404218202 ) ) ;
#22107=CARTESIAN_POINT ( 'NONE',  ( 16.11562500061451786, 3.027376345333613106, -5.243569643749998122 ) ) ;
#22109=ADVANCED_FACE ( 'NONE', ( #32235 ), #45514, .F. ) ;
#22110=CARTESIAN_POINT ( 'NONE',  ( 26.59687500061451360, 6.054752690667223547, 3.707466751127219781E-16 ) ) ;
#22111=CARTESIAN_POINT ( 'NONE',  ( 2.910968003956619921, -4.065258101981855887, 3.311910103879776024 ) ) ;
#22112=CARTESIAN_POINT ( 'NONE',  ( 14.97187500061451892, 3.027376345333611329, 5.243569643749999010 ) ) ;
#22113=CARTESIAN_POINT ( 'NONE',  ( 13.61250000122903359, -4.330127018922190985, -2.500000000000001332 ) ) ;
#22115=EDGE_CURVE ( 'NONE', #4158, #13105, #36571, .T. ) ;
#22116=CARTESIAN_POINT ( 'NONE',  ( 9.001249775931846008E-16, 18.62187500061451573, -25.09994784771203058 ) ) ;
#22117=CARTESIAN_POINT ( 'NONE',  ( 21.38437500061451502, -4.541064518000419881, 2.621784821874995952 ) ) ;
#22118=CARTESIAN_POINT ( 'NONE',  ( 19.57500000122903216, 2.886751345948129099, -4.999999999999998224 ) ) ;
#22119=( BOUNDED_CURVE ( )  B_SPLINE_CURVE ( 2, ( #41982, #58949, #36435, #7995, #20519, #2818, #48991 ),
 .UNSPECIFIED., .F., .F. ) 
 B_SPLINE_CURVE_WITH_KNOTS ( ( 3, 2, 2, 3 ),
 ( 0.3583333333333333925, 0.3611111111111111605, 0.3638888888888888729, 0.3666666666666666408 ),
 .UNSPECIFIED. ) 
 CURVE ( )  GEOMETRIC_REPRESENTATION_ITEM ( )  RATIONAL_B_SPLINE_CURVE ( ( 0.9999999999999973355, 0.8660254037844413721, 1.000000000000000000, 0.8660254037844387076, 1.000000000000000000, 0.8660254037844387076, 1.000000000000000000 ) ) 
 REPRESENTATION_ITEM ( '' )  );
#22120=CARTESIAN_POINT ( 'NONE',  ( 16.88437500061451502, -4.541064518000419881, 2.621784821874995952 ) ) ;
#22121=CARTESIAN_POINT ( 'NONE',  ( -4.243569643749997233, 11.79687500061451999, 32.45002607614398471 ) ) ;
#22122=CARTESIAN_POINT ( 'NONE',  ( 16.79062500061451857, -3.027376345333614438, 5.243569643749998122 ) ) ;
#22123=ORIENTED_EDGE ( 'NONE', *, *, #43393, .F. ) ;
#22124=ORIENTED_EDGE ( 'NONE', *, *, #10210, .F. ) ;
#22125=CARTESIAN_POINT ( 'NONE',  ( 19.38749999999999929, -2.886751345948125991, -5.000000000000000000 ) ) ;
#22126=DIRECTION ( 'NONE',  ( -1.000000000000000000, -0.000000000000000000, -0.000000000000000000 ) ) ;
#22127=CARTESIAN_POINT ( 'NONE',  ( 24.10312500061451502, -4.541064518000417216, -2.621784821875001281 ) ) ;
#22128=CARTESIAN_POINT ( 'NONE',  ( 6.590625000614518392, -3.027376345333610441, -5.243569643749999898 ) ) ;
#22129=CARTESIAN_POINT ( 'NONE',  ( 16.23750000122903359, -4.330127018922194537, 2.499999999999995559 ) ) ;
#22130=CARTESIAN_POINT ( 'NONE',  ( 23.61562500061451431, -6.054752690667223547, -1.112240025338166033E-15 ) ) ;
#22131=CARTESIAN_POINT ( 'NONE',  ( 20.66250000000000142, -5.773502691896255534, -1.060575238724906372E-15 ) ) ;
#22132=CARTESIAN_POINT ( 'NONE',  ( 25.04062500061451502, -3.027376345333610441, -5.243569643749999898 ) ) ;
#22133=CARTESIAN_POINT ( 'NONE',  ( 5.353125000614515905, 4.541064518000418104, -2.621784821874998173 ) ) ;
#22134=ORIENTED_EDGE ( 'NONE', *, *, #69513, .F. ) ;
#22135=CARTESIAN_POINT ( 'NONE',  ( 7.347880794884118750E-16, 20.00000000000000000, 36.00000000000000000 ) ) ;
#22136=CARTESIAN_POINT ( 'NONE',  ( -5.810221930991193690E-16, 14.60000000122903252, 26.00000000000000355 ) ) ;
#22138=CARTESIAN_POINT ( 'NONE',  ( 1.626862140677534273E-15, 18.76250000000000284, 34.00000000000000000 ) ) ;
#22139=CARTESIAN_POINT ( 'NONE',  ( 3.999999999999999112, 12.23750000122903359, -30.00000000000000000 ) ) ;
#22140=CARTESIAN_POINT ( 'NONE',  ( 4.243569643749999898, 17.34687500061451715, -27.54997392385601529 ) ) ;
#22142=CARTESIAN_POINT ( 'NONE',  ( 8.212500000000000355, 2.886751345948129099, -4.999999999999998224 ) ) ;
#22143=CARTESIAN_POINT ( 'NONE',  ( 5.925000001229033586, -5.773502691896255534, -1.060575238724906372E-15 ) ) ;
#22144=CARTESIAN_POINT ( 'NONE',  ( 13.39687500061451608, -3.027376345333610441, -5.243569643749999898 ) ) ;
#22145=CARTESIAN_POINT ( 'NONE',  ( 24.48750000122903359, 6.123233995736764310E-16, -4.999999999999998224 ) ) ;
#22146=CARTESIAN_POINT ( 'NONE',  ( 3.759375000614517681, 0.000000000000000000, 5.243569643749999010 ) ) ;
#22147=CARTESIAN_POINT ( 'NONE',  ( 28.16250000000000142, 2.886751345948119329, 5.000000000000014211 ) ) ;
#22148=CARTESIAN_POINT ( 'NONE',  ( 10.00000000000000000, 1.224646799147353256E-15, -10.00000000000000888 ) ) ;
#22149=CARTESIAN_POINT ( 'NONE',  ( 10.09687500061451715, -3.027376345333614438, 5.243569643749998122 ) ) ;
#22150=CARTESIAN_POINT ( 'NONE',  ( 3.999999999999998668, 17.22500000122903430, -32.30940107675850470 ) ) ;
#22151=CARTESIAN_POINT ( 'NONE',  ( 19.94062500061451715, -3.027376345333614438, 5.243569643749998122 ) ) ;
#22153=CARTESIAN_POINT ( 'NONE',  ( 4.243569643749999898, 18.19062500061459176, 32.45002607614398471 ) ) ;
#22154=CARTESIAN_POINT ( 'NONE',  ( 24.12187500061451217, -6.054752690667223547, -1.112240025338166033E-15 ) ) ;
#22155=CARTESIAN_POINT ( 'NONE',  ( 2.867942972713479755, -4.095717654485441450, 3.274159358307527690 ) ) ;
#22156=CARTESIAN_POINT ( 'NONE',  ( 28.01250000122903216, -4.330127018922190985, -2.500000000000001332 ) ) ;
#22158=CARTESIAN_POINT ( 'NONE',  ( 24.62812500061451715, 6.421520780324663323E-16, -5.243569643749999010 ) ) ;
#22159=CARTESIAN_POINT ( 'NONE',  ( 15.59062500061451573, -3.027376345333610441, -5.243569643749999898 ) ) ;
#22161=CARTESIAN_POINT ( 'NONE',  ( 10.80937500061451928, 4.541064518000418104, -2.621784821874998173 ) ) ;
#22163=CARTESIAN_POINT ( 'NONE',  ( 24.07500000122903216, 2.886751345948129099, -4.999999999999998224 ) ) ;
#22165=CARTESIAN_POINT ( 'NONE',  ( 13.05937500061451750, 4.541064518000418104, -2.621784821874998173 ) ) ;
#22167=CARTESIAN_POINT ( 'NONE',  ( -3.137519842735245283E-14, 11.56250000000000178, 34.00000000000000000 ) ) ;
#22168=CARTESIAN_POINT ( 'NONE',  ( -2.000000000000000000, 12.27500000000000036, -33.46410161513775705 ) ) ;
#22169=CARTESIAN_POINT ( 'NONE',  ( 24.49687500061451573, -3.027376345333614438, 5.243569643749998122 ) ) ;
#22170=CARTESIAN_POINT ( 'NONE',  ( 17.63437500061451502, 4.541064518000418104, 2.621784821874999949 ) ) ;
#22172=CARTESIAN_POINT ( 'NONE',  ( 28.46249999999999858, 2.886751345948129099, -4.999999999999998224 ) ) ;
#22173=CARTESIAN_POINT ( 'NONE',  ( 4.387500001229033053, 4.330127018922191873, 2.499999999999999556 ) ) ;
#22174=CARTESIAN_POINT ( 'NONE',  ( 4.837500000000001243, -2.886751345948129988, 4.999999999999997335 ) ) ;
#22176=CARTESIAN_POINT ( 'NONE',  ( 19.94062500061451715, -3.027376345333614438, 5.243569643749998122 ) ) ;
#22177=CARTESIAN_POINT ( 'NONE',  ( 10.53750000000000320, 5.773502691896255534, 3.535250795749688894E-16 ) ) ;
#22178=CARTESIAN_POINT ( 'NONE',  ( 2.878125000614517592, -4.541064518000419881, 2.621784821874995952 ) ) ;
#22179=CARTESIAN_POINT ( 'NONE',  ( 16.83749999999999858, 5.773502691896255534, 3.535250795749688894E-16 ) ) ;
#22180=CARTESIAN_POINT ( 'NONE',  ( -4.243569643749997233, 11.74062500061451786, 32.45002607614398471 ) ) ;
#22182=CARTESIAN_POINT ( 'NONE',  ( 19.72500000122903074, 2.886751345948126879, 4.999999999999999112 ) ) ;
#22183=CARTESIAN_POINT ( 'NONE',  ( -3.999999999999999112, 10.06250000000000178, -32.30940107675850470 ) ) ;
#22184=CARTESIAN_POINT ( 'NONE',  ( 27.15937500061451360, 0.000000000000000000, 5.243569643749999010 ) ) ;
#22185=EDGE_LOOP ( 'NONE', ( #62352, #5121, #41248, #61150 ) ) ;
#22186=CARTESIAN_POINT ( 'NONE',  ( 16.26562500061451289, 3.027376345333611329, 5.243569643749999010 ) ) ;
#22187=CARTESIAN_POINT ( 'NONE',  ( 21.14062500061451289, 6.054752690667223547, 3.707466751127219781E-16 ) ) ;
#22188=CARTESIAN_POINT ( 'NONE',  ( 22.92187500061451644, 3.027376345333613106, -5.243569643749998122 ) ) ;
#22189=CARTESIAN_POINT ( 'NONE',  ( 5.475000000000000533, 6.123233995736764310E-16, -4.999999999999998224 ) ) ;
#22190=CARTESIAN_POINT ( 'NONE',  ( 9.478125000614515017, 4.541064518000418104, 2.621784821874999949 ) ) ;
#22191=CARTESIAN_POINT ( 'NONE',  ( 25.34062500061451217, -3.027376345333614438, 5.243569643749998122 ) ) ;
#22192=CARTESIAN_POINT ( 'NONE',  ( 13.84687500061451537, -3.027376345333610441, -5.243569643749999898 ) ) ;
#22193=CARTESIAN_POINT ( 'NONE',  ( 18.87187500061451573, 3.027376345333613106, -5.243569643749998122 ) ) ;
#22195=CARTESIAN_POINT ( 'NONE',  ( 2.121784821874999061, 17.40312500061451573, 26.32496088578401583 ) ) ;
#22196=CARTESIAN_POINT ( 'NONE',  ( 21.11250000122903359, 0.000000000000000000, 4.999999999999998224 ) ) ;
#22198=CARTESIAN_POINT ( 'NONE',  ( 12.70312500061451821, 0.000000000000000000, 5.243569643749999010 ) ) ;
#22199=CARTESIAN_POINT ( 'NONE',  ( 5.071875000614519458, 3.027376345333611329, 5.243569643749999010 ) ) ;
#22200=CARTESIAN_POINT ( 'NONE',  ( 5.671875000614519102, -6.054752690667223547, -1.112240025338166033E-15 ) ) ;
#22201=ORIENTED_EDGE ( 'NONE', *, *, #45751, .T. ) ;
#22202=CARTESIAN_POINT ( 'NONE',  ( 26.89687500061451431, -3.027376345333610441, -5.243569643749999898 ) ) ;
#22203=CARTESIAN_POINT ( 'NONE',  ( 20.39062500061451644, -3.027376345333614438, 5.243569643749998122 ) ) ;
#22204=CARTESIAN_POINT ( 'NONE',  ( 28.68750000122903288, 4.330127018922191873, 2.499999999999999556 ) ) ;
#22205=CARTESIAN_POINT ( 'NONE',  ( 28.94062500061452070, -3.027376345333614438, 5.243569643749998122 ) ) ;
#22206=CARTESIAN_POINT ( 'NONE',  ( 23.18437500061451573, -4.541064518000419881, 2.621784821874995952 ) ) ;
#22207=CARTESIAN_POINT ( 'NONE',  ( 18.51562500061451289, 3.027376345333611329, 5.243569643749999010 ) ) ;
#22208=CARTESIAN_POINT ( 'NONE',  ( -4.243569643749997233, 18.54687500061451289, 32.45002607614398471 ) ) ;
#22209=CARTESIAN_POINT ( 'NONE',  ( 24.29062500061451502, 6.054752690667223547, 3.707466751127219781E-16 ) ) ;
#22210=CARTESIAN_POINT ( 'NONE',  ( 5.287500001229035185, 4.330127018922191873, 2.499999999999999556 ) ) ;
#22211=ORIENTED_EDGE ( 'NONE', *, *, #50947, .T. ) ;
#22212=CARTESIAN_POINT ( 'NONE',  ( 27.22499999999999787, 4.330127018922191873, 2.499999999999999556 ) ) ;
#22213=CARTESIAN_POINT ( 'NONE',  ( 8.484601909799253346E-16, 16.51249999999999929, -25.38119784648299770 ) ) ;
#22215=CARTESIAN_POINT ( 'NONE',  ( 5.859375000614519102, 4.541064518000418104, -2.621784821874998173 ) ) ;
#22216=CARTESIAN_POINT ( 'NONE',  ( 12.17812500061451608, 4.541064518000418104, 2.621784821874999949 ) ) ;
#22217=CARTESIAN_POINT ( 'NONE',  ( 7.096875000614517148, -3.027376345333610441, -5.243569643749999898 ) ) ;
#22218=CARTESIAN_POINT ( 'NONE',  ( 24.67500000122903359, 2.886751345948126879, 4.999999999999999112 ) ) ;
#22219=CARTESIAN_POINT ( 'NONE',  ( 14.78437500061451715, 6.421520780324663323E-16, -5.243569643749999010 ) ) ;
#22220=CARTESIAN_POINT ( 'NONE',  ( 3.609375000614516882, 4.541064518000418104, -2.621784821874998173 ) ) ;
#22221=CARTESIAN_POINT ( 'NONE',  ( 28.27499999999999858, -4.330127018922194537, 2.499999999999995559 ) ) ;
#22222=CARTESIAN_POINT ( 'NONE',  ( 27.30937500061451573, -4.541064518000417216, -2.621784821875001281 ) ) ;
#22223=CARTESIAN_POINT ( 'NONE',  ( 2.840625000614518392, -3.027376345333614438, 5.243569643749998122 ) ) ;
#22224=CARTESIAN_POINT ( 'NONE',  ( 12.40312500061451573, -4.541064518000417216, -2.621784821875001281 ) ) ;
#22225=EDGE_LOOP ( 'NONE', ( #26581, #22134, #64367, #49664 ) ) ;
#22226=CARTESIAN_POINT ( 'NONE',  ( 9.778125000614517504, 6.421520780324663323E-16, -5.243569643749999010 ) ) ;
#22227=CARTESIAN_POINT ( 'NONE',  ( 8.953125000614518214, 4.541064518000418104, -2.621784821874998173 ) ) ;
#22230=CARTESIAN_POINT ( 'NONE',  ( 16.01249999999999929, 2.886751345948126879, 4.999999999999999112 ) ) ;
#22231=EDGE_CURVE ( 'NONE', #5140, #12584, #62030, .T. ) ;
#22232=CARTESIAN_POINT ( 'NONE',  ( 15.15937500061451715, -4.541064518000417216, -2.621784821875001281 ) ) ;
#22233=CARTESIAN_POINT ( 'NONE',  ( 14.06250000122903288, -4.330127018922190985, -2.500000000000001332 ) ) ;
#22235=CARTESIAN_POINT ( 'NONE',  ( 19.99687500061451573, -3.027376345333614438, 5.243569643749998122 ) ) ;
#22236=CARTESIAN_POINT ( 'NONE',  ( 2.121784821874999061, 15.15312500061451750, -33.67503911421598417 ) ) ;
#22239=DIRECTION ( 'NONE',  ( 0.000000000000000000, 0.000000000000000000, 1.000000000000000000 ) ) ;
#22240=MANIFOLD_SOLID_BREP ( 'Thread3', #65457 ) ;
#22241=CARTESIAN_POINT ( 'NONE',  ( 25.90312500061451573, -4.541064518000417216, -2.621784821875001281 ) ) ;
#22242=CARTESIAN_POINT ( 'NONE',  ( -1.071796769724490339, 19.64240381056766438, -26.00000000000000355 ) ) ;
#22244=CARTESIAN_POINT ( 'NONE',  ( 27.22499999999999787, 4.330127018922191873, 2.499999999999999556 ) ) ;
#22245=CARTESIAN_POINT ( 'NONE',  ( 9.065625000614517148, 3.027376345333611329, 5.243569643749999010 ) ) ;
#22247=CARTESIAN_POINT ( 'NONE',  ( 22.58437500061451431, 4.541064518000418104, 2.621784821874999949 ) ) ;
#22249=CARTESIAN_POINT ( 'NONE',  ( 6.178125000614518747, 6.421520780324663323E-16, -5.243569643749999010 ) ) ;
#22250=CARTESIAN_POINT ( 'NONE',  ( 10.35937500061451644, 4.541064518000418104, -2.621784821874998173 ) ) ;
#22252=CARTESIAN_POINT ( 'NONE',  ( 21.45937500061451786, -4.541064518000417216, -2.621784821875001281 ) ) ;
#22253=CARTESIAN_POINT ( 'NONE',  ( 30.00000000000000000, 0.000000000000000000, 0.000000000000000000 ) ) ;
#22254=CARTESIAN_POINT ( 'NONE',  ( 29.81250000000000000, 2.886751345948129099, -4.999999999999998224 ) ) ;
#22255=CARTESIAN_POINT ( 'NONE',  ( 5.625000000000001776, 4.330127018922191873, 2.499999999999999556 ) ) ;
#22256=CARTESIAN_POINT ( 'NONE',  ( 15.37500000122903465, -5.773502691896255534, -1.060575238724906372E-15 ) ) ;
#22258=CARTESIAN_POINT ( 'NONE',  ( 12.90000000000000213, 0.000000000000000000, 4.999999999999998224 ) ) ;
#22260=CARTESIAN_POINT ( 'NONE',  ( 12.52500000000000213, -4.330127018922194537, 2.499999999999995559 ) ) ;
#22261=CARTESIAN_POINT ( 'NONE',  ( 27.29062500061451502, -3.027376345333610441, -5.243569643749999898 ) ) ;
#22262=CARTESIAN_POINT ( 'NONE',  ( 16.87500000000000000, 4.330127018922191873, 2.499999999999999556 ) ) ;
#22263=CARTESIAN_POINT ( 'NONE',  ( 9.712500001229033231, 4.330127018922192761, -2.499999999999997780 ) ) ;
#22264=CARTESIAN_POINT ( 'NONE',  ( 9.928125000614517859, 4.541064518000418104, 2.621784821874999949 ) ) ;
#22265=CARTESIAN_POINT ( 'NONE',  ( 9.187500000000001776, 5.773502691896255534, 3.535250795749688894E-16 ) ) ;
#22266=CARTESIAN_POINT ( 'NONE',  ( -5.810221930991193690E-16, 15.50000000122903465, 26.00000000000000355 ) ) ;
#22267=CARTESIAN_POINT ( 'NONE',  ( -4.243569643749997233, 14.04687500061451999, -27.54997392385601174 ) ) ;
#22268=CARTESIAN_POINT ( 'NONE',  ( 27.18750000122903288, 6.123233995736764310E-16, -4.999999999999998224 ) ) ;
#22270=CARTESIAN_POINT ( 'NONE',  ( 8.250000000000000000, 4.330127018922192761, -2.499999999999997780 ) ) ;
#22271=CARTESIAN_POINT ( 'NONE',  ( -2.000000000000000000, 12.72499999999999964, 26.53589838486224650 ) ) ;
#22272=EDGE_LOOP ( 'NONE', ( #65872, #49571, #44174, #29777 ) ) ;
#22273=CARTESIAN_POINT ( 'NONE',  ( 24.40312500061451573, 0.000000000000000000, 5.243569643749999010 ) ) ;
#22274=CARTESIAN_POINT ( 'NONE',  ( 4.210772704977717495, -2.696194641284411109, 4.497291047846275980 ) ) ;
#22275=CARTESIAN_POINT ( 'NONE',  ( 19.05000000122903003, -2.886751345948193048, -4.999999999999883649 ) ) ;
#22276=CARTESIAN_POINT ( 'NONE',  ( 22.43437500061451573, 6.421520780324663323E-16, -5.243569643749999010 ) ) ;
#22277=CARTESIAN_POINT ( 'NONE',  ( 15.66562500061451857, 3.027376345333613106, -5.243569643749998122 ) ) ;
#22278=CARTESIAN_POINT ( 'NONE',  ( 4.243569643749999898, 10.99062500061459424, -27.54997392385601529 ) ) ;
#22279=CARTESIAN_POINT ( 'NONE',  ( 7.753125000614518036, 0.000000000000000000, 5.243569643749999010 ) ) ;
#22280=CARTESIAN_POINT ( 'NONE',  ( 29.36250000122903003, -4.330127018922190985, -2.500000000000001332 ) ) ;
#22282=CARTESIAN_POINT ( 'NONE',  ( 18.55312500061451431, 0.000000000000000000, 5.243569643749999010 ) ) ;
#22283=CARTESIAN_POINT ( 'NONE',  ( 13.35000000000000142, 0.000000000000000000, 4.999999999999998224 ) ) ;
#22285=CARTESIAN_POINT ( 'NONE',  ( 14.52187500061451608, 3.027376345333611329, 5.243569643749999010 ) ) ;
#22286=CARTESIAN_POINT ( 'NONE',  ( 15.27187500061451786, 3.027376345333613106, -5.243569643749998122 ) ) ;
#22287=CARTESIAN_POINT ( 'NONE',  ( 22.73437500061451644, -4.541064518000419881, 2.621784821874995952 ) ) ;
#22289=CARTESIAN_POINT ( 'NONE',  ( 3.365625000614516082, -6.054752690667223547, -1.112240025338166033E-15 ) ) ;
#22290=CARTESIAN_POINT ( 'NONE',  ( 26.16562500061451502, 3.027376345333611329, 5.243569643749999010 ) ) ;
#22291=CARTESIAN_POINT ( 'NONE',  ( 27.70312500061451289, -4.541064518000417216, -2.621784821875001281 ) ) ;
#22292=CARTESIAN_POINT ( 'NONE',  ( -5.810221930991193690E-16, 10.55000000122903359, -34.00000000000000000 ) ) ;
#22293=CARTESIAN_POINT ( 'NONE',  ( -2.828200636599751609E-16, 16.28749999999999787, 25.38119784648299770 ) ) ;
#22294=CARTESIAN_POINT ( 'NONE',  ( 4.771875000614516971, -6.054752690667223547, -1.112240025338166033E-15 ) ) ;
#22295=CARTESIAN_POINT ( 'NONE',  ( 11.25000000122903288, -2.886751345948129988, 4.999999999999997335 ) ) ;
#22296=CARTESIAN_POINT ( 'NONE',  ( 6.937500001229033764, 6.123233995736764310E-16, -4.999999999999998224 ) ) ;
#22297=CARTESIAN_POINT ( 'NONE',  ( 3.628125000614518036, 4.541064518000418104, 2.621784821874999949 ) ) ;
#22300=CARTESIAN_POINT ( 'NONE',  ( 12.60937500061451821, 4.541064518000418104, -2.621784821874998173 ) ) ;
#22302=ORIENTED_EDGE ( 'NONE', *, *, #11801, .F. ) ;
#22303=CARTESIAN_POINT ( 'NONE',  ( 20.99062500061451431, -3.027376345333610441, -5.243569643749999898 ) ) ;
#22304=CARTESIAN_POINT ( 'NONE',  ( 13.09687500061451892, 6.054752690667223547, 3.707466751127219781E-16 ) ) ;
#22305=CARTESIAN_POINT ( 'NONE',  ( 4.378125000614518925, 6.421520780324663323E-16, -5.243569643749999010 ) ) ;
#22306=CARTESIAN_POINT ( 'NONE',  ( 21.60937500061451644, 4.541064518000418104, -2.621784821874998173 ) ) ;
#22307=CARTESIAN_POINT ( 'NONE',  ( 11.03437500061451715, -4.541064518000419881, 2.621784821874995952 ) ) ;
#22308=CARTESIAN_POINT ( 'NONE',  ( 4.790625000614518569, -3.027376345333610441, -5.243569643749999898 ) ) ;
#22310=CARTESIAN_POINT ( 'NONE',  ( 6.562500001229032875, 4.330127018922192761, -2.499999999999997780 ) ) ;
#22311=CARTESIAN_POINT ( 'NONE',  ( 20.84062500061451573, -3.027376345333614438, 5.243569643749998122 ) ) ;
#22312=CARTESIAN_POINT ( 'NONE',  ( 7.087500001229034119, 4.330127018922191873, 2.499999999999999556 ) ) ;
#22313=CARTESIAN_POINT ( 'NONE',  ( 17.42812500061451786, 6.421520780324663323E-16, -5.243569643749999010 ) ) ;
#22314=CARTESIAN_POINT ( 'NONE',  ( 15.96562500061451573, -6.054752690667223547, -1.112240025338166033E-15 ) ) ;
#22316=CARTESIAN_POINT ( 'NONE',  ( 16.50000000000000000, 0.000000000000000000, 4.999999999999998224 ) ) ;
#22317=CARTESIAN_POINT ( 'NONE',  ( 9.337500001229033231, 4.330127018922191873, 2.499999999999999556 ) ) ;
#22318=CARTESIAN_POINT ( 'NONE',  ( 6.703125000614516438, 4.541064518000418104, -2.621784821874998173 ) ) ;
#22319=EDGE_CURVE ( 'NONE', #35328, #5464, #1195, .T. ) ;
#22320=CARTESIAN_POINT ( 'NONE',  ( 20.06250000122903643, 4.330127018922192761, -2.499999999999997780 ) ) ;
#22322=CARTESIAN_POINT ( 'NONE',  ( -4.243569643749997233, 11.34687500061451892, -27.54997392385601174 ) ) ;
#22323=CARTESIAN_POINT ( 'NONE',  ( 21.41250000000000142, 2.886751345948126879, 4.999999999999998224 ) ) ;
#22324=CARTESIAN_POINT ( 'NONE',  ( 3.637500001229036162, -4.330127018922194537, 2.499999999999995559 ) ) ;
#22325=CARTESIAN_POINT ( 'NONE',  ( 4.134375000614517681, 4.541064518000418104, 2.621784821874999949 ) ) ;
#22326=CARTESIAN_POINT ( 'NONE',  ( 21.27187500061451786, 3.027376345333611329, 5.243569643749999010 ) ) ;
#22327=( BOUNDED_CURVE ( )  B_SPLINE_CURVE ( 2, ( #15163, #65045, #8532, #36244, #48435, #47328, #31436 ),
 .UNSPECIFIED., .F., .F. ) 
 B_SPLINE_CURVE_WITH_KNOTS ( ( 3, 2, 2, 3 ),
 ( 0.2999999999999999889, 0.3027777777777777568, 0.3055555555555555802, 0.3083333333333333481 ),
 .UNSPECIFIED. ) 
 CURVE ( )  GEOMETRIC_REPRESENTATION_ITEM ( )  RATIONAL_B_SPLINE_CURVE ( ( 1.000000000000000000, 0.8660254037844387076, 1.000000000000000000, 0.8660254037844387076, 1.000000000000000000, 0.8660254037844387076, 1.000000000000000000 ) ) 
 REPRESENTATION_ITEM ( '' )  );
#22328=CARTESIAN_POINT ( 'NONE',  ( -3.999999999999999112, 15.05000000000000071, 30.00000000000000000 ) ) ;
#22329=CARTESIAN_POINT ( 'NONE',  ( 16.82812500061451644, -4.541064518000419881, 2.621784821874995952 ) ) ;
#22331=CARTESIAN_POINT ( 'NONE',  ( 14.02499999999999858, 6.123233995736764310E-16, -4.999999999999998224 ) ) ;
#22333=CARTESIAN_POINT ( 'NONE',  ( 28.35937500061451289, 4.541064518000418104, -2.621784821874998173 ) ) ;
#22335=CARTESIAN_POINT ( 'NONE',  ( 13.22812500061451502, -4.541064518000419881, 2.621784821874995952 ) ) ;
#22336=CARTESIAN_POINT ( 'NONE',  ( 11.29687500061451644, 6.054752690667223547, 3.707466751127219781E-16 ) ) ;
#22338=CARTESIAN_POINT ( 'NONE',  ( 2.883025145109703313, -4.085149263999829472, -3.067080541767196245 ) ) ;
#22339=CARTESIAN_POINT ( 'NONE',  ( 22.75312500061451360, -4.541064518000417216, -2.621784821875001281 ) ) ;
#22341=DIRECTION ( 'NONE',  ( -1.000000000000000000, -0.000000000000000000, -0.000000000000000000 ) ) ;
#22342=CARTESIAN_POINT ( 'NONE',  ( 11.36250000000000071, 2.886751345948129099, -4.999999999999998224 ) ) ;
#22343=CARTESIAN_POINT ( 'NONE',  ( 20.96250000122903145, 4.330127018922192761, -2.499999999999997780 ) ) ;
#22344=CARTESIAN_POINT ( 'NONE',  ( 15.96562500061451573, -6.054752690667223547, -1.112240025338166033E-15 ) ) ;
#22347=CARTESIAN_POINT ( 'NONE',  ( 19.23749999999999716, -2.886751345948129988, 4.999999999999997335 ) ) ;
#22348=CARTESIAN_POINT ( 'NONE',  ( 23.32499999999999929, -4.330127018922194537, 2.499999999999995559 ) ) ;
#22349=CARTESIAN_POINT ( 'NONE',  ( 22.35937500061451644, -4.541064518000417216, -2.621784821875001281 ) ) ;
#22350=CARTESIAN_POINT ( 'NONE',  ( 26.42812500061451431, 6.421520780324663323E-16, -5.243569643749999010 ) ) ;
#22353=CARTESIAN_POINT ( 'NONE',  ( 9.478125000614515017, 4.541064518000418104, 2.621784821874999949 ) ) ;
#22354=CARTESIAN_POINT ( 'NONE',  ( 6.375000000000001776, 6.123233995736764310E-16, -4.999999999999998224 ) ) ;
#22355=CARTESIAN_POINT ( 'NONE',  ( 13.57500000000000107, 6.123233995736764310E-16, -4.999999999999998224 ) ) ;
#22356=CARTESIAN_POINT ( 'NONE',  ( 4.243569643749999898, 19.57812500061451644, 30.00000000000000000 ) ) ;
#22357=CARTESIAN_POINT ( 'NONE',  ( 4.059375000614519280, 4.541064518000418104, -2.621784821874998173 ) ) ;
#22358=CARTESIAN_POINT ( 'NONE',  ( 28.80937500061451573, 4.541064518000418104, -2.621784821874998173 ) ) ;
#22359=ORIENTED_EDGE ( 'NONE', *, *, #26472, .F. ) ;
#22360=CARTESIAN_POINT ( 'NONE',  ( 23.72812500061451502, 6.421520780324663323E-16, -5.243569643749999010 ) ) ;
#22361=CARTESIAN_POINT ( 'NONE',  ( 25.54687500061451644, -3.027376345333610441, -5.243569643749999898 ) ) ;
#22362=CARTESIAN_POINT ( 'NONE',  ( 2.121784821875001281, 19.50312500061459176, -26.32496088578401938 ) ) ;
#22363=CARTESIAN_POINT ( 'NONE',  ( 11.96250000000000213, 2.886751345948126879, 4.999999999999999112 ) ) ;
#22364=CARTESIAN_POINT ( 'NONE',  ( 8.053125000614516082, 4.541064518000418104, -2.621784821874998173 ) ) ;
#22365=CARTESIAN_POINT ( 'NONE',  ( 3.829234068599516760, 3.215278937808554005, 3.875698639894808117 ) ) ;
#22367=CARTESIAN_POINT ( 'NONE',  ( 27.10312500061451502, 0.000000000000000000, 5.243569643749999010 ) ) ;
#22370=CARTESIAN_POINT ( 'NONE',  ( 4.040625000614517681, 6.054752690667223547, 3.707466751127219781E-16 ) ) ;
#22371=CARTESIAN_POINT ( 'NONE',  ( 20.40937500061451715, 0.000000000000000000, 5.243569643749999010 ) ) ;
#22372=CARTESIAN_POINT ( 'NONE',  ( 4.243569643749999898, 15.09687500061451892, 32.45002607614398471 ) ) ;
#22373=CARTESIAN_POINT ( 'NONE',  ( 21.64687500061451786, 6.054752690667223547, 3.707466751127219781E-16 ) ) ;
#22374=CARTESIAN_POINT ( 'NONE',  ( 29.37187500061451928, 3.027376345333611329, 5.243569643749999010 ) ) ;
#22375=CARTESIAN_POINT ( 'NONE',  ( 4.243569643749999898, 19.59687500061451360, 32.45002607614398471 ) ) ;
#22376=CARTESIAN_POINT ( 'NONE',  ( 9.890625000614516438, 6.054752690667223547, 3.707466751127219781E-16 ) ) ;
#22377=CARTESIAN_POINT ( 'NONE',  ( 2.812500001229033320, -4.330127018922190985, -2.500000000000001332 ) ) ;
#22378=EDGE_CURVE ( 'NONE', #61146, #18509, #56836, .T. ) ;
#22379=CARTESIAN_POINT ( 'NONE',  ( 7.209375000614519635, 4.541064518000418104, -2.621784821874998173 ) ) ;
#22382=CARTESIAN_POINT ( 'NONE',  ( 6.853125000614516793, 0.000000000000000000, 5.243569643749999010 ) ) ;
#22383=CARTESIAN_POINT ( 'NONE',  ( 12.57187500061451857, 3.027376345333613106, -5.243569643749998122 ) ) ;
#22384=CARTESIAN_POINT ( 'NONE',  ( 18.67500000122903714, 2.886751345948129099, -4.999999999999998224 ) ) ;
#22385=CARTESIAN_POINT ( 'NONE',  ( 7.396875000614519635, -3.027376345333614438, 5.243569643749998122 ) ) ;
#22386=CARTESIAN_POINT ( 'NONE',  ( 9.178125000614517859, -4.541064518000419881, 2.621784821874995952 ) ) ;
#22389=CARTESIAN_POINT ( 'NONE',  ( 19.88437500061451857, 4.541064518000418104, 2.621784821874999949 ) ) ;
#22390=CARTESIAN_POINT ( 'NONE',  ( 18.07499999999999929, 6.123233995736764310E-16, -4.999999999999998224 ) ) ;
#22391=CARTESIAN_POINT ( 'NONE',  ( 28.04062500061451502, -3.027376345333614438, 5.243569643749998122 ) ) ;
#22392=CARTESIAN_POINT ( 'NONE',  ( 12.74062500061451786, -3.027376345333614438, 5.243569643749998122 ) ) ;
#22394=CARTESIAN_POINT ( 'NONE',  ( 4.243569643749999898, 11.98437500061451821, -30.00000000000000000 ) ) ;
#22396=CARTESIAN_POINT ( 'NONE',  ( 12.63750000122903394, -4.330127018922194537, 2.499999999999995559 ) ) ;
#22397=CARTESIAN_POINT ( 'NONE',  ( 27.44062500061451715, 6.054752690667223547, 3.707466751127219781E-16 ) ) ;
#22398=CARTESIAN_POINT ( 'NONE',  ( 2.121784821874999061, 15.15312500061451750, -33.67503911421598417 ) ) ;
#22399=CARTESIAN_POINT ( 'NONE',  ( 15.67500000122903181, 2.886751345948126879, 4.999999999999999112 ) ) ;
#22400=CARTESIAN_POINT ( 'NONE',  ( 12.37500000000000000, 4.330127018922191873, 2.499999999999999556 ) ) ;
#22401=CARTESIAN_POINT ( 'NONE',  ( -1.071796769724491005, 13.60759618943233384, 26.00000000000000355 ) ) ;
#22402=CARTESIAN_POINT ( 'NONE',  ( 22.07812500061451644, 4.541064518000418104, 2.621784821874999949 ) ) ;
#22403=CARTESIAN_POINT ( 'NONE',  ( 7.096875000614518036, -3.027376345333610441, -5.243569643749999898 ) ) ;
#22405=CARTESIAN_POINT ( 'NONE',  ( 6.825000001229034829, -5.773502691896255534, -1.060575238724906372E-15 ) ) ;
#22406=CARTESIAN_POINT ( 'NONE',  ( 15.33750000122903323, -4.330127018922194537, 2.499999999999995559 ) ) ;
#22407=CARTESIAN_POINT ( 'NONE',  ( 12.44062500061451537, -3.027376345333610441, -5.243569643749999898 ) ) ;
#22408=CARTESIAN_POINT ( 'NONE',  ( 17.31562500061451715, -6.054752690667223547, -1.112240025338166033E-15 ) ) ;
#22409=CARTESIAN_POINT ( 'NONE',  ( 25.35000000122903074, -2.886751345948125991, -5.000000000000000000 ) ) ;
#22410=CARTESIAN_POINT ( 'NONE',  ( 29.21250000122903145, 0.000000000000000000, 4.999999999999998224 ) ) ;
#22411=CARTESIAN_POINT ( 'NONE',  ( 22.98749999999999716, -2.886751345948125991, -5.000000000000000000 ) ) ;
#22412=CARTESIAN_POINT ( 'NONE',  ( 24.87187500061451573, 3.027376345333611329, 5.243569643749999010 ) ) ;
#22413=CARTESIAN_POINT ( 'NONE',  ( 25.80000000122903359, -2.886751345948109559, -5.000000000000028422 ) ) ;
#22414=CARTESIAN_POINT ( 'NONE',  ( 9.375000001229036428, 2.886751345948126879, 4.999999999999999112 ) ) ;
#22415=CARTESIAN_POINT ( 'NONE',  ( 28.47187500061451715, 3.027376345333611329, 5.243569643749999010 ) ) ;
#22416=CARTESIAN_POINT ( 'NONE',  ( 4.884375000614518569, 6.421520780324663323E-16, -5.243569643749999010 ) ) ;
#22417=CARTESIAN_POINT ( 'NONE',  ( 23.42812500061451786, 4.541064518000418104, 2.621784821874999949 ) ) ;
#22419=CARTESIAN_POINT ( 'NONE',  ( 4.544497808834801589, -2.085075457992688897, -4.544497808831748920 ) ) ;
#22420=CARTESIAN_POINT ( 'NONE',  ( 9.159375000614515372, 0.000000000000000000, 5.243569643749999010 ) ) ;
#22421=DIRECTION ( 'NONE',  ( -1.000000000000000000, -0.000000000000000000, -0.000000000000000000 ) ) ;
#22422=CARTESIAN_POINT ( 'NONE',  ( 3.234375000614516438, 4.541064518000418104, 2.621784821874999949 ) ) ;
#22423=CARTESIAN_POINT ( 'NONE',  ( 5.559375000614517504, 0.000000000000000000, 5.243569643749999010 ) ) ;
#22425=CARTESIAN_POINT ( 'NONE',  ( 27.72187500061451715, -6.054752690667223547, -1.112240025338166033E-15 ) ) ;
#22427=CARTESIAN_POINT ( 'NONE',  ( 19.38749999999999929, -2.886751345948125991, -5.000000000000000000 ) ) ;
#22428=ORIENTED_EDGE ( 'NONE', *, *, #8538, .T. ) ;
#22429=CARTESIAN_POINT ( 'NONE',  ( 26.73749999999999716, 5.773502691896255534, 3.535250795749688894E-16 ) ) ;
#22430=CARTESIAN_POINT ( 'NONE',  ( 27.90937500061451715, 4.541064518000418104, -2.621784821874998173 ) ) ;
#22431=ORIENTED_EDGE ( 'NONE', *, *, #53850, .T. ) ;
#22432=CARTESIAN_POINT ( 'NONE',  ( 14.50312500061451537, 0.000000000000000000, 5.243569643749999010 ) ) ;
#22433=CARTESIAN_POINT ( 'NONE',  ( 7.378125000614518036, -4.541064518000419881, 2.621784821874995952 ) ) ;
#22435=CARTESIAN_POINT ( 'NONE',  ( 5.259375000614518569, -4.541064518000417216, -2.621784821875001281 ) ) ;
#22436=CARTESIAN_POINT ( 'NONE',  ( 18.82500000122903216, 2.886751345948126879, 4.999999999999999112 ) ) ;
#22437=CARTESIAN_POINT ( 'NONE',  ( 23.88749999999999929, -2.886751345948125991, -5.000000000000000000 ) ) ;
#22438=CARTESIAN_POINT ( 'NONE',  ( 7.996875000614519280, -3.027376345333610441, -5.243569643749999898 ) ) ;
#22439=CARTESIAN_POINT ( 'NONE',  ( 12.45937500061451786, -4.541064518000417216, -2.621784821875001281 ) ) ;
#22440=CARTESIAN_POINT ( 'NONE',  ( 21.12187500061451573, 3.027376345333613106, -5.243569643749998122 ) ) ;
#22443=CARTESIAN_POINT ( 'NONE',  ( 3.721875000614518036, 3.027376345333611329, 5.243569643749999010 ) ) ;
#22445=CARTESIAN_POINT ( 'NONE',  ( 7.284375000614518036, 4.541064518000418104, 2.621784821874999949 ) ) ;
#22446=CARTESIAN_POINT ( 'NONE',  ( 20.62499999999999645, -4.330127018922194537, 2.499999999999995559 ) ) ;
#22447=CARTESIAN_POINT ( 'NONE',  ( 14.99062500061451786, -3.027376345333614438, 5.243569643749998122 ) ) ;
#22451=CARTESIAN_POINT ( 'NONE',  ( 10.45312500061451644, 0.000000000000000000, 5.243569643749999010 ) ) ;
#22452=CARTESIAN_POINT ( 'NONE',  ( 26.97187500061451360, 3.027376345333613106, -5.243569643749998122 ) ) ;
#22454=CARTESIAN_POINT ( 'NONE',  ( 28.20937500061451786, -4.541064518000417216, -2.621784821875001281 ) ) ;
#22455=CARTESIAN_POINT ( 'NONE',  ( 9.600000000000001421, 4.330127018922192761, -2.499999999999997780 ) ) ;
#22456=CARTESIAN_POINT ( 'NONE',  ( -2.000000000000000000, 14.63750000122903394, 26.53589838486224650 ) ) ;
#22457=CARTESIAN_POINT ( 'NONE',  ( 8.700000001229032165, -2.886751345948125991, -5.000000000000000000 ) ) ;
#22458=CARTESIAN_POINT ( 'NONE',  ( 18.94687500061451502, 6.054752690667223547, 3.707466751127219781E-16 ) ) ;
#22459=CARTESIAN_POINT ( 'NONE',  ( 14.97187500061451892, 3.027376345333611329, 5.243569643749999010 ) ) ;
#22462=CARTESIAN_POINT ( 'NONE',  ( 14.27812500061451573, 6.421520780324663323E-16, -5.243569643749999010 ) ) ;
#22463=CARTESIAN_POINT ( 'NONE',  ( 25.12500000122903288, 2.886751345948126879, 4.999999999999999112 ) ) ;
#22464=CARTESIAN_POINT ( 'NONE',  ( 16.17187500061451644, 3.027376345333613106, -5.243569643749998122 ) ) ;
#22465=CARTESIAN_POINT ( 'NONE',  ( 7.612500001229035362, 0.000000000000000000, 4.999999999999998224 ) ) ;
#22466=CARTESIAN_POINT ( 'NONE',  ( 16.67812500061451786, 4.541064518000418104, 2.621784821874999949 ) ) ;
#22468=CARTESIAN_POINT ( 'NONE',  ( 25.65937500061451715, 4.541064518000418104, -2.621784821874998173 ) ) ;
#22469=CARTESIAN_POINT ( 'NONE',  ( -4.243569643749999898, 11.25312500061451892, 30.00000000000000000 ) ) ;
#22470=CARTESIAN_POINT ( 'NONE',  ( 15.23437500061451644, 6.421520780324663323E-16, -5.243569643749999010 ) ) ;
#22471=CARTESIAN_POINT ( 'NONE',  ( 14.25000000122903465, 5.773502691896255534, 3.535250795749688894E-16 ) ) ;
#22472=CYLINDRICAL_SURFACE ( 'NONE', #4495, 3.999999999999996447 ) ;
#22473=CARTESIAN_POINT ( 'NONE',  ( -2.121784821874999949, 18.88437500061451857, -33.67503911421598417 ) ) ;
#22475=CARTESIAN_POINT ( 'NONE',  ( 19.05937500061451928, 0.000000000000000000, 5.243569643749999010 ) ) ;
#22476=CARTESIAN_POINT ( 'NONE',  ( 19.91250000122903074, -4.330127018922190985, -2.500000000000001332 ) ) ;
#22477=CARTESIAN_POINT ( 'NONE',  ( 15.75937500061451857, 4.541064518000418104, -2.621784821874998173 ) ) ;
#22478=CARTESIAN_POINT ( 'NONE',  ( 4.243569643749999898, 11.49687500061451928, 32.45002607614398471 ) ) ;
#22479=CARTESIAN_POINT ( 'NONE',  ( 21.67500000122903359, -5.773502691896255534, -1.060575238724906372E-15 ) ) ;
#22480=CARTESIAN_POINT ( 'NONE',  ( 18.47812500061451857, 4.541064518000418104, 2.621784821874999949 ) ) ;
#22481=ORIENTED_EDGE ( 'NONE', *, *, #25529, .F. ) ;
#22482=ORIENTED_EDGE ( 'NONE', *, *, #7942, .T. ) ;
#22483=CARTESIAN_POINT ( 'NONE',  ( 21.11249999999999716, -5.773502691896255534, -1.060575238724906372E-15 ) ) ;
#22485=CARTESIAN_POINT ( 'NONE',  ( 22.79062500061451502, -3.027376345333610441, -5.243569643749999898 ) ) ;
#22486=CARTESIAN_POINT ( 'NONE',  ( 4.003125000614518925, 4.541064518000418104, -2.621784821874998173 ) ) ;
#22487=CARTESIAN_POINT ( 'NONE',  ( 18.56250000122903288, -4.330127018922190985, -2.500000000000001332 ) ) ;
#22488=CARTESIAN_POINT ( 'NONE',  ( 21.51562500061451644, 3.027376345333613106, -5.243569643749998122 ) ) ;
#22489=( BOUNDED_CURVE ( )  B_SPLINE_CURVE ( 2, ( #68848, #1617, #57020, #62926, #6425, #24126, #28958 ),
 .UNSPECIFIED., .F., .F. ) 
 B_SPLINE_CURVE_WITH_KNOTS ( ( 3, 2, 2, 3 ),
 ( 0.7916666666666666297, 0.7944444444444443976, 0.7972222222222222765, 0.8000000000000000444 ),
 .UNSPECIFIED. ) 
 CURVE ( )  GEOMETRIC_REPRESENTATION_ITEM ( )  RATIONAL_B_SPLINE_CURVE ( ( 1.000000000000000000, 0.8660254037844387076, 1.000000000000000000, 0.8660254037844387076, 1.000000000000000000, 0.8660254037844387076, 1.000000000000000000 ) ) 
 REPRESENTATION_ITEM ( '' )  );
#22490=CARTESIAN_POINT ( 'NONE',  ( 26.46562500061451573, 3.027376345333613106, -5.243569643749998122 ) ) ;
#22491=CARTESIAN_POINT ( 'NONE',  ( 6.478125000614516793, -4.541064518000419881, 2.621784821874995952 ) ) ;
#22492=ORIENTED_EDGE ( 'NONE', *, *, #21050, .F. ) ;
#22493=CARTESIAN_POINT ( 'NONE',  ( 29.09999999999999787, 0.000000000000000000, 4.999999999999998224 ) ) ;
#22494=CARTESIAN_POINT ( 'NONE',  ( -1.999999999999997113, 10.28750000122903430, -26.53589838486224295 ) ) ;
#22497=CARTESIAN_POINT ( 'NONE',  ( 3.999999999999999112, 10.43750000122903465, -30.00000000000000000 ) ) ;
#22498=CARTESIAN_POINT ( 'NONE',  ( 4.243569643749999898, 19.18437500061451928, -30.00000000000000000 ) ) ;
#22499=EDGE_CURVE ( 'NONE', #26592, #72158, #69576, .T. ) ;
#22500=CARTESIAN_POINT ( 'NONE',  ( 6.937500001229033764, 6.123233995736764310E-16, -4.999999999999998224 ) ) ;
#22501=CARTESIAN_POINT ( 'NONE',  ( 7.350000000000002309, 4.330127018922192761, -2.499999999999997780 ) ) ;
#22502=CARTESIAN_POINT ( 'NONE',  ( 4.387500001229033053, 4.330127018922191873, 2.499999999999999556 ) ) ;
#22503=CARTESIAN_POINT ( 'NONE',  ( 11.44687500061451857, -3.027376345333614438, 5.243569643749998122 ) ) ;
#22504=CARTESIAN_POINT ( 'NONE',  ( 19.38750000122903216, -4.330127018922194537, 2.499999999999995559 ) ) ;
#22507=CARTESIAN_POINT ( 'NONE',  ( 10.58437500061451964, -4.541064518000419881, 2.621784821874995952 ) ) ;
#22508=CARTESIAN_POINT ( 'NONE',  ( 29.83125000061451715, 0.000000000000000000, 5.243569643749999010 ) ) ;
#22510=CARTESIAN_POINT ( 'NONE',  ( 18.89062500061451644, 6.054752690667223547, 3.707466751127219781E-16 ) ) ;
#22511=CARTESIAN_POINT ( 'NONE',  ( 1.071796769724489895, 14.46740381056766545, 26.00000000000000355 ) ) ;
#22512=CARTESIAN_POINT ( 'NONE',  ( 9.001249775931846008E-16, 17.21562500061459744, 34.90005215228797653 ) ) ;
#22513=CARTESIAN_POINT ( 'NONE',  ( 21.90937500061451715, -4.541064518000417216, -2.621784821875001281 ) ) ;
#22514=FACE_OUTER_BOUND ( 'NONE', #11022, .T. ) ;
#22515=CARTESIAN_POINT ( 'NONE',  ( 27.93750000122903288, -4.330127018922194537, 2.499999999999995559 ) ) ;
#22517=CARTESIAN_POINT ( 'NONE',  ( 25.19062500061451715, 6.054752690667223547, 3.707466751127219781E-16 ) ) ;
#22518=CARTESIAN_POINT ( 'NONE',  ( 15.40312500061451573, 0.000000000000000000, 5.243569643749999010 ) ) ;
#22520=CARTESIAN_POINT ( 'NONE',  ( 11.18437500061451928, 6.421520780324663323E-16, -5.243569643749999010 ) ) ;
#22521=CARTESIAN_POINT ( 'NONE',  ( 28.68749999999999645, -2.886751345948129988, 4.999999999999997335 ) ) ;
#22522=CARTESIAN_POINT ( 'NONE',  ( 25.31250000122903288, -4.330127018922190985, -2.500000000000001332 ) ) ;
#22523=CARTESIAN_POINT ( 'NONE',  ( 3.871875000614519280, -6.054752690667223547, -1.112240025338166033E-15 ) ) ;
#22524=CARTESIAN_POINT ( 'NONE',  ( 15.42187500061451821, 3.027376345333611329, 5.243569643749999010 ) ) ;
#22525=CARTESIAN_POINT ( 'NONE',  ( 29.48437500061451644, -4.541064518000419881, 2.621784821874995952 ) ) ;
#22527=CARTESIAN_POINT ( 'NONE',  ( 1.626862140677534273E-15, 12.46250000000000213, -26.00000000000000355 ) ) ;
#22528=CARTESIAN_POINT ( 'NONE',  ( 22.47187500061451715, 3.027376345333613106, -5.243569643749998122 ) ) ;
#22529=CARTESIAN_POINT ( 'NONE',  ( 13.92187500061451644, 3.027376345333613106, -5.243569643749998122 ) ) ;
#22531=CARTESIAN_POINT ( 'NONE',  ( 28.23750000000000426, -2.886751345948129988, 4.999999999999997335 ) ) ;
#22532=CARTESIAN_POINT ( 'NONE',  ( 2.962500001229034119, 4.330127018922192761, -2.499999999999997780 ) ) ;
#22534=CARTESIAN_POINT ( 'NONE',  ( 17.87812500061451715, 6.421520780324663323E-16, -5.243569643749999010 ) ) ;
#22535=CARTESIAN_POINT ( 'NONE',  ( 6.337499999999998579, -2.886751345948125991, -5.000000000000000000 ) ) ;
#22537=CARTESIAN_POINT ( 'NONE',  ( 17.02499999999999858, -4.330127018922194537, 2.499999999999995559 ) ) ;
#22538=CARTESIAN_POINT ( 'NONE',  ( -4.243569643749999898, 12.15312500061451573, 30.00000000000000000 ) ) ;
#22540=CARTESIAN_POINT ( 'NONE',  ( 21.33750000122903145, 6.123233995736764310E-16, -4.999999999999998224 ) ) ;
#22542=CARTESIAN_POINT ( 'NONE',  ( 26.52187500061451431, 3.027376345333613106, -5.243569643749998122 ) ) ;
#22543=ORIENTED_EDGE ( 'NONE', *, *, #62922, .T. ) ;
#22544=CARTESIAN_POINT ( 'NONE',  ( 21.96562500061451573, 3.027376345333613106, -5.243569643749998122 ) ) ;
#22545=CARTESIAN_POINT ( 'NONE',  ( 22.62187500061451573, 3.027376345333611329, 5.243569643749999010 ) ) ;
#22546=CARTESIAN_POINT ( 'NONE',  ( 5.924999999999999822, 6.123233995736764310E-16, -4.999999999999998224 ) ) ;
#22547=CARTESIAN_POINT ( 'NONE',  ( 10.15312500061451750, -4.541064518000417216, -2.621784821875001281 ) ) ;
#22548=CARTESIAN_POINT ( 'NONE',  ( 24.21562500061451573, 3.027376345333613106, -5.243569643749998122 ) ) ;
#22549=CARTESIAN_POINT ( 'NONE',  ( 13.88437500061451679, 6.421520780324663323E-16, -5.243569643749999010 ) ) ;
#22550=CARTESIAN_POINT ( 'NONE',  ( 18.08437500061451431, 4.541064518000418104, 2.621784821874999949 ) ) ;
#22551=LINE ( 'NONE', #56536, #21510 ) ;
#22552=CARTESIAN_POINT ( 'NONE',  ( -2.121784821874999949, 17.47812500061451502, 26.32496088578401938 ) ) ;
#22553=CARTESIAN_POINT ( 'NONE',  ( 22.35000000122903074, 5.773502691896255534, 3.535250795749688894E-16 ) ) ;
#22555=CARTESIAN_POINT ( 'NONE',  ( 11.09062500061451573, -3.027376345333610441, -5.243569643749999898 ) ) ;
#22556=CARTESIAN_POINT ( 'NONE',  ( 5.896875000614518747, 6.054752690667223547, 3.707466751127219781E-16 ) ) ;
#22557=CARTESIAN_POINT ( 'NONE',  ( 3.759375000614517681, 0.000000000000000000, 5.243569643749999010 ) ) ;
#22558=ORIENTED_EDGE ( 'NONE', *, *, #6300, .F. ) ;
#22560=CARTESIAN_POINT ( 'NONE',  ( 27.64687500061452141, -3.027376345333614438, 5.243569643749998122 ) ) ;
#22561=CARTESIAN_POINT ( 'NONE',  ( 16.86562500061451786, -6.054752690667223547, -1.112240025338166033E-15 ) ) ;
#22562=CARTESIAN_POINT ( 'NONE',  ( 27.37500000122903288, 2.886751345948126879, 4.999999999999999112 ) ) ;
#22563=CARTESIAN_POINT ( 'NONE',  ( 28.00312500061451715, 0.000000000000000000, 5.243569643749999010 ) ) ;
#22564=CARTESIAN_POINT ( 'NONE',  ( 24.45937500061451786, 0.000000000000000000, 5.243569643749999010 ) ) ;
#22565=CARTESIAN_POINT ( 'NONE',  ( 17.12812500061451715, 4.541064518000418104, 2.621784821874999949 ) ) ;
#22566=CARTESIAN_POINT ( 'NONE',  ( 2.121784821875001281, 19.10937500061451644, 33.67503911421598417 ) ) ;
#22567=CARTESIAN_POINT ( 'NONE',  ( 24.51562500061451289, -6.054752690667223547, -1.112240025338166033E-15 ) ) ;
#22568=CARTESIAN_POINT ( 'NONE',  ( 5.325000001229033941, 2.886751345948126879, 4.999999999999999112 ) ) ;
#22570=CARTESIAN_POINT ( 'NONE',  ( 27.75000000000000000, 0.000000000000000000, 4.999999999999998224 ) ) ;
#22571=CARTESIAN_POINT ( 'NONE',  ( 1.999999999999998668, 14.45000000000000107, -33.46410161513775705 ) ) ;
#22573=CARTESIAN_POINT ( 'NONE',  ( 4.734375000614518214, -4.541064518000419881, 2.621784821874995952 ) ) ;
#22574=CARTESIAN_POINT ( 'NONE',  ( 10.52812500061451750, -4.541064518000419881, 2.621784821874995952 ) ) ;
#22575=CARTESIAN_POINT ( 'NONE',  ( 5.934375000614517504, 4.541064518000418104, 2.621784821874999949 ) ) ;
#22576=CARTESIAN_POINT ( 'NONE',  ( 24.37500000122903288, -5.773502691896255534, -1.060575238724906372E-15 ) ) ;
#22577=CARTESIAN_POINT ( 'NONE',  ( 14.63437500061451679, -4.541064518000419881, 2.621784821874995952 ) ) ;
#22578=CARTESIAN_POINT ( 'NONE',  ( 28.82812500061451644, 4.541064518000418104, 2.621784821874999949 ) ) ;
#22579=CARTESIAN_POINT ( 'NONE',  ( 27.26249999999999929, 2.886751345948126879, 4.999999999999999112 ) ) ;
#22580=CARTESIAN_POINT ( 'NONE',  ( 3.590625000614518836, 6.054752690667223547, 3.707466751127219781E-16 ) ) ;
#22581=CARTESIAN_POINT ( 'NONE',  ( 12.85312500061451502, -4.541064518000417216, -2.621784821875001281 ) ) ;
#22583=CARTESIAN_POINT ( 'NONE',  ( 8.915625000614515017, 3.027376345333613106, -5.243569643749998122 ) ) ;
#22584=CARTESIAN_POINT ( 'NONE',  ( 5.990625000614517859, -3.027376345333614438, 5.243569643749998122 ) ) ;
#22586=DIRECTION ( 'NONE',  ( 0.000000000000000000, 0.000000000000000000, 1.000000000000000000 ) ) ;
#22587=CARTESIAN_POINT ( 'NONE',  ( 14.62500000000000000, 4.330127018922191873, 2.499999999999999556 ) ) ;
#22588=CARTESIAN_POINT ( 'NONE',  ( 17.18437500061451573, 4.541064518000418104, 2.621784821874999949 ) ) ;
#22589=CARTESIAN_POINT ( 'NONE',  ( 12.22500000122903430, -5.773502691896255534, -1.060575238724906372E-15 ) ) ;
#22591=CARTESIAN_POINT ( 'NONE',  ( 20.74687500061451573, 6.054752690667223547, 3.707466751127219781E-16 ) ) ;
#22592=CARTESIAN_POINT ( 'NONE',  ( 2.121784821874999061, 12.90312500061451750, -33.67503911421598417 ) ) ;
#22595=CARTESIAN_POINT ( 'NONE',  ( 30.00000000000000000, 0.000000000000000000, 0.000000000000000000 ) ) ;
#22596=ADVANCED_FACE ( 'NONE', ( #2610 ), #52855, .F. ) ;
#22597=CARTESIAN_POINT ( 'NONE',  ( 27.47812500061451502, 4.541064518000418104, 2.621784821874999949 ) ) ;
#22598=CARTESIAN_POINT ( 'NONE',  ( 29.78437500061451715, 4.541064518000418104, 2.621784821874999949 ) ) ;
#22599=CARTESIAN_POINT ( 'NONE',  ( 23.25000000000000000, 0.000000000000000000, 4.999999999999998224 ) ) ;
#22600=CARTESIAN_POINT ( 'NONE',  ( 9.778125000614517504, 6.421520780324663323E-16, -5.243569643749999010 ) ) ;
#22602=CARTESIAN_POINT ( 'NONE',  ( 18.72187500061451360, -6.054752690667223547, -1.112240025338166033E-15 ) ) ;
#22604=CARTESIAN_POINT ( 'NONE',  ( 4.153125000614515727, 0.000000000000000000, 5.243569643749999010 ) ) ;
#22605=CARTESIAN_POINT ( 'NONE',  ( 9.946875000614516793, 6.054752690667223547, 3.707466751127219781E-16 ) ) ;
#22606=ORIENTED_EDGE ( 'NONE', *, *, #54179, .F. ) ;
#22607=CARTESIAN_POINT ( 'NONE',  ( 21.68437500061451573, 4.541064518000418104, 2.621784821874999949 ) ) ;
#22609=CARTESIAN_POINT ( 'NONE',  ( 29.32499999999999929, 6.123233995736764310E-16, -4.999999999999998224 ) ) ;
#22610=CARTESIAN_POINT ( 'NONE',  ( 5.775000000000002132, -4.330127018922194537, 2.499999999999995559 ) ) ;
#22611=CARTESIAN_POINT ( 'NONE',  ( 15.75000000122902932, -2.886751345948129988, 4.999999999999997335 ) ) ;
#22615=ORIENTED_EDGE ( 'NONE', *, *, #7766, .T. ) ;
#22616=CARTESIAN_POINT ( 'NONE',  ( 12.63749999999999929, -2.886751345948125991, -5.000000000000000000 ) ) ;
#22617=CARTESIAN_POINT ( 'NONE',  ( 25.82812500061451644, -4.541064518000419881, 2.621784821874995952 ) ) ;
#22618=CARTESIAN_POINT ( 'NONE',  ( 17.25000000000000000, 4.330127018922192761, -2.499999999999997780 ) ) ;
#22619=CARTESIAN_POINT ( 'NONE',  ( 10.16250000122903252, 4.330127018922192761, -2.499999999999997780 ) ) ;
#22620=CARTESIAN_POINT ( 'NONE',  ( 8.878125000614515372, 6.421520780324663323E-16, -5.243569643749999010 ) ) ;
#22621=CARTESIAN_POINT ( 'NONE',  ( 8.512499999999999289, -5.773502691896255534, -1.060575238724906372E-15 ) ) ;
#22623=CARTESIAN_POINT ( 'NONE',  ( 4.243569643749999898, 14.68437500061451750, -30.00000000000000000 ) ) ;
#22624=CARTESIAN_POINT ( 'NONE',  ( 28.95000000122903572, -2.886751345948125991, -5.000000000000000000 ) ) ;
#22626=CARTESIAN_POINT ( 'NONE',  ( 8.550000000000002487, -4.330127018922190985, -2.500000000000001332 ) ) ;
#22627=DIRECTION ( 'NONE',  ( -1.000000000000000000, -0.000000000000000000, -0.000000000000000000 ) ) ;
#22629=CARTESIAN_POINT ( 'NONE',  ( 23.57812500061451289, -4.541064518000419881, 2.621784821874995952 ) ) ;
#22630=CARTESIAN_POINT ( 'NONE',  ( 14.55000000122903181, -2.886751345948125991, -5.000000000000000000 ) ) ;
#22631=CARTESIAN_POINT ( 'NONE',  ( 28.75312500061451715, 4.541064518000418104, -2.621784821874998173 ) ) ;
#22632=CARTESIAN_POINT ( 'NONE',  ( 19.08750000122903145, 6.123233995736764310E-16, -4.999999999999998224 ) ) ;
#22633=CARTESIAN_POINT ( 'NONE',  ( 19.80937500061451573, 4.541064518000418104, -2.621784821874998173 ) ) ;
#22634=CARTESIAN_POINT ( 'NONE',  ( 17.20312500061451644, 0.000000000000000000, 5.243569643749999010 ) ) ;
#22635=CARTESIAN_POINT ( 'NONE',  ( 2.121784821874999061, 12.00312500061459531, -33.67503911421598417 ) ) ;
#22636=CARTESIAN_POINT ( 'NONE',  ( 7.228125000614517681, 4.541064518000418104, 2.621784821874999949 ) ) ;
#22637=CARTESIAN_POINT ( 'NONE',  ( 28.01250000122903216, -4.330127018922190985, -2.500000000000001332 ) ) ;
#22639=CARTESIAN_POINT ( 'NONE',  ( 19.75312500061451360, 4.541064518000418104, -2.621784821874998173 ) ) ;
#22640=FACE_OUTER_BOUND ( 'NONE', #36245, .T. ) ;
#22642=CARTESIAN_POINT ( 'NONE',  ( 13.28437500061451715, -4.541064518000419881, 2.621784821874995952 ) ) ;
#22643=CARTESIAN_POINT ( 'NONE',  ( 10.88437500061451679, 4.541064518000418104, 2.621784821874999949 ) ) ;
#22644=CARTESIAN_POINT ( 'NONE',  ( 21.27187500061451786, 3.027376345333611329, 5.243569643749999010 ) ) ;
#22645=ORIENTED_EDGE ( 'NONE', *, *, #45774, .F. ) ;
#22647=CARTESIAN_POINT ( 'NONE',  ( 26.57812500061451644, 4.541064518000418104, 2.621784821874999949 ) ) ;
#22648=EDGE_CURVE ( 'NONE', #493, #47295, #9808, .T. ) ;
#22649=CARTESIAN_POINT ( 'NONE',  ( 23.27812500061451573, 6.421520780324663323E-16, -5.243569643749999010 ) ) ;
#22650=DIRECTION ( 'NONE',  ( -1.000000000000000000, -0.000000000000000000, -0.000000000000000000 ) ) ;
#22651=CARTESIAN_POINT ( 'NONE',  ( -3.999999999999999556, 17.26249999999999929, 27.69059892324149530 ) ) ;
#22652=CARTESIAN_POINT ( 'NONE',  ( 3.946875000614517681, -3.027376345333610441, -5.243569643749999898 ) ) ;
#22653=CARTESIAN_POINT ( 'NONE',  ( 10.98750000122903536, 6.123233995736764310E-16, -4.999999999999998224 ) ) ;
#22654=CARTESIAN_POINT ( 'NONE',  ( 6.900000001229035007, -2.886751345948125991, -5.000000000000000000 ) ) ;
#22655=CARTESIAN_POINT ( 'NONE',  ( 28.46250000122903145, -4.330127018922190985, -2.500000000000001332 ) ) ;
#22658=CARTESIAN_POINT ( 'NONE',  ( 11.37187500061451750, 3.027376345333611329, 5.243569643749999010 ) ) ;
#22660=CARTESIAN_POINT ( 'NONE',  ( 19.30312500061451786, 4.541064518000418104, -2.621784821874998173 ) ) ;
#22661=CARTESIAN_POINT ( 'NONE',  ( 13.20937500061451786, 0.000000000000000000, 5.243569643749999010 ) ) ;
#22662=CARTESIAN_POINT ( 'NONE',  ( 3.815625000614518036, -6.054752690667223547, -1.112240025338166033E-15 ) ) ;
#22663=CARTESIAN_POINT ( 'NONE',  ( 23.22187500061451715, -6.054752690667223547, -1.112240025338166033E-15 ) ) ;
#22664=CARTESIAN_POINT ( 'NONE',  ( 10.92187500061451644, 3.027376345333611329, 5.243569643749999010 ) ) ;
#22665=CARTESIAN_POINT ( 'NONE',  ( 5.315625000614516260, 3.027376345333613106, -5.243569643749998122 ) ) ;
#22667=CARTESIAN_POINT ( 'NONE',  ( 5.437500001229035540, -4.330127018922194537, 2.499999999999995559 ) ) ;
#22668=CARTESIAN_POINT ( 'NONE',  ( 20.91562500061451502, -6.054752690667223547, -1.112240025338166033E-15 ) ) ;
#22669=CARTESIAN_POINT ( 'NONE',  ( 8.775000001229033231, 2.886751345948129099, -4.999999999999998224 ) ) ;
#22670=CARTESIAN_POINT ( 'NONE',  ( 17.99062500061451786, 6.054752690667223547, 3.707466751127219781E-16 ) ) ;
#22671=CARTESIAN_POINT ( 'NONE',  ( 13.37812500061451715, 6.421520780324663323E-16, -5.243569643749999010 ) ) ;
#22673=CARTESIAN_POINT ( 'NONE',  ( 12.33750000000000036, 5.773502691896255534, 3.535250795749688894E-16 ) ) ;
#22674=CARTESIAN_POINT ( 'NONE',  ( 9.075000001229033941, -5.773502691896255534, -1.060575238724906372E-15 ) ) ;
#22675=CARTESIAN_POINT ( 'NONE',  ( 4.453125000614517326, 4.541064518000418104, -2.621784821874998173 ) ) ;
#22677=CARTESIAN_POINT ( 'NONE',  ( 21.90000000122903145, 5.773502691896255534, 3.535250795749688894E-16 ) ) ;
#22679=CARTESIAN_POINT ( 'NONE',  ( 2.121784821875001281, 10.55937500061451750, -26.32496088578401938 ) ) ;
#22680=CARTESIAN_POINT ( 'NONE',  ( 21.30000000000000071, 4.330127018922192761, -2.499999999999997780 ) ) ;
#22681=DIRECTION ( 'NONE',  ( 0.000000000000000000, 0.000000000000000000, -1.000000000000000000 ) ) ;
#22683=CARTESIAN_POINT ( 'NONE',  ( 21.83437500061451786, -4.541064518000419881, 2.621784821874995952 ) ) ;
#22684=CARTESIAN_POINT ( 'NONE',  ( 3.999999999999999112, 18.53750000122903430, 30.00000000000000000 ) ) ;
#22685=CARTESIAN_POINT ( 'NONE',  ( 16.26562500061451289, 3.027376345333611329, 5.243569643749999010 ) ) ;
#22689=CARTESIAN_POINT ( 'NONE',  ( 25.28437500061451715, 4.541064518000418104, 2.621784821874999949 ) ) ;
#22691=CARTESIAN_POINT ( 'NONE',  ( 11.42812500061451608, -4.541064518000419881, 2.621784821874995952 ) ) ;
#22692=CARTESIAN_POINT ( 'NONE',  ( 9.946875000614516793, 6.054752690667223547, 3.707466751127219781E-16 ) ) ;
#22694=CARTESIAN_POINT ( 'NONE',  ( 29.24062500061451431, 6.054752690667223547, 3.707466751127219781E-16 ) ) ;
#22695=CARTESIAN_POINT ( 'NONE',  ( 21.85312500061451502, -4.541064518000417216, -2.621784821875001281 ) ) ;
#22696=CARTESIAN_POINT ( 'NONE',  ( 0.000000000000000000, 20.00000000000000000, 30.00000000000000000 ) ) ;
#22697=CARTESIAN_POINT ( 'NONE',  ( -3.999999999999997335, 12.95000000122903216, 32.30940107675850470 ) ) ;
#22698=CARTESIAN_POINT ( 'NONE',  ( 12.90000000000000213, 0.000000000000000000, 4.999999999999998224 ) ) ;
#22699=CARTESIAN_POINT ( 'NONE',  ( 22.46250000122903501, 0.000000000000000000, 4.999999999999998224 ) ) ;
#22700=CARTESIAN_POINT ( 'NONE',  ( 16.49062500061451786, -3.027376345333610441, -5.243569643749999898 ) ) ;
#22703=CARTESIAN_POINT ( 'NONE',  ( 21.03750000000000142, -2.886751345948129988, 4.999999999999997335 ) ) ;
#22704=CARTESIAN_POINT ( 'NONE',  ( 24.14999999999999858, 0.000000000000000000, 4.999999999999998224 ) ) ;
#22705=CARTESIAN_POINT ( 'NONE',  ( 21.19687500061451502, 6.054752690667223547, 3.707466751127219781E-16 ) ) ;
#22706=CARTESIAN_POINT ( 'NONE',  ( 25.26562500061451289, 3.027376345333611329, 5.243569643749999010 ) ) ;
#22709=LINE ( 'NONE', #6093, #40729 ) ;
#22710=CARTESIAN_POINT ( 'NONE',  ( 8.653125000614515727, 0.000000000000000000, 5.243569643749999010 ) ) ;
#22711=CARTESIAN_POINT ( 'NONE',  ( 15.78749999999999964, -2.886751345948125991, -5.000000000000000000 ) ) ;
#22712=CARTESIAN_POINT ( 'NONE',  ( -3.000416591977282496E-16, 17.44062500061451360, 25.09994784771203058 ) ) ;
#22713=CARTESIAN_POINT ( 'NONE',  ( 4.134375000614517681, 4.541064518000418104, 2.621784821874999949 ) ) ;
#22714=CARTESIAN_POINT ( 'NONE',  ( 26.52187500061451431, 3.027376345333613106, -5.243569643749998122 ) ) ;
#22715=ORIENTED_EDGE ( 'NONE', *, *, #49507, .T. ) ;
#22716=CARTESIAN_POINT ( 'NONE',  ( 23.39062500061451289, 6.054752690667223547, 3.707466751127219781E-16 ) ) ;
#22717=CARTESIAN_POINT ( 'NONE',  ( 25.20937500061451431, 4.541064518000418104, -2.621784821874998173 ) ) ;
#22718=CARTESIAN_POINT ( 'NONE',  ( -2.121784821874996840, 19.42812500061459247, -26.32496088578401583 ) ) ;
#22719=CARTESIAN_POINT ( 'NONE',  ( 11.25000000000000000, -4.330127018922190985, -2.500000000000001332 ) ) ;
#22720=CARTESIAN_POINT ( 'NONE',  ( 8.728125000614518569, -4.541064518000419881, 2.621784821874995952 ) ) ;
#22721=DIRECTION ( 'NONE',  ( -0.000000000000000000, -1.000000000000000000, -0.000000000000000000 ) ) ;
#22723=CARTESIAN_POINT ( 'NONE',  ( 27.40312500061451573, 4.541064518000418104, -2.621784821874998173 ) ) ;
#22724=CARTESIAN_POINT ( 'NONE',  ( -3.999999999999997335, 18.23750000000000071, 32.30940107675850470 ) ) ;
#22726=CARTESIAN_POINT ( 'NONE',  ( 3.328125000614516438, -4.541064518000419881, 2.621784821874995952 ) ) ;
#22727=CARTESIAN_POINT ( 'NONE',  ( 18.79687500061451644, -3.027376345333610441, -5.243569643749999898 ) ) ;
#22728=CARTESIAN_POINT ( 'NONE',  ( -2.121784821874996840, 14.53437500061451715, 33.67503911421598417 ) ) ;
#22729=CARTESIAN_POINT ( 'NONE',  ( 19.95937500061451786, 0.000000000000000000, 5.243569643749999010 ) ) ;
#22730=CARTESIAN_POINT ( 'NONE',  ( 29.33437500061451431, 4.541064518000418104, 2.621784821874999949 ) ) ;
#22731=CARTESIAN_POINT ( 'NONE',  ( -4.243569643749999898, 19.82187500061451857, 27.54997392385601529 ) ) ;
#22732=CARTESIAN_POINT ( 'NONE',  ( 10.64062500061451644, -3.027376345333610441, -5.243569643749999898 ) ) ;
#22733=CARTESIAN_POINT ( 'NONE',  ( 2.662500001229036073, 0.000000000000000000, 4.999999999999998224 ) ) ;
#22734=EDGE_CURVE ( 'NONE', #19796, #34387, #5515, .T. ) ;
#22736=CARTESIAN_POINT ( 'NONE',  ( 5.821875000614519458, 3.027376345333613106, -5.243569643749998122 ) ) ;
#22737=DIRECTION ( 'NONE',  ( -0.000000000000000000, -1.000000000000000000, -0.000000000000000000 ) ) ;
#22738=CARTESIAN_POINT ( 'NONE',  ( 7.753125000614518036, 0.000000000000000000, 5.243569643749999010 ) ) ;
#22739=CARTESIAN_POINT ( 'NONE',  ( 13.02187500061451608, 3.027376345333613106, -5.243569643749998122 ) ) ;
#22741=CARTESIAN_POINT ( 'NONE',  ( 17.96250000122903501, 0.000000000000000000, 4.999999999999998224 ) ) ;
#22742=CARTESIAN_POINT ( 'NONE',  ( 8.371875000614515727, -6.054752690667223547, -1.112240025338166033E-15 ) ) ;
#22743=CARTESIAN_POINT ( 'NONE',  ( 9.965625000614517504, 3.027376345333611329, 5.243569643749999010 ) ) ;
#22746=CARTESIAN_POINT ( 'NONE',  ( 19.73437500061451644, 6.421520780324663323E-16, -5.243569643749999010 ) ) ;
#22747=CARTESIAN_POINT ( 'NONE',  ( 9.075000001229033941, -5.773502691896255534, -1.060575238724906372E-15 ) ) ;
#22748=CARTESIAN_POINT ( 'NONE',  ( 26.31562500061451715, -6.054752690667223547, -1.112240025338166033E-15 ) ) ;
#22750=CARTESIAN_POINT ( 'NONE',  ( 13.00312500061451537, 4.541064518000418104, -2.621784821874998173 ) ) ;
#22751=CARTESIAN_POINT ( 'NONE',  ( 28.73437500061451644, 6.421520780324663323E-16, -5.243569643749999010 ) ) ;
#22753=CARTESIAN_POINT ( 'NONE',  ( 13.95000000122903572, -2.886751345948129988, 4.999999999999997335 ) ) ;
#22754=CARTESIAN_POINT ( 'NONE',  ( 28.15312500061451573, -4.541064518000417216, -2.621784821875001281 ) ) ;
#22755=CARTESIAN_POINT ( 'NONE',  ( 2.121784821875001281, 15.90312500061451573, -26.32496088578401938 ) ) ;
#22756=CARTESIAN_POINT ( 'NONE',  ( 16.01250000122903216, 4.330127018922192761, -2.499999999999997780 ) ) ;
#22757=CARTESIAN_POINT ( 'NONE',  ( 13.27500000000000213, 4.330127018922191873, 2.499999999999999556 ) ) ;
#22758=CARTESIAN_POINT ( 'NONE',  ( 23.39062500061451289, 6.054752690667223547, 3.707466751127219781E-16 ) ) ;
#22759=CARTESIAN_POINT ( 'NONE',  ( 8.821875000614518569, -6.054752690667223547, -1.112240025338166033E-15 ) ) ;
#22760=CARTESIAN_POINT ( 'NONE',  ( 7.725000001229034297, -5.773502691896255534, -1.060575238724906372E-15 ) ) ;
#22761=CARTESIAN_POINT ( 'NONE',  ( 16.76250000122903216, -4.330127018922190985, -2.500000000000001332 ) ) ;
#22762=CARTESIAN_POINT ( 'NONE',  ( 12.10312500061451857, 4.541064518000418104, -2.621784821874998173 ) ) ;
#22763=CARTESIAN_POINT ( 'NONE',  ( 15.59062500061451573, -3.027376345333610441, -5.243569643749999898 ) ) ;
#22764=( BOUNDED_CURVE ( )  B_SPLINE_CURVE ( 3, ( #1063, #41658, #63095, #23930 ),
 .UNSPECIFIED., .F., .F. ) 
 B_SPLINE_CURVE_WITH_KNOTS ( ( 4, 4 ),
 ( 0.000000000000000000, 1.570796326794896780 ),
 .UNSPECIFIED. ) 
 CURVE ( )  GEOMETRIC_REPRESENTATION_ITEM ( )  RATIONAL_B_SPLINE_CURVE ( ( 1.000000000000000000, 0.8047378541243649375, 0.8047378541243649375, 1.000000000000000000 ) ) 
 REPRESENTATION_ITEM ( '' )  );
#22765=CARTESIAN_POINT ( 'NONE',  ( 27.15000000122902790, -2.886751345948125991, -5.000000000000000000 ) ) ;
#22766=CARTESIAN_POINT ( 'NONE',  ( 21.71249999999999858, 2.886751345948129099, -4.999999999999998224 ) ) ;
#22767=CARTESIAN_POINT ( 'NONE',  ( 24.08437500061451786, -4.541064518000419881, 2.621784821874995952 ) ) ;
#22768=CARTESIAN_POINT ( 'NONE',  ( -5.810221930991193690E-16, 12.35000000122903430, 26.00000000000000355 ) ) ;
#22769=CARTESIAN_POINT ( 'NONE',  ( 10.12500000122903465, 2.886751345948129099, -4.999999999999998224 ) ) ;
#22770=CARTESIAN_POINT ( 'NONE',  ( 27.72187500061451715, -6.054752690667223547, -1.112240025338166033E-15 ) ) ;
#22771=CARTESIAN_POINT ( 'NONE',  ( 5.071875000614519458, 3.027376345333611329, 5.243569643749999010 ) ) ;
#22772=CARTESIAN_POINT ( 'NONE',  ( 23.24062500061451786, -3.027376345333610441, -5.243569643749999898 ) ) ;
#22773=( BOUNDED_CURVE ( )  B_SPLINE_CURVE ( 2, ( #34299, #57562, #46490, #12506, #68666, #68305, #69029 ),
 .UNSPECIFIED., .F., .F. ) 
 B_SPLINE_CURVE_WITH_KNOTS ( ( 3, 2, 2, 3 ),
 ( 0.8583333333333332815, 0.8611111111111111605, 0.8638888888888889284, 0.8666666666666666963 ),
 .UNSPECIFIED. ) 
 CURVE ( )  GEOMETRIC_REPRESENTATION_ITEM ( )  RATIONAL_B_SPLINE_CURVE ( ( 1.000000000000000000, 0.8660254037844387076, 1.000000000000000000, 0.8660254037844387076, 1.000000000000000000, 0.8660254037844387076, 1.000000000000000000 ) ) 
 REPRESENTATION_ITEM ( '' )  );
#22775=CARTESIAN_POINT ( 'NONE',  ( 6.937499999999999112, 5.773502691896255534, 3.535250795749688401E-16 ) ) ;
#22776=CARTESIAN_POINT ( 'NONE',  ( 9.646875000614516082, -3.027376345333614438, 5.243569643749998122 ) ) ;
#22778=CARTESIAN_POINT ( 'NONE',  ( 4.059375000614519280, 4.541064518000418104, -2.621784821874998173 ) ) ;
#22779=CARTESIAN_POINT ( 'NONE',  ( 6.046875000614519102, -3.027376345333614438, 5.243569643749998122 ) ) ;
#22780=DIRECTION ( 'NONE',  ( -0.000000000000000000, -1.000000000000000000, -0.000000000000000000 ) ) ;
#22781=CARTESIAN_POINT ( 'NONE',  ( 26.10937500061451644, 4.541064518000418104, -2.621784821874998173 ) ) ;
#22782=CARTESIAN_POINT ( 'NONE',  ( 4.243569643749999898, 10.57812500061459637, 30.00000000000000000 ) ) ;
#22783=CARTESIAN_POINT ( 'NONE',  ( 20.13749999999999929, -2.886751345948129988, 4.999999999999997335 ) ) ;
#22784=VERTEX_POINT ( 'NONE', #41767 ) ;
#22785=CARTESIAN_POINT ( 'NONE',  ( 27.89999999999999858, -4.330127018922190985, -2.500000000000001332 ) ) ;
#22786=CARTESIAN_POINT ( 'NONE',  ( 28.62187500061451573, -6.054752690667223547, -1.112240025338166033E-15 ) ) ;
#22787=VERTEX_POINT ( 'NONE', #21416 ) ;
#22788=CARTESIAN_POINT ( 'NONE',  ( 15.85312500061451857, 0.000000000000000000, 5.243569643749999010 ) ) ;
#22789=CARTESIAN_POINT ( 'NONE',  ( 7.415625000614516793, -6.054752690667223547, -1.112240025338166033E-15 ) ) ;
#22791=CARTESIAN_POINT ( 'NONE',  ( 5.559375000614517504, 0.000000000000000000, 5.243569643749999010 ) ) ;
#22792=CARTESIAN_POINT ( 'NONE',  ( 18.71250000122903145, 4.330127018922192761, -2.499999999999997780 ) ) ;
#22793=CARTESIAN_POINT ( 'NONE',  ( 23.06250000000000355, 2.886751345948129099, -4.999999999999998224 ) ) ;
#22794=CARTESIAN_POINT ( 'NONE',  ( -5.810221930991193690E-16, 14.03750000000000142, -34.00000000000000000 ) ) ;
#22795=CARTESIAN_POINT ( 'NONE',  ( 6.309375000614517504, 4.541064518000418104, -2.621784821874998173 ) ) ;
#22796=CARTESIAN_POINT ( 'NONE',  ( 11.82187500061451679, 3.027376345333611329, 5.243569643749999010 ) ) ;
#22797=CARTESIAN_POINT ( 'NONE',  ( 21.45937500061451786, -4.541064518000417216, -2.621784821875001281 ) ) ;
#22799=CARTESIAN_POINT ( 'NONE',  ( 1.592000809091587073E-14, 16.28750000000000142, 26.00000000000000000 ) ) ;
#22801=CARTESIAN_POINT ( 'NONE',  ( 5.034375000614519813, 4.541064518000418104, 2.621784821874999949 ) ) ;
#22802=CARTESIAN_POINT ( 'NONE',  ( 6.496875000614517504, -3.027376345333614438, 5.243569643749998122 ) ) ;
#22803=CARTESIAN_POINT ( 'NONE',  ( 19.53749999999999432, 5.773502691896255534, 3.535250795749688894E-16 ) ) ;
#22804=CARTESIAN_POINT ( 'NONE',  ( 15.36562500061451608, 3.027376345333611329, 5.243569643749999010 ) ) ;
#22808=CARTESIAN_POINT ( 'NONE',  ( 10.71562500061451928, 3.027376345333613106, -5.243569643749998122 ) ) ;
#22809=CARTESIAN_POINT ( 'NONE',  ( 26.33437500061451431, -4.541064518000419881, 2.621784821874995952 ) ) ;
#22811=CARTESIAN_POINT ( 'NONE',  ( 27.83437500061451786, 6.421520780324663323E-16, -5.243569643749999010 ) ) ;
#22812=CARTESIAN_POINT ( 'NONE',  ( 10.53750000000000320, 5.773502691896255534, 3.535250795749688894E-16 ) ) ;
#22813=CARTESIAN_POINT ( 'NONE',  ( -3.999999999999999112, 15.16250000122903252, 30.00000000000000000 ) ) ;
#22814=CARTESIAN_POINT ( 'NONE',  ( 8.437500001229034652, 4.330127018922191873, 2.499999999999999556 ) ) ;
#22815=CARTESIAN_POINT ( 'NONE',  ( 20.22187500061451715, 3.027376345333613106, -5.243569643749998122 ) ) ;
#22816=CARTESIAN_POINT ( 'NONE',  ( 13.54687500061451999, 6.054752690667223547, 3.707466751127219781E-16 ) ) ;
#22817=CARTESIAN_POINT ( 'NONE',  ( 5.857864376269048101, 9.999999999999992895, 5.857864376269048101 ) ) ;
#22819=CARTESIAN_POINT ( 'NONE',  ( 13.86562500061451431, 3.027376345333613106, -5.243569643749998122 ) ) ;
#22820=CARTESIAN_POINT ( 'NONE',  ( 27.37500000122903288, 2.886751345948126879, 4.999999999999999112 ) ) ;
#22821=CARTESIAN_POINT ( 'NONE',  ( 14.85937500061451644, 4.541064518000418104, -2.621784821874998173 ) ) ;
#22822=CARTESIAN_POINT ( 'NONE',  ( 3.103125000614517237, 4.541064518000418104, -2.621784821874998173 ) ) ;
#22823=CARTESIAN_POINT ( 'NONE',  ( 17.39062500061451644, -3.027376345333610441, -5.243569643749999898 ) ) ;
#22824=CYLINDRICAL_SURFACE ( 'NONE', #22085, 4.000000000000000000 ) ;
#22825=CARTESIAN_POINT ( 'NONE',  ( 25.73437500061451644, 4.541064518000418104, 2.621784821874999949 ) ) ;
#22826=CARTESIAN_POINT ( 'NONE',  ( -2.121784821874999949, 10.72812500061451679, 26.32496088578401938 ) ) ;
#22827=CARTESIAN_POINT ( 'NONE',  ( 15.60937500061451644, -4.541064518000417216, -2.621784821875001281 ) ) ;
#22828=CARTESIAN_POINT ( 'NONE',  ( 14.47500000122903430, -5.773502691896255534, -1.060575238724906372E-15 ) ) ;
#22829=CYLINDRICAL_SURFACE ( 'NONE', #20963, 4.999999999999998224 ) ;
#22830=CARTESIAN_POINT ( 'NONE',  ( -2.121784821874999949, 16.63437500061451857, -33.67503911421598417 ) ) ;
#22831=CARTESIAN_POINT ( 'NONE',  ( 19.28437500061451360, 6.421520780324663323E-16, -5.243569643749999010 ) ) ;
#22832=CARTESIAN_POINT ( 'NONE',  ( 20.21250000122903145, 0.000000000000000000, 4.999999999999998224 ) ) ;
#22833=CARTESIAN_POINT ( 'NONE',  ( 15.83437500061451608, 4.541064518000418104, 2.621784821874999949 ) ) ;
#22834=CARTESIAN_POINT ( 'NONE',  ( -4.243569643749997233, 11.34687500061451892, 32.45002607614398471 ) ) ;
#22835=CARTESIAN_POINT ( 'NONE',  ( 23.25000000122903288, 5.773502691896255534, 3.535250795749688894E-16 ) ) ;
#22836=CARTESIAN_POINT ( 'NONE',  ( 14.54062500061451679, -3.027376345333614438, 5.243569643749998122 ) ) ;
#22837=CARTESIAN_POINT ( 'NONE',  ( 29.50312500061451360, -4.541064518000417216, -2.621784821875001281 ) ) ;
#22838=VERTEX_POINT ( 'NONE', #43973 ) ;
#22840=CARTESIAN_POINT ( 'NONE',  ( 21.37499999999999645, 4.330127018922191873, 2.499999999999999556 ) ) ;
#22841=CARTESIAN_POINT ( 'NONE',  ( -1.999999999999997113, 17.93750000122903288, 33.46410161513775705 ) ) ;
#22842=CARTESIAN_POINT ( 'NONE',  ( 3.861486210907942418, 3.177525289277529197, 31.07754487038764424 ) ) ;
#22843=CARTESIAN_POINT ( 'NONE',  ( 14.58750000122903323, 6.123233995736764310E-16, -4.999999999999998224 ) ) ;
#22844=CARTESIAN_POINT ( 'NONE',  ( 19.49062500061451431, -3.027376345333614438, 5.243569643749998122 ) ) ;
#22845=CARTESIAN_POINT ( 'NONE',  ( 22.82812500061451644, 6.421520780324663323E-16, -5.243569643749999010 ) ) ;
#22846=CARTESIAN_POINT ( 'NONE',  ( 6.628125000614517148, 6.421520780324663323E-16, -5.243569643749999010 ) ) ;
#22847=CARTESIAN_POINT ( 'NONE',  ( 29.02499999999999858, 4.330127018922191873, 2.499999999999999556 ) ) ;
#22849=CARTESIAN_POINT ( 'NONE',  ( 29.78437500061451715, 4.541064518000418104, 2.621784821874999949 ) ) ;
#22850=CARTESIAN_POINT ( 'NONE',  ( -2.000000000000000000, 12.38750000122903394, -33.46410161513775705 ) ) ;
#22851=CARTESIAN_POINT ( 'NONE',  ( -4.243569643749997233, 17.64687500061452141, -27.54997392385601174 ) ) ;
#22852=CARTESIAN_POINT ( 'NONE',  ( 7.012500001229035718, 4.330127018922192761, -2.499999999999997780 ) ) ;
#22853=CARTESIAN_POINT ( 'NONE',  ( 7.837499999999999467, 5.773502691896255534, 3.535250795749688894E-16 ) ) ;
#22855=CARTESIAN_POINT ( 'NONE',  ( 3.450000001229036162, 5.773502691896255534, 3.535250795749688894E-16 ) ) ;
#22856=CARTESIAN_POINT ( 'NONE',  ( 11.29687500061451644, 6.054752690667223547, 3.707466751127219781E-16 ) ) ;
#22857=CARTESIAN_POINT ( 'NONE',  ( 12.44999999999999929, 0.000000000000000000, 4.999999999999998224 ) ) ;
#22858=CARTESIAN_POINT ( 'NONE',  ( 4.096875000614518925, 6.054752690667223547, 3.707466751127219781E-16 ) ) ;
#22859=CARTESIAN_POINT ( 'NONE',  ( 12.82500000122903394, 2.886751345948129099, -4.999999999999997335 ) ) ;
#22860=CARTESIAN_POINT ( 'NONE',  ( 1.071796769724490783, 19.34509619066136565, 34.00000000000000000 ) ) ;
#22861=CARTESIAN_POINT ( 'NONE',  ( 9.946875000614516793, 6.054752690667223547, 3.707466751127219781E-16 ) ) ;
#22862=CARTESIAN_POINT ( 'NONE',  ( 14.22187500061451537, -6.054752690667223547, -1.112240025338166033E-15 ) ) ;
#22863=CARTESIAN_POINT ( 'NONE',  ( 4.517629703274214314, -3.565318894049279930, 3.824686530321367517 ) ) ;
#22864=CARTESIAN_POINT ( 'NONE',  ( 2.121784821875001281, 16.80312500061459247, 33.67503911421598417 ) ) ;
#22865=CARTESIAN_POINT ( 'NONE',  ( 21.04687500061451644, -3.027376345333610441, -5.243569643749999898 ) ) ;
#22866=CARTESIAN_POINT ( 'NONE',  ( 26.36250000122903003, 4.330127018922192761, -2.499999999999997780 ) ) ;
#22868=CARTESIAN_POINT ( 'NONE',  ( 23.54062500061451146, -3.027376345333614438, 5.243569643749998122 ) ) ;
#22869=CARTESIAN_POINT ( 'NONE',  ( 16.41562500061451857, -6.054752690667223547, -1.112240025338166033E-15 ) ) ;
#22871=CARTESIAN_POINT ( 'NONE',  ( 13.02187500061451608, 3.027376345333613106, -5.243569643749998122 ) ) ;
#22872=CARTESIAN_POINT ( 'NONE',  ( 28.31250000000000000, -5.773502691896255534, -1.060575238724906372E-15 ) ) ;
#22873=CARTESIAN_POINT ( 'NONE',  ( 25.38750000122903216, 6.123233995736764310E-16, -4.999999999999998224 ) ) ;
#22874=VECTOR ( 'NONE', #13580, 1000.000000000000227 ) ;
#22875=CARTESIAN_POINT ( 'NONE',  ( 4.134375000614517681, 4.541064518000418104, 2.621784821874999949 ) ) ;
#22876=CARTESIAN_POINT ( 'NONE',  ( 13.99687500061451928, 6.054752690667223547, 3.707466751127219781E-16 ) ) ;
#22877=CARTESIAN_POINT ( 'NONE',  ( 29.33437500061451431, 4.541064518000418104, 2.621784821874999949 ) ) ;
#22880=CARTESIAN_POINT ( 'NONE',  ( 23.48437500061451644, 4.541064518000418104, 2.621784821874999949 ) ) ;
#22881=CARTESIAN_POINT ( 'NONE',  ( 13.65937500061451715, 0.000000000000000000, 5.243569643749999010 ) ) ;
#22883=CARTESIAN_POINT ( 'NONE',  ( 25.57499999999999929, -4.330127018922194537, 2.499999999999995559 ) ) ;
#22884=CARTESIAN_POINT ( 'NONE',  ( 3.750000001229034652, -2.886751345948125991, -5.000000000000000000 ) ) ;
#22886=CARTESIAN_POINT ( 'NONE',  ( 16.22812500061451857, 4.541064518000418104, 2.621784821874999949 ) ) ;
#22887=CARTESIAN_POINT ( 'NONE',  ( 7.762500000000001954, 2.886751345948129099, -4.999999999999998224 ) ) ;
#22888=CARTESIAN_POINT ( 'NONE',  ( 13.50000000122903288, -2.886751345948130876, 4.999999999999996447 ) ) ;
#22889=CARTESIAN_POINT ( 'NONE',  ( 16.72500000000000142, 6.123233995736764310E-16, -4.999999999999998224 ) ) ;
#22890=CARTESIAN_POINT ( 'NONE',  ( -2.121784821874999949, 13.87812500061451715, 26.32496088578401938 ) ) ;
#22892=CARTESIAN_POINT ( 'NONE',  ( 21.67500000122903359, -5.773502691896255534, -1.060575238724906372E-15 ) ) ;
#22893=CARTESIAN_POINT ( 'NONE',  ( 2.695452854360187445, 9.631537354464013490, 24.63599347216290170 ) ) ;
#22894=CARTESIAN_POINT ( 'NONE',  ( 26.14687500061451431, 6.054752690667223547, 3.707466751127219781E-16 ) ) ;
#22896=CARTESIAN_POINT ( 'NONE',  ( 21.21562500061451573, 3.027376345333611329, 5.243569643749999010 ) ) ;
#22897=CARTESIAN_POINT ( 'NONE',  ( 21.30937500061451573, 0.000000000000000000, 5.243569643749999010 ) ) ;
#22898=CARTESIAN_POINT ( 'NONE',  ( 7.124999999999999112, -4.330127018922194537, 2.499999999999995559 ) ) ;
#22899=CARTESIAN_POINT ( 'NONE',  ( 10.26562500061451644, 3.027376345333613106, -5.243569643749998122 ) ) ;
#22900=CARTESIAN_POINT ( 'NONE',  ( 23.35312500061451857, 4.541064518000418104, -2.621784821874998173 ) ) ;
#22901=CARTESIAN_POINT ( 'NONE',  ( 12.04687500061451821, -3.027376345333610441, -5.243569643749999898 ) ) ;
#22902=CARTESIAN_POINT ( 'NONE',  ( 17.14687500061451786, 6.054752690667223547, 3.707466751127219781E-16 ) ) ;
#22903=CARTESIAN_POINT ( 'NONE',  ( 4.465851277537014496, 2.248593419656078840, -4.736966354317482697 ) ) ;
#22904=CARTESIAN_POINT ( 'NONE',  ( 9.001249775931846008E-16, 17.66562500061451502, 34.90005215228797653 ) ) ;
#22905=ADVANCED_FACE ( 'NONE', ( #48419 ), #38047, .F. ) ;
#22906=CARTESIAN_POINT ( 'NONE',  ( 21.48750000122903003, 4.330127018922191873, 2.499999999999999556 ) ) ;
#22908=CARTESIAN_POINT ( 'NONE',  ( 11.05312500061451608, -4.541064518000417216, -2.621784821875001281 ) ) ;
#22909=CARTESIAN_POINT ( 'NONE',  ( 4.921875000614518214, 3.027376345333613106, -5.243569643749998122 ) ) ;
#22910=CARTESIAN_POINT ( 'NONE',  ( 3.984375000614517326, 6.421520780324663323E-16, -5.243569643749999010 ) ) ;
#22911=( BOUNDED_CURVE ( )  B_SPLINE_CURVE ( 2, ( #11021, #33187, #33542, #56093, #50551, #5484, #73079 ),
 .UNSPECIFIED., .F., .F. ) 
 B_SPLINE_CURVE_WITH_KNOTS ( ( 3, 2, 2, 3 ),
 ( 0.7500000000000000000, 0.7527777777777777679, 0.7555555555555555358, 0.7583333333333333037 ),
 .UNSPECIFIED. ) 
 CURVE ( )  GEOMETRIC_REPRESENTATION_ITEM ( )  RATIONAL_B_SPLINE_CURVE ( ( 1.000000000000000000, 0.8660254037844387076, 1.000000000000000000, 0.8660254037844387076, 1.000000000000000000, 0.8660254037844387076, 1.000000000000000000 ) ) 
 REPRESENTATION_ITEM ( '' )  );
#22913=CARTESIAN_POINT ( 'NONE',  ( 26.55937500061451573, 4.541064518000418104, -2.621784821874998173 ) ) ;
#22914=CARTESIAN_POINT ( 'NONE',  ( 16.11562500061451786, 3.027376345333613106, -5.243569643749998122 ) ) ;
#22915=CARTESIAN_POINT ( 'NONE',  ( 26.88750000122903216, 4.330127018922191873, 2.499999999999999556 ) ) ;
#22916=CARTESIAN_POINT ( 'NONE',  ( 27.96562500061451928, 3.027376345333611329, 5.243569643749999010 ) ) ;
#22917=CARTESIAN_POINT ( 'NONE',  ( 21.87187500061451573, -6.054752690667223547, -1.112240025338166033E-15 ) ) ;
#22918=CARTESIAN_POINT ( 'NONE',  ( 16.60312500061451857, 4.541064518000418104, -2.621784821874998173 ) ) ;
#22919=CARTESIAN_POINT ( 'NONE',  ( 2.121784821875001281, 19.55937500061451573, 33.67503911421598417 ) ) ;
#22920=CARTESIAN_POINT ( 'NONE',  ( 21.74062500061451431, -3.027376345333614438, 5.243569643749998122 ) ) ;
#22921=CARTESIAN_POINT ( 'NONE',  ( 4.387500001229033053, 4.330127018922191873, 2.499999999999999556 ) ) ;
#22922=ORIENTED_EDGE ( 'NONE', *, *, #26612, .F. ) ;
#22923=CARTESIAN_POINT ( 'NONE',  ( 28.42499999999999716, 6.123233995736764310E-16, -4.999999999999998224 ) ) ;
#22924=CARTESIAN_POINT ( 'NONE',  ( -1.999999999999997113, 13.32499999999999929, -26.53589838486224295 ) ) ;
#22926=CARTESIAN_POINT ( 'NONE',  ( 28.52812500061451573, -4.541064518000419881, 2.621784821874995952 ) ) ;
#22927=CARTESIAN_POINT ( 'NONE',  ( 10.90312500061451928, 0.000000000000000000, 5.243569643749999010 ) ) ;
#22928=CARTESIAN_POINT ( 'NONE',  ( 23.28750000122903430, 4.330127018922191873, 2.499999999999999556 ) ) ;
#22929=CARTESIAN_POINT ( 'NONE',  ( 12.64687500061451786, 6.054752690667223547, 3.707466751127219781E-16 ) ) ;
#22930=CARTESIAN_POINT ( 'NONE',  ( 27.06562500061451004, 3.027376345333611329, 5.243569643749999010 ) ) ;
#22931=CARTESIAN_POINT ( 'NONE',  ( 27.03750000000000142, -2.886751345948125991, -5.000000000000000000 ) ) ;
#22932=CARTESIAN_POINT ( 'NONE',  ( 3.999999999999999112, 18.53750000122903430, -30.00000000000000000 ) ) ;
#22933=CARTESIAN_POINT ( 'NONE',  ( 2.803125000614518747, 0.000000000000000000, 5.243569643749999010 ) ) ;
#22934=CARTESIAN_POINT ( 'NONE',  ( 11.99062500061451608, -3.027376345333610441, -5.243569643749999898 ) ) ;
#22936=CARTESIAN_POINT ( 'NONE',  ( 11.20312500061451644, 4.541064518000418104, -2.621784821874998173 ) ) ;
#22937=AXIS2_PLACEMENT_3D ( 'NONE', #34491, #58098, #23404 ) ;
#22938=CARTESIAN_POINT ( 'NONE',  ( 5.165625000614518569, -6.054752690667223547, -1.112240025338166033E-15 ) ) ;
#22940=LINE ( 'NONE', #34754, #13759 ) ;
#22941=CARTESIAN_POINT ( 'NONE',  ( 15.63749999999999751, -2.886751345948129988, 4.999999999999997335 ) ) ;
#22943=CARTESIAN_POINT ( 'NONE',  ( 15.94687500061451502, -3.027376345333614438, 5.243569643749998122 ) ) ;
#22944=CARTESIAN_POINT ( 'NONE',  ( 10.95000000122903394, -2.886751345948125991, -5.000000000000000000 ) ) ;
#22945=CARTESIAN_POINT ( 'NONE',  ( 20.44687500061451857, -3.027376345333614438, 5.243569643749998122 ) ) ;
#22947=CARTESIAN_POINT ( 'NONE',  ( 21.90937500061451715, -4.541064518000417216, -2.621784821875001281 ) ) ;
#22948=CARTESIAN_POINT ( 'NONE',  ( -2.121784821874999949, 15.22812500061451679, -33.67503911421598417 ) ) ;
#22950=CARTESIAN_POINT ( 'NONE',  ( 1.592000809091587073E-14, 16.73750000000000071, 26.00000000000000000 ) ) ;
#22952=CARTESIAN_POINT ( 'NONE',  ( 26.91562500061451146, 3.027376345333613106, -5.243569643749998122 ) ) ;
#22953=CARTESIAN_POINT ( 'NONE',  ( 28.99687500061451573, -3.027376345333614438, 5.243569643749998122 ) ) ;
#22954=ADVANCED_FACE ( 'NONE', ( #42871 ), #66127, .F. ) ;
#22956=CARTESIAN_POINT ( 'NONE',  ( 25.12499999999999645, -4.330127018922194537, 2.499999999999995559 ) ) ;
#22957=CARTESIAN_POINT ( 'NONE',  ( 8.090625000614515727, 6.054752690667223547, 3.707466751127219781E-16 ) ) ;
#22959=CARTESIAN_POINT ( 'NONE',  ( 20.22187500061451715, 3.027376345333613106, -5.243569643749998122 ) ) ;
#22961=CARTESIAN_POINT ( 'NONE',  ( 5.953125000614519102, 0.000000000000000000, 5.243569643749999010 ) ) ;
#22962=CARTESIAN_POINT ( 'NONE',  ( 10.05937500061451750, 0.000000000000000000, 5.243569643749999010 ) ) ;
#22963=VERTEX_POINT ( 'NONE', #20685 ) ;
#22964=CARTESIAN_POINT ( 'NONE',  ( 21.87187500061451573, -6.054752690667223547, -1.112240025338166033E-15 ) ) ;
#22966=CARTESIAN_POINT ( 'NONE',  ( 29.02499999999999858, 4.330127018922191873, 2.499999999999999556 ) ) ;
#22967=CARTESIAN_POINT ( 'NONE',  ( 29.85937500061451644, 0.000000000000000000, 5.243569643749999010 ) ) ;
#22968=CARTESIAN_POINT ( 'NONE',  ( 15.60000000122903607, 5.773502691896255534, 3.535250795749688894E-16 ) ) ;
#22969=DIRECTION ( 'NONE',  ( -1.000000000000000000, -0.000000000000000000, -0.000000000000000000 ) ) ;
#22970=CARTESIAN_POINT ( 'NONE',  ( 17.17500000000000071, 6.123233995736764310E-16, -4.999999999999998224 ) ) ;
#22971=VERTEX_POINT ( 'NONE', #15875 ) ;
#22972=CARTESIAN_POINT ( 'NONE',  ( 13.08750000000000036, -2.886751345948125991, -5.000000000000000000 ) ) ;
#22974=CARTESIAN_POINT ( 'NONE',  ( 23.39062500061451289, 6.054752690667223547, 3.707466751127219781E-16 ) ) ;
#22975=CARTESIAN_POINT ( 'NONE',  ( 14.96250000000000036, 2.886751345948129099, -4.999999999999998224 ) ) ;
#22976=CARTESIAN_POINT ( 'NONE',  ( 11.13750000122903216, 4.330127018922191873, 2.499999999999999556 ) ) ;
#22977=CARTESIAN_POINT ( 'NONE',  ( 9.815625000614518925, 3.027376345333613106, -5.243569643749998122 ) ) ;
#22978=CARTESIAN_POINT ( 'NONE',  ( 8.287499999999999645, 5.773502691896255534, 3.535250795749688894E-16 ) ) ;
#22980=CARTESIAN_POINT ( 'NONE',  ( 28.50000000122903288, -2.886751345948125991, -5.000000000000000000 ) ) ;
#22982=CARTESIAN_POINT ( 'NONE',  ( 7.012500000000001066, 2.886751345948126879, 4.999999999999999112 ) ) ;
#22984=AXIS2_PLACEMENT_3D ( 'NONE', #56718, #68904, #62273 ) ;
#22986=CARTESIAN_POINT ( 'NONE',  ( 22.75312500061451360, -4.541064518000417216, -2.621784821875001281 ) ) ;
#22987=CARTESIAN_POINT ( 'NONE',  ( 29.09062500061451573, -3.027376345333610441, -5.243569643749999898 ) ) ;
#22988=CARTESIAN_POINT ( 'NONE',  ( 29.59687500061451715, -3.027376345333610441, -5.243569643749999898 ) ) ;
#22989=CARTESIAN_POINT ( 'NONE',  ( 18.98437500061451644, 4.541064518000418104, 2.621784821874999949 ) ) ;
#22990=CARTESIAN_POINT ( 'NONE',  ( 16.67812500061451786, 4.541064518000418104, 2.621784821874999949 ) ) ;
#22991=CARTESIAN_POINT ( 'NONE',  ( 2.121784821874999061, 11.10312500061459318, -33.67503911421598417 ) ) ;
#22992=CARTESIAN_POINT ( 'NONE',  ( 5.765625000614519102, 3.027376345333613106, -5.243569643749998122 ) ) ;
#22994=CARTESIAN_POINT ( 'NONE',  ( 2.878125000614517592, -4.541064518000419881, 2.621784821874995952 ) ) ;
#22996=CARTESIAN_POINT ( 'NONE',  ( 19.00312500061451715, 0.000000000000000000, 5.243569643749999010 ) ) ;
#22997=CARTESIAN_POINT ( 'NONE',  ( 4.898587196589411843E-16, 20.00000000000000000, -26.00000000000000000 ) ) ;
#22998=CARTESIAN_POINT ( 'NONE',  ( 4.387500001229033053, 4.330127018922191873, 2.499999999999999556 ) ) ;
#22999=CARTESIAN_POINT ( 'NONE',  ( 12.68437500061451573, 4.541064518000418104, 2.621784821874999949 ) ) ;
#23000=CARTESIAN_POINT ( 'NONE',  ( 11.52187500061451608, -6.054752690667223547, -1.112240025338166033E-15 ) ) ;
#23001=CARTESIAN_POINT ( 'NONE',  ( 19.39687500061451786, 6.054752690667223547, 3.707466751127219781E-16 ) ) ;
#23002=ORIENTED_EDGE ( 'NONE', *, *, #72525, .F. ) ;
#23003=CARTESIAN_POINT ( 'NONE',  ( -4.513148444473918275, 8.924709038934331318, 26.04167052991142839 ) ) ;
#23004=CARTESIAN_POINT ( 'NONE',  ( 24.02812500061451573, -4.541064518000419881, 2.621784821874995952 ) ) ;
#23006=CARTESIAN_POINT ( 'NONE',  ( 17.97187500061451715, 3.027376345333613106, -5.243569643749998122 ) ) ;
#23007=CARTESIAN_POINT ( 'NONE',  ( 24.85312500061451502, 0.000000000000000000, 5.243569643749999010 ) ) ;
#23008=CARTESIAN_POINT ( 'NONE',  ( 3.999999999999998668, 12.16250000000000320, -32.30940107675850470 ) ) ;
#23009=CARTESIAN_POINT ( 'NONE',  ( 3.999999999999998668, 17.56250000000000000, 27.69059892324149175 ) ) ;
#23010=CARTESIAN_POINT ( 'NONE',  ( 5.484375000614518214, 4.541064518000418104, 2.621784821874999949 ) ) ;
#23011=CARTESIAN_POINT ( 'NONE',  ( 11.13750000122903216, 4.330127018922191873, 2.499999999999999556 ) ) ;
#23013=CARTESIAN_POINT ( 'NONE',  ( 7.387500001229032165, 6.123233995736764310E-16, -4.999999999999998224 ) ) ;
#23014=CARTESIAN_POINT ( 'NONE',  ( 8.484601909799253346E-16, 19.66249999999999787, -25.38119784648299770 ) ) ;
#23015=CARTESIAN_POINT ( 'NONE',  ( 27.18750000122903288, 6.123233995736764310E-16, -4.999999999999998224 ) ) ;
#23018=CARTESIAN_POINT ( 'NONE',  ( 10.43437500061451750, 4.541064518000418104, 2.621784821874999949 ) ) ;
#23020=EDGE_CURVE ( 'NONE', #66787, #35925, #13035, .T. ) ;
#23021=CARTESIAN_POINT ( 'NONE',  ( 16.34062500061451573, -3.027376345333614438, 5.243569643749998122 ) ) ;
#23022=CARTESIAN_POINT ( 'NONE',  ( 12.53437500061451537, 6.421520780324663323E-16, -5.243569643749999010 ) ) ;
#23023=CARTESIAN_POINT ( 'NONE',  ( 28.95000000122903572, -2.886751345948125991, -5.000000000000000000 ) ) ;
#23024=CARTESIAN_POINT ( 'NONE',  ( 20.78437500061451715, 4.541064518000418104, 2.621784821874999949 ) ) ;
#23025=CARTESIAN_POINT ( 'NONE',  ( 10.62187500061451928, -6.054752690667223547, -1.112240025338166033E-15 ) ) ;
#23026=CARTESIAN_POINT ( 'NONE',  ( 3.069550706496567027, -3.946908300287443883, -3.323927455962977895 ) ) ;
#23027=CARTESIAN_POINT ( 'NONE',  ( 11.88750000122903216, 6.123233995736764310E-16, -4.999999999999998224 ) ) ;
#23028=CARTESIAN_POINT ( 'NONE',  ( 6.450000001229034829, -2.886751345948125991, -5.000000000000000000 ) ) ;
#23029=CARTESIAN_POINT ( 'NONE',  ( 20.72812500061451502, 4.541064518000418104, 2.621784821874999949 ) ) ;
#23031=CARTESIAN_POINT ( 'NONE',  ( 5.175000001229033586, 2.886751345948129099, -4.999999999999998224 ) ) ;
#23032=CARTESIAN_POINT ( 'NONE',  ( 16.75312500061451715, 0.000000000000000000, 5.243569643749999010 ) ) ;
#23033=CARTESIAN_POINT ( 'NONE',  ( 13.82812500061451466, 6.421520780324663323E-16, -5.243569643749999010 ) ) ;
#23035=CARTESIAN_POINT ( 'NONE',  ( 14.02499999999999858, 6.123233995736764310E-16, -4.999999999999998224 ) ) ;
#23036=CARTESIAN_POINT ( 'NONE',  ( 9.525000001229033231, -5.773502691896255534, -1.060575238724906372E-15 ) ) ;
#23037=CARTESIAN_POINT ( 'NONE',  ( 6.778125000614518392, 4.541064518000418104, 2.621784821874999949 ) ) ;
#23038=CARTESIAN_POINT ( 'NONE',  ( 19.31250000122903288, 0.000000000000000000, 4.999999999999998224 ) ) ;
#23041=CARTESIAN_POINT ( 'NONE',  ( 9.001249775931846008E-16, 12.32187500061451857, -25.09994784771203058 ) ) ;
#23044=CARTESIAN_POINT ( 'NONE',  ( 18.60937500061451644, 0.000000000000000000, 5.243569643749999010 ) ) ;
#23048=CARTESIAN_POINT ( 'NONE',  ( 16.94062500061451715, -3.027376345333610441, -5.243569643749999898 ) ) ;
#23051=CARTESIAN_POINT ( 'NONE',  ( 29.44687500061451857, -3.027376345333614438, 5.243569643749998122 ) ) ;
#23052=CARTESIAN_POINT ( 'NONE',  ( 27.23437500061451644, -4.541064518000419881, 2.621784821874995952 ) ) ;
#23054=CARTESIAN_POINT ( 'NONE',  ( 12.96562500061451750, 3.027376345333613106, -5.243569643749998122 ) ) ;
#23056=CARTESIAN_POINT ( 'NONE',  ( 10.58437500061451964, -4.541064518000419881, 2.621784821874995952 ) ) ;
#23057=ORIENTED_EDGE ( 'NONE', *, *, #3230, .F. ) ;
#23058=FACE_OUTER_BOUND ( 'NONE', #34611, .T. ) ;
#23059=CARTESIAN_POINT ( 'NONE',  ( 20.35312500061451502, 0.000000000000000000, 5.243569643749999010 ) ) ;
#23061=CARTESIAN_POINT ( 'NONE',  ( 20.88749999999999929, 5.773502691896255534, 3.535250795749688401E-16 ) ) ;
#23062=CARTESIAN_POINT ( 'NONE',  ( 10.53750000000000320, 5.773502691896255534, 3.535250795749688894E-16 ) ) ;
#23063=CARTESIAN_POINT ( 'NONE',  ( 22.61250000122903003, -4.330127018922190985, -2.500000000000001332 ) ) ;
#23064=CARTESIAN_POINT ( 'NONE',  ( 15.62812500061451537, 6.421520780324663323E-16, -5.243569643749999010 ) ) ;
#23067=CARTESIAN_POINT ( 'NONE',  ( 19.53749999999999432, 5.773502691896255534, 3.535250795749688894E-16 ) ) ;
#23068=CARTESIAN_POINT ( 'NONE',  ( 21.60000000000000142, -4.330127018922190985, -2.500000000000001332 ) ) ;
#23069=CARTESIAN_POINT ( 'NONE',  ( 20.33437500061451786, 4.541064518000418104, 2.621784821874999949 ) ) ;
#23070=CARTESIAN_POINT ( 'NONE',  ( 24.66562500061451502, 3.027376345333613106, -5.243569643749998122 ) ) ;
#23073=CARTESIAN_POINT ( 'NONE',  ( 8.203125000614518214, 0.000000000000000000, 5.243569643749999010 ) ) ;
#23074=CARTESIAN_POINT ( 'NONE',  ( 14.17500000000000071, 4.330127018922191873, 2.499999999999999556 ) ) ;
#23075=CARTESIAN_POINT ( 'NONE',  ( 9.001249775931846008E-16, 17.21562500061451928, 34.90005215228797653 ) ) ;
#23076=CARTESIAN_POINT ( 'NONE',  ( 29.57812500061451644, 6.421520780324663323E-16, -5.243569643749999010 ) ) ;
#23077=CARTESIAN_POINT ( 'NONE',  ( 26.33437500061451431, -4.541064518000419881, 2.621784821874995952 ) ) ;
#23079=CARTESIAN_POINT ( 'NONE',  ( 25.07812500061451644, 6.421520780324663323E-16, -5.243569643749999010 ) ) ;
#23080=CARTESIAN_POINT ( 'NONE',  ( 24.19687500061451857, -3.027376345333610441, -5.243569643749999898 ) ) ;
#23081=CARTESIAN_POINT ( 'NONE',  ( 4.243569643749999898, 19.09062500061459389, -27.54997392385601529 ) ) ;
#23082=CARTESIAN_POINT ( 'NONE',  ( 11.66249999999999964, -5.773502691896255534, -1.060575238724906372E-15 ) ) ;
#23083=CARTESIAN_POINT ( 'NONE',  ( 8.990625000614516082, 6.054752690667223547, 3.707466751127219781E-16 ) ) ;
#23085=CARTESIAN_POINT ( 'NONE',  ( 28.90312500061451217, 0.000000000000000000, 5.243569643749999010 ) ) ;
#23086=CARTESIAN_POINT ( 'NONE',  ( 26.91562500061451502, 3.027376345333612662, -5.243569643749998122 ) ) ;
#23087=CARTESIAN_POINT ( 'NONE',  ( 12.56250000122903465, 0.000000000000000000, 4.999999999999998224 ) ) ;
#23089=CARTESIAN_POINT ( 'NONE',  ( 19.54687500061451644, -3.027376345333614438, 5.243569643749998122 ) ) ;
#23090=CARTESIAN_POINT ( 'NONE',  ( 2.121784821875001281, 14.60937500061451821, 33.67503911421598417 ) ) ;
#23091=CARTESIAN_POINT ( 'NONE',  ( 19.69687500061451857, -3.027376345333610441, -5.243569643749999898 ) ) ;
#23092=CARTESIAN_POINT ( 'NONE',  ( 28.32187500061451502, 3.027376345333613106, -5.243569643749998122 ) ) ;
#23093=CARTESIAN_POINT ( 'NONE',  ( 4.243569643749999898, 16.93437500061451573, 30.00000000000000000 ) ) ;
#23094=CARTESIAN_POINT ( 'NONE',  ( 9.140625000614518214, -3.027376345333614438, 5.243569643749998122 ) ) ;
#23095=DIRECTION ( 'NONE',  ( 0.000000000000000000, 0.000000000000000000, 1.000000000000000000 ) ) ;
#23096=CARTESIAN_POINT ( 'NONE',  ( 4.771875000614516971, -6.054752690667223547, -1.112240025338166033E-15 ) ) ;
#23097=CARTESIAN_POINT ( 'NONE',  ( 1.626862140677534273E-15, 15.61250000000000071, -26.00000000000000355 ) ) ;
#23098=CARTESIAN_POINT ( 'NONE',  ( 7.378125000614518036, -4.541064518000419881, 2.621784821874995952 ) ) ;
#23099=CARTESIAN_POINT ( 'NONE',  ( 10.95937500061451964, 0.000000000000000000, 5.243569643749999010 ) ) ;
#23100=CARTESIAN_POINT ( 'NONE',  ( 0.000000000000000000, 0.000000000000000000, 0.000000000000000000 ) ) ;
#23101=CARTESIAN_POINT ( 'NONE',  ( 19.20000000122903572, 5.773502691896255534, 3.535250795749688894E-16 ) ) ;
#23102=CARTESIAN_POINT ( 'NONE',  ( 5.371875000614516615, 3.027376345333613106, -5.243569643749998122 ) ) ;
#23103=CARTESIAN_POINT ( 'NONE',  ( 7.040625000614517681, -3.027376345333610441, -5.243569643749999898 ) ) ;
#23104=CARTESIAN_POINT ( 'NONE',  ( 5.428125000614517859, 4.541064518000418104, 2.621784821874999949 ) ) ;
#23106=CARTESIAN_POINT ( 'NONE',  ( 19.95937500061451786, 0.000000000000000000, 5.243569643749999010 ) ) ;
#23107=CARTESIAN_POINT ( 'NONE',  ( 3.999999999999999112, 13.13750000122903394, 30.00000000000000000 ) ) ;
#23108=ORIENTED_EDGE ( 'NONE', *, *, #47762, .F. ) ;
#23109=CARTESIAN_POINT ( 'NONE',  ( 24.25312500061451715, 4.541064518000418104, -2.621784821874998173 ) ) ;
#23110=CARTESIAN_POINT ( 'NONE',  ( 11.76562500061451644, 3.027376345333611329, 5.243569643749999010 ) ) ;
#23111=CARTESIAN_POINT ( 'NONE',  ( 29.85937500061451644, 0.000000000000000000, 5.243569643749999010 ) ) ;
#23112=CARTESIAN_POINT ( 'NONE',  ( 11.61562500061451608, 3.027376345333613106, -5.243569643749998122 ) ) ;
#23114=CARTESIAN_POINT ( 'NONE',  ( 11.70000000122903216, -2.886751345948129988, 4.999999999999997335 ) ) ;
#23116=CARTESIAN_POINT ( 'NONE',  ( 28.49062500061451431, -3.027376345333614438, 5.243569643749998122 ) ) ;
#23117=CARTESIAN_POINT ( 'NONE',  ( 4.243569643749999010, 12.86562500061451608, -32.45002607614398471 ) ) ;
#23118=CARTESIAN_POINT ( 'NONE',  ( 14.66250000122903252, 4.330127018922192761, -2.499999999999997780 ) ) ;
#23119=AXIS2_PLACEMENT_3D ( 'NONE', #26256, #71321, #66141 ) ;
#23120=CARTESIAN_POINT ( 'NONE',  ( 11.70000000000000284, -4.330127018922190985, -2.500000000000001332 ) ) ;
#23121=CARTESIAN_POINT ( 'NONE',  ( 21.55312500061451431, 4.541064518000418104, -2.621784821874998173 ) ) ;
#23122=CARTESIAN_POINT ( 'NONE',  ( 8.146875000614516082, 6.054752690667223547, 3.707466751127219781E-16 ) ) ;
#23123=CARTESIAN_POINT ( 'NONE',  ( 7.462500001229035007, 4.330127018922192761, -2.499999999999997780 ) ) ;
#23124=CARTESIAN_POINT ( 'NONE',  ( 15.60000000122903607, 5.773502691896255534, 3.535250795749688894E-16 ) ) ;
#23125=CARTESIAN_POINT ( 'NONE',  ( 12.59062500061451573, 6.054752690667223547, 3.707466751127219781E-16 ) ) ;
#23127=CARTESIAN_POINT ( 'NONE',  ( 16.30312500061451786, 0.000000000000000000, 5.243569643749999010 ) ) ;
#23128=CARTESIAN_POINT ( 'NONE',  ( 26.10000000122903430, -2.886751345948129988, 4.999999999999997335 ) ) ;
#23129=CARTESIAN_POINT ( 'NONE',  ( 20.06250000000000000, 2.886751345948126879, 4.999999999999999112 ) ) ;
#23130=CARTESIAN_POINT ( 'NONE',  ( 22.24687500061451217, -3.027376345333614438, 5.243569643749998122 ) ) ;
#23132=CARTESIAN_POINT ( 'NONE',  ( 9.562500001229032875, -4.330127018922190985, -2.500000000000001332 ) ) ;
#23133=CARTESIAN_POINT ( 'NONE',  ( 8.371875000614515727, -6.054752690667223547, -1.112240025338166033E-15 ) ) ;
#23134=CARTESIAN_POINT ( 'NONE',  ( 27.94687500061451502, 6.054752690667223547, 3.707466751127219781E-16 ) ) ;
#23135=EDGE_CURVE ( 'NONE', #45736, #70526, #27620, .T. ) ;
#23136=CARTESIAN_POINT ( 'NONE',  ( 3.534375000614518036, 6.421520780324663323E-16, -5.243569643749999010 ) ) ;
#23137=CARTESIAN_POINT ( 'NONE',  ( 23.69062500061451004, -3.027376345333610441, -5.243569643749999898 ) ) ;
#23139=CARTESIAN_POINT ( 'NONE',  ( 4.625252677371872068, -1.901857634188764745, -4.625252677371872068 ) ) ;
#23140=CARTESIAN_POINT ( 'NONE',  ( 8.221875000614518925, 3.027376345333611329, 5.243569643749999010 ) ) ;
#23141=CARTESIAN_POINT ( 'NONE',  ( 4.993151921736298959, -0.2997683513397194077, 5.126451599955896832 ) ) ;
#23142=CARTESIAN_POINT ( 'NONE',  ( 27.32812500061451644, 6.421520780324663323E-16, -5.243569643749999010 ) ) ;
#23143=CARTESIAN_POINT ( 'NONE',  ( 7.584375000614516082, 6.421520780324663323E-16, -5.243569643749999010 ) ) ;
#23144=CARTESIAN_POINT ( 'NONE',  ( 6.600000000000001421, 0.000000000000000000, 4.999999999999998224 ) ) ;
#23146=CARTESIAN_POINT ( 'NONE',  ( 25.35937500061451644, 0.000000000000000000, 5.243569643749999010 ) ) ;
#23148=CARTESIAN_POINT ( 'NONE',  ( 19.04999999999999716, 4.330127018922192761, -2.499999999999997780 ) ) ;
#23149=ORIENTED_EDGE ( 'NONE', *, *, #43888, .T. ) ;
#23150=CARTESIAN_POINT ( 'NONE',  ( 27.15000000000000213, 4.330127018922192761, -2.499999999999997780 ) ) ;
#23151=CARTESIAN_POINT ( 'NONE',  ( 27.98437500061451289, 4.541064518000418104, 2.621784821874999949 ) ) ;
#23153=CARTESIAN_POINT ( 'NONE',  ( 15.62812500061451537, 6.421520780324663323E-16, -5.243569643749999010 ) ) ;
#23154=CARTESIAN_POINT ( 'NONE',  ( 9.290625000614515017, -3.027376345333610441, -5.243569643749999898 ) ) ;
#23156=CARTESIAN_POINT ( 'NONE',  ( 5.034375000614519813, 4.541064518000418104, 2.621784821874999949 ) ) ;
#23157=CARTESIAN_POINT ( 'NONE',  ( 17.66250000122903430, -4.330127018922190985, -2.500000000000001332 ) ) ;
#23158=CARTESIAN_POINT ( 'NONE',  ( 21.52499999999999858, -4.330127018922194537, 2.499999999999995559 ) ) ;
#23159=CARTESIAN_POINT ( 'NONE',  ( 29.17500000000000071, -4.330127018922194537, 2.499999999999995559 ) ) ;
#23160=CARTESIAN_POINT ( 'NONE',  ( 5.671875000614519102, -6.054752690667223547, -1.112240025338166033E-15 ) ) ;
#23161=CARTESIAN_POINT ( 'NONE',  ( 12.72187500061451537, 3.027376345333611329, 5.243569643749999010 ) ) ;
#23162=CARTESIAN_POINT ( 'NONE',  ( 22.80937500061451573, -4.541064518000417216, -2.621784821875001281 ) ) ;
#23164=CARTESIAN_POINT ( 'NONE',  ( 3.421875000614516882, -6.054752690667223547, -1.112240025338166033E-15 ) ) ;
#23165=( BOUNDED_CURVE ( )  B_SPLINE_CURVE ( 2, ( #40110, #43003, #20082, #53724, #48918, #2385, #31922 ),
 .UNSPECIFIED., .F., .F. ) 
 B_SPLINE_CURVE_WITH_KNOTS ( ( 3, 2, 2, 3 ),
 ( 0.4833333333333333925, 0.4861111111111111605, 0.4888888888888888729, 0.4916666666666666408 ),
 .UNSPECIFIED. ) 
 CURVE ( )  GEOMETRIC_REPRESENTATION_ITEM ( )  RATIONAL_B_SPLINE_CURVE ( ( 0.9999999999999973355, 0.8660254037844413721, 1.000000000000000000, 0.8660254037844387076, 1.000000000000000000, 0.8660254037844387076, 1.000000000000000000 ) ) 
 REPRESENTATION_ITEM ( '' )  );
#23166=CARTESIAN_POINT ( 'NONE',  ( 7.584375000614516082, 6.421520780324663323E-16, -5.243569643749999010 ) ) ;
#23167=CARTESIAN_POINT ( 'NONE',  ( 18.41250000000000142, -5.773502691896255534, -1.060575238724906372E-15 ) ) ;
#23168=CARTESIAN_POINT ( 'NONE',  ( 16.37812500061451715, -4.541064518000419881, 2.621784821874995952 ) ) ;
#23170=CARTESIAN_POINT ( 'NONE',  ( 24.93750000122903288, 6.123233995736764310E-16, -4.999999999999998224 ) ) ;
#23172=CARTESIAN_POINT ( 'NONE',  ( 11.12812500061451715, 6.421520780324663323E-16, -5.243569643749999010 ) ) ;
#23173=CARTESIAN_POINT ( 'NONE',  ( 25.62187500061451573, 3.027376345333613106, -5.243569643749998122 ) ) ;
#23174=CARTESIAN_POINT ( 'NONE',  ( -3.999999999999999112, 19.62500000122903288, 27.69059892324149885 ) ) ;
#23175=CARTESIAN_POINT ( 'NONE',  ( 25.50937500061451502, -4.541064518000417216, -2.621784821875001281 ) ) ;
#23176=CARTESIAN_POINT ( 'NONE',  ( 6.637500000000001066, -2.886751345948129988, 4.999999999999997335 ) ) ;
#23177=CARTESIAN_POINT ( 'NONE',  ( -1.999999999999997113, 12.98750000122903359, 33.46410161513775705 ) ) ;
#23178=CARTESIAN_POINT ( 'NONE',  ( 9.375000001229036428, 2.886751345948126879, 4.999999999999999112 ) ) ;
#23179=CARTESIAN_POINT ( 'NONE',  ( 20.48437500061451289, -4.541064518000419881, 2.621784821874995952 ) ) ;
#23180=CARTESIAN_POINT ( 'NONE',  ( 10.73437500061451644, 6.421520780324663323E-16, -5.243569643749999010 ) ) ;
#23181=CARTESIAN_POINT ( 'NONE',  ( -2.081578678577455488, 4.574985540471381285, -33.45664977638282522 ) ) ;
#23183=CARTESIAN_POINT ( 'NONE',  ( 15.06562500061451537, -6.054752690667223547, -1.112240025338166033E-15 ) ) ;
#23184=CARTESIAN_POINT ( 'NONE',  ( 25.57500000122903216, 2.886751345948126879, 4.999999999999999112 ) ) ;
#23185=CARTESIAN_POINT ( 'NONE',  ( 13.32187500061451502, -6.054752690667223547, -1.112240025338166033E-15 ) ) ;
#23186=CARTESIAN_POINT ( 'NONE',  ( 3.242103837493086330E-14, 12.80000000122903536, 26.00000000000000711 ) ) ;
#23187=CARTESIAN_POINT ( 'NONE',  ( 17.87812500061451715, 6.421520780324663323E-16, -5.243569643749999010 ) ) ;
#23188=DIRECTION ( 'NONE',  ( 0.000000000000000000, 0.000000000000000000, 1.000000000000000000 ) ) ;
#23189=CARTESIAN_POINT ( 'NONE',  ( 26.40937500061451715, -4.541064518000417216, -2.621784821875001281 ) ) ;
#23190=CARTESIAN_POINT ( 'NONE',  ( -2.121784821874996840, 10.87812500061451715, 33.67503911421598417 ) ) ;
#23191=CARTESIAN_POINT ( 'NONE',  ( 11.51250000122903216, 4.330127018922192761, -2.499999999999997780 ) ) ;
#23193=CARTESIAN_POINT ( 'NONE',  ( -4.243569643749999898, 18.05937500061451928, -30.00000000000000000 ) ) ;
#23194=CARTESIAN_POINT ( 'NONE',  ( 17.97187500061451715, 3.027376345333613106, -5.243569643749998122 ) ) ;
#23195=CARTESIAN_POINT ( 'NONE',  ( 20.66250000122903074, 0.000000000000000000, 4.999999999999998224 ) ) ;
#23197=CARTESIAN_POINT ( 'NONE',  ( 14.52187500061451608, 3.027376345333611329, 5.243569643749999010 ) ) ;
#23198=CARTESIAN_POINT ( 'NONE',  ( -2.121784821874999949, 19.72812500061451857, -33.67503911421598417 ) ) ;
#23199=CARTESIAN_POINT ( 'NONE',  ( 23.10000000122903074, -2.886751345948125991, -5.000000000000000000 ) ) ;
#23200=AXIS2_PLACEMENT_3D ( 'NONE', #23300, #62466, #40667 ) ;
#23201=CARTESIAN_POINT ( 'NONE',  ( 14.95312500061451644, 0.000000000000000000, 5.243569643749999010 ) ) ;
#23202=CARTESIAN_POINT ( 'NONE',  ( 25.50000000000000000, 0.000000000000000000, 4.999999999999998224 ) ) ;
#23203=ORIENTED_EDGE ( 'NONE', *, *, #45494, .F. ) ;
#23205=CARTESIAN_POINT ( 'NONE',  ( 20.32499999999999929, 6.123233995736764310E-16, -4.999999999999998224 ) ) ;
#23206=CARTESIAN_POINT ( 'NONE',  ( -3.137519842735245283E-14, 14.37500000122903288, 34.00000000000000000 ) ) ;
#23207=CARTESIAN_POINT ( 'NONE',  ( 0.5511252142286459099, 4.971455555459576736, 33.96427100478815220 ) ) ;
#23208=CARTESIAN_POINT ( 'NONE',  ( 14.77500000122903501, 2.886751345948126879, 4.999999999999999112 ) ) ;
#23209=CARTESIAN_POINT ( 'NONE',  ( 20.20312500061451644, 4.541064518000418104, -2.621784821874998173 ) ) ;
#23210=CARTESIAN_POINT ( 'NONE',  ( 24.10312500061451502, -4.541064518000417216, -2.621784821875001281 ) ) ;
#23211=CARTESIAN_POINT ( 'NONE',  ( 4.190625000614518925, -3.027376345333614438, 5.243569643749998122 ) ) ;
#23212=CARTESIAN_POINT ( 'NONE',  ( 28.76249999999999929, -5.773502691896255534, -1.060575238724906372E-15 ) ) ;
#23213=CARTESIAN_POINT ( 'NONE',  ( -1.071796769724491005, 10.12009619066136956, -34.00000000000000000 ) ) ;
#23214=( BOUNDED_CURVE ( )  B_SPLINE_CURVE ( 2, ( #36290, #21116, #30743, #59909, #9315, #58804, #8214, #20747, #20008 ),
 .UNSPECIFIED., .F., .F. ) 
 B_SPLINE_CURVE_WITH_KNOTS ( ( 3, 2, 2, 2, 3 ),
 ( 0.4456521739130435145, 0.4492753623188405765, 0.4565217391304347561, 0.4637681159420289911, 0.4673913043478261087 ),
 .UNSPECIFIED. ) 
 CURVE ( )  GEOMETRIC_REPRESENTATION_ITEM ( )  RATIONAL_B_SPLINE_CURVE ( ( 0.9330127018922194093, 0.9330127018922198534, 1.000000000000000000, 0.8660254037844387076, 1.000000000000000000, 0.8660254037844387076, 1.000000000000000000, 0.9330127018922188542, 0.9330127018922194093 ) ) 
 REPRESENTATION_ITEM ( '' )  );
#23216=CARTESIAN_POINT ( 'NONE',  ( 29.52187500061451431, -6.054752690667223547, -1.112240025338166033E-15 ) ) ;
#23217=CARTESIAN_POINT ( 'NONE',  ( -1.999999999999997113, 10.73750000122903536, -26.53589838486224295 ) ) ;
#23218=CARTESIAN_POINT ( 'NONE',  ( -2.121784821874999949, 18.88437500061451857, -33.67503911421598417 ) ) ;
#23219=CARTESIAN_POINT ( 'NONE',  ( 6.787500001229032520, -4.330127018922194537, 2.499999999999995559 ) ) ;
#23220=CARTESIAN_POINT ( 'NONE',  ( 9.225000000000001421, 4.330127018922191873, 2.499999999999999556 ) ) ;
#23221=EDGE_CURVE ( 'NONE', #48240, #30519, #44234, .T. ) ;
#23222=CARTESIAN_POINT ( 'NONE',  ( 3.600000001229033408, -2.886751345948129988, 4.999999999999997335 ) ) ;
#23223=CARTESIAN_POINT ( 'NONE',  ( 12.60937500061451821, 4.541064518000418104, -2.621784821874998173 ) ) ;
#23224=CARTESIAN_POINT ( 'NONE',  ( 3.985236265425895485, -3.020202436759538589, 3.985236265425895485 ) ) ;
#23225=CARTESIAN_POINT ( 'NONE',  ( 3.609375000614516882, 4.541064518000418104, -2.621784821874998173 ) ) ;
#23227=CARTESIAN_POINT ( 'NONE',  ( 29.43750000122903288, 6.123233995736764310E-16, -4.999999999999998224 ) ) ;
#23228=CARTESIAN_POINT ( 'NONE',  ( 10.92187500061451644, 3.027376345333611329, 5.243569643749999010 ) ) ;
#23229=CARTESIAN_POINT ( 'NONE',  ( 13.95937500061451786, 4.541064518000418104, -2.621784821874998173 ) ) ;
#23230=CARTESIAN_POINT ( 'NONE',  ( 3.516709882973403367, -4.011040265794256321, 3.052674468439771527 ) ) ;
#23232=CARTESIAN_POINT ( 'NONE',  ( 6.712500000000000355, -5.773502691896255534, -1.060575238724906372E-15 ) ) ;
#23233=AXIS2_PLACEMENT_3D ( 'NONE', #35669, #1349, #40505 ) ;
#23234=CARTESIAN_POINT ( 'NONE',  ( -2.121784821874996840, 17.17812500061459247, 33.67503911421598417 ) ) ;
#23235=CARTESIAN_POINT ( 'NONE',  ( 22.39687500061451075, -3.027376345333610441, -5.243569643749999898 ) ) ;
#23236=CARTESIAN_POINT ( 'NONE',  ( 2.816105206925325177, -4.131560564441517869, 3.074222403557641758 ) ) ;
#23237=CARTESIAN_POINT ( 'NONE',  ( 27.03750000122903430, -4.330127018922194537, 2.499999999999995559 ) ) ;
#23239=CARTESIAN_POINT ( 'NONE',  ( 22.90312500061451573, 4.541064518000418104, -2.621784821874998173 ) ) ;
#23240=CARTESIAN_POINT ( 'NONE',  ( 14.57812500061451644, -4.541064518000419881, 2.621784821874995952 ) ) ;
#23242=CARTESIAN_POINT ( 'NONE',  ( 12.15937500061451892, 4.541064518000418104, -2.621784821874998173 ) ) ;
#23243=CARTESIAN_POINT ( 'NONE',  ( 29.09999999999999787, 0.000000000000000000, 4.999999999999998224 ) ) ;
#23244=CARTESIAN_POINT ( 'NONE',  ( 24.86250000122903359, -4.330127018922190985, -2.500000000000001332 ) ) ;
#23245=DIRECTION ( 'NONE',  ( -0.000000000000000000, -1.000000000000000000, -0.000000000000000000 ) ) ;
#23246=CARTESIAN_POINT ( 'NONE',  ( 12.30937500061451573, 0.000000000000000000, 5.243569643749999010 ) ) ;
#23247=CARTESIAN_POINT ( 'NONE',  ( 28.02187500061451431, 3.027376345333611329, 5.243569643749999010 ) ) ;
#23248=LINE ( 'NONE', #45799, #53696 ) ;
#23250=CARTESIAN_POINT ( 'NONE',  ( 23.07187500061451857, 3.027376345333611329, 5.243569643749999010 ) ) ;
#23251=CARTESIAN_POINT ( 'NONE',  ( 15.30937500061451750, 4.541064518000418104, -2.621784821874998173 ) ) ;
#23253=CARTESIAN_POINT ( 'NONE',  ( 26.62500000000000000, 6.123233995736764310E-16, -4.999999999999998224 ) ) ;
#23254=CARTESIAN_POINT ( 'NONE',  ( 2.700000001229035718, -2.886751345948129988, 4.999999999999997335 ) ) ;
#23256=CARTESIAN_POINT ( 'NONE',  ( 16.11562500061451786, 3.027376345333613106, -5.243569643749998122 ) ) ;
#23257=CARTESIAN_POINT ( 'NONE',  ( 8.062500000000000000, -5.773502691896255534, -1.060575238724906372E-15 ) ) ;
#23258=CARTESIAN_POINT ( 'NONE',  ( 15.59999999999999964, 0.000000000000000000, 4.999999999999998224 ) ) ;
#23259=CARTESIAN_POINT ( 'NONE',  ( 16.05000000000000071, 0.000000000000000000, 4.999999999999998224 ) ) ;
#23260=CARTESIAN_POINT ( 'NONE',  ( 9.001249775931846008E-16, 12.26562500061451644, 34.90005215228797653 ) ) ;
#23262=CARTESIAN_POINT ( 'NONE',  ( 27.64687500061452141, -3.027376345333614438, 5.243569643749998122 ) ) ;
#23263=VERTEX_POINT ( 'NONE', #56054 ) ;
#23264=CARTESIAN_POINT ( 'NONE',  ( 22.56562500061451715, 3.027376345333611329, 5.243569643749999010 ) ) ;
#23265=CARTESIAN_POINT ( 'NONE',  ( 23.22187500061451715, -6.054752690667223547, -1.112240025338166033E-15 ) ) ;
#23266=CARTESIAN_POINT ( 'NONE',  ( 4.987500000000002487, -2.886751345948125991, -5.000000000000000000 ) ) ;
#23267=CARTESIAN_POINT ( 'NONE',  ( 7.453125000614516438, -4.541064518000417216, -2.621784821875001281 ) ) ;
#23268=CARTESIAN_POINT ( 'NONE',  ( 24.47812500061451502, -4.541064518000419881, 2.621784821874995952 ) ) ;
#23269=CARTESIAN_POINT ( 'NONE',  ( 12.00937500061451857, -4.541064518000417216, -2.621784821875001281 ) ) ;
#23270=CARTESIAN_POINT ( 'NONE',  ( 15.64687500061451608, -3.027376345333610441, -5.243569643749999898 ) ) ;
#23271=CARTESIAN_POINT ( 'NONE',  ( 4.243569643749999898, 16.87812500061451715, 30.00000000000000000 ) ) ;
#23272=CARTESIAN_POINT ( 'NONE',  ( 18.45000000122903216, -2.886751345948129988, 4.999999999999997335 ) ) ;
#23274=CARTESIAN_POINT ( 'NONE',  ( 9.815625000614517148, 3.027376345333612662, -5.243569643749998122 ) ) ;
#23275=CARTESIAN_POINT ( 'NONE',  ( 6.496875000614517504, -3.027376345333614438, 5.243569643749998122 ) ) ;
#23276=CARTESIAN_POINT ( 'NONE',  ( 4.246875000614519280, -3.027376345333614438, 5.243569643749998122 ) ) ;
#23277=VERTEX_POINT ( 'NONE', #44973 ) ;
#23278=CARTESIAN_POINT ( 'NONE',  ( 24.53437500061451715, -4.541064518000419881, 2.621784821874995952 ) ) ;
#23279=CARTESIAN_POINT ( 'NONE',  ( 17.57812500061451644, 4.541064518000418104, 2.621784821874999949 ) ) ;
#23280=CARTESIAN_POINT ( 'NONE',  ( 26.58750000122903145, -4.330127018922194537, 2.499999999999995559 ) ) ;
#23282=CARTESIAN_POINT ( 'NONE',  ( 28.67812500061451431, 6.421520780324663323E-16, -5.243569643749999010 ) ) ;
#23283=CARTESIAN_POINT ( 'NONE',  ( 22.13437500061451502, 4.541064518000418104, 2.621784821874999949 ) ) ;
#23284=CARTESIAN_POINT ( 'NONE',  ( 17.99062500061451786, 6.054752690667223547, 3.707466751127219781E-16 ) ) ;
#23285=CARTESIAN_POINT ( 'NONE',  ( 4.243569643749999898, 19.18437500061451928, 30.00000000000000000 ) ) ;
#23286=ADVANCED_FACE ( 'NONE', ( #46418 ), #2434, .T. ) ;
#23287=CARTESIAN_POINT ( 'NONE',  ( 22.60312500061451857, 0.000000000000000000, 5.243569643749999010 ) ) ;
#23288=CARTESIAN_POINT ( 'NONE',  ( 2.850000001229036073, -2.886751345948125991, -5.000000000000000000 ) ) ;
#23289=ORIENTED_EDGE ( 'NONE', *, *, #61121, .T. ) ;
#23290=CARTESIAN_POINT ( 'NONE',  ( 26.84999999999999787, 0.000000000000000000, 4.999999999999998224 ) ) ;
#23291=CARTESIAN_POINT ( 'NONE',  ( -3.999999999999999556, 12.31250000000000000, -32.30940107675850470 ) ) ;
#23293=CARTESIAN_POINT ( 'NONE',  ( 28.37812500061451715, 4.541064518000418104, 2.621784821874999949 ) ) ;
#23294=CARTESIAN_POINT ( 'NONE',  ( 10.49062500061451431, -3.027376345333614438, 5.243569643749998122 ) ) ;
#23295=CARTESIAN_POINT ( 'NONE',  ( 21.56250000122903288, 0.000000000000000000, 4.999999999999998224 ) ) ;
#23296=CARTESIAN_POINT ( 'NONE',  ( 27.55312500061451786, 0.000000000000000000, 5.243569643749999010 ) ) ;
#23297=CARTESIAN_POINT ( 'NONE',  ( 28.23750000000000426, -2.886751345948129988, 4.999999999999997335 ) ) ;
#23298=CARTESIAN_POINT ( 'NONE',  ( 1.999999999999998668, 17.71250000122903501, -33.46410161513775705 ) ) ;
#23299=EDGE_CURVE ( 'NONE', #71417, #9906, #55574, .T. ) ;
#23300=CARTESIAN_POINT ( 'NONE',  ( 30.00000000000000000, 0.000000000000000000, 0.000000000000000000 ) ) ;
#23301=CARTESIAN_POINT ( 'NONE',  ( 10.94062500061451537, -3.027376345333614438, 5.243569643749998122 ) ) ;
#23302=ORIENTED_EDGE ( 'NONE', *, *, #62588, .F. ) ;
#23303=CARTESIAN_POINT ( 'NONE',  ( 6.815625000614517148, 3.027376345333611329, 5.243569643749999010 ) ) ;
#23304=CARTESIAN_POINT ( 'NONE',  ( 6.028125000614517504, -4.541064518000419881, 2.621784821874995952 ) ) ;
#23306=EDGE_CURVE ( 'NONE', #35963, #5936, #59092, .T. ) ;
#23307=CARTESIAN_POINT ( 'NONE',  ( 2.737500001229034474, -4.330127018922194537, 2.499999999999995559 ) ) ;
#23308=CARTESIAN_POINT ( 'NONE',  ( 14.88750000000000107, -2.886751345948125991, -5.000000000000000000 ) ) ;
#23309=CARTESIAN_POINT ( 'NONE',  ( 15.42187500061451821, 3.027376345333611329, 5.243569643749999010 ) ) ;
#23310=CARTESIAN_POINT ( 'NONE',  ( 12.07500000122903216, 2.886751345948126879, 4.999999999999999112 ) ) ;
#23311=CARTESIAN_POINT ( 'NONE',  ( 18.34687500061451715, -3.027376345333610441, -5.243569643749999898 ) ) ;
#23313=CARTESIAN_POINT ( 'NONE',  ( 21.60937500061451644, 4.541064518000418104, -2.621784821874998173 ) ) ;
#23314=CARTESIAN_POINT ( 'NONE',  ( 4.243569643749999010, 15.11562500061451608, -32.45002607614398471 ) ) ;
#23317=CARTESIAN_POINT ( 'NONE',  ( 4.169580978743460342, 2.759455464706926708, 4.458747374224691029 ) ) ;
#23318=CARTESIAN_POINT ( 'NONE',  ( 26.20312500061451644, 0.000000000000000000, 5.243569643749999010 ) ) ;
#23319=DIRECTION ( 'NONE',  ( -1.000000000000000000, -0.000000000000000000, -0.000000000000000000 ) ) ;
#23320=CARTESIAN_POINT ( 'NONE',  ( 27.94687500061451502, 6.054752690667223547, 3.707466751127219781E-16 ) ) ;
#23322=CARTESIAN_POINT ( 'NONE',  ( 23.51249999999999574, 2.886751345948129099, -4.999999999999998224 ) ) ;
#23323=CARTESIAN_POINT ( 'NONE',  ( 6.703125000614516438, 4.541064518000418104, -2.621784821874998173 ) ) ;
#23325=CARTESIAN_POINT ( 'NONE',  ( 19.05937500061451928, 0.000000000000000000, 5.243569643749999010 ) ) ;
#23327=CARTESIAN_POINT ( 'NONE',  ( 5.915625000614515905, 3.027376345333611329, 5.243569643749999010 ) ) ;
#23328=CARTESIAN_POINT ( 'NONE',  ( 11.85937500061451644, 0.000000000000000000, 5.243569643749999010 ) ) ;
#23329=VERTEX_POINT ( 'NONE', #58932 ) ;
#23330=CARTESIAN_POINT ( 'NONE',  ( 22.05937500061451573, 4.541064518000418104, -2.621784821874998173 ) ) ;
#23332=CARTESIAN_POINT ( 'NONE',  ( 29.09999999999999787, 0.000000000000000000, 4.999999999999998224 ) ) ;
#23333=CARTESIAN_POINT ( 'NONE',  ( 28.80937500061451573, 4.541064518000418104, -2.621784821874998173 ) ) ;
#23336=CARTESIAN_POINT ( 'NONE',  ( 10.80000000000000071, -4.330127018922190985, -2.500000000000001332 ) ) ;
#23337=VERTEX_POINT ( 'NONE', #40516 ) ;
#23338=CARTESIAN_POINT ( 'NONE',  ( 11.10000000000000142, 0.000000000000000000, 4.999999999999998224 ) ) ;
#23340=CARTESIAN_POINT ( 'NONE',  ( 24.40312500061451573, 0.000000000000000000, 5.243569643749999010 ) ) ;
#23341=CARTESIAN_POINT ( 'NONE',  ( 13.61250000000000071, 2.886751345948129099, -4.999999999999998224 ) ) ;
#23343=CARTESIAN_POINT ( 'NONE',  ( 10.12500000122903465, 2.886751345948129099, -4.999999999999998224 ) ) ;
#23344=CARTESIAN_POINT ( 'NONE',  ( 8.728125000614518569, -4.541064518000419881, 2.621784821874995952 ) ) ;
#23345=CARTESIAN_POINT ( 'NONE',  ( 24.00000000000000000, 4.330127018922192761, -2.499999999999997780 ) ) ;
#23346=CARTESIAN_POINT ( 'NONE',  ( 20.31562500061451715, 3.027376345333611329, 5.243569643749999010 ) ) ;
#23348=CARTESIAN_POINT ( 'NONE',  ( 28.31250000122903288, 0.000000000000000000, 4.999999999999998224 ) ) ;
#23350=CARTESIAN_POINT ( 'NONE',  ( 6.750000000000002665, -4.330127018922190985, -2.500000000000001332 ) ) ;
#23352=CARTESIAN_POINT ( 'NONE',  ( 20.87812500061451715, -4.541064518000419881, 2.621784821874995952 ) ) ;
#23353=CARTESIAN_POINT ( 'NONE',  ( 29.16562500061451502, 3.027376345333613106, -5.243569643749998122 ) ) ;
#23354=DIRECTION ( 'NONE',  ( -1.000000000000000000, -0.000000000000000000, -0.000000000000000000 ) ) ;
#23355=CARTESIAN_POINT ( 'NONE',  ( 18.53437500061451715, 4.541064518000418104, 2.621784821874999949 ) ) ;
#23356=CARTESIAN_POINT ( 'NONE',  ( 16.00312500061451715, -4.541064518000417216, -2.621784821875001281 ) ) ;
#23357=CARTESIAN_POINT ( 'NONE',  ( 1.626862140677534273E-15, 12.01250000000000107, 34.00000000000000000 ) ) ;
#23358=CARTESIAN_POINT ( 'NONE',  ( 4.565625000614516260, 3.027376345333611329, 5.243569643749999010 ) ) ;
#23359=CARTESIAN_POINT ( 'NONE',  ( 28.68750000122903288, 4.330127018922191873, 2.499999999999999556 ) ) ;
#23361=CARTESIAN_POINT ( 'NONE',  ( 18.36562500061451431, 3.027376345333612662, -5.243569643749998122 ) ) ;
#23362=CARTESIAN_POINT ( 'NONE',  ( 3.999999999999999112, 13.92500000000000071, 30.00000000000000000 ) ) ;
#23363=CARTESIAN_POINT ( 'NONE',  ( 3.825000001229032609, 2.886751345948129099, -4.999999999999998224 ) ) ;
#23364=CARTESIAN_POINT ( 'NONE',  ( 13.92187500061451644, 3.027376345333613106, -5.243569643749998122 ) ) ;
#23365=CARTESIAN_POINT ( 'NONE',  ( 12.83437500061451786, -4.541064518000419881, 2.621784821874995952 ) ) ;
#23366=CARTESIAN_POINT ( 'NONE',  ( 19.99687500061451573, -3.027376345333614438, 5.243569643749998122 ) ) ;
#23368=CARTESIAN_POINT ( 'NONE',  ( -5.798826918071312342, 8.147596131390990593, 28.40867891430389847 ) ) ;
#23369=CARTESIAN_POINT ( 'NONE',  ( 24.81562500061451715, 3.027376345333611329, 5.243569643749999010 ) ) ;
#23370=CARTESIAN_POINT ( 'NONE',  ( 17.85937500061451999, -4.541064518000417216, -2.621784821875001281 ) ) ;
#23371=CARTESIAN_POINT ( 'NONE',  ( 23.20312500061451644, -4.541064518000417216, -2.621784821875001281 ) ) ;
#23372=CARTESIAN_POINT ( 'NONE',  ( 30.00000000000000000, 0.000000000000000000, 0.000000000000000000 ) ) ;
#23373=CARTESIAN_POINT ( 'NONE',  ( 3.999999999999999112, 15.72500000000000320, 30.00000000000000000 ) ) ;
#23374=CARTESIAN_POINT ( 'NONE',  ( 28.90312500061451217, 0.000000000000000000, 5.243569643749999010 ) ) ;
#23375=CARTESIAN_POINT ( 'NONE',  ( 10.20000000122903572, 5.773502691896255534, 3.535250795749688894E-16 ) ) ;
#23376=CARTESIAN_POINT ( 'NONE',  ( 6.787500001229032520, -4.330127018922194537, 2.499999999999995559 ) ) ;
#23377=CARTESIAN_POINT ( 'NONE',  ( -2.828200636599751609E-16, 19.88749999999999929, -34.61880215351700230 ) ) ;
#23378=CARTESIAN_POINT ( 'NONE',  ( 28.05000000122903359, -2.886751345948125991, -5.000000000000000000 ) ) ;
#23381=CARTESIAN_POINT ( 'NONE',  ( 8.784375000614518925, -4.541064518000419881, 2.621784821874995952 ) ) ;
#23382=CARTESIAN_POINT ( 'NONE',  ( -3.137519842735245283E-14, 14.71250000000000213, -26.00000000000000711 ) ) ;
#23383=CARTESIAN_POINT ( 'NONE',  ( 17.39062500061451644, -3.027376345333610441, -5.243569643749999898 ) ) ;
#23384=CARTESIAN_POINT ( 'NONE',  ( 11.97187500061451892, -6.054752690667223547, -1.112240025338166033E-15 ) ) ;
#23385=CARTESIAN_POINT ( 'NONE',  ( 28.57500000122903572, 2.886751345948129099, -4.999999999999998224 ) ) ;
#23386=CARTESIAN_POINT ( 'NONE',  ( 19.80937500061451573, 4.541064518000418104, -2.621784821874998173 ) ) ;
#23387=CARTESIAN_POINT ( 'NONE',  ( 8.409375000614518925, -4.541064518000417216, -2.621784821875001281 ) ) ;
#23388=CARTESIAN_POINT ( 'NONE',  ( 3.928125000614516527, 6.421520780324663323E-16, -5.243569643749999010 ) ) ;
#23389=EDGE_CURVE ( 'NONE', #45611, #55464, #35682, .T. ) ;
#23390=CARTESIAN_POINT ( 'NONE',  ( 7.453125000614516438, -4.541064518000417216, -2.621784821875001281 ) ) ;
#23391=CARTESIAN_POINT ( 'NONE',  ( 19.30312500061451786, 4.541064518000418104, -2.621784821874998173 ) ) ;
#23392=ORIENTED_EDGE ( 'NONE', *, *, #37730, .T. ) ;
#23393=CARTESIAN_POINT ( 'NONE',  ( 4.837500001229035895, 4.330127018922191873, 2.499999999999999556 ) ) ;
#23394=CARTESIAN_POINT ( 'NONE',  ( 14.35312500061451679, 4.541064518000418104, -2.621784821874998173 ) ) ;
#23395=CARTESIAN_POINT ( 'NONE',  ( 12.70312500061451821, 0.000000000000000000, 5.243569643749999010 ) ) ;
#23397=CARTESIAN_POINT ( 'NONE',  ( 13.27500000000000213, 4.330127018922191873, 2.499999999999999556 ) ) ;
#23398=CARTESIAN_POINT ( 'NONE',  ( 7.950000001229033053, 5.773502691896255534, 3.535250795749688894E-16 ) ) ;
#23399=CARTESIAN_POINT ( 'NONE',  ( 6.665625000614515905, 3.027376345333613106, -5.243569643749998122 ) ) ;
#23400=( BOUNDED_CURVE ( )  B_SPLINE_CURVE ( 2, ( #7712, #30246, #52779, #47238, #64217, #36151, #8078 ),
 .UNSPECIFIED., .F., .F. ) 
 B_SPLINE_CURVE_WITH_KNOTS ( ( 3, 2, 2, 3 ),
 ( 0.4750000000000000333, 0.4777777777777778567, 0.4805555555555556246, 0.4833333333333333925 ),
 .UNSPECIFIED. ) 
 CURVE ( )  GEOMETRIC_REPRESENTATION_ITEM ( )  RATIONAL_B_SPLINE_CURVE ( ( 0.9999999999999973355, 0.8660254037844413721, 1.000000000000000000, 0.8660254037844387076, 1.000000000000000000, 0.8660254037844360431, 1.000000000000002665 ) ) 
 REPRESENTATION_ITEM ( '' )  );
#23401=CARTESIAN_POINT ( 'NONE',  ( 19.20000000122903572, 5.773502691896255534, 3.535250795749688894E-16 ) ) ;
#23403=CARTESIAN_POINT ( 'NONE',  ( 2.121784821875001281, 11.45937500061451786, -26.32496088578401938 ) ) ;
#23404=DIRECTION ( 'NONE',  ( 0.000000000000000000, 0.000000000000000000, -1.000000000000000000 ) ) ;
#23405=CARTESIAN_POINT ( 'NONE',  ( 3.487500001229035362, 4.330127018922191873, 2.499999999999999556 ) ) ;
#23406=ADVANCED_FACE ( 'NONE', ( #23870 ), #18313, .F. ) ;
#23407=CARTESIAN_POINT ( 'NONE',  ( -1.071796769724475906, 11.35759618943233562, -34.00000000000000711 ) ) ;
#23408=CARTESIAN_POINT ( 'NONE',  ( -1.071796769724475906, 13.15759618943233100, 25.99999999999999289 ) ) ;
#23409=CARTESIAN_POINT ( 'NONE',  ( 18.68437500061451928, -4.541064518000419881, 2.621784821874995952 ) ) ;
#23410=CARTESIAN_POINT ( 'NONE',  ( 30.00000000000000000, 6.123233995736764310E-16, -4.999999999999998224 ) ) ;
#23411=CARTESIAN_POINT ( 'NONE',  ( 15.10312500061451502, -4.541064518000417216, -2.621784821875001281 ) ) ;
#23413=DIRECTION ( 'NONE',  ( -0.000000000000000000, -1.000000000000000000, -0.000000000000000000 ) ) ;
#23414=CARTESIAN_POINT ( 'NONE',  ( 29.78437500061451715, 4.541064518000418104, 2.621784821874999949 ) ) ;
#23415=CARTESIAN_POINT ( 'NONE',  ( 26.07187500061451857, 3.027376345333613106, -5.243569643749998122 ) ) ;
#23417=CARTESIAN_POINT ( 'NONE',  ( 12.02812500061451573, 6.421520780324663323E-16, -5.243569643749999010 ) ) ;
#23418=CARTESIAN_POINT ( 'NONE',  ( 11.70937500061451608, 4.541064518000418104, -2.621784821874998173 ) ) ;
#23419=ORIENTED_EDGE ( 'NONE', *, *, #47483, .F. ) ;
#23420=CARTESIAN_POINT ( 'NONE',  ( 2.964777361493091679, -4.026176250088806086, -3.359304602455296607 ) ) ;
#23421=CARTESIAN_POINT ( 'NONE',  ( 21.06562500061451715, 3.027376345333613106, -5.243569643749998122 ) ) ;
#23424=EDGE_CURVE ( 'NONE', #40395, #493, #41597, .T. ) ;
#23425=CARTESIAN_POINT ( 'NONE',  ( 10.16249999999999964, 2.886751345948126879, 4.999999999999999112 ) ) ;
#23426=CARTESIAN_POINT ( 'NONE',  ( 20.92500000122903714, 2.886751345948129099, -4.999999999999998224 ) ) ;
#23427=CARTESIAN_POINT ( 'NONE',  ( 15.02812500061451750, -4.541064518000419881, 2.621784821874995952 ) ) ;
#23429=ORIENTED_EDGE ( 'NONE', *, *, #7307, .T. ) ;
#23430=CARTESIAN_POINT ( 'NONE',  ( 18.52499999999999858, 6.123233995736764310E-16, -4.999999999999998224 ) ) ;
#23431=CARTESIAN_POINT ( 'NONE',  ( 22.50000000000000000, -4.330127018922190985, -2.500000000000001332 ) ) ;
#23432=CARTESIAN_POINT ( 'NONE',  ( 20.03437500061451715, -4.541064518000419881, 2.621784821874995952 ) ) ;
#23433=CARTESIAN_POINT ( 'NONE',  ( 24.81562500061451715, 3.027376345333611329, 5.243569643749999010 ) ) ;
#23434=ORIENTED_EDGE ( 'NONE', *, *, #56915, .F. ) ;
#23435=CARTESIAN_POINT ( 'NONE',  ( -3.999999999999999112, 16.96250000122903145, 30.00000000000000000 ) ) ;
#23436=CARTESIAN_POINT ( 'NONE',  ( 9.178125000614517859, -4.541064518000419881, 2.621784821874995952 ) ) ;
#23438=CARTESIAN_POINT ( 'NONE',  ( 14.92500000000000071, 6.123233995736764310E-16, -4.999999999999998224 ) ) ;
#23439=CARTESIAN_POINT ( 'NONE',  ( 4.243569643749999898, 16.42812500061451786, 30.00000000000000000 ) ) ;
#23440=CARTESIAN_POINT ( 'NONE',  ( 29.65312500061451573, 4.541064518000418104, -2.621784821874998173 ) ) ;
#23442=CARTESIAN_POINT ( 'NONE',  ( 27.04687500061451644, 6.054752690667223547, 3.707466751127219781E-16 ) ) ;
#23443=ORIENTED_EDGE ( 'NONE', *, *, #71959, .T. ) ;
#23444=CARTESIAN_POINT ( 'NONE',  ( 23.84062500061451928, 6.054752690667223547, 3.707466751127219781E-16 ) ) ;
#23445=CARTESIAN_POINT ( 'NONE',  ( 24.75937500061451502, 4.541064518000418104, -2.621784821874998173 ) ) ;
#23446=CARTESIAN_POINT ( 'NONE',  ( -3.000416591977282496E-16, 18.79062500061459318, -34.90005215228797653 ) ) ;
#23447=CARTESIAN_POINT ( 'NONE',  ( 12.03749999999999964, -2.886751345948129988, 4.999999999999997335 ) ) ;
#23448=CARTESIAN_POINT ( 'NONE',  ( 9.140625000614518214, -3.027376345333614438, 5.243569643749998122 ) ) ;
#23450=CARTESIAN_POINT ( 'NONE',  ( 29.20312500061451644, 4.541064518000418104, -2.621784821874998173 ) ) ;
#23451=CARTESIAN_POINT ( 'NONE',  ( 26.50312500061451360, 4.541064518000418104, -2.621784821874998173 ) ) ;
#23455=CARTESIAN_POINT ( 'NONE',  ( 20.33437500061451786, 4.541064518000418104, 2.621784821874999949 ) ) ;
#23456=CARTESIAN_POINT ( 'NONE',  ( -3.000416591977282496E-16, 12.99687500061451750, 25.09994784771203058 ) ) ;
#23457=CARTESIAN_POINT ( 'NONE',  ( 20.25937500061451857, 4.541064518000418104, -2.621784821874998173 ) ) ;
#23458=CARTESIAN_POINT ( 'NONE',  ( 26.78437500061451360, -4.541064518000419881, 2.621784821874995952 ) ) ;
#23459=CARTESIAN_POINT ( 'NONE',  ( 2.121784821875001281, 16.40937500061452070, 33.67503911421598417 ) ) ;
#23460=CARTESIAN_POINT ( 'NONE',  ( 6.553125000614518747, -4.541064518000417216, -2.621784821875001281 ) ) ;
#23461=CARTESIAN_POINT ( 'NONE',  ( -2.556497649636125342E-15, 19.21250000000000213, 34.00000000000000000 ) ) ;
#23462=CARTESIAN_POINT ( 'NONE',  ( 3.609375000614516882, 4.541064518000418104, -2.621784821874998173 ) ) ;
#23463=DIRECTION ( 'NONE',  ( 0.000000000000000000, 0.000000000000000000, 1.000000000000000000 ) ) ;
#23464=CARTESIAN_POINT ( 'NONE',  ( 5.690625000614516260, -3.027376345333610441, -5.243569643749999898 ) ) ;
#23465=CARTESIAN_POINT ( 'NONE',  ( 9.121875000614517504, 3.027376345333611329, 5.243569643749999010 ) ) ;
#23466=( NAMED_UNIT ( * ) PLANE_ANGLE_UNIT ( ) SI_UNIT ( $, .RADIAN. ) );
#23467=CARTESIAN_POINT ( 'NONE',  ( 18.37500000122903288, 2.886751345948126879, 4.999999999999999112 ) ) ;
#23468=CARTESIAN_POINT ( 'NONE',  ( 6.309375000614517504, 4.541064518000418104, -2.621784821874998173 ) ) ;
#23469=CARTESIAN_POINT ( 'NONE',  ( 7.528125000614515727, 6.421520780324663323E-16, -5.243569643749999010 ) ) ;
#23470=CARTESIAN_POINT ( 'NONE',  ( 4.844509297411973670, 1.237226603047926421, -5.095516945469514170 ) ) ;
#23472=CARTESIAN_POINT ( 'NONE',  ( 17.82187500061451502, -6.054752690667223547, -1.112240025338166033E-15 ) ) ;
#23473=CARTESIAN_POINT ( 'NONE',  ( 0.000000000000000000, 20.00000000000000000, -30.00000000000000000 ) ) ;
#23474=VERTEX_POINT ( 'NONE', #64484 ) ;
#23475=CARTESIAN_POINT ( 'NONE',  ( 24.21562500061451573, 3.027376345333613106, -5.243569643749998122 ) ) ;
#23476=CARTESIAN_POINT ( 'NONE',  ( 10.82812500061451644, 4.541064518000418104, 2.621784821874999949 ) ) ;
#23477=CARTESIAN_POINT ( 'NONE',  ( 26.52187500061451431, 3.027376345333612662, -5.243569643749998122 ) ) ;
#23478=CARTESIAN_POINT ( 'NONE',  ( 10.56562500061451715, -6.054752690667223547, -1.112240025338166033E-15 ) ) ;
#23479=CARTESIAN_POINT ( 'NONE',  ( 4.243569643749999898, 10.63437500061451857, -30.00000000000000000 ) ) ;
#23480=CARTESIAN_POINT ( 'NONE',  ( 13.08750000122903323, -4.330127018922194537, 2.499999999999995559 ) ) ;
#23481=CARTESIAN_POINT ( 'NONE',  ( 26.46562500061451573, 3.027376345333613106, -5.243569643749998122 ) ) ;
#23482=CARTESIAN_POINT ( 'NONE',  ( 4.243569643749999898, 11.92812500061451608, -30.00000000000000000 ) ) ;
#23483=CARTESIAN_POINT ( 'NONE',  ( 13.53750000122903430, -4.330127018922194537, 2.499999999999995559 ) ) ;
#23484=CARTESIAN_POINT ( 'NONE',  ( 11.10000000000000142, 0.000000000000000000, 4.999999999999998224 ) ) ;
#23485=CARTESIAN_POINT ( 'NONE',  ( 21.21562500061451573, 3.027376345333611329, 5.243569643749999010 ) ) ;
#23486=CARTESIAN_POINT ( 'NONE',  ( 5.709375000614517859, -4.541064518000417216, -2.621784821875001281 ) ) ;
#23487=CARTESIAN_POINT ( 'NONE',  ( 19.57500000000000284, 4.330127018922191873, 2.499999999999999556 ) ) ;
#23488=CARTESIAN_POINT ( 'NONE',  ( 9.000000001229034652, -2.886751345948129988, 4.999999999999997335 ) ) ;
#23489=CARTESIAN_POINT ( 'NONE',  ( 16.91250000122903430, 4.330127018922192761, -2.499999999999997780 ) ) ;
#23490=CARTESIAN_POINT ( 'NONE',  ( 13.30312500061451786, -4.541064518000417216, -2.621784821875001281 ) ) ;
#23491=CARTESIAN_POINT ( 'NONE',  ( 15.74062500061451608, 6.054752690667223547, 3.707466751127219781E-16 ) ) ;
#23492=CARTESIAN_POINT ( 'NONE',  ( 26.81250000122903288, 4.330127018922192761, -2.499999999999997780 ) ) ;
#23493=CARTESIAN_POINT ( 'NONE',  ( 19.98749999999999716, 5.773502691896255534, 3.535250795749688894E-16 ) ) ;
#23494=CARTESIAN_POINT ( 'NONE',  ( 23.59687500061451715, -3.027376345333614438, 5.243569643749998122 ) ) ;
#23496=CARTESIAN_POINT ( 'NONE',  ( 10.35000000122903074, -2.886751345948129988, 4.999999999999997335 ) ) ;
#23497=CARTESIAN_POINT ( 'NONE',  ( 9.496875000614517504, 6.054752690667223547, 3.707466751127219781E-16 ) ) ;
#23498=CARTESIAN_POINT ( 'NONE',  ( 25.62187500061451573, 3.027376345333613106, -5.243569643749998122 ) ) ;
#23499=CARTESIAN_POINT ( 'NONE',  ( 3.721875000614518036, 3.027376345333611329, 5.243569643749999010 ) ) ;
#23500=CARTESIAN_POINT ( 'NONE',  ( 24.17812500061451786, 6.421520780324663323E-16, -5.243569643749999010 ) ) ;
#23501=CARTESIAN_POINT ( 'NONE',  ( 26.25937500061451857, 0.000000000000000000, 5.243569643749999010 ) ) ;
#23503=CARTESIAN_POINT ( 'NONE',  ( 3.193392017337676414, -3.847432258030384578, 3.242174253483891544 ) ) ;
#23504=CARTESIAN_POINT ( 'NONE',  ( 6.909375000614518036, 0.000000000000000000, 5.243569643749999010 ) ) ;
#23505=CARTESIAN_POINT ( 'NONE',  ( -1.394453263437886801E-15, 19.32500000122903216, 33.99999999999999289 ) ) ;
#23506=CARTESIAN_POINT ( 'NONE',  ( 28.22812500061451502, 6.421520780324663323E-16, -5.243569643749999010 ) ) ;
#23507=CARTESIAN_POINT ( 'NONE',  ( 6.534375000614517148, -4.541064518000419881, 2.621784821874995952 ) ) ;
#23508=CARTESIAN_POINT ( 'NONE',  ( 25.72499999999999787, 6.123233995736764310E-16, -4.999999999999998224 ) ) ;
#23510=CARTESIAN_POINT ( 'NONE',  ( 18.26249999999999929, 2.886751345948126879, 4.999999999999999112 ) ) ;
#23512=CARTESIAN_POINT ( 'NONE',  ( 27.86249999999999716, -5.773502691896255534, -1.060575238724906372E-15 ) ) ;
#23513=CARTESIAN_POINT ( 'NONE',  ( 29.07187500061451502, -6.054752690667223547, -1.112240025338166033E-15 ) ) ;
#23514=ORIENTED_EDGE ( 'NONE', *, *, #4619, .T. ) ;
#23515=CARTESIAN_POINT ( 'NONE',  ( 15.66562500061451857, 3.027376345333613106, -5.243569643749998122 ) ) ;
#23516=CARTESIAN_POINT ( 'NONE',  ( 6.553125000614518747, -4.541064518000417216, -2.621784821875001281 ) ) ;
#23518=CARTESIAN_POINT ( 'NONE',  ( 4.771875000614516971, -6.054752690667223547, -1.112240025338166033E-15 ) ) ;
#23519=CARTESIAN_POINT ( 'NONE',  ( 14.81250000122903288, 0.000000000000000000, 4.999999999999998224 ) ) ;
#23520=CARTESIAN_POINT ( 'NONE',  ( 21.41250000000000497, 2.886751345948126879, 4.999999999999999112 ) ) ;
#23521=CARTESIAN_POINT ( 'NONE',  ( 29.43750000000000000, 5.773502691896255534, 3.535250795749688894E-16 ) ) ;
#23522=CARTESIAN_POINT ( 'NONE',  ( 4.321875000614517681, -6.054752690667223547, -1.112240025338166033E-15 ) ) ;
#23523=CARTESIAN_POINT ( 'NONE',  ( 8.184375000614515727, 4.541064518000418104, 2.621784821874999949 ) ) ;
#23524=CARTESIAN_POINT ( 'NONE',  ( 20.89687500061452141, -3.027376345333614438, 5.243569643749998122 ) ) ;
#23525=CARTESIAN_POINT ( 'NONE',  ( 4.898587196589411843E-16, 20.00000000000000000, 33.99999999999999289 ) ) ;
#23526=ORIENTED_EDGE ( 'NONE', *, *, #27624, .F. ) ;
#23527=CARTESIAN_POINT ( 'NONE',  ( 2.971875000614517592, -6.054752690667223547, -1.112240025338166033E-15 ) ) ;
#23528=CARTESIAN_POINT ( 'NONE',  ( 5.512499999999999289, 2.886751345948129099, -4.999999999999998224 ) ) ;
#23529=CARTESIAN_POINT ( 'NONE',  ( 6.384375000614516793, 4.541064518000418104, 2.621784821874999949 ) ) ;
#23530=CARTESIAN_POINT ( 'NONE',  ( 18.63749999999999929, 5.773502691896255534, 3.535250795749688894E-16 ) ) ;
#23531=CARTESIAN_POINT ( 'NONE',  ( 15.59062500061451573, -3.027376345333610441, -5.243569643749999898 ) ) ;
#23533=CARTESIAN_POINT ( 'NONE',  ( 4.169580978743460342, 2.759455464706926708, 4.458747374224691029 ) ) ;
#23535=CARTESIAN_POINT ( 'NONE',  ( 10.22812500061451679, 6.421520780324663323E-16, -5.243569643749999010 ) ) ;
#23536=CARTESIAN_POINT ( 'NONE',  ( 27.23437500061451644, -4.541064518000419881, 2.621784821874995952 ) ) ;
#23537=CARTESIAN_POINT ( 'NONE',  ( 2.121784821875001281, 19.55937500061451573, 33.67503911421598417 ) ) ;
#23538=CARTESIAN_POINT ( 'NONE',  ( 26.85937500061451644, -4.541064518000417216, -2.621784821875001281 ) ) ;
#23539=CARTESIAN_POINT ( 'NONE',  ( 7.612500000000000711, -5.773502691896255534, -1.060575238724906372E-15 ) ) ;
#23540=CARTESIAN_POINT ( 'NONE',  ( -3.999999999999999112, 13.36250000122903359, 30.00000000000000000 ) ) ;
#23541=CARTESIAN_POINT ( 'NONE',  ( 14.42812500061451786, 4.541064518000418104, 2.621784821874999949 ) ) ;
#23542=CARTESIAN_POINT ( 'NONE',  ( 7.575000001229033053, 2.886751345948126879, 4.999999999999999112 ) ) ;
#23543=CARTESIAN_POINT ( 'NONE',  ( 18.34687500061451715, -3.027376345333610441, -5.243569643749999898 ) ) ;
#23544=CARTESIAN_POINT ( 'NONE',  ( 12.45937500061451786, -4.541064518000417216, -2.621784821875001281 ) ) ;
#23545=CARTESIAN_POINT ( 'NONE',  ( 4.898587196589411843E-16, 20.00000000000000000, -26.00000000000000000 ) ) ;
#23546=ORIENTED_EDGE ( 'NONE', *, *, #20108, .F. ) ;
#23547=CARTESIAN_POINT ( 'NONE',  ( 14.12812500061451715, -4.541064518000419881, 2.621784821874995952 ) ) ;
#23548=CARTESIAN_POINT ( 'NONE',  ( 26.32500000122903216, 2.886751345948129099, -4.999999999999998224 ) ) ;
#23549=CARTESIAN_POINT ( 'NONE',  ( 13.35937500061451821, -4.541064518000417216, -2.621784821875001281 ) ) ;
#23552=CARTESIAN_POINT ( 'NONE',  ( 15.06562500061451537, -6.054752690667223547, -1.112240025338166033E-15 ) ) ;
#23554=CARTESIAN_POINT ( 'NONE',  ( 23.93437500061451573, 4.541064518000418104, 2.621784821874999949 ) ) ;
#23555=CARTESIAN_POINT ( 'NONE',  ( -1.473776270879187500, 9.816672227264547246, 25.95083297442941017 ) ) ;
#23557=CARTESIAN_POINT ( 'NONE',  ( 10.98750000122903536, 6.123233995736764310E-16, -4.999999999999998224 ) ) ;
#23559=CARTESIAN_POINT ( 'NONE',  ( 20.66250000122903074, 0.000000000000000000, 4.999999999999998224 ) ) ;
#23560=CARTESIAN_POINT ( 'NONE',  ( 2.121784821875001281, 17.30937500061451573, -26.32496088578401938 ) ) ;
#23561=( BOUNDED_CURVE ( )  B_SPLINE_CURVE ( 2, ( #60780, #10912, #38999, #48988, #67083, #66335, #55983 ),
 .UNSPECIFIED., .F., .F. ) 
 B_SPLINE_CURVE_WITH_KNOTS ( ( 3, 2, 2, 3 ),
 ( 0.8166666666666666519, 0.8194444444444444198, 0.8222222222222222987, 0.8250000000000000666 ),
 .UNSPECIFIED. ) 
 CURVE ( )  GEOMETRIC_REPRESENTATION_ITEM ( )  RATIONAL_B_SPLINE_CURVE ( ( 1.000000000000000000, 0.8660254037844387076, 1.000000000000000000, 0.8660254037844387076, 1.000000000000000000, 0.8660254037844333785, 1.000000000000005329 ) ) 
 REPRESENTATION_ITEM ( '' )  );
#23562=CARTESIAN_POINT ( 'NONE',  ( 17.37187500061451573, -6.054752690667223547, -1.112240025338166033E-15 ) ) ;
#23563=CARTESIAN_POINT ( 'NONE',  ( 19.76250000122903216, 0.000000000000000000, 4.999999999999998224 ) ) ;
#23564=ADVANCED_FACE ( 'NONE', ( #63400 ), #12785, .F. ) ;
#23565=CARTESIAN_POINT ( 'NONE',  ( 15.79687500061451821, 6.054752690667223547, 3.707466751127219781E-16 ) ) ;
#23566=CARTESIAN_POINT ( 'NONE',  ( 4.243569643749999898, 10.18437500061451750, 30.00000000000000000 ) ) ;
#23567=CARTESIAN_POINT ( 'NONE',  ( 19.01250000122903216, -4.330127018922190985, -2.500000000000001332 ) ) ;
#23568=CARTESIAN_POINT ( 'NONE',  ( 15.21562500061451750, 3.027376345333613106, -5.243569643749998122 ) ) ;
#23569=CARTESIAN_POINT ( 'NONE',  ( 29.57812500061451644, 6.421520780324663323E-16, -5.243569643749999010 ) ) ;
#23572=CARTESIAN_POINT ( 'NONE',  ( 18.33749999999999858, -2.886751345948129988, 4.999999999999997335 ) ) ;
#23574=CARTESIAN_POINT ( 'NONE',  ( 2.485350534231654862, 4.344988454211105022, 33.14460541871455490 ) ) ;
#23575=CARTESIAN_POINT ( 'NONE',  ( 15.75000000122902932, -2.886751345948129988, 4.999999999999997335 ) ) ;
#23576=CARTESIAN_POINT ( 'NONE',  ( 27.72187500061451715, -6.054752690667223547, -1.112240025338166033E-15 ) ) ;
#23577=CARTESIAN_POINT ( 'NONE',  ( 20.46562500061451928, -6.054752690667223547, -1.112240025338166033E-15 ) ) ;
#23578=CARTESIAN_POINT ( 'NONE',  ( 21.96562500061451573, 3.027376345333613106, -5.243569643749998122 ) ) ;
#23579=CARTESIAN_POINT ( 'NONE',  ( 3.590625000614518836, 6.054752690667223547, 3.707466751127219781E-16 ) ) ;
#23580=CARTESIAN_POINT ( 'NONE',  ( 28.04999999999999716, 4.330127018922192761, -2.499999999999997780 ) ) ;
#23581=CARTESIAN_POINT ( 'NONE',  ( 4.000000000000000000, 11.75000000122903643, 32.30940107675849760 ) ) ;
#23584=CARTESIAN_POINT ( 'NONE',  ( -3.999999999999997335, 12.50000000122903465, -27.69059892324149175 ) ) ;
#23585=CARTESIAN_POINT ( 'NONE',  ( -4.243569643749999898, 16.67187500061451644, -32.45002607614398471 ) ) ;
#23586=CARTESIAN_POINT ( 'NONE',  ( 5.100000001229034297, -2.886751345948125991, -5.000000000000000000 ) ) ;
#23587=CARTESIAN_POINT ( 'NONE',  ( 5.062500000000000888, 2.886751345948129099, -4.999999999999998224 ) ) ;
#23588=CARTESIAN_POINT ( 'NONE',  ( 3.337500001229034563, 6.123233995736764310E-16, -4.999999999999998224 ) ) ;
#23589=CARTESIAN_POINT ( 'NONE',  ( 9.909375000614517148, 4.541064518000418104, -2.621784821874998173 ) ) ;
#23590=CARTESIAN_POINT ( 'NONE',  ( 23.81250000122903288, 0.000000000000000000, 4.999999999999998224 ) ) ;
#23591=CYLINDRICAL_SURFACE ( 'NONE', #68081, 4.999999999999998224 ) ;
#23593=CARTESIAN_POINT ( 'NONE',  ( -1.071796769724490561, 19.57009619066136707, -34.00000000000000000 ) ) ;
#23594=CARTESIAN_POINT ( 'NONE',  ( 6.609375000614519102, -4.541064518000417216, -2.621784821875001281 ) ) ;
#23595=CARTESIAN_POINT ( 'NONE',  ( 12.45937500061451786, -4.541064518000417216, -2.621784821875001281 ) ) ;
#23596=CARTESIAN_POINT ( 'NONE',  ( 5.587500000000003020, 5.773502691896255534, 3.535250795749688894E-16 ) ) ;
#23597=( BOUNDED_CURVE ( )  B_SPLINE_CURVE ( 2, ( #35631, #46731, #2034, #24545, #953, #63702, #69623, #13093, #58152 ),
 .UNSPECIFIED., .F., .F. ) 
 B_SPLINE_CURVE_WITH_KNOTS ( ( 3, 2, 2, 2, 3 ),
 ( 0.3586956521739130821, 0.3623188405797101441, 0.3695652173913043237, 0.3768115942028985588, 0.3804347826086956763 ),
 .UNSPECIFIED. ) 
 CURVE ( )  GEOMETRIC_REPRESENTATION_ITEM ( )  RATIONAL_B_SPLINE_CURVE ( ( 0.9330127018922194093, 0.9330127018922198534, 1.000000000000000000, 0.8660254037844387076, 1.000000000000000000, 0.8660254037844387076, 1.000000000000000000, 0.9330127018922188542, 0.9330127018922194093 ) ) 
 REPRESENTATION_ITEM ( '' )  );
#23598=CARTESIAN_POINT ( 'NONE',  ( -4.243569643749999898, 17.51562500061459460, 27.54997392385601529 ) ) ;
#23599=CARTESIAN_POINT ( 'NONE',  ( 21.42187500061451644, -6.054752690667223547, -1.112240025338166033E-15 ) ) ;
#23600=DIRECTION ( 'NONE',  ( 0.000000000000000000, 0.000000000000000000, -1.000000000000000000 ) ) ;
#23601=CARTESIAN_POINT ( 'NONE',  ( 26.51250000122903216, 0.000000000000000000, 4.999999999999998224 ) ) ;
#23603=CARTESIAN_POINT ( 'NONE',  ( 22.19062500061451715, -3.027376345333614438, 5.243569643749998122 ) ) ;
#23604=CARTESIAN_POINT ( 'NONE',  ( 13.67812500061451786, -4.541064518000419881, 2.621784821874995952 ) ) ;
#23606=CARTESIAN_POINT ( 'NONE',  ( 11.37187500061451750, 3.027376345333611329, 5.243569643749999010 ) ) ;
#23607=CARTESIAN_POINT ( 'NONE',  ( 28.19999999999999929, 0.000000000000000000, 4.999999999999998224 ) ) ;
#23608=CARTESIAN_POINT ( 'NONE',  ( 21.52500000122903145, 2.886751345948126879, 4.999999999999999112 ) ) ;
#23610=CARTESIAN_POINT ( 'NONE',  ( 12.45937500061451786, -4.541064518000417216, -2.621784821875001281 ) ) ;
#23613=CARTESIAN_POINT ( 'NONE',  ( 22.92187500061451644, 3.027376345333613106, -5.243569643749998122 ) ) ;
#23614=CARTESIAN_POINT ( 'NONE',  ( 13.13437500061451857, 4.541064518000418104, 2.621784821874999949 ) ) ;
#23616=CARTESIAN_POINT ( 'NONE',  ( 25.50000000000000000, 0.000000000000000000, 4.999999999999998224 ) ) ;
#23619=CARTESIAN_POINT ( 'NONE',  ( 16.94062500061451715, -3.027376345333610441, -5.243569643749999898 ) ) ;
#23620=CARTESIAN_POINT ( 'NONE',  ( 6.637500000000001066, -2.886751345948129988, 4.999999999999997335 ) ) ;
#23621=CARTESIAN_POINT ( 'NONE',  ( 3.999999999999998668, 13.62500000122903465, 27.69059892324149530 ) ) ;
#23622=CARTESIAN_POINT ( 'NONE',  ( 14.88750000000000107, -2.886751345948125991, -5.000000000000000000 ) ) ;
#23623=CARTESIAN_POINT ( 'NONE',  ( 2.121784821875001281, 11.40312500061451750, 33.67503911421598417 ) ) ;
#23624=( BOUNDED_CURVE ( )  B_SPLINE_CURVE ( 2, ( #4114, #15532, #54711, #27735, #21810, #16268, #38823, #10007, #49541 ),
 .UNSPECIFIED., .F., .F. ) 
 B_SPLINE_CURVE_WITH_KNOTS ( ( 3, 2, 2, 2, 3 ),
 ( 0.2500000000000000000, 0.2536231884057971175, 0.2608695652173912971, 0.2681159420289855322, 0.2717391304347826497 ),
 .UNSPECIFIED. ) 
 CURVE ( )  GEOMETRIC_REPRESENTATION_ITEM ( )  RATIONAL_B_SPLINE_CURVE ( ( 0.9330127018922194093, 0.9330127018922190762, 1.000000000000000000, 0.8660254037844387076, 1.000000000000000000, 0.8660254037844387076, 1.000000000000000000, 0.9330127018922188542, 0.9330127018922194093 ) ) 
 REPRESENTATION_ITEM ( '' )  );
#23626=CARTESIAN_POINT ( 'NONE',  ( 23.59687500061451715, -3.027376345333614438, 5.243569643749998122 ) ) ;
#23627=VERTEX_POINT ( 'NONE', #41241 ) ;
#23628=CARTESIAN_POINT ( 'NONE',  ( 21.51562500061451644, 3.027376345333613106, -5.243569643749998122 ) ) ;
#23629=CARTESIAN_POINT ( 'NONE',  ( 20.97187500061451715, -6.054752690667223547, -1.112240025338166033E-15 ) ) ;
#23630=CARTESIAN_POINT ( 'NONE',  ( 4.724999999999999645, 4.330127018922191873, 2.499999999999999556 ) ) ;
#23631=CARTESIAN_POINT ( 'NONE',  ( 6.178125000614518747, 6.421520780324663323E-16, -5.243569643749999010 ) ) ;
#23632=CARTESIAN_POINT ( 'NONE',  ( 21.10312500061451502, 4.541064518000418104, -2.621784821874998173 ) ) ;
#23633=CARTESIAN_POINT ( 'NONE',  ( 12.27187500061451786, 3.027376345333611329, 5.243569643749999010 ) ) ;
#23634=CARTESIAN_POINT ( 'NONE',  ( 16.99687500061451573, -3.027376345333610441, -5.243569643749999898 ) ) ;
#23635=CARTESIAN_POINT ( 'NONE',  ( -2.121784821874996840, 17.62812500061451715, 33.67503911421598417 ) ) ;
#23636=CARTESIAN_POINT ( 'NONE',  ( 19.31250000122903288, 0.000000000000000000, 4.999999999999998224 ) ) ;
#23638=CARTESIAN_POINT ( 'NONE',  ( 10.19062500061451715, -3.027376345333610441, -5.243569643749999898 ) ) ;
#23639=CARTESIAN_POINT ( 'NONE',  ( 5.446875000614518569, 6.054752690667223547, 3.707466751127219781E-16 ) ) ;
#23640=CARTESIAN_POINT ( 'NONE',  ( 5.746875000614517504, -3.027376345333610441, -5.243569643749999898 ) ) ;
#23641=CARTESIAN_POINT ( 'NONE',  ( 25.99687500061451928, -3.027376345333610441, -5.243569643749999898 ) ) ;
#23642=CARTESIAN_POINT ( 'NONE',  ( 16.75312500061451715, 0.000000000000000000, 5.243569643749999010 ) ) ;
#23643=CARTESIAN_POINT ( 'NONE',  ( 27.45000000122903572, -2.886751345948129988, 4.999999999999997335 ) ) ;
#23644=EDGE_CURVE ( 'NONE', #46924, #26808, #7608, .T. ) ;
#23645=CARTESIAN_POINT ( 'NONE',  ( 24.47812500061451502, -4.541064518000419881, 2.621784821874995952 ) ) ;
#23646=CARTESIAN_POINT ( 'NONE',  ( 22.35937500061451644, -4.541064518000417216, -2.621784821875001281 ) ) ;
#23647=CARTESIAN_POINT ( 'NONE',  ( 17.72812500061451502, -4.541064518000419881, 2.621784821874995952 ) ) ;
#23648=CARTESIAN_POINT ( 'NONE',  ( -3.000416591977282496E-16, 17.49687500061451573, 25.09994784771203058 ) ) ;
#23649=( BOUNDED_CURVE ( )  B_SPLINE_CURVE ( 2, ( #48134, #36675, #65483, #9342, #24854, #26331, #64382, #30411, #25597 ),
 .UNSPECIFIED., .F., .F. ) 
 B_SPLINE_CURVE_WITH_KNOTS ( ( 3, 2, 2, 2, 3 ),
 ( 0.4891304347826087029, 0.4927536231884058204, 0.5000000000000000000, 0.5072463768115942351, 0.5108695652173913526 ),
 .UNSPECIFIED. ) 
 CURVE ( )  GEOMETRIC_REPRESENTATION_ITEM ( )  RATIONAL_B_SPLINE_CURVE ( ( 0.9330127018922194093, 0.9330127018922194093, 1.000000000000000000, 0.8660254037844387076, 1.000000000000000000, 0.8660254037844387076, 1.000000000000000000, 0.9330127018922182991, 0.9330127018922192983 ) ) 
 REPRESENTATION_ITEM ( '' )  );
#23650=CARTESIAN_POINT ( 'NONE',  ( 21.32812500061451644, -4.541064518000419881, 2.621784821874995952 ) ) ;
#23653=CARTESIAN_POINT ( 'NONE',  ( 25.46249999999999858, 2.886751345948126879, 4.999999999999999112 ) ) ;
#23654=CARTESIAN_POINT ( 'NONE',  ( 8.484601909799253346E-16, 12.91249999999999964, -25.38119784648299770 ) ) ;
#23656=CARTESIAN_POINT ( 'NONE',  ( 29.76562500061451644, 3.027376345333611329, 5.243569643749999010 ) ) ;
#23657=CARTESIAN_POINT ( 'NONE',  ( 10.60312500061451679, -4.541064518000417216, -2.621784821875001281 ) ) ;
#23658=CARTESIAN_POINT ( 'NONE',  ( 23.06250000122903288, -4.330127018922190985, -2.500000000000001332 ) ) ;
#23659=CARTESIAN_POINT ( 'NONE',  ( 26.80312500061451431, -4.541064518000417216, -2.621784821875001281 ) ) ;
#23660=CARTESIAN_POINT ( 'NONE',  ( 26.96249999999999858, -5.773502691896255534, -1.060575238724906372E-15 ) ) ;
#23661=CARTESIAN_POINT ( 'NONE',  ( 8.484601909799253346E-16, 16.17500000122903003, -25.38119784648299770 ) ) ;
#23662=CARTESIAN_POINT ( 'NONE',  ( 29.72812500061451502, 4.541064518000418104, 2.621784821874999949 ) ) ;
#23663=CARTESIAN_POINT ( 'NONE',  ( 11.61562500061451608, 3.027376345333613106, -5.243569643749998122 ) ) ;
#23664=EDGE_LOOP ( 'NONE', ( #30910, #51367, #27739, #53940 ) ) ;
#23665=CARTESIAN_POINT ( 'NONE',  ( 25.22812500061451502, 4.541064518000418104, 2.621784821874999949 ) ) ;
#23666=CARTESIAN_POINT ( 'NONE',  ( 7.565625000614518036, 3.027376345333613106, -5.243569643749998122 ) ) ;
#23667=CARTESIAN_POINT ( 'NONE',  ( 6.703125000614516438, 4.541064518000418104, -2.621784821874998173 ) ) ;
#23669=CARTESIAN_POINT ( 'NONE',  ( 4.640987789384291240, -1.860506746819186041, 4.902426613311977377 ) ) ;
#23670=CARTESIAN_POINT ( 'NONE',  ( 16.23750000000000071, -2.886751345948125991, -5.000000000000000000 ) ) ;
#23671=CARTESIAN_POINT ( 'NONE',  ( 15.08437500061451786, -4.541064518000419881, 2.621784821874995952 ) ) ;
#23672=CARTESIAN_POINT ( 'NONE',  ( 12.45000000122903394, 5.773502691896255534, 3.535250795749688894E-16 ) ) ;
#23673=CARTESIAN_POINT ( 'NONE',  ( 16.02187500061451786, -6.054752690667223547, -1.112240025338166033E-15 ) ) ;
#23675=CARTESIAN_POINT ( 'NONE',  ( 20.25937500061451857, 4.541064518000418104, -2.621784821874998173 ) ) ;
#23676=CARTESIAN_POINT ( 'NONE',  ( 9.001249775931846008E-16, 14.06562500061451715, -25.09994784771203058 ) ) ;
#23680=CARTESIAN_POINT ( 'NONE',  ( 25.15312500061451217, 4.541064518000418104, -2.621784821874998173 ) ) ;
#23681=CARTESIAN_POINT ( 'NONE',  ( 27.45937500061451786, 4.541064518000418104, -2.621784821874998173 ) ) ;
#23682=CARTESIAN_POINT ( 'NONE',  ( 24.41250000000000142, 2.886751345948129099, -4.999999999999998224 ) ) ;
#23683=CARTESIAN_POINT ( 'NONE',  ( 7.678125000614516082, 4.541064518000418104, 2.621784821874999949 ) ) ;
#23685=CARTESIAN_POINT ( 'NONE',  ( 19.24687500061452283, -3.027376345333610441, -5.243569643749999898 ) ) ;
#23687=CARTESIAN_POINT ( 'NONE',  ( 6.328125000614515550, 4.541064518000418104, 2.621784821874999949 ) ) ;
#23688=CARTESIAN_POINT ( 'NONE',  ( 8.221875000614518925, 3.027376345333611329, 5.243569643749999010 ) ) ;
#23690=CARTESIAN_POINT ( 'NONE',  ( 19.84687500061451360, 6.054752690667223547, 3.707466751127219781E-16 ) ) ;
#23691=CYLINDRICAL_SURFACE ( 'NONE', #4261, 4.999999999999998224 ) ;
#23692=CARTESIAN_POINT ( 'NONE',  ( 26.09999999999999787, -4.330127018922190985, -2.500000000000001332 ) ) ;
#23693=CARTESIAN_POINT ( 'NONE',  ( 29.67187500061451644, 3.027376345333613106, -5.243569643749998122 ) ) ;
#23697=CARTESIAN_POINT ( 'NONE',  ( 10.42500000000000071, 6.123233995736764310E-16, -4.999999999999998224 ) ) ;
#23699=CARTESIAN_POINT ( 'NONE',  ( 25.45312500061451644, -4.541064518000417216, -2.621784821875001281 ) ) ;
#23700=CARTESIAN_POINT ( 'NONE',  ( 13.35000000000000142, 0.000000000000000000, 4.999999999999998224 ) ) ;
#23701=CARTESIAN_POINT ( 'NONE',  ( 10.61250000122903536, 4.330127018922192761, -2.499999999999997780 ) ) ;
#23702=CARTESIAN_POINT ( 'NONE',  ( 9.478125000614515017, 4.541064518000418104, 2.621784821874999949 ) ) ;
#23703=CARTESIAN_POINT ( 'NONE',  ( 22.31250000000000000, 2.886751345948126879, 4.999999999999999112 ) ) ;
#23704=CARTESIAN_POINT ( 'NONE',  ( 20.69062500061451715, 6.054752690667223547, 3.707466751127219781E-16 ) ) ;
#23705=CARTESIAN_POINT ( 'NONE',  ( 26.25000000122903288, -2.886751345948125991, -5.000000000000000000 ) ) ;
#23707=CARTESIAN_POINT ( 'NONE',  ( 8.287499999999999645, 5.773502691896255534, 3.535250795749688894E-16 ) ) ;
#23708=ORIENTED_EDGE ( 'NONE', *, *, #798, .F. ) ;
#23709=CARTESIAN_POINT ( 'NONE',  ( 23.05312500061451431, 0.000000000000000000, 5.243569643749999010 ) ) ;
#23710=CARTESIAN_POINT ( 'NONE',  ( 29.69062500061451715, 6.054752690667223547, 3.707466751127219781E-16 ) ) ;
#23711=CARTESIAN_POINT ( 'NONE',  ( 26.18437500061451573, 4.541064518000418104, 2.621784821874999949 ) ) ;
#23712=CARTESIAN_POINT ( 'NONE',  ( 18.00937500061451502, 4.541064518000418104, -2.621784821874998173 ) ) ;
#23713=ADVANCED_FACE ( 'NONE', ( #27812 ), #61412, .F. ) ;
#23714=CARTESIAN_POINT ( 'NONE',  ( 13.26562500061451644, -6.054752690667223547, -1.112240025338166033E-15 ) ) ;
#23716=CARTESIAN_POINT ( 'NONE',  ( 25.61250000122903359, 0.000000000000000000, 4.999999999999998224 ) ) ;
#23718=CARTESIAN_POINT ( 'NONE',  ( 15.70312500061451644, 4.541064518000418104, -2.621784821874998173 ) ) ;
#23719=CARTESIAN_POINT ( 'NONE',  ( 30.00000000000000000, 0.000000000000000000, 0.000000000000000000 ) ) ;
#23720=CARTESIAN_POINT ( 'NONE',  ( 2.925000001229034918, 2.886751345948129099, -4.999999999999998224 ) ) ;
#23721=CARTESIAN_POINT ( 'NONE',  ( 11.93437500061451573, -4.541064518000419881, 2.621784821874995952 ) ) ;
#23722=CARTESIAN_POINT ( 'NONE',  ( 11.55937500061451928, -4.541064518000417216, -2.621784821875001281 ) ) ;
#23723=CARTESIAN_POINT ( 'NONE',  ( 18.98437500061451644, 4.541064518000418104, 2.621784821874999949 ) ) ;
#23724=VERTEX_POINT ( 'NONE', #33341 ) ;
#23725=CARTESIAN_POINT ( 'NONE',  ( 30.00000000000000000, 6.123233995736764310E-16, -4.999999999999998224 ) ) ;
#23726=CARTESIAN_POINT ( 'NONE',  ( 24.62812500061451715, 6.421520780324663323E-16, -5.243569643749999010 ) ) ;
#23727=CARTESIAN_POINT ( 'NONE',  ( 19.95937500061451786, 0.000000000000000000, 5.243569643749999010 ) ) ;
#23728=CARTESIAN_POINT ( 'NONE',  ( 24.81562500061451715, 3.027376345333611329, 5.243569643749999010 ) ) ;
#23730=CARTESIAN_POINT ( 'NONE',  ( -3.999999999999997335, 14.63750000000000107, 32.30940107675850470 ) ) ;
#23731=CARTESIAN_POINT ( 'NONE',  ( 29.76562500061451644, 3.027376345333611329, 5.243569643749999010 ) ) ;
#23732=CARTESIAN_POINT ( 'NONE',  ( 9.825000001229033941, 2.886751345948126879, 4.999999999999999112 ) ) ;
#23733=CARTESIAN_POINT ( 'NONE',  ( 4.762500001229033941, 4.330127018922192761, -2.499999999999997780 ) ) ;
#23735=CARTESIAN_POINT ( 'NONE',  ( 27.22500000122903430, 2.886751345948129099, -4.999999999999998224 ) ) ;
#23738=CARTESIAN_POINT ( 'NONE',  ( 10.58437500061451964, -4.541064518000419881, 2.621784821874995952 ) ) ;
#23739=CARTESIAN_POINT ( 'NONE',  ( 24.52499999999999858, 4.330127018922191873, 2.499999999999999556 ) ) ;
#23740=CARTESIAN_POINT ( 'NONE',  ( 17.76562500061451644, -6.054752690667223547, -1.112240025338166033E-15 ) ) ;
#23741=CARTESIAN_POINT ( 'NONE',  ( 10.39687500061451786, 6.054752690667223547, 3.707466751127219781E-16 ) ) ;
#23742=CARTESIAN_POINT ( 'NONE',  ( 28.27500000122903145, 2.886751345948126879, 4.999999999999999112 ) ) ;
#23743=CARTESIAN_POINT ( 'NONE',  ( 19.35937500061451644, 4.541064518000418104, -2.621784821874998173 ) ) ;
#23744=CARTESIAN_POINT ( 'NONE',  ( 8.484375000614518214, 6.421520780324663323E-16, -5.243569643749999010 ) ) ;
#23745=CARTESIAN_POINT ( 'NONE',  ( 14.88750000122903394, -4.330127018922194537, 2.499999999999995559 ) ) ;
#23747=CARTESIAN_POINT ( 'NONE',  ( 8.165625000614516793, 3.027376345333611329, 5.243569643749999010 ) ) ;
#23748=CARTESIAN_POINT ( 'NONE',  ( 18.44062500061451715, 6.054752690667223547, 3.707466751127219781E-16 ) ) ;
#23750=CARTESIAN_POINT ( 'NONE',  ( 5.400000001229032343, -2.886751345948129988, 4.999999999999997335 ) ) ;
#23751=CARTESIAN_POINT ( 'NONE',  ( 15.14062500061451644, -3.027376345333610441, -5.243569643749999898 ) ) ;
#23752=CARTESIAN_POINT ( 'NONE',  ( 13.75312500061451715, -4.541064518000417216, -2.621784821875001281 ) ) ;
#23754=CARTESIAN_POINT ( 'NONE',  ( 14.47499999999999964, 6.123233995736764310E-16, -4.999999999999998224 ) ) ;
#23755=CARTESIAN_POINT ( 'NONE',  ( 10.08750000122903323, 6.123233995736764310E-16, -4.999999999999998224 ) ) ;
#23756=CARTESIAN_POINT ( 'NONE',  ( 5.615625000614517859, -6.054752690667223547, -1.112240025338166033E-15 ) ) ;
#23757=CARTESIAN_POINT ( 'NONE',  ( 18.00000000122903288, -2.886751345948129988, 4.999999999999997335 ) ) ;
#23759=CARTESIAN_POINT ( 'NONE',  ( 2.121784821875001281, 11.00937500061451857, -26.32496088578401938 ) ) ;
#23762=CARTESIAN_POINT ( 'NONE',  ( 28.38750000122903216, -4.330127018922194537, 2.499999999999995559 ) ) ;
#23763=CARTESIAN_POINT ( 'NONE',  ( 7.320879633048903241E-15, 17.75000000122903288, 26.00000000000000355 ) ) ;
#23764=CARTESIAN_POINT ( 'NONE',  ( 18.45937500061451431, 4.541064518000418104, -2.621784821874998173 ) ) ;
#23765=AXIS2_PLACEMENT_3D ( 'NONE', #23100, #68190, #46012 ) ;
#23767=EDGE_CURVE ( 'NONE', #33656, #47420, #18517, .T. ) ;
#23768=CARTESIAN_POINT ( 'NONE',  ( 14.46562500061451750, 3.027376345333611329, 5.243569643749999010 ) ) ;
#23770=CYLINDRICAL_SURFACE ( 'NONE', #62519, 5.999999999999998224 ) ;
#23771=CARTESIAN_POINT ( 'NONE',  ( 25.80937500061451928, 0.000000000000000000, 5.243569643749999010 ) ) ;
#23773=CARTESIAN_POINT ( 'NONE',  ( 13.52812500061451750, 4.541064518000418104, 2.621784821874999949 ) ) ;
#23774=CARTESIAN_POINT ( 'NONE',  ( 16.69687500061451502, 6.054752690667223547, 3.707466751127219781E-16 ) ) ;
#23776=CARTESIAN_POINT ( 'NONE',  ( 26.99062500061451431, 6.054752690667223547, 3.707466751127219781E-16 ) ) ;
#23777=CARTESIAN_POINT ( 'NONE',  ( 20.69062500061451715, 6.054752690667223547, 3.707466751127219781E-16 ) ) ;
#23778=CARTESIAN_POINT ( 'NONE',  ( 3.101989702391181769, 3.921444007319114355, -3.480999103934488748 ) ) ;
#23779=ADVANCED_FACE ( 'NONE', ( #67340 ), #60303, .F. ) ;
#23781=CARTESIAN_POINT ( 'NONE',  ( 10.65000000000000036, 0.000000000000000000, 4.999999999999998224 ) ) ;
#23782=CARTESIAN_POINT ( 'NONE',  ( 18.48750000122903359, -4.330127018922194537, 2.499999999999995559 ) ) ;
#23783=CARTESIAN_POINT ( 'NONE',  ( 6.937500001229033764, 6.123233995736764310E-16, -4.999999999999998224 ) ) ;
#23786=CARTESIAN_POINT ( 'NONE',  ( 17.25000000000000000, 4.330127018922192761, -2.499999999999997780 ) ) ;
#23787=ADVANCED_FACE ( 'NONE', ( #16700 ), #39258, .F. ) ;
#23788=CARTESIAN_POINT ( 'NONE',  ( 20.66250000000000142, -5.773502691896255534, -1.060575238724906372E-15 ) ) ;
#23789=CARTESIAN_POINT ( 'NONE',  ( 19.58437500061451786, -4.541064518000419881, 2.621784821874995952 ) ) ;
#23790=CARTESIAN_POINT ( 'NONE',  ( 24.29062500061451502, 6.054752690667223547, 3.707466751127219781E-16 ) ) ;
#23793=CARTESIAN_POINT ( 'NONE',  ( 7.753125000614518036, 0.000000000000000000, 5.243569643749999010 ) ) ;
#23794=CARTESIAN_POINT ( 'NONE',  ( 3.234375000614516438, 4.541064518000418104, 2.621784821874999949 ) ) ;
#23795=CARTESIAN_POINT ( 'NONE',  ( 15.56250000000000000, 2.886751345948126879, 4.999999999999999112 ) ) ;
#23796=CARTESIAN_POINT ( 'NONE',  ( -2.121784821874999949, 16.57812500061451644, 26.32496088578401938 ) ) ;
#23797=CARTESIAN_POINT ( 'NONE',  ( 28.49062500061451431, -3.027376345333614438, 5.243569643749998122 ) ) ;
#23800=CARTESIAN_POINT ( 'NONE',  ( 25.24687500061451573, 6.054752690667223547, 3.707466751127219781E-16 ) ) ;
#23801=ORIENTED_EDGE ( 'NONE', *, *, #2612, .F. ) ;
#23802=CARTESIAN_POINT ( 'NONE',  ( 22.60312500061451857, 0.000000000000000000, 5.243569643749999010 ) ) ;
#23803=CARTESIAN_POINT ( 'NONE',  ( 23.07187500061451857, 3.027376345333611329, 5.243569643749999010 ) ) ;
#23804=CARTESIAN_POINT ( 'NONE',  ( 9.001249775931846008E-16, 16.76562500061459460, -25.09994784771203058 ) ) ;
#23805=CARTESIAN_POINT ( 'NONE',  ( 11.58750000000000036, -2.886751345948129988, 4.999999999999997335 ) ) ;
#23806=CARTESIAN_POINT ( 'NONE',  ( 5.390625000614518214, 6.054752690667223547, 3.707466751127219781E-16 ) ) ;
#23808=CARTESIAN_POINT ( 'NONE',  ( 23.12812500061451360, -4.541064518000419881, 2.621784821874995952 ) ) ;
#23811=CARTESIAN_POINT ( 'NONE',  ( 18.19687500061451502, -3.027376345333614438, 5.243569643749998122 ) ) ;
#23812=CARTESIAN_POINT ( 'NONE',  ( 4.243569643749999898, 12.88437500061451857, 30.00000000000000000 ) ) ;
#23813=CARTESIAN_POINT ( 'NONE',  ( 18.49687500061452283, 6.054752690667223547, 3.707466751127219781E-16 ) ) ;
#23814=CARTESIAN_POINT ( 'NONE',  ( 26.40937500061451715, -4.541064518000417216, -2.621784821875001281 ) ) ;
#23815=CARTESIAN_POINT ( 'NONE',  ( -4.243569643749999898, 16.67187500061451644, 27.54997392385601529 ) ) ;
#23816=CARTESIAN_POINT ( 'NONE',  ( 7.040625000614517681, -3.027376345333610441, -5.243569643749999898 ) ) ;
#23817=CARTESIAN_POINT ( 'NONE',  ( -1.071796769724487453, 18.10759618943233207, -34.00000000000000000 ) ) ;
#23818=CARTESIAN_POINT ( 'NONE',  ( 4.659375000614518925, 0.000000000000000000, 5.243569643749999010 ) ) ;
#23819=CARTESIAN_POINT ( 'NONE',  ( 25.83750000122903501, 6.123233995736764310E-16, -4.999999999999998224 ) ) ;
#23820=CARTESIAN_POINT ( 'NONE',  ( 6.028125000614517504, -4.541064518000419881, 2.621784821874995952 ) ) ;
#23821=CARTESIAN_POINT ( 'NONE',  ( 10.43437500061451750, 4.541064518000418104, 2.621784821874999949 ) ) ;
#23822=CARTESIAN_POINT ( 'NONE',  ( 15.52500000122903323, 2.886751345948129099, -4.999999999999998224 ) ) ;
#23823=CARTESIAN_POINT ( 'NONE',  ( 5.409375000614516260, 4.541064518000418104, -2.621784821874998173 ) ) ;
#23824=CARTESIAN_POINT ( 'NONE',  ( 7.790625000614518569, -3.027376345333614438, 5.243569643749998122 ) ) ;
#23825=CARTESIAN_POINT ( 'NONE',  ( 5.053125000614517859, 0.000000000000000000, 5.243569643749999010 ) ) ;
#23827=CARTESIAN_POINT ( 'NONE',  ( 17.78437500061451715, -4.541064518000419881, 2.621784821874995952 ) ) ;
#23828=CARTESIAN_POINT ( 'NONE',  ( -1.071796769724491005, 10.45759618943233527, 26.00000000000000355 ) ) ;
#23830=CARTESIAN_POINT ( 'NONE',  ( 24.96562500061451573, -6.054752690667223547, -1.112240025338166033E-15 ) ) ;
#23831=CARTESIAN_POINT ( 'NONE',  ( 8.915625000614515017, 3.027376345333613106, -5.243569643749998122 ) ) ;
#23832=EDGE_CURVE ( 'NONE', #39133, #57884, #47571, .T. ) ;
#23833=CARTESIAN_POINT ( 'NONE',  ( 26.37187500061451573, -6.054752690667223547, -1.112240025338166033E-15 ) ) ;
#23834=CARTESIAN_POINT ( 'NONE',  ( 9.890625000614516438, 6.054752690667223547, 3.707466751127219781E-16 ) ) ;
#23835=DIRECTION ( 'NONE',  ( 0.000000000000000000, 1.000000000000000000, -0.000000000000000000 ) ) ;
#23836=CARTESIAN_POINT ( 'NONE',  ( 9.637500001229033941, 6.123233995736764310E-16, -4.999999999999998224 ) ) ;
#23837=( BOUNDED_CURVE ( )  B_SPLINE_CURVE ( 2, ( #21600, #11618, #39704, #44154, #66683, #16058, #10527, #12691, #28967 ),
 .UNSPECIFIED., .F., .F. ) 
 B_SPLINE_CURVE_WITH_KNOTS ( ( 3, 2, 2, 2, 3 ),
 ( 0.4673913043478261087, 0.4710144927536231707, 0.4782608695652174058, 0.4855072463768115854, 0.4891304347826087029 ),
 .UNSPECIFIED. ) 
 CURVE ( )  GEOMETRIC_REPRESENTATION_ITEM ( )  RATIONAL_B_SPLINE_CURVE ( ( 0.9330127018922194093, 0.9330127018922198534, 1.000000000000000000, 0.8660254037844387076, 1.000000000000000000, 0.8660254037844387076, 1.000000000000000000, 0.9330127018922194093, 0.9330127018922194093 ) ) 
 REPRESENTATION_ITEM ( '' )  );
#23838=CARTESIAN_POINT ( 'NONE',  ( 24.40312500061451573, 0.000000000000000000, 5.243569643749999010 ) ) ;
#23839=AXIS2_PLACEMENT_3D ( 'NONE', #16923, #5497, #11033 ) ;
#23840=CARTESIAN_POINT ( 'NONE',  ( -4.243569643749997233, 13.99062500061451786, -27.54997392385601174 ) ) ;
#23841=CARTESIAN_POINT ( 'NONE',  ( 12.90000000122903145, 5.773502691896255534, 3.535250795749688894E-16 ) ) ;
#23842=CARTESIAN_POINT ( 'NONE',  ( 21.85312500061451502, -4.541064518000417216, -2.621784821875001281 ) ) ;
#23843=CARTESIAN_POINT ( 'NONE',  ( 11.51250000000000107, 2.886751345948126879, 4.999999999999999112 ) ) ;
#23844=CARTESIAN_POINT ( 'NONE',  ( 20.91562500061451502, -6.054752690667223547, -1.112240025338166033E-15 ) ) ;
#23845=CARTESIAN_POINT ( 'NONE',  ( 6.159375000614517148, -4.541064518000417216, -2.621784821875001281 ) ) ;
#23846=CARTESIAN_POINT ( 'NONE',  ( 19.94999999999999929, 4.330127018922192761, -2.499999999999997780 ) ) ;
#23847=CARTESIAN_POINT ( 'NONE',  ( 6.750000001229033764, -2.886751345948129988, 4.999999999999997335 ) ) ;
#23848=CARTESIAN_POINT ( 'NONE',  ( 16.50000000122903288, 5.773502691896255534, 3.535250795749688894E-16 ) ) ;
#23849=CARTESIAN_POINT ( 'NONE',  ( 12.77812500061451750, -4.541064518000419881, 2.621784821874995952 ) ) ;
#23850=CARTESIAN_POINT ( 'NONE',  ( 16.64062500061451289, 6.054752690667223547, 3.707466751127219781E-16 ) ) ;
#23851=CARTESIAN_POINT ( 'NONE',  ( 25.65000000122903145, -2.886751345948129988, 4.999999999999997335 ) ) ;
#23852=CARTESIAN_POINT ( 'NONE',  ( 20.02500000000000213, 4.330127018922191873, 2.499999999999999556 ) ) ;
#23853=CARTESIAN_POINT ( 'NONE',  ( 22.88437500061451857, 6.421520780324663323E-16, -5.243569643749999010 ) ) ;
#23855=CARTESIAN_POINT ( 'NONE',  ( 11.02500000122903501, 2.886751345948129099, -4.999999999999998224 ) ) ;
#23856=CARTESIAN_POINT ( 'NONE',  ( 9.046875000614518214, 6.054752690667223547, 3.707466751127219781E-16 ) ) ;
#23857=CARTESIAN_POINT ( 'NONE',  ( 25.02187500061451431, -6.054752690667223547, -1.112240025338166033E-15 ) ) ;
#23858=CARTESIAN_POINT ( 'NONE',  ( 3.834375000614519635, -4.541064518000419881, 2.621784821874995952 ) ) ;
#23859=CARTESIAN_POINT ( 'NONE',  ( 22.11562500061451786, 3.027376345333611329, 5.243569643749999010 ) ) ;
#23860=CARTESIAN_POINT ( 'NONE',  ( 25.95937500061451431, -4.541064518000417216, -2.621784821875001281 ) ) ;
#23863=CARTESIAN_POINT ( 'NONE',  ( 6.759375000614516793, 4.541064518000418104, -2.621784821874998173 ) ) ;
#23864=CARTESIAN_POINT ( 'NONE',  ( 18.62812500061451715, -4.541064518000419881, 2.621784821874995952 ) ) ;
#23865=ORIENTED_EDGE ( 'NONE', *, *, #23767, .T. ) ;
#23867=CARTESIAN_POINT ( 'NONE',  ( 28.30312500061451431, 4.541064518000418104, -2.621784821874998173 ) ) ;
#23868=CARTESIAN_POINT ( 'NONE',  ( 3.384375000614517237, -4.541064518000419881, 2.621784821874995952 ) ) ;
#23869=CARTESIAN_POINT ( 'NONE',  ( -2.000000000000000000, 14.52500000000000036, 26.53589838486224650 ) ) ;
#23870=FACE_OUTER_BOUND ( 'NONE', #46060, .T. ) ;
#23871=CARTESIAN_POINT ( 'NONE',  ( 16.35000000000000142, 4.330127018922192761, -2.499999999999997780 ) ) ;
#23872=CARTESIAN_POINT ( 'NONE',  ( 21.29062500061451502, -3.027376345333614438, 5.243569643749998122 ) ) ;
#23873=ORIENTED_EDGE ( 'NONE', *, *, #26612, .T. ) ;
#23874=CARTESIAN_POINT ( 'NONE',  ( 24.37500000000000000, 6.123233995736764310E-16, -4.999999999999998224 ) ) ;
#23876=CARTESIAN_POINT ( 'NONE',  ( 26.18437500061451573, 4.541064518000418104, 2.621784821874999949 ) ) ;
#23877=VERTEX_POINT ( 'NONE', #35149 ) ;
#23878=CARTESIAN_POINT ( 'NONE',  ( 16.22812500061451857, 4.541064518000418104, 2.621784821874999949 ) ) ;
#23879=CARTESIAN_POINT ( 'NONE',  ( 6.703125000614516438, 4.541064518000418104, -2.621784821874998173 ) ) ;
#23881=CARTESIAN_POINT ( 'NONE',  ( 28.11562500061451431, -6.054752690667223547, -1.112240025338166033E-15 ) ) ;
#23882=CARTESIAN_POINT ( 'NONE',  ( 14.43750000122903288, -4.330127018922194537, 2.499999999999995559 ) ) ;
#23883=CARTESIAN_POINT ( 'NONE',  ( 21.78750000000000142, 5.773502691896255534, 3.535250795749688894E-16 ) ) ;
#23884=CARTESIAN_POINT ( 'NONE',  ( 28.27499999999999858, -4.330127018922194537, 2.499999999999995559 ) ) ;
#23885=CARTESIAN_POINT ( 'NONE',  ( 5.146875000614517859, -3.027376345333614438, 5.243569643749998122 ) ) ;
#23886=CARTESIAN_POINT ( 'NONE',  ( 10.35937500061451644, 4.541064518000418104, -2.621784821874998173 ) ) ;
#23887=CARTESIAN_POINT ( 'NONE',  ( 19.47187500061451360, 3.027376345333611329, 5.243569643749999010 ) ) ;
#23888=CARTESIAN_POINT ( 'NONE',  ( 10.05000000122903181, -2.886751345948126435, -5.000000000000000000 ) ) ;
#23889=ORIENTED_EDGE ( 'NONE', *, *, #16221, .F. ) ;
#23890=CARTESIAN_POINT ( 'NONE',  ( 5.146875000614517859, -3.027376345333614438, 5.243569643749998122 ) ) ;
#23891=CARTESIAN_POINT ( 'NONE',  ( 3.937500000000000444, -2.886751345948129988, 4.999999999999997335 ) ) ;
#23892=CARTESIAN_POINT ( 'NONE',  ( 5.184375000614516615, -4.541064518000419881, 2.621784821874995952 ) ) ;
#23893=CARTESIAN_POINT ( 'NONE',  ( 19.34999999999999787, -4.330127018922190985, -2.500000000000001332 ) ) ;
#23894=CARTESIAN_POINT ( 'NONE',  ( 16.22812500061451857, 4.541064518000418104, 2.621784821874999949 ) ) ;
#23898=CARTESIAN_POINT ( 'NONE',  ( 8.990625000614516082, 6.054752690667223547, 3.707466751127219781E-16 ) ) ;
#23899=CARTESIAN_POINT ( 'NONE',  ( 27.60937500061451644, 0.000000000000000000, 5.243569643749999010 ) ) ;
#23900=CARTESIAN_POINT ( 'NONE',  ( -2.121784821874996840, 18.58437500061451786, 33.67503911421598417 ) ) ;
#23901=CARTESIAN_POINT ( 'NONE',  ( 27.15937500061451360, 0.000000000000000000, 5.243569643749999010 ) ) ;
#23902=CARTESIAN_POINT ( 'NONE',  ( 7.800000000000001599, 4.330127018922192761, -2.499999999999997780 ) ) ;
#23903=CARTESIAN_POINT ( 'NONE',  ( -3.999999999999999112, 12.01250000122903394, 30.00000000000000000 ) ) ;
#23904=CARTESIAN_POINT ( 'NONE',  ( 14.72812500061451679, 6.421520780324663323E-16, -5.243569643749999010 ) ) ;
#23905=CARTESIAN_POINT ( 'NONE',  ( 7.237500001229035362, -4.330127018922194537, 2.499999999999995559 ) ) ;
#23906=CARTESIAN_POINT ( 'NONE',  ( 18.75937500061451857, -4.541064518000417216, -2.621784821875001281 ) ) ;
#23907=CARTESIAN_POINT ( 'NONE',  ( 12.42187500061451821, -6.054752690667223547, -1.112240025338166033E-15 ) ) ;
#23908=CARTESIAN_POINT ( 'NONE',  ( 0.000000000000000000, 10.00000000000000000, 0.000000000000000000 ) ) ;
#23909=EDGE_LOOP ( 'NONE', ( #42599, #2794, #8934, #12780 ) ) ;
#23910=CARTESIAN_POINT ( 'NONE',  ( 13.19062500061451537, -3.027376345333614438, 5.243569643749998122 ) ) ;
#23911=CARTESIAN_POINT ( 'NONE',  ( 25.05000000122903714, 5.773502691896255534, 3.535250795749688894E-16 ) ) ;
#23912=CARTESIAN_POINT ( 'NONE',  ( 12.00937500061451857, -4.541064518000417216, -2.621784821875001281 ) ) ;
#23913=CARTESIAN_POINT ( 'NONE',  ( 30.00000000000000000, 0.000000000000000000, 4.999999999999998224 ) ) ;
#23914=CARTESIAN_POINT ( 'NONE',  ( 15.17812500061451608, 6.421520780324663323E-16, -5.243569643749999010 ) ) ;
#23916=CARTESIAN_POINT ( 'NONE',  ( 23.59687500061451715, -3.027376345333614438, 5.243569643749998122 ) ) ;
#23917=FACE_OUTER_BOUND ( 'NONE', #35256, .T. ) ;
#23918=CARTESIAN_POINT ( 'NONE',  ( 11.96250000122903501, 4.330127018922192761, -2.499999999999997780 ) ) ;
#23919=CARTESIAN_POINT ( 'NONE',  ( 20.43750000122903643, 6.123233995736764310E-16, -4.999999999999998224 ) ) ;
#23920=CARTESIAN_POINT ( 'NONE',  ( -3.000416591977282496E-16, 16.59687500061452070, -34.90005215228797653 ) ) ;
#23921=CARTESIAN_POINT ( 'NONE',  ( 17.85937500061451999, -4.541064518000417216, -2.621784821875001281 ) ) ;
#23922=CARTESIAN_POINT ( 'NONE',  ( 18.48750000122903359, -4.330127018922194537, 2.499999999999995559 ) ) ;
#23923=CARTESIAN_POINT ( 'NONE',  ( 15.19687500061451857, -3.027376345333610441, -5.243569643749999898 ) ) ;
#23924=CARTESIAN_POINT ( 'NONE',  ( -1.473772837211104525, 9.872922166578584680, 25.95083099200021337 ) ) ;
#23925=CARTESIAN_POINT ( 'NONE',  ( 20.28750000122903074, -4.330127018922194537, 2.499999999999995559 ) ) ;
#23926=CARTESIAN_POINT ( 'NONE',  ( 14.12812500061451715, -4.541064518000419881, 2.621784821874995952 ) ) ;
#23928=ORIENTED_EDGE ( 'NONE', *, *, #66238, .T. ) ;
#23929=CARTESIAN_POINT ( 'NONE',  ( 18.00000000000000355, -4.330127018922190985, -2.500000000000001332 ) ) ;
#23930=CARTESIAN_POINT ( 'NONE',  ( 0.000000000000000000, 10.00000000000000000, 0.000000000000000000 ) ) ;
#23931=CARTESIAN_POINT ( 'NONE',  ( 4.078125000614517326, 4.541064518000418104, 2.621784821874999949 ) ) ;
#23932=ADVANCED_FACE ( 'NONE', ( #12615 ), #23691, .F. ) ;
#23933=CARTESIAN_POINT ( 'NONE',  ( 14.10000000122903252, -2.886751345948125991, -5.000000000000000000 ) ) ;
#23934=CARTESIAN_POINT ( 'NONE',  ( 27.64687500061452141, -3.027376345333614438, 5.243569643749998122 ) ) ;
#23935=CARTESIAN_POINT ( 'NONE',  ( 20.12812500061451715, 6.421520780324663323E-16, -5.243569643749999010 ) ) ;
#23936=CARTESIAN_POINT ( 'NONE',  ( 22.60312500061451857, 0.000000000000000000, 5.243569643749999010 ) ) ;
#23937=CARTESIAN_POINT ( 'NONE',  ( 2.915625000614516793, -6.054752690667223547, -1.112240025338166033E-15 ) ) ;
#23938=CARTESIAN_POINT ( 'NONE',  ( 27.97500000000000142, 6.123233995736764310E-16, -4.999999999999998224 ) ) ;
#23939=CARTESIAN_POINT ( 'NONE',  ( -3.999999999999999112, 10.17500000122903359, -32.30940107675850470 ) ) ;
#23943=CARTESIAN_POINT ( 'NONE',  ( 2.121784821874999061, 15.65937500061451892, -33.67503911421598417 ) ) ;
#23944=CARTESIAN_POINT ( 'NONE',  ( 7.162500001229032520, 0.000000000000000000, 4.999999999999998224 ) ) ;
#23945=CARTESIAN_POINT ( 'NONE',  ( 5.250000000000000888, 0.000000000000000000, 4.999999999999998224 ) ) ;
#23946=CARTESIAN_POINT ( 'NONE',  ( 2.887500001229035274, 6.123233995736764310E-16, -4.999999999999998224 ) ) ;
#23947=CARTESIAN_POINT ( 'NONE',  ( 10.84687500061451892, 6.054752690667223547, 3.707466751127219781E-16 ) ) ;
#23948=CARTESIAN_POINT ( 'NONE',  ( 29.01562500061451644, -6.054752690667223547, -1.112240025338166033E-15 ) ) ;
#23950=LINE ( 'NONE', #25041, #60954 ) ;
#23952=CARTESIAN_POINT ( 'NONE',  ( 8.484375000614518214, 6.421520780324663323E-16, -5.243569643749999010 ) ) ;
#23953=CARTESIAN_POINT ( 'NONE',  ( 11.44687500061451857, -3.027376345333614438, 5.243569643749998122 ) ) ;
#23954=CARTESIAN_POINT ( 'NONE',  ( 7.687500000000000000, -2.886751345948125991, -5.000000000000000000 ) ) ;
#23955=CARTESIAN_POINT ( 'NONE',  ( 9.001249775931846008E-16, 14.96562500061459389, 34.90005215228797653 ) ) ;
#23956=CARTESIAN_POINT ( 'NONE',  ( 21.98437500061451644, 6.421520780324663323E-16, -5.243569643749999010 ) ) ;
#23957=EDGE_CURVE ( 'NONE', #50074, #20630, #56947, .T. ) ;
#23959=CARTESIAN_POINT ( 'NONE',  ( 6.412500000000001421, 2.886751345948129099, -4.999999999999998224 ) ) ;
#23960=CARTESIAN_POINT ( 'NONE',  ( 25.91250000122903074, 4.330127018922192761, -2.499999999999997780 ) ) ;
#23962=CARTESIAN_POINT ( 'NONE',  ( 21.51562500061451644, 3.027376345333613106, -5.243569643749998122 ) ) ;
#23963=CARTESIAN_POINT ( 'NONE',  ( 14.16562500061451679, -6.054752690667223547, -1.112240025338166033E-15 ) ) ;
#23965=CARTESIAN_POINT ( 'NONE',  ( 9.009375000614518569, 4.541064518000418104, -2.621784821874998173 ) ) ;
#23966=CARTESIAN_POINT ( 'NONE',  ( 29.32499999999999929, 6.123233995736764310E-16, -4.999999999999998224 ) ) ;
#23967=CARTESIAN_POINT ( 'NONE',  ( 21.90000000122903145, 5.773502691896255534, 3.535250795749688894E-16 ) ) ;
#23968=DIRECTION ( 'NONE',  ( 0.000000000000000000, 0.000000000000000000, -1.000000000000000000 ) ) ;
#23969=CARTESIAN_POINT ( 'NONE',  ( 12.87187500061451750, -6.054752690667223547, -1.112240025338166033E-15 ) ) ;
#23970=CARTESIAN_POINT ( 'NONE',  ( 28.69687500061451502, -3.027376345333610441, -5.243569643749999898 ) ) ;
#23972=CARTESIAN_POINT ( 'NONE',  ( -3.999999999999997335, 14.63750000000000107, 32.30940107675850470 ) ) ;
#23973=CARTESIAN_POINT ( 'NONE',  ( 21.19687500061451502, 6.054752690667223547, 3.707466751127219781E-16 ) ) ;
#23974=CARTESIAN_POINT ( 'NONE',  ( 14.74687500061451573, -3.027376345333610441, -5.243569643749999898 ) ) ;
#23976=CARTESIAN_POINT ( 'NONE',  ( 26.51249999999999929, -5.773502691896255534, -1.060575238724906372E-15 ) ) ;
#23978=CARTESIAN_POINT ( 'NONE',  ( 2.121784821875001281, 14.60937500061451821, -26.32496088578401938 ) ) ;
#23980=CARTESIAN_POINT ( 'NONE',  ( 17.50312500061451715, 4.541064518000418104, -2.621784821874998173 ) ) ;
#23981=CARTESIAN_POINT ( 'NONE',  ( 7.425000000000000711, 4.330127018922191873, 2.499999999999999556 ) ) ;
#23982=( BOUNDED_CURVE ( )  B_SPLINE_CURVE ( 3, ( #42567, #37019, #59543, #63997 ),
 .UNSPECIFIED., .F., .F. ) 
 B_SPLINE_CURVE_WITH_KNOTS ( ( 4, 4 ),
 ( 3.315795346099966956, 3.411714352141634876 ),
 .UNSPECIFIED. ) 
 CURVE ( )  GEOMETRIC_REPRESENTATION_ITEM ( )  RATIONAL_B_SPLINE_CURVE ( ( 1.000000000000000000, 0.9992334423044004765, 0.9992334423044004765, 1.000000000000000000 ) ) 
 REPRESENTATION_ITEM ( '' )  );
#23983=CARTESIAN_POINT ( 'NONE',  ( 12.18750000122903465, -4.330127018922194537, 2.499999999999995559 ) ) ;
#23984=CARTESIAN_POINT ( 'NONE',  ( 14.13750000000000107, 5.773502691896255534, 3.535250795749688894E-16 ) ) ;
#23985=CARTESIAN_POINT ( 'NONE',  ( -0.7368814052146555049, 9.803648494990884643, 25.82089852767304095 ) ) ;
#23986=CARTESIAN_POINT ( 'NONE',  ( 14.47500000122903430, -5.773502691896255534, -1.060575238724906372E-15 ) ) ;
#23987=CARTESIAN_POINT ( 'NONE',  ( 24.68437500061451573, 6.421520780324663323E-16, -5.243569643749999010 ) ) ;
#23988=VERTEX_POINT ( 'NONE', #62856 ) ;
#23989=CARTESIAN_POINT ( 'NONE',  ( 19.34062500061451573, 6.054752690667223547, 3.707466751127219781E-16 ) ) ;
#23990=CARTESIAN_POINT ( 'NONE',  ( 20.37187500061451573, 3.027376345333611329, 5.243569643749999010 ) ) ;
#23991=CARTESIAN_POINT ( 'NONE',  ( 5.025000000000002132, 6.123233995736764310E-16, -4.999999999999998224 ) ) ;
#23992=CARTESIAN_POINT ( 'NONE',  ( 8.315625000614515372, -6.054752690667223547, -1.112240025338166033E-15 ) ) ;
#23993=CARTESIAN_POINT ( 'NONE',  ( 22.86562500061451431, 3.027376345333613106, -5.243569643749998122 ) ) ;
#23994=CARTESIAN_POINT ( 'NONE',  ( 13.39687500061451608, -3.027376345333610441, -5.243569643749999898 ) ) ;
#23995=CARTESIAN_POINT ( 'NONE',  ( 17.74687500061451928, -3.027376345333614438, 5.243569643749998122 ) ) ;
#23996=CARTESIAN_POINT ( 'NONE',  ( -4.243569643749999898, 16.16562500061451857, 27.54997392385601529 ) ) ;
#23997=CARTESIAN_POINT ( 'NONE',  ( 19.12500000122903288, 2.886751345948129099, -4.999999999999998224 ) ) ;
#23999=CARTESIAN_POINT ( 'NONE',  ( 10.49062500061451608, -3.027376345333614438, 5.243569643749998122 ) ) ;
#24000=CARTESIAN_POINT ( 'NONE',  ( 3.009375000614516793, -4.541064518000417216, -2.621784821875001281 ) ) ;
#24001=CARTESIAN_POINT ( 'NONE',  ( 29.35312500061451502, 0.000000000000000000, 5.243569643749999010 ) ) ;
#24002=CARTESIAN_POINT ( 'NONE',  ( 25.65937500061451715, 4.541064518000418104, -2.621784821874998173 ) ) ;
#24003=CARTESIAN_POINT ( 'NONE',  ( 16.71562500061451573, 3.027376345333611329, 5.243569643749999010 ) ) ;
#24004=CARTESIAN_POINT ( 'NONE',  ( 27.22500000122903430, 2.886751345948129099, -4.999999999999998224 ) ) ;
#24005=CARTESIAN_POINT ( 'NONE',  ( 25.56562500061452070, 3.027376345333613106, -5.243569643749998122 ) ) ;
#24006=CARTESIAN_POINT ( 'NONE',  ( 22.80937500061451573, -4.541064518000417216, -2.621784821875001281 ) ) ;
#24007=CARTESIAN_POINT ( 'NONE',  ( 16.97812500061451502, 6.421520780324663323E-16, -5.243569643749999010 ) ) ;
#24008=CARTESIAN_POINT ( 'NONE',  ( -4.243569643749999898, 17.15937500061451715, 30.00000000000000000 ) ) ;
#24009=CARTESIAN_POINT ( 'NONE',  ( 23.31562500061451715, 3.027376345333613106, -5.243569643749998122 ) ) ;
#24011=CARTESIAN_POINT ( 'NONE',  ( 24.78750000000000497, -2.886751345948125991, -5.000000000000000000 ) ) ;
#24012=CARTESIAN_POINT ( 'NONE',  ( 4.000000000000000000, 12.98749999999999893, -27.69059892324149530 ) ) ;
#24014=CARTESIAN_POINT ( 'NONE',  ( 3.009375000614516793, -4.541064518000417216, -2.621784821875001281 ) ) ;
#24015=CARTESIAN_POINT ( 'NONE',  ( 10.41562500061451679, 3.027376345333611329, 5.243569643749999010 ) ) ;
#24016=CARTESIAN_POINT ( 'NONE',  ( 22.08750000122903501, -4.330127018922194537, 2.499999999999995559 ) ) ;
#24017=CARTESIAN_POINT ( 'NONE',  ( 26.99062500061451431, 6.054752690667223547, 3.707466751127219781E-16 ) ) ;
#24018=CARTESIAN_POINT ( 'NONE',  ( 26.51249999999999929, -5.773502691896255534, -1.060575238724906372E-15 ) ) ;
#24019=CARTESIAN_POINT ( 'NONE',  ( -3.999999999999997335, 16.55000000122903003, -27.69059892324149175 ) ) ;
#24020=CARTESIAN_POINT ( 'NONE',  ( 29.69062500061451715, 6.054752690667223547, 3.707466751127219781E-16 ) ) ;
#24021=CARTESIAN_POINT ( 'NONE',  ( 10.11562500061451608, -6.054752690667223547, -1.112240025338166033E-15 ) ) ;
#24023=CARTESIAN_POINT ( 'NONE',  ( 26.42812500061451431, 6.421520780324663323E-16, -5.243569643749999010 ) ) ;
#24024=CARTESIAN_POINT ( 'NONE',  ( 8.878125000614515372, 6.421520780324663323E-16, -5.243569643749999010 ) ) ;
#24026=CARTESIAN_POINT ( 'NONE',  ( 7.115625000614516082, 3.027376345333613106, -5.243569643749998122 ) ) ;
#24028=CARTESIAN_POINT ( 'NONE',  ( 4.652730581016856881, -1.830942677413806896, 4.913544636837456459 ) ) ;
#24029=( BOUNDED_CURVE ( )  B_SPLINE_CURVE ( 2, ( #51147, #11982, #72592, #57033, #56680, #28975, #34505 ),
 .UNSPECIFIED., .F., .F. ) 
 B_SPLINE_CURVE_WITH_KNOTS ( ( 3, 2, 2, 3 ),
 ( 0.7583333333333333037, 0.7611111111111110716, 0.7638888888888889506, 0.7666666666666668295 ),
 .UNSPECIFIED. ) 
 CURVE ( )  GEOMETRIC_REPRESENTATION_ITEM ( )  RATIONAL_B_SPLINE_CURVE ( ( 1.000000000000000000, 0.8660254037844387076, 1.000000000000000000, 0.8660254037844387076, 1.000000000000000000, 0.8660254037844333785, 1.000000000000005329 ) ) 
 REPRESENTATION_ITEM ( '' )  );
#24030=CARTESIAN_POINT ( 'NONE',  ( 14.21249999999999858, 2.886751345948126879, 4.999999999999999112 ) ) ;
#24031=( BOUNDED_SURFACE ( )  B_SPLINE_SURFACE ( 1, 2, ( 
 ( #14991, #48257, #38254, #16444, #27916, #61516, #50450, #55261, #39001, #67447, #4298, #44554, #10914, #67085, #5017, #26823, #55985, #37893, #49357, #33440, #5378, #61159, #21625, #16809, #43450, #72976, #9821, #44183, #22358, #10554, #32353, #20896, #71887, #65972, #44910, #39365, #15352, #61881, #27551, #11287, #33808, #56351, #5741, #28275, #60412, #4657, #72614, #50083, #71521, #54891, #33082, #21260, #55621, #27186, #43813, #66713, #66338, #15716, #60783, #10189, #21996, #49720, #32724, #72248, #16087, #38635, #56699, #46351, #209, #17173, #11647, #45634, #45267, #51168, #572, #23442, #68885, #52252, #63687, #39733, #51892, #62250, #35255, #69251, #57055, #68167, #6099, #18613, #35616, #22714, #58136, #28630, #34162, #67800, #23077, #13077, #17530, #18242, #24164, #934, #6462, #1290, #45988, #1655, #40815, #34892, #40092, #62606, #12002, #34525, #28997, #51534, #68525, #17886, #40446, #57776, #62962, #12358, #57421, #63331, #7186, #6825, #29359, #23800, #12719, #29714, #46716, #41178, #7542, #50807, #52975, #69965, #24889, #18971, #31542, #13811, #59967, #30076, #64050, #19336, #14906, #9010, #53338, #70331, #37074, #24531, #59230, #36351, #54082, #47434, #31167, #2020, #69610, #47075, #2736, #52614, #30805, #58865, #41891, #19707, #64418, #8275, #2371, #41531, #71064, #25631, #13430, #20068, #53709, #35980, #7908, #3479, #64783, #8638, #37447, #25998, #30446, #58499, #25253, #47802, #14174, #48537, #42260, #3102, #36708, #48168, #70693, #20439, #42988, #42624, #65148, #14538, #65520, #59598, #4933, #44828, #67363, #55538, #22276, #15269, #27837, #43727, #16726, #72162, #66999, #50369, #10828, #44096, #38549, #10469, #61072, #16000, #5291, #48903, #31907, #32999, #65888, #26738, #10107, #27103, #43365, #60327, #37807, #27468, #66250, #21541, #49635, #55177, #16361, #15628, #61435, #72894, #39281, #49999, #66623, #32271, #32637, #38915, #33363, #9737, #55900, #54804, #4573, #72524, #3843, #9375, #54444, #4210, #49272, #21913, #26364, #44469, #71805, #21174, #71434, #38170, #60694, #20810, #45550, #11563, #34079, #28549, #56619, #50725, #63242, #68079, #19529, #61793, #22633, #51083, #47619, #40726, #11917, #28906, #68802, #56270, #17798, #17448, #12636, #6014, #62877, #33725, #28196, #5660, #34442, #11198, #62520, #40005, #480, #51444, #22989, #56970, #6374, #128, #29629, #57336, #45183, #51804, #12273, #67715, #39648, #35171, #23355, #40358, #70151, #57695, #62167, #17087, #846, #45904, #68435, #7100, #34804, #6740, #29274, #1207, #23712, #52166, #1569, #46262, #18158, #25076, #32462, #30994, #37629, #4402, #26931, #15093, #54996, #47996, #60518, #3298, #49456, #31731, #26557, #9923, #43551, #3663, #71249, #43187, #20628, #48726, #37996, #8459, #64609, #65707, #25452, #59420, #42813, #59790, #2922, #19899, #70524, #60152, #25825, #54269, #9196, #14726, #49097, #48362, #20999, #71990, #42087, #9562, #26186, #64974, #65336, #71626, #31364, #13995, #66073, #37268, #32095, #15451, #36534, #54626, #70888, #59054, #8828, #4032, #53527, #42452, #14365, #36900, #53905, #20261, #27653, #61262, #61618, #10656, #5119, #44289, #15820, #62350, #16908, #38364, #11386, #22459, #27290, #72348, #45367, #56092, #73078, #6202, #306, #21729, #60890, #66818, #51270, #5483, #67903, #50192, #67545, #67188, #33186, #43918, #11746, #34263, #16191, #11020, #4757, #56796, #10295, #39463, #28729, #21364, #61985, #66444, #49824, #39836, #55725, #32826, #33541, #5839, #55364, #22816, #28022, #50550, #45009, #33905, #56449, #17274, #38742, #72717, #28371, #22100, #44658, #16549, #39101, #50908, #51636, #57158, #52356, #57530, #12824, #40925, #46455, #58243, #35000, #52716, #64154, #13541, #1759, #63438, #23544, #23907, #30186, #24634, #1037, #68993, #18352, #68269, #7647, #45734, #6570, #46094, #63792, #2123, #29821, #68630, #17992, #24273, #40551, #6930, #35358, #29461, #63068, #12471, #51997, #1398, #62712, #47180, #57882, #30552, #673, #34629, #29101, #7292, #69712, #46822, #69359, #18717, #41281, #13182, #19080, #35721, #41635, #36089, #58609, #8016, #23180, #17631, #40191, #12106, #59707, #58971, #37549, #19443, #8378, #71168, #65624, #42733, #3212, #71544, #24998, #54547, #64524, #25741, #48643, #65252, #13918, #2474, #53449, #47541, #15012, #20540, #70070, #9483, #9114, #3949, #60071, #43097, #32012, #20917, #42004, #36818, #54185, #31652, #26104, #36456, #14642, #15374, #37182, #8744, #26473, #48278, #49011, #2839, #42369, #43469, #3582, #59333, #25368, #65993, #30908, #37916, #47912, #60434, #70441, #19817, #64891, #14281, #31276, #53819, #70802, #20178, #9844, #53078, #45287, #71908, #33460, #43835, #16830, #50828, #38657, #49742, #60804, #229, #17193, #54912, #39754, #10211, #21281, #49378, #4320, #67821, #32745, #50469, #5762, #55642, #61181, #56006, #5037, #56371, #22379, #16463, #55283, #26845, #66362, #4677, #27207, #38276, #10576, #72270, #22019, #44930, #15737, #62272, #10936, #33103, #16106, #32373, #21647, #44204, #66735, #27573, #50105, #72635, #44574, #67106, #67467, #39022, #61536, #5399, #27936, #72997, #39383, #61902, #11307, #33828, #28294, #22736, #40111, #12735, #68186, #51553, #29731, #41194, #1671, #63703, #68544, #52269, #7558, #17550, #57793, #24180, #7202, #18260, #62626, #69267, #51188, #12021, #46733, #18630, #1309, #34912, #30093, #56717, #13094, #23096, #57440, #35632, #23818, #45654, #34182, #34545, #6119, #58153, #52630, #28649, #2035, #40833, #24546, #47091, #69624, #18986, #41548, #591, #17904, #35272, #63350, #11666, #57074, #46369, #6482, #68903, #40466, #29016, #6843, #954, #23462, #46008, #62981, #12377, #29378, #51911, #43006, #30461, #65535, #69981, #59613, #13446, #52990, #24905, #58879, #58513, #64433, #13825, #36723, #9027, #14921 ),
 ( #42639, #36366, #25269, #8653, #47816, #8289, #30820, #53352, #2750, #2387, #37463, #70346, #19723, #42274, #47449, #59982, #64797, #20826, #64065, #19351, #14188, #48921, #9393, #59245, #31183, #71079, #7924, #20083, #53725, #31923, #3117, #65163, #35995, #41908, #25647, #48184, #70708, #14555, #37089, #31558, #54098, #3495, #26014, #48552, #20453, #54459, #3858, #26380, #71452, #44485, #49287, #21192, #67379, #4950, #21929, #28211, #22291, #43743, #60343, #15646, #143, #27484, #16741, #72180, #16378, #16017, #32654, #65904, #11214, #56286, #66268, #10488, #26755, #33740, #32286, #38933, #5675, #50740, #61451, #43380, #71820, #61811, #4589, #15284, #33015, #27853, #37824, #44843, #50017, #72541, #67017, #10845, #33379, #39296, #9752, #54820, #55915, #38186, #60711, #44113, #61089, #4228, #10123, #55195, #5310, #27118, #55554, #50384, #38565, #72909, #49652, #21559, #66640, #35545, #1222, #12287, #45566, #45919, #52182, #46641, #497, #17813, #68451, #17103, #29644, #67729, #28565, #68098, #12650, #1584, #51819, #17463, #23007, #23728, #40022, #56986, #40374, #6392, #62536, #28924, #40742, #18543, #51101, #68817, #63258, #18173, #29289, #11933, #7115, #62182, #34458, #35185, #57711, #34822, #62893, #41107, #39663, #24093, #34095, #57350, #69182, #6756, #56635, #45198, #51461, #11579, #63617, #13007, #6031, #58065, #46278, #7474, #30000, #52543, #22649, #864, #23371, #58794, #3028, #8568, #48100, #69540, #64714, #37375, #14098, #30733, #54012, #25180, #70623, #2303, #64347, #3408, #25559, #8204, #24818, #25928, #41461, #48468, #7839, #19998, #24457, #63980, #35903, #69896, #18899, #47365, #19262, #47723, #42551, #70992, #14834, #13362, #65078, #58428, #59525, #20368, #53265, #41816, #30376, #42919, #59899, #47005, #9304, #52905, #13738, #36280, #2663, #31838, #70262, #14469, #65442, #19633, #42190, #37003, #36638, #1950, #8938, #59160, #31096, #53635, #31469, #26669, #49202, #60255, #10034, #71736, #44026, #44401, #3769, #11125, #32932, #55107, #38102, #61724, #48831, #16654, #37735, #66548, #50302, #9669, #55470, #32202, #21106, #72453, #10762, #66927, #33295, #4862, #27036, #5220, #16296, #38477, #54736, #26294, #71361, #43659, #66181, #4138, #32569, #15559, #15927, #38850, #20736, #54374, #27398, #4507, #60624, #43294, #65815, #39212, #49567, #61001, #72824, #72089, #49928, #21473, #10400, #21837, #55833, #61365, #27762, #22207, #44761, #67296, #15197, #6674, #51737, #29202, #40290, #39572, #18091, #59, #62096, #1137, #46192, #23284, #56901, #52097, #5590, #35101, #45113, #6306, #23647, #45833, #67648, #56197, #34012, #28127, #68733, #40652, #50655, #63172, #62812, #57626, #12567, #7030, #29560, #1502, #22565, #17380, #34732, #12204, #24007, #17014, #68370, #69096, #17731, #62451, #46555, #28834, #18458, #56549, #22918, #41022, #57261, #39938, #5943, #63538, #11490, #33652, #28476, #51013, #409, #45475, #68008, #11849, #34368, #51373, #776, #58709, #31013, #14385, #25845, #52459, #14016, #24372, #70543, #31384, #19179, #30288, #41379, #53924, #70909, #35458, #20281, #63890, #1866, #29919, #57981, #48382, #13280, #53546, #59441, #36191, #41732, #36555, #8120, #36920, #2942, #70173, #35819, #7391, #46920, #58341, #7751, #18816, #64260, #52820, #2577, #25471, #69458, #42835, #64630, #13647, #69813, #12924, #2222, #24735, #47279, #25096, #8848, #30648, #59075, #53180, #47640, #48017, #42472, #19918, #64995, #19550, #3319, #42107, #8479, #38385, #10312, #60908, #72007, #71271, #49842, #31754, #20649, #32844, #4775, #55015, #15471, #11683, #37289, #67836, #3684, #38015, #55381, #4420, #26208, #14747, #65726, #59812, #27309, #72367, #9217, #21747, #21382, #17209, #45302, #39771, #62287, #34198, #54291, #49117, #66462, #43938, #56732, #48747, #26949, #28665, #49475, #21018, #6135, #60537, #51204, #15112, #54647, #606, #15839, #71645, #37649, #23112, #43206, #65357, #60172, #9581, #32113, #4051, #26577, #43571, #66092, #9944, #32482, #18275, #63717, #47107, #58529, #12036, #46749, #57089, #30109, #64080, #51927, #62998, #968, #13462, #30477, #68204, #53006, #23478, #34561, #62641, #17565, #7939, #46024, #13109, #19001, #68918, #1324, #12392, #69283, #40127, #6497, #29033, #40849, #2401, #46384, #23834, #34928, #12752, #57455, #29393, #68561, #51568, #36011, #41209, #17919, #35647, #18645, #40482, #6860, #69639, #7218, #24195, #45669, #24561, #63367, #35287, #57809, #29747, #52285, #41562, #1686, #58169, #7574, #52643, #2050, #65920, #37839, #47834, #65180, #8306, #15300, #13841, #20468, #60359, #9768, #71094, #32302, #30836, #43397, #59261, #54837, #14571, #9408, #24922, #26396, #59630, #54112, #26029, #3510, #31573, #20843, #64450, #47464, #48568, #53369, #42291, #25665, #42656, #58896, #2766, #25288, #43022, #8670, #37104, #9043, #70724, #31938, #31201, #3873, #69997, #19366, #65550, #14939, #70364, #48202, #54475, #48938, #19742, #20099, #37478, #41924, #71467, #36380, #64815, #14205, #59998, #36741, #53743, #3136, #55212, #55932, #49670, #38582, #21946, #61107, #27136, #72197, #44130, #21576, #66285, #5691, #10504, #34113, #4244, #38202, #66657, #62200, #56301, #27499, #44502, #11233, #71837, #33396, #33032, #28226, #15663, #61828, #22665, #55571, #16034, #32671, #45215, #11596, #26771, #49303, #4605, #60728, #21208, #43760, #39680, #4966, #22308, #50756, #50033, #72558, #5328, #67035, #159, #67396, #61468, #16395, #10139, #38950, #10863, #27869, #50401, #72926, #44860, #16758, #39316, #33756, #67749, #17121, #40391, #23388, #58081, #51118, #13023, #68114, #6774, #18558, #40040, #68834, #17480, #28942, #63275, #52198, #12667, #1599, #45937, #35204, #41123, #62554, #40760, #57726, #18190, #1240, #11950, #7131, #515, #34475, #29661, #24110, #29306, #62910 ) ),
 .UNSPECIFIED., .F., .F., .F. ) 
 B_SPLINE_SURFACE_WITH_KNOTS ( ( 2, 2 ),
 ( 3, 2, 2, 2, 2, 2, 2, 2, 2, 2, 2, 2, 2, 2, 2, 2, 2, 2, 2, 2, 2, 2, 2, 2, 2, 2, 2, 2, 2, 2, 2, 2, 2, 2, 2, 2, 2, 2, 2, 2, 2, 2, 2, 2, 2, 2, 2, 2, 2, 2, 2, 2, 2, 2, 2, 2, 2, 2, 2, 2, 2, 2, 2, 2, 2, 2, 2, 2, 2, 2, 2, 2, 2, 2, 2, 2, 2, 2, 2, 2, 2, 2, 2, 2, 2, 2, 2, 2, 2, 2, 2, 2, 2, 2, 2, 2, 2, 2, 2, 2, 2, 2, 2, 2, 2, 2, 2, 2, 2, 2, 2, 2, 2, 2, 2, 2, 2, 2, 2, 2, 2, 2, 2, 2, 2, 2, 2, 2, 2, 2, 2, 2, 2, 2, 2, 2, 2, 2, 2, 2, 2, 2, 2, 2, 2, 2, 2, 2, 2, 2, 2, 2, 2, 2, 2, 2, 2, 2, 2, 2, 2, 2, 2, 2, 2, 2, 2, 2, 2, 2, 2, 2, 2, 2, 2, 2, 2, 2, 2, 2, 2, 2, 2, 2, 2, 2, 2, 2, 2, 2, 2, 2, 2, 2, 2, 2, 2, 2, 2, 2, 2, 2, 2, 2, 2, 2, 2, 2, 2, 2, 2, 2, 2, 2, 2, 2, 2, 2, 2, 2, 2, 2, 2, 2, 2, 2, 2, 2, 2, 2, 2, 2, 2, 2, 2, 2, 2, 2, 2, 2, 2, 2, 2, 2, 2, 2, 2, 2, 2, 2, 2, 2, 2, 2, 2, 2, 2, 2, 2, 2, 2, 2, 2, 2, 2, 2, 2, 2, 2, 2, 2, 2, 2, 2, 2, 2, 2, 2, 2, 2, 2, 2, 2, 2, 2, 2, 2, 2, 2, 2, 2, 2, 2, 2, 2, 2, 2, 2, 2, 2, 2, 2, 2, 2, 2, 2, 2, 2, 2, 2, 2, 2, 2, 2, 2, 2, 2, 2, 2, 2, 2, 2, 2, 2, 2, 2, 2, 2, 2, 2, 2, 2, 2, 2, 2, 2, 2, 2, 2, 2, 2, 2, 2, 2, 2, 2, 2, 2, 2, 2, 2, 2, 2, 2, 2, 2, 2, 2, 2, 2, 3 ),
 ( 0.000000000000000000, 1.000000000000000000 ),
 ( 0.000000000000000000, 0.002777777777777777884, 0.005555555555555555768, 0.008333333333333333218, 0.01111111111111111154, 0.01388888888888888812, 0.01666666666666666644, 0.01944444444444444475, 0.02222222222222222307, 0.02500000000000000139, 0.02777777777777777624, 0.03055555555555555455, 0.03333333333333333287, 0.03611111111111110772, 0.03888888888888888951, 0.04166666666666666435, 0.04444444444444444614, 0.04722222222222222099, 0.05000000000000000278, 0.05277777777777777762, 0.05555555555555555247, 0.05833333333333333426, 0.06111111111111110911, 0.06388888888888888395, 0.06666666666666666574, 0.06944444444444444753, 0.07222222222222221544, 0.07499999999999999722, 0.07777777777777777901, 0.08055555555555556080, 0.08333333333333332871, 0.08611111111111111049, 0.08888888888888889228, 0.09166666666666666019, 0.09444444444444444198, 0.09722222222222222376, 0.1000000000000000056, 0.1027777777777777735, 0.1055555555555555552, 0.1083333333333333370, 0.1111111111111111049, 0.1138888888888888867, 0.1166666666666666685, 0.1194444444444444503, 0.1222222222222222182, 0.1250000000000000000, 0.1277777777777777679, 0.1305555555555555636, 0.1333333333333333315, 0.1361111111111110994, 0.1388888888888888951, 0.1416666666666666630, 0.1444444444444444309, 0.1472222222222222265, 0.1499999999999999944, 0.1527777777777777901, 0.1555555555555555580, 0.1583333333333333259, 0.1611111111111111216, 0.1638888888888888895, 0.1666666666666666574, 0.1694444444444444531, 0.1722222222222222210, 0.1749999999999999889, 0.1777777777777777846, 0.1805555555555555525, 0.1833333333333333204, 0.1861111111111111160, 0.1888888888888888840, 0.1916666666666666796, 0.1944444444444444475, 0.1972222222222222154, 0.2000000000000000111, 0.2027777777777777790, 0.2055555555555555469, 0.2083333333333333426, 0.2111111111111111105, 0.2138888888888888784, 0.2166666666666666741, 0.2194444444444444420, 0.2222222222222222099, 0.2250000000000000056, 0.2277777777777777735, 0.2305555555555555691, 0.2333333333333333370, 0.2361111111111111049, 0.2388888888888889006, 0.2416666666666666685, 0.2444444444444444364, 0.2472222222222222321, 0.2500000000000000000, 0.2527777777777777679, 0.2555555555555555358, 0.2583333333333333592, 0.2611111111111111271, 0.2638888888888888951, 0.2666666666666666630, 0.2694444444444444309, 0.2722222222222221988, 0.2750000000000000222, 0.2777777777777777901, 0.2805555555555555580, 0.2833333333333333259, 0.2861111111111110938, 0.2888888888888888618, 0.2916666666666666852, 0.2944444444444444531, 0.2972222222222222210, 0.2999999999999999889, 0.3027777777777777568, 0.3055555555555555802, 0.3083333333333333481, 0.3111111111111111160, 0.3138888888888888840, 0.3166666666666666519, 0.3194444444444444198, 0.3222222222222222432, 0.3250000000000000111, 0.3277777777777777790, 0.3305555555555555469, 0.3333333333333333148, 0.3361111111111111382, 0.3388888888888889062, 0.3416666666666666741, 0.3444444444444444420, 0.3472222222222222099, 0.3499999999999999778, 0.3527777777777778012, 0.3555555555555555691, 0.3583333333333333370, 0.3611111111111111049, 0.3638888888888888729, 0.3666666666666666408, 0.3694444444444444642, 0.3722222222222222321, 0.3750000000000000000, 0.3777777777777777679, 0.3805555555555555358, 0.3833333333333333592, 0.3861111111111111271, 0.3888888888888888951, 0.3916666666666666630, 0.3944444444444444309, 0.3972222222222221988, 0.4000000000000000222, 0.4027777777777777901, 0.4055555555555555580, 0.4083333333333333259, 0.4111111111111110938, 0.4138888888888888618, 0.4166666666666666852, 0.4194444444444444531, 0.4222222222222222210, 0.4249999999999999889, 0.4277777777777777568, 0.4305555555555555802, 0.4333333333333333481, 0.4361111111111111160, 0.4388888888888888840, 0.4416666666666666519, 0.4444444444444444198, 0.4472222222222222432, 0.4500000000000000111, 0.4527777777777777790, 0.4555555555555555469, 0.4583333333333333148, 0.4611111111111111382, 0.4638888888888889062, 0.4666666666666666741, 0.4694444444444444420, 0.4722222222222222099, 0.4749999999999999778, 0.4777777777777778012, 0.4805555555555555691, 0.4833333333333333370, 0.4861111111111111049, 0.4888888888888888729, 0.4916666666666666408, 0.4944444444444444642, 0.4972222222222222321, 0.5000000000000000000, 0.5027777777777777679, 0.5055555555555555358, 0.5083333333333333037, 0.5111111111111110716, 0.5138888888888888395, 0.5166666666666667185, 0.5194444444444444864, 0.5222222222222222543, 0.5250000000000000222, 0.5277777777777777901, 0.5305555555555555580, 0.5333333333333333259, 0.5361111111111110938, 0.5388888888888888618, 0.5416666666666666297, 0.5444444444444443976, 0.5472222222222222765, 0.5500000000000000444, 0.5527777777777778123, 0.5555555555555555802, 0.5583333333333333481, 0.5611111111111111160, 0.5638888888888888840, 0.5666666666666666519, 0.5694444444444444198, 0.5722222222222221877, 0.5749999999999999556, 0.5777777777777777235, 0.5805555555555556024, 0.5833333333333333703, 0.5861111111111111382, 0.5888888888888889062, 0.5916666666666666741, 0.5944444444444444420, 0.5972222222222222099, 0.5999999999999999778, 0.6027777777777777457, 0.6055555555555555136, 0.6083333333333332815, 0.6111111111111111605, 0.6138888888888889284, 0.6166666666666666963, 0.6194444444444444642, 0.6222222222222222321, 0.6250000000000000000, 0.6277777777777777679, 0.6305555555555555358, 0.6333333333333333037, 0.6361111111111110716, 0.6388888888888888395, 0.6416666666666667185, 0.6444444444444444864, 0.6472222222222222543, 0.6500000000000000222, 0.6527777777777777901, 0.6555555555555555580, 0.6583333333333333259, 0.6611111111111110938, 0.6638888888888888618, 0.6666666666666666297, 0.6694444444444443976, 0.6722222222222222765, 0.6750000000000000444, 0.6777777777777778123, 0.6805555555555555802, 0.6833333333333333481, 0.6861111111111111160, 0.6888888888888888840, 0.6916666666666666519, 0.6944444444444444198, 0.6972222222222221877, 0.6999999999999999556, 0.7027777777777777235, 0.7055555555555556024, 0.7083333333333333703, 0.7111111111111111382, 0.7138888888888889062, 0.7166666666666666741, 0.7194444444444444420, 0.7222222222222222099, 0.7249999999999999778, 0.7277777777777777457, 0.7305555555555555136, 0.7333333333333332815, 0.7361111111111111605, 0.7388888888888889284, 0.7416666666666666963, 0.7444444444444444642, 0.7472222222222222321, 0.7500000000000000000, 0.7527777777777777679, 0.7555555555555555358, 0.7583333333333333037, 0.7611111111111110716, 0.7638888888888888395, 0.7666666666666667185, 0.7694444444444444864, 0.7722222222222222543, 0.7750000000000000222, 0.7777777777777777901, 0.7805555555555555580, 0.7833333333333333259, 0.7861111111111110938, 0.7888888888888888618, 0.7916666666666666297, 0.7944444444444443976, 0.7972222222222222765, 0.8000000000000000444, 0.8027777777777778123, 0.8055555555555555802, 0.8083333333333333481, 0.8111111111111111160, 0.8138888888888888840, 0.8166666666666666519, 0.8194444444444444198, 0.8222222222222221877, 0.8249999999999999556, 0.8277777777777777235, 0.8305555555555556024, 0.8333333333333333703, 0.8361111111111111382, 0.8388888888888889062, 0.8416666666666666741, 0.8444444444444444420, 0.8472222222222222099, 0.8499999999999999778, 0.8527777777777777457, 0.8555555555555555136, 0.8583333333333332815, 0.8611111111111111605, 0.8638888888888889284, 0.8666666666666666963, 0.8694444444444444642, 0.8722222222222222321, 0.8750000000000000000, 0.8777777777777777679, 0.8805555555555555358, 0.8833333333333333037, 0.8861111111111110716, 0.8888888888888888395, 0.8916666666666667185, 0.8944444444444444864, 0.8972222222222222543, 0.9000000000000000222, 0.9027777777777777901, 0.9055555555555555580, 0.9083333333333333259, 0.9111111111111110938, 0.9138888888888888618, 0.9166666666666666297, 0.9194444444444443976, 0.9222222222222222765, 0.9250000000000000444, 0.9277777777777778123, 0.9305555555555555802, 0.9333333333333333481, 0.9361111111111111160, 0.9388888888888888840, 0.9416666666666666519, 0.9444444444444444198, 0.9472222222222221877, 0.9499999999999999556, 0.9527777777777777235, 0.9555555555555556024, 0.9583333333333333703, 0.9611111111111111382, 0.9638888888888889062, 0.9666666666666666741, 0.9694444444444444420, 0.9722222222222222099, 0.9749999999999999778, 0.9777777777777777457, 0.9805555555555555136, 0.9833333333333332815, 0.9861111111111111605, 0.9888888888888889284, 0.9916666666666666963, 0.9944444444444444642, 0.9972222222222222321, 1.000000000000000000 ),
 .UNSPECIFIED. ) 
 GEOMETRIC_REPRESENTATION_ITEM ( )  RATIONAL_B_SPLINE_SURFACE ( (
 ( 1.000000000000000000, 0.8660254037844387076, 1.000000000000000000, 0.8660254037844387076, 1.000000000000000000, 0.8660254037844387076, 1.000000000000000000, 0.8660254037844387076, 1.000000000000000000, 0.8660254037844387076, 1.000000000000000000, 0.8660254037844387076, 1.000000000000000000, 0.8660254037844387076, 1.000000000000000000, 0.8660254037844387076, 1.000000000000000000, 0.8660254037844387076, 1.000000000000000000, 0.8660254037844387076, 1.000000000000000000, 0.8660254037844387076, 1.000000000000000000, 0.8660254037844387076, 1.000000000000000000, 0.8660254037844387076, 1.000000000000000000, 0.8660254037844387076, 1.000000000000000000, 0.8660254037844387076, 1.000000000000000000, 0.8660254037844387076, 1.000000000000000000, 0.8660254037844387076, 1.000000000000000000, 0.8660254037844387076, 1.000000000000000000, 0.8660254037844387076, 1.000000000000000000, 0.8660254037844387076, 1.000000000000000000, 0.8660254037844387076, 1.000000000000000000, 0.8660254037844387076, 1.000000000000000000, 0.8660254037844387076, 1.000000000000000000, 0.8660254037844387076, 1.000000000000000000, 0.8660254037844387076, 1.000000000000000000, 0.8660254037844387076, 1.000000000000000000, 0.8660254037844387076, 1.000000000000000000, 0.8660254037844387076, 1.000000000000000000, 0.8660254037844387076, 1.000000000000000000, 0.8660254037844387076, 1.000000000000000000, 0.8660254037844387076, 1.000000000000000000, 0.8660254037844387076, 1.000000000000000000, 0.8660254037844387076, 1.000000000000000000, 0.8660254037844387076, 1.000000000000000000, 0.8660254037844387076, 1.000000000000000000, 0.8660254037844387076, 1.000000000000000000, 0.8660254037844387076, 1.000000000000000000, 0.8660254037844387076, 1.000000000000000000, 0.8660254037844387076, 1.000000000000000000, 0.8660254037844387076, 1.000000000000000000, 0.8660254037844387076, 1.000000000000000000, 0.8660254037844387076, 1.000000000000000000, 0.8660254037844387076, 1.000000000000000000, 0.8660254037844387076, 1.000000000000000000, 0.8660254037844387076, 1.000000000000000000, 0.8660254037844387076, 1.000000000000000000, 0.8660254037844387076, 1.000000000000000000, 0.8660254037844387076, 1.000000000000000000, 0.8660254037844387076, 1.000000000000000000, 0.8660254037844387076, 1.000000000000000000, 0.8660254037844387076, 1.000000000000000000, 0.8660254037844387076, 1.000000000000000000, 0.8660254037844387076, 1.000000000000000000, 0.8660254037844387076, 1.000000000000000000, 0.8660254037844387076, 1.000000000000000000, 0.8660254037844387076, 1.000000000000000000, 0.8660254037844387076, 1.000000000000000000, 0.8660254037844387076, 1.000000000000000000, 0.8660254037844387076, 1.000000000000000000, 0.8660254037844387076, 1.000000000000000000, 0.8660254037844387076, 1.000000000000000000, 0.8660254037844387076, 1.000000000000000000, 0.8660254037844387076, 1.000000000000000000, 0.8660254037844387076, 1.000000000000000000, 0.8660254037844387076, 1.000000000000000000, 0.8660254037844387076, 1.000000000000000000, 0.8660254037844387076, 1.000000000000000000, 0.8660254037844387076, 1.000000000000000000, 0.8660254037844387076, 1.000000000000000000, 0.8660254037844387076, 1.000000000000000000, 0.8660254037844387076, 1.000000000000000000, 0.8660254037844387076, 1.000000000000000000, 0.8660254037844387076, 1.000000000000000000, 0.8660254037844387076, 1.000000000000000000, 0.8660254037844387076, 1.000000000000000000, 0.8660254037844387076, 1.000000000000000000, 0.8660254037844387076, 1.000000000000000000, 0.8660254037844387076, 1.000000000000000000, 0.8660254037844387076, 1.000000000000000000, 0.8660254037844387076, 1.000000000000000000, 0.8660254037844387076, 1.000000000000000000, 0.8660254037844387076, 1.000000000000000000, 0.8660254037844387076, 1.000000000000000000, 0.8660254037844387076, 1.000000000000000000, 0.8660254037844387076, 1.000000000000000000, 0.8660254037844387076, 1.000000000000000000, 0.8660254037844387076, 1.000000000000000000, 0.8660254037844387076, 1.000000000000000000, 0.8660254037844387076, 1.000000000000000000, 0.8660254037844387076, 1.000000000000000000, 0.8660254037844387076, 1.000000000000000000, 0.8660254037844387076, 1.000000000000000000, 0.8660254037844387076, 1.000000000000000000, 0.8660254037844387076, 1.000000000000000000, 0.8660254037844387076, 1.000000000000000000, 0.8660254037844387076, 1.000000000000000000, 0.8660254037844387076, 1.000000000000000000, 0.8660254037844387076, 1.000000000000000000, 0.8660254037844387076, 1.000000000000000000, 0.8660254037844387076, 1.000000000000000000, 0.8660254037844387076, 1.000000000000000000, 0.8660254037844387076, 1.000000000000000000, 0.8660254037844387076, 1.000000000000000000, 0.8660254037844387076, 1.000000000000000000, 0.8660254037844387076, 1.000000000000000000, 0.8660254037844387076, 1.000000000000000000, 0.8660254037844387076, 1.000000000000000000, 0.8660254037844387076, 1.000000000000000000, 0.8660254037844387076, 1.000000000000000000, 0.8660254037844387076, 1.000000000000000000, 0.8660254037844387076, 1.000000000000000000, 0.8660254037844387076, 1.000000000000000000, 0.8660254037844387076, 1.000000000000000000, 0.8660254037844387076, 1.000000000000000000, 0.8660254037844387076, 1.000000000000000000, 0.8660254037844387076, 1.000000000000000000, 0.8660254037844387076, 1.000000000000000000, 0.8660254037844387076, 1.000000000000000000, 0.8660254037844387076, 1.000000000000000000, 0.8660254037844387076, 1.000000000000000000, 0.8660254037844387076, 1.000000000000000000, 0.8660254037844387076, 1.000000000000000000, 0.8660254037844387076, 1.000000000000000000, 0.8660254037844387076, 1.000000000000000000, 0.8660254037844387076, 1.000000000000000000, 0.8660254037844387076, 1.000000000000000000, 0.8660254037844387076, 1.000000000000000000, 0.8660254037844387076, 1.000000000000000000, 0.8660254037844387076, 1.000000000000000000, 0.8660254037844387076, 1.000000000000000000, 0.8660254037844387076, 1.000000000000000000, 0.8660254037844387076, 1.000000000000000000, 0.8660254037844387076, 1.000000000000000000, 0.8660254037844387076, 1.000000000000000000, 0.8660254037844387076, 1.000000000000000000, 0.8660254037844387076, 1.000000000000000000, 0.8660254037844387076, 1.000000000000000000, 0.8660254037844387076, 1.000000000000000000, 0.8660254037844387076, 1.000000000000000000, 0.8660254037844387076, 1.000000000000000000, 0.8660254037844387076, 1.000000000000000000, 0.8660254037844387076, 1.000000000000000000, 0.8660254037844387076, 1.000000000000000000, 0.8660254037844387076, 1.000000000000000000, 0.8660254037844387076, 1.000000000000000000, 0.8660254037844387076, 1.000000000000000000, 0.8660254037844387076, 1.000000000000000000, 0.8660254037844387076, 1.000000000000000000, 0.8660254037844387076, 1.000000000000000000, 0.8660254037844387076, 1.000000000000000000, 0.8660254037844387076, 1.000000000000000000, 0.8660254037844387076, 1.000000000000000000, 0.8660254037844387076, 1.000000000000000000, 0.8660254037844387076, 1.000000000000000000, 0.8660254037844387076, 1.000000000000000000, 0.8660254037844387076, 1.000000000000000000, 0.8660254037844387076, 1.000000000000000000, 0.8660254037844387076, 1.000000000000000000, 0.8660254037844387076, 1.000000000000000000, 0.8660254037844387076, 1.000000000000000000, 0.8660254037844387076, 1.000000000000000000, 0.8660254037844387076, 1.000000000000000000, 0.8660254037844387076, 1.000000000000000000, 0.8660254037844387076, 1.000000000000000000, 0.8660254037844387076, 1.000000000000000000, 0.8660254037844387076, 1.000000000000000000, 0.8660254037844387076, 1.000000000000000000, 0.8660254037844387076, 1.000000000000000000, 0.8660254037844387076, 1.000000000000000000, 0.8660254037844387076, 1.000000000000000000, 0.8660254037844387076, 1.000000000000000000, 0.8660254037844387076, 1.000000000000000000, 0.8660254037844387076, 1.000000000000000000, 0.8660254037844387076, 1.000000000000000000, 0.8660254037844387076, 1.000000000000000000, 0.8660254037844387076, 1.000000000000000000, 0.8660254037844387076, 1.000000000000000000, 0.8660254037844387076, 1.000000000000000000, 0.8660254037844387076, 1.000000000000000000, 0.8660254037844387076, 1.000000000000000000, 0.8660254037844387076, 1.000000000000000000, 0.8660254037844387076, 1.000000000000000000, 0.8660254037844387076, 1.000000000000000000, 0.8660254037844387076, 1.000000000000000000, 0.8660254037844387076, 1.000000000000000000, 0.8660254037844387076, 1.000000000000000000, 0.8660254037844387076, 1.000000000000000000, 0.8660254037844387076, 1.000000000000000000, 0.8660254037844387076, 1.000000000000000000, 0.8660254037844387076, 1.000000000000000000, 0.8660254037844387076, 1.000000000000000000, 0.8660254037844387076, 1.000000000000000000, 0.8660254037844387076, 1.000000000000000000, 0.8660254037844387076, 1.000000000000000000, 0.8660254037844387076, 1.000000000000000000, 0.8660254037844387076, 1.000000000000000000, 0.8660254037844387076, 1.000000000000000000, 0.8660254037844387076, 1.000000000000000000, 0.8660254037844387076, 1.000000000000000000, 0.8660254037844387076, 1.000000000000000000, 0.8660254037844387076, 1.000000000000000000, 0.8660254037844387076, 1.000000000000000000, 0.8660254037844387076, 1.000000000000000000, 0.8660254037844387076, 1.000000000000000000, 0.8660254037844387076, 1.000000000000000000, 0.8660254037844387076, 1.000000000000000000, 0.8660254037844387076, 1.000000000000000000, 0.8660254037844387076, 1.000000000000000000, 0.8660254037844387076, 1.000000000000000000, 0.8660254037844387076, 1.000000000000000000, 0.8660254037844387076, 1.000000000000000000, 0.8660254037844387076, 1.000000000000000000, 0.8660254037844387076, 1.000000000000000000, 0.8660254037844387076, 1.000000000000000000, 0.8660254037844387076, 1.000000000000000000, 0.8660254037844387076, 1.000000000000000000, 0.8660254037844387076, 1.000000000000000000, 0.8660254037844387076, 1.000000000000000000, 0.8660254037844387076, 1.000000000000000000, 0.8660254037844387076, 1.000000000000000000, 0.8660254037844387076, 1.000000000000000000, 0.8660254037844387076, 1.000000000000000000, 0.8660254037844387076, 1.000000000000000000, 0.8660254037844387076, 1.000000000000000000, 0.8660254037844387076, 1.000000000000000000, 0.8660254037844387076, 1.000000000000000000, 0.8660254037844387076, 1.000000000000000000, 0.8660254037844387076, 1.000000000000000000, 0.8660254037844387076, 1.000000000000000000, 0.8660254037844387076, 1.000000000000000000, 0.8660254037844387076, 1.000000000000000000, 0.8660254037844387076, 1.000000000000000000, 0.8660254037844387076, 1.000000000000000000, 0.8660254037844387076, 1.000000000000000000, 0.8660254037844387076, 1.000000000000000000, 0.8660254037844387076, 1.000000000000000000, 0.8660254037844387076, 1.000000000000000000, 0.8660254037844387076, 1.000000000000000000, 0.8660254037844387076, 1.000000000000000000, 0.8660254037844387076, 1.000000000000000000, 0.8660254037844387076, 1.000000000000000000, 0.8660254037844387076, 1.000000000000000000, 0.8660254037844387076, 1.000000000000000000, 0.8660254037844387076, 1.000000000000000000, 0.8660254037844387076, 1.000000000000000000, 0.8660254037844387076, 1.000000000000000000, 0.8660254037844387076, 1.000000000000000000, 0.8660254037844387076, 1.000000000000000000, 0.8660254037844387076, 1.000000000000000000, 0.8660254037844387076, 1.000000000000000000, 0.8660254037844387076, 1.000000000000000000, 0.8660254037844387076, 1.000000000000000000, 0.8660254037844387076, 1.000000000000000000, 0.8660254037844387076, 1.000000000000000000, 0.8660254037844387076, 1.000000000000000000, 0.8660254037844387076, 1.000000000000000000, 0.8660254037844387076, 1.000000000000000000, 0.8660254037844387076, 1.000000000000000000, 0.8660254037844387076, 1.000000000000000000, 0.8660254037844387076, 1.000000000000000000, 0.8660254037844387076, 1.000000000000000000, 0.8660254037844387076, 1.000000000000000000, 0.8660254037844387076, 1.000000000000000000, 0.8660254037844387076, 1.000000000000000000, 0.8660254037844387076, 1.000000000000000000, 0.8660254037844387076, 1.000000000000000000, 0.8660254037844387076, 1.000000000000000000, 0.8660254037844387076, 1.000000000000000000, 0.8660254037844387076, 1.000000000000000000, 0.8660254037844387076, 1.000000000000000000, 0.8660254037844387076, 1.000000000000000000, 0.8660254037844387076, 1.000000000000000000, 0.8660254037844387076, 1.000000000000000000, 0.8660254037844387076, 1.000000000000000000, 0.8660254037844387076, 1.000000000000000000, 0.8660254037844387076, 1.000000000000000000, 0.8660254037844387076, 1.000000000000000000, 0.8660254037844387076, 1.000000000000000000, 0.8660254037844387076, 1.000000000000000000, 0.8660254037844387076, 1.000000000000000000, 0.8660254037844387076, 1.000000000000000000, 0.8660254037844387076, 1.000000000000000000, 0.8660254037844387076, 1.000000000000000000, 0.8660254037844387076, 1.000000000000000000, 0.8660254037844387076, 1.000000000000000000, 0.8660254037844387076, 1.000000000000000000, 0.8660254037844387076, 1.000000000000000000, 0.8660254037844387076, 1.000000000000000000, 0.8660254037844387076, 1.000000000000000000, 0.8660254037844387076, 1.000000000000000000, 0.8660254037844387076, 1.000000000000000000, 0.8660254037844387076, 1.000000000000000000, 0.8660254037844387076, 1.000000000000000000, 0.8660254037844387076, 1.000000000000000000, 0.8660254037844387076, 1.000000000000000000, 0.8660254037844387076, 1.000000000000000000, 0.8660254037844387076, 1.000000000000000000, 0.8660254037844387076, 1.000000000000000000, 0.8660254037844387076, 1.000000000000000000, 0.8660254037844387076, 1.000000000000000000, 0.8660254037844387076, 1.000000000000000000, 0.8660254037844387076, 1.000000000000000000, 0.8660254037844387076, 1.000000000000000000, 0.8660254037844387076, 1.000000000000000000, 0.8660254037844387076, 1.000000000000000000, 0.8660254037844387076, 1.000000000000000000, 0.8660254037844387076, 1.000000000000000000, 0.8660254037844387076, 1.000000000000000000, 0.8660254037844387076, 1.000000000000000000, 0.8660254037844387076, 1.000000000000000000, 0.8660254037844387076, 1.000000000000000000, 0.8660254037844387076, 1.000000000000000000, 0.8660254037844387076, 1.000000000000000000, 0.8660254037844387076, 1.000000000000000000, 0.8660254037844387076, 1.000000000000000000, 0.8660254037844387076, 1.000000000000000000, 0.8660254037844387076, 1.000000000000000000, 0.8660254037844387076, 1.000000000000000000, 0.8660254037844387076, 1.000000000000000000, 0.8660254037844387076, 1.000000000000000000, 0.8660254037844387076, 1.000000000000000000, 0.8660254037844387076, 1.000000000000000000, 0.8660254037844387076, 1.000000000000000000, 0.8660254037844387076, 1.000000000000000000, 0.8660254037844387076, 1.000000000000000000, 0.8660254037844387076, 1.000000000000000000, 0.8660254037844387076, 1.000000000000000000, 0.8660254037844387076, 1.000000000000000000, 0.8660254037844387076, 1.000000000000000000, 0.8660254037844387076, 1.000000000000000000, 0.8660254037844387076, 1.000000000000000000, 0.8660254037844387076, 1.000000000000000000, 0.8660254037844387076, 1.000000000000000000, 0.8660254037844387076, 1.000000000000000000, 0.8660254037844387076, 1.000000000000000000, 0.8660254037844387076, 1.000000000000000000, 0.8660254037844387076, 1.000000000000000000, 0.8660254037844387076, 1.000000000000000000, 0.8660254037844387076, 1.000000000000000000, 0.8660254037844387076, 1.000000000000000000, 0.8660254037844387076, 1.000000000000000000, 0.8660254037844387076, 1.000000000000000000, 0.8660254037844387076, 1.000000000000000000, 0.8660254037844387076, 1.000000000000000000, 0.8660254037844387076, 1.000000000000000000, 0.8660254037844387076, 1.000000000000000000, 0.8660254037844387076, 1.000000000000000000, 0.8660254037844387076, 1.000000000000000000, 0.8660254037844387076, 1.000000000000000000, 0.8660254037844387076, 1.000000000000000000, 0.8660254037844387076, 1.000000000000000000, 0.8660254037844387076, 1.000000000000000000, 0.8660254037844387076, 1.000000000000000000, 0.8660254037844387076, 1.000000000000000000, 0.8660254037844387076, 1.000000000000000000, 0.8660254037844387076, 1.000000000000000000, 0.8660254037844387076, 1.000000000000000000, 0.8660254037844387076, 1.000000000000000000, 0.8660254037844387076, 1.000000000000000000, 0.8660254037844387076, 1.000000000000000000),
 ( 1.000000000000000000, 0.8660254037844387076, 1.000000000000000000, 0.8660254037844387076, 1.000000000000000000, 0.8660254037844387076, 1.000000000000000000, 0.8660254037844387076, 1.000000000000000000, 0.8660254037844387076, 1.000000000000000000, 0.8660254037844387076, 1.000000000000000000, 0.8660254037844387076, 1.000000000000000000, 0.8660254037844387076, 1.000000000000000000, 0.8660254037844387076, 1.000000000000000000, 0.8660254037844387076, 1.000000000000000000, 0.8660254037844387076, 1.000000000000000000, 0.8660254037844387076, 1.000000000000000000, 0.8660254037844387076, 1.000000000000000000, 0.8660254037844387076, 1.000000000000000000, 0.8660254037844387076, 1.000000000000000000, 0.8660254037844387076, 1.000000000000000000, 0.8660254037844387076, 1.000000000000000000, 0.8660254037844387076, 1.000000000000000000, 0.8660254037844387076, 1.000000000000000000, 0.8660254037844387076, 1.000000000000000000, 0.8660254037844387076, 1.000000000000000000, 0.8660254037844387076, 1.000000000000000000, 0.8660254037844387076, 1.000000000000000000, 0.8660254037844387076, 1.000000000000000000, 0.8660254037844387076, 1.000000000000000000, 0.8660254037844387076, 1.000000000000000000, 0.8660254037844387076, 1.000000000000000000, 0.8660254037844387076, 1.000000000000000000, 0.8660254037844387076, 1.000000000000000000, 0.8660254037844387076, 1.000000000000000000, 0.8660254037844387076, 1.000000000000000000, 0.8660254037844387076, 1.000000000000000000, 0.8660254037844387076, 1.000000000000000000, 0.8660254037844387076, 1.000000000000000000, 0.8660254037844387076, 1.000000000000000000, 0.8660254037844387076, 1.000000000000000000, 0.8660254037844387076, 1.000000000000000000, 0.8660254037844387076, 1.000000000000000000, 0.8660254037844387076, 1.000000000000000000, 0.8660254037844387076, 1.000000000000000000, 0.8660254037844387076, 1.000000000000000000, 0.8660254037844387076, 1.000000000000000000, 0.8660254037844387076, 1.000000000000000000, 0.8660254037844387076, 1.000000000000000000, 0.8660254037844387076, 1.000000000000000000, 0.8660254037844387076, 1.000000000000000000, 0.8660254037844387076, 1.000000000000000000, 0.8660254037844387076, 1.000000000000000000, 0.8660254037844387076, 1.000000000000000000, 0.8660254037844387076, 1.000000000000000000, 0.8660254037844387076, 1.000000000000000000, 0.8660254037844387076, 1.000000000000000000, 0.8660254037844387076, 1.000000000000000000, 0.8660254037844387076, 1.000000000000000000, 0.8660254037844387076, 1.000000000000000000, 0.8660254037844387076, 1.000000000000000000, 0.8660254037844387076, 1.000000000000000000, 0.8660254037844387076, 1.000000000000000000, 0.8660254037844387076, 1.000000000000000000, 0.8660254037844387076, 1.000000000000000000, 0.8660254037844387076, 1.000000000000000000, 0.8660254037844387076, 1.000000000000000000, 0.8660254037844387076, 1.000000000000000000, 0.8660254037844387076, 1.000000000000000000, 0.8660254037844387076, 1.000000000000000000, 0.8660254037844387076, 1.000000000000000000, 0.8660254037844387076, 1.000000000000000000, 0.8660254037844387076, 1.000000000000000000, 0.8660254037844387076, 1.000000000000000000, 0.8660254037844387076, 1.000000000000000000, 0.8660254037844387076, 1.000000000000000000, 0.8660254037844387076, 1.000000000000000000, 0.8660254037844387076, 1.000000000000000000, 0.8660254037844387076, 1.000000000000000000, 0.8660254037844387076, 1.000000000000000000, 0.8660254037844387076, 1.000000000000000000, 0.8660254037844387076, 1.000000000000000000, 0.8660254037844387076, 1.000000000000000000, 0.8660254037844387076, 1.000000000000000000, 0.8660254037844387076, 1.000000000000000000, 0.8660254037844387076, 1.000000000000000000, 0.8660254037844387076, 1.000000000000000000, 0.8660254037844387076, 1.000000000000000000, 0.8660254037844387076, 1.000000000000000000, 0.8660254037844387076, 1.000000000000000000, 0.8660254037844387076, 1.000000000000000000, 0.8660254037844387076, 1.000000000000000000, 0.8660254037844387076, 1.000000000000000000, 0.8660254037844387076, 1.000000000000000000, 0.8660254037844387076, 1.000000000000000000, 0.8660254037844387076, 1.000000000000000000, 0.8660254037844387076, 1.000000000000000000, 0.8660254037844387076, 1.000000000000000000, 0.8660254037844387076, 1.000000000000000000, 0.8660254037844387076, 1.000000000000000000, 0.8660254037844387076, 1.000000000000000000, 0.8660254037844387076, 1.000000000000000000, 0.8660254037844387076, 1.000000000000000000, 0.8660254037844387076, 1.000000000000000000, 0.8660254037844387076, 1.000000000000000000, 0.8660254037844387076, 1.000000000000000000, 0.8660254037844387076, 1.000000000000000000, 0.8660254037844387076, 1.000000000000000000, 0.8660254037844387076, 1.000000000000000000, 0.8660254037844387076, 1.000000000000000000, 0.8660254037844387076, 1.000000000000000000, 0.8660254037844387076, 1.000000000000000000, 0.8660254037844387076, 1.000000000000000000, 0.8660254037844387076, 1.000000000000000000, 0.8660254037844387076, 1.000000000000000000, 0.8660254037844387076, 1.000000000000000000, 0.8660254037844387076, 1.000000000000000000, 0.8660254037844387076, 1.000000000000000000, 0.8660254037844387076, 1.000000000000000000, 0.8660254037844387076, 1.000000000000000000, 0.8660254037844387076, 1.000000000000000000, 0.8660254037844387076, 1.000000000000000000, 0.8660254037844387076, 1.000000000000000000, 0.8660254037844387076, 1.000000000000000000, 0.8660254037844387076, 1.000000000000000000, 0.8660254037844387076, 1.000000000000000000, 0.8660254037844387076, 1.000000000000000000, 0.8660254037844387076, 1.000000000000000000, 0.8660254037844387076, 1.000000000000000000, 0.8660254037844387076, 1.000000000000000000, 0.8660254037844387076, 1.000000000000000000, 0.8660254037844387076, 1.000000000000000000, 0.8660254037844387076, 1.000000000000000000, 0.8660254037844387076, 1.000000000000000000, 0.8660254037844387076, 1.000000000000000000, 0.8660254037844387076, 1.000000000000000000, 0.8660254037844387076, 1.000000000000000000, 0.8660254037844387076, 1.000000000000000000, 0.8660254037844387076, 1.000000000000000000, 0.8660254037844387076, 1.000000000000000000, 0.8660254037844387076, 1.000000000000000000, 0.8660254037844387076, 1.000000000000000000, 0.8660254037844387076, 1.000000000000000000, 0.8660254037844387076, 1.000000000000000000, 0.8660254037844387076, 1.000000000000000000, 0.8660254037844387076, 1.000000000000000000, 0.8660254037844387076, 1.000000000000000000, 0.8660254037844387076, 1.000000000000000000, 0.8660254037844387076, 1.000000000000000000, 0.8660254037844387076, 1.000000000000000000, 0.8660254037844387076, 1.000000000000000000, 0.8660254037844387076, 1.000000000000000000, 0.8660254037844387076, 1.000000000000000000, 0.8660254037844387076, 1.000000000000000000, 0.8660254037844387076, 1.000000000000000000, 0.8660254037844387076, 1.000000000000000000, 0.8660254037844387076, 1.000000000000000000, 0.8660254037844387076, 1.000000000000000000, 0.8660254037844387076, 1.000000000000000000, 0.8660254037844387076, 1.000000000000000000, 0.8660254037844387076, 1.000000000000000000, 0.8660254037844387076, 1.000000000000000000, 0.8660254037844387076, 1.000000000000000000, 0.8660254037844387076, 1.000000000000000000, 0.8660254037844387076, 1.000000000000000000, 0.8660254037844387076, 1.000000000000000000, 0.8660254037844387076, 1.000000000000000000, 0.8660254037844387076, 1.000000000000000000, 0.8660254037844387076, 1.000000000000000000, 0.8660254037844387076, 1.000000000000000000, 0.8660254037844387076, 1.000000000000000000, 0.8660254037844387076, 1.000000000000000000, 0.8660254037844387076, 1.000000000000000000, 0.8660254037844387076, 1.000000000000000000, 0.8660254037844387076, 1.000000000000000000, 0.8660254037844387076, 1.000000000000000000, 0.8660254037844387076, 1.000000000000000000, 0.8660254037844387076, 1.000000000000000000, 0.8660254037844387076, 1.000000000000000000, 0.8660254037844387076, 1.000000000000000000, 0.8660254037844387076, 1.000000000000000000, 0.8660254037844387076, 1.000000000000000000, 0.8660254037844387076, 1.000000000000000000, 0.8660254037844387076, 1.000000000000000000, 0.8660254037844387076, 1.000000000000000000, 0.8660254037844387076, 1.000000000000000000, 0.8660254037844387076, 1.000000000000000000, 0.8660254037844387076, 1.000000000000000000, 0.8660254037844387076, 1.000000000000000000, 0.8660254037844387076, 1.000000000000000000, 0.8660254037844387076, 1.000000000000000000, 0.8660254037844387076, 1.000000000000000000, 0.8660254037844387076, 1.000000000000000000, 0.8660254037844387076, 1.000000000000000000, 0.8660254037844387076, 1.000000000000000000, 0.8660254037844387076, 1.000000000000000000, 0.8660254037844387076, 1.000000000000000000, 0.8660254037844387076, 1.000000000000000000, 0.8660254037844387076, 1.000000000000000000, 0.8660254037844387076, 1.000000000000000000, 0.8660254037844387076, 1.000000000000000000, 0.8660254037844387076, 1.000000000000000000, 0.8660254037844387076, 1.000000000000000000, 0.8660254037844387076, 1.000000000000000000, 0.8660254037844387076, 1.000000000000000000, 0.8660254037844387076, 1.000000000000000000, 0.8660254037844387076, 1.000000000000000000, 0.8660254037844387076, 1.000000000000000000, 0.8660254037844387076, 1.000000000000000000, 0.8660254037844387076, 1.000000000000000000, 0.8660254037844387076, 1.000000000000000000, 0.8660254037844387076, 1.000000000000000000, 0.8660254037844387076, 1.000000000000000000, 0.8660254037844387076, 1.000000000000000000, 0.8660254037844387076, 1.000000000000000000, 0.8660254037844387076, 1.000000000000000000, 0.8660254037844387076, 1.000000000000000000, 0.8660254037844387076, 1.000000000000000000, 0.8660254037844387076, 1.000000000000000000, 0.8660254037844387076, 1.000000000000000000, 0.8660254037844387076, 1.000000000000000000, 0.8660254037844387076, 1.000000000000000000, 0.8660254037844387076, 1.000000000000000000, 0.8660254037844387076, 1.000000000000000000, 0.8660254037844387076, 1.000000000000000000, 0.8660254037844387076, 1.000000000000000000, 0.8660254037844387076, 1.000000000000000000, 0.8660254037844387076, 1.000000000000000000, 0.8660254037844387076, 1.000000000000000000, 0.8660254037844387076, 1.000000000000000000, 0.8660254037844387076, 1.000000000000000000, 0.8660254037844387076, 1.000000000000000000, 0.8660254037844387076, 1.000000000000000000, 0.8660254037844387076, 1.000000000000000000, 0.8660254037844387076, 1.000000000000000000, 0.8660254037844387076, 1.000000000000000000, 0.8660254037844387076, 1.000000000000000000, 0.8660254037844387076, 1.000000000000000000, 0.8660254037844387076, 1.000000000000000000, 0.8660254037844387076, 1.000000000000000000, 0.8660254037844387076, 1.000000000000000000, 0.8660254037844387076, 1.000000000000000000, 0.8660254037844387076, 1.000000000000000000, 0.8660254037844387076, 1.000000000000000000, 0.8660254037844387076, 1.000000000000000000, 0.8660254037844387076, 1.000000000000000000, 0.8660254037844387076, 1.000000000000000000, 0.8660254037844387076, 1.000000000000000000, 0.8660254037844387076, 1.000000000000000000, 0.8660254037844387076, 1.000000000000000000, 0.8660254037844387076, 1.000000000000000000, 0.8660254037844387076, 1.000000000000000000, 0.8660254037844387076, 1.000000000000000000, 0.8660254037844387076, 1.000000000000000000, 0.8660254037844387076, 1.000000000000000000, 0.8660254037844387076, 1.000000000000000000, 0.8660254037844387076, 1.000000000000000000, 0.8660254037844387076, 1.000000000000000000, 0.8660254037844387076, 1.000000000000000000, 0.8660254037844387076, 1.000000000000000000, 0.8660254037844387076, 1.000000000000000000, 0.8660254037844387076, 1.000000000000000000, 0.8660254037844387076, 1.000000000000000000, 0.8660254037844387076, 1.000000000000000000, 0.8660254037844387076, 1.000000000000000000, 0.8660254037844387076, 1.000000000000000000, 0.8660254037844387076, 1.000000000000000000, 0.8660254037844387076, 1.000000000000000000, 0.8660254037844387076, 1.000000000000000000, 0.8660254037844387076, 1.000000000000000000, 0.8660254037844387076, 1.000000000000000000, 0.8660254037844387076, 1.000000000000000000, 0.8660254037844387076, 1.000000000000000000, 0.8660254037844387076, 1.000000000000000000, 0.8660254037844387076, 1.000000000000000000, 0.8660254037844387076, 1.000000000000000000, 0.8660254037844387076, 1.000000000000000000, 0.8660254037844387076, 1.000000000000000000, 0.8660254037844387076, 1.000000000000000000, 0.8660254037844387076, 1.000000000000000000, 0.8660254037844387076, 1.000000000000000000, 0.8660254037844387076, 1.000000000000000000, 0.8660254037844387076, 1.000000000000000000, 0.8660254037844387076, 1.000000000000000000, 0.8660254037844387076, 1.000000000000000000, 0.8660254037844387076, 1.000000000000000000, 0.8660254037844387076, 1.000000000000000000, 0.8660254037844387076, 1.000000000000000000, 0.8660254037844387076, 1.000000000000000000, 0.8660254037844387076, 1.000000000000000000, 0.8660254037844387076, 1.000000000000000000, 0.8660254037844387076, 1.000000000000000000, 0.8660254037844387076, 1.000000000000000000, 0.8660254037844387076, 1.000000000000000000, 0.8660254037844387076, 1.000000000000000000, 0.8660254037844387076, 1.000000000000000000, 0.8660254037844387076, 1.000000000000000000, 0.8660254037844387076, 1.000000000000000000, 0.8660254037844387076, 1.000000000000000000, 0.8660254037844387076, 1.000000000000000000, 0.8660254037844387076, 1.000000000000000000, 0.8660254037844387076, 1.000000000000000000, 0.8660254037844387076, 1.000000000000000000, 0.8660254037844387076, 1.000000000000000000, 0.8660254037844387076, 1.000000000000000000, 0.8660254037844387076, 1.000000000000000000, 0.8660254037844387076, 1.000000000000000000, 0.8660254037844387076, 1.000000000000000000, 0.8660254037844387076, 1.000000000000000000, 0.8660254037844387076, 1.000000000000000000, 0.8660254037844387076, 1.000000000000000000, 0.8660254037844387076, 1.000000000000000000, 0.8660254037844387076, 1.000000000000000000, 0.8660254037844387076, 1.000000000000000000, 0.8660254037844387076, 1.000000000000000000, 0.8660254037844387076, 1.000000000000000000, 0.8660254037844387076, 1.000000000000000000, 0.8660254037844387076, 1.000000000000000000, 0.8660254037844387076, 1.000000000000000000, 0.8660254037844387076, 1.000000000000000000, 0.8660254037844387076, 1.000000000000000000, 0.8660254037844387076, 1.000000000000000000, 0.8660254037844387076, 1.000000000000000000, 0.8660254037844387076, 1.000000000000000000, 0.8660254037844387076, 1.000000000000000000, 0.8660254037844387076, 1.000000000000000000, 0.8660254037844387076, 1.000000000000000000, 0.8660254037844387076, 1.000000000000000000, 0.8660254037844387076, 1.000000000000000000, 0.8660254037844387076, 1.000000000000000000, 0.8660254037844387076, 1.000000000000000000, 0.8660254037844387076, 1.000000000000000000, 0.8660254037844387076, 1.000000000000000000, 0.8660254037844387076, 1.000000000000000000, 0.8660254037844387076, 1.000000000000000000, 0.8660254037844387076, 1.000000000000000000, 0.8660254037844387076, 1.000000000000000000, 0.8660254037844387076, 1.000000000000000000, 0.8660254037844387076, 1.000000000000000000, 0.8660254037844387076, 1.000000000000000000, 0.8660254037844387076, 1.000000000000000000, 0.8660254037844387076, 1.000000000000000000, 0.8660254037844387076, 1.000000000000000000, 0.8660254037844387076, 1.000000000000000000, 0.8660254037844387076, 1.000000000000000000, 0.8660254037844387076, 1.000000000000000000, 0.8660254037844387076, 1.000000000000000000, 0.8660254037844387076, 1.000000000000000000, 0.8660254037844387076, 1.000000000000000000, 0.8660254037844387076, 1.000000000000000000, 0.8660254037844387076, 1.000000000000000000, 0.8660254037844387076, 1.000000000000000000, 0.8660254037844387076, 1.000000000000000000, 0.8660254037844387076, 1.000000000000000000, 0.8660254037844387076, 1.000000000000000000, 0.8660254037844387076, 1.000000000000000000, 0.8660254037844387076, 1.000000000000000000, 0.8660254037844387076, 1.000000000000000000, 0.8660254037844387076, 1.000000000000000000, 0.8660254037844387076, 1.000000000000000000, 0.8660254037844387076, 1.000000000000000000, 0.8660254037844387076, 1.000000000000000000, 0.8660254037844387076, 1.000000000000000000, 0.8660254037844387076, 1.000000000000000000, 0.8660254037844387076, 1.000000000000000000) ) ) 
 REPRESENTATION_ITEM ( '' )  SURFACE ( )  );
#24032=CARTESIAN_POINT ( 'NONE',  ( 14.74687500061451573, -3.027376345333610441, -5.243569643749999898 ) ) ;
#24033=CARTESIAN_POINT ( 'NONE',  ( 10.80000000122903536, -2.886751345948129988, 4.999999999999997335 ) ) ;
#24034=CARTESIAN_POINT ( 'NONE',  ( 16.77187500061451786, 3.027376345333611329, 5.243569643749999010 ) ) ;
#24036=CARTESIAN_POINT ( 'NONE',  ( 9.046875000614518214, 6.054752690667223547, 3.707466751127219781E-16 ) ) ;
#24037=CARTESIAN_POINT ( 'NONE',  ( 9.001249775931846008E-16, 10.91562500061451857, -25.09994784771203058 ) ) ;
#24038=CARTESIAN_POINT ( 'NONE',  ( 3.999999999999999112, 16.62500000000000000, 30.00000000000000000 ) ) ;
#24040=CYLINDRICAL_SURFACE ( 'NONE', #51281, 4.999999999999998224 ) ;
#24041=CARTESIAN_POINT ( 'NONE',  ( 25.11562500061451431, 3.027376345333613106, -5.243569643749998122 ) ) ;
#24043=ADVANCED_FACE ( 'NONE', ( #51783 ), #41069, .F. ) ;
#24044=CARTESIAN_POINT ( 'NONE',  ( 28.39687500061452141, 6.054752690667223547, 3.707466751127219781E-16 ) ) ;
#24045=CARTESIAN_POINT ( 'NONE',  ( 23.77499999999999858, -4.330127018922194537, 2.499999999999995559 ) ) ;
#24047=( BOUNDED_CURVE ( )  B_SPLINE_CURVE ( 3, ( #44175, #60774, #15342, #5372 ),
 .UNSPECIFIED., .F., .F. ) 
 B_SPLINE_CURVE_WITH_KNOTS ( ( 4, 4 ),
 ( 0.9384417405046960869, 1.570796326794896780 ),
 .UNSPECIFIED. ) 
 CURVE ( )  GEOMETRIC_REPRESENTATION_ITEM ( )  RATIONAL_B_SPLINE_CURVE ( ( 1.000000000000000000, 0.9669539835197179523, 0.9669539835197179523, 1.000000000000000000 ) ) 
 REPRESENTATION_ITEM ( '' )  );
#24048=CARTESIAN_POINT ( 'NONE',  ( 7.640625000614517326, 6.054752690667223547, 3.707466751127219781E-16 ) ) ;
#24050=CARTESIAN_POINT ( 'NONE',  ( 18.34687500061451715, -3.027376345333610441, -5.243569643749999898 ) ) ;
#24052=CARTESIAN_POINT ( 'NONE',  ( 3.290625000614516793, -3.027376345333614438, 5.243569643749998122 ) ) ;
#24053=CARTESIAN_POINT ( 'NONE',  ( 9.459375000614517859, 4.541064518000418104, -2.621784821874998173 ) ) ;
#24055=CARTESIAN_POINT ( 'NONE',  ( 19.92187500061451644, 3.027376345333611329, 5.243569643749999010 ) ) ;
#24057=CARTESIAN_POINT ( 'NONE',  ( 26.43750000000000000, -2.886751345948129988, 4.999999999999997335 ) ) ;
#24058=CARTESIAN_POINT ( 'NONE',  ( 3.712499999999999911, 2.886751345948129099, -4.999999999999998224 ) ) ;
#24061=ORIENTED_EDGE ( 'NONE', *, *, #54124, .T. ) ;
#24062=CARTESIAN_POINT ( 'NONE',  ( 10.08749999999999858, 5.773502691896255534, 3.535250795749688894E-16 ) ) ;
#24064=CARTESIAN_POINT ( 'NONE',  ( 23.99062500061451786, -3.027376345333614438, 5.243569643749998122 ) ) ;
#24065=CARTESIAN_POINT ( 'NONE',  ( 13.08750000000000036, -2.886751345948125991, -5.000000000000000000 ) ) ;
#24067=CARTESIAN_POINT ( 'NONE',  ( 8.212500001229035007, -4.330127018922190985, -2.500000000000001332 ) ) ;
#24068=CARTESIAN_POINT ( 'NONE',  ( 6.478125000614516793, -4.541064518000419881, 2.621784821874995952 ) ) ;
#24069=CARTESIAN_POINT ( 'NONE',  ( 22.19999999999999574, 4.330127018922192761, -2.499999999999997780 ) ) ;
#24070=CARTESIAN_POINT ( 'NONE',  ( 19.75312500061451360, 4.541064518000418104, -2.621784821874998173 ) ) ;
#24072=CARTESIAN_POINT ( 'NONE',  ( 25.27500000122903145, -5.773502691896255534, -1.060575238724906372E-15 ) ) ;
#24074=CARTESIAN_POINT ( 'NONE',  ( 4.500000000000000888, -4.330127018922190985, -2.500000000000001332 ) ) ;
#24075=ORIENTED_EDGE ( 'NONE', *, *, #12791, .F. ) ;
#24076=CARTESIAN_POINT ( 'NONE',  ( 22.71562500061451573, -6.054752690667223547, -1.112240025338166033E-15 ) ) ;
#24077=CARTESIAN_POINT ( 'NONE',  ( 3.422429900546629877, -3.645130117820770455, -3.769356580772429410 ) ) ;
#24078=CARTESIAN_POINT ( 'NONE',  ( 27.57187500061451857, 3.027376345333611329, 5.243569643749999010 ) ) ;
#24079=CARTESIAN_POINT ( 'NONE',  ( 14.76562500061451821, 3.027376345333613106, -5.243569643749998122 ) ) ;
#24081=CARTESIAN_POINT ( 'NONE',  ( 27.30000000122903359, 5.773502691896255534, 3.535250795749688894E-16 ) ) ;
#24083=CARTESIAN_POINT ( 'NONE',  ( 16.41562500061451857, -6.054752690667223547, -1.112240025338166033E-15 ) ) ;
#24085=CARTESIAN_POINT ( 'NONE',  ( 6.000000001229031987, -2.886751345948126435, -5.000000000000000000 ) ) ;
#24086=CARTESIAN_POINT ( 'NONE',  ( 12.49687500061451573, -3.027376345333610441, -5.243569643749999898 ) ) ;
#24087=CARTESIAN_POINT ( 'NONE',  ( 11.07187500061451679, -6.054752690667223547, -1.112240025338166033E-15 ) ) ;
#24088=CARTESIAN_POINT ( 'NONE',  ( 20.52187500061451786, -6.054752690667223547, -1.112240025338166033E-15 ) ) ;
#24089=EDGE_LOOP ( 'NONE', ( #10180, #57904, #36336, #6323 ) ) ;
#24090=CARTESIAN_POINT ( 'NONE',  ( 0.000000000000000000, 10.00000000000000000, 24.00000000000000000 ) ) ;
#24091=CARTESIAN_POINT ( 'NONE',  ( 23.24062500061451786, -3.027376345333610441, -5.243569643749999898 ) ) ;
#24092=CARTESIAN_POINT ( 'NONE',  ( 18.68437500061451928, -4.541064518000419881, 2.621784821874995952 ) ) ;
#24093=CARTESIAN_POINT ( 'NONE',  ( 23.91562500061451502, 3.027376345333611329, 5.243569643749999010 ) ) ;
#24094=CARTESIAN_POINT ( 'NONE',  ( 0.000000000000000000, 20.00000000000000000, 24.00000000000000000 ) ) ;
#24095=CARTESIAN_POINT ( 'NONE',  ( 8.484601909799253346E-16, 15.16250000000000142, 34.61880215351700230 ) ) ;
#24096=AXIS2_PLACEMENT_3D ( 'NONE', #5520, #28058, #50586 ) ;
#24097=CARTESIAN_POINT ( 'NONE',  ( 29.50312500061451360, -4.541064518000417216, -2.621784821875001281 ) ) ;
#24098=CARTESIAN_POINT ( 'NONE',  ( 8.662500001229034297, -4.330127018922190985, -2.500000000000001332 ) ) ;
#24099=CARTESIAN_POINT ( 'NONE',  ( 4.687500001229034652, 6.123233995736764310E-16, -4.999999999999998224 ) ) ;
#24101=CARTESIAN_POINT ( 'NONE',  ( 27.75000000122903288, 5.773502691896255534, 3.535250795749688894E-16 ) ) ;
#24103=CARTESIAN_POINT ( 'NONE',  ( 10.32187500061451679, 3.027376345333613106, -5.243569643749998122 ) ) ;
#24105=CARTESIAN_POINT ( 'NONE',  ( 17.01562500061451644, 3.027376345333613106, -5.243569643749998122 ) ) ;
#24106=CARTESIAN_POINT ( 'NONE',  ( 10.09687500061451715, -3.027376345333614438, 5.243569643749998122 ) ) ;
#24107=CARTESIAN_POINT ( 'NONE',  ( 2.953125000614516438, -4.541064518000417216, -2.621784821875001281 ) ) ;
#24108=CARTESIAN_POINT ( 'NONE',  ( 18.87187500061452283, 3.027376345333612662, -5.243569643749998122 ) ) ;
#24109=CARTESIAN_POINT ( 'NONE',  ( 7.471875000614519813, -6.054752690667223547, -1.112240025338166033E-15 ) ) ;
#24110=CARTESIAN_POINT ( 'NONE',  ( 2.878125000614517592, -4.541064518000419881, 2.621784821874995952 ) ) ;
#24112=CARTESIAN_POINT ( 'NONE',  ( 8.053125000614516082, 4.541064518000418104, -2.621784821874998173 ) ) ;
#24113=CARTESIAN_POINT ( 'NONE',  ( 17.87812500061451715, 6.421520780324663323E-16, -5.243569643749999010 ) ) ;
#24115=CARTESIAN_POINT ( 'NONE',  ( 6.675000001229034474, 2.886751345948126879, 4.999999999999999112 ) ) ;
#24116=CARTESIAN_POINT ( 'NONE',  ( 15.51562500061451644, -6.054752690667223547, -1.112240025338166033E-15 ) ) ;
#24117=CARTESIAN_POINT ( 'NONE',  ( 12.06562500061451537, 3.027376345333613106, -5.243569643749998122 ) ) ;
#24119=CARTESIAN_POINT ( 'NONE',  ( 12.75000000000000178, 4.330127018922192761, -2.499999999999997780 ) ) ;
#24120=CARTESIAN_POINT ( 'NONE',  ( 5.550000001229032698, -2.886751345948125991, -5.000000000000000000 ) ) ;
#24122=CARTESIAN_POINT ( 'NONE',  ( 15.19687500061451857, -3.027376345333610441, -5.243569643749999898 ) ) ;
#24123=CARTESIAN_POINT ( 'NONE',  ( 17.55000000122903359, -2.886751345948129988, 4.999999999999997335 ) ) ;
#24125=CARTESIAN_POINT ( 'NONE',  ( 4.243569643749999010, 19.16562500061451857, -32.45002607614398471 ) ) ;
#24126=CARTESIAN_POINT ( 'NONE',  ( 8.437500000000000000, -2.886751345948130876, 4.999999999999996447 ) ) ;
#24127=CARTESIAN_POINT ( 'NONE',  ( 23.51250000122903216, -4.330127018922190985, -2.500000000000001332 ) ) ;
#24129=CYLINDRICAL_SURFACE ( 'NONE', #13693, 4.999999999999998224 ) ;
#24130=CARTESIAN_POINT ( 'NONE',  ( 19.50937500061451857, 0.000000000000000000, 5.243569643749999010 ) ) ;
#24131=CARTESIAN_POINT ( 'NONE',  ( 21.52500000122903145, 2.886751345948126879, 4.999999999999998224 ) ) ;
#24132=EDGE_CURVE ( 'NONE', #36091, #16314, #17775, .T. ) ;
#24133=CARTESIAN_POINT ( 'NONE',  ( 13.41562500061451502, 3.027376345333613106, -5.243569643749998122 ) ) ;
#24135=CARTESIAN_POINT ( 'NONE',  ( 26.70937500061451431, 0.000000000000000000, 5.243569643749999010 ) ) ;
#24137=CARTESIAN_POINT ( 'NONE',  ( 9.365625000614519635, 3.027376345333613106, -5.243569643749998122 ) ) ;
#24138=CARTESIAN_POINT ( 'NONE',  ( 14.74687500061451573, -3.027376345333610441, -5.243569643749999898 ) ) ;
#24140=CARTESIAN_POINT ( 'NONE',  ( 28.00312500061451715, 0.000000000000000000, 5.243569643749999010 ) ) ;
#24141=CARTESIAN_POINT ( 'NONE',  ( 19.45312500061451644, 0.000000000000000000, 5.243569643749999010 ) ) ;
#24142=CARTESIAN_POINT ( 'NONE',  ( 29.54062500061451502, -3.027376345333610441, -5.243569643749999898 ) ) ;
#24143=CARTESIAN_POINT ( 'NONE',  ( -3.137519842735245283E-14, 14.71250000000000213, 34.00000000000000000 ) ) ;
#24144=CARTESIAN_POINT ( 'NONE',  ( 10.61250000000000071, 2.886751345948126879, 4.999999999999999112 ) ) ;
#24145=CARTESIAN_POINT ( 'NONE',  ( 18.30000000122903359, 5.773502691896255534, 3.535250795749688894E-16 ) ) ;
#24146=CARTESIAN_POINT ( 'NONE',  ( 23.28750000122903430, 4.330127018922191873, 2.499999999999999556 ) ) ;
#24148=VERTEX_POINT ( 'NONE', #51422 ) ;
#24149=CARTESIAN_POINT ( 'NONE',  ( 16.83749999999999858, 5.773502691896255534, 3.535250795749688894E-16 ) ) ;
#24150=CARTESIAN_POINT ( 'NONE',  ( 21.78750000000000142, 5.773502691896255534, 3.535250795749688894E-16 ) ) ;
#24151=CARTESIAN_POINT ( 'NONE',  ( 20.18437500061451573, 6.421520780324663323E-16, -5.243569643749999010 ) ) ;
#24152=CARTESIAN_POINT ( 'NONE',  ( 25.52812500061451573, 6.421520780324663323E-16, -5.243569643749999010 ) ) ;
#24153=VECTOR ( 'NONE', #53142, 1000.000000000000000 ) ;
#24155=DIRECTION ( 'NONE',  ( 0.000000000000000000, 0.000000000000000000, -1.000000000000000000 ) ) ;
#24156=CARTESIAN_POINT ( 'NONE',  ( 4.978125000614518569, 4.541064518000418104, 2.621784821874999949 ) ) ;
#24157=CARTESIAN_POINT ( 'NONE',  ( 3.159375000614518036, 4.541064518000418104, -2.621784821874998173 ) ) ;
#24158=CARTESIAN_POINT ( 'NONE',  ( 12.63749999999999929, -2.886751345948125991, -5.000000000000000000 ) ) ;
#24159=CARTESIAN_POINT ( 'NONE',  ( -2.121784821874996840, 17.17812500061451786, 33.67503911421598417 ) ) ;
#24160=CARTESIAN_POINT ( 'NONE',  ( 28.07812500061451289, -4.541064518000419881, 2.621784821874995952 ) ) ;
#24162=AXIS2_PLACEMENT_3D ( 'NONE', #11879, #18488, #35132 ) ;
#24164=CARTESIAN_POINT ( 'NONE',  ( 26.18437500061451573, 4.541064518000418104, 2.621784821874999949 ) ) ;
#24166=CARTESIAN_POINT ( 'NONE',  ( 22.67812500061451431, -4.541064518000419881, 2.621784821874995952 ) ) ;
#24167=CARTESIAN_POINT ( 'NONE',  ( 22.88437500061451857, 6.421520780324663323E-16, -5.243569643749999010 ) ) ;
#24168=CARTESIAN_POINT ( 'NONE',  ( -4.243569643749998122, 15.79062500061459495, -27.54997392385601174 ) ) ;
#24169=CARTESIAN_POINT ( 'NONE',  ( 6.140625000614516438, -3.027376345333610441, -5.243569643749999898 ) ) ;
#24170=CARTESIAN_POINT ( 'NONE',  ( 3.727827348360245097, 3.332161949968362347, -3.727827348360304605 ) ) ;
#24171=CARTESIAN_POINT ( 'NONE',  ( 24.66562500061451502, 3.027376345333612662, -5.243569643749998122 ) ) ;
#24174=CARTESIAN_POINT ( 'NONE',  ( 17.07187500061451502, 3.027376345333613106, -5.243569643749998122 ) ) ;
#24175=CARTESIAN_POINT ( 'NONE',  ( 19.20937500061451786, -4.541064518000417216, -2.621784821875001281 ) ) ;
#24176=CARTESIAN_POINT ( 'NONE',  ( 27.57187500061451857, 3.027376345333611329, 5.243569643749999010 ) ) ;
#24177=CARTESIAN_POINT ( 'NONE',  ( 9.001249775931846008E-16, 16.82187500061451857, 34.90005215228797653 ) ) ;
#24178=CARTESIAN_POINT ( 'NONE',  ( 8.353125000614518569, -4.541064518000417216, -2.621784821875001281 ) ) ;
#24179=CARTESIAN_POINT ( 'NONE',  ( -3.999999999999999112, 19.09999999999999787, 30.00000000000000000 ) ) ;
#24180=CARTESIAN_POINT ( 'NONE',  ( 5.296875000614518214, -3.027376345333610441, -5.243569643749999898 ) ) ;
#24182=CARTESIAN_POINT ( 'NONE',  ( 4.153125000614515727, 0.000000000000000000, 5.243569643749999010 ) ) ;
#24183=CARTESIAN_POINT ( 'NONE',  ( 10.47187500061451715, 3.027376345333611329, 5.243569643749999010 ) ) ;
#24184=CARTESIAN_POINT ( 'NONE',  ( 17.58750000122903145, -4.330127018922194537, 2.499999999999995559 ) ) ;
#24185=CARTESIAN_POINT ( 'NONE',  ( 4.584375000614516971, 4.541064518000418104, 2.621784821874999949 ) ) ;
#24186=CARTESIAN_POINT ( 'NONE',  ( 7.753125000614518036, 0.000000000000000000, 5.243569643749999010 ) ) ;
#24189=CARTESIAN_POINT ( 'NONE',  ( 16.73437500061451644, 4.541064518000418104, 2.621784821874999949 ) ) ;
#24190=CARTESIAN_POINT ( 'NONE',  ( 30.00000000000000000, 0.000000000000000000, 0.000000000000000000 ) ) ;
#24192=CARTESIAN_POINT ( 'NONE',  ( 24.62812500061451715, 6.421520780324663323E-16, -5.243569643749999010 ) ) ;
#24193=CARTESIAN_POINT ( 'NONE',  ( 10.71562500061451928, 3.027376345333613106, -5.243569643749998122 ) ) ;
#24194=CARTESIAN_POINT ( 'NONE',  ( 27.49687500061451573, 6.054752690667223547, 3.707466751127219781E-16 ) ) ;
#24195=CARTESIAN_POINT ( 'NONE',  ( 9.290625000614515017, -3.027376345333610441, -5.243569643749999898 ) ) ;
#24196=CARTESIAN_POINT ( 'NONE',  ( 2.121784821875001281, 10.10937500061451821, -26.32496088578401938 ) ) ;
#24197=CARTESIAN_POINT ( 'NONE',  ( 11.62500000122903465, 2.886751345948126879, 4.999999999999999112 ) ) ;
#24199=CARTESIAN_POINT ( 'NONE',  ( 24.89062500061451644, -3.027376345333614438, 5.243569643749998122 ) ) ;
#24200=CARTESIAN_POINT ( 'NONE',  ( 9.001249775931846008E-16, 14.06562500061451715, -25.09994784771203058 ) ) ;
#24201=CARTESIAN_POINT ( 'NONE',  ( 13.31250000122903288, 4.330127018922192761, -2.499999999999997780 ) ) ;
#24202=CARTESIAN_POINT ( 'NONE',  ( 22.00312500061451360, 4.541064518000418104, -2.621784821874998173 ) ) ;
#24204=CARTESIAN_POINT ( 'NONE',  ( 10.23750000000000071, -2.886751345948129988, 4.999999999999997335 ) ) ;
#24205=CARTESIAN_POINT ( 'NONE',  ( 20.84062500061451573, -3.027376345333614438, 5.243569643749998122 ) ) ;
#24206=CARTESIAN_POINT ( 'NONE',  ( 5.184375000614516615, -4.541064518000419881, 2.621784821874995952 ) ) ;
#24207=CARTESIAN_POINT ( 'NONE',  ( 21.03750000000000142, -2.886751345948129988, 4.999999999999997335 ) ) ;
#24208=CARTESIAN_POINT ( 'NONE',  ( 14.88750000122903394, -4.330127018922194537, 2.499999999999995559 ) ) ;
#24210=CARTESIAN_POINT ( 'NONE',  ( 9.328125000614518214, 6.421520780324663323E-16, -5.243569643749999010 ) ) ;
#24211=CARTESIAN_POINT ( 'NONE',  ( 16.07812500061451289, 6.421520780324663323E-16, -5.243569643749999010 ) ) ;
#24213=CARTESIAN_POINT ( 'NONE',  ( 25.91250000122903074, 4.330127018922192761, -2.499999999999997780 ) ) ;
#24215=CARTESIAN_POINT ( 'NONE',  ( 22.50937500061451857, 4.541064518000418104, -2.621784821874998173 ) ) ;
#24218=CARTESIAN_POINT ( 'NONE',  ( 8.550000001229031810, -2.886751345948129988, 4.999999999999997335 ) ) ;
#24219=CARTESIAN_POINT ( 'NONE',  ( 9.646875000614516082, -3.027376345333614438, 5.243569643749998122 ) ) ;
#24220=CARTESIAN_POINT ( 'NONE',  ( 24.98437500061451644, -4.541064518000419881, 2.621784821874995952 ) ) ;
#24222=CARTESIAN_POINT ( 'NONE',  ( 22.07812500061451644, 4.541064518000418104, 2.621784821874999949 ) ) ;
#24223=CARTESIAN_POINT ( 'NONE',  ( 27.57187500061451857, 3.027376345333611329, 5.243569643749999010 ) ) ;
#24225=DIRECTION ( 'NONE',  ( -0.000000000000000000, -1.000000000000000000, -0.000000000000000000 ) ) ;
#24226=CARTESIAN_POINT ( 'NONE',  ( 8.859375000614518214, -4.541064518000417216, -2.621784821875001281 ) ) ;
#24227=CARTESIAN_POINT ( 'NONE',  ( 20.05312500061451431, -4.541064518000417216, -2.621784821875001281 ) ) ;
#24230=CARTESIAN_POINT ( 'NONE',  ( 26.91562500061451146, 3.027376345333613106, -5.243569643749998122 ) ) ;
#24231=CARTESIAN_POINT ( 'NONE',  ( 3.571875000614517237, 3.027376345333613106, -5.243569643749998122 ) ) ;
#24232=CARTESIAN_POINT ( 'NONE',  ( 4.898587196589411843E-16, 20.00000000000000000, -26.00000000000000000 ) ) ;
#24233=DIRECTION ( 'NONE',  ( -0.000000000000000000, -1.000000000000000000, -0.000000000000000000 ) ) ;
#24234=CARTESIAN_POINT ( 'NONE',  ( 16.12500000000000000, -4.330127018922194537, 2.499999999999995559 ) ) ;
#24235=CARTESIAN_POINT ( 'NONE',  ( 20.31562500061451715, 3.027376345333611329, 5.243569643749999010 ) ) ;
#24236=VERTEX_POINT ( 'NONE', #63220 ) ;
#24237=CARTESIAN_POINT ( 'NONE',  ( 25.31250000000000000, 2.886751345948129099, -4.999999999999998224 ) ) ;
#24238=EDGE_CURVE ( 'NONE', #63984, #30207, #71097, .T. ) ;
#24239=CARTESIAN_POINT ( 'NONE',  ( 26.74687500061451573, -3.027376345333614438, 5.243569643749998122 ) ) ;
#24240=ORIENTED_EDGE ( 'NONE', *, *, #66190, .T. ) ;
#24241=CARTESIAN_POINT ( 'NONE',  ( 13.45312500061451466, 4.541064518000418104, -2.621784821874998173 ) ) ;
#24242=CARTESIAN_POINT ( 'NONE',  ( 4.940625000614515372, 6.054752690667223547, 3.707466751127219781E-16 ) ) ;
#24244=CARTESIAN_POINT ( 'NONE',  ( 29.12812500061451715, 6.421520780324663323E-16, -5.243569643749999010 ) ) ;
#24245=CARTESIAN_POINT ( 'NONE',  ( 16.27500000122903501, -5.773502691896255534, -1.060575238724906372E-15 ) ) ;
#24246=AXIS2_PLACEMENT_3D ( 'NONE', #47923, #2483, #53089 ) ;
#24247=CARTESIAN_POINT ( 'NONE',  ( 20.85000000000000142, 4.330127018922192761, -2.499999999999997780 ) ) ;
#24248=CARTESIAN_POINT ( 'NONE',  ( 28.35000000000000142, -4.330127018922190985, -2.500000000000001332 ) ) ;
#24249=CARTESIAN_POINT ( 'NONE',  ( 5.409375000614516260, 4.541064518000418104, -2.621784821874998173 ) ) ;
#24250=CARTESIAN_POINT ( 'NONE',  ( 9.946875000614516793, 6.054752690667223547, 3.707466751127219781E-16 ) ) ;
#24251=CARTESIAN_POINT ( 'NONE',  ( 18.53437500061451715, 4.541064518000418104, 2.621784821874999949 ) ) ;
#24253=VERTEX_POINT ( 'NONE', #25890 ) ;
#24254=CARTESIAN_POINT ( 'NONE',  ( 2.934375000614518392, -4.541064518000419881, 2.621784821874995952 ) ) ;
#24255=CARTESIAN_POINT ( 'NONE',  ( 3.975000000000002753, -4.330127018922194537, 2.499999999999995559 ) ) ;
#24256=CARTESIAN_POINT ( 'NONE',  ( 5.034375000614519813, 4.541064518000418104, 2.621784821874999949 ) ) ;
#24257=CARTESIAN_POINT ( 'NONE',  ( 17.81250000000000355, 2.886751345948126879, 4.999999999999999112 ) ) ;
#24258=CARTESIAN_POINT ( 'NONE',  ( 13.45312500061451466, 4.541064518000418104, -2.621784821874998173 ) ) ;
#24259=CARTESIAN_POINT ( 'NONE',  ( 1.999999999999998668, 14.11250000122903359, 26.53589838486224650 ) ) ;
#24260=CARTESIAN_POINT ( 'NONE',  ( 20.40000000122903145, -2.886751345948125991, -5.000000000000000000 ) ) ;
#24261=CARTESIAN_POINT ( 'NONE',  ( -1.999999999999997113, 13.43750000122903465, 33.46410161513775705 ) ) ;
#24263=CARTESIAN_POINT ( 'NONE',  ( 6.853125000614516793, 0.000000000000000000, 5.243569643749999010 ) ) ;
#24264=CARTESIAN_POINT ( 'NONE',  ( 24.15937500061451715, -4.541064518000417216, -2.621784821875001281 ) ) ;
#24265=CARTESIAN_POINT ( 'NONE',  ( 27.15000000122902435, -2.886751345948092684, -5.000000000000057732 ) ) ;
#24266=CARTESIAN_POINT ( 'NONE',  ( 26.22187500061451715, 3.027376345333611329, 5.243569643749999010 ) ) ;
#24267=CARTESIAN_POINT ( 'NONE',  ( 6.412500000000001421, 2.886751345948129099, -4.999999999999998224 ) ) ;
#24268=CARTESIAN_POINT ( 'NONE',  ( -3.999999999999997335, 12.50000000122903465, 32.30940107675850470 ) ) ;
#24269=CARTESIAN_POINT ( 'NONE',  ( 15.32812500061451644, 4.541064518000418104, 2.621784821874999949 ) ) ;
#24270=CARTESIAN_POINT ( 'NONE',  ( 7.650000001229034119, -2.886751345948129988, 4.999999999999997335 ) ) ;
#24272=CARTESIAN_POINT ( 'NONE',  ( 17.74687500061451928, -3.027376345333614438, 5.243569643749998122 ) ) ;
#24273=CARTESIAN_POINT ( 'NONE',  ( 11.82187500061451679, 3.027376345333611329, 5.243569643749999010 ) ) ;
#24275=ORIENTED_EDGE ( 'NONE', *, *, #1251, .T. ) ;
#24276=CARTESIAN_POINT ( 'NONE',  ( 11.57812500061451644, 6.421520780324663323E-16, -5.243569643749999010 ) ) ;
#24278=CARTESIAN_POINT ( 'NONE',  ( 4.000000000000000000, 12.20000000122903394, -27.69059892324149885 ) ) ;
#24279=CARTESIAN_POINT ( 'NONE',  ( 24.41250000122903430, -4.330127018922190985, -2.500000000000001332 ) ) ;
#24280=CARTESIAN_POINT ( 'NONE',  ( 12.19687500061451679, 6.054752690667223547, 3.707466751127219781E-16 ) ) ;
#24281=CARTESIAN_POINT ( 'NONE',  ( 14.05312500061451431, 0.000000000000000000, 5.243569643749999010 ) ) ;
#24282=CARTESIAN_POINT ( 'NONE',  ( 4.000000000000000000, 18.83749999999999858, -27.69059892324149885 ) ) ;
#24283=CARTESIAN_POINT ( 'NONE',  ( 23.29687500061451644, -3.027376345333610441, -5.243569643749999898 ) ) ;
#24285=CARTESIAN_POINT ( 'NONE',  ( 5.400000000000002132, -4.330127018922190985, -2.500000000000001332 ) ) ;
#24287=CARTESIAN_POINT ( 'NONE',  ( 4.243569643749999898, 16.48437500061451644, -30.00000000000000000 ) ) ;
#24288=CARTESIAN_POINT ( 'NONE',  ( 15.64687500061451608, -3.027376345333610441, -5.243569643749999898 ) ) ;
#24289=CARTESIAN_POINT ( 'NONE',  ( 17.47500000122903430, 2.886751345948126879, 4.999999999999999112 ) ) ;
#24290=CARTESIAN_POINT ( 'NONE',  ( 13.28437500061451715, -4.541064518000419881, 2.621784821874995952 ) ) ;
#24291=CARTESIAN_POINT ( 'NONE',  ( -4.243569643749999898, 19.31562500061451715, -32.45002607614398471 ) ) ;
#24292=CARTESIAN_POINT ( 'NONE',  ( 20.06250000122903643, 4.330127018922192761, -2.499999999999997780 ) ) ;
#24293=CARTESIAN_POINT ( 'NONE',  ( 15.92812500061451608, -4.541064518000419881, 2.621784821874995952 ) ) ;
#24296=CARTESIAN_POINT ( 'NONE',  ( 19.20000000000000284, 0.000000000000000000, 4.999999999999998224 ) ) ;
#24297=DIRECTION ( 'NONE',  ( 1.000000000000000000, 0.000000000000000000, -0.000000000000000000 ) ) ;
#24298=CARTESIAN_POINT ( 'NONE',  ( 12.53437500061451537, 6.421520780324663323E-16, -5.243569643749999010 ) ) ;
#24299=CARTESIAN_POINT ( 'NONE',  ( 3.035814067847288467, 3.972922589466866938, -3.271563712840051874 ) ) ;
#24300=CARTESIAN_POINT ( 'NONE',  ( 12.52500000122903145, 2.886751345948126879, 4.999999999999999112 ) ) ;
#24301=CARTESIAN_POINT ( 'NONE',  ( 19.95000000122903572, -2.886751345948125991, -5.000000000000000000 ) ) ;
#24302=CARTESIAN_POINT ( 'NONE',  ( 19.07812500061451644, -4.541064518000419881, 2.621784821874995952 ) ) ;
#24304=CARTESIAN_POINT ( 'NONE',  ( 23.54062500061451146, -3.027376345333614438, 5.243569643749998122 ) ) ;
#24305=CARTESIAN_POINT ( 'NONE',  ( 3.215625000614518836, 3.027376345333611329, 5.243569643749999010 ) ) ;
#24306=CARTESIAN_POINT ( 'NONE',  ( 27.78749999999999787, -2.886751345948129988, 4.999999999999997335 ) ) ;
#24308=AXIS2_PLACEMENT_3D ( 'NONE', #48841, #25938, #59536 ) ;
#24310=CARTESIAN_POINT ( 'NONE',  ( 4.080569135018654592, -2.889455923578380769, -4.080569135022440896 ) ) ;
#24311=CARTESIAN_POINT ( 'NONE',  ( -4.243569643749999898, 16.70937500061451786, -30.00000000000000000 ) ) ;
#24312=CARTESIAN_POINT ( 'NONE',  ( 3.900000001229034563, 5.773502691896255534, 3.535250795749688894E-16 ) ) ;
#24313=CARTESIAN_POINT ( 'NONE',  ( 5.587500000000003020, 5.773502691896255534, 3.535250795749688894E-16 ) ) ;
#24314=CARTESIAN_POINT ( 'NONE',  ( 10.80937500061451928, 4.541064518000418104, -2.621784821874998173 ) ) ;
#24315=CARTESIAN_POINT ( 'NONE',  ( 28.64062500061451289, -3.027376345333610441, -5.243569643749999898 ) ) ;
#24317=CARTESIAN_POINT ( 'NONE',  ( -4.384844337767558109, 8.988619951912522055, -34.09994685707254547 ) ) ;
#24318=DIRECTION ( 'NONE',  ( 1.000000000000000000, 0.000000000000000000, 0.000000000000000000 ) ) ;
#24319=CARTESIAN_POINT ( 'NONE',  ( 8.221875000614518925, 3.027376345333611329, 5.243569643749999010 ) ) ;
#24320=CARTESIAN_POINT ( 'NONE',  ( 11.10937500061451644, -4.541064518000417216, -2.621784821875001281 ) ) ;
#24321=CARTESIAN_POINT ( 'NONE',  ( 7.237500000000000711, -2.886751345948125991, -5.000000000000000000 ) ) ;
#24322=CARTESIAN_POINT ( 'NONE',  ( 4.243569643749999898, 15.52812500061459566, 30.00000000000000000 ) ) ;
#24323=CARTESIAN_POINT ( 'NONE',  ( 4.875000000000000888, -4.330127018922194537, 2.499999999999995559 ) ) ;
#24324=CARTESIAN_POINT ( 'NONE',  ( 6.712500000000000355, -5.773502691896255534, -1.060575238724906372E-15 ) ) ;
#24326=CARTESIAN_POINT ( 'NONE',  ( 22.45312500061451644, 4.541064518000418104, -2.621784821874998173 ) ) ;
#24327=CARTESIAN_POINT ( 'NONE',  ( 13.22812500061451502, -4.541064518000419881, 2.621784821874995952 ) ) ;
#24329=CARTESIAN_POINT ( 'NONE',  ( 8.484375000614518214, 6.421520780324663323E-16, -5.243569643749999010 ) ) ;
#24330=CARTESIAN_POINT ( 'NONE',  ( 26.36249999999999716, 2.886751345948126879, 4.999999999999999112 ) ) ;
#24331=CARTESIAN_POINT ( 'NONE',  ( 23.58750000122903145, 6.123233995736764310E-16, -4.999999999999998224 ) ) ;
#24332=CARTESIAN_POINT ( 'NONE',  ( 4.898587196589411843E-16, 20.00000000000000000, -26.00000000000000000 ) ) ;
#24333=CARTESIAN_POINT ( 'NONE',  ( 12.90937500061451537, -4.541064518000417216, -2.621784821875001281 ) ) ;
#24334=CARTESIAN_POINT ( 'NONE',  ( 25.88437500061451502, -4.541064518000419881, 2.621784821874995952 ) ) ;
#24335=CARTESIAN_POINT ( 'NONE',  ( 3.796875000614517326, -3.027376345333614438, 5.243569643749998122 ) ) ;
#24337=CARTESIAN_POINT ( 'NONE',  ( 0.000000000000000000, 20.00000000000000000, 26.00000000000000000 ) ) ;
#24338=CARTESIAN_POINT ( 'NONE',  ( 19.54687500061451644, -3.027376345333614438, 5.243569643749998122 ) ) ;
#24339=CARTESIAN_POINT ( 'NONE',  ( 12.49687500061451573, -3.027376345333610441, -5.243569643749999898 ) ) ;
#24341=CARTESIAN_POINT ( 'NONE',  ( 24.67500000000000071, -4.330127018922194537, 2.499999999999995559 ) ) ;
#24343=CARTESIAN_POINT ( 'NONE',  ( 4.243569643749999010, 11.12187500061451928, -32.45002607614398471 ) ) ;
#24345=CARTESIAN_POINT ( 'NONE',  ( 13.67812500061451786, -4.541064518000419881, 2.621784821874995952 ) ) ;
#24346=CARTESIAN_POINT ( 'NONE',  ( 5.362500000000003375, -5.773502691896255534, -1.060575238724906372E-15 ) ) ;
#24347=CYLINDRICAL_SURFACE ( 'NONE', #11328, 4.000000000000000000 ) ;
#24349=CARTESIAN_POINT ( 'NONE',  ( 13.87500000000000178, -4.330127018922194537, 2.499999999999995559 ) ) ;
#24350=CARTESIAN_POINT ( 'NONE',  ( 2.121784821874999061, 10.20312500061451821, 26.32496088578401583 ) ) ;
#24351=CARTESIAN_POINT ( 'NONE',  ( 13.35000000122903430, 5.773502691896255534, 3.535250795749688894E-16 ) ) ;
#24352=CARTESIAN_POINT ( 'NONE',  ( 25.39687500061451431, -3.027376345333614438, 5.243569643749998122 ) ) ;
#24354=ORIENTED_EDGE ( 'NONE', *, *, #50295, .F. ) ;
#24355=CARTESIAN_POINT ( 'NONE',  ( 19.30312500061451786, 4.541064518000418104, -2.621784821874998173 ) ) ;
#24356=CARTESIAN_POINT ( 'NONE',  ( 19.54687500061451644, -3.027376345333614438, 5.243569643749998122 ) ) ;
#24357=CARTESIAN_POINT ( 'NONE',  ( 5.137500000000000178, 5.773502691896255534, 3.535250795749688894E-16 ) ) ;
#24358=CARTESIAN_POINT ( 'NONE',  ( 7.115625000614516082, 3.027376345333613106, -5.243569643749998122 ) ) ;
#24359=CARTESIAN_POINT ( 'NONE',  ( 21.47812500061451502, 6.421520780324663323E-16, -5.243569643749999010 ) ) ;
#24360=CARTESIAN_POINT ( 'NONE',  ( 15.94687500061451502, -3.027376345333614438, 5.243569643749998122 ) ) ;
#24361=CARTESIAN_POINT ( 'NONE',  ( -2.121784821874999949, 14.32812500061451644, 26.32496088578401938 ) ) ;
#24362=CARTESIAN_POINT ( 'NONE',  ( 19.98750000122903359, 6.123233995736764310E-16, -4.999999999999998224 ) ) ;
#24364=CARTESIAN_POINT ( 'NONE',  ( 9.890625000614514661, 6.054752690667223547, 3.707466751127219781E-16 ) ) ;
#24365=CARTESIAN_POINT ( 'NONE',  ( 4.059375000614519280, 4.541064518000418104, -2.621784821874998173 ) ) ;
#24366=CARTESIAN_POINT ( 'NONE',  ( 28.30312500061451431, 4.541064518000418104, -2.621784821874998173 ) ) ;
#24367=CARTESIAN_POINT ( 'NONE',  ( 24.72187500061451360, 3.027376345333613106, -5.243569643749998122 ) ) ;
#24368=CARTESIAN_POINT ( 'NONE',  ( 15.62812500061451537, 6.421520780324663323E-16, -5.243569643749999010 ) ) ;
#24369=CARTESIAN_POINT ( 'NONE',  ( 25.35000000122903074, -2.886751345948125991, -5.000000000000000000 ) ) ;
#24370=CARTESIAN_POINT ( 'NONE',  ( 24.74062500061451786, 6.054752690667223547, 3.707466751127219781E-16 ) ) ;
#24371=CARTESIAN_POINT ( 'NONE',  ( 18.57187500061451857, 3.027376345333611329, 5.243569643749999010 ) ) ;
#24372=CARTESIAN_POINT ( 'NONE',  ( 15.74062500061451608, 6.054752690667223547, 3.707466751127219781E-16 ) ) ;
#24373=CARTESIAN_POINT ( 'NONE',  ( 4.243569643749999898, 18.28437500061451715, 30.00000000000000000 ) ) ;
#24374=CARTESIAN_POINT ( 'NONE',  ( 21.17812500061451431, 4.541064518000418104, 2.621784821874999949 ) ) ;
#24375=CARTESIAN_POINT ( 'NONE',  ( 2.887500001229035274, 6.123233995736764310E-16, -4.999999999999998224 ) ) ;
#24376=ORIENTED_EDGE ( 'NONE', *, *, #53010, .F. ) ;
#24377=CARTESIAN_POINT ( 'NONE',  ( 24.63749999999999574, -2.886751345948129988, 4.999999999999997335 ) ) ;
#24378=CARTESIAN_POINT ( 'NONE',  ( 8.484601909799253346E-16, 10.66250000000000142, -25.38119784648299770 ) ) ;
#24380=CARTESIAN_POINT ( 'NONE',  ( 28.71562500061451573, 3.027376345333613106, -5.243569643749998122 ) ) ;
#24381=CARTESIAN_POINT ( 'NONE',  ( 7.565625000614518036, 3.027376345333613106, -5.243569643749998122 ) ) ;
#24382=CARTESIAN_POINT ( 'NONE',  ( 23.32500000122903572, 2.886751345948126879, 4.999999999999999112 ) ) ;
#24383=EDGE_CURVE ( 'NONE', #40816, #14839, #17354, .T. ) ;
#24384=CARTESIAN_POINT ( 'NONE',  ( 27.25312500061451360, -4.541064518000417216, -2.621784821875001281 ) ) ;
#24385=CARTESIAN_POINT ( 'NONE',  ( 25.34999999999999787, 4.330127018922192761, -2.499999999999997780 ) ) ;
#24386=CARTESIAN_POINT ( 'NONE',  ( -1.999999999999997113, 16.13750000122903216, -26.53589838486224295 ) ) ;
#24387=CARTESIAN_POINT ( 'NONE',  ( 29.61562500061451431, 3.027376345333613106, -5.243569643749998122 ) ) ;
#24388=CARTESIAN_POINT ( 'NONE',  ( 9.815625000614518925, 3.027376345333613106, -5.243569643749998122 ) ) ;
#24389=ORIENTED_EDGE ( 'NONE', *, *, #66002, .F. ) ;
#24390=CARTESIAN_POINT ( 'NONE',  ( 25.71562500061451573, 3.027376345333611329, 5.243569643749999010 ) ) ;
#24391=CARTESIAN_POINT ( 'NONE',  ( 7.678125000614516082, 4.541064518000418104, 2.621784821874999949 ) ) ;
#24392=CARTESIAN_POINT ( 'NONE',  ( 4.565625000614516260, 3.027376345333611329, 5.243569643749999010 ) ) ;
#24395=FACE_OUTER_BOUND ( 'NONE', #34091, .T. ) ;
#24396=CARTESIAN_POINT ( 'NONE',  ( 14.17500000000000071, 4.330127018922191873, 2.499999999999999556 ) ) ;
#24397=CARTESIAN_POINT ( 'NONE',  ( 13.32187500061451502, -6.054752690667223547, -1.112240025338166033E-15 ) ) ;
#24398=CARTESIAN_POINT ( 'NONE',  ( 8.850000001229034297, 5.773502691896255534, 3.535250795749688894E-16 ) ) ;
#24399=CARTESIAN_POINT ( 'NONE',  ( 17.93437500061451928, 6.421520780324663323E-16, -5.243569643749999010 ) ) ;
#24401=CARTESIAN_POINT ( 'NONE',  ( 7.471875000614519813, -6.054752690667223547, -1.112240025338166033E-15 ) ) ;
#24402=CARTESIAN_POINT ( 'NONE',  ( 4.243569643749999898, 11.02812500061451750, -30.00000000000000000 ) ) ;
#24403=CARTESIAN_POINT ( 'NONE',  ( 7.462499999999999467, 2.886751345948193936, 4.999999999999883649 ) ) ;
#24406=CARTESIAN_POINT ( 'NONE',  ( 23.69062500061451004, -3.027376345333610441, -5.243569643749999898 ) ) ;
#24407=CARTESIAN_POINT ( 'NONE',  ( -3.999999999999999112, 17.37500000122903288, 27.69059892324149885 ) ) ;
#24408=CARTESIAN_POINT ( 'NONE',  ( 27.38437500061451857, 6.421520780324663323E-16, -5.243569643749999010 ) ) ;
#24409=( BOUNDED_CURVE ( )  B_SPLINE_CURVE ( 2, ( #43744, #26756, #38566, #43381, #55196, #4590, #61090 ),
 .UNSPECIFIED., .F., .F. ) 
 B_SPLINE_CURVE_WITH_KNOTS ( ( 3, 2, 2, 3 ),
 ( 0.7833333333333334370, 0.7861111111111112049, 0.7888888888888888618, 0.7916666666666666297 ),
 .UNSPECIFIED. ) 
 CURVE ( )  GEOMETRIC_REPRESENTATION_ITEM ( )  RATIONAL_B_SPLINE_CURVE ( ( 0.9999999999999946709, 0.8660254037844440367, 1.000000000000000000, 0.8660254037844387076, 1.000000000000000000, 0.8660254037844387076, 1.000000000000000000 ) ) 
 REPRESENTATION_ITEM ( '' )  );
#24410=CARTESIAN_POINT ( 'NONE',  ( 20.99999999999999645, 0.000000000000000000, 4.999999999999998224 ) ) ;
#24411=CARTESIAN_POINT ( 'NONE',  ( 7.715625000614515727, 3.027376345333611329, 5.243569643749999010 ) ) ;
#24413=CARTESIAN_POINT ( 'NONE',  ( 15.87187500061451573, 3.027376345333611329, 5.243569643749999010 ) ) ;
#24415=CARTESIAN_POINT ( 'NONE',  ( 4.003125000614518925, 4.541064518000418104, -2.621784821874998173 ) ) ;
#24416=CARTESIAN_POINT ( 'NONE',  ( 7.546875000614517326, -3.027376345333610441, -5.243569643749999898 ) ) ;
#24418=CARTESIAN_POINT ( 'NONE',  ( 20.22187500061451715, 3.027376345333613106, -5.243569643749998122 ) ) ;
#24419=CARTESIAN_POINT ( 'NONE',  ( 21.56250000000000000, -5.773502691896255534, -1.060575238724906372E-15 ) ) ;
#24420=CARTESIAN_POINT ( 'NONE',  ( 26.73749999999999716, 5.773502691896255534, 3.535250795749688894E-16 ) ) ;
#24421=CARTESIAN_POINT ( 'NONE',  ( 28.39687500061452141, 6.054752690667223547, 3.707466751127219781E-16 ) ) ;
#24423=CARTESIAN_POINT ( 'NONE',  ( 27.75000000000000000, 0.000000000000000000, 4.999999999999998224 ) ) ;
#24425=CARTESIAN_POINT ( 'NONE',  ( 9.899999999999998579, -4.330127018922190985, -2.500000000000001332 ) ) ;
#24427=CARTESIAN_POINT ( 'NONE',  ( 23.01562500061451644, 3.027376345333611329, 5.243569643749999010 ) ) ;
#24428=CARTESIAN_POINT ( 'NONE',  ( 14.02499999999999858, 6.123233995736764310E-16, -4.999999999999998224 ) ) ;
#24429=CARTESIAN_POINT ( 'NONE',  ( 7.350000001229033408, -2.886751345948125991, -5.000000000000000000 ) ) ;
#24430=CARTESIAN_POINT ( 'NONE',  ( 6.365625000614518747, 3.027376345333611329, 5.243569643749999010 ) ) ;
#24431=CARTESIAN_POINT ( 'NONE',  ( 22.72499999999999787, 4.330127018922191873, 2.499999999999999556 ) ) ;
#24432=CARTESIAN_POINT ( 'NONE',  ( 21.92812500061451431, 6.421520780324663323E-16, -5.243569643749999010 ) ) ;
#24433=CARTESIAN_POINT ( 'NONE',  ( 12.18749999999999822, -2.886751345948193048, -4.999999999999883649 ) ) ;
#24434=CARTESIAN_POINT ( 'NONE',  ( 24.63750000122903216, 4.330127018922191873, 2.499999999999999556 ) ) ;
#24436=CARTESIAN_POINT ( 'NONE',  ( 5.475000000000000533, 6.123233995736764310E-16, -4.999999999999998224 ) ) ;
#24437=VERTEX_POINT ( 'NONE', #70587 ) ;
#24438=CARTESIAN_POINT ( 'NONE',  ( 21.66562500061451502, 3.027376345333611329, 5.243569643749999010 ) ) ;
#24439=CARTESIAN_POINT ( 'NONE',  ( 27.55312500061451786, 0.000000000000000000, 5.243569643749999010 ) ) ;
#24440=CARTESIAN_POINT ( 'NONE',  ( 28.09687500061451360, -3.027376345333614438, 5.243569643749998122 ) ) ;
#24441=CARTESIAN_POINT ( 'NONE',  ( 13.97812500061451679, 4.541064518000418104, 2.621784821874999949 ) ) ;
#24442=CARTESIAN_POINT ( 'NONE',  ( -0.7368881354385758975, 9.803648613939513368, -34.17910028561248481 ) ) ;
#24443=AXIS2_PLACEMENT_3D ( 'NONE', #18890, #8196, #36272 ) ;
#24444=CARTESIAN_POINT ( 'NONE',  ( 26.55000000122902648, -2.886751345948129988, 4.999999999999997335 ) ) ;
#24446=CARTESIAN_POINT ( 'NONE',  ( 16.79062500061451857, -3.027376345333614438, 5.243569643749998122 ) ) ;
#24447=CARTESIAN_POINT ( 'NONE',  ( 3.999999999999999112, 14.48750000122903536, -30.00000000000000000 ) ) ;
#24448=CARTESIAN_POINT ( 'NONE',  ( 3.300000001229034918, -2.886751345948125991, -5.000000000000000000 ) ) ;
#24449=CARTESIAN_POINT ( 'NONE',  ( 10.28437500061451715, 6.421520780324663323E-16, -5.243569643749999010 ) ) ;
#24450=CARTESIAN_POINT ( 'NONE',  ( 8.859375000614518214, -4.541064518000417216, -2.621784821875001281 ) ) ;
#24451=CARTESIAN_POINT ( 'NONE',  ( 18.04687500061451999, 6.054752690667223547, 3.707466751127219781E-16 ) ) ;
#24453=CARTESIAN_POINT ( 'NONE',  ( -4.384844337767561662, 8.988619951912520278, 25.90005314292746519 ) ) ;
#24454=CARTESIAN_POINT ( 'NONE',  ( 22.94062500061451715, 6.054752690667223547, 3.707466751127219781E-16 ) ) ;
#24455=B_SPLINE_CURVE_WITH_KNOTS ( 'NONE', 3,
 ( #58203, #64114, #24956, #19402, #41961, #64483, #36415, #53406, #58931, #2798 ),
 .UNSPECIFIED., .F., .F.,
 ( 4, 3, 3, 4 ),
 ( 2.168404344971008868E-19, 0.0001572649580503299096, 0.0003035751770480561132, 0.0004501423746267203254 ),
 .UNSPECIFIED. ) ;
#24456=CARTESIAN_POINT ( 'NONE',  ( 18.19687500061451502, -3.027376345333614438, 5.243569643749998122 ) ) ;
#24457=CARTESIAN_POINT ( 'NONE',  ( 22.30312500061451431, -4.541064518000417216, -2.621784821875001281 ) ) ;
#24458=CARTESIAN_POINT ( 'NONE',  ( 30.00000000000000000, 0.000000000000000000, 4.999999999999998224 ) ) ;
#24459=CARTESIAN_POINT ( 'NONE',  ( -1.999999999999997113, 14.67500000000000071, 33.46410161513775705 ) ) ;
#24460=CARTESIAN_POINT ( 'NONE',  ( 3.084375000614519191, 6.421520780324663323E-16, -5.243569643749999010 ) ) ;
#24461=CARTESIAN_POINT ( 'NONE',  ( 8.437500001229034652, 4.330127018922191873, 2.499999999999999556 ) ) ;
#24463=CARTESIAN_POINT ( 'NONE',  ( 3.412500001229032964, 4.330127018922192761, -2.499999999999997780 ) ) ;
#24465=CARTESIAN_POINT ( 'NONE',  ( 27.78750000122903074, 4.330127018922191873, 2.499999999999999556 ) ) ;
#24467=CARTESIAN_POINT ( 'NONE',  ( 10.13437500061451679, -4.541064518000419881, 2.621784821874995952 ) ) ;
#24469=CARTESIAN_POINT ( 'NONE',  ( 15.44062500061451537, -3.027376345333614438, 5.243569643749998122 ) ) ;
#24470=CARTESIAN_POINT ( 'NONE',  ( 12.12187500061451573, 3.027376345333613106, -5.243569643749998122 ) ) ;
#24471=EDGE_CURVE ( 'NONE', #39486, #63581, #5075, .T. ) ;
#24472=CARTESIAN_POINT ( 'NONE',  ( 29.40000000122903145, -2.886751345948125991, -5.000000000000000000 ) ) ;
#24474=CARTESIAN_POINT ( 'NONE',  ( 18.83437500061451431, 6.421520780324663323E-16, -5.243569643749999010 ) ) ;
#24475=CARTESIAN_POINT ( 'NONE',  ( 6.984375000614516438, -4.541064518000419881, 2.621784821874995952 ) ) ;
#24476=CARTESIAN_POINT ( 'NONE',  ( 7.265625000614516438, 3.027376345333611329, 5.243569643749999010 ) ) ;
#24477=( BOUNDED_CURVE ( )  B_SPLINE_CURVE ( 2, ( #66695, #66321, #61140, #10536, #21978, #9075, #31610, #6806, #33424 ),
 .UNSPECIFIED., .F., .F. ) 
 B_SPLINE_CURVE_WITH_KNOTS ( ( 3, 2, 2, 2, 3 ),
 ( 0.1195652173913043514, 0.1231884057971014551, 0.1304347826086956486, 0.1376811594202898559, 0.1413043478260869734 ),
 .UNSPECIFIED. ) 
 CURVE ( )  GEOMETRIC_REPRESENTATION_ITEM ( )  RATIONAL_B_SPLINE_CURVE ( ( 0.9330127018922194093, 0.9330127018922194093, 1.000000000000000000, 0.8660254037844387076, 1.000000000000000000, 0.8660254037844387076, 1.000000000000000000, 0.9330127018922190762, 0.9330127018922194093 ) ) 
 REPRESENTATION_ITEM ( '' )  );
#24478=CARTESIAN_POINT ( 'NONE',  ( 17.39062500061451644, -3.027376345333610441, -5.243569643749999898 ) ) ;
#24479=EDGE_CURVE ( 'NONE', #59218, #48662, #35140, .T. ) ;
#24481=CARTESIAN_POINT ( 'NONE',  ( 6.150000001229033231, 5.773502691896255534, 3.535250795749688894E-16 ) ) ;
#24482=CARTESIAN_POINT ( 'NONE',  ( 15.77812500061451573, 4.541064518000418104, 2.621784821874999949 ) ) ;
#24483=CARTESIAN_POINT ( 'NONE',  ( 10.52812500061451750, -4.541064518000419881, 2.621784821874995952 ) ) ;
#24485=CARTESIAN_POINT ( 'NONE',  ( 11.06250000000000000, 2.886751345948126879, 4.999999999999999112 ) ) ;
#24486=CARTESIAN_POINT ( 'NONE',  ( 7.612500001229035362, 0.000000000000000000, 4.999999999999998224 ) ) ;
#24488=CARTESIAN_POINT ( 'NONE',  ( 14.55937500061451573, 0.000000000000000000, 5.243569643749999010 ) ) ;
#24489=CARTESIAN_POINT ( 'NONE',  ( 17.32500000122903216, 2.886751345948129099, -4.999999999999998224 ) ) ;
#24491=CARTESIAN_POINT ( 'NONE',  ( -3.000416591977282496E-16, 19.69062500061451360, -34.90005215228797653 ) ) ;
#24494=AXIS2_PLACEMENT_3D ( 'NONE', #71894, #28282, #33448 ) ;
#24496=CARTESIAN_POINT ( 'NONE',  ( 3.849931240356728512, 3.190302406438068505, 3.849931240356827544 ) ) ;
#24497=CARTESIAN_POINT ( 'NONE',  ( 18.83437500061451431, 6.421520780324663323E-16, -5.243569643749999010 ) ) ;
#24498=CARTESIAN_POINT ( 'NONE',  ( 10.76250000122903572, 0.000000000000000000, 4.999999999999998224 ) ) ;
#24499=CARTESIAN_POINT ( 'NONE',  ( 13.49062500061451608, 6.054752690667223547, 3.707466751127219781E-16 ) ) ;
#24502=CARTESIAN_POINT ( 'NONE',  ( 24.12187500061451217, -6.054752690667223547, -1.112240025338166033E-15 ) ) ;
#24504=CARTESIAN_POINT ( 'NONE',  ( 10.37812500061451715, 4.541064518000418104, 2.621784821874999949 ) ) ;
#24505=CARTESIAN_POINT ( 'NONE',  ( 15.53437500061451715, -4.541064518000419881, 2.621784821874995952 ) ) ;
#24507=CARTESIAN_POINT ( 'NONE',  ( 26.14687500061451431, 6.054752690667223547, 3.707466751127219781E-16 ) ) ;
#24508=CARTESIAN_POINT ( 'NONE',  ( 26.35312500061451857, -4.541064518000417216, -2.621784821875001281 ) ) ;
#24509=CARTESIAN_POINT ( 'NONE',  ( 19.34062500061451573, 6.054752690667223547, 3.707466751127219781E-16 ) ) ;
#24511=CARTESIAN_POINT ( 'NONE',  ( 0.000000000000000000, 20.00000000000000000, 30.00000000000000000 ) ) ;
#24512=CARTESIAN_POINT ( 'NONE',  ( 9.337500000000000355, -2.886751345948129988, 4.999999999999997335 ) ) ;
#24513=CARTESIAN_POINT ( 'NONE',  ( 20.51250000122903216, 4.330127018922192761, -2.499999999999997780 ) ) ;
#24514=CARTESIAN_POINT ( 'NONE',  ( -3.999999999999999112, 18.72500000122903074, -32.30940107675850470 ) ) ;
#24517=CARTESIAN_POINT ( 'NONE',  ( 18.37500000000000355, -4.330127018922194537, 2.499999999999995559 ) ) ;
#24518=CARTESIAN_POINT ( 'NONE',  ( 20.24999999999999645, -4.330127018922190985, -2.500000000000001332 ) ) ;
#24519=CARTESIAN_POINT ( 'NONE',  ( 18.72187500061451360, -6.054752690667223547, -1.112240025338166033E-15 ) ) ;
#24520=CARTESIAN_POINT ( 'NONE',  ( 14.57812500061451644, -4.541064518000419881, 2.621784821874995952 ) ) ;
#24523=CARTESIAN_POINT ( 'NONE',  ( 6.253125000614517148, 4.541064518000418104, -2.621784821874998173 ) ) ;
#24524=CARTESIAN_POINT ( 'NONE',  ( -5.810221930991193690E-16, 15.50000000122903465, 26.00000000000000355 ) ) ;
#24525=CARTESIAN_POINT ( 'NONE',  ( 12.93750000000000178, -2.886751345948129988, 4.999999999999997335 ) ) ;
#24527=CARTESIAN_POINT ( 'NONE',  ( 9.001249775931846008E-16, 14.06562500061451715, 34.90005215228797653 ) ) ;
#24528=CARTESIAN_POINT ( 'NONE',  ( 28.52812500061451573, -4.541064518000419881, 2.621784821874995952 ) ) ;
#24531=CARTESIAN_POINT ( 'NONE',  ( 24.42187500061451999, 3.027376345333611329, 5.243569643749999010 ) ) ;
#24533=CARTESIAN_POINT ( 'NONE',  ( 22.52812500061451573, 4.541064518000418104, 2.621784821874999949 ) ) ;
#24534=CARTESIAN_POINT ( 'NONE',  ( 23.29687500061451644, -3.027376345333610441, -5.243569643749999898 ) ) ;
#24535=CARTESIAN_POINT ( 'NONE',  ( 2.121784821875001281, 16.35312500061459318, -26.32496088578401938 ) ) ;
#24536=CARTESIAN_POINT ( 'NONE',  ( 6.403125000614517504, 0.000000000000000000, 5.243569643749999010 ) ) ;
#24538=CARTESIAN_POINT ( 'NONE',  ( 24.85312500061451502, 0.000000000000000000, 5.243569643749999010 ) ) ;
#24541=CARTESIAN_POINT ( 'NONE',  ( 16.80937500061451573, 0.000000000000000000, 5.243569643749999010 ) ) ;
#24542=CARTESIAN_POINT ( 'NONE',  ( 26.07187500061451857, 3.027376345333613106, -5.243569643749998122 ) ) ;
#24543=CARTESIAN_POINT ( 'NONE',  ( -4.243569643749998122, 16.29687500061451644, 32.45002607614398471 ) ) ;
#24544=CARTESIAN_POINT ( 'NONE',  ( 6.478125000614516793, -4.541064518000419881, 2.621784821874995952 ) ) ;
#24545=CARTESIAN_POINT ( 'NONE',  ( 3.999999999999998668, 16.21250000000000213, 27.69059892324149530 ) ) ;
#24546=CARTESIAN_POINT ( 'NONE',  ( 4.284375000614518925, -4.541064518000419881, 2.621784821874995952 ) ) ;
#24548=CARTESIAN_POINT ( 'NONE',  ( 5.165625000614518569, -6.054752690667223547, -1.112240025338166033E-15 ) ) ;
#24549=CARTESIAN_POINT ( 'NONE',  ( 10.39687500061451786, 6.054752690667223547, 3.707466751127219781E-16 ) ) ;
#24550=CARTESIAN_POINT ( 'NONE',  ( 17.47500000122903430, 2.886751345948126879, 4.999999999999999112 ) ) ;
#24551=CARTESIAN_POINT ( 'NONE',  ( 6.496875000614517504, -3.027376345333614438, 5.243569643749998122 ) ) ;
#24552=CARTESIAN_POINT ( 'NONE',  ( 8.465625000614515727, 3.027376345333613106, -5.243569643749998122 ) ) ;
#24555=CARTESIAN_POINT ( 'NONE',  ( 15.68437500061451573, 6.421520780324663323E-16, -5.243569643749999010 ) ) ;
#24556=CARTESIAN_POINT ( 'NONE',  ( -3.999999999999999112, 10.55000000000000249, 30.00000000000000000 ) ) ;
#24557=ORIENTED_EDGE ( 'NONE', *, *, #19020, .F. ) ;
#24558=CARTESIAN_POINT ( 'NONE',  ( 25.41562500061451146, -6.054752690667223547, -1.112240025338166033E-15 ) ) ;
#24559=CARTESIAN_POINT ( 'NONE',  ( 10.22812500061451679, 6.421520780324663323E-16, -5.243569643749999010 ) ) ;
#24560=CARTESIAN_POINT ( 'NONE',  ( 26.93437500061451573, 6.421520780324663323E-16, -5.243569643749999010 ) ) ;
#24561=CARTESIAN_POINT ( 'NONE',  ( 9.215625000614515727, -6.054752690667223547, -1.112240025338166033E-15 ) ) ;
#24563=CARTESIAN_POINT ( 'NONE',  ( 9.825000001229033941, 2.886751345948126879, 4.999999999999999112 ) ) ;
#24564=CARTESIAN_POINT ( 'NONE',  ( 24.66562500061451502, 3.027376345333613106, -5.243569643749998122 ) ) ;
#24566=CARTESIAN_POINT ( 'NONE',  ( 9.001249775931846008E-16, 13.61562500061451786, -25.09994784771203058 ) ) ;
#24567=CARTESIAN_POINT ( 'NONE',  ( 13.57500000122903572, -5.773502691896255534, -1.060575238724906372E-15 ) ) ;
#24568=CARTESIAN_POINT ( 'NONE',  ( 20.91562500061451502, -6.054752690667223547, -1.112240025338166033E-15 ) ) ;
#24569=CARTESIAN_POINT ( 'NONE',  ( 17.99062500061451786, 6.054752690667223547, 3.707466751127219781E-16 ) ) ;
#24570=CARTESIAN_POINT ( 'NONE',  ( 4.929824033517008708, 3.348239201030694723, -4.687818875421011278 ) ) ;
#24571=CARTESIAN_POINT ( 'NONE',  ( 20.73750000000000071, -2.886751345948125991, -5.000000000000000000 ) ) ;
#24572=CARTESIAN_POINT ( 'NONE',  ( 13.72500000122903074, 2.886751345948129099, -4.999999999999998224 ) ) ;
#24573=CARTESIAN_POINT ( 'NONE',  ( 9.778125000614517504, 6.421520780324663323E-16, -5.243569643749999010 ) ) ;
#24574=CARTESIAN_POINT ( 'NONE',  ( 14.54062500061451679, -3.027376345333614438, 5.243569643749998122 ) ) ;
#24575=CARTESIAN_POINT ( 'NONE',  ( 26.85000000122903430, 5.773502691896255534, 3.535250795749688894E-16 ) ) ;
#24576=CARTESIAN_POINT ( 'NONE',  ( 20.63437500061451857, 6.421520780324663323E-16, -5.243569643749999010 ) ) ;
#24578=CARTESIAN_POINT ( 'NONE',  ( 7.050000001229036251, 5.773502691896255534, 3.535250795749688894E-16 ) ) ;
#24579=CARTESIAN_POINT ( 'NONE',  ( 6.196875000614515905, -3.027376345333610441, -5.243569643749999898 ) ) ;
#24580=CARTESIAN_POINT ( 'NONE',  ( 26.18437500061451573, 4.541064518000418104, 2.621784821874999949 ) ) ;
#24582=CARTESIAN_POINT ( 'NONE',  ( 21.36562500061451431, -6.054752690667223547, -1.112240025338166033E-15 ) ) ;
#24583=CARTESIAN_POINT ( 'NONE',  ( 25.92187500061451999, -6.054752690667223547, -1.112240025338166033E-15 ) ) ;
#24586=CARTESIAN_POINT ( 'NONE',  ( 6.037500001229035185, 6.123233995736764310E-16, -4.999999999999998224 ) ) ;
#24587=CARTESIAN_POINT ( 'NONE',  ( 8.709375000614517859, 0.000000000000000000, 5.243569643749999010 ) ) ;
#24588=CARTESIAN_POINT ( 'NONE',  ( 16.90312500061451573, -4.541064518000417216, -2.621784821875001281 ) ) ;
#24589=VERTEX_POINT ( 'NONE', #71696 ) ;
#24590=FACE_OUTER_BOUND ( 'NONE', #58393, .T. ) ;
#24591=CARTESIAN_POINT ( 'NONE',  ( 27.81562500061452070, 3.027376345333613106, -5.243569643749998122 ) ) ;
#24592=CARTESIAN_POINT ( 'NONE',  ( 4.359375000614517326, -4.541064518000417216, -2.621784821875001281 ) ) ;
#24593=CARTESIAN_POINT ( 'NONE',  ( -1.487416814333745711E-14, 16.06250000000000000, -26.00000000000000000 ) ) ;
#24594=CARTESIAN_POINT ( 'NONE',  ( 3.628460635209542318, 3.440231774957711153, -3.861774003208584549 ) ) ;
#24595=CARTESIAN_POINT ( 'NONE',  ( 16.83749999999999858, 5.773502691896255534, 3.535250795749688894E-16 ) ) ;
#24596=CARTESIAN_POINT ( 'NONE',  ( 21.10312500061451502, 4.541064518000418104, -2.621784821874998173 ) ) ;
#24597=ORIENTED_EDGE ( 'NONE', *, *, #25641, .T. ) ;
#24598=CARTESIAN_POINT ( 'NONE',  ( 25.98750000000000071, -2.886751345948129988, 4.999999999999997335 ) ) ;
#24599=CARTESIAN_POINT ( 'NONE',  ( 25.43437500061451573, -4.541064518000419881, 2.621784821874995952 ) ) ;
#24601=ORIENTED_EDGE ( 'NONE', *, *, #6663, .T. ) ;
#24602=CARTESIAN_POINT ( 'NONE',  ( 13.04062500061451502, 6.054752690667223547, 3.707466751127219781E-16 ) ) ;
#24603=CARTESIAN_POINT ( 'NONE',  ( 5.465625000614517504, 3.027376345333611329, 5.243569643749999010 ) ) ;
#24605=CARTESIAN_POINT ( 'NONE',  ( 3.046875000614519990, -3.027376345333610441, -5.243569643749999898 ) ) ;
#24606=EDGE_CURVE ( 'NONE', #30066, #37881, #53177, .T. ) ;
#24607=CARTESIAN_POINT ( 'NONE',  ( 14.70000000122903394, 5.773502691896255534, 3.535250795749688894E-16 ) ) ;
#24608=CARTESIAN_POINT ( 'NONE',  ( 20.17499999999999716, -4.330127018922194537, 2.499999999999995559 ) ) ;
#24609=CARTESIAN_POINT ( 'NONE',  ( 29.09999999999999787, 0.000000000000000000, 4.999999999999998224 ) ) ;
#24610=CARTESIAN_POINT ( 'NONE',  ( 5.746875000614517504, -3.027376345333610441, -5.243569643749999898 ) ) ;
#24611=CARTESIAN_POINT ( 'NONE',  ( 8.784375000614518925, -4.541064518000419881, 2.621784821874995952 ) ) ;
#24612=CARTESIAN_POINT ( 'NONE',  ( 20.33437500061451786, 4.541064518000418104, 2.621784821874999949 ) ) ;
#24613=CARTESIAN_POINT ( 'NONE',  ( -1.999999999999997113, 17.37500000000000000, -26.53589838486224295 ) ) ;
#24614=ORIENTED_EDGE ( 'NONE', *, *, #56333, .F. ) ;
#24615=CARTESIAN_POINT ( 'NONE',  ( 28.15312500061451573, -4.541064518000417216, -2.621784821875001281 ) ) ;
#24616=CARTESIAN_POINT ( 'NONE',  ( 29.22187500061451715, 3.027376345333613106, -5.243569643749998122 ) ) ;
#24617=CARTESIAN_POINT ( 'NONE',  ( 5.596875000614516260, -3.027376345333614438, 5.243569643749998122 ) ) ;
#24618=CARTESIAN_POINT ( 'NONE',  ( 16.94999999999999929, 0.000000000000000000, 4.999999999999998224 ) ) ;
#24619=CARTESIAN_POINT ( 'NONE',  ( 14.46562500061451750, 3.027376345333611329, 5.243569643749999010 ) ) ;
#24622=CARTESIAN_POINT ( 'NONE',  ( 19.31250000122903288, 0.000000000000000000, 4.999999999999998224 ) ) ;
#24625=CARTESIAN_POINT ( 'NONE',  ( 7.603125000614517681, 4.541064518000418104, -2.621784821874998173 ) ) ;
#24626=CARTESIAN_POINT ( 'NONE',  ( 23.74687500061451573, -3.027376345333610441, -5.243569643749999898 ) ) ;
#24627=EDGE_CURVE ( 'NONE', #71409, #5357, #17765, .T. ) ;
#24628=CYLINDRICAL_SURFACE ( 'NONE', #17195, 4.999999999999998224 ) ;
#24629=CARTESIAN_POINT ( 'NONE',  ( 27.00937500061451857, 4.541064518000418104, -2.621784821874998173 ) ) ;
#24630=CARTESIAN_POINT ( 'NONE',  ( 8.437500000000000000, -2.886751345948129988, 4.999999999999997335 ) ) ;
#24631=CARTESIAN_POINT ( 'NONE',  ( 2.000000000000001332, 12.61250000122903536, 33.46410161513774995 ) ) ;
#24632=CARTESIAN_POINT ( 'NONE',  ( 13.75312500061451715, -4.541064518000417216, -2.621784821875001281 ) ) ;
#24633=CARTESIAN_POINT ( 'NONE',  ( 7.087500001229034119, 4.330127018922191873, 2.499999999999999556 ) ) ;
#24634=CARTESIAN_POINT ( 'NONE',  ( 12.34687500061452070, -3.027376345333614438, 5.243569643749998122 ) ) ;
#24635=CARTESIAN_POINT ( 'NONE',  ( -1.349117715399773765, 4.821506530989289274, -26.22488606966763314 ) ) ;
#24637=CARTESIAN_POINT ( 'NONE',  ( 12.44062500061451537, -3.027376345333610441, -5.243569643749999898 ) ) ;
#24639=CARTESIAN_POINT ( 'NONE',  ( 24.90000000122903145, -2.886751345948125991, -5.000000000000000000 ) ) ;
#24640=CARTESIAN_POINT ( 'NONE',  ( 13.05937500061451750, 4.541064518000418104, -2.621784821874998173 ) ) ;
#24641=CARTESIAN_POINT ( 'NONE',  ( 14.84062500061451750, 6.054752690667223547, 3.707466751127219781E-16 ) ) ;
#24643=CARTESIAN_POINT ( 'NONE',  ( 4.779258346327469376, 1.469247991000700582, 4.779258346327429408 ) ) ;
#24644=CARTESIAN_POINT ( 'NONE',  ( 24.23437500061451644, 6.421520780324663323E-16, -5.243569643749999010 ) ) ;
#24646=CARTESIAN_POINT ( 'NONE',  ( -3.999999999999997335, 19.58750000000000213, 32.30940107675850470 ) ) ;
#24647=CARTESIAN_POINT ( 'NONE',  ( -2.121784821874996840, 14.98437500061451644, -26.32496088578401583 ) ) ;
#24648=CARTESIAN_POINT ( 'NONE',  ( 16.20937500061451786, 4.541064518000418104, -2.621784821874998173 ) ) ;
#24649=CARTESIAN_POINT ( 'NONE',  ( 17.66250000122903430, -4.330127018922190985, -2.500000000000001332 ) ) ;
#24650=CARTESIAN_POINT ( 'NONE',  ( 12.60937500061451821, 4.541064518000418104, -2.621784821874998173 ) ) ;
#24651=CARTESIAN_POINT ( 'NONE',  ( 2.121784821874999061, 10.25937500061451857, 26.32496088578401583 ) ) ;
#24652=CARTESIAN_POINT ( 'NONE',  ( 20.10000000122903074, 5.773502691896255534, 3.535250795749688894E-16 ) ) ;
#24653=CARTESIAN_POINT ( 'NONE',  ( 13.41562500061451502, 3.027376345333613106, -5.243569643749998122 ) ) ;
#24654=ORIENTED_EDGE ( 'NONE', *, *, #24697, .F. ) ;
#24655=ORIENTED_EDGE ( 'NONE', *, *, #46671, .T. ) ;
#24656=CARTESIAN_POINT ( 'NONE',  ( 19.01249999999999929, 2.886751345948129099, -4.999999999999998224 ) ) ;
#24658=CARTESIAN_POINT ( 'NONE',  ( 11.78437500061451892, 4.541064518000418104, 2.621784821874999949 ) ) ;
#24659=CARTESIAN_POINT ( 'NONE',  ( 3.062382790376843467, 3.952479298030559640, -3.370876042629931568 ) ) ;
#24660=CARTESIAN_POINT ( 'NONE',  ( 13.12500000122903288, -5.773502691896255534, -1.060575238724906372E-15 ) ) ;
#24661=CARTESIAN_POINT ( 'NONE',  ( 21.11250000122903359, 0.000000000000000000, 4.999999999999998224 ) ) ;
#24662=CARTESIAN_POINT ( 'NONE',  ( 17.61562500061451786, 3.027376345333611329, 5.243569643749999010 ) ) ;
#24663=CARTESIAN_POINT ( 'NONE',  ( 21.21562500061451573, 3.027376345333611329, 5.243569643749999010 ) ) ;
#24664=CARTESIAN_POINT ( 'NONE',  ( 29.02500000122903145, 2.886751345948129099, -4.999999999999998224 ) ) ;
#24665=CARTESIAN_POINT ( 'NONE',  ( 28.61249999999999716, 2.886751345948126879, 4.999999999999999112 ) ) ;
#24668=CARTESIAN_POINT ( 'NONE',  ( 27.23437500061451644, -4.541064518000419881, 2.621784821874995952 ) ) ;
#24669=CARTESIAN_POINT ( 'NONE',  ( 4.016637241357584820, -2.977687906974178400, -4.152725646678794291 ) ) ;
#24670=CARTESIAN_POINT ( 'NONE',  ( -4.243569643749997233, 14.94687500061451679, -27.54997392385601174 ) ) ;
#24671=CARTESIAN_POINT ( 'NONE',  ( 3.112500001229034918, 0.000000000000000000, 4.999999999999998224 ) ) ;
#24672=CARTESIAN_POINT ( 'NONE',  ( 5.775000000000002132, -4.330127018922194537, 2.499999999999995559 ) ) ;
#24674=CARTESIAN_POINT ( 'NONE',  ( 10.05937500061451750, 0.000000000000000000, 5.243569643749999010 ) ) ;
#24675=CARTESIAN_POINT ( 'NONE',  ( 28.07812500061451289, -4.541064518000419881, 2.621784821874995952 ) ) ;
#24676=CARTESIAN_POINT ( 'NONE',  ( 30.00000000000000000, 0.000000000000000000, 0.000000000000000000 ) ) ;
#24677=CARTESIAN_POINT ( 'NONE',  ( -3.517994946560662139, 9.362281625417800512, -25.13577631594603190 ) ) ;
#24678=CARTESIAN_POINT ( 'NONE',  ( 8.362500000000002487, 2.886751345948126879, 4.999999999999998224 ) ) ;
#24679=CARTESIAN_POINT ( 'NONE',  ( 7.396875000614519635, -3.027376345333614438, 5.243569643749998122 ) ) ;
#24680=CARTESIAN_POINT ( 'NONE',  ( 10.62187500061451928, -6.054752690667223547, -1.112240025338166033E-15 ) ) ;
#24681=CARTESIAN_POINT ( 'NONE',  ( 4.912499999999999645, -5.773502691896255534, -1.060575238724906372E-15 ) ) ;
#24682=CARTESIAN_POINT ( 'NONE',  ( 2.121784821874999061, 14.70312500061459460, 26.32496088578401583 ) ) ;
#24684=( BOUNDED_CURVE ( )  B_SPLINE_CURVE ( 2, ( #12999, #35535, #58056, #1941, #24447, #46995, #69531, #72356, #61625 ),
 .UNSPECIFIED., .F., .F. ) 
 B_SPLINE_CURVE_WITH_KNOTS ( ( 3, 2, 2, 2, 3 ),
 ( 0.4891304347826087029, 0.4927536231884058204, 0.5000000000000000000, 0.5072463768115942351, 0.5108695652173913526 ),
 .UNSPECIFIED. ) 
 CURVE ( )  GEOMETRIC_REPRESENTATION_ITEM ( )  RATIONAL_B_SPLINE_CURVE ( ( 0.9330127018922194093, 0.9330127018922194093, 1.000000000000000000, 0.8660254037844387076, 1.000000000000000000, 0.8660254037844387076, 1.000000000000000000, 0.9330127018922182991, 0.9330127018922192983 ) ) 
 REPRESENTATION_ITEM ( '' )  );
#24685=CARTESIAN_POINT ( 'NONE',  ( 7.124999999999999112, -4.330127018922194537, 2.499999999999995559 ) ) ;
#24686=ADVANCED_FACE ( 'NONE', ( #49165 ), #65775, .F. ) ;
#24688=CARTESIAN_POINT ( 'NONE',  ( 21.02812500061451573, 6.421520780324663323E-16, -5.243569643749999010 ) ) ;
#24689=CARTESIAN_POINT ( 'NONE',  ( 12.92812500061451786, 6.421520780324663323E-16, -5.243569643749999010 ) ) ;
#24691=CARTESIAN_POINT ( 'NONE',  ( 9.759375000614516793, -4.541064518000417216, -2.621784821875001281 ) ) ;
#24692=CARTESIAN_POINT ( 'NONE',  ( 26.73749999999999716, 5.773502691896255534, 3.535250795749688894E-16 ) ) ;
#24693=CARTESIAN_POINT ( 'NONE',  ( 22.38750000122903216, 4.330127018922191873, 2.499999999999999556 ) ) ;
#24695=CARTESIAN_POINT ( 'NONE',  ( 11.55937500061451928, -4.541064518000417216, -2.621784821875001281 ) ) ;
#24696=CARTESIAN_POINT ( 'NONE',  ( 25.73437500061451644, 4.541064518000418104, 2.621784821874999949 ) ) ;
#24697=EDGE_CURVE ( 'NONE', #54370, #18194, #338, .T. ) ;
#24698=CARTESIAN_POINT ( 'NONE',  ( 3.121875000614518836, 3.027376345333613106, -5.243569643749998122 ) ) ;
#24699=CARTESIAN_POINT ( 'NONE',  ( -1.999999999999997113, 12.98750000122903359, -26.53589838486224295 ) ) ;
#24700=CARTESIAN_POINT ( 'NONE',  ( 20.63437500061451857, 6.421520780324663323E-16, -5.243569643749999010 ) ) ;
#24701=CARTESIAN_POINT ( 'NONE',  ( 12.15937500061451892, 4.541064518000418104, -2.621784821874998173 ) ) ;
#24703=CARTESIAN_POINT ( 'NONE',  ( 22.38749999999999929, -2.886751345948129988, 4.999999999999997335 ) ) ;
#24705=CARTESIAN_POINT ( 'NONE',  ( -4.243569643749999898, 11.75937500061451857, -30.00000000000000000 ) ) ;
#24707=CARTESIAN_POINT ( 'NONE',  ( 14.42812500061451786, 4.541064518000418104, 2.621784821874999949 ) ) ;
#24708=CARTESIAN_POINT ( 'NONE',  ( 4.800000000000002487, 0.000000000000000000, 4.999999999999998224 ) ) ;
#24711=CARTESIAN_POINT ( 'NONE',  ( -3.999999999999999112, 19.66250000122903430, -30.00000000000000000 ) ) ;
#24712=CARTESIAN_POINT ( 'NONE',  ( 15.63749999999999751, -2.886751345948129988, 4.999999999999997335 ) ) ;
#24713=CARTESIAN_POINT ( 'NONE',  ( -1.999999999999997113, 19.28750000122903430, 33.46410161513775705 ) ) ;
#24714=CARTESIAN_POINT ( 'NONE',  ( 13.01250000122903394, 0.000000000000000000, 4.999999999999998224 ) ) ;
#24715=CARTESIAN_POINT ( 'NONE',  ( 23.70937500061451786, -4.541064518000417216, -2.621784821875001281 ) ) ;
#24716=CARTESIAN_POINT ( 'NONE',  ( -1.071796769724483234, 16.30759618943233491, -34.00000000000000711 ) ) ;
#24718=CARTESIAN_POINT ( 'NONE',  ( 18.59062500061451573, -3.027376345333614438, 5.243569643749998122 ) ) ;
#24719=CARTESIAN_POINT ( 'NONE',  ( 3.628125000614518036, 4.541064518000418104, 2.621784821874999949 ) ) ;
#24720=CARTESIAN_POINT ( 'NONE',  ( 18.94687500061451502, 6.054752690667223547, 3.707466751127219781E-16 ) ) ;
#24721=CARTESIAN_POINT ( 'NONE',  ( 3.637500000000001954, -2.886751345948125991, -5.000000000000000000 ) ) ;
#24722=CARTESIAN_POINT ( 'NONE',  ( 6.140625000614516438, -3.027376345333610441, -5.243569643749999898 ) ) ;
#24723=CARTESIAN_POINT ( 'NONE',  ( 22.64062500061451644, -3.027376345333614438, 5.243569643749998122 ) ) ;
#24724=CARTESIAN_POINT ( 'NONE',  ( -4.243569643749999898, 15.26562500061451644, 27.54997392385601529 ) ) ;
#24725=CARTESIAN_POINT ( 'NONE',  ( 18.03750000122903430, -4.330127018922194537, 2.499999999999995559 ) ) ;
#24727=CARTESIAN_POINT ( 'NONE',  ( 10.67812500061451608, 6.421520780324663323E-16, -5.243569643749999010 ) ) ;
#24728=CARTESIAN_POINT ( 'NONE',  ( 2.896875000614518747, -3.027376345333614438, 5.243569643749998122 ) ) ;
#24729=CARTESIAN_POINT ( 'NONE',  ( 3.346875000614518036, -3.027376345333614438, 5.243569643749998122 ) ) ;
#24730=CARTESIAN_POINT ( 'NONE',  ( 23.18437500061451573, -4.541064518000419881, 2.621784821874995952 ) ) ;
#24731=CARTESIAN_POINT ( 'NONE',  ( 15.25312500061451715, 4.541064518000418104, -2.621784821874998173 ) ) ;
#24732=CARTESIAN_POINT ( 'NONE',  ( 25.46250000122903501, 4.330127018922192761, -2.499999999999997780 ) ) ;
#24733=CARTESIAN_POINT ( 'NONE',  ( 25.45312500061451644, -4.541064518000417216, -2.621784821875001281 ) ) ;
#24734=CARTESIAN_POINT ( 'NONE',  ( 18.30937500061451928, -4.541064518000417216, -2.621784821875001281 ) ) ;
#24735=CARTESIAN_POINT ( 'NONE',  ( 14.16562500061451679, -6.054752690667223547, -1.112240025338166033E-15 ) ) ;
#24736=CARTESIAN_POINT ( 'NONE',  ( -2.121784821874999949, 16.18437500061451573, 26.32496088578401938 ) ) ;
#24737=CARTESIAN_POINT ( 'NONE',  ( 19.07812500061451644, -4.541064518000419881, 2.621784821874995952 ) ) ;
#24740=CARTESIAN_POINT ( 'NONE',  ( 24.29999999999999716, -4.330127018922190985, -2.500000000000001332 ) ) ;
#24741=CARTESIAN_POINT ( 'NONE',  ( 4.000000000000000000, 11.18750000000000178, -27.69059892324149530 ) ) ;
#24743=CARTESIAN_POINT ( 'NONE',  ( 27.89062500061451289, 6.054752690667223547, 3.707466751127219781E-16 ) ) ;
#24744=CARTESIAN_POINT ( 'NONE',  ( 8.090625000614515727, 6.054752690667223547, 3.707466751127219781E-16 ) ) ;
#24745=CARTESIAN_POINT ( 'NONE',  ( 20.43750000122903643, 6.123233995736764310E-16, -4.999999999999998224 ) ) ;
#24746=ADVANCED_FACE ( 'NONE', ( #33971 ), #12605, .T. ) ;
#24747=CARTESIAN_POINT ( 'NONE',  ( 24.47812500061451502, -4.541064518000419881, 2.621784821874995952 ) ) ;
#24748=CARTESIAN_POINT ( 'NONE',  ( 24.97499999999999787, 4.330127018922191873, 2.499999999999999556 ) ) ;
#24749=CARTESIAN_POINT ( 'NONE',  ( 3.999999999999998668, 14.97500000122903430, -32.30940107675850470 ) ) ;
#24750=CARTESIAN_POINT ( 'NONE',  ( -3.999999999999999112, 12.46250000122903323, 30.00000000000000000 ) ) ;
#24751=CARTESIAN_POINT ( 'NONE',  ( 9.515625000614518214, 3.027376345333611329, 5.243569643749999010 ) ) ;
#24753=CARTESIAN_POINT ( 'NONE',  ( 25.79062500061451502, -3.027376345333614438, 5.243569643749998122 ) ) ;
#24754=CARTESIAN_POINT ( 'NONE',  ( 4.715625000614516615, -6.054752690667223547, -1.112240025338166033E-15 ) ) ;
#24756=VECTOR ( 'NONE', #31423, 1000.000000000000000 ) ;
#24757=CARTESIAN_POINT ( 'NONE',  ( 17.81250000122903288, 4.330127018922192761, -2.499999999999997780 ) ) ;
#24758=CARTESIAN_POINT ( 'NONE',  ( 14.10000000000000142, 4.330127018922192761, -2.499999999999997780 ) ) ;
#24759=CARTESIAN_POINT ( 'NONE',  ( 13.24687500061451750, -3.027376345333614438, 5.243569643749998122 ) ) ;
#24760=CARTESIAN_POINT ( 'NONE',  ( 9.075000001229033941, -5.773502691896255534, -1.060575238724906372E-15 ) ) ;
#24761=CARTESIAN_POINT ( 'NONE',  ( 16.99687500061451573, -3.027376345333610441, -5.243569643749999898 ) ) ;
#24763=CARTESIAN_POINT ( 'NONE',  ( 8.746875000614515727, -3.027376345333614438, 5.243569643749998122 ) ) ;
#24764=CARTESIAN_POINT ( 'NONE',  ( 4.243569643749999898, 12.79062500061451679, -27.54997392385601529 ) ) ;
#24765=CARTESIAN_POINT ( 'NONE',  ( 1.626862140677534273E-15, 12.01250000000000284, -26.00000000000000355 ) ) ;
#24767=ORIENTED_EDGE ( 'NONE', *, *, #68132, .F. ) ;
#24768=CARTESIAN_POINT ( 'NONE',  ( 24.74062500061451786, 6.054752690667223547, 3.707466751127219781E-16 ) ) ;
#24769=CARTESIAN_POINT ( 'NONE',  ( 21.15000000122903145, -2.886751345948130876, 4.999999999999996447 ) ) ;
#24770=CARTESIAN_POINT ( 'NONE',  ( 25.58437500061451431, 6.421520780324663323E-16, -5.243569643749999010 ) ) ;
#24771=CARTESIAN_POINT ( 'NONE',  ( 28.24687500061451573, -3.027376345333610441, -5.243569643749999898 ) ) ;
#24772=CARTESIAN_POINT ( 'NONE',  ( 21.18749999999999645, -2.886751345948125991, -5.000000000000000000 ) ) ;
#24773=CARTESIAN_POINT ( 'NONE',  ( 6.365625000614518747, 3.027376345333611329, 5.243569643749999010 ) ) ;
#24775=CARTESIAN_POINT ( 'NONE',  ( 15.53437500061451715, -4.541064518000419881, 2.621784821874995952 ) ) ;
#24777=CARTESIAN_POINT ( 'NONE',  ( 3.778125000614519280, -4.541064518000419881, 2.621784821874995952 ) ) ;
#24778=CARTESIAN_POINT ( 'NONE',  ( 7.959375000614516971, -4.541064518000417216, -2.621784821875001281 ) ) ;
#24779=CARTESIAN_POINT ( 'NONE',  ( 19.09687500061451360, -3.027376345333614438, 5.243569643749998122 ) ) ;
#24781=CARTESIAN_POINT ( 'NONE',  ( 27.18750000000000000, 5.773502691896255534, 3.535250795749688894E-16 ) ) ;
#24782=CARTESIAN_POINT ( 'NONE',  ( 28.13437500061451502, -4.541064518000419881, 2.621784821874995952 ) ) ;
#24783=CARTESIAN_POINT ( 'NONE',  ( 1.071796769724491893, 10.23259618943233384, -26.00000000000000355 ) ) ;
#24784=CARTESIAN_POINT ( 'NONE',  ( 29.39999999999999858, 4.330127018922192761, -2.499999999999997780 ) ) ;
#24786=CARTESIAN_POINT ( 'NONE',  ( 10.57500000000000107, 4.330127018922191873, 2.499999999999999556 ) ) ;
#24788=CARTESIAN_POINT ( 'NONE',  ( 22.41562500061451502, 3.027376345333613106, -5.243569643749998122 ) ) ;
#24789=CARTESIAN_POINT ( 'NONE',  ( 11.10000000000000142, 0.000000000000000000, 4.999999999999998224 ) ) ;
#24790=EDGE_CURVE ( 'NONE', #36195, #38197, #4289, .T. ) ;
#24791=CARTESIAN_POINT ( 'NONE',  ( 9.300000001229035362, 5.773502691896255534, 3.535250795749688894E-16 ) ) ;
#24792=CARTESIAN_POINT ( 'NONE',  ( 6.628125000614517148, 6.421520780324663323E-16, -5.243569643749999010 ) ) ;
#24793=CARTESIAN_POINT ( 'NONE',  ( 22.46250000000000213, -5.773502691896255534, -1.060575238724906372E-15 ) ) ;
#24794=CARTESIAN_POINT ( 'NONE',  ( 20.24062500061451431, 6.054752690667223547, 3.707466751127219781E-16 ) ) ;
#24795=CARTESIAN_POINT ( 'NONE',  ( 14.73749999999999893, -2.886751345948063374, 5.000000000000112799 ) ) ;
#24796=CARTESIAN_POINT ( 'NONE',  ( 25.12500000122903288, 2.886751345948126879, 4.999999999999999112 ) ) ;
#24798=CARTESIAN_POINT ( 'NONE',  ( 4.200000000000001954, 4.330127018922192761, -2.499999999999997780 ) ) ;
#24800=CARTESIAN_POINT ( 'NONE',  ( 20.65312500061451573, 4.541064518000418104, -2.621784821874998173 ) ) ;
#24801=CARTESIAN_POINT ( 'NONE',  ( 26.46562500061451573, 3.027376345333613106, -5.243569643749998122 ) ) ;
#24802=CARTESIAN_POINT ( 'NONE',  ( 28.05937500061451573, 0.000000000000000000, 5.243569643749999010 ) ) ;
#24803=CARTESIAN_POINT ( 'NONE',  ( 14.09062500061451750, -3.027376345333614438, 5.243569643749998122 ) ) ;
#24804=CARTESIAN_POINT ( 'NONE',  ( 28.34062500061451928, 6.054752690667223547, 3.707466751127219781E-16 ) ) ;
#24805=CARTESIAN_POINT ( 'NONE',  ( 9.403125000614517504, 4.541064518000418104, -2.621784821874998173 ) ) ;
#24806=CARTESIAN_POINT ( 'NONE',  ( 26.28750000122903430, 6.123233995736764310E-16, -4.999999999999998224 ) ) ;
#24808=CARTESIAN_POINT ( 'NONE',  ( 17.80312500061451786, -4.541064518000417216, -2.621784821875001281 ) ) ;
#24810=CARTESIAN_POINT ( 'NONE',  ( 29.78437500061451715, 4.541064518000418104, 2.621784821874999949 ) ) ;
#24811=CARTESIAN_POINT ( 'NONE',  ( 10.09687500061451715, -3.027376345333614438, 5.243569643749998122 ) ) ;
#24812=CARTESIAN_POINT ( 'NONE',  ( 8.709375000614517859, 0.000000000000000000, 5.243569643749999010 ) ) ;
#24813=CARTESIAN_POINT ( 'NONE',  ( 18.68437500061451928, -4.541064518000419881, 2.621784821874995952 ) ) ;
#24815=CARTESIAN_POINT ( 'NONE',  ( 29.59687500061451715, -3.027376345333610441, -5.243569643749999898 ) ) ;
#24816=CARTESIAN_POINT ( 'NONE',  ( 22.04062500061451502, 6.054752690667223547, 3.707466751127219781E-16 ) ) ;
#24817=CARTESIAN_POINT ( 'NONE',  ( 15.49687500061451750, -3.027376345333614438, 5.243569643749998122 ) ) ;
#24818=CARTESIAN_POINT ( 'NONE',  ( 22.52812500061451573, 4.541064518000418104, 2.621784821874999949 ) ) ;
#24819=CARTESIAN_POINT ( 'NONE',  ( 2.000000000000001332, 14.75000000000000178, 33.46410161513774995 ) ) ;
#24820=CARTESIAN_POINT ( 'NONE',  ( 29.16562500061451502, 3.027376345333613106, -5.243569643749998122 ) ) ;
#24821=CARTESIAN_POINT ( 'NONE',  ( 9.637500001229033941, 6.123233995736764310E-16, -4.999999999999998224 ) ) ;
#24822=ORIENTED_EDGE ( 'NONE', *, *, #39310, .F. ) ;
#24823=CARTESIAN_POINT ( 'NONE',  ( 5.550000001229032698, -2.886751345948125991, -5.000000000000000000 ) ) ;
#24824=CARTESIAN_POINT ( 'NONE',  ( -3.999999999999999112, 16.85000000000000142, -30.00000000000000000 ) ) ;
#24825=CARTESIAN_POINT ( 'NONE',  ( 25.61250000122903359, 0.000000000000000000, 4.999999999999998224 ) ) ;
#24827=CARTESIAN_POINT ( 'NONE',  ( 6.496875000614517504, -3.027376345333614438, 5.243569643749998122 ) ) ;
#24828=CARTESIAN_POINT ( 'NONE',  ( 1.999999999999998668, 10.06250000122903465, 26.53589838486224650 ) ) ;
#24829=CARTESIAN_POINT ( 'NONE',  ( 14.84062500061451750, 6.054752690667223547, 3.707466751127219781E-16 ) ) ;
#24830=CARTESIAN_POINT ( 'NONE',  ( 10.13437500061451679, -4.541064518000419881, 2.621784821874995952 ) ) ;
#24831=CARTESIAN_POINT ( 'NONE',  ( 27.63750000122903216, 6.123233995736764310E-16, -4.999999999999998224 ) ) ;
#24832=CARTESIAN_POINT ( 'NONE',  ( 17.29687500061451999, -3.027376345333614438, 5.243569643749998122 ) ) ;
#24833=CARTESIAN_POINT ( 'NONE',  ( 8.559375000614515727, 4.541064518000418104, -2.621784821874998173 ) ) ;
#24835=CARTESIAN_POINT ( 'NONE',  ( 8.615625000614517859, 3.027376345333611329, 5.243569643749999010 ) ) ;
#24836=CARTESIAN_POINT ( 'NONE',  ( 17.84062500061451573, -3.027376345333610441, -5.243569643749999898 ) ) ;
#24837=ORIENTED_EDGE ( 'NONE', *, *, #71773, .F. ) ;
#24838=CARTESIAN_POINT ( 'NONE',  ( 14.65312500061451573, -4.541064518000417216, -2.621784821875001281 ) ) ;
#24839=CARTESIAN_POINT ( 'NONE',  ( 10.97812500061451679, -4.541064518000419881, 2.621784821874995952 ) ) ;
#24840=B_SPLINE_CURVE_WITH_KNOTS ( 'NONE', 3,
 ( #36978, #59500, #30706, #70234, #14075, #29978, #8913, #47697, #35522, #31444 ),
 .UNSPECIFIED., .F., .F.,
 ( 4, 3, 3, 4 ),
 ( 0.000000000000000000, 0.0001572314549002369448, 0.0003212513203110487804, 0.0004853362698026408980 ),
 .UNSPECIFIED. ) ;
#24842=CARTESIAN_POINT ( 'NONE',  ( 10.91250000000000320, 2.886751345948129099, -4.999999999999998224 ) ) ;
#24843=EDGE_CURVE ( 'NONE', #56056, #65447, #57913, .T. ) ;
#24844=CARTESIAN_POINT ( 'NONE',  ( 6.787500001229032520, -4.330127018922194537, 2.499999999999995559 ) ) ;
#24845=( BOUNDED_CURVE ( )  B_SPLINE_CURVE ( 2, ( #45411, #51313, #5526, #11430, #22504, #35042, #29144 ),
 .UNSPECIFIED., .F., .F. ) 
 B_SPLINE_CURVE_WITH_KNOTS ( ( 3, 2, 2, 3 ),
 ( 0.3750000000000000000, 0.3777777777777777679, 0.3805555555555554803, 0.3833333333333333037 ),
 .UNSPECIFIED. ) 
 CURVE ( )  GEOMETRIC_REPRESENTATION_ITEM ( )  RATIONAL_B_SPLINE_CURVE ( ( 1.000000000000000000, 0.8660254037844387076, 1.000000000000000000, 0.8660254037844387076, 1.000000000000000000, 0.8660254037844413721, 0.9999999999999973355 ) ) 
 REPRESENTATION_ITEM ( '' )  );
#24846=CARTESIAN_POINT ( 'NONE',  ( 13.80937500061451750, -4.541064518000417216, -2.621784821875001281 ) ) ;
#24847=CARTESIAN_POINT ( 'NONE',  ( 15.93750000122903110, 6.123233995736764310E-16, -4.999999999999998224 ) ) ;
#24849=CARTESIAN_POINT ( 'NONE',  ( -2.121784821874999949, 19.72812500061451857, -33.67503911421598417 ) ) ;
#24850=CARTESIAN_POINT ( 'NONE',  ( -3.137519842735245283E-14, 12.57500000122903572, -26.00000000000000711 ) ) ;
#24852=CARTESIAN_POINT ( 'NONE',  ( 23.40000000122902790, -2.886751345948114000, 5.000000000000024869 ) ) ;
#24854=CARTESIAN_POINT ( 'NONE',  ( 3.999999999999999112, 14.48750000122903536, 30.00000000000000000 ) ) ;
#24855=CARTESIAN_POINT ( 'NONE',  ( 15.42187500061451821, 3.027376345333611329, 5.243569643749999010 ) ) ;
#24856=CARTESIAN_POINT ( 'NONE',  ( 28.94999999999999929, 4.330127018922192761, -2.499999999999997780 ) ) ;
#24857=CARTESIAN_POINT ( 'NONE',  ( 13.19062500061451537, -3.027376345333614438, 5.243569643749998122 ) ) ;
#24859=CARTESIAN_POINT ( 'NONE',  ( 24.57187500061451502, -6.054752690667223547, -1.112240025338166033E-15 ) ) ;
#24861=CARTESIAN_POINT ( 'NONE',  ( 10.90312500061451928, 0.000000000000000000, 5.243569643749999010 ) ) ;
#24862=CARTESIAN_POINT ( 'NONE',  ( 15.94687500061451502, -3.027376345333614438, 5.243569643749998122 ) ) ;
#24864=CARTESIAN_POINT ( 'NONE',  ( 27.42187500061451644, 3.027376345333613106, -5.243569643749998122 ) ) ;
#24865=CARTESIAN_POINT ( 'NONE',  ( 28.49062500061451431, -3.027376345333614438, 5.243569643749998122 ) ) ;
#24866=CARTESIAN_POINT ( 'NONE',  ( 17.46562500061451217, 3.027376345333613106, -5.243569643749998122 ) ) ;
#24867=DIRECTION ( 'NONE',  ( -0.000000000000000000, -1.000000000000000000, -0.000000000000000000 ) ) ;
#24868=CARTESIAN_POINT ( 'NONE',  ( 1.071796769724476572, 14.73259618943233562, 34.00000000000000000 ) ) ;
#24869=CARTESIAN_POINT ( 'NONE',  ( 7.500000000000000000, 0.000000000000000000, 4.999999999999998224 ) ) ;
#24870=CARTESIAN_POINT ( 'NONE',  ( 19.31250000122903288, 0.000000000000000000, 4.999999999999998224 ) ) ;
#24871=CARTESIAN_POINT ( 'NONE',  ( -2.556497649636125342E-15, 18.87500000122903288, -26.00000000000000000 ) ) ;
#24874=CARTESIAN_POINT ( 'NONE',  ( 16.91250000000000142, 2.886751345948126879, 4.999999999999999112 ) ) ;
#24875=CARTESIAN_POINT ( 'NONE',  ( 20.10000000000000142, 0.000000000000000000, 4.999999999999998224 ) ) ;
#24876=CARTESIAN_POINT ( 'NONE',  ( 19.47187500061451360, 3.027376345333611329, 5.243569643749999010 ) ) ;
#24877=CARTESIAN_POINT ( 'NONE',  ( 12.66562500061451502, 3.027376345333611329, 5.243569643749999010 ) ) ;
#24878=EDGE_CURVE ( 'NONE', #9351, #69502, #12241, .T. ) ;
#24879=ORIENTED_EDGE ( 'NONE', *, *, #66576, .F. ) ;
#24881=CARTESIAN_POINT ( 'NONE',  ( 6.403125000614517504, 0.000000000000000000, 5.243569643749999010 ) ) ;
#24883=CARTESIAN_POINT ( 'NONE',  ( 12.44999999999999929, 0.000000000000000000, 4.999999999999998224 ) ) ;
#24885=CARTESIAN_POINT ( 'NONE',  ( 2.121784821875001281, 15.45312500061451644, 33.67503911421598417 ) ) ;
#24886=CARTESIAN_POINT ( 'NONE',  ( 26.20312500061451644, 0.000000000000000000, 5.243569643749999010 ) ) ;
#24889=CARTESIAN_POINT ( 'NONE',  ( 24.90937500061451715, 0.000000000000000000, 5.243569643749999010 ) ) ;
#24890=ORIENTED_EDGE ( 'NONE', *, *, #66396, .F. ) ;
#24891=CARTESIAN_POINT ( 'NONE',  ( 20.91562500061451502, -6.054752690667223547, -1.112240025338166033E-15 ) ) ;
#24892=CARTESIAN_POINT ( 'NONE',  ( 22.58437500061451431, 4.541064518000418104, 2.621784821874999949 ) ) ;
#24893=CARTESIAN_POINT ( 'NONE',  ( -2.121784821874996840, 16.72812500061459673, -26.32496088578401583 ) ) ;
#24894=CARTESIAN_POINT ( 'NONE',  ( 5.428125000614517859, 4.541064518000418104, 2.621784821874999949 ) ) ;
#24896=CARTESIAN_POINT ( 'NONE',  ( 24.14062500061451289, -3.027376345333610441, -5.243569643749999898 ) ) ;
#24899=CARTESIAN_POINT ( 'NONE',  ( 16.62187500061451573, 3.027376345333613106, -5.243569643749998122 ) ) ;
#24900=CARTESIAN_POINT ( 'NONE',  ( 25.20937500061451431, 4.541064518000418104, -2.621784821874998173 ) ) ;
#24901=CARTESIAN_POINT ( 'NONE',  ( -2.121784821874996840, 14.08437500061451786, 33.67503911421598417 ) ) ;
#24902=CARTESIAN_POINT ( 'NONE',  ( 6.665625000614515905, 3.027376345333613106, -5.243569643749998122 ) ) ;
#24903=CARTESIAN_POINT ( 'NONE',  ( 28.49062500061451431, -3.027376345333614438, 5.243569643749998122 ) ) ;
#24905=CARTESIAN_POINT ( 'NONE',  ( 3.121875000614518836, 3.027376345333613106, -5.243569643749998122 ) ) ;
#24907=CARTESIAN_POINT ( 'NONE',  ( 5.128125000614516260, -4.541064518000419881, 2.621784821874995952 ) ) ;
#24908=CARTESIAN_POINT ( 'NONE',  ( 10.77187500061451786, 3.027376345333613106, -5.243569643749998122 ) ) ;
#24910=CARTESIAN_POINT ( 'NONE',  ( 16.01250000122903216, 4.330127018922192761, -2.499999999999997780 ) ) ;
#24911=CARTESIAN_POINT ( 'NONE',  ( 29.65312500061451573, 4.541064518000418104, -2.621784821874998173 ) ) ;
#24912=CARTESIAN_POINT ( 'NONE',  ( 4.565625000614516260, 3.027376345333611329, 5.243569643749999010 ) ) ;
#24915=AXIS2_PLACEMENT_3D ( 'NONE', #28784, #11440, #5537 ) ;
#24916=CARTESIAN_POINT ( 'NONE',  ( 15.98437500061451821, -4.541064518000419881, 2.621784821874995952 ) ) ;
#24917=DIRECTION ( 'NONE',  ( -1.000000000000000000, -0.000000000000000000, -0.000000000000000000 ) ) ;
#24919=CARTESIAN_POINT ( 'NONE',  ( 21.70312500061451644, 0.000000000000000000, 5.243569643749999010 ) ) ;
#24920=CARTESIAN_POINT ( 'NONE',  ( 9.290625000614515017, -3.027376345333610441, -5.243569643749999898 ) ) ;
#24921=CARTESIAN_POINT ( 'NONE',  ( 23.93437500061451573, 4.541064518000418104, 2.621784821874999949 ) ) ;
#24922=CARTESIAN_POINT ( 'NONE',  ( 8.090625000614515727, 6.054752690667223547, 3.707466751127219781E-16 ) ) ;
#24923=CARTESIAN_POINT ( 'NONE',  ( 16.38750000122903216, 6.123233995736764310E-16, -4.999999999999998224 ) ) ;
#24924=CARTESIAN_POINT ( 'NONE',  ( 9.300000001229035362, 5.773502691896255534, 3.535250795749688894E-16 ) ) ;
#24925=CARTESIAN_POINT ( 'NONE',  ( 23.84062500061451928, 6.054752690667223547, 3.707466751127219781E-16 ) ) ;
#24926=CARTESIAN_POINT ( 'NONE',  ( -2.121784821874999949, 10.72812500061451679, -33.67503911421598417 ) ) ;
#24927=CARTESIAN_POINT ( 'NONE',  ( 13.68750000122903288, 6.123233995736764310E-16, -4.999999999999998224 ) ) ;
#24928=CARTESIAN_POINT ( 'NONE',  ( 22.90312500061451573, 4.541064518000418104, -2.621784821874998173 ) ) ;
#24929=CARTESIAN_POINT ( 'NONE',  ( 17.35312500061451502, -4.541064518000417216, -2.621784821875001281 ) ) ;
#24931=CARTESIAN_POINT ( 'NONE',  ( 18.00000000000000355, -4.330127018922190985, -2.500000000000001332 ) ) ;
#24932=CARTESIAN_POINT ( 'NONE',  ( 12.67500000122903536, -5.773502691896255534, -1.060575238724906372E-15 ) ) ;
#24933=CARTESIAN_POINT ( 'NONE',  ( 11.12812500061451715, 6.421520780324663323E-16, -5.243569643749999010 ) ) ;
#24935=CARTESIAN_POINT ( 'NONE',  ( 13.04062500061451502, 6.054752690667223547, 3.707466751127219781E-16 ) ) ;
#24936=CARTESIAN_POINT ( 'NONE',  ( 23.43750000122902932, -4.330127018922194537, 2.499999999999995559 ) ) ;
#24937=CARTESIAN_POINT ( 'NONE',  ( 22.02187500061452141, 3.027376345333613106, -5.243569643749998122 ) ) ;
#24938=CARTESIAN_POINT ( 'NONE',  ( 21.42187500061451644, -6.054752690667223547, -1.112240025338166033E-15 ) ) ;
#24939=CYLINDRICAL_SURFACE ( 'NONE', #67843, 4.999999999999998224 ) ;
#24940=CARTESIAN_POINT ( 'NONE',  ( 8.025000001229035007, 2.886751345948126879, 4.999999999999999112 ) ) ;
#24941=CARTESIAN_POINT ( 'NONE',  ( 6.571875000614517681, -6.054752690667223547, -1.112240025338166033E-15 ) ) ;
#24942=CARTESIAN_POINT ( 'NONE',  ( 24.68437500061451573, 6.421520780324663323E-16, -5.243569643749999010 ) ) ;
#24943=DIRECTION ( 'NONE',  ( -0.000000000000000000, -0.000000000000000000, -1.000000000000000000 ) ) ;
#24945=CARTESIAN_POINT ( 'NONE',  ( 22.22812500061451502, -4.541064518000419881, 2.621784821874995952 ) ) ;
#24946=CARTESIAN_POINT ( 'NONE',  ( 27.27187500061451431, -6.054752690667223547, -1.112240025338166033E-15 ) ) ;
#24948=CARTESIAN_POINT ( 'NONE',  ( 3.241876093077143306, -3.806644978545103530, 3.422667876732838010 ) ) ;
#24949=CARTESIAN_POINT ( 'NONE',  ( 27.71250000122903145, 4.330127018922192761, -2.499999999999997780 ) ) ;
#24950=CARTESIAN_POINT ( 'NONE',  ( 5.746875000614517504, -3.027376345333610441, -5.243569643749999898 ) ) ;
#24951=CARTESIAN_POINT ( 'NONE',  ( 16.56562500061451715, 3.027376345333613106, -5.243569643749998122 ) ) ;
#24952=ORIENTED_EDGE ( 'NONE', *, *, #3046, .T. ) ;
#24953=CARTESIAN_POINT ( 'NONE',  ( 11.32500000000000107, 6.123233995736764310E-16, -4.999999999999998224 ) ) ;
#24954=CARTESIAN_POINT ( 'NONE',  ( 25.19062500061451715, 6.054752690667223547, 3.707466751127219781E-16 ) ) ;
#24955=CARTESIAN_POINT ( 'NONE',  ( 3.759375000614517681, 0.000000000000000000, 5.243569643749999010 ) ) ;
#24956=CARTESIAN_POINT ( 'NONE',  ( 4.670535407306061870, 1.785677299253563444, 4.864229956990654635 ) ) ;
#24957=CARTESIAN_POINT ( 'NONE',  ( 17.17500000000000071, 6.123233995736764310E-16, -4.999999999999998224 ) ) ;
#24958=CARTESIAN_POINT ( 'NONE',  ( 20.01562500061451644, -6.054752690667223547, -1.112240025338166033E-15 ) ) ;
#24960=CARTESIAN_POINT ( 'NONE',  ( 23.73749999999999716, -2.886751345948129988, 4.999999999999997335 ) ) ;
#24961=CARTESIAN_POINT ( 'NONE',  ( 25.05937500061451573, -4.541064518000417216, -2.621784821875001281 ) ) ;
#24963=VERTEX_POINT ( 'NONE', #5737 ) ;
#24965=CARTESIAN_POINT ( 'NONE',  ( 13.49062500061451608, 6.054752690667223547, 3.707466751127219781E-16 ) ) ;
#24966=CARTESIAN_POINT ( 'NONE',  ( 5.915625000614515905, 3.027376345333611329, 5.243569643749999010 ) ) ;
#24968=CARTESIAN_POINT ( 'NONE',  ( 28.64062500061451289, -3.027376345333610441, -5.243569643749999898 ) ) ;
#24969=CARTESIAN_POINT ( 'NONE',  ( 14.51250000122903394, -4.330127018922190985, -2.500000000000001332 ) ) ;
#24970=CARTESIAN_POINT ( 'NONE',  ( 19.04999999999999716, 4.330127018922192761, -2.499999999999997780 ) ) ;
#24971=CARTESIAN_POINT ( 'NONE',  ( 27.71250000000000568, 2.886751345948126879, 4.999999999999999112 ) ) ;
#24972=CARTESIAN_POINT ( 'NONE',  ( 4.192336996406676342, -2.724758798235080715, 4.480034832487019614 ) ) ;
#24973=CARTESIAN_POINT ( 'NONE',  ( 10.32187500061451679, 3.027376345333613106, -5.243569643749998122 ) ) ;
#24974=CARTESIAN_POINT ( 'NONE',  ( 18.72187500061451360, -6.054752690667223547, -1.112240025338166033E-15 ) ) ;
#24975=CARTESIAN_POINT ( 'NONE',  ( 2.000000000000001332, 11.26250000122903394, 33.46410161513774995 ) ) ;
#24976=ORIENTED_EDGE ( 'NONE', *, *, #3997, .F. ) ;
#24977=CARTESIAN_POINT ( 'NONE',  ( 29.80312500061451431, 0.000000000000000000, 5.243569643749999010 ) ) ;
#24978=CARTESIAN_POINT ( 'NONE',  ( 29.48437500061451644, -4.541064518000419881, 2.621784821874995952 ) ) ;
#24979=CARTESIAN_POINT ( 'NONE',  ( 5.071875000614519458, 3.027376345333611329, 5.243569643749999010 ) ) ;
#24980=CARTESIAN_POINT ( 'NONE',  ( 15.67500000000000071, -4.330127018922194537, 2.499999999999995559 ) ) ;
#24981=CARTESIAN_POINT ( 'NONE',  ( 14.05312500061451431, 0.000000000000000000, 5.243569643749999010 ) ) ;
#24983=CARTESIAN_POINT ( 'NONE',  ( 4.964961267422091318, 0.6791209066532012395, -5.083749661835663680 ) ) ;
#24985=CARTESIAN_POINT ( 'NONE',  ( 17.96250000122903501, 0.000000000000000000, 4.999999999999998224 ) ) ;
#24986=CARTESIAN_POINT ( 'NONE',  ( 0.4082266053725523425, 9.993705886960393414, 24.01047330894736831 ) ) ;
#24988=CARTESIAN_POINT ( 'NONE',  ( 7.978125000614517681, 6.421520780324663323E-16, -5.243569643749999010 ) ) ;
#24989=CARTESIAN_POINT ( 'NONE',  ( 23.33437500061451786, 6.421520780324663323E-16, -5.243569643749999010 ) ) ;
#24990=EDGE_CURVE ( 'NONE', #66446, #1783, #5011, .T. ) ;
#24991=CARTESIAN_POINT ( 'NONE',  ( 27.11250000122903359, -4.330127018922190985, -2.500000000000001332 ) ) ;
#24992=CARTESIAN_POINT ( 'NONE',  ( 24.30937500061451573, 4.541064518000418104, -2.621784821874998173 ) ) ;
#24993=CARTESIAN_POINT ( 'NONE',  ( 6.187500000000002665, -2.886751345948129988, 4.999999999999997335 ) ) ;
#24994=CARTESIAN_POINT ( 'NONE',  ( -2.000000000000000000, 9.687500001229034652, 26.53589838486224650 ) ) ;
#24995=CARTESIAN_POINT ( 'NONE',  ( 13.52812500061451750, 4.541064518000418104, 2.621784821874999949 ) ) ;
#24996=CARTESIAN_POINT ( 'NONE',  ( 5.662500001229035185, 4.330127018922192761, -2.499999999999997780 ) ) ;
#24998=CARTESIAN_POINT ( 'NONE',  ( 10.20937500061451786, -4.541064518000417216, -2.621784821875001281 ) ) ;
#24999=CARTESIAN_POINT ( 'NONE',  ( 1.071796769724497445, 15.02990381179670010, 26.00000000000000355 ) ) ;
#25001=CARTESIAN_POINT ( 'NONE',  ( 12.47812500061451502, 6.421520780324663323E-16, -5.243569643749999010 ) ) ;
#25003=CARTESIAN_POINT ( 'NONE',  ( 24.22500000122903430, 2.886751345948126879, 4.999999999999999112 ) ) ;
#25004=CARTESIAN_POINT ( 'NONE',  ( 9.534375000614517148, 4.541064518000418104, 2.621784821874999949 ) ) ;
#25005=CARTESIAN_POINT ( 'NONE',  ( 14.91562500061451679, 3.027376345333611329, 5.243569643749999010 ) ) ;
#25007=CARTESIAN_POINT ( 'NONE',  ( 22.80937500061451573, -4.541064518000417216, -2.621784821875001281 ) ) ;
#25010=CARTESIAN_POINT ( 'NONE',  ( 20.62500000122903643, 2.886751345948161074, 4.999999999999941380 ) ) ;
#25011=CARTESIAN_POINT ( 'NONE',  ( -4.243569643749999898, 14.00937500061451857, -30.00000000000000000 ) ) ;
#25012=CARTESIAN_POINT ( 'NONE',  ( 16.43437500061451573, -4.541064518000419881, 2.621784821874995952 ) ) ;
#25013=CARTESIAN_POINT ( 'NONE',  ( 17.32500000122903216, 2.886751345948129099, -4.999999999999998224 ) ) ;
#25014=CARTESIAN_POINT ( 'NONE',  ( 11.89687500061451608, -3.027376345333614438, 5.243569643749998122 ) ) ;
#25015=CARTESIAN_POINT ( 'NONE',  ( 4.243569643749999898, 18.22812500061451502, -30.00000000000000000 ) ) ;
#25016=CARTESIAN_POINT ( 'NONE',  ( 21.15000000122903145, -2.886751345948129988, 4.999999999999997335 ) ) ;
#25017=CARTESIAN_POINT ( 'NONE',  ( 12.25312500061451537, 0.000000000000000000, 5.243569643749999010 ) ) ;
#25018=ORIENTED_EDGE ( 'NONE', *, *, #69109, .F. ) ;
#25019=ORIENTED_EDGE ( 'NONE', *, *, #15748, .F. ) ;
#25020=CARTESIAN_POINT ( 'NONE',  ( 15.78749999999999964, -2.886751345948125991, -5.000000000000000000 ) ) ;
#25021=CARTESIAN_POINT ( 'NONE',  ( 19.08750000122903145, 6.123233995736764310E-16, -4.999999999999998224 ) ) ;
#25022=CARTESIAN_POINT ( 'NONE',  ( 13.05937500061451750, 4.541064518000418104, -2.621784821874998173 ) ) ;
#25023=CARTESIAN_POINT ( 'NONE',  ( 3.182906284435134125, 3.860443623060027640, 27.56482146223813601 ) ) ;
#25024=CARTESIAN_POINT ( 'NONE',  ( 12.37500000122903465, 2.886751345948129099, -4.999999999999998224 ) ) ;
#25025=CARTESIAN_POINT ( 'NONE',  ( 20.36250000122903359, -4.330127018922190985, -2.500000000000001332 ) ) ;
#25026=CARTESIAN_POINT ( 'NONE',  ( 16.45312500061451289, -4.541064518000417216, -2.621784821875001281 ) ) ;
#25027=CARTESIAN_POINT ( 'NONE',  ( 20.84062500061451573, -3.027376345333614438, 5.243569643749998122 ) ) ;
#25028=CARTESIAN_POINT ( 'NONE',  ( 28.61250000122903359, 4.330127018922192761, -2.499999999999997780 ) ) ;
#25029=CARTESIAN_POINT ( 'NONE',  ( 28.35000000000000142, -4.330127018922190985, -2.500000000000001332 ) ) ;
#25030=DIRECTION ( 'NONE',  ( -0.000000000000000000, -1.000000000000000000, -0.000000000000000000 ) ) ;
#25032=CARTESIAN_POINT ( 'NONE',  ( 28.50937500061451502, 0.000000000000000000, 5.243569643749999010 ) ) ;
#25033=CARTESIAN_POINT ( 'NONE',  ( -3.999999999999999556, 9.725000001229034297, -32.30940107675850470 ) ) ;
#25034=CARTESIAN_POINT ( 'NONE',  ( 9.001249775931846008E-16, 16.82187500061451857, -25.09994784771203058 ) ) ;
#25035=CARTESIAN_POINT ( 'NONE',  ( 2.850000001229036073, -2.886751345948125991, -5.000000000000000000 ) ) ;
#25036=CARTESIAN_POINT ( 'NONE',  ( 6.337499999999998579, -2.886751345948125991, -5.000000000000000000 ) ) ;
#25037=CARTESIAN_POINT ( 'NONE',  ( 2.850000001229036073, -2.886751345948125991, -5.000000000000000000 ) ) ;
#25038=CARTESIAN_POINT ( 'NONE',  ( 10.65937500061451715, -4.541064518000417216, -2.621784821875001281 ) ) ;
#25039=CARTESIAN_POINT ( 'NONE',  ( 29.12812500061451715, 6.421520780324663323E-16, -5.243569643749999010 ) ) ;
#25041=CARTESIAN_POINT ( 'NONE',  ( 30.00000000000000000, 6.123233995736764310E-16, -4.999999999999998224 ) ) ;
#25042=CARTESIAN_POINT ( 'NONE',  ( 3.999999999999998668, 17.67500000122903359, -32.30940107675850470 ) ) ;
#25043=EDGE_CURVE ( 'NONE', #5464, #45340, #17169, .T. ) ;
#25044=CARTESIAN_POINT ( 'NONE',  ( 8.596875000614518925, 6.054752690667223547, 3.707466751127219781E-16 ) ) ;
#25045=CARTESIAN_POINT ( 'NONE',  ( 10.99687500061451750, -3.027376345333614438, 5.243569643749998122 ) ) ;
#25046=CARTESIAN_POINT ( 'NONE',  ( 5.175000000000002487, 4.330127018922191873, 2.499999999999999556 ) ) ;
#25047=CARTESIAN_POINT ( 'NONE',  ( -2.121784821874999949, 15.22812500061459495, 26.32496088578401938 ) ) ;
#25049=CARTESIAN_POINT ( 'NONE',  ( 7.575000000000001954, -4.330127018922194537, 2.499999999999995559 ) ) ;
#25051=CARTESIAN_POINT ( 'NONE',  ( 20.57812500061451644, 6.421520780324663323E-16, -5.243569643749999010 ) ) ;
#25052=CARTESIAN_POINT ( 'NONE',  ( 12.70312500061451821, 0.000000000000000000, 5.243569643749999010 ) ) ;
#25054=CARTESIAN_POINT ( 'NONE',  ( 9.384375000614518569, 6.421520780324663323E-16, -5.243569643749999010 ) ) ;
#25055=CARTESIAN_POINT ( 'NONE',  ( 25.31250000000000000, 2.886751345948129099, -4.999999999999998224 ) ) ;
#25056=CARTESIAN_POINT ( 'NONE',  ( 21.82500000122903572, 2.886751345948129099, -4.999999999999998224 ) ) ;
#25057=LINE ( 'NONE', #70866, #34317 ) ;
#25058=CARTESIAN_POINT ( 'NONE',  ( 8.709375000614517859, 0.000000000000000000, 5.243569643749999010 ) ) ;
#25059=CARTESIAN_POINT ( 'NONE',  ( 27.12187500061451573, 3.027376345333611329, 5.243569643749999010 ) ) ;
#25062=CARTESIAN_POINT ( 'NONE',  ( 19.13437500061451857, -4.541064518000419881, 2.621784821874995952 ) ) ;
#25063=CARTESIAN_POINT ( 'NONE',  ( 12.57187500061451857, 3.027376345333613106, -5.243569643749998122 ) ) ;
#25065=CARTESIAN_POINT ( 'NONE',  ( 23.73749999999999716, -2.886751345948129988, 4.999999999999997335 ) ) ;
#25067=CARTESIAN_POINT ( 'NONE',  ( -4.243569643749999898, 13.07187500061452035, -32.45002607614398471 ) ) ;
#25069=CARTESIAN_POINT ( 'NONE',  ( 15.77812500061451573, 4.541064518000418104, 2.621784821874999949 ) ) ;
#25070=CARTESIAN_POINT ( 'NONE',  ( 5.062500000000000888, 2.886751345948129099, -4.999999999999998224 ) ) ;
#25072=CARTESIAN_POINT ( 'NONE',  ( 13.53749999999999964, -2.886751345948125991, -5.000000000000000000 ) ) ;
#25073=CARTESIAN_POINT ( 'NONE',  ( -4.243569643749999898, 10.76562500061451644, 27.54997392385601529 ) ) ;
#25074=CARTESIAN_POINT ( 'NONE',  ( 13.46250000122903323, 0.000000000000000000, 4.999999999999998224 ) ) ;
#25075=CARTESIAN_POINT ( 'NONE',  ( 24.12187500061451217, -6.054752690667223547, -1.112240025338166033E-15 ) ) ;
#25076=CARTESIAN_POINT ( 'NONE',  ( 17.82187500061451502, -6.054752690667223547, -1.112240025338166033E-15 ) ) ;
#25078=ORIENTED_EDGE ( 'NONE', *, *, #38684, .T. ) ;
#25079=CARTESIAN_POINT ( 'NONE',  ( 19.71562500061451928, 3.027376345333613106, -5.243569643749998122 ) ) ;
#25080=CARTESIAN_POINT ( 'NONE',  ( 4.528125000614516615, 4.541064518000418104, 2.621784821874999949 ) ) ;
#25081=CARTESIAN_POINT ( 'NONE',  ( 17.44687500061451857, -3.027376345333610441, -5.243569643749999898 ) ) ;
#25082=CARTESIAN_POINT ( 'NONE',  ( 28.73437500061451644, 6.421520780324663323E-16, -5.243569643749999010 ) ) ;
#25083=CARTESIAN_POINT ( 'NONE',  ( 4.640625000614518214, -3.027376345333614438, 5.243569643749998122 ) ) ;
#25084=CARTESIAN_POINT ( 'NONE',  ( 22.07812500061451644, 4.541064518000418104, 2.621784821874999949 ) ) ;
#25085=CARTESIAN_POINT ( 'NONE',  ( 4.243569643749999898, 14.62812500061451715, 30.00000000000000000 ) ) ;
#25086=CARTESIAN_POINT ( 'NONE',  ( 15.67500000122903181, 2.886751345948126879, 4.999999999999999112 ) ) ;
#25088=CARTESIAN_POINT ( 'NONE',  ( 7.190625000614518036, 6.054752690667223547, 3.707466751127219781E-16 ) ) ;
#25089=CARTESIAN_POINT ( 'NONE',  ( 13.57500000000000107, 6.123233995736764310E-16, -4.999999999999998224 ) ) ;
#25090=CARTESIAN_POINT ( 'NONE',  ( 28.97812500061451502, -4.541064518000419881, 2.621784821874995952 ) ) ;
#25091=CARTESIAN_POINT ( 'NONE',  ( 23.97187500061451360, 3.027376345333611329, 5.243569643749999010 ) ) ;
#25092=CARTESIAN_POINT ( 'NONE',  ( 15.51562500061451644, -6.054752690667223547, -1.112240025338166033E-15 ) ) ;
#25093=CARTESIAN_POINT ( 'NONE',  ( 24.63750000122903216, 4.330127018922191873, 2.499999999999999556 ) ) ;
#25094=CARTESIAN_POINT ( 'NONE',  ( 24.44062500061451715, -3.027376345333614438, 5.243569643749998122 ) ) ;
#25095=CARTESIAN_POINT ( 'NONE',  ( 19.35937500061451644, 4.541064518000418104, -2.621784821874998173 ) ) ;
#25096=CARTESIAN_POINT ( 'NONE',  ( 14.09062500061451750, -3.027376345333614438, 5.243569643749998122 ) ) ;
#25097=CARTESIAN_POINT ( 'NONE',  ( -4.243569643749997233, 18.09687500061452070, 32.45002607614398471 ) ) ;
#25098=CARTESIAN_POINT ( 'NONE',  ( 20.84062500061451573, -3.027376345333614438, 5.243569643749998122 ) ) ;
#25099=CARTESIAN_POINT ( 'NONE',  ( 29.42812500061451431, -4.541064518000419881, 2.621784821874995952 ) ) ;
#25101=CARTESIAN_POINT ( 'NONE',  ( 25.94999999999999929, 0.000000000000000000, 4.999999999999998224 ) ) ;
#25102=CARTESIAN_POINT ( 'NONE',  ( -4.243569643749999898, 19.40937500061451715, -30.00000000000000000 ) ) ;
#25104=CARTESIAN_POINT ( 'NONE',  ( 27.32812500061451644, 6.421520780324663323E-16, -5.243569643749999010 ) ) ;
#25105=CARTESIAN_POINT ( 'NONE',  ( 8.840625000614515727, -3.027376345333610441, -5.243569643749999898 ) ) ;
#25106=CARTESIAN_POINT ( 'NONE',  ( 20.17500000122903359, 2.886751345948126879, 4.999999999999999112 ) ) ;
#25107=CARTESIAN_POINT ( 'NONE',  ( 25.49062500061451786, -3.027376345333610441, -5.243569643749999898 ) ) ;
#25108=CARTESIAN_POINT ( 'NONE',  ( 25.94999999999999929, 0.000000000000000000, 4.999999999999998224 ) ) ;
#25109=CARTESIAN_POINT ( 'NONE',  ( 3.999999999999999112, 16.28750000122903430, -30.00000000000000000 ) ) ;
#25110=CARTESIAN_POINT ( 'NONE',  ( 27.32812500061451644, 6.421520780324663323E-16, -5.243569643749999010 ) ) ;
#25111=CARTESIAN_POINT ( 'NONE',  ( 7.865625000614516971, -6.054752690667223547, -1.112240025338166033E-15 ) ) ;
#25112=ORIENTED_EDGE ( 'NONE', *, *, #29363, .T. ) ;
#25113=EDGE_CURVE ( 'NONE', #403, #10458, #32406, .T. ) ;
#25114=CARTESIAN_POINT ( 'NONE',  ( 26.31562500061451715, -6.054752690667223547, -1.112240025338166033E-15 ) ) ;
#25115=CARTESIAN_POINT ( 'NONE',  ( 5.353125000614515905, 4.541064518000418104, -2.621784821874998173 ) ) ;
#25117=DIRECTION ( 'NONE',  ( 0.000000000000000000, 0.000000000000000000, 1.000000000000000000 ) ) ;
#25118=CARTESIAN_POINT ( 'NONE',  ( 13.76250000000000107, 2.886751345948126879, 4.999999999999999112 ) ) ;
#25120=CARTESIAN_POINT ( 'NONE',  ( 14.25937500061451679, -4.541064518000417216, -2.621784821875001281 ) ) ;
#25121=CARTESIAN_POINT ( 'NONE',  ( 9.262500001229033941, 4.330127018922192761, -2.499999999999997780 ) ) ;
#25122=CARTESIAN_POINT ( 'NONE',  ( 17.07187500061451502, 3.027376345333613106, -5.243569643749998122 ) ) ;
#25124=CARTESIAN_POINT ( 'NONE',  ( 7.584375000614516082, 6.421520780324663323E-16, -5.243569643749999010 ) ) ;
#25125=CARTESIAN_POINT ( 'NONE',  ( -2.121784821874999949, 11.62812500061451715, -33.67503911421598417 ) ) ;
#25126=CARTESIAN_POINT ( 'NONE',  ( 20.10000000000000142, 0.000000000000000000, 4.999999999999998224 ) ) ;
#25130=CARTESIAN_POINT ( 'NONE',  ( 23.91562500061451502, 3.027376345333611329, 5.243569643749999010 ) ) ;
#25131=CARTESIAN_POINT ( 'NONE',  ( 2.121784821874999061, 10.25937500061451857, 26.32496088578401583 ) ) ;
#25133=CARTESIAN_POINT ( 'NONE',  ( 26.78437500061451360, -4.541064518000419881, 2.621784821874995952 ) ) ;
#25134=CARTESIAN_POINT ( 'NONE',  ( 29.55937500061451573, -4.541064518000417216, -2.621784821875001281 ) ) ;
#25135=CARTESIAN_POINT ( 'NONE',  ( 5.015625000614518214, 3.027376345333611329, 5.243569643749999010 ) ) ;
#25137=CARTESIAN_POINT ( 'NONE',  ( 17.82187500061451502, -6.054752690667223547, -1.112240025338166033E-15 ) ) ;
#25139=CARTESIAN_POINT ( 'NONE',  ( 3.365625000614516082, -6.054752690667223547, -1.112240025338166033E-15 ) ) ;
#25140=CARTESIAN_POINT ( 'NONE',  ( 7.171875000614517326, 3.027376345333613106, -5.243569643749998122 ) ) ;
#25141=CARTESIAN_POINT ( 'NONE',  ( 19.99687500061451573, -3.027376345333614438, 5.243569643749998122 ) ) ;
#25143=CARTESIAN_POINT ( 'NONE',  ( 26.28749999999999432, 5.773502691896255534, 3.535250795749688894E-16 ) ) ;
#25144=CARTESIAN_POINT ( 'NONE',  ( 26.78437500061451360, -4.541064518000419881, 2.621784821874995952 ) ) ;
#25145=EDGE_CURVE ( 'NONE', #755, #35328, #62664, .T. ) ;
#25147=CARTESIAN_POINT ( 'NONE',  ( 29.88749999999999929, 5.773502691896255534, 3.535250795749688894E-16 ) ) ;
#25149=CARTESIAN_POINT ( 'NONE',  ( 8.400000000000000355, 0.000000000000000000, 4.999999999999998224 ) ) ;
#25151=CARTESIAN_POINT ( 'NONE',  ( 23.12812500061451360, -4.541064518000419881, 2.621784821874995952 ) ) ;
#25152=CARTESIAN_POINT ( 'NONE',  ( 11.32500000000000107, 6.123233995736764310E-16, -4.999999999999998224 ) ) ;
#25153=CARTESIAN_POINT ( 'NONE',  ( 8.287500001229034297, 6.123233995736764310E-16, -4.999999999999998224 ) ) ;
#25154=CARTESIAN_POINT ( 'NONE',  ( 6.590625000614518392, -3.027376345333610441, -5.243569643749999898 ) ) ;
#25155=CARTESIAN_POINT ( 'NONE',  ( 22.87500000000000000, -4.330127018922194537, 2.499999999999995559 ) ) ;
#25156=CARTESIAN_POINT ( 'NONE',  ( 18.55312500061451431, 0.000000000000000000, 5.243569643749999010 ) ) ;
#25157=CARTESIAN_POINT ( 'NONE',  ( 25.57500000122903216, 2.886751345948126879, 4.999999999999999112 ) ) ;
#25159=CARTESIAN_POINT ( 'NONE',  ( 4.912499999999999645, -5.773502691896255534, -1.060575238724906372E-15 ) ) ;
#25160=ORIENTED_EDGE ( 'NONE', *, *, #23644, .T. ) ;
#25161=CARTESIAN_POINT ( 'NONE',  ( 18.89062500061451644, 6.054752690667223547, 3.707466751127219781E-16 ) ) ;
#25162=CARTESIAN_POINT ( 'NONE',  ( 27.10312500061451502, 0.000000000000000000, 5.243569643749999010 ) ) ;
#25163=CARTESIAN_POINT ( 'NONE',  ( 27.53437500061451360, 4.541064518000418104, 2.621784821874999949 ) ) ;
#25164=CARTESIAN_POINT ( 'NONE',  ( 8.437500000000000000, -2.886751345948129988, 4.999999999999997335 ) ) ;
#25165=CARTESIAN_POINT ( 'NONE',  ( 14.69062500061451537, -3.027376345333610441, -5.243569643749999898 ) ) ;
#25166=CARTESIAN_POINT ( 'NONE',  ( 29.61562500061451431, 3.027376345333613106, -5.243569643749998122 ) ) ;
#25167=CARTESIAN_POINT ( 'NONE',  ( 8.540625000614518569, 6.054752690667223547, 3.707466751127219781E-16 ) ) ;
#25168=DIRECTION ( 'NONE',  ( 0.000000000000000000, 0.000000000000000000, -1.000000000000000000 ) ) ;
#25169=CARTESIAN_POINT ( 'NONE',  ( 4.243569643749999898, 13.33437500061451786, 30.00000000000000000 ) ) ;
#25170=CARTESIAN_POINT ( 'NONE',  ( 25.27500000122903145, -5.773502691896255534, -1.060575238724906372E-15 ) ) ;
#25172=CARTESIAN_POINT ( 'NONE',  ( 14.12812500061451715, -4.541064518000419881, 2.621784821874995952 ) ) ;
#25174=CARTESIAN_POINT ( 'NONE',  ( 9.271875000614516082, -6.054752690667223547, -1.112240025338166033E-15 ) ) ;
#25175=CARTESIAN_POINT ( 'NONE',  ( 9.384375000614518569, 6.421520780324663323E-16, -5.243569643749999010 ) ) ;
#25176=CARTESIAN_POINT ( 'NONE',  ( 18.42187500061451644, 3.027376345333613106, -5.243569643749998122 ) ) ;
#25177=EDGE_LOOP ( 'NONE', ( #25861, #1118, #34844, #60542 ) ) ;
#25178=CARTESIAN_POINT ( 'NONE',  ( 20.87812500061451715, -4.541064518000419881, 2.621784821874995952 ) ) ;
#25179=CARTESIAN_POINT ( 'NONE',  ( 16.35937500061451644, 0.000000000000000000, 5.243569643749999010 ) ) ;
#25180=CARTESIAN_POINT ( 'NONE',  ( 22.79062500061451502, -3.027376345333610441, -5.243569643749999898 ) ) ;
#25181=CARTESIAN_POINT ( 'NONE',  ( 2.000000000000001332, 13.85000000000000142, 33.46410161513774995 ) ) ;
#25182=CARTESIAN_POINT ( 'NONE',  ( 27.29062500061451502, -3.027376345333610441, -5.243569643749999898 ) ) ;
#25183=CARTESIAN_POINT ( 'NONE',  ( 7.800000001229035362, -2.886751345948125991, -5.000000000000000000 ) ) ;
#25184=ORIENTED_EDGE ( 'NONE', *, *, #5473, .T. ) ;
#25185=CARTESIAN_POINT ( 'NONE',  ( 3.675000001229035362, -5.773502691896255534, -1.060575238724906372E-15 ) ) ;
#25186=CARTESIAN_POINT ( 'NONE',  ( 3.999999999999998668, 18.01249999999999929, -32.30940107675850470 ) ) ;
#25187=CARTESIAN_POINT ( 'NONE',  ( 23.70000000122903216, 5.773502691896255534, 3.535250795749688894E-16 ) ) ;
#25189=CARTESIAN_POINT ( 'NONE',  ( 8.109375000614518214, 4.541064518000418104, -2.621784821874998173 ) ) ;
#25190=CARTESIAN_POINT ( 'NONE',  ( 4.307019252286369060, 2.539784937741765614, -4.371005586624799655 ) ) ;
#25191=CARTESIAN_POINT ( 'NONE',  ( 15.55312500061451608, -4.541064518000417216, -2.621784821875001281 ) ) ;
#25192=CARTESIAN_POINT ( 'NONE',  ( 8.821875000614518569, -6.054752690667223547, -1.112240025338166033E-15 ) ) ;
#25193=CARTESIAN_POINT ( 'NONE',  ( 26.92500000122903359, 2.886751345948126879, 4.999999999999999112 ) ) ;
#25194=CARTESIAN_POINT ( 'NONE',  ( 18.45937500061451431, 4.541064518000418104, -2.621784821874998173 ) ) ;
#25195=CARTESIAN_POINT ( 'NONE',  ( 4.396875000614516971, -3.027376345333610441, -5.243569643749999898 ) ) ;
#25197=CARTESIAN_POINT ( 'NONE',  ( 5.915625000614515905, 3.027376345333611329, 5.243569643749999010 ) ) ;
#25198=CARTESIAN_POINT ( 'NONE',  ( 18.74062500061451431, -3.027376345333610441, -5.243569643749999898 ) ) ;
#25199=ORIENTED_EDGE ( 'NONE', *, *, #11122, .F. ) ;
#25200=CARTESIAN_POINT ( 'NONE',  ( 11.46562500061451573, -6.054752690667223547, -1.112240025338166033E-15 ) ) ;
#25201=CARTESIAN_POINT ( 'NONE',  ( 6.225000001229036073, 2.886751345948126879, 4.999999999999999112 ) ) ;
#25202=CARTESIAN_POINT ( 'NONE',  ( 10.45312500061451644, 0.000000000000000000, 5.243569643749999010 ) ) ;
#25204=CARTESIAN_POINT ( 'NONE',  ( 11.02500000000000036, 4.330127018922191873, 2.499999999999999556 ) ) ;
#25205=CARTESIAN_POINT ( 'NONE',  ( 5.812500001229035540, 0.000000000000000000, 4.999999999999998224 ) ) ;
#25206=CARTESIAN_POINT ( 'NONE',  ( 19.76250000000000639, -5.773502691896255534, -1.060575238724906372E-15 ) ) ;
#25207=EDGE_CURVE ( 'NONE', #10170, #67346, #35687, .T. ) ;
#25208=CARTESIAN_POINT ( 'NONE',  ( 15.60937500061451644, -4.541064518000417216, -2.621784821875001281 ) ) ;
#25209=CARTESIAN_POINT ( 'NONE',  ( 14.88750000122903394, -4.330127018922194537, 2.499999999999995559 ) ) ;
#25211=CARTESIAN_POINT ( 'NONE',  ( 2.226602359779148887, 9.807522476441999260, -34.70164361699148259 ) ) ;
#25213=CARTESIAN_POINT ( 'NONE',  ( 3.999999999999998668, 14.97500000122903252, -32.30940107675850470 ) ) ;
#25215=DIRECTION ( 'NONE',  ( 0.000000000000000000, 0.000000000000000000, -1.000000000000000000 ) ) ;
#25216=CARTESIAN_POINT ( 'NONE',  ( 3.891749269447642767, -3.139164435342899129, -4.200087063816749122 ) ) ;
#25217=CARTESIAN_POINT ( 'NONE',  ( 16.32187500061451502, 3.027376345333611329, 5.243569643749999010 ) ) ;
#25218=APPLICATION_CONTEXT ( 'automotive_design' ) ;
#25219=CARTESIAN_POINT ( 'NONE',  ( 28.38749999999999929, -2.886751345948125991, -5.000000000000000000 ) ) ;
#25220=CARTESIAN_POINT ( 'NONE',  ( 12.06562500061451537, 3.027376345333613106, -5.243569643749998122 ) ) ;
#25222=CARTESIAN_POINT ( 'NONE',  ( 23.03437500061451715, 4.541064518000418104, 2.621784821874999949 ) ) ;
#25224=CARTESIAN_POINT ( 'NONE',  ( 10.45312500061451644, 0.000000000000000000, 5.243569643749999010 ) ) ;
#25225=CARTESIAN_POINT ( 'NONE',  ( 15.34687500061451537, 6.054752690667223547, 3.707466751127219781E-16 ) ) ;
#25226=ORIENTED_EDGE ( 'NONE', *, *, #30129, .F. ) ;
#25227=CARTESIAN_POINT ( 'NONE',  ( 25.17187500061451644, 3.027376345333613106, -5.243569643749998122 ) ) ;
#25228=CARTESIAN_POINT ( 'NONE',  ( 27.25312500061451360, -4.541064518000417216, -2.621784821875001281 ) ) ;
#25229=CARTESIAN_POINT ( 'NONE',  ( 18.59062500061451573, -3.027376345333614438, 5.243569643749998122 ) ) ;
#25230=CARTESIAN_POINT ( 'NONE',  ( 28.86562500061451786, 3.027376345333611329, 5.243569643749999010 ) ) ;
#25232=CARTESIAN_POINT ( 'NONE',  ( 6.787500000000001421, -2.886751345948125991, -5.000000000000000000 ) ) ;
#25233=CARTESIAN_POINT ( 'NONE',  ( 18.90000000122902790, -2.886751345948129988, 4.999999999999997335 ) ) ;
#25234=CARTESIAN_POINT ( 'NONE',  ( -3.999999999999997335, 18.80000000122903003, -27.69059892324149530 ) ) ;
#25236=EDGE_LOOP ( 'NONE', ( #59080, #2948, #31606, #30664, #37305, #20434, #38714, #5198, #43902, #58025, #32633, #35601, #63440, #50070, #41430, #72977, #61728, #71874, #45980, #24376, #769, #5004, #7035, #4585, #31028, #63688, #9404, #37069, #1281, #58032, #34424, #60706, #21035, #15793, #11829, #33123, #20132, #44546, #23801, #67273, #56190, #25284, #55707, #34779, #7293, #1882, #21814, #66239 ) ) ;
#25237=CARTESIAN_POINT ( 'NONE',  ( 14.84999999999999964, -4.330127018922190985, -2.500000000000001332 ) ) ;
#25238=CARTESIAN_POINT ( 'NONE',  ( 19.68750000000000355, -2.886751345948129988, 4.999999999999997335 ) ) ;
#25239=CARTESIAN_POINT ( 'NONE',  ( 15.68437500061451573, 6.421520780324663323E-16, -5.243569643749999010 ) ) ;
#25240=CARTESIAN_POINT ( 'NONE',  ( 13.34062500061451750, -3.027376345333610441, -5.243569643749999898 ) ) ;
#25241=VERTEX_POINT ( 'NONE', #45263 ) ;
#25242=CARTESIAN_POINT ( 'NONE',  ( 4.243569643749999898, 16.03437500061451715, -30.00000000000000000 ) ) ;
#25243=CARTESIAN_POINT ( 'NONE',  ( 5.953125000614519102, 0.000000000000000000, 5.243569643749999010 ) ) ;
#25245=CARTESIAN_POINT ( 'NONE',  ( 11.70000000000000284, -4.330127018922190985, -2.500000000000001332 ) ) ;
#25248=ORIENTED_EDGE ( 'NONE', *, *, #643, .T. ) ;
#25249=CARTESIAN_POINT ( 'NONE',  ( 2.121784821875001281, 15.90312500061451573, 33.67503911421598417 ) ) ;
#25250=CARTESIAN_POINT ( 'NONE',  ( 26.72812500061451502, -4.541064518000419881, 2.621784821874995952 ) ) ;
#25253=CARTESIAN_POINT ( 'NONE',  ( 23.18437500061451573, -4.541064518000419881, 2.621784821874995952 ) ) ;
#25254=CARTESIAN_POINT ( 'NONE',  ( 20.54062500061451502, -3.027376345333610441, -5.243569643749999898 ) ) ;
#25256=CARTESIAN_POINT ( 'NONE',  ( -4.243569643749999898, 15.71562500061459211, -32.45002607614398471 ) ) ;
#25257=CARTESIAN_POINT ( 'NONE',  ( 23.85000000122903430, -2.886751345948129988, 4.999999999999997335 ) ) ;
#25259=CARTESIAN_POINT ( 'NONE',  ( 6.365625000614518747, 3.027376345333611329, 5.243569643749999010 ) ) ;
#25261=CARTESIAN_POINT ( 'NONE',  ( 23.50312500061451360, 0.000000000000000000, 5.243569643749999010 ) ) ;
#25264=CARTESIAN_POINT ( 'NONE',  ( 17.18437500061451573, 4.541064518000418104, 2.621784821874999949 ) ) ;
#25265=CARTESIAN_POINT ( 'NONE',  ( 25.32187500061451857, 3.027376345333611329, 5.243569643749999010 ) ) ;
#25266=CARTESIAN_POINT ( 'NONE',  ( -4.243569643749999898, 15.35937500061451644, 30.00000000000000000 ) ) ;
#25267=CARTESIAN_POINT ( 'NONE',  ( 5.840625000614516615, 6.054752690667223547, 3.707466751127219781E-16 ) ) ;
#25268=CARTESIAN_POINT ( 'NONE',  ( 29.65312500061451573, 4.541064518000418104, -2.621784821874998173 ) ) ;
#25269=CARTESIAN_POINT ( 'NONE',  ( 29.72812500061451502, 4.541064518000418104, 2.621784821874999949 ) ) ;
#25270=CARTESIAN_POINT ( 'NONE',  ( 0.000000000000000000, 10.00000000000000000, -36.00000000000000000 ) ) ;
#25271=CARTESIAN_POINT ( 'NONE',  ( 3.382222646665033139, 4.052127219167644512, 2.981509777668850614 ) ) ;
#25272=CARTESIAN_POINT ( 'NONE',  ( 2.840625000614518392, -3.027376345333614438, 5.243569643749998122 ) ) ;
#25273=CARTESIAN_POINT ( 'NONE',  ( 6.759375000614516793, 4.541064518000418104, -2.621784821874998173 ) ) ;
#25275=CARTESIAN_POINT ( 'NONE',  ( 17.88750000122903216, 4.330127018922191873, 2.499999999999999556 ) ) ;
#25276=CARTESIAN_POINT ( 'NONE',  ( 4.134375000614517681, 4.541064518000418104, 2.621784821874999949 ) ) ;
#25277=B_SPLINE_CURVE_WITH_KNOTS ( 'NONE', 3,
 ( #19478, #65654, #35754, #69744 ),
 .UNSPECIFIED., .F., .F.,
 ( 4, 4 ),
 ( 8.673617379884034509E-19, 0.001150238639792624086 ),
 .UNSPECIFIED. ) ;
#25278=CARTESIAN_POINT ( 'NONE',  ( 11.55000000122903181, 5.773502691896255534, 3.535250795749688894E-16 ) ) ;
#25279=CARTESIAN_POINT ( 'NONE',  ( 4.303125000614516971, -4.541064518000417216, -2.621784821875001281 ) ) ;
#25282=CARTESIAN_POINT ( 'NONE',  ( 14.93437500061451750, 4.541064518000418104, 2.621784821874999949 ) ) ;
#25284=ORIENTED_EDGE ( 'NONE', *, *, #826, .F. ) ;
#25285=CARTESIAN_POINT ( 'NONE',  ( 22.30312500061451431, -4.541064518000417216, -2.621784821875001281 ) ) ;
#25286=CARTESIAN_POINT ( 'NONE',  ( 8.203125000614518214, 0.000000000000000000, 5.243569643749999010 ) ) ;
#25287=CARTESIAN_POINT ( 'NONE',  ( 25.13437500061451502, 6.421520780324663323E-16, -5.243569643749999010 ) ) ;
#25288=CARTESIAN_POINT ( 'NONE',  ( 7.453125000614516438, -4.541064518000417216, -2.621784821875001281 ) ) ;
#25289=CYLINDRICAL_SURFACE ( 'NONE', #40350, 4.000000000000000000 ) ;
#25290=( BOUNDED_CURVE ( )  B_SPLINE_CURVE ( 2, ( #35757, #58278, #69747, #19115, #12507, #36126, #8053, #30587, #2510 ),
 .UNSPECIFIED., .F., .F. ) 
 B_SPLINE_CURVE_WITH_KNOTS ( ( 3, 2, 2, 2, 3 ),
 ( 0.5326086956521739468, 0.5362318840579710644, 0.5434782608695651884, 0.5507246376811594235, 0.5543478260869565410 ),
 .UNSPECIFIED. ) 
 CURVE ( )  GEOMETRIC_REPRESENTATION_ITEM ( )  RATIONAL_B_SPLINE_CURVE ( ( 0.9330127018922194093, 0.9330127018922194093, 1.000000000000000000, 0.8660254037844387076, 1.000000000000000000, 0.8660254037844387076, 1.000000000000000000, 0.9330127018922194093, 0.9330127018922194093 ) ) 
 REPRESENTATION_ITEM ( '' )  );
#25291=CARTESIAN_POINT ( 'NONE',  ( 11.17500000122903536, 2.886751345948126879, 4.999999999999999112 ) ) ;
#25292=CARTESIAN_POINT ( 'NONE',  ( 24.51562500061451289, -6.054752690667223547, -1.112240025338166033E-15 ) ) ;
#25293=CARTESIAN_POINT ( 'NONE',  ( 4.000000000000000000, 19.40000000122903856, -27.69059892324149530 ) ) ;
#25294=CARTESIAN_POINT ( 'NONE',  ( 9.825000001229033941, 2.886751345948126879, 4.999999999999999112 ) ) ;
#25295=CARTESIAN_POINT ( 'NONE',  ( 20.65312500061451573, 4.541064518000418104, -2.621784821874998173 ) ) ;
#25296=CARTESIAN_POINT ( 'NONE',  ( 16.86562500061451786, -6.054752690667223547, -1.112240025338166033E-15 ) ) ;
#25298=CARTESIAN_POINT ( 'NONE',  ( 18.45000000000000284, -4.330127018922190985, -2.500000000000001332 ) ) ;
#25299=CARTESIAN_POINT ( 'NONE',  ( 14.36250000122903359, 0.000000000000000000, 4.999999999999998224 ) ) ;
#25300=CARTESIAN_POINT ( 'NONE',  ( 11.50312500061451892, -4.541064518000417216, -2.621784821875001281 ) ) ;
#25302=CARTESIAN_POINT ( 'NONE',  ( 13.19062500061451537, -3.027376345333614438, 5.243569643749998122 ) ) ;
#25303=CARTESIAN_POINT ( 'NONE',  ( 24.41250000122903430, -4.330127018922190985, -2.500000000000001332 ) ) ;
#25305=CARTESIAN_POINT ( 'NONE',  ( 21.57187500061451502, 3.027376345333613106, -5.243569643749998122 ) ) ;
#25306=CARTESIAN_POINT ( 'NONE',  ( 20.52187500061451786, -6.054752690667223547, -1.112240025338166033E-15 ) ) ;
#25308=CARTESIAN_POINT ( 'NONE',  ( 8.587500001229035007, -4.330127018922194537, 2.499999999999995559 ) ) ;
#25309=CARTESIAN_POINT ( 'NONE',  ( 6.534375000614517148, -4.541064518000419881, 2.621784821874995952 ) ) ;
#25310=CARTESIAN_POINT ( 'NONE',  ( 23.33437500061451786, 6.421520780324663323E-16, -5.243569643749999010 ) ) ;
#25311=CARTESIAN_POINT ( 'NONE',  ( 10.46250000000000036, 2.886751345948129099, -4.999999999999997335 ) ) ;
#25312=AXIS2_PLACEMENT_3D ( 'NONE', #35322, #1721, #46783 ) ;
#25313=CARTESIAN_POINT ( 'NONE',  ( 21.29062500061451502, -3.027376345333614438, 5.243569643749998122 ) ) ;
#25314=CARTESIAN_POINT ( 'NONE',  ( 24.15937500061451715, -4.541064518000417216, -2.621784821875001281 ) ) ;
#25318=CARTESIAN_POINT ( 'NONE',  ( 5.221875000614519813, -6.054752690667223547, -1.112240025338166033E-15 ) ) ;
#25319=CARTESIAN_POINT ( 'NONE',  ( 18.17812500061451786, -4.541064518000419881, 2.621784821874995952 ) ) ;
#25322=CARTESIAN_POINT ( 'NONE',  ( 11.43750000000000000, 5.773502691896255534, 3.535250795749688401E-16 ) ) ;
#25323=CARTESIAN_POINT ( 'NONE',  ( 24.81562500061451715, 3.027376345333611329, 5.243569643749999010 ) ) ;
#25324=CARTESIAN_POINT ( 'NONE',  ( 0.000000000000000000, 20.00000000000000000, 30.00000000000000000 ) ) ;
#25325=CARTESIAN_POINT ( 'NONE',  ( 1.626862140677534273E-15, 17.86250000000000071, -26.00000000000000355 ) ) ;
#25326=CARTESIAN_POINT ( 'NONE',  ( 3.999818103236636890, 3.000242528463001435, -30.14366030220596571 ) ) ;
#25327=CARTESIAN_POINT ( 'NONE',  ( 14.51250000000000107, 2.886751345948129099, -4.999999999999998224 ) ) ;
#25328=CARTESIAN_POINT ( 'NONE',  ( 25.53750000122903074, 4.330127018922191873, 2.499999999999999556 ) ) ;
#25329=CARTESIAN_POINT ( 'NONE',  ( 21.51562500061451644, 3.027376345333613106, -5.243569643749998122 ) ) ;
#25330=EDGE_LOOP ( 'NONE', ( #72511, #29285, #30049, #68871 ) ) ;
#25331=CARTESIAN_POINT ( 'NONE',  ( 25.42500000000000071, 4.330127018922191873, 2.499999999999999556 ) ) ;
#25333=CARTESIAN_POINT ( 'NONE',  ( 23.78437500061451360, 6.421520780324663323E-16, -5.243569643749999010 ) ) ;
#25334=EDGE_LOOP ( 'NONE', ( #43739, #72236, #21987, #71059 ) ) ;
#25335=CARTESIAN_POINT ( 'NONE',  ( 4.898587196589411843E-16, 20.00000000000000000, 33.99999999999999289 ) ) ;
#25336=CARTESIAN_POINT ( 'NONE',  ( 12.62812500061451537, 4.541064518000418104, 2.621784821874999949 ) ) ;
#25337=CARTESIAN_POINT ( 'NONE',  ( 3.928125000614516527, 6.421520780324663323E-16, -5.243569643749999010 ) ) ;
#25339=CARTESIAN_POINT ( 'NONE',  ( 28.26562500061451289, 3.027376345333613106, -5.243569643749998122 ) ) ;
#25340=CARTESIAN_POINT ( 'NONE',  ( 14.06250000122903288, -4.330127018922190985, -2.500000000000001332 ) ) ;
#25341=CARTESIAN_POINT ( 'NONE',  ( 18.59999999999999787, 4.330127018922192761, -2.499999999999997780 ) ) ;
#25342=CARTESIAN_POINT ( 'NONE',  ( 27.86249999999999716, -5.773502691896255534, -1.060575238724906372E-15 ) ) ;
#25343=CARTESIAN_POINT ( 'NONE',  ( 3.009375000614516793, -4.541064518000417216, -2.621784821875001281 ) ) ;
#25344=CARTESIAN_POINT ( 'NONE',  ( 6.684375000614518392, 6.421520780324663323E-16, -5.243569643749999010 ) ) ;
#25345=CARTESIAN_POINT ( 'NONE',  ( 20.44687500061451857, -3.027376345333614438, 5.243569643749998122 ) ) ;
#25346=CARTESIAN_POINT ( 'NONE',  ( 26.13749999999999929, -2.886751345948109559, -5.000000000000028422 ) ) ;
#25348=CARTESIAN_POINT ( 'NONE',  ( 27.66562500061451146, -6.054752690667223547, -1.112240025338166033E-15 ) ) ;
#25349=CARTESIAN_POINT ( 'NONE',  ( 29.55937500061451573, -4.541064518000417216, -2.621784821875001281 ) ) ;
#25350=CARTESIAN_POINT ( 'NONE',  ( 3.609375000614516882, 4.541064518000418104, -2.621784821874998173 ) ) ;
#25351=CARTESIAN_POINT ( 'NONE',  ( 15.48749999999999893, 5.773502691896255534, 3.535250795749688894E-16 ) ) ;
#25352=CARTESIAN_POINT ( 'NONE',  ( 14.80312500061451608, 4.541064518000418104, -2.621784821874998173 ) ) ;
#25354=CARTESIAN_POINT ( 'NONE',  ( 5.000000000000000000, 6.176262757673013563E-16, -5.043301270189223473 ) ) ;
#25355=CARTESIAN_POINT ( 'NONE',  ( 27.07499999999999929, 6.123233995736764310E-16, -4.999999999999998224 ) ) ;
#25356=CARTESIAN_POINT ( 'NONE',  ( 17.43750000122903288, 4.330127018922191873, 2.499999999999999556 ) ) ;
#25359=CARTESIAN_POINT ( 'NONE',  ( 6.815625000614517148, 3.027376345333611329, 5.243569643749999010 ) ) ;
#25360=CARTESIAN_POINT ( 'NONE',  ( 23.52187500061451786, 3.027376345333611329, 5.243569643749999010 ) ) ;
#25361=CARTESIAN_POINT ( 'NONE',  ( 9.001249775931846008E-16, 16.37187500061451573, 34.90005215228797653 ) ) ;
#25362=EDGE_CURVE ( 'NONE', #67359, #4004, #62956, .T. ) ;
#25363=CARTESIAN_POINT ( 'NONE',  ( 24.79687500061451999, 6.054752690667223547, 3.707466751127219781E-16 ) ) ;
#25364=CARTESIAN_POINT ( 'NONE',  ( 5.962500000000002132, 2.886751345948129099, -4.999999999999998224 ) ) ;
#25365=CARTESIAN_POINT ( 'NONE',  ( -1.999999999999997113, 11.63750000122903394, 33.46410161513775705 ) ) ;
#25366=CARTESIAN_POINT ( 'NONE',  ( 12.02812500061451573, 6.421520780324663323E-16, -5.243569643749999010 ) ) ;
#25367=CARTESIAN_POINT ( 'NONE',  ( 5.175000001229033586, 2.886751345948129099, -4.999999999999998224 ) ) ;
#25368=CARTESIAN_POINT ( 'NONE',  ( 8.784375000614518925, -4.541064518000419881, 2.621784821874995952 ) ) ;
#25369=CARTESIAN_POINT ( 'NONE',  ( -2.065650683794913789, 4.559369103593685857, -26.56528590568888504 ) ) ;
#25371=CARTESIAN_POINT ( 'NONE',  ( 11.76562500061451644, 3.027376345333611329, 5.243569643749999010 ) ) ;
#25372=LINE ( 'NONE', #35362, #53257 ) ;
#25373=CARTESIAN_POINT ( 'NONE',  ( 22.80000000122903359, 5.773502691896255534, 3.535250795749688894E-16 ) ) ;
#25374=CARTESIAN_POINT ( 'NONE',  ( 9.571875000614518569, 3.027376345333611329, 5.243569643749999010 ) ) ;
#25375=CARTESIAN_POINT ( 'NONE',  ( 11.39062500061451644, -3.027376345333614438, 5.243569643749998122 ) ) ;
#25377=CARTESIAN_POINT ( 'NONE',  ( 21.53437500061451715, 6.421520780324663323E-16, -5.243569643749999010 ) ) ;
#25379=VECTOR ( 'NONE', #53047, 1000.000000000000000 ) ;
#25382=CARTESIAN_POINT ( 'NONE',  ( -4.243569643749998122, 13.59687500061451892, -27.54997392385601174 ) ) ;
#25383=CARTESIAN_POINT ( 'NONE',  ( 15.53437500061451715, -4.541064518000419881, 2.621784821874995952 ) ) ;
#25384=CARTESIAN_POINT ( 'NONE',  ( 17.25000000122903288, -2.886751345948125991, -5.000000000000000000 ) ) ;
#25385=AXIS2_PLACEMENT_3D ( 'NONE', #26451, #19057, #70780 ) ;
#25386=CARTESIAN_POINT ( 'NONE',  ( 11.44687500061451857, -3.027376345333614438, 5.243569643749998122 ) ) ;
#25387=CARTESIAN_POINT ( 'NONE',  ( 2.121784821874999061, 18.75312500061451715, -33.67503911421598417 ) ) ;
#25388=CARTESIAN_POINT ( 'NONE',  ( 17.85000000122903430, 5.773502691896255534, 3.535250795749688894E-16 ) ) ;
#25389=CARTESIAN_POINT ( 'NONE',  ( 11.76562500061451644, 3.027376345333611329, 5.243569643749999010 ) ) ;
#25391=VECTOR ( 'NONE', #44191, 1000.000000000000000 ) ;
#25392=CARTESIAN_POINT ( 'NONE',  ( 16.53750000000000142, -2.886751345948129988, 4.999999999999997335 ) ) ;
#25393=DIRECTION ( 'NONE',  ( 0.000000000000000000, 0.000000000000000000, 1.000000000000000000 ) ) ;
#25394=CARTESIAN_POINT ( 'NONE',  ( 12.15937500061451892, 4.541064518000418104, -2.621784821874998173 ) ) ;
#25395=CYLINDRICAL_SURFACE ( 'NONE', #20861, 4.999999999999998224 ) ;
#25396=CARTESIAN_POINT ( 'NONE',  ( 13.31250000122903288, 4.330127018922192761, -2.499999999999997780 ) ) ;
#25397=CARTESIAN_POINT ( 'NONE',  ( 20.10000000122903074, 5.773502691896255534, 3.535250795749688894E-16 ) ) ;
#25398=CARTESIAN_POINT ( 'NONE',  ( 17.46562500061451217, 3.027376345333613106, -5.243569643749998122 ) ) ;
#25399=CARTESIAN_POINT ( 'NONE',  ( 20.12812500061451715, 6.421520780324663323E-16, -5.243569643749999010 ) ) ;
#25400=CARTESIAN_POINT ( 'NONE',  ( 28.05000000122903359, -2.886751345948125991, -5.000000000000000000 ) ) ;
#25401=EDGE_CURVE ( 'NONE', #10265, #48564, #32904, .T. ) ;
#25402=CARTESIAN_POINT ( 'NONE',  ( 25.01249999999999929, 2.886751345948126879, 4.999999999999999112 ) ) ;
#25403=DIRECTION ( 'NONE',  ( 0.000000000000000000, 0.000000000000000000, -1.000000000000000000 ) ) ;
#25405=CARTESIAN_POINT ( 'NONE',  ( 29.10937500061451644, -4.541064518000417216, -2.621784821875001281 ) ) ;
#25407=CARTESIAN_POINT ( 'NONE',  ( 9.001249775931846008E-16, 14.12187500061451750, -25.09994784771203058 ) ) ;
#25408=CARTESIAN_POINT ( 'NONE',  ( 4.050000001229035362, -2.886751345948129988, 4.999999999999997335 ) ) ;
#25409=CARTESIAN_POINT ( 'NONE',  ( 29.85937500061451644, 0.000000000000000000, 5.243569643749999010 ) ) ;
#25410=CARTESIAN_POINT ( 'NONE',  ( 6.571875000614517681, -6.054752690667223547, -1.112240025338166033E-15 ) ) ;
#25411=CARTESIAN_POINT ( 'NONE',  ( 27.77812500061451573, 6.421520780324663323E-16, -5.243569643749999010 ) ) ;
#25412=CARTESIAN_POINT ( 'NONE',  ( 4.809375000614516615, -4.541064518000417216, -2.621784821875001281 ) ) ;
#25413=CARTESIAN_POINT ( 'NONE',  ( 14.36249999999999893, -5.773502691896255534, -1.060575238724906372E-15 ) ) ;
#25414=CARTESIAN_POINT ( 'NONE',  ( 7.500000000000000000, 0.000000000000000000, 4.999999999999998224 ) ) ;
#25415=CARTESIAN_POINT ( 'NONE',  ( 5.184375000614516615, -4.541064518000419881, 2.621784821874995952 ) ) ;
#25416=CARTESIAN_POINT ( 'NONE',  ( 12.04687500061451821, -3.027376345333610441, -5.243569643749999898 ) ) ;
#25417=CARTESIAN_POINT ( 'NONE',  ( 4.949999999999999289, -4.330127018922190985, -2.500000000000001332 ) ) ;
#25418=VECTOR ( 'NONE', #56358, 1000.000000000000000 ) ;
#25419=CARTESIAN_POINT ( 'NONE',  ( -2.121784821874996840, 14.47812500061459495, 33.67503911421598417 ) ) ;
#25421=CARTESIAN_POINT ( 'NONE',  ( 6.299999999999999822, -4.330127018922190985, -2.500000000000001332 ) ) ;
#25423=CARTESIAN_POINT ( 'NONE',  ( 20.72812500061451502, 4.541064518000418104, 2.621784821874999949 ) ) ;
#25424=CARTESIAN_POINT ( 'NONE',  ( 9.928125000614517859, 4.541064518000418104, 2.621784821874999949 ) ) ;
#25426=CARTESIAN_POINT ( 'NONE',  ( 9.684375000614517504, -4.541064518000419881, 2.621784821874995952 ) ) ;
#25427=CARTESIAN_POINT ( 'NONE',  ( 25.12499999999999645, -4.330127018922194537, 2.499999999999995559 ) ) ;
#25428=CARTESIAN_POINT ( 'NONE',  ( 21.26250000122903572, -4.330127018922190985, -2.500000000000001332 ) ) ;
#25429=CARTESIAN_POINT ( 'NONE',  ( 28.30312500061451431, 4.541064518000418104, -2.621784821874998173 ) ) ;
#25430=DIRECTION ( 'NONE',  ( 0.000000000000000000, 0.000000000000000000, -1.000000000000000000 ) ) ;
#25431=AXIS2_PLACEMENT_3D ( 'NONE', #50625, #45084, #33982 ) ;
#25432=CARTESIAN_POINT ( 'NONE',  ( 9.871875000614517504, 3.027376345333613106, -5.243569643749998122 ) ) ;
#25433=CARTESIAN_POINT ( 'NONE',  ( 14.78437500061451715, 6.421520780324663323E-16, -5.243569643749999010 ) ) ;
#25434=CARTESIAN_POINT ( 'NONE',  ( 26.44687500061451502, -3.027376345333610441, -5.243569643749999898 ) ) ;
#25437=CARTESIAN_POINT ( 'NONE',  ( 21.15937500061451715, 4.541064518000418104, -2.621784821874998173 ) ) ;
#25438=CARTESIAN_POINT ( 'NONE',  ( 12.87187500061451750, -6.054752690667223547, -1.112240025338166033E-15 ) ) ;
#25440=CARTESIAN_POINT ( 'NONE',  ( 23.96249999999999858, 2.886751345948129099, -4.999999999999998224 ) ) ;
#25442=CARTESIAN_POINT ( 'NONE',  ( -4.243569643749999898, 11.72187500061451892, -32.45002607614398471 ) ) ;
#25444=CARTESIAN_POINT ( 'NONE',  ( 14.31562500061451537, 3.027376345333613106, -5.243569643749998122 ) ) ;
#25445=CARTESIAN_POINT ( 'NONE',  ( 3.600000000000002309, -4.330127018922190985, -2.500000000000001332 ) ) ;
#25446=FACE_OUTER_BOUND ( 'NONE', #34479, .T. ) ;
#25447=CARTESIAN_POINT ( 'NONE',  ( 25.72499999999999787, 6.123233995736764310E-16, -4.999999999999998224 ) ) ;
#25448=CARTESIAN_POINT ( 'NONE',  ( 11.66249999999999964, -5.773502691896255534, -1.060575238724906372E-15 ) ) ;
#25449=CARTESIAN_POINT ( 'NONE',  ( -1.999999999999997113, 17.48750000122903359, 33.46410161513775705 ) ) ;
#25450=CARTESIAN_POINT ( 'NONE',  ( 11.43750000122903465, 6.123233995736764310E-16, -4.999999999999998224 ) ) ;
#25451=CARTESIAN_POINT ( 'NONE',  ( 22.39687500061451075, -3.027376345333610441, -5.243569643749999898 ) ) ;
#25452=CARTESIAN_POINT ( 'NONE',  ( 16.88437500061451502, -4.541064518000419881, 2.621784821874995952 ) ) ;
#25453=CARTESIAN_POINT ( 'NONE',  ( -3.999999999999997335, 16.43750000000000000, -27.69059892324149530 ) ) ;
#25455=CARTESIAN_POINT ( 'NONE',  ( 19.37812500061451715, 4.541064518000418104, 2.621784821874999949 ) ) ;
#25456=CARTESIAN_POINT ( 'NONE',  ( 4.303125000614516971, -4.541064518000417216, -2.621784821875001281 ) ) ;
#25457=CARTESIAN_POINT ( 'NONE',  ( 16.88437500061451502, -4.541064518000419881, 2.621784821874995952 ) ) ;
#25458=CARTESIAN_POINT ( 'NONE',  ( 28.54687500061451644, -3.027376345333614438, 5.243569643749998122 ) ) ;
#25459=CARTESIAN_POINT ( 'NONE',  ( 4.715625000614516615, -6.054752690667223547, -1.112240025338166033E-15 ) ) ;
#25460=CARTESIAN_POINT ( 'NONE',  ( 20.54062500061451502, -3.027376345333610441, -5.243569643749999898 ) ) ;
#25461=CARTESIAN_POINT ( 'NONE',  ( 2.121784821874999061, 15.15312500061451750, 26.32496088578401583 ) ) ;
#25462=CARTESIAN_POINT ( 'NONE',  ( 17.13750000122903216, -4.330127018922194537, 2.499999999999995559 ) ) ;
#25464=CARTESIAN_POINT ( 'NONE',  ( 6.628125000614517148, 6.421520780324663323E-16, -5.243569643749999010 ) ) ;
#25465=CARTESIAN_POINT ( 'NONE',  ( 29.46562500061451573, -6.054752690667223547, -1.112240025338166033E-15 ) ) ;
#25466=CARTESIAN_POINT ( 'NONE',  ( 24.12187500061451217, -6.054752690667223547, -1.112240025338166033E-15 ) ) ;
#25467=CARTESIAN_POINT ( 'NONE',  ( 14.12812500061451715, -4.541064518000419881, 2.621784821874995952 ) ) ;
#25468=CARTESIAN_POINT ( 'NONE',  ( 24.45000000122903572, -2.886751345948125991, -5.000000000000000000 ) ) ;
#25469=CARTESIAN_POINT ( 'NONE',  ( 24.02812500061451573, -4.541064518000419881, 2.621784821874995952 ) ) ;
#25470=CARTESIAN_POINT ( 'NONE',  ( 20.18437500061451573, 6.421520780324663323E-16, -5.243569643749999010 ) ) ;
#25471=CARTESIAN_POINT ( 'NONE',  ( 14.46562500061451750, 3.027376345333611329, 5.243569643749999010 ) ) ;
#25472=CARTESIAN_POINT ( 'NONE',  ( -2.121784821874996840, 14.98437500061451644, 33.67503911421598417 ) ) ;
#25473=CARTESIAN_POINT ( 'NONE',  ( 20.09062500061451573, -3.027376345333610441, -5.243569643749999898 ) ) ;
#25474=CARTESIAN_POINT ( 'NONE',  ( 29.20312500061451644, 4.541064518000418104, -2.621784821874998173 ) ) ;
#25477=CARTESIAN_POINT ( 'NONE',  ( 23.47499999999999787, 6.123233995736764310E-16, -4.999999999999998224 ) ) ;
#25478=CARTESIAN_POINT ( 'NONE',  ( 2.000000000000001332, 11.15000000000000213, -26.53589838486224650 ) ) ;
#25479=CARTESIAN_POINT ( 'NONE',  ( 13.05000000122903536, -2.886751345948130876, 4.999999999999996447 ) ) ;
#25480=CARTESIAN_POINT ( 'NONE',  ( 26.27812500061451573, -4.541064518000419881, 2.621784821874995952 ) ) ;
#25481=CARTESIAN_POINT ( 'NONE',  ( 8.428125000614517859, 6.421520780324663323E-16, -5.243569643749999010 ) ) ;
#25482=CARTESIAN_POINT ( 'NONE',  ( 19.50000000122903288, -2.886751345948125991, -5.000000000000000000 ) ) ;
#25483=CARTESIAN_POINT ( 'NONE',  ( 26.01562500061451289, 3.027376345333613106, -5.243569643749998122 ) ) ;
#25484=CARTESIAN_POINT ( 'NONE',  ( 25.76249999999999929, 2.886751345948129099, -4.999999999999998224 ) ) ;
#25485=CARTESIAN_POINT ( 'NONE',  ( 27.25312500061451360, -4.541064518000417216, -2.621784821875001281 ) ) ;
#25486=CARTESIAN_POINT ( 'NONE',  ( 7.490625000614516082, -3.027376345333610441, -5.243569643749999898 ) ) ;
#25488=EDGE_CURVE ( 'NONE', #9351, #1970, #33331, .T. ) ;
#25490=CARTESIAN_POINT ( 'NONE',  ( 23.05312500061451431, 0.000000000000000000, 5.243569643749999010 ) ) ;
#25491=CARTESIAN_POINT ( 'NONE',  ( 4.303125000614516971, -4.541064518000417216, -2.621784821875001281 ) ) ;
#25495=CARTESIAN_POINT ( 'NONE',  ( 13.87500000000000178, -4.330127018922194537, 2.499999999999995559 ) ) ;
#25497=CARTESIAN_POINT ( 'NONE',  ( 14.55937500061451573, 0.000000000000000000, 5.243569643749999010 ) ) ;
#25498=CARTESIAN_POINT ( 'NONE',  ( 9.562500001229032875, -4.330127018922190985, -2.500000000000001332 ) ) ;
#25499=CARTESIAN_POINT ( 'NONE',  ( 15.64687500061451608, -3.027376345333610441, -5.243569643749999898 ) ) ;
#25501=CARTESIAN_POINT ( 'NONE',  ( 9.309375000614517504, -4.541064518000417216, -2.621784821875001281 ) ) ;
#25502=CARTESIAN_POINT ( 'NONE',  ( -3.000416591977282496E-16, 11.59062500061451750, -34.90005215228797653 ) ) ;
#25504=CARTESIAN_POINT ( 'NONE',  ( 13.69687500061451679, -3.027376345333614438, 5.243569643749998122 ) ) ;
#25505=DIRECTION ( 'NONE',  ( -1.000000000000000000, -0.000000000000000000, -0.000000000000000000 ) ) ;
#25506=CARTESIAN_POINT ( 'NONE',  ( 21.44062500061452070, -3.027376345333610441, -5.243569643749999898 ) ) ;
#25508=CARTESIAN_POINT ( 'NONE',  ( 21.30000000122903359, -2.886751345948126435, -5.000000000000000000 ) ) ;
#25509=CARTESIAN_POINT ( 'NONE',  ( 25.95937500061451431, -4.541064518000417216, -2.621784821875001281 ) ) ;
#25510=CARTESIAN_POINT ( 'NONE',  ( 4.978125000614518569, 4.541064518000418104, 2.621784821874999949 ) ) ;
#25512=CARTESIAN_POINT ( 'NONE',  ( 17.18437500061451573, 4.541064518000418104, 2.621784821874999949 ) ) ;
#25514=CARTESIAN_POINT ( 'NONE',  ( 29.10000000122903074, 5.773502691896255534, 3.535250795749688894E-16 ) ) ;
#25515=CARTESIAN_POINT ( 'NONE',  ( 6.759375000614516793, 4.541064518000418104, -2.621784821874998173 ) ) ;
#25516=CARTESIAN_POINT ( 'NONE',  ( 16.09687500061452070, -3.027376345333610441, -5.243569643749999898 ) ) ;
#25518=CARTESIAN_POINT ( 'NONE',  ( 25.01249999999999929, 2.886751345948126879, 4.999999999999999112 ) ) ;
#25519=CARTESIAN_POINT ( 'NONE',  ( 27.75937500061451502, -4.541064518000417216, -2.621784821875001281 ) ) ;
#25521=CARTESIAN_POINT ( 'NONE',  ( 5.737500001229033586, 4.330127018922191873, 2.499999999999999556 ) ) ;
#25522=ORIENTED_EDGE ( 'NONE', *, *, #15421, .T. ) ;
#25523=CARTESIAN_POINT ( 'NONE',  ( 8.625000000000000000, 6.123233995736764310E-16, -4.999999999999998224 ) ) ;
#25525=CARTESIAN_POINT ( 'NONE',  ( 21.74062500061451431, -3.027376345333614438, 5.243569643749998122 ) ) ;
#25526=CARTESIAN_POINT ( 'NONE',  ( 11.51250000000000107, 2.886751345948126879, 4.999999999999999112 ) ) ;
#25527=CARTESIAN_POINT ( 'NONE',  ( 5.990625000614517859, -3.027376345333614438, 5.243569643749998122 ) ) ;
#25528=CARTESIAN_POINT ( 'NONE',  ( 19.16250000000000142, 2.886751345948126879, 4.999999999999999112 ) ) ;
#25529=EDGE_CURVE ( 'NONE', #63939, #68252, #35609, .T. ) ;
#25530=CARTESIAN_POINT ( 'NONE',  ( 19.30312500061451786, 4.541064518000418104, -2.621784821874998173 ) ) ;
#25531=CARTESIAN_POINT ( 'NONE',  ( 28.53750000122903074, 6.123233995736764310E-16, -4.999999999999998224 ) ) ;
#25532=CARTESIAN_POINT ( 'NONE',  ( 23.51250000122903216, -4.330127018922190985, -2.500000000000001332 ) ) ;
#25534=CARTESIAN_POINT ( 'NONE',  ( 4.425000000000001599, -4.330127018922194537, 2.499999999999995559 ) ) ;
#25535=ADVANCED_FACE ( 'NONE', ( #40440 ), #58492, .F. ) ;
#25536=ORIENTED_EDGE ( 'NONE', *, *, #15762, .T. ) ;
#25537=CARTESIAN_POINT ( 'NONE',  ( 20.27812500061451573, 4.541064518000418104, 2.621784821874999949 ) ) ;
#25538=CARTESIAN_POINT ( 'NONE',  ( 26.69062500061451715, -3.027376345333614438, 5.243569643749998122 ) ) ;
#25539=CARTESIAN_POINT ( 'NONE',  ( 24.04687500061451644, -3.027376345333614438, 5.243569643749998122 ) ) ;
#25540=CARTESIAN_POINT ( 'NONE',  ( 7.950000000000001954, 0.000000000000000000, 4.999999999999998224 ) ) ;
#25541=CARTESIAN_POINT ( 'NONE',  ( 12.14062500061451821, 6.054752690667223547, 3.707466751127219781E-16 ) ) ;
#25542=CARTESIAN_POINT ( 'NONE',  ( 28.56562500061451715, -6.054752690667223547, -1.112240025338166033E-15 ) ) ;
#25543=CARTESIAN_POINT ( 'NONE',  ( 16.92187500061451999, -6.054752690667223547, -1.112240025338166033E-15 ) ) ;
#25544=CARTESIAN_POINT ( 'NONE',  ( 9.065625000614517148, 3.027376345333611329, 5.243569643749999010 ) ) ;
#25545=CARTESIAN_POINT ( 'NONE',  ( 7.125000001229032875, 2.886751345948193936, 4.999999999999883649 ) ) ;
#25546=CARTESIAN_POINT ( 'NONE',  ( -4.243569643749999898, 12.65937500061451715, 30.00000000000000000 ) ) ;
#25547=( BOUNDED_CURVE ( )  B_SPLINE_CURVE ( 2, ( #22632, #22275, #39280, #5290, #49998, #45903, #33724 ),
 .UNSPECIFIED., .F., .F. ) 
 B_SPLINE_CURVE_WITH_KNOTS ( ( 3, 2, 2, 3 ),
 ( 0.3916666666666667740, 0.3944444444444444864, 0.3972222222222221433, 0.3999999999999999112 ),
 .UNSPECIFIED. ) 
 CURVE ( )  GEOMETRIC_REPRESENTATION_ITEM ( )  RATIONAL_B_SPLINE_CURVE ( ( 0.9999999999999946709, 0.8660254037844440367, 1.000000000000000000, 0.8660254037844387076, 1.000000000000000000, 0.8660254037844440367, 0.9999999999999946709 ) ) 
 REPRESENTATION_ITEM ( '' )  );
#25548=CARTESIAN_POINT ( 'NONE',  ( 24.33750000122903145, -4.330127018922194537, 2.499999999999995559 ) ) ;
#25550=CARTESIAN_POINT ( 'NONE',  ( 13.26562500061451289, -6.054752690667223547, -1.112240025338166033E-15 ) ) ;
#25551=CARTESIAN_POINT ( 'NONE',  ( 10.50937500061451679, 0.000000000000000000, 5.243569643749999010 ) ) ;
#25552=CARTESIAN_POINT ( 'NONE',  ( 9.459375000614517859, 4.541064518000418104, -2.621784821874998173 ) ) ;
#25553=CARTESIAN_POINT ( 'NONE',  ( 17.25937500061451502, 0.000000000000000000, 5.243569643749999010 ) ) ;
#25556=CARTESIAN_POINT ( 'NONE',  ( 7.285825576177820915E-16, 10.00000000000000000, 36.00000000000000000 ) ) ;
#25557=CARTESIAN_POINT ( 'NONE',  ( 22.45312500061451644, 4.541064518000418104, -2.621784821874998173 ) ) ;
#25558=CARTESIAN_POINT ( 'NONE',  ( 16.20937500061451786, 4.541064518000418104, -2.621784821874998173 ) ) ;
#25559=CARTESIAN_POINT ( 'NONE',  ( 22.60312500061451857, 0.000000000000000000, 5.243569643749999010 ) ) ;
#25560=CARTESIAN_POINT ( 'NONE',  ( 1.999999999999998668, 13.10000000000000142, 26.53589838486224650 ) ) ;
#25561=CARTESIAN_POINT ( 'NONE',  ( 27.17812500061451786, -4.541064518000419881, 2.621784821874995952 ) ) ;
#25562=CARTESIAN_POINT ( 'NONE',  ( 6.750000001229033764, -2.886751345948129988, 4.999999999999997335 ) ) ;
#25563=VERTEX_POINT ( 'NONE', #13422 ) ;
#25564=CARTESIAN_POINT ( 'NONE',  ( 30.00000000000000000, 0.000000000000000000, 4.999999999999998224 ) ) ;
#25565=CARTESIAN_POINT ( 'NONE',  ( -2.000000000000000000, 19.02499999999999858, -33.46410161513775705 ) ) ;
#25566=CARTESIAN_POINT ( 'NONE',  ( 24.18750000122903288, 4.330127018922191873, 2.499999999999999556 ) ) ;
#25569=CARTESIAN_POINT ( 'NONE',  ( 6.946875000614517681, -3.027376345333614438, 5.243569643749998122 ) ) ;
#25570=CARTESIAN_POINT ( 'NONE',  ( 12.78749999999999787, 5.773502691896255534, 3.535250795749688401E-16 ) ) ;
#25571=CARTESIAN_POINT ( 'NONE',  ( 14.61562500061451608, -6.054752690667223547, -1.112240025338166033E-15 ) ) ;
#25572=CARTESIAN_POINT ( 'NONE',  ( 8.071875000614518569, 3.027376345333613106, -5.243569643749998122 ) ) ;
#25573=CARTESIAN_POINT ( 'NONE',  ( 26.13750000122903216, -4.330127018922194537, 2.499999999999995559 ) ) ;
#25574=CARTESIAN_POINT ( 'NONE',  ( 17.14687500061451786, 6.054752690667223547, 3.707466751127219781E-16 ) ) ;
#25575=CARTESIAN_POINT ( 'NONE',  ( 4.546875000614517326, 6.054752690667223547, 3.707466751127219781E-16 ) ) ;
#25576=CARTESIAN_POINT ( 'NONE',  ( 0.000000000000000000, 20.00000000000000000, 26.00000000000000000 ) ) ;
#25577=CARTESIAN_POINT ( 'NONE',  ( 5.840625000614516615, 6.054752690667223547, 3.707466751127219781E-16 ) ) ;
#25578=CARTESIAN_POINT ( 'NONE',  ( 14.31562500061451537, 3.027376345333613106, -5.243569643749998122 ) ) ;
#25579=( BOUNDED_CURVE ( )  B_SPLINE_CURVE ( 2, ( #69372, #63451, #2484, #31290, #41646, #19455, #35371 ),
 .UNSPECIFIED., .F., .F. ) 
 B_SPLINE_CURVE_WITH_KNOTS ( ( 3, 2, 2, 3 ),
 ( 0.2250000000000000611, 0.2277777777777778290, 0.2305555555555555969, 0.2333333333333333648 ),
 .UNSPECIFIED. ) 
 CURVE ( )  GEOMETRIC_REPRESENTATION_ITEM ( )  RATIONAL_B_SPLINE_CURVE ( ( 0.9999999999999973355, 0.8660254037844413721, 1.000000000000000000, 0.8660254037844387076, 1.000000000000000000, 0.8660254037844373753, 1.000000000000001332 ) ) 
 REPRESENTATION_ITEM ( '' )  );
#25580=EDGE_LOOP ( 'NONE', ( #12646, #39818, #13345, #62161 ) ) ;
#25581=CARTESIAN_POINT ( 'NONE',  ( 12.21562500061451573, 3.027376345333611329, 5.243569643749999010 ) ) ;
#25582=CARTESIAN_POINT ( 'NONE',  ( 4.725000001229034297, 2.886751345948129099, -4.999999999999998224 ) ) ;
#25583=CARTESIAN_POINT ( 'NONE',  ( 9.703125000614514661, -4.541064518000417216, -2.621784821875001281 ) ) ;
#25585=CARTESIAN_POINT ( 'NONE',  ( 10.01250000000000107, 2.886751345948129099, -4.999999999999998224 ) ) ;
#25586=CARTESIAN_POINT ( 'NONE',  ( 5.137500001229033941, 6.123233995736764310E-16, -4.999999999999998224 ) ) ;
#25587=CARTESIAN_POINT ( 'NONE',  ( 19.20000000000000284, 0.000000000000000000, 4.999999999999998224 ) ) ;
#25588=CARTESIAN_POINT ( 'NONE',  ( 15.98437500061451821, -4.541064518000419881, 2.621784821874995952 ) ) ;
#25589=CARTESIAN_POINT ( 'NONE',  ( 16.08750000122903501, 4.330127018922191873, 2.499999999999999556 ) ) ;
#25591=( BOUNDED_CURVE ( )  B_SPLINE_CURVE ( 2, ( #44797, #66964, #43694, #66216, #71771, #54770, #15963 ),
 .UNSPECIFIED., .F., .F. ) 
 B_SPLINE_CURVE_WITH_KNOTS ( ( 3, 2, 2, 3 ),
 ( 0.2083333333333332871, 0.2111111111111110827, 0.2138888888888889062, 0.2166666666666667296 ),
 .UNSPECIFIED. ) 
 CURVE ( )  GEOMETRIC_REPRESENTATION_ITEM ( )  RATIONAL_B_SPLINE_CURVE ( ( 1.000000000000002665, 0.8660254037844360431, 1.000000000000000000, 0.8660254037844387076, 1.000000000000000000, 0.8660254037844360431, 1.000000000000002665 ) ) 
 REPRESENTATION_ITEM ( '' )  );
#25592=CARTESIAN_POINT ( 'NONE',  ( 4.243569643749999010, 18.26562500061451644, -32.45002607614398471 ) ) ;
#25594=FACE_OUTER_BOUND ( 'NONE', #39293, .T. ) ;
#25595=CARTESIAN_POINT ( 'NONE',  ( 29.35312500061451502, 0.000000000000000000, 5.243569643749999010 ) ) ;
#25596=CARTESIAN_POINT ( 'NONE',  ( 3.366080804335946919, -3.697228694398128290, 3.718268762498968094 ) ) ;
#25597=CARTESIAN_POINT ( 'NONE',  ( -3.137519842735245283E-14, 14.37500000122903288, 34.00000000000000000 ) ) ;
#25598=CARTESIAN_POINT ( 'NONE',  ( 16.47187500061452070, -6.054752690667223547, -1.112240025338166033E-15 ) ) ;
#25599=CARTESIAN_POINT ( 'NONE',  ( 29.36250000000000071, 2.886751345948129099, -4.999999999999998224 ) ) ;
#25600=CARTESIAN_POINT ( 'NONE',  ( 11.65312500061451573, 4.541064518000418104, -2.621784821874998173 ) ) ;
#25602=CARTESIAN_POINT ( 'NONE',  ( 25.05937500061451573, -4.541064518000417216, -2.621784821875001281 ) ) ;
#25604=CARTESIAN_POINT ( 'NONE',  ( 9.028125000614517504, 4.541064518000418104, 2.621784821874999949 ) ) ;
#25605=CARTESIAN_POINT ( 'NONE',  ( 12.08437500061451608, 6.421520780324663323E-16, -5.243569643749999010 ) ) ;
#25606=ORIENTED_EDGE ( 'NONE', *, *, #17223, .T. ) ;
#25607=CARTESIAN_POINT ( 'NONE',  ( 24.27187500061452141, 3.027376345333613106, -5.243569643749998122 ) ) ;
#25608=CARTESIAN_POINT ( 'NONE',  ( 27.74062500061451431, -3.027376345333610441, -5.243569643749999898 ) ) ;
#25610=CARTESIAN_POINT ( 'NONE',  ( 6.375000000000001776, 6.123233995736764310E-16, -4.999999999999998224 ) ) ;
#25612=CARTESIAN_POINT ( 'NONE',  ( 16.98750000122903359, 4.330127018922191873, 2.499999999999999556 ) ) ;
#25613=CARTESIAN_POINT ( 'NONE',  ( 27.18750000122903288, 6.123233995736764310E-16, -4.999999999999998224 ) ) ;
#25616=CARTESIAN_POINT ( 'NONE',  ( 16.16250000000000142, -5.773502691896255534, -1.060575238724906372E-15 ) ) ;
#25617=CARTESIAN_POINT ( 'NONE',  ( 20.17499999999999716, -4.330127018922194537, 2.499999999999995559 ) ) ;
#25618=CARTESIAN_POINT ( 'NONE',  ( 12.70312500061451821, 0.000000000000000000, 5.243569643749999010 ) ) ;
#25621=CARTESIAN_POINT ( 'NONE',  ( -4.243569643749997233, 15.84687500061451715, -27.54997392385601174 ) ) ;
#25622=CARTESIAN_POINT ( 'NONE',  ( 5.990625000614517859, -3.027376345333614438, 5.243569643749998122 ) ) ;
#25624=CARTESIAN_POINT ( 'NONE',  ( 12.37500000000000000, 4.330127018922191873, 2.499999999999999556 ) ) ;
#25627=CARTESIAN_POINT ( 'NONE',  ( 9.001249775931846008E-16, 15.41562500061451679, 34.90005215228797653 ) ) ;
#25628=CARTESIAN_POINT ( 'NONE',  ( 27.70312500061451289, -4.541064518000417216, -2.621784821875001281 ) ) ;
#25631=CARTESIAN_POINT ( 'NONE',  ( 23.67187500061451999, -6.054752690667223547, -1.112240025338166033E-15 ) ) ;
#25632=CARTESIAN_POINT ( 'NONE',  ( 18.47812500061451857, 4.541064518000418104, 2.621784821874999949 ) ) ;
#25633=CARTESIAN_POINT ( 'NONE',  ( -2.121784821874999949, 13.42812500061459602, -33.67503911421598417 ) ) ;
#25634=CARTESIAN_POINT ( 'NONE',  ( 23.02500000122903145, -5.773502691896255534, -1.060575238724906372E-15 ) ) ;
#25635=CARTESIAN_POINT ( 'NONE',  ( 4.265625000614517326, -6.054752690667223547, -1.112240025338166033E-15 ) ) ;
#25637=CARTESIAN_POINT ( 'NONE',  ( 20.50312500061451715, -4.541064518000417216, -2.621784821875001281 ) ) ;
#25640=CARTESIAN_POINT ( 'NONE',  ( 17.52187500061451431, 3.027376345333613106, -5.243569643749998122 ) ) ;
#25641=EDGE_CURVE ( 'NONE', #48104, #71409, #37646, .T. ) ;
#25642=CARTESIAN_POINT ( 'NONE',  ( 16.77187500061451786, 3.027376345333611329, 5.243569643749999010 ) ) ;
#25643=CARTESIAN_POINT ( 'NONE',  ( 23.82187500061451502, 3.027376345333613106, -5.243569643749998122 ) ) ;
#25644=CARTESIAN_POINT ( 'NONE',  ( 9.001249775931846008E-16, 13.22187500061451892, 34.90005215228797653 ) ) ;
#25645=CARTESIAN_POINT ( 'NONE',  ( 5.765625000614519102, 3.027376345333613106, -5.243569643749998122 ) ) ;
#25646=CARTESIAN_POINT ( 'NONE',  ( 28.67812500061451431, 6.421520780324663323E-16, -5.243569643749999010 ) ) ;
#25647=CARTESIAN_POINT ( 'NONE',  ( 28.52812500061451573, -4.541064518000419881, 2.621784821874995952 ) ) ;
#25649=CARTESIAN_POINT ( 'NONE',  ( 3.923201271487455344, -3.982966846201708488, -3.588438345016263131 ) ) ;
#25650=CARTESIAN_POINT ( 'NONE',  ( 3.628125000614518036, 4.541064518000418104, 2.621784821874999949 ) ) ;
#25651=CARTESIAN_POINT ( 'NONE',  ( 7.209375000614519635, 4.541064518000418104, -2.621784821874998173 ) ) ;
#25653=CARTESIAN_POINT ( 'NONE',  ( 15.45000000122903216, -2.886751345948125991, -5.000000000000000000 ) ) ;
#25654=CARTESIAN_POINT ( 'NONE',  ( 3.684375000614518836, 4.541064518000418104, 2.621784821874999949 ) ) ;
#25655=CARTESIAN_POINT ( 'NONE',  ( 11.17500000122903536, 2.886751345948126879, 4.999999999999999112 ) ) ;
#25656=CARTESIAN_POINT ( 'NONE',  ( 4.453125000614517326, 4.541064518000418104, -2.621784821874998173 ) ) ;
#25659=CARTESIAN_POINT ( 'NONE',  ( 13.28437500061451715, -4.541064518000419881, 2.621784821874995952 ) ) ;
#25660=FACE_OUTER_BOUND ( 'NONE', #9039, .T. ) ;
#25661=ORIENTED_EDGE ( 'NONE', *, *, #56109, .F. ) ;
#25662=CARTESIAN_POINT ( 'NONE',  ( 23.27812500061451573, 6.421520780324663323E-16, -5.243569643749999010 ) ) ;
#25663=CARTESIAN_POINT ( 'NONE',  ( 6.928125000614516082, -4.541064518000419881, 2.621784821874995952 ) ) ;
#25664=CARTESIAN_POINT ( 'NONE',  ( 23.89687500061451786, 6.054752690667223547, 3.707466751127219781E-16 ) ) ;
#25665=CARTESIAN_POINT ( 'NONE',  ( 7.603125000614517681, 4.541064518000418104, -2.621784821874998173 ) ) ;
#25667=CARTESIAN_POINT ( 'NONE',  ( 8.812500001229034652, 4.330127018922192761, -2.499999999999997780 ) ) ;
#25668=CARTESIAN_POINT ( 'NONE',  ( 23.35312500061451857, 4.541064518000418104, -2.621784821874998173 ) ) ;
#25669=CARTESIAN_POINT ( 'NONE',  ( -4.243569643749999898, 11.66562500061451679, -32.45002607614398471 ) ) ;
#25670=CARTESIAN_POINT ( 'NONE',  ( 11.47500000122903252, 2.886751345948129099, -4.999999999999998224 ) ) ;
#25671=CARTESIAN_POINT ( 'NONE',  ( 18.81562500061452070, 3.027376345333613106, -5.243569643749998122 ) ) ;
#25672=CARTESIAN_POINT ( 'NONE',  ( 17.12812500061451715, 4.541064518000418104, 2.621784821874999949 ) ) ;
#25674=CARTESIAN_POINT ( 'NONE',  ( 17.36249999999999716, 2.886751345948126879, 4.999999999999999112 ) ) ;
#25675=CARTESIAN_POINT ( 'NONE',  ( 14.32500000122903394, 2.886751345948126879, 4.999999999999999112 ) ) ;
#25678=CARTESIAN_POINT ( 'NONE',  ( 10.97812500061451679, -4.541064518000419881, 2.621784821874995952 ) ) ;
#25679=CARTESIAN_POINT ( 'NONE',  ( 14.57812500061451644, -4.541064518000419881, 2.621784821874995952 ) ) ;
#25680=AXIS2_PLACEMENT_3D ( 'NONE', #64748, #2700, #25215 ) ;
#25681=CARTESIAN_POINT ( 'NONE',  ( 23.06250000122903288, -4.330127018922190985, -2.500000000000001332 ) ) ;
#25682=CARTESIAN_POINT ( 'NONE',  ( 21.98437500061451644, 6.421520780324663323E-16, -5.243569643749999010 ) ) ;
#25683=CARTESIAN_POINT ( 'NONE',  ( 20.48437500061451289, -4.541064518000419881, 2.621784821874995952 ) ) ;
#25686=CARTESIAN_POINT ( 'NONE',  ( 6.937500001229033764, 6.123233995736764310E-16, -4.999999999999998224 ) ) ;
#25687=CARTESIAN_POINT ( 'NONE',  ( 7.059375000614518392, -4.541064518000417216, -2.621784821875001281 ) ) ;
#25688=CARTESIAN_POINT ( 'NONE',  ( 23.85937500061451644, 4.541064518000418104, -2.621784821874998173 ) ) ;
#25690=CARTESIAN_POINT ( 'NONE',  ( 18.70312500061451644, -4.541064518000417216, -2.621784821875001281 ) ) ;
#25691=CARTESIAN_POINT ( 'NONE',  ( 25.20937500061451431, 4.541064518000418104, -2.621784821874998173 ) ) ;
#25693=DIRECTION ( 'NONE',  ( -0.4999999999999975575, 0.000000000000000000, -0.8660254037844400399 ) ) ;
#25694=CARTESIAN_POINT ( 'NONE',  ( 4.321875000614517681, -6.054752690667223547, -1.112240025338166033E-15 ) ) ;
#25695=CARTESIAN_POINT ( 'NONE',  ( 16.86562500061451786, -6.054752690667223547, -1.112240025338166033E-15 ) ) ;
#25696=VERTEX_POINT ( 'NONE', #59222 ) ;
#25697=CARTESIAN_POINT ( 'NONE',  ( 0.000000000000000000, 20.00000000000000000, 30.00000000000000000 ) ) ;
#25698=CARTESIAN_POINT ( 'NONE',  ( 25.94062500061451715, -3.027376345333610441, -5.243569643749999898 ) ) ;
#25699=CARTESIAN_POINT ( 'NONE',  ( -1.999999999999997113, 10.73750000122903536, -26.53589838486224295 ) ) ;
#25701=CARTESIAN_POINT ( 'NONE',  ( 14.10000000000000142, 4.330127018922192761, -2.499999999999997780 ) ) ;
#25702=CARTESIAN_POINT ( 'NONE',  ( 24.18750000122903288, 4.330127018922191873, 2.499999999999999556 ) ) ;
#25703=CARTESIAN_POINT ( 'NONE',  ( 18.47812500061451857, 4.541064518000418104, 2.621784821874999949 ) ) ;
#25704=ORIENTED_EDGE ( 'NONE', *, *, #15134, .T. ) ;
#25705=CARTESIAN_POINT ( 'NONE',  ( 22.34999999999999787, 0.000000000000000000, 4.999999999999998224 ) ) ;
#25706=CARTESIAN_POINT ( 'NONE',  ( 24.83437500061451431, 4.541064518000418104, 2.621784821874999949 ) ) ;
#25707=ORIENTED_EDGE ( 'NONE', *, *, #17544, .T. ) ;
#25708=CARTESIAN_POINT ( 'NONE',  ( 13.38750000122903394, 4.330127018922191873, 2.499999999999999556 ) ) ;
#25709=CARTESIAN_POINT ( 'NONE',  ( 12.21562500061451573, 3.027376345333611329, 5.243569643749999010 ) ) ;
#25710=CARTESIAN_POINT ( 'NONE',  ( 3.965625000614515727, 3.027376345333613106, -5.243569643749998122 ) ) ;
#25712=CARTESIAN_POINT ( 'NONE',  ( 26.09062500061451573, 6.054752690667223547, 3.707466751127219781E-16 ) ) ;
#25713=CARTESIAN_POINT ( 'NONE',  ( 11.88750000122903216, 6.123233995736764310E-16, -4.999999999999998224 ) ) ;
#25714=CARTESIAN_POINT ( 'NONE',  ( 20.02500000000000213, 4.330127018922191873, 2.499999999999999556 ) ) ;
#25715=CARTESIAN_POINT ( 'NONE',  ( 25.68750000000000000, -2.886751345948125991, -5.000000000000000000 ) ) ;
#25716=CARTESIAN_POINT ( 'NONE',  ( 3.268712465558684332, -4.091009155385299856, -2.914164288643219081 ) ) ;
#25717=CARTESIAN_POINT ( 'NONE',  ( 7.884375000614517681, -4.541064518000419881, 2.621784821874995952 ) ) ;
#25718=CARTESIAN_POINT ( 'NONE',  ( 16.20937500061451786, 4.541064518000418104, -2.621784821874998173 ) ) ;
#25720=ORIENTED_EDGE ( 'NONE', *, *, #56271, .T. ) ;
#25721=CARTESIAN_POINT ( 'NONE',  ( 27.51562500061451644, 3.027376345333611329, 5.243569643749999010 ) ) ;
#25722=CARTESIAN_POINT ( 'NONE',  ( 26.55937500061451573, 4.541064518000418104, -2.621784821874998173 ) ) ;
#25723=CARTESIAN_POINT ( 'NONE',  ( 2.896875000614518747, -3.027376345333614438, 5.243569643749998122 ) ) ;
#25725=CARTESIAN_POINT ( 'NONE',  ( 15.00000000000000000, 4.330127018922192761, -2.499999999999997780 ) ) ;
#25726=CARTESIAN_POINT ( 'NONE',  ( 13.97812500061451679, 4.541064518000418104, 2.621784821874999949 ) ) ;
#25728=CARTESIAN_POINT ( 'NONE',  ( 29.27812500061451573, 4.541064518000418104, 2.621784821874999949 ) ) ;
#25729=CARTESIAN_POINT ( 'NONE',  ( 18.75000000122903288, 5.773502691896255534, 3.535250795749688894E-16 ) ) ;
#25732=CARTESIAN_POINT ( 'NONE',  ( 4.753125000614515372, -4.541064518000417216, -2.621784821875001281 ) ) ;
#25733=CARTESIAN_POINT ( 'NONE',  ( 24.94687500061451502, -3.027376345333614438, 5.243569643749998122 ) ) ;
#25735=CARTESIAN_POINT ( 'NONE',  ( 4.243569643749999898, 17.38437500061451502, 30.00000000000000000 ) ) ;
#25736=CARTESIAN_POINT ( 'NONE',  ( 24.27187500061452141, 3.027376345333613106, -5.243569643749998122 ) ) ;
#25737=CARTESIAN_POINT ( 'NONE',  ( 5.025000000000002132, 6.123233995736764310E-16, -4.999999999999998224 ) ) ;
#25738=CARTESIAN_POINT ( 'NONE',  ( 3.999999999999998668, 10.92500000122903536, 27.69059892324149175 ) ) ;
#25739=CARTESIAN_POINT ( 'NONE',  ( 11.39062500061451644, -3.027376345333614438, 5.243569643749998122 ) ) ;
#25740=CARTESIAN_POINT ( 'NONE',  ( 3.337500001229034563, 6.123233995736764310E-16, -4.999999999999998224 ) ) ;
#25741=CARTESIAN_POINT ( 'NONE',  ( 10.09687500061451715, -3.027376345333614438, 5.243569643749998122 ) ) ;
#25742=CARTESIAN_POINT ( 'NONE',  ( -1.092898315830475919, 4.886665047895959013, -26.14245196482272604 ) ) ;
#25744=CARTESIAN_POINT ( 'NONE',  ( 10.45312500061451644, 0.000000000000000000, 5.243569643749999010 ) ) ;
#25745=CARTESIAN_POINT ( 'NONE',  ( 14.37187500061451928, 3.027376345333613106, -5.243569643749998122 ) ) ;
#25747=CARTESIAN_POINT ( 'NONE',  ( 22.46250000122903501, 0.000000000000000000, 4.999999999999998224 ) ) ;
#25748=CARTESIAN_POINT ( 'NONE',  ( 10.95937500061451964, 0.000000000000000000, 5.243569643749999010 ) ) ;
#25749=CARTESIAN_POINT ( 'NONE',  ( 13.45312500061451466, 4.541064518000418104, -2.621784821874998173 ) ) ;
#25751=CARTESIAN_POINT ( 'NONE',  ( 20.63437500061451857, 6.421520780324663323E-16, -5.243569643749999010 ) ) ;
#25753=CARTESIAN_POINT ( 'NONE',  ( -1.071796769724488563, 12.10490381179670116, -26.00000000000000000 ) ) ;
#25755=CARTESIAN_POINT ( 'NONE',  ( -2.121784821874999949, 13.48437500061451821, -33.67503911421598417 ) ) ;
#25756=CARTESIAN_POINT ( 'NONE',  ( 14.93437500061451750, 4.541064518000418104, 2.621784821874999949 ) ) ;
#25757=CARTESIAN_POINT ( 'NONE',  ( 14.96250000122903323, -4.330127018922190985, -2.500000000000001332 ) ) ;
#25758=CARTESIAN_POINT ( 'NONE',  ( 12.23437500061451821, 4.541064518000418104, 2.621784821874999949 ) ) ;
#25759=CARTESIAN_POINT ( 'NONE',  ( 4.243569643749999010, 18.26562500061451644, -32.45002607614398471 ) ) ;
#25760=CARTESIAN_POINT ( 'NONE',  ( 17.43750000122903288, 4.330127018922191873, 2.499999999999999556 ) ) ;
#25761=CARTESIAN_POINT ( 'NONE',  ( 11.46562500061451573, -6.054752690667223547, -1.112240025338166033E-15 ) ) ;
#25763=CARTESIAN_POINT ( 'NONE',  ( 16.01249999999999929, 2.886751345948126879, 4.999999999999999112 ) ) ;
#25764=CARTESIAN_POINT ( 'NONE',  ( 18.03749999999999787, -2.886751345948126435, -5.000000000000000000 ) ) ;
#25765=CARTESIAN_POINT ( 'NONE',  ( 10.92187500061451644, 3.027376345333611329, 5.243569643749999010 ) ) ;
#25767=CARTESIAN_POINT ( 'NONE',  ( 12.07500000122903216, 2.886751345948126879, 4.999999999999999112 ) ) ;
#25768=CARTESIAN_POINT ( 'NONE',  ( 20.40000000122903145, -2.886751345948125991, -5.000000000000000000 ) ) ;
#25769=CARTESIAN_POINT ( 'NONE',  ( 18.62812500061451715, -4.541064518000419881, 2.621784821874995952 ) ) ;
#25770=CARTESIAN_POINT ( 'NONE',  ( 20.09062500061451573, -3.027376345333610441, -5.243569643749999898 ) ) ;
#25771=CARTESIAN_POINT ( 'NONE',  ( 27.56250000122902932, -4.330127018922190985, -2.500000000000001332 ) ) ;
#25772=CARTESIAN_POINT ( 'NONE',  ( 3.965625000614515727, 3.027376345333613106, -5.243569643749998122 ) ) ;
#25773=CARTESIAN_POINT ( 'NONE',  ( 24.71250000000000213, -5.773502691896255534, -1.060575238724906372E-15 ) ) ;
#25774=DIRECTION ( 'NONE',  ( -0.000000000000000000, -1.000000000000000000, -0.000000000000000000 ) ) ;
#25776=CARTESIAN_POINT ( 'NONE',  ( 28.35937500061451289, 4.541064518000418104, -2.621784821874998173 ) ) ;
#25777=CARTESIAN_POINT ( 'NONE',  ( -3.000416591977282496E-16, 12.99687500061451750, -34.90005215228797653 ) ) ;
#25778=EDGE_CURVE ( 'NONE', #55885, #7649, #28162, .T. ) ;
#25779=CARTESIAN_POINT ( 'NONE',  ( 3.750000001229034652, -2.886751345948125991, -5.000000000000000000 ) ) ;
#25780=CARTESIAN_POINT ( 'NONE',  ( 3.750000000000000000, 4.330127018922192761, -2.499999999999997780 ) ) ;
#25781=( BOUNDED_CURVE ( )  B_SPLINE_CURVE ( 2, ( #54685, #55055, #14787, #42873, #70948, #61314, #54329 ),
 .UNSPECIFIED., .F., .F. ) 
 B_SPLINE_CURVE_WITH_KNOTS ( ( 3, 2, 2, 3 ),
 ( 0.008333333333333315870, 0.01111111111111108898, 0.01388888888888885863, 0.01666666666666663174 ),
 .UNSPECIFIED. ) 
 CURVE ( )  GEOMETRIC_REPRESENTATION_ITEM ( )  RATIONAL_B_SPLINE_CURVE ( ( 1.000000000000000888, 0.8660254037844378194, 1.000000000000000000, 0.8660254037844387076, 1.000000000000000000, 0.8660254037844403729, 0.9999999999999983347 ) ) 
 REPRESENTATION_ITEM ( '' )  );
#25782=CARTESIAN_POINT ( 'NONE',  ( 16.38749999999999929, 5.773502691896255534, 3.535250795749688401E-16 ) ) ;
#25783=CARTESIAN_POINT ( 'NONE',  ( 8.146875000614516082, 6.054752690667223547, 3.707466751127219781E-16 ) ) ;
#25784=CARTESIAN_POINT ( 'NONE',  ( 25.04062500061451502, -3.027376345333610441, -5.243569643749999898 ) ) ;
#25785=CYLINDRICAL_SURFACE ( 'NONE', #58978, 4.000000000000000000 ) ;
#25786=CARTESIAN_POINT ( 'NONE',  ( -1.964573642069360249, 9.807014569943699911, -24.32727479091799694 ) ) ;
#25787=CARTESIAN_POINT ( 'NONE',  ( -1.071796769724490339, 19.30490381179669868, 34.00000000000000000 ) ) ;
#25788=CARTESIAN_POINT ( 'NONE',  ( 5.034375000614519813, 4.541064518000418104, 2.621784821874999949 ) ) ;
#25789=CARTESIAN_POINT ( 'NONE',  ( 9.271875000614516082, -6.054752690667223547, -1.112240025338166033E-15 ) ) ;
#25790=CARTESIAN_POINT ( 'NONE',  ( 4.200000000000001954, 4.330127018922192761, -2.499999999999997780 ) ) ;
#25791=CARTESIAN_POINT ( 'NONE',  ( 4.243569643749999898, 11.44062500061459708, 32.45002607614398471 ) ) ;
#25792=CARTESIAN_POINT ( 'NONE',  ( 29.09999999999999787, 0.000000000000000000, 4.999999999999998224 ) ) ;
#25793=CARTESIAN_POINT ( 'NONE',  ( 5.325000000000000178, -4.330127018922194537, 2.499999999999995559 ) ) ;
#25796=CARTESIAN_POINT ( 'NONE',  ( 19.64062500061451644, -3.027376345333610441, -5.243569643749999898 ) ) ;
#25797=CARTESIAN_POINT ( 'NONE',  ( 9.815625000614518925, 3.027376345333613106, -5.243569643749998122 ) ) ;
#25799=CARTESIAN_POINT ( 'NONE',  ( 5.934375000614517504, 4.541064518000418104, 2.621784821874999949 ) ) ;
#25800=CARTESIAN_POINT ( 'NONE',  ( 26.51249999999999929, -5.773502691896255534, -1.060575238724906372E-15 ) ) ;
#25801=CARTESIAN_POINT ( 'NONE',  ( 19.98750000122903359, 6.123233995736764310E-16, -4.999999999999998224 ) ) ;
#25802=CARTESIAN_POINT ( 'NONE',  ( 28.37812500061451715, 4.541064518000418104, 2.621784821874999949 ) ) ;
#25804=CARTESIAN_POINT ( 'NONE',  ( 9.309375000614517504, -4.541064518000417216, -2.621784821875001281 ) ) ;
#25805=CARTESIAN_POINT ( 'NONE',  ( 13.88437500061451679, 6.421520780324663323E-16, -5.243569643749999010 ) ) ;
#25806=CARTESIAN_POINT ( 'NONE',  ( 23.18437500061451573, -4.541064518000419881, 2.621784821874995952 ) ) ;
#25809=CARTESIAN_POINT ( 'NONE',  ( 20.55937500061451573, -4.541064518000417216, -2.621784821875001281 ) ) ;
#25810=CARTESIAN_POINT ( 'NONE',  ( 12.68437500061451573, 4.541064518000418104, 2.621784821874999949 ) ) ;
#25812=CARTESIAN_POINT ( 'NONE',  ( 24.41250000000000142, 2.886751345948129099, -4.999999999999998224 ) ) ;
#25814=CARTESIAN_POINT ( 'NONE',  ( -4.243569643749999898, 11.30937500061451928, -30.00000000000000000 ) ) ;
#25816=CARTESIAN_POINT ( 'NONE',  ( 14.35312500061451679, 4.541064518000418104, -2.621784821874998173 ) ) ;
#25817=CARTESIAN_POINT ( 'NONE',  ( 5.212500000000002132, 2.886751345948126879, 4.999999999999999112 ) ) ;
#25820=CARTESIAN_POINT ( 'NONE',  ( 11.77500000000000036, 6.123233995736764310E-16, -4.999999999999998224 ) ) ;
#25822=CARTESIAN_POINT ( 'NONE',  ( -1.999999999999997113, 18.38750000122903572, 33.46410161513775705 ) ) ;
#25823=CARTESIAN_POINT ( 'NONE',  ( 12.11250000122903181, 0.000000000000000000, 4.999999999999998224 ) ) ;
#25824=CARTESIAN_POINT ( 'NONE',  ( 22.95937500061451431, 4.541064518000418104, -2.621784821874998173 ) ) ;
#25825=CARTESIAN_POINT ( 'NONE',  ( 16.58437500061451786, 6.421520780324663323E-16, -5.243569643749999010 ) ) ;
#25828=CARTESIAN_POINT ( 'NONE',  ( 17.91562500061451502, 3.027376345333613106, -5.243569643749998122 ) ) ;
#25829=CARTESIAN_POINT ( 'NONE',  ( 3.065625000614517592, 3.027376345333613106, -5.243569643749998122 ) ) ;
#25830=CARTESIAN_POINT ( 'NONE',  ( 18.34687500061451715, -3.027376345333610441, -5.243569643749999898 ) ) ;
#25831=CARTESIAN_POINT ( 'NONE',  ( 28.24687500061451573, -3.027376345333610441, -5.243569643749999898 ) ) ;
#25832=CARTESIAN_POINT ( 'NONE',  ( 4.565625000614516260, 3.027376345333611329, 5.243569643749999010 ) ) ;
#25833=CARTESIAN_POINT ( 'NONE',  ( 18.96562500061451573, 3.027376345333611329, 5.243569643749999010 ) ) ;
#25834=CARTESIAN_POINT ( 'NONE',  ( -4.243569643749999898, 13.01562500061451999, 27.54997392385601529 ) ) ;
#25835=CARTESIAN_POINT ( 'NONE',  ( 17.21250000122903145, -4.330127018922190985, -2.500000000000001332 ) ) ;
#25837=CARTESIAN_POINT ( 'NONE',  ( 8.165625000614518569, 3.027376345333611329, 5.243569643749999010 ) ) ;
#25838=CARTESIAN_POINT ( 'NONE',  ( 25.97812500061451502, 6.421520780324663323E-16, -5.243569643749999010 ) ) ;
#25839=CARTESIAN_POINT ( 'NONE',  ( 9.074999999999999289, 6.123233995736764310E-16, -4.999999999999998224 ) ) ;
#25840=CARTESIAN_POINT ( 'NONE',  ( 24.08437500061451786, -4.541064518000419881, 2.621784821874995952 ) ) ;
#25841=CARTESIAN_POINT ( 'NONE',  ( 13.82812500061451466, 6.421520780324663323E-16, -5.243569643749999010 ) ) ;
#25842=CARTESIAN_POINT ( 'NONE',  ( 25.98750000122903003, 4.330127018922191873, 2.499999999999999556 ) ) ;
#25843=CARTESIAN_POINT ( 'NONE',  ( 23.05312500061451431, 0.000000000000000000, 5.243569643749999010 ) ) ;
#25844=CARTESIAN_POINT ( 'NONE',  ( 18.90937500061451360, 4.541064518000418104, -2.621784821874998173 ) ) ;
#25845=CARTESIAN_POINT ( 'NONE',  ( 15.85312500061451857, 0.000000000000000000, 5.243569643749999010 ) ) ;
#25846=CARTESIAN_POINT ( 'NONE',  ( -4.243569643749999898, 14.00937500061451857, 30.00000000000000000 ) ) ;
#25847=CARTESIAN_POINT ( 'NONE',  ( 20.95312500061451999, -4.541064518000417216, -2.621784821875001281 ) ) ;
#25848=CARTESIAN_POINT ( 'NONE',  ( 28.97812500061451502, -4.541064518000419881, 2.621784821874995952 ) ) ;
#25850=VERTEX_POINT ( 'NONE', #47427 ) ;
#25851=CARTESIAN_POINT ( 'NONE',  ( 23.09999999999999787, 4.330127018922192761, -2.499999999999997780 ) ) ;
#25852=CARTESIAN_POINT ( 'NONE',  ( -3.999999999999999112, 11.00000000000000178, -30.00000000000000000 ) ) ;
#25853=CARTESIAN_POINT ( 'NONE',  ( 21.56250000122903288, 0.000000000000000000, 4.999999999999998224 ) ) ;
#25854=CARTESIAN_POINT ( 'NONE',  ( 27.96562500061451928, 3.027376345333611329, 5.243569643749999010 ) ) ;
#25855=CARTESIAN_POINT ( 'NONE',  ( 8.765625000614518214, -6.054752690667223547, -1.112240025338166033E-15 ) ) ;
#25856=CARTESIAN_POINT ( 'NONE',  ( 19.08750000122903145, 6.123233995736764310E-16, -4.999999999999998224 ) ) ;
#25857=CARTESIAN_POINT ( 'NONE',  ( 25.00312500061451715, -4.541064518000417216, -2.621784821875001281 ) ) ;
#25858=CARTESIAN_POINT ( 'NONE',  ( 22.64999999999999858, 4.330127018922192761, -2.499999999999997780 ) ) ;
#25859=CARTESIAN_POINT ( 'NONE',  ( 27.85312500061451502, 4.541064518000418104, -2.621784821874998173 ) ) ;
#25860=CARTESIAN_POINT ( 'NONE',  ( 8.465625000614515727, 3.027376345333613106, -5.243569643749998122 ) ) ;
#25861=ORIENTED_EDGE ( 'NONE', *, *, #27838, .T. ) ;
#25862=CARTESIAN_POINT ( 'NONE',  ( 22.60312500061451857, 0.000000000000000000, 5.243569643749999010 ) ) ;
#25863=CARTESIAN_POINT ( 'NONE',  ( 4.115625000614516082, 3.027376345333611329, 5.243569643749999010 ) ) ;
#25865=CARTESIAN_POINT ( 'NONE',  ( 4.228125000614517681, -4.541064518000419881, 2.621784821874995952 ) ) ;
#25866=CARTESIAN_POINT ( 'NONE',  ( 2.000000000000001332, 13.96250000122903323, -26.53589838486224650 ) ) ;
#25867=LINE ( 'NONE', #43230, #11408 ) ;
#25868=CARTESIAN_POINT ( 'NONE',  ( 11.17500000000000071, -4.330127018922194537, 2.499999999999995559 ) ) ;
#25869=CARTESIAN_POINT ( 'NONE',  ( 11.67187500061451821, 3.027376345333613106, -5.243569643749998122 ) ) ;
#25870=CARTESIAN_POINT ( 'NONE',  ( 9.412500001229034297, 0.000000000000000000, 4.999999999999998224 ) ) ;
#25871=CARTESIAN_POINT ( 'NONE',  ( 14.67187500061451821, -6.054752690667223547, -1.112240025338166033E-15 ) ) ;
#25873=CARTESIAN_POINT ( 'NONE',  ( 5.746875000614517504, -3.027376345333610441, -5.243569643749999898 ) ) ;
#25874=CARTESIAN_POINT ( 'NONE',  ( -6.275039685470489619E-15, 18.31250000000000000, 33.99999999999999289 ) ) ;
#25875=CARTESIAN_POINT ( 'NONE',  ( 4.898587196589411843E-16, 20.00000000000000000, 33.99999999999999289 ) ) ;
#25876=CARTESIAN_POINT ( 'NONE',  ( 12.27187500061451786, 3.027376345333611329, 5.243569643749999010 ) ) ;
#25877=CARTESIAN_POINT ( 'NONE',  ( 30.00000000000000000, 0.000000000000000000, 0.000000000000000000 ) ) ;
#25878=CARTESIAN_POINT ( 'NONE',  ( 21.81562500061451004, -6.054752690667223547, -1.112240025338166033E-15 ) ) ;
#25879=CARTESIAN_POINT ( 'NONE',  ( -3.000416591977282496E-16, 10.74687500061451928, 25.09994784771203058 ) ) ;
#25880=CARTESIAN_POINT ( 'NONE',  ( -2.121784821874999949, 19.27812500061459033, 26.32496088578401938 ) ) ;
#25881=CARTESIAN_POINT ( 'NONE',  ( 26.14687500061451431, 6.054752690667223547, 3.707466751127219781E-16 ) ) ;
#25883=CARTESIAN_POINT ( 'NONE',  ( 5.465625000614517504, 3.027376345333611329, 5.243569643749999010 ) ) ;
#25885=CARTESIAN_POINT ( 'NONE',  ( 17.70937500061451431, 0.000000000000000000, 5.243569643749999010 ) ) ;
#25887=CARTESIAN_POINT ( 'NONE',  ( 26.66250000122903430, -4.330127018922190985, -2.500000000000001332 ) ) ;
#25888=CARTESIAN_POINT ( 'NONE',  ( 7.021875000614518747, -6.054752690667223547, -1.112240025338166033E-15 ) ) ;
#25889=CARTESIAN_POINT ( 'NONE',  ( 16.77187500061451786, 3.027376345333611329, 5.243569643749999010 ) ) ;
#25890=CARTESIAN_POINT ( 'NONE',  ( 8.625000000000000000, 6.123233995736764310E-16, -4.999999999999998224 ) ) ;
#25891=CARTESIAN_POINT ( 'NONE',  ( 24.67500000000000071, -4.330127018922194537, 2.499999999999995559 ) ) ;
#25892=CARTESIAN_POINT ( 'NONE',  ( 2.775000001229033675, -5.773502691896255534, -1.060575238724906372E-15 ) ) ;
#25893=CARTESIAN_POINT ( 'NONE',  ( 27.00937500061451857, 4.541064518000418104, -2.621784821874998173 ) ) ;
#25895=LINE ( 'NONE', #20702, #7952 ) ;
#25896=CARTESIAN_POINT ( 'NONE',  ( 9.187500000000001776, 5.773502691896255534, 3.535250795749688894E-16 ) ) ;
#25898=CARTESIAN_POINT ( 'NONE',  ( 22.15312500061451573, 0.000000000000000000, 5.243569643749999010 ) ) ;
#25899=CARTESIAN_POINT ( 'NONE',  ( 10.61250000000000071, 2.886751345948126879, 4.999999999999999112 ) ) ;
#25900=CARTESIAN_POINT ( 'NONE',  ( 3.590625000614518836, 6.054752690667223547, 3.707466751127219781E-16 ) ) ;
#25901=CARTESIAN_POINT ( 'NONE',  ( 20.06250000000000000, 2.886751345948126879, 4.999999999999999112 ) ) ;
#25903=CARTESIAN_POINT ( 'NONE',  ( 19.11562500061451431, -6.054752690667223547, -1.112240025338166033E-15 ) ) ;
#25905=CARTESIAN_POINT ( 'NONE',  ( 23.17500000122903359, 2.886751345948129099, -4.999999999999998224 ) ) ;
#25907=CARTESIAN_POINT ( 'NONE',  ( 3.562500000000000444, -5.773502691896255534, -1.060575238724906372E-15 ) ) ;
#25908=ORIENTED_EDGE ( 'NONE', *, *, #64257, .T. ) ;
#25909=CARTESIAN_POINT ( 'NONE',  ( 19.00312500061451715, 0.000000000000000000, 5.243569643749999010 ) ) ;
#25910=CARTESIAN_POINT ( 'NONE',  ( 23.35312500061451857, 4.541064518000418104, -2.621784821874998173 ) ) ;
#25911=CARTESIAN_POINT ( 'NONE',  ( 24.72187500061451360, 3.027376345333613106, -5.243569643749998122 ) ) ;
#25912=CARTESIAN_POINT ( 'NONE',  ( 9.712500000000002132, 2.886751345948126879, 4.999999999999999112 ) ) ;
#25913=CARTESIAN_POINT ( 'NONE',  ( 12.29062500061451857, -3.027376345333614438, 5.243569643749998122 ) ) ;
#25914=CARTESIAN_POINT ( 'NONE',  ( 26.12812500061451360, 4.541064518000418104, 2.621784821874999949 ) ) ;
#25915=CARTESIAN_POINT ( 'NONE',  ( 16.43437500061451573, -4.541064518000419881, 2.621784821874995952 ) ) ;
#25916=CARTESIAN_POINT ( 'NONE',  ( 9.253125000614517148, -4.541064518000417216, -2.621784821875001281 ) ) ;
#25918=CARTESIAN_POINT ( 'NONE',  ( 2.121784821874999061, 11.15937500061451715, 26.32496088578401583 ) ) ;
#25919=CARTESIAN_POINT ( 'NONE',  ( 24.00000000122902932, -2.886751345948125991, -5.000000000000000000 ) ) ;
#25921=CARTESIAN_POINT ( 'NONE',  ( 15.51562500061451644, -6.054752690667223547, -1.112240025338166033E-15 ) ) ;
#25922=CARTESIAN_POINT ( 'NONE',  ( 7.171875000614517326, 3.027376345333613106, -5.243569643749998122 ) ) ;
#25923=CARTESIAN_POINT ( 'NONE',  ( 10.47187500061451715, 3.027376345333611329, 5.243569643749999010 ) ) ;
#25925=CARTESIAN_POINT ( 'NONE',  ( 29.82187500061451502, 3.027376345333611329, 5.243569643749999010 ) ) ;
#25926=CARTESIAN_POINT ( 'NONE',  ( 20.80312500061451431, 0.000000000000000000, 5.243569643749999010 ) ) ;
#25927=CARTESIAN_POINT ( 'NONE',  ( 17.48437500061451999, 6.421520780324663323E-16, -5.243569643749999010 ) ) ;
#25928=CARTESIAN_POINT ( 'NONE',  ( 22.49062500061451431, 6.054752690667223547, 3.707466751127219781E-16 ) ) ;
#25929=CARTESIAN_POINT ( 'NONE',  ( 4.000000000000000000, 12.08750000000000036, 32.30940107675849049 ) ) ;
#25930=CARTESIAN_POINT ( 'NONE',  ( 27.10312500061451502, 0.000000000000000000, 5.243569643749999010 ) ) ;
#25931=CARTESIAN_POINT ( 'NONE',  ( 7.650000001229034119, -2.886751345948129988, 4.999999999999997335 ) ) ;
#25932=EDGE_LOOP ( 'NONE', ( #42248, #67012, #67220, #16570 ) ) ;
#25933=DIRECTION ( 'NONE',  ( -0.000000000000000000, -0.000000000000000000, -1.000000000000000000 ) ) ;
#25934=CARTESIAN_POINT ( 'NONE',  ( 1.999999999999998668, 18.50000000000000000, -33.46410161513775705 ) ) ;
#25935=CARTESIAN_POINT ( 'NONE',  ( 25.38750000122903216, 6.123233995736764310E-16, -4.999999999999998224 ) ) ;
#25937=CARTESIAN_POINT ( 'NONE',  ( 6.984375000614516438, -4.541064518000419881, 2.621784821874995952 ) ) ;
#25938=DIRECTION ( 'NONE',  ( 0.000000000000000000, 1.000000000000000000, 0.000000000000000000 ) ) ;
#25939=CARTESIAN_POINT ( 'NONE',  ( 15.77812500061451573, 4.541064518000418104, 2.621784821874999949 ) ) ;
#25940=CARTESIAN_POINT ( 'NONE',  ( 9.271875000614516082, -6.054752690667223547, -1.112240025338166033E-15 ) ) ;
#25941=CARTESIAN_POINT ( 'NONE',  ( 27.93750000122903288, -4.330127018922194537, 2.499999999999995559 ) ) ;
#25942=CARTESIAN_POINT ( 'NONE',  ( 17.74687500061451928, -3.027376345333614438, 5.243569643749998122 ) ) ;
#25943=CARTESIAN_POINT ( 'NONE',  ( 5.409375000614516260, 4.541064518000418104, -2.621784821874998173 ) ) ;
#25945=CARTESIAN_POINT ( 'NONE',  ( 5.203125000614518214, -4.541064518000417216, -2.621784821875001281 ) ) ;
#25946=CARTESIAN_POINT ( 'NONE',  ( 15.32812500061451644, 4.541064518000418104, 2.621784821874999949 ) ) ;
#25948=CARTESIAN_POINT ( 'NONE',  ( 11.76562500061451644, 3.027376345333611329, 5.243569643749999010 ) ) ;
#25949=CARTESIAN_POINT ( 'NONE',  ( 5.550000001229032698, -2.886751345948125991, -5.000000000000000000 ) ) ;
#25950=CARTESIAN_POINT ( 'NONE',  ( 10.71562500061451928, 3.027376345333613106, -5.243569643749998122 ) ) ;
#25952=CARTESIAN_POINT ( 'NONE',  ( 10.31250000000000355, -5.773502691896255534, -1.060575238724906372E-15 ) ) ;
#25953=CARTESIAN_POINT ( 'NONE',  ( 3.337500001229034563, 6.123233995736764310E-16, -4.999999999999998224 ) ) ;
#25954=CARTESIAN_POINT ( 'NONE',  ( 17.62500000000000000, 6.123233995736764310E-16, -4.999999999999998224 ) ) ;
#25955=CARTESIAN_POINT ( 'NONE',  ( 17.70937500061451431, 0.000000000000000000, 5.243569643749999010 ) ) ;
#25956=CARTESIAN_POINT ( 'NONE',  ( 15.18750000122903465, 4.330127018922191873, 2.499999999999999556 ) ) ;
#25958=CARTESIAN_POINT ( 'NONE',  ( -3.000416591977282496E-16, 15.64062500061451644, -34.90005215228797653 ) ) ;
#25960=CARTESIAN_POINT ( 'NONE',  ( 2.775000001229034119, -5.773502691896255534, -1.060575238724906372E-15 ) ) ;
#25961=CARTESIAN_POINT ( 'NONE',  ( 28.90312500061451217, 0.000000000000000000, 5.243569643749999010 ) ) ;
#25963=CYLINDRICAL_SURFACE ( 'NONE', #10146, 4.999999999999998224 ) ;
#25964=CARTESIAN_POINT ( 'NONE',  ( 16.39687500061451786, -3.027376345333614438, 5.243569643749998122 ) ) ;
#25965=CARTESIAN_POINT ( 'NONE',  ( 28.80000000000000071, -4.330127018922190985, -2.500000000000001332 ) ) ;
#25966=CARTESIAN_POINT ( 'NONE',  ( 11.09062500061451573, -3.027376345333610441, -5.243569643749999898 ) ) ;
#25968=CARTESIAN_POINT ( 'NONE',  ( 24.98437500061451644, -4.541064518000419881, 2.621784821874995952 ) ) ;
#25970=CARTESIAN_POINT ( 'NONE',  ( 7.528125000614515727, 6.421520780324663323E-16, -5.243569643749999010 ) ) ;
#25971=CARTESIAN_POINT ( 'NONE',  ( 12.57187500061451857, 3.027376345333613106, -5.243569643749998122 ) ) ;
#25972=ORIENTED_EDGE ( 'NONE', *, *, #24990, .T. ) ;
#25973=CARTESIAN_POINT ( 'NONE',  ( 23.82187500061451502, 3.027376345333613106, -5.243569643749998122 ) ) ;
#25974=CARTESIAN_POINT ( 'NONE',  ( 28.19062500061451715, -3.027376345333610441, -5.243569643749999898 ) ) ;
#25976=CARTESIAN_POINT ( 'NONE',  ( 24.63749999999999929, -2.886751345948163738, 4.999999999999939604 ) ) ;
#25977=( BOUNDED_CURVE ( )  B_SPLINE_CURVE ( 2, ( #69434, #2552, #64231, #1476, #23983, #29536, #35076 ),
 .UNSPECIFIED., .F., .F. ) 
 B_SPLINE_CURVE_WITH_KNOTS ( ( 3, 2, 2, 3 ),
 ( 0.6416666666666668295, 0.6444444444444445974, 0.6472222222222223653, 0.6500000000000001332 ),
 .UNSPECIFIED. ) 
 CURVE ( )  GEOMETRIC_REPRESENTATION_ITEM ( )  RATIONAL_B_SPLINE_CURVE ( ( 0.9999999999999946709, 0.8660254037844440367, 1.000000000000000000, 0.8660254037844387076, 1.000000000000000000, 0.8660254037844333785, 1.000000000000005329 ) ) 
 REPRESENTATION_ITEM ( '' )  );
#25978=CARTESIAN_POINT ( 'NONE',  ( 7.537500000000002309, -2.886751345948129988, 4.999999999999997335 ) ) ;
#25979=CARTESIAN_POINT ( 'NONE',  ( 17.73750000122903359, 6.123233995736764310E-16, -4.999999999999998224 ) ) ;
#25982=ORIENTED_EDGE ( 'NONE', *, *, #65786, .T. ) ;
#25983=CARTESIAN_POINT ( 'NONE',  ( 14.92500000000000071, 6.123233995736764310E-16, -4.999999999999998224 ) ) ;
#25984=CARTESIAN_POINT ( 'NONE',  ( 18.26249999999999929, 2.886751345948126879, 4.999999999999999112 ) ) ;
#25985=CARTESIAN_POINT ( 'NONE',  ( 13.56562500061451892, 3.027376345333611329, 5.243569643749999010 ) ) ;
#25986=ORIENTED_EDGE ( 'NONE', *, *, #26717, .T. ) ;
#25987=CARTESIAN_POINT ( 'NONE',  ( 3.722978149461063424, -3.926822905430812582, -3.198543215468592216 ) ) ;
#25988=CARTESIAN_POINT ( 'NONE',  ( -2.121784821874996840, 16.33437500061451786, -26.32496088578401583 ) ) ;
#25989=CARTESIAN_POINT ( 'NONE',  ( 4.040625000614517681, 6.054752690667223547, 3.707466751127219781E-16 ) ) ;
#25991=CARTESIAN_POINT ( 'NONE',  ( 9.750000000000001776, 0.000000000000000000, 4.999999999999998224 ) ) ;
#25994=CARTESIAN_POINT ( 'NONE',  ( 9.001249775931846008E-16, 14.51562500061451466, 34.90005215228797653 ) ) ;
#25995=CARTESIAN_POINT ( 'NONE',  ( 27.17812500061451786, -4.541064518000419881, 2.621784821874995952 ) ) ;
#25998=CARTESIAN_POINT ( 'NONE',  ( 23.29687500061451644, -3.027376345333610441, -5.243569643749999898 ) ) ;
#25999=CARTESIAN_POINT ( 'NONE',  ( 19.71562500061451928, 3.027376345333613106, -5.243569643749998122 ) ) ;
#26000=CARTESIAN_POINT ( 'NONE',  ( -3.000416591977282496E-16, 14.74062500061459424, -34.90005215228797653 ) ) ;
#26001=CARTESIAN_POINT ( 'NONE',  ( 24.37500000122903288, -5.773502691896255534, -1.060575238724906372E-15 ) ) ;
#26002=CARTESIAN_POINT ( 'NONE',  ( 3.740625000614516527, -3.027376345333614438, 5.243569643749998122 ) ) ;
#26004=CARTESIAN_POINT ( 'NONE',  ( 21.40312500061451573, -4.541064518000417216, -2.621784821875001281 ) ) ;
#26007=CARTESIAN_POINT ( 'NONE',  ( 17.85937500061451999, -4.541064518000417216, -2.621784821875001281 ) ) ;
#26008=CARTESIAN_POINT ( 'NONE',  ( 15.72187500061451892, 3.027376345333613106, -5.243569643749998122 ) ) ;
#26009=CARTESIAN_POINT ( 'NONE',  ( 25.39687500061451431, -3.027376345333614438, 5.243569643749998122 ) ) ;
#26010=CARTESIAN_POINT ( 'NONE',  ( -4.243569643749998122, 15.39687500061451786, 32.45002607614398471 ) ) ;
#26011=CARTESIAN_POINT ( 'NONE',  ( 4.828125000614518214, 6.421520780324663323E-16, -5.243569643749999010 ) ) ;
#26012=CARTESIAN_POINT ( 'NONE',  ( 27.85312500061451502, 4.541064518000418104, -2.621784821874998173 ) ) ;
#26013=( BOUNDED_CURVE ( )  B_SPLINE_CURVE ( 2, ( #68553, #33836, #51196, #28301, #34553, #51919, #57081 ),
 .UNSPECIFIED., .F., .F. ) 
 B_SPLINE_CURVE_WITH_KNOTS ( ( 3, 2, 2, 3 ),
 ( 0.9431886200030490386, 0.9444444444444444198, 0.9472222222222221877, 0.9483504900823832573 ),
 .UNSPECIFIED. ) 
 CURVE ( )  GEOMETRIC_REPRESENTATION_ITEM ( )  RATIONAL_B_SPLINE_CURVE ( ( 0.9336275693722517754, 0.9394305139167113960, 1.000000000000000000, 0.8660254037844387076, 1.000000000000000000, 0.9455826768442929797, 0.9353714217504458528 ) ) 
 REPRESENTATION_ITEM ( '' )  );
#26014=CARTESIAN_POINT ( 'NONE',  ( 28.22812500061451502, 6.421520780324663323E-16, -5.243569643749999010 ) ) ;
#26015=CARTESIAN_POINT ( 'NONE',  ( 1.999999999999998668, 19.84999999999999787, 26.53589838486224650 ) ) ;
#26016=CARTESIAN_POINT ( 'NONE',  ( 6.384375000614516793, 4.541064518000418104, 2.621784821874999949 ) ) ;
#26018=CARTESIAN_POINT ( 'NONE',  ( 13.20000000122903394, -2.886751345948125991, -5.000000000000000000 ) ) ;
#26019=CARTESIAN_POINT ( 'NONE',  ( 9.712500001229033231, 4.330127018922192761, -2.499999999999997780 ) ) ;
#26020=CARTESIAN_POINT ( 'NONE',  ( 6.028125000614517504, -4.541064518000419881, 2.621784821874995952 ) ) ;
#26023=CARTESIAN_POINT ( 'NONE',  ( 13.13437500061451857, 4.541064518000418104, 2.621784821874999949 ) ) ;
#26024=CARTESIAN_POINT ( 'NONE',  ( 0.000000000000000000, 20.00000000000000000, -30.00000000000000000 ) ) ;
#26026=CARTESIAN_POINT ( 'NONE',  ( 23.35312500061451857, 4.541064518000418104, -2.621784821874998173 ) ) ;
#26027=CARTESIAN_POINT ( 'NONE',  ( 7.153125000614518392, 4.541064518000418104, -2.621784821874998173 ) ) ;
#26028=CARTESIAN_POINT ( 'NONE',  ( 23.74687500061451573, -3.027376345333610441, -5.243569643749999898 ) ) ;
#26029=CARTESIAN_POINT ( 'NONE',  ( 7.940625000614518036, -3.027376345333610441, -5.243569643749999898 ) ) ;
#26031=CARTESIAN_POINT ( 'NONE',  ( 7.687500001229033764, -4.330127018922194537, 2.499999999999995559 ) ) ;
#26032=CARTESIAN_POINT ( 'NONE',  ( 22.45312500061451644, 4.541064518000418104, -2.621784821874998173 ) ) ;
#26033=CARTESIAN_POINT ( 'NONE',  ( 9.001249775931846008E-16, 10.01562500061451644, -25.09994784771203058 ) ) ;
#26034=CARTESIAN_POINT ( 'NONE',  ( 10.12500000122903465, 2.886751345948129099, -4.999999999999998224 ) ) ;
#26035=( BOUNDED_CURVE ( )  B_SPLINE_CURVE ( 2, ( #41919, #46744, #47102, #64444, #13836, #20838, #15657, #71462, #64810 ),
 .UNSPECIFIED., .F., .F. ) 
 B_SPLINE_CURVE_WITH_KNOTS ( ( 3, 2, 2, 2, 3 ),
 ( 0.1847826086956521896, 0.1884057971014492794, 0.1956521739130434867, 0.2028985507246376940, 0.2065217391304347838 ),
 .UNSPECIFIED. ) 
 CURVE ( )  GEOMETRIC_REPRESENTATION_ITEM ( )  RATIONAL_B_SPLINE_CURVE ( ( 0.9330127018922194093, 0.9330127018922196314, 1.000000000000000000, 0.8660254037844387076, 1.000000000000000000, 0.8660254037844387076, 1.000000000000000000, 0.9330127018922194093, 0.9330127018922194093 ) ) 
 REPRESENTATION_ITEM ( '' )  );
#26036=CARTESIAN_POINT ( 'NONE',  ( 19.60312500061451502, -4.541064518000417216, -2.621784821875001281 ) ) ;
#26037=CARTESIAN_POINT ( 'NONE',  ( 17.31562500061451715, -6.054752690667223547, -1.112240025338166033E-15 ) ) ;
#26039=CARTESIAN_POINT ( 'NONE',  ( 19.08750000000000213, 5.773502691896255534, 3.535250795749688894E-16 ) ) ;
#26040=CARTESIAN_POINT ( 'NONE',  ( 10.87500000122903288, -5.773502691896255534, -1.060575238724906372E-15 ) ) ;
#26041=CARTESIAN_POINT ( 'NONE',  ( 7.490625000614516082, -3.027376345333610441, -5.243569643749999898 ) ) ;
#26042=CARTESIAN_POINT ( 'NONE',  ( 12.29062500061451857, -3.027376345333614438, 5.243569643749998122 ) ) ;
#26043=EDGE_CURVE ( 'NONE', #45851, #14969, #73032, .T. ) ;
#26044=CARTESIAN_POINT ( 'NONE',  ( 24.18750000122903288, 4.330127018922191873, 2.499999999999999556 ) ) ;
#26045=CARTESIAN_POINT ( 'NONE',  ( 22.39687500061451075, -3.027376345333610441, -5.243569643749999898 ) ) ;
#26047=CARTESIAN_POINT ( 'NONE',  ( 4.500000001229034652, -2.886751345948129988, 4.999999999999997335 ) ) ;
#26048=CARTESIAN_POINT ( 'NONE',  ( 6.084375000614518747, -4.541064518000419881, 2.621784821874995952 ) ) ;
#26049=CARTESIAN_POINT ( 'NONE',  ( 22.95937500061451431, 4.541064518000418104, -2.621784821874998173 ) ) ;
#26052=CARTESIAN_POINT ( 'NONE',  ( 17.84062500061451573, -3.027376345333610441, -5.243569643749999898 ) ) ;
#26053=CARTESIAN_POINT ( 'NONE',  ( 23.33437500061451786, 6.421520780324663323E-16, -5.243569643749999010 ) ) ;
#26055=CARTESIAN_POINT ( 'NONE',  ( 3.459375000614519635, -4.541064518000417216, -2.621784821875001281 ) ) ;
#26056=CARTESIAN_POINT ( 'NONE',  ( -3.999999999999999112, 13.36250000122903359, -30.00000000000000000 ) ) ;
#26057=CARTESIAN_POINT ( 'NONE',  ( 5.184375000614516615, -4.541064518000419881, 2.621784821874995952 ) ) ;
#26058=CARTESIAN_POINT ( 'NONE',  ( 15.89062500061451289, -3.027376345333614438, 5.243569643749998122 ) ) ;
#26059=CARTESIAN_POINT ( 'NONE',  ( 13.54687500061451999, 6.054752690667223547, 3.707466751127219781E-16 ) ) ;
#26062=CARTESIAN_POINT ( 'NONE',  ( 26.24062500061451431, -3.027376345333614438, 5.243569643749998122 ) ) ;
#26063=CARTESIAN_POINT ( 'NONE',  ( 30.00000000000000000, 0.000000000000000000, 4.999999999999998224 ) ) ;
#26064=CARTESIAN_POINT ( 'NONE',  ( 3.965171583692859603, 3.045884815923804556, 3.965171583692790325 ) ) ;
#26065=CARTESIAN_POINT ( 'NONE',  ( 13.53749999999999964, -2.886751345948125991, -5.000000000000000000 ) ) ;
#26066=CARTESIAN_POINT ( 'NONE',  ( 24.97500000122903430, 2.886751345948129099, -4.999999999999998224 ) ) ;
#26067=CARTESIAN_POINT ( 'NONE',  ( 18.81562500061452070, 3.027376345333613106, -5.243569643749998122 ) ) ;
#26068=ORIENTED_EDGE ( 'NONE', *, *, #59373, .F. ) ;
#26069=CARTESIAN_POINT ( 'NONE',  ( 22.68750000000000000, 5.773502691896255534, 3.535250795749688894E-16 ) ) ;
#26070=CARTESIAN_POINT ( 'NONE',  ( 23.52187500061451786, 3.027376345333611329, 5.243569643749999010 ) ) ;
#26072=CARTESIAN_POINT ( 'NONE',  ( 18.18750000122903288, 6.123233995736764310E-16, -4.999999999999998224 ) ) ;
#26073=CARTESIAN_POINT ( 'NONE',  ( 10.37812500061451715, 4.541064518000418104, 2.621784821874999949 ) ) ;
#26074=CARTESIAN_POINT ( 'NONE',  ( 3.103125000614517237, 4.541064518000418104, -2.621784821874998173 ) ) ;
#26076=CARTESIAN_POINT ( 'NONE',  ( 27.96562500061451928, 3.027376345333611329, 5.243569643749999010 ) ) ;
#26077=CARTESIAN_POINT ( 'NONE',  ( 19.16250000000000142, 2.886751345948126879, 4.999999999999999112 ) ) ;
#26078=CARTESIAN_POINT ( 'NONE',  ( 26.96249999999999858, -5.773502691896255534, -1.060575238724906372E-15 ) ) ;
#26079=CARTESIAN_POINT ( 'NONE',  ( 3.262500001229035718, -4.330127018922190985, -2.500000000000001332 ) ) ;
#26080=CARTESIAN_POINT ( 'NONE',  ( 7.659375000614518036, 4.541064518000418104, -2.621784821874998173 ) ) ;
#26081=CARTESIAN_POINT ( 'NONE',  ( 17.85937500061451999, -4.541064518000417216, -2.621784821875001281 ) ) ;
#26082=CARTESIAN_POINT ( 'NONE',  ( 3.999999999999999112, 11.33750000122903501, 30.00000000000000000 ) ) ;
#26084=CARTESIAN_POINT ( 'NONE',  ( 25.82812500061451644, -4.541064518000419881, 2.621784821874995952 ) ) ;
#26085=CARTESIAN_POINT ( 'NONE',  ( 27.08437500061451786, 4.541064518000418104, 2.621784821874999949 ) ) ;
#26088=CARTESIAN_POINT ( 'NONE',  ( 13.50000000000000178, -4.330127018922190985, -2.500000000000001332 ) ) ;
#26089=CARTESIAN_POINT ( 'NONE',  ( 11.99062500061451608, -3.027376345333610441, -5.243569643749999898 ) ) ;
#26092=CARTESIAN_POINT ( 'NONE',  ( 28.75312500061451715, 4.541064518000418104, -2.621784821874998173 ) ) ;
#26093=CARTESIAN_POINT ( 'NONE',  ( 18.37500000122903288, 2.886751345948126879, 4.999999999999999112 ) ) ;
#26096=CARTESIAN_POINT ( 'NONE',  ( 6.253125000614517148, 4.541064518000418104, -2.621784821874998173 ) ) ;
#26097=CARTESIAN_POINT ( 'NONE',  ( 21.57187500061451502, 3.027376345333613106, -5.243569643749998122 ) ) ;
#26098=CARTESIAN_POINT ( 'NONE',  ( -4.243569643749999898, 17.15937500061451715, 30.00000000000000000 ) ) ;
#26099=CARTESIAN_POINT ( 'NONE',  ( 23.74687500061451573, -3.027376345333610441, -5.243569643749999898 ) ) ;
#26100=CARTESIAN_POINT ( 'NONE',  ( 4.987500000000002487, -2.886751345948125991, -5.000000000000000000 ) ) ;
#26101=CARTESIAN_POINT ( 'NONE',  ( 3.999999999999999112, 10.88750000122903394, 30.00000000000000000 ) ) ;
#26102=CARTESIAN_POINT ( 'NONE',  ( 13.11562500061451786, 3.027376345333611329, 5.243569643749999010 ) ) ;
#26103=CARTESIAN_POINT ( 'NONE',  ( 3.750000001229034652, -2.886751345948125991, -5.000000000000000000 ) ) ;
#26104=CARTESIAN_POINT ( 'NONE',  ( 9.309375000614517504, -4.541064518000417216, -2.621784821875001281 ) ) ;
#26105=CARTESIAN_POINT ( 'NONE',  ( 3.999999999999999112, 14.93750000122903288, 30.00000000000000000 ) ) ;
#26106=CARTESIAN_POINT ( 'NONE',  ( 10.67812500061451608, 6.421520780324663323E-16, -5.243569643749999010 ) ) ;
#26107=CARTESIAN_POINT ( 'NONE',  ( 14.03437500061451715, 4.541064518000418104, 2.621784821874999949 ) ) ;
#26109=CARTESIAN_POINT ( 'NONE',  ( 21.15000000122903145, -2.886751345948129988, 4.999999999999997335 ) ) ;
#26110=CARTESIAN_POINT ( 'NONE',  ( 11.55937500061451928, -4.541064518000417216, -2.621784821875001281 ) ) ;
#26111=CARTESIAN_POINT ( 'NONE',  ( 12.77812500061451750, -4.541064518000419881, 2.621784821874995952 ) ) ;
#26113=CARTESIAN_POINT ( 'NONE',  ( 21.87187500061451573, -6.054752690667223547, -1.112240025338166033E-15 ) ) ;
#26117=CARTESIAN_POINT ( 'NONE',  ( 4.243569643749999898, 14.19687500061452035, -27.54997392385601529 ) ) ;
#26118=CARTESIAN_POINT ( 'NONE',  ( 16.31250000122903288, -4.330127018922190985, -2.500000000000001332 ) ) ;
#26119=CARTESIAN_POINT ( 'NONE',  ( 10.35937500061451644, 4.541064518000418104, -2.621784821874998173 ) ) ;
#26120=CARTESIAN_POINT ( 'NONE',  ( -3.000416591977282496E-16, 18.34062500061451928, -34.90005215228797653 ) ) ;
#26121=CARTESIAN_POINT ( 'NONE',  ( 17.17500000122903359, -5.773502691896255534, -1.060575238724906372E-15 ) ) ;
#26122=CARTESIAN_POINT ( 'NONE',  ( 13.22812500061451502, -4.541064518000419881, 2.621784821874995952 ) ) ;
#26124=CARTESIAN_POINT ( 'NONE',  ( 16.46249999999999503, 2.886751345948126879, 4.999999999999999112 ) ) ;
#26125=CARTESIAN_POINT ( 'NONE',  ( 5.025000001229035895, -5.773502691896255534, -1.060575238724906372E-15 ) ) ;
#26126=CARTESIAN_POINT ( 'NONE',  ( 9.121875000614517504, 3.027376345333611329, 5.243569643749999010 ) ) ;
#26127=CARTESIAN_POINT ( 'NONE',  ( 4.342984975361706468, -2.477595912125914790, -4.621313785610477787 ) ) ;
#26128=CARTESIAN_POINT ( 'NONE',  ( 11.13750000122903216, 4.330127018922191873, 2.499999999999999556 ) ) ;
#26129=CARTESIAN_POINT ( 'NONE',  ( 18.33750000122903501, 4.330127018922191873, 2.499999999999999556 ) ) ;
#26130=CARTESIAN_POINT ( 'NONE',  ( 16.64062500061451289, 6.054752690667223547, 3.707466751127219781E-16 ) ) ;
#26131=CARTESIAN_POINT ( 'NONE',  ( 20.65312500061451573, 4.541064518000418104, -2.621784821874998173 ) ) ;
#26132=CARTESIAN_POINT ( 'NONE',  ( 28.01250000122903216, -4.330127018922190985, -2.500000000000001332 ) ) ;
#26133=CARTESIAN_POINT ( 'NONE',  ( 3.853125000614517681, -4.541064518000417216, -2.621784821875001281 ) ) ;
#26134=CARTESIAN_POINT ( 'NONE',  ( 25.23749999999999716, -2.886751345948125991, -5.000000000000000000 ) ) ;
#26137=CARTESIAN_POINT ( 'NONE',  ( 29.33437500061451431, 4.541064518000418104, 2.621784821874999949 ) ) ;
#26138=CARTESIAN_POINT ( 'NONE',  ( 11.73750000000000071, -2.886751345948126435, -5.000000000000000000 ) ) ;
#26139=CARTESIAN_POINT ( 'NONE',  ( 11.96250000122903501, 4.330127018922192761, -2.499999999999997780 ) ) ;
#26140=CARTESIAN_POINT ( 'NONE',  ( 29.55937500061451573, -4.541064518000417216, -2.621784821875001281 ) ) ;
#26143=CARTESIAN_POINT ( 'NONE',  ( 7.959375000614516971, -4.541064518000417216, -2.621784821875001281 ) ) ;
#26144=CARTESIAN_POINT ( 'NONE',  ( 24.96562500061451573, -6.054752690667223547, -1.112240025338166033E-15 ) ) ;
#26146=CARTESIAN_POINT ( 'NONE',  ( -2.152738742430647445, 9.767338418468105132, -24.39599078399185217 ) ) ;
#26147=CARTESIAN_POINT ( 'NONE',  ( 3.723272892789626365, -3.337319327924350265, 3.976188005925537450 ) ) ;
#26148=CARTESIAN_POINT ( 'NONE',  ( 4.359375000614517326, -4.541064518000417216, -2.621784821875001281 ) ) ;
#26149=CARTESIAN_POINT ( 'NONE',  ( 8.109375000614518214, 4.541064518000418104, -2.621784821874998173 ) ) ;
#26150=CARTESIAN_POINT ( 'NONE',  ( 5.325000000000000178, -4.330127018922194537, 2.499999999999995559 ) ) ;
#26151=CARTESIAN_POINT ( 'NONE',  ( 4.243569643749999898, 11.89062500061459460, 32.45002607614398471 ) ) ;
#26152=CARTESIAN_POINT ( 'NONE',  ( 20.69999999999999929, -4.330127018922190985, -2.500000000000001332 ) ) ;
#26154=CARTESIAN_POINT ( 'NONE',  ( 29.32499999999999929, 6.123233995736764310E-16, -4.999999999999998224 ) ) ;
#26156=CARTESIAN_POINT ( 'NONE',  ( 4.050000000000001599, -4.330127018922190985, -2.500000000000001332 ) ) ;
#26158=ORIENTED_EDGE ( 'NONE', *, *, #40501, .F. ) ;
#26159=CARTESIAN_POINT ( 'NONE',  ( 21.25312500061451715, 0.000000000000000000, 5.243569643749999010 ) ) ;
#26160=CARTESIAN_POINT ( 'NONE',  ( 9.665625000614515017, -6.054752690667223547, -1.112240025338166033E-15 ) ) ;
#26162=CARTESIAN_POINT ( 'NONE',  ( 6.421875000614519102, 3.027376345333611329, 5.243569643749999010 ) ) ;
#26163=CARTESIAN_POINT ( 'NONE',  ( 24.52499999999999858, 4.330127018922191873, 2.499999999999999556 ) ) ;
#26164=CARTESIAN_POINT ( 'NONE',  ( 20.73750000122903359, -4.330127018922194537, 2.499999999999995559 ) ) ;
#26165=CARTESIAN_POINT ( 'NONE',  ( 27.92812500061451431, 4.541064518000418104, 2.621784821874999949 ) ) ;
#26166=CARTESIAN_POINT ( 'NONE',  ( 9.946875000614516793, 6.054752690667223547, 3.707466751127219781E-16 ) ) ;
#26167=CARTESIAN_POINT ( 'NONE',  ( 13.28437500061451715, -4.541064518000419881, 2.621784821874995952 ) ) ;
#26168=CARTESIAN_POINT ( 'NONE',  ( 24.98437500061451644, -4.541064518000419881, 2.621784821874995952 ) ) ;
#26169=CARTESIAN_POINT ( 'NONE',  ( 3.999999999999999112, 18.08750000122903501, -30.00000000000000000 ) ) ;
#26171=CARTESIAN_POINT ( 'NONE',  ( 18.68437500061451928, -4.541064518000419881, 2.621784821874995952 ) ) ;
#26172=CARTESIAN_POINT ( 'NONE',  ( 9.121875000614517504, 3.027376345333611329, 5.243569643749999010 ) ) ;
#26174=CARTESIAN_POINT ( 'NONE',  ( 23.66250000000000142, 2.886751345948126879, 4.999999999999999112 ) ) ;
#26176=CARTESIAN_POINT ( 'NONE',  ( -3.999999999999999112, 9.725000001229036073, -32.30940107675850470 ) ) ;
#26178=CARTESIAN_POINT ( 'NONE',  ( 11.54062500061451857, -3.027376345333610441, -5.243569643749999898 ) ) ;
#26179=CARTESIAN_POINT ( 'NONE',  ( 3.262500000000001510, 2.886751345948129099, -4.999999999999998224 ) ) ;
#26180=DIRECTION ( 'NONE',  ( -0.000000000000000000, -1.000000000000000000, -0.000000000000000000 ) ) ;
#26182=CARTESIAN_POINT ( 'NONE',  ( 11.32500000000000107, 6.123233995736764310E-16, -4.999999999999998224 ) ) ;
#26183=CARTESIAN_POINT ( 'NONE',  ( -2.828200636599751609E-16, 19.10000000122903074, 25.38119784648299770 ) ) ;
#26184=CARTESIAN_POINT ( 'NONE',  ( 10.42500000122903536, -5.773502691896255534, -1.060575238724906372E-15 ) ) ;
#26185=CARTESIAN_POINT ( 'NONE',  ( 21.60937500061451644, 4.541064518000418104, -2.621784821874998173 ) ) ;
#26186=CARTESIAN_POINT ( 'NONE',  ( 16.20937500061451786, 4.541064518000418104, -2.621784821874998173 ) ) ;
#26188=VERTEX_POINT ( 'NONE', #66902 ) ;
#26189=CARTESIAN_POINT ( 'NONE',  ( 17.01562500061451644, 3.027376345333613106, -5.243569643749998122 ) ) ;
#26190=CARTESIAN_POINT ( 'NONE',  ( 28.83750000122903145, -4.330127018922194537, 2.499999999999995559 ) ) ;
#26191=CARTESIAN_POINT ( 'NONE',  ( 16.95937500061451786, -4.541064518000417216, -2.621784821875001281 ) ) ;
#26192=CARTESIAN_POINT ( 'NONE',  ( 29.55937500061451573, -4.541064518000417216, -2.621784821875001281 ) ) ;
#26193=CARTESIAN_POINT ( 'NONE',  ( 5.615625000614517859, -6.054752690667223547, -1.112240025338166033E-15 ) ) ;
#26194=CARTESIAN_POINT ( 'NONE',  ( 18.40312500061451573, 4.541064518000418104, -2.621784821874998173 ) ) ;
#26196=CARTESIAN_POINT ( 'NONE',  ( 28.13437500061451502, -4.541064518000419881, 2.621784821874995952 ) ) ;
#26197=CARTESIAN_POINT ( 'NONE',  ( -3.000416591977282496E-16, 13.84062500061451928, 25.09994784771203058 ) ) ;
#26198=CARTESIAN_POINT ( 'NONE',  ( 16.31250000122903288, -4.330127018922190985, -2.500000000000001332 ) ) ;
#26200=CARTESIAN_POINT ( 'NONE',  ( 7.640625000614517326, 6.054752690667223547, 3.707466751127219781E-16 ) ) ;
#26201=CARTESIAN_POINT ( 'NONE',  ( 26.95312500061451644, 4.541064518000418104, -2.621784821874998173 ) ) ;
#26202=CARTESIAN_POINT ( 'NONE',  ( 9.750000001229032875, 5.773502691896255534, 3.535250795749688401E-16 ) ) ;
#26203=CARTESIAN_POINT ( 'NONE',  ( 22.02187500061452141, 3.027376345333613106, -5.243569643749998122 ) ) ;
#26204=CARTESIAN_POINT ( 'NONE',  ( 11.99062500061451608, -3.027376345333610441, -5.243569643749999898 ) ) ;
#26205=CARTESIAN_POINT ( 'NONE',  ( 22.38750000122903216, 4.330127018922191873, 2.499999999999999556 ) ) ;
#26206=CARTESIAN_POINT ( 'NONE',  ( 23.27812500061451573, 6.421520780324663323E-16, -5.243569643749999010 ) ) ;
#26207=CARTESIAN_POINT ( 'NONE',  ( 16.77187500061451786, 3.027376345333611329, 5.243569643749999010 ) ) ;
#26208=CARTESIAN_POINT ( 'NONE',  ( 12.85312500061451502, -4.541064518000417216, -2.621784821875001281 ) ) ;
#26209=CARTESIAN_POINT ( 'NONE',  ( -3.000416591977282496E-16, 14.79687500061451821, 25.09994784771203058 ) ) ;
#26210=CARTESIAN_POINT ( 'NONE',  ( 20.87812500061451715, -4.541064518000419881, 2.621784821874995952 ) ) ;
#26211=CARTESIAN_POINT ( 'NONE',  ( 10.16250000000000320, 2.886751345948126879, 4.999999999999998224 ) ) ;
#26212=VERTEX_POINT ( 'NONE', #9646 ) ;
#26213=ORIENTED_EDGE ( 'NONE', *, *, #14786, .F. ) ;
#26214=CARTESIAN_POINT ( 'NONE',  ( 23.92499999999999716, 6.123233995736764310E-16, -4.999999999999998224 ) ) ;
#26215=CARTESIAN_POINT ( 'NONE',  ( -2.121784821874999949, 18.43437500061451928, -33.67503911421598417 ) ) ;
#26217=CARTESIAN_POINT ( 'NONE',  ( 25.94062500061451715, -3.027376345333610441, -5.243569643749999898 ) ) ;
#26218=CARTESIAN_POINT ( 'NONE',  ( 4.528125000614516615, 4.541064518000418104, 2.621784821874999949 ) ) ;
#26219=CARTESIAN_POINT ( 'NONE',  ( 19.27500000122903145, 2.886751345948126879, 4.999999999999999112 ) ) ;
#26220=CARTESIAN_POINT ( 'NONE',  ( 24.14062500061451289, -3.027376345333610441, -5.243569643749999898 ) ) ;
#26221=CARTESIAN_POINT ( 'NONE',  ( 23.28750000000000142, -2.886751345948129988, 4.999999999999997335 ) ) ;
#26222=CARTESIAN_POINT ( 'NONE',  ( 28.04062500061451502, -3.027376345333614438, 5.243569643749998122 ) ) ;
#26223=CARTESIAN_POINT ( 'NONE',  ( 7.190625000614518036, 6.054752690667223547, 3.707466751127219781E-16 ) ) ;
#26226=VECTOR ( 'NONE', #35186, 1000.000000000000000 ) ;
#26227=CARTESIAN_POINT ( 'NONE',  ( 23.50312500061451360, 0.000000000000000000, 5.243569643749999010 ) ) ;
#26228=CARTESIAN_POINT ( 'NONE',  ( 6.028125000614517504, -4.541064518000419881, 2.621784821874995952 ) ) ;
#26230=LINE ( 'NONE', #48768, #9926 ) ;
#26231=CARTESIAN_POINT ( 'NONE',  ( 4.000000000000000000, 13.10000000122903430, -27.69059892324149530 ) ) ;
#26232=CARTESIAN_POINT ( 'NONE',  ( 19.65000000000000213, 0.000000000000000000, 4.999999999999998224 ) ) ;
#26233=EDGE_CURVE ( 'NONE', #64681, #24253, #65792, .T. ) ;
#26234=CARTESIAN_POINT ( 'NONE',  ( 9.825000000000001066, -4.330127018922194537, 2.499999999999995559 ) ) ;
#26235=CARTESIAN_POINT ( 'NONE',  ( 11.33437500061451608, 4.541064518000418104, 2.621784821874999949 ) ) ;
#26236=CARTESIAN_POINT ( 'NONE',  ( 6.562500001229032875, 4.330127018922192761, -2.499999999999997780 ) ) ;
#26237=CARTESIAN_POINT ( 'NONE',  ( 13.62187500061451750, 3.027376345333611329, 5.243569643749999010 ) ) ;
#26239=CARTESIAN_POINT ( 'NONE',  ( 6.834375000614518747, 4.541064518000418104, 2.621784821874999949 ) ) ;
#26240=CARTESIAN_POINT ( 'NONE',  ( -2.121784821874999949, 10.27812500061451750, -33.67503911421598417 ) ) ;
#26241=CARTESIAN_POINT ( 'NONE',  ( 1.626862140677534273E-15, 9.875000001229034652, -26.00000000000000355 ) ) ;
#26242=CARTESIAN_POINT ( 'NONE',  ( 12.45937500061451786, -4.541064518000417216, -2.621784821875001281 ) ) ;
#26243=DIRECTION ( 'NONE',  ( -0.000000000000000000, -1.000000000000000000, -0.000000000000000000 ) ) ;
#26244=CARTESIAN_POINT ( 'NONE',  ( 21.89062500061451289, -3.027376345333610441, -5.243569643749999898 ) ) ;
#26245=CARTESIAN_POINT ( 'NONE',  ( 4.243569643749999898, 11.04687500061451644, 32.45002607614398471 ) ) ;
#26247=CARTESIAN_POINT ( 'NONE',  ( 27.08437500061451786, 4.541064518000418104, 2.621784821874999949 ) ) ;
#26248=CARTESIAN_POINT ( 'NONE',  ( -5.000000000000000000, 0.000000000000000000, -50.00000000000000000 ) ) ;
#26249=CARTESIAN_POINT ( 'NONE',  ( 5.128125000614516260, -4.541064518000419881, 2.621784821874995952 ) ) ;
#26251=CARTESIAN_POINT ( 'NONE',  ( 14.97187500061451892, 3.027376345333611329, 5.243569643749999010 ) ) ;
#26252=CARTESIAN_POINT ( 'NONE',  ( 26.17500000122903359, -5.773502691896255534, -1.060575238724906372E-15 ) ) ;
#26253=CARTESIAN_POINT ( 'NONE',  ( 28.05000000122903359, -2.886751345948125991, -5.000000000000000000 ) ) ;
#26254=CARTESIAN_POINT ( 'NONE',  ( 5.596875000614516260, -3.027376345333614438, 5.243569643749998122 ) ) ;
#26255=CARTESIAN_POINT ( 'NONE',  ( 16.73437500061451644, 4.541064518000418104, 2.621784821874999949 ) ) ;
#26256=CARTESIAN_POINT ( 'NONE',  ( 30.00000000000000000, 0.000000000000000000, 0.000000000000000000 ) ) ;
#26257=CARTESIAN_POINT ( 'NONE',  ( 23.81250000000000000, -5.773502691896255534, -1.060575238724906372E-15 ) ) ;
#26258=CARTESIAN_POINT ( 'NONE',  ( 2.700000001229035718, -2.886751345948129988, 4.999999999999997335 ) ) ;
#26259=CARTESIAN_POINT ( 'NONE',  ( 27.45937500061451786, 4.541064518000418104, -2.621784821874998173 ) ) ;
#26261=FACE_OUTER_BOUND ( 'NONE', #10856, .T. ) ;
#26262=CARTESIAN_POINT ( 'NONE',  ( 6.975000000000002309, 4.330127018922191873, 2.499999999999999556 ) ) ;
#26264=CARTESIAN_POINT ( 'NONE',  ( 18.81562500061452070, 3.027376345333613106, -5.243569643749998122 ) ) ;
#26265=CARTESIAN_POINT ( 'NONE',  ( 11.73750000000000249, -2.886751345948125991, -5.000000000000000000 ) ) ;
#26266=CARTESIAN_POINT ( 'NONE',  ( 3.553125000614516082, 4.541064518000418104, -2.621784821874998173 ) ) ;
#26267=CARTESIAN_POINT ( 'NONE',  ( 18.89999999999999858, -4.330127018922190985, -2.500000000000001332 ) ) ;
#26268=CARTESIAN_POINT ( 'NONE',  ( 19.15312500061451573, -4.541064518000417216, -2.621784821875001281 ) ) ;
#26269=CARTESIAN_POINT ( 'NONE',  ( 15.63750000122903216, 4.330127018922191873, 2.499999999999999556 ) ) ;
#26270=CARTESIAN_POINT ( 'NONE',  ( 22.42500000122903359, 2.886751345948126879, 4.999999999999999112 ) ) ;
#26272=CARTESIAN_POINT ( 'NONE',  ( 29.25937500061451502, 4.541064518000418104, -2.621784821874998173 ) ) ;
#26273=ORIENTED_EDGE ( 'NONE', *, *, #62569, .T. ) ;
#26274=CARTESIAN_POINT ( 'NONE',  ( 18.59062500061451573, -3.027376345333614438, 5.243569643749998122 ) ) ;
#26275=CARTESIAN_POINT ( 'NONE',  ( 25.52812500061451573, 6.421520780324663323E-16, -5.243569643749999010 ) ) ;
#26276=CARTESIAN_POINT ( 'NONE',  ( 25.13437500061451502, 6.421520780324663323E-16, -5.243569643749999010 ) ) ;
#26277=CARTESIAN_POINT ( 'NONE',  ( 8.587500000000002132, -2.886751345948125991, -5.000000000000000000 ) ) ;
#26278=CARTESIAN_POINT ( 'NONE',  ( 12.51562500061451821, 3.027376345333613106, -5.243569643749998122 ) ) ;
#26279=CARTESIAN_POINT ( 'NONE',  ( 25.75312500061451715, 0.000000000000000000, 5.243569643749999010 ) ) ;
#26280=CARTESIAN_POINT ( 'NONE',  ( 16.80937500061451573, 0.000000000000000000, 5.243569643749999010 ) ) ;
#26281=CARTESIAN_POINT ( 'NONE',  ( 7.903125000614515727, -4.541064518000417216, -2.621784821875001281 ) ) ;
#26282=DIRECTION ( 'NONE',  ( -0.000000000000000000, -1.000000000000000000, -0.000000000000000000 ) ) ;
#26283=CARTESIAN_POINT ( 'NONE',  ( -0.7368881354385758975, 9.859898613939513723, 25.82089971438751519 ) ) ;
#26284=CARTESIAN_POINT ( 'NONE',  ( 22.91250000122903430, 0.000000000000000000, 4.999999999999998224 ) ) ;
#26286=CARTESIAN_POINT ( 'NONE',  ( 14.65312500061451573, -4.541064518000417216, -2.621784821875001281 ) ) ;
#26287=CARTESIAN_POINT ( 'NONE',  ( 7.884375000614517681, -4.541064518000419881, 2.621784821874995952 ) ) ;
#26288=CARTESIAN_POINT ( 'NONE',  ( 7.246875000614518392, 6.054752690667223547, 3.707466751127219781E-16 ) ) ;
#26289=ORIENTED_EDGE ( 'NONE', *, *, #51085, .F. ) ;
#26290=EDGE_CURVE ( 'NONE', #30796, #50879, #61570, .T. ) ;
#26291=CARTESIAN_POINT ( 'NONE',  ( 29.14687500061451075, -3.027376345333610441, -5.243569643749999898 ) ) ;
#26292=CARTESIAN_POINT ( 'NONE',  ( 22.67812500061451431, -4.541064518000419881, 2.621784821874995952 ) ) ;
#26293=CARTESIAN_POINT ( 'NONE',  ( 16.54687500061451644, -3.027376345333610441, -5.243569643749999898 ) ) ;
#26294=CARTESIAN_POINT ( 'NONE',  ( 19.56562500061451715, -6.054752690667223547, -1.112240025338166033E-15 ) ) ;
#26295=CARTESIAN_POINT ( 'NONE',  ( 3.999999999999998668, 11.26250000000000107, 27.69059892324149175 ) ) ;
#26296=CARTESIAN_POINT ( 'NONE',  ( 26.31562500061451715, -6.054752690667223547, -1.112240025338166033E-15 ) ) ;
#26297=CARTESIAN_POINT ( 'NONE',  ( 8.025000001229035007, 2.886751345948126879, 4.999999999999999112 ) ) ;
#26298=ORIENTED_EDGE ( 'NONE', *, *, #13854, .F. ) ;
#26299=CARTESIAN_POINT ( 'NONE',  ( 29.84999999999999787, 4.330127018922192761, -2.499999999999997780 ) ) ;
#26300=CARTESIAN_POINT ( 'NONE',  ( -1.999999999999997113, 18.27499999999999858, -26.53589838486224295 ) ) ;
#26301=CARTESIAN_POINT ( 'NONE',  ( 24.33750000122903145, -4.330127018922194537, 2.499999999999995559 ) ) ;
#26303=CARTESIAN_POINT ( 'NONE',  ( 6.646875000614518747, -3.027376345333610441, -5.243569643749999898 ) ) ;
#26304=CARTESIAN_POINT ( 'NONE',  ( 30.00000000000000000, 0.000000000000000000, 0.000000000000000000 ) ) ;
#26305=CARTESIAN_POINT ( 'NONE',  ( 13.07812500061451821, 4.541064518000418104, 2.621784821874999949 ) ) ;
#26306=CARTESIAN_POINT ( 'NONE',  ( 8.596875000614518925, 6.054752690667223547, 3.707466751127219781E-16 ) ) ;
#26307=CARTESIAN_POINT ( 'NONE',  ( 27.30000000122903359, 5.773502691896255534, 3.535250795749688894E-16 ) ) ;
#26308=CARTESIAN_POINT ( 'NONE',  ( 16.69687500061451502, 6.054752690667223547, 3.707466751127219781E-16 ) ) ;
#26309=CARTESIAN_POINT ( 'NONE',  ( 5.071875000614519458, 3.027376345333611329, 5.243569643749999010 ) ) ;
#26310=CARTESIAN_POINT ( 'NONE',  ( -5.810221930991193690E-16, 10.88749999999999929, 26.00000000000000355 ) ) ;
#26311=CARTESIAN_POINT ( 'NONE',  ( 5.653125000614517504, -4.541064518000417216, -2.621784821875001281 ) ) ;
#26312=CARTESIAN_POINT ( 'NONE',  ( 16.15312500061451573, 4.541064518000418104, -2.621784821874998173 ) ) ;
#26313=ORIENTED_EDGE ( 'NONE', *, *, #3226, .T. ) ;
#26314=CARTESIAN_POINT ( 'NONE',  ( 11.61562500061451608, 3.027376345333613106, -5.243569643749998122 ) ) ;
#26315=CARTESIAN_POINT ( 'NONE',  ( 5.775000001229033231, 2.886751345948126879, 4.999999999999999112 ) ) ;
#26316=CARTESIAN_POINT ( 'NONE',  ( 8.615625000614517859, 3.027376345333611329, 5.243569643749999010 ) ) ;
#26318=CARTESIAN_POINT ( 'NONE',  ( 8.775000000000002132, 4.330127018922191873, 2.499999999999999556 ) ) ;
#26319=CARTESIAN_POINT ( 'NONE',  ( 3.187500001229033764, -4.330127018922194537, 2.499999999999995559 ) ) ;
#26321=CARTESIAN_POINT ( 'NONE',  ( 17.06250000000000000, -5.773502691896255534, -1.060575238724906372E-15 ) ) ;
#26323=CARTESIAN_POINT ( 'NONE',  ( 17.48437500061451999, 6.421520780324663323E-16, -5.243569643749999010 ) ) ;
#26324=CARTESIAN_POINT ( 'NONE',  ( 15.90000000122903501, -2.886751345948125991, -5.000000000000000000 ) ) ;
#26326=CARTESIAN_POINT ( 'NONE',  ( -2.121784821874999949, 15.67812500061451608, -33.67503911421598417 ) ) ;
#26327=CARTESIAN_POINT ( 'NONE',  ( 3.228971818887576006, 3.817556940351970685, 3.594618424259643508 ) ) ;
#26329=CARTESIAN_POINT ( 'NONE',  ( 28.11562500061451431, -6.054752690667223547, -1.112240025338166033E-15 ) ) ;
#26330=CARTESIAN_POINT ( 'NONE',  ( 20.02500000122902790, 2.886751345948095793, -5.000000000000055067 ) ) ;
#26331=CARTESIAN_POINT ( 'NONE',  ( 4.000000000000000000, 14.45000000122903572, 32.30940107675849760 ) ) ;
#26332=CARTESIAN_POINT ( 'NONE',  ( 15.12187500061451750, -6.054752690667223547, -1.112240025338166033E-15 ) ) ;
#26333=CARTESIAN_POINT ( 'NONE',  ( 29.21249999999999858, -5.773502691896255534, -1.060575238724906372E-15 ) ) ;
#26334=CARTESIAN_POINT ( 'NONE',  ( 12.77812500061451750, -4.541064518000419881, 2.621784821874995952 ) ) ;
#26336=CARTESIAN_POINT ( 'NONE',  ( 21.23437500061451644, 4.541064518000418104, 2.621784821874999949 ) ) ;
#26338=CARTESIAN_POINT ( 'NONE',  ( 8.390625000614518214, -3.027376345333610441, -5.243569643749999898 ) ) ;
#26339=CARTESIAN_POINT ( 'NONE',  ( 13.92187500061451644, 3.027376345333613106, -5.243569643749998122 ) ) ;
#26341=CARTESIAN_POINT ( 'NONE',  ( 23.33437500061451786, 6.421520780324663323E-16, -5.243569643749999010 ) ) ;
#26342=CARTESIAN_POINT ( 'NONE',  ( 27.06562500061451004, 3.027376345333611329, 5.243569643749999010 ) ) ;
#26343=FACE_BOUND ( 'NONE', #62914, .T. ) ;
#26344=CARTESIAN_POINT ( 'NONE',  ( 8.099999999999999645, -4.330127018922190985, -2.500000000000001332 ) ) ;
#26345=CARTESIAN_POINT ( 'NONE',  ( 17.70000000122903216, -2.886751345948125991, -5.000000000000000000 ) ) ;
#26346=CARTESIAN_POINT ( 'NONE',  ( 7.320879633048903241E-15, 17.75000000122903288, -34.00000000000000000 ) ) ;
#26349=CARTESIAN_POINT ( 'NONE',  ( 15.90000000000000036, 4.330127018922192761, -2.499999999999997780 ) ) ;
#26350=CARTESIAN_POINT ( 'NONE',  ( 18.33749999999999858, -2.886751345948129988, 4.999999999999997335 ) ) ;
#26351=CARTESIAN_POINT ( 'NONE',  ( 12.02812500061451573, 6.421520780324663323E-16, -5.243569643749999010 ) ) ;
#26352=VERTEX_POINT ( 'NONE', #29810 ) ;
#26353=CARTESIAN_POINT ( 'NONE',  ( -2.000000000000000000, 10.92500000000000071, -33.46410161513775705 ) ) ;
#26354=CARTESIAN_POINT ( 'NONE',  ( 4.243569643749999010, 16.52187500061451786, -32.45002607614398471 ) ) ;
#26355=CARTESIAN_POINT ( 'NONE',  ( 4.228125000614517681, -4.541064518000419881, 2.621784821874995952 ) ) ;
#26357=CARTESIAN_POINT ( 'NONE',  ( 10.01250000000000107, 2.886751345948129099, -4.999999999999998224 ) ) ;
#26358=CARTESIAN_POINT ( 'NONE',  ( 20.77500000000000213, 6.123233995736764310E-16, -4.999999999999998224 ) ) ;
#26359=ORIENTED_EDGE ( 'NONE', *, *, #27838, .F. ) ;
#26360=CARTESIAN_POINT ( 'NONE',  ( 2.121784821875001281, 13.20312500061451821, 33.67503911421598417 ) ) ;
#26361=CARTESIAN_POINT ( 'NONE',  ( 25.90312500061451573, -4.541064518000417216, -2.621784821875001281 ) ) ;
#26362=LINE ( 'NONE', #61070, #49028 ) ;
#26363=FACE_OUTER_BOUND ( 'NONE', #42619, .T. ) ;
#26364=CARTESIAN_POINT ( 'NONE',  ( 20.48437500061451289, -4.541064518000419881, 2.621784821874995952 ) ) ;
#26365=CARTESIAN_POINT ( 'NONE',  ( 19.19062500061452070, -3.027376345333610441, -5.243569643749999898 ) ) ;
#26366=CARTESIAN_POINT ( 'NONE',  ( 4.243569643749999898, 13.27812500061459566, -30.00000000000000000 ) ) ;
#26367=CARTESIAN_POINT ( 'NONE',  ( 24.52500000122903145, 2.886751345948129099, -4.999999999999998224 ) ) ;
#26368=CARTESIAN_POINT ( 'NONE',  ( 3.140625000614516882, 6.054752690667223547, 3.707466751127219781E-16 ) ) ;
#26370=CARTESIAN_POINT ( 'NONE',  ( 21.44062500061452070, -3.027376345333610441, -5.243569643749999898 ) ) ;
#26373=( BOUNDED_CURVE ( )  B_SPLINE_CURVE ( 2, ( #49671, #10140, #33033, #27500, #26397, #48939, #72198 ),
 .UNSPECIFIED., .F., .F. ) 
 B_SPLINE_CURVE_WITH_KNOTS ( ( 3, 2, 2, 3 ),
 ( 0.8499999999999999778, 0.8527777777777777457, 0.8555555555555555136, 0.8583333333333332815 ),
 .UNSPECIFIED. ) 
 CURVE ( )  GEOMETRIC_REPRESENTATION_ITEM ( )  RATIONAL_B_SPLINE_CURVE ( ( 1.000000000000000000, 0.8660254037844387076, 1.000000000000000000, 0.8660254037844387076, 1.000000000000000000, 0.8660254037844387076, 1.000000000000000000 ) ) 
 REPRESENTATION_ITEM ( '' )  );
#26374=CARTESIAN_POINT ( 'NONE',  ( 14.48437500061451821, 4.541064518000418104, 2.621784821874999949 ) ) ;
#26375=CARTESIAN_POINT ( 'NONE',  ( 15.23437500061451644, 6.421520780324663323E-16, -5.243569643749999010 ) ) ;
#26376=CARTESIAN_POINT ( 'NONE',  ( 25.77187500061451075, 3.027376345333611329, 5.243569643749999010 ) ) ;
#26377=CARTESIAN_POINT ( 'NONE',  ( -2.121784821874999949, 14.83437500061451786, 26.32496088578401938 ) ) ;
#26378=CARTESIAN_POINT ( 'NONE',  ( 4.940625000614515372, 6.054752690667223547, 3.707466751127219781E-16 ) ) ;
#26379=CARTESIAN_POINT ( 'NONE',  ( 28.94062500061452070, -3.027376345333614438, 5.243569643749998122 ) ) ;
#26380=CARTESIAN_POINT ( 'NONE',  ( 28.04062500061451502, -3.027376345333614438, 5.243569643749998122 ) ) ;
#26381=CARTESIAN_POINT ( 'NONE',  ( 3.999999999999999112, 16.28750000122903430, -30.00000000000000000 ) ) ;
#26382=CARTESIAN_POINT ( 'NONE',  ( -2.000000000000000000, 19.92500000000000071, 26.53589838486224650 ) ) ;
#26383=CARTESIAN_POINT ( 'NONE',  ( 7.134375000614516793, 6.421520780324663323E-16, -5.243569643749999010 ) ) ;
#26385=CARTESIAN_POINT ( 'NONE',  ( 15.07500000122903394, 2.886751345948129099, -4.999999999999998224 ) ) ;
#26386=CARTESIAN_POINT ( 'NONE',  ( 10.42500000122903536, -5.773502691896255534, -1.060575238724906372E-15 ) ) ;
#26387=CARTESIAN_POINT ( 'NONE',  ( 4.603125000614518569, 0.000000000000000000, 5.243569643749999010 ) ) ;
#26390=CARTESIAN_POINT ( 'NONE',  ( 13.58437500061451786, 4.541064518000418104, 2.621784821874999949 ) ) ;
#26391=CARTESIAN_POINT ( 'NONE',  ( 21.03750000000000142, -2.886751345948096681, 5.000000000000054179 ) ) ;
#26393=CARTESIAN_POINT ( 'NONE',  ( 22.67812500061451431, -4.541064518000419881, 2.621784821874995952 ) ) ;
#26394=CARTESIAN_POINT ( 'NONE',  ( 8.278125000614515727, -4.541064518000419881, 2.621784821874995952 ) ) ;
#26395=CARTESIAN_POINT ( 'NONE',  ( 25.69687500061451502, 6.054752690667223547, 3.707466751127219781E-16 ) ) ;
#26396=CARTESIAN_POINT ( 'NONE',  ( 8.053125000614516082, 4.541064518000418104, -2.621784821874998173 ) ) ;
#26397=CARTESIAN_POINT ( 'NONE',  ( 6.562500001229032875, 4.330127018922192761, -2.499999999999997780 ) ) ;
#26398=CARTESIAN_POINT ( 'NONE',  ( 8.512500001229033941, 0.000000000000000000, 4.999999999999998224 ) ) ;
#26399=CARTESIAN_POINT ( 'NONE',  ( 23.69062500061451004, -3.027376345333610441, -5.243569643749999898 ) ) ;
#26400=CARTESIAN_POINT ( 'NONE',  ( -4.243569643749999898, 10.76562500061451644, -32.45002607614398471 ) ) ;
#26401=CARTESIAN_POINT ( 'NONE',  ( 10.65000000122903323, 5.773502691896255534, 3.535250795749688894E-16 ) ) ;
#26402=CARTESIAN_POINT ( 'NONE',  ( 18.70312500061451644, -4.541064518000417216, -2.621784821875001281 ) ) ;
#26403=CARTESIAN_POINT ( 'NONE',  ( 14.46562500061451750, 3.027376345333611329, 5.243569643749999010 ) ) ;
#26405=CARTESIAN_POINT ( 'NONE',  ( 14.84999999999999964, -4.330127018922190985, -2.500000000000001332 ) ) ;
#26406=CARTESIAN_POINT ( 'NONE',  ( 10.27500000122903323, 2.886751345948126879, 4.999999999999999112 ) ) ;
#26407=CARTESIAN_POINT ( 'NONE',  ( 7.565625000614518036, 3.027376345333613106, -5.243569643749998122 ) ) ;
#26408=CARTESIAN_POINT ( 'NONE',  ( 11.42812500061451608, -4.541064518000419881, 2.621784821874995952 ) ) ;
#26409=EDGE_CURVE ( 'NONE', #12792, #45611, #58338, .T. ) ;
#26410=CARTESIAN_POINT ( 'NONE',  ( 22.16250000122903074, -4.330127018922190985, -2.500000000000001332 ) ) ;
#26411=CARTESIAN_POINT ( 'NONE',  ( 19.39687500061451786, 6.054752690667223547, 3.707466751127219781E-16 ) ) ;
#26413=CARTESIAN_POINT ( 'NONE',  ( 4.312500001229034652, 4.330127018922192761, -2.499999999999997780 ) ) ;
#26415=CARTESIAN_POINT ( 'NONE',  ( 4.846875000614519813, -3.027376345333610441, -5.243569643749999898 ) ) ;
#26416=CARTESIAN_POINT ( 'NONE',  ( 24.38437500061451502, 4.541064518000418104, 2.621784821874999949 ) ) ;
#26417=( BOUNDED_CURVE ( )  B_SPLINE_CURVE ( 2, ( #17695, #21, #17343, #39533, #56156, #38811, #34697 ),
 .UNSPECIFIED., .F., .F. ) 
 B_SPLINE_CURVE_WITH_KNOTS ( ( 3, 2, 2, 3 ),
 ( 0.4249999999999999889, 0.4277777777777777568, 0.4305555555555555802, 0.4333333333333333481 ),
 .UNSPECIFIED. ) 
 CURVE ( )  GEOMETRIC_REPRESENTATION_ITEM ( )  RATIONAL_B_SPLINE_CURVE ( ( 1.000000000000000000, 0.8660254037844387076, 1.000000000000000000, 0.8660254037844387076, 1.000000000000000000, 0.8660254037844387076, 1.000000000000000000 ) ) 
 REPRESENTATION_ITEM ( '' )  );
#26419=CARTESIAN_POINT ( 'NONE',  ( 19.71562500061451928, 3.027376345333613106, -5.243569643749998122 ) ) ;
#26420=CARTESIAN_POINT ( 'NONE',  ( 25.43437500061451573, -4.541064518000419881, 2.621784821874995952 ) ) ;
#26422=CARTESIAN_POINT ( 'NONE',  ( 12.33750000122903145, 6.123233995736764310E-16, -4.999999999999998224 ) ) ;
#26423=LINE ( 'NONE', #48964, #44273 ) ;
#26424=CARTESIAN_POINT ( 'NONE',  ( 4.584375000614516971, 4.541064518000418104, 2.621784821874999949 ) ) ;
#26426=CARTESIAN_POINT ( 'NONE',  ( 15.06562500061451537, -6.054752690667223547, -1.112240025338166033E-15 ) ) ;
#26427=CARTESIAN_POINT ( 'NONE',  ( 13.47187500061451537, 3.027376345333613106, -5.243569643749998122 ) ) ;
#26429=CARTESIAN_POINT ( 'NONE',  ( 9.225000000000001421, 4.330127018922191873, 2.499999999999999556 ) ) ;
#26430=CARTESIAN_POINT ( 'NONE',  ( 26.05312500061451431, 4.541064518000418104, -2.621784821874998173 ) ) ;
#26431=CARTESIAN_POINT ( 'NONE',  ( 3.447219858367251533, 3.621695079390137018, -3.577502417051553696 ) ) ;
#26432=CARTESIAN_POINT ( 'NONE',  ( -3.999999999999997335, 11.60000000122903430, -27.69059892324149530 ) ) ;
#26433=CARTESIAN_POINT ( 'NONE',  ( 13.98750000000000249, -2.886751345948125991, -5.000000000000000000 ) ) ;
#26434=CARTESIAN_POINT ( 'NONE',  ( 23.96250000122903145, -4.330127018922190985, -2.500000000000001332 ) ) ;
#26435=CARTESIAN_POINT ( 'NONE',  ( 18.44062500061451715, 6.054752690667223547, 3.707466751127219781E-16 ) ) ;
#26437=CARTESIAN_POINT ( 'NONE',  ( 23.17500000000000071, 4.330127018922191873, 2.499999999999999556 ) ) ;
#26438=CARTESIAN_POINT ( 'NONE',  ( 23.97187500061451360, 3.027376345333611329, 5.243569643749999010 ) ) ;
#26440=VERTEX_POINT ( 'NONE', #18705 ) ;
#26441=CARTESIAN_POINT ( 'NONE',  ( 3.002593080208402654, -3.998053875910604127, -3.392725720445497473 ) ) ;
#26442=CARTESIAN_POINT ( 'NONE',  ( 11.01562500061451821, -6.054752690667223547, -1.112240025338166033E-15 ) ) ;
#26443=CARTESIAN_POINT ( 'NONE',  ( 2.915625000614516793, -6.054752690667223547, -1.112240025338166033E-15 ) ) ;
#26445=CARTESIAN_POINT ( 'NONE',  ( 27.92812500061451431, 4.541064518000418104, 2.621784821874999949 ) ) ;
#26446=CARTESIAN_POINT ( 'NONE',  ( 18.07499999999999929, 6.123233995736764310E-16, -4.999999999999998224 ) ) ;
#26447=CARTESIAN_POINT ( 'NONE',  ( 25.94999999999999929, 0.000000000000000000, 4.999999999999998224 ) ) ;
#26448=CARTESIAN_POINT ( 'NONE',  ( 4.000000000000000000, 10.73750000000000071, -27.69059892324149885 ) ) ;
#26449=CARTESIAN_POINT ( 'NONE',  ( 7.246875000614518392, 6.054752690667223547, 3.707466751127219781E-16 ) ) ;
#26450=CARTESIAN_POINT ( 'NONE',  ( 18.00937500061451502, 4.541064518000418104, -2.621784821874998173 ) ) ;
#26451=CARTESIAN_POINT ( 'NONE',  ( 30.00000000000000000, 0.000000000000000000, 0.000000000000000000 ) ) ;
#26452=ORIENTED_EDGE ( 'NONE', *, *, #72086, .F. ) ;
#26453=CARTESIAN_POINT ( 'NONE',  ( 27.47812500061451502, 4.541064518000418104, 2.621784821874999949 ) ) ;
#26454=CARTESIAN_POINT ( 'NONE',  ( 26.89687500061451431, -3.027376345333610441, -5.243569643749999898 ) ) ;
#26456=CARTESIAN_POINT ( 'NONE',  ( 13.42499999999999893, -4.330127018922194537, 2.499999999999995559 ) ) ;
#26457=CARTESIAN_POINT ( 'NONE',  ( 10.37812500061451715, 4.541064518000418104, 2.621784821874999949 ) ) ;
#26460=CARTESIAN_POINT ( 'NONE',  ( -0.7368881354385758975, 9.803648613939513368, -34.17910028561248481 ) ) ;
#26461=CARTESIAN_POINT ( 'NONE',  ( 16.08750000122903501, 4.330127018922191873, 2.499999999999999556 ) ) ;
#26462=CARTESIAN_POINT ( 'NONE',  ( 15.15000000122903323, 5.773502691896255534, 3.535250795749688401E-16 ) ) ;
#26464=CARTESIAN_POINT ( 'NONE',  ( 4.415625000614518569, 3.027376345333613106, -5.243569643749998122 ) ) ;
#26465=CARTESIAN_POINT ( 'NONE',  ( 22.02187500061452141, 3.027376345333613106, -5.243569643749998122 ) ) ;
#26466=CARTESIAN_POINT ( 'NONE',  ( 4.243569643749999898, 18.24687500061451928, 32.45002607614398471 ) ) ;
#26467=CARTESIAN_POINT ( 'NONE',  ( 23.18437500061451573, -4.541064518000419881, 2.621784821874995952 ) ) ;
#26468=CARTESIAN_POINT ( 'NONE',  ( 4.575000000000002842, 6.123233995736764310E-16, -4.999999999999998224 ) ) ;
#26469=CARTESIAN_POINT ( 'NONE',  ( -3.999999999999997335, 10.70000000122903394, 32.30940107675850470 ) ) ;
#26470=CARTESIAN_POINT ( 'NONE',  ( 12.25312500061451537, 0.000000000000000000, 5.243569643749999010 ) ) ;
#26471=CARTESIAN_POINT ( 'NONE',  ( 4.950000001229033941, -2.886751345948129988, 4.999999999999997335 ) ) ;
#26472=EDGE_CURVE ( 'NONE', #18997, #32666, #41269, .T. ) ;
#26473=CARTESIAN_POINT ( 'NONE',  ( 9.084375000614517859, 4.541064518000418104, 2.621784821874999949 ) ) ;
#26474=CARTESIAN_POINT ( 'NONE',  ( 9.440625000614517148, 6.054752690667223547, 3.707466751127219781E-16 ) ) ;
#26475=CARTESIAN_POINT ( 'NONE',  ( 13.99687500061451928, 6.054752690667223547, 3.707466751127219781E-16 ) ) ;
#26477=CARTESIAN_POINT ( 'NONE',  ( 21.33750000122903145, 6.123233995736764310E-16, -4.999999999999998224 ) ) ;
#26478=CARTESIAN_POINT ( 'NONE',  ( 10.13437500061451679, -4.541064518000419881, 2.621784821874995952 ) ) ;
#26479=CARTESIAN_POINT ( 'NONE',  ( 13.15312500061451750, 0.000000000000000000, 5.243569643749999010 ) ) ;
#26481=CARTESIAN_POINT ( 'NONE',  ( 21.83437500061451786, -4.541064518000419881, 2.621784821874995952 ) ) ;
#26482=CARTESIAN_POINT ( 'NONE',  ( 25.50000000122903288, 5.773502691896255534, 3.535250795749688401E-16 ) ) ;
#26483=CARTESIAN_POINT ( 'NONE',  ( -3.963752180954429605, 3.047823949009539124, 30.55459436224499115 ) ) ;
#26484=CARTESIAN_POINT ( 'NONE',  ( 3.274239950736235638, 3.778839813355128641, -3.307020945026925673 ) ) ;
#26485=CARTESIAN_POINT ( 'NONE',  ( 2.121784821875001281, 11.45937500061451786, -26.32496088578401938 ) ) ;
#26486=CARTESIAN_POINT ( 'NONE',  ( 15.63750000122903216, 4.330127018922191873, 2.499999999999999556 ) ) ;
#26487=CARTESIAN_POINT ( 'NONE',  ( 10.54687500061451644, -3.027376345333614438, 5.243569643749998122 ) ) ;
#26488=CARTESIAN_POINT ( 'NONE',  ( -3.000416591977282496E-16, 17.44062500061451360, -34.90005215228797653 ) ) ;
#26489=CARTESIAN_POINT ( 'NONE',  ( 18.15000000122903501, -2.886751345948125991, -5.000000000000000000 ) ) ;
#26490=CARTESIAN_POINT ( 'NONE',  ( 10.86562500061451431, 3.027376345333611329, 5.243569643749999010 ) ) ;
#26492=CARTESIAN_POINT ( 'NONE',  ( 15.07499999999999929, 4.330127018922191873, 2.499999999999999556 ) ) ;
#26493=CARTESIAN_POINT ( 'NONE',  ( 4.678147931978664076, 1.767710935909229342, -4.678147931978664076 ) ) ;
#26494=CARTESIAN_POINT ( 'NONE',  ( 10.80937500061451928, 4.541064518000418104, -2.621784821874998173 ) ) ;
#26496=CARTESIAN_POINT ( 'NONE',  ( 2.972982959257041813, 4.020181188108474579, -3.027672370053282158 ) ) ;
#26497=CARTESIAN_POINT ( 'NONE',  ( 9.337500001229033231, 4.330127018922191873, 2.499999999999999556 ) ) ;
#26498=CARTESIAN_POINT ( 'NONE',  ( 18.11250000122903359, -4.330127018922190985, -2.500000000000001332 ) ) ;
#26500=CARTESIAN_POINT ( 'NONE',  ( 14.57812500061451644, -4.541064518000419881, 2.621784821874995952 ) ) ;
#26501=CARTESIAN_POINT ( 'NONE',  ( 18.81562500061452070, 3.027376345333613106, -5.243569643749998122 ) ) ;
#26502=CARTESIAN_POINT ( 'NONE',  ( 28.91250000122903074, -4.330127018922190985, -2.500000000000001332 ) ) ;
#26504=CARTESIAN_POINT ( 'NONE',  ( 29.51250000122903216, 4.330127018922192761, -2.499999999999997780 ) ) ;
#26505=CARTESIAN_POINT ( 'NONE',  ( 24.03750000000000142, 5.773502691896255534, 3.535250795749688894E-16 ) ) ;
#26507=AXIS2_PLACEMENT_3D ( 'NONE', #64746, #35938, #58461 ) ;
#26509=CARTESIAN_POINT ( 'NONE',  ( 24.90937500061451715, 0.000000000000000000, 5.243569643749999010 ) ) ;
#26511=CARTESIAN_POINT ( 'NONE',  ( 13.08750000122903323, -4.330127018922194537, 2.499999999999995559 ) ) ;
#26512=CARTESIAN_POINT ( 'NONE',  ( 29.52187500061451431, -6.054752690667223547, -1.112240025338166033E-15 ) ) ;
#26515=CARTESIAN_POINT ( 'NONE',  ( 6.346875000614517148, 6.054752690667223547, 3.707466751127219781E-16 ) ) ;
#26516=B_SPLINE_CURVE_WITH_KNOTS ( 'NONE', 3,
 ( #2201, #47259, #71991, #60891, #66819, #9924, #45010, #16192, #54997, #21365 ),
 .UNSPECIFIED., .F., .F.,
 ( 4, 3, 3, 4 ),
 ( 1.914080865847744861E-16, 2.812508936123897185E-05, 5.625017725354377072E-05, 0.0001049420589380106804 ),
 .UNSPECIFIED. ) ;
#26517=CARTESIAN_POINT ( 'NONE',  ( 26.39062500061451644, -3.027376345333610441, -5.243569643749999898 ) ) ;
#26518=CARTESIAN_POINT ( 'NONE',  ( -6.275039685470489619E-15, 17.97500000122903074, -26.00000000000000355 ) ) ;
#26519=CARTESIAN_POINT ( 'NONE',  ( -1.585543809737899990, 9.875380255848552835, -24.20988672647330731 ) ) ;
#26521=CARTESIAN_POINT ( 'NONE',  ( 6.421875000614519102, 3.027376345333611329, 5.243569643749999010 ) ) ;
#26522=CARTESIAN_POINT ( 'NONE',  ( 9.984375000614518214, 4.541064518000418104, 2.621784821874999949 ) ) ;
#26523=CARTESIAN_POINT ( 'NONE',  ( 29.40937500061451715, 0.000000000000000000, 5.243569643749999010 ) ) ;
#26524=CARTESIAN_POINT ( 'NONE',  ( 4.243569643749999010, 11.96562500061459389, 27.54997392385601174 ) ) ;
#26525=CARTESIAN_POINT ( 'NONE',  ( 22.01249999999999574, -5.773502691896255534, -1.060575238724906372E-15 ) ) ;
#26526=CARTESIAN_POINT ( 'NONE',  ( 29.85937500061451644, 0.000000000000000000, 5.243569643749999010 ) ) ;
#26528=CARTESIAN_POINT ( 'NONE',  ( 18.10312500061451502, 0.000000000000000000, 5.243569643749999010 ) ) ;
#26529=CARTESIAN_POINT ( 'NONE',  ( 11.09062500061451573, -3.027376345333610441, -5.243569643749999898 ) ) ;
#26531=CARTESIAN_POINT ( 'NONE',  ( 8.109375000614518214, 4.541064518000418104, -2.621784821874998173 ) ) ;
#26532=CARTESIAN_POINT ( 'NONE',  ( 24.71250000000000213, -5.773502691896255534, -1.060575238724906372E-15 ) ) ;
#26533=CARTESIAN_POINT ( 'NONE',  ( 20.66250000122903074, 0.000000000000000000, 4.999999999999998224 ) ) ;
#26536=CARTESIAN_POINT ( 'NONE',  ( 8.521875000614516082, 3.027376345333613106, -5.243569643749998122 ) ) ;
#26537=CARTESIAN_POINT ( 'NONE',  ( 14.10937500061451644, 0.000000000000000000, 5.243569643749999010 ) ) ;
#26538=CARTESIAN_POINT ( 'NONE',  ( 25.28437500061451715, 4.541064518000418104, 2.621784821874999949 ) ) ;
#26541=CARTESIAN_POINT ( 'NONE',  ( 18.49687500061452283, 6.054752690667223547, 3.707466751127219781E-16 ) ) ;
#26543=CARTESIAN_POINT ( 'NONE',  ( 8.296875000614516438, -3.027376345333614438, 5.243569643749998122 ) ) ;
#26545=CARTESIAN_POINT ( 'NONE',  ( 20.02500000000000213, 4.330127018922191873, 2.499999999999999556 ) ) ;
#26547=CARTESIAN_POINT ( 'NONE',  ( 29.88749999999999929, 5.773502691896255534, 3.535250795749688401E-16 ) ) ;
#26549=CARTESIAN_POINT ( 'NONE',  ( 13.00312500061451537, 4.541064518000418104, -2.621784821874998173 ) ) ;
#26550=CARTESIAN_POINT ( 'NONE',  ( 28.62187500061451573, -6.054752690667223547, -1.112240025338166033E-15 ) ) ;
#26551=DIRECTION ( 'NONE',  ( 0.000000000000000000, 0.000000000000000000, -1.000000000000000000 ) ) ;
#26553=CARTESIAN_POINT ( 'NONE',  ( 11.62500000000000000, -4.330127018922194537, 2.499999999999995559 ) ) ;
#26554=CARTESIAN_POINT ( 'NONE',  ( -2.000000000000000000, 18.23750000122903359, 26.53589838486224650 ) ) ;
#26555=CARTESIAN_POINT ( 'NONE',  ( 12.60000000122903430, -2.886751345948129988, 4.999999999999997335 ) ) ;
#26556=CARTESIAN_POINT ( 'NONE',  ( 21.94687500061451857, -3.027376345333610441, -5.243569643749999898 ) ) ;
#26557=CARTESIAN_POINT ( 'NONE',  ( 17.33437500061451431, -4.541064518000419881, 2.621784821874995952 ) ) ;
#26560=CARTESIAN_POINT ( 'NONE',  ( 17.09062500061451573, 6.054752690667223547, 3.707466751127219781E-16 ) ) ;
#26561=CARTESIAN_POINT ( 'NONE',  ( 27.86250000122903359, 0.000000000000000000, 4.999999999999998224 ) ) ;
#26562=CARTESIAN_POINT ( 'NONE',  ( 17.63437500061451502, 4.541064518000418104, 2.621784821874999949 ) ) ;
#26563=CARTESIAN_POINT ( 'NONE',  ( 5.840625000614516615, 6.054752690667223547, 3.707466751127219781E-16 ) ) ;
#26564=CARTESIAN_POINT ( 'NONE',  ( 20.12812500061451715, 6.421520780324663323E-16, -5.243569643749999010 ) ) ;
#26565=CARTESIAN_POINT ( 'NONE',  ( -1.071796769724496556, 16.94240381056766509, -26.00000000000000355 ) ) ;
#26566=CARTESIAN_POINT ( 'NONE',  ( 28.09687500061451360, -3.027376345333614438, 5.243569643749998122 ) ) ;
#26567=CARTESIAN_POINT ( 'NONE',  ( -2.121784821874999949, 13.42812500061451786, 26.32496088578401938 ) ) ;
#26568=CARTESIAN_POINT ( 'NONE',  ( 15.90000000122903501, -2.886751345948125991, -5.000000000000000000 ) ) ;
#26570=CARTESIAN_POINT ( 'NONE',  ( 27.17812500061451786, -4.541064518000419881, 2.621784821874995952 ) ) ;
#26571=CARTESIAN_POINT ( 'NONE',  ( -3.999999999999999112, 9.762500001229033941, 30.00000000000000000 ) ) ;
#26572=ADVANCED_FACE ( 'NONE', ( #35 ), #58960, .F. ) ;
#26573=CARTESIAN_POINT ( 'NONE',  ( 20.74687500061451573, 6.054752690667223547, 3.707466751127219781E-16 ) ) ;
#26574=CARTESIAN_POINT ( 'NONE',  ( 21.90000000122903145, 5.773502691896255534, 3.535250795749688894E-16 ) ) ;
#26575=CARTESIAN_POINT ( 'NONE',  ( 23.50312500061451360, 0.000000000000000000, 5.243569643749999010 ) ) ;
#26576=CARTESIAN_POINT ( 'NONE',  ( 17.70937500061451431, 0.000000000000000000, 5.243569643749999010 ) ) ;
#26577=CARTESIAN_POINT ( 'NONE',  ( 11.35312500061451679, 0.000000000000000000, 5.243569643749999010 ) ) ;
#26578=CARTESIAN_POINT ( 'NONE',  ( 4.243569643749999898, 14.68437500061451750, 30.00000000000000000 ) ) ;
#26579=CARTESIAN_POINT ( 'NONE',  ( 17.46562500061451217, 3.027376345333613106, -5.243569643749998122 ) ) ;
#26580=CARTESIAN_POINT ( 'NONE',  ( 29.12812500061451715, 6.421520780324663323E-16, -5.243569643749999010 ) ) ;
#26581=ORIENTED_EDGE ( 'NONE', *, *, #13122, .F. ) ;
#26582=CARTESIAN_POINT ( 'NONE',  ( 22.34999999999999787, 0.000000000000000000, 4.999999999999998224 ) ) ;
#26583=CARTESIAN_POINT ( 'NONE',  ( 9.001249775931846008E-16, 18.62187500061451928, -25.09994784771203058 ) ) ;
#26584=CARTESIAN_POINT ( 'NONE',  ( 3.999999999999999112, 18.08750000122903501, 30.00000000000000000 ) ) ;
#26585=CARTESIAN_POINT ( 'NONE',  ( 25.56562500061452070, 3.027376345333613106, -5.243569643749998122 ) ) ;
#26586=CARTESIAN_POINT ( 'NONE',  ( 6.553125000614518747, -4.541064518000417216, -2.621784821875001281 ) ) ;
#26587=CARTESIAN_POINT ( 'NONE',  ( 18.00000000122903288, -2.886751345948129988, 4.999999999999997335 ) ) ;
#26588=CARTESIAN_POINT ( 'NONE',  ( 22.22812500061451502, -4.541064518000419881, 2.621784821874995952 ) ) ;
#26589=CARTESIAN_POINT ( 'NONE',  ( 22.23750000000000071, 5.773502691896255534, 3.535250795749688894E-16 ) ) ;
#26590=CARTESIAN_POINT ( 'NONE',  ( 28.15312500061451573, -4.541064518000417216, -2.621784821875001281 ) ) ;
#26591=CARTESIAN_POINT ( 'NONE',  ( 7.978125000614517681, 6.421520780324663323E-16, -5.243569643749999010 ) ) ;
#26592=VERTEX_POINT ( 'NONE', #54537 ) ;
#26593=CARTESIAN_POINT ( 'NONE',  ( 23.99062500061451786, -3.027376345333614438, 5.243569643749998122 ) ) ;
#26594=CARTESIAN_POINT ( 'NONE',  ( 3.478125000614517237, 6.421520780324663323E-16, -5.243569643749999010 ) ) ;
#26598=CARTESIAN_POINT ( 'NONE',  ( 2.000000000000001332, 14.41250000122903430, -26.53589838486224650 ) ) ;
#26599=AXIS2_PLACEMENT_3D ( 'NONE', #45173, #11908, #51073 ) ;
#26600=EDGE_CURVE ( 'NONE', #53550, #42330, #63102, .T. ) ;
#26601=CARTESIAN_POINT ( 'NONE',  ( 10.42500000000000071, 6.123233995736764310E-16, -4.999999999999998224 ) ) ;
#26603=CARTESIAN_POINT ( 'NONE',  ( 10.54687500061451644, -3.027376345333614438, 5.243569643749998122 ) ) ;
#26604=CARTESIAN_POINT ( 'NONE',  ( 5.475000001229035185, -5.773502691896255534, -1.060575238724906372E-15 ) ) ;
#26605=CARTESIAN_POINT ( 'NONE',  ( 14.22187500061451537, -6.054752690667223547, -1.112240025338166033E-15 ) ) ;
#26606=CARTESIAN_POINT ( 'NONE',  ( 4.996875000614516615, 6.054752690667223547, 3.707466751127219781E-16 ) ) ;
#26609=CARTESIAN_POINT ( 'NONE',  ( 30.00000000000000000, 0.000000000000000000, 4.999999999999998224 ) ) ;
#26610=CARTESIAN_POINT ( 'NONE',  ( 13.24687500061451750, -3.027376345333614438, 5.243569643749998122 ) ) ;
#26611=CARTESIAN_POINT ( 'NONE',  ( 6.262500001229034829, 0.000000000000000000, 4.999999999999998224 ) ) ;
#26612=EDGE_CURVE ( 'NONE', #37421, #9597, #65923, .T. ) ;
#26613=CARTESIAN_POINT ( 'NONE',  ( 22.94062500061451715, 6.054752690667223547, 3.707466751127219781E-16 ) ) ;
#26614=CARTESIAN_POINT ( 'NONE',  ( -4.243569643749999898, 10.37187500061451750, 27.54997392385601529 ) ) ;
#26615=CARTESIAN_POINT ( 'NONE',  ( 4.243569643749999010, 19.61562500061459602, 27.54997392385601174 ) ) ;
#26616=CARTESIAN_POINT ( 'NONE',  ( 23.74687500061451573, -3.027376345333610441, -5.243569643749999898 ) ) ;
#26617=CARTESIAN_POINT ( 'NONE',  ( -1.071796769724491005, 13.72009619066136921, -34.00000000000000000 ) ) ;
#26618=CARTESIAN_POINT ( 'NONE',  ( 5.540625000614515905, -3.027376345333614438, 5.243569643749998122 ) ) ;
#26620=CARTESIAN_POINT ( 'NONE',  ( 23.91562500061451502, 3.027376345333611329, 5.243569643749999010 ) ) ;
#26621=CARTESIAN_POINT ( 'NONE',  ( 18.32812500061451644, 6.421520780324663323E-16, -5.243569643749999010 ) ) ;
#26623=CARTESIAN_POINT ( 'NONE',  ( 15.23437500061451644, 6.421520780324663323E-16, -5.243569643749999010 ) ) ;
#26625=CARTESIAN_POINT ( 'NONE',  ( 27.90000000122903145, -2.886751345948129988, 4.999999999999997335 ) ) ;
#26626=CARTESIAN_POINT ( 'NONE',  ( 7.134375000614516793, 6.421520780324663323E-16, -5.243569643749999010 ) ) ;
#26627=CARTESIAN_POINT ( 'NONE',  ( 17.55937500061451573, 4.541064518000418104, -2.621784821874998173 ) ) ;
#26629=CARTESIAN_POINT ( 'NONE',  ( 23.58749999999999858, 5.773502691896255534, 3.535250795749688894E-16 ) ) ;
#26630=CARTESIAN_POINT ( 'NONE',  ( 3.037500001229032964, 4.330127018922191873, 2.499999999999999556 ) ) ;
#26631=CARTESIAN_POINT ( 'NONE',  ( 24.19687500061451857, -3.027376345333610441, -5.243569643749999898 ) ) ;
#26632=CARTESIAN_POINT ( 'NONE',  ( 16.02187500061451786, -6.054752690667223547, -1.112240025338166033E-15 ) ) ;
#26634=CARTESIAN_POINT ( 'NONE',  ( 27.00000000000000000, -4.330127018922190985, -2.500000000000001332 ) ) ;
#26636=CARTESIAN_POINT ( 'NONE',  ( 7.500000000000000000, 0.000000000000000000, 4.999999999999998224 ) ) ;
#26638=CARTESIAN_POINT ( 'NONE',  ( 20.09062500061451573, -3.027376345333610441, -5.243569643749999898 ) ) ;
#26639=CARTESIAN_POINT ( 'NONE',  ( 9.937500000000001776, -2.886751345948125991, -5.000000000000000000 ) ) ;
#26640=CARTESIAN_POINT ( 'NONE',  ( 3.140625000614516882, 6.054752690667223547, 3.707466751127219781E-16 ) ) ;
#26641=CARTESIAN_POINT ( 'NONE',  ( 20.32499999999999929, 6.123233995736764310E-16, -4.999999999999998224 ) ) ;
#26643=CARTESIAN_POINT ( 'NONE',  ( 22.01250000122903216, 0.000000000000000000, 4.999999999999998224 ) ) ;
#26645=CARTESIAN_POINT ( 'NONE',  ( 28.92187500061451644, 3.027376345333611329, 5.243569643749999010 ) ) ;
#26646=AXIS2_PLACEMENT_3D ( 'NONE', #8755, #51563, #62636 ) ;
#26648=CARTESIAN_POINT ( 'NONE',  ( 16.60312500061451857, 4.541064518000418104, -2.621784821874998173 ) ) ;
#26649=CARTESIAN_POINT ( 'NONE',  ( 23.95312500061451289, 0.000000000000000000, 5.243569643749999010 ) ) ;
#26650=CARTESIAN_POINT ( 'NONE',  ( 24.19687500061451857, -3.027376345333610441, -5.243569643749999898 ) ) ;
#26651=CARTESIAN_POINT ( 'NONE',  ( 9.825000000000001066, -4.330127018922194537, 2.499999999999995559 ) ) ;
#26652=CARTESIAN_POINT ( 'NONE',  ( 11.91562500061451857, -6.054752690667223547, -1.112240025338166033E-15 ) ) ;
#26653=CARTESIAN_POINT ( 'NONE',  ( 27.66562500061451146, -6.054752690667223547, -1.112240025338166033E-15 ) ) ;
#26654=CARTESIAN_POINT ( 'NONE',  ( 15.08437500061451786, -4.541064518000419881, 2.621784821874995952 ) ) ;
#26655=CARTESIAN_POINT ( 'NONE',  ( 19.88437500061451857, 4.541064518000418104, 2.621784821874999949 ) ) ;
#26657=CARTESIAN_POINT ( 'NONE',  ( -3.000416591977282496E-16, 10.74687500061451928, 25.09994784771203058 ) ) ;
#26659=CARTESIAN_POINT ( 'NONE',  ( 22.72500000122903430, 2.886751345948129099, -4.999999999999998224 ) ) ;
#26661=CARTESIAN_POINT ( 'NONE',  ( 13.97812500061451679, 4.541064518000418104, 2.621784821874999949 ) ) ;
#26662=CARTESIAN_POINT ( 'NONE',  ( 7.059375000614518392, -4.541064518000417216, -2.621784821875001281 ) ) ;
#26663=CARTESIAN_POINT ( 'NONE',  ( 8.371875000614515727, -6.054752690667223547, -1.112240025338166033E-15 ) ) ;
#26664=ORIENTED_EDGE ( 'NONE', *, *, #48794, .F. ) ;
#26665=CARTESIAN_POINT ( 'NONE',  ( 26.74687500061451573, -3.027376345333614438, 5.243569643749998122 ) ) ;
#26666=CARTESIAN_POINT ( 'NONE',  ( 20.35312500061451502, 0.000000000000000000, 5.243569643749999010 ) ) ;
#26667=( BOUNDED_SURFACE ( )  B_SPLINE_SURFACE ( 1, 2, ( 
 ( #42956, #42592, #13396, #30414, #8243, #41497, #59937, #31876, #64385, #8606, #2339, #9344, #31135, #2703, #52941, #65117, #35943, #25599, #54411, #70661, #53303, #26333, #53676, #3446, #47765, #20036, #37041, #65485, #24856, #20408, #14875, #31511, #25965, #59565, #14508, #54052, #47402, #71033, #58465, #19303, #37414, #3811, #30773, #25219, #48872, #13776, #19673, #36317, #64751, #58833, #70301, #42227, #7877, #14142, #36677, #18938, #3070, #43333, #27800, #27435, #72860, #37774, #66588, #71774, #56233, #66218, #33689, #16330, #55144, #44435, #65855, #61039, #5627, #38138, #22244, #60293, #38885, #71402, #15965, #4542, #26706, #21875, #27071, #21143, #50337, #43697, #44798, #10797, #28163, #20776, #9704, #32238, #15595, #15237, #60661, #10075, #44061, #10437, #49602, #4177, #55870, #38516, #32606, #5257, #39248, #72129, #21508, #32967, #55507, #72489, #61402, #4900, #49966, #54772, #49240, #66965, #33332, #67331, #16691, #61761, #11165, #51774, #57663, #93, #58018, #56937, #29241, #51050, #63210, #45151, #22956, #45516, #56585, #447, #5982, #7069, #67683, #17054, #1174, #46230, #29598, #34409, #7427, #39612, #12961, #34046, #40325, #46594, #28512, #23682, #68047, #17416, #68769, #52134, #40692, #1537, #6342, #17766, #39974, #62487, #62132, #28873, #18126, #12606, #11524, #35139, #24045, #11884, #51412, #69136, #12240, #18495, #814, #23322, #45871, #41060, #63574, #62847, #50691, #35498, #22599, #68404, #34772, #57304, #6709, #71956, #43885, #52858, #71216, #13317, #21332, #20593, #13687, #41416, #54596, #52494, #37599, #66411, #9530, #64299, #38329, #43150, #15420, #59756, #32063, #49063, #54963, #63932, #30328, #20965, #3999, #69495, #1905, #26525, #35856, #43519, #37963, #48693, #71591, #7790, #58379, #66042, #36231, #65673, #15062, #3630, #60485, #2258, #18854, #4368, #9891, #26898, #9163, #32427, #60120, #24772, #15788, #49423, #60858, #29954, #24410, #46959, #47316, #69849, #19216, #41770, #31698, #54233, #26152, #61229, #61951, #10261, #16515, #10623, #33153, #73045, #32793, #68235, #72685, #72316, #11713, #67155, #40158, #22783, #27987, #39068, #28697, #61582, #11355, #33506, #56055, #4724, #39430, #10985, #34230, #27621, #33873, #55330, #49791, #27258, #5447, #21697, #50517, #22427, #50155, #56764, #56416, #44254, #66785, #22067, #16158, #51236, #23148, #55690, #44974, #38710, #639, #67512, #16876, #5086, #5807, #44626, #28338, #45702, #50875, #273, #17599, #45335, #67870, #17242, #39802, #62318, #6168, #23510, #63032, #52678, #63754, #29067, #12073, #13143, #46059, #2086, #47143, #7255, #35683, #40517, #68593, #41242, #46419, #1722, #29783, #35323, #69674, #12431, #51603, #13502, #58205, #36049, #68957, #19040, #46784, #34965, #24957, #58570, #30513, #41598, #7977, #53040, #7609, #17955, #57492, #24595, #64117, #18679, #6896, #29427, #30146, #62678, #18314, #51963, #1362, #52319, #34595, #47501, #23871, #1003, #2435, #40885, #19405, #70032, #24234, #63401, #57123, #12786, #6534, #57845, #69319, #36417, #71129, #48237, #65955, #59294, #43059, #13878, #8340, #58933, #65214, #71871, #42692, #70762, #8704, #9076, #31237, #19777, #30869, #20137, #60033, #37512, #53408, #31972, #65584, #47873, #42327, #15335, #3542, #54508, #3174, #14604, #37140, #60395, #9803, #31612, #41963, #25327, #54148, #37875, #70401, #14974, #64852, #53778, #9444, #71503, #3911, #20879, #25701, #43433, #32336, #26433, #48974, #54874, #4279, #48604, #14240, #26805, #2800, #36778, #49339, #64485, #59668, #26065, #20502, #32709, #21979, #66696, #67069, #44166, #50066, #21611, #10174, #16068, #15699, #33791, #61863, #66322, #50790, #50435, #22698, #60767, #16427, #38618, #6082, #61142, #56683, #39349, #5000, #67430, #38238, #10897, #28614, #10537, #45250, #55246, #11269, #21243, #38985, #27533, #49705, #44894, #72596, #33065, #193, #55604, #67783, #56334, #51151, #43796, #4641, #27171, #44538, #72233, #61500, #33425, #55967, #5362, #27900, #72960, #5724, #22342, #16792, #28259, #62234, #17157, #39716, #11630, #34146, #1638, #41159, #6807, #7168, #62590, #17514, #45617, #35959, #28979, #18595, #47056, #23781, #24144, #7524, #23062, #7891, #29341, #52234, #916, #13058, #68151, #45971, #68505, #6444, #23425, #51517, #30057, #40075, #11986, #46697, #69233, #52595, #57402, #30427, #34509, #58480, #18223, #51873, #18952, #1272, #63668, #46333, #68867, #57038, #29696, #40797, #24512, #17868, #35597, #40427, #62944, #12338, #63310, #552, #12701, #35238, #34873, #57759, #58116, #2002, #69590, #41512, #64031, #13410, #69946, #42967, #54062, #58846, #30786, #3823, #14519, #65497, #14154, #3082, #8618, #71413, #20789, #42603, #52955, #26344, #3458, #47416, #64399, #42240, #2352, #43345, #65867, #2716, #20048, #36332, #15249, #65129, #36688, #13791, #25978, #24869, #59577, #37786, #31522, #59210, #60306, #37052, #37425, #31147, #48517, #71044, #48883, #8256, #53317, #14886, #20419, #19316, #41870, #59948, #25232, #9355, #31888, #70673, #54423, #47778, #70313, #9717, #53688, #8990, #19686, #25610, #64764, #48148, #71786, #56247, #55881, #5638, #15977, #61772, #16341, #4553, #67693, #28175, #105, #11176, #50702, #22610, #50348, #38150, #27082, #22255, #33700, #61415, #55156, #10087, #10808, #32250, #38527, #32617, #49613, #21890, #54783, #17065, #21519, #21154, #45162, #61049, #62143, #44809, #39625, #10449, #4189, #38896, #72140, #26718, #49251, #43708, #66229, #15608, #60673, #72872, #44074, #66603, #67342, #32978, #33343, #55518, #4911, #5269, #27447, #49977, #72501, #44447, #66976, #27814, #16703, #39260, #459, #12972, #68415, #41427, #24058, #29253, #17777, #29965, #40336, #12617, #34783, #57316, #5993, #40704, #62858, #35510, #28885, #35151, #56597, #51062, #28523, #6720, #11537, #12252 ),
 ( #22967, #51785, #56949, #1185, #34421, #23693, #11896, #45528, #6353, #68059, #46604, #52145, #17426, #41071, #63222, #58029, #39986, #46241, #51424, #69506, #825, #46970, #29609, #68781, #57674, #62498, #18137, #18866, #23333, #7439, #45883, #1548, #34057, #7080, #69147, #18506, #63585, #52506, #1917, #24421, #36242, #37340, #3372, #71324, #13328, #30340, #24782, #58756, #58390, #64309, #13699, #36602, #2991, #47685, #69859, #42151, #25519, #65043, #31434, #70221, #70589, #52868, #7803, #35867, #26259, #19226, #8902, #59863, #14063, #14433, #70958, #2267, #20699, #19595, #42517, #8166, #25893, #47326, #30695, #53226, #41780, #2623, #25144, #20331, #64678, #59123, #36968, #59490, #42884, #8530, #63943, #31059, #48796, #53596, #48064, #9267, #19964, #53974, #48433, #65407, #14797, #31802, #54340, #3734, #26999, #44722, #39170, #33257, #50261, #61327, #16257, #49890, #49168, #27723, #9632, #71699, #10725, #38812, #55068, #49529, #72415, #54699, #43989, #15522, #15891, #66144, #72053, #43622, #32166, #38064, #37697, #55795, #5185, #15160, #72786, #21797, #67257, #4104, #38437, #60588, #28089, #9997, #5551, #22169, #21432, #16615, #60219, #32893, #50617, #32532, #61686, #26631, #11085, #43257, #60963, #66510, #21071, #66889, #10362, #4469, #33613, #55433, #56157, #22, #65778, #4825, #27359, #44362, #17344, #16977, #22880, #45438, #68336, #34698, #6270, #28440, #6997, #17696, #39903, #29528, #63504, #23250, #62416, #39534, #12534, #23613, #50975, #372, #46521, #57227, #35068, #56865, #45800, #51339, #40988, #12891, #12170, #22528, #69062, #46159, #62059, #33974, #11815, #45075, #35424, #57948, #67971, #62778, #5906, #7356, #6642, #28798, #56513, #68699, #67611, #29169, #29885, #1106, #741, #52423, #51703, #52063, #40257, #18059, #40619, #18422, #34332, #63139, #57594, #1467, #11453, #23973, #25437, #58307, #14350, #59403, #19513, #47980, #52785, #7718, #53512, #58674, #13980, #42071, #47605, #8812, #24700, #41346, #25809, #70508, #48347, #8084, #31349, #59039, #47244, #37253, #70872, #42798, #53890, #20246, #65320, #19884, #30252, #69776, #64959, #3281, #30979, #19144, #2186, #2906, #1829, #30614, #41698, #64222, #64592, #24338, #59775, #13611, #63856, #14710, #53144, #31716, #36885, #36519, #2543, #9181, #25062, #42437, #70135, #8443, #69424, #46886, #18781, #13246, #36156, #35784, #3648, #71234, #26171, #37980, #5103, #60502, #43537, #26541, #54981, #49082, #60137, #20613, #66058, #60875, #10279, #4742, #9908, #4017, #27276, #38726, #15436, #54611, #32445, #49441, #66428, #32810, #4386, #21348, #43172, #48712, #65691, #10641, #37615, #55348, #44272, #26916, #43904, #49809, #15078, #55709, #71975, #15806, #9546, #72334, #32080, #71611, #20984, #38347, #21714, #66804, #16175, #61247, #33171, #54251, #36324, #23774, #58472, #35591, #53310, #46690, #30420, #1267, #68861, #46326, #52588, #59204, #30048, #58110, #69227, #69583, #18588, #7161, #18217, #7517, #47409, #24862, #40791, #19309, #52948, #35232, #29690, #2709, #64024, #41862, #63661, #1994, #24505, #47771, #70307, #18945, #29335, #25225, #2345, #63303, #12695, #41153, #51865, #19680, #42233, #52227, #41504, #57753, #64758, #13403, #13052, #1631, #69939, #24138, #35951, #14148, #7884, #47049, #36683, #64392, #13782, #58839, #8249, #30779, #32612, #42598, #8985, #71781, #9711, #48143, #31141, #32245, #65124, #21149, #66224, #26339, #54778, #59572, #14514, #60300, #65491, #20783, #48878, #54417, #15603, #31517, #70667, #55150, #4184, #38144, #43703, #60668, #14881, #10082, #4548, #27077, #49608, #26712, #49246, #15243, #37047, #72135, #20043, #54058, #21515, #44069, #20414, #37420, #37780, #3453, #9350, #25971, #3818, #48512, #59943, #71039, #42962, #31883, #3077, #66596, #15972, #53682, #38522, #8612, #25605, #71408, #43339, #65861, #45878, #55876, #23328, #5988, #44804, #34052, #55513, #50697, #68410, #27809, #62493, #49972, #28518, #61045, #5633, #67337, #16336, #11532, #16697, #61409, #39981, #33338, #34416, #453, #17772, #10443, #27442, #21882, #5263, #4906, #10803, #50343, #33695, #99, #39255, #66971, #45523, #56242, #72867, #68053, #28879, #61767, #22250, #11171, #11891, #56944, #51419, #51058, #38891, #28170, #22962, #17422, #17060, #22605, #45157, #39620, #32973, #67689, #62138, #56592, #6348, #72497, #44442, #820, #29248, #41776, #24053, #70217, #52864, #58024, #46600, #58752, #19222, #63580, #7434, #47322, #34778, #69501, #69142, #64305, #57669, #41422, #12247, #6715, #57311, #12967, #40332, #41066, #18501, #40699, #13695, #12612, #36238, #2264, #47681, #62853, #51780, #1180, #35146, #23688, #63217, #7075, #35505, #52501, #29960, #46236, #24778, #1912, #29604, #69855, #8162, #68776, #18132, #1543, #52140, #63938, #7798, #24416, #46965, #18861, #13323, #35862, #2619, #58385, #30336, #30691, #53222, #25140, #26626, #42147, #26995, #25888, #71318, #19961, #32161, #14059, #65037, #14428, #25515, #42513, #48060, #49163, #36598, #64674, #49524, #20694, #20325, #3367, #19591, #59119, #55064, #2987, #9262, #15517, #70585, #43253, #36963, #59485, #37692, #71694, #9628, #21066, #48428, #43617, #38059, #54694, #66139, #60215, #65773, #26254, #8897, #4097, #8526, #31429, #60584, #15155, #53969, #70954, #48791, #31055, #42879, #65402, #14793, #37335, #59858, #31797, #53592, #54335, #3729, #9992, #32527, #4465, #28434, #28084, #367, #38432, #67252, #72410, #56859, #66884, #34327, #16972, #55790, #45070, #66505, #61681, #6265, #38807, #22875, #60956, #39528, #72049, #16610, #5180, #27354, #22523, #28793, #55428, #11080, #67966, #49885, #16, #4820, #61322, #62054, #50971, #11449, #45432, #27717, #17339, #39898, #33969, #5901, #56508, #67607, #5546, #21792, #62411, #10358, #44358, #11810, #21427, #10720 ) ),
 .UNSPECIFIED., .F., .F., .F. ) 
 B_SPLINE_SURFACE_WITH_KNOTS ( ( 2, 2 ),
 ( 3, 2, 2, 2, 2, 2, 2, 2, 2, 2, 2, 2, 2, 2, 2, 2, 2, 2, 2, 2, 2, 2, 2, 2, 2, 2, 2, 2, 2, 2, 2, 2, 2, 2, 2, 2, 2, 2, 2, 2, 2, 2, 2, 2, 2, 2, 2, 2, 2, 2, 2, 2, 2, 2, 2, 2, 2, 2, 2, 2, 2, 2, 2, 2, 2, 2, 2, 2, 2, 2, 2, 2, 2, 2, 2, 2, 2, 2, 2, 2, 2, 2, 2, 2, 2, 2, 2, 2, 2, 2, 2, 2, 2, 2, 2, 2, 2, 2, 2, 2, 2, 2, 2, 2, 2, 2, 2, 2, 2, 2, 2, 2, 2, 2, 2, 2, 2, 2, 2, 2, 2, 2, 2, 2, 2, 2, 2, 2, 2, 2, 2, 2, 2, 2, 2, 2, 2, 2, 2, 2, 2, 2, 2, 2, 2, 2, 2, 2, 2, 2, 2, 2, 2, 2, 2, 2, 2, 2, 2, 2, 2, 2, 2, 2, 2, 2, 2, 2, 2, 2, 2, 2, 2, 2, 2, 2, 2, 2, 2, 2, 2, 2, 2, 2, 2, 2, 2, 2, 2, 2, 2, 2, 2, 2, 2, 2, 2, 2, 2, 2, 2, 2, 2, 2, 2, 2, 2, 2, 2, 2, 2, 2, 2, 2, 2, 2, 2, 2, 2, 2, 2, 2, 2, 2, 2, 2, 2, 2, 2, 2, 2, 2, 2, 2, 2, 2, 2, 2, 2, 2, 2, 2, 2, 2, 2, 2, 2, 2, 2, 2, 2, 2, 2, 2, 2, 2, 2, 2, 2, 2, 2, 2, 2, 2, 2, 2, 2, 2, 2, 2, 2, 2, 2, 2, 2, 2, 2, 2, 2, 2, 2, 2, 2, 2, 2, 2, 2, 2, 2, 2, 2, 2, 2, 2, 2, 2, 2, 2, 2, 2, 2, 2, 2, 2, 2, 2, 2, 2, 2, 2, 2, 2, 2, 2, 2, 2, 2, 2, 2, 2, 2, 2, 2, 2, 2, 2, 2, 2, 2, 2, 2, 2, 2, 2, 2, 2, 2, 2, 2, 2, 2, 2, 2, 2, 2, 2, 2, 2, 2, 2, 2, 2, 2, 2, 2, 2, 2, 2, 2, 2, 3 ),
 ( 0.000000000000000000, 1.000000000000000000 ),
 ( 0.000000000000000000, 0.002777777777777777884, 0.005555555555555555768, 0.008333333333333333218, 0.01111111111111111154, 0.01388888888888888812, 0.01666666666666666644, 0.01944444444444444475, 0.02222222222222222307, 0.02500000000000000139, 0.02777777777777777624, 0.03055555555555555455, 0.03333333333333333287, 0.03611111111111110772, 0.03888888888888888951, 0.04166666666666666435, 0.04444444444444444614, 0.04722222222222222099, 0.05000000000000000278, 0.05277777777777777762, 0.05555555555555555247, 0.05833333333333333426, 0.06111111111111110911, 0.06388888888888888395, 0.06666666666666666574, 0.06944444444444444753, 0.07222222222222221544, 0.07499999999999999722, 0.07777777777777777901, 0.08055555555555556080, 0.08333333333333332871, 0.08611111111111111049, 0.08888888888888889228, 0.09166666666666666019, 0.09444444444444444198, 0.09722222222222222376, 0.1000000000000000056, 0.1027777777777777735, 0.1055555555555555552, 0.1083333333333333370, 0.1111111111111111049, 0.1138888888888888867, 0.1166666666666666685, 0.1194444444444444503, 0.1222222222222222182, 0.1250000000000000000, 0.1277777777777777679, 0.1305555555555555636, 0.1333333333333333315, 0.1361111111111110994, 0.1388888888888888951, 0.1416666666666666630, 0.1444444444444444309, 0.1472222222222222265, 0.1499999999999999944, 0.1527777777777777901, 0.1555555555555555580, 0.1583333333333333259, 0.1611111111111111216, 0.1638888888888888895, 0.1666666666666666574, 0.1694444444444444531, 0.1722222222222222210, 0.1749999999999999889, 0.1777777777777777846, 0.1805555555555555525, 0.1833333333333333204, 0.1861111111111111160, 0.1888888888888888840, 0.1916666666666666796, 0.1944444444444444475, 0.1972222222222222154, 0.2000000000000000111, 0.2027777777777777790, 0.2055555555555555469, 0.2083333333333333426, 0.2111111111111111105, 0.2138888888888888784, 0.2166666666666666741, 0.2194444444444444420, 0.2222222222222222099, 0.2250000000000000056, 0.2277777777777777735, 0.2305555555555555691, 0.2333333333333333370, 0.2361111111111111049, 0.2388888888888889006, 0.2416666666666666685, 0.2444444444444444364, 0.2472222222222222321, 0.2500000000000000000, 0.2527777777777777679, 0.2555555555555555358, 0.2583333333333333592, 0.2611111111111111271, 0.2638888888888888951, 0.2666666666666666630, 0.2694444444444444309, 0.2722222222222221988, 0.2750000000000000222, 0.2777777777777777901, 0.2805555555555555580, 0.2833333333333333259, 0.2861111111111110938, 0.2888888888888888618, 0.2916666666666666852, 0.2944444444444444531, 0.2972222222222222210, 0.2999999999999999889, 0.3027777777777777568, 0.3055555555555555802, 0.3083333333333333481, 0.3111111111111111160, 0.3138888888888888840, 0.3166666666666666519, 0.3194444444444444198, 0.3222222222222222432, 0.3250000000000000111, 0.3277777777777777790, 0.3305555555555555469, 0.3333333333333333148, 0.3361111111111111382, 0.3388888888888889062, 0.3416666666666666741, 0.3444444444444444420, 0.3472222222222222099, 0.3499999999999999778, 0.3527777777777778012, 0.3555555555555555691, 0.3583333333333333370, 0.3611111111111111049, 0.3638888888888888729, 0.3666666666666666408, 0.3694444444444444642, 0.3722222222222222321, 0.3750000000000000000, 0.3777777777777777679, 0.3805555555555555358, 0.3833333333333333592, 0.3861111111111111271, 0.3888888888888888951, 0.3916666666666666630, 0.3944444444444444309, 0.3972222222222221988, 0.4000000000000000222, 0.4027777777777777901, 0.4055555555555555580, 0.4083333333333333259, 0.4111111111111110938, 0.4138888888888888618, 0.4166666666666666852, 0.4194444444444444531, 0.4222222222222222210, 0.4249999999999999889, 0.4277777777777777568, 0.4305555555555555802, 0.4333333333333333481, 0.4361111111111111160, 0.4388888888888888840, 0.4416666666666666519, 0.4444444444444444198, 0.4472222222222222432, 0.4500000000000000111, 0.4527777777777777790, 0.4555555555555555469, 0.4583333333333333148, 0.4611111111111111382, 0.4638888888888889062, 0.4666666666666666741, 0.4694444444444444420, 0.4722222222222222099, 0.4749999999999999778, 0.4777777777777778012, 0.4805555555555555691, 0.4833333333333333370, 0.4861111111111111049, 0.4888888888888888729, 0.4916666666666666408, 0.4944444444444444642, 0.4972222222222222321, 0.5000000000000000000, 0.5027777777777777679, 0.5055555555555555358, 0.5083333333333333037, 0.5111111111111110716, 0.5138888888888888395, 0.5166666666666667185, 0.5194444444444444864, 0.5222222222222222543, 0.5250000000000000222, 0.5277777777777777901, 0.5305555555555555580, 0.5333333333333333259, 0.5361111111111110938, 0.5388888888888888618, 0.5416666666666666297, 0.5444444444444443976, 0.5472222222222222765, 0.5500000000000000444, 0.5527777777777778123, 0.5555555555555555802, 0.5583333333333333481, 0.5611111111111111160, 0.5638888888888888840, 0.5666666666666666519, 0.5694444444444444198, 0.5722222222222221877, 0.5749999999999999556, 0.5777777777777777235, 0.5805555555555556024, 0.5833333333333333703, 0.5861111111111111382, 0.5888888888888889062, 0.5916666666666666741, 0.5944444444444444420, 0.5972222222222222099, 0.5999999999999999778, 0.6027777777777777457, 0.6055555555555555136, 0.6083333333333332815, 0.6111111111111111605, 0.6138888888888889284, 0.6166666666666666963, 0.6194444444444444642, 0.6222222222222222321, 0.6250000000000000000, 0.6277777777777777679, 0.6305555555555555358, 0.6333333333333333037, 0.6361111111111110716, 0.6388888888888888395, 0.6416666666666667185, 0.6444444444444444864, 0.6472222222222222543, 0.6500000000000000222, 0.6527777777777777901, 0.6555555555555555580, 0.6583333333333333259, 0.6611111111111110938, 0.6638888888888888618, 0.6666666666666666297, 0.6694444444444443976, 0.6722222222222222765, 0.6750000000000000444, 0.6777777777777778123, 0.6805555555555555802, 0.6833333333333333481, 0.6861111111111111160, 0.6888888888888888840, 0.6916666666666666519, 0.6944444444444444198, 0.6972222222222221877, 0.6999999999999999556, 0.7027777777777777235, 0.7055555555555556024, 0.7083333333333333703, 0.7111111111111111382, 0.7138888888888889062, 0.7166666666666666741, 0.7194444444444444420, 0.7222222222222222099, 0.7249999999999999778, 0.7277777777777777457, 0.7305555555555555136, 0.7333333333333332815, 0.7361111111111111605, 0.7388888888888889284, 0.7416666666666666963, 0.7444444444444444642, 0.7472222222222222321, 0.7500000000000000000, 0.7527777777777777679, 0.7555555555555555358, 0.7583333333333333037, 0.7611111111111110716, 0.7638888888888888395, 0.7666666666666667185, 0.7694444444444444864, 0.7722222222222222543, 0.7750000000000000222, 0.7777777777777777901, 0.7805555555555555580, 0.7833333333333333259, 0.7861111111111110938, 0.7888888888888888618, 0.7916666666666666297, 0.7944444444444443976, 0.7972222222222222765, 0.8000000000000000444, 0.8027777777777778123, 0.8055555555555555802, 0.8083333333333333481, 0.8111111111111111160, 0.8138888888888888840, 0.8166666666666666519, 0.8194444444444444198, 0.8222222222222221877, 0.8249999999999999556, 0.8277777777777777235, 0.8305555555555556024, 0.8333333333333333703, 0.8361111111111111382, 0.8388888888888889062, 0.8416666666666666741, 0.8444444444444444420, 0.8472222222222222099, 0.8499999999999999778, 0.8527777777777777457, 0.8555555555555555136, 0.8583333333333332815, 0.8611111111111111605, 0.8638888888888889284, 0.8666666666666666963, 0.8694444444444444642, 0.8722222222222222321, 0.8750000000000000000, 0.8777777777777777679, 0.8805555555555555358, 0.8833333333333333037, 0.8861111111111110716, 0.8888888888888888395, 0.8916666666666667185, 0.8944444444444444864, 0.8972222222222222543, 0.9000000000000000222, 0.9027777777777777901, 0.9055555555555555580, 0.9083333333333333259, 0.9111111111111110938, 0.9138888888888888618, 0.9166666666666666297, 0.9194444444444443976, 0.9222222222222222765, 0.9250000000000000444, 0.9277777777777778123, 0.9305555555555555802, 0.9333333333333333481, 0.9361111111111111160, 0.9388888888888888840, 0.9416666666666666519, 0.9444444444444444198, 0.9472222222222221877, 0.9499999999999999556, 0.9527777777777777235, 0.9555555555555556024, 0.9583333333333333703, 0.9611111111111111382, 0.9638888888888889062, 0.9666666666666666741, 0.9694444444444444420, 0.9722222222222222099, 0.9749999999999999778, 0.9777777777777777457, 0.9805555555555555136, 0.9833333333333332815, 0.9861111111111111605, 0.9888888888888889284, 0.9916666666666666963, 0.9944444444444444642, 0.9972222222222222321, 1.000000000000000000 ),
 .UNSPECIFIED. ) 
 GEOMETRIC_REPRESENTATION_ITEM ( )  RATIONAL_B_SPLINE_SURFACE ( (
 ( 1.000000000000000000, 0.8660254037844387076, 1.000000000000000000, 0.8660254037844387076, 1.000000000000000000, 0.8660254037844387076, 1.000000000000000000, 0.8660254037844387076, 1.000000000000000000, 0.8660254037844387076, 1.000000000000000000, 0.8660254037844387076, 1.000000000000000000, 0.8660254037844387076, 1.000000000000000000, 0.8660254037844387076, 1.000000000000000000, 0.8660254037844387076, 1.000000000000000000, 0.8660254037844387076, 1.000000000000000000, 0.8660254037844387076, 1.000000000000000000, 0.8660254037844387076, 1.000000000000000000, 0.8660254037844387076, 1.000000000000000000, 0.8660254037844387076, 1.000000000000000000, 0.8660254037844387076, 1.000000000000000000, 0.8660254037844387076, 1.000000000000000000, 0.8660254037844387076, 1.000000000000000000, 0.8660254037844387076, 1.000000000000000000, 0.8660254037844387076, 1.000000000000000000, 0.8660254037844387076, 1.000000000000000000, 0.8660254037844387076, 1.000000000000000000, 0.8660254037844387076, 1.000000000000000000, 0.8660254037844387076, 1.000000000000000000, 0.8660254037844387076, 1.000000000000000000, 0.8660254037844387076, 1.000000000000000000, 0.8660254037844387076, 1.000000000000000000, 0.8660254037844387076, 1.000000000000000000, 0.8660254037844387076, 1.000000000000000000, 0.8660254037844387076, 1.000000000000000000, 0.8660254037844387076, 1.000000000000000000, 0.8660254037844387076, 1.000000000000000000, 0.8660254037844387076, 1.000000000000000000, 0.8660254037844387076, 1.000000000000000000, 0.8660254037844387076, 1.000000000000000000, 0.8660254037844387076, 1.000000000000000000, 0.8660254037844387076, 1.000000000000000000, 0.8660254037844387076, 1.000000000000000000, 0.8660254037844387076, 1.000000000000000000, 0.8660254037844387076, 1.000000000000000000, 0.8660254037844387076, 1.000000000000000000, 0.8660254037844387076, 1.000000000000000000, 0.8660254037844387076, 1.000000000000000000, 0.8660254037844387076, 1.000000000000000000, 0.8660254037844387076, 1.000000000000000000, 0.8660254037844387076, 1.000000000000000000, 0.8660254037844387076, 1.000000000000000000, 0.8660254037844387076, 1.000000000000000000, 0.8660254037844387076, 1.000000000000000000, 0.8660254037844387076, 1.000000000000000000, 0.8660254037844387076, 1.000000000000000000, 0.8660254037844387076, 1.000000000000000000, 0.8660254037844387076, 1.000000000000000000, 0.8660254037844387076, 1.000000000000000000, 0.8660254037844387076, 1.000000000000000000, 0.8660254037844387076, 1.000000000000000000, 0.8660254037844387076, 1.000000000000000000, 0.8660254037844387076, 1.000000000000000000, 0.8660254037844387076, 1.000000000000000000, 0.8660254037844387076, 1.000000000000000000, 0.8660254037844387076, 1.000000000000000000, 0.8660254037844387076, 1.000000000000000000, 0.8660254037844387076, 1.000000000000000000, 0.8660254037844387076, 1.000000000000000000, 0.8660254037844387076, 1.000000000000000000, 0.8660254037844387076, 1.000000000000000000, 0.8660254037844387076, 1.000000000000000000, 0.8660254037844387076, 1.000000000000000000, 0.8660254037844387076, 1.000000000000000000, 0.8660254037844387076, 1.000000000000000000, 0.8660254037844387076, 1.000000000000000000, 0.8660254037844387076, 1.000000000000000000, 0.8660254037844387076, 1.000000000000000000, 0.8660254037844387076, 1.000000000000000000, 0.8660254037844387076, 1.000000000000000000, 0.8660254037844387076, 1.000000000000000000, 0.8660254037844387076, 1.000000000000000000, 0.8660254037844387076, 1.000000000000000000, 0.8660254037844387076, 1.000000000000000000, 0.8660254037844387076, 1.000000000000000000, 0.8660254037844387076, 1.000000000000000000, 0.8660254037844387076, 1.000000000000000000, 0.8660254037844387076, 1.000000000000000000, 0.8660254037844387076, 1.000000000000000000, 0.8660254037844387076, 1.000000000000000000, 0.8660254037844387076, 1.000000000000000000, 0.8660254037844387076, 1.000000000000000000, 0.8660254037844387076, 1.000000000000000000, 0.8660254037844387076, 1.000000000000000000, 0.8660254037844387076, 1.000000000000000000, 0.8660254037844387076, 1.000000000000000000, 0.8660254037844387076, 1.000000000000000000, 0.8660254037844387076, 1.000000000000000000, 0.8660254037844387076, 1.000000000000000000, 0.8660254037844387076, 1.000000000000000000, 0.8660254037844387076, 1.000000000000000000, 0.8660254037844387076, 1.000000000000000000, 0.8660254037844387076, 1.000000000000000000, 0.8660254037844387076, 1.000000000000000000, 0.8660254037844387076, 1.000000000000000000, 0.8660254037844387076, 1.000000000000000000, 0.8660254037844387076, 1.000000000000000000, 0.8660254037844387076, 1.000000000000000000, 0.8660254037844387076, 1.000000000000000000, 0.8660254037844387076, 1.000000000000000000, 0.8660254037844387076, 1.000000000000000000, 0.8660254037844387076, 1.000000000000000000, 0.8660254037844387076, 1.000000000000000000, 0.8660254037844387076, 1.000000000000000000, 0.8660254037844387076, 1.000000000000000000, 0.8660254037844387076, 1.000000000000000000, 0.8660254037844387076, 1.000000000000000000, 0.8660254037844387076, 1.000000000000000000, 0.8660254037844387076, 1.000000000000000000, 0.8660254037844387076, 1.000000000000000000, 0.8660254037844387076, 1.000000000000000000, 0.8660254037844387076, 1.000000000000000000, 0.8660254037844387076, 1.000000000000000000, 0.8660254037844387076, 1.000000000000000000, 0.8660254037844387076, 1.000000000000000000, 0.8660254037844387076, 1.000000000000000000, 0.8660254037844387076, 1.000000000000000000, 0.8660254037844387076, 1.000000000000000000, 0.8660254037844387076, 1.000000000000000000, 0.8660254037844387076, 1.000000000000000000, 0.8660254037844387076, 1.000000000000000000, 0.8660254037844387076, 1.000000000000000000, 0.8660254037844387076, 1.000000000000000000, 0.8660254037844387076, 1.000000000000000000, 0.8660254037844387076, 1.000000000000000000, 0.8660254037844387076, 1.000000000000000000, 0.8660254037844387076, 1.000000000000000000, 0.8660254037844387076, 1.000000000000000000, 0.8660254037844387076, 1.000000000000000000, 0.8660254037844387076, 1.000000000000000000, 0.8660254037844387076, 1.000000000000000000, 0.8660254037844387076, 1.000000000000000000, 0.8660254037844387076, 1.000000000000000000, 0.8660254037844387076, 1.000000000000000000, 0.8660254037844387076, 1.000000000000000000, 0.8660254037844387076, 1.000000000000000000, 0.8660254037844387076, 1.000000000000000000, 0.8660254037844387076, 1.000000000000000000, 0.8660254037844387076, 1.000000000000000000, 0.8660254037844387076, 1.000000000000000000, 0.8660254037844387076, 1.000000000000000000, 0.8660254037844387076, 1.000000000000000000, 0.8660254037844387076, 1.000000000000000000, 0.8660254037844387076, 1.000000000000000000, 0.8660254037844387076, 1.000000000000000000, 0.8660254037844387076, 1.000000000000000000, 0.8660254037844387076, 1.000000000000000000, 0.8660254037844387076, 1.000000000000000000, 0.8660254037844387076, 1.000000000000000000, 0.8660254037844387076, 1.000000000000000000, 0.8660254037844387076, 1.000000000000000000, 0.8660254037844387076, 1.000000000000000000, 0.8660254037844387076, 1.000000000000000000, 0.8660254037844387076, 1.000000000000000000, 0.8660254037844387076, 1.000000000000000000, 0.8660254037844387076, 1.000000000000000000, 0.8660254037844387076, 1.000000000000000000, 0.8660254037844387076, 1.000000000000000000, 0.8660254037844387076, 1.000000000000000000, 0.8660254037844387076, 1.000000000000000000, 0.8660254037844387076, 1.000000000000000000, 0.8660254037844387076, 1.000000000000000000, 0.8660254037844387076, 1.000000000000000000, 0.8660254037844387076, 1.000000000000000000, 0.8660254037844387076, 1.000000000000000000, 0.8660254037844387076, 1.000000000000000000, 0.8660254037844387076, 1.000000000000000000, 0.8660254037844387076, 1.000000000000000000, 0.8660254037844387076, 1.000000000000000000, 0.8660254037844387076, 1.000000000000000000, 0.8660254037844387076, 1.000000000000000000, 0.8660254037844387076, 1.000000000000000000, 0.8660254037844387076, 1.000000000000000000, 0.8660254037844387076, 1.000000000000000000, 0.8660254037844387076, 1.000000000000000000, 0.8660254037844387076, 1.000000000000000000, 0.8660254037844387076, 1.000000000000000000, 0.8660254037844387076, 1.000000000000000000, 0.8660254037844387076, 1.000000000000000000, 0.8660254037844387076, 1.000000000000000000, 0.8660254037844387076, 1.000000000000000000, 0.8660254037844387076, 1.000000000000000000, 0.8660254037844387076, 1.000000000000000000, 0.8660254037844387076, 1.000000000000000000, 0.8660254037844387076, 1.000000000000000000, 0.8660254037844387076, 1.000000000000000000, 0.8660254037844387076, 1.000000000000000000, 0.8660254037844387076, 1.000000000000000000, 0.8660254037844387076, 1.000000000000000000, 0.8660254037844387076, 1.000000000000000000, 0.8660254037844387076, 1.000000000000000000, 0.8660254037844387076, 1.000000000000000000, 0.8660254037844387076, 1.000000000000000000, 0.8660254037844387076, 1.000000000000000000, 0.8660254037844387076, 1.000000000000000000, 0.8660254037844387076, 1.000000000000000000, 0.8660254037844387076, 1.000000000000000000, 0.8660254037844387076, 1.000000000000000000, 0.8660254037844387076, 1.000000000000000000, 0.8660254037844387076, 1.000000000000000000, 0.8660254037844387076, 1.000000000000000000, 0.8660254037844387076, 1.000000000000000000, 0.8660254037844387076, 1.000000000000000000, 0.8660254037844387076, 1.000000000000000000, 0.8660254037844387076, 1.000000000000000000, 0.8660254037844387076, 1.000000000000000000, 0.8660254037844387076, 1.000000000000000000, 0.8660254037844387076, 1.000000000000000000, 0.8660254037844387076, 1.000000000000000000, 0.8660254037844387076, 1.000000000000000000, 0.8660254037844387076, 1.000000000000000000, 0.8660254037844387076, 1.000000000000000000, 0.8660254037844387076, 1.000000000000000000, 0.8660254037844387076, 1.000000000000000000, 0.8660254037844387076, 1.000000000000000000, 0.8660254037844387076, 1.000000000000000000, 0.8660254037844387076, 1.000000000000000000, 0.8660254037844387076, 1.000000000000000000, 0.8660254037844387076, 1.000000000000000000, 0.8660254037844387076, 1.000000000000000000, 0.8660254037844387076, 1.000000000000000000, 0.8660254037844387076, 1.000000000000000000, 0.8660254037844387076, 1.000000000000000000, 0.8660254037844387076, 1.000000000000000000, 0.8660254037844387076, 1.000000000000000000, 0.8660254037844387076, 1.000000000000000000, 0.8660254037844387076, 1.000000000000000000, 0.8660254037844387076, 1.000000000000000000, 0.8660254037844387076, 1.000000000000000000, 0.8660254037844387076, 1.000000000000000000, 0.8660254037844387076, 1.000000000000000000, 0.8660254037844387076, 1.000000000000000000, 0.8660254037844387076, 1.000000000000000000, 0.8660254037844387076, 1.000000000000000000, 0.8660254037844387076, 1.000000000000000000, 0.8660254037844387076, 1.000000000000000000, 0.8660254037844387076, 1.000000000000000000, 0.8660254037844387076, 1.000000000000000000, 0.8660254037844387076, 1.000000000000000000, 0.8660254037844387076, 1.000000000000000000, 0.8660254037844387076, 1.000000000000000000, 0.8660254037844387076, 1.000000000000000000, 0.8660254037844387076, 1.000000000000000000, 0.8660254037844387076, 1.000000000000000000, 0.8660254037844387076, 1.000000000000000000, 0.8660254037844387076, 1.000000000000000000, 0.8660254037844387076, 1.000000000000000000, 0.8660254037844387076, 1.000000000000000000, 0.8660254037844387076, 1.000000000000000000, 0.8660254037844387076, 1.000000000000000000, 0.8660254037844387076, 1.000000000000000000, 0.8660254037844387076, 1.000000000000000000, 0.8660254037844387076, 1.000000000000000000, 0.8660254037844387076, 1.000000000000000000, 0.8660254037844387076, 1.000000000000000000, 0.8660254037844387076, 1.000000000000000000, 0.8660254037844387076, 1.000000000000000000, 0.8660254037844387076, 1.000000000000000000, 0.8660254037844387076, 1.000000000000000000, 0.8660254037844387076, 1.000000000000000000, 0.8660254037844387076, 1.000000000000000000, 0.8660254037844387076, 1.000000000000000000, 0.8660254037844387076, 1.000000000000000000, 0.8660254037844387076, 1.000000000000000000, 0.8660254037844387076, 1.000000000000000000, 0.8660254037844387076, 1.000000000000000000, 0.8660254037844387076, 1.000000000000000000, 0.8660254037844387076, 1.000000000000000000, 0.8660254037844387076, 1.000000000000000000, 0.8660254037844387076, 1.000000000000000000, 0.8660254037844387076, 1.000000000000000000, 0.8660254037844387076, 1.000000000000000000, 0.8660254037844387076, 1.000000000000000000, 0.8660254037844387076, 1.000000000000000000, 0.8660254037844387076, 1.000000000000000000, 0.8660254037844387076, 1.000000000000000000, 0.8660254037844387076, 1.000000000000000000, 0.8660254037844387076, 1.000000000000000000, 0.8660254037844387076, 1.000000000000000000, 0.8660254037844387076, 1.000000000000000000, 0.8660254037844387076, 1.000000000000000000, 0.8660254037844387076, 1.000000000000000000, 0.8660254037844387076, 1.000000000000000000, 0.8660254037844387076, 1.000000000000000000, 0.8660254037844387076, 1.000000000000000000, 0.8660254037844387076, 1.000000000000000000, 0.8660254037844387076, 1.000000000000000000, 0.8660254037844387076, 1.000000000000000000, 0.8660254037844387076, 1.000000000000000000, 0.8660254037844387076, 1.000000000000000000, 0.8660254037844387076, 1.000000000000000000, 0.8660254037844387076, 1.000000000000000000, 0.8660254037844387076, 1.000000000000000000, 0.8660254037844387076, 1.000000000000000000, 0.8660254037844387076, 1.000000000000000000, 0.8660254037844387076, 1.000000000000000000, 0.8660254037844387076, 1.000000000000000000, 0.8660254037844387076, 1.000000000000000000, 0.8660254037844387076, 1.000000000000000000, 0.8660254037844387076, 1.000000000000000000, 0.8660254037844387076, 1.000000000000000000, 0.8660254037844387076, 1.000000000000000000, 0.8660254037844387076, 1.000000000000000000, 0.8660254037844387076, 1.000000000000000000, 0.8660254037844387076, 1.000000000000000000, 0.8660254037844387076, 1.000000000000000000, 0.8660254037844387076, 1.000000000000000000, 0.8660254037844387076, 1.000000000000000000, 0.8660254037844387076, 1.000000000000000000, 0.8660254037844387076, 1.000000000000000000, 0.8660254037844387076, 1.000000000000000000, 0.8660254037844387076, 1.000000000000000000, 0.8660254037844387076, 1.000000000000000000, 0.8660254037844387076, 1.000000000000000000, 0.8660254037844387076, 1.000000000000000000, 0.8660254037844387076, 1.000000000000000000, 0.8660254037844387076, 1.000000000000000000, 0.8660254037844387076, 1.000000000000000000, 0.8660254037844387076, 1.000000000000000000, 0.8660254037844387076, 1.000000000000000000, 0.8660254037844387076, 1.000000000000000000, 0.8660254037844387076, 1.000000000000000000, 0.8660254037844387076, 1.000000000000000000, 0.8660254037844387076, 1.000000000000000000, 0.8660254037844387076, 1.000000000000000000, 0.8660254037844387076, 1.000000000000000000, 0.8660254037844387076, 1.000000000000000000, 0.8660254037844387076, 1.000000000000000000, 0.8660254037844387076, 1.000000000000000000, 0.8660254037844387076, 1.000000000000000000, 0.8660254037844387076, 1.000000000000000000, 0.8660254037844387076, 1.000000000000000000, 0.8660254037844387076, 1.000000000000000000, 0.8660254037844387076, 1.000000000000000000, 0.8660254037844387076, 1.000000000000000000, 0.8660254037844387076, 1.000000000000000000, 0.8660254037844387076, 1.000000000000000000, 0.8660254037844387076, 1.000000000000000000, 0.8660254037844387076, 1.000000000000000000, 0.8660254037844387076, 1.000000000000000000, 0.8660254037844387076, 1.000000000000000000, 0.8660254037844387076, 1.000000000000000000, 0.8660254037844387076, 1.000000000000000000, 0.8660254037844387076, 1.000000000000000000, 0.8660254037844387076, 1.000000000000000000, 0.8660254037844387076, 1.000000000000000000, 0.8660254037844387076, 1.000000000000000000, 0.8660254037844387076, 1.000000000000000000, 0.8660254037844387076, 1.000000000000000000, 0.8660254037844387076, 1.000000000000000000, 0.8660254037844387076, 1.000000000000000000, 0.8660254037844387076, 1.000000000000000000, 0.8660254037844387076, 1.000000000000000000, 0.8660254037844387076, 1.000000000000000000, 0.8660254037844387076, 1.000000000000000000, 0.8660254037844387076, 1.000000000000000000),
 ( 1.000000000000000000, 0.8660254037844387076, 1.000000000000000000, 0.8660254037844387076, 1.000000000000000000, 0.8660254037844387076, 1.000000000000000000, 0.8660254037844387076, 1.000000000000000000, 0.8660254037844387076, 1.000000000000000000, 0.8660254037844387076, 1.000000000000000000, 0.8660254037844387076, 1.000000000000000000, 0.8660254037844387076, 1.000000000000000000, 0.8660254037844387076, 1.000000000000000000, 0.8660254037844387076, 1.000000000000000000, 0.8660254037844387076, 1.000000000000000000, 0.8660254037844387076, 1.000000000000000000, 0.8660254037844387076, 1.000000000000000000, 0.8660254037844387076, 1.000000000000000000, 0.8660254037844387076, 1.000000000000000000, 0.8660254037844387076, 1.000000000000000000, 0.8660254037844387076, 1.000000000000000000, 0.8660254037844387076, 1.000000000000000000, 0.8660254037844387076, 1.000000000000000000, 0.8660254037844387076, 1.000000000000000000, 0.8660254037844387076, 1.000000000000000000, 0.8660254037844387076, 1.000000000000000000, 0.8660254037844387076, 1.000000000000000000, 0.8660254037844387076, 1.000000000000000000, 0.8660254037844387076, 1.000000000000000000, 0.8660254037844387076, 1.000000000000000000, 0.8660254037844387076, 1.000000000000000000, 0.8660254037844387076, 1.000000000000000000, 0.8660254037844387076, 1.000000000000000000, 0.8660254037844387076, 1.000000000000000000, 0.8660254037844387076, 1.000000000000000000, 0.8660254037844387076, 1.000000000000000000, 0.8660254037844387076, 1.000000000000000000, 0.8660254037844387076, 1.000000000000000000, 0.8660254037844387076, 1.000000000000000000, 0.8660254037844387076, 1.000000000000000000, 0.8660254037844387076, 1.000000000000000000, 0.8660254037844387076, 1.000000000000000000, 0.8660254037844387076, 1.000000000000000000, 0.8660254037844387076, 1.000000000000000000, 0.8660254037844387076, 1.000000000000000000, 0.8660254037844387076, 1.000000000000000000, 0.8660254037844387076, 1.000000000000000000, 0.8660254037844387076, 1.000000000000000000, 0.8660254037844387076, 1.000000000000000000, 0.8660254037844387076, 1.000000000000000000, 0.8660254037844387076, 1.000000000000000000, 0.8660254037844387076, 1.000000000000000000, 0.8660254037844387076, 1.000000000000000000, 0.8660254037844387076, 1.000000000000000000, 0.8660254037844387076, 1.000000000000000000, 0.8660254037844387076, 1.000000000000000000, 0.8660254037844387076, 1.000000000000000000, 0.8660254037844387076, 1.000000000000000000, 0.8660254037844387076, 1.000000000000000000, 0.8660254037844387076, 1.000000000000000000, 0.8660254037844387076, 1.000000000000000000, 0.8660254037844387076, 1.000000000000000000, 0.8660254037844387076, 1.000000000000000000, 0.8660254037844387076, 1.000000000000000000, 0.8660254037844387076, 1.000000000000000000, 0.8660254037844387076, 1.000000000000000000, 0.8660254037844387076, 1.000000000000000000, 0.8660254037844387076, 1.000000000000000000, 0.8660254037844387076, 1.000000000000000000, 0.8660254037844387076, 1.000000000000000000, 0.8660254037844387076, 1.000000000000000000, 0.8660254037844387076, 1.000000000000000000, 0.8660254037844387076, 1.000000000000000000, 0.8660254037844387076, 1.000000000000000000, 0.8660254037844387076, 1.000000000000000000, 0.8660254037844387076, 1.000000000000000000, 0.8660254037844387076, 1.000000000000000000, 0.8660254037844387076, 1.000000000000000000, 0.8660254037844387076, 1.000000000000000000, 0.8660254037844387076, 1.000000000000000000, 0.8660254037844387076, 1.000000000000000000, 0.8660254037844387076, 1.000000000000000000, 0.8660254037844387076, 1.000000000000000000, 0.8660254037844387076, 1.000000000000000000, 0.8660254037844387076, 1.000000000000000000, 0.8660254037844387076, 1.000000000000000000, 0.8660254037844387076, 1.000000000000000000, 0.8660254037844387076, 1.000000000000000000, 0.8660254037844387076, 1.000000000000000000, 0.8660254037844387076, 1.000000000000000000, 0.8660254037844387076, 1.000000000000000000, 0.8660254037844387076, 1.000000000000000000, 0.8660254037844387076, 1.000000000000000000, 0.8660254037844387076, 1.000000000000000000, 0.8660254037844387076, 1.000000000000000000, 0.8660254037844387076, 1.000000000000000000, 0.8660254037844387076, 1.000000000000000000, 0.8660254037844387076, 1.000000000000000000, 0.8660254037844387076, 1.000000000000000000, 0.8660254037844387076, 1.000000000000000000, 0.8660254037844387076, 1.000000000000000000, 0.8660254037844387076, 1.000000000000000000, 0.8660254037844387076, 1.000000000000000000, 0.8660254037844387076, 1.000000000000000000, 0.8660254037844387076, 1.000000000000000000, 0.8660254037844387076, 1.000000000000000000, 0.8660254037844387076, 1.000000000000000000, 0.8660254037844387076, 1.000000000000000000, 0.8660254037844387076, 1.000000000000000000, 0.8660254037844387076, 1.000000000000000000, 0.8660254037844387076, 1.000000000000000000, 0.8660254037844387076, 1.000000000000000000, 0.8660254037844387076, 1.000000000000000000, 0.8660254037844387076, 1.000000000000000000, 0.8660254037844387076, 1.000000000000000000, 0.8660254037844387076, 1.000000000000000000, 0.8660254037844387076, 1.000000000000000000, 0.8660254037844387076, 1.000000000000000000, 0.8660254037844387076, 1.000000000000000000, 0.8660254037844387076, 1.000000000000000000, 0.8660254037844387076, 1.000000000000000000, 0.8660254037844387076, 1.000000000000000000, 0.8660254037844387076, 1.000000000000000000, 0.8660254037844387076, 1.000000000000000000, 0.8660254037844387076, 1.000000000000000000, 0.8660254037844387076, 1.000000000000000000, 0.8660254037844387076, 1.000000000000000000, 0.8660254037844387076, 1.000000000000000000, 0.8660254037844387076, 1.000000000000000000, 0.8660254037844387076, 1.000000000000000000, 0.8660254037844387076, 1.000000000000000000, 0.8660254037844387076, 1.000000000000000000, 0.8660254037844387076, 1.000000000000000000, 0.8660254037844387076, 1.000000000000000000, 0.8660254037844387076, 1.000000000000000000, 0.8660254037844387076, 1.000000000000000000, 0.8660254037844387076, 1.000000000000000000, 0.8660254037844387076, 1.000000000000000000, 0.8660254037844387076, 1.000000000000000000, 0.8660254037844387076, 1.000000000000000000, 0.8660254037844387076, 1.000000000000000000, 0.8660254037844387076, 1.000000000000000000, 0.8660254037844387076, 1.000000000000000000, 0.8660254037844387076, 1.000000000000000000, 0.8660254037844387076, 1.000000000000000000, 0.8660254037844387076, 1.000000000000000000, 0.8660254037844387076, 1.000000000000000000, 0.8660254037844387076, 1.000000000000000000, 0.8660254037844387076, 1.000000000000000000, 0.8660254037844387076, 1.000000000000000000, 0.8660254037844387076, 1.000000000000000000, 0.8660254037844387076, 1.000000000000000000, 0.8660254037844387076, 1.000000000000000000, 0.8660254037844387076, 1.000000000000000000, 0.8660254037844387076, 1.000000000000000000, 0.8660254037844387076, 1.000000000000000000, 0.8660254037844387076, 1.000000000000000000, 0.8660254037844387076, 1.000000000000000000, 0.8660254037844387076, 1.000000000000000000, 0.8660254037844387076, 1.000000000000000000, 0.8660254037844387076, 1.000000000000000000, 0.8660254037844387076, 1.000000000000000000, 0.8660254037844387076, 1.000000000000000000, 0.8660254037844387076, 1.000000000000000000, 0.8660254037844387076, 1.000000000000000000, 0.8660254037844387076, 1.000000000000000000, 0.8660254037844387076, 1.000000000000000000, 0.8660254037844387076, 1.000000000000000000, 0.8660254037844387076, 1.000000000000000000, 0.8660254037844387076, 1.000000000000000000, 0.8660254037844387076, 1.000000000000000000, 0.8660254037844387076, 1.000000000000000000, 0.8660254037844387076, 1.000000000000000000, 0.8660254037844387076, 1.000000000000000000, 0.8660254037844387076, 1.000000000000000000, 0.8660254037844387076, 1.000000000000000000, 0.8660254037844387076, 1.000000000000000000, 0.8660254037844387076, 1.000000000000000000, 0.8660254037844387076, 1.000000000000000000, 0.8660254037844387076, 1.000000000000000000, 0.8660254037844387076, 1.000000000000000000, 0.8660254037844387076, 1.000000000000000000, 0.8660254037844387076, 1.000000000000000000, 0.8660254037844387076, 1.000000000000000000, 0.8660254037844387076, 1.000000000000000000, 0.8660254037844387076, 1.000000000000000000, 0.8660254037844387076, 1.000000000000000000, 0.8660254037844387076, 1.000000000000000000, 0.8660254037844387076, 1.000000000000000000, 0.8660254037844387076, 1.000000000000000000, 0.8660254037844387076, 1.000000000000000000, 0.8660254037844387076, 1.000000000000000000, 0.8660254037844387076, 1.000000000000000000, 0.8660254037844387076, 1.000000000000000000, 0.8660254037844387076, 1.000000000000000000, 0.8660254037844387076, 1.000000000000000000, 0.8660254037844387076, 1.000000000000000000, 0.8660254037844387076, 1.000000000000000000, 0.8660254037844387076, 1.000000000000000000, 0.8660254037844387076, 1.000000000000000000, 0.8660254037844387076, 1.000000000000000000, 0.8660254037844387076, 1.000000000000000000, 0.8660254037844387076, 1.000000000000000000, 0.8660254037844387076, 1.000000000000000000, 0.8660254037844387076, 1.000000000000000000, 0.8660254037844387076, 1.000000000000000000, 0.8660254037844387076, 1.000000000000000000, 0.8660254037844387076, 1.000000000000000000, 0.8660254037844387076, 1.000000000000000000, 0.8660254037844387076, 1.000000000000000000, 0.8660254037844387076, 1.000000000000000000, 0.8660254037844387076, 1.000000000000000000, 0.8660254037844387076, 1.000000000000000000, 0.8660254037844387076, 1.000000000000000000, 0.8660254037844387076, 1.000000000000000000, 0.8660254037844387076, 1.000000000000000000, 0.8660254037844387076, 1.000000000000000000, 0.8660254037844387076, 1.000000000000000000, 0.8660254037844387076, 1.000000000000000000, 0.8660254037844387076, 1.000000000000000000, 0.8660254037844387076, 1.000000000000000000, 0.8660254037844387076, 1.000000000000000000, 0.8660254037844387076, 1.000000000000000000, 0.8660254037844387076, 1.000000000000000000, 0.8660254037844387076, 1.000000000000000000, 0.8660254037844387076, 1.000000000000000000, 0.8660254037844387076, 1.000000000000000000, 0.8660254037844387076, 1.000000000000000000, 0.8660254037844387076, 1.000000000000000000, 0.8660254037844387076, 1.000000000000000000, 0.8660254037844387076, 1.000000000000000000, 0.8660254037844387076, 1.000000000000000000, 0.8660254037844387076, 1.000000000000000000, 0.8660254037844387076, 1.000000000000000000, 0.8660254037844387076, 1.000000000000000000, 0.8660254037844387076, 1.000000000000000000, 0.8660254037844387076, 1.000000000000000000, 0.8660254037844387076, 1.000000000000000000, 0.8660254037844387076, 1.000000000000000000, 0.8660254037844387076, 1.000000000000000000, 0.8660254037844387076, 1.000000000000000000, 0.8660254037844387076, 1.000000000000000000, 0.8660254037844387076, 1.000000000000000000, 0.8660254037844387076, 1.000000000000000000, 0.8660254037844387076, 1.000000000000000000, 0.8660254037844387076, 1.000000000000000000, 0.8660254037844387076, 1.000000000000000000, 0.8660254037844387076, 1.000000000000000000, 0.8660254037844387076, 1.000000000000000000, 0.8660254037844387076, 1.000000000000000000, 0.8660254037844387076, 1.000000000000000000, 0.8660254037844387076, 1.000000000000000000, 0.8660254037844387076, 1.000000000000000000, 0.8660254037844387076, 1.000000000000000000, 0.8660254037844387076, 1.000000000000000000, 0.8660254037844387076, 1.000000000000000000, 0.8660254037844387076, 1.000000000000000000, 0.8660254037844387076, 1.000000000000000000, 0.8660254037844387076, 1.000000000000000000, 0.8660254037844387076, 1.000000000000000000, 0.8660254037844387076, 1.000000000000000000, 0.8660254037844387076, 1.000000000000000000, 0.8660254037844387076, 1.000000000000000000, 0.8660254037844387076, 1.000000000000000000, 0.8660254037844387076, 1.000000000000000000, 0.8660254037844387076, 1.000000000000000000, 0.8660254037844387076, 1.000000000000000000, 0.8660254037844387076, 1.000000000000000000, 0.8660254037844387076, 1.000000000000000000, 0.8660254037844387076, 1.000000000000000000, 0.8660254037844387076, 1.000000000000000000, 0.8660254037844387076, 1.000000000000000000, 0.8660254037844387076, 1.000000000000000000, 0.8660254037844387076, 1.000000000000000000, 0.8660254037844387076, 1.000000000000000000, 0.8660254037844387076, 1.000000000000000000, 0.8660254037844387076, 1.000000000000000000, 0.8660254037844387076, 1.000000000000000000, 0.8660254037844387076, 1.000000000000000000, 0.8660254037844387076, 1.000000000000000000, 0.8660254037844387076, 1.000000000000000000, 0.8660254037844387076, 1.000000000000000000, 0.8660254037844387076, 1.000000000000000000, 0.8660254037844387076, 1.000000000000000000, 0.8660254037844387076, 1.000000000000000000, 0.8660254037844387076, 1.000000000000000000, 0.8660254037844387076, 1.000000000000000000, 0.8660254037844387076, 1.000000000000000000, 0.8660254037844387076, 1.000000000000000000, 0.8660254037844387076, 1.000000000000000000, 0.8660254037844387076, 1.000000000000000000, 0.8660254037844387076, 1.000000000000000000, 0.8660254037844387076, 1.000000000000000000, 0.8660254037844387076, 1.000000000000000000, 0.8660254037844387076, 1.000000000000000000, 0.8660254037844387076, 1.000000000000000000, 0.8660254037844387076, 1.000000000000000000, 0.8660254037844387076, 1.000000000000000000, 0.8660254037844387076, 1.000000000000000000, 0.8660254037844387076, 1.000000000000000000, 0.8660254037844387076, 1.000000000000000000, 0.8660254037844387076, 1.000000000000000000, 0.8660254037844387076, 1.000000000000000000, 0.8660254037844387076, 1.000000000000000000, 0.8660254037844387076, 1.000000000000000000, 0.8660254037844387076, 1.000000000000000000, 0.8660254037844387076, 1.000000000000000000, 0.8660254037844387076, 1.000000000000000000, 0.8660254037844387076, 1.000000000000000000, 0.8660254037844387076, 1.000000000000000000, 0.8660254037844387076, 1.000000000000000000, 0.8660254037844387076, 1.000000000000000000, 0.8660254037844387076, 1.000000000000000000, 0.8660254037844387076, 1.000000000000000000, 0.8660254037844387076, 1.000000000000000000, 0.8660254037844387076, 1.000000000000000000, 0.8660254037844387076, 1.000000000000000000, 0.8660254037844387076, 1.000000000000000000, 0.8660254037844387076, 1.000000000000000000, 0.8660254037844387076, 1.000000000000000000, 0.8660254037844387076, 1.000000000000000000, 0.8660254037844387076, 1.000000000000000000, 0.8660254037844387076, 1.000000000000000000, 0.8660254037844387076, 1.000000000000000000, 0.8660254037844387076, 1.000000000000000000, 0.8660254037844387076, 1.000000000000000000, 0.8660254037844387076, 1.000000000000000000, 0.8660254037844387076, 1.000000000000000000, 0.8660254037844387076, 1.000000000000000000, 0.8660254037844387076, 1.000000000000000000, 0.8660254037844387076, 1.000000000000000000, 0.8660254037844387076, 1.000000000000000000, 0.8660254037844387076, 1.000000000000000000, 0.8660254037844387076, 1.000000000000000000, 0.8660254037844387076, 1.000000000000000000, 0.8660254037844387076, 1.000000000000000000, 0.8660254037844387076, 1.000000000000000000, 0.8660254037844387076, 1.000000000000000000, 0.8660254037844387076, 1.000000000000000000, 0.8660254037844387076, 1.000000000000000000, 0.8660254037844387076, 1.000000000000000000, 0.8660254037844387076, 1.000000000000000000, 0.8660254037844387076, 1.000000000000000000, 0.8660254037844387076, 1.000000000000000000, 0.8660254037844387076, 1.000000000000000000, 0.8660254037844387076, 1.000000000000000000, 0.8660254037844387076, 1.000000000000000000, 0.8660254037844387076, 1.000000000000000000, 0.8660254037844387076, 1.000000000000000000, 0.8660254037844387076, 1.000000000000000000, 0.8660254037844387076, 1.000000000000000000, 0.8660254037844387076, 1.000000000000000000, 0.8660254037844387076, 1.000000000000000000, 0.8660254037844387076, 1.000000000000000000, 0.8660254037844387076, 1.000000000000000000, 0.8660254037844387076, 1.000000000000000000, 0.8660254037844387076, 1.000000000000000000, 0.8660254037844387076, 1.000000000000000000, 0.8660254037844387076, 1.000000000000000000, 0.8660254037844387076, 1.000000000000000000, 0.8660254037844387076, 1.000000000000000000, 0.8660254037844387076, 1.000000000000000000, 0.8660254037844387076, 1.000000000000000000, 0.8660254037844387076, 1.000000000000000000) ) ) 
 REPRESENTATION_ITEM ( '' )  SURFACE ( )  );
#26668=CARTESIAN_POINT ( 'NONE',  ( 23.25937500061451857, -4.541064518000417216, -2.621784821875001281 ) ) ;
#26669=CARTESIAN_POINT ( 'NONE',  ( 20.76562500061451644, 3.027376345333611329, 5.243569643749999010 ) ) ;
#26670=CARTESIAN_POINT ( 'NONE',  ( 4.000000000000000000, 12.53749999999999964, 32.30940107675849049 ) ) ;
#26671=CARTESIAN_POINT ( 'NONE',  ( 25.82812500061451644, -4.541064518000419881, 2.621784821874995952 ) ) ;
#26672=CARTESIAN_POINT ( 'NONE',  ( 6.600000001229032520, 5.773502691896255534, 3.535250795749688894E-16 ) ) ;
#26673=VECTOR ( 'NONE', #39067, 1000.000000000000000 ) ;
#26674=ORIENTED_EDGE ( 'NONE', *, *, #13592, .F. ) ;
#26675=CARTESIAN_POINT ( 'NONE',  ( 22.46250000122903501, 0.000000000000000000, 4.999999999999998224 ) ) ;
#26676=CARTESIAN_POINT ( 'NONE',  ( 4.000000000000000000, 14.33750000000000213, -27.69059892324149530 ) ) ;
#26677=CARTESIAN_POINT ( 'NONE',  ( 22.80000000122903359, 5.773502691896255534, 3.535250795749688894E-16 ) ) ;
#26679=CARTESIAN_POINT ( 'NONE',  ( 4.509375000614518569, 4.541064518000418104, -2.621784821874998173 ) ) ;
#26680=CARTESIAN_POINT ( 'NONE',  ( 23.36250000000000071, -5.773502691896255534, -1.060575238724906372E-15 ) ) ;
#26681=CARTESIAN_POINT ( 'NONE',  ( 12.51562500061451821, 3.027376345333613106, -5.243569643749998122 ) ) ;
#26682=CARTESIAN_POINT ( 'NONE',  ( 8.334375000614516082, -4.541064518000419881, 2.621784821874995952 ) ) ;
#26683=CARTESIAN_POINT ( 'NONE',  ( 23.81250000122903288, 0.000000000000000000, 4.999999999999998224 ) ) ;
#26684=CARTESIAN_POINT ( 'NONE',  ( 14.33437500061451786, 6.421520780324663323E-16, -5.243569643749999010 ) ) ;
#26685=CARTESIAN_POINT ( 'NONE',  ( 2.859375000614519546, 0.000000000000000000, 5.243569643749999010 ) ) ;
#26686=CARTESIAN_POINT ( 'NONE',  ( 8.025000001229035007, 2.886751345948126879, 4.999999999999998224 ) ) ;
#26687=CARTESIAN_POINT ( 'NONE',  ( 4.303125000614516971, -4.541064518000417216, -2.621784821875001281 ) ) ;
#26688=CARTESIAN_POINT ( 'NONE',  ( 14.27812500061451573, 6.421520780324663323E-16, -5.243569643749999010 ) ) ;
#26690=CARTESIAN_POINT ( 'NONE',  ( 11.95312500061451644, -4.541064518000417216, -2.621784821875001281 ) ) ;
#26691=CARTESIAN_POINT ( 'NONE',  ( 9.103125000614515017, 0.000000000000000000, 5.243569643749999010 ) ) ;
#26693=CARTESIAN_POINT ( 'NONE',  ( 8.175000000000002487, 6.123233995736764310E-16, -4.999999999999998224 ) ) ;
#26694=CARTESIAN_POINT ( 'NONE',  ( 4.237500001229036251, 6.123233995736764310E-16, -4.999999999999998224 ) ) ;
#26695=CARTESIAN_POINT ( 'NONE',  ( 18.59999999999999787, 4.330127018922192761, -2.499999999999997780 ) ) ;
#26696=CARTESIAN_POINT ( 'NONE',  ( 19.35937500061451644, 4.541064518000418104, -2.621784821874998173 ) ) ;
#26697=CARTESIAN_POINT ( 'NONE',  ( 13.20000000122903394, -2.886751345948125991, -5.000000000000000000 ) ) ;
#26699=AXIS2_PLACEMENT_3D ( 'NONE', #35581, #39057, #58102 ) ;
#26700=CARTESIAN_POINT ( 'NONE',  ( -3.000416591977282496E-16, 16.99062500061451786, -34.90005215228797653 ) ) ;
#26703=CARTESIAN_POINT ( 'NONE',  ( 28.67812500061451431, 6.421520780324663323E-16, -5.243569643749999010 ) ) ;
#26704=FACE_OUTER_BOUND ( 'NONE', #13431, .T. ) ;
#26705=CARTESIAN_POINT ( 'NONE',  ( 13.47187500061451537, 3.027376345333613106, -5.243569643749998122 ) ) ;
#26706=CARTESIAN_POINT ( 'NONE',  ( 27.00000000000000000, -4.330127018922190985, -2.500000000000001332 ) ) ;
#26707=CARTESIAN_POINT ( 'NONE',  ( 10.75312500061451715, 4.541064518000418104, -2.621784821874998173 ) ) ;
#26709=CARTESIAN_POINT ( 'NONE',  ( 20.29687500061451644, 6.054752690667223547, 3.707466751127219781E-16 ) ) ;
#26711=CARTESIAN_POINT ( 'NONE',  ( 7.978125000614517681, 6.421520780324663323E-16, -5.243569643749999010 ) ) ;
#26712=CARTESIAN_POINT ( 'NONE',  ( 13.09687500061451892, 6.054752690667223547, 3.707466751127219781E-16 ) ) ;
#26713=ORIENTED_EDGE ( 'NONE', *, *, #25401, .F. ) ;
#26714=CARTESIAN_POINT ( 'NONE',  ( 23.70937500061451786, -4.541064518000417216, -2.621784821875001281 ) ) ;
#26715=CARTESIAN_POINT ( 'NONE',  ( 3.943546631589882168, 3.074146327801218881, -29.31700319132604093 ) ) ;
#26716=CARTESIAN_POINT ( 'NONE',  ( 8.849999999999999645, 0.000000000000000000, 4.999999999999998224 ) ) ;
#26717=EDGE_CURVE ( 'NONE', #40294, #47010, #3202, .T. ) ;
#26718=CARTESIAN_POINT ( 'NONE',  ( 4.724999999999999645, 4.330127018922191873, 2.499999999999999556 ) ) ;
#26719=CARTESIAN_POINT ( 'NONE',  ( 18.03750000122903430, -4.330127018922194537, 2.499999999999995559 ) ) ;
#26723=CARTESIAN_POINT ( 'NONE',  ( 16.12500000000000000, -4.330127018922194537, 2.499999999999995559 ) ) ;
#26724=CARTESIAN_POINT ( 'NONE',  ( 16.23750000000000071, -2.886751345948125991, -5.000000000000000000 ) ) ;
#26725=CARTESIAN_POINT ( 'NONE',  ( 12.44062500061451537, -3.027376345333610441, -5.243569643749999898 ) ) ;
#26726=ORIENTED_EDGE ( 'NONE', *, *, #4619, .F. ) ;
#26727=CARTESIAN_POINT ( 'NONE',  ( 24.60000000000000142, 0.000000000000000000, 4.999999999999998224 ) ) ;
#26728=CARTESIAN_POINT ( 'NONE',  ( -2.121784821874996840, 18.13437500061451502, -26.32496088578401583 ) ) ;
#26729=CARTESIAN_POINT ( 'NONE',  ( 29.32500000122903216, -5.773502691896255534, -1.060575238724906372E-15 ) ) ;
#26731=CARTESIAN_POINT ( 'NONE',  ( 10.87500000000000000, 6.123233995736764310E-16, -4.999999999999998224 ) ) ;
#26732=CARTESIAN_POINT ( 'NONE',  ( 3.765213524098920406, 3.290336489363023365, -3.765213524098920406 ) ) ;
#26733=EDGE_LOOP ( 'NONE', ( #44456, #67314, #8613, #14622 ) ) ;
#26734=CARTESIAN_POINT ( 'NONE',  ( 9.001249775931846008E-16, 11.81562500061451715, 34.90005215228797653 ) ) ;
#26735=CARTESIAN_POINT ( 'NONE',  ( 24.06562500061451715, -6.054752690667223547, -1.112240025338166033E-15 ) ) ;
#26736=CARTESIAN_POINT ( 'NONE',  ( 3.593020343235445058, 3.477097182003509257, 3.793492915512545416 ) ) ;
#26738=CARTESIAN_POINT ( 'NONE',  ( 21.72187500061451715, 3.027376345333611329, 5.243569643749999010 ) ) ;
#26739=CARTESIAN_POINT ( 'NONE',  ( 19.90312500061451573, 0.000000000000000000, 5.243569643749999010 ) ) ;
#26740=EDGE_CURVE ( 'NONE', #59952, #62607, #43825, .T. ) ;
#26741=CARTESIAN_POINT ( 'NONE',  ( 4.243569643749999898, 15.07812500061459460, -30.00000000000000000 ) ) ;
#26742=CARTESIAN_POINT ( 'NONE',  ( 23.13750000122903216, 6.123233995736764310E-16, -4.999999999999998224 ) ) ;
#26743=CARTESIAN_POINT ( 'NONE',  ( 4.790625000614518569, -3.027376345333610441, -5.243569643749999898 ) ) ;
#26745=CARTESIAN_POINT ( 'NONE',  ( 20.91562500061451502, -6.054752690667223547, -1.112240025338166033E-15 ) ) ;
#26748=CARTESIAN_POINT ( 'NONE',  ( 15.72187500061451892, 3.027376345333613106, -5.243569643749998122 ) ) ;
#26749=CARTESIAN_POINT ( 'NONE',  ( 15.38437500061451679, 4.541064518000418104, 2.621784821874999949 ) ) ;
#26750=CARTESIAN_POINT ( 'NONE',  ( 23.48437500061451644, 4.541064518000418104, 2.621784821874999949 ) ) ;
#26751=CARTESIAN_POINT ( 'NONE',  ( -4.243569643749998122, 11.79687500061451999, 32.45002607614398471 ) ) ;
#26752=CARTESIAN_POINT ( 'NONE',  ( 6.140625000614516438, -3.027376345333610441, -5.243569643749999898 ) ) ;
#26753=CARTESIAN_POINT ( 'NONE',  ( 25.37812500061451715, -4.541064518000419881, 2.621784821874995952 ) ) ;
#26755=CARTESIAN_POINT ( 'NONE',  ( 27.10312500061451502, 0.000000000000000000, 5.243569643749999010 ) ) ;
#26756=CARTESIAN_POINT ( 'NONE',  ( 8.475000001229034297, 2.886751345948193936, 4.999999999999883649 ) ) ;
#26757=CARTESIAN_POINT ( 'NONE',  ( 8.484601909799253346E-16, 19.21250000000000213, 34.61880215351700230 ) ) ;
#26758=CARTESIAN_POINT ( 'NONE',  ( 6.121875000614517504, -6.054752690667223547, -1.112240025338166033E-15 ) ) ;
#26760=CARTESIAN_POINT ( 'NONE',  ( 14.58750000122903323, 6.123233995736764310E-16, -4.999999999999998224 ) ) ;
#26761=CARTESIAN_POINT ( 'NONE',  ( 9.600000001229034297, -2.886751345948125991, -5.000000000000000000 ) ) ;
#26762=CARTESIAN_POINT ( 'NONE',  ( 3.065625000614517592, 3.027376345333613106, -5.243569643749998122 ) ) ;
#26765=CARTESIAN_POINT ( 'NONE',  ( 14.82187500061451679, 3.027376345333613106, -5.243569643749998122 ) ) ;
#26766=CARTESIAN_POINT ( 'NONE',  ( 7.575000000000001954, -4.330127018922194537, 2.499999999999995559 ) ) ;
#26767=VERTEX_POINT ( 'NONE', #42721 ) ;
#26768=CARTESIAN_POINT ( 'NONE',  ( 20.20312500061451644, 4.541064518000418104, -2.621784821874998173 ) ) ;
#26769=CARTESIAN_POINT ( 'NONE',  ( 7.040625000614517681, -3.027376345333610441, -5.243569643749999898 ) ) ;
#26770=CARTESIAN_POINT ( 'NONE',  ( 22.47187500061452070, 3.027376345333612662, -5.243569643749998122 ) ) ;
#26771=CARTESIAN_POINT ( 'NONE',  ( 5.090625000614516615, -3.027376345333614438, 5.243569643749998122 ) ) ;
#26773=CARTESIAN_POINT ( 'NONE',  ( 7.612500001229035362, 0.000000000000000000, 4.999999999999998224 ) ) ;
#26774=CARTESIAN_POINT ( 'NONE',  ( 21.92812500061451431, 6.421520780324663323E-16, -5.243569643749999010 ) ) ;
#26775=CARTESIAN_POINT ( 'NONE',  ( 1.999999999999998668, 17.26250000122903572, -33.46410161513775705 ) ) ;
#26776=CARTESIAN_POINT ( 'NONE',  ( 11.55000000122903181, 5.773502691896255534, 3.535250795749688894E-16 ) ) ;
#26777=CARTESIAN_POINT ( 'NONE',  ( 20.12812500061451715, 6.421520780324663323E-16, -5.243569643749999010 ) ) ;
#26778=CARTESIAN_POINT ( 'NONE',  ( 14.99062500061451786, -3.027376345333614438, 5.243569643749998122 ) ) ;
#26780=CARTESIAN_POINT ( 'NONE',  ( 16.19999999999999929, -4.330127018922190985, -2.500000000000001332 ) ) ;
#26781=CARTESIAN_POINT ( 'NONE',  ( 12.11250000122903181, 0.000000000000000000, 4.999999999999998224 ) ) ;
#26782=CARTESIAN_POINT ( 'NONE',  ( 8.915625000614515017, 3.027376345333613106, -5.243569643749998122 ) ) ;
#26783=CARTESIAN_POINT ( 'NONE',  ( 11.84062500061451750, -3.027376345333614438, 5.243569643749998122 ) ) ;
#26784=CARTESIAN_POINT ( 'NONE',  ( 21.18750000122903288, -4.330127018922194537, 2.499999999999995559 ) ) ;
#26785=CARTESIAN_POINT ( 'NONE',  ( 20.10937500061451289, -4.541064518000417216, -2.621784821875001281 ) ) ;
#26787=CARTESIAN_POINT ( 'NONE',  ( 6.525000001229033231, 2.886751345948129099, -4.999999999999998224 ) ) ;
#26788=AXIS2_PLACEMENT_3D ( 'NONE', #72725, #26939, #21737 ) ;
#26789=CARTESIAN_POINT ( 'NONE',  ( 4.884375000614518569, 6.421520780324663323E-16, -5.243569643749999010 ) ) ;
#26790=CARTESIAN_POINT ( 'NONE',  ( 23.93437500061451573, 4.541064518000418104, 2.621784821874999949 ) ) ;
#26791=CARTESIAN_POINT ( 'NONE',  ( -1.487416814333745711E-14, 15.16250000000000142, 34.00000000000000000 ) ) ;
#26792=CARTESIAN_POINT ( 'NONE',  ( 18.21562500061451573, -6.054752690667223547, -1.112240025338166033E-15 ) ) ;
#26793=CARTESIAN_POINT ( 'NONE',  ( 24.04687500061451644, -3.027376345333614438, 5.243569643749998122 ) ) ;
#26795=CARTESIAN_POINT ( 'NONE',  ( 29.73281250092177430, 0.000000000000000000, 5.121784821874998173 ) ) ;
#26796=CARTESIAN_POINT ( 'NONE',  ( 27.98437500061451289, 4.541064518000418104, 2.621784821874999949 ) ) ;
#26798=CARTESIAN_POINT ( 'NONE',  ( 15.85312500061451857, 0.000000000000000000, 5.243569643749999010 ) ) ;
#26799=CARTESIAN_POINT ( 'NONE',  ( 14.33437500061451786, 6.421520780324663323E-16, -5.243569643749999010 ) ) ;
#26801=CARTESIAN_POINT ( 'NONE',  ( 22.42500000122903003, 2.886751345948093572, 5.000000000000056843 ) ) ;
#26802=CARTESIAN_POINT ( 'NONE',  ( 22.11562500061451786, 3.027376345333611329, 5.243569643749999010 ) ) ;
#26803=CARTESIAN_POINT ( 'NONE',  ( 3.999999999999999112, 13.02500000000000213, -30.00000000000000000 ) ) ;
#26805=CARTESIAN_POINT ( 'NONE',  ( 13.76250000000000107, 2.886751345948126879, 4.999999999999999112 ) ) ;
#26806=CARTESIAN_POINT ( 'NONE',  ( 23.17500000122903359, 2.886751345948129099, -4.999999999999998224 ) ) ;
#26807=CARTESIAN_POINT ( 'NONE',  ( 19.26562500061451644, 3.027376345333613106, -5.243569643749998122 ) ) ;
#26808=VERTEX_POINT ( 'NONE', #65242 ) ;
#26809=CARTESIAN_POINT ( 'NONE',  ( 21.63749999999999929, -2.886751345948125991, -5.000000000000000000 ) ) ;
#26811=CARTESIAN_POINT ( 'NONE',  ( 22.92187500061451644, 3.027376345333613106, -5.243569643749998122 ) ) ;
#26813=DIRECTION ( 'NONE',  ( -0.000000000000000000, -1.000000000000000000, -0.000000000000000000 ) ) ;
#26814=CARTESIAN_POINT ( 'NONE',  ( 9.928125000614517859, 4.541064518000418104, 2.621784821874999949 ) ) ;
#26815=DIRECTION ( 'NONE',  ( -1.000000000000000000, -0.000000000000000000, -0.000000000000000000 ) ) ;
#26817=CARTESIAN_POINT ( 'NONE',  ( 26.24062500061451431, -3.027376345333614438, 5.243569643749998122 ) ) ;
#26818=CARTESIAN_POINT ( 'NONE',  ( 18.22499999999999787, 4.330127018922191873, 2.499999999999999556 ) ) ;
#26819=CARTESIAN_POINT ( 'NONE',  ( 24.63749999999999574, -2.886751345948129988, 4.999999999999997335 ) ) ;
#26820=CARTESIAN_POINT ( 'NONE',  ( 2.121784821874999061, 19.20312500061451644, 26.32496088578401583 ) ) ;
#26821=CARTESIAN_POINT ( 'NONE',  ( 5.821875000614519458, 3.027376345333613106, -5.243569643749998122 ) ) ;
#26822=CARTESIAN_POINT ( 'NONE',  ( 17.10937500061451999, 4.541064518000418104, -2.621784821874998173 ) ) ;
#26823=CARTESIAN_POINT ( 'NONE',  ( 29.29687500061451644, 6.054752690667223547, 3.707466751127219781E-16 ) ) ;
#26824=VERTEX_POINT ( 'NONE', #3571 ) ;
#26825=CARTESIAN_POINT ( 'NONE',  ( 25.75312500061451715, 0.000000000000000000, 5.243569643749999010 ) ) ;
#26826=CARTESIAN_POINT ( 'NONE',  ( 28.77187500061451431, 3.027376345333613106, -5.243569643749998122 ) ) ;
#26828=CARTESIAN_POINT ( 'NONE',  ( 12.90000000000000213, 0.000000000000000000, 4.999999999999998224 ) ) ;
#26829=CARTESIAN_POINT ( 'NONE',  ( 11.31562500061451892, 3.027376345333611329, 5.243569643749999010 ) ) ;
#26830=LINE ( 'NONE', #72983, #25418 ) ;
#26831=CARTESIAN_POINT ( 'NONE',  ( 19.50000000000000000, 4.330127018922192761, -2.499999999999997780 ) ) ;
#26832=CARTESIAN_POINT ( 'NONE',  ( 29.39062500061451644, -3.027376345333614438, 5.243569643749998122 ) ) ;
#26833=CARTESIAN_POINT ( 'NONE',  ( 16.16250000122903430, 0.000000000000000000, 4.999999999999998224 ) ) ;
#26836=CARTESIAN_POINT ( 'NONE',  ( 4.903125000614516615, 4.541064518000418104, -2.621784821874998173 ) ) ;
#26837=CARTESIAN_POINT ( 'NONE',  ( 20.70937500061451786, 4.541064518000418104, -2.621784821874998173 ) ) ;
#26838=CARTESIAN_POINT ( 'NONE',  ( 2.121784821875001281, 15.95937500061451608, 33.67503911421598417 ) ) ;
#26839=CARTESIAN_POINT ( 'NONE',  ( 20.55937500061451573, -4.541064518000417216, -2.621784821875001281 ) ) ;
#26840=CARTESIAN_POINT ( 'NONE',  ( 28.77187500061451431, 3.027376345333613106, -5.243569643749998122 ) ) ;
#26841=CARTESIAN_POINT ( 'NONE',  ( -3.000416591977282496E-16, 19.29687500061451644, 25.09994784771203058 ) ) ;
#26842=CARTESIAN_POINT ( 'NONE',  ( 12.36562500061451608, -6.054752690667223547, -1.112240025338166033E-15 ) ) ;
#26843=CARTESIAN_POINT ( 'NONE',  ( 4.312500001229034652, 4.330127018922192761, -2.499999999999997780 ) ) ;
#26844=EDGE_CURVE ( 'NONE', #13883, #35438, #68301, .T. ) ;
#26845=CARTESIAN_POINT ( 'NONE',  ( 7.096875000614517148, -3.027376345333610441, -5.243569643749999898 ) ) ;
#26846=CARTESIAN_POINT ( 'NONE',  ( 3.882866153107933371, 3.150134987115559060, -3.987202789055975582 ) ) ;
#26847=CARTESIAN_POINT ( 'NONE',  ( 8.953125000614518214, 4.541064518000418104, -2.621784821874998173 ) ) ;
#26848=CARTESIAN_POINT ( 'NONE',  ( 13.65937500061451715, 0.000000000000000000, 5.243569643749999010 ) ) ;
#26850=CARTESIAN_POINT ( 'NONE',  ( 22.01250000122903216, 0.000000000000000000, 4.999999999999998224 ) ) ;
#26851=CARTESIAN_POINT ( 'NONE',  ( 8.484375000614518214, 6.421520780324663323E-16, -5.243569643749999010 ) ) ;
#26852=CARTESIAN_POINT ( 'NONE',  ( 12.59062500061451573, 6.054752690667223547, 3.707466751127219781E-16 ) ) ;
#26854=CARTESIAN_POINT ( 'NONE',  ( 22.54687500061451999, 6.054752690667223547, 3.707466751127219781E-16 ) ) ;
#26856=CARTESIAN_POINT ( 'NONE',  ( -3.964499721297434665, 3.046849790701494420, 29.45062293401495879 ) ) ;
#26859=CARTESIAN_POINT ( 'NONE',  ( 4.243569643749999010, 11.57187500061451679, -32.45002607614398471 ) ) ;
#26860=CARTESIAN_POINT ( 'NONE',  ( 14.43750000122903288, -4.330127018922194537, 2.499999999999995559 ) ) ;
#26861=CARTESIAN_POINT ( 'NONE',  ( 9.001249775931846008E-16, 15.86562500061451608, -25.09994784771203058 ) ) ;
#26862=CARTESIAN_POINT ( 'NONE',  ( 16.53750000122903430, 4.330127018922191873, 2.499999999999999556 ) ) ;
#26863=CARTESIAN_POINT ( 'NONE',  ( 10.00312500061451715, 0.000000000000000000, 5.243569643749999010 ) ) ;
#26865=CARTESIAN_POINT ( 'NONE',  ( 13.87500000000000178, -4.330127018922194537, 2.499999999999995559 ) ) ;
#26867=CARTESIAN_POINT ( 'NONE',  ( 23.27812500061451573, 6.421520780324663323E-16, -5.243569643749999010 ) ) ;
#26868=CARTESIAN_POINT ( 'NONE',  ( 11.07187500061451679, -6.054752690667223547, -1.112240025338166033E-15 ) ) ;
#26869=CARTESIAN_POINT ( 'NONE',  ( 4.390052511545366798, -2.393233949706693675, -4.665573943098876519 ) ) ;
#26870=CARTESIAN_POINT ( 'NONE',  ( 11.28750000122903252, -4.330127018922194537, 2.499999999999995559 ) ) ;
#26871=CARTESIAN_POINT ( 'NONE',  ( 18.93750000122903288, -4.330127018922194537, 2.499999999999995559 ) ) ;
#26872=( BOUNDED_CURVE ( )  B_SPLINE_CURVE ( 2, ( #34676, #29147, #51682, #1086, #59019, #13961, #64572 ),
 .UNSPECIFIED., .F., .F. ) 
 B_SPLINE_CURVE_WITH_KNOTS ( ( 3, 2, 2, 3 ),
 ( 0.4666666666666667296, 0.4694444444444444975, 0.4722222222222222654, 0.4750000000000000333 ),
 .UNSPECIFIED. ) 
 CURVE ( )  GEOMETRIC_REPRESENTATION_ITEM ( )  RATIONAL_B_SPLINE_CURVE ( ( 0.9999999999999973355, 0.8660254037844413721, 1.000000000000000000, 0.8660254037844387076, 1.000000000000000000, 0.8660254037844360431, 1.000000000000002665 ) ) 
 REPRESENTATION_ITEM ( '' )  );
#26873=CARTESIAN_POINT ( 'NONE',  ( 15.62812500061451537, 6.421520780324663323E-16, -5.243569643749999010 ) ) ;
#26874=CARTESIAN_POINT ( 'NONE',  ( 18.17812500061451786, -4.541064518000419881, 2.621784821874995952 ) ) ;
#26875=CARTESIAN_POINT ( 'NONE',  ( 25.23750000122903359, -4.330127018922194537, 2.499999999999995559 ) ) ;
#26877=CARTESIAN_POINT ( 'NONE',  ( 28.83750000122903145, -4.330127018922194537, 2.499999999999995559 ) ) ;
#26878=CARTESIAN_POINT ( 'NONE',  ( 25.57499999999999929, -4.330127018922194537, 2.499999999999995559 ) ) ;
#26880=CARTESIAN_POINT ( 'NONE',  ( 26.55937500061451573, 4.541064518000418104, -2.621784821874998173 ) ) ;
#26882=CARTESIAN_POINT ( 'NONE',  ( 13.20000000122903394, -2.886751345948125991, -5.000000000000000000 ) ) ;
#26883=CARTESIAN_POINT ( 'NONE',  ( 4.237500000000001599, 5.773502691896255534, 3.535250795749688894E-16 ) ) ;
#26884=EDGE_CURVE ( 'NONE', #100, #32704, #61933, .T. ) ;
#26887=CARTESIAN_POINT ( 'NONE',  ( 8.334375000614516082, -4.541064518000419881, 2.621784821874995952 ) ) ;
#26888=CARTESIAN_POINT ( 'NONE',  ( 25.82812500061451644, -4.541064518000419881, 2.621784821874995952 ) ) ;
#26889=LINE ( 'NONE', #43512, #71972 ) ;
#26891=CARTESIAN_POINT ( 'NONE',  ( 9.834375000614517859, 6.421520780324663323E-16, -5.243569643749999010 ) ) ;
#26892=DIRECTION ( 'NONE',  ( 0.000000000000000000, 0.000000000000000000, 1.000000000000000000 ) ) ;
#26893=CARTESIAN_POINT ( 'NONE',  ( 28.94062500061452070, -3.027376345333614438, 5.243569643749998122 ) ) ;
#26894=CARTESIAN_POINT ( 'NONE',  ( 8.521875000614516082, 3.027376345333613106, -5.243569643749998122 ) ) ;
#26895=CARTESIAN_POINT ( 'NONE',  ( 29.55937500061451573, -4.541064518000417216, -2.621784821875001281 ) ) ;
#26897=CARTESIAN_POINT ( 'NONE',  ( -4.243569643749999898, 12.15312500061459211, 30.00000000000000000 ) ) ;
#26898=CARTESIAN_POINT ( 'NONE',  ( 21.33749999999999858, 5.773502691896255534, 3.535250795749688894E-16 ) ) ;
#26899=EDGE_LOOP ( 'NONE', ( #9688, #40175, #15552, #56565 ) ) ;
#26900=CARTESIAN_POINT ( 'NONE',  ( 20.66250000122903074, 0.000000000000000000, 4.999999999999998224 ) ) ;
#26901=CARTESIAN_POINT ( 'NONE',  ( 3.712499999999999911, 2.886751345948129099, -4.999999999999998224 ) ) ;
#26902=VERTEX_POINT ( 'NONE', #54174 ) ;
#26903=CARTESIAN_POINT ( 'NONE',  ( 17.95312500061451644, 4.541064518000418104, -2.621784821874998173 ) ) ;
#26904=CARTESIAN_POINT ( 'NONE',  ( 11.61562500061451608, 3.027376345333613106, -5.243569643749998122 ) ) ;
#26906=CARTESIAN_POINT ( 'NONE',  ( 6.946875000614517681, -3.027376345333614438, 5.243569643749998122 ) ) ;
#26907=CARTESIAN_POINT ( 'NONE',  ( 19.46250000122903145, -4.330127018922190985, -2.500000000000001332 ) ) ;
#26908=CARTESIAN_POINT ( 'NONE',  ( 15.71250000000000036, -5.773502691896255534, -1.060575238724906372E-15 ) ) ;
#26909=CARTESIAN_POINT ( 'NONE',  ( 5.896875000614518747, 6.054752690667223547, 3.707466751127219781E-16 ) ) ;
#26910=CARTESIAN_POINT ( 'NONE',  ( 14.37187500061451928, 3.027376345333613106, -5.243569643749998122 ) ) ;
#26911=CARTESIAN_POINT ( 'NONE',  ( 24.72187500061451360, 3.027376345333613106, -5.243569643749998122 ) ) ;
#26913=CYLINDRICAL_SURFACE ( 'NONE', #60753, 4.000000000000000000 ) ;
#26914=ORIENTED_EDGE ( 'NONE', *, *, #40712, .T. ) ;
#26916=CARTESIAN_POINT ( 'NONE',  ( 17.44687500061451857, -3.027376345333610441, -5.243569643749999898 ) ) ;
#26917=CARTESIAN_POINT ( 'NONE',  ( 10.39687500061451786, 6.054752690667223547, 3.707466751127219781E-16 ) ) ;
#26919=CARTESIAN_POINT ( 'NONE',  ( 20.10000000000000142, 0.000000000000000000, 4.999999999999998224 ) ) ;
#26921=CARTESIAN_POINT ( 'NONE',  ( -4.243569643749997233, 9.996875000614517504, -27.54997392385601174 ) ) ;
#26923=CARTESIAN_POINT ( 'NONE',  ( 12.62812500061451537, 4.541064518000418104, 2.621784821874999949 ) ) ;
#26924=CARTESIAN_POINT ( 'NONE',  ( 28.92187500061451644, 3.027376345333611329, 5.243569643749999010 ) ) ;
#26926=CARTESIAN_POINT ( 'NONE',  ( 29.07187500061451502, -6.054752690667223547, -1.112240025338166033E-15 ) ) ;
#26927=CARTESIAN_POINT ( 'NONE',  ( 13.08750000000000036, -2.886751345948125991, -5.000000000000000000 ) ) ;
#26928=CARTESIAN_POINT ( 'NONE',  ( 8.484601909799253346E-16, 17.97500000122903785, 34.61880215351700230 ) ) ;
#26929=CARTESIAN_POINT ( 'NONE',  ( 11.28750000122903252, -4.330127018922194537, 2.499999999999995559 ) ) ;
#26930=CARTESIAN_POINT ( 'NONE',  ( 23.29687500061451644, -3.027376345333610441, -5.243569643749999898 ) ) ;
#26931=CARTESIAN_POINT ( 'NONE',  ( 17.63437500061451502, 4.541064518000418104, 2.621784821874999949 ) ) ;
#26933=EDGE_LOOP ( 'NONE', ( #35340, #3929, #54271, #31366 ) ) ;
#26934=CARTESIAN_POINT ( 'NONE',  ( 17.46562500061451217, 3.027376345333613106, -5.243569643749998122 ) ) ;
#26935=CARTESIAN_POINT ( 'NONE',  ( 28.35000000122903430, -2.886751345948129988, 4.999999999999997335 ) ) ;
#26936=CARTESIAN_POINT ( 'NONE',  ( 15.19687500061451857, -3.027376345333610441, -5.243569643749999898 ) ) ;
#26937=CARTESIAN_POINT ( 'NONE',  ( 5.948646956027292099, 8.038298999021534996, -29.19102198739167875 ) ) ;
#26938=CARTESIAN_POINT ( 'NONE',  ( 20.27812500061451573, 4.541064518000418104, 2.621784821874999949 ) ) ;
#26939=DIRECTION ( 'NONE',  ( -0.000000000000000000, -0.000000000000000000, -1.000000000000000000 ) ) ;
#26940=CARTESIAN_POINT ( 'NONE',  ( 28.73437500061451644, 6.421520780324663323E-16, -5.243569643749999010 ) ) ;
#26941=CARTESIAN_POINT ( 'NONE',  ( -3.000416591977282496E-16, 12.94062500061451537, 25.09994784771203058 ) ) ;
#26942=CARTESIAN_POINT ( 'NONE',  ( 16.77187500061451786, 3.027376345333611329, 5.243569643749999010 ) ) ;
#26943=CARTESIAN_POINT ( 'NONE',  ( 13.68750000122903288, 6.123233995736764310E-16, -4.999999999999998224 ) ) ;
#26945=CARTESIAN_POINT ( 'NONE',  ( 4.243569643749999898, 19.14687500061451431, -27.54997392385601529 ) ) ;
#26946=CARTESIAN_POINT ( 'NONE',  ( 20.07187500061451857, -6.054752690667223547, -1.112240025338166033E-15 ) ) ;
#26947=CARTESIAN_POINT ( 'NONE',  ( 21.37500000122902932, 2.886751345948129099, -4.999999999999998224 ) ) ;
#26948=CARTESIAN_POINT ( 'NONE',  ( 17.37187500061451573, -6.054752690667223547, -1.112240025338166033E-15 ) ) ;
#26949=CARTESIAN_POINT ( 'NONE',  ( 12.10312500061451857, 4.541064518000418104, -2.621784821874998173 ) ) ;
#26950=CARTESIAN_POINT ( 'NONE',  ( -4.243569643749999898, 15.32187500061451679, 27.54997392385601529 ) ) ;
#26951=CARTESIAN_POINT ( 'NONE',  ( 18.44062500061451715, 6.054752690667223547, 3.707466751127219781E-16 ) ) ;
#26952=VERTEX_POINT ( 'NONE', #70431 ) ;
#26953=CARTESIAN_POINT ( 'NONE',  ( 23.17500000000000071, 4.330127018922191873, 2.499999999999999556 ) ) ;
#26954=CARTESIAN_POINT ( 'NONE',  ( 4.243569643749999010, 18.77187500061451786, -32.45002607614398471 ) ) ;
#26955=CARTESIAN_POINT ( 'NONE',  ( 3.843527511662434559, -3.198147656327572808, -4.075615451639215792 ) ) ;
#26956=CARTESIAN_POINT ( 'NONE',  ( 23.54062500061451146, -3.027376345333614438, 5.243569643749998122 ) ) ;
#26957=CARTESIAN_POINT ( 'NONE',  ( 6.403125000614517504, 0.000000000000000000, 5.243569643749999010 ) ) ;
#26958=CARTESIAN_POINT ( 'NONE',  ( 18.45000000122903216, -2.886751345948129988, 4.999999999999997335 ) ) ;
#26959=CARTESIAN_POINT ( 'NONE',  ( 23.50312500061451360, 0.000000000000000000, 5.243569643749999010 ) ) ;
#26960=CARTESIAN_POINT ( 'NONE',  ( 23.09999999999999787, 4.330127018922192761, -2.499999999999997780 ) ) ;
#26961=CARTESIAN_POINT ( 'NONE',  ( 25.82812500061451644, -4.541064518000419881, 2.621784821874995952 ) ) ;
#26962=CARTESIAN_POINT ( 'NONE',  ( 4.565625000614516260, 3.027376345333611329, 5.243569643749999010 ) ) ;
#26963=ORIENTED_EDGE ( 'NONE', *, *, #63735, .F. ) ;
#26964=CARTESIAN_POINT ( 'NONE',  ( 24.06562500061451715, -6.054752690667223547, -1.112240025338166033E-15 ) ) ;
#26965=CARTESIAN_POINT ( 'NONE',  ( 3.328125000614516438, -4.541064518000419881, 2.621784821874995952 ) ) ;
#26967=CARTESIAN_POINT ( 'NONE',  ( 1.071796769724489895, 18.96740381056766722, 26.00000000000000355 ) ) ;
#26968=CARTESIAN_POINT ( 'NONE',  ( 4.000000000000000000, 14.00000000122903288, -27.69059892324149530 ) ) ;
#26969=CARTESIAN_POINT ( 'NONE',  ( -4.243569643749999898, 19.82187500061451857, -32.45002607614398471 ) ) ;
#26970=CARTESIAN_POINT ( 'NONE',  ( 10.87500000000000000, 6.123233995736764310E-16, -4.999999999999998224 ) ) ;
#26972=CARTESIAN_POINT ( 'NONE',  ( 10.65937500061451715, -4.541064518000417216, -2.621784821875001281 ) ) ;
#26973=CARTESIAN_POINT ( 'NONE',  ( 7.425000001229034474, 2.886751345948129099, -4.999999999999998224 ) ) ;
#26974=CARTESIAN_POINT ( 'NONE',  ( 13.92187500061451644, 3.027376345333613106, -5.243569643749998122 ) ) ;
#26975=CARTESIAN_POINT ( 'NONE',  ( 5.071875000614519458, 3.027376345333611329, 5.243569643749999010 ) ) ;
#26977=CARTESIAN_POINT ( 'NONE',  ( 0.000000000000000000, 20.00000000000000000, -30.00000000000000000 ) ) ;
#26978=CARTESIAN_POINT ( 'NONE',  ( 11.82187500061451679, 3.027376345333611329, 5.243569643749999010 ) ) ;
#26980=CYLINDRICAL_SURFACE ( 'NONE', #1771, 4.999999999999998224 ) ;
#26981=CARTESIAN_POINT ( 'NONE',  ( 20.95312500061451999, -4.541064518000417216, -2.621784821875001281 ) ) ;
#26982=CARTESIAN_POINT ( 'NONE',  ( 16.61250000000000071, -5.773502691896255534, -1.060575238724906372E-15 ) ) ;
#26983=CARTESIAN_POINT ( 'NONE',  ( 9.001249775931846008E-16, 19.01562500061459104, 34.90005215228797653 ) ) ;
#26984=CARTESIAN_POINT ( 'NONE',  ( 22.80937500061451573, -4.541064518000417216, -2.621784821875001281 ) ) ;
#26985=EDGE_CURVE ( 'NONE', #21477, #62607, #45653, .T. ) ;
#26986=FACE_OUTER_BOUND ( 'NONE', #35744, .T. ) ;
#26987=CARTESIAN_POINT ( 'NONE',  ( 29.47500000122903430, 2.886751345948129099, -4.999999999999998224 ) ) ;
#26989=CARTESIAN_POINT ( 'NONE',  ( 24.36562500061451786, 3.027376345333611329, 5.243569643749999010 ) ) ;
#26990=CARTESIAN_POINT ( 'NONE',  ( 17.01562500061451644, 3.027376345333613106, -5.243569643749998122 ) ) ;
#26992=CARTESIAN_POINT ( 'NONE',  ( 15.15937500061451715, -4.541064518000417216, -2.621784821875001281 ) ) ;
#26994=CARTESIAN_POINT ( 'NONE',  ( 28.42500000122904069, -5.773502691896255534, -1.060575238724906372E-15 ) ) ;
#26995=CARTESIAN_POINT ( 'NONE',  ( 7.059375000614518392, -4.541064518000417216, -2.621784821875001281 ) ) ;
#26996=CARTESIAN_POINT ( 'NONE',  ( 14.07187500061451679, 3.027376345333611329, 5.243569643749999010 ) ) ;
#26997=CARTESIAN_POINT ( 'NONE',  ( 4.849242802210273595, -1.218730718756773967, -5.100017238597982505 ) ) ;
#26998=CARTESIAN_POINT ( 'NONE',  ( 4.462500001229035007, 0.000000000000000000, 4.999999999999998224 ) ) ;
#26999=CARTESIAN_POINT ( 'NONE',  ( 25.95937500061451431, -4.541064518000417216, -2.621784821875001281 ) ) ;
#27000=CARTESIAN_POINT ( 'NONE',  ( 17.82187500061451502, -6.054752690667223547, -1.112240025338166033E-15 ) ) ;
#27002=CARTESIAN_POINT ( 'NONE',  ( 28.53749999999999787, 5.773502691896255534, 3.535250795749688894E-16 ) ) ;
#27003=CARTESIAN_POINT ( 'NONE',  ( 5.850000000000001421, -4.330127018922190985, -2.500000000000001332 ) ) ;
#27005=CARTESIAN_POINT ( 'NONE',  ( 18.96562500061451573, 3.027376345333611329, 5.243569643749999010 ) ) ;
#27006=CARTESIAN_POINT ( 'NONE',  ( 8.737500000000002487, 5.773502691896255534, 3.535250795749688894E-16 ) ) ;
#27007=CARTESIAN_POINT ( 'NONE',  ( 4.865625000614517859, 3.027376345333613106, -5.243569643749998122 ) ) ;
#27008=CARTESIAN_POINT ( 'NONE',  ( 20.54999999999999716, 0.000000000000000000, 4.999999999999998224 ) ) ;
#27009=CARTESIAN_POINT ( 'NONE',  ( 3.807538167735159185, -3.240779705755961526, 4.122180188640082399 ) ) ;
#27010=CARTESIAN_POINT ( 'NONE',  ( 22.12500000122903288, -5.773502691896255534, -1.060575238724906372E-15 ) ) ;
#27011=CARTESIAN_POINT ( 'NONE',  ( 0.8036833610285047946, 9.975469519845873378, 35.95937231738776063 ) ) ;
#27012=CARTESIAN_POINT ( 'NONE',  ( 3.000000000000002665, 0.000000000000000000, 4.999999999999998224 ) ) ;
#27014=CARTESIAN_POINT ( 'NONE',  ( 16.82812500061451644, -4.541064518000419881, 2.621784821874995952 ) ) ;
#27015=CARTESIAN_POINT ( 'NONE',  ( 23.20312500061451644, -4.541064518000417216, -2.621784821875001281 ) ) ;
#27016=CARTESIAN_POINT ( 'NONE',  ( 24.42187500061451999, 3.027376345333611329, 5.243569643749999010 ) ) ;
#27017=CARTESIAN_POINT ( 'NONE',  ( 6.899999999999999467, 4.330127018922192761, -2.499999999999997780 ) ) ;
#27018=CARTESIAN_POINT ( 'NONE',  ( 10.71562500061451928, 3.027376345333613106, -5.243569643749998122 ) ) ;
#27019=CARTESIAN_POINT ( 'NONE',  ( 26.46562500061451573, 3.027376345333613106, -5.243569643749998122 ) ) ;
#27020=CARTESIAN_POINT ( 'NONE',  ( 15.00937500061451679, 0.000000000000000000, 5.243569643749999010 ) ) ;
#27021=CARTESIAN_POINT ( 'NONE',  ( 19.32187500061451857, 3.027376345333613106, -5.243569643749998122 ) ) ;
#27023=CARTESIAN_POINT ( 'NONE',  ( -3.000416591977282496E-16, 19.69062500061451360, 25.09994784771203058 ) ) ;
#27024=EDGE_CURVE ( 'NONE', #58126, #56216, #7866, .T. ) ;
#27025=CARTESIAN_POINT ( 'NONE',  ( 24.93750000122903288, 6.123233995736764310E-16, -4.999999999999998224 ) ) ;
#27027=CARTESIAN_POINT ( 'NONE',  ( 11.84062500061451573, -3.027376345333614438, 5.243569643749998122 ) ) ;
#27028=CARTESIAN_POINT ( 'NONE',  ( 9.084375000614517859, 4.541064518000418104, 2.621784821874999949 ) ) ;
#27029=CARTESIAN_POINT ( 'NONE',  ( 7.209375000614519635, 4.541064518000418104, -2.621784821874998173 ) ) ;
#27030=VERTEX_POINT ( 'NONE', #33817 ) ;
#27031=CARTESIAN_POINT ( 'NONE',  ( 27.98437500061451289, 4.541064518000418104, 2.621784821874999949 ) ) ;
#27032=CARTESIAN_POINT ( 'NONE',  ( 19.07812500061451644, -4.541064518000419881, 2.621784821874995952 ) ) ;
#27033=CARTESIAN_POINT ( 'NONE',  ( 3.178125000614515638, 4.541064518000418104, 2.621784821874999949 ) ) ;
#27034=CARTESIAN_POINT ( 'NONE',  ( 3.196875000614516793, 6.054752690667223547, 3.707466751127219781E-16 ) ) ;
#27035=CARTESIAN_POINT ( 'NONE',  ( 24.08437500061451786, -4.541064518000419881, 2.621784821874995952 ) ) ;
#27036=CARTESIAN_POINT ( 'NONE',  ( 19.75312500061451360, 4.541064518000418104, -2.621784821874998173 ) ) ;
#27037=CARTESIAN_POINT ( 'NONE',  ( 3.999999999999999112, 11.22500000000000142, 30.00000000000000000 ) ) ;
#27038=CARTESIAN_POINT ( 'NONE',  ( 25.41562500061451146, -6.054752690667223547, -1.112240025338166033E-15 ) ) ;
#27039=CARTESIAN_POINT ( 'NONE',  ( 4.650000001229035895, -2.886751345948125991, -5.000000000000000000 ) ) ;
#27040=ORIENTED_EDGE ( 'NONE', *, *, #34911, .F. ) ;
#27041=CARTESIAN_POINT ( 'NONE',  ( 3.075000001229035718, 2.886751345948126879, 4.999999999999999112 ) ) ;
#27042=CARTESIAN_POINT ( 'NONE',  ( -1.999999999999997113, 16.47500000000000142, -26.53589838486224295 ) ) ;
#27044=CARTESIAN_POINT ( 'NONE',  ( 5.071875000614519458, 3.027376345333611329, 5.243569643749999010 ) ) ;
#27045=CARTESIAN_POINT ( 'NONE',  ( 25.27499999999999858, 6.123233995736764310E-16, -4.999999999999998224 ) ) ;
#27046=CARTESIAN_POINT ( 'NONE',  ( 13.37812500061451715, 6.421520780324663323E-16, -5.243569643749999010 ) ) ;
#27047=CARTESIAN_POINT ( 'NONE',  ( 6.534375000614517148, -4.541064518000419881, 2.621784821874995952 ) ) ;
#27048=CARTESIAN_POINT ( 'NONE',  ( 23.92500000122903359, -5.773502691896255534, -1.060575238724906372E-15 ) ) ;
#27049=CARTESIAN_POINT ( 'NONE',  ( 13.99687500061451928, 6.054752690667223547, 3.707466751127219781E-16 ) ) ;
#27050=CARTESIAN_POINT ( 'NONE',  ( 3.571875000614517237, 3.027376345333613106, -5.243569643749998122 ) ) ;
#27051=CARTESIAN_POINT ( 'NONE',  ( 1.626862140677534273E-15, 18.76250000000000284, 34.00000000000000000 ) ) ;
#27052=CARTESIAN_POINT ( 'NONE',  ( 2.953125000614516438, -4.541064518000417216, -2.621784821875001281 ) ) ;
#27053=CARTESIAN_POINT ( 'NONE',  ( 14.95312500061451644, 0.000000000000000000, 5.243569643749999010 ) ) ;
#27054=ORIENTED_EDGE ( 'NONE', *, *, #69433, .T. ) ;
#27055=CARTESIAN_POINT ( 'NONE',  ( 10.64062500061451644, -3.027376345333610441, -5.243569643749999898 ) ) ;
#27056=CARTESIAN_POINT ( 'NONE',  ( 7.715625000614515727, 3.027376345333611329, 5.243569643749999010 ) ) ;
#27058=CARTESIAN_POINT ( 'NONE',  ( 9.525000000000002132, 6.123233995736764310E-16, -4.999999999999998224 ) ) ;
#27059=CARTESIAN_POINT ( 'NONE',  ( 3.375000001229033320, 2.886751345948129099, -4.999999999999998224 ) ) ;
#27060=CARTESIAN_POINT ( 'NONE',  ( 17.51249999999999929, -5.773502691896255534, -1.060575238724906372E-15 ) ) ;
#27061=CARTESIAN_POINT ( 'NONE',  ( 18.45937500061451431, 4.541064518000418104, -2.621784821874998173 ) ) ;
#27062=CARTESIAN_POINT ( 'NONE',  ( 14.10000000122903252, -2.886751345948125991, -5.000000000000000000 ) ) ;
#27064=CARTESIAN_POINT ( 'NONE',  ( 9.001249775931846008E-16, 16.31562500061451715, -25.09994784771203058 ) ) ;
#27066=CARTESIAN_POINT ( 'NONE',  ( 28.86562500061451786, 3.027376345333611329, 5.243569643749999010 ) ) ;
#27069=CARTESIAN_POINT ( 'NONE',  ( 13.02187500061451608, 3.027376345333613106, -5.243569643749998122 ) ) ;
#27070=ADVANCED_FACE ( 'NONE', ( #16819 ), #72625, .F. ) ;
#27071=CARTESIAN_POINT ( 'NONE',  ( 26.92499999999999716, -4.330127018922194537, 2.499999999999995559 ) ) ;
#27072=CARTESIAN_POINT ( 'NONE',  ( 10.30312500061451431, 4.541064518000418104, -2.621784821874998173 ) ) ;
#27074=CARTESIAN_POINT ( 'NONE',  ( 21.87187500061451573, -6.054752690667223547, -1.112240025338166033E-15 ) ) ;
#27076=CARTESIAN_POINT ( 'NONE',  ( 8.653125000614515727, 0.000000000000000000, 5.243569643749999010 ) ) ;
#27077=CARTESIAN_POINT ( 'NONE',  ( 13.17187500061451999, 3.027376345333611329, 5.243569643749999010 ) ) ;
#27078=VERTEX_POINT ( 'NONE', #33451 ) ;
#27079=CARTESIAN_POINT ( 'NONE',  ( 22.65937500061451715, 0.000000000000000000, 5.243569643749999010 ) ) ;
#27080=CARTESIAN_POINT ( 'NONE',  ( 0.2755985575760799833, 4.994312242614637576, -26.00710267647355778 ) ) ;
#27082=CARTESIAN_POINT ( 'NONE',  ( 5.662500000000000533, 2.886751345948126879, 4.999999999999999112 ) ) ;
#27083=CARTESIAN_POINT ( 'NONE',  ( 16.42500000122903359, 2.886751345948129099, -4.999999999999998224 ) ) ;
#27085=CARTESIAN_POINT ( 'NONE',  ( -2.556497649636125342E-15, 19.21250000000000213, -26.00000000000000000 ) ) ;
#27086=ORIENTED_EDGE ( 'NONE', *, *, #38503, .T. ) ;
#27087=CARTESIAN_POINT ( 'NONE',  ( 13.04999999999999893, -4.330127018922190985, -2.500000000000001332 ) ) ;
#27088=CARTESIAN_POINT ( 'NONE',  ( 15.75000000000000000, -4.330127018922190985, -2.500000000000001332 ) ) ;
#27089=CARTESIAN_POINT ( 'NONE',  ( 13.46250000122903323, 0.000000000000000000, 4.999999999999998224 ) ) ;
#27090=CARTESIAN_POINT ( 'NONE',  ( 10.64062500061451644, -3.027376345333610441, -5.243569643749999898 ) ) ;
#27091=( BOUNDED_CURVE ( )  B_SPLINE_CURVE ( 2, ( #28245, #55591, #179, #54858, #22684, #45235, #67768, #4267, #71857 ),
 .UNSPECIFIED., .F., .F. ) 
 B_SPLINE_CURVE_WITH_KNOTS ( ( 3, 2, 2, 2, 3 ),
 ( 0.09782608695652174335, 0.1014492753623188470, 0.1086956521739130405, 0.1159420289855072478, 0.1195652173913043514 ),
 .UNSPECIFIED. ) 
 CURVE ( )  GEOMETRIC_REPRESENTATION_ITEM ( )  RATIONAL_B_SPLINE_CURVE ( ( 0.9330127018922194093, 0.9330127018922194093, 1.000000000000000000, 0.8660254037844387076, 1.000000000000000000, 0.8660254037844387076, 1.000000000000000000, 0.9330127018922194093, 0.9330127018922194093 ) ) 
 REPRESENTATION_ITEM ( '' )  );
#27092=ORIENTED_EDGE ( 'NONE', *, *, #6241, .F. ) ;
#27094=CARTESIAN_POINT ( 'NONE',  ( -4.243569643749997233, 15.39687500061451786, -27.54997392385601174 ) ) ;
#27095=CARTESIAN_POINT ( 'NONE',  ( 3.665625000614517681, 3.027376345333611329, 5.243569643749999010 ) ) ;
#27097=CARTESIAN_POINT ( 'NONE',  ( 10.91250000000000320, 2.886751345948129099, -4.999999999999998224 ) ) ;
#27098=CARTESIAN_POINT ( 'NONE',  ( 3.100832673336169520, 3.922389953441107302, 3.244276004801022850 ) ) ;
#27100=CARTESIAN_POINT ( 'NONE',  ( 23.12812500061451360, -4.541064518000419881, 2.621784821874995952 ) ) ;
#27103=CARTESIAN_POINT ( 'NONE',  ( 21.64687500061451786, 6.054752690667223547, 3.707466751127219781E-16 ) ) ;
#27104=CARTESIAN_POINT ( 'NONE',  ( 18.29062500061451502, -3.027376345333610441, -5.243569643749999898 ) ) ;
#27105=CARTESIAN_POINT ( 'NONE',  ( 4.243569643749999898, 13.72812500061459318, -30.00000000000000000 ) ) ;
#27106=CARTESIAN_POINT ( 'NONE',  ( 6.178125000614518747, 6.421520780324663323E-16, -5.243569643749999010 ) ) ;
#27107=CARTESIAN_POINT ( 'NONE',  ( 4.603125000614518569, 0.000000000000000000, 5.243569643749999010 ) ) ;
#27109=CARTESIAN_POINT ( 'NONE',  ( 21.02812500061451573, 6.421520780324663323E-16, -5.243569643749999010 ) ) ;
#27112=CARTESIAN_POINT ( 'NONE',  ( 14.59687500061452070, -3.027376345333614438, 5.243569643749998122 ) ) ;
#27113=CARTESIAN_POINT ( 'NONE',  ( 14.44687500061451679, 6.054752690667223547, 3.707466751127219781E-16 ) ) ;
#27114=CARTESIAN_POINT ( 'NONE',  ( 21.90937500061451715, -4.541064518000417216, -2.621784821875001281 ) ) ;
#27115=ORIENTED_EDGE ( 'NONE', *, *, #52167, .F. ) ;
#27116=CARTESIAN_POINT ( 'NONE',  ( -4.243569643749999898, 11.72187500061451892, 27.54997392385601529 ) ) ;
#27117=CARTESIAN_POINT ( 'NONE',  ( 26.46562500061451573, 3.027376345333613106, -5.243569643749998122 ) ) ;
#27118=CARTESIAN_POINT ( 'NONE',  ( 25.86562500061451431, -6.054752690667223547, -1.112240025338166033E-15 ) ) ;
#27119=CARTESIAN_POINT ( 'NONE',  ( 1.592000809091587073E-14, 16.40000000122903501, -34.00000000000000000 ) ) ;
#27120=CARTESIAN_POINT ( 'NONE',  ( -3.999999999999997335, 18.68750000000000000, 32.30940107675850470 ) ) ;
#27121=CARTESIAN_POINT ( 'NONE',  ( 4.284375000614518925, -4.541064518000419881, 2.621784821874995952 ) ) ;
#27123=CARTESIAN_POINT ( 'NONE',  ( 13.12500000122903288, -5.773502691896255534, -1.060575238724906372E-15 ) ) ;
#27124=CARTESIAN_POINT ( 'NONE',  ( 9.262500001229033941, 4.330127018922192761, -2.499999999999997780 ) ) ;
#27125=CARTESIAN_POINT ( 'NONE',  ( 29.02500000122903145, 2.886751345948129099, -4.999999999999998224 ) ) ;
#27128=CARTESIAN_POINT ( 'NONE',  ( 12.23437500061451821, 4.541064518000418104, 2.621784821874999949 ) ) ;
#27132=CARTESIAN_POINT ( 'NONE',  ( 19.49062500061451431, -3.027376345333614438, 5.243569643749998122 ) ) ;
#27133=CARTESIAN_POINT ( 'NONE',  ( 12.30937500061451573, 0.000000000000000000, 5.243569643749999010 ) ) ;
#27134=CARTESIAN_POINT ( 'NONE',  ( 5.015625000614518214, 3.027376345333611329, 5.243569643749999010 ) ) ;
#27135=CARTESIAN_POINT ( 'NONE',  ( 22.35937500061451644, -4.541064518000417216, -2.621784821875001281 ) ) ;
#27136=CARTESIAN_POINT ( 'NONE',  ( 6.140625000614516438, -3.027376345333610441, -5.243569643749999898 ) ) ;
#27137=CYLINDRICAL_SURFACE ( 'NONE', #4979, 3.999999999999996447 ) ;
#27138=CARTESIAN_POINT ( 'NONE',  ( 7.537500001229033408, 4.330127018922191873, 2.499999999999999556 ) ) ;
#27139=CARTESIAN_POINT ( 'NONE',  ( 22.90312500061451573, 4.541064518000418104, -2.621784821874998173 ) ) ;
#27140=CARTESIAN_POINT ( 'NONE',  ( -2.000000000000000000, 17.78750000122903430, -33.46410161513775705 ) ) ;
#27141=CARTESIAN_POINT ( 'NONE',  ( 8.737500001229033586, 6.123233995736764310E-16, -4.999999999999998224 ) ) ;
#27142=CARTESIAN_POINT ( 'NONE',  ( 18.29062500061451502, -3.027376345333610441, -5.243569643749999898 ) ) ;
#27143=CARTESIAN_POINT ( 'NONE',  ( 15.59062500061451573, -3.027376345333610441, -5.243569643749999898 ) ) ;
#27145=CARTESIAN_POINT ( 'NONE',  ( 14.62500000000000000, 4.330127018922191873, 2.499999999999999556 ) ) ;
#27146=CARTESIAN_POINT ( 'NONE',  ( 11.51250000122903216, 4.330127018922192761, -2.499999999999997780 ) ) ;
#27147=CARTESIAN_POINT ( 'NONE',  ( 9.065625000614517148, 3.027376345333611329, 5.243569643749999010 ) ) ;
#27148=CARTESIAN_POINT ( 'NONE',  ( 11.95312500061451644, -4.541064518000417216, -2.621784821875001281 ) ) ;
#27149=CARTESIAN_POINT ( 'NONE',  ( 20.13750000122903216, 4.330127018922191873, 2.499999999999999556 ) ) ;
#27150=CARTESIAN_POINT ( 'NONE',  ( -2.121784821874999949, 13.03437500061451715, -33.67503911421598417 ) ) ;
#27151=CARTESIAN_POINT ( 'NONE',  ( 20.29687500061451644, 6.054752690667223547, 3.707466751127219781E-16 ) ) ;
#27153=CARTESIAN_POINT ( 'NONE',  ( 4.650000001229035895, -2.886751345948125991, -5.000000000000000000 ) ) ;
#27154=CARTESIAN_POINT ( 'NONE',  ( 3.121875000614518836, 3.027376345333613106, -5.243569643749998122 ) ) ;
#27155=CARTESIAN_POINT ( 'NONE',  ( 19.92187500061451644, 3.027376345333611329, 5.243569643749999010 ) ) ;
#27158=CARTESIAN_POINT ( 'NONE',  ( 18.62812500061451715, -4.541064518000419881, 2.621784821874995952 ) ) ;
#27160=LINE ( 'NONE', #66311, #48405 ) ;
#27161=DIRECTION ( 'NONE',  ( -0.000000000000000000, -1.000000000000000000, -0.000000000000000000 ) ) ;
#27162=CARTESIAN_POINT ( 'NONE',  ( 28.95937500061451431, 0.000000000000000000, 5.243569643749999010 ) ) ;
#27164=CARTESIAN_POINT ( 'NONE',  ( 14.76562500061451821, 3.027376345333613106, -5.243569643749998122 ) ) ;
#27165=CARTESIAN_POINT ( 'NONE',  ( 14.37187500061451928, 3.027376345333613106, -5.243569643749998122 ) ) ;
#27166=ORIENTED_EDGE ( 'NONE', *, *, #31908, .T. ) ;
#27168=CARTESIAN_POINT ( 'NONE',  ( 22.30312500061451431, -4.541064518000417216, -2.621784821875001281 ) ) ;
#27171=CARTESIAN_POINT ( 'NONE',  ( 11.73750000000000249, -2.886751345948125991, -5.000000000000000000 ) ) ;
#27172=CARTESIAN_POINT ( 'NONE',  ( 23.55000000122903359, -2.886751345948125991, -5.000000000000000000 ) ) ;
#27173=CARTESIAN_POINT ( 'NONE',  ( 18.59062500061451573, -3.027376345333614438, 5.243569643749998122 ) ) ;
#27174=ORIENTED_EDGE ( 'NONE', *, *, #4477, .T. ) ;
#27175=CARTESIAN_POINT ( 'NONE',  ( 18.93750000000000000, -2.886751345948125991, -5.000000000000000000 ) ) ;
#27176=CARTESIAN_POINT ( 'NONE',  ( 21.72187500061451715, 3.027376345333611329, 5.243569643749999010 ) ) ;
#27179=CARTESIAN_POINT ( 'NONE',  ( 11.61562500061451608, 3.027376345333613106, -5.243569643749998122 ) ) ;
#27182=CARTESIAN_POINT ( 'NONE',  ( 16.83749999999999858, 5.773502691896255534, 3.535250795749688894E-16 ) ) ;
#27183=CARTESIAN_POINT ( 'NONE',  ( 25.27499999999999858, 6.123233995736764310E-16, -4.999999999999998224 ) ) ;
#27184=FACE_OUTER_BOUND ( 'NONE', #35863, .T. ) ;
#27185=CARTESIAN_POINT ( 'NONE',  ( 4.621875000614516615, 3.027376345333611329, 5.243569643749999010 ) ) ;
#27186=CARTESIAN_POINT ( 'NONE',  ( 27.87187500061451573, 3.027376345333613106, -5.243569643749998122 ) ) ;
#27188=CARTESIAN_POINT ( 'NONE',  ( 26.84062500061451573, -3.027376345333610441, -5.243569643749999898 ) ) ;
#27189=CARTESIAN_POINT ( 'NONE',  ( 26.63437500061451857, 4.541064518000418104, 2.621784821874999949 ) ) ;
#27190=CARTESIAN_POINT ( 'NONE',  ( 3.384375000614517237, -4.541064518000419881, 2.621784821874995952 ) ) ;
#27191=CARTESIAN_POINT ( 'NONE',  ( 12.86250000000000071, 2.886751345948126879, 4.999999999999999112 ) ) ;
#27192=CARTESIAN_POINT ( 'NONE',  ( 10.82812500061451644, 4.541064518000418104, 2.621784821874999949 ) ) ;
#27193=CARTESIAN_POINT ( 'NONE',  ( 0.000000000000000000, 20.00000000000000000, 30.00000000000000000 ) ) ;
#27194=CARTESIAN_POINT ( 'NONE',  ( 1.071796769724490117, 19.23259618943233917, -26.00000000000000000 ) ) ;
#27195=CARTESIAN_POINT ( 'NONE',  ( 29.50312500061451360, -4.541064518000417216, -2.621784821875001281 ) ) ;
#27196=CARTESIAN_POINT ( 'NONE',  ( 16.72500000122903430, -5.773502691896255534, -1.060575238724906372E-15 ) ) ;
#27199=CARTESIAN_POINT ( 'NONE',  ( 5.990625000614517859, -3.027376345333614438, 5.243569643749998122 ) ) ;
#27200=CARTESIAN_POINT ( 'NONE',  ( 22.13437500061451502, 4.541064518000418104, 2.621784821874999949 ) ) ;
#27201=CARTESIAN_POINT ( 'NONE',  ( -4.243569643749997233, 14.49687500061451928, 32.45002607614398471 ) ) ;
#27202=CARTESIAN_POINT ( 'NONE',  ( 21.60937500061451644, 4.541064518000418104, -2.621784821874998173 ) ) ;
#27203=CARTESIAN_POINT ( 'NONE',  ( 3.149999999999999911, -4.330127018922190985, -2.500000000000001332 ) ) ;
#27204=CARTESIAN_POINT ( 'NONE',  ( -4.243569643749998122, 19.44687500061451857, 32.45002607614398471 ) ) ;
#27205=CARTESIAN_POINT ( 'NONE',  ( 8.915625000614515017, 3.027376345333613106, -5.243569643749998122 ) ) ;
#27206=FACE_OUTER_BOUND ( 'NONE', #60553, .T. ) ;
#27207=CARTESIAN_POINT ( 'NONE',  ( 6.984375000614516438, -4.541064518000419881, 2.621784821874995952 ) ) ;
#27209=CARTESIAN_POINT ( 'NONE',  ( 6.403125000614517504, 0.000000000000000000, 5.243569643749999010 ) ) ;
#27210=CARTESIAN_POINT ( 'NONE',  ( 12.12187500061451573, 3.027376345333613106, -5.243569643749998122 ) ) ;
#27212=CARTESIAN_POINT ( 'NONE',  ( 22.53750000122903430, -4.330127018922194537, 2.499999999999995559 ) ) ;
#27213=CARTESIAN_POINT ( 'NONE',  ( 8.634375000614518569, 4.541064518000418104, 2.621784821874999949 ) ) ;
#27214=CARTESIAN_POINT ( 'NONE',  ( 11.01562500061451821, -6.054752690667223547, -1.112240025338166033E-15 ) ) ;
#27216=CARTESIAN_POINT ( 'NONE',  ( 18.83437500061451431, 6.421520780324663323E-16, -5.243569643749999010 ) ) ;
#27217=CARTESIAN_POINT ( 'NONE',  ( 9.528763966825557376E-15, 17.41249999999999787, -26.00000000000000000 ) ) ;
#27218=CARTESIAN_POINT ( 'NONE',  ( 21.78750000122903074, 6.123233995736764310E-16, -4.999999999999998224 ) ) ;
#27219=CARTESIAN_POINT ( 'NONE',  ( 28.17187500061451644, -6.054752690667223547, -1.112240025338166033E-15 ) ) ;
#27220=CARTESIAN_POINT ( 'NONE',  ( -2.121784821874999949, 12.13437500061451857, -33.67503911421598417 ) ) ;
#27221=CARTESIAN_POINT ( 'NONE',  ( 14.85000000122903252, -2.886751345948129988, 4.999999999999997335 ) ) ;
#27222=CARTESIAN_POINT ( 'NONE',  ( 4.243569643749999898, 16.39062500061451999, -27.54997392385601529 ) ) ;
#27223=CARTESIAN_POINT ( 'NONE',  ( 14.25000000122903465, 5.773502691896255534, 3.535250795749688894E-16 ) ) ;
#27224=CARTESIAN_POINT ( 'NONE',  ( 9.703125000614514661, -4.541064518000417216, -2.621784821875001281 ) ) ;
#27226=CARTESIAN_POINT ( 'NONE',  ( 13.53749999999999964, -2.886751345948125991, -5.000000000000000000 ) ) ;
#27228=CARTESIAN_POINT ( 'NONE',  ( 22.00312500061451360, 4.541064518000418104, -2.621784821874998173 ) ) ;
#27229=CARTESIAN_POINT ( 'NONE',  ( 6.834375000614518747, 4.541064518000418104, 2.621784821874999949 ) ) ;
#27231=CARTESIAN_POINT ( 'NONE',  ( 11.02500000122903501, 2.886751345948129099, -4.999999999999998224 ) ) ;
#27232=CARTESIAN_POINT ( 'NONE',  ( 18.00000000122903288, -2.886751345948129988, 4.999999999999997335 ) ) ;
#27233=CARTESIAN_POINT ( 'NONE',  ( 15.14062500061451644, -3.027376345333610441, -5.243569643749999898 ) ) ;
#27234=CARTESIAN_POINT ( 'NONE',  ( 18.66562500061451146, -6.054752690667223547, -1.112240025338166033E-15 ) ) ;
#27235=CARTESIAN_POINT ( 'NONE',  ( 26.02500000122903145, 2.886751345948126879, 4.999999999999999112 ) ) ;
#27237=CARTESIAN_POINT ( 'NONE',  ( 28.08750000122903145, 6.123233995736764310E-16, -4.999999999999998224 ) ) ;
#27238=CARTESIAN_POINT ( 'NONE',  ( 23.25000000000000000, 0.000000000000000000, 4.999999999999998224 ) ) ;
#27240=CARTESIAN_POINT ( 'NONE',  ( 25.39687500061451431, -3.027376345333614438, 5.243569643749998122 ) ) ;
#27241=CARTESIAN_POINT ( 'NONE',  ( 18.22500000122903074, 2.886751345948129099, -4.999999999999997335 ) ) ;
#27242=CARTESIAN_POINT ( 'NONE',  ( 12.60000000122903430, -2.886751345948129988, 4.999999999999997335 ) ) ;
#27244=CARTESIAN_POINT ( 'NONE',  ( 27.57187500061451857, 3.027376345333611329, 5.243569643749999010 ) ) ;
#27245=( BOUNDED_CURVE ( )  B_SPLINE_CURVE ( 2, ( #39054, #22413, #39416, #33138, #61567, #27607, #12055 ),
 .UNSPECIFIED., .F., .F. ) 
 B_SPLINE_CURVE_WITH_KNOTS ( ( 3, 2, 2, 3 ),
 ( 0.1416666666666666352, 0.1444444444444444031, 0.1472222222222221710, 0.1499999999999999389 ),
 .UNSPECIFIED. ) 
 CURVE ( )  GEOMETRIC_REPRESENTATION_ITEM ( )  RATIONAL_B_SPLINE_CURVE ( ( 1.000000000000001332, 0.8660254037844373753, 1.000000000000000000, 0.8660254037844387076, 1.000000000000000000, 0.8660254037844413721, 0.9999999999999973355 ) ) 
 REPRESENTATION_ITEM ( '' )  );
#27246=EDGE_CURVE ( 'NONE', #66704, #44084, #42832, .T. ) ;
#27248=CARTESIAN_POINT ( 'NONE',  ( 5.334375000614517859, 6.421520780324663323E-16, -5.243569643749999010 ) ) ;
#27249=CARTESIAN_POINT ( 'NONE',  ( 25.49062500061451786, -3.027376345333610441, -5.243569643749999898 ) ) ;
#27251=CARTESIAN_POINT ( 'NONE',  ( 1.999999999999998668, 19.84999999999999787, -33.46410161513775705 ) ) ;
#27252=CARTESIAN_POINT ( 'NONE',  ( 10.77187500061451786, 3.027376345333613106, -5.243569643749998122 ) ) ;
#27253=CARTESIAN_POINT ( 'NONE',  ( 3.632573829565322487, -3.435821811263616521, 3.669822893043289014 ) ) ;
#27254=CARTESIAN_POINT ( 'NONE',  ( 3.421875000614516882, -6.054752690667223547, -1.112240025338166033E-15 ) ) ;
#27255=CARTESIAN_POINT ( 'NONE',  ( 9.384375000614518569, 6.421520780324663323E-16, -5.243569643749999010 ) ) ;
#27256=CARTESIAN_POINT ( 'NONE',  ( 28.80937500061451573, 4.541064518000418104, -2.621784821874998173 ) ) ;
#27257=CARTESIAN_POINT ( 'NONE',  ( 4.243569643749999898, 12.82812500061459637, 30.00000000000000000 ) ) ;
#27258=CARTESIAN_POINT ( 'NONE',  ( 19.53749999999999432, 5.773502691896255534, 3.535250795749688894E-16 ) ) ;
#27259=ORIENTED_EDGE ( 'NONE', *, *, #28959, .F. ) ;
#27260=CARTESIAN_POINT ( 'NONE',  ( -1.071796769724488563, 17.84240381056766367, -26.00000000000000000 ) ) ;
#27261=EDGE_CURVE ( 'NONE', #45340, #26440, #30517, .T. ) ;
#27262=CARTESIAN_POINT ( 'NONE',  ( 3.562500000000000444, -5.773502691896255534, -1.060575238724906372E-15 ) ) ;
#27264=CARTESIAN_POINT ( 'NONE',  ( 17.20312500061451644, 0.000000000000000000, 5.243569643749999010 ) ) ;
#27265=CARTESIAN_POINT ( 'NONE',  ( 8.615625000614517859, 3.027376345333611329, 5.243569643749999010 ) ) ;
#27267=CARTESIAN_POINT ( 'NONE',  ( 7.621875000614519280, 3.027376345333613106, -5.243569643749998122 ) ) ;
#27268=CARTESIAN_POINT ( 'NONE',  ( 17.55000000122903359, -2.886751345948129988, 4.999999999999997335 ) ) ;
#27270=CARTESIAN_POINT ( 'NONE',  ( 7.884375000614517681, -4.541064518000419881, 2.621784821874995952 ) ) ;
#27271=CARTESIAN_POINT ( 'NONE',  ( 12.79687500061451821, -3.027376345333614438, 5.243569643749998122 ) ) ;
#27272=CARTESIAN_POINT ( 'NONE',  ( 24.83437500061451431, 4.541064518000418104, 2.621784821874999949 ) ) ;
#27276=CARTESIAN_POINT ( 'NONE',  ( 18.08437500061451431, 4.541064518000418104, 2.621784821874999949 ) ) ;
#27277=CARTESIAN_POINT ( 'NONE',  ( 8.896875000614517859, -3.027376345333610441, -5.243569643749999898 ) ) ;
#27279=CARTESIAN_POINT ( 'NONE',  ( 21.44999999999999929, 0.000000000000000000, 4.999999999999998224 ) ) ;
#27281=CARTESIAN_POINT ( 'NONE',  ( 30.00000000000000000, 0.000000000000000000, 4.999999999999998224 ) ) ;
#27283=CARTESIAN_POINT ( 'NONE',  ( 13.22812500061451502, -4.541064518000419881, 2.621784821874995952 ) ) ;
#27284=CARTESIAN_POINT ( 'NONE',  ( 3.000000000000002665, 0.000000000000000000, 4.999999999999998224 ) ) ;
#27285=CARTESIAN_POINT ( 'NONE',  ( 28.24687500061451573, -3.027376345333610441, -5.243569643749999898 ) ) ;
#27286=CARTESIAN_POINT ( 'NONE',  ( 9.225000000000001421, 4.330127018922191873, 2.499999999999999556 ) ) ;
#27287=CARTESIAN_POINT ( 'NONE',  ( 3.999999999999998668, 16.32500000122903216, 27.69059892324149175 ) ) ;
#27288=CARTESIAN_POINT ( 'NONE',  ( 8.775000001229033231, 2.886751345948129099, -4.999999999999998224 ) ) ;
#27289=CARTESIAN_POINT ( 'NONE',  ( 20.03437500061451715, -4.541064518000419881, 2.621784821874995952 ) ) ;
#27290=CARTESIAN_POINT ( 'NONE',  ( 14.93437500061451750, 4.541064518000418104, 2.621784821874999949 ) ) ;
#27291=CARTESIAN_POINT ( 'NONE',  ( 0.000000000000000000, 20.00000000000000000, 30.00000000000000000 ) ) ;
#27293=CARTESIAN_POINT ( 'NONE',  ( 16.11562500061451786, 3.027376345333613106, -5.243569643749998122 ) ) ;
#27294=CARTESIAN_POINT ( 'NONE',  ( 27.97500000122903074, -5.773502691896255534, -1.060575238724906372E-15 ) ) ;
#27295=CARTESIAN_POINT ( 'NONE',  ( 14.33437500061451786, 6.421520780324663323E-16, -5.243569643749999010 ) ) ;
#27296=CARTESIAN_POINT ( 'NONE',  ( 1.587219675395663998, 9.875134926496690113, -24.21030195342116187 ) ) ;
#27297=CARTESIAN_POINT ( 'NONE',  ( 17.27812500061451217, -4.541064518000419881, 2.621784821874995952 ) ) ;
#27299=CARTESIAN_POINT ( 'NONE',  ( 28.95937500061451431, 0.000000000000000000, 5.243569643749999010 ) ) ;
#27300=CARTESIAN_POINT ( 'NONE',  ( 2.121784821875001281, 13.65312500061451750, 33.67503911421598417 ) ) ;
#27301=CARTESIAN_POINT ( 'NONE',  ( 16.20937500061451786, 4.541064518000418104, -2.621784821874998173 ) ) ;
#27302=CARTESIAN_POINT ( 'NONE',  ( 13.35000000122903430, 5.773502691896255534, 3.535250795749688894E-16 ) ) ;
#27304=CARTESIAN_POINT ( 'NONE',  ( 3.329819492037558781, -3.729919858448222048, 3.685474251491927866 ) ) ;
#27305=CARTESIAN_POINT ( 'NONE',  ( 19.62187500061451573, -6.054752690667223547, -1.112240025338166033E-15 ) ) ;
#27306=CARTESIAN_POINT ( 'NONE',  ( 22.50000000122903288, -2.886751345948129988, 4.999999999999997335 ) ) ;
#27307=( BOUNDED_CURVE ( )  B_SPLINE_CURVE ( 2, ( #73060, #9905, #17257, #39083, #61244, #44269, #67885, #54978, #22799 ),
 .UNSPECIFIED., .F., .F. ) 
 B_SPLINE_CURVE_WITH_KNOTS ( ( 3, 2, 2, 2, 3 ),
 ( 0.3369565217391304324, 0.3405797101449275499, 0.3478260869565217295, 0.3550724637681159646, 0.3586956521739130821 ),
 .UNSPECIFIED. ) 
 CURVE ( )  GEOMETRIC_REPRESENTATION_ITEM ( )  RATIONAL_B_SPLINE_CURVE ( ( 0.9330127018922194093, 0.9330127018922194093, 1.000000000000000000, 0.8660254037844387076, 1.000000000000000000, 0.8660254037844387076, 1.000000000000000000, 0.9330127018922188542, 0.9330127018922194093 ) ) 
 REPRESENTATION_ITEM ( '' )  );
#27308=CARTESIAN_POINT ( 'NONE',  ( 17.74687500061451928, -3.027376345333614438, 5.243569643749998122 ) ) ;
#27309=CARTESIAN_POINT ( 'NONE',  ( 12.70312500061451821, 0.000000000000000000, 5.243569643749999010 ) ) ;
#27310=CARTESIAN_POINT ( 'NONE',  ( 4.243569643749999898, 12.84687500061451715, 32.45002607614398471 ) ) ;
#27311=CARTESIAN_POINT ( 'NONE',  ( 18.06562500061451715, 3.027376345333611329, 5.243569643749999010 ) ) ;
#27312=ORIENTED_EDGE ( 'NONE', *, *, #25778, .F. ) ;
#27313=VERTEX_POINT ( 'NONE', #32886 ) ;
#27314=CARTESIAN_POINT ( 'NONE',  ( 21.33749999999999858, 5.773502691896255534, 3.535250795749688894E-16 ) ) ;
#27316=CARTESIAN_POINT ( 'NONE',  ( 25.15312500061451217, 4.541064518000418104, -2.621784821874998173 ) ) ;
#27317=CARTESIAN_POINT ( 'NONE',  ( 6.478125000614516793, -4.541064518000419881, 2.621784821874995952 ) ) ;
#27318=CARTESIAN_POINT ( 'NONE',  ( 18.60000000122903430, -2.886751345948125991, -5.000000000000000000 ) ) ;
#27319=CARTESIAN_POINT ( 'NONE',  ( 23.09062500061451573, -3.027376345333614438, 5.243569643749998122 ) ) ;
#27320=CARTESIAN_POINT ( 'NONE',  ( 22.27499999999999858, 4.330127018922191873, 2.499999999999999556 ) ) ;
#27321=CARTESIAN_POINT ( 'NONE',  ( 25.86562500061451431, -6.054752690667223547, -1.112240025338166033E-15 ) ) ;
#27322=CARTESIAN_POINT ( 'NONE',  ( 6.365625000614518747, 3.027376345333611329, 5.243569643749999010 ) ) ;
#27324=CARTESIAN_POINT ( 'NONE',  ( 29.47499999999999787, 4.330127018922191873, 2.499999999999999556 ) ) ;
#27327=CARTESIAN_POINT ( 'NONE',  ( 1.071796769724476572, 12.93259618943233313, 34.00000000000000000 ) ) ;
#27328=EDGE_CURVE ( 'NONE', #71040, #10011, #2692, .T. ) ;
#27329=CARTESIAN_POINT ( 'NONE',  ( 8.484601909799253346E-16, 13.47500000122903430, -25.38119784648299770 ) ) ;
#27331=CARTESIAN_POINT ( 'NONE',  ( 4.243569643749999010, 19.22187500061452070, -32.45002607614398471 ) ) ;
#27332=CARTESIAN_POINT ( 'NONE',  ( 11.73750000000000249, -2.886751345948125991, -5.000000000000000000 ) ) ;
#27333=CARTESIAN_POINT ( 'NONE',  ( 11.74687500061451573, 6.054752690667223547, 3.707466751127219781E-16 ) ) ;
#27334=CARTESIAN_POINT ( 'NONE',  ( 7.125000001229033764, 2.886751345948126879, 4.999999999999999112 ) ) ;
#27335=CARTESIAN_POINT ( 'NONE',  ( 13.05937500061451750, 4.541064518000418104, -2.621784821874998173 ) ) ;
#27336=CARTESIAN_POINT ( 'NONE',  ( 6.496875000614517504, -3.027376345333614438, 5.243569643749998122 ) ) ;
#27337=CARTESIAN_POINT ( 'NONE',  ( 4.243569643749999010, 10.16562500061451857, -32.45002607614398471 ) ) ;
#27339=CARTESIAN_POINT ( 'NONE',  ( 9.384375000614518569, 6.421520780324663323E-16, -5.243569643749999010 ) ) ;
#27340=CARTESIAN_POINT ( 'NONE',  ( 13.19999999999999929, 4.330127018922192761, -2.499999999999997780 ) ) ;
#27341=CARTESIAN_POINT ( 'NONE',  ( 18.47812500061451857, 4.541064518000418104, 2.621784821874999949 ) ) ;
#27342=CARTESIAN_POINT ( 'NONE',  ( -1.071796769724491005, 12.37009619066136956, -34.00000000000000000 ) ) ;
#27343=CARTESIAN_POINT ( 'NONE',  ( 4.243569643749999898, 19.09062500061459389, 32.45002607614398471 ) ) ;
#27344=CARTESIAN_POINT ( 'NONE',  ( 23.40937500061451715, 4.541064518000418104, -2.621784821874998173 ) ) ;
#27345=CARTESIAN_POINT ( 'NONE',  ( 3.999999999999999112, 19.32500000000000284, 30.00000000000000000 ) ) ;
#27346=CARTESIAN_POINT ( 'NONE',  ( 28.20000000122903216, 5.773502691896255534, 3.535250795749688894E-16 ) ) ;
#27348=CARTESIAN_POINT ( 'NONE',  ( 25.37812500061451715, -4.541064518000419881, 2.621784821874995952 ) ) ;
#27349=CARTESIAN_POINT ( 'NONE',  ( 18.70312500061451644, -4.541064518000417216, -2.621784821875001281 ) ) ;
#27351=CARTESIAN_POINT ( 'NONE',  ( 13.92187500061451644, 3.027376345333613106, -5.243569643749998122 ) ) ;
#27352=CARTESIAN_POINT ( 'NONE',  ( 7.350000001229033408, -2.886751345948193048, -4.999999999999883649 ) ) ;
#27353=CARTESIAN_POINT ( 'NONE',  ( 25.68750000122903288, -4.330127018922194537, 2.499999999999995559 ) ) ;
#27354=CARTESIAN_POINT ( 'NONE',  ( 3.909375000614518481, -4.541064518000417216, -2.621784821875001281 ) ) ;
#27355=CARTESIAN_POINT ( 'NONE',  ( 14.48437500061451821, 4.541064518000418104, 2.621784821874999949 ) ) ;
#27357=CARTESIAN_POINT ( 'NONE',  ( 3.065815551951259543, -3.949781639713015657, 3.065815551951216467 ) ) ;
#27358=CARTESIAN_POINT ( 'NONE',  ( 3.112500001229034918, 0.000000000000000000, 4.999999999999998224 ) ) ;
#27359=CARTESIAN_POINT ( 'NONE',  ( 23.63437500061451502, -4.541064518000419881, 2.621784821874995952 ) ) ;
#27360=CARTESIAN_POINT ( 'NONE',  ( 16.54687500061451644, -3.027376345333610441, -5.243569643749999898 ) ) ;
#27362=CARTESIAN_POINT ( 'NONE',  ( 27.48749999999999716, -2.886751345948125991, -5.000000000000000000 ) ) ;
#27363=CARTESIAN_POINT ( 'NONE',  ( 4.612500001229032698, -4.330127018922190985, -2.500000000000001332 ) ) ;
#27364=CARTESIAN_POINT ( 'NONE',  ( 5.437500000000001776, -2.886751345948125991, -5.000000000000000000 ) ) ;
#27366=CARTESIAN_POINT ( 'NONE',  ( 19.19062500061452070, -3.027376345333610441, -5.243569643749999898 ) ) ;
#27367=CARTESIAN_POINT ( 'NONE',  ( 10.35000000000000142, -4.330127018922190985, -2.500000000000001332 ) ) ;
#27368=CARTESIAN_POINT ( 'NONE',  ( 5.353125000614515905, 4.541064518000418104, -2.621784821874998173 ) ) ;
#27369=CARTESIAN_POINT ( 'NONE',  ( 17.66249999999999787, 2.886751345948129099, -4.999999999999998224 ) ) ;
#27371=CARTESIAN_POINT ( 'NONE',  ( 20.58750000122903145, 4.330127018922191873, 2.499999999999999556 ) ) ;
#27372=CARTESIAN_POINT ( 'NONE',  ( 5.378878668797007379, 8.432125716319056608, 27.31293200927705911 ) ) ;
#27373=CARTESIAN_POINT ( 'NONE',  ( 29.22187500061451715, 3.027376345333613106, -5.243569643749998122 ) ) ;
#27374=ORIENTED_EDGE ( 'NONE', *, *, #21176, .F. ) ;
#27375=CARTESIAN_POINT ( 'NONE',  ( 17.35312500061451502, -4.541064518000417216, -2.621784821875001281 ) ) ;
#27376=CARTESIAN_POINT ( 'NONE',  ( 25.26562500061451289, 3.027376345333611329, 5.243569643749999010 ) ) ;
#27377=CARTESIAN_POINT ( 'NONE',  ( 23.14687500061451786, -3.027376345333614438, 5.243569643749998122 ) ) ;
#27378=CARTESIAN_POINT ( 'NONE',  ( 6.225000000000001421, -4.330127018922194537, 2.499999999999995559 ) ) ;
#27379=CARTESIAN_POINT ( 'NONE',  ( 8.428125000614517859, 6.421520780324663323E-16, -5.243569643749999010 ) ) ;
#27380=CARTESIAN_POINT ( 'NONE',  ( 25.15312500061451217, 4.541064518000418104, -2.621784821874998173 ) ) ;
#27381=CARTESIAN_POINT ( 'NONE',  ( 15.72187500061451892, 3.027376345333613106, -5.243569643749998122 ) ) ;
#27382=CARTESIAN_POINT ( 'NONE',  ( 18.83437500061451431, 6.421520780324663323E-16, -5.243569643749999010 ) ) ;
#27383=CARTESIAN_POINT ( 'NONE',  ( 4.421718391856483521, 2.334208790866869609, -4.695382105235059278 ) ) ;
#27384=CARTESIAN_POINT ( 'NONE',  ( -2.121784821874996840, 10.48437500061451821, 33.67503911421598417 ) ) ;
#27385=CARTESIAN_POINT ( 'NONE',  ( 20.88750000122903572, 6.123233995736764310E-16, -4.999999999999998224 ) ) ;
#27387=CARTESIAN_POINT ( 'NONE',  ( 10.82812500061451644, 4.541064518000418104, 2.621784821874999949 ) ) ;
#27388=CARTESIAN_POINT ( 'NONE',  ( 7.809375000614519280, 0.000000000000000000, 5.243569643749999010 ) ) ;
#27389=CARTESIAN_POINT ( 'NONE',  ( 7.096875000614517148, -3.027376345333610441, -5.243569643749999898 ) ) ;
#27390=ORIENTED_EDGE ( 'NONE', *, *, #27534, .F. ) ;
#27391=CARTESIAN_POINT ( 'NONE',  ( 28.43437500061451573, 4.541064518000418104, 2.621784821874999949 ) ) ;
#27392=CARTESIAN_POINT ( 'NONE',  ( 18.89062500061451644, 6.054752690667223547, 3.707466751127219781E-16 ) ) ;
#27393=CARTESIAN_POINT ( 'NONE',  ( 29.13750000122903216, 4.330127018922191873, 2.499999999999999556 ) ) ;
#27394=ADVANCED_FACE ( 'NONE', ( #4463 ), #48013, .T. ) ;
#27395=CARTESIAN_POINT ( 'NONE',  ( 28.49062500061451431, -3.027376345333614438, 5.243569643749998122 ) ) ;
#27396=AXIS2_PLACEMENT_3D ( 'NONE', #12393, #23835, #28666 ) ;
#27397=CARTESIAN_POINT ( 'NONE',  ( 24.90937500061451715, 0.000000000000000000, 5.243569643749999010 ) ) ;
#27398=CARTESIAN_POINT ( 'NONE',  ( 19.15312500061451573, -4.541064518000417216, -2.621784821875001281 ) ) ;
#27399=CARTESIAN_POINT ( 'NONE',  ( 4.243569643749999010, 19.67187500061451644, 27.54997392385601174 ) ) ;
#27400=CARTESIAN_POINT ( 'NONE',  ( 25.67812500061451431, 4.541064518000418104, 2.621784821874999949 ) ) ;
#27401=CARTESIAN_POINT ( 'NONE',  ( 4.875000001229034652, 2.886751345948126879, 4.999999999999999112 ) ) ;
#27402=EDGE_LOOP ( 'NONE', ( #18862, #36998, #25972, #45756 ) ) ;
#27403=CARTESIAN_POINT ( 'NONE',  ( 26.62500000000000000, 6.123233995736764310E-16, -4.999999999999998224 ) ) ;
#27404=CARTESIAN_POINT ( 'NONE',  ( 4.000000000000000000, 16.58750000000000213, -27.69059892324149530 ) ) ;
#27406=CARTESIAN_POINT ( 'NONE',  ( 4.059375000614519280, 4.541064518000418104, -2.621784821874998173 ) ) ;
#27407=CARTESIAN_POINT ( 'NONE',  ( 11.69062500061451360, 6.054752690667223547, 3.707466751127219781E-16 ) ) ;
#27408=CARTESIAN_POINT ( 'NONE',  ( 6.084375000614518747, -4.541064518000419881, 2.621784821874995952 ) ) ;
#27409=CARTESIAN_POINT ( 'NONE',  ( 24.93750000122903288, 6.123233995736764310E-16, -4.999999999999998224 ) ) ;
#27410=CARTESIAN_POINT ( 'NONE',  ( 15.30937500061451750, 4.541064518000418104, -2.621784821874998173 ) ) ;
#27411=CARTESIAN_POINT ( 'NONE',  ( 29.46562500061451573, -6.054752690667223547, -1.112240025338166033E-15 ) ) ;
#27412=CARTESIAN_POINT ( 'NONE',  ( 29.13749999999999929, -2.886751345948129988, 4.999999999999997335 ) ) ;
#27413=CARTESIAN_POINT ( 'NONE',  ( 27.57187500061451857, 3.027376345333611329, 5.243569643749999010 ) ) ;
#27414=CARTESIAN_POINT ( 'NONE',  ( 3.328125000614516438, -4.541064518000419881, 2.621784821874995952 ) ) ;
#27415=CARTESIAN_POINT ( 'NONE',  ( 13.64062500061451644, -3.027376345333614438, 5.243569643749998122 ) ) ;
#27416=VERTEX_POINT ( 'NONE', #12532 ) ;
#27417=CARTESIAN_POINT ( 'NONE',  ( 11.09062500061451573, -3.027376345333610441, -5.243569643749999898 ) ) ;
#27418=CARTESIAN_POINT ( 'NONE',  ( 8.765625000614518214, -6.054752690667223547, -1.112240025338166033E-15 ) ) ;
#27420=CARTESIAN_POINT ( 'NONE',  ( 8.137500000000002842, -2.886751345948125991, -5.000000000000000000 ) ) ;
#27423=CARTESIAN_POINT ( 'NONE',  ( 16.91250000000000142, 2.886751345948126879, 4.999999999999999112 ) ) ;
#27424=CARTESIAN_POINT ( 'NONE',  ( 17.85937500061451999, -4.541064518000417216, -2.621784821875001281 ) ) ;
#27425=CARTESIAN_POINT ( 'NONE',  ( 14.32500000122903394, 2.886751345948126879, 4.999999999999999112 ) ) ;
#27427=CARTESIAN_POINT ( 'NONE',  ( -4.243569643749997233, 15.79062500061451857, -27.54997392385601174 ) ) ;
#27430=CARTESIAN_POINT ( 'NONE',  ( 25.94062500061451715, -3.027376345333610441, -5.243569643749999898 ) ) ;
#27432=CARTESIAN_POINT ( 'NONE',  ( 20.21250000122903145, 0.000000000000000000, 4.999999999999998224 ) ) ;
#27433=FACE_OUTER_BOUND ( 'NONE', #48934, .T. ) ;
#27434=CARTESIAN_POINT ( 'NONE',  ( 12.72187500061451537, 3.027376345333611329, 5.243569643749999010 ) ) ;
#27435=CARTESIAN_POINT ( 'NONE',  ( 27.78749999999999787, -2.886751345948129988, 4.999999999999997335 ) ) ;
#27436=CARTESIAN_POINT ( 'NONE',  ( 10.37812500061451715, 4.541064518000418104, 2.621784821874999949 ) ) ;
#27439=CARTESIAN_POINT ( 'NONE',  ( 21.45937500061451786, -4.541064518000417216, -2.621784821875001281 ) ) ;
#27441=CARTESIAN_POINT ( 'NONE',  ( 7.003125000614518036, -4.541064518000417216, -2.621784821875001281 ) ) ;
#27442=CARTESIAN_POINT ( 'NONE',  ( 10.95937500061451964, 0.000000000000000000, 5.243569643749999010 ) ) ;
#27443=ORIENTED_EDGE ( 'NONE', *, *, #62569, .F. ) ;
#27444=CARTESIAN_POINT ( 'NONE',  ( 21.72187500061451715, 3.027376345333611329, 5.243569643749999010 ) ) ;
#27445=CARTESIAN_POINT ( 'NONE',  ( 3.182906284435136790, 3.860443623060027640, -32.43517853776187110 ) ) ;
#27447=CARTESIAN_POINT ( 'NONE',  ( 4.162499999999999645, 2.886751345948129099, -4.999999999999998224 ) ) ;
#27448=CARTESIAN_POINT ( 'NONE',  ( 14.77500000122903501, 2.886751345948126879, 4.999999999999999112 ) ) ;
#27450=CARTESIAN_POINT ( 'NONE',  ( 3.791863662739624274, -3.259105699911376774, 4.107706494585713131 ) ) ;
#27452=CARTESIAN_POINT ( 'NONE',  ( 13.35000000000000142, 0.000000000000000000, 4.999999999999998224 ) ) ;
#27453=CARTESIAN_POINT ( 'NONE',  ( 15.45000000000000107, 4.330127018922192761, -2.499999999999997780 ) ) ;
#27454=CARTESIAN_POINT ( 'NONE',  ( 12.26250000122903394, -4.330127018922190985, -2.500000000000001332 ) ) ;
#27455=CARTESIAN_POINT ( 'NONE',  ( 10.34062500061451750, 6.054752690667223547, 3.707466751127219781E-16 ) ) ;
#27457=CARTESIAN_POINT ( 'NONE',  ( 9.750000000000001776, 0.000000000000000000, 4.999999999999998224 ) ) ;
#27458=CARTESIAN_POINT ( 'NONE',  ( 0.000000000000000000, 20.00000000000000000, -30.00000000000000000 ) ) ;
#27459=CARTESIAN_POINT ( 'NONE',  ( 4.243569643749999898, 15.58437500061451786, -30.00000000000000000 ) ) ;
#27460=CARTESIAN_POINT ( 'NONE',  ( 3.215625000614518836, 3.027376345333611329, 5.243569643749999010 ) ) ;
#27462=CARTESIAN_POINT ( 'NONE',  ( 10.98750000000000071, 5.773502691896255534, 3.535250795749688894E-16 ) ) ;
#27463=CARTESIAN_POINT ( 'NONE',  ( 3.801890562635342086, 3.247887812877087832, -3.801890562635342086 ) ) ;
#27464=EDGE_LOOP ( 'NONE', ( #7668, #48244, #37998, #50910 ) ) ;
#27465=CARTESIAN_POINT ( 'NONE',  ( 23.84062500061451928, 6.054752690667223547, 3.707466751127219781E-16 ) ) ;
#27466=CARTESIAN_POINT ( 'NONE',  ( 4.247151432104769420, -2.638504256727666863, 4.531370421416291983 ) ) ;
#27467=CARTESIAN_POINT ( 'NONE',  ( 29.29687500061451644, 6.054752690667223547, 3.707466751127219781E-16 ) ) ;
#27468=CARTESIAN_POINT ( 'NONE',  ( 21.49687500061451573, -3.027376345333610441, -5.243569643749999898 ) ) ;
#27469=CARTESIAN_POINT ( 'NONE',  ( 16.37812500061451715, -4.541064518000419881, 2.621784821874995952 ) ) ;
#27470=CARTESIAN_POINT ( 'NONE',  ( 2.121784821875001281, 12.30312500061459247, -26.32496088578401938 ) ) ;
#27471=CARTESIAN_POINT ( 'NONE',  ( 5.578125000614518214, -4.541064518000419881, 2.621784821874995952 ) ) ;
#27472=CARTESIAN_POINT ( 'NONE',  ( 28.05000000122903359, -2.886751345948125991, -5.000000000000000000 ) ) ;
#27474=CARTESIAN_POINT ( 'NONE',  ( 19.94062500061451715, -3.027376345333614438, 5.243569643749998122 ) ) ;
#27477=CARTESIAN_POINT ( 'NONE',  ( 14.07187500061451679, 3.027376345333611329, 5.243569643749999010 ) ) ;
#27478=CARTESIAN_POINT ( 'NONE',  ( 13.77187500061451786, -6.054752690667223547, -1.112240025338166033E-15 ) ) ;
#27479=CARTESIAN_POINT ( 'NONE',  ( 21.75937500061451502, 0.000000000000000000, 5.243569643749999010 ) ) ;
#27480=ORIENTED_EDGE ( 'NONE', *, *, #67858, .F. ) ;
#27481=CARTESIAN_POINT ( 'NONE',  ( -4.243569643749999898, 12.20937500061451608, 30.00000000000000000 ) ) ;
#27482=CARTESIAN_POINT ( 'NONE',  ( 2.953125000614516438, -4.541064518000417216, -2.621784821875001281 ) ) ;
#27483=CARTESIAN_POINT ( 'NONE',  ( 26.95312500061451644, 4.541064518000418104, -2.621784821874998173 ) ) ;
#27484=CARTESIAN_POINT ( 'NONE',  ( 27.51562500061451644, 3.027376345333611329, 5.243569643749999010 ) ) ;
#27485=CARTESIAN_POINT ( 'NONE',  ( -3.999999999999999112, 20.00000000000000000, 30.00000000000000000 ) ) ;
#27486=CARTESIAN_POINT ( 'NONE',  ( 4.734375000614518214, -4.541064518000419881, 2.621784821874995952 ) ) ;
#27487=CARTESIAN_POINT ( 'NONE',  ( 12.48750000122903359, 4.330127018922191873, 2.499999999999999556 ) ) ;
#27488=CARTESIAN_POINT ( 'NONE',  ( 9.375000001229036428, 2.886751345948126879, 4.999999999999999112 ) ) ;
#27489=CARTESIAN_POINT ( 'NONE',  ( 28.68750000122903288, 4.330127018922191873, 2.499999999999999556 ) ) ;
#27492=CARTESIAN_POINT ( 'NONE',  ( 12.64687500061451608, 6.054752690667223547, 3.707466751127219781E-16 ) ) ;
#27494=ORIENTED_EDGE ( 'NONE', *, *, #58732, .F. ) ;
#27495=CARTESIAN_POINT ( 'NONE',  ( 20.24062500061451431, 6.054752690667223547, 3.707466751127219781E-16 ) ) ;
#27496=CARTESIAN_POINT ( 'NONE',  ( 14.18437500061451750, -4.541064518000419881, 2.621784821874995952 ) ) ;
#27497=CARTESIAN_POINT ( 'NONE',  ( 5.653125000614517504, -4.541064518000417216, -2.621784821875001281 ) ) ;
#27498=CARTESIAN_POINT ( 'NONE',  ( 21.64687500061451786, 6.054752690667223547, 3.707466751127219781E-16 ) ) ;
#27499=CARTESIAN_POINT ( 'NONE',  ( 5.653125000614517504, -4.541064518000417216, -2.621784821875001281 ) ) ;
#27500=CARTESIAN_POINT ( 'NONE',  ( 6.600000001229032520, 5.773502691896255534, 3.535250795749688401E-16 ) ) ;
#27501=CARTESIAN_POINT ( 'NONE',  ( 5.662500001229035185, 4.330127018922192761, -2.499999999999997780 ) ) ;
#27502=EDGE_CURVE ( 'NONE', #18316, #70559, #23248, .T. ) ;
#27503=CARTESIAN_POINT ( 'NONE',  ( 19.94062500061451715, -3.027376345333614438, 5.243569643749998122 ) ) ;
#27504=CARTESIAN_POINT ( 'NONE',  ( 8.925000001229033586, 2.886751345948126879, 4.999999999999999112 ) ) ;
#27505=CARTESIAN_POINT ( 'NONE',  ( 16.22812500061451857, 4.541064518000418104, 2.621784821874999949 ) ) ;
#27506=CARTESIAN_POINT ( 'NONE',  ( 15.92812500061451608, -4.541064518000419881, 2.621784821874995952 ) ) ;
#27508=CARTESIAN_POINT ( 'NONE',  ( 16.12500000000000000, -4.330127018922194537, 2.499999999999995559 ) ) ;
#27509=CARTESIAN_POINT ( 'NONE',  ( 10.65000000122903323, 5.773502691896255534, 3.535250795749688894E-16 ) ) ;
#27510=CARTESIAN_POINT ( 'NONE',  ( 6.890625000614516438, -3.027376345333614438, 5.243569643749998122 ) ) ;
#27511=CARTESIAN_POINT ( 'NONE',  ( 10.26562500061451644, 3.027376345333613106, -5.243569643749998122 ) ) ;
#27512=CARTESIAN_POINT ( 'NONE',  ( 20.92500000122903714, 2.886751345948129099, -4.999999999999998224 ) ) ;
#27513=CARTESIAN_POINT ( 'NONE',  ( -4.243569643749999898, 13.52187500061451786, -32.45002607614398471 ) ) ;
#27514=CARTESIAN_POINT ( 'NONE',  ( 4.547618213146977340, -2.078260952684914731, 4.652852879716590451 ) ) ;
#27515=CARTESIAN_POINT ( 'NONE',  ( 4.912500001229034297, 0.000000000000000000, 4.999999999999998224 ) ) ;
#27516=CARTESIAN_POINT ( 'NONE',  ( 4.246875000614519280, -3.027376345333614438, 5.243569643749998122 ) ) ;
#27517=CARTESIAN_POINT ( 'NONE',  ( 21.57187500061451502, 3.027376345333613106, -5.243569643749998122 ) ) ;
#27519=CARTESIAN_POINT ( 'NONE',  ( 16.07812500061451289, 6.421520780324663323E-16, -5.243569643749999010 ) ) ;
#27521=CARTESIAN_POINT ( 'NONE',  ( 1.626862140677534273E-15, 13.81250000000000000, -26.00000000000000355 ) ) ;
#27523=CARTESIAN_POINT ( 'NONE',  ( 28.73437500061451644, 6.421520780324663323E-16, -5.243569643749999010 ) ) ;
#27525=CARTESIAN_POINT ( 'NONE',  ( 14.61562500061451608, -6.054752690667223547, -1.112240025338166033E-15 ) ) ;
#27526=CARTESIAN_POINT ( 'NONE',  ( 12.87187500061451750, -6.054752690667223547, -1.112240025338166033E-15 ) ) ;
#27527=ORIENTED_EDGE ( 'NONE', *, *, #58189, .T. ) ;
#27528=CARTESIAN_POINT ( 'NONE',  ( 29.12812500061451715, 6.421520780324663323E-16, -5.243569643749999010 ) ) ;
#27529=CARTESIAN_POINT ( 'NONE',  ( 23.46562500061451573, 3.027376345333611329, 5.243569643749999010 ) ) ;
#27530=CARTESIAN_POINT ( 'NONE',  ( 17.58750000122903145, -4.330127018922194537, 2.499999999999995559 ) ) ;
#27531=CARTESIAN_POINT ( 'NONE',  ( 28.57500000122903572, 2.886751345948099789, -5.000000000000048850 ) ) ;
#27532=EDGE_CURVE ( 'NONE', #12792, #13938, #68697, .T. ) ;
#27533=CARTESIAN_POINT ( 'NONE',  ( 12.18750000000000000, -2.886751345948125991, -5.000000000000000000 ) ) ;
#27534=EDGE_CURVE ( 'NONE', #27030, #18997, #7426, .T. ) ;
#27535=CARTESIAN_POINT ( 'NONE',  ( 22.50000000122903288, -2.886751345948129988, 4.999999999999997335 ) ) ;
#27536=CARTESIAN_POINT ( 'NONE',  ( 15.89062500061451289, -3.027376345333614438, 5.243569643749998122 ) ) ;
#27538=VERTEX_POINT ( 'NONE', #31714 ) ;
#27539=CARTESIAN_POINT ( 'NONE',  ( 20.58750000000000213, -2.886751345948129988, 4.999999999999997335 ) ) ;
#27540=CARTESIAN_POINT ( 'NONE',  ( 22.20937500061451431, 0.000000000000000000, 5.243569643749999010 ) ) ;
#27541=CARTESIAN_POINT ( 'NONE',  ( 26.99062500061451431, 6.054752690667223547, 3.707466751127219781E-16 ) ) ;
#27543=CARTESIAN_POINT ( 'NONE',  ( 19.94999999999999929, 4.330127018922192761, -2.499999999999997780 ) ) ;
#27544=CARTESIAN_POINT ( 'NONE',  ( 9.628125000614517148, -4.541064518000419881, 2.621784821874995952 ) ) ;
#27545=CARTESIAN_POINT ( 'NONE',  ( 0.000000000000000000, 0.000000000000000000, 50.00000000000000000 ) ) ;
#27547=CARTESIAN_POINT ( 'NONE',  ( 17.32499999999999929, 4.330127018922191873, 2.499999999999999556 ) ) ;
#27548=CARTESIAN_POINT ( 'NONE',  ( 23.43750000000000000, -2.886751345948125991, -5.000000000000000000 ) ) ;
#27549=CARTESIAN_POINT ( 'NONE',  ( 2.121784821874999061, 19.65312500061451573, 26.32496088578401583 ) ) ;
#27550=CARTESIAN_POINT ( 'NONE',  ( 3.646875000614520079, 6.054752690667223547, 3.707466751127219781E-16 ) ) ;
#27551=CARTESIAN_POINT ( 'NONE',  ( 28.43437500061451573, 4.541064518000418104, 2.621784821874999949 ) ) ;
#27552=ORIENTED_EDGE ( 'NONE', *, *, #14692, .T. ) ;
#27553=CARTESIAN_POINT ( 'NONE',  ( 23.91562500061451502, 3.027376345333611329, 5.243569643749999010 ) ) ;
#27554=CARTESIAN_POINT ( 'NONE',  ( 25.95937500061451431, -4.541064518000417216, -2.621784821875001281 ) ) ;
#27555=CARTESIAN_POINT ( 'NONE',  ( 4.243569643749999898, 18.67812500061459247, -30.00000000000000000 ) ) ;
#27556=VECTOR ( 'NONE', #22721, 1000.000000000000000 ) ;
#27557=CARTESIAN_POINT ( 'NONE',  ( 13.68750000000000178, 5.773502691896255534, 3.535250795749688894E-16 ) ) ;
#27558=CARTESIAN_POINT ( 'NONE',  ( 12.21562500061451573, 3.027376345333611329, 5.243569643749999010 ) ) ;
#27559=FACE_OUTER_BOUND ( 'NONE', #33737, .T. ) ;
#27560=CARTESIAN_POINT ( 'NONE',  ( 7.087499999999999467, -2.886751345948130876, 4.999999999999996447 ) ) ;
#27561=CARTESIAN_POINT ( 'NONE',  ( 25.79062500061451502, -3.027376345333614438, 5.243569643749998122 ) ) ;
#27562=CARTESIAN_POINT ( 'NONE',  ( 16.31250000122903288, -4.330127018922190985, -2.500000000000001332 ) ) ;
#27563=CARTESIAN_POINT ( 'NONE',  ( 0.000000000000000000, 20.00000000000000000, 30.00000000000000000 ) ) ;
#27565=CARTESIAN_POINT ( 'NONE',  ( 2.803125000614518747, 0.000000000000000000, 5.243569643749999010 ) ) ;
#27566=CARTESIAN_POINT ( 'NONE',  ( 21.15937500061451715, 4.541064518000418104, -2.621784821874998173 ) ) ;
#27567=CARTESIAN_POINT ( 'NONE',  ( 4.243569643749999010, 13.82187500061451857, 27.54997392385601174 ) ) ;
#27568=CARTESIAN_POINT ( 'NONE',  ( 22.47187500061451715, 3.027376345333613106, -5.243569643749998122 ) ) ;
#27569=CARTESIAN_POINT ( 'NONE',  ( 3.862500000000001155, 2.886751345948126879, 4.999999999999999112 ) ) ;
#27571=CARTESIAN_POINT ( 'NONE',  ( 8.765625000614518214, -6.054752690667223547, -1.112240025338166033E-15 ) ) ;
#27572=CYLINDRICAL_SURFACE ( 'NONE', #39529, 5.000000000000000000 ) ;
#27573=CARTESIAN_POINT ( 'NONE',  ( 6.421875000614519102, 3.027376345333611329, 5.243569643749999010 ) ) ;
#27575=CARTESIAN_POINT ( 'NONE',  ( 8.128125000614515372, 4.541064518000418104, 2.621784821874999949 ) ) ;
#27576=CARTESIAN_POINT ( 'NONE',  ( 12.45937500061451786, -4.541064518000417216, -2.621784821875001281 ) ) ;
#27577=CYLINDRICAL_SURFACE ( 'NONE', #9605, 4.999999999999998224 ) ;
#27578=CARTESIAN_POINT ( 'NONE',  ( 18.45000000122903216, -2.886751345948129988, 4.999999999999997335 ) ) ;
#27579=CARTESIAN_POINT ( 'NONE',  ( 8.746875000614515727, -3.027376345333614438, 5.243569643749998122 ) ) ;
#27580=CARTESIAN_POINT ( 'NONE',  ( 10.07812500061451644, -4.541064518000419881, 2.621784821874995952 ) ) ;
#27581=CARTESIAN_POINT ( 'NONE',  ( 6.778125000614518392, 4.541064518000418104, 2.621784821874999949 ) ) ;
#27583=CARTESIAN_POINT ( 'NONE',  ( 18.34687500061451715, -3.027376345333610441, -5.243569643749999898 ) ) ;
#27584=CARTESIAN_POINT ( 'NONE',  ( 1.071796769724491893, 13.04509619066137027, 33.99999999999999289 ) ) ;
#27585=CARTESIAN_POINT ( 'NONE',  ( 12.21562500061451573, 3.027376345333611329, 5.243569643749999010 ) ) ;
#27586=EDGE_CURVE ( 'NONE', #64681, #23474, #14979, .T. ) ;
#27587=CARTESIAN_POINT ( 'NONE',  ( 28.65937500061451715, -4.541064518000417216, -2.621784821875001281 ) ) ;
#27588=CARTESIAN_POINT ( 'NONE',  ( 4.243569643749999898, 11.04687500061451644, -27.54997392385601529 ) ) ;
#27589=CARTESIAN_POINT ( 'NONE',  ( 11.81250000122903465, -4.330127018922190985, -2.500000000000001332 ) ) ;
#27590=CARTESIAN_POINT ( 'NONE',  ( 4.243569643749999898, 16.42812500061451786, -30.00000000000000000 ) ) ;
#27591=CARTESIAN_POINT ( 'NONE',  ( 15.45000000122903216, -2.886751345948125991, -5.000000000000000000 ) ) ;
#27592=CARTESIAN_POINT ( 'NONE',  ( 10.22812500061451679, 6.421520780324663323E-16, -5.243569643749999010 ) ) ;
#27594=CARTESIAN_POINT ( 'NONE',  ( 13.16249999999999964, 2.886751345948129099, -4.999999999999998224 ) ) ;
#27596=CARTESIAN_POINT ( 'NONE',  ( 22.52812500061451573, 4.541064518000418104, 2.621784821874999949 ) ) ;
#27597=CARTESIAN_POINT ( 'NONE',  ( 8.034375000614518925, 6.421520780324663323E-16, -5.243569643749999010 ) ) ;
#27598=CARTESIAN_POINT ( 'NONE',  ( 10.83750000122903501, -4.330127018922194537, 2.499999999999995559 ) ) ;
#27599=CARTESIAN_POINT ( 'NONE',  ( 18.45000000122903216, -2.886751345948129988, 4.999999999999997335 ) ) ;
#27600=CARTESIAN_POINT ( 'NONE',  ( 16.34062500061451573, -3.027376345333614438, 5.243569643749998122 ) ) ;
#27601=CARTESIAN_POINT ( 'NONE',  ( 19.04062500061451146, -3.027376345333614438, 5.243569643749998122 ) ) ;
#27602=CARTESIAN_POINT ( 'NONE',  ( 25.20000000122903216, -2.886751345948129988, 4.999999999999997335 ) ) ;
#27603=CARTESIAN_POINT ( 'NONE',  ( 28.76250000122903216, 0.000000000000000000, 4.999999999999998224 ) ) ;
#27604=CARTESIAN_POINT ( 'NONE',  ( 22.16250000000000142, 2.886751345948129099, -4.999999999999998224 ) ) ;
#27606=CARTESIAN_POINT ( 'NONE',  ( 26.44687500061451502, -3.027376345333610441, -5.243569643749999898 ) ) ;
#27607=CARTESIAN_POINT ( 'NONE',  ( 25.65000000122903856, -2.886751345948163738, 4.999999999999939604 ) ) ;
#27608=CARTESIAN_POINT ( 'NONE',  ( 12.22500000122903430, -5.773502691896255534, -1.060575238724906372E-15 ) ) ;
#27609=CARTESIAN_POINT ( 'NONE',  ( 27.15937500061451360, 0.000000000000000000, 5.243569643749999010 ) ) ;
#27610=CARTESIAN_POINT ( 'NONE',  ( 4.546875000614517326, 6.054752690667223547, 3.707466751127219781E-16 ) ) ;
#27611=CARTESIAN_POINT ( 'NONE',  ( 24.06562500061451715, -6.054752690667223547, -1.112240025338166033E-15 ) ) ;
#27613=CARTESIAN_POINT ( 'NONE',  ( 3.486133158594716510E-16, 19.88749999999999929, -34.00000000000000000 ) ) ;
#27614=CARTESIAN_POINT ( 'NONE',  ( 9.909375000614517148, 4.541064518000418104, -2.621784821874998173 ) ) ;
#27615=B_SPLINE_CURVE_WITH_KNOTS ( 'NONE', 3,
 ( #70943, #20314, #54679, #9251, #42867, #37323, #72037, #48780, #15143, #14781 ),
 .UNSPECIFIED., .F., .F.,
 ( 4, 3, 3, 4 ),
 ( 6.133173666733496745E-19, 2.812507128105724141E-05, 5.625014365164849055E-05, 9.987238900461527181E-05 ),
 .UNSPECIFIED. ) ;
#27617=CARTESIAN_POINT ( 'NONE',  ( 3.046875000614519990, -3.027376345333610441, -5.243569643749999898 ) ) ;
#27618=CARTESIAN_POINT ( 'NONE',  ( 7.546875000614517326, -3.027376345333610441, -5.243569643749999898 ) ) ;
#27619=CARTESIAN_POINT ( 'NONE',  ( 27.94687500061451502, 6.054752690667223547, 3.707466751127219781E-16 ) ) ;
#27620=LINE ( 'NONE', #44625, #26673 ) ;
#27621=CARTESIAN_POINT ( 'NONE',  ( 19.68750000000000355, -2.886751345948129988, 4.999999999999997335 ) ) ;
#27622=ORIENTED_EDGE ( 'NONE', *, *, #11874, .T. ) ;
#27623=CARTESIAN_POINT ( 'NONE',  ( 26.58750000000000213, -2.886751345948125991, -5.000000000000000000 ) ) ;
#27624=EDGE_CURVE ( 'NONE', #35328, #28339, #53888, .T. ) ;
#27625=CARTESIAN_POINT ( 'NONE',  ( 28.09687500061451360, -3.027376345333614438, 5.243569643749998122 ) ) ;
#27626=ORIENTED_EDGE ( 'NONE', *, *, #36651, .F. ) ;
#27627=CARTESIAN_POINT ( 'NONE',  ( 17.12812500061451715, 4.541064518000418104, 2.621784821874999949 ) ) ;
#27628=CARTESIAN_POINT ( 'NONE',  ( 7.603125000614517681, 4.541064518000418104, -2.621784821874998173 ) ) ;
#27630=CARTESIAN_POINT ( 'NONE',  ( 5.709375000614517859, -4.541064518000417216, -2.621784821875001281 ) ) ;
#27631=CARTESIAN_POINT ( 'NONE',  ( 18.78750000122903430, 4.330127018922191873, 2.499999999999999556 ) ) ;
#27633=CARTESIAN_POINT ( 'NONE',  ( 7.471875000614519813, -6.054752690667223547, -1.112240025338166033E-15 ) ) ;
#27634=CARTESIAN_POINT ( 'NONE',  ( 10.99687500061451750, -3.027376345333614438, 5.243569643749998122 ) ) ;
#27635=CARTESIAN_POINT ( 'NONE',  ( 20.67187500061451289, 3.027376345333613106, -5.243569643749998122 ) ) ;
#27636=ORIENTED_EDGE ( 'NONE', *, *, #52167, .T. ) ;
#27638=CARTESIAN_POINT ( 'NONE',  ( 6.346875000614517148, 6.054752690667223547, 3.707466751127219781E-16 ) ) ;
#27640=CARTESIAN_POINT ( 'NONE',  ( 20.28750000000000142, -2.886751345948125991, -5.000000000000000000 ) ) ;
#27641=CARTESIAN_POINT ( 'NONE',  ( 17.39062500061451644, -3.027376345333610441, -5.243569643749999898 ) ) ;
#27643=CARTESIAN_POINT ( 'NONE',  ( 2.121784821874999061, 10.70937500061451964, -33.67503911421598417 ) ) ;
#27645=CARTESIAN_POINT ( 'NONE',  ( 12.25312500061451537, 0.000000000000000000, 5.243569643749999010 ) ) ;
#27646=CARTESIAN_POINT ( 'NONE',  ( 28.02187500061451431, 3.027376345333611329, 5.243569643749999010 ) ) ;
#27648=CARTESIAN_POINT ( 'NONE',  ( 28.65937500061451715, -4.541064518000417216, -2.621784821875001281 ) ) ;
#27649=CARTESIAN_POINT ( 'NONE',  ( 10.72500000000000142, -4.330127018922194537, 2.499999999999995559 ) ) ;
#27650=CARTESIAN_POINT ( 'NONE',  ( -2.000000000000000000, 15.98750000122903181, 26.53589838486224650 ) ) ;
#27651=CARTESIAN_POINT ( 'NONE',  ( 8.850000001229034297, 5.773502691896255534, 3.535250795749688894E-16 ) ) ;
#27652=CARTESIAN_POINT ( 'NONE',  ( 20.40937500061451715, 0.000000000000000000, 5.243569643749999010 ) ) ;
#27653=CARTESIAN_POINT ( 'NONE',  ( 15.38437500061451679, 4.541064518000418104, 2.621784821874999949 ) ) ;
#27654=CARTESIAN_POINT ( 'NONE',  ( -3.999999999999999112, 12.31250000000000000, 27.69059892324149885 ) ) ;
#27655=VERTEX_POINT ( 'NONE', #9179 ) ;
#27656=CARTESIAN_POINT ( 'NONE',  ( 15.59062500061451573, -3.027376345333610441, -5.243569643749999898 ) ) ;
#27657=CARTESIAN_POINT ( 'NONE',  ( 29.47500000122903430, 2.886751345948129099, -4.999999999999998224 ) ) ;
#27658=CARTESIAN_POINT ( 'NONE',  ( 16.13437500061451502, 6.421520780324663323E-16, -5.243569643749999010 ) ) ;
#27660=CARTESIAN_POINT ( 'NONE',  ( 18.06562500061451715, 3.027376345333611329, 5.243569643749999010 ) ) ;
#27661=DIRECTION ( 'NONE',  ( -0.000000000000000000, -1.000000000000000000, -0.000000000000000000 ) ) ;
#27662=CARTESIAN_POINT ( 'NONE',  ( 26.93437500061451573, 6.421520780324663323E-16, -5.243569643749999010 ) ) ;
#27663=CYLINDRICAL_SURFACE ( 'NONE', #8917, 4.000000000000000000 ) ;
#27664=CARTESIAN_POINT ( 'NONE',  ( 15.19687500061451857, -3.027376345333610441, -5.243569643749999898 ) ) ;
#27665=CARTESIAN_POINT ( 'NONE',  ( 14.92500000122903181, -5.773502691896255534, -1.060575238724906372E-15 ) ) ;
#27667=CARTESIAN_POINT ( 'NONE',  ( 3.323491336998473322, -3.735569206101108986, 3.679756774564975519 ) ) ;
#27668=CARTESIAN_POINT ( 'NONE',  ( 19.54687500061451644, -3.027376345333614438, 5.243569643749998122 ) ) ;
#27669=CARTESIAN_POINT ( 'NONE',  ( 22.01250000122903216, 0.000000000000000000, 4.999999999999998224 ) ) ;
#27671=CARTESIAN_POINT ( 'NONE',  ( 18.15937500061451715, 0.000000000000000000, 5.243569643749999010 ) ) ;
#27672=CARTESIAN_POINT ( 'NONE',  ( 4.243569643749999898, 11.53437500061451892, 30.00000000000000000 ) ) ;
#27673=CARTESIAN_POINT ( 'NONE',  ( 18.21562500061451573, -6.054752690667223547, -1.112240025338166033E-15 ) ) ;
#27674=ORIENTED_EDGE ( 'NONE', *, *, #7253, .T. ) ;
#27675=VERTEX_POINT ( 'NONE', #2904 ) ;
#27676=CARTESIAN_POINT ( 'NONE',  ( 20.40000000000000213, 4.330127018922192761, -2.499999999999997780 ) ) ;
#27677=CARTESIAN_POINT ( 'NONE',  ( 28.08750000122903145, 6.123233995736764310E-16, -4.999999999999998224 ) ) ;
#27678=CARTESIAN_POINT ( 'NONE',  ( 23.46562500061451573, 3.027376345333611329, 5.243569643749999010 ) ) ;
#27679=CARTESIAN_POINT ( 'NONE',  ( 5.803125000614517859, 4.541064518000418104, -2.621784821874998173 ) ) ;
#27680=CARTESIAN_POINT ( 'NONE',  ( 16.31250000122903288, -4.330127018922190985, -2.500000000000001332 ) ) ;
#27681=CARTESIAN_POINT ( 'NONE',  ( 21.96562500061451573, 3.027376345333613106, -5.243569643749998122 ) ) ;
#27682=CARTESIAN_POINT ( 'NONE',  ( 19.68750000000000355, -2.886751345948129988, 4.999999999999997335 ) ) ;
#27683=( BOUNDED_CURVE ( )  B_SPLINE_CURVE ( 2, ( #53672, #14137, #52576, #19298, #52215, #18933, #18208 ),
 .UNSPECIFIED., .F., .F. ) 
 B_SPLINE_CURVE_WITH_KNOTS ( ( 3, 2, 2, 3 ),
 ( 0.2416666666666666963, 0.2444444444444444642, 0.2472222222222222321, 0.2500000000000000000 ),
 .UNSPECIFIED. ) 
 CURVE ( )  GEOMETRIC_REPRESENTATION_ITEM ( )  RATIONAL_B_SPLINE_CURVE ( ( 0.9999999999999986677, 0.8660254037844400399, 1.000000000000000000, 0.8660254037844387076, 1.000000000000000000, 0.8660254037844387076, 1.000000000000000000 ) ) 
 REPRESENTATION_ITEM ( '' )  );
#27684=CARTESIAN_POINT ( 'NONE',  ( 26.16562500061451502, 3.027376345333611329, 5.243569643749999010 ) ) ;
#27685=CARTESIAN_POINT ( 'NONE',  ( 5.765625000614519102, 3.027376345333613106, -5.243569643749998122 ) ) ;
#27686=ORIENTED_EDGE ( 'NONE', *, *, #61290, .F. ) ;
#27687=CARTESIAN_POINT ( 'NONE',  ( -5.810221930991193690E-16, 14.48749999999999893, -34.00000000000000000 ) ) ;
#27688=CARTESIAN_POINT ( 'NONE',  ( 2.953125000614516438, -4.541064518000417216, -2.621784821875001281 ) ) ;
#27690=CARTESIAN_POINT ( 'NONE',  ( 2.000000000000001332, 18.80000000000000071, 33.46410161513774995 ) ) ;
#27691=CARTESIAN_POINT ( 'NONE',  ( -2.828200636599751609E-16, 10.55000000122903359, -34.61880215351700230 ) ) ;
#27692=CARTESIAN_POINT ( 'NONE',  ( -2.121784821874996840, 19.48437500061451644, -26.32496088578401583 ) ) ;
#27693=CARTESIAN_POINT ( 'NONE',  ( 9.000000000000001776, -4.330127018922190985, -2.500000000000001332 ) ) ;
#27694=CARTESIAN_POINT ( 'NONE',  ( 9.721875000614517148, -6.054752690667223547, -1.112240025338166033E-15 ) ) ;
#27695=CARTESIAN_POINT ( 'NONE',  ( 6.337500001229033231, -4.330127018922194537, 2.499999999999995559 ) ) ;
#27696=CARTESIAN_POINT ( 'NONE',  ( 12.27187500061451786, 3.027376345333611329, 5.243569643749999010 ) ) ;
#27697=CARTESIAN_POINT ( 'NONE',  ( 3.159375000614518036, 4.541064518000418104, -2.621784821874998173 ) ) ;
#27698=CARTESIAN_POINT ( 'NONE',  ( 1.071796769724490117, 18.89509619066136992, 33.99999999999999289 ) ) ;
#27699=VECTOR ( 'NONE', #33048, 1000.000000000000000 ) ;
#27700=CARTESIAN_POINT ( 'NONE',  ( 0.000000000000000000, -10.00000000000000000, 0.000000000000000000 ) ) ;
#27701=CARTESIAN_POINT ( 'NONE',  ( 9.046875000614518214, 6.054752690667223547, 3.707466751127219781E-16 ) ) ;
#27702=CARTESIAN_POINT ( 'NONE',  ( 1.626862140677534273E-15, 18.76250000000000284, -26.00000000000000355 ) ) ;
#27703=CARTESIAN_POINT ( 'NONE',  ( 20.61562500061451431, 3.027376345333613106, -5.243569643749998122 ) ) ;
#27704=CARTESIAN_POINT ( 'NONE',  ( 4.612500001229032698, -4.330127018922190985, -2.500000000000001332 ) ) ;
#27705=CARTESIAN_POINT ( 'NONE',  ( -4.243569643749999898, 17.96562500061459389, 27.54997392385601529 ) ) ;
#27706=CARTESIAN_POINT ( 'NONE',  ( 22.88437500061451857, 6.421520780324663323E-16, -5.243569643749999010 ) ) ;
#27707=CARTESIAN_POINT ( 'NONE',  ( 9.525000000000002132, 6.123233995736764310E-16, -4.999999999999998224 ) ) ;
#27708=CARTESIAN_POINT ( 'NONE',  ( 29.55000000122903003, 5.773502691896255534, 3.535250795749688894E-16 ) ) ;
#27711=CARTESIAN_POINT ( 'NONE',  ( 24.96562500061451573, -6.054752690667223547, -1.112240025338166033E-15 ) ) ;
#27712=CARTESIAN_POINT ( 'NONE',  ( 15.66562500061451857, 3.027376345333613106, -5.243569643749998122 ) ) ;
#27714=CARTESIAN_POINT ( 'NONE',  ( 13.69687500061451679, -3.027376345333614438, 5.243569643749998122 ) ) ;
#27716=CARTESIAN_POINT ( 'NONE',  ( 24.56250000122903288, 4.330127018922192761, -2.499999999999997780 ) ) ;
#27717=CARTESIAN_POINT ( 'NONE',  ( 3.384375000614517237, -4.541064518000419881, 2.621784821874995952 ) ) ;
#27719=CARTESIAN_POINT ( 'NONE',  ( 13.17187500061451999, 3.027376345333611329, 5.243569643749999010 ) ) ;
#27720=CARTESIAN_POINT ( 'NONE',  ( 14.96250000000000036, 2.886751345948129099, -4.999999999999997335 ) ) ;
#27721=CARTESIAN_POINT ( 'NONE',  ( 30.00000000000000000, 0.000000000000000000, 0.000000000000000000 ) ) ;
#27722=CARTESIAN_POINT ( 'NONE',  ( -5.810221930991193690E-16, 11.90000000122903501, 26.00000000000000355 ) ) ;
#27723=CARTESIAN_POINT ( 'NONE',  ( 25.62187500061451573, 3.027376345333613106, -5.243569643749998122 ) ) ;
#27724=CARTESIAN_POINT ( 'NONE',  ( 15.49687500061451750, -3.027376345333614438, 5.243569643749998122 ) ) ;
#27726=CARTESIAN_POINT ( 'NONE',  ( 27.15000000000000213, 4.330127018922192761, -2.499999999999997780 ) ) ;
#27727=CARTESIAN_POINT ( 'NONE',  ( 4.275000001229035895, 2.886751345948129099, -4.999999999999998224 ) ) ;
#27728=CARTESIAN_POINT ( 'NONE',  ( 6.675000000000000711, -4.330127018922194537, 2.499999999999995559 ) ) ;
#27730=CARTESIAN_POINT ( 'NONE',  ( 20.50312500061451715, -4.541064518000417216, -2.621784821875001281 ) ) ;
#27731=CARTESIAN_POINT ( 'NONE',  ( 9.150000000000002132, 4.330127018922192761, -2.499999999999997780 ) ) ;
#27732=CARTESIAN_POINT ( 'NONE',  ( -5.810221930991193690E-16, 13.70000000122903394, 26.00000000000000355 ) ) ;
#27734=CARTESIAN_POINT ( 'NONE',  ( 17.58749999999999858, -2.886751345948125991, -5.000000000000000000 ) ) ;
#27735=CARTESIAN_POINT ( 'NONE',  ( -3.999999999999997335, 17.33749999999999858, 32.30940107675850470 ) ) ;
#27736=CARTESIAN_POINT ( 'NONE',  ( 20.25000000122903288, -2.886751345948129988, 4.999999999999997335 ) ) ;
#27738=CARTESIAN_POINT ( 'NONE',  ( 27.23437500061451644, -4.541064518000419881, 2.621784821874995952 ) ) ;
#27739=ORIENTED_EDGE ( 'NONE', *, *, #53141, .T. ) ;
#27740=CARTESIAN_POINT ( 'NONE',  ( 16.04062500061451857, -3.027376345333610441, -5.243569643749999898 ) ) ;
#27741=CARTESIAN_POINT ( 'NONE',  ( 22.07812500061451644, 4.541064518000418104, 2.621784821874999949 ) ) ;
#27742=CARTESIAN_POINT ( 'NONE',  ( 23.59687500061451715, -3.027376345333614438, 5.243569643749998122 ) ) ;
#27743=CARTESIAN_POINT ( 'NONE',  ( 7.200000000000001954, -4.330127018922190985, -2.500000000000001332 ) ) ;
#27744=CARTESIAN_POINT ( 'NONE',  ( 8.353125000614518569, -4.541064518000417216, -2.621784821875001281 ) ) ;
#27745=CARTESIAN_POINT ( 'NONE',  ( 23.57812500061451289, -4.541064518000419881, 2.621784821874995952 ) ) ;
#27746=CARTESIAN_POINT ( 'NONE',  ( 14.07187500061451679, 3.027376345333611329, 5.243569643749999010 ) ) ;
#27747=CARTESIAN_POINT ( 'NONE',  ( 19.28437500061451360, 6.421520780324663323E-16, -5.243569643749999010 ) ) ;
#27748=CARTESIAN_POINT ( 'NONE',  ( -5.810221930991193690E-16, 12.35000000122903430, -34.00000000000000000 ) ) ;
#27749=CARTESIAN_POINT ( 'NONE',  ( -2.121784821874996840, 18.97812500061451857, 33.67503911421598417 ) ) ;
#27750=CARTESIAN_POINT ( 'NONE',  ( 20.62500000122903288, 2.886751345948126879, 4.999999999999999112 ) ) ;
#27752=CARTESIAN_POINT ( 'NONE',  ( 12.66562500061451502, 3.027376345333611329, 5.243569643749999010 ) ) ;
#27753=CARTESIAN_POINT ( 'NONE',  ( 6.009375000614519458, 0.000000000000000000, 5.243569643749999010 ) ) ;
#27754=CARTESIAN_POINT ( 'NONE',  ( 6.271875000614517859, 3.027376345333613106, -5.243569643749998122 ) ) ;
#27756=CARTESIAN_POINT ( 'NONE',  ( 27.57187500061451857, 3.027376345333611329, 5.243569643749999010 ) ) ;
#27757=CARTESIAN_POINT ( 'NONE',  ( 19.30312500061451786, 4.541064518000418104, -2.621784821874998173 ) ) ;
#27758=CARTESIAN_POINT ( 'NONE',  ( 28.95000000122903572, -2.886751345948125991, -5.000000000000000000 ) ) ;
#27759=EDGE_CURVE ( 'NONE', #61054, #16658, #48709, .T. ) ;
#27760=CARTESIAN_POINT ( 'NONE',  ( 26.87812500061451360, 6.421520780324663323E-16, -5.243569643749999010 ) ) ;
#27761=CARTESIAN_POINT ( 'NONE',  ( 23.29687500061451644, -3.027376345333610441, -5.243569643749999898 ) ) ;
#27762=CARTESIAN_POINT ( 'NONE',  ( 18.55312500061451431, 0.000000000000000000, 5.243569643749999010 ) ) ;
#27763=CARTESIAN_POINT ( 'NONE',  ( 4.243569643749999898, 18.73437500061451644, 30.00000000000000000 ) ) ;
#27764=CARTESIAN_POINT ( 'NONE',  ( 24.44062500061451715, -3.027376345333614438, 5.243569643749998122 ) ) ;
#27765=CARTESIAN_POINT ( 'NONE',  ( 5.062500001229035540, -4.330127018922190985, -2.500000000000001332 ) ) ;
#27767=CARTESIAN_POINT ( 'NONE',  ( 28.61249999999999716, 2.886751345948126879, 4.999999999999999112 ) ) ;
#27768=CARTESIAN_POINT ( 'NONE',  ( 4.000000000000000000, 15.23750000000000071, -27.69059892324149530 ) ) ;
#27770=CARTESIAN_POINT ( 'NONE',  ( 4.884375000614518569, 6.421520780324663323E-16, -5.243569643749999010 ) ) ;
#27771=CARTESIAN_POINT ( 'NONE',  ( 12.36562500061451608, -6.054752690667223547, -1.112240025338166033E-15 ) ) ;
#27772=CARTESIAN_POINT ( 'NONE',  ( 6.159375000614517148, -4.541064518000417216, -2.621784821875001281 ) ) ;
#27773=CARTESIAN_POINT ( 'NONE',  ( 24.97500000122903430, 2.886751345948129099, -4.999999999999998224 ) ) ;
#27774=AXIS2_PLACEMENT_3D ( 'NONE', #45261, #46343, #24155 ) ;
#27775=CARTESIAN_POINT ( 'NONE',  ( 16.13437500061451502, 6.421520780324663323E-16, -5.243569643749999010 ) ) ;
#27776=CARTESIAN_POINT ( 'NONE',  ( 29.42812500061451431, -4.541064518000419881, 2.621784821874995952 ) ) ;
#27777=CARTESIAN_POINT ( 'NONE',  ( 27.00000000000000000, -4.330127018922190985, -2.500000000000001332 ) ) ;
#27778=CARTESIAN_POINT ( 'NONE',  ( 25.95937500061451431, -4.541064518000417216, -2.621784821875001281 ) ) ;
#27779=CARTESIAN_POINT ( 'NONE',  ( 4.153125000614515727, 0.000000000000000000, 5.243569643749999010 ) ) ;
#27780=CARTESIAN_POINT ( 'NONE',  ( 13.56562500061451892, 3.027376345333611329, 5.243569643749999010 ) ) ;
#27781=ORIENTED_EDGE ( 'NONE', *, *, #33711, .T. ) ;
#27782=AXIS2_PLACEMENT_3D ( 'NONE', #29781, #52317, #1720 ) ;
#27783=CARTESIAN_POINT ( 'NONE',  ( 11.24062500061451608, 6.054752690667223547, 3.707466751127219781E-16 ) ) ;
#27784=AXIS2_PLACEMENT_3D ( 'NONE', #18985, #64064, #23095 ) ;
#27785=CARTESIAN_POINT ( 'NONE',  ( 9.290625000614515017, -3.027376345333610441, -5.243569643749999898 ) ) ;
#27788=CARTESIAN_POINT ( 'NONE',  ( 16.50000000000000000, 0.000000000000000000, 4.999999999999998224 ) ) ;
#27789=CARTESIAN_POINT ( 'NONE',  ( 16.20937500061451786, 4.541064518000418104, -2.621784821874998173 ) ) ;
#27790=CARTESIAN_POINT ( 'NONE',  ( 12.71250000122903145, -4.330127018922190985, -2.500000000000001332 ) ) ;
#27792=CARTESIAN_POINT ( 'NONE',  ( 22.02187500061452141, 3.027376345333613106, -5.243569643749998122 ) ) ;
#27793=CARTESIAN_POINT ( 'NONE',  ( -4.243569643749999898, 13.01562500061451999, -32.45002607614398471 ) ) ;
#27794=DIRECTION ( 'NONE',  ( -0.000000000000000000, -1.000000000000000000, -0.000000000000000000 ) ) ;
#27797=CARTESIAN_POINT ( 'NONE',  ( 27.89062500061451289, 6.054752690667223547, 3.707466751127219781E-16 ) ) ;
#27798=CARTESIAN_POINT ( 'NONE',  ( 0.000000000000000000, 20.00000000000000000, -33.99999999999999289 ) ) ;
#27799=DIRECTION ( 'NONE',  ( 1.000000000000000000, 0.000000000000000000, 0.000000000000000000 ) ) ;
#27800=CARTESIAN_POINT ( 'NONE',  ( 27.82499999999999929, -4.330127018922194537, 2.499999999999995559 ) ) ;
#27802=CARTESIAN_POINT ( 'NONE',  ( 10.22812500061451679, 6.421520780324663323E-16, -5.243569643749999010 ) ) ;
#27804=CARTESIAN_POINT ( 'NONE',  ( 20.67187500061451289, 3.027376345333613106, -5.243569643749998122 ) ) ;
#27807=AXIS2_PLACEMENT_3D ( 'NONE', #4751, #49818, #26551 ) ;
#27808=CARTESIAN_POINT ( 'NONE',  ( 5.203125000614518214, -4.541064518000417216, -2.621784821875001281 ) ) ;
#27809=CARTESIAN_POINT ( 'NONE',  ( 11.59687500061451892, -3.027376345333610441, -5.243569643749999898 ) ) ;
#27810=ORIENTED_EDGE ( 'NONE', *, *, #39698, .T. ) ;
#27811=CARTESIAN_POINT ( 'NONE',  ( 22.02187500061452141, 3.027376345333613106, -5.243569643749998122 ) ) ;
#27812=FACE_OUTER_BOUND ( 'NONE', #30421, .T. ) ;
#27813=CARTESIAN_POINT ( 'NONE',  ( 28.91250000000000497, 2.886751345948129099, -4.999999999999998224 ) ) ;
#27814=CARTESIAN_POINT ( 'NONE',  ( 3.975000000000002753, -4.330127018922194537, 2.499999999999995559 ) ) ;
#27815=CARTESIAN_POINT ( 'NONE',  ( 15.63750000122903216, 4.330127018922191873, 2.499999999999999556 ) ) ;
#27817=CARTESIAN_POINT ( 'NONE',  ( 17.36250000000000071, 2.886751345948161074, 4.999999999999941380 ) ) ;
#27819=CARTESIAN_POINT ( 'NONE',  ( 13.57500000000000107, 6.123233995736764310E-16, -4.999999999999998224 ) ) ;
#27820=CARTESIAN_POINT ( 'NONE',  ( 17.47499999999999787, -4.330127018922194537, 2.499999999999995559 ) ) ;
#27822=CARTESIAN_POINT ( 'NONE',  ( 12.30000000122903181, -2.886751345948125991, -5.000000000000000000 ) ) ;
#27823=CARTESIAN_POINT ( 'NONE',  ( 10.26562500061451644, 3.027376345333613106, -5.243569643749998122 ) ) ;
#27824=VECTOR ( 'NONE', #19685, 1000.000000000000000 ) ;
#27825=CARTESIAN_POINT ( 'NONE',  ( 8.699999999999999289, 4.330127018922192761, -2.499999999999997780 ) ) ;
#27826=CARTESIAN_POINT ( 'NONE',  ( 26.17500000000000071, 6.123233995736764310E-16, -4.999999999999998224 ) ) ;
#27827=CARTESIAN_POINT ( 'NONE',  ( 4.243569643749999898, 15.54687500061451644, -27.54997392385601529 ) ) ;
#27828=CARTESIAN_POINT ( 'NONE',  ( 27.30000000122903359, 5.773502691896255534, 3.535250795749688894E-16 ) ) ;
#27830=CARTESIAN_POINT ( 'NONE',  ( 6.412500000000001421, 2.886751345948129099, -4.999999999999998224 ) ) ;
#27833=CARTESIAN_POINT ( 'NONE',  ( 24.66562500061451502, 3.027376345333613106, -5.243569643749998122 ) ) ;
#27834=CARTESIAN_POINT ( 'NONE',  ( 1.071796769724491893, 13.38259618943233598, -26.00000000000000355 ) ) ;
#27836=FACE_OUTER_BOUND ( 'NONE', #16941, .T. ) ;
#27837=CARTESIAN_POINT ( 'NONE',  ( 22.35937500061451644, -4.541064518000417216, -2.621784821875001281 ) ) ;
#27838=EDGE_CURVE ( 'NONE', #69794, #68418, #52750, .T. ) ;
#27839=CARTESIAN_POINT ( 'NONE',  ( 15.77812500061451573, 4.541064518000418104, 2.621784821874999949 ) ) ;
#27840=CARTESIAN_POINT ( 'NONE',  ( 4.243569643749999010, 10.61562500061459602, -32.45002607614398471 ) ) ;
#27841=CARTESIAN_POINT ( 'NONE',  ( 7.678125000614516082, 4.541064518000418104, 2.621784821874999949 ) ) ;
#27842=CARTESIAN_POINT ( 'NONE',  ( 28.42500000122904069, -5.773502691896255534, -1.060575238724906372E-15 ) ) ;
#27844=CARTESIAN_POINT ( 'NONE',  ( 19.67812500061451786, 6.421520780324663323E-16, -5.243569643749999010 ) ) ;
#27847=CARTESIAN_POINT ( 'NONE',  ( 14.70937500061451786, -4.541064518000417216, -2.621784821875001281 ) ) ;
#27848=CARTESIAN_POINT ( 'NONE',  ( 13.54687500061451999, 6.054752690667223547, 3.707466751127219781E-16 ) ) ;
#27849=CARTESIAN_POINT ( 'NONE',  ( 21.60937500061451644, 4.541064518000418104, -2.621784821874998173 ) ) ;
#27851=CARTESIAN_POINT ( 'NONE',  ( 3.703125000614516882, 0.000000000000000000, 5.243569643749999010 ) ) ;
#27852=CARTESIAN_POINT ( 'NONE',  ( 26.72812500061451502, -4.541064518000419881, 2.621784821874995952 ) ) ;
#27853=CARTESIAN_POINT ( 'NONE',  ( 26.61562500061451786, 3.027376345333611329, 5.243569643749999010 ) ) ;
#27854=CARTESIAN_POINT ( 'NONE',  ( 8.484601909799253346E-16, 17.41250000000000142, 34.61880215351700230 ) ) ;
#27855=CARTESIAN_POINT ( 'NONE',  ( 5.409375000614516260, 4.541064518000418104, -2.621784821874998173 ) ) ;
#27857=CARTESIAN_POINT ( 'NONE',  ( 12.63750000122903394, -4.330127018922194537, 2.499999999999995559 ) ) ;
#27858=CARTESIAN_POINT ( 'NONE',  ( 6.187500001229032875, 4.330127018922191873, 2.499999999999999556 ) ) ;
#27859=CARTESIAN_POINT ( 'NONE',  ( 28.76250000122903216, 0.000000000000000000, 4.999999999999998224 ) ) ;
#27862=CARTESIAN_POINT ( 'NONE',  ( 12.45937500061451786, -4.541064518000417216, -2.621784821875001281 ) ) ;
#27863=ORIENTED_EDGE ( 'NONE', *, *, #65098, .T. ) ;
#27864=CARTESIAN_POINT ( 'NONE',  ( 20.65312500061451573, 4.541064518000418104, -2.621784821874998173 ) ) ;
#27865=CARTESIAN_POINT ( 'NONE',  ( 14.25937500061451679, -4.541064518000417216, -2.621784821875001281 ) ) ;
#27866=CARTESIAN_POINT ( 'NONE',  ( 4.753125000614515372, -4.541064518000417216, -2.621784821875001281 ) ) ;
#27867=CARTESIAN_POINT ( 'NONE',  ( 21.42187500061451644, -6.054752690667223547, -1.112240025338166033E-15 ) ) ;
#27868=CARTESIAN_POINT ( 'NONE',  ( 9.384375000614518569, 6.421520780324663323E-16, -5.243569643749999010 ) ) ;
#27869=CARTESIAN_POINT ( 'NONE',  ( 4.303125000614516971, -4.541064518000417216, -2.621784821875001281 ) ) ;
#27871=CARTESIAN_POINT ( 'NONE',  ( 5.062500001229035540, -4.330127018922190985, -2.500000000000001332 ) ) ;
#27872=CARTESIAN_POINT ( 'NONE',  ( 19.00312500061451715, 0.000000000000000000, 5.243569643749999010 ) ) ;
#27873=CARTESIAN_POINT ( 'NONE',  ( 7.537500001229033408, 4.330127018922191873, 2.499999999999999556 ) ) ;
#27874=CARTESIAN_POINT ( 'NONE',  ( 18.17812500061451786, -4.541064518000419881, 2.621784821874995952 ) ) ;
#27875=CARTESIAN_POINT ( 'NONE',  ( 15.47812500061451679, -4.541064518000419881, 2.621784821874995952 ) ) ;
#27877=CARTESIAN_POINT ( 'NONE',  ( 15.67500000000000071, -4.330127018922194537, 2.499999999999995559 ) ) ;
#27878=CARTESIAN_POINT ( 'NONE',  ( 9.412500001229034297, 0.000000000000000000, 4.999999999999998224 ) ) ;
#27879=CARTESIAN_POINT ( 'NONE',  ( 4.490625000614516971, 6.054752690667223547, 3.707466751127219781E-16 ) ) ;
#27880=CARTESIAN_POINT ( 'NONE',  ( 20.73750000122903359, -4.330127018922194537, 2.499999999999995559 ) ) ;
#27882=CARTESIAN_POINT ( 'NONE',  ( 4.243569643749999010, 11.57187500061451679, -32.45002607614398471 ) ) ;
#27883=CARTESIAN_POINT ( 'NONE',  ( 3.187500001229033764, -4.330127018922194537, 2.499999999999995559 ) ) ;
#27884=CARTESIAN_POINT ( 'NONE',  ( 4.171875000614517326, 3.027376345333611329, 5.243569643749999010 ) ) ;
#27885=CARTESIAN_POINT ( 'NONE',  ( 21.53437500061451715, 6.421520780324663323E-16, -5.243569643749999010 ) ) ;
#27888=CARTESIAN_POINT ( 'NONE',  ( 15.32812500061451644, 4.541064518000418104, 2.621784821874999949 ) ) ;
#27891=CARTESIAN_POINT ( 'NONE',  ( 29.10937500061451644, -4.541064518000417216, -2.621784821875001281 ) ) ;
#27893=CARTESIAN_POINT ( 'NONE',  ( 11.87812500061451537, -4.541064518000419881, 2.621784821874995952 ) ) ;
#27894=CARTESIAN_POINT ( 'NONE',  ( 11.14687500061451608, -3.027376345333610441, -5.243569643749999898 ) ) ;
#27895=ORIENTED_EDGE ( 'NONE', *, *, #20120, .F. ) ;
#27896=CARTESIAN_POINT ( 'NONE',  ( 28.75312500061451715, 4.541064518000418104, -2.621784821874998173 ) ) ;
#27897=CARTESIAN_POINT ( 'NONE',  ( 23.16562500061451502, -6.054752690667223547, -1.112240025338166033E-15 ) ) ;
#27898=CYLINDRICAL_SURFACE ( 'NONE', #1500, 5.999999999999998224 ) ;
#27899=LINE ( 'NONE', #51870, #10096 ) ;
#27900=CARTESIAN_POINT ( 'NONE',  ( 11.47499999999999964, 4.330127018922191873, 2.499999999999999556 ) ) ;
#27901=CARTESIAN_POINT ( 'NONE',  ( 21.26250000122903572, -4.330127018922190985, -2.500000000000001332 ) ) ;
#27902=CARTESIAN_POINT ( 'NONE',  ( 16.79062500061451857, -3.027376345333614438, 5.243569643749998122 ) ) ;
#27904=ORIENTED_EDGE ( 'NONE', *, *, #38380, .T. ) ;
#27905=CARTESIAN_POINT ( 'NONE',  ( 20.85000000000000142, 4.330127018922192761, -2.499999999999997780 ) ) ;
#27907=CARTESIAN_POINT ( 'NONE',  ( 23.92499999999999716, 6.123233995736764310E-16, -4.999999999999998224 ) ) ;
#27908=CARTESIAN_POINT ( 'NONE',  ( 20.74687500061451573, 6.054752690667223547, 3.707466751127219781E-16 ) ) ;
#27909=CARTESIAN_POINT ( 'NONE',  ( 26.54062500061451146, 6.054752690667223547, 3.707466751127219781E-16 ) ) ;
#27910=VERTEX_POINT ( 'NONE', #50532 ) ;
#27911=CARTESIAN_POINT ( 'NONE',  ( 4.000000000000000000, 17.93750000000000355, -27.69059892324149885 ) ) ;
#27912=CARTESIAN_POINT ( 'NONE',  ( 9.215625000614515727, -6.054752690667223547, -1.112240025338166033E-15 ) ) ;
#27913=CARTESIAN_POINT ( 'NONE',  ( 16.42500000000000071, 4.330127018922191873, 2.499999999999999556 ) ) ;
#27914=CARTESIAN_POINT ( 'NONE',  ( 7.687500001229033764, -4.330127018922194537, 2.499999999999995559 ) ) ;
#27915=CARTESIAN_POINT ( 'NONE',  ( 4.584375000614516971, 4.541064518000418104, 2.621784821874999949 ) ) ;
#27916=CARTESIAN_POINT ( 'NONE',  ( 29.70937500061451431, 4.541064518000418104, -2.621784821874998173 ) ) ;
#27918=CARTESIAN_POINT ( 'NONE',  ( 24.14062500061451289, -3.027376345333610441, -5.243569643749999898 ) ) ;
#27919=CARTESIAN_POINT ( 'NONE',  ( 25.73437500061451644, 4.541064518000418104, 2.621784821874999949 ) ) ;
#27920=CARTESIAN_POINT ( 'NONE',  ( 4.243569643749999010, 19.16562500061459318, -32.45002607614398471 ) ) ;
#27921=CARTESIAN_POINT ( 'NONE',  ( 11.02500000000000036, 4.330127018922191873, 2.499999999999999556 ) ) ;
#27922=CARTESIAN_POINT ( 'NONE',  ( 8.203125000614518214, 0.000000000000000000, 5.243569643749999010 ) ) ;
#27923=CARTESIAN_POINT ( 'NONE',  ( 6.112500000000001599, 2.886751345948126879, 4.999999999999998224 ) ) ;
#27924=CARTESIAN_POINT ( 'NONE',  ( 19.42499999999999716, 6.123233995736764310E-16, -4.999999999999998224 ) ) ;
#27925=CARTESIAN_POINT ( 'NONE',  ( 25.64062500061451644, 6.054752690667223547, 3.707466751127219781E-16 ) ) ;
#27926=CARTESIAN_POINT ( 'NONE',  ( 12.71250000122903145, -4.330127018922190985, -2.500000000000001332 ) ) ;
#27928=CARTESIAN_POINT ( 'NONE',  ( 3.478125000614517237, 6.421520780324663323E-16, -5.243569643749999010 ) ) ;
#27929=CARTESIAN_POINT ( 'NONE',  ( 20.07187500061451857, -6.054752690667223547, -1.112240025338166033E-15 ) ) ;
#27930=CARTESIAN_POINT ( 'NONE',  ( -2.121784821874996840, 15.43437500061451928, 33.67503911421598417 ) ) ;
#27931=CARTESIAN_POINT ( 'NONE',  ( 21.98437500061451644, 6.421520780324663323E-16, -5.243569643749999010 ) ) ;
#27932=CARTESIAN_POINT ( 'NONE',  ( 3.412500000000002309, 2.886751345948126879, 4.999999999999999112 ) ) ;
#27933=CARTESIAN_POINT ( 'NONE',  ( 2.121784821875001281, 19.55937500061451573, 33.67503911421598417 ) ) ;
#27934=CARTESIAN_POINT ( 'NONE',  ( 10.41562500061451679, 3.027376345333611329, 5.243569643749999010 ) ) ;
#27935=LINE ( 'NONE', #11665, #30074 ) ;
#27936=CARTESIAN_POINT ( 'NONE',  ( 6.084375000614518747, -4.541064518000419881, 2.621784821874995952 ) ) ;
#27937=CYLINDRICAL_SURFACE ( 'NONE', #37184, 4.999999999999998224 ) ;
#27938=CARTESIAN_POINT ( 'NONE',  ( 7.078125000614516438, 6.421520780324663323E-16, -5.243569643749999010 ) ) ;
#27939=CARTESIAN_POINT ( 'NONE',  ( 12.68437500061451573, 4.541064518000418104, 2.621784821874999949 ) ) ;
#27940=( NAMED_UNIT ( * ) SI_UNIT ( $, .STERADIAN. ) SOLID_ANGLE_UNIT ( ) );
#27941=CARTESIAN_POINT ( 'NONE',  ( 19.98750000122903359, 6.123233995736764310E-16, -4.999999999999998224 ) ) ;
#27942=CARTESIAN_POINT ( 'NONE',  ( 8.596875000614518925, 6.054752690667223547, 3.707466751127219781E-16 ) ) ;
#27943=CARTESIAN_POINT ( 'NONE',  ( 9.365625000614519635, 3.027376345333613106, -5.243569643749998122 ) ) ;
#27946=CARTESIAN_POINT ( 'NONE',  ( 18.42187500061451644, 3.027376345333613106, -5.243569643749998122 ) ) ;
#27947=CARTESIAN_POINT ( 'NONE',  ( 4.442661813835188767, 2.294285635476659646, 4.469955633307156617 ) ) ;
#27948=CARTESIAN_POINT ( 'NONE',  ( 27.47812500061451502, 4.541064518000418104, 2.621784821874999949 ) ) ;
#27949=( BOUNDED_CURVE ( )  B_SPLINE_CURVE ( 2, ( #64033, #35599, #58848, #52957, #47058, #40799, #12340, #57404, #35240 ),
 .UNSPECIFIED., .F., .F. ) 
 B_SPLINE_CURVE_WITH_KNOTS ( ( 3, 2, 2, 2, 3 ),
 ( 0.9456521739130434590, 0.9492753623188405765, 0.9565217391304348116, 0.9637681159420289356, 0.9662083058201528241 ),
 .UNSPECIFIED. ) 
 CURVE ( )  GEOMETRIC_REPRESENTATION_ITEM ( )  RATIONAL_B_SPLINE_CURVE ( ( 0.9330127018922194093, 0.9330127018922194093, 1.000000000000000000, 0.8660254037844387076, 1.000000000000000000, 0.8660254037844387076, 1.000000000000000000, 0.9548845634016894790, 0.9401540307620559478 ) ) 
 REPRESENTATION_ITEM ( '' )  );
#27950=CARTESIAN_POINT ( 'NONE',  ( 11.12812500061451715, 6.421520780324663323E-16, -5.243569643749999010 ) ) ;
#27951=EDGE_CURVE ( 'NONE', #22963, #51457, #27307, .T. ) ;
#27952=CARTESIAN_POINT ( 'NONE',  ( 29.82187500061451502, 3.027376345333611329, 5.243569643749999010 ) ) ;
#27953=CARTESIAN_POINT ( 'NONE',  ( -2.121784821874999949, 13.03437500061451715, -33.67503911421598417 ) ) ;
#27954=CARTESIAN_POINT ( 'NONE',  ( 12.33750000122903145, 6.123233995736764310E-16, -4.999999999999998224 ) ) ;
#27955=CARTESIAN_POINT ( 'NONE',  ( 27.59062500061451573, -3.027376345333614438, 5.243569643749998122 ) ) ;
#27956=CARTESIAN_POINT ( 'NONE',  ( 2.121784821875001281, 16.35312500061451857, -26.32496088578401938 ) ) ;
#27957=CARTESIAN_POINT ( 'NONE',  ( 15.30000000122903359, -2.886751345948129988, 4.999999999999997335 ) ) ;
#27958=CARTESIAN_POINT ( 'NONE',  ( 13.08750000000000036, -2.886751345948125991, -5.000000000000000000 ) ) ;
#27959=AXIS2_PLACEMENT_3D ( 'NONE', #8822, #65331, #43182 ) ;
#27960=CARTESIAN_POINT ( 'NONE',  ( 22.67812500061451431, -4.541064518000419881, 2.621784821874995952 ) ) ;
#27961=CARTESIAN_POINT ( 'NONE',  ( 6.684375000614518392, 6.421520780324663323E-16, -5.243569643749999010 ) ) ;
#27962=EDGE_CURVE ( 'NONE', #65794, #15563, #44787, .T. ) ;
#27963=CARTESIAN_POINT ( 'NONE',  ( 8.437500001229034652, 4.330127018922191873, 2.499999999999999556 ) ) ;
#27964=CARTESIAN_POINT ( 'NONE',  ( 16.61250000122903359, 0.000000000000000000, 4.999999999999998224 ) ) ;
#27965=CARTESIAN_POINT ( 'NONE',  ( 13.86562500061451431, 3.027376345333613106, -5.243569643749998122 ) ) ;
#27966=CARTESIAN_POINT ( 'NONE',  ( 17.39062500061451644, -3.027376345333610441, -5.243569643749999898 ) ) ;
#27967=CARTESIAN_POINT ( 'NONE',  ( 26.43750000122903288, 4.330127018922191873, 2.499999999999999556 ) ) ;
#27968=( BOUNDED_CURVE ( )  B_SPLINE_CURVE ( 3, ( #53932, #20656, #3691, #32121 ),
 .UNSPECIFIED., .F., .T. ) 
 B_SPLINE_CURVE_WITH_KNOTS ( ( 4, 4 ),
 ( 4.133880465060611797, 4.712388980384689674 ),
 .UNSPECIFIED. ) 
 CURVE ( )  GEOMETRIC_REPRESENTATION_ITEM ( )  RATIONAL_B_SPLINE_CURVE ( ( 1.000000000000000000, 0.9723045704793149557, 0.9723045704793149557, 1.000000000000000000 ) ) 
 REPRESENTATION_ITEM ( '' )  );
#27969=CARTESIAN_POINT ( 'NONE',  ( 29.10000000122903074, 5.773502691896255534, 3.535250795749688894E-16 ) ) ;
#27970=CARTESIAN_POINT ( 'NONE',  ( 23.40000000000000213, -4.330127018922190985, -2.500000000000001332 ) ) ;
#27971=CARTESIAN_POINT ( 'NONE',  ( 25.69687500061451502, 6.054752690667223547, 3.707466751127219781E-16 ) ) ;
#27972=DIRECTION ( 'NONE',  ( 0.000000000000000000, 0.000000000000000000, 1.000000000000000000 ) ) ;
#27973=CARTESIAN_POINT ( 'NONE',  ( 9.675000001229035362, 2.886751345948129099, -4.999999999999998224 ) ) ;
#27974=CARTESIAN_POINT ( 'NONE',  ( 26.93437500061451573, 6.421520780324663323E-16, -5.243569643749999010 ) ) ;
#27976=CARTESIAN_POINT ( 'NONE',  ( 5.784375000614517148, 6.421520780324663323E-16, -5.243569643749999010 ) ) ;
#27977=CARTESIAN_POINT ( 'NONE',  ( 24.02812500061451573, -4.541064518000419881, 2.621784821874995952 ) ) ;
#27981=CARTESIAN_POINT ( 'NONE',  ( 11.37187500061451750, 3.027376345333611329, 5.243569643749999010 ) ) ;
#27982=CARTESIAN_POINT ( 'NONE',  ( 4.453125000614517326, 4.541064518000418104, -2.621784821874998173 ) ) ;
#27983=CARTESIAN_POINT ( 'NONE',  ( 3.984375000614517326, 6.421520780324663323E-16, -5.243569643749999010 ) ) ;
#27984=CARTESIAN_POINT ( 'NONE',  ( 5.784375000614517148, 6.421520780324663323E-16, -5.243569643749999010 ) ) ;
#27985=CARTESIAN_POINT ( 'NONE',  ( 29.07187500061451502, -6.054752690667223547, -1.112240025338166033E-15 ) ) ;
#27986=CARTESIAN_POINT ( 'NONE',  ( 4.243569643749999898, 10.99062500061459424, 32.45002607614398471 ) ) ;
#27987=CARTESIAN_POINT ( 'NONE',  ( 20.10000000000000142, 0.000000000000000000, 4.999999999999998224 ) ) ;
#27989=CARTESIAN_POINT ( 'NONE',  ( 26.17500000000000071, 6.123233995736764310E-16, -4.999999999999998224 ) ) ;
#27990=ADVANCED_FACE ( 'NONE', ( #11001 ), #26913, .F. ) ;
#27991=CARTESIAN_POINT ( 'NONE',  ( 28.80937500061451573, 4.541064518000418104, -2.621784821874998173 ) ) ;
#27992=ORIENTED_EDGE ( 'NONE', *, *, #11628, .F. ) ;
#27993=CARTESIAN_POINT ( 'NONE',  ( 18.74062500061451431, -3.027376345333610441, -5.243569643749999898 ) ) ;
#27994=CARTESIAN_POINT ( 'NONE',  ( 7.453125000614516438, -4.541064518000417216, -2.621784821875001281 ) ) ;
#27996=CARTESIAN_POINT ( 'NONE',  ( 3.646875000614520079, 6.054752690667223547, 3.707466751127219781E-16 ) ) ;
#27997=CARTESIAN_POINT ( 'NONE',  ( 18.26250000122903216, 4.330127018922192761, -2.499999999999997780 ) ) ;
#27998=CARTESIAN_POINT ( 'NONE',  ( 24.18750000000000355, -2.886751345948129988, 4.999999999999997335 ) ) ;
#27999=CARTESIAN_POINT ( 'NONE',  ( 16.05000000000000071, 0.000000000000000000, 4.999999999999998224 ) ) ;
#28000=CARTESIAN_POINT ( 'NONE',  ( 8.146875000614516082, 6.054752690667223547, 3.707466751127219781E-16 ) ) ;
#28001=CARTESIAN_POINT ( 'NONE',  ( 10.84687500061451892, 6.054752690667223547, 3.707466751127219781E-16 ) ) ;
#28002=CARTESIAN_POINT ( 'NONE',  ( 21.79687500061451644, -3.027376345333614438, 5.243569643749998122 ) ) ;
#28004=ORIENTED_EDGE ( 'NONE', *, *, #53941, .F. ) ;
#28005=CARTESIAN_POINT ( 'NONE',  ( 3.384375000614517237, -4.541064518000419881, 2.621784821874995952 ) ) ;
#28007=CARTESIAN_POINT ( 'NONE',  ( 7.246875000614518392, 6.054752690667223547, 3.707466751127219781E-16 ) ) ;
#28009=CARTESIAN_POINT ( 'NONE',  ( 21.18749999999999645, -2.886751345948125991, -5.000000000000000000 ) ) ;
#28010=CARTESIAN_POINT ( 'NONE',  ( 17.16562500061451502, 3.027376345333611329, 5.243569643749999010 ) ) ;
#28014=CARTESIAN_POINT ( 'NONE',  ( 9.028125000614517504, 4.541064518000418104, 2.621784821874999949 ) ) ;
#28015=CARTESIAN_POINT ( 'NONE',  ( 26.59687500061451360, 6.054752690667223547, 3.707466751127219781E-16 ) ) ;
#28017=CARTESIAN_POINT ( 'NONE',  ( 28.69687500061451502, -3.027376345333610441, -5.243569643749999898 ) ) ;
#28018=CARTESIAN_POINT ( 'NONE',  ( 9.150000000000002132, 4.330127018922192761, -2.499999999999997780 ) ) ;
#28019=CARTESIAN_POINT ( 'NONE',  ( -2.828200636599751609E-16, 15.05000000122903536, 25.38119784648299770 ) ) ;
#28020=CARTESIAN_POINT ( 'NONE',  ( 9.525000001229033231, -5.773502691896255534, -1.060575238724906372E-15 ) ) ;
#28021=CARTESIAN_POINT ( 'NONE',  ( 19.92187500061451644, 3.027376345333611329, 5.243569643749999010 ) ) ;
#28022=CARTESIAN_POINT ( 'NONE',  ( 13.50937500061451679, 4.541064518000418104, -2.621784821874998173 ) ) ;
#28023=CARTESIAN_POINT ( 'NONE',  ( 0.000000000000000000, 20.00000000000000000, -30.00000000000000000 ) ) ;
#28024=ORIENTED_EDGE ( 'NONE', *, *, #55282, .T. ) ;
#28025=CARTESIAN_POINT ( 'NONE',  ( 13.90312500061451750, 4.541064518000418104, -2.621784821874998173 ) ) ;
#28026=CARTESIAN_POINT ( 'NONE',  ( 25.91250000122903074, 4.330127018922192761, -2.499999999999997780 ) ) ;
#28027=CARTESIAN_POINT ( 'NONE',  ( 14.03437500061451715, 4.541064518000418104, 2.621784821874999949 ) ) ;
#28028=CARTESIAN_POINT ( 'NONE',  ( 1.968632615237262629, 9.806224642577898720, -24.32863725417373857 ) ) ;
#28029=CARTESIAN_POINT ( 'NONE',  ( 18.21562500061451573, -6.054752690667223547, -1.112240025338166033E-15 ) ) ;
#28030=DIRECTION ( 'NONE',  ( -1.000000000000000000, -0.000000000000000000, -0.000000000000000000 ) ) ;
#28031=CARTESIAN_POINT ( 'NONE',  ( 26.67187500061451644, 3.027376345333611329, 5.243569643749999010 ) ) ;
#28032=CARTESIAN_POINT ( 'NONE',  ( -3.000416591977282496E-16, 11.59062500061451750, 25.09994784771203058 ) ) ;
#28033=CARTESIAN_POINT ( 'NONE',  ( 15.87187500061451573, 3.027376345333611329, 5.243569643749999010 ) ) ;
#28034=CARTESIAN_POINT ( 'NONE',  ( 14.85000000122903252, -2.886751345948129988, 4.999999999999997335 ) ) ;
#28036=CARTESIAN_POINT ( 'NONE',  ( 3.336147517545859920, -3.724270626431634312, 3.691191611388044524 ) ) ;
#28037=CARTESIAN_POINT ( 'NONE',  ( 21.00937500061451857, -4.541064518000417216, -2.621784821875001281 ) ) ;
#28038=CARTESIAN_POINT ( 'NONE',  ( 20.43750000122903643, 6.123233995736764310E-16, -4.999999999999998224 ) ) ;
#28039=CARTESIAN_POINT ( 'NONE',  ( 14.44687500061451679, 6.054752690667223547, 3.707466751127219781E-16 ) ) ;
#28040=CARTESIAN_POINT ( 'NONE',  ( 2.121784821874999061, 12.05937500061451750, 26.32496088578401583 ) ) ;
#28041=CARTESIAN_POINT ( 'NONE',  ( 22.16250000122903074, -4.330127018922190985, -2.500000000000001332 ) ) ;
#28042=CARTESIAN_POINT ( 'NONE',  ( 16.37812500061451715, -4.541064518000419881, 2.621784821874995952 ) ) ;
#28044=ORIENTED_EDGE ( 'NONE', *, *, #13788, .F. ) ;
#28045=CARTESIAN_POINT ( 'NONE',  ( 19.42499999999999716, 6.123233995736764310E-16, -4.999999999999998224 ) ) ;
#28046=CARTESIAN_POINT ( 'NONE',  ( -4.243569643749999898, 19.85937500061451644, -30.00000000000000000 ) ) ;
#28047=CARTESIAN_POINT ( 'NONE',  ( 25.37812500061451715, -4.541064518000419881, 2.621784821874995952 ) ) ;
#28048=CARTESIAN_POINT ( 'NONE',  ( 1.838027276006278798, 4.657088507379086195, 33.56272475032025682 ) ) ;
#28049=EDGE_CURVE ( 'NONE', #48298, #69560, #64604, .T. ) ;
#28050=CARTESIAN_POINT ( 'NONE',  ( 16.38750000122903216, 6.123233995736764310E-16, -4.999999999999998224 ) ) ;
#28051=CARTESIAN_POINT ( 'NONE',  ( 22.75312500061451360, -4.541064518000417216, -2.621784821875001281 ) ) ;
#28052=CARTESIAN_POINT ( 'NONE',  ( 24.55312500061451786, -4.541064518000417216, -2.621784821875001281 ) ) ;
#28053=CARTESIAN_POINT ( 'NONE',  ( 4.865625000614517859, 3.027376345333613106, -5.243569643749998122 ) ) ;
#28054=ORIENTED_EDGE ( 'NONE', *, *, #60470, .T. ) ;
#28055=CARTESIAN_POINT ( 'NONE',  ( 29.17500000000000071, -4.330127018922194537, 2.499999999999995559 ) ) ;
#28056=CARTESIAN_POINT ( 'NONE',  ( 3.628125000614518036, 4.541064518000418104, 2.621784821874999949 ) ) ;
#28058=DIRECTION ( 'NONE',  ( -0.000000000000000000, -1.000000000000000000, -0.000000000000000000 ) ) ;
#28059=CARTESIAN_POINT ( 'NONE',  ( -2.828200636599751609E-16, 11.00000000122903288, -34.61880215351700230 ) ) ;
#28060=CARTESIAN_POINT ( 'NONE',  ( 2.121784821875001281, 17.75937500061451502, -26.32496088578401938 ) ) ;
#28061=CARTESIAN_POINT ( 'NONE',  ( 7.575000000000001954, -4.330127018922194537, 2.499999999999995559 ) ) ;
#28062=CARTESIAN_POINT ( 'NONE',  ( 5.025000001229035895, -5.773502691896255534, -1.060575238724906372E-15 ) ) ;
#28063=CARTESIAN_POINT ( 'NONE',  ( 12.34687500061452070, -3.027376345333614438, 5.243569643749998122 ) ) ;
#28065=CARTESIAN_POINT ( 'NONE',  ( 4.434375000614519280, 6.421520780324663323E-16, -5.243569643749999010 ) ) ;
#28068=CARTESIAN_POINT ( 'NONE',  ( 10.05937500061451750, 0.000000000000000000, 5.243569643749999010 ) ) ;
#28069=CARTESIAN_POINT ( 'NONE',  ( 1.999999999999998668, 17.26250000122903572, -33.46410161513775705 ) ) ;
#28070=CARTESIAN_POINT ( 'NONE',  ( 19.82812500061451644, 4.541064518000418104, 2.621784821874999949 ) ) ;
#28071=CARTESIAN_POINT ( 'NONE',  ( 16.64999999999999858, -4.330127018922190985, -2.500000000000001332 ) ) ;
#28072=CARTESIAN_POINT ( 'NONE',  ( -4.243569643749999898, 18.00312500061459176, 30.00000000000000000 ) ) ;
#28073=CARTESIAN_POINT ( 'NONE',  ( 22.92187500061451644, 3.027376345333613106, -5.243569643749998122 ) ) ;
#28076=CARTESIAN_POINT ( 'NONE',  ( 28.42500000122904069, -5.773502691896255534, -1.060575238724906372E-15 ) ) ;
#28078=CARTESIAN_POINT ( 'NONE',  ( 24.55312500061451786, -4.541064518000417216, -2.621784821875001281 ) ) ;
#28079=CARTESIAN_POINT ( 'NONE',  ( 15.02812500061451750, -4.541064518000419881, 2.621784821874995952 ) ) ;
#28081=CARTESIAN_POINT ( 'NONE',  ( 10.84687500061451892, 6.054752690667223547, 3.707466751127219781E-16 ) ) ;
#28082=CARTESIAN_POINT ( 'NONE',  ( 28.61249999999999716, 2.886751345948126879, 4.999999999999999112 ) ) ;
#28083=CARTESIAN_POINT ( 'NONE',  ( 23.77500000122903145, 2.886751345948126879, 4.999999999999999112 ) ) ;
#28084=CARTESIAN_POINT ( 'NONE',  ( 4.696875000614518569, -3.027376345333614438, 5.243569643749998122 ) ) ;
#28085=CARTESIAN_POINT ( 'NONE',  ( 14.29687500061451821, -3.027376345333610441, -5.243569643749999898 ) ) ;
#28086=CARTESIAN_POINT ( 'NONE',  ( 28.77187500061451431, 3.027376345333613106, -5.243569643749998122 ) ) ;
#28087=CARTESIAN_POINT ( 'NONE',  ( 3.160880256176461511, -3.874123901750303300, -3.160880256176591185 ) ) ;
#28089=CARTESIAN_POINT ( 'NONE',  ( 24.60937500061451644, -4.541064518000417216, -2.621784821875001281 ) ) ;
#28090=CARTESIAN_POINT ( 'NONE',  ( 15.08437500061451786, -4.541064518000419881, 2.621784821874995952 ) ) ;
#28092=CARTESIAN_POINT ( 'NONE',  ( 28.35000000000000142, -4.330127018922190985, -2.500000000000001332 ) ) ;
#28093=CARTESIAN_POINT ( 'NONE',  ( 3.037500001229032964, 4.330127018922191873, 2.499999999999999556 ) ) ;
#28095=CARTESIAN_POINT ( 'NONE',  ( 16.79062500061451857, -3.027376345333614438, 5.243569643749998122 ) ) ;
#28096=CARTESIAN_POINT ( 'NONE',  ( 8.324999999999999289, 4.330127018922191873, 2.499999999999999556 ) ) ;
#28098=CARTESIAN_POINT ( 'NONE',  ( 16.23750000000000071, -2.886751345948125991, -5.000000000000000000 ) ) ;
#28099=CARTESIAN_POINT ( 'NONE',  ( -2.121784821874999949, 12.97812500061451679, 26.32496088578401938 ) ) ;
#28100=DIRECTION ( 'NONE',  ( 0.000000000000000000, 0.000000000000000000, 1.000000000000000000 ) ) ;
#28101=CARTESIAN_POINT ( 'NONE',  ( 21.11250000122903359, 0.000000000000000000, 4.999999999999998224 ) ) ;
#28102=CARTESIAN_POINT ( 'NONE',  ( -1.071796769724488563, 10.19240381056766687, -26.00000000000000000 ) ) ;
#28103=CARTESIAN_POINT ( 'NONE',  ( 26.63437500061451857, 4.541064518000418104, 2.621784821874999949 ) ) ;
#28105=CARTESIAN_POINT ( 'NONE',  ( 17.05312500061451786, 4.541064518000418104, -2.621784821874998173 ) ) ;
#28106=CARTESIAN_POINT ( 'NONE',  ( 22.30312500061451431, -4.541064518000417216, -2.621784821875001281 ) ) ;
#28107=CARTESIAN_POINT ( 'NONE',  ( 22.02187500061452141, 3.027376345333613106, -5.243569643749998122 ) ) ;
#28108=CARTESIAN_POINT ( 'NONE',  ( 7.575000000000001954, -4.330127018922194537, 2.499999999999995559 ) ) ;
#28109=CARTESIAN_POINT ( 'NONE',  ( 9.103125000614515017, 0.000000000000000000, 5.243569643749999010 ) ) ;
#28110=CARTESIAN_POINT ( 'NONE',  ( 24.29062500061451502, 6.054752690667223547, 3.707466751127219781E-16 ) ) ;
#28111=CARTESIAN_POINT ( 'NONE',  ( 14.40937500061451715, 4.541064518000418104, -2.621784821874998173 ) ) ;
#28112=CARTESIAN_POINT ( 'NONE',  ( 20.18437500061451573, 6.421520780324663323E-16, -5.243569643749999010 ) ) ;
#28113=LINE ( 'NONE', #49554, #6234 ) ;
#28114=CARTESIAN_POINT ( 'NONE',  ( 2.121784821875001281, 18.60312500061451857, 33.67503911421598417 ) ) ;
#28115=CARTESIAN_POINT ( 'NONE',  ( 22.20000000122903216, -2.886751345948125991, -5.000000000000000000 ) ) ;
#28117=CARTESIAN_POINT ( 'NONE',  ( 11.46562500061451573, -6.054752690667223547, -1.112240025338166033E-15 ) ) ;
#28118=CARTESIAN_POINT ( 'NONE',  ( 6.234375000614519102, 6.421520780324663323E-16, -5.243569643749999010 ) ) ;
#28119=CARTESIAN_POINT ( 'NONE',  ( 5.934375000614517504, 4.541064518000418104, 2.621784821874999949 ) ) ;
#28120=( BOUNDED_CURVE ( )  B_SPLINE_CURVE ( 2, ( #52843, #35124, #41401, #1890, #24757, #19200, #18112 ),
 .UNSPECIFIED., .F., .F. ) 
 B_SPLINE_CURVE_WITH_KNOTS ( ( 3, 2, 2, 3 ),
 ( 0.4333333333333333481, 0.4361111111111111160, 0.4388888888888888840, 0.4416666666666666519 ),
 .UNSPECIFIED. ) 
 CURVE ( )  GEOMETRIC_REPRESENTATION_ITEM ( )  RATIONAL_B_SPLINE_CURVE ( ( 1.000000000000000000, 0.8660254037844387076, 1.000000000000000000, 0.8660254037844387076, 1.000000000000000000, 0.8660254037844387076, 1.000000000000000000 ) ) 
 REPRESENTATION_ITEM ( '' )  );
#28121=ORIENTED_EDGE ( 'NONE', *, *, #24238, .F. ) ;
#28122=CARTESIAN_POINT ( 'NONE',  ( 27.04687500061451644, 6.054752690667223547, 3.707466751127219781E-16 ) ) ;
#28123=CARTESIAN_POINT ( 'NONE',  ( 19.52812500061451573, -4.541064518000419881, 2.621784821874995952 ) ) ;
#28124=CARTESIAN_POINT ( 'NONE',  ( 27.86250000122903359, 0.000000000000000000, 4.999999999999998224 ) ) ;
#28125=CARTESIAN_POINT ( 'NONE',  ( 26.65312500061451573, 0.000000000000000000, 5.243569643749999010 ) ) ;
#28126=CARTESIAN_POINT ( 'NONE',  ( 25.05937500061451573, -4.541064518000417216, -2.621784821875001281 ) ) ;
#28127=CARTESIAN_POINT ( 'NONE',  ( 17.54062500061451502, 6.054752690667223547, 3.707466751127219781E-16 ) ) ;
#28128=CARTESIAN_POINT ( 'NONE',  ( -4.243569643749999898, 19.40937500061451715, 30.00000000000000000 ) ) ;
#28129=CARTESIAN_POINT ( 'NONE',  ( 24.17812500061451786, 6.421520780324663323E-16, -5.243569643749999010 ) ) ;
#28130=CARTESIAN_POINT ( 'NONE',  ( 5.362500001229033586, 0.000000000000000000, 4.999999999999998224 ) ) ;
#28132=CARTESIAN_POINT ( 'NONE',  ( 28.68749999999999645, -2.886751345948129988, 4.999999999999997335 ) ) ;
#28133=CARTESIAN_POINT ( 'NONE',  ( 3.999999999999999112, 16.17500000000000071, -30.00000000000000000 ) ) ;
#28135=CARTESIAN_POINT ( 'NONE',  ( 4.584375000614516971, 4.541064518000418104, 2.621784821874999949 ) ) ;
#28136=CARTESIAN_POINT ( 'NONE',  ( 11.20312500061451644, 4.541064518000418104, -2.621784821874998173 ) ) ;
#28137=CARTESIAN_POINT ( 'NONE',  ( 6.384375000614516793, 4.541064518000418104, 2.621784821874999949 ) ) ;
#28138=CARTESIAN_POINT ( 'NONE',  ( 24.26250000122903216, 0.000000000000000000, 4.999999999999998224 ) ) ;
#28139=CARTESIAN_POINT ( 'NONE',  ( 15.04687500061451644, -3.027376345333614438, 5.243569643749998122 ) ) ;
#28140=CARTESIAN_POINT ( 'NONE',  ( 29.54062500061451502, -3.027376345333610441, -5.243569643749999898 ) ) ;
#28141=CARTESIAN_POINT ( 'NONE',  ( 28.42499999999999716, 6.123233995736764310E-16, -4.999999999999998224 ) ) ;
#28142=CARTESIAN_POINT ( 'NONE',  ( 27.42187500061451644, 3.027376345333613106, -5.243569643749998122 ) ) ;
#28143=CYLINDRICAL_SURFACE ( 'NONE', #18437, 4.999999999999998224 ) ;
#28144=CARTESIAN_POINT ( 'NONE',  ( 14.01562500061451644, 3.027376345333611329, 5.243569643749999010 ) ) ;
#28146=CARTESIAN_POINT ( 'NONE',  ( 8.990625000614516082, 6.054752690667223547, 3.707466751127219781E-16 ) ) ;
#28147=CARTESIAN_POINT ( 'NONE',  ( 6.440625000614517148, -3.027376345333614438, 5.243569643749998122 ) ) ;
#28149=FACE_OUTER_BOUND ( 'NONE', #41074, .T. ) ;
#28150=CARTESIAN_POINT ( 'NONE',  ( 16.35000000000000142, 4.330127018922192761, -2.499999999999997780 ) ) ;
#28151=CARTESIAN_POINT ( 'NONE',  ( 15.98437500061451821, -4.541064518000419881, 2.621784821874995952 ) ) ;
#28152=CARTESIAN_POINT ( 'NONE',  ( 12.11250000122903181, 0.000000000000000000, 4.999999999999998224 ) ) ;
#28153=EDGE_CURVE ( 'NONE', #17794, #69491, #50890, .T. ) ;
#28155=CARTESIAN_POINT ( 'NONE',  ( 20.67187500061451289, 3.027376345333613106, -5.243569643749998122 ) ) ;
#28156=CARTESIAN_POINT ( 'NONE',  ( -3.000416591977282496E-16, 15.19062500061451715, -34.90005215228797653 ) ) ;
#28157=CARTESIAN_POINT ( 'NONE',  ( -1.071796769724496556, 16.94240381056766509, 33.99999999999998579 ) ) ;
#28160=CARTESIAN_POINT ( 'NONE',  ( 25.97812500061451502, 6.421520780324663323E-16, -5.243569643749999010 ) ) ;
#28161=FACE_OUTER_BOUND ( 'NONE', #11558, .T. ) ;
#28162=( BOUNDED_CURVE ( )  B_SPLINE_CURVE ( 2, ( #71056, #30439, #52968, #3470, #2364, #8268, #48895 ),
 .UNSPECIFIED., .F., .F. ) 
 B_SPLINE_CURVE_WITH_KNOTS ( ( 3, 2, 2, 3 ),
 ( 0.7249999999999999778, 0.7277777777777777457, 0.7305555555555555136, 0.7333333333333332815 ),
 .UNSPECIFIED. ) 
 CURVE ( )  GEOMETRIC_REPRESENTATION_ITEM ( )  RATIONAL_B_SPLINE_CURVE ( ( 1.000000000000000000, 0.8660254037844387076, 1.000000000000000000, 0.8660254037844387076, 1.000000000000000000, 0.8660254037844387076, 1.000000000000000000 ) ) 
 REPRESENTATION_ITEM ( '' )  );
#28163=CARTESIAN_POINT ( 'NONE',  ( 26.69999999999999929, 4.330127018922192761, -2.499999999999997780 ) ) ;
#28165=CARTESIAN_POINT ( 'NONE',  ( 8.503125000614515372, 4.541064518000418104, -2.621784821874998173 ) ) ;
#28167=CARTESIAN_POINT ( 'NONE',  ( 19.20937500061451786, -4.541064518000417216, -2.621784821875001281 ) ) ;
#28169=CARTESIAN_POINT ( 'NONE',  ( 4.228125000614517681, -4.541064518000419881, 2.621784821874995952 ) ) ;
#28170=CARTESIAN_POINT ( 'NONE',  ( 10.09687500061451715, -3.027376345333614438, 5.243569643749998122 ) ) ;
#28172=CARTESIAN_POINT ( 'NONE',  ( 20.89687500061452141, -3.027376345333614438, 5.243569643749998122 ) ) ;
#28174=CARTESIAN_POINT ( 'NONE',  ( 29.13749999999999929, -2.886751345948129988, 4.999999999999997335 ) ) ;
#28175=CARTESIAN_POINT ( 'NONE',  ( 5.924999999999999822, 6.123233995736764310E-16, -4.999999999999998224 ) ) ;
#28176=CARTESIAN_POINT ( 'NONE',  ( 14.96250000122903323, -4.330127018922190985, -2.500000000000001332 ) ) ;
#28178=ORIENTED_EDGE ( 'NONE', *, *, #63321, .F. ) ;
#28179=CARTESIAN_POINT ( 'NONE',  ( 13.79999999999999893, 0.000000000000000000, 4.999999999999998224 ) ) ;
#28180=CARTESIAN_POINT ( 'NONE',  ( 25.86562500061451431, -6.054752690667223547, -1.112240025338166033E-15 ) ) ;
#28181=CARTESIAN_POINT ( 'NONE',  ( 16.72500000000000142, 6.123233995736764310E-16, -4.999999999999998224 ) ) ;
#28182=CARTESIAN_POINT ( 'NONE',  ( 10.38750000122903572, -4.330127018922194537, 2.499999999999995559 ) ) ;
#28183=CARTESIAN_POINT ( 'NONE',  ( 8.240625000614516082, -3.027376345333614438, 5.243569643749998122 ) ) ;
#28184=CARTESIAN_POINT ( 'NONE',  ( 8.887499999999999289, -2.886751345948129988, 4.999999999999997335 ) ) ;
#28185=CARTESIAN_POINT ( 'NONE',  ( 30.00000000000000000, 0.000000000000000000, 0.000000000000000000 ) ) ;
#28186=CARTESIAN_POINT ( 'NONE',  ( 4.243569643749999898, 15.09687500061451892, -27.54997392385601529 ) ) ;
#28187=CARTESIAN_POINT ( 'NONE',  ( 27.03750000122903430, -4.330127018922194537, 2.499999999999995559 ) ) ;
#28189=CARTESIAN_POINT ( 'NONE',  ( 7.762500000000001954, 2.886751345948129099, -4.999999999999998224 ) ) ;
#28190=CARTESIAN_POINT ( 'NONE',  ( -3.999999999999999112, 12.80000000000000071, 30.00000000000000000 ) ) ;
#28192=CARTESIAN_POINT ( 'NONE',  ( 23.61562500061451431, -6.054752690667223547, -1.112240025338166033E-15 ) ) ;
#28193=CARTESIAN_POINT ( 'NONE',  ( 12.78750000122903430, 6.123233995736764310E-16, -4.999999999999998224 ) ) ;
#28194=CARTESIAN_POINT ( 'NONE',  ( 28.60312500061451502, -4.541064518000417216, -2.621784821875001281 ) ) ;
#28195=CARTESIAN_POINT ( 'NONE',  ( 29.82187500061451502, 3.027376345333611329, 5.243569643749999010 ) ) ;
#28196=CARTESIAN_POINT ( 'NONE',  ( 19.28437500061451360, 6.421520780324663323E-16, -5.243569643749999010 ) ) ;
#28197=CARTESIAN_POINT ( 'NONE',  ( 17.46562500061451217, 3.027376345333613106, -5.243569643749998122 ) ) ;
#28198=CARTESIAN_POINT ( 'NONE',  ( -2.121784821874996840, 10.42812500061459424, -26.32496088578401583 ) ) ;
#28199=CARTESIAN_POINT ( 'NONE',  ( 6.590625000614518392, -3.027376345333610441, -5.243569643749999898 ) ) ;
#28200=CARTESIAN_POINT ( 'NONE',  ( 27.41250000122903430, 0.000000000000000000, 4.999999999999998224 ) ) ;
#28202=CARTESIAN_POINT ( 'NONE',  ( 20.09062500061451573, -3.027376345333610441, -5.243569643749999898 ) ) ;
#28203=CARTESIAN_POINT ( 'NONE',  ( 13.57500000000000107, 6.123233995736764310E-16, -4.999999999999998224 ) ) ;
#28205=CARTESIAN_POINT ( 'NONE',  ( 13.47187500061451537, 3.027376345333613106, -5.243569643749998122 ) ) ;
#28206=CARTESIAN_POINT ( 'NONE',  ( 12.30937500061451573, 0.000000000000000000, 5.243569643749999010 ) ) ;
#28207=CARTESIAN_POINT ( 'NONE',  ( 21.34687500061451715, -3.027376345333614438, 5.243569643749998122 ) ) ;
#28208=EDGE_LOOP ( 'NONE', ( #58448, #53327, #53161, #26313 ) ) ;
#28209=CARTESIAN_POINT ( 'NONE',  ( 2.878125000614517592, -4.541064518000419881, 2.621784821874995952 ) ) ;
#28210=CARTESIAN_POINT ( 'NONE',  ( 25.52812500061451573, 6.421520780324663323E-16, -5.243569643749999010 ) ) ;
#28211=CARTESIAN_POINT ( 'NONE',  ( 27.74062500061451431, -3.027376345333610441, -5.243569643749999898 ) ) ;
#28212=FACE_OUTER_BOUND ( 'NONE', #7885, .T. ) ;
#28213=CARTESIAN_POINT ( 'NONE',  ( -1.999999999999997113, 16.02500000000000213, 33.46410161513775705 ) ) ;
#28214=CARTESIAN_POINT ( 'NONE',  ( 5.559375000614517504, 0.000000000000000000, 5.243569643749999010 ) ) ;
#28215=CARTESIAN_POINT ( 'NONE',  ( 12.56250000122903465, 0.000000000000000000, 4.999999999999998224 ) ) ;
#28216=CARTESIAN_POINT ( 'NONE',  ( 8.100000001229034297, -2.886751345948129988, 4.999999999999997335 ) ) ;
#28217=CARTESIAN_POINT ( 'NONE',  ( 3.853125000614517681, -4.541064518000417216, -2.621784821875001281 ) ) ;
#28220=CARTESIAN_POINT ( 'NONE',  ( 11.03437500061451715, -4.541064518000419881, 2.621784821874995952 ) ) ;
#28221=CARTESIAN_POINT ( 'NONE',  ( 18.85312500061451502, 4.541064518000418104, -2.621784821874998173 ) ) ;
#28222=CARTESIAN_POINT ( 'NONE',  ( 12.87187500061451750, -6.054752690667223547, -1.112240025338166033E-15 ) ) ;
#28223=CARTESIAN_POINT ( 'NONE',  ( 4.190625000614518925, -3.027376345333614438, 5.243569643749998122 ) ) ;
#28224=CARTESIAN_POINT ( 'NONE',  ( 23.03437500061451715, 4.541064518000418104, 2.621784821874999949 ) ) ;
#28225=CARTESIAN_POINT ( 'NONE',  ( 8.784375000614518925, -4.541064518000419881, 2.621784821874995952 ) ) ;
#28226=CARTESIAN_POINT ( 'NONE',  ( 5.428125000614517859, 4.541064518000418104, 2.621784821874999949 ) ) ;
#28228=CARTESIAN_POINT ( 'NONE',  ( 6.525000001229033231, 2.886751345948129099, -4.999999999999998224 ) ) ;
#28229=CARTESIAN_POINT ( 'NONE',  ( 20.61562500061451431, 3.027376345333613106, -5.243569643749998122 ) ) ;
#28230=CARTESIAN_POINT ( 'NONE',  ( 7.012500001229035718, 4.330127018922192761, -2.499999999999997780 ) ) ;
#28231=CARTESIAN_POINT ( 'NONE',  ( 16.90312500061451573, -4.541064518000417216, -2.621784821875001281 ) ) ;
#28232=CARTESIAN_POINT ( 'NONE',  ( 13.07812500061451821, 4.541064518000418104, 2.621784821874999949 ) ) ;
#28234=CARTESIAN_POINT ( 'NONE',  ( 13.64999999999999858, 4.330127018922192761, -2.499999999999997780 ) ) ;
#28235=CARTESIAN_POINT ( 'NONE',  ( 9.300000001229035362, 5.773502691896255534, 3.535250795749688894E-16 ) ) ;
#28236=CARTESIAN_POINT ( 'NONE',  ( 6.740625000614516082, 6.054752690667223547, 3.707466751127219781E-16 ) ) ;
#28237=CARTESIAN_POINT ( 'NONE',  ( 19.83750000122903145, -4.330127018922194537, 2.499999999999995559 ) ) ;
#28239=CARTESIAN_POINT ( 'NONE',  ( 4.243569643749999898, 11.98437500061451821, -30.00000000000000000 ) ) ;
#28240=CARTESIAN_POINT ( 'NONE',  ( 4.898734551532200499, 1.001199177798645534, 4.898734551532190729 ) ) ;
#28241=EDGE_CURVE ( 'NONE', #16088, #55534, #72179, .T. ) ;
#28242=CARTESIAN_POINT ( 'NONE',  ( 3.787500001229033408, 6.123233995736764310E-16, -4.999999999999998224 ) ) ;
#28244=CARTESIAN_POINT ( 'NONE',  ( 21.60937500061451644, 4.541064518000418104, -2.621784821874998173 ) ) ;
#28245=CARTESIAN_POINT ( 'NONE',  ( -5.810221930991193690E-16, 18.65000000122903501, 26.00000000000000355 ) ) ;
#28246=CARTESIAN_POINT ( 'NONE',  ( 17.16562500061451502, 3.027376345333611329, 5.243569643749999010 ) ) ;
#28249=CARTESIAN_POINT ( 'NONE',  ( 4.500000000000000888, -4.330127018922190985, -2.500000000000001332 ) ) ;
#28250=CARTESIAN_POINT ( 'NONE',  ( 28.09687500061451360, -3.027376345333614438, 5.243569643749998122 ) ) ;
#28252=CARTESIAN_POINT ( 'NONE',  ( 11.69062500061451360, 6.054752690667223547, 3.707466751127219781E-16 ) ) ;
#28253=CARTESIAN_POINT ( 'NONE',  ( 10.20937500061451786, -4.541064518000417216, -2.621784821875001281 ) ) ;
#28255=CARTESIAN_POINT ( 'NONE',  ( 29.76562500061451644, 3.027376345333611329, 5.243569643749999010 ) ) ;
#28256=CARTESIAN_POINT ( 'NONE',  ( 21.89062500061451289, -3.027376345333610441, -5.243569643749999898 ) ) ;
#28258=CARTESIAN_POINT ( 'NONE',  ( -5.810221930991193690E-16, 15.50000000122903465, -34.00000000000000000 ) ) ;
#28259=CARTESIAN_POINT ( 'NONE',  ( 11.28749999999999787, -2.886751345948125991, -5.000000000000000000 ) ) ;
#28260=CARTESIAN_POINT ( 'NONE',  ( 22.42500000122903359, 2.886751345948126879, 4.999999999999999112 ) ) ;
#28261=CARTESIAN_POINT ( 'NONE',  ( 16.97812500061451502, 6.421520780324663323E-16, -5.243569643749999010 ) ) ;
#28263=EDGE_LOOP ( 'NONE', ( #2841, #44322, #26359, #33069 ) ) ;
#28264=CARTESIAN_POINT ( 'NONE',  ( 18.97499999999999787, 6.123233995736764310E-16, -4.999999999999998224 ) ) ;
#28265=CARTESIAN_POINT ( 'NONE',  ( 24.93750000000000355, 5.773502691896255534, 3.535250795749688894E-16 ) ) ;
#28266=CARTESIAN_POINT ( 'NONE',  ( 21.23437500061451644, 4.541064518000418104, 2.621784821874999949 ) ) ;
#28267=CARTESIAN_POINT ( 'NONE',  ( 26.35312500061451857, -4.541064518000417216, -2.621784821875001281 ) ) ;
#28268=ORIENTED_EDGE ( 'NONE', *, *, #10575, .F. ) ;
#28269=CARTESIAN_POINT ( 'NONE',  ( -1.999999999999997113, 17.03750000122903430, 33.46410161513775705 ) ) ;
#28270=CARTESIAN_POINT ( 'NONE',  ( 8.803125000614517859, -4.541064518000417216, -2.621784821875001281 ) ) ;
#28271=CARTESIAN_POINT ( 'NONE',  ( 0.000000000000000000, 20.00000000000000000, -33.99999999999999289 ) ) ;
#28272=CARTESIAN_POINT ( 'NONE',  ( 15.45000000000000107, 4.330127018922192761, -2.499999999999997780 ) ) ;
#28273=CARTESIAN_POINT ( 'NONE',  ( -4.243569643749999898, 18.00312500061451715, 30.00000000000000000 ) ) ;
#28274=CARTESIAN_POINT ( 'NONE',  ( 5.296875000614518214, -3.027376345333610441, -5.243569643749999898 ) ) ;
#28275=CARTESIAN_POINT ( 'NONE',  ( 28.24687500061451573, -3.027376345333610441, -5.243569643749999898 ) ) ;
#28276=EDGE_LOOP ( 'NONE', ( #17061, #18319, #61264, #10091 ) ) ;
#28277=CARTESIAN_POINT ( 'NONE',  ( 24.96562500061451573, -6.054752690667223547, -1.112240025338166033E-15 ) ) ;
#28278=CARTESIAN_POINT ( 'NONE',  ( 26.29687500061451644, -3.027376345333614438, 5.243569643749998122 ) ) ;
#28279=CARTESIAN_POINT ( 'NONE',  ( -4.243569643749999898, 18.86562500061459247, -32.45002607614398471 ) ) ;
#28280=CARTESIAN_POINT ( 'NONE',  ( 10.76250000000000107, -5.773502691896255534, -1.060575238724906372E-15 ) ) ;
#28281=CARTESIAN_POINT ( 'NONE',  ( 8.428125000614517859, 6.421520780324663323E-16, -5.243569643749999010 ) ) ;
#28282=DIRECTION ( 'NONE',  ( -1.000000000000000000, -0.000000000000000000, -0.000000000000000000 ) ) ;
#28283=CARTESIAN_POINT ( 'NONE',  ( 19.53749999999999432, 5.773502691896255534, 3.535250795749688401E-16 ) ) ;
#28284=CARTESIAN_POINT ( 'NONE',  ( 26.69062500061451715, -3.027376345333614438, 5.243569643749998122 ) ) ;
#28287=CARTESIAN_POINT ( 'NONE',  ( 3.140625000614516882, 6.054752690667223547, 3.707466751127219781E-16 ) ) ;
#28288=CARTESIAN_POINT ( 'NONE',  ( 20.25937500061451857, 4.541064518000418104, -2.621784821874998173 ) ) ;
#28289=CARTESIAN_POINT ( 'NONE',  ( -4.243569643749997233, 14.94687500061451679, 32.45002607614398471 ) ) ;
#28290=CARTESIAN_POINT ( 'NONE',  ( 21.45937500061451786, -4.541064518000417216, -2.621784821875001281 ) ) ;
#28291=CARTESIAN_POINT ( 'NONE',  ( 3.637500000000001954, -2.886751345948125991, -5.000000000000000000 ) ) ;
#28292=CARTESIAN_POINT ( 'NONE',  ( 9.001249775931846008E-16, 18.62187500061451573, 34.90005215228797653 ) ) ;
#28293=CARTESIAN_POINT ( 'NONE',  ( 9.515625000614518214, 3.027376345333611329, 5.243569643749999010 ) ) ;
#28294=CARTESIAN_POINT ( 'NONE',  ( 5.859375000614519102, 4.541064518000418104, -2.621784821874998173 ) ) ;
#28296=CARTESIAN_POINT ( 'NONE',  ( 7.265625000614516438, 3.027376345333611329, 5.243569643749999010 ) ) ;
#28297=CARTESIAN_POINT ( 'NONE',  ( 11.40937500061451892, 0.000000000000000000, 5.243569643749999010 ) ) ;
#28298=CARTESIAN_POINT ( 'NONE',  ( 18.15000000122903501, -2.886751345948125991, -5.000000000000000000 ) ) ;
#28299=CARTESIAN_POINT ( 'NONE',  ( 8.821875000614518569, -6.054752690667223547, -1.112240025338166033E-15 ) ) ;
#28300=CARTESIAN_POINT ( 'NONE',  ( 8.990625000614516082, 6.054752690667223547, 3.707466751127219781E-16 ) ) ;
#28301=CARTESIAN_POINT ( 'NONE',  ( 4.125000001229034652, -5.773502691896255534, -1.060575238724906372E-15 ) ) ;
#28303=CARTESIAN_POINT ( 'NONE',  ( 20.10937500061451289, -4.541064518000417216, -2.621784821875001281 ) ) ;
#28304=CARTESIAN_POINT ( 'NONE',  ( 4.486351857634337748, 2.207646840049596992, 4.593693573296974364 ) ) ;
#28305=CARTESIAN_POINT ( 'NONE',  ( 26.80312500061451431, -4.541064518000417216, -2.621784821875001281 ) ) ;
#28306=CARTESIAN_POINT ( 'NONE',  ( 12.29062500061451857, -3.027376345333614438, 5.243569643749998122 ) ) ;
#28307=CARTESIAN_POINT ( 'NONE',  ( 29.14687500061451431, -3.027376345333610441, -5.243569643749999898 ) ) ;
#28308=CARTESIAN_POINT ( 'NONE',  ( 13.27500000122903323, 2.886751345948129099, -4.999999999999998224 ) ) ;
#28310=CARTESIAN_POINT ( 'NONE',  ( 26.72812500061451502, -4.541064518000419881, 2.621784821874995952 ) ) ;
#28311=CARTESIAN_POINT ( 'NONE',  ( -4.243569643749999898, 14.81562500061451715, -32.45002607614398471 ) ) ;
#28312=CARTESIAN_POINT ( 'NONE',  ( 16.05000000122903359, 5.773502691896255534, 3.535250795749688894E-16 ) ) ;
#28313=CARTESIAN_POINT ( 'NONE',  ( 13.76250000000000107, 2.886751345948126879, 4.999999999999999112 ) ) ;
#28314=CARTESIAN_POINT ( 'NONE',  ( 21.70312500061451644, 0.000000000000000000, 5.243569643749999010 ) ) ;
#28315=CARTESIAN_POINT ( 'NONE',  ( 8.259375000614518569, 0.000000000000000000, 5.243569643749999010 ) ) ;
#28316=CARTESIAN_POINT ( 'NONE',  ( 8.062500001229034652, 0.000000000000000000, 4.999999999999998224 ) ) ;
#28317=CARTESIAN_POINT ( 'NONE',  ( 17.32500000122903216, 2.886751345948129099, -4.999999999999998224 ) ) ;
#28318=CARTESIAN_POINT ( 'NONE',  ( 13.07812500061451821, 4.541064518000418104, 2.621784821874999949 ) ) ;
#28320=CARTESIAN_POINT ( 'NONE',  ( 16.86562500061451786, -6.054752690667223547, -1.112240025338166033E-15 ) ) ;
#28321=CARTESIAN_POINT ( 'NONE',  ( 28.50000000122903288, -2.886751345948125991, -5.000000000000000000 ) ) ;
#28322=CARTESIAN_POINT ( 'NONE',  ( 23.69999999999999929, 0.000000000000000000, 4.999999999999998224 ) ) ;
#28323=CARTESIAN_POINT ( 'NONE',  ( 23.37187500061451573, 3.027376345333613106, -5.243569643749998122 ) ) ;
#28324=CARTESIAN_POINT ( 'NONE',  ( 10.38750000122903572, -4.330127018922194537, 2.499999999999995559 ) ) ;
#28325=CARTESIAN_POINT ( 'NONE',  ( 28.09687500061451360, -3.027376345333614438, 5.243569643749998122 ) ) ;
#28326=CARTESIAN_POINT ( 'NONE',  ( 5.709375000614517859, -4.541064518000417216, -2.621784821875001281 ) ) ;
#28327=CARTESIAN_POINT ( 'NONE',  ( 24.77812500061451217, 4.541064518000418104, 2.621784821874999949 ) ) ;
#28329=CARTESIAN_POINT ( 'NONE',  ( 1.071796769724490339, 19.86740381056766225, -34.00000000000000000 ) ) ;
#28330=CARTESIAN_POINT ( 'NONE',  ( 9.121875000614517504, 3.027376345333611329, 5.243569643749999010 ) ) ;
#28332=CARTESIAN_POINT ( 'NONE',  ( 3.684375000614518836, 4.541064518000418104, 2.621784821874999949 ) ) ;
#28333=CARTESIAN_POINT ( 'NONE',  ( 5.634375000614519458, -4.541064518000419881, 2.621784821874995952 ) ) ;
#28335=CARTESIAN_POINT ( 'NONE',  ( 25.84687500061451360, -3.027376345333614438, 5.243569643749998122 ) ) ;
#28336=EDGE_CURVE ( 'NONE', #54892, #33433, #12089, .T. ) ;
#28338=CARTESIAN_POINT ( 'NONE',  ( 18.67500000000000071, 4.330127018922191873, 2.499999999999999556 ) ) ;
#28339=VERTEX_POINT ( 'NONE', #6550 ) ;
#28340=CARTESIAN_POINT ( 'NONE',  ( 26.88749999999999574, -2.886751345948129988, 4.999999999999997335 ) ) ;
#28341=CARTESIAN_POINT ( 'NONE',  ( 29.82187500061451502, 3.027376345333611329, 5.243569643749999010 ) ) ;
#28342=ORIENTED_EDGE ( 'NONE', *, *, #16791, .F. ) ;
#28343=CARTESIAN_POINT ( 'NONE',  ( 16.15312500061451573, 4.541064518000418104, -2.621784821874998173 ) ) ;
#28344=CARTESIAN_POINT ( 'NONE',  ( 8.203125000614518214, 0.000000000000000000, 5.243569643749999010 ) ) ;
#28346=CARTESIAN_POINT ( 'NONE',  ( 5.296875000614518214, -3.027376345333610441, -5.243569643749999898 ) ) ;
#28347=CARTESIAN_POINT ( 'NONE',  ( 17.21250000122903145, -4.330127018922190985, -2.500000000000001332 ) ) ;
#28348=CARTESIAN_POINT ( 'NONE',  ( 22.61250000000000071, 2.886751345948129099, -4.999999999999998224 ) ) ;
#28350=CARTESIAN_POINT ( 'NONE',  ( 6.421875000614519102, 3.027376345333611329, 5.243569643749999010 ) ) ;
#28351=CARTESIAN_POINT ( 'NONE',  ( 12.57187500061451857, 3.027376345333613106, -5.243569643749998122 ) ) ;
#28352=CARTESIAN_POINT ( 'NONE',  ( 21.68437500061451573, 4.541064518000418104, 2.621784821874999949 ) ) ;
#28353=CARTESIAN_POINT ( 'NONE',  ( -1.071796769724491005, 14.50759618943233420, -34.00000000000000000 ) ) ;
#28355=CARTESIAN_POINT ( 'NONE',  ( 3.309375000614518836, 0.000000000000000000, 5.243569643749999010 ) ) ;
#28356=( BOUNDED_CURVE ( )  B_SPLINE_CURVE ( 2, ( #14314, #20575, #64190, #59366, #58642, #42765, #65285 ),
 .UNSPECIFIED., .F., .F. ) 
 B_SPLINE_CURVE_WITH_KNOTS ( ( 3, 2, 2, 3 ),
 ( 0.05833333333333334120, 0.06111111111111110911, 0.06388888888888888395, 0.06666666666666665186 ),
 .UNSPECIFIED. ) 
 CURVE ( )  GEOMETRIC_REPRESENTATION_ITEM ( )  RATIONAL_B_SPLINE_CURVE ( ( 0.9999999999999995559, 0.8660254037844390407, 1.000000000000000000, 0.8660254037844387076, 1.000000000000000000, 0.8660254037844393737, 0.9999999999999993339 ) ) 
 REPRESENTATION_ITEM ( '' )  );
#28357=CARTESIAN_POINT ( 'NONE',  ( 5.934375000614517504, 4.541064518000418104, 2.621784821874999949 ) ) ;
#28358=CARTESIAN_POINT ( 'NONE',  ( 18.00000000000000355, -4.330127018922190985, -2.500000000000001332 ) ) ;
#28359=CARTESIAN_POINT ( 'NONE',  ( 15.47812500061451679, -4.541064518000419881, 2.621784821874995952 ) ) ;
#28363=CARTESIAN_POINT ( 'NONE',  ( 11.05312500061451608, -4.541064518000417216, -2.621784821875001281 ) ) ;
#28364=CARTESIAN_POINT ( 'NONE',  ( 26.03437500061451715, 6.421520780324663323E-16, -5.243569643749999010 ) ) ;
#28366=CARTESIAN_POINT ( 'NONE',  ( 29.48437500061451644, -4.541064518000419881, 2.621784821874995952 ) ) ;
#28367=CARTESIAN_POINT ( 'NONE',  ( 9.937500000000001776, -2.886751345948125991, -5.000000000000000000 ) ) ;
#28368=CARTESIAN_POINT ( 'NONE',  ( 3.999999999999999112, 14.48750000122903536, 30.00000000000000000 ) ) ;
#28369=CARTESIAN_POINT ( 'NONE',  ( 8.512500001229033941, 0.000000000000000000, 4.999999999999998224 ) ) ;
#28370=CARTESIAN_POINT ( 'NONE',  ( 20.52187500061451786, -6.054752690667223547, -1.112240025338166033E-15 ) ) ;
#28371=CARTESIAN_POINT ( 'NONE',  ( 13.20937500061451786, 0.000000000000000000, 5.243569643749999010 ) ) ;
#28372=CARTESIAN_POINT ( 'NONE',  ( 23.36250000122903359, 0.000000000000000000, 4.999999999999998224 ) ) ;
#28373=ORIENTED_EDGE ( 'NONE', *, *, #70404, .F. ) ;
#28374=CARTESIAN_POINT ( 'NONE',  ( 15.47812500061451679, -4.541064518000419881, 2.621784821874995952 ) ) ;
#28375=CARTESIAN_POINT ( 'NONE',  ( 26.73750000122903003, 6.123233995736764310E-16, -4.999999999999998224 ) ) ;
#28376=CARTESIAN_POINT ( 'NONE',  ( 14.78437500061451715, 6.421520780324663323E-16, -5.243569643749999010 ) ) ;
#28377=CARTESIAN_POINT ( 'NONE',  ( 3.685019977366421173, 9.302529035819388170, -25.24908463647652823 ) ) ;
#28378=CARTESIAN_POINT ( 'NONE',  ( 17.61562500061451786, 3.027376345333611329, 5.243569643749999010 ) ) ;
#28379=CARTESIAN_POINT ( 'NONE',  ( 30.00000000000000000, 0.000000000000000000, 4.999999999999998224 ) ) ;
#28380=CARTESIAN_POINT ( 'NONE',  ( 26.44687500061451502, -3.027376345333610441, -5.243569643749999898 ) ) ;
#28381=CARTESIAN_POINT ( 'NONE',  ( 2.121784821874999061, 10.65312500061451750, 26.32496088578401583 ) ) ;
#28382=CARTESIAN_POINT ( 'NONE',  ( 15.15937500061451715, -4.541064518000417216, -2.621784821875001281 ) ) ;
#28383=CARTESIAN_POINT ( 'NONE',  ( 13.12500000122903288, -5.773502691896255534, -1.060575238724906372E-15 ) ) ;
#28384=CARTESIAN_POINT ( 'NONE',  ( 0.000000000000000000, 20.00000000000000000, -30.00000000000000000 ) ) ;
#28385=CARTESIAN_POINT ( 'NONE',  ( -3.000416591977282496E-16, 19.74687500061451928, -34.90005215228797653 ) ) ;
#28386=CARTESIAN_POINT ( 'NONE',  ( 19.17187500061451999, -6.054752690667223547, -1.112240025338166033E-15 ) ) ;
#28387=CARTESIAN_POINT ( 'NONE',  ( 19.38750000122903216, -4.330127018922194537, 2.499999999999995559 ) ) ;
#28388=( BOUNDED_CURVE ( )  B_SPLINE_CURVE ( 2, ( #12837, #57894, #59345, #58984, #8389, #29833, #2850 ),
 .UNSPECIFIED., .F., .F. ) 
 B_SPLINE_CURVE_WITH_KNOTS ( ( 3, 2, 2, 3 ),
 ( 0.9346169692731971512, 0.9361111111111111160, 0.9388888888888888840, 0.9402232515920995182 ),
 .UNSPECIFIED. ) 
 CURVE ( )  GEOMETRIC_REPRESENTATION_ITEM ( )  RATIONAL_B_SPLINE_CURVE ( ( 0.9333974052703135627, 0.9279362622076117173, 1.000000000000000000, 0.8660254037844387076, 1.000000000000000000, 0.9356425464276099113, 0.9331159465740572756 ) ) 
 REPRESENTATION_ITEM ( '' )  );
#28389=CARTESIAN_POINT ( 'NONE',  ( 15.68437500061451573, 6.421520780324663323E-16, -5.243569643749999010 ) ) ;
#28390=CARTESIAN_POINT ( 'NONE',  ( 9.001249775931846008E-16, 11.87187500061451750, 34.90005215228797653 ) ) ;
#28391=CARTESIAN_POINT ( 'NONE',  ( 21.41250000122903074, 4.330127018922192761, -2.499999999999997780 ) ) ;
#28392=CARTESIAN_POINT ( 'NONE',  ( 14.76562500061451821, 3.027376345333613106, -5.243569643749998122 ) ) ;
#28393=CARTESIAN_POINT ( 'NONE',  ( 28.94062500061452070, -3.027376345333614438, 5.243569643749998122 ) ) ;
#28394=ORIENTED_EDGE ( 'NONE', *, *, #38051, .F. ) ;
#28396=CARTESIAN_POINT ( 'NONE',  ( 20.43749999999999645, 5.773502691896255534, 3.535250795749688894E-16 ) ) ;
#28398=CARTESIAN_POINT ( 'NONE',  ( 3.365625000614516082, -6.054752690667223547, -1.112240025338166033E-15 ) ) ;
#28399=CARTESIAN_POINT ( 'NONE',  ( 16.01250000122903216, 4.330127018922192761, -2.499999999999997780 ) ) ;
#28400=CARTESIAN_POINT ( 'NONE',  ( 19.82812500061451644, 4.541064518000418104, 2.621784821874999949 ) ) ;
#28401=EDGE_CURVE ( 'NONE', #20653, #66446, #16494, .T. ) ;
#28402=CARTESIAN_POINT ( 'NONE',  ( 24.96562500061451573, -6.054752690667223547, -1.112240025338166033E-15 ) ) ;
#28403=CARTESIAN_POINT ( 'NONE',  ( 6.103125000614515905, -4.541064518000417216, -2.621784821875001281 ) ) ;
#28404=CARTESIAN_POINT ( 'NONE',  ( 29.58749999999999858, -2.886751345948129988, 4.999999999999997335 ) ) ;
#28406=( BOUNDED_CURVE ( )  B_SPLINE_CURVE ( 2, ( #3868, #49298, #14933, #38196, #70359, #20463, #37834 ),
 .UNSPECIFIED., .F., .F. ) 
 B_SPLINE_CURVE_WITH_KNOTS ( ( 3, 2, 2, 3 ),
 ( 0.6666666666666666297, 0.6694444444444443976, 0.6722222222222222765, 0.6750000000000000444 ),
 .UNSPECIFIED. ) 
 CURVE ( )  GEOMETRIC_REPRESENTATION_ITEM ( )  RATIONAL_B_SPLINE_CURVE ( ( 1.000000000000000000, 0.8660254037844387076, 1.000000000000000000, 0.8660254037844387076, 1.000000000000000000, 0.8660254037844387076, 1.000000000000000000 ) ) 
 REPRESENTATION_ITEM ( '' )  );
#28408=CARTESIAN_POINT ( 'NONE',  ( 11.17500000122903536, 2.886751345948126879, 4.999999999999998224 ) ) ;
#28409=CARTESIAN_POINT ( 'NONE',  ( 4.000000000000000000, 11.75000000122903643, -27.69059892324149530 ) ) ;
#28410=CARTESIAN_POINT ( 'NONE',  ( 9.001249775931846008E-16, 19.07187500061451502, -25.09994784771203058 ) ) ;
#28411=CARTESIAN_POINT ( 'NONE',  ( 6.600000001229032520, 5.773502691896255534, 3.535250795749688894E-16 ) ) ;
#28412=CARTESIAN_POINT ( 'NONE',  ( 8.137500000000002842, -2.886751345948125991, -5.000000000000000000 ) ) ;
#28413=CARTESIAN_POINT ( 'NONE',  ( 3.750000001229034652, -2.886751345948125991, -5.000000000000000000 ) ) ;
#28414=CARTESIAN_POINT ( 'NONE',  ( 12.15937500061451892, 4.541064518000418104, -2.621784821874998173 ) ) ;
#28415=CARTESIAN_POINT ( 'NONE',  ( 29.80312500061451431, 0.000000000000000000, 5.243569643749999010 ) ) ;
#28416=CARTESIAN_POINT ( 'NONE',  ( 3.543100117577441033, 4.136409934384715825, -3.322667120213021796 ) ) ;
#28418=CARTESIAN_POINT ( 'NONE',  ( -3.999999999999999112, 19.62500000122903288, -32.30940107675850470 ) ) ;
#28419=CARTESIAN_POINT ( 'NONE',  ( 9.496875000614517504, 6.054752690667223547, 3.707466751127219781E-16 ) ) ;
#28420=CARTESIAN_POINT ( 'NONE',  ( 3.619842856578028734, -3.449164782042274169, -3.619842856578066481 ) ) ;
#28422=CARTESIAN_POINT ( 'NONE',  ( -3.000416591977282496E-16, 16.54062500061459673, 25.09994784771203058 ) ) ;
#28423=CARTESIAN_POINT ( 'NONE',  ( 21.19687500061451502, 6.054752690667223547, 3.707466751127219781E-16 ) ) ;
#28425=CARTESIAN_POINT ( 'NONE',  ( 2.791126035847173448, -4.148447354374293461, 2.973833421074890904 ) ) ;
#28426=CARTESIAN_POINT ( 'NONE',  ( 29.66250000122903074, 0.000000000000000000, 4.999999999999998224 ) ) ;
#28428=CARTESIAN_POINT ( 'NONE',  ( 22.71562500061451573, -6.054752690667223547, -1.112240025338166033E-15 ) ) ;
#28429=CARTESIAN_POINT ( 'NONE',  ( 15.55312500061451608, -4.541064518000417216, -2.621784821875001281 ) ) ;
#28431=CARTESIAN_POINT ( 'NONE',  ( 11.40937500061451892, 0.000000000000000000, 5.243569643749999010 ) ) ;
#28432=CARTESIAN_POINT ( 'NONE',  ( 28.91250000000000497, 2.886751345948129099, -4.999999999999998224 ) ) ;
#28433=CARTESIAN_POINT ( 'NONE',  ( 24.93750000122903288, 6.123233995736764310E-16, -4.999999999999998224 ) ) ;
#28434=CARTESIAN_POINT ( 'NONE',  ( 4.734375000614518214, -4.541064518000419881, 2.621784821874995952 ) ) ;
#28435=CARTESIAN_POINT ( 'NONE',  ( 14.67187500061451821, -6.054752690667223547, -1.112240025338166033E-15 ) ) ;
#28436=CARTESIAN_POINT ( 'NONE',  ( 29.85937500061451644, 0.000000000000000000, 5.243569643749999010 ) ) ;
#28438=ADVANCED_FACE ( 'NONE', ( #51253 ), #68610, .F. ) ;
#28440=CARTESIAN_POINT ( 'NONE',  ( 23.29687500061451644, -3.027376345333610441, -5.243569643749999898 ) ) ;
#28441=CARTESIAN_POINT ( 'NONE',  ( 13.80937500061451750, -4.541064518000417216, -2.621784821875001281 ) ) ;
#28443=CARTESIAN_POINT ( 'NONE',  ( 25.80000000000000071, 4.330127018922192761, -2.499999999999997780 ) ) ;
#28444=DIRECTION ( 'NONE',  ( 0.000000000000000000, 0.000000000000000000, -1.000000000000000000 ) ) ;
#28446=CARTESIAN_POINT ( 'NONE',  ( 16.41562500061451857, -6.054752690667223547, -1.112240025338166033E-15 ) ) ;
#28447=CARTESIAN_POINT ( 'NONE',  ( 6.262500000000000178, -5.773502691896255534, -1.060575238724906372E-15 ) ) ;
#28448=CARTESIAN_POINT ( 'NONE',  ( 2.915625000614516793, -6.054752690667223547, -1.112240025338166033E-15 ) ) ;
#28449=CARTESIAN_POINT ( 'NONE',  ( 16.42500000000000071, 4.330127018922191873, 2.499999999999999556 ) ) ;
#28450=CARTESIAN_POINT ( 'NONE',  ( -3.000416591977282496E-16, 13.84062500061451928, 25.09994784771203058 ) ) ;
#28452=CARTESIAN_POINT ( 'NONE',  ( 21.71250000122903501, -4.330127018922190985, -2.500000000000001332 ) ) ;
#28454=CARTESIAN_POINT ( 'NONE',  ( 26.25937500061451857, 0.000000000000000000, 5.243569643749999010 ) ) ;
#28456=CARTESIAN_POINT ( 'NONE',  ( 21.44062500061452070, -3.027376345333610441, -5.243569643749999898 ) ) ;
#28457=CARTESIAN_POINT ( 'NONE',  ( 21.42187500061451644, -6.054752690667223547, -1.112240025338166033E-15 ) ) ;
#28458=CARTESIAN_POINT ( 'NONE',  ( 7.724999999999999645, 6.123233995736764310E-16, -4.999999999999998224 ) ) ;
#28459=CARTESIAN_POINT ( 'NONE',  ( 9.028125000614517504, 4.541064518000418104, 2.621784821874999949 ) ) ;
#28460=CARTESIAN_POINT ( 'NONE',  ( 23.95312500061451289, 0.000000000000000000, 5.243569643749999010 ) ) ;
#28461=CARTESIAN_POINT ( 'NONE',  ( 12.45937500061451786, -4.541064518000417216, -2.621784821875001281 ) ) ;
#28462=CARTESIAN_POINT ( 'NONE',  ( 16.09687500061452070, -3.027376345333610441, -5.243569643749999898 ) ) ;
#28463=CARTESIAN_POINT ( 'NONE',  ( 4.411272977760241965, 2.353862934769528348, -4.685547128476531320 ) ) ;
#28464=CARTESIAN_POINT ( 'NONE',  ( -2.121784821874996840, 18.52812500061451928, 33.67503911421598417 ) ) ;
#28465=CARTESIAN_POINT ( 'NONE',  ( 22.05000000122903714, -2.886751345948129988, 4.999999999999997335 ) ) ;
#28467=CARTESIAN_POINT ( 'NONE',  ( 11.57812500061451644, 6.421520780324663323E-16, -5.243569643749999010 ) ) ;
#28468=CARTESIAN_POINT ( 'NONE',  ( 5.034375000614519813, 4.541064518000418104, 2.621784821874999949 ) ) ;
#28469=CARTESIAN_POINT ( 'NONE',  ( 4.171875000614517326, 3.027376345333611329, 5.243569643749999010 ) ) ;
#28471=CARTESIAN_POINT ( 'NONE',  ( 24.75937500061451502, 4.541064518000418104, -2.621784821874998173 ) ) ;
#28472=CARTESIAN_POINT ( 'NONE',  ( 17.35312500061451502, -4.541064518000417216, -2.621784821875001281 ) ) ;
#28473=CARTESIAN_POINT ( 'NONE',  ( 28.27500000122903145, 2.886751345948126879, 4.999999999999999112 ) ) ;
#28474=CARTESIAN_POINT ( 'NONE',  ( 26.76562500061451644, -6.054752690667223547, -1.112240025338166033E-15 ) ) ;
#28475=CARTESIAN_POINT ( 'NONE',  ( 22.43437500061451573, 6.421520780324663323E-16, -5.243569643749999010 ) ) ;
#28476=CARTESIAN_POINT ( 'NONE',  ( 16.30312500061451786, 0.000000000000000000, 5.243569643749999010 ) ) ;
#28477=CARTESIAN_POINT ( 'NONE',  ( 9.001249775931846008E-16, 19.52187500061451786, 34.90005215228797653 ) ) ;
#28478=CARTESIAN_POINT ( 'NONE',  ( 22.86562500061451431, 3.027376345333613106, -5.243569643749998122 ) ) ;
#28479=CARTESIAN_POINT ( 'NONE',  ( 5.212500001229032343, 4.330127018922192761, -2.499999999999997780 ) ) ;
#28481=CARTESIAN_POINT ( 'NONE',  ( 27.15000000000000213, 4.330127018922192761, -2.499999999999997780 ) ) ;
#28482=CARTESIAN_POINT ( 'NONE',  ( 3.999999999999999112, 12.57500000000000107, -30.00000000000000000 ) ) ;
#28484=CARTESIAN_POINT ( 'NONE',  ( 28.45312500061451289, 0.000000000000000000, 5.243569643749999010 ) ) ;
#28485=CARTESIAN_POINT ( 'NONE',  ( 11.39062500061451644, -3.027376345333614438, 5.243569643749998122 ) ) ;
#28486=CARTESIAN_POINT ( 'NONE',  ( 21.45000000122903216, 5.773502691896255534, 3.535250795749688894E-16 ) ) ;
#28487=CARTESIAN_POINT ( 'NONE',  ( 13.13437500061451857, 4.541064518000418104, 2.621784821874999949 ) ) ;
#28488=CARTESIAN_POINT ( 'NONE',  ( 27.32812500061451644, 6.421520780324663323E-16, -5.243569643749999010 ) ) ;
#28490=CARTESIAN_POINT ( 'NONE',  ( 28.46249999999999858, 2.886751345948129099, -4.999999999999998224 ) ) ;
#28491=EDGE_CURVE ( 'NONE', #46707, #47914, #49954, .T. ) ;
#28492=CARTESIAN_POINT ( 'NONE',  ( -3.999999999999997335, 19.25000000122903288, -27.69059892324149175 ) ) ;
#28493=CARTESIAN_POINT ( 'NONE',  ( 14.58750000122903323, 6.123233995736764310E-16, -4.999999999999998224 ) ) ;
#28494=CARTESIAN_POINT ( 'NONE',  ( 12.29062500061451857, -3.027376345333614438, 5.243569643749998122 ) ) ;
#28495=ORIENTED_EDGE ( 'NONE', *, *, #22734, .T. ) ;
#28496=CARTESIAN_POINT ( 'NONE',  ( 9.028125000614517504, 4.541064518000418104, 2.621784821874999949 ) ) ;
#28497=CARTESIAN_POINT ( 'NONE',  ( 6.553125000614518747, -4.541064518000417216, -2.621784821875001281 ) ) ;
#28499=CARTESIAN_POINT ( 'NONE',  ( 14.96250000000000036, 2.886751345948129099, -4.999999999999998224 ) ) ;
#28500=CARTESIAN_POINT ( 'NONE',  ( 16.73437500061451644, 4.541064518000418104, 2.621784821874999949 ) ) ;
#28501=CARTESIAN_POINT ( 'NONE',  ( 11.02500000122903501, 2.886751345948129099, -4.999999999999998224 ) ) ;
#28502=CARTESIAN_POINT ( 'NONE',  ( 19.84687500061451360, 6.054752690667223547, 3.707466751127219781E-16 ) ) ;
#28504=CARTESIAN_POINT ( 'NONE',  ( 19.80937500061451573, 4.541064518000418104, -2.621784821874998173 ) ) ;
#28505=CARTESIAN_POINT ( 'NONE',  ( -2.121784821874996840, 13.57812500061451644, -26.32496088578401583 ) ) ;
#28506=FACE_OUTER_BOUND ( 'NONE', #14416, .T. ) ;
#28508=DIRECTION ( 'NONE',  ( -1.000000000000000000, -0.000000000000000000, -0.000000000000000000 ) ) ;
#28509=CARTESIAN_POINT ( 'NONE',  ( 27.40312500061451573, 4.541064518000418104, -2.621784821874998173 ) ) ;
#28510=CARTESIAN_POINT ( 'NONE',  ( 30.00000000000000000, 0.000000000000000000, 0.000000000000000000 ) ) ;
#28511=CARTESIAN_POINT ( 'NONE',  ( 27.64687500061452141, -3.027376345333614438, 5.243569643749998122 ) ) ;
#28512=CARTESIAN_POINT ( 'NONE',  ( 24.44999999999999929, 4.330127018922192761, -2.499999999999997780 ) ) ;
#28513=CARTESIAN_POINT ( 'NONE',  ( 8.128125000614515372, 4.541064518000418104, 2.621784821874999949 ) ) ;
#28515=CARTESIAN_POINT ( 'NONE',  ( 17.93437500061451928, 6.421520780324663323E-16, -5.243569643749999010 ) ) ;
#28517=CARTESIAN_POINT ( 'NONE',  ( 6.065625000614516260, -6.054752690667223547, -1.112240025338166033E-15 ) ) ;
#28518=CARTESIAN_POINT ( 'NONE',  ( 11.48437500061451644, -4.541064518000419881, 2.621784821874995952 ) ) ;
#28519=ORIENTED_EDGE ( 'NONE', *, *, #60253, .F. ) ;
#28520=CARTESIAN_POINT ( 'NONE',  ( 22.24687500061451217, -3.027376345333614438, 5.243569643749998122 ) ) ;
#28521=CARTESIAN_POINT ( 'NONE',  ( 30.00000000000000000, 6.123233995736764310E-16, -4.999999999999998224 ) ) ;
#28522=CARTESIAN_POINT ( 'NONE',  ( 29.17500000000000071, -4.330127018922194537, 2.499999999999995559 ) ) ;
#28523=CARTESIAN_POINT ( 'NONE',  ( 3.112500000000000711, -5.773502691896255534, -1.060575238724906372E-15 ) ) ;
#28524=CARTESIAN_POINT ( 'NONE',  ( 14.17500000122903536, 2.886751345948129099, -4.999999999999998224 ) ) ;
#28525=CARTESIAN_POINT ( 'NONE',  ( 2.000000000000001332, 12.16250000122903430, 33.46410161513774995 ) ) ;
#28526=CARTESIAN_POINT ( 'NONE',  ( 22.01250000122903216, 0.000000000000000000, 4.999999999999998224 ) ) ;
#28527=CARTESIAN_POINT ( 'NONE',  ( 3.309375000614518836, 0.000000000000000000, 5.243569643749999010 ) ) ;
#28529=CARTESIAN_POINT ( 'NONE',  ( 13.42499999999999893, -4.330127018922194537, 2.499999999999995559 ) ) ;
#28530=CARTESIAN_POINT ( 'NONE',  ( 24.32812500061451289, 4.541064518000418104, 2.621784821874999949 ) ) ;
#28531=CARTESIAN_POINT ( 'NONE',  ( 15.18750000000000000, -2.886751345948129988, 4.999999999999997335 ) ) ;
#28532=( BOUNDED_CURVE ( )  B_SPLINE_CURVE ( 2, ( #72761, #5886, #67591, #352, #11432, #22859, #45413 ),
 .UNSPECIFIED., .F., .F. ) 
 B_SPLINE_CURVE_WITH_KNOTS ( ( 3, 2, 2, 3 ),
 ( 0.6166666666666666963, 0.6194444444444444642, 0.6222222222222222321, 0.6250000000000000000 ),
 .UNSPECIFIED. ) 
 CURVE ( )  GEOMETRIC_REPRESENTATION_ITEM ( )  RATIONAL_B_SPLINE_CURVE ( ( 1.000000000000000000, 0.8660254037844387076, 1.000000000000000000, 0.8660254037844387076, 1.000000000000000000, 0.8660254037844387076, 1.000000000000000000 ) ) 
 REPRESENTATION_ITEM ( '' )  );
#28534=CARTESIAN_POINT ( 'NONE',  ( 9.450000001229033941, -2.886751345948129988, 4.999999999999997335 ) ) ;
#28535=CARTESIAN_POINT ( 'NONE',  ( 8.840625000614515727, -3.027376345333610441, -5.243569643749999898 ) ) ;
#28536=CARTESIAN_POINT ( 'NONE',  ( 8.324999999999999289, 4.330127018922191873, 2.499999999999999556 ) ) ;
#28537=CARTESIAN_POINT ( 'NONE',  ( 16.01250000122903216, 4.330127018922192761, -2.499999999999997780 ) ) ;
#28539=CARTESIAN_POINT ( 'NONE',  ( -2.121784821874996840, 13.63437500061451857, -26.32496088578401583 ) ) ;
#28540=CARTESIAN_POINT ( 'NONE',  ( 28.35000000122903430, -2.886751345948129988, 4.999999999999997335 ) ) ;
#28542=CARTESIAN_POINT ( 'NONE',  ( 6.975000000000002309, 4.330127018922191873, 2.499999999999999556 ) ) ;
#28543=CARTESIAN_POINT ( 'NONE',  ( 30.00000000000000000, 0.000000000000000000, 4.999999999999998224 ) ) ;
#28544=ORIENTED_EDGE ( 'NONE', *, *, #40932, .T. ) ;
#28545=CARTESIAN_POINT ( 'NONE',  ( 20.72812500061451502, 4.541064518000418104, 2.621784821874999949 ) ) ;
#28546=CARTESIAN_POINT ( 'NONE',  ( 13.12500000122903288, -5.773502691896255534, -1.060575238724906372E-15 ) ) ;
#28547=CARTESIAN_POINT ( 'NONE',  ( 28.49062500061451431, -3.027376345333614438, 5.243569643749998122 ) ) ;
#28548=FACE_OUTER_BOUND ( 'NONE', #6100, .T. ) ;
#28549=CARTESIAN_POINT ( 'NONE',  ( 20.07187500061451857, -6.054752690667223547, -1.112240025338166033E-15 ) ) ;
#28550=CARTESIAN_POINT ( 'NONE',  ( 17.50312500061451715, 4.541064518000418104, -2.621784821874998173 ) ) ;
#28551=CARTESIAN_POINT ( 'NONE',  ( -2.121784821874999949, 12.52812500061459211, -33.67503911421598417 ) ) ;
#28552=CARTESIAN_POINT ( 'NONE',  ( 5.803125000614517859, 4.541064518000418104, -2.621784821874998173 ) ) ;
#28553=CARTESIAN_POINT ( 'NONE',  ( 29.02500000122903145, 2.886751345948129099, -4.999999999999998224 ) ) ;
#28555=CARTESIAN_POINT ( 'NONE',  ( 19.30312500061451786, 4.541064518000418104, -2.621784821874998173 ) ) ;
#28556=CARTESIAN_POINT ( 'NONE',  ( 1.999999999999998668, 14.00000000000000178, 26.53589838486224650 ) ) ;
#28557=CARTESIAN_POINT ( 'NONE',  ( 3.562500001229033764, 0.000000000000000000, 4.999999999999998224 ) ) ;
#28558=CARTESIAN_POINT ( 'NONE',  ( 12.53437500061451537, 6.421520780324663323E-16, -5.243569643749999010 ) ) ;
#28559=CARTESIAN_POINT ( 'NONE',  ( 11.48437500061451644, -4.541064518000419881, 2.621784821874995952 ) ) ;
#28560=CARTESIAN_POINT ( 'NONE',  ( 19.43437500061451928, 4.541064518000418104, 2.621784821874999949 ) ) ;
#28561=ORIENTED_EDGE ( 'NONE', *, *, #32854, .F. ) ;
#28563=CARTESIAN_POINT ( 'NONE',  ( 24.70312500061451644, 4.541064518000418104, -2.621784821874998173 ) ) ;
#28564=CARTESIAN_POINT ( 'NONE',  ( 19.02187500061451786, 3.027376345333611329, 5.243569643749999010 ) ) ;
#28565=CARTESIAN_POINT ( 'NONE',  ( 25.07812500061451644, 6.421520780324663323E-16, -5.243569643749999010 ) ) ;
#28567=CARTESIAN_POINT ( 'NONE',  ( -3.999999999999999112, 16.40000000000000213, 30.00000000000000000 ) ) ;
#28568=CARTESIAN_POINT ( 'NONE',  ( 4.471875000614518925, 3.027376345333613106, -5.243569643749998122 ) ) ;
#28569=CARTESIAN_POINT ( 'NONE',  ( 12.37500000122903465, 2.886751345948129099, -4.999999999999998224 ) ) ;
#28570=CARTESIAN_POINT ( 'NONE',  ( 7.725000001229034297, -5.773502691896255534, -1.060575238724906372E-15 ) ) ;
#28571=CARTESIAN_POINT ( 'NONE',  ( 27.11250000122903359, -4.330127018922190985, -2.500000000000001332 ) ) ;
#28574=CARTESIAN_POINT ( 'NONE',  ( 13.02187500061451608, 3.027376345333613106, -5.243569643749998122 ) ) ;
#28575=FACE_OUTER_BOUND ( 'NONE', #38523, .T. ) ;
#28576=CARTESIAN_POINT ( 'NONE',  ( 16.45312500061451289, -4.541064518000417216, -2.621784821875001281 ) ) ;
#28577=CARTESIAN_POINT ( 'NONE',  ( 13.47187500061451537, 3.027376345333613106, -5.243569643749998122 ) ) ;
#28578=CARTESIAN_POINT ( 'NONE',  ( 5.128125000614516260, -4.541064518000419881, 2.621784821874995952 ) ) ;
#28579=CARTESIAN_POINT ( 'NONE',  ( 20.22187500061451715, 3.027376345333612662, -5.243569643749998122 ) ) ;
#28580=CARTESIAN_POINT ( 'NONE',  ( 9.346875000614517148, -3.027376345333610441, -5.243569643749999898 ) ) ;
#28581=CARTESIAN_POINT ( 'NONE',  ( 14.85000000122903252, -2.886751345948130876, 4.999999999999996447 ) ) ;
#28582=CARTESIAN_POINT ( 'NONE',  ( -3.999999999999999112, 17.71249999999999858, 27.69059892324149885 ) ) ;
#28583=CARTESIAN_POINT ( 'NONE',  ( 6.225000001229036073, 2.886751345948126879, 4.999999999999999112 ) ) ;
#28584=CARTESIAN_POINT ( 'NONE',  ( 19.75312500061451360, 4.541064518000418104, -2.621784821874998173 ) ) ;
#28585=ADVANCED_FACE ( 'NONE', ( #7271 ), #57140, .F. ) ;
#28586=CARTESIAN_POINT ( 'NONE',  ( 8.212500001229035007, -4.330127018922190985, -2.500000000000001332 ) ) ;
#28587=CARTESIAN_POINT ( 'NONE',  ( 17.01562500061451644, 3.027376345333613106, -5.243569643749998122 ) ) ;
#28588=CARTESIAN_POINT ( 'NONE',  ( 14.16562500061451679, -6.054752690667223547, -1.112240025338166033E-15 ) ) ;
#28590=CARTESIAN_POINT ( 'NONE',  ( 13.19999999999999929, 4.330127018922192761, -2.499999999999997780 ) ) ;
#28591=CARTESIAN_POINT ( 'NONE',  ( 10.12500000122903465, 2.886751345948129099, -4.999999999999998224 ) ) ;
#28592=CARTESIAN_POINT ( 'NONE',  ( 6.028125000614517504, -4.541064518000419881, 2.621784821874995952 ) ) ;
#28594=CARTESIAN_POINT ( 'NONE',  ( 18.03750000122903430, -4.330127018922194537, 2.499999999999995559 ) ) ;
#28596=CARTESIAN_POINT ( 'NONE',  ( -3.000416591977282496E-16, 10.29687500061451644, -34.90005215228797653 ) ) ;
#28597=CARTESIAN_POINT ( 'NONE',  ( 4.530078317929211451, -2.116641477924516401, 4.600875075901697642 ) ) ;
#28598=CARTESIAN_POINT ( 'NONE',  ( 30.00000000000000000, 0.000000000000000000, 0.000000000000000000 ) ) ;
#28599=CARTESIAN_POINT ( 'NONE',  ( 2.859375000614519546, 0.000000000000000000, 5.243569643749999010 ) ) ;
#28600=CARTESIAN_POINT ( 'NONE',  ( 21.04687500061451644, -3.027376345333610441, -5.243569643749999898 ) ) ;
#28601=CARTESIAN_POINT ( 'NONE',  ( 10.68750000122903288, 4.330127018922191873, 2.499999999999999556 ) ) ;
#28602=CARTESIAN_POINT ( 'NONE',  ( 17.05312500061451786, 4.541064518000418104, -2.621784821874998173 ) ) ;
#28604=CARTESIAN_POINT ( 'NONE',  ( -3.999999999999999112, 15.46250000000000036, -32.30940107675850470 ) ) ;
#28605=CARTESIAN_POINT ( 'NONE',  ( -1.999999999999997113, 15.57500000000000284, 33.46410161513775705 ) ) ;
#28606=CARTESIAN_POINT ( 'NONE',  ( 27.45937500061451786, 4.541064518000418104, -2.621784821874998173 ) ) ;
#28608=CARTESIAN_POINT ( 'NONE',  ( 12.25312500061451537, 0.000000000000000000, 5.243569643749999010 ) ) ;
#28609=CARTESIAN_POINT ( 'NONE',  ( 11.44687500061451857, -3.027376345333614438, 5.243569643749998122 ) ) ;
#28610=ORIENTED_EDGE ( 'NONE', *, *, #40314, .F. ) ;
#28611=CARTESIAN_POINT ( 'NONE',  ( 19.26562500061451644, 3.027376345333613106, -5.243569643749998122 ) ) ;
#28612=CARTESIAN_POINT ( 'NONE',  ( 3.242103837493086330E-14, 11.00000000122903288, -34.00000000000000000 ) ) ;
#28613=CARTESIAN_POINT ( 'NONE',  ( 20.99999999999999645, 0.000000000000000000, 4.999999999999998224 ) ) ;
#28614=CARTESIAN_POINT ( 'NONE',  ( 12.44999999999999929, 0.000000000000000000, 4.999999999999998224 ) ) ;
#28615=CARTESIAN_POINT ( 'NONE',  ( 22.27500000122903145, 2.886751345948129099, -4.999999999999998224 ) ) ;
#28616=CARTESIAN_POINT ( 'NONE',  ( 15.59062500061451573, -3.027376345333610441, -5.243569643749999898 ) ) ;
#28618=ORIENTED_EDGE ( 'NONE', *, *, #24132, .T. ) ;
#28619=CARTESIAN_POINT ( 'NONE',  ( 20.32499999999999929, 6.123233995736764310E-16, -4.999999999999998224 ) ) ;
#28620=CARTESIAN_POINT ( 'NONE',  ( 23.47499999999999787, 6.123233995736764310E-16, -4.999999999999998224 ) ) ;
#28621=CARTESIAN_POINT ( 'NONE',  ( 20.52187500061451786, -6.054752690667223547, -1.112240025338166033E-15 ) ) ;
#28622=CARTESIAN_POINT ( 'NONE',  ( 25.97812500061451502, 6.421520780324663323E-16, -5.243569643749999010 ) ) ;
#28625=CARTESIAN_POINT ( 'NONE',  ( 9.290625000614515017, -3.027376345333610441, -5.243569643749999898 ) ) ;
#28627=CARTESIAN_POINT ( 'NONE',  ( 15.63749999999999751, -2.886751345948129988, 4.999999999999997335 ) ) ;
#28628=CARTESIAN_POINT ( 'NONE',  ( -2.121784821874996840, 18.07812500061451644, 33.67503911421598417 ) ) ;
#28629=CARTESIAN_POINT ( 'NONE',  ( 29.24062500061451431, 6.054752690667223547, 3.707466751127219781E-16 ) ) ;
#28630=CARTESIAN_POINT ( 'NONE',  ( 26.44687500061451502, -3.027376345333610441, -5.243569643749999898 ) ) ;
#28632=CARTESIAN_POINT ( 'NONE',  ( 22.94062500061451715, 6.054752690667223547, 3.707466751127219781E-16 ) ) ;
#28633=CARTESIAN_POINT ( 'NONE',  ( 24.83437500061451431, 4.541064518000418104, 2.621784821874999949 ) ) ;
#28634=CARTESIAN_POINT ( 'NONE',  ( -2.121784821874999949, 18.37812500061459531, -33.67503911421598417 ) ) ;
#28635=CARTESIAN_POINT ( 'NONE',  ( 12.41249999999999964, 2.886751345948126879, 4.999999999999999112 ) ) ;
#28636=CARTESIAN_POINT ( 'NONE',  ( 8.953125000614518214, 4.541064518000418104, -2.621784821874998173 ) ) ;
#28637=CARTESIAN_POINT ( 'NONE',  ( 3.739591918817028127, 3.929519787406462239, -3.193872078864750996 ) ) ;
#28638=CARTESIAN_POINT ( 'NONE',  ( 3.999999999999999112, 11.22500000000000142, 30.00000000000000000 ) ) ;
#28639=CARTESIAN_POINT ( 'NONE',  ( 26.39062500061451644, -3.027376345333610441, -5.243569643749999898 ) ) ;
#28642=CARTESIAN_POINT ( 'NONE',  ( 18.49687500061452283, 6.054752690667223547, 3.707466751127219781E-16 ) ) ;
#28643=CARTESIAN_POINT ( 'NONE',  ( 4.243569643749999898, 14.23437500061451821, 30.00000000000000000 ) ) ;
#28644=CARTESIAN_POINT ( 'NONE',  ( 18.87187500061451573, 3.027376345333613106, -5.243569643749998122 ) ) ;
#28645=CARTESIAN_POINT ( 'NONE',  ( 28.24687500061451573, -3.027376345333610441, -5.243569643749999898 ) ) ;
#28646=CARTESIAN_POINT ( 'NONE',  ( 2.121784821875001281, 17.75937500061451502, 33.67503911421598417 ) ) ;
#28647=CARTESIAN_POINT ( 'NONE',  ( 9.290625000614515017, -3.027376345333610441, -5.243569643749999898 ) ) ;
#28648=CARTESIAN_POINT ( 'NONE',  ( 4.000000000000000000, 17.15000000122903145, 32.30940107675849760 ) ) ;
#28649=CARTESIAN_POINT ( 'NONE',  ( 4.396875000614516971, -3.027376345333610441, -5.243569643749999898 ) ) ;
#28650=LINE ( 'NONE', #62982, #14764 ) ;
#28651=CARTESIAN_POINT ( 'NONE',  ( 7.903125000614515727, -4.541064518000417216, -2.621784821875001281 ) ) ;
#28652=CARTESIAN_POINT ( 'NONE',  ( 11.33437500061451608, 4.541064518000418104, 2.621784821874999949 ) ) ;
#28654=CARTESIAN_POINT ( 'NONE',  ( 20.13750000122903216, 4.330127018922191873, 2.499999999999999556 ) ) ;
#28655=CARTESIAN_POINT ( 'NONE',  ( 5.934375000614517504, 4.541064518000418104, 2.621784821874999949 ) ) ;
#28656=CARTESIAN_POINT ( 'NONE',  ( 7.378125000614518036, -4.541064518000419881, 2.621784821874995952 ) ) ;
#28657=CARTESIAN_POINT ( 'NONE',  ( 5.653125000614517504, -4.541064518000417216, -2.621784821875001281 ) ) ;
#28659=CARTESIAN_POINT ( 'NONE',  ( 17.97187500061451715, 3.027376345333613106, -5.243569643749998122 ) ) ;
#28660=CARTESIAN_POINT ( 'NONE',  ( 8.962500001229033231, 0.000000000000000000, 4.999999999999998224 ) ) ;
#28661=ORIENTED_EDGE ( 'NONE', *, *, #65329, .F. ) ;
#28662=CARTESIAN_POINT ( 'NONE',  ( 25.56562500061452070, 3.027376345333613106, -5.243569643749998122 ) ) ;
#28663=CARTESIAN_POINT ( 'NONE',  ( 12.10312500061451857, 4.541064518000418104, -2.621784821874998173 ) ) ;
#28664=CARTESIAN_POINT ( 'NONE',  ( 29.52187500061451431, -6.054752690667223547, -1.112240025338166033E-15 ) ) ;
#28665=CARTESIAN_POINT ( 'NONE',  ( 12.06562500061451537, 3.027376345333613106, -5.243569643749998122 ) ) ;
#28666=DIRECTION ( 'NONE',  ( 0.000000000000000000, 0.000000000000000000, -1.000000000000000000 ) ) ;
#28667=CARTESIAN_POINT ( 'NONE',  ( 11.85000000122903430, -2.886751345948125991, -5.000000000000000000 ) ) ;
#28668=CARTESIAN_POINT ( 'NONE',  ( 27.51562500061451644, 3.027376345333611329, 5.243569643749999010 ) ) ;
#28669=EDGE_CURVE ( 'NONE', #23627, #11718, #50048, .T. ) ;
#28670=CARTESIAN_POINT ( 'NONE',  ( -4.243569643749999898, 12.15312500061451573, -30.00000000000000000 ) ) ;
#28671=CARTESIAN_POINT ( 'NONE',  ( 15.90000000122903501, -2.886751345948125991, -5.000000000000000000 ) ) ;
#28672=CARTESIAN_POINT ( 'NONE',  ( 11.92500000000000071, 4.330127018922191873, 2.499999999999999556 ) ) ;
#28673=CARTESIAN_POINT ( 'NONE',  ( 19.86562500061451786, 3.027376345333611329, 5.243569643749999010 ) ) ;
#28674=CARTESIAN_POINT ( 'NONE',  ( 8.859375000614518214, -4.541064518000417216, -2.621784821875001281 ) ) ;
#28675=CARTESIAN_POINT ( 'NONE',  ( 8.325000001229033941, 2.886751345948129099, -4.999999999999998224 ) ) ;
#28676=CARTESIAN_POINT ( 'NONE',  ( 17.36250000122903359, 4.330127018922192761, -2.499999999999997780 ) ) ;
#28677=CARTESIAN_POINT ( 'NONE',  ( 12.55312500061451786, 4.541064518000418104, -2.621784821874998173 ) ) ;
#28678=CARTESIAN_POINT ( 'NONE',  ( 15.89062500061451289, -3.027376345333614438, 5.243569643749998122 ) ) ;
#28679=CARTESIAN_POINT ( 'NONE',  ( 26.77500000122903145, 2.886751345948129099, -4.999999999999998224 ) ) ;
#28680=CARTESIAN_POINT ( 'NONE',  ( 23.51249999999999574, 2.886751345948129099, -4.999999999999998224 ) ) ;
#28681=CARTESIAN_POINT ( 'NONE',  ( 24.38437500061451502, 4.541064518000418104, 2.621784821874999949 ) ) ;
#28684=CARTESIAN_POINT ( 'NONE',  ( 10.65000000122903323, 5.773502691896255534, 3.535250795749688894E-16 ) ) ;
#28685=CARTESIAN_POINT ( 'NONE',  ( 27.90937500061451715, 4.541064518000418104, -2.621784821874998173 ) ) ;
#28686=CARTESIAN_POINT ( 'NONE',  ( 3.271875000614519635, 3.027376345333611329, 5.243569643749999010 ) ) ;
#28687=CARTESIAN_POINT ( 'NONE',  ( 23.31562500061451715, 3.027376345333613106, -5.243569643749998122 ) ) ;
#28689=CARTESIAN_POINT ( 'NONE',  ( 4.411272977760241965, 2.353862934769528348, -4.685547128476531320 ) ) ;
#28690=CARTESIAN_POINT ( 'NONE',  ( 6.984375000614516438, -4.541064518000419881, 2.621784821874995952 ) ) ;
#28691=CARTESIAN_POINT ( 'NONE',  ( -5.810221930991193690E-16, 10.43750000000000000, 26.00000000000000355 ) ) ;
#28692=CARTESIAN_POINT ( 'NONE',  ( 26.42812500061451431, 6.421520780324663323E-16, -5.243569643749999010 ) ) ;
#28693=CARTESIAN_POINT ( 'NONE',  ( 6.346875000614517148, 6.054752690667223547, 3.707466751127219781E-16 ) ) ;
#28695=CARTESIAN_POINT ( 'NONE',  ( 25.58437500061451431, 6.421520780324663323E-16, -5.243569643749999010 ) ) ;
#28696=CARTESIAN_POINT ( 'NONE',  ( -0.7368881354385758975, 9.803648613939513368, 25.82089971438751519 ) ) ;
#28697=CARTESIAN_POINT ( 'NONE',  ( 20.02500000000000213, 4.330127018922191873, 2.499999999999999556 ) ) ;
#28698=VERTEX_POINT ( 'NONE', #7626 ) ;
#28699=CARTESIAN_POINT ( 'NONE',  ( 27.18750000000000000, 5.773502691896255534, 3.535250795749688894E-16 ) ) ;
#28700=CARTESIAN_POINT ( 'NONE',  ( 28.13437500061451502, -4.541064518000419881, 2.621784821874995952 ) ) ;
#28703=CARTESIAN_POINT ( 'NONE',  ( 15.51562500061451644, -6.054752690667223547, -1.112240025338166033E-15 ) ) ;
#28704=CARTESIAN_POINT ( 'NONE',  ( 7.528125000614515727, 6.421520780324663323E-16, -5.243569643749999010 ) ) ;
#28706=CARTESIAN_POINT ( 'NONE',  ( 5.671875000614519102, -6.054752690667223547, -1.112240025338166033E-15 ) ) ;
#28707=CARTESIAN_POINT ( 'NONE',  ( 16.80000000122903359, -2.886751345948125991, -5.000000000000000000 ) ) ;
#28708=CARTESIAN_POINT ( 'NONE',  ( 21.93750000000000000, -2.886751345948129988, 4.999999999999997335 ) ) ;
#28709=CARTESIAN_POINT ( 'NONE',  ( 29.47499999999999787, 4.330127018922191873, 2.499999999999999556 ) ) ;
#28710=CARTESIAN_POINT ( 'NONE',  ( 5.709375000614517859, -4.541064518000417216, -2.621784821875001281 ) ) ;
#28711=CARTESIAN_POINT ( 'NONE',  ( 10.58437500061451964, -4.541064518000419881, 2.621784821874995952 ) ) ;
#28712=CARTESIAN_POINT ( 'NONE',  ( 21.15937500061451715, 4.541064518000418104, -2.621784821874998173 ) ) ;
#28713=CARTESIAN_POINT ( 'NONE',  ( 1.592000809091587073E-14, 15.05000000122903714, -34.00000000000000000 ) ) ;
#28714=EDGE_LOOP ( 'NONE', ( #15353, #43314, #10766, #57691 ) ) ;
#28715=CARTESIAN_POINT ( 'NONE',  ( 4.434375000614519280, 6.421520780324663323E-16, -5.243569643749999010 ) ) ;
#28716=CARTESIAN_POINT ( 'NONE',  ( 8.109375000614518214, 4.541064518000418104, -2.621784821874998173 ) ) ;
#28717=CARTESIAN_POINT ( 'NONE',  ( 17.84999999999999787, 0.000000000000000000, 4.999999999999998224 ) ) ;
#28718=CARTESIAN_POINT ( 'NONE',  ( 15.21562500061451750, 3.027376345333613106, -5.243569643749998122 ) ) ;
#28721=CARTESIAN_POINT ( 'NONE',  ( 10.86562500061451431, 3.027376345333611329, 5.243569643749999010 ) ) ;
#28722=CARTESIAN_POINT ( 'NONE',  ( 25.69687500061451502, 6.054752690667223547, 3.707466751127219781E-16 ) ) ;
#28724=CARTESIAN_POINT ( 'NONE',  ( 26.18437500061451573, 4.541064518000418104, 2.621784821874999949 ) ) ;
#28725=CARTESIAN_POINT ( 'NONE',  ( 8.925000000000002487, -4.330127018922194537, 2.499999999999995559 ) ) ;
#28726=CARTESIAN_POINT ( 'NONE',  ( -3.999999999999997335, 16.10000000122903430, 32.30940107675850470 ) ) ;
#28727=CARTESIAN_POINT ( 'NONE',  ( 8.100000001229034297, -2.886751345948129988, 4.999999999999997335 ) ) ;
#28728=CARTESIAN_POINT ( 'NONE',  ( 19.47187500061451360, 3.027376345333611329, 5.243569643749999010 ) ) ;
#28729=CARTESIAN_POINT ( 'NONE',  ( 13.95937500061451786, 4.541064518000418104, -2.621784821874998173 ) ) ;
#28730=CARTESIAN_POINT ( 'NONE',  ( -0.2805529113108836126, 4.994030452822313393, -33.99254504240288099 ) ) ;
#28731=VERTEX_POINT ( 'NONE', #46800 ) ;
#28732=CARTESIAN_POINT ( 'NONE',  ( 15.81562500061451537, 3.027376345333611329, 5.243569643749999010 ) ) ;
#28733=CARTESIAN_POINT ( 'NONE',  ( 25.95000000122903216, 5.773502691896255534, 3.535250795749688894E-16 ) ) ;
#28734=CARTESIAN_POINT ( 'NONE',  ( 12.83437500061451786, -4.541064518000419881, 2.621784821874995952 ) ) ;
#28735=CARTESIAN_POINT ( 'NONE',  ( 0.000000000000000000, 10.00000000000000000, -36.00000000000000000 ) ) ;
#28736=CARTESIAN_POINT ( 'NONE',  ( 16.34062500061451573, -3.027376345333614438, 5.243569643749998122 ) ) ;
#28737=EDGE_CURVE ( 'NONE', #45391, #52475, #54686, .T. ) ;
#28739=CARTESIAN_POINT ( 'NONE',  ( 25.17187500061451644, 3.027376345333613106, -5.243569643749998122 ) ) ;
#28740=CARTESIAN_POINT ( 'NONE',  ( 4.243569643749999898, 11.02812500061451750, 30.00000000000000000 ) ) ;
#28741=CARTESIAN_POINT ( 'NONE',  ( 16.17187500061451644, 3.027376345333613106, -5.243569643749998122 ) ) ;
#28742=CARTESIAN_POINT ( 'NONE',  ( 12.86250000122903359, 4.330127018922192761, -2.499999999999997780 ) ) ;
#28743=CYLINDRICAL_SURFACE ( 'NONE', #55157, 4.999999999999998224 ) ;
#28744=CARTESIAN_POINT ( 'NONE',  ( -3.000416591977282496E-16, 17.94687500061451502, -34.90005215228797653 ) ) ;
#28745=( BOUNDED_CURVE ( )  B_SPLINE_CURVE ( 2, ( #30681, #65763, #37682, #60205, #9617, #14783, #32149, #3357, #59848 ),
 .UNSPECIFIED., .F., .F. ) 
 B_SPLINE_CURVE_WITH_KNOTS ( ( 3, 2, 2, 2, 3 ),
 ( 0.7934782608695651884, 0.7971014492753623060, 0.8043478260869565410, 0.8115942028985507761, 0.8152173913043478937 ),
 .UNSPECIFIED. ) 
 CURVE ( )  GEOMETRIC_REPRESENTATION_ITEM ( )  RATIONAL_B_SPLINE_CURVE ( ( 0.9330127018922194093, 0.9330127018922194093, 1.000000000000000000, 0.8660254037844387076, 1.000000000000000000, 0.8660254037844387076, 1.000000000000000000, 0.9330127018922182991, 0.9330127018922192983 ) ) 
 REPRESENTATION_ITEM ( '' )  );
#28746=CARTESIAN_POINT ( 'NONE',  ( 17.48437500061451999, 6.421520780324663323E-16, -5.243569643749999010 ) ) ;
#28747=CARTESIAN_POINT ( 'NONE',  ( 20.85000000122903430, -2.886751345948125991, -5.000000000000000000 ) ) ;
#28748=CARTESIAN_POINT ( 'NONE',  ( 14.78437500061451715, 6.421520780324663323E-16, -5.243569643749999010 ) ) ;
#28749=CARTESIAN_POINT ( 'NONE',  ( 4.243569643749999010, 12.02187500061451786, 27.54997392385601174 ) ) ;
#28750=CARTESIAN_POINT ( 'NONE',  ( 21.48750000122903003, 4.330127018922191873, 2.499999999999999556 ) ) ;
#28751=CARTESIAN_POINT ( 'NONE',  ( 14.27812500061451573, 6.421520780324663323E-16, -5.243569643749999010 ) ) ;
#28752=CARTESIAN_POINT ( 'NONE',  ( 29.69062500061451715, 6.054752690667223547, 3.707466751127219781E-16 ) ) ;
#28753=VERTEX_POINT ( 'NONE', #1738 ) ;
#28754=ORIENTED_EDGE ( 'NONE', *, *, #23389, .T. ) ;
#28755=CARTESIAN_POINT ( 'NONE',  ( 21.15000000000000213, -4.330127018922190985, -2.500000000000001332 ) ) ;
#28756=DIRECTION ( 'NONE',  ( -1.000000000000000000, -0.000000000000000000, -0.000000000000000000 ) ) ;
#28757=CARTESIAN_POINT ( 'NONE',  ( 3.665625000614517681, 3.027376345333611329, 5.243569643749999010 ) ) ;
#28758=CARTESIAN_POINT ( 'NONE',  ( 13.87500000122903465, 2.886751345948126879, 4.999999999999999112 ) ) ;
#28759=CARTESIAN_POINT ( 'NONE',  ( 20.35312500061451502, 0.000000000000000000, 5.243569643749999010 ) ) ;
#28760=CARTESIAN_POINT ( 'NONE',  ( 23.65312500061451573, -4.541064518000417216, -2.621784821875001281 ) ) ;
#28762=CARTESIAN_POINT ( 'NONE',  ( 4.490625000614516971, 6.054752690667223547, 3.707466751127219781E-16 ) ) ;
#28763=CARTESIAN_POINT ( 'NONE',  ( 28.98750000000000071, 5.773502691896255534, 3.535250795749688894E-16 ) ) ;
#28764=CARTESIAN_POINT ( 'NONE',  ( 4.779258346327469376, 1.469247991000700582, 4.779258346327429408 ) ) ;
#28766=CARTESIAN_POINT ( 'NONE',  ( 29.55937500061451573, -4.541064518000417216, -2.621784821875001281 ) ) ;
#28767=CARTESIAN_POINT ( 'NONE',  ( -3.999999999999997335, 11.60000000122903430, -27.69059892324149175 ) ) ;
#28768=CARTESIAN_POINT ( 'NONE',  ( 4.243569643749999898, 18.28437500061451715, -30.00000000000000000 ) ) ;
#28769=CARTESIAN_POINT ( 'NONE',  ( 5.775000001229033231, 2.886751345948126879, 4.999999999999999112 ) ) ;
#28770=CARTESIAN_POINT ( 'NONE',  ( 7.650000000000000355, -4.330127018922190985, -2.500000000000001332 ) ) ;
#28771=CARTESIAN_POINT ( 'NONE',  ( 5.175000001229033586, 2.886751345948129099, -4.999999999999998224 ) ) ;
#28772=CARTESIAN_POINT ( 'NONE',  ( 11.10937500061451644, -4.541064518000417216, -2.621784821875001281 ) ) ;
#28774=CARTESIAN_POINT ( 'NONE',  ( 4.659375000614518925, 0.000000000000000000, 5.243569643749999010 ) ) ;
#28775=CARTESIAN_POINT ( 'NONE',  ( 1.071796769724490783, 19.07990381179670081, 26.00000000000000355 ) ) ;
#28776=CARTESIAN_POINT ( 'NONE',  ( 29.66250000122903074, 0.000000000000000000, 4.999999999999998224 ) ) ;
#28777=CARTESIAN_POINT ( 'NONE',  ( 11.07187500061451679, -6.054752690667223547, -1.112240025338166033E-15 ) ) ;
#28778=CARTESIAN_POINT ( 'NONE',  ( 14.78437500061451715, 6.421520780324663323E-16, -5.243569643749999010 ) ) ;
#28779=CARTESIAN_POINT ( 'NONE',  ( -2.000000000000000000, 18.57500000000000284, -33.46410161513775705 ) ) ;
#28780=CARTESIAN_POINT ( 'NONE',  ( 7.724999999999999645, 6.123233995736764310E-16, -4.999999999999998224 ) ) ;
#28781=( BOUNDED_CURVE ( )  B_SPLINE_CURVE ( 2, ( #39882, #68315, #45780, #56843, #40968, #353, #69039, #22860, #17675 ),
 .UNSPECIFIED., .F., .F. ) 
 B_SPLINE_CURVE_WITH_KNOTS ( ( 3, 2, 2, 2, 3 ),
 ( 0.01086956521739130578, 0.01449275362318840597, 0.02173913043478260809, 0.02898550724637680848, 0.03260869565217391908 ),
 .UNSPECIFIED. ) 
 CURVE ( )  GEOMETRIC_REPRESENTATION_ITEM ( )  RATIONAL_B_SPLINE_CURVE ( ( 0.9330127018922194093, 0.9330127018922194093, 1.000000000000000000, 0.8660254037844387076, 1.000000000000000000, 0.8660254037844387076, 1.000000000000000000, 0.9330127018922191873, 0.9330127018922192983 ) ) 
 REPRESENTATION_ITEM ( '' )  );
#28782=CARTESIAN_POINT ( 'NONE',  ( -3.000416591977282496E-16, 17.44062500061459176, 25.09994784771203058 ) ) ;
#28783=CARTESIAN_POINT ( 'NONE',  ( 21.75937500061451502, 0.000000000000000000, 5.243569643749999010 ) ) ;
#28784=CARTESIAN_POINT ( 'NONE',  ( 0.000000000000000000, 20.00000000000000000, -30.00000000000000000 ) ) ;
#28785=CARTESIAN_POINT ( 'NONE',  ( 26.13750000122903216, -4.330127018922194537, 2.499999999999995559 ) ) ;
#28787=CARTESIAN_POINT ( 'NONE',  ( 22.79062500061451502, -3.027376345333610441, -5.243569643749999898 ) ) ;
#28788=CARTESIAN_POINT ( 'NONE',  ( 15.29062500061451679, 6.054752690667223547, 3.707466751127219781E-16 ) ) ;
#28790=CARTESIAN_POINT ( 'NONE',  ( 12.12187500061451573, 3.027376345333613106, -5.243569643749998122 ) ) ;
#28791=CARTESIAN_POINT ( 'NONE',  ( 28.23750000000000426, -2.886751345948129988, 4.999999999999997335 ) ) ;
#28792=CARTESIAN_POINT ( 'NONE',  ( 24.60000000122903430, 5.773502691896255534, 3.535250795749688894E-16 ) ) ;
#28793=CARTESIAN_POINT ( 'NONE',  ( 3.834375000614519635, -4.541064518000419881, 2.621784821874995952 ) ) ;
#28794=CARTESIAN_POINT ( 'NONE',  ( 11.37187500061451750, 3.027376345333611329, 5.243569643749999010 ) ) ;
#28795=CARTESIAN_POINT ( 'NONE',  ( 28.20937500061451786, -4.541064518000417216, -2.621784821875001281 ) ) ;
#28796=CARTESIAN_POINT ( 'NONE',  ( 3.384375000614517237, -4.541064518000419881, 2.621784821874995952 ) ) ;
#28798=CARTESIAN_POINT ( 'NONE',  ( 21.94687500061451857, -3.027376345333610441, -5.243569643749999898 ) ) ;
#28799=CARTESIAN_POINT ( 'NONE',  ( 13.32187500061451502, -6.054752690667223547, -1.112240025338166033E-15 ) ) ;
#28801=CARTESIAN_POINT ( 'NONE',  ( 26.25000000000000000, 4.330127018922192761, -2.499999999999997780 ) ) ;
#28802=CARTESIAN_POINT ( 'NONE',  ( 4.537500001229034297, -4.330127018922194537, 2.499999999999995559 ) ) ;
#28804=CARTESIAN_POINT ( 'NONE',  ( 17.65312500061451573, 0.000000000000000000, 5.243569643749999010 ) ) ;
#28805=CARTESIAN_POINT ( 'NONE',  ( 6.899999999999999467, 4.330127018922192761, -2.499999999999997780 ) ) ;
#28806=EDGE_CURVE ( 'NONE', #41505, #27416, #3788, .T. ) ;
#28807=CARTESIAN_POINT ( 'NONE',  ( 13.46250000122903323, 0.000000000000000000, 4.999999999999998224 ) ) ;
#28808=CARTESIAN_POINT ( 'NONE',  ( 16.98750000000000426, -2.886751345948129988, 4.999999999999997335 ) ) ;
#28809=CARTESIAN_POINT ( 'NONE',  ( 4.243569643749999898, 12.37812500061451715, 30.00000000000000000 ) ) ;
#28810=( BOUNDED_CURVE ( )  B_SPLINE_CURVE ( 2, ( #35163, #28897, #57687, #34432, #28537, #5650, #68794 ),
 .UNSPECIFIED., .F., .F. ) 
 B_SPLINE_CURVE_WITH_KNOTS ( ( 3, 2, 2, 3 ),
 ( 0.5000000000000000000, 0.5027777777777777679, 0.5055555555555556468, 0.5083333333333334147 ),
 .UNSPECIFIED. ) 
 CURVE ( )  GEOMETRIC_REPRESENTATION_ITEM ( )  RATIONAL_B_SPLINE_CURVE ( ( 1.000000000000000000, 0.8660254037844387076, 1.000000000000000000, 0.8660254037844387076, 1.000000000000000000, 0.8660254037844333785, 1.000000000000005329 ) ) 
 REPRESENTATION_ITEM ( '' )  );
#28812=CARTESIAN_POINT ( 'NONE',  ( 21.56250000122903288, 0.000000000000000000, 4.999999999999998224 ) ) ;
#28813=CARTESIAN_POINT ( 'NONE',  ( 26.78437500061451360, -4.541064518000419881, 2.621784821874995952 ) ) ;
#28815=CARTESIAN_POINT ( 'NONE',  ( 22.37812500061451360, 6.421520780324663323E-16, -5.243569643749999010 ) ) ;
#28816=CARTESIAN_POINT ( 'NONE',  ( 22.20937500061451431, 0.000000000000000000, 5.243569643749999010 ) ) ;
#28817=CARTESIAN_POINT ( 'NONE',  ( 4.650000000000001243, 4.330127018922192761, -2.499999999999997780 ) ) ;
#28818=CARTESIAN_POINT ( 'NONE',  ( 6.628125000614517148, 6.421520780324663323E-16, -5.243569643749999010 ) ) ;
#28819=CARTESIAN_POINT ( 'NONE',  ( 25.26562500061451289, 3.027376345333611329, 5.243569643749999010 ) ) ;
#28820=CARTESIAN_POINT ( 'NONE',  ( 12.64687500061451608, 6.054752690667223547, 3.707466751127219781E-16 ) ) ;
#28821=CARTESIAN_POINT ( 'NONE',  ( 15.68437500061451573, 6.421520780324663323E-16, -5.243569643749999010 ) ) ;
#28822=CARTESIAN_POINT ( 'NONE',  ( 4.243569643749999010, 16.91562500061451502, 27.54997392385601174 ) ) ;
#28823=CARTESIAN_POINT ( 'NONE',  ( 21.63750000122903572, -4.330127018922194537, 2.499999999999995559 ) ) ;
#28825=CARTESIAN_POINT ( 'NONE',  ( 9.928125000614517859, 4.541064518000418104, 2.621784821874999949 ) ) ;
#28826=CARTESIAN_POINT ( 'NONE',  ( 6.309375000614517504, 4.541064518000418104, -2.621784821874998173 ) ) ;
#28827=CARTESIAN_POINT ( 'NONE',  ( 4.546875000614517326, 6.054752690667223547, 3.707466751127219781E-16 ) ) ;
#28829=CARTESIAN_POINT ( 'NONE',  ( 26.40937500061451715, -4.541064518000417216, -2.621784821875001281 ) ) ;
#28830=CARTESIAN_POINT ( 'NONE',  ( 17.54062500061451502, 6.054752690667223547, 3.707466751127219781E-16 ) ) ;
#28831=CARTESIAN_POINT ( 'NONE',  ( 28.42500000122904069, -5.773502691896255534, -1.060575238724906372E-15 ) ) ;
#28832=CARTESIAN_POINT ( 'NONE',  ( 28.07812500061451289, -4.541064518000419881, 2.621784821874995952 ) ) ;
#28833=CARTESIAN_POINT ( 'NONE',  ( 20.78437500061451715, 4.541064518000418104, 2.621784821874999949 ) ) ;
#28834=CARTESIAN_POINT ( 'NONE',  ( 16.71562500061451573, 3.027376345333611329, 5.243569643749999010 ) ) ;
#28835=CARTESIAN_POINT ( 'NONE',  ( -2.121784821874999949, 18.88437500061451857, 26.32496088578401938 ) ) ;
#28836=( BOUNDED_CURVE ( )  B_SPLINE_CURVE ( 2, ( #51922, #1319, #69992, #58164, #24556, #8301, #2396, #23828, #40477 ),
 .UNSPECIFIED., .F., .F. ) 
 B_SPLINE_CURVE_WITH_KNOTS ( ( 3, 2, 2, 2, 3 ),
 ( 0.9021739130434782705, 0.9057971014492753881, 0.9130434782608695121, 0.9202898550724637472, 0.9239130434782608647 ),
 .UNSPECIFIED. ) 
 CURVE ( )  GEOMETRIC_REPRESENTATION_ITEM ( )  RATIONAL_B_SPLINE_CURVE ( ( 0.9330127018922194093, 0.9330127018922194093, 1.000000000000000000, 0.8660254037844387076, 1.000000000000000000, 0.8660254037844387076, 1.000000000000000000, 0.9330127018922194093, 0.9330127018922194093 ) ) 
 REPRESENTATION_ITEM ( '' )  );
#28837=CARTESIAN_POINT ( 'NONE',  ( 22.19062500061451715, -3.027376345333614438, 5.243569643749998122 ) ) ;
#28839=ORIENTED_EDGE ( 'NONE', *, *, #28401, .F. ) ;
#28840=CARTESIAN_POINT ( 'NONE',  ( 26.96249999999999858, -5.773502691896255534, -1.060575238724906372E-15 ) ) ;
#28841=CARTESIAN_POINT ( 'NONE',  ( 1.999999999999998668, 13.10000000000000142, -33.46410161513775705 ) ) ;
#28843=CARTESIAN_POINT ( 'NONE',  ( 29.80312500061451431, 0.000000000000000000, 5.243569643749999010 ) ) ;
#28844=CARTESIAN_POINT ( 'NONE',  ( 9.515625000614518214, 3.027376345333611329, 5.243569643749999010 ) ) ;
#28845=CARTESIAN_POINT ( 'NONE',  ( 22.80000000122903359, 5.773502691896255534, 3.535250795749688894E-16 ) ) ;
#28846=EDGE_CURVE ( 'NONE', #2372, #65643, #22119, .T. ) ;
#28847=CARTESIAN_POINT ( 'NONE',  ( 27.74062500061451431, -3.027376345333610441, -5.243569643749999898 ) ) ;
#28848=CARTESIAN_POINT ( 'NONE',  ( 26.69999999999999929, 4.330127018922192761, -2.499999999999997780 ) ) ;
#28849=CARTESIAN_POINT ( 'NONE',  ( 4.000000000000000000, 18.05000000122903359, -27.69059892324149530 ) ) ;
#28850=CARTESIAN_POINT ( 'NONE',  ( -0.7157356635157281488, 9.902086024390941432, -34.05916648805959568 ) ) ;
#28851=CARTESIAN_POINT ( 'NONE',  ( 11.72812500061451857, 4.541064518000418104, 2.621784821874999949 ) ) ;
#28852=ORIENTED_EDGE ( 'NONE', *, *, #58732, .T. ) ;
#28853=CARTESIAN_POINT ( 'NONE',  ( 8.653125000614515727, 0.000000000000000000, 5.243569643749999010 ) ) ;
#28854=CARTESIAN_POINT ( 'NONE',  ( 7.078125000614516438, 6.421520780324663323E-16, -5.243569643749999010 ) ) ;
#28856=EDGE_CURVE ( 'NONE', #21346, #38296, #36764, .T. ) ;
#28857=CYLINDRICAL_SURFACE ( 'NONE', #42037, 3.999999999999996447 ) ;
#28858=CARTESIAN_POINT ( 'NONE',  ( 15.45000000000000107, 4.330127018922192761, -2.499999999999997780 ) ) ;
#28860=CARTESIAN_POINT ( 'NONE',  ( 15.34687500061451537, 6.054752690667223547, 3.707466751127219781E-16 ) ) ;
#28861=CARTESIAN_POINT ( 'NONE',  ( 10.31250000122903288, 0.000000000000000000, 4.999999999999998224 ) ) ;
#28862=CARTESIAN_POINT ( 'NONE',  ( 18.38437500061451857, 6.421520780324663323E-16, -5.243569643749999010 ) ) ;
#28864=CARTESIAN_POINT ( 'NONE',  ( 21.04687500061451644, -3.027376345333610441, -5.243569643749999898 ) ) ;
#28865=CARTESIAN_POINT ( 'NONE',  ( 2.121784821875001281, 13.65312500061451750, -26.32496088578401938 ) ) ;
#28866=CARTESIAN_POINT ( 'NONE',  ( 7.350000000000002309, 4.330127018922192761, -2.499999999999997780 ) ) ;
#28868=CARTESIAN_POINT ( 'NONE',  ( 20.77500000000000213, 6.123233995736764310E-16, -4.999999999999998224 ) ) ;
#28869=CARTESIAN_POINT ( 'NONE',  ( 27.17812500061451786, -4.541064518000419881, 2.621784821874995952 ) ) ;
#28870=CARTESIAN_POINT ( 'NONE',  ( 5.175000001229032698, 2.886751345948062486, -5.000000000000113687 ) ) ;
#28871=CARTESIAN_POINT ( 'NONE',  ( 29.18437500061451573, 6.421520780324663323E-16, -5.243569643749999010 ) ) ;
#28873=CARTESIAN_POINT ( 'NONE',  ( 23.96249999999999858, 2.886751345948129099, -4.999999999999998224 ) ) ;
#28874=CARTESIAN_POINT ( 'NONE',  ( 6.740625000614516082, 6.054752690667223547, 3.707466751127219781E-16 ) ) ;
#28876=CARTESIAN_POINT ( 'NONE',  ( 18.79687500061451644, -3.027376345333610441, -5.243569643749999898 ) ) ;
#28878=CARTESIAN_POINT ( 'NONE',  ( 5.053125000614517859, 0.000000000000000000, 5.243569643749999010 ) ) ;
#28879=CARTESIAN_POINT ( 'NONE',  ( 10.43437500061451750, 4.541064518000418104, 2.621784821874999949 ) ) ;
#28880=ORIENTED_EDGE ( 'NONE', *, *, #35886, .T. ) ;
#28881=CARTESIAN_POINT ( 'NONE',  ( 21.12187500061451573, 3.027376345333613106, -5.243569643749998122 ) ) ;
#28882=DIRECTION ( 'NONE',  ( -1.000000000000000000, -0.000000000000000000, -0.000000000000000000 ) ) ;
#28883=CARTESIAN_POINT ( 'NONE',  ( 27.89999999999999858, -4.330127018922190985, -2.500000000000001332 ) ) ;
#28885=CARTESIAN_POINT ( 'NONE',  ( 3.262500000000001510, 2.886751345948129099, -4.999999999999998224 ) ) ;
#28889=CARTESIAN_POINT ( 'NONE',  ( 9.712500000000002132, 2.886751345948126879, 4.999999999999999112 ) ) ;
#28891=CARTESIAN_POINT ( 'NONE',  ( 24.81562500061451715, 3.027376345333611329, 5.243569643749999010 ) ) ;
#28892=CARTESIAN_POINT ( 'NONE',  ( 14.13750000000000107, 5.773502691896255534, 3.535250795749688894E-16 ) ) ;
#28893=CARTESIAN_POINT ( 'NONE',  ( 11.10000000122903252, 5.773502691896255534, 3.535250795749688894E-16 ) ) ;
#28894=CARTESIAN_POINT ( 'NONE',  ( 7.828125000614517326, -4.541064518000419881, 2.621784821874995952 ) ) ;
#28895=CARTESIAN_POINT ( 'NONE',  ( 24.48749999999999716, 5.773502691896255534, 3.535250795749688894E-16 ) ) ;
#28896=CARTESIAN_POINT ( 'NONE',  ( 20.99062500061451431, -3.027376345333610441, -5.243569643749999898 ) ) ;
#28897=CARTESIAN_POINT ( 'NONE',  ( 16.12500000122903288, 2.886751345948126879, 4.999999999999998224 ) ) ;
#28898=CARTESIAN_POINT ( 'NONE',  ( 28.38750000122903216, -4.330127018922194537, 2.499999999999995559 ) ) ;
#28900=CARTESIAN_POINT ( 'NONE',  ( 8.212500000000000355, 2.886751345948129099, -4.999999999999998224 ) ) ;
#28901=VECTOR ( 'NONE', #29102, 1000.000000000000000 ) ;
#28903=CARTESIAN_POINT ( 'NONE',  ( 22.79062500061451502, -3.027376345333610441, -5.243569643749999898 ) ) ;
#28904=CARTESIAN_POINT ( 'NONE',  ( 3.401703127296281881, -3.664590583214551778, -3.702615937477313768 ) ) ;
#28905=CARTESIAN_POINT ( 'NONE',  ( 28.50937500061451502, 0.000000000000000000, 5.243569643749999010 ) ) ;
#28906=CARTESIAN_POINT ( 'NONE',  ( 19.62187500061451573, -6.054752690667223547, -1.112240025338166033E-15 ) ) ;
#28907=CARTESIAN_POINT ( 'NONE',  ( 16.34062500061451573, -3.027376345333614438, 5.243569643749998122 ) ) ;
#28908=CARTESIAN_POINT ( 'NONE',  ( 4.243569643749999010, 10.16562500061459673, -32.45002607614398471 ) ) ;
#28909=CARTESIAN_POINT ( 'NONE',  ( 5.015625000614518214, 3.027376345333611329, 5.243569643749999010 ) ) ;
#28911=CARTESIAN_POINT ( 'NONE',  ( 27.63750000122903216, 6.123233995736764310E-16, -4.999999999999998224 ) ) ;
#28913=CARTESIAN_POINT ( 'NONE',  ( 18.02812500061451573, 4.541064518000418104, 2.621784821874999949 ) ) ;
#28914=CYLINDRICAL_SURFACE ( 'NONE', #2062, 4.999999999999998224 ) ;
#28915=CARTESIAN_POINT ( 'NONE',  ( 3.637500001229036162, -4.330127018922194537, 2.499999999999995559 ) ) ;
#28916=CARTESIAN_POINT ( 'NONE',  ( 12.08437500061451608, 6.421520780324663323E-16, -5.243569643749999010 ) ) ;
#28917=CARTESIAN_POINT ( 'NONE',  ( 13.20937500061451786, 0.000000000000000000, 5.243569643749999010 ) ) ;
#28918=CARTESIAN_POINT ( 'NONE',  ( 21.12187500061451573, 3.027376345333613106, -5.243569643749998122 ) ) ;
#28920=CARTESIAN_POINT ( 'NONE',  ( -5.605356288733176484, 8.281802244057956841, 32.14897154774516252 ) ) ;
#28921=CARTESIAN_POINT ( 'NONE',  ( 24.77812500061451217, 4.541064518000418104, 2.621784821874999949 ) ) ;
#28922=VECTOR ( 'NONE', #34330, 1000.000000000000000 ) ;
#28923=CARTESIAN_POINT ( 'NONE',  ( 17.89687500061451431, -3.027376345333610441, -5.243569643749999898 ) ) ;
#28924=CARTESIAN_POINT ( 'NONE',  ( 24.59062500061451573, -3.027376345333610441, -5.243569643749999898 ) ) ;
#28926=CARTESIAN_POINT ( 'NONE',  ( 3.999999999999998668, 16.21250000000000213, 27.69059892324149175 ) ) ;
#28927=CARTESIAN_POINT ( 'NONE',  ( 29.27812500061451573, 4.541064518000418104, 2.621784821874999949 ) ) ;
#28928=CARTESIAN_POINT ( 'NONE',  ( 11.47500000122903252, 2.886751345948129099, -4.999999999999998224 ) ) ;
#28929=VECTOR ( 'NONE', #36443, 1000.000000000000000 ) ;
#28930=CARTESIAN_POINT ( 'NONE',  ( 7.237500001229035362, -4.330127018922194537, 2.499999999999995559 ) ) ;
#28931=CARTESIAN_POINT ( 'NONE',  ( -3.999999999999997335, 19.13750000000000284, -27.69059892324149175 ) ) ;
#28932=CARTESIAN_POINT ( 'NONE',  ( 26.62500000122903288, -5.773502691896255534, -1.060575238724906372E-15 ) ) ;
#28935=CARTESIAN_POINT ( 'NONE',  ( 8.859375000614518214, -4.541064518000417216, -2.621784821875001281 ) ) ;
#28936=CARTESIAN_POINT ( 'NONE',  ( 17.66250000000000142, 2.886751345948162850, -4.999999999999940492 ) ) ;
#28937=CARTESIAN_POINT ( 'NONE',  ( 17.99062500061451786, 6.054752690667223547, 3.707466751127219781E-16 ) ) ;
#28938=CARTESIAN_POINT ( 'NONE',  ( 10.17187500061451999, -6.054752690667223547, -1.112240025338166033E-15 ) ) ;
#28939=CARTESIAN_POINT ( 'NONE',  ( 29.58750000122903501, 4.330127018922191873, 2.499999999999999556 ) ) ;
#28940=CARTESIAN_POINT ( 'NONE',  ( 20.03437500061451715, -4.541064518000419881, 2.621784821874995952 ) ) ;
#28941=CARTESIAN_POINT ( 'NONE',  ( 7.584375000614516082, 6.421520780324663323E-16, -5.243569643749999010 ) ) ;
#28942=CARTESIAN_POINT ( 'NONE',  ( 3.553125000614516082, 4.541064518000418104, -2.621784821874998173 ) ) ;
#28943=CARTESIAN_POINT ( 'NONE',  ( 5.700000000000000178, 0.000000000000000000, 4.999999999999998224 ) ) ;
#28944=CARTESIAN_POINT ( 'NONE',  ( 9.140625000614518214, -3.027376345333614438, 5.243569643749998122 ) ) ;
#28945=CARTESIAN_POINT ( 'NONE',  ( 19.49062500061451431, -3.027376345333614438, 5.243569643749998122 ) ) ;
#28947=CARTESIAN_POINT ( 'NONE',  ( 6.262500001229034829, 0.000000000000000000, 4.999999999999998224 ) ) ;
#28948=CARTESIAN_POINT ( 'NONE',  ( 14.42812500061451786, 4.541064518000418104, 2.621784821874999949 ) ) ;
#28949=CARTESIAN_POINT ( 'NONE',  ( 13.45312500061451466, 4.541064518000418104, -2.621784821874998173 ) ) ;
#28951=CARTESIAN_POINT ( 'NONE',  ( 14.43750000000000000, -2.886751345948125991, -5.000000000000000000 ) ) ;
#28952=CARTESIAN_POINT ( 'NONE',  ( 8.887500001229033941, 4.330127018922191873, 2.499999999999999556 ) ) ;
#28953=CARTESIAN_POINT ( 'NONE',  ( 5.128125000614516260, -4.541064518000419881, 2.621784821874995952 ) ) ;
#28954=CARTESIAN_POINT ( 'NONE',  ( 17.51250000122903216, 0.000000000000000000, 4.999999999999998224 ) ) ;
#28957=CARTESIAN_POINT ( 'NONE',  ( 9.001249775931846008E-16, 10.52187500061451964, -25.09994784771203058 ) ) ;
#28958=CARTESIAN_POINT ( 'NONE',  ( 8.400000000000000355, 0.000000000000000000, 4.999999999999998224 ) ) ;
#28959=EDGE_CURVE ( 'NONE', #54151, #16881, #47128, .T. ) ;
#28960=CARTESIAN_POINT ( 'NONE',  ( 4.050000001229035362, -2.886751345948129988, 4.999999999999997335 ) ) ;
#28961=CARTESIAN_POINT ( 'NONE',  ( -1.071796769724504328, 11.54240381056766829, -26.00000000000001066 ) ) ;
#28962=CARTESIAN_POINT ( 'NONE',  ( 18.15937500061451715, 0.000000000000000000, 5.243569643749999010 ) ) ;
#28963=CARTESIAN_POINT ( 'NONE',  ( 10.72500000122903252, 2.886751345948126879, 4.999999999999998224 ) ) ;
#28965=CARTESIAN_POINT ( 'NONE',  ( 13.60312500061451679, 0.000000000000000000, 5.243569643749999010 ) ) ;
#28967=CARTESIAN_POINT ( 'NONE',  ( -5.810221930991193690E-16, 14.60000000122903252, 26.00000000000000355 ) ) ;
#28968=CARTESIAN_POINT ( 'NONE',  ( 28.84687500061452070, 6.054752690667223547, 3.707466751127219781E-16 ) ) ;
#28969=CARTESIAN_POINT ( 'NONE',  ( 26.97187500061451360, 3.027376345333613106, -5.243569643749998122 ) ) ;
#28971=CARTESIAN_POINT ( 'NONE',  ( 12.10312500061451857, 4.541064518000418104, -2.621784821874998173 ) ) ;
#28972=AXIS2_PLACEMENT_3D ( 'NONE', #58030, #12974, #68416 ) ;
#28973=CARTESIAN_POINT ( 'NONE',  ( 10.43437500061451750, 4.541064518000418104, 2.621784821874999949 ) ) ;
#28974=ORIENTED_EDGE ( 'NONE', *, *, #28669, .F. ) ;
#28975=CARTESIAN_POINT ( 'NONE',  ( 9.337499999999998579, -2.886751345948063374, 5.000000000000112799 ) ) ;
#28976=CARTESIAN_POINT ( 'NONE',  ( 19.19062500061452070, -3.027376345333610441, -5.243569643749999898 ) ) ;
#28977=CARTESIAN_POINT ( 'NONE',  ( 3.114445430177177343, 3.911558880626788248, -3.492103232390192602 ) ) ;
#28978=CARTESIAN_POINT ( 'NONE',  ( 1.999999999999998668, 14.90000000000000036, 26.53589838486224650 ) ) ;
#28979=CARTESIAN_POINT ( 'NONE',  ( 10.76250000000000107, -5.773502691896255534, -1.060575238724906372E-15 ) ) ;
#28980=CARTESIAN_POINT ( 'NONE',  ( 22.35000000122903074, 5.773502691896255534, 3.535250795749688894E-16 ) ) ;
#28981=CARTESIAN_POINT ( 'NONE',  ( 15.06562500061451537, -6.054752690667223547, -1.112240025338166033E-15 ) ) ;
#28984=CARTESIAN_POINT ( 'NONE',  ( 18.75000000000000000, 0.000000000000000000, 4.999999999999998224 ) ) ;
#28985=CARTESIAN_POINT ( 'NONE',  ( 22.57499999999999929, 6.123233995736764310E-16, -4.999999999999998224 ) ) ;
#28986=CARTESIAN_POINT ( 'NONE',  ( 19.28437500061451360, 6.421520780324663323E-16, -5.243569643749999010 ) ) ;
#28987=CARTESIAN_POINT ( 'NONE',  ( 25.45312500061451644, -4.541064518000417216, -2.621784821875001281 ) ) ;
#28988=ADVANCED_FACE ( 'NONE', ( #65231 ), #71146, .F. ) ;
#28989=EDGE_LOOP ( 'NONE', ( #602, #31448, #53821, #28974 ) ) ;
#28990=CARTESIAN_POINT ( 'NONE',  ( 27.93750000122903288, -4.330127018922194537, 2.499999999999995559 ) ) ;
#28991=CARTESIAN_POINT ( 'NONE',  ( 7.190625000614518036, 6.054752690667223547, 3.707466751127219781E-16 ) ) ;
#28993=CARTESIAN_POINT ( 'NONE',  ( 13.61250000000000071, 2.886751345948129099, -4.999999999999998224 ) ) ;
#28994=CARTESIAN_POINT ( 'NONE',  ( -4.243569643749999898, 16.65312500061451573, 30.00000000000000000 ) ) ;
#28995=CARTESIAN_POINT ( 'NONE',  ( 28.15312500061451573, -4.541064518000417216, -2.621784821875001281 ) ) ;
#28997=CARTESIAN_POINT ( 'NONE',  ( 25.73437500061451644, 4.541064518000418104, 2.621784821874999949 ) ) ;
#28999=CARTESIAN_POINT ( 'NONE',  ( 22.79062500061451502, -3.027376345333610441, -5.243569643749999898 ) ) ;
#29000=CARTESIAN_POINT ( 'NONE',  ( 25.02187500061451431, -6.054752690667223547, -1.112240025338166033E-15 ) ) ;
#29001=CARTESIAN_POINT ( 'NONE',  ( -4.243569643749999898, 19.80312500061451786, -30.00000000000000000 ) ) ;
#29002=CARTESIAN_POINT ( 'NONE',  ( 11.51250000000000107, 2.886751345948126879, 4.999999999999999112 ) ) ;
#29003=CARTESIAN_POINT ( 'NONE',  ( 9.028125000614517504, 4.541064518000418104, 2.621784821874999949 ) ) ;
#29005=CARTESIAN_POINT ( 'NONE',  ( 29.57812500061451644, 6.421520780324663323E-16, -5.243569643749999010 ) ) ;
#29006=CARTESIAN_POINT ( 'NONE',  ( 26.27812500061451573, -4.541064518000419881, 2.621784821874995952 ) ) ;
#29009=CARTESIAN_POINT ( 'NONE',  ( 18.34687500061451715, -3.027376345333610441, -5.243569643749999898 ) ) ;
#29010=CARTESIAN_POINT ( 'NONE',  ( 2.121784821875001281, 11.45937500061451786, 33.67503911421598417 ) ) ;
#29011=CARTESIAN_POINT ( 'NONE',  ( 19.09687500061451360, -3.027376345333614438, 5.243569643749998122 ) ) ;
#29012=CARTESIAN_POINT ( 'NONE',  ( 27.83437500061451786, 6.421520780324663323E-16, -5.243569643749999010 ) ) ;
#29013=CARTESIAN_POINT ( 'NONE',  ( -2.121784821874996840, 17.23437500061451999, 33.67503911421598417 ) ) ;
#29014=CARTESIAN_POINT ( 'NONE',  ( 7.153125000614518392, 4.541064518000418104, -2.621784821874998173 ) ) ;
#29015=FACE_OUTER_BOUND ( 'NONE', #63332, .T. ) ;
#29016=CARTESIAN_POINT ( 'NONE',  ( 3.721875000614518036, 3.027376345333611329, 5.243569643749999010 ) ) ;
#29017=CARTESIAN_POINT ( 'NONE',  ( 1.592000809091587073E-14, 15.95000000122903394, -34.00000000000000000 ) ) ;
#29018=AXIS2_PLACEMENT_3D ( 'NONE', #23473, #46019, #52279 ) ;
#29019=CARTESIAN_POINT ( 'NONE',  ( 6.253125000614517148, 4.541064518000418104, -2.621784821874998173 ) ) ;
#29020=CARTESIAN_POINT ( 'NONE',  ( 9.046875000614518214, 6.054752690667223547, 3.707466751127219781E-16 ) ) ;
#29021=CARTESIAN_POINT ( 'NONE',  ( 19.61250000122903359, 4.330127018922192761, -2.499999999999997780 ) ) ;
#29022=CARTESIAN_POINT ( 'NONE',  ( 6.721875000614518925, 3.027376345333613106, -5.243569643749998122 ) ) ;
#29023=CARTESIAN_POINT ( 'NONE',  ( 6.665625000614515905, 3.027376345333613106, -5.243569643749998122 ) ) ;
#29026=CARTESIAN_POINT ( 'NONE',  ( 15.53437500061451715, -4.541064518000419881, 2.621784821874995952 ) ) ;
#29029=CARTESIAN_POINT ( 'NONE',  ( 23.46562500061451573, 3.027376345333611329, 5.243569643749999010 ) ) ;
#29030=CARTESIAN_POINT ( 'NONE',  ( 10.04062500061451502, -3.027376345333614438, 5.243569643749998122 ) ) ;
#29031=CARTESIAN_POINT ( 'NONE',  ( 26.78437500061451360, -4.541064518000419881, 2.621784821874995952 ) ) ;
#29032=APPLICATION_CONTEXT ( 'automotive_design' ) ;
#29033=CARTESIAN_POINT ( 'NONE',  ( 10.04062500061451502, -3.027376345333614438, 5.243569643749998122 ) ) ;
#29034=DIRECTION ( 'NONE',  ( -1.000000000000000000, -0.000000000000000000, -0.000000000000000000 ) ) ;
#29035=CARTESIAN_POINT ( 'NONE',  ( 13.38750000122903394, 4.330127018922191873, 2.499999999999999556 ) ) ;
#29036=( BOUNDED_CURVE ( )  B_SPLINE_CURVE ( 2, ( #60756, #32698, #4630, #44883, #50423, #72949, #539 ),
 .UNSPECIFIED., .F., .F. ) 
 B_SPLINE_CURVE_WITH_KNOTS ( ( 3, 2, 2, 3 ),
 ( 0.2500000000000000000, 0.2527777777777777679, 0.2555555555555554803, 0.2583333333333333037 ),
 .UNSPECIFIED. ) 
 CURVE ( )  GEOMETRIC_REPRESENTATION_ITEM ( )  RATIONAL_B_SPLINE_CURVE ( ( 1.000000000000000000, 0.8660254037844387076, 1.000000000000000000, 0.8660254037844387076, 1.000000000000000000, 0.8660254037844413721, 0.9999999999999973355 ) ) 
 REPRESENTATION_ITEM ( '' )  );
#29037=CARTESIAN_POINT ( 'NONE',  ( 27.29062500061451502, -3.027376345333610441, -5.243569643749999898 ) ) ;
#29038=CARTESIAN_POINT ( 'NONE',  ( 9.001249775931846008E-16, 13.16562500061451857, -25.09994784771203058 ) ) ;
#29039=CARTESIAN_POINT ( 'NONE',  ( 13.80000000122903181, 5.773502691896255534, 3.535250795749688894E-16 ) ) ;
#29040=CARTESIAN_POINT ( 'NONE',  ( 11.32500000000000107, 6.123233995736764310E-16, -4.999999999999998224 ) ) ;
#29041=CARTESIAN_POINT ( 'NONE',  ( 20.42812500061451431, -4.541064518000419881, 2.621784821874995952 ) ) ;
#29042=CARTESIAN_POINT ( 'NONE',  ( 6.384375000614516793, 4.541064518000418104, 2.621784821874999949 ) ) ;
#29043=CARTESIAN_POINT ( 'NONE',  ( 19.76250000000000639, -5.773502691896255534, -1.060575238724906372E-15 ) ) ;
#29044=CARTESIAN_POINT ( 'NONE',  ( 6.937500001229033764, 6.123233995736764310E-16, -4.999999999999998224 ) ) ;
#29045=CARTESIAN_POINT ( 'NONE',  ( 16.53750000122903430, 4.330127018922191873, 2.499999999999999556 ) ) ;
#29046=CARTESIAN_POINT ( 'NONE',  ( 12.66562500061451502, 3.027376345333611329, 5.243569643749999010 ) ) ;
#29047=CARTESIAN_POINT ( 'NONE',  ( 15.14062500061451644, -3.027376345333610441, -5.243569643749999898 ) ) ;
#29048=CARTESIAN_POINT ( 'NONE',  ( 25.35000000122903074, -2.886751345948125991, -5.000000000000000000 ) ) ;
#29049=CARTESIAN_POINT ( 'NONE',  ( 20.62499999999999645, -4.330127018922194537, 2.499999999999995559 ) ) ;
#29050=CARTESIAN_POINT ( 'NONE',  ( 22.84687500061451715, -3.027376345333610441, -5.243569643749999898 ) ) ;
#29051=DIRECTION ( 'NONE',  ( -1.000000000000000000, -0.000000000000000000, -0.000000000000000000 ) ) ;
#29052=CARTESIAN_POINT ( 'NONE',  ( 10.31250000122903288, 0.000000000000000000, 4.999999999999998224 ) ) ;
#29053=CARTESIAN_POINT ( 'NONE',  ( 9.459375000614517859, 4.541064518000418104, -2.621784821874998173 ) ) ;
#29054=CARTESIAN_POINT ( 'NONE',  ( 26.22187500061451715, 3.027376345333611329, 5.243569643749999010 ) ) ;
#29055=CARTESIAN_POINT ( 'NONE',  ( 3.796875000614517326, -3.027376345333614438, 5.243569643749998122 ) ) ;
#29056=CARTESIAN_POINT ( 'NONE',  ( 22.90312500061451573, 4.541064518000418104, -2.621784821874998173 ) ) ;
#29057=CARTESIAN_POINT ( 'NONE',  ( 26.52187500061451431, 3.027376345333613106, -5.243569643749998122 ) ) ;
#29060=VECTOR ( 'NONE', #1869, 1000.000000000000000 ) ;
#29061=CARTESIAN_POINT ( 'NONE',  ( 8.446875000614518569, -3.027376345333610441, -5.243569643749999898 ) ) ;
#29063=CARTESIAN_POINT ( 'NONE',  ( 28.49062500061451431, -3.027376345333614438, 5.243569643749998122 ) ) ;
#29064=CARTESIAN_POINT ( 'NONE',  ( 7.359375000614516438, 0.000000000000000000, 5.243569643749999010 ) ) ;
#29065=CARTESIAN_POINT ( 'NONE',  ( 25.80000000000000071, 4.330127018922192761, -2.499999999999997780 ) ) ;
#29066=CARTESIAN_POINT ( 'NONE',  ( -2.121784821874996840, 9.978125000614596729, 33.67503911421598417 ) ) ;
#29067=CARTESIAN_POINT ( 'NONE',  ( 18.11250000000000071, 2.886751345948129099, -4.999999999999998224 ) ) ;
#29069=CARTESIAN_POINT ( 'NONE',  ( 28.27499999999999858, -4.330127018922194537, 2.499999999999995559 ) ) ;
#29070=CARTESIAN_POINT ( 'NONE',  ( 29.67187500061451644, 3.027376345333613106, -5.243569643749998122 ) ) ;
#29072=ORIENTED_EDGE ( 'NONE', *, *, #47483, .T. ) ;
#29073=CARTESIAN_POINT ( 'NONE',  ( 16.04062500061451857, -3.027376345333610441, -5.243569643749999898 ) ) ;
#29074=CARTESIAN_POINT ( 'NONE',  ( 5.878125000614517148, 4.541064518000418104, 2.621784821874999949 ) ) ;
#29076=CARTESIAN_POINT ( 'NONE',  ( 5.409375000614516260, 4.541064518000418104, -2.621784821874998173 ) ) ;
#29077=CARTESIAN_POINT ( 'NONE',  ( 15.03750000122903252, 6.123233995736764310E-16, -4.999999999999998224 ) ) ;
#29078=CARTESIAN_POINT ( 'NONE',  ( 21.33749999999999858, 5.773502691896255534, 3.535250795749688894E-16 ) ) ;
#29079=CARTESIAN_POINT ( 'NONE',  ( 28.87499999999999645, 6.123233995736764310E-16, -4.999999999999998224 ) ) ;
#29080=CARTESIAN_POINT ( 'NONE',  ( 5.634375000614519458, -4.541064518000419881, 2.621784821874995952 ) ) ;
#29081=CARTESIAN_POINT ( 'NONE',  ( 8.259375000614518569, 0.000000000000000000, 5.243569643749999010 ) ) ;
#29082=CARTESIAN_POINT ( 'NONE',  ( 21.04687500061451644, -3.027376345333610441, -5.243569643749999898 ) ) ;
#29083=CARTESIAN_POINT ( 'NONE',  ( 0.000000000000000000, 20.00000000000000000, -30.00000000000000000 ) ) ;
#29084=EDGE_LOOP ( 'NONE', ( #52976, #59546, #56880, #33027 ) ) ;
#29085=CARTESIAN_POINT ( 'NONE',  ( 5.071875000614519458, 3.027376345333611329, 5.243569643749999010 ) ) ;
#29086=CARTESIAN_POINT ( 'NONE',  ( 5.662500000000000533, 2.886751345948126879, 4.999999999999999112 ) ) ;
#29087=CARTESIAN_POINT ( 'NONE',  ( 6.609375000614519102, -4.541064518000417216, -2.621784821875001281 ) ) ;
#29088=CARTESIAN_POINT ( 'NONE',  ( 17.47499999999999787, -4.330127018922194537, 2.499999999999995559 ) ) ;
#29089=CARTESIAN_POINT ( 'NONE',  ( 16.49062500061451786, -3.027376345333610441, -5.243569643749999898 ) ) ;
#29091=CARTESIAN_POINT ( 'NONE',  ( 4.206670228171102366, 2.702577582867563333, 4.419125496164216571 ) ) ;
#29093=CARTESIAN_POINT ( 'NONE',  ( 9.328125000614518214, 6.421520780324663323E-16, -5.243569643749999010 ) ) ;
#29094=CARTESIAN_POINT ( 'NONE',  ( 27.83437500061451786, 6.421520780324663323E-16, -5.243569643749999010 ) ) ;
#29095=CARTESIAN_POINT ( 'NONE',  ( 0.000000000000000000, 20.00000000000000000, -30.00000000000000000 ) ) ;
#29096=CARTESIAN_POINT ( 'NONE',  ( 26.63437500061451857, 4.541064518000418104, 2.621784821874999949 ) ) ;
#29097=CARTESIAN_POINT ( 'NONE',  ( 8.324999999999999289, 4.330127018922191873, 2.499999999999999556 ) ) ;
#29098=CARTESIAN_POINT ( 'NONE',  ( 4.000000000000000000, 13.55000000122903359, 32.30940107675849049 ) ) ;
#29099=CARTESIAN_POINT ( 'NONE',  ( 6.675000001229034474, 2.886751345948126879, 4.999999999999999112 ) ) ;
#29100=CARTESIAN_POINT ( 'NONE',  ( 18.23437500061451999, -4.541064518000419881, 2.621784821874995952 ) ) ;
#29101=CARTESIAN_POINT ( 'NONE',  ( 11.25937500061451679, 4.541064518000418104, -2.621784821874998173 ) ) ;
#29102=DIRECTION ( 'NONE',  ( -1.000000000000000000, -0.000000000000000000, -0.000000000000000000 ) ) ;
#29103=EDGE_LOOP ( 'NONE', ( #11049, #57332, #66201, #62373 ) ) ;
#29104=CARTESIAN_POINT ( 'NONE',  ( 14.50312500061451537, 0.000000000000000000, 5.243569643749999010 ) ) ;
#29105=CARTESIAN_POINT ( 'NONE',  ( 25.35000000122903074, -2.886751345948125991, -5.000000000000000000 ) ) ;
#29106=CARTESIAN_POINT ( 'NONE',  ( 13.77187500061451786, -6.054752690667223547, -1.112240025338166033E-15 ) ) ;
#29109=CARTESIAN_POINT ( 'NONE',  ( 14.46562500061451750, 3.027376345333611329, 5.243569643749999010 ) ) ;
#29111=CARTESIAN_POINT ( 'NONE',  ( 25.95937500061451431, -4.541064518000417216, -2.621784821875001281 ) ) ;
#29112=CARTESIAN_POINT ( 'NONE',  ( 2.886376055866514356, -4.082748248927369872, 3.290317514273759958 ) ) ;
#29113=CARTESIAN_POINT ( 'NONE',  ( 11.58750000122903501, 4.330127018922191873, 2.499999999999999556 ) ) ;
#29116=CARTESIAN_POINT ( 'NONE',  ( 2.121784821875001281, 16.40937500061452070, -26.32496088578401938 ) ) ;
#29117=CARTESIAN_POINT ( 'NONE',  ( 17.74687500061451928, -3.027376345333614438, 5.243569643749998122 ) ) ;
#29118=CARTESIAN_POINT ( 'NONE',  ( 20.10000000122903074, 5.773502691896255534, 3.535250795749688894E-16 ) ) ;
#29119=CARTESIAN_POINT ( 'NONE',  ( 14.18437500061451750, -4.541064518000419881, 2.621784821874995952 ) ) ;
#29120=CARTESIAN_POINT ( 'NONE',  ( 2.121784821875001281, 10.55937500061451750, 33.67503911421598417 ) ) ;
#29121=CARTESIAN_POINT ( 'NONE',  ( 22.35000000122903074, 5.773502691896255534, 3.535250795749688894E-16 ) ) ;
#29123=CARTESIAN_POINT ( 'NONE',  ( 14.87812500061451537, 4.541064518000418104, 2.621784821874999949 ) ) ;
#29124=CARTESIAN_POINT ( 'NONE',  ( 29.65312500061451573, 4.541064518000418104, -2.621784821874998173 ) ) ;
#29127=CARTESIAN_POINT ( 'NONE',  ( 19.23749999999999716, -2.886751345948129988, 4.999999999999997335 ) ) ;
#29129=CARTESIAN_POINT ( 'NONE',  ( 3.780892357739493281, 3.275126314170738517, 31.33023311637936459 ) ) ;
#29130=CARTESIAN_POINT ( 'NONE',  ( 15.60000000122903607, 5.773502691896255534, 3.535250795749688894E-16 ) ) ;
#29131=CARTESIAN_POINT ( 'NONE',  ( 19.64062500061451644, -3.027376345333610441, -5.243569643749999898 ) ) ;
#29132=CARTESIAN_POINT ( 'NONE',  ( 22.00312500061451360, 4.541064518000418104, -2.621784821874998173 ) ) ;
#29133=CARTESIAN_POINT ( 'NONE',  ( 3.928125000614516527, 6.421520780324663323E-16, -5.243569643749999010 ) ) ;
#29134=CARTESIAN_POINT ( 'NONE',  ( 26.58750000000000213, -2.886751345948125991, -5.000000000000000000 ) ) ;
#29137=CARTESIAN_POINT ( 'NONE',  ( 0.000000000000000000, 20.00000000000000000, 26.00000000000000000 ) ) ;
#29138=CARTESIAN_POINT ( 'NONE',  ( -2.000000000000000000, 10.13750000122903572, -33.46410161513775705 ) ) ;
#29139=CARTESIAN_POINT ( 'NONE',  ( -4.243569643749997233, 15.39687500061451786, -27.54997392385601174 ) ) ;
#29140=CARTESIAN_POINT ( 'NONE',  ( 5.175000001229033586, 2.886751345948129099, -4.999999999999998224 ) ) ;
#29141=CARTESIAN_POINT ( 'NONE',  ( 9.375000000000001776, -4.330127018922194537, 2.499999999999995559 ) ) ;
#29142=CARTESIAN_POINT ( 'NONE',  ( 4.725000001229034297, 2.886751345948129099, -4.999999999999998224 ) ) ;
#29143=CARTESIAN_POINT ( 'NONE',  ( 8.784375000614518925, -4.541064518000419881, 2.621784821874995952 ) ) ;
#29144=CARTESIAN_POINT ( 'NONE',  ( 19.31250000122903288, 0.000000000000000000, 4.999999999999998224 ) ) ;
#29145=CARTESIAN_POINT ( 'NONE',  ( 24.71250000122903145, 0.000000000000000000, 4.999999999999998224 ) ) ;
#29146=CARTESIAN_POINT ( 'NONE',  ( -1.974232797588181931, 9.810253314282340042, -35.67951850763265043 ) ) ;
#29147=CARTESIAN_POINT ( 'NONE',  ( 17.02500000122903145, 2.886751345948161074, 4.999999999999941380 ) ) ;
#29148=ADVANCED_FACE ( 'NONE', ( #42710 ), #24031, .T. ) ;
#29149=CARTESIAN_POINT ( 'NONE',  ( 7.134375000614516793, 6.421520780324663323E-16, -5.243569643749999010 ) ) ;
#29150=CARTESIAN_POINT ( 'NONE',  ( 12.57187500061451857, 3.027376345333613106, -5.243569643749998122 ) ) ;
#29151=CARTESIAN_POINT ( 'NONE',  ( 3.525000000000000355, -4.330127018922194537, 2.499999999999995559 ) ) ;
#29152=CARTESIAN_POINT ( 'NONE',  ( 6.112499999999999822, 2.886751345948126879, 4.999999999999999112 ) ) ;
#29153=VECTOR ( 'NONE', #54208, 1000.000000000000000 ) ;
#29154=CARTESIAN_POINT ( 'NONE',  ( 4.243569643749999010, 17.36562500061459602, 27.54997392385601174 ) ) ;
#29155=CARTESIAN_POINT ( 'NONE',  ( 22.20937500061451431, 0.000000000000000000, 5.243569643749999010 ) ) ;
#29156=CARTESIAN_POINT ( 'NONE',  ( 1.626862140677534273E-15, 11.11250000000000071, -26.00000000000000355 ) ) ;
#29157=CARTESIAN_POINT ( 'NONE',  ( 25.80000000122903714, -2.886751345948125991, -5.000000000000000000 ) ) ;
#29159=CARTESIAN_POINT ( 'NONE',  ( 23.72812500061451502, 6.421520780324663323E-16, -5.243569643749999010 ) ) ;
#29160=CARTESIAN_POINT ( 'NONE',  ( 13.30312500061451786, -4.541064518000417216, -2.621784821875001281 ) ) ;
#29162=CARTESIAN_POINT ( 'NONE',  ( 12.57187500061451857, 3.027376345333613106, -5.243569643749998122 ) ) ;
#29163=CARTESIAN_POINT ( 'NONE',  ( 29.58749999999999858, -2.886751345948129988, 4.999999999999997335 ) ) ;
#29164=CARTESIAN_POINT ( 'NONE',  ( 21.67500000122903359, -5.773502691896255534, -1.060575238724906372E-15 ) ) ;
#29165=DIRECTION ( 'NONE',  ( 0.000000000000000000, 0.000000000000000000, -1.000000000000000000 ) ) ;
#29166=CARTESIAN_POINT ( 'NONE',  ( 11.40937500061451892, 0.000000000000000000, 5.243569643749999010 ) ) ;
#29167=CARTESIAN_POINT ( 'NONE',  ( 28.17187500061451644, -6.054752690667223547, -1.112240025338166033E-15 ) ) ;
#29168=CARTESIAN_POINT ( 'NONE',  ( -3.999999999999997335, 12.38750000000000107, -27.69059892324149530 ) ) ;
#29169=CARTESIAN_POINT ( 'NONE',  ( 21.79687500061451644, -3.027376345333614438, 5.243569643749998122 ) ) ;
#29170=CARTESIAN_POINT ( 'NONE',  ( 13.17187500061451999, 3.027376345333611329, 5.243569643749999010 ) ) ;
#29172=CARTESIAN_POINT ( 'NONE',  ( 25.31250000000000000, 2.886751345948129099, -4.999999999999998224 ) ) ;
#29175=CARTESIAN_POINT ( 'NONE',  ( 18.29062500061451502, -3.027376345333610441, -5.243569643749999898 ) ) ;
#29176=CARTESIAN_POINT ( 'NONE',  ( 7.462500000000001243, 2.886751345948126879, 4.999999999999999112 ) ) ;
#29177=( BOUNDED_CURVE ( )  B_SPLINE_CURVE ( 2, ( #39317, #50757, #51481, #160, #6048, #62555, #28943 ),
 .UNSPECIFIED., .F., .F. ) 
 B_SPLINE_CURVE_WITH_KNOTS ( ( 3, 2, 2, 3 ),
 ( 0.8916666666666667185, 0.8944444444444444864, 0.8972222222222223653, 0.9000000000000001332 ),
 .UNSPECIFIED. ) 
 CURVE ( )  GEOMETRIC_REPRESENTATION_ITEM ( )  RATIONAL_B_SPLINE_CURVE ( ( 1.000000000000000000, 0.8660254037844387076, 1.000000000000000000, 0.8660254037844387076, 1.000000000000000000, 0.8660254037844333785, 1.000000000000005329 ) ) 
 REPRESENTATION_ITEM ( '' )  );
#29178=CARTESIAN_POINT ( 'NONE',  ( 2.953125000614516438, -4.541064518000417216, -2.621784821875001281 ) ) ;
#29179=CARTESIAN_POINT ( 'NONE',  ( 15.07499999999999929, 4.330127018922191873, 2.499999999999999556 ) ) ;
#29180=CARTESIAN_POINT ( 'NONE',  ( 4.243569643749999898, 11.44062500061451715, 32.45002607614398471 ) ) ;
#29182=CARTESIAN_POINT ( 'NONE',  ( 26.55937500061451573, 4.541064518000418104, -2.621784821874998173 ) ) ;
#29183=ORIENTED_EDGE ( 'NONE', *, *, #57737, .T. ) ;
#29184=CARTESIAN_POINT ( 'NONE',  ( 22.86562500061451431, 3.027376345333613106, -5.243569643749998122 ) ) ;
#29185=CARTESIAN_POINT ( 'NONE',  ( 20.07187500061451857, -6.054752690667223547, -1.112240025338166033E-15 ) ) ;
#29186=CARTESIAN_POINT ( 'NONE',  ( 4.762499999999999289, 2.886751345948126879, 4.999999999999999112 ) ) ;
#29187=CARTESIAN_POINT ( 'NONE',  ( 7.040625000614517681, -3.027376345333610441, -5.243569643749999898 ) ) ;
#29188=CARTESIAN_POINT ( 'NONE',  ( 21.77812500061451928, -4.541064518000419881, 2.621784821874995952 ) ) ;
#29189=CARTESIAN_POINT ( 'NONE',  ( 11.59687500061451892, -3.027376345333610441, -5.243569643749999898 ) ) ;
#29190=CARTESIAN_POINT ( 'NONE',  ( 17.07187500061451502, 3.027376345333613106, -5.243569643749998122 ) ) ;
#29191=CARTESIAN_POINT ( 'NONE',  ( 4.243569643749999898, 16.84062500061451573, 32.45002607614398471 ) ) ;
#29192=CARTESIAN_POINT ( 'NONE',  ( 20.10000000122903074, 5.773502691896255534, 3.535250795749688894E-16 ) ) ;
#29194=CARTESIAN_POINT ( 'NONE',  ( 9.665625000614516793, -6.054752690667223547, -1.112240025338166033E-15 ) ) ;
#29195=CARTESIAN_POINT ( 'NONE',  ( 6.121875000614517504, -6.054752690667223547, -1.112240025338166033E-15 ) ) ;
#29196=CARTESIAN_POINT ( 'NONE',  ( 4.471875000614518925, 3.027376345333613106, -5.243569643749998122 ) ) ;
#29197=CARTESIAN_POINT ( 'NONE',  ( 25.24687500061451573, 6.054752690667223547, 3.707466751127219781E-16 ) ) ;
#29198=CARTESIAN_POINT ( 'NONE',  ( 16.60312500061451857, 4.541064518000418104, -2.621784821874998173 ) ) ;
#29199=CARTESIAN_POINT ( 'NONE',  ( 26.62500000122903288, -5.773502691896255534, -1.060575238724906372E-15 ) ) ;
#29200=CARTESIAN_POINT ( 'NONE',  ( 25.79062500061451502, -3.027376345333614438, 5.243569643749998122 ) ) ;
#29201=CARTESIAN_POINT ( 'NONE',  ( 22.24687500061451217, -3.027376345333614438, 5.243569643749998122 ) ) ;
#29202=CARTESIAN_POINT ( 'NONE',  ( 18.29062500061451502, -3.027376345333610441, -5.243569643749999898 ) ) ;
#29203=CARTESIAN_POINT ( 'NONE',  ( 4.243569643749999898, 16.48437500061451644, 30.00000000000000000 ) ) ;
#29204=CARTESIAN_POINT ( 'NONE',  ( 22.79062500061451502, -3.027376345333610441, -5.243569643749999898 ) ) ;
#29206=VERTEX_POINT ( 'NONE', #57003 ) ;
#29207=CARTESIAN_POINT ( 'NONE',  ( 25.38749999999999929, 5.773502691896255534, 3.535250795749688894E-16 ) ) ;
#29208=CARTESIAN_POINT ( 'NONE',  ( -3.999999999999999556, 13.21250000000000213, -32.30940107675850470 ) ) ;
#29210=CARTESIAN_POINT ( 'NONE',  ( 28.26562500061451289, 3.027376345333613106, -5.243569643749998122 ) ) ;
#29211=CARTESIAN_POINT ( 'NONE',  ( 9.178125000614517859, -4.541064518000419881, 2.621784821874995952 ) ) ;
#29212=CARTESIAN_POINT ( 'NONE',  ( 22.42500000122903359, 2.886751345948126879, 4.999999999999999112 ) ) ;
#29213=CARTESIAN_POINT ( 'NONE',  ( 28.37812500061451715, 4.541064518000418104, 2.621784821874999949 ) ) ;
#29214=CARTESIAN_POINT ( 'NONE',  ( 26.62500000000000000, 6.123233995736764310E-16, -4.999999999999998224 ) ) ;
#29215=CARTESIAN_POINT ( 'NONE',  ( -3.999999999999999556, 17.37500000122903288, -32.30940107675850470 ) ) ;
#29216=CARTESIAN_POINT ( 'NONE',  ( 25.31250000122903288, -4.330127018922190985, -2.500000000000001332 ) ) ;
#29217=CARTESIAN_POINT ( 'NONE',  ( 10.04062500061451502, -3.027376345333614438, 5.243569643749998122 ) ) ;
#29219=EDGE_CURVE ( 'NONE', #43350, #32246, #40438, .T. ) ;
#29220=CARTESIAN_POINT ( 'NONE',  ( 26.46562500061451573, 3.027376345333613106, -5.243569643749998122 ) ) ;
#29221=CARTESIAN_POINT ( 'NONE',  ( 7.753125000614518036, 0.000000000000000000, 5.243569643749999010 ) ) ;
#29222=CARTESIAN_POINT ( 'NONE',  ( 6.403125000614517504, 0.000000000000000000, 5.243569643749999010 ) ) ;
#29225=CYLINDRICAL_SURFACE ( 'NONE', #17296, 3.999999999999996447 ) ;
#29226=( BOUNDED_CURVE ( )  B_SPLINE_CURVE ( 2, ( #46414, #51230, #12426, #17236, #62671, #11708, #17593 ),
 .UNSPECIFIED., .F., .F. ) 
 B_SPLINE_CURVE_WITH_KNOTS ( ( 3, 2, 2, 3 ),
 ( 0.5166666666666666075, 0.5194444444444443754, 0.5222222222222222543, 0.5250000000000000222 ),
 .UNSPECIFIED. ) 
 CURVE ( )  GEOMETRIC_REPRESENTATION_ITEM ( )  RATIONAL_B_SPLINE_CURVE ( ( 1.000000000000005329, 0.8660254037844333785, 1.000000000000000000, 0.8660254037844387076, 1.000000000000000000, 0.8660254037844387076, 1.000000000000000000 ) ) 
 REPRESENTATION_ITEM ( '' )  );
#29227=CARTESIAN_POINT ( 'NONE',  ( 15.52500000000000036, 4.330127018922191873, 2.499999999999999556 ) ) ;
#29228=EDGE_CURVE ( 'NONE', #9597, #55622, #54263, .T. ) ;
#29229=( BOUNDED_CURVE ( )  B_SPLINE_CURVE ( 2, ( #9856, #19830, #32023, #54559, #49025 ),
 .UNSPECIFIED., .F., .F. ) 
 B_SPLINE_CURVE_WITH_KNOTS ( ( 3, 2, 3 ),
 ( 0.000000000000000000, 0.007246376811594202987, 0.01086956521739130578 ),
 .UNSPECIFIED. ) 
 CURVE ( )  GEOMETRIC_REPRESENTATION_ITEM ( )  RATIONAL_B_SPLINE_CURVE ( ( 1.000000000000000000, 0.8660254037844387076, 1.000000000000000000, 0.9330127018922192983, 0.9330127018922194093 ) ) 
 REPRESENTATION_ITEM ( '' )  );
#29230=CARTESIAN_POINT ( 'NONE',  ( 15.27187500061451786, 3.027376345333613106, -5.243569643749998122 ) ) ;
#29231=CARTESIAN_POINT ( 'NONE',  ( 11.70000000122903216, -2.886751345948129988, 4.999999999999997335 ) ) ;
#29232=CARTESIAN_POINT ( 'NONE',  ( 18.12187500061451573, 3.027376345333611329, 5.243569643749999010 ) ) ;
#29234=CARTESIAN_POINT ( 'NONE',  ( 21.87187500061451573, -6.054752690667223547, -1.112240025338166033E-15 ) ) ;
#29235=CARTESIAN_POINT ( 'NONE',  ( -2.121784821874999949, 13.42812500061451786, -33.67503911421598417 ) ) ;
#29239=CARTESIAN_POINT ( 'NONE',  ( 24.06562500061451715, -6.054752690667223547, -1.112240025338166033E-15 ) ) ;
#29240=CARTESIAN_POINT ( 'NONE',  ( 27.49687500061451217, 6.054752690667223547, 3.707466751127219781E-16 ) ) ;
#29241=CARTESIAN_POINT ( 'NONE',  ( 25.27499999999999858, 6.123233995736764310E-16, -4.999999999999998224 ) ) ;
#29243=CARTESIAN_POINT ( 'NONE',  ( 7.603125000614517681, 4.541064518000418104, -2.621784821874998173 ) ) ;
#29245=CARTESIAN_POINT ( 'NONE',  ( 19.13437500061451857, -4.541064518000419881, 2.621784821874995952 ) ) ;
#29247=CARTESIAN_POINT ( 'NONE',  ( 4.490625000614516971, 6.054752690667223547, 3.707466751127219781E-16 ) ) ;
#29248=CARTESIAN_POINT ( 'NONE',  ( 9.534375000614517148, 4.541064518000418104, 2.621784821874999949 ) ) ;
#29250=CARTESIAN_POINT ( 'NONE',  ( 18.64687500061451786, -3.027376345333614438, 5.243569643749998122 ) ) ;
#29251=CARTESIAN_POINT ( 'NONE',  ( 13.80000000122903536, 5.773502691896255534, 3.535250795749688401E-16 ) ) ;
#29252=CARTESIAN_POINT ( 'NONE',  ( 29.55000000000000071, 0.000000000000000000, 4.999999999999998224 ) ) ;
#29253=CARTESIAN_POINT ( 'NONE',  ( 3.675000000000001155, 6.123233995736764310E-16, -4.999999999999998224 ) ) ;
#29257=ORIENTED_EDGE ( 'NONE', *, *, #55418, .T. ) ;
#29258=CARTESIAN_POINT ( 'NONE',  ( 9.825000000000001066, -4.330127018922194537, 2.499999999999995559 ) ) ;
#29260=CARTESIAN_POINT ( 'NONE',  ( 24.29062500061451502, 6.054752690667223547, 3.707466751127219781E-16 ) ) ;
#29261=CARTESIAN_POINT ( 'NONE',  ( 13.46249999999999858, -5.773502691896255534, -1.060575238724906372E-15 ) ) ;
#29262=CARTESIAN_POINT ( 'NONE',  ( 10.76250000122903572, 0.000000000000000000, 4.999999999999998224 ) ) ;
#29263=CARTESIAN_POINT ( 'NONE',  ( 8.953125000614518214, 4.541064518000418104, -2.621784821874998173 ) ) ;
#29264=CARTESIAN_POINT ( 'NONE',  ( 25.05000000000000071, 0.000000000000000000, 4.999999999999998224 ) ) ;
#29265=CARTESIAN_POINT ( 'NONE',  ( 20.72812500061451502, 4.541064518000418104, 2.621784821874999949 ) ) ;
#29266=DIRECTION ( 'NONE',  ( 0.000000000000000000, 0.000000000000000000, 1.000000000000000000 ) ) ;
#29267=CARTESIAN_POINT ( 'NONE',  ( 27.41250000122903430, 0.000000000000000000, 4.999999999999998224 ) ) ;
#29269=CARTESIAN_POINT ( 'NONE',  ( 7.537500000000002309, -2.886751345948129988, 4.999999999999997335 ) ) ;
#29270=ORIENTED_EDGE ( 'NONE', *, *, #27261, .T. ) ;
#29271=CARTESIAN_POINT ( 'NONE',  ( 22.22812500061451502, -4.541064518000419881, 2.621784821874995952 ) ) ;
#29272=CARTESIAN_POINT ( 'NONE',  ( 3.303520312748406962, -3.753280843300089487, -3.373494653866986770 ) ) ;
#29273=CARTESIAN_POINT ( 'NONE',  ( 28.32187500061451502, 3.027376345333613106, -5.243569643749998122 ) ) ;
#29274=CARTESIAN_POINT ( 'NONE',  ( 18.08437500061451431, 4.541064518000418104, 2.621784821874999949 ) ) ;
#29275=CARTESIAN_POINT ( 'NONE',  ( 15.10312500061451502, -4.541064518000417216, -2.621784821875001281 ) ) ;
#29277=CARTESIAN_POINT ( 'NONE',  ( 27.33750000122903145, 4.330127018922191873, 2.499999999999999556 ) ) ;
#29279=CARTESIAN_POINT ( 'NONE',  ( 15.81562500061451537, 3.027376345333611329, 5.243569643749999010 ) ) ;
#29281=CARTESIAN_POINT ( 'NONE',  ( 2.812500001229033320, -4.330127018922190985, -2.500000000000001332 ) ) ;
#29282=CARTESIAN_POINT ( 'NONE',  ( 11.89687500061451608, -3.027376345333614438, 5.243569643749998122 ) ) ;
#29283=CARTESIAN_POINT ( 'NONE',  ( 11.93437500061451573, -4.541064518000419881, 2.621784821874995952 ) ) ;
#29284=CARTESIAN_POINT ( 'NONE',  ( 19.05937500061451928, 0.000000000000000000, 5.243569643749999010 ) ) ;
#29285=ORIENTED_EDGE ( 'NONE', *, *, #23020, .T. ) ;
#29286=CARTESIAN_POINT ( 'NONE',  ( 24.11250000122903359, 4.330127018922192761, -2.499999999999997780 ) ) ;
#29287=CARTESIAN_POINT ( 'NONE',  ( 23.76562500061451644, 3.027376345333613106, -5.243569643749998122 ) ) ;
#29288=CARTESIAN_POINT ( 'NONE',  ( 18.64687500061451786, -3.027376345333614438, 5.243569643749998122 ) ) ;
#29289=CARTESIAN_POINT ( 'NONE',  ( 24.32812500061451289, 4.541064518000418104, 2.621784821874999949 ) ) ;
#29290=CARTESIAN_POINT ( 'NONE',  ( 2.000000000000001332, 12.05000000000000249, -26.53589838486224650 ) ) ;
#29291=CARTESIAN_POINT ( 'NONE',  ( -3.999999999999997335, 14.18750000000000000, 32.30940107675850470 ) ) ;
#29292=CARTESIAN_POINT ( 'NONE',  ( 28.37812500061451715, 4.541064518000418104, 2.621784821874999949 ) ) ;
#29293=CARTESIAN_POINT ( 'NONE',  ( 10.12500000122903465, 2.886751345948129099, -4.999999999999998224 ) ) ;
#29294=CARTESIAN_POINT ( 'NONE',  ( 6.562500001229032875, 4.330127018922192761, -2.499999999999997780 ) ) ;
#29296=CARTESIAN_POINT ( 'NONE',  ( 28.20000000122903216, 5.773502691896255534, 3.535250795749688894E-16 ) ) ;
#29299=CARTESIAN_POINT ( 'NONE',  ( 8.709375000614517859, 0.000000000000000000, 5.243569643749999010 ) ) ;
#29300=CARTESIAN_POINT ( 'NONE',  ( 1.626862140677534273E-15, 15.27500000122903501, 34.00000000000000000 ) ) ;
#29301=CARTESIAN_POINT ( 'NONE',  ( 17.20312500061451644, 0.000000000000000000, 5.243569643749999010 ) ) ;
#29302=CARTESIAN_POINT ( 'NONE',  ( 11.93437500061451573, -4.541064518000419881, 2.621784821874995952 ) ) ;
#29303=CARTESIAN_POINT ( 'NONE',  ( 3.365625000614516082, -6.054752690667223547, -1.112240025338166033E-15 ) ) ;
#29304=CARTESIAN_POINT ( 'NONE',  ( 19.32187500061451857, 3.027376345333612662, -5.243569643749998122 ) ) ;
#29305=CARTESIAN_POINT ( 'NONE',  ( 7.321875000614516793, 3.027376345333611329, 5.243569643749999010 ) ) ;
#29306=CARTESIAN_POINT ( 'NONE',  ( 2.840625000614518392, -3.027376345333614438, 5.243569643749998122 ) ) ;
#29308=CARTESIAN_POINT ( 'NONE',  ( 7.415625000614516793, -6.054752690667223547, -1.112240025338166033E-15 ) ) ;
#29309=CARTESIAN_POINT ( 'NONE',  ( 17.95312500061451644, 4.541064518000418104, -2.621784821874998173 ) ) ;
#29310=EDGE_LOOP ( 'NONE', ( #21238, #37203, #55190 ) ) ;
#29311=CARTESIAN_POINT ( 'NONE',  ( 5.137500001229033941, 6.123233995736764310E-16, -4.999999999999998224 ) ) ;
#29312=CARTESIAN_POINT ( 'NONE',  ( 14.99062500061451786, -3.027376345333614438, 5.243569643749998122 ) ) ;
#29313=CARTESIAN_POINT ( 'NONE',  ( 13.41562500061451502, 3.027376345333613106, -5.243569643749998122 ) ) ;
#29315=CARTESIAN_POINT ( 'NONE',  ( 13.57500000000000107, 6.123233995736764310E-16, -4.999999999999998224 ) ) ;
#29316=CARTESIAN_POINT ( 'NONE',  ( 7.800000001229035362, -2.886751345948125991, -5.000000000000000000 ) ) ;
#29317=CARTESIAN_POINT ( 'NONE',  ( 4.678125000614516971, -4.541064518000419881, 2.621784821874995952 ) ) ;
#29318=EDGE_CURVE ( 'NONE', #32246, #35438, #19283, .T. ) ;
#29319=EDGE_CURVE ( 'NONE', #69237, #33272, #6589, .T. ) ;
#29320=CARTESIAN_POINT ( 'NONE',  ( 19.65000000122902790, 5.773502691896255534, 3.535250795749688894E-16 ) ) ;
#29322=CARTESIAN_POINT ( 'NONE',  ( -3.000416591977282496E-16, 11.19687500061451679, -34.90005215228797653 ) ) ;
#29323=CARTESIAN_POINT ( 'NONE',  ( 0.000000000000000000, 20.00000000000000000, 30.00000000000000000 ) ) ;
#29324=CARTESIAN_POINT ( 'NONE',  ( 3.825000001229032609, 2.886751345948129099, -4.999999999999998224 ) ) ;
#29326=DIRECTION ( 'NONE',  ( 0.000000000000000000, 0.000000000000000000, 1.000000000000000000 ) ) ;
#29327=CARTESIAN_POINT ( 'NONE',  ( 17.74687500061451928, -3.027376345333614438, 5.243569643749998122 ) ) ;
#29328=LINE ( 'NONE', #69220, #20929 ) ;
#29329=CARTESIAN_POINT ( 'NONE',  ( 14.69062500061451537, -3.027376345333610441, -5.243569643749999898 ) ) ;
#29331=CARTESIAN_POINT ( 'NONE',  ( 15.93750000122903110, 6.123233995736764310E-16, -4.999999999999998224 ) ) ;
#29332=CARTESIAN_POINT ( 'NONE',  ( 25.92187500061451999, -6.054752690667223547, -1.112240025338166033E-15 ) ) ;
#29334=CARTESIAN_POINT ( 'NONE',  ( 13.15312500061451750, 0.000000000000000000, 5.243569643749999010 ) ) ;
#29335=CARTESIAN_POINT ( 'NONE',  ( 15.38437500061451679, 4.541064518000418104, 2.621784821874999949 ) ) ;
#29336=ORIENTED_EDGE ( 'NONE', *, *, #9782, .T. ) ;
#29337=CARTESIAN_POINT ( 'NONE',  ( 28.52812500061451573, -4.541064518000419881, 2.621784821874995952 ) ) ;
#29338=CARTESIAN_POINT ( 'NONE',  ( 21.40312500061451573, -4.541064518000417216, -2.621784821875001281 ) ) ;
#29339=CARTESIAN_POINT ( 'NONE',  ( 29.24062500061451431, 6.054752690667223547, 3.707466751127219781E-16 ) ) ;
#29340=CARTESIAN_POINT ( 'NONE',  ( 3.999999999999999112, 15.38750000122903394, -30.00000000000000000 ) ) ;
#29341=CARTESIAN_POINT ( 'NONE',  ( 10.46249999999999858, 2.886751345948129099, -4.999999999999998224 ) ) ;
#29342=CARTESIAN_POINT ( 'NONE',  ( 20.02500000122903145, 2.886751345948129099, -4.999999999999998224 ) ) ;
#29345=ORIENTED_EDGE ( 'NONE', *, *, #24132, .F. ) ;
#29346=CARTESIAN_POINT ( 'NONE',  ( 17.81250000000000355, 2.886751345948126879, 4.999999999999999112 ) ) ;
#29347=CARTESIAN_POINT ( 'NONE',  ( 20.36249999999999716, 2.886751345948129099, -4.999999999999998224 ) ) ;
#29348=CARTESIAN_POINT ( 'NONE',  ( 18.90937500061451360, 4.541064518000418104, -2.621784821874998173 ) ) ;
#29349=CARTESIAN_POINT ( 'NONE',  ( 25.60312500061451502, 4.541064518000418104, -2.621784821874998173 ) ) ;
#29350=ORIENTED_EDGE ( 'NONE', *, *, #3296, .T. ) ;
#29352=CARTESIAN_POINT ( 'NONE',  ( 8.503125000614515372, 4.541064518000418104, -2.621784821874998173 ) ) ;
#29353=CARTESIAN_POINT ( 'NONE',  ( 3.196875000614517237, 6.054752690667223547, 3.707466751127219781E-16 ) ) ;
#29354=CARTESIAN_POINT ( 'NONE',  ( 14.69999999999999929, 0.000000000000000000, 4.999999999999998224 ) ) ;
#29355=CARTESIAN_POINT ( 'NONE',  ( 2.121784821874999061, 17.40312500061451573, 26.32496088578401583 ) ) ;
#29356=CARTESIAN_POINT ( 'NONE',  ( 29.20312500061451644, 4.541064518000418104, -2.621784821874998173 ) ) ;
#29359=CARTESIAN_POINT ( 'NONE',  ( 25.28437500061451715, 4.541064518000418104, 2.621784821874999949 ) ) ;
#29360=ORIENTED_EDGE ( 'NONE', *, *, #71944, .F. ) ;
#29361=CARTESIAN_POINT ( 'NONE',  ( 21.40312500061451573, -4.541064518000417216, -2.621784821875001281 ) ) ;
#29362=CARTESIAN_POINT ( 'NONE',  ( 23.82187500061451502, 3.027376345333613106, -5.243569643749998122 ) ) ;
#29363=EDGE_CURVE ( 'NONE', #31619, #66176, #11083, .T. ) ;
#29364=CARTESIAN_POINT ( 'NONE',  ( -4.243569643749998122, 16.69062500061459531, -27.54997392385601174 ) ) ;
#29365=CARTESIAN_POINT ( 'NONE',  ( 11.28749999999999787, -2.886751345948125991, -5.000000000000000000 ) ) ;
#29366=CARTESIAN_POINT ( 'NONE',  ( 9.290625000614515017, -3.027376345333610441, -5.243569643749999898 ) ) ;
#29367=CARTESIAN_POINT ( 'NONE',  ( 3.750000000000000000, 4.330127018922192761, -2.499999999999997780 ) ) ;
#29368=CARTESIAN_POINT ( 'NONE',  ( 24.77812500061451217, 4.541064518000418104, 2.621784821874999949 ) ) ;
#29371=CARTESIAN_POINT ( 'NONE',  ( 19.17187500061451999, -6.054752690667223547, -1.112240025338166033E-15 ) ) ;
#29372=CARTESIAN_POINT ( 'NONE',  ( 2.121784821875001281, 12.80937500061451928, 33.67503911421598417 ) ) ;
#29373=CARTESIAN_POINT ( 'NONE',  ( 20.37187500061451573, 3.027376345333611329, 5.243569643749999010 ) ) ;
#29374=CARTESIAN_POINT ( 'NONE',  ( 27.94687500061451502, 6.054752690667223547, 3.707466751127219781E-16 ) ) ;
#29375=CARTESIAN_POINT ( 'NONE',  ( 4.243569643749999010, 16.52187500061451786, 27.54997392385601174 ) ) ;
#29376=CARTESIAN_POINT ( 'NONE',  ( 7.340625000614518392, -3.027376345333614438, 5.243569643749998122 ) ) ;
#29377=CARTESIAN_POINT ( 'NONE',  ( 1.999999999999998668, 10.51250000122903572, -33.46410161513775705 ) ) ;
#29378=CARTESIAN_POINT ( 'NONE',  ( 3.459375000614519635, -4.541064518000417216, -2.621784821875001281 ) ) ;
#29379=CARTESIAN_POINT ( 'NONE',  ( 26.02500000122903145, 2.886751345948110892, 5.000000000000026645 ) ) ;
#29380=CARTESIAN_POINT ( 'NONE',  ( 4.790625000614518569, -3.027376345333610441, -5.243569643749999898 ) ) ;
#29381=CARTESIAN_POINT ( 'NONE',  ( 8.746875000614515727, -3.027376345333614438, 5.243569643749998122 ) ) ;
#29382=CARTESIAN_POINT ( 'NONE',  ( 15.63750000122903216, 4.330127018922191873, 2.499999999999999556 ) ) ;
#29383=CARTESIAN_POINT ( 'NONE',  ( 6.534375000614517148, -4.541064518000419881, 2.621784821874995952 ) ) ;
#29384=CARTESIAN_POINT ( 'NONE',  ( 6.815625000614517148, 3.027376345333611329, 5.243569643749999010 ) ) ;
#29387=CARTESIAN_POINT ( 'NONE',  ( 17.63437500061451502, 4.541064518000418104, 2.621784821874999949 ) ) ;
#29389=VERTEX_POINT ( 'NONE', #38435 ) ;
#29390=CARTESIAN_POINT ( 'NONE',  ( 25.75312500061451715, 0.000000000000000000, 5.243569643749999010 ) ) ;
#29391=CARTESIAN_POINT ( 'NONE',  ( 10.11562500061451608, -6.054752690667223547, -1.112240025338166033E-15 ) ) ;
#29392=CARTESIAN_POINT ( 'NONE',  ( 26.40937500061451715, -4.541064518000417216, -2.621784821875001281 ) ) ;
#29393=CARTESIAN_POINT ( 'NONE',  ( 9.740625000614516082, -3.027376345333610441, -5.243569643749999898 ) ) ;
#29394=LINE ( 'NONE', #34562, #62754 ) ;
#29395=CARTESIAN_POINT ( 'NONE',  ( 11.43750000122903465, 6.123233995736764310E-16, -4.999999999999998224 ) ) ;
#29396=CARTESIAN_POINT ( 'NONE',  ( 26.16562500061451502, 3.027376345333611329, 5.243569643749999010 ) ) ;
#29397=CARTESIAN_POINT ( 'NONE',  ( 4.243569643749999898, 13.69062500061451537, -27.54997392385601529 ) ) ;
#29398=CARTESIAN_POINT ( 'NONE',  ( 12.00000000122903465, 5.773502691896255534, 3.535250795749688894E-16 ) ) ;
#29399=CARTESIAN_POINT ( 'NONE',  ( 21.51562500061451644, 3.027376345333613106, -5.243569643749998122 ) ) ;
#29400=CARTESIAN_POINT ( 'NONE',  ( 12.07499999999999929, -4.330127018922194537, 2.499999999999995559 ) ) ;
#29401=CARTESIAN_POINT ( 'NONE',  ( 20.65312500061451573, 4.541064518000418104, -2.621784821874998173 ) ) ;
#29402=CARTESIAN_POINT ( 'NONE',  ( 5.296875000614517326, -3.027376345333610441, -5.243569643749999898 ) ) ;
#29403=CARTESIAN_POINT ( 'NONE',  ( 20.81250000000000000, 2.886751345948129099, -4.999999999999998224 ) ) ;
#29404=CARTESIAN_POINT ( 'NONE',  ( 7.050000001229036251, 5.773502691896255534, 3.535250795749688894E-16 ) ) ;
#29405=CARTESIAN_POINT ( 'NONE',  ( 15.15000000122903323, 5.773502691896255534, 3.535250795749688894E-16 ) ) ;
#29406=CARTESIAN_POINT ( 'NONE',  ( 12.51562500061451821, 3.027376345333613106, -5.243569643749998122 ) ) ;
#29407=CARTESIAN_POINT ( 'NONE',  ( 16.67812500061451786, 4.541064518000418104, 2.621784821874999949 ) ) ;
#29409=CARTESIAN_POINT ( 'NONE',  ( 25.80000000122903714, -2.886751345948125991, -5.000000000000000000 ) ) ;
#29410=CARTESIAN_POINT ( 'NONE',  ( 19.53749999999999432, 5.773502691896255534, 3.535250795749688894E-16 ) ) ;
#29411=CARTESIAN_POINT ( 'NONE',  ( 23.89687500061451786, 6.054752690667223547, 3.707466751127219781E-16 ) ) ;
#29413=CARTESIAN_POINT ( 'NONE',  ( 9.337500001229033231, 4.330127018922191873, 2.499999999999999556 ) ) ;
#29414=CARTESIAN_POINT ( 'NONE',  ( 7.734375000614517326, 4.541064518000418104, 2.621784821874999949 ) ) ;
#29415=CARTESIAN_POINT ( 'NONE',  ( 25.05937500061451573, -4.541064518000417216, -2.621784821875001281 ) ) ;
#29417=CARTESIAN_POINT ( 'NONE',  ( 21.66562500061451502, 3.027376345333611329, 5.243569643749999010 ) ) ;
#29418=CARTESIAN_POINT ( 'NONE',  ( 26.70937500061451431, 0.000000000000000000, 5.243569643749999010 ) ) ;
#29420=CARTESIAN_POINT ( 'NONE',  ( 8.746875000614515727, -3.027376345333614438, 5.243569643749998122 ) ) ;
#29421=CARTESIAN_POINT ( 'NONE',  ( 19.97812500061451502, -4.541064518000419881, 2.621784821874995952 ) ) ;
#29423=CARTESIAN_POINT ( 'NONE',  ( 27.74062500061451431, -3.027376345333610441, -5.243569643749999898 ) ) ;
#29424=CARTESIAN_POINT ( 'NONE',  ( 5.071875000614519458, 3.027376345333611329, 5.243569643749999010 ) ) ;
#29425=CARTESIAN_POINT ( 'NONE',  ( 22.72500000122903785, 2.886751345948162850, -4.999999999999940492 ) ) ;
#29427=CARTESIAN_POINT ( 'NONE',  ( 16.68750000000000000, -2.886751345948125991, -5.000000000000000000 ) ) ;
#29428=VERTEX_POINT ( 'NONE', #44719 ) ;
#29429=CARTESIAN_POINT ( 'NONE',  ( 24.03750000000000142, 5.773502691896255534, 3.535250795749688894E-16 ) ) ;
#29430=CARTESIAN_POINT ( 'NONE',  ( 26.33437500061451431, -4.541064518000419881, 2.621784821874995952 ) ) ;
#29431=VERTEX_POINT ( 'NONE', #16254 ) ;
#29432=CARTESIAN_POINT ( 'NONE',  ( 15.96562500061451573, -6.054752690667223547, -1.112240025338166033E-15 ) ) ;
#29433=CARTESIAN_POINT ( 'NONE',  ( 6.178125000614518747, 6.421520780324663323E-16, -5.243569643749999010 ) ) ;
#29435=CARTESIAN_POINT ( 'NONE',  ( 29.72812500061451502, 4.541064518000418104, 2.621784821874999949 ) ) ;
#29436=CARTESIAN_POINT ( 'NONE',  ( 15.45000000122903216, -2.886751345948125991, -5.000000000000000000 ) ) ;
#29437=CARTESIAN_POINT ( 'NONE',  ( 20.99999999999999645, 0.000000000000000000, 4.999999999999998224 ) ) ;
#29438=CARTESIAN_POINT ( 'NONE',  ( 28.31250000000000000, -5.773502691896255534, -1.060575238724906372E-15 ) ) ;
#29439=CARTESIAN_POINT ( 'NONE',  ( 5.559375000614517504, 0.000000000000000000, 5.243569643749999010 ) ) ;
#29440=CARTESIAN_POINT ( 'NONE',  ( 9.496875000614517504, 6.054752690667223547, 3.707466751127219781E-16 ) ) ;
#29441=CARTESIAN_POINT ( 'NONE',  ( 19.50937500061451857, 0.000000000000000000, 5.243569643749999010 ) ) ;
#29442=ORIENTED_EDGE ( 'NONE', *, *, #4248, .T. ) ;
#29443=CARTESIAN_POINT ( 'NONE',  ( 5.184375000614516615, -4.541064518000419881, 2.621784821874995952 ) ) ;
#29444=CARTESIAN_POINT ( 'NONE',  ( 3.487500000000000711, -2.886751345948129988, 4.999999999999997335 ) ) ;
#29445=CARTESIAN_POINT ( 'NONE',  ( 5.634375000614519458, -4.541064518000419881, 2.621784821874995952 ) ) ;
#29446=CARTESIAN_POINT ( 'NONE',  ( 18.78749999999999432, -2.886751345948129988, 4.999999999999997335 ) ) ;
#29447=CARTESIAN_POINT ( 'NONE',  ( 15.96562500061451573, -6.054752690667223547, -1.112240025338166033E-15 ) ) ;
#29451=CARTESIAN_POINT ( 'NONE',  ( 9.065625000614517148, 3.027376345333611329, 5.243569643749999010 ) ) ;
#29452=CARTESIAN_POINT ( 'NONE',  ( 27.08437500061451786, 4.541064518000418104, 2.621784821874999949 ) ) ;
#29453=CARTESIAN_POINT ( 'NONE',  ( 2.121784821874999061, 18.80937500061451928, 26.32496088578401583 ) ) ;
#29454=CARTESIAN_POINT ( 'NONE',  ( 27.19687500061451857, -3.027376345333614438, 5.243569643749998122 ) ) ;
#29455=CARTESIAN_POINT ( 'NONE',  ( 7.912499999999999645, 2.886751345948126879, 4.999999999999999112 ) ) ;
#29456=CARTESIAN_POINT ( 'NONE',  ( 3.999999999999999112, 12.23750000122903359, 30.00000000000000000 ) ) ;
#29457=CARTESIAN_POINT ( 'NONE',  ( 15.77812500061451573, 4.541064518000418104, 2.621784821874999949 ) ) ;
#29458=CARTESIAN_POINT ( 'NONE',  ( 7.350000001229033408, -2.886751345948125991, -5.000000000000000000 ) ) ;
#29460=CARTESIAN_POINT ( 'NONE',  ( 18.27187500061451431, -6.054752690667223547, -1.112240025338166033E-15 ) ) ;
#29461=CARTESIAN_POINT ( 'NONE',  ( 11.67187500061451821, 3.027376345333613106, -5.243569643749998122 ) ) ;
#29462=CARTESIAN_POINT ( 'NONE',  ( -2.506492529888154408, 4.347006505069263227, -33.15646410307740410 ) ) ;
#29464=CARTESIAN_POINT ( 'NONE',  ( 12.74062500061451786, -3.027376345333614438, 5.243569643749998122 ) ) ;
#29465=CARTESIAN_POINT ( 'NONE',  ( 24.93750000122903288, 6.123233995736764310E-16, -4.999999999999998224 ) ) ;
#29466=CARTESIAN_POINT ( 'NONE',  ( 13.17187500061451999, 3.027376345333611329, 5.243569643749999010 ) ) ;
#29468=CARTESIAN_POINT ( 'NONE',  ( 15.74062500061451608, 6.054752690667223547, 3.707466751127219781E-16 ) ) ;
#29470=CARTESIAN_POINT ( 'NONE',  ( 23.70937500061451786, -4.541064518000417216, -2.621784821875001281 ) ) ;
#29471=DIRECTION ( 'NONE',  ( 0.000000000000000000, 0.000000000000000000, -1.000000000000000000 ) ) ;
#29472=CARTESIAN_POINT ( 'NONE',  ( 11.73750000122903181, -4.330127018922194537, 2.499999999999995559 ) ) ;
#29475=CARTESIAN_POINT ( 'NONE',  ( -3.000416591977282496E-16, 17.04687500061451999, -34.90005215228797653 ) ) ;
#29476=CARTESIAN_POINT ( 'NONE',  ( 17.63437500061451502, 4.541064518000418104, 2.621784821874999949 ) ) ;
#29477=CARTESIAN_POINT ( 'NONE',  ( 18.78750000122903430, 4.330127018922191873, 2.499999999999999556 ) ) ;
#29478=CARTESIAN_POINT ( 'NONE',  ( 13.47187500061451537, 3.027376345333613106, -5.243569643749998122 ) ) ;
#29479=ADVANCED_FACE ( 'NONE', ( #66508 ), #61325, .F. ) ;
#29480=CARTESIAN_POINT ( 'NONE',  ( -3.000416591977282496E-16, 10.74687500061451928, 25.09994784771203058 ) ) ;
#29481=CARTESIAN_POINT ( 'NONE',  ( 20.58750000122903145, 4.330127018922191873, 2.499999999999999556 ) ) ;
#29482=CARTESIAN_POINT ( 'NONE',  ( 14.24062500061451608, -3.027376345333610441, -5.243569643749999898 ) ) ;
#29484=VERTEX_POINT ( 'NONE', #55793 ) ;
#29485=CARTESIAN_POINT ( 'NONE',  ( 18.11250000000000071, 2.886751345948129099, -4.999999999999998224 ) ) ;
#29486=CARTESIAN_POINT ( 'NONE',  ( 3.590625000614518836, 6.054752690667223547, 3.707466751127219781E-16 ) ) ;
#29487=CARTESIAN_POINT ( 'NONE',  ( 14.32500000122903394, 2.886751345948126879, 4.999999999999999112 ) ) ;
#29488=CARTESIAN_POINT ( 'NONE',  ( 26.89687500061451431, -3.027376345333610441, -5.243569643749999898 ) ) ;
#29489=CARTESIAN_POINT ( 'NONE',  ( 20.05312500061451431, -4.541064518000417216, -2.621784821875001281 ) ) ;
#29490=CARTESIAN_POINT ( 'NONE',  ( 23.69062500061451004, -3.027376345333610441, -5.243569643749999898 ) ) ;
#29491=CARTESIAN_POINT ( 'NONE',  ( 3.028125000614518392, 6.421520780324663323E-16, -5.243569643749999010 ) ) ;
#29492=EDGE_CURVE ( 'NONE', #15264, #21571, #33611, .T. ) ;
#29493=CARTESIAN_POINT ( 'NONE',  ( 26.51249999999999929, -5.773502691896255534, -1.060575238724906372E-15 ) ) ;
#29494=CARTESIAN_POINT ( 'NONE',  ( 4.650000000000001243, 4.330127018922192761, -2.499999999999997780 ) ) ;
#29496=DIRECTION ( 'NONE',  ( -0.000000000000000000, -1.000000000000000000, -0.000000000000000000 ) ) ;
#29498=CARTESIAN_POINT ( 'NONE',  ( 9.001249775931846008E-16, 15.92187500061451821, -25.09994784771203058 ) ) ;
#29499=CARTESIAN_POINT ( 'NONE',  ( 5.475000001229035185, -5.773502691896255534, -1.060575238724906372E-15 ) ) ;
#29500=CARTESIAN_POINT ( 'NONE',  ( 5.287500000000000533, -2.886751345948129988, 4.999999999999997335 ) ) ;
#29501=ADVANCED_FACE ( 'NONE', ( #39532 ), #67969, .F. ) ;
#29502=CARTESIAN_POINT ( 'NONE',  ( 4.125000001229034652, -5.773502691896255534, -1.060575238724906372E-15 ) ) ;
#29503=CARTESIAN_POINT ( 'NONE',  ( 8.746875000614515727, -3.027376345333614438, 5.243569643749998122 ) ) ;
#29504=CARTESIAN_POINT ( 'NONE',  ( 28.41562500061451502, 3.027376345333611329, 5.243569643749999010 ) ) ;
#29505=CARTESIAN_POINT ( 'NONE',  ( 4.000000000000000000, 10.73750000000000071, 32.30940107675849760 ) ) ;
#29506=CARTESIAN_POINT ( 'NONE',  ( 5.475000001229035185, -5.773502691896255534, -1.060575238724906372E-15 ) ) ;
#29508=CARTESIAN_POINT ( 'NONE',  ( 7.584375000614516082, 6.421520780324663323E-16, -5.243569643749999010 ) ) ;
#29509=CARTESIAN_POINT ( 'NONE',  ( 11.03437500061451715, -4.541064518000419881, 2.621784821874995952 ) ) ;
#29510=CARTESIAN_POINT ( 'NONE',  ( 6.524999999999999467, 4.330127018922191873, 2.499999999999999556 ) ) ;
#29511=CARTESIAN_POINT ( 'NONE',  ( 2.121784821875001281, 15.45312500061459460, 33.67503911421598417 ) ) ;
#29512=CARTESIAN_POINT ( 'NONE',  ( 21.68437500061451573, 4.541064518000418104, 2.621784821874999949 ) ) ;
#29514=CARTESIAN_POINT ( 'NONE',  ( 5.700000000000000178, 0.000000000000000000, 4.999999999999998224 ) ) ;
#29515=CARTESIAN_POINT ( 'NONE',  ( 27.41250000122903430, 0.000000000000000000, 4.999999999999998224 ) ) ;
#29517=CARTESIAN_POINT ( 'NONE',  ( 23.50312500061451360, 0.000000000000000000, 5.243569643749999010 ) ) ;
#29518=CARTESIAN_POINT ( 'NONE',  ( 11.95312500061451644, -4.541064518000417216, -2.621784821875001281 ) ) ;
#29520=CARTESIAN_POINT ( 'NONE',  ( 12.45937500061451786, -4.541064518000417216, -2.621784821875001281 ) ) ;
#29521=CARTESIAN_POINT ( 'NONE',  ( 28.98750000000000071, 5.773502691896255534, 3.535250795749688894E-16 ) ) ;
#29522=CARTESIAN_POINT ( 'NONE',  ( 22.05000000122903714, -2.886751345948129988, 4.999999999999997335 ) ) ;
#29524=CARTESIAN_POINT ( 'NONE',  ( 10.65937500061451715, -4.541064518000417216, -2.621784821875001281 ) ) ;
#29525=CARTESIAN_POINT ( 'NONE',  ( 29.52187500061451431, -6.054752690667223547, -1.112240025338166033E-15 ) ) ;
#29526=CARTESIAN_POINT ( 'NONE',  ( 2.896875000614518747, -3.027376345333614438, 5.243569643749998122 ) ) ;
#29527=DIRECTION ( 'NONE',  ( 0.000000000000000000, 0.000000000000000000, 1.000000000000000000 ) ) ;
#29528=CARTESIAN_POINT ( 'NONE',  ( 23.14687500061451786, -3.027376345333614438, 5.243569643749998122 ) ) ;
#29529=CARTESIAN_POINT ( 'NONE',  ( 14.48437500061451821, 4.541064518000418104, 2.621784821874999949 ) ) ;
#29531=CARTESIAN_POINT ( 'NONE',  ( 26.77499999999999858, 4.330127018922191873, 2.499999999999999556 ) ) ;
#29534=CARTESIAN_POINT ( 'NONE',  ( 17.12812500061451715, 4.541064518000418104, 2.621784821874999949 ) ) ;
#29535=CARTESIAN_POINT ( 'NONE',  ( 7.500000000000000000, 0.000000000000000000, 4.999999999999998224 ) ) ;
#29536=CARTESIAN_POINT ( 'NONE',  ( 12.15000000122903145, -2.886751345948063374, 5.000000000000112799 ) ) ;
#29537=CARTESIAN_POINT ( 'NONE',  ( 15.26249999999999929, -5.773502691896255534, -1.060575238724906372E-15 ) ) ;
#29538=CARTESIAN_POINT ( 'NONE',  ( 9.001249775931846008E-16, 10.46562500061451928, 34.90005215228797653 ) ) ;
#29540=CARTESIAN_POINT ( 'NONE',  ( 25.69687500061451502, 6.054752690667223547, 3.707466751127219781E-16 ) ) ;
#29541=VERTEX_POINT ( 'NONE', #19 ) ;
#29542=CARTESIAN_POINT ( 'NONE',  ( 20.27812500061451573, 4.541064518000418104, 2.621784821874999949 ) ) ;
#29543=CARTESIAN_POINT ( 'NONE',  ( 20.70937500061451786, 4.541064518000418104, -2.621784821874998173 ) ) ;
#29544=CARTESIAN_POINT ( 'NONE',  ( 3.187500000000002220, -2.886751345948125991, -5.000000000000000000 ) ) ;
#29545=CARTESIAN_POINT ( 'NONE',  ( 7.603125000614517681, 4.541064518000418104, -2.621784821874998173 ) ) ;
#29546=CARTESIAN_POINT ( 'NONE',  ( 20.80312500061451431, 0.000000000000000000, 5.243569643749999010 ) ) ;
#29547=CARTESIAN_POINT ( 'NONE',  ( 12.30937500061451573, 0.000000000000000000, 5.243569643749999010 ) ) ;
#29548=CARTESIAN_POINT ( 'NONE',  ( 16.39687500061451786, -3.027376345333614438, 5.243569643749998122 ) ) ;
#29549=CARTESIAN_POINT ( 'NONE',  ( -2.121784821874999949, 16.57812500061451644, 26.32496088578401938 ) ) ;
#29550=CARTESIAN_POINT ( 'NONE',  ( 20.17500000122903359, 2.886751345948126879, 4.999999999999999112 ) ) ;
#29552=CARTESIAN_POINT ( 'NONE',  ( 8.653125000614515727, 0.000000000000000000, 5.243569643749999010 ) ) ;
#29553=CARTESIAN_POINT ( 'NONE',  ( 3.384375000614517237, -4.541064518000419881, 2.621784821874995952 ) ) ;
#29554=CARTESIAN_POINT ( 'NONE',  ( 4.959375000614516971, 4.541064518000418104, -2.621784821874998173 ) ) ;
#29555=CARTESIAN_POINT ( 'NONE',  ( 26.29687500061451644, -3.027376345333614438, 5.243569643749998122 ) ) ;
#29556=CARTESIAN_POINT ( 'NONE',  ( 17.87812500061451715, 6.421520780324663323E-16, -5.243569643749999010 ) ) ;
#29557=CARTESIAN_POINT ( 'NONE',  ( 26.17500000122903359, -5.773502691896255534, -1.060575238724906372E-15 ) ) ;
#29558=CARTESIAN_POINT ( 'NONE',  ( 25.04062500061451502, -3.027376345333610441, -5.243569643749999898 ) ) ;
#29559=CARTESIAN_POINT ( 'NONE',  ( 21.72187500061451715, 3.027376345333611329, 5.243569643749999010 ) ) ;
#29560=CARTESIAN_POINT ( 'NONE',  ( 17.20312500061451644, 0.000000000000000000, 5.243569643749999010 ) ) ;
#29561=CARTESIAN_POINT ( 'NONE',  ( 4.243569643749999898, 17.34687500061451715, 32.45002607614398471 ) ) ;
#29562=CARTESIAN_POINT ( 'NONE',  ( 23.12812500061451360, -4.541064518000419881, 2.621784821874995952 ) ) ;
#29563=LINE ( 'NONE', #12207, #52669 ) ;
#29565=CARTESIAN_POINT ( 'NONE',  ( 25.34999999999999787, 4.330127018922192761, -2.499999999999997780 ) ) ;
#29566=CARTESIAN_POINT ( 'NONE',  ( 3.999999999999999112, 13.92500000000000071, -30.00000000000000000 ) ) ;
#29569=CARTESIAN_POINT ( 'NONE',  ( 3.459375000614519635, -4.541064518000417216, -2.621784821875001281 ) ) ;
#29570=CARTESIAN_POINT ( 'NONE',  ( 9.703125000614514661, -4.541064518000417216, -2.621784821875001281 ) ) ;
#29571=CARTESIAN_POINT ( 'NONE',  ( 23.25000000122903288, 5.773502691896255534, 3.535250795749688894E-16 ) ) ;
#29572=CARTESIAN_POINT ( 'NONE',  ( 26.65312500061451573, 0.000000000000000000, 5.243569643749999010 ) ) ;
#29573=CARTESIAN_POINT ( 'NONE',  ( 24.89999999999999858, 4.330127018922192761, -2.499999999999997780 ) ) ;
#29574=CARTESIAN_POINT ( 'NONE',  ( -3.999999999999997335, 16.10000000122903430, -27.69059892324149175 ) ) ;
#29575=CARTESIAN_POINT ( 'NONE',  ( 29.42812500061451431, -4.541064518000419881, 2.621784821874995952 ) ) ;
#29576=CARTESIAN_POINT ( 'NONE',  ( 9.853125000614516793, 4.541064518000418104, -2.621784821874998173 ) ) ;
#29577=ORIENTED_EDGE ( 'NONE', *, *, #15596, .T. ) ;
#29578=EDGE_CURVE ( 'NONE', #8958, #17518, #62241, .T. ) ;
#29579=CARTESIAN_POINT ( 'NONE',  ( 25.26562500061451289, 3.027376345333611329, 5.243569643749999010 ) ) ;
#29580=CARTESIAN_POINT ( 'NONE',  ( 7.603125000614517681, 4.541064518000418104, -2.621784821874998173 ) ) ;
#29581=CARTESIAN_POINT ( 'NONE',  ( 5.803125000614517859, 4.541064518000418104, -2.621784821874998173 ) ) ;
#29583=CARTESIAN_POINT ( 'NONE',  ( 4.635052905075760954, -1.875242991712875451, 4.896808582233176388 ) ) ;
#29584=CARTESIAN_POINT ( 'NONE',  ( 13.31250000000000178, 2.886751345948126879, 4.999999999999999112 ) ) ;
#29585=CARTESIAN_POINT ( 'NONE',  ( 14.67187500061451821, -6.054752690667223547, -1.112240025338166033E-15 ) ) ;
#29586=CARTESIAN_POINT ( 'NONE',  ( 10.23750000122903359, 4.330127018922191873, 2.499999999999999556 ) ) ;
#29587=CARTESIAN_POINT ( 'NONE',  ( 17.55937500061451573, 4.541064518000418104, -2.621784821874998173 ) ) ;
#29589=CARTESIAN_POINT ( 'NONE',  ( 8.146875000614516082, 6.054752690667223547, 3.707466751127219781E-16 ) ) ;
#29590=CARTESIAN_POINT ( 'NONE',  ( -4.243569643749999898, 10.76562500061451644, -32.45002607614398471 ) ) ;
#29593=ORIENTED_EDGE ( 'NONE', *, *, #21830, .F. ) ;
#29594=CARTESIAN_POINT ( 'NONE',  ( 24.55312500061451786, -4.541064518000417216, -2.621784821875001281 ) ) ;
#29596=CARTESIAN_POINT ( 'NONE',  ( 29.33437500061451431, 4.541064518000418104, 2.621784821874999949 ) ) ;
#29597=( BOUNDED_CURVE ( )  B_SPLINE_CURVE ( 2, ( #2923, #60153, #43188, #25453, #71250, #65708, #37630, #24716, #30267 ),
 .UNSPECIFIED., .F., .F. ) 
 B_SPLINE_CURVE_WITH_KNOTS ( ( 3, 2, 2, 2, 3 ),
 ( 0.3369565217391304324, 0.3405797101449275499, 0.3478260869565217295, 0.3550724637681159646, 0.3586956521739130821 ),
 .UNSPECIFIED. ) 
 CURVE ( )  GEOMETRIC_REPRESENTATION_ITEM ( )  RATIONAL_B_SPLINE_CURVE ( ( 0.9330127018922194093, 0.9330127018922194093, 1.000000000000000000, 0.8660254037844387076, 1.000000000000000000, 0.8660254037844387076, 1.000000000000000000, 0.9330127018922188542, 0.9330127018922194093 ) ) 
 REPRESENTATION_ITEM ( '' )  );
#29598=CARTESIAN_POINT ( 'NONE',  ( 24.75000000000000000, -4.330127018922190985, -2.500000000000001332 ) ) ;
#29599=CARTESIAN_POINT ( 'NONE',  ( 7.190625000614518036, 6.054752690667223547, 3.707466751127219781E-16 ) ) ;
#29601=CARTESIAN_POINT ( 'NONE',  ( 18.83437500061451431, 6.421520780324663323E-16, -5.243569643749999010 ) ) ;
#29603=CARTESIAN_POINT ( 'NONE',  ( 28.57500000122903572, 2.886751345948129099, -4.999999999999998224 ) ) ;
#29604=CARTESIAN_POINT ( 'NONE',  ( 7.884375000614517681, -4.541064518000419881, 2.621784821874995952 ) ) ;
#29605=ORIENTED_EDGE ( 'NONE', *, *, #3025, .T. ) ;
#29606=CARTESIAN_POINT ( 'NONE',  ( 18.42187500061451644, 3.027376345333613106, -5.243569643749998122 ) ) ;
#29608=CARTESIAN_POINT ( 'NONE',  ( 26.96249999999999858, -5.773502691896255534, -1.060575238724906372E-15 ) ) ;
#29609=CARTESIAN_POINT ( 'NONE',  ( 29.03437500061451715, -4.541064518000419881, 2.621784821874995952 ) ) ;
#29610=CARTESIAN_POINT ( 'NONE',  ( -5.810221930991193690E-16, 10.43750000000000000, -34.00000000000000000 ) ) ;
#29613=CARTESIAN_POINT ( 'NONE',  ( 9.412499999999999645, -5.773502691896255534, -1.060575238724906372E-15 ) ) ;
#29615=CARTESIAN_POINT ( 'NONE',  ( 24.62812500061451715, 6.421520780324663323E-16, -5.243569643749999010 ) ) ;
#29616=CARTESIAN_POINT ( 'NONE',  ( 13.95000000000000107, -4.330127018922190985, -2.500000000000001332 ) ) ;
#29617=CARTESIAN_POINT ( 'NONE',  ( 8.025000001229035007, 2.886751345948126879, 4.999999999999999112 ) ) ;
#29618=CARTESIAN_POINT ( 'NONE',  ( 7.115625000614516082, 3.027376345333613106, -5.243569643749998122 ) ) ;
#29619=CARTESIAN_POINT ( 'NONE',  ( 21.44999999999999929, 0.000000000000000000, 4.999999999999998224 ) ) ;
#29620=EDGE_CURVE ( 'NONE', #33795, #52020, #11338, .T. ) ;
#29621=CARTESIAN_POINT ( 'NONE',  ( 19.79062500061451502, 6.054752690667223547, 3.707466751127219781E-16 ) ) ;
#29622=CARTESIAN_POINT ( 'NONE',  ( 26.36250000122903003, 4.330127018922192761, -2.499999999999997780 ) ) ;
#29624=CARTESIAN_POINT ( 'NONE',  ( 4.837500000000001243, -2.886751345948129988, 4.999999999999997335 ) ) ;
#29625=ORIENTED_EDGE ( 'NONE', *, *, #5562, .T. ) ;
#29626=CARTESIAN_POINT ( 'NONE',  ( 21.36562500061451431, -6.054752690667223547, -1.112240025338166033E-15 ) ) ;
#29627=CARTESIAN_POINT ( 'NONE',  ( 3.275492200589926739, -3.777717676570560901, -3.275492200590059078 ) ) ;
#29628=CARTESIAN_POINT ( 'NONE',  ( 28.24687500061451573, -3.027376345333610441, -5.243569643749999898 ) ) ;
#29629=CARTESIAN_POINT ( 'NONE',  ( 18.83437500061451431, 6.421520780324663323E-16, -5.243569643749999010 ) ) ;
#29630=CARTESIAN_POINT ( 'NONE',  ( 14.84062500061451750, 6.054752690667223547, 3.707466751127219781E-16 ) ) ;
#29631=CARTESIAN_POINT ( 'NONE',  ( 2.121784821874999061, 10.20312500061459460, -33.67503911421598417 ) ) ;
#29632=CARTESIAN_POINT ( 'NONE',  ( 26.02500000122903145, 2.886751345948126879, 4.999999999999999112 ) ) ;
#29634=CARTESIAN_POINT ( 'NONE',  ( 17.01562500061451644, 3.027376345333612662, -5.243569643749998122 ) ) ;
#29635=CARTESIAN_POINT ( 'NONE',  ( 1.071796769724488119, 18.33259618943233704, -26.00000000000000000 ) ) ;
#29636=CARTESIAN_POINT ( 'NONE',  ( 4.350000001229033408, 5.773502691896255534, 3.535250795749688894E-16 ) ) ;
#29637=CARTESIAN_POINT ( 'NONE',  ( 13.32187500061451502, -6.054752690667223547, -1.112240025338166033E-15 ) ) ;
#29638=CARTESIAN_POINT ( 'NONE',  ( 12.72187500061451537, 3.027376345333611329, 5.243569643749999010 ) ) ;
#29639=CARTESIAN_POINT ( 'NONE',  ( 19.92187500061451644, 3.027376345333611329, 5.243569643749999010 ) ) ;
#29640=ORIENTED_EDGE ( 'NONE', *, *, #49317, .F. ) ;
#29641=CARTESIAN_POINT ( 'NONE',  ( 9.787499999999999645, -2.886751345948130876, 4.999999999999996447 ) ) ;
#29642=CARTESIAN_POINT ( 'NONE',  ( 23.72812500061451502, 6.421520780324663323E-16, -5.243569643749999010 ) ) ;
#29643=CARTESIAN_POINT ( 'NONE',  ( 19.69687500061451857, -3.027376345333610441, -5.243569643749999898 ) ) ;
#29644=CARTESIAN_POINT ( 'NONE',  ( 25.15312500061451217, 4.541064518000418104, -2.621784821874998173 ) ) ;
#29645=CARTESIAN_POINT ( 'NONE',  ( 3.999999999999999112, 18.98750000122903359, -30.00000000000000000 ) ) ;
#29646=CARTESIAN_POINT ( 'NONE',  ( 3.999999999999999112, 15.27500000000000036, 30.00000000000000000 ) ) ;
#29647=CARTESIAN_POINT ( 'NONE',  ( 3.534375000614518036, 6.421520780324663323E-16, -5.243569643749999010 ) ) ;
#29648=CARTESIAN_POINT ( 'NONE',  ( 8.925000001229033586, 2.886751345948126879, 4.999999999999999112 ) ) ;
#29649=CARTESIAN_POINT ( 'NONE',  ( 5.212500001229032343, 4.330127018922192761, -2.499999999999997780 ) ) ;
#29651=CARTESIAN_POINT ( 'NONE',  ( 28.12500000122902932, 2.886751345948129099, -4.999999999999998224 ) ) ;
#29653=ADVANCED_FACE ( 'NONE', ( #36101 ), #12485, .F. ) ;
#29654=CARTESIAN_POINT ( 'NONE',  ( 10.17187500061451999, -6.054752690667223547, -1.112240025338166033E-15 ) ) ;
#29656=CARTESIAN_POINT ( 'NONE',  ( 16.90312500061451573, -4.541064518000417216, -2.621784821875001281 ) ) ;
#29657=CARTESIAN_POINT ( 'NONE',  ( 10.92187500061451644, 3.027376345333611329, 5.243569643749999010 ) ) ;
#29658=CARTESIAN_POINT ( 'NONE',  ( 28.46250000122903145, -4.330127018922190985, -2.500000000000001332 ) ) ;
#29659=CARTESIAN_POINT ( 'NONE',  ( 18.72187500061451360, -6.054752690667223547, -1.112240025338166033E-15 ) ) ;
#29660=CARTESIAN_POINT ( 'NONE',  ( 7.921875000614517326, -6.054752690667223547, -1.112240025338166033E-15 ) ) ;
#29661=CARTESIAN_POINT ( 'NONE',  ( 2.915625000614516793, -6.054752690667223547, -1.112240025338166033E-15 ) ) ;
#29662=CARTESIAN_POINT ( 'NONE',  ( 11.70000000122903216, -2.886751345948130876, 4.999999999999996447 ) ) ;
#29663=CARTESIAN_POINT ( 'NONE',  ( 7.978125000614517681, 6.421520780324663323E-16, -5.243569643749999010 ) ) ;
#29664=( BOUNDED_CURVE ( )  B_SPLINE_CURVE ( 2, ( #23559, #25010, #19456, #42016, #47552, #64537, #23919 ),
 .UNSPECIFIED., .F., .F. ) 
 B_SPLINE_CURVE_WITH_KNOTS ( ( 3, 2, 2, 3 ),
 ( 0.3333333333333333703, 0.3361111111111111382, 0.3388888888888889062, 0.3416666666666666186 ),
 .UNSPECIFIED. ) 
 CURVE ( )  GEOMETRIC_REPRESENTATION_ITEM ( )  RATIONAL_B_SPLINE_CURVE ( ( 0.9999999999999973355, 0.8660254037844413721, 1.000000000000000000, 0.8660254037844387076, 1.000000000000000000, 0.8660254037844413721, 0.9999999999999973355 ) ) 
 REPRESENTATION_ITEM ( '' )  );
#29665=CARTESIAN_POINT ( 'NONE',  ( 17.24062500061451786, -3.027376345333614438, 5.243569643749998122 ) ) ;
#29667=CARTESIAN_POINT ( 'NONE',  ( 5.287500001229035185, 4.330127018922191873, 2.499999999999999556 ) ) ;
#29668=CARTESIAN_POINT ( 'NONE',  ( 13.90312500061451750, 4.541064518000418104, -2.621784821874998173 ) ) ;
#29669=CARTESIAN_POINT ( 'NONE',  ( 13.97812500061451679, 4.541064518000418104, 2.621784821874999949 ) ) ;
#29671=CARTESIAN_POINT ( 'NONE',  ( 13.72500000000000142, 4.330127018922191873, 2.499999999999999556 ) ) ;
#29672=CARTESIAN_POINT ( 'NONE',  ( 5.512500001229033941, -4.330127018922190985, -2.500000000000001332 ) ) ;
#29674=CARTESIAN_POINT ( 'NONE',  ( 16.13437500061451502, 6.421520780324663323E-16, -5.243569643749999010 ) ) ;
#29675=CARTESIAN_POINT ( 'NONE',  ( 17.66250000122903430, -4.330127018922190985, -2.500000000000001332 ) ) ;
#29677=CARTESIAN_POINT ( 'NONE',  ( -3.000416591977282496E-16, 19.24062500061451431, -34.90005215228797653 ) ) ;
#29679=CARTESIAN_POINT ( 'NONE',  ( 23.55000000122903359, -2.886751345948159742, -4.999999999999942268 ) ) ;
#29680=CARTESIAN_POINT ( 'NONE',  ( 3.046343057529203424, 3.964819538874875704, 3.046343057529141696 ) ) ;
#29681=CARTESIAN_POINT ( 'NONE',  ( 3.242103837493086330E-14, 13.13749999999999929, 26.00000000000000711 ) ) ;
#29682=CARTESIAN_POINT ( 'NONE',  ( 19.54687500061451644, -3.027376345333614438, 5.243569643749998122 ) ) ;
#29684=CARTESIAN_POINT ( 'NONE',  ( 14.42812500061451786, 4.541064518000418104, 2.621784821874999949 ) ) ;
#29686=CARTESIAN_POINT ( 'NONE',  ( 15.75000000122903643, -2.886751345948197045, 4.999999999999880096 ) ) ;
#29687=CARTESIAN_POINT ( 'NONE',  ( 25.99687500061451928, -3.027376345333610441, -5.243569643749999898 ) ) ;
#29689=CARTESIAN_POINT ( 'NONE',  ( 9.740625000614516082, -3.027376345333610441, -5.243569643749999898 ) ) ;
#29690=CARTESIAN_POINT ( 'NONE',  ( 15.75937500061451857, 4.541064518000418104, -2.621784821874998173 ) ) ;
#29691=VERTEX_POINT ( 'NONE', #6943 ) ;
#29692=CARTESIAN_POINT ( 'NONE',  ( 26.42812500061451431, 6.421520780324663323E-16, -5.243569643749999010 ) ) ;
#29693=CARTESIAN_POINT ( 'NONE',  ( 19.60312500061451502, -4.541064518000417216, -2.621784821875001281 ) ) ;
#29694=CARTESIAN_POINT ( 'NONE',  ( 18.89999999999999858, -4.330127018922190985, -2.500000000000001332 ) ) ;
#29695=CARTESIAN_POINT ( 'NONE',  ( -3.999999999999999112, 14.26250000122903572, -30.00000000000000000 ) ) ;
#29696=CARTESIAN_POINT ( 'NONE',  ( 9.412499999999999645, -5.773502691896255534, -1.060575238724906372E-15 ) ) ;
#29697=CARTESIAN_POINT ( 'NONE',  ( 18.75000000122903288, 5.773502691896255534, 3.535250795749688894E-16 ) ) ;
#29698=CARTESIAN_POINT ( 'NONE',  ( 3.999999999999999112, 10.32500000000000107, 30.00000000000000000 ) ) ;
#29701=CARTESIAN_POINT ( 'NONE',  ( 18.30000000000000071, 0.000000000000000000, 4.999999999999998224 ) ) ;
#29702=CARTESIAN_POINT ( 'NONE',  ( 21.30000000000000071, 4.330127018922192761, -2.499999999999997780 ) ) ;
#29703=CARTESIAN_POINT ( 'NONE',  ( 18.98437500061451644, 4.541064518000418104, 2.621784821874999949 ) ) ;
#29704=CARTESIAN_POINT ( 'NONE',  ( 24.51562500061451289, -6.054752690667223547, -1.112240025338166033E-15 ) ) ;
#29705=ORIENTED_EDGE ( 'NONE', *, *, #32955, .T. ) ;
#29706=CARTESIAN_POINT ( 'NONE',  ( 1.592000809091587073E-14, 16.85000000122903785, 26.00000000000000000 ) ) ;
#29707=CARTESIAN_POINT ( 'NONE',  ( 5.015625000614518214, 3.027376345333611329, 5.243569643749999010 ) ) ;
#29709=CARTESIAN_POINT ( 'NONE',  ( 14.55000000000000071, 4.330127018922192761, -2.499999999999997780 ) ) ;
#29710=CARTESIAN_POINT ( 'NONE',  ( 2.121784821875001281, 18.60312500061451857, 33.67503911421598417 ) ) ;
#29711=CARTESIAN_POINT ( 'NONE',  ( 28.90312500061451217, 0.000000000000000000, 5.243569643749999010 ) ) ;
#29714=CARTESIAN_POINT ( 'NONE',  ( 25.17187500061451644, 3.027376345333613106, -5.243569643749998122 ) ) ;
#29716=CARTESIAN_POINT ( 'NONE',  ( 21.21562500061451573, 3.027376345333611329, 5.243569643749999010 ) ) ;
#29717=CARTESIAN_POINT ( 'NONE',  ( 23.22187500061451715, -6.054752690667223547, -1.112240025338166033E-15 ) ) ;
#29718=CARTESIAN_POINT ( 'NONE',  ( 2.121784821874999061, 16.95312500061459460, -33.67503911421598417 ) ) ;
#29719=CARTESIAN_POINT ( 'NONE',  ( 7.340625000614518392, -3.027376345333614438, 5.243569643749998122 ) ) ;
#29721=CARTESIAN_POINT ( 'NONE',  ( 23.72812500061451502, 6.421520780324663323E-16, -5.243569643749999010 ) ) ;
#29724=CARTESIAN_POINT ( 'NONE',  ( 17.78437500061451715, -4.541064518000419881, 2.621784821874995952 ) ) ;
#29726=CARTESIAN_POINT ( 'NONE',  ( 19.13437500061451857, -4.541064518000419881, 2.621784821874995952 ) ) ;
#29727=CARTESIAN_POINT ( 'NONE',  ( 26.25937500061451857, 0.000000000000000000, 5.243569643749999010 ) ) ;
#29728=CARTESIAN_POINT ( 'NONE',  ( 2.121784821875001281, 17.30937500061451573, 33.67503911421598417 ) ) ;
#29729=CARTESIAN_POINT ( 'NONE',  ( 8.690625000614515372, -3.027376345333614438, 5.243569643749998122 ) ) ;
#29731=CARTESIAN_POINT ( 'NONE',  ( 5.634375000614519458, -4.541064518000419881, 2.621784821874995952 ) ) ;
#29733=CARTESIAN_POINT ( 'NONE',  ( 4.640625000614518214, -3.027376345333614438, 5.243569643749998122 ) ) ;
#29734=CARTESIAN_POINT ( 'NONE',  ( 10.80937500061451928, 4.541064518000418104, -2.621784821874998173 ) ) ;
#29736=CARTESIAN_POINT ( 'NONE',  ( 16.50000000122903288, 5.773502691896255534, 3.535250795749688894E-16 ) ) ;
#29737=CARTESIAN_POINT ( 'NONE',  ( 4.659375000614518925, 0.000000000000000000, 5.243569643749999010 ) ) ;
#29738=CARTESIAN_POINT ( 'NONE',  ( 6.290625000614517681, 6.054752690667223547, 3.707466751127219781E-16 ) ) ;
#29741=CARTESIAN_POINT ( 'NONE',  ( 17.22187500061451715, 3.027376345333611329, 5.243569643749999010 ) ) ;
#29742=FACE_OUTER_BOUND ( 'NONE', #53429, .T. ) ;
#29743=ORIENTED_EDGE ( 'NONE', *, *, #18362, .F. ) ;
#29744=CARTESIAN_POINT ( 'NONE',  ( 25.07812500061451644, 6.421520780324663323E-16, -5.243569643749999010 ) ) ;
#29745=CARTESIAN_POINT ( 'NONE',  ( 8.653125000614515727, 0.000000000000000000, 5.243569643749999010 ) ) ;
#29746=CARTESIAN_POINT ( 'NONE',  ( 26.55937500061451573, 4.541064518000418104, -2.621784821874998173 ) ) ;
#29747=CARTESIAN_POINT ( 'NONE',  ( 9.065625000614517148, 3.027376345333611329, 5.243569643749999010 ) ) ;
#29749=CARTESIAN_POINT ( 'NONE',  ( 11.21250000122903501, 0.000000000000000000, 4.999999999999998224 ) ) ;
#29750=CARTESIAN_POINT ( 'NONE',  ( 25.41562500061451146, -6.054752690667223547, -1.112240025338166033E-15 ) ) ;
#29752=CARTESIAN_POINT ( 'NONE',  ( -2.121784821874996840, 12.67812500061451786, -26.32496088578401583 ) ) ;
#29753=CARTESIAN_POINT ( 'NONE',  ( 11.66250000122903430, 0.000000000000000000, 4.999999999999998224 ) ) ;
#29754=CARTESIAN_POINT ( 'NONE',  ( 22.86562500061451431, 3.027376345333613106, -5.243569643749998122 ) ) ;
#29755=CARTESIAN_POINT ( 'NONE',  ( 10.65000000000000036, 0.000000000000000000, 4.999999999999998224 ) ) ;
#29756=CARTESIAN_POINT ( 'NONE',  ( 19.26562500061451644, 3.027376345333613106, -5.243569643749998122 ) ) ;
#29757=CARTESIAN_POINT ( 'NONE',  ( 5.071875000614518569, 3.027376345333611329, 5.243569643749999010 ) ) ;
#29758=CARTESIAN_POINT ( 'NONE',  ( 20.36249999999999716, 2.886751345948129099, -4.999999999999998224 ) ) ;
#29759=CARTESIAN_POINT ( 'NONE',  ( 13.35000000122903430, 5.773502691896255534, 3.535250795749688894E-16 ) ) ;
#29760=CARTESIAN_POINT ( 'NONE',  ( 9.928125000614517859, 4.541064518000418104, 2.621784821874999949 ) ) ;
#29761=CARTESIAN_POINT ( 'NONE',  ( 15.47812500061451679, -4.541064518000419881, 2.621784821874995952 ) ) ;
#29762=CARTESIAN_POINT ( 'NONE',  ( 24.93750000122903288, 6.123233995736764310E-16, -4.999999999999998224 ) ) ;
#29763=CARTESIAN_POINT ( 'NONE',  ( 22.58437500061451431, 4.541064518000418104, 2.621784821874999949 ) ) ;
#29766=CARTESIAN_POINT ( 'NONE',  ( 6.600000001229032520, 5.773502691896255534, 3.535250795749688894E-16 ) ) ;
#29767=EDGE_CURVE ( 'NONE', #24148, #68292, #14118, .T. ) ;
#29768=CARTESIAN_POINT ( 'NONE',  ( 9.271875000614516082, -6.054752690667223547, -1.112240025338166033E-15 ) ) ;
#29769=CARTESIAN_POINT ( 'NONE',  ( 26.78437500061451360, -4.541064518000419881, 2.621784821874995952 ) ) ;
#29771=CARTESIAN_POINT ( 'NONE',  ( 20.31562500061451715, 3.027376345333611329, 5.243569643749999010 ) ) ;
#29772=CARTESIAN_POINT ( 'NONE',  ( 25.58437500061451431, 6.421520780324663323E-16, -5.243569643749999010 ) ) ;
#29775=CARTESIAN_POINT ( 'NONE',  ( 7.809375000614519280, 0.000000000000000000, 5.243569643749999010 ) ) ;
#29776=CARTESIAN_POINT ( 'NONE',  ( 20.09062500061451573, -3.027376345333610441, -5.243569643749999898 ) ) ;
#29777=ORIENTED_EDGE ( 'NONE', *, *, #33488, .T. ) ;
#29778=CARTESIAN_POINT ( 'NONE',  ( 0.000000000000000000, 20.00000000000000000, 30.00000000000000000 ) ) ;
#29779=CARTESIAN_POINT ( 'NONE',  ( 27.44062500061451715, 6.054752690667223547, 3.707466751127219781E-16 ) ) ;
#29780=CARTESIAN_POINT ( 'NONE',  ( 5.184375000614516615, -4.541064518000419881, 2.621784821874995952 ) ) ;
#29781=CARTESIAN_POINT ( 'NONE',  ( 0.000000000000000000, 20.00000000000000000, -30.00000000000000000 ) ) ;
#29782=CARTESIAN_POINT ( 'NONE',  ( 30.00000000000000000, 6.123233995736764310E-16, -4.999999999999998224 ) ) ;
#29783=CARTESIAN_POINT ( 'NONE',  ( 17.62500000000000000, 6.123233995736764310E-16, -4.999999999999998224 ) ) ;
#29784=CARTESIAN_POINT ( 'NONE',  ( 21.59062500061451928, 6.054752690667223547, 3.707466751127219781E-16 ) ) ;
#29785=VERTEX_POINT ( 'NONE', #41293 ) ;
#29786=CARTESIAN_POINT ( 'NONE',  ( 25.80000000000000071, 4.330127018922192761, -2.499999999999997780 ) ) ;
#29787=CARTESIAN_POINT ( 'NONE',  ( 25.84687500061451360, -3.027376345333614438, 5.243569643749998122 ) ) ;
#29789=AXIS2_PLACEMENT_3D ( 'NONE', #41867, #17866, #46330 ) ;
#29790=CARTESIAN_POINT ( 'NONE',  ( 12.44062500061451537, -3.027376345333610441, -5.243569643749999898 ) ) ;
#29791=CARTESIAN_POINT ( 'NONE',  ( 6.515625000614516438, -6.054752690667223547, -1.112240025338166033E-15 ) ) ;
#29793=CARTESIAN_POINT ( 'NONE',  ( 28.67812500061451431, 6.421520780324663323E-16, -5.243569643749999010 ) ) ;
#29794=CARTESIAN_POINT ( 'NONE',  ( 15.07500000122903394, 2.886751345948129099, -4.999999999999998224 ) ) ;
#29795=CARTESIAN_POINT ( 'NONE',  ( 22.98749999999999716, -2.886751345948125991, -5.000000000000000000 ) ) ;
#29796=CARTESIAN_POINT ( 'NONE',  ( 29.32499999999999929, 6.123233995736764310E-16, -4.999999999999998224 ) ) ;
#29797=CARTESIAN_POINT ( 'NONE',  ( 4.096875000614518925, 6.054752690667223547, 3.707466751127219781E-16 ) ) ;
#29798=CARTESIAN_POINT ( 'NONE',  ( 9.121875000614517504, 3.027376345333611329, 5.243569643749999010 ) ) ;
#29799=CARTESIAN_POINT ( 'NONE',  ( 19.13437500061451857, -4.541064518000419881, 2.621784821874995952 ) ) ;
#29802=CARTESIAN_POINT ( 'NONE',  ( 28.45312500061451289, 0.000000000000000000, 5.243569643749999010 ) ) ;
#29803=CARTESIAN_POINT ( 'NONE',  ( 4.312500000000000000, 2.886751345948126879, 4.999999999999999112 ) ) ;
#29804=EDGE_CURVE ( 'NONE', #72082, #964, #29664, .T. ) ;
#29805=CARTESIAN_POINT ( 'NONE',  ( 4.621875000614516615, 3.027376345333611329, 5.243569643749999010 ) ) ;
#29806=CARTESIAN_POINT ( 'NONE',  ( 19.68750000000000355, -2.886751345948129988, 4.999999999999997335 ) ) ;
#29807=CARTESIAN_POINT ( 'NONE',  ( 13.04062500061451502, 6.054752690667223547, 3.707466751127219781E-16 ) ) ;
#29809=CARTESIAN_POINT ( 'NONE',  ( 0.000000000000000000, 20.00000000000000000, 30.00000000000000000 ) ) ;
#29810=CARTESIAN_POINT ( 'NONE',  ( 5.000000000000000000, 6.176262757673013563E-16, -5.043301270189223473 ) ) ;
#29812=CARTESIAN_POINT ( 'NONE',  ( 7.153125000614518392, 4.541064518000418104, -2.621784821874998173 ) ) ;
#29813=CARTESIAN_POINT ( 'NONE',  ( 24.45937500061451786, 0.000000000000000000, 5.243569643749999010 ) ) ;
#29814=CARTESIAN_POINT ( 'NONE',  ( -4.243569643749999898, 18.47187500061451715, 27.54997392385601529 ) ) ;
#29815=CARTESIAN_POINT ( 'NONE',  ( 26.44687500061451502, -3.027376345333610441, -5.243569643749999898 ) ) ;
#29816=CARTESIAN_POINT ( 'NONE',  ( 8.212500000000000355, 2.886751345948129099, -4.999999999999998224 ) ) ;
#29817=CARTESIAN_POINT ( 'NONE',  ( -3.999999999999999556, 14.22500000122903430, 27.69059892324149530 ) ) ;
#29818=CARTESIAN_POINT ( 'NONE',  ( 14.39062500061451821, 6.054752690667223547, 3.707466751127219781E-16 ) ) ;
#29819=CARTESIAN_POINT ( 'NONE',  ( 7.312500001229033764, -4.330127018922190985, -2.500000000000001332 ) ) ;
#29820=CARTESIAN_POINT ( 'NONE',  ( 17.48437500061451999, 6.421520780324663323E-16, -5.243569643749999010 ) ) ;
#29821=CARTESIAN_POINT ( 'NONE',  ( 11.93437500061451573, -4.541064518000419881, 2.621784821874995952 ) ) ;
#29822=DIRECTION ( 'NONE',  ( -0.000000000000000000, -1.000000000000000000, -0.000000000000000000 ) ) ;
#29823=ORIENTED_EDGE ( 'NONE', *, *, #47090, .F. ) ;
#29824=CARTESIAN_POINT ( 'NONE',  ( 11.50312500061451892, -4.541064518000417216, -2.621784821875001281 ) ) ;
#29825=CARTESIAN_POINT ( 'NONE',  ( 29.21250000122903145, 0.000000000000000000, 4.999999999999998224 ) ) ;
#29826=CARTESIAN_POINT ( 'NONE',  ( 23.32500000122903572, 2.886751345948126879, 4.999999999999999112 ) ) ;
#29827=CARTESIAN_POINT ( 'NONE',  ( 13.62187500061451750, 3.027376345333611329, 5.243569643749999010 ) ) ;
#29828=CARTESIAN_POINT ( 'NONE',  ( 15.32812500061451644, 4.541064518000418104, 2.621784821874999949 ) ) ;
#29829=CARTESIAN_POINT ( 'NONE',  ( 2.000000000000001332, 16.55000000000000071, -26.53589838486224650 ) ) ;
#29830=CARTESIAN_POINT ( 'NONE',  ( 23.48437500061451644, 4.541064518000418104, 2.621784821874999949 ) ) ;
#29832=CARTESIAN_POINT ( 'NONE',  ( 12.30000000122903181, -2.886751345948125991, -5.000000000000000000 ) ) ;
#29833=CARTESIAN_POINT ( 'NONE',  ( 4.295826441391526807, 3.688361401553225338, -3.611570655833856502 ) ) ;
#29835=CARTESIAN_POINT ( 'NONE',  ( 4.243569643749999898, 16.93437500061451573, -30.00000000000000000 ) ) ;
#29836=CARTESIAN_POINT ( 'NONE',  ( 18.79687500061451644, -3.027376345333610441, -5.243569643749999898 ) ) ;
#29837=CARTESIAN_POINT ( 'NONE',  ( 17.73750000122903359, 6.123233995736764310E-16, -4.999999999999998224 ) ) ;
#29838=CARTESIAN_POINT ( 'NONE',  ( 13.13437500061451857, 4.541064518000418104, 2.621784821874999949 ) ) ;
#29839=CARTESIAN_POINT ( 'NONE',  ( -4.243569643749997233, 10.44687500061451857, 32.45002607614398471 ) ) ;
#29840=CARTESIAN_POINT ( 'NONE',  ( 19.98750000122903359, 6.123233995736764310E-16, -4.999999999999998224 ) ) ;
#29841=CARTESIAN_POINT ( 'NONE',  ( 13.86562500061451431, 3.027376345333613106, -5.243569643749998122 ) ) ;
#29843=VERTEX_POINT ( 'NONE', #69006 ) ;
#29844=CARTESIAN_POINT ( 'NONE',  ( 17.13749999999999929, -2.886751345948125991, -5.000000000000000000 ) ) ;
#29846=CARTESIAN_POINT ( 'NONE',  ( 13.43437500061451750, 6.421520780324663323E-16, -5.243569643749999010 ) ) ;
#29847=DIRECTION ( 'NONE',  ( -0.000000000000000000, -0.000000000000000000, -1.000000000000000000 ) ) ;
#29848=CARTESIAN_POINT ( 'NONE',  ( 15.82500000122903216, -5.773502691896255534, -1.060575238724906372E-15 ) ) ;
#29849=CARTESIAN_POINT ( 'NONE',  ( 27.68437500061451573, -4.541064518000419881, 2.621784821874995952 ) ) ;
#29850=CARTESIAN_POINT ( 'NONE',  ( 21.06562500061451715, 3.027376345333613106, -5.243569643749998122 ) ) ;
#29851=CARTESIAN_POINT ( 'NONE',  ( 22.45312500061451644, 4.541064518000418104, -2.621784821874998173 ) ) ;
#29852=CARTESIAN_POINT ( 'NONE',  ( 29.32500000122903216, -5.773502691896255534, -1.060575238724906372E-15 ) ) ;
#29853=CARTESIAN_POINT ( 'NONE',  ( 28.53749999999999787, 5.773502691896255534, 3.535250795749688894E-16 ) ) ;
#29854=CARTESIAN_POINT ( 'NONE',  ( -2.000000000000000000, 10.13750000122903572, -33.46410161513775705 ) ) ;
#29856=CARTESIAN_POINT ( 'NONE',  ( 0.000000000000000000, 20.00000000000000000, -30.00000000000000000 ) ) ;
#29857=CARTESIAN_POINT ( 'NONE',  ( -1.999999999999997113, 9.837500001229035007, -26.53589838486224295 ) ) ;
#29858=CARTESIAN_POINT ( 'NONE',  ( 2.121784821874999061, 15.20937500061451786, -33.67503911421598417 ) ) ;
#29859=CARTESIAN_POINT ( 'NONE',  ( 7.312500001229033764, -4.330127018922190985, -2.500000000000001332 ) ) ;
#29860=CARTESIAN_POINT ( 'NONE',  ( 5.512499999999999289, 2.886751345948129099, -4.999999999999998224 ) ) ;
#29862=CARTESIAN_POINT ( 'NONE',  ( 9.796875000614519990, -3.027376345333610441, -5.243569643749999898 ) ) ;
#29863=CARTESIAN_POINT ( 'NONE',  ( 28.30312500061451431, 4.541064518000418104, -2.621784821874998173 ) ) ;
#29865=CARTESIAN_POINT ( 'NONE',  ( 30.00000000000000000, 0.000000000000000000, 0.000000000000000000 ) ) ;
#29866=CARTESIAN_POINT ( 'NONE',  ( 7.546875000614517326, -3.027376345333610441, -5.243569643749999898 ) ) ;
#29867=CARTESIAN_POINT ( 'NONE',  ( 12.38437500061451857, -4.541064518000419881, 2.621784821874995952 ) ) ;
#29868=CARTESIAN_POINT ( 'NONE',  ( 6.037500000000001421, 5.773502691896255534, 3.535250795749688894E-16 ) ) ;
#29869=CARTESIAN_POINT ( 'NONE',  ( -4.243569643749999898, 13.91562500061459140, 27.54997392385601529 ) ) ;
#29871=( BOUNDED_CURVE ( )  B_SPLINE_CURVE ( 2, ( #48721, #66068, #71244, #20623, #54621, #65701, #14360, #15088, #3292 ),
 .UNSPECIFIED., .F., .F. ) 
 B_SPLINE_CURVE_WITH_KNOTS ( ( 3, 2, 2, 2, 3 ),
 ( 0.9239130434782608647, 0.9275362318840579823, 0.9347826086956522174, 0.9420289855072463414, 0.9456521739130434590 ),
 .UNSPECIFIED. ) 
 CURVE ( )  GEOMETRIC_REPRESENTATION_ITEM ( )  RATIONAL_B_SPLINE_CURVE ( ( 0.9330127018922194093, 0.9330127018922194093, 1.000000000000000000, 0.8660254037844387076, 1.000000000000000000, 0.8660254037844387076, 1.000000000000000000, 0.9330127018922194093, 0.9330127018922194093 ) ) 
 REPRESENTATION_ITEM ( '' )  );
#29872=CARTESIAN_POINT ( 'NONE',  ( 7.537500000000002309, -2.886751345948129988, 4.999999999999997335 ) ) ;
#29873=CARTESIAN_POINT ( 'NONE',  ( 26.10000000122903430, -2.886751345948129988, 4.999999999999997335 ) ) ;
#29875=CARTESIAN_POINT ( 'NONE',  ( 23.84062500061451928, 6.054752690667223547, 3.707466751127219781E-16 ) ) ;
#29876=CARTESIAN_POINT ( 'NONE',  ( 13.26562500061451644, -6.054752690667223547, -1.112240025338166033E-15 ) ) ;
#29878=CARTESIAN_POINT ( 'NONE',  ( 8.634375000614518569, 4.541064518000418104, 2.621784821874999949 ) ) ;
#29879=CARTESIAN_POINT ( 'NONE',  ( 26.84999999999999787, 0.000000000000000000, 4.999999999999998224 ) ) ;
#29880=CARTESIAN_POINT ( 'NONE',  ( 23.06250000122903288, -4.330127018922190985, -2.500000000000001332 ) ) ;
#29881=CARTESIAN_POINT ( 'NONE',  ( 12.12187500061451573, 3.027376345333613106, -5.243569643749998122 ) ) ;
#29882=CARTESIAN_POINT ( 'NONE',  ( 26.07187500061451857, 3.027376345333613106, -5.243569643749998122 ) ) ;
#29883=CARTESIAN_POINT ( 'NONE',  ( 3.234375000614516438, 4.541064518000418104, 2.621784821874999949 ) ) ;
#29884=CARTESIAN_POINT ( 'NONE',  ( 4.000000000000000000, 13.55000000122903359, -27.69059892324149885 ) ) ;
#29885=CARTESIAN_POINT ( 'NONE',  ( 21.75937500061451502, 0.000000000000000000, 5.243569643749999010 ) ) ;
#29886=CARTESIAN_POINT ( 'NONE',  ( 11.74687500061451573, 6.054752690667223547, 3.707466751127219781E-16 ) ) ;
#29888=CARTESIAN_POINT ( 'NONE',  ( 25.12499999999999645, -4.330127018922194537, 2.499999999999995559 ) ) ;
#29890=CARTESIAN_POINT ( 'NONE',  ( -3.000416591977282496E-16, 12.54687500061451999, -34.90005215228797653 ) ) ;
#29892=CARTESIAN_POINT ( 'NONE',  ( 15.70312500061451644, 4.541064518000418104, -2.621784821874998173 ) ) ;
#29893=CARTESIAN_POINT ( 'NONE',  ( 6.000000000000001776, 4.330127018922192761, -2.499999999999997780 ) ) ;
#29894=DIRECTION ( 'NONE',  ( 0.000000000000000000, 0.000000000000000000, -1.000000000000000000 ) ) ;
#29896=CARTESIAN_POINT ( 'NONE',  ( 14.77500000000000036, -4.330127018922194537, 2.499999999999995559 ) ) ;
#29898=CARTESIAN_POINT ( 'NONE',  ( 4.243569643749999898, 11.02812500061451750, 30.00000000000000000 ) ) ;
#29899=CARTESIAN_POINT ( 'NONE',  ( 14.13750000122903394, 6.123233995736764310E-16, -4.999999999999998224 ) ) ;
#29900=CARTESIAN_POINT ( 'NONE',  ( 24.79687500061451999, 6.054752690667223547, 3.707466751127219781E-16 ) ) ;
#29902=CARTESIAN_POINT ( 'NONE',  ( 20.54062500061451502, -3.027376345333610441, -5.243569643749999898 ) ) ;
#29903=CARTESIAN_POINT ( 'NONE',  ( 19.58437500061451786, -4.541064518000419881, 2.621784821874995952 ) ) ;
#29904=CARTESIAN_POINT ( 'NONE',  ( 5.175000000000002487, 4.330127018922191873, 2.499999999999999556 ) ) ;
#29905=CARTESIAN_POINT ( 'NONE',  ( 7.340625000614518392, -3.027376345333614438, 5.243569643749998122 ) ) ;
#29906=CARTESIAN_POINT ( 'NONE',  ( 22.49062500061451431, 6.054752690667223547, 3.707466751127219781E-16 ) ) ;
#29907=CARTESIAN_POINT ( 'NONE',  ( 17.59687500061451715, 6.054752690667223547, 3.707466751127219781E-16 ) ) ;
#29908=CARTESIAN_POINT ( 'NONE',  ( 4.243569643749999010, 14.66562500061451857, 27.54997392385601174 ) ) ;
#29909=CARTESIAN_POINT ( 'NONE',  ( 19.46250000122903145, -4.330127018922190985, -2.500000000000001332 ) ) ;
#29911=CARTESIAN_POINT ( 'NONE',  ( 8.428125000614517859, 6.421520780324663323E-16, -5.243569643749999010 ) ) ;
#29913=CARTESIAN_POINT ( 'NONE',  ( 29.31562500061451715, 3.027376345333611329, 5.243569643749999010 ) ) ;
#29914=CARTESIAN_POINT ( 'NONE',  ( 25.54687500061451644, -3.027376345333610441, -5.243569643749999898 ) ) ;
#29915=CARTESIAN_POINT ( 'NONE',  ( 16.49062500061451786, -3.027376345333610441, -5.243569643749999898 ) ) ;
#29916=CARTESIAN_POINT ( 'NONE',  ( 24.75000000122902932, -2.886751345948129988, 4.999999999999997335 ) ) ;
#29917=CARTESIAN_POINT ( 'NONE',  ( 25.41562500061451146, -6.054752690667223547, -1.112240025338166033E-15 ) ) ;
#29918=CARTESIAN_POINT ( 'NONE',  ( 22.65937500061451715, 0.000000000000000000, 5.243569643749999010 ) ) ;
#29919=CARTESIAN_POINT ( 'NONE',  ( 15.29062500061451679, 6.054752690667223547, 3.707466751127219781E-16 ) ) ;
#29920=CARTESIAN_POINT ( 'NONE',  ( -4.243569643749999898, 16.70937500061451786, 30.00000000000000000 ) ) ;
#29921=CARTESIAN_POINT ( 'NONE',  ( 21.44062500061452070, -3.027376345333610441, -5.243569643749999898 ) ) ;
#29922=CARTESIAN_POINT ( 'NONE',  ( 2.925000001229034918, 2.886751345948129099, -4.999999999999998224 ) ) ;
#29924=CARTESIAN_POINT ( 'NONE',  ( 24.67500000000000071, -4.330127018922194537, 2.499999999999995559 ) ) ;
#29925=CARTESIAN_POINT ( 'NONE',  ( -3.999999999999999112, 13.70000000000000107, -30.00000000000000000 ) ) ;
#29927=CARTESIAN_POINT ( 'NONE',  ( 2.896875000614518747, -3.027376345333614438, 5.243569643749998122 ) ) ;
#29928=CARTESIAN_POINT ( 'NONE',  ( 8.315625000614515372, -6.054752690667223547, -1.112240025338166033E-15 ) ) ;
#29929=CARTESIAN_POINT ( 'NONE',  ( 22.57500000122903572, -5.773502691896255534, -1.060575238724906372E-15 ) ) ;
#29930=CARTESIAN_POINT ( 'NONE',  ( 26.12812500061451360, 4.541064518000418104, 2.621784821874999949 ) ) ;
#29931=CARTESIAN_POINT ( 'NONE',  ( 24.52499999999999858, 4.330127018922191873, 2.499999999999999556 ) ) ;
#29932=CARTESIAN_POINT ( 'NONE',  ( -2.000000000000000000, 15.08750000122903501, -33.46410161513775705 ) ) ;
#29933=CARTESIAN_POINT ( 'NONE',  ( -2.000000000000000000, 15.53750000122903430, -33.46410161513775705 ) ) ;
#29934=CARTESIAN_POINT ( 'NONE',  ( 10.41562500061451679, 3.027376345333611329, 5.243569643749999010 ) ) ;
#29936=CARTESIAN_POINT ( 'NONE',  ( 26.76562500061451644, -6.054752690667223547, -1.112240025338166033E-15 ) ) ;
#29937=CARTESIAN_POINT ( 'NONE',  ( 6.928125000614516082, -4.541064518000419881, 2.621784821874995952 ) ) ;
#29938=CARTESIAN_POINT ( 'NONE',  ( 3.740625000614516527, -3.027376345333614438, 5.243569643749998122 ) ) ;
#29940=CARTESIAN_POINT ( 'NONE',  ( 4.670675770459133069, -1.784685619568015635, 4.930540594781983366 ) ) ;
#29941=CARTESIAN_POINT ( 'NONE',  ( 12.86250000000000071, 2.886751345948126879, 4.999999999999999112 ) ) ;
#29942=CARTESIAN_POINT ( 'NONE',  ( 12.83437500061451786, -4.541064518000419881, 2.621784821874995952 ) ) ;
#29943=CARTESIAN_POINT ( 'NONE',  ( 9.900000001229033231, -2.886751345948129988, 4.999999999999997335 ) ) ;
#29944=CARTESIAN_POINT ( 'NONE',  ( 16.05937500061451573, -4.541064518000417216, -2.621784821875001281 ) ) ;
#29946=CARTESIAN_POINT ( 'NONE',  ( 7.659375000614518036, 4.541064518000418104, -2.621784821874998173 ) ) ;
#29947=CARTESIAN_POINT ( 'NONE',  ( 4.243569643749999898, 10.57812500061451821, -30.00000000000000000 ) ) ;
#29948=CARTESIAN_POINT ( 'NONE',  ( 4.000000000000000000, 16.58750000000000213, 32.30940107675849760 ) ) ;
#29951=CARTESIAN_POINT ( 'NONE',  ( 23.61562500061451431, -6.054752690667223547, -1.112240025338166033E-15 ) ) ;
#29953=CARTESIAN_POINT ( 'NONE',  ( 28.80937500061451573, 4.541064518000418104, -2.621784821874998173 ) ) ;
#29954=CARTESIAN_POINT ( 'NONE',  ( 21.03750000000000142, -2.886751345948129988, 4.999999999999997335 ) ) ;
#29955=CARTESIAN_POINT ( 'NONE',  ( 7.865625000614516971, -6.054752690667223547, -1.112240025338166033E-15 ) ) ;
#29957=CARTESIAN_POINT ( 'NONE',  ( 16.05937500061451573, -4.541064518000417216, -2.621784821875001281 ) ) ;
#29959=CARTESIAN_POINT ( 'NONE',  ( 29.32500000122903216, -5.773502691896255534, -1.060575238724906372E-15 ) ) ;
#29960=CARTESIAN_POINT ( 'NONE',  ( 8.034375000614518925, 6.421520780324663323E-16, -5.243569643749999010 ) ) ;
#29961=ORIENTED_EDGE ( 'NONE', *, *, #38656, .T. ) ;
#29962=CARTESIAN_POINT ( 'NONE',  ( 18.27187500061451431, -6.054752690667223547, -1.112240025338166033E-15 ) ) ;
#29964=CARTESIAN_POINT ( 'NONE',  ( 26.06250000000000000, -5.773502691896255534, -1.060575238724906372E-15 ) ) ;
#29965=CARTESIAN_POINT ( 'NONE',  ( 3.600000000000002309, -4.330127018922190985, -2.500000000000001332 ) ) ;
#29966=CARTESIAN_POINT ( 'NONE',  ( 30.00000000000000000, 0.000000000000000000, 0.000000000000000000 ) ) ;
#29967=CARTESIAN_POINT ( 'NONE',  ( 10.72500000000000142, -4.330127018922194537, 2.499999999999995559 ) ) ;
#29969=CARTESIAN_POINT ( 'NONE',  ( 10.35000000000000142, -4.330127018922190985, -2.500000000000001332 ) ) ;
#29971=CARTESIAN_POINT ( 'NONE',  ( 23.57812500061451289, -4.541064518000419881, 2.621784821874995952 ) ) ;
#29972=CARTESIAN_POINT ( 'NONE',  ( 14.32500000000000107, -4.330127018922194537, 2.499999999999995559 ) ) ;
#29973=CARTESIAN_POINT ( 'NONE',  ( 7.425000001229034474, 2.886751345948129099, -4.999999999999998224 ) ) ;
#29974=CARTESIAN_POINT ( 'NONE',  ( 6.665625000614515905, 3.027376345333613106, -5.243569643749998122 ) ) ;
#29975=CARTESIAN_POINT ( 'NONE',  ( 22.68750000000000000, 5.773502691896255534, 3.535250795749688894E-16 ) ) ;
#29977=CARTESIAN_POINT ( 'NONE',  ( 20.35312500061451502, 0.000000000000000000, 5.243569643749999010 ) ) ;
#29978=CARTESIAN_POINT ( 'NONE',  ( 4.117801095115578569, -2.836267711383653634, 4.249660802484540589 ) ) ;
#29979=CARTESIAN_POINT ( 'NONE',  ( 25.23750000122903359, -4.330127018922194537, 2.499999999999995559 ) ) ;
#29981=CARTESIAN_POINT ( 'NONE',  ( 5.812500000000001776, -5.773502691896255534, -1.060575238724906372E-15 ) ) ;
#29983=CARTESIAN_POINT ( 'NONE',  ( 21.02812500061451573, 6.421520780324663323E-16, -5.243569643749999010 ) ) ;
#29984=CARTESIAN_POINT ( 'NONE',  ( 27.89062500061451289, 6.054752690667223547, 3.707466751127219781E-16 ) ) ;
#29985=CARTESIAN_POINT ( 'NONE',  ( 27.19687500061451857, -3.027376345333614438, 5.243569643749998122 ) ) ;
#29986=CARTESIAN_POINT ( 'NONE',  ( 14.99062500061451786, -3.027376345333614438, 5.243569643749998122 ) ) ;
#29988=CARTESIAN_POINT ( 'NONE',  ( 26.17500000122903359, -5.773502691896255534, -1.060575238724906372E-15 ) ) ;
#29990=CARTESIAN_POINT ( 'NONE',  ( 16.82812500061451644, -4.541064518000419881, 2.621784821874995952 ) ) ;
#29991=CARTESIAN_POINT ( 'NONE',  ( -1.999999999999997113, 16.92500000000000426, -26.53589838486224295 ) ) ;
#29992=CARTESIAN_POINT ( 'NONE',  ( 5.812500001229035540, 0.000000000000000000, 4.999999999999998224 ) ) ;
#29993=CARTESIAN_POINT ( 'NONE',  ( 9.684375000614517504, -4.541064518000419881, 2.621784821874995952 ) ) ;
#29994=CARTESIAN_POINT ( 'NONE',  ( 10.17187500061451999, -6.054752690667223547, -1.112240025338166033E-15 ) ) ;
#29995=CARTESIAN_POINT ( 'NONE',  ( 20.97187500061451715, -6.054752690667223547, -1.112240025338166033E-15 ) ) ;
#29997=CARTESIAN_POINT ( 'NONE',  ( -3.039972894299037609, 9.532883912050410302, 24.81249067399576447 ) ) ;
#29998=CARTESIAN_POINT ( 'NONE',  ( 23.05312500061451431, 0.000000000000000000, 5.243569643749999010 ) ) ;
#29999=CARTESIAN_POINT ( 'NONE',  ( 18.90937500061451360, 4.541064518000418104, -2.621784821874998173 ) ) ;
#30000=CARTESIAN_POINT ( 'NONE',  ( 23.35312500061451857, 4.541064518000418104, -2.621784821874998173 ) ) ;
#30002=CARTESIAN_POINT ( 'NONE',  ( 1.999999999999998668, 14.45000000000000107, 26.53589838486224650 ) ) ;
#30003=VECTOR ( 'NONE', #61214, 1000.000000000000000 ) ;
#30004=CARTESIAN_POINT ( 'NONE',  ( 29.42812500061451431, -4.541064518000419881, 2.621784821874995952 ) ) ;
#30005=CARTESIAN_POINT ( 'NONE',  ( 9.900000001229033231, -2.886751345948129988, 4.999999999999997335 ) ) ;
#30007=CARTESIAN_POINT ( 'NONE',  ( 4.200000001229033053, -2.886751345948125991, -5.000000000000000000 ) ) ;
#30008=CARTESIAN_POINT ( 'NONE',  ( -3.999999999999999112, 19.55000000000000071, -30.00000000000000000 ) ) ;
#30009=CARTESIAN_POINT ( 'NONE',  ( 28.27500000122903145, 2.886751345948126879, 4.999999999999999112 ) ) ;
#30011=CARTESIAN_POINT ( 'NONE',  ( 10.20937500061451786, -4.541064518000417216, -2.621784821875001281 ) ) ;
#30012=CARTESIAN_POINT ( 'NONE',  ( 3.999999999999998668, 10.02500000122903323, 27.69059892324149530 ) ) ;
#30013=CARTESIAN_POINT ( 'NONE',  ( 17.16562500061451502, 3.027376345333611329, 5.243569643749999010 ) ) ;
#30014=CARTESIAN_POINT ( 'NONE',  ( 10.05937500061451750, 0.000000000000000000, 5.243569643749999010 ) ) ;
#30015=CARTESIAN_POINT ( 'NONE',  ( 28.91250000122903074, -4.330127018922190985, -2.500000000000001332 ) ) ;
#30016=CARTESIAN_POINT ( 'NONE',  ( 18.94687500061451857, 6.054752690667223547, 3.707466751127219781E-16 ) ) ;
#30017=CARTESIAN_POINT ( 'NONE',  ( 7.434375000614519280, -4.541064518000419881, 2.621784821874995952 ) ) ;
#30018=CARTESIAN_POINT ( 'NONE',  ( 8.390625000614518214, -3.027376345333610441, -5.243569643749999898 ) ) ;
#30019=CARTESIAN_POINT ( 'NONE',  ( 17.72812500061451502, -4.541064518000419881, 2.621784821874995952 ) ) ;
#30022=CARTESIAN_POINT ( 'NONE',  ( 5.512500001229033941, -4.330127018922190985, -2.500000000000001332 ) ) ;
#30023=CARTESIAN_POINT ( 'NONE',  ( 15.06562500061451537, -6.054752690667223547, -1.112240025338166033E-15 ) ) ;
#30024=CARTESIAN_POINT ( 'NONE',  ( 10.30312500061451431, 4.541064518000418104, -2.621784821874998173 ) ) ;
#30026=CARTESIAN_POINT ( 'NONE',  ( 10.95000000000000107, 4.330127018922192761, -2.499999999999997780 ) ) ;
#30027=CARTESIAN_POINT ( 'NONE',  ( 7.725000001229034297, -5.773502691896255534, -1.060575238724906372E-15 ) ) ;
#30028=( BOUNDED_CURVE ( )  B_SPLINE_CURVE ( 2, ( #14955, #60014, #9425, #43412, #65937, #9785, #32318 ),
 .UNSPECIFIED., .F., .F. ) 
 B_SPLINE_CURVE_WITH_KNOTS ( ( 3, 2, 2, 3 ),
 ( 0.9257108577306782937, 0.9277777777777778123, 0.9305555555555555802, 0.9323466298429085031 ),
 .UNSPECIFIED. ) 
 CURVE ( )  GEOMETRIC_REPRESENTATION_ITEM ( )  RATIONAL_B_SPLINE_CURVE ( ( 0.9489772546989883040, 0.9003106796607971418, 1.000000000000000000, 0.8660254037844387076, 1.000000000000000000, 0.9136149564015341173, 0.9386297746918415008 ) ) 
 REPRESENTATION_ITEM ( '' )  );
#30029=ADVANCED_FACE ( 'NONE', ( #70815 ), #20190, .F. ) ;
#30030=CARTESIAN_POINT ( 'NONE',  ( 14.63437500061451679, -4.541064518000419881, 2.621784821874995952 ) ) ;
#30031=CARTESIAN_POINT ( 'NONE',  ( 17.36250000122903359, 4.330127018922192761, -2.499999999999997780 ) ) ;
#30032=B_SPLINE_CURVE_WITH_KNOTS ( 'NONE', 3,
 ( #44205, #56007, #33461, #65994, #32374, #4321, #26846, #71909, #10212, #50106 ),
 .UNSPECIFIED., .F., .F.,
 ( 4, 3, 3, 4 ),
 ( 1.795354992613655247E-16, 0.0001572292605084571135, 0.0003224816258534031780, 0.0004877840086384408781 ),
 .UNSPECIFIED. ) ;
#30035=CARTESIAN_POINT ( 'NONE',  ( 2.121784821875001281, 17.70312500061451644, -26.32496088578401938 ) ) ;
#30037=CARTESIAN_POINT ( 'NONE',  ( 3.242103837493086330E-14, 11.00000000122903288, -34.00000000000000000 ) ) ;
#30038=CARTESIAN_POINT ( 'NONE',  ( 4.607378645714853782, 3.612521970890910872, 4.230067690458080953 ) ) ;
#30039=CARTESIAN_POINT ( 'NONE',  ( 17.33437500061451431, -4.541064518000419881, 2.621784821874995952 ) ) ;
#30042=CARTESIAN_POINT ( 'NONE',  ( 14.27812500061451573, 6.421520780324663323E-16, -5.243569643749999010 ) ) ;
#30044=DIRECTION ( 'NONE',  ( -1.000000000000000000, -0.000000000000000000, -0.000000000000000000 ) ) ;
#30045=CARTESIAN_POINT ( 'NONE',  ( 25.73437500061451644, 4.541064518000418104, 2.621784821874999949 ) ) ;
#30047=CARTESIAN_POINT ( 'NONE',  ( 10.07812500061451644, -4.541064518000419881, 2.621784821874995952 ) ) ;
#30048=CARTESIAN_POINT ( 'NONE',  ( 16.28437500061452070, 4.541064518000418104, 2.621784821874999949 ) ) ;
#30049=ORIENTED_EDGE ( 'NONE', *, *, #54952, .T. ) ;
#30050=CARTESIAN_POINT ( 'NONE',  ( 27.23437500061451644, -4.541064518000419881, 2.621784821874995952 ) ) ;
#30051=CARTESIAN_POINT ( 'NONE',  ( 28.67812500061451431, 6.421520780324663323E-16, -5.243569643749999010 ) ) ;
#30052=CARTESIAN_POINT ( 'NONE',  ( 19.90312500061451573, 0.000000000000000000, 5.243569643749999010 ) ) ;
#30053=CARTESIAN_POINT ( 'NONE',  ( 28.97812500061451502, -4.541064518000419881, 2.621784821874995952 ) ) ;
#30054=EDGE_CURVE ( 'NONE', #14839, #1970, #46585, .T. ) ;
#30055=CARTESIAN_POINT ( 'NONE',  ( 2.000000000000001332, 14.75000000000000178, 33.46410161513774995 ) ) ;
#30057=CARTESIAN_POINT ( 'NONE',  ( 10.08749999999999858, 5.773502691896255534, 3.535250795749688894E-16 ) ) ;
#30058=CARTESIAN_POINT ( 'NONE',  ( 20.47500000122903074, 2.886751345948129099, -4.999999999999998224 ) ) ;
#30059=CARTESIAN_POINT ( 'NONE',  ( 0.000000000000000000, 20.00000000000000000, 30.00000000000000000 ) ) ;
#30062=CARTESIAN_POINT ( 'NONE',  ( 18.22499999999999787, 4.330127018922191873, 2.499999999999999556 ) ) ;
#30063=CARTESIAN_POINT ( 'NONE',  ( 20.54999999999999716, 0.000000000000000000, 4.999999999999998224 ) ) ;
#30064=CARTESIAN_POINT ( 'NONE',  ( 18.49687500061452283, 6.054752690667223547, 3.707466751127219781E-16 ) ) ;
#30065=CARTESIAN_POINT ( 'NONE',  ( 14.61562500061451608, -6.054752690667223547, -1.112240025338166033E-15 ) ) ;
#30066=VERTEX_POINT ( 'NONE', #47925 ) ;
#30067=CARTESIAN_POINT ( 'NONE',  ( 3.637500001229036162, -4.330127018922194537, 2.499999999999995559 ) ) ;
#30068=CARTESIAN_POINT ( 'NONE',  ( 6.815625000614517148, 3.027376345333611329, 5.243569643749999010 ) ) ;
#30069=CARTESIAN_POINT ( 'NONE',  ( 12.03749999999999964, -2.886751345948129988, 4.999999999999997335 ) ) ;
#30071=CARTESIAN_POINT ( 'NONE',  ( -2.121784821874996840, 16.27812500061451573, 33.67503911421598417 ) ) ;
#30072=CARTESIAN_POINT ( 'NONE',  ( 28.67812500061451431, 6.421520780324663323E-16, -5.243569643749999010 ) ) ;
#30074=VECTOR ( 'NONE', #67820, 1000.000000000000000 ) ;
#30076=CARTESIAN_POINT ( 'NONE',  ( 24.72187500061451360, 3.027376345333613106, -5.243569643749998122 ) ) ;
#30078=CARTESIAN_POINT ( 'NONE',  ( 22.49062500061451431, 6.054752690667223547, 3.707466751127219781E-16 ) ) ;
#30079=CARTESIAN_POINT ( 'NONE',  ( 23.18437500061451573, -4.541064518000419881, 2.621784821874995952 ) ) ;
#30080=CARTESIAN_POINT ( 'NONE',  ( -3.000416591977282496E-16, 15.64062500061459282, -34.90005215228797653 ) ) ;
#30081=CARTESIAN_POINT ( 'NONE',  ( 5.690625000614516260, -3.027376345333610441, -5.243569643749999898 ) ) ;
#30083=CARTESIAN_POINT ( 'NONE',  ( 24.47812500061451502, -4.541064518000419881, 2.621784821874995952 ) ) ;
#30086=CARTESIAN_POINT ( 'NONE',  ( 17.37187500061451573, -6.054752690667223547, -1.112240025338166033E-15 ) ) ;
#30087=CARTESIAN_POINT ( 'NONE',  ( 18.94687500061451502, 6.054752690667223547, 3.707466751127219781E-16 ) ) ;
#30088=CARTESIAN_POINT ( 'NONE',  ( 26.18437500061451573, 4.541064518000418104, 2.621784821874999949 ) ) ;
#30089=CARTESIAN_POINT ( 'NONE',  ( -2.121784821874996840, 15.43437500061451928, 33.67503911421598417 ) ) ;
#30090=CARTESIAN_POINT ( 'NONE',  ( 7.303125000614516082, 0.000000000000000000, 5.243569643749999010 ) ) ;
#30091=CARTESIAN_POINT ( 'NONE',  ( -1.071796769724491005, 19.00759618943233775, 26.00000000000000355 ) ) ;
#30093=CARTESIAN_POINT ( 'NONE',  ( 4.884375000614518569, 6.421520780324663323E-16, -5.243569643749999010 ) ) ;
#30095=CARTESIAN_POINT ( 'NONE',  ( 4.040625000614517681, 6.054752690667223547, 3.707466751127219781E-16 ) ) ;
#30096=CARTESIAN_POINT ( 'NONE',  ( 9.309375000614517504, -4.541064518000417216, -2.621784821875001281 ) ) ;
#30098=CARTESIAN_POINT ( 'NONE',  ( 17.62500000122903288, -5.773502691896255534, -1.060575238724906372E-15 ) ) ;
#30099=CARTESIAN_POINT ( 'NONE',  ( 4.434375000614519280, 6.421520780324663323E-16, -5.243569643749999010 ) ) ;
#30100=CARTESIAN_POINT ( 'NONE',  ( 7.865625000614516971, -6.054752690667223547, -1.112240025338166033E-15 ) ) ;
#30103=CARTESIAN_POINT ( 'NONE',  ( 17.70937500061451431, 0.000000000000000000, 5.243569643749999010 ) ) ;
#30106=CARTESIAN_POINT ( 'NONE',  ( 23.84062500061451928, 6.054752690667223547, 3.707466751127219781E-16 ) ) ;
#30107=CARTESIAN_POINT ( 'NONE',  ( 10.60312500061451679, -4.541064518000417216, -2.621784821875001281 ) ) ;
#30108=CARTESIAN_POINT ( 'NONE',  ( 25.99687500061451928, -3.027376345333610441, -5.243569643749999898 ) ) ;
#30109=CARTESIAN_POINT ( 'NONE',  ( 10.90312500061451928, 0.000000000000000000, 5.243569643749999010 ) ) ;
#30111=CARTESIAN_POINT ( 'NONE',  ( 10.46250000122903323, -4.330127018922190985, -2.500000000000001332 ) ) ;
#30112=CARTESIAN_POINT ( 'NONE',  ( 25.56562500061452070, 3.027376345333613106, -5.243569643749998122 ) ) ;
#30113=CARTESIAN_POINT ( 'NONE',  ( -4.243569643749997233, 12.19062500061451715, -27.54997392385601174 ) ) ;
#30114=CARTESIAN_POINT ( 'NONE',  ( 13.61250000122903359, -4.330127018922190985, -2.500000000000001332 ) ) ;
#30115=CARTESIAN_POINT ( 'NONE',  ( 20.99062500061451431, -3.027376345333610441, -5.243569643749999898 ) ) ;
#30117=CARTESIAN_POINT ( 'NONE',  ( 21.36562500061451431, -6.054752690667223547, -1.112240025338166033E-15 ) ) ;
#30119=CARTESIAN_POINT ( 'NONE',  ( 21.18749999999999645, -2.886751345948125991, -5.000000000000000000 ) ) ;
#30120=CARTESIAN_POINT ( 'NONE',  ( 14.21250000122903323, 4.330127018922192761, -2.499999999999997780 ) ) ;
#30122=CARTESIAN_POINT ( 'NONE',  ( 10.56562500061451715, -6.054752690667223547, -1.112240025338166033E-15 ) ) ;
#30123=CARTESIAN_POINT ( 'NONE',  ( 13.26562500061451644, -6.054752690667223547, -1.112240025338166033E-15 ) ) ;
#30124=AXIS2_PLACEMENT_3D ( 'NONE', #3100, #70691, #9008 ) ;
#30125=CARTESIAN_POINT ( 'NONE',  ( 25.57500000122903216, 2.886751345948126879, 4.999999999999999112 ) ) ;
#30126=VECTOR ( 'NONE', #69072, 1000.000000000000000 ) ;
#30127=CARTESIAN_POINT ( 'NONE',  ( 21.83437500061451786, -4.541064518000419881, 2.621784821874995952 ) ) ;
#30129=EDGE_CURVE ( 'NONE', #63662, #56329, #71920, .T. ) ;
#30130=CARTESIAN_POINT ( 'NONE',  ( 8.775000001229033231, 2.886751345948129099, -4.999999999999998224 ) ) ;
#30131=CARTESIAN_POINT ( 'NONE',  ( 7.959375000614516971, -4.541064518000417216, -2.621784821875001281 ) ) ;
#30132=CARTESIAN_POINT ( 'NONE',  ( 26.82187500061451857, -6.054752690667223547, -1.112240025338166033E-15 ) ) ;
#30133=EDGE_CURVE ( 'NONE', #49995, #11143, #29229, .T. ) ;
#30134=CARTESIAN_POINT ( 'NONE',  ( 3.384375000614517237, -4.541064518000419881, 2.621784821874995952 ) ) ;
#30135=CARTESIAN_POINT ( 'NONE',  ( 22.37812500061451360, 6.421520780324663323E-16, -5.243569643749999010 ) ) ;
#30136=CARTESIAN_POINT ( 'NONE',  ( 27.49687500061451217, 6.054752690667223547, 3.707466751127219781E-16 ) ) ;
#30139=CARTESIAN_POINT ( 'NONE',  ( 8.109375000614518214, 4.541064518000418104, -2.621784821874998173 ) ) ;
#30140=CARTESIAN_POINT ( 'NONE',  ( 16.82812500061451644, -4.541064518000419881, 2.621784821874995952 ) ) ;
#30142=CARTESIAN_POINT ( 'NONE',  ( 2.867942972713479755, -4.095717654485441450, 3.274159358307527690 ) ) ;
#30143=CARTESIAN_POINT ( 'NONE',  ( 27.51562500061451644, 3.027376345333611329, 5.243569643749999010 ) ) ;
#30144=CARTESIAN_POINT ( 'NONE',  ( 4.696875000614518569, -3.027376345333614438, 5.243569643749998122 ) ) ;
#30146=CARTESIAN_POINT ( 'NONE',  ( 16.64999999999999858, -4.330127018922190985, -2.500000000000001332 ) ) ;
#30147=CARTESIAN_POINT ( 'NONE',  ( 20.65312500061451573, 4.541064518000418104, -2.621784821874998173 ) ) ;
#30148=ORIENTED_EDGE ( 'NONE', *, *, #53983, .T. ) ;
#30149=CARTESIAN_POINT ( 'NONE',  ( 24.52499999999999858, 4.330127018922191873, 2.499999999999999556 ) ) ;
#30150=CARTESIAN_POINT ( 'NONE',  ( 25.54687500061451644, -3.027376345333610441, -5.243569643749999898 ) ) ;
#30151=ORIENTED_EDGE ( 'NONE', *, *, #32136, .F. ) ;
#30152=CARTESIAN_POINT ( 'NONE',  ( 13.34062500061451750, -3.027376345333610441, -5.243569643749999898 ) ) ;
#30153=CARTESIAN_POINT ( 'NONE',  ( 5.053125000614517859, 0.000000000000000000, 5.243569643749999010 ) ) ;
#30155=CARTESIAN_POINT ( 'NONE',  ( 3.421875000614516882, -6.054752690667223547, -1.112240025338166033E-15 ) ) ;
#30156=CARTESIAN_POINT ( 'NONE',  ( 15.00000000122903465, -2.886751345948125991, -5.000000000000000000 ) ) ;
#30158=CARTESIAN_POINT ( 'NONE',  ( 20.66250000000000142, -5.773502691896255534, -1.060575238724906372E-15 ) ) ;
#30159=CARTESIAN_POINT ( 'NONE',  ( 29.55000000000000071, 0.000000000000000000, 4.999999999999998224 ) ) ;
#30160=CARTESIAN_POINT ( 'NONE',  ( 3.684375000614518836, 4.541064518000418104, 2.621784821874999949 ) ) ;
#30161=CARTESIAN_POINT ( 'NONE',  ( 8.821875000614518569, -6.054752690667223547, -1.112240025338166033E-15 ) ) ;
#30162=CARTESIAN_POINT ( 'NONE',  ( 18.94687500061451502, 6.054752690667223547, 3.707466751127219781E-16 ) ) ;
#30165=CARTESIAN_POINT ( 'NONE',  ( 28.37812500061451715, 4.541064518000418104, 2.621784821874999949 ) ) ;
#30166=CARTESIAN_POINT ( 'NONE',  ( 29.82187500061451502, 3.027376345333611329, 5.243569643749999010 ) ) ;
#30168=CARTESIAN_POINT ( 'NONE',  ( 3.834375000614519635, -4.541064518000419881, 2.621784821874995952 ) ) ;
#30170=CARTESIAN_POINT ( 'NONE',  ( 15.82499999999999929, 6.123233995736764310E-16, -4.999999999999998224 ) ) ;
#30171=CARTESIAN_POINT ( 'NONE',  ( 13.34062500061451750, -3.027376345333610441, -5.243569643749999898 ) ) ;
#30172=CARTESIAN_POINT ( 'NONE',  ( 1.071796769724491893, 13.94509619066136707, 33.99999999999999289 ) ) ;
#30174=CARTESIAN_POINT ( 'NONE',  ( 19.53750000122903430, 6.123233995736764310E-16, -4.999999999999998224 ) ) ;
#30175=CARTESIAN_POINT ( 'NONE',  ( 3.038088735723376566, 9.529008066655457299, 24.82235102052792541 ) ) ;
#30177=CARTESIAN_POINT ( 'NONE',  ( 8.203125000614518214, 0.000000000000000000, 5.243569643749999010 ) ) ;
#30178=CARTESIAN_POINT ( 'NONE',  ( 24.27187500061452141, 3.027376345333613106, -5.243569643749998122 ) ) ;
#30179=CARTESIAN_POINT ( 'NONE',  ( 26.96250000122903145, 0.000000000000000000, 4.999999999999998224 ) ) ;
#30180=CARTESIAN_POINT ( 'NONE',  ( 27.38437500061451857, 6.421520780324663323E-16, -5.243569643749999010 ) ) ;
#30181=CARTESIAN_POINT ( 'NONE',  ( 7.425000000000000711, 4.330127018922191873, 2.499999999999999556 ) ) ;
#30182=CARTESIAN_POINT ( 'NONE',  ( 3.999999999999998668, 13.17500000122903359, 27.69059892324149175 ) ) ;
#30183=CARTESIAN_POINT ( 'NONE',  ( 15.06562500061451537, -6.054752690667223547, -1.112240025338166033E-15 ) ) ;
#30184=CARTESIAN_POINT ( 'NONE',  ( 6.450000001229034829, -2.886751345948125991, -5.000000000000000000 ) ) ;
#30186=CARTESIAN_POINT ( 'NONE',  ( 12.38437500061451857, -4.541064518000419881, 2.621784821874995952 ) ) ;
#30188=ORIENTED_EDGE ( 'NONE', *, *, #17491, .F. ) ;
#30189=CARTESIAN_POINT ( 'NONE',  ( 11.84062500061451750, -3.027376345333614438, 5.243569643749998122 ) ) ;
#30190=AXIS2_PLACEMENT_3D ( 'NONE', #72399, #9254, #55053 ) ;
#30192=CARTESIAN_POINT ( 'NONE',  ( 23.73750000122903359, 4.330127018922191873, 2.499999999999999556 ) ) ;
#30193=CARTESIAN_POINT ( 'NONE',  ( 11.93437500061451573, -4.541064518000419881, 2.621784821874995952 ) ) ;
#30194=CARTESIAN_POINT ( 'NONE',  ( 14.69062500061451537, -3.027376345333610441, -5.243569643749999898 ) ) ;
#30196=CARTESIAN_POINT ( 'NONE',  ( 24.79687500061451999, 6.054752690667223547, 3.707466751127219781E-16 ) ) ;
#30199=CARTESIAN_POINT ( 'NONE',  ( 0.000000000000000000, 20.00000000000000000, 30.00000000000000000 ) ) ;
#30200=CARTESIAN_POINT ( 'NONE',  ( -4.243569643749999898, 17.57187500061451502, -32.45002607614398471 ) ) ;
#30201=CARTESIAN_POINT ( 'NONE',  ( 15.68437500061451573, 6.421520780324663323E-16, -5.243569643749999010 ) ) ;
#30202=CARTESIAN_POINT ( 'NONE',  ( 17.81250000122903288, 4.330127018922192761, -2.499999999999997780 ) ) ;
#30203=CARTESIAN_POINT ( 'NONE',  ( 13.24687500061451750, -3.027376345333614438, 5.243569643749998122 ) ) ;
#30204=CARTESIAN_POINT ( 'NONE',  ( -4.243569643749999898, 10.37187500061451750, 27.54997392385601529 ) ) ;
#30205=CARTESIAN_POINT ( 'NONE',  ( 20.47500000122903074, 2.886751345948129099, -4.999999999999998224 ) ) ;
#30206=CARTESIAN_POINT ( 'NONE',  ( 13.45312500061451466, 4.541064518000418104, -2.621784821874998173 ) ) ;
#30207=VERTEX_POINT ( 'NONE', #59346 ) ;
#30208=VERTEX_POINT ( 'NONE', #37561 ) ;
#30209=CARTESIAN_POINT ( 'NONE',  ( 17.51249999999999929, -5.773502691896255534, -1.060575238724906372E-15 ) ) ;
#30210=CARTESIAN_POINT ( 'NONE',  ( 11.93437500061451573, -4.541064518000419881, 2.621784821874995952 ) ) ;
#30211=CARTESIAN_POINT ( 'NONE',  ( 1.095284332908920577, 4.886121113889973167, 26.14314022704991203 ) ) ;
#30212=CARTESIAN_POINT ( 'NONE',  ( 12.93750000122903465, 4.330127018922191873, 2.499999999999999556 ) ) ;
#30213=CARTESIAN_POINT ( 'NONE',  ( 21.37500000122902932, 2.886751345948129099, -4.999999999999998224 ) ) ;
#30214=CARTESIAN_POINT ( 'NONE',  ( 18.02812500061451573, 4.541064518000418104, 2.621784821874999949 ) ) ;
#30215=CARTESIAN_POINT ( 'NONE',  ( 23.80312500061451786, 4.541064518000418104, -2.621784821874998173 ) ) ;
#30216=CARTESIAN_POINT ( 'NONE',  ( 29.13750000122903216, 4.330127018922191873, 2.499999999999999556 ) ) ;
#30217=CARTESIAN_POINT ( 'NONE',  ( 28.01249999999999574, 2.886751345948129099, -4.999999999999998224 ) ) ;
#30219=AXIS2_PLACEMENT_3D ( 'NONE', #26024, #48933, #21202 ) ;
#30221=CARTESIAN_POINT ( 'NONE',  ( 27.60937500061451644, 0.000000000000000000, 5.243569643749999010 ) ) ;
#30222=CARTESIAN_POINT ( 'NONE',  ( 4.003764151685233585, -2.995052564723633903, -4.167540328934556726 ) ) ;
#30223=CARTESIAN_POINT ( 'NONE',  ( 4.243569643749999898, 15.09687500061451892, -27.54997392385601529 ) ) ;
#30224=CARTESIAN_POINT ( 'NONE',  ( 3.262500001229035718, -4.330127018922190985, -2.500000000000001332 ) ) ;
#30225=CARTESIAN_POINT ( 'NONE',  ( 6.899999999999999467, 4.330127018922192761, -2.499999999999997780 ) ) ;
#30227=CARTESIAN_POINT ( 'NONE',  ( 2.929078911596073365, -4.327287789770789317, 2.992056976644557942 ) ) ;
#30228=CARTESIAN_POINT ( 'NONE',  ( 10.09687500061451715, -3.027376345333614438, 5.243569643749998122 ) ) ;
#30229=CARTESIAN_POINT ( 'NONE',  ( 29.61562500061451431, 3.027376345333613106, -5.243569643749998122 ) ) ;
#30230=CARTESIAN_POINT ( 'NONE',  ( 1.626862140677534273E-15, 10.66249999999999964, 34.00000000000000000 ) ) ;
#30231=CARTESIAN_POINT ( 'NONE',  ( -5.191270968837354616, 8.550562458943611333, -26.96705733337210376 ) ) ;
#30232=DIRECTION ( 'NONE',  ( 0.000000000000000000, 0.000000000000000000, 1.000000000000000000 ) ) ;
#30233=CARTESIAN_POINT ( 'NONE',  ( 7.246875000614518392, 6.054752690667223547, 3.707466751127219781E-16 ) ) ;
#30234=CARTESIAN_POINT ( 'NONE',  ( 11.89687500061451608, -3.027376345333614438, 5.243569643749998122 ) ) ;
#30235=CARTESIAN_POINT ( 'NONE',  ( 7.087499999999999467, -2.886751345948129988, 4.999999999999997335 ) ) ;
#30236=CARTESIAN_POINT ( 'NONE',  ( 4.243569643749999898, 14.62812500061459531, 30.00000000000000000 ) ) ;
#30238=CARTESIAN_POINT ( 'NONE',  ( 7.087499999999999467, -2.886751345948129988, 4.999999999999997335 ) ) ;
#30240=CARTESIAN_POINT ( 'NONE',  ( 19.11562500061451431, -6.054752690667223547, -1.112240025338166033E-15 ) ) ;
#30241=CARTESIAN_POINT ( 'NONE',  ( 13.49062500061451608, 6.054752690667223547, 3.707466751127219781E-16 ) ) ;
#30243=CARTESIAN_POINT ( 'NONE',  ( 10.13437500061451679, -4.541064518000419881, 2.621784821874995952 ) ) ;
#30244=CARTESIAN_POINT ( 'NONE',  ( 25.83749999999999858, 5.773502691896255534, 3.535250795749688894E-16 ) ) ;
#30245=CARTESIAN_POINT ( 'NONE',  ( 22.76250000122903216, 4.330127018922192761, -2.499999999999997780 ) ) ;
#30246=CARTESIAN_POINT ( 'NONE',  ( 17.13749999999999929, -2.886751345948159742, -4.999999999999942268 ) ) ;
#30247=CARTESIAN_POINT ( 'NONE',  ( 12.23437500061451821, 4.541064518000418104, 2.621784821874999949 ) ) ;
#30248=CARTESIAN_POINT ( 'NONE',  ( 27.45937500061451786, 4.541064518000418104, -2.621784821874998173 ) ) ;
#30250=CARTESIAN_POINT ( 'NONE',  ( 3.346875000614518036, -3.027376345333614438, 5.243569643749998122 ) ) ;
#30251=CARTESIAN_POINT ( 'NONE',  ( 24.37500000122903288, -5.773502691896255534, -1.060575238724906372E-15 ) ) ;
#30252=CARTESIAN_POINT ( 'NONE',  ( 20.03437500061451715, -4.541064518000419881, 2.621784821874995952 ) ) ;
#30253=CARTESIAN_POINT ( 'NONE',  ( 11.37187500061451750, 3.027376345333611329, 5.243569643749999010 ) ) ;
#30255=CARTESIAN_POINT ( 'NONE',  ( 23.81250000000000000, -5.773502691896255534, -1.060575238724906372E-15 ) ) ;
#30257=CARTESIAN_POINT ( 'NONE',  ( 2.121784821875001281, 11.00937500061451857, -26.32496088578401938 ) ) ;
#30259=CARTESIAN_POINT ( 'NONE',  ( 15.25312500061451715, 4.541064518000418104, -2.621784821874998173 ) ) ;
#30260=CARTESIAN_POINT ( 'NONE',  ( 5.475000000000000533, 6.123233995736764310E-16, -4.999999999999998224 ) ) ;
#30261=CARTESIAN_POINT ( 'NONE',  ( 6.937500001229033764, 6.123233995736764310E-16, -4.999999999999998224 ) ) ;
#30262=CARTESIAN_POINT ( 'NONE',  ( -3.999999999999997335, 13.28749999999999964, -27.69059892324149530 ) ) ;
#30263=CARTESIAN_POINT ( 'NONE',  ( 15.18750000000000000, -2.886751345948129988, 4.999999999999997335 ) ) ;
#30264=CARTESIAN_POINT ( 'NONE',  ( 4.243569643749999010, 10.16562500061451857, 27.54997392385601174 ) ) ;
#30265=CARTESIAN_POINT ( 'NONE',  ( 14.81250000122903288, 0.000000000000000000, 4.999999999999998224 ) ) ;
#30266=CARTESIAN_POINT ( 'NONE',  ( 24.27187500061452141, 3.027376345333613106, -5.243569643749998122 ) ) ;
#30267=CARTESIAN_POINT ( 'NONE',  ( 1.592000809091587073E-14, 16.28750000000000142, -34.00000000000000000 ) ) ;
#30268=EDGE_LOOP ( 'NONE', ( #63748, #25160, #52739, #26298 ) ) ;
#30269=CARTESIAN_POINT ( 'NONE',  ( 18.70312500061451644, -4.541064518000417216, -2.621784821875001281 ) ) ;
#30270=CARTESIAN_POINT ( 'NONE',  ( 4.865625000614517859, 3.027376345333613106, -5.243569643749998122 ) ) ;
#30271=CARTESIAN_POINT ( 'NONE',  ( 19.05937500061451928, 0.000000000000000000, 5.243569643749999010 ) ) ;
#30272=CARTESIAN_POINT ( 'NONE',  ( 3.487500000000000711, -2.886751345948129988, 4.999999999999997335 ) ) ;
#30273=CARTESIAN_POINT ( 'NONE',  ( 6.440625000614517148, -3.027376345333614438, 5.243569643749998122 ) ) ;
#30274=CARTESIAN_POINT ( 'NONE',  ( 20.69062500061451715, 6.054752690667223547, 3.707466751127219781E-16 ) ) ;
#30275=EDGE_CURVE ( 'NONE', #6226, #65099, #36467, .T. ) ;
#30276=CARTESIAN_POINT ( 'NONE',  ( -4.243569643749997233, 14.44062500061451715, 32.45002607614398471 ) ) ;
#30277=CARTESIAN_POINT ( 'NONE',  ( 19.76250000122903216, 0.000000000000000000, 4.999999999999998224 ) ) ;
#30279=CARTESIAN_POINT ( 'NONE',  ( 9.028125000614517504, 4.541064518000418104, 2.621784821874999949 ) ) ;
#30280=CARTESIAN_POINT ( 'NONE',  ( 3.871875000614519280, -6.054752690667223547, -1.112240025338166033E-15 ) ) ;
#30281=CARTESIAN_POINT ( 'NONE',  ( 29.54062500061451502, -3.027376345333610441, -5.243569643749999898 ) ) ;
#30282=CARTESIAN_POINT ( 'NONE',  ( 22.54687500061451999, 6.054752690667223547, 3.707466751127219781E-16 ) ) ;
#30283=CARTESIAN_POINT ( 'NONE',  ( 15.36562500061451608, 3.027376345333611329, 5.243569643749999010 ) ) ;
#30284=CARTESIAN_POINT ( 'NONE',  ( 24.00000000122902932, -2.886751345948125991, -5.000000000000000000 ) ) ;
#30286=CARTESIAN_POINT ( 'NONE',  ( 24.51562500061451289, -6.054752690667223547, -1.112240025338166033E-15 ) ) ;
#30287=CARTESIAN_POINT ( 'NONE',  ( 19.05937500061451928, 0.000000000000000000, 5.243569643749999010 ) ) ;
#30288=CARTESIAN_POINT ( 'NONE',  ( 15.59062500061451573, -3.027376345333610441, -5.243569643749999898 ) ) ;
#30289=CARTESIAN_POINT ( 'NONE',  ( -2.121784821874999949, 16.63437500061451857, 26.32496088578401938 ) ) ;
#30290=CARTESIAN_POINT ( 'NONE',  ( 20.80312500061451431, 0.000000000000000000, 5.243569643749999010 ) ) ;
#30293=CARTESIAN_POINT ( 'NONE',  ( 24.71250000000000213, -5.773502691896255534, -1.060575238724906372E-15 ) ) ;
#30294=CARTESIAN_POINT ( 'NONE',  ( -1.999999999999997113, 10.17500000000000249, -26.53589838486224295 ) ) ;
#30296=CARTESIAN_POINT ( 'NONE',  ( 25.71562500061451573, 3.027376345333611329, 5.243569643749999010 ) ) ;
#30297=CARTESIAN_POINT ( 'NONE',  ( 6.628125000614517148, 6.421520780324663323E-16, -5.243569643749999010 ) ) ;
#30298=CARTESIAN_POINT ( 'NONE',  ( 18.63750000122903216, 6.123233995736764310E-16, -4.999999999999998224 ) ) ;
#30300=CARTESIAN_POINT ( 'NONE',  ( 24.59062500061451573, -3.027376345333610441, -5.243569643749999898 ) ) ;
#30301=CARTESIAN_POINT ( 'NONE',  ( 26.43750000000000000, -2.886751345948129988, 4.999999999999997335 ) ) ;
#30302=CARTESIAN_POINT ( 'NONE',  ( -2.828200636599751609E-16, 15.05000000122903536, -34.61880215351700230 ) ) ;
#30303=FACE_OUTER_BOUND ( 'NONE', #38018, .T. ) ;
#30304=CARTESIAN_POINT ( 'NONE',  ( 10.75312500061451715, 4.541064518000418104, -2.621784821874998173 ) ) ;
#30305=VERTEX_POINT ( 'NONE', #9127 ) ;
#30306=CARTESIAN_POINT ( 'NONE',  ( 26.01562500061451289, 3.027376345333613106, -5.243569643749998122 ) ) ;
#30307=CARTESIAN_POINT ( 'NONE',  ( 8.465625000614515727, 3.027376345333613106, -5.243569643749998122 ) ) ;
#30310=CARTESIAN_POINT ( 'NONE',  ( 13.12500000000000178, 6.123233995736764310E-16, -4.999999999999998224 ) ) ;
#30311=ADVANCED_FACE ( 'NONE', ( #58985 ), #31663, .F. ) ;
#30312=CARTESIAN_POINT ( 'NONE',  ( 13.46249999999999858, -5.773502691896255534, -1.060575238724906372E-15 ) ) ;
#30313=EDGE_CURVE ( 'NONE', #2494, #38561, #37214, .T. ) ;
#30315=CARTESIAN_POINT ( 'NONE',  ( 14.29687500061451821, -3.027376345333610441, -5.243569643749999898 ) ) ;
#30316=CARTESIAN_POINT ( 'NONE',  ( 8.400000001229035007, 5.773502691896255534, 3.535250795749688894E-16 ) ) ;
#30317=CARTESIAN_POINT ( 'NONE',  ( 18.08437500061451431, 4.541064518000418104, 2.621784821874999949 ) ) ;
#30319=CARTESIAN_POINT ( 'NONE',  ( 7.921875000614517326, -6.054752690667223547, -1.112240025338166033E-15 ) ) ;
#30320=CARTESIAN_POINT ( 'NONE',  ( 9.001249775931846008E-16, 11.36562500061451786, -25.09994784771203058 ) ) ;
#30323=CYLINDRICAL_SURFACE ( 'NONE', #46578, 4.999999999999998224 ) ;
#30324=CARTESIAN_POINT ( 'NONE',  ( 25.41562500061451146, -6.054752690667223547, -1.112240025338166033E-15 ) ) ;
#30325=CARTESIAN_POINT ( 'NONE',  ( 21.11250000122903359, 0.000000000000000000, 4.999999999999998224 ) ) ;
#30326=CARTESIAN_POINT ( 'NONE',  ( 26.10937500061451644, 4.541064518000418104, -2.621784821874998173 ) ) ;
#30327=CARTESIAN_POINT ( 'NONE',  ( 29.33437500061451431, 4.541064518000418104, 2.621784821874999949 ) ) ;
#30328=CARTESIAN_POINT ( 'NONE',  ( 22.19999999999999574, 4.330127018922192761, -2.499999999999997780 ) ) ;
#30329=CARTESIAN_POINT ( 'NONE',  ( 6.215625000614517504, 3.027376345333613106, -5.243569643749998122 ) ) ;
#30330=B_SPLINE_CURVE_WITH_KNOTS ( 'NONE', 3,
 ( #9731, #49630, #4568, #4928, #27098, #44463, #48897, #37801, #61067, #65882 ),
 .UNSPECIFIED., .F., .F.,
 ( 4, 3, 3, 4 ),
 ( 4.336808689942017255E-19, 0.0001572269111698576115, 0.0003144536816620901835, 0.0005496948180016699662 ),
 .UNSPECIFIED. ) ;
#30332=( BOUNDED_CURVE ( )  B_SPLINE_CURVE ( 1, ( #12861, #40958 ),
 .UNSPECIFIED., .F., .F. ) 
 B_SPLINE_CURVE_WITH_KNOTS ( ( 2, 2 ),
 ( 0.000000000000000000, 1.000000000000000000 ),
 .UNSPECIFIED. ) 
 CURVE ( )  GEOMETRIC_REPRESENTATION_ITEM ( )  RATIONAL_B_SPLINE_CURVE ( ( 0.9401540970596797830, 0.9401540970596797830 ) ) 
 REPRESENTATION_ITEM ( '' )  );
#30333=CARTESIAN_POINT ( 'NONE',  ( 16.17187500061451644, 3.027376345333613106, -5.243569643749998122 ) ) ;
#30335=CARTESIAN_POINT ( 'NONE',  ( 3.890625000614517326, -3.027376345333610441, -5.243569643749999898 ) ) ;
#30336=CARTESIAN_POINT ( 'NONE',  ( 7.284375000614518036, 4.541064518000418104, 2.621784821874999949 ) ) ;
#30337=CARTESIAN_POINT ( 'NONE',  ( 18.00937500061451502, 4.541064518000418104, -2.621784821874998173 ) ) ;
#30339=CARTESIAN_POINT ( 'NONE',  ( 27.37500000000000000, -4.330127018922194537, 2.499999999999995559 ) ) ;
#30340=CARTESIAN_POINT ( 'NONE',  ( 28.17187500061451644, -6.054752690667223547, -1.112240025338166033E-15 ) ) ;
#30342=CARTESIAN_POINT ( 'NONE',  ( 3.328125000614516438, -4.541064518000419881, 2.621784821874995952 ) ) ;
#30343=ORIENTED_EDGE ( 'NONE', *, *, #69330, .F. ) ;
#30344=CARTESIAN_POINT ( 'NONE',  ( 11.58750000000000036, -2.886751345948129988, 4.999999999999997335 ) ) ;
#30346=CARTESIAN_POINT ( 'NONE',  ( 21.06562500061451715, 3.027376345333613106, -5.243569643749998122 ) ) ;
#30347=CARTESIAN_POINT ( 'NONE',  ( 12.03749999999999964, -2.886751345948129988, 4.999999999999997335 ) ) ;
#30348=CARTESIAN_POINT ( 'NONE',  ( 8.362500001229031810, 4.330127018922192761, -2.499999999999997780 ) ) ;
#30349=CARTESIAN_POINT ( 'NONE',  ( 5.653125000614517504, -4.541064518000417216, -2.621784821875001281 ) ) ;
#30350=CARTESIAN_POINT ( 'NONE',  ( 20.85000000000000142, 4.330127018922192761, -2.499999999999997780 ) ) ;
#30351=CARTESIAN_POINT ( 'NONE',  ( 21.74062500061451431, -3.027376345333614438, 5.243569643749998122 ) ) ;
#30352=CARTESIAN_POINT ( 'NONE',  ( 24.41250000122903430, -4.330127018922190985, -2.500000000000001332 ) ) ;
#30354=CARTESIAN_POINT ( 'NONE',  ( 5.924999999999999822, 6.123233995736764310E-16, -4.999999999999998224 ) ) ;
#30355=ORIENTED_EDGE ( 'NONE', *, *, #336, .T. ) ;
#30356=CARTESIAN_POINT ( 'NONE',  ( 18.44062500061451715, 6.054752690667223547, 3.707466751127219781E-16 ) ) ;
#30357=CARTESIAN_POINT ( 'NONE',  ( 27.02812500061451573, 4.541064518000418104, 2.621784821874999949 ) ) ;
#30358=CARTESIAN_POINT ( 'NONE',  ( 26.44687500061451502, -3.027376345333610441, -5.243569643749999898 ) ) ;
#30359=CARTESIAN_POINT ( 'NONE',  ( 14.95312500061451644, 0.000000000000000000, 5.243569643749999010 ) ) ;
#30360=CARTESIAN_POINT ( 'NONE',  ( 29.46562500061451573, -6.054752690667223547, -1.112240025338166033E-15 ) ) ;
#30361=CARTESIAN_POINT ( 'NONE',  ( 9.703125000614514661, -4.541064518000417216, -2.621784821875001281 ) ) ;
#30363=AXIS2_PLACEMENT_3D ( 'NONE', #17854, #40060, #51137 ) ;
#30364=CARTESIAN_POINT ( 'NONE',  ( 27.26250000122903216, 4.330127018922192761, -2.499999999999997780 ) ) ;
#30366=CARTESIAN_POINT ( 'NONE',  ( 17.57812500061451644, 4.541064518000418104, 2.621784821874999949 ) ) ;
#30368=CARTESIAN_POINT ( 'NONE',  ( 28.99687500061451573, -3.027376345333614438, 5.243569643749998122 ) ) ;
#30369=CARTESIAN_POINT ( 'NONE',  ( 11.52187500061451608, -6.054752690667223547, -1.112240025338166033E-15 ) ) ;
#30370=CARTESIAN_POINT ( 'NONE',  ( 10.65937500061451715, -4.541064518000417216, -2.621784821875001281 ) ) ;
#30371=CARTESIAN_POINT ( 'NONE',  ( 18.72187500061451360, -6.054752690667223547, -1.112240025338166033E-15 ) ) ;
#30372=ORIENTED_EDGE ( 'NONE', *, *, #6970, .T. ) ;
#30373=CARTESIAN_POINT ( 'NONE',  ( 3.046343057529203424, 3.964819538874875704, 3.046343057529141696 ) ) ;
#30374=CARTESIAN_POINT ( 'NONE',  ( 22.22812500061451502, -4.541064518000419881, 2.621784821874995952 ) ) ;
#30375=CARTESIAN_POINT ( 'NONE',  ( 16.50937500061451502, -4.541064518000417216, -2.621784821875001281 ) ) ;
#30376=CARTESIAN_POINT ( 'NONE',  ( 21.62812500061451360, 4.541064518000418104, 2.621784821874999949 ) ) ;
#30377=CARTESIAN_POINT ( 'NONE',  ( 8.484601909799253346E-16, 14.26250000000000107, 34.61880215351700230 ) ) ;
#30378=CARTESIAN_POINT ( 'NONE',  ( 3.046875000614519990, -3.027376345333610441, -5.243569643749999898 ) ) ;
#30379=CARTESIAN_POINT ( 'NONE',  ( 9.000000001229034652, -2.886751345948129988, 4.999999999999997335 ) ) ;
#30381=CARTESIAN_POINT ( 'NONE',  ( 4.275000001229035895, 2.886751345948129099, -4.999999999999998224 ) ) ;
#30382=CARTESIAN_POINT ( 'NONE',  ( 3.999999999999999112, 18.42500000000000071, -30.00000000000000000 ) ) ;
#30383=CARTESIAN_POINT ( 'NONE',  ( 25.01250000122903216, 4.330127018922192761, -2.499999999999997780 ) ) ;
#30385=CARTESIAN_POINT ( 'NONE',  ( 9.046875000614518214, 6.054752690667223547, 3.707466751127219781E-16 ) ) ;
#30387=CARTESIAN_POINT ( 'NONE',  ( 16.00312500061451715, -4.541064518000417216, -2.621784821875001281 ) ) ;
#30388=CARTESIAN_POINT ( 'NONE',  ( 10.50937500061451679, 0.000000000000000000, 5.243569643749999010 ) ) ;
#30389=CARTESIAN_POINT ( 'NONE',  ( 2.990625000614519191, -3.027376345333610441, -5.243569643749999898 ) ) ;
#30390=CARTESIAN_POINT ( 'NONE',  ( 18.23437500061451999, -4.541064518000419881, 2.621784821874995952 ) ) ;
#30391=CARTESIAN_POINT ( 'NONE',  ( 7.396875000614519635, -3.027376345333614438, 5.243569643749998122 ) ) ;
#30392=CARTESIAN_POINT ( 'NONE',  ( 1.999999999999998668, 17.60000000000000142, -33.46410161513775705 ) ) ;
#30393=CARTESIAN_POINT ( 'NONE',  ( 8.690625000614515372, -3.027376345333614438, 5.243569643749998122 ) ) ;
#30394=CARTESIAN_POINT ( 'NONE',  ( 18.77812500061451573, 6.421520780324663323E-16, -5.243569643749999010 ) ) ;
#30395=VERTEX_POINT ( 'NONE', #605 ) ;
#30397=CARTESIAN_POINT ( 'NONE',  ( 14.87812500061451537, 4.541064518000418104, 2.621784821874999949 ) ) ;
#30398=CARTESIAN_POINT ( 'NONE',  ( 10.86562500061451431, 3.027376345333611329, 5.243569643749999010 ) ) ;
#30400=CARTESIAN_POINT ( 'NONE',  ( 12.07499999999999929, -4.330127018922194537, 2.499999999999995559 ) ) ;
#30401=CARTESIAN_POINT ( 'NONE',  ( 6.300000001229033586, -2.886751345948129988, 4.999999999999997335 ) ) ;
#30403=CARTESIAN_POINT ( 'NONE',  ( 13.95937500061451786, 4.541064518000418104, -2.621784821874998173 ) ) ;
#30404=CARTESIAN_POINT ( 'NONE',  ( 16.76250000122903216, -4.330127018922190985, -2.500000000000001332 ) ) ;
#30406=CARTESIAN_POINT ( 'NONE',  ( 9.001249775931846008E-16, 18.56562500061451715, -25.09994784771203058 ) ) ;
#30407=CARTESIAN_POINT ( 'NONE',  ( 16.16250000122903430, 0.000000000000000000, 4.999999999999998224 ) ) ;
#30408=CARTESIAN_POINT ( 'NONE',  ( -1.487416814333745711E-14, 14.82500000122903572, -26.00000000000000000 ) ) ;
#30409=VECTOR ( 'NONE', #50814, 1000.000000000000000 ) ;
#30410=CARTESIAN_POINT ( 'NONE',  ( 9.525000001229035007, -5.773502691896255534, -1.060575238724906372E-15 ) ) ;
#30411=CARTESIAN_POINT ( 'NONE',  ( 1.071796769724476572, 14.39509619066136636, 34.00000000000000000 ) ) ;
#30412=CARTESIAN_POINT ( 'NONE',  ( 18.98437500061451644, 4.541064518000418104, 2.621784821874999949 ) ) ;
#30414=CARTESIAN_POINT ( 'NONE',  ( 29.88749999999999929, 5.773502691896255534, 3.535250795749688894E-16 ) ) ;
#30415=CARTESIAN_POINT ( 'NONE',  ( 13.94062500061451892, 6.054752690667223547, 3.707466751127219781E-16 ) ) ;
#30417=CARTESIAN_POINT ( 'NONE',  ( 22.99687500061451573, 6.054752690667223547, 3.707466751127219781E-16 ) ) ;
#30419=CARTESIAN_POINT ( 'NONE',  ( 9.440625000614517148, 6.054752690667223547, 3.707466751127219781E-16 ) ) ;
#30420=CARTESIAN_POINT ( 'NONE',  ( 16.50937500061451502, -4.541064518000417216, -2.621784821875001281 ) ) ;
#30421=EDGE_LOOP ( 'NONE', ( #63254, #49792, #29183, #25982 ) ) ;
#30422=CARTESIAN_POINT ( 'NONE',  ( 26.63437500061451857, 4.541064518000418104, 2.621784821874999949 ) ) ;
#30423=CARTESIAN_POINT ( 'NONE',  ( 28.41562500061451502, 3.027376345333611329, 5.243569643749999010 ) ) ;
#30424=CARTESIAN_POINT ( 'NONE',  ( 16.82812500061451644, -4.541064518000419881, 2.621784821874995952 ) ) ;
#30425=CARTESIAN_POINT ( 'NONE',  ( 18.78749999999999787, -2.886751345948096681, 5.000000000000054179 ) ) ;
#30426=DIRECTION ( 'NONE',  ( -1.000000000000000000, -0.000000000000000000, -0.000000000000000000 ) ) ;
#30427=CARTESIAN_POINT ( 'NONE',  ( 9.825000000000001066, -4.330127018922194537, 2.499999999999995559 ) ) ;
#30428=CARTESIAN_POINT ( 'NONE',  ( 19.95000000122903572, -2.886751345948125991, -5.000000000000000000 ) ) ;
#30429=CARTESIAN_POINT ( 'NONE',  ( -6.275039685470489619E-15, 17.97500000122903074, -26.00000000000000355 ) ) ;
#30431=ORIENTED_EDGE ( 'NONE', *, *, #47837, .T. ) ;
#30432=CARTESIAN_POINT ( 'NONE',  ( 18.14999999999999858, 4.330127018922192761, -2.499999999999997780 ) ) ;
#30433=CARTESIAN_POINT ( 'NONE',  ( 19.23749999999999716, -2.886751345948129988, 4.999999999999997335 ) ) ;
#30434=CARTESIAN_POINT ( 'NONE',  ( 18.23437500061451999, -4.541064518000419881, 2.621784821874995952 ) ) ;
#30435=CARTESIAN_POINT ( 'NONE',  ( 13.86562500061451431, 3.027376345333613106, -5.243569643749998122 ) ) ;
#30438=CARTESIAN_POINT ( 'NONE',  ( 7.040625000614517681, -3.027376345333610441, -5.243569643749999898 ) ) ;
#30439=CARTESIAN_POINT ( 'NONE',  ( 10.38750000000000107, -2.886751345948126435, -5.000000000000000000 ) ) ;
#30440=CARTESIAN_POINT ( 'NONE',  ( 12.71250000000000036, 2.886751345948129099, -4.999999999999998224 ) ) ;
#30442=CARTESIAN_POINT ( 'NONE',  ( -2.121784821874996840, 14.92812500061451608, 33.67503911421598417 ) ) ;
#30443=CARTESIAN_POINT ( 'NONE',  ( 27.51562500061451644, 3.027376345333611329, 5.243569643749999010 ) ) ;
#30446=CARTESIAN_POINT ( 'NONE',  ( 23.25937500061451857, -4.541064518000417216, -2.621784821875001281 ) ) ;
#30447=EDGE_LOOP ( 'NONE', ( #20095, #42840, #2720, #42111 ) ) ;
#30448=CARTESIAN_POINT ( 'NONE',  ( 20.95312500061451999, -4.541064518000417216, -2.621784821875001281 ) ) ;
#30449=CARTESIAN_POINT ( 'NONE',  ( 22.92187500061451644, 3.027376345333613106, -5.243569643749998122 ) ) ;
#30450=CARTESIAN_POINT ( 'NONE',  ( 4.243569643749999898, 15.52812500061459389, -30.00000000000000000 ) ) ;
#30451=CARTESIAN_POINT ( 'NONE',  ( 6.665625000614515905, 3.027376345333613106, -5.243569643749998122 ) ) ;
#30453=CARTESIAN_POINT ( 'NONE',  ( 24.32812500061451289, 4.541064518000418104, 2.621784821874999949 ) ) ;
#30456=CARTESIAN_POINT ( 'NONE',  ( 17.44687500061451857, -3.027376345333610441, -5.243569643749999898 ) ) ;
#30457=CARTESIAN_POINT ( 'NONE',  ( 24.27187500061452141, 3.027376345333613106, -5.243569643749998122 ) ) ;
#30458=CARTESIAN_POINT ( 'NONE',  ( -4.243569643749999898, 14.45937500061451964, 30.00000000000000000 ) ) ;
#30459=CARTESIAN_POINT ( 'NONE',  ( 6.703125000614516438, 4.541064518000418104, -2.621784821874998173 ) ) ;
#30460=CARTESIAN_POINT ( 'NONE',  ( 29.46562500061451573, -6.054752690667223547, -1.112240025338166033E-15 ) ) ;
#30461=CARTESIAN_POINT ( 'NONE',  ( 3.346875000614518036, -3.027376345333614438, 5.243569643749998122 ) ) ;
#30463=CARTESIAN_POINT ( 'NONE',  ( 4.715625000614516615, -6.054752690667223547, -1.112240025338166033E-15 ) ) ;
#30464=CARTESIAN_POINT ( 'NONE',  ( 8.859375000614518214, -4.541064518000417216, -2.621784821875001281 ) ) ;
#30466=CARTESIAN_POINT ( 'NONE',  ( 16.98750000122903359, 4.330127018922191873, 2.499999999999999556 ) ) ;
#30467=CARTESIAN_POINT ( 'NONE',  ( 2.859375000614519546, 0.000000000000000000, 5.243569643749999010 ) ) ;
#30468=CARTESIAN_POINT ( 'NONE',  ( 5.465625000614517504, 3.027376345333611329, 5.243569643749999010 ) ) ;
#30471=CARTESIAN_POINT ( 'NONE',  ( 17.03437500061451715, 6.421520780324663323E-16, -5.243569643749999010 ) ) ;
#30474=CARTESIAN_POINT ( 'NONE',  ( 22.75312500061451360, -4.541064518000417216, -2.621784821875001281 ) ) ;
#30475=CARTESIAN_POINT ( 'NONE',  ( 9.553125000614517859, 0.000000000000000000, 5.243569643749999010 ) ) ;
#30476=CARTESIAN_POINT ( 'NONE',  ( 25.84687500061451715, -3.027376345333614438, 5.243569643749998122 ) ) ;
#30477=CARTESIAN_POINT ( 'NONE',  ( 10.67812500061451608, 6.421520780324663323E-16, -5.243569643749999010 ) ) ;
#30478=CARTESIAN_POINT ( 'NONE',  ( 20.36249999999999716, 2.886751345948095793, -5.000000000000055067 ) ) ;
#30479=( BOUNDED_CURVE ( )  B_SPLINE_CURVE ( 3, ( #23908, #22817, #307, #46095 ),
 .UNSPECIFIED., .F., .F. ) 
 B_SPLINE_CURVE_WITH_KNOTS ( ( 4, 4 ),
 ( 1.570796326794896558, 3.141592653589793116 ),
 .UNSPECIFIED. ) 
 CURVE ( )  GEOMETRIC_REPRESENTATION_ITEM ( )  RATIONAL_B_SPLINE_CURVE ( ( 1.000000000000000000, 0.8047378541243649375, 0.8047378541243649375, 1.000000000000000000 ) ) 
 REPRESENTATION_ITEM ( '' )  );
#30480=CARTESIAN_POINT ( 'NONE',  ( 9.412500001229034297, 0.000000000000000000, 4.999999999999998224 ) ) ;
#30481=CARTESIAN_POINT ( 'NONE',  ( 25.49062500061451786, -3.027376345333610441, -5.243569643749999898 ) ) ;
#30482=CARTESIAN_POINT ( 'NONE',  ( 2.121784821874999061, 10.65312500061451750, -33.67503911421598417 ) ) ;
#30483=CARTESIAN_POINT ( 'NONE',  ( 12.11250000122903181, 0.000000000000000000, 4.999999999999998224 ) ) ;
#30484=CARTESIAN_POINT ( 'NONE',  ( 22.49062500061451431, 6.054752690667223547, 3.707466751127219781E-16 ) ) ;
#30485=CARTESIAN_POINT ( 'NONE',  ( 17.57812500061451644, 4.541064518000418104, 2.621784821874999949 ) ) ;
#30486=CARTESIAN_POINT ( 'NONE',  ( 6.534375000614517148, -4.541064518000419881, 2.621784821874995952 ) ) ;
#30487=EDGE_CURVE ( 'NONE', #29484, #48852, #59415, .T. ) ;
#30488=CARTESIAN_POINT ( 'NONE',  ( 18.11250000000000071, 2.886751345948129099, -4.999999999999998224 ) ) ;
#30489=CARTESIAN_POINT ( 'NONE',  ( 12.86250000122903359, 4.330127018922192761, -2.499999999999997780 ) ) ;
#30490=CARTESIAN_POINT ( 'NONE',  ( 9.890625000614516438, 6.054752690667223547, 3.707466751127219781E-16 ) ) ;
#30491=CARTESIAN_POINT ( 'NONE',  ( 13.34062500061451750, -3.027376345333610441, -5.243569643749999898 ) ) ;
#30492=CARTESIAN_POINT ( 'NONE',  ( 24.11250000122903359, 4.330127018922192761, -2.499999999999997780 ) ) ;
#30493=CARTESIAN_POINT ( 'NONE',  ( 20.82187500061451857, 3.027376345333611329, 5.243569643749999010 ) ) ;
#30494=CARTESIAN_POINT ( 'NONE',  ( 21.45937500061451786, -4.541064518000417216, -2.621784821875001281 ) ) ;
#30495=CARTESIAN_POINT ( 'NONE',  ( 30.00000000000000000, 0.000000000000000000, 4.999999999999998224 ) ) ;
#30496=CARTESIAN_POINT ( 'NONE',  ( 8.362500001229031810, 4.330127018922192761, -2.499999999999997780 ) ) ;
#30497=CARTESIAN_POINT ( 'NONE',  ( 6.984375000614516438, -4.541064518000419881, 2.621784821874995952 ) ) ;
#30498=CARTESIAN_POINT ( 'NONE',  ( 25.47187500061451715, -6.054752690667223547, -1.112240025338166033E-15 ) ) ;
#30499=CARTESIAN_POINT ( 'NONE',  ( 4.584099534023079237, 1.997112472210624379, -4.621249760862988332 ) ) ;
#30500=CARTESIAN_POINT ( 'NONE',  ( 20.76562500061451644, 3.027376345333611329, 5.243569643749999010 ) ) ;
#30501=CARTESIAN_POINT ( 'NONE',  ( 27.72187500061451715, -6.054752690667223547, -1.112240025338166033E-15 ) ) ;
#30505=CARTESIAN_POINT ( 'NONE',  ( 6.571875000614517681, -6.054752690667223547, -1.112240025338166033E-15 ) ) ;
#30506=CARTESIAN_POINT ( 'NONE',  ( 16.75312500061451715, 0.000000000000000000, 5.243569643749999010 ) ) ;
#30507=VERTEX_POINT ( 'NONE', #40491 ) ;
#30508=CARTESIAN_POINT ( 'NONE',  ( 22.98750000000000071, -2.886751345948092684, -5.000000000000057732 ) ) ;
#30509=CARTESIAN_POINT ( 'NONE',  ( 25.22812500061451502, 4.541064518000418104, 2.621784821874999949 ) ) ;
#30510=CARTESIAN_POINT ( 'NONE',  ( 4.209375000614516971, 0.000000000000000000, 5.243569643749999010 ) ) ;
#30511=CARTESIAN_POINT ( 'NONE',  ( 10.31250000122903288, 0.000000000000000000, 4.999999999999998224 ) ) ;
#30513=CARTESIAN_POINT ( 'NONE',  ( 17.10000000000000142, -4.330127018922190985, -2.500000000000001332 ) ) ;
#30514=CARTESIAN_POINT ( 'NONE',  ( 20.16562500061451146, 3.027376345333613106, -5.243569643749998122 ) ) ;
#30515=ORIENTED_EDGE ( 'NONE', *, *, #10064, .F. ) ;
#30516=CARTESIAN_POINT ( 'NONE',  ( 24.11249999999999716, 2.886751345948126879, 4.999999999999999112 ) ) ;
#30517=( BOUNDED_CURVE ( )  B_SPLINE_CURVE ( 2, ( #38057, #60953, #32525, #10718, #49883, #43982, #60213 ),
 .UNSPECIFIED., .F., .F. ) 
 B_SPLINE_CURVE_WITH_KNOTS ( ( 3, 2, 2, 3 ),
 ( 0.4833333333333333925, 0.4861111111111111605, 0.4888888888888888729, 0.4916666666666666408 ),
 .UNSPECIFIED. ) 
 CURVE ( )  GEOMETRIC_REPRESENTATION_ITEM ( )  RATIONAL_B_SPLINE_CURVE ( ( 0.9999999999999973355, 0.8660254037844413721, 1.000000000000000000, 0.8660254037844387076, 1.000000000000000000, 0.8660254037844387076, 1.000000000000000000 ) ) 
 REPRESENTATION_ITEM ( '' )  );
#30518=CARTESIAN_POINT ( 'NONE',  ( 25.17187500061451644, 3.027376345333613106, -5.243569643749998122 ) ) ;
#30519=VERTEX_POINT ( 'NONE', #63006 ) ;
#30520=CARTESIAN_POINT ( 'NONE',  ( 3.015485575276906527, -3.988347017152381824, -3.404139683571346442 ) ) ;
#30521=CARTESIAN_POINT ( 'NONE',  ( 11.99062500061451608, -3.027376345333610441, -5.243569643749999898 ) ) ;
#30522=CARTESIAN_POINT ( 'NONE',  ( 6.253125000614517148, 4.541064518000418104, -2.621784821874998173 ) ) ;
#30524=CARTESIAN_POINT ( 'NONE',  ( 29.50312500061451360, -4.541064518000417216, -2.621784821875001281 ) ) ;
#30525=CARTESIAN_POINT ( 'NONE',  ( 14.58750000122903323, 6.123233995736764310E-16, -4.999999999999998224 ) ) ;
#30526=CARTESIAN_POINT ( 'NONE',  ( 19.20000000000000284, 0.000000000000000000, 4.999999999999998224 ) ) ;
#30527=CARTESIAN_POINT ( 'NONE',  ( 26.39999999999999858, 0.000000000000000000, 4.999999999999998224 ) ) ;
#30528=CARTESIAN_POINT ( 'NONE',  ( 3.346875000614518036, -3.027376345333614438, 5.243569643749998122 ) ) ;
#30529=CARTESIAN_POINT ( 'NONE',  ( 9.684375000614517504, -4.541064518000419881, 2.621784821874995952 ) ) ;
#30530=CARTESIAN_POINT ( 'NONE',  ( 20.07187500061451857, -6.054752690667223547, -1.112240025338166033E-15 ) ) ;
#30531=CARTESIAN_POINT ( 'NONE',  ( -3.999999999999997335, 13.85000000122903607, 32.30940107675850470 ) ) ;
#30532=VERTEX_POINT ( 'NONE', #58537 ) ;
#30533=CARTESIAN_POINT ( 'NONE',  ( 28.67812500061451431, 6.421520780324663323E-16, -5.243569643749999010 ) ) ;
#30534=CARTESIAN_POINT ( 'NONE',  ( 3.337499999999999911, 5.773502691896255534, 3.535250795749688894E-16 ) ) ;
#30535=CARTESIAN_POINT ( 'NONE',  ( 4.884375000614518569, 6.421520780324663323E-16, -5.243569643749999010 ) ) ;
#30536=CARTESIAN_POINT ( 'NONE',  ( 17.32499999999999929, 4.330127018922191873, 2.499999999999999556 ) ) ;
#30537=CARTESIAN_POINT ( 'NONE',  ( 13.75312500061451715, -4.541064518000417216, -2.621784821875001281 ) ) ;
#30540=CARTESIAN_POINT ( 'NONE',  ( 18.30000000122903359, 5.773502691896255534, 3.535250795749688894E-16 ) ) ;
#30541=CARTESIAN_POINT ( 'NONE',  ( 3.203127373816012646, 9.474626018533117033, 24.92290371183301900 ) ) ;
#30543=CARTESIAN_POINT ( 'NONE',  ( 7.565625000614518036, 3.027376345333613106, -5.243569643749998122 ) ) ;
#30544=CARTESIAN_POINT ( 'NONE',  ( 23.44687500061451502, 6.054752690667223547, 3.707466751127219781E-16 ) ) ;
#30545=CARTESIAN_POINT ( 'NONE',  ( 4.243569643749999898, 19.18437500061451928, 30.00000000000000000 ) ) ;
#30546=CARTESIAN_POINT ( 'NONE',  ( 23.25937500061451857, -4.541064518000417216, -2.621784821875001281 ) ) ;
#30547=CARTESIAN_POINT ( 'NONE',  ( 6.825000000000001066, 6.123233995736764310E-16, -4.999999999999998224 ) ) ;
#30548=CARTESIAN_POINT ( 'NONE',  ( -1.999999999999997113, 10.28750000122903430, 33.46410161513775705 ) ) ;
#30549=CARTESIAN_POINT ( 'NONE',  ( 13.64062500061451644, -3.027376345333614438, 5.243569643749998122 ) ) ;
#30550=CARTESIAN_POINT ( 'NONE',  ( 5.812500001229035540, 0.000000000000000000, 4.999999999999998224 ) ) ;
#30552=CARTESIAN_POINT ( 'NONE',  ( 11.37187500061451750, 3.027376345333611329, 5.243569643749999010 ) ) ;
#30553=CARTESIAN_POINT ( 'NONE',  ( -1.839935159944503518, 4.656359355287978730, -26.43822482402454455 ) ) ;
#30555=CARTESIAN_POINT ( 'NONE',  ( 12.59062500061451573, 6.054752690667223547, 3.707466751127219781E-16 ) ) ;
#30556=CARTESIAN_POINT ( 'NONE',  ( 3.433818815427341686, -3.634411862891160361, -3.779699544484016016 ) ) ;
#30557=CARTESIAN_POINT ( 'NONE',  ( 24.03750000122903430, 6.123233995736764310E-16, -4.999999999999998224 ) ) ;
#30558=CARTESIAN_POINT ( 'NONE',  ( 10.32187500061451679, 3.027376345333613106, -5.243569643749998122 ) ) ;
#30559=CARTESIAN_POINT ( 'NONE',  ( 14.01562500061451644, 3.027376345333611329, 5.243569643749999010 ) ) ;
#30561=CARTESIAN_POINT ( 'NONE',  ( 24.04687500061451644, -3.027376345333614438, 5.243569643749998122 ) ) ;
#30564=CARTESIAN_POINT ( 'NONE',  ( -1.071796769724490117, 19.45759618943232994, 26.00000000000000000 ) ) ;
#30565=CARTESIAN_POINT ( 'NONE',  ( 2.121784821875001281, 15.05937500061451928, -26.32496088578401938 ) ) ;
#30566=CARTESIAN_POINT ( 'NONE',  ( 14.59687500061452070, -3.027376345333614438, 5.243569643749998122 ) ) ;
#30567=CARTESIAN_POINT ( 'NONE',  ( 18.30000000122903359, 5.773502691896255534, 3.535250795749688894E-16 ) ) ;
#30568=CARTESIAN_POINT ( 'NONE',  ( 13.17187500061451999, 3.027376345333611329, 5.243569643749999010 ) ) ;
#30569=CARTESIAN_POINT ( 'NONE',  ( 4.243569643749999898, 17.77812500061451928, -30.00000000000000000 ) ) ;
#30570=CARTESIAN_POINT ( 'NONE',  ( 20.40000000122903145, -2.886751345948125991, -5.000000000000000000 ) ) ;
#30571=CARTESIAN_POINT ( 'NONE',  ( 12.55312500061451786, 4.541064518000418104, -2.621784821874998173 ) ) ;
#30574=CARTESIAN_POINT ( 'NONE',  ( 19.08750000000000213, 5.773502691896255534, 3.535250795749688894E-16 ) ) ;
#30575=CARTESIAN_POINT ( 'NONE',  ( 1.626862140677534273E-15, 17.52500000122903145, -26.00000000000000355 ) ) ;
#30576=CARTESIAN_POINT ( 'NONE',  ( 11.40937500061451892, 0.000000000000000000, 5.243569643749999010 ) ) ;
#30577=DIRECTION ( 'NONE',  ( -1.000000000000000000, -0.000000000000000000, -0.000000000000000000 ) ) ;
#30578=CARTESIAN_POINT ( 'NONE',  ( 13.35000000122903430, 5.773502691896255534, 3.535250795749688894E-16 ) ) ;
#30579=CARTESIAN_POINT ( 'NONE',  ( 20.55000000122903359, 5.773502691896255534, 3.535250795749688894E-16 ) ) ;
#30580=CARTESIAN_POINT ( 'NONE',  ( 16.52812500061451573, 6.421520780324663323E-16, -5.243569643749999010 ) ) ;
#30581=CARTESIAN_POINT ( 'NONE',  ( 21.14062500061451289, 6.054752690667223547, 3.707466751127219781E-16 ) ) ;
#30582=CARTESIAN_POINT ( 'NONE',  ( 28.12500000122902932, 2.886751345948129099, -4.999999999999998224 ) ) ;
#30583=CARTESIAN_POINT ( 'NONE',  ( 26.96249999999999858, -5.773502691896255534, -1.060575238724906372E-15 ) ) ;
#30586=CARTESIAN_POINT ( 'NONE',  ( 27.15937500061451360, 0.000000000000000000, 5.243569643749999010 ) ) ;
#30587=CARTESIAN_POINT ( 'NONE',  ( 1.071796769724491893, 14.28259618943233455, -26.00000000000000355 ) ) ;
#30588=CARTESIAN_POINT ( 'NONE',  ( -4.243569643749997233, 16.29687500061451644, -27.54997392385601174 ) ) ;
#30590=CARTESIAN_POINT ( 'NONE',  ( 3.000000001229032875, 5.773502691896255534, 3.535250795749688894E-16 ) ) ;
#30591=CARTESIAN_POINT ( 'NONE',  ( 5.662500000000000533, 2.886751345948126879, 4.999999999999999112 ) ) ;
#30592=CARTESIAN_POINT ( 'NONE',  ( 9.234375000614518214, -4.541064518000419881, 2.621784821874995952 ) ) ;
#30593=CARTESIAN_POINT ( 'NONE',  ( 28.15312500061451573, -4.541064518000417216, -2.621784821875001281 ) ) ;
#30594=CARTESIAN_POINT ( 'NONE',  ( -1.487416814333745711E-14, 14.82500000122903572, 34.00000000000000000 ) ) ;
#30596=CARTESIAN_POINT ( 'NONE',  ( 8.287499999999999645, 5.773502691896255534, 3.535250795749688401E-16 ) ) ;
#30597=CARTESIAN_POINT ( 'NONE',  ( 6.871875000614517504, 3.027376345333611329, 5.243569643749999010 ) ) ;
#30598=CARTESIAN_POINT ( 'NONE',  ( 11.97187500061451892, -6.054752690667223547, -1.112240025338166033E-15 ) ) ;
#30599=CARTESIAN_POINT ( 'NONE',  ( 3.562500000000000444, -5.773502691896255534, -1.060575238724906372E-15 ) ) ;
#30600=CARTESIAN_POINT ( 'NONE',  ( -4.243569643749998122, 13.99062500061459602, 32.45002607614398471 ) ) ;
#30601=CARTESIAN_POINT ( 'NONE',  ( 3.999999999999998668, 18.01249999999999929, 27.69059892324149530 ) ) ;
#30602=CARTESIAN_POINT ( 'NONE',  ( 7.050000000000000711, 0.000000000000000000, 4.999999999999998224 ) ) ;
#30604=CARTESIAN_POINT ( 'NONE',  ( 19.45312500061451644, 0.000000000000000000, 5.243569643749999010 ) ) ;
#30605=CARTESIAN_POINT ( 'NONE',  ( 14.09062500061451750, -3.027376345333614438, 5.243569643749998122 ) ) ;
#30607=CARTESIAN_POINT ( 'NONE',  ( 10.54687500061451644, -3.027376345333614438, 5.243569643749998122 ) ) ;
#30608=CARTESIAN_POINT ( 'NONE',  ( 25.42500000000000071, 4.330127018922191873, 2.499999999999999556 ) ) ;
#30609=CARTESIAN_POINT ( 'NONE',  ( 22.53750000122903430, -4.330127018922194537, 2.499999999999995559 ) ) ;
#30610=CARTESIAN_POINT ( 'NONE',  ( 9.234375000614518214, -4.541064518000419881, 2.621784821874995952 ) ) ;
#30611=CARTESIAN_POINT ( 'NONE',  ( 25.39687500061451431, -3.027376345333614438, 5.243569643749998122 ) ) ;
#30612=CARTESIAN_POINT ( 'NONE',  ( 30.00000000000000000, 6.123233995736764310E-16, -4.999999999999998224 ) ) ;
#30613=CARTESIAN_POINT ( 'NONE',  ( 3.242103837493086330E-14, 12.80000000122903536, -34.00000000000000000 ) ) ;
#30614=CARTESIAN_POINT ( 'NONE',  ( 19.69687500061451857, -3.027376345333610441, -5.243569643749999898 ) ) ;
#30615=CARTESIAN_POINT ( 'NONE',  ( 12.04687500061451821, -3.027376345333610441, -5.243569643749999898 ) ) ;
#30617=CARTESIAN_POINT ( 'NONE',  ( 22.57499999999999929, 6.123233995736764310E-16, -4.999999999999998224 ) ) ;
#30619=CARTESIAN_POINT ( 'NONE',  ( -2.121784821874999949, 12.13437500061451857, -33.67503911421598417 ) ) ;
#30621=CARTESIAN_POINT ( 'NONE',  ( 14.99062500061451786, -3.027376345333614438, 5.243569643749998122 ) ) ;
#30622=CARTESIAN_POINT ( 'NONE',  ( 4.687500000000000000, 5.773502691896255534, 3.535250795749688894E-16 ) ) ;
#30624=CARTESIAN_POINT ( 'NONE',  ( 13.64999999999999858, 4.330127018922192761, -2.499999999999997780 ) ) ;
#30625=CARTESIAN_POINT ( 'NONE',  ( -2.000000000000000000, 19.58750000122903501, 26.53589838486224650 ) ) ;
#30626=CARTESIAN_POINT ( 'NONE',  ( 13.20000000122903394, -2.886751345948125991, -5.000000000000000000 ) ) ;
#30627=CARTESIAN_POINT ( 'NONE',  ( 24.30937500061451573, 4.541064518000418104, -2.621784821874998173 ) ) ;
#30630=CARTESIAN_POINT ( 'NONE',  ( 19.41562500061451146, 3.027376345333611329, 5.243569643749999010 ) ) ;
#30631=CARTESIAN_POINT ( 'NONE',  ( 4.378125000614518925, 6.421520780324663323E-16, -5.243569643749999010 ) ) ;
#30632=CARTESIAN_POINT ( 'NONE',  ( 20.18437500061451573, 6.421520780324663323E-16, -5.243569643749999010 ) ) ;
#30633=CARTESIAN_POINT ( 'NONE',  ( 29.25937500061451502, 4.541064518000418104, -2.621784821874998173 ) ) ;
#30634=CARTESIAN_POINT ( 'NONE',  ( 4.190625000614518925, -3.027376345333614438, 5.243569643749998122 ) ) ;
#30635=CARTESIAN_POINT ( 'NONE',  ( 21.74062500061451431, -3.027376345333614438, 5.243569643749998122 ) ) ;
#30636=CARTESIAN_POINT ( 'NONE',  ( -4.243569643749999898, 14.85312500061451679, 30.00000000000000000 ) ) ;
#30637=CARTESIAN_POINT ( 'NONE',  ( 19.57500000122903216, 2.886751345948129099, -4.999999999999998224 ) ) ;
#30639=CARTESIAN_POINT ( 'NONE',  ( 8.203125000614518214, 0.000000000000000000, 5.243569643749999010 ) ) ;
#30640=CARTESIAN_POINT ( 'NONE',  ( 3.346875000614518036, -3.027376345333614438, 5.243569643749998122 ) ) ;
#30641=CARTESIAN_POINT ( 'NONE',  ( 2.859375000614519546, 0.000000000000000000, 5.243569643749999010 ) ) ;
#30642=ADVANCED_FACE ( 'NONE', ( #59228 ), #53707, .F. ) ;
#30643=CARTESIAN_POINT ( 'NONE',  ( 22.62187500061451573, 3.027376345333611329, 5.243569643749999010 ) ) ;
#30644=CARTESIAN_POINT ( 'NONE',  ( 14.61562500061451608, -6.054752690667223547, -1.112240025338166033E-15 ) ) ;
#30645=CARTESIAN_POINT ( 'NONE',  ( 24.93750000122903288, 6.123233995736764310E-16, -4.999999999999998224 ) ) ;
#30646=CARTESIAN_POINT ( 'NONE',  ( 25.94062500061451715, -3.027376345333610441, -5.243569643749999898 ) ) ;
#30647=CARTESIAN_POINT ( 'NONE',  ( 19.73437500061451644, 6.421520780324663323E-16, -5.243569643749999010 ) ) ;
#30648=CARTESIAN_POINT ( 'NONE',  ( 14.01562500061451644, 3.027376345333611329, 5.243569643749999010 ) ) ;
#30649=CARTESIAN_POINT ( 'NONE',  ( -2.121784821874999949, 17.08437500061451786, 26.32496088578401938 ) ) ;
#30650=CARTESIAN_POINT ( 'NONE',  ( 19.37812500061451715, 4.541064518000418104, 2.621784821874999949 ) ) ;
#30652=ORIENTED_EDGE ( 'NONE', *, *, #30487, .T. ) ;
#30653=CARTESIAN_POINT ( 'NONE',  ( 25.23749999999999716, -2.886751345948125991, -5.000000000000000000 ) ) ;
#30654=CARTESIAN_POINT ( 'NONE',  ( 8.484601909799253346E-16, 11.11250000000000071, -25.38119784648299770 ) ) ;
#30656=CARTESIAN_POINT ( 'NONE',  ( 27.17812500061451786, -4.541064518000419881, 2.621784821874995952 ) ) ;
#30657=CARTESIAN_POINT ( 'NONE',  ( 7.790625000614518569, -3.027376345333614438, 5.243569643749998122 ) ) ;
#30658=CARTESIAN_POINT ( 'NONE',  ( 19.95000000122903572, -2.886751345948125991, -5.000000000000000000 ) ) ;
#30659=CARTESIAN_POINT ( 'NONE',  ( 25.34062500061451217, -3.027376345333614438, 5.243569643749998122 ) ) ;
#30660=CARTESIAN_POINT ( 'NONE',  ( 24.48749999999999716, 5.773502691896255534, 3.535250795749688894E-16 ) ) ;
#30661=CARTESIAN_POINT ( 'NONE',  ( -1.999999999999997113, 15.68750000122903465, -26.53589838486224295 ) ) ;
#30662=CARTESIAN_POINT ( 'NONE',  ( 28.07812500061451289, -4.541064518000419881, 2.621784821874995952 ) ) ;
#30663=CARTESIAN_POINT ( 'NONE',  ( 10.71562500061451928, 3.027376345333613106, -5.243569643749998122 ) ) ;
#30664=ORIENTED_EDGE ( 'NONE', *, *, #26043, .F. ) ;
#30665=CARTESIAN_POINT ( 'NONE',  ( 26.39062500061451644, -3.027376345333610441, -5.243569643749999898 ) ) ;
#30666=CARTESIAN_POINT ( 'NONE',  ( 5.015625000614518214, 3.027376345333611329, 5.243569643749999010 ) ) ;
#30668=DIRECTION ( 'NONE',  ( 0.000000000000000000, 0.000000000000000000, -1.000000000000000000 ) ) ;
#30669=CARTESIAN_POINT ( 'NONE',  ( 12.18750000000000000, -2.886751345948125991, -5.000000000000000000 ) ) ;
#30670=( BOUNDED_CURVE ( )  B_SPLINE_CURVE ( 2, ( #38616, #16067, #11266, #67068, #61139, #62231, #66693, #55602, #72958 ),
 .UNSPECIFIED., .F., .F. ) 
 B_SPLINE_CURVE_WITH_KNOTS ( ( 3, 2, 2, 2, 3 ),
 ( 0.8369565217391304879, 0.8405797101449274944, 0.8478260869565217295, 0.8550724637681159646, 0.8586956521739130821 ),
 .UNSPECIFIED. ) 
 CURVE ( )  GEOMETRIC_REPRESENTATION_ITEM ( )  RATIONAL_B_SPLINE_CURVE ( ( 0.9330127018922192983, 0.9330127018922202975, 1.000000000000000000, 0.8660254037844387076, 1.000000000000000000, 0.8660254037844387076, 1.000000000000000000, 0.9330127018922194093, 0.9330127018922194093 ) ) 
 REPRESENTATION_ITEM ( '' )  );
#30671=CARTESIAN_POINT ( 'NONE',  ( 13.35937500061451821, -4.541064518000417216, -2.621784821875001281 ) ) ;
#30672=CARTESIAN_POINT ( 'NONE',  ( 9.450000001229033941, -2.886751345948129988, 4.999999999999997335 ) ) ;
#30673=CARTESIAN_POINT ( 'NONE',  ( 17.48437500061451999, 6.421520780324663323E-16, -5.243569643749999010 ) ) ;
#30675=CARTESIAN_POINT ( 'NONE',  ( 8.334375000614516082, -4.541064518000419881, 2.621784821874995952 ) ) ;
#30676=CARTESIAN_POINT ( 'NONE',  ( -2.121784821874996840, 11.77812500061451750, -26.32496088578401583 ) ) ;
#30677=CARTESIAN_POINT ( 'NONE',  ( 20.24999999999999645, -4.330127018922190985, -2.500000000000001332 ) ) ;
#30679=EDGE_CURVE ( 'NONE', #32129, #5008, #52541, .T. ) ;
#30680=CARTESIAN_POINT ( 'NONE',  ( 23.99062500061451786, -3.027376345333614438, 5.243569643749998122 ) ) ;
#30681=CARTESIAN_POINT ( 'NONE',  ( -5.810221930991193690E-16, 11.78749999999999964, 26.00000000000000355 ) ) ;
#30683=CARTESIAN_POINT ( 'NONE',  ( -1.071796769724487453, 17.32009619066136707, 26.00000000000000000 ) ) ;
#30684=CARTESIAN_POINT ( 'NONE',  ( 25.09687500061451715, -3.027376345333610441, -5.243569643749999898 ) ) ;
#30685=CARTESIAN_POINT ( 'NONE',  ( 28.05937500061451573, 0.000000000000000000, 5.243569643749999010 ) ) ;
#30686=CARTESIAN_POINT ( 'NONE',  ( 4.078125000614517326, 4.541064518000418104, 2.621784821874999949 ) ) ;
#30688=CARTESIAN_POINT ( 'NONE',  ( 16.73437500061451644, 4.541064518000418104, 2.621784821874999949 ) ) ;
#30690=CARTESIAN_POINT ( 'NONE',  ( 3.965625000614515727, 3.027376345333613106, -5.243569643749998122 ) ) ;
#30691=CARTESIAN_POINT ( 'NONE',  ( 7.246875000614518392, 6.054752690667223547, 3.707466751127219781E-16 ) ) ;
#30692=CARTESIAN_POINT ( 'NONE',  ( 19.24687500061452283, -3.027376345333610441, -5.243569643749999898 ) ) ;
#30694=CARTESIAN_POINT ( 'NONE',  ( 26.62500000000000000, 6.123233995736764310E-16, -4.999999999999998224 ) ) ;
#30695=CARTESIAN_POINT ( 'NONE',  ( 26.93437500061451573, 6.421520780324663323E-16, -5.243569643749999010 ) ) ;
#30696=CARTESIAN_POINT ( 'NONE',  ( 14.36250000122903359, 0.000000000000000000, 4.999999999999998224 ) ) ;
#30698=CARTESIAN_POINT ( 'NONE',  ( 7.987500000000000711, -2.886751345948129988, 4.999999999999997335 ) ) ;
#30700=CARTESIAN_POINT ( 'NONE',  ( 22.75312500061451360, -4.541064518000417216, -2.621784821875001281 ) ) ;
#30701=CARTESIAN_POINT ( 'NONE',  ( 12.26249999999999929, 2.886751345948129099, -4.999999999999998224 ) ) ;
#30702=CARTESIAN_POINT ( 'NONE',  ( 8.737500001229033586, 6.123233995736764310E-16, -4.999999999999998224 ) ) ;
#30703=CARTESIAN_POINT ( 'NONE',  ( 5.615625000614517859, -6.054752690667223547, -1.112240025338166033E-15 ) ) ;
#30704=CARTESIAN_POINT ( 'NONE',  ( 21.22500000000000142, 6.123233995736764310E-16, -4.999999999999998224 ) ) ;
#30705=CARTESIAN_POINT ( 'NONE',  ( 18.40312500061451573, 4.541064518000418104, -2.621784821874998173 ) ) ;
#30706=CARTESIAN_POINT ( 'NONE',  ( 4.162909324394188815, -2.769634124722277768, 4.389987815956644113 ) ) ;
#30707=CARTESIAN_POINT ( 'NONE',  ( 25.72500000122903074, -5.773502691896255534, -1.060575238724906372E-15 ) ) ;
#30709=CARTESIAN_POINT ( 'NONE',  ( 4.125000000000000000, 6.123233995736764310E-16, -4.999999999999998224 ) ) ;
#30711=CARTESIAN_POINT ( 'NONE',  ( 19.45312500061451644, 0.000000000000000000, 5.243569643749999010 ) ) ;
#30712=CARTESIAN_POINT ( 'NONE',  ( 27.59062500061451573, -3.027376345333614438, 5.243569643749998122 ) ) ;
#30713=CARTESIAN_POINT ( 'NONE',  ( 26.33437500061451431, -4.541064518000419881, 2.621784821874995952 ) ) ;
#30714=CARTESIAN_POINT ( 'NONE',  ( 9.449999999999999289, -4.330127018922190985, -2.500000000000001332 ) ) ;
#30715=CARTESIAN_POINT ( 'NONE',  ( 13.52812500061451750, 4.541064518000418104, 2.621784821874999949 ) ) ;
#30716=CARTESIAN_POINT ( 'NONE',  ( 1.999999999999998668, 11.30000000000000071, 26.53589838486224650 ) ) ;
#30717=CARTESIAN_POINT ( 'NONE',  ( 10.04062500061451502, -3.027376345333614438, 5.243569643749998122 ) ) ;
#30718=DIRECTION ( 'NONE',  ( -1.000000000000000000, -0.000000000000000000, -0.000000000000000000 ) ) ;
#30719=CARTESIAN_POINT ( 'NONE',  ( 2.121784821875001281, 12.35937500061451821, 33.67503911421598417 ) ) ;
#30720=( BOUNDED_CURVE ( )  B_SPLINE_CURVE ( 2, ( #66346, #15724, #32732, #33815, #38643, #27560, #50091 ),
 .UNSPECIFIED., .F., .F. ) 
 B_SPLINE_CURVE_WITH_KNOTS ( ( 3, 2, 2, 3 ),
 ( 0.8416666666666667851, 0.8444444444444445530, 0.8472222222222222099, 0.8499999999999999778 ),
 .UNSPECIFIED. ) 
 CURVE ( )  GEOMETRIC_REPRESENTATION_ITEM ( )  RATIONAL_B_SPLINE_CURVE ( ( 0.9999999999999946709, 0.8660254037844440367, 1.000000000000000000, 0.8660254037844387076, 1.000000000000000000, 0.8660254037844387076, 1.000000000000000000 ) ) 
 REPRESENTATION_ITEM ( '' )  );
#30721=CARTESIAN_POINT ( 'NONE',  ( 25.31250000122903288, -4.330127018922190985, -2.500000000000001332 ) ) ;
#30723=CARTESIAN_POINT ( 'NONE',  ( 17.35312500061451502, -4.541064518000417216, -2.621784821875001281 ) ) ;
#30724=CARTESIAN_POINT ( 'NONE',  ( 8.137500000000002842, -2.886751345948126435, -5.000000000000000000 ) ) ;
#30725=EDGE_CURVE ( 'NONE', #15843, #68418, #38605, .T. ) ;
#30726=CARTESIAN_POINT ( 'NONE',  ( 9.346875000614517148, -3.027376345333610441, -5.243569643749999898 ) ) ;
#30727=CARTESIAN_POINT ( 'NONE',  ( 10.77187500061451786, 3.027376345333613106, -5.243569643749998122 ) ) ;
#30728=CARTESIAN_POINT ( 'NONE',  ( 17.67187500061451644, 3.027376345333611329, 5.243569643749999010 ) ) ;
#30729=ORIENTED_EDGE ( 'NONE', *, *, #61885, .T. ) ;
#30730=CARTESIAN_POINT ( 'NONE',  ( 15.29999999999999893, -4.330127018922190985, -2.500000000000001332 ) ) ;
#30731=CARTESIAN_POINT ( 'NONE',  ( 22.15312500061451573, 0.000000000000000000, 5.243569643749999010 ) ) ;
#30732=CARTESIAN_POINT ( 'NONE',  ( 17.03437500061451715, 6.421520780324663323E-16, -5.243569643749999010 ) ) ;
#30733=CARTESIAN_POINT ( 'NONE',  ( 22.86562500061451431, 3.027376345333613106, -5.243569643749998122 ) ) ;
#30734=CARTESIAN_POINT ( 'NONE',  ( -3.999999999999997335, 13.28749999999999964, 32.30940107675850470 ) ) ;
#30735=CARTESIAN_POINT ( 'NONE',  ( 28.11562500061451431, -6.054752690667223547, -1.112240025338166033E-15 ) ) ;
#30736=CARTESIAN_POINT ( 'NONE',  ( 7.687500001229033764, -4.330127018922194537, 2.499999999999995559 ) ) ;
#30738=CARTESIAN_POINT ( 'NONE',  ( 4.987500001229032698, -4.330127018922194537, 2.499999999999995559 ) ) ;
#30739=CARTESIAN_POINT ( 'NONE',  ( 3.999999999999998668, 17.11250000000000071, -32.30940107675850470 ) ) ;
#30740=CARTESIAN_POINT ( 'NONE',  ( 23.81250000122903288, 0.000000000000000000, 4.999999999999998224 ) ) ;
#30742=CARTESIAN_POINT ( 'NONE',  ( 8.221875000614518925, 3.027376345333611329, 5.243569643749999010 ) ) ;
#30743=CARTESIAN_POINT ( 'NONE',  ( 1.999999999999998668, 15.35000000000000142, 26.53589838486224650 ) ) ;
#30744=CARTESIAN_POINT ( 'NONE',  ( 15.17812500061451608, 6.421520780324663323E-16, -5.243569643749999010 ) ) ;
#30745=CARTESIAN_POINT ( 'NONE',  ( 9.646875000614516082, -3.027376345333614438, 5.243569643749998122 ) ) ;
#30746=CARTESIAN_POINT ( 'NONE',  ( 27.15000000122902790, -2.886751345948125991, -5.000000000000000000 ) ) ;
#30747=CARTESIAN_POINT ( 'NONE',  ( 17.03437500061451715, 6.421520780324663323E-16, -5.243569643749999010 ) ) ;
#30748=CARTESIAN_POINT ( 'NONE',  ( 4.696875000614518569, -3.027376345333614438, 5.243569643749998122 ) ) ;
#30750=CARTESIAN_POINT ( 'NONE',  ( 4.415625000614518569, 3.027376345333613106, -5.243569643749998122 ) ) ;
#30751=CARTESIAN_POINT ( 'NONE',  ( 18.55312500061451431, 0.000000000000000000, 5.243569643749999010 ) ) ;
#30752=( BOUNDED_CURVE ( )  B_SPLINE_CURVE ( 2, ( #25355, #52704, #47901, #52344, #8730, #35346, #2110 ),
 .UNSPECIFIED., .F., .F. ) 
 B_SPLINE_CURVE_WITH_KNOTS ( ( 3, 2, 2, 3 ),
 ( 0.1083333333333333648, 0.1111111111111111327, 0.1138888888888889006, 0.1166666666666666824 ),
 .UNSPECIFIED. ) 
 CURVE ( )  GEOMETRIC_REPRESENTATION_ITEM ( )  RATIONAL_B_SPLINE_CURVE ( ( 0.9999999999999986677, 0.8660254037844400399, 1.000000000000000000, 0.8660254037844387076, 1.000000000000000000, 0.8660254037844380415, 1.000000000000000666 ) ) 
 REPRESENTATION_ITEM ( '' )  );
#30753=ORIENTED_EDGE ( 'NONE', *, *, #68178, .F. ) ;
#30754=CARTESIAN_POINT ( 'NONE',  ( 11.87812500061451537, -4.541064518000419881, 2.621784821874995952 ) ) ;
#30755=CARTESIAN_POINT ( 'NONE',  ( 6.000000001229033764, -2.886751345948125991, -5.000000000000000000 ) ) ;
#30756=CARTESIAN_POINT ( 'NONE',  ( 11.50312500061451892, -4.541064518000417216, -2.621784821875001281 ) ) ;
#30758=CARTESIAN_POINT ( 'NONE',  ( 10.20000000000000107, 0.000000000000000000, 4.999999999999998224 ) ) ;
#30759=CARTESIAN_POINT ( 'NONE',  ( 5.962500001229033231, -4.330127018922190985, -2.500000000000001332 ) ) ;
#30760=CARTESIAN_POINT ( 'NONE',  ( 20.58750000000000213, -2.886751345948129988, 4.999999999999997335 ) ) ;
#30761=CARTESIAN_POINT ( 'NONE',  ( 15.04687500061451644, -3.027376345333614438, 5.243569643749998122 ) ) ;
#30762=CARTESIAN_POINT ( 'NONE',  ( 15.07500000122903394, 2.886751345948129099, -4.999999999999998224 ) ) ;
#30764=( BOUNDED_CURVE ( )  B_SPLINE_CURVE ( 2, ( #10587, #73006, #5773, #44215, #66747, #16474, #22390 ),
 .UNSPECIFIED., .F., .F. ) 
 B_SPLINE_CURVE_WITH_KNOTS ( ( 3, 2, 2, 3 ),
 ( 0.4333333333333333481, 0.4361111111111111160, 0.4388888888888888840, 0.4416666666666666519 ),
 .UNSPECIFIED. ) 
 CURVE ( )  GEOMETRIC_REPRESENTATION_ITEM ( )  RATIONAL_B_SPLINE_CURVE ( ( 1.000000000000000000, 0.8660254037844387076, 1.000000000000000000, 0.8660254037844387076, 1.000000000000000000, 0.8660254037844387076, 1.000000000000000000 ) ) 
 REPRESENTATION_ITEM ( '' )  );
#30765=CARTESIAN_POINT ( 'NONE',  ( 2.121784821875001281, 19.50312500061451360, -26.32496088578401938 ) ) ;
#30766=CARTESIAN_POINT ( 'NONE',  ( 1.592000809091587073E-14, 15.95000000122903394, 26.00000000000000000 ) ) ;
#30768=FACE_OUTER_BOUND ( 'NONE', #21712, .T. ) ;
#30769=FACE_OUTER_BOUND ( 'NONE', #19241, .T. ) ;
#30770=CARTESIAN_POINT ( 'NONE',  ( 3.906976797710813631, -3.120192015497321059, -4.214200603120166200 ) ) ;
#30771=CARTESIAN_POINT ( 'NONE',  ( 16.65937500061452070, 4.541064518000418104, -2.621784821874998173 ) ) ;
#30773=CARTESIAN_POINT ( 'NONE',  ( 28.42499999999999716, 6.123233995736764310E-16, -4.999999999999998224 ) ) ;
#30774=CARTESIAN_POINT ( 'NONE',  ( 11.50312500061451892, -4.541064518000417216, -2.621784821875001281 ) ) ;
#30776=CARTESIAN_POINT ( 'NONE',  ( 24.15937500061451715, -4.541064518000417216, -2.621784821875001281 ) ) ;
#30778=CARTESIAN_POINT ( 'NONE',  ( 9.515625000614518214, 3.027376345333611329, 5.243569643749999010 ) ) ;
#30779=CARTESIAN_POINT ( 'NONE',  ( 14.37187500061451928, 3.027376345333613106, -5.243569643749998122 ) ) ;
#30780=ORIENTED_EDGE ( 'NONE', *, *, #3046, .F. ) ;
#30781=CARTESIAN_POINT ( 'NONE',  ( 25.73437500061451644, 4.541064518000418104, 2.621784821874999949 ) ) ;
#30782=CARTESIAN_POINT ( 'NONE',  ( 27.47812500061451502, 4.541064518000418104, 2.621784821874999949 ) ) ;
#30783=CARTESIAN_POINT ( 'NONE',  ( 19.07812500061451644, -4.541064518000419881, 2.621784821874995952 ) ) ;
#30784=CARTESIAN_POINT ( 'NONE',  ( 28.00312500061451715, 0.000000000000000000, 5.243569643749999010 ) ) ;
#30785=CARTESIAN_POINT ( 'NONE',  ( 1.071796769724505438, 12.77990381179669832, -33.99999999999999289 ) ) ;
#30786=CARTESIAN_POINT ( 'NONE',  ( 8.512499999999999289, -5.773502691896255534, -1.060575238724906372E-15 ) ) ;
#30787=CARTESIAN_POINT ( 'NONE',  ( 18.60000000122903430, -2.886751345948125991, -5.000000000000000000 ) ) ;
#30788=LINE ( 'NONE', #19689, #44338 ) ;
#30790=ORIENTED_EDGE ( 'NONE', *, *, #59478, .F. ) ;
#30791=CARTESIAN_POINT ( 'NONE',  ( 15.86250000000000249, 2.886751345948129099, -4.999999999999998224 ) ) ;
#30793=CARTESIAN_POINT ( 'NONE',  ( 18.14999999999999858, 4.330127018922192761, -2.499999999999997780 ) ) ;
#30794=CARTESIAN_POINT ( 'NONE',  ( 15.98437500061451821, -4.541064518000419881, 2.621784821874995952 ) ) ;
#30795=CARTESIAN_POINT ( 'NONE',  ( 12.92812500061451786, 6.421520780324663323E-16, -5.243569643749999010 ) ) ;
#30796=VERTEX_POINT ( 'NONE', #32269 ) ;
#30798=CARTESIAN_POINT ( 'NONE',  ( 7.003125000614518036, -4.541064518000417216, -2.621784821875001281 ) ) ;
#30799=CARTESIAN_POINT ( 'NONE',  ( 12.30000000000000249, 4.330127018922192761, -2.499999999999997780 ) ) ;
#30801=CARTESIAN_POINT ( 'NONE',  ( -2.121784821874999949, 14.32812500061451644, 26.32496088578401938 ) ) ;
#30802=CARTESIAN_POINT ( 'NONE',  ( 26.91562500061451146, 3.027376345333613106, -5.243569643749998122 ) ) ;
#30805=CARTESIAN_POINT ( 'NONE',  ( 24.00937500061451502, 0.000000000000000000, 5.243569643749999010 ) ) ;
#30806=CARTESIAN_POINT ( 'NONE',  ( 20.65312500061451573, 4.541064518000418104, -2.621784821874998173 ) ) ;
#30807=CARTESIAN_POINT ( 'NONE',  ( -2.121784821874996840, 17.17812500061459602, -26.32496088578401583 ) ) ;
#30808=CARTESIAN_POINT ( 'NONE',  ( 22.80000000122903359, 5.773502691896255534, 3.535250795749688894E-16 ) ) ;
#30809=CARTESIAN_POINT ( 'NONE',  ( 7.490625000614516082, -3.027376345333610441, -5.243569643749999898 ) ) ;
#30811=CARTESIAN_POINT ( 'NONE',  ( 23.46562500061451573, 3.027376345333611329, 5.243569643749999010 ) ) ;
#30814=CARTESIAN_POINT ( 'NONE',  ( 15.94687500061451502, -3.027376345333614438, 5.243569643749998122 ) ) ;
#30815=CARTESIAN_POINT ( 'NONE',  ( 24.53437500061451715, -4.541064518000419881, 2.621784821874995952 ) ) ;
#30816=CARTESIAN_POINT ( 'NONE',  ( 4.243569643749999898, 14.68437500061451750, 30.00000000000000000 ) ) ;
#30817=CARTESIAN_POINT ( 'NONE',  ( 5.240625000614516971, -3.027376345333610441, -5.243569643749999898 ) ) ;
#30818=CARTESIAN_POINT ( 'NONE',  ( 28.22812500061451502, 6.421520780324663323E-16, -5.243569643749999010 ) ) ;
#30819=EDGE_CURVE ( 'NONE', #35463, #11388, #7705, .T. ) ;
#30820=CARTESIAN_POINT ( 'NONE',  ( 29.57812500061451644, 6.421520780324663323E-16, -5.243569643749999010 ) ) ;
#30821=DIRECTION ( 'NONE',  ( 0.000000000000000000, 0.000000000000000000, -1.000000000000000000 ) ) ;
#30822=CARTESIAN_POINT ( 'NONE',  ( 3.807538167735159185, -3.240779705755961526, 4.122180188640082399 ) ) ;
#30823=CARTESIAN_POINT ( 'NONE',  ( 2.878125000614517592, -4.541064518000419881, 2.621784821874995952 ) ) ;
#30824=CARTESIAN_POINT ( 'NONE',  ( 7.921875000614517326, -6.054752690667223547, -1.112240025338166033E-15 ) ) ;
#30825=CARTESIAN_POINT ( 'NONE',  ( 16.95000000122903216, 5.773502691896255534, 3.535250795749688894E-16 ) ) ;
#30826=CARTESIAN_POINT ( 'NONE',  ( 3.234375000614516438, 4.541064518000418104, 2.621784821874999949 ) ) ;
#30827=CARTESIAN_POINT ( 'NONE',  ( 4.828125000614518214, 6.421520780324663323E-16, -5.243569643749999010 ) ) ;
#30830=CARTESIAN_POINT ( 'NONE',  ( 13.43437500061451750, 6.421520780324663323E-16, -5.243569643749999010 ) ) ;
#30831=CARTESIAN_POINT ( 'NONE',  ( 27.52500000000000213, 6.123233995736764310E-16, -4.999999999999998224 ) ) ;
#30832=VERTEX_POINT ( 'NONE', #15267 ) ;
#30833=CARTESIAN_POINT ( 'NONE',  ( 22.71562500061451573, -6.054752690667223547, -1.112240025338166033E-15 ) ) ;
#30834=CARTESIAN_POINT ( 'NONE',  ( 6.478125000614516793, -4.541064518000419881, 2.621784821874995952 ) ) ;
#30835=CARTESIAN_POINT ( 'NONE',  ( 25.17187500061451644, 3.027376345333612662, -5.243569643749998122 ) ) ;
#30836=CARTESIAN_POINT ( 'NONE',  ( 8.315625000614515372, -6.054752690667223547, -1.112240025338166033E-15 ) ) ;
#30837=CARTESIAN_POINT ( 'NONE',  ( 3.504965621013899746, 3.565840152826760256, 3.504965621013765631 ) ) ;
#30838=CARTESIAN_POINT ( 'NONE',  ( 10.12500000122903465, 2.886751345948129099, -4.999999999999998224 ) ) ;
#30839=CARTESIAN_POINT ( 'NONE',  ( 25.30312500061451431, 0.000000000000000000, 5.243569643749999010 ) ) ;
#30840=CARTESIAN_POINT ( 'NONE',  ( 4.243569643749999010, 10.61562500061451786, -32.45002607614398471 ) ) ;
#30841=CARTESIAN_POINT ( 'NONE',  ( 9.562500001229032875, -4.330127018922190985, -2.500000000000001332 ) ) ;
#30842=CARTESIAN_POINT ( 'NONE',  ( 23.27812500061451573, 6.421520780324663323E-16, -5.243569643749999010 ) ) ;
#30843=CARTESIAN_POINT ( 'NONE',  ( 18.06562500061451715, 3.027376345333611329, 5.243569643749999010 ) ) ;
#30845=CARTESIAN_POINT ( 'NONE',  ( 19.20000000000000284, 0.000000000000000000, 4.999999999999998224 ) ) ;
#30846=CARTESIAN_POINT ( 'NONE',  ( 14.92500000122903181, -5.773502691896255534, -1.060575238724906372E-15 ) ) ;
#30847=CARTESIAN_POINT ( 'NONE',  ( 11.16562500061451679, 3.027376345333613106, -5.243569643749998122 ) ) ;
#30848=CARTESIAN_POINT ( 'NONE',  ( 12.55312500061451786, 4.541064518000418104, -2.621784821874998173 ) ) ;
#30849=CARTESIAN_POINT ( 'NONE',  ( 23.62500000122902932, 2.886751345948129099, -4.999999999999998224 ) ) ;
#30850=CARTESIAN_POINT ( 'NONE',  ( 23.03437500061451715, 4.541064518000418104, 2.621784821874999949 ) ) ;
#30851=CARTESIAN_POINT ( 'NONE',  ( 21.87187500061451573, -6.054752690667223547, -1.112240025338166033E-15 ) ) ;
#30853=CARTESIAN_POINT ( 'NONE',  ( 7.425000001229034474, 2.886751345948129099, -4.999999999999998224 ) ) ;
#30854=CARTESIAN_POINT ( 'NONE',  ( 5.784375000614517148, 6.421520780324663323E-16, -5.243569643749999010 ) ) ;
#30855=CARTESIAN_POINT ( 'NONE',  ( 22.73437500061451644, -4.541064518000419881, 2.621784821874995952 ) ) ;
#30856=CARTESIAN_POINT ( 'NONE',  ( 26.70000000122903216, -2.886751345948142422, -4.999999999999970690 ) ) ;
#30857=CARTESIAN_POINT ( 'NONE',  ( 21.77812500061451928, -4.541064518000419881, 2.621784821874995952 ) ) ;
#30858=CARTESIAN_POINT ( 'NONE',  ( 25.02187500061451431, -6.054752690667223547, -1.112240025338166033E-15 ) ) ;
#30861=CARTESIAN_POINT ( 'NONE',  ( 1.999999999999998668, 15.80000000000000071, 26.53589838486224650 ) ) ;
#30862=CARTESIAN_POINT ( 'NONE',  ( 6.009375000614519458, 0.000000000000000000, 5.243569643749999010 ) ) ;
#30863=CARTESIAN_POINT ( 'NONE',  ( 17.05312500061451786, 4.541064518000418104, -2.621784821874998173 ) ) ;
#30864=VERTEX_POINT ( 'NONE', #9373 ) ;
#30865=CARTESIAN_POINT ( 'NONE',  ( 25.23750000000000071, -2.886751345948142422, -4.999999999999970690 ) ) ;
#30866=CARTESIAN_POINT ( 'NONE',  ( 25.37812500061451715, -4.541064518000419881, 2.621784821874995952 ) ) ;
#30867=CARTESIAN_POINT ( 'NONE',  ( 5.034375000614519813, 4.541064518000418104, 2.621784821874999949 ) ) ;
#30869=CARTESIAN_POINT ( 'NONE',  ( 15.22500000000000142, -4.330127018922194537, 2.499999999999995559 ) ) ;
#30870=CARTESIAN_POINT ( 'NONE',  ( 19.97812500061451502, -4.541064518000419881, 2.621784821874995952 ) ) ;
#30871=ORIENTED_EDGE ( 'NONE', *, *, #29228, .F. ) ;
#30872=CARTESIAN_POINT ( 'NONE',  ( 23.62500000000000000, 4.330127018922191873, 2.499999999999999556 ) ) ;
#30873=CARTESIAN_POINT ( 'NONE',  ( 27.42187500061451644, 3.027376345333613106, -5.243569643749998122 ) ) ;
#30876=CARTESIAN_POINT ( 'NONE',  ( 13.79062500061451502, -3.027376345333610441, -5.243569643749999898 ) ) ;
#30877=CARTESIAN_POINT ( 'NONE',  ( 25.01250000122903216, 4.330127018922192761, -2.499999999999997780 ) ) ;
#30879=CARTESIAN_POINT ( 'NONE',  ( 2.934375000614518392, -4.541064518000419881, 2.621784821874995952 ) ) ;
#30880=CARTESIAN_POINT ( 'NONE',  ( 12.71250000122903145, -4.330127018922190985, -2.500000000000001332 ) ) ;
#30881=CARTESIAN_POINT ( 'NONE',  ( 18.63749999999999929, 5.773502691896255534, 3.535250795749688894E-16 ) ) ;
#30882=CARTESIAN_POINT ( 'NONE',  ( 26.36249999999999716, 2.886751345948126879, 4.999999999999999112 ) ) ;
#30884=CARTESIAN_POINT ( 'NONE',  ( 6.721875000614518925, 3.027376345333613106, -5.243569643749998122 ) ) ;
#30885=CARTESIAN_POINT ( 'NONE',  ( 18.19687500061451502, -3.027376345333614438, 5.243569643749998122 ) ) ;
#30888=CARTESIAN_POINT ( 'NONE',  ( 29.01562500061451644, -6.054752690667223547, -1.112240025338166033E-15 ) ) ;
#30889=CARTESIAN_POINT ( 'NONE',  ( 3.750000000000000000, 4.330127018922192761, -2.499999999999997780 ) ) ;
#30890=CARTESIAN_POINT ( 'NONE',  ( 3.684375000614518836, 4.541064518000418104, 2.621784821874999949 ) ) ;
#30891=CARTESIAN_POINT ( 'NONE',  ( 15.86250000000000249, 2.886751345948129099, -4.999999999999998224 ) ) ;
#30892=CARTESIAN_POINT ( 'NONE',  ( 12.66562500061451502, 3.027376345333611329, 5.243569643749999010 ) ) ;
#30894=CARTESIAN_POINT ( 'NONE',  ( 5.000000000001397105, 0.3395091859857997107, -5.050874639569527424 ) ) ;
#30895=CARTESIAN_POINT ( 'NONE',  ( 17.58750000122903145, -4.330127018922194537, 2.499999999999995559 ) ) ;
#30896=CARTESIAN_POINT ( 'NONE',  ( -5.810221930991193690E-16, 13.25000000122903465, 26.00000000000000355 ) ) ;
#30898=CARTESIAN_POINT ( 'NONE',  ( 6.928125000614516082, -4.541064518000419881, 2.621784821874995952 ) ) ;
#30899=CARTESIAN_POINT ( 'NONE',  ( 23.59687500061451715, -3.027376345333614438, 5.243569643749998122 ) ) ;
#30901=CARTESIAN_POINT ( 'NONE',  ( 4.243569643749999010, 17.87187500061451573, 27.54997392385601174 ) ) ;
#30902=CARTESIAN_POINT ( 'NONE',  ( 24.23437500061451644, 6.421520780324663323E-16, -5.243569643749999010 ) ) ;
#30903=CARTESIAN_POINT ( 'NONE',  ( 5.137500000000000178, 5.773502691896255534, 3.535250795749688894E-16 ) ) ;
#30904=CARTESIAN_POINT ( 'NONE',  ( -3.999999999999999112, 10.21250000122903501, 30.00000000000000000 ) ) ;
#30905=CARTESIAN_POINT ( 'NONE',  ( 12.81562500061451537, -6.054752690667223547, -1.112240025338166033E-15 ) ) ;
#30906=CARTESIAN_POINT ( 'NONE',  ( 4.575000001229033941, -5.773502691896255534, -1.060575238724906372E-15 ) ) ;
#30908=CARTESIAN_POINT ( 'NONE',  ( 8.709375000614517859, 0.000000000000000000, 5.243569643749999010 ) ) ;
#30910=ORIENTED_EDGE ( 'NONE', *, *, #69831, .F. ) ;
#30911=CARTESIAN_POINT ( 'NONE',  ( 12.10312500061451857, 4.541064518000418104, -2.621784821874998173 ) ) ;
#30913=CARTESIAN_POINT ( 'NONE',  ( 22.83750000122903501, 4.330127018922191873, 2.499999999999999556 ) ) ;
#30914=CARTESIAN_POINT ( 'NONE',  ( 10.47187500061451715, 3.027376345333611329, 5.243569643749999010 ) ) ;
#30915=CARTESIAN_POINT ( 'NONE',  ( 12.29062500061451857, -3.027376345333614438, 5.243569643749998122 ) ) ;
#30917=CARTESIAN_POINT ( 'NONE',  ( 21.04687500061451644, -3.027376345333610441, -5.243569643749999898 ) ) ;
#30918=CARTESIAN_POINT ( 'NONE',  ( 1.592000809091587073E-14, 15.95000000122903394, 26.00000000000000000 ) ) ;
#30920=CARTESIAN_POINT ( 'NONE',  ( 3.249167837762792832, 3.800382659950008790, -3.347690552023643296 ) ) ;
#30921=CARTESIAN_POINT ( 'NONE',  ( 9.001249775931846008E-16, 14.57187500061451679, -25.09994784771203058 ) ) ;
#30922=CARTESIAN_POINT ( 'NONE',  ( 15.87187500061451573, 3.027376345333611329, 5.243569643749999010 ) ) ;
#30923=CARTESIAN_POINT ( 'NONE',  ( 18.15000000122903501, -2.886751345948125991, -5.000000000000000000 ) ) ;
#30924=CARTESIAN_POINT ( 'NONE',  ( 11.59687500061451892, -3.027376345333610441, -5.243569643749999898 ) ) ;
#30925=CARTESIAN_POINT ( 'NONE',  ( 4.243569643749999010, 18.71562500061451217, -32.45002607614398471 ) ) ;
#30926=CARTESIAN_POINT ( 'NONE',  ( 16.98750000122903359, 4.330127018922191873, 2.499999999999999556 ) ) ;
#30927=CARTESIAN_POINT ( 'NONE',  ( 11.99062500061451608, -3.027376345333610441, -5.243569643749999898 ) ) ;
#30928=ORIENTED_EDGE ( 'NONE', *, *, #22319, .T. ) ;
#30929=CARTESIAN_POINT ( 'NONE',  ( 15.93750000000000000, 5.773502691896255534, 3.535250795749688894E-16 ) ) ;
#30930=CARTESIAN_POINT ( 'NONE',  ( 17.92500000000000071, -4.330127018922194537, 2.499999999999995559 ) ) ;
#30931=CARTESIAN_POINT ( 'NONE',  ( 12.72187500061451537, 3.027376345333611329, 5.243569643749999010 ) ) ;
#30933=CARTESIAN_POINT ( 'NONE',  ( 13.16250000122903430, -4.330127018922190985, -2.500000000000001332 ) ) ;
#30934=CARTESIAN_POINT ( 'NONE',  ( 21.45000000122903216, 5.773502691896255534, 3.535250795749688894E-16 ) ) ;
#30935=CARTESIAN_POINT ( 'NONE',  ( 17.54062500061451502, 6.054752690667223547, 3.707466751127219781E-16 ) ) ;
#30936=CARTESIAN_POINT ( 'NONE',  ( 19.94062500061451715, -3.027376345333614438, 5.243569643749998122 ) ) ;
#30937=CARTESIAN_POINT ( 'NONE',  ( 27.37500000122903288, 2.886751345948126879, 4.999999999999999112 ) ) ;
#30938=CARTESIAN_POINT ( 'NONE',  ( 25.19999999999999929, -4.330127018922190985, -2.500000000000001332 ) ) ;
#30939=LINE ( 'NONE', #71200, #43052 ) ;
#30941=CARTESIAN_POINT ( 'NONE',  ( 27.87187500061451573, 3.027376345333613106, -5.243569643749998122 ) ) ;
#30942=CARTESIAN_POINT ( 'NONE',  ( 4.038036497978814587, -2.948822205205740676, -4.128098832493389381 ) ) ;
#30943=CARTESIAN_POINT ( 'NONE',  ( -4.243569643749999898, 14.42187500061451644, -32.45002607614398471 ) ) ;
#30944=CARTESIAN_POINT ( 'NONE',  ( 3.187500001229033764, -4.330127018922194537, 2.499999999999995559 ) ) ;
#30945=CARTESIAN_POINT ( 'NONE',  ( 6.487499999999999822, 5.773502691896255534, 3.535250795749688894E-16 ) ) ;
#30947=EDGE_CURVE ( 'NONE', #68526, #14829, #1416, .T. ) ;
#30948=CARTESIAN_POINT ( 'NONE',  ( 2.737500001229034474, -4.330127018922194537, 2.499999999999995559 ) ) ;
#30949=CARTESIAN_POINT ( 'NONE',  ( 7.209375000614519635, 4.541064518000418104, -2.621784821874998173 ) ) ;
#30950=VECTOR ( 'NONE', #24867, 1000.000000000000000 ) ;
#30951=B_SPLINE_CURVE_WITH_KNOTS ( 'NONE', 3,
 ( #56797, #1038, #28730, #51271, #50909, #674, #61986, #23181, #29462, #51998, #11387, #45735, #1399, #45368, #68994, #40552, #51637, #6571, #62713, #18353, #12107, #63069, #63439, #40926, #35001, #33906, #58972, #8745, #3213, #2124, #52717, #25369, #30553, #24635, #25742, #53450, #70071, #48279, #47913, #2840 ),
 .UNSPECIFIED., .F., .F.,
 ( 4, 2, 2, 2, 2, 2, 2, 2, 2, 2, 2, 2, 2, 2, 2, 2, 2, 2, 2, 4 ),
 ( 0.02627519828802198087, 0.02668902850173000482, 0.02710285871543802530, 0.02793051914285407319, 0.02958583999768617245, 0.03041350042510221341, 0.03124116085251825783, 0.03206882127993430226, 0.03248265149364232274, 0.03289648170735034322, 0.03331031192105836369, 0.03372414213476638417, 0.03455180256218243207, 0.03537946298959847302, 0.03620712341701451398, 0.03703478384443055493, 0.03786244427184659589, 0.03869010469926264378, 0.03910393491297066426, 0.03951776512667868474 ),
 .UNSPECIFIED. ) ;
#30952=CARTESIAN_POINT ( 'NONE',  ( 27.51562500061451644, 3.027376345333611329, 5.243569643749999010 ) ) ;
#30957=CARTESIAN_POINT ( 'NONE',  ( 5.334375000614517859, 6.421520780324663323E-16, -5.243569643749999010 ) ) ;
#30958=CARTESIAN_POINT ( 'NONE',  ( 10.05937500061451750, 0.000000000000000000, 5.243569643749999010 ) ) ;
#30959=CARTESIAN_POINT ( 'NONE',  ( 3.825000000000001954, 4.330127018922191873, 2.499999999999999556 ) ) ;
#30960=CARTESIAN_POINT ( 'NONE',  ( 4.243569643749999898, 15.07812500061459460, 30.00000000000000000 ) ) ;
#30962=EDGE_CURVE ( 'NONE', #66791, #54370, #26362, .T. ) ;
#30963=CARTESIAN_POINT ( 'NONE',  ( 7.312500000000000000, 2.886751345948129099, -4.999999999999998224 ) ) ;
#30965=CARTESIAN_POINT ( 'NONE',  ( 20.20312500061451644, 4.541064518000418104, -2.621784821874998173 ) ) ;
#30966=CARTESIAN_POINT ( 'NONE',  ( 10.11562500061451608, -6.054752690667223547, -1.112240025338166033E-15 ) ) ;
#30968=CARTESIAN_POINT ( 'NONE',  ( 8.596875000614518925, 6.054752690667223547, 3.707466751127219781E-16 ) ) ;
#30969=CARTESIAN_POINT ( 'NONE',  ( 25.57499999999999929, -4.330127018922194537, 2.499999999999995559 ) ) ;
#30970=CARTESIAN_POINT ( 'NONE',  ( 19.16250000122903430, 4.330127018922192761, -2.499999999999997780 ) ) ;
#30971=CARTESIAN_POINT ( 'NONE',  ( 26.95312500061451644, 4.541064518000418104, -2.621784821874998173 ) ) ;
#30973=CARTESIAN_POINT ( 'NONE',  ( 10.05937500061451750, 0.000000000000000000, 5.243569643749999010 ) ) ;
#30974=CARTESIAN_POINT ( 'NONE',  ( 13.77187500061451786, -6.054752690667223547, -1.112240025338166033E-15 ) ) ;
#30975=CARTESIAN_POINT ( 'NONE',  ( 27.68437500061451573, -4.541064518000419881, 2.621784821874995952 ) ) ;
#30976=EDGE_CURVE ( 'NONE', #10804, #65099, #57478, .T. ) ;
#30978=CARTESIAN_POINT ( 'NONE',  ( 1.071796769724489895, 13.67990381179670045, -34.00000000000000000 ) ) ;
#30979=CARTESIAN_POINT ( 'NONE',  ( 19.88437500061451857, 4.541064518000418104, 2.621784821874999949 ) ) ;
#30980=CARTESIAN_POINT ( 'NONE',  ( 12.19687500061451679, 6.054752690667223547, 3.707466751127219781E-16 ) ) ;
#30982=CARTESIAN_POINT ( 'NONE',  ( 22.19999999999999574, 4.330127018922192761, -2.499999999999997780 ) ) ;
#30984=CARTESIAN_POINT ( 'NONE',  ( -4.243569643749999898, 12.17187500061451999, -32.45002607614398471 ) ) ;
#30986=CARTESIAN_POINT ( 'NONE',  ( 15.29062500061451679, 6.054752690667223547, 3.707466751127219781E-16 ) ) ;
#30987=CARTESIAN_POINT ( 'NONE',  ( 4.462500000000001243, -5.773502691896255534, -1.060575238724906372E-15 ) ) ;
#30988=CARTESIAN_POINT ( 'NONE',  ( 6.900000001229033231, -2.886751345948193048, -4.999999999999883649 ) ) ;
#30989=CARTESIAN_POINT ( 'NONE',  ( 25.53749999999999787, -2.886751345948114000, 5.000000000000024869 ) ) ;
#30990=CARTESIAN_POINT ( 'NONE',  ( 12.26249999999999929, 2.886751345948129099, -4.999999999999998224 ) ) ;
#30991=CARTESIAN_POINT ( 'NONE',  ( -3.999999999999999556, 18.27500000122903501, 27.69059892324149530 ) ) ;
#30992=CARTESIAN_POINT ( 'NONE',  ( 12.63750000122903394, -4.330127018922194537, 2.499999999999995559 ) ) ;
#30993=CARTESIAN_POINT ( 'NONE',  ( 25.32187500061451857, 3.027376345333611329, 5.243569643749999010 ) ) ;
#30994=CARTESIAN_POINT ( 'NONE',  ( 17.74687500061451928, -3.027376345333614438, 5.243569643749998122 ) ) ;
#30996=ORIENTED_EDGE ( 'NONE', *, *, #60294, .T. ) ;
#30997=CARTESIAN_POINT ( 'NONE',  ( 19.07812500061451644, -4.541064518000419881, 2.621784821874995952 ) ) ;
#30998=CARTESIAN_POINT ( 'NONE',  ( 3.965625000614515727, 3.027376345333613106, -5.243569643749998122 ) ) ;
#30999=CARTESIAN_POINT ( 'NONE',  ( 17.82187500061451502, -6.054752690667223547, -1.112240025338166033E-15 ) ) ;
#31000=CARTESIAN_POINT ( 'NONE',  ( 28.43437500061451573, 4.541064518000418104, 2.621784821874999949 ) ) ;
#31001=CARTESIAN_POINT ( 'NONE',  ( 5.315625000614516260, 3.027376345333613106, -5.243569643749998122 ) ) ;
#31002=CARTESIAN_POINT ( 'NONE',  ( 19.22812500061451502, 6.421520780324663323E-16, -5.243569643749999010 ) ) ;
#31003=CARTESIAN_POINT ( 'NONE',  ( 4.243569643749999898, 15.04062500061451679, 32.45002607614398471 ) ) ;
#31004=CARTESIAN_POINT ( 'NONE',  ( 16.65000000122903501, -2.886751345948129988, 4.999999999999997335 ) ) ;
#31006=CARTESIAN_POINT ( 'NONE',  ( 6.890625000614516438, -3.027376345333614438, 5.243569643749998122 ) ) ;
#31007=CARTESIAN_POINT ( 'NONE',  ( 3.234375000614516438, 4.541064518000418104, 2.621784821874999949 ) ) ;
#31008=CARTESIAN_POINT ( 'NONE',  ( 23.29687500061451644, -3.027376345333610441, -5.243569643749999898 ) ) ;
#31009=CARTESIAN_POINT ( 'NONE',  ( 13.52812500061451750, 4.541064518000418104, 2.621784821874999949 ) ) ;
#31010=CARTESIAN_POINT ( 'NONE',  ( 25.01250000122903216, 4.330127018922192761, -2.499999999999997780 ) ) ;
#31011=CARTESIAN_POINT ( 'NONE',  ( 24.10312500061451502, -4.541064518000417216, -2.621784821875001281 ) ) ;
#31012=CARTESIAN_POINT ( 'NONE',  ( 19.24687500061452283, -3.027376345333610441, -5.243569643749999898 ) ) ;
#31013=CARTESIAN_POINT ( 'NONE',  ( 15.92812500061451608, -4.541064518000419881, 2.621784821874995952 ) ) ;
#31014=CARTESIAN_POINT ( 'NONE',  ( -4.243569643749999898, 15.77187500061451608, 27.54997392385601529 ) ) ;
#31015=CARTESIAN_POINT ( 'NONE',  ( 19.82812500061451644, 4.541064518000418104, 2.621784821874999949 ) ) ;
#31017=VERTEX_POINT ( 'NONE', #72893 ) ;
#31018=CARTESIAN_POINT ( 'NONE',  ( 21.86250000000000071, 2.886751345948126879, 4.999999999999999112 ) ) ;
#31019=CARTESIAN_POINT ( 'NONE',  ( -2.828200636599751609E-16, 11.78749999999999964, -34.61880215351700230 ) ) ;
#31020=CARTESIAN_POINT ( 'NONE',  ( 12.67499999999999893, 6.123233995736764310E-16, -4.999999999999998224 ) ) ;
#31021=CARTESIAN_POINT ( 'NONE',  ( 26.76562500061451644, -6.054752690667223547, -1.112240025338166033E-15 ) ) ;
#31022=CARTESIAN_POINT ( 'NONE',  ( 8.953125000614518214, 4.541064518000418104, -2.621784821874998173 ) ) ;
#31023=CARTESIAN_POINT ( 'NONE',  ( 20.96250000122903145, 4.330127018922192761, -2.499999999999997780 ) ) ;
#31024=CARTESIAN_POINT ( 'NONE',  ( 24.55312500061451786, -4.541064518000417216, -2.621784821875001281 ) ) ;
#31025=CARTESIAN_POINT ( 'NONE',  ( 24.86250000000000071, 2.886751345948129099, -4.999999999999998224 ) ) ;
#31026=CARTESIAN_POINT ( 'NONE',  ( 27.06562500061451004, 3.027376345333611329, 5.243569643749999010 ) ) ;
#31027=CARTESIAN_POINT ( 'NONE',  ( 8.053125000614516082, 4.541064518000418104, -2.621784821874998173 ) ) ;
#31028=ORIENTED_EDGE ( 'NONE', *, *, #48081, .F. ) ;
#31029=CARTESIAN_POINT ( 'NONE',  ( 23.54062500061451146, -3.027376345333614438, 5.243569643749998122 ) ) ;
#31030=CARTESIAN_POINT ( 'NONE',  ( 5.203125000614518214, -4.541064518000417216, -2.621784821875001281 ) ) ;
#31032=CARTESIAN_POINT ( 'NONE',  ( 2.878125000614517592, -4.541064518000419881, 2.621784821874995952 ) ) ;
#31033=CARTESIAN_POINT ( 'NONE',  ( -3.000416591977282496E-16, 19.74687500061451928, -34.90005215228797653 ) ) ;
#31034=CARTESIAN_POINT ( 'NONE',  ( 12.75000000000000178, 4.330127018922192761, -2.499999999999997780 ) ) ;
#31035=CARTESIAN_POINT ( 'NONE',  ( 14.70937500061451786, -4.541064518000417216, -2.621784821875001281 ) ) ;
#31036=CARTESIAN_POINT ( 'NONE',  ( 8.250000001229034652, -2.886751345948125991, -5.000000000000000000 ) ) ;
#31037=CARTESIAN_POINT ( 'NONE',  ( 15.68437500061451573, 6.421520780324663323E-16, -5.243569643749999010 ) ) ;
#31039=CARTESIAN_POINT ( 'NONE',  ( 7.209375000614519635, 4.541064518000418104, -2.621784821874998173 ) ) ;
#31040=CARTESIAN_POINT ( 'NONE',  ( -3.000416591977282496E-16, 12.04062500061451857, -34.90005215228797653 ) ) ;
#31042=CARTESIAN_POINT ( 'NONE',  ( 13.09687500061451892, 6.054752690667223547, 3.707466751127219781E-16 ) ) ;
#31044=CARTESIAN_POINT ( 'NONE',  ( 22.26562500061451644, -6.054752690667223547, -1.112240025338166033E-15 ) ) ;
#31045=CARTESIAN_POINT ( 'NONE',  ( 2.121784821875001281, 10.10937500061451821, 33.67503911421598417 ) ) ;
#31047=CARTESIAN_POINT ( 'NONE',  ( 26.82187500061451857, -6.054752690667223547, -1.112240025338166033E-15 ) ) ;
#31048=EDGE_CURVE ( 'NONE', #5287, #62948, #43851, .T. ) ;
#31049=CARTESIAN_POINT ( 'NONE',  ( 29.25937500061451502, 4.541064518000418104, -2.621784821874998173 ) ) ;
#31050=CARTESIAN_POINT ( 'NONE',  ( 4.115625000614516082, 3.027376345333611329, 5.243569643749999010 ) ) ;
#31052=CARTESIAN_POINT ( 'NONE',  ( 17.14687500061451786, 6.054752690667223547, 3.707466751127219781E-16 ) ) ;
#31054=CARTESIAN_POINT ( 'NONE',  ( 3.515625000614516882, 3.027376345333613106, -5.243569643749998122 ) ) ;
#31055=CARTESIAN_POINT ( 'NONE',  ( 5.221875000614519813, -6.054752690667223547, -1.112240025338166033E-15 ) ) ;
#31056=CARTESIAN_POINT ( 'NONE',  ( 17.40937500061451715, -4.541064518000417216, -2.621784821875001281 ) ) ;
#31058=CARTESIAN_POINT ( 'NONE',  ( 25.31250000000000000, 2.886751345948129099, -4.999999999999998224 ) ) ;
#31059=CARTESIAN_POINT ( 'NONE',  ( 26.44687500061451502, -3.027376345333610441, -5.243569643749999898 ) ) ;
#31062=EDGE_LOOP ( 'NONE', ( #47745, #42971, #49479, #56614 ) ) ;
#31063=CARTESIAN_POINT ( 'NONE',  ( 7.387500000000001066, 5.773502691896255534, 3.535250795749688894E-16 ) ) ;
#31065=CARTESIAN_POINT ( 'NONE',  ( 22.19062500061451715, -3.027376345333614438, 5.243569643749998122 ) ) ;
#31066=CARTESIAN_POINT ( 'NONE',  ( 12.30000000000000249, 4.330127018922192761, -2.499999999999997780 ) ) ;
#31067=CARTESIAN_POINT ( 'NONE',  ( 8.925000001229033586, 2.886751345948126879, 4.999999999999999112 ) ) ;
#31068=CARTESIAN_POINT ( 'NONE',  ( 6.703125000614516438, 4.541064518000418104, -2.621784821874998173 ) ) ;
#31069=CARTESIAN_POINT ( 'NONE',  ( 21.03750000000000142, -2.886751345948129988, 4.999999999999997335 ) ) ;
#31070=CARTESIAN_POINT ( 'NONE',  ( 18.06562500061451715, 3.027376345333611329, 5.243569643749999010 ) ) ;
#31072=CARTESIAN_POINT ( 'NONE',  ( 22.46250000122903501, 0.000000000000000000, 4.999999999999998224 ) ) ;
#31074=CARTESIAN_POINT ( 'NONE',  ( 4.687500000000000000, 5.773502691896255534, 3.535250795749688894E-16 ) ) ;
#31076=CARTESIAN_POINT ( 'NONE',  ( 19.30312500061451786, 4.541064518000418104, -2.621784821874998173 ) ) ;
#31077=CARTESIAN_POINT ( 'NONE',  ( 26.12812500061451360, 4.541064518000418104, 2.621784821874999949 ) ) ;
#31078=CARTESIAN_POINT ( 'NONE',  ( 24.75937500061451502, 4.541064518000418104, -2.621784821874998173 ) ) ;
#31079=CARTESIAN_POINT ( 'NONE',  ( 8.812500000000000000, 2.886751345948126879, 4.999999999999999112 ) ) ;
#31080=CARTESIAN_POINT ( 'NONE',  ( 12.77812500061451750, -4.541064518000419881, 2.621784821874995952 ) ) ;
#31081=CARTESIAN_POINT ( 'NONE',  ( 27.92812500061451431, 4.541064518000418104, 2.621784821874999949 ) ) ;
#31082=CARTESIAN_POINT ( 'NONE',  ( 9.665625000614515017, -6.054752690667223547, -1.112240025338166033E-15 ) ) ;
#31084=CARTESIAN_POINT ( 'NONE',  ( -2.121784821874999949, 12.58437500061451786, 26.32496088578401938 ) ) ;
#31085=EDGE_CURVE ( 'NONE', #5008, #32129, #67901, .T. ) ;
#31086=CARTESIAN_POINT ( 'NONE',  ( 24.60000000122903430, 5.773502691896255534, 3.535250795749688894E-16 ) ) ;
#31088=CARTESIAN_POINT ( 'NONE',  ( 13.34062500061451750, -3.027376345333610441, -5.243569643749999898 ) ) ;
#31089=CARTESIAN_POINT ( 'NONE',  ( 11.48437500061451644, -4.541064518000419881, 2.621784821874995952 ) ) ;
#31090=CARTESIAN_POINT ( 'NONE',  ( 8.596875000614518925, 6.054752690667223547, 3.707466751127219781E-16 ) ) ;
#31091=CARTESIAN_POINT ( 'NONE',  ( 17.14687500061451786, 6.054752690667223547, 3.707466751127219781E-16 ) ) ;
#31094=CARTESIAN_POINT ( 'NONE',  ( 21.74062500061451431, -3.027376345333614438, 5.243569643749998122 ) ) ;
#31095=CARTESIAN_POINT ( 'NONE',  ( 17.07187500061451502, 3.027376345333613106, -5.243569643749998122 ) ) ;
#31096=CARTESIAN_POINT ( 'NONE',  ( 20.87812500061451715, -4.541064518000419881, 2.621784821874995952 ) ) ;
#31097=CARTESIAN_POINT ( 'NONE',  ( 3.999999999999998668, 11.71250000000000036, 27.69059892324149175 ) ) ;
#31098=CARTESIAN_POINT ( 'NONE',  ( 26.54062500061451146, 6.054752690667223547, 3.707466751127219781E-16 ) ) ;
#31099=CARTESIAN_POINT ( 'NONE',  ( 6.712500001229034119, 0.000000000000000000, 4.999999999999998224 ) ) ;
#31100=ORIENTED_EDGE ( 'NONE', *, *, #26717, .F. ) ;
#31101=CARTESIAN_POINT ( 'NONE',  ( 5.100000001229034297, -2.886751345948125991, -5.000000000000000000 ) ) ;
#31102=CARTESIAN_POINT ( 'NONE',  ( 3.999999999999999112, 17.97500000000000142, -30.00000000000000000 ) ) ;
#31103=CARTESIAN_POINT ( 'NONE',  ( 25.20000000122903216, -2.886751345948129988, 4.999999999999997335 ) ) ;
#31105=CARTESIAN_POINT ( 'NONE',  ( 7.471875000614519813, -6.054752690667223547, -1.112240025338166033E-15 ) ) ;
#31106=CARTESIAN_POINT ( 'NONE',  ( 4.897546610576117843, 1.006994139586731674, -5.145967878999484491 ) ) ;
#31107=ADVANCED_FACE ( 'NONE', ( #16724 ), #1841, .T. ) ;
#31108=CARTESIAN_POINT ( 'NONE',  ( 15.02812500061451750, -4.541064518000419881, 2.621784821874995952 ) ) ;
#31109=CARTESIAN_POINT ( 'NONE',  ( 8.559375000614515727, 4.541064518000418104, -2.621784821874998173 ) ) ;
#31110=CARTESIAN_POINT ( 'NONE',  ( 26.70000000122903572, -2.886751345948125991, -5.000000000000000000 ) ) ;
#31111=CARTESIAN_POINT ( 'NONE',  ( 16.80937500061451573, 0.000000000000000000, 5.243569643749999010 ) ) ;
#31112=CARTESIAN_POINT ( 'NONE',  ( 3.946875000614517681, -3.027376345333610441, -5.243569643749999898 ) ) ;
#31113=FACE_OUTER_BOUND ( 'NONE', #22272, .T. ) ;
#31114=( BOUNDED_CURVE ( )  B_SPLINE_CURVE ( 2, ( #4, #22511, #16961, #39514, #62042, #33955, #56495, #62020, #5872 ),
 .UNSPECIFIED., .F., .F. ) 
 B_SPLINE_CURVE_WITH_KNOTS ( ( 3, 2, 2, 2, 3 ),
 ( 0.5326086956521739468, 0.5362318840579710644, 0.5434782608695651884, 0.5507246376811594235, 0.5543478260869565410 ),
 .UNSPECIFIED. ) 
 CURVE ( )  GEOMETRIC_REPRESENTATION_ITEM ( )  RATIONAL_B_SPLINE_CURVE ( ( 0.9330127018922194093, 0.9330127018922194093, 1.000000000000000000, 0.8660254037844387076, 1.000000000000000000, 0.8660254037844387076, 1.000000000000000000, 0.9330127018922194093, 0.9330127018922194093 ) ) 
 REPRESENTATION_ITEM ( '' )  );
#31115=CARTESIAN_POINT ( 'NONE',  ( 4.940625000614515372, 6.054752690667223547, 3.707466751127219781E-16 ) ) ;
#31116=CARTESIAN_POINT ( 'NONE',  ( 15.36562500061451608, 3.027376345333611329, 5.243569643749999010 ) ) ;
#31117=ORIENTED_EDGE ( 'NONE', *, *, #56957, .T. ) ;
#31118=CARTESIAN_POINT ( 'NONE',  ( 13.07812500061451821, 4.541064518000418104, 2.621784821874999949 ) ) ;
#31119=CARTESIAN_POINT ( 'NONE',  ( 5.250000001229035540, 5.773502691896255534, 3.535250795749688894E-16 ) ) ;
#31120=CARTESIAN_POINT ( 'NONE',  ( 11.95312500061451644, -4.541064518000417216, -2.621784821875001281 ) ) ;
#31122=CARTESIAN_POINT ( 'NONE',  ( 10.23750000000000071, -2.886751345948129988, 4.999999999999997335 ) ) ;
#31123=CARTESIAN_POINT ( 'NONE',  ( 6.225000001229036073, 2.886751345948126879, 4.999999999999999112 ) ) ;
#31124=CARTESIAN_POINT ( 'NONE',  ( 19.23749999999999716, -2.886751345948129988, 4.999999999999997335 ) ) ;
#31125=CARTESIAN_POINT ( 'NONE',  ( 15.15937500061451715, -4.541064518000417216, -2.621784821875001281 ) ) ;
#31126=CARTESIAN_POINT ( 'NONE',  ( 17.02500000122903145, 2.886751345948126879, 4.999999999999999112 ) ) ;
#31128=CARTESIAN_POINT ( 'NONE',  ( -2.121784821874996840, 19.42812500061451786, -26.32496088578401583 ) ) ;
#31129=CARTESIAN_POINT ( 'NONE',  ( 3.211236255978536125, 3.832487665771286522, 3.578695418803822470 ) ) ;
#31134=CARTESIAN_POINT ( 'NONE',  ( 15.00937500061451679, 0.000000000000000000, 5.243569643749999010 ) ) ;
#31135=CARTESIAN_POINT ( 'NONE',  ( 29.55000000000000071, 0.000000000000000000, 4.999999999999998224 ) ) ;
#31136=CARTESIAN_POINT ( 'NONE',  ( 11.84062500061451750, -3.027376345333614438, 5.243569643749998122 ) ) ;
#31138=CARTESIAN_POINT ( 'NONE',  ( 23.14687500061451786, -3.027376345333614438, 5.243569643749998122 ) ) ;
#31140=CARTESIAN_POINT ( 'NONE',  ( 11.05312500061451608, -4.541064518000417216, -2.621784821875001281 ) ) ;
#31141=CARTESIAN_POINT ( 'NONE',  ( 14.10937500061451644, 0.000000000000000000, 5.243569643749999010 ) ) ;
#31143=CARTESIAN_POINT ( 'NONE',  ( 24.57187500061451502, -6.054752690667223547, -1.112240025338166033E-15 ) ) ;
#31144=CARTESIAN_POINT ( 'NONE',  ( 27.21562500061451928, -6.054752690667223547, -1.112240025338166033E-15 ) ) ;
#31145=CARTESIAN_POINT ( 'NONE',  ( 28.64999999999999858, 0.000000000000000000, 4.999999999999998224 ) ) ;
#31146=( BOUNDED_CURVE ( )  B_SPLINE_CURVE ( 2, ( #1858, #41725, #8113, #52452, #46548, #2569, #25089 ),
 .UNSPECIFIED., .F., .F. ) 
 B_SPLINE_CURVE_WITH_KNOTS ( ( 3, 2, 2, 3 ),
 ( 0.5999999999999999778, 0.6027777777777777457, 0.6055555555555555136, 0.6083333333333332815 ),
 .UNSPECIFIED. ) 
 CURVE ( )  GEOMETRIC_REPRESENTATION_ITEM ( )  RATIONAL_B_SPLINE_CURVE ( ( 1.000000000000000000, 0.8660254037844387076, 1.000000000000000000, 0.8660254037844387076, 1.000000000000000000, 0.8660254037844387076, 1.000000000000000000 ) ) 
 REPRESENTATION_ITEM ( '' )  );
#31147=CARTESIAN_POINT ( 'NONE',  ( 7.200000000000001954, -4.330127018922190985, -2.500000000000001332 ) ) ;
#31148=CARTESIAN_POINT ( 'NONE',  ( 16.80000000122903359, -2.886751345948125991, -5.000000000000000000 ) ) ;
#31151=ORIENTED_EDGE ( 'NONE', *, *, #40764, .T. ) ;
#31152=CARTESIAN_POINT ( 'NONE',  ( 16.23750000000000071, -2.886751345948125991, -5.000000000000000000 ) ) ;
#31153=CARTESIAN_POINT ( 'NONE',  ( 18.78749999999999432, -2.886751345948129988, 4.999999999999997335 ) ) ;
#31154=CARTESIAN_POINT ( 'NONE',  ( 13.04062500061451502, 6.054752690667223547, 3.707466751127219781E-16 ) ) ;
#31157=CARTESIAN_POINT ( 'NONE',  ( -2.121784821874999949, 16.63437500061451857, -33.67503911421598417 ) ) ;
#31158=CARTESIAN_POINT ( 'NONE',  ( 6.478125000614516793, -4.541064518000419881, 2.621784821874995952 ) ) ;
#31160=CARTESIAN_POINT ( 'NONE',  ( 13.27500000000000213, 4.330127018922191873, 2.499999999999999556 ) ) ;
#31163=CARTESIAN_POINT ( 'NONE',  ( -4.243569643749999898, 16.20312500061451644, 30.00000000000000000 ) ) ;
#31164=CARTESIAN_POINT ( 'NONE',  ( 27.89062500061451289, 6.054752690667223547, 3.707466751127219781E-16 ) ) ;
#31167=CARTESIAN_POINT ( 'NONE',  ( 24.23437500061451644, 6.421520780324663323E-16, -5.243569643749999010 ) ) ;
#31168=CARTESIAN_POINT ( 'NONE',  ( 18.14062500061451644, -3.027376345333614438, 5.243569643749998122 ) ) ;
#31169=CARTESIAN_POINT ( 'NONE',  ( -4.243569643749998122, 13.54062500061459140, -27.54997392385601174 ) ) ;
#31170=CARTESIAN_POINT ( 'NONE',  ( 23.81250000122903288, 0.000000000000000000, 4.999999999999998224 ) ) ;
#31171=CARTESIAN_POINT ( 'NONE',  ( 4.678125000614516971, -4.541064518000419881, 2.621784821874995952 ) ) ;
#31173=CARTESIAN_POINT ( 'NONE',  ( 21.70312500061451644, 0.000000000000000000, 5.243569643749999010 ) ) ;
#31176=CARTESIAN_POINT ( 'NONE',  ( 18.42187500061451644, 3.027376345333613106, -5.243569643749998122 ) ) ;
#31177=CARTESIAN_POINT ( 'NONE',  ( 15.98437500061451821, -4.541064518000419881, 2.621784821874995952 ) ) ;
#31178=CARTESIAN_POINT ( 'NONE',  ( 23.97187500061451360, 3.027376345333611329, 5.243569643749999010 ) ) ;
#31179=CARTESIAN_POINT ( 'NONE',  ( -4.243569643749998122, 13.14687500061451786, 32.45002607614398471 ) ) ;
#31180=CARTESIAN_POINT ( 'NONE',  ( 4.415625000614518569, 3.027376345333613106, -5.243569643749998122 ) ) ;
#31181=FACE_OUTER_BOUND ( 'NONE', #34868, .T. ) ;
#31182=( BOUNDED_CURVE ( )  B_SPLINE_CURVE ( 2, ( #70968, #37351, #20341, #42894, #59873, #9278, #31812, #3744, #48806 ),
 .UNSPECIFIED., .F., .F. ) 
 B_SPLINE_CURVE_WITH_KNOTS ( ( 3, 2, 2, 2, 3 ),
 ( 0.07608695652173913526, 0.07971014492753622505, 0.08695652173913043237, 0.09420289855072463969, 0.09782608695652174335 ),
 .UNSPECIFIED. ) 
 CURVE ( )  GEOMETRIC_REPRESENTATION_ITEM ( )  RATIONAL_B_SPLINE_CURVE ( ( 0.9330127018922192983, 0.9330127018922194093, 1.000000000000000000, 0.8660254037844387076, 1.000000000000000000, 0.8660254037844387076, 1.000000000000000000, 0.9330127018922194093, 0.9330127018922194093 ) ) 
 REPRESENTATION_ITEM ( '' )  );
#31183=CARTESIAN_POINT ( 'NONE',  ( 28.90312500061451217, 0.000000000000000000, 5.243569643749999010 ) ) ;
#31184=FACE_OUTER_BOUND ( 'NONE', #61447, .T. ) ;
#31185=CARTESIAN_POINT ( 'NONE',  ( 1.071796769724505438, 12.77990381179669832, 26.00000000000001421 ) ) ;
#31186=CARTESIAN_POINT ( 'NONE',  ( 3.853125000614517681, -4.541064518000417216, -2.621784821875001281 ) ) ;
#31187=CARTESIAN_POINT ( 'NONE',  ( 7.546875000614517326, -3.027376345333610441, -5.243569643749999898 ) ) ;
#31189=CARTESIAN_POINT ( 'NONE',  ( 15.15000000122903323, 5.773502691896255534, 3.535250795749688894E-16 ) ) ;
#31190=CARTESIAN_POINT ( 'NONE',  ( 3.534375000614518036, 6.421520780324663323E-16, -5.243569643749999010 ) ) ;
#31191=CARTESIAN_POINT ( 'NONE',  ( 11.85000000122903430, -2.886751345948125991, -5.000000000000000000 ) ) ;
#31192=CARTESIAN_POINT ( 'NONE',  ( 4.640625000614518214, -3.027376345333614438, 5.243569643749998122 ) ) ;
#31195=CARTESIAN_POINT ( 'NONE',  ( 13.20937500061451786, 0.000000000000000000, 5.243569643749999010 ) ) ;
#31196=DIRECTION ( 'NONE',  ( 0.000000000000000000, 0.000000000000000000, -1.000000000000000000 ) ) ;
#31197=VERTEX_POINT ( 'NONE', #37696 ) ;
#31198=CARTESIAN_POINT ( 'NONE',  ( 22.60312500061451857, 0.000000000000000000, 5.243569643749999010 ) ) ;
#31199=CARTESIAN_POINT ( 'NONE',  ( 7.378125000614518036, -4.541064518000419881, 2.621784821874995952 ) ) ;
#31200=CARTESIAN_POINT ( 'NONE',  ( 25.58437500061451431, 6.421520780324663323E-16, -5.243569643749999010 ) ) ;
#31201=CARTESIAN_POINT ( 'NONE',  ( 7.190625000614518036, 6.054752690667223547, 3.707466751127219781E-16 ) ) ;
#31202=CYLINDRICAL_SURFACE ( 'NONE', #51011, 4.999999999999998224 ) ;
#31203=CARTESIAN_POINT ( 'NONE',  ( 8.250000001229034652, -2.886751345948125991, -5.000000000000000000 ) ) ;
#31204=CARTESIAN_POINT ( 'NONE',  ( 23.76562500061451644, 3.027376345333613106, -5.243569643749998122 ) ) ;
#31205=CARTESIAN_POINT ( 'NONE',  ( 9.001249775931846008E-16, 11.36562500061451786, -25.09994784771203058 ) ) ;
#31206=CARTESIAN_POINT ( 'NONE',  ( 9.900000001229033231, -2.886751345948129988, 4.999999999999997335 ) ) ;
#31208=CARTESIAN_POINT ( 'NONE',  ( 19.82812500061451644, 4.541064518000418104, 2.621784821874999949 ) ) ;
#31209=CARTESIAN_POINT ( 'NONE',  ( 17.20312500061451644, 0.000000000000000000, 5.243569643749999010 ) ) ;
#31211=CARTESIAN_POINT ( 'NONE',  ( 18.78749999999999432, -2.886751345948129988, 4.999999999999997335 ) ) ;
#31212=CARTESIAN_POINT ( 'NONE',  ( 12.78750000122903430, 6.123233995736764310E-16, -4.999999999999998224 ) ) ;
#31213=CARTESIAN_POINT ( 'NONE',  ( 9.478125000614515017, 4.541064518000418104, 2.621784821874999949 ) ) ;
#31214=CARTESIAN_POINT ( 'NONE',  ( 14.61562500061451608, -6.054752690667223547, -1.112240025338166033E-15 ) ) ;
#31215=CARTESIAN_POINT ( 'NONE',  ( 22.46250000122903501, 0.000000000000000000, 4.999999999999998224 ) ) ;
#31216=CARTESIAN_POINT ( 'NONE',  ( 22.58437500061451431, 4.541064518000418104, 2.621784821874999949 ) ) ;
#31217=CARTESIAN_POINT ( 'NONE',  ( 20.85937500061451644, 0.000000000000000000, 5.243569643749999010 ) ) ;
#31219=CARTESIAN_POINT ( 'NONE',  ( 7.200000001229035718, -2.886751345948129988, 4.999999999999997335 ) ) ;
#31220=CARTESIAN_POINT ( 'NONE',  ( 6.384375000614516793, 4.541064518000418104, 2.621784821874999949 ) ) ;
#31221=CARTESIAN_POINT ( 'NONE',  ( 23.48437500061451644, 4.541064518000418104, 2.621784821874999949 ) ) ;
#31222=EDGE_CURVE ( 'NONE', #3749, #6439, #31596, .T. ) ;
#31223=VECTOR ( 'NONE', #47978, 1000.000000000000000 ) ;
#31224=CARTESIAN_POINT ( 'NONE',  ( 19.34062500061451573, 6.054752690667223547, 3.707466751127219781E-16 ) ) ;
#31225=CARTESIAN_POINT ( 'NONE',  ( 23.70937500061451786, -4.541064518000417216, -2.621784821875001281 ) ) ;
#31227=LINE ( 'NONE', #26795, #31493 ) ;
#31229=CARTESIAN_POINT ( 'NONE',  ( 6.271875000614517859, 3.027376345333613106, -5.243569643749998122 ) ) ;
#31230=CARTESIAN_POINT ( 'NONE',  ( 17.39062500061451644, -3.027376345333610441, -5.243569643749999898 ) ) ;
#31231=VECTOR ( 'NONE', #15869, 1000.000000000000000 ) ;
#31232=ORIENTED_EDGE ( 'NONE', *, *, #19011, .T. ) ;
#31234=CARTESIAN_POINT ( 'NONE',  ( 25.34062500061451217, -3.027376345333614438, 5.243569643749998122 ) ) ;
#31237=CARTESIAN_POINT ( 'NONE',  ( 15.29999999999999893, -4.330127018922190985, -2.500000000000001332 ) ) ;
#31238=CARTESIAN_POINT ( 'NONE',  ( 25.12500000122903288, 2.886751345948126879, 4.999999999999999112 ) ) ;
#31239=CARTESIAN_POINT ( 'NONE',  ( 18.51562500061451289, 3.027376345333611329, 5.243569643749999010 ) ) ;
#31241=CARTESIAN_POINT ( 'NONE',  ( 22.05000000000000071, -4.330127018922190985, -2.500000000000001332 ) ) ;
#31242=CARTESIAN_POINT ( 'NONE',  ( 24.72187500061451360, 3.027376345333613106, -5.243569643749998122 ) ) ;
#31244=DIRECTION ( 'NONE',  ( -1.000000000000000000, -0.000000000000000000, -0.000000000000000000 ) ) ;
#31245=CARTESIAN_POINT ( 'NONE',  ( 12.74062500061451786, -3.027376345333614438, 5.243569643749998122 ) ) ;
#31246=CARTESIAN_POINT ( 'NONE',  ( 3.403125000614518836, -4.541064518000417216, -2.621784821875001281 ) ) ;
#31248=CARTESIAN_POINT ( 'NONE',  ( 26.20312500061451644, 0.000000000000000000, 5.243569643749999010 ) ) ;
#31249=CARTESIAN_POINT ( 'NONE',  ( 11.92500000122903181, 2.886751345948129099, -4.999999999999998224 ) ) ;
#31250=CARTESIAN_POINT ( 'NONE',  ( 19.98749999999999716, 5.773502691896255534, 3.535250795749688894E-16 ) ) ;
#31251=CARTESIAN_POINT ( 'NONE',  ( 27.67499999999999716, 4.330127018922191873, 2.499999999999999556 ) ) ;
#31253=CARTESIAN_POINT ( 'NONE',  ( 5.896875000614518747, 6.054752690667223547, 3.707466751127219781E-16 ) ) ;
#31254=CARTESIAN_POINT ( 'NONE',  ( 17.22187500061451715, 3.027376345333611329, 5.243569643749999010 ) ) ;
#31256=ORIENTED_EDGE ( 'NONE', *, *, #23957, .F. ) ;
#31257=CARTESIAN_POINT ( 'NONE',  ( 29.57812500061451644, 6.421520780324663323E-16, -5.243569643749999010 ) ) ;
#31258=CARTESIAN_POINT ( 'NONE',  ( 26.78437500061451360, -4.541064518000419881, 2.621784821874995952 ) ) ;
#31260=CARTESIAN_POINT ( 'NONE',  ( 15.33750000000000036, -2.886751345948125991, -5.000000000000000000 ) ) ;
#31261=CARTESIAN_POINT ( 'NONE',  ( 14.76562500061451821, 3.027376345333613106, -5.243569643749998122 ) ) ;
#31262=CARTESIAN_POINT ( 'NONE',  ( -3.999999999999999112, 15.05000000000000071, -30.00000000000000000 ) ) ;
#31263=CARTESIAN_POINT ( 'NONE',  ( 0.000000000000000000, 20.00000000000000000, 26.00000000000000000 ) ) ;
#31264=CARTESIAN_POINT ( 'NONE',  ( -3.137519842735245283E-14, 11.56250000000000178, -26.00000000000000711 ) ) ;
#31265=CARTESIAN_POINT ( 'NONE',  ( 19.12500000122903288, 2.886751345948129099, -4.999999999999998224 ) ) ;
#31266=CARTESIAN_POINT ( 'NONE',  ( 15.11250000122903359, 4.330127018922192761, -2.499999999999997780 ) ) ;
#31268=CARTESIAN_POINT ( 'NONE',  ( 7.753125000614518036, 0.000000000000000000, 5.243569643749999010 ) ) ;
#31269=CARTESIAN_POINT ( 'NONE',  ( 25.24687500061451573, 6.054752690667223547, 3.707466751127219781E-16 ) ) ;
#31270=CARTESIAN_POINT ( 'NONE',  ( -4.243569643749997233, 16.74687500061451928, 32.45002607614398471 ) ) ;
#31271=CARTESIAN_POINT ( 'NONE',  ( 24.08437500061451786, -4.541064518000419881, 2.621784821874995952 ) ) ;
#31272=CARTESIAN_POINT ( 'NONE',  ( 4.837500000000001243, -2.886751345948129988, 4.999999999999997335 ) ) ;
#31273=CARTESIAN_POINT ( 'NONE',  ( -2.000000000000000000, 11.48750000122903359, 26.53589838486224650 ) ) ;
#31274=CARTESIAN_POINT ( 'NONE',  ( 12.32812500061451821, -4.541064518000419881, 2.621784821874995952 ) ) ;
#31275=CARTESIAN_POINT ( 'NONE',  ( 3.375000001229033320, 2.886751345948129099, -4.999999999999998224 ) ) ;
#31276=CARTESIAN_POINT ( 'NONE',  ( 8.409375000614518925, -4.541064518000417216, -2.621784821875001281 ) ) ;
#31277=CARTESIAN_POINT ( 'NONE',  ( 3.947751918878622757, -3.068428716296062841, 3.947751918878600108 ) ) ;
#31279=VECTOR ( 'NONE', #29822, 1000.000000000000000 ) ;
#31280=CARTESIAN_POINT ( 'NONE',  ( 10.26562500061451644, 3.027376345333613106, -5.243569643749998122 ) ) ;
#31281=CARTESIAN_POINT ( 'NONE',  ( 14.67187500061451821, -6.054752690667223547, -1.112240025338166033E-15 ) ) ;
#31283=CARTESIAN_POINT ( 'NONE',  ( 20.70000000122903216, -2.886751345948129988, 4.999999999999997335 ) ) ;
#31284=CARTESIAN_POINT ( 'NONE',  ( 10.73437500061451644, 6.421520780324663323E-16, -5.243569643749999010 ) ) ;
#31285=CARTESIAN_POINT ( 'NONE',  ( 13.26562500061451644, -6.054752690667223547, -1.112240025338166033E-15 ) ) ;
#31287=CARTESIAN_POINT ( 'NONE',  ( 20.74687500061451573, 6.054752690667223547, 3.707466751127219781E-16 ) ) ;
#31288=CARTESIAN_POINT ( 'NONE',  ( -1.487416814333745711E-14, 15.72500000122903430, 34.00000000000000000 ) ) ;
#31290=CARTESIAN_POINT ( 'NONE',  ( 23.81250000000000000, -5.773502691896255534, -1.060575238724906372E-15 ) ) ;
#31292=CARTESIAN_POINT ( 'NONE',  ( 2.121784821874999061, 13.85937500061451821, -33.67503911421598417 ) ) ;
#31293=CARTESIAN_POINT ( 'NONE',  ( 16.69687500061451502, 6.054752690667223547, 3.707466751127219781E-16 ) ) ;
#31294=CARTESIAN_POINT ( 'NONE',  ( 15.26250000122903216, 0.000000000000000000, 4.999999999999998224 ) ) ;
#31295=CARTESIAN_POINT ( 'NONE',  ( 12.34687500061452070, -3.027376345333614438, 5.243569643749998122 ) ) ;
#31296=CARTESIAN_POINT ( 'NONE',  ( -4.243569643749997233, 18.04062500061451857, -27.54997392385601174 ) ) ;
#31297=CARTESIAN_POINT ( 'NONE',  ( 17.40000000122903145, 5.773502691896255534, 3.535250795749688894E-16 ) ) ;
#31298=CARTESIAN_POINT ( 'NONE',  ( 12.89062500061451821, -3.027376345333610441, -5.243569643749999898 ) ) ;
#31301=CARTESIAN_POINT ( 'NONE',  ( 16.05000000000000071, 0.000000000000000000, 4.999999999999998224 ) ) ;
#31303=CARTESIAN_POINT ( 'NONE',  ( 9.271875000614519635, -6.054752690667223547, -1.112240025338166033E-15 ) ) ;
#31304=CARTESIAN_POINT ( 'NONE',  ( 0.5593513097472442297, 4.976037924071838425, 26.02984368186838893 ) ) ;
#31305=CARTESIAN_POINT ( 'NONE',  ( 11.73750000122903181, -4.330127018922194537, 2.499999999999995559 ) ) ;
#31306=CARTESIAN_POINT ( 'NONE',  ( 21.22500000122903074, -5.773502691896255534, -1.060575238724906372E-15 ) ) ;
#31307=CARTESIAN_POINT ( 'NONE',  ( 16.90312500061451573, -4.541064518000417216, -2.621784821875001281 ) ) ;
#31308=CARTESIAN_POINT ( 'NONE',  ( 20.91562500061451502, -6.054752690667223547, -1.112240025338166033E-15 ) ) ;
#31309=CARTESIAN_POINT ( 'NONE',  ( 27.90000000122903145, -2.886751345948129988, 4.999999999999997335 ) ) ;
#31310=CARTESIAN_POINT ( 'NONE',  ( 4.303125000614516971, -4.541064518000417216, -2.621784821875001281 ) ) ;
#31311=CARTESIAN_POINT ( 'NONE',  ( 24.78750000000000497, -2.886751345948125991, -5.000000000000000000 ) ) ;
#31312=CARTESIAN_POINT ( 'NONE',  ( 0.000000000000000000, -10.00000000000000000, 0.000000000000000000 ) ) ;
#31314=CARTESIAN_POINT ( 'NONE',  ( 27.75937500061451502, -4.541064518000417216, -2.621784821875001281 ) ) ;
#31315=CARTESIAN_POINT ( 'NONE',  ( -3.000416591977282496E-16, 14.34687500061451715, -34.90005215228797653 ) ) ;
#31316=CARTESIAN_POINT ( 'NONE',  ( 3.300000001229034918, -2.886751345948125991, -5.000000000000000000 ) ) ;
#31317=CARTESIAN_POINT ( 'NONE',  ( 3.787500000000002753, 5.773502691896255534, 3.535250795749688894E-16 ) ) ;
#31320=CARTESIAN_POINT ( 'NONE',  ( 6.909375000614518036, 0.000000000000000000, 5.243569643749999010 ) ) ;
#31321=CARTESIAN_POINT ( 'NONE',  ( 25.11562500061451431, 3.027376345333613106, -5.243569643749998122 ) ) ;
#31322=CARTESIAN_POINT ( 'NONE',  ( 14.43750000000000000, -2.886751345948126435, -5.000000000000000000 ) ) ;
#31324=CARTESIAN_POINT ( 'NONE',  ( -1.999999999999997113, 19.28750000122903430, 33.46410161513775705 ) ) ;
#31325=CARTESIAN_POINT ( 'NONE',  ( 4.659375000614518925, 0.000000000000000000, 5.243569643749999010 ) ) ;
#31326=CARTESIAN_POINT ( 'NONE',  ( 8.221875000614518925, 3.027376345333611329, 5.243569643749999010 ) ) ;
#31327=CARTESIAN_POINT ( 'NONE',  ( 3.187500000000002220, -2.886751345948125991, -5.000000000000000000 ) ) ;
#31329=CARTESIAN_POINT ( 'NONE',  ( -2.121784821874999949, 11.62812500061459531, 26.32496088578401938 ) ) ;
#31330=CARTESIAN_POINT ( 'NONE',  ( 20.73750000122903359, -4.330127018922194537, 2.499999999999995559 ) ) ;
#31331=CARTESIAN_POINT ( 'NONE',  ( 3.750000000000000000, 4.330127018922192761, -2.499999999999997780 ) ) ;
#31335=CARTESIAN_POINT ( 'NONE',  ( 19.86562500061451786, 3.027376345333611329, 5.243569643749999010 ) ) ;
#31336=CARTESIAN_POINT ( 'NONE',  ( 10.07812500061451644, -4.541064518000419881, 2.621784821874995952 ) ) ;
#31338=CARTESIAN_POINT ( 'NONE',  ( 9.721875000614517148, -6.054752690667223547, -1.112240025338166033E-15 ) ) ;
#31339=CARTESIAN_POINT ( 'NONE',  ( 26.96249999999999858, -5.773502691896255534, -1.060575238724906372E-15 ) ) ;
#31340=CARTESIAN_POINT ( 'NONE',  ( 20.06250000122903643, 4.330127018922192761, -2.499999999999997780 ) ) ;
#31341=CARTESIAN_POINT ( 'NONE',  ( 28.49062500061451431, -3.027376345333614438, 5.243569643749998122 ) ) ;
#31343=VECTOR ( 'NONE', #9357, 1000.000000000000000 ) ;
#31344=CARTESIAN_POINT ( 'NONE',  ( 8.409375000614518925, -4.541064518000417216, -2.621784821875001281 ) ) ;
#31345=CARTESIAN_POINT ( 'NONE',  ( 14.25937500061451679, -4.541064518000417216, -2.621784821875001281 ) ) ;
#31346=CARTESIAN_POINT ( 'NONE',  ( 26.10937500061451644, 4.541064518000418104, -2.621784821874998173 ) ) ;
#31347=CARTESIAN_POINT ( 'NONE',  ( 8.587500001229035007, -4.330127018922194537, 2.499999999999995559 ) ) ;
#31349=CARTESIAN_POINT ( 'NONE',  ( 20.40937500061451715, 0.000000000000000000, 5.243569643749999010 ) ) ;
#31350=CARTESIAN_POINT ( 'NONE',  ( 12.30937500061451573, 0.000000000000000000, 5.243569643749999010 ) ) ;
#31352=CARTESIAN_POINT ( 'NONE',  ( 24.48749999999999716, 5.773502691896255534, 3.535250795749688894E-16 ) ) ;
#31354=CARTESIAN_POINT ( 'NONE',  ( 2.121784821874999061, 12.95937500061451786, -33.67503911421598417 ) ) ;
#31356=CARTESIAN_POINT ( 'NONE',  ( 14.65312500061451573, -4.541064518000417216, -2.621784821875001281 ) ) ;
#31357=CARTESIAN_POINT ( 'NONE',  ( 3.862500000000001155, 2.886751345948126879, 4.999999999999999112 ) ) ;
#31359=CARTESIAN_POINT ( 'NONE',  ( 4.276577733362700862, 2.590537181842085257, -4.276577733362700862 ) ) ;
#31360=CARTESIAN_POINT ( 'NONE',  ( 12.82499999999999929, 4.330127018922191873, 2.499999999999999556 ) ) ;
#31361=CARTESIAN_POINT ( 'NONE',  ( -2.828200636599751609E-16, 18.65000000122903501, 25.38119784648299770 ) ) ;
#31362=CARTESIAN_POINT ( 'NONE',  ( 10.98750000122903536, 6.123233995736764310E-16, -4.999999999999998224 ) ) ;
#31363=CARTESIAN_POINT ( 'NONE',  ( 23.25937500061451857, -4.541064518000417216, -2.621784821875001281 ) ) ;
#31364=CARTESIAN_POINT ( 'NONE',  ( 16.05937500061451573, -4.541064518000417216, -2.621784821875001281 ) ) ;
#31366=ORIENTED_EDGE ( 'NONE', *, *, #6059, .F. ) ;
#31367=CARTESIAN_POINT ( 'NONE',  ( 17.65312500061451573, 0.000000000000000000, 5.243569643749999010 ) ) ;
#31368=CARTESIAN_POINT ( 'NONE',  ( 3.440625000614518036, -3.027376345333610441, -5.243569643749999898 ) ) ;
#31369=CARTESIAN_POINT ( 'NONE',  ( 16.77187500061451786, 3.027376345333611329, 5.243569643749999010 ) ) ;
#31370=CARTESIAN_POINT ( 'NONE',  ( 29.07187500061451502, -6.054752690667223547, -1.112240025338166033E-15 ) ) ;
#31371=CARTESIAN_POINT ( 'NONE',  ( 5.428125000614517859, 4.541064518000418104, 2.621784821874999949 ) ) ;
#31372=CARTESIAN_POINT ( 'NONE',  ( 20.61562500061451431, 3.027376345333613106, -5.243569643749998122 ) ) ;
#31373=CARTESIAN_POINT ( 'NONE',  ( 4.243569643749999898, 15.49062500061451786, 32.45002607614398471 ) ) ;
#31374=CARTESIAN_POINT ( 'NONE',  ( 15.41250000122903252, -4.330127018922190985, -2.500000000000001332 ) ) ;
#31376=CARTESIAN_POINT ( 'NONE',  ( 6.515625000614516438, -6.054752690667223547, -1.112240025338166033E-15 ) ) ;
#31377=CARTESIAN_POINT ( 'NONE',  ( 3.459375000614519635, -4.541064518000417216, -2.621784821875001281 ) ) ;
#31378=CARTESIAN_POINT ( 'NONE',  ( 4.000000000000000000, 18.95000000122903216, -27.69059892324149885 ) ) ;
#31379=CARTESIAN_POINT ( 'NONE',  ( 23.59687500061451715, -3.027376345333614438, 5.243569643749998122 ) ) ;
#31380=CARTESIAN_POINT ( 'NONE',  ( 14.72812500061451679, 6.421520780324663323E-16, -5.243569643749999010 ) ) ;
#31381=CARTESIAN_POINT ( 'NONE',  ( 24.33750000122903145, -4.330127018922194537, 2.499999999999995559 ) ) ;
#31382=CARTESIAN_POINT ( 'NONE',  ( 22.86562500061451431, 3.027376345333613106, -5.243569643749998122 ) ) ;
#31383=CARTESIAN_POINT ( 'NONE',  ( 19.69687500061451857, -3.027376345333610441, -5.243569643749999898 ) ) ;
#31384=CARTESIAN_POINT ( 'NONE',  ( 15.66562500061451857, 3.027376345333613106, -5.243569643749998122 ) ) ;
#31385=CARTESIAN_POINT ( 'NONE',  ( -2.121784821874996840, 14.08437500061451786, 33.67503911421598417 ) ) ;
#31386=AXIS2_PLACEMENT_3D ( 'NONE', #3131, #54832, #31196 ) ;
#31387=CARTESIAN_POINT ( 'NONE',  ( 18.96562500061451573, 3.027376345333611329, 5.243569643749999010 ) ) ;
#31388=CARTESIAN_POINT ( 'NONE',  ( 10.12500000000000178, 4.330127018922191873, 2.499999999999999556 ) ) ;
#31389=ORIENTED_EDGE ( 'NONE', *, *, #67466, .T. ) ;
#31391=CARTESIAN_POINT ( 'NONE',  ( 22.98749999999999716, -2.886751345948125991, -5.000000000000000000 ) ) ;
#31392=CARTESIAN_POINT ( 'NONE',  ( -1.999999999999997113, 10.62500000000000000, -26.53589838486224295 ) ) ;
#31393=CARTESIAN_POINT ( 'NONE',  ( 27.25312500061451360, -4.541064518000417216, -2.621784821875001281 ) ) ;
#31394=CARTESIAN_POINT ( 'NONE',  ( 7.303125000614516082, 0.000000000000000000, 5.243569643749999010 ) ) ;
#31395=CARTESIAN_POINT ( 'NONE',  ( 20.13750000122903216, 4.330127018922191873, 2.499999999999999556 ) ) ;
#31396=CARTESIAN_POINT ( 'NONE',  ( 24.06562500061451715, -6.054752690667223547, -1.112240025338166033E-15 ) ) ;
#31397=CARTESIAN_POINT ( 'NONE',  ( 22.50000000000000000, -4.330127018922190985, -2.500000000000001332 ) ) ;
#31398=CARTESIAN_POINT ( 'NONE',  ( 27.81562500061452070, 3.027376345333613106, -5.243569643749998122 ) ) ;
#31399=CARTESIAN_POINT ( 'NONE',  ( 8.540625000614518569, 6.054752690667223547, 3.707466751127219781E-16 ) ) ;
#31400=( BOUNDED_CURVE ( )  B_SPLINE_CURVE ( 2, ( #1627, #6432, #68493, #58106, #46685, #57026, #68139 ),
 .UNSPECIFIED., .F., .F. ) 
 B_SPLINE_CURVE_WITH_KNOTS ( ( 3, 2, 2, 3 ),
 ( 0.2583333333333333037, 0.2611111111111110716, 0.2638888888888888395, 0.2666666666666666075 ),
 .UNSPECIFIED. ) 
 CURVE ( )  GEOMETRIC_REPRESENTATION_ITEM ( )  RATIONAL_B_SPLINE_CURVE ( ( 1.000000000000002665, 0.8660254037844360431, 1.000000000000000000, 0.8660254037844387076, 1.000000000000000000, 0.8660254037844413721, 0.9999999999999973355 ) ) 
 REPRESENTATION_ITEM ( '' )  );
#31401=ORIENTED_EDGE ( 'NONE', *, *, #43004, .T. ) ;
#31402=CARTESIAN_POINT ( 'NONE',  ( 23.20312500061451644, -4.541064518000417216, -2.621784821875001281 ) ) ;
#31403=CARTESIAN_POINT ( 'NONE',  ( 4.490625000614516971, 6.054752690667223547, 3.707466751127219781E-16 ) ) ;
#31405=CARTESIAN_POINT ( 'NONE',  ( 3.028125000614518392, 6.421520780324663323E-16, -5.243569643749999010 ) ) ;
#31406=CARTESIAN_POINT ( 'NONE',  ( -1.999999999999997113, 14.78750000122903252, -26.53589838486224295 ) ) ;
#31407=EDGE_CURVE ( 'NONE', #17509, #29541, #18841, .T. ) ;
#31408=CARTESIAN_POINT ( 'NONE',  ( -3.999999999999999112, 10.17500000122903359, 27.69059892324149885 ) ) ;
#31409=CARTESIAN_POINT ( 'NONE',  ( 10.05000000000000071, 4.330127018922192761, -2.499999999999997780 ) ) ;
#31410=CARTESIAN_POINT ( 'NONE',  ( 10.35937500061451644, 4.541064518000418104, -2.621784821874998173 ) ) ;
#31411=CARTESIAN_POINT ( 'NONE',  ( 9.337500001229033231, 4.330127018922191873, 2.499999999999999556 ) ) ;
#31412=CARTESIAN_POINT ( 'NONE',  ( 14.93437500061451750, 4.541064518000418104, 2.621784821874999949 ) ) ;
#31414=CARTESIAN_POINT ( 'NONE',  ( 6.571875000614517681, -6.054752690667223547, -1.112240025338166033E-15 ) ) ;
#31415=CARTESIAN_POINT ( 'NONE',  ( -2.121784821874996840, 9.978125000614518569, -26.32496088578401583 ) ) ;
#31416=LINE ( 'NONE', #70203, #32410 ) ;
#31417=CARTESIAN_POINT ( 'NONE',  ( 13.02187500061451608, 3.027376345333613106, -5.243569643749998122 ) ) ;
#31418=CARTESIAN_POINT ( 'NONE',  ( 21.82500000122903572, 2.886751345948095793, -5.000000000000055067 ) ) ;
#31419=CARTESIAN_POINT ( 'NONE',  ( 22.07812500061451644, 4.541064518000418104, 2.621784821874999949 ) ) ;
#31420=CARTESIAN_POINT ( 'NONE',  ( -3.000416591977282496E-16, 11.19687500061451679, 25.09994784771203058 ) ) ;
#31422=CARTESIAN_POINT ( 'NONE',  ( 26.03437500061451715, 6.421520780324663323E-16, -5.243569643749999010 ) ) ;
#31423=DIRECTION ( 'NONE',  ( -0.000000000000000000, -1.000000000000000000, -0.000000000000000000 ) ) ;
#31424=CARTESIAN_POINT ( 'NONE',  ( 5.278125000614516615, 6.421520780324663323E-16, -5.243569643749999010 ) ) ;
#31426=CARTESIAN_POINT ( 'NONE',  ( 16.47187500061452070, -6.054752690667223547, -1.112240025338166033E-15 ) ) ;
#31428=CARTESIAN_POINT ( 'NONE',  ( 27.18750000122903288, 6.123233995736764310E-16, -4.999999999999998224 ) ) ;
#31429=CARTESIAN_POINT ( 'NONE',  ( 5.446875000614518569, 6.054752690667223547, 3.707466751127219781E-16 ) ) ;
#31430=CARTESIAN_POINT ( 'NONE',  ( 16.88437500061451502, -4.541064518000419881, 2.621784821874995952 ) ) ;
#31431=CARTESIAN_POINT ( 'NONE',  ( 4.819830401275195797, -1.330621173773433918, -5.072058569993805222 ) ) ;
#31432=CARTESIAN_POINT ( 'NONE',  ( 23.96249999999999858, 2.886751345948129099, -4.999999999999998224 ) ) ;
#31433=CARTESIAN_POINT ( 'NONE',  ( 3.637500001229036162, -4.330127018922194537, 2.499999999999995559 ) ) ;
#31434=CARTESIAN_POINT ( 'NONE',  ( 27.68437500061451573, -4.541064518000419881, 2.621784821874995952 ) ) ;
#31436=CARTESIAN_POINT ( 'NONE',  ( 21.67500000000000071, 6.123233995736764310E-16, -4.999999999999998224 ) ) ;
#31437=CARTESIAN_POINT ( 'NONE',  ( 6.862500000000002487, 2.886751345948129099, -4.999999999999998224 ) ) ;
#31439=CARTESIAN_POINT ( 'NONE',  ( 22.90312500061451573, 4.541064518000418104, -2.621784821874998173 ) ) ;
#31440=CARTESIAN_POINT ( 'NONE',  ( 12.00000000000000000, 0.000000000000000000, 4.999999999999998224 ) ) ;
#31441=CARTESIAN_POINT ( 'NONE',  ( 4.303125000614516971, -4.541064518000417216, -2.621784821875001281 ) ) ;
#31442=CARTESIAN_POINT ( 'NONE',  ( 19.87500000000000000, 6.123233995736764310E-16, -4.999999999999998224 ) ) ;
#31443=CARTESIAN_POINT ( 'NONE',  ( 18.81562500061452070, 3.027376345333613106, -5.243569643749998122 ) ) ;
#31444=CARTESIAN_POINT ( 'NONE',  ( 4.057522967627288146, -2.921730200955767298, 4.057522967627288146 ) ) ;
#31445=CARTESIAN_POINT ( 'NONE',  ( 23.55000000122903359, -2.886751345948125991, -5.000000000000000000 ) ) ;
#31447=CARTESIAN_POINT ( 'NONE',  ( 3.787500000000002753, 5.773502691896255534, 3.535250795749688894E-16 ) ) ;
#31448=ORIENTED_EDGE ( 'NONE', *, *, #9880, .F. ) ;
#31449=CARTESIAN_POINT ( 'NONE',  ( 20.57812500061451644, 6.421520780324663323E-16, -5.243569643749999010 ) ) ;
#31450=CARTESIAN_POINT ( 'NONE',  ( 26.91562500061451146, 3.027376345333613106, -5.243569643749998122 ) ) ;
#31451=CARTESIAN_POINT ( 'NONE',  ( 24.98437500061451644, -4.541064518000419881, 2.621784821874995952 ) ) ;
#31452=CARTESIAN_POINT ( 'NONE',  ( 8.512499999999999289, -5.773502691896255534, -1.060575238724906372E-15 ) ) ;
#31453=CARTESIAN_POINT ( 'NONE',  ( 11.39062500061451644, -3.027376345333614438, 5.243569643749998122 ) ) ;
#31454=CARTESIAN_POINT ( 'NONE',  ( 26.84062500061451573, -3.027376345333610441, -5.243569643749999898 ) ) ;
#31455=CARTESIAN_POINT ( 'NONE',  ( 16.47187500061452070, -6.054752690667223547, -1.112240025338166033E-15 ) ) ;
#31456=CARTESIAN_POINT ( 'NONE',  ( 9.628125000614517148, -4.541064518000419881, 2.621784821874995952 ) ) ;
#31458=CARTESIAN_POINT ( 'NONE',  ( -2.121784821874999949, 11.23437500061451821, 26.32496088578401938 ) ) ;
#31459=CARTESIAN_POINT ( 'NONE',  ( 23.25000000122903288, 5.773502691896255534, 3.535250795749688894E-16 ) ) ;
#31461=CARTESIAN_POINT ( 'NONE',  ( 15.44062500061451892, -3.027376345333614438, 5.243569643749998122 ) ) ;
#31462=CARTESIAN_POINT ( 'NONE',  ( 9.721875000614517148, -6.054752690667223547, -1.112240025338166033E-15 ) ) ;
#31463=CARTESIAN_POINT ( 'NONE',  ( 9.571875000614518569, 3.027376345333611329, 5.243569643749999010 ) ) ;
#31465=CARTESIAN_POINT ( 'NONE',  ( -1.964573642069356252, 9.807014569943703464, 35.67272520908200306 ) ) ;
#31466=CARTESIAN_POINT ( 'NONE',  ( 21.36562500061451431, -6.054752690667223547, -1.112240025338166033E-15 ) ) ;
#31467=EDGE_CURVE ( 'NONE', #30832, #48258, #26417, .T. ) ;
#31468=CARTESIAN_POINT ( 'NONE',  ( 17.52187500061451431, 3.027376345333613106, -5.243569643749998122 ) ) ;
#31469=CARTESIAN_POINT ( 'NONE',  ( 20.80312500061451431, 0.000000000000000000, 5.243569643749999010 ) ) ;
#31470=CARTESIAN_POINT ( 'NONE',  ( -3.999999999999999556, 11.41250000000000142, 27.69059892324149530 ) ) ;
#31471=CARTESIAN_POINT ( 'NONE',  ( 26.05312500061451431, 4.541064518000418104, -2.621784821874998173 ) ) ;
#31472=CARTESIAN_POINT ( 'NONE',  ( 6.075000001229034829, 2.886751345948129099, -4.999999999999998224 ) ) ;
#31474=CARTESIAN_POINT ( 'NONE',  ( 29.36250000000000071, 2.886751345948129099, -4.999999999999998224 ) ) ;
#31475=CARTESIAN_POINT ( 'NONE',  ( 4.000000000000000000, 17.03750000000000142, -27.69059892324149530 ) ) ;
#31476=AXIS2_PLACEMENT_3D ( 'NONE', #70826, #20200, #25393 ) ;
#31477=CARTESIAN_POINT ( 'NONE',  ( 25.23750000122903359, -4.330127018922194537, 2.499999999999995559 ) ) ;
#31480=CARTESIAN_POINT ( 'NONE',  ( 5.971875000614516260, 3.027376345333611329, 5.243569643749999010 ) ) ;
#31481=CARTESIAN_POINT ( 'NONE',  ( 23.43750000000000000, -2.886751345948142422, -4.999999999999970690 ) ) ;
#31482=CARTESIAN_POINT ( 'NONE',  ( 15.51562500061451644, -6.054752690667223547, -1.112240025338166033E-15 ) ) ;
#31483=CARTESIAN_POINT ( 'NONE',  ( 8.146875000614516082, 6.054752690667223547, 3.707466751127219781E-16 ) ) ;
#31484=CARTESIAN_POINT ( 'NONE',  ( 25.95000000122903216, 5.773502691896255534, 3.535250795749688894E-16 ) ) ;
#31485=CARTESIAN_POINT ( 'NONE',  ( 16.84687500061452070, -3.027376345333614438, 5.243569643749998122 ) ) ;
#31486=CARTESIAN_POINT ( 'NONE',  ( 6.196875000614515905, -3.027376345333610441, -5.243569643749999898 ) ) ;
#31487=DIRECTION ( 'NONE',  ( -0.000000000000000000, -1.000000000000000000, -0.000000000000000000 ) ) ;
#31488=EDGE_CURVE ( 'NONE', #3749, #26440, #45074, .T. ) ;
#31489=CARTESIAN_POINT ( 'NONE',  ( 4.753125000614515372, -4.541064518000417216, -2.621784821875001281 ) ) ;
#31490=CARTESIAN_POINT ( 'NONE',  ( 15.14062500061451644, -3.027376345333610441, -5.243569643749999898 ) ) ;
#31491=ORIENTED_EDGE ( 'NONE', *, *, #68597, .F. ) ;
#31492=CARTESIAN_POINT ( 'NONE',  ( 12.96562500061451750, 3.027376345333613106, -5.243569643749998122 ) ) ;
#31493=VECTOR ( 'NONE', #25693, 1000.000000000000227 ) ;
#31494=CARTESIAN_POINT ( 'NONE',  ( 5.625000001229036428, 2.886751345948129099, -4.999999999999998224 ) ) ;
#31495=CARTESIAN_POINT ( 'NONE',  ( 10.11562500061451608, -6.054752690667223547, -1.112240025338166033E-15 ) ) ;
#31497=CARTESIAN_POINT ( 'NONE',  ( 11.47499999999999964, 4.330127018922191873, 2.499999999999999556 ) ) ;
#31498=CARTESIAN_POINT ( 'NONE',  ( 3.750000001229034652, -2.886751345948125991, -5.000000000000000000 ) ) ;
#31499=CARTESIAN_POINT ( 'NONE',  ( 18.07499999999999929, 6.123233995736764310E-16, -4.999999999999998224 ) ) ;
#31500=CARTESIAN_POINT ( 'NONE',  ( 19.54687500061451644, -3.027376345333614438, 5.243569643749998122 ) ) ;
#31501=CARTESIAN_POINT ( 'NONE',  ( 15.86250000122903181, -4.330127018922190985, -2.500000000000001332 ) ) ;
#31503=CARTESIAN_POINT ( 'NONE',  ( -2.121784821874999949, 17.02812500061451573, -33.67503911421598417 ) ) ;
#31504=CARTESIAN_POINT ( 'NONE',  ( 12.11250000122903181, 0.000000000000000000, 4.999999999999998224 ) ) ;
#31505=CARTESIAN_POINT ( 'NONE',  ( 2.814937200665621919, -4.236319168869982832, -2.662479962439228132 ) ) ;
#31506=CARTESIAN_POINT ( 'NONE',  ( 29.39062500061451289, -3.027376345333614438, 5.243569643749998122 ) ) ;
#31507=EDGE_CURVE ( 'NONE', #22068, #23988, #61810, .T. ) ;
#31508=CARTESIAN_POINT ( 'NONE',  ( 4.826610586788474322, 1.315217771577623873, 4.826610586788474322 ) ) ;
#31510=CARTESIAN_POINT ( 'NONE',  ( 16.80937500061451573, 0.000000000000000000, 5.243569643749999010 ) ) ;
#31511=CARTESIAN_POINT ( 'NONE',  ( 28.83749999999999858, -2.886751345948125991, -5.000000000000000000 ) ) ;
#31512=CARTESIAN_POINT ( 'NONE',  ( 12.66562500061451502, 3.027376345333611329, 5.243569643749999010 ) ) ;
#31514=CARTESIAN_POINT ( 'NONE',  ( 23.63437500061451502, -4.541064518000419881, 2.621784821874995952 ) ) ;
#31516=CARTESIAN_POINT ( 'NONE',  ( 8.690625000614515372, -3.027376345333614438, 5.243569643749998122 ) ) ;
#31517=CARTESIAN_POINT ( 'NONE',  ( 13.54687500061451999, 6.054752690667223547, 3.707466751127219781E-16 ) ) ;
#31519=CARTESIAN_POINT ( 'NONE',  ( 24.08437500061451786, -4.541064518000419881, 2.621784821874995952 ) ) ;
#31520=CARTESIAN_POINT ( 'NONE',  ( 28.56562500061451715, -6.054752690667223547, -1.112240025338166033E-15 ) ) ;
#31522=CARTESIAN_POINT ( 'NONE',  ( 7.387500000000001066, 5.773502691896255534, 3.535250795749688894E-16 ) ) ;
#31524=CARTESIAN_POINT ( 'NONE',  ( 17.66250000122903430, -4.330127018922190985, -2.500000000000001332 ) ) ;
#31526=ORIENTED_EDGE ( 'NONE', *, *, #57166, .T. ) ;
#31527=CARTESIAN_POINT ( 'NONE',  ( 16.19999999999999929, -4.330127018922190985, -2.500000000000001332 ) ) ;
#31528=CARTESIAN_POINT ( 'NONE',  ( 18.89999999999999858, -4.330127018922190985, -2.500000000000001332 ) ) ;
#31529=CARTESIAN_POINT ( 'NONE',  ( 14.69062500061451537, -3.027376345333610441, -5.243569643749999898 ) ) ;
#31530=ORIENTED_EDGE ( 'NONE', *, *, #16880, .F. ) ;
#31532=CARTESIAN_POINT ( 'NONE',  ( 2.121784821875001281, 16.40937500061452070, -26.32496088578401938 ) ) ;
#31533=CARTESIAN_POINT ( 'NONE',  ( 3.553125000614516082, 4.541064518000418104, -2.621784821874998173 ) ) ;
#31535=CARTESIAN_POINT ( 'NONE',  ( 13.16249999999999964, 2.886751345948129099, -4.999999999999998224 ) ) ;
#31537=ORIENTED_EDGE ( 'NONE', *, *, #15860, .T. ) ;
#31538=CARTESIAN_POINT ( 'NONE',  ( -2.121784821874996840, 15.37812500061451892, 33.67503911421598417 ) ) ;
#31539=CARTESIAN_POINT ( 'NONE',  ( 26.24062500061451431, -3.027376345333614438, 5.243569643749998122 ) ) ;
#31542=CARTESIAN_POINT ( 'NONE',  ( 24.83437500061451431, 4.541064518000418104, 2.621784821874999949 ) ) ;
#31543=CARTESIAN_POINT ( 'NONE',  ( 17.99062500061451786, 6.054752690667223547, 3.707466751127219781E-16 ) ) ;
#31544=CARTESIAN_POINT ( 'NONE',  ( 4.243569643749999898, 14.17812500061459247, -30.00000000000000000 ) ) ;
#31545=CARTESIAN_POINT ( 'NONE',  ( 23.55000000122903359, -2.886751345948125991, -5.000000000000000000 ) ) ;
#31546=CARTESIAN_POINT ( 'NONE',  ( 3.965625000614515727, 3.027376345333613106, -5.243569643749998122 ) ) ;
#31548=CARTESIAN_POINT ( 'NONE',  ( 20.61562500061451431, 3.027376345333612662, -5.243569643749998122 ) ) ;
#31551=( BOUNDED_CURVE ( )  B_SPLINE_CURVE ( 2, ( #43836, #66363, #9484, #32746, #15738, #34913, #57075, #34546, #23097 ),
 .UNSPECIFIED., .F., .F. ) 
 B_SPLINE_CURVE_WITH_KNOTS ( ( 3, 2, 2, 2, 3 ),
 ( 0.4021739130434782705, 0.4057971014492753881, 0.4130434782608695676, 0.4202898550724637472, 0.4239130434782608647 ),
 .UNSPECIFIED. ) 
 CURVE ( )  GEOMETRIC_REPRESENTATION_ITEM ( )  RATIONAL_B_SPLINE_CURVE ( ( 0.9330127018922194093, 0.9330127018922194093, 1.000000000000000000, 0.8660254037844387076, 1.000000000000000000, 0.8660254037844387076, 1.000000000000000000, 0.9330127018922194093, 0.9330127018922194093 ) ) 
 REPRESENTATION_ITEM ( '' )  );
#31552=CARTESIAN_POINT ( 'NONE',  ( 16.69687500061451502, 6.054752690667223547, 3.707466751127219781E-16 ) ) ;
#31553=CARTESIAN_POINT ( 'NONE',  ( 16.92187500061451999, -6.054752690667223547, -1.112240025338166033E-15 ) ) ;
#31554=CARTESIAN_POINT ( 'NONE',  ( 25.99687500061451928, -3.027376345333610441, -5.243569643749999898 ) ) ;
#31555=CARTESIAN_POINT ( 'NONE',  ( -4.243569643749999898, 13.97187500061451715, 27.54997392385601529 ) ) ;
#31556=CARTESIAN_POINT ( 'NONE',  ( 6.065625000614516260, -6.054752690667223547, -1.112240025338166033E-15 ) ) ;
#31557=CARTESIAN_POINT ( 'NONE',  ( 28.11562500061451431, -6.054752690667223547, -1.112240025338166033E-15 ) ) ;
#31558=CARTESIAN_POINT ( 'NONE',  ( 28.34062500061451928, 6.054752690667223547, 3.707466751127219781E-16 ) ) ;
#31560=CARTESIAN_POINT ( 'NONE',  ( 8.484601909799253346E-16, 18.31250000000000355, 34.61880215351700230 ) ) ;
#31561=CARTESIAN_POINT ( 'NONE',  ( 7.809375000614519280, 0.000000000000000000, 5.243569643749999010 ) ) ;
#31562=CARTESIAN_POINT ( 'NONE',  ( 13.27500000122903323, 2.886751345948129099, -4.999999999999998224 ) ) ;
#31563=CARTESIAN_POINT ( 'NONE',  ( 9.000000001229034652, -2.886751345948129988, 4.999999999999997335 ) ) ;
#31564=CARTESIAN_POINT ( 'NONE',  ( 6.065625000614516260, -6.054752690667223547, -1.112240025338166033E-15 ) ) ;
#31567=CARTESIAN_POINT ( 'NONE',  ( 13.84687500061451537, -3.027376345333610441, -5.243569643749999898 ) ) ;
#31568=FACE_OUTER_BOUND ( 'NONE', #68876, .T. ) ;
#31570=CARTESIAN_POINT ( 'NONE',  ( 22.15312500061451573, 0.000000000000000000, 5.243569643749999010 ) ) ;
#31571=CARTESIAN_POINT ( 'NONE',  ( 7.115625000614516082, 3.027376345333613106, -5.243569643749998122 ) ) ;
#31572=CARTESIAN_POINT ( 'NONE',  ( 23.78437500061451360, 6.421520780324663323E-16, -5.243569643749999010 ) ) ;
#31573=CARTESIAN_POINT ( 'NONE',  ( 7.865625000614516971, -6.054752690667223547, -1.112240025338166033E-15 ) ) ;
#31574=CARTESIAN_POINT ( 'NONE',  ( 20.54999999999999716, 0.000000000000000000, 4.999999999999998224 ) ) ;
#31575=CARTESIAN_POINT ( 'NONE',  ( 8.887500001229033941, 4.330127018922191873, 2.499999999999999556 ) ) ;
#31577=CARTESIAN_POINT ( 'NONE',  ( 21.70312500061451644, 0.000000000000000000, 5.243569643749999010 ) ) ;
#31578=CARTESIAN_POINT ( 'NONE',  ( -2.121784821874999949, 10.27812500061451750, -33.67503911421598417 ) ) ;
#31579=CARTESIAN_POINT ( 'NONE',  ( 11.36250000122903536, -4.330127018922190985, -2.500000000000001332 ) ) ;
#31580=CARTESIAN_POINT ( 'NONE',  ( 20.50312500061451715, -4.541064518000417216, -2.621784821875001281 ) ) ;
#31581=CARTESIAN_POINT ( 'NONE',  ( 18.96562500061451573, 3.027376345333611329, 5.243569643749999010 ) ) ;
#31583=CARTESIAN_POINT ( 'NONE',  ( 17.10000000000000142, -4.330127018922190985, -2.500000000000001332 ) ) ;
#31584=CARTESIAN_POINT ( 'NONE',  ( 10.95000000122903394, -2.886751345948125991, -5.000000000000000000 ) ) ;
#31585=VECTOR ( 'NONE', #63264, 1000.000000000000000 ) ;
#31586=CARTESIAN_POINT ( 'NONE',  ( 6.853125000614516793, 0.000000000000000000, 5.243569643749999010 ) ) ;
#31587=CARTESIAN_POINT ( 'NONE',  ( 12.36562500061451608, -6.054752690667223547, -1.112240025338166033E-15 ) ) ;
#31588=AXIS2_PLACEMENT_3D ( 'NONE', #21140, #48868, #55501 ) ;
#31589=CARTESIAN_POINT ( 'NONE',  ( 24.03750000122903430, 6.123233995736764310E-16, -4.999999999999998224 ) ) ;
#31590=CARTESIAN_POINT ( 'NONE',  ( 22.88437500061451857, 6.421520780324663323E-16, -5.243569643749999010 ) ) ;
#31592=CARTESIAN_POINT ( 'NONE',  ( 6.037500001229035185, 6.123233995736764310E-16, -4.999999999999998224 ) ) ;
#31593=( BOUNDED_CURVE ( )  B_SPLINE_CURVE ( 2, ( #64202, #19125, #41679, #25042, #13589, #48324, #36136, #53491, #20222 ),
 .UNSPECIFIED., .F., .F. ) 
 B_SPLINE_CURVE_WITH_KNOTS ( ( 3, 2, 2, 2, 3 ),
 ( 0.1847826086956521896, 0.1884057971014492794, 0.1956521739130434867, 0.2028985507246376940, 0.2065217391304347838 ),
 .UNSPECIFIED. ) 
 CURVE ( )  GEOMETRIC_REPRESENTATION_ITEM ( )  RATIONAL_B_SPLINE_CURVE ( ( 0.9330127018922194093, 0.9330127018922196314, 1.000000000000000000, 0.8660254037844387076, 1.000000000000000000, 0.8660254037844387076, 1.000000000000000000, 0.9330127018922194093, 0.9330127018922194093 ) ) 
 REPRESENTATION_ITEM ( '' )  );
#31594=CARTESIAN_POINT ( 'NONE',  ( 7.321875000614516793, 3.027376345333611329, 5.243569643749999010 ) ) ;
#31595=CARTESIAN_POINT ( 'NONE',  ( 24.00937500061451502, 0.000000000000000000, 5.243569643749999010 ) ) ;
#31596=( BOUNDED_CURVE ( )  B_SPLINE_CURVE ( 2, ( #9631, #32165, #66143, #33612, #66888, #12169, #57226 ),
 .UNSPECIFIED., .F., .F. ) 
 B_SPLINE_CURVE_WITH_KNOTS ( ( 3, 2, 2, 3 ),
 ( 0.4750000000000000333, 0.4777777777777778567, 0.4805555555555556246, 0.4833333333333333925 ),
 .UNSPECIFIED. ) 
 CURVE ( )  GEOMETRIC_REPRESENTATION_ITEM ( )  RATIONAL_B_SPLINE_CURVE ( ( 0.9999999999999973355, 0.8660254037844413721, 1.000000000000000000, 0.8660254037844387076, 1.000000000000000000, 0.8660254037844360431, 1.000000000000002665 ) ) 
 REPRESENTATION_ITEM ( '' )  );
#31597=CARTESIAN_POINT ( 'NONE',  ( 4.324156358178267823, -2.510600649150880770, -4.568139011954959194 ) ) ;
#31598=CARTESIAN_POINT ( 'NONE',  ( 17.87812500061451715, 6.421520780324663323E-16, -5.243569643749999010 ) ) ;
#31599=CARTESIAN_POINT ( 'NONE',  ( 23.78437500061451360, 6.421520780324663323E-16, -5.243569643749999010 ) ) ;
#31601=CARTESIAN_POINT ( 'NONE',  ( 12.52500000122903145, 2.886751345948126879, 4.999999999999998224 ) ) ;
#31602=CYLINDRICAL_SURFACE ( 'NONE', #32446, 4.999999999999998224 ) ;
#31603=CARTESIAN_POINT ( 'NONE',  ( 4.884375000614518569, 6.421520780324663323E-16, -5.243569643749999010 ) ) ;
#31604=CARTESIAN_POINT ( 'NONE',  ( 17.95312500061451644, 4.541064518000418104, -2.621784821874998173 ) ) ;
#31605=CARTESIAN_POINT ( 'NONE',  ( 12.79687500061451821, -3.027376345333614438, 5.243569643749998122 ) ) ;
#31606=ORIENTED_EDGE ( 'NONE', *, *, #3230, .T. ) ;
#31607=CARTESIAN_POINT ( 'NONE',  ( 22.16250000000000142, 2.886751345948095793, -5.000000000000055067 ) ) ;
#31608=CARTESIAN_POINT ( 'NONE',  ( 25.67812500061451431, 4.541064518000418104, 2.621784821874999949 ) ) ;
#31610=CARTESIAN_POINT ( 'NONE',  ( -2.000000000000000000, 18.23750000122903359, 26.53589838486224650 ) ) ;
#31612=CARTESIAN_POINT ( 'NONE',  ( 14.58750000000000036, 5.773502691896255534, 3.535250795749688894E-16 ) ) ;
#31613=CARTESIAN_POINT ( 'NONE',  ( 24.30000000122903359, -2.886751345948129988, 4.999999999999997335 ) ) ;
#31614=CARTESIAN_POINT ( 'NONE',  ( 18.77812500061451573, 6.421520780324663323E-16, -5.243569643749999010 ) ) ;
#31616=CARTESIAN_POINT ( 'NONE',  ( 22.08749999999999858, -2.886751345948125991, -5.000000000000000000 ) ) ;
#31617=CARTESIAN_POINT ( 'NONE',  ( 23.55937500061451573, 0.000000000000000000, 5.243569643749999010 ) ) ;
#31618=( BOUNDED_CURVE ( )  B_SPLINE_CURVE ( 2, ( #60940, #49509, #38792, #8885, #27340, #44341, #21413 ),
 .UNSPECIFIED., .F., .T. ) 
 B_SPLINE_CURVE_WITH_KNOTS ( ( 3, 2, 2, 3 ),
 ( 0.6166666666666666963, 0.6194444444444444642, 0.6222222222222222321, 0.6250000000000000000 ),
 .UNSPECIFIED. ) 
 CURVE ( )  GEOMETRIC_REPRESENTATION_ITEM ( )  RATIONAL_B_SPLINE_CURVE ( ( 1.000000000000000000, 0.8660254037844387076, 1.000000000000000000, 0.8660254037844387076, 1.000000000000000000, 0.8660254037844387076, 1.000000000000000000 ) ) 
 REPRESENTATION_ITEM ( '' )  );
#31619=VERTEX_POINT ( 'NONE', #40256 ) ;
#31621=CARTESIAN_POINT ( 'NONE',  ( 11.12812500061451715, 6.421520780324663323E-16, -5.243569643749999010 ) ) ;
#31622=CARTESIAN_POINT ( 'NONE',  ( 4.678125000614516971, -4.541064518000419881, 2.621784821874995952 ) ) ;
#31624=CARTESIAN_POINT ( 'NONE',  ( 26.65312500061451573, 0.000000000000000000, 5.243569643749999010 ) ) ;
#31625=CARTESIAN_POINT ( 'NONE',  ( 19.68750000000000355, -2.886751345948129988, 4.999999999999997335 ) ) ;
#31626=CARTESIAN_POINT ( 'NONE',  ( 27.37500000000000000, -4.330127018922194537, 2.499999999999995559 ) ) ;
#31627=CARTESIAN_POINT ( 'NONE',  ( 3.384375000614517237, -4.541064518000419881, 2.621784821874995952 ) ) ;
#31628=CARTESIAN_POINT ( 'NONE',  ( 7.771875000614516971, 3.027376345333611329, 5.243569643749999010 ) ) ;
#31629=CARTESIAN_POINT ( 'NONE',  ( 17.70937500061451431, 0.000000000000000000, 5.243569643749999010 ) ) ;
#31630=CARTESIAN_POINT ( 'NONE',  ( -3.999999999999999112, 13.81250000122903465, 30.00000000000000000 ) ) ;
#31631=VERTEX_POINT ( 'NONE', #67970 ) ;
#31632=CARTESIAN_POINT ( 'NONE',  ( 25.86562500061451431, -6.054752690667223547, -1.112240025338166033E-15 ) ) ;
#31633=CARTESIAN_POINT ( 'NONE',  ( 28.35937500061451289, 4.541064518000418104, -2.621784821874998173 ) ) ;
#31634=CARTESIAN_POINT ( 'NONE',  ( 7.387500001229032165, 6.123233995736764310E-16, -4.999999999999998224 ) ) ;
#31636=CARTESIAN_POINT ( 'NONE',  ( 15.52500000000000036, 4.330127018922191873, 2.499999999999999556 ) ) ;
#31637=CARTESIAN_POINT ( 'NONE',  ( 12.02812500061451573, 6.421520780324663323E-16, -5.243569643749999010 ) ) ;
#31640=CARTESIAN_POINT ( 'NONE',  ( 28.15312500061451573, -4.541064518000417216, -2.621784821875001281 ) ) ;
#31641=CARTESIAN_POINT ( 'NONE',  ( 17.25000000122903288, -2.886751345948125991, -5.000000000000000000 ) ) ;
#31644=CARTESIAN_POINT ( 'NONE',  ( 4.715625000614516615, -6.054752690667223547, -1.112240025338166033E-15 ) ) ;
#31645=CARTESIAN_POINT ( 'NONE',  ( 22.05937500061451573, 4.541064518000418104, -2.621784821874998173 ) ) ;
#31646=CARTESIAN_POINT ( 'NONE',  ( 4.243569643749999898, 17.79687500061451999, 32.45002607614398471 ) ) ;
#31647=CARTESIAN_POINT ( 'NONE',  ( 24.15937500061451715, -4.541064518000417216, -2.621784821875001281 ) ) ;
#31648=CARTESIAN_POINT ( 'NONE',  ( 4.949999999999999289, -4.330127018922190985, -2.500000000000001332 ) ) ;
#31649=CARTESIAN_POINT ( 'NONE',  ( 4.000000000000000000, 11.75000000122903643, 32.30940107675849049 ) ) ;
#31650=CARTESIAN_POINT ( 'NONE',  ( 13.07812500061451821, 4.541064518000418104, 2.621784821874999949 ) ) ;
#31651=CARTESIAN_POINT ( 'NONE',  ( 4.762500001229033941, 4.330127018922192761, -2.499999999999997780 ) ) ;
#31652=CARTESIAN_POINT ( 'NONE',  ( 9.346875000614517148, -3.027376345333610441, -5.243569643749999898 ) ) ;
#31654=CARTESIAN_POINT ( 'NONE',  ( 9.703125000614514661, -4.541064518000417216, -2.621784821875001281 ) ) ;
#31655=CARTESIAN_POINT ( 'NONE',  ( 14.59687500061452070, -3.027376345333614438, 5.243569643749998122 ) ) ;
#31656=CARTESIAN_POINT ( 'NONE',  ( 20.96250000122903145, 4.330127018922192761, -2.499999999999997780 ) ) ;
#31657=CARTESIAN_POINT ( 'NONE',  ( 10.69687500061451679, -3.027376345333610441, -5.243569643749999898 ) ) ;
#31658=CARTESIAN_POINT ( 'NONE',  ( 11.72812500061451857, 4.541064518000418104, 2.621784821874999949 ) ) ;
#31660=CARTESIAN_POINT ( 'NONE',  ( 20.48437500061451289, -4.541064518000419881, 2.621784821874995952 ) ) ;
#31662=CARTESIAN_POINT ( 'NONE',  ( -0.2761983717765542079, 4.994289515549795944, 33.99286899158064301 ) ) ;
#31663=CYLINDRICAL_SURFACE ( 'NONE', #47850, 3.999999999999996447 ) ;
#31664=ADVANCED_FACE ( 'NONE', ( #11814 ), #34331, .F. ) ;
#31665=CARTESIAN_POINT ( 'NONE',  ( 4.243569643749999010, 15.17187500061451644, -32.45002607614398471 ) ) ;
#31666=CARTESIAN_POINT ( 'NONE',  ( 16.38750000122903216, 6.123233995736764310E-16, -4.999999999999998224 ) ) ;
#31667=CARTESIAN_POINT ( 'NONE',  ( 9.534375000614517148, 4.541064518000418104, 2.621784821874999949 ) ) ;
#31668=CARTESIAN_POINT ( 'NONE',  ( 2.121784821874999061, 17.85312500061451502, -33.67503911421598417 ) ) ;
#31669=CARTESIAN_POINT ( 'NONE',  ( 17.02500000122903145, 2.886751345948126879, 4.999999999999999112 ) ) ;
#31670=CARTESIAN_POINT ( 'NONE',  ( 13.52812500061451750, 4.541064518000418104, 2.621784821874999949 ) ) ;
#31671=ORIENTED_EDGE ( 'NONE', *, *, #13788, .T. ) ;
#31672=CARTESIAN_POINT ( 'NONE',  ( 16.91250000000000142, 2.886751345948126879, 4.999999999999999112 ) ) ;
#31674=CARTESIAN_POINT ( 'NONE',  ( 11.25937500061451679, 4.541064518000418104, -2.621784821874998173 ) ) ;
#31675=CARTESIAN_POINT ( 'NONE',  ( 17.84999999999999787, 0.000000000000000000, 4.999999999999998224 ) ) ;
#31676=CARTESIAN_POINT ( 'NONE',  ( 13.72500000122903074, 2.886751345948129099, -4.999999999999998224 ) ) ;
#31677=CARTESIAN_POINT ( 'NONE',  ( 20.21250000122903145, 0.000000000000000000, 4.999999999999998224 ) ) ;
#31678=CARTESIAN_POINT ( 'NONE',  ( 18.77812500061451573, 6.421520780324663323E-16, -5.243569643749999010 ) ) ;
#31679=CARTESIAN_POINT ( 'NONE',  ( 20.42812500061451431, -4.541064518000419881, 2.621784821874995952 ) ) ;
#31680=CARTESIAN_POINT ( 'NONE',  ( 28.95000000122903572, -2.886751345948125991, -5.000000000000000000 ) ) ;
#31681=CARTESIAN_POINT ( 'NONE',  ( 4.453125000614517326, 4.541064518000418104, -2.621784821874998173 ) ) ;
#31682=CARTESIAN_POINT ( 'NONE',  ( 24.56250000000000000, 2.886751345948126879, 4.999999999999999112 ) ) ;
#31683=DIRECTION ( 'NONE',  ( 0.000000000000000000, 0.000000000000000000, 1.000000000000000000 ) ) ;
#31685=CARTESIAN_POINT ( 'NONE',  ( 27.94687500061451502, 6.054752690667223547, 3.707466751127219781E-16 ) ) ;
#31686=CARTESIAN_POINT ( 'NONE',  ( 4.837500001229035895, 4.330127018922191873, 2.499999999999999556 ) ) ;
#31687=CARTESIAN_POINT ( 'NONE',  ( 29.44687500061451857, -3.027376345333614438, 5.243569643749998122 ) ) ;
#31688=CARTESIAN_POINT ( 'NONE',  ( 22.80000000000000071, 0.000000000000000000, 4.999999999999998224 ) ) ;
#31689=CARTESIAN_POINT ( 'NONE',  ( 7.321875000614516793, 3.027376345333611329, 5.243569643749999010 ) ) ;
#31690=CARTESIAN_POINT ( 'NONE',  ( 26.80312500061451431, -4.541064518000417216, -2.621784821875001281 ) ) ;
#31694=CARTESIAN_POINT ( 'NONE',  ( 4.846875000614519813, -3.027376345333610441, -5.243569643749999898 ) ) ;
#31695=CARTESIAN_POINT ( 'NONE',  ( 9.121875000614517504, 3.027376345333611329, 5.243569643749999010 ) ) ;
#31696=CARTESIAN_POINT ( 'NONE',  ( 3.637500000000001954, -2.886751345948125991, -5.000000000000000000 ) ) ;
#31697=CARTESIAN_POINT ( 'NONE',  ( -4.243569643749999898, 12.56562500061459531, 27.54997392385601529 ) ) ;
#31698=CARTESIAN_POINT ( 'NONE',  ( 20.77500000000000213, 6.123233995736764310E-16, -4.999999999999998224 ) ) ;
#31699=CARTESIAN_POINT ( 'NONE',  ( -1.999999999999997113, 17.82499999999999929, -26.53589838486224295 ) ) ;
#31700=CARTESIAN_POINT ( 'NONE',  ( 5.250000000000000888, 0.000000000000000000, 4.999999999999998224 ) ) ;
#31703=CARTESIAN_POINT ( 'NONE',  ( 20.61562500061451431, 3.027376345333613106, -5.243569643749998122 ) ) ;
#31704=CARTESIAN_POINT ( 'NONE',  ( 9.740625000614516082, -3.027376345333610441, -5.243569643749999898 ) ) ;
#31706=CARTESIAN_POINT ( 'NONE',  ( 7.509375000614517681, -4.541064518000417216, -2.621784821875001281 ) ) ;
#31707=CARTESIAN_POINT ( 'NONE',  ( 23.25000000000000000, 0.000000000000000000, 4.999999999999998224 ) ) ;
#31708=CARTESIAN_POINT ( 'NONE',  ( 19.01250000122903216, -4.330127018922190985, -2.500000000000001332 ) ) ;
#31709=CARTESIAN_POINT ( 'NONE',  ( 27.17812500061451786, -4.541064518000419881, 2.621784821874995952 ) ) ;
#31710=CARTESIAN_POINT ( 'NONE',  ( 4.000000000000000000, 10.85000000122903430, 32.30940107675849760 ) ) ;
#31711=CARTESIAN_POINT ( 'NONE',  ( 8.821875000614518569, -6.054752690667223547, -1.112240025338166033E-15 ) ) ;
#31712=CARTESIAN_POINT ( 'NONE',  ( 13.92187500061451644, 3.027376345333613106, -5.243569643749998122 ) ) ;
#31713=CARTESIAN_POINT ( 'NONE',  ( 24.23437500061451644, 6.421520780324663323E-16, -5.243569643749999010 ) ) ;
#31714=CARTESIAN_POINT ( 'NONE',  ( 3.734827092922140768, -3.324314453528163682, -3.734827092927292203 ) ) ;
#31716=CARTESIAN_POINT ( 'NONE',  ( 19.32187500061451857, 3.027376345333613106, -5.243569643749998122 ) ) ;
#31717=CARTESIAN_POINT ( 'NONE',  ( 9.046875000614518214, 6.054752690667223547, 3.707466751127219781E-16 ) ) ;
#31719=CARTESIAN_POINT ( 'NONE',  ( 22.87500000000000000, -4.330127018922194537, 2.499999999999995559 ) ) ;
#31721=CARTESIAN_POINT ( 'NONE',  ( -4.243569643749999898, 10.40937500061451892, -30.00000000000000000 ) ) ;
#31723=CARTESIAN_POINT ( 'NONE',  ( 12.32812500061451821, -4.541064518000419881, 2.621784821874995952 ) ) ;
#31724=CARTESIAN_POINT ( 'NONE',  ( 28.35937500061451289, 4.541064518000418104, -2.621784821874998173 ) ) ;
#31725=CARTESIAN_POINT ( 'NONE',  ( -3.999999999999999112, 19.21250000122903501, -30.00000000000000000 ) ) ;
#31726=PLANE ( 'NONE',  #17280 ) ;
#31727=CARTESIAN_POINT ( 'NONE',  ( 11.40000000000000036, 4.330127018922192761, -2.499999999999997780 ) ) ;
#31728=CARTESIAN_POINT ( 'NONE',  ( -3.999999999999997335, 17.90000000122903501, 32.30940107675850470 ) ) ;
#31729=CARTESIAN_POINT ( 'NONE',  ( 10.46250000122903323, -4.330127018922190985, -2.500000000000001332 ) ) ;
#31730=CARTESIAN_POINT ( 'NONE',  ( 21.68437500061451573, 4.541064518000418104, 2.621784821874999949 ) ) ;
#31731=CARTESIAN_POINT ( 'NONE',  ( 17.37187500061451573, -6.054752690667223547, -1.112240025338166033E-15 ) ) ;
#31733=ORIENTED_EDGE ( 'NONE', *, *, #38503, .F. ) ;
#31734=CARTESIAN_POINT ( 'NONE',  ( 17.24062500061451786, -3.027376345333614438, 5.243569643749998122 ) ) ;
#31735=CARTESIAN_POINT ( 'NONE',  ( 28.23750000122903359, 4.330127018922191873, 2.499999999999999556 ) ) ;
#31736=CARTESIAN_POINT ( 'NONE',  ( 17.07187500061451502, 3.027376345333613106, -5.243569643749998122 ) ) ;
#31737=CARTESIAN_POINT ( 'NONE',  ( 27.98437500061451289, 4.541064518000418104, 2.621784821874999949 ) ) ;
#31738=CARTESIAN_POINT ( 'NONE',  ( 4.828125000614518214, 6.421520780324663323E-16, -5.243569643749999010 ) ) ;
#31739=CARTESIAN_POINT ( 'NONE',  ( 20.39062500061451644, -3.027376345333614438, 5.243569643749998122 ) ) ;
#31740=CARTESIAN_POINT ( 'NONE',  ( 29.14687500061451075, -3.027376345333610441, -5.243569643749999898 ) ) ;
#31741=CARTESIAN_POINT ( 'NONE',  ( 2.121784821875001281, 12.75312500061451715, 33.67503911421598417 ) ) ;
#31742=CARTESIAN_POINT ( 'NONE',  ( 16.91250000122903430, 4.330127018922192761, -2.499999999999997780 ) ) ;
#31745=CARTESIAN_POINT ( 'NONE',  ( 7.903125000614515727, -4.541064518000417216, -2.621784821875001281 ) ) ;
#31746=CARTESIAN_POINT ( 'NONE',  ( 27.96562500061451928, 3.027376345333611329, 5.243569643749999010 ) ) ;
#31747=CARTESIAN_POINT ( 'NONE',  ( 9.787500001229036073, 4.330127018922191873, 2.499999999999999556 ) ) ;
#31748=CARTESIAN_POINT ( 'NONE',  ( 22.24687500061451217, -3.027376345333614438, 5.243569643749998122 ) ) ;
#31749=CARTESIAN_POINT ( 'NONE',  ( 11.61562500061451608, 3.027376345333613106, -5.243569643749998122 ) ) ;
#31750=CARTESIAN_POINT ( 'NONE',  ( 23.10000000122903074, -2.886751345948125991, -5.000000000000000000 ) ) ;
#31751=EDGE_CURVE ( 'NONE', #1870, #24236, #9392, .T. ) ;
#31752=CARTESIAN_POINT ( 'NONE',  ( 23.54062500061451146, -3.027376345333614438, 5.243569643749998122 ) ) ;
#31753=CARTESIAN_POINT ( 'NONE',  ( 18.64687500061451786, -3.027376345333614438, 5.243569643749998122 ) ) ;
#31754=CARTESIAN_POINT ( 'NONE',  ( 13.34062500061451750, -3.027376345333610441, -5.243569643749999898 ) ) ;
#31755=CARTESIAN_POINT ( 'NONE',  ( -4.243569643749997233, 15.39687500061451786, 32.45002607614398471 ) ) ;
#31756=CARTESIAN_POINT ( 'NONE',  ( 19.60312500061451502, -4.541064518000417216, -2.621784821875001281 ) ) ;
#31758=ORIENTED_EDGE ( 'NONE', *, *, #1146, .T. ) ;
#31760=CARTESIAN_POINT ( 'NONE',  ( 21.78750000000000142, 5.773502691896255534, 3.535250795749688894E-16 ) ) ;
#31761=CARTESIAN_POINT ( 'NONE',  ( 4.243569643749999898, 19.63437500061451857, -30.00000000000000000 ) ) ;
#31762=CARTESIAN_POINT ( 'NONE',  ( 1.071796769724488119, 17.99509619066137134, 33.99999999999999289 ) ) ;
#31763=CARTESIAN_POINT ( 'NONE',  ( 26.57812500061451644, 4.541064518000418104, 2.621784821874999949 ) ) ;
#31764=CARTESIAN_POINT ( 'NONE',  ( 5.878125000614517148, 4.541064518000418104, 2.621784821874999949 ) ) ;
#31765=CARTESIAN_POINT ( 'NONE',  ( 18.93750000122903288, -4.330127018922194537, 2.499999999999995559 ) ) ;
#31766=CARTESIAN_POINT ( 'NONE',  ( 25.64062500061451644, 6.054752690667223547, 3.707466751127219781E-16 ) ) ;
#31767=CARTESIAN_POINT ( 'NONE',  ( 23.96249999999999858, 2.886751345948129099, -4.999999999999998224 ) ) ;
#31768=EDGE_CURVE ( 'NONE', #7627, #6226, #34842, .T. ) ;
#31769=CARTESIAN_POINT ( 'NONE',  ( 27.92812500061451431, 4.541064518000418104, 2.621784821874999949 ) ) ;
#31770=CARTESIAN_POINT ( 'NONE',  ( 8.503125000614515372, 4.541064518000418104, -2.621784821874998173 ) ) ;
#31772=CARTESIAN_POINT ( 'NONE',  ( 22.67812500061451431, -4.541064518000419881, 2.621784821874995952 ) ) ;
#31773=CARTESIAN_POINT ( 'NONE',  ( 5.990625000614517859, -3.027376345333614438, 5.243569643749998122 ) ) ;
#31775=CARTESIAN_POINT ( 'NONE',  ( 2.803125000614518747, 0.000000000000000000, 5.243569643749999010 ) ) ;
#31776=CARTESIAN_POINT ( 'NONE',  ( -2.000000000000000000, 14.18750000122903288, -33.46410161513775705 ) ) ;
#31777=CARTESIAN_POINT ( 'NONE',  ( 11.58750000000000036, -2.886751345948129988, 4.999999999999997335 ) ) ;
#31778=CARTESIAN_POINT ( 'NONE',  ( 10.09687500061451715, -3.027376345333614438, 5.243569643749998122 ) ) ;
#31779=CARTESIAN_POINT ( 'NONE',  ( 6.300000001229033586, -2.886751345948129988, 4.999999999999997335 ) ) ;
#31780=CARTESIAN_POINT ( 'NONE',  ( 13.95937500061451786, 4.541064518000418104, -2.621784821874998173 ) ) ;
#31782=CARTESIAN_POINT ( 'NONE',  ( 5.821875000614519458, 3.027376345333613106, -5.243569643749998122 ) ) ;
#31783=CARTESIAN_POINT ( 'NONE',  ( -4.243569643749999898, 9.865625000614517859, -32.45002607614398471 ) ) ;
#31785=CARTESIAN_POINT ( 'NONE',  ( 11.93437500061451573, -4.541064518000419881, 2.621784821874995952 ) ) ;
#31786=CYLINDRICAL_SURFACE ( 'NONE', #54808, 3.999999999999996447 ) ;
#31787=CARTESIAN_POINT ( 'NONE',  ( 21.29062500061451502, -3.027376345333614438, 5.243569643749998122 ) ) ;
#31788=CARTESIAN_POINT ( 'NONE',  ( 4.243569643749999010, 11.12187500061451928, 27.54997392385601174 ) ) ;
#31789=CARTESIAN_POINT ( 'NONE',  ( 9.001249775931846008E-16, 18.56562500061459531, 34.90005215228797653 ) ) ;
#31790=CARTESIAN_POINT ( 'NONE',  ( 25.24687500061451573, 6.054752690667223547, 3.707466751127219781E-16 ) ) ;
#31792=CARTESIAN_POINT ( 'NONE',  ( 3.815625000614518036, -6.054752690667223547, -1.112240025338166033E-15 ) ) ;
#31794=CARTESIAN_POINT ( 'NONE',  ( 14.48437500061451821, 4.541064518000418104, 2.621784821874999949 ) ) ;
#31795=CARTESIAN_POINT ( 'NONE',  ( 29.92500000000000071, 4.330127018922191873, 2.499999999999999556 ) ) ;
#31796=CARTESIAN_POINT ( 'NONE',  ( 28.16250000122903074, 4.330127018922192761, -2.499999999999997780 ) ) ;
#31797=CARTESIAN_POINT ( 'NONE',  ( 4.996875000614516615, 6.054752690667223547, 3.707466751127219781E-16 ) ) ;
#31798=CARTESIAN_POINT ( 'NONE',  ( 17.74687500061451928, -3.027376345333614438, 5.243569643749998122 ) ) ;
#31800=CARTESIAN_POINT ( 'NONE',  ( 24.11249999999999716, 2.886751345948126879, 4.999999999999999112 ) ) ;
#31801=CARTESIAN_POINT ( 'NONE',  ( 2.962500001229034119, 4.330127018922192761, -2.499999999999997780 ) ) ;
#31802=CARTESIAN_POINT ( 'NONE',  ( 26.07187500061451857, 3.027376345333613106, -5.243569643749998122 ) ) ;
#31804=CARTESIAN_POINT ( 'NONE',  ( 14.32500000122903216, 2.886751345948193936, 4.999999999999883649 ) ) ;
#31805=CARTESIAN_POINT ( 'NONE',  ( 8.137500000000002842, -2.886751345948125991, -5.000000000000000000 ) ) ;
#31807=CARTESIAN_POINT ( 'NONE',  ( 21.89062500061451289, -3.027376345333610441, -5.243569643749999898 ) ) ;
#31808=CARTESIAN_POINT ( 'NONE',  ( 11.40000000000000036, 4.330127018922192761, -2.499999999999997780 ) ) ;
#31809=CARTESIAN_POINT ( 'NONE',  ( 4.003125000614518925, 4.541064518000418104, -2.621784821874998173 ) ) ;
#31810=CARTESIAN_POINT ( 'NONE',  ( 20.40000000000000213, 4.330127018922192761, -2.499999999999997780 ) ) ;
#31811=CARTESIAN_POINT ( 'NONE',  ( 17.91562500061451502, 3.027376345333613106, -5.243569643749998122 ) ) ;
#31812=CARTESIAN_POINT ( 'NONE',  ( -2.000000000000000000, 18.68750000122903288, 26.53589838486224650 ) ) ;
#31813=CARTESIAN_POINT ( 'NONE',  ( 22.76250000122903216, 4.330127018922192761, -2.499999999999997780 ) ) ;
#31815=CARTESIAN_POINT ( 'NONE',  ( 29.70937500061451431, 4.541064518000418104, -2.621784821874998173 ) ) ;
#31817=CARTESIAN_POINT ( 'NONE',  ( 19.64062500061451644, -3.027376345333610441, -5.243569643749999898 ) ) ;
#31818=CARTESIAN_POINT ( 'NONE',  ( 24.92812500061451431, -4.541064518000419881, 2.621784821874995952 ) ) ;
#31819=CARTESIAN_POINT ( 'NONE',  ( 25.47187500061451715, -6.054752690667223547, -1.112240025338166033E-15 ) ) ;
#31820=CARTESIAN_POINT ( 'NONE',  ( 9.487500000000000711, -2.886751345948125991, -5.000000000000000000 ) ) ;
#31821=CARTESIAN_POINT ( 'NONE',  ( 12.40312500061451573, -4.541064518000417216, -2.621784821875001281 ) ) ;
#31822=CARTESIAN_POINT ( 'NONE',  ( 25.90312500061451573, -4.541064518000417216, -2.621784821875001281 ) ) ;
#31823=CARTESIAN_POINT ( 'NONE',  ( 17.59687500061451715, 6.054752690667223547, 3.707466751127219781E-16 ) ) ;
#31824=CARTESIAN_POINT ( 'NONE',  ( 7.978125000614517681, 6.421520780324663323E-16, -5.243569643749999010 ) ) ;
#31826=CARTESIAN_POINT ( 'NONE',  ( -4.243569643749999898, 10.85937500061451821, 30.00000000000000000 ) ) ;
#31827=CARTESIAN_POINT ( 'NONE',  ( 23.02500000122903145, -5.773502691896255534, -1.060575238724906372E-15 ) ) ;
#31829=CARTESIAN_POINT ( 'NONE',  ( 14.91562500061451679, 3.027376345333611329, 5.243569643749999010 ) ) ;
#31830=CARTESIAN_POINT ( 'NONE',  ( 8.184375000614515727, 4.541064518000418104, 2.621784821874999949 ) ) ;
#31831=CARTESIAN_POINT ( 'NONE',  ( 6.196875000614515905, -3.027376345333610441, -5.243569643749999898 ) ) ;
#31832=ORIENTED_EDGE ( 'NONE', *, *, #22734, .F. ) ;
#31833=CARTESIAN_POINT ( 'NONE',  ( -4.112406224592624504, 9.116497278081070021, 34.37320649897247193 ) ) ;
#31834=CARTESIAN_POINT ( 'NONE',  ( 22.00312500061451360, 4.541064518000418104, -2.621784821874998173 ) ) ;
#31835=( BOUNDED_SURFACE ( )  B_SPLINE_SURFACE ( 1, 2, ( 
 ( #16186, #55720, #33181, #50184, #67183, #39458, #72712, #22095, #4397, #10290, #28366, #72343, #61613, #16544, #67540, #39096, #11381, #60885, #49819, #5478, #4752, #26926, #11015, #17269, #44653, #33536, #43913, #5114, #33900, #56086, #61979, #28017, #27648, #50545, #32456, #49451, #66813, #67897, #9918, #16903, #38358, #73073, #21724, #27285, #22454, #44283, #56444, #5834, #50902, #32820, #39830, #38737, #301, #71985, #22811, #61257, #45362, #54991, #21359, #66438, #63786, #19073, #62345, #17626, #51631, #11741, #30180, #2117, #51265, #18710, #1032, #29454, #23901, #40919, #52711, #12464, #24629, #6924, #51991, #57876, #23538, #69707, #1392, #46815, #47174, #46449, #29096, #1753, #6564, #34258, #7286, #29815, #68987, #52350, #69353, #18344, #56791, #24266, #28724, #40186, #63431, #6196, #46088, #12818, #41275, #68624, #35352, #63061, #13176, #17986, #57523, #40545, #35715, #667, #58237, #7642, #23175, #45729, #34994, #68264, #62707, #12101, #34622, #57153, #64886, #54180, #13912, #53814, #36812, #36451, #20172, #48273, #36084, #8738, #70797, #25363, #42726, #65247, #9109, #14274, #14636, #58604, #58965, #54542, #2834, #59327, #19811, #13536, #24992, #25736, #30902, #37177, #31647, #53444, #31271, #8373, #41999, #59702, #47907, #3576, #20535, #43091, #64149, #26099, #3207, #8011, #48637, #2468, #9478, #64519, #41630, #71162, #65619, #15007, #70436, #42364, #30546, #53073, #26467, #37544, #60066, #32007, #3944, #49006, #71537, #47536, #70065, #19438, #60799, #33456, #38271, #5756, #16458, #61531, #33098, #39016, #5394, #27568, #15369, #10929, #60428, #71903, #10570, #37911, #10205, #55637, #50464, #55277, #5031, #21642, #27931, #32740, #16101, #4672, #67100, #56366, #56000, #72992, #44925, #22373, #27202, #67461, #66730, #16824, #28290, #49737, #44199, #39378, #66355, #50100, #38651, #15732, #72630, #22014, #9839, #61175, #44570, #72264, #61897, #11302, #33823, #50821, #20912, #32368, #43464, #65988, #54906, #4314, #26839, #49373, #21276, #43830, #62620, #29373, #63344, #12016, #23457, #40106, #586, #1304, #6476, #12730, #52264, #1666, #22729, #40828, #17900, #39749, #68539, #34176, #41189, #23091, #224, #7197, #35266, #51905, #45648, #34539, #67816, #45282, #58148, #57788, #34907, #17189, #24175, #6113, #29726, #29011, #57069, #46727, #69262, #30087, #62266, #28644, #51548, #11661, #63698, #13089, #56712, #18624, #949, #40460, #57435, #23813, #35627, #46003, #7553, #62976, #51182, #12372, #68182, #46364, #17545, #68898, #6838, #18255, #2030, #47086, #36360, #37458, #52625, #14548, #7919, #70703, #19346, #47444, #42634, #69976, #54093, #47811, #2745, #30456, #9387, #52985, #69619, #65158, #20078, #58508, #25264, #41903, #2381, #53720, #65530, #70341, #19717, #31553, #59977, #64428, #24541, #25642, #18981, #42269, #14916, #24899, #3112, #48547, #64792, #71074, #14183, #13820, #41542, #9022, #59239, #8648, #37084, #58874, #36718, #8284, #64060, #59608, #31177, #30814, #13441, #48179, #3490, #35990, #20449, #26008, #53347, #42999, #43737, #4583, #50379, #10117, #66633, #44479, #26749, #67010, #37819, #22286, #26375, #15639, #16011, #49282, #33374, #48914, #71445, #67373, #16371, #4221, #32647, #38926, #72535, #31918, #4944, #44838, #61445, #49646, #55188, #61805, #38180, #27113, #72173, #21553, #38559, #10839, #44107, #61082, #20820, #32281, #72904, #21186, #10480, #33009, #55910, #55548, #5303, #9747, #71815, #27478, #66262, #43375, #50011, #39291, #21923, #27848, #60704, #16736, #54454, #3853, #65899, #15279, #60338, #54815, #28917, #11927, #41101, #17458, #56980, #34452, #51455, #68445, #40736, #858, #23365, #5670, #11574, #29638, #491, #62886, #17807, #46272, #40368, #12644, #62177, #51094, #6750, #6025, #28206, #12281, #18537, #45913, #34814, #45193, #6384, #35180, #57344, #63252, #29283, #51813, #1216, #33735, #50735, #68091, #69176, #11208, #68811, #39658, #23722, #23000, #28559, #18167, #45560, #57704, #7109, #52176, #34089, #56281, #56630, #137, #1578, #24087, #17098, #46634, #40016, #62530, #22643, #67725, #13732, #30727, #42546, #70987, #30370, #63611, #36632, #58059, #53259, #25923, #13356, #64708, #59520, #2657, #8933, #58788, #52899, #29994, #19993, #70254, #19627, #53629, #69890, #36274, #47358, #20363, #70619, #8198, #63973, #35539, #42183, #59154, #1944, #31463, #36997, #7468, #25552, #2297, #25175, #54006, #41810, #47716, #3021, #58421, #48095, #69534, #3402, #52535, #19255, #14092, #7833, #65073, #24450, #46999, #48463, #14464, #24812, #8562, #64340, #31090, #13002, #18893, #41455, #35897, #60994, #26663, #38468, #15551, #55463, #50294, #54730, #66175, #4855, #15191, #55100, #38094, #37729, #21464, #49560, #37370, #10026, #72081, #49197, #44018, #66540, #10393, #60617, #15920, #59893, #60249, #55825, #4133, #32562, #21100, #14828, #26288, #27029, #32197, #32925, #27389, #71730, #4500, #9664, #43289, #49921, #43651, #72445, #21829, #44394, #65437, #66919, #16288, #9298, #38843, #3764, #10755, #65809, #42914, #61358, #33286, #5213, #27754, #72817, #31831, #54369, #48825, #71356, #20730, #16647, #1131, #28119, #51730, #51004, #11482, #46186, #23640, #52090, #22200, #50648, #34005, #44754, #63165, #35095, #11116, #68725, #56542, #62444, #56893, #768, #12560, #45468, #57620, #39930, #11842, #17723, #5935, #29554, #34361, #6668, #7023, #6298, #62089, #34724, #39564, #67288, #40283, #62804, #28827, #12197, #29196, #51366, #39203, #57254, #61717, #52, #23276, #33645, #28469, #45826, #18085, #402, #68362, #22910, #40646, #56189, #5582, #67641, #68000, #22557, #45105, #17007, #17373, #64987, #8473, #19171, #2214, #31377, #7745, #47272, #24729, #41726, #58703, #31007, #64253, #13641, #69090, #1859, #19912, #63883, #53173, #8114, #36549, #30641 ),
 ( #59433, #64623, #36185, #18451, #53540, #7382, #2936, #30281, #13274, #25465, #48009, #1495, #24001, #29913, #35812, #46549, #42465, #14378, #63531, #70537, #58334, #2570, #25090, #47633, #36913, #69806, #8841, #70166, #19543, #42101, #52814, #41016, #14010, #59068, #12918, #35451, #41373, #57975, #18809, #52453, #24366, #46913, #69452, #73007, #39395, #61547, #48375, #22391, #20274, #31746, #44586, #70902, #43200, #67118, #11319, #15106, #16475, #54640, #61914, #71263, #50117, #65720, #27948, #17206, #50481, #44940, #5774, #67478, #37642, #16841, #26570, #33840, #62284, #60165, #4045, #56381, #26201, #39033, #54283, #20643, #28305, #48740, #42826, #10949, #11679, #22029, #33470, #14740, #72646, #50840, #56018, #240, #5410, #22748, #45299, #3311, #65350, #9575, #39767, #53918, #67833, #9210, #25838, #32107, #37282, #59804, #3677, #35644, #29390, #57452, #62638, #64077, #34558, #28662, #46746, #1683, #40123, #24558, #34195, #68915, #12748, #47104, #6856, #69636, #51924, #1321, #29744, #68557, #41559, #23830, #18642, #18998, #46381, #965, #69280, #51565, #56729, #52281, #24192, #18272, #41206, #63714, #40846, #51201, #13106, #603, #12033, #63364, #23109, #23475, #35284, #58166, #17916, #57806, #34925, #7570, #46021, #7215, #40479, #30106, #6131, #52640, #2047, #45666, #68199, #62994, #17562, #57086, #6494, #29029, #12389, #36738, #26026, #58893, #25662, #8667, #8303, #65177, #20096, #7936, #53740, #42653, #70361, #14568, #37101, #54109, #59258, #59627, #30474, #30833, #26393, #47831, #31198, #64812, #58526, #69994, #70721, #2763, #9040, #3507, #25285, #3133, #53366, #13838, #31570, #19738, #42288, #48565, #19363, #3870, #53003, #14202, #71091, #48198, #14936, #2398, #24919, #48935, #20465, #43019, #65547, #37475, #59995, #13459, #9405, #71464, #31935, #54472, #20840, #43394, #36007, #47461, #41921, #64446, #36377, #22303, #33028, #4962, #60356, #66281, #11228, #55208, #44497, #72554, #27864, #21942, #67391, #43756, #32667, #61463, #60724, #9765, #67030, #154, #55567, #27495, #26768, #16030, #16753, #16389, #44855, #38945, #38578, #10500, #15297, #32299, #49665, #50751, #65916, #50396, #21204, #10858, #4601, #10135, #55927, #27132, #39311, #61102, #50029, #15659, #22660, #38198, #54834, #5323, #33391, #72921, #37836, #61823, #72193, #33751, #5686, #56296, #28221, #4241, #49300, #21572, #71834, #44126, #66653, #34835, #7484, #68109, #46288, #41118, #57361, #63629, #40386, #34470, #11591, #1594, #51831, #1235, #35198, #51474, #17825, #28937, #1962, #52193, #68463, #45577, #17116, #23740, #18185, #56647, #13018, #18553, #62195, #7126, #56998, #62905, #35556, #23383, #6768, #57721, #68829, #58076, #29301, #30013, #12299, #6405, #34108, #24105, #40755, #63270, #29656, #876, #12662, #45932, #45210, #46653, #69193, #17475, #39675, #52556, #67744, #6042, #28576, #51113, #510, #23021, #40035, #62549, #11945, #2675, #59171, #37014, #19274, #59538, #30387, #14847, #18912, #8215, #8579, #41828, #25939, #41472, #63992, #59910, #8948, #69907, #25191, #31482, #65089, #24469, #70634, #37386, #54024, #42201, #47735, #54385, #30744, #70274, #19645, #64725, #31108, #3419, #14110, #36649, #13373, #24829, #42930, #13749, #3040, #53647, #48479, #25571, #71003, #2314, #64359, #20009, #36291, #35915, #48111, #31849, #42562, #14480, #58440, #20379, #65454, #9316, #47017, #69552, #7851, #52916, #47377, #58805, #53276, #61733, #3780, #38859, #32213, #21847, #43670, #71747, #66936, #21117, #5230, #72099, #27046, #54747, #33662, #4149, #71373, #16305, #44410, #61374, #26305, #10771, #49213, #4871, #16663, #49577, #44036, #55842, #11134, #66193, #48842, #49938, #20748, #66558, #39221, #26681, #43305, #72462, #33304, #27771, #50311, #60634, #72833, #21484, #22216, #65826, #15571, #15938, #44770, #38113, #38487, #61011, #10046, #55479, #10409, #15208, #32941, #27407, #32580, #67305, #37748, #60266, #9680, #55118, #4517, #28485, #69106, #17390, #51383, #34378, #28136, #39582, #40299, #45485, #12213, #46201, #68017, #6315, #22927, #56558, #57272, #62460, #68742, #35110, #57634, #5599, #23657, #785, #22574, #23294, #17023, #24015, #5953, #56206, #63181, #18100, #34742, #51022, #39947, #50664, #68, #41031, #40661, #17740, #45122, #7040, #62106, #12576, #11858, #56910, #29570, #52106, #12933, #67657, #11499, #28844, #34021, #46564, #18468, #1511, #62821, #63547, #418, #6683, #29211, #45843, #68379, #51747, #1148, #53189, #31022, #69822, #42845, #25105, #19928, #25855, #47649, #2231, #48027, #52829, #20290, #53556, #2953, #70181, #25481, #42482, #42115, #29928, #70553, #1875, #13290, #19559, #52468, #24744, #64639, #65005, #19188, #14025, #36200, #14393, #47288, #30657, #41741, #8489, #36930, #59451, #36565, #24381, #8858, #46929, #35827, #59085, #69467, #64269, #31394, #53934, #13658, #3329, #58718, #48392, #8130, #2586, #70920, #65366, #35468, #57990, #7400, #18825, #41388, #63900, #58350, #7761, #30297, #22128, #26586, #38024, #27317, #60182, #26957, #9954, #9591, #66470, #21391, #9227, #55025, #43947, #71655, #15847, #38393, #55389, #60547, #60917, #31764, #32123, #27679, #49126, #32490, #66102, #59822, #71281, #72015, #4060, #10320, #4783, #21028, #4428, #54657, #15122, #32852, #43581, #49849, #66846, #16216, #37299, #72375, #49484, #54301, #21755, #48757, #55750, #37659, #14755, #44316, #38769, #61288, #15481, #10681, #3693, #26218, #72742, #33211, #5144, #20658, #50217, #43217, #44683, #65737, #56474, #18020, #68655, #23931, #67214, #22486, #5866, #16575, #35025, #6955, #1064, #51297, #57553, #39127, #28757, #45760, #29486, #17303, #52023, #11774, #34290, #62738, #28398, #1425, #56822, #51662, #61642, #6229, #33932, #6599, #11415, #11044, #12130, #34657, #698, #62013, #40576, #33570 ) ),
 .UNSPECIFIED., .F., .F., .F. ) 
 B_SPLINE_SURFACE_WITH_KNOTS ( ( 2, 2 ),
 ( 3, 2, 2, 2, 2, 2, 2, 2, 2, 2, 2, 2, 2, 2, 2, 2, 2, 2, 2, 2, 2, 2, 2, 2, 2, 2, 2, 2, 2, 2, 2, 2, 2, 2, 2, 2, 2, 2, 2, 2, 2, 2, 2, 2, 2, 2, 2, 2, 2, 2, 2, 2, 2, 2, 2, 2, 2, 2, 2, 2, 2, 2, 2, 2, 2, 2, 2, 2, 2, 2, 2, 2, 2, 2, 2, 2, 2, 2, 2, 2, 2, 2, 2, 2, 2, 2, 2, 2, 2, 2, 2, 2, 2, 2, 2, 2, 2, 2, 2, 2, 2, 2, 2, 2, 2, 2, 2, 2, 2, 2, 2, 2, 2, 2, 2, 2, 2, 2, 2, 2, 2, 2, 2, 2, 2, 2, 2, 2, 2, 2, 2, 2, 2, 2, 2, 2, 2, 2, 2, 2, 2, 2, 2, 2, 2, 2, 2, 2, 2, 2, 2, 2, 2, 2, 2, 2, 2, 2, 2, 2, 2, 2, 2, 2, 2, 2, 2, 2, 2, 2, 2, 2, 2, 2, 2, 2, 2, 2, 2, 2, 2, 2, 2, 2, 2, 2, 2, 2, 2, 2, 2, 2, 2, 2, 2, 2, 2, 2, 2, 2, 2, 2, 2, 2, 2, 2, 2, 2, 2, 2, 2, 2, 2, 2, 2, 2, 2, 2, 2, 2, 2, 2, 2, 2, 2, 2, 2, 2, 2, 2, 2, 2, 2, 2, 2, 2, 2, 2, 2, 2, 2, 2, 2, 2, 2, 2, 2, 2, 2, 2, 2, 2, 2, 2, 2, 2, 2, 2, 2, 2, 2, 2, 2, 2, 2, 2, 2, 2, 2, 2, 2, 2, 2, 2, 2, 2, 2, 2, 2, 2, 2, 2, 2, 2, 2, 2, 2, 2, 2, 2, 2, 2, 2, 2, 2, 2, 2, 2, 2, 2, 2, 2, 2, 2, 2, 2, 2, 2, 2, 2, 2, 2, 2, 2, 2, 2, 2, 2, 2, 2, 2, 2, 2, 2, 2, 2, 2, 2, 2, 2, 2, 2, 2, 2, 2, 2, 2, 2, 2, 2, 2, 2, 2, 2, 2, 2, 2, 2, 2, 2, 2, 2, 2, 2, 2, 2, 2, 2, 2, 2, 3 ),
 ( 0.000000000000000000, 1.000000000000000000 ),
 ( 0.000000000000000000, 0.002777777777777777884, 0.005555555555555555768, 0.008333333333333333218, 0.01111111111111111154, 0.01388888888888888812, 0.01666666666666666644, 0.01944444444444444475, 0.02222222222222222307, 0.02500000000000000139, 0.02777777777777777624, 0.03055555555555555455, 0.03333333333333333287, 0.03611111111111110772, 0.03888888888888888951, 0.04166666666666666435, 0.04444444444444444614, 0.04722222222222222099, 0.05000000000000000278, 0.05277777777777777762, 0.05555555555555555247, 0.05833333333333333426, 0.06111111111111110911, 0.06388888888888888395, 0.06666666666666666574, 0.06944444444444444753, 0.07222222222222221544, 0.07499999999999999722, 0.07777777777777777901, 0.08055555555555556080, 0.08333333333333332871, 0.08611111111111111049, 0.08888888888888889228, 0.09166666666666666019, 0.09444444444444444198, 0.09722222222222222376, 0.1000000000000000056, 0.1027777777777777735, 0.1055555555555555552, 0.1083333333333333370, 0.1111111111111111049, 0.1138888888888888867, 0.1166666666666666685, 0.1194444444444444503, 0.1222222222222222182, 0.1250000000000000000, 0.1277777777777777679, 0.1305555555555555636, 0.1333333333333333315, 0.1361111111111110994, 0.1388888888888888951, 0.1416666666666666630, 0.1444444444444444309, 0.1472222222222222265, 0.1499999999999999944, 0.1527777777777777901, 0.1555555555555555580, 0.1583333333333333259, 0.1611111111111111216, 0.1638888888888888895, 0.1666666666666666574, 0.1694444444444444531, 0.1722222222222222210, 0.1749999999999999889, 0.1777777777777777846, 0.1805555555555555525, 0.1833333333333333204, 0.1861111111111111160, 0.1888888888888888840, 0.1916666666666666796, 0.1944444444444444475, 0.1972222222222222154, 0.2000000000000000111, 0.2027777777777777790, 0.2055555555555555469, 0.2083333333333333426, 0.2111111111111111105, 0.2138888888888888784, 0.2166666666666666741, 0.2194444444444444420, 0.2222222222222222099, 0.2250000000000000056, 0.2277777777777777735, 0.2305555555555555691, 0.2333333333333333370, 0.2361111111111111049, 0.2388888888888889006, 0.2416666666666666685, 0.2444444444444444364, 0.2472222222222222321, 0.2500000000000000000, 0.2527777777777777679, 0.2555555555555555358, 0.2583333333333333592, 0.2611111111111111271, 0.2638888888888888951, 0.2666666666666666630, 0.2694444444444444309, 0.2722222222222221988, 0.2750000000000000222, 0.2777777777777777901, 0.2805555555555555580, 0.2833333333333333259, 0.2861111111111110938, 0.2888888888888888618, 0.2916666666666666852, 0.2944444444444444531, 0.2972222222222222210, 0.2999999999999999889, 0.3027777777777777568, 0.3055555555555555802, 0.3083333333333333481, 0.3111111111111111160, 0.3138888888888888840, 0.3166666666666666519, 0.3194444444444444198, 0.3222222222222222432, 0.3250000000000000111, 0.3277777777777777790, 0.3305555555555555469, 0.3333333333333333148, 0.3361111111111111382, 0.3388888888888889062, 0.3416666666666666741, 0.3444444444444444420, 0.3472222222222222099, 0.3499999999999999778, 0.3527777777777778012, 0.3555555555555555691, 0.3583333333333333370, 0.3611111111111111049, 0.3638888888888888729, 0.3666666666666666408, 0.3694444444444444642, 0.3722222222222222321, 0.3750000000000000000, 0.3777777777777777679, 0.3805555555555555358, 0.3833333333333333592, 0.3861111111111111271, 0.3888888888888888951, 0.3916666666666666630, 0.3944444444444444309, 0.3972222222222221988, 0.4000000000000000222, 0.4027777777777777901, 0.4055555555555555580, 0.4083333333333333259, 0.4111111111111110938, 0.4138888888888888618, 0.4166666666666666852, 0.4194444444444444531, 0.4222222222222222210, 0.4249999999999999889, 0.4277777777777777568, 0.4305555555555555802, 0.4333333333333333481, 0.4361111111111111160, 0.4388888888888888840, 0.4416666666666666519, 0.4444444444444444198, 0.4472222222222222432, 0.4500000000000000111, 0.4527777777777777790, 0.4555555555555555469, 0.4583333333333333148, 0.4611111111111111382, 0.4638888888888889062, 0.4666666666666666741, 0.4694444444444444420, 0.4722222222222222099, 0.4749999999999999778, 0.4777777777777778012, 0.4805555555555555691, 0.4833333333333333370, 0.4861111111111111049, 0.4888888888888888729, 0.4916666666666666408, 0.4944444444444444642, 0.4972222222222222321, 0.5000000000000000000, 0.5027777777777777679, 0.5055555555555555358, 0.5083333333333333037, 0.5111111111111110716, 0.5138888888888888395, 0.5166666666666667185, 0.5194444444444444864, 0.5222222222222222543, 0.5250000000000000222, 0.5277777777777777901, 0.5305555555555555580, 0.5333333333333333259, 0.5361111111111110938, 0.5388888888888888618, 0.5416666666666666297, 0.5444444444444443976, 0.5472222222222222765, 0.5500000000000000444, 0.5527777777777778123, 0.5555555555555555802, 0.5583333333333333481, 0.5611111111111111160, 0.5638888888888888840, 0.5666666666666666519, 0.5694444444444444198, 0.5722222222222221877, 0.5749999999999999556, 0.5777777777777777235, 0.5805555555555556024, 0.5833333333333333703, 0.5861111111111111382, 0.5888888888888889062, 0.5916666666666666741, 0.5944444444444444420, 0.5972222222222222099, 0.5999999999999999778, 0.6027777777777777457, 0.6055555555555555136, 0.6083333333333332815, 0.6111111111111111605, 0.6138888888888889284, 0.6166666666666666963, 0.6194444444444444642, 0.6222222222222222321, 0.6250000000000000000, 0.6277777777777777679, 0.6305555555555555358, 0.6333333333333333037, 0.6361111111111110716, 0.6388888888888888395, 0.6416666666666667185, 0.6444444444444444864, 0.6472222222222222543, 0.6500000000000000222, 0.6527777777777777901, 0.6555555555555555580, 0.6583333333333333259, 0.6611111111111110938, 0.6638888888888888618, 0.6666666666666666297, 0.6694444444444443976, 0.6722222222222222765, 0.6750000000000000444, 0.6777777777777778123, 0.6805555555555555802, 0.6833333333333333481, 0.6861111111111111160, 0.6888888888888888840, 0.6916666666666666519, 0.6944444444444444198, 0.6972222222222221877, 0.6999999999999999556, 0.7027777777777777235, 0.7055555555555556024, 0.7083333333333333703, 0.7111111111111111382, 0.7138888888888889062, 0.7166666666666666741, 0.7194444444444444420, 0.7222222222222222099, 0.7249999999999999778, 0.7277777777777777457, 0.7305555555555555136, 0.7333333333333332815, 0.7361111111111111605, 0.7388888888888889284, 0.7416666666666666963, 0.7444444444444444642, 0.7472222222222222321, 0.7500000000000000000, 0.7527777777777777679, 0.7555555555555555358, 0.7583333333333333037, 0.7611111111111110716, 0.7638888888888888395, 0.7666666666666667185, 0.7694444444444444864, 0.7722222222222222543, 0.7750000000000000222, 0.7777777777777777901, 0.7805555555555555580, 0.7833333333333333259, 0.7861111111111110938, 0.7888888888888888618, 0.7916666666666666297, 0.7944444444444443976, 0.7972222222222222765, 0.8000000000000000444, 0.8027777777777778123, 0.8055555555555555802, 0.8083333333333333481, 0.8111111111111111160, 0.8138888888888888840, 0.8166666666666666519, 0.8194444444444444198, 0.8222222222222221877, 0.8249999999999999556, 0.8277777777777777235, 0.8305555555555556024, 0.8333333333333333703, 0.8361111111111111382, 0.8388888888888889062, 0.8416666666666666741, 0.8444444444444444420, 0.8472222222222222099, 0.8499999999999999778, 0.8527777777777777457, 0.8555555555555555136, 0.8583333333333332815, 0.8611111111111111605, 0.8638888888888889284, 0.8666666666666666963, 0.8694444444444444642, 0.8722222222222222321, 0.8750000000000000000, 0.8777777777777777679, 0.8805555555555555358, 0.8833333333333333037, 0.8861111111111110716, 0.8888888888888888395, 0.8916666666666667185, 0.8944444444444444864, 0.8972222222222222543, 0.9000000000000000222, 0.9027777777777777901, 0.9055555555555555580, 0.9083333333333333259, 0.9111111111111110938, 0.9138888888888888618, 0.9166666666666666297, 0.9194444444444443976, 0.9222222222222222765, 0.9250000000000000444, 0.9277777777777778123, 0.9305555555555555802, 0.9333333333333333481, 0.9361111111111111160, 0.9388888888888888840, 0.9416666666666666519, 0.9444444444444444198, 0.9472222222222221877, 0.9499999999999999556, 0.9527777777777777235, 0.9555555555555556024, 0.9583333333333333703, 0.9611111111111111382, 0.9638888888888889062, 0.9666666666666666741, 0.9694444444444444420, 0.9722222222222222099, 0.9749999999999999778, 0.9777777777777777457, 0.9805555555555555136, 0.9833333333333332815, 0.9861111111111111605, 0.9888888888888889284, 0.9916666666666666963, 0.9944444444444444642, 0.9972222222222222321, 1.000000000000000000 ),
 .UNSPECIFIED. ) 
 GEOMETRIC_REPRESENTATION_ITEM ( )  RATIONAL_B_SPLINE_SURFACE ( (
 ( 1.000000000000000000, 0.8660254037844387076, 1.000000000000000000, 0.8660254037844387076, 1.000000000000000000, 0.8660254037844387076, 1.000000000000000000, 0.8660254037844387076, 1.000000000000000000, 0.8660254037844387076, 1.000000000000000000, 0.8660254037844387076, 1.000000000000000000, 0.8660254037844387076, 1.000000000000000000, 0.8660254037844387076, 1.000000000000000000, 0.8660254037844387076, 1.000000000000000000, 0.8660254037844387076, 1.000000000000000000, 0.8660254037844387076, 1.000000000000000000, 0.8660254037844387076, 1.000000000000000000, 0.8660254037844387076, 1.000000000000000000, 0.8660254037844387076, 1.000000000000000000, 0.8660254037844387076, 1.000000000000000000, 0.8660254037844387076, 1.000000000000000000, 0.8660254037844387076, 1.000000000000000000, 0.8660254037844387076, 1.000000000000000000, 0.8660254037844387076, 1.000000000000000000, 0.8660254037844387076, 1.000000000000000000, 0.8660254037844387076, 1.000000000000000000, 0.8660254037844387076, 1.000000000000000000, 0.8660254037844387076, 1.000000000000000000, 0.8660254037844387076, 1.000000000000000000, 0.8660254037844387076, 1.000000000000000000, 0.8660254037844387076, 1.000000000000000000, 0.8660254037844387076, 1.000000000000000000, 0.8660254037844387076, 1.000000000000000000, 0.8660254037844387076, 1.000000000000000000, 0.8660254037844387076, 1.000000000000000000, 0.8660254037844387076, 1.000000000000000000, 0.8660254037844387076, 1.000000000000000000, 0.8660254037844387076, 1.000000000000000000, 0.8660254037844387076, 1.000000000000000000, 0.8660254037844387076, 1.000000000000000000, 0.8660254037844387076, 1.000000000000000000, 0.8660254037844387076, 1.000000000000000000, 0.8660254037844387076, 1.000000000000000000, 0.8660254037844387076, 1.000000000000000000, 0.8660254037844387076, 1.000000000000000000, 0.8660254037844387076, 1.000000000000000000, 0.8660254037844387076, 1.000000000000000000, 0.8660254037844387076, 1.000000000000000000, 0.8660254037844387076, 1.000000000000000000, 0.8660254037844387076, 1.000000000000000000, 0.8660254037844387076, 1.000000000000000000, 0.8660254037844387076, 1.000000000000000000, 0.8660254037844387076, 1.000000000000000000, 0.8660254037844387076, 1.000000000000000000, 0.8660254037844387076, 1.000000000000000000, 0.8660254037844387076, 1.000000000000000000, 0.8660254037844387076, 1.000000000000000000, 0.8660254037844387076, 1.000000000000000000, 0.8660254037844387076, 1.000000000000000000, 0.8660254037844387076, 1.000000000000000000, 0.8660254037844387076, 1.000000000000000000, 0.8660254037844387076, 1.000000000000000000, 0.8660254037844387076, 1.000000000000000000, 0.8660254037844387076, 1.000000000000000000, 0.8660254037844387076, 1.000000000000000000, 0.8660254037844387076, 1.000000000000000000, 0.8660254037844387076, 1.000000000000000000, 0.8660254037844387076, 1.000000000000000000, 0.8660254037844387076, 1.000000000000000000, 0.8660254037844387076, 1.000000000000000000, 0.8660254037844387076, 1.000000000000000000, 0.8660254037844387076, 1.000000000000000000, 0.8660254037844387076, 1.000000000000000000, 0.8660254037844387076, 1.000000000000000000, 0.8660254037844387076, 1.000000000000000000, 0.8660254037844387076, 1.000000000000000000, 0.8660254037844387076, 1.000000000000000000, 0.8660254037844387076, 1.000000000000000000, 0.8660254037844387076, 1.000000000000000000, 0.8660254037844387076, 1.000000000000000000, 0.8660254037844387076, 1.000000000000000000, 0.8660254037844387076, 1.000000000000000000, 0.8660254037844387076, 1.000000000000000000, 0.8660254037844387076, 1.000000000000000000, 0.8660254037844387076, 1.000000000000000000, 0.8660254037844387076, 1.000000000000000000, 0.8660254037844387076, 1.000000000000000000, 0.8660254037844387076, 1.000000000000000000, 0.8660254037844387076, 1.000000000000000000, 0.8660254037844387076, 1.000000000000000000, 0.8660254037844387076, 1.000000000000000000, 0.8660254037844387076, 1.000000000000000000, 0.8660254037844387076, 1.000000000000000000, 0.8660254037844387076, 1.000000000000000000, 0.8660254037844387076, 1.000000000000000000, 0.8660254037844387076, 1.000000000000000000, 0.8660254037844387076, 1.000000000000000000, 0.8660254037844387076, 1.000000000000000000, 0.8660254037844387076, 1.000000000000000000, 0.8660254037844387076, 1.000000000000000000, 0.8660254037844387076, 1.000000000000000000, 0.8660254037844387076, 1.000000000000000000, 0.8660254037844387076, 1.000000000000000000, 0.8660254037844387076, 1.000000000000000000, 0.8660254037844387076, 1.000000000000000000, 0.8660254037844387076, 1.000000000000000000, 0.8660254037844387076, 1.000000000000000000, 0.8660254037844387076, 1.000000000000000000, 0.8660254037844387076, 1.000000000000000000, 0.8660254037844387076, 1.000000000000000000, 0.8660254037844387076, 1.000000000000000000, 0.8660254037844387076, 1.000000000000000000, 0.8660254037844387076, 1.000000000000000000, 0.8660254037844387076, 1.000000000000000000, 0.8660254037844387076, 1.000000000000000000, 0.8660254037844387076, 1.000000000000000000, 0.8660254037844387076, 1.000000000000000000, 0.8660254037844387076, 1.000000000000000000, 0.8660254037844387076, 1.000000000000000000, 0.8660254037844387076, 1.000000000000000000, 0.8660254037844387076, 1.000000000000000000, 0.8660254037844387076, 1.000000000000000000, 0.8660254037844387076, 1.000000000000000000, 0.8660254037844387076, 1.000000000000000000, 0.8660254037844387076, 1.000000000000000000, 0.8660254037844387076, 1.000000000000000000, 0.8660254037844387076, 1.000000000000000000, 0.8660254037844387076, 1.000000000000000000, 0.8660254037844387076, 1.000000000000000000, 0.8660254037844387076, 1.000000000000000000, 0.8660254037844387076, 1.000000000000000000, 0.8660254037844387076, 1.000000000000000000, 0.8660254037844387076, 1.000000000000000000, 0.8660254037844387076, 1.000000000000000000, 0.8660254037844387076, 1.000000000000000000, 0.8660254037844387076, 1.000000000000000000, 0.8660254037844387076, 1.000000000000000000, 0.8660254037844387076, 1.000000000000000000, 0.8660254037844387076, 1.000000000000000000, 0.8660254037844387076, 1.000000000000000000, 0.8660254037844387076, 1.000000000000000000, 0.8660254037844387076, 1.000000000000000000, 0.8660254037844387076, 1.000000000000000000, 0.8660254037844387076, 1.000000000000000000, 0.8660254037844387076, 1.000000000000000000, 0.8660254037844387076, 1.000000000000000000, 0.8660254037844387076, 1.000000000000000000, 0.8660254037844387076, 1.000000000000000000, 0.8660254037844387076, 1.000000000000000000, 0.8660254037844387076, 1.000000000000000000, 0.8660254037844387076, 1.000000000000000000, 0.8660254037844387076, 1.000000000000000000, 0.8660254037844387076, 1.000000000000000000, 0.8660254037844387076, 1.000000000000000000, 0.8660254037844387076, 1.000000000000000000, 0.8660254037844387076, 1.000000000000000000, 0.8660254037844387076, 1.000000000000000000, 0.8660254037844387076, 1.000000000000000000, 0.8660254037844387076, 1.000000000000000000, 0.8660254037844387076, 1.000000000000000000, 0.8660254037844387076, 1.000000000000000000, 0.8660254037844387076, 1.000000000000000000, 0.8660254037844387076, 1.000000000000000000, 0.8660254037844387076, 1.000000000000000000, 0.8660254037844387076, 1.000000000000000000, 0.8660254037844387076, 1.000000000000000000, 0.8660254037844387076, 1.000000000000000000, 0.8660254037844387076, 1.000000000000000000, 0.8660254037844387076, 1.000000000000000000, 0.8660254037844387076, 1.000000000000000000, 0.8660254037844387076, 1.000000000000000000, 0.8660254037844387076, 1.000000000000000000, 0.8660254037844387076, 1.000000000000000000, 0.8660254037844387076, 1.000000000000000000, 0.8660254037844387076, 1.000000000000000000, 0.8660254037844387076, 1.000000000000000000, 0.8660254037844387076, 1.000000000000000000, 0.8660254037844387076, 1.000000000000000000, 0.8660254037844387076, 1.000000000000000000, 0.8660254037844387076, 1.000000000000000000, 0.8660254037844387076, 1.000000000000000000, 0.8660254037844387076, 1.000000000000000000, 0.8660254037844387076, 1.000000000000000000, 0.8660254037844387076, 1.000000000000000000, 0.8660254037844387076, 1.000000000000000000, 0.8660254037844387076, 1.000000000000000000, 0.8660254037844387076, 1.000000000000000000, 0.8660254037844387076, 1.000000000000000000, 0.8660254037844387076, 1.000000000000000000, 0.8660254037844387076, 1.000000000000000000, 0.8660254037844387076, 1.000000000000000000, 0.8660254037844387076, 1.000000000000000000, 0.8660254037844387076, 1.000000000000000000, 0.8660254037844387076, 1.000000000000000000, 0.8660254037844387076, 1.000000000000000000, 0.8660254037844387076, 1.000000000000000000, 0.8660254037844387076, 1.000000000000000000, 0.8660254037844387076, 1.000000000000000000, 0.8660254037844387076, 1.000000000000000000, 0.8660254037844387076, 1.000000000000000000, 0.8660254037844387076, 1.000000000000000000, 0.8660254037844387076, 1.000000000000000000, 0.8660254037844387076, 1.000000000000000000, 0.8660254037844387076, 1.000000000000000000, 0.8660254037844387076, 1.000000000000000000, 0.8660254037844387076, 1.000000000000000000, 0.8660254037844387076, 1.000000000000000000, 0.8660254037844387076, 1.000000000000000000, 0.8660254037844387076, 1.000000000000000000, 0.8660254037844387076, 1.000000000000000000, 0.8660254037844387076, 1.000000000000000000, 0.8660254037844387076, 1.000000000000000000, 0.8660254037844387076, 1.000000000000000000, 0.8660254037844387076, 1.000000000000000000, 0.8660254037844387076, 1.000000000000000000, 0.8660254037844387076, 1.000000000000000000, 0.8660254037844387076, 1.000000000000000000, 0.8660254037844387076, 1.000000000000000000, 0.8660254037844387076, 1.000000000000000000, 0.8660254037844387076, 1.000000000000000000, 0.8660254037844387076, 1.000000000000000000, 0.8660254037844387076, 1.000000000000000000, 0.8660254037844387076, 1.000000000000000000, 0.8660254037844387076, 1.000000000000000000, 0.8660254037844387076, 1.000000000000000000, 0.8660254037844387076, 1.000000000000000000, 0.8660254037844387076, 1.000000000000000000, 0.8660254037844387076, 1.000000000000000000, 0.8660254037844387076, 1.000000000000000000, 0.8660254037844387076, 1.000000000000000000, 0.8660254037844387076, 1.000000000000000000, 0.8660254037844387076, 1.000000000000000000, 0.8660254037844387076, 1.000000000000000000, 0.8660254037844387076, 1.000000000000000000, 0.8660254037844387076, 1.000000000000000000, 0.8660254037844387076, 1.000000000000000000, 0.8660254037844387076, 1.000000000000000000, 0.8660254037844387076, 1.000000000000000000, 0.8660254037844387076, 1.000000000000000000, 0.8660254037844387076, 1.000000000000000000, 0.8660254037844387076, 1.000000000000000000, 0.8660254037844387076, 1.000000000000000000, 0.8660254037844387076, 1.000000000000000000, 0.8660254037844387076, 1.000000000000000000, 0.8660254037844387076, 1.000000000000000000, 0.8660254037844387076, 1.000000000000000000, 0.8660254037844387076, 1.000000000000000000, 0.8660254037844387076, 1.000000000000000000, 0.8660254037844387076, 1.000000000000000000, 0.8660254037844387076, 1.000000000000000000, 0.8660254037844387076, 1.000000000000000000, 0.8660254037844387076, 1.000000000000000000, 0.8660254037844387076, 1.000000000000000000, 0.8660254037844387076, 1.000000000000000000, 0.8660254037844387076, 1.000000000000000000, 0.8660254037844387076, 1.000000000000000000, 0.8660254037844387076, 1.000000000000000000, 0.8660254037844387076, 1.000000000000000000, 0.8660254037844387076, 1.000000000000000000, 0.8660254037844387076, 1.000000000000000000, 0.8660254037844387076, 1.000000000000000000, 0.8660254037844387076, 1.000000000000000000, 0.8660254037844387076, 1.000000000000000000, 0.8660254037844387076, 1.000000000000000000, 0.8660254037844387076, 1.000000000000000000, 0.8660254037844387076, 1.000000000000000000, 0.8660254037844387076, 1.000000000000000000, 0.8660254037844387076, 1.000000000000000000, 0.8660254037844387076, 1.000000000000000000, 0.8660254037844387076, 1.000000000000000000, 0.8660254037844387076, 1.000000000000000000, 0.8660254037844387076, 1.000000000000000000, 0.8660254037844387076, 1.000000000000000000, 0.8660254037844387076, 1.000000000000000000, 0.8660254037844387076, 1.000000000000000000, 0.8660254037844387076, 1.000000000000000000, 0.8660254037844387076, 1.000000000000000000, 0.8660254037844387076, 1.000000000000000000, 0.8660254037844387076, 1.000000000000000000, 0.8660254037844387076, 1.000000000000000000, 0.8660254037844387076, 1.000000000000000000, 0.8660254037844387076, 1.000000000000000000, 0.8660254037844387076, 1.000000000000000000, 0.8660254037844387076, 1.000000000000000000, 0.8660254037844387076, 1.000000000000000000, 0.8660254037844387076, 1.000000000000000000, 0.8660254037844387076, 1.000000000000000000, 0.8660254037844387076, 1.000000000000000000, 0.8660254037844387076, 1.000000000000000000, 0.8660254037844387076, 1.000000000000000000, 0.8660254037844387076, 1.000000000000000000, 0.8660254037844387076, 1.000000000000000000, 0.8660254037844387076, 1.000000000000000000, 0.8660254037844387076, 1.000000000000000000, 0.8660254037844387076, 1.000000000000000000, 0.8660254037844387076, 1.000000000000000000, 0.8660254037844387076, 1.000000000000000000, 0.8660254037844387076, 1.000000000000000000, 0.8660254037844387076, 1.000000000000000000, 0.8660254037844387076, 1.000000000000000000, 0.8660254037844387076, 1.000000000000000000, 0.8660254037844387076, 1.000000000000000000, 0.8660254037844387076, 1.000000000000000000, 0.8660254037844387076, 1.000000000000000000, 0.8660254037844387076, 1.000000000000000000, 0.8660254037844387076, 1.000000000000000000, 0.8660254037844387076, 1.000000000000000000, 0.8660254037844387076, 1.000000000000000000, 0.8660254037844387076, 1.000000000000000000, 0.8660254037844387076, 1.000000000000000000, 0.8660254037844387076, 1.000000000000000000, 0.8660254037844387076, 1.000000000000000000, 0.8660254037844387076, 1.000000000000000000, 0.8660254037844387076, 1.000000000000000000, 0.8660254037844387076, 1.000000000000000000, 0.8660254037844387076, 1.000000000000000000, 0.8660254037844387076, 1.000000000000000000, 0.8660254037844387076, 1.000000000000000000, 0.8660254037844387076, 1.000000000000000000, 0.8660254037844387076, 1.000000000000000000, 0.8660254037844387076, 1.000000000000000000, 0.8660254037844387076, 1.000000000000000000, 0.8660254037844387076, 1.000000000000000000, 0.8660254037844387076, 1.000000000000000000, 0.8660254037844387076, 1.000000000000000000, 0.8660254037844387076, 1.000000000000000000, 0.8660254037844387076, 1.000000000000000000, 0.8660254037844387076, 1.000000000000000000, 0.8660254037844387076, 1.000000000000000000, 0.8660254037844387076, 1.000000000000000000, 0.8660254037844387076, 1.000000000000000000, 0.8660254037844387076, 1.000000000000000000, 0.8660254037844387076, 1.000000000000000000, 0.8660254037844387076, 1.000000000000000000, 0.8660254037844387076, 1.000000000000000000, 0.8660254037844387076, 1.000000000000000000, 0.8660254037844387076, 1.000000000000000000, 0.8660254037844387076, 1.000000000000000000, 0.8660254037844387076, 1.000000000000000000, 0.8660254037844387076, 1.000000000000000000, 0.8660254037844387076, 1.000000000000000000, 0.8660254037844387076, 1.000000000000000000, 0.8660254037844387076, 1.000000000000000000, 0.8660254037844387076, 1.000000000000000000, 0.8660254037844387076, 1.000000000000000000, 0.8660254037844387076, 1.000000000000000000, 0.8660254037844387076, 1.000000000000000000, 0.8660254037844387076, 1.000000000000000000, 0.8660254037844387076, 1.000000000000000000, 0.8660254037844387076, 1.000000000000000000, 0.8660254037844387076, 1.000000000000000000, 0.8660254037844387076, 1.000000000000000000, 0.8660254037844387076, 1.000000000000000000, 0.8660254037844387076, 1.000000000000000000, 0.8660254037844387076, 1.000000000000000000, 0.8660254037844387076, 1.000000000000000000, 0.8660254037844387076, 1.000000000000000000, 0.8660254037844387076, 1.000000000000000000, 0.8660254037844387076, 1.000000000000000000, 0.8660254037844387076, 1.000000000000000000, 0.8660254037844387076, 1.000000000000000000, 0.8660254037844387076, 1.000000000000000000, 0.8660254037844387076, 1.000000000000000000, 0.8660254037844387076, 1.000000000000000000, 0.8660254037844387076, 1.000000000000000000),
 ( 1.000000000000000000, 0.8660254037844387076, 1.000000000000000000, 0.8660254037844387076, 1.000000000000000000, 0.8660254037844387076, 1.000000000000000000, 0.8660254037844387076, 1.000000000000000000, 0.8660254037844387076, 1.000000000000000000, 0.8660254037844387076, 1.000000000000000000, 0.8660254037844387076, 1.000000000000000000, 0.8660254037844387076, 1.000000000000000000, 0.8660254037844387076, 1.000000000000000000, 0.8660254037844387076, 1.000000000000000000, 0.8660254037844387076, 1.000000000000000000, 0.8660254037844387076, 1.000000000000000000, 0.8660254037844387076, 1.000000000000000000, 0.8660254037844387076, 1.000000000000000000, 0.8660254037844387076, 1.000000000000000000, 0.8660254037844387076, 1.000000000000000000, 0.8660254037844387076, 1.000000000000000000, 0.8660254037844387076, 1.000000000000000000, 0.8660254037844387076, 1.000000000000000000, 0.8660254037844387076, 1.000000000000000000, 0.8660254037844387076, 1.000000000000000000, 0.8660254037844387076, 1.000000000000000000, 0.8660254037844387076, 1.000000000000000000, 0.8660254037844387076, 1.000000000000000000, 0.8660254037844387076, 1.000000000000000000, 0.8660254037844387076, 1.000000000000000000, 0.8660254037844387076, 1.000000000000000000, 0.8660254037844387076, 1.000000000000000000, 0.8660254037844387076, 1.000000000000000000, 0.8660254037844387076, 1.000000000000000000, 0.8660254037844387076, 1.000000000000000000, 0.8660254037844387076, 1.000000000000000000, 0.8660254037844387076, 1.000000000000000000, 0.8660254037844387076, 1.000000000000000000, 0.8660254037844387076, 1.000000000000000000, 0.8660254037844387076, 1.000000000000000000, 0.8660254037844387076, 1.000000000000000000, 0.8660254037844387076, 1.000000000000000000, 0.8660254037844387076, 1.000000000000000000, 0.8660254037844387076, 1.000000000000000000, 0.8660254037844387076, 1.000000000000000000, 0.8660254037844387076, 1.000000000000000000, 0.8660254037844387076, 1.000000000000000000, 0.8660254037844387076, 1.000000000000000000, 0.8660254037844387076, 1.000000000000000000, 0.8660254037844387076, 1.000000000000000000, 0.8660254037844387076, 1.000000000000000000, 0.8660254037844387076, 1.000000000000000000, 0.8660254037844387076, 1.000000000000000000, 0.8660254037844387076, 1.000000000000000000, 0.8660254037844387076, 1.000000000000000000, 0.8660254037844387076, 1.000000000000000000, 0.8660254037844387076, 1.000000000000000000, 0.8660254037844387076, 1.000000000000000000, 0.8660254037844387076, 1.000000000000000000, 0.8660254037844387076, 1.000000000000000000, 0.8660254037844387076, 1.000000000000000000, 0.8660254037844387076, 1.000000000000000000, 0.8660254037844387076, 1.000000000000000000, 0.8660254037844387076, 1.000000000000000000, 0.8660254037844387076, 1.000000000000000000, 0.8660254037844387076, 1.000000000000000000, 0.8660254037844387076, 1.000000000000000000, 0.8660254037844387076, 1.000000000000000000, 0.8660254037844387076, 1.000000000000000000, 0.8660254037844387076, 1.000000000000000000, 0.8660254037844387076, 1.000000000000000000, 0.8660254037844387076, 1.000000000000000000, 0.8660254037844387076, 1.000000000000000000, 0.8660254037844387076, 1.000000000000000000, 0.8660254037844387076, 1.000000000000000000, 0.8660254037844387076, 1.000000000000000000, 0.8660254037844387076, 1.000000000000000000, 0.8660254037844387076, 1.000000000000000000, 0.8660254037844387076, 1.000000000000000000, 0.8660254037844387076, 1.000000000000000000, 0.8660254037844387076, 1.000000000000000000, 0.8660254037844387076, 1.000000000000000000, 0.8660254037844387076, 1.000000000000000000, 0.8660254037844387076, 1.000000000000000000, 0.8660254037844387076, 1.000000000000000000, 0.8660254037844387076, 1.000000000000000000, 0.8660254037844387076, 1.000000000000000000, 0.8660254037844387076, 1.000000000000000000, 0.8660254037844387076, 1.000000000000000000, 0.8660254037844387076, 1.000000000000000000, 0.8660254037844387076, 1.000000000000000000, 0.8660254037844387076, 1.000000000000000000, 0.8660254037844387076, 1.000000000000000000, 0.8660254037844387076, 1.000000000000000000, 0.8660254037844387076, 1.000000000000000000, 0.8660254037844387076, 1.000000000000000000, 0.8660254037844387076, 1.000000000000000000, 0.8660254037844387076, 1.000000000000000000, 0.8660254037844387076, 1.000000000000000000, 0.8660254037844387076, 1.000000000000000000, 0.8660254037844387076, 1.000000000000000000, 0.8660254037844387076, 1.000000000000000000, 0.8660254037844387076, 1.000000000000000000, 0.8660254037844387076, 1.000000000000000000, 0.8660254037844387076, 1.000000000000000000, 0.8660254037844387076, 1.000000000000000000, 0.8660254037844387076, 1.000000000000000000, 0.8660254037844387076, 1.000000000000000000, 0.8660254037844387076, 1.000000000000000000, 0.8660254037844387076, 1.000000000000000000, 0.8660254037844387076, 1.000000000000000000, 0.8660254037844387076, 1.000000000000000000, 0.8660254037844387076, 1.000000000000000000, 0.8660254037844387076, 1.000000000000000000, 0.8660254037844387076, 1.000000000000000000, 0.8660254037844387076, 1.000000000000000000, 0.8660254037844387076, 1.000000000000000000, 0.8660254037844387076, 1.000000000000000000, 0.8660254037844387076, 1.000000000000000000, 0.8660254037844387076, 1.000000000000000000, 0.8660254037844387076, 1.000000000000000000, 0.8660254037844387076, 1.000000000000000000, 0.8660254037844387076, 1.000000000000000000, 0.8660254037844387076, 1.000000000000000000, 0.8660254037844387076, 1.000000000000000000, 0.8660254037844387076, 1.000000000000000000, 0.8660254037844387076, 1.000000000000000000, 0.8660254037844387076, 1.000000000000000000, 0.8660254037844387076, 1.000000000000000000, 0.8660254037844387076, 1.000000000000000000, 0.8660254037844387076, 1.000000000000000000, 0.8660254037844387076, 1.000000000000000000, 0.8660254037844387076, 1.000000000000000000, 0.8660254037844387076, 1.000000000000000000, 0.8660254037844387076, 1.000000000000000000, 0.8660254037844387076, 1.000000000000000000, 0.8660254037844387076, 1.000000000000000000, 0.8660254037844387076, 1.000000000000000000, 0.8660254037844387076, 1.000000000000000000, 0.8660254037844387076, 1.000000000000000000, 0.8660254037844387076, 1.000000000000000000, 0.8660254037844387076, 1.000000000000000000, 0.8660254037844387076, 1.000000000000000000, 0.8660254037844387076, 1.000000000000000000, 0.8660254037844387076, 1.000000000000000000, 0.8660254037844387076, 1.000000000000000000, 0.8660254037844387076, 1.000000000000000000, 0.8660254037844387076, 1.000000000000000000, 0.8660254037844387076, 1.000000000000000000, 0.8660254037844387076, 1.000000000000000000, 0.8660254037844387076, 1.000000000000000000, 0.8660254037844387076, 1.000000000000000000, 0.8660254037844387076, 1.000000000000000000, 0.8660254037844387076, 1.000000000000000000, 0.8660254037844387076, 1.000000000000000000, 0.8660254037844387076, 1.000000000000000000, 0.8660254037844387076, 1.000000000000000000, 0.8660254037844387076, 1.000000000000000000, 0.8660254037844387076, 1.000000000000000000, 0.8660254037844387076, 1.000000000000000000, 0.8660254037844387076, 1.000000000000000000, 0.8660254037844387076, 1.000000000000000000, 0.8660254037844387076, 1.000000000000000000, 0.8660254037844387076, 1.000000000000000000, 0.8660254037844387076, 1.000000000000000000, 0.8660254037844387076, 1.000000000000000000, 0.8660254037844387076, 1.000000000000000000, 0.8660254037844387076, 1.000000000000000000, 0.8660254037844387076, 1.000000000000000000, 0.8660254037844387076, 1.000000000000000000, 0.8660254037844387076, 1.000000000000000000, 0.8660254037844387076, 1.000000000000000000, 0.8660254037844387076, 1.000000000000000000, 0.8660254037844387076, 1.000000000000000000, 0.8660254037844387076, 1.000000000000000000, 0.8660254037844387076, 1.000000000000000000, 0.8660254037844387076, 1.000000000000000000, 0.8660254037844387076, 1.000000000000000000, 0.8660254037844387076, 1.000000000000000000, 0.8660254037844387076, 1.000000000000000000, 0.8660254037844387076, 1.000000000000000000, 0.8660254037844387076, 1.000000000000000000, 0.8660254037844387076, 1.000000000000000000, 0.8660254037844387076, 1.000000000000000000, 0.8660254037844387076, 1.000000000000000000, 0.8660254037844387076, 1.000000000000000000, 0.8660254037844387076, 1.000000000000000000, 0.8660254037844387076, 1.000000000000000000, 0.8660254037844387076, 1.000000000000000000, 0.8660254037844387076, 1.000000000000000000, 0.8660254037844387076, 1.000000000000000000, 0.8660254037844387076, 1.000000000000000000, 0.8660254037844387076, 1.000000000000000000, 0.8660254037844387076, 1.000000000000000000, 0.8660254037844387076, 1.000000000000000000, 0.8660254037844387076, 1.000000000000000000, 0.8660254037844387076, 1.000000000000000000, 0.8660254037844387076, 1.000000000000000000, 0.8660254037844387076, 1.000000000000000000, 0.8660254037844387076, 1.000000000000000000, 0.8660254037844387076, 1.000000000000000000, 0.8660254037844387076, 1.000000000000000000, 0.8660254037844387076, 1.000000000000000000, 0.8660254037844387076, 1.000000000000000000, 0.8660254037844387076, 1.000000000000000000, 0.8660254037844387076, 1.000000000000000000, 0.8660254037844387076, 1.000000000000000000, 0.8660254037844387076, 1.000000000000000000, 0.8660254037844387076, 1.000000000000000000, 0.8660254037844387076, 1.000000000000000000, 0.8660254037844387076, 1.000000000000000000, 0.8660254037844387076, 1.000000000000000000, 0.8660254037844387076, 1.000000000000000000, 0.8660254037844387076, 1.000000000000000000, 0.8660254037844387076, 1.000000000000000000, 0.8660254037844387076, 1.000000000000000000, 0.8660254037844387076, 1.000000000000000000, 0.8660254037844387076, 1.000000000000000000, 0.8660254037844387076, 1.000000000000000000, 0.8660254037844387076, 1.000000000000000000, 0.8660254037844387076, 1.000000000000000000, 0.8660254037844387076, 1.000000000000000000, 0.8660254037844387076, 1.000000000000000000, 0.8660254037844387076, 1.000000000000000000, 0.8660254037844387076, 1.000000000000000000, 0.8660254037844387076, 1.000000000000000000, 0.8660254037844387076, 1.000000000000000000, 0.8660254037844387076, 1.000000000000000000, 0.8660254037844387076, 1.000000000000000000, 0.8660254037844387076, 1.000000000000000000, 0.8660254037844387076, 1.000000000000000000, 0.8660254037844387076, 1.000000000000000000, 0.8660254037844387076, 1.000000000000000000, 0.8660254037844387076, 1.000000000000000000, 0.8660254037844387076, 1.000000000000000000, 0.8660254037844387076, 1.000000000000000000, 0.8660254037844387076, 1.000000000000000000, 0.8660254037844387076, 1.000000000000000000, 0.8660254037844387076, 1.000000000000000000, 0.8660254037844387076, 1.000000000000000000, 0.8660254037844387076, 1.000000000000000000, 0.8660254037844387076, 1.000000000000000000, 0.8660254037844387076, 1.000000000000000000, 0.8660254037844387076, 1.000000000000000000, 0.8660254037844387076, 1.000000000000000000, 0.8660254037844387076, 1.000000000000000000, 0.8660254037844387076, 1.000000000000000000, 0.8660254037844387076, 1.000000000000000000, 0.8660254037844387076, 1.000000000000000000, 0.8660254037844387076, 1.000000000000000000, 0.8660254037844387076, 1.000000000000000000, 0.8660254037844387076, 1.000000000000000000, 0.8660254037844387076, 1.000000000000000000, 0.8660254037844387076, 1.000000000000000000, 0.8660254037844387076, 1.000000000000000000, 0.8660254037844387076, 1.000000000000000000, 0.8660254037844387076, 1.000000000000000000, 0.8660254037844387076, 1.000000000000000000, 0.8660254037844387076, 1.000000000000000000, 0.8660254037844387076, 1.000000000000000000, 0.8660254037844387076, 1.000000000000000000, 0.8660254037844387076, 1.000000000000000000, 0.8660254037844387076, 1.000000000000000000, 0.8660254037844387076, 1.000000000000000000, 0.8660254037844387076, 1.000000000000000000, 0.8660254037844387076, 1.000000000000000000, 0.8660254037844387076, 1.000000000000000000, 0.8660254037844387076, 1.000000000000000000, 0.8660254037844387076, 1.000000000000000000, 0.8660254037844387076, 1.000000000000000000, 0.8660254037844387076, 1.000000000000000000, 0.8660254037844387076, 1.000000000000000000, 0.8660254037844387076, 1.000000000000000000, 0.8660254037844387076, 1.000000000000000000, 0.8660254037844387076, 1.000000000000000000, 0.8660254037844387076, 1.000000000000000000, 0.8660254037844387076, 1.000000000000000000, 0.8660254037844387076, 1.000000000000000000, 0.8660254037844387076, 1.000000000000000000, 0.8660254037844387076, 1.000000000000000000, 0.8660254037844387076, 1.000000000000000000, 0.8660254037844387076, 1.000000000000000000, 0.8660254037844387076, 1.000000000000000000, 0.8660254037844387076, 1.000000000000000000, 0.8660254037844387076, 1.000000000000000000, 0.8660254037844387076, 1.000000000000000000, 0.8660254037844387076, 1.000000000000000000, 0.8660254037844387076, 1.000000000000000000, 0.8660254037844387076, 1.000000000000000000, 0.8660254037844387076, 1.000000000000000000, 0.8660254037844387076, 1.000000000000000000, 0.8660254037844387076, 1.000000000000000000, 0.8660254037844387076, 1.000000000000000000, 0.8660254037844387076, 1.000000000000000000, 0.8660254037844387076, 1.000000000000000000, 0.8660254037844387076, 1.000000000000000000, 0.8660254037844387076, 1.000000000000000000, 0.8660254037844387076, 1.000000000000000000, 0.8660254037844387076, 1.000000000000000000, 0.8660254037844387076, 1.000000000000000000, 0.8660254037844387076, 1.000000000000000000, 0.8660254037844387076, 1.000000000000000000, 0.8660254037844387076, 1.000000000000000000, 0.8660254037844387076, 1.000000000000000000, 0.8660254037844387076, 1.000000000000000000, 0.8660254037844387076, 1.000000000000000000, 0.8660254037844387076, 1.000000000000000000, 0.8660254037844387076, 1.000000000000000000, 0.8660254037844387076, 1.000000000000000000, 0.8660254037844387076, 1.000000000000000000, 0.8660254037844387076, 1.000000000000000000, 0.8660254037844387076, 1.000000000000000000, 0.8660254037844387076, 1.000000000000000000, 0.8660254037844387076, 1.000000000000000000, 0.8660254037844387076, 1.000000000000000000, 0.8660254037844387076, 1.000000000000000000, 0.8660254037844387076, 1.000000000000000000, 0.8660254037844387076, 1.000000000000000000, 0.8660254037844387076, 1.000000000000000000, 0.8660254037844387076, 1.000000000000000000, 0.8660254037844387076, 1.000000000000000000, 0.8660254037844387076, 1.000000000000000000, 0.8660254037844387076, 1.000000000000000000, 0.8660254037844387076, 1.000000000000000000, 0.8660254037844387076, 1.000000000000000000, 0.8660254037844387076, 1.000000000000000000, 0.8660254037844387076, 1.000000000000000000, 0.8660254037844387076, 1.000000000000000000, 0.8660254037844387076, 1.000000000000000000, 0.8660254037844387076, 1.000000000000000000, 0.8660254037844387076, 1.000000000000000000, 0.8660254037844387076, 1.000000000000000000, 0.8660254037844387076, 1.000000000000000000, 0.8660254037844387076, 1.000000000000000000, 0.8660254037844387076, 1.000000000000000000, 0.8660254037844387076, 1.000000000000000000, 0.8660254037844387076, 1.000000000000000000, 0.8660254037844387076, 1.000000000000000000, 0.8660254037844387076, 1.000000000000000000, 0.8660254037844387076, 1.000000000000000000, 0.8660254037844387076, 1.000000000000000000, 0.8660254037844387076, 1.000000000000000000, 0.8660254037844387076, 1.000000000000000000, 0.8660254037844387076, 1.000000000000000000, 0.8660254037844387076, 1.000000000000000000, 0.8660254037844387076, 1.000000000000000000, 0.8660254037844387076, 1.000000000000000000, 0.8660254037844387076, 1.000000000000000000, 0.8660254037844387076, 1.000000000000000000, 0.8660254037844387076, 1.000000000000000000, 0.8660254037844387076, 1.000000000000000000, 0.8660254037844387076, 1.000000000000000000, 0.8660254037844387076, 1.000000000000000000, 0.8660254037844387076, 1.000000000000000000, 0.8660254037844387076, 1.000000000000000000, 0.8660254037844387076, 1.000000000000000000, 0.8660254037844387076, 1.000000000000000000, 0.8660254037844387076, 1.000000000000000000, 0.8660254037844387076, 1.000000000000000000, 0.8660254037844387076, 1.000000000000000000, 0.8660254037844387076, 1.000000000000000000, 0.8660254037844387076, 1.000000000000000000, 0.8660254037844387076, 1.000000000000000000, 0.8660254037844387076, 1.000000000000000000) ) ) 
 REPRESENTATION_ITEM ( '' )  SURFACE ( )  );
#31837=CARTESIAN_POINT ( 'NONE',  ( 17.37187500061451573, -6.054752690667223547, -1.112240025338166033E-15 ) ) ;
#31838=CARTESIAN_POINT ( 'NONE',  ( 21.29062500061451502, -3.027376345333614438, 5.243569643749998122 ) ) ;
#31839=CARTESIAN_POINT ( 'NONE',  ( 2.000000000000001332, 12.50000000000000000, 33.46410161513774995 ) ) ;
#31840=CARTESIAN_POINT ( 'NONE',  ( 27.47812500061451502, 4.541064518000418104, 2.621784821874999949 ) ) ;
#31841=CARTESIAN_POINT ( 'NONE',  ( 6.862500001229034474, -4.330127018922190985, -2.500000000000001332 ) ) ;
#31843=CYLINDRICAL_SURFACE ( 'NONE', #58094, 4.999999999999998224 ) ;
#31844=CARTESIAN_POINT ( 'NONE',  ( -3.999999999999997335, 16.88749999999999929, -27.69059892324149175 ) ) ;
#31845=CARTESIAN_POINT ( 'NONE',  ( 24.41250000122903430, -4.330127018922190985, -2.500000000000001332 ) ) ;
#31847=CARTESIAN_POINT ( 'NONE',  ( 7.584375000614516082, 6.421520780324663323E-16, -5.243569643749999010 ) ) ;
#31848=CYLINDRICAL_SURFACE ( 'NONE', #1910, 4.999999999999998224 ) ;
#31849=CARTESIAN_POINT ( 'NONE',  ( 14.31562500061451537, 3.027376345333613106, -5.243569643749998122 ) ) ;
#31850=CARTESIAN_POINT ( 'NONE',  ( 7.846875000614518036, -3.027376345333614438, 5.243569643749998122 ) ) ;
#31851=CARTESIAN_POINT ( 'NONE',  ( 27.00000000122903288, -2.886751345948129988, 4.999999999999997335 ) ) ;
#31852=CARTESIAN_POINT ( 'NONE',  ( 17.59687500061451715, 6.054752690667223547, 3.707466751127219781E-16 ) ) ;
#31853=CARTESIAN_POINT ( 'NONE',  ( 5.709375000614517859, -4.541064518000417216, -2.621784821875001281 ) ) ;
#31854=FACE_OUTER_BOUND ( 'NONE', #26933, .T. ) ;
#31855=CARTESIAN_POINT ( 'NONE',  ( 6.178125000614518747, 6.421520780324663323E-16, -5.243569643749999010 ) ) ;
#31856=CARTESIAN_POINT ( 'NONE',  ( 16.49062500061451786, -3.027376345333610441, -5.243569643749999898 ) ) ;
#31857=ORIENTED_EDGE ( 'NONE', *, *, #67743, .F. ) ;
#31858=CARTESIAN_POINT ( 'NONE',  ( 11.80312500061451608, 0.000000000000000000, 5.243569643749999010 ) ) ;
#31859=CARTESIAN_POINT ( 'NONE',  ( 5.962500001229033231, -4.330127018922190985, -2.500000000000001332 ) ) ;
#31860=CARTESIAN_POINT ( 'NONE',  ( 7.828125000614517326, -4.541064518000419881, 2.621784821874995952 ) ) ;
#31862=CARTESIAN_POINT ( 'NONE',  ( 9.600000000000001421, 4.330127018922192761, -2.499999999999997780 ) ) ;
#31863=CARTESIAN_POINT ( 'NONE',  ( 3.900000001229034563, 5.773502691896255534, 3.535250795749688894E-16 ) ) ;
#31864=CARTESIAN_POINT ( 'NONE',  ( 18.82500000000000284, -4.330127018922194537, 2.499999999999995559 ) ) ;
#31865=CARTESIAN_POINT ( 'NONE',  ( 18.38437500061451857, 6.421520780324663323E-16, -5.243569643749999010 ) ) ;
#31866=CARTESIAN_POINT ( 'NONE',  ( 15.15000000122903323, 5.773502691896255534, 3.535250795749688894E-16 ) ) ;
#31868=CARTESIAN_POINT ( 'NONE',  ( -2.121784821874996840, 16.72812500061451857, -26.32496088578401583 ) ) ;
#31869=DIRECTION ( 'NONE',  ( 1.000000000000000000, 0.000000000000000000, 0.000000000000000000 ) ) ;
#31871=CARTESIAN_POINT ( 'NONE',  ( 3.617702362022032325, -3.451409801779584452, 3.617702362022032325 ) ) ;
#31872=CARTESIAN_POINT ( 'NONE',  ( 28.19062500061451715, -3.027376345333610441, -5.243569643749999898 ) ) ;
#31873=DIRECTION ( 'NONE',  ( -0.000000000000000000, -1.000000000000000000, -0.000000000000000000 ) ) ;
#31875=CARTESIAN_POINT ( 'NONE',  ( 17.10937500061451999, 4.541064518000418104, -2.621784821874998173 ) ) ;
#31876=CARTESIAN_POINT ( 'NONE',  ( 29.73750000000000071, -2.886751345948125991, -5.000000000000000000 ) ) ;
#31877=EDGE_CURVE ( 'NONE', #1400, #52020, #52422, .T. ) ;
#31878=CARTESIAN_POINT ( 'NONE',  ( 10.64062500061451644, -3.027376345333610441, -5.243569643749999898 ) ) ;
#31880=CARTESIAN_POINT ( 'NONE',  ( 20.48437500061451289, -4.541064518000419881, 2.621784821874995952 ) ) ;
#31882=CARTESIAN_POINT ( 'NONE',  ( 8.053125000614516082, 4.541064518000418104, -2.621784821874998173 ) ) ;
#31883=CARTESIAN_POINT ( 'NONE',  ( 12.34687500061452070, -3.027376345333614438, 5.243569643749998122 ) ) ;
#31885=CARTESIAN_POINT ( 'NONE',  ( 23.29687500061451644, -3.027376345333610441, -5.243569643749999898 ) ) ;
#31886=CARTESIAN_POINT ( 'NONE',  ( 28.15312500061451573, -4.541064518000417216, -2.621784821875001281 ) ) ;
#31888=CARTESIAN_POINT ( 'NONE',  ( 6.712500000000000355, -5.773502691896255534, -1.060575238724906372E-15 ) ) ;
#31889=CARTESIAN_POINT ( 'NONE',  ( 17.25000000122903288, -2.886751345948125991, -5.000000000000000000 ) ) ;
#31890=DIRECTION ( 'NONE',  ( -1.000000000000000000, -0.000000000000000000, -0.000000000000000000 ) ) ;
#31893=CARTESIAN_POINT ( 'NONE',  ( 15.41250000000000142, 2.886751345948129099, -4.999999999999998224 ) ) ;
#31894=CARTESIAN_POINT ( 'NONE',  ( 19.34999999999999787, -4.330127018922190985, -2.500000000000001332 ) ) ;
#31895=CARTESIAN_POINT ( 'NONE',  ( 10.86562500061451431, 3.027376345333611329, 5.243569643749999010 ) ) ;
#31896=ORIENTED_EDGE ( 'NONE', *, *, #20969, .F. ) ;
#31897=CARTESIAN_POINT ( 'NONE',  ( -3.999999999999997335, 11.03749999999999964, -27.69059892324149530 ) ) ;
#31898=CARTESIAN_POINT ( 'NONE',  ( -4.243569643749999898, 17.60937500061451999, -30.00000000000000000 ) ) ;
#31899=CARTESIAN_POINT ( 'NONE',  ( 3.028125000614518392, 6.421520780324663323E-16, -5.243569643749999010 ) ) ;
#31900=CARTESIAN_POINT ( 'NONE',  ( 9.112500000000000711, 2.886751345948129099, -4.999999999999998224 ) ) ;
#31903=CARTESIAN_POINT ( 'NONE',  ( 4.243569643749999898, 11.92812500061451608, 30.00000000000000000 ) ) ;
#31904=CARTESIAN_POINT ( 'NONE',  ( 27.74062500061451431, -3.027376345333610441, -5.243569643749999898 ) ) ;
#31907=CARTESIAN_POINT ( 'NONE',  ( 21.83437500061451786, -4.541064518000419881, 2.621784821874995952 ) ) ;
#31908=EDGE_CURVE ( 'NONE', #11892, #32497, #53143, .T. ) ;
#31909=CARTESIAN_POINT ( 'NONE',  ( 18.02812500061451573, 4.541064518000418104, 2.621784821874999949 ) ) ;
#31910=CARTESIAN_POINT ( 'NONE',  ( -4.243569643749998122, 14.44062500061459531, -27.54997392385601174 ) ) ;
#31911=CARTESIAN_POINT ( 'NONE',  ( 22.38750000122903216, 4.330127018922191873, 2.499999999999999556 ) ) ;
#31912=CARTESIAN_POINT ( 'NONE',  ( 3.590625000614518836, 6.054752690667223547, 3.707466751127219781E-16 ) ) ;
#31914=CARTESIAN_POINT ( 'NONE',  ( 22.49062500061451431, 6.054752690667223547, 3.707466751127219781E-16 ) ) ;
#31917=CARTESIAN_POINT ( 'NONE',  ( 15.60937500061451644, -4.541064518000417216, -2.621784821875001281 ) ) ;
#31918=CARTESIAN_POINT ( 'NONE',  ( 14.74687500061451573, -3.027376345333610441, -5.243569643749999898 ) ) ;
#31919=CARTESIAN_POINT ( 'NONE',  ( 24.30937500061451573, 4.541064518000418104, -2.621784821874998173 ) ) ;
#31920=CARTESIAN_POINT ( 'NONE',  ( 4.243569643749999898, 13.33437500061451786, 30.00000000000000000 ) ) ;
#31921=CARTESIAN_POINT ( 'NONE',  ( 5.803125000614517859, 4.541064518000418104, -2.621784821874998173 ) ) ;
#31922=CARTESIAN_POINT ( 'NONE',  ( 16.38750000122903216, 6.123233995736764310E-16, -4.999999999999998224 ) ) ;
#31923=CARTESIAN_POINT ( 'NONE',  ( 28.71562500061451573, 3.027376345333613106, -5.243569643749998122 ) ) ;
#31924=CARTESIAN_POINT ( 'NONE',  ( 3.999999999999998668, 19.47500000122903430, -32.30940107675850470 ) ) ;
#31925=CARTESIAN_POINT ( 'NONE',  ( -2.000000000000000000, 18.12500000000000355, 26.53589838486224650 ) ) ;
#31926=CARTESIAN_POINT ( 'NONE',  ( 6.796875000614516438, 6.054752690667223547, 3.707466751127219781E-16 ) ) ;
#31927=CARTESIAN_POINT ( 'NONE',  ( 14.21250000122903323, 4.330127018922192761, -2.499999999999997780 ) ) ;
#31928=CARTESIAN_POINT ( 'NONE',  ( 10.12500000122903465, 2.886751345948129099, -4.999999999999998224 ) ) ;
#31929=CARTESIAN_POINT ( 'NONE',  ( 5.765625000614519102, 3.027376345333613106, -5.243569643749998122 ) ) ;
#31932=CARTESIAN_POINT ( 'NONE',  ( 14.18437500061451750, -4.541064518000419881, 2.621784821874995952 ) ) ;
#31933=CARTESIAN_POINT ( 'NONE',  ( 21.07499999999999929, -4.330127018922194537, 2.499999999999995559 ) ) ;
#31934=ORIENTED_EDGE ( 'NONE', *, *, #37808, .T. ) ;
#31935=CARTESIAN_POINT ( 'NONE',  ( 21.32812500061451644, -4.541064518000419881, 2.621784821874995952 ) ) ;
#31936=CARTESIAN_POINT ( 'NONE',  ( 6.703125000614516438, 4.541064518000418104, -2.621784821874998173 ) ) ;
#31937=CARTESIAN_POINT ( 'NONE',  ( 25.24687500061451573, 6.054752690667223547, 3.707466751127219781E-16 ) ) ;
#31938=CARTESIAN_POINT ( 'NONE',  ( 7.228125000614517681, 4.541064518000418104, 2.621784821874999949 ) ) ;
#31940=CARTESIAN_POINT ( 'NONE',  ( 7.200000001229035718, -2.886751345948129988, 4.999999999999997335 ) ) ;
#31941=EDGE_CURVE ( 'NONE', #36195, #45966, #69788, .T. ) ;
#31942=CARTESIAN_POINT ( 'NONE',  ( 22.26562500061451644, -6.054752690667223547, -1.112240025338166033E-15 ) ) ;
#31943=CARTESIAN_POINT ( 'NONE',  ( -2.000000000000000000, 19.58750000122903501, -33.46410161513775705 ) ) ;
#31944=CARTESIAN_POINT ( 'NONE',  ( 11.02500000122903501, 2.886751345948129099, -4.999999999999998224 ) ) ;
#31945=CARTESIAN_POINT ( 'NONE',  ( 19.07812500061451644, -4.541064518000419881, 2.621784821874995952 ) ) ;
#31946=CARTESIAN_POINT ( 'NONE',  ( 18.59062500061451573, -3.027376345333614438, 5.243569643749998122 ) ) ;
#31948=CARTESIAN_POINT ( 'NONE',  ( 18.71249999999999858, 2.886751345948126879, 4.999999999999999112 ) ) ;
#31949=CARTESIAN_POINT ( 'NONE',  ( 12.45000000122903394, 5.773502691896255534, 3.535250795749688894E-16 ) ) ;
#31950=CARTESIAN_POINT ( 'NONE',  ( 8.128125000614515372, 4.541064518000418104, 2.621784821874999949 ) ) ;
#31951=CARTESIAN_POINT ( 'NONE',  ( 11.46562500061451573, -6.054752690667223547, -1.112240025338166033E-15 ) ) ;
#31952=CARTESIAN_POINT ( 'NONE',  ( 22.23750000122903003, 6.123233995736764310E-16, -4.999999999999998224 ) ) ;
#31953=CARTESIAN_POINT ( 'NONE',  ( 21.72187500061451715, 3.027376345333611329, 5.243569643749999010 ) ) ;
#31955=CARTESIAN_POINT ( 'NONE',  ( 4.762500001229033941, 4.330127018922192761, -2.499999999999997780 ) ) ;
#31956=CARTESIAN_POINT ( 'NONE',  ( 4.396875000614516971, -3.027376345333610441, -5.243569643749999898 ) ) ;
#31957=CARTESIAN_POINT ( 'NONE',  ( 23.55937500061451573, 0.000000000000000000, 5.243569643749999010 ) ) ;
#31958=CARTESIAN_POINT ( 'NONE',  ( 4.305309508024516063, -2.542763747326308277, -4.514440081878920985 ) ) ;
#31959=CARTESIAN_POINT ( 'NONE',  ( 18.29062500061451502, -3.027376345333610441, -5.243569643749999898 ) ) ;
#31960=CARTESIAN_POINT ( 'NONE',  ( 24.90937500061451715, 0.000000000000000000, 5.243569643749999010 ) ) ;
#31962=CARTESIAN_POINT ( 'NONE',  ( -1.071796769724504328, 11.20490381179670081, -26.00000000000001066 ) ) ;
#31964=CARTESIAN_POINT ( 'NONE',  ( 6.421875000614519102, 3.027376345333611329, 5.243569643749999010 ) ) ;
#31965=CARTESIAN_POINT ( 'NONE',  ( 15.21562500061451750, 3.027376345333613106, -5.243569643749998122 ) ) ;
#31966=CARTESIAN_POINT ( 'NONE',  ( 12.60937500061451821, 4.541064518000418104, -2.621784821874998173 ) ) ;
#31967=ORIENTED_EDGE ( 'NONE', *, *, #44349, .T. ) ;
#31969=CARTESIAN_POINT ( 'NONE',  ( 24.47812500061451502, -4.541064518000419881, 2.621784821874995952 ) ) ;
#31970=CARTESIAN_POINT ( 'NONE',  ( -3.137519842735245283E-14, 12.91250000000000142, -26.00000000000000711 ) ) ;
#31972=CARTESIAN_POINT ( 'NONE',  ( 15.03749999999999964, 5.773502691896255534, 3.535250795749688894E-16 ) ) ;
#31973=CARTESIAN_POINT ( 'NONE',  ( 25.08750000122903145, 4.330127018922191873, 2.499999999999999556 ) ) ;
#31974=CARTESIAN_POINT ( 'NONE',  ( 19.45312500061451644, 0.000000000000000000, 5.243569643749999010 ) ) ;
#31976=CARTESIAN_POINT ( 'NONE',  ( 23.58749999999999858, 5.773502691896255534, 3.535250795749688894E-16 ) ) ;
#31977=( BOUNDED_CURVE ( )  B_SPLINE_CURVE ( 2, ( #62537, #68818, #11215, #23008, #33741, #144, #29290, #5311, #68452 ),
 .UNSPECIFIED., .F., .F. ) 
 B_SPLINE_CURVE_WITH_KNOTS ( ( 3, 2, 2, 2, 3 ),
 ( 0.7500000000000000000, 0.7536231884057971175, 0.7608695652173913526, 0.7681159420289854767, 0.7717391304347825942 ),
 .UNSPECIFIED. ) 
 CURVE ( )  GEOMETRIC_REPRESENTATION_ITEM ( )  RATIONAL_B_SPLINE_CURVE ( ( 0.9330127018922194093, 0.9330127018922194093, 1.000000000000000000, 0.8660254037844387076, 1.000000000000000000, 0.8660254037844387076, 1.000000000000000000, 0.9330127018922194093, 0.9330127018922194093 ) ) 
 REPRESENTATION_ITEM ( '' )  );
#31979=CARTESIAN_POINT ( 'NONE',  ( 24.42187500061451999, 3.027376345333611329, 5.243569643749999010 ) ) ;
#31981=CARTESIAN_POINT ( 'NONE',  ( 2.983212779636571277, -4.012535546436136968, -3.375586037630073033 ) ) ;
#31982=CARTESIAN_POINT ( 'NONE',  ( 10.94062500061451537, -3.027376345333614438, 5.243569643749998122 ) ) ;
#31983=CARTESIAN_POINT ( 'NONE',  ( 3.178125000614515638, 4.541064518000418104, 2.621784821874999949 ) ) ;
#31985=CARTESIAN_POINT ( 'NONE',  ( 27.66562500061451146, -6.054752690667223547, -1.112240025338166033E-15 ) ) ;
#31986=CARTESIAN_POINT ( 'NONE',  ( 16.68750000000000000, -2.886751345948125991, -5.000000000000000000 ) ) ;
#31987=CARTESIAN_POINT ( 'NONE',  ( 25.57499999999999929, -4.330127018922194537, 2.499999999999995559 ) ) ;
#31988=CARTESIAN_POINT ( 'NONE',  ( 3.999999999999998668, 10.81250000000000178, -32.30940107675850470 ) ) ;
#31989=CARTESIAN_POINT ( 'NONE',  ( 7.846875000614518036, -3.027376345333614438, 5.243569643749998122 ) ) ;
#31990=CARTESIAN_POINT ( 'NONE',  ( 16.88437500061451502, -4.541064518000419881, 2.621784821874995952 ) ) ;
#31993=CARTESIAN_POINT ( 'NONE',  ( 26.35312500061451857, -4.541064518000417216, -2.621784821875001281 ) ) ;
#31994=CARTESIAN_POINT ( 'NONE',  ( 26.93437500061451573, 6.421520780324663323E-16, -5.243569643749999010 ) ) ;
#31996=CARTESIAN_POINT ( 'NONE',  ( 13.79999999999999893, 0.000000000000000000, 4.999999999999998224 ) ) ;
#31997=CARTESIAN_POINT ( 'NONE',  ( 10.67812500061451608, 6.421520780324663323E-16, -5.243569643749999010 ) ) ;
#31999=CARTESIAN_POINT ( 'NONE',  ( 25.83750000122903501, 6.123233995736764310E-16, -4.999999999999998224 ) ) ;
#32000=CARTESIAN_POINT ( 'NONE',  ( 28.11562500061451431, -6.054752690667223547, -1.112240025338166033E-15 ) ) ;
#32001=CARTESIAN_POINT ( 'NONE',  ( 15.18750000122903465, 4.330127018922191873, 2.499999999999999556 ) ) ;
#32004=CARTESIAN_POINT ( 'NONE',  ( 4.640625000614518214, -3.027376345333614438, 5.243569643749998122 ) ) ;
#32005=CARTESIAN_POINT ( 'NONE',  ( 21.49687500061451573, -3.027376345333610441, -5.243569643749999898 ) ) ;
#32006=CARTESIAN_POINT ( 'NONE',  ( -2.121784821874996840, 18.13437500061451502, 33.67503911421598417 ) ) ;
#32007=CARTESIAN_POINT ( 'NONE',  ( 23.07187500061451857, 3.027376345333611329, 5.243569643749999010 ) ) ;
#32008=CARTESIAN_POINT ( 'NONE',  ( 4.724999999999999645, 4.330127018922191873, 2.499999999999999556 ) ) ;
#32009=CARTESIAN_POINT ( 'NONE',  ( -2.828200636599751609E-16, 11.00000000122903288, 25.38119784648299770 ) ) ;
#32010=CARTESIAN_POINT ( 'NONE',  ( 12.21562500061451573, 3.027376345333611329, 5.243569643749999010 ) ) ;
#32011=CARTESIAN_POINT ( 'NONE',  ( 4.800000001229032698, 5.773502691896255534, 3.535250795749688894E-16 ) ) ;
#32012=CARTESIAN_POINT ( 'NONE',  ( 9.534375000614517148, 4.541064518000418104, 2.621784821874999949 ) ) ;
#32014=CARTESIAN_POINT ( 'NONE',  ( 9.928125000614517859, 4.541064518000418104, 2.621784821874999949 ) ) ;
#32015=CARTESIAN_POINT ( 'NONE',  ( 15.04687500061451644, -3.027376345333614438, 5.243569643749998122 ) ) ;
#32016=CARTESIAN_POINT ( 'NONE',  ( 21.97500000122903074, 2.886751345948126879, 4.999999999999999112 ) ) ;
#32017=CARTESIAN_POINT ( 'NONE',  ( 11.40937500061451892, 0.000000000000000000, 5.243569643749999010 ) ) ;
#32018=CARTESIAN_POINT ( 'NONE',  ( 11.46562500061451573, -6.054752690667223547, -1.112240025338166033E-15 ) ) ;
#32020=CARTESIAN_POINT ( 'NONE',  ( 20.33437500061451786, 4.541064518000418104, 2.621784821874999949 ) ) ;
#32023=CARTESIAN_POINT ( 'NONE',  ( -2.000000000000000000, 19.92500000000000071, -33.46410161513775705 ) ) ;
#32024=CARTESIAN_POINT ( 'NONE',  ( 4.243569643749999010, 15.62187500061451928, -32.45002607614398471 ) ) ;
#32025=CARTESIAN_POINT ( 'NONE',  ( 16.35000000122903430, -2.886751345948125991, -5.000000000000000000 ) ) ;
#32026=CARTESIAN_POINT ( 'NONE',  ( 10.32187500061451679, 3.027376345333613106, -5.243569643749998122 ) ) ;
#32027=CARTESIAN_POINT ( 'NONE',  ( 4.243569643749999898, 16.87812500061451715, -30.00000000000000000 ) ) ;
#32028=CARTESIAN_POINT ( 'NONE',  ( 17.77500000122903145, 2.886751345948129099, -4.999999999999998224 ) ) ;
#32029=CARTESIAN_POINT ( 'NONE',  ( 9.328125000614518214, 6.421520780324663323E-16, -5.243569643749999010 ) ) ;
#32031=CARTESIAN_POINT ( 'NONE',  ( 15.37500000000000000, 6.123233995736764310E-16, -4.999999999999998224 ) ) ;
#32032=CARTESIAN_POINT ( 'NONE',  ( 29.17500000000000071, -4.330127018922194537, 2.499999999999995559 ) ) ;
#32033=CARTESIAN_POINT ( 'NONE',  ( 10.54687500061451644, -3.027376345333614438, 5.243569643749998122 ) ) ;
#32034=CARTESIAN_POINT ( 'NONE',  ( 28.08750000122903145, 6.123233995736764310E-16, -4.999999999999998224 ) ) ;
#32035=EDGE_CURVE ( 'NONE', #48144, #32339, #64591, .T. ) ;
#32036=CARTESIAN_POINT ( 'NONE',  ( 9.450000001229033941, -2.886751345948129988, 4.999999999999997335 ) ) ;
#32037=CARTESIAN_POINT ( 'NONE',  ( 18.52500000122903145, -5.773502691896255534, -1.060575238724906372E-15 ) ) ;
#32038=( BOUNDED_CURVE ( )  B_SPLINE_CURVE ( 1, ( #72035, #66867 ),
 .UNSPECIFIED., .F., .F. ) 
 B_SPLINE_CURVE_WITH_KNOTS ( ( 2, 2 ),
 ( 0.000000000000000000, 1.000000000000000000 ),
 .UNSPECIFIED. ) 
 CURVE ( )  GEOMETRIC_REPRESENTATION_ITEM ( )  RATIONAL_B_SPLINE_CURVE ( ( 0.9401540804572410259, 0.9401540804572410259 ) ) 
 REPRESENTATION_ITEM ( '' )  );
#32039=EDGE_CURVE ( 'NONE', #37430, #47010, #39157, .T. ) ;
#32040=CARTESIAN_POINT ( 'NONE',  ( 14.39062500061451821, 6.054752690667223547, 3.707466751127219781E-16 ) ) ;
#32041=CARTESIAN_POINT ( 'NONE',  ( 18.70312500061451644, -4.541064518000417216, -2.621784821875001281 ) ) ;
#32042=CARTESIAN_POINT ( 'NONE',  ( 28.72500000122903074, 2.886751345948126879, 4.999999999999999112 ) ) ;
#32044=CARTESIAN_POINT ( 'NONE',  ( 3.140625000614516882, 6.054752690667223547, 3.707466751127219781E-16 ) ) ;
#32045=CARTESIAN_POINT ( 'NONE',  ( 24.11249999999999716, 2.886751345948126879, 4.999999999999999112 ) ) ;
#32048=CARTESIAN_POINT ( 'NONE',  ( 26.18437500061451573, 4.541064518000418104, 2.621784821874999949 ) ) ;
#32049=CARTESIAN_POINT ( 'NONE',  ( 1.999999999999998668, 17.60000000000000142, 26.53589838486224650 ) ) ;
#32050=CARTESIAN_POINT ( 'NONE',  ( 13.50000000122903288, -2.886751345948129988, 4.999999999999997335 ) ) ;
#32051=CARTESIAN_POINT ( 'NONE',  ( 4.312500000000000000, 2.886751345948126879, 4.999999999999999112 ) ) ;
#32053=( BOUNDED_CURVE ( )  B_SPLINE_CURVE ( 2, ( #37709, #32906, #26269, #54351, #60598, #66155, #4836 ),
 .UNSPECIFIED., .F., .F. ) 
 B_SPLINE_CURVE_WITH_KNOTS ( ( 3, 2, 2, 3 ),
 ( 0.5166666666666666075, 0.5194444444444443754, 0.5222222222222222543, 0.5250000000000000222 ),
 .UNSPECIFIED. ) 
 CURVE ( )  GEOMETRIC_REPRESENTATION_ITEM ( )  RATIONAL_B_SPLINE_CURVE ( ( 1.000000000000005329, 0.8660254037844333785, 1.000000000000000000, 0.8660254037844387076, 1.000000000000000000, 0.8660254037844387076, 1.000000000000000000 ) ) 
 REPRESENTATION_ITEM ( '' )  );
#32054=CARTESIAN_POINT ( 'NONE',  ( 6.946875000614517681, -3.027376345333614438, 5.243569643749998122 ) ) ;
#32055=CARTESIAN_POINT ( 'NONE',  ( 24.92812500061451431, -4.541064518000419881, 2.621784821874995952 ) ) ;
#32058=CARTESIAN_POINT ( 'NONE',  ( 5.709375000614517859, -4.541064518000417216, -2.621784821875001281 ) ) ;
#32059=CARTESIAN_POINT ( 'NONE',  ( 7.659375000614518036, 4.541064518000418104, -2.621784821874998173 ) ) ;
#32060=CARTESIAN_POINT ( 'NONE',  ( 3.787500000000002753, 5.773502691896255534, 3.535250795749688894E-16 ) ) ;
#32062=CARTESIAN_POINT ( 'NONE',  ( 2.121784821875001281, 13.20312500061459637, 33.67503911421598417 ) ) ;
#32063=CARTESIAN_POINT ( 'NONE',  ( 22.34999999999999787, 0.000000000000000000, 4.999999999999998224 ) ) ;
#32065=CARTESIAN_POINT ( 'NONE',  ( 28.76249999999999929, -5.773502691896255534, -1.060575238724906372E-15 ) ) ;
#32066=CARTESIAN_POINT ( 'NONE',  ( 3.000000000000002665, 0.000000000000000000, 4.999999999999998224 ) ) ;
#32067=ORIENTED_EDGE ( 'NONE', *, *, #35738, .T. ) ;
#32068=CARTESIAN_POINT ( 'NONE',  ( 18.66562500061451146, -6.054752690667223547, -1.112240025338166033E-15 ) ) ;
#32069=CARTESIAN_POINT ( 'NONE',  ( 10.67812500061451608, 6.421520780324663323E-16, -5.243569643749999010 ) ) ;
#32071=CARTESIAN_POINT ( 'NONE',  ( 6.346875000614517148, 6.054752690667223547, 3.707466751127219781E-16 ) ) ;
#32072=CARTESIAN_POINT ( 'NONE',  ( 22.68750000000000000, 5.773502691896255534, 3.535250795749688894E-16 ) ) ;
#32073=CARTESIAN_POINT ( 'NONE',  ( 19.76250000122903216, 0.000000000000000000, 4.999999999999998224 ) ) ;
#32074=DIRECTION ( 'NONE',  ( -1.000000000000000000, -0.000000000000000000, -0.000000000000000000 ) ) ;
#32075=CARTESIAN_POINT ( 'NONE',  ( 9.459375000614517859, 4.541064518000418104, -2.621784821874998173 ) ) ;
#32076=CARTESIAN_POINT ( 'NONE',  ( 14.89687500061451786, 6.054752690667223547, 3.707466751127219781E-16 ) ) ;
#32077=CARTESIAN_POINT ( 'NONE',  ( 24.34687500061451715, 6.054752690667223547, 3.707466751127219781E-16 ) ) ;
#32080=CARTESIAN_POINT ( 'NONE',  ( 17.10937500061451999, 4.541064518000418104, -2.621784821874998173 ) ) ;
#32081=CARTESIAN_POINT ( 'NONE',  ( 9.759375000614516793, -4.541064518000417216, -2.621784821875001281 ) ) ;
#32083=CARTESIAN_POINT ( 'NONE',  ( 20.81250000000000000, 2.886751345948129099, -4.999999999999998224 ) ) ;
#32085=CARTESIAN_POINT ( 'NONE',  ( -4.243569643749997233, 10.89687500061451786, -27.54997392385601174 ) ) ;
#32087=CARTESIAN_POINT ( 'NONE',  ( 11.27812500061451573, 4.541064518000418104, 2.621784821874999949 ) ) ;
#32088=CARTESIAN_POINT ( 'NONE',  ( 29.14687500061451075, -3.027376345333610441, -5.243569643749999898 ) ) ;
#32090=CARTESIAN_POINT ( 'NONE',  ( 7.320879633048903241E-15, 17.75000000122903288, -34.00000000000000000 ) ) ;
#32091=CARTESIAN_POINT ( 'NONE',  ( 12.44999999999999929, 0.000000000000000000, 4.999999999999998224 ) ) ;
#32092=CARTESIAN_POINT ( 'NONE',  ( 3.999999999999999112, 17.63750000122903572, 30.00000000000000000 ) ) ;
#32093=CARTESIAN_POINT ( 'NONE',  ( 12.52500000122903145, 2.886751345948126879, 4.999999999999999112 ) ) ;
#32094=CARTESIAN_POINT ( 'NONE',  ( 21.27187500061451786, 3.027376345333611329, 5.243569643749999010 ) ) ;
#32095=CARTESIAN_POINT ( 'NONE',  ( 15.90937500061451892, 0.000000000000000000, 5.243569643749999010 ) ) ;
#32097=CARTESIAN_POINT ( 'NONE',  ( 16.71562500061451573, 3.027376345333611329, 5.243569643749999010 ) ) ;
#32098=CARTESIAN_POINT ( 'NONE',  ( 28.53750000122903074, 6.123233995736764310E-16, -4.999999999999998224 ) ) ;
#32099=CARTESIAN_POINT ( 'NONE',  ( 16.99687500061451573, -3.027376345333610441, -5.243569643749999898 ) ) ;
#32100=CARTESIAN_POINT ( 'NONE',  ( 3.553125000614516082, 4.541064518000418104, -2.621784821874998173 ) ) ;
#32101=CARTESIAN_POINT ( 'NONE',  ( 18.29062500061451502, -3.027376345333610441, -5.243569643749999898 ) ) ;
#32102=CARTESIAN_POINT ( 'NONE',  ( -1.487416814333745711E-14, 16.96250000000000213, -26.00000000000000000 ) ) ;
#32103=CARTESIAN_POINT ( 'NONE',  ( 29.25937500061451502, 4.541064518000418104, -2.621784821874998173 ) ) ;
#32104=CARTESIAN_POINT ( 'NONE',  ( -4.243569643749999898, 12.11562500061451608, 27.54997392385601529 ) ) ;
#32105=CARTESIAN_POINT ( 'NONE',  ( 17.02500000122903145, 2.886751345948126879, 4.999999999999999112 ) ) ;
#32107=CARTESIAN_POINT ( 'NONE',  ( 25.94062500061451715, -3.027376345333610441, -5.243569643749999898 ) ) ;
#32109=CARTESIAN_POINT ( 'NONE',  ( 19.50937500061451857, 0.000000000000000000, 5.243569643749999010 ) ) ;
#32110=CARTESIAN_POINT ( 'NONE',  ( 22.08750000122903501, -4.330127018922194537, 2.499999999999995559 ) ) ;
#32111=CARTESIAN_POINT ( 'NONE',  ( 23.46562500061451573, 3.027376345333611329, 5.243569643749999010 ) ) ;
#32112=CARTESIAN_POINT ( 'NONE',  ( 16.95937500061451786, -4.541064518000417216, -2.621784821875001281 ) ) ;
#32113=CARTESIAN_POINT ( 'NONE',  ( 11.42812500061451608, -4.541064518000419881, 2.621784821874995952 ) ) ;
#32114=CARTESIAN_POINT ( 'NONE',  ( 4.243569643749999898, 15.54687500061451644, 32.45002607614398471 ) ) ;
#32115=CARTESIAN_POINT ( 'NONE',  ( 17.05312500061451786, 4.541064518000418104, -2.621784821874998173 ) ) ;
#32116=CARTESIAN_POINT ( 'NONE',  ( 28.67812500061451431, 6.421520780324663323E-16, -5.243569643749999010 ) ) ;
#32119=CARTESIAN_POINT ( 'NONE',  ( 22.80000000000000071, 0.000000000000000000, 4.999999999999998224 ) ) ;
#32120=CARTESIAN_POINT ( 'NONE',  ( 2.121784821875001281, 18.20937500061451786, -26.32496088578401938 ) ) ;
#32121=CARTESIAN_POINT ( 'NONE',  ( 0.000000000000000000, -4.999999999999998224, 0.000000000000000000 ) ) ;
#32122=CARTESIAN_POINT ( 'NONE',  ( 25.49062500061451786, -3.027376345333610441, -5.243569643749999898 ) ) ;
#32123=CARTESIAN_POINT ( 'NONE',  ( 5.840625000614516615, 6.054752690667223547, 3.707466751127219781E-16 ) ) ;
#32124=CARTESIAN_POINT ( 'NONE',  ( 16.46250000122903501, 4.330127018922192761, -2.499999999999997780 ) ) ;
#32125=CARTESIAN_POINT ( 'NONE',  ( 21.44062500061452070, -3.027376345333610441, -5.243569643749999898 ) ) ;
#32126=CARTESIAN_POINT ( 'NONE',  ( 23.06250000000000355, 2.886751345948129099, -4.999999999999998224 ) ) ;
#32127=CARTESIAN_POINT ( 'NONE',  ( 26.72812500061451502, -4.541064518000419881, 2.621784821874995952 ) ) ;
#32128=CARTESIAN_POINT ( 'NONE',  ( 7.265625000614516438, 3.027376345333611329, 5.243569643749999010 ) ) ;
#32129=VERTEX_POINT ( 'NONE', #44971 ) ;
#32130=B_SPLINE_CURVE_WITH_KNOTS ( 'NONE', 3,
 ( #42690, #70760, #3540, #14972, #43431, #43057, #26431, #59292, #4278, #20135 ),
 .UNSPECIFIED., .F., .F.,
 ( 4, 3, 3, 4 ),
 ( 0.000000000000000000, 0.0001572273160846694696, 0.0003144546168236625494, 0.0005074023328272463454 ),
 .UNSPECIFIED. ) ;
#32131=CARTESIAN_POINT ( 'NONE',  ( 23.12812500061451360, -4.541064518000419881, 2.621784821874995952 ) ) ;
#32132=CARTESIAN_POINT ( 'NONE',  ( 6.253125000614517148, 4.541064518000418104, -2.621784821874998173 ) ) ;
#32134=CARTESIAN_POINT ( 'NONE',  ( 3.590625000614518836, 6.054752690667223547, 3.707466751127219781E-16 ) ) ;
#32135=CARTESIAN_POINT ( 'NONE',  ( -3.999999999999999112, 12.91250000122903430, -30.00000000000000000 ) ) ;
#32136=EDGE_CURVE ( 'NONE', #62008, #24437, #8956, .T. ) ;
#32137=DIRECTION ( 'NONE',  ( -0.000000000000000000, -1.000000000000000000, -0.000000000000000000 ) ) ;
#32138=CARTESIAN_POINT ( 'NONE',  ( 10.57500000000000107, 4.330127018922191873, 2.499999999999999556 ) ) ;
#32139=CARTESIAN_POINT ( 'NONE',  ( 12.42187500061451821, -6.054752690667223547, -1.112240025338166033E-15 ) ) ;
#32140=CARTESIAN_POINT ( 'NONE',  ( 5.550000001229032698, -2.886751345948125991, -5.000000000000000000 ) ) ;
#32141=CARTESIAN_POINT ( 'NONE',  ( 14.63437500061451679, -4.541064518000419881, 2.621784821874995952 ) ) ;
#32142=CARTESIAN_POINT ( 'NONE',  ( 5.221875000614519813, -6.054752690667223547, -1.112240025338166033E-15 ) ) ;
#32143=CARTESIAN_POINT ( 'NONE',  ( 1.999999999999998668, 18.50000000000000000, 26.53589838486224650 ) ) ;
#32144=CARTESIAN_POINT ( 'NONE',  ( 19.72499999999999787, -4.330127018922194537, 2.499999999999995559 ) ) ;
#32145=CARTESIAN_POINT ( 'NONE',  ( 13.73437500061451821, -4.541064518000419881, 2.621784821874995952 ) ) ;
#32147=CARTESIAN_POINT ( 'NONE',  ( 22.97812500061451857, 4.541064518000418104, 2.621784821874999949 ) ) ;
#32149=CARTESIAN_POINT ( 'NONE',  ( 2.000000000000001332, 11.60000000000000142, 33.46410161513774995 ) ) ;
#32150=CARTESIAN_POINT ( 'NONE',  ( 30.00000000000000000, 0.000000000000000000, 0.000000000000000000 ) ) ;
#32151=CARTESIAN_POINT ( 'NONE',  ( 23.44687500061451502, 6.054752690667223547, 3.707466751127219781E-16 ) ) ;
#32154=CARTESIAN_POINT ( 'NONE',  ( 4.190625000614518925, -3.027376345333614438, 5.243569643749998122 ) ) ;
#32156=CARTESIAN_POINT ( 'NONE',  ( 23.99062500061451786, -3.027376345333614438, 5.243569643749998122 ) ) ;
#32157=CARTESIAN_POINT ( 'NONE',  ( 17.80312500061451786, -4.541064518000417216, -2.621784821875001281 ) ) ;
#32158=CARTESIAN_POINT ( 'NONE',  ( 14.63437500061451679, -4.541064518000419881, 2.621784821874995952 ) ) ;
#32160=CARTESIAN_POINT ( 'NONE',  ( 28.12500000122902932, 2.886751345948129099, -4.999999999999998224 ) ) ;
#32161=CARTESIAN_POINT ( 'NONE',  ( 6.909375000614518036, 0.000000000000000000, 5.243569643749999010 ) ) ;
#32162=CARTESIAN_POINT ( 'NONE',  ( 16.92187500061451999, -6.054752690667223547, -1.112240025338166033E-15 ) ) ;
#32164=CARTESIAN_POINT ( 'NONE',  ( 24.82499999999999929, 6.123233995736764310E-16, -4.999999999999998224 ) ) ;
#32165=CARTESIAN_POINT ( 'NONE',  ( 16.80000000122903359, -2.886751345948159742, -4.999999999999942268 ) ) ;
#32166=CARTESIAN_POINT ( 'NONE',  ( 25.05937500061451573, -4.541064518000417216, -2.621784821875001281 ) ) ;
#32167=CARTESIAN_POINT ( 'NONE',  ( 16.28437500061452070, 4.541064518000418104, 2.621784821874999949 ) ) ;
#32170=CARTESIAN_POINT ( 'NONE',  ( 8.925000000000002487, -4.330127018922194537, 2.499999999999995559 ) ) ;
#32172=CARTESIAN_POINT ( 'NONE',  ( 20.57812500061451644, 6.421520780324663323E-16, -5.243569643749999010 ) ) ;
#32173=CARTESIAN_POINT ( 'NONE',  ( 8.250000000000000000, 4.330127018922192761, -2.499999999999997780 ) ) ;
#32174=CARTESIAN_POINT ( 'NONE',  ( 3.253125000614518036, 0.000000000000000000, 5.243569643749999010 ) ) ;
#32175=CARTESIAN_POINT ( 'NONE',  ( 19.83750000000000213, -2.886751345948125991, -5.000000000000000000 ) ) ;
#32176=CARTESIAN_POINT ( 'NONE',  ( 18.14062500061451644, -3.027376345333614438, 5.243569643749998122 ) ) ;
#32179=CARTESIAN_POINT ( 'NONE',  ( 24.22500000122903430, 2.886751345948126879, 4.999999999999999112 ) ) ;
#32181=CARTESIAN_POINT ( 'NONE',  ( 28.65937500061451715, -4.541064518000417216, -2.621784821875001281 ) ) ;
#32182=ORIENTED_EDGE ( 'NONE', *, *, #67378, .F. ) ;
#32183=CARTESIAN_POINT ( 'NONE',  ( 17.46562500061451217, 3.027376345333613106, -5.243569643749998122 ) ) ;
#32184=CARTESIAN_POINT ( 'NONE',  ( 24.44062500061451715, -3.027376345333614438, 5.243569643749998122 ) ) ;
#32185=CARTESIAN_POINT ( 'NONE',  ( 24.68437500061451573, 6.421520780324663323E-16, -5.243569643749999010 ) ) ;
#32186=CARTESIAN_POINT ( 'NONE',  ( 9.037499999999999645, -2.886751345948125991, -5.000000000000000000 ) ) ;
#32187=CARTESIAN_POINT ( 'NONE',  ( 11.01562500061451821, -6.054752690667223547, -1.112240025338166033E-15 ) ) ;
#32188=CARTESIAN_POINT ( 'NONE',  ( 27.51562500061451644, 3.027376345333611329, 5.243569643749999010 ) ) ;
#32189=CARTESIAN_POINT ( 'NONE',  ( 18.15937500061451715, 0.000000000000000000, 5.243569643749999010 ) ) ;
#32190=CARTESIAN_POINT ( 'NONE',  ( 19.39687500061451786, 6.054752690667223547, 3.707466751127219781E-16 ) ) ;
#32191=CARTESIAN_POINT ( 'NONE',  ( 3.041898612738912711, -3.968258880967949320, 3.108631698898131734 ) ) ;
#32192=CARTESIAN_POINT ( 'NONE',  ( -4.243569643749997233, 10.89687500061451786, 32.45002607614398471 ) ) ;
#32193=CARTESIAN_POINT ( 'NONE',  ( 22.87500000122903288, 2.886751345948126879, 4.999999999999999112 ) ) ;
#32195=CARTESIAN_POINT ( 'NONE',  ( 13.82812500061451466, 6.421520780324663323E-16, -5.243569643749999010 ) ) ;
#32196=CARTESIAN_POINT ( 'NONE',  ( 7.996875000614519280, -3.027376345333610441, -5.243569643749999898 ) ) ;
#32197=CARTESIAN_POINT ( 'NONE',  ( 7.171875000614517326, 3.027376345333613106, -5.243569643749998122 ) ) ;
#32198=ORIENTED_EDGE ( 'NONE', *, *, #33236, .T. ) ;
#32199=CARTESIAN_POINT ( 'NONE',  ( 28.17187500061451644, -6.054752690667223547, -1.112240025338166033E-15 ) ) ;
#32200=CARTESIAN_POINT ( 'NONE',  ( 19.86562500061451786, 3.027376345333611329, 5.243569643749999010 ) ) ;
#32201=CARTESIAN_POINT ( 'NONE',  ( 23.97187500061451360, 3.027376345333611329, 5.243569643749999010 ) ) ;
#32202=CARTESIAN_POINT ( 'NONE',  ( 20.01562500061451644, -6.054752690667223547, -1.112240025338166033E-15 ) ) ;
#32203=CARTESIAN_POINT ( 'NONE',  ( 2.000000000000001332, 11.60000000000000142, 33.46410161513774995 ) ) ;
#32204=CARTESIAN_POINT ( 'NONE',  ( 25.97812500061451502, 6.421520780324663323E-16, -5.243569643749999010 ) ) ;
#32205=CARTESIAN_POINT ( 'NONE',  ( 8.175000001229031810, -5.773502691896255534, -1.060575238724906372E-15 ) ) ;
#32206=ORIENTED_EDGE ( 'NONE', *, *, #60575, .T. ) ;
#32207=DIRECTION ( 'NONE',  ( 0.000000000000000000, 0.000000000000000000, 1.000000000000000000 ) ) ;
#32208=CARTESIAN_POINT ( 'NONE',  ( -3.999999999999999112, 15.94999999999999929, -30.00000000000000000 ) ) ;
#32209=CARTESIAN_POINT ( 'NONE',  ( 23.28750000122903430, 4.330127018922191873, 2.499999999999999556 ) ) ;
#32211=CARTESIAN_POINT ( 'NONE',  ( 3.984375000614517326, 6.421520780324663323E-16, -5.243569643749999010 ) ) ;
#32212=CARTESIAN_POINT ( 'NONE',  ( 12.71250000000000036, 2.886751345948062486, -5.000000000000113687 ) ) ;
#32213=CARTESIAN_POINT ( 'NONE',  ( 13.67812500061451786, -4.541064518000419881, 2.621784821874995952 ) ) ;
#32214=CARTESIAN_POINT ( 'NONE',  ( 9.121875000614517504, 3.027376345333611329, 5.243569643749999010 ) ) ;
#32215=CARTESIAN_POINT ( 'NONE',  ( 26.81250000122903288, 4.330127018922192761, -2.499999999999997780 ) ) ;
#32216=CARTESIAN_POINT ( 'NONE',  ( 14.52187500061451786, 3.027376345333611329, 5.243569643749999010 ) ) ;
#32217=CARTESIAN_POINT ( 'NONE',  ( 5.034375000614519813, 4.541064518000418104, 2.621784821874999949 ) ) ;
#32218=FACE_OUTER_BOUND ( 'NONE', #59944, .T. ) ;
#32219=CARTESIAN_POINT ( 'NONE',  ( 4.828125000614518214, 6.421520780324663323E-16, -5.243569643749999010 ) ) ;
#32220=CARTESIAN_POINT ( 'NONE',  ( 15.10312500061451502, -4.541064518000417216, -2.621784821875001281 ) ) ;
#32222=CARTESIAN_POINT ( 'NONE',  ( 11.35312500061451679, 0.000000000000000000, 5.243569643749999010 ) ) ;
#32223=CARTESIAN_POINT ( 'NONE',  ( 8.128125000614515372, 4.541064518000418104, 2.621784821874999949 ) ) ;
#32225=CARTESIAN_POINT ( 'NONE',  ( 9.150000000000002132, 4.330127018922192761, -2.499999999999997780 ) ) ;
#32226=CARTESIAN_POINT ( 'NONE',  ( 4.312500001229034652, 4.330127018922192761, -2.499999999999997780 ) ) ;
#32227=CARTESIAN_POINT ( 'NONE',  ( 18.30000000000000071, 0.000000000000000000, 4.999999999999998224 ) ) ;
#32228=CARTESIAN_POINT ( 'NONE',  ( 17.29687500061451999, -3.027376345333614438, 5.243569643749998122 ) ) ;
#32229=CARTESIAN_POINT ( 'NONE',  ( 14.70000000122903394, 5.773502691896255534, 3.535250795749688894E-16 ) ) ;
#32231=CARTESIAN_POINT ( 'NONE',  ( 9.001249775931846008E-16, 16.76562500061451999, -25.09994784771203058 ) ) ;
#32234=CARTESIAN_POINT ( 'NONE',  ( 29.24062500061451431, 6.054752690667223547, 3.707466751127219781E-16 ) ) ;
#32235=FACE_OUTER_BOUND ( 'NONE', #19310, .T. ) ;
#32236=CARTESIAN_POINT ( 'NONE',  ( 29.67187500061451644, 3.027376345333613106, -5.243569643749998122 ) ) ;
#32237=CARTESIAN_POINT ( 'NONE',  ( 16.92187500061451999, -6.054752690667223547, -1.112240025338166033E-15 ) ) ;
#32238=CARTESIAN_POINT ( 'NONE',  ( 26.58750000000000213, -2.886751345948125991, -5.000000000000000000 ) ) ;
#32239=EDGE_CURVE ( 'NONE', #13801, #58433, #40883, .T. ) ;
#32240=CARTESIAN_POINT ( 'NONE',  ( 11.01562500061451821, -6.054752690667223547, -1.112240025338166033E-15 ) ) ;
#32242=CARTESIAN_POINT ( 'NONE',  ( 20.97187500061451715, -6.054752690667223547, -1.112240025338166033E-15 ) ) ;
#32244=CARTESIAN_POINT ( 'NONE',  ( 6.478125000614516793, -4.541064518000419881, 2.621784821874995952 ) ) ;
#32245=CARTESIAN_POINT ( 'NONE',  ( 14.07187500061451679, 3.027376345333611329, 5.243569643749999010 ) ) ;
#32246=VERTEX_POINT ( 'NONE', #6532 ) ;
#32247=CARTESIAN_POINT ( 'NONE',  ( 24.38437500061451502, 4.541064518000418104, 2.621784821874999949 ) ) ;
#32248=CARTESIAN_POINT ( 'NONE',  ( 3.964577175323932057, 3.046748717458610312, -29.45119415667360840 ) ) ;
#32249=CARTESIAN_POINT ( 'NONE',  ( 24.67500000000000071, -4.330127018922194537, 2.499999999999995559 ) ) ;
#32250=CARTESIAN_POINT ( 'NONE',  ( 5.400000000000002132, -4.330127018922190985, -2.500000000000001332 ) ) ;
#32251=CARTESIAN_POINT ( 'NONE',  ( 17.92500000122903359, 2.886751345948126879, 4.999999999999999112 ) ) ;
#32254=ORIENTED_EDGE ( 'NONE', *, *, #18853, .T. ) ;
#32255=CARTESIAN_POINT ( 'NONE',  ( 14.73749999999999893, -2.886751345948129988, 4.999999999999997335 ) ) ;
#32256=CARTESIAN_POINT ( 'NONE',  ( 15.97499999999999964, 4.330127018922191873, 2.499999999999999556 ) ) ;
#32257=CARTESIAN_POINT ( 'NONE',  ( 12.32812500061451821, -4.541064518000419881, 2.621784821874995952 ) ) ;
#32258=( BOUNDED_CURVE ( )  B_SPLINE_CURVE ( 2, ( #47254, #69787, #19154, #72890, #28190, #62160, #22271, #11557, #61788 ),
 .UNSPECIFIED., .F., .F. ) 
 B_SPLINE_CURVE_WITH_KNOTS ( ( 3, 2, 2, 2, 3 ),
 ( 0.6847826086956522174, 0.6884057971014492239, 0.6956521739130434590, 0.7028985507246376940, 0.7065217391304348116 ),
 .UNSPECIFIED. ) 
 CURVE ( )  GEOMETRIC_REPRESENTATION_ITEM ( )  RATIONAL_B_SPLINE_CURVE ( ( 0.9330127018922192983, 0.9330127018922202975, 1.000000000000000000, 0.8660254037844387076, 1.000000000000000000, 0.8660254037844387076, 1.000000000000000000, 0.9330127018922194093, 0.9330127018922194093 ) ) 
 REPRESENTATION_ITEM ( '' )  );
#32260=CARTESIAN_POINT ( 'NONE',  ( -2.000000000000000000, 16.88750000122903572, -33.46410161513775705 ) ) ;
#32261=CARTESIAN_POINT ( 'NONE',  ( 4.243569643749999898, 16.44687500061451857, -27.54997392385601529 ) ) ;
#32262=CARTESIAN_POINT ( 'NONE',  ( 29.66250000122903074, 0.000000000000000000, 4.999999999999998224 ) ) ;
#32264=CARTESIAN_POINT ( 'NONE',  ( 10.35000000000000142, -4.330127018922190985, -2.500000000000001332 ) ) ;
#32266=ORIENTED_EDGE ( 'NONE', *, *, #71724, .F. ) ;
#32267=CARTESIAN_POINT ( 'NONE',  ( -2.121784821874996840, 13.12812500061451715, 33.67503911421598417 ) ) ;
#32268=CARTESIAN_POINT ( 'NONE',  ( 23.35312500061451857, 4.541064518000418104, -2.621784821874998173 ) ) ;
#32269=CARTESIAN_POINT ( 'NONE',  ( 7.285825576177820915E-16, 10.00000000000000000, 36.00000000000000000 ) ) ;
#32271=CARTESIAN_POINT ( 'NONE',  ( 21.04687500061451644, -3.027376345333610441, -5.243569643749999898 ) ) ;
#32272=CARTESIAN_POINT ( 'NONE',  ( 20.05312500061451431, -4.541064518000417216, -2.621784821875001281 ) ) ;
#32273=CARTESIAN_POINT ( 'NONE',  ( -2.121784821874996840, 14.47812500061459318, -26.32496088578401583 ) ) ;
#32274=CARTESIAN_POINT ( 'NONE',  ( 23.32500000122903572, 2.886751345948126879, 4.999999999999999112 ) ) ;
#32275=CARTESIAN_POINT ( 'NONE',  ( 4.078125000614517326, 4.541064518000418104, 2.621784821874999949 ) ) ;
#32277=CARTESIAN_POINT ( 'NONE',  ( 21.81562500061451004, -6.054752690667223547, -1.112240025338166033E-15 ) ) ;
#32280=CARTESIAN_POINT ( 'NONE',  ( 16.13437500061451502, 6.421520780324663323E-16, -5.243569643749999010 ) ) ;
#32281=CARTESIAN_POINT ( 'NONE',  ( 14.14687500061451786, -3.027376345333614438, 5.243569643749998122 ) ) ;
#32282=CARTESIAN_POINT ( 'NONE',  ( 23.52187500061451786, 3.027376345333611329, 5.243569643749999010 ) ) ;
#32283=CARTESIAN_POINT ( 'NONE',  ( -4.243569643749998122, 12.69687500061451857, 32.45002607614398471 ) ) ;
#32284=CARTESIAN_POINT ( 'NONE',  ( 4.003125000614518925, 4.541064518000418104, -2.621784821874998173 ) ) ;
#32285=CARTESIAN_POINT ( 'NONE',  ( 25.90312500061451573, -4.541064518000417216, -2.621784821875001281 ) ) ;
#32286=CARTESIAN_POINT ( 'NONE',  ( 27.02812500061451573, 4.541064518000418104, 2.621784821874999949 ) ) ;
#32288=CARTESIAN_POINT ( 'NONE',  ( -3.999999999999999112, 19.09999999999999787, 30.00000000000000000 ) ) ;
#32289=CARTESIAN_POINT ( 'NONE',  ( 7.359375000614516438, 0.000000000000000000, 5.243569643749999010 ) ) ;
#32291=CARTESIAN_POINT ( 'NONE',  ( 15.37500000122903465, -5.773502691896255534, -1.060575238724906372E-15 ) ) ;
#32292=CARTESIAN_POINT ( 'NONE',  ( 9.637500001229033941, 6.123233995736764310E-16, -4.999999999999998224 ) ) ;
#32293=CARTESIAN_POINT ( 'NONE',  ( 29.40000000122903145, -2.886751345948125991, -5.000000000000000000 ) ) ;
#32296=CARTESIAN_POINT ( 'NONE',  ( 15.15937500061451715, -4.541064518000417216, -2.621784821875001281 ) ) ;
#32299=CARTESIAN_POINT ( 'NONE',  ( 19.86562500061451786, 3.027376345333611329, 5.243569643749999010 ) ) ;
#32300=CARTESIAN_POINT ( 'NONE',  ( 6.178125000614518747, 6.421520780324663323E-16, -5.243569643749999010 ) ) ;
#32301=CARTESIAN_POINT ( 'NONE',  ( 24.08437500061451786, -4.541064518000419881, 2.621784821874995952 ) ) ;
#32302=CARTESIAN_POINT ( 'NONE',  ( 8.353125000614518569, -4.541064518000417216, -2.621784821875001281 ) ) ;
#32304=CARTESIAN_POINT ( 'NONE',  ( 7.125000001229033764, 2.886751345948126879, 4.999999999999999112 ) ) ;
#32306=CARTESIAN_POINT ( 'NONE',  ( 22.67812500061451431, -4.541064518000419881, 2.621784821874995952 ) ) ;
#32307=CARTESIAN_POINT ( 'NONE',  ( 1.999999999999998668, 18.16250000122903074, -33.46410161513775705 ) ) ;
#32308=CARTESIAN_POINT ( 'NONE',  ( 11.17500000122903536, 2.886751345948126879, 4.999999999999999112 ) ) ;
#32309=CARTESIAN_POINT ( 'NONE',  ( 19.04062500061451146, -3.027376345333614438, 5.243569643749998122 ) ) ;
#32310=CARTESIAN_POINT ( 'NONE',  ( 15.02812500061451750, -4.541064518000419881, 2.621784821874995952 ) ) ;
#32312=CARTESIAN_POINT ( 'NONE',  ( 16.87500000000000000, 4.330127018922191873, 2.499999999999999556 ) ) ;
#32313=CARTESIAN_POINT ( 'NONE',  ( 11.10000000122903252, 5.773502691896255534, 3.535250795749688894E-16 ) ) ;
#32314=CARTESIAN_POINT ( 'NONE',  ( 8.090625000614515727, 6.054752690667223547, 3.707466751127219781E-16 ) ) ;
#32315=CARTESIAN_POINT ( 'NONE',  ( 12.14062500061451821, 6.054752690667223547, 3.707466751127219781E-16 ) ) ;
#32316=CARTESIAN_POINT ( 'NONE',  ( 19.80000000122903359, -2.886751345948129988, 4.999999999999997335 ) ) ;
#32317=CARTESIAN_POINT ( 'NONE',  ( 19.80937500061451573, 4.541064518000418104, -2.621784821874998173 ) ) ;
#32318=CARTESIAN_POINT ( 'NONE',  ( 4.629056002857023344, -1.889931353889065413, 4.891133006415133266 ) ) ;
#32319=EDGE_CURVE ( 'NONE', #61054, #23329, #65031, .T. ) ;
#32320=CARTESIAN_POINT ( 'NONE',  ( 6.487500001229034474, 6.123233995736764310E-16, -4.999999999999998224 ) ) ;
#32321=CARTESIAN_POINT ( 'NONE',  ( 5.221875000614519813, -6.054752690667223547, -1.112240025338166033E-15 ) ) ;
#32322=CARTESIAN_POINT ( 'NONE',  ( 22.05937500061451573, 4.541064518000418104, -2.621784821874998173 ) ) ;
#32323=CARTESIAN_POINT ( 'NONE',  ( 18.44062500061451715, 6.054752690667223547, 3.707466751127219781E-16 ) ) ;
#32324=CARTESIAN_POINT ( 'NONE',  ( 23.18437500061451573, -4.541064518000419881, 2.621784821874995952 ) ) ;
#32327=CARTESIAN_POINT ( 'NONE',  ( 29.82187500061451502, 3.027376345333611329, 5.243569643749999010 ) ) ;
#32329=CARTESIAN_POINT ( 'NONE',  ( 14.01562500061451644, 3.027376345333611329, 5.243569643749999010 ) ) ;
#32330=CARTESIAN_POINT ( 'NONE',  ( 12.38437500061451857, -4.541064518000419881, 2.621784821874995952 ) ) ;
#32333=CARTESIAN_POINT ( 'NONE',  ( 23.84062500061451928, 6.054752690667223547, 3.707466751127219781E-16 ) ) ;
#32334=CARTESIAN_POINT ( 'NONE',  ( 11.55000000000000071, 0.000000000000000000, 4.999999999999998224 ) ) ;
#32335=CARTESIAN_POINT ( 'NONE',  ( 30.00000000000000000, 0.000000000000000000, 4.999999999999998224 ) ) ;
#32336=CARTESIAN_POINT ( 'NONE',  ( 14.02499999999999858, 6.123233995736764310E-16, -4.999999999999998224 ) ) ;
#32337=CARTESIAN_POINT ( 'NONE',  ( 23.73750000122903359, 4.330127018922191873, 2.499999999999999556 ) ) ;
#32338=CARTESIAN_POINT ( 'NONE',  ( 18.74062500061451431, -3.027376345333610441, -5.243569643749999898 ) ) ;
#32339=VERTEX_POINT ( 'NONE', #6894 ) ;
#32340=CARTESIAN_POINT ( 'NONE',  ( 21.60000000000000142, -4.330127018922190985, -2.500000000000001332 ) ) ;
#32341=CARTESIAN_POINT ( 'NONE',  ( 23.37187500061451573, 3.027376345333613106, -5.243569643749998122 ) ) ;
#32342=ORIENTED_EDGE ( 'NONE', *, *, #28737, .T. ) ;
#32344=CARTESIAN_POINT ( 'NONE',  ( 10.60312500061451679, -4.541064518000417216, -2.621784821875001281 ) ) ;
#32345=CARTESIAN_POINT ( 'NONE',  ( 4.415625000614518569, 3.027376345333613106, -5.243569643749998122 ) ) ;
#32347=CARTESIAN_POINT ( 'NONE',  ( 26.46562500061451573, 3.027376345333613106, -5.243569643749998122 ) ) ;
#32348=CARTESIAN_POINT ( 'NONE',  ( 16.27499999999999858, 6.123233995736764310E-16, -4.999999999999998224 ) ) ;
#32349=CARTESIAN_POINT ( 'NONE',  ( 23.62500000000000000, 4.330127018922191873, 2.499999999999999556 ) ) ;
#32350=CARTESIAN_POINT ( 'NONE',  ( 30.00000000000000000, 6.123233995736764310E-16, -4.999999999999998224 ) ) ;
#32351=CARTESIAN_POINT ( 'NONE',  ( 7.396875000614519635, -3.027376345333614438, 5.243569643749998122 ) ) ;
#32352=CARTESIAN_POINT ( 'NONE',  ( 18.15937500061451715, 0.000000000000000000, 5.243569643749999010 ) ) ;
#32353=CARTESIAN_POINT ( 'NONE',  ( 28.73437500061451644, 6.421520780324663323E-16, -5.243569643749999010 ) ) ;
#32354=ORIENTED_EDGE ( 'NONE', *, *, #51501, .T. ) ;
#32355=CARTESIAN_POINT ( 'NONE',  ( 27.29062500061451502, -3.027376345333610441, -5.243569643749999898 ) ) ;
#32356=CARTESIAN_POINT ( 'NONE',  ( 27.49687500061451217, 6.054752690667223547, 3.707466751127219781E-16 ) ) ;
#32357=CARTESIAN_POINT ( 'NONE',  ( 2.859375000614519546, 0.000000000000000000, 5.243569643749999010 ) ) ;
#32358=CARTESIAN_POINT ( 'NONE',  ( 13.46249999999999858, -5.773502691896255534, -1.060575238724906372E-15 ) ) ;
#32359=CARTESIAN_POINT ( 'NONE',  ( 10.11562500061451608, -6.054752690667223547, -1.112240025338166033E-15 ) ) ;
#32360=CARTESIAN_POINT ( 'NONE',  ( 30.00000000000000000, 0.000000000000000000, 0.000000000000000000 ) ) ;
#32362=CARTESIAN_POINT ( 'NONE',  ( 28.60312500061451502, -4.541064518000417216, -2.621784821875001281 ) ) ;
#32363=CARTESIAN_POINT ( 'NONE',  ( 15.93750000122903110, 6.123233995736764310E-16, -4.999999999999998224 ) ) ;
#32365=CARTESIAN_POINT ( 'NONE',  ( 6.028125000614517504, -4.541064518000419881, 2.621784821874995952 ) ) ;
#32366=CARTESIAN_POINT ( 'NONE',  ( 22.92187500061451644, 3.027376345333613106, -5.243569643749998122 ) ) ;
#32367=CARTESIAN_POINT ( 'NONE',  ( 4.243569643749999898, 15.99687500061451573, 32.45002607614398471 ) ) ;
#32368=CARTESIAN_POINT ( 'NONE',  ( 20.74687500061451573, 6.054752690667223547, 3.707466751127219781E-16 ) ) ;
#32369=CARTESIAN_POINT ( 'NONE',  ( 5.587500000000003020, 5.773502691896255534, 3.535250795749688894E-16 ) ) ;
#32370=CARTESIAN_POINT ( 'NONE',  ( -3.000416591977282496E-16, 19.74687500061451928, 25.09994784771203058 ) ) ;
#32371=CARTESIAN_POINT ( 'NONE',  ( 13.04062500061451502, 6.054752690667223547, 3.707466751127219781E-16 ) ) ;
#32372=CARTESIAN_POINT ( 'NONE',  ( 4.050000001229035362, -2.886751345948129988, 4.999999999999997335 ) ) ;
#32373=CARTESIAN_POINT ( 'NONE',  ( 6.571875000614517681, -6.054752690667223547, -1.112240025338166033E-15 ) ) ;
#32374=CARTESIAN_POINT ( 'NONE',  ( 3.913234685210329467, 3.112428286967196200, -4.086165593540687091 ) ) ;
#32375=CARTESIAN_POINT ( 'NONE',  ( 10.79062500061451679, 6.054752690667223547, 3.707466751127219781E-16 ) ) ;
#32376=CARTESIAN_POINT ( 'NONE',  ( 15.23437500061451644, 6.421520780324663323E-16, -5.243569643749999010 ) ) ;
#32378=CARTESIAN_POINT ( 'NONE',  ( 20.43750000122903643, 6.123233995736764310E-16, -4.999999999999998224 ) ) ;
#32379=CARTESIAN_POINT ( 'NONE',  ( 7.546875000614517326, -3.027376345333610441, -5.243569643749999898 ) ) ;
#32380=CARTESIAN_POINT ( 'NONE',  ( 12.96562500061451750, 3.027376345333613106, -5.243569643749998122 ) ) ;
#32382=CARTESIAN_POINT ( 'NONE',  ( 21.94687500061451857, -3.027376345333610441, -5.243569643749999898 ) ) ;
#32384=CARTESIAN_POINT ( 'NONE',  ( -3.027546007007307249, 3.984809627175307067, 27.37408915144584398 ) ) ;
#32386=CARTESIAN_POINT ( 'NONE',  ( -2.121784821874996840, 12.73437500061451821, -26.32496088578401583 ) ) ;
#32387=CARTESIAN_POINT ( 'NONE',  ( 14.58750000122903323, 6.123233995736764310E-16, -4.999999999999998224 ) ) ;
#32388=EDGE_CURVE ( 'NONE', #38296, #49458, #12179, .T. ) ;
#32389=CARTESIAN_POINT ( 'NONE',  ( -3.000416591977282496E-16, 15.19062500061451715, -34.90005215228797653 ) ) ;
#32390=CARTESIAN_POINT ( 'NONE',  ( 18.18750000122903288, 6.123233995736764310E-16, -4.999999999999998224 ) ) ;
#32391=CARTESIAN_POINT ( 'NONE',  ( 10.56562500061451715, -6.054752690667223547, -1.112240025338166033E-15 ) ) ;
#32392=VECTOR ( 'NONE', #33410, 1000.000000000000000 ) ;
#32394=CARTESIAN_POINT ( 'NONE',  ( 16.27499999999999858, 6.123233995736764310E-16, -4.999999999999998224 ) ) ;
#32396=CARTESIAN_POINT ( 'NONE',  ( 21.59062500061451928, 6.054752690667223547, 3.707466751127219781E-16 ) ) ;
#32397=CARTESIAN_POINT ( 'NONE',  ( 9.984375000614518214, 4.541064518000418104, 2.621784821874999949 ) ) ;
#32398=EDGE_CURVE ( 'NONE', #70091, #17423, #46704, .T. ) ;
#32399=DIRECTION ( 'NONE',  ( -1.000000000000000000, -0.000000000000000000, -0.000000000000000000 ) ) ;
#32400=CARTESIAN_POINT ( 'NONE',  ( 9.225000001229034297, 2.886751345948129099, -4.999999999999998224 ) ) ;
#32401=CARTESIAN_POINT ( 'NONE',  ( 19.01250000122903216, -4.330127018922190985, -2.500000000000001332 ) ) ;
#32402=CARTESIAN_POINT ( 'NONE',  ( 16.07812500061451289, 6.421520780324663323E-16, -5.243569643749999010 ) ) ;
#32403=EDGE_CURVE ( 'NONE', #43953, #57884, #63399, .T. ) ;
#32404=CARTESIAN_POINT ( 'NONE',  ( 17.16562500061451502, 3.027376345333611329, 5.243569643749999010 ) ) ;
#32405=CARTESIAN_POINT ( 'NONE',  ( 25.31250000122903288, -4.330127018922190985, -2.500000000000001332 ) ) ;
#32406=CIRCLE ( 'NONE', #65397, 5.000000000000000000 ) ;
#32407=CARTESIAN_POINT ( 'NONE',  ( 29.28750000122903074, -4.330127018922194537, 2.499999999999995559 ) ) ;
#32408=CARTESIAN_POINT ( 'NONE',  ( 25.87500000000000000, 4.330127018922191873, 2.499999999999999556 ) ) ;
#32410=VECTOR ( 'NONE', #70941, 1000.000000000000000 ) ;
#32411=CARTESIAN_POINT ( 'NONE',  ( 26.74687500061451573, -3.027376345333614438, 5.243569643749998122 ) ) ;
#32413=CARTESIAN_POINT ( 'NONE',  ( 11.92500000122903181, 2.886751345948129099, -4.999999999999998224 ) ) ;
#32414=CARTESIAN_POINT ( 'NONE',  ( 3.000000000000002665, 0.000000000000000000, 4.999999999999998224 ) ) ;
#32415=( BOUNDED_CURVE ( )  B_SPLINE_CURVE ( 2, ( #39697, #72943, #176, #67412, #17137, #39331, #61845 ),
 .UNSPECIFIED., .F., .F. ) 
 B_SPLINE_CURVE_WITH_KNOTS ( ( 3, 2, 2, 3 ),
 ( 0.2166666666666667296, 0.2194444444444444975, 0.2222222222222222654, 0.2250000000000000611 ),
 .UNSPECIFIED. ) 
 CURVE ( )  GEOMETRIC_REPRESENTATION_ITEM ( )  RATIONAL_B_SPLINE_CURVE ( ( 0.9999999999999973355, 0.8660254037844413721, 1.000000000000000000, 0.8660254037844387076, 1.000000000000000000, 0.8660254037844360431, 1.000000000000002665 ) ) 
 REPRESENTATION_ITEM ( '' )  );
#32417=CARTESIAN_POINT ( 'NONE',  ( 6.384375000614516793, 4.541064518000418104, 2.621784821874999949 ) ) ;
#32418=CARTESIAN_POINT ( 'NONE',  ( 26.31562500061451715, -6.054752690667223547, -1.112240025338166033E-15 ) ) ;
#32419=CARTESIAN_POINT ( 'NONE',  ( 4.869423765992945796, -1.135214599616954256, -5.119209941160161037 ) ) ;
#32420=CARTESIAN_POINT ( 'NONE',  ( 4.000000000000000000, 10.40000000122903323, 32.30940107675849760 ) ) ;
#32422=CARTESIAN_POINT ( 'NONE',  ( 5.221875000614519813, -6.054752690667223547, -1.112240025338166033E-15 ) ) ;
#32423=CARTESIAN_POINT ( 'NONE',  ( 9.721875000614517148, -6.054752690667223547, -1.112240025338166033E-15 ) ) ;
#32424=CARTESIAN_POINT ( 'NONE',  ( 29.44687500061451857, -3.027376345333614438, 5.243569643749998122 ) ) ;
#32425=EDGE_CURVE ( 'NONE', #13717, #57266, #4646, .T. ) ;
#32426=CARTESIAN_POINT ( 'NONE',  ( -3.000416591977282496E-16, 11.59062500061459389, 25.09994784771203058 ) ) ;
#32427=CARTESIAN_POINT ( 'NONE',  ( 21.26249999999999574, 2.886751345948129099, -4.999999999999998224 ) ) ;
#32428=CARTESIAN_POINT ( 'NONE',  ( 29.13749999999999929, -2.886751345948129988, 4.999999999999997335 ) ) ;
#32429=CARTESIAN_POINT ( 'NONE',  ( 5.137500000000000178, 5.773502691896255534, 3.535250795749688894E-16 ) ) ;
#32431=CARTESIAN_POINT ( 'NONE',  ( 17.91562500061451502, 3.027376345333613106, -5.243569643749998122 ) ) ;
#32432=CARTESIAN_POINT ( 'NONE',  ( 10.90312500061451928, 0.000000000000000000, 5.243569643749999010 ) ) ;
#32434=CARTESIAN_POINT ( 'NONE',  ( 7.209375000614519635, 4.541064518000418104, -2.621784821874998173 ) ) ;
#32435=CARTESIAN_POINT ( 'NONE',  ( 23.13749999999999929, 5.773502691896255534, 3.535250795749688894E-16 ) ) ;
#32436=CARTESIAN_POINT ( 'NONE',  ( 19.68750000122903288, 4.330127018922191873, 2.499999999999999556 ) ) ;
#32438=CARTESIAN_POINT ( 'NONE',  ( 15.63749999999999751, -2.886751345948063374, 5.000000000000112799 ) ) ;
#32439=CARTESIAN_POINT ( 'NONE',  ( 8.184375000614515727, 4.541064518000418104, 2.621784821874999949 ) ) ;
#32440=CARTESIAN_POINT ( 'NONE',  ( 12.94687500061451857, -3.027376345333610441, -5.243569643749999898 ) ) ;
#32441=CARTESIAN_POINT ( 'NONE',  ( 24.30937500061451573, 4.541064518000418104, -2.621784821874998173 ) ) ;
#32442=CARTESIAN_POINT ( 'NONE',  ( 0.000000000000000000, 20.00000000000000000, 30.00000000000000000 ) ) ;
#32445=CARTESIAN_POINT ( 'NONE',  ( 17.93437500061451928, 6.421520780324663323E-16, -5.243569643749999010 ) ) ;
#32446=AXIS2_PLACEMENT_3D ( 'NONE', #36770, #59287, #2791 ) ;
#32447=CARTESIAN_POINT ( 'NONE',  ( 9.271875000614516082, -6.054752690667223547, -1.112240025338166033E-15 ) ) ;
#32449=CARTESIAN_POINT ( 'NONE',  ( 21.26249999999999574, 2.886751345948129099, -4.999999999999998224 ) ) ;
#32453=CARTESIAN_POINT ( 'NONE',  ( 12.17812500061451608, 4.541064518000418104, 2.621784821874999949 ) ) ;
#32454=CARTESIAN_POINT ( 'NONE',  ( 28.54687500061451644, -3.027376345333614438, 5.243569643749998122 ) ) ;
#32455=CARTESIAN_POINT ( 'NONE',  ( 6.825000001229035718, -5.773502691896255534, -1.060575238724906372E-15 ) ) ;
#32456=CARTESIAN_POINT ( 'NONE',  ( 28.58437500061451786, -4.541064518000419881, 2.621784821874995952 ) ) ;
#32457=CARTESIAN_POINT ( 'NONE',  ( 11.17500000000000071, -4.330127018922194537, 2.499999999999995559 ) ) ;
#32458=CARTESIAN_POINT ( 'NONE',  ( -1.999999999999997113, 17.93750000122903288, 33.46410161513775705 ) ) ;
#32459=CARTESIAN_POINT ( 'NONE',  ( 11.66250000122903430, 0.000000000000000000, 4.999999999999998224 ) ) ;
#32461=CARTESIAN_POINT ( 'NONE',  ( 22.58437500061451431, 4.541064518000418104, 2.621784821874999949 ) ) ;
#32462=CARTESIAN_POINT ( 'NONE',  ( 17.78437500061451715, -4.541064518000419881, 2.621784821874995952 ) ) ;
#32463=CARTESIAN_POINT ( 'NONE',  ( -5.810221930991193690E-16, 12.23750000000000071, 26.00000000000000355 ) ) ;
#32464=ORIENTED_EDGE ( 'NONE', *, *, #47732, .F. ) ;
#32465=CARTESIAN_POINT ( 'NONE',  ( 16.07812500061451289, 6.421520780324663323E-16, -5.243569643749999010 ) ) ;
#32467=CARTESIAN_POINT ( 'NONE',  ( 28.98750000122903359, 6.123233995736764310E-16, -4.999999999999998224 ) ) ;
#32468=CARTESIAN_POINT ( 'NONE',  ( 18.04687500061451999, 6.054752690667223547, 3.707466751127219781E-16 ) ) ;
#32469=CARTESIAN_POINT ( 'NONE',  ( 5.375648687660713243, 8.434199909737650103, -27.30640515792645928 ) ) ;
#32470=CARTESIAN_POINT ( 'NONE',  ( 19.90312500061451573, 0.000000000000000000, 5.243569643749999010 ) ) ;
#32471=LINE ( 'NONE', #55004, #18529 ) ;
#32472=CARTESIAN_POINT ( 'NONE',  ( 29.40937500061451715, 0.000000000000000000, 5.243569643749999010 ) ) ;
#32473=CARTESIAN_POINT ( 'NONE',  ( -4.243569643749999898, 13.91562500061451679, 27.54997392385601529 ) ) ;
#32474=CARTESIAN_POINT ( 'NONE',  ( 17.48437500061451999, 6.421520780324663323E-16, -5.243569643749999010 ) ) ;
#32475=CARTESIAN_POINT ( 'NONE',  ( 15.22500000122903252, 2.886751345948126879, 4.999999999999999112 ) ) ;
#32477=CARTESIAN_POINT ( 'NONE',  ( -4.243569643749999898, 19.40937500061451715, -30.00000000000000000 ) ) ;
#32478=CARTESIAN_POINT ( 'NONE',  ( 20.25937500061451857, 4.541064518000418104, -2.621784821874998173 ) ) ;
#32479=CARTESIAN_POINT ( 'NONE',  ( 22.27500000122903145, 2.886751345948129099, -4.999999999999998224 ) ) ;
#32481=CARTESIAN_POINT ( 'NONE',  ( 17.44687500061451857, -3.027376345333610441, -5.243569643749999898 ) ) ;
#32482=CARTESIAN_POINT ( 'NONE',  ( 11.20312500061451644, 4.541064518000418104, -2.621784821874998173 ) ) ;
#32483=CARTESIAN_POINT ( 'NONE',  ( -2.121784821874996840, 13.63437500061451857, 33.67503911421598417 ) ) ;
#32484=CARTESIAN_POINT ( 'NONE',  ( 17.27812500061451217, -4.541064518000419881, 2.621784821874995952 ) ) ;
#32486=CARTESIAN_POINT ( 'NONE',  ( 23.81250000000000000, -5.773502691896255534, -1.060575238724906372E-15 ) ) ;
#32487=CARTESIAN_POINT ( 'NONE',  ( 4.243569643749999898, 18.73437500061451644, -30.00000000000000000 ) ) ;
#32488=CARTESIAN_POINT ( 'NONE',  ( 12.48749999999999893, -2.886751345948063374, 5.000000000000112799 ) ) ;
#32489=CARTESIAN_POINT ( 'NONE',  ( 25.67812500061451431, 4.541064518000418104, 2.621784821874999949 ) ) ;
#32490=CARTESIAN_POINT ( 'NONE',  ( 5.728125000614515905, 6.421520780324663323E-16, -5.243569643749999010 ) ) ;
#32491=CARTESIAN_POINT ( 'NONE',  ( 18.26250000122903216, 4.330127018922192761, -2.499999999999997780 ) ) ;
#32492=CARTESIAN_POINT ( 'NONE',  ( 23.16562500061451502, -6.054752690667223547, -1.112240025338166033E-15 ) ) ;
#32493=CARTESIAN_POINT ( 'NONE',  ( 23.92499999999999716, 6.123233995736764310E-16, -4.999999999999998224 ) ) ;
#32495=CARTESIAN_POINT ( 'NONE',  ( 26.27812500061451573, -4.541064518000419881, 2.621784821874995952 ) ) ;
#32496=CARTESIAN_POINT ( 'NONE',  ( 9.290625000614515017, -3.027376345333610441, -5.243569643749999898 ) ) ;
#32497=VERTEX_POINT ( 'NONE', #58568 ) ;
#32498=CARTESIAN_POINT ( 'NONE',  ( 22.34062500061451573, -3.027376345333610441, -5.243569643749999898 ) ) ;
#32499=CARTESIAN_POINT ( 'NONE',  ( 3.103125000614517237, 4.541064518000418104, -2.621784821874998173 ) ) ;
#32500=VECTOR ( 'NONE', #49450, 1000.000000000000000 ) ;
#32502=CARTESIAN_POINT ( 'NONE',  ( -1.071796769724475906, 11.02009619066136636, 25.99999999999999289 ) ) ;
#32503=CARTESIAN_POINT ( 'NONE',  ( -3.999999999999997335, 14.75000000122903288, -27.69059892324149175 ) ) ;
#32504=CARTESIAN_POINT ( 'NONE',  ( 11.47499999999999964, 4.330127018922191873, 2.499999999999999556 ) ) ;
#32505=VECTOR ( 'NONE', #55794, 1000.000000000000000 ) ;
#32506=CARTESIAN_POINT ( 'NONE',  ( 10.92187500061451644, 3.027376345333611329, 5.243569643749999010 ) ) ;
#32507=CARTESIAN_POINT ( 'NONE',  ( 6.937500001229033764, 6.123233995736764310E-16, -4.999999999999998224 ) ) ;
#32508=CARTESIAN_POINT ( 'NONE',  ( 15.34687500061451537, 6.054752690667223547, 3.707466751127219781E-16 ) ) ;
#32509=CARTESIAN_POINT ( 'NONE',  ( 6.721875000614518925, 3.027376345333613106, -5.243569643749998122 ) ) ;
#32511=CARTESIAN_POINT ( 'NONE',  ( 1.626862140677534273E-15, 10.77500000122903323, 34.00000000000000000 ) ) ;
#32512=CARTESIAN_POINT ( 'NONE',  ( 12.42187500061451821, -6.054752690667223547, -1.112240025338166033E-15 ) ) ;
#32513=FACE_OUTER_BOUND ( 'NONE', #28276, .T. ) ;
#32514=CARTESIAN_POINT ( 'NONE',  ( 21.40312500061451573, -4.541064518000417216, -2.621784821875001281 ) ) ;
#32515=CARTESIAN_POINT ( 'NONE',  ( -3.999999999999997335, 12.50000000122903465, -27.69059892324149530 ) ) ;
#32516=CARTESIAN_POINT ( 'NONE',  ( 4.243569643749999898, 18.64062500061459104, 32.45002607614398471 ) ) ;
#32517=CARTESIAN_POINT ( 'NONE',  ( 22.62187500061451573, 3.027376345333611329, 5.243569643749999010 ) ) ;
#32519=CARTESIAN_POINT ( 'NONE',  ( 27.78750000122903074, 4.330127018922191873, 2.499999999999999556 ) ) ;
#32521=CARTESIAN_POINT ( 'NONE',  ( 25.82812500061451644, -4.541064518000419881, 2.621784821874995952 ) ) ;
#32522=CARTESIAN_POINT ( 'NONE',  ( 17.31562500061451715, -6.054752690667223547, -1.112240025338166033E-15 ) ) ;
#32524=CARTESIAN_POINT ( 'NONE',  ( 14.37187500061451928, 3.027376345333613106, -5.243569643749998122 ) ) ;
#32525=CARTESIAN_POINT ( 'NONE',  ( 16.87500000000000000, 4.330127018922191873, 2.499999999999999556 ) ) ;
#32526=CARTESIAN_POINT ( 'NONE',  ( 28.20000000122903216, 5.773502691896255534, 3.535250795749688894E-16 ) ) ;
#32527=CARTESIAN_POINT ( 'NONE',  ( 4.809375000614516615, -4.541064518000417216, -2.621784821875001281 ) ) ;
#32528=CARTESIAN_POINT ( 'NONE',  ( 15.79687500061451821, 6.054752690667223547, 3.707466751127219781E-16 ) ) ;
#32529=CARTESIAN_POINT ( 'NONE',  ( 16.12500000000000000, -4.330127018922194537, 2.499999999999995559 ) ) ;
#32530=EDGE_CURVE ( 'NONE', #50028, #45391, #69377, .T. ) ;
#32531=CARTESIAN_POINT ( 'NONE',  ( 4.725000001229034297, 2.886751345948129099, -4.999999999999998224 ) ) ;
#32532=CARTESIAN_POINT ( 'NONE',  ( 24.27187500061452141, 3.027376345333613106, -5.243569643749998122 ) ) ;
#32533=CARTESIAN_POINT ( 'NONE',  ( 17.52187500061451431, 3.027376345333613106, -5.243569643749998122 ) ) ;
#32535=CARTESIAN_POINT ( 'NONE',  ( 29.13749999999999929, -2.886751345948129988, 4.999999999999997335 ) ) ;
#32536=CARTESIAN_POINT ( 'NONE',  ( 5.962500000000002132, 2.886751345948129099, -4.999999999999998224 ) ) ;
#32538=CARTESIAN_POINT ( 'NONE',  ( 20.76562500061451644, 3.027376345333611329, 5.243569643749999010 ) ) ;
#32539=CARTESIAN_POINT ( 'NONE',  ( 8.625000000000000000, 6.123233995736764310E-16, -4.999999999999998224 ) ) ;
#32540=CARTESIAN_POINT ( 'NONE',  ( 4.903125000614516615, 4.541064518000418104, -2.621784821874998173 ) ) ;
#32541=CARTESIAN_POINT ( 'NONE',  ( 20.24999999999999645, -4.330127018922190985, -2.500000000000001332 ) ) ;
#32543=CARTESIAN_POINT ( 'NONE',  ( 24.33750000122903145, -4.330127018922194537, 2.499999999999995559 ) ) ;
#32544=CARTESIAN_POINT ( 'NONE',  ( 5.192387018522387265, 8.549830518147031100, 33.03071326595781443 ) ) ;
#32545=CARTESIAN_POINT ( 'NONE',  ( 3.037500000000002309, -2.886751345948129988, 4.999999999999997335 ) ) ;
#32548=CARTESIAN_POINT ( 'NONE',  ( 18.29062500061451502, -3.027376345333610441, -5.243569643749999898 ) ) ;
#32549=CARTESIAN_POINT ( 'NONE',  ( 23.27812500061451573, 6.421520780324663323E-16, -5.243569643749999010 ) ) ;
#32550=CARTESIAN_POINT ( 'NONE',  ( 23.67187500061451999, -6.054752690667223547, -1.112240025338166033E-15 ) ) ;
#32551=CARTESIAN_POINT ( 'NONE',  ( 6.524999999999999467, 4.330127018922191873, 2.499999999999999556 ) ) ;
#32552=CARTESIAN_POINT ( 'NONE',  ( 12.81562500061451537, -6.054752690667223547, -1.112240025338166033E-15 ) ) ;
#32553=CARTESIAN_POINT ( 'NONE',  ( 25.64062500061451644, 6.054752690667223547, 3.707466751127219781E-16 ) ) ;
#32554=CARTESIAN_POINT ( 'NONE',  ( 15.27187500061451786, 3.027376345333613106, -5.243569643749998122 ) ) ;
#32555=CARTESIAN_POINT ( 'NONE',  ( 20.40937500061451715, 0.000000000000000000, 5.243569643749999010 ) ) ;
#32556=CARTESIAN_POINT ( 'NONE',  ( 21.11250000122903359, 0.000000000000000000, 4.999999999999998224 ) ) ;
#32557=CARTESIAN_POINT ( 'NONE',  ( 2.121784821875001281, 10.55937500061451750, 33.67503911421598417 ) ) ;
#32558=CARTESIAN_POINT ( 'NONE',  ( 23.92500000122903359, -5.773502691896255534, -1.060575238724906372E-15 ) ) ;
#32560=CARTESIAN_POINT ( 'NONE',  ( 14.80312500061451608, 4.541064518000418104, -2.621784821874998173 ) ) ;
#32561=CARTESIAN_POINT ( 'NONE',  ( 6.871875000614517504, 3.027376345333611329, 5.243569643749999010 ) ) ;
#32562=CARTESIAN_POINT ( 'NONE',  ( 7.359375000614516438, 0.000000000000000000, 5.243569643749999010 ) ) ;
#32564=CARTESIAN_POINT ( 'NONE',  ( 28.09687500061451360, -3.027376345333614438, 5.243569643749998122 ) ) ;
#32565=CARTESIAN_POINT ( 'NONE',  ( 18.85312500061451502, 4.541064518000418104, -2.621784821874998173 ) ) ;
#32566=CARTESIAN_POINT ( 'NONE',  ( 29.62500000122903288, 2.886751345948126879, 4.999999999999999112 ) ) ;
#32567=CARTESIAN_POINT ( 'NONE',  ( 29.46562500061451573, -6.054752690667223547, -1.112240025338166033E-15 ) ) ;
#32568=CARTESIAN_POINT ( 'NONE',  ( 24.04687500061451644, -3.027376345333614438, 5.243569643749998122 ) ) ;
#32569=CARTESIAN_POINT ( 'NONE',  ( 19.37812500061451715, 4.541064518000418104, 2.621784821874999949 ) ) ;
#32570=CARTESIAN_POINT ( 'NONE',  ( -3.999999999999999112, 11.00000000000000178, 30.00000000000000000 ) ) ;
#32571=CARTESIAN_POINT ( 'NONE',  ( 24.14062500061451289, -3.027376345333610441, -5.243569643749999898 ) ) ;
#32572=CARTESIAN_POINT ( 'NONE',  ( 5.700000001229033941, 5.773502691896255534, 3.535250795749688894E-16 ) ) ;
#32573=ORIENTED_EDGE ( 'NONE', *, *, #10710, .T. ) ;
#32574=CARTESIAN_POINT ( 'NONE',  ( 29.06250000000000000, 2.886751345948126879, 4.999999999999999112 ) ) ;
#32575=CARTESIAN_POINT ( 'NONE',  ( -1.999999999999997113, 15.57500000000000284, -26.53589838486224295 ) ) ;
#32576=CARTESIAN_POINT ( 'NONE',  ( 22.57500000122903572, -5.773502691896255534, -1.060575238724906372E-15 ) ) ;
#32578=CARTESIAN_POINT ( 'NONE',  ( 5.259375000614518569, -4.541064518000417216, -2.621784821875001281 ) ) ;
#32579=CARTESIAN_POINT ( 'NONE',  ( 28.97812500061451502, -4.541064518000419881, 2.621784821874995952 ) ) ;
#32580=CARTESIAN_POINT ( 'NONE',  ( 11.65312500061451573, 4.541064518000418104, -2.621784821874998173 ) ) ;
#32581=CARTESIAN_POINT ( 'NONE',  ( 5.746875000614517504, -3.027376345333610441, -5.243569643749999898 ) ) ;
#32582=CARTESIAN_POINT ( 'NONE',  ( 24.18750000122903288, 4.330127018922191873, 2.499999999999999556 ) ) ;
#32583=CARTESIAN_POINT ( 'NONE',  ( 14.85937500061451644, 4.541064518000418104, -2.621784821874998173 ) ) ;
#32584=CARTESIAN_POINT ( 'NONE',  ( 29.01562500061451644, -6.054752690667223547, -1.112240025338166033E-15 ) ) ;
#32585=CARTESIAN_POINT ( 'NONE',  ( 7.950000001229033053, 5.773502691896255534, 3.535250795749688401E-16 ) ) ;
#32586=CARTESIAN_POINT ( 'NONE',  ( 3.028125000614518392, 6.421520780324663323E-16, -5.243569643749999010 ) ) ;
#32587=CARTESIAN_POINT ( 'NONE',  ( 15.25312500061451715, 4.541064518000418104, -2.621784821874998173 ) ) ;
#32589=ORIENTED_EDGE ( 'NONE', *, *, #26409, .T. ) ;
#32590=CARTESIAN_POINT ( 'NONE',  ( 9.103125000614515017, 0.000000000000000000, 5.243569643749999010 ) ) ;
#32591=CARTESIAN_POINT ( 'NONE',  ( 8.203125000614518214, 0.000000000000000000, 5.243569643749999010 ) ) ;
#32593=CARTESIAN_POINT ( 'NONE',  ( 8.699999999999999289, 4.330127018922192761, -2.499999999999997780 ) ) ;
#32594=CARTESIAN_POINT ( 'NONE',  ( 5.025000001229035895, -5.773502691896255534, -1.060575238724906372E-15 ) ) ;
#32595=CARTESIAN_POINT ( 'NONE',  ( 18.75000000000000000, 0.000000000000000000, 4.999999999999998224 ) ) ;
#32596=CARTESIAN_POINT ( 'NONE',  ( 19.50937500061451857, 0.000000000000000000, 5.243569643749999010 ) ) ;
#32597=CARTESIAN_POINT ( 'NONE',  ( 13.57500000122903572, -5.773502691896255534, -1.060575238724906372E-15 ) ) ;
#32599=CARTESIAN_POINT ( 'NONE',  ( -4.243569643749999898, 16.20312500061451644, -30.00000000000000000 ) ) ;
#32601=CARTESIAN_POINT ( 'NONE',  ( 3.486133158594716510E-16, 19.55000000122903359, 26.00000000000000355 ) ) ;
#32602=CARTESIAN_POINT ( 'NONE',  ( 29.12812500061451715, 6.421520780324663323E-16, -5.243569643749999010 ) ) ;
#32603=CARTESIAN_POINT ( 'NONE',  ( 3.999999999999999112, 19.77500000000000213, 30.00000000000000000 ) ) ;
#32604=CARTESIAN_POINT ( 'NONE',  ( 3.999999999999999112, 16.17500000000000071, -30.00000000000000000 ) ) ;
#32605=CARTESIAN_POINT ( 'NONE',  ( 13.05937500061451750, 4.541064518000418104, -2.621784821874998173 ) ) ;
#32606=CARTESIAN_POINT ( 'NONE',  ( 26.17500000000000071, 6.123233995736764310E-16, -4.999999999999998224 ) ) ;
#32607=CARTESIAN_POINT ( 'NONE',  ( 8.953125000614518214, 4.541064518000418104, -2.621784821874998173 ) ) ;
#32609=CARTESIAN_POINT ( 'NONE',  ( 21.08437500061451786, 6.421520780324663323E-16, -5.243569643749999010 ) ) ;
#32611=CARTESIAN_POINT ( 'NONE',  ( 7.565625000614518036, 3.027376345333613106, -5.243569643749998122 ) ) ;
#32612=CARTESIAN_POINT ( 'NONE',  ( 14.33437500061451786, 6.421520780324663323E-16, -5.243569643749999010 ) ) ;
#32614=CARTESIAN_POINT ( 'NONE',  ( 22.69687500061451857, -3.027376345333614438, 5.243569643749998122 ) ) ;
#32615=CARTESIAN_POINT ( 'NONE',  ( 1.838027276006276800, 4.657088507379087083, -26.43727524967973608 ) ) ;
#32617=CARTESIAN_POINT ( 'NONE',  ( 5.325000000000000178, -4.330127018922194537, 2.499999999999995559 ) ) ;
#32618=CARTESIAN_POINT ( 'NONE',  ( 16.27500000122903501, -5.773502691896255534, -1.060575238724906372E-15 ) ) ;
#32619=LINE ( 'NONE', #38152, #64351 ) ;
#32620=CARTESIAN_POINT ( 'NONE',  ( 19.08749999999999858, 5.773502691896255534, 3.535250795749688401E-16 ) ) ;
#32621=ORIENTED_EDGE ( 'NONE', *, *, #68031, .F. ) ;
#32622=CARTESIAN_POINT ( 'NONE',  ( 12.82499999999999929, 4.330127018922191873, 2.499999999999999556 ) ) ;
#32623=CARTESIAN_POINT ( 'NONE',  ( 16.91250000000000142, 2.886751345948126879, 4.999999999999999112 ) ) ;
#32624=CARTESIAN_POINT ( 'NONE',  ( 13.76250000122903394, 4.330127018922192761, -2.499999999999997780 ) ) ;
#32625=CARTESIAN_POINT ( 'NONE',  ( 10.75312500061451715, 4.541064518000418104, -2.621784821874998173 ) ) ;
#32628=CARTESIAN_POINT ( 'NONE',  ( -3.000416591977282496E-16, 13.89687500061451786, -34.90005215228797653 ) ) ;
#32629=CARTESIAN_POINT ( 'NONE',  ( 3.703125000614516882, 0.000000000000000000, 5.243569643749999010 ) ) ;
#32631=CARTESIAN_POINT ( 'NONE',  ( 9.899999999999998579, -4.330127018922190985, -2.500000000000001332 ) ) ;
#32632=DIRECTION ( 'NONE',  ( -1.000000000000000000, -0.000000000000000000, -0.000000000000000000 ) ) ;
#32633=ORIENTED_EDGE ( 'NONE', *, *, #1892, .F. ) ;
#32634=CARTESIAN_POINT ( 'NONE',  ( 24.89062500061451644, -3.027376345333614438, 5.243569643749998122 ) ) ;
#32635=CARTESIAN_POINT ( 'NONE',  ( 4.196964255440878588, -2.717639258240006406, 4.484364939275536699 ) ) ;
#32637=CARTESIAN_POINT ( 'NONE',  ( 21.00937500061451857, -4.541064518000417216, -2.621784821875001281 ) ) ;
#32638=CARTESIAN_POINT ( 'NONE',  ( 18.77812500061451573, 6.421520780324663323E-16, -5.243569643749999010 ) ) ;
#32639=CARTESIAN_POINT ( 'NONE',  ( 2.121784821875001281, 15.00312500061459531, -26.32496088578401938 ) ) ;
#32640=CARTESIAN_POINT ( 'NONE',  ( 6.515625000614516438, -6.054752690667223547, -1.112240025338166033E-15 ) ) ;
#32641=CARTESIAN_POINT ( 'NONE',  ( 5.278125000614516615, 6.421520780324663323E-16, -5.243569643749999010 ) ) ;
#32643=CARTESIAN_POINT ( 'NONE',  ( 20.54062500061451502, -3.027376345333610441, -5.243569643749999898 ) ) ;
#32646=CARTESIAN_POINT ( 'NONE',  ( 15.53437500061451715, -4.541064518000419881, 2.621784821874995952 ) ) ;
#32647=CARTESIAN_POINT ( 'NONE',  ( 14.85937500061451644, 4.541064518000418104, -2.621784821874998173 ) ) ;
#32648=CARTESIAN_POINT ( 'NONE',  ( 22.80937500061451573, -4.541064518000417216, -2.621784821875001281 ) ) ;
#32650=CARTESIAN_POINT ( 'NONE',  ( 4.243569643749999010, 11.57187500061451679, 27.54997392385601174 ) ) ;
#32651=CARTESIAN_POINT ( 'NONE',  ( -1.071796769724491005, 14.62009619066136779, -34.00000000000000000 ) ) ;
#32652=CARTESIAN_POINT ( 'NONE',  ( 27.51562500061451644, 3.027376345333611329, 5.243569643749999010 ) ) ;
#32653=EDGE_CURVE ( 'NONE', #19034, #14527, #24455, .T. ) ;
#32654=CARTESIAN_POINT ( 'NONE',  ( 27.32812500061451644, 6.421520780324663323E-16, -5.243569643749999010 ) ) ;
#32655=CARTESIAN_POINT ( 'NONE',  ( 2.000000000000001332, 16.21250000122903501, -26.53589838486224650 ) ) ;
#32656=CARTESIAN_POINT ( 'NONE',  ( -2.828200636599751609E-16, 19.43750000000000000, 25.38119784648299770 ) ) ;
#32657=AXIS2_PLACEMENT_3D ( 'NONE', #58730, #12591, #1160 ) ;
#32658=CARTESIAN_POINT ( 'NONE',  ( 3.684375000614518836, 4.541064518000418104, 2.621784821874999949 ) ) ;
#32659=CARTESIAN_POINT ( 'NONE',  ( 14.43750000122903288, -4.330127018922194537, 2.499999999999995559 ) ) ;
#32660=CARTESIAN_POINT ( 'NONE',  ( 9.937500001229032875, -4.330127018922194537, 2.499999999999995559 ) ) ;
#32661=CARTESIAN_POINT ( 'NONE',  ( 3.515625000614516882, 3.027376345333613106, -5.243569643749998122 ) ) ;
#32664=CARTESIAN_POINT ( 'NONE',  ( 10.95937500061451964, 0.000000000000000000, 5.243569643749999010 ) ) ;
#32666=VERTEX_POINT ( 'NONE', #25325 ) ;
#32667=CARTESIAN_POINT ( 'NONE',  ( 20.50312500061451715, -4.541064518000417216, -2.621784821875001281 ) ) ;
#32668=CARTESIAN_POINT ( 'NONE',  ( 14.78437500061451715, 6.421520780324663323E-16, -5.243569643749999010 ) ) ;
#32669=CARTESIAN_POINT ( 'NONE',  ( 5.390625000614518214, 6.054752690667223547, 3.707466751127219781E-16 ) ) ;
#32670=CARTESIAN_POINT ( 'NONE',  ( 21.90937500061451715, -4.541064518000417216, -2.621784821875001281 ) ) ;
#32671=CARTESIAN_POINT ( 'NONE',  ( 5.203125000614518214, -4.541064518000417216, -2.621784821875001281 ) ) ;
#32673=CARTESIAN_POINT ( 'NONE',  ( 7.912500001229033408, 4.330127018922192761, -2.499999999999997780 ) ) ;
#32674=CARTESIAN_POINT ( 'NONE',  ( 22.97812500061451857, 4.541064518000418104, 2.621784821874999949 ) ) ;
#32676=CARTESIAN_POINT ( 'NONE',  ( -3.999999999999997335, 18.80000000122903359, -27.69059892324149175 ) ) ;
#32677=CARTESIAN_POINT ( 'NONE',  ( 7.875000001229034652, 2.886751345948129099, -4.999999999999998224 ) ) ;
#32678=CARTESIAN_POINT ( 'NONE',  ( 19.52812500061451573, -4.541064518000419881, 2.621784821874995952 ) ) ;
#32679=CARTESIAN_POINT ( 'NONE',  ( 14.76562500061451821, 3.027376345333613106, -5.243569643749998122 ) ) ;
#32681=CARTESIAN_POINT ( 'NONE',  ( 15.33750000000000036, -2.886751345948125991, -5.000000000000000000 ) ) ;
#32682=CARTESIAN_POINT ( 'NONE',  ( 12.56250000122903465, 0.000000000000000000, 4.999999999999998224 ) ) ;
#32683=CARTESIAN_POINT ( 'NONE',  ( 7.003125000614518036, -4.541064518000417216, -2.621784821875001281 ) ) ;
#32684=CARTESIAN_POINT ( 'NONE',  ( 11.27812500061451573, 4.541064518000418104, 2.621784821874999949 ) ) ;
#32686=CARTESIAN_POINT ( 'NONE',  ( 21.00000000122903288, 5.773502691896255534, 3.535250795749688894E-16 ) ) ;
#32687=CARTESIAN_POINT ( 'NONE',  ( 2.121784821874999061, 13.40937500061451892, -33.67503911421598417 ) ) ;
#32688=CARTESIAN_POINT ( 'NONE',  ( 20.52187500061451786, -6.054752690667223547, -1.112240025338166033E-15 ) ) ;
#32689=CARTESIAN_POINT ( 'NONE',  ( 4.990567482066851746, 0.3502114279239787464, 5.133889258466388661 ) ) ;
#32690=VECTOR ( 'NONE', #7334, 1000.000000000000000 ) ;
#32691=CARTESIAN_POINT ( 'NONE',  ( 5.437500001229035540, -4.330127018922194537, 2.499999999999995559 ) ) ;
#32693=CARTESIAN_POINT ( 'NONE',  ( 3.384375000614517237, -4.541064518000419881, 2.621784821874995952 ) ) ;
#32694=CARTESIAN_POINT ( 'NONE',  ( 21.23437500061451644, 4.541064518000418104, 2.621784821874999949 ) ) ;
#32695=( BOUNDED_CURVE ( )  B_SPLINE_CURVE ( 2, ( #32102, #26565, #29991, #49105, #46631, #1575, #15459, #18533, #41098 ),
 .UNSPECIFIED., .F., .F. ) 
 B_SPLINE_CURVE_WITH_KNOTS ( ( 3, 2, 2, 2, 3 ),
 ( 0.2934782608695652439, 0.2971014492753623060, 0.3043478260869565410, 0.3115942028985507206, 0.3152173913043478382 ),
 .UNSPECIFIED. ) 
 CURVE ( )  GEOMETRIC_REPRESENTATION_ITEM ( )  RATIONAL_B_SPLINE_CURVE ( ( 0.9330127018922194093, 0.9330127018922198534, 1.000000000000000000, 0.8660254037844387076, 1.000000000000000000, 0.8660254037844387076, 1.000000000000000000, 0.9330127018922188542, 0.9330127018922194093 ) ) 
 REPRESENTATION_ITEM ( '' )  );
#32696=CARTESIAN_POINT ( 'NONE',  ( 19.75312500061451360, 4.541064518000418104, -2.621784821874998173 ) ) ;
#32698=CARTESIAN_POINT ( 'NONE',  ( 23.21250000000000213, 2.886751345948126879, 4.999999999999998224 ) ) ;
#32699=CARTESIAN_POINT ( 'NONE',  ( 13.12500000000000178, 6.123233995736764310E-16, -4.999999999999998224 ) ) ;
#32700=CARTESIAN_POINT ( 'NONE',  ( 29.85937500061451644, 0.000000000000000000, 5.243569643749999010 ) ) ;
#32702=CARTESIAN_POINT ( 'NONE',  ( 15.66562500061451857, 3.027376345333613106, -5.243569643749998122 ) ) ;
#32703=CARTESIAN_POINT ( 'NONE',  ( 12.12187500061451573, 3.027376345333613106, -5.243569643749998122 ) ) ;
#32704=VERTEX_POINT ( 'NONE', #8703 ) ;
#32705=CARTESIAN_POINT ( 'NONE',  ( 3.999999999999999112, 17.07499999999999929, -30.00000000000000000 ) ) ;
#32706=CARTESIAN_POINT ( 'NONE',  ( 22.37812500061451360, 6.421520780324663323E-16, -5.243569643749999010 ) ) ;
#32708=CARTESIAN_POINT ( 'NONE',  ( 14.66249999999999787, 2.886751345948193936, 4.999999999999883649 ) ) ;
#32709=CARTESIAN_POINT ( 'NONE',  ( 13.46249999999999858, -5.773502691896255534, -1.060575238724906372E-15 ) ) ;
#32710=CARTESIAN_POINT ( 'NONE',  ( 24.45000000122903572, -2.886751345948125991, -5.000000000000000000 ) ) ;
#32711=CARTESIAN_POINT ( 'NONE',  ( 17.76562500061451644, -6.054752690667223547, -1.112240025338166033E-15 ) ) ;
#32713=CARTESIAN_POINT ( 'NONE',  ( 21.97500000000000142, -4.330127018922194537, 2.499999999999995559 ) ) ;
#32714=CARTESIAN_POINT ( 'NONE',  ( 23.93437500061451573, 4.541064518000418104, 2.621784821874999949 ) ) ;
#32717=CARTESIAN_POINT ( 'NONE',  ( 11.42812500061451608, -4.541064518000419881, 2.621784821874995952 ) ) ;
#32720=CARTESIAN_POINT ( 'NONE',  ( 18.03749999999999787, -2.886751345948125991, -5.000000000000000000 ) ) ;
#32721=CARTESIAN_POINT ( 'NONE',  ( 23.47499999999999787, 6.123233995736764310E-16, -4.999999999999998224 ) ) ;
#32723=CARTESIAN_POINT ( 'NONE',  ( 5.559375000614517504, 0.000000000000000000, 5.243569643749999010 ) ) ;
#32724=CARTESIAN_POINT ( 'NONE',  ( 27.53437500061451360, 4.541064518000418104, 2.621784821874999949 ) ) ;
#32725=VERTEX_POINT ( 'NONE', #48236 ) ;
#32726=CARTESIAN_POINT ( 'NONE',  ( 25.26562500061451289, 3.027376345333611329, 5.243569643749999010 ) ) ;
#32727=CARTESIAN_POINT ( 'NONE',  ( 27.60937500061451644, 0.000000000000000000, 5.243569643749999010 ) ) ;
#32729=CARTESIAN_POINT ( 'NONE',  ( 13.01249999999999929, -5.773502691896255534, -1.060575238724906372E-15 ) ) ;
#32730=CARTESIAN_POINT ( 'NONE',  ( 11.27812500061451573, 4.541064518000418104, 2.621784821874999949 ) ) ;
#32731=CARTESIAN_POINT ( 'NONE',  ( 30.00000000000000000, 0.000000000000000000, 4.999999999999998224 ) ) ;
#32732=CARTESIAN_POINT ( 'NONE',  ( 7.200000000000001954, -4.330127018922190985, -2.500000000000001332 ) ) ;
#32733=CARTESIAN_POINT ( 'NONE',  ( 29.42812500061451431, -4.541064518000419881, 2.621784821874995952 ) ) ;
#32734=CARTESIAN_POINT ( 'NONE',  ( 15.97500000122903430, 2.886751345948129099, -4.999999999999998224 ) ) ;
#32737=CARTESIAN_POINT ( 'NONE',  ( 4.303125000614516971, -4.541064518000417216, -2.621784821875001281 ) ) ;
#32738=CARTESIAN_POINT ( 'NONE',  ( 22.17187500061451644, 3.027376345333611329, 5.243569643749999010 ) ) ;
#32739=CARTESIAN_POINT ( 'NONE',  ( -2.121784821874999949, 14.83437500061451786, 26.32496088578401938 ) ) ;
#32740=CARTESIAN_POINT ( 'NONE',  ( 21.94687500061451857, -3.027376345333610441, -5.243569643749999898 ) ) ;
#32741=CARTESIAN_POINT ( 'NONE',  ( 29.44687500061451857, -3.027376345333614438, 5.243569643749998122 ) ) ;
#32742=CARTESIAN_POINT ( 'NONE',  ( -2.121784821874996840, 18.58437500061451786, 33.67503911421598417 ) ) ;
#32743=CARTESIAN_POINT ( 'NONE',  ( 9.365625000614519635, 3.027376345333613106, -5.243569643749998122 ) ) ;
#32744=CARTESIAN_POINT ( 'NONE',  ( 2.925000001229034918, 2.886751345948129099, -4.999999999999998224 ) ) ;
#32745=CARTESIAN_POINT ( 'NONE',  ( 7.509375000614517681, -4.541064518000417216, -2.621784821875001281 ) ) ;
#32746=CARTESIAN_POINT ( 'NONE',  ( 3.999999999999998668, 15.76250000000000107, -32.30940107675850470 ) ) ;
#32747=CARTESIAN_POINT ( 'NONE',  ( 10.56562500061451715, -6.054752690667223547, -1.112240025338166033E-15 ) ) ;
#32748=CARTESIAN_POINT ( 'NONE',  ( 15.34687500061451537, 6.054752690667223547, 3.707466751127219781E-16 ) ) ;
#32750=CARTESIAN_POINT ( 'NONE',  ( 21.26250000122903572, -4.330127018922190985, -2.500000000000001332 ) ) ;
#32751=CARTESIAN_POINT ( 'NONE',  ( 7.771875000614516971, 3.027376345333611329, 5.243569643749999010 ) ) ;
#32752=CARTESIAN_POINT ( 'NONE',  ( 10.11562500061451608, -6.054752690667223547, -1.112240025338166033E-15 ) ) ;
#32753=EDGE_CURVE ( 'NONE', #30305, #30532, #42691, .T. ) ;
#32755=CARTESIAN_POINT ( 'NONE',  ( 19.54687500061451644, -3.027376345333614438, 5.243569643749998122 ) ) ;
#32756=CARTESIAN_POINT ( 'NONE',  ( 25.53750000122903074, 4.330127018922191873, 2.499999999999999556 ) ) ;
#32757=CARTESIAN_POINT ( 'NONE',  ( -4.243569643749999898, 19.80312500061451786, -30.00000000000000000 ) ) ;
#32758=CARTESIAN_POINT ( 'NONE',  ( 29.10937500061451644, -4.541064518000417216, -2.621784821875001281 ) ) ;
#32759=CARTESIAN_POINT ( 'NONE',  ( 9.001249775931846008E-16, 10.97187500061451715, -25.09994784771203058 ) ) ;
#32760=CARTESIAN_POINT ( 'NONE',  ( 15.11250000122903359, 4.330127018922192761, -2.499999999999997780 ) ) ;
#32761=CARTESIAN_POINT ( 'NONE',  ( -4.243569643749999898, 14.36562500061451786, -32.45002607614398471 ) ) ;
#32762=CARTESIAN_POINT ( 'NONE',  ( 15.60000000122903607, 5.773502691896255534, 3.535250795749688894E-16 ) ) ;
#32763=CARTESIAN_POINT ( 'NONE',  ( 9.815625000614518925, 3.027376345333613106, -5.243569643749998122 ) ) ;
#32764=ORIENTED_EDGE ( 'NONE', *, *, #13900, .T. ) ;
#32765=CARTESIAN_POINT ( 'NONE',  ( 13.35000000000000142, 0.000000000000000000, 4.999999999999998224 ) ) ;
#32767=CARTESIAN_POINT ( 'NONE',  ( 23.46562500061451573, 3.027376345333611329, 5.243569643749999010 ) ) ;
#32768=CARTESIAN_POINT ( 'NONE',  ( 10.77187500061451786, 3.027376345333612662, -5.243569643749998122 ) ) ;
#32770=CARTESIAN_POINT ( 'NONE',  ( 10.87500000122903288, -5.773502691896255534, -1.060575238724906372E-15 ) ) ;
#32771=CARTESIAN_POINT ( 'NONE',  ( 18.97500000122903074, -5.773502691896255534, -1.060575238724906372E-15 ) ) ;
#32772=CARTESIAN_POINT ( 'NONE',  ( 16.04062500061451857, -3.027376345333610441, -5.243569643749999898 ) ) ;
#32773=CARTESIAN_POINT ( 'NONE',  ( 17.72812500061451502, -4.541064518000419881, 2.621784821874995952 ) ) ;
#32774=CARTESIAN_POINT ( 'NONE',  ( 26.25000000122903288, -2.886751345948125991, -5.000000000000000000 ) ) ;
#32775=CARTESIAN_POINT ( 'NONE',  ( 28.20000000122903216, 5.773502691896255534, 3.535250795749688894E-16 ) ) ;
#32776=CARTESIAN_POINT ( 'NONE',  ( 21.82499999999999574, 4.330127018922191873, 2.499999999999999556 ) ) ;
#32778=CARTESIAN_POINT ( 'NONE',  ( 25.73437500061451644, 4.541064518000418104, 2.621784821874999949 ) ) ;
#32779=CARTESIAN_POINT ( 'NONE',  ( -1.999999999999997113, 16.02500000000000213, 33.46410161513775705 ) ) ;
#32780=CARTESIAN_POINT ( 'NONE',  ( 11.62500000122903465, 2.886751345948126879, 4.999999999999999112 ) ) ;
#32781=CARTESIAN_POINT ( 'NONE',  ( 27.98437500061451289, 4.541064518000418104, 2.621784821874999949 ) ) ;
#32783=CARTESIAN_POINT ( 'NONE',  ( 5.521875000614517859, 3.027376345333611329, 5.243569643749999010 ) ) ;
#32784=CARTESIAN_POINT ( 'NONE',  ( 26.09062500061451573, 6.054752690667223547, 3.707466751127219781E-16 ) ) ;
#32785=CARTESIAN_POINT ( 'NONE',  ( 4.771875000614516971, -6.054752690667223547, -1.112240025338166033E-15 ) ) ;
#32787=CARTESIAN_POINT ( 'NONE',  ( 10.20937500061451786, -4.541064518000417216, -2.621784821875001281 ) ) ;
#32788=CARTESIAN_POINT ( 'NONE',  ( 22.23750000122903003, 6.123233995736764310E-16, -4.999999999999998224 ) ) ;
#32789=CARTESIAN_POINT ( 'NONE',  ( 3.946875000614517681, -3.027376345333610441, -5.243569643749999898 ) ) ;
#32790=CARTESIAN_POINT ( 'NONE',  ( 7.884375000614517681, -4.541064518000419881, 2.621784821874995952 ) ) ;
#32791=CARTESIAN_POINT ( 'NONE',  ( 28.65937500061451715, -4.541064518000417216, -2.621784821875001281 ) ) ;
#32792=CARTESIAN_POINT ( 'NONE',  ( 2.121784821874999061, 12.00312500061459531, 26.32496088578401583 ) ) ;
#32793=CARTESIAN_POINT ( 'NONE',  ( 20.40000000000000213, 4.330127018922192761, -2.499999999999997780 ) ) ;
#32795=CARTESIAN_POINT ( 'NONE',  ( 29.06250000000000000, 2.886751345948126879, 4.999999999999999112 ) ) ;
#32796=CARTESIAN_POINT ( 'NONE',  ( 4.012500000000001954, -5.773502691896255534, -1.060575238724906372E-15 ) ) ;
#32797=ADVANCED_FACE ( 'NONE', ( #37139 ), #59667, .F. ) ;
#32799=CARTESIAN_POINT ( 'NONE',  ( 17.31562500061451715, -6.054752690667223547, -1.112240025338166033E-15 ) ) ;
#32800=CARTESIAN_POINT ( 'NONE',  ( 7.940625000614518036, -3.027376345333610441, -5.243569643749999898 ) ) ;
#32802=CARTESIAN_POINT ( 'NONE',  ( 7.021875000614518747, -6.054752690667223547, -1.112240025338166033E-15 ) ) ;
#32803=CARTESIAN_POINT ( 'NONE',  ( 16.83750000122903145, 6.123233995736764310E-16, -4.999999999999998224 ) ) ;
#32804=CARTESIAN_POINT ( 'NONE',  ( 7.546875000614517326, -3.027376345333610441, -5.243569643749999898 ) ) ;
#32805=CARTESIAN_POINT ( 'NONE',  ( 12.87187500061451750, -6.054752690667223547, -1.112240025338166033E-15 ) ) ;
#32806=CARTESIAN_POINT ( 'NONE',  ( 23.07187500061451857, 3.027376345333611329, 5.243569643749999010 ) ) ;
#32808=EDGE_LOOP ( 'NONE', ( #56553, #27895, #55249, #45585 ) ) ;
#32810=CARTESIAN_POINT ( 'NONE',  ( 17.82187500061451502, -6.054752690667223547, -1.112240025338166033E-15 ) ) ;
#32811=CARTESIAN_POINT ( 'NONE',  ( 9.609375000614518214, 0.000000000000000000, 5.243569643749999010 ) ) ;
#32813=CARTESIAN_POINT ( 'NONE',  ( 21.30000000000000071, 4.330127018922192761, -2.499999999999997780 ) ) ;
#32817=CARTESIAN_POINT ( 'NONE',  ( 13.30312500061451786, -4.541064518000417216, -2.621784821875001281 ) ) ;
#32818=CARTESIAN_POINT ( 'NONE',  ( 3.374999999999999556, 4.330127018922191873, 2.499999999999999556 ) ) ;
#32819=CARTESIAN_POINT ( 'NONE',  ( -3.999999999999997335, 19.25000000122903288, -27.69059892324149530 ) ) ;
#32820=CARTESIAN_POINT ( 'NONE',  ( 28.02187500061451431, 3.027376345333611329, 5.243569643749999010 ) ) ;
#32821=CARTESIAN_POINT ( 'NONE',  ( 10.87500000000000000, 6.123233995736764310E-16, -4.999999999999998224 ) ) ;
#32822=CARTESIAN_POINT ( 'NONE',  ( -3.999999999999999556, 16.47500000122903430, 27.69059892324149530 ) ) ;
#32823=CARTESIAN_POINT ( 'NONE',  ( 8.925000001229033586, 2.886751345948126879, 4.999999999999999112 ) ) ;
#32824=B_SPLINE_CURVE_WITH_KNOTS ( 'NONE', 3,
 ( #13864, #48591, #3529, #19763, #14227, #14590, #19388, #8690, #53393, #53765 ),
 .UNSPECIFIED., .F., .F.,
 ( 4, 3, 3, 4 ),
 ( 5.217251150924370361E-16, 0.0001572577921159111416, 0.0003064946508897742989, 0.0004559760873501511732 ),
 .UNSPECIFIED. ) ;
#32825=CARTESIAN_POINT ( 'NONE',  ( 21.42187500061451644, -6.054752690667223547, -1.112240025338166033E-15 ) ) ;
#32826=CARTESIAN_POINT ( 'NONE',  ( 13.69687500061451679, -3.027376345333614438, 5.243569643749998122 ) ) ;
#32827=LINE ( 'NONE', #44659, #10036 ) ;
#32829=CARTESIAN_POINT ( 'NONE',  ( 16.64062500061451289, 6.054752690667223547, 3.707466751127219781E-16 ) ) ;
#32830=CARTESIAN_POINT ( 'NONE',  ( 28.05000000122903359, -2.886751345948125991, -5.000000000000000000 ) ) ;
#32831=CARTESIAN_POINT ( 'NONE',  ( 15.34687500061451537, 6.054752690667223547, 3.707466751127219781E-16 ) ) ;
#32833=CARTESIAN_POINT ( 'NONE',  ( 16.22812500061451857, 4.541064518000418104, 2.621784821874999949 ) ) ;
#32835=CARTESIAN_POINT ( 'NONE',  ( 29.33437500061451431, 4.541064518000418104, 2.621784821874999949 ) ) ;
#32836=CARTESIAN_POINT ( 'NONE',  ( -2.121784821874996840, 11.77812500061451750, 33.67503911421598417 ) ) ;
#32837=CARTESIAN_POINT ( 'NONE',  ( 18.34687500061451715, -3.027376345333610441, -5.243569643749999898 ) ) ;
#32838=CARTESIAN_POINT ( 'NONE',  ( 13.80000000122903181, 5.773502691896255534, 3.535250795749688894E-16 ) ) ;
#32840=CARTESIAN_POINT ( 'NONE',  ( 3.317152244841671926, -3.741199378463153646, 3.674032409778095420 ) ) ;
#32841=CARTESIAN_POINT ( 'NONE',  ( 19.84687500061451360, 6.054752690667223547, 3.707466751127219781E-16 ) ) ;
#32842=CARTESIAN_POINT ( 'NONE',  ( 21.33750000122903145, 6.123233995736764310E-16, -4.999999999999998224 ) ) ;
#32843=CARTESIAN_POINT ( 'NONE',  ( 18.19687500061451502, -3.027376345333614438, 5.243569643749998122 ) ) ;
#32844=CARTESIAN_POINT ( 'NONE',  ( 13.26562500061451644, -6.054752690667223547, -1.112240025338166033E-15 ) ) ;
#32845=CARTESIAN_POINT ( 'NONE',  ( -3.000416591977282496E-16, 12.09687500061451715, 25.09994784771203058 ) ) ;
#32846=CARTESIAN_POINT ( 'NONE',  ( 18.55312500061451431, 0.000000000000000000, 5.243569643749999010 ) ) ;
#32847=ORIENTED_EDGE ( 'NONE', *, *, #35944, .T. ) ;
#32848=ORIENTED_EDGE ( 'NONE', *, *, #6200, .F. ) ;
#32849=CARTESIAN_POINT ( 'NONE',  ( 19.50000000000000000, 4.330127018922192761, -2.499999999999997780 ) ) ;
#32850=CARTESIAN_POINT ( 'NONE',  ( 7.162500001229032520, 0.000000000000000000, 4.999999999999998224 ) ) ;
#32851=CARTESIAN_POINT ( 'NONE',  ( 25.26562500061451289, 3.027376345333611329, 5.243569643749999010 ) ) ;
#32852=CARTESIAN_POINT ( 'NONE',  ( 5.278125000614516615, 6.421520780324663323E-16, -5.243569643749999010 ) ) ;
#32853=CARTESIAN_POINT ( 'NONE',  ( 17.21250000122903145, -4.330127018922190985, -2.500000000000001332 ) ) ;
#32854=EDGE_CURVE ( 'NONE', #72158, #885, #38617, .T. ) ;
#32855=CARTESIAN_POINT ( 'NONE',  ( 23.20312500061451644, -4.541064518000417216, -2.621784821875001281 ) ) ;
#32856=CARTESIAN_POINT ( 'NONE',  ( 22.42500000000000071, -4.330127018922194537, 2.499999999999995559 ) ) ;
#32858=CARTESIAN_POINT ( 'NONE',  ( 24.81562500061451715, 3.027376345333611329, 5.243569643749999010 ) ) ;
#32859=CARTESIAN_POINT ( 'NONE',  ( 5.090625000614516615, -3.027376345333614438, 5.243569643749998122 ) ) ;
#32860=EDGE_LOOP ( 'NONE', ( #10097, #66465, #46663, #19637 ) ) ;
#32861=CARTESIAN_POINT ( 'NONE',  ( 29.69999999999999574, -4.330127018922190985, -2.500000000000001332 ) ) ;
#32862=CARTESIAN_POINT ( 'NONE',  ( 4.003125000614518925, 4.541064518000418104, -2.621784821874998173 ) ) ;
#32864=CARTESIAN_POINT ( 'NONE',  ( 4.000000000000000000, 12.98749999999999893, 32.30940107675849760 ) ) ;
#32865=CARTESIAN_POINT ( 'NONE',  ( -3.999999999999999112, 14.26250000122903572, -30.00000000000000000 ) ) ;
#32866=CARTESIAN_POINT ( 'NONE',  ( -2.121784821874999949, 18.43437500061451928, -33.67503911421598417 ) ) ;
#32867=CARTESIAN_POINT ( 'NONE',  ( 10.08749999999999858, 5.773502691896255534, 3.535250795749688894E-16 ) ) ;
#32868=CARTESIAN_POINT ( 'NONE',  ( 12.15937500061451892, 4.541064518000418104, -2.621784821874998173 ) ) ;
#32869=CARTESIAN_POINT ( 'NONE',  ( 7.575000001229033053, 2.886751345948126879, 4.999999999999999112 ) ) ;
#32870=CARTESIAN_POINT ( 'NONE',  ( 12.98437500061451821, 6.421520780324663323E-16, -5.243569643749999010 ) ) ;
#32871=CARTESIAN_POINT ( 'NONE',  ( 6.946875000614517681, -3.027376345333614438, 5.243569643749998122 ) ) ;
#32873=FACE_OUTER_BOUND ( 'NONE', #57085, .T. ) ;
#32874=CARTESIAN_POINT ( 'NONE',  ( 9.571875000614518569, 3.027376345333611329, 5.243569643749999010 ) ) ;
#32875=CARTESIAN_POINT ( 'NONE',  ( 20.50312500061451715, -4.541064518000417216, -2.621784821875001281 ) ) ;
#32877=CARTESIAN_POINT ( 'NONE',  ( -4.243569643749999898, 19.76562500061459104, 27.54997392385601529 ) ) ;
#32878=CARTESIAN_POINT ( 'NONE',  ( 24.27187500061452141, 3.027376345333613106, -5.243569643749998122 ) ) ;
#32880=CARTESIAN_POINT ( 'NONE',  ( 28.46250000122903145, -4.330127018922190985, -2.500000000000001332 ) ) ;
#32882=CARTESIAN_POINT ( 'NONE',  ( 25.60312500061451502, 4.541064518000418104, -2.621784821874998173 ) ) ;
#32883=CARTESIAN_POINT ( 'NONE',  ( 16.94062500061451715, -3.027376345333610441, -5.243569643749999898 ) ) ;
#32885=CARTESIAN_POINT ( 'NONE',  ( 13.62187500061451750, 3.027376345333611329, 5.243569643749999010 ) ) ;
#32886=CARTESIAN_POINT ( 'NONE',  ( 7.347880794884120722E-16, 20.00000000000000000, 36.00000000000000000 ) ) ;
#32887=CARTESIAN_POINT ( 'NONE',  ( 26.85000000122903430, 5.773502691896255534, 3.535250795749688894E-16 ) ) ;
#32888=CARTESIAN_POINT ( 'NONE',  ( 0.000000000000000000, 20.00000000000000000, 30.00000000000000000 ) ) ;
#32889=CARTESIAN_POINT ( 'NONE',  ( 14.33437500061451786, 6.421520780324663323E-16, -5.243569643749999010 ) ) ;
#32890=CARTESIAN_POINT ( 'NONE',  ( 15.03749999999999964, 5.773502691896255534, 3.535250795749688401E-16 ) ) ;
#32892=CARTESIAN_POINT ( 'NONE',  ( 4.425000001229032698, 2.886751345948126879, 4.999999999999999112 ) ) ;
#32893=CARTESIAN_POINT ( 'NONE',  ( 24.34687500061451715, 6.054752690667223547, 3.707466751127219781E-16 ) ) ;
#32894=CARTESIAN_POINT ( 'NONE',  ( 17.14687500061451786, 6.054752690667223547, 3.707466751127219781E-16 ) ) ;
#32896=CARTESIAN_POINT ( 'NONE',  ( 27.75000000000000000, 0.000000000000000000, 4.999999999999998224 ) ) ;
#32897=CARTESIAN_POINT ( 'NONE',  ( 2.887500001229035274, 6.123233995736764310E-16, -4.999999999999998224 ) ) ;
#32898=CARTESIAN_POINT ( 'NONE',  ( 6.112499999999999822, 2.886751345948126879, 4.999999999999999112 ) ) ;
#32900=CARTESIAN_POINT ( 'NONE',  ( 19.71562500061451928, 3.027376345333613106, -5.243569643749998122 ) ) ;
#32901=CARTESIAN_POINT ( 'NONE',  ( 9.825000000000001066, -4.330127018922194537, 2.499999999999995559 ) ) ;
#32903=CARTESIAN_POINT ( 'NONE',  ( 4.753125000614515372, -4.541064518000417216, -2.621784821875001281 ) ) ;
#32904=( BOUNDED_CURVE ( )  B_SPLINE_CURVE ( 2, ( #24524, #57051, #6819, #17880, #46710, #68163, #63680, #52246, #6457 ),
 .UNSPECIFIED., .F., .F. ) 
 B_SPLINE_CURVE_WITH_KNOTS ( ( 3, 2, 2, 2, 3 ),
 ( 0.4021739130434782705, 0.4057971014492753881, 0.4130434782608695676, 0.4202898550724637472, 0.4239130434782608647 ),
 .UNSPECIFIED. ) 
 CURVE ( )  GEOMETRIC_REPRESENTATION_ITEM ( )  RATIONAL_B_SPLINE_CURVE ( ( 0.9330127018922194093, 0.9330127018922194093, 1.000000000000000000, 0.8660254037844387076, 1.000000000000000000, 0.8660254037844387076, 1.000000000000000000, 0.9330127018922194093, 0.9330127018922194093 ) ) 
 REPRESENTATION_ITEM ( '' )  );
#32905=CARTESIAN_POINT ( 'NONE',  ( 17.17500000000000071, 6.123233995736764310E-16, -4.999999999999998224 ) ) ;
#32906=CARTESIAN_POINT ( 'NONE',  ( 15.67500000122903359, 2.886751345948060266, 5.000000000000114575 ) ) ;
#32907=CARTESIAN_POINT ( 'NONE',  ( 20.77500000122903145, -5.773502691896255534, -1.060575238724906372E-15 ) ) ;
#32909=CARTESIAN_POINT ( 'NONE',  ( 28.69687500061451502, -3.027376345333610441, -5.243569643749999898 ) ) ;
#32910=EDGE_LOOP ( 'NONE', ( #37934, #56952, #72288, #27552 ) ) ;
#32911=CARTESIAN_POINT ( 'NONE',  ( 16.22812500061451857, 4.541064518000418104, 2.621784821874999949 ) ) ;
#32912=CARTESIAN_POINT ( 'NONE',  ( 25.22812500061451502, 4.541064518000418104, 2.621784821874999949 ) ) ;
#32913=CARTESIAN_POINT ( 'NONE',  ( 21.87187500061451573, -6.054752690667223547, -1.112240025338166033E-15 ) ) ;
#32914=CARTESIAN_POINT ( 'NONE',  ( 7.237500000000000711, -2.886751345948125991, -5.000000000000000000 ) ) ;
#32915=CARTESIAN_POINT ( 'NONE',  ( 10.56562500061451715, -6.054752690667223547, -1.112240025338166033E-15 ) ) ;
#32916=CARTESIAN_POINT ( 'NONE',  ( 27.74062500061451431, -3.027376345333610441, -5.243569643749999898 ) ) ;
#32917=CARTESIAN_POINT ( 'NONE',  ( 14.48437500061451821, 4.541064518000418104, 2.621784821874999949 ) ) ;
#32918=CARTESIAN_POINT ( 'NONE',  ( 19.17187500061451999, -6.054752690667223547, -1.112240025338166033E-15 ) ) ;
#32919=CARTESIAN_POINT ( 'NONE',  ( 4.000000000000000000, 11.75000000122903643, -27.69059892324149885 ) ) ;
#32920=CARTESIAN_POINT ( 'NONE',  ( 4.243569643749999898, 10.14687500061451786, 32.45002607614398471 ) ) ;
#32921=CARTESIAN_POINT ( 'NONE',  ( 21.97500000122903074, 2.886751345948126879, 4.999999999999999112 ) ) ;
#32923=CARTESIAN_POINT ( 'NONE',  ( 11.12812500061451715, 6.421520780324663323E-16, -5.243569643749999010 ) ) ;
#32924=CARTESIAN_POINT ( 'NONE',  ( 7.959375000614516971, -4.541064518000417216, -2.621784821875001281 ) ) ;
#32925=CARTESIAN_POINT ( 'NONE',  ( 7.134375000614516793, 6.421520780324663323E-16, -5.243569643749999010 ) ) ;
#32927=CARTESIAN_POINT ( 'NONE',  ( 28.54687500061451644, -3.027376345333614438, 5.243569643749998122 ) ) ;
#32928=CARTESIAN_POINT ( 'NONE',  ( 19.37812500061451715, 4.541064518000418104, 2.621784821874999949 ) ) ;
#32929=CARTESIAN_POINT ( 'NONE',  ( 28.53750000122903074, 6.123233995736764310E-16, -4.999999999999998224 ) ) ;
#32930=CARTESIAN_POINT ( 'NONE',  ( 3.759375000614517681, 0.000000000000000000, 5.243569643749999010 ) ) ;
#32931=CARTESIAN_POINT ( 'NONE',  ( 24.49687500061451573, -3.027376345333614438, 5.243569643749998122 ) ) ;
#32932=CARTESIAN_POINT ( 'NONE',  ( 20.42812500061451431, -4.541064518000419881, 2.621784821874995952 ) ) ;
#32933=CARTESIAN_POINT ( 'NONE',  ( 4.243569643749999898, 18.69687500061451857, 32.45002607614398471 ) ) ;
#32934=CARTESIAN_POINT ( 'NONE',  ( 23.84062500061451928, 6.054752690667223547, 3.707466751127219781E-16 ) ) ;
#32935=CARTESIAN_POINT ( 'NONE',  ( 3.675000001229035362, -5.773502691896255534, -1.060575238724906372E-15 ) ) ;
#32936=VERTEX_POINT ( 'NONE', #55603 ) ;
#32937=CARTESIAN_POINT ( 'NONE',  ( 4.465851277537014496, 2.248593419656078840, -4.736966354317482697 ) ) ;
#32938=CARTESIAN_POINT ( 'NONE',  ( -2.000000000000000000, 15.42500000000000071, -33.46410161513775705 ) ) ;
#32940=CARTESIAN_POINT ( 'NONE',  ( 4.134375000614517681, 4.541064518000418104, 2.621784821874999949 ) ) ;
#32941=CARTESIAN_POINT ( 'NONE',  ( 11.72812500061451857, 4.541064518000418104, 2.621784821874999949 ) ) ;
#32942=CARTESIAN_POINT ( 'NONE',  ( 7.021875000614518747, -6.054752690667223547, -1.112240025338166033E-15 ) ) ;
#32943=CARTESIAN_POINT ( 'NONE',  ( 25.46250000122903501, 4.330127018922192761, -2.499999999999997780 ) ) ;
#32944=CARTESIAN_POINT ( 'NONE',  ( 15.53437500061451715, -4.541064518000419881, 2.621784821874995952 ) ) ;
#32945=CARTESIAN_POINT ( 'NONE',  ( 28.45312500061451289, 0.000000000000000000, 5.243569643749999010 ) ) ;
#32946=CARTESIAN_POINT ( 'NONE',  ( 29.09999999999999787, 0.000000000000000000, 4.999999999999998224 ) ) ;
#32947=CARTESIAN_POINT ( 'NONE',  ( 25.77187500061451075, 3.027376345333611329, 5.243569643749999010 ) ) ;
#32949=CARTESIAN_POINT ( 'NONE',  ( 12.81562500061451537, -6.054752690667223547, -1.112240025338166033E-15 ) ) ;
#32951=CARTESIAN_POINT ( 'NONE',  ( 10.90312500061451928, 0.000000000000000000, 5.243569643749999010 ) ) ;
#32952=CARTESIAN_POINT ( 'NONE',  ( 8.840625000614515727, -3.027376345333610441, -5.243569643749999898 ) ) ;
#32954=CARTESIAN_POINT ( 'NONE',  ( 9.637499999999999289, 5.773502691896255534, 3.535250795749688894E-16 ) ) ;
#32955=EDGE_CURVE ( 'NONE', #61789, #51427, #11764, .T. ) ;
#32956=CARTESIAN_POINT ( 'NONE',  ( 3.037500001229032964, 4.330127018922191873, 2.499999999999999556 ) ) ;
#32957=CARTESIAN_POINT ( 'NONE',  ( 17.25000000000000000, 4.330127018922192761, -2.499999999999997780 ) ) ;
#32958=CARTESIAN_POINT ( 'NONE',  ( 18.72187500061451360, -6.054752690667223547, -1.112240025338166033E-15 ) ) ;
#32959=CARTESIAN_POINT ( 'NONE',  ( 14.77500000122903501, 2.886751345948126879, 4.999999999999999112 ) ) ;
#32961=CARTESIAN_POINT ( 'NONE',  ( -4.243569643749999898, 15.75312500061451537, -30.00000000000000000 ) ) ;
#32962=CARTESIAN_POINT ( 'NONE',  ( 17.28750000122903430, 6.123233995736764310E-16, -4.999999999999998224 ) ) ;
#32963=CARTESIAN_POINT ( 'NONE',  ( 29.46562500061451573, -6.054752690667223547, -1.112240025338166033E-15 ) ) ;
#32964=DIRECTION ( 'NONE',  ( 0.000000000000000000, 0.000000000000000000, 1.000000000000000000 ) ) ;
#32966=CARTESIAN_POINT ( 'NONE',  ( 12.79687500061451821, -3.027376345333614438, 5.243569643749998122 ) ) ;
#32967=CARTESIAN_POINT ( 'NONE',  ( 25.98750000000000071, -2.886751345948129988, 4.999999999999997335 ) ) ;
#32968=CARTESIAN_POINT ( 'NONE',  ( 8.878125000614515372, 6.421520780324663323E-16, -5.243569643749999010 ) ) ;
#32970=CARTESIAN_POINT ( 'NONE',  ( 20.85937500061451644, 0.000000000000000000, 5.243569643749999010 ) ) ;
#32972=CARTESIAN_POINT ( 'NONE',  ( 7.265625000614516438, 3.027376345333611329, 5.243569643749999010 ) ) ;
#32973=CARTESIAN_POINT ( 'NONE',  ( 9.834375000614517859, 6.421520780324663323E-16, -5.243569643749999010 ) ) ;
#32974=VERTEX_POINT ( 'NONE', #26064 ) ;
#32975=CARTESIAN_POINT ( 'NONE',  ( 20.97187500061451715, -6.054752690667223547, -1.112240025338166033E-15 ) ) ;
#32976=CARTESIAN_POINT ( 'NONE',  ( 3.859048791629765773, 3.180512981247727300, -31.08635514026660474 ) ) ;
#32978=CARTESIAN_POINT ( 'NONE',  ( 4.349999999999999645, 0.000000000000000000, 4.999999999999998224 ) ) ;
#32979=CARTESIAN_POINT ( 'NONE',  ( 14.62500000122903288, 2.886751345948129099, -4.999999999999998224 ) ) ;
#32982=ORIENTED_EDGE ( 'NONE', *, *, #17622, .T. ) ;
#32983=CARTESIAN_POINT ( 'NONE',  ( 12.00000000000000000, 0.000000000000000000, 4.999999999999998224 ) ) ;
#32984=CARTESIAN_POINT ( 'NONE',  ( 16.76249999999999929, 2.886751345948129099, -4.999999999999998224 ) ) ;
#32985=CARTESIAN_POINT ( 'NONE',  ( 12.56250000122903465, 0.000000000000000000, 4.999999999999998224 ) ) ;
#32986=CARTESIAN_POINT ( 'NONE',  ( 10.52812500061451750, -4.541064518000419881, 2.621784821874995952 ) ) ;
#32987=ORIENTED_EDGE ( 'NONE', *, *, #42238, .F. ) ;
#32988=CARTESIAN_POINT ( 'NONE',  ( 9.862500000000000711, -5.773502691896255534, -1.060575238724906372E-15 ) ) ;
#32989=CARTESIAN_POINT ( 'NONE',  ( 18.45000000122903216, -2.886751345948096681, 5.000000000000054179 ) ) ;
#32990=CARTESIAN_POINT ( 'NONE',  ( 2.121784821875001281, 14.15937500061451715, -26.32496088578401938 ) ) ;
#32991=CARTESIAN_POINT ( 'NONE',  ( 3.590625000614518836, 6.054752690667223547, 3.707466751127219781E-16 ) ) ;
#32993=CARTESIAN_POINT ( 'NONE',  ( 8.925000000000002487, -4.330127018922194537, 2.499999999999995559 ) ) ;
#32994=CARTESIAN_POINT ( 'NONE',  ( 3.900000001229035451, 5.773502691896255534, 3.535250795749688401E-16 ) ) ;
#32995=ORIENTED_EDGE ( 'NONE', *, *, #33946, .T. ) ;
#32996=CARTESIAN_POINT ( 'NONE',  ( 24.96562500061451573, -6.054752690667223547, -1.112240025338166033E-15 ) ) ;
#32997=CARTESIAN_POINT ( 'NONE',  ( 1.071796769724489895, 13.56740381056766687, -34.00000000000000000 ) ) ;
#32999=CARTESIAN_POINT ( 'NONE',  ( 21.79687500061451644, -3.027376345333614438, 5.243569643749998122 ) ) ;
#33000=CARTESIAN_POINT ( 'NONE',  ( 16.75312500061451715, 0.000000000000000000, 5.243569643749999010 ) ) ;
#33001=CARTESIAN_POINT ( 'NONE',  ( -4.243569643749999898, 12.15312500061459389, -30.00000000000000000 ) ) ;
#33002=CARTESIAN_POINT ( 'NONE',  ( 5.878125000614517148, 4.541064518000418104, 2.621784821874999949 ) ) ;
#33003=CARTESIAN_POINT ( 'NONE',  ( 28.76250000122903216, 0.000000000000000000, 4.999999999999998224 ) ) ;
#33005=CARTESIAN_POINT ( 'NONE',  ( 20.24062500061451786, 6.054752690667223547, 3.707466751127219781E-16 ) ) ;
#33008=CARTESIAN_POINT ( 'NONE',  ( 14.18437500061451750, -4.541064518000419881, 2.621784821874995952 ) ) ;
#33009=CARTESIAN_POINT ( 'NONE',  ( 13.99687500061451928, 6.054752690667223547, 3.707466751127219781E-16 ) ) ;
#33010=CARTESIAN_POINT ( 'NONE',  ( 21.79687500061451644, -3.027376345333614438, 5.243569643749998122 ) ) ;
#33012=CARTESIAN_POINT ( 'NONE',  ( 4.243569643749999010, 12.02187500061451786, 27.54997392385601174 ) ) ;
#33013=CARTESIAN_POINT ( 'NONE',  ( 3.628125000614518036, 4.541064518000418104, 2.621784821874999949 ) ) ;
#33014=CARTESIAN_POINT ( 'NONE',  ( 25.75312500061451715, 0.000000000000000000, 5.243569643749999010 ) ) ;
#33015=CARTESIAN_POINT ( 'NONE',  ( 26.65312500061451573, 0.000000000000000000, 5.243569643749999010 ) ) ;
#33017=CARTESIAN_POINT ( 'NONE',  ( 3.999999999999999112, 18.42500000000000071, 30.00000000000000000 ) ) ;
#33018=CARTESIAN_POINT ( 'NONE',  ( 5.821875000614519458, 3.027376345333613106, -5.243569643749998122 ) ) ;
#33020=CARTESIAN_POINT ( 'NONE',  ( 12.90000000122903145, 5.773502691896255534, 3.535250795749688894E-16 ) ) ;
#33021=CARTESIAN_POINT ( 'NONE',  ( 8.250000001229034652, -2.886751345948125991, -5.000000000000000000 ) ) ;
#33022=CARTESIAN_POINT ( 'NONE',  ( 2.915625000614516793, -6.054752690667223547, -1.112240025338166033E-15 ) ) ;
#33025=CARTESIAN_POINT ( 'NONE',  ( 11.89687500061451608, -3.027376345333614438, 5.243569643749998122 ) ) ;
#33027=ORIENTED_EDGE ( 'NONE', *, *, #56499, .F. ) ;
#33028=CARTESIAN_POINT ( 'NONE',  ( 20.95312500061451999, -4.541064518000417216, -2.621784821875001281 ) ) ;
#33029=CARTESIAN_POINT ( 'NONE',  ( 12.72187500061451537, 3.027376345333611329, 5.243569643749999010 ) ) ;
#33030=CARTESIAN_POINT ( 'NONE',  ( 5.465625000614517504, 3.027376345333611329, 5.243569643749999010 ) ) ;
#33031=CARTESIAN_POINT ( 'NONE',  ( 22.62187500061451573, 3.027376345333611329, 5.243569643749999010 ) ) ;
#33032=CARTESIAN_POINT ( 'NONE',  ( 5.465625000614517504, 3.027376345333611329, 5.243569643749999010 ) ) ;
#33033=CARTESIAN_POINT ( 'NONE',  ( 6.637500001229035718, 4.330127018922191873, 2.499999999999999556 ) ) ;
#33034=CARTESIAN_POINT ( 'NONE',  ( 6.675000001229034474, 2.886751345948126879, 4.999999999999999112 ) ) ;
#33035=CARTESIAN_POINT ( 'NONE',  ( 20.31562500061451715, 3.027376345333611329, 5.243569643749999010 ) ) ;
#33036=CARTESIAN_POINT ( 'NONE',  ( 2.000000000000001332, 17.56250000122903288, -26.53589838486224650 ) ) ;
#33037=CARTESIAN_POINT ( 'NONE',  ( 7.912500001229033408, 4.330127018922192761, -2.499999999999997780 ) ) ;
#33038=CARTESIAN_POINT ( 'NONE',  ( 16.37812500061451715, -4.541064518000419881, 2.621784821874995952 ) ) ;
#33039=CARTESIAN_POINT ( 'NONE',  ( 14.80312500061451608, 4.541064518000418104, -2.621784821874998173 ) ) ;
#33041=CARTESIAN_POINT ( 'NONE',  ( 15.75000000000000000, -4.330127018922190985, -2.500000000000001332 ) ) ;
#33042=CARTESIAN_POINT ( 'NONE',  ( 12.48750000122903359, 4.330127018922191873, 2.499999999999999556 ) ) ;
#33043=CARTESIAN_POINT ( 'NONE',  ( 8.353125000614518569, -4.541064518000417216, -2.621784821875001281 ) ) ;
#33044=CARTESIAN_POINT ( 'NONE',  ( 10.64062500061451644, -3.027376345333610441, -5.243569643749999898 ) ) ;
#33046=CARTESIAN_POINT ( 'NONE',  ( 21.67500000122903359, -5.773502691896255534, -1.060575238724906372E-15 ) ) ;
#33047=CARTESIAN_POINT ( 'NONE',  ( -4.243569643749999898, 12.65937500061451715, -30.00000000000000000 ) ) ;
#33048=DIRECTION ( 'NONE',  ( -0.000000000000000000, -1.000000000000000000, -0.000000000000000000 ) ) ;
#33049=CARTESIAN_POINT ( 'NONE',  ( 4.537500001229034297, -4.330127018922194537, 2.499999999999995559 ) ) ;
#33050=CARTESIAN_POINT ( 'NONE',  ( 3.796875000614517326, -3.027376345333614438, 5.243569643749998122 ) ) ;
#33051=CARTESIAN_POINT ( 'NONE',  ( 20.89687500061452141, -3.027376345333614438, 5.243569643749998122 ) ) ;
#33052=( BOUNDED_CURVE ( )  B_SPLINE_CURVE ( 2, ( #54146, #10172, #25699, #60766, #14238, #60030, #71501, #54872, #48235 ),
 .UNSPECIFIED., .F., .F. ) 
 B_SPLINE_CURVE_WITH_KNOTS ( ( 3, 2, 2, 2, 3 ),
 ( 0.8586956521739130821, 0.8623188405797101996, 0.8695652173913043237, 0.8768115942028985588, 0.8804347826086956763 ),
 .UNSPECIFIED. ) 
 CURVE ( )  GEOMETRIC_REPRESENTATION_ITEM ( )  RATIONAL_B_SPLINE_CURVE ( ( 0.9330127018922194093, 0.9330127018922194093, 1.000000000000000000, 0.8660254037844387076, 1.000000000000000000, 0.8660254037844387076, 1.000000000000000000, 0.9330127018922194093, 0.9330127018922194093 ) ) 
 REPRESENTATION_ITEM ( '' )  );
#33053=CARTESIAN_POINT ( 'NONE',  ( 16.71562500061451573, 3.027376345333611329, 5.243569643749999010 ) ) ;
#33055=CARTESIAN_POINT ( 'NONE',  ( -3.999999999999997335, 15.53750000000000142, -27.69059892324149530 ) ) ;
#33057=CARTESIAN_POINT ( 'NONE',  ( 28.84687500061452070, 6.054752690667223547, 3.707466751127219781E-16 ) ) ;
#33059=CARTESIAN_POINT ( 'NONE',  ( 14.39062500061451821, 6.054752690667223547, 3.707466751127219781E-16 ) ) ;
#33060=CARTESIAN_POINT ( 'NONE',  ( 14.07187500061451679, 3.027376345333611329, 5.243569643749999010 ) ) ;
#33062=CARTESIAN_POINT ( 'NONE',  ( 3.999999999999998668, 17.11250000000000071, -32.30940107675850470 ) ) ;
#33063=CARTESIAN_POINT ( 'NONE',  ( 21.74062500061451431, -3.027376345333614438, 5.243569643749998122 ) ) ;
#33064=CARTESIAN_POINT ( 'NONE',  ( -1.999999999999997113, 11.63750000122903394, -26.53589838486224295 ) ) ;
#33065=CARTESIAN_POINT ( 'NONE',  ( 12.03749999999999964, -2.886751345948129988, 4.999999999999997335 ) ) ;
#33066=CARTESIAN_POINT ( 'NONE',  ( 21.00000000122903288, 5.773502691896255534, 3.535250795749688894E-16 ) ) ;
#33067=CARTESIAN_POINT ( 'NONE',  ( 16.60312500061451857, 4.541064518000418104, -2.621784821874998173 ) ) ;
#33069=ORIENTED_EDGE ( 'NONE', *, *, #16136, .F. ) ;
#33070=CARTESIAN_POINT ( 'NONE',  ( 21.11249999999999716, -5.773502691896255534, -1.060575238724906372E-15 ) ) ;
#33071=CARTESIAN_POINT ( 'NONE',  ( 22.28437500061451715, -4.541064518000419881, 2.621784821874995952 ) ) ;
#33072=CARTESIAN_POINT ( 'NONE',  ( 27.32812500061451644, 6.421520780324663323E-16, -5.243569643749999010 ) ) ;
#33074=VERTEX_POINT ( 'NONE', #4640 ) ;
#33075=CARTESIAN_POINT ( 'NONE',  ( 3.999999999999999112, 17.97500000000000142, -30.00000000000000000 ) ) ;
#33076=CARTESIAN_POINT ( 'NONE',  ( 10.82812500061451644, 4.541064518000418104, 2.621784821874999949 ) ) ;
#33079=CARTESIAN_POINT ( 'NONE',  ( 17.73750000000000071, 5.773502691896255534, 3.535250795749688894E-16 ) ) ;
#33080=CARTESIAN_POINT ( 'NONE',  ( 24.71250000000000213, -5.773502691896255534, -1.060575238724906372E-15 ) ) ;
#33081=CARTESIAN_POINT ( 'NONE',  ( 4.096875000614518925, 6.054752690667223547, 3.707466751127219781E-16 ) ) ;
#33082=CARTESIAN_POINT ( 'NONE',  ( 27.98437500061451289, 4.541064518000418104, 2.621784821874999949 ) ) ;
#33084=CARTESIAN_POINT ( 'NONE',  ( 26.99062500061451431, 6.054752690667223547, 3.707466751127219781E-16 ) ) ;
#33085=CARTESIAN_POINT ( 'NONE',  ( 25.99687500061451928, -3.027376345333610441, -5.243569643749999898 ) ) ;
#33086=CARTESIAN_POINT ( 'NONE',  ( -4.243569643749998122, 17.59062500061459389, -27.54997392385601174 ) ) ;
#33087=CARTESIAN_POINT ( 'NONE',  ( 14.43750000000000000, -2.886751345948125991, -5.000000000000000000 ) ) ;
#33088=CARTESIAN_POINT ( 'NONE',  ( 12.14062500061451821, 6.054752690667223547, 3.707466751127219781E-16 ) ) ;
#33090=DIRECTION ( 'NONE',  ( 0.000000000000000000, 0.000000000000000000, -1.000000000000000000 ) ) ;
#33091=CARTESIAN_POINT ( 'NONE',  ( 27.92812500061451431, 4.541064518000418104, 2.621784821874999949 ) ) ;
#33092=CARTESIAN_POINT ( 'NONE',  ( 15.71250000122903501, 0.000000000000000000, 4.999999999999998224 ) ) ;
#33095=CARTESIAN_POINT ( 'NONE',  ( 5.728125000614515905, 6.421520780324663323E-16, -5.243569643749999010 ) ) ;
#33096=CARTESIAN_POINT ( 'NONE',  ( 22.09687500061451715, 6.054752690667223547, 3.707466751127219781E-16 ) ) ;
#33097=CARTESIAN_POINT ( 'NONE',  ( -2.121784821874999949, 13.93437500061451750, 26.32496088578401938 ) ) ;
#33098=CARTESIAN_POINT ( 'NONE',  ( 22.58437500061451431, 4.541064518000418104, 2.621784821874999949 ) ) ;
#33099=CARTESIAN_POINT ( 'NONE',  ( 3.487500000000000711, -2.886751345948129988, 4.999999999999997335 ) ) ;
#33100=CARTESIAN_POINT ( 'NONE',  ( 4.243569643749999010, 19.22187500061452070, 27.54997392385601174 ) ) ;
#33101=CARTESIAN_POINT ( 'NONE',  ( 8.840625000614515727, -3.027376345333610441, -5.243569643749999898 ) ) ;
#33102=CARTESIAN_POINT ( 'NONE',  ( 1.999999999999998668, 17.26250000122903572, 26.53589838486224650 ) ) ;
#33103=CARTESIAN_POINT ( 'NONE',  ( 6.646875000614518747, -3.027376345333610441, -5.243569643749999898 ) ) ;
#33105=CARTESIAN_POINT ( 'NONE',  ( 8.615625000614517859, 3.027376345333611329, 5.243569643749999010 ) ) ;
#33106=CARTESIAN_POINT ( 'NONE',  ( 13.17187500061451999, 3.027376345333611329, 5.243569643749999010 ) ) ;
#33108=CARTESIAN_POINT ( 'NONE',  ( 19.83750000122903145, -4.330127018922194537, 2.499999999999995559 ) ) ;
#33109=CARTESIAN_POINT ( 'NONE',  ( 7.696875000614516793, 6.054752690667223547, 3.707466751127219781E-16 ) ) ;
#33110=CARTESIAN_POINT ( 'NONE',  ( 10.67812500061451608, 6.421520780324663323E-16, -5.243569643749999010 ) ) ;
#33111=CARTESIAN_POINT ( 'NONE',  ( 6.290625000614517681, 6.054752690667223547, 3.707466751127219781E-16 ) ) ;
#33113=CARTESIAN_POINT ( 'NONE',  ( 18.72187500061451360, -6.054752690667223547, -1.112240025338166033E-15 ) ) ;
#33114=CARTESIAN_POINT ( 'NONE',  ( 4.500855584045652336, 2.177941268590406043, 4.634382331106658093 ) ) ;
#33115=( BOUNDED_CURVE ( )  B_SPLINE_CURVE ( 2, ( #28764, #57192, #68664, #69027, #29494, #56829, #12138 ),
 .UNSPECIFIED., .F., .F. ) 
 B_SPLINE_CURVE_WITH_KNOTS ( ( 3, 2, 2, 3 ),
 ( 0.9341357058143047176, 0.9361111111111111160, 0.9388888888888888840, 0.9405958805770093800 ),
 .UNSPECIFIED. ) 
 CURVE ( )  GEOMETRIC_REPRESENTATION_ITEM ( )  RATIONAL_B_SPLINE_CURVE ( ( 0.9449585719455479982, 0.9047245142793810535, 1.000000000000000000, 0.8660254037844387076, 1.000000000000000000, 0.9176703320226651250, 0.9365266264699128040 ) ) 
 REPRESENTATION_ITEM ( '' )  );
#33116=CARTESIAN_POINT ( 'NONE',  ( 12.40312500061451573, -4.541064518000417216, -2.621784821875001281 ) ) ;
#33117=CARTESIAN_POINT ( 'NONE',  ( 28.32187500061451502, 3.027376345333612662, -5.243569643749998122 ) ) ;
#33118=CARTESIAN_POINT ( 'NONE',  ( 4.243569643749999010, 12.02187500061451786, -32.45002607614398471 ) ) ;
#33119=CARTESIAN_POINT ( 'NONE',  ( 12.07500000122903216, 2.886751345948126879, 4.999999999999999112 ) ) ;
#33120=CARTESIAN_POINT ( 'NONE',  ( 4.243569643749999010, 14.21562500061451928, -32.45002607614398471 ) ) ;
#33121=CARTESIAN_POINT ( 'NONE',  ( 14.13750000122903394, 6.123233995736764310E-16, -4.999999999999998224 ) ) ;
#33122=CARTESIAN_POINT ( 'NONE',  ( 10.26562500061451644, 3.027376345333613106, -5.243569643749998122 ) ) ;
#33123=ORIENTED_EDGE ( 'NONE', *, *, #28491, .F. ) ;
#33124=CARTESIAN_POINT ( 'NONE',  ( 14.43750000000000000, -2.886751345948125991, -5.000000000000000000 ) ) ;
#33126=CARTESIAN_POINT ( 'NONE',  ( 22.97812500061451857, 4.541064518000418104, 2.621784821874999949 ) ) ;
#33127=CARTESIAN_POINT ( 'NONE',  ( 7.884375000614517681, -4.541064518000419881, 2.621784821874995952 ) ) ;
#33128=CARTESIAN_POINT ( 'NONE',  ( 10.91250000122903252, -4.330127018922190985, -2.500000000000001332 ) ) ;
#33129=CARTESIAN_POINT ( 'NONE',  ( 17.47500000122903430, 2.886751345948126879, 4.999999999999999112 ) ) ;
#33130=CARTESIAN_POINT ( 'NONE',  ( 16.11562500061451786, 3.027376345333613106, -5.243569643749998122 ) ) ;
#33131=CARTESIAN_POINT ( 'NONE',  ( 17.95312500061451644, 4.541064518000418104, -2.621784821874998173 ) ) ;
#33132=CARTESIAN_POINT ( 'NONE',  ( 25.72500000122903074, -5.773502691896255534, -1.060575238724906372E-15 ) ) ;
#33133=( BOUNDED_CURVE ( )  B_SPLINE_CURVE ( 2, ( #27281, #20619, #10285, #26547, #49446, #37258, #20989 ),
 .UNSPECIFIED., .F., .F. ) 
 B_SPLINE_CURVE_WITH_KNOTS ( ( 3, 2, 2, 3 ),
 ( 0.000000000000000000, 0.002777777777777771812, 0.005555555555555543625, 0.008333333333333315870 ),
 .UNSPECIFIED. ) 
 CURVE ( )  GEOMETRIC_REPRESENTATION_ITEM ( )  RATIONAL_B_SPLINE_CURVE ( ( 1.000000000000000000, 0.8660254037844387076, 1.000000000000000000, 0.8660254037844387076, 1.000000000000000000, 0.8660254037844395958, 0.9999999999999991118 ) ) 
 REPRESENTATION_ITEM ( '' )  );
#33134=CARTESIAN_POINT ( 'NONE',  ( 27.67500000122903359, 2.886751345948129099, -4.999999999999998224 ) ) ;
#33135=CARTESIAN_POINT ( 'NONE',  ( 21.75000000000000000, 4.330127018922192761, -2.499999999999997780 ) ) ;
#33137=CARTESIAN_POINT ( 'NONE',  ( 25.43437500061451573, -4.541064518000419881, 2.621784821874995952 ) ) ;
#33138=CARTESIAN_POINT ( 'NONE',  ( 25.72500000122903074, -5.773502691896255534, -1.060575238724906372E-15 ) ) ;
#33139=CARTESIAN_POINT ( 'NONE',  ( 11.88750000122903216, 6.123233995736764310E-16, -4.999999999999998224 ) ) ;
#33140=CARTESIAN_POINT ( 'NONE',  ( 28.24687500061451573, -3.027376345333610441, -5.243569643749999898 ) ) ;
#33141=CARTESIAN_POINT ( 'NONE',  ( 22.68750000000000000, 5.773502691896255534, 3.535250795749688401E-16 ) ) ;
#33142=CARTESIAN_POINT ( 'NONE',  ( 6.159375000614517148, -4.541064518000417216, -2.621784821875001281 ) ) ;
#33143=CARTESIAN_POINT ( 'NONE',  ( 22.60312500061451857, 0.000000000000000000, 5.243569643749999010 ) ) ;
#33144=( BOUNDED_CURVE ( )  B_SPLINE_CURVE ( 2, ( #46379, #18640, #53001, #41204, #63712, #53364, #30831 ),
 .UNSPECIFIED., .F., .F. ) 
 B_SPLINE_CURVE_WITH_KNOTS ( ( 3, 2, 2, 3 ),
 ( 0.08333333333333328707, 0.08611111111111106886, 0.08888888888888883677, 0.09166666666666660468 ),
 .UNSPECIFIED. ) 
 CURVE ( )  GEOMETRIC_REPRESENTATION_ITEM ( )  RATIONAL_B_SPLINE_CURVE ( ( 1.000000000000001998, 0.8660254037844365982, 1.000000000000000000, 0.8660254037844387076, 1.000000000000000000, 0.8660254037844413721, 0.9999999999999973355 ) ) 
 REPRESENTATION_ITEM ( '' )  );
#33146=CARTESIAN_POINT ( 'NONE',  ( 3.999999999999999112, 19.77500000000000213, -30.00000000000000000 ) ) ;
#33147=CARTESIAN_POINT ( 'NONE',  ( 11.22187500061451892, 3.027376345333613106, -5.243569643749998122 ) ) ;
#33148=CARTESIAN_POINT ( 'NONE',  ( 14.92500000000000071, 6.123233995736764310E-16, -4.999999999999998224 ) ) ;
#33149=CARTESIAN_POINT ( 'NONE',  ( 3.159375000614518036, 4.541064518000418104, -2.621784821874998173 ) ) ;
#33150=CARTESIAN_POINT ( 'NONE',  ( 5.671875000614519102, -6.054752690667223547, -1.112240025338166033E-15 ) ) ;
#33151=CARTESIAN_POINT ( 'NONE',  ( 28.95937500061451431, 0.000000000000000000, 5.243569643749999010 ) ) ;
#33152=CARTESIAN_POINT ( 'NONE',  ( -4.243569643749999898, 9.903125000614593887, 30.00000000000000000 ) ) ;
#33153=CARTESIAN_POINT ( 'NONE',  ( 20.47500000000000142, 4.330127018922191873, 2.499999999999999556 ) ) ;
#33155=CARTESIAN_POINT ( 'NONE',  ( 26.62500000000000000, 6.123233995736764310E-16, -4.999999999999998224 ) ) ;
#33156=CARTESIAN_POINT ( 'NONE',  ( 28.65937500061451715, -4.541064518000417216, -2.621784821875001281 ) ) ;
#33158=ORIENTED_EDGE ( 'NONE', *, *, #65932, .F. ) ;
#33159=CARTESIAN_POINT ( 'NONE',  ( 18.36562500061451431, 3.027376345333613106, -5.243569643749998122 ) ) ;
#33160=CARTESIAN_POINT ( 'NONE',  ( 8.465625000614515727, 3.027376345333613106, -5.243569643749998122 ) ) ;
#33162=CARTESIAN_POINT ( 'NONE',  ( 4.171875000614517326, 3.027376345333611329, 5.243569643749999010 ) ) ;
#33163=CARTESIAN_POINT ( 'NONE',  ( 16.98750000122903359, 4.330127018922191873, 2.499999999999999556 ) ) ;
#33164=CARTESIAN_POINT ( 'NONE',  ( 1.999999999999998668, 14.00000000000000178, -33.46410161513775705 ) ) ;
#33165=CARTESIAN_POINT ( 'NONE',  ( 6.534375000614517148, -4.541064518000419881, 2.621784821874995952 ) ) ;
#33166=CARTESIAN_POINT ( 'NONE',  ( 12.38437500061451857, -4.541064518000419881, 2.621784821874995952 ) ) ;
#33167=CARTESIAN_POINT ( 'NONE',  ( 24.57187500061451502, -6.054752690667223547, -1.112240025338166033E-15 ) ) ;
#33168=CARTESIAN_POINT ( 'NONE',  ( -3.999999999999999112, 14.60000000000000142, -30.00000000000000000 ) ) ;
#33171=CARTESIAN_POINT ( 'NONE',  ( 16.80937500061451573, 0.000000000000000000, 5.243569643749999010 ) ) ;
#33172=CARTESIAN_POINT ( 'NONE',  ( 10.17187500061451999, -6.054752690667223547, -1.112240025338166033E-15 ) ) ;
#33174=CARTESIAN_POINT ( 'NONE',  ( 21.52499999999999858, -4.330127018922194537, 2.499999999999995559 ) ) ;
#33176=DIRECTION ( 'NONE',  ( -0.000000000000000000, -1.000000000000000000, -0.000000000000000000 ) ) ;
#33178=CARTESIAN_POINT ( 'NONE',  ( 11.57812500061451644, 6.421520780324663323E-16, -5.243569643749999010 ) ) ;
#33179=CARTESIAN_POINT ( 'NONE',  ( 29.85937500061451644, 0.000000000000000000, 5.243569643749999010 ) ) ;
#33181=CARTESIAN_POINT ( 'NONE',  ( 29.78437500061451715, 4.541064518000418104, 2.621784821874999949 ) ) ;
#33182=CARTESIAN_POINT ( 'NONE',  ( 9.862500000000000711, -5.773502691896255534, -1.060575238724906372E-15 ) ) ;
#33183=CARTESIAN_POINT ( 'NONE',  ( -2.000000000000000000, 16.43750000122903643, 26.53589838486224650 ) ) ;
#33184=CARTESIAN_POINT ( 'NONE',  ( 9.112500001229033586, -4.330127018922190985, -2.500000000000001332 ) ) ;
#33185=CARTESIAN_POINT ( 'NONE',  ( 20.25937500061451857, 4.541064518000418104, -2.621784821874998173 ) ) ;
#33186=CARTESIAN_POINT ( 'NONE',  ( 14.33437500061451786, 6.421520780324663323E-16, -5.243569643749999010 ) ) ;
#33187=CARTESIAN_POINT ( 'NONE',  ( 9.375000001229036428, 2.886751345948126879, 4.999999999999998224 ) ) ;
#33188=EDGE_LOOP ( 'NONE', ( #22481, #72317, #9721, #25720 ) ) ;
#33189=CARTESIAN_POINT ( 'NONE',  ( 15.21562500061451750, 3.027376345333613106, -5.243569643749998122 ) ) ;
#33190=CARTESIAN_POINT ( 'NONE',  ( 2.803125000614518747, 0.000000000000000000, 5.243569643749999010 ) ) ;
#33191=CARTESIAN_POINT ( 'NONE',  ( 16.32187500061451502, 3.027376345333611329, 5.243569643749999010 ) ) ;
#33192=CARTESIAN_POINT ( 'NONE',  ( 2.878125000614517592, -4.541064518000419881, 2.621784821874995952 ) ) ;
#33193=CARTESIAN_POINT ( 'NONE',  ( 16.60312500061451857, 4.541064518000418104, -2.621784821874998173 ) ) ;
#33194=CARTESIAN_POINT ( 'NONE',  ( 18.03750000122903430, -4.330127018922194537, 2.499999999999995559 ) ) ;
#33195=CARTESIAN_POINT ( 'NONE',  ( 27.49687500061451217, 6.054752690667223547, 3.707466751127219781E-16 ) ) ;
#33196=CARTESIAN_POINT ( 'NONE',  ( 4.243569643749999898, 10.12812500061451715, 30.00000000000000000 ) ) ;
#33197=CARTESIAN_POINT ( 'NONE',  ( 15.79687500061451821, 6.054752690667223547, 3.707466751127219781E-16 ) ) ;
#33198=CARTESIAN_POINT ( 'NONE',  ( 13.57500000122903572, -5.773502691896255534, -1.060575238724906372E-15 ) ) ;
#33200=CARTESIAN_POINT ( 'NONE',  ( 9.001249775931846008E-16, 18.17187500061451999, -25.09994784771203058 ) ) ;
#33201=CARTESIAN_POINT ( 'NONE',  ( 20.22187500061451715, 3.027376345333613106, -5.243569643749998122 ) ) ;
#33202=CARTESIAN_POINT ( 'NONE',  ( 21.93750000122903288, 4.330127018922191873, 2.499999999999999556 ) ) ;
#33203=CARTESIAN_POINT ( 'NONE',  ( 15.87187500061451573, 3.027376345333611329, 5.243569643749999010 ) ) ;
#33204=CARTESIAN_POINT ( 'NONE',  ( -3.000416591977282496E-16, 12.54687500061451999, 25.09994784771203058 ) ) ;
#33205=CARTESIAN_POINT ( 'NONE',  ( 17.65312500061451573, 0.000000000000000000, 5.243569643749999010 ) ) ;
#33206=ORIENTED_EDGE ( 'NONE', *, *, #3605, .F. ) ;
#33208=CARTESIAN_POINT ( 'NONE',  ( 20.99999999999999645, 0.000000000000000000, 4.999999999999998224 ) ) ;
#33209=CARTESIAN_POINT ( 'NONE',  ( 17.47499999999999787, -4.330127018922194537, 2.499999999999995559 ) ) ;
#33210=CARTESIAN_POINT ( 'NONE',  ( 23.91562500061451502, 3.027376345333611329, 5.243569643749999010 ) ) ;
#33211=CARTESIAN_POINT ( 'NONE',  ( 4.453125000614517326, 4.541064518000418104, -2.621784821874998173 ) ) ;
#33212=CARTESIAN_POINT ( 'NONE',  ( 17.70000000122903216, -2.886751345948125991, -5.000000000000000000 ) ) ;
#33213=CARTESIAN_POINT ( 'NONE',  ( 22.11562500061451786, 3.027376345333611329, 5.243569643749999010 ) ) ;
#33214=CARTESIAN_POINT ( 'NONE',  ( 19.91250000000000142, 2.886751345948129099, -4.999999999999998224 ) ) ;
#33215=CARTESIAN_POINT ( 'NONE',  ( 25.30312500061451431, 0.000000000000000000, 5.243569643749999010 ) ) ;
#33216=CARTESIAN_POINT ( 'NONE',  ( 6.890625000614516438, -3.027376345333614438, 5.243569643749998122 ) ) ;
#33218=EDGE_CURVE ( 'NONE', #49981, #55550, #14553, .T. ) ;
#33220=CARTESIAN_POINT ( 'NONE',  ( 3.178125000614515638, 4.541064518000418104, 2.621784821874999949 ) ) ;
#33221=EDGE_CURVE ( 'NONE', #64403, #18194, #38984, .T. ) ;
#33223=CARTESIAN_POINT ( 'NONE',  ( 1.999999999999998668, 18.95000000000000284, 26.53589838486224650 ) ) ;
#33224=CARTESIAN_POINT ( 'NONE',  ( 3.999999999999999112, 10.88750000122903394, -30.00000000000000000 ) ) ;
#33225=CARTESIAN_POINT ( 'NONE',  ( 2.121784821874999061, 17.45937500061451786, -33.67503911421598417 ) ) ;
#33226=STYLED_ITEM ( 'NONE', ( #72638 ), #47954 ) ;
#33227=CARTESIAN_POINT ( 'NONE',  ( 8.849999999999999645, 0.000000000000000000, 4.999999999999998224 ) ) ;
#33228=EDGE_CURVE ( 'NONE', #14078, #4525, #16926, .T. ) ;
#33229=CARTESIAN_POINT ( 'NONE',  ( 7.996875000614519280, -3.027376345333610441, -5.243569643749999898 ) ) ;
#33230=CARTESIAN_POINT ( 'NONE',  ( 6.900000001229035007, -2.886751345948125991, -5.000000000000000000 ) ) ;
#33231=CARTESIAN_POINT ( 'NONE',  ( 13.02187500061451608, 3.027376345333613106, -5.243569643749998122 ) ) ;
#33233=CARTESIAN_POINT ( 'NONE',  ( 3.234375000614516438, 4.541064518000418104, 2.621784821874999949 ) ) ;
#33234=CARTESIAN_POINT ( 'NONE',  ( 3.999999999999999112, 18.98750000122903359, 30.00000000000000000 ) ) ;
#33235=CARTESIAN_POINT ( 'NONE',  ( 19.79999999999999716, -4.330127018922190985, -2.500000000000001332 ) ) ;
#33236=EDGE_CURVE ( 'NONE', #46607, #59952, #24477, .T. ) ;
#33237=CARTESIAN_POINT ( 'NONE',  ( 9.271875000614516082, -6.054752690667223547, -1.112240025338166033E-15 ) ) ;
#33238=CARTESIAN_POINT ( 'NONE',  ( 20.99999999999999645, 0.000000000000000000, 4.999999999999998224 ) ) ;
#33239=CARTESIAN_POINT ( 'NONE',  ( 20.57812500061451644, 6.421520780324663323E-16, -5.243569643749999010 ) ) ;
#33240=CARTESIAN_POINT ( 'NONE',  ( 4.575000001229033053, -5.773502691896255534, -1.060575238724906372E-15 ) ) ;
#33241=CARTESIAN_POINT ( 'NONE',  ( 2.121784821874999061, 16.05312500061459247, 26.32496088578401583 ) ) ;
#33242=CARTESIAN_POINT ( 'NONE',  ( 23.67187500061451999, -6.054752690667223547, -1.112240025338166033E-15 ) ) ;
#33243=CARTESIAN_POINT ( 'NONE',  ( 4.311958327294343363, 2.531208285321026263, 4.311958327294242999 ) ) ;
#33244=CARTESIAN_POINT ( 'NONE',  ( 2.803125000614518747, 0.000000000000000000, 5.243569643749999010 ) ) ;
#33246=CARTESIAN_POINT ( 'NONE',  ( 25.64062500061451644, 6.054752690667223547, 3.707466751127219781E-16 ) ) ;
#33247=CARTESIAN_POINT ( 'NONE',  ( 16.64062500061451289, 6.054752690667223547, 3.707466751127219781E-16 ) ) ;
#33249=CARTESIAN_POINT ( 'NONE',  ( 15.19687500061451857, -3.027376345333610441, -5.243569643749999898 ) ) ;
#33251=CARTESIAN_POINT ( 'NONE',  ( 25.87500000122903288, 2.886751345948129099, -4.999999999999998224 ) ) ;
#33252=FACE_OUTER_BOUND ( 'NONE', #50582, .T. ) ;
#33253=CARTESIAN_POINT ( 'NONE',  ( 13.24687500061451750, -3.027376345333614438, 5.243569643749998122 ) ) ;
#33254=CARTESIAN_POINT ( 'NONE',  ( -1.999999999999997113, 11.97500000000000142, 33.46410161513775705 ) ) ;
#33255=DIRECTION ( 'NONE',  ( 0.000000000000000000, 0.000000000000000000, 1.000000000000000000 ) ) ;
#33256=CARTESIAN_POINT ( 'NONE',  ( -1.071796769724491005, 12.25759618943233775, -34.00000000000000000 ) ) ;
#33257=CARTESIAN_POINT ( 'NONE',  ( 25.84687500061451360, -3.027376345333614438, 5.243569643749998122 ) ) ;
#33258=CARTESIAN_POINT ( 'NONE',  ( 15.60937500061451644, -4.541064518000417216, -2.621784821875001281 ) ) ;
#33260=CARTESIAN_POINT ( 'NONE',  ( 27.71250000000000568, 2.886751345948126879, 4.999999999999999112 ) ) ;
#33261=CARTESIAN_POINT ( 'NONE',  ( 3.637500001229036162, -4.330127018922194537, 2.499999999999995559 ) ) ;
#33262=CARTESIAN_POINT ( 'NONE',  ( 4.500000000000000888, -4.330127018922190985, -2.500000000000001332 ) ) ;
#33264=CARTESIAN_POINT ( 'NONE',  ( 19.79062500061451502, 6.054752690667223547, 3.707466751127219781E-16 ) ) ;
#33265=CARTESIAN_POINT ( 'NONE',  ( 8.699999999999999289, 4.330127018922192761, -2.499999999999997780 ) ) ;
#33267=CARTESIAN_POINT ( 'NONE',  ( 17.73750000000000071, 5.773502691896255534, 3.535250795749688894E-16 ) ) ;
#33269=CARTESIAN_POINT ( 'NONE',  ( 20.06250000122903643, 4.330127018922192761, -2.499999999999997780 ) ) ;
#33270=CARTESIAN_POINT ( 'NONE',  ( 2.692168354449049339, 9.632460402479559036, 35.36566372828262672 ) ) ;
#33271=CARTESIAN_POINT ( 'NONE',  ( 27.27187500061451431, -6.054752690667223547, -1.112240025338166033E-15 ) ) ;
#33272=VERTEX_POINT ( 'NONE', #50789 ) ;
#33273=CARTESIAN_POINT ( 'NONE',  ( 17.65312500061451573, 0.000000000000000000, 5.243569643749999010 ) ) ;
#33274=CARTESIAN_POINT ( 'NONE',  ( 23.50312500061451360, 0.000000000000000000, 5.243569643749999010 ) ) ;
#33275=CARTESIAN_POINT ( 'NONE',  ( 23.40937500061451715, 4.541064518000418104, -2.621784821874998173 ) ) ;
#33276=CARTESIAN_POINT ( 'NONE',  ( 5.700000000000000178, 0.000000000000000000, 4.999999999999998224 ) ) ;
#33277=CARTESIAN_POINT ( 'NONE',  ( 8.803125000614517859, -4.541064518000417216, -2.621784821875001281 ) ) ;
#33278=CARTESIAN_POINT ( 'NONE',  ( 24.59062500061451573, -3.027376345333610441, -5.243569643749999898 ) ) ;
#33279=CARTESIAN_POINT ( 'NONE',  ( 15.87187500061451573, 3.027376345333611329, 5.243569643749999010 ) ) ;
#33280=CARTESIAN_POINT ( 'NONE',  ( 20.22187500061451715, 3.027376345333613106, -5.243569643749998122 ) ) ;
#33281=CARTESIAN_POINT ( 'NONE',  ( 4.243569643749999898, 11.04687500061451999, 32.45002607614398471 ) ) ;
#33282=CARTESIAN_POINT ( 'NONE',  ( 20.70000000122903216, -2.886751345948129988, 4.999999999999997335 ) ) ;
#33284=CARTESIAN_POINT ( 'NONE',  ( 11.99062500061451608, -3.027376345333610441, -5.243569643749999898 ) ) ;
#33285=CARTESIAN_POINT ( 'NONE',  ( 8.709375000614517859, 0.000000000000000000, 5.243569643749999010 ) ) ;
#33286=CARTESIAN_POINT ( 'NONE',  ( 6.346875000614517148, 6.054752690667223547, 3.707466751127219781E-16 ) ) ;
#33288=ORIENTED_EDGE ( 'NONE', *, *, #1071, .F. ) ;
#33289=CARTESIAN_POINT ( 'NONE',  ( 27.30937500061451573, -4.541064518000417216, -2.621784821875001281 ) ) ;
#33290=CARTESIAN_POINT ( 'NONE',  ( 19.67812500061451786, 6.421520780324663323E-16, -5.243569643749999010 ) ) ;
#33291=CARTESIAN_POINT ( 'NONE',  ( 29.51250000122903216, 4.330127018922192761, -2.499999999999997780 ) ) ;
#33292=CARTESIAN_POINT ( 'NONE',  ( 28.64062500061451289, -3.027376345333610441, -5.243569643749999898 ) ) ;
#33293=VECTOR ( 'NONE', #4951, 1000.000000000000000 ) ;
#33294=CARTESIAN_POINT ( 'NONE',  ( 24.34687500061451715, 6.054752690667223547, 3.707466751127219781E-16 ) ) ;
#33295=CARTESIAN_POINT ( 'NONE',  ( 19.82812500061451644, 4.541064518000418104, 2.621784821874999949 ) ) ;
#33296=CARTESIAN_POINT ( 'NONE',  ( 2.000000000000001332, 10.25000000000000000, 33.46410161513774995 ) ) ;
#33297=CARTESIAN_POINT ( 'NONE',  ( 24.66562500061451502, 3.027376345333613106, -5.243569643749998122 ) ) ;
#33298=CARTESIAN_POINT ( 'NONE',  ( 5.250000001229035540, 5.773502691896255534, 3.535250795749688894E-16 ) ) ;
#33299=ORIENTED_EDGE ( 'NONE', *, *, #36205, .T. ) ;
#33300=CARTESIAN_POINT ( 'NONE',  ( 28.12499999999999645, 4.330127018922191873, 2.499999999999999556 ) ) ;
#33301=CARTESIAN_POINT ( 'NONE',  ( 3.999999999999999112, 15.27500000000000036, -30.00000000000000000 ) ) ;
#33303=CARTESIAN_POINT ( 'NONE',  ( 3.684375000614518836, 4.541064518000418104, 2.621784821874999949 ) ) ;
#33304=CARTESIAN_POINT ( 'NONE',  ( 12.40312500061451573, -4.541064518000417216, -2.621784821875001281 ) ) ;
#33305=CARTESIAN_POINT ( 'NONE',  ( 6.346875000614517148, 6.054752690667223547, 3.707466751127219781E-16 ) ) ;
#33306=CARTESIAN_POINT ( 'NONE',  ( 24.03750000122903430, 6.123233995736764310E-16, -4.999999999999998224 ) ) ;
#33307=CARTESIAN_POINT ( 'NONE',  ( 14.18437500061451750, -4.541064518000419881, 2.621784821874995952 ) ) ;
#33308=CARTESIAN_POINT ( 'NONE',  ( 3.309375000614518836, 0.000000000000000000, 5.243569643749999010 ) ) ;
#33309=CARTESIAN_POINT ( 'NONE',  ( 7.912500001229033408, 4.330127018922192761, -2.499999999999997780 ) ) ;
#33310=CARTESIAN_POINT ( 'NONE',  ( 25.88437500061451502, -4.541064518000419881, 2.621784821874995952 ) ) ;
#33311=CARTESIAN_POINT ( 'NONE',  ( 3.103125000614517237, 4.541064518000418104, -2.621784821874998173 ) ) ;
#33312=CARTESIAN_POINT ( 'NONE',  ( 12.32812500061451821, -4.541064518000419881, 2.621784821874995952 ) ) ;
#33313=ORIENTED_EDGE ( 'NONE', *, *, #2528, .T. ) ;
#33314=CARTESIAN_POINT ( 'NONE',  ( 9.890625000614516438, 6.054752690667223547, 3.707466751127219781E-16 ) ) ;
#33315=CARTESIAN_POINT ( 'NONE',  ( 8.915625000614515017, 3.027376345333613106, -5.243569643749998122 ) ) ;
#33317=CARTESIAN_POINT ( 'NONE',  ( 2.775000001229033675, -5.773502691896255534, -1.060575238724906372E-15 ) ) ;
#33318=CARTESIAN_POINT ( 'NONE',  ( 15.67500000000000071, -4.330127018922194537, 2.499999999999995559 ) ) ;
#33319=EDGE_CURVE ( 'NONE', #58630, #20653, #34395, .T. ) ;
#33320=CARTESIAN_POINT ( 'NONE',  ( 16.24687500061451573, 6.054752690667223547, 3.707466751127219781E-16 ) ) ;
#33321=CARTESIAN_POINT ( 'NONE',  ( 12.93750000122903465, 4.330127018922191873, 2.499999999999999556 ) ) ;
#33323=CARTESIAN_POINT ( 'NONE',  ( 20.10937500061451289, -4.541064518000417216, -2.621784821875001281 ) ) ;
#33324=CARTESIAN_POINT ( 'NONE',  ( 2.121784821874999061, 13.35312500061451679, -33.67503911421598417 ) ) ;
#33325=DIRECTION ( 'NONE',  ( 0.000000000000000000, 0.000000000000000000, -1.000000000000000000 ) ) ;
#33328=CARTESIAN_POINT ( 'NONE',  ( 26.69062500061451715, -3.027376345333614438, 5.243569643749998122 ) ) ;
#33329=CARTESIAN_POINT ( 'NONE',  ( -1.394453263437886604E-15, 19.66249999999999787, 33.99999999999999289 ) ) ;
#33331=( BOUNDED_CURVE ( )  B_SPLINE_CURVE ( 2, ( #69245, #47068, #23794, #29353, #24157, #46345, #2013 ),
 .UNSPECIFIED., .F., .F. ) 
 B_SPLINE_CURVE_WITH_KNOTS ( ( 3, 2, 2, 3 ),
 ( 0.9854705224330112534, 0.9861111111111111605, 0.9888888888888889284, 0.9894640555095505219 ),
 .UNSPECIFIED. ) 
 CURVE ( )  GEOMETRIC_REPRESENTATION_ITEM ( )  RATIONAL_B_SPLINE_CURVE ( ( 0.9524577574850663364, 0.9691038605840708309, 1.000000000000000000, 0.8660254037844387076, 1.000000000000000000, 0.9722592223264697742, 0.9560064545842259509 ) ) 
 REPRESENTATION_ITEM ( '' )  );
#33332=CARTESIAN_POINT ( 'NONE',  ( 25.64999999999999858, -4.330127018922190985, -2.500000000000001332 ) ) ;
#33333=CARTESIAN_POINT ( 'NONE',  ( 10.19062500061451892, -3.027376345333610441, -5.243569643749999898 ) ) ;
#33335=CARTESIAN_POINT ( 'NONE',  ( 21.90937500061451715, -4.541064518000417216, -2.621784821875001281 ) ) ;
#33337=CARTESIAN_POINT ( 'NONE',  ( 4.828125000614518214, 6.421520780324663323E-16, -5.243569643749999010 ) ) ;
#33338=CARTESIAN_POINT ( 'NONE',  ( 11.14687500061451608, -3.027376345333610441, -5.243569643749999898 ) ) ;
#33340=CARTESIAN_POINT ( 'NONE',  ( 21.83437500061451786, -4.541064518000419881, 2.621784821874995952 ) ) ;
#33341=CARTESIAN_POINT ( 'NONE',  ( 23.13750000122903216, 6.123233995736764310E-16, -4.999999999999998224 ) ) ;
#33342=CARTESIAN_POINT ( 'NONE',  ( 29.47499999999999787, 4.330127018922191873, 2.499999999999999556 ) ) ;
#33343=CARTESIAN_POINT ( 'NONE',  ( 4.312500000000000000, 2.886751345948126879, 4.999999999999999112 ) ) ;
#33345=CARTESIAN_POINT ( 'NONE',  ( 15.03750000122903252, 6.123233995736764310E-16, -4.999999999999998224 ) ) ;
#33347=ORIENTED_EDGE ( 'NONE', *, *, #6059, .T. ) ;
#33348=CARTESIAN_POINT ( 'NONE',  ( 11.62500000000000000, -4.330127018922194537, 2.499999999999995559 ) ) ;
#33349=CARTESIAN_POINT ( 'NONE',  ( 15.86250000000000249, 2.886751345948129099, -4.999999999999998224 ) ) ;
#33350=CARTESIAN_POINT ( 'NONE',  ( 13.12500000122903288, -5.773502691896255534, -1.060575238724906372E-15 ) ) ;
#33351=CARTESIAN_POINT ( 'NONE',  ( 10.79062500061451679, 6.054752690667223547, 3.707466751127219781E-16 ) ) ;
#33352=CARTESIAN_POINT ( 'NONE',  ( 9.525000000000002132, 6.123233995736764310E-16, -4.999999999999998224 ) ) ;
#33353=CARTESIAN_POINT ( 'NONE',  ( 1.592000809091587073E-14, 16.85000000122903785, -34.00000000000000000 ) ) ;
#33354=CARTESIAN_POINT ( 'NONE',  ( -3.000416591977282496E-16, 14.34687500061451715, -34.90005215228797653 ) ) ;
#33355=CARTESIAN_POINT ( 'NONE',  ( 28.65000000122903145, 5.773502691896255534, 3.535250795749688894E-16 ) ) ;
#33357=CARTESIAN_POINT ( 'NONE',  ( 6.787500000000001421, -2.886751345948125991, -5.000000000000000000 ) ) ;
#33359=VERTEX_POINT ( 'NONE', #67782 ) ;
#33360=CARTESIAN_POINT ( 'NONE',  ( 23.65312500061451573, -4.541064518000417216, -2.621784821875001281 ) ) ;
#33362=CARTESIAN_POINT ( 'NONE',  ( 29.10937500061451644, -4.541064518000417216, -2.621784821875001281 ) ) ;
#33363=CARTESIAN_POINT ( 'NONE',  ( 20.93437500061451573, -4.541064518000419881, 2.621784821874995952 ) ) ;
#33364=CARTESIAN_POINT ( 'NONE',  ( 17.05312500061451786, 4.541064518000418104, -2.621784821874998173 ) ) ;
#33365=EDGE_CURVE ( 'NONE', #66904, #68293, #41949, .T. ) ;
#33366=CARTESIAN_POINT ( 'NONE',  ( -2.121784821874999949, 12.07812500061459637, -33.67503911421598417 ) ) ;
#33367=CARTESIAN_POINT ( 'NONE',  ( 7.603125000614517681, 4.541064518000418104, -2.621784821874998173 ) ) ;
#33368=CARTESIAN_POINT ( 'NONE',  ( 28.53750000122903074, 6.123233995736764310E-16, -4.999999999999998224 ) ) ;
#33370=CARTESIAN_POINT ( 'NONE',  ( 19.60312500061451502, -4.541064518000417216, -2.621784821875001281 ) ) ;
#33373=CARTESIAN_POINT ( 'NONE',  ( 15.30937500061451750, 4.541064518000418104, -2.621784821874998173 ) ) ;
#33374=CARTESIAN_POINT ( 'NONE',  ( 15.08437500061451786, -4.541064518000419881, 2.621784821874995952 ) ) ;
#33375=CARTESIAN_POINT ( 'NONE',  ( 22.43437500061451573, 6.421520780324663323E-16, -5.243569643749999010 ) ) ;
#33376=ORIENTED_EDGE ( 'NONE', *, *, #14874, .F. ) ;
#33378=CARTESIAN_POINT ( 'NONE',  ( 26.80312500061451431, -4.541064518000417216, -2.621784821875001281 ) ) ;
#33379=CARTESIAN_POINT ( 'NONE',  ( 26.35312500061451857, -4.541064518000417216, -2.621784821875001281 ) ) ;
#33381=CARTESIAN_POINT ( 'NONE',  ( -3.999999999999999556, 17.71249999999999858, 27.69059892324149530 ) ) ;
#33382=CARTESIAN_POINT ( 'NONE',  ( 5.334375000614517859, 6.421520780324663323E-16, -5.243569643749999010 ) ) ;
#33383=CARTESIAN_POINT ( 'NONE',  ( 11.36250000122903536, -4.330127018922190985, -2.500000000000001332 ) ) ;
#33384=CARTESIAN_POINT ( 'NONE',  ( 6.262500001229034829, 0.000000000000000000, 4.999999999999998224 ) ) ;
#33385=CARTESIAN_POINT ( 'NONE',  ( 3.365625000614516082, -6.054752690667223547, -1.112240025338166033E-15 ) ) ;
#33388=CARTESIAN_POINT ( 'NONE',  ( 12.94687500061451857, -3.027376345333610441, -5.243569643749999898 ) ) ;
#33390=ORIENTED_EDGE ( 'NONE', *, *, #37910, .F. ) ;
#33391=CARTESIAN_POINT ( 'NONE',  ( 19.15312500061451573, -4.541064518000417216, -2.621784821875001281 ) ) ;
#33392=CARTESIAN_POINT ( 'NONE',  ( 14.03437500061451715, 4.541064518000418104, 2.621784821874999949 ) ) ;
#33393=CARTESIAN_POINT ( 'NONE',  ( 4.490625000614516971, 6.054752690667223547, 3.707466751127219781E-16 ) ) ;
#33394=CARTESIAN_POINT ( 'NONE',  ( 22.28437500061451715, -4.541064518000419881, 2.621784821874995952 ) ) ;
#33395=CARTESIAN_POINT ( 'NONE',  ( 10.69687500061451679, -3.027376345333610441, -5.243569643749999898 ) ) ;
#33396=CARTESIAN_POINT ( 'NONE',  ( 5.503125000614516260, 0.000000000000000000, 5.243569643749999010 ) ) ;
#33397=CARTESIAN_POINT ( 'NONE',  ( 10.76250000122903572, 0.000000000000000000, 4.999999999999998224 ) ) ;
#33398=CARTESIAN_POINT ( 'NONE',  ( 5.475000001229035185, -5.773502691896255534, -1.060575238724906372E-15 ) ) ;
#33399=CARTESIAN_POINT ( 'NONE',  ( 19.11562500061451431, -6.054752690667223547, -1.112240025338166033E-15 ) ) ;
#33400=CARTESIAN_POINT ( 'NONE',  ( 7.312500001229033764, -4.330127018922190985, -2.500000000000001332 ) ) ;
#33401=CARTESIAN_POINT ( 'NONE',  ( 17.39062500061451644, -3.027376345333610441, -5.243569643749999898 ) ) ;
#33402=CARTESIAN_POINT ( 'NONE',  ( 15.10312500061451502, -4.541064518000417216, -2.621784821875001281 ) ) ;
#33404=CARTESIAN_POINT ( 'NONE',  ( 16.05000000000000071, 0.000000000000000000, 4.999999999999998224 ) ) ;
#33405=CARTESIAN_POINT ( 'NONE',  ( 8.625000001229034652, -5.773502691896255534, -1.060575238724906372E-15 ) ) ;
#33406=CARTESIAN_POINT ( 'NONE',  ( 4.903125000614516615, 4.541064518000418104, -2.621784821874998173 ) ) ;
#33407=CARTESIAN_POINT ( 'NONE',  ( 20.81250000122903643, -4.330127018922190985, -2.500000000000001332 ) ) ;
#33409=CARTESIAN_POINT ( 'NONE',  ( 9.001249775931846008E-16, 13.67187500061451999, -25.09994784771203058 ) ) ;
#33410=DIRECTION ( 'NONE',  ( -1.000000000000000000, -0.000000000000000000, -0.000000000000000000 ) ) ;
#33411=CARTESIAN_POINT ( 'NONE',  ( 3.225000001229033408, -5.773502691896255534, -1.060575238724906372E-15 ) ) ;
#33412=CARTESIAN_POINT ( 'NONE',  ( 4.659375000614518925, 0.000000000000000000, 5.243569643749999010 ) ) ;
#33413=CARTESIAN_POINT ( 'NONE',  ( 20.40937500061451715, 0.000000000000000000, 5.243569643749999010 ) ) ;
#33414=CARTESIAN_POINT ( 'NONE',  ( 15.36562500061451608, 3.027376345333611329, 5.243569643749999010 ) ) ;
#33416=CARTESIAN_POINT ( 'NONE',  ( 26.77499999999999858, 4.330127018922191873, 2.499999999999999556 ) ) ;
#33417=CARTESIAN_POINT ( 'NONE',  ( 29.22187500061451715, 3.027376345333613106, -5.243569643749998122 ) ) ;
#33419=CARTESIAN_POINT ( 'NONE',  ( 13.75312500061451715, -4.541064518000417216, -2.621784821875001281 ) ) ;
#33420=CARTESIAN_POINT ( 'NONE',  ( 10.73437500061451644, 6.421520780324663323E-16, -5.243569643749999010 ) ) ;
#33421=ORIENTED_EDGE ( 'NONE', *, *, #55194, .F. ) ;
#33422=CARTESIAN_POINT ( 'NONE',  ( 29.31562500061451715, 3.027376345333611329, 5.243569643749999010 ) ) ;
#33423=CARTESIAN_POINT ( 'NONE',  ( 22.60312500061451857, 0.000000000000000000, 5.243569643749999010 ) ) ;
#33424=CARTESIAN_POINT ( 'NONE',  ( 7.320879633048903241E-15, 18.20000000122903216, 26.00000000000000355 ) ) ;
#33425=CARTESIAN_POINT ( 'NONE',  ( 11.58750000000000036, -2.886751345948129988, 4.999999999999997335 ) ) ;
#33426=CARTESIAN_POINT ( 'NONE',  ( 22.57500000122903572, -5.773502691896255534, -1.060575238724906372E-15 ) ) ;
#33427=CARTESIAN_POINT ( 'NONE',  ( 16.90312500061451573, -4.541064518000417216, -2.621784821875001281 ) ) ;
#33429=ORIENTED_EDGE ( 'NONE', *, *, #72450, .F. ) ;
#33430=CARTESIAN_POINT ( 'NONE',  ( 20.02500000000000213, 4.330127018922191873, 2.499999999999999556 ) ) ;
#33431=CARTESIAN_POINT ( 'NONE',  ( 21.64687500061451786, 6.054752690667223547, 3.707466751127219781E-16 ) ) ;
#33432=CARTESIAN_POINT ( 'NONE',  ( 26.61562500061451786, 3.027376345333611329, 5.243569643749999010 ) ) ;
#33433=VERTEX_POINT ( 'NONE', #12337 ) ;
#33434=CARTESIAN_POINT ( 'NONE',  ( 7.978125000614517681, 6.421520780324663323E-16, -5.243569643749999010 ) ) ;
#33435=CARTESIAN_POINT ( 'NONE',  ( 6.150000000000003020, 0.000000000000000000, 4.999999999999998224 ) ) ;
#33436=CARTESIAN_POINT ( 'NONE',  ( 17.88749999999999929, -2.886751345948129988, 4.999999999999997335 ) ) ;
#33437=CARTESIAN_POINT ( 'NONE',  ( 25.08749999999999858, -2.886751345948129988, 4.999999999999997335 ) ) ;
#33438=CARTESIAN_POINT ( 'NONE',  ( 3.479729569495786379, -3.590471016896914946, -3.821457900550485398 ) ) ;
#33439=CARTESIAN_POINT ( 'NONE',  ( 4.509375000614518569, 4.541064518000418104, -2.621784821874998173 ) ) ;
#33440=CARTESIAN_POINT ( 'NONE',  ( 29.14687500061451075, -3.027376345333610441, -5.243569643749999898 ) ) ;
#33441=ORIENTED_EDGE ( 'NONE', *, *, #38783, .F. ) ;
#33442=CARTESIAN_POINT ( 'NONE',  ( 24.74062500061451786, 6.054752690667223547, 3.707466751127219781E-16 ) ) ;
#33443=CARTESIAN_POINT ( 'NONE',  ( 24.30937500061451573, 4.541064518000418104, -2.621784821874998173 ) ) ;
#33444=EDGE_CURVE ( 'NONE', #26592, #2667, #27899, .T. ) ;
#33446=CARTESIAN_POINT ( 'NONE',  ( 13.27500000000000213, 4.330127018922191873, 2.499999999999999556 ) ) ;
#33447=CARTESIAN_POINT ( 'NONE',  ( 9.703125000614514661, -4.541064518000417216, -2.621784821875001281 ) ) ;
#33448=DIRECTION ( 'NONE',  ( 0.000000000000000000, 0.000000000000000000, 1.000000000000000000 ) ) ;
#33449=DIRECTION ( 'NONE',  ( 0.000000000000000000, 1.000000000000000000, -0.000000000000000000 ) ) ;
#33450=CARTESIAN_POINT ( 'NONE',  ( 25.26562500061451644, 3.027376345333611329, 5.243569643749999010 ) ) ;
#33451=CARTESIAN_POINT ( 'NONE',  ( 20.32499999999999929, 6.123233995736764310E-16, -4.999999999999998224 ) ) ;
#33453=CARTESIAN_POINT ( 'NONE',  ( 3.778125000614519280, -4.541064518000419881, 2.621784821874995952 ) ) ;
#33454=CARTESIAN_POINT ( 'NONE',  ( 19.58437500061451786, -4.541064518000419881, 2.621784821874995952 ) ) ;
#33455=CARTESIAN_POINT ( 'NONE',  ( -4.243569643749997233, 13.59687500061451715, 32.45002607614398471 ) ) ;
#33456=CARTESIAN_POINT ( 'NONE',  ( 22.77187500061451786, -6.054752690667223547, -1.112240025338166033E-15 ) ) ;
#33457=CARTESIAN_POINT ( 'NONE',  ( 29.85937500061451644, 0.000000000000000000, 5.243569643749999010 ) ) ;
#33458=CARTESIAN_POINT ( 'NONE',  ( 9.703125000614514661, -4.541064518000417216, -2.621784821875001281 ) ) ;
#33459=CARTESIAN_POINT ( 'NONE',  ( -2.000000000000000000, 15.08750000122903501, 26.53589838486224650 ) ) ;
#33460=CARTESIAN_POINT ( 'NONE',  ( 8.109375000614518214, 4.541064518000418104, -2.621784821874998173 ) ) ;
#33461=CARTESIAN_POINT ( 'NONE',  ( 3.943184062799388823, 3.074387202984122602, -4.182138569239902459 ) ) ;
#33462=CARTESIAN_POINT ( 'NONE',  ( 7.978125000614517681, 6.421520780324663323E-16, -5.243569643749999010 ) ) ;
#33463=CARTESIAN_POINT ( 'NONE',  ( 13.20937500061451786, 0.000000000000000000, 5.243569643749999010 ) ) ;
#33464=CARTESIAN_POINT ( 'NONE',  ( 18.75000000122903288, 5.773502691896255534, 3.535250795749688894E-16 ) ) ;
#33465=CARTESIAN_POINT ( 'NONE',  ( 8.971875000614515372, 3.027376345333613106, -5.243569643749998122 ) ) ;
#33466=CARTESIAN_POINT ( 'NONE',  ( 9.853125000614516793, 4.541064518000418104, -2.621784821874998173 ) ) ;
#33467=CARTESIAN_POINT ( 'NONE',  ( 5.128125000614516260, -4.541064518000419881, 2.621784821874995952 ) ) ;
#33469=CARTESIAN_POINT ( 'NONE',  ( 18.27187500061451431, -6.054752690667223547, -1.112240025338166033E-15 ) ) ;
#33470=CARTESIAN_POINT ( 'NONE',  ( 26.57812500061451644, 4.541064518000418104, 2.621784821874999949 ) ) ;
#33471=CARTESIAN_POINT ( 'NONE',  ( 11.24062500061451608, 6.054752690667223547, 3.707466751127219781E-16 ) ) ;
#33472=CARTESIAN_POINT ( 'NONE',  ( 29.44687500061451502, -3.027376345333614438, 5.243569643749998122 ) ) ;
#33473=CARTESIAN_POINT ( 'NONE',  ( 4.243569643749999898, 12.88437500061451857, -30.00000000000000000 ) ) ;
#33474=CARTESIAN_POINT ( 'NONE',  ( 13.72500000122903074, 2.886751345948129099, -4.999999999999998224 ) ) ;
#33475=CARTESIAN_POINT ( 'NONE',  ( 28.41562500061451502, 3.027376345333611329, 5.243569643749999010 ) ) ;
#33476=CARTESIAN_POINT ( 'NONE',  ( -4.243569643749999898, 16.20312500061451644, -30.00000000000000000 ) ) ;
#33477=CARTESIAN_POINT ( 'NONE',  ( 16.31250000122903288, -4.330127018922190985, -2.500000000000001332 ) ) ;
#33478=CARTESIAN_POINT ( 'NONE',  ( 13.50000000000000178, -4.330127018922190985, -2.500000000000001332 ) ) ;
#33479=CARTESIAN_POINT ( 'NONE',  ( 10.31250000122903288, 0.000000000000000000, 4.999999999999998224 ) ) ;
#33480=CARTESIAN_POINT ( 'NONE',  ( 23.61562500061451431, -6.054752690667223547, -1.112240025338166033E-15 ) ) ;
#33481=CARTESIAN_POINT ( 'NONE',  ( 8.071875000614518569, 3.027376345333612662, -5.243569643749998122 ) ) ;
#33482=CARTESIAN_POINT ( 'NONE',  ( 9.525000001229033231, -5.773502691896255534, -1.060575238724906372E-15 ) ) ;
#33483=CARTESIAN_POINT ( 'NONE',  ( 19.76250000122903216, 0.000000000000000000, 4.999999999999998224 ) ) ;
#33484=CARTESIAN_POINT ( 'NONE',  ( 14.31562500061451537, 3.027376345333613106, -5.243569643749998122 ) ) ;
#33486=CARTESIAN_POINT ( 'NONE',  ( 19.19062500061452070, -3.027376345333610441, -5.243569643749999898 ) ) ;
#33487=CARTESIAN_POINT ( 'NONE',  ( 25.91250000122903074, 4.330127018922192761, -2.499999999999997780 ) ) ;
#33488=EDGE_CURVE ( 'NONE', #885, #11117, #39598, .T. ) ;
#33489=CARTESIAN_POINT ( 'NONE',  ( 29.17500000122903714, 2.886751345948126879, 4.999999999999999112 ) ) ;
#33490=CARTESIAN_POINT ( 'NONE',  ( 22.76249999999999574, 2.886751345948126879, 4.999999999999999112 ) ) ;
#33491=CARTESIAN_POINT ( 'NONE',  ( 25.09687500061451715, -3.027376345333610441, -5.243569643749999898 ) ) ;
#33493=CARTESIAN_POINT ( 'NONE',  ( 10.91250000122903252, -4.330127018922190985, -2.500000000000001332 ) ) ;
#33494=CARTESIAN_POINT ( 'NONE',  ( 27.04687500061451644, 6.054752690667223547, 3.707466751127219781E-16 ) ) ;
#33495=CARTESIAN_POINT ( 'NONE',  ( -3.999999999999999112, 13.21250000000000213, 27.69059892324149885 ) ) ;
#33496=CARTESIAN_POINT ( 'NONE',  ( 3.871875000614519280, -6.054752690667223547, -1.112240025338166033E-15 ) ) ;
#33497=CARTESIAN_POINT ( 'NONE',  ( 23.05312500061451431, 0.000000000000000000, 5.243569643749999010 ) ) ;
#33499=LINE ( 'NONE', #39061, #66882 ) ;
#33500=CARTESIAN_POINT ( 'NONE',  ( 9.196875000614518569, -3.027376345333614438, 5.243569643749998122 ) ) ;
#33501=CARTESIAN_POINT ( 'NONE',  ( 4.924325218087134637, -0.8666147624583920850, 4.924325218087160394 ) ) ;
#33502=CARTESIAN_POINT ( 'NONE',  ( 3.459375000614519635, -4.541064518000417216, -2.621784821875001281 ) ) ;
#33503=CARTESIAN_POINT ( 'NONE',  ( 6.871875000614517504, 3.027376345333611329, 5.243569643749999010 ) ) ;
#33504=CARTESIAN_POINT ( 'NONE',  ( 28.24687500061451573, -3.027376345333610441, -5.243569643749999898 ) ) ;
#33505=CARTESIAN_POINT ( 'NONE',  ( -4.243569643749998122, 9.940625000614591755, 32.45002607614398471 ) ) ;
#33506=CARTESIAN_POINT ( 'NONE',  ( 19.91250000000000142, 2.886751345948129099, -4.999999999999998224 ) ) ;
#33508=CARTESIAN_POINT ( 'NONE',  ( 26.25000000000000000, 4.330127018922192761, -2.499999999999997780 ) ) ;
#33509=CARTESIAN_POINT ( 'NONE',  ( 28.50937500061451502, 0.000000000000000000, 5.243569643749999010 ) ) ;
#33511=CARTESIAN_POINT ( 'NONE',  ( 16.97812500061451502, 6.421520780324663323E-16, -5.243569643749999010 ) ) ;
#33512=CARTESIAN_POINT ( 'NONE',  ( 8.390625000614518214, -3.027376345333610441, -5.243569643749999898 ) ) ;
#33514=CARTESIAN_POINT ( 'NONE',  ( 3.796875000614517326, -3.027376345333614438, 5.243569643749998122 ) ) ;
#33515=CARTESIAN_POINT ( 'NONE',  ( 17.73750000122903359, 6.123233995736764310E-16, -4.999999999999998224 ) ) ;
#33516=CARTESIAN_POINT ( 'NONE',  ( 25.42500000000000071, 4.330127018922191873, 2.499999999999999556 ) ) ;
#33517=CARTESIAN_POINT ( 'NONE',  ( 15.59999999999999964, 0.000000000000000000, 4.999999999999998224 ) ) ;
#33518=CARTESIAN_POINT ( 'NONE',  ( 6.496875000614517504, -3.027376345333614438, 5.243569643749998122 ) ) ;
#33519=CARTESIAN_POINT ( 'NONE',  ( 11.37187500061451750, 3.027376345333611329, 5.243569643749999010 ) ) ;
#33520=CARTESIAN_POINT ( 'NONE',  ( 22.95937500061451431, 4.541064518000418104, -2.621784821874998173 ) ) ;
#33523=CARTESIAN_POINT ( 'NONE',  ( 3.571875000614517237, 3.027376345333613106, -5.243569643749998122 ) ) ;
#33526=CARTESIAN_POINT ( 'NONE',  ( 7.134375000614516793, 6.421520780324663323E-16, -5.243569643749999010 ) ) ;
#33528=CARTESIAN_POINT ( 'NONE',  ( 21.60000000000000142, -4.330127018922190985, -2.500000000000001332 ) ) ;
#33529=CARTESIAN_POINT ( 'NONE',  ( 15.51562500061451644, -6.054752690667223547, -1.112240025338166033E-15 ) ) ;
#33533=CARTESIAN_POINT ( 'NONE',  ( 9.140625000614518214, -3.027376345333614438, 5.243569643749998122 ) ) ;
#33534=CARTESIAN_POINT ( 'NONE',  ( 25.95937500061451431, -4.541064518000417216, -2.621784821875001281 ) ) ;
#33536=CARTESIAN_POINT ( 'NONE',  ( 28.92187500061451644, 3.027376345333611329, 5.243569643749999010 ) ) ;
#33537=CARTESIAN_POINT ( 'NONE',  ( 11.02500000000000036, 4.330127018922191873, 2.499999999999999556 ) ) ;
#33538=CARTESIAN_POINT ( 'NONE',  ( 1.999999999999998668, 16.36250000122903359, 26.53589838486224650 ) ) ;
#33539=CARTESIAN_POINT ( 'NONE',  ( 9.037500001229034297, -4.330127018922194537, 2.499999999999995559 ) ) ;
#33540=CARTESIAN_POINT ( 'NONE',  ( 19.09687500061451360, -3.027376345333614438, 5.243569643749998122 ) ) ;
#33541=CARTESIAN_POINT ( 'NONE',  ( 13.65937500061451715, 0.000000000000000000, 5.243569643749999010 ) ) ;
#33542=CARTESIAN_POINT ( 'NONE',  ( 9.337500001229033231, 4.330127018922191873, 2.499999999999999556 ) ) ;
#33545=CARTESIAN_POINT ( 'NONE',  ( 14.24062500061451608, -3.027376345333610441, -5.243569643749999898 ) ) ;
#33546=CARTESIAN_POINT ( 'NONE',  ( 25.23750000122903359, -4.330127018922194537, 2.499999999999995559 ) ) ;
#33547=CARTESIAN_POINT ( 'NONE',  ( 15.23437500061451644, 6.421520780324663323E-16, -5.243569643749999010 ) ) ;
#33548=CARTESIAN_POINT ( 'NONE',  ( 4.519730000842647755, 8.925305311771484895, -26.03535200691664642 ) ) ;
#33549=CARTESIAN_POINT ( 'NONE',  ( 16.41562500061451857, -6.054752690667223547, -1.112240025338166033E-15 ) ) ;
#33551=CARTESIAN_POINT ( 'NONE',  ( 27.27187500061451431, -6.054752690667223547, -1.112240025338166033E-15 ) ) ;
#33552=CARTESIAN_POINT ( 'NONE',  ( 9.001249775931846008E-16, 10.46562500061451928, 34.90005215228797653 ) ) ;
#33553=CARTESIAN_POINT ( 'NONE',  ( 14.78437500061451715, 6.421520780324663323E-16, -5.243569643749999010 ) ) ;
#33554=CARTESIAN_POINT ( 'NONE',  ( 14.66250000122903252, 4.330127018922192761, -2.499999999999997780 ) ) ;
#33555=DIRECTION ( 'NONE',  ( -0.000000000000000000, -1.000000000000000000, -0.000000000000000000 ) ) ;
#33556=CARTESIAN_POINT ( 'NONE',  ( 3.360320061989407137, -3.702473467127644469, 3.713053667660598745 ) ) ;
#33557=CARTESIAN_POINT ( 'NONE',  ( 19.99687500061451573, -3.027376345333614438, 5.243569643749998122 ) ) ;
#33558=CARTESIAN_POINT ( 'NONE',  ( 21.11250000122903359, 0.000000000000000000, 4.999999999999998224 ) ) ;
#33560=VECTOR ( 'NONE', #13501, 1000.000000000000000 ) ;
#33561=CARTESIAN_POINT ( 'NONE',  ( 17.55937500061451573, 4.541064518000418104, -2.621784821874998173 ) ) ;
#33562=CARTESIAN_POINT ( 'NONE',  ( 4.243569643749999898, 13.29687500061451644, 32.45002607614398471 ) ) ;
#33563=CARTESIAN_POINT ( 'NONE',  ( 16.45312500061451289, -4.541064518000417216, -2.621784821875001281 ) ) ;
#33564=ORIENTED_EDGE ( 'NONE', *, *, #51473, .F. ) ;
#33565=VERTEX_POINT ( 'NONE', #72959 ) ;
#33566=AXIS2_PLACEMENT_3D ( 'NONE', #51044, #18121, #51405 ) ;
#33567=CARTESIAN_POINT ( 'NONE',  ( 19.79999999999999716, -4.330127018922190985, -2.500000000000001332 ) ) ;
#33568=CARTESIAN_POINT ( 'NONE',  ( 17.43750000000000000, -2.886751345948096681, 5.000000000000054179 ) ) ;
#33569=CARTESIAN_POINT ( 'NONE',  ( 25.52812500061451573, 6.421520780324663323E-16, -5.243569643749999010 ) ) ;
#33570=CARTESIAN_POINT ( 'NONE',  ( 2.803125000614518747, 0.000000000000000000, 5.243569643749999010 ) ) ;
#33571=CARTESIAN_POINT ( 'NONE',  ( 17.02500000122903145, 2.886751345948126879, 4.999999999999999112 ) ) ;
#33572=CARTESIAN_POINT ( 'NONE',  ( 21.66562500061451502, 3.027376345333611329, 5.243569643749999010 ) ) ;
#33573=CARTESIAN_POINT ( 'NONE',  ( 26.05312500061451431, 4.541064518000418104, -2.621784821874998173 ) ) ;
#33574=CARTESIAN_POINT ( 'NONE',  ( 6.065625000614516260, -6.054752690667223547, -1.112240025338166033E-15 ) ) ;
#33576=EDGE_CURVE ( 'NONE', #42322, #62008, #915, .T. ) ;
#33579=( BOUNDED_CURVE ( )  B_SPLINE_CURVE ( 2, ( #425, #17396, #4523, #40304, #69113, #12582, #29933, #19193, #47293 ),
 .UNSPECIFIED., .F., .F. ) 
 B_SPLINE_CURVE_WITH_KNOTS ( ( 3, 2, 2, 2, 3 ),
 ( 0.3804347826086956763, 0.3840579710144927383, 0.3913043478260869734, 0.3985507246376811530, 0.4021739130434782705 ),
 .UNSPECIFIED. ) 
 CURVE ( )  GEOMETRIC_REPRESENTATION_ITEM ( )  RATIONAL_B_SPLINE_CURVE ( ( 0.9330127018922194093, 0.9330127018922198534, 1.000000000000000000, 0.8660254037844387076, 1.000000000000000000, 0.8660254037844387076, 1.000000000000000000, 0.9330127018922194093, 0.9330127018922194093 ) ) 
 REPRESENTATION_ITEM ( '' )  );
#33582=CARTESIAN_POINT ( 'NONE',  ( -3.999999999999999112, 11.56250000122903465, -30.00000000000000000 ) ) ;
#33583=CARTESIAN_POINT ( 'NONE',  ( 4.243569643749999010, 18.32187500061451502, -32.45002607614398471 ) ) ;
#33584=CARTESIAN_POINT ( 'NONE',  ( 7.687500000000000000, -2.886751345948125991, -5.000000000000000000 ) ) ;
#33585=CARTESIAN_POINT ( 'NONE',  ( 3.525000001229034119, 2.886751345948126879, 4.999999999999999112 ) ) ;
#33586=CARTESIAN_POINT ( 'NONE',  ( 12.68437500061451573, 4.541064518000418104, 2.621784821874999949 ) ) ;
#33587=CARTESIAN_POINT ( 'NONE',  ( 1.999999999999998668, 16.81250000122903643, -33.46410161513775705 ) ) ;
#33588=CARTESIAN_POINT ( 'NONE',  ( 2.859375000614519546, 0.000000000000000000, 5.243569643749999010 ) ) ;
#33591=CARTESIAN_POINT ( 'NONE',  ( -3.999999999999997335, 10.70000000122903394, 32.30940107675850470 ) ) ;
#33592=CARTESIAN_POINT ( 'NONE',  ( 8.971875000614515372, 3.027376345333613106, -5.243569643749998122 ) ) ;
#33594=CARTESIAN_POINT ( 'NONE',  ( 20.42812500061451431, -4.541064518000419881, 2.621784821874995952 ) ) ;
#33595=CARTESIAN_POINT ( 'NONE',  ( 16.68750000000000000, -2.886751345948126435, -5.000000000000000000 ) ) ;
#33596=CARTESIAN_POINT ( 'NONE',  ( -2.121784821874999949, 17.92812500061459602, 26.32496088578401938 ) ) ;
#33597=CARTESIAN_POINT ( 'NONE',  ( 22.58437500061451431, 4.541064518000418104, 2.621784821874999949 ) ) ;
#33598=CYLINDRICAL_SURFACE ( 'NONE', #24915, 3.999999999999996447 ) ;
#33599=CARTESIAN_POINT ( 'NONE',  ( 29.02500000122903145, 2.886751345948129099, -4.999999999999998224 ) ) ;
#33600=AXIS2_PLACEMENT_3D ( 'NONE', #29083, #51618, #1019 ) ;
#33602=CARTESIAN_POINT ( 'NONE',  ( 26.20312500061451644, 0.000000000000000000, 5.243569643749999010 ) ) ;
#33603=CARTESIAN_POINT ( 'NONE',  ( 15.70312500061451644, 4.541064518000418104, -2.621784821874998173 ) ) ;
#33605=CARTESIAN_POINT ( 'NONE',  ( 10.95937500061451964, 0.000000000000000000, 5.243569643749999010 ) ) ;
#33606=CARTESIAN_POINT ( 'NONE',  ( 28.27499999999999858, -4.330127018922194537, 2.499999999999995559 ) ) ;
#33607=CARTESIAN_POINT ( 'NONE',  ( 25.46250000122903501, 4.330127018922192761, -2.499999999999997780 ) ) ;
#33609=CARTESIAN_POINT ( 'NONE',  ( 15.12187500061451750, -6.054752690667223547, -1.112240025338166033E-15 ) ) ;
#33610=CARTESIAN_POINT ( 'NONE',  ( 29.07187500061451502, -6.054752690667223547, -1.112240025338166033E-15 ) ) ;
#33611=LINE ( 'NONE', #15889, #11213 ) ;
#33612=CARTESIAN_POINT ( 'NONE',  ( 16.72500000122903430, -5.773502691896255534, -1.060575238724906372E-15 ) ) ;
#33613=CARTESIAN_POINT ( 'NONE',  ( 23.85937500061451644, 4.541064518000418104, -2.621784821874998173 ) ) ;
#33614=CARTESIAN_POINT ( 'NONE',  ( 15.34687500061451537, 6.054752690667223547, 3.707466751127219781E-16 ) ) ;
#33616=CARTESIAN_POINT ( 'NONE',  ( 29.09999999999999787, 0.000000000000000000, 4.999999999999998224 ) ) ;
#33617=CARTESIAN_POINT ( 'NONE',  ( 4.312500001229034652, 4.330127018922192761, -2.499999999999997780 ) ) ;
#33618=CARTESIAN_POINT ( 'NONE',  ( 5.100000000000000533, 4.330127018922192761, -2.499999999999997780 ) ) ;
#33620=CARTESIAN_POINT ( 'NONE',  ( 19.52812500061451573, -4.541064518000419881, 2.621784821874995952 ) ) ;
#33621=CARTESIAN_POINT ( 'NONE',  ( 9.562500000000001776, 2.886751345948129099, -4.999999999999998224 ) ) ;
#33622=FACE_OUTER_BOUND ( 'NONE', #63314, .T. ) ;
#33623=CARTESIAN_POINT ( 'NONE',  ( 17.25000000000000000, 4.330127018922192761, -2.499999999999997780 ) ) ;
#33624=CARTESIAN_POINT ( 'NONE',  ( -4.243569643749997233, 12.64062500061451999, 32.45002607614398471 ) ) ;
#33626=CARTESIAN_POINT ( 'NONE',  ( 21.97500000122903074, 2.886751345948126879, 4.999999999999999112 ) ) ;
#33628=CARTESIAN_POINT ( 'NONE',  ( 27.68437500061451573, -4.541064518000419881, 2.621784821874995952 ) ) ;
#33630=CARTESIAN_POINT ( 'NONE',  ( 16.97812500061451502, 6.421520780324663323E-16, -5.243569643749999010 ) ) ;
#33631=CARTESIAN_POINT ( 'NONE',  ( 22.82812500061451644, 6.421520780324663323E-16, -5.243569643749999010 ) ) ;
#33632=B_SPLINE_CURVE_WITH_KNOTS ( 'NONE', 3,
 ( #24090, #46637, #494, #41104, #7471, #62533, #29997, #52538, #1947, #24453, #23003, #45563, #47002, #69537, #34455, #18896, #23368, #63976, #40371, #13359, #56983, #45916, #62889, #17810, #68448, #6387, #28920, #12284, #34817, #57347, #13735, #31833, #48097, #14466, #14830, #43291, #64711, #14095, #31465, #8565, #36635, #65075, #8201, #36999, #42548, #25556 ),
 .UNSPECIFIED., .F., .F.,
 ( 4, 2, 2, 2, 2, 2, 2, 2, 2, 2, 2, 2, 2, 2, 2, 2, 2, 2, 2, 2, 2, 2, 4 ),
 ( 0.000000000000000000, 0.001203096460345648173, 0.002406192920691296346, 0.003609289381036944518, 0.004812385841382592691, 0.005413934071555414826, 0.006015482301728236093, 0.007218578762073870822, 0.008421675222419504683, 0.009023223452592316410, 0.009624771682765129871, 0.01082786814311074639, 0.01142941637328355291, 0.01203096460345635769, 0.01323406106380197247, 0.01443715752414758725, 0.01503870575432038684, 0.01564025398449318469, 0.01684335044483878038, 0.01744489867501157823, 0.01804644690518437608, 0.01864799513535717046, 0.01924954336552996831 ),
 .UNSPECIFIED. ) ;
#33633=CARTESIAN_POINT ( 'NONE',  ( 22.73437500061451644, -4.541064518000419881, 2.621784821874995952 ) ) ;
#33634=CARTESIAN_POINT ( 'NONE',  ( 5.962500000000002132, 2.886751345948129099, -4.999999999999998224 ) ) ;
#33635=CARTESIAN_POINT ( 'NONE',  ( 10.19062500061451892, -3.027376345333610441, -5.243569643749999898 ) ) ;
#33636=CARTESIAN_POINT ( 'NONE',  ( 24.44062500061451715, -3.027376345333614438, 5.243569643749998122 ) ) ;
#33637=CARTESIAN_POINT ( 'NONE',  ( 15.60937500061451644, -4.541064518000417216, -2.621784821875001281 ) ) ;
#33638=CARTESIAN_POINT ( 'NONE',  ( 19.99687500061451573, -3.027376345333614438, 5.243569643749998122 ) ) ;
#33640=CARTESIAN_POINT ( 'NONE',  ( -2.121784821874999949, 17.02812500061451573, 26.32496088578401938 ) ) ;
#33641=CARTESIAN_POINT ( 'NONE',  ( 20.40000000122903145, -2.886751345948125991, -5.000000000000000000 ) ) ;
#33643=CARTESIAN_POINT ( 'NONE',  ( 12.25312500061451537, 0.000000000000000000, 5.243569643749999010 ) ) ;
#33644=CARTESIAN_POINT ( 'NONE',  ( 6.084375000614518747, -4.541064518000419881, 2.621784821874995952 ) ) ;
#33645=CARTESIAN_POINT ( 'NONE',  ( 4.209375000614516971, 0.000000000000000000, 5.243569643749999010 ) ) ;
#33646=ORIENTED_EDGE ( 'NONE', *, *, #40344, .F. ) ;
#33647=CARTESIAN_POINT ( 'NONE',  ( 28.92187500061451644, 3.027376345333611329, 5.243569643749999010 ) ) ;
#33648=CARTESIAN_POINT ( 'NONE',  ( 19.90312500061451573, 0.000000000000000000, 5.243569643749999010 ) ) ;
#33649=CARTESIAN_POINT ( 'NONE',  ( 27.75000000122903288, 5.773502691896255534, 3.535250795749688894E-16 ) ) ;
#33650=CARTESIAN_POINT ( 'NONE',  ( 26.72812500061451502, -4.541064518000419881, 2.621784821874995952 ) ) ;
#33651=CARTESIAN_POINT ( 'NONE',  ( 25.17187500061451644, 3.027376345333613106, -5.243569643749998122 ) ) ;
#33652=CARTESIAN_POINT ( 'NONE',  ( 16.34062500061451573, -3.027376345333614438, 5.243569643749998122 ) ) ;
#33653=CARTESIAN_POINT ( 'NONE',  ( 3.999999999999999112, 10.32500000000000107, 30.00000000000000000 ) ) ;
#33654=CARTESIAN_POINT ( 'NONE',  ( 25.26562500061451289, 3.027376345333611329, 5.243569643749999010 ) ) ;
#33655=CARTESIAN_POINT ( 'NONE',  ( 4.237500001229036251, 6.123233995736764310E-16, -4.999999999999998224 ) ) ;
#33656=VERTEX_POINT ( 'NONE', #17513 ) ;
#33657=CARTESIAN_POINT ( 'NONE',  ( 27.29999999999999716, 0.000000000000000000, 4.999999999999998224 ) ) ;
#33658=CARTESIAN_POINT ( 'NONE',  ( -3.999999999999999112, 14.60000000000000142, -30.00000000000000000 ) ) ;
#33661=CARTESIAN_POINT ( 'NONE',  ( 4.959375000614516971, 4.541064518000418104, -2.621784821874998173 ) ) ;
#33662=CARTESIAN_POINT ( 'NONE',  ( 13.30312500061451786, -4.541064518000417216, -2.621784821875001281 ) ) ;
#33663=CARTESIAN_POINT ( 'NONE',  ( 7.171875000614517326, 3.027376345333613106, -5.243569643749998122 ) ) ;
#33664=CARTESIAN_POINT ( 'NONE',  ( 25.57500000122903216, 2.886751345948126879, 4.999999999999999112 ) ) ;
#33666=CARTESIAN_POINT ( 'NONE',  ( 14.07187500061451679, 3.027376345333611329, 5.243569643749999010 ) ) ;
#33667=CARTESIAN_POINT ( 'NONE',  ( 3.084375000614519191, 6.421520780324663323E-16, -5.243569643749999010 ) ) ;
#33668=CARTESIAN_POINT ( 'NONE',  ( 27.86249999999999716, -5.773502691896255534, -1.060575238724906372E-15 ) ) ;
#33669=CARTESIAN_POINT ( 'NONE',  ( 27.34687500061451360, -3.027376345333610441, -5.243569643749999898 ) ) ;
#33671=CARTESIAN_POINT ( 'NONE',  ( 13.86562500061451431, 3.027376345333613106, -5.243569643749998122 ) ) ;
#33672=ORIENTED_EDGE ( 'NONE', *, *, #69921, .T. ) ;
#33674=CARTESIAN_POINT ( 'NONE',  ( 10.34062500061451750, 6.054752690667223547, 3.707466751127219781E-16 ) ) ;
#33675=AXIS2_PLACEMENT_3D ( 'NONE', #65580, #20876, #65951 ) ;
#33676=CARTESIAN_POINT ( 'NONE',  ( 6.590625000614518392, -3.027376345333610441, -5.243569643749999898 ) ) ;
#33678=CARTESIAN_POINT ( 'NONE',  ( 16.08749999999999503, -2.886751345948129988, 4.999999999999997335 ) ) ;
#33679=CARTESIAN_POINT ( 'NONE',  ( 17.22187500061451715, 3.027376345333611329, 5.243569643749999010 ) ) ;
#33680=CARTESIAN_POINT ( 'NONE',  ( 13.87500000122903465, 2.886751345948126879, 4.999999999999999112 ) ) ;
#33682=CARTESIAN_POINT ( 'NONE',  ( 21.23437500061451644, 4.541064518000418104, 2.621784821874999949 ) ) ;
#33683=CARTESIAN_POINT ( 'NONE',  ( -2.121784821874999949, 12.97812500061451679, -33.67503911421598417 ) ) ;
#33685=CARTESIAN_POINT ( 'NONE',  ( 4.162457142321725811, 2.770219694541247168, 4.452085545162252522 ) ) ;
#33686=CARTESIAN_POINT ( 'NONE',  ( 27.74062500061451431, -3.027376345333610441, -5.243569643749999898 ) ) ;
#33687=CARTESIAN_POINT ( 'NONE',  ( 5.137500001229033941, 6.123233995736764310E-16, -4.999999999999998224 ) ) ;
#33689=CARTESIAN_POINT ( 'NONE',  ( 27.52500000000000213, 6.123233995736764310E-16, -4.999999999999998224 ) ) ;
#33690=CARTESIAN_POINT ( 'NONE',  ( 8.428125000614517859, 6.421520780324663323E-16, -5.243569643749999010 ) ) ;
#33692=CARTESIAN_POINT ( 'NONE',  ( 18.12187500061451573, 3.027376345333611329, 5.243569643749999010 ) ) ;
#33694=CARTESIAN_POINT ( 'NONE',  ( 5.578125000614518214, -4.541064518000419881, 2.621784821874995952 ) ) ;
#33695=CARTESIAN_POINT ( 'NONE',  ( 10.73437500061451644, 6.421520780324663323E-16, -5.243569643749999010 ) ) ;
#33696=ORIENTED_EDGE ( 'NONE', *, *, #50010, .F. ) ;
#33697=CARTESIAN_POINT ( 'NONE',  ( 22.39687500061451075, -3.027376345333610441, -5.243569643749999898 ) ) ;
#33698=CARTESIAN_POINT ( 'NONE',  ( 3.992467690304758232, 3.010110221998377078, -30.28122918867793700 ) ) ;
#33699=CARTESIAN_POINT ( 'NONE',  ( 29.92500000000000071, 4.330127018922191873, 2.499999999999999556 ) ) ;
#33700=CARTESIAN_POINT ( 'NONE',  ( 5.587500000000003020, 5.773502691896255534, 3.535250795749688894E-16 ) ) ;
#33701=CARTESIAN_POINT ( 'NONE',  ( 15.22500000122903252, 2.886751345948126879, 4.999999999999999112 ) ) ;
#33703=CARTESIAN_POINT ( 'NONE',  ( 18.97499999999999787, 6.123233995736764310E-16, -4.999999999999998224 ) ) ;
#33704=ORIENTED_EDGE ( 'NONE', *, *, #12479, .F. ) ;
#33705=CARTESIAN_POINT ( 'NONE',  ( 13.01249999999999929, -5.773502691896255534, -1.060575238724906372E-15 ) ) ;
#33706=CARTESIAN_POINT ( 'NONE',  ( 28.00312500061451715, 0.000000000000000000, 5.243569643749999010 ) ) ;
#33707=CARTESIAN_POINT ( 'NONE',  ( 16.64999999999999858, -4.330127018922190985, -2.500000000000001332 ) ) ;
#33708=( BOUNDED_CURVE ( )  B_SPLINE_CURVE ( 1, ( #53031, #57115 ),
 .UNSPECIFIED., .F., .F. ) 
 B_SPLINE_CURVE_WITH_KNOTS ( ( 2, 2 ),
 ( 0.000000000000000000, 1.000000000000000000 ),
 .UNSPECIFIED. ) 
 CURVE ( )  GEOMETRIC_REPRESENTATION_ITEM ( )  RATIONAL_B_SPLINE_CURVE ( ( 0.9401542295229587953, 0.9401542295229587953 ) ) 
 REPRESENTATION_ITEM ( '' )  );
#33709=CARTESIAN_POINT ( 'NONE',  ( 11.51250000122903216, 4.330127018922192761, -2.499999999999997780 ) ) ;
#33710=CARTESIAN_POINT ( 'NONE',  ( 9.440625000614517148, 6.054752690667223547, 3.707466751127219781E-16 ) ) ;
#33711=EDGE_CURVE ( 'NONE', #60995, #37430, #57045, .T. ) ;
#33713=CARTESIAN_POINT ( 'NONE',  ( 7.837499999999999467, 5.773502691896255534, 3.535250795749688894E-16 ) ) ;
#33714=CARTESIAN_POINT ( 'NONE',  ( -5.810221930991193690E-16, 18.98750000000000071, 26.00000000000000355 ) ) ;
#33715=CARTESIAN_POINT ( 'NONE',  ( -4.243569643749999898, 15.32187500061451679, -32.45002607614398471 ) ) ;
#33716=CARTESIAN_POINT ( 'NONE',  ( 27.86250000122903359, 0.000000000000000000, 4.999999999999998224 ) ) ;
#33718=CARTESIAN_POINT ( 'NONE',  ( 8.025000000000000355, -4.330127018922194537, 2.499999999999995559 ) ) ;
#33721=CARTESIAN_POINT ( 'NONE',  ( 23.99062500061451786, -3.027376345333614438, 5.243569643749998122 ) ) ;
#33722=CARTESIAN_POINT ( 'NONE',  ( 28.86562500061451786, 3.027376345333611329, 5.243569643749999010 ) ) ;
#33724=CARTESIAN_POINT ( 'NONE',  ( 18.86250000122903359, 0.000000000000000000, 4.999999999999998224 ) ) ;
#33725=CARTESIAN_POINT ( 'NONE',  ( 19.32187500061451857, 3.027376345333613106, -5.243569643749998122 ) ) ;
#33726=CARTESIAN_POINT ( 'NONE',  ( 17.09062500061451573, 6.054752690667223547, 3.707466751127219781E-16 ) ) ;
#33727=CARTESIAN_POINT ( 'NONE',  ( 2.121784821875001281, 10.50312500061459531, -26.32496088578401938 ) ) ;
#33728=CARTESIAN_POINT ( 'NONE',  ( 6.740625000614516082, 6.054752690667223547, 3.707466751127219781E-16 ) ) ;
#33729=CARTESIAN_POINT ( 'NONE',  ( 29.25000000122903288, -2.886751345948129988, 4.999999999999997335 ) ) ;
#33731=CARTESIAN_POINT ( 'NONE',  ( 19.22812500061451502, 6.421520780324663323E-16, -5.243569643749999010 ) ) ;
#33732=FACE_OUTER_BOUND ( 'NONE', #3906, .T. ) ;
#33734=CARTESIAN_POINT ( 'NONE',  ( 13.73437500061451821, -4.541064518000419881, 2.621784821874995952 ) ) ;
#33735=CARTESIAN_POINT ( 'NONE',  ( 11.82187500061451679, 3.027376345333611329, 5.243569643749999010 ) ) ;
#33736=CARTESIAN_POINT ( 'NONE',  ( 21.42187500061451644, -6.054752690667223547, -1.112240025338166033E-15 ) ) ;
#33737=EDGE_LOOP ( 'NONE', ( #51378, #56344, #62599, #7979 ) ) ;
#33738=CARTESIAN_POINT ( 'NONE',  ( 2.803125000614518747, 0.000000000000000000, 5.243569643749999010 ) ) ;
#33739=CARTESIAN_POINT ( 'NONE',  ( 25.60312500061451502, 4.541064518000418104, -2.621784821874998173 ) ) ;
#33740=CARTESIAN_POINT ( 'NONE',  ( 27.06562500061451004, 3.027376345333611329, 5.243569643749999010 ) ) ;
#33741=CARTESIAN_POINT ( 'NONE',  ( 3.999999999999999112, 12.12500000000000000, -30.00000000000000000 ) ) ;
#33742=CARTESIAN_POINT ( 'NONE',  ( -2.828200636599751609E-16, 17.63749999999999929, 25.38119784648299770 ) ) ;
#33743=CARTESIAN_POINT ( 'NONE',  ( 5.709375000614517859, -4.541064518000417216, -2.621784821875001281 ) ) ;
#33744=CARTESIAN_POINT ( 'NONE',  ( 12.07500000122903216, 2.886751345948126879, 4.999999999999999112 ) ) ;
#33745=CARTESIAN_POINT ( 'NONE',  ( 6.225000001229036073, 2.886751345948126879, 4.999999999999999112 ) ) ;
#33746=CARTESIAN_POINT ( 'NONE',  ( 3.815625000614518036, -6.054752690667223547, -1.112240025338166033E-15 ) ) ;
#33749=CARTESIAN_POINT ( 'NONE',  ( 12.08437500061451608, 6.421520780324663323E-16, -5.243569643749999010 ) ) ;
#33751=CARTESIAN_POINT ( 'NONE',  ( 18.96562500061451573, 3.027376345333611329, 5.243569643749999010 ) ) ;
#33752=CARTESIAN_POINT ( 'NONE',  ( 13.54687500061451999, 6.054752690667223547, 3.707466751127219781E-16 ) ) ;
#33753=CARTESIAN_POINT ( 'NONE',  ( 3.928125000614516527, 6.421520780324663323E-16, -5.243569643749999010 ) ) ;
#33754=CARTESIAN_POINT ( 'NONE',  ( 22.32187500061451857, -6.054752690667223547, -1.112240025338166033E-15 ) ) ;
#33755=CARTESIAN_POINT ( 'NONE',  ( 10.05937500061451750, 0.000000000000000000, 5.243569643749999010 ) ) ;
#33756=CARTESIAN_POINT ( 'NONE',  ( 4.078125000614517326, 4.541064518000418104, 2.621784821874999949 ) ) ;
#33758=CARTESIAN_POINT ( 'NONE',  ( 4.875000001229034652, 2.886751345948126879, 4.999999999999999112 ) ) ;
#33759=CARTESIAN_POINT ( 'NONE',  ( 20.57812500061451644, 6.421520780324663323E-16, -5.243569643749999010 ) ) ;
#33760=CARTESIAN_POINT ( 'NONE',  ( 8.437500001229034652, 4.330127018922191873, 2.499999999999999556 ) ) ;
#33761=CARTESIAN_POINT ( 'NONE',  ( 16.49062500061451786, -3.027376345333610441, -5.243569643749999898 ) ) ;
#33763=CARTESIAN_POINT ( 'NONE',  ( 15.81562500061451537, 3.027376345333611329, 5.243569643749999010 ) ) ;
#33765=CARTESIAN_POINT ( 'NONE',  ( 16.08749999999999503, -2.886751345948129988, 4.999999999999997335 ) ) ;
#33766=CARTESIAN_POINT ( 'NONE',  ( 9.225000001229034297, 2.886751345948129099, -4.999999999999998224 ) ) ;
#33767=ADVANCED_FACE ( 'NONE', ( #2001 ), #42239, .F. ) ;
#33768=CARTESIAN_POINT ( 'NONE',  ( 4.940625000614515372, 6.054752690667223547, 3.707466751127219781E-16 ) ) ;
#33770=CARTESIAN_POINT ( 'NONE',  ( 20.17500000122903359, 2.886751345948126879, 4.999999999999999112 ) ) ;
#33772=CARTESIAN_POINT ( 'NONE',  ( -4.243569643749997233, 12.24687500061451928, -27.54997392385601174 ) ) ;
#33774=CARTESIAN_POINT ( 'NONE',  ( 0.000000000000000000, 20.00000000000000000, -30.00000000000000000 ) ) ;
#33776=CARTESIAN_POINT ( 'NONE',  ( 21.75937500061451502, 0.000000000000000000, 5.243569643749999010 ) ) ;
#33777=CARTESIAN_POINT ( 'NONE',  ( 12.44999999999999929, 0.000000000000000000, 4.999999999999998224 ) ) ;
#33778=CARTESIAN_POINT ( 'NONE',  ( 17.65312500061451573, 0.000000000000000000, 5.243569643749999010 ) ) ;
#33780=CARTESIAN_POINT ( 'NONE',  ( 11.10000000000000142, 0.000000000000000000, 4.999999999999998224 ) ) ;
#33782=CARTESIAN_POINT ( 'NONE',  ( 27.90937500061451715, 4.541064518000418104, -2.621784821874998173 ) ) ;
#33784=CARTESIAN_POINT ( 'NONE',  ( 12.51562500061451821, 3.027376345333613106, -5.243569643749998122 ) ) ;
#33785=CARTESIAN_POINT ( 'NONE',  ( 10.88437500061451679, 4.541064518000418104, 2.621784821874999949 ) ) ;
#33786=ORIENTED_EDGE ( 'NONE', *, *, #40515, .F. ) ;
#33787=CARTESIAN_POINT ( 'NONE',  ( -3.999999999999999112, 14.11250000000000071, -32.30940107675850470 ) ) ;
#33788=CARTESIAN_POINT ( 'NONE',  ( 23.42812500061451786, 4.541064518000418104, 2.621784821874999949 ) ) ;
#33791=CARTESIAN_POINT ( 'NONE',  ( 13.08750000000000036, -2.886751345948125991, -5.000000000000000000 ) ) ;
#33792=CARTESIAN_POINT ( 'NONE',  ( 21.07500000122903572, 2.886751345948126879, 4.999999999999999112 ) ) ;
#33793=CARTESIAN_POINT ( 'NONE',  ( 15.85312500061451857, 0.000000000000000000, 5.243569643749999010 ) ) ;
#33795=VERTEX_POINT ( 'NONE', #35237 ) ;
#33796=CARTESIAN_POINT ( 'NONE',  ( 20.92500000000000071, 4.330127018922191873, 2.499999999999999556 ) ) ;
#33797=CARTESIAN_POINT ( 'NONE',  ( 24.33749999999999858, -2.886751345948125991, -5.000000000000000000 ) ) ;
#33798=CARTESIAN_POINT ( 'NONE',  ( 21.83437500061451786, -4.541064518000419881, 2.621784821874995952 ) ) ;
#33799=CARTESIAN_POINT ( 'NONE',  ( 24.10312500061451502, -4.541064518000417216, -2.621784821875001281 ) ) ;
#33802=CARTESIAN_POINT ( 'NONE',  ( 7.903125000614515727, -4.541064518000417216, -2.621784821875001281 ) ) ;
#33804=VECTOR ( 'NONE', #51388, 1000.000000000000000 ) ;
#33805=CARTESIAN_POINT ( 'NONE',  ( 14.96250000000000036, 2.886751345948129099, -4.999999999999998224 ) ) ;
#33806=CARTESIAN_POINT ( 'NONE',  ( 3.578157825243565515, -3.492515161539162527, -3.678572976455726895 ) ) ;
#33807=CARTESIAN_POINT ( 'NONE',  ( 5.034375000614519813, 4.541064518000418104, 2.621784821874999949 ) ) ;
#33808=CARTESIAN_POINT ( 'NONE',  ( 28.35937500061451289, 4.541064518000418104, -2.621784821874998173 ) ) ;
#33809=ORIENTED_EDGE ( 'NONE', *, *, #36205, .F. ) ;
#33810=CARTESIAN_POINT ( 'NONE',  ( 24.81562500061451715, 3.027376345333611329, 5.243569643749999010 ) ) ;
#33811=CARTESIAN_POINT ( 'NONE',  ( 25.88437500061451502, -4.541064518000419881, 2.621784821874995952 ) ) ;
#33812=CARTESIAN_POINT ( 'NONE',  ( -2.121784821874999949, 17.92812500061459602, -33.67503911421598417 ) ) ;
#33813=CARTESIAN_POINT ( 'NONE',  ( 11.10000000000000142, 0.000000000000000000, 4.999999999999998224 ) ) ;
#33814=CARTESIAN_POINT ( 'NONE',  ( 8.540625000614518569, 6.054752690667223547, 3.707466751127219781E-16 ) ) ;
#33815=CARTESIAN_POINT ( 'NONE',  ( 7.162500000000001421, -5.773502691896255534, -1.060575238724906372E-15 ) ) ;
#33816=CARTESIAN_POINT ( 'NONE',  ( 26.05312500061451431, 4.541064518000418104, -2.621784821874998173 ) ) ;
#33817=CARTESIAN_POINT ( 'NONE',  ( 7.320879633048903241E-15, 18.20000000122903216, -34.00000000000000000 ) ) ;
#33819=CARTESIAN_POINT ( 'NONE',  ( 3.065625000614517592, 3.027376345333613106, -5.243569643749998122 ) ) ;
#33820=CARTESIAN_POINT ( 'NONE',  ( 19.09687500061451360, -3.027376345333614438, 5.243569643749998122 ) ) ;
#33821=CARTESIAN_POINT ( 'NONE',  ( 4.243569643749999010, 15.17187500061451644, 27.54997392385601174 ) ) ;
#33823=CARTESIAN_POINT ( 'NONE',  ( 20.85937500061451644, 0.000000000000000000, 5.243569643749999010 ) ) ;
#33824=CARTESIAN_POINT ( 'NONE',  ( 3.337499999999999911, 5.773502691896255534, 3.535250795749688894E-16 ) ) ;
#33825=CARTESIAN_POINT ( 'NONE',  ( -2.121784821874996840, 19.48437500061451644, 33.67503911421598417 ) ) ;
#33826=CARTESIAN_POINT ( 'NONE',  ( 9.628125000614517148, -4.541064518000419881, 2.621784821874995952 ) ) ;
#33827=DIRECTION ( 'NONE',  ( -1.000000000000000000, 0.000000000000000000, 0.000000000000000000 ) ) ;
#33828=CARTESIAN_POINT ( 'NONE',  ( 5.896875000614518747, 6.054752690667223547, 3.707466751127219781E-16 ) ) ;
#33830=CARTESIAN_POINT ( 'NONE',  ( 6.553125000614518747, -4.541064518000417216, -2.621784821875001281 ) ) ;
#33831=CARTESIAN_POINT ( 'NONE',  ( 12.94687500061451857, -3.027376345333610441, -5.243569643749999898 ) ) ;
#33832=( LENGTH_UNIT ( ) NAMED_UNIT ( * ) SI_UNIT ( .MILLI., .METRE. ) );
#33833=CARTESIAN_POINT ( 'NONE',  ( 18.22500000122903430, 2.886751345948129099, -4.999999999999998224 ) ) ;
#33834=CARTESIAN_POINT ( 'NONE',  ( 6.984375000614516438, -4.541064518000419881, 2.621784821874995952 ) ) ;
#33835=CARTESIAN_POINT ( 'NONE',  ( 8.953125000614518214, 4.541064518000418104, -2.621784821874998173 ) ) ;
#33836=CARTESIAN_POINT ( 'NONE',  ( 4.178128910459903089, -3.728570022149966690, -3.541927282058038973 ) ) ;
#33838=CARTESIAN_POINT ( 'NONE',  ( 20.14687500061451786, -3.027376345333610441, -5.243569643749999898 ) ) ;
#33839=CARTESIAN_POINT ( 'NONE',  ( 9.037500001229034297, -4.330127018922194537, 2.499999999999995559 ) ) ;
#33840=CARTESIAN_POINT ( 'NONE',  ( 27.14062500061451644, -3.027376345333614438, 5.243569643749998122 ) ) ;
#33841=CARTESIAN_POINT ( 'NONE',  ( 11.54062500061451857, -3.027376345333610441, -5.243569643749999898 ) ) ;
#33842=CARTESIAN_POINT ( 'NONE',  ( 29.70937500061451431, 4.541064518000418104, -2.621784821874998173 ) ) ;
#33843=CARTESIAN_POINT ( 'NONE',  ( 4.243569643749999898, 10.14687500061451786, -27.54997392385601529 ) ) ;
#33844=CARTESIAN_POINT ( 'NONE',  ( 13.50000000122903288, -2.886751345948129988, 4.999999999999997335 ) ) ;
#33845=CARTESIAN_POINT ( 'NONE',  ( 27.85312500061451502, 4.541064518000418104, -2.621784821874998173 ) ) ;
#33846=CARTESIAN_POINT ( 'NONE',  ( -2.121784821874999949, 16.12812500061451715, -33.67503911421598417 ) ) ;
#33847=CARTESIAN_POINT ( 'NONE',  ( 14.51250000122903394, -4.330127018922190985, -2.500000000000001332 ) ) ;
#33848=CARTESIAN_POINT ( 'NONE',  ( 12.26249999999999929, 2.886751345948129099, -4.999999999999998224 ) ) ;
#33849=CARTESIAN_POINT ( 'NONE',  ( 23.09062500061451573, -3.027376345333614438, 5.243569643749998122 ) ) ;
#33850=CARTESIAN_POINT ( 'NONE',  ( 8.334375000614516082, -4.541064518000419881, 2.621784821874995952 ) ) ;
#33851=CARTESIAN_POINT ( 'NONE',  ( 8.737500001229033586, 6.123233995736764310E-16, -4.999999999999998224 ) ) ;
#33852=CARTESIAN_POINT ( 'NONE',  ( 16.08750000122903501, 4.330127018922191873, 2.499999999999999556 ) ) ;
#33853=CARTESIAN_POINT ( 'NONE',  ( 13.41562500061451502, 3.027376345333613106, -5.243569643749998122 ) ) ;
#33854=CARTESIAN_POINT ( 'NONE',  ( 16.11562500061451786, 3.027376345333613106, -5.243569643749998122 ) ) ;
#33855=CARTESIAN_POINT ( 'NONE',  ( 27.90000000122903145, -2.886751345948129988, 4.999999999999997335 ) ) ;
#33856=CARTESIAN_POINT ( 'NONE',  ( 22.19999999999999574, 4.330127018922192761, -2.499999999999997780 ) ) ;
#33857=CARTESIAN_POINT ( 'NONE',  ( 23.10937500061451644, 0.000000000000000000, 5.243569643749999010 ) ) ;
#33858=CARTESIAN_POINT ( 'NONE',  ( 18.26250000122903216, 4.330127018922192761, -2.499999999999997780 ) ) ;
#33860=CARTESIAN_POINT ( 'NONE',  ( 10.98750000122903536, 6.123233995736764310E-16, -4.999999999999998224 ) ) ;
#33861=CARTESIAN_POINT ( 'NONE',  ( 28.02187500061451431, 3.027376345333611329, 5.243569643749999010 ) ) ;
#33862=CARTESIAN_POINT ( 'NONE',  ( 4.771875000614516971, -6.054752690667223547, -1.112240025338166033E-15 ) ) ;
#33863=CARTESIAN_POINT ( 'NONE',  ( 22.49062500061451431, 6.054752690667223547, 3.707466751127219781E-16 ) ) ;
#33866=CARTESIAN_POINT ( 'NONE',  ( 9.271875000614516082, -6.054752690667223547, -1.112240025338166033E-15 ) ) ;
#33868=CARTESIAN_POINT ( 'NONE',  ( 29.31562500061451715, 3.027376345333611329, 5.243569643749999010 ) ) ;
#33869=CARTESIAN_POINT ( 'NONE',  ( 6.009375000614519458, 0.000000000000000000, 5.243569643749999010 ) ) ;
#33870=CARTESIAN_POINT ( 'NONE',  ( 25.91249999999999787, 2.886751345948093572, 5.000000000000056843 ) ) ;
#33871=CARTESIAN_POINT ( 'NONE',  ( 28.73437500061451644, 6.421520780324663323E-16, -5.243569643749999010 ) ) ;
#33872=CARTESIAN_POINT ( 'NONE',  ( -4.243569643749999898, 10.80312500061459602, 30.00000000000000000 ) ) ;
#33873=CARTESIAN_POINT ( 'NONE',  ( 19.65000000000000213, 0.000000000000000000, 4.999999999999998224 ) ) ;
#33874=ORIENTED_EDGE ( 'NONE', *, *, #64752, .T. ) ;
#33875=CARTESIAN_POINT ( 'NONE',  ( 27.11249999999999716, 2.886751345948129099, -4.999999999999998224 ) ) ;
#33876=CARTESIAN_POINT ( 'NONE',  ( 28.02187500061451431, 3.027376345333611329, 5.243569643749999010 ) ) ;
#33878=CARTESIAN_POINT ( 'NONE',  ( 15.36562500061451608, 3.027376345333611329, 5.243569643749999010 ) ) ;
#33879=CARTESIAN_POINT ( 'NONE',  ( 9.403125000614517504, 4.541064518000418104, -2.621784821874998173 ) ) ;
#33881=CARTESIAN_POINT ( 'NONE',  ( 3.684375000614518836, 4.541064518000418104, 2.621784821874999949 ) ) ;
#33882=CARTESIAN_POINT ( 'NONE',  ( 17.81250000122903288, 4.330127018922192761, -2.499999999999997780 ) ) ;
#33883=CARTESIAN_POINT ( 'NONE',  ( 22.76249999999999574, 2.886751345948126879, 4.999999999999999112 ) ) ;
#33885=CARTESIAN_POINT ( 'NONE',  ( 6.759375000614516793, 4.541064518000418104, -2.621784821874998173 ) ) ;
#33886=CARTESIAN_POINT ( 'NONE',  ( 10.65937500061451715, -4.541064518000417216, -2.621784821875001281 ) ) ;
#33887=CARTESIAN_POINT ( 'NONE',  ( 22.54687500061451999, 6.054752690667223547, 3.707466751127219781E-16 ) ) ;
#33888=CARTESIAN_POINT ( 'NONE',  ( -1.071796769724504328, 14.69240381056766687, -26.00000000000001066 ) ) ;
#33889=VERTEX_POINT ( 'NONE', #46695 ) ;
#33890=CARTESIAN_POINT ( 'NONE',  ( 3.496875000614518836, -3.027376345333610441, -5.243569643749999898 ) ) ;
#33891=CARTESIAN_POINT ( 'NONE',  ( 5.971875000614516260, 3.027376345333611329, 5.243569643749999010 ) ) ;
#33892=CARTESIAN_POINT ( 'NONE',  ( 18.86249999999999716, -5.773502691896255534, -1.060575238724906372E-15 ) ) ;
#33893=CARTESIAN_POINT ( 'NONE',  ( 16.26562500061451289, 3.027376345333611329, 5.243569643749999010 ) ) ;
#33895=ADVANCED_FACE ( 'NONE', ( #19315 ), #69589, .F. ) ;
#33897=CARTESIAN_POINT ( 'NONE',  ( 9.590625000614517504, -3.027376345333614438, 5.243569643749998122 ) ) ;
#33898=CARTESIAN_POINT ( 'NONE',  ( 26.82187500061451857, -6.054752690667223547, -1.112240025338166033E-15 ) ) ;
#33900=CARTESIAN_POINT ( 'NONE',  ( 28.80937500061451573, 4.541064518000418104, -2.621784821874998173 ) ) ;
#33901=CARTESIAN_POINT ( 'NONE',  ( 8.887499999999999289, -2.886751345948129988, 4.999999999999997335 ) ) ;
#33902=CARTESIAN_POINT ( 'NONE',  ( -3.999999999999999556, 16.02500000122903501, 27.69059892324149530 ) ) ;
#33903=CARTESIAN_POINT ( 'NONE',  ( 9.637500001229033941, 6.123233995736764310E-16, -4.999999999999998224 ) ) ;
#33904=CARTESIAN_POINT ( 'NONE',  ( 18.87187500061451573, 3.027376345333613106, -5.243569643749998122 ) ) ;
#33905=CARTESIAN_POINT ( 'NONE',  ( 13.39687500061451608, -3.027376345333610441, -5.243569643749999898 ) ) ;
#33906=CARTESIAN_POINT ( 'NONE',  ( -3.578127771932956058, 3.495591672637165637, -28.19363475146253251 ) ) ;
#33908=CARTESIAN_POINT ( 'NONE',  ( 13.67812500061451786, -4.541064518000419881, 2.621784821874995952 ) ) ;
#33909=CARTESIAN_POINT ( 'NONE',  ( 26.40000000122902790, 5.773502691896255534, 3.535250795749688894E-16 ) ) ;
#33910=CARTESIAN_POINT ( 'NONE',  ( 15.57187500061451679, -6.054752690667223547, -1.112240025338166033E-15 ) ) ;
#33911=B_SPLINE_CURVE_WITH_KNOTS ( 'NONE', 3,
 ( #14505, #19301, #25216, #3809, #41854, #30770, #47763, #8604, #20033, #71029 ),
 .UNSPECIFIED., .F., .F.,
 ( 4, 3, 3, 4 ),
 ( 0.000000000000000000, 2.812508172722986163E-05, 5.625016478268387503E-05, 0.0001066165372333795924 ),
 .UNSPECIFIED. ) ;
#33912=CARTESIAN_POINT ( 'NONE',  ( 4.763386231524737724, 8.796087519298451340, -33.66842538561026288 ) ) ;
#33913=CARTESIAN_POINT ( 'NONE',  ( 17.72812500061451502, -4.541064518000419881, 2.621784821874995952 ) ) ;
#33914=FACE_BOUND ( 'NONE', #12788, .T. ) ;
#33915=CARTESIAN_POINT ( 'NONE',  ( 26.22187500061451715, 3.027376345333611329, 5.243569643749999010 ) ) ;
#33916=CARTESIAN_POINT ( 'NONE',  ( -3.000416591977282496E-16, 10.69062500061451715, 25.09994784771203058 ) ) ;
#33917=CARTESIAN_POINT ( 'NONE',  ( 15.57187500061451679, -6.054752690667223547, -1.112240025338166033E-15 ) ) ;
#33918=CARTESIAN_POINT ( 'NONE',  ( 13.95000000122903572, -2.886751345948129988, 4.999999999999997335 ) ) ;
#33920=CARTESIAN_POINT ( 'NONE',  ( 4.243569643749999898, 18.69687500061451857, -27.54997392385601529 ) ) ;
#33921=( BOUNDED_CURVE ( )  B_SPLINE_CURVE ( 2, ( #2036, #36724, #13826, #41909, #69982, #47092, #14556 ),
 .UNSPECIFIED., .F., .F. ) 
 B_SPLINE_CURVE_WITH_KNOTS ( ( 3, 2, 2, 3 ),
 ( 0.9514076071890844588, 0.9527777777777777235, 0.9555555555555556024, 0.9567839273083657003 ),
 .UNSPECIFIED. ) 
 CURVE ( )  GEOMETRIC_REPRESENTATION_ITEM ( )  RATIONAL_B_SPLINE_CURVE ( ( 0.9330248690816613788, 0.9339155015080172761, 1.000000000000000000, 0.8660254037844387076, 1.000000000000000000, 0.9407545805492795177, 0.9339074489089478348 ) ) 
 REPRESENTATION_ITEM ( '' )  );
#33922=CARTESIAN_POINT ( 'NONE',  ( 18.68437500061451928, -4.541064518000419881, 2.621784821874995952 ) ) ;
#33923=CARTESIAN_POINT ( 'NONE',  ( 20.32500000122903572, -5.773502691896255534, -1.060575238724906372E-15 ) ) ;
#33924=CARTESIAN_POINT ( 'NONE',  ( 15.12187500061451750, -6.054752690667223547, -1.112240025338166033E-15 ) ) ;
#33925=CARTESIAN_POINT ( 'NONE',  ( 2.121784821875001281, 11.90937500061451892, 33.67503911421598417 ) ) ;
#33926=CARTESIAN_POINT ( 'NONE',  ( 22.38750000122903216, 4.330127018922191873, 2.499999999999999556 ) ) ;
#33927=CARTESIAN_POINT ( 'NONE',  ( 14.84062500061451750, 6.054752690667223547, 3.707466751127219781E-16 ) ) ;
#33928=VERTEX_POINT ( 'NONE', #14153 ) ;
#33929=ORIENTED_EDGE ( 'NONE', *, *, #41045, .T. ) ;
#33930=CARTESIAN_POINT ( 'NONE',  ( 21.75000000000000000, 4.330127018922192761, -2.499999999999997780 ) ) ;
#33932=CARTESIAN_POINT ( 'NONE',  ( 3.140625000614516882, 6.054752690667223547, 3.707466751127219781E-16 ) ) ;
#33933=CARTESIAN_POINT ( 'NONE',  ( 16.20000000122903216, -2.886751345948129988, 4.999999999999997335 ) ) ;
#33934=CARTESIAN_POINT ( 'NONE',  ( 21.02812500061451573, 6.421520780324663323E-16, -5.243569643749999010 ) ) ;
#33935=CARTESIAN_POINT ( 'NONE',  ( 25.26562500061451289, 3.027376345333611329, 5.243569643749999010 ) ) ;
#33936=CARTESIAN_POINT ( 'NONE',  ( 4.715625000614516615, -6.054752690667223547, -1.112240025338166033E-15 ) ) ;
#33937=CARTESIAN_POINT ( 'NONE',  ( 29.21249999999999858, -5.773502691896255534, -1.060575238724906372E-15 ) ) ;
#33941=CARTESIAN_POINT ( 'NONE',  ( 2.000000000000001332, 10.81250000122903465, -26.53589838486224650 ) ) ;
#33942=CARTESIAN_POINT ( 'NONE',  ( -2.121784821874996840, 17.68437500061451928, -26.32496088578401583 ) ) ;
#33943=CARTESIAN_POINT ( 'NONE',  ( 5.287500001229035185, 4.330127018922191873, 2.499999999999999556 ) ) ;
#33945=CARTESIAN_POINT ( 'NONE',  ( 7.162500000000001421, -5.773502691896255534, -1.060575238724906372E-15 ) ) ;
#33946=EDGE_CURVE ( 'NONE', #24236, #60873, #36761, .T. ) ;
#33947=CARTESIAN_POINT ( 'NONE',  ( 3.862500001229035362, 4.330127018922192761, -2.499999999999997780 ) ) ;
#33948=CARTESIAN_POINT ( 'NONE',  ( 11.33437500061451608, 4.541064518000418104, 2.621784821874999949 ) ) ;
#33949=LINE ( 'NONE', #50237, #63071 ) ;
#33950=CARTESIAN_POINT ( 'NONE',  ( 3.628125000614518036, 4.541064518000418104, 2.621784821874999949 ) ) ;
#33952=CARTESIAN_POINT ( 'NONE',  ( -5.810221930991193690E-16, 10.88750000000000107, -34.00000000000000000 ) ) ;
#33953=CARTESIAN_POINT ( 'NONE',  ( 10.13437500061451679, -4.541064518000419881, 2.621784821874995952 ) ) ;
#33954=CARTESIAN_POINT ( 'NONE',  ( -1.071796769724487453, 18.55759618943233491, -34.00000000000000000 ) ) ;
#33955=CARTESIAN_POINT ( 'NONE',  ( 4.000000000000000000, 14.33750000000000213, 32.30940107675849760 ) ) ;
#33956=( BOUNDED_CURVE ( )  B_SPLINE_CURVE ( 2, ( #44203, #72996, #33102, #39753, #56716, #28648, #71907, #72634, #22018 ),
 .UNSPECIFIED., .F., .F. ) 
 B_SPLINE_CURVE_WITH_KNOTS ( ( 3, 2, 2, 2, 3 ),
 ( 0.2282608695652174058, 0.2318840579710144956, 0.2391304347826087029, 0.2463768115942029102, 0.2500000000000000000 ),
 .UNSPECIFIED. ) 
 CURVE ( )  GEOMETRIC_REPRESENTATION_ITEM ( )  RATIONAL_B_SPLINE_CURVE ( ( 0.9330127018922194093, 0.9330127018922196314, 1.000000000000000000, 0.8660254037844387076, 1.000000000000000000, 0.8660254037844387076, 1.000000000000000000, 0.9330127018922196314, 0.9330127018922194093 ) ) 
 REPRESENTATION_ITEM ( '' )  );
#33957=CARTESIAN_POINT ( 'NONE',  ( -4.243569643749999898, 16.61562500061459247, 27.54997392385601529 ) ) ;
#33958=CARTESIAN_POINT ( 'NONE',  ( 21.60937500061451644, 4.541064518000418104, -2.621784821874998173 ) ) ;
#33959=CARTESIAN_POINT ( 'NONE',  ( 2.771473848796851769, -4.161669585790501280, 2.894079486085709529 ) ) ;
#33961=CARTESIAN_POINT ( 'NONE',  ( 27.82500000122903572, 2.886751345948126879, 4.999999999999999112 ) ) ;
#33963=CARTESIAN_POINT ( 'NONE',  ( 23.42812500061451786, 4.541064518000418104, 2.621784821874999949 ) ) ;
#33964=CARTESIAN_POINT ( 'NONE',  ( 15.44062500061451537, -3.027376345333614438, 5.243569643749998122 ) ) ;
#33966=CARTESIAN_POINT ( 'NONE',  ( 12.42187500061451821, -6.054752690667223547, -1.112240025338166033E-15 ) ) ;
#33967=CARTESIAN_POINT ( 'NONE',  ( 28.38749999999999929, -2.886751345948125991, -5.000000000000000000 ) ) ;
#33968=CARTESIAN_POINT ( 'NONE',  ( 25.65000000122903145, -2.886751345948129988, 4.999999999999997335 ) ) ;
#33969=CARTESIAN_POINT ( 'NONE',  ( 3.271875000614519635, 3.027376345333611329, 5.243569643749999010 ) ) ;
#33970=CARTESIAN_POINT ( 'NONE',  ( 13.92187500061451644, 3.027376345333613106, -5.243569643749998122 ) ) ;
#33971=FACE_OUTER_BOUND ( 'NONE', #70757, .T. ) ;
#33972=CARTESIAN_POINT ( 'NONE',  ( 8.287500001229034297, 6.123233995736764310E-16, -4.999999999999998224 ) ) ;
#33973=CARTESIAN_POINT ( 'NONE',  ( -3.999999999999997335, 12.05000000122903359, 32.30940107675850470 ) ) ;
#33974=CARTESIAN_POINT ( 'NONE',  ( 22.32187500061451502, -6.054752690667223547, -1.112240025338166033E-15 ) ) ;
#33975=CARTESIAN_POINT ( 'NONE',  ( 15.19687500061451857, -3.027376345333610441, -5.243569643749999898 ) ) ;
#33977=CARTESIAN_POINT ( 'NONE',  ( 27.18750000000000000, 5.773502691896255534, 3.535250795749688894E-16 ) ) ;
#33978=CARTESIAN_POINT ( 'NONE',  ( 3.525000001229034119, 2.886751345948126879, 4.999999999999999112 ) ) ;
#33980=CARTESIAN_POINT ( 'NONE',  ( 16.52812500061451573, 6.421520780324663323E-16, -5.243569643749999010 ) ) ;
#33981=CARTESIAN_POINT ( 'NONE',  ( 6.487499999999999822, 5.773502691896255534, 3.535250795749688894E-16 ) ) ;
#33982=DIRECTION ( 'NONE',  ( 0.000000000000000000, 0.000000000000000000, -1.000000000000000000 ) ) ;
#33983=CARTESIAN_POINT ( 'NONE',  ( 17.96250000000000213, -5.773502691896255534, -1.060575238724906372E-15 ) ) ;
#33984=EDGE_CURVE ( 'NONE', #20497, #16648, #47125, .T. ) ;
#33985=CARTESIAN_POINT ( 'NONE',  ( -2.121784821874996840, 12.22812500061451857, 33.67503911421598417 ) ) ;
#33986=( BOUNDED_CURVE ( )  B_SPLINE_CURVE ( 2, ( #27702, #67954, #11796, #39513, #34313, #56846, #28779, #33954, #62760 ),
 .UNSPECIFIED., .F., .T. ) 
 B_SPLINE_CURVE_WITH_KNOTS ( ( 3, 2, 2, 2, 3 ),
 ( 0.1195652173913043514, 0.1231884057971014551, 0.1304347826086956486, 0.1376811594202898559, 0.1413043478260869734 ),
 .UNSPECIFIED. ) 
 CURVE ( )  GEOMETRIC_REPRESENTATION_ITEM ( )  RATIONAL_B_SPLINE_CURVE ( ( 0.9330127018922194093, 0.9330127018922194093, 1.000000000000000000, 0.8660254037844387076, 1.000000000000000000, 0.8660254037844387076, 1.000000000000000000, 0.9330127018922190762, 0.9330127018922194093 ) ) 
 REPRESENTATION_ITEM ( '' )  );
#33987=FACE_OUTER_BOUND ( 'NONE', #70326, .T. ) ;
#33988=CARTESIAN_POINT ( 'NONE',  ( 20.66250000122903074, 0.000000000000000000, 4.999999999999998224 ) ) ;
#33990=CARTESIAN_POINT ( 'NONE',  ( 28.24687500061451573, -3.027376345333610441, -5.243569643749999898 ) ) ;
#33991=VERTEX_POINT ( 'NONE', #47415 ) ;
#33992=CARTESIAN_POINT ( 'NONE',  ( 21.59062500061451928, 6.054752690667223547, 3.707466751127219781E-16 ) ) ;
#33993=CARTESIAN_POINT ( 'NONE',  ( 22.84687500061451715, -3.027376345333610441, -5.243569643749999898 ) ) ;
#33994=CARTESIAN_POINT ( 'NONE',  ( 7.762500000000001954, 2.886751345948129099, -4.999999999999998224 ) ) ;
#33995=CARTESIAN_POINT ( 'NONE',  ( 9.740625000614516082, -3.027376345333610441, -5.243569643749999898 ) ) ;
#33996=CARTESIAN_POINT ( 'NONE',  ( 24.96562500061451573, -6.054752690667223547, -1.112240025338166033E-15 ) ) ;
#33997=CARTESIAN_POINT ( 'NONE',  ( 11.82187500061451679, 3.027376345333611329, 5.243569643749999010 ) ) ;
#33998=CARTESIAN_POINT ( 'NONE',  ( 17.37187500061451573, -6.054752690667223547, -1.112240025338166033E-15 ) ) ;
#33999=CARTESIAN_POINT ( 'NONE',  ( 30.00000000000000000, 0.000000000000000000, 0.000000000000000000 ) ) ;
#34000=CARTESIAN_POINT ( 'NONE',  ( -3.000416591977282496E-16, 16.54062500061451857, 25.09994784771203058 ) ) ;
#34001=CARTESIAN_POINT ( 'NONE',  ( 20.28750000122903074, -4.330127018922194537, 2.499999999999995559 ) ) ;
#34003=CARTESIAN_POINT ( 'NONE',  ( 11.80312500061451608, 0.000000000000000000, 5.243569643749999010 ) ) ;
#34004=CARTESIAN_POINT ( 'NONE',  ( 5.146875000614517859, -3.027376345333614438, 5.243569643749998122 ) ) ;
#34005=CARTESIAN_POINT ( 'NONE',  ( 5.596875000614516260, -3.027376345333614438, 5.243569643749998122 ) ) ;
#34007=CARTESIAN_POINT ( 'NONE',  ( 26.03437500061451715, 6.421520780324663323E-16, -5.243569643749999010 ) ) ;
#34008=CARTESIAN_POINT ( 'NONE',  ( 16.90312500061451573, -4.541064518000417216, -2.621784821875001281 ) ) ;
#34009=CARTESIAN_POINT ( 'NONE',  ( 27.78750000122903074, 4.330127018922191873, 2.499999999999999556 ) ) ;
#34010=CARTESIAN_POINT ( 'NONE',  ( 27.21562500061451928, -6.054752690667223547, -1.112240025338166033E-15 ) ) ;
#34011=CARTESIAN_POINT ( 'NONE',  ( 20.82187500061451857, 3.027376345333611329, 5.243569643749999010 ) ) ;
#34012=CARTESIAN_POINT ( 'NONE',  ( 17.57812500061451644, 4.541064518000418104, 2.621784821874999949 ) ) ;
#34013=CARTESIAN_POINT ( 'NONE',  ( -3.000416591977282496E-16, 18.39687500061451786, 25.09994784771203058 ) ) ;
#34014=CARTESIAN_POINT ( 'NONE',  ( 23.61562500061451431, -6.054752690667223547, -1.112240025338166033E-15 ) ) ;
#34015=CARTESIAN_POINT ( 'NONE',  ( 5.137500001229033941, 6.123233995736764310E-16, -4.999999999999998224 ) ) ;
#34017=CARTESIAN_POINT ( 'NONE',  ( 28.38749999999999929, -2.886751345948125991, -5.000000000000000000 ) ) ;
#34018=CARTESIAN_POINT ( 'NONE',  ( 8.484601909799253346E-16, 13.36250000000000071, -25.38119784648299770 ) ) ;
#34020=CARTESIAN_POINT ( 'NONE',  ( 29.72812500061451502, 4.541064518000418104, 2.621784821874999949 ) ) ;
#34021=CARTESIAN_POINT ( 'NONE',  ( 9.478125000614515017, 4.541064518000418104, 2.621784821874999949 ) ) ;
#34022=CARTESIAN_POINT ( 'NONE',  ( 21.86250000122903003, 4.330127018922192761, -2.499999999999997780 ) ) ;
#34023=CARTESIAN_POINT ( 'NONE',  ( 13.32187500061451502, -6.054752690667223547, -1.112240025338166033E-15 ) ) ;
#34024=CARTESIAN_POINT ( 'NONE',  ( 2.934375000614518392, -4.541064518000419881, 2.621784821874995952 ) ) ;
#34025=CARTESIAN_POINT ( 'NONE',  ( 26.77499999999999858, 4.330127018922191873, 2.499999999999999556 ) ) ;
#34026=CARTESIAN_POINT ( 'NONE',  ( 14.73750000122903359, 4.330127018922191873, 2.499999999999999556 ) ) ;
#34027=CARTESIAN_POINT ( 'NONE',  ( 14.09062500061451750, -3.027376345333614438, 5.243569643749998122 ) ) ;
#34029=CARTESIAN_POINT ( 'NONE',  ( 9.665625000614515017, -6.054752690667223547, -1.112240025338166033E-15 ) ) ;
#34030=CARTESIAN_POINT ( 'NONE',  ( 5.503125000614516260, 0.000000000000000000, 5.243569643749999010 ) ) ;
#34033=CARTESIAN_POINT ( 'NONE',  ( 15.29999999999999893, -4.330127018922190985, -2.500000000000001332 ) ) ;
#34034=CARTESIAN_POINT ( 'NONE',  ( 16.13437500061451502, 6.421520780324663323E-16, -5.243569643749999010 ) ) ;
#34035=CARTESIAN_POINT ( 'NONE',  ( 11.73750000122903181, -4.330127018922194537, 2.499999999999995559 ) ) ;
#34036=CARTESIAN_POINT ( 'NONE',  ( 18.72187500061451360, -6.054752690667223547, -1.112240025338166033E-15 ) ) ;
#34038=CARTESIAN_POINT ( 'NONE',  ( 20.85937500061451644, 0.000000000000000000, 5.243569643749999010 ) ) ;
#34039=CARTESIAN_POINT ( 'NONE',  ( -4.243569643749999898, 13.50312500061451715, -30.00000000000000000 ) ) ;
#34040=CARTESIAN_POINT ( 'NONE',  ( 21.00000000122903288, 5.773502691896255534, 3.535250795749688401E-16 ) ) ;
#34043=CARTESIAN_POINT ( 'NONE',  ( 26.42812500061451431, 6.421520780324663323E-16, -5.243569643749999010 ) ) ;
#34044=CARTESIAN_POINT ( 'NONE',  ( 5.250000001229035540, 5.773502691896255534, 3.535250795749688401E-16 ) ) ;
#34045=CARTESIAN_POINT ( 'NONE',  ( 29.03437500061451715, -4.541064518000419881, 2.621784821874995952 ) ) ;
#34046=CARTESIAN_POINT ( 'NONE',  ( 24.56250000000000000, 2.886751345948126879, 4.999999999999999112 ) ) ;
#34047=CARTESIAN_POINT ( 'NONE',  ( 9.178125000614517859, -4.541064518000419881, 2.621784821874995952 ) ) ;
#34049=CARTESIAN_POINT ( 'NONE',  ( 18.98437500061451644, 4.541064518000418104, 2.621784821874999949 ) ) ;
#34051=CARTESIAN_POINT ( 'NONE',  ( 5.390625000614518214, 6.054752690667223547, 3.707466751127219781E-16 ) ) ;
#34052=CARTESIAN_POINT ( 'NONE',  ( 11.74687500061451573, 6.054752690667223547, 3.707466751127219781E-16 ) ) ;
#34054=CARTESIAN_POINT ( 'NONE',  ( 22.62187500061451573, 3.027376345333611329, 5.243569643749999010 ) ) ;
#34056=CARTESIAN_POINT ( 'NONE',  ( 28.80000000000000071, -4.330127018922190985, -2.500000000000001332 ) ) ;
#34057=CARTESIAN_POINT ( 'NONE',  ( 28.65937500061451715, -4.541064518000417216, -2.621784821875001281 ) ) ;
#34058=CARTESIAN_POINT ( 'NONE',  ( 13.98750000122903359, -4.330127018922194537, 2.499999999999995559 ) ) ;
#34059=CARTESIAN_POINT ( 'NONE',  ( 3.776121927792477351, -3.277331717486649421, 4.093179622544351304 ) ) ;
#34061=CARTESIAN_POINT ( 'NONE',  ( 13.38750000000000107, -2.886751345948129988, 4.999999999999997335 ) ) ;
#34062=CARTESIAN_POINT ( 'NONE',  ( 23.80312500061451786, 4.541064518000418104, -2.621784821874998173 ) ) ;
#34063=CARTESIAN_POINT ( 'NONE',  ( 14.24999999999999822, 0.000000000000000000, 4.999999999999998224 ) ) ;
#34064=CARTESIAN_POINT ( 'NONE',  ( 9.487500001229033586, -4.330127018922194537, 2.499999999999995559 ) ) ;
#34065=CARTESIAN_POINT ( 'NONE',  ( 7.940625000614518036, -3.027376345333610441, -5.243569643749999898 ) ) ;
#34067=CARTESIAN_POINT ( 'NONE',  ( 8.175000000000002487, 6.123233995736764310E-16, -4.999999999999998224 ) ) ;
#34068=CARTESIAN_POINT ( 'NONE',  ( 27.29999999999999716, 0.000000000000000000, 4.999999999999998224 ) ) ;
#34069=CARTESIAN_POINT ( 'NONE',  ( 2.121784821875001281, 13.70937500061451786, -26.32496088578401938 ) ) ;
#34070=CARTESIAN_POINT ( 'NONE',  ( 28.05000000122903359, -2.886751345948125991, -5.000000000000000000 ) ) ;
#34072=CARTESIAN_POINT ( 'NONE',  ( 7.312500000000000000, 2.886751345948129099, -4.999999999999998224 ) ) ;
#34074=EDGE_LOOP ( 'NONE', ( #65587, #37518, #37507, #52639 ) ) ;
#34075=CARTESIAN_POINT ( 'NONE',  ( 20.95312500061451999, -4.541064518000417216, -2.621784821875001281 ) ) ;
#34076=CARTESIAN_POINT ( 'NONE',  ( 14.43750000122903288, -4.330127018922194537, 2.499999999999995559 ) ) ;
#34077=CARTESIAN_POINT ( 'NONE',  ( 0.000000000000000000, 0.000000000000000000, 50.00000000000000000 ) ) ;
#34078=DIRECTION ( 'NONE',  ( -0.000000000000000000, -1.000000000000000000, -0.000000000000000000 ) ) ;
#34079=CARTESIAN_POINT ( 'NONE',  ( 20.10937500061451289, -4.541064518000417216, -2.621784821875001281 ) ) ;
#34080=CARTESIAN_POINT ( 'NONE',  ( 17.54062500061451502, 6.054752690667223547, 3.707466751127219781E-16 ) ) ;
#34081=CARTESIAN_POINT ( 'NONE',  ( 9.001249775931846008E-16, 12.71562500061459211, -25.09994784771203058 ) ) ;
#34082=CARTESIAN_POINT ( 'NONE',  ( 6.478125000614516793, -4.541064518000419881, 2.621784821874995952 ) ) ;
#34083=CARTESIAN_POINT ( 'NONE',  ( 27.97500000122903074, -5.773502691896255534, -1.060575238724906372E-15 ) ) ;
#34085=CARTESIAN_POINT ( 'NONE',  ( 20.27812500061451573, 4.541064518000418104, 2.621784821874999949 ) ) ;
#34086=CARTESIAN_POINT ( 'NONE',  ( 2.000000000000001332, 11.26250000122903394, -26.53589838486224650 ) ) ;
#34087=CARTESIAN_POINT ( 'NONE',  ( 4.275000001229035895, 2.886751345948129099, -4.999999999999998224 ) ) ;
#34088=CARTESIAN_POINT ( 'NONE',  ( 12.75937500061451857, 0.000000000000000000, 5.243569643749999010 ) ) ;
#34089=CARTESIAN_POINT ( 'NONE',  ( 11.25937500061451679, 4.541064518000418104, -2.621784821874998173 ) ) ;
#34090=CARTESIAN_POINT ( 'NONE',  ( 20.85937500061451644, 0.000000000000000000, 5.243569643749999010 ) ) ;
#34091=EDGE_LOOP ( 'NONE', ( #66246, #62147, #7756, #53 ) ) ;
#34092=CARTESIAN_POINT ( 'NONE',  ( 3.815625000614518036, -6.054752690667223547, -1.112240025338166033E-15 ) ) ;
#34093=CARTESIAN_POINT ( 'NONE',  ( 24.85312500061451502, 0.000000000000000000, 5.243569643749999010 ) ) ;
#34094=CARTESIAN_POINT ( 'NONE',  ( 19.99687500061451573, -3.027376345333614438, 5.243569643749998122 ) ) ;
#34095=CARTESIAN_POINT ( 'NONE',  ( 23.87812500061451715, 4.541064518000418104, 2.621784821874999949 ) ) ;
#34096=CARTESIAN_POINT ( 'NONE',  ( 19.76250000122903216, 0.000000000000000000, 4.999999999999998224 ) ) ;
#34097=CARTESIAN_POINT ( 'NONE',  ( 1.999999999999998668, 16.69999999999999929, 26.53589838486224650 ) ) ;
#34098=CARTESIAN_POINT ( 'NONE',  ( 3.759375000614517681, 0.000000000000000000, 5.243569643749999010 ) ) ;
#34100=CARTESIAN_POINT ( 'NONE',  ( 12.93750000122903465, 4.330127018922191873, 2.499999999999999556 ) ) ;
#34101=CARTESIAN_POINT ( 'NONE',  ( 6.337500001229033231, -4.330127018922194537, 2.499999999999995559 ) ) ;
#34102=CARTESIAN_POINT ( 'NONE',  ( 3.999999999999999112, 19.32500000000000284, -30.00000000000000000 ) ) ;
#34103=CARTESIAN_POINT ( 'NONE',  ( 26.77500000122903145, 2.886751345948129099, -4.999999999999998224 ) ) ;
#34106=CARTESIAN_POINT ( 'NONE',  ( 10.73437500061451644, 6.421520780324663323E-16, -5.243569643749999010 ) ) ;
#34108=CARTESIAN_POINT ( 'NONE',  ( 17.05312500061451786, 4.541064518000418104, -2.621784821874998173 ) ) ;
#34109=CARTESIAN_POINT ( 'NONE',  ( 13.80937500061451750, -4.541064518000417216, -2.621784821875001281 ) ) ;
#34110=CARTESIAN_POINT ( 'NONE',  ( 4.078125000614517326, 4.541064518000418104, 2.621784821874999949 ) ) ;
#34111=CARTESIAN_POINT ( 'NONE',  ( 22.73437500061451644, -4.541064518000419881, 2.621784821874995952 ) ) ;
#34112=CARTESIAN_POINT ( 'NONE',  ( 8.896875000614517859, -3.027376345333610441, -5.243569643749999898 ) ) ;
#34113=CARTESIAN_POINT ( 'NONE',  ( 5.878125000614517148, 4.541064518000418104, 2.621784821874999949 ) ) ;
#34115=CARTESIAN_POINT ( 'NONE',  ( 6.112500001229034474, 4.330127018922192761, -2.499999999999997780 ) ) ;
#34116=CARTESIAN_POINT ( 'NONE',  ( 19.71562500061451928, 3.027376345333613106, -5.243569643749998122 ) ) ;
#34117=CARTESIAN_POINT ( 'NONE',  ( 6.900000001229035007, -2.886751345948125991, -5.000000000000000000 ) ) ;
#34118=CARTESIAN_POINT ( 'NONE',  ( 17.50312500061451715, 4.541064518000418104, -2.621784821874998173 ) ) ;
#34119=CARTESIAN_POINT ( 'NONE',  ( 13.11562500061451786, 3.027376345333611329, 5.243569643749999010 ) ) ;
#34121=CARTESIAN_POINT ( 'NONE',  ( 13.68750000000000178, 5.773502691896255534, 3.535250795749688894E-16 ) ) ;
#34122=CARTESIAN_POINT ( 'NONE',  ( 8.587500001229035007, -4.330127018922194537, 2.499999999999995559 ) ) ;
#34123=CARTESIAN_POINT ( 'NONE',  ( 5.053125000614517859, 0.000000000000000000, 5.243569643749999010 ) ) ;
#34124=EDGE_CURVE ( 'NONE', #48852, #53469, #5884, .T. ) ;
#34125=CARTESIAN_POINT ( 'NONE',  ( 19.05000000122903359, -2.886751345948125991, -5.000000000000000000 ) ) ;
#34127=CARTESIAN_POINT ( 'NONE',  ( -4.243569643749999898, 11.30937500061451928, -30.00000000000000000 ) ) ;
#34129=CARTESIAN_POINT ( 'NONE',  ( 3.450000001229036162, 5.773502691896255534, 3.535250795749688894E-16 ) ) ;
#34130=CARTESIAN_POINT ( 'NONE',  ( 28.53750000122903074, 6.123233995736764310E-16, -4.999999999999998224 ) ) ;
#34131=CARTESIAN_POINT ( 'NONE',  ( 20.03437500061451715, -4.541064518000419881, 2.621784821874995952 ) ) ;
#34133=CARTESIAN_POINT ( 'NONE',  ( 15.81562500061451537, 3.027376345333611329, 5.243569643749999010 ) ) ;
#34135=CARTESIAN_POINT ( 'NONE',  ( 10.91250000000000142, 2.886751345948062486, -5.000000000000113687 ) ) ;
#34136=CARTESIAN_POINT ( 'NONE',  ( 25.17187500061451644, 3.027376345333613106, -5.243569643749998122 ) ) ;
#34138=CARTESIAN_POINT ( 'NONE',  ( 12.40312500061451573, -4.541064518000417216, -2.621784821875001281 ) ) ;
#34139=CARTESIAN_POINT ( 'NONE',  ( 9.609375000614518214, 0.000000000000000000, 5.243569643749999010 ) ) ;
#34141=CARTESIAN_POINT ( 'NONE',  ( 29.57812500061451644, 6.421520780324663323E-16, -5.243569643749999010 ) ) ;
#34142=CARTESIAN_POINT ( 'NONE',  ( 20.46562500061451928, -6.054752690667223547, -1.112240025338166033E-15 ) ) ;
#34144=EDGE_CURVE ( 'NONE', #69611, #30395, #2715, .T. ) ;
#34146=CARTESIAN_POINT ( 'NONE',  ( 11.10000000000000142, 0.000000000000000000, 4.999999999999998224 ) ) ;
#34147=CARTESIAN_POINT ( 'NONE',  ( 21.56250000122903288, 0.000000000000000000, 4.999999999999998224 ) ) ;
#34148=CARTESIAN_POINT ( 'NONE',  ( 15.51562500061451644, -6.054752690667223547, -1.112240025338166033E-15 ) ) ;
#34151=CARTESIAN_POINT ( 'NONE',  ( 20.28750000000000142, -2.886751345948125991, -5.000000000000000000 ) ) ;
#34152=CARTESIAN_POINT ( 'NONE',  ( 23.58749999999999858, 5.773502691896255534, 3.535250795749688894E-16 ) ) ;
#34153=CARTESIAN_POINT ( 'NONE',  ( 21.08437500061451786, 6.421520780324663323E-16, -5.243569643749999010 ) ) ;
#34154=CARTESIAN_POINT ( 'NONE',  ( 26.31562500061451715, -6.054752690667223547, -1.112240025338166033E-15 ) ) ;
#34155=VERTEX_POINT ( 'NONE', #31145 ) ;
#34156=DIRECTION ( 'NONE',  ( -1.000000000000000000, -0.000000000000000000, -0.000000000000000000 ) ) ;
#34157=CARTESIAN_POINT ( 'NONE',  ( 7.603125000614517681, 4.541064518000418104, -2.621784821874998173 ) ) ;
#34158=CARTESIAN_POINT ( 'NONE',  ( 3.275654489317120444, 3.777613493092820462, 3.573368934894253002 ) ) ;
#34159=CARTESIAN_POINT ( 'NONE',  ( 14.32500000000000107, -4.330127018922194537, 2.499999999999995559 ) ) ;
#34160=CARTESIAN_POINT ( 'NONE',  ( 4.243569643749999010, 18.26562500061451644, 27.54997392385601174 ) ) ;
#34161=CARTESIAN_POINT ( 'NONE',  ( 3.946875000614517681, -3.027376345333610441, -5.243569643749999898 ) ) ;
#34162=CARTESIAN_POINT ( 'NONE',  ( 26.40937500061451715, -4.541064518000417216, -2.621784821875001281 ) ) ;
#34164=CARTESIAN_POINT ( 'NONE',  ( 24.10312500061451502, -4.541064518000417216, -2.621784821875001281 ) ) ;
#34165=CARTESIAN_POINT ( 'NONE',  ( 24.23437500061451644, 6.421520780324663323E-16, -5.243569643749999010 ) ) ;
#34166=CARTESIAN_POINT ( 'NONE',  ( 2.121784821875001281, 18.60312500061459673, -26.32496088578401938 ) ) ;
#34167=CARTESIAN_POINT ( 'NONE',  ( 12.07499999999999929, -4.330127018922194537, 2.499999999999995559 ) ) ;
#34168=CARTESIAN_POINT ( 'NONE',  ( 8.128125000614515372, 4.541064518000418104, 2.621784821874999949 ) ) ;
#34170=CARTESIAN_POINT ( 'NONE',  ( 29.09062500061451573, -3.027376345333610441, -5.243569643749999898 ) ) ;
#34171=CARTESIAN_POINT ( 'NONE',  ( 26.42812500061451431, 6.421520780324663323E-16, -5.243569643749999010 ) ) ;
#34172=DIRECTION ( 'NONE',  ( 0.000000000000000000, 0.000000000000000000, -1.000000000000000000 ) ) ;
#34174=CARTESIAN_POINT ( 'NONE',  ( 20.59687500061451360, -3.027376345333610441, -5.243569643749999898 ) ) ;
#34175=CARTESIAN_POINT ( 'NONE',  ( 4.243569643749999898, 15.13437500061451679, 30.00000000000000000 ) ) ;
#34176=CARTESIAN_POINT ( 'NONE',  ( 19.77187500061451786, 3.027376345333613106, -5.243569643749998122 ) ) ;
#34177=CARTESIAN_POINT ( 'NONE',  ( 26.52187500061451431, 3.027376345333613106, -5.243569643749998122 ) ) ;
#34179=CARTESIAN_POINT ( 'NONE',  ( -3.000416591977282496E-16, 16.59687500061452070, 25.09994784771203058 ) ) ;
#34180=CARTESIAN_POINT ( 'NONE',  ( 10.60312500061451679, -4.541064518000417216, -2.621784821875001281 ) ) ;
#34182=CARTESIAN_POINT ( 'NONE',  ( 4.584375000614516971, 4.541064518000418104, 2.621784821874999949 ) ) ;
#34183=LINE ( 'NONE', #955, #56065 ) ;
#34184=CARTESIAN_POINT ( 'NONE',  ( 8.765625000614518214, -6.054752690667223547, -1.112240025338166033E-15 ) ) ;
#34185=CARTESIAN_POINT ( 'NONE',  ( 11.03437500061451715, -4.541064518000419881, 2.621784821874995952 ) ) ;
#34186=SURFACE_SIDE_STYLE ('',( #68549 ) ) ;
#34187=CARTESIAN_POINT ( 'NONE',  ( 19.65000000122902790, 5.773502691896255534, 3.535250795749688894E-16 ) ) ;
#34188=CARTESIAN_POINT ( 'NONE',  ( 6.609375000614519102, -4.541064518000417216, -2.621784821875001281 ) ) ;
#34189=CARTESIAN_POINT ( 'NONE',  ( 10.22812500061451679, 6.421520780324663323E-16, -5.243569643749999010 ) ) ;
#34190=CARTESIAN_POINT ( 'NONE',  ( 5.015625000614518214, 3.027376345333611329, 5.243569643749999010 ) ) ;
#34192=CARTESIAN_POINT ( 'NONE',  ( 19.84687500061451360, 6.054752690667223547, 3.707466751127219781E-16 ) ) ;
#34193=CARTESIAN_POINT ( 'NONE',  ( 9.000000001229032875, -2.886751345948063374, 5.000000000000112799 ) ) ;
#34194=ORIENTED_EDGE ( 'NONE', *, *, #12308, .F. ) ;
#34195=CARTESIAN_POINT ( 'NONE',  ( 25.37812500061451715, -4.541064518000419881, 2.621784821874995952 ) ) ;
#34196=CARTESIAN_POINT ( 'NONE',  ( 13.07812500061451821, 4.541064518000418104, 2.621784821874999949 ) ) ;
#34197=CARTESIAN_POINT ( 'NONE',  ( 29.55937500061451573, -4.541064518000417216, -2.621784821875001281 ) ) ;
#34198=CARTESIAN_POINT ( 'NONE',  ( 12.36562500061451608, -6.054752690667223547, -1.112240025338166033E-15 ) ) ;
#34199=CARTESIAN_POINT ( 'NONE',  ( 4.243569643749999010, 10.22187500061451892, -32.45002607614398471 ) ) ;
#34200=CARTESIAN_POINT ( 'NONE',  ( 13.53750000122903430, -4.330127018922194537, 2.499999999999995559 ) ) ;
#34201=( BOUNDED_CURVE ( )  B_SPLINE_CURVE ( 2, ( #39442, #49434, #15799, #44986, #61963, #21707, #61240 ),
 .UNSPECIFIED., .F., .F. ) 
 B_SPLINE_CURVE_WITH_KNOTS ( ( 3, 2, 2, 3 ),
 ( 0.2083333333333332871, 0.2111111111111110827, 0.2138888888888889062, 0.2166666666666667296 ),
 .UNSPECIFIED. ) 
 CURVE ( )  GEOMETRIC_REPRESENTATION_ITEM ( )  RATIONAL_B_SPLINE_CURVE ( ( 1.000000000000002665, 0.8660254037844360431, 1.000000000000000000, 0.8660254037844387076, 1.000000000000000000, 0.8660254037844360431, 1.000000000000002665 ) ) 
 REPRESENTATION_ITEM ( '' )  );
#34202=CARTESIAN_POINT ( 'NONE',  ( 27.36562500061451786, 3.027376345333613106, -5.243569643749998122 ) ) ;
#34203=CARTESIAN_POINT ( 'NONE',  ( 4.243569643749999010, 12.41562500061451857, -32.45002607614398471 ) ) ;
#34204=CARTESIAN_POINT ( 'NONE',  ( 14.92500000122903181, -5.773502691896255534, -1.060575238724906372E-15 ) ) ;
#34205=CARTESIAN_POINT ( 'NONE',  ( 14.28750000000000142, -2.886751345948129988, 4.999999999999997335 ) ) ;
#34206=CARTESIAN_POINT ( 'NONE',  ( 20.16562500061451146, 3.027376345333613106, -5.243569643749998122 ) ) ;
#34207=CARTESIAN_POINT ( 'NONE',  ( 7.209375000614519635, 4.541064518000418104, -2.621784821874998173 ) ) ;
#34208=CARTESIAN_POINT ( 'NONE',  ( 7.950000001229033053, 5.773502691896255534, 3.535250795749688894E-16 ) ) ;
#34209=CARTESIAN_POINT ( 'NONE',  ( 17.13750000122903216, -4.330127018922194537, 2.499999999999995559 ) ) ;
#34210=CARTESIAN_POINT ( 'NONE',  ( 13.37812500061451715, 6.421520780324663323E-16, -5.243569643749999010 ) ) ;
#34211=CARTESIAN_POINT ( 'NONE',  ( 14.87812500061451537, 4.541064518000418104, 2.621784821874999949 ) ) ;
#34212=CARTESIAN_POINT ( 'NONE',  ( 26.92500000122903359, 2.886751345948126879, 4.999999999999999112 ) ) ;
#34213=CARTESIAN_POINT ( 'NONE',  ( 22.61250000000000071, 2.886751345948129099, -4.999999999999998224 ) ) ;
#34214=CARTESIAN_POINT ( 'NONE',  ( 24.23437500061451644, 6.421520780324663323E-16, -5.243569643749999010 ) ) ;
#34215=CYLINDRICAL_SURFACE ( 'NONE', #6395, 4.999999999999998224 ) ;
#34216=CARTESIAN_POINT ( 'NONE',  ( 10.76250000122903572, 0.000000000000000000, 4.999999999999998224 ) ) ;
#34217=CARTESIAN_POINT ( 'NONE',  ( 28.58437500061451786, -4.541064518000419881, 2.621784821874995952 ) ) ;
#34219=CARTESIAN_POINT ( 'NONE',  ( 4.096875000614518925, 6.054752690667223547, 3.707466751127219781E-16 ) ) ;
#34220=CARTESIAN_POINT ( 'NONE',  ( 24.32812500061451289, 4.541064518000418104, 2.621784821874999949 ) ) ;
#34222=FACE_OUTER_BOUND ( 'NONE', #56818, .T. ) ;
#34223=CARTESIAN_POINT ( 'NONE',  ( 10.99687500061451750, -3.027376345333614438, 5.243569643749998122 ) ) ;
#34224=CARTESIAN_POINT ( 'NONE',  ( 25.94999999999999929, 0.000000000000000000, 4.999999999999998224 ) ) ;
#34225=CARTESIAN_POINT ( 'NONE',  ( 28.97812500061451502, -4.541064518000419881, 2.621784821874995952 ) ) ;
#34226=CARTESIAN_POINT ( 'NONE',  ( 6.309375000614517504, 4.541064518000418104, -2.621784821874998173 ) ) ;
#34228=CARTESIAN_POINT ( 'NONE',  ( 26.40937500061451715, -4.541064518000417216, -2.621784821875001281 ) ) ;
#34229=CARTESIAN_POINT ( 'NONE',  ( -3.000416591977282496E-16, 11.14062500061459637, 25.09994784771203058 ) ) ;
#34230=CARTESIAN_POINT ( 'NONE',  ( 19.72499999999999787, -4.330127018922194537, 2.499999999999995559 ) ) ;
#34232=CARTESIAN_POINT ( 'NONE',  ( 26.96249999999999858, -5.773502691896255534, -1.060575238724906372E-15 ) ) ;
#34233=CARTESIAN_POINT ( 'NONE',  ( 28.35937500061451289, 4.541064518000418104, -2.621784821874998173 ) ) ;
#34234=ORIENTED_EDGE ( 'NONE', *, *, #34124, .F. ) ;
#34235=CARTESIAN_POINT ( 'NONE',  ( 16.49062500061451786, -3.027376345333610441, -5.243569643749999898 ) ) ;
#34236=CARTESIAN_POINT ( 'NONE',  ( 8.315625000614515372, -6.054752690667223547, -1.112240025338166033E-15 ) ) ;
#34238=CARTESIAN_POINT ( 'NONE',  ( 5.446875000614518569, 6.054752690667223547, 3.707466751127219781E-16 ) ) ;
#34239=CARTESIAN_POINT ( 'NONE',  ( 17.28750000122903430, 6.123233995736764310E-16, -4.999999999999998224 ) ) ;
#34240=CARTESIAN_POINT ( 'NONE',  ( 22.05000000000000071, -4.330127018922190985, -2.500000000000001332 ) ) ;
#34241=CARTESIAN_POINT ( 'NONE',  ( 1.510657702057710734E-15, 19.43750000000000000, -33.99999999999999289 ) ) ;
#34242=CARTESIAN_POINT ( 'NONE',  ( 3.909375000614518481, -4.541064518000417216, -2.621784821875001281 ) ) ;
#34243=CARTESIAN_POINT ( 'NONE',  ( 10.95937500061451964, 0.000000000000000000, 5.243569643749999010 ) ) ;
#34244=CARTESIAN_POINT ( 'NONE',  ( 22.05937500061451573, 4.541064518000418104, -2.621784821874998173 ) ) ;
#34245=CARTESIAN_POINT ( 'NONE',  ( 1.592000809091587073E-14, 17.18750000000000355, -34.00000000000000000 ) ) ;
#34246=ORIENTED_EDGE ( 'NONE', *, *, #42591, .F. ) ;
#34247=CARTESIAN_POINT ( 'NONE',  ( 4.771875000614516971, -6.054752690667223547, -1.112240025338166033E-15 ) ) ;
#34248=CARTESIAN_POINT ( 'NONE',  ( 8.146875000614516082, 6.054752690667223547, 3.707466751127219781E-16 ) ) ;
#34250=CARTESIAN_POINT ( 'NONE',  ( 19.42499999999999716, 6.123233995736764310E-16, -4.999999999999998224 ) ) ;
#34251=CARTESIAN_POINT ( 'NONE',  ( 16.30312500061451786, 0.000000000000000000, 5.243569643749999010 ) ) ;
#34253=FACE_OUTER_BOUND ( 'NONE', #41128, .T. ) ;
#34255=CARTESIAN_POINT ( 'NONE',  ( 10.60312500061451679, -4.541064518000417216, -2.621784821875001281 ) ) ;
#34256=CARTESIAN_POINT ( 'NONE',  ( 27.12187500061451573, 3.027376345333611329, 5.243569643749999010 ) ) ;
#34258=CARTESIAN_POINT ( 'NONE',  ( 26.52187500061451431, 3.027376345333613106, -5.243569643749998122 ) ) ;
#34259=CARTESIAN_POINT ( 'NONE',  ( 8.775000000000002132, 4.330127018922191873, 2.499999999999999556 ) ) ;
#34260=CARTESIAN_POINT ( 'NONE',  ( -1.999999999999997113, 16.13750000122903216, 33.46410161513775705 ) ) ;
#34261=CARTESIAN_POINT ( 'NONE',  ( 8.250000001229034652, -2.886751345948125991, -5.000000000000000000 ) ) ;
#34262=CARTESIAN_POINT ( 'NONE',  ( 20.70937500061451786, 4.541064518000418104, -2.621784821874998173 ) ) ;
#34263=CARTESIAN_POINT ( 'NONE',  ( 14.22187500061451537, -6.054752690667223547, -1.112240025338166033E-15 ) ) ;
#34266=CARTESIAN_POINT ( 'NONE',  ( 15.85312500061451857, 0.000000000000000000, 5.243569643749999010 ) ) ;
#34267=CARTESIAN_POINT ( 'NONE',  ( 26.28750000122903430, 6.123233995736764310E-16, -4.999999999999998224 ) ) ;
#34268=CARTESIAN_POINT ( 'NONE',  ( 14.14687500061451786, -3.027376345333614438, 5.243569643749998122 ) ) ;
#34269=CARTESIAN_POINT ( 'NONE',  ( 4.096875000614518925, 6.054752690667223547, 3.707466751127219781E-16 ) ) ;
#34270=CARTESIAN_POINT ( 'NONE',  ( 16.71562500061451573, 3.027376345333611329, 5.243569643749999010 ) ) ;
#34273=CARTESIAN_POINT ( 'NONE',  ( 25.24687500061451573, 6.054752690667223547, 3.707466751127219781E-16 ) ) ;
#34274=CARTESIAN_POINT ( 'NONE',  ( -0.7368881354385758975, 9.803648613939515144, 25.82089971438751519 ) ) ;
#34275=CARTESIAN_POINT ( 'NONE',  ( 15.94687500061451502, -3.027376345333614438, 5.243569643749998122 ) ) ;
#34276=CARTESIAN_POINT ( 'NONE',  ( 11.21250000122903501, 0.000000000000000000, 4.999999999999998224 ) ) ;
#34278=CARTESIAN_POINT ( 'NONE',  ( -4.243569643749999898, 15.77187500061451608, -32.45002607614398471 ) ) ;
#34279=CARTESIAN_POINT ( 'NONE',  ( 17.78437500061451715, -4.541064518000419881, 2.621784821874995952 ) ) ;
#34280=CARTESIAN_POINT ( 'NONE',  ( 21.15000000122903145, -2.886751345948129988, 4.999999999999997335 ) ) ;
#34281=CARTESIAN_POINT ( 'NONE',  ( 14.07187500061451679, 3.027376345333611329, 5.243569643749999010 ) ) ;
#34282=CARTESIAN_POINT ( 'NONE',  ( -2.121784821874999949, 11.23437500061451821, 26.32496088578401938 ) ) ;
#34283=CARTESIAN_POINT ( 'NONE',  ( 22.83750000122903501, 4.330127018922191873, 2.499999999999999556 ) ) ;
#34284=CARTESIAN_POINT ( 'NONE',  ( 15.06562500061451537, -6.054752690667223547, -1.112240025338166033E-15 ) ) ;
#34285=CARTESIAN_POINT ( 'NONE',  ( 0.000000000000000000, 20.00000000000000000, -30.00000000000000000 ) ) ;
#34286=ORIENTED_EDGE ( 'NONE', *, *, #10471, .T. ) ;
#34288=CARTESIAN_POINT ( 'NONE',  ( 20.13749999999999929, -2.886751345948129988, 4.999999999999997335 ) ) ;
#34289=CARTESIAN_POINT ( 'NONE',  ( -1.071796769724487453, 17.77009619066136636, 26.00000000000000000 ) ) ;
#34290=CARTESIAN_POINT ( 'NONE',  ( 3.440625000614518036, -3.027376345333610441, -5.243569643749999898 ) ) ;
#34291=CARTESIAN_POINT ( 'NONE',  ( 16.12500000122903288, 2.886751345948126879, 4.999999999999999112 ) ) ;
#34292=CARTESIAN_POINT ( 'NONE',  ( 20.87812500061451715, -4.541064518000419881, 2.621784821874995952 ) ) ;
#34293=ADVANCED_FACE ( 'NONE', ( #26343, #10447 ), #71043, .T. ) ;
#34294=CARTESIAN_POINT ( 'NONE',  ( 22.52812500061451573, 4.541064518000418104, 2.621784821874999949 ) ) ;
#34295=CARTESIAN_POINT ( 'NONE',  ( 4.078125000614517326, 4.541064518000418104, 2.621784821874999949 ) ) ;
#34296=CARTESIAN_POINT ( 'NONE',  ( 28.87499999999999645, 6.123233995736764310E-16, -4.999999999999998224 ) ) ;
#34297=DIRECTION ( 'NONE',  ( -0.000000000000000000, -1.000000000000000000, -0.000000000000000000 ) ) ;
#34299=CARTESIAN_POINT ( 'NONE',  ( 6.487500001229034474, 6.123233995736764310E-16, -4.999999999999998224 ) ) ;
#34300=CARTESIAN_POINT ( 'NONE',  ( -3.999999999999999112, 12.01250000122903394, -30.00000000000000000 ) ) ;
#34301=CARTESIAN_POINT ( 'NONE',  ( -2.121784821874996840, 17.23437500061451999, -26.32496088578401583 ) ) ;
#34303=CARTESIAN_POINT ( 'NONE',  ( 6.150000001229033231, 5.773502691896255534, 3.535250795749688894E-16 ) ) ;
#34304=CARTESIAN_POINT ( 'NONE',  ( 8.099999999999999645, -4.330127018922190985, -2.500000000000001332 ) ) ;
#34305=CARTESIAN_POINT ( 'NONE',  ( 4.275000001229035895, 2.886751345948129099, -4.999999999999998224 ) ) ;
#34306=CARTESIAN_POINT ( 'NONE',  ( 11.22187500061451892, 3.027376345333613106, -5.243569643749998122 ) ) ;
#34307=CARTESIAN_POINT ( 'NONE',  ( 2.000000000000001332, 16.66250000122903430, -26.53589838486224650 ) ) ;
#34308=CARTESIAN_POINT ( 'NONE',  ( 3.346875000614518036, -3.027376345333614438, 5.243569643749998122 ) ) ;
#34309=CARTESIAN_POINT ( 'NONE',  ( 1.510657702057710734E-15, 19.10000000122903430, 26.00000000000000000 ) ) ;
#34311=CARTESIAN_POINT ( 'NONE',  ( 10.99687500061451750, -3.027376345333614438, 5.243569643749998122 ) ) ;
#34312=CARTESIAN_POINT ( 'NONE',  ( 14.03437500061451715, 4.541064518000418104, 2.621784821874999949 ) ) ;
#34313=CARTESIAN_POINT ( 'NONE',  ( -3.999999999999999112, 18.64999999999999858, -30.00000000000000000 ) ) ;
#34314=CARTESIAN_POINT ( 'NONE',  ( 6.825000000000001066, 6.123233995736764310E-16, -4.999999999999998224 ) ) ;
#34315=CARTESIAN_POINT ( 'NONE',  ( 9.001249775931846008E-16, 17.66562500061459318, 34.90005215228797653 ) ) ;
#34316=CARTESIAN_POINT ( 'NONE',  ( 22.43437500061451573, 6.421520780324663323E-16, -5.243569643749999010 ) ) ;
#34317=VECTOR ( 'NONE', #53507, 1000.000000000000000 ) ;
#34319=CARTESIAN_POINT ( 'NONE',  ( 26.32500000122903216, 2.886751345948129099, -4.999999999999998224 ) ) ;
#34321=CARTESIAN_POINT ( 'NONE',  ( 23.01562500061451644, 3.027376345333611329, 5.243569643749999010 ) ) ;
#34322=CARTESIAN_POINT ( 'NONE',  ( 16.15312500061451573, 4.541064518000418104, -2.621784821874998173 ) ) ;
#34324=CARTESIAN_POINT ( 'NONE',  ( 12.04687500061451821, -3.027376345333610441, -5.243569643749999898 ) ) ;
#34325=CARTESIAN_POINT ( 'NONE',  ( 27.44999999999999929, -4.330127018922190985, -2.500000000000001332 ) ) ;
#34326=CARTESIAN_POINT ( 'NONE',  ( 25.61250000122903359, 0.000000000000000000, 4.999999999999998224 ) ) ;
#34327=CARTESIAN_POINT ( 'NONE',  ( 4.434375000614519280, 6.421520780324663323E-16, -5.243569643749999010 ) ) ;
#34328=CARTESIAN_POINT ( 'NONE',  ( 14.70937500061451786, -4.541064518000417216, -2.621784821875001281 ) ) ;
#34329=CARTESIAN_POINT ( 'NONE',  ( 28.32187500061451502, 3.027376345333613106, -5.243569643749998122 ) ) ;
#34330=DIRECTION ( 'NONE',  ( -1.000000000000000000, -0.000000000000000000, -0.000000000000000000 ) ) ;
#34331=CYLINDRICAL_SURFACE ( 'NONE', #11255, 4.999999999999998224 ) ;
#34332=CARTESIAN_POINT ( 'NONE',  ( 21.38437500061451502, -4.541064518000419881, 2.621784821874995952 ) ) ;
#34333=CARTESIAN_POINT ( 'NONE',  ( 14.93437500061451750, 4.541064518000418104, 2.621784821874999949 ) ) ;
#34335=CARTESIAN_POINT ( 'NONE',  ( 26.06250000000000000, -5.773502691896255534, -1.060575238724906372E-15 ) ) ;
#34336=CARTESIAN_POINT ( 'NONE',  ( 2.850000001229036073, -2.886751345948125991, -5.000000000000000000 ) ) ;
#34338=CARTESIAN_POINT ( 'NONE',  ( 17.01562500061451644, 3.027376345333613106, -5.243569643749998122 ) ) ;
#34339=CARTESIAN_POINT ( 'NONE',  ( 6.112499999999999822, 2.886751345948126879, 4.999999999999999112 ) ) ;
#34340=( BOUNDED_CURVE ( )  B_SPLINE_CURVE ( 2, ( #16831, #61903, #592, #5763, #11667, #50829, #62627, #12022, #29017 ),
 .UNSPECIFIED., .F., .F. ) 
 B_SPLINE_CURVE_WITH_KNOTS ( ( 3, 2, 2, 2, 3 ),
 ( 0.3369565217391304324, 0.3405797101449275499, 0.3478260869565217295, 0.3550724637681159646, 0.3586956521739130821 ),
 .UNSPECIFIED. ) 
 CURVE ( )  GEOMETRIC_REPRESENTATION_ITEM ( )  RATIONAL_B_SPLINE_CURVE ( ( 0.9330127018922194093, 0.9330127018922194093, 1.000000000000000000, 0.8660254037844387076, 1.000000000000000000, 0.8660254037844387076, 1.000000000000000000, 0.9330127018922188542, 0.9330127018922194093 ) ) 
 REPRESENTATION_ITEM ( '' )  );
#34341=CARTESIAN_POINT ( 'NONE',  ( 15.56249999999999822, 2.886751345948193936, 4.999999999999883649 ) ) ;
#34342=CARTESIAN_POINT ( 'NONE',  ( 16.68750000000000000, -2.886751345948125991, -5.000000000000000000 ) ) ;
#34343=CARTESIAN_POINT ( 'NONE',  ( -4.243569643749999898, 12.60312500061451679, 30.00000000000000000 ) ) ;
#34345=CARTESIAN_POINT ( 'NONE',  ( 21.00000000122903288, 5.773502691896255534, 3.535250795749688894E-16 ) ) ;
#34346=CARTESIAN_POINT ( 'NONE',  ( 27.00937500061451857, 4.541064518000418104, -2.621784821874998173 ) ) ;
#34348=CARTESIAN_POINT ( 'NONE',  ( 20.91562500061451502, -6.054752690667223547, -1.112240025338166033E-15 ) ) ;
#34349=CARTESIAN_POINT ( 'NONE',  ( 21.23437500061451644, 4.541064518000418104, 2.621784821874999949 ) ) ;
#34350=CARTESIAN_POINT ( 'NONE',  ( 3.712499999999999911, 2.886751345948129099, -4.999999999999998224 ) ) ;
#34351=CARTESIAN_POINT ( 'NONE',  ( 8.615625000614517859, 3.027376345333611329, 5.243569643749999010 ) ) ;
#34352=CARTESIAN_POINT ( 'NONE',  ( 23.31562500061451715, 3.027376345333613106, -5.243569643749998122 ) ) ;
#34353=CARTESIAN_POINT ( 'NONE',  ( 11.89687500061451608, -3.027376345333614438, 5.243569643749998122 ) ) ;
#34354=CARTESIAN_POINT ( 'NONE',  ( 17.85937500061451999, -4.541064518000417216, -2.621784821875001281 ) ) ;
#34356=CARTESIAN_POINT ( 'NONE',  ( 4.243569643749999898, 17.77812500061451928, 30.00000000000000000 ) ) ;
#34357=CARTESIAN_POINT ( 'NONE',  ( 21.37500000122902932, 2.886751345948129099, -4.999999999999998224 ) ) ;
#34359=CARTESIAN_POINT ( 'NONE',  ( 12.62812500061451537, 4.541064518000418104, 2.621784821874999949 ) ) ;
#34360=CARTESIAN_POINT ( 'NONE',  ( 4.584375000614516971, 4.541064518000418104, 2.621784821874999949 ) ) ;
#34361=CARTESIAN_POINT ( 'NONE',  ( 4.921875000614518214, 3.027376345333613106, -5.243569643749998122 ) ) ;
#34363=CARTESIAN_POINT ( 'NONE',  ( 24.27187500061452141, 3.027376345333613106, -5.243569643749998122 ) ) ;
#34364=CARTESIAN_POINT ( 'NONE',  ( 15.96562500061451573, -6.054752690667223547, -1.112240025338166033E-15 ) ) ;
#34365=CARTESIAN_POINT ( 'NONE',  ( 26.77500000122903145, 2.886751345948129099, -4.999999999999998224 ) ) ;
#34366=CARTESIAN_POINT ( 'NONE',  ( 27.51562500061451644, 3.027376345333611329, 5.243569643749999010 ) ) ;
#34367=CARTESIAN_POINT ( 'NONE',  ( 21.30937500061451573, 0.000000000000000000, 5.243569643749999010 ) ) ;
#34368=CARTESIAN_POINT ( 'NONE',  ( 16.07812500061451289, 6.421520780324663323E-16, -5.243569643749999010 ) ) ;
#34369=CARTESIAN_POINT ( 'NONE',  ( -2.121784821874999949, 19.78437500061451715, 26.32496088578401938 ) ) ;
#34370=CARTESIAN_POINT ( 'NONE',  ( 22.52812500061451573, 4.541064518000418104, 2.621784821874999949 ) ) ;
#34373=CARTESIAN_POINT ( 'NONE',  ( 27.97500000000000142, 6.123233995736764310E-16, -4.999999999999998224 ) ) ;
#34374=CARTESIAN_POINT ( 'NONE',  ( 2.000000000000001332, 12.95000000000000107, -26.53589838486224650 ) ) ;
#34376=CARTESIAN_POINT ( 'NONE',  ( 28.41562500061451502, 3.027376345333611329, 5.243569643749999010 ) ) ;
#34377=EDGE_CURVE ( 'NONE', #12584, #3838, #54252, .T. ) ;
#34378=CARTESIAN_POINT ( 'NONE',  ( 11.24062500061451608, 6.054752690667223547, 3.707466751127219781E-16 ) ) ;
#34379=CARTESIAN_POINT ( 'NONE',  ( 22.76250000122903216, 4.330127018922192761, -2.499999999999997780 ) ) ;
#34380=CARTESIAN_POINT ( 'NONE',  ( 12.34687500061451892, -3.027376345333614438, 5.243569643749998122 ) ) ;
#34381=CARTESIAN_POINT ( 'NONE',  ( 28.15312500061451573, -4.541064518000417216, -2.621784821875001281 ) ) ;
#34383=CARTESIAN_POINT ( 'NONE',  ( 28.19999999999999929, 0.000000000000000000, 4.999999999999998224 ) ) ;
#34384=CARTESIAN_POINT ( 'NONE',  ( 8.484601909799253346E-16, 17.97500000122903785, -25.38119784648299770 ) ) ;
#34385=CYLINDRICAL_SURFACE ( 'NONE', #23200, 4.999999999999998224 ) ;
#34386=CARTESIAN_POINT ( 'NONE',  ( 11.84062500061451750, -3.027376345333614438, 5.243569643749998122 ) ) ;
#34387=VERTEX_POINT ( 'NONE', #4188 ) ;
#34388=CARTESIAN_POINT ( 'NONE',  ( 8.840625000614515727, -3.027376345333610441, -5.243569643749999898 ) ) ;
#34389=CARTESIAN_POINT ( 'NONE',  ( 5.653125000614517504, -4.541064518000417216, -2.621784821875001281 ) ) ;
#34392=EDGE_CURVE ( 'NONE', #29843, #24253, #14113, .T. ) ;
#34394=CARTESIAN_POINT ( 'NONE',  ( 16.16250000000000142, -5.773502691896255534, -1.060575238724906372E-15 ) ) ;
#34395=( BOUNDED_CURVE ( )  B_SPLINE_CURVE ( 2, ( #28258, #45248, #11267, #55965, #29340, #6081, #40426, #68504, #34872 ),
 .UNSPECIFIED., .F., .F. ) 
 B_SPLINE_CURVE_WITH_KNOTS ( ( 3, 2, 2, 2, 3 ),
 ( 0.4021739130434782705, 0.4057971014492753881, 0.4130434782608695676, 0.4202898550724637472, 0.4239130434782608647 ),
 .UNSPECIFIED. ) 
 CURVE ( )  GEOMETRIC_REPRESENTATION_ITEM ( )  RATIONAL_B_SPLINE_CURVE ( ( 0.9330127018922194093, 0.9330127018922194093, 1.000000000000000000, 0.8660254037844387076, 1.000000000000000000, 0.8660254037844387076, 1.000000000000000000, 0.9330127018922194093, 0.9330127018922194093 ) ) 
 REPRESENTATION_ITEM ( '' )  );
#34397=CARTESIAN_POINT ( 'NONE',  ( 15.45937500061451608, 0.000000000000000000, 5.243569643749999010 ) ) ;
#34398=CARTESIAN_POINT ( 'NONE',  ( 11.32500000122903394, -5.773502691896255534, -1.060575238724906372E-15 ) ) ;
#34399=CARTESIAN_POINT ( 'NONE',  ( 18.49687500061452283, 6.054752690667223547, 3.707466751127219781E-16 ) ) ;
#34401=CARTESIAN_POINT ( 'NONE',  ( 21.79687500061451644, -3.027376345333614438, 5.243569643749998122 ) ) ;
#34402=CARTESIAN_POINT ( 'NONE',  ( 4.243569643749999010, 14.21562500061451928, -32.45002607614398471 ) ) ;
#34406=CARTESIAN_POINT ( 'NONE',  ( 27.51562500061451644, 3.027376345333611329, 5.243569643749999010 ) ) ;
#34407=CARTESIAN_POINT ( 'NONE',  ( -3.999999999999997335, 19.58750000000000213, -27.69059892324149530 ) ) ;
#34408=CARTESIAN_POINT ( 'NONE',  ( 29.59687500061451715, -3.027376345333610441, -5.243569643749999898 ) ) ;
#34409=CARTESIAN_POINT ( 'NONE',  ( 24.71250000000000213, -5.773502691896255534, -1.060575238724906372E-15 ) ) ;
#34411=CARTESIAN_POINT ( 'NONE',  ( 7.903125000614515727, -4.541064518000417216, -2.621784821875001281 ) ) ;
#34413=CARTESIAN_POINT ( 'NONE',  ( 19.62187500061451573, -6.054752690667223547, -1.112240025338166033E-15 ) ) ;
#34415=CARTESIAN_POINT ( 'NONE',  ( 5.428125000614517859, 4.541064518000418104, 2.621784821874999949 ) ) ;
#34416=CARTESIAN_POINT ( 'NONE',  ( 11.10937500061451644, -4.541064518000417216, -2.621784821875001281 ) ) ;
#34417=ORIENTED_EDGE ( 'NONE', *, *, #44436, .T. ) ;
#34418=CARTESIAN_POINT ( 'NONE',  ( 20.29687500061451644, 6.054752690667223547, 3.707466751127219781E-16 ) ) ;
#34419=DIRECTION ( 'NONE',  ( -0.000000000000000000, -1.000000000000000000, -0.000000000000000000 ) ) ;
#34420=CARTESIAN_POINT ( 'NONE',  ( 28.01249999999999574, 2.886751345948129099, -4.999999999999998224 ) ) ;
#34421=CARTESIAN_POINT ( 'NONE',  ( 29.70937500061451431, 4.541064518000418104, -2.621784821874998173 ) ) ;
#34422=LINE ( 'NONE', #61052, #57286 ) ;
#34424=ORIENTED_EDGE ( 'NONE', *, *, #50947, .F. ) ;
#34425=CARTESIAN_POINT ( 'NONE',  ( 9.375000000000001776, -4.330127018922194537, 2.499999999999995559 ) ) ;
#34427=CARTESIAN_POINT ( 'NONE',  ( 24.25312500061451715, 4.541064518000418104, -2.621784821874998173 ) ) ;
#34428=CARTESIAN_POINT ( 'NONE',  ( 14.81250000000000000, -5.773502691896255534, -1.060575238724906372E-15 ) ) ;
#34429=CARTESIAN_POINT ( 'NONE',  ( 11.58750000122903501, 4.330127018922191873, 2.499999999999999556 ) ) ;
#34430=CARTESIAN_POINT ( 'NONE',  ( 9.028125000614517504, 4.541064518000418104, 2.621784821874999949 ) ) ;
#34431=CARTESIAN_POINT ( 'NONE',  ( 7.950000000000001954, 0.000000000000000000, 4.999999999999998224 ) ) ;
#34432=CARTESIAN_POINT ( 'NONE',  ( 16.05000000122903359, 5.773502691896255534, 3.535250795749688401E-16 ) ) ;
#34434=CARTESIAN_POINT ( 'NONE',  ( 28.20000000122903216, 5.773502691896255534, 3.535250795749688894E-16 ) ) ;
#34436=CARTESIAN_POINT ( 'NONE',  ( 7.987500000000000711, -2.886751345948129988, 4.999999999999997335 ) ) ;
#34437=CYLINDRICAL_SURFACE ( 'NONE', #16129, 4.999999999999998224 ) ;
#34439=CARTESIAN_POINT ( 'NONE',  ( 21.44062500061452070, -3.027376345333610441, -5.243569643749999898 ) ) ;
#34440=CARTESIAN_POINT ( 'NONE',  ( 3.332049138959096268, -3.727976942097309010, -3.471129952855481093 ) ) ;
#34441=CARTESIAN_POINT ( 'NONE',  ( 28.54687500061451644, -3.027376345333614438, 5.243569643749998122 ) ) ;
#34442=CARTESIAN_POINT ( 'NONE',  ( 19.20937500061451786, -4.541064518000417216, -2.621784821875001281 ) ) ;
#34443=CARTESIAN_POINT ( 'NONE',  ( 17.39062500061451644, -3.027376345333610441, -5.243569643749999898 ) ) ;
#34444=CARTESIAN_POINT ( 'NONE',  ( 4.243569643749999898, 11.92812500061459424, -30.00000000000000000 ) ) ;
#34445=CARTESIAN_POINT ( 'NONE',  ( 4.940625000614515372, 6.054752690667223547, 3.707466751127219781E-16 ) ) ;
#34446=CARTESIAN_POINT ( 'NONE',  ( 2.840625000614518392, -3.027376345333614438, 5.243569643749998122 ) ) ;
#34448=CARTESIAN_POINT ( 'NONE',  ( 18.40312500061451573, 4.541064518000418104, -2.621784821874998173 ) ) ;
#34449=DIRECTION ( 'NONE',  ( -1.000000000000000000, -0.000000000000000000, -0.000000000000000000 ) ) ;
#34450=CARTESIAN_POINT ( 'NONE',  ( 3.675000001229035362, -5.773502691896255534, -1.060575238724906372E-15 ) ) ;
#34451=CARTESIAN_POINT ( 'NONE',  ( 12.12187500061451573, 3.027376345333613106, -5.243569643749998122 ) ) ;
#34452=CARTESIAN_POINT ( 'NONE',  ( 13.02187500061451608, 3.027376345333613106, -5.243569643749998122 ) ) ;
#34453=CARTESIAN_POINT ( 'NONE',  ( 19.84687500061451360, 6.054752690667223547, 3.707466751127219781E-16 ) ) ;
#34455=CARTESIAN_POINT ( 'NONE',  ( -5.376511845580211890, 8.433624770265598869, 27.30849239394979122 ) ) ;
#34456=CARTESIAN_POINT ( 'NONE',  ( 24.51562500061451289, -6.054752690667223547, -1.112240025338166033E-15 ) ) ;
#34457=CARTESIAN_POINT ( 'NONE',  ( 18.49687500061452283, 6.054752690667223547, 3.707466751127219781E-16 ) ) ;
#34458=CARTESIAN_POINT ( 'NONE',  ( 24.17812500061451786, 6.421520780324663323E-16, -5.243569643749999010 ) ) ;
#34459=CARTESIAN_POINT ( 'NONE',  ( 27.18750000000000000, 5.773502691896255534, 3.535250795749688401E-16 ) ) ;
#34460=CARTESIAN_POINT ( 'NONE',  ( 8.484601909799253346E-16, 16.06250000000000000, 34.61880215351700230 ) ) ;
#34461=CARTESIAN_POINT ( 'NONE',  ( 29.61562500061451431, 3.027376345333613106, -5.243569643749998122 ) ) ;
#34462=CARTESIAN_POINT ( 'NONE',  ( 10.83750000122903501, -4.330127018922194537, 2.499999999999995559 ) ) ;
#34463=CARTESIAN_POINT ( 'NONE',  ( 7.312500001229033764, -4.330127018922190985, -2.500000000000001332 ) ) ;
#34464=FACE_OUTER_BOUND ( 'NONE', #25236, .T. ) ;
#34465=CARTESIAN_POINT ( 'NONE',  ( 28.31250000122903288, 0.000000000000000000, 4.999999999999998224 ) ) ;
#34468=CARTESIAN_POINT ( 'NONE',  ( 10.47187500061451715, 3.027376345333611329, 5.243569643749999010 ) ) ;
#34470=CARTESIAN_POINT ( 'NONE',  ( 18.29062500061451502, -3.027376345333610441, -5.243569643749999898 ) ) ;
#34471=CARTESIAN_POINT ( 'NONE',  ( 12.08437500061451608, 6.421520780324663323E-16, -5.243569643749999010 ) ) ;
#34472=CARTESIAN_POINT ( 'NONE',  ( 3.140625000614516882, 6.054752690667223547, 3.707466751127219781E-16 ) ) ;
#34473=CARTESIAN_POINT ( 'NONE',  ( 20.33437500061451786, 4.541064518000418104, 2.621784821874999949 ) ) ;
#34474=CARTESIAN_POINT ( 'NONE',  ( 7.096875000614517148, -3.027376345333610441, -5.243569643749999898 ) ) ;
#34475=CARTESIAN_POINT ( 'NONE',  ( 2.953125000614516438, -4.541064518000417216, -2.621784821875001281 ) ) ;
#34477=CARTESIAN_POINT ( 'NONE',  ( 10.07812500061451644, -4.541064518000419881, 2.621784821874995952 ) ) ;
#34478=CARTESIAN_POINT ( 'NONE',  ( 20.54062500061451502, -3.027376345333610441, -5.243569643749999898 ) ) ;
#34479=EDGE_LOOP ( 'NONE', ( #15253, #18674, #9300, #53415 ) ) ;
#34480=CARTESIAN_POINT ( 'NONE',  ( 6.525000001229033231, 2.886751345948129099, -4.999999999999998224 ) ) ;
#34481=CARTESIAN_POINT ( 'NONE',  ( 14.46562500061451750, 3.027376345333611329, 5.243569643749999010 ) ) ;
#34482=CARTESIAN_POINT ( 'NONE',  ( 13.26562500061451644, -6.054752690667223547, -1.112240025338166033E-15 ) ) ;
#34484=CARTESIAN_POINT ( 'NONE',  ( 12.41249999999999964, 2.886751345948126879, 4.999999999999999112 ) ) ;
#34485=CARTESIAN_POINT ( 'NONE',  ( 9.187500001229034652, 6.123233995736764310E-16, -4.999999999999998224 ) ) ;
#34486=CARTESIAN_POINT ( 'NONE',  ( 5.765625000614519102, 3.027376345333613106, -5.243569643749998122 ) ) ;
#34488=CARTESIAN_POINT ( 'NONE',  ( 18.33750000122903501, 4.330127018922191873, 2.499999999999999556 ) ) ;
#34490=CARTESIAN_POINT ( 'NONE',  ( 2.121784821874999061, 10.25937500061451857, -33.67503911421598417 ) ) ;
#34491=CARTESIAN_POINT ( 'NONE',  ( 0.000000000000000000, 20.00000000000000000, 30.00000000000000000 ) ) ;
#34492=CARTESIAN_POINT ( 'NONE',  ( 2.887500001229035274, 6.123233995736764310E-16, -4.999999999999998224 ) ) ;
#34494=CARTESIAN_POINT ( 'NONE',  ( 19.32187500061451857, 3.027376345333613106, -5.243569643749998122 ) ) ;
#34495=CARTESIAN_POINT ( 'NONE',  ( 1.592000809091587073E-14, 16.40000000122903501, 26.00000000000000000 ) ) ;
#34496=CARTESIAN_POINT ( 'NONE',  ( 16.75312500061451715, 0.000000000000000000, 5.243569643749999010 ) ) ;
#34498=CARTESIAN_POINT ( 'NONE',  ( 30.00000000000000000, 0.000000000000000000, 4.999999999999998224 ) ) ;
#34499=CARTESIAN_POINT ( 'NONE',  ( 28.92187500061451644, 3.027376345333611329, 5.243569643749999010 ) ) ;
#34500=CARTESIAN_POINT ( 'NONE',  ( 26.67187500061451644, 3.027376345333611329, 5.243569643749999010 ) ) ;
#34502=CARTESIAN_POINT ( 'NONE',  ( 12.32812500061451821, -4.541064518000419881, 2.621784821874995952 ) ) ;
#34503=CARTESIAN_POINT ( 'NONE',  ( 9.984375000614518214, 4.541064518000418104, 2.621784821874999949 ) ) ;
#34504=ORIENTED_EDGE ( 'NONE', *, *, #38215, .T. ) ;
#34505=CARTESIAN_POINT ( 'NONE',  ( 9.299999999999998934, 0.000000000000000000, 4.999999999999998224 ) ) ;
#34506=CARTESIAN_POINT ( 'NONE',  ( 19.37812500061451715, 4.541064518000418104, 2.621784821874999949 ) ) ;
#34507=CARTESIAN_POINT ( 'NONE',  ( 0.000000000000000000, 20.00000000000000000, -30.00000000000000000 ) ) ;
#34509=CARTESIAN_POINT ( 'NONE',  ( 9.787499999999999645, -2.886751345948129988, 4.999999999999997335 ) ) ;
#34510=CARTESIAN_POINT ( 'NONE',  ( 21.11250000122903359, 0.000000000000000000, 4.999999999999998224 ) ) ;
#34511=CARTESIAN_POINT ( 'NONE',  ( 16.07812500061451289, 6.421520780324663323E-16, -5.243569643749999010 ) ) ;
#34514=CARTESIAN_POINT ( 'NONE',  ( 19.50000000000000000, 4.330127018922192761, -2.499999999999997780 ) ) ;
#34515=CARTESIAN_POINT ( 'NONE',  ( 22.01249999999999574, -5.773502691896255534, -1.060575238724906372E-15 ) ) ;
#34516=CARTESIAN_POINT ( 'NONE',  ( 21.60937500061451644, 4.541064518000418104, -2.621784821874998173 ) ) ;
#34517=CARTESIAN_POINT ( 'NONE',  ( 25.37812500061451715, -4.541064518000419881, 2.621784821874995952 ) ) ;
#34518=ORIENTED_EDGE ( 'NONE', *, *, #48920, .T. ) ;
#34520=CARTESIAN_POINT ( 'NONE',  ( 7.265625000614516438, 3.027376345333611329, 5.243569643749999010 ) ) ;
#34522=CARTESIAN_POINT ( 'NONE',  ( 13.83749999999999858, -2.886751345948129988, 4.999999999999997335 ) ) ;
#34523=CARTESIAN_POINT ( 'NONE',  ( 9.001249775931846008E-16, 16.76562500061451999, 34.90005215228797653 ) ) ;
#34524=CARTESIAN_POINT ( 'NONE',  ( 28.97812500061451502, -4.541064518000419881, 2.621784821874995952 ) ) ;
#34525=CARTESIAN_POINT ( 'NONE',  ( 25.77187500061451075, 3.027376345333611329, 5.243569643749999010 ) ) ;
#34526=EDGE_LOOP ( 'NONE', ( #57629, #21626, #22615, #55173 ) ) ;
#34527=CARTESIAN_POINT ( 'NONE',  ( 22.97812500061451857, 4.541064518000418104, 2.621784821874999949 ) ) ;
#34528=CARTESIAN_POINT ( 'NONE',  ( 25.62187500061451573, 3.027376345333613106, -5.243569643749998122 ) ) ;
#34529=CARTESIAN_POINT ( 'NONE',  ( 4.243569643749999010, 18.71562500061458678, -32.45002607614398471 ) ) ;
#34530=CARTESIAN_POINT ( 'NONE',  ( 11.36250000000000071, 2.886751345948129099, -4.999999999999998224 ) ) ;
#34531=CARTESIAN_POINT ( 'NONE',  ( 9.103125000614515017, 0.000000000000000000, 5.243569643749999010 ) ) ;
#34533=CARTESIAN_POINT ( 'NONE',  ( 28.75312500061451715, 4.541064518000418104, -2.621784821874998173 ) ) ;
#34534=CARTESIAN_POINT ( 'NONE',  ( 25.97812500061451502, 6.421520780324663323E-16, -5.243569643749999010 ) ) ;
#34537=CARTESIAN_POINT ( 'NONE',  ( 18.64687500061451786, -3.027376345333614438, 5.243569643749998122 ) ) ;
#34538=CARTESIAN_POINT ( 'NONE',  ( -2.121784821874996840, 11.38437500061451679, 33.67503911421598417 ) ) ;
#34539=CARTESIAN_POINT ( 'NONE',  ( 19.47187500061451360, 3.027376345333611329, 5.243569643749999010 ) ) ;
#34540=CARTESIAN_POINT ( 'NONE',  ( 28.35937500061451289, 4.541064518000418104, -2.621784821874998173 ) ) ;
#34541=CARTESIAN_POINT ( 'NONE',  ( 4.243569643749999010, 17.42187500061451999, 27.54997392385601174 ) ) ;
#34542=CARTESIAN_POINT ( 'NONE',  ( 6.815625000614517148, 3.027376345333611329, 5.243569643749999010 ) ) ;
#34543=CARTESIAN_POINT ( 'NONE',  ( -3.999999999999999112, 18.16250000000000142, -32.30940107675850470 ) ) ;
#34545=CARTESIAN_POINT ( 'NONE',  ( 4.546875000614517326, 6.054752690667223547, 3.707466751127219781E-16 ) ) ;
#34546=CARTESIAN_POINT ( 'NONE',  ( 1.071796769724491893, 15.63259618943233598, -26.00000000000000355 ) ) ;
#34547=CARTESIAN_POINT ( 'NONE',  ( 6.890625000614516438, -3.027376345333614438, 5.243569643749998122 ) ) ;
#34548=CARTESIAN_POINT ( 'NONE',  ( 12.30937500061451573, 0.000000000000000000, 5.243569643749999010 ) ) ;
#34549=FILL_AREA_STYLE ('',( #11311 ) ) ;
#34550=CARTESIAN_POINT ( 'NONE',  ( 18.41250000122903430, 0.000000000000000000, 4.999999999999998224 ) ) ;
#34551=CARTESIAN_POINT ( 'NONE',  ( 6.684375000614518392, 6.421520780324663323E-16, -5.243569643749999010 ) ) ;
#34552=CARTESIAN_POINT ( 'NONE',  ( 8.428125000614517859, 6.421520780324663323E-16, -5.243569643749999010 ) ) ;
#34553=CARTESIAN_POINT ( 'NONE',  ( 4.087500001229035007, -4.330127018922194537, 2.499999999999995559 ) ) ;
#34555=CARTESIAN_POINT ( 'NONE',  ( 15.57187500061451679, -6.054752690667223547, -1.112240025338166033E-15 ) ) ;
#34558=CARTESIAN_POINT ( 'NONE',  ( 25.60312500061451502, 4.541064518000418104, -2.621784821874998173 ) ) ;
#34559=CARTESIAN_POINT ( 'NONE',  ( 10.64062500061451644, -3.027376345333610441, -5.243569643749999898 ) ) ;
#34560=CARTESIAN_POINT ( 'NONE',  ( 27.87187500061451573, 3.027376345333612662, -5.243569643749998122 ) ) ;
#34561=CARTESIAN_POINT ( 'NONE',  ( 10.52812500061451750, -4.541064518000419881, 2.621784821874995952 ) ) ;
#34562=CARTESIAN_POINT ( 'NONE',  ( 30.00000000000000000, 0.000000000000000000, 4.999999999999998224 ) ) ;
#34563=CARTESIAN_POINT ( 'NONE',  ( 13.61250000122903359, -4.330127018922190985, -2.500000000000001332 ) ) ;
#34564=CARTESIAN_POINT ( 'NONE',  ( 26.95312500061451644, 4.541064518000418104, -2.621784821874998173 ) ) ;
#34565=CARTESIAN_POINT ( 'NONE',  ( -3.000416591977282496E-16, 12.04062500061451857, -34.90005215228797653 ) ) ;
#34566=CARTESIAN_POINT ( 'NONE',  ( 12.71250000122903145, -4.330127018922190985, -2.500000000000001332 ) ) ;
#34567=CARTESIAN_POINT ( 'NONE',  ( 10.98750000000000071, 5.773502691896255534, 3.535250795749688894E-16 ) ) ;
#34568=CARTESIAN_POINT ( 'NONE',  ( 20.61562500061451431, 3.027376345333613106, -5.243569643749998122 ) ) ;
#34569=CARTESIAN_POINT ( 'NONE',  ( 7.171875000614516438, 3.027376345333612662, -5.243569643749998122 ) ) ;
#34571=CARTESIAN_POINT ( 'NONE',  ( 19.65000000000000213, 0.000000000000000000, 4.999999999999998224 ) ) ;
#34572=CARTESIAN_POINT ( 'NONE',  ( 6.862500001229034474, -4.330127018922190985, -2.500000000000001332 ) ) ;
#34573=CARTESIAN_POINT ( 'NONE',  ( 15.48750000122903359, 6.123233995736764310E-16, -4.999999999999998224 ) ) ;
#34574=CARTESIAN_POINT ( 'NONE',  ( 13.11562500061451786, 3.027376345333611329, 5.243569643749999010 ) ) ;
#34575=CARTESIAN_POINT ( 'NONE',  ( 16.56562500061451715, 3.027376345333613106, -5.243569643749998122 ) ) ;
#34576=CARTESIAN_POINT ( 'NONE',  ( 26.28750000122903430, 6.123233995736764310E-16, -4.999999999999998224 ) ) ;
#34577=CARTESIAN_POINT ( 'NONE',  ( 20.73750000000000071, -2.886751345948125991, -5.000000000000000000 ) ) ;
#34578=CARTESIAN_POINT ( 'NONE',  ( 23.44687500061451502, 6.054752690667223547, 3.707466751127219781E-16 ) ) ;
#34580=CARTESIAN_POINT ( 'NONE',  ( 9.112500001229033586, -4.330127018922190985, -2.500000000000001332 ) ) ;
#34581=CARTESIAN_POINT ( 'NONE',  ( 9.946875000614516793, 6.054752690667223547, 3.707466751127219781E-16 ) ) ;
#34582=CARTESIAN_POINT ( 'NONE',  ( 25.13437500061451502, 6.421520780324663323E-16, -5.243569643749999010 ) ) ;
#34584=CARTESIAN_POINT ( 'NONE',  ( 23.76562500061451644, 3.027376345333613106, -5.243569643749998122 ) ) ;
#34585=CARTESIAN_POINT ( 'NONE',  ( 27.30937500061451573, -4.541064518000417216, -2.621784821875001281 ) ) ;
#34588=CARTESIAN_POINT ( 'NONE',  ( 8.896875000614517859, -3.027376345333610441, -5.243569643749999898 ) ) ;
#34590=CARTESIAN_POINT ( 'NONE',  ( 26.99062500061451431, 6.054752690667223547, 3.707466751127219781E-16 ) ) ;
#34591=CARTESIAN_POINT ( 'NONE',  ( 5.709375000614517859, -4.541064518000417216, -2.621784821875001281 ) ) ;
#34592=CARTESIAN_POINT ( 'NONE',  ( 1.592000809091587073E-14, 16.40000000122903501, -34.00000000000000000 ) ) ;
#34593=CARTESIAN_POINT ( 'NONE',  ( 25.13437500061451502, 6.421520780324663323E-16, -5.243569643749999010 ) ) ;
#34594=CARTESIAN_POINT ( 'NONE',  ( 2.121784821875001281, 10.05312500061459424, 33.67503911421598417 ) ) ;
#34595=CARTESIAN_POINT ( 'NONE',  ( 16.42500000000000071, 4.330127018922191873, 2.499999999999999556 ) ) ;
#34597=CARTESIAN_POINT ( 'NONE',  ( 27.63749999999999929, 5.773502691896255534, 3.535250795749688894E-16 ) ) ;
#34598=CARTESIAN_POINT ( 'NONE',  ( 27.45937500061451786, 4.541064518000418104, -2.621784821874998173 ) ) ;
#34600=CARTESIAN_POINT ( 'NONE',  ( 16.30312500061451786, 0.000000000000000000, 5.243569643749999010 ) ) ;
#34601=CARTESIAN_POINT ( 'NONE',  ( 6.890625000614516438, -3.027376345333614438, 5.243569643749998122 ) ) ;
#34603=CARTESIAN_POINT ( 'NONE',  ( 3.759375000614517681, 0.000000000000000000, 5.243569643749999010 ) ) ;
#34604=CARTESIAN_POINT ( 'NONE',  ( 14.66250000122903252, 4.330127018922192761, -2.499999999999997780 ) ) ;
#34605=CARTESIAN_POINT ( 'NONE',  ( 21.48750000000000071, -2.886751345948129988, 4.999999999999997335 ) ) ;
#34606=CARTESIAN_POINT ( 'NONE',  ( 29.88749999999999929, 5.773502691896255534, 3.535250795749688894E-16 ) ) ;
#34607=CARTESIAN_POINT ( 'NONE',  ( 5.371875000614516615, 3.027376345333613106, -5.243569643749998122 ) ) ;
#34608=CARTESIAN_POINT ( 'NONE',  ( 10.09687500061451715, -3.027376345333614438, 5.243569643749998122 ) ) ;
#34609=CARTESIAN_POINT ( 'NONE',  ( 22.77187500061451786, -6.054752690667223547, -1.112240025338166033E-15 ) ) ;
#34611=EDGE_LOOP ( 'NONE', ( #10499, #6890, #58589, #21385 ) ) ;
#34612=CARTESIAN_POINT ( 'NONE',  ( 4.921875000614518214, 3.027376345333613106, -5.243569643749998122 ) ) ;
#34613=CARTESIAN_POINT ( 'NONE',  ( 7.546875000614517326, -3.027376345333610441, -5.243569643749999898 ) ) ;
#34614=CARTESIAN_POINT ( 'NONE',  ( 17.51249999999999929, -5.773502691896255534, -1.060575238724906372E-15 ) ) ;
#34615=CARTESIAN_POINT ( 'NONE',  ( 15.70312500061451644, 4.541064518000418104, -2.621784821874998173 ) ) ;
#34619=CARTESIAN_POINT ( 'NONE',  ( 9.403125000614517504, 4.541064518000418104, -2.621784821874998173 ) ) ;
#34620=CARTESIAN_POINT ( 'NONE',  ( 26.25937500061451857, 0.000000000000000000, 5.243569643749999010 ) ) ;
#34622=CARTESIAN_POINT ( 'NONE',  ( 25.28437500061451715, 4.541064518000418104, 2.621784821874999949 ) ) ;
#34623=CARTESIAN_POINT ( 'NONE',  ( 7.837499999999999467, 5.773502691896255534, 3.535250795749688894E-16 ) ) ;
#34624=CARTESIAN_POINT ( 'NONE',  ( -3.999999999999999556, 12.87500000122903465, 27.69059892324149530 ) ) ;
#34625=CARTESIAN_POINT ( 'NONE',  ( 7.162500001229032520, 0.000000000000000000, 4.999999999999998224 ) ) ;
#34626=( BOUNDED_CURVE ( )  B_SPLINE_CURVE ( 2, ( #45603, #24131, #12324, #57023, #46681, #7509, #62931 ),
 .UNSPECIFIED., .F., .F. ) 
 B_SPLINE_CURVE_WITH_KNOTS ( ( 3, 2, 2, 3 ),
 ( 0.2999999999999999889, 0.3027777777777777568, 0.3055555555555555802, 0.3083333333333333481 ),
 .UNSPECIFIED. ) 
 CURVE ( )  GEOMETRIC_REPRESENTATION_ITEM ( )  RATIONAL_B_SPLINE_CURVE ( ( 1.000000000000000000, 0.8660254037844387076, 1.000000000000000000, 0.8660254037844387076, 1.000000000000000000, 0.8660254037844387076, 1.000000000000000000 ) ) 
 REPRESENTATION_ITEM ( '' )  );
#34627=ADVANCED_FACE ( 'NONE', ( #5267 ), #61798, .T. ) ;
#34628=CARTESIAN_POINT ( 'NONE',  ( 16.62187500061451573, 3.027376345333613106, -5.243569643749998122 ) ) ;
#34629=CARTESIAN_POINT ( 'NONE',  ( 11.29687500061451644, 6.054752690667223547, 3.707466751127219781E-16 ) ) ;
#34632=CARTESIAN_POINT ( 'NONE',  ( 15.70312500061451644, 4.541064518000418104, -2.621784821874998173 ) ) ;
#34633=CARTESIAN_POINT ( 'NONE',  ( 25.76250000122903216, -4.330127018922190985, -2.500000000000001332 ) ) ;
#34634=CARTESIAN_POINT ( 'NONE',  ( 12.90937500061451537, -4.541064518000417216, -2.621784821875001281 ) ) ;
#34635=CARTESIAN_POINT ( 'NONE',  ( -3.137519842735245283E-14, 12.57500000122903572, 34.00000000000000000 ) ) ;
#34636=CARTESIAN_POINT ( 'NONE',  ( 13.75312500061451715, -4.541064518000417216, -2.621784821875001281 ) ) ;
#34637=EDGE_CURVE ( 'NONE', #59354, #30864, #31146, .T. ) ;
#34639=CARTESIAN_POINT ( 'NONE',  ( 25.47187500061451715, -6.054752690667223547, -1.112240025338166033E-15 ) ) ;
#34640=CARTESIAN_POINT ( 'NONE',  ( 2.892512340070121812, -4.078410086807788382, 3.295700467049730520 ) ) ;
#34641=CARTESIAN_POINT ( 'NONE',  ( 11.92500000122903181, 2.886751345948129099, -4.999999999999998224 ) ) ;
#34644=CARTESIAN_POINT ( 'NONE',  ( -2.121784821874996840, 16.78437500061452070, -26.32496088578401583 ) ) ;
#34645=EDGE_CURVE ( 'NONE', #14992, #44258, #47632, .T. ) ;
#34646=CARTESIAN_POINT ( 'NONE',  ( 19.13437500061451857, -4.541064518000419881, 2.621784821874995952 ) ) ;
#34647=CARTESIAN_POINT ( 'NONE',  ( 20.17500000122903359, 2.886751345948126879, 4.999999999999999112 ) ) ;
#34648=CARTESIAN_POINT ( 'NONE',  ( 14.55937500061451573, 0.000000000000000000, 5.243569643749999010 ) ) ;
#34649=CARTESIAN_POINT ( 'NONE',  ( -3.000416591977282496E-16, 10.29687500061451644, 25.09994784771203058 ) ) ;
#34650=CARTESIAN_POINT ( 'NONE',  ( 22.91250000122903430, 0.000000000000000000, 4.999999999999998224 ) ) ;
#34651=CARTESIAN_POINT ( 'NONE',  ( 15.70312500061451644, 4.541064518000418104, -2.621784821874998173 ) ) ;
#34652=CARTESIAN_POINT ( 'NONE',  ( 29.09062500061451573, -3.027376345333610441, -5.243569643749999898 ) ) ;
#34653=VERTEX_POINT ( 'NONE', #64622 ) ;
#34655=CARTESIAN_POINT ( 'NONE',  ( 19.27500000000000213, -4.330127018922194537, 2.499999999999995559 ) ) ;
#34657=CARTESIAN_POINT ( 'NONE',  ( 2.953125000614516438, -4.541064518000417216, -2.621784821875001281 ) ) ;
#34658=CARTESIAN_POINT ( 'NONE',  ( 15.71250000122903501, 0.000000000000000000, 4.999999999999998224 ) ) ;
#34659=CARTESIAN_POINT ( 'NONE',  ( 20.65312500061451573, 4.541064518000418104, -2.621784821874998173 ) ) ;
#34660=CARTESIAN_POINT ( 'NONE',  ( 22.07812500061451644, 4.541064518000418104, 2.621784821874999949 ) ) ;
#34661=CARTESIAN_POINT ( 'NONE',  ( 2.878125000614517592, -4.541064518000419881, 2.621784821874995952 ) ) ;
#34662=CARTESIAN_POINT ( 'NONE',  ( 27.26249999999999929, 2.886751345948126879, 4.999999999999999112 ) ) ;
#34663=CARTESIAN_POINT ( 'NONE',  ( 2.000000000000001332, 11.71250000122903501, 33.46410161513774995 ) ) ;
#34665=CARTESIAN_POINT ( 'NONE',  ( 29.40937500061451715, 0.000000000000000000, 5.243569643749999010 ) ) ;
#34666=CARTESIAN_POINT ( 'NONE',  ( -1.999999999999997113, 12.08750000122903501, -26.53589838486224295 ) ) ;
#34667=CARTESIAN_POINT ( 'NONE',  ( 4.243569643749999010, 16.97187500061451360, -32.45002607614398471 ) ) ;
#34668=EDGE_CURVE ( 'NONE', #66446, #33991, #16920, .T. ) ;
#34669=CARTESIAN_POINT ( 'NONE',  ( 5.212500001229032343, 4.330127018922192761, -2.499999999999997780 ) ) ;
#34670=CARTESIAN_POINT ( 'NONE',  ( 8.962500000000002132, -5.773502691896255534, -1.060575238724906372E-15 ) ) ;
#34671=CARTESIAN_POINT ( 'NONE',  ( 5.062500001229035540, -4.330127018922190985, -2.500000000000001332 ) ) ;
#34672=CARTESIAN_POINT ( 'NONE',  ( 8.934375000614517504, 6.421520780324663323E-16, -5.243569643749999010 ) ) ;
#34673=CARTESIAN_POINT ( 'NONE',  ( 3.947751918878622757, -3.068428716296062841, 3.947751918878600108 ) ) ;
#34674=CARTESIAN_POINT ( 'NONE',  ( 3.571875000614517237, 3.027376345333613106, -5.243569643749998122 ) ) ;
#34675=CARTESIAN_POINT ( 'NONE',  ( 28.08749999999999858, 5.773502691896255534, 3.535250795749688401E-16 ) ) ;
#34676=CARTESIAN_POINT ( 'NONE',  ( 17.06250000122903288, 0.000000000000000000, 4.999999999999998224 ) ) ;
#34677=CARTESIAN_POINT ( 'NONE',  ( 7.996875000614519280, -3.027376345333610441, -5.243569643749999898 ) ) ;
#34678=CARTESIAN_POINT ( 'NONE',  ( 13.43437500061451750, 6.421520780324663323E-16, -5.243569643749999010 ) ) ;
#34680=CARTESIAN_POINT ( 'NONE',  ( 6.787500000000001421, -2.886751345948125991, -5.000000000000000000 ) ) ;
#34681=CARTESIAN_POINT ( 'NONE',  ( 4.243569643749999898, 17.77812500061459744, 30.00000000000000000 ) ) ;
#34682=CARTESIAN_POINT ( 'NONE',  ( 20.70937500061451786, 4.541064518000418104, -2.621784821874998173 ) ) ;
#34684=CARTESIAN_POINT ( 'NONE',  ( 25.98750000122903003, 4.330127018922191873, 2.499999999999999556 ) ) ;
#34686=CARTESIAN_POINT ( 'NONE',  ( 21.96562500061451573, 3.027376345333613106, -5.243569643749998122 ) ) ;
#34687=CARTESIAN_POINT ( 'NONE',  ( 16.45312500061451289, -4.541064518000417216, -2.621784821875001281 ) ) ;
#34689=CARTESIAN_POINT ( 'NONE',  ( 12.64687500061451608, 6.054752690667223547, 3.707466751127219781E-16 ) ) ;
#34690=CARTESIAN_POINT ( 'NONE',  ( 29.66249999999999432, -5.773502691896255534, -1.060575238724906372E-15 ) ) ;
#34691=CARTESIAN_POINT ( 'NONE',  ( 26.02500000122903145, 2.886751345948126879, 4.999999999999999112 ) ) ;
#34694=CARTESIAN_POINT ( 'NONE',  ( 11.59687500061451892, -3.027376345333610441, -5.243569643749999898 ) ) ;
#34695=CARTESIAN_POINT ( 'NONE',  ( 29.74687500061451217, 6.054752690667223547, 3.707466751127219781E-16 ) ) ;
#34696=CARTESIAN_POINT ( 'NONE',  ( 3.609375000614516882, 4.541064518000418104, -2.621784821874998173 ) ) ;
#34697=CARTESIAN_POINT ( 'NONE',  ( 18.30000000000000071, 0.000000000000000000, 4.999999999999998224 ) ) ;
#34698=CARTESIAN_POINT ( 'NONE',  ( 23.37187500061451573, 3.027376345333613106, -5.243569643749998122 ) ) ;
#34699=CARTESIAN_POINT ( 'NONE',  ( 15.23437500061451644, 6.421520780324663323E-16, -5.243569643749999010 ) ) ;
#34701=CARTESIAN_POINT ( 'NONE',  ( 25.61250000000000071, -5.773502691896255534, -1.060575238724906372E-15 ) ) ;
#34704=CARTESIAN_POINT ( 'NONE',  ( 17.39062500061451644, -3.027376345333610441, -5.243569643749999898 ) ) ;
#34705=CARTESIAN_POINT ( 'NONE',  ( 6.937499999999999112, 5.773502691896255534, 3.535250795749688894E-16 ) ) ;
#34706=CARTESIAN_POINT ( 'NONE',  ( 1.626862140677534273E-15, 13.47500000122903252, 34.00000000000000000 ) ) ;
#34707=CARTESIAN_POINT ( 'NONE',  ( 14.43750000000000000, -2.886751345948125991, -5.000000000000000000 ) ) ;
#34708=CARTESIAN_POINT ( 'NONE',  ( 9.001249775931846008E-16, 10.01562500061451644, 34.90005215228797653 ) ) ;
#34710=CARTESIAN_POINT ( 'NONE',  ( 26.07187500061451857, 3.027376345333613106, -5.243569643749998122 ) ) ;
#34711=ORIENTED_EDGE ( 'NONE', *, *, #63337, .F. ) ;
#34712=CARTESIAN_POINT ( 'NONE',  ( 20.80312500061451431, 0.000000000000000000, 5.243569643749999010 ) ) ;
#34713=CARTESIAN_POINT ( 'NONE',  ( 20.44687500061451857, -3.027376345333614438, 5.243569643749998122 ) ) ;
#34714=CARTESIAN_POINT ( 'NONE',  ( 3.975000000000002753, -4.330127018922194537, 2.499999999999995559 ) ) ;
#34715=CARTESIAN_POINT ( 'NONE',  ( 6.778125000614518392, 4.541064518000418104, 2.621784821874999949 ) ) ;
#34716=CARTESIAN_POINT ( 'NONE',  ( 23.27812500061451573, 6.421520780324663323E-16, -5.243569643749999010 ) ) ;
#34717=CARTESIAN_POINT ( 'NONE',  ( 13.47187500061451537, 3.027376345333613106, -5.243569643749998122 ) ) ;
#34718=CARTESIAN_POINT ( 'NONE',  ( 16.65937500061452070, 4.541064518000418104, -2.621784821874998173 ) ) ;
#34719=CARTESIAN_POINT ( 'NONE',  ( 9.001249775931846008E-16, 17.21562500061451928, 34.90005215228797653 ) ) ;
#34720=CARTESIAN_POINT ( 'NONE',  ( 17.88750000122903216, 4.330127018922191873, 2.499999999999999556 ) ) ;
#34722=CARTESIAN_POINT ( 'NONE',  ( 8.878125000614515372, 6.421520780324663323E-16, -5.243569643749999010 ) ) ;
#34723=CARTESIAN_POINT ( 'NONE',  ( 4.659375000614518925, 0.000000000000000000, 5.243569643749999010 ) ) ;
#34724=CARTESIAN_POINT ( 'NONE',  ( 4.734375000614518214, -4.541064518000419881, 2.621784821874995952 ) ) ;
#34727=CARTESIAN_POINT ( 'NONE',  ( 25.58437500061451431, 6.421520780324663323E-16, -5.243569643749999010 ) ) ;
#34728=CARTESIAN_POINT ( 'NONE',  ( 16.94062500061451715, -3.027376345333610441, -5.243569643749999898 ) ) ;
#34729=CARTESIAN_POINT ( 'NONE',  ( 27.93750000122903288, -4.330127018922194537, 2.499999999999995559 ) ) ;
#34730=CARTESIAN_POINT ( 'NONE',  ( 27.14062500061451644, -3.027376345333614438, 5.243569643749998122 ) ) ;
#34731=CARTESIAN_POINT ( 'NONE',  ( 22.17187500061451644, 3.027376345333611329, 5.243569643749999010 ) ) ;
#34732=CARTESIAN_POINT ( 'NONE',  ( 17.05312500061451786, 4.541064518000418104, -2.621784821874998173 ) ) ;
#34733=CARTESIAN_POINT ( 'NONE',  ( 4.243569643749999898, 16.89687500061451786, 32.45002607614398471 ) ) ;
#34734=CARTESIAN_POINT ( 'NONE',  ( 21.70312500061451644, 0.000000000000000000, 5.243569643749999010 ) ) ;
#34735=DIRECTION ( 'NONE',  ( 0.000000000000000000, 0.000000000000000000, 1.000000000000000000 ) ) ;
#34736=ORIENTED_EDGE ( 'NONE', *, *, #57642, .F. ) ;
#34737=ORIENTED_EDGE ( 'NONE', *, *, #56333, .T. ) ;
#34738=CARTESIAN_POINT ( 'NONE',  ( 25.83749999999999858, 5.773502691896255534, 3.535250795749688894E-16 ) ) ;
#34739=CARTESIAN_POINT ( 'NONE',  ( 3.999999999999998668, 13.96250000000000213, -32.30940107675850470 ) ) ;
#34740=CARTESIAN_POINT ( 'NONE',  ( 7.320879633048903241E-15, 18.20000000122903216, 26.00000000000000355 ) ) ;
#34741=CARTESIAN_POINT ( 'NONE',  ( 3.309375000614518836, 0.000000000000000000, 5.243569643749999010 ) ) ;
#34742=CARTESIAN_POINT ( 'NONE',  ( 10.22812500061451679, 6.421520780324663323E-16, -5.243569643749999010 ) ) ;
#34743=CARTESIAN_POINT ( 'NONE',  ( 22.35000000122903074, 5.773502691896255534, 3.535250795749688894E-16 ) ) ;
#34744=CARTESIAN_POINT ( 'NONE',  ( 28.22812500061451502, 6.421520780324663323E-16, -5.243569643749999010 ) ) ;
#34745=CARTESIAN_POINT ( 'NONE',  ( 27.41250000000000142, -5.773502691896255534, -1.060575238724906372E-15 ) ) ;
#34746=CARTESIAN_POINT ( 'NONE',  ( 3.999999999999999112, 18.98750000122903359, -30.00000000000000000 ) ) ;
#34747=DIRECTION ( 'NONE',  ( -0.9848080501874559856, 0.000000000000000000, 0.1736464922939166267 ) ) ;
#34748=CARTESIAN_POINT ( 'NONE',  ( 9.890625000614516438, 6.054752690667223547, 3.707466751127219781E-16 ) ) ;
#34750=CARTESIAN_POINT ( 'NONE',  ( 8.765625000614518214, -6.054752690667223547, -1.112240025338166033E-15 ) ) ;
#34751=VECTOR ( 'NONE', #57382, 1000.000000000000000 ) ;
#34752=CARTESIAN_POINT ( 'NONE',  ( 5.278125000614516615, 6.421520780324663323E-16, -5.243569643749999010 ) ) ;
#34754=CARTESIAN_POINT ( 'NONE',  ( 30.00000000000000000, 0.000000000000000000, 4.999999999999998224 ) ) ;
#34755=CARTESIAN_POINT ( 'NONE',  ( 14.47499999999999964, 6.123233995736764310E-16, -4.999999999999998224 ) ) ;
#34756=VECTOR ( 'NONE', #70400, 1000.000000000000000 ) ;
#34757=CARTESIAN_POINT ( 'NONE',  ( 15.87187500061451573, 3.027376345333611329, 5.243569643749999010 ) ) ;
#34758=CARTESIAN_POINT ( 'NONE',  ( 11.51250000122903216, 4.330127018922192761, -2.499999999999997780 ) ) ;
#34759=CARTESIAN_POINT ( 'NONE',  ( 18.57187500061451857, 3.027376345333611329, 5.243569643749999010 ) ) ;
#34761=CARTESIAN_POINT ( 'NONE',  ( 21.49687500061451573, -3.027376345333610441, -5.243569643749999898 ) ) ;
#34762=CARTESIAN_POINT ( 'NONE',  ( 2.121784821874999061, 14.25312500061451715, -33.67503911421598417 ) ) ;
#34763=VECTOR ( 'NONE', #5081, 1000.000000000000000 ) ;
#34766=CARTESIAN_POINT ( 'NONE',  ( 1.071796769724489895, 11.76740381056766616, -34.00000000000000000 ) ) ;
#34767=EDGE_CURVE ( 'NONE', #8342, #48969, #52936, .T. ) ;
#34768=CARTESIAN_POINT ( 'NONE',  ( 24.85312500061451502, 0.000000000000000000, 5.243569643749999010 ) ) ;
#34769=CARTESIAN_POINT ( 'NONE',  ( 24.86250000000000426, 2.886751345948146419, -4.999999999999968914 ) ) ;
#34770=CARTESIAN_POINT ( 'NONE',  ( 27.79687500061451999, -3.027376345333610441, -5.243569643749999898 ) ) ;
#34771=( BOUNDED_CURVE ( )  B_SPLINE_CURVE ( 2, ( #31504, #59559, #55770, #69927, #48864, #47759, #19296 ),
 .UNSPECIFIED., .F., .F. ) 
 B_SPLINE_CURVE_WITH_KNOTS ( ( 3, 2, 2, 3 ),
 ( 0.6500000000000001332, 0.6527777777777779011, 0.6555555555555556690, 0.6583333333333334370 ),
 .UNSPECIFIED. ) 
 CURVE ( )  GEOMETRIC_REPRESENTATION_ITEM ( )  RATIONAL_B_SPLINE_CURVE ( ( 0.9999999999999946709, 0.8660254037844440367, 1.000000000000000000, 0.8660254037844387076, 1.000000000000000000, 0.8660254037844333785, 1.000000000000005329 ) ) 
 REPRESENTATION_ITEM ( '' )  );
#34772=CARTESIAN_POINT ( 'NONE',  ( 23.17500000000000071, 4.330127018922191873, 2.499999999999999556 ) ) ;
#34773=CARTESIAN_POINT ( 'NONE',  ( 7.265625000614516438, 3.027376345333611329, 5.243569643749999010 ) ) ;
#34775=CARTESIAN_POINT ( 'NONE',  ( 19.69687500061451857, -3.027376345333610441, -5.243569643749999898 ) ) ;
#34777=CARTESIAN_POINT ( 'NONE',  ( 5.128125000614516260, -4.541064518000419881, 2.621784821874995952 ) ) ;
#34778=CARTESIAN_POINT ( 'NONE',  ( 9.084375000614517859, 4.541064518000418104, 2.621784821874999949 ) ) ;
#34779=ORIENTED_EDGE ( 'NONE', *, *, #15234, .F. ) ;
#34780=CARTESIAN_POINT ( 'NONE',  ( 18.15937500061451715, 0.000000000000000000, 5.243569643749999010 ) ) ;
#34781=CARTESIAN_POINT ( 'NONE',  ( 13.87500000122903288, 2.886751345948193936, 4.999999999999883649 ) ) ;
#34782=CARTESIAN_POINT ( 'NONE',  ( 27.93750000000000000, -2.886751345948125991, -5.000000000000000000 ) ) ;
#34783=CARTESIAN_POINT ( 'NONE',  ( 3.487500000000000711, -2.886751345948129988, 4.999999999999997335 ) ) ;
#34784=CARTESIAN_POINT ( 'NONE',  ( 1.626862140677534273E-15, 16.17500000122903359, 34.00000000000000000 ) ) ;
#34787=CARTESIAN_POINT ( 'NONE',  ( 9.637499999999999289, 5.773502691896255534, 3.535250795749688894E-16 ) ) ;
#34789=CARTESIAN_POINT ( 'NONE',  ( 23.72812500061451502, 6.421520780324663323E-16, -5.243569643749999010 ) ) ;
#34790=CARTESIAN_POINT ( 'NONE',  ( 14.77500000000000036, -4.330127018922194537, 2.499999999999995559 ) ) ;
#34791=CARTESIAN_POINT ( 'NONE',  ( 11.47500000122903252, 2.886751345948129099, -4.999999999999998224 ) ) ;
#34792=CARTESIAN_POINT ( 'NONE',  ( 8.990625000614516082, 6.054752690667223547, 3.707466751127219781E-16 ) ) ;
#34793=CARTESIAN_POINT ( 'NONE',  ( 23.21250000000000213, 2.886751345948126879, 4.999999999999999112 ) ) ;
#34794=CARTESIAN_POINT ( 'NONE',  ( 21.51562500061451644, 3.027376345333613106, -5.243569643749998122 ) ) ;
#34796=CARTESIAN_POINT ( 'NONE',  ( 27.56250000122902932, -4.330127018922190985, -2.500000000000001332 ) ) ;
#34798=CARTESIAN_POINT ( 'NONE',  ( 6.524999999999999467, 4.330127018922191873, 2.499999999999999556 ) ) ;
#34800=ORIENTED_EDGE ( 'NONE', *, *, #42990, .F. ) ;
#34801=CARTESIAN_POINT ( 'NONE',  ( 21.10312500061451502, 4.541064518000418104, -2.621784821874998173 ) ) ;
#34802=CARTESIAN_POINT ( 'NONE',  ( 28.07812500061451289, -4.541064518000419881, 2.621784821874995952 ) ) ;
#34803=CARTESIAN_POINT ( 'NONE',  ( 27.79687500061451999, -3.027376345333610441, -5.243569643749999898 ) ) ;
#34804=CARTESIAN_POINT ( 'NONE',  ( 18.15937500061451715, 0.000000000000000000, 5.243569643749999010 ) ) ;
#34805=CARTESIAN_POINT ( 'NONE',  ( 13.49062500061451608, 6.054752690667223547, 3.707466751127219781E-16 ) ) ;
#34806=CARTESIAN_POINT ( 'NONE',  ( -4.243569643749999898, 9.903125000614593887, -30.00000000000000000 ) ) ;
#34808=CARTESIAN_POINT ( 'NONE',  ( 25.23750000122903359, -4.330127018922194537, 2.499999999999995559 ) ) ;
#34810=CARTESIAN_POINT ( 'NONE',  ( 15.92812500061451608, -4.541064518000419881, 2.621784821874995952 ) ) ;
#34811=CARTESIAN_POINT ( 'NONE',  ( 1.071796769724491893, 13.83259618943233527, 33.99999999999999289 ) ) ;
#34812=CARTESIAN_POINT ( 'NONE',  ( 3.112500001229034918, 0.000000000000000000, 4.999999999999998224 ) ) ;
#34813=CARTESIAN_POINT ( 'NONE',  ( 11.97187500061451892, -6.054752690667223547, -1.112240025338166033E-15 ) ) ;
#34814=CARTESIAN_POINT ( 'NONE',  ( 12.15937500061451892, 4.541064518000418104, -2.621784821874998173 ) ) ;
#34815=CARTESIAN_POINT ( 'NONE',  ( 21.00937500061451857, -4.541064518000417216, -2.621784821875001281 ) ) ;
#34816=EDGE_LOOP ( 'NONE', ( #67440, #5642, #22543, #61504 ) ) ;
#34817=CARTESIAN_POINT ( 'NONE',  ( -5.191270968837347510, 8.550562458943613109, 33.03294266662791046 ) ) ;
#34818=CARTESIAN_POINT ( 'NONE',  ( 24.96562500061451573, -6.054752690667223547, -1.112240025338166033E-15 ) ) ;
#34821=CARTESIAN_POINT ( 'NONE',  ( 18.04687500061451999, 6.054752690667223547, 3.707466751127219781E-16 ) ) ;
#34822=CARTESIAN_POINT ( 'NONE',  ( 24.06562500061451715, -6.054752690667223547, -1.112240025338166033E-15 ) ) ;
#34824=CARTESIAN_POINT ( 'NONE',  ( 8.484601909799253346E-16, 16.96250000000000213, 34.61880215351700230 ) ) ;
#34825=CARTESIAN_POINT ( 'NONE',  ( 29.46562500061451573, -6.054752690667223547, -1.112240025338166033E-15 ) ) ;
#34826=CARTESIAN_POINT ( 'NONE',  ( 10.53750000122903252, 6.123233995736764310E-16, -4.999999999999998224 ) ) ;
#34827=VECTOR ( 'NONE', #19772, 1000.000000000000000 ) ;
#34828=CARTESIAN_POINT ( 'NONE',  ( 8.025000001229035007, 2.886751345948126879, 4.999999999999999112 ) ) ;
#34829=CARTESIAN_POINT ( 'NONE',  ( 4.000000000000000000, 19.73749999999999716, -27.69059892324149530 ) ) ;
#34830=CARTESIAN_POINT ( 'NONE',  ( 26.40000000122902790, 5.773502691896255534, 3.535250795749688894E-16 ) ) ;
#34833=CARTESIAN_POINT ( 'NONE',  ( 9.684375000614517504, -4.541064518000419881, 2.621784821874995952 ) ) ;
#34835=CARTESIAN_POINT ( 'NONE',  ( 18.59062500061451573, -3.027376345333614438, 5.243569643749998122 ) ) ;
#34836=CARTESIAN_POINT ( 'NONE',  ( 10.58437500061451964, -4.541064518000419881, 2.621784821874995952 ) ) ;
#34837=CARTESIAN_POINT ( 'NONE',  ( 28.42500000122904069, -5.773502691896255534, -1.060575238724906372E-15 ) ) ;
#34838=CARTESIAN_POINT ( 'NONE',  ( 20.55937500061451573, -4.541064518000417216, -2.621784821875001281 ) ) ;
#34839=CARTESIAN_POINT ( 'NONE',  ( 6.909375000614518036, 0.000000000000000000, 5.243569643749999010 ) ) ;
#34841=CARTESIAN_POINT ( 'NONE',  ( 8.278125000614515727, -4.541064518000419881, 2.621784821874995952 ) ) ;
#34842=( BOUNDED_CURVE ( )  B_SPLINE_CURVE ( 2, ( #53511, #30978, #69061, #7355, #41345, #29884, #18421, #40987, #63503 ),
 .UNSPECIFIED., .F., .F. ) 
 B_SPLINE_CURVE_WITH_KNOTS ( ( 3, 2, 2, 2, 3 ),
 ( 0.5760869565217391353, 0.5797101449275362528, 0.5869565217391304879, 0.5942028985507246119, 0.5978260869565217295 ),
 .UNSPECIFIED. ) 
 CURVE ( )  GEOMETRIC_REPRESENTATION_ITEM ( )  RATIONAL_B_SPLINE_CURVE ( ( 0.9330127018922194093, 0.9330127018922194093, 1.000000000000000000, 0.8660254037844387076, 1.000000000000000000, 0.8660254037844387076, 1.000000000000000000, 0.9330127018922194093, 0.9330127018922194093 ) ) 
 REPRESENTATION_ITEM ( '' )  );
#34843=CARTESIAN_POINT ( 'NONE',  ( 16.60312500061451857, 4.541064518000418104, -2.621784821874998173 ) ) ;
#34844=ORIENTED_EDGE ( 'NONE', *, *, #62019, .F. ) ;
#34845=CARTESIAN_POINT ( 'NONE',  ( 5.887500001229034829, -4.330127018922194537, 2.499999999999995559 ) ) ;
#34846=CARTESIAN_POINT ( 'NONE',  ( 15.17812500061451608, 6.421520780324663323E-16, -5.243569643749999010 ) ) ;
#34847=CARTESIAN_POINT ( 'NONE',  ( 14.24062500061451608, -3.027376345333610441, -5.243569643749999898 ) ) ;
#34849=CARTESIAN_POINT ( 'NONE',  ( 13.35000000000000142, 0.000000000000000000, 4.999999999999998224 ) ) ;
#34850=CARTESIAN_POINT ( 'NONE',  ( 7.837500001229035007, 6.123233995736764310E-16, -4.999999999999998224 ) ) ;
#34851=CARTESIAN_POINT ( 'NONE',  ( 5.240625000614516971, -3.027376345333610441, -5.243569643749999898 ) ) ;
#34852=CARTESIAN_POINT ( 'NONE',  ( 17.92500000122903359, 2.886751345948126879, 4.999999999999999112 ) ) ;
#34854=CARTESIAN_POINT ( 'NONE',  ( -4.243569643749999898, 10.37187500061451750, -32.45002607614398471 ) ) ;
#34855=DIRECTION ( 'NONE',  ( -0.000000000000000000, -1.000000000000000000, -0.000000000000000000 ) ) ;
#34856=CARTESIAN_POINT ( 'NONE',  ( 2.925000001229034918, 2.886751345948129099, -4.999999999999998224 ) ) ;
#34857=CARTESIAN_POINT ( 'NONE',  ( 6.600000000000001421, 0.000000000000000000, 4.999999999999998224 ) ) ;
#34858=CARTESIAN_POINT ( 'NONE',  ( 13.83749999999999858, -2.886751345948130876, 4.999999999999996447 ) ) ;
#34859=CARTESIAN_POINT ( 'NONE',  ( 18.04687500061451999, 6.054752690667223547, 3.707466751127219781E-16 ) ) ;
#34860=VECTOR ( 'NONE', #18780, 1000.000000000000000 ) ;
#34861=CARTESIAN_POINT ( 'NONE',  ( 13.26562500061451644, -6.054752690667223547, -1.112240025338166033E-15 ) ) ;
#34864=CARTESIAN_POINT ( 'NONE',  ( 26.18437500061451573, 4.541064518000418104, 2.621784821874999949 ) ) ;
#34866=CARTESIAN_POINT ( 'NONE',  ( 12.47812500061451502, 6.421520780324663323E-16, -5.243569643749999010 ) ) ;
#34867=CARTESIAN_POINT ( 'NONE',  ( 10.77187500061451786, 3.027376345333613106, -5.243569643749998122 ) ) ;
#34868=EDGE_LOOP ( 'NONE', ( #59205, #24075, #62735, #72370 ) ) ;
#34869=CARTESIAN_POINT ( 'NONE',  ( 29.35312500061451502, 0.000000000000000000, 5.243569643749999010 ) ) ;
#34870=CARTESIAN_POINT ( 'NONE',  ( 20.84062500061451573, -3.027376345333614438, 5.243569643749998122 ) ) ;
#34871=CARTESIAN_POINT ( 'NONE',  ( 29.46562500061451573, -6.054752690667223547, -1.112240025338166033E-15 ) ) ;
#34872=CARTESIAN_POINT ( 'NONE',  ( 1.626862140677534273E-15, 15.27500000122903501, -26.00000000000000355 ) ) ;
#34873=CARTESIAN_POINT ( 'NONE',  ( 8.962500000000002132, -5.773502691896255534, -1.060575238724906372E-15 ) ) ;
#34874=CARTESIAN_POINT ( 'NONE',  ( 19.76250000122903216, 0.000000000000000000, 4.999999999999998224 ) ) ;
#34875=CARTESIAN_POINT ( 'NONE',  ( -2.000000000000000000, 18.68750000122903288, -33.46410161513775705 ) ) ;
#34878=CARTESIAN_POINT ( 'NONE',  ( 18.41250000000000142, -5.773502691896255534, -1.060575238724906372E-15 ) ) ;
#34879=CARTESIAN_POINT ( 'NONE',  ( 20.77500000000000213, 6.123233995736764310E-16, -4.999999999999998224 ) ) ;
#34880=CARTESIAN_POINT ( 'NONE',  ( 19.54687500061451644, -3.027376345333614438, 5.243569643749998122 ) ) ;
#34881=CARTESIAN_POINT ( 'NONE',  ( 25.75312500061451715, 0.000000000000000000, 5.243569643749999010 ) ) ;
#34884=CARTESIAN_POINT ( 'NONE',  ( -1.071796769724483234, 16.87009619066137134, 25.99999999999999645 ) ) ;
#34885=CARTESIAN_POINT ( 'NONE',  ( 8.840625000614515727, -3.027376345333610441, -5.243569643749999898 ) ) ;
#34887=CARTESIAN_POINT ( 'NONE',  ( 13.95000000000000107, -4.330127018922190985, -2.500000000000001332 ) ) ;
#34888=CARTESIAN_POINT ( 'NONE',  ( 4.243569643749999898, 18.22812500061451502, 30.00000000000000000 ) ) ;
#34889=CARTESIAN_POINT ( 'NONE',  ( 3.046875000614519990, -3.027376345333610441, -5.243569643749999898 ) ) ;
#34892=CARTESIAN_POINT ( 'NONE',  ( 25.92187500061451999, -6.054752690667223547, -1.112240025338166033E-15 ) ) ;
#34894=CARTESIAN_POINT ( 'NONE',  ( 24.89062500061451644, -3.027376345333614438, 5.243569643749998122 ) ) ;
#34895=CARTESIAN_POINT ( 'NONE',  ( 23.10937500061451644, 0.000000000000000000, 5.243569643749999010 ) ) ;
#34896=CARTESIAN_POINT ( 'NONE',  ( -3.000416591977282496E-16, 17.44062500061459176, -34.90005215228797653 ) ) ;
#34897=CARTESIAN_POINT ( 'NONE',  ( 10.57500000000000107, 4.330127018922191873, 2.499999999999999556 ) ) ;
#34898=ADVANCED_FACE ( 'NONE', ( #25594 ), #37408, .F. ) ;
#34899=CARTESIAN_POINT ( 'NONE',  ( 8.615625000614517859, 3.027376345333611329, 5.243569643749999010 ) ) ;
#34901=CARTESIAN_POINT ( 'NONE',  ( 28.11562500061451431, -6.054752690667223547, -1.112240025338166033E-15 ) ) ;
#34902=CARTESIAN_POINT ( 'NONE',  ( 23.57812500061451289, -4.541064518000419881, 2.621784821874995952 ) ) ;
#34905=CARTESIAN_POINT ( 'NONE',  ( 19.62187500061451573, -6.054752690667223547, -1.112240025338166033E-15 ) ) ;
#34906=CARTESIAN_POINT ( 'NONE',  ( -4.243569643749999898, 11.72187500061451892, 27.54997392385601529 ) ) ;
#34907=CARTESIAN_POINT ( 'NONE',  ( 19.28437500061451360, 6.421520780324663323E-16, -5.243569643749999010 ) ) ;
#34908=CARTESIAN_POINT ( 'NONE',  ( 26.67187500061451644, 3.027376345333611329, 5.243569643749999010 ) ) ;
#34909=CARTESIAN_POINT ( 'NONE',  ( 4.243569643749999010, 16.07187500061451857, 27.54997392385601174 ) ) ;
#34910=CARTESIAN_POINT ( 'NONE',  ( 7.903125000614515727, -4.541064518000417216, -2.621784821875001281 ) ) ;
#34911=EDGE_CURVE ( 'NONE', #68252, #16431, #57037, .T. ) ;
#34912=CARTESIAN_POINT ( 'NONE',  ( 4.921875000614518214, 3.027376345333613106, -5.243569643749998122 ) ) ;
#34913=CARTESIAN_POINT ( 'NONE',  ( 4.000000000000000000, 15.68750000000000000, -27.69059892324149885 ) ) ;
#34914=AXIS2_PLACEMENT_3D ( 'NONE', #63991, #52915, #51830 ) ;
#34915=CARTESIAN_POINT ( 'NONE',  ( 5.503125000614516260, 0.000000000000000000, 5.243569643749999010 ) ) ;
#34916=CARTESIAN_POINT ( 'NONE',  ( 9.234375000614518214, -4.541064518000419881, 2.621784821874995952 ) ) ;
#34917=CARTESIAN_POINT ( 'NONE',  ( 16.87500000122903288, 2.886751345948129099, -4.999999999999998224 ) ) ;
#34918=CARTESIAN_POINT ( 'NONE',  ( 5.521875000614517859, 3.027376345333611329, 5.243569643749999010 ) ) ;
#34919=CARTESIAN_POINT ( 'NONE',  ( 6.515625000614516438, -6.054752690667223547, -1.112240025338166033E-15 ) ) ;
#34920=CARTESIAN_POINT ( 'NONE',  ( 5.540625000614515905, -3.027376345333614438, 5.243569643749998122 ) ) ;
#34922=CARTESIAN_POINT ( 'NONE',  ( 16.50937500061451502, -4.541064518000417216, -2.621784821875001281 ) ) ;
#34923=CARTESIAN_POINT ( 'NONE',  ( -3.305247878049081707E-15, 5.000000000000034639, -34.00000000000004263 ) ) ;
#34924=EDGE_LOOP ( 'NONE', ( #3819, #1367, #68499, #17300 ) ) ;
#34925=CARTESIAN_POINT ( 'NONE',  ( 24.02812500061451573, -4.541064518000419881, 2.621784821874995952 ) ) ;
#34926=CARTESIAN_POINT ( 'NONE',  ( 8.953125000614518214, 4.541064518000418104, -2.621784821874998173 ) ) ;
#34927=CARTESIAN_POINT ( 'NONE',  ( 27.00937500061451857, 4.541064518000418104, -2.621784821874998173 ) ) ;
#34928=CARTESIAN_POINT ( 'NONE',  ( 9.853125000614516793, 4.541064518000418104, -2.621784821874998173 ) ) ;
#34929=CARTESIAN_POINT ( 'NONE',  ( -4.243569643749999898, 9.921875000614516438, -32.45002607614398471 ) ) ;
#34931=CARTESIAN_POINT ( 'NONE',  ( 10.98750000122903536, 6.123233995736764310E-16, -4.999999999999998224 ) ) ;
#34932=CARTESIAN_POINT ( 'NONE',  ( 26.31562500061451715, -6.054752690667223547, -1.112240025338166033E-15 ) ) ;
#34933=CARTESIAN_POINT ( 'NONE',  ( 2.121784821875001281, 13.20312500061451821, -26.32496088578401938 ) ) ;
#34934=CARTESIAN_POINT ( 'NONE',  ( 12.33750000122903145, 6.123233995736764310E-16, -4.999999999999998224 ) ) ;
#34935=CARTESIAN_POINT ( 'NONE',  ( 21.10312500061451502, 4.541064518000418104, -2.621784821874998173 ) ) ;
#34936=CARTESIAN_POINT ( 'NONE',  ( 10.16249999999999964, 2.886751345948126879, 4.999999999999999112 ) ) ;
#34937=CARTESIAN_POINT ( 'NONE',  ( 20.09062500061451573, -3.027376345333610441, -5.243569643749999898 ) ) ;
#34938=CARTESIAN_POINT ( 'NONE',  ( 4.959375000614516971, 4.541064518000418104, -2.621784821874998173 ) ) ;
#34939=CARTESIAN_POINT ( 'NONE',  ( 21.26249999999999574, 2.886751345948129099, -4.999999999999998224 ) ) ;
#34940=CARTESIAN_POINT ( 'NONE',  ( 7.537500001229033408, 4.330127018922191873, 2.499999999999999556 ) ) ;
#34941=CARTESIAN_POINT ( 'NONE',  ( 15.52500000122903323, 2.886751345948129099, -4.999999999999998224 ) ) ;
#34942=CARTESIAN_POINT ( 'NONE',  ( 13.52812500061451750, 4.541064518000418104, 2.621784821874999949 ) ) ;
#34943=CARTESIAN_POINT ( 'NONE',  ( 14.80312500061451608, 4.541064518000418104, -2.621784821874998173 ) ) ;
#34944=CARTESIAN_POINT ( 'NONE',  ( 25.23750000122903359, -4.330127018922194537, 2.499999999999995559 ) ) ;
#34945=CARTESIAN_POINT ( 'NONE',  ( 20.40000000000000213, 4.330127018922192761, -2.499999999999997780 ) ) ;
#34946=CARTESIAN_POINT ( 'NONE',  ( 22.95937500061451431, 4.541064518000418104, -2.621784821874998173 ) ) ;
#34948=CARTESIAN_POINT ( 'NONE',  ( 11.13750000122903216, 4.330127018922191873, 2.499999999999999556 ) ) ;
#34949=CARTESIAN_POINT ( 'NONE',  ( 9.609375000614518214, 0.000000000000000000, 5.243569643749999010 ) ) ;
#34950=CARTESIAN_POINT ( 'NONE',  ( 25.09687500061451715, -3.027376345333610441, -5.243569643749999898 ) ) ;
#34951=CARTESIAN_POINT ( 'NONE',  ( 3.196875000614516793, 6.054752690667223547, 3.707466751127219781E-16 ) ) ;
#34952=CARTESIAN_POINT ( 'NONE',  ( 20.39062500061451644, -3.027376345333614438, 5.243569643749998122 ) ) ;
#34953=CARTESIAN_POINT ( 'NONE',  ( 26.74687500061451573, -3.027376345333614438, 5.243569643749998122 ) ) ;
#34956=VECTOR ( 'NONE', #70940, 1000.000000000000000 ) ;
#34957=CARTESIAN_POINT ( 'NONE',  ( 7.584375000614516082, 6.421520780324663323E-16, -5.243569643749999010 ) ) ;
#34958=CARTESIAN_POINT ( 'NONE',  ( 18.66562500061451146, -6.054752690667223547, -1.112240025338166033E-15 ) ) ;
#34960=CARTESIAN_POINT ( 'NONE',  ( 4.550098044277414822, 3.654122216399865675, 4.158013951629233595 ) ) ;
#34961=CARTESIAN_POINT ( 'NONE',  ( 28.00312500061451715, 0.000000000000000000, 5.243569643749999010 ) ) ;
#34962=CARTESIAN_POINT ( 'NONE',  ( 3.421875000614516882, -6.054752690667223547, -1.112240025338166033E-15 ) ) ;
#34963=CARTESIAN_POINT ( 'NONE',  ( 22.80000000122903359, 5.773502691896255534, 3.535250795749688401E-16 ) ) ;
#34965=CARTESIAN_POINT ( 'NONE',  ( 17.21249999999999858, 2.886751345948129099, -4.999999999999998224 ) ) ;
#34967=CARTESIAN_POINT ( 'NONE',  ( 24.82499999999999929, 6.123233995736764310E-16, -4.999999999999998224 ) ) ;
#34968=CARTESIAN_POINT ( 'NONE',  ( 27.08437500061451786, 4.541064518000418104, 2.621784821874999949 ) ) ;
#34970=CARTESIAN_POINT ( 'NONE',  ( 16.34062500061451573, -3.027376345333614438, 5.243569643749998122 ) ) ;
#34971=CARTESIAN_POINT ( 'NONE',  ( 7.078125000614516438, 6.421520780324663323E-16, -5.243569643749999010 ) ) ;
#34973=CARTESIAN_POINT ( 'NONE',  ( 29.76562500061451644, 3.027376345333611329, 5.243569643749999010 ) ) ;
#34974=CARTESIAN_POINT ( 'NONE',  ( 16.12500000122903288, 2.886751345948126879, 4.999999999999999112 ) ) ;
#34975=CARTESIAN_POINT ( 'NONE',  ( 20.92500000000000071, 4.330127018922191873, 2.499999999999999556 ) ) ;
#34976=CARTESIAN_POINT ( 'NONE',  ( 29.84999999999999787, 4.330127018922192761, -2.499999999999997780 ) ) ;
#34977=CARTESIAN_POINT ( 'NONE',  ( 4.471875000614518925, 3.027376345333613106, -5.243569643749998122 ) ) ;
#34978=CARTESIAN_POINT ( 'NONE',  ( 9.459375000614517859, 4.541064518000418104, -2.621784821874998173 ) ) ;
#34979=CARTESIAN_POINT ( 'NONE',  ( 21.64687500061451786, 6.054752690667223547, 3.707466751127219781E-16 ) ) ;
#34980=EDGE_CURVE ( 'NONE', #55912, #39861, #65112, .T. ) ;
#34982=ORIENTED_EDGE ( 'NONE', *, *, #13710, .T. ) ;
#34983=CARTESIAN_POINT ( 'NONE',  ( 3.121875000614518836, 3.027376345333613106, -5.243569643749998122 ) ) ;
#34984=CARTESIAN_POINT ( 'NONE',  ( 5.025000000000002132, 6.123233995736764310E-16, -4.999999999999998224 ) ) ;
#34985=CARTESIAN_POINT ( 'NONE',  ( 7.659375000614518036, 4.541064518000418104, -2.621784821874998173 ) ) ;
#34986=CARTESIAN_POINT ( 'NONE',  ( 19.04999999999999716, 4.330127018922192761, -2.499999999999997780 ) ) ;
#34987=CARTESIAN_POINT ( 'NONE',  ( 15.14062500061451644, -3.027376345333610441, -5.243569643749999898 ) ) ;
#34989=CARTESIAN_POINT ( 'NONE',  ( 24.90000000122903501, -2.886751345948142422, -4.999999999999970690 ) ) ;
#34991=CARTESIAN_POINT ( 'NONE',  ( 10.94062500061451537, -3.027376345333614438, 5.243569643749998122 ) ) ;
#34992=CARTESIAN_POINT ( 'NONE',  ( 27.00937500061451857, 4.541064518000418104, -2.621784821874998173 ) ) ;
#34993=CARTESIAN_POINT ( 'NONE',  ( 9.001249775931846008E-16, 19.07187500061451502, 34.90005215228797653 ) ) ;
#34994=CARTESIAN_POINT ( 'NONE',  ( 25.43437500061451573, -4.541064518000419881, 2.621784821874995952 ) ) ;
#34995=CARTESIAN_POINT ( 'NONE',  ( 7.950000000000001954, 0.000000000000000000, 4.999999999999998224 ) ) ;
#34996=CARTESIAN_POINT ( 'NONE',  ( -2.828200636599751609E-16, 12.35000000122903430, 25.38119784648299770 ) ) ;
#34997=CARTESIAN_POINT ( 'NONE',  ( 13.82812500061451466, 6.421520780324663323E-16, -5.243569643749999010 ) ) ;
#34998=CARTESIAN_POINT ( 'NONE',  ( 7.500000001229034652, 5.773502691896255534, 3.535250795749688894E-16 ) ) ;
#34999=CARTESIAN_POINT ( 'NONE',  ( 18.60937500061451644, 0.000000000000000000, 5.243569643749999010 ) ) ;
#35000=CARTESIAN_POINT ( 'NONE',  ( 12.68437500061451573, 4.541064518000418104, 2.621784821874999949 ) ) ;
#35001=CARTESIAN_POINT ( 'NONE',  ( -3.779748323423378853, 3.276532024208882010, -28.66603734123481573 ) ) ;
#35003=CARTESIAN_POINT ( 'NONE',  ( 13.22812500061451502, -4.541064518000419881, 2.621784821874995952 ) ) ;
#35004=CARTESIAN_POINT ( 'NONE',  ( 26.88750000122903216, 4.330127018922191873, 2.499999999999999556 ) ) ;
#35005=CARTESIAN_POINT ( 'NONE',  ( 13.73437500061451821, -4.541064518000419881, 2.621784821874995952 ) ) ;
#35006=CARTESIAN_POINT ( 'NONE',  ( 15.36562500061451608, 3.027376345333611329, 5.243569643749999010 ) ) ;
#35008=CARTESIAN_POINT ( 'NONE',  ( 24.42187500061451999, 3.027376345333611329, 5.243569643749999010 ) ) ;
#35009=CYLINDRICAL_SURFACE ( 'NONE', #71474, 4.000000000000000000 ) ;
#35010=CARTESIAN_POINT ( 'NONE',  ( 12.78750000122903430, 6.123233995736764310E-16, -4.999999999999998224 ) ) ;
#35013=CARTESIAN_POINT ( 'NONE',  ( 2.121784821874999061, 17.90937500061451715, -33.67503911421598417 ) ) ;
#35014=CARTESIAN_POINT ( 'NONE',  ( 18.45937500061451431, 4.541064518000418104, -2.621784821874998173 ) ) ;
#35015=CARTESIAN_POINT ( 'NONE',  ( 19.01250000122903216, -4.330127018922190985, -2.500000000000001332 ) ) ;
#35016=CARTESIAN_POINT ( 'NONE',  ( 13.62187500061451750, 3.027376345333611329, 5.243569643749999010 ) ) ;
#35017=CARTESIAN_POINT ( 'NONE',  ( -4.243569643749999898, 9.959375000614517859, 30.00000000000000000 ) ) ;
#35018=CARTESIAN_POINT ( 'NONE',  ( 18.78750000122903430, 4.330127018922191873, 2.499999999999999556 ) ) ;
#35019=VECTOR ( 'NONE', #61663, 1000.000000000000000 ) ;
#35020=CARTESIAN_POINT ( 'NONE',  ( 16.15312500061451573, 4.541064518000418104, -2.621784821874998173 ) ) ;
#35021=ORIENTED_EDGE ( 'NONE', *, *, #33319, .F. ) ;
#35023=CARTESIAN_POINT ( 'NONE',  ( 19.04999999999999716, 4.330127018922192761, -2.499999999999997780 ) ) ;
#35025=CARTESIAN_POINT ( 'NONE',  ( 3.890625000614517326, -3.027376345333610441, -5.243569643749999898 ) ) ;
#35026=CARTESIAN_POINT ( 'NONE',  ( 14.92500000122903181, -5.773502691896255534, -1.060575238724906372E-15 ) ) ;
#35027=CARTESIAN_POINT ( 'NONE',  ( 26.25937500061451857, 0.000000000000000000, 5.243569643749999010 ) ) ;
#35028=CARTESIAN_POINT ( 'NONE',  ( 20.69062500061451715, 6.054752690667223547, 3.707466751127219781E-16 ) ) ;
#35029=CARTESIAN_POINT ( 'NONE',  ( 21.89062500061451289, -3.027376345333610441, -5.243569643749999898 ) ) ;
#35030=CARTESIAN_POINT ( 'NONE',  ( 4.040625000614517681, 6.054752690667223547, 3.707466751127219781E-16 ) ) ;
#35031=CARTESIAN_POINT ( 'NONE',  ( 26.69999999999999929, 4.330127018922192761, -2.499999999999997780 ) ) ;
#35036=CARTESIAN_POINT ( 'NONE',  ( -3.000416591977282496E-16, 17.04687500061451644, -34.90005215228797653 ) ) ;
#35037=CARTESIAN_POINT ( 'NONE',  ( 6.075000001229034829, 2.886751345948129099, -4.999999999999998224 ) ) ;
#35038=CARTESIAN_POINT ( 'NONE',  ( 5.850000000000001421, -4.330127018922190985, -2.500000000000001332 ) ) ;
#35039=EDGE_CURVE ( 'NONE', #3790, #20937, #4214, .T. ) ;
#35040=CARTESIAN_POINT ( 'NONE',  ( 2.962500001229034119, 4.330127018922192761, -2.499999999999997780 ) ) ;
#35041=CARTESIAN_POINT ( 'NONE',  ( 9.009375000614518569, 4.541064518000418104, -2.621784821874998173 ) ) ;
#35042=CARTESIAN_POINT ( 'NONE',  ( 19.35000000122903430, -2.886751345948163738, 4.999999999999939604 ) ) ;
#35043=CARTESIAN_POINT ( 'NONE',  ( 27.63750000122903216, 6.123233995736764310E-16, -4.999999999999998224 ) ) ;
#35044=CARTESIAN_POINT ( 'NONE',  ( -5.999929701724457054, 8.000052723701786661, -30.20526279067533792 ) ) ;
#35045=CARTESIAN_POINT ( 'NONE',  ( 30.00000000000000000, 0.000000000000000000, 0.000000000000000000 ) ) ;
#35046=CARTESIAN_POINT ( 'NONE',  ( 8.784375000614518925, -4.541064518000419881, 2.621784821874995952 ) ) ;
#35047=CARTESIAN_POINT ( 'NONE',  ( 11.40937500061451892, 0.000000000000000000, 5.243569643749999010 ) ) ;
#35048=CARTESIAN_POINT ( 'NONE',  ( 7.350000000000002309, 4.330127018922192761, -2.499999999999997780 ) ) ;
#35049=CARTESIAN_POINT ( 'NONE',  ( 4.243569643749999898, 14.14062500061459460, 32.45002607614398471 ) ) ;
#35050=CARTESIAN_POINT ( 'NONE',  ( 22.13437500061451502, 4.541064518000418104, 2.621784821874999949 ) ) ;
#35053=CARTESIAN_POINT ( 'NONE',  ( 6.450000000000001066, 4.330127018922192761, -2.499999999999997780 ) ) ;
#35054=CARTESIAN_POINT ( 'NONE',  ( 26.28750000122903430, 6.123233995736764310E-16, -4.999999999999998224 ) ) ;
#35056=CARTESIAN_POINT ( 'NONE',  ( 21.62812500061451360, 4.541064518000418104, 2.621784821874999949 ) ) ;
#35057=CARTESIAN_POINT ( 'NONE',  ( 13.04062500061451502, 6.054752690667223547, 3.707466751127219781E-16 ) ) ;
#35059=CARTESIAN_POINT ( 'NONE',  ( 11.67187500061451821, 3.027376345333613106, -5.243569643749998122 ) ) ;
#35060=CARTESIAN_POINT ( 'NONE',  ( 28.94999999999999929, 4.330127018922192761, -2.499999999999997780 ) ) ;
#35061=CARTESIAN_POINT ( 'NONE',  ( 22.50000000122903288, -2.886751345948129988, 4.999999999999997335 ) ) ;
#35063=CARTESIAN_POINT ( 'NONE',  ( 10.69687500061451679, -3.027376345333610441, -5.243569643749999898 ) ) ;
#35064=CARTESIAN_POINT ( 'NONE',  ( 27.98437500061451289, 4.541064518000418104, 2.621784821874999949 ) ) ;
#35067=CARTESIAN_POINT ( 'NONE',  ( -3.999999999999997335, 12.95000000122903216, -27.69059892324149530 ) ) ;
#35068=CARTESIAN_POINT ( 'NONE',  ( 22.73437500061451644, -4.541064518000419881, 2.621784821874995952 ) ) ;
#35069=CARTESIAN_POINT ( 'NONE',  ( 13.05937500061451750, 4.541064518000418104, -2.621784821874998173 ) ) ;
#35071=CARTESIAN_POINT ( 'NONE',  ( 26.02499999999999858, -4.330127018922194537, 2.499999999999995559 ) ) ;
#35074=CARTESIAN_POINT ( 'NONE',  ( 16.45312500061451289, -4.541064518000417216, -2.621784821875001281 ) ) ;
#35075=CARTESIAN_POINT ( 'NONE',  ( 7.612500000000000711, -5.773502691896255534, -1.060575238724906372E-15 ) ) ;
#35076=CARTESIAN_POINT ( 'NONE',  ( 12.11250000122903181, 0.000000000000000000, 4.999999999999998224 ) ) ;
#35077=CARTESIAN_POINT ( 'NONE',  ( 15.86250000000000249, 2.886751345948129099, -4.999999999999998224 ) ) ;
#35078=CARTESIAN_POINT ( 'NONE',  ( -4.243569643749997233, 9.940625000614515372, 32.45002607614398471 ) ) ;
#35079=CARTESIAN_POINT ( 'NONE',  ( 0.000000000000000000, 20.00000000000000000, 26.00000000000000000 ) ) ;
#35080=CARTESIAN_POINT ( 'NONE',  ( 24.15937500061451715, -4.541064518000417216, -2.621784821875001281 ) ) ;
#35081=ORIENTED_EDGE ( 'NONE', *, *, #63436, .F. ) ;
#35082=CARTESIAN_POINT ( 'NONE',  ( 21.25312500061451715, 0.000000000000000000, 5.243569643749999010 ) ) ;
#35083=CARTESIAN_POINT ( 'NONE',  ( 20.52187500061451786, -6.054752690667223547, -1.112240025338166033E-15 ) ) ;
#35084=CARTESIAN_POINT ( 'NONE',  ( 3.412500000000002309, 2.886751345948126879, 4.999999999999999112 ) ) ;
#35085=CARTESIAN_POINT ( 'NONE',  ( 7.753125000614518036, 0.000000000000000000, 5.243569643749999010 ) ) ;
#35086=CARTESIAN_POINT ( 'NONE',  ( 22.26562500061451644, -6.054752690667223547, -1.112240025338166033E-15 ) ) ;
#35087=CARTESIAN_POINT ( 'NONE',  ( 12.94687500061451857, -3.027376345333610441, -5.243569643749999898 ) ) ;
#35088=CARTESIAN_POINT ( 'NONE',  ( 17.78437500061451715, -4.541064518000419881, 2.621784821874995952 ) ) ;
#35089=CARTESIAN_POINT ( 'NONE',  ( -4.243569643749999898, 16.65312500061451573, 30.00000000000000000 ) ) ;
#35091=CARTESIAN_POINT ( 'NONE',  ( 18.11250000122903359, -4.330127018922190985, -2.500000000000001332 ) ) ;
#35093=CARTESIAN_POINT ( 'NONE',  ( 8.690625000614515372, -3.027376345333614438, 5.243569643749998122 ) ) ;
#35094=CARTESIAN_POINT ( 'NONE',  ( 4.434375000614519280, 6.421520780324663323E-16, -5.243569643749999010 ) ) ;
#35095=CARTESIAN_POINT ( 'NONE',  ( 5.484375000614518214, 4.541064518000418104, 2.621784821874999949 ) ) ;
#35096=CARTESIAN_POINT ( 'NONE',  ( 25.02187500061451431, -6.054752690667223547, -1.112240025338166033E-15 ) ) ;
#35097=CARTESIAN_POINT ( 'NONE',  ( 16.82812500061451644, -4.541064518000419881, 2.621784821874995952 ) ) ;
#35098=CARTESIAN_POINT ( 'NONE',  ( 26.66250000122903430, -4.330127018922190985, -2.500000000000001332 ) ) ;
#35099=CARTESIAN_POINT ( 'NONE',  ( 26.16562500061451502, 3.027376345333611329, 5.243569643749999010 ) ) ;
#35100=CARTESIAN_POINT ( 'NONE',  ( 22.20937500061451431, 0.000000000000000000, 5.243569643749999010 ) ) ;
#35101=CARTESIAN_POINT ( 'NONE',  ( 17.84062500061451573, -3.027376345333610441, -5.243569643749999898 ) ) ;
#35102=CARTESIAN_POINT ( 'NONE',  ( 4.243569643749999010, 17.42187500061451999, 27.54997392385601174 ) ) ;
#35103=CARTESIAN_POINT ( 'NONE',  ( 23.20312500061451644, -4.541064518000417216, -2.621784821875001281 ) ) ;
#35106=CARTESIAN_POINT ( 'NONE',  ( 25.91250000000000142, 2.886751345948126879, 4.999999999999999112 ) ) ;
#35107=CARTESIAN_POINT ( 'NONE',  ( 1.999999999999998668, 13.55000000000000071, -33.46410161513775705 ) ) ;
#35109=CARTESIAN_POINT ( 'NONE',  ( 29.24062500061451431, 6.054752690667223547, 3.707466751127219781E-16 ) ) ;
#35110=CARTESIAN_POINT ( 'NONE',  ( 10.71562500061451928, 3.027376345333613106, -5.243569643749998122 ) ) ;
#35111=CARTESIAN_POINT ( 'NONE',  ( 22.72500000122903430, 2.886751345948129099, -4.999999999999998224 ) ) ;
#35112=AXIS2_PLACEMENT_3D ( 'NONE', #13929, #40937, #52368 ) ;
#35113=CARTESIAN_POINT ( 'NONE',  ( 27.51562500061451644, 3.027376345333611329, 5.243569643749999010 ) ) ;
#35114=CARTESIAN_POINT ( 'NONE',  ( 25.91250000000000142, 2.886751345948126879, 4.999999999999999112 ) ) ;
#35115=CARTESIAN_POINT ( 'NONE',  ( 2.000000000000001332, 16.66250000122903430, -26.53589838486224650 ) ) ;
#35116=CARTESIAN_POINT ( 'NONE',  ( -1.999999999999997113, 12.53750000122903430, 33.46410161513775705 ) ) ;
#35117=CARTESIAN_POINT ( 'NONE',  ( 9.665625000614515017, -6.054752690667223547, -1.112240025338166033E-15 ) ) ;
#35118=ORIENTED_EDGE ( 'NONE', *, *, #66833, .F. ) ;
#35119=CARTESIAN_POINT ( 'NONE',  ( 25.67812500061451431, 4.541064518000418104, 2.621784821874999949 ) ) ;
#35120=CARTESIAN_POINT ( 'NONE',  ( 8.353125000614518569, -4.541064518000417216, -2.621784821875001281 ) ) ;
#35122=CARTESIAN_POINT ( 'NONE',  ( 6.478125000614516793, -4.541064518000419881, 2.621784821874995952 ) ) ;
#35124=CARTESIAN_POINT ( 'NONE',  ( 17.92500000122903359, 2.886751345948126879, 4.999999999999998224 ) ) ;
#35125=CARTESIAN_POINT ( 'NONE',  ( 13.23750000000000071, 5.773502691896255534, 3.535250795749688894E-16 ) ) ;
#35126=CARTESIAN_POINT ( 'NONE',  ( 13.65937500061451715, 0.000000000000000000, 5.243569643749999010 ) ) ;
#35127=CARTESIAN_POINT ( 'NONE',  ( 12.00000000122903465, 5.773502691896255534, 3.535250795749688894E-16 ) ) ;
#35128=CARTESIAN_POINT ( 'NONE',  ( 16.95937500061451786, -4.541064518000417216, -2.621784821875001281 ) ) ;
#35130=CARTESIAN_POINT ( 'NONE',  ( 9.384375000614518569, 6.421520780324663323E-16, -5.243569643749999010 ) ) ;
#35131=CARTESIAN_POINT ( 'NONE',  ( 4.243569643749999010, 11.96562500061451750, -32.45002607614398471 ) ) ;
#35132=DIRECTION ( 'NONE',  ( 0.000000000000000000, 0.000000000000000000, 1.000000000000000000 ) ) ;
#35135=CARTESIAN_POINT ( 'NONE',  ( 24.29062500061451502, 6.054752690667223547, 3.707466751127219781E-16 ) ) ;
#35136=CARTESIAN_POINT ( 'NONE',  ( -1.394453263437886604E-15, 19.66249999999999787, -26.00000000000000000 ) ) ;
#35137=CARTESIAN_POINT ( 'NONE',  ( 28.84687500061452070, 6.054752690667223547, 3.707466751127219781E-16 ) ) ;
#35139=CARTESIAN_POINT ( 'NONE',  ( 23.81250000000000000, -5.773502691896255534, -1.060575238724906372E-15 ) ) ;
#35140=B_SPLINE_CURVE_WITH_KNOTS ( 'NONE', 3,
 ( #36965, #31431, #53971, #4467, #50259, #26997, #43619, #66886, #38061, #60958 ),
 .UNSPECIFIED., .F., .F.,
 ( 4, 3, 3, 4 ),
 ( 2.168404344971008868E-19, 0.0001125111793028066998, 0.0001785213024883201523, 0.0002445501373023005053 ),
 .UNSPECIFIED. ) ;
#35141=CARTESIAN_POINT ( 'NONE',  ( 5.690625000614516260, -3.027376345333610441, -5.243569643749999898 ) ) ;
#35143=CARTESIAN_POINT ( 'NONE',  ( 19.39687500061451786, 6.054752690667223547, 3.707466751127219781E-16 ) ) ;
#35145=CARTESIAN_POINT ( 'NONE',  ( 28.61250000122903359, 4.330127018922192761, -2.499999999999997780 ) ) ;
#35146=CARTESIAN_POINT ( 'NONE',  ( 8.259375000614518569, 0.000000000000000000, 5.243569643749999010 ) ) ;
#35148=CARTESIAN_POINT ( 'NONE',  ( 18.79687500061451644, -3.027376345333610441, -5.243569643749999898 ) ) ;
#35149=CARTESIAN_POINT ( 'NONE',  ( 13.23750000122903359, 6.123233995736764310E-16, -4.999999999999998224 ) ) ;
#35150=CARTESIAN_POINT ( 'NONE',  ( 27.63749999999999929, 5.773502691896255534, 3.535250795749688894E-16 ) ) ;
#35151=CARTESIAN_POINT ( 'NONE',  ( 3.225000000000002309, 6.123233995736764310E-16, -4.999999999999998224 ) ) ;
#35152=CARTESIAN_POINT ( 'NONE',  ( 1.071796769724491893, 12.14509619066136814, 33.99999999999999289 ) ) ;
#35154=ORIENTED_EDGE ( 'NONE', *, *, #52783, .F. ) ;
#35155=CARTESIAN_POINT ( 'NONE',  ( 10.72500000000000142, -4.330127018922194537, 2.499999999999995559 ) ) ;
#35157=CARTESIAN_POINT ( 'NONE',  ( 24.70312500061451644, 4.541064518000418104, -2.621784821874998173 ) ) ;
#35158=CARTESIAN_POINT ( 'NONE',  ( 13.79999999999999893, 0.000000000000000000, 4.999999999999998224 ) ) ;
#35159=CARTESIAN_POINT ( 'NONE',  ( 10.42500000122903536, -5.773502691896255534, -1.060575238724906372E-15 ) ) ;
#35160=CARTESIAN_POINT ( 'NONE',  ( 8.203125000614518214, 0.000000000000000000, 5.243569643749999010 ) ) ;
#35161=CARTESIAN_POINT ( 'NONE',  ( 21.97500000000000142, -4.330127018922194537, 2.499999999999995559 ) ) ;
#35162=CARTESIAN_POINT ( 'NONE',  ( 20.09062500061451573, -3.027376345333610441, -5.243569643749999898 ) ) ;
#35163=CARTESIAN_POINT ( 'NONE',  ( 16.16250000122903430, 0.000000000000000000, 4.999999999999998224 ) ) ;
#35164=CARTESIAN_POINT ( 'NONE',  ( 26.51250000122903216, 0.000000000000000000, 4.999999999999998224 ) ) ;
#35166=CARTESIAN_POINT ( 'NONE',  ( 5.549999999999998934, 4.330127018922192761, -2.499999999999997780 ) ) ;
#35168=CARTESIAN_POINT ( 'NONE',  ( 21.81562500061451004, -6.054752690667223547, -1.112240025338166033E-15 ) ) ;
#35169=CARTESIAN_POINT ( 'NONE',  ( 29.76562500061451644, 3.027376345333611329, 5.243569643749999010 ) ) ;
#35170=CARTESIAN_POINT ( 'NONE',  ( 26.78437500061451360, -4.541064518000419881, 2.621784821874995952 ) ) ;
#35171=CARTESIAN_POINT ( 'NONE',  ( 18.57187500061451857, 3.027376345333611329, 5.243569643749999010 ) ) ;
#35172=CARTESIAN_POINT ( 'NONE',  ( 13.15312500061451750, 0.000000000000000000, 5.243569643749999010 ) ) ;
#35174=CARTESIAN_POINT ( 'NONE',  ( 25.16250000122903074, 0.000000000000000000, 4.999999999999998224 ) ) ;
#35176=CARTESIAN_POINT ( 'NONE',  ( 15.89062500061451644, -3.027376345333614438, 5.243569643749998122 ) ) ;
#35177=CARTESIAN_POINT ( 'NONE',  ( 1.071796769724476572, 11.24509619066136779, -25.99999999999999289 ) ) ;
#35178=CARTESIAN_POINT ( 'NONE',  ( 6.037500001229035185, 6.123233995736764310E-16, -4.999999999999998224 ) ) ;
#35179=CARTESIAN_POINT ( 'NONE',  ( 11.74687500061451573, 6.054752690667223547, 3.707466751127219781E-16 ) ) ;
#35180=CARTESIAN_POINT ( 'NONE',  ( 12.04687500061451821, -3.027376345333610441, -5.243569643749999898 ) ) ;
#35181=CARTESIAN_POINT ( 'NONE',  ( 19.54687500061451644, -3.027376345333614438, 5.243569643749998122 ) ) ;
#35182=ORIENTED_EDGE ( 'NONE', *, *, #68596, .T. ) ;
#35183=CARTESIAN_POINT ( 'NONE',  ( 23.31562500061451715, 3.027376345333613106, -5.243569643749998122 ) ) ;
#35184=CARTESIAN_POINT ( 'NONE',  ( 19.09687500061451360, -3.027376345333614438, 5.243569643749998122 ) ) ;
#35185=CARTESIAN_POINT ( 'NONE',  ( 24.14062500061451289, -3.027376345333610441, -5.243569643749999898 ) ) ;
#35186=DIRECTION ( 'NONE',  ( -1.000000000000000000, -0.000000000000000000, -0.000000000000000000 ) ) ;
#35187=CARTESIAN_POINT ( 'NONE',  ( -3.999999999999997335, 15.53749999999999964, 32.30940107675850470 ) ) ;
#35188=CARTESIAN_POINT ( 'NONE',  ( 3.346875000614518036, -3.027376345333614438, 5.243569643749998122 ) ) ;
#35189=CARTESIAN_POINT ( 'NONE',  ( 9.150000001229033231, -2.886751345948125991, -5.000000000000000000 ) ) ;
#35190=CARTESIAN_POINT ( 'NONE',  ( 4.087500001229035007, -4.330127018922194537, 2.499999999999995559 ) ) ;
#35192=CARTESIAN_POINT ( 'NONE',  ( 26.06250000122903288, 0.000000000000000000, 4.999999999999998224 ) ) ;
#35195=CARTESIAN_POINT ( 'NONE',  ( 9.871875000614517504, 3.027376345333613106, -5.243569643749998122 ) ) ;
#35197=EDGE_CURVE ( 'NONE', #42898, #22963, #38132, .T. ) ;
#35198=CARTESIAN_POINT ( 'NONE',  ( 18.10312500061451502, 0.000000000000000000, 5.243569643749999010 ) ) ;
#35199=CARTESIAN_POINT ( 'NONE',  ( 12.04687500061451821, -3.027376345333610441, -5.243569643749999898 ) ) ;
#35200=CARTESIAN_POINT ( 'NONE',  ( 29.10000000122903074, 5.773502691896255534, 3.535250795749688894E-16 ) ) ;
#35201=ADVANCED_FACE ( 'NONE', ( #72483 ), #60654, .F. ) ;
#35202=CARTESIAN_POINT ( 'NONE',  ( 18.98437500061451644, 4.541064518000418104, 2.621784821874999949 ) ) ;
#35203=CARTESIAN_POINT ( 'NONE',  ( 7.509375000614517681, -4.541064518000417216, -2.621784821875001281 ) ) ;
#35204=CARTESIAN_POINT ( 'NONE',  ( 3.328125000614516438, -4.541064518000419881, 2.621784821874995952 ) ) ;
#35205=CARTESIAN_POINT ( 'NONE',  ( -1.071796769724487453, 17.65759618943233633, 26.00000000000000000 ) ) ;
#35206=CARTESIAN_POINT ( 'NONE',  ( 8.353125000614518569, -4.541064518000417216, -2.621784821875001281 ) ) ;
#35207=CARTESIAN_POINT ( 'NONE',  ( 17.46562500061451217, 3.027376345333613106, -5.243569643749998122 ) ) ;
#35208=ORIENTED_EDGE ( 'NONE', *, *, #5562, .F. ) ;
#35209=CARTESIAN_POINT ( 'NONE',  ( 5.362500001229033586, 0.000000000000000000, 4.999999999999998224 ) ) ;
#35210=CARTESIAN_POINT ( 'NONE',  ( 13.97812500061451679, 4.541064518000418104, 2.621784821874999949 ) ) ;
#35211=CARTESIAN_POINT ( 'NONE',  ( 12.14062500061451821, 6.054752690667223547, 3.707466751127219781E-16 ) ) ;
#35213=CARTESIAN_POINT ( 'NONE',  ( 13.31250000000000178, 2.886751345948126879, 4.999999999999999112 ) ) ;
#35214=CARTESIAN_POINT ( 'NONE',  ( 7.162500001229032520, 0.000000000000000000, 4.999999999999998224 ) ) ;
#35215=CARTESIAN_POINT ( 'NONE',  ( 3.553125000614516082, 4.541064518000418104, -2.621784821874998173 ) ) ;
#35217=CARTESIAN_POINT ( 'NONE',  ( 18.60000000122903430, -2.886751345948125991, -5.000000000000000000 ) ) ;
#35219=CARTESIAN_POINT ( 'NONE',  ( -4.243569643749999898, 11.27187500061451608, -32.45002607614398471 ) ) ;
#35223=CARTESIAN_POINT ( 'NONE',  ( -3.999999999999999112, 13.25000000000000178, 30.00000000000000000 ) ) ;
#35224=CARTESIAN_POINT ( 'NONE',  ( 17.52187500061451431, 3.027376345333613106, -5.243569643749998122 ) ) ;
#35226=CARTESIAN_POINT ( 'NONE',  ( 14.05312500061451431, 0.000000000000000000, 5.243569643749999010 ) ) ;
#35228=LINE ( 'NONE', #1263, #24756 ) ;
#35229=CARTESIAN_POINT ( 'NONE',  ( 25.58437500061451431, 6.421520780324663323E-16, -5.243569643749999010 ) ) ;
#35231=CARTESIAN_POINT ( 'NONE',  ( 13.30312500061451786, -4.541064518000417216, -2.621784821875001281 ) ) ;
#35232=CARTESIAN_POINT ( 'NONE',  ( 15.79687500061451821, 6.054752690667223547, 3.707466751127219781E-16 ) ) ;
#35233=ORIENTED_EDGE ( 'NONE', *, *, #37992, .F. ) ;
#35234=CARTESIAN_POINT ( 'NONE',  ( 26.76562500061451644, -6.054752690667223547, -1.112240025338166033E-15 ) ) ;
#35235=CARTESIAN_POINT ( 'NONE',  ( 19.75312500061451360, 4.541064518000418104, -2.621784821874998173 ) ) ;
#35236=CARTESIAN_POINT ( 'NONE',  ( 29.09062500061451573, -3.027376345333610441, -5.243569643749999898 ) ) ;
#35237=CARTESIAN_POINT ( 'NONE',  ( -1.394453263437886801E-15, 19.66249999999999787, 33.99999999999999289 ) ) ;
#35238=CARTESIAN_POINT ( 'NONE',  ( 9.000000000000001776, -4.330127018922190985, -2.500000000000001332 ) ) ;
#35239=CARTESIAN_POINT ( 'NONE',  ( 18.82500000122903216, 2.886751345948126879, 4.999999999999999112 ) ) ;
#35240=CARTESIAN_POINT ( 'NONE',  ( -0.6945831915928805111, 10.00052343484236772, 26.06076730949330411 ) ) ;
#35242=ORIENTED_EDGE ( 'NONE', *, *, #46955, .F. ) ;
#35243=CARTESIAN_POINT ( 'NONE',  ( 18.26249999999999929, 2.886751345948126879, 4.999999999999999112 ) ) ;
#35244=CARTESIAN_POINT ( 'NONE',  ( 21.41250000000000497, 2.886751345948126879, 4.999999999999999112 ) ) ;
#35245=CARTESIAN_POINT ( 'NONE',  ( 19.20937500061451786, -4.541064518000417216, -2.621784821875001281 ) ) ;
#35246=CARTESIAN_POINT ( 'NONE',  ( 24.14062500061451289, -3.027376345333610441, -5.243569643749999898 ) ) ;
#35247=ORIENTED_EDGE ( 'NONE', *, *, #51473, .T. ) ;
#35248=CARTESIAN_POINT ( 'NONE',  ( 5.353125000614515905, 4.541064518000418104, -2.621784821874998173 ) ) ;
#35250=CARTESIAN_POINT ( 'NONE',  ( 15.00000000000000000, 4.330127018922192761, -2.499999999999997780 ) ) ;
#35251=CARTESIAN_POINT ( 'NONE',  ( 4.243569643749999010, 17.36562500061451786, 27.54997392385601174 ) ) ;
#35252=CARTESIAN_POINT ( 'NONE',  ( 29.80312500061451431, 0.000000000000000000, 5.243569643749999010 ) ) ;
#35255=CARTESIAN_POINT ( 'NONE',  ( 26.78437500061451360, -4.541064518000419881, 2.621784821874995952 ) ) ;
#35256=EDGE_LOOP ( 'NONE', ( #21125, #73100, #58950, #33206, #44030, #38993 ) ) ;
#35257=CARTESIAN_POINT ( 'NONE',  ( 22.64062500061451644, -3.027376345333614438, 5.243569643749998122 ) ) ;
#35258=CARTESIAN_POINT ( 'NONE',  ( 22.43437500061451573, 6.421520780324663323E-16, -5.243569643749999010 ) ) ;
#35259=CARTESIAN_POINT ( 'NONE',  ( 4.243569643749999898, 17.29062500061459318, -27.54997392385601529 ) ) ;
#35260=CARTESIAN_POINT ( 'NONE',  ( 7.003125000614518036, -4.541064518000417216, -2.621784821875001281 ) ) ;
#35262=CARTESIAN_POINT ( 'NONE',  ( 24.74062500061451786, 6.054752690667223547, 3.707466751127219781E-16 ) ) ;
#35265=CARTESIAN_POINT ( 'NONE',  ( 16.24687500061451573, 6.054752690667223547, 3.707466751127219781E-16 ) ) ;
#35266=CARTESIAN_POINT ( 'NONE',  ( 19.58437500061451786, -4.541064518000419881, 2.621784821874995952 ) ) ;
#35267=CARTESIAN_POINT ( 'NONE',  ( 27.60937500061451644, 0.000000000000000000, 5.243569643749999010 ) ) ;
#35268=CARTESIAN_POINT ( 'NONE',  ( 2.121784821875001281, 15.50937500061451857, 33.67503911421598417 ) ) ;
#35269=CARTESIAN_POINT ( 'NONE',  ( 7.453125000614516438, -4.541064518000417216, -2.621784821875001281 ) ) ;
#35270=CYLINDRICAL_SURFACE ( 'NONE', #50195, 4.999999999999998224 ) ;
#35272=CARTESIAN_POINT ( 'NONE',  ( 4.021875000614516082, 3.027376345333613106, -5.243569643749998122 ) ) ;
#35273=CARTESIAN_POINT ( 'NONE',  ( 8.737500001229033586, 6.123233995736764310E-16, -4.999999999999998224 ) ) ;
#35274=CARTESIAN_POINT ( 'NONE',  ( 6.065625000614516260, -6.054752690667223547, -1.112240025338166033E-15 ) ) ;
#35275=CARTESIAN_POINT ( 'NONE',  ( 8.596875000614518925, 6.054752690667223547, 3.707466751127219781E-16 ) ) ;
#35276=CARTESIAN_POINT ( 'NONE',  ( 16.80000000122903359, -2.886751345948125991, -5.000000000000000000 ) ) ;
#35277=CARTESIAN_POINT ( 'NONE',  ( 5.634375000614519458, -4.541064518000419881, 2.621784821874995952 ) ) ;
#35278=CARTESIAN_POINT ( 'NONE',  ( 6.778125000614518392, 4.541064518000418104, 2.621784821874999949 ) ) ;
#35281=CARTESIAN_POINT ( 'NONE',  ( 17.74687500061451928, -3.027376345333614438, 5.243569643749998122 ) ) ;
#35284=CARTESIAN_POINT ( 'NONE',  ( 24.17812500061451786, 6.421520780324663323E-16, -5.243569643749999010 ) ) ;
#35285=CARTESIAN_POINT ( 'NONE',  ( 10.79062500061451679, 6.054752690667223547, 3.707466751127219781E-16 ) ) ;
#35286=CARTESIAN_POINT ( 'NONE',  ( 27.45937500061451786, 4.541064518000418104, -2.621784821874998173 ) ) ;
#35287=CARTESIAN_POINT ( 'NONE',  ( 9.140625000614518214, -3.027376345333614438, 5.243569643749998122 ) ) ;
#35288=CARTESIAN_POINT ( 'NONE',  ( -3.000416591977282496E-16, 10.74687500061451928, -34.90005215228797653 ) ) ;
#35289=CARTESIAN_POINT ( 'NONE',  ( 11.47500000122903252, 2.886751345948129099, -4.999999999999998224 ) ) ;
#35291=CARTESIAN_POINT ( 'NONE',  ( 25.82812500061451644, -4.541064518000419881, 2.621784821874995952 ) ) ;
#35292=CARTESIAN_POINT ( 'NONE',  ( 9.001249775931846008E-16, 12.71562500061451750, -25.09994784771203058 ) ) ;
#35293=CARTESIAN_POINT ( 'NONE',  ( 12.18750000122903465, -4.330127018922194537, 2.499999999999995559 ) ) ;
#35294=CARTESIAN_POINT ( 'NONE',  ( 22.30312500061451431, -4.541064518000417216, -2.621784821875001281 ) ) ;
#35295=CARTESIAN_POINT ( 'NONE',  ( 11.02500000000000036, 4.330127018922191873, 2.499999999999999556 ) ) ;
#35296=CARTESIAN_POINT ( 'NONE',  ( 19.30312500061451786, 4.541064518000418104, -2.621784821874998173 ) ) ;
#35297=CARTESIAN_POINT ( 'NONE',  ( 6.196875000614517681, -3.027376345333610441, -5.243569643749999898 ) ) ;
#35298=CARTESIAN_POINT ( 'NONE',  ( 21.60000000000000142, -4.330127018922190985, -2.500000000000001332 ) ) ;
#35299=CARTESIAN_POINT ( 'NONE',  ( 12.71250000122903145, -4.330127018922190985, -2.500000000000001332 ) ) ;
#35300=CARTESIAN_POINT ( 'NONE',  ( 13.94062500061451892, 6.054752690667223547, 3.707466751127219781E-16 ) ) ;
#35301=CARTESIAN_POINT ( 'NONE',  ( 16.34062500061451573, -3.027376345333614438, 5.243569643749998122 ) ) ;
#35302=CARTESIAN_POINT ( 'NONE',  ( 25.12500000122903288, 2.886751345948126879, 4.999999999999999112 ) ) ;
#35303=CARTESIAN_POINT ( 'NONE',  ( 21.41250000000000497, 2.886751345948126879, 4.999999999999999112 ) ) ;
#35304=CARTESIAN_POINT ( 'NONE',  ( 23.97187500061451360, 3.027376345333611329, 5.243569643749999010 ) ) ;
#35305=FACE_OUTER_BOUND ( 'NONE', #60177, .T. ) ;
#35306=CARTESIAN_POINT ( 'NONE',  ( 6.712500001229034119, 0.000000000000000000, 4.999999999999998224 ) ) ;
#35307=CARTESIAN_POINT ( 'NONE',  ( 9.009375000614518569, 4.541064518000418104, -2.621784821874998173 ) ) ;
#35308=CARTESIAN_POINT ( 'NONE',  ( 25.39687500061451431, -3.027376345333614438, 5.243569643749998122 ) ) ;
#35309=EDGE_CURVE ( 'NONE', #12269, #23263, #13671, .T. ) ;
#35310=CARTESIAN_POINT ( 'NONE',  ( 30.00000000000000000, 0.000000000000000000, 4.999999999999998224 ) ) ;
#35311=CARTESIAN_POINT ( 'NONE',  ( 21.51562500061451644, 3.027376345333613106, -5.243569643749998122 ) ) ;
#35312=CARTESIAN_POINT ( 'NONE',  ( 27.83437500061451786, 6.421520780324663323E-16, -5.243569643749999010 ) ) ;
#35314=CARTESIAN_POINT ( 'NONE',  ( 18.71250000000000213, 2.886751345948161074, 4.999999999999941380 ) ) ;
#35315=CARTESIAN_POINT ( 'NONE',  ( 8.409375000614518925, -4.541064518000417216, -2.621784821875001281 ) ) ;
#35316=CARTESIAN_POINT ( 'NONE',  ( 18.51562500061451289, 3.027376345333611329, 5.243569643749999010 ) ) ;
#35318=DIRECTION ( 'NONE',  ( -0.000000000000000000, -1.000000000000000000, -0.000000000000000000 ) ) ;
#35319=CARTESIAN_POINT ( 'NONE',  ( 28.52812500061451573, -4.541064518000419881, 2.621784821874995952 ) ) ;
#35320=CARTESIAN_POINT ( 'NONE',  ( 3.159375000614518036, 4.541064518000418104, -2.621784821874998173 ) ) ;
#35321=CARTESIAN_POINT ( 'NONE',  ( 22.87500000122903288, 2.886751345948126879, 4.999999999999998224 ) ) ;
#35322=CARTESIAN_POINT ( 'NONE',  ( 30.00000000000000000, 0.000000000000000000, 0.000000000000000000 ) ) ;
#35323=CARTESIAN_POINT ( 'NONE',  ( 17.58749999999999858, -2.886751345948125991, -5.000000000000000000 ) ) ;
#35324=CARTESIAN_POINT ( 'NONE',  ( 21.36562500061451431, -6.054752690667223547, -1.112240025338166033E-15 ) ) ;
#35326=CARTESIAN_POINT ( 'NONE',  ( 24.60000000000000142, 0.000000000000000000, 4.999999999999998224 ) ) ;
#35327=CARTESIAN_POINT ( 'NONE',  ( 26.10937500061451644, 4.541064518000418104, -2.621784821874998173 ) ) ;
#35328=VERTEX_POINT ( 'NONE', #32962 ) ;
#35329=CARTESIAN_POINT ( 'NONE',  ( 16.00312500061451715, -4.541064518000417216, -2.621784821875001281 ) ) ;
#35330=CARTESIAN_POINT ( 'NONE',  ( 5.015625000614518214, 3.027376345333611329, 5.243569643749999010 ) ) ;
#35332=CARTESIAN_POINT ( 'NONE',  ( 29.31562500061451715, 3.027376345333611329, 5.243569643749999010 ) ) ;
#35333=CARTESIAN_POINT ( 'NONE',  ( 16.16250000122903430, 0.000000000000000000, 4.999999999999998224 ) ) ;
#35334=CARTESIAN_POINT ( 'NONE',  ( 22.23750000000000071, 5.773502691896255534, 3.535250795749688894E-16 ) ) ;
#35335=CARTESIAN_POINT ( 'NONE',  ( 28.19999999999999929, 0.000000000000000000, 4.999999999999998224 ) ) ;
#35336=CARTESIAN_POINT ( 'NONE',  ( 5.334375000614517859, 6.421520780324663323E-16, -5.243569643749999010 ) ) ;
#35337=CARTESIAN_POINT ( 'NONE',  ( 9.609375000614518214, 0.000000000000000000, 5.243569643749999010 ) ) ;
#35338=CARTESIAN_POINT ( 'NONE',  ( 19.20937500061451786, -4.541064518000417216, -2.621784821875001281 ) ) ;
#35339=CARTESIAN_POINT ( 'NONE',  ( -2.000000000000000000, 15.08750000122903501, -33.46410161513775705 ) ) ;
#35340=ORIENTED_EDGE ( 'NONE', *, *, #49345, .T. ) ;
#35341=CARTESIAN_POINT ( 'NONE',  ( 28.11562500061451431, -6.054752690667223547, -1.112240025338166033E-15 ) ) ;
#35342=CARTESIAN_POINT ( 'NONE',  ( 3.112500000000000711, -5.773502691896255534, -1.060575238724906372E-15 ) ) ;
#35343=CARTESIAN_POINT ( 'NONE',  ( 4.696875000614518569, -3.027376345333614438, 5.243569643749998122 ) ) ;
#35344=CARTESIAN_POINT ( 'NONE',  ( 18.11250000000000071, 2.886751345948129099, -4.999999999999998224 ) ) ;
#35345=CARTESIAN_POINT ( 'NONE',  ( 12.55312500061451786, 4.541064518000418104, -2.621784821874998173 ) ) ;
#35346=CARTESIAN_POINT ( 'NONE',  ( 26.88749999999999929, -2.886751345948121994, 5.000000000000011546 ) ) ;
#35347=CARTESIAN_POINT ( 'NONE',  ( 4.763386231524743053, 8.796087519298447788, 26.33157461438974423 ) ) ;
#35349=CARTESIAN_POINT ( 'NONE',  ( 7.340625000614518392, -3.027376345333614438, 5.243569643749998122 ) ) ;
#35350=CARTESIAN_POINT ( 'NONE',  ( 24.98437500061451644, -4.541064518000419881, 2.621784821874995952 ) ) ;
#35351=CARTESIAN_POINT ( 'NONE',  ( 19.68750000122903288, 4.330127018922191873, 2.499999999999999556 ) ) ;
#35352=CARTESIAN_POINT ( 'NONE',  ( 25.88437500061451502, -4.541064518000419881, 2.621784821874995952 ) ) ;
#35353=CARTESIAN_POINT ( 'NONE',  ( 6.562500000000001776, 2.886751345948126879, 4.999999999999999112 ) ) ;
#35354=CARTESIAN_POINT ( 'NONE',  ( -3.999999999999999556, 13.32500000122903572, 27.69059892324149530 ) ) ;
#35355=CARTESIAN_POINT ( 'NONE',  ( 15.70312500061451644, 4.541064518000418104, -2.621784821874998173 ) ) ;
#35356=CARTESIAN_POINT ( 'NONE',  ( 6.150000001229033231, 5.773502691896255534, 3.535250795749688894E-16 ) ) ;
#35357=CARTESIAN_POINT ( 'NONE',  ( 16.92187500061451999, -6.054752690667223547, -1.112240025338166033E-15 ) ) ;
#35358=CARTESIAN_POINT ( 'NONE',  ( 11.70937500061451608, 4.541064518000418104, -2.621784821874998173 ) ) ;
#35359=DIRECTION ( 'NONE',  ( -0.000000000000000000, -1.000000000000000000, -0.000000000000000000 ) ) ;
#35361=CARTESIAN_POINT ( 'NONE',  ( 11.72812500061451857, 4.541064518000418104, 2.621784821874999949 ) ) ;
#35362=CARTESIAN_POINT ( 'NONE',  ( 30.00000000000000000, 0.000000000000000000, 4.999999999999998224 ) ) ;
#35363=CARTESIAN_POINT ( 'NONE',  ( 23.55000000122903359, -2.886751345948125991, -5.000000000000000000 ) ) ;
#35364=CARTESIAN_POINT ( 'NONE',  ( 12.27187500061451786, 3.027376345333611329, 5.243569643749999010 ) ) ;
#35365=CARTESIAN_POINT ( 'NONE',  ( 3.834375000614519635, -4.541064518000419881, 2.621784821874995952 ) ) ;
#35366=CARTESIAN_POINT ( 'NONE',  ( 14.42812500061451786, 4.541064518000418104, 2.621784821874999949 ) ) ;
#35368=CARTESIAN_POINT ( 'NONE',  ( 23.25937500061451857, -4.541064518000417216, -2.621784821875001281 ) ) ;
#35369=DIRECTION ( 'NONE',  ( -1.000000000000000000, -0.000000000000000000, -0.000000000000000000 ) ) ;
#35370=CARTESIAN_POINT ( 'NONE',  ( 12.60000000122903430, -2.886751345948129988, 4.999999999999997335 ) ) ;
#35371=CARTESIAN_POINT ( 'NONE',  ( 23.69999999999999929, 0.000000000000000000, 4.999999999999998224 ) ) ;
#35373=CARTESIAN_POINT ( 'NONE',  ( 4.243569643749999898, 17.38437500061451502, -30.00000000000000000 ) ) ;
#35374=CARTESIAN_POINT ( 'NONE',  ( 18.19687500061451502, -3.027376345333614438, 5.243569643749998122 ) ) ;
#35375=CARTESIAN_POINT ( 'NONE',  ( 17.10000000122903430, -2.886751345948129988, 4.999999999999997335 ) ) ;
#35376=CARTESIAN_POINT ( 'NONE',  ( 12.68437500061451573, 4.541064518000418104, 2.621784821874999949 ) ) ;
#35377=CARTESIAN_POINT ( 'NONE',  ( -2.121784821874996840, 10.48437500061451821, 33.67503911421598417 ) ) ;
#35378=CARTESIAN_POINT ( 'NONE',  ( 20.92500000122903714, 2.886751345948129099, -4.999999999999998224 ) ) ;
#35379=CARTESIAN_POINT ( 'NONE',  ( 13.97812500061451679, 4.541064518000418104, 2.621784821874999949 ) ) ;
#35380=ORIENTED_EDGE ( 'NONE', *, *, #73023, .F. ) ;
#35382=CARTESIAN_POINT ( 'NONE',  ( 18.97499999999999787, 6.123233995736764310E-16, -4.999999999999998224 ) ) ;
#35384=CARTESIAN_POINT ( 'NONE',  ( 4.027123420325200875, 2.963623535648654883, 4.154172641102294783 ) ) ;
#35385=CARTESIAN_POINT ( 'NONE',  ( 15.97500000122903430, 2.886751345948129099, -4.999999999999998224 ) ) ;
#35386=CARTESIAN_POINT ( 'NONE',  ( 26.55937500061451573, 4.541064518000418104, -2.621784821874998173 ) ) ;
#35387=CARTESIAN_POINT ( 'NONE',  ( 19.22812500061451502, 6.421520780324663323E-16, -5.243569643749999010 ) ) ;
#35388=CARTESIAN_POINT ( 'NONE',  ( 22.71562500061451573, -6.054752690667223547, -1.112240025338166033E-15 ) ) ;
#35389=CARTESIAN_POINT ( 'NONE',  ( 29.55000000122903003, 5.773502691896255534, 3.535250795749688894E-16 ) ) ;
#35390=CARTESIAN_POINT ( 'NONE',  ( 28.23750000000000426, -2.886751345948129988, 4.999999999999997335 ) ) ;
#35391=CARTESIAN_POINT ( 'NONE',  ( 3.999999999999998668, 11.82500000122903394, 27.69059892324149530 ) ) ;
#35393=CARTESIAN_POINT ( 'NONE',  ( 12.78750000122903430, 6.123233995736764310E-16, -4.999999999999998224 ) ) ;
#35394=CARTESIAN_POINT ( 'NONE',  ( 4.243569643749999010, 15.62187500061451928, -32.45002607614398471 ) ) ;
#35395=CARTESIAN_POINT ( 'NONE',  ( 5.887500001229034829, -4.330127018922194537, 2.499999999999995559 ) ) ;
#35396=CARTESIAN_POINT ( 'NONE',  ( 5.737499999999998934, -2.886751345948129988, 4.999999999999997335 ) ) ;
#35398=CARTESIAN_POINT ( 'NONE',  ( 2.971875000614517592, -6.054752690667223547, -1.112240025338166033E-15 ) ) ;
#35399=CARTESIAN_POINT ( 'NONE',  ( 10.02187500061451964, 3.027376345333611329, 5.243569643749999010 ) ) ;
#35400=CARTESIAN_POINT ( 'NONE',  ( 29.39062500061451289, -3.027376345333614438, 5.243569643749998122 ) ) ;
#35401=CARTESIAN_POINT ( 'NONE',  ( 27.41250000122903430, 0.000000000000000000, 4.999999999999998224 ) ) ;
#35402=CARTESIAN_POINT ( 'NONE',  ( -5.790145606462772321, 8.153486631126842354, -28.41457251781636728 ) ) ;
#35404=CARTESIAN_POINT ( 'NONE',  ( 8.521875000614516082, 3.027376345333613106, -5.243569643749998122 ) ) ;
#35405=CARTESIAN_POINT ( 'NONE',  ( 11.33437500061451608, 4.541064518000418104, 2.621784821874999949 ) ) ;
#35406=CARTESIAN_POINT ( 'NONE',  ( 6.412500000000001421, 2.886751345948129099, -4.999999999999998224 ) ) ;
#35407=CARTESIAN_POINT ( 'NONE',  ( -4.243569643749999898, 14.81562500061459531, 27.54997392385601529 ) ) ;
#35408=( BOUNDED_SURFACE ( )  B_SPLINE_SURFACE ( 1, 2, ( 
 ( #25564, #10405, #20003, #43299, #26299, #48105, #20373, #42556, #54379, #38482, #65083, #70628, #14474, #42924, #4512, #14840, #72094, #31474, #21478, #65448, #37380, #54741, #44031, #37008, #10040, #32574, #59904, #9309, #45838, #11130, #51018, #10767, #50660, #61370, #5948, #28132, #62817, #27767, #414, #62456, #11854, #72458, #22923, #34017, #21843, #12209, #50307, #55838, #11495, #40295, #33300, #67653, #5225, #56554, #34373, #45118, #64, #45481, #72829, #39578, #22570, #68013, #17385, #16301, #66932, #62101, #44766, #38855, #39943, #44406, #5595, #56906, #33657, #55475, #22212, #67301, #28481, #16659, #51379, #39217, #6311, #28840, #781, #61729, #23290, #56202, #68375, #17736, #4867, #17019, #27403, #49933, #46197, #41384, #68738, #69102, #52464, #69463, #63178, #18464, #57630, #42112, #13653, #70177, #64635, #36196, #69818, #63543, #25101, #35106, #18821, #34738, #19554, #51743, #1871, #35464, #57267, #52102, #1142, #12929, #47645, #23653, #6679, #29207, #29565, #58714, #46560, #30653, #18096, #8126, #1507, #12572, #63896, #2582, #40657, #35823, #57986, #41027, #7036, #24011, #7396, #30293, #29924, #24377, #46925, #58346, #13286, #7757, #52825, #2227, #41737, #64265, #24740, #47284, #19184, #53185, #43943, #8854, #14389, #43213, #72012, #19924, #26214, #42478, #3325, #32486, #8485, #4056, #37295, #20654, #37655, #70916, #36926, #54653, #25477, #71651, #48753, #3689, #59818, #59447, #49480, #70549, #26953, #2949, #25851, #48023, #65001, #31391, #65733, #53930, #60543, #71277, #32119, #15118, #54297, #21387, #14021, #15476, #48388, #36561, #60178, #9587, #20287, #42841, #26582, #49122, #65362, #21024, #43577, #14752, #66098, #38020, #9949, #59081, #4425, #55021, #9223, #31018, #53552, #31760, #33930, #10678, #11413, #45392, #60914, #56472, #16933, #73101, #17301, #67568, #22840, #27314, #44313, #44680, #50574, #66843, #28755, #22483, #38766, #55747, #33208, #61285, #67211, #56115, #5864, #11041, #39488, #49847, #67928, #5141, #696, #72372, #331, #16572, #39124, #28396, #27676, #39862, #23205, #50934, #10317, #62374, #11772, #34288, #56820, #62010, #6227, #5507, #61639, #51295, #16213, #45033, #33567, #66467, #15844, #21752, #4780, #38390, #50214, #72739, #32849, #55386, #28045, #22125, #1423, #45758, #34655, #29127, #24296, #36111, #1062, #30574, #35023, #24656, #35382, #69017, #35745, #6953, #41303, #53100, #51660, #63813, #18018, #47202, #2496, #13205, #18380, #12495, #68294, #69733, #40574, #23572, #1786, #13567, #62736, #46844, #40948, #29485, #17654, #58632, #23929, #58265, #46117, #63462, #68654, #69384, #12849, #40214, #63094, #7671, #52740, #2145, #12128, #30209, #18739, #57184, #6597, #57551, #52022, #19102, #46479, #57905, #7314, #29844, #52379, #64179, #41657, #8039, #48299, #31672, #48663, #8767, #47935, #65644, #36476, #9502, #59727, #14662, #70825, #25392, #60455, #26124, #9863, #37935, #37205, #20199, #32394, #43489, #53470, #43120, #8400, #15032, #31301, #25763, #71188, #30929, #54934, #9135, #54205, #25020, #2862, #47562, #42753, #59355, #70092, #70464, #20938, #64547, #3602, #20562, #32031, #64913, #37569, #42026, #60093, #54567, #3970, #42391, #26492, #15393, #58994, #49035, #19839, #53841, #65274, #71563, #14303, #3236, #36841, #19469, #66013, #13940, #11689, #5782, #39405, #33124, #67844, #4696, #39041, #34205, #62293, #21302, #44596, #5057, #4340, #21667, #43856, #55661, #17216, #66381, #26865, #49396, #72289, #28313, #16127, #249, #60825, #71927, #44224, #27226, #33478, #15757, #10231, #16484, #32765, #66757, #22757, #38297, #67486, #27594, #10957, #27958, #61201, #49763, #44949, #55302, #61923, #61555, #67127, #50126, #38680, #39777, #5420, #10596, #72657, #56028, #22037, #50490, #45308, #73016, #22400, #16849, #11329, #33848, #56392, #50849, #68210, #35656, #29400, #1331, #56739, #40133, #28672, #57462, #46031, #7581, #62647, #41216, #23120, #46391, #63375, #52292, #51575, #23843, #612, #68926, #18283, #12759, #29040, #1693, #63724, #17571, #40858, #12044, #23484, #6868, #35295, #34567, #68567, #57096, #6141, #69291, #51212, #45674, #6505, #974, #29755, #17926, #57816, #58176, #40489, #63004, #51934, #13116, #46756, #12401, #7226, #24204, #18654, #34936, #38537, #72151, #49624, #44457, #51072, #61424, #45540, #32988, #470, #66988, #27457, #5649, #17438, #66612, #50713, #72884, #33352, #6364, #39995, #5279, #45172, #4922, #44818, #55528, #116, #22265, #56960, #21901, #67703, #56607, #6003, #15988, #17075, #28184, #61061, #55890, #21530, #62509, #27825, #39636, #49988, #67352, #72512, #22621, #16715, #44085, #16350, #62154, #28536, #22978, #10459, #11551, #34067, #38905, #10818, #50357, #39270, #68069, #34431, #61782, #11186, #33713, #56258, #11907, #18767, #59025, #35772, #7702, #25049, #29872, #8426, #64943, #19499, #52049, #47592, #30963, #70121, #2529, #36143, #13967, #24685, #30238, #30602, #12877, #19131, #52771, #42056, #64579, #69045, #46507, #41685, #24324, #18408, #36505, #1453, #58295, #53498, #63843, #35053, #23959, #40974, #13597, #25421, #63489, #19869, #46873, #2890, #47230, #2173, #47964, #69412, #53129, #42422, #35410, #70491, #7342, #57580, #6983, #29514, #69763, #1817, #57935, #52409, #41333, #13234, #64208, #58662, #8070, #25793, #66044, #31700, #60861, #71594, #32429, #49065, #54598, #72320, #21700, #15792, #42782, #36868, #4003, #37966, #65302, #59758, #20968, #54966, #20230, #43522, #43889, #71218, #9893, #49426, #15422, #14335, #4727, #10264, #70856, #21335, #53873, #48695, #4371, #26156, #32796, #14693, #38332, #9165, #37235, #60487, #55333, #31331, #26901, #37601, #20595, #44257, #27262, #43154, #71961, #54235, #9532, #3632, #66414, #60123, #59387, #65675, #49794, #8797, #3265, #48331, #15064, #32066 ),
 ( #26526, #28341, #56421, #39434, #67158, #29070, #67873, #51606, #6537, #5810, #61954, #1006, #12076, #22070, #11717, #50158, #56767, #50520, #67515, #39805, #72688, #23513, #50878, #277, #66790, #44629, #16161, #11358, #27991, #38713, #16518, #62681, #33156, #22786, #62321, #642, #33509, #45338, #10627, #17245, #34233, #6171, #10989, #51240, #57126, #5089, #28700, #27625, #73048, #33876, #23151, #39071, #22430, #61586, #61232, #45705, #55694, #56058, #68239, #17602, #44977, #5451, #16879, #40162, #34598, #30873, #63036, #13147, #46788, #2805, #63405, #12434, #1726, #58937, #34968, #68598, #46063, #40890, #47506, #8344, #53413, #70036, #7982, #24239, #36422, #46423, #7614, #17958, #40520, #57495, #35688, #69323, #6899, #12790, #29430, #18683, #51967, #1366, #23876, #68961, #35327, #19409, #57850, #41968, #18318, #64490, #7259, #29787, #2090, #13882, #52324, #47147, #41246, #63758, #58209, #30150, #52684, #41602, #24599, #69678, #19044, #64121, #13507, #36054, #58574, #30518, #53044, #2439, #24961, #20884, #3916, #42333, #55251, #20143, #25706, #54513, #10179, #31242, #37517, #53783, #48979, #43438, #71876, #65219, #48609, #31979, #71508, #9081, #48243, #65960, #36783, #9809, #60038, #14980, #71134, #70767, #60772, #26438, #32714, #38243, #9449, #20507, #25333, #43802, #3179, #15340, #8709, #37880, #31617, #26070, #60401, #42697, #47878, #32341, #54879, #70407, #14609, #19783, #43064, #59673, #64857, #37147, #21248, #14245, #4285, #26811, #49344, #54153, #66327, #59299, #15705, #3548, #65589, #21985, #62242, #68158, #16074, #11278, #38624, #38991, #22349, #39356, #33071, #61506, #27540, #11993, #56690, #67790, #10903, #5369, #50797, #61148, #62597, #61870, #33798, #4647, #10543, #27176, #44901, #33431, #34516, #55610, #559, #44172, #56342, #200, #11638, #44544, #5731, #21617, #28266, #22705, #45257, #67075, #34153, #17521, #5006, #17164, #50072, #55975, #67438, #39723, #72604, #27908, #16434, #49710, #6090, #40083, #72238, #28621, #51158, #50442, #66702, #72967, #23069, #16799, #45624, #924, #24151, #57766, #13799, #1279, #23432, #12708, #69953, #45978, #6451, #57046, #51881, #58488, #68874, #52962, #40434, #7897, #23789, #34880, #13065, #24876, #68513, #58123, #7175, #40804, #28986, #47423, #35245, #52602, #12345, #52241, #62951, #7531, #29703, #64406, #29348, #2008, #64038, #13417, #17875, #24519, #35604, #57409, #51524, #46340, #6814, #30064, #41877, #18230, #69240, #63317, #47063, #69597, #30434, #1645, #46705, #63675, #18959, #18602, #41166, #41519, #35966, #2359, #19323, #27000, #9998, #37698, #72787, #38438, #22170, #50262, #49530, #32533, #44723, #55796, #65779, #55434, #20700, #43258, #72054, #15161, #60964, #32894, #10726, #4105, #60589, #43990, #10363, #21072, #60220, #4826, #47785, #21798, #21433, #66511, #55069, #9633, #67258, #27360, #36339, #58853, #15892, #4470, #8263, #5186, #32167, #49891, #54700, #72416, #43623, #38065, #44363, #26632, #30794, #66890, #16258, #53324, #49169, #2723, #38813, #71700, #25239, #66145, #33258, #71325, #61328, #27724, #15523, #56514, #742, #33614, #23251, #17697, #34699, #33975, #1107, #6998, #28090, #45801, #50618, #50976, #34333, #51340, #45076, #373, #39535, #23974, #68700, #52064, #46522, #18060, #51704, #45439, #29529, #16978, #68337, #16616, #1468, #56158, #56866, #17345, #39171, #5907, #5552, #67972, #61687, #23, #11086, #22529, #11454, #40620, #28441, #12535, #67612, #63140, #22881, #62060, #40258, #57595, #39904, #62779, #62417, #11816, #6271, #28799, #12171, #57228, #6643, #29170, #23614, #46160, #35069, #3282, #41347, #64594, #2907, #25438, #12892, #13981, #47606, #35425, #25810, #63857, #69425, #25063, #53891, #24339, #52786, #18782, #69063, #47981, #31350, #18423, #70509, #30980, #24701, #59405, #13247, #30615, #40989, #63505, #57949, #36157, #69778, #7357, #35785, #29886, #47245, #8813, #52425, #1831, #46887, #58308, #19885, #7719, #64960, #30253, #42438, #2187, #19145, #70136, #36886, #41699, #19514, #64223, #13612, #58675, #8085, #53145, #36520, #2544, #42072, #59040, #8444, #53513, #14351, #20615, #43906, #55349, #4743, #65321, #66429, #26917, #14712, #5104, #43173, #48713, #4387, #33172, #54253, #60503, #3649, #71976, #15807, #21715, #15079, #71612, #54982, #21349, #32081, #71235, #38349, #59776, #32811, #9909, #37981, #20985, #65692, #10642, #49442, #55710, #61248, #32447, #43538, #48348, #66805, #26172, #60876, #31717, #10280, #54612, #49084, #27277, #37616, #70873, #49810, #72335, #20247, #60138, #42799, #66059, #9547, #37254, #4018, #44274, #9182, #16176, #38728, #26543, #15437, #11732, #44643, #34248, #28716, #45720, #44994, #12092, #17976, #39087, #56781, #61604, #61970, #45354, #62336, #293, #34985, #73064, #23166, #34613, #57143, #67173, #68255, #6187, #16534, #57513, #22445, #28007, #51256, #12454, #33526, #39821, #56076, #658, #17617, #1023, #67531, #50893, #40177, #62696, #11372, #50536, #6555, #11005, #29087, #51622, #17260, #22802, #16894, #63052, #23529, #27638, #40536, #46079, #67888, #50174, #68614, #5467, #72702, #39449, #22084, #33891, #28357, #56435, #5825, #64874, #41619, #13525, #6915, #63421, #29445, #24617, #41263, #14262, #12808, #2822, #46439, #36072, #2456, #13899, #46804, #64138, #23892, #58592, #7999, #24979, #24256, #64507, #70424, #18335, #30535, #40908, #63775, #47164, #53062, #35343, #13163, #29805, #36801, #58953, #42351, #51983, #8361, #41987, #35704, #19799, #7275, #47524, #1382, #68978, #57866, #69696, #7631, #52340, #69340, #1742, #58226, #18699, #30168, #52700, #2106, #19061, #30890, #70053, #25350, #19426, #53432, #36439, #47896, #15356, #27190, #3196, #60416, #9465, #43081, #16091, #49725, #14995, #54895, #14625, #54529, #65235, #9825, #25723, #32357 ) ),
 .UNSPECIFIED., .F., .F., .F. ) 
 B_SPLINE_SURFACE_WITH_KNOTS ( ( 2, 2 ),
 ( 3, 2, 2, 2, 2, 2, 2, 2, 2, 2, 2, 2, 2, 2, 2, 2, 2, 2, 2, 2, 2, 2, 2, 2, 2, 2, 2, 2, 2, 2, 2, 2, 2, 2, 2, 2, 2, 2, 2, 2, 2, 2, 2, 2, 2, 2, 2, 2, 2, 2, 2, 2, 2, 2, 2, 2, 2, 2, 2, 2, 2, 2, 2, 2, 2, 2, 2, 2, 2, 2, 2, 2, 2, 2, 2, 2, 2, 2, 2, 2, 2, 2, 2, 2, 2, 2, 2, 2, 2, 2, 2, 2, 2, 2, 2, 2, 2, 2, 2, 2, 2, 2, 2, 2, 2, 2, 2, 2, 2, 2, 2, 2, 2, 2, 2, 2, 2, 2, 2, 2, 2, 2, 2, 2, 2, 2, 2, 2, 2, 2, 2, 2, 2, 2, 2, 2, 2, 2, 2, 2, 2, 2, 2, 2, 2, 2, 2, 2, 2, 2, 2, 2, 2, 2, 2, 2, 2, 2, 2, 2, 2, 2, 2, 2, 2, 2, 2, 2, 2, 2, 2, 2, 2, 2, 2, 2, 2, 2, 2, 2, 2, 2, 2, 2, 2, 2, 2, 2, 2, 2, 2, 2, 2, 2, 2, 2, 2, 2, 2, 2, 2, 2, 2, 2, 2, 2, 2, 2, 2, 2, 2, 2, 2, 2, 2, 2, 2, 2, 2, 2, 2, 2, 2, 2, 2, 2, 2, 2, 2, 2, 2, 2, 2, 2, 2, 2, 2, 2, 2, 2, 2, 2, 2, 2, 2, 2, 2, 2, 2, 2, 2, 2, 2, 2, 2, 2, 2, 2, 2, 2, 2, 2, 2, 2, 2, 2, 2, 2, 2, 2, 2, 2, 2, 2, 2, 2, 2, 2, 2, 2, 2, 2, 2, 2, 2, 2, 2, 2, 2, 2, 2, 2, 2, 2, 2, 2, 2, 2, 2, 2, 2, 2, 2, 2, 2, 2, 2, 2, 2, 2, 2, 2, 2, 2, 2, 2, 2, 2, 2, 2, 2, 2, 2, 2, 2, 2, 2, 2, 2, 2, 2, 2, 2, 2, 2, 2, 2, 2, 2, 2, 2, 2, 2, 2, 2, 2, 2, 2, 2, 2, 2, 2, 2, 2, 2, 2, 2, 2, 2, 2, 3 ),
 ( 0.000000000000000000, 1.000000000000000000 ),
 ( 0.000000000000000000, 0.002777777777777777884, 0.005555555555555555768, 0.008333333333333333218, 0.01111111111111111154, 0.01388888888888888812, 0.01666666666666666644, 0.01944444444444444475, 0.02222222222222222307, 0.02500000000000000139, 0.02777777777777777624, 0.03055555555555555455, 0.03333333333333333287, 0.03611111111111110772, 0.03888888888888888951, 0.04166666666666666435, 0.04444444444444444614, 0.04722222222222222099, 0.05000000000000000278, 0.05277777777777777762, 0.05555555555555555247, 0.05833333333333333426, 0.06111111111111110911, 0.06388888888888888395, 0.06666666666666666574, 0.06944444444444444753, 0.07222222222222221544, 0.07499999999999999722, 0.07777777777777777901, 0.08055555555555556080, 0.08333333333333332871, 0.08611111111111111049, 0.08888888888888889228, 0.09166666666666666019, 0.09444444444444444198, 0.09722222222222222376, 0.1000000000000000056, 0.1027777777777777735, 0.1055555555555555552, 0.1083333333333333370, 0.1111111111111111049, 0.1138888888888888867, 0.1166666666666666685, 0.1194444444444444503, 0.1222222222222222182, 0.1250000000000000000, 0.1277777777777777679, 0.1305555555555555636, 0.1333333333333333315, 0.1361111111111110994, 0.1388888888888888951, 0.1416666666666666630, 0.1444444444444444309, 0.1472222222222222265, 0.1499999999999999944, 0.1527777777777777901, 0.1555555555555555580, 0.1583333333333333259, 0.1611111111111111216, 0.1638888888888888895, 0.1666666666666666574, 0.1694444444444444531, 0.1722222222222222210, 0.1749999999999999889, 0.1777777777777777846, 0.1805555555555555525, 0.1833333333333333204, 0.1861111111111111160, 0.1888888888888888840, 0.1916666666666666796, 0.1944444444444444475, 0.1972222222222222154, 0.2000000000000000111, 0.2027777777777777790, 0.2055555555555555469, 0.2083333333333333426, 0.2111111111111111105, 0.2138888888888888784, 0.2166666666666666741, 0.2194444444444444420, 0.2222222222222222099, 0.2250000000000000056, 0.2277777777777777735, 0.2305555555555555691, 0.2333333333333333370, 0.2361111111111111049, 0.2388888888888889006, 0.2416666666666666685, 0.2444444444444444364, 0.2472222222222222321, 0.2500000000000000000, 0.2527777777777777679, 0.2555555555555555358, 0.2583333333333333592, 0.2611111111111111271, 0.2638888888888888951, 0.2666666666666666630, 0.2694444444444444309, 0.2722222222222221988, 0.2750000000000000222, 0.2777777777777777901, 0.2805555555555555580, 0.2833333333333333259, 0.2861111111111110938, 0.2888888888888888618, 0.2916666666666666852, 0.2944444444444444531, 0.2972222222222222210, 0.2999999999999999889, 0.3027777777777777568, 0.3055555555555555802, 0.3083333333333333481, 0.3111111111111111160, 0.3138888888888888840, 0.3166666666666666519, 0.3194444444444444198, 0.3222222222222222432, 0.3250000000000000111, 0.3277777777777777790, 0.3305555555555555469, 0.3333333333333333148, 0.3361111111111111382, 0.3388888888888889062, 0.3416666666666666741, 0.3444444444444444420, 0.3472222222222222099, 0.3499999999999999778, 0.3527777777777778012, 0.3555555555555555691, 0.3583333333333333370, 0.3611111111111111049, 0.3638888888888888729, 0.3666666666666666408, 0.3694444444444444642, 0.3722222222222222321, 0.3750000000000000000, 0.3777777777777777679, 0.3805555555555555358, 0.3833333333333333592, 0.3861111111111111271, 0.3888888888888888951, 0.3916666666666666630, 0.3944444444444444309, 0.3972222222222221988, 0.4000000000000000222, 0.4027777777777777901, 0.4055555555555555580, 0.4083333333333333259, 0.4111111111111110938, 0.4138888888888888618, 0.4166666666666666852, 0.4194444444444444531, 0.4222222222222222210, 0.4249999999999999889, 0.4277777777777777568, 0.4305555555555555802, 0.4333333333333333481, 0.4361111111111111160, 0.4388888888888888840, 0.4416666666666666519, 0.4444444444444444198, 0.4472222222222222432, 0.4500000000000000111, 0.4527777777777777790, 0.4555555555555555469, 0.4583333333333333148, 0.4611111111111111382, 0.4638888888888889062, 0.4666666666666666741, 0.4694444444444444420, 0.4722222222222222099, 0.4749999999999999778, 0.4777777777777778012, 0.4805555555555555691, 0.4833333333333333370, 0.4861111111111111049, 0.4888888888888888729, 0.4916666666666666408, 0.4944444444444444642, 0.4972222222222222321, 0.5000000000000000000, 0.5027777777777777679, 0.5055555555555555358, 0.5083333333333333037, 0.5111111111111110716, 0.5138888888888888395, 0.5166666666666667185, 0.5194444444444444864, 0.5222222222222222543, 0.5250000000000000222, 0.5277777777777777901, 0.5305555555555555580, 0.5333333333333333259, 0.5361111111111110938, 0.5388888888888888618, 0.5416666666666666297, 0.5444444444444443976, 0.5472222222222222765, 0.5500000000000000444, 0.5527777777777778123, 0.5555555555555555802, 0.5583333333333333481, 0.5611111111111111160, 0.5638888888888888840, 0.5666666666666666519, 0.5694444444444444198, 0.5722222222222221877, 0.5749999999999999556, 0.5777777777777777235, 0.5805555555555556024, 0.5833333333333333703, 0.5861111111111111382, 0.5888888888888889062, 0.5916666666666666741, 0.5944444444444444420, 0.5972222222222222099, 0.5999999999999999778, 0.6027777777777777457, 0.6055555555555555136, 0.6083333333333332815, 0.6111111111111111605, 0.6138888888888889284, 0.6166666666666666963, 0.6194444444444444642, 0.6222222222222222321, 0.6250000000000000000, 0.6277777777777777679, 0.6305555555555555358, 0.6333333333333333037, 0.6361111111111110716, 0.6388888888888888395, 0.6416666666666667185, 0.6444444444444444864, 0.6472222222222222543, 0.6500000000000000222, 0.6527777777777777901, 0.6555555555555555580, 0.6583333333333333259, 0.6611111111111110938, 0.6638888888888888618, 0.6666666666666666297, 0.6694444444444443976, 0.6722222222222222765, 0.6750000000000000444, 0.6777777777777778123, 0.6805555555555555802, 0.6833333333333333481, 0.6861111111111111160, 0.6888888888888888840, 0.6916666666666666519, 0.6944444444444444198, 0.6972222222222221877, 0.6999999999999999556, 0.7027777777777777235, 0.7055555555555556024, 0.7083333333333333703, 0.7111111111111111382, 0.7138888888888889062, 0.7166666666666666741, 0.7194444444444444420, 0.7222222222222222099, 0.7249999999999999778, 0.7277777777777777457, 0.7305555555555555136, 0.7333333333333332815, 0.7361111111111111605, 0.7388888888888889284, 0.7416666666666666963, 0.7444444444444444642, 0.7472222222222222321, 0.7500000000000000000, 0.7527777777777777679, 0.7555555555555555358, 0.7583333333333333037, 0.7611111111111110716, 0.7638888888888888395, 0.7666666666666667185, 0.7694444444444444864, 0.7722222222222222543, 0.7750000000000000222, 0.7777777777777777901, 0.7805555555555555580, 0.7833333333333333259, 0.7861111111111110938, 0.7888888888888888618, 0.7916666666666666297, 0.7944444444444443976, 0.7972222222222222765, 0.8000000000000000444, 0.8027777777777778123, 0.8055555555555555802, 0.8083333333333333481, 0.8111111111111111160, 0.8138888888888888840, 0.8166666666666666519, 0.8194444444444444198, 0.8222222222222221877, 0.8249999999999999556, 0.8277777777777777235, 0.8305555555555556024, 0.8333333333333333703, 0.8361111111111111382, 0.8388888888888889062, 0.8416666666666666741, 0.8444444444444444420, 0.8472222222222222099, 0.8499999999999999778, 0.8527777777777777457, 0.8555555555555555136, 0.8583333333333332815, 0.8611111111111111605, 0.8638888888888889284, 0.8666666666666666963, 0.8694444444444444642, 0.8722222222222222321, 0.8750000000000000000, 0.8777777777777777679, 0.8805555555555555358, 0.8833333333333333037, 0.8861111111111110716, 0.8888888888888888395, 0.8916666666666667185, 0.8944444444444444864, 0.8972222222222222543, 0.9000000000000000222, 0.9027777777777777901, 0.9055555555555555580, 0.9083333333333333259, 0.9111111111111110938, 0.9138888888888888618, 0.9166666666666666297, 0.9194444444444443976, 0.9222222222222222765, 0.9250000000000000444, 0.9277777777777778123, 0.9305555555555555802, 0.9333333333333333481, 0.9361111111111111160, 0.9388888888888888840, 0.9416666666666666519, 0.9444444444444444198, 0.9472222222222221877, 0.9499999999999999556, 0.9527777777777777235, 0.9555555555555556024, 0.9583333333333333703, 0.9611111111111111382, 0.9638888888888889062, 0.9666666666666666741, 0.9694444444444444420, 0.9722222222222222099, 0.9749999999999999778, 0.9777777777777777457, 0.9805555555555555136, 0.9833333333333332815, 0.9861111111111111605, 0.9888888888888889284, 0.9916666666666666963, 0.9944444444444444642, 0.9972222222222222321, 1.000000000000000000 ),
 .UNSPECIFIED. ) 
 GEOMETRIC_REPRESENTATION_ITEM ( )  RATIONAL_B_SPLINE_SURFACE ( (
 ( 1.000000000000000000, 0.8660254037844387076, 1.000000000000000000, 0.8660254037844387076, 1.000000000000000000, 0.8660254037844387076, 1.000000000000000000, 0.8660254037844387076, 1.000000000000000000, 0.8660254037844387076, 1.000000000000000000, 0.8660254037844387076, 1.000000000000000000, 0.8660254037844387076, 1.000000000000000000, 0.8660254037844387076, 1.000000000000000000, 0.8660254037844387076, 1.000000000000000000, 0.8660254037844387076, 1.000000000000000000, 0.8660254037844387076, 1.000000000000000000, 0.8660254037844387076, 1.000000000000000000, 0.8660254037844387076, 1.000000000000000000, 0.8660254037844387076, 1.000000000000000000, 0.8660254037844387076, 1.000000000000000000, 0.8660254037844387076, 1.000000000000000000, 0.8660254037844387076, 1.000000000000000000, 0.8660254037844387076, 1.000000000000000000, 0.8660254037844387076, 1.000000000000000000, 0.8660254037844387076, 1.000000000000000000, 0.8660254037844387076, 1.000000000000000000, 0.8660254037844387076, 1.000000000000000000, 0.8660254037844387076, 1.000000000000000000, 0.8660254037844387076, 1.000000000000000000, 0.8660254037844387076, 1.000000000000000000, 0.8660254037844387076, 1.000000000000000000, 0.8660254037844387076, 1.000000000000000000, 0.8660254037844387076, 1.000000000000000000, 0.8660254037844387076, 1.000000000000000000, 0.8660254037844387076, 1.000000000000000000, 0.8660254037844387076, 1.000000000000000000, 0.8660254037844387076, 1.000000000000000000, 0.8660254037844387076, 1.000000000000000000, 0.8660254037844387076, 1.000000000000000000, 0.8660254037844387076, 1.000000000000000000, 0.8660254037844387076, 1.000000000000000000, 0.8660254037844387076, 1.000000000000000000, 0.8660254037844387076, 1.000000000000000000, 0.8660254037844387076, 1.000000000000000000, 0.8660254037844387076, 1.000000000000000000, 0.8660254037844387076, 1.000000000000000000, 0.8660254037844387076, 1.000000000000000000, 0.8660254037844387076, 1.000000000000000000, 0.8660254037844387076, 1.000000000000000000, 0.8660254037844387076, 1.000000000000000000, 0.8660254037844387076, 1.000000000000000000, 0.8660254037844387076, 1.000000000000000000, 0.8660254037844387076, 1.000000000000000000, 0.8660254037844387076, 1.000000000000000000, 0.8660254037844387076, 1.000000000000000000, 0.8660254037844387076, 1.000000000000000000, 0.8660254037844387076, 1.000000000000000000, 0.8660254037844387076, 1.000000000000000000, 0.8660254037844387076, 1.000000000000000000, 0.8660254037844387076, 1.000000000000000000, 0.8660254037844387076, 1.000000000000000000, 0.8660254037844387076, 1.000000000000000000, 0.8660254037844387076, 1.000000000000000000, 0.8660254037844387076, 1.000000000000000000, 0.8660254037844387076, 1.000000000000000000, 0.8660254037844387076, 1.000000000000000000, 0.8660254037844387076, 1.000000000000000000, 0.8660254037844387076, 1.000000000000000000, 0.8660254037844387076, 1.000000000000000000, 0.8660254037844387076, 1.000000000000000000, 0.8660254037844387076, 1.000000000000000000, 0.8660254037844387076, 1.000000000000000000, 0.8660254037844387076, 1.000000000000000000, 0.8660254037844387076, 1.000000000000000000, 0.8660254037844387076, 1.000000000000000000, 0.8660254037844387076, 1.000000000000000000, 0.8660254037844387076, 1.000000000000000000, 0.8660254037844387076, 1.000000000000000000, 0.8660254037844387076, 1.000000000000000000, 0.8660254037844387076, 1.000000000000000000, 0.8660254037844387076, 1.000000000000000000, 0.8660254037844387076, 1.000000000000000000, 0.8660254037844387076, 1.000000000000000000, 0.8660254037844387076, 1.000000000000000000, 0.8660254037844387076, 1.000000000000000000, 0.8660254037844387076, 1.000000000000000000, 0.8660254037844387076, 1.000000000000000000, 0.8660254037844387076, 1.000000000000000000, 0.8660254037844387076, 1.000000000000000000, 0.8660254037844387076, 1.000000000000000000, 0.8660254037844387076, 1.000000000000000000, 0.8660254037844387076, 1.000000000000000000, 0.8660254037844387076, 1.000000000000000000, 0.8660254037844387076, 1.000000000000000000, 0.8660254037844387076, 1.000000000000000000, 0.8660254037844387076, 1.000000000000000000, 0.8660254037844387076, 1.000000000000000000, 0.8660254037844387076, 1.000000000000000000, 0.8660254037844387076, 1.000000000000000000, 0.8660254037844387076, 1.000000000000000000, 0.8660254037844387076, 1.000000000000000000, 0.8660254037844387076, 1.000000000000000000, 0.8660254037844387076, 1.000000000000000000, 0.8660254037844387076, 1.000000000000000000, 0.8660254037844387076, 1.000000000000000000, 0.8660254037844387076, 1.000000000000000000, 0.8660254037844387076, 1.000000000000000000, 0.8660254037844387076, 1.000000000000000000, 0.8660254037844387076, 1.000000000000000000, 0.8660254037844387076, 1.000000000000000000, 0.8660254037844387076, 1.000000000000000000, 0.8660254037844387076, 1.000000000000000000, 0.8660254037844387076, 1.000000000000000000, 0.8660254037844387076, 1.000000000000000000, 0.8660254037844387076, 1.000000000000000000, 0.8660254037844387076, 1.000000000000000000, 0.8660254037844387076, 1.000000000000000000, 0.8660254037844387076, 1.000000000000000000, 0.8660254037844387076, 1.000000000000000000, 0.8660254037844387076, 1.000000000000000000, 0.8660254037844387076, 1.000000000000000000, 0.8660254037844387076, 1.000000000000000000, 0.8660254037844387076, 1.000000000000000000, 0.8660254037844387076, 1.000000000000000000, 0.8660254037844387076, 1.000000000000000000, 0.8660254037844387076, 1.000000000000000000, 0.8660254037844387076, 1.000000000000000000, 0.8660254037844387076, 1.000000000000000000, 0.8660254037844387076, 1.000000000000000000, 0.8660254037844387076, 1.000000000000000000, 0.8660254037844387076, 1.000000000000000000, 0.8660254037844387076, 1.000000000000000000, 0.8660254037844387076, 1.000000000000000000, 0.8660254037844387076, 1.000000000000000000, 0.8660254037844387076, 1.000000000000000000, 0.8660254037844387076, 1.000000000000000000, 0.8660254037844387076, 1.000000000000000000, 0.8660254037844387076, 1.000000000000000000, 0.8660254037844387076, 1.000000000000000000, 0.8660254037844387076, 1.000000000000000000, 0.8660254037844387076, 1.000000000000000000, 0.8660254037844387076, 1.000000000000000000, 0.8660254037844387076, 1.000000000000000000, 0.8660254037844387076, 1.000000000000000000, 0.8660254037844387076, 1.000000000000000000, 0.8660254037844387076, 1.000000000000000000, 0.8660254037844387076, 1.000000000000000000, 0.8660254037844387076, 1.000000000000000000, 0.8660254037844387076, 1.000000000000000000, 0.8660254037844387076, 1.000000000000000000, 0.8660254037844387076, 1.000000000000000000, 0.8660254037844387076, 1.000000000000000000, 0.8660254037844387076, 1.000000000000000000, 0.8660254037844387076, 1.000000000000000000, 0.8660254037844387076, 1.000000000000000000, 0.8660254037844387076, 1.000000000000000000, 0.8660254037844387076, 1.000000000000000000, 0.8660254037844387076, 1.000000000000000000, 0.8660254037844387076, 1.000000000000000000, 0.8660254037844387076, 1.000000000000000000, 0.8660254037844387076, 1.000000000000000000, 0.8660254037844387076, 1.000000000000000000, 0.8660254037844387076, 1.000000000000000000, 0.8660254037844387076, 1.000000000000000000, 0.8660254037844387076, 1.000000000000000000, 0.8660254037844387076, 1.000000000000000000, 0.8660254037844387076, 1.000000000000000000, 0.8660254037844387076, 1.000000000000000000, 0.8660254037844387076, 1.000000000000000000, 0.8660254037844387076, 1.000000000000000000, 0.8660254037844387076, 1.000000000000000000, 0.8660254037844387076, 1.000000000000000000, 0.8660254037844387076, 1.000000000000000000, 0.8660254037844387076, 1.000000000000000000, 0.8660254037844387076, 1.000000000000000000, 0.8660254037844387076, 1.000000000000000000, 0.8660254037844387076, 1.000000000000000000, 0.8660254037844387076, 1.000000000000000000, 0.8660254037844387076, 1.000000000000000000, 0.8660254037844387076, 1.000000000000000000, 0.8660254037844387076, 1.000000000000000000, 0.8660254037844387076, 1.000000000000000000, 0.8660254037844387076, 1.000000000000000000, 0.8660254037844387076, 1.000000000000000000, 0.8660254037844387076, 1.000000000000000000, 0.8660254037844387076, 1.000000000000000000, 0.8660254037844387076, 1.000000000000000000, 0.8660254037844387076, 1.000000000000000000, 0.8660254037844387076, 1.000000000000000000, 0.8660254037844387076, 1.000000000000000000, 0.8660254037844387076, 1.000000000000000000, 0.8660254037844387076, 1.000000000000000000, 0.8660254037844387076, 1.000000000000000000, 0.8660254037844387076, 1.000000000000000000, 0.8660254037844387076, 1.000000000000000000, 0.8660254037844387076, 1.000000000000000000, 0.8660254037844387076, 1.000000000000000000, 0.8660254037844387076, 1.000000000000000000, 0.8660254037844387076, 1.000000000000000000, 0.8660254037844387076, 1.000000000000000000, 0.8660254037844387076, 1.000000000000000000, 0.8660254037844387076, 1.000000000000000000, 0.8660254037844387076, 1.000000000000000000, 0.8660254037844387076, 1.000000000000000000, 0.8660254037844387076, 1.000000000000000000, 0.8660254037844387076, 1.000000000000000000, 0.8660254037844387076, 1.000000000000000000, 0.8660254037844387076, 1.000000000000000000, 0.8660254037844387076, 1.000000000000000000, 0.8660254037844387076, 1.000000000000000000, 0.8660254037844387076, 1.000000000000000000, 0.8660254037844387076, 1.000000000000000000, 0.8660254037844387076, 1.000000000000000000, 0.8660254037844387076, 1.000000000000000000, 0.8660254037844387076, 1.000000000000000000, 0.8660254037844387076, 1.000000000000000000, 0.8660254037844387076, 1.000000000000000000, 0.8660254037844387076, 1.000000000000000000, 0.8660254037844387076, 1.000000000000000000, 0.8660254037844387076, 1.000000000000000000, 0.8660254037844387076, 1.000000000000000000, 0.8660254037844387076, 1.000000000000000000, 0.8660254037844387076, 1.000000000000000000, 0.8660254037844387076, 1.000000000000000000, 0.8660254037844387076, 1.000000000000000000, 0.8660254037844387076, 1.000000000000000000, 0.8660254037844387076, 1.000000000000000000, 0.8660254037844387076, 1.000000000000000000, 0.8660254037844387076, 1.000000000000000000, 0.8660254037844387076, 1.000000000000000000, 0.8660254037844387076, 1.000000000000000000, 0.8660254037844387076, 1.000000000000000000, 0.8660254037844387076, 1.000000000000000000, 0.8660254037844387076, 1.000000000000000000, 0.8660254037844387076, 1.000000000000000000, 0.8660254037844387076, 1.000000000000000000, 0.8660254037844387076, 1.000000000000000000, 0.8660254037844387076, 1.000000000000000000, 0.8660254037844387076, 1.000000000000000000, 0.8660254037844387076, 1.000000000000000000, 0.8660254037844387076, 1.000000000000000000, 0.8660254037844387076, 1.000000000000000000, 0.8660254037844387076, 1.000000000000000000, 0.8660254037844387076, 1.000000000000000000, 0.8660254037844387076, 1.000000000000000000, 0.8660254037844387076, 1.000000000000000000, 0.8660254037844387076, 1.000000000000000000, 0.8660254037844387076, 1.000000000000000000, 0.8660254037844387076, 1.000000000000000000, 0.8660254037844387076, 1.000000000000000000, 0.8660254037844387076, 1.000000000000000000, 0.8660254037844387076, 1.000000000000000000, 0.8660254037844387076, 1.000000000000000000, 0.8660254037844387076, 1.000000000000000000, 0.8660254037844387076, 1.000000000000000000, 0.8660254037844387076, 1.000000000000000000, 0.8660254037844387076, 1.000000000000000000, 0.8660254037844387076, 1.000000000000000000, 0.8660254037844387076, 1.000000000000000000, 0.8660254037844387076, 1.000000000000000000, 0.8660254037844387076, 1.000000000000000000, 0.8660254037844387076, 1.000000000000000000, 0.8660254037844387076, 1.000000000000000000, 0.8660254037844387076, 1.000000000000000000, 0.8660254037844387076, 1.000000000000000000, 0.8660254037844387076, 1.000000000000000000, 0.8660254037844387076, 1.000000000000000000, 0.8660254037844387076, 1.000000000000000000, 0.8660254037844387076, 1.000000000000000000, 0.8660254037844387076, 1.000000000000000000, 0.8660254037844387076, 1.000000000000000000, 0.8660254037844387076, 1.000000000000000000, 0.8660254037844387076, 1.000000000000000000, 0.8660254037844387076, 1.000000000000000000, 0.8660254037844387076, 1.000000000000000000, 0.8660254037844387076, 1.000000000000000000, 0.8660254037844387076, 1.000000000000000000, 0.8660254037844387076, 1.000000000000000000, 0.8660254037844387076, 1.000000000000000000, 0.8660254037844387076, 1.000000000000000000, 0.8660254037844387076, 1.000000000000000000, 0.8660254037844387076, 1.000000000000000000, 0.8660254037844387076, 1.000000000000000000, 0.8660254037844387076, 1.000000000000000000, 0.8660254037844387076, 1.000000000000000000, 0.8660254037844387076, 1.000000000000000000, 0.8660254037844387076, 1.000000000000000000, 0.8660254037844387076, 1.000000000000000000, 0.8660254037844387076, 1.000000000000000000, 0.8660254037844387076, 1.000000000000000000, 0.8660254037844387076, 1.000000000000000000, 0.8660254037844387076, 1.000000000000000000, 0.8660254037844387076, 1.000000000000000000, 0.8660254037844387076, 1.000000000000000000, 0.8660254037844387076, 1.000000000000000000, 0.8660254037844387076, 1.000000000000000000, 0.8660254037844387076, 1.000000000000000000, 0.8660254037844387076, 1.000000000000000000, 0.8660254037844387076, 1.000000000000000000, 0.8660254037844387076, 1.000000000000000000, 0.8660254037844387076, 1.000000000000000000, 0.8660254037844387076, 1.000000000000000000, 0.8660254037844387076, 1.000000000000000000, 0.8660254037844387076, 1.000000000000000000, 0.8660254037844387076, 1.000000000000000000, 0.8660254037844387076, 1.000000000000000000, 0.8660254037844387076, 1.000000000000000000, 0.8660254037844387076, 1.000000000000000000, 0.8660254037844387076, 1.000000000000000000, 0.8660254037844387076, 1.000000000000000000, 0.8660254037844387076, 1.000000000000000000, 0.8660254037844387076, 1.000000000000000000, 0.8660254037844387076, 1.000000000000000000, 0.8660254037844387076, 1.000000000000000000, 0.8660254037844387076, 1.000000000000000000, 0.8660254037844387076, 1.000000000000000000, 0.8660254037844387076, 1.000000000000000000, 0.8660254037844387076, 1.000000000000000000, 0.8660254037844387076, 1.000000000000000000, 0.8660254037844387076, 1.000000000000000000, 0.8660254037844387076, 1.000000000000000000, 0.8660254037844387076, 1.000000000000000000, 0.8660254037844387076, 1.000000000000000000, 0.8660254037844387076, 1.000000000000000000, 0.8660254037844387076, 1.000000000000000000, 0.8660254037844387076, 1.000000000000000000, 0.8660254037844387076, 1.000000000000000000, 0.8660254037844387076, 1.000000000000000000, 0.8660254037844387076, 1.000000000000000000, 0.8660254037844387076, 1.000000000000000000, 0.8660254037844387076, 1.000000000000000000, 0.8660254037844387076, 1.000000000000000000, 0.8660254037844387076, 1.000000000000000000, 0.8660254037844387076, 1.000000000000000000, 0.8660254037844387076, 1.000000000000000000, 0.8660254037844387076, 1.000000000000000000, 0.8660254037844387076, 1.000000000000000000, 0.8660254037844387076, 1.000000000000000000, 0.8660254037844387076, 1.000000000000000000, 0.8660254037844387076, 1.000000000000000000, 0.8660254037844387076, 1.000000000000000000, 0.8660254037844387076, 1.000000000000000000, 0.8660254037844387076, 1.000000000000000000, 0.8660254037844387076, 1.000000000000000000, 0.8660254037844387076, 1.000000000000000000, 0.8660254037844387076, 1.000000000000000000, 0.8660254037844387076, 1.000000000000000000, 0.8660254037844387076, 1.000000000000000000, 0.8660254037844387076, 1.000000000000000000, 0.8660254037844387076, 1.000000000000000000, 0.8660254037844387076, 1.000000000000000000, 0.8660254037844387076, 1.000000000000000000, 0.8660254037844387076, 1.000000000000000000, 0.8660254037844387076, 1.000000000000000000, 0.8660254037844387076, 1.000000000000000000, 0.8660254037844387076, 1.000000000000000000, 0.8660254037844387076, 1.000000000000000000, 0.8660254037844387076, 1.000000000000000000, 0.8660254037844387076, 1.000000000000000000, 0.8660254037844387076, 1.000000000000000000, 0.8660254037844387076, 1.000000000000000000, 0.8660254037844387076, 1.000000000000000000, 0.8660254037844387076, 1.000000000000000000, 0.8660254037844387076, 1.000000000000000000, 0.8660254037844387076, 1.000000000000000000),
 ( 1.000000000000000000, 0.8660254037844387076, 1.000000000000000000, 0.8660254037844387076, 1.000000000000000000, 0.8660254037844387076, 1.000000000000000000, 0.8660254037844387076, 1.000000000000000000, 0.8660254037844387076, 1.000000000000000000, 0.8660254037844387076, 1.000000000000000000, 0.8660254037844387076, 1.000000000000000000, 0.8660254037844387076, 1.000000000000000000, 0.8660254037844387076, 1.000000000000000000, 0.8660254037844387076, 1.000000000000000000, 0.8660254037844387076, 1.000000000000000000, 0.8660254037844387076, 1.000000000000000000, 0.8660254037844387076, 1.000000000000000000, 0.8660254037844387076, 1.000000000000000000, 0.8660254037844387076, 1.000000000000000000, 0.8660254037844387076, 1.000000000000000000, 0.8660254037844387076, 1.000000000000000000, 0.8660254037844387076, 1.000000000000000000, 0.8660254037844387076, 1.000000000000000000, 0.8660254037844387076, 1.000000000000000000, 0.8660254037844387076, 1.000000000000000000, 0.8660254037844387076, 1.000000000000000000, 0.8660254037844387076, 1.000000000000000000, 0.8660254037844387076, 1.000000000000000000, 0.8660254037844387076, 1.000000000000000000, 0.8660254037844387076, 1.000000000000000000, 0.8660254037844387076, 1.000000000000000000, 0.8660254037844387076, 1.000000000000000000, 0.8660254037844387076, 1.000000000000000000, 0.8660254037844387076, 1.000000000000000000, 0.8660254037844387076, 1.000000000000000000, 0.8660254037844387076, 1.000000000000000000, 0.8660254037844387076, 1.000000000000000000, 0.8660254037844387076, 1.000000000000000000, 0.8660254037844387076, 1.000000000000000000, 0.8660254037844387076, 1.000000000000000000, 0.8660254037844387076, 1.000000000000000000, 0.8660254037844387076, 1.000000000000000000, 0.8660254037844387076, 1.000000000000000000, 0.8660254037844387076, 1.000000000000000000, 0.8660254037844387076, 1.000000000000000000, 0.8660254037844387076, 1.000000000000000000, 0.8660254037844387076, 1.000000000000000000, 0.8660254037844387076, 1.000000000000000000, 0.8660254037844387076, 1.000000000000000000, 0.8660254037844387076, 1.000000000000000000, 0.8660254037844387076, 1.000000000000000000, 0.8660254037844387076, 1.000000000000000000, 0.8660254037844387076, 1.000000000000000000, 0.8660254037844387076, 1.000000000000000000, 0.8660254037844387076, 1.000000000000000000, 0.8660254037844387076, 1.000000000000000000, 0.8660254037844387076, 1.000000000000000000, 0.8660254037844387076, 1.000000000000000000, 0.8660254037844387076, 1.000000000000000000, 0.8660254037844387076, 1.000000000000000000, 0.8660254037844387076, 1.000000000000000000, 0.8660254037844387076, 1.000000000000000000, 0.8660254037844387076, 1.000000000000000000, 0.8660254037844387076, 1.000000000000000000, 0.8660254037844387076, 1.000000000000000000, 0.8660254037844387076, 1.000000000000000000, 0.8660254037844387076, 1.000000000000000000, 0.8660254037844387076, 1.000000000000000000, 0.8660254037844387076, 1.000000000000000000, 0.8660254037844387076, 1.000000000000000000, 0.8660254037844387076, 1.000000000000000000, 0.8660254037844387076, 1.000000000000000000, 0.8660254037844387076, 1.000000000000000000, 0.8660254037844387076, 1.000000000000000000, 0.8660254037844387076, 1.000000000000000000, 0.8660254037844387076, 1.000000000000000000, 0.8660254037844387076, 1.000000000000000000, 0.8660254037844387076, 1.000000000000000000, 0.8660254037844387076, 1.000000000000000000, 0.8660254037844387076, 1.000000000000000000, 0.8660254037844387076, 1.000000000000000000, 0.8660254037844387076, 1.000000000000000000, 0.8660254037844387076, 1.000000000000000000, 0.8660254037844387076, 1.000000000000000000, 0.8660254037844387076, 1.000000000000000000, 0.8660254037844387076, 1.000000000000000000, 0.8660254037844387076, 1.000000000000000000, 0.8660254037844387076, 1.000000000000000000, 0.8660254037844387076, 1.000000000000000000, 0.8660254037844387076, 1.000000000000000000, 0.8660254037844387076, 1.000000000000000000, 0.8660254037844387076, 1.000000000000000000, 0.8660254037844387076, 1.000000000000000000, 0.8660254037844387076, 1.000000000000000000, 0.8660254037844387076, 1.000000000000000000, 0.8660254037844387076, 1.000000000000000000, 0.8660254037844387076, 1.000000000000000000, 0.8660254037844387076, 1.000000000000000000, 0.8660254037844387076, 1.000000000000000000, 0.8660254037844387076, 1.000000000000000000, 0.8660254037844387076, 1.000000000000000000, 0.8660254037844387076, 1.000000000000000000, 0.8660254037844387076, 1.000000000000000000, 0.8660254037844387076, 1.000000000000000000, 0.8660254037844387076, 1.000000000000000000, 0.8660254037844387076, 1.000000000000000000, 0.8660254037844387076, 1.000000000000000000, 0.8660254037844387076, 1.000000000000000000, 0.8660254037844387076, 1.000000000000000000, 0.8660254037844387076, 1.000000000000000000, 0.8660254037844387076, 1.000000000000000000, 0.8660254037844387076, 1.000000000000000000, 0.8660254037844387076, 1.000000000000000000, 0.8660254037844387076, 1.000000000000000000, 0.8660254037844387076, 1.000000000000000000, 0.8660254037844387076, 1.000000000000000000, 0.8660254037844387076, 1.000000000000000000, 0.8660254037844387076, 1.000000000000000000, 0.8660254037844387076, 1.000000000000000000, 0.8660254037844387076, 1.000000000000000000, 0.8660254037844387076, 1.000000000000000000, 0.8660254037844387076, 1.000000000000000000, 0.8660254037844387076, 1.000000000000000000, 0.8660254037844387076, 1.000000000000000000, 0.8660254037844387076, 1.000000000000000000, 0.8660254037844387076, 1.000000000000000000, 0.8660254037844387076, 1.000000000000000000, 0.8660254037844387076, 1.000000000000000000, 0.8660254037844387076, 1.000000000000000000, 0.8660254037844387076, 1.000000000000000000, 0.8660254037844387076, 1.000000000000000000, 0.8660254037844387076, 1.000000000000000000, 0.8660254037844387076, 1.000000000000000000, 0.8660254037844387076, 1.000000000000000000, 0.8660254037844387076, 1.000000000000000000, 0.8660254037844387076, 1.000000000000000000, 0.8660254037844387076, 1.000000000000000000, 0.8660254037844387076, 1.000000000000000000, 0.8660254037844387076, 1.000000000000000000, 0.8660254037844387076, 1.000000000000000000, 0.8660254037844387076, 1.000000000000000000, 0.8660254037844387076, 1.000000000000000000, 0.8660254037844387076, 1.000000000000000000, 0.8660254037844387076, 1.000000000000000000, 0.8660254037844387076, 1.000000000000000000, 0.8660254037844387076, 1.000000000000000000, 0.8660254037844387076, 1.000000000000000000, 0.8660254037844387076, 1.000000000000000000, 0.8660254037844387076, 1.000000000000000000, 0.8660254037844387076, 1.000000000000000000, 0.8660254037844387076, 1.000000000000000000, 0.8660254037844387076, 1.000000000000000000, 0.8660254037844387076, 1.000000000000000000, 0.8660254037844387076, 1.000000000000000000, 0.8660254037844387076, 1.000000000000000000, 0.8660254037844387076, 1.000000000000000000, 0.8660254037844387076, 1.000000000000000000, 0.8660254037844387076, 1.000000000000000000, 0.8660254037844387076, 1.000000000000000000, 0.8660254037844387076, 1.000000000000000000, 0.8660254037844387076, 1.000000000000000000, 0.8660254037844387076, 1.000000000000000000, 0.8660254037844387076, 1.000000000000000000, 0.8660254037844387076, 1.000000000000000000, 0.8660254037844387076, 1.000000000000000000, 0.8660254037844387076, 1.000000000000000000, 0.8660254037844387076, 1.000000000000000000, 0.8660254037844387076, 1.000000000000000000, 0.8660254037844387076, 1.000000000000000000, 0.8660254037844387076, 1.000000000000000000, 0.8660254037844387076, 1.000000000000000000, 0.8660254037844387076, 1.000000000000000000, 0.8660254037844387076, 1.000000000000000000, 0.8660254037844387076, 1.000000000000000000, 0.8660254037844387076, 1.000000000000000000, 0.8660254037844387076, 1.000000000000000000, 0.8660254037844387076, 1.000000000000000000, 0.8660254037844387076, 1.000000000000000000, 0.8660254037844387076, 1.000000000000000000, 0.8660254037844387076, 1.000000000000000000, 0.8660254037844387076, 1.000000000000000000, 0.8660254037844387076, 1.000000000000000000, 0.8660254037844387076, 1.000000000000000000, 0.8660254037844387076, 1.000000000000000000, 0.8660254037844387076, 1.000000000000000000, 0.8660254037844387076, 1.000000000000000000, 0.8660254037844387076, 1.000000000000000000, 0.8660254037844387076, 1.000000000000000000, 0.8660254037844387076, 1.000000000000000000, 0.8660254037844387076, 1.000000000000000000, 0.8660254037844387076, 1.000000000000000000, 0.8660254037844387076, 1.000000000000000000, 0.8660254037844387076, 1.000000000000000000, 0.8660254037844387076, 1.000000000000000000, 0.8660254037844387076, 1.000000000000000000, 0.8660254037844387076, 1.000000000000000000, 0.8660254037844387076, 1.000000000000000000, 0.8660254037844387076, 1.000000000000000000, 0.8660254037844387076, 1.000000000000000000, 0.8660254037844387076, 1.000000000000000000, 0.8660254037844387076, 1.000000000000000000, 0.8660254037844387076, 1.000000000000000000, 0.8660254037844387076, 1.000000000000000000, 0.8660254037844387076, 1.000000000000000000, 0.8660254037844387076, 1.000000000000000000, 0.8660254037844387076, 1.000000000000000000, 0.8660254037844387076, 1.000000000000000000, 0.8660254037844387076, 1.000000000000000000, 0.8660254037844387076, 1.000000000000000000, 0.8660254037844387076, 1.000000000000000000, 0.8660254037844387076, 1.000000000000000000, 0.8660254037844387076, 1.000000000000000000, 0.8660254037844387076, 1.000000000000000000, 0.8660254037844387076, 1.000000000000000000, 0.8660254037844387076, 1.000000000000000000, 0.8660254037844387076, 1.000000000000000000, 0.8660254037844387076, 1.000000000000000000, 0.8660254037844387076, 1.000000000000000000, 0.8660254037844387076, 1.000000000000000000, 0.8660254037844387076, 1.000000000000000000, 0.8660254037844387076, 1.000000000000000000, 0.8660254037844387076, 1.000000000000000000, 0.8660254037844387076, 1.000000000000000000, 0.8660254037844387076, 1.000000000000000000, 0.8660254037844387076, 1.000000000000000000, 0.8660254037844387076, 1.000000000000000000, 0.8660254037844387076, 1.000000000000000000, 0.8660254037844387076, 1.000000000000000000, 0.8660254037844387076, 1.000000000000000000, 0.8660254037844387076, 1.000000000000000000, 0.8660254037844387076, 1.000000000000000000, 0.8660254037844387076, 1.000000000000000000, 0.8660254037844387076, 1.000000000000000000, 0.8660254037844387076, 1.000000000000000000, 0.8660254037844387076, 1.000000000000000000, 0.8660254037844387076, 1.000000000000000000, 0.8660254037844387076, 1.000000000000000000, 0.8660254037844387076, 1.000000000000000000, 0.8660254037844387076, 1.000000000000000000, 0.8660254037844387076, 1.000000000000000000, 0.8660254037844387076, 1.000000000000000000, 0.8660254037844387076, 1.000000000000000000, 0.8660254037844387076, 1.000000000000000000, 0.8660254037844387076, 1.000000000000000000, 0.8660254037844387076, 1.000000000000000000, 0.8660254037844387076, 1.000000000000000000, 0.8660254037844387076, 1.000000000000000000, 0.8660254037844387076, 1.000000000000000000, 0.8660254037844387076, 1.000000000000000000, 0.8660254037844387076, 1.000000000000000000, 0.8660254037844387076, 1.000000000000000000, 0.8660254037844387076, 1.000000000000000000, 0.8660254037844387076, 1.000000000000000000, 0.8660254037844387076, 1.000000000000000000, 0.8660254037844387076, 1.000000000000000000, 0.8660254037844387076, 1.000000000000000000, 0.8660254037844387076, 1.000000000000000000, 0.8660254037844387076, 1.000000000000000000, 0.8660254037844387076, 1.000000000000000000, 0.8660254037844387076, 1.000000000000000000, 0.8660254037844387076, 1.000000000000000000, 0.8660254037844387076, 1.000000000000000000, 0.8660254037844387076, 1.000000000000000000, 0.8660254037844387076, 1.000000000000000000, 0.8660254037844387076, 1.000000000000000000, 0.8660254037844387076, 1.000000000000000000, 0.8660254037844387076, 1.000000000000000000, 0.8660254037844387076, 1.000000000000000000, 0.8660254037844387076, 1.000000000000000000, 0.8660254037844387076, 1.000000000000000000, 0.8660254037844387076, 1.000000000000000000, 0.8660254037844387076, 1.000000000000000000, 0.8660254037844387076, 1.000000000000000000, 0.8660254037844387076, 1.000000000000000000, 0.8660254037844387076, 1.000000000000000000, 0.8660254037844387076, 1.000000000000000000, 0.8660254037844387076, 1.000000000000000000, 0.8660254037844387076, 1.000000000000000000, 0.8660254037844387076, 1.000000000000000000, 0.8660254037844387076, 1.000000000000000000, 0.8660254037844387076, 1.000000000000000000, 0.8660254037844387076, 1.000000000000000000, 0.8660254037844387076, 1.000000000000000000, 0.8660254037844387076, 1.000000000000000000, 0.8660254037844387076, 1.000000000000000000, 0.8660254037844387076, 1.000000000000000000, 0.8660254037844387076, 1.000000000000000000, 0.8660254037844387076, 1.000000000000000000, 0.8660254037844387076, 1.000000000000000000, 0.8660254037844387076, 1.000000000000000000, 0.8660254037844387076, 1.000000000000000000, 0.8660254037844387076, 1.000000000000000000, 0.8660254037844387076, 1.000000000000000000, 0.8660254037844387076, 1.000000000000000000, 0.8660254037844387076, 1.000000000000000000, 0.8660254037844387076, 1.000000000000000000, 0.8660254037844387076, 1.000000000000000000, 0.8660254037844387076, 1.000000000000000000, 0.8660254037844387076, 1.000000000000000000, 0.8660254037844387076, 1.000000000000000000, 0.8660254037844387076, 1.000000000000000000, 0.8660254037844387076, 1.000000000000000000, 0.8660254037844387076, 1.000000000000000000, 0.8660254037844387076, 1.000000000000000000, 0.8660254037844387076, 1.000000000000000000, 0.8660254037844387076, 1.000000000000000000, 0.8660254037844387076, 1.000000000000000000, 0.8660254037844387076, 1.000000000000000000, 0.8660254037844387076, 1.000000000000000000, 0.8660254037844387076, 1.000000000000000000, 0.8660254037844387076, 1.000000000000000000, 0.8660254037844387076, 1.000000000000000000, 0.8660254037844387076, 1.000000000000000000, 0.8660254037844387076, 1.000000000000000000, 0.8660254037844387076, 1.000000000000000000, 0.8660254037844387076, 1.000000000000000000, 0.8660254037844387076, 1.000000000000000000, 0.8660254037844387076, 1.000000000000000000, 0.8660254037844387076, 1.000000000000000000, 0.8660254037844387076, 1.000000000000000000, 0.8660254037844387076, 1.000000000000000000, 0.8660254037844387076, 1.000000000000000000, 0.8660254037844387076, 1.000000000000000000, 0.8660254037844387076, 1.000000000000000000, 0.8660254037844387076, 1.000000000000000000, 0.8660254037844387076, 1.000000000000000000, 0.8660254037844387076, 1.000000000000000000, 0.8660254037844387076, 1.000000000000000000, 0.8660254037844387076, 1.000000000000000000, 0.8660254037844387076, 1.000000000000000000, 0.8660254037844387076, 1.000000000000000000, 0.8660254037844387076, 1.000000000000000000, 0.8660254037844387076, 1.000000000000000000, 0.8660254037844387076, 1.000000000000000000, 0.8660254037844387076, 1.000000000000000000, 0.8660254037844387076, 1.000000000000000000, 0.8660254037844387076, 1.000000000000000000, 0.8660254037844387076, 1.000000000000000000, 0.8660254037844387076, 1.000000000000000000, 0.8660254037844387076, 1.000000000000000000, 0.8660254037844387076, 1.000000000000000000, 0.8660254037844387076, 1.000000000000000000, 0.8660254037844387076, 1.000000000000000000, 0.8660254037844387076, 1.000000000000000000, 0.8660254037844387076, 1.000000000000000000, 0.8660254037844387076, 1.000000000000000000, 0.8660254037844387076, 1.000000000000000000, 0.8660254037844387076, 1.000000000000000000, 0.8660254037844387076, 1.000000000000000000, 0.8660254037844387076, 1.000000000000000000, 0.8660254037844387076, 1.000000000000000000, 0.8660254037844387076, 1.000000000000000000, 0.8660254037844387076, 1.000000000000000000, 0.8660254037844387076, 1.000000000000000000, 0.8660254037844387076, 1.000000000000000000, 0.8660254037844387076, 1.000000000000000000, 0.8660254037844387076, 1.000000000000000000, 0.8660254037844387076, 1.000000000000000000, 0.8660254037844387076, 1.000000000000000000, 0.8660254037844387076, 1.000000000000000000, 0.8660254037844387076, 1.000000000000000000, 0.8660254037844387076, 1.000000000000000000, 0.8660254037844387076, 1.000000000000000000, 0.8660254037844387076, 1.000000000000000000) ) ) 
 REPRESENTATION_ITEM ( '' )  SURFACE ( )  );
#35410=CARTESIAN_POINT ( 'NONE',  ( 5.887500000000000178, -2.886751345948125991, -5.000000000000000000 ) ) ;
#35411=CARTESIAN_POINT ( 'NONE',  ( 26.62500000122903288, -5.773502691896255534, -1.060575238724906372E-15 ) ) ;
#35413=CARTESIAN_POINT ( 'NONE',  ( 22.34062500061451573, -3.027376345333610441, -5.243569643749999898 ) ) ;
#35414=CARTESIAN_POINT ( 'NONE',  ( 14.05312500061451431, 0.000000000000000000, 5.243569643749999010 ) ) ;
#35416=CARTESIAN_POINT ( 'NONE',  ( 8.709375000614517859, 0.000000000000000000, 5.243569643749999010 ) ) ;
#35417=CARTESIAN_POINT ( 'NONE',  ( 26.39999999999999858, 0.000000000000000000, 4.999999999999998224 ) ) ;
#35418=CARTESIAN_POINT ( 'NONE',  ( 23.21250000122903501, 4.330127018922192761, -2.499999999999997780 ) ) ;
#35419=CARTESIAN_POINT ( 'NONE',  ( 8.062500001229034652, 0.000000000000000000, 4.999999999999998224 ) ) ;
#35420=CARTESIAN_POINT ( 'NONE',  ( 11.22187500061451892, 3.027376345333613106, -5.243569643749998122 ) ) ;
#35421=CARTESIAN_POINT ( 'NONE',  ( 26.48437500061451644, 6.421520780324663323E-16, -5.243569643749999010 ) ) ;
#35422=CARTESIAN_POINT ( 'NONE',  ( 3.159375000614518036, 4.541064518000418104, -2.621784821874998173 ) ) ;
#35424=CARTESIAN_POINT ( 'NONE',  ( 22.20937500061451431, 0.000000000000000000, 5.243569643749999010 ) ) ;
#35425=CARTESIAN_POINT ( 'NONE',  ( 12.72187500061451537, 3.027376345333611329, 5.243569643749999010 ) ) ;
#35427=CARTESIAN_POINT ( 'NONE',  ( 24.75000000000000000, -4.330127018922190985, -2.500000000000001332 ) ) ;
#35429=CARTESIAN_POINT ( 'NONE',  ( 2.121784821874999061, 12.05937500061451750, -33.67503911421598417 ) ) ;
#35431=CARTESIAN_POINT ( 'NONE',  ( 14.16562500061451679, -6.054752690667223547, -1.112240025338166033E-15 ) ) ;
#35432=CARTESIAN_POINT ( 'NONE',  ( 6.975000000000002309, 4.330127018922191873, 2.499999999999999556 ) ) ;
#35434=CARTESIAN_POINT ( 'NONE',  ( 14.10000000000000142, 4.330127018922192761, -2.499999999999997780 ) ) ;
#35435=CARTESIAN_POINT ( 'NONE',  ( 8.484601909799253346E-16, 19.32500000122902861, 34.61880215351700230 ) ) ;
#35436=CARTESIAN_POINT ( 'NONE',  ( 14.85000000122903252, -2.886751345948129988, 4.999999999999997335 ) ) ;
#35437=CARTESIAN_POINT ( 'NONE',  ( 24.53437500061451715, -4.541064518000419881, 2.621784821874995952 ) ) ;
#35438=VERTEX_POINT ( 'NONE', #61755 ) ;
#35439=CARTESIAN_POINT ( 'NONE',  ( 20.65312500061451573, 4.541064518000418104, -2.621784821874998173 ) ) ;
#35440=CARTESIAN_POINT ( 'NONE',  ( 19.77187500061451786, 3.027376345333613106, -5.243569643749998122 ) ) ;
#35441=CARTESIAN_POINT ( 'NONE',  ( 5.100000000000000533, 4.330127018922192761, -2.499999999999997780 ) ) ;
#35442=CARTESIAN_POINT ( 'NONE',  ( 7.678125000614516082, 4.541064518000418104, 2.621784821874999949 ) ) ;
#35443=CARTESIAN_POINT ( 'NONE',  ( 22.45312500061451644, 4.541064518000418104, -2.621784821874998173 ) ) ;
#35444=CARTESIAN_POINT ( 'NONE',  ( 11.93437500061451573, -4.541064518000419881, 2.621784821874995952 ) ) ;
#35445=CARTESIAN_POINT ( 'NONE',  ( 16.62187500061451573, 3.027376345333613106, -5.243569643749998122 ) ) ;
#35446=CARTESIAN_POINT ( 'NONE',  ( -2.121784821874996840, 15.37812500061451892, 33.67503911421598417 ) ) ;
#35447=CARTESIAN_POINT ( 'NONE',  ( 18.82500000122903216, 2.886751345948126879, 4.999999999999999112 ) ) ;
#35449=CARTESIAN_POINT ( 'NONE',  ( 8.465625000614515727, 3.027376345333612662, -5.243569643749998122 ) ) ;
#35450=CARTESIAN_POINT ( 'NONE',  ( 3.646875000614520079, 6.054752690667223547, 3.707466751127219781E-16 ) ) ;
#35451=CARTESIAN_POINT ( 'NONE',  ( 28.49062500061451431, -3.027376345333614438, 5.243569643749998122 ) ) ;
#35452=CARTESIAN_POINT ( 'NONE',  ( 24.94687500061451502, -3.027376345333614438, 5.243569643749998122 ) ) ;
#35453=CARTESIAN_POINT ( 'NONE',  ( 18.06562500061451715, 3.027376345333611329, 5.243569643749999010 ) ) ;
#35454=CARTESIAN_POINT ( 'NONE',  ( 25.23750000122903359, -4.330127018922194537, 2.499999999999995559 ) ) ;
#35455=EDGE_CURVE ( 'NONE', #69491, #46824, #62233, .T. ) ;
#35456=CARTESIAN_POINT ( 'NONE',  ( 26.31562500061451715, -6.054752690667223547, -1.112240025338166033E-15 ) ) ;
#35457=CARTESIAN_POINT ( 'NONE',  ( 21.38437500061451502, -4.541064518000419881, 2.621784821874995952 ) ) ;
#35458=CARTESIAN_POINT ( 'NONE',  ( 15.44062500061451537, -3.027376345333614438, 5.243569643749998122 ) ) ;
#35459=CARTESIAN_POINT ( 'NONE',  ( 4.243569643749999010, 17.87187500061451573, 27.54997392385601174 ) ) ;
#35461=CARTESIAN_POINT ( 'NONE',  ( 22.04062500061451502, 6.054752690667223547, 3.707466751127219781E-16 ) ) ;
#35462=CARTESIAN_POINT ( 'NONE',  ( 3.375000001229033320, 2.886751345948129099, -4.999999999999998224 ) ) ;
#35463=VERTEX_POINT ( 'NONE', #40686 ) ;
#35464=CARTESIAN_POINT ( 'NONE',  ( 25.68750000000000000, -2.886751345948125991, -5.000000000000000000 ) ) ;
#35465=CARTESIAN_POINT ( 'NONE',  ( 4.000000000000000000, 13.88750000000000107, -27.69059892324149530 ) ) ;
#35467=CARTESIAN_POINT ( 'NONE',  ( 28.97812500061451502, -4.541064518000419881, 2.621784821874995952 ) ) ;
#35468=CARTESIAN_POINT ( 'NONE',  ( 6.928125000614516082, -4.541064518000419881, 2.621784821874995952 ) ) ;
#35469=CARTESIAN_POINT ( 'NONE',  ( 21.41250000122903074, 4.330127018922192761, -2.499999999999997780 ) ) ;
#35470=( BOUNDED_SURFACE ( )  B_SPLINE_SURFACE ( 1, 2, ( 
 ( #58419, #21373, #24810, #15460, #65716, #2295, #9934, #60899, #52896, #43560, #38005, #60527, #32472, #43927, #32835, #7831, #32103, #66453, #4766, #31740, #55005, #4411, #47356, #30368, #27299, #41453, #49833, #69888, #54636, #48735, #26940, #4041, #19253, #41808, #65345, #63971, #14735, #49465, #15102, #13354, #71998, #35895, #54278, #59799, #37277, #9205, #26196, #26566, #18891, #3672, #71258, #20638, #37638, #43196, #60161, #9571, #49106, #71635, #21008, #15830, #66082, #38375, #10302, #33195, #61626, #57168, #10665, #5849, #55734, #33551, #45019, #39845, #45743, #39110, #17284, #56458, #682, #5128, #27662, #67197, #68278, #11028, #5492, #56101, #39472, #28031, #50560, #22110, #66828, #40200, #56805, #28380, #23189, #17640, #50201, #72726, #62722, #33915, #50918, #6580, #51279, #44667, #16200, #16559, #29111, #316, #12115, #73087, #45377, #67554, #22825, #61272, #22468, #16917, #61995, #11395, #67913, #34639, #62359, #11755, #72357, #21738, #44299, #34273, #6211, #28739, #38751, #35730, #57538, #69369, #8388, #46465, #52006, #7657, #52726, #30196, #58251, #47549, #12481, #42013, #57891, #46831, #69002, #52365, #18726, #35008, #58981, #13927, #36465, #63448, #24644, #7300, #58618, #41290, #12834, #30561, #64533, #51645, #23554, #53088, #47189, #1769, #6939, #69720, #29470, #1046, #46102, #23916, #18364, #1407, #29830, #40934, #63801, #41644, #19089, #24283, #35368, #68639, #13191, #2132, #18002, #2482, #64163, #13551, #36098, #40560, #8025, #63079, #25007, #70078, #19453, #20926, #60443, #14651, #49022, #26854, #36829, #3958, #54194, #59716, #15746, #15383, #37925, #70451, #59343, #71552, #43478, #20550, #3591, #49386, #2848, #32382, #42379, #26113, #26481, #43107, #64901, #53458, #66003, #38285, #54556, #9853, #25377, #54922, #60080, #4330, #71917, #21292, #43844, #66371, #60813, #48288, #65633, #47922, #15020, #30917, #19827, #65262, #3222, #9123, #37558, #14291, #8754, #31287, #20187, #53829, #25751, #37192, #70812, #42742, #31660, #48652, #71177, #9491, #32020, #66746, #238, #51198, #44214, #33838, #28303, #5772, #50838, #11676, #23106, #49751, #22389, #34192, #45663, #22027, #22746, #45296, #16116, #21656, #68196, #32755, #17559, #61192, #44938, #39031, #67830, #67476, #38668, #10586, #72279, #55292, #16473, #11317, #56016, #56726, #17203, #16839, #4686, #39764, #27216, #44584, #50115, #33113, #55651, #61545, #39393, #40120, #10221, #5047, #67116, #27946, #10947, #27583, #72644, #33469, #5409, #50479, #6128, #73005, #61912, #56380, #62281, #28659, #601, #962, #69277, #23472, #23827, #35281, #30103, #36004, #29387, #7567, #46743, #64074, #46018, #17913, #57449, #58523, #51921, #68912, #1318, #29741, #46378, #18270, #12386, #57083, #30471, #47101, #18639, #13456, #7933, #68555, #40476, #53000, #24189, #41203, #47458, #41557, #62991, #6491, #34922, #19361, #63711, #2395, #40843, #35641, #57803, #13103, #51562, #63361, #12745, #6853, #52278, #7212, #24916, #1680, #58163, #69991, #62635, #12030, #52638, #2044, #24555, #69633, #18995, #34555, #29026, #71830, #36735, #42285, #71088, #43016, #20462, #48562, #37833, #2760, #32296, #48195, #37098, #59256, #42650, #59623, #25282, #49297, #4238, #26765, #53737, #14932, #70718, #48932, #9037, #3130, #20837, #54831, #41918, #13835, #43390, #37472, #65174, #70358, #59992, #47828, #31932, #14565, #20093, #14199, #64443, #8300, #65914, #19735, #9402, #31567, #64809, #54469, #9762, #8664, #65545, #3867, #26390, #71461, #15294, #36374, #30830, #54106, #60353, #58890, #25659, #53363, #31195, #3504, #26023, #6040, #43753, #28574, #72190, #33388, #50026, #56294, #5320, #55205, #4598, #10132, #66278, #27492, #22300, #67027, #45208, #11225, #27862, #21569, #15656, #38195, #66650, #16027, #27128, #72551, #38575, #10854, #33749, #39307, #44494, #61099, #51111, #33025, #4959, #21201, #152, #55924, #61460, #21938, #56645, #10497, #11589, #55563, #50393, #50749, #5684, #22658, #16387, #61820, #17114, #49662, #67388, #38942, #72918, #60722, #28220, #67741, #32664, #44123, #39673, #62193, #44852, #16750, #34106, #45576, #1960, #11943, #23738, #69191, #12660, #34468, #23018, #18551, #7849, #24103, #58074, #68107, #30011, #29654, #24467, #7483, #63626, #13016, #41470, #47015, #17823, #35195, #17473, #63268, #35554, #52554, #34833, #45930, #51829, #57719, #41116, #46651, #874, #62903, #69550, #18909, #63990, #13372, #40033, #7124, #35913, #58438, #12298, #30385, #508, #56996, #6403, #62546, #28935, #51471, #23381, #52191, #29299, #68461, #1593, #40384, #57359, #6765, #1233, #46286, #68827, #18184, #40753, #42928, #37012, #30742, #2312, #47374, #25189, #47733, #58803, #8577, #70272, #42560, #65452, #71001, #3038, #19643, #37746, #64723, #36647, #52914, #31847, #65087, #20007, #31105, #15206, #42199, #43304, #14108, #14478, #9314, #14844, #54383, #59169, #20377, #48840, #8213, #25937, #25569, #53645, #60264, #37385, #59908, #19272, #53274, #3778, #26303, #59535, #48109, #71371, #24827, #20746, #64357, #70632, #48477, #8947, #13748, #69905, #65824, #9678, #3417, #41826, #36289, #2672, #31480, #54022, #39220, #22215, #44769, #67, #5598, #49575, #44409, #54745, #21846, #67304, #16662, #66556, #4515, #10408, #66935, #50310, #5229, #32578, #21482, #11133, #55841, #38485, #27044, #17022, #71745, #33661, #38111, #27770, #4870, #15569, #61732, #22573, #66191, #72832, #56205, #28135, #50663, #26679, #72097, #44034, #60632, #61009, #15936, #16304, #45121, #67656, #55478, #32940, #39581, #27406, #49937, #32211, #62105, #38858, #72461, #61373, #4147, #10770, #49211, #33303, #21115, #43668, #10044, #55116, #68378, #29569, #7399, #17389, #57633, #34741, #40298, #69466, #69105, #18467, #51021, #39946, #52105, #24014, #1147, #57271, #29927, #56557 ),
 ( #28843, #23656, #34020, #46200, #46563, #41030, #45842, #56909, #62820, #68741, #1510, #7039, #11857, #784, #63546, #35109, #17739, #6314, #18824, #417, #12932, #62459, #35467, #6682, #68016, #57989, #52467, #45484, #1874, #24380, #46928, #41387, #11498, #5951, #22926, #18099, #28484, #34376, #23293, #51382, #12212, #29210, #51746, #40660, #63180, #12575, #41740, #2952, #19558, #25854, #48026, #24743, #47287, #52828, #35826, #70180, #65004, #36564, #14754, #53933, #70552, #64268, #13289, #2230, #19927, #69821, #25104, #59084, #31393, #37298, #30656, #8857, #42481, #65365, #19187, #13657, #58717, #59821, #53188, #42114, #2585, #31021, #47648, #64638, #36199, #58349, #31763, #48391, #14392, #9226, #54300, #8129, #14024, #3692, #25480, #36929, #48756, #42844, #8488, #7760, #53555, #20657, #59450, #26217, #3328, #70919, #20289, #71280, #63899, #30296, #32489, #66101, #10319, #26585, #33569, #32122, #38768, #5509, #28047, #50576, #21754, #32851, #72374, #10680, #27316, #49125, #60916, #73103, #38023, #43580, #44315, #66845, #16215, #49848, #39126, #4059, #56117, #49483, #38392, #60546, #43946, #55388, #71654, #43216, #65736, #15121, #55024, #61287, #72014, #50216, #4782, #4427, #22127, #37658, #60181, #9590, #44682, #33210, #66469, #21027, #55749, #15479, #5143, #15846, #54656, #72741, #9953, #26956, #21390, #27678, #67213, #16574, #61641, #11043, #30842, #68925, #57815, #41215, #7225, #46390, #18281, #63374, #40857, #12399, #24928, #29754, #53376, #22485, #57461, #12758, #8313, #67570, #53013, #52650, #47471, #30484, #13469, #36017, #64456, #70003, #35294, #35655, #45035, #13115, #58535, #7947, #52291, #1692, #24202, #58175, #41569, #69645, #23842, #46755, #2407, #47113, #69290, #18653, #16935, #62012, #19373, #29399, #19007, #63723, #6867, #41930, #13847, #51933, #64087, #36388, #58901, #39490, #34935, #1330, #7580, #30115, #2056, #24568, #14577, #43402, #37845, #36748, #14211, #60736, #25295, #10145, #53748, #14946, #31580, #60366, #60005, #59268, #8676, #64822, #47841, #9049, #3881, #48574, #26777, #65927, #9415, #3145, #70370, #19748, #48208, #70730, #31208, #54119, #20107, #65556, #15307, #20850, #26036, #42662, #32678, #37110, #59636, #2772, #54843, #37484, #43028, #3515, #38208, #65187, #66291, #71102, #31945, #32309, #9775, #4252, #20475, #49309, #71843, #25671, #48945, #54481, #26402, #42297, #21214, #43767, #71473, #15671, #166, #67754, #44866, #5334, #521, #27142, #56658, #66663, #27874, #50761, #67402, #16040, #4612, #22670, #62560, #5695, #39686, #16763, #45221, #17126, #50407, #21950, #40048, #67041, #38955, #55217, #34118, #39321, #22313, #33401, #17486, #50038, #45587, #72564, #61834, #11601, #62205, #6052, #61473, #28587, #51124, #61114, #28231, #72931, #10868, #11956, #23032, #68121, #21582, #10511, #49676, #72205, #11239, #33761, #44136, #38588, #33038, #55578, #56306, #4971, #27505, #44507, #16401, #55938, #41838, #58087, #18922, #6416, #64002, #63640, #35926, #41482, #24482, #47026, #2323, #7860, #51843, #46665, #57011, #24116, #69561, #13382, #68839, #6780, #12673, #69205, #52566, #7495, #34846, #23751, #58449, #30023, #40767, #29312, #19286, #887, #30397, #40397, #1973, #7138, #17836, #52926, #24838, #68474, #47386, #69916, #64368, #34481, #28948, #51487, #23394, #18564, #45943, #62916, #46300, #12311, #57372, #1246, #18196, #63281, #35210, #57732, #29668, #41130, #52204, #1605, #13029, #35568, #70283, #2684, #58815, #20018, #14856, #59547, #37757, #3792, #71012, #64734, #36301, #8226, #59179, #8588, #19654, #42572, #31118, #20390, #42210, #31492, #43679, #53657, #14122, #42939, #37395, #65464, #59919, #9689, #47747, #4160, #65100, #8959, #3050, #14489, #54033, #36660, #21126, #49223, #71757, #25581, #9325, #37023, #20757, #3428, #48120, #65835, #26690, #13758, #30754, #15218, #31858, #25948, #70643, #54393, #48488, #26314, #48853, #53285, #43315, #25200, #71383, #60275, #32222, #54756, #72472, #27783, #22936, #428, #38497, #27417, #10781, #49948, #15949, #61023, #32951, #10420, #55128, #67667, #21858, #66202, #15580, #27055, #55488, #51032, #4526, #72845, #49585, #44420, #38868, #33674, #39591, #4882, #11144, #50321, #17033, #72109, #21493, #66947, #62114, #16315, #61385, #33314, #55852, #5241, #22226, #44782, #60643, #34029, #50674, #67315, #11507, #56566, #44046, #66569, #5962, #16673, #39231, #38122, #45132, #61743, #10058, #56217, #32590, #5610, #28496, #28146, #78, #22583, #24024, #34388, #51757, #34750, #68387, #12586, #28853, #35836, #56920, #41042, #7772, #30307, #52840, #46573, #35120, #1520, #12943, #39956, #17748, #40307, #51392, #1157, #62829, #57644, #35479, #63556, #68751, #12222, #2239, #57284, #29221, #45496, #24391, #7050, #29580, #23666, #68027, #6691, #58359, #46211, #52117, #1885, #58001, #46941, #18109, #7409, #41398, #794, #18477, #40671, #63191, #17399, #29937, #52477, #11867, #23303, #69477, #18834, #69117, #63912, #13299, #62470, #6324, #45852, #48036, #20299, #36939, #58728, #47297, #42853, #32132, #48402, #9237, #69834, #54309, #53943, #26228, #31773, #14763, #37308, #65746, #71289, #42123, #59459, #19197, #14401, #59830, #3701, #59094, #70190, #2961, #8867, #65375, #70928, #25115, #14033, #48766, #20668, #31030, #19568, #9600, #64279, #43226, #30666, #15130, #70561, #8140, #37668, #60190, #53199, #54665, #24754, #41752, #13667, #36211, #2595, #47657, #31403, #64649, #36574, #8499, #53566, #25491, #19937, #42490, #65014, #3339, #25863, #55034, #16226, #32862, #39134, #61296, #38033, #60555, #66111, #49135, #10328, #5153, #49859, #28056, #67222, #10690, #4437, #26594, #62021, #71663, #11421, #26965, #38777, #55397, #61651, #33220, #9962, #32499, #15490, #21038, #4792, #27688, #72383, #50584, #16583, #55759 ) ),
 .UNSPECIFIED., .F., .F., .F. ) 
 B_SPLINE_SURFACE_WITH_KNOTS ( ( 2, 2 ),
 ( 3, 2, 2, 2, 2, 2, 2, 2, 2, 2, 2, 2, 2, 2, 2, 2, 2, 2, 2, 2, 2, 2, 2, 2, 2, 2, 2, 2, 2, 2, 2, 2, 2, 2, 2, 2, 2, 2, 2, 2, 2, 2, 2, 2, 2, 2, 2, 2, 2, 2, 2, 2, 2, 2, 2, 2, 2, 2, 2, 2, 2, 2, 2, 2, 2, 2, 2, 2, 2, 2, 2, 2, 2, 2, 2, 2, 2, 2, 2, 2, 2, 2, 2, 2, 2, 2, 2, 2, 2, 2, 2, 2, 2, 2, 2, 2, 2, 2, 2, 2, 2, 2, 2, 2, 2, 2, 2, 2, 2, 2, 2, 2, 2, 2, 2, 2, 2, 2, 2, 2, 2, 2, 2, 2, 2, 2, 2, 2, 2, 2, 2, 2, 2, 2, 2, 2, 2, 2, 2, 2, 2, 2, 2, 2, 2, 2, 2, 2, 2, 2, 2, 2, 2, 2, 2, 2, 2, 2, 2, 2, 2, 2, 2, 2, 2, 2, 2, 2, 2, 2, 2, 2, 2, 2, 2, 2, 2, 2, 2, 2, 2, 2, 2, 2, 2, 2, 2, 2, 2, 2, 2, 2, 2, 2, 2, 2, 2, 2, 2, 2, 2, 2, 2, 2, 2, 2, 2, 2, 2, 2, 2, 2, 2, 2, 2, 2, 2, 2, 2, 2, 2, 2, 2, 2, 2, 2, 2, 2, 2, 2, 2, 2, 2, 2, 2, 2, 2, 2, 2, 2, 2, 2, 2, 2, 2, 2, 2, 2, 2, 2, 2, 2, 2, 2, 2, 2, 2, 2, 2, 2, 2, 2, 2, 2, 2, 2, 2, 2, 2, 2, 2, 2, 2, 2, 2, 2, 2, 2, 2, 2, 2, 2, 2, 2, 2, 2, 2, 2, 2, 2, 2, 2, 2, 2, 2, 2, 2, 2, 2, 2, 2, 2, 2, 2, 2, 2, 2, 2, 2, 2, 2, 2, 2, 2, 2, 2, 2, 2, 2, 2, 2, 2, 2, 2, 2, 2, 2, 2, 2, 2, 2, 2, 2, 2, 2, 2, 2, 2, 2, 2, 2, 2, 2, 2, 2, 2, 2, 2, 2, 2, 2, 2, 2, 2, 2, 2, 2, 2, 2, 2, 3 ),
 ( 0.000000000000000000, 1.000000000000000000 ),
 ( 0.000000000000000000, 0.002777777777777777884, 0.005555555555555555768, 0.008333333333333333218, 0.01111111111111111154, 0.01388888888888888812, 0.01666666666666666644, 0.01944444444444444475, 0.02222222222222222307, 0.02500000000000000139, 0.02777777777777777624, 0.03055555555555555455, 0.03333333333333333287, 0.03611111111111110772, 0.03888888888888888951, 0.04166666666666666435, 0.04444444444444444614, 0.04722222222222222099, 0.05000000000000000278, 0.05277777777777777762, 0.05555555555555555247, 0.05833333333333333426, 0.06111111111111110911, 0.06388888888888888395, 0.06666666666666666574, 0.06944444444444444753, 0.07222222222222221544, 0.07499999999999999722, 0.07777777777777777901, 0.08055555555555556080, 0.08333333333333332871, 0.08611111111111111049, 0.08888888888888889228, 0.09166666666666666019, 0.09444444444444444198, 0.09722222222222222376, 0.1000000000000000056, 0.1027777777777777735, 0.1055555555555555552, 0.1083333333333333370, 0.1111111111111111049, 0.1138888888888888867, 0.1166666666666666685, 0.1194444444444444503, 0.1222222222222222182, 0.1250000000000000000, 0.1277777777777777679, 0.1305555555555555636, 0.1333333333333333315, 0.1361111111111110994, 0.1388888888888888951, 0.1416666666666666630, 0.1444444444444444309, 0.1472222222222222265, 0.1499999999999999944, 0.1527777777777777901, 0.1555555555555555580, 0.1583333333333333259, 0.1611111111111111216, 0.1638888888888888895, 0.1666666666666666574, 0.1694444444444444531, 0.1722222222222222210, 0.1749999999999999889, 0.1777777777777777846, 0.1805555555555555525, 0.1833333333333333204, 0.1861111111111111160, 0.1888888888888888840, 0.1916666666666666796, 0.1944444444444444475, 0.1972222222222222154, 0.2000000000000000111, 0.2027777777777777790, 0.2055555555555555469, 0.2083333333333333426, 0.2111111111111111105, 0.2138888888888888784, 0.2166666666666666741, 0.2194444444444444420, 0.2222222222222222099, 0.2250000000000000056, 0.2277777777777777735, 0.2305555555555555691, 0.2333333333333333370, 0.2361111111111111049, 0.2388888888888889006, 0.2416666666666666685, 0.2444444444444444364, 0.2472222222222222321, 0.2500000000000000000, 0.2527777777777777679, 0.2555555555555555358, 0.2583333333333333592, 0.2611111111111111271, 0.2638888888888888951, 0.2666666666666666630, 0.2694444444444444309, 0.2722222222222221988, 0.2750000000000000222, 0.2777777777777777901, 0.2805555555555555580, 0.2833333333333333259, 0.2861111111111110938, 0.2888888888888888618, 0.2916666666666666852, 0.2944444444444444531, 0.2972222222222222210, 0.2999999999999999889, 0.3027777777777777568, 0.3055555555555555802, 0.3083333333333333481, 0.3111111111111111160, 0.3138888888888888840, 0.3166666666666666519, 0.3194444444444444198, 0.3222222222222222432, 0.3250000000000000111, 0.3277777777777777790, 0.3305555555555555469, 0.3333333333333333148, 0.3361111111111111382, 0.3388888888888889062, 0.3416666666666666741, 0.3444444444444444420, 0.3472222222222222099, 0.3499999999999999778, 0.3527777777777778012, 0.3555555555555555691, 0.3583333333333333370, 0.3611111111111111049, 0.3638888888888888729, 0.3666666666666666408, 0.3694444444444444642, 0.3722222222222222321, 0.3750000000000000000, 0.3777777777777777679, 0.3805555555555555358, 0.3833333333333333592, 0.3861111111111111271, 0.3888888888888888951, 0.3916666666666666630, 0.3944444444444444309, 0.3972222222222221988, 0.4000000000000000222, 0.4027777777777777901, 0.4055555555555555580, 0.4083333333333333259, 0.4111111111111110938, 0.4138888888888888618, 0.4166666666666666852, 0.4194444444444444531, 0.4222222222222222210, 0.4249999999999999889, 0.4277777777777777568, 0.4305555555555555802, 0.4333333333333333481, 0.4361111111111111160, 0.4388888888888888840, 0.4416666666666666519, 0.4444444444444444198, 0.4472222222222222432, 0.4500000000000000111, 0.4527777777777777790, 0.4555555555555555469, 0.4583333333333333148, 0.4611111111111111382, 0.4638888888888889062, 0.4666666666666666741, 0.4694444444444444420, 0.4722222222222222099, 0.4749999999999999778, 0.4777777777777778012, 0.4805555555555555691, 0.4833333333333333370, 0.4861111111111111049, 0.4888888888888888729, 0.4916666666666666408, 0.4944444444444444642, 0.4972222222222222321, 0.5000000000000000000, 0.5027777777777777679, 0.5055555555555555358, 0.5083333333333333037, 0.5111111111111110716, 0.5138888888888888395, 0.5166666666666667185, 0.5194444444444444864, 0.5222222222222222543, 0.5250000000000000222, 0.5277777777777777901, 0.5305555555555555580, 0.5333333333333333259, 0.5361111111111110938, 0.5388888888888888618, 0.5416666666666666297, 0.5444444444444443976, 0.5472222222222222765, 0.5500000000000000444, 0.5527777777777778123, 0.5555555555555555802, 0.5583333333333333481, 0.5611111111111111160, 0.5638888888888888840, 0.5666666666666666519, 0.5694444444444444198, 0.5722222222222221877, 0.5749999999999999556, 0.5777777777777777235, 0.5805555555555556024, 0.5833333333333333703, 0.5861111111111111382, 0.5888888888888889062, 0.5916666666666666741, 0.5944444444444444420, 0.5972222222222222099, 0.5999999999999999778, 0.6027777777777777457, 0.6055555555555555136, 0.6083333333333332815, 0.6111111111111111605, 0.6138888888888889284, 0.6166666666666666963, 0.6194444444444444642, 0.6222222222222222321, 0.6250000000000000000, 0.6277777777777777679, 0.6305555555555555358, 0.6333333333333333037, 0.6361111111111110716, 0.6388888888888888395, 0.6416666666666667185, 0.6444444444444444864, 0.6472222222222222543, 0.6500000000000000222, 0.6527777777777777901, 0.6555555555555555580, 0.6583333333333333259, 0.6611111111111110938, 0.6638888888888888618, 0.6666666666666666297, 0.6694444444444443976, 0.6722222222222222765, 0.6750000000000000444, 0.6777777777777778123, 0.6805555555555555802, 0.6833333333333333481, 0.6861111111111111160, 0.6888888888888888840, 0.6916666666666666519, 0.6944444444444444198, 0.6972222222222221877, 0.6999999999999999556, 0.7027777777777777235, 0.7055555555555556024, 0.7083333333333333703, 0.7111111111111111382, 0.7138888888888889062, 0.7166666666666666741, 0.7194444444444444420, 0.7222222222222222099, 0.7249999999999999778, 0.7277777777777777457, 0.7305555555555555136, 0.7333333333333332815, 0.7361111111111111605, 0.7388888888888889284, 0.7416666666666666963, 0.7444444444444444642, 0.7472222222222222321, 0.7500000000000000000, 0.7527777777777777679, 0.7555555555555555358, 0.7583333333333333037, 0.7611111111111110716, 0.7638888888888888395, 0.7666666666666667185, 0.7694444444444444864, 0.7722222222222222543, 0.7750000000000000222, 0.7777777777777777901, 0.7805555555555555580, 0.7833333333333333259, 0.7861111111111110938, 0.7888888888888888618, 0.7916666666666666297, 0.7944444444444443976, 0.7972222222222222765, 0.8000000000000000444, 0.8027777777777778123, 0.8055555555555555802, 0.8083333333333333481, 0.8111111111111111160, 0.8138888888888888840, 0.8166666666666666519, 0.8194444444444444198, 0.8222222222222221877, 0.8249999999999999556, 0.8277777777777777235, 0.8305555555555556024, 0.8333333333333333703, 0.8361111111111111382, 0.8388888888888889062, 0.8416666666666666741, 0.8444444444444444420, 0.8472222222222222099, 0.8499999999999999778, 0.8527777777777777457, 0.8555555555555555136, 0.8583333333333332815, 0.8611111111111111605, 0.8638888888888889284, 0.8666666666666666963, 0.8694444444444444642, 0.8722222222222222321, 0.8750000000000000000, 0.8777777777777777679, 0.8805555555555555358, 0.8833333333333333037, 0.8861111111111110716, 0.8888888888888888395, 0.8916666666666667185, 0.8944444444444444864, 0.8972222222222222543, 0.9000000000000000222, 0.9027777777777777901, 0.9055555555555555580, 0.9083333333333333259, 0.9111111111111110938, 0.9138888888888888618, 0.9166666666666666297, 0.9194444444444443976, 0.9222222222222222765, 0.9250000000000000444, 0.9277777777777778123, 0.9305555555555555802, 0.9333333333333333481, 0.9361111111111111160, 0.9388888888888888840, 0.9416666666666666519, 0.9444444444444444198, 0.9472222222222221877, 0.9499999999999999556, 0.9527777777777777235, 0.9555555555555556024, 0.9583333333333333703, 0.9611111111111111382, 0.9638888888888889062, 0.9666666666666666741, 0.9694444444444444420, 0.9722222222222222099, 0.9749999999999999778, 0.9777777777777777457, 0.9805555555555555136, 0.9833333333333332815, 0.9861111111111111605, 0.9888888888888889284, 0.9916666666666666963, 0.9944444444444444642, 0.9972222222222222321, 1.000000000000000000 ),
 .UNSPECIFIED. ) 
 GEOMETRIC_REPRESENTATION_ITEM ( )  RATIONAL_B_SPLINE_SURFACE ( (
 ( 1.000000000000000000, 0.8660254037844387076, 1.000000000000000000, 0.8660254037844387076, 1.000000000000000000, 0.8660254037844387076, 1.000000000000000000, 0.8660254037844387076, 1.000000000000000000, 0.8660254037844387076, 1.000000000000000000, 0.8660254037844387076, 1.000000000000000000, 0.8660254037844387076, 1.000000000000000000, 0.8660254037844387076, 1.000000000000000000, 0.8660254037844387076, 1.000000000000000000, 0.8660254037844387076, 1.000000000000000000, 0.8660254037844387076, 1.000000000000000000, 0.8660254037844387076, 1.000000000000000000, 0.8660254037844387076, 1.000000000000000000, 0.8660254037844387076, 1.000000000000000000, 0.8660254037844387076, 1.000000000000000000, 0.8660254037844387076, 1.000000000000000000, 0.8660254037844387076, 1.000000000000000000, 0.8660254037844387076, 1.000000000000000000, 0.8660254037844387076, 1.000000000000000000, 0.8660254037844387076, 1.000000000000000000, 0.8660254037844387076, 1.000000000000000000, 0.8660254037844387076, 1.000000000000000000, 0.8660254037844387076, 1.000000000000000000, 0.8660254037844387076, 1.000000000000000000, 0.8660254037844387076, 1.000000000000000000, 0.8660254037844387076, 1.000000000000000000, 0.8660254037844387076, 1.000000000000000000, 0.8660254037844387076, 1.000000000000000000, 0.8660254037844387076, 1.000000000000000000, 0.8660254037844387076, 1.000000000000000000, 0.8660254037844387076, 1.000000000000000000, 0.8660254037844387076, 1.000000000000000000, 0.8660254037844387076, 1.000000000000000000, 0.8660254037844387076, 1.000000000000000000, 0.8660254037844387076, 1.000000000000000000, 0.8660254037844387076, 1.000000000000000000, 0.8660254037844387076, 1.000000000000000000, 0.8660254037844387076, 1.000000000000000000, 0.8660254037844387076, 1.000000000000000000, 0.8660254037844387076, 1.000000000000000000, 0.8660254037844387076, 1.000000000000000000, 0.8660254037844387076, 1.000000000000000000, 0.8660254037844387076, 1.000000000000000000, 0.8660254037844387076, 1.000000000000000000, 0.8660254037844387076, 1.000000000000000000, 0.8660254037844387076, 1.000000000000000000, 0.8660254037844387076, 1.000000000000000000, 0.8660254037844387076, 1.000000000000000000, 0.8660254037844387076, 1.000000000000000000, 0.8660254037844387076, 1.000000000000000000, 0.8660254037844387076, 1.000000000000000000, 0.8660254037844387076, 1.000000000000000000, 0.8660254037844387076, 1.000000000000000000, 0.8660254037844387076, 1.000000000000000000, 0.8660254037844387076, 1.000000000000000000, 0.8660254037844387076, 1.000000000000000000, 0.8660254037844387076, 1.000000000000000000, 0.8660254037844387076, 1.000000000000000000, 0.8660254037844387076, 1.000000000000000000, 0.8660254037844387076, 1.000000000000000000, 0.8660254037844387076, 1.000000000000000000, 0.8660254037844387076, 1.000000000000000000, 0.8660254037844387076, 1.000000000000000000, 0.8660254037844387076, 1.000000000000000000, 0.8660254037844387076, 1.000000000000000000, 0.8660254037844387076, 1.000000000000000000, 0.8660254037844387076, 1.000000000000000000, 0.8660254037844387076, 1.000000000000000000, 0.8660254037844387076, 1.000000000000000000, 0.8660254037844387076, 1.000000000000000000, 0.8660254037844387076, 1.000000000000000000, 0.8660254037844387076, 1.000000000000000000, 0.8660254037844387076, 1.000000000000000000, 0.8660254037844387076, 1.000000000000000000, 0.8660254037844387076, 1.000000000000000000, 0.8660254037844387076, 1.000000000000000000, 0.8660254037844387076, 1.000000000000000000, 0.8660254037844387076, 1.000000000000000000, 0.8660254037844387076, 1.000000000000000000, 0.8660254037844387076, 1.000000000000000000, 0.8660254037844387076, 1.000000000000000000, 0.8660254037844387076, 1.000000000000000000, 0.8660254037844387076, 1.000000000000000000, 0.8660254037844387076, 1.000000000000000000, 0.8660254037844387076, 1.000000000000000000, 0.8660254037844387076, 1.000000000000000000, 0.8660254037844387076, 1.000000000000000000, 0.8660254037844387076, 1.000000000000000000, 0.8660254037844387076, 1.000000000000000000, 0.8660254037844387076, 1.000000000000000000, 0.8660254037844387076, 1.000000000000000000, 0.8660254037844387076, 1.000000000000000000, 0.8660254037844387076, 1.000000000000000000, 0.8660254037844387076, 1.000000000000000000, 0.8660254037844387076, 1.000000000000000000, 0.8660254037844387076, 1.000000000000000000, 0.8660254037844387076, 1.000000000000000000, 0.8660254037844387076, 1.000000000000000000, 0.8660254037844387076, 1.000000000000000000, 0.8660254037844387076, 1.000000000000000000, 0.8660254037844387076, 1.000000000000000000, 0.8660254037844387076, 1.000000000000000000, 0.8660254037844387076, 1.000000000000000000, 0.8660254037844387076, 1.000000000000000000, 0.8660254037844387076, 1.000000000000000000, 0.8660254037844387076, 1.000000000000000000, 0.8660254037844387076, 1.000000000000000000, 0.8660254037844387076, 1.000000000000000000, 0.8660254037844387076, 1.000000000000000000, 0.8660254037844387076, 1.000000000000000000, 0.8660254037844387076, 1.000000000000000000, 0.8660254037844387076, 1.000000000000000000, 0.8660254037844387076, 1.000000000000000000, 0.8660254037844387076, 1.000000000000000000, 0.8660254037844387076, 1.000000000000000000, 0.8660254037844387076, 1.000000000000000000, 0.8660254037844387076, 1.000000000000000000, 0.8660254037844387076, 1.000000000000000000, 0.8660254037844387076, 1.000000000000000000, 0.8660254037844387076, 1.000000000000000000, 0.8660254037844387076, 1.000000000000000000, 0.8660254037844387076, 1.000000000000000000, 0.8660254037844387076, 1.000000000000000000, 0.8660254037844387076, 1.000000000000000000, 0.8660254037844387076, 1.000000000000000000, 0.8660254037844387076, 1.000000000000000000, 0.8660254037844387076, 1.000000000000000000, 0.8660254037844387076, 1.000000000000000000, 0.8660254037844387076, 1.000000000000000000, 0.8660254037844387076, 1.000000000000000000, 0.8660254037844387076, 1.000000000000000000, 0.8660254037844387076, 1.000000000000000000, 0.8660254037844387076, 1.000000000000000000, 0.8660254037844387076, 1.000000000000000000, 0.8660254037844387076, 1.000000000000000000, 0.8660254037844387076, 1.000000000000000000, 0.8660254037844387076, 1.000000000000000000, 0.8660254037844387076, 1.000000000000000000, 0.8660254037844387076, 1.000000000000000000, 0.8660254037844387076, 1.000000000000000000, 0.8660254037844387076, 1.000000000000000000, 0.8660254037844387076, 1.000000000000000000, 0.8660254037844387076, 1.000000000000000000, 0.8660254037844387076, 1.000000000000000000, 0.8660254037844387076, 1.000000000000000000, 0.8660254037844387076, 1.000000000000000000, 0.8660254037844387076, 1.000000000000000000, 0.8660254037844387076, 1.000000000000000000, 0.8660254037844387076, 1.000000000000000000, 0.8660254037844387076, 1.000000000000000000, 0.8660254037844387076, 1.000000000000000000, 0.8660254037844387076, 1.000000000000000000, 0.8660254037844387076, 1.000000000000000000, 0.8660254037844387076, 1.000000000000000000, 0.8660254037844387076, 1.000000000000000000, 0.8660254037844387076, 1.000000000000000000, 0.8660254037844387076, 1.000000000000000000, 0.8660254037844387076, 1.000000000000000000, 0.8660254037844387076, 1.000000000000000000, 0.8660254037844387076, 1.000000000000000000, 0.8660254037844387076, 1.000000000000000000, 0.8660254037844387076, 1.000000000000000000, 0.8660254037844387076, 1.000000000000000000, 0.8660254037844387076, 1.000000000000000000, 0.8660254037844387076, 1.000000000000000000, 0.8660254037844387076, 1.000000000000000000, 0.8660254037844387076, 1.000000000000000000, 0.8660254037844387076, 1.000000000000000000, 0.8660254037844387076, 1.000000000000000000, 0.8660254037844387076, 1.000000000000000000, 0.8660254037844387076, 1.000000000000000000, 0.8660254037844387076, 1.000000000000000000, 0.8660254037844387076, 1.000000000000000000, 0.8660254037844387076, 1.000000000000000000, 0.8660254037844387076, 1.000000000000000000, 0.8660254037844387076, 1.000000000000000000, 0.8660254037844387076, 1.000000000000000000, 0.8660254037844387076, 1.000000000000000000, 0.8660254037844387076, 1.000000000000000000, 0.8660254037844387076, 1.000000000000000000, 0.8660254037844387076, 1.000000000000000000, 0.8660254037844387076, 1.000000000000000000, 0.8660254037844387076, 1.000000000000000000, 0.8660254037844387076, 1.000000000000000000, 0.8660254037844387076, 1.000000000000000000, 0.8660254037844387076, 1.000000000000000000, 0.8660254037844387076, 1.000000000000000000, 0.8660254037844387076, 1.000000000000000000, 0.8660254037844387076, 1.000000000000000000, 0.8660254037844387076, 1.000000000000000000, 0.8660254037844387076, 1.000000000000000000, 0.8660254037844387076, 1.000000000000000000, 0.8660254037844387076, 1.000000000000000000, 0.8660254037844387076, 1.000000000000000000, 0.8660254037844387076, 1.000000000000000000, 0.8660254037844387076, 1.000000000000000000, 0.8660254037844387076, 1.000000000000000000, 0.8660254037844387076, 1.000000000000000000, 0.8660254037844387076, 1.000000000000000000, 0.8660254037844387076, 1.000000000000000000, 0.8660254037844387076, 1.000000000000000000, 0.8660254037844387076, 1.000000000000000000, 0.8660254037844387076, 1.000000000000000000, 0.8660254037844387076, 1.000000000000000000, 0.8660254037844387076, 1.000000000000000000, 0.8660254037844387076, 1.000000000000000000, 0.8660254037844387076, 1.000000000000000000, 0.8660254037844387076, 1.000000000000000000, 0.8660254037844387076, 1.000000000000000000, 0.8660254037844387076, 1.000000000000000000, 0.8660254037844387076, 1.000000000000000000, 0.8660254037844387076, 1.000000000000000000, 0.8660254037844387076, 1.000000000000000000, 0.8660254037844387076, 1.000000000000000000, 0.8660254037844387076, 1.000000000000000000, 0.8660254037844387076, 1.000000000000000000, 0.8660254037844387076, 1.000000000000000000, 0.8660254037844387076, 1.000000000000000000, 0.8660254037844387076, 1.000000000000000000, 0.8660254037844387076, 1.000000000000000000, 0.8660254037844387076, 1.000000000000000000, 0.8660254037844387076, 1.000000000000000000, 0.8660254037844387076, 1.000000000000000000, 0.8660254037844387076, 1.000000000000000000, 0.8660254037844387076, 1.000000000000000000, 0.8660254037844387076, 1.000000000000000000, 0.8660254037844387076, 1.000000000000000000, 0.8660254037844387076, 1.000000000000000000, 0.8660254037844387076, 1.000000000000000000, 0.8660254037844387076, 1.000000000000000000, 0.8660254037844387076, 1.000000000000000000, 0.8660254037844387076, 1.000000000000000000, 0.8660254037844387076, 1.000000000000000000, 0.8660254037844387076, 1.000000000000000000, 0.8660254037844387076, 1.000000000000000000, 0.8660254037844387076, 1.000000000000000000, 0.8660254037844387076, 1.000000000000000000, 0.8660254037844387076, 1.000000000000000000, 0.8660254037844387076, 1.000000000000000000, 0.8660254037844387076, 1.000000000000000000, 0.8660254037844387076, 1.000000000000000000, 0.8660254037844387076, 1.000000000000000000, 0.8660254037844387076, 1.000000000000000000, 0.8660254037844387076, 1.000000000000000000, 0.8660254037844387076, 1.000000000000000000, 0.8660254037844387076, 1.000000000000000000, 0.8660254037844387076, 1.000000000000000000, 0.8660254037844387076, 1.000000000000000000, 0.8660254037844387076, 1.000000000000000000, 0.8660254037844387076, 1.000000000000000000, 0.8660254037844387076, 1.000000000000000000, 0.8660254037844387076, 1.000000000000000000, 0.8660254037844387076, 1.000000000000000000, 0.8660254037844387076, 1.000000000000000000, 0.8660254037844387076, 1.000000000000000000, 0.8660254037844387076, 1.000000000000000000, 0.8660254037844387076, 1.000000000000000000, 0.8660254037844387076, 1.000000000000000000, 0.8660254037844387076, 1.000000000000000000, 0.8660254037844387076, 1.000000000000000000, 0.8660254037844387076, 1.000000000000000000, 0.8660254037844387076, 1.000000000000000000, 0.8660254037844387076, 1.000000000000000000, 0.8660254037844387076, 1.000000000000000000, 0.8660254037844387076, 1.000000000000000000, 0.8660254037844387076, 1.000000000000000000, 0.8660254037844387076, 1.000000000000000000, 0.8660254037844387076, 1.000000000000000000, 0.8660254037844387076, 1.000000000000000000, 0.8660254037844387076, 1.000000000000000000, 0.8660254037844387076, 1.000000000000000000, 0.8660254037844387076, 1.000000000000000000, 0.8660254037844387076, 1.000000000000000000, 0.8660254037844387076, 1.000000000000000000, 0.8660254037844387076, 1.000000000000000000, 0.8660254037844387076, 1.000000000000000000, 0.8660254037844387076, 1.000000000000000000, 0.8660254037844387076, 1.000000000000000000, 0.8660254037844387076, 1.000000000000000000, 0.8660254037844387076, 1.000000000000000000, 0.8660254037844387076, 1.000000000000000000, 0.8660254037844387076, 1.000000000000000000, 0.8660254037844387076, 1.000000000000000000, 0.8660254037844387076, 1.000000000000000000, 0.8660254037844387076, 1.000000000000000000, 0.8660254037844387076, 1.000000000000000000, 0.8660254037844387076, 1.000000000000000000, 0.8660254037844387076, 1.000000000000000000, 0.8660254037844387076, 1.000000000000000000, 0.8660254037844387076, 1.000000000000000000, 0.8660254037844387076, 1.000000000000000000, 0.8660254037844387076, 1.000000000000000000, 0.8660254037844387076, 1.000000000000000000, 0.8660254037844387076, 1.000000000000000000, 0.8660254037844387076, 1.000000000000000000, 0.8660254037844387076, 1.000000000000000000, 0.8660254037844387076, 1.000000000000000000, 0.8660254037844387076, 1.000000000000000000, 0.8660254037844387076, 1.000000000000000000, 0.8660254037844387076, 1.000000000000000000, 0.8660254037844387076, 1.000000000000000000, 0.8660254037844387076, 1.000000000000000000, 0.8660254037844387076, 1.000000000000000000, 0.8660254037844387076, 1.000000000000000000, 0.8660254037844387076, 1.000000000000000000, 0.8660254037844387076, 1.000000000000000000, 0.8660254037844387076, 1.000000000000000000, 0.8660254037844387076, 1.000000000000000000, 0.8660254037844387076, 1.000000000000000000, 0.8660254037844387076, 1.000000000000000000, 0.8660254037844387076, 1.000000000000000000, 0.8660254037844387076, 1.000000000000000000, 0.8660254037844387076, 1.000000000000000000, 0.8660254037844387076, 1.000000000000000000, 0.8660254037844387076, 1.000000000000000000, 0.8660254037844387076, 1.000000000000000000, 0.8660254037844387076, 1.000000000000000000, 0.8660254037844387076, 1.000000000000000000, 0.8660254037844387076, 1.000000000000000000, 0.8660254037844387076, 1.000000000000000000, 0.8660254037844387076, 1.000000000000000000, 0.8660254037844387076, 1.000000000000000000, 0.8660254037844387076, 1.000000000000000000, 0.8660254037844387076, 1.000000000000000000, 0.8660254037844387076, 1.000000000000000000, 0.8660254037844387076, 1.000000000000000000, 0.8660254037844387076, 1.000000000000000000, 0.8660254037844387076, 1.000000000000000000, 0.8660254037844387076, 1.000000000000000000, 0.8660254037844387076, 1.000000000000000000, 0.8660254037844387076, 1.000000000000000000, 0.8660254037844387076, 1.000000000000000000, 0.8660254037844387076, 1.000000000000000000, 0.8660254037844387076, 1.000000000000000000, 0.8660254037844387076, 1.000000000000000000, 0.8660254037844387076, 1.000000000000000000, 0.8660254037844387076, 1.000000000000000000, 0.8660254037844387076, 1.000000000000000000, 0.8660254037844387076, 1.000000000000000000, 0.8660254037844387076, 1.000000000000000000, 0.8660254037844387076, 1.000000000000000000, 0.8660254037844387076, 1.000000000000000000, 0.8660254037844387076, 1.000000000000000000, 0.8660254037844387076, 1.000000000000000000, 0.8660254037844387076, 1.000000000000000000, 0.8660254037844387076, 1.000000000000000000, 0.8660254037844387076, 1.000000000000000000, 0.8660254037844387076, 1.000000000000000000, 0.8660254037844387076, 1.000000000000000000, 0.8660254037844387076, 1.000000000000000000, 0.8660254037844387076, 1.000000000000000000, 0.8660254037844387076, 1.000000000000000000, 0.8660254037844387076, 1.000000000000000000, 0.8660254037844387076, 1.000000000000000000, 0.8660254037844387076, 1.000000000000000000, 0.8660254037844387076, 1.000000000000000000, 0.8660254037844387076, 1.000000000000000000, 0.8660254037844387076, 1.000000000000000000, 0.8660254037844387076, 1.000000000000000000, 0.8660254037844387076, 1.000000000000000000),
 ( 1.000000000000000000, 0.8660254037844387076, 1.000000000000000000, 0.8660254037844387076, 1.000000000000000000, 0.8660254037844387076, 1.000000000000000000, 0.8660254037844387076, 1.000000000000000000, 0.8660254037844387076, 1.000000000000000000, 0.8660254037844387076, 1.000000000000000000, 0.8660254037844387076, 1.000000000000000000, 0.8660254037844387076, 1.000000000000000000, 0.8660254037844387076, 1.000000000000000000, 0.8660254037844387076, 1.000000000000000000, 0.8660254037844387076, 1.000000000000000000, 0.8660254037844387076, 1.000000000000000000, 0.8660254037844387076, 1.000000000000000000, 0.8660254037844387076, 1.000000000000000000, 0.8660254037844387076, 1.000000000000000000, 0.8660254037844387076, 1.000000000000000000, 0.8660254037844387076, 1.000000000000000000, 0.8660254037844387076, 1.000000000000000000, 0.8660254037844387076, 1.000000000000000000, 0.8660254037844387076, 1.000000000000000000, 0.8660254037844387076, 1.000000000000000000, 0.8660254037844387076, 1.000000000000000000, 0.8660254037844387076, 1.000000000000000000, 0.8660254037844387076, 1.000000000000000000, 0.8660254037844387076, 1.000000000000000000, 0.8660254037844387076, 1.000000000000000000, 0.8660254037844387076, 1.000000000000000000, 0.8660254037844387076, 1.000000000000000000, 0.8660254037844387076, 1.000000000000000000, 0.8660254037844387076, 1.000000000000000000, 0.8660254037844387076, 1.000000000000000000, 0.8660254037844387076, 1.000000000000000000, 0.8660254037844387076, 1.000000000000000000, 0.8660254037844387076, 1.000000000000000000, 0.8660254037844387076, 1.000000000000000000, 0.8660254037844387076, 1.000000000000000000, 0.8660254037844387076, 1.000000000000000000, 0.8660254037844387076, 1.000000000000000000, 0.8660254037844387076, 1.000000000000000000, 0.8660254037844387076, 1.000000000000000000, 0.8660254037844387076, 1.000000000000000000, 0.8660254037844387076, 1.000000000000000000, 0.8660254037844387076, 1.000000000000000000, 0.8660254037844387076, 1.000000000000000000, 0.8660254037844387076, 1.000000000000000000, 0.8660254037844387076, 1.000000000000000000, 0.8660254037844387076, 1.000000000000000000, 0.8660254037844387076, 1.000000000000000000, 0.8660254037844387076, 1.000000000000000000, 0.8660254037844387076, 1.000000000000000000, 0.8660254037844387076, 1.000000000000000000, 0.8660254037844387076, 1.000000000000000000, 0.8660254037844387076, 1.000000000000000000, 0.8660254037844387076, 1.000000000000000000, 0.8660254037844387076, 1.000000000000000000, 0.8660254037844387076, 1.000000000000000000, 0.8660254037844387076, 1.000000000000000000, 0.8660254037844387076, 1.000000000000000000, 0.8660254037844387076, 1.000000000000000000, 0.8660254037844387076, 1.000000000000000000, 0.8660254037844387076, 1.000000000000000000, 0.8660254037844387076, 1.000000000000000000, 0.8660254037844387076, 1.000000000000000000, 0.8660254037844387076, 1.000000000000000000, 0.8660254037844387076, 1.000000000000000000, 0.8660254037844387076, 1.000000000000000000, 0.8660254037844387076, 1.000000000000000000, 0.8660254037844387076, 1.000000000000000000, 0.8660254037844387076, 1.000000000000000000, 0.8660254037844387076, 1.000000000000000000, 0.8660254037844387076, 1.000000000000000000, 0.8660254037844387076, 1.000000000000000000, 0.8660254037844387076, 1.000000000000000000, 0.8660254037844387076, 1.000000000000000000, 0.8660254037844387076, 1.000000000000000000, 0.8660254037844387076, 1.000000000000000000, 0.8660254037844387076, 1.000000000000000000, 0.8660254037844387076, 1.000000000000000000, 0.8660254037844387076, 1.000000000000000000, 0.8660254037844387076, 1.000000000000000000, 0.8660254037844387076, 1.000000000000000000, 0.8660254037844387076, 1.000000000000000000, 0.8660254037844387076, 1.000000000000000000, 0.8660254037844387076, 1.000000000000000000, 0.8660254037844387076, 1.000000000000000000, 0.8660254037844387076, 1.000000000000000000, 0.8660254037844387076, 1.000000000000000000, 0.8660254037844387076, 1.000000000000000000, 0.8660254037844387076, 1.000000000000000000, 0.8660254037844387076, 1.000000000000000000, 0.8660254037844387076, 1.000000000000000000, 0.8660254037844387076, 1.000000000000000000, 0.8660254037844387076, 1.000000000000000000, 0.8660254037844387076, 1.000000000000000000, 0.8660254037844387076, 1.000000000000000000, 0.8660254037844387076, 1.000000000000000000, 0.8660254037844387076, 1.000000000000000000, 0.8660254037844387076, 1.000000000000000000, 0.8660254037844387076, 1.000000000000000000, 0.8660254037844387076, 1.000000000000000000, 0.8660254037844387076, 1.000000000000000000, 0.8660254037844387076, 1.000000000000000000, 0.8660254037844387076, 1.000000000000000000, 0.8660254037844387076, 1.000000000000000000, 0.8660254037844387076, 1.000000000000000000, 0.8660254037844387076, 1.000000000000000000, 0.8660254037844387076, 1.000000000000000000, 0.8660254037844387076, 1.000000000000000000, 0.8660254037844387076, 1.000000000000000000, 0.8660254037844387076, 1.000000000000000000, 0.8660254037844387076, 1.000000000000000000, 0.8660254037844387076, 1.000000000000000000, 0.8660254037844387076, 1.000000000000000000, 0.8660254037844387076, 1.000000000000000000, 0.8660254037844387076, 1.000000000000000000, 0.8660254037844387076, 1.000000000000000000, 0.8660254037844387076, 1.000000000000000000, 0.8660254037844387076, 1.000000000000000000, 0.8660254037844387076, 1.000000000000000000, 0.8660254037844387076, 1.000000000000000000, 0.8660254037844387076, 1.000000000000000000, 0.8660254037844387076, 1.000000000000000000, 0.8660254037844387076, 1.000000000000000000, 0.8660254037844387076, 1.000000000000000000, 0.8660254037844387076, 1.000000000000000000, 0.8660254037844387076, 1.000000000000000000, 0.8660254037844387076, 1.000000000000000000, 0.8660254037844387076, 1.000000000000000000, 0.8660254037844387076, 1.000000000000000000, 0.8660254037844387076, 1.000000000000000000, 0.8660254037844387076, 1.000000000000000000, 0.8660254037844387076, 1.000000000000000000, 0.8660254037844387076, 1.000000000000000000, 0.8660254037844387076, 1.000000000000000000, 0.8660254037844387076, 1.000000000000000000, 0.8660254037844387076, 1.000000000000000000, 0.8660254037844387076, 1.000000000000000000, 0.8660254037844387076, 1.000000000000000000, 0.8660254037844387076, 1.000000000000000000, 0.8660254037844387076, 1.000000000000000000, 0.8660254037844387076, 1.000000000000000000, 0.8660254037844387076, 1.000000000000000000, 0.8660254037844387076, 1.000000000000000000, 0.8660254037844387076, 1.000000000000000000, 0.8660254037844387076, 1.000000000000000000, 0.8660254037844387076, 1.000000000000000000, 0.8660254037844387076, 1.000000000000000000, 0.8660254037844387076, 1.000000000000000000, 0.8660254037844387076, 1.000000000000000000, 0.8660254037844387076, 1.000000000000000000, 0.8660254037844387076, 1.000000000000000000, 0.8660254037844387076, 1.000000000000000000, 0.8660254037844387076, 1.000000000000000000, 0.8660254037844387076, 1.000000000000000000, 0.8660254037844387076, 1.000000000000000000, 0.8660254037844387076, 1.000000000000000000, 0.8660254037844387076, 1.000000000000000000, 0.8660254037844387076, 1.000000000000000000, 0.8660254037844387076, 1.000000000000000000, 0.8660254037844387076, 1.000000000000000000, 0.8660254037844387076, 1.000000000000000000, 0.8660254037844387076, 1.000000000000000000, 0.8660254037844387076, 1.000000000000000000, 0.8660254037844387076, 1.000000000000000000, 0.8660254037844387076, 1.000000000000000000, 0.8660254037844387076, 1.000000000000000000, 0.8660254037844387076, 1.000000000000000000, 0.8660254037844387076, 1.000000000000000000, 0.8660254037844387076, 1.000000000000000000, 0.8660254037844387076, 1.000000000000000000, 0.8660254037844387076, 1.000000000000000000, 0.8660254037844387076, 1.000000000000000000, 0.8660254037844387076, 1.000000000000000000, 0.8660254037844387076, 1.000000000000000000, 0.8660254037844387076, 1.000000000000000000, 0.8660254037844387076, 1.000000000000000000, 0.8660254037844387076, 1.000000000000000000, 0.8660254037844387076, 1.000000000000000000, 0.8660254037844387076, 1.000000000000000000, 0.8660254037844387076, 1.000000000000000000, 0.8660254037844387076, 1.000000000000000000, 0.8660254037844387076, 1.000000000000000000, 0.8660254037844387076, 1.000000000000000000, 0.8660254037844387076, 1.000000000000000000, 0.8660254037844387076, 1.000000000000000000, 0.8660254037844387076, 1.000000000000000000, 0.8660254037844387076, 1.000000000000000000, 0.8660254037844387076, 1.000000000000000000, 0.8660254037844387076, 1.000000000000000000, 0.8660254037844387076, 1.000000000000000000, 0.8660254037844387076, 1.000000000000000000, 0.8660254037844387076, 1.000000000000000000, 0.8660254037844387076, 1.000000000000000000, 0.8660254037844387076, 1.000000000000000000, 0.8660254037844387076, 1.000000000000000000, 0.8660254037844387076, 1.000000000000000000, 0.8660254037844387076, 1.000000000000000000, 0.8660254037844387076, 1.000000000000000000, 0.8660254037844387076, 1.000000000000000000, 0.8660254037844387076, 1.000000000000000000, 0.8660254037844387076, 1.000000000000000000, 0.8660254037844387076, 1.000000000000000000, 0.8660254037844387076, 1.000000000000000000, 0.8660254037844387076, 1.000000000000000000, 0.8660254037844387076, 1.000000000000000000, 0.8660254037844387076, 1.000000000000000000, 0.8660254037844387076, 1.000000000000000000, 0.8660254037844387076, 1.000000000000000000, 0.8660254037844387076, 1.000000000000000000, 0.8660254037844387076, 1.000000000000000000, 0.8660254037844387076, 1.000000000000000000, 0.8660254037844387076, 1.000000000000000000, 0.8660254037844387076, 1.000000000000000000, 0.8660254037844387076, 1.000000000000000000, 0.8660254037844387076, 1.000000000000000000, 0.8660254037844387076, 1.000000000000000000, 0.8660254037844387076, 1.000000000000000000, 0.8660254037844387076, 1.000000000000000000, 0.8660254037844387076, 1.000000000000000000, 0.8660254037844387076, 1.000000000000000000, 0.8660254037844387076, 1.000000000000000000, 0.8660254037844387076, 1.000000000000000000, 0.8660254037844387076, 1.000000000000000000, 0.8660254037844387076, 1.000000000000000000, 0.8660254037844387076, 1.000000000000000000, 0.8660254037844387076, 1.000000000000000000, 0.8660254037844387076, 1.000000000000000000, 0.8660254037844387076, 1.000000000000000000, 0.8660254037844387076, 1.000000000000000000, 0.8660254037844387076, 1.000000000000000000, 0.8660254037844387076, 1.000000000000000000, 0.8660254037844387076, 1.000000000000000000, 0.8660254037844387076, 1.000000000000000000, 0.8660254037844387076, 1.000000000000000000, 0.8660254037844387076, 1.000000000000000000, 0.8660254037844387076, 1.000000000000000000, 0.8660254037844387076, 1.000000000000000000, 0.8660254037844387076, 1.000000000000000000, 0.8660254037844387076, 1.000000000000000000, 0.8660254037844387076, 1.000000000000000000, 0.8660254037844387076, 1.000000000000000000, 0.8660254037844387076, 1.000000000000000000, 0.8660254037844387076, 1.000000000000000000, 0.8660254037844387076, 1.000000000000000000, 0.8660254037844387076, 1.000000000000000000, 0.8660254037844387076, 1.000000000000000000, 0.8660254037844387076, 1.000000000000000000, 0.8660254037844387076, 1.000000000000000000, 0.8660254037844387076, 1.000000000000000000, 0.8660254037844387076, 1.000000000000000000, 0.8660254037844387076, 1.000000000000000000, 0.8660254037844387076, 1.000000000000000000, 0.8660254037844387076, 1.000000000000000000, 0.8660254037844387076, 1.000000000000000000, 0.8660254037844387076, 1.000000000000000000, 0.8660254037844387076, 1.000000000000000000, 0.8660254037844387076, 1.000000000000000000, 0.8660254037844387076, 1.000000000000000000, 0.8660254037844387076, 1.000000000000000000, 0.8660254037844387076, 1.000000000000000000, 0.8660254037844387076, 1.000000000000000000, 0.8660254037844387076, 1.000000000000000000, 0.8660254037844387076, 1.000000000000000000, 0.8660254037844387076, 1.000000000000000000, 0.8660254037844387076, 1.000000000000000000, 0.8660254037844387076, 1.000000000000000000, 0.8660254037844387076, 1.000000000000000000, 0.8660254037844387076, 1.000000000000000000, 0.8660254037844387076, 1.000000000000000000, 0.8660254037844387076, 1.000000000000000000, 0.8660254037844387076, 1.000000000000000000, 0.8660254037844387076, 1.000000000000000000, 0.8660254037844387076, 1.000000000000000000, 0.8660254037844387076, 1.000000000000000000, 0.8660254037844387076, 1.000000000000000000, 0.8660254037844387076, 1.000000000000000000, 0.8660254037844387076, 1.000000000000000000, 0.8660254037844387076, 1.000000000000000000, 0.8660254037844387076, 1.000000000000000000, 0.8660254037844387076, 1.000000000000000000, 0.8660254037844387076, 1.000000000000000000, 0.8660254037844387076, 1.000000000000000000, 0.8660254037844387076, 1.000000000000000000, 0.8660254037844387076, 1.000000000000000000, 0.8660254037844387076, 1.000000000000000000, 0.8660254037844387076, 1.000000000000000000, 0.8660254037844387076, 1.000000000000000000, 0.8660254037844387076, 1.000000000000000000, 0.8660254037844387076, 1.000000000000000000, 0.8660254037844387076, 1.000000000000000000, 0.8660254037844387076, 1.000000000000000000, 0.8660254037844387076, 1.000000000000000000, 0.8660254037844387076, 1.000000000000000000, 0.8660254037844387076, 1.000000000000000000, 0.8660254037844387076, 1.000000000000000000, 0.8660254037844387076, 1.000000000000000000, 0.8660254037844387076, 1.000000000000000000, 0.8660254037844387076, 1.000000000000000000, 0.8660254037844387076, 1.000000000000000000, 0.8660254037844387076, 1.000000000000000000, 0.8660254037844387076, 1.000000000000000000, 0.8660254037844387076, 1.000000000000000000, 0.8660254037844387076, 1.000000000000000000, 0.8660254037844387076, 1.000000000000000000, 0.8660254037844387076, 1.000000000000000000, 0.8660254037844387076, 1.000000000000000000, 0.8660254037844387076, 1.000000000000000000, 0.8660254037844387076, 1.000000000000000000, 0.8660254037844387076, 1.000000000000000000, 0.8660254037844387076, 1.000000000000000000, 0.8660254037844387076, 1.000000000000000000, 0.8660254037844387076, 1.000000000000000000, 0.8660254037844387076, 1.000000000000000000, 0.8660254037844387076, 1.000000000000000000, 0.8660254037844387076, 1.000000000000000000, 0.8660254037844387076, 1.000000000000000000, 0.8660254037844387076, 1.000000000000000000, 0.8660254037844387076, 1.000000000000000000, 0.8660254037844387076, 1.000000000000000000, 0.8660254037844387076, 1.000000000000000000, 0.8660254037844387076, 1.000000000000000000, 0.8660254037844387076, 1.000000000000000000, 0.8660254037844387076, 1.000000000000000000, 0.8660254037844387076, 1.000000000000000000, 0.8660254037844387076, 1.000000000000000000, 0.8660254037844387076, 1.000000000000000000, 0.8660254037844387076, 1.000000000000000000, 0.8660254037844387076, 1.000000000000000000, 0.8660254037844387076, 1.000000000000000000, 0.8660254037844387076, 1.000000000000000000, 0.8660254037844387076, 1.000000000000000000, 0.8660254037844387076, 1.000000000000000000, 0.8660254037844387076, 1.000000000000000000, 0.8660254037844387076, 1.000000000000000000, 0.8660254037844387076, 1.000000000000000000, 0.8660254037844387076, 1.000000000000000000, 0.8660254037844387076, 1.000000000000000000, 0.8660254037844387076, 1.000000000000000000, 0.8660254037844387076, 1.000000000000000000, 0.8660254037844387076, 1.000000000000000000, 0.8660254037844387076, 1.000000000000000000, 0.8660254037844387076, 1.000000000000000000, 0.8660254037844387076, 1.000000000000000000, 0.8660254037844387076, 1.000000000000000000, 0.8660254037844387076, 1.000000000000000000, 0.8660254037844387076, 1.000000000000000000, 0.8660254037844387076, 1.000000000000000000, 0.8660254037844387076, 1.000000000000000000, 0.8660254037844387076, 1.000000000000000000, 0.8660254037844387076, 1.000000000000000000, 0.8660254037844387076, 1.000000000000000000, 0.8660254037844387076, 1.000000000000000000, 0.8660254037844387076, 1.000000000000000000, 0.8660254037844387076, 1.000000000000000000, 0.8660254037844387076, 1.000000000000000000, 0.8660254037844387076, 1.000000000000000000, 0.8660254037844387076, 1.000000000000000000, 0.8660254037844387076, 1.000000000000000000, 0.8660254037844387076, 1.000000000000000000, 0.8660254037844387076, 1.000000000000000000) ) ) 
 REPRESENTATION_ITEM ( '' )  SURFACE ( )  );
#35471=CARTESIAN_POINT ( 'NONE',  ( 26.31562500061451715, -6.054752690667223547, -1.112240025338166033E-15 ) ) ;
#35472=CARTESIAN_POINT ( 'NONE',  ( 24.82499999999999929, 6.123233995736764310E-16, -4.999999999999998224 ) ) ;
#35473=CARTESIAN_POINT ( 'NONE',  ( -3.999999999999999112, 15.16250000122903252, -30.00000000000000000 ) ) ;
#35474=EDGE_CURVE ( 'NONE', #58564, #37474, #48927, .T. ) ;
#35475=CARTESIAN_POINT ( 'NONE',  ( 29.09062500061451573, -3.027376345333610441, -5.243569643749999898 ) ) ;
#35476=CARTESIAN_POINT ( 'NONE',  ( 11.20312500061451644, 4.541064518000418104, -2.621784821874998173 ) ) ;
#35478=CARTESIAN_POINT ( 'NONE',  ( 25.04062500061451502, -3.027376345333610441, -5.243569643749999898 ) ) ;
#35479=CARTESIAN_POINT ( 'NONE',  ( 7.978125000614517681, 6.421520780324663323E-16, -5.243569643749999010 ) ) ;
#35480=CARTESIAN_POINT ( 'NONE',  ( 4.040625000614517681, 6.054752690667223547, 3.707466751127219781E-16 ) ) ;
#35482=ADVANCED_FACE ( 'NONE', ( #28506 ), #68398, .F. ) ;
#35483=CARTESIAN_POINT ( 'NONE',  ( 30.00000000000000000, 0.000000000000000000, 0.000000000000000000 ) ) ;
#35484=CARTESIAN_POINT ( 'NONE',  ( 12.71250000000000036, 2.886751345948129099, -4.999999999999998224 ) ) ;
#35486=CARTESIAN_POINT ( 'NONE',  ( 13.17187500061451999, 3.027376345333611329, 5.243569643749999010 ) ) ;
#35487=CARTESIAN_POINT ( 'NONE',  ( 10.38750000122903572, -4.330127018922194537, 2.499999999999995559 ) ) ;
#35488=CARTESIAN_POINT ( 'NONE',  ( 16.62187500061451573, 3.027376345333613106, -5.243569643749998122 ) ) ;
#35490=CARTESIAN_POINT ( 'NONE',  ( 9.271875000614516082, -6.054752690667223547, -1.112240025338166033E-15 ) ) ;
#35491=CARTESIAN_POINT ( 'NONE',  ( -2.121784821874999949, 12.52812500061451573, -33.67503911421598417 ) ) ;
#35494=DIRECTION ( 'NONE',  ( -1.000000000000000000, -0.000000000000000000, -0.000000000000000000 ) ) ;
#35495=CARTESIAN_POINT ( 'NONE',  ( 24.66562500061451502, 3.027376345333613106, -5.243569643749998122 ) ) ;
#35496=CARTESIAN_POINT ( 'NONE',  ( 11.17500000000000071, -4.330127018922194537, 2.499999999999995559 ) ) ;
#35497=CARTESIAN_POINT ( 'NONE',  ( 27.68437500061451573, -4.541064518000419881, 2.621784821874995952 ) ) ;
#35498=CARTESIAN_POINT ( 'NONE',  ( 23.28750000000000142, -2.886751345948129988, 4.999999999999997335 ) ) ;
#35499=CARTESIAN_POINT ( 'NONE',  ( 6.778125000614518392, 4.541064518000418104, 2.621784821874999949 ) ) ;
#35501=( BOUNDED_CURVE ( )  B_SPLINE_CURVE ( 2, ( #71089, #14200, #8665, #53738, #26766, #59993, #54470 ),
 .UNSPECIFIED., .F., .F. ) 
 B_SPLINE_CURVE_WITH_KNOTS ( ( 3, 2, 2, 3 ),
 ( 0.8250000000000000666, 0.8277777777777778345, 0.8305555555555557135, 0.8333333333333334814 ),
 .UNSPECIFIED. ) 
 CURVE ( )  GEOMETRIC_REPRESENTATION_ITEM ( )  RATIONAL_B_SPLINE_CURVE ( ( 0.9999999999999946709, 0.8660254037844440367, 1.000000000000000000, 0.8660254037844387076, 1.000000000000000000, 0.8660254037844333785, 1.000000000000005329 ) ) 
 REPRESENTATION_ITEM ( '' )  );
#35502=CARTESIAN_POINT ( 'NONE',  ( 15.98437500061451821, -4.541064518000419881, 2.621784821874995952 ) ) ;
#35504=CARTESIAN_POINT ( 'NONE',  ( 3.065625000614517592, 3.027376345333613106, -5.243569643749998122 ) ) ;
#35505=CARTESIAN_POINT ( 'NONE',  ( 8.109375000614518214, 4.541064518000418104, -2.621784821874998173 ) ) ;
#35506=ORIENTED_EDGE ( 'NONE', *, *, #1706, .T. ) ;
#35507=CARTESIAN_POINT ( 'NONE',  ( 19.32187500061451857, 3.027376345333613106, -5.243569643749998122 ) ) ;
#35508=CARTESIAN_POINT ( 'NONE',  ( 21.48750000000000071, -2.886751345948130876, 4.999999999999996447 ) ) ;
#35509=CARTESIAN_POINT ( 'NONE',  ( 26.84999999999999787, 0.000000000000000000, 4.999999999999998224 ) ) ;
#35510=CARTESIAN_POINT ( 'NONE',  ( 3.300000000000000711, 4.330127018922192761, -2.499999999999997780 ) ) ;
#35512=CARTESIAN_POINT ( 'NONE',  ( 27.89999999999999858, -4.330127018922190985, -2.500000000000001332 ) ) ;
#35514=CARTESIAN_POINT ( 'NONE',  ( 11.13750000000000284, -2.886751345948129988, 4.999999999999997335 ) ) ;
#35516=CARTESIAN_POINT ( 'NONE',  ( 25.19062500061451715, 6.054752690667223547, 3.707466751127219781E-16 ) ) ;
#35517=CARTESIAN_POINT ( 'NONE',  ( 14.69999999999999929, 0.000000000000000000, 4.999999999999998224 ) ) ;
#35518=CARTESIAN_POINT ( 'NONE',  ( 8.475000001229034297, 2.886751345948126879, 4.999999999999999112 ) ) ;
#35519=CARTESIAN_POINT ( 'NONE',  ( 7.190625000614518036, 6.054752690667223547, 3.707466751127219781E-16 ) ) ;
#35520=CARTESIAN_POINT ( 'NONE',  ( 22.76249999999999574, 2.886751345948126879, 4.999999999999999112 ) ) ;
#35521=CARTESIAN_POINT ( 'NONE',  ( 20.65312500061451573, 4.541064518000418104, -2.621784821874998173 ) ) ;
#35522=CARTESIAN_POINT ( 'NONE',  ( 4.072484567436527314, -2.900952432071136400, 4.105854893343868994 ) ) ;
#35523=CARTESIAN_POINT ( 'NONE',  ( 24.78750000122903074, -4.330127018922194537, 2.499999999999995559 ) ) ;
#35525=CARTESIAN_POINT ( 'NONE',  ( 5.850000000000001421, -4.330127018922190985, -2.500000000000001332 ) ) ;
#35527=CARTESIAN_POINT ( 'NONE',  ( 21.29062500061451502, -3.027376345333614438, 5.243569643749998122 ) ) ;
#35528=CARTESIAN_POINT ( 'NONE',  ( 27.85312500061451502, 4.541064518000418104, -2.621784821874998173 ) ) ;
#35529=CARTESIAN_POINT ( 'NONE',  ( 27.27187500061451431, -6.054752690667223547, -1.112240025338166033E-15 ) ) ;
#35530=CARTESIAN_POINT ( 'NONE',  ( 14.35312500061451679, 4.541064518000418104, -2.621784821874998173 ) ) ;
#35531=CARTESIAN_POINT ( 'NONE',  ( -4.243569643749999898, 9.865625000614594242, -32.45002607614398471 ) ) ;
#35532=CARTESIAN_POINT ( 'NONE',  ( 25.01250000122903216, 4.330127018922192761, -2.499999999999997780 ) ) ;
#35534=CARTESIAN_POINT ( 'NONE',  ( 17.61562500061451786, 3.027376345333611329, 5.243569643749999010 ) ) ;
#35535=CARTESIAN_POINT ( 'NONE',  ( 1.071796769724489895, 14.57990381179669903, -34.00000000000000000 ) ) ;
#35537=CARTESIAN_POINT ( 'NONE',  ( 2.887500001229035274, 6.123233995736764310E-16, -4.999999999999998224 ) ) ;
#35538=CARTESIAN_POINT ( 'NONE',  ( 10.39687500061451786, 6.054752690667223547, 3.707466751127219781E-16 ) ) ;
#35539=CARTESIAN_POINT ( 'NONE',  ( 9.721875000614517148, -6.054752690667223547, -1.112240025338166033E-15 ) ) ;
#35540=CARTESIAN_POINT ( 'NONE',  ( 18.87187500061451573, 3.027376345333613106, -5.243569643749998122 ) ) ;
#35541=ORIENTED_EDGE ( 'NONE', *, *, #9144, .F. ) ;
#35542=CARTESIAN_POINT ( 'NONE',  ( 9.862499999999997158, -5.773502691896255534, -1.060575238724906372E-15 ) ) ;
#35543=CARTESIAN_POINT ( 'NONE',  ( 23.69062500061451004, -3.027376345333610441, -5.243569643749999898 ) ) ;
#35544=CARTESIAN_POINT ( 'NONE',  ( 18.94687500061451502, 6.054752690667223547, 3.707466751127219781E-16 ) ) ;
#35545=CARTESIAN_POINT ( 'NONE',  ( 25.56562500061452070, 3.027376345333613106, -5.243569643749998122 ) ) ;
#35547=CARTESIAN_POINT ( 'NONE',  ( -3.999999999999999112, 14.60000000000000142, 30.00000000000000000 ) ) ;
#35548=CARTESIAN_POINT ( 'NONE',  ( 29.57812500061451644, 6.421520780324663323E-16, -5.243569643749999010 ) ) ;
#35549=CARTESIAN_POINT ( 'NONE',  ( 10.61250000122903536, 4.330127018922192761, -2.499999999999997780 ) ) ;
#35550=CARTESIAN_POINT ( 'NONE',  ( 4.162500001229033408, -4.330127018922190985, -2.500000000000001332 ) ) ;
#35551=CARTESIAN_POINT ( 'NONE',  ( -3.999999999999999112, 20.00000000000000000, -30.00000000000000000 ) ) ;
#35552=CARTESIAN_POINT ( 'NONE',  ( 27.97500000122903074, -5.773502691896255534, -1.060575238724906372E-15 ) ) ;
#35554=CARTESIAN_POINT ( 'NONE',  ( 9.759375000614516793, -4.541064518000417216, -2.621784821875001281 ) ) ;
#35556=CARTESIAN_POINT ( 'NONE',  ( 17.42812500061451786, 6.421520780324663323E-16, -5.243569643749999010 ) ) ;
#35557=CARTESIAN_POINT ( 'NONE',  ( 11.74687500061451573, 6.054752690667223547, 3.707466751127219781E-16 ) ) ;
#35558=CARTESIAN_POINT ( 'NONE',  ( 29.43750000122903288, 6.123233995736764310E-16, -4.999999999999998224 ) ) ;
#35559=CARTESIAN_POINT ( 'NONE',  ( 20.85937500061451644, 0.000000000000000000, 5.243569643749999010 ) ) ;
#35560=CARTESIAN_POINT ( 'NONE',  ( 6.946875000614517681, -3.027376345333614438, 5.243569643749998122 ) ) ;
#35561=CARTESIAN_POINT ( 'NONE',  ( 3.115864988711636752, -3.910524711353453142, -3.240904574695108842 ) ) ;
#35562=CARTESIAN_POINT ( 'NONE',  ( -5.810221930991193690E-16, 14.03750000000000142, 26.00000000000000355 ) ) ;
#35564=CARTESIAN_POINT ( 'NONE',  ( 8.240625000614516082, -3.027376345333614438, 5.243569643749998122 ) ) ;
#35565=CARTESIAN_POINT ( 'NONE',  ( 18.17812500061451786, -4.541064518000419881, 2.621784821874995952 ) ) ;
#35567=CARTESIAN_POINT ( 'NONE',  ( 6.075000001229034829, 2.886751345948129099, -4.999999999999998224 ) ) ;
#35568=CARTESIAN_POINT ( 'NONE',  ( 13.71562500061451750, -6.054752690667223547, -1.112240025338166033E-15 ) ) ;
#35569=CARTESIAN_POINT ( 'NONE',  ( 11.05312500061451608, -4.541064518000417216, -2.621784821875001281 ) ) ;
#35571=CARTESIAN_POINT ( 'NONE',  ( 13.79999999999999893, 0.000000000000000000, 4.999999999999998224 ) ) ;
#35572=CARTESIAN_POINT ( 'NONE',  ( 7.500000001229034652, 5.773502691896255534, 3.535250795749688894E-16 ) ) ;
#35573=CARTESIAN_POINT ( 'NONE',  ( 15.42187500061451821, 3.027376345333611329, 5.243569643749999010 ) ) ;
#35574=CARTESIAN_POINT ( 'NONE',  ( 18.37500000122903288, 2.886751345948126879, 4.999999999999999112 ) ) ;
#35576=CARTESIAN_POINT ( 'NONE',  ( -4.243569643749999898, 17.96562500061451573, -32.45002607614398471 ) ) ;
#35577=CARTESIAN_POINT ( 'NONE',  ( 4.080569135018654592, -2.889455923578380769, -4.080569135022440896 ) ) ;
#35578=CARTESIAN_POINT ( 'NONE',  ( 6.712500001229034119, 0.000000000000000000, 4.999999999999998224 ) ) ;
#35580=CARTESIAN_POINT ( 'NONE',  ( 4.866467007518584076, 1.159079983394287972, 4.866467007518584076 ) ) ;
#35581=CARTESIAN_POINT ( 'NONE',  ( 30.00000000000000000, 0.000000000000000000, 0.000000000000000000 ) ) ;
#35582=CARTESIAN_POINT ( 'NONE',  ( 17.37187500061451573, -6.054752690667223547, -1.112240025338166033E-15 ) ) ;
#35585=CARTESIAN_POINT ( 'NONE',  ( 14.99062500061451786, -3.027376345333614438, 5.243569643749998122 ) ) ;
#35587=DIRECTION ( 'NONE',  ( -1.000000000000000000, -0.000000000000000000, -0.000000000000000000 ) ) ;
#35588=CARTESIAN_POINT ( 'NONE',  ( 26.33437500061451431, -4.541064518000419881, 2.621784821874995952 ) ) ;
#35590=CARTESIAN_POINT ( 'NONE',  ( 10.30312500061451431, 4.541064518000418104, -2.621784821874998173 ) ) ;
#35591=CARTESIAN_POINT ( 'NONE',  ( 16.62187500061451573, 3.027376345333613106, -5.243569643749998122 ) ) ;
#35593=CARTESIAN_POINT ( 'NONE',  ( 26.61562500061451786, 3.027376345333611329, 5.243569643749999010 ) ) ;
#35594=CARTESIAN_POINT ( 'NONE',  ( 19.56562500061451715, -6.054752690667223547, -1.112240025338166033E-15 ) ) ;
#35595=CARTESIAN_POINT ( 'NONE',  ( 1.071796769724476572, 12.59509619066136921, -25.99999999999999289 ) ) ;
#35597=CARTESIAN_POINT ( 'NONE',  ( 9.262499999999999289, 2.886751345948126879, 4.999999999999999112 ) ) ;
#35598=CARTESIAN_POINT ( 'NONE',  ( 20.10000000122903074, 5.773502691896255534, 3.535250795749688894E-16 ) ) ;
#35599=CARTESIAN_POINT ( 'NONE',  ( -1.071796769724488563, 10.19240381056766687, 34.00000000000000000 ) ) ;
#35601=ORIENTED_EDGE ( 'NONE', *, *, #35886, .F. ) ;
#35602=CARTESIAN_POINT ( 'NONE',  ( 16.68750000000000000, -2.886751345948125991, -5.000000000000000000 ) ) ;
#35603=CARTESIAN_POINT ( 'NONE',  ( 21.52499999999999858, -4.330127018922194537, 2.499999999999995559 ) ) ;
#35604=CARTESIAN_POINT ( 'NONE',  ( 18.68437500061451928, -4.541064518000419881, 2.621784821874995952 ) ) ;
#35605=CARTESIAN_POINT ( 'NONE',  ( 14.27812500061451573, 6.421520780324663323E-16, -5.243569643749999010 ) ) ;
#35607=CYLINDRICAL_SURFACE ( 'NONE', #27774, 4.000000000000000000 ) ;
#35608=CARTESIAN_POINT ( 'NONE',  ( 7.078125000614516438, 6.421520780324663323E-16, -5.243569643749999010 ) ) ;
#35609=LINE ( 'NONE', #51529, #563 ) ;
#35610=CARTESIAN_POINT ( 'NONE',  ( 12.59999999999999964, -4.330127018922190985, -2.500000000000001332 ) ) ;
#35612=CARTESIAN_POINT ( 'NONE',  ( 4.243569643749999898, 18.64062500061451644, 32.45002607614398471 ) ) ;
#35613=CARTESIAN_POINT ( 'NONE',  ( 3.009375000614516793, -4.541064518000417216, -2.621784821875001281 ) ) ;
#35616=CARTESIAN_POINT ( 'NONE',  ( 26.55937500061451573, 4.541064518000418104, -2.621784821874998173 ) ) ;
#35617=ORIENTED_EDGE ( 'NONE', *, *, #60470, .F. ) ;
#35618=CARTESIAN_POINT ( 'NONE',  ( 21.10312500061451502, 4.541064518000418104, -2.621784821874998173 ) ) ;
#35619=CARTESIAN_POINT ( 'NONE',  ( 22.24687500061451217, -3.027376345333614438, 5.243569643749998122 ) ) ;
#35620=CARTESIAN_POINT ( 'NONE',  ( 9.001249775931846008E-16, 15.41562500061459495, -25.09994784771203058 ) ) ;
#35621=CARTESIAN_POINT ( 'NONE',  ( 5.765625000614519102, 3.027376345333613106, -5.243569643749998122 ) ) ;
#35623=CARTESIAN_POINT ( 'NONE',  ( 23.69062500061451004, -3.027376345333610441, -5.243569643749999898 ) ) ;
#35626=CARTESIAN_POINT ( 'NONE',  ( 16.69687500061451502, 6.054752690667223547, 3.707466751127219781E-16 ) ) ;
#35627=CARTESIAN_POINT ( 'NONE',  ( 18.45937500061451431, 4.541064518000418104, -2.621784821874998173 ) ) ;
#35628=CARTESIAN_POINT ( 'NONE',  ( 28.02187500061451431, 3.027376345333611329, 5.243569643749999010 ) ) ;
#35629=CARTESIAN_POINT ( 'NONE',  ( -4.243569643749998122, 15.84687500061451892, 32.45002607614398471 ) ) ;
#35630=CARTESIAN_POINT ( 'NONE',  ( 6.515625000614516438, -6.054752690667223547, -1.112240025338166033E-15 ) ) ;
#35631=CARTESIAN_POINT ( 'NONE',  ( 1.592000809091587073E-14, 16.28750000000000142, 26.00000000000000000 ) ) ;
#35632=CARTESIAN_POINT ( 'NONE',  ( 4.696875000614518569, -3.027376345333614438, 5.243569643749998122 ) ) ;
#35634=CARTESIAN_POINT ( 'NONE',  ( 4.678125000614516971, -4.541064518000419881, 2.621784821874995952 ) ) ;
#35635=CARTESIAN_POINT ( 'NONE',  ( 9.796875000614519990, -3.027376345333610441, -5.243569643749999898 ) ) ;
#35636=CARTESIAN_POINT ( 'NONE',  ( 17.32500000122903216, 2.886751345948129099, -4.999999999999998224 ) ) ;
#35637=CARTESIAN_POINT ( 'NONE',  ( 4.959375000614516971, 4.541064518000418104, -2.621784821874998173 ) ) ;
#35638=CARTESIAN_POINT ( 'NONE',  ( 8.203125000614518214, 0.000000000000000000, 5.243569643749999010 ) ) ;
#35641=CARTESIAN_POINT ( 'NONE',  ( 16.32187500061451502, 3.027376345333611329, 5.243569643749999010 ) ) ;
#35642=DIRECTION ( 'NONE',  ( -0.000000000000000000, -1.000000000000000000, -0.000000000000000000 ) ) ;
#35644=CARTESIAN_POINT ( 'NONE',  ( 25.79062500061451502, -3.027376345333614438, 5.243569643749998122 ) ) ;
#35645=CARTESIAN_POINT ( 'NONE',  ( 10.52812500061451750, -4.541064518000419881, 2.621784821874995952 ) ) ;
#35646=CARTESIAN_POINT ( 'NONE',  ( 26.97187500061451004, 3.027376345333612662, -5.243569643749998122 ) ) ;
#35647=CARTESIAN_POINT ( 'NONE',  ( 9.515625000614518214, 3.027376345333611329, 5.243569643749999010 ) ) ;
#35648=CARTESIAN_POINT ( 'NONE',  ( 26.28750000122903430, 6.123233995736764310E-16, -4.999999999999998224 ) ) ;
#35649=( BOUNDED_CURVE ( )  B_SPLINE_CURVE ( 2, ( #54138, #31601, #60022, #9434, #71493, #13868, #26422 ),
 .UNSPECIFIED., .F., .F. ) 
 B_SPLINE_CURVE_WITH_KNOTS ( ( 3, 2, 2, 3 ),
 ( 0.6333333333333333037, 0.6361111111111110716, 0.6388888888888889506, 0.6416666666666668295 ),
 .UNSPECIFIED. ) 
 CURVE ( )  GEOMETRIC_REPRESENTATION_ITEM ( )  RATIONAL_B_SPLINE_CURVE ( ( 1.000000000000000000, 0.8660254037844387076, 1.000000000000000000, 0.8660254037844387076, 1.000000000000000000, 0.8660254037844333785, 1.000000000000005329 ) ) 
 REPRESENTATION_ITEM ( '' )  );
#35650=CARTESIAN_POINT ( 'NONE',  ( 10.35000000122903074, -2.886751345948129988, 4.999999999999997335 ) ) ;
#35651=EDGE_CURVE ( 'NONE', #46824, #22963, #11335, .T. ) ;
#35652=CARTESIAN_POINT ( 'NONE',  ( 24.44062500061451715, -3.027376345333614438, 5.243569643749998122 ) ) ;
#35653=CARTESIAN_POINT ( 'NONE',  ( 4.243569643749999010, 13.31562500061451537, -32.45002607614398471 ) ) ;
#35654=CARTESIAN_POINT ( 'NONE',  ( 11.58750000122903501, 4.330127018922191873, 2.499999999999999556 ) ) ;
#35655=CARTESIAN_POINT ( 'NONE',  ( 22.26562500061451644, -6.054752690667223547, -1.112240025338166033E-15 ) ) ;
#35656=CARTESIAN_POINT ( 'NONE',  ( 12.11250000000000249, -5.773502691896255534, -1.060575238724906372E-15 ) ) ;
#35657=CARTESIAN_POINT ( 'NONE',  ( 20.35312500061451502, 0.000000000000000000, 5.243569643749999010 ) ) ;
#35659=CARTESIAN_POINT ( 'NONE',  ( 20.10000000000000142, 0.000000000000000000, 4.999999999999998224 ) ) ;
#35660=CARTESIAN_POINT ( 'NONE',  ( 13.80000000122903181, 5.773502691896255534, 3.535250795749688894E-16 ) ) ;
#35661=CARTESIAN_POINT ( 'NONE',  ( 11.42812500061451608, -4.541064518000419881, 2.621784821874995952 ) ) ;
#35662=CARTESIAN_POINT ( 'NONE',  ( 14.05312500061451431, 0.000000000000000000, 5.243569643749999010 ) ) ;
#35663=CARTESIAN_POINT ( 'NONE',  ( 25.61250000122903359, 0.000000000000000000, 4.999999999999998224 ) ) ;
#35664=CARTESIAN_POINT ( 'NONE',  ( 21.12187500061451573, 3.027376345333613106, -5.243569643749998122 ) ) ;
#35665=CARTESIAN_POINT ( 'NONE',  ( 3.507483327083503521, -3.563363679198468859, 3.507483327083555924 ) ) ;
#35666=CARTESIAN_POINT ( 'NONE',  ( 8.625000001229034652, -5.773502691896255534, -1.060575238724906372E-15 ) ) ;
#35667=CARTESIAN_POINT ( 'NONE',  ( 8.784375000614518925, -4.541064518000419881, 2.621784821874995952 ) ) ;
#35668=CARTESIAN_POINT ( 'NONE',  ( 26.03437500061451715, 6.421520780324663323E-16, -5.243569643749999010 ) ) ;
#35669=CARTESIAN_POINT ( 'NONE',  ( 30.00000000000000000, 0.000000000000000000, 0.000000000000000000 ) ) ;
#35670=CARTESIAN_POINT ( 'NONE',  ( 20.35312500061451502, 0.000000000000000000, 5.243569643749999010 ) ) ;
#35671=CARTESIAN_POINT ( 'NONE',  ( 26.44687500061451502, -3.027376345333610441, -5.243569643749999898 ) ) ;
#35673=CARTESIAN_POINT ( 'NONE',  ( 18.59999999999999787, 4.330127018922192761, -2.499999999999997780 ) ) ;
#35674=CARTESIAN_POINT ( 'NONE',  ( 8.184375000614515727, 4.541064518000418104, 2.621784821874999949 ) ) ;
#35675=CARTESIAN_POINT ( 'NONE',  ( 17.76562500061451644, -6.054752690667223547, -1.112240025338166033E-15 ) ) ;
#35677=CARTESIAN_POINT ( 'NONE',  ( -3.999999999999999112, 12.80000000000000071, -30.00000000000000000 ) ) ;
#35678=CARTESIAN_POINT ( 'NONE',  ( 28.56562500061451715, -6.054752690667223547, -1.112240025338166033E-15 ) ) ;
#35679=CARTESIAN_POINT ( 'NONE',  ( 3.984375000614517326, 6.421520780324663323E-16, -5.243569643749999010 ) ) ;
#35681=EDGE_CURVE ( 'NONE', #66787, #37790, #65813, .T. ) ;
#35682=LINE ( 'NONE', #58204, #12347 ) ;
#35683=CARTESIAN_POINT ( 'NONE',  ( 17.84999999999999787, 0.000000000000000000, 4.999999999999998224 ) ) ;
#35684=CARTESIAN_POINT ( 'NONE',  ( 21.47812500061451502, 6.421520780324663323E-16, -5.243569643749999010 ) ) ;
#35686=CARTESIAN_POINT ( 'NONE',  ( 25.34999999999999787, 4.330127018922192761, -2.499999999999997780 ) ) ;
#35687=( BOUNDED_CURVE ( )  B_SPLINE_CURVE ( 2, ( #22354, #21990, #50077, #44549, #67080, #16439, #33435 ),
 .UNSPECIFIED., .F., .F. ) 
 B_SPLINE_CURVE_WITH_KNOTS ( ( 3, 2, 2, 3 ),
 ( 0.8750000000000000000, 0.8777777777777777679, 0.8805555555555555358, 0.8833333333333333037 ),
 .UNSPECIFIED. ) 
 CURVE ( )  GEOMETRIC_REPRESENTATION_ITEM ( )  RATIONAL_B_SPLINE_CURVE ( ( 1.000000000000000000, 0.8660254037844387076, 1.000000000000000000, 0.8660254037844387076, 1.000000000000000000, 0.8660254037844387076, 1.000000000000000000 ) ) 
 REPRESENTATION_ITEM ( '' )  );
#35688=CARTESIAN_POINT ( 'NONE',  ( 26.48437500061451644, 6.421520780324663323E-16, -5.243569643749999010 ) ) ;
#35689=ORIENTED_EDGE ( 'NONE', *, *, #531, .F. ) ;
#35691=CARTESIAN_POINT ( 'NONE',  ( 13.56562500061451892, 3.027376345333611329, 5.243569643749999010 ) ) ;
#35692=CARTESIAN_POINT ( 'NONE',  ( 5.840625000614516615, 6.054752690667223547, 3.707466751127219781E-16 ) ) ;
#35694=CARTESIAN_POINT ( 'NONE',  ( 3.234375000614516438, 4.541064518000418104, 2.621784821874999949 ) ) ;
#35695=CARTESIAN_POINT ( 'NONE',  ( 16.08750000122903501, 4.330127018922191873, 2.499999999999999556 ) ) ;
#35696=CARTESIAN_POINT ( 'NONE',  ( 20.40000000000000213, 4.330127018922192761, -2.499999999999997780 ) ) ;
#35697=CARTESIAN_POINT ( 'NONE',  ( 28.98750000000000071, 5.773502691896255534, 3.535250795749688894E-16 ) ) ;
#35698=CARTESIAN_POINT ( 'NONE',  ( 3.834375000614519635, -4.541064518000419881, 2.621784821874995952 ) ) ;
#35699=CARTESIAN_POINT ( 'NONE',  ( 10.05937500061451750, 0.000000000000000000, 5.243569643749999010 ) ) ;
#35700=CARTESIAN_POINT ( 'NONE',  ( 18.57187500061451857, 3.027376345333611329, 5.243569643749999010 ) ) ;
#35701=ORIENTED_EDGE ( 'NONE', *, *, #30976, .T. ) ;
#35702=CARTESIAN_POINT ( 'NONE',  ( 2.896875000614518747, -3.027376345333614438, 5.243569643749998122 ) ) ;
#35703=CARTESIAN_POINT ( 'NONE',  ( 4.349999999999999645, 0.000000000000000000, 4.999999999999998224 ) ) ;
#35704=CARTESIAN_POINT ( 'NONE',  ( 4.359375000614517326, -4.541064518000417216, -2.621784821875001281 ) ) ;
#35705=CARTESIAN_POINT ( 'NONE',  ( 15.18750000000000000, -2.886751345948129988, 4.999999999999997335 ) ) ;
#35706=CARTESIAN_POINT ( 'NONE',  ( 13.00312500061451537, 4.541064518000418104, -2.621784821874998173 ) ) ;
#35709=CARTESIAN_POINT ( 'NONE',  ( 18.60000000122903430, -2.886751345948125991, -5.000000000000000000 ) ) ;
#35712=CARTESIAN_POINT ( 'NONE',  ( 8.503125000614515372, 4.541064518000418104, -2.621784821874998173 ) ) ;
#35713=CARTESIAN_POINT ( 'NONE',  ( 24.42187500061451999, 3.027376345333611329, 5.243569643749999010 ) ) ;
#35714=CARTESIAN_POINT ( 'NONE',  ( 19.57500000122903216, 2.886751345948129099, -4.999999999999997335 ) ) ;
#35715=CARTESIAN_POINT ( 'NONE',  ( 25.65937500061451715, 4.541064518000418104, -2.621784821874998173 ) ) ;
#35716=CARTESIAN_POINT ( 'NONE',  ( 8.025000000000000355, -4.330127018922194537, 2.499999999999995559 ) ) ;
#35717=CARTESIAN_POINT ( 'NONE',  ( -2.000000000000000000, 12.38750000122903394, 26.53589838486224650 ) ) ;
#35718=CARTESIAN_POINT ( 'NONE',  ( 14.24062500061451608, -3.027376345333610441, -5.243569643749999898 ) ) ;
#35719=CARTESIAN_POINT ( 'NONE',  ( 5.850000001229035185, -2.886751345948129988, 4.999999999999997335 ) ) ;
#35720=CARTESIAN_POINT ( 'NONE',  ( 17.78437500061451715, -4.541064518000419881, 2.621784821874995952 ) ) ;
#35721=CARTESIAN_POINT ( 'NONE',  ( 10.92187500061451644, 3.027376345333611329, 5.243569643749999010 ) ) ;
#35724=CARTESIAN_POINT ( 'NONE',  ( 11.35312500061451679, 0.000000000000000000, 5.243569643749999010 ) ) ;
#35725=CARTESIAN_POINT ( 'NONE',  ( 29.02500000122903145, 2.886751345948160630, -4.999999999999943157 ) ) ;
#35726=CARTESIAN_POINT ( 'NONE',  ( 23.02500000122903145, -5.773502691896255534, -1.060575238724906372E-15 ) ) ;
#35727=CARTESIAN_POINT ( 'NONE',  ( 13.50937500061451679, 4.541064518000418104, -2.621784821874998173 ) ) ;
#35728=CARTESIAN_POINT ( 'NONE',  ( 15.14062500061451644, -3.027376345333610441, -5.243569643749999898 ) ) ;
#35729=CARTESIAN_POINT ( 'NONE',  ( 11.66250000122903430, 0.000000000000000000, 4.999999999999998224 ) ) ;
#35730=CARTESIAN_POINT ( 'NONE',  ( 25.09687500061451715, -3.027376345333610441, -5.243569643749999898 ) ) ;
#35735=CARTESIAN_POINT ( 'NONE',  ( 2.121784821874999061, 16.10937500061451644, -33.67503911421598417 ) ) ;
#35736=CARTESIAN_POINT ( 'NONE',  ( 16.09687500061452070, -3.027376345333610441, -5.243569643749999898 ) ) ;
#35737=CARTESIAN_POINT ( 'NONE',  ( 18.41250000122903430, 0.000000000000000000, 4.999999999999998224 ) ) ;
#35738=EDGE_CURVE ( 'NONE', #37161, #58014, #41946, .T. ) ;
#35739=CARTESIAN_POINT ( 'NONE',  ( 12.98437500061451821, 6.421520780324663323E-16, -5.243569643749999010 ) ) ;
#35740=CARTESIAN_POINT ( 'NONE',  ( 4.243569643749999010, 19.16562500061451857, -32.45002607614398471 ) ) ;
#35741=CARTESIAN_POINT ( 'NONE',  ( 20.73750000122903359, -4.330127018922194537, 2.499999999999995559 ) ) ;
#35742=CARTESIAN_POINT ( 'NONE',  ( 13.67812500061451786, -4.541064518000419881, 2.621784821874995952 ) ) ;
#35743=VERTEX_POINT ( 'NONE', #12955 ) ;
#35744=EDGE_LOOP ( 'NONE', ( #65011, #48077, #40572, #66160 ) ) ;
#35745=CARTESIAN_POINT ( 'NONE',  ( 18.89999999999999858, -4.330127018922190985, -2.500000000000001332 ) ) ;
#35746=CARTESIAN_POINT ( 'NONE',  ( 13.54687500061451821, 6.054752690667223547, 3.707466751127219781E-16 ) ) ;
#35747=DIRECTION ( 'NONE',  ( 0.000000000000000000, 0.000000000000000000, 1.000000000000000000 ) ) ;
#35748=CARTESIAN_POINT ( 'NONE',  ( 11.66250000122903430, 0.000000000000000000, 4.999999999999998224 ) ) ;
#35749=CARTESIAN_POINT ( 'NONE',  ( 21.93750000122903288, 4.330127018922191873, 2.499999999999999556 ) ) ;
#35750=CARTESIAN_POINT ( 'NONE',  ( 17.31562500061451715, -6.054752690667223547, -1.112240025338166033E-15 ) ) ;
#35751=CARTESIAN_POINT ( 'NONE',  ( 23.46562500061451573, 3.027376345333611329, 5.243569643749999010 ) ) ;
#35752=CARTESIAN_POINT ( 'NONE',  ( 4.153125000614515727, 0.000000000000000000, 5.243569643749999010 ) ) ;
#35753=CARTESIAN_POINT ( 'NONE',  ( 27.15000000000000213, 4.330127018922192761, -2.499999999999997780 ) ) ;
#35754=CARTESIAN_POINT ( 'NONE',  ( 5.000000000001367795, -0.3826438005438348444, -5.034765704839666789 ) ) ;
#35756=FACE_OUTER_BOUND ( 'NONE', #34924, .T. ) ;
#35757=CARTESIAN_POINT ( 'NONE',  ( -5.810221930991193690E-16, 14.48749999999999893, -34.00000000000000000 ) ) ;
#35758=CARTESIAN_POINT ( 'NONE',  ( 2.121784821874999061, 17.00937500061451857, -33.67503911421598417 ) ) ;
#35759=CARTESIAN_POINT ( 'NONE',  ( 4.312500001229034652, 4.330127018922192761, -2.499999999999997780 ) ) ;
#35760=CARTESIAN_POINT ( 'NONE',  ( 5.175000000000002487, 4.330127018922191873, 2.499999999999999556 ) ) ;
#35761=CARTESIAN_POINT ( 'NONE',  ( 3.695974187897780983, 4.072863115247815635, 3.432733439617522642 ) ) ;
#35762=CARTESIAN_POINT ( 'NONE',  ( 10.47187500061451715, 3.027376345333611329, 5.243569643749999010 ) ) ;
#35763=CARTESIAN_POINT ( 'NONE',  ( 29.46562500061451573, -6.054752690667223547, -1.112240025338166033E-15 ) ) ;
#35764=DIRECTION ( 'NONE',  ( -0.000000000000000000, -1.000000000000000000, -0.000000000000000000 ) ) ;
#35766=CYLINDRICAL_SURFACE ( 'NONE', #64242, 4.999999999999998224 ) ;
#35767=CARTESIAN_POINT ( 'NONE',  ( 6.834375000614518747, 4.541064518000418104, 2.621784821874999949 ) ) ;
#35768=CARTESIAN_POINT ( 'NONE',  ( 10.09687500061451715, -3.027376345333614438, 5.243569643749998122 ) ) ;
#35769=CARTESIAN_POINT ( 'NONE',  ( 5.850000000000001421, -4.330127018922190985, -2.500000000000001332 ) ) ;
#35770=CARTESIAN_POINT ( 'NONE',  ( 2.121784821875001281, 15.90312500061459211, 33.67503911421598417 ) ) ;
#35772=CARTESIAN_POINT ( 'NONE',  ( 7.650000000000000355, -4.330127018922190985, -2.500000000000001332 ) ) ;
#35774=CARTESIAN_POINT ( 'NONE',  ( 19.22812500061451502, 6.421520780324663323E-16, -5.243569643749999010 ) ) ;
#35775=CARTESIAN_POINT ( 'NONE',  ( 12.55312500061451786, 4.541064518000418104, -2.621784821874998173 ) ) ;
#35777=CARTESIAN_POINT ( 'NONE',  ( 10.47187500061451715, 3.027376345333611329, 5.243569643749999010 ) ) ;
#35778=CARTESIAN_POINT ( 'NONE',  ( 26.69999999999999929, 4.330127018922192761, -2.499999999999997780 ) ) ;
#35779=CARTESIAN_POINT ( 'NONE',  ( 23.13750000122903216, 6.123233995736764310E-16, -4.999999999999998224 ) ) ;
#35780=CARTESIAN_POINT ( 'NONE',  ( 11.82187500061451679, 3.027376345333611329, 5.243569643749999010 ) ) ;
#35781=CARTESIAN_POINT ( 'NONE',  ( 25.62187500061451573, 3.027376345333613106, -5.243569643749998122 ) ) ;
#35783=CARTESIAN_POINT ( 'NONE',  ( 24.48750000122903359, 6.123233995736764310E-16, -4.999999999999998224 ) ) ;
#35784=CARTESIAN_POINT ( 'NONE',  ( 18.79687500061451644, -3.027376345333610441, -5.243569643749999898 ) ) ;
#35785=CARTESIAN_POINT ( 'NONE',  ( 11.78437500061451892, 4.541064518000418104, 2.621784821874999949 ) ) ;
#35787=CARTESIAN_POINT ( 'NONE',  ( 23.92499999999999716, 6.123233995736764310E-16, -4.999999999999998224 ) ) ;
#35789=CARTESIAN_POINT ( 'NONE',  ( 2.121784821874999061, 11.15937500061451715, -33.67503911421598417 ) ) ;
#35791=CARTESIAN_POINT ( 'NONE',  ( 15.66562500061451857, 3.027376345333613106, -5.243569643749998122 ) ) ;
#35792=CARTESIAN_POINT ( 'NONE',  ( 4.275000000000001243, 4.330127018922191873, 2.499999999999999556 ) ) ;
#35794=CARTESIAN_POINT ( 'NONE',  ( 1.626862140677534273E-15, 14.26250000000000107, -26.00000000000000355 ) ) ;
#35795=CARTESIAN_POINT ( 'NONE',  ( 14.66249999999999964, 2.886751345948126879, 4.999999999999999112 ) ) ;
#35796=CARTESIAN_POINT ( 'NONE',  ( -3.999999999999999556, 19.17500000122903359, 27.69059892324149530 ) ) ;
#35797=CARTESIAN_POINT ( 'NONE',  ( 14.66250000122903252, 4.330127018922192761, -2.499999999999997780 ) ) ;
#35799=CARTESIAN_POINT ( 'NONE',  ( 25.17187500061451644, 3.027376345333613106, -5.243569643749998122 ) ) ;
#35801=CARTESIAN_POINT ( 'NONE',  ( 19.26562500061451644, 3.027376345333613106, -5.243569643749998122 ) ) ;
#35802=CARTESIAN_POINT ( 'NONE',  ( 4.040625000614517681, 6.054752690667223547, 3.707466751127219781E-16 ) ) ;
#35803=CARTESIAN_POINT ( 'NONE',  ( 19.24687500061452283, -3.027376345333610441, -5.243569643749999898 ) ) ;
#35804=CARTESIAN_POINT ( 'NONE',  ( 3.825000000000001954, 4.330127018922191873, 2.499999999999999556 ) ) ;
#35805=CARTESIAN_POINT ( 'NONE',  ( 6.590625000614518392, -3.027376345333610441, -5.243569643749999898 ) ) ;
#35806=CARTESIAN_POINT ( 'NONE',  ( 20.95312500061451999, -4.541064518000417216, -2.621784821875001281 ) ) ;
#35807=CARTESIAN_POINT ( 'NONE',  ( 4.243569643749999010, 16.01562500061451644, 27.54997392385601174 ) ) ;
#35808=CARTESIAN_POINT ( 'NONE',  ( 18.33750000122903501, 4.330127018922191873, 2.499999999999999556 ) ) ;
#35810=CARTESIAN_POINT ( 'NONE',  ( 10.00312500061451715, 0.000000000000000000, 5.243569643749999010 ) ) ;
#35811=CARTESIAN_POINT ( 'NONE',  ( 2.934375000614518392, -4.541064518000419881, 2.621784821874995952 ) ) ;
#35812=CARTESIAN_POINT ( 'NONE',  ( 29.27812500061451573, 4.541064518000418104, 2.621784821874999949 ) ) ;
#35813=CARTESIAN_POINT ( 'NONE',  ( 22.09687500061451715, 6.054752690667223547, 3.707466751127219781E-16 ) ) ;
#35814=CARTESIAN_POINT ( 'NONE',  ( 15.70312500061451644, 4.541064518000418104, -2.621784821874998173 ) ) ;
#35815=CARTESIAN_POINT ( 'NONE',  ( 24.11250000122903359, 4.330127018922192761, -2.499999999999997780 ) ) ;
#35816=EDGE_CURVE ( 'NONE', #72158, #14259, #18839, .T. ) ;
#35817=CARTESIAN_POINT ( 'NONE',  ( 24.62812500061451715, 6.421520780324663323E-16, -5.243569643749999010 ) ) ;
#35818=CARTESIAN_POINT ( 'NONE',  ( 19.39687500061451786, 6.054752690667223547, 3.707466751127219781E-16 ) ) ;
#35819=CARTESIAN_POINT ( 'NONE',  ( 14.80312500061451608, 4.541064518000418104, -2.621784821874998173 ) ) ;
#35820=CARTESIAN_POINT ( 'NONE',  ( 2.121784821874999061, 17.00937500061451857, 26.32496088578401583 ) ) ;
#35821=CARTESIAN_POINT ( 'NONE',  ( 21.06562500061451715, 3.027376345333613106, -5.243569643749998122 ) ) ;
#35822=ORIENTED_EDGE ( 'NONE', *, *, #69064, .F. ) ;
#35823=CARTESIAN_POINT ( 'NONE',  ( 24.93750000000000355, 5.773502691896255534, 3.535250795749688894E-16 ) ) ;
#35824=CARTESIAN_POINT ( 'NONE',  ( 2.000000000000001332, 10.25000000000000000, -26.53589838486224650 ) ) ;
#35826=CARTESIAN_POINT ( 'NONE',  ( 27.77812500061451573, 6.421520780324663323E-16, -5.243569643749999010 ) ) ;
#35827=CARTESIAN_POINT ( 'NONE',  ( 7.453125000614516438, -4.541064518000417216, -2.621784821875001281 ) ) ;
#35828=CARTESIAN_POINT ( 'NONE',  ( 18.71250000122903145, 4.330127018922192761, -2.499999999999997780 ) ) ;
#35829=CARTESIAN_POINT ( 'NONE',  ( 28.30312500061451431, 4.541064518000418104, -2.621784821874998173 ) ) ;
#35830=CARTESIAN_POINT ( 'NONE',  ( 24.22500000000000142, -4.330127018922194537, 2.499999999999995559 ) ) ;
#35831=CARTESIAN_POINT ( 'NONE',  ( -2.000000000000000000, 15.53750000122903430, -33.46410161513775705 ) ) ;
#35832=CARTESIAN_POINT ( 'NONE',  ( 29.27812500061451573, 4.541064518000418104, 2.621784821874999949 ) ) ;
#35833=CARTESIAN_POINT ( 'NONE',  ( 10.64062500061451644, -3.027376345333610441, -5.243569643749999898 ) ) ;
#35835=CARTESIAN_POINT ( 'NONE',  ( 24.74062500061451786, 6.054752690667223547, 3.707466751127219781E-16 ) ) ;
#35836=CARTESIAN_POINT ( 'NONE',  ( 8.615625000614517859, 3.027376345333611329, 5.243569643749999010 ) ) ;
#35837=CARTESIAN_POINT ( 'NONE',  ( 3.553125000614516082, 4.541064518000418104, -2.621784821874998173 ) ) ;
#35839=CARTESIAN_POINT ( 'NONE',  ( 0.000000000000000000, 20.00000000000000000, -30.00000000000000000 ) ) ;
#35840=CARTESIAN_POINT ( 'NONE',  ( 12.52500000000000213, -4.330127018922194537, 2.499999999999995559 ) ) ;
#35842=CARTESIAN_POINT ( 'NONE',  ( 12.49687500061451573, -3.027376345333610441, -5.243569643749999898 ) ) ;
#35843=CARTESIAN_POINT ( 'NONE',  ( 9.937500001229032875, -4.330127018922194537, 2.499999999999995559 ) ) ;
#35844=CARTESIAN_POINT ( 'NONE',  ( 16.80937500061451573, 0.000000000000000000, 5.243569643749999010 ) ) ;
#35846=CARTESIAN_POINT ( 'NONE',  ( 7.434375000614519280, -4.541064518000419881, 2.621784821874995952 ) ) ;
#35847=CARTESIAN_POINT ( 'NONE',  ( -4.243569643749999898, 12.56562500061451715, -32.45002607614398471 ) ) ;
#35849=CARTESIAN_POINT ( 'NONE',  ( 24.48750000122903359, 6.123233995736764310E-16, -4.999999999999998224 ) ) ;
#35851=EDGE_LOOP ( 'NONE', ( #10083, #51658, #29577, #45454 ) ) ;
#35852=CARTESIAN_POINT ( 'NONE',  ( 23.50312500061451360, 0.000000000000000000, 5.243569643749999010 ) ) ;
#35853=CARTESIAN_POINT ( 'NONE',  ( 21.18750000122903288, -4.330127018922194537, 2.499999999999995559 ) ) ;
#35854=CARTESIAN_POINT ( 'NONE',  ( 26.67187500061451644, 3.027376345333611329, 5.243569643749999010 ) ) ;
#35855=CARTESIAN_POINT ( 'NONE',  ( 29.07187500061451502, -6.054752690667223547, -1.112240025338166033E-15 ) ) ;
#35856=CARTESIAN_POINT ( 'NONE',  ( 21.97500000000000142, -4.330127018922194537, 2.499999999999995559 ) ) ;
#35857=CARTESIAN_POINT ( 'NONE',  ( 6.478125000614516793, -4.541064518000419881, 2.621784821874995952 ) ) ;
#35859=CARTESIAN_POINT ( 'NONE',  ( 17.25937500061451502, 0.000000000000000000, 5.243569643749999010 ) ) ;
#35861=CARTESIAN_POINT ( 'NONE',  ( 3.590625000614518836, 6.054752690667223547, 3.707466751127219781E-16 ) ) ;
#35862=CARTESIAN_POINT ( 'NONE',  ( 7.396875000614519635, -3.027376345333614438, 5.243569643749998122 ) ) ;
#35863=EDGE_LOOP ( 'NONE', ( #21842, #49247, #47521, #6225, #66606, #21997, #47369, #32198, #72877, #41302, #792, #28495, #53034, #24952, #68652, #59674, #48835, #13145, #10297, #36840, #8918, #27810, #58631, #63600, #46421, #42334, #33929, #61987, #34417, #32589, #64759, #42348, #52524, #32354, #11542, #68386, #37894, #53098, #4276, #34737, #32982, #41600, #47701, #18614, #72591, #62558, #10230, #43436 ) ) ;
#35864=CARTESIAN_POINT ( 'NONE',  ( 19.65937500061451360, -4.541064518000417216, -2.621784821875001281 ) ) ;
#35866=CARTESIAN_POINT ( 'NONE',  ( 27.67499999999999716, 4.330127018922191873, 2.499999999999999556 ) ) ;
#35867=CARTESIAN_POINT ( 'NONE',  ( 27.49687500061451217, 6.054752690667223547, 3.707466751127219781E-16 ) ) ;
#35870=CARTESIAN_POINT ( 'NONE',  ( 10.23750000000000071, -2.886751345948129988, 4.999999999999997335 ) ) ;
#35872=CARTESIAN_POINT ( 'NONE',  ( 22.26562500061451644, -6.054752690667223547, -1.112240025338166033E-15 ) ) ;
#35873=CARTESIAN_POINT ( 'NONE',  ( 12.82499999999999929, 4.330127018922191873, 2.499999999999999556 ) ) ;
#35874=CARTESIAN_POINT ( 'NONE',  ( 9.225000001229034297, 2.886751345948129099, -4.999999999999998224 ) ) ;
#35875=CARTESIAN_POINT ( 'NONE',  ( 5.465625000614517504, 3.027376345333611329, 5.243569643749999010 ) ) ;
#35876=CARTESIAN_POINT ( 'NONE',  ( 22.83749999999999858, -2.886751345948129988, 4.999999999999997335 ) ) ;
#35877=CARTESIAN_POINT ( 'NONE',  ( 20.39062500061451644, -3.027376345333614438, 5.243569643749998122 ) ) ;
#35878=CARTESIAN_POINT ( 'NONE',  ( 23.51249999999999929, 2.886751345948112668, -5.000000000000024869 ) ) ;
#35879=CARTESIAN_POINT ( 'NONE',  ( 24.48750000122903359, 6.123233995736764310E-16, -4.999999999999998224 ) ) ;
#35881=CARTESIAN_POINT ( 'NONE',  ( 5.362500000000003375, -5.773502691896255534, -1.060575238724906372E-15 ) ) ;
#35882=ORIENTED_EDGE ( 'NONE', *, *, #19281, .F. ) ;
#35883=CARTESIAN_POINT ( 'NONE',  ( 19.60312500061451502, -4.541064518000417216, -2.621784821875001281 ) ) ;
#35884=CARTESIAN_POINT ( 'NONE',  ( 26.09062500061451573, 6.054752690667223547, 3.707466751127219781E-16 ) ) ;
#35885=CARTESIAN_POINT ( 'NONE',  ( 26.67187500061451644, 3.027376345333611329, 5.243569643749999010 ) ) ;
#35886=EDGE_CURVE ( 'NONE', #58433, #44258, #9379, .T. ) ;
#35887=CARTESIAN_POINT ( 'NONE',  ( 14.46562500061451750, 3.027376345333611329, 5.243569643749999010 ) ) ;
#35888=CARTESIAN_POINT ( 'NONE',  ( 9.515625000614518214, 3.027376345333611329, 5.243569643749999010 ) ) ;
#35890=( BOUNDED_SURFACE ( )  B_SPLINE_SURFACE ( 1, 2, ( 
 ( #14187, #53351, #2749, #70345, #25268, #19350, #54458, #36722, #60342, #30460, #64432, #19721, #15283, #41907, #37088, #13824, #64796, #3116, #71078, #3857, #42273, #48551, #14552, #26379, #36364, #58878, #47815, #71449, #59243, #8652, #25646, #70707, #48183, #42638, #65162, #24903, #20824, #14920, #59612, #43379, #65903, #8288, #30818, #37823, #9026, #31557, #52989, #9391, #54097, #47448, #3494, #69980, #26012, #65534, #37462, #59981, #55553, #61450, #71819, #16016, #72178, #32652, #50016, #66267, #141, #21191, #5307, #45197, #67728, #17102, #10844, #72540, #38931, #50383, #67015, #15644, #27483, #39662, #4588, #10122, #33378, #55914, #27852, #16376, #5674, #43742, #22647, #38564, #4949, #27117, #10485, #21928, #38185, #60709, #55193, #72908, #66638, #22290, #61087, #16740, #44484, #44112, #61809, #9751, #32285, #44842, #67377, #49651, #33014, #21558, #39295, #11212, #33739, #56285, #28210, #50739, #54819, #4225, #26753, #49286, #1948, #40739, #51817, #11931, #12285, #17461, #7113, #45564, #52180, #34818, #56633, #69180, #34093, #23369, #28921, #40020, #28563, #68449, #23726, #18897, #69538, #34456, #45917, #6754, #17811, #56984, #6388, #51459, #862, #51098, #63615, #40372, #62181, #11578, #23004, #62890, #47003, #495, #68815, #68095, #57348, #29287, #29642, #35543, #1220, #1582, #46276, #13005, #62534, #18171, #63256, #58063, #12648, #35183, #57708, #24091, #46638, #18541, #41105, #6029, #29998, #7472, #52539, #24454, #14831, #47362, #19259, #65440, #3024, #19996, #26292, #20366, #41814, #58425, #13736, #71359, #25557, #37373, #70259, #14467, #14096, #42549, #30374, #47720, #30731, #64344, #8566, #24816, #31834, #52903, #37000, #3767, #48829, #41459, #65076, #31094, #70621, #8936, #48098, #69894, #59158, #63977, #36278, #58792, #59523, #31466, #54010, #3405, #59896, #2301, #54372, #19631, #36636, #8202, #42187, #53633, #53263, #2661, #25178, #64712, #25926, #48466, #70990, #42917, #9302, #13360, #35901, #7837, #66178, #5586, #60252, #22203, #26666, #16291, #43292, #9667, #54734, #15554, #4136, #44397, #38846, #61361, #10758, #44757, #33648, #32200, #21833, #49200, #5216, #39206, #33290, #55828, #71733, #21103, #28123, #65812, #50651, #43655, #32928, #49563, #27757, #4858, #38098, #60620, #10030, #15194, #27032, #66923, #66544, #67292, #50298, #27392, #32565, #37733, #55103, #4503, #72084, #21467, #44021, #15923, #10396, #72820, #16650, #38473, #60997, #20733, #55466, #49924, #72448, #61720, #11119, #56192, #51369, #35453, #68003, #63533, #17376, #62807, #29556, #63168, #52092, #56896, #18087, #69092, #5938, #46188, #23279, #28830, #57977, #57622, #7025, #39567, #28472, #40648, #12563, #12200, #45829, #18454, #45108, #1497, #11485, #68365, #68727, #34728, #34008, #22561, #35097, #7385, #23642, #24003, #67644, #46551, #29198, #41018, #12920, #29915, #55, #17010, #62092, #39933, #57257, #56545, #6670, #51008, #405, #22914, #45471, #62447, #11845, #34364, #6302, #51732, #771, #17727, #1133, #40286, #35814, #41375, #24368, #58705, #53542, #25092, #3314, #42468, #36551, #30283, #1861, #46916, #24731, #47274, #58336, #8116, #69808, #42103, #64991, #70539, #2572, #19173, #37285, #64255, #36187, #52455, #31380, #64625, #19545, #30644, #14743, #41728, #42830, #13643, #14012, #8844, #14381, #53920, #53175, #19914, #48378, #7747, #25467, #47635, #70169, #59808, #36916, #59436, #18811, #52816, #25841, #70905, #59071, #8475, #20277, #69454, #65353, #63885, #31009, #48011, #2938, #13276, #2218, #9213, #40124, #56382, #17207, #3680, #62285, #61915, #34196, #39768, #22750, #45300, #604, #6132, #50118, #44941, #54286, #22392, #67834, #11680, #67119, #5049, #10950, #67479, #50841, #5775, #33116, #22030, #56730, #28306, #39034, #27585, #17563, #71267, #28663, #38670, #241, #26204, #21658, #66748, #72648, #16118, #51202, #23110, #45667, #68200, #62639, #31749, #44216, #33841, #61193, #48743, #10588, #55653, #44587, #61548, #16476, #33471, #56019, #5411, #27950, #50482, #73008, #16842, #39396, #11320, #57087, #13460, #23476, #35285, #7571, #24193, #46022, #34559, #30107, #19364, #35645, #69637, #6495, #41560, #41207, #36008, #18999, #2048, #24559, #53004, #58527, #29391, #46747, #29030, #1684, #47105, #64078, #46382, #57453, #63365, #69281, #52641, #58167, #12390, #1322, #7937, #30475, #18273, #6857, #69995, #51566, #2399, #17917, #24920, #966, #68558, #40480, #51925, #62995, #47462, #41922, #12034, #34926, #23831, #68916, #40847, #13107, #12749, #57807, #7216, #29745, #52282, #18643, #63715, #49301, #13839, #71835, #42289, #3508, #20097, #26394, #48566, #25286, #47832, #53367, #36378, #70722, #65548, #37102, #15298, #54473, #71092, #64813, #58894, #8304, #36739, #59259, #70362, #42654, #8668, #54110, #3871, #9406, #14569, #31199, #21205, #3134, #48199, #64447, #43395, #26027, #31571, #65178, #26769, #53741, #54835, #25663, #20466, #20841, #48936, #65917, #59628, #31936, #60357, #19739, #37476, #9041, #4242, #30834, #43020, #14937, #14203, #59996, #71465, #37837, #9766, #32300, #2764, #38200, #50753, #15661, #4964, #10502, #21574, #10137, #50031, #5325, #512, #51115, #16032, #27497, #61465, #72556, #66655, #38580, #33030, #61104, #32669, #45212, #21944, #43758, #66283, #4603, #55569, #28578, #55210, #50398, #27134, #44499, #16391, #11230, #17118, #67032, #61825, #27866, #67746, #49667, #72195, #38947, #39677, #10860, #33393, #55929, #72923, #22305, #44857, #67393, #60726, #11593, #28223, #16755, #62197, #34110, #44128, #39313, #56649, #33753, #56298, #5688, #22662, #156, #6044, #68465, #52918, #57723, #69554, #51833, #69195, #68831, #1596, #11947, #29303, #12301, #45934, #63272, #6407, #13375, #34472, #18555, #58442, #7853, #30389, #24107, #12664, #52195, #63631, #7128 ),
 ( #57000, #17827, #28939, #46655, #41120, #13020, #35558, #24472, #46290, #41474, #68111, #47019, #51476, #18187, #58078, #35200, #878, #45579, #7486, #23023, #30015, #52558, #17477, #1964, #18914, #63994, #35917, #40037, #62551, #23385, #40388, #62907, #29658, #34837, #57363, #6770, #1237, #23742, #40757, #53649, #65092, #20381, #48481, #2677, #64727, #54387, #25941, #8581, #47737, #60268, #41830, #3782, #8218, #71005, #24831, #64361, #36293, #70276, #58807, #42932, #65456, #14849, #37388, #26307, #15210, #13751, #3421, #30746, #59912, #20750, #9318, #31851, #53278, #25193, #9682, #47379, #32215, #19647, #14482, #31110, #48845, #59540, #42203, #14112, #36652, #69909, #3042, #71375, #48113, #43308, #65828, #8950, #59173, #19276, #25573, #70636, #20011, #42564, #37016, #31484, #54026, #37750, #2316, #4873, #21486, #39583, #66560, #38489, #54749, #33664, #44412, #21849, #32943, #17025, #49579, #45124, #72101, #66938, #11136, #44772, #56208, #61013, #72835, #50666, #60636, #27773, #27409, #10411, #62107, #39223, #61735, #21119, #10048, #22218, #67307, #16307, #38861, #44038, #55481, #4519, #49216, #22576, #5601, #61376, #28138, #70, #32582, #55120, #67659, #10773, #33306, #11500, #4151, #27048, #71749, #15940, #26683, #55844, #43672, #49940, #50313, #72464, #5232, #66195, #16665, #15573, #38115, #1149, #17391, #24382, #22928, #29571, #69468, #18826, #41389, #12577, #23658, #63182, #1512, #18101, #39948, #51748, #63901, #28845, #34379, #35111, #57635, #7041, #40662, #29929, #68018, #46930, #40300, #29212, #51384, #34743, #46202, #62461, #11859, #56911, #52107, #17741, #24016, #62822, #41032, #68743, #68380, #12934, #34022, #56559, #46565, #69107, #6316, #57273, #786, #18469, #23295, #63548, #6684, #28486, #35469, #5954, #12214, #45844, #57991, #419, #7401, #52469, #51023, #45486, #1876, #47650, #31023, #70182, #36201, #58719, #53190, #8131, #2232, #14756, #19560, #43218, #13291, #47289, #2587, #71282, #24745, #19929, #69823, #42116, #59086, #53935, #59823, #25106, #31395, #70554, #37300, #19189, #41742, #30658, #9228, #64640, #14026, #36566, #53557, #64270, #13659, #8490, #65006, #2954, #59452, #25482, #20291, #48028, #42483, #65367, #3694, #26219, #14394, #36931, #8859, #3330, #25856, #48393, #70921, #42846, #31765, #7762, #54302, #58351, #48758, #20660, #35828, #52830, #30298, #27318, #22487, #73105, #38025, #26958, #10321, #49485, #15482, #60548, #32491, #9955, #54658, #67215, #72016, #65738, #15123, #26587, #55026, #50578, #4061, #72376, #49127, #21392, #38394, #33212, #39128, #4429, #10682, #49850, #16576, #71656, #21029, #43948, #61643, #66471, #15848, #60918, #32853, #55390, #4784, #21756, #60183, #33571, #50218, #44317, #11045, #56119, #43582, #66103, #5511, #66847, #16217, #37660, #44684, #38770, #9592, #61289, #32124, #55751, #28050, #5145, #27680, #72744, #22129, #33933, #51298, #34291, #67931, #12131, #28399, #35385, #56476, #40577, #7317, #29848, #52384, #23575, #34658, #1065, #12498, #29130, #50937, #62739, #1790, #39865, #45395, #46120, #68657, #18021, #51663, #40950, #5867, #57908, #699, #40218, #62377, #45761, #63097, #35026, #63465, #333, #45037, #23208, #57187, #11776, #68297, #6600, #22843, #17657, #17304, #57554, #12852, #56823, #6956, #29487, #52024, #1426, #46482, #67572, #11416, #23933, #6230, #69020, #16937, #18383, #39492, #28758, #62014, #9139, #46848, #31676, #2149, #36479, #53104, #59359, #8404, #58269, #7676, #13209, #69388, #30578, #25396, #70096, #48304, #14308, #30933, #24660, #18743, #41307, #69737, #19106, #30212, #2501, #41661, #13943, #36844, #42395, #47566, #64183, #54209, #36116, #8043, #24300, #3239, #58998, #64552, #25024, #59731, #13571, #14666, #58636, #53474, #53845, #8771, #25767, #19472, #64917, #20203, #52744, #70468, #42030, #2866, #63817, #31305, #70829, #35748, #47206, #42758, #65278, #47939, #19844, #37209, #48667, #5061, #15036, #26870, #72293, #15763, #37573, #26128, #21671, #10961, #27231, #61205, #71193, #33128, #32770, #27598, #10600, #66761, #16133, #44601, #50130, #20942, #38302, #20566, #66386, #38685, #55665, #37940, #49039, #54940, #60831, #44229, #71568, #4345, #10237, #72662, #49768, #3974, #66018, #22041, #67132, #9868, #43493, #61559, #43124, #16488, #9506, #39045, #49401, #60097, #33482, #3606, #32036, #65647, #54571, #26497, #15398, #60459, #32400, #71932, #4701, #21307, #43861, #55307, #23488, #17930, #16853, #67490, #41839, #5424, #64369, #33851, #68213, #11692, #40493, #40136, #39409, #61927, #44952, #27963, #62296, #57100, #28675, #6872, #46035, #62651, #56395, #50494, #73020, #28316, #50853, #11333, #34208, #252, #45677, #68571, #978, #6145, #22760, #13760, #67847, #39780, #56032, #34940, #17574, #23123, #56742, #18288, #45312, #46395, #17219, #12048, #12405, #63009, #57466, #51215, #29404, #51938, #5785, #29044, #615, #34572, #22405, #1335, #23847, #6509, #51579, #68930, #37396, #59548, #42573, #71384, #8227, #54394, #2685, #65101, #20391, #8960, #25201, #58816, #42940, #37758, #71013, #59920, #30755, #31859, #3429, #3793, #9326, #14857, #26315, #20758, #48854, #59180, #31494, #36302, #25949, #43316, #65836, #20019, #48121, #15219, #65465, #14490, #31119, #53286, #64735, #60276, #8589, #47748, #48489, #53658, #70284, #19656, #3051, #42211, #14123, #36661, #25582, #70644, #37024, #54034, #41099, #12642, #62884, #68089, #57702, #22998, #29636, #12279, #34087, #46632, #11572, #856, #6382, #17456, #6022, #45911, #1214, #69532, #46997, #11925, #23363, #57342, #68442, #62528, #34450, #28915, #56978, #28557, #63609, #17805, #39656, #62175, #488, #51453, #24448, #51092, #46270, #45558, #40365, #34812, #7107, #13000, #6748, #52174, #23720, #35537, #40014, #29281, #51811, #58057, #68809, #18165 ) ),
 .UNSPECIFIED., .F., .F., .F. ) 
 B_SPLINE_SURFACE_WITH_KNOTS ( ( 2, 2 ),
 ( 3, 2, 2, 2, 2, 2, 2, 2, 2, 2, 2, 2, 2, 2, 2, 2, 2, 2, 2, 2, 2, 2, 2, 2, 2, 2, 2, 2, 2, 2, 2, 2, 2, 2, 2, 2, 2, 2, 2, 2, 2, 2, 2, 2, 2, 2, 2, 2, 2, 2, 2, 2, 2, 2, 2, 2, 2, 2, 2, 2, 2, 2, 2, 2, 2, 2, 2, 2, 2, 2, 2, 2, 2, 2, 2, 2, 2, 2, 2, 2, 2, 2, 2, 2, 2, 2, 2, 2, 2, 2, 2, 2, 2, 2, 2, 2, 2, 2, 2, 2, 2, 2, 2, 2, 2, 2, 2, 2, 2, 2, 2, 2, 2, 2, 2, 2, 2, 2, 2, 2, 2, 2, 2, 2, 2, 2, 2, 2, 2, 2, 2, 2, 2, 2, 2, 2, 2, 2, 2, 2, 2, 2, 2, 2, 2, 2, 2, 2, 2, 2, 2, 2, 2, 2, 2, 2, 2, 2, 2, 2, 2, 2, 2, 2, 2, 2, 2, 2, 2, 2, 2, 2, 2, 2, 2, 2, 2, 2, 2, 2, 2, 2, 2, 2, 2, 2, 2, 2, 2, 2, 2, 2, 2, 2, 2, 2, 2, 2, 2, 2, 2, 2, 2, 2, 2, 2, 2, 2, 2, 2, 2, 2, 2, 2, 2, 2, 2, 2, 2, 2, 2, 2, 2, 2, 2, 2, 2, 2, 2, 2, 2, 2, 2, 2, 2, 2, 2, 2, 2, 2, 2, 2, 2, 2, 2, 2, 2, 2, 2, 2, 2, 2, 2, 2, 2, 2, 2, 2, 2, 2, 2, 2, 2, 2, 2, 2, 2, 2, 2, 2, 2, 2, 2, 2, 2, 2, 2, 2, 2, 2, 2, 2, 2, 2, 2, 2, 2, 2, 2, 2, 2, 2, 2, 2, 2, 2, 2, 2, 2, 2, 2, 2, 2, 2, 2, 2, 2, 2, 2, 2, 2, 2, 2, 2, 2, 2, 2, 2, 2, 2, 2, 2, 2, 2, 2, 2, 2, 2, 2, 2, 2, 2, 2, 2, 2, 2, 2, 2, 2, 2, 2, 2, 2, 2, 2, 2, 2, 2, 2, 2, 2, 2, 2, 2, 2, 2, 2, 2, 2, 2, 3 ),
 ( 0.000000000000000000, 1.000000000000000000 ),
 ( 0.000000000000000000, 0.002777777777777777884, 0.005555555555555555768, 0.008333333333333333218, 0.01111111111111111154, 0.01388888888888888812, 0.01666666666666666644, 0.01944444444444444475, 0.02222222222222222307, 0.02500000000000000139, 0.02777777777777777624, 0.03055555555555555455, 0.03333333333333333287, 0.03611111111111110772, 0.03888888888888888951, 0.04166666666666666435, 0.04444444444444444614, 0.04722222222222222099, 0.05000000000000000278, 0.05277777777777777762, 0.05555555555555555247, 0.05833333333333333426, 0.06111111111111110911, 0.06388888888888888395, 0.06666666666666666574, 0.06944444444444444753, 0.07222222222222221544, 0.07499999999999999722, 0.07777777777777777901, 0.08055555555555556080, 0.08333333333333332871, 0.08611111111111111049, 0.08888888888888889228, 0.09166666666666666019, 0.09444444444444444198, 0.09722222222222222376, 0.1000000000000000056, 0.1027777777777777735, 0.1055555555555555552, 0.1083333333333333370, 0.1111111111111111049, 0.1138888888888888867, 0.1166666666666666685, 0.1194444444444444503, 0.1222222222222222182, 0.1250000000000000000, 0.1277777777777777679, 0.1305555555555555636, 0.1333333333333333315, 0.1361111111111110994, 0.1388888888888888951, 0.1416666666666666630, 0.1444444444444444309, 0.1472222222222222265, 0.1499999999999999944, 0.1527777777777777901, 0.1555555555555555580, 0.1583333333333333259, 0.1611111111111111216, 0.1638888888888888895, 0.1666666666666666574, 0.1694444444444444531, 0.1722222222222222210, 0.1749999999999999889, 0.1777777777777777846, 0.1805555555555555525, 0.1833333333333333204, 0.1861111111111111160, 0.1888888888888888840, 0.1916666666666666796, 0.1944444444444444475, 0.1972222222222222154, 0.2000000000000000111, 0.2027777777777777790, 0.2055555555555555469, 0.2083333333333333426, 0.2111111111111111105, 0.2138888888888888784, 0.2166666666666666741, 0.2194444444444444420, 0.2222222222222222099, 0.2250000000000000056, 0.2277777777777777735, 0.2305555555555555691, 0.2333333333333333370, 0.2361111111111111049, 0.2388888888888889006, 0.2416666666666666685, 0.2444444444444444364, 0.2472222222222222321, 0.2500000000000000000, 0.2527777777777777679, 0.2555555555555555358, 0.2583333333333333592, 0.2611111111111111271, 0.2638888888888888951, 0.2666666666666666630, 0.2694444444444444309, 0.2722222222222221988, 0.2750000000000000222, 0.2777777777777777901, 0.2805555555555555580, 0.2833333333333333259, 0.2861111111111110938, 0.2888888888888888618, 0.2916666666666666852, 0.2944444444444444531, 0.2972222222222222210, 0.2999999999999999889, 0.3027777777777777568, 0.3055555555555555802, 0.3083333333333333481, 0.3111111111111111160, 0.3138888888888888840, 0.3166666666666666519, 0.3194444444444444198, 0.3222222222222222432, 0.3250000000000000111, 0.3277777777777777790, 0.3305555555555555469, 0.3333333333333333148, 0.3361111111111111382, 0.3388888888888889062, 0.3416666666666666741, 0.3444444444444444420, 0.3472222222222222099, 0.3499999999999999778, 0.3527777777777778012, 0.3555555555555555691, 0.3583333333333333370, 0.3611111111111111049, 0.3638888888888888729, 0.3666666666666666408, 0.3694444444444444642, 0.3722222222222222321, 0.3750000000000000000, 0.3777777777777777679, 0.3805555555555555358, 0.3833333333333333592, 0.3861111111111111271, 0.3888888888888888951, 0.3916666666666666630, 0.3944444444444444309, 0.3972222222222221988, 0.4000000000000000222, 0.4027777777777777901, 0.4055555555555555580, 0.4083333333333333259, 0.4111111111111110938, 0.4138888888888888618, 0.4166666666666666852, 0.4194444444444444531, 0.4222222222222222210, 0.4249999999999999889, 0.4277777777777777568, 0.4305555555555555802, 0.4333333333333333481, 0.4361111111111111160, 0.4388888888888888840, 0.4416666666666666519, 0.4444444444444444198, 0.4472222222222222432, 0.4500000000000000111, 0.4527777777777777790, 0.4555555555555555469, 0.4583333333333333148, 0.4611111111111111382, 0.4638888888888889062, 0.4666666666666666741, 0.4694444444444444420, 0.4722222222222222099, 0.4749999999999999778, 0.4777777777777778012, 0.4805555555555555691, 0.4833333333333333370, 0.4861111111111111049, 0.4888888888888888729, 0.4916666666666666408, 0.4944444444444444642, 0.4972222222222222321, 0.5000000000000000000, 0.5027777777777777679, 0.5055555555555555358, 0.5083333333333333037, 0.5111111111111110716, 0.5138888888888888395, 0.5166666666666667185, 0.5194444444444444864, 0.5222222222222222543, 0.5250000000000000222, 0.5277777777777777901, 0.5305555555555555580, 0.5333333333333333259, 0.5361111111111110938, 0.5388888888888888618, 0.5416666666666666297, 0.5444444444444443976, 0.5472222222222222765, 0.5500000000000000444, 0.5527777777777778123, 0.5555555555555555802, 0.5583333333333333481, 0.5611111111111111160, 0.5638888888888888840, 0.5666666666666666519, 0.5694444444444444198, 0.5722222222222221877, 0.5749999999999999556, 0.5777777777777777235, 0.5805555555555556024, 0.5833333333333333703, 0.5861111111111111382, 0.5888888888888889062, 0.5916666666666666741, 0.5944444444444444420, 0.5972222222222222099, 0.5999999999999999778, 0.6027777777777777457, 0.6055555555555555136, 0.6083333333333332815, 0.6111111111111111605, 0.6138888888888889284, 0.6166666666666666963, 0.6194444444444444642, 0.6222222222222222321, 0.6250000000000000000, 0.6277777777777777679, 0.6305555555555555358, 0.6333333333333333037, 0.6361111111111110716, 0.6388888888888888395, 0.6416666666666667185, 0.6444444444444444864, 0.6472222222222222543, 0.6500000000000000222, 0.6527777777777777901, 0.6555555555555555580, 0.6583333333333333259, 0.6611111111111110938, 0.6638888888888888618, 0.6666666666666666297, 0.6694444444444443976, 0.6722222222222222765, 0.6750000000000000444, 0.6777777777777778123, 0.6805555555555555802, 0.6833333333333333481, 0.6861111111111111160, 0.6888888888888888840, 0.6916666666666666519, 0.6944444444444444198, 0.6972222222222221877, 0.6999999999999999556, 0.7027777777777777235, 0.7055555555555556024, 0.7083333333333333703, 0.7111111111111111382, 0.7138888888888889062, 0.7166666666666666741, 0.7194444444444444420, 0.7222222222222222099, 0.7249999999999999778, 0.7277777777777777457, 0.7305555555555555136, 0.7333333333333332815, 0.7361111111111111605, 0.7388888888888889284, 0.7416666666666666963, 0.7444444444444444642, 0.7472222222222222321, 0.7500000000000000000, 0.7527777777777777679, 0.7555555555555555358, 0.7583333333333333037, 0.7611111111111110716, 0.7638888888888888395, 0.7666666666666667185, 0.7694444444444444864, 0.7722222222222222543, 0.7750000000000000222, 0.7777777777777777901, 0.7805555555555555580, 0.7833333333333333259, 0.7861111111111110938, 0.7888888888888888618, 0.7916666666666666297, 0.7944444444444443976, 0.7972222222222222765, 0.8000000000000000444, 0.8027777777777778123, 0.8055555555555555802, 0.8083333333333333481, 0.8111111111111111160, 0.8138888888888888840, 0.8166666666666666519, 0.8194444444444444198, 0.8222222222222221877, 0.8249999999999999556, 0.8277777777777777235, 0.8305555555555556024, 0.8333333333333333703, 0.8361111111111111382, 0.8388888888888889062, 0.8416666666666666741, 0.8444444444444444420, 0.8472222222222222099, 0.8499999999999999778, 0.8527777777777777457, 0.8555555555555555136, 0.8583333333333332815, 0.8611111111111111605, 0.8638888888888889284, 0.8666666666666666963, 0.8694444444444444642, 0.8722222222222222321, 0.8750000000000000000, 0.8777777777777777679, 0.8805555555555555358, 0.8833333333333333037, 0.8861111111111110716, 0.8888888888888888395, 0.8916666666666667185, 0.8944444444444444864, 0.8972222222222222543, 0.9000000000000000222, 0.9027777777777777901, 0.9055555555555555580, 0.9083333333333333259, 0.9111111111111110938, 0.9138888888888888618, 0.9166666666666666297, 0.9194444444444443976, 0.9222222222222222765, 0.9250000000000000444, 0.9277777777777778123, 0.9305555555555555802, 0.9333333333333333481, 0.9361111111111111160, 0.9388888888888888840, 0.9416666666666666519, 0.9444444444444444198, 0.9472222222222221877, 0.9499999999999999556, 0.9527777777777777235, 0.9555555555555556024, 0.9583333333333333703, 0.9611111111111111382, 0.9638888888888889062, 0.9666666666666666741, 0.9694444444444444420, 0.9722222222222222099, 0.9749999999999999778, 0.9777777777777777457, 0.9805555555555555136, 0.9833333333333332815, 0.9861111111111111605, 0.9888888888888889284, 0.9916666666666666963, 0.9944444444444444642, 0.9972222222222222321, 1.000000000000000000 ),
 .UNSPECIFIED. ) 
 GEOMETRIC_REPRESENTATION_ITEM ( )  RATIONAL_B_SPLINE_SURFACE ( (
 ( 1.000000000000000000, 0.8660254037844387076, 1.000000000000000000, 0.8660254037844387076, 1.000000000000000000, 0.8660254037844387076, 1.000000000000000000, 0.8660254037844387076, 1.000000000000000000, 0.8660254037844387076, 1.000000000000000000, 0.8660254037844387076, 1.000000000000000000, 0.8660254037844387076, 1.000000000000000000, 0.8660254037844387076, 1.000000000000000000, 0.8660254037844387076, 1.000000000000000000, 0.8660254037844387076, 1.000000000000000000, 0.8660254037844387076, 1.000000000000000000, 0.8660254037844387076, 1.000000000000000000, 0.8660254037844387076, 1.000000000000000000, 0.8660254037844387076, 1.000000000000000000, 0.8660254037844387076, 1.000000000000000000, 0.8660254037844387076, 1.000000000000000000, 0.8660254037844387076, 1.000000000000000000, 0.8660254037844387076, 1.000000000000000000, 0.8660254037844387076, 1.000000000000000000, 0.8660254037844387076, 1.000000000000000000, 0.8660254037844387076, 1.000000000000000000, 0.8660254037844387076, 1.000000000000000000, 0.8660254037844387076, 1.000000000000000000, 0.8660254037844387076, 1.000000000000000000, 0.8660254037844387076, 1.000000000000000000, 0.8660254037844387076, 1.000000000000000000, 0.8660254037844387076, 1.000000000000000000, 0.8660254037844387076, 1.000000000000000000, 0.8660254037844387076, 1.000000000000000000, 0.8660254037844387076, 1.000000000000000000, 0.8660254037844387076, 1.000000000000000000, 0.8660254037844387076, 1.000000000000000000, 0.8660254037844387076, 1.000000000000000000, 0.8660254037844387076, 1.000000000000000000, 0.8660254037844387076, 1.000000000000000000, 0.8660254037844387076, 1.000000000000000000, 0.8660254037844387076, 1.000000000000000000, 0.8660254037844387076, 1.000000000000000000, 0.8660254037844387076, 1.000000000000000000, 0.8660254037844387076, 1.000000000000000000, 0.8660254037844387076, 1.000000000000000000, 0.8660254037844387076, 1.000000000000000000, 0.8660254037844387076, 1.000000000000000000, 0.8660254037844387076, 1.000000000000000000, 0.8660254037844387076, 1.000000000000000000, 0.8660254037844387076, 1.000000000000000000, 0.8660254037844387076, 1.000000000000000000, 0.8660254037844387076, 1.000000000000000000, 0.8660254037844387076, 1.000000000000000000, 0.8660254037844387076, 1.000000000000000000, 0.8660254037844387076, 1.000000000000000000, 0.8660254037844387076, 1.000000000000000000, 0.8660254037844387076, 1.000000000000000000, 0.8660254037844387076, 1.000000000000000000, 0.8660254037844387076, 1.000000000000000000, 0.8660254037844387076, 1.000000000000000000, 0.8660254037844387076, 1.000000000000000000, 0.8660254037844387076, 1.000000000000000000, 0.8660254037844387076, 1.000000000000000000, 0.8660254037844387076, 1.000000000000000000, 0.8660254037844387076, 1.000000000000000000, 0.8660254037844387076, 1.000000000000000000, 0.8660254037844387076, 1.000000000000000000, 0.8660254037844387076, 1.000000000000000000, 0.8660254037844387076, 1.000000000000000000, 0.8660254037844387076, 1.000000000000000000, 0.8660254037844387076, 1.000000000000000000, 0.8660254037844387076, 1.000000000000000000, 0.8660254037844387076, 1.000000000000000000, 0.8660254037844387076, 1.000000000000000000, 0.8660254037844387076, 1.000000000000000000, 0.8660254037844387076, 1.000000000000000000, 0.8660254037844387076, 1.000000000000000000, 0.8660254037844387076, 1.000000000000000000, 0.8660254037844387076, 1.000000000000000000, 0.8660254037844387076, 1.000000000000000000, 0.8660254037844387076, 1.000000000000000000, 0.8660254037844387076, 1.000000000000000000, 0.8660254037844387076, 1.000000000000000000, 0.8660254037844387076, 1.000000000000000000, 0.8660254037844387076, 1.000000000000000000, 0.8660254037844387076, 1.000000000000000000, 0.8660254037844387076, 1.000000000000000000, 0.8660254037844387076, 1.000000000000000000, 0.8660254037844387076, 1.000000000000000000, 0.8660254037844387076, 1.000000000000000000, 0.8660254037844387076, 1.000000000000000000, 0.8660254037844387076, 1.000000000000000000, 0.8660254037844387076, 1.000000000000000000, 0.8660254037844387076, 1.000000000000000000, 0.8660254037844387076, 1.000000000000000000, 0.8660254037844387076, 1.000000000000000000, 0.8660254037844387076, 1.000000000000000000, 0.8660254037844387076, 1.000000000000000000, 0.8660254037844387076, 1.000000000000000000, 0.8660254037844387076, 1.000000000000000000, 0.8660254037844387076, 1.000000000000000000, 0.8660254037844387076, 1.000000000000000000, 0.8660254037844387076, 1.000000000000000000, 0.8660254037844387076, 1.000000000000000000, 0.8660254037844387076, 1.000000000000000000, 0.8660254037844387076, 1.000000000000000000, 0.8660254037844387076, 1.000000000000000000, 0.8660254037844387076, 1.000000000000000000, 0.8660254037844387076, 1.000000000000000000, 0.8660254037844387076, 1.000000000000000000, 0.8660254037844387076, 1.000000000000000000, 0.8660254037844387076, 1.000000000000000000, 0.8660254037844387076, 1.000000000000000000, 0.8660254037844387076, 1.000000000000000000, 0.8660254037844387076, 1.000000000000000000, 0.8660254037844387076, 1.000000000000000000, 0.8660254037844387076, 1.000000000000000000, 0.8660254037844387076, 1.000000000000000000, 0.8660254037844387076, 1.000000000000000000, 0.8660254037844387076, 1.000000000000000000, 0.8660254037844387076, 1.000000000000000000, 0.8660254037844387076, 1.000000000000000000, 0.8660254037844387076, 1.000000000000000000, 0.8660254037844387076, 1.000000000000000000, 0.8660254037844387076, 1.000000000000000000, 0.8660254037844387076, 1.000000000000000000, 0.8660254037844387076, 1.000000000000000000, 0.8660254037844387076, 1.000000000000000000, 0.8660254037844387076, 1.000000000000000000, 0.8660254037844387076, 1.000000000000000000, 0.8660254037844387076, 1.000000000000000000, 0.8660254037844387076, 1.000000000000000000, 0.8660254037844387076, 1.000000000000000000, 0.8660254037844387076, 1.000000000000000000, 0.8660254037844387076, 1.000000000000000000, 0.8660254037844387076, 1.000000000000000000, 0.8660254037844387076, 1.000000000000000000, 0.8660254037844387076, 1.000000000000000000, 0.8660254037844387076, 1.000000000000000000, 0.8660254037844387076, 1.000000000000000000, 0.8660254037844387076, 1.000000000000000000, 0.8660254037844387076, 1.000000000000000000, 0.8660254037844387076, 1.000000000000000000, 0.8660254037844387076, 1.000000000000000000, 0.8660254037844387076, 1.000000000000000000, 0.8660254037844387076, 1.000000000000000000, 0.8660254037844387076, 1.000000000000000000, 0.8660254037844387076, 1.000000000000000000, 0.8660254037844387076, 1.000000000000000000, 0.8660254037844387076, 1.000000000000000000, 0.8660254037844387076, 1.000000000000000000, 0.8660254037844387076, 1.000000000000000000, 0.8660254037844387076, 1.000000000000000000, 0.8660254037844387076, 1.000000000000000000, 0.8660254037844387076, 1.000000000000000000, 0.8660254037844387076, 1.000000000000000000, 0.8660254037844387076, 1.000000000000000000, 0.8660254037844387076, 1.000000000000000000, 0.8660254037844387076, 1.000000000000000000, 0.8660254037844387076, 1.000000000000000000, 0.8660254037844387076, 1.000000000000000000, 0.8660254037844387076, 1.000000000000000000, 0.8660254037844387076, 1.000000000000000000, 0.8660254037844387076, 1.000000000000000000, 0.8660254037844387076, 1.000000000000000000, 0.8660254037844387076, 1.000000000000000000, 0.8660254037844387076, 1.000000000000000000, 0.8660254037844387076, 1.000000000000000000, 0.8660254037844387076, 1.000000000000000000, 0.8660254037844387076, 1.000000000000000000, 0.8660254037844387076, 1.000000000000000000, 0.8660254037844387076, 1.000000000000000000, 0.8660254037844387076, 1.000000000000000000, 0.8660254037844387076, 1.000000000000000000, 0.8660254037844387076, 1.000000000000000000, 0.8660254037844387076, 1.000000000000000000, 0.8660254037844387076, 1.000000000000000000, 0.8660254037844387076, 1.000000000000000000, 0.8660254037844387076, 1.000000000000000000, 0.8660254037844387076, 1.000000000000000000, 0.8660254037844387076, 1.000000000000000000, 0.8660254037844387076, 1.000000000000000000, 0.8660254037844387076, 1.000000000000000000, 0.8660254037844387076, 1.000000000000000000, 0.8660254037844387076, 1.000000000000000000, 0.8660254037844387076, 1.000000000000000000, 0.8660254037844387076, 1.000000000000000000, 0.8660254037844387076, 1.000000000000000000, 0.8660254037844387076, 1.000000000000000000, 0.8660254037844387076, 1.000000000000000000, 0.8660254037844387076, 1.000000000000000000, 0.8660254037844387076, 1.000000000000000000, 0.8660254037844387076, 1.000000000000000000, 0.8660254037844387076, 1.000000000000000000, 0.8660254037844387076, 1.000000000000000000, 0.8660254037844387076, 1.000000000000000000, 0.8660254037844387076, 1.000000000000000000, 0.8660254037844387076, 1.000000000000000000, 0.8660254037844387076, 1.000000000000000000, 0.8660254037844387076, 1.000000000000000000, 0.8660254037844387076, 1.000000000000000000, 0.8660254037844387076, 1.000000000000000000, 0.8660254037844387076, 1.000000000000000000, 0.8660254037844387076, 1.000000000000000000, 0.8660254037844387076, 1.000000000000000000, 0.8660254037844387076, 1.000000000000000000, 0.8660254037844387076, 1.000000000000000000, 0.8660254037844387076, 1.000000000000000000, 0.8660254037844387076, 1.000000000000000000, 0.8660254037844387076, 1.000000000000000000, 0.8660254037844387076, 1.000000000000000000, 0.8660254037844387076, 1.000000000000000000, 0.8660254037844387076, 1.000000000000000000, 0.8660254037844387076, 1.000000000000000000, 0.8660254037844387076, 1.000000000000000000, 0.8660254037844387076, 1.000000000000000000, 0.8660254037844387076, 1.000000000000000000, 0.8660254037844387076, 1.000000000000000000, 0.8660254037844387076, 1.000000000000000000, 0.8660254037844387076, 1.000000000000000000, 0.8660254037844387076, 1.000000000000000000, 0.8660254037844387076, 1.000000000000000000, 0.8660254037844387076, 1.000000000000000000, 0.8660254037844387076, 1.000000000000000000, 0.8660254037844387076, 1.000000000000000000, 0.8660254037844387076, 1.000000000000000000, 0.8660254037844387076, 1.000000000000000000, 0.8660254037844387076, 1.000000000000000000, 0.8660254037844387076, 1.000000000000000000, 0.8660254037844387076, 1.000000000000000000, 0.8660254037844387076, 1.000000000000000000, 0.8660254037844387076, 1.000000000000000000, 0.8660254037844387076, 1.000000000000000000, 0.8660254037844387076, 1.000000000000000000, 0.8660254037844387076, 1.000000000000000000, 0.8660254037844387076, 1.000000000000000000, 0.8660254037844387076, 1.000000000000000000, 0.8660254037844387076, 1.000000000000000000, 0.8660254037844387076, 1.000000000000000000, 0.8660254037844387076, 1.000000000000000000, 0.8660254037844387076, 1.000000000000000000, 0.8660254037844387076, 1.000000000000000000, 0.8660254037844387076, 1.000000000000000000, 0.8660254037844387076, 1.000000000000000000, 0.8660254037844387076, 1.000000000000000000, 0.8660254037844387076, 1.000000000000000000, 0.8660254037844387076, 1.000000000000000000, 0.8660254037844387076, 1.000000000000000000, 0.8660254037844387076, 1.000000000000000000, 0.8660254037844387076, 1.000000000000000000, 0.8660254037844387076, 1.000000000000000000, 0.8660254037844387076, 1.000000000000000000, 0.8660254037844387076, 1.000000000000000000, 0.8660254037844387076, 1.000000000000000000, 0.8660254037844387076, 1.000000000000000000, 0.8660254037844387076, 1.000000000000000000, 0.8660254037844387076, 1.000000000000000000, 0.8660254037844387076, 1.000000000000000000, 0.8660254037844387076, 1.000000000000000000, 0.8660254037844387076, 1.000000000000000000, 0.8660254037844387076, 1.000000000000000000, 0.8660254037844387076, 1.000000000000000000, 0.8660254037844387076, 1.000000000000000000, 0.8660254037844387076, 1.000000000000000000, 0.8660254037844387076, 1.000000000000000000, 0.8660254037844387076, 1.000000000000000000, 0.8660254037844387076, 1.000000000000000000, 0.8660254037844387076, 1.000000000000000000, 0.8660254037844387076, 1.000000000000000000, 0.8660254037844387076, 1.000000000000000000, 0.8660254037844387076, 1.000000000000000000, 0.8660254037844387076, 1.000000000000000000, 0.8660254037844387076, 1.000000000000000000, 0.8660254037844387076, 1.000000000000000000, 0.8660254037844387076, 1.000000000000000000, 0.8660254037844387076, 1.000000000000000000, 0.8660254037844387076, 1.000000000000000000, 0.8660254037844387076, 1.000000000000000000, 0.8660254037844387076, 1.000000000000000000, 0.8660254037844387076, 1.000000000000000000, 0.8660254037844387076, 1.000000000000000000, 0.8660254037844387076, 1.000000000000000000, 0.8660254037844387076, 1.000000000000000000, 0.8660254037844387076, 1.000000000000000000, 0.8660254037844387076, 1.000000000000000000, 0.8660254037844387076, 1.000000000000000000, 0.8660254037844387076, 1.000000000000000000, 0.8660254037844387076, 1.000000000000000000, 0.8660254037844387076, 1.000000000000000000, 0.8660254037844387076, 1.000000000000000000, 0.8660254037844387076, 1.000000000000000000, 0.8660254037844387076, 1.000000000000000000, 0.8660254037844387076, 1.000000000000000000, 0.8660254037844387076, 1.000000000000000000, 0.8660254037844387076, 1.000000000000000000, 0.8660254037844387076, 1.000000000000000000, 0.8660254037844387076, 1.000000000000000000, 0.8660254037844387076, 1.000000000000000000, 0.8660254037844387076, 1.000000000000000000, 0.8660254037844387076, 1.000000000000000000, 0.8660254037844387076, 1.000000000000000000, 0.8660254037844387076, 1.000000000000000000, 0.8660254037844387076, 1.000000000000000000, 0.8660254037844387076, 1.000000000000000000, 0.8660254037844387076, 1.000000000000000000, 0.8660254037844387076, 1.000000000000000000, 0.8660254037844387076, 1.000000000000000000, 0.8660254037844387076, 1.000000000000000000, 0.8660254037844387076, 1.000000000000000000, 0.8660254037844387076, 1.000000000000000000, 0.8660254037844387076, 1.000000000000000000, 0.8660254037844387076, 1.000000000000000000, 0.8660254037844387076, 1.000000000000000000, 0.8660254037844387076, 1.000000000000000000, 0.8660254037844387076, 1.000000000000000000, 0.8660254037844387076, 1.000000000000000000, 0.8660254037844387076, 1.000000000000000000, 0.8660254037844387076, 1.000000000000000000, 0.8660254037844387076, 1.000000000000000000, 0.8660254037844387076, 1.000000000000000000, 0.8660254037844387076, 1.000000000000000000, 0.8660254037844387076, 1.000000000000000000, 0.8660254037844387076, 1.000000000000000000, 0.8660254037844387076, 1.000000000000000000, 0.8660254037844387076, 1.000000000000000000, 0.8660254037844387076, 1.000000000000000000, 0.8660254037844387076, 1.000000000000000000, 0.8660254037844387076, 1.000000000000000000, 0.8660254037844387076, 1.000000000000000000, 0.8660254037844387076, 1.000000000000000000, 0.8660254037844387076, 1.000000000000000000, 0.8660254037844387076, 1.000000000000000000, 0.8660254037844387076, 1.000000000000000000, 0.8660254037844387076, 1.000000000000000000, 0.8660254037844387076, 1.000000000000000000, 0.8660254037844387076, 1.000000000000000000, 0.8660254037844387076, 1.000000000000000000, 0.8660254037844387076, 1.000000000000000000, 0.8660254037844387076, 1.000000000000000000, 0.8660254037844387076, 1.000000000000000000, 0.8660254037844387076, 1.000000000000000000, 0.8660254037844387076, 1.000000000000000000, 0.8660254037844387076, 1.000000000000000000, 0.8660254037844387076, 1.000000000000000000, 0.8660254037844387076, 1.000000000000000000, 0.8660254037844387076, 1.000000000000000000, 0.8660254037844387076, 1.000000000000000000, 0.8660254037844387076, 1.000000000000000000, 0.8660254037844387076, 1.000000000000000000, 0.8660254037844387076, 1.000000000000000000, 0.8660254037844387076, 1.000000000000000000, 0.8660254037844387076, 1.000000000000000000, 0.8660254037844387076, 1.000000000000000000, 0.8660254037844387076, 1.000000000000000000, 0.8660254037844387076, 1.000000000000000000, 0.8660254037844387076, 1.000000000000000000, 0.8660254037844387076, 1.000000000000000000, 0.8660254037844387076, 1.000000000000000000, 0.8660254037844387076, 1.000000000000000000, 0.8660254037844387076, 1.000000000000000000, 0.8660254037844387076, 1.000000000000000000, 0.8660254037844387076, 1.000000000000000000, 0.8660254037844387076, 1.000000000000000000, 0.8660254037844387076, 1.000000000000000000),
 ( 1.000000000000000000, 0.8660254037844387076, 1.000000000000000000, 0.8660254037844387076, 1.000000000000000000, 0.8660254037844387076, 1.000000000000000000, 0.8660254037844387076, 1.000000000000000000, 0.8660254037844387076, 1.000000000000000000, 0.8660254037844387076, 1.000000000000000000, 0.8660254037844387076, 1.000000000000000000, 0.8660254037844387076, 1.000000000000000000, 0.8660254037844387076, 1.000000000000000000, 0.8660254037844387076, 1.000000000000000000, 0.8660254037844387076, 1.000000000000000000, 0.8660254037844387076, 1.000000000000000000, 0.8660254037844387076, 1.000000000000000000, 0.8660254037844387076, 1.000000000000000000, 0.8660254037844387076, 1.000000000000000000, 0.8660254037844387076, 1.000000000000000000, 0.8660254037844387076, 1.000000000000000000, 0.8660254037844387076, 1.000000000000000000, 0.8660254037844387076, 1.000000000000000000, 0.8660254037844387076, 1.000000000000000000, 0.8660254037844387076, 1.000000000000000000, 0.8660254037844387076, 1.000000000000000000, 0.8660254037844387076, 1.000000000000000000, 0.8660254037844387076, 1.000000000000000000, 0.8660254037844387076, 1.000000000000000000, 0.8660254037844387076, 1.000000000000000000, 0.8660254037844387076, 1.000000000000000000, 0.8660254037844387076, 1.000000000000000000, 0.8660254037844387076, 1.000000000000000000, 0.8660254037844387076, 1.000000000000000000, 0.8660254037844387076, 1.000000000000000000, 0.8660254037844387076, 1.000000000000000000, 0.8660254037844387076, 1.000000000000000000, 0.8660254037844387076, 1.000000000000000000, 0.8660254037844387076, 1.000000000000000000, 0.8660254037844387076, 1.000000000000000000, 0.8660254037844387076, 1.000000000000000000, 0.8660254037844387076, 1.000000000000000000, 0.8660254037844387076, 1.000000000000000000, 0.8660254037844387076, 1.000000000000000000, 0.8660254037844387076, 1.000000000000000000, 0.8660254037844387076, 1.000000000000000000, 0.8660254037844387076, 1.000000000000000000, 0.8660254037844387076, 1.000000000000000000, 0.8660254037844387076, 1.000000000000000000, 0.8660254037844387076, 1.000000000000000000, 0.8660254037844387076, 1.000000000000000000, 0.8660254037844387076, 1.000000000000000000, 0.8660254037844387076, 1.000000000000000000, 0.8660254037844387076, 1.000000000000000000, 0.8660254037844387076, 1.000000000000000000, 0.8660254037844387076, 1.000000000000000000, 0.8660254037844387076, 1.000000000000000000, 0.8660254037844387076, 1.000000000000000000, 0.8660254037844387076, 1.000000000000000000, 0.8660254037844387076, 1.000000000000000000, 0.8660254037844387076, 1.000000000000000000, 0.8660254037844387076, 1.000000000000000000, 0.8660254037844387076, 1.000000000000000000, 0.8660254037844387076, 1.000000000000000000, 0.8660254037844387076, 1.000000000000000000, 0.8660254037844387076, 1.000000000000000000, 0.8660254037844387076, 1.000000000000000000, 0.8660254037844387076, 1.000000000000000000, 0.8660254037844387076, 1.000000000000000000, 0.8660254037844387076, 1.000000000000000000, 0.8660254037844387076, 1.000000000000000000, 0.8660254037844387076, 1.000000000000000000, 0.8660254037844387076, 1.000000000000000000, 0.8660254037844387076, 1.000000000000000000, 0.8660254037844387076, 1.000000000000000000, 0.8660254037844387076, 1.000000000000000000, 0.8660254037844387076, 1.000000000000000000, 0.8660254037844387076, 1.000000000000000000, 0.8660254037844387076, 1.000000000000000000, 0.8660254037844387076, 1.000000000000000000, 0.8660254037844387076, 1.000000000000000000, 0.8660254037844387076, 1.000000000000000000, 0.8660254037844387076, 1.000000000000000000, 0.8660254037844387076, 1.000000000000000000, 0.8660254037844387076, 1.000000000000000000, 0.8660254037844387076, 1.000000000000000000, 0.8660254037844387076, 1.000000000000000000, 0.8660254037844387076, 1.000000000000000000, 0.8660254037844387076, 1.000000000000000000, 0.8660254037844387076, 1.000000000000000000, 0.8660254037844387076, 1.000000000000000000, 0.8660254037844387076, 1.000000000000000000, 0.8660254037844387076, 1.000000000000000000, 0.8660254037844387076, 1.000000000000000000, 0.8660254037844387076, 1.000000000000000000, 0.8660254037844387076, 1.000000000000000000, 0.8660254037844387076, 1.000000000000000000, 0.8660254037844387076, 1.000000000000000000, 0.8660254037844387076, 1.000000000000000000, 0.8660254037844387076, 1.000000000000000000, 0.8660254037844387076, 1.000000000000000000, 0.8660254037844387076, 1.000000000000000000, 0.8660254037844387076, 1.000000000000000000, 0.8660254037844387076, 1.000000000000000000, 0.8660254037844387076, 1.000000000000000000, 0.8660254037844387076, 1.000000000000000000, 0.8660254037844387076, 1.000000000000000000, 0.8660254037844387076, 1.000000000000000000, 0.8660254037844387076, 1.000000000000000000, 0.8660254037844387076, 1.000000000000000000, 0.8660254037844387076, 1.000000000000000000, 0.8660254037844387076, 1.000000000000000000, 0.8660254037844387076, 1.000000000000000000, 0.8660254037844387076, 1.000000000000000000, 0.8660254037844387076, 1.000000000000000000, 0.8660254037844387076, 1.000000000000000000, 0.8660254037844387076, 1.000000000000000000, 0.8660254037844387076, 1.000000000000000000, 0.8660254037844387076, 1.000000000000000000, 0.8660254037844387076, 1.000000000000000000, 0.8660254037844387076, 1.000000000000000000, 0.8660254037844387076, 1.000000000000000000, 0.8660254037844387076, 1.000000000000000000, 0.8660254037844387076, 1.000000000000000000, 0.8660254037844387076, 1.000000000000000000, 0.8660254037844387076, 1.000000000000000000, 0.8660254037844387076, 1.000000000000000000, 0.8660254037844387076, 1.000000000000000000, 0.8660254037844387076, 1.000000000000000000, 0.8660254037844387076, 1.000000000000000000, 0.8660254037844387076, 1.000000000000000000, 0.8660254037844387076, 1.000000000000000000, 0.8660254037844387076, 1.000000000000000000, 0.8660254037844387076, 1.000000000000000000, 0.8660254037844387076, 1.000000000000000000, 0.8660254037844387076, 1.000000000000000000, 0.8660254037844387076, 1.000000000000000000, 0.8660254037844387076, 1.000000000000000000, 0.8660254037844387076, 1.000000000000000000, 0.8660254037844387076, 1.000000000000000000, 0.8660254037844387076, 1.000000000000000000, 0.8660254037844387076, 1.000000000000000000, 0.8660254037844387076, 1.000000000000000000, 0.8660254037844387076, 1.000000000000000000, 0.8660254037844387076, 1.000000000000000000, 0.8660254037844387076, 1.000000000000000000, 0.8660254037844387076, 1.000000000000000000, 0.8660254037844387076, 1.000000000000000000, 0.8660254037844387076, 1.000000000000000000, 0.8660254037844387076, 1.000000000000000000, 0.8660254037844387076, 1.000000000000000000, 0.8660254037844387076, 1.000000000000000000, 0.8660254037844387076, 1.000000000000000000, 0.8660254037844387076, 1.000000000000000000, 0.8660254037844387076, 1.000000000000000000, 0.8660254037844387076, 1.000000000000000000, 0.8660254037844387076, 1.000000000000000000, 0.8660254037844387076, 1.000000000000000000, 0.8660254037844387076, 1.000000000000000000, 0.8660254037844387076, 1.000000000000000000, 0.8660254037844387076, 1.000000000000000000, 0.8660254037844387076, 1.000000000000000000, 0.8660254037844387076, 1.000000000000000000, 0.8660254037844387076, 1.000000000000000000, 0.8660254037844387076, 1.000000000000000000, 0.8660254037844387076, 1.000000000000000000, 0.8660254037844387076, 1.000000000000000000, 0.8660254037844387076, 1.000000000000000000, 0.8660254037844387076, 1.000000000000000000, 0.8660254037844387076, 1.000000000000000000, 0.8660254037844387076, 1.000000000000000000, 0.8660254037844387076, 1.000000000000000000, 0.8660254037844387076, 1.000000000000000000, 0.8660254037844387076, 1.000000000000000000, 0.8660254037844387076, 1.000000000000000000, 0.8660254037844387076, 1.000000000000000000, 0.8660254037844387076, 1.000000000000000000, 0.8660254037844387076, 1.000000000000000000, 0.8660254037844387076, 1.000000000000000000, 0.8660254037844387076, 1.000000000000000000, 0.8660254037844387076, 1.000000000000000000, 0.8660254037844387076, 1.000000000000000000, 0.8660254037844387076, 1.000000000000000000, 0.8660254037844387076, 1.000000000000000000, 0.8660254037844387076, 1.000000000000000000, 0.8660254037844387076, 1.000000000000000000, 0.8660254037844387076, 1.000000000000000000, 0.8660254037844387076, 1.000000000000000000, 0.8660254037844387076, 1.000000000000000000, 0.8660254037844387076, 1.000000000000000000, 0.8660254037844387076, 1.000000000000000000, 0.8660254037844387076, 1.000000000000000000, 0.8660254037844387076, 1.000000000000000000, 0.8660254037844387076, 1.000000000000000000, 0.8660254037844387076, 1.000000000000000000, 0.8660254037844387076, 1.000000000000000000, 0.8660254037844387076, 1.000000000000000000, 0.8660254037844387076, 1.000000000000000000, 0.8660254037844387076, 1.000000000000000000, 0.8660254037844387076, 1.000000000000000000, 0.8660254037844387076, 1.000000000000000000, 0.8660254037844387076, 1.000000000000000000, 0.8660254037844387076, 1.000000000000000000, 0.8660254037844387076, 1.000000000000000000, 0.8660254037844387076, 1.000000000000000000, 0.8660254037844387076, 1.000000000000000000, 0.8660254037844387076, 1.000000000000000000, 0.8660254037844387076, 1.000000000000000000, 0.8660254037844387076, 1.000000000000000000, 0.8660254037844387076, 1.000000000000000000, 0.8660254037844387076, 1.000000000000000000, 0.8660254037844387076, 1.000000000000000000, 0.8660254037844387076, 1.000000000000000000, 0.8660254037844387076, 1.000000000000000000, 0.8660254037844387076, 1.000000000000000000, 0.8660254037844387076, 1.000000000000000000, 0.8660254037844387076, 1.000000000000000000, 0.8660254037844387076, 1.000000000000000000, 0.8660254037844387076, 1.000000000000000000, 0.8660254037844387076, 1.000000000000000000, 0.8660254037844387076, 1.000000000000000000, 0.8660254037844387076, 1.000000000000000000, 0.8660254037844387076, 1.000000000000000000, 0.8660254037844387076, 1.000000000000000000, 0.8660254037844387076, 1.000000000000000000, 0.8660254037844387076, 1.000000000000000000, 0.8660254037844387076, 1.000000000000000000, 0.8660254037844387076, 1.000000000000000000, 0.8660254037844387076, 1.000000000000000000, 0.8660254037844387076, 1.000000000000000000, 0.8660254037844387076, 1.000000000000000000, 0.8660254037844387076, 1.000000000000000000, 0.8660254037844387076, 1.000000000000000000, 0.8660254037844387076, 1.000000000000000000, 0.8660254037844387076, 1.000000000000000000, 0.8660254037844387076, 1.000000000000000000, 0.8660254037844387076, 1.000000000000000000, 0.8660254037844387076, 1.000000000000000000, 0.8660254037844387076, 1.000000000000000000, 0.8660254037844387076, 1.000000000000000000, 0.8660254037844387076, 1.000000000000000000, 0.8660254037844387076, 1.000000000000000000, 0.8660254037844387076, 1.000000000000000000, 0.8660254037844387076, 1.000000000000000000, 0.8660254037844387076, 1.000000000000000000, 0.8660254037844387076, 1.000000000000000000, 0.8660254037844387076, 1.000000000000000000, 0.8660254037844387076, 1.000000000000000000, 0.8660254037844387076, 1.000000000000000000, 0.8660254037844387076, 1.000000000000000000, 0.8660254037844387076, 1.000000000000000000, 0.8660254037844387076, 1.000000000000000000, 0.8660254037844387076, 1.000000000000000000, 0.8660254037844387076, 1.000000000000000000, 0.8660254037844387076, 1.000000000000000000, 0.8660254037844387076, 1.000000000000000000, 0.8660254037844387076, 1.000000000000000000, 0.8660254037844387076, 1.000000000000000000, 0.8660254037844387076, 1.000000000000000000, 0.8660254037844387076, 1.000000000000000000, 0.8660254037844387076, 1.000000000000000000, 0.8660254037844387076, 1.000000000000000000, 0.8660254037844387076, 1.000000000000000000, 0.8660254037844387076, 1.000000000000000000, 0.8660254037844387076, 1.000000000000000000, 0.8660254037844387076, 1.000000000000000000, 0.8660254037844387076, 1.000000000000000000, 0.8660254037844387076, 1.000000000000000000, 0.8660254037844387076, 1.000000000000000000, 0.8660254037844387076, 1.000000000000000000, 0.8660254037844387076, 1.000000000000000000, 0.8660254037844387076, 1.000000000000000000, 0.8660254037844387076, 1.000000000000000000, 0.8660254037844387076, 1.000000000000000000, 0.8660254037844387076, 1.000000000000000000, 0.8660254037844387076, 1.000000000000000000, 0.8660254037844387076, 1.000000000000000000, 0.8660254037844387076, 1.000000000000000000, 0.8660254037844387076, 1.000000000000000000, 0.8660254037844387076, 1.000000000000000000, 0.8660254037844387076, 1.000000000000000000, 0.8660254037844387076, 1.000000000000000000, 0.8660254037844387076, 1.000000000000000000, 0.8660254037844387076, 1.000000000000000000, 0.8660254037844387076, 1.000000000000000000, 0.8660254037844387076, 1.000000000000000000, 0.8660254037844387076, 1.000000000000000000, 0.8660254037844387076, 1.000000000000000000, 0.8660254037844387076, 1.000000000000000000, 0.8660254037844387076, 1.000000000000000000, 0.8660254037844387076, 1.000000000000000000, 0.8660254037844387076, 1.000000000000000000, 0.8660254037844387076, 1.000000000000000000, 0.8660254037844387076, 1.000000000000000000, 0.8660254037844387076, 1.000000000000000000, 0.8660254037844387076, 1.000000000000000000, 0.8660254037844387076, 1.000000000000000000, 0.8660254037844387076, 1.000000000000000000, 0.8660254037844387076, 1.000000000000000000, 0.8660254037844387076, 1.000000000000000000, 0.8660254037844387076, 1.000000000000000000, 0.8660254037844387076, 1.000000000000000000, 0.8660254037844387076, 1.000000000000000000, 0.8660254037844387076, 1.000000000000000000, 0.8660254037844387076, 1.000000000000000000, 0.8660254037844387076, 1.000000000000000000, 0.8660254037844387076, 1.000000000000000000, 0.8660254037844387076, 1.000000000000000000, 0.8660254037844387076, 1.000000000000000000, 0.8660254037844387076, 1.000000000000000000, 0.8660254037844387076, 1.000000000000000000, 0.8660254037844387076, 1.000000000000000000, 0.8660254037844387076, 1.000000000000000000, 0.8660254037844387076, 1.000000000000000000, 0.8660254037844387076, 1.000000000000000000, 0.8660254037844387076, 1.000000000000000000, 0.8660254037844387076, 1.000000000000000000, 0.8660254037844387076, 1.000000000000000000, 0.8660254037844387076, 1.000000000000000000, 0.8660254037844387076, 1.000000000000000000, 0.8660254037844387076, 1.000000000000000000, 0.8660254037844387076, 1.000000000000000000, 0.8660254037844387076, 1.000000000000000000, 0.8660254037844387076, 1.000000000000000000, 0.8660254037844387076, 1.000000000000000000, 0.8660254037844387076, 1.000000000000000000, 0.8660254037844387076, 1.000000000000000000, 0.8660254037844387076, 1.000000000000000000, 0.8660254037844387076, 1.000000000000000000, 0.8660254037844387076, 1.000000000000000000, 0.8660254037844387076, 1.000000000000000000, 0.8660254037844387076, 1.000000000000000000, 0.8660254037844387076, 1.000000000000000000, 0.8660254037844387076, 1.000000000000000000, 0.8660254037844387076, 1.000000000000000000, 0.8660254037844387076, 1.000000000000000000, 0.8660254037844387076, 1.000000000000000000, 0.8660254037844387076, 1.000000000000000000, 0.8660254037844387076, 1.000000000000000000, 0.8660254037844387076, 1.000000000000000000, 0.8660254037844387076, 1.000000000000000000, 0.8660254037844387076, 1.000000000000000000, 0.8660254037844387076, 1.000000000000000000, 0.8660254037844387076, 1.000000000000000000, 0.8660254037844387076, 1.000000000000000000, 0.8660254037844387076, 1.000000000000000000, 0.8660254037844387076, 1.000000000000000000, 0.8660254037844387076, 1.000000000000000000, 0.8660254037844387076, 1.000000000000000000, 0.8660254037844387076, 1.000000000000000000, 0.8660254037844387076, 1.000000000000000000, 0.8660254037844387076, 1.000000000000000000, 0.8660254037844387076, 1.000000000000000000, 0.8660254037844387076, 1.000000000000000000, 0.8660254037844387076, 1.000000000000000000, 0.8660254037844387076, 1.000000000000000000, 0.8660254037844387076, 1.000000000000000000, 0.8660254037844387076, 1.000000000000000000, 0.8660254037844387076, 1.000000000000000000, 0.8660254037844387076, 1.000000000000000000, 0.8660254037844387076, 1.000000000000000000, 0.8660254037844387076, 1.000000000000000000, 0.8660254037844387076, 1.000000000000000000, 0.8660254037844387076, 1.000000000000000000) ) ) 
 REPRESENTATION_ITEM ( '' )  SURFACE ( )  );
#35891=CARTESIAN_POINT ( 'NONE',  ( 26.66250000122903430, -4.330127018922190985, -2.500000000000001332 ) ) ;
#35893=CARTESIAN_POINT ( 'NONE',  ( 17.20312500061451644, 0.000000000000000000, 5.243569643749999010 ) ) ;
#35894=CARTESIAN_POINT ( 'NONE',  ( 8.062500000000000000, -5.773502691896255534, -1.060575238724906372E-15 ) ) ;
#35895=CARTESIAN_POINT ( 'NONE',  ( 28.32187500061451502, 3.027376345333613106, -5.243569643749998122 ) ) ;
#35896=CARTESIAN_POINT ( 'NONE',  ( 9.909375000614517148, 4.541064518000418104, -2.621784821874998173 ) ) ;
#35897=CARTESIAN_POINT ( 'NONE',  ( 8.446875000614518569, -3.027376345333610441, -5.243569643749999898 ) ) ;
#35898=CARTESIAN_POINT ( 'NONE',  ( 17.40937500061451715, -4.541064518000417216, -2.621784821875001281 ) ) ;
#35899=ORIENTED_EDGE ( 'NONE', *, *, #34668, .T. ) ;
#35900=CARTESIAN_POINT ( 'NONE',  ( 24.18750000122903288, 4.330127018922191873, 2.499999999999999556 ) ) ;
#35901=CARTESIAN_POINT ( 'NONE',  ( 20.57812500061451644, 6.421520780324663323E-16, -5.243569643749999010 ) ) ;
#35902=CARTESIAN_POINT ( 'NONE',  ( 17.33437500061451431, -4.541064518000419881, 2.621784821874995952 ) ) ;
#35903=CARTESIAN_POINT ( 'NONE',  ( 22.22812500061451502, -4.541064518000419881, 2.621784821874995952 ) ) ;
#35904=CARTESIAN_POINT ( 'NONE',  ( 4.000000000000000000, 13.43750000000000000, 32.30940107675849049 ) ) ;
#35905=VECTOR ( 'NONE', #54404, 1000.000000000000000 ) ;
#35906=CARTESIAN_POINT ( 'NONE',  ( 28.75312500061451715, 4.541064518000418104, -2.621784821874998173 ) ) ;
#35907=CARTESIAN_POINT ( 'NONE',  ( 10.50000000122903465, -2.886751345948125991, -5.000000000000000000 ) ) ;
#35908=ORIENTED_EDGE ( 'NONE', *, *, #12056, .F. ) ;
#35909=CARTESIAN_POINT ( 'NONE',  ( 4.537500001229034297, -4.330127018922194537, 2.499999999999995559 ) ) ;
#35910=CARTESIAN_POINT ( 'NONE',  ( -3.999999999999999556, 17.26249999999999929, -32.30940107675850470 ) ) ;
#35911=CARTESIAN_POINT ( 'NONE',  ( 24.11250000122903359, 4.330127018922192761, -2.499999999999997780 ) ) ;
#35913=CARTESIAN_POINT ( 'NONE',  ( 9.159375000614515372, 0.000000000000000000, 5.243569643749999010 ) ) ;
#35915=CARTESIAN_POINT ( 'NONE',  ( 14.39062500061451821, 6.054752690667223547, 3.707466751127219781E-16 ) ) ;
#35916=CARTESIAN_POINT ( 'NONE',  ( 11.40937500061451892, 0.000000000000000000, 5.243569643749999010 ) ) ;
#35917=CARTESIAN_POINT ( 'NONE',  ( 28.68750000122903288, 4.330127018922191873, 2.499999999999999556 ) ) ;
#35918=VECTOR ( 'NONE', #47134, 1000.000000000000000 ) ;
#35919=CARTESIAN_POINT ( 'NONE',  ( 18.53437500061451715, 4.541064518000418104, 2.621784821874999949 ) ) ;
#35920=CARTESIAN_POINT ( 'NONE',  ( 6.609375000614519102, -4.541064518000417216, -2.621784821875001281 ) ) ;
#35921=CARTESIAN_POINT ( 'NONE',  ( 7.320879633048903241E-15, 17.63749999999999218, -34.00000000000000000 ) ) ;
#35922=CARTESIAN_POINT ( 'NONE',  ( 6.965625000614518392, -6.054752690667223547, -1.112240025338166033E-15 ) ) ;
#35923=CARTESIAN_POINT ( 'NONE',  ( 16.82812500061451644, -4.541064518000419881, 2.621784821874995952 ) ) ;
#35925=VERTEX_POINT ( 'NONE', #2249 ) ;
#35926=CARTESIAN_POINT ( 'NONE',  ( 15.85312500061451857, 0.000000000000000000, 5.243569643749999010 ) ) ;
#35928=CARTESIAN_POINT ( 'NONE',  ( 11.39062500061451644, -3.027376345333614438, 5.243569643749998122 ) ) ;
#35930=CARTESIAN_POINT ( 'NONE',  ( 10.68750000000000000, -2.886751345948129988, 4.999999999999997335 ) ) ;
#35931=CARTESIAN_POINT ( 'NONE',  ( 7.387500001229032165, 6.123233995736764310E-16, -4.999999999999998224 ) ) ;
#35932=CARTESIAN_POINT ( 'NONE',  ( 14.48437500061451821, 4.541064518000418104, 2.621784821874999949 ) ) ;
#35933=CARTESIAN_POINT ( 'NONE',  ( 15.82500000122903216, -5.773502691896255534, -1.060575238724906372E-15 ) ) ;
#35935=( BOUNDED_CURVE ( )  B_SPLINE_CURVE ( 2, ( #6041, #10855, #11944, #55925, #61821, #66651, #50027, #16028, #11226 ),
 .UNSPECIFIED., .F., .F. ) 
 B_SPLINE_CURVE_WITH_KNOTS ( ( 3, 2, 2, 2, 3 ),
 ( 0.4891304347826087029, 0.4927536231884058204, 0.5000000000000000000, 0.5072463768115942351, 0.5108695652173913526 ),
 .UNSPECIFIED. ) 
 CURVE ( )  GEOMETRIC_REPRESENTATION_ITEM ( )  RATIONAL_B_SPLINE_CURVE ( ( 0.9330127018922194093, 0.9330127018922194093, 1.000000000000000000, 0.8660254037844387076, 1.000000000000000000, 0.8660254037844387076, 1.000000000000000000, 0.9330127018922182991, 0.9330127018922192983 ) ) 
 REPRESENTATION_ITEM ( '' )  );
#35936=CARTESIAN_POINT ( 'NONE',  ( -2.121784821874999949, 18.37812500061451715, -33.67503911421598417 ) ) ;
#35937=CARTESIAN_POINT ( 'NONE',  ( 16.27500000122903501, -5.773502691896255534, -1.060575238724906372E-15 ) ) ;
#35938=DIRECTION ( 'NONE',  ( -1.000000000000000000, -0.000000000000000000, -0.000000000000000000 ) ) ;
#35939=DIRECTION ( 'NONE',  ( -1.000000000000000000, -0.000000000000000000, -0.000000000000000000 ) ) ;
#35940=CARTESIAN_POINT ( 'NONE',  ( 3.387317645811362521, -3.677893962807537775, 3.685928698369520973 ) ) ;
#35941=CARTESIAN_POINT ( 'NONE',  ( 4.633613603196540254, 1.878729617659674167, 4.895446622381335544 ) ) ;
#35942=CARTESIAN_POINT ( 'NONE',  ( 18.72187500061451360, -6.054752690667223547, -1.112240025338166033E-15 ) ) ;
#35943=CARTESIAN_POINT ( 'NONE',  ( 29.39999999999999858, 4.330127018922192761, -2.499999999999997780 ) ) ;
#35944=EDGE_CURVE ( 'NONE', #46701, #33889, #1715, .T. ) ;
#35945=CARTESIAN_POINT ( 'NONE',  ( 13.15312500061451750, 0.000000000000000000, 5.243569643749999010 ) ) ;
#35947=CARTESIAN_POINT ( 'NONE',  ( 24.08437500061451786, -4.541064518000419881, 2.621784821874995952 ) ) ;
#35949=VECTOR ( 'NONE', #40500, 1000.000000000000000 ) ;
#35950=CARTESIAN_POINT ( 'NONE',  ( 9.178125000614517859, -4.541064518000419881, 2.621784821874995952 ) ) ;
#35951=CARTESIAN_POINT ( 'NONE',  ( 14.70937500061451786, -4.541064518000417216, -2.621784821875001281 ) ) ;
#35952=ORIENTED_EDGE ( 'NONE', *, *, #16469, .T. ) ;
#35953=CARTESIAN_POINT ( 'NONE',  ( 25.50937500061451502, -4.541064518000417216, -2.621784821875001281 ) ) ;
#35954=CARTESIAN_POINT ( 'NONE',  ( 28.26562500061451289, 3.027376345333613106, -5.243569643749998122 ) ) ;
#35955=CARTESIAN_POINT ( 'NONE',  ( 18.10312500061451502, 0.000000000000000000, 5.243569643749999010 ) ) ;
#35956=CARTESIAN_POINT ( 'NONE',  ( 4.898587196589411843E-16, 20.00000000000000000, 33.99999999999999289 ) ) ;
#35959=CARTESIAN_POINT ( 'NONE',  ( 10.80000000000000071, -4.330127018922190985, -2.500000000000001332 ) ) ;
#35960=CARTESIAN_POINT ( 'NONE',  ( 18.97500000122903074, -5.773502691896255534, -1.060575238724906372E-15 ) ) ;
#35963=VERTEX_POINT ( 'NONE', #42865 ) ;
#35964=CARTESIAN_POINT ( 'NONE',  ( 17.73750000000000071, 5.773502691896255534, 3.535250795749688894E-16 ) ) ;
#35965=CARTESIAN_POINT ( 'NONE',  ( 21.86250000000000071, 2.886751345948126879, 4.999999999999999112 ) ) ;
#35966=CARTESIAN_POINT ( 'NONE',  ( 17.93437500061451928, 6.421520780324663323E-16, -5.243569643749999010 ) ) ;
#35967=CARTESIAN_POINT ( 'NONE',  ( 13.15312500061451750, 0.000000000000000000, 5.243569643749999010 ) ) ;
#35970=CARTESIAN_POINT ( 'NONE',  ( 1.071796769724489895, 18.62990381179669797, -34.00000000000000000 ) ) ;
#35971=CARTESIAN_POINT ( 'NONE',  ( 5.503125000614516260, 0.000000000000000000, 5.243569643749999010 ) ) ;
#35973=CARTESIAN_POINT ( 'NONE',  ( 13.04999999999999893, -4.330127018922190985, -2.500000000000001332 ) ) ;
#35975=CARTESIAN_POINT ( 'NONE',  ( 9.001249775931846008E-16, 16.31562500061451715, 34.90005215228797653 ) ) ;
#35976=CARTESIAN_POINT ( 'NONE',  ( 29.39062500061451289, -3.027376345333614438, 5.243569643749998122 ) ) ;
#35980=CARTESIAN_POINT ( 'NONE',  ( 23.52187500061451786, 3.027376345333611329, 5.243569643749999010 ) ) ;
#35981=ORIENTED_EDGE ( 'NONE', *, *, #54670, .F. ) ;
#35982=CARTESIAN_POINT ( 'NONE',  ( 21.47812500061451502, 6.421520780324663323E-16, -5.243569643749999010 ) ) ;
#35983=CARTESIAN_POINT ( 'NONE',  ( 22.80937500061451573, -4.541064518000417216, -2.621784821875001281 ) ) ;
#35984=CARTESIAN_POINT ( 'NONE',  ( -3.000416591977282496E-16, 16.54062500061459673, -34.90005215228797653 ) ) ;
#35985=CARTESIAN_POINT ( 'NONE',  ( 7.303125000614516082, 0.000000000000000000, 5.243569643749999010 ) ) ;
#35987=CARTESIAN_POINT ( 'NONE',  ( 24.51562500061451289, -6.054752690667223547, -1.112240025338166033E-15 ) ) ;
#35990=CARTESIAN_POINT ( 'NONE',  ( 15.79687500061451821, 6.054752690667223547, 3.707466751127219781E-16 ) ) ;
#35991=CARTESIAN_POINT ( 'NONE',  ( 23.67187500061451999, -6.054752690667223547, -1.112240025338166033E-15 ) ) ;
#35992=CARTESIAN_POINT ( 'NONE',  ( 2.121784821875001281, 14.60937500061451821, 33.67503911421598417 ) ) ;
#35993=CARTESIAN_POINT ( 'NONE',  ( 8.128125000614515372, 4.541064518000418104, 2.621784821874999949 ) ) ;
#35995=CARTESIAN_POINT ( 'NONE',  ( 28.60312500061451502, -4.541064518000417216, -2.621784821875001281 ) ) ;
#35996=CARTESIAN_POINT ( 'NONE',  ( 0.000000000000000000, 20.00000000000000000, 30.00000000000000000 ) ) ;
#35997=CARTESIAN_POINT ( 'NONE',  ( 5.315625000614516260, 3.027376345333613106, -5.243569643749998122 ) ) ;
#35998=CARTESIAN_POINT ( 'NONE',  ( 8.559375000614515727, 4.541064518000418104, -2.621784821874998173 ) ) ;
#35999=CARTESIAN_POINT ( 'NONE',  ( 16.61250000122903359, 0.000000000000000000, 4.999999999999998224 ) ) ;
#36000=CARTESIAN_POINT ( 'NONE',  ( 3.871875000614519280, -6.054752690667223547, -1.112240025338166033E-15 ) ) ;
#36001=CARTESIAN_POINT ( 'NONE',  ( 6.965625000614518392, -6.054752690667223547, -1.112240025338166033E-15 ) ) ;
#36004=CARTESIAN_POINT ( 'NONE',  ( 17.67187500061451644, 3.027376345333611329, 5.243569643749999010 ) ) ;
#36007=CARTESIAN_POINT ( 'NONE',  ( 21.17812500061451431, 4.541064518000418104, 2.621784821874999949 ) ) ;
#36008=CARTESIAN_POINT ( 'NONE',  ( 10.34062500061451750, 6.054752690667223547, 3.707466751127219781E-16 ) ) ;
#36010=CARTESIAN_POINT ( 'NONE',  ( 27.57187500061451857, 3.027376345333611329, 5.243569643749999010 ) ) ;
#36011=CARTESIAN_POINT ( 'NONE',  ( 9.628125000614517148, -4.541064518000419881, 2.621784821874995952 ) ) ;
#36012=FACE_OUTER_BOUND ( 'NONE', #1647, .T. ) ;
#36013=CARTESIAN_POINT ( 'NONE',  ( 9.562500001229032875, -4.330127018922190985, -2.500000000000001332 ) ) ;
#36014=CARTESIAN_POINT ( 'NONE',  ( 24.10312500061451502, -4.541064518000417216, -2.621784821875001281 ) ) ;
#36015=CARTESIAN_POINT ( 'NONE',  ( -4.243569643749999898, 9.903125000614517504, -30.00000000000000000 ) ) ;
#36016=CARTESIAN_POINT ( 'NONE',  ( 13.12500000122903288, -5.773502691896255534, -1.060575238724906372E-15 ) ) ;
#36017=CARTESIAN_POINT ( 'NONE',  ( 22.41562500061451502, 3.027376345333613106, -5.243569643749998122 ) ) ;
#36019=CARTESIAN_POINT ( 'NONE',  ( 18.25312500061451715, -4.541064518000417216, -2.621784821875001281 ) ) ;
#36020=CARTESIAN_POINT ( 'NONE',  ( 5.146875000614517859, -3.027376345333614438, 5.243569643749998122 ) ) ;
#36021=CARTESIAN_POINT ( 'NONE',  ( 18.37500000000000355, -4.330127018922194537, 2.499999999999995559 ) ) ;
#36022=CARTESIAN_POINT ( 'NONE',  ( 12.97500000122903252, 2.886751345948126879, 4.999999999999999112 ) ) ;
#36024=CARTESIAN_POINT ( 'NONE',  ( 11.54062500061451857, -3.027376345333610441, -5.243569643749999898 ) ) ;
#36025=CARTESIAN_POINT ( 'NONE',  ( 13.67812500061451786, -4.541064518000419881, 2.621784821874995952 ) ) ;
#36027=CARTESIAN_POINT ( 'NONE',  ( 26.02500000122903145, 2.886751345948126879, 4.999999999999999112 ) ) ;
#36029=CARTESIAN_POINT ( 'NONE',  ( 21.64687500061451786, 6.054752690667223547, 3.707466751127219781E-16 ) ) ;
#36030=CARTESIAN_POINT ( 'NONE',  ( 22.13437500061451502, 4.541064518000418104, 2.621784821874999949 ) ) ;
#36032=CARTESIAN_POINT ( 'NONE',  ( 7.837500001229035007, 6.123233995736764310E-16, -4.999999999999998224 ) ) ;
#36033=CARTESIAN_POINT ( 'NONE',  ( 7.509375000614517681, -4.541064518000417216, -2.621784821875001281 ) ) ;
#36034=CARTESIAN_POINT ( 'NONE',  ( 26.14687500061451431, 6.054752690667223547, 3.707466751127219781E-16 ) ) ;
#36035=CARTESIAN_POINT ( 'NONE',  ( 3.459375000614519635, -4.541064518000417216, -2.621784821875001281 ) ) ;
#36036=CARTESIAN_POINT ( 'NONE',  ( 21.96562500061451573, 3.027376345333613106, -5.243569643749998122 ) ) ;
#36037=CARTESIAN_POINT ( 'NONE',  ( 27.15937500061451360, 0.000000000000000000, 5.243569643749999010 ) ) ;
#36041=CARTESIAN_POINT ( 'NONE',  ( 7.096875000614517148, -3.027376345333610441, -5.243569643749999898 ) ) ;
#36042=CARTESIAN_POINT ( 'NONE',  ( 17.65312500061451573, 0.000000000000000000, 5.243569643749999010 ) ) ;
#36045=CARTESIAN_POINT ( 'NONE',  ( 27.96562500061451928, 3.027376345333611329, 5.243569643749999010 ) ) ;
#36046=CARTESIAN_POINT ( 'NONE',  ( 5.221875000614519813, -6.054752690667223547, -1.112240025338166033E-15 ) ) ;
#36047=CARTESIAN_POINT ( 'NONE',  ( -3.999999999999997335, 15.98750000000000249, -27.69059892324149530 ) ) ;
#36048=CARTESIAN_POINT ( 'NONE',  ( 0.000000000000000000, 20.00000000000000000, -30.00000000000000000 ) ) ;
#36049=CARTESIAN_POINT ( 'NONE',  ( 17.36249999999999716, 2.886751345948126879, 4.999999999999999112 ) ) ;
#36050=CARTESIAN_POINT ( 'NONE',  ( 20.20312500061451644, 4.541064518000418104, -2.621784821874998173 ) ) ;
#36052=CARTESIAN_POINT ( 'NONE',  ( 23.85000000000000142, -4.330127018922190985, -2.500000000000001332 ) ) ;
#36054=CARTESIAN_POINT ( 'NONE',  ( 25.24687500061451573, 6.054752690667223547, 3.707466751127219781E-16 ) ) ;
#36057=CARTESIAN_POINT ( 'NONE',  ( 13.19062500061451537, -3.027376345333614438, 5.243569643749998122 ) ) ;
#36058=CARTESIAN_POINT ( 'NONE',  ( 6.478125000614516793, -4.541064518000419881, 2.621784821874995952 ) ) ;
#36060=CARTESIAN_POINT ( 'NONE',  ( 28.94062500061452070, -3.027376345333614438, 5.243569643749998122 ) ) ;
#36061=CARTESIAN_POINT ( 'NONE',  ( 14.96250000122903323, -4.330127018922190985, -2.500000000000001332 ) ) ;
#36062=AXIS2_PLACEMENT_3D ( 'NONE', #24190, #24917, #7213 ) ;
#36063=CARTESIAN_POINT ( 'NONE',  ( 19.34999999999999787, -4.330127018922190985, -2.500000000000001332 ) ) ;
#36064=CARTESIAN_POINT ( 'NONE',  ( 27.78749999999999787, -2.886751345948129988, 4.999999999999997335 ) ) ;
#36065=CARTESIAN_POINT ( 'NONE',  ( 3.121875000614518836, 3.027376345333613106, -5.243569643749998122 ) ) ;
#36066=CARTESIAN_POINT ( 'NONE',  ( 8.559375000614515727, 4.541064518000418104, -2.621784821874998173 ) ) ;
#36067=CARTESIAN_POINT ( 'NONE',  ( 19.58437500061451786, -4.541064518000419881, 2.621784821874995952 ) ) ;
#36069=ORIENTED_EDGE ( 'NONE', *, *, #54349, .T. ) ;
#36070=CARTESIAN_POINT ( 'NONE',  ( 28.94062500061452070, -3.027376345333614438, 5.243569643749998122 ) ) ;
#36071=CARTESIAN_POINT ( 'NONE',  ( 3.562500000000000444, -5.773502691896255534, -1.060575238724906372E-15 ) ) ;
#36072=CARTESIAN_POINT ( 'NONE',  ( 5.371875000614516615, 3.027376345333613106, -5.243569643749998122 ) ) ;
#36073=CARTESIAN_POINT ( 'NONE',  ( 16.05000000000000071, 0.000000000000000000, 4.999999999999998224 ) ) ;
#36074=CARTESIAN_POINT ( 'NONE',  ( 13.71562500061451750, -6.054752690667223547, -1.112240025338166033E-15 ) ) ;
#36076=CYLINDRICAL_SURFACE ( 'NONE', #3262, 3.999999999999996447 ) ;
#36077=CARTESIAN_POINT ( 'NONE',  ( 18.48750000122903359, -4.330127018922194537, 2.499999999999995559 ) ) ;
#36080=CARTESIAN_POINT ( 'NONE',  ( 8.803125000614517859, -4.541064518000417216, -2.621784821875001281 ) ) ;
#36081=CARTESIAN_POINT ( 'NONE',  ( 24.68437500061451573, 6.421520780324663323E-16, -5.243569643749999010 ) ) ;
#36083=CARTESIAN_POINT ( 'NONE',  ( -4.243569643749999898, 19.85937500061451644, 30.00000000000000000 ) ) ;
#36084=CARTESIAN_POINT ( 'NONE',  ( 24.90937500061451715, 0.000000000000000000, 5.243569643749999010 ) ) ;
#36085=CARTESIAN_POINT ( 'NONE',  ( 8.400000000000000355, 0.000000000000000000, 4.999999999999998224 ) ) ;
#36086=CARTESIAN_POINT ( 'NONE',  ( 4.000000000000000000, 14.00000000122903288, 32.30940107675849049 ) ) ;
#36087=CARTESIAN_POINT ( 'NONE',  ( 14.09062500061451750, -3.027376345333614438, 5.243569643749998122 ) ) ;
#36088=CARTESIAN_POINT ( 'NONE',  ( 6.975000001229032520, 2.886751345948129099, -4.999999999999998224 ) ) ;
#36089=CARTESIAN_POINT ( 'NONE',  ( 10.84687500061451892, 6.054752690667223547, 3.707466751127219781E-16 ) ) ;
#36090=CARTESIAN_POINT ( 'NONE',  ( 3.869872862876293507, -3.166083388853397906, 4.043238470916601379 ) ) ;
#36091=VERTEX_POINT ( 'NONE', #13310 ) ;
#36092=CARTESIAN_POINT ( 'NONE',  ( 13.15312500061451750, 0.000000000000000000, 5.243569643749999010 ) ) ;
#36094=CARTESIAN_POINT ( 'NONE',  ( 24.11250000122903359, 4.330127018922192761, -2.499999999999997780 ) ) ;
#36095=CARTESIAN_POINT ( 'NONE',  ( 11.22187500061451892, 3.027376345333613106, -5.243569643749998122 ) ) ;
#36096=CARTESIAN_POINT ( 'NONE',  ( 14.57812500061451644, -4.541064518000419881, 2.621784821874995952 ) ) ;
#36098=CARTESIAN_POINT ( 'NONE',  ( 22.95937500061451431, 4.541064518000418104, -2.621784821874998173 ) ) ;
#36099=CARTESIAN_POINT ( 'NONE',  ( 3.999999999999999112, 15.83750000122903501, 30.00000000000000000 ) ) ;
#36100=CYLINDRICAL_SURFACE ( 'NONE', #43407, 4.999999999999998224 ) ;
#36101=FACE_OUTER_BOUND ( 'NONE', #55262, .T. ) ;
#36102=CARTESIAN_POINT ( 'NONE',  ( 9.001249775931846008E-16, 14.12187500061451750, -25.09994784771203058 ) ) ;
#36103=CARTESIAN_POINT ( 'NONE',  ( 14.67187500061451821, -6.054752690667223547, -1.112240025338166033E-15 ) ) ;
#36104=CARTESIAN_POINT ( 'NONE',  ( 17.28750000122903430, 6.123233995736764310E-16, -4.999999999999998224 ) ) ;
#36105=CARTESIAN_POINT ( 'NONE',  ( 13.35937500061451821, -4.541064518000417216, -2.621784821875001281 ) ) ;
#36106=CARTESIAN_POINT ( 'NONE',  ( -4.243569643749997233, 10.89687500061451786, 32.45002607614398471 ) ) ;
#36107=CARTESIAN_POINT ( 'NONE',  ( 20.77500000122903145, -5.773502691896255534, -1.060575238724906372E-15 ) ) ;
#36108=CARTESIAN_POINT ( 'NONE',  ( 12.17812500061451608, 4.541064518000418104, 2.621784821874999949 ) ) ;
#36111=CARTESIAN_POINT ( 'NONE',  ( 19.16250000000000142, 2.886751345948126879, 4.999999999999999112 ) ) ;
#36113=CARTESIAN_POINT ( 'NONE',  ( 11.55937500061451928, -4.541064518000417216, -2.621784821875001281 ) ) ;
#36114=DIRECTION ( 'NONE',  ( -1.000000000000000000, -0.000000000000000000, -0.000000000000000000 ) ) ;
#36116=CARTESIAN_POINT ( 'NONE',  ( 12.60000000122903430, -2.886751345948129988, 4.999999999999997335 ) ) ;
#36117=CARTESIAN_POINT ( 'NONE',  ( 21.78750000122903074, 6.123233995736764310E-16, -4.999999999999998224 ) ) ;
#36118=CARTESIAN_POINT ( 'NONE',  ( 18.32812500061451644, 6.421520780324663323E-16, -5.243569643749999010 ) ) ;
#36119=CARTESIAN_POINT ( 'NONE',  ( 21.55312500061451431, 4.541064518000418104, -2.621784821874998173 ) ) ;
#36120=CARTESIAN_POINT ( 'NONE',  ( 26.62500000122903288, -5.773502691896255534, -1.060575238724906372E-15 ) ) ;
#36121=CARTESIAN_POINT ( 'NONE',  ( 26.55000000000000071, -4.330127018922190985, -2.500000000000001332 ) ) ;
#36123=VECTOR ( 'NONE', #7507, 1000.000000000000000 ) ;
#36125=CARTESIAN_POINT ( 'NONE',  ( 27.98437500061451289, 4.541064518000418104, 2.621784821874999949 ) ) ;
#36126=CARTESIAN_POINT ( 'NONE',  ( 4.000000000000000000, 14.33750000000000213, -27.69059892324149885 ) ) ;
#36127=CARTESIAN_POINT ( 'NONE',  ( 9.001249775931846008E-16, 16.37187500061451573, -25.09994784771203058 ) ) ;
#36128=CARTESIAN_POINT ( 'NONE',  ( 3.150000001229034119, -2.886751345948129988, 4.999999999999997335 ) ) ;
#36129=CARTESIAN_POINT ( 'NONE',  ( 6.299999999999999822, -4.330127018922190985, -2.500000000000001332 ) ) ;
#36130=( BOUNDED_CURVE ( )  B_SPLINE_CURVE ( 2, ( #4087, #38798, #49514, #43975, #27345, #21782, #10711, #66495, #3722 ),
 .UNSPECIFIED., .F., .F. ) 
 B_SPLINE_CURVE_WITH_KNOTS ( ( 3, 2, 2, 2, 3 ),
 ( 0.05434782608695652717, 0.05797101449275362389, 0.06521739130434782428, 0.07246376811594203160, 0.07608695652173913526 ),
 .UNSPECIFIED. ) 
 CURVE ( )  GEOMETRIC_REPRESENTATION_ITEM ( )  RATIONAL_B_SPLINE_CURVE ( ( 0.9330127018922194093, 0.9330127018922194093, 1.000000000000000000, 0.8660254037844387076, 1.000000000000000000, 0.8660254037844387076, 1.000000000000000000, 0.9330127018922191873, 0.9330127018922192983 ) ) 
 REPRESENTATION_ITEM ( '' )  );
#36132=CARTESIAN_POINT ( 'NONE',  ( 9.421875000614519990, 3.027376345333613106, -5.243569643749998122 ) ) ;
#36133=CARTESIAN_POINT ( 'NONE',  ( 28.75312500061451715, 4.541064518000418104, -2.621784821874998173 ) ) ;
#36135=CARTESIAN_POINT ( 'NONE',  ( -5.605356288733176484, 8.281802244057951512, -27.85102845225483748 ) ) ;
#36136=CARTESIAN_POINT ( 'NONE',  ( 2.000000000000001332, 17.56250000122903288, -26.53589838486224650 ) ) ;
#36137=CARTESIAN_POINT ( 'NONE',  ( 7.284375000614518036, 4.541064518000418104, 2.621784821874999949 ) ) ;
#36138=CARTESIAN_POINT ( 'NONE',  ( 12.19687500061451679, 6.054752690667223547, 3.707466751127219781E-16 ) ) ;
#36139=CARTESIAN_POINT ( 'NONE',  ( 4.237500000000001599, 5.773502691896255534, 3.535250795749688894E-16 ) ) ;
#36140=CARTESIAN_POINT ( 'NONE',  ( -4.243569643749999898, 14.40312500061459389, 30.00000000000000000 ) ) ;
#36141=EDGE_CURVE ( 'NONE', #33565, #66841, #31416, .T. ) ;
#36143=CARTESIAN_POINT ( 'NONE',  ( 7.200000000000001954, -4.330127018922190985, -2.500000000000001332 ) ) ;
#36145=CARTESIAN_POINT ( 'NONE',  ( 20.50312500061451715, -4.541064518000417216, -2.621784821875001281 ) ) ;
#36146=CARTESIAN_POINT ( 'NONE',  ( 13.71562500061451750, -6.054752690667223547, -1.112240025338166033E-15 ) ) ;
#36148=CARTESIAN_POINT ( 'NONE',  ( 10.28437500061451715, 6.421520780324663323E-16, -5.243569643749999010 ) ) ;
#36149=CARTESIAN_POINT ( 'NONE',  ( 25.64999999999999858, -4.330127018922190985, -2.500000000000001332 ) ) ;
#36150=CARTESIAN_POINT ( 'NONE',  ( 22.61250000122903003, -4.330127018922190985, -2.500000000000001332 ) ) ;
#36151=CARTESIAN_POINT ( 'NONE',  ( 16.98750000000000426, -2.886751345948096681, 5.000000000000054179 ) ) ;
#36152=CARTESIAN_POINT ( 'NONE',  ( 12.38437500061451857, -4.541064518000419881, 2.621784821874995952 ) ) ;
#36153=CARTESIAN_POINT ( 'NONE',  ( 25.84687500061451360, -3.027376345333614438, 5.243569643749998122 ) ) ;
#36154=CARTESIAN_POINT ( 'NONE',  ( 3.646875000614520079, 6.054752690667223547, 3.707466751127219781E-16 ) ) ;
#36155=CARTESIAN_POINT ( 'NONE',  ( 30.00000000000000000, 0.000000000000000000, 4.999999999999998224 ) ) ;
#36156=CARTESIAN_POINT ( 'NONE',  ( 18.83437500061451431, 6.421520780324663323E-16, -5.243569643749999010 ) ) ;
#36157=CARTESIAN_POINT ( 'NONE',  ( 11.89687500061451608, -3.027376345333614438, 5.243569643749998122 ) ) ;
#36159=CARTESIAN_POINT ( 'NONE',  ( 22.80000000000000071, 0.000000000000000000, 4.999999999999998224 ) ) ;
#36161=CARTESIAN_POINT ( 'NONE',  ( 2.121784821875001281, 13.25937500061451857, -26.32496088578401938 ) ) ;
#36163=CARTESIAN_POINT ( 'NONE',  ( 14.01562500061451644, 3.027376345333611329, 5.243569643749999010 ) ) ;
#36164=CARTESIAN_POINT ( 'NONE',  ( 4.387500000000002842, -2.886751345948129988, 4.999999999999997335 ) ) ;
#36165=CARTESIAN_POINT ( 'NONE',  ( 29.80312500061451431, 0.000000000000000000, 5.243569643749999010 ) ) ;
#36167=CARTESIAN_POINT ( 'NONE',  ( 14.92500000000000071, 6.123233995736764310E-16, -4.999999999999998224 ) ) ;
#36168=CARTESIAN_POINT ( 'NONE',  ( -3.999999999999999112, 19.66250000122903430, 30.00000000000000000 ) ) ;
#36169=CARTESIAN_POINT ( 'NONE',  ( 13.23750000122903359, 6.123233995736764310E-16, -4.999999999999998224 ) ) ;
#36170=CARTESIAN_POINT ( 'NONE',  ( 25.54687500061451644, -3.027376345333610441, -5.243569643749999898 ) ) ;
#36171=CARTESIAN_POINT ( 'NONE',  ( 20.40000000122903501, -2.886751345948092684, -5.000000000000057732 ) ) ;
#36174=CARTESIAN_POINT ( 'NONE',  ( 20.20312500061451644, 4.541064518000418104, -2.621784821874998173 ) ) ;
#36175=CARTESIAN_POINT ( 'NONE',  ( 4.715625000614516615, -6.054752690667223547, -1.112240025338166033E-15 ) ) ;
#36176=CARTESIAN_POINT ( 'NONE',  ( 18.87187500061451573, 3.027376345333613106, -5.243569643749998122 ) ) ;
#36177=CARTESIAN_POINT ( 'NONE',  ( 28.39687500061452141, 6.054752690667223547, 3.707466751127219781E-16 ) ) ;
#36178=CARTESIAN_POINT ( 'NONE',  ( 6.928125000614516082, -4.541064518000419881, 2.621784821874995952 ) ) ;
#36179=CARTESIAN_POINT ( 'NONE',  ( 22.79062500061451502, -3.027376345333610441, -5.243569643749999898 ) ) ;
#36180=CARTESIAN_POINT ( 'NONE',  ( 2.121784821875001281, 15.90312500061451573, 33.67503911421598417 ) ) ;
#36181=CARTESIAN_POINT ( 'NONE',  ( 18.67500000122903714, 2.886751345948129099, -4.999999999999998224 ) ) ;
#36183=CARTESIAN_POINT ( 'NONE',  ( 8.278125000614515727, -4.541064518000419881, 2.621784821874995952 ) ) ;
#36184=CARTESIAN_POINT ( 'NONE',  ( 3.459375000614519635, -4.541064518000417216, -2.621784821875001281 ) ) ;
#36185=CARTESIAN_POINT ( 'NONE',  ( 29.72812500061451502, 4.541064518000418104, 2.621784821874999949 ) ) ;
#36186=CARTESIAN_POINT ( 'NONE',  ( 21.87187500061451573, -6.054752690667223547, -1.112240025338166033E-15 ) ) ;
#36187=CARTESIAN_POINT ( 'NONE',  ( 14.80312500061451608, 4.541064518000418104, -2.621784821874998173 ) ) ;
#36188=CARTESIAN_POINT ( 'NONE',  ( 23.85000000122903430, -2.886751345948129988, 4.999999999999997335 ) ) ;
#36189=CARTESIAN_POINT ( 'NONE',  ( 24.85312500061451502, 0.000000000000000000, 5.243569643749999010 ) ) ;
#36190=CARTESIAN_POINT ( 'NONE',  ( 19.92187500061451644, 3.027376345333611329, 5.243569643749999010 ) ) ;
#36191=CARTESIAN_POINT ( 'NONE',  ( 15.06562500061451537, -6.054752690667223547, -1.112240025338166033E-15 ) ) ;
#36192=CARTESIAN_POINT ( 'NONE',  ( 2.121784821874999061, 16.10937500061451644, 26.32496088578401583 ) ) ;
#36193=CARTESIAN_POINT ( 'NONE',  ( 20.31562500061451715, 3.027376345333611329, 5.243569643749999010 ) ) ;
#36194=CARTESIAN_POINT ( 'NONE',  ( 29.50312500061451360, -4.541064518000417216, -2.621784821875001281 ) ) ;
#36195=VERTEX_POINT ( 'NONE', #35849 ) ;
#36196=CARTESIAN_POINT ( 'NONE',  ( 26.06250000000000000, -5.773502691896255534, -1.060575238724906372E-15 ) ) ;
#36197=CARTESIAN_POINT ( 'NONE',  ( 1.999999999999998668, 11.30000000000000071, -33.46410161513775705 ) ) ;
#36199=CARTESIAN_POINT ( 'NONE',  ( 26.65312500061451573, 0.000000000000000000, 5.243569643749999010 ) ) ;
#36200=CARTESIAN_POINT ( 'NONE',  ( 7.903125000614515727, -4.541064518000417216, -2.621784821875001281 ) ) ;
#36201=CARTESIAN_POINT ( 'NONE',  ( 20.88750000122903572, 6.123233995736764310E-16, -4.999999999999998224 ) ) ;
#36202=CARTESIAN_POINT ( 'NONE',  ( 24.66562500061451502, 3.027376345333613106, -5.243569643749998122 ) ) ;
#36203=CARTESIAN_POINT ( 'NONE',  ( 24.75000000000000000, -4.330127018922190985, -2.500000000000001332 ) ) ;
#36204=CARTESIAN_POINT ( 'NONE',  ( 3.999999999999998668, 15.42500000122903359, -32.30940107675850470 ) ) ;
#36205=EDGE_CURVE ( 'NONE', #27078, #43803, #21226, .T. ) ;
#36206=CARTESIAN_POINT ( 'NONE',  ( 28.37812500061451715, 4.541064518000418104, 2.621784821874999949 ) ) ;
#36207=CARTESIAN_POINT ( 'NONE',  ( 11.54062500061451857, -3.027376345333610441, -5.243569643749999898 ) ) ;
#36208=ORIENTED_EDGE ( 'NONE', *, *, #4157, .F. ) ;
#36209=B_SPLINE_CURVE_WITH_KNOTS ( 'NONE', 3,
 ( #22155, #50248, #40603, #56143, #23236, #51688, #28425, #33959, #6256, #50962 ),
 .UNSPECIFIED., .F., .F.,
 ( 4, 3, 3, 4 ),
 ( 1.837010936913719881E-16, 0.0001572264585416875324, 0.0003144530955621989074, 0.0005640517951500036587 ),
 .UNSPECIFIED. ) ;
#36210=CARTESIAN_POINT ( 'NONE',  ( 25.45312500061451644, -4.541064518000417216, -2.621784821875001281 ) ) ;
#36211=CARTESIAN_POINT ( 'NONE',  ( 4.603125000614518569, 0.000000000000000000, 5.243569643749999010 ) ) ;
#36213=PLANE ( 'NONE',  #69206 ) ;
#36216=CARTESIAN_POINT ( 'NONE',  ( 12.26249999999999929, 2.886751345948129099, -4.999999999999998224 ) ) ;
#36217=CARTESIAN_POINT ( 'NONE',  ( 14.63437500061451679, -4.541064518000419881, 2.621784821874995952 ) ) ;
#36218=CARTESIAN_POINT ( 'NONE',  ( 7.725000001229034297, -5.773502691896255534, -1.060575238724906372E-15 ) ) ;
#36219=CARTESIAN_POINT ( 'NONE',  ( 17.33437500061451431, -4.541064518000419881, 2.621784821874995952 ) ) ;
#36221=CARTESIAN_POINT ( 'NONE',  ( 9.009375000614518569, 4.541064518000418104, -2.621784821874998173 ) ) ;
#36222=CARTESIAN_POINT ( 'NONE',  ( -3.000416591977282496E-16, 12.49062500061451608, -34.90005215228797653 ) ) ;
#36223=DIRECTION ( 'NONE',  ( 0.000000000000000000, 0.000000000000000000, 1.000000000000000000 ) ) ;
#36225=VERTEX_POINT ( 'NONE', #47668 ) ;
#36226=CARTESIAN_POINT ( 'NONE',  ( 24.14062500061451289, -3.027376345333610441, -5.243569643749999898 ) ) ;
#36227=CARTESIAN_POINT ( 'NONE',  ( -2.121784821874999949, 11.23437500061451821, 26.32496088578401938 ) ) ;
#36228=CARTESIAN_POINT ( 'NONE',  ( 21.26250000122903572, -4.330127018922190985, -2.500000000000001332 ) ) ;
#36229=CARTESIAN_POINT ( 'NONE',  ( 25.13437500061451502, 6.421520780324663323E-16, -5.243569643749999010 ) ) ;
#36230=CARTESIAN_POINT ( 'NONE',  ( 28.17187500061451644, -6.054752690667223547, -1.112240025338166033E-15 ) ) ;
#36231=CARTESIAN_POINT ( 'NONE',  ( 21.67500000000000071, 6.123233995736764310E-16, -4.999999999999998224 ) ) ;
#36232=ADVANCED_FACE ( 'NONE', ( #42134 ), #64660, .F. ) ;
#36233=CARTESIAN_POINT ( 'NONE',  ( 5.428125000614517859, 4.541064518000418104, 2.621784821874999949 ) ) ;
#36235=CARTESIAN_POINT ( 'NONE',  ( 16.80937500061451573, 0.000000000000000000, 5.243569643749999010 ) ) ;
#36237=CARTESIAN_POINT ( 'NONE',  ( 29.51250000122903216, 4.330127018922192761, -2.499999999999997780 ) ) ;
#36238=CARTESIAN_POINT ( 'NONE',  ( 8.484375000614518214, 6.421520780324663323E-16, -5.243569643749999010 ) ) ;
#36239=CARTESIAN_POINT ( 'NONE',  ( 20.18437500061451573, 6.421520780324663323E-16, -5.243569643749999010 ) ) ;
#36241=CARTESIAN_POINT ( 'NONE',  ( 26.69999999999999929, 4.330127018922192761, -2.499999999999997780 ) ) ;
#36242=CARTESIAN_POINT ( 'NONE',  ( 28.35937500061451289, 4.541064518000418104, -2.621784821874998173 ) ) ;
#36243=CARTESIAN_POINT ( 'NONE',  ( 3.486133158594716510E-16, 19.88749999999999929, 26.00000000000000355 ) ) ;
#36244=CARTESIAN_POINT ( 'NONE',  ( 21.78750000000000142, 5.773502691896255534, 3.535250795749688401E-16 ) ) ;
#36245=EDGE_LOOP ( 'NONE', ( #72430, #24061, #31671, #63363 ) ) ;
#36246=CARTESIAN_POINT ( 'NONE',  ( 8.025000000000000355, -4.330127018922194537, 2.499999999999995559 ) ) ;
#36248=CARTESIAN_POINT ( 'NONE',  ( 20.99062500061451431, -3.027376345333610441, -5.243569643749999898 ) ) ;
#36249=CARTESIAN_POINT ( 'NONE',  ( 10.91250000000000320, 2.886751345948129099, -4.999999999999998224 ) ) ;
#36250=CARTESIAN_POINT ( 'NONE',  ( 8.812500001229034652, 4.330127018922192761, -2.499999999999997780 ) ) ;
#36251=CARTESIAN_POINT ( 'NONE',  ( 5.915625000614515905, 3.027376345333611329, 5.243569643749999010 ) ) ;
#36252=CARTESIAN_POINT ( 'NONE',  ( 21.37499999999999645, 4.330127018922191873, 2.499999999999999556 ) ) ;
#36253=CARTESIAN_POINT ( 'NONE',  ( 21.89062500061451289, -3.027376345333610441, -5.243569643749999898 ) ) ;
#36255=CARTESIAN_POINT ( 'NONE',  ( 26.70000000122903572, -2.886751345948125991, -5.000000000000000000 ) ) ;
#36257=CARTESIAN_POINT ( 'NONE',  ( 3.937500000000000444, -2.886751345948129988, 4.999999999999997335 ) ) ;
#36259=CARTESIAN_POINT ( 'NONE',  ( 20.12812500061451715, 6.421520780324663323E-16, -5.243569643749999010 ) ) ;
#36260=CARTESIAN_POINT ( 'NONE',  ( 27.25312500061451360, -4.541064518000417216, -2.621784821875001281 ) ) ;
#36261=CARTESIAN_POINT ( 'NONE',  ( 26.55937500061451573, 4.541064518000418104, -2.621784821874998173 ) ) ;
#36262=CARTESIAN_POINT ( 'NONE',  ( 12.37500000000000000, 4.330127018922191873, 2.499999999999999556 ) ) ;
#36263=CARTESIAN_POINT ( 'NONE',  ( 13.67812500061451786, -4.541064518000419881, 2.621784821874995952 ) ) ;
#36264=CARTESIAN_POINT ( 'NONE',  ( 28.22812500061451502, 6.421520780324663323E-16, -5.243569643749999010 ) ) ;
#36265=CARTESIAN_POINT ( 'NONE',  ( 10.19062500061451892, -3.027376345333610441, -5.243569643749999898 ) ) ;
#36267=CARTESIAN_POINT ( 'NONE',  ( -3.000416591977282496E-16, 12.54687500061451999, 25.09994784771203058 ) ) ;
#36269=CARTESIAN_POINT ( 'NONE',  ( 25.65000000122903145, -2.886751345948129988, 4.999999999999997335 ) ) ;
#36271=CARTESIAN_POINT ( 'NONE',  ( 17.54062500061451502, 6.054752690667223547, 3.707466751127219781E-16 ) ) ;
#36272=DIRECTION ( 'NONE',  ( 0.000000000000000000, 0.000000000000000000, -1.000000000000000000 ) ) ;
#36273=CARTESIAN_POINT ( 'NONE',  ( 11.29687500061451644, 6.054752690667223547, 3.707466751127219781E-16 ) ) ;
#36274=CARTESIAN_POINT ( 'NONE',  ( 9.946875000614516793, 6.054752690667223547, 3.707466751127219781E-16 ) ) ;
#36275=CARTESIAN_POINT ( 'NONE',  ( 17.52187500061451431, 3.027376345333613106, -5.243569643749998122 ) ) ;
#36276=ORIENTED_EDGE ( 'NONE', *, *, #54349, .F. ) ;
#36277=CARTESIAN_POINT ( 'NONE',  ( 29.40937500061451715, 0.000000000000000000, 5.243569643749999010 ) ) ;
#36278=CARTESIAN_POINT ( 'NONE',  ( 21.47812500061451502, 6.421520780324663323E-16, -5.243569643749999010 ) ) ;
#36279=CARTESIAN_POINT ( 'NONE',  ( 15.34687500061451537, 6.054752690667223547, 3.707466751127219781E-16 ) ) ;
#36280=CARTESIAN_POINT ( 'NONE',  ( 21.36562500061451431, -6.054752690667223547, -1.112240025338166033E-15 ) ) ;
#36281=CARTESIAN_POINT ( 'NONE',  ( 3.999999999999999112, 13.47500000000000142, 30.00000000000000000 ) ) ;
#36282=CARTESIAN_POINT ( 'NONE',  ( 26.76562500061451644, -6.054752690667223547, -1.112240025338166033E-15 ) ) ;
#36283=CARTESIAN_POINT ( 'NONE',  ( 9.450000001229033941, -2.886751345948129988, 4.999999999999997335 ) ) ;
#36284=ORIENTED_EDGE ( 'NONE', *, *, #26884, .T. ) ;
#36285=CARTESIAN_POINT ( 'NONE',  ( 4.237500001229036251, 6.123233995736764310E-16, -4.999999999999998224 ) ) ;
#36286=CARTESIAN_POINT ( 'NONE',  ( 3.999999999999999112, 18.87500000000000000, -30.00000000000000000 ) ) ;
#36287=CARTESIAN_POINT ( 'NONE',  ( 24.71250000122903145, 0.000000000000000000, 4.999999999999998224 ) ) ;
#36289=CARTESIAN_POINT ( 'NONE',  ( 6.046875000614519102, -3.027376345333614438, 5.243569643749998122 ) ) ;
#36290=CARTESIAN_POINT ( 'NONE',  ( 1.592000809091587073E-14, 15.38750000000000284, 26.00000000000000000 ) ) ;
#36291=CARTESIAN_POINT ( 'NONE',  ( 14.42812500061451786, 4.541064518000418104, 2.621784821874999949 ) ) ;
#36292=CARTESIAN_POINT ( 'NONE',  ( 8.521875000614516082, 3.027376345333613106, -5.243569643749998122 ) ) ;
#36293=CARTESIAN_POINT ( 'NONE',  ( 27.56250000122902932, -4.330127018922190985, -2.500000000000001332 ) ) ;
#36294=CARTESIAN_POINT ( 'NONE',  ( 16.47187500061452070, -6.054752690667223547, -1.112240025338166033E-15 ) ) ;
#36295=CARTESIAN_POINT ( 'NONE',  ( 5.521875000614517859, 3.027376345333611329, 5.243569643749999010 ) ) ;
#36296=LINE ( 'NONE', #25576, #65119 ) ;
#36297=( BOUNDED_CURVE ( )  B_SPLINE_CURVE ( 2, ( #50245, #11068, #27704, #33240, #50958, #22863, #67595 ),
 .UNSPECIFIED., .F., .F. ) 
 B_SPLINE_CURVE_WITH_KNOTS ( ( 3, 2, 2, 3 ),
 ( 0.9259902657761827083, 0.9277777777777778123, 0.9305555555555555802, 0.9321263668030935756 ),
 .UNSPECIFIED. ) 
 CURVE ( )  GEOMETRIC_REPRESENTATION_ITEM ( )  RATIONAL_B_SPLINE_CURVE ( ( 0.9385307109133473880, 0.9137867684880971453, 1.000000000000000000, 0.8660254037844387076, 1.000000000000000000, 0.9242384310568843020, 0.9341619918451884441 ) ) 
 REPRESENTATION_ITEM ( '' )  );
#36298=CARTESIAN_POINT ( 'NONE',  ( 6.665625000614515905, 3.027376345333613106, -5.243569643749998122 ) ) ;
#36299=CARTESIAN_POINT ( 'NONE',  ( 18.06562500061451715, 3.027376345333611329, 5.243569643749999010 ) ) ;
#36301=CARTESIAN_POINT ( 'NONE',  ( 13.30312500061451786, -4.541064518000417216, -2.621784821875001281 ) ) ;
#36302=CARTESIAN_POINT ( 'NONE',  ( 5.587500001229033231, 6.123233995736764310E-16, -4.999999999999998224 ) ) ;
#36303=CARTESIAN_POINT ( 'NONE',  ( 11.61562500061451608, 3.027376345333613106, -5.243569643749998122 ) ) ;
#36305=CARTESIAN_POINT ( 'NONE',  ( 12.03749999999999964, -2.886751345948129988, 4.999999999999997335 ) ) ;
#36306=CARTESIAN_POINT ( 'NONE',  ( 6.187500001229032875, 4.330127018922191873, 2.499999999999999556 ) ) ;
#36307=CARTESIAN_POINT ( 'NONE',  ( 14.97187500061451892, 3.027376345333611329, 5.243569643749999010 ) ) ;
#36308=CARTESIAN_POINT ( 'NONE',  ( 15.97500000122903430, 2.886751345948129099, -4.999999999999998224 ) ) ;
#36310=CARTESIAN_POINT ( 'NONE',  ( 2.121784821875001281, 19.05312500061451431, -26.32496088578401938 ) ) ;
#36313=CARTESIAN_POINT ( 'NONE',  ( 4.359375000614517326, -4.541064518000417216, -2.621784821875001281 ) ) ;
#36315=CARTESIAN_POINT ( 'NONE',  ( 4.898734551532200499, 1.001199177798645534, 4.898734551532190729 ) ) ;
#36316=CARTESIAN_POINT ( 'NONE',  ( 14.89687500061451786, 6.054752690667223547, 3.707466751127219781E-16 ) ) ;
#36317=CARTESIAN_POINT ( 'NONE',  ( 28.23750000000000426, -2.886751345948129988, 4.999999999999997335 ) ) ;
#36318=EDGE_CURVE ( 'NONE', #48564, #63279, #3353, .T. ) ;
#36319=CARTESIAN_POINT ( 'NONE',  ( 13.97812500061451679, 4.541064518000418104, 2.621784821874999949 ) ) ;
#36321=CARTESIAN_POINT ( 'NONE',  ( 24.87187500061451573, 3.027376345333611329, 5.243569643749999010 ) ) ;
#36323=CARTESIAN_POINT ( 'NONE',  ( 11.12812500061451715, 6.421520780324663323E-16, -5.243569643749999010 ) ) ;
#36324=CARTESIAN_POINT ( 'NONE',  ( 16.73437500061451644, 4.541064518000418104, 2.621784821874999949 ) ) ;
#36325=ORIENTED_EDGE ( 'NONE', *, *, #10637, .F. ) ;
#36326=CARTESIAN_POINT ( 'NONE',  ( 25.92187500061451999, -6.054752690667223547, -1.112240025338166033E-15 ) ) ;
#36327=CARTESIAN_POINT ( 'NONE',  ( 28.30312500061451431, 4.541064518000418104, -2.621784821874998173 ) ) ;
#36328=CARTESIAN_POINT ( 'NONE',  ( 18.89062500061451644, 6.054752690667223547, 3.707466751127219781E-16 ) ) ;
#36329=CARTESIAN_POINT ( 'NONE',  ( 28.90312500061451217, 0.000000000000000000, 5.243569643749999010 ) ) ;
#36330=CARTESIAN_POINT ( 'NONE',  ( 4.854756222371646501, 1.196571399816914738, -5.105259861685001788 ) ) ;
#36331=( BOUNDED_CURVE ( )  B_SPLINE_CURVE ( 2, ( #18761, #24678, #47225, #30596, #2884, #59380, #70849 ),
 .UNSPECIFIED., .F., .F. ) 
 B_SPLINE_CURVE_WITH_KNOTS ( ( 3, 2, 2, 3 ),
 ( 0.8000000000000000444, 0.8027777777777778123, 0.8055555555555555802, 0.8083333333333333481 ),
 .UNSPECIFIED. ) 
 CURVE ( )  GEOMETRIC_REPRESENTATION_ITEM ( )  RATIONAL_B_SPLINE_CURVE ( ( 1.000000000000000000, 0.8660254037844387076, 1.000000000000000000, 0.8660254037844387076, 1.000000000000000000, 0.8660254037844387076, 1.000000000000000000 ) ) 
 REPRESENTATION_ITEM ( '' )  );
#36332=CARTESIAN_POINT ( 'NONE',  ( 7.724999999999999645, 6.123233995736764310E-16, -4.999999999999998224 ) ) ;
#36333=CARTESIAN_POINT ( 'NONE',  ( 18.63750000122903216, 6.123233995736764310E-16, -4.999999999999998224 ) ) ;
#36334=CARTESIAN_POINT ( 'NONE',  ( 1.626862140677534273E-15, 10.21250000000000036, 34.00000000000000000 ) ) ;
#36336=ORIENTED_EDGE ( 'NONE', *, *, #63436, .T. ) ;
#36337=CARTESIAN_POINT ( 'NONE',  ( 17.62500000000000000, 6.123233995736764310E-16, -4.999999999999998224 ) ) ;
#36338=CARTESIAN_POINT ( 'NONE',  ( 19.98749999999999716, 5.773502691896255534, 3.535250795749688894E-16 ) ) ;
#36339=CARTESIAN_POINT ( 'NONE',  ( 16.50937500061451502, -4.541064518000417216, -2.621784821875001281 ) ) ;
#36340=CARTESIAN_POINT ( 'NONE',  ( 13.26562500061451644, -6.054752690667223547, -1.112240025338166033E-15 ) ) ;
#36341=ORIENTED_EDGE ( 'NONE', *, *, #69921, .F. ) ;
#36342=CARTESIAN_POINT ( 'NONE',  ( 5.465625000614517504, 3.027376345333611329, 5.243569643749999010 ) ) ;
#36344=CARTESIAN_POINT ( 'NONE',  ( 13.19999999999999929, 4.330127018922192761, -2.499999999999997780 ) ) ;
#36346=CARTESIAN_POINT ( 'NONE',  ( -4.243569643749999898, 14.40312500061451750, 30.00000000000000000 ) ) ;
#36347=CARTESIAN_POINT ( 'NONE',  ( 26.39062500061451644, -3.027376345333610441, -5.243569643749999898 ) ) ;
#36348=MECHANICAL_DESIGN_GEOMETRIC_PRESENTATION_REPRESENTATION('',(#13656),#15568);
#36351=CARTESIAN_POINT ( 'NONE',  ( 24.34687500061451715, 6.054752690667223547, 3.707466751127219781E-16 ) ) ;
#36352=CARTESIAN_POINT ( 'NONE',  ( 20.84062500061451573, -3.027376345333614438, 5.243569643749998122 ) ) ;
#36354=CARTESIAN_POINT ( 'NONE',  ( 4.243569643749999898, 15.49062500061459779, -27.54997392385601529 ) ) ;
#36355=CARTESIAN_POINT ( 'NONE',  ( 7.190625000614518036, 6.054752690667223547, 3.707466751127219781E-16 ) ) ;
#36357=CARTESIAN_POINT ( 'NONE',  ( 23.61562500061451786, -6.054752690667223547, -1.112240025338166033E-15 ) ) ;
#36360=CARTESIAN_POINT ( 'NONE',  ( 17.93437500061451928, 6.421520780324663323E-16, -5.243569643749999010 ) ) ;
#36361=CARTESIAN_POINT ( 'NONE',  ( 25.05937500061451573, -4.541064518000417216, -2.621784821875001281 ) ) ;
#36362=CARTESIAN_POINT ( 'NONE',  ( -4.243569643749998122, 14.94687500061451679, 32.45002607614398471 ) ) ;
#36363=CARTESIAN_POINT ( 'NONE',  ( 4.378125000614518925, 6.421520780324663323E-16, -5.243569643749999010 ) ) ;
#36364=CARTESIAN_POINT ( 'NONE',  ( 28.90312500061451217, 0.000000000000000000, 5.243569643749999010 ) ) ;
#36365=( BOUNDED_CURVE ( )  B_SPLINE_CURVE ( 2, ( #67704, #56961, #57328, #51436, #838, #68427, #46254 ),
 .UNSPECIFIED., .F., .F. ) 
 B_SPLINE_CURVE_WITH_KNOTS ( ( 3, 2, 2, 3 ),
 ( 0.3999999999999999112, 0.4027777777777777346, 0.4055555555555555580, 0.4083333333333333814 ),
 .UNSPECIFIED. ) 
 CURVE ( )  GEOMETRIC_REPRESENTATION_ITEM ( )  RATIONAL_B_SPLINE_CURVE ( ( 1.000000000000005329, 0.8660254037844333785, 1.000000000000000000, 0.8660254037844387076, 1.000000000000000000, 0.8660254037844360431, 1.000000000000002665 ) ) 
 REPRESENTATION_ITEM ( '' )  );
#36366=CARTESIAN_POINT ( 'NONE',  ( 29.76562500061451644, 3.027376345333611329, 5.243569643749999010 ) ) ;
#36367=CARTESIAN_POINT ( 'NONE',  ( 5.878125000614517148, 4.541064518000418104, 2.621784821874999949 ) ) ;
#36368=CARTESIAN_POINT ( 'NONE',  ( 9.196875000614518569, -3.027376345333614438, 5.243569643749998122 ) ) ;
#36369=CARTESIAN_POINT ( 'NONE',  ( 16.65000000122903501, -2.886751345948129988, 4.999999999999997335 ) ) ;
#36370=CARTESIAN_POINT ( 'NONE',  ( 3.909375000614518481, -4.541064518000417216, -2.621784821875001281 ) ) ;
#36371=CARTESIAN_POINT ( 'NONE',  ( 5.203125000614518214, -4.541064518000417216, -2.621784821875001281 ) ) ;
#36374=CARTESIAN_POINT ( 'NONE',  ( 13.47187500061451537, 3.027376345333613106, -5.243569643749998122 ) ) ;
#36377=CARTESIAN_POINT ( 'NONE',  ( 21.02812500061451573, 6.421520780324663323E-16, -5.243569643749999010 ) ) ;
#36378=CARTESIAN_POINT ( 'NONE',  ( 8.090625000614515727, 6.054752690667223547, 3.707466751127219781E-16 ) ) ;
#36379=CARTESIAN_POINT ( 'NONE',  ( 23.55937500061451573, 0.000000000000000000, 5.243569643749999010 ) ) ;
#36380=CARTESIAN_POINT ( 'NONE',  ( 6.628125000614517148, 6.421520780324663323E-16, -5.243569643749999010 ) ) ;
#36382=CARTESIAN_POINT ( 'NONE',  ( 10.57500000122903572, 2.886751345948129099, -4.999999999999998224 ) ) ;
#36383=ADVANCED_FACE ( 'NONE', ( #63925 ), #65388, .F. ) ;
#36384=CARTESIAN_POINT ( 'NONE',  ( 25.86562500061451431, -6.054752690667223547, -1.112240025338166033E-15 ) ) ;
#36385=CARTESIAN_POINT ( 'NONE',  ( -2.828200636599751609E-16, 19.55000000122903359, -34.61880215351700230 ) ) ;
#36386=CARTESIAN_POINT ( 'NONE',  ( 9.787500001229036073, 4.330127018922191873, 2.499999999999999556 ) ) ;
#36388=CARTESIAN_POINT ( 'NONE',  ( 21.21562500061451573, 3.027376345333611329, 5.243569643749999010 ) ) ;
#36389=EDGE_CURVE ( 'NONE', #16272, #53042, #21673, .T. ) ;
#36390=CARTESIAN_POINT ( 'NONE',  ( 18.74062500061451431, -3.027376345333610441, -5.243569643749999898 ) ) ;
#36391=CARTESIAN_POINT ( 'NONE',  ( 6.009375000614519458, 0.000000000000000000, 5.243569643749999010 ) ) ;
#36392=CARTESIAN_POINT ( 'NONE',  ( 18.03749999999999787, -2.886751345948125991, -5.000000000000000000 ) ) ;
#36393=CARTESIAN_POINT ( 'NONE',  ( 14.73750000122903359, 4.330127018922191873, 2.499999999999999556 ) ) ;
#36394=CARTESIAN_POINT ( 'NONE',  ( 10.49062500061451431, -3.027376345333614438, 5.243569643749998122 ) ) ;
#36395=CARTESIAN_POINT ( 'NONE',  ( 12.70312500061451821, 0.000000000000000000, 5.243569643749999010 ) ) ;
#36397=CARTESIAN_POINT ( 'NONE',  ( 23.47500000122903430, -5.773502691896255534, -1.060575238724906372E-15 ) ) ;
#36398=CARTESIAN_POINT ( 'NONE',  ( 21.68437500061451573, 4.541064518000418104, 2.621784821874999949 ) ) ;
#36399=CARTESIAN_POINT ( 'NONE',  ( 21.72187500061451715, 3.027376345333611329, 5.243569643749999010 ) ) ;
#36401=EDGE_CURVE ( 'NONE', #52021, #72145, #32038, .T. ) ;
#36402=CARTESIAN_POINT ( 'NONE',  ( 7.687500001229033764, -4.330127018922194537, 2.499999999999995559 ) ) ;
#36403=CARTESIAN_POINT ( 'NONE',  ( 7.284375000614518036, 4.541064518000418104, 2.621784821874999949 ) ) ;
#36404=CARTESIAN_POINT ( 'NONE',  ( 23.44687500061451502, 6.054752690667223547, 3.707466751127219781E-16 ) ) ;
#36405=CARTESIAN_POINT ( 'NONE',  ( 4.465851277537014496, 2.248593419656078840, -4.736966354317482697 ) ) ;
#36406=CARTESIAN_POINT ( 'NONE',  ( 20.65312500061451573, 4.541064518000418104, -2.621784821874998173 ) ) ;
#36407=CARTESIAN_POINT ( 'NONE',  ( 24.42187500061451999, 3.027376345333611329, 5.243569643749999010 ) ) ;
#36409=CARTESIAN_POINT ( 'NONE',  ( -1.071796769724488563, 13.45490381179670081, -26.00000000000000000 ) ) ;
#36410=CARTESIAN_POINT ( 'NONE',  ( 6.121875000614517504, -6.054752690667223547, -1.112240025338166033E-15 ) ) ;
#36411=CARTESIAN_POINT ( 'NONE',  ( 17.31562500061451715, -6.054752690667223547, -1.112240025338166033E-15 ) ) ;
#36412=VERTEX_POINT ( 'NONE', #71675 ) ;
#36413=CARTESIAN_POINT ( 'NONE',  ( 24.96562500061451573, -6.054752690667223547, -1.112240025338166033E-15 ) ) ;
#36414=CARTESIAN_POINT ( 'NONE',  ( 4.171875000614517326, 3.027376345333611329, 5.243569643749999010 ) ) ;
#36415=CARTESIAN_POINT ( 'NONE',  ( 4.735359408593126318, 1.605107869101089380, 4.812405942391664304 ) ) ;
#36416=CARTESIAN_POINT ( 'NONE',  ( 3.649209776892925472, 3.418079578393367068, -3.833452633727637338 ) ) ;
#36417=CARTESIAN_POINT ( 'NONE',  ( 15.86250000000000249, 2.886751345948129099, -4.999999999999998224 ) ) ;
#36418=CARTESIAN_POINT ( 'NONE',  ( 19.86562500061451786, 3.027376345333611329, 5.243569643749999010 ) ) ;
#36419=EDGE_LOOP ( 'NONE', ( #56768, #56059, #54663, #59792, #2924, #40001, #18599, #8250, #16173, #58490, #56632, #60723, #31758, #48119, #20017, #22201, #41966, #56243, #38388, #43553, #59313, #28852, #24655, #55331, #51390, #22482, #7611, #43678, #43298, #9363, #20144, #52377, #15341, #30729, #72615, #70768, #21366, #42555, #20784, #27674, #44070, #13564, #64491, #22102, #5273, #26273, #44812, #36692, #13872, #38154, #10027, #23149, #29442, #58047, #50320, #21150, #36982, #56966, #13896, #30928, #13565, #14465, #10658, #40573, #1716, #48622, #21110, #59521, #23873, #11180, #7260, #1356, #25536, #46115, #20741, #31967, #39838, #56919, #61768, #10756, #57319, #54154, #23289, #3169, #70405, #15116, #21529, #48521, #39122, #32573, #8986, #32342, #47161, #36785, #54787, #42209, #67567, #43212, #52901, #11913, #70316, #46424, #40880, #73080, #3831, #64035, #3765, #12090, #7835, #7455, #61583, #58798, #52337, #19901, #28394, #46986 ) ) ;
#36420=CARTESIAN_POINT ( 'NONE',  ( 24.14999999999999858, 0.000000000000000000, 4.999999999999998224 ) ) ;
#36421=EDGE_CURVE ( 'NONE', #54892, #26952, #16052, .T. ) ;
#36422=CARTESIAN_POINT ( 'NONE',  ( 26.70937500061451431, 0.000000000000000000, 5.243569643749999010 ) ) ;
#36424=CARTESIAN_POINT ( 'NONE',  ( 2.996142289009378956, -4.002898508228532215, -3.387016711638999311 ) ) ;
#36425=CARTESIAN_POINT ( 'NONE',  ( 12.59062500061451573, 6.054752690667223547, 3.707466751127219781E-16 ) ) ;
#36428=CARTESIAN_POINT ( 'NONE',  ( 28.79062500061451502, 6.054752690667223547, 3.707466751127219781E-16 ) ) ;
#36429=CARTESIAN_POINT ( 'NONE',  ( 14.10000000122903252, -2.886751345948125991, -5.000000000000000000 ) ) ;
#36430=CARTESIAN_POINT ( 'NONE',  ( 20.28750000000000142, -2.886751345948125991, -5.000000000000000000 ) ) ;
#36431=CARTESIAN_POINT ( 'NONE',  ( 26.51249999999999929, -5.773502691896255534, -1.060575238724906372E-15 ) ) ;
#36432=CARTESIAN_POINT ( 'NONE',  ( 29.43750000122903288, 6.123233995736764310E-16, -4.999999999999998224 ) ) ;
#36433=CARTESIAN_POINT ( 'NONE',  ( 5.934375000614517504, 4.541064518000418104, 2.621784821874999949 ) ) ;
#36434=CARTESIAN_POINT ( 'NONE',  ( 18.83437500061451431, 6.421520780324663323E-16, -5.243569643749999010 ) ) ;
#36435=CARTESIAN_POINT ( 'NONE',  ( 19.91250000122903074, -4.330127018922190985, -2.500000000000001332 ) ) ;
#36437=CARTESIAN_POINT ( 'NONE',  ( 28.49062500061451431, -3.027376345333614438, 5.243569643749998122 ) ) ;
#36438=CARTESIAN_POINT ( 'NONE',  ( 29.03437500061451715, -4.541064518000419881, 2.621784821874995952 ) ) ;
#36439=CARTESIAN_POINT ( 'NONE',  ( 3.496875000614518836, -3.027376345333610441, -5.243569643749999898 ) ) ;
#36440=CARTESIAN_POINT ( 'NONE',  ( 17.13749999999999929, -2.886751345948125991, -5.000000000000000000 ) ) ;
#36441=CARTESIAN_POINT ( 'NONE',  ( 13.67812500061451786, -4.541064518000419881, 2.621784821874995952 ) ) ;
#36442=CARTESIAN_POINT ( 'NONE',  ( 0.000000000000000000, 20.00000000000000000, 30.00000000000000000 ) ) ;
#36443=DIRECTION ( 'NONE',  ( -0.000000000000000000, -1.000000000000000000, -0.000000000000000000 ) ) ;
#36445=CARTESIAN_POINT ( 'NONE',  ( 18.11250000122903359, -4.330127018922190985, -2.500000000000001332 ) ) ;
#36448=CARTESIAN_POINT ( 'NONE',  ( 8.315625000614515372, -6.054752690667223547, -1.112240025338166033E-15 ) ) ;
#36449=CARTESIAN_POINT ( 'NONE',  ( 23.22187500061451715, -6.054752690667223547, -1.112240025338166033E-15 ) ) ;
#36450=CARTESIAN_POINT ( 'NONE',  ( -3.000416591977282496E-16, 18.84687500061452070, 25.09994784771203058 ) ) ;
#36451=CARTESIAN_POINT ( 'NONE',  ( 25.02187500061451431, -6.054752690667223547, -1.112240025338166033E-15 ) ) ;
#36452=CARTESIAN_POINT ( 'NONE',  ( 6.112499999999999822, 2.886751345948126879, 4.999999999999999112 ) ) ;
#36453=CARTESIAN_POINT ( 'NONE',  ( -3.999999999999999112, 10.66250000122903430, 30.00000000000000000 ) ) ;
#36454=CARTESIAN_POINT ( 'NONE',  ( 14.84062500061451750, 6.054752690667223547, 3.707466751127219781E-16 ) ) ;
#36455=CARTESIAN_POINT ( 'NONE',  ( 3.900000001229034563, 5.773502691896255534, 3.535250795749688894E-16 ) ) ;
#36456=CARTESIAN_POINT ( 'NONE',  ( 9.271875000614516082, -6.054752690667223547, -1.112240025338166033E-15 ) ) ;
#36457=CARTESIAN_POINT ( 'NONE',  ( -1.487416814333745711E-14, 14.82500000122903572, 34.00000000000000000 ) ) ;
#36459=CARTESIAN_POINT ( 'NONE',  ( 13.00312500061451537, 4.541064518000418104, -2.621784821874998173 ) ) ;
#36460=CARTESIAN_POINT ( 'NONE',  ( 3.999999999999998668, 12.27500000122903501, -32.30940107675850470 ) ) ;
#36461=CARTESIAN_POINT ( 'NONE',  ( 24.82500000122902861, -5.773502691896255534, -1.060575238724906372E-15 ) ) ;
#36462=CARTESIAN_POINT ( 'NONE',  ( 9.609375000614518214, 0.000000000000000000, 5.243569643749999010 ) ) ;
#36463=CARTESIAN_POINT ( 'NONE',  ( 11.54062500061451857, -3.027376345333610441, -5.243569643749999898 ) ) ;
#36465=CARTESIAN_POINT ( 'NONE',  ( 24.30937500061451573, 4.541064518000418104, -2.621784821874998173 ) ) ;
#36467=LINE ( 'NONE', #64904, #58426 ) ;
#36468=CARTESIAN_POINT ( 'NONE',  ( 2.121784821874999061, 14.75937500061451679, -33.67503911421598417 ) ) ;
#36469=CARTESIAN_POINT ( 'NONE',  ( 16.77187500061451786, 3.027376345333611329, 5.243569643749999010 ) ) ;
#36470=CARTESIAN_POINT ( 'NONE',  ( 18.52500000122903145, -5.773502691896255534, -1.060575238724906372E-15 ) ) ;
#36471=CARTESIAN_POINT ( 'NONE',  ( 11.67187500061451821, 3.027376345333613106, -5.243569643749998122 ) ) ;
#36472=CARTESIAN_POINT ( 'NONE',  ( -4.243569643749997233, 17.59062500061451928, -27.54997392385601174 ) ) ;
#36473=CARTESIAN_POINT ( 'NONE',  ( 20.43750000122903643, 6.123233995736764310E-16, -4.999999999999998224 ) ) ;
#36474=CARTESIAN_POINT ( 'NONE',  ( 12.32812500061451821, -4.541064518000419881, 2.621784821874995952 ) ) ;
#36476=CARTESIAN_POINT ( 'NONE',  ( 16.72500000000000142, 6.123233995736764310E-16, -4.999999999999998224 ) ) ;
#36477=CARTESIAN_POINT ( 'NONE',  ( 11.48437500061451644, -4.541064518000419881, 2.621784821874995952 ) ) ;
#36478=CARTESIAN_POINT ( 'NONE',  ( 22.50000000000000000, -4.330127018922190985, -2.500000000000001332 ) ) ;
#36479=CARTESIAN_POINT ( 'NONE',  ( 13.65000000122903323, -2.886751345948125991, -5.000000000000000000 ) ) ;
#36480=CARTESIAN_POINT ( 'NONE',  ( 21.30000000122903359, -2.886751345948125991, -5.000000000000000000 ) ) ;
#36481=CARTESIAN_POINT ( 'NONE',  ( 18.70312500061451644, -4.541064518000417216, -2.621784821875001281 ) ) ;
#36482=EDGE_CURVE ( 'NONE', #10458, #19994, #16237, .T. ) ;
#36483=CARTESIAN_POINT ( 'NONE',  ( 20.16562500061451146, 3.027376345333613106, -5.243569643749998122 ) ) ;
#36484=CARTESIAN_POINT ( 'NONE',  ( 27.63750000122903216, 6.123233995736764310E-16, -4.999999999999998224 ) ) ;
#36485=CARTESIAN_POINT ( 'NONE',  ( 26.13749999999999929, -2.886751345948125991, -5.000000000000000000 ) ) ;
#36486=CARTESIAN_POINT ( 'NONE',  ( 0.000000000000000000, 20.00000000000000000, -30.00000000000000000 ) ) ;
#36488=CARTESIAN_POINT ( 'NONE',  ( 28.77187500061451431, 3.027376345333613106, -5.243569643749998122 ) ) ;
#36489=CARTESIAN_POINT ( 'NONE',  ( 28.87499999999999645, 6.123233995736764310E-16, -4.999999999999998224 ) ) ;
#36490=CARTESIAN_POINT ( 'NONE',  ( 4.243569643749999898, 13.78437500061451715, -30.00000000000000000 ) ) ;
#36491=CARTESIAN_POINT ( 'NONE',  ( 3.375000001229033320, 2.886751345948129099, -4.999999999999998224 ) ) ;
#36492=CARTESIAN_POINT ( 'NONE',  ( 6.937499999999999112, 5.773502691896255534, 3.535250795749688894E-16 ) ) ;
#36494=CARTESIAN_POINT ( 'NONE',  ( 7.734375000614517326, 4.541064518000418104, 2.621784821874999949 ) ) ;
#36495=CARTESIAN_POINT ( 'NONE',  ( 29.05312500061451431, -4.541064518000417216, -2.621784821875001281 ) ) ;
#36496=CARTESIAN_POINT ( 'NONE',  ( 3.999999999999998668, 10.81250000000000178, 27.69059892324149530 ) ) ;
#36497=CARTESIAN_POINT ( 'NONE',  ( -0.4074127065224517064, 10.00000000000000178, -36.00000000000000711 ) ) ;
#36499=CARTESIAN_POINT ( 'NONE',  ( 5.821875000614519458, 3.027376345333613106, -5.243569643749998122 ) ) ;
#36500=CARTESIAN_POINT ( 'NONE',  ( 10.32187500061451679, 3.027376345333613106, -5.243569643749998122 ) ) ;
#36501=CARTESIAN_POINT ( 'NONE',  ( 3.412500000000002309, 2.886751345948126879, 4.999999999999999112 ) ) ;
#36502=EDGE_CURVE ( 'NONE', #12747, #47914, #49506, .T. ) ;
#36503=CARTESIAN_POINT ( 'NONE',  ( 4.243569643749999010, 13.76562500061459460, 27.54997392385601174 ) ) ;
#36505=CARTESIAN_POINT ( 'NONE',  ( 6.637500000000001066, -2.886751345948129988, 4.999999999999997335 ) ) ;
#36507=CARTESIAN_POINT ( 'NONE',  ( 20.99062500061451431, -3.027376345333610441, -5.243569643749999898 ) ) ;
#36508=CARTESIAN_POINT ( 'NONE',  ( 12.06562500061451537, 3.027376345333613106, -5.243569643749998122 ) ) ;
#36510=CARTESIAN_POINT ( 'NONE',  ( 8.821875000614518569, -6.054752690667223547, -1.112240025338166033E-15 ) ) ;
#36511=CARTESIAN_POINT ( 'NONE',  ( 27.03750000000000142, -2.886751345948125991, -5.000000000000000000 ) ) ;
#36512=CARTESIAN_POINT ( 'NONE',  ( 21.71250000122903501, -4.330127018922190985, -2.500000000000001332 ) ) ;
#36513=DIRECTION ( 'NONE',  ( -0.000000000000000000, -1.000000000000000000, -0.000000000000000000 ) ) ;
#36514=CARTESIAN_POINT ( 'NONE',  ( 9.571875000614518569, 3.027376345333611329, 5.243569643749999010 ) ) ;
#36515=CARTESIAN_POINT ( 'NONE',  ( 26.74687500061451573, -3.027376345333614438, 5.243569643749998122 ) ) ;
#36516=CARTESIAN_POINT ( 'NONE',  ( 1.071796769724488119, 17.99509619066137134, -26.00000000000000000 ) ) ;
#36518=CARTESIAN_POINT ( 'NONE',  ( 1.626862140677534273E-15, 13.02500000122903323, -26.00000000000000355 ) ) ;
#36519=CARTESIAN_POINT ( 'NONE',  ( 19.24687500061452283, -3.027376345333610441, -5.243569643749999898 ) ) ;
#36520=CARTESIAN_POINT ( 'NONE',  ( 10.88437500061451679, 4.541064518000418104, 2.621784821874999949 ) ) ;
#36522=CARTESIAN_POINT ( 'NONE',  ( 22.98749999999999716, -2.886751345948125991, -5.000000000000000000 ) ) ;
#36524=CARTESIAN_POINT ( 'NONE',  ( 4.243569643749999898, 12.39687500061451608, -27.54997392385601529 ) ) ;
#36526=CARTESIAN_POINT ( 'NONE',  ( 14.91562500061451679, 3.027376345333611329, 5.243569643749999010 ) ) ;
#36527=CARTESIAN_POINT ( 'NONE',  ( 4.949999999999999289, -4.330127018922190985, -2.500000000000001332 ) ) ;
#36529=CARTESIAN_POINT ( 'NONE',  ( 25.68750000000000355, -2.886751345948159742, -4.999999999999942268 ) ) ;
#36530=CARTESIAN_POINT ( 'NONE',  ( 11.55000000000000071, 0.000000000000000000, 4.999999999999998224 ) ) ;
#36531=CARTESIAN_POINT ( 'NONE',  ( -3.999999999999999556, 16.92500000122903359, 27.69059892324149530 ) ) ;
#36532=CARTESIAN_POINT ( 'NONE',  ( 12.86250000122903359, 4.330127018922192761, -2.499999999999997780 ) ) ;
#36533=CARTESIAN_POINT ( 'NONE',  ( 24.19687500061451857, -3.027376345333610441, -5.243569643749999898 ) ) ;
#36534=CARTESIAN_POINT ( 'NONE',  ( 15.83437500061451608, 4.541064518000418104, 2.621784821874999949 ) ) ;
#36536=ORIENTED_EDGE ( 'NONE', *, *, #69202, .T. ) ;
#36537=CARTESIAN_POINT ( 'NONE',  ( 19.79062500061451502, 6.054752690667223547, 3.707466751127219781E-16 ) ) ;
#36538=CARTESIAN_POINT ( 'NONE',  ( 3.590625000614518836, 6.054752690667223547, 3.707466751127219781E-16 ) ) ;
#36539=CARTESIAN_POINT ( 'NONE',  ( 17.55937500061451573, 4.541064518000418104, -2.621784821874998173 ) ) ;
#36540=CARTESIAN_POINT ( 'NONE',  ( 28.50937500061451502, 0.000000000000000000, 5.243569643749999010 ) ) ;
#36541=CARTESIAN_POINT ( 'NONE',  ( 5.765625000614519102, 3.027376345333613106, -5.243569643749998122 ) ) ;
#36542=CARTESIAN_POINT ( 'NONE',  ( 21.29062500061451502, -3.027376345333614438, 5.243569643749998122 ) ) ;
#36543=CARTESIAN_POINT ( 'NONE',  ( -3.000416591977282496E-16, 16.09062500061451573, 25.09994784771203058 ) ) ;
#36544=CARTESIAN_POINT ( 'NONE',  ( 15.56250000122903465, 4.330127018922192761, -2.499999999999997780 ) ) ;
#36546=CARTESIAN_POINT ( 'NONE',  ( 6.365625000614518747, 3.027376345333611329, 5.243569643749999010 ) ) ;
#36547=ADVANCED_FACE ( 'NONE', ( #21411 ), #43601, .F. ) ;
#36548=CARTESIAN_POINT ( 'NONE',  ( 3.759375000614517681, 0.000000000000000000, 5.243569643749999010 ) ) ;
#36549=CARTESIAN_POINT ( 'NONE',  ( 2.896875000614518747, -3.027376345333614438, 5.243569643749998122 ) ) ;
#36550=CARTESIAN_POINT ( 'NONE',  ( 22.43437500061451573, 6.421520780324663323E-16, -5.243569643749999010 ) ) ;
#36551=CARTESIAN_POINT ( 'NONE',  ( 15.40312500061451573, 0.000000000000000000, 5.243569643749999010 ) ) ;
#36552=CARTESIAN_POINT ( 'NONE',  ( 25.42500000122903359, 2.886751345948129099, -4.999999999999998224 ) ) ;
#36553=CARTESIAN_POINT ( 'NONE',  ( 24.25312500061451715, 4.541064518000418104, -2.621784821874998173 ) ) ;
#36554=CARTESIAN_POINT ( 'NONE',  ( 19.20937500061451786, -4.541064518000417216, -2.621784821875001281 ) ) ;
#36555=CARTESIAN_POINT ( 'NONE',  ( 14.99062500061451786, -3.027376345333614438, 5.243569643749998122 ) ) ;
#36556=CARTESIAN_POINT ( 'NONE',  ( -2.121784821874996840, 15.43437500061451928, 33.67503911421598417 ) ) ;
#36557=CARTESIAN_POINT ( 'NONE',  ( 19.26562500061451644, 3.027376345333613106, -5.243569643749998122 ) ) ;
#36559=ORIENTED_EDGE ( 'NONE', *, *, #29318, .F. ) ;
#36561=CARTESIAN_POINT ( 'NONE',  ( 22.53750000000000142, -2.886751345948125991, -5.000000000000000000 ) ) ;
#36562=CARTESIAN_POINT ( 'NONE',  ( -4.243569643749999898, 19.82187500061451857, -32.45002607614398471 ) ) ;
#36564=CARTESIAN_POINT ( 'NONE',  ( 27.66562500061451146, -6.054752690667223547, -1.112240025338166033E-15 ) ) ;
#36565=CARTESIAN_POINT ( 'NONE',  ( 7.603125000614517681, 4.541064518000418104, -2.621784821874998173 ) ) ;
#36566=CARTESIAN_POINT ( 'NONE',  ( 19.80000000122903359, -2.886751345948129988, 4.999999999999997335 ) ) ;
#36567=CARTESIAN_POINT ( 'NONE',  ( 24.92812500061451431, -4.541064518000419881, 2.621784821874995952 ) ) ;
#36568=CARTESIAN_POINT ( 'NONE',  ( 25.61250000000000071, -5.773502691896255534, -1.060575238724906372E-15 ) ) ;
#36569=CARTESIAN_POINT ( 'NONE',  ( 28.71562500061451573, 3.027376345333613106, -5.243569643749998122 ) ) ;
#36570=CARTESIAN_POINT ( 'NONE',  ( 9.028125000614517504, 4.541064518000418104, 2.621784821874999949 ) ) ;
#36571=( BOUNDED_CURVE ( )  B_SPLINE_CURVE ( 2, ( #50689, #40323, #17763, #34044, #5980, #28870, #33687 ),
 .UNSPECIFIED., .F., .F. ) 
 B_SPLINE_CURVE_WITH_KNOTS ( ( 3, 2, 2, 3 ),
 ( 0.9000000000000001332, 0.9027777777777779011, 0.9055555555555556690, 0.9083333333333334370 ),
 .UNSPECIFIED. ) 
 CURVE ( )  GEOMETRIC_REPRESENTATION_ITEM ( )  RATIONAL_B_SPLINE_CURVE ( ( 0.9999999999999946709, 0.8660254037844440367, 1.000000000000000000, 0.8660254037844387076, 1.000000000000000000, 0.8660254037844333785, 1.000000000000005329 ) ) 
 REPRESENTATION_ITEM ( '' )  );
#36573=CARTESIAN_POINT ( 'NONE',  ( 25.56562500061452070, 3.027376345333613106, -5.243569643749998122 ) ) ;
#36574=CARTESIAN_POINT ( 'NONE',  ( 4.415625000614518569, 3.027376345333613106, -5.243569643749998122 ) ) ;
#36576=CARTESIAN_POINT ( 'NONE',  ( 4.078125000614517326, 4.541064518000418104, 2.621784821874999949 ) ) ;
#36577=CARTESIAN_POINT ( 'NONE',  ( -3.999999999999997335, 13.73749999999999893, -27.69059892324149530 ) ) ;
#36578=CARTESIAN_POINT ( 'NONE',  ( 12.90000000000000213, 0.000000000000000000, 4.999999999999998224 ) ) ;
#36579=CARTESIAN_POINT ( 'NONE',  ( 13.95937500061451786, 4.541064518000418104, -2.621784821874998173 ) ) ;
#36580=CARTESIAN_POINT ( 'NONE',  ( 9.787500001229036073, 4.330127018922191873, 2.499999999999999556 ) ) ;
#36581=CARTESIAN_POINT ( 'NONE',  ( 16.24687500061451573, 6.054752690667223547, 3.707466751127219781E-16 ) ) ;
#36583=CARTESIAN_POINT ( 'NONE',  ( 8.071875000614518569, 3.027376345333613106, -5.243569643749998122 ) ) ;
#36584=CARTESIAN_POINT ( 'NONE',  ( 4.243569643749999010, 12.86562500061451608, -32.45002607614398471 ) ) ;
#36585=CARTESIAN_POINT ( 'NONE',  ( -5.810221930991193690E-16, 11.78749999999999964, -34.00000000000000000 ) ) ;
#36586=CARTESIAN_POINT ( 'NONE',  ( 11.74687500061451573, 6.054752690667223547, 3.707466751127219781E-16 ) ) ;
#36587=FACE_OUTER_BOUND ( 'NONE', #8564, .T. ) ;
#36588=CARTESIAN_POINT ( 'NONE',  ( 21.70312500061451644, 0.000000000000000000, 5.243569643749999010 ) ) ;
#36589=LINE ( 'NONE', #20684, #55757 ) ;
#36591=CARTESIAN_POINT ( 'NONE',  ( 26.52187500061451431, 3.027376345333613106, -5.243569643749998122 ) ) ;
#36592=CARTESIAN_POINT ( 'NONE',  ( 28.73437500061451644, 6.421520780324663323E-16, -5.243569643749999010 ) ) ;
#36593=CARTESIAN_POINT ( 'NONE',  ( 3.928125000614516527, 6.421520780324663323E-16, -5.243569643749999010 ) ) ;
#36595=CARTESIAN_POINT ( 'NONE',  ( 17.74687500061451928, -3.027376345333614438, 5.243569643749998122 ) ) ;
#36597=CARTESIAN_POINT ( 'NONE',  ( 28.72500000122903074, 2.886751345948126879, 4.999999999999999112 ) ) ;
#36598=CARTESIAN_POINT ( 'NONE',  ( 6.609375000614519102, -4.541064518000417216, -2.621784821875001281 ) ) ;
#36599=CARTESIAN_POINT ( 'NONE',  ( 17.33437500061451431, -4.541064518000419881, 2.621784821874995952 ) ) ;
#36601=CARTESIAN_POINT ( 'NONE',  ( 25.61250000000000071, -5.773502691896255534, -1.060575238724906372E-15 ) ) ;
#36602=CARTESIAN_POINT ( 'NONE',  ( 27.94687500061451502, 6.054752690667223547, 3.707466751127219781E-16 ) ) ;
#36604=CARTESIAN_POINT ( 'NONE',  ( 14.13750000122903394, 6.123233995736764310E-16, -4.999999999999998224 ) ) ;
#36605=VERTEX_POINT ( 'NONE', #26241 ) ;
#36606=CARTESIAN_POINT ( 'NONE',  ( 7.837499999999999467, 5.773502691896255534, 3.535250795749688894E-16 ) ) ;
#36608=CARTESIAN_POINT ( 'NONE',  ( 22.49062500061451431, 6.054752690667223547, 3.707466751127219781E-16 ) ) ;
#36609=CARTESIAN_POINT ( 'NONE',  ( 10.80000000000000071, -4.330127018922190985, -2.500000000000001332 ) ) ;
#36610=CARTESIAN_POINT ( 'NONE',  ( 7.500000001229034652, 5.773502691896255534, 3.535250795749688894E-16 ) ) ;
#36611=CARTESIAN_POINT ( 'NONE',  ( 7.040625000614517681, -3.027376345333610441, -5.243569643749999898 ) ) ;
#36612=CARTESIAN_POINT ( 'NONE',  ( 22.08749999999999858, -2.886751345948125991, -5.000000000000000000 ) ) ;
#36613=CARTESIAN_POINT ( 'NONE',  ( 18.17812500061451786, -4.541064518000419881, 2.621784821874995952 ) ) ;
#36614=CARTESIAN_POINT ( 'NONE',  ( 1.980717643099229042, -4.701347860447535609, -1.980717643099229042 ) ) ;
#36615=CARTESIAN_POINT ( 'NONE',  ( 26.47500000122903074, 2.886751345948126879, 4.999999999999999112 ) ) ;
#36616=CARTESIAN_POINT ( 'NONE',  ( 1.626862140677534273E-15, 10.21250000000000036, -26.00000000000000355 ) ) ;
#36617=CARTESIAN_POINT ( 'NONE',  ( 5.137500000000000178, 5.773502691896255534, 3.535250795749688894E-16 ) ) ;
#36618=ORIENTED_EDGE ( 'NONE', *, *, #16676, .F. ) ;
#36619=CARTESIAN_POINT ( 'NONE',  ( 20.16562500061451146, 3.027376345333613106, -5.243569643749998122 ) ) ;
#36620=CARTESIAN_POINT ( 'NONE',  ( 27.62812500061451360, -4.541064518000419881, 2.621784821874995952 ) ) ;
#36621=CARTESIAN_POINT ( 'NONE',  ( 24.83437500061451431, 4.541064518000418104, 2.621784821874999949 ) ) ;
#36622=CARTESIAN_POINT ( 'NONE',  ( 8.212500000000000355, 2.886751345948129099, -4.999999999999998224 ) ) ;
#36623=CARTESIAN_POINT ( 'NONE',  ( 12.70312500061451821, 0.000000000000000000, 5.243569643749999010 ) ) ;
#36624=CARTESIAN_POINT ( 'NONE',  ( 28.82812500061451644, 4.541064518000418104, 2.621784821874999949 ) ) ;
#36625=CARTESIAN_POINT ( 'NONE',  ( 8.690625000614515372, -3.027376345333614438, 5.243569643749998122 ) ) ;
#36626=CARTESIAN_POINT ( 'NONE',  ( 2.994107990571896138, -4.004412234122908920, 3.194628461336531888 ) ) ;
#36627=CARTESIAN_POINT ( 'NONE',  ( -2.121784821874996840, 11.83437500061451786, 33.67503911421598417 ) ) ;
#36628=CARTESIAN_POINT ( 'NONE',  ( 23.96250000122903145, -4.330127018922190985, -2.500000000000001332 ) ) ;
#36630=CARTESIAN_POINT ( 'NONE',  ( 13.45312500061451466, 4.541064518000418104, -2.621784821874998173 ) ) ;
#36631=CARTESIAN_POINT ( 'NONE',  ( 10.54687500061451644, -3.027376345333614438, 5.243569643749998122 ) ) ;
#36632=CARTESIAN_POINT ( 'NONE',  ( 10.58437500061451964, -4.541064518000419881, 2.621784821874995952 ) ) ;
#36633=CARTESIAN_POINT ( 'NONE',  ( 17.70937500061451431, 0.000000000000000000, 5.243569643749999010 ) ) ;
#36634=ORIENTED_EDGE ( 'NONE', *, *, #29767, .T. ) ;
#36635=CARTESIAN_POINT ( 'NONE',  ( -1.393485112971533768, 9.904374691868486735, 35.83932025239862185 ) ) ;
#36636=CARTESIAN_POINT ( 'NONE',  ( 21.10312500061451502, 4.541064518000418104, -2.621784821874998173 ) ) ;
#36637=CARTESIAN_POINT ( 'NONE',  ( 17.40937500061451715, -4.541064518000417216, -2.621784821875001281 ) ) ;
#36638=CARTESIAN_POINT ( 'NONE',  ( 21.02812500061451573, 6.421520780324663323E-16, -5.243569643749999010 ) ) ;
#36639=CARTESIAN_POINT ( 'NONE',  ( -3.999999999999999556, 14.56250000000000000, 27.69059892324149530 ) ) ;
#36640=CARTESIAN_POINT ( 'NONE',  ( 26.57812500061451644, 4.541064518000418104, 2.621784821874999949 ) ) ;
#36641=CARTESIAN_POINT ( 'NONE',  ( 7.237500001229035362, -4.330127018922194537, 2.499999999999995559 ) ) ;
#36643=CARTESIAN_POINT ( 'NONE',  ( 3.750000001229034652, -2.886751345948125991, -5.000000000000000000 ) ) ;
#36644=CARTESIAN_POINT ( 'NONE',  ( 1.999999999999998668, 17.60000000000000142, -33.46410161513775705 ) ) ;
#36645=CARTESIAN_POINT ( 'NONE',  ( 24.52500000122903145, 2.886751345948129099, -4.999999999999998224 ) ) ;
#36647=CARTESIAN_POINT ( 'NONE',  ( 7.659375000614518036, 4.541064518000418104, -2.621784821874998173 ) ) ;
#36649=CARTESIAN_POINT ( 'NONE',  ( 14.91562500061451679, 3.027376345333611329, 5.243569643749999010 ) ) ;
#36650=CARTESIAN_POINT ( 'NONE',  ( 8.896875000614517859, -3.027376345333610441, -5.243569643749999898 ) ) ;
#36651=EDGE_CURVE ( 'NONE', #69502, #35463, #41511, .T. ) ;
#36652=CARTESIAN_POINT ( 'NONE',  ( 26.51250000122903216, 0.000000000000000000, 4.999999999999998224 ) ) ;
#36653=CARTESIAN_POINT ( 'NONE',  ( 16.35937500061451644, 0.000000000000000000, 5.243569643749999010 ) ) ;
#36654=CARTESIAN_POINT ( 'NONE',  ( 4.021875000614516082, 3.027376345333613106, -5.243569643749998122 ) ) ;
#36655=LINE ( 'NONE', #13024, #17923 ) ;
#36656=CARTESIAN_POINT ( 'NONE',  ( 6.328125000614515550, 4.541064518000418104, 2.621784821874999949 ) ) ;
#36657=CARTESIAN_POINT ( 'NONE',  ( 14.35312500061451679, 4.541064518000418104, -2.621784821874998173 ) ) ;
#36658=ADVANCED_FACE ( 'NONE', ( #32873 ), #72763, .F. ) ;
#36659=VERTEX_POINT ( 'NONE', #4805 ) ;
#36660=CARTESIAN_POINT ( 'NONE',  ( 12.36562500061451608, -6.054752690667223547, -1.112240025338166033E-15 ) ) ;
#36661=CARTESIAN_POINT ( 'NONE',  ( 4.762500001229033941, 4.330127018922192761, -2.499999999999997780 ) ) ;
#36662=CARTESIAN_POINT ( 'NONE',  ( 9.965625000614517504, 3.027376345333611329, 5.243569643749999010 ) ) ;
#36664=CARTESIAN_POINT ( 'NONE',  ( 9.937500000000001776, -2.886751345948125991, -5.000000000000000000 ) ) ;
#36665=CARTESIAN_POINT ( 'NONE',  ( 7.650000001229034119, -2.886751345948129988, 4.999999999999997335 ) ) ;
#36666=CARTESIAN_POINT ( 'NONE',  ( 21.18749999999999645, -2.886751345948125991, -5.000000000000000000 ) ) ;
#36667=CARTESIAN_POINT ( 'NONE',  ( 14.33437500061451786, 6.421520780324663323E-16, -5.243569643749999010 ) ) ;
#36668=CARTESIAN_POINT ( 'NONE',  ( 15.48750000122903359, 6.123233995736764310E-16, -4.999999999999998224 ) ) ;
#36670=CARTESIAN_POINT ( 'NONE',  ( 2.121784821874999061, 18.75312500061451715, -33.67503911421598417 ) ) ;
#36673=DIRECTION ( 'NONE',  ( -0.000000000000000000, -1.000000000000000000, -0.000000000000000000 ) ) ;
#36674=CARTESIAN_POINT ( 'NONE',  ( 1.071796769724505438, 10.97990381179670116, -33.99999999999999289 ) ) ;
#36675=CARTESIAN_POINT ( 'NONE',  ( 1.071796769724489895, 14.57990381179669903, 26.00000000000000355 ) ) ;
#36676=CARTESIAN_POINT ( 'NONE',  ( 15.15937500061451715, -4.541064518000417216, -2.621784821875001281 ) ) ;
#36677=CARTESIAN_POINT ( 'NONE',  ( 27.97500000000000142, 6.123233995736764310E-16, -4.999999999999998224 ) ) ;
#36678=CARTESIAN_POINT ( 'NONE',  ( 12.44062500061451537, -3.027376345333610441, -5.243569643749999898 ) ) ;
#36680=CARTESIAN_POINT ( 'NONE',  ( 24.83437500061451431, 4.541064518000418104, 2.621784821874999949 ) ) ;
#36682=CARTESIAN_POINT ( 'NONE',  ( 9.140625000614518214, -3.027376345333614438, 5.243569643749998122 ) ) ;
#36683=CARTESIAN_POINT ( 'NONE',  ( 14.55937500061451573, 0.000000000000000000, 5.243569643749999010 ) ) ;
#36684=ORIENTED_EDGE ( 'NONE', *, *, #21207, .F. ) ;
#36685=CARTESIAN_POINT ( 'NONE',  ( 24.75937500061451502, 4.541064518000418104, -2.621784821874998173 ) ) ;
#36686=CARTESIAN_POINT ( 'NONE',  ( 26.91562500061451146, 3.027376345333613106, -5.243569643749998122 ) ) ;
#36687=CARTESIAN_POINT ( 'NONE',  ( 27.29062500061451502, -3.027376345333610441, -5.243569643749999898 ) ) ;
#36688=CARTESIAN_POINT ( 'NONE',  ( 7.612500000000000711, -5.773502691896255534, -1.060575238724906372E-15 ) ) ;
#36689=CARTESIAN_POINT ( 'NONE',  ( 17.96250000122903501, 0.000000000000000000, 4.999999999999998224 ) ) ;
#36692=ORIENTED_EDGE ( 'NONE', *, *, #28846, .T. ) ;
#36693=CARTESIAN_POINT ( 'NONE',  ( 14.06250000000000000, 2.886751345948129099, -4.999999999999998224 ) ) ;
#36694=CARTESIAN_POINT ( 'NONE',  ( 19.31250000000000000, -5.773502691896255534, -1.060575238724906372E-15 ) ) ;
#36695=CARTESIAN_POINT ( 'NONE',  ( 13.11562500061451786, 3.027376345333611329, 5.243569643749999010 ) ) ;
#36696=EDGE_LOOP ( 'NONE', ( #52549, #14882, #57493, #45390 ) ) ;
#36697=CARTESIAN_POINT ( 'NONE',  ( 28.42499999999999716, 6.123233995736764310E-16, -4.999999999999998224 ) ) ;
#36698=CARTESIAN_POINT ( 'NONE',  ( -4.243569643749999898, 18.05937500061451928, -30.00000000000000000 ) ) ;
#36699=CARTESIAN_POINT ( 'NONE',  ( 6.178125000614518747, 6.421520780324663323E-16, -5.243569643749999010 ) ) ;
#36701=CARTESIAN_POINT ( 'NONE',  ( 11.13750000000000284, -2.886751345948129988, 4.999999999999997335 ) ) ;
#36704=CARTESIAN_POINT ( 'NONE',  ( -2.121784821874999949, 15.22812500061451679, 26.32496088578401938 ) ) ;
#36705=CARTESIAN_POINT ( 'NONE',  ( 25.52812500061451573, 6.421520780324663323E-16, -5.243569643749999010 ) ) ;
#36708=CARTESIAN_POINT ( 'NONE',  ( 22.95937500061451431, 4.541064518000418104, -2.621784821874998173 ) ) ;
#36709=CARTESIAN_POINT ( 'NONE',  ( 19.04062500061451146, -3.027376345333614438, 5.243569643749998122 ) ) ;
#36710=CARTESIAN_POINT ( 'NONE',  ( 4.243569643749999010, 14.21562500061459389, -32.45002607614398471 ) ) ;
#36711=CARTESIAN_POINT ( 'NONE',  ( 24.11250000122903359, 4.330127018922192761, -2.499999999999997780 ) ) ;
#36712=CARTESIAN_POINT ( 'NONE',  ( 6.065625000614516260, -6.054752690667223547, -1.112240025338166033E-15 ) ) ;
#36714=CARTESIAN_POINT ( 'NONE',  ( 22.56562500061451715, 3.027376345333611329, 5.243569643749999010 ) ) ;
#36717=( BOUNDED_CURVE ( )  B_SPLINE_CURVE ( 2, ( #35921, #58445, #30392, #52921, #69912, #37391, #10414, #3424, #4522 ),
 .UNSPECIFIED., .F., .F. ) 
 B_SPLINE_CURVE_WITH_KNOTS ( ( 3, 2, 2, 2, 3 ),
 ( 0.2282608695652174058, 0.2318840579710144956, 0.2391304347826087029, 0.2463768115942029102, 0.2500000000000000000 ),
 .UNSPECIFIED. ) 
 CURVE ( )  GEOMETRIC_REPRESENTATION_ITEM ( )  RATIONAL_B_SPLINE_CURVE ( ( 0.9330127018922194093, 0.9330127018922196314, 1.000000000000000000, 0.8660254037844387076, 1.000000000000000000, 0.8660254037844387076, 1.000000000000000000, 0.9330127018922196314, 0.9330127018922194093 ) ) 
 REPRESENTATION_ITEM ( '' )  );
#36718=CARTESIAN_POINT ( 'NONE',  ( 16.13437500061451502, 6.421520780324663323E-16, -5.243569643749999010 ) ) ;
#36719=CARTESIAN_POINT ( 'NONE',  ( 24.34687500061451715, 6.054752690667223547, 3.707466751127219781E-16 ) ) ;
#36720=CARTESIAN_POINT ( 'NONE',  ( 2.121784821875001281, 13.25937500061451857, 33.67503911421598417 ) ) ;
#36721=CARTESIAN_POINT ( 'NONE',  ( 4.753125000614515372, -4.541064518000417216, -2.621784821875001281 ) ) ;
#36722=CARTESIAN_POINT ( 'NONE',  ( 29.54062500061451502, -3.027376345333610441, -5.243569643749999898 ) ) ;
#36723=CARTESIAN_POINT ( 'NONE',  ( 2.934375000614518392, -4.541064518000419881, 2.621784821874995952 ) ) ;
#36724=CARTESIAN_POINT ( 'NONE',  ( 4.292152659130343828, 3.669920861174119864, 3.643510608689493058 ) ) ;
#36725=CARTESIAN_POINT ( 'NONE',  ( 3.909375000614518481, -4.541064518000417216, -2.621784821875001281 ) ) ;
#36726=CARTESIAN_POINT ( 'NONE',  ( 2.803125000614518747, 0.000000000000000000, 5.243569643749999010 ) ) ;
#36727=CARTESIAN_POINT ( 'NONE',  ( 7.471875000614519813, -6.054752690667223547, -1.112240025338166033E-15 ) ) ;
#36728=CARTESIAN_POINT ( 'NONE',  ( 14.40000000122903323, -2.886751345948129988, 4.999999999999997335 ) ) ;
#36729=CARTESIAN_POINT ( 'NONE',  ( 3.271875000614519635, 3.027376345333611329, 5.243569643749999010 ) ) ;
#36730=CARTESIAN_POINT ( 'NONE',  ( 10.87500000122903288, -5.773502691896255534, -1.060575238724906372E-15 ) ) ;
#36731=CARTESIAN_POINT ( 'NONE',  ( 5.315625000614516260, 3.027376345333613106, -5.243569643749998122 ) ) ;
#36735=CARTESIAN_POINT ( 'NONE',  ( 15.45937500061451608, 0.000000000000000000, 5.243569643749999010 ) ) ;
#36737=ORIENTED_EDGE ( 'NONE', *, *, #45774, .T. ) ;
#36738=CARTESIAN_POINT ( 'NONE',  ( 23.39062500061451289, 6.054752690667223547, 3.707466751127219781E-16 ) ) ;
#36739=CARTESIAN_POINT ( 'NONE',  ( 7.715625000614515727, 3.027376345333611329, 5.243569643749999010 ) ) ;
#36740=CARTESIAN_POINT ( 'NONE',  ( 25.65937500061451715, 4.541064518000418104, -2.621784821874998173 ) ) ;
#36741=CARTESIAN_POINT ( 'NONE',  ( 6.478125000614516793, -4.541064518000419881, 2.621784821874995952 ) ) ;
#36742=CARTESIAN_POINT ( 'NONE',  ( -4.243569643749999898, 19.80312500061451786, 30.00000000000000000 ) ) ;
#36743=CARTESIAN_POINT ( 'NONE',  ( 7.350000001229033408, -2.886751345948125991, -5.000000000000000000 ) ) ;
#36744=CARTESIAN_POINT ( 'NONE',  ( 24.36562500061451786, 3.027376345333611329, 5.243569643749999010 ) ) ;
#36745=EDGE_CURVE ( 'NONE', #17299, #22971, #59404, .T. ) ;
#36746=CARTESIAN_POINT ( 'NONE',  ( -4.243569643749999898, 9.865625000614517859, -32.45002607614398471 ) ) ;
#36747=CARTESIAN_POINT ( 'NONE',  ( 11.21250000122903501, 0.000000000000000000, 4.999999999999998224 ) ) ;
#36748=CARTESIAN_POINT ( 'NONE',  ( 20.76562500061451644, 3.027376345333611329, 5.243569643749999010 ) ) ;
#36749=CARTESIAN_POINT ( 'NONE',  ( 17.46562500061451217, 3.027376345333613106, -5.243569643749998122 ) ) ;
#36751=CARTESIAN_POINT ( 'NONE',  ( 17.47499999999999787, -4.330127018922194537, 2.499999999999995559 ) ) ;
#36752=CARTESIAN_POINT ( 'NONE',  ( 13.20000000122903394, -2.886751345948125991, -5.000000000000000000 ) ) ;
#36753=CARTESIAN_POINT ( 'NONE',  ( 9.703125000614514661, -4.541064518000417216, -2.621784821875001281 ) ) ;
#36754=AXIS2_PLACEMENT_3D ( 'NONE', #61185, #15015, #4324 ) ;
#36755=CARTESIAN_POINT ( 'NONE',  ( 12.59062500061451573, 6.054752690667223547, 3.707466751127219781E-16 ) ) ;
#36756=CARTESIAN_POINT ( 'NONE',  ( 22.87500000122903288, 2.886751345948126879, 4.999999999999999112 ) ) ;
#36757=CARTESIAN_POINT ( 'NONE',  ( 21.79687500061451644, -3.027376345333614438, 5.243569643749998122 ) ) ;
#36758=CARTESIAN_POINT ( 'NONE',  ( 21.00937500061451857, -4.541064518000417216, -2.621784821875001281 ) ) ;
#36760=CARTESIAN_POINT ( 'NONE',  ( 7.350000001229033408, -2.886751345948125991, -5.000000000000000000 ) ) ;
#36761=( BOUNDED_CURVE ( )  B_SPLINE_CURVE ( 2, ( #13057, #30785, #70312, #18951, #2351, #63309, #48147, #35595, #41510 ),
 .UNSPECIFIED., .F., .F. ) 
 B_SPLINE_CURVE_WITH_KNOTS ( ( 3, 2, 2, 2, 3 ),
 ( 0.6630434782608696231, 0.6666666666666666297, 0.6739130434782608647, 0.6811594202898550998, 0.6847826086956522174 ),
 .UNSPECIFIED. ) 
 CURVE ( )  GEOMETRIC_REPRESENTATION_ITEM ( )  RATIONAL_B_SPLINE_CURVE ( ( 0.9330127018922192983, 0.9330127018922202975, 1.000000000000000000, 0.8660254037844387076, 1.000000000000000000, 0.8660254037844387076, 1.000000000000000000, 0.9330127018922182991, 0.9330127018922192983 ) ) 
 REPRESENTATION_ITEM ( '' )  );
#36762=CARTESIAN_POINT ( 'NONE',  ( 5.296875000614518214, -3.027376345333610441, -5.243569643749999898 ) ) ;
#36763=CARTESIAN_POINT ( 'NONE',  ( 23.67187500061451999, -6.054752690667223547, -1.112240025338166033E-15 ) ) ;
#36764=( BOUNDED_CURVE ( )  B_SPLINE_CURVE ( 2, ( #60050, #25346, #8357, #47520, #9461, #3928, #41615 ),
 .UNSPECIFIED., .F., .F. ) 
 B_SPLINE_CURVE_WITH_KNOTS ( ( 3, 2, 2, 3 ),
 ( 0.1416666666666666352, 0.1444444444444444031, 0.1472222222222221710, 0.1499999999999999389 ),
 .UNSPECIFIED. ) 
 CURVE ( )  GEOMETRIC_REPRESENTATION_ITEM ( )  RATIONAL_B_SPLINE_CURVE ( ( 1.000000000000001332, 0.8660254037844373753, 1.000000000000000000, 0.8660254037844387076, 1.000000000000000000, 0.8660254037844413721, 0.9999999999999973355 ) ) 
 REPRESENTATION_ITEM ( '' )  );
#36766=CARTESIAN_POINT ( 'NONE',  ( 17.80312500061451786, -4.541064518000417216, -2.621784821875001281 ) ) ;
#36767=CARTESIAN_POINT ( 'NONE',  ( 24.45937500061451786, 0.000000000000000000, 5.243569643749999010 ) ) ;
#36769=CARTESIAN_POINT ( 'NONE',  ( 30.00000000000000000, 0.000000000000000000, 4.999999999999998224 ) ) ;
#36770=CARTESIAN_POINT ( 'NONE',  ( 30.00000000000000000, 0.000000000000000000, 0.000000000000000000 ) ) ;
#36771=CARTESIAN_POINT ( 'NONE',  ( 5.034375000614519813, 4.541064518000418104, 2.621784821874999949 ) ) ;
#36772=CARTESIAN_POINT ( 'NONE',  ( 17.57812500061451644, 4.541064518000418104, 2.621784821874999949 ) ) ;
#36773=ORIENTED_EDGE ( 'NONE', *, *, #41845, .F. ) ;
#36774=CARTESIAN_POINT ( 'NONE',  ( 25.19999999999999929, -4.330127018922190985, -2.500000000000001332 ) ) ;
#36775=CARTESIAN_POINT ( 'NONE',  ( 24.59062500061451573, -3.027376345333610441, -5.243569643749999898 ) ) ;
#36776=CARTESIAN_POINT ( 'NONE',  ( 3.999999999999999112, 17.07499999999999929, 30.00000000000000000 ) ) ;
#36778=CARTESIAN_POINT ( 'NONE',  ( 13.68750000000000178, 5.773502691896255534, 3.535250795749688894E-16 ) ) ;
#36779=CARTESIAN_POINT ( 'NONE',  ( 27.63750000122903216, 6.123233995736764310E-16, -4.999999999999998224 ) ) ;
#36780=CARTESIAN_POINT ( 'NONE',  ( 21.70312500061451644, 0.000000000000000000, 5.243569643749999010 ) ) ;
#36782=CARTESIAN_POINT ( 'NONE',  ( 23.13749999999999929, 5.773502691896255534, 3.535250795749688894E-16 ) ) ;
#36783=CARTESIAN_POINT ( 'NONE',  ( 24.23437500061451644, 6.421520780324663323E-16, -5.243569643749999010 ) ) ;
#36784=( BOUNDED_CURVE ( )  B_SPLINE_CURVE ( 2, ( #15618, #38160, #49625, #9726, #55167, #71795, #32260, #60683, #33353 ),
 .UNSPECIFIED., .F., .F. ) 
 B_SPLINE_CURVE_WITH_KNOTS ( ( 3, 2, 2, 2, 3 ),
 ( 0.2500000000000000000, 0.2536231884057971175, 0.2608695652173912971, 0.2681159420289855322, 0.2717391304347826497 ),
 .UNSPECIFIED. ) 
 CURVE ( )  GEOMETRIC_REPRESENTATION_ITEM ( )  RATIONAL_B_SPLINE_CURVE ( ( 0.9330127018922194093, 0.9330127018922190762, 1.000000000000000000, 0.8660254037844387076, 1.000000000000000000, 0.8660254037844387076, 1.000000000000000000, 0.9330127018922188542, 0.9330127018922194093 ) ) 
 REPRESENTATION_ITEM ( '' )  );
#36785=ORIENTED_EDGE ( 'NONE', *, *, #21442, .T. ) ;
#36787=CARTESIAN_POINT ( 'NONE',  ( 13.41562500061451502, 3.027376345333613106, -5.243569643749998122 ) ) ;
#36788=CARTESIAN_POINT ( 'NONE',  ( 3.628125000614518036, 4.541064518000418104, 2.621784821874999949 ) ) ;
#36790=CARTESIAN_POINT ( 'NONE',  ( 25.67812500061451431, 4.541064518000418104, 2.621784821874999949 ) ) ;
#36791=CARTESIAN_POINT ( 'NONE',  ( 12.97500000122903252, 2.886751345948126879, 4.999999999999999112 ) ) ;
#36792=CARTESIAN_POINT ( 'NONE',  ( 18.45000000000000284, -4.330127018922190985, -2.500000000000001332 ) ) ;
#36793=CARTESIAN_POINT ( 'NONE',  ( 26.47499999999999787, -4.330127018922194537, 2.499999999999995559 ) ) ;
#36794=DIRECTION ( 'NONE',  ( -0.000000000000000000, -1.000000000000000000, -0.000000000000000000 ) ) ;
#36795=CARTESIAN_POINT ( 'NONE',  ( 6.946875000614517681, -3.027376345333614438, 5.243569643749998122 ) ) ;
#36796=CARTESIAN_POINT ( 'NONE',  ( 16.28437500061452070, 4.541064518000418104, 2.621784821874999949 ) ) ;
#36797=B_SPLINE_CURVE_WITH_KNOTS ( 'NONE', 3,
 ( #40512, #6529, #23141, #67506, #39063, #33501 ),
 .UNSPECIFIED., .F., .F.,
 ( 4, 2, 4 ),
 ( 0.001054571168816651220, 0.001510402992670096395, 0.001966234816523541352 ),
 .UNSPECIFIED. ) ;
#36798=ORIENTED_EDGE ( 'NONE', *, *, #36141, .T. ) ;
#36799=CARTESIAN_POINT ( 'NONE',  ( 29.27812500061451573, 4.541064518000418104, 2.621784821874999949 ) ) ;
#36800=CARTESIAN_POINT ( 'NONE',  ( 4.125000000000000000, 6.123233995736764310E-16, -4.999999999999998224 ) ) ;
#36801=CARTESIAN_POINT ( 'NONE',  ( 4.584375000614516971, 4.541064518000418104, 2.621784821874999949 ) ) ;
#36802=CARTESIAN_POINT ( 'NONE',  ( 16.50000000000000000, 0.000000000000000000, 4.999999999999998224 ) ) ;
#36803=CARTESIAN_POINT ( 'NONE',  ( 12.77812500061451750, -4.541064518000419881, 2.621784821874995952 ) ) ;
#36806=CARTESIAN_POINT ( 'NONE',  ( 18.15000000122903501, -2.886751345948125991, -5.000000000000000000 ) ) ;
#36807=DIRECTION ( 'NONE',  ( 0.000000000000000000, 0.000000000000000000, -1.000000000000000000 ) ) ;
#36809=CARTESIAN_POINT ( 'NONE',  ( 8.053125000614516082, 4.541064518000418104, -2.621784821874998173 ) ) ;
#36810=CARTESIAN_POINT ( 'NONE',  ( 24.83437500061451431, 4.541064518000418104, 2.621784821874999949 ) ) ;
#36811=CARTESIAN_POINT ( 'NONE',  ( 4.243569643749999010, 17.42187500061451999, 27.54997392385601174 ) ) ;
#36812=CARTESIAN_POINT ( 'NONE',  ( 25.05937500061451573, -4.541064518000417216, -2.621784821875001281 ) ) ;
#36813=CARTESIAN_POINT ( 'NONE',  ( 5.512499999999999289, 2.886751345948129099, -4.999999999999998224 ) ) ;
#36815=CARTESIAN_POINT ( 'NONE',  ( 12.66562500061451502, 3.027376345333611329, 5.243569643749999010 ) ) ;
#36816=CARTESIAN_POINT ( 'NONE',  ( 5.475000001229035185, -5.773502691896255534, -1.060575238724906372E-15 ) ) ;
#36817=VECTOR ( 'NONE', #22650, 1000.000000000000000 ) ;
#36818=CARTESIAN_POINT ( 'NONE',  ( 9.421875000614519990, 3.027376345333613106, -5.243569643749998122 ) ) ;
#36821=CARTESIAN_POINT ( 'NONE',  ( 10.41562500061451679, 3.027376345333611329, 5.243569643749999010 ) ) ;
#36822=CARTESIAN_POINT ( 'NONE',  ( 15.27187500061451786, 3.027376345333613106, -5.243569643749998122 ) ) ;
#36824=CARTESIAN_POINT ( 'NONE',  ( 22.72500000122903430, 2.886751345948129099, -4.999999999999998224 ) ) ;
#36825=CARTESIAN_POINT ( 'NONE',  ( 9.309375000614517504, -4.541064518000417216, -2.621784821875001281 ) ) ;
#36826=CARTESIAN_POINT ( 'NONE',  ( 11.09062500061451573, -3.027376345333610441, -5.243569643749999898 ) ) ;
#36827=EDGE_CURVE ( 'NONE', #10011, #63961, #72394, .T. ) ;
#36829=CARTESIAN_POINT ( 'NONE',  ( 22.50937500061451857, 4.541064518000418104, -2.621784821874998173 ) ) ;
#36832=CARTESIAN_POINT ( 'NONE',  ( 30.00000000000000000, 0.000000000000000000, 0.000000000000000000 ) ) ;
#36833=CARTESIAN_POINT ( 'NONE',  ( 2.121784821874999061, 15.65937500061451892, -33.67503911421598417 ) ) ;
#36834=CARTESIAN_POINT ( 'NONE',  ( 14.97187500061451892, 3.027376345333611329, 5.243569643749999010 ) ) ;
#36835=CARTESIAN_POINT ( 'NONE',  ( 16.53750000122903430, 4.330127018922191873, 2.499999999999999556 ) ) ;
#36836=CARTESIAN_POINT ( 'NONE',  ( 11.14687500061451608, -3.027376345333610441, -5.243569643749999898 ) ) ;
#36837=CARTESIAN_POINT ( 'NONE',  ( 4.243569643749999898, 18.19062500061451360, -27.54997392385601529 ) ) ;
#36838=CARTESIAN_POINT ( 'NONE',  ( 17.92500000122903359, 2.886751345948126879, 4.999999999999999112 ) ) ;
#36839=CARTESIAN_POINT ( 'NONE',  ( 12.92812500061451786, 6.421520780324663323E-16, -5.243569643749999010 ) ) ;
#36840=ORIENTED_EDGE ( 'NONE', *, *, #3964, .T. ) ;
#36841=CARTESIAN_POINT ( 'NONE',  ( 14.69999999999999929, 0.000000000000000000, 4.999999999999998224 ) ) ;
#36842=CARTESIAN_POINT ( 'NONE',  ( 9.421875000614518214, 3.027376345333612662, -5.243569643749998122 ) ) ;
#36843=CARTESIAN_POINT ( 'NONE',  ( -10.00000000000000000, 0.000000000000000000, 50.00000000000000000 ) ) ;
#36844=CARTESIAN_POINT ( 'NONE',  ( 12.78750000122903430, 6.123233995736764310E-16, -4.999999999999998224 ) ) ;
#36845=CARTESIAN_POINT ( 'NONE',  ( 20.81250000122903643, -4.330127018922190985, -2.500000000000001332 ) ) ;
#36846=CARTESIAN_POINT ( 'NONE',  ( 17.84062500061451573, -3.027376345333610441, -5.243569643749999898 ) ) ;
#36847=CARTESIAN_POINT ( 'NONE',  ( 21.62812500061451360, 4.541064518000418104, 2.621784821874999949 ) ) ;
#36848=CARTESIAN_POINT ( 'NONE',  ( 26.92500000122903359, 2.886751345948126879, 4.999999999999999112 ) ) ;
#36849=CARTESIAN_POINT ( 'NONE',  ( 25.98750000000000071, -2.886751345948129988, 4.999999999999997335 ) ) ;
#36850=CARTESIAN_POINT ( 'NONE',  ( 30.00000000000000000, 0.000000000000000000, 0.000000000000000000 ) ) ;
#36852=CARTESIAN_POINT ( 'NONE',  ( 28.05937500061451573, 0.000000000000000000, 5.243569643749999010 ) ) ;
#36853=FACE_OUTER_BOUND ( 'NONE', #43663, .T. ) ;
#36854=CARTESIAN_POINT ( 'NONE',  ( -4.243569643749999898, 13.10937500061451821, -30.00000000000000000 ) ) ;
#36855=CARTESIAN_POINT ( 'NONE',  ( 3.712500001229034563, -4.330127018922190985, -2.500000000000001332 ) ) ;
#36856=CARTESIAN_POINT ( 'NONE',  ( 4.575000000000002842, 6.123233995736764310E-16, -4.999999999999998224 ) ) ;
#36858=CARTESIAN_POINT ( 'NONE',  ( 7.509375000614517681, -4.541064518000417216, -2.621784821875001281 ) ) ;
#36860=CARTESIAN_POINT ( 'NONE',  ( 29.54062500061451502, -3.027376345333610441, -5.243569643749999898 ) ) ;
#36861=CARTESIAN_POINT ( 'NONE',  ( -0.4071169142669905927, 9.993716716995059812, -24.01045583075348233 ) ) ;
#36863=CARTESIAN_POINT ( 'NONE',  ( 4.734375000614518214, -4.541064518000419881, 2.621784821874995952 ) ) ;
#36864=CARTESIAN_POINT ( 'NONE',  ( 8.896875000614517859, -3.027376345333610441, -5.243569643749999898 ) ) ;
#36865=CARTESIAN_POINT ( 'NONE',  ( 3.262500000000001510, 2.886751345948129099, -4.999999999999998224 ) ) ;
#36866=CARTESIAN_POINT ( 'NONE',  ( -4.243569643749999898, 11.66562500061459495, 27.54997392385601529 ) ) ;
#36867=CARTESIAN_POINT ( 'NONE',  ( 29.47499999999999787, 4.330127018922191873, 2.499999999999999556 ) ) ;
#36868=CARTESIAN_POINT ( 'NONE',  ( 4.875000000000000888, -4.330127018922194537, 2.499999999999995559 ) ) ;
#36869=EDGE_CURVE ( 'NONE', #11718, #41592, #11758, .T. ) ;
#36871=CARTESIAN_POINT ( 'NONE',  ( 20.27812500061451573, 4.541064518000418104, 2.621784821874999949 ) ) ;
#36872=CARTESIAN_POINT ( 'NONE',  ( 10.79062500061451679, 6.054752690667223547, 3.707466751127219781E-16 ) ) ;
#36874=CARTESIAN_POINT ( 'NONE',  ( 9.421875000614519990, 3.027376345333613106, -5.243569643749998122 ) ) ;
#36875=CARTESIAN_POINT ( 'NONE',  ( 26.77499999999999858, 4.330127018922191873, 2.499999999999999556 ) ) ;
#36876=CARTESIAN_POINT ( 'NONE',  ( 19.42500000122903714, -5.773502691896255534, -1.060575238724906372E-15 ) ) ;
#36877=CARTESIAN_POINT ( 'NONE',  ( 28.34062500061451928, 6.054752690667223547, 3.707466751127219781E-16 ) ) ;
#36879=CARTESIAN_POINT ( 'NONE',  ( 8.484375000614518214, 6.421520780324663323E-16, -5.243569643749999010 ) ) ;
#36880=CARTESIAN_POINT ( 'NONE',  ( 14.55937500061451573, 0.000000000000000000, 5.243569643749999010 ) ) ;
#36881=CARTESIAN_POINT ( 'NONE',  ( 26.67187500061451644, 3.027376345333611329, 5.243569643749999010 ) ) ;
#36882=ADVANCED_FACE ( 'NONE', ( #11793 ), #68678, .F. ) ;
#36885=CARTESIAN_POINT ( 'NONE',  ( 19.28437500061451360, 6.421520780324663323E-16, -5.243569643749999010 ) ) ;
#36886=CARTESIAN_POINT ( 'NONE',  ( 11.18437500061451928, 6.421520780324663323E-16, -5.243569643749999010 ) ) ;
#36888=CARTESIAN_POINT ( 'NONE',  ( 24.37500000000000000, 6.123233995736764310E-16, -4.999999999999998224 ) ) ;
#36890=CARTESIAN_POINT ( 'NONE',  ( -2.121784821874996840, 12.28437500061451892, -26.32496088578401583 ) ) ;
#36892=CARTESIAN_POINT ( 'NONE',  ( 15.40312500061451573, 0.000000000000000000, 5.243569643749999010 ) ) ;
#36893=CARTESIAN_POINT ( 'NONE',  ( 3.637500000000001954, -2.886751345948125991, -5.000000000000000000 ) ) ;
#36896=CARTESIAN_POINT ( 'NONE',  ( 12.33750000000000036, 5.773502691896255534, 3.535250795749688894E-16 ) ) ;
#36897=CARTESIAN_POINT ( 'NONE',  ( 1.999999999999998668, 18.61250000122903359, 26.53589838486224650 ) ) ;
#36898=CARTESIAN_POINT ( 'NONE',  ( 10.68750000122903288, 4.330127018922191873, 2.499999999999999556 ) ) ;
#36899=CARTESIAN_POINT ( 'NONE',  ( 22.50937500061451857, 4.541064518000418104, -2.621784821874998173 ) ) ;
#36900=CARTESIAN_POINT ( 'NONE',  ( 15.49687500061451750, -3.027376345333614438, 5.243569643749998122 ) ) ;
#36902=ORIENTED_EDGE ( 'NONE', *, *, #50559, .F. ) ;
#36903=CARTESIAN_POINT ( 'NONE',  ( 16.82812500061451644, -4.541064518000419881, 2.621784821874995952 ) ) ;
#36904=CARTESIAN_POINT ( 'NONE',  ( 5.090625000614516615, -3.027376345333614438, 5.243569643749998122 ) ) ;
#36905=CARTESIAN_POINT ( 'NONE',  ( 18.38437500061451857, 6.421520780324663323E-16, -5.243569643749999010 ) ) ;
#36906=CARTESIAN_POINT ( 'NONE',  ( 27.94687500061451502, 6.054752690667223547, 3.707466751127219781E-16 ) ) ;
#36907=CARTESIAN_POINT ( 'NONE',  ( 3.740625000614516527, -3.027376345333614438, 5.243569643749998122 ) ) ;
#36908=CARTESIAN_POINT ( 'NONE',  ( 19.52812500061451573, -4.541064518000419881, 2.621784821874995952 ) ) ;
#36909=CARTESIAN_POINT ( 'NONE',  ( 9.001249775931846008E-16, 14.51562500061451466, 34.90005215228797653 ) ) ;
#36910=CARTESIAN_POINT ( 'NONE',  ( 16.27500000122903501, -5.773502691896255534, -1.060575238724906372E-15 ) ) ;
#36912=CARTESIAN_POINT ( 'NONE',  ( 6.253125000614517148, 4.541064518000418104, -2.621784821874998173 ) ) ;
#36913=CARTESIAN_POINT ( 'NONE',  ( 28.90312500061451217, 0.000000000000000000, 5.243569643749999010 ) ) ;
#36915=CARTESIAN_POINT ( 'NONE',  ( 22.50937500061451857, 4.541064518000418104, -2.621784821874998173 ) ) ;
#36916=CARTESIAN_POINT ( 'NONE',  ( 13.97812500061451679, 4.541064518000418104, 2.621784821874999949 ) ) ;
#36917=CARTESIAN_POINT ( 'NONE',  ( 25.38750000122903216, 6.123233995736764310E-16, -4.999999999999998224 ) ) ;
#36918=CARTESIAN_POINT ( 'NONE',  ( 22.26562500061451644, -6.054752690667223547, -1.112240025338166033E-15 ) ) ;
#36919=CARTESIAN_POINT ( 'NONE',  ( 19.62187500061451573, -6.054752690667223547, -1.112240025338166033E-15 ) ) ;
#36920=CARTESIAN_POINT ( 'NONE',  ( 14.91562500061451679, 3.027376345333611329, 5.243569643749999010 ) ) ;
#36921=CARTESIAN_POINT ( 'NONE',  ( 4.243569643749999898, 14.19687500061451857, 32.45002607614398471 ) ) ;
#36922=CARTESIAN_POINT ( 'NONE',  ( 20.16562500061451146, 3.027376345333613106, -5.243569643749998122 ) ) ;
#36923=CARTESIAN_POINT ( 'NONE',  ( 29.80312500061451431, 0.000000000000000000, 5.243569643749999010 ) ) ;
#36925=ORIENTED_EDGE ( 'NONE', *, *, #61652, .F. ) ;
#36926=CARTESIAN_POINT ( 'NONE',  ( 23.55000000000000071, 4.330127018922192761, -2.499999999999997780 ) ) ;
#36927=CARTESIAN_POINT ( 'NONE',  ( -1.999999999999997113, 11.07500000000000107, -26.53589838486224295 ) ) ;
#36928=CARTESIAN_POINT ( 'NONE',  ( 3.779449423378813400, -3.273493860712442860, -3.876766845908668824 ) ) ;
#36929=CARTESIAN_POINT ( 'NONE',  ( 26.24062500061451431, -3.027376345333614438, 5.243569643749998122 ) ) ;
#36930=CARTESIAN_POINT ( 'NONE',  ( 7.678125000614516082, 4.541064518000418104, 2.621784821874999949 ) ) ;
#36931=CARTESIAN_POINT ( 'NONE',  ( 19.20000000122903572, 5.773502691896255534, 3.535250795749688894E-16 ) ) ;
#36932=EDGE_CURVE ( 'NONE', #1400, #38366, #28781, .T. ) ;
#36933=CARTESIAN_POINT ( 'NONE',  ( 25.15312500061451217, 4.541064518000418104, -2.621784821874998173 ) ) ;
#36934=CARTESIAN_POINT ( 'NONE',  ( 22.08749999999999858, -2.886751345948125991, -5.000000000000000000 ) ) ;
#36935=CARTESIAN_POINT ( 'NONE',  ( 28.34062500061451928, 6.054752690667223547, 3.707466751127219781E-16 ) ) ;
#36936=CARTESIAN_POINT ( 'NONE',  ( 8.990625000614516082, 6.054752690667223547, 3.707466751127219781E-16 ) ) ;
#36938=CARTESIAN_POINT ( 'NONE',  ( 24.02812500061451573, -4.541064518000419881, 2.621784821874995952 ) ) ;
#36939=CARTESIAN_POINT ( 'NONE',  ( 6.403125000614517504, 0.000000000000000000, 5.243569643749999010 ) ) ;
#36941=CARTESIAN_POINT ( 'NONE',  ( 4.115625000614516082, 3.027376345333611329, 5.243569643749999010 ) ) ;
#36942=CARTESIAN_POINT ( 'NONE',  ( 2.000000000000001332, 13.51250000122903394, -26.53589838486224650 ) ) ;
#36944=CARTESIAN_POINT ( 'NONE',  ( 11.51250000000000107, 2.886751345948126879, 4.999999999999999112 ) ) ;
#36945=CARTESIAN_POINT ( 'NONE',  ( 10.50937500061451679, 0.000000000000000000, 5.243569643749999010 ) ) ;
#36946=CARTESIAN_POINT ( 'NONE',  ( 8.062500001229034652, 0.000000000000000000, 4.999999999999998224 ) ) ;
#36947=CARTESIAN_POINT ( 'NONE',  ( 14.78437500061451715, 6.421520780324663323E-16, -5.243569643749999010 ) ) ;
#36949=CARTESIAN_POINT ( 'NONE',  ( 6.534375000614517148, -4.541064518000419881, 2.621784821874995952 ) ) ;
#36950=CARTESIAN_POINT ( 'NONE',  ( 9.001249775931846008E-16, 10.46562500061451928, -25.09994784771203058 ) ) ;
#36951=CARTESIAN_POINT ( 'NONE',  ( 30.00000000000000000, 0.000000000000000000, 0.000000000000000000 ) ) ;
#36952=CARTESIAN_POINT ( 'NONE',  ( 12.94687500061451857, -3.027376345333610441, -5.243569643749999898 ) ) ;
#36953=CARTESIAN_POINT ( 'NONE',  ( 22.04062500061451502, 6.054752690667223547, 3.707466751127219781E-16 ) ) ;
#36954=CARTESIAN_POINT ( 'NONE',  ( 9.001249775931846008E-16, 10.52187500061451964, 34.90005215228797653 ) ) ;
#36956=CARTESIAN_POINT ( 'NONE',  ( 27.23437500061451644, -4.541064518000419881, 2.621784821874995952 ) ) ;
#36958=CARTESIAN_POINT ( 'NONE',  ( 3.365625000614516082, -6.054752690667223547, -1.112240025338166033E-15 ) ) ;
#36960=CARTESIAN_POINT ( 'NONE',  ( 17.67187500061451644, 3.027376345333611329, 5.243569643749999010 ) ) ;
#36962=CARTESIAN_POINT ( 'NONE',  ( 27.22500000122903430, 2.886751345948129099, -4.999999999999998224 ) ) ;
#36963=CARTESIAN_POINT ( 'NONE',  ( 6.084375000614518747, -4.541064518000419881, 2.621784821874995952 ) ) ;
#36964=CARTESIAN_POINT ( 'NONE',  ( 16.80937500061451573, 0.000000000000000000, 5.243569643749999010 ) ) ;
#36965=CARTESIAN_POINT ( 'NONE',  ( 4.809916128174254624, -1.365542690628744449, -5.062639209831853115 ) ) ;
#36966=CARTESIAN_POINT ( 'NONE',  ( 23.62500000000000000, 4.330127018922191873, 2.499999999999999556 ) ) ;
#36967=CARTESIAN_POINT ( 'NONE',  ( 4.687500001229034652, 6.123233995736764310E-16, -4.999999999999998224 ) ) ;
#36968=CARTESIAN_POINT ( 'NONE',  ( 26.63437500061451857, 4.541064518000418104, 2.621784821874999949 ) ) ;
#36970=CARTESIAN_POINT ( 'NONE',  ( 6.899999999999999467, 4.330127018922192761, -2.499999999999997780 ) ) ;
#36972=CARTESIAN_POINT ( 'NONE',  ( 23.20312500061451644, -4.541064518000417216, -2.621784821875001281 ) ) ;
#36973=CARTESIAN_POINT ( 'NONE',  ( 12.07499999999999929, -4.330127018922194537, 2.499999999999995559 ) ) ;
#36975=CARTESIAN_POINT ( 'NONE',  ( 7.453125000614516438, -4.541064518000417216, -2.621784821875001281 ) ) ;
#36976=CARTESIAN_POINT ( 'NONE',  ( 18.56250000000000000, 2.886751345948129099, -4.999999999999998224 ) ) ;
#36977=CARTESIAN_POINT ( 'NONE',  ( 18.51562500061451289, 3.027376345333611329, 5.243569643749999010 ) ) ;
#36978=CARTESIAN_POINT ( 'NONE',  ( 4.192336996406676342, -2.724758798235080715, 4.480034832487019614 ) ) ;
#36979=CARTESIAN_POINT ( 'NONE',  ( 23.62500000122902932, 2.886751345948129099, -4.999999999999998224 ) ) ;
#36981=CARTESIAN_POINT ( 'NONE',  ( 29.82187500061451502, 3.027376345333611329, 5.243569643749999010 ) ) ;
#36982=ORIENTED_EDGE ( 'NONE', *, *, #52495, .T. ) ;
#36983=CARTESIAN_POINT ( 'NONE',  ( 20.61562500061451431, 3.027376345333613106, -5.243569643749998122 ) ) ;
#36984=CARTESIAN_POINT ( 'NONE',  ( 25.86562500061451431, -6.054752690667223547, -1.112240025338166033E-15 ) ) ;
#36985=CARTESIAN_POINT ( 'NONE',  ( 23.85937500061451644, 4.541064518000418104, -2.621784821874998173 ) ) ;
#36986=CARTESIAN_POINT ( 'NONE',  ( 7.875000000000000000, 4.330127018922191873, 2.499999999999999556 ) ) ;
#36987=CARTESIAN_POINT ( 'NONE',  ( 12.66562500061451502, 3.027376345333611329, 5.243569643749999010 ) ) ;
#36988=CARTESIAN_POINT ( 'NONE',  ( 27.85312500061451502, 4.541064518000418104, -2.621784821874998173 ) ) ;
#36989=CARTESIAN_POINT ( 'NONE',  ( 16.95937500061451786, -4.541064518000417216, -2.621784821875001281 ) ) ;
#36990=CARTESIAN_POINT ( 'NONE',  ( 8.390625000614518214, -3.027376345333610441, -5.243569643749999898 ) ) ;
#36992=CARTESIAN_POINT ( 'NONE',  ( -4.243569643749997233, 11.34687500061451892, 32.45002607614398471 ) ) ;
#36993=CARTESIAN_POINT ( 'NONE',  ( 24.48750000122903359, 6.123233995736764310E-16, -4.999999999999998224 ) ) ;
#36995=CARTESIAN_POINT ( 'NONE',  ( 13.71562500061451750, -6.054752690667223547, -1.112240025338166033E-15 ) ) ;
#36996=CARTESIAN_POINT ( 'NONE',  ( 10.35937500061451644, 4.541064518000418104, -2.621784821874998173 ) ) ;
#36997=CARTESIAN_POINT ( 'NONE',  ( 9.534375000614517148, 4.541064518000418104, 2.621784821874999949 ) ) ;
#36998=ORIENTED_EDGE ( 'NONE', *, *, #34668, .F. ) ;
#36999=CARTESIAN_POINT ( 'NONE',  ( -0.4071169142669882612, 9.993716716995061589, 35.98954416924652122 ) ) ;
#37000=CARTESIAN_POINT ( 'NONE',  ( 21.92812500061451431, 6.421520780324663323E-16, -5.243569643749999010 ) ) ;
#37002=CARTESIAN_POINT ( 'NONE',  ( 16.84687500061451715, -3.027376345333614438, 5.243569643749998122 ) ) ;
#37003=CARTESIAN_POINT ( 'NONE',  ( 21.06562500061451715, 3.027376345333613106, -5.243569643749998122 ) ) ;
#37004=CARTESIAN_POINT ( 'NONE',  ( 1.999999999999998668, 12.20000000000000107, 26.53589838486224650 ) ) ;
#37005=CARTESIAN_POINT ( 'NONE',  ( 26.27812500061451573, -4.541064518000419881, 2.621784821874995952 ) ) ;
#37006=CARTESIAN_POINT ( 'NONE',  ( 6.637500001229035718, 4.330127018922191873, 2.499999999999999556 ) ) ;
#37007=ORIENTED_EDGE ( 'NONE', *, *, #20885, .T. ) ;
#37008=CARTESIAN_POINT ( 'NONE',  ( 29.13749999999999929, -2.886751345948129988, 4.999999999999997335 ) ) ;
#37009=CARTESIAN_POINT ( 'NONE',  ( 1.999999999999998668, 18.05000000000000071, -33.46410161513775705 ) ) ;
#37010=CARTESIAN_POINT ( 'NONE',  ( 25.68750000122903288, -4.330127018922194537, 2.499999999999995559 ) ) ;
#37012=CARTESIAN_POINT ( 'NONE',  ( 8.259375000614518569, 0.000000000000000000, 5.243569643749999010 ) ) ;
#37013=DIRECTION ( 'NONE',  ( 0.000000000000000000, 0.000000000000000000, 1.000000000000000000 ) ) ;
#37014=CARTESIAN_POINT ( 'NONE',  ( 16.11562500061451786, 3.027376345333613106, -5.243569643749998122 ) ) ;
#37015=CARTESIAN_POINT ( 'NONE',  ( 7.546875000614517326, -3.027376345333610441, -5.243569643749999898 ) ) ;
#37016=CARTESIAN_POINT ( 'NONE',  ( 25.98750000122903003, 4.330127018922191873, 2.499999999999999556 ) ) ;
#37017=CARTESIAN_POINT ( 'NONE',  ( 18.04687500061451999, 6.054752690667223547, 3.707466751127219781E-16 ) ) ;
#37018=CARTESIAN_POINT ( 'NONE',  ( 4.621875000614516615, 3.027376345333611329, 5.243569643749999010 ) ) ;
#37019=CARTESIAN_POINT ( 'NONE',  ( 4.896606315213732685, -1.024120609751041799, 4.896606315213732685 ) ) ;
#37020=CARTESIAN_POINT ( 'NONE',  ( 6.215625000614517504, 3.027376345333613106, -5.243569643749998122 ) ) ;
#37021=CARTESIAN_POINT ( 'NONE',  ( 15.92812500061451608, -4.541064518000419881, 2.621784821874995952 ) ) ;
#37023=CARTESIAN_POINT ( 'NONE',  ( 12.14062500061451821, 6.054752690667223547, 3.707466751127219781E-16 ) ) ;
#37024=CARTESIAN_POINT ( 'NONE',  ( 4.650000001229035895, -2.886751345948125991, -5.000000000000000000 ) ) ;
#37025=CARTESIAN_POINT ( 'NONE',  ( 9.590625000614517504, -3.027376345333614438, 5.243569643749998122 ) ) ;
#37027=CARTESIAN_POINT ( 'NONE',  ( 11.81250000000000000, 2.886751345948129099, -4.999999999999998224 ) ) ;
#37029=CARTESIAN_POINT ( 'NONE',  ( 5.175000001229033586, 2.886751345948129099, -4.999999999999998224 ) ) ;
#37030=CARTESIAN_POINT ( 'NONE',  ( 21.48750000000000071, -2.886751345948129988, 4.999999999999997335 ) ) ;
#37031=CARTESIAN_POINT ( 'NONE',  ( 15.53437500061451715, -4.541064518000419881, 2.621784821874995952 ) ) ;
#37032=CARTESIAN_POINT ( 'NONE',  ( 16.27500000122903501, -5.773502691896255534, -1.060575238724906372E-15 ) ) ;
#37034=CARTESIAN_POINT ( 'NONE',  ( 2.121784821875001281, 18.60312500061451857, -26.32496088578401938 ) ) ;
#37035=CARTESIAN_POINT ( 'NONE',  ( -1.999999999999997113, 16.13750000122903216, 33.46410161513775705 ) ) ;
#37036=DIRECTION ( 'NONE',  ( -0.000000000000000000, -1.000000000000000000, -0.000000000000000000 ) ) ;
#37037=LINE ( 'NONE', #42953, #2898 ) ;
#37038=CARTESIAN_POINT ( 'NONE',  ( 10.87500000000000000, 6.123233995736764310E-16, -4.999999999999998224 ) ) ;
#37040=CARTESIAN_POINT ( 'NONE',  ( 16.17187500061451644, 3.027376345333613106, -5.243569643749998122 ) ) ;
#37041=CARTESIAN_POINT ( 'NONE',  ( 29.02499999999999858, 4.330127018922191873, 2.499999999999999556 ) ) ;
#37042=CARTESIAN_POINT ( 'NONE',  ( 12.51562500061451821, 3.027376345333613106, -5.243569643749998122 ) ) ;
#37044=CARTESIAN_POINT ( 'NONE',  ( 23.52187500061451786, 3.027376345333611329, 5.243569643749999010 ) ) ;
#37046=CARTESIAN_POINT ( 'NONE',  ( 7.603125000614517681, 4.541064518000418104, -2.621784821874998173 ) ) ;
#37047=CARTESIAN_POINT ( 'NONE',  ( 12.98437500061451821, 6.421520780324663323E-16, -5.243569643749999010 ) ) ;
#37048=VERTEX_POINT ( 'NONE', #18401 ) ;
#37049=CARTESIAN_POINT ( 'NONE',  ( 25.02187500061451431, -6.054752690667223547, -1.112240025338166033E-15 ) ) ;
#37050=CARTESIAN_POINT ( 'NONE',  ( 27.10312500061451502, 0.000000000000000000, 5.243569643749999010 ) ) ;
#37051=DIRECTION ( 'NONE',  ( 0.000000000000000000, 1.000000000000000000, 0.000000000000000000 ) ) ;
#37052=CARTESIAN_POINT ( 'NONE',  ( 7.275000000000000355, 6.123233995736764310E-16, -4.999999999999998224 ) ) ;
#37053=CARTESIAN_POINT ( 'NONE',  ( 17.32500000122903216, 2.886751345948129099, -4.999999999999998224 ) ) ;
#37054=CARTESIAN_POINT ( 'NONE',  ( -3.999999999999997335, 17.90000000122903501, -27.69059892324149530 ) ) ;
#37055=CARTESIAN_POINT ( 'NONE',  ( 0.000000000000000000, 20.00000000000000000, -30.00000000000000000 ) ) ;
#37056=VERTEX_POINT ( 'NONE', #6620 ) ;
#37057=EDGE_CURVE ( 'NONE', #22838, #68526, #19277, .T. ) ;
#37058=CARTESIAN_POINT ( 'NONE',  ( 15.03749999999999964, 5.773502691896255534, 3.535250795749688894E-16 ) ) ;
#37059=CARTESIAN_POINT ( 'NONE',  ( 18.41250000000000142, -5.773502691896255534, -1.060575238724906372E-15 ) ) ;
#37060=CARTESIAN_POINT ( 'NONE',  ( 12.96562500061451750, 3.027376345333613106, -5.243569643749998122 ) ) ;
#37063=CARTESIAN_POINT ( 'NONE',  ( 9.001249775931846008E-16, 17.72187500061451715, -25.09994784771203058 ) ) ;
#37064=CARTESIAN_POINT ( 'NONE',  ( 29.25000000122903288, -2.886751345948129988, 4.999999999999997335 ) ) ;
#37066=CARTESIAN_POINT ( 'NONE',  ( 11.36250000000000071, 2.886751345948129099, -4.999999999999998224 ) ) ;
#37069=ORIENTED_EDGE ( 'NONE', *, *, #19260, .F. ) ;
#37070=CARTESIAN_POINT ( 'NONE',  ( 4.243569643749999898, 15.94062500061451537, 32.45002607614398471 ) ) ;
#37071=CARTESIAN_POINT ( 'NONE',  ( 27.81562500061452070, 3.027376345333613106, -5.243569643749998122 ) ) ;
#37074=CARTESIAN_POINT ( 'NONE',  ( 24.45937500061451786, 0.000000000000000000, 5.243569643749999010 ) ) ;
#37075=CARTESIAN_POINT ( 'NONE',  ( 18.40312500061451573, 4.541064518000418104, -2.621784821874998173 ) ) ;
#37076=CARTESIAN_POINT ( 'NONE',  ( 2.121784821874999061, 13.35312500061459495, -33.67503911421598417 ) ) ;
#37077=CARTESIAN_POINT ( 'NONE',  ( 24.30000000122903359, -2.886751345948129988, 4.999999999999997335 ) ) ;
#37078=CARTESIAN_POINT ( 'NONE',  ( 4.940625000614515372, 6.054752690667223547, 3.707466751127219781E-16 ) ) ;
#37080=CARTESIAN_POINT ( 'NONE',  ( 22.30312500061451431, -4.541064518000417216, -2.621784821875001281 ) ) ;
#37083=CARTESIAN_POINT ( 'NONE',  ( 18.57187500061451857, 3.027376345333611329, 5.243569643749999010 ) ) ;
#37084=CARTESIAN_POINT ( 'NONE',  ( 16.20937500061451786, 4.541064518000418104, -2.621784821874998173 ) ) ;
#37085=CARTESIAN_POINT ( 'NONE',  ( 23.85937500061451644, 4.541064518000418104, -2.621784821874998173 ) ) ;
#37086=CARTESIAN_POINT ( 'NONE',  ( -3.000416591977282496E-16, 15.24687500061451928, 25.09994784771203058 ) ) ;
#37087=CARTESIAN_POINT ( 'NONE',  ( 6.028125000614517504, -4.541064518000419881, 2.621784821874995952 ) ) ;
#37088=CARTESIAN_POINT ( 'NONE',  ( 29.27812500061451573, 4.541064518000418104, 2.621784821874999949 ) ) ;
#37089=CARTESIAN_POINT ( 'NONE',  ( 28.37812500061451715, 4.541064518000418104, 2.621784821874999949 ) ) ;
#37091=CARTESIAN_POINT ( 'NONE',  ( -2.000000000000000000, 19.47499999999999787, 26.53589838486224650 ) ) ;
#37092=CARTESIAN_POINT ( 'NONE',  ( 7.396875000614519635, -3.027376345333614438, 5.243569643749998122 ) ) ;
#37093=CARTESIAN_POINT ( 'NONE',  ( 14.92500000122903181, -5.773502691896255534, -1.060575238724906372E-15 ) ) ;
#37094=CARTESIAN_POINT ( 'NONE',  ( 9.075000001229033941, -5.773502691896255534, -1.060575238724906372E-15 ) ) ;
#37095=CARTESIAN_POINT ( 'NONE',  ( 4.378125000614518925, 6.421520780324663323E-16, -5.243569643749999010 ) ) ;
#37098=CARTESIAN_POINT ( 'NONE',  ( 15.08437500061451786, -4.541064518000419881, 2.621784821874995952 ) ) ;
#37099=CARTESIAN_POINT ( 'NONE',  ( 21.18749999999999645, -2.886751345948126435, -5.000000000000000000 ) ) ;
#37101=CARTESIAN_POINT ( 'NONE',  ( 22.90312500061451573, 4.541064518000418104, -2.621784821874998173 ) ) ;
#37102=CARTESIAN_POINT ( 'NONE',  ( 7.978125000614517681, 6.421520780324663323E-16, -5.243569643749999010 ) ) ;
#37103=CARTESIAN_POINT ( 'NONE',  ( 23.37187500061451573, 3.027376345333612662, -5.243569643749998122 ) ) ;
#37104=CARTESIAN_POINT ( 'NONE',  ( 7.340625000614518392, -3.027376345333614438, 5.243569643749998122 ) ) ;
#37106=CARTESIAN_POINT ( 'NONE',  ( 8.287500001229034297, 6.123233995736764310E-16, -4.999999999999998224 ) ) ;
#37107=CARTESIAN_POINT ( 'NONE',  ( 21.85312500061451502, -4.541064518000417216, -2.621784821875001281 ) ) ;
#37108=CARTESIAN_POINT ( 'NONE',  ( 9.001249775931846008E-16, 10.91562500061451857, -25.09994784771203058 ) ) ;
#37109=CARTESIAN_POINT ( 'NONE',  ( 10.20000000122903572, 5.773502691896255534, 3.535250795749688894E-16 ) ) ;
#37110=CARTESIAN_POINT ( 'NONE',  ( 19.49062500061451431, -3.027376345333614438, 5.243569643749998122 ) ) ;
#37111=CARTESIAN_POINT ( 'NONE',  ( 18.40312500061451573, 4.541064518000418104, -2.621784821874998173 ) ) ;
#37113=CARTESIAN_POINT ( 'NONE',  ( 18.18750000000000000, 5.773502691896255534, 3.535250795749688894E-16 ) ) ;
#37114=CARTESIAN_POINT ( 'NONE',  ( 12.41250000122903430, 4.330127018922192761, -2.499999999999997780 ) ) ;
#37115=CARTESIAN_POINT ( 'NONE',  ( 10.11562500061451608, -6.054752690667223547, -1.112240025338166033E-15 ) ) ;
#37116=CARTESIAN_POINT ( 'NONE',  ( 13.49062500061451608, 6.054752690667223547, 3.707466751127219781E-16 ) ) ;
#37117=CARTESIAN_POINT ( 'NONE',  ( 23.70000000122903216, 5.773502691896255534, 3.535250795749688894E-16 ) ) ;
#37119=CARTESIAN_POINT ( 'NONE',  ( 22.17187500061451644, 3.027376345333611329, 5.243569643749999010 ) ) ;
#37121=CARTESIAN_POINT ( 'NONE',  ( 5.775000001229033231, 2.886751345948126879, 4.999999999999999112 ) ) ;
#37122=CARTESIAN_POINT ( 'NONE',  ( 6.946875000614517681, -3.027376345333614438, 5.243569643749998122 ) ) ;
#37123=CARTESIAN_POINT ( 'NONE',  ( 23.52187500061451786, 3.027376345333611329, 5.243569643749999010 ) ) ;
#37124=CARTESIAN_POINT ( 'NONE',  ( 26.73750000122903003, 6.123233995736764310E-16, -4.999999999999998224 ) ) ;
#37126=CARTESIAN_POINT ( 'NONE',  ( 17.95312500061451644, 4.541064518000418104, -2.621784821874998173 ) ) ;
#37127=CARTESIAN_POINT ( 'NONE',  ( 24.12187500061451217, -6.054752690667223547, -1.112240025338166033E-15 ) ) ;
#37129=CARTESIAN_POINT ( 'NONE',  ( 9.412500001229034297, 0.000000000000000000, 4.999999999999998224 ) ) ;
#37130=CARTESIAN_POINT ( 'NONE',  ( 27.82500000122903572, 2.886751345948119329, 5.000000000000014211 ) ) ;
#37131=CARTESIAN_POINT ( 'NONE',  ( 5.671875000614519102, -6.054752690667223547, -1.112240025338166033E-15 ) ) ;
#37132=CARTESIAN_POINT ( 'NONE',  ( 16.15312500061451573, 4.541064518000418104, -2.621784821874998173 ) ) ;
#37133=AXIS2_PLACEMENT_3D ( 'NONE', #2522, #71586, #26892 ) ;
#37134=CARTESIAN_POINT ( 'NONE',  ( 14.25937500061451679, -4.541064518000417216, -2.621784821875001281 ) ) ;
#37137=CARTESIAN_POINT ( 'NONE',  ( 24.02812500061451573, -4.541064518000419881, 2.621784821874995952 ) ) ;
#37139=FACE_OUTER_BOUND ( 'NONE', #39931, .T. ) ;
#37140=CARTESIAN_POINT ( 'NONE',  ( 14.69999999999999929, 0.000000000000000000, 4.999999999999998224 ) ) ;
#37141=EDGE_CURVE ( 'NONE', #72227, #30208, #40596, .T. ) ;
#37142=CARTESIAN_POINT ( 'NONE',  ( 23.88750000122903216, -4.330127018922194537, 2.499999999999995559 ) ) ;
#37143=CARTESIAN_POINT ( 'NONE',  ( 18.92812500061451431, 4.541064518000418104, 2.621784821874999949 ) ) ;
#37144=VERTEX_POINT ( 'NONE', #33952 ) ;
#37145=CARTESIAN_POINT ( 'NONE',  ( 21.82499999999999574, 4.330127018922191873, 2.499999999999999556 ) ) ;
#37146=( BOUNDED_CURVE ( )  B_SPLINE_CURVE ( 2, ( #46314, #63650, #36313, #53299, #19669, #46677, #2699 ),
 .UNSPECIFIED., .F., .F. ) 
 B_SPLINE_CURVE_WITH_KNOTS ( ( 3, 2, 2, 3 ),
 ( 0.9429157369121473620, 0.9444444444444444198, 0.9472222222222221877, 0.9486015587049059228 ),
 .UNSPECIFIED. ) 
 CURVE ( )  GEOMETRIC_REPRESENTATION_ITEM ( )  RATIONAL_B_SPLINE_CURVE ( ( 0.9336915734631608954, 0.9262691292263730558, 1.000000000000000000, 0.8660254037844387076, 1.000000000000000000, 0.9334734226073392316, 0.9330158706060402984 ) ) 
 REPRESENTATION_ITEM ( '' )  );
#37147=CARTESIAN_POINT ( 'NONE',  ( 23.07187500061451857, 3.027376345333611329, 5.243569643749999010 ) ) ;
#37148=EDGE_CURVE ( 'NONE', #5464, #3749, #26872, .T. ) ;
#37151=CARTESIAN_POINT ( 'NONE',  ( 13.07812500061451821, 4.541064518000418104, 2.621784821874999949 ) ) ;
#37152=CARTESIAN_POINT ( 'NONE',  ( 3.553125000614516082, 4.541064518000418104, -2.621784821874998173 ) ) ;
#37154=CARTESIAN_POINT ( 'NONE',  ( 27.06562500061451004, 3.027376345333611329, 5.243569643749999010 ) ) ;
#37155=CARTESIAN_POINT ( 'NONE',  ( 19.53749999999999432, 5.773502691896255534, 3.535250795749688894E-16 ) ) ;
#37156=CARTESIAN_POINT ( 'NONE',  ( 26.81250000000000000, 2.886751345948126879, 4.999999999999999112 ) ) ;
#37157=CARTESIAN_POINT ( 'NONE',  ( 3.421875000614516882, -6.054752690667223547, -1.112240025338166033E-15 ) ) ;
#37158=CARTESIAN_POINT ( 'NONE',  ( 7.471875000614519813, -6.054752690667223547, -1.112240025338166033E-15 ) ) ;
#37159=CARTESIAN_POINT ( 'NONE',  ( 17.97187500061451715, 3.027376345333613106, -5.243569643749998122 ) ) ;
#37161=VERTEX_POINT ( 'NONE', #25414 ) ;
#37162=CARTESIAN_POINT ( 'NONE',  ( 27.32812500061451644, 6.421520780324663323E-16, -5.243569643749999010 ) ) ;
#37163=CARTESIAN_POINT ( 'NONE',  ( 27.27187500061451431, -6.054752690667223547, -1.112240025338166033E-15 ) ) ;
#37165=CARTESIAN_POINT ( 'NONE',  ( 15.97499999999999964, 4.330127018922191873, 2.499999999999999556 ) ) ;
#37166=CARTESIAN_POINT ( 'NONE',  ( 10.41562500061451679, 3.027376345333611329, 5.243569643749999010 ) ) ;
#37167=CARTESIAN_POINT ( 'NONE',  ( -3.999999999999997335, 15.08750000000000036, -27.69059892324149530 ) ) ;
#37169=CARTESIAN_POINT ( 'NONE',  ( 29.57812500061451644, 6.421520780324663323E-16, -5.243569643749999010 ) ) ;
#37170=CARTESIAN_POINT ( 'NONE',  ( 18.07500000122903216, -5.773502691896255534, -1.060575238724906372E-15 ) ) ;
#37171=CARTESIAN_POINT ( 'NONE',  ( 3.065815551951259543, -3.949781639713015657, 3.065815551951216467 ) ) ;
#37173=CARTESIAN_POINT ( 'NONE',  ( 6.103125000614515905, -4.541064518000417216, -2.621784821875001281 ) ) ;
#37174=CARTESIAN_POINT ( 'NONE',  ( 22.47187500061451715, 3.027376345333613106, -5.243569643749998122 ) ) ;
#37176=CARTESIAN_POINT ( 'NONE',  ( 2.121784821874999061, 17.45937500061451786, 26.32496088578401583 ) ) ;
#37177=CARTESIAN_POINT ( 'NONE',  ( 24.19687500061451857, -3.027376345333610441, -5.243569643749999898 ) ) ;
#37178=CARTESIAN_POINT ( 'NONE',  ( 3.975000000000002753, -4.330127018922194537, 2.499999999999995559 ) ) ;
#37179=CARTESIAN_POINT ( 'NONE',  ( -2.000000000000000000, 10.58750000122903323, 26.53589838486224650 ) ) ;
#37180=CARTESIAN_POINT ( 'NONE',  ( 11.16562500061451679, 3.027376345333613106, -5.243569643749998122 ) ) ;
#37181=CARTESIAN_POINT ( 'NONE',  ( 3.262500001229035718, -4.330127018922190985, -2.500000000000001332 ) ) ;
#37182=CARTESIAN_POINT ( 'NONE',  ( 9.159375000614515372, 0.000000000000000000, 5.243569643749999010 ) ) ;
#37184=AXIS2_PLACEMENT_3D ( 'NONE', #39023, #49012, #38658 ) ;
#37185=CARTESIAN_POINT ( 'NONE',  ( 9.778125000614517504, 6.421520780324663323E-16, -5.243569643749999010 ) ) ;
#37186=CARTESIAN_POINT ( 'NONE',  ( 14.40937500061451715, 4.541064518000418104, -2.621784821874998173 ) ) ;
#37187=CARTESIAN_POINT ( 'NONE',  ( 4.898587196589411843E-16, 20.00000000000000000, 33.99999999999999289 ) ) ;
#37188=CARTESIAN_POINT ( 'NONE',  ( 22.57500000122903572, -5.773502691896255534, -1.060575238724906372E-15 ) ) ;
#37189=CARTESIAN_POINT ( 'NONE',  ( 9.421875000614519990, 3.027376345333613106, -5.243569643749998122 ) ) ;
#37190=CARTESIAN_POINT ( 'NONE',  ( 12.81562500061451537, -6.054752690667223547, -1.112240025338166033E-15 ) ) ;
#37192=CARTESIAN_POINT ( 'NONE',  ( 20.59687500061451360, -3.027376345333610441, -5.243569643749999898 ) ) ;
#37195=CARTESIAN_POINT ( 'NONE',  ( -3.999999999999999112, 12.01250000122903394, -30.00000000000000000 ) ) ;
#37197=CARTESIAN_POINT ( 'NONE',  ( -2.121784821874996840, 14.08437500061451786, -26.32496088578401583 ) ) ;
#37198=CARTESIAN_POINT ( 'NONE',  ( 14.13750000122903394, 6.123233995736764310E-16, -4.999999999999998224 ) ) ;
#37199=CARTESIAN_POINT ( 'NONE',  ( 9.834375000614517859, 6.421520780324663323E-16, -5.243569643749999010 ) ) ;
#37200=CARTESIAN_POINT ( 'NONE',  ( 4.243569643749999898, 16.84062500061451573, -27.54997392385601529 ) ) ;
#37201=CARTESIAN_POINT ( 'NONE',  ( 17.81250000122903288, 4.330127018922192761, -2.499999999999997780 ) ) ;
#37202=CARTESIAN_POINT ( 'NONE',  ( 11.80312500061451608, 0.000000000000000000, 5.243569643749999010 ) ) ;
#37203=ORIENTED_EDGE ( 'NONE', *, *, #51099, .T. ) ;
#37205=CARTESIAN_POINT ( 'NONE',  ( 16.35000000000000142, 4.330127018922192761, -2.499999999999997780 ) ) ;
#37207=CARTESIAN_POINT ( 'NONE',  ( 10.35937500061451644, 4.541064518000418104, -2.621784821874998173 ) ) ;
#37208=LINE ( 'NONE', #9138, #29153 ) ;
#37209=CARTESIAN_POINT ( 'NONE',  ( 11.43750000122903465, 6.123233995736764310E-16, -4.999999999999998224 ) ) ;
#37210=CARTESIAN_POINT ( 'NONE',  ( 20.77500000122903145, -5.773502691896255534, -1.060575238724906372E-15 ) ) ;
#37211=CARTESIAN_POINT ( 'NONE',  ( 16.97812500061451502, 6.421520780324663323E-16, -5.243569643749999010 ) ) ;
#37212=CARTESIAN_POINT ( 'NONE',  ( 21.51562500061451644, 3.027376345333613106, -5.243569643749998122 ) ) ;
#37213=CARTESIAN_POINT ( 'NONE',  ( 27.00000000122903288, -2.886751345948129988, 4.999999999999997335 ) ) ;
#37214=( BOUNDED_CURVE ( )  B_SPLINE_CURVE ( 2, ( #71180, #43110, #66006, #49389, #39770, #22031, #39397 ),
 .UNSPECIFIED., .F., .F. ) 
 B_SPLINE_CURVE_WITH_KNOTS ( ( 3, 2, 2, 3 ),
 ( 0.9939769717443815988, 0.9944444444444444642, 0.9972222222222222321, 0.9976335333330554889 ),
 .UNSPECIFIED. ) 
 CURVE ( )  GEOMETRIC_REPRESENTATION_ITEM ( )  RATIONAL_B_SPLINE_CURVE ( ( 0.9624955293375538901, 0.9774533921562205130, 1.000000000000000000, 0.8660254037844387076, 1.000000000000000000, 0.9801621136025704395, 0.9661990982304526909 ) ) 
 REPRESENTATION_ITEM ( '' )  );
#37215=CARTESIAN_POINT ( 'NONE',  ( 3.328125000614516438, -4.541064518000419881, 2.621784821874995952 ) ) ;
#37216=CARTESIAN_POINT ( 'NONE',  ( 25.76249999999999929, 2.886751345948129099, -4.999999999999998224 ) ) ;
#37219=CARTESIAN_POINT ( 'NONE',  ( 28.73437500061451644, 6.421520780324663323E-16, -5.243569643749999010 ) ) ;
#37220=DIRECTION ( 'NONE',  ( 0.000000000000000000, 0.000000000000000000, -1.000000000000000000 ) ) ;
#37221=CARTESIAN_POINT ( 'NONE',  ( 4.725000001229034297, 2.886751345948129099, -4.999999999999998224 ) ) ;
#37222=CARTESIAN_POINT ( 'NONE',  ( 3.525000000000000355, -4.330127018922194537, 2.499999999999995559 ) ) ;
#37223=CARTESIAN_POINT ( 'NONE',  ( 7.546875000614517326, -3.027376345333610441, -5.243569643749999898 ) ) ;
#37224=CARTESIAN_POINT ( 'NONE',  ( 25.60312500061451502, 4.541064518000418104, -2.621784821874998173 ) ) ;
#37226=CARTESIAN_POINT ( 'NONE',  ( -1.004196803065525945, 9.951383199219650422, -24.08129654815694920 ) ) ;
#37228=CARTESIAN_POINT ( 'NONE',  ( 22.01250000122903216, 0.000000000000000000, 4.999999999999998224 ) ) ;
#37229=CARTESIAN_POINT ( 'NONE',  ( 4.584375000614516971, 4.541064518000418104, 2.621784821874999949 ) ) ;
#37230=CARTESIAN_POINT ( 'NONE',  ( 8.484375000614518214, 6.421520780324663323E-16, -5.243569643749999010 ) ) ;
#37231=CARTESIAN_POINT ( 'NONE',  ( 3.525000000000000355, -4.330127018922194537, 2.499999999999995559 ) ) ;
#37232=VECTOR ( 'NONE', #50274, 1000.000000000000000 ) ;
#37233=CARTESIAN_POINT ( 'NONE',  ( 9.001249775931846008E-16, 11.36562500061459602, 34.90005215228797653 ) ) ;
#37234=CARTESIAN_POINT ( 'NONE',  ( 20.77500000122903145, -5.773502691896255534, -1.060575238724906372E-15 ) ) ;
#37235=CARTESIAN_POINT ( 'NONE',  ( 3.862500000000001155, 2.886751345948126879, 4.999999999999999112 ) ) ;
#37236=AXIS2_PLACEMENT_3D ( 'NONE', #24511, #70672, #40796 ) ;
#37237=EDGE_CURVE ( 'NONE', #22838, #30519, #42416, .T. ) ;
#37240=CARTESIAN_POINT ( 'NONE',  ( 19.26562500061451644, 3.027376345333613106, -5.243569643749998122 ) ) ;
#37241=CARTESIAN_POINT ( 'NONE',  ( 10.82812500061451644, 4.541064518000418104, 2.621784821874999949 ) ) ;
#37243=CARTESIAN_POINT ( 'NONE',  ( 7.696875000614516793, 6.054752690667223547, 3.707466751127219781E-16 ) ) ;
#37244=CARTESIAN_POINT ( 'NONE',  ( 24.44999999999999929, 4.330127018922192761, -2.499999999999997780 ) ) ;
#37245=CARTESIAN_POINT ( 'NONE',  ( 20.25000000122903288, -2.886751345948129988, 4.999999999999997335 ) ) ;
#37246=CARTESIAN_POINT ( 'NONE',  ( 27.74062500061451431, -3.027376345333610441, -5.243569643749999898 ) ) ;
#37248=CARTESIAN_POINT ( 'NONE',  ( 9.534375000614517148, 4.541064518000418104, 2.621784821874999949 ) ) ;
#37249=CARTESIAN_POINT ( 'NONE',  ( 13.39687500061451608, -3.027376345333610441, -5.243569643749999898 ) ) ;
#37250=CARTESIAN_POINT ( 'NONE',  ( 24.68437500061451573, 6.421520780324663323E-16, -5.243569643749999010 ) ) ;
#37253=CARTESIAN_POINT ( 'NONE',  ( 20.29687500061451644, 6.054752690667223547, 3.707466751127219781E-16 ) ) ;
#37254=CARTESIAN_POINT ( 'NONE',  ( 8.521875000614516082, 3.027376345333613106, -5.243569643749998122 ) ) ;
#37256=CARTESIAN_POINT ( 'NONE',  ( 22.50000000000000000, -4.330127018922190985, -2.500000000000001332 ) ) ;
#37258=CARTESIAN_POINT ( 'NONE',  ( 29.81249999999999645, 2.886751345948139313, -4.999999999999980460 ) ) ;
#37260=CARTESIAN_POINT ( 'NONE',  ( 11.80312500061451608, 0.000000000000000000, 5.243569643749999010 ) ) ;
#37261=CARTESIAN_POINT ( 'NONE',  ( 5.587500000000003020, 5.773502691896255534, 3.535250795749688894E-16 ) ) ;
#37262=CARTESIAN_POINT ( 'NONE',  ( 6.712500001229034119, 0.000000000000000000, 4.999999999999998224 ) ) ;
#37264=CARTESIAN_POINT ( 'NONE',  ( 11.88749999999999751, 5.773502691896255534, 3.535250795749688894E-16 ) ) ;
#37265=CARTESIAN_POINT ( 'NONE',  ( 3.999999999999998668, 17.22500000122903785, 27.69059892324149175 ) ) ;
#37266=CARTESIAN_POINT ( 'NONE',  ( 11.25000000122903288, -2.886751345948129988, 4.999999999999997335 ) ) ;
#37267=CARTESIAN_POINT ( 'NONE',  ( 21.72187500061451715, 3.027376345333611329, 5.243569643749999010 ) ) ;
#37268=CARTESIAN_POINT ( 'NONE',  ( 15.94687500061451502, -3.027376345333614438, 5.243569643749998122 ) ) ;
#37270=ORIENTED_EDGE ( 'NONE', *, *, #63369, .T. ) ;
#37271=CARTESIAN_POINT ( 'NONE',  ( 17.39062500061451644, -3.027376345333610441, -5.243569643749999898 ) ) ;
#37272=CARTESIAN_POINT ( 'NONE',  ( 28.42500000122904069, -5.773502691896255534, -1.060575238724906372E-15 ) ) ;
#37273=CARTESIAN_POINT ( 'NONE',  ( 17.52187500061451431, 3.027376345333613106, -5.243569643749998122 ) ) ;
#37274=CARTESIAN_POINT ( 'NONE',  ( 28.35937500061451289, 4.541064518000418104, -2.621784821874998173 ) ) ;
#37275=CARTESIAN_POINT ( 'NONE',  ( 3.965625000614515727, 3.027376345333613106, -5.243569643749998122 ) ) ;
#37276=CARTESIAN_POINT ( 'NONE',  ( 19.19062500061452070, -3.027376345333610441, -5.243569643749999898 ) ) ;
#37277=CARTESIAN_POINT ( 'NONE',  ( 28.20937500061451786, -4.541064518000417216, -2.621784821875001281 ) ) ;
#37278=CARTESIAN_POINT ( 'NONE',  ( -2.121784821874996840, 12.67812500061451786, 33.67503911421598417 ) ) ;
#37279=CARTESIAN_POINT ( 'NONE',  ( 17.73750000122903359, 6.123233995736764310E-16, -4.999999999999998224 ) ) ;
#37281=CARTESIAN_POINT ( 'NONE',  ( 8.053125000614516082, 4.541064518000418104, -2.621784821874998173 ) ) ;
#37282=CARTESIAN_POINT ( 'NONE',  ( 25.90312500061451573, -4.541064518000417216, -2.621784821875001281 ) ) ;
#37283=CARTESIAN_POINT ( 'NONE',  ( 9.037499999999997868, -2.886751345948193048, -4.999999999999883649 ) ) ;
#37284=CARTESIAN_POINT ( 'NONE',  ( 23.85937500061451644, 4.541064518000418104, -2.621784821874998173 ) ) ;
#37285=CARTESIAN_POINT ( 'NONE',  ( 14.87812500061451537, 4.541064518000418104, 2.621784821874999949 ) ) ;
#37286=CARTESIAN_POINT ( 'NONE',  ( 23.32500000122903572, 2.886751345948126879, 4.999999999999999112 ) ) ;
#37287=CARTESIAN_POINT ( 'NONE',  ( 23.01562500061451644, 3.027376345333611329, 5.243569643749999010 ) ) ;
#37288=CARTESIAN_POINT ( 'NONE',  ( 20.63437500061451857, 6.421520780324663323E-16, -5.243569643749999010 ) ) ;
#37289=CARTESIAN_POINT ( 'NONE',  ( 13.07812500061451821, 4.541064518000418104, 2.621784821874999949 ) ) ;
#37290=CARTESIAN_POINT ( 'NONE',  ( 4.243569643749999010, 14.72187500061451715, 27.54997392385601174 ) ) ;
#37291=CARTESIAN_POINT ( 'NONE',  ( 20.91562500061451502, -6.054752690667223547, -1.112240025338166033E-15 ) ) ;
#37294=ORIENTED_EDGE ( 'NONE', *, *, #39744, .T. ) ;
#37295=CARTESIAN_POINT ( 'NONE',  ( 23.69999999999999929, 0.000000000000000000, 4.999999999999998224 ) ) ;
#37296=CARTESIAN_POINT ( 'NONE',  ( 3.999999999999999112, 11.67500000000000071, -30.00000000000000000 ) ) ;
#37297=CARTESIAN_POINT ( 'NONE',  ( 2.000000000000001332, 18.01250000122903572, 33.46410161513774995 ) ) ;
#37298=CARTESIAN_POINT ( 'NONE',  ( 27.21562500061451928, -6.054752690667223547, -1.112240025338166033E-15 ) ) ;
#37299=CARTESIAN_POINT ( 'NONE',  ( 5.090625000614516615, -3.027376345333614438, 5.243569643749998122 ) ) ;
#37300=CARTESIAN_POINT ( 'NONE',  ( 20.06250000122903643, 4.330127018922192761, -2.499999999999997780 ) ) ;
#37301=CARTESIAN_POINT ( 'NONE',  ( 25.75312500061451715, 0.000000000000000000, 5.243569643749999010 ) ) ;
#37302=CARTESIAN_POINT ( 'NONE',  ( 21.93750000000000000, -2.886751345948129988, 4.999999999999997335 ) ) ;
#37303=CARTESIAN_POINT ( 'NONE',  ( 28.30312500061451431, 4.541064518000418104, -2.621784821874998173 ) ) ;
#37304=CARTESIAN_POINT ( 'NONE',  ( 7.940625000614518036, -3.027376345333610441, -5.243569643749999898 ) ) ;
#37305=ORIENTED_EDGE ( 'NONE', *, *, #43499, .F. ) ;
#37306=EDGE_CURVE ( 'NONE', #38366, #67359, #64593, .T. ) ;
#37307=CARTESIAN_POINT ( 'NONE',  ( 22.30312500061451431, -4.541064518000417216, -2.621784821875001281 ) ) ;
#37308=CARTESIAN_POINT ( 'NONE',  ( 5.915625000614515905, 3.027376345333611329, 5.243569643749999010 ) ) ;
#37310=CARTESIAN_POINT ( 'NONE',  ( 4.040625000614517681, 6.054752690667223547, 3.707466751127219781E-16 ) ) ;
#37311=CARTESIAN_POINT ( 'NONE',  ( 3.999999999999999112, 14.03750000122903430, -30.00000000000000000 ) ) ;
#37313=CARTESIAN_POINT ( 'NONE',  ( 11.84999999999999964, 4.330127018922192761, -2.499999999999997780 ) ) ;
#37314=CARTESIAN_POINT ( 'NONE',  ( 10.47187500061451715, 3.027376345333611329, 5.243569643749999010 ) ) ;
#37315=CARTESIAN_POINT ( 'NONE',  ( 7.837500001229035007, 6.123233995736764310E-16, -4.999999999999998224 ) ) ;
#37316=CARTESIAN_POINT ( 'NONE',  ( 14.18437500061451750, -4.541064518000419881, 2.621784821874995952 ) ) ;
#37318=CARTESIAN_POINT ( 'NONE',  ( 5.971875000614516260, 3.027376345333611329, 5.243569643749999010 ) ) ;
#37319=CARTESIAN_POINT ( 'NONE',  ( -1.473776270879187500, 9.816672227264547246, -34.04916702557058983 ) ) ;
#37321=ADVANCED_FACE ( 'NONE', ( #58288 ), #35766, .F. ) ;
#37322=CARTESIAN_POINT ( 'NONE',  ( 12.68437500061451573, 4.541064518000418104, 2.621784821874999949 ) ) ;
#37323=CARTESIAN_POINT ( 'NONE',  ( 3.678818219770688902, 3.386201399061161688, 4.003588590596459440 ) ) ;
#37324=CARTESIAN_POINT ( 'NONE',  ( 22.86562500061451431, 3.027376345333613106, -5.243569643749998122 ) ) ;
#37325=CARTESIAN_POINT ( 'NONE',  ( -2.121784821874999949, 9.884375000614518569, 26.32496088578401938 ) ) ;
#37326=CARTESIAN_POINT ( 'NONE',  ( 4.243569643749999898, 18.67812500061459602, 30.00000000000000000 ) ) ;
#37327=CARTESIAN_POINT ( 'NONE',  ( 24.98437500061451644, -4.541064518000419881, 2.621784821874995952 ) ) ;
#37328=CARTESIAN_POINT ( 'NONE',  ( 30.00000000000000000, 0.000000000000000000, 0.000000000000000000 ) ) ;
#37329=CARTESIAN_POINT ( 'NONE',  ( 4.865625000614517859, 3.027376345333613106, -5.243569643749998122 ) ) ;
#37331=CARTESIAN_POINT ( 'NONE',  ( 13.43437500061451750, 6.421520780324663323E-16, -5.243569643749999010 ) ) ;
#37333=AXIS2_PLACEMENT_3D ( 'NONE', #5256, #16690, #5626 ) ;
#37334=CARTESIAN_POINT ( 'NONE',  ( 28.08750000122903145, 6.123233995736764310E-16, -4.999999999999998224 ) ) ;
#37335=CARTESIAN_POINT ( 'NONE',  ( 5.071875000614519458, 3.027376345333611329, 5.243569643749999010 ) ) ;
#37336=CARTESIAN_POINT ( 'NONE',  ( 16.39687500061451786, -3.027376345333614438, 5.243569643749998122 ) ) ;
#37337=CARTESIAN_POINT ( 'NONE',  ( -3.999999999999999112, 11.90000000000000036, 30.00000000000000000 ) ) ;
#37338=CARTESIAN_POINT ( 'NONE',  ( 24.93750000000000355, 5.773502691896255534, 3.535250795749688894E-16 ) ) ;
#37339=CARTESIAN_POINT ( 'NONE',  ( 4.087500001229035007, -4.330127018922194537, 2.499999999999995559 ) ) ;
#37340=CARTESIAN_POINT ( 'NONE',  ( 28.32187500061451502, 3.027376345333613106, -5.243569643749998122 ) ) ;
#37342=CARTESIAN_POINT ( 'NONE',  ( 29.62500000000000000, -4.330127018922194537, 2.499999999999995559 ) ) ;
#37343=CARTESIAN_POINT ( 'NONE',  ( 7.762500000000001954, 2.886751345948129099, -4.999999999999998224 ) ) ;
#37345=CARTESIAN_POINT ( 'NONE',  ( 21.36562500061451431, -6.054752690667223547, -1.112240025338166033E-15 ) ) ;
#37346=CARTESIAN_POINT ( 'NONE',  ( 11.84999999999999964, 4.330127018922192761, -2.499999999999997780 ) ) ;
#37348=CARTESIAN_POINT ( 'NONE',  ( 4.415625000614518569, 3.027376345333613106, -5.243569643749998122 ) ) ;
#37349=CARTESIAN_POINT ( 'NONE',  ( 20.51249999999999929, 2.886751345948126879, 4.999999999999999112 ) ) ;
#37350=CARTESIAN_POINT ( 'NONE',  ( 18.02812500061451573, 4.541064518000418104, 2.621784821874999949 ) ) ;
#37351=CARTESIAN_POINT ( 'NONE',  ( -1.071796769724490783, 18.85490381179670649, 34.00000000000000000 ) ) ;
#37352=CARTESIAN_POINT ( 'NONE',  ( 23.47500000122903430, -5.773502691896255534, -1.060575238724906372E-15 ) ) ;
#37354=CARTESIAN_POINT ( 'NONE',  ( 3.412500000000002309, 2.886751345948126879, 4.999999999999999112 ) ) ;
#37355=ORIENTED_EDGE ( 'NONE', *, *, #17544, .F. ) ;
#37356=CARTESIAN_POINT ( 'NONE',  ( 20.46562500061451928, -6.054752690667223547, -1.112240025338166033E-15 ) ) ;
#37357=CARTESIAN_POINT ( 'NONE',  ( 24.02812500061451573, -4.541064518000419881, 2.621784821874995952 ) ) ;
#37358=CARTESIAN_POINT ( 'NONE',  ( 24.27187500061452141, 3.027376345333613106, -5.243569643749998122 ) ) ;
#37359=CARTESIAN_POINT ( 'NONE',  ( 9.337500000000000355, -2.886751345948129988, 4.999999999999997335 ) ) ;
#37360=CARTESIAN_POINT ( 'NONE',  ( 12.32812500061451821, -4.541064518000419881, 2.621784821874995952 ) ) ;
#37361=CARTESIAN_POINT ( 'NONE',  ( 25.67812500061451431, 4.541064518000418104, 2.621784821874999949 ) ) ;
#37362=CARTESIAN_POINT ( 'NONE',  ( 17.03437500061451715, 6.421520780324663323E-16, -5.243569643749999010 ) ) ;
#37363=CARTESIAN_POINT ( 'NONE',  ( 8.015625000614518214, 3.027376345333613106, -5.243569643749998122 ) ) ;
#37365=CARTESIAN_POINT ( 'NONE',  ( 2.226602359779148887, 9.807522476441999260, 25.29835638300850320 ) ) ;
#37366=CARTESIAN_POINT ( 'NONE',  ( 23.77500000122903145, 2.886751345948126879, 4.999999999999999112 ) ) ;
#37368=CARTESIAN_POINT ( 'NONE',  ( 15.17812500061451608, 6.421520780324663323E-16, -5.243569643749999010 ) ) ;
#37369=CARTESIAN_POINT ( 'NONE',  ( 9.046875000614518214, 6.054752690667223547, 3.707466751127219781E-16 ) ) ;
#37370=CARTESIAN_POINT ( 'NONE',  ( 7.846875000614518036, -3.027376345333614438, 5.243569643749998122 ) ) ;
#37372=CARTESIAN_POINT ( 'NONE',  ( -6.275039685470489619E-15, 17.97500000122903074, 33.99999999999999289 ) ) ;
#37373=CARTESIAN_POINT ( 'NONE',  ( 22.41562500061451502, 3.027376345333613106, -5.243569643749998122 ) ) ;
#37374=CARTESIAN_POINT ( 'NONE',  ( 16.77187500061451786, 3.027376345333611329, 5.243569643749999010 ) ) ;
#37375=CARTESIAN_POINT ( 'NONE',  ( 22.94062500061451715, 6.054752690667223547, 3.707466751127219781E-16 ) ) ;
#37376=CARTESIAN_POINT ( 'NONE',  ( 3.999999999999998668, 13.06250000000000355, 27.69059892324149175 ) ) ;
#37377=CARTESIAN_POINT ( 'NONE',  ( 28.19062500061451715, -3.027376345333610441, -5.243569643749999898 ) ) ;
#37378=CARTESIAN_POINT ( 'NONE',  ( 8.062500001229034652, 0.000000000000000000, 4.999999999999998224 ) ) ;
#37379=ORIENTED_EDGE ( 'NONE', *, *, #9276, .F. ) ;
#37380=CARTESIAN_POINT ( 'NONE',  ( 29.25000000000000000, -4.330127018922190985, -2.500000000000001332 ) ) ;
#37381=CARTESIAN_POINT ( 'NONE',  ( 1.999999999999998668, 17.15000000000000213, -33.46410161513775705 ) ) ;
#37383=CARTESIAN_POINT ( 'NONE',  ( 25.12500000122903288, 2.886751345948126879, 4.999999999999999112 ) ) ;
#37385=CARTESIAN_POINT ( 'NONE',  ( 6.834375000614518747, 4.541064518000418104, 2.621784821874999949 ) ) ;
#37386=CARTESIAN_POINT ( 'NONE',  ( 15.36562500061451608, 3.027376345333611329, 5.243569643749999010 ) ) ;
#37387=CARTESIAN_POINT ( 'NONE',  ( 7.771875000614516971, 3.027376345333611329, 5.243569643749999010 ) ) ;
#37388=CARTESIAN_POINT ( 'NONE',  ( 27.33750000122903145, 4.330127018922191873, 2.499999999999999556 ) ) ;
#37389=CARTESIAN_POINT ( 'NONE',  ( 17.89687500061451431, -3.027376345333610441, -5.243569643749999898 ) ) ;
#37390=CARTESIAN_POINT ( 'NONE',  ( 5.671875000614519102, -6.054752690667223547, -1.112240025338166033E-15 ) ) ;
#37391=CARTESIAN_POINT ( 'NONE',  ( 4.000000000000000000, 17.48750000000000071, -27.69059892324149885 ) ) ;
#37392=CARTESIAN_POINT ( 'NONE',  ( 5.240625000614516971, -3.027376345333610441, -5.243569643749999898 ) ) ;
#37393=CARTESIAN_POINT ( 'NONE',  ( 15.51562500061451644, -6.054752690667223547, -1.112240025338166033E-15 ) ) ;
#37394=ORIENTED_EDGE ( 'NONE', *, *, #61111, .T. ) ;
#37395=CARTESIAN_POINT ( 'NONE',  ( 12.77812500061451750, -4.541064518000419881, 2.621784821874995952 ) ) ;
#37396=CARTESIAN_POINT ( 'NONE',  ( 6.600000001229032520, 5.773502691896255534, 3.535250795749688894E-16 ) ) ;
#37397=CARTESIAN_POINT ( 'NONE',  ( 8.315625000614515372, -6.054752690667223547, -1.112240025338166033E-15 ) ) ;
#37399=CARTESIAN_POINT ( 'NONE',  ( 8.437500000000000000, -2.886751345948129988, 4.999999999999997335 ) ) ;
#37400=CARTESIAN_POINT ( 'NONE',  ( 3.712500001229034563, -4.330127018922190985, -2.500000000000001332 ) ) ;
#37401=CARTESIAN_POINT ( 'NONE',  ( 18.22499999999999787, 4.330127018922191873, 2.499999999999999556 ) ) ;
#37402=EDGE_CURVE ( 'NONE', #26902, #57550, #36331, .T. ) ;
#37403=CARTESIAN_POINT ( 'NONE',  ( 18.60937500061451644, 0.000000000000000000, 5.243569643749999010 ) ) ;
#37404=CARTESIAN_POINT ( 'NONE',  ( 15.60000000122903607, 5.773502691896255534, 3.535250795749688894E-16 ) ) ;
#37406=CARTESIAN_POINT ( 'NONE',  ( 2.121784821874999061, 15.60312500061451857, -33.67503911421598417 ) ) ;
#37407=CARTESIAN_POINT ( 'NONE',  ( -1.394453263437886801E-15, 19.66249999999999787, -26.00000000000000000 ) ) ;
#37408=CYLINDRICAL_SURFACE ( 'NONE', #26507, 4.999999999999998224 ) ;
#37409=DIRECTION ( 'NONE',  ( -1.000000000000000000, -0.000000000000000000, -0.000000000000000000 ) ) ;
#37410=CARTESIAN_POINT ( 'NONE',  ( 28.30312500061451431, 4.541064518000418104, -2.621784821874998173 ) ) ;
#37413=CARTESIAN_POINT ( 'NONE',  ( 15.60937500061451644, -4.541064518000417216, -2.621784821875001281 ) ) ;
#37414=CARTESIAN_POINT ( 'NONE',  ( 28.49999999999999645, 4.330127018922192761, -2.499999999999997780 ) ) ;
#37415=CARTESIAN_POINT ( 'NONE',  ( 11.80312500061451608, 0.000000000000000000, 5.243569643749999010 ) ) ;
#37417=CARTESIAN_POINT ( 'NONE',  ( 24.72187500061451360, 3.027376345333613106, -5.243569643749998122 ) ) ;
#37419=CARTESIAN_POINT ( 'NONE',  ( 8.278125000614515727, -4.541064518000419881, 2.621784821874995952 ) ) ;
#37420=CARTESIAN_POINT ( 'NONE',  ( 12.72187500061451537, 3.027376345333611329, 5.243569643749999010 ) ) ;
#37421=VERTEX_POINT ( 'NONE', #69756 ) ;
#37422=CARTESIAN_POINT ( 'NONE',  ( 24.79687500061451999, 6.054752690667223547, 3.707466751127219781E-16 ) ) ;
#37423=CARTESIAN_POINT ( 'NONE',  ( 28.30312500061451431, 4.541064518000418104, -2.621784821874998173 ) ) ;
#37425=CARTESIAN_POINT ( 'NONE',  ( 7.237500000000000711, -2.886751345948125991, -5.000000000000000000 ) ) ;
#37427=CARTESIAN_POINT ( 'NONE',  ( 15.78750000122903430, -4.330127018922194537, 2.499999999999995559 ) ) ;
#37428=CARTESIAN_POINT ( 'NONE',  ( 27.33750000122903145, 4.330127018922191873, 2.499999999999999556 ) ) ;
#37429=CARTESIAN_POINT ( 'NONE',  ( 0.000000000000000000, 20.00000000000000000, 26.00000000000000000 ) ) ;
#37430=VERTEX_POINT ( 'NONE', #41326 ) ;
#37431=CARTESIAN_POINT ( 'NONE',  ( 15.78749999999999964, -2.886751345948125991, -5.000000000000000000 ) ) ;
#37432=CARTESIAN_POINT ( 'NONE',  ( 20.06250000000000000, 2.886751345948126879, 4.999999999999999112 ) ) ;
#37433=CARTESIAN_POINT ( 'NONE',  ( 10.30312500061451431, 4.541064518000418104, -2.621784821874998173 ) ) ;
#37434=( BOUNDED_CURVE ( )  B_SPLINE_CURVE ( 2, ( #72876, #72143, #45165, #32620, #21522, #11179, #33703 ),
 .UNSPECIFIED., .F., .F. ) 
 B_SPLINE_CURVE_WITH_KNOTS ( ( 3, 2, 2, 3 ),
 ( 0.3999999999999999112, 0.4027777777777777346, 0.4055555555555555580, 0.4083333333333333814 ),
 .UNSPECIFIED. ) 
 CURVE ( )  GEOMETRIC_REPRESENTATION_ITEM ( )  RATIONAL_B_SPLINE_CURVE ( ( 1.000000000000005329, 0.8660254037844333785, 1.000000000000000000, 0.8660254037844387076, 1.000000000000000000, 0.8660254037844360431, 1.000000000000002665 ) ) 
 REPRESENTATION_ITEM ( '' )  );
#37435=ORIENTED_EDGE ( 'NONE', *, *, #73023, .T. ) ;
#37436=CARTESIAN_POINT ( 'NONE',  ( 3.675000001229035362, -5.773502691896255534, -1.060575238724906372E-15 ) ) ;
#37437=CARTESIAN_POINT ( 'NONE',  ( 9.001249775931846008E-16, 17.27187500061451786, -25.09994784771203058 ) ) ;
#37438=CARTESIAN_POINT ( 'NONE',  ( 3.853125000614517681, -4.541064518000417216, -2.621784821875001281 ) ) ;
#37440=CARTESIAN_POINT ( 'NONE',  ( 10.61250000000000071, 2.886751345948126879, 4.999999999999999112 ) ) ;
#37441=CARTESIAN_POINT ( 'NONE',  ( 3.366080804335946919, -3.697228694398128290, 3.718268762498968094 ) ) ;
#37442=EDGE_LOOP ( 'NONE', ( #44092, #38775, #21908, #17872 ) ) ;
#37443=CARTESIAN_POINT ( 'NONE',  ( 4.243569643749999898, 14.17812500061451608, 30.00000000000000000 ) ) ;
#37444=CARTESIAN_POINT ( 'NONE',  ( 27.40312500061451573, 4.541064518000418104, -2.621784821874998173 ) ) ;
#37445=CARTESIAN_POINT ( 'NONE',  ( 29.21250000122903145, 0.000000000000000000, 4.999999999999998224 ) ) ;
#37447=CARTESIAN_POINT ( 'NONE',  ( 23.33437500061451786, 6.421520780324663323E-16, -5.243569643749999010 ) ) ;
#37448=CARTESIAN_POINT ( 'NONE',  ( 18.06562500061451715, 3.027376345333611329, 5.243569643749999010 ) ) ;
#37449=EDGE_CURVE ( 'NONE', #11892, #2226, #31593, .T. ) ;
#37450=CARTESIAN_POINT ( 'NONE',  ( 4.243569643749999898, 12.82812500061459460, -30.00000000000000000 ) ) ;
#37451=CARTESIAN_POINT ( 'NONE',  ( 24.00000000122902932, -2.886751345948125991, -5.000000000000000000 ) ) ;
#37452=CARTESIAN_POINT ( 'NONE',  ( 3.403125000614518836, -4.541064518000417216, -2.621784821875001281 ) ) ;
#37454=CARTESIAN_POINT ( 'NONE',  ( 22.15312500061451573, 0.000000000000000000, 5.243569643749999010 ) ) ;
#37457=CARTESIAN_POINT ( 'NONE',  ( 14.74687500061451573, -3.027376345333610441, -5.243569643749999898 ) ) ;
#37458=CARTESIAN_POINT ( 'NONE',  ( 17.89687500061451431, -3.027376345333610441, -5.243569643749999898 ) ) ;
#37459=CARTESIAN_POINT ( 'NONE',  ( 24.72187500061451360, 3.027376345333613106, -5.243569643749998122 ) ) ;
#37460=CARTESIAN_POINT ( 'NONE',  ( 4.243569643749999010, 13.82187500061451857, 27.54997392385601174 ) ) ;
#37461=CARTESIAN_POINT ( 'NONE',  ( 5.203125000614518214, -4.541064518000417216, -2.621784821875001281 ) ) ;
#37462=CARTESIAN_POINT ( 'NONE',  ( 27.77812500061451573, 6.421520780324663323E-16, -5.243569643749999010 ) ) ;
#37463=CARTESIAN_POINT ( 'NONE',  ( 29.42812500061451431, -4.541064518000419881, 2.621784821874995952 ) ) ;
#37464=CARTESIAN_POINT ( 'NONE',  ( 1.626862140677534273E-15, 16.17500000122903359, -26.00000000000000355 ) ) ;
#37465=CARTESIAN_POINT ( 'NONE',  ( -3.999999999999999112, 19.55000000000000071, 30.00000000000000000 ) ) ;
#37466=CARTESIAN_POINT ( 'NONE',  ( 7.621875000614519280, 3.027376345333613106, -5.243569643749998122 ) ) ;
#37467=CARTESIAN_POINT ( 'NONE',  ( 14.96250000122903323, -4.330127018922190985, -2.500000000000001332 ) ) ;
#37468=CARTESIAN_POINT ( 'NONE',  ( 8.662500001229034297, -4.330127018922190985, -2.500000000000001332 ) ) ;
#37469=CARTESIAN_POINT ( 'NONE',  ( 4.753125000614515372, -4.541064518000417216, -2.621784821875001281 ) ) ;
#37472=CARTESIAN_POINT ( 'NONE',  ( 14.37187500061451928, 3.027376345333613106, -5.243569643749998122 ) ) ;
#37474=VERTEX_POINT ( 'NONE', #70486 ) ;
#37475=CARTESIAN_POINT ( 'NONE',  ( 21.51562500061451644, 3.027376345333613106, -5.243569643749998122 ) ) ;
#37476=CARTESIAN_POINT ( 'NONE',  ( 6.590625000614518392, -3.027376345333610441, -5.243569643749999898 ) ) ;
#37477=CARTESIAN_POINT ( 'NONE',  ( 24.49687500061451573, -3.027376345333614438, 5.243569643749998122 ) ) ;
#37478=CARTESIAN_POINT ( 'NONE',  ( 6.740625000614516082, 6.054752690667223547, 3.707466751127219781E-16 ) ) ;
#37480=CARTESIAN_POINT ( 'NONE',  ( 7.312500001229033764, -4.330127018922190985, -2.500000000000001332 ) ) ;
#37481=CARTESIAN_POINT ( 'NONE',  ( 22.64062500061451644, -3.027376345333614438, 5.243569643749998122 ) ) ;
#37482=CARTESIAN_POINT ( 'NONE',  ( -4.243569643749997233, 10.39062500061451644, -27.54997392385601174 ) ) ;
#37483=CARTESIAN_POINT ( 'NONE',  ( 10.16250000122903252, 4.330127018922192761, -2.499999999999997780 ) ) ;
#37484=CARTESIAN_POINT ( 'NONE',  ( 19.34062500061451573, 6.054752690667223547, 3.707466751127219781E-16 ) ) ;
#37485=CARTESIAN_POINT ( 'NONE',  ( 18.92812500061451431, 4.541064518000418104, 2.621784821874999949 ) ) ;
#37487=CARTESIAN_POINT ( 'NONE',  ( 18.86249999999999716, -5.773502691896255534, -1.060575238724906372E-15 ) ) ;
#37488=CARTESIAN_POINT ( 'NONE',  ( 10.61250000122903536, 4.330127018922192761, -2.499999999999997780 ) ) ;
#37490=CARTESIAN_POINT ( 'NONE',  ( 8.653125000614515727, 0.000000000000000000, 5.243569643749999010 ) ) ;
#37491=CARTESIAN_POINT ( 'NONE',  ( 11.69062500061451360, 6.054752690667223547, 3.707466751127219781E-16 ) ) ;
#37492=CARTESIAN_POINT ( 'NONE',  ( 22.31250000122903288, 4.330127018922192761, -2.499999999999997780 ) ) ;
#37493=CARTESIAN_POINT ( 'NONE',  ( 22.32187500061451502, -6.054752690667223547, -1.112240025338166033E-15 ) ) ;
#37495=CARTESIAN_POINT ( 'NONE',  ( 4.837500001229035895, 4.330127018922191873, 2.499999999999999556 ) ) ;
#37496=CARTESIAN_POINT ( 'NONE',  ( 5.934375000614517504, 4.541064518000418104, 2.621784821874999949 ) ) ;
#37497=CARTESIAN_POINT ( 'NONE',  ( 22.43437500061451573, 6.421520780324663323E-16, -5.243569643749999010 ) ) ;
#37498=CARTESIAN_POINT ( 'NONE',  ( 21.78750000122903074, 6.123233995736764310E-16, -4.999999999999998224 ) ) ;
#37499=CARTESIAN_POINT ( 'NONE',  ( 19.26562500061451644, 3.027376345333613106, -5.243569643749998122 ) ) ;
#37500=CARTESIAN_POINT ( 'NONE',  ( 25.28437500061451715, 4.541064518000418104, 2.621784821874999949 ) ) ;
#37502=CARTESIAN_POINT ( 'NONE',  ( -3.137519842735245283E-14, 11.22500000122903430, -26.00000000000000711 ) ) ;
#37503=CARTESIAN_POINT ( 'NONE',  ( -2.000000000000000000, 13.28750000122903430, -33.46410161513775705 ) ) ;
#37504=CARTESIAN_POINT ( 'NONE',  ( 5.071875000614519458, 3.027376345333611329, 5.243569643749999010 ) ) ;
#37505=CARTESIAN_POINT ( 'NONE',  ( 15.70312500061451644, 4.541064518000418104, -2.621784821874998173 ) ) ;
#37506=CARTESIAN_POINT ( 'NONE',  ( 13.80937500061451750, -4.541064518000417216, -2.621784821875001281 ) ) ;
#37507=ORIENTED_EDGE ( 'NONE', *, *, #60732, .T. ) ;
#37508=CARTESIAN_POINT ( 'NONE',  ( 9.187500000000001776, 5.773502691896255534, 3.535250795749688401E-16 ) ) ;
#37509=CARTESIAN_POINT ( 'NONE',  ( 23.95312500061451289, 0.000000000000000000, 5.243569643749999010 ) ) ;
#37510=CARTESIAN_POINT ( 'NONE',  ( -1.487416814333745711E-14, 16.96250000000000213, 34.00000000000000000 ) ) ;
#37511=CARTESIAN_POINT ( 'NONE',  ( -1.071796769724491005, 11.47009619066136565, -34.00000000000000000 ) ) ;
#37512=CARTESIAN_POINT ( 'NONE',  ( 15.11249999999999893, 2.886751345948126879, 4.999999999999999112 ) ) ;
#37513=CARTESIAN_POINT ( 'NONE',  ( 23.43750000122902932, -4.330127018922194537, 2.499999999999995559 ) ) ;
#37514=CARTESIAN_POINT ( 'NONE',  ( 17.95312500061451644, 4.541064518000418104, -2.621784821874998173 ) ) ;
#37516=CARTESIAN_POINT ( 'NONE',  ( 21.89999999999999858, 0.000000000000000000, 4.999999999999998224 ) ) ;
#37517=CARTESIAN_POINT ( 'NONE',  ( 24.68437500061451573, 6.421520780324663323E-16, -5.243569643749999010 ) ) ;
#37518=ORIENTED_EDGE ( 'NONE', *, *, #26233, .T. ) ;
#37519=CYLINDRICAL_SURFACE ( 'NONE', #6511, 4.999999999999998224 ) ;
#37520=CARTESIAN_POINT ( 'NONE',  ( 10.56562500061451715, -6.054752690667223547, -1.112240025338166033E-15 ) ) ;
#37521=CARTESIAN_POINT ( 'NONE',  ( 4.040625000614517681, 6.054752690667223547, 3.707466751127219781E-16 ) ) ;
#37523=CARTESIAN_POINT ( 'NONE',  ( 27.59062500061451573, -3.027376345333614438, 5.243569643749998122 ) ) ;
#37524=CARTESIAN_POINT ( 'NONE',  ( 18.14999999999999858, 4.330127018922192761, -2.499999999999997780 ) ) ;
#37525=CARTESIAN_POINT ( 'NONE',  ( 27.63749999999999929, 5.773502691896255534, 3.535250795749688894E-16 ) ) ;
#37527=CARTESIAN_POINT ( 'NONE',  ( 6.459375000614518747, 0.000000000000000000, 5.243569643749999010 ) ) ;
#37528=CARTESIAN_POINT ( 'NONE',  ( 17.48437500061451999, 6.421520780324663323E-16, -5.243569643749999010 ) ) ;
#37530=CARTESIAN_POINT ( 'NONE',  ( 25.37812500061451715, -4.541064518000419881, 2.621784821874995952 ) ) ;
#37531=CARTESIAN_POINT ( 'NONE',  ( 26.97187500061451360, 3.027376345333613106, -5.243569643749998122 ) ) ;
#37533=CARTESIAN_POINT ( 'NONE',  ( 14.36249999999999893, -5.773502691896255534, -1.060575238724906372E-15 ) ) ;
#37534=CARTESIAN_POINT ( 'NONE',  ( 11.87812500061451537, -4.541064518000419881, 2.621784821874995952 ) ) ;
#37537=CARTESIAN_POINT ( 'NONE',  ( 28.52812500061451573, -4.541064518000419881, 2.621784821874995952 ) ) ;
#37538=CARTESIAN_POINT ( 'NONE',  ( 15.22500000122903252, 2.886751345948126879, 4.999999999999999112 ) ) ;
#37541=CARTESIAN_POINT ( 'NONE',  ( 4.678125000614516971, -4.541064518000419881, 2.621784821874995952 ) ) ;
#37542=CARTESIAN_POINT ( 'NONE',  ( 21.34687500061451715, -3.027376345333614438, 5.243569643749998122 ) ) ;
#37543=CARTESIAN_POINT ( 'NONE',  ( 2.121784821875001281, 18.20937500061451786, 33.67503911421598417 ) ) ;
#37544=CARTESIAN_POINT ( 'NONE',  ( 23.14687500061451786, -3.027376345333614438, 5.243569643749998122 ) ) ;
#37545=CARTESIAN_POINT ( 'NONE',  ( 4.462500000000001243, -5.773502691896255534, -1.060575238724906372E-15 ) ) ;
#37546=CARTESIAN_POINT ( 'NONE',  ( -3.999999999999999556, 11.52500000122903501, 27.69059892324149530 ) ) ;
#37547=CARTESIAN_POINT ( 'NONE',  ( 12.29062500061451857, -3.027376345333614438, 5.243569643749998122 ) ) ;
#37548=CARTESIAN_POINT ( 'NONE',  ( 5.250000001229035540, 5.773502691896255534, 3.535250795749688894E-16 ) ) ;
#37549=CARTESIAN_POINT ( 'NONE',  ( 10.50937500061451679, 0.000000000000000000, 5.243569643749999010 ) ) ;
#37550=CARTESIAN_POINT ( 'NONE',  ( 11.21250000122903501, 0.000000000000000000, 4.999999999999998224 ) ) ;
#37551=CARTESIAN_POINT ( 'NONE',  ( 9.590625000614517504, -3.027376345333614438, 5.243569643749998122 ) ) ;
#37552=CARTESIAN_POINT ( 'NONE',  ( 14.93437500061451750, 4.541064518000418104, 2.621784821874999949 ) ) ;
#37553=CARTESIAN_POINT ( 'NONE',  ( 25.50000000000000000, 0.000000000000000000, 4.999999999999998224 ) ) ;
#37554=CARTESIAN_POINT ( 'NONE',  ( 20.47500000122903074, 2.886751345948129099, -4.999999999999998224 ) ) ;
#37555=CARTESIAN_POINT ( 'NONE',  ( 10.80937500061451928, 4.541064518000418104, -2.621784821874998173 ) ) ;
#37556=CARTESIAN_POINT ( 'NONE',  ( 12.74062500061451786, -3.027376345333614438, 5.243569643749998122 ) ) ;
#37558=CARTESIAN_POINT ( 'NONE',  ( 20.85937500061451644, 0.000000000000000000, 5.243569643749999010 ) ) ;
#37559=CARTESIAN_POINT ( 'NONE',  ( 25.46250000122903501, 4.330127018922192761, -2.499999999999997780 ) ) ;
#37560=CARTESIAN_POINT ( 'NONE',  ( -1.090676731616020634, 4.887066358488520557, 26.14194573437305635 ) ) ;
#37561=CARTESIAN_POINT ( 'NONE',  ( 17.62500000000000000, 6.123233995736764310E-16, -4.999999999999998224 ) ) ;
#37562=CARTESIAN_POINT ( 'NONE',  ( 4.243569643749999898, 13.33437500061451786, -30.00000000000000000 ) ) ;
#37563=CARTESIAN_POINT ( 'NONE',  ( 15.48750000122903359, 6.123233995736764310E-16, -4.999999999999998224 ) ) ;
#37564=CARTESIAN_POINT ( 'NONE',  ( 9.984375000614518214, 4.541064518000418104, 2.621784821874999949 ) ) ;
#37565=CARTESIAN_POINT ( 'NONE',  ( -4.243569643749997233, 17.14062500061451644, -27.54997392385601174 ) ) ;
#37566=CARTESIAN_POINT ( 'NONE',  ( 17.62500000122903288, -5.773502691896255534, -1.060575238724906372E-15 ) ) ;
#37567=CARTESIAN_POINT ( 'NONE',  ( 10.45312500061451644, 0.000000000000000000, 5.243569643749999010 ) ) ;
#37568=ORIENTED_EDGE ( 'NONE', *, *, #48397, .F. ) ;
#37569=CARTESIAN_POINT ( 'NONE',  ( 15.29999999999999893, -4.330127018922190985, -2.500000000000001332 ) ) ;
#37570=CARTESIAN_POINT ( 'NONE',  ( -3.999999999999999112, 17.41250000122903430, -30.00000000000000000 ) ) ;
#37571=CARTESIAN_POINT ( 'NONE',  ( 9.609375000614518214, 0.000000000000000000, 5.243569643749999010 ) ) ;
#37572=CARTESIAN_POINT ( 'NONE',  ( -3.999999999999999112, 14.22500000122903430, 27.69059892324149885 ) ) ;
#37573=CARTESIAN_POINT ( 'NONE',  ( 11.17500000122903536, 2.886751345948126879, 4.999999999999999112 ) ) ;
#37574=CARTESIAN_POINT ( 'NONE',  ( 19.50000000122903288, -2.886751345948125991, -5.000000000000000000 ) ) ;
#37575=CARTESIAN_POINT ( 'NONE',  ( 14.72812500061451679, 6.421520780324663323E-16, -5.243569643749999010 ) ) ;
#37576=CARTESIAN_POINT ( 'NONE',  ( 20.46562500061451928, -6.054752690667223547, -1.112240025338166033E-15 ) ) ;
#37577=CARTESIAN_POINT ( 'NONE',  ( 28.23750000122903359, 4.330127018922191873, 2.499999999999999556 ) ) ;
#37579=CARTESIAN_POINT ( 'NONE',  ( 29.66250000122903074, 0.000000000000000000, 4.999999999999998224 ) ) ;
#37580=CARTESIAN_POINT ( 'NONE',  ( 24.22500000000000142, -4.330127018922194537, 2.499999999999995559 ) ) ;
#37584=CARTESIAN_POINT ( 'NONE',  ( 27.68437500061451573, -4.541064518000419881, 2.621784821874995952 ) ) ;
#37586=CARTESIAN_POINT ( 'NONE',  ( 13.61250000122903359, -4.330127018922190985, -2.500000000000001332 ) ) ;
#37587=CARTESIAN_POINT ( 'NONE',  ( 4.200000000000001954, 4.330127018922192761, -2.499999999999997780 ) ) ;
#37588=( BOUNDED_CURVE ( )  B_SPLINE_CURVE ( 2, ( #3985, #49050, #55316, #66395, #65288, #37949, #14676, #60468, #3617 ),
 .UNSPECIFIED., .F., .F. ) 
 B_SPLINE_CURVE_WITH_KNOTS ( ( 3, 2, 2, 2, 3 ),
 ( 0.7065217391304348116, 0.7101449275362319291, 0.7173913043478260532, 0.7246376811594202882, 0.7282608695652174058 ),
 .UNSPECIFIED. ) 
 CURVE ( )  GEOMETRIC_REPRESENTATION_ITEM ( )  RATIONAL_B_SPLINE_CURVE ( ( 0.9330127018922194093, 0.9330127018922194093, 1.000000000000000000, 0.8660254037844387076, 1.000000000000000000, 0.8660254037844387076, 1.000000000000000000, 0.9330127018922194093, 0.9330127018922194093 ) ) 
 REPRESENTATION_ITEM ( '' )  );
#37589=FACE_BOUND ( 'NONE', #14934, .T. ) ;
#37590=CARTESIAN_POINT ( 'NONE',  ( 6.721875000614518925, 3.027376345333613106, -5.243569643749998122 ) ) ;
#37591=CARTESIAN_POINT ( 'NONE',  ( 26.99062500061451431, 6.054752690667223547, 3.707466751127219781E-16 ) ) ;
#37593=CARTESIAN_POINT ( 'NONE',  ( 3.999999999999999112, 10.43750000122903465, 30.00000000000000000 ) ) ;
#37595=CARTESIAN_POINT ( 'NONE',  ( 4.884375000614518569, 6.421520780324663323E-16, -5.243569643749999010 ) ) ;
#37596=CARTESIAN_POINT ( 'NONE',  ( 9.534375000614517148, 4.541064518000418104, 2.621784821874999949 ) ) ;
#37597=CARTESIAN_POINT ( 'NONE',  ( 4.762499999999999289, 2.886751345948126879, 4.999999999999999112 ) ) ;
#37598=CARTESIAN_POINT ( 'NONE',  ( 4.243569643749999898, 12.37812500061459353, 30.00000000000000000 ) ) ;
#37599=CARTESIAN_POINT ( 'NONE',  ( 22.64999999999999858, 4.330127018922192761, -2.499999999999997780 ) ) ;
#37600=CARTESIAN_POINT ( 'NONE',  ( 28.80000000000000071, -4.330127018922190985, -2.500000000000001332 ) ) ;
#37601=CARTESIAN_POINT ( 'NONE',  ( 3.675000000000001155, 6.123233995736764310E-16, -4.999999999999998224 ) ) ;
#37602=EDGE_LOOP ( 'NONE', ( #71428, #70187, #58525, #18243 ) ) ;
#37603=CARTESIAN_POINT ( 'NONE',  ( 18.40312500061451573, 4.541064518000418104, -2.621784821874998173 ) ) ;
#37604=CARTESIAN_POINT ( 'NONE',  ( 11.31562500061451892, 3.027376345333611329, 5.243569643749999010 ) ) ;
#37606=CARTESIAN_POINT ( 'NONE',  ( 6.534375000614517148, -4.541064518000419881, 2.621784821874995952 ) ) ;
#37607=CARTESIAN_POINT ( 'NONE',  ( 24.03750000000000142, 5.773502691896255534, 3.535250795749688894E-16 ) ) ;
#37608=CARTESIAN_POINT ( 'NONE',  ( 20.21250000122903145, 0.000000000000000000, 4.999999999999998224 ) ) ;
#37610=CARTESIAN_POINT ( 'NONE',  ( 10.28437500061451715, 6.421520780324663323E-16, -5.243569643749999010 ) ) ;
#37611=CARTESIAN_POINT ( 'NONE',  ( 13.69687500061451679, -3.027376345333614438, 5.243569643749998122 ) ) ;
#37612=CARTESIAN_POINT ( 'NONE',  ( 23.59687500061451715, -3.027376345333614438, 5.243569643749998122 ) ) ;
#37615=CARTESIAN_POINT ( 'NONE',  ( 17.55937500061451573, 4.541064518000418104, -2.621784821874998173 ) ) ;
#37616=CARTESIAN_POINT ( 'NONE',  ( 8.859375000614518214, -4.541064518000417216, -2.621784821875001281 ) ) ;
#37618=CARTESIAN_POINT ( 'NONE',  ( 20.47500000000000142, 4.330127018922191873, 2.499999999999999556 ) ) ;
#37622=CARTESIAN_POINT ( 'NONE',  ( 11.31562500061451892, 3.027376345333611329, 5.243569643749999010 ) ) ;
#37623=CARTESIAN_POINT ( 'NONE',  ( 28.58437500061451786, -4.541064518000419881, 2.621784821874995952 ) ) ;
#37625=CARTESIAN_POINT ( 'NONE',  ( 12.41249999999999964, 2.886751345948126879, 4.999999999999999112 ) ) ;
#37626=CARTESIAN_POINT ( 'NONE',  ( 1.999999999999998668, 17.71250000122903501, 26.53589838486224650 ) ) ;
#37627=CARTESIAN_POINT ( 'NONE',  ( 12.37500000122903465, 2.886751345948129099, -4.999999999999998224 ) ) ;
#37628=CARTESIAN_POINT ( 'NONE',  ( 21.45937500061451786, -4.541064518000417216, -2.621784821875001281 ) ) ;
#37629=CARTESIAN_POINT ( 'NONE',  ( 17.70937500061451431, 0.000000000000000000, 5.243569643749999010 ) ) ;
#37630=CARTESIAN_POINT ( 'NONE',  ( -2.000000000000000000, 16.32499999999999929, -33.46410161513775705 ) ) ;
#37631=ORIENTED_EDGE ( 'NONE', *, *, #32039, .T. ) ;
#37632=CARTESIAN_POINT ( 'NONE',  ( 16.90312500061451573, -4.541064518000417216, -2.621784821875001281 ) ) ;
#37633=CARTESIAN_POINT ( 'NONE',  ( 29.40000000122903145, -2.886751345948125991, -5.000000000000000000 ) ) ;
#37634=CARTESIAN_POINT ( 'NONE',  ( 17.67187500061451644, 3.027376345333611329, 5.243569643749999010 ) ) ;
#37635=CARTESIAN_POINT ( 'NONE',  ( 3.665625000614517681, 3.027376345333611329, 5.243569643749999010 ) ) ;
#37636=CARTESIAN_POINT ( 'NONE',  ( 18.36562500061451431, 3.027376345333613106, -5.243569643749998122 ) ) ;
#37637=CARTESIAN_POINT ( 'NONE',  ( 30.00000000000000000, 0.000000000000000000, 4.999999999999998224 ) ) ;
#37638=CARTESIAN_POINT ( 'NONE',  ( 27.90937500061451715, 4.541064518000418104, -2.621784821874998173 ) ) ;
#37639=CARTESIAN_POINT ( 'NONE',  ( -4.243569643749999898, 12.15312500061451573, 30.00000000000000000 ) ) ;
#37640=CARTESIAN_POINT ( 'NONE',  ( 16.42500000122903359, 2.886751345948129099, -4.999999999999998224 ) ) ;
#37642=CARTESIAN_POINT ( 'NONE',  ( 27.25312500061451360, -4.541064518000417216, -2.621784821875001281 ) ) ;
#37643=CARTESIAN_POINT ( 'NONE',  ( 0.000000000000000000, 20.00000000000000000, 30.00000000000000000 ) ) ;
#37644=CARTESIAN_POINT ( 'NONE',  ( 19.80937500061451573, 4.541064518000418104, -2.621784821874998173 ) ) ;
#37645=CARTESIAN_POINT ( 'NONE',  ( 22.65000000122903856, -2.886751345948125991, -5.000000000000000000 ) ) ;
#37646=( BOUNDED_CURVE ( )  B_SPLINE_CURVE ( 2, ( #51164, #567, #45629, #40088, #62602, #11998, #65880, #58858, #48529 ),
 .UNSPECIFIED., .F., .F. ) 
 B_SPLINE_CURVE_WITH_KNOTS ( ( 3, 2, 2, 2, 3 ),
 ( 0.7500000000000000000, 0.7536231884057971175, 0.7608695652173913526, 0.7681159420289854767, 0.7717391304347825942 ),
 .UNSPECIFIED. ) 
 CURVE ( )  GEOMETRIC_REPRESENTATION_ITEM ( )  RATIONAL_B_SPLINE_CURVE ( ( 0.9330127018922194093, 0.9330127018922194093, 1.000000000000000000, 0.8660254037844387076, 1.000000000000000000, 0.8660254037844387076, 1.000000000000000000, 0.9330127018922194093, 0.9330127018922194093 ) ) 
 REPRESENTATION_ITEM ( '' )  );
#37647=CARTESIAN_POINT ( 'NONE',  ( 22.90312500061451573, 4.541064518000418104, -2.621784821874998173 ) ) ;
#37648=CARTESIAN_POINT ( 'NONE',  ( 17.93437500061451928, 6.421520780324663323E-16, -5.243569643749999010 ) ) ;
#37649=CARTESIAN_POINT ( 'NONE',  ( 11.65312500061451573, 4.541064518000418104, -2.621784821874998173 ) ) ;
#37650=CARTESIAN_POINT ( 'NONE',  ( 2.121784821874999061, 15.20937500061451786, 26.32496088578401583 ) ) ;
#37651=CARTESIAN_POINT ( 'NONE',  ( 19.75312500061451360, 4.541064518000418104, -2.621784821874998173 ) ) ;
#37652=CARTESIAN_POINT ( 'NONE',  ( 28.75312500061451715, 4.541064518000418104, -2.621784821874998173 ) ) ;
#37654=ORIENTED_EDGE ( 'NONE', *, *, #63887, .T. ) ;
#37655=CARTESIAN_POINT ( 'NONE',  ( 23.62500000000000000, 4.330127018922191873, 2.499999999999999556 ) ) ;
#37656=CARTESIAN_POINT ( 'NONE',  ( 9.001249775931846008E-16, 19.07187500061451502, -25.09994784771203058 ) ) ;
#37657=CARTESIAN_POINT ( 'NONE',  ( 13.20000000122903394, -2.886751345948126435, -5.000000000000000000 ) ) ;
#37658=CARTESIAN_POINT ( 'NONE',  ( 24.06562500061451715, -6.054752690667223547, -1.112240025338166033E-15 ) ) ;
#37659=CARTESIAN_POINT ( 'NONE',  ( 4.828125000614518214, 6.421520780324663323E-16, -5.243569643749999010 ) ) ;
#37660=CARTESIAN_POINT ( 'NONE',  ( 16.65000000122903501, -2.886751345948129988, 4.999999999999997335 ) ) ;
#37661=CARTESIAN_POINT ( 'NONE',  ( 23.46562500061451573, 3.027376345333611329, 5.243569643749999010 ) ) ;
#37662=CARTESIAN_POINT ( 'NONE',  ( 21.86250000000000071, 2.886751345948126879, 4.999999999999999112 ) ) ;
#37663=CARTESIAN_POINT ( 'NONE',  ( 27.17812500061451786, -4.541064518000419881, 2.621784821874995952 ) ) ;
#37664=CARTESIAN_POINT ( 'NONE',  ( 8.578125000614518214, 4.541064518000418104, 2.621784821874999949 ) ) ;
#37666=ADVANCED_FACE ( 'NONE', ( #65296 ), #57929, .F. ) ;
#37667=CARTESIAN_POINT ( 'NONE',  ( 23.31562500061451715, 3.027376345333613106, -5.243569643749998122 ) ) ;
#37668=CARTESIAN_POINT ( 'NONE',  ( 4.865625000614517859, 3.027376345333613106, -5.243569643749998122 ) ) ;
#37670=CARTESIAN_POINT ( 'NONE',  ( 4.415625000614518569, 3.027376345333613106, -5.243569643749998122 ) ) ;
#37671=CARTESIAN_POINT ( 'NONE',  ( -1.999999999999997113, 12.53750000122903430, -26.53589838486224295 ) ) ;
#37672=CARTESIAN_POINT ( 'NONE',  ( -3.999999999999999112, 10.51250000000000107, -32.30940107675850470 ) ) ;
#37673=CARTESIAN_POINT ( 'NONE',  ( 10.53750000000000320, 5.773502691896255534, 3.535250795749688894E-16 ) ) ;
#37674=CARTESIAN_POINT ( 'NONE',  ( 11.29687500061451644, 6.054752690667223547, 3.707466751127219781E-16 ) ) ;
#37675=CARTESIAN_POINT ( 'NONE',  ( 7.237500001229035362, -4.330127018922194537, 2.499999999999995559 ) ) ;
#37676=CARTESIAN_POINT ( 'NONE',  ( 15.08437500061451786, -4.541064518000419881, 2.621784821874995952 ) ) ;
#37677=CARTESIAN_POINT ( 'NONE',  ( 7.059375000614518392, -4.541064518000417216, -2.621784821875001281 ) ) ;
#37678=CARTESIAN_POINT ( 'NONE',  ( 30.00000000000000000, 0.000000000000000000, 0.000000000000000000 ) ) ;
#37680=CARTESIAN_POINT ( 'NONE',  ( 13.35937500061451821, -4.541064518000417216, -2.621784821875001281 ) ) ;
#37681=CARTESIAN_POINT ( 'NONE',  ( 20.99062500061451431, -3.027376345333610441, -5.243569643749999898 ) ) ;
#37682=CARTESIAN_POINT ( 'NONE',  ( 1.999999999999998668, 11.75000000000000178, 26.53589838486224650 ) ) ;
#37684=CARTESIAN_POINT ( 'NONE',  ( 23.52187500061451786, 3.027376345333611329, 5.243569643749999010 ) ) ;
#37686=CARTESIAN_POINT ( 'NONE',  ( 4.453125000614517326, 4.541064518000418104, -2.621784821874998173 ) ) ;
#37688=CARTESIAN_POINT ( 'NONE',  ( 18.62812500061451715, -4.541064518000419881, 2.621784821874995952 ) ) ;
#37689=CARTESIAN_POINT ( 'NONE',  ( 14.22187500061451537, -6.054752690667223547, -1.112240025338166033E-15 ) ) ;
#37690=CARTESIAN_POINT ( 'NONE',  ( 26.06250000122903288, 0.000000000000000000, 4.999999999999998224 ) ) ;
#37691=CARTESIAN_POINT ( 'NONE',  ( 27.67500000122903359, 2.886751345948129099, -4.999999999999998224 ) ) ;
#37692=CARTESIAN_POINT ( 'NONE',  ( 6.009375000614519458, 0.000000000000000000, 5.243569643749999010 ) ) ;
#37693=CARTESIAN_POINT ( 'NONE',  ( 17.25937500061451502, 0.000000000000000000, 5.243569643749999010 ) ) ;
#37695=CARTESIAN_POINT ( 'NONE',  ( 23.36250000000000071, -5.773502691896255534, -1.060575238724906372E-15 ) ) ;
#37696=CARTESIAN_POINT ( 'NONE',  ( 5.000000000000000888, 2.882564675336284927E-11, 5.151554443534156036 ) ) ;
#37697=CARTESIAN_POINT ( 'NONE',  ( 24.98437500061451644, -4.541064518000419881, 2.621784821874995952 ) ) ;
#37698=CARTESIAN_POINT ( 'NONE',  ( 17.74687500061451928, -3.027376345333614438, 5.243569643749998122 ) ) ;
#37700=CARTESIAN_POINT ( 'NONE',  ( 5.812500001229035540, 0.000000000000000000, 4.999999999999998224 ) ) ;
#37701=CARTESIAN_POINT ( 'NONE',  ( 9.000000000000001776, -4.330127018922190985, -2.500000000000001332 ) ) ;
#37703=CARTESIAN_POINT ( 'NONE',  ( 18.74062500061451431, -3.027376345333610441, -5.243569643749999898 ) ) ;
#37704=CARTESIAN_POINT ( 'NONE',  ( 8.212500000000000355, 2.886751345948129099, -4.999999999999998224 ) ) ;
#37705=CARTESIAN_POINT ( 'NONE',  ( 4.153125000614515727, 0.000000000000000000, 5.243569643749999010 ) ) ;
#37706=CARTESIAN_POINT ( 'NONE',  ( 20.43749999999999645, 5.773502691896255534, 3.535250795749688894E-16 ) ) ;
#37707=EDGE_CURVE ( 'NONE', #2091, #39103, #21692, .T. ) ;
#37708=CARTESIAN_POINT ( 'NONE',  ( 19.67812500061451786, 6.421520780324663323E-16, -5.243569643749999010 ) ) ;
#37709=CARTESIAN_POINT ( 'NONE',  ( 15.71250000122903501, 0.000000000000000000, 4.999999999999998224 ) ) ;
#37710=CARTESIAN_POINT ( 'NONE',  ( 22.31250000122903288, 4.330127018922192761, -2.499999999999997780 ) ) ;
#37712=CARTESIAN_POINT ( 'NONE',  ( 3.374999999999999556, 4.330127018922191873, 2.499999999999999556 ) ) ;
#37713=EDGE_CURVE ( 'NONE', #42330, #329, #58903, .T. ) ;
#37714=ORIENTED_EDGE ( 'NONE', *, *, #50142, .F. ) ;
#37715=CARTESIAN_POINT ( 'NONE',  ( 18.17812500061451786, -4.541064518000419881, 2.621784821874995952 ) ) ;
#37716=CARTESIAN_POINT ( 'NONE',  ( 25.00312500061451715, -4.541064518000417216, -2.621784821875001281 ) ) ;
#37717=CARTESIAN_POINT ( 'NONE',  ( 25.28437500061451715, 4.541064518000418104, 2.621784821874999949 ) ) ;
#37718=CARTESIAN_POINT ( 'NONE',  ( 8.137500000000002842, -2.886751345948125991, -5.000000000000000000 ) ) ;
#37719=CARTESIAN_POINT ( 'NONE',  ( 11.72812500061451857, 4.541064518000418104, 2.621784821874999949 ) ) ;
#37720=CARTESIAN_POINT ( 'NONE',  ( 26.87812500061451360, 6.421520780324663323E-16, -5.243569643749999010 ) ) ;
#37721=CARTESIAN_POINT ( 'NONE',  ( 17.93437500061451928, 6.421520780324663323E-16, -5.243569643749999010 ) ) ;
#37722=CARTESIAN_POINT ( 'NONE',  ( 18.04687500061451999, 6.054752690667223547, 3.707466751127219781E-16 ) ) ;
#37723=CARTESIAN_POINT ( 'NONE',  ( 6.937500001229033764, 6.123233995736764310E-16, -4.999999999999998224 ) ) ;
#37724=CARTESIAN_POINT ( 'NONE',  ( 4.243569643749999898, 19.12812500061451715, 30.00000000000000000 ) ) ;
#37725=CARTESIAN_POINT ( 'NONE',  ( 23.85000000122903430, -2.886751345948129988, 4.999999999999997335 ) ) ;
#37727=CARTESIAN_POINT ( 'NONE',  ( 14.20312500061451644, -4.541064518000417216, -2.621784821875001281 ) ) ;
#37728=CARTESIAN_POINT ( 'NONE',  ( 7.359375000614516438, 0.000000000000000000, 5.243569643749999010 ) ) ;
#37729=CARTESIAN_POINT ( 'NONE',  ( 7.959375000614516971, -4.541064518000417216, -2.621784821875001281 ) ) ;
#37730=EDGE_CURVE ( 'NONE', #38159, #11468, #3993, .T. ) ;
#37732=CARTESIAN_POINT ( 'NONE',  ( -5.810221930991193690E-16, 13.58750000000000036, 26.00000000000000355 ) ) ;
#37733=CARTESIAN_POINT ( 'NONE',  ( 18.81562500061452070, 3.027376345333613106, -5.243569643749998122 ) ) ;
#37734=CARTESIAN_POINT ( 'NONE',  ( 23.52187500061451786, 3.027376345333611329, 5.243569643749999010 ) ) ;
#37735=CARTESIAN_POINT ( 'NONE',  ( 20.20312500061451644, 4.541064518000418104, -2.621784821874998173 ) ) ;
#37736=CARTESIAN_POINT ( 'NONE',  ( -3.999999999999997335, 11.93750000000000355, 32.30940107675850470 ) ) ;
#37737=CARTESIAN_POINT ( 'NONE',  ( 26.09062500061451573, 6.054752690667223547, 3.707466751127219781E-16 ) ) ;
#37738=CARTESIAN_POINT ( 'NONE',  ( 7.575000001229033053, 2.886751345948126879, 4.999999999999999112 ) ) ;
#37740=CARTESIAN_POINT ( 'NONE',  ( 3.225000001229033408, -5.773502691896255534, -1.060575238724906372E-15 ) ) ;
#37741=CARTESIAN_POINT ( 'NONE',  ( 1.999999999999998668, 14.90000000000000036, -33.46410161513775705 ) ) ;
#37742=CARTESIAN_POINT ( 'NONE',  ( 23.02500000122903145, -5.773502691896255534, -1.060575238724906372E-15 ) ) ;
#37744=VECTOR ( 'NONE', #35587, 1000.000000000000000 ) ;
#37746=CARTESIAN_POINT ( 'NONE',  ( 7.734375000614517326, 4.541064518000418104, 2.621784821874999949 ) ) ;
#37748=CARTESIAN_POINT ( 'NONE',  ( 11.57812500061451644, 6.421520780324663323E-16, -5.243569643749999010 ) ) ;
#37749=CARTESIAN_POINT ( 'NONE',  ( 7.434375000614519280, -4.541064518000419881, 2.621784821874995952 ) ) ;
#37750=CARTESIAN_POINT ( 'NONE',  ( 25.87500000122903288, 2.886751345948129099, -4.999999999999998224 ) ) ;
#37751=CARTESIAN_POINT ( 'NONE',  ( 14.67187500061451821, -6.054752690667223547, -1.112240025338166033E-15 ) ) ;
#37752=CARTESIAN_POINT ( 'NONE',  ( 3.909375000614518481, -4.541064518000417216, -2.621784821875001281 ) ) ;
#37754=CARTESIAN_POINT ( 'NONE',  ( 5.428125000614517859, 4.541064518000418104, 2.621784821874999949 ) ) ;
#37755=CARTESIAN_POINT ( 'NONE',  ( 14.42812500061451786, 4.541064518000418104, 2.621784821874999949 ) ) ;
#37756=ORIENTED_EDGE ( 'NONE', *, *, #3316, .T. ) ;
#37757=CARTESIAN_POINT ( 'NONE',  ( 13.45312500061451466, 4.541064518000418104, -2.621784821874998173 ) ) ;
#37758=CARTESIAN_POINT ( 'NONE',  ( 6.112500001229034474, 4.330127018922192761, -2.499999999999997780 ) ) ;
#37759=CARTESIAN_POINT ( 'NONE',  ( 7.603125000614517681, 4.541064518000418104, -2.621784821874998173 ) ) ;
#37761=CARTESIAN_POINT ( 'NONE',  ( 8.849999999999999645, 0.000000000000000000, 4.999999999999998224 ) ) ;
#37762=CARTESIAN_POINT ( 'NONE',  ( 3.112500001229034918, 0.000000000000000000, 4.999999999999998224 ) ) ;
#37763=CARTESIAN_POINT ( 'NONE',  ( 18.33749999999999858, -2.886751345948129988, 4.999999999999997335 ) ) ;
#37764=CARTESIAN_POINT ( 'NONE',  ( 18.12187500061451573, 3.027376345333611329, 5.243569643749999010 ) ) ;
#37765=CARTESIAN_POINT ( 'NONE',  ( 14.66250000122903252, 4.330127018922192761, -2.499999999999997780 ) ) ;
#37767=CARTESIAN_POINT ( 'NONE',  ( -3.000416591977282496E-16, 16.54062500061451857, -34.90005215228797653 ) ) ;
#37768=CARTESIAN_POINT ( 'NONE',  ( -2.000000000000000000, 15.98750000122903181, 26.53589838486224650 ) ) ;
#37769=CARTESIAN_POINT ( 'NONE',  ( 4.898587196589411843E-16, 20.00000000000000000, 33.99999999999999289 ) ) ;
#37771=CARTESIAN_POINT ( 'NONE',  ( 29.57812500061451644, 6.421520780324663323E-16, -5.243569643749999010 ) ) ;
#37772=DIRECTION ( 'NONE',  ( 0.000000000000000000, 0.000000000000000000, 1.000000000000000000 ) ) ;
#37773=CARTESIAN_POINT ( 'NONE',  ( 16.02187500061451786, -6.054752690667223547, -1.112240025338166033E-15 ) ) ;
#37774=CARTESIAN_POINT ( 'NONE',  ( 27.71250000000000568, 2.886751345948126879, 4.999999999999999112 ) ) ;
#37775=CARTESIAN_POINT ( 'NONE',  ( 12.10312500061451857, 4.541064518000418104, -2.621784821874998173 ) ) ;
#37777=CARTESIAN_POINT ( 'NONE',  ( 20.33437500061451786, 4.541064518000418104, 2.621784821874999949 ) ) ;
#37779=CARTESIAN_POINT ( 'NONE',  ( 8.015625000614518214, 3.027376345333613106, -5.243569643749998122 ) ) ;
#37780=CARTESIAN_POINT ( 'NONE',  ( 12.68437500061451573, 4.541064518000418104, 2.621784821874999949 ) ) ;
#37782=CARTESIAN_POINT ( 'NONE',  ( 23.18437500061451573, -4.541064518000419881, 2.621784821874995952 ) ) ;
#37783=CARTESIAN_POINT ( 'NONE',  ( 2.483674929639045459, 4.345807424128182994, -33.14570507670406130 ) ) ;
#37784=CARTESIAN_POINT ( 'NONE',  ( 26.91562500061451146, 3.027376345333613106, -5.243569643749998122 ) ) ;
#37786=CARTESIAN_POINT ( 'NONE',  ( 7.425000000000000711, 4.330127018922191873, 2.499999999999999556 ) ) ;
#37787=CARTESIAN_POINT ( 'NONE',  ( 16.83750000122903145, 6.123233995736764310E-16, -4.999999999999998224 ) ) ;
#37790=VERTEX_POINT ( 'NONE', #15056 ) ;
#37791=CARTESIAN_POINT ( 'NONE',  ( 15.18750000000000000, -2.886751345948129988, 4.999999999999997335 ) ) ;
#37792=CARTESIAN_POINT ( 'NONE',  ( 17.84999999999999787, 0.000000000000000000, 4.999999999999998224 ) ) ;
#37793=CARTESIAN_POINT ( 'NONE',  ( 11.20312500061451644, 4.541064518000418104, -2.621784821874998173 ) ) ;
#37796=CARTESIAN_POINT ( 'NONE',  ( 26.21250000000000213, 2.886751345948146419, -4.999999999999968914 ) ) ;
#37797=CARTESIAN_POINT ( 'NONE',  ( -2.121784821874996840, 17.23437500061451999, -26.32496088578401583 ) ) ;
#37798=CARTESIAN_POINT ( 'NONE',  ( 3.103125000614517237, 4.541064518000418104, -2.621784821874998173 ) ) ;
#37800=CARTESIAN_POINT ( 'NONE',  ( 9.562500000000001776, 2.886751345948129099, -4.999999999999998224 ) ) ;
#37801=CARTESIAN_POINT ( 'NONE',  ( 3.150046044403394419, 3.883032850835071770, 3.416330326112916982 ) ) ;
#37803=CARTESIAN_POINT ( 'NONE',  ( 9.001249775931846008E-16, 13.61562500061451786, 34.90005215228797653 ) ) ;
#37804=CARTESIAN_POINT ( 'NONE',  ( 25.67812500061451431, 4.541064518000418104, 2.621784821874999949 ) ) ;
#37807=CARTESIAN_POINT ( 'NONE',  ( 21.53437500061451715, 6.421520780324663323E-16, -5.243569643749999010 ) ) ;
#37808=EDGE_CURVE ( 'NONE', #55534, #15843, #55400, .T. ) ;
#37809=CARTESIAN_POINT ( 'NONE',  ( 19.30312500061451786, 4.541064518000418104, -2.621784821874998173 ) ) ;
#37810=CARTESIAN_POINT ( 'NONE',  ( 4.243569643749999898, 14.14062500061459460, -27.54997392385601529 ) ) ;
#37811=CARTESIAN_POINT ( 'NONE',  ( 23.92500000122903359, -5.773502691896255534, -1.060575238724906372E-15 ) ) ;
#37812=CARTESIAN_POINT ( 'NONE',  ( 4.903125000614516615, 4.541064518000418104, -2.621784821874998173 ) ) ;
#37814=CARTESIAN_POINT ( 'NONE',  ( 22.19062500061451004, -3.027376345333614438, 5.243569643749998122 ) ) ;
#37817=CARTESIAN_POINT ( 'NONE',  ( 15.64687500061451608, -3.027376345333610441, -5.243569643749999898 ) ) ;
#37818=EDGE_CURVE ( 'NONE', #30507, #14890, #39152, .T. ) ;
#37819=CARTESIAN_POINT ( 'NONE',  ( 15.30937500061451750, 4.541064518000418104, -2.621784821874998173 ) ) ;
#37820=CARTESIAN_POINT ( 'NONE',  ( 21.53437500061451715, 6.421520780324663323E-16, -5.243569643749999010 ) ) ;
#37821=CARTESIAN_POINT ( 'NONE',  ( -4.243569643749999898, 12.17187500061451999, 27.54997392385601529 ) ) ;
#37822=CARTESIAN_POINT ( 'NONE',  ( 4.040625000614517681, 6.054752690667223547, 3.707466751127219781E-16 ) ) ;
#37823=CARTESIAN_POINT ( 'NONE',  ( 28.19062500061451715, -3.027376345333610441, -5.243569643749999898 ) ) ;
#37824=CARTESIAN_POINT ( 'NONE',  ( 26.57812500061451644, 4.541064518000418104, 2.621784821874999949 ) ) ;
#37825=CARTESIAN_POINT ( 'NONE',  ( 1.626862140677534273E-15, 14.26250000000000107, 34.00000000000000000 ) ) ;
#37826=CARTESIAN_POINT ( 'NONE',  ( -3.999999999999999556, 18.16250000000000497, 27.69059892324149530 ) ) ;
#37827=CARTESIAN_POINT ( 'NONE',  ( 6.196875000614515905, -3.027376345333610441, -5.243569643749999898 ) ) ;
#37828=CARTESIAN_POINT ( 'NONE',  ( 15.41250000122903252, -4.330127018922190985, -2.500000000000001332 ) ) ;
#37829=CARTESIAN_POINT ( 'NONE',  ( 8.437500001229034652, 4.330127018922191873, 2.499999999999999556 ) ) ;
#37830=CARTESIAN_POINT ( 'NONE',  ( 4.265625000614517326, -6.054752690667223547, -1.112240025338166033E-15 ) ) ;
#37833=CARTESIAN_POINT ( 'NONE',  ( 15.23437500061451644, 6.421520780324663323E-16, -5.243569643749999010 ) ) ;
#37834=CARTESIAN_POINT ( 'NONE',  ( 11.77500000000000036, 6.123233995736764310E-16, -4.999999999999998224 ) ) ;
#37835=EDGE_LOOP ( 'NONE', ( #28178, #36208, #62993, #34504 ) ) ;
#37836=CARTESIAN_POINT ( 'NONE',  ( 19.07812500061451644, -4.541064518000419881, 2.621784821874995952 ) ) ;
#37837=CARTESIAN_POINT ( 'NONE',  ( 6.253125000614517148, 4.541064518000418104, -2.621784821874998173 ) ) ;
#37838=CARTESIAN_POINT ( 'NONE',  ( 24.27187500061451786, 3.027376345333612662, -5.243569643749998122 ) ) ;
#37839=CARTESIAN_POINT ( 'NONE',  ( 8.728125000614518569, -4.541064518000419881, 2.621784821874995952 ) ) ;
#37841=CARTESIAN_POINT ( 'NONE',  ( 7.987500001229032698, 4.330127018922191873, 2.499999999999999556 ) ) ;
#37842=CARTESIAN_POINT ( 'NONE',  ( 22.41562500061451502, 3.027376345333613106, -5.243569643749998122 ) ) ;
#37843=CARTESIAN_POINT ( 'NONE',  ( 4.000000000000000000, 18.95000000122903216, -27.69059892324149530 ) ) ;
#37844=CARTESIAN_POINT ( 'NONE',  ( 10.87500000122903288, -5.773502691896255534, -1.060575238724906372E-15 ) ) ;
#37845=CARTESIAN_POINT ( 'NONE',  ( 20.80312500061451431, 0.000000000000000000, 5.243569643749999010 ) ) ;
#37846=CARTESIAN_POINT ( 'NONE',  ( 15.85312500061451857, 0.000000000000000000, 5.243569643749999010 ) ) ;
#37848=CARTESIAN_POINT ( 'NONE',  ( 16.38749999999999929, 5.773502691896255534, 3.535250795749688894E-16 ) ) ;
#37849=CARTESIAN_POINT ( 'NONE',  ( 11.43750000122903465, 6.123233995736764310E-16, -4.999999999999998224 ) ) ;
#37852=CARTESIAN_POINT ( 'NONE',  ( 8.840625000614515727, -3.027376345333610441, -5.243569643749999898 ) ) ;
#37853=CARTESIAN_POINT ( 'NONE',  ( 10.86562500061451431, 3.027376345333611329, 5.243569643749999010 ) ) ;
#37854=CARTESIAN_POINT ( 'NONE',  ( 20.51250000122903216, 4.330127018922192761, -2.499999999999997780 ) ) ;
#37855=CARTESIAN_POINT ( 'NONE',  ( 19.92187500061451644, 3.027376345333611329, 5.243569643749999010 ) ) ;
#37857=CARTESIAN_POINT ( 'NONE',  ( 6.112500001229034474, 4.330127018922192761, -2.499999999999997780 ) ) ;
#37858=CARTESIAN_POINT ( 'NONE',  ( 4.059375000614519280, 4.541064518000418104, -2.621784821874998173 ) ) ;
#37859=CARTESIAN_POINT ( 'NONE',  ( 23.07187500061451857, 3.027376345333611329, 5.243569643749999010 ) ) ;
#37862=CARTESIAN_POINT ( 'NONE',  ( 26.51250000122903216, 0.000000000000000000, 4.999999999999998224 ) ) ;
#37863=CARTESIAN_POINT ( 'NONE',  ( 18.77812500061451573, 6.421520780324663323E-16, -5.243569643749999010 ) ) ;
#37864=CARTESIAN_POINT ( 'NONE',  ( 23.29687500061451644, -3.027376345333610441, -5.243569643749999898 ) ) ;
#37866=CARTESIAN_POINT ( 'NONE',  ( 4.603329117574985752, 1.951758446961684434, -4.603329117574985752 ) ) ;
#37867=CARTESIAN_POINT ( 'NONE',  ( 28.17187500061451644, -6.054752690667223547, -1.112240025338166033E-15 ) ) ;
#37869=CARTESIAN_POINT ( 'NONE',  ( 16.00312500061451715, -4.541064518000417216, -2.621784821875001281 ) ) ;
#37870=CARTESIAN_POINT ( 'NONE',  ( 13.24687500061451750, -3.027376345333614438, 5.243569643749998122 ) ) ;
#37872=CARTESIAN_POINT ( 'NONE',  ( 9.150000000000002132, 4.330127018922192761, -2.499999999999997780 ) ) ;
#37873=CARTESIAN_POINT ( 'NONE',  ( 21.81562500061451004, -6.054752690667223547, -1.112240025338166033E-15 ) ) ;
#37874=CARTESIAN_POINT ( 'NONE',  ( 2.000000000000001332, 12.95000000000000107, -26.53589838486224650 ) ) ;
#37875=CARTESIAN_POINT ( 'NONE',  ( 14.43750000000000000, -2.886751345948125991, -5.000000000000000000 ) ) ;
#37876=CARTESIAN_POINT ( 'NONE',  ( 24.90000000122903145, -2.886751345948125991, -5.000000000000000000 ) ) ;
#37877=CARTESIAN_POINT ( 'NONE',  ( 18.62812500061451715, -4.541064518000419881, 2.621784821874995952 ) ) ;
#37878=ORIENTED_EDGE ( 'NONE', *, *, #50272, .T. ) ;
#37879=CARTESIAN_POINT ( 'NONE',  ( 21.78750000000000142, 5.773502691896255534, 3.535250795749688894E-16 ) ) ;
#37880=CARTESIAN_POINT ( 'NONE',  ( 23.59687500061451715, -3.027376345333614438, 5.243569643749998122 ) ) ;
#37881=VERTEX_POINT ( 'NONE', #33148 ) ;
#37882=CARTESIAN_POINT ( 'NONE',  ( 21.22500000000000142, 6.123233995736764310E-16, -4.999999999999998224 ) ) ;
#37883=CARTESIAN_POINT ( 'NONE',  ( 10.22812500061451679, 6.421520780324663323E-16, -5.243569643749999010 ) ) ;
#37884=CARTESIAN_POINT ( 'NONE',  ( 3.065625000614517592, 3.027376345333613106, -5.243569643749998122 ) ) ;
#37886=CARTESIAN_POINT ( 'NONE',  ( 27.14062500061451644, -3.027376345333614438, 5.243569643749998122 ) ) ;
#37888=CARTESIAN_POINT ( 'NONE',  ( 17.92500000000000071, -4.330127018922194537, 2.499999999999995559 ) ) ;
#37889=CARTESIAN_POINT ( 'NONE',  ( 24.37500000000000000, 6.123233995736764310E-16, -4.999999999999998224 ) ) ;
#37890=CARTESIAN_POINT ( 'NONE',  ( 4.243569643749999010, 19.16562500061451857, 27.54997392385601174 ) ) ;
#37891=CARTESIAN_POINT ( 'NONE',  ( 6.009375000614519458, 0.000000000000000000, 5.243569643749999010 ) ) ;
#37892=CARTESIAN_POINT ( 'NONE',  ( 17.52187500061451431, 3.027376345333613106, -5.243569643749998122 ) ) ;
#37893=CARTESIAN_POINT ( 'NONE',  ( 29.22187500061451715, 3.027376345333613106, -5.243569643749998122 ) ) ;
#37894=ORIENTED_EDGE ( 'NONE', *, *, #40409, .T. ) ;
#37896=CARTESIAN_POINT ( 'NONE',  ( 25.79062500061451502, -3.027376345333614438, 5.243569643749998122 ) ) ;
#37897=CARTESIAN_POINT ( 'NONE',  ( 28.32187500061451502, 3.027376345333613106, -5.243569643749998122 ) ) ;
#37898=DIRECTION ( 'NONE',  ( -0.000000000000000000, -1.000000000000000000, -0.000000000000000000 ) ) ;
#37899=CARTESIAN_POINT ( 'NONE',  ( 13.23750000000000071, 5.773502691896255534, 3.535250795749688894E-16 ) ) ;
#37900=CARTESIAN_POINT ( 'NONE',  ( 10.15312500061451750, -4.541064518000417216, -2.621784821875001281 ) ) ;
#37903=CARTESIAN_POINT ( 'NONE',  ( 29.61562500061451431, 3.027376345333612662, -5.243569643749998122 ) ) ;
#37904=CARTESIAN_POINT ( 'NONE',  ( 15.45000000122903216, -2.886751345948125991, -5.000000000000000000 ) ) ;
#37905=CARTESIAN_POINT ( 'NONE',  ( 3.103072119908869997, -3.920863138419562244, 3.103072119908869997 ) ) ;
#37907=CARTESIAN_POINT ( 'NONE',  ( 6.328125000614515550, 4.541064518000418104, 2.621784821874999949 ) ) ;
#37908=CARTESIAN_POINT ( 'NONE',  ( 21.64687500061451786, 6.054752690667223547, 3.707466751127219781E-16 ) ) ;
#37909=CARTESIAN_POINT ( 'NONE',  ( -4.243569643749999898, 16.22187500061452070, 27.54997392385601529 ) ) ;
#37910=EDGE_CURVE ( 'NONE', #12976, #32725, #55685, .T. ) ;
#37911=CARTESIAN_POINT ( 'NONE',  ( 22.24687500061451217, -3.027376345333614438, 5.243569643749998122 ) ) ;
#37912=CARTESIAN_POINT ( 'NONE',  ( 5.175000000000002487, 4.330127018922191873, 2.499999999999999556 ) ) ;
#37913=CARTESIAN_POINT ( 'NONE',  ( -3.999999999999997335, 11.60000000122903430, 32.30940107675850470 ) ) ;
#37914=CARTESIAN_POINT ( 'NONE',  ( 11.84062500061451750, -3.027376345333614438, 5.243569643749998122 ) ) ;
#37915=CARTESIAN_POINT ( 'NONE',  ( 4.687500001229034652, 6.123233995736764310E-16, -4.999999999999998224 ) ) ;
#37916=CARTESIAN_POINT ( 'NONE',  ( 8.671875000614518214, 3.027376345333611329, 5.243569643749999010 ) ) ;
#37917=CARTESIAN_POINT ( 'NONE',  ( 0.000000000000000000, 20.00000000000000000, -30.00000000000000000 ) ) ;
#37918=CARTESIAN_POINT ( 'NONE',  ( 9.965625000614517504, 3.027376345333611329, 5.243569643749999010 ) ) ;
#37919=CARTESIAN_POINT ( 'NONE',  ( 15.12187500061451750, -6.054752690667223547, -1.112240025338166033E-15 ) ) ;
#37920=DIRECTION ( 'NONE',  ( 0.000000000000000000, 0.000000000000000000, 1.000000000000000000 ) ) ;
#37921=CARTESIAN_POINT ( 'NONE',  ( 20.51250000122903216, 4.330127018922192761, -2.499999999999997780 ) ) ;
#37922=CARTESIAN_POINT ( 'NONE',  ( 8.409375000614518925, -4.541064518000417216, -2.621784821875001281 ) ) ;
#37923=CARTESIAN_POINT ( 'NONE',  ( 11.24062500061451608, 6.054752690667223547, 3.707466751127219781E-16 ) ) ;
#37925=CARTESIAN_POINT ( 'NONE',  ( 22.28437500061451715, -4.541064518000419881, 2.621784821874995952 ) ) ;
#37926=CARTESIAN_POINT ( 'NONE',  ( 25.57500000122903572, 2.886751345948093572, 5.000000000000056843 ) ) ;
#37927=CARTESIAN_POINT ( 'NONE',  ( -3.779748323423379297, 3.276532024208883342, 31.33396265876518783 ) ) ;
#37928=DIRECTION ( 'NONE',  ( 0.000000000000000000, 0.000000000000000000, -1.000000000000000000 ) ) ;
#37929=CARTESIAN_POINT ( 'NONE',  ( 4.243569643749999898, 12.39687500061451786, -27.54997392385601529 ) ) ;
#37930=CARTESIAN_POINT ( 'NONE',  ( 14.92500000122903181, -5.773502691896255534, -1.060575238724906372E-15 ) ) ;
#37931=CARTESIAN_POINT ( 'NONE',  ( 2.121784821875001281, 18.15312500061451928, -26.32496088578401938 ) ) ;
#37932=CARTESIAN_POINT ( 'NONE',  ( 18.45000000122903216, -2.886751345948129988, 4.999999999999997335 ) ) ;
#37933=CARTESIAN_POINT ( 'NONE',  ( 10.52812500061451750, -4.541064518000419881, 2.621784821874995952 ) ) ;
#37934=ORIENTED_EDGE ( 'NONE', *, *, #32753, .F. ) ;
#37935=CARTESIAN_POINT ( 'NONE',  ( 16.38749999999999929, 5.773502691896255534, 3.535250795749688894E-16 ) ) ;
#37936=CARTESIAN_POINT ( 'NONE',  ( 29.13749999999999574, -2.886751345948092240, 5.000000000000060396 ) ) ;
#37937=CARTESIAN_POINT ( 'NONE',  ( 23.31562500061451715, 3.027376345333613106, -5.243569643749998122 ) ) ;
#37938=CARTESIAN_POINT ( 'NONE',  ( 11.33437500061451608, 4.541064518000418104, 2.621784821874999949 ) ) ;
#37939=CARTESIAN_POINT ( 'NONE',  ( 4.379101211152973683, -2.413214113851987364, -4.655270838772533004 ) ) ;
#37940=CARTESIAN_POINT ( 'NONE',  ( 10.38750000122903572, -4.330127018922194537, 2.499999999999995559 ) ) ;
#37941=CARTESIAN_POINT ( 'NONE',  ( 19.46250000122903145, -4.330127018922190985, -2.500000000000001332 ) ) ;
#37942=CARTESIAN_POINT ( 'NONE',  ( 16.00312500061451715, -4.541064518000417216, -2.621784821875001281 ) ) ;
#37943=CARTESIAN_POINT ( 'NONE',  ( 17.84062500061451573, -3.027376345333610441, -5.243569643749999898 ) ) ;
#37944=CARTESIAN_POINT ( 'NONE',  ( 25.83750000122903501, 6.123233995736764310E-16, -4.999999999999998224 ) ) ;
#37945=CARTESIAN_POINT ( 'NONE',  ( 29.40000000122903145, -2.886751345948125991, -5.000000000000000000 ) ) ;
#37946=CARTESIAN_POINT ( 'NONE',  ( 23.96249999999999858, 2.886751345948129099, -4.999999999999998224 ) ) ;
#37948=CARTESIAN_POINT ( 'NONE',  ( 26.22187500061451715, 3.027376345333611329, 5.243569643749999010 ) ) ;
#37949=CARTESIAN_POINT ( 'NONE',  ( 4.000000000000000000, 12.53749999999999964, -27.69059892324149885 ) ) ;
#37951=CARTESIAN_POINT ( 'NONE',  ( 13.27500000122903323, 2.886751345948129099, -4.999999999999998224 ) ) ;
#37952=CARTESIAN_POINT ( 'NONE',  ( 3.037500000000002309, -2.886751345948129988, 4.999999999999997335 ) ) ;
#37954=CARTESIAN_POINT ( 'NONE',  ( 6.796875000614516438, 6.054752690667223547, 3.707466751127219781E-16 ) ) ;
#37955=CARTESIAN_POINT ( 'NONE',  ( 26.84062500061451573, -3.027376345333610441, -5.243569643749999898 ) ) ;
#37959=CARTESIAN_POINT ( 'NONE',  ( 5.446875000614518569, 6.054752690667223547, 3.707466751127219781E-16 ) ) ;
#37960=CARTESIAN_POINT ( 'NONE',  ( 8.671875000614518214, 3.027376345333611329, 5.243569643749999010 ) ) ;
#37961=CARTESIAN_POINT ( 'NONE',  ( 28.09687500061451360, -3.027376345333614438, 5.243569643749998122 ) ) ;
#37962=CARTESIAN_POINT ( 'NONE',  ( -4.243569643749999898, 11.25312500061459531, 30.00000000000000000 ) ) ;
#37963=CARTESIAN_POINT ( 'NONE',  ( 21.89999999999999858, 0.000000000000000000, 4.999999999999998224 ) ) ;
#37964=CARTESIAN_POINT ( 'NONE',  ( 4.021830710287673583, -2.971297458697284011, 4.021830710287673583 ) ) ;
#37965=CARTESIAN_POINT ( 'NONE',  ( 29.92500000000000071, 4.330127018922191873, 2.499999999999999556 ) ) ;
#37966=CARTESIAN_POINT ( 'NONE',  ( 4.800000000000002487, 0.000000000000000000, 4.999999999999998224 ) ) ;
#37968=CARTESIAN_POINT ( 'NONE',  ( 18.92812500061451431, 4.541064518000418104, 2.621784821874999949 ) ) ;
#37969=CARTESIAN_POINT ( 'NONE',  ( 11.05312500061451608, -4.541064518000417216, -2.621784821875001281 ) ) ;
#37971=CARTESIAN_POINT ( 'NONE',  ( 7.996875000614519280, -3.027376345333610441, -5.243569643749999898 ) ) ;
#37972=CARTESIAN_POINT ( 'NONE',  ( 22.61250000000000071, 2.886751345948129099, -4.999999999999998224 ) ) ;
#37973=CARTESIAN_POINT ( 'NONE',  ( 21.03750000122903074, 4.330127018922191873, 2.499999999999999556 ) ) ;
#37975=CARTESIAN_POINT ( 'NONE',  ( 6.196875000614515905, -3.027376345333610441, -5.243569643749999898 ) ) ;
#37976=CARTESIAN_POINT ( 'NONE',  ( 13.05937500061451750, 4.541064518000418104, -2.621784821874998173 ) ) ;
#37977=CARTESIAN_POINT ( 'NONE',  ( 23.40937500061451715, 4.541064518000418104, -2.621784821874998173 ) ) ;
#37978=VERTEX_POINT ( 'NONE', #28691 ) ;
#37980=CARTESIAN_POINT ( 'NONE',  ( 18.64687500061451786, -3.027376345333614438, 5.243569643749998122 ) ) ;
#37981=CARTESIAN_POINT ( 'NONE',  ( 9.534375000614517148, 4.541064518000418104, 2.621784821874999949 ) ) ;
#37983=CARTESIAN_POINT ( 'NONE',  ( 22.08749999999999858, -2.886751345948125991, -5.000000000000000000 ) ) ;
#37985=CARTESIAN_POINT ( 'NONE',  ( 4.243569643749999898, 10.18437500061451750, -30.00000000000000000 ) ) ;
#37987=CARTESIAN_POINT ( 'NONE',  ( 12.40312500061451573, -4.541064518000417216, -2.621784821875001281 ) ) ;
#37988=CARTESIAN_POINT ( 'NONE',  ( 29.59687500061451715, -3.027376345333610441, -5.243569643749999898 ) ) ;
#37989=CARTESIAN_POINT ( 'NONE',  ( 4.898587196589411843E-16, 20.00000000000000000, -26.00000000000000000 ) ) ;
#37991=CARTESIAN_POINT ( 'NONE',  ( 11.51250000000000107, 2.886751345948126879, 4.999999999999999112 ) ) ;
#37992=EDGE_CURVE ( 'NONE', #7272, #48969, #43905, .T. ) ;
#37993=CARTESIAN_POINT ( 'NONE',  ( -2.000000000000000000, 17.78750000122903430, 26.53589838486224650 ) ) ;
#37994=CARTESIAN_POINT ( 'NONE',  ( 12.41250000122903430, 4.330127018922192761, -2.499999999999997780 ) ) ;
#37995=CARTESIAN_POINT ( 'NONE',  ( 23.22187500061451715, -6.054752690667223547, -1.112240025338166033E-15 ) ) ;
#37996=CARTESIAN_POINT ( 'NONE',  ( 17.03437500061451715, 6.421520780324663323E-16, -5.243569643749999010 ) ) ;
#37997=DIRECTION ( 'NONE',  ( 0.000000000000000000, 0.000000000000000000, -1.000000000000000000 ) ) ;
#37998=ORIENTED_EDGE ( 'NONE', *, *, #30313, .F. ) ;
#37999=CARTESIAN_POINT ( 'NONE',  ( 18.36562500061451431, 3.027376345333613106, -5.243569643749998122 ) ) ;
#38000=CARTESIAN_POINT ( 'NONE',  ( 29.55000000122903003, 5.773502691896255534, 3.535250795749688894E-16 ) ) ;
#38001=CARTESIAN_POINT ( 'NONE',  ( 17.59687500061451715, 6.054752690667223547, 3.707466751127219781E-16 ) ) ;
#38002=CARTESIAN_POINT ( 'NONE',  ( 3.140625000614516882, 6.054752690667223547, 3.707466751127219781E-16 ) ) ;
#38003=CARTESIAN_POINT ( 'NONE',  ( 18.74062500061451431, -3.027376345333610441, -5.243569643749999898 ) ) ;
#38005=CARTESIAN_POINT ( 'NONE',  ( 29.48437500061451644, -4.541064518000419881, 2.621784821874995952 ) ) ;
#38006=CARTESIAN_POINT ( 'NONE',  ( 9.001249775931846008E-16, 12.26562500061451644, 34.90005215228797653 ) ) ;
#38007=CARTESIAN_POINT ( 'NONE',  ( 18.08437500061451431, 4.541064518000418104, 2.621784821874999949 ) ) ;
#38008=CARTESIAN_POINT ( 'NONE',  ( 16.68750000122903288, -4.330127018922194537, 2.499999999999995559 ) ) ;
#38010=CARTESIAN_POINT ( 'NONE',  ( 3.366080804335946919, -3.697228694398128290, 3.718268762498968094 ) ) ;
#38011=CARTESIAN_POINT ( 'NONE',  ( 20.33437500061451786, 4.541064518000418104, 2.621784821874999949 ) ) ;
#38012=CARTESIAN_POINT ( 'NONE',  ( 21.60000000122903430, -2.886751345948129988, 4.999999999999997335 ) ) ;
#38013=CARTESIAN_POINT ( 'NONE',  ( 23.39062500061451289, 6.054752690667223547, 3.707466751127219781E-16 ) ) ;
#38014=CARTESIAN_POINT ( 'NONE',  ( 17.89687500061451431, -3.027376345333610441, -5.243569643749999898 ) ) ;
#38015=CARTESIAN_POINT ( 'NONE',  ( 12.96562500061451750, 3.027376345333613106, -5.243569643749998122 ) ) ;
#38016=CARTESIAN_POINT ( 'NONE',  ( -2.121784821874999949, 15.28437500061451892, 26.32496088578401938 ) ) ;
#38017=CARTESIAN_POINT ( 'NONE',  ( 17.50312500061451715, 4.541064518000418104, -2.621784821874998173 ) ) ;
#38018=EDGE_LOOP ( 'NONE', ( #71926, #5018, #11995, #23057 ) ) ;
#38020=CARTESIAN_POINT ( 'NONE',  ( 22.08749999999999858, -2.886751345948125991, -5.000000000000000000 ) ) ;
#38021=CARTESIAN_POINT ( 'NONE',  ( 2.121784821875001281, 19.10937500061451644, -26.32496088578401938 ) ) ;
#38022=CARTESIAN_POINT ( 'NONE',  ( 12.63749999999999751, -2.886751345948193048, -4.999999999999883649 ) ) ;
#38023=CARTESIAN_POINT ( 'NONE',  ( 25.00312500061451715, -4.541064518000417216, -2.621784821875001281 ) ) ;
#38024=CARTESIAN_POINT ( 'NONE',  ( 6.515625000614516438, -6.054752690667223547, -1.112240025338166033E-15 ) ) ;
#38025=CARTESIAN_POINT ( 'NONE',  ( 18.48750000122903359, -4.330127018922194537, 2.499999999999995559 ) ) ;
#38026=CARTESIAN_POINT ( 'NONE',  ( 21.29062500061451502, -3.027376345333614438, 5.243569643749998122 ) ) ;
#38027=CARTESIAN_POINT ( 'NONE',  ( 23.77499999999999858, -4.330127018922194537, 2.499999999999995559 ) ) ;
#38029=CARTESIAN_POINT ( 'NONE',  ( 25.41562500061451146, -6.054752690667223547, -1.112240025338166033E-15 ) ) ;
#38030=CARTESIAN_POINT ( 'NONE',  ( 6.928125000614516082, -4.541064518000419881, 2.621784821874995952 ) ) ;
#38032=CARTESIAN_POINT ( 'NONE',  ( 22.64062500061451644, -3.027376345333614438, 5.243569643749998122 ) ) ;
#38033=CARTESIAN_POINT ( 'NONE',  ( 3.890625000614517326, -3.027376345333610441, -5.243569643749999898 ) ) ;
#38036=CARTESIAN_POINT ( 'NONE',  ( 4.000000000000000000, 12.65000000122903501, -27.69059892324149530 ) ) ;
#38037=CARTESIAN_POINT ( 'NONE',  ( 10.49999999999999822, 4.330127018922192761, -2.499999999999997780 ) ) ;
#38038=CARTESIAN_POINT ( 'NONE',  ( 11.70937500061451608, 4.541064518000418104, -2.621784821874998173 ) ) ;
#38039=CARTESIAN_POINT ( 'NONE',  ( 7.650000001229034119, -2.886751345948129988, 4.999999999999997335 ) ) ;
#38040=CARTESIAN_POINT ( 'NONE',  ( 14.55937500061451573, 0.000000000000000000, 5.243569643749999010 ) ) ;
#38041=CARTESIAN_POINT ( 'NONE',  ( 5.634375000614519458, -4.541064518000419881, 2.621784821874995952 ) ) ;
#38042=CARTESIAN_POINT ( 'NONE',  ( -0.7368881354385758975, 9.803648613939515144, -34.17910028561248481 ) ) ;
#38043=CARTESIAN_POINT ( 'NONE',  ( 11.37187500061451750, 3.027376345333611329, 5.243569643749999010 ) ) ;
#38044=CYLINDRICAL_SURFACE ( 'NONE', #52424, 4.999999999999998224 ) ;
#38045=CARTESIAN_POINT ( 'NONE',  ( 23.12812500061451360, -4.541064518000419881, 2.621784821874995952 ) ) ;
#38047=CYLINDRICAL_SURFACE ( 'NONE', #66639, 4.999999999999998224 ) ;
#38048=CARTESIAN_POINT ( 'NONE',  ( 24.60937500061451644, -4.541064518000417216, -2.621784821875001281 ) ) ;
#38050=CARTESIAN_POINT ( 'NONE',  ( 28.05000000122903359, -2.886751345948125991, -5.000000000000000000 ) ) ;
#38051=EDGE_CURVE ( 'NONE', #31197, #6716, #36797, .T. ) ;
#38053=CARTESIAN_POINT ( 'NONE',  ( 26.12812500061451360, 4.541064518000418104, 2.621784821874999949 ) ) ;
#38054=CARTESIAN_POINT ( 'NONE',  ( 17.20312500061451644, 0.000000000000000000, 5.243569643749999010 ) ) ;
#38056=CARTESIAN_POINT ( 'NONE',  ( 14.74687500061451573, -3.027376345333610441, -5.243569643749999898 ) ) ;
#38057=CARTESIAN_POINT ( 'NONE',  ( 16.94999999999999929, 0.000000000000000000, 4.999999999999998224 ) ) ;
#38058=CARTESIAN_POINT ( 'NONE',  ( 28.35000000122903430, -2.886751345948129988, 4.999999999999997335 ) ) ;
#38059=CARTESIAN_POINT ( 'NONE',  ( 5.784375000614517148, 6.421520780324663323E-16, -5.243569643749999010 ) ) ;
#38060=CARTESIAN_POINT ( 'NONE',  ( 17.48437500061451999, 6.421520780324663323E-16, -5.243569643749999010 ) ) ;
#38061=CARTESIAN_POINT ( 'NONE',  ( 4.864538933187982472, -1.156167748881617108, -5.114563458357813452 ) ) ;
#38062=CARTESIAN_POINT ( 'NONE',  ( 25.05000000000000071, 0.000000000000000000, 4.999999999999998224 ) ) ;
#38063=CARTESIAN_POINT ( 'NONE',  ( 3.937500001229034208, 4.330127018922191873, 2.499999999999999556 ) ) ;
#38064=CARTESIAN_POINT ( 'NONE',  ( 25.02187500061451431, -6.054752690667223547, -1.112240025338166033E-15 ) ) ;
#38065=CARTESIAN_POINT ( 'NONE',  ( 16.09687500061452070, -3.027376345333610441, -5.243569643749999898 ) ) ;
#38067=CARTESIAN_POINT ( 'NONE',  ( 27.67499999999999716, 4.330127018922191873, 2.499999999999999556 ) ) ;
#38068=CARTESIAN_POINT ( 'NONE',  ( 4.912499999999999645, -5.773502691896255534, -1.060575238724906372E-15 ) ) ;
#38070=CARTESIAN_POINT ( 'NONE',  ( 19.86562500061451786, 3.027376345333611329, 5.243569643749999010 ) ) ;
#38071=CARTESIAN_POINT ( 'NONE',  ( 10.12500000000000178, 4.330127018922191873, 2.499999999999999556 ) ) ;
#38072=CARTESIAN_POINT ( 'NONE',  ( 3.028125000614518392, 6.421520780324663323E-16, -5.243569643749999010 ) ) ;
#38074=CARTESIAN_POINT ( 'NONE',  ( 18.75000000000000000, 0.000000000000000000, 4.999999999999998224 ) ) ;
#38075=EDGE_CURVE ( 'NONE', #68271, #54526, #64165, .T. ) ;
#38077=CARTESIAN_POINT ( 'NONE',  ( 22.23750000122903003, 6.123233995736764310E-16, -4.999999999999998224 ) ) ;
#38078=CARTESIAN_POINT ( 'NONE',  ( 3.979525575715635810, 9.178911176227739332, 34.50663612706885175 ) ) ;
#38079=CARTESIAN_POINT ( 'NONE',  ( 28.62187500061451573, -6.054752690667223547, -1.112240025338166033E-15 ) ) ;
#38080=VERTEX_POINT ( 'NONE', #45696 ) ;
#38081=CARTESIAN_POINT ( 'NONE',  ( 18.25312500061451715, -4.541064518000417216, -2.621784821875001281 ) ) ;
#38082=CARTESIAN_POINT ( 'NONE',  ( 23.39062500061451289, 6.054752690667223547, 3.707466751127219781E-16 ) ) ;
#38083=CARTESIAN_POINT ( 'NONE',  ( 25.95937500061451431, -4.541064518000417216, -2.621784821875001281 ) ) ;
#38084=CARTESIAN_POINT ( 'NONE',  ( 7.350000000000002309, 4.330127018922192761, -2.499999999999997780 ) ) ;
#38085=CARTESIAN_POINT ( 'NONE',  ( 10.97812500061451679, -4.541064518000419881, 2.621784821874995952 ) ) ;
#38086=CARTESIAN_POINT ( 'NONE',  ( 26.27812500061451573, -4.541064518000419881, 2.621784821874995952 ) ) ;
#38087=CARTESIAN_POINT ( 'NONE',  ( 13.69687500061451679, -3.027376345333614438, 5.243569643749998122 ) ) ;
#38088=CARTESIAN_POINT ( 'NONE',  ( 18.90937500061451360, 4.541064518000418104, -2.621784821874998173 ) ) ;
#38089=CARTESIAN_POINT ( 'NONE',  ( -2.121784821874999949, 18.82812500061451644, 26.32496088578401938 ) ) ;
#38090=CARTESIAN_POINT ( 'NONE',  ( 24.37500000122903288, -5.773502691896255534, -1.060575238724906372E-15 ) ) ;
#38092=CARTESIAN_POINT ( 'NONE',  ( 14.99062500061452141, -3.027376345333614438, 5.243569643749998122 ) ) ;
#38093=CARTESIAN_POINT ( 'NONE',  ( 7.771875000614516971, 3.027376345333611329, 5.243569643749999010 ) ) ;
#38094=CARTESIAN_POINT ( 'NONE',  ( 7.996875000614519280, -3.027376345333610441, -5.243569643749999898 ) ) ;
#38095=EDGE_CURVE ( 'NONE', #33889, #46701, #8881, .T. ) ;
#38097=CARTESIAN_POINT ( 'NONE',  ( 28.35937500061451289, 4.541064518000418104, -2.621784821874998173 ) ) ;
#38098=CARTESIAN_POINT ( 'NONE',  ( 19.22812500061451502, 6.421520780324663323E-16, -5.243569643749999010 ) ) ;
#38099=CARTESIAN_POINT ( 'NONE',  ( 29.10000000122903074, 5.773502691896255534, 3.535250795749688894E-16 ) ) ;
#38100=CARTESIAN_POINT ( 'NONE',  ( 3.009375000614516793, -4.541064518000417216, -2.621784821875001281 ) ) ;
#38101=CARTESIAN_POINT ( 'NONE',  ( 24.38437500061451502, 4.541064518000418104, 2.621784821874999949 ) ) ;
#38102=CARTESIAN_POINT ( 'NONE',  ( 20.35312500061451502, 0.000000000000000000, 5.243569643749999010 ) ) ;
#38103=CARTESIAN_POINT ( 'NONE',  ( -3.999999999999999556, 12.76250000000000284, 27.69059892324149530 ) ) ;
#38104=CARTESIAN_POINT ( 'NONE',  ( 25.22812500061451502, 4.541064518000418104, 2.621784821874999949 ) ) ;
#38105=CARTESIAN_POINT ( 'NONE',  ( 6.337500001229033231, -4.330127018922194537, 2.499999999999995559 ) ) ;
#38107=FACE_OUTER_BOUND ( 'NONE', #53269, .T. ) ;
#38108=CARTESIAN_POINT ( 'NONE',  ( -3.999999999999997335, 15.08750000000000036, -27.69059892324149175 ) ) ;
#38109=CARTESIAN_POINT ( 'NONE',  ( 22.53750000122903430, -4.330127018922194537, 2.499999999999995559 ) ) ;
#38111=CARTESIAN_POINT ( 'NONE',  ( 4.921875000614518214, 3.027376345333613106, -5.243569643749998122 ) ) ;
#38112=CARTESIAN_POINT ( 'NONE',  ( 25.38749999999999929, 5.773502691896255534, 3.535250795749688401E-16 ) ) ;
#38113=CARTESIAN_POINT ( 'NONE',  ( 11.99062500061451608, -3.027376345333610441, -5.243569643749999898 ) ) ;
#38114=CARTESIAN_POINT ( 'NONE',  ( 5.784375000614517148, 6.421520780324663323E-16, -5.243569643749999010 ) ) ;
#38115=CARTESIAN_POINT ( 'NONE',  ( 23.43750000122902932, -4.330127018922194537, 2.499999999999995559 ) ) ;
#38116=CARTESIAN_POINT ( 'NONE',  ( 15.64687500061451608, -3.027376345333610441, -5.243569643749999898 ) ) ;
#38117=CARTESIAN_POINT ( 'NONE',  ( 3.346875000614518036, -3.027376345333614438, 5.243569643749998122 ) ) ;
#38118=CARTESIAN_POINT ( 'NONE',  ( 8.062500001229034652, 0.000000000000000000, 4.999999999999998224 ) ) ;
#38119=CARTESIAN_POINT ( 'NONE',  ( 5.015625000614518214, 3.027376345333611329, 5.243569643749999010 ) ) ;
#38120=CARTESIAN_POINT ( 'NONE',  ( 15.44062500061451537, -3.027376345333614438, 5.243569643749998122 ) ) ;
#38122=CARTESIAN_POINT ( 'NONE',  ( 9.290625000614515017, -3.027376345333610441, -5.243569643749999898 ) ) ;
#38123=CARTESIAN_POINT ( 'NONE',  ( 7.903125000614515727, -4.541064518000417216, -2.621784821875001281 ) ) ;
#38125=CARTESIAN_POINT ( 'NONE',  ( 8.099999999999999645, -4.330127018922190985, -2.500000000000001332 ) ) ;
#38126=CARTESIAN_POINT ( 'NONE',  ( 4.087500001229035007, -4.330127018922194537, 2.499999999999995559 ) ) ;
#38127=CARTESIAN_POINT ( 'NONE',  ( 18.11250000000000071, 2.886751345948129099, -4.999999999999998224 ) ) ;
#38128=CARTESIAN_POINT ( 'NONE',  ( 17.37187500061451573, -6.054752690667223547, -1.112240025338166033E-15 ) ) ;
#38129=CARTESIAN_POINT ( 'NONE',  ( 12.90000000122903145, 5.773502691896255534, 3.535250795749688894E-16 ) ) ;
#38131=CARTESIAN_POINT ( 'NONE',  ( 2.121784821874999061, 16.95312500061451999, -33.67503911421598417 ) ) ;
#38132=LINE ( 'NONE', #37769, #5315 ) ;
#38134=FACE_OUTER_BOUND ( 'NONE', #44781, .T. ) ;
#38135=CARTESIAN_POINT ( 'NONE',  ( 20.10000000122903074, 5.773502691896255534, 3.535250795749688401E-16 ) ) ;
#38136=CARTESIAN_POINT ( 'NONE',  ( 1.999999999999998668, 16.25000000000000000, -33.46410161513775705 ) ) ;
#38137=CARTESIAN_POINT ( 'NONE',  ( 14.74687500061451573, -3.027376345333610441, -5.243569643749999898 ) ) ;
#38138=CARTESIAN_POINT ( 'NONE',  ( 27.26249999999999929, 2.886751345948126879, 4.999999999999999112 ) ) ;
#38139=CARTESIAN_POINT ( 'NONE',  ( 12.59062500061451573, 6.054752690667223547, 3.707466751127219781E-16 ) ) ;
#38141=CARTESIAN_POINT ( 'NONE',  ( 21.83437500061451786, -4.541064518000419881, 2.621784821874995952 ) ) ;
#38143=CARTESIAN_POINT ( 'NONE',  ( 7.865625000614516971, -6.054752690667223547, -1.112240025338166033E-15 ) ) ;
#38144=CARTESIAN_POINT ( 'NONE',  ( 13.39687500061451608, -3.027376345333610441, -5.243569643749999898 ) ) ;
#38145=ORIENTED_EDGE ( 'NONE', *, *, #24790, .F. ) ;
#38146=CARTESIAN_POINT ( 'NONE',  ( 22.80937500061451573, -4.541064518000417216, -2.621784821875001281 ) ) ;
#38147=CARTESIAN_POINT ( 'NONE',  ( 29.02499999999999858, 4.330127018922191873, 2.499999999999999556 ) ) ;
#38149=CARTESIAN_POINT ( 'NONE',  ( 8.775000000000002132, 4.330127018922191873, 2.499999999999999556 ) ) ;
#38150=CARTESIAN_POINT ( 'NONE',  ( 5.700000000000000178, 0.000000000000000000, 4.999999999999998224 ) ) ;
#38151=CARTESIAN_POINT ( 'NONE',  ( 16.72500000122903430, -5.773502691896255534, -1.060575238724906372E-15 ) ) ;
#38152=CARTESIAN_POINT ( 'NONE',  ( 30.00000000000000000, 0.000000000000000000, 9.999999999999998224 ) ) ;
#38153=CARTESIAN_POINT ( 'NONE',  ( 17.39999999999999858, 0.000000000000000000, 4.999999999999998224 ) ) ;
#38154=ORIENTED_EDGE ( 'NONE', *, *, #61508, .T. ) ;
#38155=CARTESIAN_POINT ( 'NONE',  ( 13.53749999999999964, -2.886751345948125991, -5.000000000000000000 ) ) ;
#38156=CARTESIAN_POINT ( 'NONE',  ( 17.62500000000000000, 6.123233995736764310E-16, -4.999999999999998224 ) ) ;
#38157=CARTESIAN_POINT ( 'NONE',  ( 13.72500000122903074, 2.886751345948129099, -4.999999999999998224 ) ) ;
#38158=CARTESIAN_POINT ( 'NONE',  ( 12.36562500061451608, -6.054752690667223547, -1.112240025338166033E-15 ) ) ;
#38159=VERTEX_POINT ( 'NONE', #56050 ) ;
#38160=CARTESIAN_POINT ( 'NONE',  ( -1.071796769724485010, 17.05490381179669868, -25.99999999999999289 ) ) ;
#38161=CARTESIAN_POINT ( 'NONE',  ( 2.121784821874999061, 17.00937500061451857, -33.67503911421598417 ) ) ;
#38162=CARTESIAN_POINT ( 'NONE',  ( 4.453125000614517326, 4.541064518000418104, -2.621784821874998173 ) ) ;
#38164=CARTESIAN_POINT ( 'NONE',  ( 10.20000000000000107, 0.000000000000000000, 4.999999999999998224 ) ) ;
#38165=DIRECTION ( 'NONE',  ( 0.000000000000000000, 0.000000000000000000, -1.000000000000000000 ) ) ;
#38167=CARTESIAN_POINT ( 'NONE',  ( 23.69062500061451004, -3.027376345333610441, -5.243569643749999898 ) ) ;
#38170=CARTESIAN_POINT ( 'NONE',  ( 20.29687500061451644, 6.054752690667223547, 3.707466751127219781E-16 ) ) ;
#38171=CARTESIAN_POINT ( 'NONE',  ( 20.09062500061451573, -3.027376345333610441, -5.243569643749999898 ) ) ;
#38172=CARTESIAN_POINT ( 'NONE',  ( -4.243569643749998122, 13.09062500061459389, -27.54997392385601174 ) ) ;
#38173=CARTESIAN_POINT ( 'NONE',  ( 7.303125000614516082, 0.000000000000000000, 5.243569643749999010 ) ) ;
#38174=CARTESIAN_POINT ( 'NONE',  ( 4.528125000614516615, 4.541064518000418104, 2.621784821874999949 ) ) ;
#38176=CARTESIAN_POINT ( 'NONE',  ( 21.62812500061451360, 4.541064518000418104, 2.621784821874999949 ) ) ;
#38177=CYLINDRICAL_SURFACE ( 'NONE', #15023, 3.999999999999996447 ) ;
#38179=CARTESIAN_POINT ( 'NONE',  ( 14.33437500061451786, 6.421520780324663323E-16, -5.243569643749999010 ) ) ;
#38180=CARTESIAN_POINT ( 'NONE',  ( 14.48437500061451821, 4.541064518000418104, 2.621784821874999949 ) ) ;
#38181=CARTESIAN_POINT ( 'NONE',  ( 22.32187500061451502, -6.054752690667223547, -1.112240025338166033E-15 ) ) ;
#38182=VERTEX_POINT ( 'NONE', #73038 ) ;
#38183=CARTESIAN_POINT ( 'NONE',  ( -4.243569643749998122, 11.34687500061451892, 32.45002607614398471 ) ) ;
#38184=CARTESIAN_POINT ( 'NONE',  ( 3.778125000614519280, -4.541064518000419881, 2.621784821874995952 ) ) ;
#38185=CARTESIAN_POINT ( 'NONE',  ( 26.35312500061451857, -4.541064518000417216, -2.621784821875001281 ) ) ;
#38186=CARTESIAN_POINT ( 'NONE',  ( 26.16562500061451502, 3.027376345333611329, 5.243569643749999010 ) ) ;
#38189=CARTESIAN_POINT ( 'NONE',  ( 4.809375000614516615, -4.541064518000417216, -2.621784821875001281 ) ) ;
#38190=CARTESIAN_POINT ( 'NONE',  ( 15.26250000122903216, 0.000000000000000000, 4.999999999999998224 ) ) ;
#38191=CARTESIAN_POINT ( 'NONE',  ( 9.112500001229033586, -4.330127018922190985, -2.500000000000001332 ) ) ;
#38192=CARTESIAN_POINT ( 'NONE',  ( 29.13750000122903216, 4.330127018922191873, 2.499999999999999556 ) ) ;
#38195=CARTESIAN_POINT ( 'NONE',  ( 12.34687500061452070, -3.027376345333614438, 5.243569643749998122 ) ) ;
#38196=CARTESIAN_POINT ( 'NONE',  ( 11.88749999999999929, 5.773502691896255534, 3.535250795749688401E-16 ) ) ;
#38197=VERTEX_POINT ( 'NONE', #5442 ) ;
#38198=CARTESIAN_POINT ( 'NONE',  ( 19.26562500061451644, 3.027376345333613106, -5.243569643749998122 ) ) ;
#38199=CARTESIAN_POINT ( 'NONE',  ( 16.84687500061451715, -3.027376345333614438, 5.243569643749998122 ) ) ;
#38200=CARTESIAN_POINT ( 'NONE',  ( 6.103125000614515905, -4.541064518000417216, -2.621784821875001281 ) ) ;
#38201=CARTESIAN_POINT ( 'NONE',  ( 21.23437500061451644, 4.541064518000418104, 2.621784821874999949 ) ) ;
#38202=CARTESIAN_POINT ( 'NONE',  ( 5.803125000614517859, 4.541064518000418104, -2.621784821874998173 ) ) ;
#38204=CARTESIAN_POINT ( 'NONE',  ( 7.725000001229034297, -5.773502691896255534, -1.060575238724906372E-15 ) ) ;
#38205=CARTESIAN_POINT ( 'NONE',  ( 23.65312500061451573, -4.541064518000417216, -2.621784821875001281 ) ) ;
#38206=CARTESIAN_POINT ( 'NONE',  ( -3.999999999999999112, 18.76250000122903216, -30.00000000000000000 ) ) ;
#38207=CARTESIAN_POINT ( 'NONE',  ( 6.787500001229032520, -4.330127018922194537, 2.499999999999995559 ) ) ;
#38208=CARTESIAN_POINT ( 'NONE',  ( 19.22812500061451502, 6.421520780324663323E-16, -5.243569643749999010 ) ) ;
#38209=CARTESIAN_POINT ( 'NONE',  ( 14.57812500061451644, -4.541064518000419881, 2.621784821874995952 ) ) ;
#38211=CARTESIAN_POINT ( 'NONE',  ( 15.48749999999999893, 5.773502691896255534, 3.535250795749688894E-16 ) ) ;
#38212=CARTESIAN_POINT ( 'NONE',  ( 11.13750000122903216, 4.330127018922191873, 2.499999999999999556 ) ) ;
#38213=CARTESIAN_POINT ( 'NONE',  ( 8.540625000614518569, 6.054752690667223547, 3.707466751127219781E-16 ) ) ;
#38214=CARTESIAN_POINT ( 'NONE',  ( 11.31562500061451892, 3.027376345333611329, 5.243569643749999010 ) ) ;
#38215=EDGE_CURVE ( 'NONE', #18194, #18095, #29226, .T. ) ;
#38216=CARTESIAN_POINT ( 'NONE',  ( 21.03750000122903074, 4.330127018922191873, 2.499999999999999556 ) ) ;
#38217=CARTESIAN_POINT ( 'NONE',  ( 4.243569643749999898, 14.64687500061451964, -27.54997392385601529 ) ) ;
#38218=CARTESIAN_POINT ( 'NONE',  ( 20.14687500061451786, -3.027376345333610441, -5.243569643749999898 ) ) ;
#38219=CARTESIAN_POINT ( 'NONE',  ( 21.26249999999999574, 2.886751345948129099, -4.999999999999997335 ) ) ;
#38220=CARTESIAN_POINT ( 'NONE',  ( 4.987500001229032698, -4.330127018922194537, 2.499999999999995559 ) ) ;
#38221=CARTESIAN_POINT ( 'NONE',  ( 5.259375000614518569, -4.541064518000417216, -2.621784821875001281 ) ) ;
#38222=CARTESIAN_POINT ( 'NONE',  ( 21.79687500061451644, -3.027376345333614438, 5.243569643749998122 ) ) ;
#38223=CARTESIAN_POINT ( 'NONE',  ( 5.212500000000002132, 2.886751345948126879, 4.999999999999998224 ) ) ;
#38224=CARTESIAN_POINT ( 'NONE',  ( 18.85312500061451502, 4.541064518000418104, -2.621784821874998173 ) ) ;
#38227=CARTESIAN_POINT ( 'NONE',  ( 4.544497808834801589, -2.085075457992688897, -4.544497808831748920 ) ) ;
#38228=CARTESIAN_POINT ( 'NONE',  ( 27.60937500061451644, 0.000000000000000000, 5.243569643749999010 ) ) ;
#38231=CARTESIAN_POINT ( 'NONE',  ( 13.86562500061451431, 3.027376345333613106, -5.243569643749998122 ) ) ;
#38232=CARTESIAN_POINT ( 'NONE',  ( 13.69687500061451679, -3.027376345333614438, 5.243569643749998122 ) ) ;
#38233=ORIENTED_EDGE ( 'NONE', *, *, #33218, .F. ) ;
#38235=CARTESIAN_POINT ( 'NONE',  ( 22.94062500061451715, 6.054752690667223547, 3.707466751127219781E-16 ) ) ;
#38237=CARTESIAN_POINT ( 'NONE',  ( 1.626862140677534273E-15, 11.67500000122903181, -26.00000000000000355 ) ) ;
#38238=CARTESIAN_POINT ( 'NONE',  ( 12.52500000000000213, -4.330127018922194537, 2.499999999999995559 ) ) ;
#38239=CARTESIAN_POINT ( 'NONE',  ( 23.10000000122903074, -2.886751345948125991, -5.000000000000000000 ) ) ;
#38240=CARTESIAN_POINT ( 'NONE',  ( 18.02812500061451573, 4.541064518000418104, 2.621784821874999949 ) ) ;
#38241=ORIENTED_EDGE ( 'NONE', *, *, #24606, .T. ) ;
#38242=CARTESIAN_POINT ( 'NONE',  ( 21.26249999999999574, 2.886751345948129099, -4.999999999999998224 ) ) ;
#38243=CARTESIAN_POINT ( 'NONE',  ( 23.89687500061451786, 6.054752690667223547, 3.707466751127219781E-16 ) ) ;
#38245=CARTESIAN_POINT ( 'NONE',  ( 19.98749999999999716, 5.773502691896255534, 3.535250795749688401E-16 ) ) ;
#38246=CARTESIAN_POINT ( 'NONE',  ( 9.815625000614518925, 3.027376345333613106, -5.243569643749998122 ) ) ;
#38249=CARTESIAN_POINT ( 'NONE',  ( 16.12500000000000000, -4.330127018922194537, 2.499999999999995559 ) ) ;
#38250=CARTESIAN_POINT ( 'NONE',  ( 24.78750000000000497, -2.886751345948125991, -5.000000000000000000 ) ) ;
#38251=CARTESIAN_POINT ( 'NONE',  ( 4.243569643749999898, 19.09062500061451573, 32.45002607614398471 ) ) ;
#38252=CARTESIAN_POINT ( 'NONE',  ( 3.984375000614517326, 6.421520780324663323E-16, -5.243569643749999010 ) ) ;
#38253=CARTESIAN_POINT ( 'NONE',  ( 16.32187500061451502, 3.027376345333611329, 5.243569643749999010 ) ) ;
#38254=CARTESIAN_POINT ( 'NONE',  ( 29.78437500061451715, 4.541064518000418104, 2.621784821874999949 ) ) ;
#38256=CARTESIAN_POINT ( 'NONE',  ( 25.30312500061451431, 0.000000000000000000, 5.243569643749999010 ) ) ;
#38257=CARTESIAN_POINT ( 'NONE',  ( 27.15937500061451360, 0.000000000000000000, 5.243569643749999010 ) ) ;
#38260=CARTESIAN_POINT ( 'NONE',  ( 14.92500000000000071, 6.123233995736764310E-16, -4.999999999999998224 ) ) ;
#38261=CARTESIAN_POINT ( 'NONE',  ( 12.47812500061451502, 6.421520780324663323E-16, -5.243569643749999010 ) ) ;
#38262=CARTESIAN_POINT ( 'NONE',  ( 3.722276561693393937, 3.338418630728691827, 4.014037966420130665 ) ) ;
#38263=CARTESIAN_POINT ( 'NONE',  ( 3.242103837493086330E-14, 11.33750000000000213, 26.00000000000000711 ) ) ;
#38264=CARTESIAN_POINT ( 'NONE',  ( 28.00312500061451715, 0.000000000000000000, 5.243569643749999010 ) ) ;
#38265=CARTESIAN_POINT ( 'NONE',  ( 15.75000000122902932, -2.886751345948129988, 4.999999999999997335 ) ) ;
#38268=CARTESIAN_POINT ( 'NONE',  ( 4.378125000614518925, 6.421520780324663323E-16, -5.243569643749999010 ) ) ;
#38269=CARTESIAN_POINT ( 'NONE',  ( 21.60937500061451644, 4.541064518000418104, -2.621784821874998173 ) ) ;
#38270=CARTESIAN_POINT ( 'NONE',  ( 2.121784821874999061, 16.55937500061451573, 26.32496088578401583 ) ) ;
#38271=CARTESIAN_POINT ( 'NONE',  ( 22.73437500061451644, -4.541064518000419881, 2.621784821874995952 ) ) ;
#38272=CARTESIAN_POINT ( 'NONE',  ( 29.63437500061451502, 6.421520780324663323E-16, -5.243569643749999010 ) ) ;
#38273=CARTESIAN_POINT ( 'NONE',  ( -4.243569643749998122, 18.09687500061451715, 32.45002607614398471 ) ) ;
#38274=CARTESIAN_POINT ( 'NONE',  ( 11.27812500061451573, 4.541064518000418104, 2.621784821874999949 ) ) ;
#38275=CARTESIAN_POINT ( 'NONE',  ( 3.150000001229034119, -2.886751345948129988, 4.999999999999997335 ) ) ;
#38276=CARTESIAN_POINT ( 'NONE',  ( 6.946875000614517681, -3.027376345333614438, 5.243569643749998122 ) ) ;
#38278=CARTESIAN_POINT ( 'NONE',  ( 8.840625000614515727, -3.027376345333610441, -5.243569643749999898 ) ) ;
#38279=CARTESIAN_POINT ( 'NONE',  ( 13.28437500061451715, -4.541064518000419881, 2.621784821874995952 ) ) ;
#38281=CARTESIAN_POINT ( 'NONE',  ( 21.82500000122903572, 2.886751345948129099, -4.999999999999998224 ) ) ;
#38282=CARTESIAN_POINT ( 'NONE',  ( 7.171875000614517326, 3.027376345333613106, -5.243569643749998122 ) ) ;
#38283=CARTESIAN_POINT ( 'NONE',  ( 10.49062500061451431, -3.027376345333614438, 5.243569643749998122 ) ) ;
#38285=CARTESIAN_POINT ( 'NONE',  ( 21.64687500061451786, 6.054752690667223547, 3.707466751127219781E-16 ) ) ;
#38286=FACE_OUTER_BOUND ( 'NONE', #62334, .T. ) ;
#38288=CARTESIAN_POINT ( 'NONE',  ( -0.6906555412606038002, 4.953935347589259131, 33.94230526677440452 ) ) ;
#38289=CARTESIAN_POINT ( 'NONE',  ( 29.22187500061451715, 3.027376345333612662, -5.243569643749998122 ) ) ;
#38290=CARTESIAN_POINT ( 'NONE',  ( -3.000416591977282496E-16, 11.19687500061451679, -34.90005215228797653 ) ) ;
#38291=CARTESIAN_POINT ( 'NONE',  ( 16.08750000122903501, 4.330127018922191873, 2.499999999999999556 ) ) ;
#38292=CARTESIAN_POINT ( 'NONE',  ( -4.243569643749997233, 14.44062500061451715, -27.54997392385601174 ) ) ;
#38293=CARTESIAN_POINT ( 'NONE',  ( 18.67500000122903714, 2.886751345948129099, -4.999999999999998224 ) ) ;
#38294=CARTESIAN_POINT ( 'NONE',  ( 10.97812500061451679, -4.541064518000419881, 2.621784821874995952 ) ) ;
#38296=VERTEX_POINT ( 'NONE', #34224 ) ;
#38297=CARTESIAN_POINT ( 'NONE',  ( 13.23750000000000071, 5.773502691896255534, 3.535250795749688894E-16 ) ) ;
#38298=CARTESIAN_POINT ( 'NONE',  ( -1.999999999999997113, 13.77500000000000036, 33.46410161513775705 ) ) ;
#38299=CARTESIAN_POINT ( 'NONE',  ( 23.87812500061451715, 4.541064518000418104, 2.621784821874999949 ) ) ;
#38300=CARTESIAN_POINT ( 'NONE',  ( 10.09687500061451715, -3.027376345333614438, 5.243569643749998122 ) ) ;
#38302=CARTESIAN_POINT ( 'NONE',  ( 10.57500000122903572, 2.886751345948129099, -4.999999999999998224 ) ) ;
#38303=CARTESIAN_POINT ( 'NONE',  ( 18.41250000122903430, 0.000000000000000000, 4.999999999999998224 ) ) ;
#38305=CARTESIAN_POINT ( 'NONE',  ( 15.59062500061451573, -3.027376345333610441, -5.243569643749999898 ) ) ;
#38306=CARTESIAN_POINT ( 'NONE',  ( 17.87812500061451715, 6.421520780324663323E-16, -5.243569643749999010 ) ) ;
#38307=CARTESIAN_POINT ( 'NONE',  ( 26.58750000122903145, -4.330127018922194537, 2.499999999999995559 ) ) ;
#38308=( BOUNDED_CURVE ( )  B_SPLINE_CURVE ( 2, ( #71155, #20165, #9832, #10563, #43458, #37903, #37169, #48999, #27195, #54899, #32733, #26832, #71530, #20905, #25728, #70790, #60059, #4665, #54172, #15000, #71896, #48266, #43823, #65981, #42719, #15361, #59695, #44192, #26092, #3200, #10198, #66347, #32362, #3569, #37537, #65240, #14629, #61168, #15725, #60421, #9102, #21269, #9470, #4307, #31640, #32000, #55270, #49366, #38264, #48630, #33091, #54535, #3937, #60792, #49730, #20527, #72257, #21634, #66723, #16095, #38644, #5750, #68534, #218, #22723, #51177, #16818, #62971, #45276, #40101, #45997, #67809, #22367, #68176, #72985, #40455, #581, #23086, #17183, #45643, #62614, #17539, #61891, #28284, #39373, #12367, #6471, #944, #23451, #39742, #34171, #28639, #67093, #17895, #29006, #72623, #12011, #67455, #50816, #55630, #33816, #51543, #34534, #11296, #57064, #62259, #5024, #27561, #56360, #11656, #50092, #27925, #56707, #6108, #50458, #22007, #44563, #16452, #39010, #61525, #10923, #33450, #55994, #5387, #44919, #64789, #41185, #7549, #58143, #2027, #18978, #64425, #24538, #47082, #29368, #35262, #53344, #24171, #13437, #41539, #69973, #35987, #30083, #46723, #7916, #70337, #30453, #52982, #58871, #2378, #18620, #24896, #52621, #47441, #42266, #69258, #69616, #19343, #7193, #64057, #58506, #41898, #29721, #35623, #13817, #36357, #34902, #8281, #25261, #30811, #2742, #47808, #57429, #63694, #19714, #6833, #51900, #1298, #23808, #46359, #68893, #13085, #18250, #40823, #63340, #12726, #1662, #57784, #52259, #20445, #4217, #66257, #15635, #36714, #54811, #31914, #53716, #9382, #48175, #55184, #37080, #65895, #43733, #37814, #37454, #54450, #59236, #8644, #71070, #72169, #14180, #49278, #42630, #32277, #54088, #48910, #31173, #42995, #38176, #3849, #59973, #65154, #3486, #26370, #26004, #59604, #3108, #60700, #48543, #71441, #20816, #15275, #4579, #43371, #27109, #60334, #9743, #26745, #65526, #21548, #71811, #49642, #21181, #14912, #10113, #31548, #44103, #32643, #25637, #70699, #20074, #14544, #9018, #61078, #34085, #33005, #44475, #5298, #4940, #28202, #21919, #45189, #39654, #27474, #11923, #40012, #50731, #55906, #22639, #56626, #27844, #16732, #33370, #67006, #67721, #72900, #6020, #45556, #68087, #16006, #28555, #854, #33731, #134, #50006, #39287, #17454, #17094, #22996, #62173, #61801, #11204, #38555, #10476, #50375, #51451, #66629, #51090, #16367, #11570, #22282, #44834, #67369, #62526, #34448, #23361, #55544, #38922, #56277, #5666, #486, #56976, #72531, #6380, #28913, #61441, #10834, #58785, #69172, #12998, #24808, #63608, #41451, #7105, #53255, #35534, #30366, #36271, #58055, #12641, #58417, #63247, #30723, #63969, #13352, #7464, #35893, #52895, #52532, #40363, #7830, #29634, #2654, #69886, #64337, #13729, #29990, #24446, #18889, #57341, #8195, #19251, #62882, #2292, #57700, #18532, #45909, #24083, #1940, #47353, #40732, #41806, #41097, #68440, #17803, #52172, #46994, #12278, #18163, #69530, #34810, #35176, #6746, #29279, #51809, #1212, #23718, #1574, #46268, #68807, #46630, #25921, #55098, #31461, #70985, #48461, #65435, #9296, #54728, #14826, #37368, #59891, #3762, #15549, #20361, #38092, #42912, #31829, #20728, #59518, #32560, #54367, #60615, #48093, #26286, #21098, #48823, #43649, #71354, #14462, #64706, #4131, #43287, #65807, #15189, #54004, #37727, #8931, #25172, #49195, #66173, #53627, #26661, #3400, #60247, #9661, #32195, #42544, #71728, #36995, #10024, #47713, #70252, #19624, #42181, #14090, #36630, #59151, #8560, #31088, #3019, #25550, #19991, #70617, #65070, #21461, #39928, #17005, #49919, #5211, #39562, #45103, #4498, #50646, #67998, #11480, #22198, #27752, #34359, #10753, #50291, #38841, #72815, #55823, #49558, #60992, #61715, #66917, #33643, #67639, #16286, #44752, #44392, #4853, #5580, #33284, #62087, #56540, #5933, #27027, #34003, #11840, #67286, #39201, #38466, #16645, #28467, #56187, #51002, #28117, #11114, #50, #72079, #44016, #61356, #62442, #66538, #400, #32923, #22555, #22908, #45466, #17371, #15918, #10391, #55461, #27387, #72443, #21827, #6296, #24727, #69804, #45824, #13272, #46184, #23999, #46547, #69088, #51364, #57252, #2212, #68723, #7021, #23638, #6666, #57973, #63163, #46911, #35810, #58332, #28825, #24364, #1493, #23274, #52088, #17721, #47270, #29194, #56891, #63881, #69450, #51728, #18083, #766, #68360, #41724, #18807, #18449, #40281, #7743, #62802, #41371, #40644, #57618, #30279, #52811, #13639, #12195, #34722, #12558, #1129, #19170, #64251, #35093, #29552, #41014, #63529, #7380, #12916, #35449, #29911, #52451, #1857, #2935, #36183, #9209, #30639, #25837, #72642, #59066, #37281, #48739, #53539, #22025, #31745, #3676, #48374, #54282, #20642, #42825, #53171, #26200, #2568, #14008, #48008, #47631, #70901, #64621, #66744, #70536, #20273, #55649, #10584, #25088, #71262, #19911, #8840, #5045, #14377, #65349, #44212, #31006, #16114, #42099, #27581, #70164, #42464, #14739, #25464, #38666, #19541, #31376, #64986, #59803, #61189, #36546, #3310, #33111, #36912, #50113, #44582, #67114, #59432, #58701, #8471, #53917, #8111, #50836, #11674, #67828, #236, #599, #46016, #56724, #28657, #10945, #16837, #34920, #5770, #68194, #23104, #51560, #45661, #17911, #67474, #56378, #12028, #11315, #33467, #17557, #23825, #34190, #50477, #57447, #39391, #16471, #23470 ),
 .UNSPECIFIED., .F., .F. ) 
 B_SPLINE_CURVE_WITH_KNOTS ( ( 3, 2, 2, 2, 2, 2, 2, 2, 2, 2, 2, 2, 2, 2, 2, 2, 2, 2, 2, 2, 2, 2, 2, 2, 2, 2, 2, 2, 2, 2, 2, 2, 2, 2, 2, 2, 2, 2, 2, 2, 2, 2, 2, 2, 2, 2, 2, 2, 2, 2, 2, 2, 2, 2, 2, 2, 2, 2, 2, 2, 2, 2, 2, 2, 2, 2, 2, 2, 2, 2, 2, 2, 2, 2, 2, 2, 2, 2, 2, 2, 2, 2, 2, 2, 2, 2, 2, 2, 2, 2, 2, 2, 2, 2, 2, 2, 2, 2, 2, 2, 2, 2, 2, 2, 2, 2, 2, 2, 2, 2, 2, 2, 2, 2, 2, 2, 2, 2, 2, 2, 2, 2, 2, 2, 2, 2, 2, 2, 2, 2, 2, 2, 2, 2, 2, 2, 2, 2, 2, 2, 2, 2, 2, 2, 2, 2, 2, 2, 2, 2, 2, 2, 2, 2, 2, 2, 2, 2, 2, 2, 2, 2, 2, 2, 2, 2, 2, 2, 2, 2, 2, 2, 2, 2, 2, 2, 2, 2, 2, 2, 2, 2, 2, 2, 2, 2, 2, 2, 2, 2, 2, 2, 2, 2, 2, 2, 2, 2, 2, 2, 2, 2, 2, 2, 2, 2, 2, 2, 2, 2, 2, 2, 2, 2, 2, 2, 2, 2, 2, 2, 2, 2, 2, 2, 2, 2, 2, 2, 2, 2, 2, 2, 2, 2, 2, 2, 2, 2, 2, 2, 2, 2, 2, 2, 2, 2, 2, 2, 2, 2, 2, 2, 2, 2, 2, 2, 2, 2, 2, 2, 2, 2, 2, 2, 2, 2, 2, 2, 2, 2, 2, 2, 2, 2, 2, 2, 2, 2, 2, 2, 2, 2, 2, 2, 2, 2, 2, 2, 2, 2, 2, 2, 2, 2, 2, 2, 2, 2, 2, 2, 2, 2, 2, 2, 2, 2, 2, 2, 2, 2, 2, 2, 2, 2, 2, 2, 2, 2, 2, 2, 2, 2, 2, 2, 2, 2, 2, 2, 2, 2, 2, 2, 2, 3 ),
 ( 0.000000000000000000, 0.002777777777777777884, 0.005555555555555555768, 0.008333333333333333218, 0.01111111111111111154, 0.01388888888888888812, 0.01666666666666666644, 0.01944444444444444475, 0.02222222222222222307, 0.02500000000000000139, 0.02777777777777777624, 0.03055555555555555455, 0.03333333333333333287, 0.03611111111111111466, 0.03888888888888888951, 0.04166666666666666435, 0.04444444444444444614, 0.04722222222222222099, 0.05000000000000000278, 0.05277777777777777762, 0.05555555555555555247, 0.05833333333333333426, 0.06111111111111110911, 0.06388888888888888395, 0.06666666666666666574, 0.06944444444444444753, 0.07222222222222222932, 0.07499999999999999722, 0.07777777777777777901, 0.08055555555555556080, 0.08333333333333332871, 0.08611111111111111049, 0.08888888888888889228, 0.09166666666666666019, 0.09444444444444444198, 0.09722222222222222376, 0.1000000000000000056, 0.1027777777777777735, 0.1055555555555555552, 0.1083333333333333370, 0.1111111111111111049, 0.1138888888888888729, 0.1166666666666666685, 0.1194444444444444503, 0.1222222222222222182, 0.1250000000000000000, 0.1277777777777777679, 0.1305555555555555636, 0.1333333333333333315, 0.1361111111111110994, 0.1388888888888888951, 0.1416666666666666630, 0.1444444444444444586, 0.1472222222222222543, 0.1499999999999999944, 0.1527777777777777901, 0.1555555555555555580, 0.1583333333333333259, 0.1611111111111111216, 0.1638888888888888895, 0.1666666666666666574, 0.1694444444444444531, 0.1722222222222222210, 0.1749999999999999889, 0.1777777777777777846, 0.1805555555555555525, 0.1833333333333333204, 0.1861111111111111160, 0.1888888888888888840, 0.1916666666666666796, 0.1944444444444444475, 0.1972222222222222154, 0.2000000000000000111, 0.2027777777777777790, 0.2055555555555555469, 0.2083333333333333426, 0.2111111111111111105, 0.2138888888888888784, 0.2166666666666666741, 0.2194444444444444420, 0.2222222222222222099, 0.2250000000000000056, 0.2277777777777777457, 0.2305555555555555414, 0.2333333333333333370, 0.2361111111111111049, 0.2388888888888889006, 0.2416666666666666685, 0.2444444444444444364, 0.2472222222222222321, 0.2500000000000000000, 0.2527777777777777679, 0.2555555555555555358, 0.2583333333333333592, 0.2611111111111111271, 0.2638888888888888951, 0.2666666666666666630, 0.2694444444444444309, 0.2722222222222221988, 0.2750000000000000222, 0.2777777777777777901, 0.2805555555555555580, 0.2833333333333333259, 0.2861111111111110938, 0.2888888888888889173, 0.2916666666666666852, 0.2944444444444445086, 0.2972222222222222210, 0.2999999999999999889, 0.3027777777777777568, 0.3055555555555555802, 0.3083333333333333481, 0.3111111111111111160, 0.3138888888888888840, 0.3166666666666666519, 0.3194444444444444198, 0.3222222222222222432, 0.3250000000000000111, 0.3277777777777777790, 0.3305555555555554914, 0.3333333333333333148, 0.3361111111111110827, 0.3388888888888889062, 0.3416666666666666741, 0.3444444444444444420, 0.3472222222222222099, 0.3499999999999999778, 0.3527777777777778012, 0.3555555555555555691, 0.3583333333333333370, 0.3611111111111111049, 0.3638888888888888729, 0.3666666666666666408, 0.3694444444444444642, 0.3722222222222222321, 0.3750000000000000000, 0.3777777777777777679, 0.3805555555555555358, 0.3833333333333333592, 0.3861111111111111271, 0.3888888888888888951, 0.3916666666666666630, 0.3944444444444444309, 0.3972222222222221988, 0.4000000000000000222, 0.4027777777777777901, 0.4055555555555555580, 0.4083333333333333259, 0.4111111111111110938, 0.4138888888888889173, 0.4166666666666666852, 0.4194444444444445086, 0.4222222222222222210, 0.4249999999999999889, 0.4277777777777777568, 0.4305555555555555802, 0.4333333333333333481, 0.4361111111111111160, 0.4388888888888888840, 0.4416666666666666519, 0.4444444444444444198, 0.4472222222222222432, 0.4500000000000000111, 0.4527777777777777790, 0.4555555555555554914, 0.4583333333333333148, 0.4611111111111110827, 0.4638888888888889062, 0.4666666666666666741, 0.4694444444444444420, 0.4722222222222222099, 0.4749999999999999778, 0.4777777777777778012, 0.4805555555555555691, 0.4833333333333333370, 0.4861111111111111049, 0.4888888888888888729, 0.4916666666666666408, 0.4944444444444444642, 0.4972222222222222321, 0.5000000000000000000, 0.5027777777777777679, 0.5055555555555555358, 0.5083333333333333037, 0.5111111111111110716, 0.5138888888888888395, 0.5166666666666667185, 0.5194444444444444864, 0.5222222222222222543, 0.5250000000000000222, 0.5277777777777777901, 0.5305555555555555580, 0.5333333333333333259, 0.5361111111111110938, 0.5388888888888888618, 0.5416666666666667407, 0.5444444444444443976, 0.5472222222222222765, 0.5500000000000000444, 0.5527777777777778123, 0.5555555555555555802, 0.5583333333333333481, 0.5611111111111111160, 0.5638888888888888840, 0.5666666666666666519, 0.5694444444444444198, 0.5722222222222221877, 0.5749999999999999556, 0.5777777777777778345, 0.5805555555555556024, 0.5833333333333333703, 0.5861111111111111382, 0.5888888888888890172, 0.5916666666666666741, 0.5944444444444444420, 0.5972222222222222099, 0.5999999999999999778, 0.6027777777777777457, 0.6055555555555555136, 0.6083333333333332815, 0.6111111111111111605, 0.6138888888888889284, 0.6166666666666666963, 0.6194444444444444642, 0.6222222222222222321, 0.6250000000000001110, 0.6277777777777777679, 0.6305555555555555358, 0.6333333333333333037, 0.6361111111111110716, 0.6388888888888888395, 0.6416666666666667185, 0.6444444444444444864, 0.6472222222222222543, 0.6500000000000000222, 0.6527777777777777901, 0.6555555555555555580, 0.6583333333333333259, 0.6611111111111109828, 0.6638888888888888618, 0.6666666666666666297, 0.6694444444444443976, 0.6722222222222221655, 0.6750000000000000444, 0.6777777777777778123, 0.6805555555555555802, 0.6833333333333333481, 0.6861111111111111160, 0.6888888888888888840, 0.6916666666666666519, 0.6944444444444444198, 0.6972222222222221877, 0.6999999999999999556, 0.7027777777777777235, 0.7055555555555556024, 0.7083333333333332593, 0.7111111111111111382, 0.7138888888888889062, 0.7166666666666666741, 0.7194444444444444420, 0.7222222222222222099, 0.7249999999999999778, 0.7277777777777777457, 0.7305555555555555136, 0.7333333333333332815, 0.7361111111111111605, 0.7388888888888889284, 0.7416666666666666963, 0.7444444444444444642, 0.7472222222222222321, 0.7500000000000000000, 0.7527777777777777679, 0.7555555555555555358, 0.7583333333333333037, 0.7611111111111110716, 0.7638888888888888395, 0.7666666666666667185, 0.7694444444444444864, 0.7722222222222222543, 0.7750000000000000222, 0.7777777777777777901, 0.7805555555555555580, 0.7833333333333333259, 0.7861111111111110938, 0.7888888888888888618, 0.7916666666666667407, 0.7944444444444443976, 0.7972222222222222765, 0.8000000000000000444, 0.8027777777777778123, 0.8055555555555555802, 0.8083333333333333481, 0.8111111111111111160, 0.8138888888888888840, 0.8166666666666666519, 0.8194444444444444198, 0.8222222222222221877, 0.8249999999999999556, 0.8277777777777778345, 0.8305555555555556024, 0.8333333333333333703, 0.8361111111111111382, 0.8388888888888890172, 0.8416666666666666741, 0.8444444444444444420, 0.8472222222222222099, 0.8499999999999999778, 0.8527777777777777457, 0.8555555555555555136, 0.8583333333333332815, 0.8611111111111111605, 0.8638888888888889284, 0.8666666666666666963, 0.8694444444444444642, 0.8722222222222222321, 0.8749999999999998890, 0.8777777777777777679, 0.8805555555555555358, 0.8833333333333333037, 0.8861111111111110716, 0.8888888888888888395, 0.8916666666666667185, 0.8944444444444444864, 0.8972222222222222543, 0.9000000000000000222, 0.9027777777777777901, 0.9055555555555555580, 0.9083333333333333259, 0.9111111111111109828, 0.9138888888888888618, 0.9166666666666666297, 0.9194444444444443976, 0.9222222222222221655, 0.9243558487027168091 ),
 .UNSPECIFIED. ) 
 CURVE ( )  GEOMETRIC_REPRESENTATION_ITEM ( )  RATIONAL_B_SPLINE_CURVE ( ( 1.000000000000000000, 0.8660254037844387076, 1.000000000000000000, 0.8660254037844387076, 1.000000000000000000, 0.8660254037844387076, 1.000000000000000000, 0.8660254037844387076, 1.000000000000000000, 0.8660254037844387076, 1.000000000000000000, 0.8660254037844387076, 1.000000000000000000, 0.8660254037844387076, 1.000000000000000000, 0.8660254037844387076, 1.000000000000000000, 0.8660254037844387076, 1.000000000000000000, 0.8660254037844387076, 1.000000000000000000, 0.8660254037844387076, 1.000000000000000000, 0.8660254037844387076, 1.000000000000000000, 0.8660254037844387076, 1.000000000000000000, 0.8660254037844387076, 1.000000000000000000, 0.8660254037844387076, 1.000000000000000000, 0.8660254037844387076, 1.000000000000000000, 0.8660254037844387076, 1.000000000000000000, 0.8660254037844387076, 1.000000000000000000, 0.8660254037844387076, 1.000000000000000000, 0.8660254037844387076, 1.000000000000000000, 0.8660254037844387076, 1.000000000000000000, 0.8660254037844387076, 1.000000000000000000, 0.8660254037844387076, 1.000000000000000000, 0.8660254037844387076, 1.000000000000000000, 0.8660254037844387076, 1.000000000000000000, 0.8660254037844387076, 1.000000000000000000, 0.8660254037844387076, 1.000000000000000000, 0.8660254037844387076, 1.000000000000000000, 0.8660254037844387076, 1.000000000000000000, 0.8660254037844387076, 1.000000000000000000, 0.8660254037844387076, 1.000000000000000000, 0.8660254037844387076, 1.000000000000000000, 0.8660254037844387076, 1.000000000000000000, 0.8660254037844387076, 1.000000000000000000, 0.8660254037844387076, 1.000000000000000000, 0.8660254037844387076, 1.000000000000000000, 0.8660254037844387076, 1.000000000000000000, 0.8660254037844387076, 1.000000000000000000, 0.8660254037844387076, 1.000000000000000000, 0.8660254037844387076, 1.000000000000000000, 0.8660254037844387076, 1.000000000000000000, 0.8660254037844387076, 1.000000000000000000, 0.8660254037844387076, 1.000000000000000000, 0.8660254037844387076, 1.000000000000000000, 0.8660254037844387076, 1.000000000000000000, 0.8660254037844387076, 1.000000000000000000, 0.8660254037844387076, 1.000000000000000000, 0.8660254037844387076, 1.000000000000000000, 0.8660254037844387076, 1.000000000000000000, 0.8660254037844387076, 1.000000000000000000, 0.8660254037844387076, 1.000000000000000000, 0.8660254037844387076, 1.000000000000000000, 0.8660254037844387076, 1.000000000000000000, 0.8660254037844387076, 1.000000000000000000, 0.8660254037844387076, 1.000000000000000000, 0.8660254037844387076, 1.000000000000000000, 0.8660254037844387076, 1.000000000000000000, 0.8660254037844387076, 1.000000000000000000, 0.8660254037844387076, 1.000000000000000000, 0.8660254037844387076, 1.000000000000000000, 0.8660254037844387076, 1.000000000000000000, 0.8660254037844387076, 1.000000000000000000, 0.8660254037844387076, 1.000000000000000000, 0.8660254037844387076, 1.000000000000000000, 0.8660254037844387076, 1.000000000000000000, 0.8660254037844387076, 1.000000000000000000, 0.8660254037844387076, 1.000000000000000000, 0.8660254037844387076, 1.000000000000000000, 0.8660254037844387076, 1.000000000000000000, 0.8660254037844387076, 1.000000000000000000, 0.8660254037844387076, 1.000000000000000000, 0.8660254037844387076, 1.000000000000000000, 0.8660254037844387076, 1.000000000000000000, 0.8660254037844387076, 1.000000000000000000, 0.8660254037844387076, 1.000000000000000000, 0.8660254037844387076, 1.000000000000000000, 0.8660254037844387076, 1.000000000000000000, 0.8660254037844387076, 1.000000000000000000, 0.8660254037844387076, 1.000000000000000000, 0.8660254037844387076, 1.000000000000000000, 0.8660254037844387076, 1.000000000000000000, 0.8660254037844387076, 1.000000000000000000, 0.8660254037844387076, 1.000000000000000000, 0.8660254037844387076, 1.000000000000000000, 0.8660254037844387076, 1.000000000000000000, 0.8660254037844387076, 1.000000000000000000, 0.8660254037844387076, 1.000000000000000000, 0.8660254037844387076, 1.000000000000000000, 0.8660254037844387076, 1.000000000000000000, 0.8660254037844387076, 1.000000000000000000, 0.8660254037844387076, 1.000000000000000000, 0.8660254037844387076, 1.000000000000000000, 0.8660254037844387076, 1.000000000000000000, 0.8660254037844387076, 1.000000000000000000, 0.8660254037844387076, 1.000000000000000000, 0.8660254037844387076, 1.000000000000000000, 0.8660254037844387076, 1.000000000000000000, 0.8660254037844387076, 1.000000000000000000, 0.8660254037844387076, 1.000000000000000000, 0.8660254037844387076, 1.000000000000000000, 0.8660254037844387076, 1.000000000000000000, 0.8660254037844387076, 1.000000000000000000, 0.8660254037844387076, 1.000000000000000000, 0.8660254037844387076, 1.000000000000000000, 0.8660254037844387076, 1.000000000000000000, 0.8660254037844387076, 1.000000000000000000, 0.8660254037844387076, 1.000000000000000000, 0.8660254037844387076, 1.000000000000000000, 0.8660254037844387076, 1.000000000000000000, 0.8660254037844387076, 1.000000000000000000, 0.8660254037844387076, 1.000000000000000000, 0.8660254037844387076, 1.000000000000000000, 0.8660254037844387076, 1.000000000000000000, 0.8660254037844387076, 1.000000000000000000, 0.8660254037844387076, 1.000000000000000000, 0.8660254037844387076, 1.000000000000000000, 0.8660254037844387076, 1.000000000000000000, 0.8660254037844387076, 1.000000000000000000, 0.8660254037844387076, 1.000000000000000000, 0.8660254037844387076, 1.000000000000000000, 0.8660254037844387076, 1.000000000000000000, 0.8660254037844387076, 1.000000000000000000, 0.8660254037844387076, 1.000000000000000000, 0.8660254037844387076, 1.000000000000000000, 0.8660254037844387076, 1.000000000000000000, 0.8660254037844387076, 1.000000000000000000, 0.8660254037844387076, 1.000000000000000000, 0.8660254037844387076, 1.000000000000000000, 0.8660254037844387076, 1.000000000000000000, 0.8660254037844387076, 1.000000000000000000, 0.8660254037844387076, 1.000000000000000000, 0.8660254037844387076, 1.000000000000000000, 0.8660254037844387076, 1.000000000000000000, 0.8660254037844387076, 1.000000000000000000, 0.8660254037844387076, 1.000000000000000000, 0.8660254037844387076, 1.000000000000000000, 0.8660254037844387076, 1.000000000000000000, 0.8660254037844387076, 1.000000000000000000, 0.8660254037844387076, 1.000000000000000000, 0.8660254037844387076, 1.000000000000000000, 0.8660254037844387076, 1.000000000000000000, 0.8660254037844387076, 1.000000000000000000, 0.8660254037844387076, 1.000000000000000000, 0.8660254037844387076, 1.000000000000000000, 0.8660254037844387076, 1.000000000000000000, 0.8660254037844387076, 1.000000000000000000, 0.8660254037844387076, 1.000000000000000000, 0.8660254037844387076, 1.000000000000000000, 0.8660254037844387076, 1.000000000000000000, 0.8660254037844387076, 1.000000000000000000, 0.8660254037844387076, 1.000000000000000000, 0.8660254037844387076, 1.000000000000000000, 0.8660254037844387076, 1.000000000000000000, 0.8660254037844387076, 1.000000000000000000, 0.8660254037844387076, 1.000000000000000000, 0.8660254037844387076, 1.000000000000000000, 0.8660254037844387076, 1.000000000000000000, 0.8660254037844387076, 1.000000000000000000, 0.8660254037844387076, 1.000000000000000000, 0.8660254037844387076, 1.000000000000000000, 0.8660254037844387076, 1.000000000000000000, 0.8660254037844387076, 1.000000000000000000, 0.8660254037844387076, 1.000000000000000000, 0.8660254037844387076, 1.000000000000000000, 0.8660254037844387076, 1.000000000000000000, 0.8660254037844387076, 1.000000000000000000, 0.8660254037844387076, 1.000000000000000000, 0.8660254037844387076, 1.000000000000000000, 0.8660254037844387076, 1.000000000000000000, 0.8660254037844387076, 1.000000000000000000, 0.8660254037844387076, 1.000000000000000000, 0.8660254037844387076, 1.000000000000000000, 0.8660254037844387076, 1.000000000000000000, 0.8660254037844387076, 1.000000000000000000, 0.8660254037844387076, 1.000000000000000000, 0.8660254037844387076, 1.000000000000000000, 0.8660254037844387076, 1.000000000000000000, 0.8660254037844387076, 1.000000000000000000, 0.8660254037844387076, 1.000000000000000000, 0.8660254037844387076, 1.000000000000000000, 0.8660254037844387076, 1.000000000000000000, 0.8660254037844387076, 1.000000000000000000, 0.8660254037844387076, 1.000000000000000000, 0.8660254037844387076, 1.000000000000000000, 0.8660254037844387076, 1.000000000000000000, 0.8660254037844387076, 1.000000000000000000, 0.8660254037844387076, 1.000000000000000000, 0.8660254037844387076, 1.000000000000000000, 0.8660254037844387076, 1.000000000000000000, 0.8660254037844387076, 1.000000000000000000, 0.8660254037844387076, 1.000000000000000000, 0.8660254037844387076, 1.000000000000000000, 0.8660254037844387076, 1.000000000000000000, 0.8660254037844387076, 1.000000000000000000, 0.8660254037844387076, 1.000000000000000000, 0.8660254037844387076, 1.000000000000000000, 0.8660254037844387076, 1.000000000000000000, 0.8660254037844387076, 1.000000000000000000, 0.8660254037844387076, 1.000000000000000000, 0.8660254037844387076, 1.000000000000000000, 0.8660254037844387076, 1.000000000000000000, 0.8660254037844387076, 1.000000000000000000, 0.8660254037844387076, 1.000000000000000000, 0.8660254037844387076, 1.000000000000000000, 0.8660254037844387076, 1.000000000000000000, 0.8660254037844387076, 1.000000000000000000, 0.8660254037844387076, 1.000000000000000000, 0.8660254037844387076, 1.000000000000000000, 0.8660254037844387076, 1.000000000000000000, 0.8660254037844387076, 1.000000000000000000, 0.8660254037844387076, 1.000000000000000000, 0.8660254037844387076, 1.000000000000000000, 0.8660254037844387076, 1.000000000000000000, 0.8660254037844387076, 1.000000000000000000, 0.8660254037844387076, 1.000000000000000000, 0.8660254037844387076, 1.000000000000000000, 0.8660254037844387076, 1.000000000000000000, 0.8660254037844387076, 1.000000000000000000, 0.8660254037844387076, 1.000000000000000000, 0.8660254037844387076, 1.000000000000000000, 0.8660254037844387076, 1.000000000000000000, 0.8660254037844387076, 1.000000000000000000, 0.8660254037844387076, 1.000000000000000000, 0.8660254037844387076, 1.000000000000000000, 0.8660254037844387076, 1.000000000000000000, 0.8660254037844387076, 1.000000000000000000, 0.8660254037844387076, 1.000000000000000000, 0.8660254037844387076, 1.000000000000000000, 0.8660254037844387076, 1.000000000000000000, 0.8660254037844387076, 1.000000000000000000, 0.8660254037844387076, 1.000000000000000000, 0.8660254037844387076, 1.000000000000000000, 0.8660254037844387076, 1.000000000000000000, 0.8660254037844387076, 1.000000000000000000, 0.8660254037844387076, 1.000000000000000000, 0.8660254037844387076, 1.000000000000000000, 0.8660254037844387076, 1.000000000000000000, 0.8660254037844387076, 1.000000000000000000, 0.8660254037844387076, 1.000000000000000000, 0.8660254037844387076, 1.000000000000000000, 0.8660254037844387076, 1.000000000000000000, 0.8660254037844387076, 1.000000000000000000, 0.8660254037844387076, 1.000000000000000000, 0.8660254037844387076, 1.000000000000000000, 0.8660254037844387076, 1.000000000000000000, 0.8660254037844387076, 1.000000000000000000, 0.8660254037844387076, 1.000000000000000000, 0.8660254037844387076, 1.000000000000000000, 0.8660254037844387076, 1.000000000000000000, 0.8660254037844387076, 1.000000000000000000, 0.8660254037844387076, 1.000000000000000000, 0.8660254037844387076, 1.000000000000000000, 0.8660254037844387076, 1.000000000000000000, 0.8660254037844387076, 1.000000000000000000, 0.8660254037844387076, 1.000000000000000000, 0.8660254037844387076, 1.000000000000000000, 0.8660254037844387076, 1.000000000000000000, 0.8660254037844387076, 1.000000000000000000, 0.8660254037844387076, 1.000000000000000000, 0.8660254037844387076, 1.000000000000000000, 0.8660254037844387076, 1.000000000000000000, 0.8660254037844387076, 1.000000000000000000, 0.8660254037844387076, 1.000000000000000000, 0.8660254037844387076, 1.000000000000000000, 0.8660254037844387076, 1.000000000000000000, 0.8660254037844387076, 1.000000000000000000, 0.8660254037844387076, 1.000000000000000000, 0.8660254037844387076, 1.000000000000000000, 0.8660254037844387076, 1.000000000000000000, 0.8660254037844387076, 1.000000000000000000, 0.8660254037844387076, 1.000000000000000000, 0.8660254037844387076, 1.000000000000000000, 0.8660254037844387076, 1.000000000000000000, 0.8660254037844387076, 1.000000000000000000, 0.8660254037844387076, 1.000000000000000000, 0.8660254037844387076, 1.000000000000000000, 0.8660254037844387076, 1.000000000000000000, 0.8660254037844387076, 1.000000000000000000, 0.8660254037844387076, 1.000000000000000000, 0.8660254037844387076, 1.000000000000000000, 0.8660254037844387076, 1.000000000000000000, 0.8660254037844387076, 1.000000000000000000, 0.8660254037844387076, 1.000000000000000000, 0.8660254037844387076, 1.000000000000000000, 0.8660254037844387076, 1.000000000000000000, 0.8660254037844387076, 1.000000000000000000, 0.8660254037844387076, 1.000000000000000000, 0.8660254037844387076, 1.000000000000000000, 0.8660254037844387076, 1.000000000000000000, 0.8660254037844387076, 1.000000000000000000, 0.8660254037844387076, 1.000000000000000000, 0.8660254037844387076, 1.000000000000000000, 0.8660254037844387076, 1.000000000000000000, 0.8660254037844387076, 1.000000000000000000, 0.8660254037844387076, 1.000000000000000000, 0.8660254037844387076, 1.000000000000000000, 0.8660254037844387076, 1.000000000000000000, 0.8660254037844387076, 1.000000000000000000, 0.8660254037844387076, 1.000000000000000000, 0.8660254037844387076, 1.000000000000000000, 0.8660254037844387076, 1.000000000000000000, 0.8660254037844387076, 1.000000000000000000, 0.8660254037844387076, 1.000000000000000000, 0.8660254037844387076, 1.000000000000000000, 0.8660254037844387076, 1.000000000000000000, 0.8660254037844387076, 1.000000000000000000, 0.8660254037844387076, 1.000000000000000000, 0.8660254037844387076, 1.000000000000000000, 0.8660254037844387076, 1.000000000000000000, 0.8660254037844387076, 1.000000000000000000, 0.8660254037844387076, 1.000000000000000000, 0.8660254037844387076, 1.000000000000000000, 0.8660254037844387076, 1.000000000000000000, 0.8660254037844387076, 1.000000000000000000, 0.8660254037844387076, 1.000000000000000000, 0.8660254037844387076, 1.000000000000000000, 0.8660254037844387076, 1.000000000000000000, 0.8660254037844387076, 1.000000000000000000, 0.8660254037844387076, 1.000000000000000000, 0.8660254037844387076, 1.000000000000000000, 0.8660254037844387076, 1.000000000000000000, 0.8660254037844387076, 1.000000000000000000, 0.8660254037844387076, 1.000000000000000000, 0.8660254037844387076, 1.000000000000000000, 0.8660254037844387076, 1.000000000000000000, 0.8660254037844387076, 1.000000000000000000, 0.8660254037844387076, 1.000000000000000000, 0.8660254037844387076, 1.000000000000000000, 0.8660254037844387076, 1.000000000000000000, 0.8660254037844387076, 1.000000000000000000, 0.8660254037844387076, 1.000000000000000000, 0.8660254037844387076, 1.000000000000000000, 0.8970933713683293398, 0.9522730444008626893 ) ) 
 REPRESENTATION_ITEM ( '' )  );
#38310=CARTESIAN_POINT ( 'NONE',  ( 29.02500000122903145, 2.886751345948129099, -4.999999999999998224 ) ) ;
#38311=CARTESIAN_POINT ( 'NONE',  ( 23.55000000000000071, 4.330127018922192761, -2.499999999999997780 ) ) ;
#38313=CARTESIAN_POINT ( 'NONE',  ( 24.64687500061451431, -3.027376345333610441, -5.243569643749999898 ) ) ;
#38314=CARTESIAN_POINT ( 'NONE',  ( 1.626862140677534273E-15, 12.01250000000000107, -26.00000000000000355 ) ) ;
#38315=CARTESIAN_POINT ( 'NONE',  ( 11.73750000122903181, -4.330127018922194537, 2.499999999999995559 ) ) ;
#38316=CARTESIAN_POINT ( 'NONE',  ( 4.612500000000002487, 2.886751345948129099, -4.999999999999998224 ) ) ;
#38318=FACE_OUTER_BOUND ( 'NONE', #72955, .T. ) ;
#38319=CARTESIAN_POINT ( 'NONE',  ( 4.734375000614518214, -4.541064518000419881, 2.621784821874995952 ) ) ;
#38320=CARTESIAN_POINT ( 'NONE',  ( 26.42812500061451431, 6.421520780324663323E-16, -5.243569643749999010 ) ) ;
#38321=( BOUNDED_CURVE ( )  B_SPLINE_CURVE ( 2, ( #60265, #9679, #3039, #25570, #42561, #32212, #54746 ),
 .UNSPECIFIED., .F., .F. ) 
 B_SPLINE_CURVE_WITH_KNOTS ( ( 3, 2, 2, 3 ),
 ( 0.6333333333333333037, 0.6361111111111110716, 0.6388888888888889506, 0.6416666666666668295 ),
 .UNSPECIFIED. ) 
 CURVE ( )  GEOMETRIC_REPRESENTATION_ITEM ( )  RATIONAL_B_SPLINE_CURVE ( ( 1.000000000000000000, 0.8660254037844387076, 1.000000000000000000, 0.8660254037844387076, 1.000000000000000000, 0.8660254037844333785, 1.000000000000005329 ) ) 
 REPRESENTATION_ITEM ( '' )  );
#38323=CARTESIAN_POINT ( 'NONE',  ( 11.33437500061451608, 4.541064518000418104, 2.621784821874999949 ) ) ;
#38324=CARTESIAN_POINT ( 'NONE',  ( 3.678016528196605073, -3.387136381216779402, 3.825344076974688257 ) ) ;
#38325=CARTESIAN_POINT ( 'NONE',  ( 3.084375000614519191, 6.421520780324663323E-16, -5.243569643749999010 ) ) ;
#38326=CARTESIAN_POINT ( 'NONE',  ( 8.821875000614518569, -6.054752690667223547, -1.112240025338166033E-15 ) ) ;
#38327=CARTESIAN_POINT ( 'NONE',  ( 28.02187500061451431, 3.027376345333611329, 5.243569643749999010 ) ) ;
#38328=CARTESIAN_POINT ( 'NONE',  ( 4.243569643749999898, 12.34062500061459389, 32.45002607614398471 ) ) ;
#38329=CARTESIAN_POINT ( 'NONE',  ( 22.50000000000000000, -4.330127018922190985, -2.500000000000001332 ) ) ;
#38330=ORIENTED_EDGE ( 'NONE', *, *, #68955, .F. ) ;
#38331=CARTESIAN_POINT ( 'NONE',  ( 29.39999999999999858, 4.330127018922192761, -2.499999999999997780 ) ) ;
#38332=CARTESIAN_POINT ( 'NONE',  ( 3.937500000000000444, -2.886751345948129988, 4.999999999999997335 ) ) ;
#38334=CARTESIAN_POINT ( 'NONE',  ( 18.47812500061451857, 4.541064518000418104, 2.621784821874999949 ) ) ;
#38335=CARTESIAN_POINT ( 'NONE',  ( 10.86562500061451431, 3.027376345333611329, 5.243569643749999010 ) ) ;
#38337=CARTESIAN_POINT ( 'NONE',  ( 6.684375000614518392, 6.421520780324663323E-16, -5.243569643749999010 ) ) ;
#38338=CARTESIAN_POINT ( 'NONE',  ( 18.11250000122903359, -4.330127018922190985, -2.500000000000001332 ) ) ;
#38341=CARTESIAN_POINT ( 'NONE',  ( 7.771875000614516971, 3.027376345333611329, 5.243569643749999010 ) ) ;
#38342=CARTESIAN_POINT ( 'NONE',  ( 12.53437500061451537, 6.421520780324663323E-16, -5.243569643749999010 ) ) ;
#38343=CARTESIAN_POINT ( 'NONE',  ( 23.82187500061451502, 3.027376345333613106, -5.243569643749998122 ) ) ;
#38344=DIRECTION ( 'NONE',  ( 0.000000000000000000, 0.000000000000000000, -1.000000000000000000 ) ) ;
#38347=CARTESIAN_POINT ( 'NONE',  ( 16.99687500061451573, -3.027376345333610441, -5.243569643749999898 ) ) ;
#38349=CARTESIAN_POINT ( 'NONE',  ( 9.684375000614517504, -4.541064518000419881, 2.621784821874995952 ) ) ;
#38351=CARTESIAN_POINT ( 'NONE',  ( 20.58750000000000213, -2.886751345948129988, 4.999999999999997335 ) ) ;
#38353=CARTESIAN_POINT ( 'NONE',  ( -4.243569643749999898, 10.82187500061451857, -32.45002607614398471 ) ) ;
#38355=CARTESIAN_POINT ( 'NONE',  ( 12.51562500061451821, 3.027376345333613106, -5.243569643749998122 ) ) ;
#38356=CARTESIAN_POINT ( 'NONE',  ( 3.337499999999999911, 5.773502691896255534, 3.535250795749688894E-16 ) ) ;
#38357=CARTESIAN_POINT ( 'NONE',  ( -1.999999999999997113, 19.28750000122903430, -26.53589838486224295 ) ) ;
#38358=CARTESIAN_POINT ( 'NONE',  ( 28.35937500061451289, 4.541064518000418104, -2.621784821874998173 ) ) ;
#38359=CARTESIAN_POINT ( 'NONE',  ( 11.06250000000000000, 2.886751345948126879, 4.999999999999999112 ) ) ;
#38360=CARTESIAN_POINT ( 'NONE',  ( -3.999999999999999556, 15.57500000122903216, 27.69059892324149530 ) ) ;
#38361=CARTESIAN_POINT ( 'NONE',  ( 11.36250000122903536, -4.330127018922190985, -2.500000000000001332 ) ) ;
#38363=CARTESIAN_POINT ( 'NONE',  ( 22.17187500061451644, 3.027376345333611329, 5.243569643749999010 ) ) ;
#38364=CARTESIAN_POINT ( 'NONE',  ( 15.04687500061451644, -3.027376345333614438, 5.243569643749998122 ) ) ;
#38366=VERTEX_POINT ( 'NONE', #23505 ) ;
#38367=CARTESIAN_POINT ( 'NONE',  ( 16.34062500061451573, -3.027376345333614438, 5.243569643749998122 ) ) ;
#38369=CARTESIAN_POINT ( 'NONE',  ( 29.17500000122903714, 2.886751345948126879, 4.999999999999999112 ) ) ;
#38370=CARTESIAN_POINT ( 'NONE',  ( 15.75937500061451857, 4.541064518000418104, -2.621784821874998173 ) ) ;
#38371=CARTESIAN_POINT ( 'NONE',  ( 2.516032931661824179, 9.680092174376738967, -24.54948276669228591 ) ) ;
#38372=CARTESIAN_POINT ( 'NONE',  ( 15.92812500061451608, -4.541064518000419881, 2.621784821874995952 ) ) ;
#38373=FACE_BOUND ( 'NONE', #7615, .T. ) ;
#38374=EDGE_CURVE ( 'NONE', #58126, #40801, #50512, .T. ) ;
#38375=CARTESIAN_POINT ( 'NONE',  ( 27.57187500061451857, 3.027376345333611329, 5.243569643749999010 ) ) ;
#38376=CARTESIAN_POINT ( 'NONE',  ( 4.243569643749999898, 13.24062500061451786, 32.45002607614398471 ) ) ;
#38377=CARTESIAN_POINT ( 'NONE',  ( 16.43437500061451573, -4.541064518000419881, 2.621784821874995952 ) ) ;
#38378=CARTESIAN_POINT ( 'NONE',  ( 15.18750000122903465, 4.330127018922191873, 2.499999999999999556 ) ) ;
#38380=EDGE_CURVE ( 'NONE', #20653, #42194, #44968, .T. ) ;
#38381=CARTESIAN_POINT ( 'NONE',  ( 2.121784821874999061, 19.25937500061451857, -33.67503911421598417 ) ) ;
#38382=CARTESIAN_POINT ( 'NONE',  ( 20.78437500061451715, 4.541064518000418104, 2.621784821874999949 ) ) ;
#38383=CARTESIAN_POINT ( 'NONE',  ( 22.87500000122903288, 2.886751345948126879, 4.999999999999999112 ) ) ;
#38384=CARTESIAN_POINT ( 'NONE',  ( 16.84687500061451715, -3.027376345333614438, 5.243569643749998122 ) ) ;
#38385=CARTESIAN_POINT ( 'NONE',  ( 13.56562500061451892, 3.027376345333611329, 5.243569643749999010 ) ) ;
#38386=CARTESIAN_POINT ( 'NONE',  ( 4.243569643749999898, 12.43437500061451750, 30.00000000000000000 ) ) ;
#38387=CARTESIAN_POINT ( 'NONE',  ( 17.16562500061451502, 3.027376345333611329, 5.243569643749999010 ) ) ;
#38388=ORIENTED_EDGE ( 'NONE', *, *, #14786, .T. ) ;
#38389=EDGE_LOOP ( 'NONE', ( #2440, #21001, #695, #25704 ) ) ;
#38390=CARTESIAN_POINT ( 'NONE',  ( 19.61249999999999716, 2.886751345948126879, 4.999999999999999112 ) ) ;
#38391=CARTESIAN_POINT ( 'NONE',  ( 30.00000000000000000, 0.000000000000000000, 4.999999999999998224 ) ) ;
#38392=CARTESIAN_POINT ( 'NONE',  ( 24.62812500061451715, 6.421520780324663323E-16, -5.243569643749999010 ) ) ;
#38393=CARTESIAN_POINT ( 'NONE',  ( 6.028125000614517504, -4.541064518000419881, 2.621784821874995952 ) ) ;
#38394=CARTESIAN_POINT ( 'NONE',  ( 17.73750000122903359, 6.123233995736764310E-16, -4.999999999999998224 ) ) ;
#38395=CARTESIAN_POINT ( 'NONE',  ( 22.52812500061451573, 4.541064518000418104, 2.621784821874999949 ) ) ;
#38396=CARTESIAN_POINT ( 'NONE',  ( 23.69999999999999929, 0.000000000000000000, 4.999999999999998224 ) ) ;
#38397=CARTESIAN_POINT ( 'NONE',  ( 25.79062500061451502, -3.027376345333614438, 5.243569643749998122 ) ) ;
#38398=CARTESIAN_POINT ( 'NONE',  ( 5.015625000614518214, 3.027376345333611329, 5.243569643749999010 ) ) ;
#38399=ORIENTED_EDGE ( 'NONE', *, *, #11801, .T. ) ;
#38400=CARTESIAN_POINT ( 'NONE',  ( 23.72812500061451502, 6.421520780324663323E-16, -5.243569643749999010 ) ) ;
#38404=CARTESIAN_POINT ( 'NONE',  ( 11.06250000122903288, 4.330127018922192761, -2.499999999999997780 ) ) ;
#38405=CARTESIAN_POINT ( 'NONE',  ( -3.999999999999999556, 12.87500000122903465, -32.30940107675850470 ) ) ;
#38406=CARTESIAN_POINT ( 'NONE',  ( -4.243569643749999898, 18.50937500061451857, -30.00000000000000000 ) ) ;
#38407=AXIS2_PLACEMENT_3D ( 'NONE', #14443, #10735, #43632 ) ;
#38408=EDGE_CURVE ( 'NONE', #71251, #20715, #51448, .T. ) ;
#38409=CARTESIAN_POINT ( 'NONE',  ( 10.35000000000000142, -4.330127018922190985, -2.500000000000001332 ) ) ;
#38411=CARTESIAN_POINT ( 'NONE',  ( 10.80937500061451928, 4.541064518000418104, -2.621784821874998173 ) ) ;
#38412=CARTESIAN_POINT ( 'NONE',  ( 6.412500001229036073, -4.330127018922190985, -2.500000000000001332 ) ) ;
#38413=CARTESIAN_POINT ( 'NONE',  ( 12.12187500061451573, 3.027376345333613106, -5.243569643749998122 ) ) ;
#38414=CARTESIAN_POINT ( 'NONE',  ( 6.384375000614516793, 4.541064518000418104, 2.621784821874999949 ) ) ;
#38416=DIRECTION ( 'NONE',  ( -0.000000000000000000, -1.000000000000000000, -0.000000000000000000 ) ) ;
#38417=CARTESIAN_POINT ( 'NONE',  ( 10.47187500061451715, 3.027376345333611329, 5.243569643749999010 ) ) ;
#38418=CARTESIAN_POINT ( 'NONE',  ( 3.617702362022032325, -3.451409801779584452, 3.617702362022032325 ) ) ;
#38419=CARTESIAN_POINT ( 'NONE',  ( 18.74062500061451431, -3.027376345333610441, -5.243569643749999898 ) ) ;
#38421=CARTESIAN_POINT ( 'NONE',  ( -4.243569643749999898, 19.35312500061459318, 30.00000000000000000 ) ) ;
#38422=CARTESIAN_POINT ( 'NONE',  ( 23.85937500061451644, 4.541064518000418104, -2.621784821874998173 ) ) ;
#38423=CARTESIAN_POINT ( 'NONE',  ( -3.999999999999999112, 13.81250000122903465, -30.00000000000000000 ) ) ;
#38424=CARTESIAN_POINT ( 'NONE',  ( 29.28750000122903074, -4.330127018922194537, 2.499999999999995559 ) ) ;
#38426=CARTESIAN_POINT ( 'NONE',  ( 24.44062500061451715, -3.027376345333614438, 5.243569643749998122 ) ) ;
#38427=CARTESIAN_POINT ( 'NONE',  ( 17.16562500061451502, 3.027376345333611329, 5.243569643749999010 ) ) ;
#38429=CARTESIAN_POINT ( 'NONE',  ( 13.80937500061451750, -4.541064518000417216, -2.621784821875001281 ) ) ;
#38431=CARTESIAN_POINT ( 'NONE',  ( 26.70000000122903572, -2.886751345948125991, -5.000000000000000000 ) ) ;
#38432=CARTESIAN_POINT ( 'NONE',  ( 4.621875000614516615, 3.027376345333611329, 5.243569643749999010 ) ) ;
#38433=CARTESIAN_POINT ( 'NONE',  ( 15.15937500061451715, -4.541064518000417216, -2.621784821875001281 ) ) ;
#38435=CARTESIAN_POINT ( 'NONE',  ( -6.275039685470489619E-15, 18.31250000000000000, -26.00000000000000355 ) ) ;
#38436=CARTESIAN_POINT ( 'NONE',  ( 3.675000001229035362, -5.773502691896255534, -1.060575238724906372E-15 ) ) ;
#38437=CARTESIAN_POINT ( 'NONE',  ( 24.68437500061451573, 6.421520780324663323E-16, -5.243569643749999010 ) ) ;
#38438=CARTESIAN_POINT ( 'NONE',  ( 17.67187500061451644, 3.027376345333611329, 5.243569643749999010 ) ) ;
#38440=CARTESIAN_POINT ( 'NONE',  ( 27.59999999999999787, 4.330127018922192761, -2.499999999999997780 ) ) ;
#38441=CARTESIAN_POINT ( 'NONE',  ( 4.125000001229034652, -5.773502691896255534, -1.060575238724906372E-15 ) ) ;
#38442=CARTESIAN_POINT ( 'NONE',  ( 5.400000000000002132, -4.330127018922190985, -2.500000000000001332 ) ) ;
#38444=CARTESIAN_POINT ( 'NONE',  ( 19.97812500061451502, -4.541064518000419881, 2.621784821874995952 ) ) ;
#38445=CARTESIAN_POINT ( 'NONE',  ( 10.05000000000000071, 4.330127018922192761, -2.499999999999997780 ) ) ;
#38446=CARTESIAN_POINT ( 'NONE',  ( 3.740625000614516527, -3.027376345333614438, 5.243569643749998122 ) ) ;
#38447=CARTESIAN_POINT ( 'NONE',  ( 19.57500000000000284, 4.330127018922191873, 2.499999999999999556 ) ) ;
#38449=CARTESIAN_POINT ( 'NONE',  ( 23.85000000122903430, -2.886751345948129988, 4.999999999999997335 ) ) ;
#38450=CARTESIAN_POINT ( 'NONE',  ( 5.989600911063004851, 8.007829439449656306, 30.40685004427880855 ) ) ;
#38451=CARTESIAN_POINT ( 'NONE',  ( 28.80937500061451573, 4.541064518000418104, -2.621784821874998173 ) ) ;
#38454=CARTESIAN_POINT ( 'NONE',  ( 18.10312500061451502, 0.000000000000000000, 5.243569643749999010 ) ) ;
#38455=CARTESIAN_POINT ( 'NONE',  ( 25.45312500061451644, -4.541064518000417216, -2.621784821875001281 ) ) ;
#38456=CARTESIAN_POINT ( 'NONE',  ( 22.54687500061451999, 6.054752690667223547, 3.707466751127219781E-16 ) ) ;
#38457=CARTESIAN_POINT ( 'NONE',  ( 7.275000000000000355, 6.123233995736764310E-16, -4.999999999999998224 ) ) ;
#38458=CARTESIAN_POINT ( 'NONE',  ( 8.540625000614518569, 6.054752690667223547, 3.707466751127219781E-16 ) ) ;
#38459=CARTESIAN_POINT ( 'NONE',  ( 27.06562500061451004, 3.027376345333611329, 5.243569643749999010 ) ) ;
#38460=CARTESIAN_POINT ( 'NONE',  ( 15.83437500061451608, 4.541064518000418104, 2.621784821874999949 ) ) ;
#38461=CARTESIAN_POINT ( 'NONE',  ( 19.62187500061451573, -6.054752690667223547, -1.112240025338166033E-15 ) ) ;
#38463=CARTESIAN_POINT ( 'NONE',  ( -4.243569643749999898, 10.82187500061451857, 27.54997392385601529 ) ) ;
#38464=CARTESIAN_POINT ( 'NONE',  ( 22.23750000122903003, 6.123233995736764310E-16, -4.999999999999998224 ) ) ;
#38466=CARTESIAN_POINT ( 'NONE',  ( 11.65312500061451573, 4.541064518000418104, -2.621784821874998173 ) ) ;
#38467=CARTESIAN_POINT ( 'NONE',  ( 7.846875000614518036, -3.027376345333614438, 5.243569643749998122 ) ) ;
#38468=CARTESIAN_POINT ( 'NONE',  ( 8.334375000614516082, -4.541064518000419881, 2.621784821874995952 ) ) ;
#38469=( BOUNDED_CURVE ( )  B_SPLINE_CURVE ( 2, ( #34309, #28775, #51315, #45779, #33234, #68314, #16593, #27698, #10701 ),
 .UNSPECIFIED., .F., .F. ) 
 B_SPLINE_CURVE_WITH_KNOTS ( ( 3, 2, 2, 2, 3 ),
 ( 0.05434782608695652717, 0.05797101449275362389, 0.06521739130434782428, 0.07246376811594203160, 0.07608695652173913526 ),
 .UNSPECIFIED. ) 
 CURVE ( )  GEOMETRIC_REPRESENTATION_ITEM ( )  RATIONAL_B_SPLINE_CURVE ( ( 0.9330127018922194093, 0.9330127018922194093, 1.000000000000000000, 0.8660254037844387076, 1.000000000000000000, 0.8660254037844387076, 1.000000000000000000, 0.9330127018922191873, 0.9330127018922192983 ) ) 
 REPRESENTATION_ITEM ( '' )  );
#38471=EDGE_CURVE ( 'NONE', #24589, #5140, #3783, .T. ) ;
#38472=CARTESIAN_POINT ( 'NONE',  ( 26.97187500061451360, 3.027376345333613106, -5.243569643749998122 ) ) ;
#38473=CARTESIAN_POINT ( 'NONE',  ( 18.44062500061451715, 6.054752690667223547, 3.707466751127219781E-16 ) ) ;
#38474=CARTESIAN_POINT ( 'NONE',  ( 29.02500000122903145, 2.886751345948129099, -4.999999999999998224 ) ) ;
#38475=CARTESIAN_POINT ( 'NONE',  ( 3.159375000614518036, 4.541064518000418104, -2.621784821874998173 ) ) ;
#38476=CARTESIAN_POINT ( 'NONE',  ( 24.75937500061451502, 4.541064518000418104, -2.621784821874998173 ) ) ;
#38477=CARTESIAN_POINT ( 'NONE',  ( 19.64062500061451644, -3.027376345333610441, -5.243569643749999898 ) ) ;
#38478=CARTESIAN_POINT ( 'NONE',  ( -2.000000000000000000, 10.92500000000000071, 26.53589838486224650 ) ) ;
#38479=CARTESIAN_POINT ( 'NONE',  ( 23.69062500061451004, -3.027376345333610441, -5.243569643749999898 ) ) ;
#38480=CARTESIAN_POINT ( 'NONE',  ( 5.737500001229033586, 4.330127018922191873, 2.499999999999999556 ) ) ;
#38482=CARTESIAN_POINT ( 'NONE',  ( 29.66249999999999432, -5.773502691896255534, -1.060575238724906372E-15 ) ) ;
#38483=CARTESIAN_POINT ( 'NONE',  ( -3.999999999999999556, 15.91249999999999964, -32.30940107675850470 ) ) ;
#38485=CARTESIAN_POINT ( 'NONE',  ( 5.109375000614518214, 0.000000000000000000, 5.243569643749999010 ) ) ;
#38486=CYLINDRICAL_SURFACE ( 'NONE', #71515, 4.999999999999998224 ) ;
#38487=CARTESIAN_POINT ( 'NONE',  ( 11.95312500061451644, -4.541064518000417216, -2.621784821875001281 ) ) ;
#38488=CARTESIAN_POINT ( 'NONE',  ( 5.484375000614518214, 4.541064518000418104, 2.621784821874999949 ) ) ;
#38489=CARTESIAN_POINT ( 'NONE',  ( 25.65000000122903145, -2.886751345948129988, 4.999999999999997335 ) ) ;
#38490=CARTESIAN_POINT ( 'NONE',  ( 15.90937500061451892, 0.000000000000000000, 5.243569643749999010 ) ) ;
#38491=CARTESIAN_POINT ( 'NONE',  ( 28.56562500061451715, -6.054752690667223547, -1.112240025338166033E-15 ) ) ;
#38492=CARTESIAN_POINT ( 'NONE',  ( 30.00000000000000000, 0.000000000000000000, 4.999999999999998224 ) ) ;
#38493=CARTESIAN_POINT ( 'NONE',  ( 26.18437500061451573, 4.541064518000418104, 2.621784821874999949 ) ) ;
#38495=CARTESIAN_POINT ( 'NONE',  ( 13.11562500061451786, 3.027376345333611329, 5.243569643749999010 ) ) ;
#38496=ORIENTED_EDGE ( 'NONE', *, *, #37306, .F. ) ;
#38497=CARTESIAN_POINT ( 'NONE',  ( 11.12812500061451715, 6.421520780324663323E-16, -5.243569643749999010 ) ) ;
#38498=CARTESIAN_POINT ( 'NONE',  ( 7.490625000614516082, -3.027376345333610441, -5.243569643749999898 ) ) ;
#38500=CARTESIAN_POINT ( 'NONE',  ( 8.925000000000002487, -4.330127018922194537, 2.499999999999995559 ) ) ;
#38501=CARTESIAN_POINT ( 'NONE',  ( 4.875000001229034652, 2.886751345948126879, 4.999999999999999112 ) ) ;
#38502=CARTESIAN_POINT ( 'NONE',  ( 17.47499999999999787, -4.330127018922194537, 2.499999999999995559 ) ) ;
#38503=EDGE_CURVE ( 'NONE', #37474, #60642, #65518, .T. ) ;
#38504=CARTESIAN_POINT ( 'NONE',  ( 18.53437500061451715, 4.541064518000418104, 2.621784821874999949 ) ) ;
#38505=CARTESIAN_POINT ( 'NONE',  ( 13.61250000122903359, -4.330127018922190985, -2.500000000000001332 ) ) ;
#38507=VECTOR ( 'NONE', #43967, 1000.000000000000000 ) ;
#38508=CARTESIAN_POINT ( 'NONE',  ( 4.243569643749999010, 15.56562500061451715, -32.45002607614398471 ) ) ;
#38509=CARTESIAN_POINT ( 'NONE',  ( 0.000000000000000000, 20.00000000000000000, -30.00000000000000000 ) ) ;
#38511=CARTESIAN_POINT ( 'NONE',  ( 28.37812500061451715, 4.541064518000418104, 2.621784821874999949 ) ) ;
#38514=CARTESIAN_POINT ( 'NONE',  ( 13.69687500061451679, -3.027376345333614438, 5.243569643749998122 ) ) ;
#38515=( BOUNDED_CURVE ( )  B_SPLINE_CURVE ( 2, ( #70298, #42224, #61400, #10794, #32603, #42954, #72487, #10434, #33329 ),
 .UNSPECIFIED., .F., .F. ) 
 B_SPLINE_CURVE_WITH_KNOTS ( ( 3, 2, 2, 2, 3 ),
 ( 0.01086956521739130578, 0.01449275362318840597, 0.02173913043478260809, 0.02898550724637680848, 0.03260869565217391908 ),
 .UNSPECIFIED. ) 
 CURVE ( )  GEOMETRIC_REPRESENTATION_ITEM ( )  RATIONAL_B_SPLINE_CURVE ( ( 0.9330127018922194093, 0.9330127018922194093, 1.000000000000000000, 0.8660254037844387076, 1.000000000000000000, 0.8660254037844387076, 1.000000000000000000, 0.9330127018922191873, 0.9330127018922192983 ) ) 
 REPRESENTATION_ITEM ( '' )  );
#38516=CARTESIAN_POINT ( 'NONE',  ( 26.21249999999999858, 2.886751345948129099, -4.999999999999998224 ) ) ;
#38517=CARTESIAN_POINT ( 'NONE',  ( 10.34062500061451750, 6.054752690667223547, 3.707466751127219781E-16 ) ) ;
#38519=CARTESIAN_POINT ( 'NONE',  ( 21.38437500061451502, -4.541064518000419881, 2.621784821874995952 ) ) ;
#38521=CARTESIAN_POINT ( 'NONE',  ( 7.790625000614518569, -3.027376345333614438, 5.243569643749998122 ) ) ;
#38522=CARTESIAN_POINT ( 'NONE',  ( 12.15937500061451892, 4.541064518000418104, -2.621784821874998173 ) ) ;
#38523=EDGE_LOOP ( 'NONE', ( #52115, #9665, #65862, #16932 ) ) ;
#38524=CARTESIAN_POINT ( 'NONE',  ( 22.43437500061451573, 6.421520780324663323E-16, -5.243569643749999010 ) ) ;
#38525=DIRECTION ( 'NONE',  ( 0.000000000000000000, 0.000000000000000000, 1.000000000000000000 ) ) ;
#38527=CARTESIAN_POINT ( 'NONE',  ( 5.362500000000003375, -5.773502691896255534, -1.060575238724906372E-15 ) ) ;
#38528=CARTESIAN_POINT ( 'NONE',  ( 14.10000000122903252, -2.886751345948125991, -5.000000000000000000 ) ) ;
#38530=CARTESIAN_POINT ( 'NONE',  ( 10.98750000122903536, 6.123233995736764310E-16, -4.999999999999998224 ) ) ;
#38532=CARTESIAN_POINT ( 'NONE',  ( 12.41249999999999964, 2.886751345948126879, 4.999999999999999112 ) ) ;
#38533=CARTESIAN_POINT ( 'NONE',  ( 17.21249999999999858, 2.886751345948129099, -4.999999999999998224 ) ) ;
#38534=CARTESIAN_POINT ( 'NONE',  ( 12.82500000122903394, 2.886751345948129099, -4.999999999999998224 ) ) ;
#38535=CARTESIAN_POINT ( 'NONE',  ( 11.27812500061451573, 4.541064518000418104, 2.621784821874999949 ) ) ;
#38537=CARTESIAN_POINT ( 'NONE',  ( 10.12500000000000178, 4.330127018922191873, 2.499999999999999556 ) ) ;
#38538=CYLINDRICAL_SURFACE ( 'NONE', #20673, 3.999999999999996447 ) ;
#38539=CARTESIAN_POINT ( 'NONE',  ( -4.243569643749999898, 13.52187500061451786, -32.45002607614398471 ) ) ;
#38540=CARTESIAN_POINT ( 'NONE',  ( 3.403125000614518836, -4.541064518000417216, -2.621784821875001281 ) ) ;
#38542=CARTESIAN_POINT ( 'NONE',  ( 8.737500000000002487, 5.773502691896255534, 3.535250795749688894E-16 ) ) ;
#38543=CARTESIAN_POINT ( 'NONE',  ( 3.862500001229035362, 4.330127018922192761, -2.499999999999997780 ) ) ;
#38545=CARTESIAN_POINT ( 'NONE',  ( 24.74062500061451786, 6.054752690667223547, 3.707466751127219781E-16 ) ) ;
#38546=CARTESIAN_POINT ( 'NONE',  ( 29.28750000122903074, -4.330127018922194537, 2.499999999999995559 ) ) ;
#38547=VECTOR ( 'NONE', #49482, 1000.000000000000000 ) ;
#38549=CARTESIAN_POINT ( 'NONE',  ( 22.05937500061451573, 4.541064518000418104, -2.621784821874998173 ) ) ;
#38550=CARTESIAN_POINT ( 'NONE',  ( 17.87812500061451715, 6.421520780324663323E-16, -5.243569643749999010 ) ) ;
#38551=CARTESIAN_POINT ( 'NONE',  ( -4.243569643749999898, 10.80312500061459424, -30.00000000000000000 ) ) ;
#38552=CARTESIAN_POINT ( 'NONE',  ( 5.653125000614517504, -4.541064518000417216, -2.621784821875001281 ) ) ;
#38553=CARTESIAN_POINT ( 'NONE',  ( 3.290625000614516793, -3.027376345333614438, 5.243569643749998122 ) ) ;
#38555=CARTESIAN_POINT ( 'NONE',  ( 18.85312500061451502, 4.541064518000418104, -2.621784821874998173 ) ) ;
#38558=CARTESIAN_POINT ( 'NONE',  ( 14.22187500061451537, -6.054752690667223547, -1.112240025338166033E-15 ) ) ;
#38559=CARTESIAN_POINT ( 'NONE',  ( 14.33437500061451786, 6.421520780324663323E-16, -5.243569643749999010 ) ) ;
#38560=CARTESIAN_POINT ( 'NONE',  ( 23.29687500061451644, -3.027376345333610441, -5.243569643749999898 ) ) ;
#38561=VERTEX_POINT ( 'NONE', #30142 ) ;
#38562=CARTESIAN_POINT ( 'NONE',  ( -3.000416591977282496E-16, 12.99687500061451750, 25.09994784771203058 ) ) ;
#38563=CARTESIAN_POINT ( 'NONE',  ( 3.590625000614518836, 6.054752690667223547, 3.707466751127219781E-16 ) ) ;
#38564=CARTESIAN_POINT ( 'NONE',  ( 26.54062500061451146, 6.054752690667223547, 3.707466751127219781E-16 ) ) ;
#38565=CARTESIAN_POINT ( 'NONE',  ( 25.75312500061451715, 0.000000000000000000, 5.243569643749999010 ) ) ;
#38566=CARTESIAN_POINT ( 'NONE',  ( 8.437500001229034652, 4.330127018922191873, 2.499999999999999556 ) ) ;
#38567=CARTESIAN_POINT ( 'NONE',  ( 3.999999999999998668, 18.91249999999999787, 27.69059892324149175 ) ) ;
#38568=CARTESIAN_POINT ( 'NONE',  ( 5.146875000614517859, -3.027376345333614438, 5.243569643749998122 ) ) ;
#38570=CARTESIAN_POINT ( 'NONE',  ( 12.18750000122903465, -4.330127018922194537, 2.499999999999995559 ) ) ;
#38571=CARTESIAN_POINT ( 'NONE',  ( 8.400000001229035007, 5.773502691896255534, 3.535250795749688894E-16 ) ) ;
#38572=CARTESIAN_POINT ( 'NONE',  ( 3.478125000614517237, 6.421520780324663323E-16, -5.243569643749999010 ) ) ;
#38575=CARTESIAN_POINT ( 'NONE',  ( 12.15937500061451892, 4.541064518000418104, -2.621784821874998173 ) ) ;
#38578=CARTESIAN_POINT ( 'NONE',  ( 19.97812500061451502, -4.541064518000419881, 2.621784821874995952 ) ) ;
#38579=CARTESIAN_POINT ( 'NONE',  ( 13.02187500061451608, 3.027376345333613106, -5.243569643749998122 ) ) ;
#38580=CARTESIAN_POINT ( 'NONE',  ( 5.503125000614516260, 0.000000000000000000, 5.243569643749999010 ) ) ;
#38581=CARTESIAN_POINT ( 'NONE',  ( 21.34687500061451715, -3.027376345333614438, 5.243569643749998122 ) ) ;
#38582=CARTESIAN_POINT ( 'NONE',  ( 6.253125000614517148, 4.541064518000418104, -2.621784821874998173 ) ) ;
#38584=CARTESIAN_POINT ( 'NONE',  ( 5.550000001229032698, -2.886751345948125991, -5.000000000000000000 ) ) ;
#38585=CARTESIAN_POINT ( 'NONE',  ( 22.15312500061451573, 0.000000000000000000, 5.243569643749999010 ) ) ;
#38586=CARTESIAN_POINT ( 'NONE',  ( 3.999999999999998668, 18.57500000122903216, -32.30940107675850470 ) ) ;
#38587=CARTESIAN_POINT ( 'NONE',  ( 7.987500001229032698, 4.330127018922191873, 2.499999999999999556 ) ) ;
#38588=CARTESIAN_POINT ( 'NONE',  ( 16.41562500061451857, -6.054752690667223547, -1.112240025338166033E-15 ) ) ;
#38589=CARTESIAN_POINT ( 'NONE',  ( 14.95312500061451644, 0.000000000000000000, 5.243569643749999010 ) ) ;
#38591=CARTESIAN_POINT ( 'NONE',  ( 16.83749999999999858, 5.773502691896255534, 3.535250795749688894E-16 ) ) ;
#38592=CARTESIAN_POINT ( 'NONE',  ( 10.57500000122903572, 2.886751345948129099, -4.999999999999998224 ) ) ;
#38593=CARTESIAN_POINT ( 'NONE',  ( 8.465625000614515727, 3.027376345333613106, -5.243569643749998122 ) ) ;
#38594=CARTESIAN_POINT ( 'NONE',  ( 10.34062500061451750, 6.054752690667223547, 3.707466751127219781E-16 ) ) ;
#38596=CARTESIAN_POINT ( 'NONE',  ( 21.78750000122903074, 6.123233995736764310E-16, -4.999999999999998224 ) ) ;
#38597=CARTESIAN_POINT ( 'NONE',  ( -2.121784821874999949, 14.38437500061451679, -33.67503911421598417 ) ) ;
#38598=DIRECTION ( 'NONE',  ( 0.000000000000000000, 0.000000000000000000, -1.000000000000000000 ) ) ;
#38599=CARTESIAN_POINT ( 'NONE',  ( 5.212500001229032343, 4.330127018922192761, -2.499999999999997780 ) ) ;
#38601=CARTESIAN_POINT ( 'NONE',  ( 4.471875000614518925, 3.027376345333613106, -5.243569643749998122 ) ) ;
#38602=CARTESIAN_POINT ( 'NONE',  ( 21.15937500061451715, 4.541064518000418104, -2.621784821874998173 ) ) ;
#38604=CARTESIAN_POINT ( 'NONE',  ( 16.64062500061451289, 6.054752690667223547, 3.707466751127219781E-16 ) ) ;
#38605=B_SPLINE_CURVE_WITH_KNOTS ( 'NONE', 3,
 ( #27466, #66997, #43725, #72160, #44826, #22274, #60325, #49270, #32635, #66248 ),
 .UNSPECIFIED., .F., .F.,
 ( 4, 3, 3, 4 ),
 ( 4.336808689942017255E-19, 5.718089424411147026E-05, 8.577416319149967013E-05, 0.0001143682889712568761 ),
 .UNSPECIFIED. ) ;
#38607=CARTESIAN_POINT ( 'NONE',  ( -1.071796769724488563, 15.59240381056766722, -26.00000000000000000 ) ) ;
#38608=FACE_OUTER_BOUND ( 'NONE', #64694, .T. ) ;
#38609=CARTESIAN_POINT ( 'NONE',  ( 29.07187500061451502, -6.054752690667223547, -1.112240025338166033E-15 ) ) ;
#38611=CARTESIAN_POINT ( 'NONE',  ( 14.54062500061451679, -3.027376345333614438, 5.243569643749998122 ) ) ;
#38612=CARTESIAN_POINT ( 'NONE',  ( 12.27187500061451786, 3.027376345333611329, 5.243569643749999010 ) ) ;
#38614=CARTESIAN_POINT ( 'NONE',  ( 22.27499999999999858, 4.330127018922191873, 2.499999999999999556 ) ) ;
#38615=CARTESIAN_POINT ( 'NONE',  ( 23.69062500061451004, -3.027376345333610441, -5.243569643749999898 ) ) ;
#38616=CARTESIAN_POINT ( 'NONE',  ( 3.242103837493086330E-14, 11.33750000000000213, -34.00000000000000000 ) ) ;
#38617=LINE ( 'NONE', #48973, #54928 ) ;
#38618=CARTESIAN_POINT ( 'NONE',  ( 12.78749999999999964, 5.773502691896255534, 3.535250795749688894E-16 ) ) ;
#38619=CARTESIAN_POINT ( 'NONE',  ( 25.27500000122903145, -5.773502691896255534, -1.060575238724906372E-15 ) ) ;
#38620=CARTESIAN_POINT ( 'NONE',  ( 19.15312500061451573, -4.541064518000417216, -2.621784821875001281 ) ) ;
#38623=CARTESIAN_POINT ( 'NONE',  ( 20.88749999999999929, 5.773502691896255534, 3.535250795749688894E-16 ) ) ;
#38624=CARTESIAN_POINT ( 'NONE',  ( 22.43437500061451573, 6.421520780324663323E-16, -5.243569643749999010 ) ) ;
#38625=CARTESIAN_POINT ( 'NONE',  ( 28.56562500061451715, -6.054752690667223547, -1.112240025338166033E-15 ) ) ;
#38627=CARTESIAN_POINT ( 'NONE',  ( 3.999999999999998668, 18.01249999999999929, -32.30940107675850470 ) ) ;
#38628=CARTESIAN_POINT ( 'NONE',  ( 10.15312500061451750, -4.541064518000417216, -2.621784821875001281 ) ) ;
#38629=CARTESIAN_POINT ( 'NONE',  ( 3.390184931900214860, 3.675138926287994767, 3.390184931900133147 ) ) ;
#38631=CARTESIAN_POINT ( 'NONE',  ( 16.87500000000000000, 4.330127018922191873, 2.499999999999999556 ) ) ;
#38632=CARTESIAN_POINT ( 'NONE',  ( 25.42500000000000071, 4.330127018922191873, 2.499999999999999556 ) ) ;
#38633=CARTESIAN_POINT ( 'NONE',  ( 3.505568899737581567, -3.565293584294087825, -3.783441448803638529 ) ) ;
#38634=CARTESIAN_POINT ( 'NONE',  ( 4.021875000614516082, 3.027376345333613106, -5.243569643749998122 ) ) ;
#38635=CARTESIAN_POINT ( 'NONE',  ( 27.42187500061451644, 3.027376345333613106, -5.243569643749998122 ) ) ;
#38636=ORIENTED_EDGE ( 'NONE', *, *, #43935, .T. ) ;
#38637=CARTESIAN_POINT ( 'NONE',  ( 25.67812500061451431, 4.541064518000418104, 2.621784821874999949 ) ) ;
#38638=CARTESIAN_POINT ( 'NONE',  ( 27.72187500061451715, -6.054752690667223547, -1.112240025338166033E-15 ) ) ;
#38639=CARTESIAN_POINT ( 'NONE',  ( -2.121784821874996840, 18.97812500061459318, -26.32496088578401583 ) ) ;
#38640=CARTESIAN_POINT ( 'NONE',  ( 14.84999999999999964, -4.330127018922190985, -2.500000000000001332 ) ) ;
#38641=CARTESIAN_POINT ( 'NONE',  ( 10.60312500061451679, -4.541064518000417216, -2.621784821875001281 ) ) ;
#38643=CARTESIAN_POINT ( 'NONE',  ( 7.124999999999999112, -4.330127018922194537, 2.499999999999995559 ) ) ;
#38644=CARTESIAN_POINT ( 'NONE',  ( 27.55312500061451786, 0.000000000000000000, 5.243569643749999010 ) ) ;
#38645=CARTESIAN_POINT ( 'NONE',  ( 16.98750000122903359, 4.330127018922191873, 2.499999999999999556 ) ) ;
#38648=CARTESIAN_POINT ( 'NONE',  ( 4.265625000614517326, -6.054752690667223547, -1.112240025338166033E-15 ) ) ;
#38649=CARTESIAN_POINT ( 'NONE',  ( 21.23437500061451644, 4.541064518000418104, 2.621784821874999949 ) ) ;
#38650=CARTESIAN_POINT ( 'NONE',  ( -3.000416591977282496E-16, 15.24687500061451928, 25.09994784771203058 ) ) ;
#38651=CARTESIAN_POINT ( 'NONE',  ( 21.23437500061451644, 4.541064518000418104, 2.621784821874999949 ) ) ;
#38652=CARTESIAN_POINT ( 'NONE',  ( 3.600000000000002309, -4.330127018922190985, -2.500000000000001332 ) ) ;
#38653=CARTESIAN_POINT ( 'NONE',  ( -4.243569643749999898, 19.85937500061451644, 30.00000000000000000 ) ) ;
#38654=CARTESIAN_POINT ( 'NONE',  ( 9.028125000614517504, 4.541064518000418104, 2.621784821874999949 ) ) ;
#38656=EDGE_CURVE ( 'NONE', #69731, #493, #44344, .T. ) ;
#38657=CARTESIAN_POINT ( 'NONE',  ( 7.959375000614516971, -4.541064518000417216, -2.621784821875001281 ) ) ;
#38658=DIRECTION ( 'NONE',  ( 0.000000000000000000, 0.000000000000000000, 1.000000000000000000 ) ) ;
#38659=ADVANCED_FACE ( 'NONE', ( #24590 ), #12781, .F. ) ;
#38660=CARTESIAN_POINT ( 'NONE',  ( 7.678125000614516082, 4.541064518000418104, 2.621784821874999949 ) ) ;
#38661=CARTESIAN_POINT ( 'NONE',  ( 12.53437500061451537, 6.421520780324663323E-16, -5.243569643749999010 ) ) ;
#38663=CARTESIAN_POINT ( 'NONE',  ( 20.81250000122903643, -4.330127018922190985, -2.500000000000001332 ) ) ;
#38664=CARTESIAN_POINT ( 'NONE',  ( 7.059375000614518392, -4.541064518000417216, -2.621784821875001281 ) ) ;
#38665=CARTESIAN_POINT ( 'NONE',  ( 10.56562500061451715, -6.054752690667223547, -1.112240025338166033E-15 ) ) ;
#38666=CARTESIAN_POINT ( 'NONE',  ( 6.590625000614520168, -3.027376345333610441, -5.243569643749999898 ) ) ;
#38668=CARTESIAN_POINT ( 'NONE',  ( 19.28437500061451360, 6.421520780324663323E-16, -5.243569643749999010 ) ) ;
#38669=CARTESIAN_POINT ( 'NONE',  ( 4.000000000000000000, 13.10000000122903430, 32.30940107675849760 ) ) ;
#38670=CARTESIAN_POINT ( 'NONE',  ( 12.06562500061451537, 3.027376345333613106, -5.243569643749998122 ) ) ;
#38672=CARTESIAN_POINT ( 'NONE',  ( 28.50937500061451502, 0.000000000000000000, 5.243569643749999010 ) ) ;
#38673=CARTESIAN_POINT ( 'NONE',  ( -4.243569643749998122, 12.69687500061451857, -27.54997392385601174 ) ) ;
#38674=EDGE_CURVE ( 'NONE', #52475, #3090, #19035, .T. ) ;
#38675=CARTESIAN_POINT ( 'NONE',  ( 15.78750000122903430, -4.330127018922194537, 2.499999999999995559 ) ) ;
#38676=CARTESIAN_POINT ( 'NONE',  ( -3.000416591977282496E-16, 14.29062500061451679, -34.90005215228797653 ) ) ;
#38677=CARTESIAN_POINT ( 'NONE',  ( 14.28750000122903430, 4.330127018922191873, 2.499999999999999556 ) ) ;
#38678=CARTESIAN_POINT ( 'NONE',  ( 11.20312500061451644, 4.541064518000418104, -2.621784821874998173 ) ) ;
#38679=ORIENTED_EDGE ( 'NONE', *, *, #33576, .T. ) ;
#38680=CARTESIAN_POINT ( 'NONE',  ( 12.75000000000000178, 4.330127018922192761, -2.499999999999997780 ) ) ;
#38682=CARTESIAN_POINT ( 'NONE',  ( 22.26562500061451644, -6.054752690667223547, -1.112240025338166033E-15 ) ) ;
#38683=CARTESIAN_POINT ( 'NONE',  ( 7.771875000614516082, 3.027376345333611329, 5.243569643749999010 ) ) ;
#38684=EDGE_CURVE ( 'NONE', #16881, #46843, #58565, .T. ) ;
#38685=CARTESIAN_POINT ( 'NONE',  ( 10.46250000122903323, -4.330127018922190985, -2.500000000000001332 ) ) ;
#38686=CARTESIAN_POINT ( 'NONE',  ( 19.05000000122903359, -2.886751345948125991, -5.000000000000000000 ) ) ;
#38687=CARTESIAN_POINT ( 'NONE',  ( 16.26562500061451289, 3.027376345333611329, 5.243569643749999010 ) ) ;
#38688=( BOUNDED_CURVE ( )  B_SPLINE_CURVE ( 2, ( #71349, #25545, #20724, #60243, #2649, #65803, #37723 ),
 .UNSPECIFIED., .F., .F. ) 
 B_SPLINE_CURVE_WITH_KNOTS ( ( 3, 2, 2, 3 ),
 ( 0.8333333333333334814, 0.8361111111111112493, 0.8388888888888890172, 0.8416666666666667851 ),
 .UNSPECIFIED. ) 
 CURVE ( )  GEOMETRIC_REPRESENTATION_ITEM ( )  RATIONAL_B_SPLINE_CURVE ( ( 0.9999999999999946709, 0.8660254037844440367, 1.000000000000000000, 0.8660254037844387076, 1.000000000000000000, 0.8660254037844333785, 1.000000000000005329 ) ) 
 REPRESENTATION_ITEM ( '' )  );
#38689=CARTESIAN_POINT ( 'NONE',  ( 19.07812500061451644, -4.541064518000419881, 2.621784821874995952 ) ) ;
#38690=CARTESIAN_POINT ( 'NONE',  ( 26.06250000122903288, 0.000000000000000000, 4.999999999999998224 ) ) ;
#38691=CARTESIAN_POINT ( 'NONE',  ( 27.26250000122903216, 4.330127018922192761, -2.499999999999997780 ) ) ;
#38692=CARTESIAN_POINT ( 'NONE',  ( 22.05000000000000071, -4.330127018922190985, -2.500000000000001332 ) ) ;
#38694=CARTESIAN_POINT ( 'NONE',  ( 26.07187500061451857, 3.027376345333613106, -5.243569643749998122 ) ) ;
#38696=CARTESIAN_POINT ( 'NONE',  ( 12.71250000122903145, -4.330127018922190985, -2.500000000000001332 ) ) ;
#38697=CARTESIAN_POINT ( 'NONE',  ( 28.99687500061451573, -3.027376345333614438, 5.243569643749998122 ) ) ;
#38698=CYLINDRICAL_SURFACE ( 'NONE', #7796, 4.999999999999998224 ) ;
#38699=CARTESIAN_POINT ( 'NONE',  ( 4.246875000614519280, -3.027376345333614438, 5.243569643749998122 ) ) ;
#38700=CARTESIAN_POINT ( 'NONE',  ( 24.62812500061451715, 6.421520780324663323E-16, -5.243569643749999010 ) ) ;
#38703=CARTESIAN_POINT ( 'NONE',  ( 9.759375000614516793, -4.541064518000417216, -2.621784821875001281 ) ) ;
#38705=CARTESIAN_POINT ( 'NONE',  ( 3.196875000614516793, 6.054752690667223547, 3.707466751127219781E-16 ) ) ;
#38706=CARTESIAN_POINT ( 'NONE',  ( 5.296875000614518214, -3.027376345333610441, -5.243569643749999898 ) ) ;
#38707=CARTESIAN_POINT ( 'NONE',  ( 27.75937500061451502, -4.541064518000417216, -2.621784821875001281 ) ) ;
#38708=CARTESIAN_POINT ( 'NONE',  ( -4.243569643749998122, 10.84062500061459389, 32.45002607614398471 ) ) ;
#38710=CARTESIAN_POINT ( 'NONE',  ( 18.93750000000000000, -2.886751345948125991, -5.000000000000000000 ) ) ;
#38712=CARTESIAN_POINT ( 'NONE',  ( 28.35000000000000142, -4.330127018922190985, -2.500000000000001332 ) ) ;
#38713=CARTESIAN_POINT ( 'NONE',  ( 28.77187500061451431, 3.027376345333613106, -5.243569643749998122 ) ) ;
#38714=ORIENTED_EDGE ( 'NONE', *, *, #68596, .F. ) ;
#38715=CARTESIAN_POINT ( 'NONE',  ( 16.94062500061451715, -3.027376345333610441, -5.243569643749999898 ) ) ;
#38716=CARTESIAN_POINT ( 'NONE',  ( 7.678125000614516082, 4.541064518000418104, 2.621784821874999949 ) ) ;
#38718=CARTESIAN_POINT ( 'NONE',  ( 5.971875000614516260, 3.027376345333611329, 5.243569643749999010 ) ) ;
#38719=CARTESIAN_POINT ( 'NONE',  ( 17.47500000122903430, 2.886751345948126879, 4.999999999999999112 ) ) ;
#38720=CARTESIAN_POINT ( 'NONE',  ( 7.509375000614517681, -4.541064518000417216, -2.621784821875001281 ) ) ;
#38721=CARTESIAN_POINT ( 'NONE',  ( 11.29687500061451644, 6.054752690667223547, 3.707466751127219781E-16 ) ) ;
#38722=CARTESIAN_POINT ( 'NONE',  ( 24.79687500061451999, 6.054752690667223547, 3.707466751127219781E-16 ) ) ;
#38726=CARTESIAN_POINT ( 'NONE',  ( 18.04687500061451999, 6.054752690667223547, 3.707466751127219781E-16 ) ) ;
#38728=CARTESIAN_POINT ( 'NONE',  ( 8.334375000614516082, -4.541064518000419881, 2.621784821874995952 ) ) ;
#38730=CARTESIAN_POINT ( 'NONE',  ( 21.97500000000000142, -4.330127018922194537, 2.499999999999995559 ) ) ;
#38732=CARTESIAN_POINT ( 'NONE',  ( -3.999999999999997335, 9.800000001229033586, -27.69059892324149530 ) ) ;
#38734=CARTESIAN_POINT ( 'NONE',  ( 11.72812500061451857, 4.541064518000418104, 2.621784821874999949 ) ) ;
#38735=CARTESIAN_POINT ( 'NONE',  ( 27.98437500061451289, 4.541064518000418104, 2.621784821874999949 ) ) ;
#38737=CARTESIAN_POINT ( 'NONE',  ( 27.94687500061451502, 6.054752690667223547, 3.707466751127219781E-16 ) ) ;
#38738=CARTESIAN_POINT ( 'NONE',  ( 10.23750000000000071, -2.886751345948129988, 4.999999999999997335 ) ) ;
#38739=CARTESIAN_POINT ( 'NONE',  ( -3.999999999999999112, 15.61250000122903359, 30.00000000000000000 ) ) ;
#38740=CARTESIAN_POINT ( 'NONE',  ( 9.787500001229036073, 4.330127018922191873, 2.499999999999999556 ) ) ;
#38741=CARTESIAN_POINT ( 'NONE',  ( 21.08437500061451786, 6.421520780324663323E-16, -5.243569643749999010 ) ) ;
#38742=CARTESIAN_POINT ( 'NONE',  ( 13.28437500061451715, -4.541064518000419881, 2.621784821874995952 ) ) ;
#38743=CARTESIAN_POINT ( 'NONE',  ( -1.071796769724488563, 12.44240381056766864, 34.00000000000000000 ) ) ;
#38744=ORIENTED_EDGE ( 'NONE', *, *, #25043, .T. ) ;
#38745=CARTESIAN_POINT ( 'NONE',  ( 15.40312500061451573, 0.000000000000000000, 5.243569643749999010 ) ) ;
#38746=CARTESIAN_POINT ( 'NONE',  ( 27.56250000122902932, -4.330127018922190985, -2.500000000000001332 ) ) ;
#38747=CARTESIAN_POINT ( 'NONE',  ( 14.44687500061451679, 6.054752690667223547, 3.707466751127219781E-16 ) ) ;
#38748=CARTESIAN_POINT ( 'NONE',  ( 2.990625000614519191, -3.027376345333610441, -5.243569643749999898 ) ) ;
#38749=CARTESIAN_POINT ( 'NONE',  ( 18.10312500061451502, 0.000000000000000000, 5.243569643749999010 ) ) ;
#38751=CARTESIAN_POINT ( 'NONE',  ( 25.13437500061451502, 6.421520780324663323E-16, -5.243569643749999010 ) ) ;
#38752=CARTESIAN_POINT ( 'NONE',  ( -2.121784821874999949, 11.62812500061451715, 26.32496088578401938 ) ) ;
#38753=CARTESIAN_POINT ( 'NONE',  ( 16.39687500061451786, -3.027376345333614438, 5.243569643749998122 ) ) ;
#38754=CARTESIAN_POINT ( 'NONE',  ( 14.17500000122903536, 2.886751345948129099, -4.999999999999998224 ) ) ;
#38756=CARTESIAN_POINT ( 'NONE',  ( 4.243569643749999898, 18.24687500061451928, -27.54997392385601529 ) ) ;
#38757=ADVANCED_FACE ( 'NONE', ( #64480 ), #47138, .F. ) ;
#38758=CARTESIAN_POINT ( 'NONE',  ( 19.92187500061451644, 3.027376345333611329, 5.243569643749999010 ) ) ;
#38759=CARTESIAN_POINT ( 'NONE',  ( 22.57500000122903572, -5.773502691896255534, -1.060575238724906372E-15 ) ) ;
#38760=( BOUNDED_CURVE ( )  B_SPLINE_CURVE ( 2, ( #28420, #356, #55775, #61667, #29151, #23230, #44703 ),
 .UNSPECIFIED., .F., .T. ) 
 B_SPLINE_CURVE_WITH_KNOTS ( ( 3, 2, 2, 3 ),
 ( 0.9770077471373426192, 0.9777777777777777457, 0.9805555555555555136, 0.9812411888349016342 ),
 .UNSPECIFIED. ) 
 CURVE ( )  GEOMETRIC_REPRESENTATION_ITEM ( )  RATIONAL_B_SPLINE_CURVE ( ( 0.9463123399370627631, 0.9628607641146736951, 1.000000000000000000, 0.8660254037844387076, 1.000000000000000000, 0.9669313209691547950, 0.9501871924685547643 ) ) 
 REPRESENTATION_ITEM ( '' )  );
#38761=CARTESIAN_POINT ( 'NONE',  ( 17.48437500061451999, 6.421520780324663323E-16, -5.243569643749999010 ) ) ;
#38762=CARTESIAN_POINT ( 'NONE',  ( 2.121784821874999061, 12.50937500061451857, 26.32496088578401583 ) ) ;
#38763=CARTESIAN_POINT ( 'NONE',  ( 17.09062500061451573, 6.054752690667223547, 3.707466751127219781E-16 ) ) ;
#38764=ORIENTED_EDGE ( 'NONE', *, *, #70404, .T. ) ;
#38765=ORIENTED_EDGE ( 'NONE', *, *, #41986, .F. ) ;
#38766=CARTESIAN_POINT ( 'NONE',  ( 21.07499999999999929, -4.330127018922194537, 2.499999999999995559 ) ) ;
#38767=CARTESIAN_POINT ( 'NONE',  ( 28.23750000122903359, 4.330127018922191873, 2.499999999999999556 ) ) ;
#38768=CARTESIAN_POINT ( 'NONE',  ( 25.45312500061451644, -4.541064518000417216, -2.621784821875001281 ) ) ;
#38769=CARTESIAN_POINT ( 'NONE',  ( 4.715625000614516615, -6.054752690667223547, -1.112240025338166033E-15 ) ) ;
#38770=CARTESIAN_POINT ( 'NONE',  ( 16.57500000122903216, 2.886751345948126879, 4.999999999999999112 ) ) ;
#38771=CARTESIAN_POINT ( 'NONE',  ( 22.97812500061451857, 4.541064518000418104, 2.621784821874999949 ) ) ;
#38772=CARTESIAN_POINT ( 'NONE',  ( 19.83750000000000213, -2.886751345948125991, -5.000000000000000000 ) ) ;
#38773=CARTESIAN_POINT ( 'NONE',  ( 26.61562500061451786, 3.027376345333611329, 5.243569643749999010 ) ) ;
#38774=CARTESIAN_POINT ( 'NONE',  ( 4.940625000614515372, 6.054752690667223547, 3.707466751127219781E-16 ) ) ;
#38775=ORIENTED_EDGE ( 'NONE', *, *, #52924, .T. ) ;
#38776=CARTESIAN_POINT ( 'NONE',  ( 26.85000000122903430, 5.773502691896255534, 3.535250795749688401E-16 ) ) ;
#38777=CARTESIAN_POINT ( 'NONE',  ( 3.290625000614516793, -3.027376345333614438, 5.243569643749998122 ) ) ;
#38778=( BOUNDED_CURVE ( )  B_SPLINE_CURVE ( 2, ( #17029, #39587, #34026, #56563, #5959, #49582, #28493 ),
 .UNSPECIFIED., .F., .F. ) 
 B_SPLINE_CURVE_WITH_KNOTS ( ( 3, 2, 2, 3 ),
 ( 0.5500000000000000444, 0.5527777777777778123, 0.5555555555555555802, 0.5583333333333333481 ),
 .UNSPECIFIED. ) 
 CURVE ( )  GEOMETRIC_REPRESENTATION_ITEM ( )  RATIONAL_B_SPLINE_CURVE ( ( 1.000000000000000000, 0.8660254037844387076, 1.000000000000000000, 0.8660254037844387076, 1.000000000000000000, 0.8660254037844387076, 1.000000000000000000 ) ) 
 REPRESENTATION_ITEM ( '' )  );
#38780=CYLINDRICAL_SURFACE ( 'NONE', #24096, 3.999999999999996447 ) ;
#38781=CARTESIAN_POINT ( 'NONE',  ( -3.999999999999997335, 10.70000000122903394, -27.69059892324149175 ) ) ;
#38782=CARTESIAN_POINT ( 'NONE',  ( -4.243569643749999898, 18.92187500061451644, -32.45002607614398471 ) ) ;
#38783=EDGE_CURVE ( 'NONE', #40333, #8864, #69371, .T. ) ;
#38784=CARTESIAN_POINT ( 'NONE',  ( 7.800000000000001599, 4.330127018922192761, -2.499999999999997780 ) ) ;
#38785=CARTESIAN_POINT ( 'NONE',  ( 8.859375000614518214, -4.541064518000417216, -2.621784821875001281 ) ) ;
#38786=CARTESIAN_POINT ( 'NONE',  ( 6.075000001229034829, 2.886751345948129099, -4.999999999999998224 ) ) ;
#38787=CARTESIAN_POINT ( 'NONE',  ( 13.09687500061451892, 6.054752690667223547, 3.707466751127219781E-16 ) ) ;
#38788=CARTESIAN_POINT ( 'NONE',  ( 4.021875000614516082, 3.027376345333613106, -5.243569643749998122 ) ) ;
#38790=CARTESIAN_POINT ( 'NONE',  ( 19.65000000000000213, 0.000000000000000000, 4.999999999999998224 ) ) ;
#38791=CARTESIAN_POINT ( 'NONE',  ( 10.17187500061451999, -6.054752690667223547, -1.112240025338166033E-15 ) ) ;
#38792=CARTESIAN_POINT ( 'NONE',  ( 13.27500000000000213, 4.330127018922191873, 2.499999999999999556 ) ) ;
#38793=EDGE_CURVE ( 'NONE', #47914, #11866, #66561, .T. ) ;
#38794=CARTESIAN_POINT ( 'NONE',  ( 19.41562500061451146, 3.027376345333611329, 5.243569643749999010 ) ) ;
#38797=CARTESIAN_POINT ( 'NONE',  ( 24.72187500061451360, 3.027376345333613106, -5.243569643749998122 ) ) ;
#38798=CARTESIAN_POINT ( 'NONE',  ( 1.071796769724490783, 19.41740381056767006, 26.00000000000000355 ) ) ;
#38799=CARTESIAN_POINT ( 'NONE',  ( 28.08750000122903145, 6.123233995736764310E-16, -4.999999999999998224 ) ) ;
#38801=CARTESIAN_POINT ( 'NONE',  ( 26.01562500061451289, 3.027376345333613106, -5.243569643749998122 ) ) ;
#38802=CARTESIAN_POINT ( 'NONE',  ( 16.56562500061451715, 3.027376345333613106, -5.243569643749998122 ) ) ;
#38804=CARTESIAN_POINT ( 'NONE',  ( 13.47187500061451537, 3.027376345333613106, -5.243569643749998122 ) ) ;
#38806=CARTESIAN_POINT ( 'NONE',  ( 25.05000000122903714, 5.773502691896255534, 3.535250795749688894E-16 ) ) ;
#38807=CARTESIAN_POINT ( 'NONE',  ( 4.171875000614517326, 3.027376345333611329, 5.243569643749999010 ) ) ;
#38808=CARTESIAN_POINT ( 'NONE',  ( 13.35937500061451821, -4.541064518000417216, -2.621784821875001281 ) ) ;
#38811=CARTESIAN_POINT ( 'NONE',  ( 18.33749999999999858, -2.886751345948130876, 4.999999999999996447 ) ) ;
#38812=CARTESIAN_POINT ( 'NONE',  ( 25.47187500061451715, -6.054752690667223547, -1.112240025338166033E-15 ) ) ;
#38813=CARTESIAN_POINT ( 'NONE',  ( 15.75937500061451857, 4.541064518000418104, -2.621784821874998173 ) ) ;
#38815=CARTESIAN_POINT ( 'NONE',  ( 27.07499999999999929, 6.123233995736764310E-16, -4.999999999999998224 ) ) ;
#38816=CARTESIAN_POINT ( 'NONE',  ( 1.071796769724489895, 10.41740381056766473, 26.00000000000000355 ) ) ;
#38817=CARTESIAN_POINT ( 'NONE',  ( 5.924999999999999822, 6.123233995736764310E-16, -4.999999999999998224 ) ) ;
#38819=CARTESIAN_POINT ( 'NONE',  ( 18.92812500061451431, 4.541064518000418104, 2.621784821874999949 ) ) ;
#38820=CARTESIAN_POINT ( 'NONE',  ( 8.925000000000002487, -4.330127018922194537, 2.499999999999995559 ) ) ;
#38821=CARTESIAN_POINT ( 'NONE',  ( 3.178125000614515638, 4.541064518000418104, 2.621784821874999949 ) ) ;
#38822=CARTESIAN_POINT ( 'NONE',  ( 17.55000000000000071, -4.330127018922190985, -2.500000000000001332 ) ) ;
#38823=CARTESIAN_POINT ( 'NONE',  ( -2.000000000000000000, 17.22500000000000142, 26.53589838486224650 ) ) ;
#38824=B_SPLINE_CURVE_WITH_KNOTS ( 'NONE', 3,
 ( #38010, #33556, #67202, #50206, #39477, #28036, #27304, #27667, #32840, #21743 ),
 .UNSPECIFIED., .F., .F.,
 ( 4, 3, 3, 4 ),
 ( 1.727079271278346568E-16, 2.812506120703778600E-05, 5.881405194855023478E-05, 8.950367042444256477E-05 ),
 .UNSPECIFIED. ) ;
#38825=CARTESIAN_POINT ( 'NONE',  ( 21.26250000122903572, -4.330127018922190985, -2.500000000000001332 ) ) ;
#38827=CARTESIAN_POINT ( 'NONE',  ( 27.79687500061451999, -3.027376345333610441, -5.243569643749999898 ) ) ;
#38828=ORIENTED_EDGE ( 'NONE', *, *, #54584, .T. ) ;
#38829=CARTESIAN_POINT ( 'NONE',  ( 16.71562500061451573, 3.027376345333611329, 5.243569643749999010 ) ) ;
#38830=CARTESIAN_POINT ( 'NONE',  ( 23.84062500061451928, 6.054752690667223547, 3.707466751127219781E-16 ) ) ;
#38831=CARTESIAN_POINT ( 'NONE',  ( 23.44687500061451502, 6.054752690667223547, 3.707466751127219781E-16 ) ) ;
#38832=CARTESIAN_POINT ( 'NONE',  ( 5.850000000000001421, -4.330127018922190985, -2.500000000000001332 ) ) ;
#38833=CARTESIAN_POINT ( 'NONE',  ( 9.365625000614519635, 3.027376345333613106, -5.243569643749998122 ) ) ;
#38834=CARTESIAN_POINT ( 'NONE',  ( 25.00312500061451715, -4.541064518000417216, -2.621784821875001281 ) ) ;
#38835=CARTESIAN_POINT ( 'NONE',  ( 14.22187500061451537, -6.054752690667223547, -1.112240025338166033E-15 ) ) ;
#38836=CARTESIAN_POINT ( 'NONE',  ( 18.49687500061452283, 6.054752690667223547, 3.707466751127219781E-16 ) ) ;
#38837=CARTESIAN_POINT ( 'NONE',  ( 30.00000000000000000, 0.000000000000000000, 4.999999999999998224 ) ) ;
#38838=CARTESIAN_POINT ( 'NONE',  ( -3.000416591977282496E-16, 19.24062500061451431, 25.09994784771203058 ) ) ;
#38839=CARTESIAN_POINT ( 'NONE',  ( 22.08750000122903501, -4.330127018922194537, 2.499999999999995559 ) ) ;
#38841=CARTESIAN_POINT ( 'NONE',  ( 12.51562500061451821, 3.027376345333612662, -5.243569643749998122 ) ) ;
#38842=CARTESIAN_POINT ( 'NONE',  ( 9.159375000614515372, 0.000000000000000000, 5.243569643749999010 ) ) ;
#38843=CARTESIAN_POINT ( 'NONE',  ( 6.571875000614517681, -6.054752690667223547, -1.112240025338166033E-15 ) ) ;
#38844=ORIENTED_EDGE ( 'NONE', *, *, #24606, .F. ) ;
#38845=CARTESIAN_POINT ( 'NONE',  ( 28.80937500061451573, 4.541064518000418104, -2.621784821874998173 ) ) ;
#38846=CARTESIAN_POINT ( 'NONE',  ( 20.05312500061451431, -4.541064518000417216, -2.621784821875001281 ) ) ;
#38847=CARTESIAN_POINT ( 'NONE',  ( 3.253125000614518036, 0.000000000000000000, 5.243569643749999010 ) ) ;
#38848=CARTESIAN_POINT ( 'NONE',  ( 28.04062500061451502, -3.027376345333614438, 5.243569643749998122 ) ) ;
#38849=CARTESIAN_POINT ( 'NONE',  ( 24.15937500061451715, -4.541064518000417216, -2.621784821875001281 ) ) ;
#38850=CARTESIAN_POINT ( 'NONE',  ( 19.26562500061451644, 3.027376345333613106, -5.243569643749998122 ) ) ;
#38851=CARTESIAN_POINT ( 'NONE',  ( -3.000416591977282496E-16, 19.29687500061451644, 25.09994784771203058 ) ) ;
#38852=CARTESIAN_POINT ( 'NONE',  ( 25.71562500061451573, 3.027376345333611329, 5.243569643749999010 ) ) ;
#38853=CARTESIAN_POINT ( 'NONE',  ( 3.525000001229034119, 2.886751345948126879, 4.999999999999999112 ) ) ;
#38855=CARTESIAN_POINT ( 'NONE',  ( 27.48749999999999716, -2.886751345948125991, -5.000000000000000000 ) ) ;
#38856=CARTESIAN_POINT ( 'NONE',  ( 3.999999999999998668, 16.21250000000000213, -32.30940107675850470 ) ) ;
#38858=CARTESIAN_POINT ( 'NONE',  ( 3.909375000614518481, -4.541064518000417216, -2.621784821875001281 ) ) ;
#38859=CARTESIAN_POINT ( 'NONE',  ( 13.71562500061451750, -6.054752690667223547, -1.112240025338166033E-15 ) ) ;
#38860=CARTESIAN_POINT ( 'NONE',  ( 6.459375000614518747, 0.000000000000000000, 5.243569643749999010 ) ) ;
#38861=CARTESIAN_POINT ( 'NONE',  ( 24.56250000122903288, 4.330127018922192761, -2.499999999999997780 ) ) ;
#38862=CARTESIAN_POINT ( 'NONE',  ( 15.72187500061451892, 3.027376345333612662, -5.243569643749998122 ) ) ;
#38863=CARTESIAN_POINT ( 'NONE',  ( 3.159375000614518036, 4.541064518000418104, -2.621784821874998173 ) ) ;
#38865=CARTESIAN_POINT ( 'NONE',  ( 25.69687500061451502, 6.054752690667223547, 3.707466751127219781E-16 ) ) ;
#38866=CARTESIAN_POINT ( 'NONE',  ( 12.55312500061451786, 4.541064518000418104, -2.621784821874998173 ) ) ;
#38868=CARTESIAN_POINT ( 'NONE',  ( 10.37812500061451715, 4.541064518000418104, 2.621784821874999949 ) ) ;
#38869=CARTESIAN_POINT ( 'NONE',  ( 7.415625000614516793, -6.054752690667223547, -1.112240025338166033E-15 ) ) ;
#38871=CARTESIAN_POINT ( 'NONE',  ( 8.550000000000002487, -4.330127018922190985, -2.500000000000001332 ) ) ;
#38872=CARTESIAN_POINT ( 'NONE',  ( 2.962500001229034119, 4.330127018922192761, -2.499999999999997780 ) ) ;
#38873=CARTESIAN_POINT ( 'NONE',  ( 18.56250000000000000, 2.886751345948129099, -4.999999999999998224 ) ) ;
#38874=CARTESIAN_POINT ( 'NONE',  ( 18.83437500061451431, 6.421520780324663323E-16, -5.243569643749999010 ) ) ;
#38875=CARTESIAN_POINT ( 'NONE',  ( 14.40000000122903323, -2.886751345948129988, 4.999999999999997335 ) ) ;
#38877=CARTESIAN_POINT ( 'NONE',  ( -2.121784821874999949, 14.77812500061451750, -33.67503911421598417 ) ) ;
#38881=EDGE_CURVE ( 'NONE', #70720, #30507, #67003, .T. ) ;
#38882=CARTESIAN_POINT ( 'NONE',  ( 27.21562500061451928, -6.054752690667223547, -1.112240025338166033E-15 ) ) ;
#38883=CARTESIAN_POINT ( 'NONE',  ( 30.00000000000000000, 0.000000000000000000, 4.999999999999998224 ) ) ;
#38884=CARTESIAN_POINT ( 'NONE',  ( 0.000000000000000000, 10.00000000000000000, 24.00000000000000000 ) ) ;
#38885=CARTESIAN_POINT ( 'NONE',  ( 27.15000000000000213, 4.330127018922192761, -2.499999999999997780 ) ) ;
#38886=CARTESIAN_POINT ( 'NONE',  ( 8.540625000614518569, 6.054752690667223547, 3.707466751127219781E-16 ) ) ;
#38888=CARTESIAN_POINT ( 'NONE',  ( 21.30937500061451573, 0.000000000000000000, 5.243569643749999010 ) ) ;
#38890=CARTESIAN_POINT ( 'NONE',  ( 5.090625000614516615, -3.027376345333614438, 5.243569643749998122 ) ) ;
#38891=CARTESIAN_POINT ( 'NONE',  ( 10.13437500061451679, -4.541064518000419881, 2.621784821874995952 ) ) ;
#38892=VERTEX_POINT ( 'NONE', #9799 ) ;
#38893=CARTESIAN_POINT ( 'NONE',  ( 22.58437500061451431, 4.541064518000418104, 2.621784821874999949 ) ) ;
#38894=CARTESIAN_POINT ( 'NONE',  ( 28.91250000000000497, 2.886751345948099789, -5.000000000000048850 ) ) ;
#38895=CARTESIAN_POINT ( 'NONE',  ( 28.94999999999999929, 4.330127018922192761, -2.499999999999997780 ) ) ;
#38896=CARTESIAN_POINT ( 'NONE',  ( 4.800000000000002487, 0.000000000000000000, 4.999999999999998224 ) ) ;
#38897=CARTESIAN_POINT ( 'NONE',  ( 14.66250000122903252, 4.330127018922192761, -2.499999999999997780 ) ) ;
#38899=CARTESIAN_POINT ( 'NONE',  ( 14.58750000122903323, 6.123233995736764310E-16, -4.999999999999998224 ) ) ;
#38901=CARTESIAN_POINT ( 'NONE',  ( 11.66249999999999964, -5.773502691896255534, -1.060575238724906372E-15 ) ) ;
#38902=CARTESIAN_POINT ( 'NONE',  ( 16.42500000000000071, 4.330127018922191873, 2.499999999999999556 ) ) ;
#38903=CARTESIAN_POINT ( 'NONE',  ( 12.33750000122903145, 6.123233995736764310E-16, -4.999999999999998224 ) ) ;
#38904=CARTESIAN_POINT ( 'NONE',  ( 10.94062500061451537, -3.027376345333614438, 5.243569643749998122 ) ) ;
#38905=CARTESIAN_POINT ( 'NONE',  ( 8.137500000000002842, -2.886751345948125991, -5.000000000000000000 ) ) ;
#38907=CARTESIAN_POINT ( 'NONE',  ( -2.121784821874999949, 15.28437500061451892, -33.67503911421598417 ) ) ;
#38908=CARTESIAN_POINT ( 'NONE',  ( 29.13750000122903216, 4.330127018922191873, 2.499999999999999556 ) ) ;
#38910=CARTESIAN_POINT ( 'NONE',  ( 10.42500000000000071, 6.123233995736764310E-16, -4.999999999999998224 ) ) ;
#38911=CARTESIAN_POINT ( 'NONE',  ( 3.486133158594716510E-16, 19.88749999999999929, -34.00000000000000000 ) ) ;
#38913=CARTESIAN_POINT ( 'NONE',  ( 24.25312500061451715, 4.541064518000418104, -2.621784821874998173 ) ) ;
#38914=CARTESIAN_POINT ( 'NONE',  ( 29.78437500061451715, 4.541064518000418104, 2.621784821874999949 ) ) ;
#38915=CARTESIAN_POINT ( 'NONE',  ( 20.97187500061451715, -6.054752690667223547, -1.112240025338166033E-15 ) ) ;
#38916=CARTESIAN_POINT ( 'NONE',  ( 16.26562500061451289, 3.027376345333611329, 5.243569643749999010 ) ) ;
#38918=CARTESIAN_POINT ( 'NONE',  ( 4.243569643749999010, 11.51562500061459282, -32.45002607614398471 ) ) ;
#38919=CARTESIAN_POINT ( 'NONE',  ( 7.565625000614518036, 3.027376345333613106, -5.243569643749998122 ) ) ;
#38920=CARTESIAN_POINT ( 'NONE',  ( 29.06250000122903288, 4.330127018922192761, -2.499999999999997780 ) ) ;
#38922=CARTESIAN_POINT ( 'NONE',  ( 18.29062500061451502, -3.027376345333610441, -5.243569643749999898 ) ) ;
#38925=CARTESIAN_POINT ( 'NONE',  ( 16.17187500061451644, 3.027376345333613106, -5.243569643749998122 ) ) ;
#38926=CARTESIAN_POINT ( 'NONE',  ( 14.82187500061451679, 3.027376345333613106, -5.243569643749998122 ) ) ;
#38927=CARTESIAN_POINT ( 'NONE',  ( 22.39687500061451075, -3.027376345333610441, -5.243569643749999898 ) ) ;
#38928=ORIENTED_EDGE ( 'NONE', *, *, #61885, .F. ) ;
#38929=CARTESIAN_POINT ( 'NONE',  ( -2.121784821874996840, 12.73437500061451821, 33.67503911421598417 ) ) ;
#38930=CARTESIAN_POINT ( 'NONE',  ( 3.403125000614518836, -4.541064518000417216, -2.621784821875001281 ) ) ;
#38931=CARTESIAN_POINT ( 'NONE',  ( 27.10312500061451502, 0.000000000000000000, 5.243569643749999010 ) ) ;
#38933=CARTESIAN_POINT ( 'NONE',  ( 26.99062500061451431, 6.054752690667223547, 3.707466751127219781E-16 ) ) ;
#38935=CARTESIAN_POINT ( 'NONE',  ( 4.000000000000000000, 17.03750000000000142, 32.30940107675849049 ) ) ;
#38936=CARTESIAN_POINT ( 'NONE',  ( 5.371875000614516615, 3.027376345333613106, -5.243569643749998122 ) ) ;
#38937=CARTESIAN_POINT ( 'NONE',  ( 11.55000000122903181, 5.773502691896255534, 3.535250795749688894E-16 ) ) ;
#38938=CARTESIAN_POINT ( 'NONE',  ( 6.412500001229036073, -4.330127018922190985, -2.500000000000001332 ) ) ;
#38939=CARTESIAN_POINT ( 'NONE',  ( 28.83750000122903145, -4.330127018922194537, 2.499999999999995559 ) ) ;
#38942=CARTESIAN_POINT ( 'NONE',  ( 11.14687500061451608, -3.027376345333610441, -5.243569643749999898 ) ) ;
#38943=DIRECTION ( 'NONE',  ( 0.000000000000000000, 0.000000000000000000, -1.000000000000000000 ) ) ;
#38945=CARTESIAN_POINT ( 'NONE',  ( 20.01562500061451644, -6.054752690667223547, -1.112240025338166033E-15 ) ) ;
#38946=CARTESIAN_POINT ( 'NONE',  ( 14.48437500061451821, 4.541064518000418104, 2.621784821874999949 ) ) ;
#38947=CARTESIAN_POINT ( 'NONE',  ( 4.603125000614518569, 0.000000000000000000, 5.243569643749999010 ) ) ;
#38948=CARTESIAN_POINT ( 'NONE',  ( 22.99687500061452283, 6.054752690667223547, 3.707466751127219781E-16 ) ) ;
#38949=CARTESIAN_POINT ( 'NONE',  ( 9.646875000614516082, -3.027376345333614438, 5.243569643749998122 ) ) ;
#38950=CARTESIAN_POINT ( 'NONE',  ( 4.378125000614518925, 6.421520780324663323E-16, -5.243569643749999010 ) ) ;
#38951=CARTESIAN_POINT ( 'NONE',  ( 10.87500000122903288, -5.773502691896255534, -1.060575238724906372E-15 ) ) ;
#38952=CARTESIAN_POINT ( 'NONE',  ( 6.337500001229033231, -4.330127018922194537, 2.499999999999995559 ) ) ;
#38953=CARTESIAN_POINT ( 'NONE',  ( 20.16562500061451146, 3.027376345333613106, -5.243569643749998122 ) ) ;
#38954=CARTESIAN_POINT ( 'NONE',  ( 8.100000001229034297, -2.886751345948129988, 4.999999999999997335 ) ) ;
#38955=CARTESIAN_POINT ( 'NONE',  ( 17.57812500061451644, 4.541064518000418104, 2.621784821874999949 ) ) ;
#38956=CARTESIAN_POINT ( 'NONE',  ( 15.25312500061451715, 4.541064518000418104, -2.621784821874998173 ) ) ;
#38958=CARTESIAN_POINT ( 'NONE',  ( 16.53750000000000142, -2.886751345948129988, 4.999999999999997335 ) ) ;
#38959=CARTESIAN_POINT ( 'NONE',  ( 8.962500001229033231, 0.000000000000000000, 4.999999999999998224 ) ) ;
#38960=CARTESIAN_POINT ( 'NONE',  ( 6.328125000614515550, 4.541064518000418104, 2.621784821874999949 ) ) ;
#38963=CARTESIAN_POINT ( 'NONE',  ( 20.62500000122903288, 2.886751345948126879, 4.999999999999999112 ) ) ;
#38965=CARTESIAN_POINT ( 'NONE',  ( 4.243569643749999898, 12.43437500061451750, -30.00000000000000000 ) ) ;
#38967=AXIS2_PLACEMENT_3D ( 'NONE', #59017, #8419, #18038 ) ;
#38969=CARTESIAN_POINT ( 'NONE',  ( 3.046875000614519990, -3.027376345333610441, -5.243569643749999898 ) ) ;
#38970=CARTESIAN_POINT ( 'NONE',  ( 20.10937500061451289, -4.541064518000417216, -2.621784821875001281 ) ) ;
#38972=CARTESIAN_POINT ( 'NONE',  ( 16.60312500061451857, 4.541064518000418104, -2.621784821874998173 ) ) ;
#38976=CARTESIAN_POINT ( 'NONE',  ( 29.29687500061451644, 6.054752690667223547, 3.707466751127219781E-16 ) ) ;
#38978=CARTESIAN_POINT ( 'NONE',  ( 13.79062500061451502, -3.027376345333610441, -5.243569643749999898 ) ) ;
#38979=CARTESIAN_POINT ( 'NONE',  ( 11.93437500061451573, -4.541064518000419881, 2.621784821874995952 ) ) ;
#38981=CARTESIAN_POINT ( 'NONE',  ( 28.90312500061451217, 0.000000000000000000, 5.243569643749999010 ) ) ;
#38982=CARTESIAN_POINT ( 'NONE',  ( 23.35312500061451857, 4.541064518000418104, -2.621784821874998173 ) ) ;
#38984=LINE ( 'NONE', #32335, #59585 ) ;
#38985=CARTESIAN_POINT ( 'NONE',  ( 12.22499999999999964, 6.123233995736764310E-16, -4.999999999999998224 ) ) ;
#38986=CARTESIAN_POINT ( 'NONE',  ( 22.31250000122903288, 4.330127018922192761, -2.499999999999997780 ) ) ;
#38987=CARTESIAN_POINT ( 'NONE',  ( 15.77812500061451573, 4.541064518000418104, 2.621784821874999949 ) ) ;
#38990=CARTESIAN_POINT ( 'NONE',  ( 20.99999999999999645, 0.000000000000000000, 4.999999999999998224 ) ) ;
#38991=CARTESIAN_POINT ( 'NONE',  ( 22.39687500061451075, -3.027376345333610441, -5.243569643749999898 ) ) ;
#38992=CARTESIAN_POINT ( 'NONE',  ( 26.72812500061451502, -4.541064518000419881, 2.621784821874995952 ) ) ;
#38993=ORIENTED_EDGE ( 'NONE', *, *, #62622, .T. ) ;
#38994=CYLINDRICAL_SURFACE ( 'NONE', #15941, 4.999999999999998224 ) ;
#38995=CARTESIAN_POINT ( 'NONE',  ( 10.04062500061451502, -3.027376345333614438, 5.243569643749998122 ) ) ;
#38996=DIRECTION ( 'NONE',  ( 1.000000000000000000, 0.000000000000000000, 0.000000000000000000 ) ) ;
#38997=CARTESIAN_POINT ( 'NONE',  ( 18.00000000000000355, -4.330127018922190985, -2.500000000000001332 ) ) ;
#38998=CARTESIAN_POINT ( 'NONE',  ( 23.32499999999999929, -4.330127018922194537, 2.499999999999995559 ) ) ;
#38999=CARTESIAN_POINT ( 'NONE',  ( 7.875000000000000000, 4.330127018922191873, 2.499999999999999556 ) ) ;
#39000=CARTESIAN_POINT ( 'NONE',  ( 4.846875000614519813, -3.027376345333610441, -5.243569643749999898 ) ) ;
#39001=CARTESIAN_POINT ( 'NONE',  ( 29.55937500061451573, -4.541064518000417216, -2.621784821875001281 ) ) ;
#39003=CARTESIAN_POINT ( 'NONE',  ( 23.20312500061451644, -4.541064518000417216, -2.621784821875001281 ) ) ;
#39004=CARTESIAN_POINT ( 'NONE',  ( 25.28437500061451715, 4.541064518000418104, 2.621784821874999949 ) ) ;
#39005=CARTESIAN_POINT ( 'NONE',  ( -3.137519842735245283E-14, 12.91250000000000142, -26.00000000000000711 ) ) ;
#39006=CARTESIAN_POINT ( 'NONE',  ( 13.16249999999999964, 2.886751345948129099, -4.999999999999998224 ) ) ;
#39007=CARTESIAN_POINT ( 'NONE',  ( 7.790625000614518569, -3.027376345333614438, 5.243569643749998122 ) ) ;
#39010=CARTESIAN_POINT ( 'NONE',  ( 25.37812500061451715, -4.541064518000419881, 2.621784821874995952 ) ) ;
#39013=CARTESIAN_POINT ( 'NONE',  ( 3.440625000614518036, -3.027376345333610441, -5.243569643749999898 ) ) ;
#39014=CARTESIAN_POINT ( 'NONE',  ( 19.05937500061451928, 0.000000000000000000, 5.243569643749999010 ) ) ;
#39015=CARTESIAN_POINT ( 'NONE',  ( 4.243569643749999898, 13.74687500061451750, 32.45002607614398471 ) ) ;
#39016=CARTESIAN_POINT ( 'NONE',  ( 22.54687500061451999, 6.054752690667223547, 3.707466751127219781E-16 ) ) ;
#39017=CARTESIAN_POINT ( 'NONE',  ( 3.525000000000000355, -4.330127018922194537, 2.499999999999995559 ) ) ;
#39018=CARTESIAN_POINT ( 'NONE',  ( -4.243569643749999898, 19.37187500061451928, 27.54997392385601529 ) ) ;
#39019=CARTESIAN_POINT ( 'NONE',  ( 10.82812500061451644, 4.541064518000418104, 2.621784821874999949 ) ) ;
#39021=ADVANCED_FACE ( 'NONE', ( #43791 ), #43429, .F. ) ;
#39022=CARTESIAN_POINT ( 'NONE',  ( 6.196875000614515905, -3.027376345333610441, -5.243569643749999898 ) ) ;
#39023=CARTESIAN_POINT ( 'NONE',  ( 30.00000000000000000, 0.000000000000000000, 0.000000000000000000 ) ) ;
#39024=CARTESIAN_POINT ( 'NONE',  ( 7.490625000614516082, -3.027376345333610441, -5.243569643749999898 ) ) ;
#39025=CARTESIAN_POINT ( 'NONE',  ( 11.63437500061451857, 6.421520780324663323E-16, -5.243569643749999010 ) ) ;
#39026=CARTESIAN_POINT ( 'NONE',  ( 19.31250000122903288, 0.000000000000000000, 4.999999999999998224 ) ) ;
#39027=CARTESIAN_POINT ( 'NONE',  ( 9.009375000614518569, 4.541064518000418104, -2.621784821874998173 ) ) ;
#39028=CARTESIAN_POINT ( 'NONE',  ( 9.515625000614518214, 3.027376345333611329, 5.243569643749999010 ) ) ;
#39031=CARTESIAN_POINT ( 'NONE',  ( 19.39687500061451786, 6.054752690667223547, 3.707466751127219781E-16 ) ) ;
#39032=CARTESIAN_POINT ( 'NONE',  ( 4.515288692908367096, 2.147595869733109897, 4.674606788361012732 ) ) ;
#39033=CARTESIAN_POINT ( 'NONE',  ( 26.91562500061451146, 3.027376345333613106, -5.243569643749998122 ) ) ;
#39034=CARTESIAN_POINT ( 'NONE',  ( 12.25312500061451537, 0.000000000000000000, 5.243569643749999010 ) ) ;
#39035=CARTESIAN_POINT ( 'NONE',  ( 29.67187500061451644, 3.027376345333612662, -5.243569643749998122 ) ) ;
#39036=CARTESIAN_POINT ( 'NONE',  ( 4.243569643749999898, 13.29687500061451999, -27.54997392385601529 ) ) ;
#39037=CARTESIAN_POINT ( 'NONE',  ( 14.02500000122903323, -5.773502691896255534, -1.060575238724906372E-15 ) ) ;
#39038=CARTESIAN_POINT ( 'NONE',  ( 27.92812500061451431, 4.541064518000418104, 2.621784821874999949 ) ) ;
#39039=CARTESIAN_POINT ( 'NONE',  ( -4.243569643749999898, 16.16562500061451857, -32.45002607614398471 ) ) ;
#39040=CARTESIAN_POINT ( 'NONE',  ( 16.27500000122903501, -5.773502691896255534, -1.060575238724906372E-15 ) ) ;
#39041=CARTESIAN_POINT ( 'NONE',  ( 14.32500000000000107, -4.330127018922194537, 2.499999999999995559 ) ) ;
#39042=CARTESIAN_POINT ( 'NONE',  ( 12.11250000122903181, 0.000000000000000000, 4.999999999999998224 ) ) ;
#39043=CARTESIAN_POINT ( 'NONE',  ( 23.12812500061451360, -4.541064518000419881, 2.621784821874995952 ) ) ;
#39044=CARTESIAN_POINT ( 'NONE',  ( 7.246875000614518392, 6.054752690667223547, 3.707466751127219781E-16 ) ) ;
#39045=CARTESIAN_POINT ( 'NONE',  ( 9.637500001229033941, 6.123233995736764310E-16, -4.999999999999998224 ) ) ;
#39046=CARTESIAN_POINT ( 'NONE',  ( 17.62500000122903288, -5.773502691896255534, -1.060575238724906372E-15 ) ) ;
#39047=CARTESIAN_POINT ( 'NONE',  ( 15.25312500061451715, 4.541064518000418104, -2.621784821874998173 ) ) ;
#39048=CARTESIAN_POINT ( 'NONE',  ( 18.59062500061451573, -3.027376345333614438, 5.243569643749998122 ) ) ;
#39049=CARTESIAN_POINT ( 'NONE',  ( 24.63750000122903216, 4.330127018922191873, 2.499999999999999556 ) ) ;
#39050=CARTESIAN_POINT ( 'NONE',  ( 28.12500000122902932, 2.886751345948129099, -4.999999999999998224 ) ) ;
#39051=CARTESIAN_POINT ( 'NONE',  ( 21.78750000000000142, 5.773502691896255534, 3.535250795749688894E-16 ) ) ;
#39053=CARTESIAN_POINT ( 'NONE',  ( 25.05937500061451573, -4.541064518000417216, -2.621784821875001281 ) ) ;
#39054=CARTESIAN_POINT ( 'NONE',  ( 25.83750000122903501, 6.123233995736764310E-16, -4.999999999999998224 ) ) ;
#39055=CARTESIAN_POINT ( 'NONE',  ( 13.05000000122903536, -2.886751345948129988, 4.999999999999997335 ) ) ;
#39056=CARTESIAN_POINT ( 'NONE',  ( 27.34687500061451360, -3.027376345333610441, -5.243569643749999898 ) ) ;
#39057=DIRECTION ( 'NONE',  ( -1.000000000000000000, -0.000000000000000000, -0.000000000000000000 ) ) ;
#39058=CARTESIAN_POINT ( 'NONE',  ( 5.484375000614518214, 4.541064518000418104, 2.621784821874999949 ) ) ;
#39059=CARTESIAN_POINT ( 'NONE',  ( 23.80312500061451786, 4.541064518000418104, -2.621784821874998173 ) ) ;
#39061=CARTESIAN_POINT ( 'NONE',  ( 30.00000000000000000, 6.123233995736764310E-16, -4.999999999999998224 ) ) ;
#39062=CARTESIAN_POINT ( 'NONE',  ( 9.684375000614517504, -4.541064518000419881, 2.621784821874995952 ) ) ;
#39063=CARTESIAN_POINT ( 'NONE',  ( 4.947905662033538654, -0.7326246900418315056, 4.992941444957970099 ) ) ;
#39064=CARTESIAN_POINT ( 'NONE',  ( 29.42812500061451431, -4.541064518000419881, 2.621784821874995952 ) ) ;
#39065=CARTESIAN_POINT ( 'NONE',  ( 7.284375000614518036, 4.541064518000418104, 2.621784821874999949 ) ) ;
#39066=CARTESIAN_POINT ( 'NONE',  ( 28.32187500061451502, 3.027376345333613106, -5.243569643749998122 ) ) ;
#39067=DIRECTION ( 'NONE',  ( -1.000000000000000000, -0.000000000000000000, -0.000000000000000000 ) ) ;
#39068=CARTESIAN_POINT ( 'NONE',  ( 20.06250000000000000, 2.886751345948126879, 4.999999999999999112 ) ) ;
#39069=ORIENTED_EDGE ( 'NONE', *, *, #53290, .T. ) ;
#39070=CARTESIAN_POINT ( 'NONE',  ( 28.23750000000000426, -2.886751345948129988, 4.999999999999997335 ) ) ;
#39071=CARTESIAN_POINT ( 'NONE',  ( 27.94687500061451502, 6.054752690667223547, 3.707466751127219781E-16 ) ) ;
#39073=CARTESIAN_POINT ( 'NONE',  ( 17.69062500061451715, -3.027376345333614438, 5.243569643749998122 ) ) ;
#39074=CARTESIAN_POINT ( 'NONE',  ( 8.728125000614518569, -4.541064518000419881, 2.621784821874995952 ) ) ;
#39076=CARTESIAN_POINT ( 'NONE',  ( 5.784375000614517148, 6.421520780324663323E-16, -5.243569643749999010 ) ) ;
#39077=CARTESIAN_POINT ( 'NONE',  ( 16.61250000122903359, 0.000000000000000000, 4.999999999999998224 ) ) ;
#39078=DIRECTION ( 'NONE',  ( -0.000000000000000000, -1.000000000000000000, -0.000000000000000000 ) ) ;
#39079=CARTESIAN_POINT ( 'NONE',  ( 7.359375000614516438, 0.000000000000000000, 5.243569643749999010 ) ) ;
#39080=CARTESIAN_POINT ( 'NONE',  ( 12.49687500061451573, -3.027376345333610441, -5.243569643749999898 ) ) ;
#39081=CARTESIAN_POINT ( 'NONE',  ( 20.59687500061451360, -3.027376345333610441, -5.243569643749999898 ) ) ;
#39082=EDGE_CURVE ( 'NONE', #11533, #11468, #1409, .T. ) ;
#39083=CARTESIAN_POINT ( 'NONE',  ( -3.999999999999997335, 16.43750000000000000, 32.30940107675850470 ) ) ;
#39085=CARTESIAN_POINT ( 'NONE',  ( 3.871875000614519280, -6.054752690667223547, -1.112240025338166033E-15 ) ) ;
#39087=CARTESIAN_POINT ( 'NONE',  ( 7.921875000614517326, -6.054752690667223547, -1.112240025338166033E-15 ) ) ;
#39089=CARTESIAN_POINT ( 'NONE',  ( 22.01249999999999574, -5.773502691896255534, -1.060575238724906372E-15 ) ) ;
#39090=CARTESIAN_POINT ( 'NONE',  ( 18.62812500061451715, -4.541064518000419881, 2.621784821874995952 ) ) ;
#39094=CARTESIAN_POINT ( 'NONE',  ( 8.915625000614515017, 3.027376345333613106, -5.243569643749998122 ) ) ;
#39095=CARTESIAN_POINT ( 'NONE',  ( 29.37187500061451928, 3.027376345333611329, 5.243569643749999010 ) ) ;
#39096=CARTESIAN_POINT ( 'NONE',  ( 29.29687500061451644, 6.054752690667223547, 3.707466751127219781E-16 ) ) ;
#39097=CARTESIAN_POINT ( 'NONE',  ( 9.899999999999998579, -4.330127018922190985, -2.500000000000001332 ) ) ;
#39098=CARTESIAN_POINT ( 'NONE',  ( 8.484601909799253346E-16, 15.72500000122903252, 34.61880215351700230 ) ) ;
#39099=CARTESIAN_POINT ( 'NONE',  ( 8.887500001229033941, 4.330127018922191873, 2.499999999999999556 ) ) ;
#39100=CARTESIAN_POINT ( 'NONE',  ( 20.67187500061451289, 3.027376345333613106, -5.243569643749998122 ) ) ;
#39101=CARTESIAN_POINT ( 'NONE',  ( 13.05937500061451750, 4.541064518000418104, -2.621784821874998173 ) ) ;
#39102=DIRECTION ( 'NONE',  ( -1.000000000000000000, -0.000000000000000000, -0.000000000000000000 ) ) ;
#39103=VERTEX_POINT ( 'NONE', #54870 ) ;
#39104=CARTESIAN_POINT ( 'NONE',  ( 14.42812500061451786, 4.541064518000418104, 2.621784821874999949 ) ) ;
#39105=CARTESIAN_POINT ( 'NONE',  ( 25.27500000122903145, -5.773502691896255534, -1.060575238724906372E-15 ) ) ;
#39106=CARTESIAN_POINT ( 'NONE',  ( 14.93437500061451750, 4.541064518000418104, 2.621784821874999949 ) ) ;
#39108=CARTESIAN_POINT ( 'NONE',  ( 16.49062500061451786, -3.027376345333610441, -5.243569643749999898 ) ) ;
#39110=CARTESIAN_POINT ( 'NONE',  ( 27.12187500061451573, 3.027376345333611329, 5.243569643749999010 ) ) ;
#39111=CARTESIAN_POINT ( 'NONE',  ( -2.121784821874999949, 11.17812500061451786, 26.32496088578401938 ) ) ;
#39112=CARTESIAN_POINT ( 'NONE',  ( 14.93437500061451750, 4.541064518000418104, 2.621784821874999949 ) ) ;
#39113=CARTESIAN_POINT ( 'NONE',  ( 15.26250000122903216, 0.000000000000000000, 4.999999999999998224 ) ) ;
#39115=CARTESIAN_POINT ( 'NONE',  ( 4.243569643749999898, 19.18437500061451928, -30.00000000000000000 ) ) ;
#39116=( BOUNDED_CURVE ( )  B_SPLINE_CURVE ( 2, ( #60047, #65600, #9458, #31988, #54522, #26448, #19054, #41612, #13517 ),
 .UNSPECIFIED., .F., .F. ) 
 B_SPLINE_CURVE_WITH_KNOTS ( ( 3, 2, 2, 2, 3 ),
 ( 0.8804347826086956763, 0.8840579710144927938, 0.8913043478260869179, 0.8985507246376811530, 0.9021739130434782705 ),
 .UNSPECIFIED. ) 
 CURVE ( )  GEOMETRIC_REPRESENTATION_ITEM ( )  RATIONAL_B_SPLINE_CURVE ( ( 0.9330127018922194093, 0.9330127018922194093, 1.000000000000000000, 0.8660254037844387076, 1.000000000000000000, 0.8660254037844387076, 1.000000000000000000, 0.9330127018922194093, 0.9330127018922194093 ) ) 
 REPRESENTATION_ITEM ( '' )  );
#39117=CARTESIAN_POINT ( 'NONE',  ( 20.37187500061451573, 3.027376345333611329, 5.243569643749999010 ) ) ;
#39118=CARTESIAN_POINT ( 'NONE',  ( 18.93750000122903288, -4.330127018922194537, 2.499999999999995559 ) ) ;
#39119=CARTESIAN_POINT ( 'NONE',  ( 17.59687500061451715, 6.054752690667223547, 3.707466751127219781E-16 ) ) ;
#39120=CARTESIAN_POINT ( 'NONE',  ( 2.121784821875001281, 12.35937500061451821, 33.67503911421598417 ) ) ;
#39121=CARTESIAN_POINT ( 'NONE',  ( 16.56562500061451715, 3.027376345333613106, -5.243569643749998122 ) ) ;
#39122=ORIENTED_EDGE ( 'NONE', *, *, #16801, .T. ) ;
#39123=ORIENTED_EDGE ( 'NONE', *, *, #56109, .T. ) ;
#39124=CARTESIAN_POINT ( 'NONE',  ( 20.47500000000000142, 4.330127018922191873, 2.499999999999999556 ) ) ;
#39125=CARTESIAN_POINT ( 'NONE',  ( 29.83125000061451715, 0.000000000000000000, 5.243569643749999010 ) ) ;
#39126=CARTESIAN_POINT ( 'NONE',  ( 24.77812500061451217, 4.541064518000418104, 2.621784821874999949 ) ) ;
#39127=CARTESIAN_POINT ( 'NONE',  ( 3.703125000614516882, 0.000000000000000000, 5.243569643749999010 ) ) ;
#39128=CARTESIAN_POINT ( 'NONE',  ( 17.66250000122903430, -4.330127018922190985, -2.500000000000001332 ) ) ;
#39129=CARTESIAN_POINT ( 'NONE',  ( 21.92812500061451431, 6.421520780324663323E-16, -5.243569643749999010 ) ) ;
#39130=CARTESIAN_POINT ( 'NONE',  ( 20.92500000000000071, 4.330127018922191873, 2.499999999999999556 ) ) ;
#39131=CARTESIAN_POINT ( 'NONE',  ( 24.66562500061451502, 3.027376345333613106, -5.243569643749998122 ) ) ;
#39132=CARTESIAN_POINT ( 'NONE',  ( 5.390625000614518214, 6.054752690667223547, 3.707466751127219781E-16 ) ) ;
#39133=VERTEX_POINT ( 'NONE', #49335 ) ;
#39134=CARTESIAN_POINT ( 'NONE',  ( 3.965625000614515727, 3.027376345333613106, -5.243569643749998122 ) ) ;
#39136=FACE_OUTER_BOUND ( 'NONE', #67832, .T. ) ;
#39137=CARTESIAN_POINT ( 'NONE',  ( -1.999999999999997113, 11.63750000122903394, -26.53589838486224295 ) ) ;
#39138=CARTESIAN_POINT ( 'NONE',  ( -2.121784821874996840, 18.58437500061451786, -26.32496088578401583 ) ) ;
#39140=CARTESIAN_POINT ( 'NONE',  ( 8.699999999999999289, 4.330127018922192761, -2.499999999999997780 ) ) ;
#39142=CARTESIAN_POINT ( 'NONE',  ( 4.612500001229032698, -4.330127018922190985, -2.500000000000001332 ) ) ;
#39143=CARTESIAN_POINT ( 'NONE',  ( 13.28437500061451715, -4.541064518000419881, 2.621784821874995952 ) ) ;
#39144=CARTESIAN_POINT ( 'NONE',  ( 23.70000000122903216, 5.773502691896255534, 3.535250795749688401E-16 ) ) ;
#39145=CARTESIAN_POINT ( 'NONE',  ( 3.084375000614519191, 6.421520780324663323E-16, -5.243569643749999010 ) ) ;
#39146=LINE ( 'NONE', #66865, #35019 ) ;
#39148=CARTESIAN_POINT ( 'NONE',  ( 9.646875000614516082, -3.027376345333614438, 5.243569643749998122 ) ) ;
#39150=CARTESIAN_POINT ( 'NONE',  ( 20.39062500061451644, -3.027376345333614438, 5.243569643749998122 ) ) ;
#39151=CARTESIAN_POINT ( 'NONE',  ( -1.071796769724504328, 12.55490381179670045, -26.00000000000001066 ) ) ;
#39152=( BOUNDED_CURVE ( )  B_SPLINE_CURVE ( 2, ( #32788, #22062, #16152, #55325, #4719, #44249, #37228 ),
 .UNSPECIFIED., .F., .F. ) 
 B_SPLINE_CURVE_WITH_KNOTS ( ( 3, 2, 2, 3 ),
 ( 0.2750000000000000777, 0.2777777777777778456, 0.2805555555555556135, 0.2833333333333333814 ),
 .UNSPECIFIED. ) 
 CURVE ( )  GEOMETRIC_REPRESENTATION_ITEM ( )  RATIONAL_B_SPLINE_CURVE ( ( 0.9999999999999973355, 0.8660254037844413721, 1.000000000000000000, 0.8660254037844387076, 1.000000000000000000, 0.8660254037844360431, 1.000000000000002665 ) ) 
 REPRESENTATION_ITEM ( '' )  );
#39153=CARTESIAN_POINT ( 'NONE',  ( -2.121784821874996840, 18.07812500061459104, 33.67503911421598417 ) ) ;
#39154=CARTESIAN_POINT ( 'NONE',  ( 24.64687500061451431, -3.027376345333610441, -5.243569643749999898 ) ) ;
#39157=( BOUNDED_CURVE ( )  B_SPLINE_CURVE ( 2, ( #40618, #6996, #12533, #23972, #5804, #45332, #23869, #17239, #56760 ),
 .UNSPECIFIED., .F., .F. ) 
 B_SPLINE_CURVE_WITH_KNOTS ( ( 3, 2, 2, 2, 3 ),
 ( 0.5108695652173913526, 0.5144927536231883591, 0.5217391304347825942, 0.5289855072463768293, 0.5326086956521739468 ),
 .UNSPECIFIED. ) 
 CURVE ( )  GEOMETRIC_REPRESENTATION_ITEM ( )  RATIONAL_B_SPLINE_CURVE ( ( 0.9330127018922192983, 0.9330127018922202975, 1.000000000000000000, 0.8660254037844387076, 1.000000000000000000, 0.8660254037844387076, 1.000000000000000000, 0.9330127018922194093, 0.9330127018922194093 ) ) 
 REPRESENTATION_ITEM ( '' )  );
#39158=CARTESIAN_POINT ( 'NONE',  ( 29.17500000122903714, 2.886751345948126879, 4.999999999999999112 ) ) ;
#39160=CARTESIAN_POINT ( 'NONE',  ( 25.94062500061451715, -3.027376345333610441, -5.243569643749999898 ) ) ;
#39161=CARTESIAN_POINT ( 'NONE',  ( 14.54062500061451679, -3.027376345333614438, 5.243569643749998122 ) ) ;
#39163=CARTESIAN_POINT ( 'NONE',  ( 11.74687500061451573, 6.054752690667223547, 3.707466751127219781E-16 ) ) ;
#39164=CARTESIAN_POINT ( 'NONE',  ( 28.49999999999999645, 4.330127018922192761, -2.499999999999997780 ) ) ;
#39165=CARTESIAN_POINT ( 'NONE',  ( 24.45000000122903572, -2.886751345948125991, -5.000000000000000000 ) ) ;
#39167=CARTESIAN_POINT ( 'NONE',  ( 14.22187500061451537, -6.054752690667223547, -1.112240025338166033E-15 ) ) ;
#39168=CARTESIAN_POINT ( 'NONE',  ( 29.55937500061451573, -4.541064518000417216, -2.621784821875001281 ) ) ;
#39169=CARTESIAN_POINT ( 'NONE',  ( 3.155232096411749065, -4.128743534138908267, -2.848806427449918743 ) ) ;
#39170=CARTESIAN_POINT ( 'NONE',  ( 25.88437500061451502, -4.541064518000419881, 2.621784821874995952 ) ) ;
#39171=CARTESIAN_POINT ( 'NONE',  ( 14.18437500061451750, -4.541064518000419881, 2.621784821874995952 ) ) ;
#39173=CARTESIAN_POINT ( 'NONE',  ( 28.19999999999999929, 0.000000000000000000, 4.999999999999998224 ) ) ;
#39174=CARTESIAN_POINT ( 'NONE',  ( 3.825000001229032609, 2.886751345948129099, -4.999999999999998224 ) ) ;
#39175=CARTESIAN_POINT ( 'NONE',  ( 5.625000000000001776, 4.330127018922191873, 2.499999999999999556 ) ) ;
#39177=CARTESIAN_POINT ( 'NONE',  ( 20.12812500061451715, 6.421520780324663323E-16, -5.243569643749999010 ) ) ;
#39178=CARTESIAN_POINT ( 'NONE',  ( 10.57500000000000107, 4.330127018922191873, 2.499999999999999556 ) ) ;
#39179=CARTESIAN_POINT ( 'NONE',  ( 15.48749999999999893, 5.773502691896255534, 3.535250795749688401E-16 ) ) ;
#39180=CARTESIAN_POINT ( 'NONE',  ( 17.81250000000000355, 2.886751345948126879, 4.999999999999999112 ) ) ;
#39181=CARTESIAN_POINT ( 'NONE',  ( -4.243569643749997233, 13.09062500061451750, 32.45002607614398471 ) ) ;
#39182=( BOUNDED_CURVE ( )  B_SPLINE_CURVE ( 2, ( #26611, #49149, #66124, #55049, #4451, #6623, #24586 ),
 .UNSPECIFIED., .F., .T. ) 
 B_SPLINE_CURVE_WITH_KNOTS ( ( 3, 2, 2, 3 ),
 ( 0.8666666666666666963, 0.8694444444444444642, 0.8722222222222222321, 0.8750000000000000000 ),
 .UNSPECIFIED. ) 
 CURVE ( )  GEOMETRIC_REPRESENTATION_ITEM ( )  RATIONAL_B_SPLINE_CURVE ( ( 1.000000000000000000, 0.8660254037844387076, 1.000000000000000000, 0.8660254037844387076, 1.000000000000000000, 0.8660254037844387076, 1.000000000000000000 ) ) 
 REPRESENTATION_ITEM ( '' )  );
#39184=CARTESIAN_POINT ( 'NONE',  ( 21.93750000122903288, 4.330127018922191873, 2.499999999999999556 ) ) ;
#39185=CARTESIAN_POINT ( 'NONE',  ( -3.999999999999999112, 10.10000000000000142, -30.00000000000000000 ) ) ;
#39186=CARTESIAN_POINT ( 'NONE',  ( 27.19687500061451857, -3.027376345333614438, 5.243569643749998122 ) ) ;
#39187=ORIENTED_EDGE ( 'NONE', *, *, #2612, .T. ) ;
#39188=CARTESIAN_POINT ( 'NONE',  ( 17.20312500061451644, 0.000000000000000000, 5.243569643749999010 ) ) ;
#39189=CARTESIAN_POINT ( 'NONE',  ( 22.04062500061451502, 6.054752690667223547, 3.707466751127219781E-16 ) ) ;
#39190=CARTESIAN_POINT ( 'NONE',  ( 22.88437500061451857, 6.421520780324663323E-16, -5.243569643749999010 ) ) ;
#39191=CARTESIAN_POINT ( 'NONE',  ( 7.050000000000000711, 0.000000000000000000, 4.999999999999998224 ) ) ;
#39192=CARTESIAN_POINT ( 'NONE',  ( 9.215625000614515727, -6.054752690667223547, -1.112240025338166033E-15 ) ) ;
#39193=CARTESIAN_POINT ( 'NONE',  ( 24.74062500061451786, 6.054752690667223547, 3.707466751127219781E-16 ) ) ;
#39194=CARTESIAN_POINT ( 'NONE',  ( 15.68437500061451573, 6.421520780324663323E-16, -5.243569643749999010 ) ) ;
#39195=CARTESIAN_POINT ( 'NONE',  ( 19.50937500061451857, 0.000000000000000000, 5.243569643749999010 ) ) ;
#39196=DIRECTION ( 'NONE',  ( -1.000000000000000000, -0.000000000000000000, -0.000000000000000000 ) ) ;
#39197=CARTESIAN_POINT ( 'NONE',  ( 2.121784821874999061, 17.85312500061451502, 26.32496088578401583 ) ) ;
#39198=EDGE_CURVE ( 'NONE', #32936, #12269, #16490, .T. ) ;
#39199=CARTESIAN_POINT ( 'NONE',  ( 21.82500000122903572, 2.886751345948129099, -4.999999999999998224 ) ) ;
#39201=CARTESIAN_POINT ( 'NONE',  ( 11.69062500061451537, 6.054752690667223547, 3.707466751127219781E-16 ) ) ;
#39202=CARTESIAN_POINT ( 'NONE',  ( 5.934375000614517504, 4.541064518000418104, 2.621784821874999949 ) ) ;
#39203=CARTESIAN_POINT ( 'NONE',  ( 4.396875000614516971, -3.027376345333610441, -5.243569643749999898 ) ) ;
#39205=CARTESIAN_POINT ( 'NONE',  ( 27.12187500061451573, 3.027376345333611329, 5.243569643749999010 ) ) ;
#39206=CARTESIAN_POINT ( 'NONE',  ( 19.71562500061451928, 3.027376345333613106, -5.243569643749998122 ) ) ;
#39207=CARTESIAN_POINT ( 'NONE',  ( 26.10000000122903430, -2.886751345948129988, 4.999999999999997335 ) ) ;
#39208=B_SPLINE_CURVE_WITH_KNOTS ( 'NONE', 3,
 ( #33438, #10552, #38633, #21623, #49354, #11285, #50081, #33806, #61878, #61157 ),
 .UNSPECIFIED., .F., .F.,
 ( 4, 3, 3, 4 ),
 ( 0.000000000000000000, 7.861372412303096113E-05, 0.0001572277528824084529, 0.0002833172372400243359 ),
 .UNSPECIFIED. ) ;
#39209=CARTESIAN_POINT ( 'NONE',  ( 26.84062500061451573, -3.027376345333610441, -5.243569643749999898 ) ) ;
#39210=VECTOR ( 'NONE', #18559, 1000.000000000000000 ) ;
#39211=CARTESIAN_POINT ( 'NONE',  ( 23.07187500061451857, 3.027376345333611329, 5.243569643749999010 ) ) ;
#39212=CARTESIAN_POINT ( 'NONE',  ( 18.96562500061451573, 3.027376345333611329, 5.243569643749999010 ) ) ;
#39213=CARTESIAN_POINT ( 'NONE',  ( -3.999999999999999112, 10.10000000000000142, 30.00000000000000000 ) ) ;
#39214=CARTESIAN_POINT ( 'NONE',  ( 24.21562500061451573, 3.027376345333613106, -5.243569643749998122 ) ) ;
#39215=CARTESIAN_POINT ( 'NONE',  ( 5.587500001229033231, 6.123233995736764310E-16, -4.999999999999998224 ) ) ;
#39216=ORIENTED_EDGE ( 'NONE', *, *, #45678, .F. ) ;
#39217=CARTESIAN_POINT ( 'NONE',  ( 27.03750000000000142, -2.886751345948125991, -5.000000000000000000 ) ) ;
#39218=CARTESIAN_POINT ( 'NONE',  ( 8.484601909799253346E-16, 14.71250000000000036, -25.38119784648299770 ) ) ;
#39220=CARTESIAN_POINT ( 'NONE',  ( 5.896875000614518747, 6.054752690667223547, 3.707466751127219781E-16 ) ) ;
#39221=CARTESIAN_POINT ( 'NONE',  ( 12.55312500061451786, 4.541064518000418104, -2.621784821874998173 ) ) ;
#39222=CARTESIAN_POINT ( 'NONE',  ( 7.284375000614518036, 4.541064518000418104, 2.621784821874999949 ) ) ;
#39223=CARTESIAN_POINT ( 'NONE',  ( 24.82500000122902861, -5.773502691896255534, -1.060575238724906372E-15 ) ) ;
#39224=CARTESIAN_POINT ( 'NONE',  ( 15.60937500061451644, -4.541064518000417216, -2.621784821875001281 ) ) ;
#39225=CARTESIAN_POINT ( 'NONE',  ( 29.05312500061451431, -4.541064518000417216, -2.621784821875001281 ) ) ;
#39226=CARTESIAN_POINT ( 'NONE',  ( 26.84999999999999787, 0.000000000000000000, 4.999999999999998224 ) ) ;
#39227=CARTESIAN_POINT ( 'NONE',  ( 27.27187500061451431, -6.054752690667223547, -1.112240025338166033E-15 ) ) ;
#39228=CARTESIAN_POINT ( 'NONE',  ( 3.703125000614516882, 0.000000000000000000, 5.243569643749999010 ) ) ;
#39229=CARTESIAN_POINT ( 'NONE',  ( 13.97812500061451679, 4.541064518000418104, 2.621784821874999949 ) ) ;
#39230=ORIENTED_EDGE ( 'NONE', *, *, #57275, .F. ) ;
#39231=CARTESIAN_POINT ( 'NONE',  ( 9.328125000614518214, 6.421520780324663323E-16, -5.243569643749999010 ) ) ;
#39232=CARTESIAN_POINT ( 'NONE',  ( 5.578125000614518214, -4.541064518000419881, 2.621784821874995952 ) ) ;
#39234=CARTESIAN_POINT ( 'NONE',  ( -0.6945863667395647534, 9.663023495605401081, 26.06076786935074097 ) ) ;
#39235=CARTESIAN_POINT ( 'NONE',  ( 15.48749999999999893, 5.773502691896255534, 3.535250795749688894E-16 ) ) ;
#39236=CARTESIAN_POINT ( 'NONE',  ( 15.53437500061451715, -4.541064518000419881, 2.621784821874995952 ) ) ;
#39237=CARTESIAN_POINT ( 'NONE',  ( 14.36250000122903359, 0.000000000000000000, 4.999999999999998224 ) ) ;
#39239=CARTESIAN_POINT ( 'NONE',  ( 21.75937500061451502, 0.000000000000000000, 5.243569643749999010 ) ) ;
#39240=CARTESIAN_POINT ( 'NONE',  ( -3.000416591977282496E-16, 13.39062500061451644, -34.90005215228797653 ) ) ;
#39243=CARTESIAN_POINT ( 'NONE',  ( 20.54999999999999716, 0.000000000000000000, 4.999999999999998224 ) ) ;
#39244=CARTESIAN_POINT ( 'NONE',  ( 26.84062500061451573, -3.027376345333610441, -5.243569643749999898 ) ) ;
#39245=CARTESIAN_POINT ( 'NONE',  ( 24.89999999999999858, 4.330127018922192761, -2.499999999999997780 ) ) ;
#39247=EDGE_CURVE ( 'NONE', #11634, #36225, #980, .T. ) ;
#39248=CARTESIAN_POINT ( 'NONE',  ( 26.09999999999999787, -4.330127018922190985, -2.500000000000001332 ) ) ;
#39249=CARTESIAN_POINT ( 'NONE',  ( 9.253125000614517148, -4.541064518000417216, -2.621784821875001281 ) ) ;
#39252=CARTESIAN_POINT ( 'NONE',  ( 21.79687500061451644, -3.027376345333614438, 5.243569643749998122 ) ) ;
#39254=CARTESIAN_POINT ( 'NONE',  ( 4.303125000614516971, -4.541064518000417216, -2.621784821875001281 ) ) ;
#39255=CARTESIAN_POINT ( 'NONE',  ( 10.65937500061451715, -4.541064518000417216, -2.621784821875001281 ) ) ;
#39256=ORIENTED_EDGE ( 'NONE', *, *, #35197, .F. ) ;
#39257=CARTESIAN_POINT ( 'NONE',  ( 20.63437500061451857, 6.421520780324663323E-16, -5.243569643749999010 ) ) ;
#39258=CYLINDRICAL_SURFACE ( 'NONE', #19389, 4.000000000000000000 ) ;
#39259=CARTESIAN_POINT ( 'NONE',  ( 29.73750000000000071, -2.886751345948125991, -5.000000000000000000 ) ) ;
#39260=CARTESIAN_POINT ( 'NONE',  ( 3.900000000000000799, 0.000000000000000000, 4.999999999999998224 ) ) ;
#39261=CARTESIAN_POINT ( 'NONE',  ( 15.33750000122903323, -4.330127018922194537, 2.499999999999995559 ) ) ;
#39262=CARTESIAN_POINT ( 'NONE',  ( 1.071796769724497445, 15.36740381056766758, -33.99999999999998579 ) ) ;
#39263=CARTESIAN_POINT ( 'NONE',  ( -2.000000000000000000, 19.02499999999999858, -33.46410161513775705 ) ) ;
#39264=EDGE_LOOP ( 'NONE', ( #66946, #9925, #62372, #9359 ) ) ;
#39265=CARTESIAN_POINT ( 'NONE',  ( 13.98750000000000249, -2.886751345948125991, -5.000000000000000000 ) ) ;
#39266=CARTESIAN_POINT ( 'NONE',  ( 25.97812500061451502, 6.421520780324663323E-16, -5.243569643749999010 ) ) ;
#39267=CARTESIAN_POINT ( 'NONE',  ( 17.43750000000000355, -2.886751345948129988, 4.999999999999997335 ) ) ;
#39268=CARTESIAN_POINT ( 'NONE',  ( 10.31250000122903288, 0.000000000000000000, 4.999999999999998224 ) ) ;
#39269=CARTESIAN_POINT ( 'NONE',  ( 7.978125000614517681, 6.421520780324663323E-16, -5.243569643749999010 ) ) ;
#39270=CARTESIAN_POINT ( 'NONE',  ( 8.025000000000000355, -4.330127018922194537, 2.499999999999995559 ) ) ;
#39272=CARTESIAN_POINT ( 'NONE',  ( -3.000416591977282496E-16, 15.69687500061451857, -34.90005215228797653 ) ) ;
#39273=CARTESIAN_POINT ( 'NONE',  ( 27.15000000122902790, -2.886751345948125991, -5.000000000000000000 ) ) ;
#39275=CARTESIAN_POINT ( 'NONE',  ( 7.875000000000000000, 4.330127018922191873, 2.499999999999999556 ) ) ;
#39277=ORIENTED_EDGE ( 'NONE', *, *, #703, .T. ) ;
#39278=CARTESIAN_POINT ( 'NONE',  ( 25.45312500061451644, -4.541064518000417216, -2.621784821875001281 ) ) ;
#39279=CARTESIAN_POINT ( 'NONE',  ( 28.94062500061452070, -3.027376345333614438, 5.243569643749998122 ) ) ;
#39280=CARTESIAN_POINT ( 'NONE',  ( 19.01250000122903216, -4.330127018922190985, -2.500000000000001332 ) ) ;
#39281=CARTESIAN_POINT ( 'NONE',  ( 21.15937500061451715, 4.541064518000418104, -2.621784821874998173 ) ) ;
#39282=CARTESIAN_POINT ( 'NONE',  ( 17.42812500061451786, 6.421520780324663323E-16, -5.243569643749999010 ) ) ;
#39283=CARTESIAN_POINT ( 'NONE',  ( 4.243569643749999010, 12.41562500061459495, -32.45002607614398471 ) ) ;
#39284=CARTESIAN_POINT ( 'NONE',  ( 6.365625000614518747, 3.027376345333611329, 5.243569643749999010 ) ) ;
#39285=CARTESIAN_POINT ( 'NONE',  ( 29.66250000122903074, 0.000000000000000000, 4.999999999999998224 ) ) ;
#39287=CARTESIAN_POINT ( 'NONE',  ( 19.11562500061451431, -6.054752690667223547, -1.112240025338166033E-15 ) ) ;
#39288=CARTESIAN_POINT ( 'NONE',  ( -5.810221930991193690E-16, 14.03750000000000142, 26.00000000000000355 ) ) ;
#39290=CARTESIAN_POINT ( 'NONE',  ( 13.35937500061451821, -4.541064518000417216, -2.621784821875001281 ) ) ;
#39291=CARTESIAN_POINT ( 'NONE',  ( 13.62187500061451750, 3.027376345333611329, 5.243569643749999010 ) ) ;
#39292=CARTESIAN_POINT ( 'NONE',  ( 21.57187500061451502, 3.027376345333613106, -5.243569643749998122 ) ) ;
#39293=EDGE_LOOP ( 'NONE', ( #40018, #32266, #72381, #2725 ) ) ;
#39294=CARTESIAN_POINT ( 'NONE',  ( 3.440625000614518036, -3.027376345333610441, -5.243569643749999898 ) ) ;
#39295=CARTESIAN_POINT ( 'NONE',  ( 25.67812500061451431, 4.541064518000418104, 2.621784821874999949 ) ) ;
#39296=CARTESIAN_POINT ( 'NONE',  ( 26.31562500061451715, -6.054752690667223547, -1.112240025338166033E-15 ) ) ;
#39298=CARTESIAN_POINT ( 'NONE',  ( -2.828200636599751609E-16, 15.83750000000000036, 25.38119784648299770 ) ) ;
#39299=CARTESIAN_POINT ( 'NONE',  ( 4.209375000614516971, 0.000000000000000000, 5.243569643749999010 ) ) ;
#39301=CARTESIAN_POINT ( 'NONE',  ( 11.02500000122903501, 2.886751345948129099, -4.999999999999998224 ) ) ;
#39302=B_SPLINE_CURVE_WITH_KNOTS ( 'NONE', 3,
 ( #56806, #6212, #22111, #17641, #40201, #34640, #29112, #51646, #1047, #68640 ),
 .UNSPECIFIED., .F., .F.,
 ( 4, 3, 3, 4 ),
 ( 0.000000000000000000, 2.812505145549477149E-05, 5.585677060009500101E-05, 8.358888089303753656E-05 ),
 .UNSPECIFIED. ) ;
#39303=CARTESIAN_POINT ( 'NONE',  ( 6.037500001229035185, 6.123233995736764310E-16, -4.999999999999998224 ) ) ;
#39304=CARTESIAN_POINT ( 'NONE',  ( 3.253125000614518036, 0.000000000000000000, 5.243569643749999010 ) ) ;
#39307=CARTESIAN_POINT ( 'NONE',  ( 12.04687500061451821, -3.027376345333610441, -5.243569643749999898 ) ) ;
#39309=VERTEX_POINT ( 'NONE', #50062 ) ;
#39310=EDGE_CURVE ( 'NONE', #2356, #11533, #24029, .T. ) ;
#39311=CARTESIAN_POINT ( 'NONE',  ( 19.45312500061451644, 0.000000000000000000, 5.243569643749999010 ) ) ;
#39312=CARTESIAN_POINT ( 'NONE',  ( 14.44687500061451679, 6.054752690667223547, 3.707466751127219781E-16 ) ) ;
#39313=CARTESIAN_POINT ( 'NONE',  ( 4.003125000614518925, 4.541064518000418104, -2.621784821874998173 ) ) ;
#39314=CARTESIAN_POINT ( 'NONE',  ( 21.87187500061451573, -6.054752690667223547, -1.112240025338166033E-15 ) ) ;
#39315=CARTESIAN_POINT ( 'NONE',  ( 10.02187500061451964, 3.027376345333611329, 5.243569643749999010 ) ) ;
#39316=CARTESIAN_POINT ( 'NONE',  ( 4.115625000614516082, 3.027376345333611329, 5.243569643749999010 ) ) ;
#39317=CARTESIAN_POINT ( 'NONE',  ( 5.924999999999999822, 6.123233995736764310E-16, -4.999999999999998224 ) ) ;
#39318=CARTESIAN_POINT ( 'NONE',  ( 5.250000001229035540, 5.773502691896255534, 3.535250795749688894E-16 ) ) ;
#39319=CARTESIAN_POINT ( 'NONE',  ( 19.22812500061451502, 6.421520780324663323E-16, -5.243569643749999010 ) ) ;
#39320=CARTESIAN_POINT ( 'NONE',  ( 9.150000001229033231, -2.886751345948125991, -5.000000000000000000 ) ) ;
#39321=CARTESIAN_POINT ( 'NONE',  ( 17.46562500061451217, 3.027376345333613106, -5.243569643749998122 ) ) ;
#39322=CARTESIAN_POINT ( 'NONE',  ( 16.75312500061451715, 0.000000000000000000, 5.243569643749999010 ) ) ;
#39324=CARTESIAN_POINT ( 'NONE',  ( 14.77500000000000036, -4.330127018922194537, 2.499999999999995559 ) ) ;
#39325=CARTESIAN_POINT ( 'NONE',  ( 8.325000001229033941, 2.886751345948129099, -4.999999999999998224 ) ) ;
#39326=CARTESIAN_POINT ( 'NONE',  ( 5.540625000614515905, -3.027376345333614438, 5.243569643749998122 ) ) ;
#39327=CARTESIAN_POINT ( 'NONE',  ( 20.02500000122903145, 2.886751345948129099, -4.999999999999998224 ) ) ;
#39329=CARTESIAN_POINT ( 'NONE',  ( -2.121784821874996840, 12.28437500061451892, -26.32496088578401583 ) ) ;
#39330=CARTESIAN_POINT ( 'NONE',  ( 4.602184248673647282, -1.954755528723157942, 4.813238914019062342 ) ) ;
#39331=CARTESIAN_POINT ( 'NONE',  ( 23.96249999999999858, 2.886751345948095793, -5.000000000000055067 ) ) ;
#39332=CARTESIAN_POINT ( 'NONE',  ( 5.034375000614519813, 4.541064518000418104, 2.621784821874999949 ) ) ;
#39333=CARTESIAN_POINT ( 'NONE',  ( 21.45937500061451786, -4.541064518000417216, -2.621784821875001281 ) ) ;
#39335=CARTESIAN_POINT ( 'NONE',  ( 5.000000000000000000, 6.123233995736766282E-16, 50.00000000000000000 ) ) ;
#39336=CARTESIAN_POINT ( 'NONE',  ( 17.35312500061451502, -4.541064518000417216, -2.621784821875001281 ) ) ;
#39340=CARTESIAN_POINT ( 'NONE',  ( 28.58437500061451786, -4.541064518000419881, 2.621784821874995952 ) ) ;
#39342=CARTESIAN_POINT ( 'NONE',  ( 13.37812500061451715, 6.421520780324663323E-16, -5.243569643749999010 ) ) ;
#39343=CARTESIAN_POINT ( 'NONE',  ( 10.50937500061451679, 0.000000000000000000, 5.243569643749999010 ) ) ;
#39345=CARTESIAN_POINT ( 'NONE',  ( 29.61562500061451431, 3.027376345333613106, -5.243569643749998122 ) ) ;
#39346=CARTESIAN_POINT ( 'NONE',  ( 23.12812500061451360, -4.541064518000419881, 2.621784821874995952 ) ) ;
#39348=CARTESIAN_POINT ( 'NONE',  ( 1.626862140677534273E-15, 13.02500000122903323, 34.00000000000000000 ) ) ;
#39349=CARTESIAN_POINT ( 'NONE',  ( 12.63749999999999929, -2.886751345948125991, -5.000000000000000000 ) ) ;
#39350=CARTESIAN_POINT ( 'NONE',  ( 21.22500000122903074, -5.773502691896255534, -1.060575238724906372E-15 ) ) ;
#39351=CARTESIAN_POINT ( 'NONE',  ( 16.94062500061451715, -3.027376345333610441, -5.243569643749999898 ) ) ;
#39354=CARTESIAN_POINT ( 'NONE',  ( 19.83750000000000213, -2.886751345948125991, -5.000000000000000000 ) ) ;
#39355=CARTESIAN_POINT ( 'NONE',  ( 24.63749999999999574, -2.886751345948129988, 4.999999999999997335 ) ) ;
#39356=CARTESIAN_POINT ( 'NONE',  ( 22.32187500061451502, -6.054752690667223547, -1.112240025338166033E-15 ) ) ;
#39357=CARTESIAN_POINT ( 'NONE',  ( 24.85312500061451502, 0.000000000000000000, 5.243569643749999010 ) ) ;
#39360=CARTESIAN_POINT ( 'NONE',  ( 8.278125000614515727, -4.541064518000419881, 2.621784821874995952 ) ) ;
#39362=CARTESIAN_POINT ( 'NONE',  ( 14.24999999999999822, 0.000000000000000000, 4.999999999999998224 ) ) ;
#39363=CARTESIAN_POINT ( 'NONE',  ( 7.800000001229035362, -2.886751345948126435, -5.000000000000000000 ) ) ;
#39364=CARTESIAN_POINT ( 'NONE',  ( 5.221875000614519813, -6.054752690667223547, -1.112240025338166033E-15 ) ) ;
#39365=CARTESIAN_POINT ( 'NONE',  ( 28.54687500061451644, -3.027376345333614438, 5.243569643749998122 ) ) ;
#39367=CARTESIAN_POINT ( 'NONE',  ( 23.35312500061451857, 4.541064518000418104, -2.621784821874998173 ) ) ;
#39368=CARTESIAN_POINT ( 'NONE',  ( 25.13437500061451502, 6.421520780324663323E-16, -5.243569643749999010 ) ) ;
#39369=CARTESIAN_POINT ( 'NONE',  ( -4.243569643749998122, 18.04062500061459318, -27.54997392385601174 ) ) ;
#39370=CARTESIAN_POINT ( 'NONE',  ( 11.40000000000000036, 4.330127018922192761, -2.499999999999997780 ) ) ;
#39371=CARTESIAN_POINT ( 'NONE',  ( 9.628125000614517148, -4.541064518000419881, 2.621784821874995952 ) ) ;
#39372=CARTESIAN_POINT ( 'NONE',  ( 3.735381814749570761, 3.323750120342865433, 3.996720557861077161 ) ) ;
#39373=CARTESIAN_POINT ( 'NONE',  ( 26.65312500061451573, 0.000000000000000000, 5.243569643749999010 ) ) ;
#39375=CARTESIAN_POINT ( 'NONE',  ( 3.253125000614518036, 0.000000000000000000, 5.243569643749999010 ) ) ;
#39376=CARTESIAN_POINT ( 'NONE',  ( 19.77187500061451786, 3.027376345333613106, -5.243569643749998122 ) ) ;
#39377=CARTESIAN_POINT ( 'NONE',  ( 4.243569643749999898, 15.58437500061451786, 30.00000000000000000 ) ) ;
#39378=CARTESIAN_POINT ( 'NONE',  ( 21.34687500061451715, -3.027376345333614438, 5.243569643749998122 ) ) ;
#39379=CARTESIAN_POINT ( 'NONE',  ( 3.825000000000001954, 4.330127018922191873, 2.499999999999999556 ) ) ;
#39380=CARTESIAN_POINT ( 'NONE',  ( 2.121784821874999061, 18.80937500061451928, 26.32496088578401583 ) ) ;
#39381=CARTESIAN_POINT ( 'NONE',  ( 9.778125000614517504, 6.421520780324663323E-16, -5.243569643749999010 ) ) ;
#39382=CARTESIAN_POINT ( 'NONE',  ( 2.737500001229034474, -4.330127018922194537, 2.499999999999995559 ) ) ;
#39383=CARTESIAN_POINT ( 'NONE',  ( 6.009375000614519458, 0.000000000000000000, 5.243569643749999010 ) ) ;
#39384=CYLINDRICAL_SURFACE ( 'NONE', #22984, 4.999999999999998224 ) ;
#39385=CARTESIAN_POINT ( 'NONE',  ( 6.665625000614515905, 3.027376345333613106, -5.243569643749998122 ) ) ;
#39386=CARTESIAN_POINT ( 'NONE',  ( 11.74687500061451573, 6.054752690667223547, 3.707466751127219781E-16 ) ) ;
#39388=CARTESIAN_POINT ( 'NONE',  ( 19.72500000122903074, 2.886751345948126879, 4.999999999999999112 ) ) ;
#39389=CARTESIAN_POINT ( 'NONE',  ( 8.709375000614517859, 0.000000000000000000, 5.243569643749999010 ) ) ;
#39390=CARTESIAN_POINT ( 'NONE',  ( 9.290625000614515017, -3.027376345333610441, -5.243569643749999898 ) ) ;
#39391=CARTESIAN_POINT ( 'NONE',  ( 4.903125000614516615, 4.541064518000418104, -2.621784821874998173 ) ) ;
#39393=CARTESIAN_POINT ( 'NONE',  ( 18.60937500061451644, 0.000000000000000000, 5.243569643749999010 ) ) ;
#39394=CARTESIAN_POINT ( 'NONE',  ( 1.626862140677534273E-15, 11.67500000122903181, 34.00000000000000000 ) ) ;
#39395=CARTESIAN_POINT ( 'NONE',  ( 28.15312500061451573, -4.541064518000417216, -2.621784821875001281 ) ) ;
#39396=CARTESIAN_POINT ( 'NONE',  ( 10.97812500061451679, -4.541064518000419881, 2.621784821874995952 ) ) ;
#39397=CARTESIAN_POINT ( 'NONE',  ( 2.867942972713479755, -4.095717654485441450, 3.274159358307528134 ) ) ;
#39398=CARTESIAN_POINT ( 'NONE',  ( -2.121784821874996840, 11.83437500061451786, -26.32496088578401583 ) ) ;
#39399=CARTESIAN_POINT ( 'NONE',  ( 12.00000000122903465, 5.773502691896255534, 3.535250795749688894E-16 ) ) ;
#39400=EDGE_CURVE ( 'NONE', #3790, #2494, #709, .T. ) ;
#39401=( BOUNDED_CURVE ( )  B_SPLINE_CURVE ( 2, ( #30696, #31804, #64311, #53228, #42886, #20333, #36604 ),
 .UNSPECIFIED., .F., .F. ) 
 B_SPLINE_CURVE_WITH_KNOTS ( ( 3, 2, 2, 3 ),
 ( 0.5666666666666667629, 0.5694444444444445308, 0.5722222222222221877, 0.5749999999999999556 ),
 .UNSPECIFIED. ) 
 CURVE ( )  GEOMETRIC_REPRESENTATION_ITEM ( )  RATIONAL_B_SPLINE_CURVE ( ( 0.9999999999999946709, 0.8660254037844440367, 1.000000000000000000, 0.8660254037844387076, 1.000000000000000000, 0.8660254037844387076, 1.000000000000000000 ) ) 
 REPRESENTATION_ITEM ( '' )  );
#39402=CARTESIAN_POINT ( 'NONE',  ( 27.14062500061451644, -3.027376345333614438, 5.243569643749998122 ) ) ;
#39403=CARTESIAN_POINT ( 'NONE',  ( -4.243569643749997233, 14.89062500061451644, -27.54997392385601174 ) ) ;
#39404=CARTESIAN_POINT ( 'NONE',  ( 14.06250000122903288, -4.330127018922190985, -2.500000000000001332 ) ) ;
#39405=CARTESIAN_POINT ( 'NONE',  ( 14.47499999999999964, 6.123233995736764310E-16, -4.999999999999998224 ) ) ;
#39406=LINE ( 'NONE', #44225, #72762 ) ;
#39407=CARTESIAN_POINT ( 'NONE',  ( 22.37812500061451360, 6.421520780324663323E-16, -5.243569643749999010 ) ) ;
#39408=CARTESIAN_POINT ( 'NONE',  ( 6.571875000614517681, -6.054752690667223547, -1.112240025338166033E-15 ) ) ;
#39409=CARTESIAN_POINT ( 'NONE',  ( 8.550000001229031810, -2.886751345948129988, 4.999999999999997335 ) ) ;
#39410=CARTESIAN_POINT ( 'NONE',  ( 16.31250000122903288, -4.330127018922190985, -2.500000000000001332 ) ) ;
#39411=CARTESIAN_POINT ( 'NONE',  ( 12.96562500061451750, 3.027376345333613106, -5.243569643749998122 ) ) ;
#39412=CARTESIAN_POINT ( 'NONE',  ( 17.24062500061451786, -3.027376345333614438, 5.243569643749998122 ) ) ;
#39413=CARTESIAN_POINT ( 'NONE',  ( 27.63750000122903216, 6.123233995736764310E-16, -4.999999999999998224 ) ) ;
#39414=CARTESIAN_POINT ( 'NONE',  ( 22.87500000000000000, -4.330127018922194537, 2.499999999999995559 ) ) ;
#39415=CARTESIAN_POINT ( 'NONE',  ( 24.57187500061451502, -6.054752690667223547, -1.112240025338166033E-15 ) ) ;
#39416=CARTESIAN_POINT ( 'NONE',  ( 25.76250000122903216, -4.330127018922190985, -2.500000000000001332 ) ) ;
#39417=CARTESIAN_POINT ( 'NONE',  ( 10.57500000122903572, 2.886751345948129099, -4.999999999999998224 ) ) ;
#39418=CARTESIAN_POINT ( 'NONE',  ( 28.32187500061451502, 3.027376345333613106, -5.243569643749998122 ) ) ;
#39419=ADVANCED_FACE ( 'NONE', ( #23058 ), #46696, .T. ) ;
#39420=CARTESIAN_POINT ( 'NONE',  ( 5.184375000614516615, -4.541064518000419881, 2.621784821874995952 ) ) ;
#39421=CARTESIAN_POINT ( 'NONE',  ( 22.52812500061451573, 4.541064518000418104, 2.621784821874999949 ) ) ;
#39423=CARTESIAN_POINT ( 'NONE',  ( 0.000000000000000000, 20.00000000000000000, -33.99999999999999289 ) ) ;
#39424=CARTESIAN_POINT ( 'NONE',  ( 10.05937500061451750, 0.000000000000000000, 5.243569643749999010 ) ) ;
#39425=CARTESIAN_POINT ( 'NONE',  ( 3.999999999999999112, 12.57500000000000107, 30.00000000000000000 ) ) ;
#39426=CARTESIAN_POINT ( 'NONE',  ( 3.271875000614519635, 3.027376345333611329, 5.243569643749999010 ) ) ;
#39427=CARTESIAN_POINT ( 'NONE',  ( 6.684375000614518392, 6.421520780324663323E-16, -5.243569643749999010 ) ) ;
#39429=CARTESIAN_POINT ( 'NONE',  ( 27.45937500061451786, 4.541064518000418104, -2.621784821874998173 ) ) ;
#39430=CARTESIAN_POINT ( 'NONE',  ( 19.79999999999999716, -4.330127018922190985, -2.500000000000001332 ) ) ;
#39432=CARTESIAN_POINT ( 'NONE',  ( 26.06250000000000000, -5.773502691896255534, -1.060575238724906372E-15 ) ) ;
#39434=CARTESIAN_POINT ( 'NONE',  ( 29.74687500061451217, 6.054752690667223547, 3.707466751127219781E-16 ) ) ;
#39436=CARTESIAN_POINT ( 'NONE',  ( 15.55312500061451608, -4.541064518000417216, -2.621784821875001281 ) ) ;
#39437=CARTESIAN_POINT ( 'NONE',  ( 7.153125000614518392, 4.541064518000418104, -2.621784821874998173 ) ) ;
#39439=CARTESIAN_POINT ( 'NONE',  ( 4.996875000614516615, 6.054752690667223547, 3.707466751127219781E-16 ) ) ;
#39440=CARTESIAN_POINT ( 'NONE',  ( 18.18750000122903288, 6.123233995736764310E-16, -4.999999999999998224 ) ) ;
#39441=CARTESIAN_POINT ( 'NONE',  ( 23.21250000000000213, 2.886751345948126879, 4.999999999999999112 ) ) ;
#39442=CARTESIAN_POINT ( 'NONE',  ( 24.03750000122903430, 6.123233995736764310E-16, -4.999999999999998224 ) ) ;
#39443=CARTESIAN_POINT ( 'NONE',  ( 7.284375000614518036, 4.541064518000418104, 2.621784821874999949 ) ) ;
#39444=CARTESIAN_POINT ( 'NONE',  ( 12.19687500061451679, 6.054752690667223547, 3.707466751127219781E-16 ) ) ;
#39445=CARTESIAN_POINT ( 'NONE',  ( 21.53437500061451715, 6.421520780324663323E-16, -5.243569643749999010 ) ) ;
#39448=CARTESIAN_POINT ( 'NONE',  ( 4.134375000614517681, 4.541064518000418104, 2.621784821874999949 ) ) ;
#39449=CARTESIAN_POINT ( 'NONE',  ( 6.046875000614519102, -3.027376345333614438, 5.243569643749998122 ) ) ;
#39450=CARTESIAN_POINT ( 'NONE',  ( 18.14999999999999858, 4.330127018922192761, -2.499999999999997780 ) ) ;
#39451=CARTESIAN_POINT ( 'NONE',  ( 15.92812500061451608, -4.541064518000419881, 2.621784821874995952 ) ) ;
#39453=CARTESIAN_POINT ( 'NONE',  ( 4.289383384044220371, 2.569665102604888673, 4.334061492837330221 ) ) ;
#39455=CARTESIAN_POINT ( 'NONE',  ( 10.00312500061451715, 0.000000000000000000, 5.243569643749999010 ) ) ;
#39456=CARTESIAN_POINT ( 'NONE',  ( 27.38437500061451857, 6.421520780324663323E-16, -5.243569643749999010 ) ) ;
#39457=FACE_OUTER_BOUND ( 'NONE', #71731, .T. ) ;
#39458=CARTESIAN_POINT ( 'NONE',  ( 29.67187500061451644, 3.027376345333613106, -5.243569643749998122 ) ) ;
#39459=CARTESIAN_POINT ( 'NONE',  ( 9.000000000000001776, -4.330127018922190985, -2.500000000000001332 ) ) ;
#39460=CARTESIAN_POINT ( 'NONE',  ( -3.999999999999999112, 14.71250000122903501, 30.00000000000000000 ) ) ;
#39461=CARTESIAN_POINT ( 'NONE',  ( 10.20000000122903572, 5.773502691896255534, 3.535250795749688894E-16 ) ) ;
#39462=CARTESIAN_POINT ( 'NONE',  ( 19.84687500061451360, 6.054752690667223547, 3.707466751127219781E-16 ) ) ;
#39463=CARTESIAN_POINT ( 'NONE',  ( 13.99687500061451928, 6.054752690667223547, 3.707466751127219781E-16 ) ) ;
#39466=CARTESIAN_POINT ( 'NONE',  ( 15.74062500061451608, 6.054752690667223547, 3.707466751127219781E-16 ) ) ;
#39467=CARTESIAN_POINT ( 'NONE',  ( 27.33750000122903145, 4.330127018922191873, 2.499999999999999556 ) ) ;
#39468=CARTESIAN_POINT ( 'NONE',  ( 15.00937500061451679, 0.000000000000000000, 5.243569643749999010 ) ) ;
#39469=CARTESIAN_POINT ( 'NONE',  ( 3.365625000614516082, -6.054752690667223547, -1.112240025338166033E-15 ) ) ;
#39470=CARTESIAN_POINT ( 'NONE',  ( 16.45312500061451289, -4.541064518000417216, -2.621784821875001281 ) ) ;
#39472=CARTESIAN_POINT ( 'NONE',  ( 26.70937500061451431, 0.000000000000000000, 5.243569643749999010 ) ) ;
#39473=CARTESIAN_POINT ( 'NONE',  ( -4.243569643749999898, 11.21562500061451750, 27.54997392385601529 ) ) ;
#39474=CARTESIAN_POINT ( 'NONE',  ( 15.27187500061451786, 3.027376345333613106, -5.243569643749998122 ) ) ;
#39475=CARTESIAN_POINT ( 'NONE',  ( 14.81250000122903288, 0.000000000000000000, 4.999999999999998224 ) ) ;
#39476=LINE ( 'NONE', #46105, #10334 ) ;
#39477=CARTESIAN_POINT ( 'NONE',  ( 3.342464638718772196, -3.718602191040201621, 3.696902112923342365 ) ) ;
#39478=CARTESIAN_POINT ( 'NONE',  ( 18.34687500061451715, -3.027376345333610441, -5.243569643749999898 ) ) ;
#39479=CARTESIAN_POINT ( 'NONE',  ( 21.18750000122903288, -4.330127018922194537, 2.499999999999995559 ) ) ;
#39481=CARTESIAN_POINT ( 'NONE',  ( 14.33437500061451786, 6.421520780324663323E-16, -5.243569643749999010 ) ) ;
#39482=CARTESIAN_POINT ( 'NONE',  ( 2.121784821874999061, 13.40937500061451892, 26.32496088578401583 ) ) ;
#39483=CARTESIAN_POINT ( 'NONE',  ( 21.60000000122903430, -2.886751345948129988, 4.999999999999997335 ) ) ;
#39484=CARTESIAN_POINT ( 'NONE',  ( 15.25312500061451715, 4.541064518000418104, -2.621784821874998173 ) ) ;
#39486=VERTEX_POINT ( 'NONE', #10209 ) ;
#39488=CARTESIAN_POINT ( 'NONE',  ( 20.77500000000000213, 6.123233995736764310E-16, -4.999999999999998224 ) ) ;
#39489=CARTESIAN_POINT ( 'NONE',  ( -1.071796769724492338, 17.95490381179670081, 34.00000000000000000 ) ) ;
#39490=CARTESIAN_POINT ( 'NONE',  ( 21.14062500061451289, 6.054752690667223547, 3.707466751127219781E-16 ) ) ;
#39491=CARTESIAN_POINT ( 'NONE',  ( 3.942105046096219478, 3.076001935233271922, 29.30868670468199255 ) ) ;
#39492=CARTESIAN_POINT ( 'NONE',  ( 13.91250000122903252, 0.000000000000000000, 4.999999999999998224 ) ) ;
#39493=CARTESIAN_POINT ( 'NONE',  ( 19.00312500061451715, 0.000000000000000000, 5.243569643749999010 ) ) ;
#39494=CARTESIAN_POINT ( 'NONE',  ( 24.32812500061451289, 4.541064518000418104, 2.621784821874999949 ) ) ;
#39495=CARTESIAN_POINT ( 'NONE',  ( 5.578125000614518214, -4.541064518000419881, 2.621784821874995952 ) ) ;
#39496=ORIENTED_EDGE ( 'NONE', *, *, #69860, .T. ) ;
#39497=CARTESIAN_POINT ( 'NONE',  ( 29.39999999999999858, 4.330127018922192761, -2.499999999999997780 ) ) ;
#39501=CARTESIAN_POINT ( 'NONE',  ( 8.484601909799253346E-16, 11.67500000122903359, -25.38119784648299770 ) ) ;
#39502=CARTESIAN_POINT ( 'NONE',  ( 4.243569643749999010, 17.42187500061451999, -32.45002607614398471 ) ) ;
#39503=CARTESIAN_POINT ( 'NONE',  ( 6.862500001229034474, -4.330127018922190985, -2.500000000000001332 ) ) ;
#39504=CARTESIAN_POINT ( 'NONE',  ( 7.200000000000001954, -4.330127018922190985, -2.500000000000001332 ) ) ;
#39505=ADVANCED_FACE ( 'NONE', ( #6117 ), #27572, .F. ) ;
#39506=CARTESIAN_POINT ( 'NONE',  ( 3.712500001229034563, -4.330127018922190985, -2.500000000000001332 ) ) ;
#39507=CARTESIAN_POINT ( 'NONE',  ( 11.37187500061451750, 3.027376345333611329, 5.243569643749999010 ) ) ;
#39508=DIRECTION ( 'NONE',  ( -1.000000000000000000, -0.000000000000000000, -0.000000000000000000 ) ) ;
#39509=CARTESIAN_POINT ( 'NONE',  ( 3.684375000614518836, 4.541064518000418104, 2.621784821874999949 ) ) ;
#39510=CYLINDRICAL_SURFACE ( 'NONE', #9030, 3.999999999999996447 ) ;
#39512=CARTESIAN_POINT ( 'NONE',  ( 10.43437500061451750, 4.541064518000418104, 2.621784821874999949 ) ) ;
#39513=CARTESIAN_POINT ( 'NONE',  ( -3.999999999999997335, 18.68750000000000000, -27.69059892324149530 ) ) ;
#39514=CARTESIAN_POINT ( 'NONE',  ( 3.999999999999998668, 14.41250000000000142, 27.69059892324149530 ) ) ;
#39516=CARTESIAN_POINT ( 'NONE',  ( 4.243569643749999010, 16.91562500061459673, 27.54997392385601174 ) ) ;
#39517=CARTESIAN_POINT ( 'NONE',  ( 22.24687500061451217, -3.027376345333614438, 5.243569643749998122 ) ) ;
#39519=CARTESIAN_POINT ( 'NONE',  ( 29.10000000122903074, 5.773502691896255534, 3.535250795749688894E-16 ) ) ;
#39522=CARTESIAN_POINT ( 'NONE',  ( 22.60312500061451857, 0.000000000000000000, 5.243569643749999010 ) ) ;
#39523=CARTESIAN_POINT ( 'NONE',  ( 16.19062500061451715, 6.054752690667223547, 3.707466751127219781E-16 ) ) ;
#39525=CARTESIAN_POINT ( 'NONE',  ( 10.69687500061451679, -3.027376345333610441, -5.243569643749999898 ) ) ;
#39526=CARTESIAN_POINT ( 'NONE',  ( 29.25000000000000000, -4.330127018922190985, -2.500000000000001332 ) ) ;
#39527=CARTESIAN_POINT ( 'NONE',  ( 25.76250000122903216, -4.330127018922190985, -2.500000000000001332 ) ) ;
#39528=CARTESIAN_POINT ( 'NONE',  ( 4.059375000614519280, 4.541064518000418104, -2.621784821874998173 ) ) ;
#39529=AXIS2_PLACEMENT_3D ( 'NONE', #16105, #61535, #33827 ) ;
#39530=CARTESIAN_POINT ( 'NONE',  ( 13.80937500061451750, -4.541064518000417216, -2.621784821875001281 ) ) ;
#39531=CARTESIAN_POINT ( 'NONE',  ( 28.99687500061451573, -3.027376345333614438, 5.243569643749998122 ) ) ;
#39532=FACE_OUTER_BOUND ( 'NONE', #7172, .T. ) ;
#39533=CARTESIAN_POINT ( 'NONE',  ( 18.41249999999999787, -5.773502691896255534, -1.060575238724906372E-15 ) ) ;
#39534=CARTESIAN_POINT ( 'NONE',  ( 22.99687500061451573, 6.054752690667223547, 3.707466751127219781E-16 ) ) ;
#39535=CARTESIAN_POINT ( 'NONE',  ( 14.78437500061451715, 6.421520780324663323E-16, -5.243569643749999010 ) ) ;
#39537=CARTESIAN_POINT ( 'NONE',  ( 28.76249999999999929, -5.773502691896255534, -1.060575238724906372E-15 ) ) ;
#39538=CARTESIAN_POINT ( 'NONE',  ( 4.425000001229032698, 2.886751345948126879, 4.999999999999999112 ) ) ;
#39540=CARTESIAN_POINT ( 'NONE',  ( 16.60312500061451857, 4.541064518000418104, -2.621784821874998173 ) ) ;
#39541=CARTESIAN_POINT ( 'NONE',  ( 7.237500000000000711, -2.886751345948125991, -5.000000000000000000 ) ) ;
#39542=( BOUNDED_CURVE ( )  B_SPLINE_CURVE ( 2, ( #61182, #55284, #60805, #5400, #50470, #44575, #71545 ),
 .UNSPECIFIED., .F., .F. ) 
 B_SPLINE_CURVE_WITH_KNOTS ( ( 3, 2, 2, 3 ),
 ( 0.8166666666666666519, 0.8194444444444444198, 0.8222222222222222987, 0.8250000000000000666 ),
 .UNSPECIFIED. ) 
 CURVE ( )  GEOMETRIC_REPRESENTATION_ITEM ( )  RATIONAL_B_SPLINE_CURVE ( ( 1.000000000000000000, 0.8660254037844387076, 1.000000000000000000, 0.8660254037844387076, 1.000000000000000000, 0.8660254037844333785, 1.000000000000005329 ) ) 
 REPRESENTATION_ITEM ( '' )  );
#39544=CARTESIAN_POINT ( 'NONE',  ( 18.30000000000000071, 0.000000000000000000, 4.999999999999998224 ) ) ;
#39545=CARTESIAN_POINT ( 'NONE',  ( 2.121784821874999061, 12.00312500061451715, 26.32496088578401583 ) ) ;
#39547=CARTESIAN_POINT ( 'NONE',  ( 20.51250000122903216, 4.330127018922192761, -2.499999999999997780 ) ) ;
#39548=CARTESIAN_POINT ( 'NONE',  ( -3.999999999999999112, 13.32500000122903216, 27.69059892324149885 ) ) ;
#39549=CARTESIAN_POINT ( 'NONE',  ( 27.04687500061451644, 6.054752690667223547, 3.707466751127219781E-16 ) ) ;
#39551=CARTESIAN_POINT ( 'NONE',  ( 21.66562500061451502, 3.027376345333611329, 5.243569643749999010 ) ) ;
#39552=CARTESIAN_POINT ( 'NONE',  ( 22.32187500061451502, -6.054752690667223547, -1.112240025338166033E-15 ) ) ;
#39553=CARTESIAN_POINT ( 'NONE',  ( 5.887500000000000178, -2.886751345948125991, -5.000000000000000000 ) ) ;
#39554=CARTESIAN_POINT ( 'NONE',  ( 10.49062500061451431, -3.027376345333614438, 5.243569643749998122 ) ) ;
#39555=CARTESIAN_POINT ( 'NONE',  ( 23.61562500061451431, -6.054752690667223547, -1.112240025338166033E-15 ) ) ;
#39556=CARTESIAN_POINT ( 'NONE',  ( 14.18437500061451750, -4.541064518000419881, 2.621784821874995952 ) ) ;
#39557=CARTESIAN_POINT ( 'NONE',  ( 17.10937500061451999, 4.541064518000418104, -2.621784821874998173 ) ) ;
#39558=CARTESIAN_POINT ( 'NONE',  ( 4.442357930815816758, 2.294658147637304690, -4.714824131856698131 ) ) ;
#39559=CARTESIAN_POINT ( 'NONE',  ( 9.001249775931846008E-16, 18.11562500061451786, 34.90005215228797653 ) ) ;
#39560=CARTESIAN_POINT ( 'NONE',  ( 22.12500000122903288, -5.773502691896255534, -1.060575238724906372E-15 ) ) ;
#39562=CARTESIAN_POINT ( 'NONE',  ( 12.92812500061451786, 6.421520780324663323E-16, -5.243569643749999010 ) ) ;
#39563=CARTESIAN_POINT ( 'NONE',  ( 5.296875000614518214, -3.027376345333610441, -5.243569643749999898 ) ) ;
#39564=CARTESIAN_POINT ( 'NONE',  ( 4.696875000614518569, -3.027376345333614438, 5.243569643749998122 ) ) ;
#39566=CARTESIAN_POINT ( 'NONE',  ( 28.95937500061451431, 0.000000000000000000, 5.243569643749999010 ) ) ;
#39567=CARTESIAN_POINT ( 'NONE',  ( 17.39062500061451644, -3.027376345333610441, -5.243569643749999898 ) ) ;
#39568=CARTESIAN_POINT ( 'NONE',  ( 28.31250000122903288, 0.000000000000000000, 4.999999999999998224 ) ) ;
#39569=ADVANCED_FACE ( 'NONE', ( #27206 ), #49741, .F. ) ;
#39570=CARTESIAN_POINT ( 'NONE',  ( 28.22812500061451502, 6.421520780324663323E-16, -5.243569643749999010 ) ) ;
#39571=CARTESIAN_POINT ( 'NONE',  ( 21.00937500061451857, -4.541064518000417216, -2.621784821875001281 ) ) ;
#39572=CARTESIAN_POINT ( 'NONE',  ( 18.21562500061451573, -6.054752690667223547, -1.112240025338166033E-15 ) ) ;
#39573=CARTESIAN_POINT ( 'NONE',  ( 2.121784821874999061, 19.25937500061451857, 26.32496088578401583 ) ) ;
#39575=CARTESIAN_POINT ( 'NONE',  ( 23.87812500061451715, 4.541064518000418104, 2.621784821874999949 ) ) ;
#39576=CARTESIAN_POINT ( 'NONE',  ( 4.012500001229033053, 0.000000000000000000, 4.999999999999998224 ) ) ;
#39577=ORIENTED_EDGE ( 'NONE', *, *, #65470, .F. ) ;
#39578=CARTESIAN_POINT ( 'NONE',  ( 27.78749999999999787, -2.886751345948129988, 4.999999999999997335 ) ) ;
#39579=CARTESIAN_POINT ( 'NONE',  ( 4.000000000000000000, 13.43750000000000000, -27.69059892324149530 ) ) ;
#39581=CARTESIAN_POINT ( 'NONE',  ( 4.096875000614518925, 6.054752690667223547, 3.707466751127219781E-16 ) ) ;
#39582=CARTESIAN_POINT ( 'NONE',  ( 11.16562500061451679, 3.027376345333613106, -5.243569643749998122 ) ) ;
#39583=CARTESIAN_POINT ( 'NONE',  ( 25.72500000122903074, -5.773502691896255534, -1.060575238724906372E-15 ) ) ;
#39584=CARTESIAN_POINT ( 'NONE',  ( 12.75937500061451857, 0.000000000000000000, 5.243569643749999010 ) ) ;
#39585=CARTESIAN_POINT ( 'NONE',  ( 29.09062500061451573, -3.027376345333610441, -5.243569643749999898 ) ) ;
#39586=CARTESIAN_POINT ( 'NONE',  ( 28.83749999999999858, -2.886751345948125991, -5.000000000000000000 ) ) ;
#39587=CARTESIAN_POINT ( 'NONE',  ( 14.77500000122903501, 2.886751345948126879, 4.999999999999998224 ) ) ;
#39588=CARTESIAN_POINT ( 'NONE',  ( 12.47812500061451502, 6.421520780324663323E-16, -5.243569643749999010 ) ) ;
#39589=ORIENTED_EDGE ( 'NONE', *, *, #7572, .F. ) ;
#39590=VECTOR ( 'NONE', #1466, 1000.000000000000000 ) ;
#39591=CARTESIAN_POINT ( 'NONE',  ( 10.30312500061451431, 4.541064518000418104, -2.621784821874998173 ) ) ;
#39592=CARTESIAN_POINT ( 'NONE',  ( 7.153125000614518392, 4.541064518000418104, -2.621784821874998173 ) ) ;
#39595=CARTESIAN_POINT ( 'NONE',  ( 14.06250000122903288, -4.330127018922190985, -2.500000000000001332 ) ) ;
#39597=CARTESIAN_POINT ( 'NONE',  ( 16.72500000000000142, 6.123233995736764310E-16, -4.999999999999998224 ) ) ;
#39598=( BOUNDED_CURVE ( )  B_SPLINE_CURVE ( 2, ( #28613, #550, #16790, #23061, #45616, #68149, #51516 ),
 .UNSPECIFIED., .F., .F. ) 
 B_SPLINE_CURVE_WITH_KNOTS ( ( 3, 2, 2, 3 ),
 ( 0.3333333333333333703, 0.3361111111111111382, 0.3388888888888889062, 0.3416666666666666186 ),
 .UNSPECIFIED. ) 
 CURVE ( )  GEOMETRIC_REPRESENTATION_ITEM ( )  RATIONAL_B_SPLINE_CURVE ( ( 0.9999999999999973355, 0.8660254037844413721, 1.000000000000000000, 0.8660254037844387076, 1.000000000000000000, 0.8660254037844413721, 0.9999999999999973355 ) ) 
 REPRESENTATION_ITEM ( '' )  );
#39599=CARTESIAN_POINT ( 'NONE',  ( 16.39687500061451786, -3.027376345333614438, 5.243569643749998122 ) ) ;
#39600=CARTESIAN_POINT ( 'NONE',  ( 12.15000000122903501, -2.886751345948129988, 4.999999999999997335 ) ) ;
#39601=CARTESIAN_POINT ( 'NONE',  ( 19.02187500061451786, 3.027376345333611329, 5.243569643749999010 ) ) ;
#39603=CARTESIAN_POINT ( 'NONE',  ( 20.97187500061451715, -6.054752690667223547, -1.112240025338166033E-15 ) ) ;
#39604=CARTESIAN_POINT ( 'NONE',  ( -4.243569643749999898, 13.46562500061451928, -32.45002607614398471 ) ) ;
#39605=CARTESIAN_POINT ( 'NONE',  ( -3.999999999999999112, 19.66250000122903430, 30.00000000000000000 ) ) ;
#39607=FACE_OUTER_BOUND ( 'NONE', #28208, .T. ) ;
#39608=CARTESIAN_POINT ( 'NONE',  ( 28.04062500061451502, -3.027376345333614438, 5.243569643749998122 ) ) ;
#39611=EDGE_CURVE ( 'NONE', #65915, #50879, #27935, .T. ) ;
#39612=CARTESIAN_POINT ( 'NONE',  ( 24.63749999999999574, -2.886751345948129988, 4.999999999999997335 ) ) ;
#39614=CARTESIAN_POINT ( 'NONE',  ( 8.203125000614518214, 0.000000000000000000, 5.243569643749999010 ) ) ;
#39616=CARTESIAN_POINT ( 'NONE',  ( 20.10937500061451289, -4.541064518000417216, -2.621784821875001281 ) ) ;
#39618=VECTOR ( 'NONE', #10289, 1000.000000000000000 ) ;
#39619=CARTESIAN_POINT ( 'NONE',  ( 6.365625000614518747, 3.027376345333611329, 5.243569643749999010 ) ) ;
#39620=CARTESIAN_POINT ( 'NONE',  ( 9.871875000614517504, 3.027376345333613106, -5.243569643749998122 ) ) ;
#39621=ORIENTED_EDGE ( 'NONE', *, *, #33444, .F. ) ;
#39622=CARTESIAN_POINT ( 'NONE',  ( 20.48437500061451289, -4.541064518000419881, 2.621784821874995952 ) ) ;
#39625=CARTESIAN_POINT ( 'NONE',  ( 4.912499999999999645, -5.773502691896255534, -1.060575238724906372E-15 ) ) ;
#39626=CARTESIAN_POINT ( 'NONE',  ( 15.15000000122903323, 5.773502691896255534, 3.535250795749688894E-16 ) ) ;
#39628=CARTESIAN_POINT ( 'NONE',  ( -3.999999999999999112, 19.09999999999999787, -30.00000000000000000 ) ) ;
#39630=CARTESIAN_POINT ( 'NONE',  ( 12.56250000000000178, -5.773502691896255534, -1.060575238724906372E-15 ) ) ;
#39631=CARTESIAN_POINT ( 'NONE',  ( 24.92812500061451431, -4.541064518000419881, 2.621784821874995952 ) ) ;
#39632=CARTESIAN_POINT ( 'NONE',  ( 16.05000000000000071, 0.000000000000000000, 4.999999999999998224 ) ) ;
#39633=CARTESIAN_POINT ( 'NONE',  ( 11.55000000122903181, 5.773502691896255534, 3.535250795749688894E-16 ) ) ;
#39634=CARTESIAN_POINT ( 'NONE',  ( 8.653125000614515727, 0.000000000000000000, 5.243569643749999010 ) ) ;
#39635=VECTOR ( 'NONE', #42100, 1000.000000000000000 ) ;
#39636=CARTESIAN_POINT ( 'NONE',  ( 8.662499999999999645, 2.886751345948129099, -4.999999999999998224 ) ) ;
#39637=DIRECTION ( 'NONE',  ( 0.000000000000000000, 0.000000000000000000, 1.000000000000000000 ) ) ;
#39638=CARTESIAN_POINT ( 'NONE',  ( -2.121784821874999949, 13.93437500061451750, -33.67503911421598417 ) ) ;
#39639=CARTESIAN_POINT ( 'NONE',  ( 26.88750000122903216, 4.330127018922191873, 2.499999999999999556 ) ) ;
#39641=CARTESIAN_POINT ( 'NONE',  ( 6.899999999999999467, 4.330127018922192761, -2.499999999999997780 ) ) ;
#39642=CARTESIAN_POINT ( 'NONE',  ( -1.071796769724475906, 13.15759618943233100, -34.00000000000000711 ) ) ;
#39644=CARTESIAN_POINT ( 'NONE',  ( 22.37812500061451360, 6.421520780324663323E-16, -5.243569643749999010 ) ) ;
#39645=CARTESIAN_POINT ( 'NONE',  ( 12.90000000122903145, 5.773502691896255534, 3.535250795749688894E-16 ) ) ;
#39646=CARTESIAN_POINT ( 'NONE',  ( 29.24062500061451431, 6.054752690667223547, 3.707466751127219781E-16 ) ) ;
#39647=CARTESIAN_POINT ( 'NONE',  ( 28.80937500061451573, 4.541064518000418104, -2.621784821874998173 ) ) ;
#39648=CARTESIAN_POINT ( 'NONE',  ( 18.60937500061451644, 0.000000000000000000, 5.243569643749999010 ) ) ;
#39649=CARTESIAN_POINT ( 'NONE',  ( 16.86562500061451786, -6.054752690667223547, -1.112240025338166033E-15 ) ) ;
#39650=CARTESIAN_POINT ( 'NONE',  ( -4.243569643749999898, 12.60312500061459318, -30.00000000000000000 ) ) ;
#39651=CARTESIAN_POINT ( 'NONE',  ( 7.528125000614515727, 6.421520780324663323E-16, -5.243569643749999010 ) ) ;
#39652=CARTESIAN_POINT ( 'NONE',  ( 27.75000000122903288, 5.773502691896255534, 3.535250795749688894E-16 ) ) ;
#39654=CARTESIAN_POINT ( 'NONE',  ( 19.97812500061451502, -4.541064518000419881, 2.621784821874995952 ) ) ;
#39656=CARTESIAN_POINT ( 'NONE',  ( 3.450000001229036162, 5.773502691896255534, 3.535250795749688894E-16 ) ) ;
#39657=CARTESIAN_POINT ( 'NONE',  ( 12.90937500061451537, -4.541064518000417216, -2.621784821875001281 ) ) ;
#39658=CARTESIAN_POINT ( 'NONE',  ( 11.59687500061451892, -3.027376345333610441, -5.243569643749999898 ) ) ;
#39659=CARTESIAN_POINT ( 'NONE',  ( 21.04687500061451644, -3.027376345333610441, -5.243569643749999898 ) ) ;
#39661=FACE_OUTER_BOUND ( 'NONE', #4134, .T. ) ;
#39662=CARTESIAN_POINT ( 'NONE',  ( 26.91562500061451146, 3.027376345333613106, -5.243569643749998122 ) ) ;
#39663=CARTESIAN_POINT ( 'NONE',  ( 23.95312500061451289, 0.000000000000000000, 5.243569643749999010 ) ) ;
#39665=CARTESIAN_POINT ( 'NONE',  ( 4.000000000000000000, 17.93750000000000355, 32.30940107675849049 ) ) ;
#39666=CARTESIAN_POINT ( 'NONE',  ( 3.796875000614517326, -3.027376345333614438, 5.243569643749998122 ) ) ;
#39667=CARTESIAN_POINT ( 'NONE',  ( 12.97500000122903252, 2.886751345948126879, 4.999999999999999112 ) ) ;
#39668=CARTESIAN_POINT ( 'NONE',  ( 7.650000001229034119, -2.886751345948129988, 4.999999999999997335 ) ) ;
#39669=CARTESIAN_POINT ( 'NONE',  ( 21.60000000122903074, -2.886751345948130876, 4.999999999999996447 ) ) ;
#39670=CARTESIAN_POINT ( 'NONE',  ( 26.32500000122903216, 2.886751345948129099, -4.999999999999998224 ) ) ;
#39673=CARTESIAN_POINT ( 'NONE',  ( 10.88437500061451679, 4.541064518000418104, 2.621784821874999949 ) ) ;
#39674=CYLINDRICAL_SURFACE ( 'NONE', #8971, 4.000000000000000000 ) ;
#39675=CARTESIAN_POINT ( 'NONE',  ( 16.60312500061451857, 4.541064518000418104, -2.621784821874998173 ) ) ;
#39676=CARTESIAN_POINT ( 'NONE',  ( 14.52187500061451608, 3.027376345333611329, 5.243569643749999010 ) ) ;
#39677=CARTESIAN_POINT ( 'NONE',  ( 4.565625000614516260, 3.027376345333611329, 5.243569643749999010 ) ) ;
#39678=CARTESIAN_POINT ( 'NONE',  ( 22.02187500061451786, 3.027376345333612662, -5.243569643749998122 ) ) ;
#39679=CARTESIAN_POINT ( 'NONE',  ( 9.796875000614519990, -3.027376345333610441, -5.243569643749999898 ) ) ;
#39680=CARTESIAN_POINT ( 'NONE',  ( 4.865625000614517859, 3.027376345333613106, -5.243569643749998122 ) ) ;
#39682=CARTESIAN_POINT ( 'NONE',  ( 5.812500001229035540, 0.000000000000000000, 4.999999999999998224 ) ) ;
#39683=EDGE_CURVE ( 'NONE', #34387, #17794, #33956, .T. ) ;
#39684=CARTESIAN_POINT ( 'NONE',  ( 20.05312500061451431, -4.541064518000417216, -2.621784821875001281 ) ) ;
#39685=CARTESIAN_POINT ( 'NONE',  ( 7.050000001229036251, 5.773502691896255534, 3.535250795749688894E-16 ) ) ;
#39686=CARTESIAN_POINT ( 'NONE',  ( 17.87812500061451715, 6.421520780324663323E-16, -5.243569643749999010 ) ) ;
#39688=CARTESIAN_POINT ( 'NONE',  ( 12.47812500061451502, 6.421520780324663323E-16, -5.243569643749999010 ) ) ;
#39690=CARTESIAN_POINT ( 'NONE',  ( 14.10000000000000142, 4.330127018922192761, -2.499999999999997780 ) ) ;
#39691=CARTESIAN_POINT ( 'NONE',  ( 9.150000001229033231, -2.886751345948125991, -5.000000000000000000 ) ) ;
#39692=CARTESIAN_POINT ( 'NONE',  ( 5.015625000614518214, 3.027376345333611329, 5.243569643749999010 ) ) ;
#39693=CARTESIAN_POINT ( 'NONE',  ( 18.30000000122903359, 5.773502691896255534, 3.535250795749688894E-16 ) ) ;
#39695=CARTESIAN_POINT ( 'NONE',  ( -2.121784821874996840, 10.48437500061451821, -26.32496088578401583 ) ) ;
#39696=DIRECTION ( 'NONE',  ( 0.000000000000000000, 0.000000000000000000, 1.000000000000000000 ) ) ;
#39697=CARTESIAN_POINT ( 'NONE',  ( 24.14999999999999858, 0.000000000000000000, 4.999999999999998224 ) ) ;
#39698=EDGE_CURVE ( 'NONE', #48564, #29785, #49083, .T. ) ;
#39700=CARTESIAN_POINT ( 'NONE',  ( 20.25937500061451857, 4.541064518000418104, -2.621784821874998173 ) ) ;
#39701=CARTESIAN_POINT ( 'NONE',  ( 10.57500000122903039, 2.886751345948062486, -5.000000000000113687 ) ) ;
#39702=CARTESIAN_POINT ( 'NONE',  ( 16.22812500061451857, 4.541064518000418104, 2.621784821874999949 ) ) ;
#39704=CARTESIAN_POINT ( 'NONE',  ( -1.999999999999997113, 14.78750000122903252, 33.46410161513775705 ) ) ;
#39705=CARTESIAN_POINT ( 'NONE',  ( 10.42500000000000071, 6.123233995736764310E-16, -4.999999999999998224 ) ) ;
#39706=CARTESIAN_POINT ( 'NONE',  ( 26.03437500061451715, 6.421520780324663323E-16, -5.243569643749999010 ) ) ;
#39708=CARTESIAN_POINT ( 'NONE',  ( 11.35312500061451679, 0.000000000000000000, 5.243569643749999010 ) ) ;
#39709=CARTESIAN_POINT ( 'NONE',  ( 10.69687500061451679, -3.027376345333610441, -5.243569643749999898 ) ) ;
#39710=ORIENTED_EDGE ( 'NONE', *, *, #1892, .T. ) ;
#39711=CARTESIAN_POINT ( 'NONE',  ( 2.843225714139721028, -4.112946153745474120, -2.917534517181566756 ) ) ;
#39712=CARTESIAN_POINT ( 'NONE',  ( 20.80312500061451431, 0.000000000000000000, 5.243569643749999010 ) ) ;
#39714=CARTESIAN_POINT ( 'NONE',  ( -2.000000000000000000, 12.83750000122903501, 26.53589838486224650 ) ) ;
#39716=CARTESIAN_POINT ( 'NONE',  ( 11.17500000000000071, -4.330127018922194537, 2.499999999999995559 ) ) ;
#39717=CARTESIAN_POINT ( 'NONE',  ( 21.71250000122903501, -4.330127018922190985, -2.500000000000001332 ) ) ;
#39718=CARTESIAN_POINT ( 'NONE',  ( 15.66562500061451857, 3.027376345333613106, -5.243569643749998122 ) ) ;
#39721=CARTESIAN_POINT ( 'NONE',  ( 20.51249999999999929, 2.886751345948126879, 4.999999999999999112 ) ) ;
#39722=CARTESIAN_POINT ( 'NONE',  ( 24.00000000000000000, 4.330127018922192761, -2.499999999999997780 ) ) ;
#39723=CARTESIAN_POINT ( 'NONE',  ( 20.82187500061451857, 3.027376345333611329, 5.243569643749999010 ) ) ;
#39724=CARTESIAN_POINT ( 'NONE',  ( 25.19062500061451715, 6.054752690667223547, 3.707466751127219781E-16 ) ) ;
#39726=CARTESIAN_POINT ( 'NONE',  ( -5.810221930991193690E-16, 13.25000000122903465, -34.00000000000000000 ) ) ;
#39727=CARTESIAN_POINT ( 'NONE',  ( 7.678125000614516082, 4.541064518000418104, 2.621784821874999949 ) ) ;
#39729=CIRCLE ( 'NONE', #16082, 5.000000000000000000 ) ;
#39730=CARTESIAN_POINT ( 'NONE',  ( 15.15000000000000036, 0.000000000000000000, 4.999999999999998224 ) ) ;
#39731=CARTESIAN_POINT ( 'NONE',  ( 9.001249775931846008E-16, 17.66562500061451502, 34.90005215228797653 ) ) ;
#39732=CARTESIAN_POINT ( 'NONE',  ( 5.634375000614519458, -4.541064518000419881, 2.621784821874995952 ) ) ;
#39733=CARTESIAN_POINT ( 'NONE',  ( 26.89687500061451431, -3.027376345333610441, -5.243569643749999898 ) ) ;
#39734=ORIENTED_EDGE ( 'NONE', *, *, #52008, .T. ) ;
#39735=CARTESIAN_POINT ( 'NONE',  ( 23.46562500061451573, 3.027376345333611329, 5.243569643749999010 ) ) ;
#39736=CARTESIAN_POINT ( 'NONE',  ( 24.53437500061451715, -4.541064518000419881, 2.621784821874995952 ) ) ;
#39737=CARTESIAN_POINT ( 'NONE',  ( 4.243569643749999898, 18.64062500061459104, -27.54997392385601529 ) ) ;
#39738=CARTESIAN_POINT ( 'NONE',  ( 10.91250000000000320, 2.886751345948129099, -4.999999999999998224 ) ) ;
#39739=CARTESIAN_POINT ( 'NONE',  ( 8.278125000614515727, -4.541064518000419881, 2.621784821874995952 ) ) ;
#39740=FACE_OUTER_BOUND ( 'NONE', #19566, .T. ) ;
#39741=CARTESIAN_POINT ( 'NONE',  ( 1.071796769724491893, 11.13259618943233420, 33.99999999999999289 ) ) ;
#39742=CARTESIAN_POINT ( 'NONE',  ( 26.46562500061451573, 3.027376345333612662, -5.243569643749998122 ) ) ;
#39744=EDGE_CURVE ( 'NONE', #65546, #50439, #56623, .T. ) ;
#39746=CARTESIAN_POINT ( 'NONE',  ( 3.215625000614518836, 3.027376345333611329, 5.243569643749999010 ) ) ;
#39747=CARTESIAN_POINT ( 'NONE',  ( 18.72187500061451360, -6.054752690667223547, -1.112240025338166033E-15 ) ) ;
#39748=CARTESIAN_POINT ( 'NONE',  ( -2.121784821874996840, 14.08437500061451786, 33.67503911421598417 ) ) ;
#39749=CARTESIAN_POINT ( 'NONE',  ( 19.84687500061451360, 6.054752690667223547, 3.707466751127219781E-16 ) ) ;
#39750=CARTESIAN_POINT ( 'NONE',  ( 29.25937500061451502, 4.541064518000418104, -2.621784821874998173 ) ) ;
#39751=CARTESIAN_POINT ( 'NONE',  ( -2.121784821874996840, 19.03437500061451715, 33.67503911421598417 ) ) ;
#39752=CARTESIAN_POINT ( 'NONE',  ( 10.15312500061451750, -4.541064518000417216, -2.621784821875001281 ) ) ;
#39753=CARTESIAN_POINT ( 'NONE',  ( 3.999999999999998668, 17.22500000122903430, 27.69059892324149530 ) ) ;
#39754=CARTESIAN_POINT ( 'NONE',  ( 7.734375000614517326, 4.541064518000418104, 2.621784821874999949 ) ) ;
#39756=CARTESIAN_POINT ( 'NONE',  ( 8.690625000614515372, -3.027376345333614438, 5.243569643749998122 ) ) ;
#39757=CARTESIAN_POINT ( 'NONE',  ( 11.97187500061451892, -6.054752690667223547, -1.112240025338166033E-15 ) ) ;
#39759=CARTESIAN_POINT ( 'NONE',  ( 18.78750000122903430, 4.330127018922191873, 2.499999999999999556 ) ) ;
#39760=CARTESIAN_POINT ( 'NONE',  ( 6.759375000614516793, 4.541064518000418104, -2.621784821874998173 ) ) ;
#39761=CARTESIAN_POINT ( 'NONE',  ( 8.765625000614518214, -6.054752690667223547, -1.112240025338166033E-15 ) ) ;
#39764=CARTESIAN_POINT ( 'NONE',  ( 18.87187500061451573, 3.027376345333613106, -5.243569643749998122 ) ) ;
#39765=CARTESIAN_POINT ( 'NONE',  ( -5.810221930991193690E-16, 14.48749999999999893, 26.00000000000000355 ) ) ;
#39767=CARTESIAN_POINT ( 'NONE',  ( 26.12812500061451360, 4.541064518000418104, 2.621784821874999949 ) ) ;
#39768=CARTESIAN_POINT ( 'NONE',  ( 13.04062500061451502, 6.054752690667223547, 3.707466751127219781E-16 ) ) ;
#39769=EDGE_CURVE ( 'NONE', #36659, #4004, #71750, .T. ) ;
#39770=CARTESIAN_POINT ( 'NONE',  ( 2.878125000614517592, -4.541064518000419881, 2.621784821874995952 ) ) ;
#39771=CARTESIAN_POINT ( 'NONE',  ( 12.44062500061451537, -3.027376345333610441, -5.243569643749999898 ) ) ;
#39772=CARTESIAN_POINT ( 'NONE',  ( -4.243569643749999898, 10.40937500061451892, -30.00000000000000000 ) ) ;
#39773=CARTESIAN_POINT ( 'NONE',  ( 13.91250000122903252, 0.000000000000000000, 4.999999999999998224 ) ) ;
#39774=CARTESIAN_POINT ( 'NONE',  ( 27.70312500061451289, -4.541064518000417216, -2.621784821875001281 ) ) ;
#39775=CARTESIAN_POINT ( 'NONE',  ( 2.121784821875001281, 15.00312500061451715, -26.32496088578401938 ) ) ;
#39776=CARTESIAN_POINT ( 'NONE',  ( 15.56250000122903465, 4.330127018922192761, -2.499999999999997780 ) ) ;
#39777=CARTESIAN_POINT ( 'NONE',  ( 12.71250000000000036, 2.886751345948129099, -4.999999999999998224 ) ) ;
#39778=CARTESIAN_POINT ( 'NONE',  ( 19.94062500061451715, -3.027376345333614438, 5.243569643749998122 ) ) ;
#39779=CARTESIAN_POINT ( 'NONE',  ( 6.871875000614517504, 3.027376345333611329, 5.243569643749999010 ) ) ;
#39780=CARTESIAN_POINT ( 'NONE',  ( 7.612500001229035362, 0.000000000000000000, 4.999999999999998224 ) ) ;
#39781=CARTESIAN_POINT ( 'NONE',  ( 16.46250000122903501, 4.330127018922192761, -2.499999999999997780 ) ) ;
#39782=CARTESIAN_POINT ( 'NONE',  ( 11.95312500061451644, -4.541064518000417216, -2.621784821875001281 ) ) ;
#39783=CARTESIAN_POINT ( 'NONE',  ( 14.95312500061451644, 0.000000000000000000, 5.243569643749999010 ) ) ;
#39784=CARTESIAN_POINT ( 'NONE',  ( 27.45000000122903572, -2.886751345948129988, 4.999999999999997335 ) ) ;
#39785=CARTESIAN_POINT ( 'NONE',  ( 22.34999999999999787, 0.000000000000000000, 4.999999999999998224 ) ) ;
#39786=CARTESIAN_POINT ( 'NONE',  ( 23.55937500061451573, 0.000000000000000000, 5.243569643749999010 ) ) ;
#39788=CARTESIAN_POINT ( 'NONE',  ( 9.637500001229033941, 6.123233995736764310E-16, -4.999999999999998224 ) ) ;
#39789=CARTESIAN_POINT ( 'NONE',  ( 27.83437500061451786, 6.421520780324663323E-16, -5.243569643749999010 ) ) ;
#39790=CARTESIAN_POINT ( 'NONE',  ( 6.234375000614519102, 6.421520780324663323E-16, -5.243569643749999010 ) ) ;
#39791=CARTESIAN_POINT ( 'NONE',  ( 23.87812500061451715, 4.541064518000418104, 2.621784821874999949 ) ) ;
#39793=CARTESIAN_POINT ( 'NONE',  ( 4.898587196589411843E-16, 20.00000000000000000, -26.00000000000000000 ) ) ;
#39794=CARTESIAN_POINT ( 'NONE',  ( 11.44687500061451857, -3.027376345333614438, 5.243569643749998122 ) ) ;
#39795=B_SPLINE_CURVE_WITH_KNOTS ( 'NONE', 3,
 ( #28240, #61125, #530, #32689, #72941, #16773 ),
 .UNSPECIFIED., .F., .F.,
 ( 4, 2, 4 ),
 ( 2.013653876781666499E-16, 0.0005272855844084262241, 0.001054571168816651220 ),
 .UNSPECIFIED. ) ;
#39796=CARTESIAN_POINT ( 'NONE',  ( 4.575260086717169550, 2.016679235498957112, 4.840250765194281435 ) ) ;
#39797=CARTESIAN_POINT ( 'NONE',  ( 3.646875000614520079, 6.054752690667223547, 3.707466751127219781E-16 ) ) ;
#39798=CARTESIAN_POINT ( 'NONE',  ( 6.271875000614517859, 3.027376345333613106, -5.243569643749998122 ) ) ;
#39799=CARTESIAN_POINT ( 'NONE',  ( 6.637500000000001066, -2.886751345948130876, 4.999999999999996447 ) ) ;
#39800=CARTESIAN_POINT ( 'NONE',  ( 26.78437500061451360, -4.541064518000419881, 2.621784821874995952 ) ) ;
#39801=CARTESIAN_POINT ( 'NONE',  ( 4.243569643749999898, 10.54062500061459495, 32.45002607614398471 ) ) ;
#39802=CARTESIAN_POINT ( 'NONE',  ( 18.37500000000000355, -4.330127018922194537, 2.499999999999995559 ) ) ;
#39803=ORIENTED_EDGE ( 'NONE', *, *, #55282, .F. ) ;
#39804=CARTESIAN_POINT ( 'NONE',  ( 27.26249999999999929, 2.886751345948126879, 4.999999999999999112 ) ) ;
#39805=CARTESIAN_POINT ( 'NONE',  ( 29.14687500061451075, -3.027376345333610441, -5.243569643749999898 ) ) ;
#39807=CARTESIAN_POINT ( 'NONE',  ( 16.60312500061451857, 4.541064518000418104, -2.621784821874998173 ) ) ;
#39808=CARTESIAN_POINT ( 'NONE',  ( 9.178125000614517859, -4.541064518000419881, 2.621784821874995952 ) ) ;
#39810=CARTESIAN_POINT ( 'NONE',  ( 5.109375000614518214, 0.000000000000000000, 5.243569643749999010 ) ) ;
#39811=CARTESIAN_POINT ( 'NONE',  ( 17.96250000122903501, 0.000000000000000000, 4.999999999999998224 ) ) ;
#39812=CARTESIAN_POINT ( 'NONE',  ( 22.42500000000000071, -4.330127018922194537, 2.499999999999995559 ) ) ;
#39813=CARTESIAN_POINT ( 'NONE',  ( 3.999999999999998668, 13.96250000000000036, -32.30940107675850470 ) ) ;
#39814=CARTESIAN_POINT ( 'NONE',  ( 3.984375000614517326, 6.421520780324663323E-16, -5.243569643749999010 ) ) ;
#39815=CARTESIAN_POINT ( 'NONE',  ( 11.85937500061451644, 0.000000000000000000, 5.243569643749999010 ) ) ;
#39816=CARTESIAN_POINT ( 'NONE',  ( 21.08437500061451786, 6.421520780324663323E-16, -5.243569643749999010 ) ) ;
#39818=ORIENTED_EDGE ( 'NONE', *, *, #44518, .F. ) ;
#39819=EDGE_CURVE ( 'NONE', #29389, #22784, #8504, .T. ) ;
#39820=CARTESIAN_POINT ( 'NONE',  ( 3.946875000614517681, -3.027376345333610441, -5.243569643749999898 ) ) ;
#39821=CARTESIAN_POINT ( 'NONE',  ( 7.096875000614517148, -3.027376345333610441, -5.243569643749999898 ) ) ;
#39823=CARTESIAN_POINT ( 'NONE',  ( 18.52499999999999858, 6.123233995736764310E-16, -4.999999999999998224 ) ) ;
#39824=CARTESIAN_POINT ( 'NONE',  ( 14.91562500061451679, 3.027376345333611329, 5.243569643749999010 ) ) ;
#39826=CYLINDRICAL_SURFACE ( 'NONE', #50483, 4.999999999999998224 ) ;
#39828=CARTESIAN_POINT ( 'NONE',  ( 10.52812500061451750, -4.541064518000419881, 2.621784821874995952 ) ) ;
#39829=CARTESIAN_POINT ( 'NONE',  ( 27.57187500061451857, 3.027376345333611329, 5.243569643749999010 ) ) ;
#39830=CARTESIAN_POINT ( 'NONE',  ( 27.98437500061451289, 4.541064518000418104, 2.621784821874999949 ) ) ;
#39831=CARTESIAN_POINT ( 'NONE',  ( 8.849999999999999645, 0.000000000000000000, 4.999999999999998224 ) ) ;
#39832=CARTESIAN_POINT ( 'NONE',  ( 1.999999999999998668, 15.01250000122903394, 26.53589838486224650 ) ) ;
#39833=CARTESIAN_POINT ( 'NONE',  ( 9.450000001229033941, -2.886751345948129988, 4.999999999999997335 ) ) ;
#39834=( BOUNDED_CURVE ( )  B_SPLINE_CURVE ( 2, ( #37700, #8905, #25521, #58758, #70960, #13701, #53976 ),
 .UNSPECIFIED., .F., .F. ) 
 B_SPLINE_CURVE_WITH_KNOTS ( ( 3, 2, 2, 3 ),
 ( 0.8833333333333333037, 0.8861111111111110716, 0.8888888888888888395, 0.8916666666666667185 ),
 .UNSPECIFIED. ) 
 CURVE ( )  GEOMETRIC_REPRESENTATION_ITEM ( )  RATIONAL_B_SPLINE_CURVE ( ( 1.000000000000000000, 0.8660254037844387076, 1.000000000000000000, 0.8660254037844387076, 1.000000000000000000, 0.8660254037844387076, 1.000000000000000000 ) ) 
 REPRESENTATION_ITEM ( '' )  );
#39835=CARTESIAN_POINT ( 'NONE',  ( 20.33437500061451786, 4.541064518000418104, 2.621784821874999949 ) ) ;
#39836=CARTESIAN_POINT ( 'NONE',  ( 13.77187500061451786, -6.054752690667223547, -1.112240025338166033E-15 ) ) ;
#39837=CARTESIAN_POINT ( 'NONE',  ( 4.898587196589411843E-16, 20.00000000000000000, -26.00000000000000000 ) ) ;
#39838=ORIENTED_EDGE ( 'NONE', *, *, #2252, .T. ) ;
#39839=CARTESIAN_POINT ( 'NONE',  ( 14.31562500061451537, 3.027376345333613106, -5.243569643749998122 ) ) ;
#39840=CARTESIAN_POINT ( 'NONE',  ( 26.43750000122903288, 4.330127018922191873, 2.499999999999999556 ) ) ;
#39841=CARTESIAN_POINT ( 'NONE',  ( 14.22187500061451537, -6.054752690667223547, -1.112240025338166033E-15 ) ) ;
#39843=CARTESIAN_POINT ( 'NONE',  ( 17.80312500061451786, -4.541064518000417216, -2.621784821875001281 ) ) ;
#39844=CARTESIAN_POINT ( 'NONE',  ( 18.15000000122903501, -2.886751345948126435, -5.000000000000000000 ) ) ;
#39845=CARTESIAN_POINT ( 'NONE',  ( 27.19687500061451857, -3.027376345333614438, 5.243569643749998122 ) ) ;
#39846=CARTESIAN_POINT ( 'NONE',  ( 4.243569643749999010, 11.51562500061451644, 27.54997392385601174 ) ) ;
#39847=ADVANCED_FACE ( 'NONE', ( #29015 ), #35270, .F. ) ;
#39848=CARTESIAN_POINT ( 'NONE',  ( 15.83437500061451608, 4.541064518000418104, 2.621784821874999949 ) ) ;
#39849=CARTESIAN_POINT ( 'NONE',  ( 14.10000000122903252, -2.886751345948125991, -5.000000000000000000 ) ) ;
#39851=CARTESIAN_POINT ( 'NONE',  ( 9.001249775931846008E-16, 15.92187500061451821, -25.09994784771203058 ) ) ;
#39852=CARTESIAN_POINT ( 'NONE',  ( 18.42187500061451644, 3.027376345333613106, -5.243569643749998122 ) ) ;
#39853=CARTESIAN_POINT ( 'NONE',  ( 19.95000000122903572, -2.886751345948125991, -5.000000000000000000 ) ) ;
#39855=CARTESIAN_POINT ( 'NONE',  ( 14.25937500061451679, -4.541064518000417216, -2.621784821875001281 ) ) ;
#39856=CARTESIAN_POINT ( 'NONE',  ( -3.000416591977282496E-16, 11.19687500061451679, 25.09994784771203058 ) ) ;
#39857=CARTESIAN_POINT ( 'NONE',  ( 23.17500000122903359, 2.886751345948129099, -4.999999999999998224 ) ) ;
#39858=CARTESIAN_POINT ( 'NONE',  ( 15.59062500061451573, -3.027376345333610441, -5.243569643749999898 ) ) ;
#39859=DIRECTION ( 'NONE',  ( 0.000000000000000000, 0.000000000000000000, -1.000000000000000000 ) ) ;
#39860=ORIENTED_EDGE ( 'NONE', *, *, #27502, .T. ) ;
#39861=VERTEX_POINT ( 'NONE', #17549 ) ;
#39862=CARTESIAN_POINT ( 'NONE',  ( 20.36249999999999716, 2.886751345948129099, -4.999999999999998224 ) ) ;
#39863=CARTESIAN_POINT ( 'NONE',  ( 15.03750000122903252, 6.123233995736764310E-16, -4.999999999999998224 ) ) ;
#39864=CARTESIAN_POINT ( 'NONE',  ( 0.1378111602261695712, 5.000000000000000000, 33.99999999999998579 ) ) ;
#39865=CARTESIAN_POINT ( 'NONE',  ( 15.45000000122903216, -2.886751345948125991, -5.000000000000000000 ) ) ;
#39866=CARTESIAN_POINT ( 'NONE',  ( 18.85312500061451502, 4.541064518000418104, -2.621784821874998173 ) ) ;
#39867=CARTESIAN_POINT ( 'NONE',  ( 23.95312500061451289, 0.000000000000000000, 5.243569643749999010 ) ) ;
#39868=CARTESIAN_POINT ( 'NONE',  ( 5.690625000614516260, -3.027376345333610441, -5.243569643749999898 ) ) ;
#39872=CARTESIAN_POINT ( 'NONE',  ( 29.82187500061451502, 3.027376345333611329, 5.243569643749999010 ) ) ;
#39873=CARTESIAN_POINT ( 'NONE',  ( -3.999999999999999556, 11.07500000122903394, -32.30940107675850470 ) ) ;
#39874=CARTESIAN_POINT ( 'NONE',  ( 4.243569643749999898, 18.73437500061451644, -30.00000000000000000 ) ) ;
#39875=CARTESIAN_POINT ( 'NONE',  ( 6.637500001229035718, 4.330127018922191873, 2.499999999999999556 ) ) ;
#39877=CARTESIAN_POINT ( 'NONE',  ( 9.299999999999998934, 0.000000000000000000, 4.999999999999998224 ) ) ;
#39878=CARTESIAN_POINT ( 'NONE',  ( 4.575000001229033941, -5.773502691896255534, -1.060575238724906372E-15 ) ) ;
#39879=CARTESIAN_POINT ( 'NONE',  ( 12.75937500061451857, 0.000000000000000000, 5.243569643749999010 ) ) ;
#39880=CARTESIAN_POINT ( 'NONE',  ( 29.76562500061451644, 3.027376345333611329, 5.243569643749999010 ) ) ;
#39881=CARTESIAN_POINT ( 'NONE',  ( 4.509375000614518569, 4.541064518000418104, -2.621784821874998173 ) ) ;
#39882=CARTESIAN_POINT ( 'NONE',  ( 3.486133158594716510E-16, 19.55000000122903359, 26.00000000000000355 ) ) ;
#39883=CARTESIAN_POINT ( 'NONE',  ( 9.459375000614517859, 4.541064518000418104, -2.621784821874998173 ) ) ;
#39884=CARTESIAN_POINT ( 'NONE',  ( 14.37187500061451928, 3.027376345333613106, -5.243569643749998122 ) ) ;
#39885=CARTESIAN_POINT ( 'NONE',  ( 1.071796769724491893, 13.94509619066136707, -26.00000000000000355 ) ) ;
#39886=CARTESIAN_POINT ( 'NONE',  ( 6.000000000000001776, 4.330127018922192761, -2.499999999999997780 ) ) ;
#39887=CARTESIAN_POINT ( 'NONE',  ( -4.243569643749998122, 16.24062500061459247, 32.45002607614398471 ) ) ;
#39888=CARTESIAN_POINT ( 'NONE',  ( 21.08437500061451786, 6.421520780324663323E-16, -5.243569643749999010 ) ) ;
#39889=CARTESIAN_POINT ( 'NONE',  ( 9.674999999999998934, 4.330127018922191873, 2.499999999999999556 ) ) ;
#39890=CARTESIAN_POINT ( 'NONE',  ( 27.37500000122903288, 2.886751345948126879, 4.999999999999999112 ) ) ;
#39892=CARTESIAN_POINT ( 'NONE',  ( 22.26562500061451644, -6.054752690667223547, -1.112240025338166033E-15 ) ) ;
#39893=CARTESIAN_POINT ( 'NONE',  ( 14.91562500061451679, 3.027376345333611329, 5.243569643749999010 ) ) ;
#39895=CARTESIAN_POINT ( 'NONE',  ( 11.59687500061451892, -3.027376345333610441, -5.243569643749999898 ) ) ;
#39896=CARTESIAN_POINT ( 'NONE',  ( 27.67499999999999716, 4.330127018922191873, 2.499999999999999556 ) ) ;
#39897=CARTESIAN_POINT ( 'NONE',  ( 24.48750000122903359, 6.123233995736764310E-16, -4.999999999999998224 ) ) ;
#39898=CARTESIAN_POINT ( 'NONE',  ( 3.309375000614518836, 0.000000000000000000, 5.243569643749999010 ) ) ;
#39899=CARTESIAN_POINT ( 'NONE',  ( 13.54687500061451999, 6.054752690667223547, 3.707466751127219781E-16 ) ) ;
#39903=CARTESIAN_POINT ( 'NONE',  ( 23.18437500061451573, -4.541064518000419881, 2.621784821874995952 ) ) ;
#39904=CARTESIAN_POINT ( 'NONE',  ( 13.50937500061451679, 4.541064518000418104, -2.621784821874998173 ) ) ;
#39906=CARTESIAN_POINT ( 'NONE',  ( 25.01249999999999929, 2.886751345948126879, 4.999999999999999112 ) ) ;
#39907=CARTESIAN_POINT ( 'NONE',  ( 3.487500001229035362, 4.330127018922191873, 2.499999999999999556 ) ) ;
#39909=CARTESIAN_POINT ( 'NONE',  ( 17.61562500061451786, 3.027376345333611329, 5.243569643749999010 ) ) ;
#39910=CARTESIAN_POINT ( 'NONE',  ( 7.837499999999999467, 5.773502691896255534, 3.535250795749688894E-16 ) ) ;
#39911=CARTESIAN_POINT ( 'NONE',  ( -1.071796769724491005, 14.05759618943233669, 26.00000000000000355 ) ) ;
#39912=CARTESIAN_POINT ( 'NONE',  ( 17.92500000000000071, -4.330127018922194537, 2.499999999999995559 ) ) ;
#39913=CARTESIAN_POINT ( 'NONE',  ( 4.243569643749999010, 13.76562500061451644, 27.54997392385601174 ) ) ;
#39915=CARTESIAN_POINT ( 'NONE',  ( 20.73750000122903359, -4.330127018922194537, 2.499999999999995559 ) ) ;
#39916=CARTESIAN_POINT ( 'NONE',  ( 27.98437500061451289, 4.541064518000418104, 2.621784821874999949 ) ) ;
#39918=CARTESIAN_POINT ( 'NONE',  ( 21.02812500061451573, 6.421520780324663323E-16, -5.243569643749999010 ) ) ;
#39919=CARTESIAN_POINT ( 'NONE',  ( 22.80937500061451573, -4.541064518000417216, -2.621784821875001281 ) ) ;
#39920=CARTESIAN_POINT ( 'NONE',  ( 3.225000000000002309, 6.123233995736764310E-16, -4.999999999999998224 ) ) ;
#39921=CARTESIAN_POINT ( 'NONE',  ( 9.553125000614517859, 0.000000000000000000, 5.243569643749999010 ) ) ;
#39922=CARTESIAN_POINT ( 'NONE',  ( 23.42812500061451786, 4.541064518000418104, 2.621784821874999949 ) ) ;
#39923=CARTESIAN_POINT ( 'NONE',  ( 13.02187500061451608, 3.027376345333613106, -5.243569643749998122 ) ) ;
#39924=CARTESIAN_POINT ( 'NONE',  ( 16.02187500061451786, -6.054752690667223547, -1.112240025338166033E-15 ) ) ;
#39925=CARTESIAN_POINT ( 'NONE',  ( 4.243569643749999010, 17.36562500061451786, 27.54997392385601174 ) ) ;
#39926=CARTESIAN_POINT ( 'NONE',  ( 20.21250000122903145, 0.000000000000000000, 4.999999999999998224 ) ) ;
#39928=CARTESIAN_POINT ( 'NONE',  ( 13.07812500061451821, 4.541064518000418104, 2.621784821874999949 ) ) ;
#39929=CARTESIAN_POINT ( 'NONE',  ( 4.809375000614516615, -4.541064518000417216, -2.621784821875001281 ) ) ;
#39930=CARTESIAN_POINT ( 'NONE',  ( 5.109375000614518214, 0.000000000000000000, 5.243569643749999010 ) ) ;
#39931=EDGE_LOOP ( 'NONE', ( #46237, #64871, #65591, #55972 ) ) ;
#39932=CARTESIAN_POINT ( 'NONE',  ( 26.07187500061451857, 3.027376345333613106, -5.243569643749998122 ) ) ;
#39933=CARTESIAN_POINT ( 'NONE',  ( 16.34062500061451573, -3.027376345333614438, 5.243569643749998122 ) ) ;
#39934=CARTESIAN_POINT ( 'NONE',  ( 27.33750000122903145, 4.330127018922191873, 2.499999999999999556 ) ) ;
#39936=CARTESIAN_POINT ( 'NONE',  ( 28.26562500061451289, 3.027376345333613106, -5.243569643749998122 ) ) ;
#39937=CARTESIAN_POINT ( 'NONE',  ( 22.50937500061451857, 4.541064518000418104, -2.621784821874998173 ) ) ;
#39938=CARTESIAN_POINT ( 'NONE',  ( 16.49062500061451786, -3.027376345333610441, -5.243569643749999898 ) ) ;
#39939=CARTESIAN_POINT ( 'NONE',  ( -2.121784821874996840, 19.03437500061451715, 33.67503911421598417 ) ) ;
#39940=CARTESIAN_POINT ( 'NONE',  ( 23.05312500061451431, 0.000000000000000000, 5.243569643749999010 ) ) ;
#39941=CARTESIAN_POINT ( 'NONE',  ( 3.750000001229034652, -2.886751345948125991, -5.000000000000000000 ) ) ;
#39942=ORIENTED_EDGE ( 'NONE', *, *, #32530, .F. ) ;
#39943=CARTESIAN_POINT ( 'NONE',  ( 27.44999999999999929, -4.330127018922190985, -2.500000000000001332 ) ) ;
#39944=CARTESIAN_POINT ( 'NONE',  ( -2.000000000000000000, 12.27500000000000036, -33.46410161513775705 ) ) ;
#39946=CARTESIAN_POINT ( 'NONE',  ( 3.084375000614519191, 6.421520780324663323E-16, -5.243569643749999010 ) ) ;
#39947=CARTESIAN_POINT ( 'NONE',  ( 10.15312500061451750, -4.541064518000417216, -2.621784821875001281 ) ) ;
#39948=CARTESIAN_POINT ( 'NONE',  ( 22.91250000122903430, 0.000000000000000000, 4.999999999999998224 ) ) ;
#39949=CARTESIAN_POINT ( 'NONE',  ( 12.57187500061452035, 3.027376345333612662, -5.243569643749998122 ) ) ;
#39950=CARTESIAN_POINT ( 'NONE',  ( 26.05312500061451431, 4.541064518000418104, -2.621784821874998173 ) ) ;
#39951=CARTESIAN_POINT ( 'NONE',  ( 27.07499999999999929, 6.123233995736764310E-16, -4.999999999999998224 ) ) ;
#39952=CARTESIAN_POINT ( 'NONE',  ( 1.999999999999998668, 18.61250000122903359, -33.46410161513775705 ) ) ;
#39953=CARTESIAN_POINT ( 'NONE',  ( 4.115625000614516082, 3.027376345333611329, 5.243569643749999010 ) ) ;
#39954=CARTESIAN_POINT ( 'NONE',  ( 11.91562500061451857, -6.054752690667223547, -1.112240025338166033E-15 ) ) ;
#39955=ORIENTED_EDGE ( 'NONE', *, *, #23306, .T. ) ;
#39956=CARTESIAN_POINT ( 'NONE',  ( 8.240625000614516082, -3.027376345333614438, 5.243569643749998122 ) ) ;
#39957=CARTESIAN_POINT ( 'NONE',  ( 6.215625000614517504, 3.027376345333613106, -5.243569643749998122 ) ) ;
#39960=CARTESIAN_POINT ( 'NONE',  ( 15.11249999999999893, 2.886751345948126879, 4.999999999999999112 ) ) ;
#39961=CARTESIAN_POINT ( 'NONE',  ( 17.25937500061451502, 0.000000000000000000, 5.243569643749999010 ) ) ;
#39962=CARTESIAN_POINT ( 'NONE',  ( 10.46250000122903323, -4.330127018922190985, -2.500000000000001332 ) ) ;
#39963=CARTESIAN_POINT ( 'NONE',  ( 19.88437500061451857, 4.541064518000418104, 2.621784821874999949 ) ) ;
#39965=CARTESIAN_POINT ( 'NONE',  ( 21.27187500061451786, 3.027376345333611329, 5.243569643749999010 ) ) ;
#39966=CARTESIAN_POINT ( 'NONE',  ( -2.121784821874996840, 14.47812500061451679, -26.32496088578401583 ) ) ;
#39969=CARTESIAN_POINT ( 'NONE',  ( -5.810221930991193690E-16, 11.78749999999999964, -34.00000000000000000 ) ) ;
#39970=CARTESIAN_POINT ( 'NONE',  ( 27.10312500061451502, 0.000000000000000000, 5.243569643749999010 ) ) ;
#39971=CARTESIAN_POINT ( 'NONE',  ( 17.13750000122903216, -4.330127018922194537, 2.499999999999995559 ) ) ;
#39972=CARTESIAN_POINT ( 'NONE',  ( 28.50937500061451502, 0.000000000000000000, 5.243569643749999010 ) ) ;
#39973=( BOUNDED_CURVE ( )  B_SPLINE_CURVE ( 2, ( #37732, #58791, #48828, #71358, #20732, #2660, #15193, #60251, #19995 ),
 .UNSPECIFIED., .F., .F. ) 
 B_SPLINE_CURVE_WITH_KNOTS ( ( 3, 2, 2, 2, 3 ),
 ( 0.6195652173913043237, 0.6231884057971014412, 0.6304347826086956763, 0.6376811594202898004, 0.6413043478260869179 ),
 .UNSPECIFIED. ) 
 CURVE ( )  GEOMETRIC_REPRESENTATION_ITEM ( )  RATIONAL_B_SPLINE_CURVE ( ( 0.9330127018922194093, 0.9330127018922194093, 1.000000000000000000, 0.8660254037844387076, 1.000000000000000000, 0.8660254037844387076, 1.000000000000000000, 0.9330127018922194093, 0.9330127018922194093 ) ) 
 REPRESENTATION_ITEM ( '' )  );
#39974=CARTESIAN_POINT ( 'NONE',  ( 24.07499999999999929, 4.330127018922191873, 2.499999999999999556 ) ) ;
#39975=EDGE_CURVE ( 'NONE', #51457, #27655, #23597, .T. ) ;
#39976=CARTESIAN_POINT ( 'NONE',  ( 6.815625000614517148, 3.027376345333611329, 5.243569643749999010 ) ) ;
#39978=CARTESIAN_POINT ( 'NONE',  ( 19.43437500061451928, 4.541064518000418104, 2.621784821874999949 ) ) ;
#39980=CARTESIAN_POINT ( 'NONE',  ( 5.690625000614516260, -3.027376345333610441, -5.243569643749999898 ) ) ;
#39981=CARTESIAN_POINT ( 'NONE',  ( 11.18437500061451928, 6.421520780324663323E-16, -5.243569643749999010 ) ) ;
#39983=CARTESIAN_POINT ( 'NONE',  ( 21.19687500061451502, 6.054752690667223547, 3.707466751127219781E-16 ) ) ;
#39985=CARTESIAN_POINT ( 'NONE',  ( 28.16249999999999787, 2.886751345948126879, 4.999999999999999112 ) ) ;
#39986=CARTESIAN_POINT ( 'NONE',  ( 29.25937500061451502, 4.541064518000418104, -2.621784821874998173 ) ) ;
#39987=DIRECTION ( 'NONE',  ( -0.000000000000000000, -1.000000000000000000, -0.000000000000000000 ) ) ;
#39989=CARTESIAN_POINT ( 'NONE',  ( 10.61250000000000071, 2.886751345948126879, 4.999999999999999112 ) ) ;
#39991=CARTESIAN_POINT ( 'NONE',  ( 25.04062500061451502, -3.027376345333610441, -5.243569643749999898 ) ) ;
#39992=CARTESIAN_POINT ( 'NONE',  ( 14.17500000000000071, 4.330127018922191873, 2.499999999999999556 ) ) ;
#39993=CARTESIAN_POINT ( 'NONE',  ( 11.02500000122903501, 2.886751345948129099, -4.999999999999998224 ) ) ;
#39994=CARTESIAN_POINT ( 'NONE',  ( 10.04062500061451502, -3.027376345333614438, 5.243569643749998122 ) ) ;
#39995=CARTESIAN_POINT ( 'NONE',  ( 9.449999999999999289, -4.330127018922190985, -2.500000000000001332 ) ) ;
#39997=CARTESIAN_POINT ( 'NONE',  ( 28.57500000122903572, 2.886751345948129099, -4.999999999999998224 ) ) ;
#39999=CARTESIAN_POINT ( 'NONE',  ( 7.575000000000001954, -4.330127018922194537, 2.499999999999995559 ) ) ;
#40001=ORIENTED_EDGE ( 'NONE', *, *, #30947, .T. ) ;
#40002=CARTESIAN_POINT ( 'NONE',  ( 21.59062500061451928, 6.054752690667223547, 3.707466751127219781E-16 ) ) ;
#40003=CARTESIAN_POINT ( 'NONE',  ( 29.01562500061451644, -6.054752690667223547, -1.112240025338166033E-15 ) ) ;
#40004=CARTESIAN_POINT ( 'NONE',  ( 29.22187500061451715, 3.027376345333613106, -5.243569643749998122 ) ) ;
#40005=CARTESIAN_POINT ( 'NONE',  ( 19.09687500061451360, -3.027376345333614438, 5.243569643749998122 ) ) ;
#40006=ADVANCED_FACE ( 'NONE', ( #590 ), #52629, .F. ) ;
#40007=CARTESIAN_POINT ( 'NONE',  ( 16.15312500061451573, 4.541064518000418104, -2.621784821874998173 ) ) ;
#40008=CARTESIAN_POINT ( 'NONE',  ( 4.243569643749999898, 10.57812500061459637, -30.00000000000000000 ) ) ;
#40009=CARTESIAN_POINT ( 'NONE',  ( 3.028125000614518392, 6.421520780324663323E-16, -5.243569643749999010 ) ) ;
#40010=CARTESIAN_POINT ( 'NONE',  ( 27.71250000122903145, 4.330127018922192761, -2.499999999999997780 ) ) ;
#40012=CARTESIAN_POINT ( 'NONE',  ( 19.86562500061451786, 3.027376345333611329, 5.243569643749999010 ) ) ;
#40014=CARTESIAN_POINT ( 'NONE',  ( 2.850000001229036073, -2.886751345948125991, -5.000000000000000000 ) ) ;
#40015=CARTESIAN_POINT ( 'NONE',  ( 13.05937500061451750, 4.541064518000418104, -2.621784821874998173 ) ) ;
#40016=CARTESIAN_POINT ( 'NONE',  ( 10.95937500061451964, 0.000000000000000000, 5.243569643749999010 ) ) ;
#40017=CARTESIAN_POINT ( 'NONE',  ( 20.22187500061451715, 3.027376345333613106, -5.243569643749998122 ) ) ;
#40018=ORIENTED_EDGE ( 'NONE', *, *, #33576, .F. ) ;
#40019=CARTESIAN_POINT ( 'NONE',  ( 2.164655401860464234, 4.642258459466365395, 2.164655401860464234 ) ) ;
#40020=CARTESIAN_POINT ( 'NONE',  ( 24.74062500061451786, 6.054752690667223547, 3.707466751127219781E-16 ) ) ;
#40021=CARTESIAN_POINT ( 'NONE',  ( 19.80937500061451573, 4.541064518000418104, -2.621784821874998173 ) ) ;
#40022=CARTESIAN_POINT ( 'NONE',  ( 24.77812500061451217, 4.541064518000418104, 2.621784821874999949 ) ) ;
#40024=CARTESIAN_POINT ( 'NONE',  ( -2.000000000000000000, 17.67500000000000071, 26.53589838486224650 ) ) ;
#40025=CARTESIAN_POINT ( 'NONE',  ( 28.56562500061451715, -6.054752690667223547, -1.112240025338166033E-15 ) ) ;
#40027=CARTESIAN_POINT ( 'NONE',  ( 11.62500000122903465, 2.886751345948126879, 4.999999999999999112 ) ) ;
#40028=CARTESIAN_POINT ( 'NONE',  ( 7.950000001229033053, 5.773502691896255534, 3.535250795749688894E-16 ) ) ;
#40029=CARTESIAN_POINT ( 'NONE',  ( 8.484601909799253346E-16, 19.21250000000000213, -25.38119784648299770 ) ) ;
#40030=CARTESIAN_POINT ( 'NONE',  ( 27.15000000122902790, -2.886751345948125991, -5.000000000000000000 ) ) ;
#40033=CARTESIAN_POINT ( 'NONE',  ( 9.234375000614518214, -4.541064518000419881, 2.621784821874995952 ) ) ;
#40035=CARTESIAN_POINT ( 'NONE',  ( 16.30312500061451786, 0.000000000000000000, 5.243569643749999010 ) ) ;
#40036=CARTESIAN_POINT ( 'NONE',  ( 13.17187500061451999, 3.027376345333611329, 5.243569643749999010 ) ) ;
#40037=CARTESIAN_POINT ( 'NONE',  ( 28.65000000122903145, 5.773502691896255534, 3.535250795749688894E-16 ) ) ;
#40038=CARTESIAN_POINT ( 'NONE',  ( 20.14687500061451786, -3.027376345333610441, -5.243569643749999898 ) ) ;
#40039=CARTESIAN_POINT ( 'NONE',  ( 6.346875000614517148, 6.054752690667223547, 3.707466751127219781E-16 ) ) ;
#40040=CARTESIAN_POINT ( 'NONE',  ( 3.665625000614517681, 3.027376345333611329, 5.243569643749999010 ) ) ;
#40042=CARTESIAN_POINT ( 'NONE',  ( 10.19062500061451892, -3.027376345333610441, -5.243569643749999898 ) ) ;
#40044=CARTESIAN_POINT ( 'NONE',  ( 19.60312500061451502, -4.541064518000417216, -2.621784821875001281 ) ) ;
#40046=B_SPLINE_CURVE_WITH_KNOTS ( 'NONE', 3,
 ( #26127, #15397, #66017, #65277, #49038, #37939, #15035, #26869, #60830, #10236 ),
 .UNSPECIFIED., .F., .F.,
 ( 4, 3, 3, 4 ),
 ( 0.000000000000000000, 5.625091169402055566E-05, 9.375822253212263134E-05, 0.0001312677523608356484 ),
 .UNSPECIFIED. ) ;
#40047=CARTESIAN_POINT ( 'NONE',  ( 5.625000001229036428, 2.886751345948129099, -4.999999999999998224 ) ) ;
#40048=CARTESIAN_POINT ( 'NONE',  ( 17.65312500061451573, 0.000000000000000000, 5.243569643749999010 ) ) ;
#40049=CARTESIAN_POINT ( 'NONE',  ( 13.49062500061451608, 6.054752690667223547, 3.707466751127219781E-16 ) ) ;
#40051=CARTESIAN_POINT ( 'NONE',  ( 12.90000000000000213, 0.000000000000000000, 4.999999999999998224 ) ) ;
#40052=CARTESIAN_POINT ( 'NONE',  ( 8.250000001229034652, -2.886751345948125991, -5.000000000000000000 ) ) ;
#40053=CARTESIAN_POINT ( 'NONE',  ( 5.578125000614518214, -4.541064518000419881, 2.621784821874995952 ) ) ;
#40054=CARTESIAN_POINT ( 'NONE',  ( 17.77500000122903145, 2.886751345948129099, -4.999999999999998224 ) ) ;
#40056=CARTESIAN_POINT ( 'NONE',  ( -2.121784821874999949, 10.33437500061451786, -33.67503911421598417 ) ) ;
#40057=CARTESIAN_POINT ( 'NONE',  ( 3.675000001229035362, -5.773502691896255534, -1.060575238724906372E-15 ) ) ;
#40059=CARTESIAN_POINT ( 'NONE',  ( 19.58437500061451786, -4.541064518000419881, 2.621784821874995952 ) ) ;
#40060=DIRECTION ( 'NONE',  ( -1.000000000000000000, -0.000000000000000000, -0.000000000000000000 ) ) ;
#40061=EDGE_CURVE ( 'NONE', #6439, #66791, #23165, .T. ) ;
#40062=CARTESIAN_POINT ( 'NONE',  ( 15.55312500061451608, -4.541064518000417216, -2.621784821875001281 ) ) ;
#40064=CARTESIAN_POINT ( 'NONE',  ( 15.86250000122903181, -4.330127018922190985, -2.500000000000001332 ) ) ;
#40065=CARTESIAN_POINT ( 'NONE',  ( 29.37187500061451928, 3.027376345333611329, 5.243569643749999010 ) ) ;
#40066=CARTESIAN_POINT ( 'NONE',  ( 27.38437500061451857, 6.421520780324663323E-16, -5.243569643749999010 ) ) ;
#40068=CARTESIAN_POINT ( 'NONE',  ( 12.29062500061451857, -3.027376345333614438, 5.243569643749998122 ) ) ;
#40069=CARTESIAN_POINT ( 'NONE',  ( 10.39687500061451786, 6.054752690667223547, 3.707466751127219781E-16 ) ) ;
#40071=CARTESIAN_POINT ( 'NONE',  ( 28.97812500061451502, -4.541064518000419881, 2.621784821874995952 ) ) ;
#40072=CARTESIAN_POINT ( 'NONE',  ( 21.02812500061451573, 6.421520780324663323E-16, -5.243569643749999010 ) ) ;
#40073=CARTESIAN_POINT ( 'NONE',  ( 3.999999999999998668, 13.17500000122903536, -32.30940107675850470 ) ) ;
#40074=ADVANCED_FACE ( 'NONE', ( #31181 ), #35890, .T. ) ;
#40075=CARTESIAN_POINT ( 'NONE',  ( 10.05000000000000071, 4.330127018922192761, -2.499999999999997780 ) ) ;
#40076=CARTESIAN_POINT ( 'NONE',  ( 21.37500000122902932, 2.886751345948129099, -4.999999999999998224 ) ) ;
#40077=CARTESIAN_POINT ( 'NONE',  ( 15.29062500061451679, 6.054752690667223547, 3.707466751127219781E-16 ) ) ;
#40080=CARTESIAN_POINT ( 'NONE',  ( 19.12500000000000000, 4.330127018922191873, 2.499999999999999556 ) ) ;
#40082=CARTESIAN_POINT ( 'NONE',  ( 21.93750000000000000, -2.886751345948129988, 4.999999999999997335 ) ) ;
#40083=CARTESIAN_POINT ( 'NONE',  ( 20.59687500061451360, -3.027376345333610441, -5.243569643749999898 ) ) ;
#40084=CARTESIAN_POINT ( 'NONE',  ( 25.41562500061451146, -6.054752690667223547, -1.112240025338166033E-15 ) ) ;
#40086=CARTESIAN_POINT ( 'NONE',  ( 28.61250000000000071, 2.886751345948143754, 4.999999999999969802 ) ) ;
#40087=CARTESIAN_POINT ( 'NONE',  ( 8.165625000614516793, 3.027376345333611329, 5.243569643749999010 ) ) ;
#40088=CARTESIAN_POINT ( 'NONE',  ( 3.999999999999998668, 12.16250000000000320, 27.69059892324149530 ) ) ;
#40089=CARTESIAN_POINT ( 'NONE',  ( 14.06250000000000000, 2.886751345948129099, -4.999999999999998224 ) ) ;
#40090=CARTESIAN_POINT ( 'NONE',  ( -4.243569643749997233, 17.59062500061451928, 32.45002607614398471 ) ) ;
#40091=CARTESIAN_POINT ( 'NONE',  ( 29.50312500061451360, -4.541064518000417216, -2.621784821875001281 ) ) ;
#40092=CARTESIAN_POINT ( 'NONE',  ( 25.88437500061451502, -4.541064518000419881, 2.621784821874995952 ) ) ;
#40093=ORIENTED_EDGE ( 'NONE', *, *, #19563, .T. ) ;
#40094=CARTESIAN_POINT ( 'NONE',  ( 23.57812500061451289, -4.541064518000419881, 2.621784821874995952 ) ) ;
#40095=CARTESIAN_POINT ( 'NONE',  ( 26.37187500061451217, -6.054752690667223547, -1.112240025338166033E-15 ) ) ;
#40096=CARTESIAN_POINT ( 'NONE',  ( 4.243569643749999010, 18.26562500061459104, -32.45002607614398471 ) ) ;
#40097=CARTESIAN_POINT ( 'NONE',  ( 11.06250000000000000, 2.886751345948126879, 4.999999999999999112 ) ) ;
#40098=CARTESIAN_POINT ( 'NONE',  ( 9.065625000614517148, 3.027376345333611329, 5.243569643749999010 ) ) ;
#40100=CARTESIAN_POINT ( 'NONE',  ( 29.54062500061451502, -3.027376345333610441, -5.243569643749999898 ) ) ;
#40101=CARTESIAN_POINT ( 'NONE',  ( 27.21562500061451573, -6.054752690667223547, -1.112240025338166033E-15 ) ) ;
#40104=CARTESIAN_POINT ( 'NONE',  ( 19.69687500061451857, -3.027376345333610441, -5.243569643749999898 ) ) ;
#40105=CARTESIAN_POINT ( 'NONE',  ( -4.243569643749997233, 15.39687500061451786, 32.45002607614398471 ) ) ;
#40106=CARTESIAN_POINT ( 'NONE',  ( 20.22187500061451715, 3.027376345333613106, -5.243569643749998122 ) ) ;
#40107=CARTESIAN_POINT ( 'NONE',  ( 27.08437500061451786, 4.541064518000418104, 2.621784821874999949 ) ) ;
#40108=CARTESIAN_POINT ( 'NONE',  ( -4.243569643749999898, 16.25937500061451857, 30.00000000000000000 ) ) ;
#40109=CARTESIAN_POINT ( 'NONE',  ( 9.403125000614517504, 4.541064518000418104, -2.621784821874998173 ) ) ;
#40110=CARTESIAN_POINT ( 'NONE',  ( 16.61250000122903359, 0.000000000000000000, 4.999999999999998224 ) ) ;
#40111=CARTESIAN_POINT ( 'NONE',  ( 5.784375000614517148, 6.421520780324663323E-16, -5.243569643749999010 ) ) ;
#40112=CARTESIAN_POINT ( 'NONE',  ( 26.06250000122903288, 0.000000000000000000, 4.999999999999998224 ) ) ;
#40113=CARTESIAN_POINT ( 'NONE',  ( 7.340625000614518392, -3.027376345333614438, 5.243569643749998122 ) ) ;
#40114=CARTESIAN_POINT ( 'NONE',  ( 12.60937500061451821, 4.541064518000418104, -2.621784821874998173 ) ) ;
#40115=CARTESIAN_POINT ( 'NONE',  ( 18.60000000122903430, -2.886751345948125991, -5.000000000000000000 ) ) ;
#40116=CARTESIAN_POINT ( 'NONE',  ( 6.421875000614519102, 3.027376345333611329, 5.243569643749999010 ) ) ;
#40117=CARTESIAN_POINT ( 'NONE',  ( 7.828125000614517326, -4.541064518000419881, 2.621784821874995952 ) ) ;
#40120=CARTESIAN_POINT ( 'NONE',  ( 18.57187500061451857, 3.027376345333611329, 5.243569643749999010 ) ) ;
#40123=CARTESIAN_POINT ( 'NONE',  ( 25.45312500061451644, -4.541064518000417216, -2.621784821875001281 ) ) ;
#40124=CARTESIAN_POINT ( 'NONE',  ( 13.30312500061451786, -4.541064518000417216, -2.621784821875001281 ) ) ;
#40125=EDGE_CURVE ( 'NONE', #72689, #40370, #15186, .T. ) ;
#40126=CARTESIAN_POINT ( 'NONE',  ( 27.75937500061451502, -4.541064518000417216, -2.621784821875001281 ) ) ;
#40127=CARTESIAN_POINT ( 'NONE',  ( 10.11562500061451608, -6.054752690667223547, -1.112240025338166033E-15 ) ) ;
#40129=CARTESIAN_POINT ( 'NONE',  ( 13.83750000122903323, 4.330127018922191873, 2.499999999999999556 ) ) ;
#40130=CARTESIAN_POINT ( 'NONE',  ( 26.50312500061451360, 4.541064518000418104, -2.621784821874998173 ) ) ;
#40131=CARTESIAN_POINT ( 'NONE',  ( 2.121784821874999061, 12.45312500061451821, -33.67503911421598417 ) ) ;
#40132=CARTESIAN_POINT ( 'NONE',  ( 14.32500000122903394, 2.886751345948126879, 4.999999999999999112 ) ) ;
#40133=CARTESIAN_POINT ( 'NONE',  ( 11.96250000000000213, 2.886751345948126879, 4.999999999999999112 ) ) ;
#40134=CARTESIAN_POINT ( 'NONE',  ( 20.50312500061451715, -4.541064518000417216, -2.621784821875001281 ) ) ;
#40135=CARTESIAN_POINT ( 'NONE',  ( 7.434375000614519280, -4.541064518000419881, 2.621784821874995952 ) ) ;
#40136=CARTESIAN_POINT ( 'NONE',  ( 8.587500001229035007, -4.330127018922194537, 2.499999999999995559 ) ) ;
#40137=CARTESIAN_POINT ( 'NONE',  ( 16.05000000122903359, 5.773502691896255534, 3.535250795749688894E-16 ) ) ;
#40138=CARTESIAN_POINT ( 'NONE',  ( 13.67812500061451786, -4.541064518000419881, 2.621784821874995952 ) ) ;
#40139=CARTESIAN_POINT ( 'NONE',  ( 14.91562500061451679, 3.027376345333611329, 5.243569643749999010 ) ) ;
#40140=CARTESIAN_POINT ( 'NONE',  ( 24.67500000122903359, 2.886751345948126879, 4.999999999999999112 ) ) ;
#40141=CARTESIAN_POINT ( 'NONE',  ( 19.83750000000000213, -2.886751345948125991, -5.000000000000000000 ) ) ;
#40142=CARTESIAN_POINT ( 'NONE',  ( 23.82187500061451502, 3.027376345333613106, -5.243569643749998122 ) ) ;
#40143=LINE ( 'NONE', #44240, #30003 ) ;
#40144=CARTESIAN_POINT ( 'NONE',  ( 9.187500001229034652, 6.123233995736764310E-16, -4.999999999999998224 ) ) ;
#40145=CARTESIAN_POINT ( 'NONE',  ( 10.05937500061451750, 0.000000000000000000, 5.243569643749999010 ) ) ;
#40146=CARTESIAN_POINT ( 'NONE',  ( 28.65937500061451715, -4.541064518000417216, -2.621784821875001281 ) ) ;
#40147=CARTESIAN_POINT ( 'NONE',  ( 4.211141394161732165, -2.695746283285643141, -4.240727999807930360 ) ) ;
#40148=CARTESIAN_POINT ( 'NONE',  ( 23.35312500061451857, 4.541064518000418104, -2.621784821874998173 ) ) ;
#40151=CARTESIAN_POINT ( 'NONE',  ( 7.734375000614517326, 4.541064518000418104, 2.621784821874999949 ) ) ;
#40153=CARTESIAN_POINT ( 'NONE',  ( 26.39062500061451644, -3.027376345333610441, -5.243569643749999898 ) ) ;
#40154=CARTESIAN_POINT ( 'NONE',  ( 6.571875000614517681, -6.054752690667223547, -1.112240025338166033E-15 ) ) ;
#40155=CARTESIAN_POINT ( 'NONE',  ( -3.999999999999999112, 16.47500000122903430, -32.30940107675850470 ) ) ;
#40156=CARTESIAN_POINT ( 'NONE',  ( 26.70937500061451431, 0.000000000000000000, 5.243569643749999010 ) ) ;
#40157=CARTESIAN_POINT ( 'NONE',  ( 2.121784821875001281, 10.50312500061459353, 33.67503911421598417 ) ) ;
#40158=CARTESIAN_POINT ( 'NONE',  ( 20.17499999999999716, -4.330127018922194537, 2.499999999999995559 ) ) ;
#40159=ORIENTED_EDGE ( 'NONE', *, *, #6614, .F. ) ;
#40160=CARTESIAN_POINT ( 'NONE',  ( 26.47499999999999787, -4.330127018922194537, 2.499999999999995559 ) ) ;
#40161=ADVANCED_FACE ( 'NONE', ( #52533 ), #35470, .T. ) ;
#40162=CARTESIAN_POINT ( 'NONE',  ( 27.49687500061451217, 6.054752690667223547, 3.707466751127219781E-16 ) ) ;
#40164=CARTESIAN_POINT ( 'NONE',  ( 15.40312500061451573, 0.000000000000000000, 5.243569643749999010 ) ) ;
#40165=CARTESIAN_POINT ( 'NONE',  ( 5.803125000614517859, 4.541064518000418104, -2.621784821874998173 ) ) ;
#40167=CARTESIAN_POINT ( 'NONE',  ( 3.946875000614517681, -3.027376345333610441, -5.243569643749999898 ) ) ;
#40168=CARTESIAN_POINT ( 'NONE',  ( 14.92500000122903181, -5.773502691896255534, -1.060575238724906372E-15 ) ) ;
#40169=CARTESIAN_POINT ( 'NONE',  ( 21.89999999999999858, 0.000000000000000000, 4.999999999999998224 ) ) ;
#40170=CARTESIAN_POINT ( 'NONE',  ( 28.91250000000000497, 2.886751345948129099, -4.999999999999998224 ) ) ;
#40171=CARTESIAN_POINT ( 'NONE',  ( 3.459375000614519635, -4.541064518000417216, -2.621784821875001281 ) ) ;
#40172=CARTESIAN_POINT ( 'NONE',  ( 8.371875000614515727, -6.054752690667223547, -1.112240025338166033E-15 ) ) ;
#40173=CARTESIAN_POINT ( 'NONE',  ( 21.27187500061451786, 3.027376345333611329, 5.243569643749999010 ) ) ;
#40174=CARTESIAN_POINT ( 'NONE',  ( -1.071796769724488563, 15.25490381179670152, -26.00000000000000000 ) ) ;
#40175=ORIENTED_EDGE ( 'NONE', *, *, #4248, .F. ) ;
#40176=CARTESIAN_POINT ( 'NONE',  ( 3.159375000614518036, 4.541064518000418104, -2.621784821874998173 ) ) ;
#40177=CARTESIAN_POINT ( 'NONE',  ( 6.834375000614518747, 4.541064518000418104, 2.621784821874999949 ) ) ;
#40178=CARTESIAN_POINT ( 'NONE',  ( 18.48750000000000071, -2.886751345948125991, -5.000000000000000000 ) ) ;
#40179=CARTESIAN_POINT ( 'NONE',  ( 17.20312500061451644, 0.000000000000000000, 5.243569643749999010 ) ) ;
#40181=CARTESIAN_POINT ( 'NONE',  ( 24.71250000122903145, 0.000000000000000000, 4.999999999999998224 ) ) ;
#40183=CARTESIAN_POINT ( 'NONE',  ( 10.07812500061451644, -4.541064518000419881, 2.621784821874995952 ) ) ;
#40184=CARTESIAN_POINT ( 'NONE',  ( 26.78437500061451360, -4.541064518000419881, 2.621784821874995952 ) ) ;
#40185=CARTESIAN_POINT ( 'NONE',  ( -5.810221930991193690E-16, 13.25000000122903465, 26.00000000000000355 ) ) ;
#40186=CARTESIAN_POINT ( 'NONE',  ( 26.14687500061451431, 6.054752690667223547, 3.707466751127219781E-16 ) ) ;
#40187=CARTESIAN_POINT ( 'NONE',  ( 6.899999999999999467, 4.330127018922192761, -2.499999999999997780 ) ) ;
#40188=CARTESIAN_POINT ( 'NONE',  ( 4.000000000000000000, 13.10000000122903430, 32.30940107675849049 ) ) ;
#40189=CARTESIAN_POINT ( 'NONE',  ( 5.587500001229033231, 6.123233995736764310E-16, -4.999999999999998224 ) ) ;
#40190=CARTESIAN_POINT ( 'NONE',  ( 19.43437500061451928, 4.541064518000418104, 2.621784821874999949 ) ) ;
#40191=CARTESIAN_POINT ( 'NONE',  ( 10.65937500061451715, -4.541064518000417216, -2.621784821875001281 ) ) ;
#40194=CARTESIAN_POINT ( 'NONE',  ( 15.10312500061451502, -4.541064518000417216, -2.621784821875001281 ) ) ;
#40195=CARTESIAN_POINT ( 'NONE',  ( 26.96250000122903145, 0.000000000000000000, 4.999999999999998224 ) ) ;
#40196=CARTESIAN_POINT ( 'NONE',  ( 13.13437500061451857, 4.541064518000418104, 2.621784821874999949 ) ) ;
#40197=CARTESIAN_POINT ( 'NONE',  ( 0.4082266053725470134, 9.993705886960393414, -35.98952669105264590 ) ) ;
#40198=CARTESIAN_POINT ( 'NONE',  ( 13.86562500061451431, 3.027376345333613106, -5.243569643749998122 ) ) ;
#40199=CARTESIAN_POINT ( 'NONE',  ( 2.000000000000001332, 18.80000000000000071, -26.53589838486224650 ) ) ;
#40200=CARTESIAN_POINT ( 'NONE',  ( 26.52187500061451431, 3.027376345333613106, -5.243569643749998122 ) ) ;
#40201=CARTESIAN_POINT ( 'NONE',  ( 2.898640642222699348, -4.074056819411355335, 3.301080373617285790 ) ) ;
#40202=CARTESIAN_POINT ( 'NONE',  ( 12.00000000122903465, 5.773502691896255534, 3.535250795749688894E-16 ) ) ;
#40203=CARTESIAN_POINT ( 'NONE',  ( 30.00000000000000000, 0.000000000000000000, 0.000000000000000000 ) ) ;
#40204=CARTESIAN_POINT ( 'NONE',  ( 9.001249775931846008E-16, 16.82187500061451857, -25.09994784771203058 ) ) ;
#40205=CARTESIAN_POINT ( 'NONE',  ( 17.70937500061451431, 0.000000000000000000, 5.243569643749999010 ) ) ;
#40206=CARTESIAN_POINT ( 'NONE',  ( 19.46250000122903145, -4.330127018922190985, -2.500000000000001332 ) ) ;
#40207=CARTESIAN_POINT ( 'NONE',  ( 14.85937500061451644, 4.541064518000418104, -2.621784821874998173 ) ) ;
#40208=CARTESIAN_POINT ( 'NONE',  ( -2.121784821874996840, 19.42812500061451786, -26.32496088578401583 ) ) ;
#40209=CARTESIAN_POINT ( 'NONE',  ( 23.32500000122903572, 2.886751345948126879, 4.999999999999999112 ) ) ;
#40210=CARTESIAN_POINT ( 'NONE',  ( 15.81562500061451537, 3.027376345333611329, 5.243569643749999010 ) ) ;
#40211=CARTESIAN_POINT ( 'NONE',  ( 29.05312500061451431, -4.541064518000417216, -2.621784821875001281 ) ) ;
#40214=CARTESIAN_POINT ( 'NONE',  ( 17.73750000000000071, 5.773502691896255534, 3.535250795749688894E-16 ) ) ;
#40216=CARTESIAN_POINT ( 'NONE',  ( 3.202568429182106602, 3.863133281671068620, 32.44766922691853495 ) ) ;
#40218=CARTESIAN_POINT ( 'NONE',  ( 15.07500000122903394, 2.886751345948129099, -4.999999999999998224 ) ) ;
#40219=CARTESIAN_POINT ( 'NONE',  ( 19.79062500061451502, 6.054752690667223547, 3.707466751127219781E-16 ) ) ;
#40220=CARTESIAN_POINT ( 'NONE',  ( 23.16562500061451502, -6.054752690667223547, -1.112240025338166033E-15 ) ) ;
#40221=CARTESIAN_POINT ( 'NONE',  ( 4.453125000614517326, 4.541064518000418104, -2.621784821874998173 ) ) ;
#40222=CARTESIAN_POINT ( 'NONE',  ( 27.71250000000000568, 2.886751345948126879, 4.999999999999999112 ) ) ;
#40223=CARTESIAN_POINT ( 'NONE',  ( 1.071796769724489895, 11.87990381179669974, 26.00000000000000355 ) ) ;
#40226=CARTESIAN_POINT ( 'NONE',  ( -3.999999999999999556, 10.17500000122903359, -32.30940107675850470 ) ) ;
#40227=CARTESIAN_POINT ( 'NONE',  ( 4.243569643749999010, 15.17187500061451644, -32.45002607614398471 ) ) ;
#40228=CARTESIAN_POINT ( 'NONE',  ( 5.587500001229033231, 6.123233995736764310E-16, -4.999999999999998224 ) ) ;
#40229=CARTESIAN_POINT ( 'NONE',  ( 7.462500000000001243, 2.886751345948126879, 4.999999999999999112 ) ) ;
#40230=CARTESIAN_POINT ( 'NONE',  ( 4.875000001229034652, 2.886751345948126879, 4.999999999999999112 ) ) ;
#40231=CARTESIAN_POINT ( 'NONE',  ( 10.20937500061451786, -4.541064518000417216, -2.621784821875001281 ) ) ;
#40232=CARTESIAN_POINT ( 'NONE',  ( 23.73750000122903359, 4.330127018922191873, 2.499999999999999556 ) ) ;
#40234=CARTESIAN_POINT ( 'NONE',  ( 29.62500000122903288, 2.886751345948126879, 4.999999999999998224 ) ) ;
#40235=CARTESIAN_POINT ( 'NONE',  ( 8.034375000614518925, 6.421520780324663323E-16, -5.243569643749999010 ) ) ;
#40236=CARTESIAN_POINT ( 'NONE',  ( 13.88437500061451679, 6.421520780324663323E-16, -5.243569643749999010 ) ) ;
#40238=CARTESIAN_POINT ( 'NONE',  ( 5.737499999999998934, -2.886751345948129988, 4.999999999999997335 ) ) ;
#40239=CARTESIAN_POINT ( 'NONE',  ( -2.121784821874996840, 16.27812500061459744, 33.67503911421598417 ) ) ;
#40240=CARTESIAN_POINT ( 'NONE',  ( 21.12187500061451573, 3.027376345333613106, -5.243569643749998122 ) ) ;
#40241=AXIS2_PLACEMENT_3D ( 'NONE', #40252, #62773, #23968 ) ;
#40243=( BOUNDED_CURVE ( )  B_SPLINE_CURVE ( 3, ( #3837, #27463, #26732, #60321 ),
 .UNSPECIFIED., .F., .F. ) 
 B_SPLINE_CURVE_WITH_KNOTS ( ( 4, 4 ),
 ( 0.6957555874851240052, 0.7294133852515908290 ),
 .UNSPECIFIED. ) 
 CURVE ( )  GEOMETRIC_REPRESENTATION_ITEM ( )  RATIONAL_B_SPLINE_CURVE ( ( 1.000000000000000000, 0.9999055982821311028, 0.9999055982821311028, 1.000000000000000000 ) ) 
 REPRESENTATION_ITEM ( '' )  );
#40244=CARTESIAN_POINT ( 'NONE',  ( 26.47500000122903074, 2.886751345948126879, 4.999999999999999112 ) ) ;
#40246=CARTESIAN_POINT ( 'NONE',  ( 22.04062500061451502, 6.054752690667223547, 3.707466751127219781E-16 ) ) ;
#40247=CARTESIAN_POINT ( 'NONE',  ( 16.60312500061451857, 4.541064518000418104, -2.621784821874998173 ) ) ;
#40249=CARTESIAN_POINT ( 'NONE',  ( 12.72187500061451537, 3.027376345333611329, 5.243569643749999010 ) ) ;
#40250=CARTESIAN_POINT ( 'NONE',  ( 29.55000000000000071, 0.000000000000000000, 4.999999999999998224 ) ) ;
#40251=CARTESIAN_POINT ( 'NONE',  ( 25.16250000122903074, 0.000000000000000000, 4.999999999999998224 ) ) ;
#40252=CARTESIAN_POINT ( 'NONE',  ( 0.000000000000000000, 20.00000000000000000, 30.00000000000000000 ) ) ;
#40253=CARTESIAN_POINT ( 'NONE',  ( 12.79687500061451821, -3.027376345333614438, 5.243569643749998122 ) ) ;
#40254=CARTESIAN_POINT ( 'NONE',  ( 28.28437500061451715, 6.421520780324663323E-16, -5.243569643749999010 ) ) ;
#40255=CARTESIAN_POINT ( 'NONE',  ( 4.898587196589411843E-16, 20.00000000000000000, 33.99999999999999289 ) ) ;
#40256=CARTESIAN_POINT ( 'NONE',  ( 11.88750000122903216, 6.123233995736764310E-16, -4.999999999999998224 ) ) ;
#40257=CARTESIAN_POINT ( 'NONE',  ( 21.53437500061451715, 6.421520780324663323E-16, -5.243569643749999010 ) ) ;
#40258=CARTESIAN_POINT ( 'NONE',  ( 13.58437500061451786, 4.541064518000418104, 2.621784821874999949 ) ) ;
#40260=CARTESIAN_POINT ( 'NONE',  ( 26.81250000000000000, 2.886751345948126879, 4.999999999999999112 ) ) ;
#40263=CARTESIAN_POINT ( 'NONE',  ( 16.97812500061451502, 6.421520780324663323E-16, -5.243569643749999010 ) ) ;
#40264=CARTESIAN_POINT ( 'NONE',  ( 5.850000000000001421, -4.330127018922190985, -2.500000000000001332 ) ) ;
#40265=CARTESIAN_POINT ( 'NONE',  ( 4.000000000000000000, 13.55000000122903359, 32.30940107675849760 ) ) ;
#40266=CARTESIAN_POINT ( 'NONE',  ( 17.84999999999999787, 0.000000000000000000, 4.999999999999998224 ) ) ;
#40267=CARTESIAN_POINT ( 'NONE',  ( 4.243569643749999898, 11.47812500061451679, 30.00000000000000000 ) ) ;
#40269=CARTESIAN_POINT ( 'NONE',  ( 26.97187500061451360, 3.027376345333613106, -5.243569643749998122 ) ) ;
#40270=ORIENTED_EDGE ( 'NONE', *, *, #45929, .T. ) ;
#40271=CARTESIAN_POINT ( 'NONE',  ( 20.84062500061451573, -3.027376345333614438, 5.243569643749998122 ) ) ;
#40272=CARTESIAN_POINT ( 'NONE',  ( 21.15937500061451715, 4.541064518000418104, -2.621784821874998173 ) ) ;
#40273=CARTESIAN_POINT ( 'NONE',  ( 4.500000000000000888, -4.330127018922190985, -2.500000000000001332 ) ) ;
#40274=CARTESIAN_POINT ( 'NONE',  ( 8.015625000614518214, 3.027376345333613106, -5.243569643749998122 ) ) ;
#40275=CARTESIAN_POINT ( 'NONE',  ( 23.87812500061451715, 4.541064518000418104, 2.621784821874999949 ) ) ;
#40276=CARTESIAN_POINT ( 'NONE',  ( 12.87187500061451750, -6.054752690667223547, -1.112240025338166033E-15 ) ) ;
#40277=CARTESIAN_POINT ( 'NONE',  ( 17.48437500061451999, 6.421520780324663323E-16, -5.243569643749999010 ) ) ;
#40278=CARTESIAN_POINT ( 'NONE',  ( -4.243569643749999898, 18.41562500061451857, 27.54997392385601529 ) ) ;
#40279=CARTESIAN_POINT ( 'NONE',  ( 19.61250000122903359, 4.330127018922192761, -2.499999999999997780 ) ) ;
#40281=CARTESIAN_POINT ( 'NONE',  ( 9.253125000614517148, -4.541064518000417216, -2.621784821875001281 ) ) ;
#40282=CARTESIAN_POINT ( 'NONE',  ( 5.371875000614516615, 3.027376345333613106, -5.243569643749998122 ) ) ;
#40283=CARTESIAN_POINT ( 'NONE',  ( 4.621875000614516615, 3.027376345333611329, 5.243569643749999010 ) ) ;
#40284=ORIENTED_EDGE ( 'NONE', *, *, #45137, .F. ) ;
#40285=CARTESIAN_POINT ( 'NONE',  ( 24.19687500061451857, -3.027376345333610441, -5.243569643749999898 ) ) ;
#40286=CARTESIAN_POINT ( 'NONE',  ( 15.74062500061451608, 6.054752690667223547, 3.707466751127219781E-16 ) ) ;
#40287=CARTESIAN_POINT ( 'NONE',  ( 26.73750000122903003, 6.123233995736764310E-16, -4.999999999999998224 ) ) ;
#40288=CARTESIAN_POINT ( 'NONE',  ( 27.40312500061451573, 4.541064518000418104, -2.621784821874998173 ) ) ;
#40289=CARTESIAN_POINT ( 'NONE',  ( 22.09687500061451715, 6.054752690667223547, 3.707466751127219781E-16 ) ) ;
#40290=CARTESIAN_POINT ( 'NONE',  ( 18.25312500061451715, -4.541064518000417216, -2.621784821875001281 ) ) ;
#40291=CARTESIAN_POINT ( 'NONE',  ( -4.243569643749999898, 17.12187500061451573, 27.54997392385601529 ) ) ;
#40292=CARTESIAN_POINT ( 'NONE',  ( 22.49062500061451431, 6.054752690667223547, 3.707466751127219781E-16 ) ) ;
#40293=CARTESIAN_POINT ( 'NONE',  ( 3.037500001229032964, 4.330127018922191873, 2.499999999999999556 ) ) ;
#40294=VERTEX_POINT ( 'NONE', #22136 ) ;
#40295=CARTESIAN_POINT ( 'NONE',  ( 28.16249999999999787, 2.886751345948126879, 4.999999999999999112 ) ) ;
#40296=CARTESIAN_POINT ( 'NONE',  ( -3.999999999999997335, 14.18750000000000000, -27.69059892324149175 ) ) ;
#40298=CARTESIAN_POINT ( 'NONE',  ( 3.271875000614519635, 3.027376345333611329, 5.243569643749999010 ) ) ;
#40299=CARTESIAN_POINT ( 'NONE',  ( 11.12812500061451715, 6.421520780324663323E-16, -5.243569643749999010 ) ) ;
#40300=CARTESIAN_POINT ( 'NONE',  ( 22.46250000122903501, 0.000000000000000000, 4.999999999999998224 ) ) ;
#40301=CARTESIAN_POINT ( 'NONE',  ( 26.91562500061451146, 3.027376345333613106, -5.243569643749998122 ) ) ;
#40302=CARTESIAN_POINT ( 'NONE',  ( 27.48749999999999716, -2.886751345948125991, -5.000000000000000000 ) ) ;
#40303=CARTESIAN_POINT ( 'NONE',  ( 8.484601909799253346E-16, 17.52500000122903501, -25.38119784648299770 ) ) ;
#40304=CARTESIAN_POINT ( 'NONE',  ( -3.999999999999997335, 15.65000000122903501, -27.69059892324149530 ) ) ;
#40305=CARTESIAN_POINT ( 'NONE',  ( 9.740625000614516082, -3.027376345333610441, -5.243569643749999898 ) ) ;
#40306=ORIENTED_EDGE ( 'NONE', *, *, #34124, .T. ) ;
#40307=CARTESIAN_POINT ( 'NONE',  ( 8.165625000614516793, 3.027376345333611329, 5.243569643749999010 ) ) ;
#40308=CARTESIAN_POINT ( 'NONE',  ( 5.128125000614516260, -4.541064518000419881, 2.621784821874995952 ) ) ;
#40310=CARTESIAN_POINT ( 'NONE',  ( 4.898587196589411843E-16, 20.00000000000000000, 33.99999999999999289 ) ) ;
#40311=CARTESIAN_POINT ( 'NONE',  ( 14.58750000000000036, 5.773502691896255534, 3.535250795749688894E-16 ) ) ;
#40312=CARTESIAN_POINT ( 'NONE',  ( 16.62187500061451573, 3.027376345333613106, -5.243569643749998122 ) ) ;
#40313=CARTESIAN_POINT ( 'NONE',  ( 11.77500000122903501, -5.773502691896255534, -1.060575238724906372E-15 ) ) ;
#40314=EDGE_CURVE ( 'NONE', #50439, #6778, #65671, .T. ) ;
#40315=CARTESIAN_POINT ( 'NONE',  ( 19.09687500061451360, -3.027376345333614438, 5.243569643749998122 ) ) ;
#40317=CARTESIAN_POINT ( 'NONE',  ( 20.48437500061451289, -4.541064518000419881, 2.621784821874995952 ) ) ;
#40318=CARTESIAN_POINT ( 'NONE',  ( -4.243569643749997233, 14.44062500061451715, -27.54997392385601174 ) ) ;
#40321=CARTESIAN_POINT ( 'NONE',  ( 4.148109664150280373, 2.791627878887652514, 4.438675071986421194 ) ) ;
#40322=CARTESIAN_POINT ( 'NONE',  ( 26.87812500061451360, 6.421520780324663323E-16, -5.243569643749999010 ) ) ;
#40323=CARTESIAN_POINT ( 'NONE',  ( 5.325000001229032165, 2.886751345948193936, 4.999999999999883649 ) ) ;
#40324=CARTESIAN_POINT ( 'NONE',  ( 29.55937500061451573, -4.541064518000417216, -2.621784821875001281 ) ) ;
#40325=CARTESIAN_POINT ( 'NONE',  ( 24.52499999999999858, 4.330127018922191873, 2.499999999999999556 ) ) ;
#40327=CARTESIAN_POINT ( 'NONE',  ( 7.490625000614516082, -3.027376345333610441, -5.243569643749999898 ) ) ;
#40329=CARTESIAN_POINT ( 'NONE',  ( 19.80937500061451573, 4.541064518000418104, -2.621784821874998173 ) ) ;
#40331=CARTESIAN_POINT ( 'NONE',  ( 4.753125000614515372, -4.541064518000417216, -2.621784821875001281 ) ) ;
#40332=CARTESIAN_POINT ( 'NONE',  ( 8.709375000614517859, 0.000000000000000000, 5.243569643749999010 ) ) ;
#40333=VERTEX_POINT ( 'NONE', #45767 ) ;
#40334=CARTESIAN_POINT ( 'NONE',  ( 18.75937500061451857, -4.541064518000417216, -2.621784821875001281 ) ) ;
#40335=CARTESIAN_POINT ( 'NONE',  ( 28.23750000000000426, -2.886751345948129988, 4.999999999999997335 ) ) ;
#40336=CARTESIAN_POINT ( 'NONE',  ( 3.562500000000000444, -5.773502691896255534, -1.060575238724906372E-15 ) ) ;
#40337=CARTESIAN_POINT ( 'NONE',  ( 2.000000000000001332, 10.25000000000000000, -26.53589838486224650 ) ) ;
#40339=EDGE_LOOP ( 'NONE', ( #14388, #65305, #50159, #33786 ) ) ;
#40340=CARTESIAN_POINT ( 'NONE',  ( 10.91250000000000320, 2.886751345948129099, -4.999999999999998224 ) ) ;
#40342=CARTESIAN_POINT ( 'NONE',  ( 25.07812500061451644, 6.421520780324663323E-16, -5.243569643749999010 ) ) ;
#40343=CARTESIAN_POINT ( 'NONE',  ( 13.83749999999999858, -2.886751345948129988, 4.999999999999997335 ) ) ;
#40344=EDGE_CURVE ( 'NONE', #27030, #22784, #52390, .T. ) ;
#40345=CARTESIAN_POINT ( 'NONE',  ( 10.01250000122903394, -4.330127018922190985, -2.500000000000001332 ) ) ;
#40346=CARTESIAN_POINT ( 'NONE',  ( 9.290625000614515017, -3.027376345333610441, -5.243569643749999898 ) ) ;
#40347=CARTESIAN_POINT ( 'NONE',  ( 24.03750000000000142, 5.773502691896255534, 3.535250795749688894E-16 ) ) ;
#40348=CARTESIAN_POINT ( 'NONE',  ( 21.36562500061451431, -6.054752690667223547, -1.112240025338166033E-15 ) ) ;
#40349=CARTESIAN_POINT ( 'NONE',  ( 0.000000000000000000, 20.00000000000000000, -30.00000000000000000 ) ) ;
#40350=AXIS2_PLACEMENT_3D ( 'NONE', #41563, #47835, #20469 ) ;
#40351=CARTESIAN_POINT ( 'NONE',  ( 28.16250000122903074, 4.330127018922192761, -2.499999999999997780 ) ) ;
#40353=CARTESIAN_POINT ( 'NONE',  ( 6.600000000000001421, 0.000000000000000000, 4.999999999999998224 ) ) ;
#40355=CARTESIAN_POINT ( 'NONE',  ( 21.06562500061451715, 3.027376345333613106, -5.243569643749998122 ) ) ;
#40356=CARTESIAN_POINT ( 'NONE',  ( 29.05312500061451431, -4.541064518000417216, -2.621784821875001281 ) ) ;
#40357=CYLINDRICAL_SURFACE ( 'NONE', #59647, 4.999999999999998224 ) ;
#40358=CARTESIAN_POINT ( 'NONE',  ( 18.49687500061452283, 6.054752690667223547, 3.707466751127219781E-16 ) ) ;
#40359=CARTESIAN_POINT ( 'NONE',  ( 13.37812500061451715, 6.421520780324663323E-16, -5.243569643749999010 ) ) ;
#40361=CARTESIAN_POINT ( 'NONE',  ( 29.10000000122903074, 5.773502691896255534, 3.535250795749688894E-16 ) ) ;
#40363=CARTESIAN_POINT ( 'NONE',  ( 17.09062500061451573, 6.054752690667223547, 3.707466751127219781E-16 ) ) ;
#40364=CARTESIAN_POINT ( 'NONE',  ( 2.000000000000001332, 13.85000000000000142, 33.46410161513774995 ) ) ;
#40365=CARTESIAN_POINT ( 'NONE',  ( 3.150000001229034119, -2.886751345948129988, 4.999999999999997335 ) ) ;
#40366=AXIS2_PLACEMENT_3D ( 'NONE', #7424, #59111, #47673 ) ;
#40367=CARTESIAN_POINT ( 'NONE',  ( 13.09687500061451892, 6.054752690667223547, 3.707466751127219781E-16 ) ) ;
#40368=CARTESIAN_POINT ( 'NONE',  ( 12.53437500061451537, 6.421520780324663323E-16, -5.243569643749999010 ) ) ;
#40369=CARTESIAN_POINT ( 'NONE',  ( 19.88437500061451857, 4.541064518000418104, 2.621784821874999949 ) ) ;
#40370=VERTEX_POINT ( 'NONE', #68303 ) ;
#40371=CARTESIAN_POINT ( 'NONE',  ( -5.948681673321857488, 8.038272906428572284, 29.19158024300208609 ) ) ;
#40372=CARTESIAN_POINT ( 'NONE',  ( 24.14062500061451289, -3.027376345333610441, -5.243569643749999898 ) ) ;
#40373=CARTESIAN_POINT ( 'NONE',  ( 19.77187500061451786, 3.027376345333613106, -5.243569643749998122 ) ) ;
#40374=CARTESIAN_POINT ( 'NONE',  ( 24.70312500061451644, 4.541064518000418104, -2.621784821874998173 ) ) ;
#40375=DIRECTION ( 'NONE',  ( -1.000000000000000000, -0.000000000000000000, -0.000000000000000000 ) ) ;
#40376=CARTESIAN_POINT ( 'NONE',  ( -1.999999999999997113, 15.57500000000000284, 33.46410161513775705 ) ) ;
#40377=CARTESIAN_POINT ( 'NONE',  ( 28.41562500061451502, 3.027376345333611329, 5.243569643749999010 ) ) ;
#40378=CARTESIAN_POINT ( 'NONE',  ( 10.23750000122903359, 4.330127018922191873, 2.499999999999999556 ) ) ;
#40379=CARTESIAN_POINT ( 'NONE',  ( 5.887500001229034829, -4.330127018922194537, 2.499999999999995559 ) ) ;
#40380=CARTESIAN_POINT ( 'NONE',  ( 1.592000809091587073E-14, 17.18750000000000355, 26.00000000000000000 ) ) ;
#40381=CARTESIAN_POINT ( 'NONE',  ( 26.58750000122903145, -4.330127018922194537, 2.499999999999995559 ) ) ;
#40384=CARTESIAN_POINT ( 'NONE',  ( 8.596875000614518925, 6.054752690667223547, 3.707466751127219781E-16 ) ) ;
#40385=CARTESIAN_POINT ( 'NONE',  ( -5.810221930991193690E-16, 10.10000000122903430, 26.00000000000000355 ) ) ;
#40386=CARTESIAN_POINT ( 'NONE',  ( 18.32812500061451644, 6.421520780324663323E-16, -5.243569643749999010 ) ) ;
#40387=CARTESIAN_POINT ( 'NONE',  ( 10.84687500061451892, 6.054752690667223547, 3.707466751127219781E-16 ) ) ;
#40388=CARTESIAN_POINT ( 'NONE',  ( 28.53750000122903074, 6.123233995736764310E-16, -4.999999999999998224 ) ) ;
#40389=CARTESIAN_POINT ( 'NONE',  ( 20.48437500061451289, -4.541064518000419881, 2.621784821874995952 ) ) ;
#40390=CARTESIAN_POINT ( 'NONE',  ( 7.959375000614516971, -4.541064518000417216, -2.621784821875001281 ) ) ;
#40391=CARTESIAN_POINT ( 'NONE',  ( 3.965625000614515727, 3.027376345333613106, -5.243569643749998122 ) ) ;
#40393=CARTESIAN_POINT ( 'NONE',  ( 8.203125000614518214, 0.000000000000000000, 5.243569643749999010 ) ) ;
#40394=CARTESIAN_POINT ( 'NONE',  ( 19.34062500061451573, 6.054752690667223547, 3.707466751127219781E-16 ) ) ;
#40395=VERTEX_POINT ( 'NONE', #50942 ) ;
#40396=CARTESIAN_POINT ( 'NONE',  ( 5.812500001229035540, 0.000000000000000000, 4.999999999999998224 ) ) ;
#40397=CARTESIAN_POINT ( 'NONE',  ( 14.84062500061451750, 6.054752690667223547, 3.707466751127219781E-16 ) ) ;
#40398=CARTESIAN_POINT ( 'NONE',  ( 12.92812500061451786, 6.421520780324663323E-16, -5.243569643749999010 ) ) ;
#40400=CARTESIAN_POINT ( 'NONE',  ( 13.87500000000000178, -4.330127018922194537, 2.499999999999995559 ) ) ;
#40401=CARTESIAN_POINT ( 'NONE',  ( 8.287500001229034297, 6.123233995736764310E-16, -4.999999999999998224 ) ) ;
#40402=CARTESIAN_POINT ( 'NONE',  ( 4.978125000614518569, 4.541064518000418104, 2.621784821874999949 ) ) ;
#40403=( BOUNDED_SURFACE ( )  B_SPLINE_SURFACE ( 1, 2, ( 
 ( #41813, #25925, #9666, #52902, #59157, #59895, #42916, #24815, #48465, #70989, #64343, #47719, #36277, #20365, #70258, #65439, #9301, #65811, #3766, #26291, #19630, #47361, #69893, #42186, #39566, #33647, #67291, #60996, #38845, #55465, #72819, #62091, #17009, #49199, #72447, #32927, #10395, #45107, #27391, #43654, #38097, #10029, #56191, #66922, #10757, #32199, #11118, #32564, #15553, #5585, #27031, #55102, #21466, #50297, #44756, #4502, #4857, #15922, #54733, #22560, #49923, #27756, #60619, #21832, #16290, #71732, #44396, #61360, #33289, #55827, #67643, #4135, #5215, #39205, #61719, #28122, #49562, #38472, #50650, #22202, #16649, #54, #72083, #26665, #21102, #44020, #66543, #66177, #22913, #68002, #45470, #63167, #28829, #57976, #68726, #29555, #1132, #62806, #6669, #12199, #12919, #39932, #34007, #23641, #62446, #40647, #11484, #57256, #69091, #51007, #17375, #52091, #24002, #46187, #34727, #29914, #56544, #1860, #7384, #11844, #18086, #7024, #12562, #29197, #51368, #1496, #63532, #5937, #46550, #35096, #57621, #35452, #18453, #68364, #41017, #770, #28471, #24367, #404, #51731, #52454, #56895, #23278, #45828, #6301, #46915, #69453, #18810, #41374, #34363, #17726, #40285, #59070, #25466, #25840, #54285, #2571, #25091, #42467, #19544, #37284, #20645, #48377, #7746, #3313, #14742, #70904, #31379, #48742, #47634, #8474, #65352, #59435, #41727, #48010, #31008, #53919, #20276, #24730, #2217, #70538, #53174, #47273, #42829, #2937, #42102, #59807, #19913, #64990, #14011, #71266, #14380, #70168, #30643, #64254, #30282, #36915, #53541, #36550, #9212, #13275, #8843, #52815, #31748, #69807, #3679, #63884, #35813, #64624, #26203, #58335, #19172, #13642, #36186, #58704, #8115, #54643, #49839, #4047, #4417, #44306, #11034, #61278, #66835, #66088, #50566, #22117, #5498, #73093, #44673, #5134, #72004, #72363, #66459, #10671, #43202, #28037, #60167, #10309, #43933, #21379, #56107, #38382, #26573, #49112, #21014, #67204, #4772, #21744, #65722, #16565, #43567, #71641, #39117, #38011, #15466, #32478, #33201, #55740, #60533, #15836, #26946, #15108, #33557, #60905, #38758, #9940, #32841, #37644, #49472, #9577, #55378, #55012, #27305, #16206, #27668, #32109, #50207, #72731, #61632, #52371, #17290, #22831, #51651, #7305, #28386, #34646, #50925, #22475, #18372, #40940, #63454, #12840, #322, #57897, #29836, #45383, #63086, #33922, #6945, #57174, #12120, #68284, #67919, #35014, #39852, #45025, #39478, #6587, #17645, #67560, #35374, #62365, #40566, #5855, #12487, #6218, #23194, #68645, #11762, #23921, #18008, #34279, #29117, #40205, #57543, #29476, #56464, #56811, #1052, #28746, #51285, #52013, #23562, #687, #1414, #46108, #46471, #45748, #16924, #69008, #62001, #11402, #62727, #64539, #42018, #13932, #38199, #1776, #36469, #8759, #31293, #53834, #7661, #8031, #48292, #70456, #19832, #25012, #41649, #60725, #8393, #2137, #47194, #24648, #13197, #58256, #35736, #53463, #19094, #70818, #58987, #42384, #30922, #53092, #70083, #2487, #3228, #30201, #24288, #2854, #52732, #25383, #46836, #47554, #59348, #41295, #69725, #64906, #14296, #47927, #19458, #20192, #69375, #66282, #43757, #64169, #36834, #25756, #15660, #10136, #13557, #32668, #18731, #63805, #36103, #58624, #30566, #6043, #39676, #38946, #39312, #44498, #55209, #68110, #72194, #27865, #61824, #27496, #67031, #72555, #50030, #33392, #44856, #155, #72922, #56297, #16031, #34109, #50397, #16754, #17117, #45578, #16390, #61464, #33752, #10859, #28577, #11946, #62196, #21573, #67745, #51114, #11592, #22661, #40036, #55928, #22304, #45211, #38579, #56648, #5324, #67392, #28222, #61103, #11229, #21943, #33029, #44127, #5687, #50752, #511, #23022, #4602, #17476, #66654, #62550, #10501, #27133, #49666, #55568, #4963, #69553, #24470, #34471, #35199, #18554, #23384, #29302, #45933, #41119, #68464, #68830, #35557, #2315, #52557, #58077, #57362, #41829, #13374, #69908, #64360, #35916, #18913, #63271, #63630, #57722, #1963, #56999, #19275, #51475, #1595, #7127, #12663, #47378, #29657, #17826, #40387, #12300, #58441, #69194, #13019, #6406, #7852, #34836, #62906, #30388, #51832, #6769, #23741, #47018, #41473, #1236, #52194, #18186, #28938, #24830, #24106, #30014, #46289, #46654, #877, #40756, #7485, #63993, #52917, #14481, #53648, #54386, #30745, #9317, #65455, #53277, #43671, #8580, #14111, #42931, #71748, #19646, #25940, #42202, #13750, #9681, #32214, #54748, #4150, #64726, #49215, #21118, #36650, #3781, #25192, #71374, #48480, #3420, #59539, #59172, #26306, #31109, #36292, #2676, #71004, #8949, #58806, #26682, #3041, #8216, #47736, #70275, #31483, #20380, #25572, #48112, #70635, #20010, #65090, #14848, #31850, #54025, #37387, #42563, #65827, #59911, #48844, #20749, #37015, #43307, #15209, #37749, #60267, #56207, #17024, #39222, #60635, #44771, #33663, #67306, #22217, #45123, #32942, #44411, #11135, #72834, #72100, #10772, #66937, #16664, #61734, #55119, #4518, #61375, #61012, #27047, #5600, #38860, #4872, #28137, #33305, #55843, #72463, #67658, #5231, #27772, #10047, #27408, #16306, #50312, #50665, #22575, #66194, #69, #15572, #38114, #32581, #10410, #49578, #21485, #44037, #66559, #15939, #38488, #55480, #49939, #21848, #50892, #16893, #1380, #46077, #29443, #23890, #68612, #29085, #22801, #657, #17259, #34612, #67171, #51981, #11003, #34247, #67887, #45353, #6913, #62335, #5465, #73062, #44992, #17973, #28715, #45719, #16532, #40534, #67530, #50534, #63050, #61969, #39448, #56434, #12091, #6552, #11371, #39820, #292, #39085, #57511, #11731, #62695, #22443, #56780, #61602, #6186, #33523, #51255, #33890, #56073, #23164, #28005, #5824, #28355, #12451, #68254, #17616, #40176, #34983, #57142, #51620, #1021, #23527, #24254, #35702, #64505 ),
 ( #24977, #63419, #3194, #41261, #46802, #2454, #31257, #52338, #58590, #1740, #46437, #42349, #64872, #14260, #36799, #69338, #8723, #53799, #18697, #13897, #57864, #30888, #7997, #36070, #19059, #63773, #58951, #13161, #68976, #12805, #30533, #41617, #18333, #59314, #58223, #36437, #29802, #8359, #30165, #47162, #19424, #7628, #52698, #2104, #24615, #35341, #53060, #13522, #64136, #53430, #40906, #47522, #7273, #41984, #69694, #70051, #2820, #25348, #47894, #70422, #19797, #25721, #26453, #9823, #14623, #20521, #37162, #32355, #59688, #60052, #43452, #60414, #54165, #9463, #48623, #33084, #4659, #61161, #55623, #27188, #60785, #54527, #54893, #48993, #66340, #48259, #10556, #42712, #65974, #71523, #3930, #3562, #31993, #71148, #70782, #49723, #20158, #65233, #72250, #10191, #20898, #4300, #15354, #15718, #9095, #31632, #26084, #37896, #26825, #49359, #38637, #71889, #43079, #65605, #14993, #21627, #21262, #43816, #37530, #44185, #38256, #32726, #66715, #55263, #16089, #67449, #23079, #17532, #55987, #28277, #61883, #34894, #68527, #33810, #574, #33442, #211, #72616, #11289, #12360, #50809, #5380, #5743, #44912, #45636, #21998, #68169, #56701, #44556, #5019, #72978, #27918, #34164, #62964, #10916, #17175, #50452, #27553, #936, #23444, #45990, #17888, #22360, #40448, #50085, #16811, #40094, #16446, #62608, #39735, #67802, #22716, #39367, #12004, #56353, #67087, #39003, #62252, #45269, #61518, #11649, #6101, #34527, #28632, #57057, #51170, #6464, #28999, #51536, #18615, #24166, #35257, #23802, #64052, #24533, #30078, #64420, #6827, #47077, #1292, #52977, #46353, #2022, #42261, #64784, #69253, #19338, #47436, #57423, #58138, #41533, #68887, #52254, #18244, #13432, #40817, #41180, #69612, #18973, #8276, #41893, #63689, #35982, #46718, #29361, #70332, #63333, #52616, #58501, #29716, #13079, #1657, #35618, #7544, #7910, #2373, #30448, #24891, #12721, #36352, #69967, #13813, #58866, #47803, #30806, #53339, #2737, #25254, #19709, #14175, #51894, #57778, #7188, #60695, #49273, #4211, #21543, #20440, #54445, #38171, #32272, #14539, #20811, #3844, #26739, #71806, #70694, #48170, #43366, #25999, #20069, #21175, #48904, #65521, #43728, #65889, #71435, #59968, #44098, #15270, #37809, #53710, #14907, #26365, #60329, #9738, #72163, #36709, #54805, #66252, #15630, #10108, #42625, #42989, #32638, #55178, #4574, #9376, #3481, #66624, #65149, #49636, #25632, #48538, #37075, #59599, #9011, #27104, #54083, #59231, #8639, #31168, #3103, #37448, #31909, #31543, #71065, #44470, #38550, #5661, #67000, #45184, #16001, #61794, #481, #55539, #21914, #34080, #28550, #28197, #39282, #34443, #61073, #6375, #11918, #72526, #22634, #11565, #50726, #33726, #33364, #56620, #68080, #10470, #6015, #39649, #67716, #17088, #33000, #11199, #22990, #4934, #16362, #51084, #45551, #129, #56272, #56971, #27469, #28907, #51445, #38916, #62168, #17449, #40007, #62521, #55901, #847, #23356, #50001, #45905, #61436, #10829, #5293, #27839, #72895, #50370, #22277, #44829, #67364, #16727, #41092, #1936, #40727, #57696, #12637, #63243, #46625, #58051, #13349, #12994, #69526, #29275, #47346, #63604, #29986, #30359, #58778, #7101, #29630, #46990, #24079, #41800, #25165, #52888, #12274, #7824, #19245, #2286, #35887, #53248, #52168, #35530, #69880, #63965, #46263, #52528, #7460, #58411, #24803, #51805, #6741, #24441, #1570, #1208, #64329, #18884, #69168, #13722, #41447, #36263, #18527, #2646, #8187, #30715, #34805, #68437, #17799, #40359, #62878, #57337, #23714, #68803, #18159, #35172, #54720, #53620, #53995, #21090, #43278, #65799, #70977, #14453, #32552, #31080, #60607, #36623, #36987, #59144, #3011, #8553, #26278, #65062, #43641, #31821, #15180, #37360, #25913, #42903, #48453, #49188, #25541, #70245, #59882, #48084, #14817, #4123, #26652, #71718, #70610, #3392, #66165, #37719, #60239, #20352, #59509, #55089, #19983, #10016, #42536, #8923, #31453, #65427, #9288, #48815, #54360, #15541, #3754, #9653, #71345, #20720, #32187, #38085, #4489, #47706, #19617, #42173, #64699, #14083, #27018, #72807, #11472, #66530, #32915, #45095, #39554, #16637, #50283, #45458, #49550, #17364, #22899, #10383, #33635, #22547, #61707, #44744, #44384, #67630, #5925, #21453, #16997, #50638, #56179, #50994, #33995, #10744, #11106, #16277, #72072, #39921, #44008, #22190, #5572, #72435, #38833, #66909, #21819, #5203, #39192, #62079, #67278, #28109, #60984, #28459, #42, #56532, #392, #62435, #61348, #33277, #67990, #55816, #11833, #56884, #34351, #15910, #38458, #55452, #4845, #27379, #49911, #27744, #23992, #7738, #1850, #57245, #63522, #46539, #46906, #41366, #40274, #17714, #12909, #68716, #62795, #63876, #18442, #35085, #13267, #35442, #41007, #29545, #13634, #57966, #7374, #23267, #57611, #69081, #29905, #52445, #41719, #6289, #6658, #18076, #24358, #18802, #29187, #52081, #63156, #36178, #69799, #7014, #69445, #34715, #1486, #759, #12551, #28818, #35805, #51721, #58327, #46177, #30273, #45817, #52806, #2207, #68353, #51356, #1122, #23631, #24722, #64246, #12188, #47265, #40637, #19165, #54632, #4039, #26563, #49103, #36541, #21005, #43557, #8466, #26193, #70159, #43193, #20268, #48369, #31371, #59061, #71256, #31001, #66079, #2563, #70895, #53912, #15457, #71632, #14002, #3670, #42094, #48733, #42458, #59427, #31738, #64616, #19906, #25459, #53534, #25083, #65343, #25832, #3305, #65713, #8106, #42820, #47626, #54276, #19536, #14733, #58695, #30634, #70531, #20636, #15099, #53166, #8835, #37275, #2930, #48003, #64981, #59797, #14372, #36907, #9203, #37635, #60158, #9568, #32100, #45374, #16914, #312, #67910, #39469, #73084, #66824, #44664, #61268, #5489, #38002, #22822, #55002, #5125, #38748, #16197, #50914, #33192, #49462, #43924 ) ),
 .UNSPECIFIED., .F., .F., .F. ) 
 B_SPLINE_SURFACE_WITH_KNOTS ( ( 2, 2 ),
 ( 3, 2, 2, 2, 2, 2, 2, 2, 2, 2, 2, 2, 2, 2, 2, 2, 2, 2, 2, 2, 2, 2, 2, 2, 2, 2, 2, 2, 2, 2, 2, 2, 2, 2, 2, 2, 2, 2, 2, 2, 2, 2, 2, 2, 2, 2, 2, 2, 2, 2, 2, 2, 2, 2, 2, 2, 2, 2, 2, 2, 2, 2, 2, 2, 2, 2, 2, 2, 2, 2, 2, 2, 2, 2, 2, 2, 2, 2, 2, 2, 2, 2, 2, 2, 2, 2, 2, 2, 2, 2, 2, 2, 2, 2, 2, 2, 2, 2, 2, 2, 2, 2, 2, 2, 2, 2, 2, 2, 2, 2, 2, 2, 2, 2, 2, 2, 2, 2, 2, 2, 2, 2, 2, 2, 2, 2, 2, 2, 2, 2, 2, 2, 2, 2, 2, 2, 2, 2, 2, 2, 2, 2, 2, 2, 2, 2, 2, 2, 2, 2, 2, 2, 2, 2, 2, 2, 2, 2, 2, 2, 2, 2, 2, 2, 2, 2, 2, 2, 2, 2, 2, 2, 2, 2, 2, 2, 2, 2, 2, 2, 2, 2, 2, 2, 2, 2, 2, 2, 2, 2, 2, 2, 2, 2, 2, 2, 2, 2, 2, 2, 2, 2, 2, 2, 2, 2, 2, 2, 2, 2, 2, 2, 2, 2, 2, 2, 2, 2, 2, 2, 2, 2, 2, 2, 2, 2, 2, 2, 2, 2, 2, 2, 2, 2, 2, 2, 2, 2, 2, 2, 2, 2, 2, 2, 2, 2, 2, 2, 2, 2, 2, 2, 2, 2, 2, 2, 2, 2, 2, 2, 2, 2, 2, 2, 2, 2, 2, 2, 2, 2, 2, 2, 2, 2, 2, 2, 2, 2, 2, 2, 2, 2, 2, 2, 2, 2, 2, 2, 2, 2, 2, 2, 2, 2, 2, 2, 2, 2, 2, 2, 2, 2, 2, 2, 2, 2, 2, 2, 2, 2, 2, 2, 2, 2, 2, 2, 2, 2, 2, 2, 2, 2, 2, 2, 2, 2, 2, 2, 2, 2, 2, 2, 2, 2, 2, 2, 2, 2, 2, 2, 2, 2, 2, 2, 2, 2, 2, 2, 2, 2, 2, 2, 2, 2, 2, 2, 2, 2, 2, 2, 3 ),
 ( 0.000000000000000000, 1.000000000000000000 ),
 ( 0.000000000000000000, 0.002777777777777777884, 0.005555555555555555768, 0.008333333333333333218, 0.01111111111111111154, 0.01388888888888888812, 0.01666666666666666644, 0.01944444444444444475, 0.02222222222222222307, 0.02500000000000000139, 0.02777777777777777624, 0.03055555555555555455, 0.03333333333333333287, 0.03611111111111110772, 0.03888888888888888951, 0.04166666666666666435, 0.04444444444444444614, 0.04722222222222222099, 0.05000000000000000278, 0.05277777777777777762, 0.05555555555555555247, 0.05833333333333333426, 0.06111111111111110911, 0.06388888888888888395, 0.06666666666666666574, 0.06944444444444444753, 0.07222222222222221544, 0.07499999999999999722, 0.07777777777777777901, 0.08055555555555556080, 0.08333333333333332871, 0.08611111111111111049, 0.08888888888888889228, 0.09166666666666666019, 0.09444444444444444198, 0.09722222222222222376, 0.1000000000000000056, 0.1027777777777777735, 0.1055555555555555552, 0.1083333333333333370, 0.1111111111111111049, 0.1138888888888888867, 0.1166666666666666685, 0.1194444444444444503, 0.1222222222222222182, 0.1250000000000000000, 0.1277777777777777679, 0.1305555555555555636, 0.1333333333333333315, 0.1361111111111110994, 0.1388888888888888951, 0.1416666666666666630, 0.1444444444444444309, 0.1472222222222222265, 0.1499999999999999944, 0.1527777777777777901, 0.1555555555555555580, 0.1583333333333333259, 0.1611111111111111216, 0.1638888888888888895, 0.1666666666666666574, 0.1694444444444444531, 0.1722222222222222210, 0.1749999999999999889, 0.1777777777777777846, 0.1805555555555555525, 0.1833333333333333204, 0.1861111111111111160, 0.1888888888888888840, 0.1916666666666666796, 0.1944444444444444475, 0.1972222222222222154, 0.2000000000000000111, 0.2027777777777777790, 0.2055555555555555469, 0.2083333333333333426, 0.2111111111111111105, 0.2138888888888888784, 0.2166666666666666741, 0.2194444444444444420, 0.2222222222222222099, 0.2250000000000000056, 0.2277777777777777735, 0.2305555555555555691, 0.2333333333333333370, 0.2361111111111111049, 0.2388888888888889006, 0.2416666666666666685, 0.2444444444444444364, 0.2472222222222222321, 0.2500000000000000000, 0.2527777777777777679, 0.2555555555555555358, 0.2583333333333333592, 0.2611111111111111271, 0.2638888888888888951, 0.2666666666666666630, 0.2694444444444444309, 0.2722222222222221988, 0.2750000000000000222, 0.2777777777777777901, 0.2805555555555555580, 0.2833333333333333259, 0.2861111111111110938, 0.2888888888888888618, 0.2916666666666666852, 0.2944444444444444531, 0.2972222222222222210, 0.2999999999999999889, 0.3027777777777777568, 0.3055555555555555802, 0.3083333333333333481, 0.3111111111111111160, 0.3138888888888888840, 0.3166666666666666519, 0.3194444444444444198, 0.3222222222222222432, 0.3250000000000000111, 0.3277777777777777790, 0.3305555555555555469, 0.3333333333333333148, 0.3361111111111111382, 0.3388888888888889062, 0.3416666666666666741, 0.3444444444444444420, 0.3472222222222222099, 0.3499999999999999778, 0.3527777777777778012, 0.3555555555555555691, 0.3583333333333333370, 0.3611111111111111049, 0.3638888888888888729, 0.3666666666666666408, 0.3694444444444444642, 0.3722222222222222321, 0.3750000000000000000, 0.3777777777777777679, 0.3805555555555555358, 0.3833333333333333592, 0.3861111111111111271, 0.3888888888888888951, 0.3916666666666666630, 0.3944444444444444309, 0.3972222222222221988, 0.4000000000000000222, 0.4027777777777777901, 0.4055555555555555580, 0.4083333333333333259, 0.4111111111111110938, 0.4138888888888888618, 0.4166666666666666852, 0.4194444444444444531, 0.4222222222222222210, 0.4249999999999999889, 0.4277777777777777568, 0.4305555555555555802, 0.4333333333333333481, 0.4361111111111111160, 0.4388888888888888840, 0.4416666666666666519, 0.4444444444444444198, 0.4472222222222222432, 0.4500000000000000111, 0.4527777777777777790, 0.4555555555555555469, 0.4583333333333333148, 0.4611111111111111382, 0.4638888888888889062, 0.4666666666666666741, 0.4694444444444444420, 0.4722222222222222099, 0.4749999999999999778, 0.4777777777777778012, 0.4805555555555555691, 0.4833333333333333370, 0.4861111111111111049, 0.4888888888888888729, 0.4916666666666666408, 0.4944444444444444642, 0.4972222222222222321, 0.5000000000000000000, 0.5027777777777777679, 0.5055555555555555358, 0.5083333333333333037, 0.5111111111111110716, 0.5138888888888888395, 0.5166666666666667185, 0.5194444444444444864, 0.5222222222222222543, 0.5250000000000000222, 0.5277777777777777901, 0.5305555555555555580, 0.5333333333333333259, 0.5361111111111110938, 0.5388888888888888618, 0.5416666666666666297, 0.5444444444444443976, 0.5472222222222222765, 0.5500000000000000444, 0.5527777777777778123, 0.5555555555555555802, 0.5583333333333333481, 0.5611111111111111160, 0.5638888888888888840, 0.5666666666666666519, 0.5694444444444444198, 0.5722222222222221877, 0.5749999999999999556, 0.5777777777777777235, 0.5805555555555556024, 0.5833333333333333703, 0.5861111111111111382, 0.5888888888888889062, 0.5916666666666666741, 0.5944444444444444420, 0.5972222222222222099, 0.5999999999999999778, 0.6027777777777777457, 0.6055555555555555136, 0.6083333333333332815, 0.6111111111111111605, 0.6138888888888889284, 0.6166666666666666963, 0.6194444444444444642, 0.6222222222222222321, 0.6250000000000000000, 0.6277777777777777679, 0.6305555555555555358, 0.6333333333333333037, 0.6361111111111110716, 0.6388888888888888395, 0.6416666666666667185, 0.6444444444444444864, 0.6472222222222222543, 0.6500000000000000222, 0.6527777777777777901, 0.6555555555555555580, 0.6583333333333333259, 0.6611111111111110938, 0.6638888888888888618, 0.6666666666666666297, 0.6694444444444443976, 0.6722222222222222765, 0.6750000000000000444, 0.6777777777777778123, 0.6805555555555555802, 0.6833333333333333481, 0.6861111111111111160, 0.6888888888888888840, 0.6916666666666666519, 0.6944444444444444198, 0.6972222222222221877, 0.6999999999999999556, 0.7027777777777777235, 0.7055555555555556024, 0.7083333333333333703, 0.7111111111111111382, 0.7138888888888889062, 0.7166666666666666741, 0.7194444444444444420, 0.7222222222222222099, 0.7249999999999999778, 0.7277777777777777457, 0.7305555555555555136, 0.7333333333333332815, 0.7361111111111111605, 0.7388888888888889284, 0.7416666666666666963, 0.7444444444444444642, 0.7472222222222222321, 0.7500000000000000000, 0.7527777777777777679, 0.7555555555555555358, 0.7583333333333333037, 0.7611111111111110716, 0.7638888888888888395, 0.7666666666666667185, 0.7694444444444444864, 0.7722222222222222543, 0.7750000000000000222, 0.7777777777777777901, 0.7805555555555555580, 0.7833333333333333259, 0.7861111111111110938, 0.7888888888888888618, 0.7916666666666666297, 0.7944444444444443976, 0.7972222222222222765, 0.8000000000000000444, 0.8027777777777778123, 0.8055555555555555802, 0.8083333333333333481, 0.8111111111111111160, 0.8138888888888888840, 0.8166666666666666519, 0.8194444444444444198, 0.8222222222222221877, 0.8249999999999999556, 0.8277777777777777235, 0.8305555555555556024, 0.8333333333333333703, 0.8361111111111111382, 0.8388888888888889062, 0.8416666666666666741, 0.8444444444444444420, 0.8472222222222222099, 0.8499999999999999778, 0.8527777777777777457, 0.8555555555555555136, 0.8583333333333332815, 0.8611111111111111605, 0.8638888888888889284, 0.8666666666666666963, 0.8694444444444444642, 0.8722222222222222321, 0.8750000000000000000, 0.8777777777777777679, 0.8805555555555555358, 0.8833333333333333037, 0.8861111111111110716, 0.8888888888888888395, 0.8916666666666667185, 0.8944444444444444864, 0.8972222222222222543, 0.9000000000000000222, 0.9027777777777777901, 0.9055555555555555580, 0.9083333333333333259, 0.9111111111111110938, 0.9138888888888888618, 0.9166666666666666297, 0.9194444444444443976, 0.9222222222222222765, 0.9250000000000000444, 0.9277777777777778123, 0.9305555555555555802, 0.9333333333333333481, 0.9361111111111111160, 0.9388888888888888840, 0.9416666666666666519, 0.9444444444444444198, 0.9472222222222221877, 0.9499999999999999556, 0.9527777777777777235, 0.9555555555555556024, 0.9583333333333333703, 0.9611111111111111382, 0.9638888888888889062, 0.9666666666666666741, 0.9694444444444444420, 0.9722222222222222099, 0.9749999999999999778, 0.9777777777777777457, 0.9805555555555555136, 0.9833333333333332815, 0.9861111111111111605, 0.9888888888888889284, 0.9916666666666666963, 0.9944444444444444642, 0.9972222222222222321, 1.000000000000000000 ),
 .UNSPECIFIED. ) 
 GEOMETRIC_REPRESENTATION_ITEM ( )  RATIONAL_B_SPLINE_SURFACE ( (
 ( 1.000000000000000000, 0.8660254037844387076, 1.000000000000000000, 0.8660254037844387076, 1.000000000000000000, 0.8660254037844387076, 1.000000000000000000, 0.8660254037844387076, 1.000000000000000000, 0.8660254037844387076, 1.000000000000000000, 0.8660254037844387076, 1.000000000000000000, 0.8660254037844387076, 1.000000000000000000, 0.8660254037844387076, 1.000000000000000000, 0.8660254037844387076, 1.000000000000000000, 0.8660254037844387076, 1.000000000000000000, 0.8660254037844387076, 1.000000000000000000, 0.8660254037844387076, 1.000000000000000000, 0.8660254037844387076, 1.000000000000000000, 0.8660254037844387076, 1.000000000000000000, 0.8660254037844387076, 1.000000000000000000, 0.8660254037844387076, 1.000000000000000000, 0.8660254037844387076, 1.000000000000000000, 0.8660254037844387076, 1.000000000000000000, 0.8660254037844387076, 1.000000000000000000, 0.8660254037844387076, 1.000000000000000000, 0.8660254037844387076, 1.000000000000000000, 0.8660254037844387076, 1.000000000000000000, 0.8660254037844387076, 1.000000000000000000, 0.8660254037844387076, 1.000000000000000000, 0.8660254037844387076, 1.000000000000000000, 0.8660254037844387076, 1.000000000000000000, 0.8660254037844387076, 1.000000000000000000, 0.8660254037844387076, 1.000000000000000000, 0.8660254037844387076, 1.000000000000000000, 0.8660254037844387076, 1.000000000000000000, 0.8660254037844387076, 1.000000000000000000, 0.8660254037844387076, 1.000000000000000000, 0.8660254037844387076, 1.000000000000000000, 0.8660254037844387076, 1.000000000000000000, 0.8660254037844387076, 1.000000000000000000, 0.8660254037844387076, 1.000000000000000000, 0.8660254037844387076, 1.000000000000000000, 0.8660254037844387076, 1.000000000000000000, 0.8660254037844387076, 1.000000000000000000, 0.8660254037844387076, 1.000000000000000000, 0.8660254037844387076, 1.000000000000000000, 0.8660254037844387076, 1.000000000000000000, 0.8660254037844387076, 1.000000000000000000, 0.8660254037844387076, 1.000000000000000000, 0.8660254037844387076, 1.000000000000000000, 0.8660254037844387076, 1.000000000000000000, 0.8660254037844387076, 1.000000000000000000, 0.8660254037844387076, 1.000000000000000000, 0.8660254037844387076, 1.000000000000000000, 0.8660254037844387076, 1.000000000000000000, 0.8660254037844387076, 1.000000000000000000, 0.8660254037844387076, 1.000000000000000000, 0.8660254037844387076, 1.000000000000000000, 0.8660254037844387076, 1.000000000000000000, 0.8660254037844387076, 1.000000000000000000, 0.8660254037844387076, 1.000000000000000000, 0.8660254037844387076, 1.000000000000000000, 0.8660254037844387076, 1.000000000000000000, 0.8660254037844387076, 1.000000000000000000, 0.8660254037844387076, 1.000000000000000000, 0.8660254037844387076, 1.000000000000000000, 0.8660254037844387076, 1.000000000000000000, 0.8660254037844387076, 1.000000000000000000, 0.8660254037844387076, 1.000000000000000000, 0.8660254037844387076, 1.000000000000000000, 0.8660254037844387076, 1.000000000000000000, 0.8660254037844387076, 1.000000000000000000, 0.8660254037844387076, 1.000000000000000000, 0.8660254037844387076, 1.000000000000000000, 0.8660254037844387076, 1.000000000000000000, 0.8660254037844387076, 1.000000000000000000, 0.8660254037844387076, 1.000000000000000000, 0.8660254037844387076, 1.000000000000000000, 0.8660254037844387076, 1.000000000000000000, 0.8660254037844387076, 1.000000000000000000, 0.8660254037844387076, 1.000000000000000000, 0.8660254037844387076, 1.000000000000000000, 0.8660254037844387076, 1.000000000000000000, 0.8660254037844387076, 1.000000000000000000, 0.8660254037844387076, 1.000000000000000000, 0.8660254037844387076, 1.000000000000000000, 0.8660254037844387076, 1.000000000000000000, 0.8660254037844387076, 1.000000000000000000, 0.8660254037844387076, 1.000000000000000000, 0.8660254037844387076, 1.000000000000000000, 0.8660254037844387076, 1.000000000000000000, 0.8660254037844387076, 1.000000000000000000, 0.8660254037844387076, 1.000000000000000000, 0.8660254037844387076, 1.000000000000000000, 0.8660254037844387076, 1.000000000000000000, 0.8660254037844387076, 1.000000000000000000, 0.8660254037844387076, 1.000000000000000000, 0.8660254037844387076, 1.000000000000000000, 0.8660254037844387076, 1.000000000000000000, 0.8660254037844387076, 1.000000000000000000, 0.8660254037844387076, 1.000000000000000000, 0.8660254037844387076, 1.000000000000000000, 0.8660254037844387076, 1.000000000000000000, 0.8660254037844387076, 1.000000000000000000, 0.8660254037844387076, 1.000000000000000000, 0.8660254037844387076, 1.000000000000000000, 0.8660254037844387076, 1.000000000000000000, 0.8660254037844387076, 1.000000000000000000, 0.8660254037844387076, 1.000000000000000000, 0.8660254037844387076, 1.000000000000000000, 0.8660254037844387076, 1.000000000000000000, 0.8660254037844387076, 1.000000000000000000, 0.8660254037844387076, 1.000000000000000000, 0.8660254037844387076, 1.000000000000000000, 0.8660254037844387076, 1.000000000000000000, 0.8660254037844387076, 1.000000000000000000, 0.8660254037844387076, 1.000000000000000000, 0.8660254037844387076, 1.000000000000000000, 0.8660254037844387076, 1.000000000000000000, 0.8660254037844387076, 1.000000000000000000, 0.8660254037844387076, 1.000000000000000000, 0.8660254037844387076, 1.000000000000000000, 0.8660254037844387076, 1.000000000000000000, 0.8660254037844387076, 1.000000000000000000, 0.8660254037844387076, 1.000000000000000000, 0.8660254037844387076, 1.000000000000000000, 0.8660254037844387076, 1.000000000000000000, 0.8660254037844387076, 1.000000000000000000, 0.8660254037844387076, 1.000000000000000000, 0.8660254037844387076, 1.000000000000000000, 0.8660254037844387076, 1.000000000000000000, 0.8660254037844387076, 1.000000000000000000, 0.8660254037844387076, 1.000000000000000000, 0.8660254037844387076, 1.000000000000000000, 0.8660254037844387076, 1.000000000000000000, 0.8660254037844387076, 1.000000000000000000, 0.8660254037844387076, 1.000000000000000000, 0.8660254037844387076, 1.000000000000000000, 0.8660254037844387076, 1.000000000000000000, 0.8660254037844387076, 1.000000000000000000, 0.8660254037844387076, 1.000000000000000000, 0.8660254037844387076, 1.000000000000000000, 0.8660254037844387076, 1.000000000000000000, 0.8660254037844387076, 1.000000000000000000, 0.8660254037844387076, 1.000000000000000000, 0.8660254037844387076, 1.000000000000000000, 0.8660254037844387076, 1.000000000000000000, 0.8660254037844387076, 1.000000000000000000, 0.8660254037844387076, 1.000000000000000000, 0.8660254037844387076, 1.000000000000000000, 0.8660254037844387076, 1.000000000000000000, 0.8660254037844387076, 1.000000000000000000, 0.8660254037844387076, 1.000000000000000000, 0.8660254037844387076, 1.000000000000000000, 0.8660254037844387076, 1.000000000000000000, 0.8660254037844387076, 1.000000000000000000, 0.8660254037844387076, 1.000000000000000000, 0.8660254037844387076, 1.000000000000000000, 0.8660254037844387076, 1.000000000000000000, 0.8660254037844387076, 1.000000000000000000, 0.8660254037844387076, 1.000000000000000000, 0.8660254037844387076, 1.000000000000000000, 0.8660254037844387076, 1.000000000000000000, 0.8660254037844387076, 1.000000000000000000, 0.8660254037844387076, 1.000000000000000000, 0.8660254037844387076, 1.000000000000000000, 0.8660254037844387076, 1.000000000000000000, 0.8660254037844387076, 1.000000000000000000, 0.8660254037844387076, 1.000000000000000000, 0.8660254037844387076, 1.000000000000000000, 0.8660254037844387076, 1.000000000000000000, 0.8660254037844387076, 1.000000000000000000, 0.8660254037844387076, 1.000000000000000000, 0.8660254037844387076, 1.000000000000000000, 0.8660254037844387076, 1.000000000000000000, 0.8660254037844387076, 1.000000000000000000, 0.8660254037844387076, 1.000000000000000000, 0.8660254037844387076, 1.000000000000000000, 0.8660254037844387076, 1.000000000000000000, 0.8660254037844387076, 1.000000000000000000, 0.8660254037844387076, 1.000000000000000000, 0.8660254037844387076, 1.000000000000000000, 0.8660254037844387076, 1.000000000000000000, 0.8660254037844387076, 1.000000000000000000, 0.8660254037844387076, 1.000000000000000000, 0.8660254037844387076, 1.000000000000000000, 0.8660254037844387076, 1.000000000000000000, 0.8660254037844387076, 1.000000000000000000, 0.8660254037844387076, 1.000000000000000000, 0.8660254037844387076, 1.000000000000000000, 0.8660254037844387076, 1.000000000000000000, 0.8660254037844387076, 1.000000000000000000, 0.8660254037844387076, 1.000000000000000000, 0.8660254037844387076, 1.000000000000000000, 0.8660254037844387076, 1.000000000000000000, 0.8660254037844387076, 1.000000000000000000, 0.8660254037844387076, 1.000000000000000000, 0.8660254037844387076, 1.000000000000000000, 0.8660254037844387076, 1.000000000000000000, 0.8660254037844387076, 1.000000000000000000, 0.8660254037844387076, 1.000000000000000000, 0.8660254037844387076, 1.000000000000000000, 0.8660254037844387076, 1.000000000000000000, 0.8660254037844387076, 1.000000000000000000, 0.8660254037844387076, 1.000000000000000000, 0.8660254037844387076, 1.000000000000000000, 0.8660254037844387076, 1.000000000000000000, 0.8660254037844387076, 1.000000000000000000, 0.8660254037844387076, 1.000000000000000000, 0.8660254037844387076, 1.000000000000000000, 0.8660254037844387076, 1.000000000000000000, 0.8660254037844387076, 1.000000000000000000, 0.8660254037844387076, 1.000000000000000000, 0.8660254037844387076, 1.000000000000000000, 0.8660254037844387076, 1.000000000000000000, 0.8660254037844387076, 1.000000000000000000, 0.8660254037844387076, 1.000000000000000000, 0.8660254037844387076, 1.000000000000000000, 0.8660254037844387076, 1.000000000000000000, 0.8660254037844387076, 1.000000000000000000, 0.8660254037844387076, 1.000000000000000000, 0.8660254037844387076, 1.000000000000000000, 0.8660254037844387076, 1.000000000000000000, 0.8660254037844387076, 1.000000000000000000, 0.8660254037844387076, 1.000000000000000000, 0.8660254037844387076, 1.000000000000000000, 0.8660254037844387076, 1.000000000000000000, 0.8660254037844387076, 1.000000000000000000, 0.8660254037844387076, 1.000000000000000000, 0.8660254037844387076, 1.000000000000000000, 0.8660254037844387076, 1.000000000000000000, 0.8660254037844387076, 1.000000000000000000, 0.8660254037844387076, 1.000000000000000000, 0.8660254037844387076, 1.000000000000000000, 0.8660254037844387076, 1.000000000000000000, 0.8660254037844387076, 1.000000000000000000, 0.8660254037844387076, 1.000000000000000000, 0.8660254037844387076, 1.000000000000000000, 0.8660254037844387076, 1.000000000000000000, 0.8660254037844387076, 1.000000000000000000, 0.8660254037844387076, 1.000000000000000000, 0.8660254037844387076, 1.000000000000000000, 0.8660254037844387076, 1.000000000000000000, 0.8660254037844387076, 1.000000000000000000, 0.8660254037844387076, 1.000000000000000000, 0.8660254037844387076, 1.000000000000000000, 0.8660254037844387076, 1.000000000000000000, 0.8660254037844387076, 1.000000000000000000, 0.8660254037844387076, 1.000000000000000000, 0.8660254037844387076, 1.000000000000000000, 0.8660254037844387076, 1.000000000000000000, 0.8660254037844387076, 1.000000000000000000, 0.8660254037844387076, 1.000000000000000000, 0.8660254037844387076, 1.000000000000000000, 0.8660254037844387076, 1.000000000000000000, 0.8660254037844387076, 1.000000000000000000, 0.8660254037844387076, 1.000000000000000000, 0.8660254037844387076, 1.000000000000000000, 0.8660254037844387076, 1.000000000000000000, 0.8660254037844387076, 1.000000000000000000, 0.8660254037844387076, 1.000000000000000000, 0.8660254037844387076, 1.000000000000000000, 0.8660254037844387076, 1.000000000000000000, 0.8660254037844387076, 1.000000000000000000, 0.8660254037844387076, 1.000000000000000000, 0.8660254037844387076, 1.000000000000000000, 0.8660254037844387076, 1.000000000000000000, 0.8660254037844387076, 1.000000000000000000, 0.8660254037844387076, 1.000000000000000000, 0.8660254037844387076, 1.000000000000000000, 0.8660254037844387076, 1.000000000000000000, 0.8660254037844387076, 1.000000000000000000, 0.8660254037844387076, 1.000000000000000000, 0.8660254037844387076, 1.000000000000000000, 0.8660254037844387076, 1.000000000000000000, 0.8660254037844387076, 1.000000000000000000, 0.8660254037844387076, 1.000000000000000000, 0.8660254037844387076, 1.000000000000000000, 0.8660254037844387076, 1.000000000000000000, 0.8660254037844387076, 1.000000000000000000, 0.8660254037844387076, 1.000000000000000000, 0.8660254037844387076, 1.000000000000000000, 0.8660254037844387076, 1.000000000000000000, 0.8660254037844387076, 1.000000000000000000, 0.8660254037844387076, 1.000000000000000000, 0.8660254037844387076, 1.000000000000000000, 0.8660254037844387076, 1.000000000000000000, 0.8660254037844387076, 1.000000000000000000, 0.8660254037844387076, 1.000000000000000000, 0.8660254037844387076, 1.000000000000000000, 0.8660254037844387076, 1.000000000000000000, 0.8660254037844387076, 1.000000000000000000, 0.8660254037844387076, 1.000000000000000000, 0.8660254037844387076, 1.000000000000000000, 0.8660254037844387076, 1.000000000000000000, 0.8660254037844387076, 1.000000000000000000, 0.8660254037844387076, 1.000000000000000000, 0.8660254037844387076, 1.000000000000000000, 0.8660254037844387076, 1.000000000000000000, 0.8660254037844387076, 1.000000000000000000, 0.8660254037844387076, 1.000000000000000000, 0.8660254037844387076, 1.000000000000000000, 0.8660254037844387076, 1.000000000000000000, 0.8660254037844387076, 1.000000000000000000, 0.8660254037844387076, 1.000000000000000000, 0.8660254037844387076, 1.000000000000000000, 0.8660254037844387076, 1.000000000000000000, 0.8660254037844387076, 1.000000000000000000, 0.8660254037844387076, 1.000000000000000000, 0.8660254037844387076, 1.000000000000000000, 0.8660254037844387076, 1.000000000000000000, 0.8660254037844387076, 1.000000000000000000, 0.8660254037844387076, 1.000000000000000000, 0.8660254037844387076, 1.000000000000000000, 0.8660254037844387076, 1.000000000000000000, 0.8660254037844387076, 1.000000000000000000, 0.8660254037844387076, 1.000000000000000000, 0.8660254037844387076, 1.000000000000000000, 0.8660254037844387076, 1.000000000000000000, 0.8660254037844387076, 1.000000000000000000, 0.8660254037844387076, 1.000000000000000000, 0.8660254037844387076, 1.000000000000000000, 0.8660254037844387076, 1.000000000000000000, 0.8660254037844387076, 1.000000000000000000, 0.8660254037844387076, 1.000000000000000000, 0.8660254037844387076, 1.000000000000000000, 0.8660254037844387076, 1.000000000000000000, 0.8660254037844387076, 1.000000000000000000, 0.8660254037844387076, 1.000000000000000000, 0.8660254037844387076, 1.000000000000000000, 0.8660254037844387076, 1.000000000000000000, 0.8660254037844387076, 1.000000000000000000, 0.8660254037844387076, 1.000000000000000000, 0.8660254037844387076, 1.000000000000000000, 0.8660254037844387076, 1.000000000000000000, 0.8660254037844387076, 1.000000000000000000, 0.8660254037844387076, 1.000000000000000000, 0.8660254037844387076, 1.000000000000000000, 0.8660254037844387076, 1.000000000000000000, 0.8660254037844387076, 1.000000000000000000, 0.8660254037844387076, 1.000000000000000000, 0.8660254037844387076, 1.000000000000000000, 0.8660254037844387076, 1.000000000000000000, 0.8660254037844387076, 1.000000000000000000, 0.8660254037844387076, 1.000000000000000000, 0.8660254037844387076, 1.000000000000000000, 0.8660254037844387076, 1.000000000000000000, 0.8660254037844387076, 1.000000000000000000, 0.8660254037844387076, 1.000000000000000000, 0.8660254037844387076, 1.000000000000000000, 0.8660254037844387076, 1.000000000000000000, 0.8660254037844387076, 1.000000000000000000, 0.8660254037844387076, 1.000000000000000000, 0.8660254037844387076, 1.000000000000000000, 0.8660254037844387076, 1.000000000000000000, 0.8660254037844387076, 1.000000000000000000, 0.8660254037844387076, 1.000000000000000000, 0.8660254037844387076, 1.000000000000000000, 0.8660254037844387076, 1.000000000000000000, 0.8660254037844387076, 1.000000000000000000, 0.8660254037844387076, 1.000000000000000000, 0.8660254037844387076, 1.000000000000000000, 0.8660254037844387076, 1.000000000000000000, 0.8660254037844387076, 1.000000000000000000, 0.8660254037844387076, 1.000000000000000000),
 ( 1.000000000000000000, 0.8660254037844387076, 1.000000000000000000, 0.8660254037844387076, 1.000000000000000000, 0.8660254037844387076, 1.000000000000000000, 0.8660254037844387076, 1.000000000000000000, 0.8660254037844387076, 1.000000000000000000, 0.8660254037844387076, 1.000000000000000000, 0.8660254037844387076, 1.000000000000000000, 0.8660254037844387076, 1.000000000000000000, 0.8660254037844387076, 1.000000000000000000, 0.8660254037844387076, 1.000000000000000000, 0.8660254037844387076, 1.000000000000000000, 0.8660254037844387076, 1.000000000000000000, 0.8660254037844387076, 1.000000000000000000, 0.8660254037844387076, 1.000000000000000000, 0.8660254037844387076, 1.000000000000000000, 0.8660254037844387076, 1.000000000000000000, 0.8660254037844387076, 1.000000000000000000, 0.8660254037844387076, 1.000000000000000000, 0.8660254037844387076, 1.000000000000000000, 0.8660254037844387076, 1.000000000000000000, 0.8660254037844387076, 1.000000000000000000, 0.8660254037844387076, 1.000000000000000000, 0.8660254037844387076, 1.000000000000000000, 0.8660254037844387076, 1.000000000000000000, 0.8660254037844387076, 1.000000000000000000, 0.8660254037844387076, 1.000000000000000000, 0.8660254037844387076, 1.000000000000000000, 0.8660254037844387076, 1.000000000000000000, 0.8660254037844387076, 1.000000000000000000, 0.8660254037844387076, 1.000000000000000000, 0.8660254037844387076, 1.000000000000000000, 0.8660254037844387076, 1.000000000000000000, 0.8660254037844387076, 1.000000000000000000, 0.8660254037844387076, 1.000000000000000000, 0.8660254037844387076, 1.000000000000000000, 0.8660254037844387076, 1.000000000000000000, 0.8660254037844387076, 1.000000000000000000, 0.8660254037844387076, 1.000000000000000000, 0.8660254037844387076, 1.000000000000000000, 0.8660254037844387076, 1.000000000000000000, 0.8660254037844387076, 1.000000000000000000, 0.8660254037844387076, 1.000000000000000000, 0.8660254037844387076, 1.000000000000000000, 0.8660254037844387076, 1.000000000000000000, 0.8660254037844387076, 1.000000000000000000, 0.8660254037844387076, 1.000000000000000000, 0.8660254037844387076, 1.000000000000000000, 0.8660254037844387076, 1.000000000000000000, 0.8660254037844387076, 1.000000000000000000, 0.8660254037844387076, 1.000000000000000000, 0.8660254037844387076, 1.000000000000000000, 0.8660254037844387076, 1.000000000000000000, 0.8660254037844387076, 1.000000000000000000, 0.8660254037844387076, 1.000000000000000000, 0.8660254037844387076, 1.000000000000000000, 0.8660254037844387076, 1.000000000000000000, 0.8660254037844387076, 1.000000000000000000, 0.8660254037844387076, 1.000000000000000000, 0.8660254037844387076, 1.000000000000000000, 0.8660254037844387076, 1.000000000000000000, 0.8660254037844387076, 1.000000000000000000, 0.8660254037844387076, 1.000000000000000000, 0.8660254037844387076, 1.000000000000000000, 0.8660254037844387076, 1.000000000000000000, 0.8660254037844387076, 1.000000000000000000, 0.8660254037844387076, 1.000000000000000000, 0.8660254037844387076, 1.000000000000000000, 0.8660254037844387076, 1.000000000000000000, 0.8660254037844387076, 1.000000000000000000, 0.8660254037844387076, 1.000000000000000000, 0.8660254037844387076, 1.000000000000000000, 0.8660254037844387076, 1.000000000000000000, 0.8660254037844387076, 1.000000000000000000, 0.8660254037844387076, 1.000000000000000000, 0.8660254037844387076, 1.000000000000000000, 0.8660254037844387076, 1.000000000000000000, 0.8660254037844387076, 1.000000000000000000, 0.8660254037844387076, 1.000000000000000000, 0.8660254037844387076, 1.000000000000000000, 0.8660254037844387076, 1.000000000000000000, 0.8660254037844387076, 1.000000000000000000, 0.8660254037844387076, 1.000000000000000000, 0.8660254037844387076, 1.000000000000000000, 0.8660254037844387076, 1.000000000000000000, 0.8660254037844387076, 1.000000000000000000, 0.8660254037844387076, 1.000000000000000000, 0.8660254037844387076, 1.000000000000000000, 0.8660254037844387076, 1.000000000000000000, 0.8660254037844387076, 1.000000000000000000, 0.8660254037844387076, 1.000000000000000000, 0.8660254037844387076, 1.000000000000000000, 0.8660254037844387076, 1.000000000000000000, 0.8660254037844387076, 1.000000000000000000, 0.8660254037844387076, 1.000000000000000000, 0.8660254037844387076, 1.000000000000000000, 0.8660254037844387076, 1.000000000000000000, 0.8660254037844387076, 1.000000000000000000, 0.8660254037844387076, 1.000000000000000000, 0.8660254037844387076, 1.000000000000000000, 0.8660254037844387076, 1.000000000000000000, 0.8660254037844387076, 1.000000000000000000, 0.8660254037844387076, 1.000000000000000000, 0.8660254037844387076, 1.000000000000000000, 0.8660254037844387076, 1.000000000000000000, 0.8660254037844387076, 1.000000000000000000, 0.8660254037844387076, 1.000000000000000000, 0.8660254037844387076, 1.000000000000000000, 0.8660254037844387076, 1.000000000000000000, 0.8660254037844387076, 1.000000000000000000, 0.8660254037844387076, 1.000000000000000000, 0.8660254037844387076, 1.000000000000000000, 0.8660254037844387076, 1.000000000000000000, 0.8660254037844387076, 1.000000000000000000, 0.8660254037844387076, 1.000000000000000000, 0.8660254037844387076, 1.000000000000000000, 0.8660254037844387076, 1.000000000000000000, 0.8660254037844387076, 1.000000000000000000, 0.8660254037844387076, 1.000000000000000000, 0.8660254037844387076, 1.000000000000000000, 0.8660254037844387076, 1.000000000000000000, 0.8660254037844387076, 1.000000000000000000, 0.8660254037844387076, 1.000000000000000000, 0.8660254037844387076, 1.000000000000000000, 0.8660254037844387076, 1.000000000000000000, 0.8660254037844387076, 1.000000000000000000, 0.8660254037844387076, 1.000000000000000000, 0.8660254037844387076, 1.000000000000000000, 0.8660254037844387076, 1.000000000000000000, 0.8660254037844387076, 1.000000000000000000, 0.8660254037844387076, 1.000000000000000000, 0.8660254037844387076, 1.000000000000000000, 0.8660254037844387076, 1.000000000000000000, 0.8660254037844387076, 1.000000000000000000, 0.8660254037844387076, 1.000000000000000000, 0.8660254037844387076, 1.000000000000000000, 0.8660254037844387076, 1.000000000000000000, 0.8660254037844387076, 1.000000000000000000, 0.8660254037844387076, 1.000000000000000000, 0.8660254037844387076, 1.000000000000000000, 0.8660254037844387076, 1.000000000000000000, 0.8660254037844387076, 1.000000000000000000, 0.8660254037844387076, 1.000000000000000000, 0.8660254037844387076, 1.000000000000000000, 0.8660254037844387076, 1.000000000000000000, 0.8660254037844387076, 1.000000000000000000, 0.8660254037844387076, 1.000000000000000000, 0.8660254037844387076, 1.000000000000000000, 0.8660254037844387076, 1.000000000000000000, 0.8660254037844387076, 1.000000000000000000, 0.8660254037844387076, 1.000000000000000000, 0.8660254037844387076, 1.000000000000000000, 0.8660254037844387076, 1.000000000000000000, 0.8660254037844387076, 1.000000000000000000, 0.8660254037844387076, 1.000000000000000000, 0.8660254037844387076, 1.000000000000000000, 0.8660254037844387076, 1.000000000000000000, 0.8660254037844387076, 1.000000000000000000, 0.8660254037844387076, 1.000000000000000000, 0.8660254037844387076, 1.000000000000000000, 0.8660254037844387076, 1.000000000000000000, 0.8660254037844387076, 1.000000000000000000, 0.8660254037844387076, 1.000000000000000000, 0.8660254037844387076, 1.000000000000000000, 0.8660254037844387076, 1.000000000000000000, 0.8660254037844387076, 1.000000000000000000, 0.8660254037844387076, 1.000000000000000000, 0.8660254037844387076, 1.000000000000000000, 0.8660254037844387076, 1.000000000000000000, 0.8660254037844387076, 1.000000000000000000, 0.8660254037844387076, 1.000000000000000000, 0.8660254037844387076, 1.000000000000000000, 0.8660254037844387076, 1.000000000000000000, 0.8660254037844387076, 1.000000000000000000, 0.8660254037844387076, 1.000000000000000000, 0.8660254037844387076, 1.000000000000000000, 0.8660254037844387076, 1.000000000000000000, 0.8660254037844387076, 1.000000000000000000, 0.8660254037844387076, 1.000000000000000000, 0.8660254037844387076, 1.000000000000000000, 0.8660254037844387076, 1.000000000000000000, 0.8660254037844387076, 1.000000000000000000, 0.8660254037844387076, 1.000000000000000000, 0.8660254037844387076, 1.000000000000000000, 0.8660254037844387076, 1.000000000000000000, 0.8660254037844387076, 1.000000000000000000, 0.8660254037844387076, 1.000000000000000000, 0.8660254037844387076, 1.000000000000000000, 0.8660254037844387076, 1.000000000000000000, 0.8660254037844387076, 1.000000000000000000, 0.8660254037844387076, 1.000000000000000000, 0.8660254037844387076, 1.000000000000000000, 0.8660254037844387076, 1.000000000000000000, 0.8660254037844387076, 1.000000000000000000, 0.8660254037844387076, 1.000000000000000000, 0.8660254037844387076, 1.000000000000000000, 0.8660254037844387076, 1.000000000000000000, 0.8660254037844387076, 1.000000000000000000, 0.8660254037844387076, 1.000000000000000000, 0.8660254037844387076, 1.000000000000000000, 0.8660254037844387076, 1.000000000000000000, 0.8660254037844387076, 1.000000000000000000, 0.8660254037844387076, 1.000000000000000000, 0.8660254037844387076, 1.000000000000000000, 0.8660254037844387076, 1.000000000000000000, 0.8660254037844387076, 1.000000000000000000, 0.8660254037844387076, 1.000000000000000000, 0.8660254037844387076, 1.000000000000000000, 0.8660254037844387076, 1.000000000000000000, 0.8660254037844387076, 1.000000000000000000, 0.8660254037844387076, 1.000000000000000000, 0.8660254037844387076, 1.000000000000000000, 0.8660254037844387076, 1.000000000000000000, 0.8660254037844387076, 1.000000000000000000, 0.8660254037844387076, 1.000000000000000000, 0.8660254037844387076, 1.000000000000000000, 0.8660254037844387076, 1.000000000000000000, 0.8660254037844387076, 1.000000000000000000, 0.8660254037844387076, 1.000000000000000000, 0.8660254037844387076, 1.000000000000000000, 0.8660254037844387076, 1.000000000000000000, 0.8660254037844387076, 1.000000000000000000, 0.8660254037844387076, 1.000000000000000000, 0.8660254037844387076, 1.000000000000000000, 0.8660254037844387076, 1.000000000000000000, 0.8660254037844387076, 1.000000000000000000, 0.8660254037844387076, 1.000000000000000000, 0.8660254037844387076, 1.000000000000000000, 0.8660254037844387076, 1.000000000000000000, 0.8660254037844387076, 1.000000000000000000, 0.8660254037844387076, 1.000000000000000000, 0.8660254037844387076, 1.000000000000000000, 0.8660254037844387076, 1.000000000000000000, 0.8660254037844387076, 1.000000000000000000, 0.8660254037844387076, 1.000000000000000000, 0.8660254037844387076, 1.000000000000000000, 0.8660254037844387076, 1.000000000000000000, 0.8660254037844387076, 1.000000000000000000, 0.8660254037844387076, 1.000000000000000000, 0.8660254037844387076, 1.000000000000000000, 0.8660254037844387076, 1.000000000000000000, 0.8660254037844387076, 1.000000000000000000, 0.8660254037844387076, 1.000000000000000000, 0.8660254037844387076, 1.000000000000000000, 0.8660254037844387076, 1.000000000000000000, 0.8660254037844387076, 1.000000000000000000, 0.8660254037844387076, 1.000000000000000000, 0.8660254037844387076, 1.000000000000000000, 0.8660254037844387076, 1.000000000000000000, 0.8660254037844387076, 1.000000000000000000, 0.8660254037844387076, 1.000000000000000000, 0.8660254037844387076, 1.000000000000000000, 0.8660254037844387076, 1.000000000000000000, 0.8660254037844387076, 1.000000000000000000, 0.8660254037844387076, 1.000000000000000000, 0.8660254037844387076, 1.000000000000000000, 0.8660254037844387076, 1.000000000000000000, 0.8660254037844387076, 1.000000000000000000, 0.8660254037844387076, 1.000000000000000000, 0.8660254037844387076, 1.000000000000000000, 0.8660254037844387076, 1.000000000000000000, 0.8660254037844387076, 1.000000000000000000, 0.8660254037844387076, 1.000000000000000000, 0.8660254037844387076, 1.000000000000000000, 0.8660254037844387076, 1.000000000000000000, 0.8660254037844387076, 1.000000000000000000, 0.8660254037844387076, 1.000000000000000000, 0.8660254037844387076, 1.000000000000000000, 0.8660254037844387076, 1.000000000000000000, 0.8660254037844387076, 1.000000000000000000, 0.8660254037844387076, 1.000000000000000000, 0.8660254037844387076, 1.000000000000000000, 0.8660254037844387076, 1.000000000000000000, 0.8660254037844387076, 1.000000000000000000, 0.8660254037844387076, 1.000000000000000000, 0.8660254037844387076, 1.000000000000000000, 0.8660254037844387076, 1.000000000000000000, 0.8660254037844387076, 1.000000000000000000, 0.8660254037844387076, 1.000000000000000000, 0.8660254037844387076, 1.000000000000000000, 0.8660254037844387076, 1.000000000000000000, 0.8660254037844387076, 1.000000000000000000, 0.8660254037844387076, 1.000000000000000000, 0.8660254037844387076, 1.000000000000000000, 0.8660254037844387076, 1.000000000000000000, 0.8660254037844387076, 1.000000000000000000, 0.8660254037844387076, 1.000000000000000000, 0.8660254037844387076, 1.000000000000000000, 0.8660254037844387076, 1.000000000000000000, 0.8660254037844387076, 1.000000000000000000, 0.8660254037844387076, 1.000000000000000000, 0.8660254037844387076, 1.000000000000000000, 0.8660254037844387076, 1.000000000000000000, 0.8660254037844387076, 1.000000000000000000, 0.8660254037844387076, 1.000000000000000000, 0.8660254037844387076, 1.000000000000000000, 0.8660254037844387076, 1.000000000000000000, 0.8660254037844387076, 1.000000000000000000, 0.8660254037844387076, 1.000000000000000000, 0.8660254037844387076, 1.000000000000000000, 0.8660254037844387076, 1.000000000000000000, 0.8660254037844387076, 1.000000000000000000, 0.8660254037844387076, 1.000000000000000000, 0.8660254037844387076, 1.000000000000000000, 0.8660254037844387076, 1.000000000000000000, 0.8660254037844387076, 1.000000000000000000, 0.8660254037844387076, 1.000000000000000000, 0.8660254037844387076, 1.000000000000000000, 0.8660254037844387076, 1.000000000000000000, 0.8660254037844387076, 1.000000000000000000, 0.8660254037844387076, 1.000000000000000000, 0.8660254037844387076, 1.000000000000000000, 0.8660254037844387076, 1.000000000000000000, 0.8660254037844387076, 1.000000000000000000, 0.8660254037844387076, 1.000000000000000000, 0.8660254037844387076, 1.000000000000000000, 0.8660254037844387076, 1.000000000000000000, 0.8660254037844387076, 1.000000000000000000, 0.8660254037844387076, 1.000000000000000000, 0.8660254037844387076, 1.000000000000000000, 0.8660254037844387076, 1.000000000000000000, 0.8660254037844387076, 1.000000000000000000, 0.8660254037844387076, 1.000000000000000000, 0.8660254037844387076, 1.000000000000000000, 0.8660254037844387076, 1.000000000000000000, 0.8660254037844387076, 1.000000000000000000, 0.8660254037844387076, 1.000000000000000000, 0.8660254037844387076, 1.000000000000000000, 0.8660254037844387076, 1.000000000000000000, 0.8660254037844387076, 1.000000000000000000, 0.8660254037844387076, 1.000000000000000000, 0.8660254037844387076, 1.000000000000000000, 0.8660254037844387076, 1.000000000000000000, 0.8660254037844387076, 1.000000000000000000, 0.8660254037844387076, 1.000000000000000000, 0.8660254037844387076, 1.000000000000000000, 0.8660254037844387076, 1.000000000000000000, 0.8660254037844387076, 1.000000000000000000, 0.8660254037844387076, 1.000000000000000000, 0.8660254037844387076, 1.000000000000000000, 0.8660254037844387076, 1.000000000000000000, 0.8660254037844387076, 1.000000000000000000, 0.8660254037844387076, 1.000000000000000000, 0.8660254037844387076, 1.000000000000000000, 0.8660254037844387076, 1.000000000000000000, 0.8660254037844387076, 1.000000000000000000, 0.8660254037844387076, 1.000000000000000000, 0.8660254037844387076, 1.000000000000000000, 0.8660254037844387076, 1.000000000000000000, 0.8660254037844387076, 1.000000000000000000, 0.8660254037844387076, 1.000000000000000000, 0.8660254037844387076, 1.000000000000000000, 0.8660254037844387076, 1.000000000000000000, 0.8660254037844387076, 1.000000000000000000, 0.8660254037844387076, 1.000000000000000000, 0.8660254037844387076, 1.000000000000000000, 0.8660254037844387076, 1.000000000000000000, 0.8660254037844387076, 1.000000000000000000, 0.8660254037844387076, 1.000000000000000000, 0.8660254037844387076, 1.000000000000000000, 0.8660254037844387076, 1.000000000000000000) ) ) 
 REPRESENTATION_ITEM ( '' )  SURFACE ( )  );
#40404=AXIS2_PLACEMENT_3D ( 'NONE', #57697, #12275, #19248 ) ;
#40405=CARTESIAN_POINT ( 'NONE',  ( 18.56250000122903288, -4.330127018922190985, -2.500000000000001332 ) ) ;
#40407=CARTESIAN_POINT ( 'NONE',  ( -4.243569643749999898, 11.72187500061451892, -32.45002607614398471 ) ) ;
#40408=CARTESIAN_POINT ( 'NONE',  ( 30.00000000000000000, 0.000000000000000000, 4.999999999999998224 ) ) ;
#40409=EDGE_CURVE ( 'NONE', #23988, #15128, #13231, .T. ) ;
#40410=CARTESIAN_POINT ( 'NONE',  ( 3.150000001229034119, -2.886751345948129988, 4.999999999999997335 ) ) ;
#40412=CARTESIAN_POINT ( 'NONE',  ( 14.02499999999999858, 6.123233995736764310E-16, -4.999999999999998224 ) ) ;
#40413=CARTESIAN_POINT ( 'NONE',  ( 19.43437500061451928, 4.541064518000418104, 2.621784821874999949 ) ) ;
#40415=CARTESIAN_POINT ( 'NONE',  ( 13.30312500061451786, -4.541064518000417216, -2.621784821875001281 ) ) ;
#40418=CARTESIAN_POINT ( 'NONE',  ( 26.93437500061451573, 6.421520780324663323E-16, -5.243569643749999010 ) ) ;
#40420=CARTESIAN_POINT ( 'NONE',  ( 13.11562500061451786, 3.027376345333611329, 5.243569643749999010 ) ) ;
#40421=CARTESIAN_POINT ( 'NONE',  ( 9.721875000614517148, -6.054752690667223547, -1.112240025338166033E-15 ) ) ;
#40422=EDGE_LOOP ( 'NONE', ( #24767, #71052, #39496, #31526 ) ) ;
#40423=CARTESIAN_POINT ( 'NONE',  ( 29.65312500061451573, 4.541064518000418104, -2.621784821874998173 ) ) ;
#40424=CARTESIAN_POINT ( 'NONE',  ( 21.29062500061451502, -3.027376345333614438, 5.243569643749998122 ) ) ;
#40425=CYLINDRICAL_SURFACE ( 'NONE', #29789, 4.999999999999998224 ) ;
#40426=CARTESIAN_POINT ( 'NONE',  ( 2.000000000000001332, 15.31250000122903465, -26.53589838486224650 ) ) ;
#40427=CARTESIAN_POINT ( 'NONE',  ( 9.225000000000001421, 4.330127018922191873, 2.499999999999999556 ) ) ;
#40428=CARTESIAN_POINT ( 'NONE',  ( 22.38750000122903216, 4.330127018922191873, 2.499999999999999556 ) ) ;
#40429=CARTESIAN_POINT ( 'NONE',  ( 17.12812500061451715, 4.541064518000418104, 2.621784821874999949 ) ) ;
#40432=CARTESIAN_POINT ( 'NONE',  ( 17.43750000000000355, -2.886751345948129988, 4.999999999999997335 ) ) ;
#40433=CARTESIAN_POINT ( 'NONE',  ( 22.23750000000000071, 5.773502691896255534, 3.535250795749688894E-16 ) ) ;
#40434=CARTESIAN_POINT ( 'NONE',  ( 19.65937500061451360, -4.541064518000417216, -2.621784821875001281 ) ) ;
#40435=CARTESIAN_POINT ( 'NONE',  ( 24.47812500061451502, -4.541064518000419881, 2.621784821874995952 ) ) ;
#40436=EDGE_LOOP ( 'NONE', ( #67029, #50212, #16520, #21023, #50381, #44975, #58741, #64342, #38765, #40905, #38330, #3323, #45042, #43340, #35233, #22302, #25661, #3049, #15474, #59422, #16571, #68611, #57128, #8345, #55565, #61230, #4779, #43065, #33288, #71506, #6595, #53631, #21250, #63395, #12494, #58572, #66568, #67642, #4649, #6723, #8037, #27040, #9798, #70988, #23546, #42168, #55727, #44805 ) ) ;
#40437=CARTESIAN_POINT ( 'NONE',  ( -5.810221930991193690E-16, 18.65000000122903501, -34.00000000000000000 ) ) ;
#40438=B_SPLINE_CURVE_WITH_KNOTS ( 'NONE', 3,
 ( #12304, #46658, #69198, #63635, #23026, #46293, #45582, #35561, #7489, #17830 ),
 .UNSPECIFIED., .F., .F.,
 ( 4, 3, 3, 4 ),
 ( 0.000000000000000000, 7.861231028638042341E-05, 0.0001572246814500608740, 0.0003053779378607085417 ),
 .UNSPECIFIED. ) ;
#40439=CARTESIAN_POINT ( 'NONE',  ( 9.365625000614519635, 3.027376345333613106, -5.243569643749998122 ) ) ;
#40440=FACE_OUTER_BOUND ( 'NONE', #16064, .T. ) ;
#40441=CARTESIAN_POINT ( 'NONE',  ( 15.86250000000000249, 2.886751345948129099, -4.999999999999998224 ) ) ;
#40442=CARTESIAN_POINT ( 'NONE',  ( -4.243569643749999898, 17.55312500061451786, 30.00000000000000000 ) ) ;
#40443=CARTESIAN_POINT ( 'NONE',  ( 3.234375000614516438, 4.541064518000418104, 2.621784821874999949 ) ) ;
#40446=CARTESIAN_POINT ( 'NONE',  ( 25.58437500061451431, 6.421520780324663323E-16, -5.243569643749999010 ) ) ;
#40448=CARTESIAN_POINT ( 'NONE',  ( 23.69062500061451004, -3.027376345333610441, -5.243569643749999898 ) ) ;
#40449=CARTESIAN_POINT ( 'NONE',  ( 22.09687500061451715, 6.054752690667223547, 3.707466751127219781E-16 ) ) ;
#40450=CARTESIAN_POINT ( 'NONE',  ( -4.243569643749999898, 17.10312500061459318, -30.00000000000000000 ) ) ;
#40451=CARTESIAN_POINT ( 'NONE',  ( 10.72500000000000142, -4.330127018922194537, 2.499999999999995559 ) ) ;
#40452=CARTESIAN_POINT ( 'NONE',  ( 8.165625000614516793, 3.027376345333611329, 5.243569643749999010 ) ) ;
#40454=FACE_OUTER_BOUND ( 'NONE', #47149, .T. ) ;
#40455=CARTESIAN_POINT ( 'NONE',  ( 26.99062500061451786, 6.054752690667223547, 3.707466751127219781E-16 ) ) ;
#40458=CARTESIAN_POINT ( 'NONE',  ( 19.43437500061451928, 4.541064518000418104, 2.621784821874999949 ) ) ;
#40459=CARTESIAN_POINT ( 'NONE',  ( -4.243569643749997233, 12.24687500061451928, 32.45002607614398471 ) ) ;
#40460=CARTESIAN_POINT ( 'NONE',  ( 18.57187500061451857, 3.027376345333611329, 5.243569643749999010 ) ) ;
#40461=CARTESIAN_POINT ( 'NONE',  ( 27.53437500061451360, 4.541064518000418104, 2.621784821874999949 ) ) ;
#40462=CARTESIAN_POINT ( 'NONE',  ( -2.121784821874996840, 16.33437500061451786, 33.67503911421598417 ) ) ;
#40463=CARTESIAN_POINT ( 'NONE',  ( 8.428125000614517859, 6.421520780324663323E-16, -5.243569643749999010 ) ) ;
#40464=CARTESIAN_POINT ( 'NONE',  ( -2.000000000000000000, 19.02499999999999858, 26.53589838486224650 ) ) ;
#40466=CARTESIAN_POINT ( 'NONE',  ( 3.759375000614517681, 0.000000000000000000, 5.243569643749999010 ) ) ;
#40467=CARTESIAN_POINT ( 'NONE',  ( 25.91250000122903074, 4.330127018922192761, -2.499999999999997780 ) ) ;
#40468=CARTESIAN_POINT ( 'NONE',  ( 4.190625000614518925, -3.027376345333614438, 5.243569643749998122 ) ) ;
#40469=CARTESIAN_POINT ( 'NONE',  ( 10.24687500061451750, -3.027376345333610441, -5.243569643749999898 ) ) ;
#40471=CARTESIAN_POINT ( 'NONE',  ( 17.02500000122903145, 2.886751345948126879, 4.999999999999999112 ) ) ;
#40472=CARTESIAN_POINT ( 'NONE',  ( 5.671875000614519102, -6.054752690667223547, -1.112240025338166033E-15 ) ) ;
#40473=CARTESIAN_POINT ( 'NONE',  ( 6.478125000614516793, -4.541064518000419881, 2.621784821874995952 ) ) ;
#40474=CARTESIAN_POINT ( 'NONE',  ( 22.80000000000000071, 0.000000000000000000, 4.999999999999998224 ) ) ;
#40476=CARTESIAN_POINT ( 'NONE',  ( 16.80937500061451573, 0.000000000000000000, 5.243569643749999010 ) ) ;
#40477=CARTESIAN_POINT ( 'NONE',  ( -5.810221930991193690E-16, 10.43750000000000000, 26.00000000000000355 ) ) ;
#40478=ORIENTED_EDGE ( 'NONE', *, *, #58225, .T. ) ;
#40479=CARTESIAN_POINT ( 'NONE',  ( 23.87812500061451715, 4.541064518000418104, 2.621784821874999949 ) ) ;
#40480=CARTESIAN_POINT ( 'NONE',  ( 9.178125000614517859, -4.541064518000419881, 2.621784821874995952 ) ) ;
#40481=CARTESIAN_POINT ( 'NONE',  ( 27.79687500061451644, -3.027376345333610441, -5.243569643749999898 ) ) ;
#40482=CARTESIAN_POINT ( 'NONE',  ( 9.440625000614517148, 6.054752690667223547, 3.707466751127219781E-16 ) ) ;
#40483=CARTESIAN_POINT ( 'NONE',  ( -4.243569643749999898, 10.37187500061451750, -32.45002607614398471 ) ) ;
#40484=CARTESIAN_POINT ( 'NONE',  ( 11.28750000122903252, -4.330127018922194537, 2.499999999999995559 ) ) ;
#40486=CARTESIAN_POINT ( 'NONE',  ( 28.07812500061451289, -4.541064518000419881, 2.621784821874995952 ) ) ;
#40487=CARTESIAN_POINT ( 'NONE',  ( 4.243569643749999010, 13.76562500061451644, -32.45002607614398471 ) ) ;
#40488=CARTESIAN_POINT ( 'NONE',  ( 13.35000000122903430, 5.773502691896255534, 3.535250795749688894E-16 ) ) ;
#40489=CARTESIAN_POINT ( 'NONE',  ( 10.49999999999999822, 4.330127018922192761, -2.499999999999997780 ) ) ;
#40490=CARTESIAN_POINT ( 'NONE',  ( 21.14062500061451289, 6.054752690667223547, 3.707466751127219781E-16 ) ) ;
#40491=CARTESIAN_POINT ( 'NONE',  ( 22.23750000122903003, 6.123233995736764310E-16, -4.999999999999998224 ) ) ;
#40492=CARTESIAN_POINT ( 'NONE',  ( 19.46249999999999858, 2.886751345948129099, -4.999999999999998224 ) ) ;
#40493=CARTESIAN_POINT ( 'NONE',  ( 8.625000001229034652, -5.773502691896255534, -1.060575238724906372E-15 ) ) ;
#40494=CARTESIAN_POINT ( 'NONE',  ( 15.97500000122903430, 2.886751345948129099, -4.999999999999998224 ) ) ;
#40495=CARTESIAN_POINT ( 'NONE',  ( 12.02812500061451573, 6.421520780324663323E-16, -5.243569643749999010 ) ) ;
#40496=CARTESIAN_POINT ( 'NONE',  ( 14.84062500061451750, 6.054752690667223547, 3.707466751127219781E-16 ) ) ;
#40497=CARTESIAN_POINT ( 'NONE',  ( 25.46250000122903501, 4.330127018922192761, -2.499999999999997780 ) ) ;
#40498=CARTESIAN_POINT ( 'NONE',  ( 19.65000000000000213, 0.000000000000000000, 4.999999999999998224 ) ) ;
#40499=CARTESIAN_POINT ( 'NONE',  ( 24.04687500061451644, -3.027376345333614438, 5.243569643749998122 ) ) ;
#40500=DIRECTION ( 'NONE',  ( -1.000000000000000000, -0.000000000000000000, -0.000000000000000000 ) ) ;
#40501=EDGE_CURVE ( 'NONE', #14527, #55334, #33115, .T. ) ;
#40502=CARTESIAN_POINT ( 'NONE',  ( 9.450000001229033941, -2.886751345948129988, 4.999999999999997335 ) ) ;
#40503=CARTESIAN_POINT ( 'NONE',  ( 8.109375000614518214, 4.541064518000418104, -2.621784821874998173 ) ) ;
#40504=CARTESIAN_POINT ( 'NONE',  ( 25.50937500061451502, -4.541064518000417216, -2.621784821875001281 ) ) ;
#40505=DIRECTION ( 'NONE',  ( 0.000000000000000000, 0.000000000000000000, 1.000000000000000000 ) ) ;
#40506=CARTESIAN_POINT ( 'NONE',  ( 21.14062500061451289, 6.054752690667223547, 3.707466751127219781E-16 ) ) ;
#40507=CARTESIAN_POINT ( 'NONE',  ( 26.59687500061451360, 6.054752690667223547, 3.707466751127219781E-16 ) ) ;
#40509=CARTESIAN_POINT ( 'NONE',  ( 3.210790684466319878, -3.832931176703135989, 3.307821435622600337 ) ) ;
#40510=CARTESIAN_POINT ( 'NONE',  ( 6.834375000614518747, 4.541064518000418104, 2.621784821874999949 ) ) ;
#40511=CARTESIAN_POINT ( 'NONE',  ( 20.69062500061451715, 6.054752690667223547, 3.707466751127219781E-16 ) ) ;
#40512=CARTESIAN_POINT ( 'NONE',  ( 5.000000000000000888, 2.882564675336284927E-11, 5.151554443534156036 ) ) ;
#40513=CARTESIAN_POINT ( 'NONE',  ( 28.71562500061451573, 3.027376345333613106, -5.243569643749998122 ) ) ;
#40514=CARTESIAN_POINT ( 'NONE',  ( 3.684375000614518836, 4.541064518000418104, 2.621784821874999949 ) ) ;
#40515=EDGE_CURVE ( 'NONE', #68271, #19034, #50806, .T. ) ;
#40516=CARTESIAN_POINT ( 'NONE',  ( 4.661467738957717266, -1.808512791952580301, -4.661467738957749241 ) ) ;
#40517=CARTESIAN_POINT ( 'NONE',  ( 17.81250000000000355, 2.886751345948126879, 4.999999999999999112 ) ) ;
#40519=CARTESIAN_POINT ( 'NONE',  ( 24.86250000000000071, 2.886751345948129099, -4.999999999999998224 ) ) ;
#40520=CARTESIAN_POINT ( 'NONE',  ( 26.55937500061451573, 4.541064518000418104, -2.621784821874998173 ) ) ;
#40521=ORIENTED_EDGE ( 'NONE', *, *, #23221, .F. ) ;
#40522=CARTESIAN_POINT ( 'NONE',  ( 14.72812500061451679, 6.421520780324663323E-16, -5.243569643749999010 ) ) ;
#40523=CARTESIAN_POINT ( 'NONE',  ( 7.003125000614518036, -4.541064518000417216, -2.621784821875001281 ) ) ;
#40525=CARTESIAN_POINT ( 'NONE',  ( 4.359375000614517326, -4.541064518000417216, -2.621784821875001281 ) ) ;
#40526=CARTESIAN_POINT ( 'NONE',  ( 14.36250000122903359, 0.000000000000000000, 4.999999999999998224 ) ) ;
#40527=CARTESIAN_POINT ( 'NONE',  ( 21.03750000000000142, -2.886751345948129988, 4.999999999999997335 ) ) ;
#40529=CARTESIAN_POINT ( 'NONE',  ( 4.171875000614517326, 3.027376345333611329, 5.243569643749999010 ) ) ;
#40530=CARTESIAN_POINT ( 'NONE',  ( 8.146875000614516082, 6.054752690667223547, 3.707466751127219781E-16 ) ) ;
#40531=CARTESIAN_POINT ( 'NONE',  ( 20.82187500061451857, 3.027376345333611329, 5.243569643749999010 ) ) ;
#40534=CARTESIAN_POINT ( 'NONE',  ( 4.321875000614517681, -6.054752690667223547, -1.112240025338166033E-15 ) ) ;
#40535=CARTESIAN_POINT ( 'NONE',  ( 5.062500000000000888, 2.886751345948129099, -4.999999999999998224 ) ) ;
#40536=CARTESIAN_POINT ( 'NONE',  ( 6.309375000614517504, 4.541064518000418104, -2.621784821874998173 ) ) ;
#40537=CARTESIAN_POINT ( 'NONE',  ( 19.01249999999999929, 2.886751345948129099, -4.999999999999998224 ) ) ;
#40538=CARTESIAN_POINT ( 'NONE',  ( 15.29062500061451679, 6.054752690667223547, 3.707466751127219781E-16 ) ) ;
#40542=CARTESIAN_POINT ( 'NONE',  ( 9.290625000614515017, -3.027376345333610441, -5.243569643749999898 ) ) ;
#40543=CARTESIAN_POINT ( 'NONE',  ( 27.79687500061451999, -3.027376345333610441, -5.243569643749999898 ) ) ;
#40544=CARTESIAN_POINT ( 'NONE',  ( 19.53750000122903430, 6.123233995736764310E-16, -4.999999999999998224 ) ) ;
#40545=CARTESIAN_POINT ( 'NONE',  ( 25.69687500061451502, 6.054752690667223547, 3.707466751127219781E-16 ) ) ;
#40546=CARTESIAN_POINT ( 'NONE',  ( 7.162500000000001421, -5.773502691896255534, -1.060575238724906372E-15 ) ) ;
#40547=CARTESIAN_POINT ( 'NONE',  ( -3.999999999999997335, 13.85000000122903607, 32.30940107675850470 ) ) ;
#40548=CARTESIAN_POINT ( 'NONE',  ( 14.01562500061451644, 3.027376345333611329, 5.243569643749999010 ) ) ;
#40549=CARTESIAN_POINT ( 'NONE',  ( 6.712500001229034119, 0.000000000000000000, 4.999999999999998224 ) ) ;
#40550=CARTESIAN_POINT ( 'NONE',  ( 18.45937500061451431, 4.541064518000418104, -2.621784821874998173 ) ) ;
#40551=CARTESIAN_POINT ( 'NONE',  ( 11.78437500061451892, 4.541064518000418104, 2.621784821874999949 ) ) ;
#40552=CARTESIAN_POINT ( 'NONE',  ( -3.943440097865042571, 3.074283834720752839, -30.68362617565046335 ) ) ;
#40554=CARTESIAN_POINT ( 'NONE',  ( 12.96562500061451750, 3.027376345333613106, -5.243569643749998122 ) ) ;
#40555=CARTESIAN_POINT ( 'NONE',  ( 25.31250000122903288, -4.330127018922190985, -2.500000000000001332 ) ) ;
#40556=CARTESIAN_POINT ( 'NONE',  ( 12.30937500061451573, 0.000000000000000000, 5.243569643749999010 ) ) ;
#40557=CARTESIAN_POINT ( 'NONE',  ( 4.027635003466097707, 2.962795348797195416, -4.326299380533228600 ) ) ;
#40558=CARTESIAN_POINT ( 'NONE',  ( 14.20312500061451644, -4.541064518000417216, -2.621784821875001281 ) ) ;
#40560=CARTESIAN_POINT ( 'NONE',  ( 22.92187500061451644, 3.027376345333613106, -5.243569643749998122 ) ) ;
#40561=CARTESIAN_POINT ( 'NONE',  ( -4.243569643749999898, 10.31562500061451715, 27.54997392385601529 ) ) ;
#40562=CARTESIAN_POINT ( 'NONE',  ( 10.83750000122903501, -4.330127018922194537, 2.499999999999995559 ) ) ;
#40564=CARTESIAN_POINT ( 'NONE',  ( 8.100000001229034297, -2.886751345948130876, 4.999999999999996447 ) ) ;
#40565=CARTESIAN_POINT ( 'NONE',  ( 4.243569643749999010, 16.07187500061451857, -32.45002607614398471 ) ) ;
#40566=CARTESIAN_POINT ( 'NONE',  ( 18.12187500061451573, 3.027376345333611329, 5.243569643749999010 ) ) ;
#40567=CARTESIAN_POINT ( 'NONE',  ( 20.06250000122903643, 4.330127018922192761, -2.499999999999997780 ) ) ;
#40568=CARTESIAN_POINT ( 'NONE',  ( 13.80937500061451750, -4.541064518000417216, -2.621784821875001281 ) ) ;
#40569=CARTESIAN_POINT ( 'NONE',  ( 4.243569643749999898, 10.14687500061451786, 32.45002607614398471 ) ) ;
#40570=CARTESIAN_POINT ( 'NONE',  ( 19.72500000122903074, 2.886751345948126879, 4.999999999999999112 ) ) ;
#40571=CARTESIAN_POINT ( 'NONE',  ( 14.91562500061451679, 3.027376345333611329, 5.243569643749999010 ) ) ;
#40572=ORIENTED_EDGE ( 'NONE', *, *, #67682, .T. ) ;
#40573=ORIENTED_EDGE ( 'NONE', *, *, #60856, .T. ) ;
#40574=CARTESIAN_POINT ( 'NONE',  ( 18.37500000000000355, -4.330127018922194537, 2.499999999999995559 ) ) ;
#40576=CARTESIAN_POINT ( 'NONE',  ( 2.840625000614518392, -3.027376345333614438, 5.243569643749998122 ) ) ;
#40577=CARTESIAN_POINT ( 'NONE',  ( 15.90000000122903501, -2.886751345948125991, -5.000000000000000000 ) ) ;
#40578=CARTESIAN_POINT ( 'NONE',  ( 26.40937500061451715, -4.541064518000417216, -2.621784821875001281 ) ) ;
#40579=CARTESIAN_POINT ( 'NONE',  ( 19.45312500061451644, 0.000000000000000000, 5.243569643749999010 ) ) ;
#40581=CARTESIAN_POINT ( 'NONE',  ( 23.31562500061451715, 3.027376345333613106, -5.243569643749998122 ) ) ;
#40582=CARTESIAN_POINT ( 'NONE',  ( 3.553125000614516082, 4.541064518000418104, -2.621784821874998173 ) ) ;
#40583=CARTESIAN_POINT ( 'NONE',  ( 28.46249999999999858, 2.886751345948129099, -4.999999999999998224 ) ) ;
#40584=CARTESIAN_POINT ( 'NONE',  ( 4.627512969954662658, 1.893775943066041245, 4.889672281578874902 ) ) ;
#40587=CARTESIAN_POINT ( 'NONE',  ( 28.72500000000000142, -4.330127018922194537, 2.499999999999995559 ) ) ;
#40588=CARTESIAN_POINT ( 'NONE',  ( 4.243569643749999898, 16.89687500061451786, -27.54997392385601529 ) ) ;
#40589=CARTESIAN_POINT ( 'NONE',  ( 6.112500001229034474, 4.330127018922192761, -2.499999999999997780 ) ) ;
#40590=CARTESIAN_POINT ( 'NONE',  ( 5.625000000000001776, 4.330127018922191873, 2.499999999999999556 ) ) ;
#40591=CARTESIAN_POINT ( 'NONE',  ( 3.150000001229034119, -2.886751345948129988, 4.999999999999997335 ) ) ;
#40592=CARTESIAN_POINT ( 'NONE',  ( 9.646875000614516082, -3.027376345333614438, 5.243569643749998122 ) ) ;
#40593=DIRECTION ( 'NONE',  ( -1.000000000000000000, -0.000000000000000000, -0.000000000000000000 ) ) ;
#40595=CARTESIAN_POINT ( 'NONE',  ( -5.989433049342593129, 8.007954590042437815, -30.40871493912334955 ) ) ;
#40596=LINE ( 'NONE', #62039, #50139 ) ;
#40597=CARTESIAN_POINT ( 'NONE',  ( 8.821875000614518569, -6.054752690667223547, -1.112240025338166033E-15 ) ) ;
#40598=CARTESIAN_POINT ( 'NONE',  ( 14.70937500061451786, -4.541064518000417216, -2.621784821875001281 ) ) ;
#40599=CARTESIAN_POINT ( 'NONE',  ( 6.299999999999999822, -4.330127018922190985, -2.500000000000001332 ) ) ;
#40600=CARTESIAN_POINT ( 'NONE',  ( -4.243569643749999898, 16.16562500061459673, 27.54997392385601529 ) ) ;
#40601=CARTESIAN_POINT ( 'NONE',  ( 20.52187500061451786, -6.054752690667223547, -1.112240025338166033E-15 ) ) ;
#40603=CARTESIAN_POINT ( 'NONE',  ( 2.841718689647413587, -4.113985430540962440, 3.174331389344874577 ) ) ;
#40604=CARTESIAN_POINT ( 'NONE',  ( 26.55000000122902648, -2.886751345948129988, 4.999999999999997335 ) ) ;
#40606=CARTESIAN_POINT ( 'NONE',  ( 22.15312500061451573, 0.000000000000000000, 5.243569643749999010 ) ) ;
#40607=CARTESIAN_POINT ( 'NONE',  ( 12.89062500061451821, -3.027376345333610441, -5.243569643749999898 ) ) ;
#40609=CARTESIAN_POINT ( 'NONE',  ( 10.99687500061451750, -3.027376345333614438, 5.243569643749998122 ) ) ;
#40610=CARTESIAN_POINT ( 'NONE',  ( 28.12499999999999645, 4.330127018922191873, 2.499999999999999556 ) ) ;
#40611=CARTESIAN_POINT ( 'NONE',  ( 23.47500000122903430, -5.773502691896255534, -1.060575238724906372E-15 ) ) ;
#40612=AXIS2_PLACEMENT_3D ( 'NONE', #43959, #60927, #1075 ) ;
#40613=DIRECTION ( 'NONE',  ( -0.000000000000000000, -1.000000000000000000, -0.000000000000000000 ) ) ;
#40614=CARTESIAN_POINT ( 'NONE',  ( 11.29687500061451644, 6.054752690667223547, 3.707466751127219781E-16 ) ) ;
#40615=CARTESIAN_POINT ( 'NONE',  ( 29.40937500061451715, 0.000000000000000000, 5.243569643749999010 ) ) ;
#40616=CARTESIAN_POINT ( 'NONE',  ( 7.320879633048903241E-15, 18.20000000122903216, -34.00000000000000000 ) ) ;
#40617=EDGE_CURVE ( 'NONE', #17518, #18233, #69395, .T. ) ;
#40618=CARTESIAN_POINT ( 'NONE',  ( -3.137519842735245283E-14, 14.71250000000000213, 34.00000000000000000 ) ) ;
#40619=CARTESIAN_POINT ( 'NONE',  ( 21.45937500061451786, -4.541064518000417216, -2.621784821875001281 ) ) ;
#40620=CARTESIAN_POINT ( 'NONE',  ( 13.84687500061451537, -3.027376345333610441, -5.243569643749999898 ) ) ;
#40621=EDGE_CURVE ( 'NONE', #48662, #26352, #25277, .T. ) ;
#40623=CARTESIAN_POINT ( 'NONE',  ( 24.93750000000000355, 5.773502691896255534, 3.535250795749688894E-16 ) ) ;
#40626=CARTESIAN_POINT ( 'NONE',  ( 16.67812500061451786, 4.541064518000418104, 2.621784821874999949 ) ) ;
#40627=CARTESIAN_POINT ( 'NONE',  ( 7.575000000000001954, -4.330127018922194537, 2.499999999999995559 ) ) ;
#40628=CARTESIAN_POINT ( 'NONE',  ( 0.000000000000000000, 20.00000000000000000, 30.00000000000000000 ) ) ;
#40629=CARTESIAN_POINT ( 'NONE',  ( 14.69999999999999929, 0.000000000000000000, 4.999999999999998224 ) ) ;
#40630=CARTESIAN_POINT ( 'NONE',  ( -4.243569643749997233, 10.39062500061451644, 32.45002607614398471 ) ) ;
#40632=CARTESIAN_POINT ( 'NONE',  ( 25.28437500061451715, 4.541064518000418104, 2.621784821874999949 ) ) ;
#40633=ORIENTED_EDGE ( 'NONE', *, *, #5973, .T. ) ;
#40634=CARTESIAN_POINT ( 'NONE',  ( 23.05312500061451431, 0.000000000000000000, 5.243569643749999010 ) ) ;
#40635=CARTESIAN_POINT ( 'NONE',  ( 20.55937500061451573, -4.541064518000417216, -2.621784821875001281 ) ) ;
#40636=CARTESIAN_POINT ( 'NONE',  ( 3.374999999999999556, 4.330127018922191873, 2.499999999999999556 ) ) ;
#40637=CARTESIAN_POINT ( 'NONE',  ( 5.990625000614517859, -3.027376345333614438, 5.243569643749998122 ) ) ;
#40638=CARTESIAN_POINT ( 'NONE',  ( 21.81562500061451004, -6.054752690667223547, -1.112240025338166033E-15 ) ) ;
#40639=CARTESIAN_POINT ( 'NONE',  ( 13.24687500061451750, -3.027376345333614438, 5.243569643749998122 ) ) ;
#40640=CARTESIAN_POINT ( 'NONE',  ( 17.44687500061451857, -3.027376345333610441, -5.243569643749999898 ) ) ;
#40641=CARTESIAN_POINT ( 'NONE',  ( 2.121784821875001281, 18.15312500061451928, 33.67503911421598417 ) ) ;
#40642=CARTESIAN_POINT ( 'NONE',  ( 18.71250000122903145, 4.330127018922192761, -2.499999999999997780 ) ) ;
#40644=CARTESIAN_POINT ( 'NONE',  ( 9.103125000614515017, 0.000000000000000000, 5.243569643749999010 ) ) ;
#40645=CARTESIAN_POINT ( 'NONE',  ( 4.996875000614516615, 6.054752690667223547, 3.707466751127219781E-16 ) ) ;
#40646=CARTESIAN_POINT ( 'NONE',  ( 3.946875000614517681, -3.027376345333610441, -5.243569643749999898 ) ) ;
#40647=CARTESIAN_POINT ( 'NONE',  ( 25.92187500061451999, -6.054752690667223547, -1.112240025338166033E-15 ) ) ;
#40648=CARTESIAN_POINT ( 'NONE',  ( 17.31562500061451715, -6.054752690667223547, -1.112240025338166033E-15 ) ) ;
#40649=CARTESIAN_POINT ( 'NONE',  ( 28.08750000122903145, 6.123233995736764310E-16, -4.999999999999998224 ) ) ;
#40650=CARTESIAN_POINT ( 'NONE',  ( 26.20312500061451644, 0.000000000000000000, 5.243569643749999010 ) ) ;
#40651=CARTESIAN_POINT ( 'NONE',  ( 21.23437500061451644, 4.541064518000418104, 2.621784821874999949 ) ) ;
#40652=CARTESIAN_POINT ( 'NONE',  ( 17.46562500061451217, 3.027376345333613106, -5.243569643749998122 ) ) ;
#40653=CARTESIAN_POINT ( 'NONE',  ( 2.121784821875001281, 18.20937500061451786, 33.67503911421598417 ) ) ;
#40654=CARTESIAN_POINT ( 'NONE',  ( 22.00312500061451360, 4.541064518000418104, -2.621784821874998173 ) ) ;
#40655=CARTESIAN_POINT ( 'NONE',  ( 3.450000001229036162, 5.773502691896255534, 3.535250795749688894E-16 ) ) ;
#40657=CARTESIAN_POINT ( 'NONE',  ( 24.97499999999999787, 4.330127018922191873, 2.499999999999999556 ) ) ;
#40658=CARTESIAN_POINT ( 'NONE',  ( -2.000000000000000000, 14.07500000000000107, -33.46410161513775705 ) ) ;
#40660=CARTESIAN_POINT ( 'NONE',  ( 28.19062500061451715, -3.027376345333610441, -5.243569643749999898 ) ) ;
#40661=CARTESIAN_POINT ( 'NONE',  ( 10.00312500061451715, 0.000000000000000000, 5.243569643749999010 ) ) ;
#40662=CARTESIAN_POINT ( 'NONE',  ( 22.61250000122903003, -4.330127018922190985, -2.500000000000001332 ) ) ;
#40664=CARTESIAN_POINT ( 'NONE',  ( 26.95312500061451644, 4.541064518000418104, -2.621784821874998173 ) ) ;
#40665=CARTESIAN_POINT ( 'NONE',  ( 27.97500000000000142, 6.123233995736764310E-16, -4.999999999999998224 ) ) ;
#40666=CARTESIAN_POINT ( 'NONE',  ( 3.999999999999998668, 16.77500000122903145, -32.30940107675850470 ) ) ;
#40667=DIRECTION ( 'NONE',  ( 0.000000000000000000, 0.000000000000000000, 1.000000000000000000 ) ) ;
#40668=CARTESIAN_POINT ( 'NONE',  ( 9.928125000614517859, 4.541064518000418104, 2.621784821874999949 ) ) ;
#40670=CARTESIAN_POINT ( 'NONE',  ( 26.05312500061451431, 4.541064518000418104, -2.621784821874998173 ) ) ;
#40671=CARTESIAN_POINT ( 'NONE',  ( 7.040625000614517681, -3.027376345333610441, -5.243569643749999898 ) ) ;
#40672=AXIS2_PLACEMENT_3D ( 'NONE', #33774, #5706, #22681 ) ;
#40673=CARTESIAN_POINT ( 'NONE',  ( 6.178125000614518747, 6.421520780324663323E-16, -5.243569643749999010 ) ) ;
#40675=FACE_BOUND ( 'NONE', #59126, .T. ) ;
#40676=CARTESIAN_POINT ( 'NONE',  ( 16.57499999999999929, -4.330127018922194537, 2.499999999999995559 ) ) ;
#40678=VECTOR ( 'NONE', #20907, 1000.000000000000000 ) ;
#40679=CARTESIAN_POINT ( 'NONE',  ( 13.80937500061451750, -4.541064518000417216, -2.621784821875001281 ) ) ;
#40680=CARTESIAN_POINT ( 'NONE',  ( 10.72500000122903252, 2.886751345948126879, 4.999999999999999112 ) ) ;
#40681=CARTESIAN_POINT ( 'NONE',  ( 15.90937500061451892, 0.000000000000000000, 5.243569643749999010 ) ) ;
#40683=CARTESIAN_POINT ( 'NONE',  ( 22.05937500061451573, 4.541064518000418104, -2.621784821874998173 ) ) ;
#40684=CARTESIAN_POINT ( 'NONE',  ( -2.121784821874999949, 12.07812500061451821, -33.67503911421598417 ) ) ;
#40686=CARTESIAN_POINT ( 'NONE',  ( 3.504965621013899746, 3.565840152826760256, 3.504965621013765631 ) ) ;
#40689=CARTESIAN_POINT ( 'NONE',  ( 25.52812500061451573, 6.421520780324663323E-16, -5.243569643749999010 ) ) ;
#40690=CARTESIAN_POINT ( 'NONE',  ( 17.25000000122903288, -2.886751345948092684, -5.000000000000057732 ) ) ;
#40691=CARTESIAN_POINT ( 'NONE',  ( 27.98437500061451289, 4.541064518000418104, 2.621784821874999949 ) ) ;
#40692=CARTESIAN_POINT ( 'NONE',  ( 24.22500000000000142, -4.330127018922194537, 2.499999999999995559 ) ) ;
#40693=CARTESIAN_POINT ( 'NONE',  ( 7.228125000614517681, 4.541064518000418104, 2.621784821874999949 ) ) ;
#40695=( BOUNDED_CURVE ( )  B_SPLINE_CURVE ( 2, ( #63269, #58075, #69551, #41827, #6404, #28936, #51472 ),
 .UNSPECIFIED., .F., .F. ) 
 B_SPLINE_CURVE_WITH_KNOTS ( ( 3, 2, 2, 3 ),
 ( 0.4500000000000001221, 0.4527777777777778345, 0.4555555555555555469, 0.4583333333333332593 ),
 .UNSPECIFIED. ) 
 CURVE ( )  GEOMETRIC_REPRESENTATION_ITEM ( )  RATIONAL_B_SPLINE_CURVE ( ( 0.9999999999999946709, 0.8660254037844440367, 1.000000000000000000, 0.8660254037844387076, 1.000000000000000000, 0.8660254037844413721, 0.9999999999999973355 ) ) 
 REPRESENTATION_ITEM ( '' )  );
#40696=CARTESIAN_POINT ( 'NONE',  ( 18.68437500061451928, -4.541064518000419881, 2.621784821874995952 ) ) ;
#40698=CARTESIAN_POINT ( 'NONE',  ( 28.68750000122903288, 4.330127018922191873, 2.499999999999999556 ) ) ;
#40699=CARTESIAN_POINT ( 'NONE',  ( 8.596875000614518925, 6.054752690667223547, 3.707466751127219781E-16 ) ) ;
#40701=CARTESIAN_POINT ( 'NONE',  ( 18.98437500061451644, 4.541064518000418104, 2.621784821874999949 ) ) ;
#40702=CARTESIAN_POINT ( 'NONE',  ( 13.76250000122903394, 4.330127018922192761, -2.499999999999997780 ) ) ;
#40703=CARTESIAN_POINT ( 'NONE',  ( 25.53750000000000142, -2.886751345948129988, 4.999999999999997335 ) ) ;
#40704=CARTESIAN_POINT ( 'NONE',  ( 3.374999999999999556, 4.330127018922191873, 2.499999999999999556 ) ) ;
#40707=VERTEX_POINT ( 'NONE', #59005 ) ;
#40708=CARTESIAN_POINT ( 'NONE',  ( 9.674999999999998934, 4.330127018922191873, 2.499999999999999556 ) ) ;
#40710=CARTESIAN_POINT ( 'NONE',  ( 25.56562500061452070, 3.027376345333613106, -5.243569643749998122 ) ) ;
#40711=CARTESIAN_POINT ( 'NONE',  ( 13.16249999999999964, 2.886751345948129099, -4.999999999999998224 ) ) ;
#40712=EDGE_CURVE ( 'NONE', #68026, #17299, #20788, .T. ) ;
#40713=CARTESIAN_POINT ( 'NONE',  ( 9.675000001229035362, 2.886751345948129099, -4.999999999999998224 ) ) ;
#40714=CARTESIAN_POINT ( 'NONE',  ( 8.540625000614518569, 6.054752690667223547, 3.707466751127219781E-16 ) ) ;
#40715=CARTESIAN_POINT ( 'NONE',  ( 21.30000000000000071, 4.330127018922192761, -2.499999999999997780 ) ) ;
#40716=CARTESIAN_POINT ( 'NONE',  ( 20.20312500061451644, 4.541064518000418104, -2.621784821874998173 ) ) ;
#40717=CARTESIAN_POINT ( 'NONE',  ( 30.00000000000000000, 0.000000000000000000, 0.000000000000000000 ) ) ;
#40718=CARTESIAN_POINT ( 'NONE',  ( 26.32500000122903216, 2.886751345948129099, -4.999999999999998224 ) ) ;
#40720=CARTESIAN_POINT ( 'NONE',  ( 6.825000000000001066, 6.123233995736764310E-16, -4.999999999999998224 ) ) ;
#40723=CARTESIAN_POINT ( 'NONE',  ( 22.19062500061451715, -3.027376345333614438, 5.243569643749998122 ) ) ;
#40724=DIRECTION ( 'NONE',  ( 1.000000000000000000, 0.000000000000000000, 0.000000000000000000 ) ) ;
#40725=CARTESIAN_POINT ( 'NONE',  ( 28.20937500061451786, -4.541064518000417216, -2.621784821875001281 ) ) ;
#40726=CARTESIAN_POINT ( 'NONE',  ( 19.69687500061451857, -3.027376345333610441, -5.243569643749999898 ) ) ;
#40727=CARTESIAN_POINT ( 'NONE',  ( 15.44062500061451537, -3.027376345333614438, 5.243569643749998122 ) ) ;
#40729=VECTOR ( 'NONE', #34156, 1000.000000000000000 ) ;
#40730=CARTESIAN_POINT ( 'NONE',  ( 26.43750000122903288, 4.330127018922191873, 2.499999999999999556 ) ) ;
#40732=CARTESIAN_POINT ( 'NONE',  ( 16.30312500061451786, 0.000000000000000000, 5.243569643749999010 ) ) ;
#40733=DIRECTION ( 'NONE',  ( 0.000000000000000000, 0.000000000000000000, 1.000000000000000000 ) ) ;
#40735=CARTESIAN_POINT ( 'NONE',  ( 11.67187500061451821, 3.027376345333613106, -5.243569643749998122 ) ) ;
#40736=CARTESIAN_POINT ( 'NONE',  ( 12.90937500061451537, -4.541064518000417216, -2.621784821875001281 ) ) ;
#40737=CARTESIAN_POINT ( 'NONE',  ( 19.13437500061451857, -4.541064518000419881, 2.621784821874995952 ) ) ;
#40738=ORIENTED_EDGE ( 'NONE', *, *, #66190, .F. ) ;
#40739=CARTESIAN_POINT ( 'NONE',  ( 25.26562500061451289, 3.027376345333611329, 5.243569643749999010 ) ) ;
#40740=VECTOR ( 'NONE', #22780, 1000.000000000000000 ) ;
#40741=CARTESIAN_POINT ( 'NONE',  ( 19.43437500061451928, 4.541064518000418104, 2.621784821874999949 ) ) ;
#40742=CARTESIAN_POINT ( 'NONE',  ( 24.55312500061451786, -4.541064518000417216, -2.621784821875001281 ) ) ;
#40743=CARTESIAN_POINT ( 'NONE',  ( 27.07499999999999929, 6.123233995736764310E-16, -4.999999999999998224 ) ) ;
#40744=CARTESIAN_POINT ( 'NONE',  ( -2.000000000000000000, 13.62500000000000178, 26.53589838486224650 ) ) ;
#40745=CARTESIAN_POINT ( 'NONE',  ( 28.22812500061451502, 6.421520780324663323E-16, -5.243569643749999010 ) ) ;
#40746=CARTESIAN_POINT ( 'NONE',  ( 10.57500000122903572, 2.886751345948129099, -4.999999999999998224 ) ) ;
#40748=CARTESIAN_POINT ( 'NONE',  ( 5.587500001229033231, 6.123233995736764310E-16, -4.999999999999998224 ) ) ;
#40750=CARTESIAN_POINT ( 'NONE',  ( 27.00000000122903288, -2.886751345948129988, 4.999999999999997335 ) ) ;
#40753=CARTESIAN_POINT ( 'NONE',  ( 8.334375000614516082, -4.541064518000419881, 2.621784821874995952 ) ) ;
#40754=CARTESIAN_POINT ( 'NONE',  ( 1.071796769724489895, 10.07990381179669903, 26.00000000000000355 ) ) ;
#40755=CARTESIAN_POINT ( 'NONE',  ( 16.97812500061451502, 6.421520780324663323E-16, -5.243569643749999010 ) ) ;
#40756=CARTESIAN_POINT ( 'NONE',  ( 9.909375000614517148, 4.541064518000418104, -2.621784821874998173 ) ) ;
#40757=CARTESIAN_POINT ( 'NONE',  ( 28.23750000122903359, 4.330127018922191873, 2.499999999999999556 ) ) ;
#40758=CARTESIAN_POINT ( 'NONE',  ( 19.13437500061451857, -4.541064518000419881, 2.621784821874995952 ) ) ;
#40759=CARTESIAN_POINT ( 'NONE',  ( 7.996875000614519280, -3.027376345333610441, -5.243569643749999898 ) ) ;
#40760=CARTESIAN_POINT ( 'NONE',  ( 3.215625000614518836, 3.027376345333611329, 5.243569643749999010 ) ) ;
#40762=CARTESIAN_POINT ( 'NONE',  ( 7.603125000614517681, 4.541064518000418104, -2.621784821874998173 ) ) ;
#40763=CARTESIAN_POINT ( 'NONE',  ( 17.61562500061451786, 3.027376345333611329, 5.243569643749999010 ) ) ;
#40764=EDGE_CURVE ( 'NONE', #33074, #17652, #30939, .T. ) ;
#40765=ORIENTED_EDGE ( 'NONE', *, *, #53394, .F. ) ;
#40766=CARTESIAN_POINT ( 'NONE',  ( 6.112500001229034474, 4.330127018922192761, -2.499999999999997780 ) ) ;
#40767=CARTESIAN_POINT ( 'NONE',  ( 15.02812500061451750, -4.541064518000419881, 2.621784821874995952 ) ) ;
#40768=CARTESIAN_POINT ( 'NONE',  ( 12.21562500061451573, 3.027376345333611329, 5.243569643749999010 ) ) ;
#40770=CARTESIAN_POINT ( 'NONE',  ( 12.78749999999999964, 5.773502691896255534, 3.535250795749688894E-16 ) ) ;
#40771=CARTESIAN_POINT ( 'NONE',  ( 6.637500001229035718, 4.330127018922191873, 2.499999999999999556 ) ) ;
#40772=CARTESIAN_POINT ( 'NONE',  ( 3.628125000614518036, 4.541064518000418104, 2.621784821874999949 ) ) ;
#40773=CARTESIAN_POINT ( 'NONE',  ( 19.16250000122903430, 4.330127018922192761, -2.499999999999997780 ) ) ;
#40775=B_SPLINE_CURVE_WITH_KNOTS ( 'NONE', 1,
 ( #21267, #5385 ),
 .UNSPECIFIED., .F., .F.,
 ( 2, 2 ),
 ( 0.000000000000000000, 1.000000000000000000 ),
 .UNSPECIFIED. ) ;
#40776=CARTESIAN_POINT ( 'NONE',  ( 2.121784821875001281, 12.35937500061451821, -26.32496088578401938 ) ) ;
#40777=LINE ( 'NONE', #40408, #34751 ) ;
#40779=CARTESIAN_POINT ( 'NONE',  ( 2.962500001229034119, 4.330127018922192761, -2.499999999999997780 ) ) ;
#40781=CARTESIAN_POINT ( 'NONE',  ( 19.17187500061451999, -6.054752690667223547, -1.112240025338166033E-15 ) ) ;
#40782=DIRECTION ( 'NONE',  ( -0.000000000000000000, -1.000000000000000000, -0.000000000000000000 ) ) ;
#40784=CARTESIAN_POINT ( 'NONE',  ( 14.54062500061451679, -3.027376345333614438, 5.243569643749998122 ) ) ;
#40786=CARTESIAN_POINT ( 'NONE',  ( 0.000000000000000000, 20.00000000000000000, -33.99999999999999289 ) ) ;
#40787=CARTESIAN_POINT ( 'NONE',  ( 25.77187500061451075, 3.027376345333611329, 5.243569643749999010 ) ) ;
#40789=CARTESIAN_POINT ( 'NONE',  ( 11.91562500061451857, -6.054752690667223547, -1.112240025338166033E-15 ) ) ;
#40791=CARTESIAN_POINT ( 'NONE',  ( 15.90937500061451892, 0.000000000000000000, 5.243569643749999010 ) ) ;
#40792=EDGE_LOOP ( 'NONE', ( #13734, #48752, #39803, #47342 ) ) ;
#40793=CARTESIAN_POINT ( 'NONE',  ( 28.56562500061451715, -6.054752690667223547, -1.112240025338166033E-15 ) ) ;
#40794=CARTESIAN_POINT ( 'NONE',  ( 21.10312500061451502, 4.541064518000418104, -2.621784821874998173 ) ) ;
#40795=CARTESIAN_POINT ( 'NONE',  ( 2.000000000000001332, 13.06250000122903465, -26.53589838486224650 ) ) ;
#40796=DIRECTION ( 'NONE',  ( 0.000000000000000000, 0.000000000000000000, -1.000000000000000000 ) ) ;
#40797=CARTESIAN_POINT ( 'NONE',  ( 9.375000000000001776, -4.330127018922194537, 2.499999999999995559 ) ) ;
#40798=CARTESIAN_POINT ( 'NONE',  ( 20.21250000122903145, 0.000000000000000000, 4.999999999999998224 ) ) ;
#40799=CARTESIAN_POINT ( 'NONE',  ( -3.999999999999999112, 10.06250000000000178, 27.69059892324149885 ) ) ;
#40801=VERTEX_POINT ( 'NONE', #47945 ) ;
#40802=CARTESIAN_POINT ( 'NONE',  ( 18.78749999999999432, -2.886751345948129988, 4.999999999999997335 ) ) ;
#40803=CARTESIAN_POINT ( 'NONE',  ( 21.56250000000000000, -5.773502691896255534, -1.060575238724906372E-15 ) ) ;
#40804=CARTESIAN_POINT ( 'NONE',  ( 19.32187500061451857, 3.027376345333613106, -5.243569643749998122 ) ) ;
#40805=CARTESIAN_POINT ( 'NONE',  ( 24.17812500061451786, 6.421520780324663323E-16, -5.243569643749999010 ) ) ;
#40807=CARTESIAN_POINT ( 'NONE',  ( 28.01250000122903216, -4.330127018922190985, -2.500000000000001332 ) ) ;
#40808=CARTESIAN_POINT ( 'NONE',  ( 5.053125000614517859, 0.000000000000000000, 5.243569643749999010 ) ) ;
#40809=DIRECTION ( 'NONE',  ( -0.000000000000000000, -1.000000000000000000, -0.000000000000000000 ) ) ;
#40810=CARTESIAN_POINT ( 'NONE',  ( 14.81250000000000000, -5.773502691896255534, -1.060575238724906372E-15 ) ) ;
#40811=CARTESIAN_POINT ( 'NONE',  ( -4.243569643749999898, 17.10312500061451502, 30.00000000000000000 ) ) ;
#40812=CARTESIAN_POINT ( 'NONE',  ( 28.22812500061451502, 6.421520780324663323E-16, -5.243569643749999010 ) ) ;
#40815=CARTESIAN_POINT ( 'NONE',  ( 25.95937500061451431, -4.541064518000417216, -2.621784821875001281 ) ) ;
#40816=VERTEX_POINT ( 'NONE', #13577 ) ;
#40817=CARTESIAN_POINT ( 'NONE',  ( 21.74062500061451431, -3.027376345333614438, 5.243569643749998122 ) ) ;
#40818=CARTESIAN_POINT ( 'NONE',  ( 22.54687500061451999, 6.054752690667223547, 3.707466751127219781E-16 ) ) ;
#40819=CARTESIAN_POINT ( 'NONE',  ( 2.121784821875001281, 15.90312500061459566, -26.32496088578401938 ) ) ;
#40820=CARTESIAN_POINT ( 'NONE',  ( 10.27499999999999858, -4.330127018922194537, 2.499999999999995559 ) ) ;
#40821=CARTESIAN_POINT ( 'NONE',  ( 6.740625000614516082, 6.054752690667223547, 3.707466751127219781E-16 ) ) ;
#40823=CARTESIAN_POINT ( 'NONE',  ( 22.94062500061451004, 6.054752690667223547, 3.707466751127219781E-16 ) ) ;
#40826=CARTESIAN_POINT ( 'NONE',  ( 17.10937500061451999, 4.541064518000418104, -2.621784821874998173 ) ) ;
#40827=CARTESIAN_POINT ( 'NONE',  ( 4.243569643749999010, 12.47187500061451715, 27.54997392385601174 ) ) ;
#40828=CARTESIAN_POINT ( 'NONE',  ( 19.92187500061451644, 3.027376345333611329, 5.243569643749999010 ) ) ;
#40829=CARTESIAN_POINT ( 'NONE',  ( 27.49687500061451217, 6.054752690667223547, 3.707466751127219781E-16 ) ) ;
#40830=CARTESIAN_POINT ( 'NONE',  ( 4.243569643749999898, 16.89687500061451786, 32.45002607614398471 ) ) ;
#40831=CARTESIAN_POINT ( 'NONE',  ( 8.615625000614517859, 3.027376345333611329, 5.243569643749999010 ) ) ;
#40832=CARTESIAN_POINT ( 'NONE',  ( -5.810221930991193690E-16, 10.55000000122903359, -34.00000000000000000 ) ) ;
#40833=CARTESIAN_POINT ( 'NONE',  ( 4.321875000614517681, -6.054752690667223547, -1.112240025338166033E-15 ) ) ;
#40834=CYLINDRICAL_SURFACE ( 'NONE', #43099, 4.999999999999998224 ) ;
#40836=CARTESIAN_POINT ( 'NONE',  ( 4.340625000614515727, -3.027376345333610441, -5.243569643749999898 ) ) ;
#40837=CARTESIAN_POINT ( 'NONE',  ( 8.709375000614517859, 0.000000000000000000, 5.243569643749999010 ) ) ;
#40838=CARTESIAN_POINT ( 'NONE',  ( 16.72500000122903430, -5.773502691896255534, -1.060575238724906372E-15 ) ) ;
#40839=CARTESIAN_POINT ( 'NONE',  ( 5.071875000614519458, 3.027376345333611329, 5.243569643749999010 ) ) ;
#40840=CARTESIAN_POINT ( 'NONE',  ( 7.715625000614515727, 3.027376345333611329, 5.243569643749999010 ) ) ;
#40843=CARTESIAN_POINT ( 'NONE',  ( 16.35937500061451644, 0.000000000000000000, 5.243569643749999010 ) ) ;
#40844=FACE_OUTER_BOUND ( 'NONE', #66852, .T. ) ;
#40846=CARTESIAN_POINT ( 'NONE',  ( 24.47812500061451502, -4.541064518000419881, 2.621784821874995952 ) ) ;
#40847=CARTESIAN_POINT ( 'NONE',  ( 8.840625000614515727, -3.027376345333610441, -5.243569643749999898 ) ) ;
#40848=CARTESIAN_POINT ( 'NONE',  ( 27.64687500061452141, -3.027376345333614438, 5.243569643749998122 ) ) ;
#40849=CARTESIAN_POINT ( 'NONE',  ( 10.00312500061451715, 0.000000000000000000, 5.243569643749999010 ) ) ;
#40850=CARTESIAN_POINT ( 'NONE',  ( 4.544497808834801589, -2.085075457992688897, -4.544497808831748920 ) ) ;
#40852=CARTESIAN_POINT ( 'NONE',  ( 10.05000000122903181, -2.886751345948125991, -5.000000000000000000 ) ) ;
#40853=CARTESIAN_POINT ( 'NONE',  ( 23.87812500061451715, 4.541064518000418104, 2.621784821874999949 ) ) ;
#40854=ADVANCED_FACE ( 'NONE', ( #58275 ), #2507, .F. ) ;
#40855=CARTESIAN_POINT ( 'NONE',  ( 2.121784821875001281, 13.65312500061451750, -26.32496088578401938 ) ) ;
#40856=CARTESIAN_POINT ( 'NONE',  ( 12.52500000122903145, 2.886751345948126879, 4.999999999999999112 ) ) ;
#40857=CARTESIAN_POINT ( 'NONE',  ( 22.97812500061451857, 4.541064518000418104, 2.621784821874999949 ) ) ;
#40858=CARTESIAN_POINT ( 'NONE',  ( 11.17500000000000071, -4.330127018922194537, 2.499999999999995559 ) ) ;
#40859=CARTESIAN_POINT ( 'NONE',  ( 19.34062500061451573, 6.054752690667223547, 3.707466751127219781E-16 ) ) ;
#40860=CARTESIAN_POINT ( 'NONE',  ( 5.371875000614516615, 3.027376345333612662, -5.243569643749998122 ) ) ;
#40861=CARTESIAN_POINT ( 'NONE',  ( 20.43749999999999645, 5.773502691896255534, 3.535250795749688894E-16 ) ) ;
#40862=CARTESIAN_POINT ( 'NONE',  ( 15.37500000122903465, -5.773502691896255534, -1.060575238724906372E-15 ) ) ;
#40863=CARTESIAN_POINT ( 'NONE',  ( 11.69062500061451360, 6.054752690667223547, 3.707466751127219781E-16 ) ) ;
#40864=CARTESIAN_POINT ( 'NONE',  ( 16.37812500061451715, -4.541064518000419881, 2.621784821874995952 ) ) ;
#40865=CARTESIAN_POINT ( 'NONE',  ( 25.98750000122903003, 4.330127018922191873, 2.499999999999999556 ) ) ;
#40866=CARTESIAN_POINT ( 'NONE',  ( 19.38749999999999929, -2.886751345948125991, -5.000000000000000000 ) ) ;
#40867=CARTESIAN_POINT ( 'NONE',  ( 22.73437500061451644, -4.541064518000419881, 2.621784821874995952 ) ) ;
#40869=CARTESIAN_POINT ( 'NONE',  ( 11.28750000122903252, -4.330127018922194537, 2.499999999999995559 ) ) ;
#40870=CARTESIAN_POINT ( 'NONE',  ( 9.234375000614518214, -4.541064518000419881, 2.621784821874995952 ) ) ;
#40871=CARTESIAN_POINT ( 'NONE',  ( 25.32187500061451857, 3.027376345333611329, 5.243569643749999010 ) ) ;
#40872=CARTESIAN_POINT ( 'NONE',  ( 15.48750000122903359, 6.123233995736764310E-16, -4.999999999999998224 ) ) ;
#40873=CARTESIAN_POINT ( 'NONE',  ( 20.84062500061451573, -3.027376345333614438, 5.243569643749998122 ) ) ;
#40874=CARTESIAN_POINT ( 'NONE',  ( 27.60937500061451644, 0.000000000000000000, 5.243569643749999010 ) ) ;
#40878=CARTESIAN_POINT ( 'NONE',  ( 7.621875000614519280, 3.027376345333613106, -5.243569643749998122 ) ) ;
#40879=CARTESIAN_POINT ( 'NONE',  ( 19.37812500061451715, 4.541064518000418104, 2.621784821874999949 ) ) ;
#40880=ORIENTED_EDGE ( 'NONE', *, *, #64083, .T. ) ;
#40881=CARTESIAN_POINT ( 'NONE',  ( 27.17812500061451786, -4.541064518000419881, 2.621784821874995952 ) ) ;
#40882=CARTESIAN_POINT ( 'NONE',  ( 3.234375000614516438, 4.541064518000418104, 2.621784821874999949 ) ) ;
#40883=LINE ( 'NONE', #63030, #40740 ) ;
#40884=DIRECTION ( 'NONE',  ( 0.000000000000000000, 0.000000000000000000, -1.000000000000000000 ) ) ;
#40885=CARTESIAN_POINT ( 'NONE',  ( 16.23750000000000071, -2.886751345948125991, -5.000000000000000000 ) ) ;
#40886=CARTESIAN_POINT ( 'NONE',  ( 21.55312500061451431, 4.541064518000418104, -2.621784821874998173 ) ) ;
#40887=VERTEX_POINT ( 'NONE', #2155 ) ;
#40888=CARTESIAN_POINT ( 'NONE',  ( 25.83749999999999858, 5.773502691896255534, 3.535250795749688894E-16 ) ) ;
#40890=CARTESIAN_POINT ( 'NONE',  ( 26.97187500061451360, 3.027376345333613106, -5.243569643749998122 ) ) ;
#40893=CARTESIAN_POINT ( 'NONE',  ( 15.32812500061451644, 4.541064518000418104, 2.621784821874999949 ) ) ;
#40894=CARTESIAN_POINT ( 'NONE',  ( 6.740625000614516082, 6.054752690667223547, 3.707466751127219781E-16 ) ) ;
#40896=CARTESIAN_POINT ( 'NONE',  ( 29.54062500061451502, -3.027376345333610441, -5.243569643749999898 ) ) ;
#40898=CARTESIAN_POINT ( 'NONE',  ( 14.25000000122903465, 5.773502691896255534, 3.535250795749688894E-16 ) ) ;
#40899=CARTESIAN_POINT ( 'NONE',  ( 21.15000000000000213, -4.330127018922190985, -2.500000000000001332 ) ) ;
#40900=CARTESIAN_POINT ( 'NONE',  ( 28.42499999999999716, 6.123233995736764310E-16, -4.999999999999998224 ) ) ;
#40901=CARTESIAN_POINT ( 'NONE',  ( 5.184375000614516615, -4.541064518000419881, 2.621784821874995952 ) ) ;
#40902=CARTESIAN_POINT ( 'NONE',  ( 8.859375000614518214, -4.541064518000417216, -2.621784821875001281 ) ) ;
#40903=CARTESIAN_POINT ( 'NONE',  ( 20.29687500061451644, 6.054752690667223547, 3.707466751127219781E-16 ) ) ;
#40904=CARTESIAN_POINT ( 'NONE',  ( 30.00000000000000000, 0.000000000000000000, 0.000000000000000000 ) ) ;
#40905=ORIENTED_EDGE ( 'NONE', *, *, #29319, .F. ) ;
#40906=CARTESIAN_POINT ( 'NONE',  ( 27.92812500061451431, 4.541064518000418104, 2.621784821874999949 ) ) ;
#40907=CARTESIAN_POINT ( 'NONE',  ( 3.187500000000002220, -2.886751345948125991, -5.000000000000000000 ) ) ;
#40908=CARTESIAN_POINT ( 'NONE',  ( 4.846875000614519813, -3.027376345333610441, -5.243569643749999898 ) ) ;
#40909=CARTESIAN_POINT ( 'NONE',  ( 18.18750000000000000, 5.773502691896255534, 3.535250795749688894E-16 ) ) ;
#40910=CARTESIAN_POINT ( 'NONE',  ( 14.01562500061451644, 3.027376345333611329, 5.243569643749999010 ) ) ;
#40912=CARTESIAN_POINT ( 'NONE',  ( 5.700000000000000178, 0.000000000000000000, 4.999999999999998224 ) ) ;
#40915=CARTESIAN_POINT ( 'NONE',  ( 8.840625000614515727, -3.027376345333610441, -5.243569643749999898 ) ) ;
#40916=CARTESIAN_POINT ( 'NONE',  ( 26.14687500061451431, 6.054752690667223547, 3.707466751127219781E-16 ) ) ;
#40917=EDGE_CURVE ( 'NONE', #32704, #100, #66688, .T. ) ;
#40918=CARTESIAN_POINT ( 'NONE',  ( -2.121784821874999949, 18.43437500061451928, 26.32496088578401938 ) ) ;
#40919=CARTESIAN_POINT ( 'NONE',  ( 27.12187500061451573, 3.027376345333611329, 5.243569643749999010 ) ) ;
#40920=CARTESIAN_POINT ( 'NONE',  ( 6.712500000000000355, -5.773502691896255534, -1.060575238724906372E-15 ) ) ;
#40921=CARTESIAN_POINT ( 'NONE',  ( 8.484601909799253346E-16, 13.47500000122903430, 34.61880215351700230 ) ) ;
#40922=CARTESIAN_POINT ( 'NONE',  ( 15.89062500061451289, -3.027376345333614438, 5.243569643749998122 ) ) ;
#40923=CARTESIAN_POINT ( 'NONE',  ( 6.187500001229032875, 4.330127018922191873, 2.499999999999999556 ) ) ;
#40924=CARTESIAN_POINT ( 'NONE',  ( 18.64687500061451786, -3.027376345333614438, 5.243569643749998122 ) ) ;
#40925=CARTESIAN_POINT ( 'NONE',  ( 12.79687500061451821, -3.027376345333614438, 5.243569643749998122 ) ) ;
#40926=CARTESIAN_POINT ( 'NONE',  ( -3.858979783667864538, 3.180598473748192490, -28.91336298736815635 ) ) ;
#40927=ORIENTED_EDGE ( 'NONE', *, *, #11525, .T. ) ;
#40928=CARTESIAN_POINT ( 'NONE',  ( 13.34062500061451750, -3.027376345333610441, -5.243569643749999898 ) ) ;
#40929=CARTESIAN_POINT ( 'NONE',  ( 24.97500000122903430, 2.886751345948129099, -4.999999999999998224 ) ) ;
#40930=CARTESIAN_POINT ( 'NONE',  ( 12.98437500061451821, 6.421520780324663323E-16, -5.243569643749999010 ) ) ;
#40931=CARTESIAN_POINT ( 'NONE',  ( 15.85312500061451857, 0.000000000000000000, 5.243569643749999010 ) ) ;
#40932=EDGE_CURVE ( 'NONE', #66981, #27675, #28356, .T. ) ;
#40933=CARTESIAN_POINT ( 'NONE',  ( 4.400918202330496243, -2.373166445152071535, -4.675799785326651303 ) ) ;
#40934=CARTESIAN_POINT ( 'NONE',  ( 23.44687500061451502, 6.054752690667223547, 3.707466751127219781E-16 ) ) ;
#40936=CARTESIAN_POINT ( 'NONE',  ( 12.93750000122903465, 4.330127018922191873, 2.499999999999999556 ) ) ;
#40937=DIRECTION ( 'NONE',  ( -1.000000000000000000, -0.000000000000000000, -0.000000000000000000 ) ) ;
#40938=CARTESIAN_POINT ( 'NONE',  ( 3.103125000614517237, 4.541064518000418104, -2.621784821874998173 ) ) ;
#40939=CARTESIAN_POINT ( 'NONE',  ( 2.121784821874999061, 17.45937500061451786, -33.67503911421598417 ) ) ;
#40940=CARTESIAN_POINT ( 'NONE',  ( 18.98437500061451644, 4.541064518000418104, 2.621784821874999949 ) ) ;
#40941=CARTESIAN_POINT ( 'NONE',  ( 16.50000000122903288, 5.773502691896255534, 3.535250795749688894E-16 ) ) ;
#40942=CARTESIAN_POINT ( 'NONE',  ( 15.45937500061451608, 0.000000000000000000, 5.243569643749999010 ) ) ;
#40944=CARTESIAN_POINT ( 'NONE',  ( 21.03750000122903074, 4.330127018922191873, 2.499999999999999556 ) ) ;
#40945=CARTESIAN_POINT ( 'NONE',  ( 14.72812500061451679, 6.421520780324663323E-16, -5.243569643749999010 ) ) ;
#40948=CARTESIAN_POINT ( 'NONE',  ( 18.14999999999999858, 4.330127018922192761, -2.499999999999997780 ) ) ;
#40949=CARTESIAN_POINT ( 'NONE',  ( 1.351293209486982505, 4.820886669536883495, 26.22567693883006967 ) ) ;
#40950=CARTESIAN_POINT ( 'NONE',  ( 15.22500000122903252, 2.886751345948126879, 4.999999999999999112 ) ) ;
#40951=CARTESIAN_POINT ( 'NONE',  ( 26.52187500061451431, 3.027376345333613106, -5.243569643749998122 ) ) ;
#40952=CARTESIAN_POINT ( 'NONE',  ( 20.01562500061451644, -6.054752690667223547, -1.112240025338166033E-15 ) ) ;
#40953=CARTESIAN_POINT ( 'NONE',  ( 22.94062500061451715, 6.054752690667223547, 3.707466751127219781E-16 ) ) ;
#40954=CARTESIAN_POINT ( 'NONE',  ( 4.003125000614518925, 4.541064518000418104, -2.621784821874998173 ) ) ;
#40955=CARTESIAN_POINT ( 'NONE',  ( 27.93750000000000000, -2.886751345948125991, -5.000000000000000000 ) ) ;
#40956=CARTESIAN_POINT ( 'NONE',  ( 0.000000000000000000, 20.00000000000000000, -33.99999999999999289 ) ) ;
#40958=CARTESIAN_POINT ( 'NONE',  ( -0.7368881354385758975, 9.803648613939515144, -34.17910028561248481 ) ) ;
#40960=CARTESIAN_POINT ( 'NONE',  ( -4.243569643749999898, 17.15937500061451715, -30.00000000000000000 ) ) ;
#40961=CARTESIAN_POINT ( 'NONE',  ( 4.987500001229032698, -4.330127018922194537, 2.499999999999995559 ) ) ;
#40962=CARTESIAN_POINT ( 'NONE',  ( 6.562500000000001776, 2.886751345948126879, 4.999999999999999112 ) ) ;
#40963=CARTESIAN_POINT ( 'NONE',  ( 16.27499999999999858, 6.123233995736764310E-16, -4.999999999999998224 ) ) ;
#40964=CARTESIAN_POINT ( 'NONE',  ( 8.709375000614517859, 0.000000000000000000, 5.243569643749999010 ) ) ;
#40965=CARTESIAN_POINT ( 'NONE',  ( 28.00312500061451715, 0.000000000000000000, 5.243569643749999010 ) ) ;
#40966=CARTESIAN_POINT ( 'NONE',  ( 27.52500000122903145, -5.773502691896255534, -1.060575238724906372E-15 ) ) ;
#40967=DIRECTION ( 'NONE',  ( -1.000000000000000000, -0.000000000000000000, -0.000000000000000000 ) ) ;
#40968=CARTESIAN_POINT ( 'NONE',  ( 3.999999999999999112, 19.43750000122903288, 30.00000000000000000 ) ) ;
#40969=CARTESIAN_POINT ( 'NONE',  ( 7.921875000614517326, -6.054752690667223547, -1.112240025338166033E-15 ) ) ;
#40970=CARTESIAN_POINT ( 'NONE',  ( 11.85937500061451644, 0.000000000000000000, 5.243569643749999010 ) ) ;
#40971=CARTESIAN_POINT ( 'NONE',  ( 5.400000000000002132, -4.330127018922190985, -2.500000000000001332 ) ) ;
#40972=CARTESIAN_POINT ( 'NONE',  ( -4.243569643749998122, 15.34062500061459744, 32.45002607614398471 ) ) ;
#40973=CARTESIAN_POINT ( 'NONE',  ( 4.912500000000000533, -5.773502691896255534, -1.060575238724906372E-15 ) ) ;
#40974=CARTESIAN_POINT ( 'NONE',  ( 6.375000000000001776, 6.123233995736764310E-16, -4.999999999999998224 ) ) ;
#40975=CARTESIAN_POINT ( 'NONE',  ( 26.81250000122903288, 4.330127018922192761, -2.499999999999997780 ) ) ;
#40977=CARTESIAN_POINT ( 'NONE',  ( 22.67812500061451431, -4.541064518000419881, 2.621784821874995952 ) ) ;
#40978=CARTESIAN_POINT ( 'NONE',  ( 13.11562500061451786, 3.027376345333611329, 5.243569643749999010 ) ) ;
#40980=CARTESIAN_POINT ( 'NONE',  ( 8.896875000614517859, -3.027376345333610441, -5.243569643749999898 ) ) ;
#40981=CARTESIAN_POINT ( 'NONE',  ( 27.33750000000000213, -2.886751345948129988, 4.999999999999997335 ) ) ;
#40982=CARTESIAN_POINT ( 'NONE',  ( 21.56250000122903288, 0.000000000000000000, 4.999999999999998224 ) ) ;
#40983=CARTESIAN_POINT ( 'NONE',  ( 7.320879633048903241E-15, 18.20000000122903216, -34.00000000000000000 ) ) ;
#40984=CARTESIAN_POINT ( 'NONE',  ( 11.33437500061451608, 4.541064518000418104, 2.621784821874999949 ) ) ;
#40985=CARTESIAN_POINT ( 'NONE',  ( 27.04687500061451644, 6.054752690667223547, 3.707466751127219781E-16 ) ) ;
#40987=CARTESIAN_POINT ( 'NONE',  ( 1.071796769724491893, 13.49509619066136779, -26.00000000000000355 ) ) ;
#40988=CARTESIAN_POINT ( 'NONE',  ( 22.58437500061451431, 4.541064518000418104, 2.621784821874999949 ) ) ;
#40989=CARTESIAN_POINT ( 'NONE',  ( 12.00937500061451857, -4.541064518000417216, -2.621784821875001281 ) ) ;
#40991=CARTESIAN_POINT ( 'NONE',  ( 24.82499999999999929, 6.123233995736764310E-16, -4.999999999999998224 ) ) ;
#40993=CARTESIAN_POINT ( 'NONE',  ( -4.243569643749999898, 15.77187500061451608, -32.45002607614398471 ) ) ;
#40995=CARTESIAN_POINT ( 'NONE',  ( 17.16562500061451502, 3.027376345333611329, 5.243569643749999010 ) ) ;
#40996=CARTESIAN_POINT ( 'NONE',  ( 7.800000000000001599, 4.330127018922192761, -2.499999999999997780 ) ) ;
#40997=ADVANCED_FACE ( 'NONE', ( #14673 ), #7682, .F. ) ;
#40999=CARTESIAN_POINT ( 'NONE',  ( 15.82499999999999929, 6.123233995736764310E-16, -4.999999999999998224 ) ) ;
#41000=CARTESIAN_POINT ( 'NONE',  ( 4.000000000000000000, 19.40000000122903856, 32.30940107675849049 ) ) ;
#41001=CARTESIAN_POINT ( 'NONE',  ( 13.80000000122903181, 5.773502691896255534, 3.535250795749688894E-16 ) ) ;
#41002=CARTESIAN_POINT ( 'NONE',  ( 25.62187500061451573, 3.027376345333613106, -5.243569643749998122 ) ) ;
#41003=ORIENTED_EDGE ( 'NONE', *, *, #57235, .F. ) ;
#41004=CARTESIAN_POINT ( 'NONE',  ( 19.97812500061451502, -4.541064518000419881, 2.621784821874995952 ) ) ;
#41005=CARTESIAN_POINT ( 'NONE',  ( 19.99687500061451573, -3.027376345333614438, 5.243569643749998122 ) ) ;
#41006=CARTESIAN_POINT ( 'NONE',  ( 3.000000000000002665, 0.000000000000000000, 4.999999999999998224 ) ) ;
#41007=CARTESIAN_POINT ( 'NONE',  ( 7.640625000614517326, 6.054752690667223547, 3.707466751127219781E-16 ) ) ;
#41008=CARTESIAN_POINT ( 'NONE',  ( 21.02812500061451573, 6.421520780324663323E-16, -5.243569643749999010 ) ) ;
#41009=CARTESIAN_POINT ( 'NONE',  ( 12.15937500061451892, 4.541064518000418104, -2.621784821874998173 ) ) ;
#41010=CARTESIAN_POINT ( 'NONE',  ( 18.00937500061451502, 4.541064518000418104, -2.621784821874998173 ) ) ;
#41011=CARTESIAN_POINT ( 'NONE',  ( 4.243569643749999898, 14.14062500061451644, 32.45002607614398471 ) ) ;
#41012=CARTESIAN_POINT ( 'NONE',  ( 18.48750000122903359, -4.330127018922194537, 2.499999999999995559 ) ) ;
#41014=CARTESIAN_POINT ( 'NONE',  ( 8.615625000614517859, 3.027376345333611329, 5.243569643749999010 ) ) ;
#41015=CARTESIAN_POINT ( 'NONE',  ( 3.796875000614517326, -3.027376345333614438, 5.243569643749998122 ) ) ;
#41016=CARTESIAN_POINT ( 'NONE',  ( 28.64062500061451289, -3.027376345333610441, -5.243569643749999898 ) ) ;
#41017=CARTESIAN_POINT ( 'NONE',  ( 24.83437500061451431, 4.541064518000418104, 2.621784821874999949 ) ) ;
#41018=CARTESIAN_POINT ( 'NONE',  ( 16.56562500061451715, 3.027376345333613106, -5.243569643749998122 ) ) ;
#41019=CARTESIAN_POINT ( 'NONE',  ( 24.56250000122903288, 4.330127018922192761, -2.499999999999997780 ) ) ;
#41020=CARTESIAN_POINT ( 'NONE',  ( 24.92812500061451431, -4.541064518000419881, 2.621784821874995952 ) ) ;
#41021=CARTESIAN_POINT ( 'NONE',  ( 21.34687500061451715, -3.027376345333614438, 5.243569643749998122 ) ) ;
#41022=CARTESIAN_POINT ( 'NONE',  ( 16.56562500061451715, 3.027376345333613106, -5.243569643749998122 ) ) ;
#41023=CARTESIAN_POINT ( 'NONE',  ( -2.121784821874999949, 17.98437500061451999, 26.32496088578401938 ) ) ;
#41024=CARTESIAN_POINT ( 'NONE',  ( 22.45312500061451644, 4.541064518000418104, -2.621784821874998173 ) ) ;
#41027=CARTESIAN_POINT ( 'NONE',  ( 24.86250000000000071, 2.886751345948129099, -4.999999999999998224 ) ) ;
#41028=CARTESIAN_POINT ( 'NONE',  ( 2.000000000000001332, 12.50000000000000000, -26.53589838486224650 ) ) ;
#41030=CARTESIAN_POINT ( 'NONE',  ( 29.61562500061451431, 3.027376345333613106, -5.243569643749998122 ) ) ;
#41031=CARTESIAN_POINT ( 'NONE',  ( 10.04062500061451502, -3.027376345333614438, 5.243569643749998122 ) ) ;
#41032=CARTESIAN_POINT ( 'NONE',  ( 22.01250000122903216, 0.000000000000000000, 4.999999999999998224 ) ) ;
#41034=CARTESIAN_POINT ( 'NONE',  ( 26.39062500061451644, -3.027376345333610441, -5.243569643749999898 ) ) ;
#41035=CARTESIAN_POINT ( 'NONE',  ( 25.31250000000000000, 2.886751345948129099, -4.999999999999998224 ) ) ;
#41036=CARTESIAN_POINT ( 'NONE',  ( 2.000000000000001332, 15.31250000122903465, -26.53589838486224650 ) ) ;
#41037=CARTESIAN_POINT ( 'NONE',  ( 29.16562500061451502, 3.027376345333613106, -5.243569643749998122 ) ) ;
#41038=CARTESIAN_POINT ( 'NONE',  ( 11.01562500061451821, -6.054752690667223547, -1.112240025338166033E-15 ) ) ;
#41041=CARTESIAN_POINT ( 'NONE',  ( 26.35312500061451857, -4.541064518000417216, -2.621784821875001281 ) ) ;
#41042=CARTESIAN_POINT ( 'NONE',  ( 8.540625000614518569, 6.054752690667223547, 3.707466751127219781E-16 ) ) ;
#41043=CARTESIAN_POINT ( 'NONE',  ( 3.215625000614518836, 3.027376345333611329, 5.243569643749999010 ) ) ;
#41045=EDGE_CURVE ( 'NONE', #55745, #54151, #46265, .T. ) ;
#41046=FACE_OUTER_BOUND ( 'NONE', #27402, .T. ) ;
#41047=CARTESIAN_POINT ( 'NONE',  ( 12.82499999999999929, 4.330127018922191873, 2.499999999999999556 ) ) ;
#41048=CARTESIAN_POINT ( 'NONE',  ( 13.28437500061451715, -4.541064518000419881, 2.621784821874995952 ) ) ;
#41049=CARTESIAN_POINT ( 'NONE',  ( 10.12500000122903465, 2.886751345948129099, -4.999999999999998224 ) ) ;
#41050=CARTESIAN_POINT ( 'NONE',  ( 15.87187500061451573, 3.027376345333611329, 5.243569643749999010 ) ) ;
#41052=CARTESIAN_POINT ( 'NONE',  ( 7.846875000614518036, -3.027376345333614438, 5.243569643749998122 ) ) ;
#41053=CARTESIAN_POINT ( 'NONE',  ( -4.243569643749999898, 10.80312500061451786, -30.00000000000000000 ) ) ;
#41057=CARTESIAN_POINT ( 'NONE',  ( 25.49062500061451786, -3.027376345333610441, -5.243569643749999898 ) ) ;
#41059=CARTESIAN_POINT ( 'NONE',  ( 27.60937500061451644, 0.000000000000000000, 5.243569643749999010 ) ) ;
#41060=CARTESIAN_POINT ( 'NONE',  ( 23.43750000000000000, -2.886751345948125991, -5.000000000000000000 ) ) ;
#41061=CARTESIAN_POINT ( 'NONE',  ( 7.078125000614516438, 6.421520780324663323E-16, -5.243569643749999010 ) ) ;
#41063=CARTESIAN_POINT ( 'NONE',  ( 18.42187500061451644, 3.027376345333613106, -5.243569643749998122 ) ) ;
#41065=CARTESIAN_POINT ( 'NONE',  ( 29.21250000122903145, 0.000000000000000000, 4.999999999999998224 ) ) ;
#41066=CARTESIAN_POINT ( 'NONE',  ( 8.671875000614518214, 3.027376345333611329, 5.243569643749999010 ) ) ;
#41067=ORIENTED_EDGE ( 'NONE', *, *, #30679, .F. ) ;
#41068=CARTESIAN_POINT ( 'NONE',  ( 18.83437500061451431, 6.421520780324663323E-16, -5.243569643749999010 ) ) ;
#41069=CYLINDRICAL_SURFACE ( 'NONE', #7774, 3.999999999999996447 ) ;
#41070=CARTESIAN_POINT ( 'NONE',  ( 27.86249999999999716, -5.773502691896255534, -1.060575238724906372E-15 ) ) ;
#41071=CARTESIAN_POINT ( 'NONE',  ( 29.37187500061451928, 3.027376345333611329, 5.243569643749999010 ) ) ;
#41072=CARTESIAN_POINT ( 'NONE',  ( 1.592000809091587073E-14, 16.85000000122903785, -34.00000000000000000 ) ) ;
#41073=CARTESIAN_POINT ( 'NONE',  ( -1.487416814333745711E-14, 15.72500000122903430, -26.00000000000000000 ) ) ;
#41074=EDGE_LOOP ( 'NONE', ( #26068, #1551, #24275, #4658 ) ) ;
#41075=CARTESIAN_POINT ( 'NONE',  ( 11.32500000000000107, 6.123233995736764310E-16, -4.999999999999998224 ) ) ;
#41077=CARTESIAN_POINT ( 'NONE',  ( 23.76562500061451644, 3.027376345333613106, -5.243569643749998122 ) ) ;
#41078=CARTESIAN_POINT ( 'NONE',  ( 15.37500000000000000, 6.123233995736764310E-16, -4.999999999999998224 ) ) ;
#41080=CARTESIAN_POINT ( 'NONE',  ( 8.587500001229035007, -4.330127018922194537, 2.499999999999995559 ) ) ;
#41081=CARTESIAN_POINT ( 'NONE',  ( 7.565625000614518036, 3.027376345333613106, -5.243569643749998122 ) ) ;
#41082=CARTESIAN_POINT ( 'NONE',  ( 20.92500000000000071, 4.330127018922191873, 2.499999999999999556 ) ) ;
#41083=CARTESIAN_POINT ( 'NONE',  ( 20.80312500061451431, 0.000000000000000000, 5.243569643749999010 ) ) ;
#41084=CARTESIAN_POINT ( 'NONE',  ( 1.012874171167973181, -4.999999999999998224, -1.012874171167973181 ) ) ;
#41085=CARTESIAN_POINT ( 'NONE',  ( 25.05000000122903714, 5.773502691896255534, 3.535250795749688894E-16 ) ) ;
#41087=CARTESIAN_POINT ( 'NONE',  ( 4.949999999999999289, -4.330127018922190985, -2.500000000000001332 ) ) ;
#41088=VERTEX_POINT ( 'NONE', #2826 ) ;
#41089=CARTESIAN_POINT ( 'NONE',  ( 21.96562500061451573, 3.027376345333613106, -5.243569643749998122 ) ) ;
#41090=CARTESIAN_POINT ( 'NONE',  ( 27.47812500061451502, 4.541064518000418104, 2.621784821874999949 ) ) ;
#41091=CARTESIAN_POINT ( 'NONE',  ( 27.72187500061451715, -6.054752690667223547, -1.112240025338166033E-15 ) ) ;
#41092=CARTESIAN_POINT ( 'NONE',  ( 15.51562500061451644, -6.054752690667223547, -1.112240025338166033E-15 ) ) ;
#41093=CYLINDRICAL_SURFACE ( 'NONE', #47468, 3.999999999999996447 ) ;
#41095=CARTESIAN_POINT ( 'NONE',  ( 25.42500000122903359, 2.886751345948129099, -4.999999999999998224 ) ) ;
#41097=CARTESIAN_POINT ( 'NONE',  ( 16.22812500061451857, 4.541064518000418104, 2.621784821874999949 ) ) ;
#41098=CARTESIAN_POINT ( 'NONE',  ( 1.592000809091587073E-14, 16.73750000000000071, -34.00000000000000000 ) ) ;
#41099=CARTESIAN_POINT ( 'NONE',  ( 4.575000001229033941, -5.773502691896255534, -1.060575238724906372E-15 ) ) ;
#41100=CARTESIAN_POINT ( 'NONE',  ( 10.84687500061451892, 6.054752690667223547, 3.707466751127219781E-16 ) ) ;
#41101=CARTESIAN_POINT ( 'NONE',  ( 13.13437500061451857, 4.541064518000418104, 2.621784821874999949 ) ) ;
#41102=CARTESIAN_POINT ( 'NONE',  ( 19.20937500061451786, -4.541064518000417216, -2.621784821875001281 ) ) ;
#41104=CARTESIAN_POINT ( 'NONE',  ( -1.587936087009578445, 9.880963660774181534, 24.20021078848421681 ) ) ;
#41105=CARTESIAN_POINT ( 'NONE',  ( 23.12812500061451360, -4.541064518000419881, 2.621784821874995952 ) ) ;
#41106=CARTESIAN_POINT ( 'NONE',  ( 19.92187500061451644, 3.027376345333611329, 5.243569643749999010 ) ) ;
#41107=CARTESIAN_POINT ( 'NONE',  ( 23.99062500061451786, -3.027376345333614438, 5.243569643749998122 ) ) ;
#41109=CARTESIAN_POINT ( 'NONE',  ( -3.999999999999999112, 14.15000000000000036, 30.00000000000000000 ) ) ;
#41110=CARTESIAN_POINT ( 'NONE',  ( 2.859375000614519546, 0.000000000000000000, 5.243569643749999010 ) ) ;
#41111=CARTESIAN_POINT ( 'NONE',  ( 9.187500001229034652, 6.123233995736764310E-16, -4.999999999999998224 ) ) ;
#41112=CARTESIAN_POINT ( 'NONE',  ( 4.725000001229034297, 2.886751345948129099, -4.999999999999998224 ) ) ;
#41114=CARTESIAN_POINT ( 'NONE',  ( 27.26250000122903216, 4.330127018922192761, -2.499999999999997780 ) ) ;
#41116=CARTESIAN_POINT ( 'NONE',  ( 9.534375000614517148, 4.541064518000418104, 2.621784821874999949 ) ) ;
#41117=CARTESIAN_POINT ( 'NONE',  ( 7.724999999999999645, 6.123233995736764310E-16, -4.999999999999998224 ) ) ;
#41118=CARTESIAN_POINT ( 'NONE',  ( 18.44062500061451715, 6.054752690667223547, 3.707466751127219781E-16 ) ) ;
#41119=CARTESIAN_POINT ( 'NONE',  ( 11.85937500061451644, 0.000000000000000000, 5.243569643749999010 ) ) ;
#41120=CARTESIAN_POINT ( 'NONE',  ( 29.51250000122903216, 4.330127018922192761, -2.499999999999997780 ) ) ;
#41121=CARTESIAN_POINT ( 'NONE',  ( 20.93437500061451573, -4.541064518000419881, 2.621784821874995952 ) ) ;
#41122=CARTESIAN_POINT ( 'NONE',  ( 7.171875000614517326, 3.027376345333613106, -5.243569643749998122 ) ) ;
#41123=CARTESIAN_POINT ( 'NONE',  ( 3.290625000614516793, -3.027376345333614438, 5.243569643749998122 ) ) ;
#41124=CARTESIAN_POINT ( 'NONE',  ( 2.000000000000001332, 16.21250000122903501, 33.46410161513774995 ) ) ;
#41125=CARTESIAN_POINT ( 'NONE',  ( 7.940625000614518036, -3.027376345333610441, -5.243569643749999898 ) ) ;
#41126=CARTESIAN_POINT ( 'NONE',  ( 17.35312500061451502, -4.541064518000417216, -2.621784821875001281 ) ) ;
#41128=EDGE_LOOP ( 'NONE', ( #66096, #17444, #17710, #28561 ) ) ;
#41129=CARTESIAN_POINT ( 'NONE',  ( 6.600000001229032520, 5.773502691896255534, 3.535250795749688894E-16 ) ) ;
#41130=CARTESIAN_POINT ( 'NONE',  ( 13.86562500061451431, 3.027376345333613106, -5.243569643749998122 ) ) ;
#41131=CARTESIAN_POINT ( 'NONE',  ( 13.79062500061451502, -3.027376345333610441, -5.243569643749999898 ) ) ;
#41133=CARTESIAN_POINT ( 'NONE',  ( 12.52500000000000213, -4.330127018922194537, 2.499999999999995559 ) ) ;
#41134=EDGE_CURVE ( 'NONE', #26352, #48852, #51719, .T. ) ;
#41135=CARTESIAN_POINT ( 'NONE',  ( 6.975000001229032520, 2.886751345948129099, -4.999999999999998224 ) ) ;
#41136=CARTESIAN_POINT ( 'NONE',  ( 14.85937500061451644, 4.541064518000418104, -2.621784821874998173 ) ) ;
#41137=CARTESIAN_POINT ( 'NONE',  ( 19.08750000122903145, 6.123233995736764310E-16, -4.999999999999998224 ) ) ;
#41139=( BOUNDED_CURVE ( )  B_SPLINE_CURVE ( 2, ( #59374, #2516, #53862, #25782, #48319, #18396, #40963 ),
 .UNSPECIFIED., .F., .F. ) 
 B_SPLINE_CURVE_WITH_KNOTS ( ( 3, 2, 2, 3 ),
 ( 0.5000000000000000000, 0.5027777777777777679, 0.5055555555555556468, 0.5083333333333334147 ),
 .UNSPECIFIED. ) 
 CURVE ( )  GEOMETRIC_REPRESENTATION_ITEM ( )  RATIONAL_B_SPLINE_CURVE ( ( 1.000000000000000000, 0.8660254037844387076, 1.000000000000000000, 0.8660254037844387076, 1.000000000000000000, 0.8660254037844333785, 1.000000000000005329 ) ) 
 REPRESENTATION_ITEM ( '' )  );
#41140=CARTESIAN_POINT ( 'NONE',  ( -2.121784821874996840, 18.07812500061451644, -26.32496088578401583 ) ) ;
#41143=CARTESIAN_POINT ( 'NONE',  ( 9.600000001229034297, -2.886751345948126435, -5.000000000000000000 ) ) ;
#41144=CARTESIAN_POINT ( 'NONE',  ( 13.98750000000000071, -2.886751345948193048, -4.999999999999883649 ) ) ;
#41145=CARTESIAN_POINT ( 'NONE',  ( 19.47187500061451360, 3.027376345333611329, 5.243569643749999010 ) ) ;
#41146=CARTESIAN_POINT ( 'NONE',  ( 10.65000000122903323, 5.773502691896255534, 3.535250795749688401E-16 ) ) ;
#41147=CARTESIAN_POINT ( 'NONE',  ( 14.16562500061451679, -6.054752690667223547, -1.112240025338166033E-15 ) ) ;
#41150=CARTESIAN_POINT ( 'NONE',  ( 25.65937500061451715, 4.541064518000418104, -2.621784821874998173 ) ) ;
#41152=CARTESIAN_POINT ( 'NONE',  ( 11.20312500061451644, 4.541064518000418104, -2.621784821874998173 ) ) ;
#41153=CARTESIAN_POINT ( 'NONE',  ( 15.19687500061451857, -3.027376345333610441, -5.243569643749999898 ) ) ;
#41155=CARTESIAN_POINT ( 'NONE',  ( 27.77812500061451573, 6.421520780324663323E-16, -5.243569643749999010 ) ) ;
#41156=CARTESIAN_POINT ( 'NONE',  ( 20.99062500061451431, -3.027376345333610441, -5.243569643749999898 ) ) ;
#41157=CARTESIAN_POINT ( 'NONE',  ( 29.42812500061451431, -4.541064518000419881, 2.621784821874995952 ) ) ;
#41158=CARTESIAN_POINT ( 'NONE',  ( 3.999999999999999112, 14.82500000000000107, 30.00000000000000000 ) ) ;
#41159=CARTESIAN_POINT ( 'NONE',  ( 11.02500000000000036, 4.330127018922191873, 2.499999999999999556 ) ) ;
#41160=CARTESIAN_POINT ( 'NONE',  ( 19.01250000122903216, -4.330127018922190985, -2.500000000000001332 ) ) ;
#41161=CARTESIAN_POINT ( 'NONE',  ( 23.32500000122903216, 2.886751345948143754, 4.999999999999969802 ) ) ;
#41163=VERTEX_POINT ( 'NONE', #31999 ) ;
#41164=CARTESIAN_POINT ( 'NONE',  ( 16.53750000000000142, -2.886751345948129988, 4.999999999999997335 ) ) ;
#41165=CARTESIAN_POINT ( 'NONE',  ( 20.69999999999999929, -4.330127018922190985, -2.500000000000001332 ) ) ;
#41166=CARTESIAN_POINT ( 'NONE',  ( 18.00937500061451502, 4.541064518000418104, -2.621784821874998173 ) ) ;
#41167=CARTESIAN_POINT ( 'NONE',  ( 14.95312500061451644, 0.000000000000000000, 5.243569643749999010 ) ) ;
#41169=ORIENTED_EDGE ( 'NONE', *, *, #65842, .T. ) ;
#41171=CARTESIAN_POINT ( 'NONE',  ( 4.903125000614516615, 4.541064518000418104, -2.621784821874998173 ) ) ;
#41172=CARTESIAN_POINT ( 'NONE',  ( 12.07499999999999929, -4.330127018922194537, 2.499999999999995559 ) ) ;
#41174=CARTESIAN_POINT ( 'NONE',  ( 4.243569643749999010, 16.91562500061451502, 27.54997392385601174 ) ) ;
#41175=CARTESIAN_POINT ( 'NONE',  ( 2.934375000614518392, -4.541064518000419881, 2.621784821874995952 ) ) ;
#41178=CARTESIAN_POINT ( 'NONE',  ( 25.09687500061451715, -3.027376345333610441, -5.243569643749999898 ) ) ;
#41179=VERTEX_POINT ( 'NONE', #3568 ) ;
#41180=CARTESIAN_POINT ( 'NONE',  ( 21.70312500061451644, 0.000000000000000000, 5.243569643749999010 ) ) ;
#41181=CARTESIAN_POINT ( 'NONE',  ( 22.28437500061451715, -4.541064518000419881, 2.621784821874995952 ) ) ;
#41182=CARTESIAN_POINT ( 'NONE',  ( -2.121784821874999949, 15.67812500061459247, -33.67503911421598417 ) ) ;
#41183=CARTESIAN_POINT ( 'NONE',  ( 7.040625000614517681, -3.027376345333610441, -5.243569643749999898 ) ) ;
#41185=CARTESIAN_POINT ( 'NONE',  ( 25.07812500061451644, 6.421520780324663323E-16, -5.243569643749999010 ) ) ;
#41188=CARTESIAN_POINT ( 'NONE',  ( 17.67187500061451644, 3.027376345333611329, 5.243569643749999010 ) ) ;
#41189=CARTESIAN_POINT ( 'NONE',  ( 19.73437500061451644, 6.421520780324663323E-16, -5.243569643749999010 ) ) ;
#41190=CARTESIAN_POINT ( 'NONE',  ( 27.12187500061451573, 3.027376345333611329, 5.243569643749999010 ) ) ;
#41191=CARTESIAN_POINT ( 'NONE',  ( -3.000416591977282496E-16, 17.49687500061451573, 25.09994784771203058 ) ) ;
#41192=CARTESIAN_POINT ( 'NONE',  ( 8.315625000614515372, -6.054752690667223547, -1.112240025338166033E-15 ) ) ;
#41193=CARTESIAN_POINT ( 'NONE',  ( 7.320879633048903241E-15, 18.08749999999999858, -34.00000000000000000 ) ) ;
#41194=CARTESIAN_POINT ( 'NONE',  ( 5.596875000614516260, -3.027376345333614438, 5.243569643749998122 ) ) ;
#41196=CARTESIAN_POINT ( 'NONE',  ( 5.465625000614517504, 3.027376345333611329, 5.243569643749999010 ) ) ;
#41197=CARTESIAN_POINT ( 'NONE',  ( 10.50937500061451679, 0.000000000000000000, 5.243569643749999010 ) ) ;
#41198=CARTESIAN_POINT ( 'NONE',  ( 17.28750000122903430, 6.123233995736764310E-16, -4.999999999999998224 ) ) ;
#41199=CARTESIAN_POINT ( 'NONE',  ( 5.596875000614516260, -3.027376345333614438, 5.243569643749998122 ) ) ;
#41200=CARTESIAN_POINT ( 'NONE',  ( 8.053125000614516082, 4.541064518000418104, -2.621784821874998173 ) ) ;
#41203=CARTESIAN_POINT ( 'NONE',  ( 16.69687500061451502, 6.054752690667223547, 3.707466751127219781E-16 ) ) ;
#41204=CARTESIAN_POINT ( 'NONE',  ( 27.63749999999999929, 5.773502691896255534, 3.535250795749688401E-16 ) ) ;
#41206=CARTESIAN_POINT ( 'NONE',  ( 24.55312500061451786, -4.541064518000417216, -2.621784821875001281 ) ) ;
#41207=CARTESIAN_POINT ( 'NONE',  ( 10.37812500061451715, 4.541064518000418104, 2.621784821874999949 ) ) ;
#41208=CARTESIAN_POINT ( 'NONE',  ( 27.94687500061451502, 6.054752690667223547, 3.707466751127219781E-16 ) ) ;
#41209=CARTESIAN_POINT ( 'NONE',  ( 9.590625000614517504, -3.027376345333614438, 5.243569643749998122 ) ) ;
#41210=CARTESIAN_POINT ( 'NONE',  ( -2.121784821874999949, 10.78437500061451715, -33.67503911421598417 ) ) ;
#41211=CARTESIAN_POINT ( 'NONE',  ( 10.42500000122903536, -5.773502691896255534, -1.060575238724906372E-15 ) ) ;
#41212=CARTESIAN_POINT ( 'NONE',  ( 24.62812500061451715, 6.421520780324663323E-16, -5.243569643749999010 ) ) ;
#41213=CARTESIAN_POINT ( 'NONE',  ( -2.121784821874999949, 13.42812500061451786, -33.67503911421598417 ) ) ;
#41214=CARTESIAN_POINT ( 'NONE',  ( 12.07500000122903216, 2.886751345948126879, 4.999999999999999112 ) ) ;
#41215=CARTESIAN_POINT ( 'NONE',  ( 23.16562500061451502, -6.054752690667223547, -1.112240025338166033E-15 ) ) ;
#41216=CARTESIAN_POINT ( 'NONE',  ( 11.73750000000000249, -2.886751345948125991, -5.000000000000000000 ) ) ;
#41217=CARTESIAN_POINT ( 'NONE',  ( 19.75312500061451360, 4.541064518000418104, -2.621784821874998173 ) ) ;
#41219=CARTESIAN_POINT ( 'NONE',  ( 21.48750000000000071, -2.886751345948129988, 4.999999999999997335 ) ) ;
#41220=CARTESIAN_POINT ( 'NONE',  ( 14.13750000122903394, 6.123233995736764310E-16, -4.999999999999998224 ) ) ;
#41221=CARTESIAN_POINT ( 'NONE',  ( 9.815625000614518925, 3.027376345333613106, -5.243569643749998122 ) ) ;
#41222=CARTESIAN_POINT ( 'NONE',  ( 16.79062500061451857, -3.027376345333614438, 5.243569643749998122 ) ) ;
#41223=CARTESIAN_POINT ( 'NONE',  ( 24.63750000122903216, 4.330127018922191873, 2.499999999999999556 ) ) ;
#41224=CARTESIAN_POINT ( 'NONE',  ( 20.29687500061451644, 6.054752690667223547, 3.707466751127219781E-16 ) ) ;
#41225=CARTESIAN_POINT ( 'NONE',  ( 7.650000001229034119, -2.886751345948129988, 4.999999999999997335 ) ) ;
#41226=CARTESIAN_POINT ( 'NONE',  ( 9.384375000614518569, 6.421520780324663323E-16, -5.243569643749999010 ) ) ;
#41227=CARTESIAN_POINT ( 'NONE',  ( 24.60937500061451644, -4.541064518000417216, -2.621784821875001281 ) ) ;
#41228=CARTESIAN_POINT ( 'NONE',  ( 2.896875000614518747, -3.027376345333614438, 5.243569643749998122 ) ) ;
#41229=EDGE_CURVE ( 'NONE', #72689, #68632, #20904, .T. ) ;
#41230=CARTESIAN_POINT ( 'NONE',  ( 21.92812500061451431, 6.421520780324663323E-16, -5.243569643749999010 ) ) ;
#41231=CARTESIAN_POINT ( 'NONE',  ( 26.89687500061451431, -3.027376345333610441, -5.243569643749999898 ) ) ;
#41233=CYLINDRICAL_SURFACE ( 'NONE', #72779, 4.999999999999998224 ) ;
#41234=CARTESIAN_POINT ( 'NONE',  ( 8.296875000614516438, -3.027376345333614438, 5.243569643749998122 ) ) ;
#41235=CARTESIAN_POINT ( 'NONE',  ( 16.26562500061451289, 3.027376345333611329, 5.243569643749999010 ) ) ;
#41237=CARTESIAN_POINT ( 'NONE',  ( -3.999999999999997335, 12.83750000000000213, -27.69059892324149530 ) ) ;
#41238=CARTESIAN_POINT ( 'NONE',  ( 26.80312500061451431, -4.541064518000417216, -2.621784821875001281 ) ) ;
#41239=CARTESIAN_POINT ( 'NONE',  ( 4.621875000614516615, 3.027376345333611329, 5.243569643749999010 ) ) ;
#41241=CARTESIAN_POINT ( 'NONE',  ( -4.243569643749999898, 19.80312500061451786, -30.00000000000000000 ) ) ;
#41242=CARTESIAN_POINT ( 'NONE',  ( 17.73750000000000071, 5.773502691896255534, 3.535250795749688894E-16 ) ) ;
#41243=CARTESIAN_POINT ( 'NONE',  ( 21.32812500061451644, -4.541064518000419881, 2.621784821874995952 ) ) ;
#41244=ORIENTED_EDGE ( 'NONE', *, *, #20037, .T. ) ;
#41245=CARTESIAN_POINT ( 'NONE',  ( 24.75000000000000000, -4.330127018922190985, -2.500000000000001332 ) ) ;
#41246=CARTESIAN_POINT ( 'NONE',  ( 25.65937500061451715, 4.541064518000418104, -2.621784821874998173 ) ) ;
#41248=ORIENTED_EDGE ( 'NONE', *, *, #24697, .T. ) ;
#41249=CARTESIAN_POINT ( 'NONE',  ( 12.70312500061451821, 0.000000000000000000, 5.243569643749999010 ) ) ;
#41250=CARTESIAN_POINT ( 'NONE',  ( 6.403125000614517504, 0.000000000000000000, 5.243569643749999010 ) ) ;
#41252=CARTESIAN_POINT ( 'NONE',  ( 29.09062500061451573, -3.027376345333610441, -5.243569643749999898 ) ) ;
#41253=CARTESIAN_POINT ( 'NONE',  ( 15.93750000122903110, 6.123233995736764310E-16, -4.999999999999998224 ) ) ;
#41254=CARTESIAN_POINT ( 'NONE',  ( 21.71249999999999858, 2.886751345948129099, -4.999999999999998224 ) ) ;
#41255=CARTESIAN_POINT ( 'NONE',  ( 28.57499999999999929, 4.330127018922191873, 2.499999999999999556 ) ) ;
#41256=CARTESIAN_POINT ( 'NONE',  ( 5.109375000614518214, 0.000000000000000000, 5.243569643749999010 ) ) ;
#41257=CARTESIAN_POINT ( 'NONE',  ( 9.984375000614518214, 4.541064518000418104, 2.621784821874999949 ) ) ;
#41258=CARTESIAN_POINT ( 'NONE',  ( 19.24687500061452283, -3.027376345333610441, -5.243569643749999898 ) ) ;
#41259=CARTESIAN_POINT ( 'NONE',  ( -3.999999999999999112, 15.16250000122903252, -30.00000000000000000 ) ) ;
#41260=ORIENTED_EDGE ( 'NONE', *, *, #43169, .F. ) ;
#41261=CARTESIAN_POINT ( 'NONE',  ( 29.69062500061451715, 6.054752690667223547, 3.707466751127219781E-16 ) ) ;
#41262=CARTESIAN_POINT ( 'NONE',  ( 29.52187500061451431, -6.054752690667223547, -1.112240025338166033E-15 ) ) ;
#41263=CARTESIAN_POINT ( 'NONE',  ( 5.559375000614517504, 0.000000000000000000, 5.243569643749999010 ) ) ;
#41264=CARTESIAN_POINT ( 'NONE',  ( 16.80000000000000071, 4.330127018922192761, -2.499999999999997780 ) ) ;
#41265=CARTESIAN_POINT ( 'NONE',  ( 14.09062500061451750, -3.027376345333614438, 5.243569643749998122 ) ) ;
#41266=CARTESIAN_POINT ( 'NONE',  ( 2.000000000000001332, 13.96250000122903323, 33.46410161513774995 ) ) ;
#41268=CARTESIAN_POINT ( 'NONE',  ( 20.32500000122903572, -5.773502691896255534, -1.060575238724906372E-15 ) ) ;
#41269=LINE ( 'NONE', #63781, #60710 ) ;
#41271=CARTESIAN_POINT ( 'NONE',  ( 6.628125000614517148, 6.421520780324663323E-16, -5.243569643749999010 ) ) ;
#41272=CARTESIAN_POINT ( 'NONE',  ( 25.09687500061451715, -3.027376345333610441, -5.243569643749999898 ) ) ;
#41274=CARTESIAN_POINT ( 'NONE',  ( 4.243569643749999010, 19.67187500061451644, 27.54997392385601174 ) ) ;
#41275=CARTESIAN_POINT ( 'NONE',  ( 25.95937500061451431, -4.541064518000417216, -2.621784821875001281 ) ) ;
#41276=CARTESIAN_POINT ( 'NONE',  ( 8.625000000000000000, 6.123233995736764310E-16, -4.999999999999998224 ) ) ;
#41277=CARTESIAN_POINT ( 'NONE',  ( 3.999999999999998668, 12.72500000122903430, 27.69059892324149175 ) ) ;
#41278=CARTESIAN_POINT ( 'NONE',  ( 14.20312500061451644, -4.541064518000417216, -2.621784821875001281 ) ) ;
#41279=CARTESIAN_POINT ( 'NONE',  ( 6.562500001229032875, 4.330127018922192761, -2.499999999999997780 ) ) ;
#41280=CARTESIAN_POINT ( 'NONE',  ( 16.80937500061451573, 0.000000000000000000, 5.243569643749999010 ) ) ;
#41281=CARTESIAN_POINT ( 'NONE',  ( 11.03437500061451715, -4.541064518000419881, 2.621784821874995952 ) ) ;
#41284=CARTESIAN_POINT ( 'NONE',  ( 12.85312500061451502, -4.541064518000417216, -2.621784821875001281 ) ) ;
#41285=CARTESIAN_POINT ( 'NONE',  ( 28.98750000122903359, 6.123233995736764310E-16, -4.999999999999998224 ) ) ;
#41286=CARTESIAN_POINT ( 'NONE',  ( 23.40000000122903145, -2.886751345948129988, 4.999999999999997335 ) ) ;
#41287=CARTESIAN_POINT ( 'NONE',  ( 13.84687500061451537, -3.027376345333610441, -5.243569643749999898 ) ) ;
#41288=CARTESIAN_POINT ( 'NONE',  ( 13.52812500061451750, 4.541064518000418104, 2.621784821874999949 ) ) ;
#41290=CARTESIAN_POINT ( 'NONE',  ( 24.12187500061451217, -6.054752690667223547, -1.112240025338166033E-15 ) ) ;
#41291=CARTESIAN_POINT ( 'NONE',  ( 3.999999999999998668, 15.87500000122903465, 27.69059892324149530 ) ) ;
#41293=CARTESIAN_POINT ( 'NONE',  ( 1.592000809091587073E-14, 15.05000000122903714, 26.00000000000000000 ) ) ;
#41294=CARTESIAN_POINT ( 'NONE',  ( 4.243569643749999898, 17.79687500061451999, -27.54997392385601529 ) ) ;
#41295=CARTESIAN_POINT ( 'NONE',  ( 15.38437500061451679, 4.541064518000418104, 2.621784821874999949 ) ) ;
#41296=CARTESIAN_POINT ( 'NONE',  ( 18.11250000122903359, -4.330127018922190985, -2.500000000000001332 ) ) ;
#41297=CARTESIAN_POINT ( 'NONE',  ( 12.49687500061451573, -3.027376345333610441, -5.243569643749999898 ) ) ;
#41298=CARTESIAN_POINT ( 'NONE',  ( 2.121784821874999061, 19.20312500061451644, -33.67503911421598417 ) ) ;
#41299=CARTESIAN_POINT ( 'NONE',  ( 19.50000000122903288, -2.886751345948125991, -5.000000000000000000 ) ) ;
#41300=CARTESIAN_POINT ( 'NONE',  ( 12.74062500061451786, -3.027376345333614438, 5.243569643749998122 ) ) ;
#41301=ORIENTED_EDGE ( 'NONE', *, *, #16676, .T. ) ;
#41302=ORIENTED_EDGE ( 'NONE', *, *, #9933, .T. ) ;
#41303=CARTESIAN_POINT ( 'NONE',  ( 18.82500000000000284, -4.330127018922194537, 2.499999999999995559 ) ) ;
#41305=CARTESIAN_POINT ( 'NONE',  ( 13.50937500061451679, 4.541064518000418104, -2.621784821874998173 ) ) ;
#41306=CARTESIAN_POINT ( 'NONE',  ( 3.980152422927321521, 3.026382568917634242, 4.011453763075421008 ) ) ;
#41307=CARTESIAN_POINT ( 'NONE',  ( 13.05000000122903536, -2.886751345948129988, 4.999999999999997335 ) ) ;
#41308=CARTESIAN_POINT ( 'NONE',  ( 21.86250000122903003, 4.330127018922192761, -2.499999999999997780 ) ) ;
#41309=CARTESIAN_POINT ( 'NONE',  ( 17.42812500061451786, 6.421520780324663323E-16, -5.243569643749999010 ) ) ;
#41310=CARTESIAN_POINT ( 'NONE',  ( 24.14062500061451289, -3.027376345333610441, -5.243569643749999898 ) ) ;
#41311=CARTESIAN_POINT ( 'NONE',  ( 29.47500000122903430, 2.886751345948129099, -4.999999999999998224 ) ) ;
#41312=CARTESIAN_POINT ( 'NONE',  ( 28.38749999999999929, -2.886751345948125991, -5.000000000000000000 ) ) ;
#41316=CARTESIAN_POINT ( 'NONE',  ( 3.939080010846523372, -3.079553322829319928, -4.243980907203444453 ) ) ;
#41317=CARTESIAN_POINT ( 'NONE',  ( 4.243569643749999898, 16.44687500061451857, -27.54997392385601529 ) ) ;
#41318=LINE ( 'NONE', #2513, #63117 ) ;
#41319=CARTESIAN_POINT ( 'NONE',  ( 5.962500000000002132, 2.886751345948129099, -4.999999999999998224 ) ) ;
#41320=( BOUNDED_CURVE ( )  B_SPLINE_CURVE ( 2, ( #30037, #36674, #47038, #65114, #52577, #8239, #1984, #41493, #64015 ),
 .UNSPECIFIED., .F., .F. ) 
 B_SPLINE_CURVE_WITH_KNOTS ( ( 3, 2, 2, 2, 3 ),
 ( 0.8369565217391304879, 0.8405797101449274944, 0.8478260869565217295, 0.8550724637681159646, 0.8586956521739130821 ),
 .UNSPECIFIED. ) 
 CURVE ( )  GEOMETRIC_REPRESENTATION_ITEM ( )  RATIONAL_B_SPLINE_CURVE ( ( 0.9330127018922192983, 0.9330127018922202975, 1.000000000000000000, 0.8660254037844387076, 1.000000000000000000, 0.8660254037844387076, 1.000000000000000000, 0.9330127018922194093, 0.9330127018922194093 ) ) 
 REPRESENTATION_ITEM ( '' )  );
#41322=CARTESIAN_POINT ( 'NONE',  ( 10.50937500061451679, 0.000000000000000000, 5.243569643749999010 ) ) ;
#41323=CARTESIAN_POINT ( 'NONE',  ( 27.36562500061451786, 3.027376345333613106, -5.243569643749998122 ) ) ;
#41325=CARTESIAN_POINT ( 'NONE',  ( 3.697207292818405211, -3.366579844074466088, -3.697207292818405211 ) ) ;
#41326=CARTESIAN_POINT ( 'NONE',  ( -3.137519842735245283E-14, 14.71250000000000213, 34.00000000000000000 ) ) ;
#41328=CARTESIAN_POINT ( 'NONE',  ( 6.984375000614516438, -4.541064518000419881, 2.621784821874995952 ) ) ;
#41329=CARTESIAN_POINT ( 'NONE',  ( 10.84687500061451892, 6.054752690667223547, 3.707466751127219781E-16 ) ) ;
#41330=CARTESIAN_POINT ( 'NONE',  ( 5.887500000000000178, -2.886751345948125991, -5.000000000000000000 ) ) ;
#41331=CARTESIAN_POINT ( 'NONE',  ( 4.243569643749999010, 15.11562500061459424, 27.54997392385601174 ) ) ;
#41332=CARTESIAN_POINT ( 'NONE',  ( 4.000000000000000000, 17.93750000000000355, 32.30940107675849760 ) ) ;
#41333=CARTESIAN_POINT ( 'NONE',  ( 5.512499999999999289, 2.886751345948129099, -4.999999999999998224 ) ) ;
#41335=CARTESIAN_POINT ( 'NONE',  ( 19.94062500061451715, -3.027376345333614438, 5.243569643749998122 ) ) ;
#41336=CARTESIAN_POINT ( 'NONE',  ( 12.96562500061451750, 3.027376345333613106, -5.243569643749998122 ) ) ;
#41338=CARTESIAN_POINT ( 'NONE',  ( 8.371875000614515727, -6.054752690667223547, -1.112240025338166033E-15 ) ) ;
#41339=CARTESIAN_POINT ( 'NONE',  ( 27.11249999999999716, 2.886751345948129099, -4.999999999999998224 ) ) ;
#41340=CARTESIAN_POINT ( 'NONE',  ( 23.10000000122903074, -2.886751345948125991, -5.000000000000000000 ) ) ;
#41341=CARTESIAN_POINT ( 'NONE',  ( -1.999999999999997113, 18.38750000122903572, -26.53589838486224295 ) ) ;
#41342=CARTESIAN_POINT ( 'NONE',  ( 12.19687500061451679, 6.054752690667223547, 3.707466751127219781E-16 ) ) ;
#41343=CARTESIAN_POINT ( 'NONE',  ( 26.52187500061451431, 3.027376345333613106, -5.243569643749998122 ) ) ;
#41345=CARTESIAN_POINT ( 'NONE',  ( 3.999999999999999112, 13.58750000122903323, -30.00000000000000000 ) ) ;
#41346=CARTESIAN_POINT ( 'NONE',  ( 20.59687500061451360, -3.027376345333610441, -5.243569643749999898 ) ) ;
#41347=CARTESIAN_POINT ( 'NONE',  ( 12.98437500061451821, 6.421520780324663323E-16, -5.243569643749999010 ) ) ;
#41349=CARTESIAN_POINT ( 'NONE',  ( 26.96249999999999858, -5.773502691896255534, -1.060575238724906372E-15 ) ) ;
#41351=CARTESIAN_POINT ( 'NONE',  ( -2.121784821874996840, 11.83437500061451786, -26.32496088578401583 ) ) ;
#41353=CARTESIAN_POINT ( 'NONE',  ( 14.12812500061451715, -4.541064518000419881, 2.621784821874995952 ) ) ;
#41354=CARTESIAN_POINT ( 'NONE',  ( 5.437500000000001776, -2.886751345948125991, -5.000000000000000000 ) ) ;
#41357=CARTESIAN_POINT ( 'NONE',  ( 15.48749999999999893, 5.773502691896255534, 3.535250795749688894E-16 ) ) ;
#41358=CARTESIAN_POINT ( 'NONE',  ( -4.243569643749999898, 10.31562500061451715, 27.54997392385601529 ) ) ;
#41359=CARTESIAN_POINT ( 'NONE',  ( 15.15000000122903323, 5.773502691896255534, 3.535250795749688894E-16 ) ) ;
#41360=CARTESIAN_POINT ( 'NONE',  ( 23.85937500061451644, 4.541064518000418104, -2.621784821874998173 ) ) ;
#41362=CARTESIAN_POINT ( 'NONE',  ( 20.12812500061451715, 6.421520780324663323E-16, -5.243569643749999010 ) ) ;
#41363=CARTESIAN_POINT ( 'NONE',  ( 4.190625000614518925, -3.027376345333614438, 5.243569643749998122 ) ) ;
#41364=CARTESIAN_POINT ( 'NONE',  ( 19.39687500061451786, 6.054752690667223547, 3.707466751127219781E-16 ) ) ;
#41365=CARTESIAN_POINT ( 'NONE',  ( 4.162499999999999645, 2.886751345948129099, -4.999999999999998224 ) ) ;
#41366=CARTESIAN_POINT ( 'NONE',  ( 8.053125000614516082, 4.541064518000418104, -2.621784821874998173 ) ) ;
#41367=CARTESIAN_POINT ( 'NONE',  ( 21.85312500061451502, -4.541064518000417216, -2.621784821875001281 ) ) ;
#41368=CARTESIAN_POINT ( 'NONE',  ( 4.243569643749999010, 15.56562500061451715, 27.54997392385601174 ) ) ;
#41369=CARTESIAN_POINT ( 'NONE',  ( 19.68750000122903288, 4.330127018922191873, 2.499999999999999556 ) ) ;
#41371=CARTESIAN_POINT ( 'NONE',  ( 9.140625000614518214, -3.027376345333614438, 5.243569643749998122 ) ) ;
#41372=CARTESIAN_POINT ( 'NONE',  ( 4.096875000614518925, 6.054752690667223547, 3.707466751127219781E-16 ) ) ;
#41373=CARTESIAN_POINT ( 'NONE',  ( 28.45312500061451289, 0.000000000000000000, 5.243569643749999010 ) ) ;
#41374=CARTESIAN_POINT ( 'NONE',  ( 24.30937500061451573, 4.541064518000418104, -2.621784821874998173 ) ) ;
#41375=CARTESIAN_POINT ( 'NONE',  ( 15.66562500061451857, 3.027376345333613106, -5.243569643749998122 ) ) ;
#41376=CARTESIAN_POINT ( 'NONE',  ( 24.37500000122903288, -5.773502691896255534, -1.060575238724906372E-15 ) ) ;
#41377=CARTESIAN_POINT ( 'NONE',  ( 24.89062500061451644, -3.027376345333614438, 5.243569643749998122 ) ) ;
#41378=CARTESIAN_POINT ( 'NONE',  ( 20.59687500061451360, -3.027376345333610441, -5.243569643749999898 ) ) ;
#41379=CARTESIAN_POINT ( 'NONE',  ( 15.55312500061451608, -4.541064518000417216, -2.621784821875001281 ) ) ;
#41380=CARTESIAN_POINT ( 'NONE',  ( 4.243569643749999010, 16.52187500061451786, 27.54997392385601174 ) ) ;
#41381=CARTESIAN_POINT ( 'NONE',  ( 23.35312500061451857, 4.541064518000418104, -2.621784821874998173 ) ) ;
#41382=CYLINDRICAL_SURFACE ( 'NONE', #70349, 4.999999999999998224 ) ;
#41384=CARTESIAN_POINT ( 'NONE',  ( 26.51249999999999929, -5.773502691896255534, -1.060575238724906372E-15 ) ) ;
#41385=CARTESIAN_POINT ( 'NONE',  ( -2.828200636599751609E-16, 10.43750000000000178, -34.61880215351700230 ) ) ;
#41387=CARTESIAN_POINT ( 'NONE',  ( 28.64062500061451289, -3.027376345333610441, -5.243569643749999898 ) ) ;
#41388=CARTESIAN_POINT ( 'NONE',  ( 6.778125000614518392, 4.541064518000418104, 2.621784821874999949 ) ) ;
#41389=CARTESIAN_POINT ( 'NONE',  ( 23.13750000122903216, 6.123233995736764310E-16, -4.999999999999998224 ) ) ;
#41390=CARTESIAN_POINT ( 'NONE',  ( 27.17812500061451786, -4.541064518000419881, 2.621784821874995952 ) ) ;
#41391=CARTESIAN_POINT ( 'NONE',  ( 24.33749999999999858, -2.886751345948125991, -5.000000000000000000 ) ) ;
#41392=CARTESIAN_POINT ( 'NONE',  ( -3.999999999999999112, 16.06250000122903288, -30.00000000000000000 ) ) ;
#41393=FACE_OUTER_BOUND ( 'NONE', #71275, .T. ) ;
#41394=CARTESIAN_POINT ( 'NONE',  ( 10.26562500061451644, 3.027376345333613106, -5.243569643749998122 ) ) ;
#41395=VERTEX_POINT ( 'NONE', #65980 ) ;
#41397=CARTESIAN_POINT ( 'NONE',  ( 25.00312500061451715, -4.541064518000417216, -2.621784821875001281 ) ) ;
#41398=CARTESIAN_POINT ( 'NONE',  ( 7.153125000614518392, 4.541064518000418104, -2.621784821874998173 ) ) ;
#41399=CARTESIAN_POINT ( 'NONE',  ( 4.340625000614515727, -3.027376345333610441, -5.243569643749999898 ) ) ;
#41401=CARTESIAN_POINT ( 'NONE',  ( 17.88750000122903216, 4.330127018922191873, 2.499999999999999556 ) ) ;
#41402=CARTESIAN_POINT ( 'NONE',  ( 13.27500000000000213, 4.330127018922191873, 2.499999999999999556 ) ) ;
#41403=CARTESIAN_POINT ( 'NONE',  ( 12.60937500061451821, 4.541064518000418104, -2.621784821874998173 ) ) ;
#41404=CARTESIAN_POINT ( 'NONE',  ( 8.887500001229033941, 4.330127018922191873, 2.499999999999999556 ) ) ;
#41405=CARTESIAN_POINT ( 'NONE',  ( 16.17187500061451644, 3.027376345333613106, -5.243569643749998122 ) ) ;
#41407=CARTESIAN_POINT ( 'NONE',  ( 8.671875000614518214, 3.027376345333611329, 5.243569643749999010 ) ) ;
#41408=CARTESIAN_POINT ( 'NONE',  ( 2.121784821875001281, 10.50312500061451715, -26.32496088578401938 ) ) ;
#41409=CARTESIAN_POINT ( 'NONE',  ( -1.999999999999997113, 11.97500000000000142, -26.53589838486224295 ) ) ;
#41411=CYLINDRICAL_SURFACE ( 'NONE', #14711, 4.999999999999998224 ) ;
#41412=CARTESIAN_POINT ( 'NONE',  ( 24.47812500061451502, -4.541064518000419881, 2.621784821874995952 ) ) ;
#41414=CARTESIAN_POINT ( 'NONE',  ( 26.22187500061451715, 3.027376345333611329, 5.243569643749999010 ) ) ;
#41415=CARTESIAN_POINT ( 'NONE',  ( 28.62187500061451573, -6.054752690667223547, -1.112240025338166033E-15 ) ) ;
#41416=CARTESIAN_POINT ( 'NONE',  ( 22.76249999999999574, 2.886751345948126879, 4.999999999999999112 ) ) ;
#41417=CARTESIAN_POINT ( 'NONE',  ( 7.003125000614518036, -4.541064518000417216, -2.621784821875001281 ) ) ;
#41419=CARTESIAN_POINT ( 'NONE',  ( 16.20937500061451786, 4.541064518000418104, -2.621784821874998173 ) ) ;
#41421=CARTESIAN_POINT ( 'NONE',  ( 3.740625000614516527, -3.027376345333614438, 5.243569643749998122 ) ) ;
#41422=CARTESIAN_POINT ( 'NONE',  ( 8.896875000614517859, -3.027376345333610441, -5.243569643749999898 ) ) ;
#41424=CARTESIAN_POINT ( 'NONE',  ( 18.45937500061451431, 4.541064518000418104, -2.621784821874998173 ) ) ;
#41426=CARTESIAN_POINT ( 'NONE',  ( 26.47499999999999787, -4.330127018922194537, 2.499999999999995559 ) ) ;
#41427=CARTESIAN_POINT ( 'NONE',  ( 3.750000000000000000, 4.330127018922192761, -2.499999999999997780 ) ) ;
#41430=ORIENTED_EDGE ( 'NONE', *, *, #58553, .F. ) ;
#41431=CARTESIAN_POINT ( 'NONE',  ( 11.43750000000000000, 5.773502691896255534, 3.535250795749688894E-16 ) ) ;
#41433=CARTESIAN_POINT ( 'NONE',  ( 21.96562500061451573, 3.027376345333613106, -5.243569643749998122 ) ) ;
#41434=CARTESIAN_POINT ( 'NONE',  ( 11.55000000000000071, 0.000000000000000000, 4.999999999999998224 ) ) ;
#41435=CARTESIAN_POINT ( 'NONE',  ( 7.725000001229034297, -5.773502691896255534, -1.060575238724906372E-15 ) ) ;
#41436=CARTESIAN_POINT ( 'NONE',  ( 7.715625000614515727, 3.027376345333611329, 5.243569643749999010 ) ) ;
#41437=CARTESIAN_POINT ( 'NONE',  ( 22.16250000000000142, 2.886751345948129099, -4.999999999999998224 ) ) ;
#41438=CARTESIAN_POINT ( 'NONE',  ( 21.10312500061451502, 4.541064518000418104, -2.621784821874998173 ) ) ;
#41439=CARTESIAN_POINT ( 'NONE',  ( 4.711411573247316298, 1.674097066322985938, -4.711411573247316298 ) ) ;
#41440=CARTESIAN_POINT ( 'NONE',  ( 25.42500000122903359, 2.886751345948129099, -4.999999999999998224 ) ) ;
#41442=CARTESIAN_POINT ( 'NONE',  ( 5.625000000000001776, 4.330127018922191873, 2.499999999999999556 ) ) ;
#41444=CARTESIAN_POINT ( 'NONE',  ( 19.67812500061451786, 6.421520780324663323E-16, -5.243569643749999010 ) ) ;
#41445=CARTESIAN_POINT ( 'NONE',  ( 27.40312500061451573, 4.541064518000418104, -2.621784821874998173 ) ) ;
#41446=CARTESIAN_POINT ( 'NONE',  ( 26.93437500061451573, 6.421520780324663323E-16, -5.243569643749999010 ) ) ;
#41447=CARTESIAN_POINT ( 'NONE',  ( 13.71562500061451750, -6.054752690667223547, -1.112240025338166033E-15 ) ) ;
#41449=CARTESIAN_POINT ( 'NONE',  ( 25.98750000122903003, 4.330127018922191873, 2.499999999999999556 ) ) ;
#41451=CARTESIAN_POINT ( 'NONE',  ( 17.72812500061451502, -4.541064518000419881, 2.621784821874995952 ) ) ;
#41452=DIRECTION ( 'NONE',  ( -1.000000000000000000, -0.000000000000000000, -0.000000000000000000 ) ) ;
#41453=CARTESIAN_POINT ( 'NONE',  ( 28.92187500061451644, 3.027376345333611329, 5.243569643749999010 ) ) ;
#41454=CARTESIAN_POINT ( 'NONE',  ( 10.20937500061451786, -4.541064518000417216, -2.621784821875001281 ) ) ;
#41455=CARTESIAN_POINT ( 'NONE',  ( 8.484375000614518214, 6.421520780324663323E-16, -5.243569643749999010 ) ) ;
#41456=CARTESIAN_POINT ( 'NONE',  ( 18.30937500061451928, -4.541064518000417216, -2.621784821875001281 ) ) ;
#41457=ORIENTED_EDGE ( 'NONE', *, *, #14874, .T. ) ;
#41458=CARTESIAN_POINT ( 'NONE',  ( 24.26250000122903216, 0.000000000000000000, 4.999999999999998224 ) ) ;
#41459=CARTESIAN_POINT ( 'NONE',  ( 21.81562500061451004, -6.054752690667223547, -1.112240025338166033E-15 ) ) ;
#41460=CARTESIAN_POINT ( 'NONE',  ( 19.35937500061451644, 4.541064518000418104, -2.621784821874998173 ) ) ;
#41461=CARTESIAN_POINT ( 'NONE',  ( 22.45312500061451644, 4.541064518000418104, -2.621784821874998173 ) ) ;
#41462=CARTESIAN_POINT ( 'NONE',  ( 3.999999999999998668, 13.96250000000000213, 27.69059892324149175 ) ) ;
#41463=CARTESIAN_POINT ( 'NONE',  ( 3.571875000614517237, 3.027376345333613106, -5.243569643749998122 ) ) ;
#41464=CARTESIAN_POINT ( 'NONE',  ( 9.975000001229034297, -5.773502691896255534, -1.060575238724906372E-15 ) ) ;
#41465=ORIENTED_EDGE ( 'NONE', *, *, #61270, .F. ) ;
#41466=CARTESIAN_POINT ( 'NONE',  ( 4.312500001229034652, 4.330127018922192761, -2.499999999999997780 ) ) ;
#41468=CARTESIAN_POINT ( 'NONE',  ( 24.82500000122902861, -5.773502691896255534, -1.060575238724906372E-15 ) ) ;
#41470=CARTESIAN_POINT ( 'NONE',  ( 9.984375000614518214, 4.541064518000418104, 2.621784821874999949 ) ) ;
#41472=CARTESIAN_POINT ( 'NONE',  ( 15.74062500061451608, 6.054752690667223547, 3.707466751127219781E-16 ) ) ;
#41473=CARTESIAN_POINT ( 'NONE',  ( 10.32187500061451679, 3.027376345333613106, -5.243569643749998122 ) ) ;
#41474=CARTESIAN_POINT ( 'NONE',  ( 29.32500000122903216, -5.773502691896255534, -1.060575238724906372E-15 ) ) ;
#41475=CARTESIAN_POINT ( 'NONE',  ( 20.44687500061451857, -3.027376345333614438, 5.243569643749998122 ) ) ;
#41476=CARTESIAN_POINT ( 'NONE',  ( 7.021875000614518747, -6.054752690667223547, -1.112240025338166033E-15 ) ) ;
#41477=CARTESIAN_POINT ( 'NONE',  ( 1.999999999999998668, 16.36250000122903359, 26.53589838486224650 ) ) ;
#41479=CARTESIAN_POINT ( 'NONE',  ( 7.828125000614517326, -4.541064518000419881, 2.621784821874995952 ) ) ;
#41480=CARTESIAN_POINT ( 'NONE',  ( 17.54062500061451502, 6.054752690667223547, 3.707466751127219781E-16 ) ) ;
#41482=CARTESIAN_POINT ( 'NONE',  ( 15.81562500061451537, 3.027376345333611329, 5.243569643749999010 ) ) ;
#41483=CARTESIAN_POINT ( 'NONE',  ( 11.42812500061451608, -4.541064518000419881, 2.621784821874995952 ) ) ;
#41485=CARTESIAN_POINT ( 'NONE',  ( 11.70000000000000284, -4.330127018922190985, -2.500000000000001332 ) ) ;
#41486=CARTESIAN_POINT ( 'NONE',  ( 6.600000001229032520, 5.773502691896255534, 3.535250795749688894E-16 ) ) ;
#41487=EDGE_CURVE ( 'NONE', #57422, #60454, #53065, .T. ) ;
#41488=CARTESIAN_POINT ( 'NONE',  ( 14.07187500061451679, 3.027376345333611329, 5.243569643749999010 ) ) ;
#41489=CARTESIAN_POINT ( 'NONE',  ( 17.25000000122903288, -2.886751345948125991, -5.000000000000000000 ) ) ;
#41491=CARTESIAN_POINT ( 'NONE',  ( -4.243569643749997233, 18.49062500061451431, -27.54997392385601174 ) ) ;
#41492=CARTESIAN_POINT ( 'NONE',  ( 16.38750000122903216, 6.123233995736764310E-16, -4.999999999999998224 ) ) ;
#41493=CARTESIAN_POINT ( 'NONE',  ( 1.071796769724491893, 10.79509619066136850, -26.00000000000000355 ) ) ;
#41494=CARTESIAN_POINT ( 'NONE',  ( 3.965171583692859603, 3.045884815923804556, 3.965171583692790325 ) ) ;
#41495=CARTESIAN_POINT ( 'NONE',  ( 17.25937500061451502, 0.000000000000000000, 5.243569643749999010 ) ) ;
#41497=CARTESIAN_POINT ( 'NONE',  ( 29.81250000000000000, 2.886751345948129099, -4.999999999999998224 ) ) ;
#41498=CARTESIAN_POINT ( 'NONE',  ( 13.34062500061451750, -3.027376345333610441, -5.243569643749999898 ) ) ;
#41501=CARTESIAN_POINT ( 'NONE',  ( 23.44687500061451502, 6.054752690667223547, 3.707466751127219781E-16 ) ) ;
#41503=CARTESIAN_POINT ( 'NONE',  ( 9.328125000614518214, 6.421520780324663323E-16, -5.243569643749999010 ) ) ;
#41504=CARTESIAN_POINT ( 'NONE',  ( 15.00937500061451679, 0.000000000000000000, 5.243569643749999010 ) ) ;
#41505=VERTEX_POINT ( 'NONE', #59319 ) ;
#41506=CARTESIAN_POINT ( 'NONE',  ( 26.22187500061451715, 3.027376345333611329, 5.243569643749999010 ) ) ;
#41507=CARTESIAN_POINT ( 'NONE',  ( 27.96562500061451928, 3.027376345333611329, 5.243569643749999010 ) ) ;
#41508=CARTESIAN_POINT ( 'NONE',  ( 18.14062500061451644, -3.027376345333614438, 5.243569643749998122 ) ) ;
#41510=CARTESIAN_POINT ( 'NONE',  ( -3.137519842735245283E-14, 12.57500000122903572, -26.00000000000000711 ) ) ;
#41511=( BOUNDED_CURVE ( )  B_SPLINE_CURVE ( 3, ( #10341, #4449, #15141, #50241 ),
 .UNSPECIFIED., .F., .F. ) 
 B_SPLINE_CURVE_WITH_KNOTS ( ( 4, 4 ),
 ( 2.315884994543730091, 2.347585424998526182 ),
 .UNSPECIFIED. ) 
 CURVE ( )  GEOMETRIC_REPRESENTATION_ITEM ( )  RATIONAL_B_SPLINE_CURVE ( ( 1.000000000000000000, 0.9999162586456273871, 0.9999162586456273871, 1.000000000000000000 ) ) 
 REPRESENTATION_ITEM ( '' )  );
#41512=CARTESIAN_POINT ( 'NONE',  ( 8.775000000000002132, 4.330127018922191873, 2.499999999999999556 ) ) ;
#41513=CARTESIAN_POINT ( 'NONE',  ( 19.23750000122903714, 4.330127018922191873, 2.499999999999999556 ) ) ;
#41514=DIRECTION ( 'NONE',  ( -1.000000000000000000, 0.000000000000000000, 0.000000000000000000 ) ) ;
#41516=ORIENTED_EDGE ( 'NONE', *, *, #48583, .T. ) ;
#41517=CARTESIAN_POINT ( 'NONE',  ( 17.02499999999999858, -4.330127018922194537, 2.499999999999995559 ) ) ;
#41518=CARTESIAN_POINT ( 'NONE',  ( 22.31250000000000000, 2.886751345948126879, 4.999999999999999112 ) ) ;
#41519=CARTESIAN_POINT ( 'NONE',  ( 17.97187500061451715, 3.027376345333613106, -5.243569643749998122 ) ) ;
#41520=CARTESIAN_POINT ( 'NONE',  ( 14.84062500061451750, 6.054752690667223547, 3.707466751127219781E-16 ) ) ;
#41521=ORIENTED_EDGE ( 'NONE', *, *, #27951, .T. ) ;
#41523=CARTESIAN_POINT ( 'NONE',  ( 6.853125000614516793, 0.000000000000000000, 5.243569643749999010 ) ) ;
#41525=CARTESIAN_POINT ( 'NONE',  ( 12.86250000000000071, 2.886751345948126879, 4.999999999999999112 ) ) ;
#41527=CARTESIAN_POINT ( 'NONE',  ( -2.121784821874996840, 14.47812500061451679, 33.67503911421598417 ) ) ;
#41528=CARTESIAN_POINT ( 'NONE',  ( 28.04062500061451502, -3.027376345333614438, 5.243569643749998122 ) ) ;
#41531=CARTESIAN_POINT ( 'NONE',  ( 23.74687500061451573, -3.027376345333610441, -5.243569643749999898 ) ) ;
#41533=CARTESIAN_POINT ( 'NONE',  ( 21.92812500061451431, 6.421520780324663323E-16, -5.243569643749999010 ) ) ;
#41534=CARTESIAN_POINT ( 'NONE',  ( 23.52187500061451786, 3.027376345333611329, 5.243569643749999010 ) ) ;
#41536=CARTESIAN_POINT ( 'NONE',  ( 4.243569643749999898, 16.39062500061459460, -27.54997392385601529 ) ) ;
#41537=CARTESIAN_POINT ( 'NONE',  ( 7.453125000614516438, -4.541064518000417216, -2.621784821875001281 ) ) ;
#41539=CARTESIAN_POINT ( 'NONE',  ( 24.59062500061451573, -3.027376345333610441, -5.243569643749999898 ) ) ;
#41542=CARTESIAN_POINT ( 'NONE',  ( 16.35937500061451644, 0.000000000000000000, 5.243569643749999010 ) ) ;
#41543=CARTESIAN_POINT ( 'NONE',  ( 27.75937500061451502, -4.541064518000417216, -2.621784821875001281 ) ) ;
#41544=CARTESIAN_POINT ( 'NONE',  ( -2.121784821874996840, 14.53437500061451715, 33.67503911421598417 ) ) ;
#41545=CARTESIAN_POINT ( 'NONE',  ( 8.240625000614516082, -3.027376345333614438, 5.243569643749998122 ) ) ;
#41546=CARTESIAN_POINT ( 'NONE',  ( 4.000000000000000000, 10.40000000122903323, -27.69059892324149885 ) ) ;
#41548=CARTESIAN_POINT ( 'NONE',  ( 4.134375000614517681, 4.541064518000418104, 2.621784821874999949 ) ) ;
#41550=CARTESIAN_POINT ( 'NONE',  ( 5.278125000614516615, 6.421520780324663323E-16, -5.243569643749999010 ) ) ;
#41551=CARTESIAN_POINT ( 'NONE',  ( 9.159375000614515372, 0.000000000000000000, 5.243569643749999010 ) ) ;
#41552=CARTESIAN_POINT ( 'NONE',  ( 16.05000000122903359, 5.773502691896255534, 3.535250795749688894E-16 ) ) ;
#41553=CARTESIAN_POINT ( 'NONE',  ( 29.76562500061451644, 3.027376345333611329, 5.243569643749999010 ) ) ;
#41554=CARTESIAN_POINT ( 'NONE',  ( 7.190625000614518036, 6.054752690667223547, 3.707466751127219781E-16 ) ) ;
#41557=CARTESIAN_POINT ( 'NONE',  ( 16.62187500061451573, 3.027376345333613106, -5.243569643749998122 ) ) ;
#41558=ORIENTED_EDGE ( 'NONE', *, *, #12308, .T. ) ;
#41559=CARTESIAN_POINT ( 'NONE',  ( 25.00312500061451715, -4.541064518000417216, -2.621784821875001281 ) ) ;
#41560=CARTESIAN_POINT ( 'NONE',  ( 10.41562500061451679, 3.027376345333611329, 5.243569643749999010 ) ) ;
#41561=CARTESIAN_POINT ( 'NONE',  ( 26.07187500061451502, 3.027376345333612662, -5.243569643749998122 ) ) ;
#41562=CARTESIAN_POINT ( 'NONE',  ( 8.990625000614516082, 6.054752690667223547, 3.707466751127219781E-16 ) ) ;
#41563=CARTESIAN_POINT ( 'NONE',  ( 0.000000000000000000, 20.00000000000000000, 30.00000000000000000 ) ) ;
#41564=CARTESIAN_POINT ( 'NONE',  ( 10.80000000122903536, -2.886751345948129988, 4.999999999999997335 ) ) ;
#41565=CARTESIAN_POINT ( 'NONE',  ( 23.91562500061451502, 3.027376345333611329, 5.243569643749999010 ) ) ;
#41567=CARTESIAN_POINT ( 'NONE',  ( -4.243569643749999898, 11.21562500061451750, -32.45002607614398471 ) ) ;
#41568=CARTESIAN_POINT ( 'NONE',  ( 12.48750000122903359, 4.330127018922191873, 2.499999999999999556 ) ) ;
#41569=CARTESIAN_POINT ( 'NONE',  ( 21.92812500061451431, 6.421520780324663323E-16, -5.243569643749999010 ) ) ;
#41570=CARTESIAN_POINT ( 'NONE',  ( 17.72812500061451502, -4.541064518000419881, 2.621784821874995952 ) ) ;
#41571=CARTESIAN_POINT ( 'NONE',  ( 4.897546610576117843, 1.006994139586731674, -5.145967878999484491 ) ) ;
#41572=CARTESIAN_POINT ( 'NONE',  ( 18.30000000000000071, 0.000000000000000000, 4.999999999999998224 ) ) ;
#41573=CARTESIAN_POINT ( 'NONE',  ( 13.27500000122903323, 2.886751345948129099, -4.999999999999998224 ) ) ;
#41574=CARTESIAN_POINT ( 'NONE',  ( 10.64062500061451644, -3.027376345333610441, -5.243569643749999898 ) ) ;
#41575=EDGE_CURVE ( 'NONE', #34387, #7528, #58957, .T. ) ;
#41576=CARTESIAN_POINT ( 'NONE',  ( 13.97812500061451679, 4.541064518000418104, 2.621784821874999949 ) ) ;
#41577=CARTESIAN_POINT ( 'NONE',  ( 26.73750000122903003, 6.123233995736764310E-16, -4.999999999999998224 ) ) ;
#41578=CARTESIAN_POINT ( 'NONE',  ( 21.19687500061451502, 6.054752690667223547, 3.707466751127219781E-16 ) ) ;
#41579=CARTESIAN_POINT ( 'NONE',  ( 22.05937500061451573, 4.541064518000418104, -2.621784821874998173 ) ) ;
#41581=CARTESIAN_POINT ( 'NONE',  ( 7.987500001229032698, 4.330127018922191873, 2.499999999999999556 ) ) ;
#41582=CARTESIAN_POINT ( 'NONE',  ( 5.521875000614517859, 3.027376345333611329, 5.243569643749999010 ) ) ;
#41583=CARTESIAN_POINT ( 'NONE',  ( 25.73437500061451644, 4.541064518000418104, 2.621784821874999949 ) ) ;
#41584=CARTESIAN_POINT ( 'NONE',  ( 15.26250000122903216, 0.000000000000000000, 4.999999999999998224 ) ) ;
#41585=CARTESIAN_POINT ( 'NONE',  ( 21.02812500061451573, 6.421520780324663323E-16, -5.243569643749999010 ) ) ;
#41586=CARTESIAN_POINT ( 'NONE',  ( 26.55937500061451573, 4.541064518000418104, -2.621784821874998173 ) ) ;
#41590=CARTESIAN_POINT ( 'NONE',  ( 7.659375000614518036, 4.541064518000418104, -2.621784821874998173 ) ) ;
#41591=CARTESIAN_POINT ( 'NONE',  ( 18.06562500061451715, 3.027376345333611329, 5.243569643749999010 ) ) ;
#41592=VERTEX_POINT ( 'NONE', #3199 ) ;
#41593=DIRECTION ( 'NONE',  ( 0.000000000000000000, 0.000000000000000000, 1.000000000000000000 ) ) ;
#41594=CARTESIAN_POINT ( 'NONE',  ( 26.54062500061451146, 6.054752690667223547, 3.707466751127219781E-16 ) ) ;
#41595=CARTESIAN_POINT ( 'NONE',  ( 3.946875000614517681, -3.027376345333610441, -5.243569643749999898 ) ) ;
#41596=CARTESIAN_POINT ( 'NONE',  ( -2.000000000000000000, 15.87500000000000000, -33.46410161513775705 ) ) ;
#41597=LINE ( 'NONE', #29782, #33560 ) ;
#41598=CARTESIAN_POINT ( 'NONE',  ( 17.06250000000000000, -5.773502691896255534, -1.060575238724906372E-15 ) ) ;
#41599=CARTESIAN_POINT ( 'NONE',  ( 20.35312500061451502, 0.000000000000000000, 5.243569643749999010 ) ) ;
#41600=ORIENTED_EDGE ( 'NONE', *, *, #36421, .T. ) ;
#41601=CARTESIAN_POINT ( 'NONE',  ( 24.33749999999999858, -2.886751345948125991, -5.000000000000000000 ) ) ;
#41602=CARTESIAN_POINT ( 'NONE',  ( 25.47187500061451715, -6.054752690667223547, -1.112240025338166033E-15 ) ) ;
#41604=VECTOR ( 'NONE', #25933, 1000.000000000000000 ) ;
#41605=CARTESIAN_POINT ( 'NONE',  ( 12.55312500061451786, 4.541064518000418104, -2.621784821874998173 ) ) ;
#41606=CARTESIAN_POINT ( 'NONE',  ( 5.390625000614518214, 6.054752690667223547, 3.707466751127219781E-16 ) ) ;
#41608=CARTESIAN_POINT ( 'NONE',  ( 29.27812500061451573, 4.541064518000418104, 2.621784821874999949 ) ) ;
#41609=CARTESIAN_POINT ( 'NONE',  ( 15.86250000122903181, -4.330127018922190985, -2.500000000000001332 ) ) ;
#41610=CARTESIAN_POINT ( 'NONE',  ( 19.50000000000000000, 4.330127018922192761, -2.499999999999997780 ) ) ;
#41611=CARTESIAN_POINT ( 'NONE',  ( 25.64999999999999858, -4.330127018922190985, -2.500000000000001332 ) ) ;
#41612=CARTESIAN_POINT ( 'NONE',  ( 1.071796769724491893, 10.68259618943233313, -26.00000000000000355 ) ) ;
#41613=CARTESIAN_POINT ( 'NONE',  ( 9.909375000614517148, 4.541064518000418104, -2.621784821874998173 ) ) ;
#41614=CARTESIAN_POINT ( 'NONE',  ( 18.98437500061451644, 4.541064518000418104, 2.621784821874999949 ) ) ;
#41615=CARTESIAN_POINT ( 'NONE',  ( 25.94999999999999929, 0.000000000000000000, 4.999999999999998224 ) ) ;
#41616=ORIENTED_EDGE ( 'NONE', *, *, #18934, .F. ) ;
#41617=CARTESIAN_POINT ( 'NONE',  ( 28.64062500061451289, -3.027376345333610441, -5.243569643749999898 ) ) ;
#41618=CARTESIAN_POINT ( 'NONE',  ( 29.07187500061451502, -6.054752690667223547, -1.112240025338166033E-15 ) ) ;
#41619=CARTESIAN_POINT ( 'NONE',  ( 5.784375000614517148, 6.421520780324663323E-16, -5.243569643749999010 ) ) ;
#41620=CARTESIAN_POINT ( 'NONE',  ( 16.61250000000000426, -5.773502691896255534, -1.060575238724906372E-15 ) ) ;
#41621=CARTESIAN_POINT ( 'NONE',  ( 13.86562500061451431, 3.027376345333613106, -5.243569643749998122 ) ) ;
#41624=CARTESIAN_POINT ( 'NONE',  ( 18.71250000122903145, 4.330127018922192761, -2.499999999999997780 ) ) ;
#41626=CARTESIAN_POINT ( 'NONE',  ( 8.540625000614518569, 6.054752690667223547, 3.707466751127219781E-16 ) ) ;
#41627=CARTESIAN_POINT ( 'NONE',  ( 24.30937500061451573, 4.541064518000418104, -2.621784821874998173 ) ) ;
#41628=CARTESIAN_POINT ( 'NONE',  ( 27.03750000122903430, -4.330127018922194537, 2.499999999999995559 ) ) ;
#41630=CARTESIAN_POINT ( 'NONE',  ( 23.48437500061451644, 4.541064518000418104, 2.621784821874999949 ) ) ;
#41631=CARTESIAN_POINT ( 'NONE',  ( 6.937499999999999112, 5.773502691896255534, 3.535250795749688894E-16 ) ) ;
#41632=CARTESIAN_POINT ( 'NONE',  ( -3.999999999999997335, 12.95000000122903572, 32.30940107675850470 ) ) ;
#41633=CARTESIAN_POINT ( 'NONE',  ( 15.10312500061451502, -4.541064518000417216, -2.621784821875001281 ) ) ;
#41634=CARTESIAN_POINT ( 'NONE',  ( 7.612500001229035362, 0.000000000000000000, 4.999999999999998224 ) ) ;
#41635=CARTESIAN_POINT ( 'NONE',  ( 10.88437500061451679, 4.541064518000418104, 2.621784821874999949 ) ) ;
#41638=CARTESIAN_POINT ( 'NONE',  ( 13.45312500061451466, 4.541064518000418104, -2.621784821874998173 ) ) ;
#41640=CARTESIAN_POINT ( 'NONE',  ( 22.91250000122903430, 0.000000000000000000, 4.999999999999998224 ) ) ;
#41641=CARTESIAN_POINT ( 'NONE',  ( 12.08437500061451608, 6.421520780324663323E-16, -5.243569643749999010 ) ) ;
#41642=CARTESIAN_POINT ( 'NONE',  ( 14.50312500061451537, 0.000000000000000000, 5.243569643749999010 ) ) ;
#41644=CARTESIAN_POINT ( 'NONE',  ( 23.37187500061451573, 3.027376345333613106, -5.243569643749998122 ) ) ;
#41645=CYLINDRICAL_SURFACE ( 'NONE', #43144, 4.999999999999998224 ) ;
#41646=CARTESIAN_POINT ( 'NONE',  ( 23.77499999999999858, -4.330127018922194537, 2.499999999999995559 ) ) ;
#41648=CARTESIAN_POINT ( 'NONE',  ( -4.243569643749999898, 15.35937500061451644, -30.00000000000000000 ) ) ;
#41649=CARTESIAN_POINT ( 'NONE',  ( 16.39687500061451786, -3.027376345333614438, 5.243569643749998122 ) ) ;
#41650=CARTESIAN_POINT ( 'NONE',  ( 17.02500000122903145, 2.886751345948126879, 4.999999999999999112 ) ) ;
#41651=CARTESIAN_POINT ( 'NONE',  ( 13.09687500061451892, 6.054752690667223547, 3.707466751127219781E-16 ) ) ;
#41652=CARTESIAN_POINT ( 'NONE',  ( 4.243569643749999898, 11.04687500061451999, 32.45002607614398471 ) ) ;
#41653=CARTESIAN_POINT ( 'NONE',  ( 19.12500000122903288, 2.886751345948129099, -4.999999999999998224 ) ) ;
#41654=CARTESIAN_POINT ( 'NONE',  ( 12.85312500061451502, -4.541064518000417216, -2.621784821875001281 ) ) ;
#41657=CARTESIAN_POINT ( 'NONE',  ( 17.02499999999999858, -4.330127018922194537, 2.499999999999995559 ) ) ;
#41658=CARTESIAN_POINT ( 'NONE',  ( 9.999999999999992895, 5.857864376269048101, -9.999999999999992895 ) ) ;
#41659=CARTESIAN_POINT ( 'NONE',  ( 11.70937500061451608, 4.541064518000418104, -2.621784821874998173 ) ) ;
#41661=CARTESIAN_POINT ( 'NONE',  ( 12.86250000122903359, 4.330127018922192761, -2.499999999999997780 ) ) ;
#41662=CARTESIAN_POINT ( 'NONE',  ( 20.66250000122903074, 0.000000000000000000, 4.999999999999998224 ) ) ;
#41663=CARTESIAN_POINT ( 'NONE',  ( 18.17812500061451786, -4.541064518000419881, 2.621784821874995952 ) ) ;
#41664=CARTESIAN_POINT ( 'NONE',  ( 21.25312500061451715, 0.000000000000000000, 5.243569643749999010 ) ) ;
#41665=CARTESIAN_POINT ( 'NONE',  ( 3.440625000614518036, -3.027376345333610441, -5.243569643749999898 ) ) ;
#41666=ADVANCED_FACE ( 'NONE', ( #49729 ), #16817, .T. ) ;
#41667=CARTESIAN_POINT ( 'NONE',  ( 26.88749999999999574, -2.886751345948129988, 4.999999999999997335 ) ) ;
#41669=CARTESIAN_POINT ( 'NONE',  ( 28.09687500061451360, -3.027376345333614438, 5.243569643749998122 ) ) ;
#41670=CARTESIAN_POINT ( 'NONE',  ( 13.01250000122903394, 0.000000000000000000, 4.999999999999998224 ) ) ;
#41671=CARTESIAN_POINT ( 'NONE',  ( -2.121784821874999949, 16.63437500061451857, -33.67503911421598417 ) ) ;
#41672=CARTESIAN_POINT ( 'NONE',  ( 4.875000001229034652, 2.886751345948126879, 4.999999999999999112 ) ) ;
#41673=CARTESIAN_POINT ( 'NONE',  ( 6.262500000000000178, -5.773502691896255534, -1.060575238724906372E-15 ) ) ;
#41675=CARTESIAN_POINT ( 'NONE',  ( 10.43437500061451750, 4.541064518000418104, 2.621784821874999949 ) ) ;
#41676=CARTESIAN_POINT ( 'NONE',  ( 28.49062500061451431, -3.027376345333614438, 5.243569643749998122 ) ) ;
#41677=CARTESIAN_POINT ( 'NONE',  ( 2.000000000000001332, 10.70000000000000107, 33.46410161513774995 ) ) ;
#41678=CARTESIAN_POINT ( 'NONE',  ( -5.672756003115389412, 8.235591643417164320, -28.03551386504724618 ) ) ;
#41679=CARTESIAN_POINT ( 'NONE',  ( 1.999999999999998668, 17.71250000122903501, -33.46410161513775705 ) ) ;
#41680=CARTESIAN_POINT ( 'NONE',  ( 7.659375000614518036, 4.541064518000418104, -2.621784821874998173 ) ) ;
#41681=CARTESIAN_POINT ( 'NONE',  ( 10.92187500061451644, 3.027376345333611329, 5.243569643749999010 ) ) ;
#41682=CARTESIAN_POINT ( 'NONE',  ( 5.025000000000002132, 6.123233995736764310E-16, -4.999999999999998224 ) ) ;
#41683=CARTESIAN_POINT ( 'NONE',  ( -2.121784821874996840, 14.02812500061459566, 33.67503911421598417 ) ) ;
#41684=CARTESIAN_POINT ( 'NONE',  ( 4.987500000000004263, -2.886751345948059377, -5.000000000000114575 ) ) ;
#41685=CARTESIAN_POINT ( 'NONE',  ( 6.750000000000002665, -4.330127018922190985, -2.500000000000001332 ) ) ;
#41687=CARTESIAN_POINT ( 'NONE',  ( 20.31562500061451715, 3.027376345333611329, 5.243569643749999010 ) ) ;
#41688=CARTESIAN_POINT ( 'NONE',  ( 13.97812500061451679, 4.541064518000418104, 2.621784821874999949 ) ) ;
#41690=CARTESIAN_POINT ( 'NONE',  ( 10.02187500061451964, 3.027376345333611329, 5.243569643749999010 ) ) ;
#41691=CARTESIAN_POINT ( 'NONE',  ( 26.17500000000000071, 6.123233995736764310E-16, -4.999999999999998224 ) ) ;
#41692=CARTESIAN_POINT ( 'NONE',  ( 23.51250000122903216, -4.330127018922190985, -2.500000000000001332 ) ) ;
#41693=CARTESIAN_POINT ( 'NONE',  ( 11.25000000122903288, -2.886751345948130876, 4.999999999999996447 ) ) ;
#41694=CARTESIAN_POINT ( 'NONE',  ( 10.92187500061451644, 3.027376345333611329, 5.243569643749999010 ) ) ;
#41695=CARTESIAN_POINT ( 'NONE',  ( 25.54687500061451644, -3.027376345333610441, -5.243569643749999898 ) ) ;
#41696=CARTESIAN_POINT ( 'NONE',  ( 4.021875000614516082, 3.027376345333613106, -5.243569643749998122 ) ) ;
#41698=CARTESIAN_POINT ( 'NONE',  ( 19.65937500061451360, -4.541064518000417216, -2.621784821875001281 ) ) ;
#41699=CARTESIAN_POINT ( 'NONE',  ( 11.14687500061451608, -3.027376345333610441, -5.243569643749999898 ) ) ;
#41701=CARTESIAN_POINT ( 'NONE',  ( 24.33749999999999858, -2.886751345948125991, -5.000000000000000000 ) ) ;
#41703=CARTESIAN_POINT ( 'NONE',  ( -3.000416591977282496E-16, 11.64687500061451786, -34.90005215228797653 ) ) ;
#41705=CARTESIAN_POINT ( 'NONE',  ( 16.00312500061451715, -4.541064518000417216, -2.621784821875001281 ) ) ;
#41706=CARTESIAN_POINT ( 'NONE',  ( 4.237500000000001599, 5.773502691896255534, 3.535250795749688894E-16 ) ) ;
#41709=CARTESIAN_POINT ( 'NONE',  ( 15.52500000000000036, 4.330127018922191873, 2.499999999999999556 ) ) ;
#41710=CARTESIAN_POINT ( 'NONE',  ( -4.243569643749999898, 10.80312500061451786, 30.00000000000000000 ) ) ;
#41711=CARTESIAN_POINT ( 'NONE',  ( 14.28750000122903430, 4.330127018922191873, 2.499999999999999556 ) ) ;
#41712=CARTESIAN_POINT ( 'NONE',  ( 24.75937500061451502, 4.541064518000418104, -2.621784821874998173 ) ) ;
#41714=EDGE_LOOP ( 'NONE', ( #24879, #27626, #52871, #10906 ) ) ;
#41715=CARTESIAN_POINT ( 'NONE',  ( 20.69062500061451715, 6.054752690667223547, 3.707466751127219781E-16 ) ) ;
#41716=CARTESIAN_POINT ( 'NONE',  ( 3.478125000614517237, 6.421520780324663323E-16, -5.243569643749999010 ) ) ;
#41717=CARTESIAN_POINT ( 'NONE',  ( 19.62187500061451573, -6.054752690667223547, -1.112240025338166033E-15 ) ) ;
#41718=CARTESIAN_POINT ( 'NONE',  ( 28.99687500061451573, -3.027376345333614438, 5.243569643749998122 ) ) ;
#41719=CARTESIAN_POINT ( 'NONE',  ( 7.265625000614516438, 3.027376345333611329, 5.243569643749999010 ) ) ;
#41720=CARTESIAN_POINT ( 'NONE',  ( 21.40312500061451573, -4.541064518000417216, -2.621784821875001281 ) ) ;
#41721=CARTESIAN_POINT ( 'NONE',  ( 4.243569643749999898, 15.07812500061451644, 30.00000000000000000 ) ) ;
#41722=CARTESIAN_POINT ( 'NONE',  ( 18.41250000122903430, 0.000000000000000000, 4.999999999999998224 ) ) ;
#41724=CARTESIAN_POINT ( 'NONE',  ( 9.365625000614519635, 3.027376345333612662, -5.243569643749998122 ) ) ;
#41725=CARTESIAN_POINT ( 'NONE',  ( 13.76250000000000107, 2.886751345948126879, 4.999999999999998224 ) ) ;
#41726=CARTESIAN_POINT ( 'NONE',  ( 3.309375000614518836, 0.000000000000000000, 5.243569643749999010 ) ) ;
#41727=CARTESIAN_POINT ( 'NONE',  ( 23.37187500061451573, 3.027376345333613106, -5.243569643749998122 ) ) ;
#41728=CARTESIAN_POINT ( 'NONE',  ( 14.54062500061451679, -3.027376345333614438, 5.243569643749998122 ) ) ;
#41729=CARTESIAN_POINT ( 'NONE',  ( 24.90000000122903145, -2.886751345948125991, -5.000000000000000000 ) ) ;
#41730=CARTESIAN_POINT ( 'NONE',  ( 26.27812500061451573, -4.541064518000419881, 2.621784821874995952 ) ) ;
#41731=CARTESIAN_POINT ( 'NONE',  ( 20.44687500061451857, -3.027376345333614438, 5.243569643749998122 ) ) ;
#41732=CARTESIAN_POINT ( 'NONE',  ( 15.02812500061451750, -4.541064518000419881, 2.621784821874995952 ) ) ;
#41733=CARTESIAN_POINT ( 'NONE',  ( 2.121784821875001281, 15.95937500061451608, 33.67503911421598417 ) ) ;
#41734=CARTESIAN_POINT ( 'NONE',  ( 19.22812500061451502, 6.421520780324663323E-16, -5.243569643749999010 ) ) ;
#41735=CARTESIAN_POINT ( 'NONE',  ( 29.39062500061451289, -3.027376345333614438, 5.243569643749998122 ) ) ;
#41737=CARTESIAN_POINT ( 'NONE',  ( 24.37500000000000000, 6.123233995736764310E-16, -4.999999999999998224 ) ) ;
#41738=CARTESIAN_POINT ( 'NONE',  ( -2.121784821874996840, 19.48437500061451644, -26.32496088578401583 ) ) ;
#41740=CARTESIAN_POINT ( 'NONE',  ( 28.07812500061451289, -4.541064518000419881, 2.621784821874995952 ) ) ;
#41741=CARTESIAN_POINT ( 'NONE',  ( 7.753125000614518036, 0.000000000000000000, 5.243569643749999010 ) ) ;
#41742=CARTESIAN_POINT ( 'NONE',  ( 19.98750000122903359, 6.123233995736764310E-16, -4.999999999999998224 ) ) ;
#41743=CARTESIAN_POINT ( 'NONE',  ( 25.22812500061451502, 4.541064518000418104, 2.621784821874999949 ) ) ;
#41744=CARTESIAN_POINT ( 'NONE',  ( 25.68750000000000000, -2.886751345948125991, -5.000000000000000000 ) ) ;
#41745=CARTESIAN_POINT ( 'NONE',  ( 4.000000000000000000, 16.25000000122903643, -27.69059892324149530 ) ) ;
#41746=CARTESIAN_POINT ( 'NONE',  ( 28.19062500061451715, -3.027376345333610441, -5.243569643749999898 ) ) ;
#41747=CARTESIAN_POINT ( 'NONE',  ( 10.34062500061451750, 6.054752690667223547, 3.707466751127219781E-16 ) ) ;
#41748=( BOUNDED_CURVE ( )  B_SPLINE_CURVE ( 2, ( #47584, #63834, #19489, #36496, #13226, #29505, #41677, #19123, #30230 ),
 .UNSPECIFIED., .F., .F. ) 
 B_SPLINE_CURVE_WITH_KNOTS ( ( 3, 2, 2, 2, 3 ),
 ( 0.8804347826086956763, 0.8840579710144927938, 0.8913043478260869179, 0.8985507246376811530, 0.9021739130434782705 ),
 .UNSPECIFIED. ) 
 CURVE ( )  GEOMETRIC_REPRESENTATION_ITEM ( )  RATIONAL_B_SPLINE_CURVE ( ( 0.9330127018922194093, 0.9330127018922194093, 1.000000000000000000, 0.8660254037844387076, 1.000000000000000000, 0.8660254037844387076, 1.000000000000000000, 0.9330127018922194093, 0.9330127018922194093 ) ) 
 REPRESENTATION_ITEM ( '' )  );
#41749=ORIENTED_EDGE ( 'NONE', *, *, #22231, .F. ) ;
#41751=CARTESIAN_POINT ( 'NONE',  ( 24.70312500061451644, 4.541064518000418104, -2.621784821874998173 ) ) ;
#41752=CARTESIAN_POINT ( 'NONE',  ( 4.678125000614516971, -4.541064518000419881, 2.621784821874995952 ) ) ;
#41754=DIRECTION ( 'NONE',  ( 0.000000000000000000, 0.000000000000000000, 1.000000000000000000 ) ) ;
#41755=CARTESIAN_POINT ( 'NONE',  ( 12.33750000000000036, 5.773502691896255534, 3.535250795749688894E-16 ) ) ;
#41756=CARTESIAN_POINT ( 'NONE',  ( 14.07187500061451679, 3.027376345333611329, 5.243569643749999010 ) ) ;
#41757=CARTESIAN_POINT ( 'NONE',  ( 7.875000001229034652, 2.886751345948129099, -4.999999999999998224 ) ) ;
#41758=CARTESIAN_POINT ( 'NONE',  ( 16.88437500061451502, -4.541064518000419881, 2.621784821874995952 ) ) ;
#41760=CARTESIAN_POINT ( 'NONE',  ( 8.634375000614518569, 4.541064518000418104, 2.621784821874999949 ) ) ;
#41761=CARTESIAN_POINT ( 'NONE',  ( 4.243569643749999898, 12.34062500061451750, -27.54997392385601529 ) ) ;
#41763=CARTESIAN_POINT ( 'NONE',  ( 20.92500000122903359, 2.886751345948129099, -4.999999999999997335 ) ) ;
#41766=CARTESIAN_POINT ( 'NONE',  ( 25.64062500061451644, 6.054752690667223547, 3.707466751127219781E-16 ) ) ;
#41767=CARTESIAN_POINT ( 'NONE',  ( 7.320879633048903241E-15, 18.08749999999999858, -34.00000000000000000 ) ) ;
#41768=CARTESIAN_POINT ( 'NONE',  ( 25.50937500061451502, -4.541064518000417216, -2.621784821875001281 ) ) ;
#41769=CARTESIAN_POINT ( 'NONE',  ( 28.77187500061451431, 3.027376345333613106, -5.243569643749998122 ) ) ;
#41770=CARTESIAN_POINT ( 'NONE',  ( 20.81250000000000000, 2.886751345948129099, -4.999999999999998224 ) ) ;
#41771=CARTESIAN_POINT ( 'NONE',  ( 3.703125000614516882, 0.000000000000000000, 5.243569643749999010 ) ) ;
#41773=CARTESIAN_POINT ( 'NONE',  ( 17.85937500061451999, -4.541064518000417216, -2.621784821875001281 ) ) ;
#41775=CARTESIAN_POINT ( 'NONE',  ( 28.91250000122903074, -4.330127018922190985, -2.500000000000001332 ) ) ;
#41776=CARTESIAN_POINT ( 'NONE',  ( 9.496875000614517504, 6.054752690667223547, 3.707466751127219781E-16 ) ) ;
#41777=CARTESIAN_POINT ( 'NONE',  ( 18.38437500061451857, 6.421520780324663323E-16, -5.243569643749999010 ) ) ;
#41779=CARTESIAN_POINT ( 'NONE',  ( 25.98750000000000071, -2.886751345948129988, 4.999999999999997335 ) ) ;
#41780=CARTESIAN_POINT ( 'NONE',  ( 26.85937500061451644, -4.541064518000417216, -2.621784821875001281 ) ) ;
#41781=FACE_OUTER_BOUND ( 'NONE', #47789, .T. ) ;
#41782=EDGE_LOOP ( 'NONE', ( #20793, #46436, #57124, #1364 ) ) ;
#41783=CARTESIAN_POINT ( 'NONE',  ( 7.462500000000001243, 2.886751345948126879, 4.999999999999999112 ) ) ;
#41785=CARTESIAN_POINT ( 'NONE',  ( 21.02812500061451573, 6.421520780324663323E-16, -5.243569643749999010 ) ) ;
#41786=CARTESIAN_POINT ( 'NONE',  ( 11.66249999999999964, -5.773502691896255534, -1.060575238724906372E-15 ) ) ;
#41787=CARTESIAN_POINT ( 'NONE',  ( 7.575000001229033053, 2.886751345948126879, 4.999999999999999112 ) ) ;
#41788=CARTESIAN_POINT ( 'NONE',  ( 7.378125000614518036, -4.541064518000419881, 2.621784821874995952 ) ) ;
#41789=CARTESIAN_POINT ( 'NONE',  ( 21.52499999999999858, -4.330127018922194537, 2.499999999999995559 ) ) ;
#41790=EDGE_CURVE ( 'NONE', #18509, #15804, #58540, .T. ) ;
#41791=CARTESIAN_POINT ( 'NONE',  ( 21.47812500061451502, 6.421520780324663323E-16, -5.243569643749999010 ) ) ;
#41792=CARTESIAN_POINT ( 'NONE',  ( 23.62500000000000000, 4.330127018922191873, 2.499999999999999556 ) ) ;
#41793=CARTESIAN_POINT ( 'NONE',  ( 25.68750000122903288, -4.330127018922194537, 2.499999999999995559 ) ) ;
#41795=CARTESIAN_POINT ( 'NONE',  ( 5.212500000000002132, 2.886751345948126879, 4.999999999999999112 ) ) ;
#41797=CARTESIAN_POINT ( 'NONE',  ( 18.32812500061451644, 6.421520780324663323E-16, -5.243569643749999010 ) ) ;
#41798=CARTESIAN_POINT ( 'NONE',  ( 25.90312500061451573, -4.541064518000417216, -2.621784821875001281 ) ) ;
#41799=CARTESIAN_POINT ( 'NONE',  ( 26.14687500061451431, 6.054752690667223547, 3.707466751127219781E-16 ) ) ;
#41800=CARTESIAN_POINT ( 'NONE',  ( 14.72812500061451679, 6.421520780324663323E-16, -5.243569643749999010 ) ) ;
#41801=CARTESIAN_POINT ( 'NONE',  ( 29.39062500061451289, -3.027376345333614438, 5.243569643749998122 ) ) ;
#41802=CARTESIAN_POINT ( 'NONE',  ( 8.615625000614517859, 3.027376345333611329, 5.243569643749999010 ) ) ;
#41804=CARTESIAN_POINT ( 'NONE',  ( 27.15000000122902790, -2.886751345948125991, -5.000000000000000000 ) ) ;
#41806=CARTESIAN_POINT ( 'NONE',  ( 16.26562500061451289, 3.027376345333611329, 5.243569643749999010 ) ) ;
#41807=CARTESIAN_POINT ( 'NONE',  ( 1.626862140677534273E-15, 12.12500000122903465, -26.00000000000000355 ) ) ;
#41808=CARTESIAN_POINT ( 'NONE',  ( 28.62187500061451573, -6.054752690667223547, -1.112240025338166033E-15 ) ) ;
#41809=CARTESIAN_POINT ( 'NONE',  ( 9.459375000614517859, 4.541064518000418104, -2.621784821874998173 ) ) ;
#41810=CARTESIAN_POINT ( 'NONE',  ( 9.309375000614517504, -4.541064518000417216, -2.621784821875001281 ) ) ;
#41811=CARTESIAN_POINT ( 'NONE',  ( 18.15937500061451715, 0.000000000000000000, 5.243569643749999010 ) ) ;
#41812=EDGE_LOOP ( 'NONE', ( #15932, #5448, #13404, #35689 ) ) ;
#41813=CARTESIAN_POINT ( 'NONE',  ( 29.85937500061451644, 0.000000000000000000, 5.243569643749999010 ) ) ;
#41814=CARTESIAN_POINT ( 'NONE',  ( 22.60312500061451857, 0.000000000000000000, 5.243569643749999010 ) ) ;
#41815=CARTESIAN_POINT ( 'NONE',  ( 15.45937500061451608, 0.000000000000000000, 5.243569643749999010 ) ) ;
#41816=CARTESIAN_POINT ( 'NONE',  ( 21.66562500061451502, 3.027376345333611329, 5.243569643749999010 ) ) ;
#41817=CARTESIAN_POINT ( 'NONE',  ( -3.999999999999999556, 15.01250000000000107, 27.69059892324149530 ) ) ;
#41818=CARTESIAN_POINT ( 'NONE',  ( 28.15312500061451573, -4.541064518000417216, -2.621784821875001281 ) ) ;
#41819=CARTESIAN_POINT ( 'NONE',  ( 9.937500001229032875, -4.330127018922194537, 2.499999999999995559 ) ) ;
#41820=VERTEX_POINT ( 'NONE', #61167 ) ;
#41821=CARTESIAN_POINT ( 'NONE',  ( 5.025000001229035895, -5.773502691896255534, -1.060575238724906372E-15 ) ) ;
#41822=CARTESIAN_POINT ( 'NONE',  ( -3.999999999999999556, 16.81250000000000000, -32.30940107675850470 ) ) ;
#41823=CARTESIAN_POINT ( 'NONE',  ( 23.77500000122903145, 2.886751345948126879, 4.999999999999999112 ) ) ;
#41826=CARTESIAN_POINT ( 'NONE',  ( 6.084375000614518747, -4.541064518000419881, 2.621784821874995952 ) ) ;
#41827=CARTESIAN_POINT ( 'NONE',  ( 17.73750000000000071, 5.773502691896255534, 3.535250795749688401E-16 ) ) ;
#41828=CARTESIAN_POINT ( 'NONE',  ( 15.81562500061451537, 3.027376345333611329, 5.243569643749999010 ) ) ;
#41829=CARTESIAN_POINT ( 'NONE',  ( 11.55937500061451928, -4.541064518000417216, -2.621784821875001281 ) ) ;
#41830=CARTESIAN_POINT ( 'NONE',  ( 27.78750000122903074, 4.330127018922191873, 2.499999999999999556 ) ) ;
#41831=CARTESIAN_POINT ( 'NONE',  ( 17.55937500061451573, 4.541064518000418104, -2.621784821874998173 ) ) ;
#41832=CARTESIAN_POINT ( 'NONE',  ( 5.634375000614519458, -4.541064518000419881, 2.621784821874995952 ) ) ;
#41833=DIRECTION ( 'NONE',  ( -1.000000000000000000, -0.000000000000000000, -0.000000000000000000 ) ) ;
#41834=CARTESIAN_POINT ( 'NONE',  ( 6.703125000614516438, 4.541064518000418104, -2.621784821874998173 ) ) ;
#41835=CARTESIAN_POINT ( 'NONE',  ( 17.31562500061451715, -6.054752690667223547, -1.112240025338166033E-15 ) ) ;
#41836=EDGE_LOOP ( 'NONE', ( #3403, #3180, #38744, #29270 ) ) ;
#41838=CARTESIAN_POINT ( 'NONE',  ( 16.07812500061451289, 6.421520780324663323E-16, -5.243569643749999010 ) ) ;
#41839=CARTESIAN_POINT ( 'NONE',  ( 8.850000001229034297, 5.773502691896255534, 3.535250795749688894E-16 ) ) ;
#41841=CARTESIAN_POINT ( 'NONE',  ( 10.19062500061451892, -3.027376345333610441, -5.243569643749999898 ) ) ;
#41843=CARTESIAN_POINT ( 'NONE',  ( 10.42500000000000071, 6.123233995736764310E-16, -4.999999999999998224 ) ) ;
#41844=CARTESIAN_POINT ( 'NONE',  ( 6.562500001229032875, 4.330127018922192761, -2.499999999999997780 ) ) ;
#41845=EDGE_CURVE ( 'NONE', #6203, #69560, #4306, .T. ) ;
#41846=CARTESIAN_POINT ( 'NONE',  ( 14.44687500061451679, 6.054752690667223547, 3.707466751127219781E-16 ) ) ;
#41847=B_SPLINE_CURVE_WITH_KNOTS ( 'NONE', 3,
 ( #23533, #67178, #6559, #29091, #11010, #46083, #73068, #16539, #39453, #61609 ),
 .UNSPECIFIED., .F., .F.,
 ( 4, 3, 3, 4 ),
 ( 4.336808689942017736E-19, 7.861678629069894031E-05, 0.0001572339239830308245, 0.0003065732708899783433 ),
 .UNSPECIFIED. ) ;
#41848=CARTESIAN_POINT ( 'NONE',  ( 16.53750000122903430, 4.330127018922191873, 2.499999999999999556 ) ) ;
#41850=CARTESIAN_POINT ( 'NONE',  ( -4.243569643749999898, 19.76562500061451644, -32.45002607614398471 ) ) ;
#41852=CARTESIAN_POINT ( 'NONE',  ( 23.36250000122903359, 0.000000000000000000, 4.999999999999998224 ) ) ;
#41854=CARTESIAN_POINT ( 'NONE',  ( 3.901908842376271558, -3.126527325029728299, -4.209502533745343555 ) ) ;
#41855=CARTESIAN_POINT ( 'NONE',  ( 16.95937500061451786, -4.541064518000417216, -2.621784821875001281 ) ) ;
#41857=CARTESIAN_POINT ( 'NONE',  ( 13.37812500061451715, 6.421520780324663323E-16, -5.243569643749999010 ) ) ;
#41859=CARTESIAN_POINT ( 'NONE',  ( 24.00937500061451502, 0.000000000000000000, 5.243569643749999010 ) ) ;
#41861=CARTESIAN_POINT ( 'NONE',  ( 11.01562500061451821, -6.054752690667223547, -1.112240025338166033E-15 ) ) ;
#41862=CARTESIAN_POINT ( 'NONE',  ( 15.64687500061451608, -3.027376345333610441, -5.243569643749999898 ) ) ;
#41864=CARTESIAN_POINT ( 'NONE',  ( 27.34687500061451360, -3.027376345333610441, -5.243569643749999898 ) ) ;
#41865=CARTESIAN_POINT ( 'NONE',  ( 27.85312500061451502, 4.541064518000418104, -2.621784821874998173 ) ) ;
#41866=CARTESIAN_POINT ( 'NONE',  ( 19.11562500061451431, -6.054752690667223547, -1.112240025338166033E-15 ) ) ;
#41867=CARTESIAN_POINT ( 'NONE',  ( 30.00000000000000000, 0.000000000000000000, 0.000000000000000000 ) ) ;
#41868=CARTESIAN_POINT ( 'NONE',  ( 4.000000000000000000, 14.78750000000000142, 32.30940107675849760 ) ) ;
#41870=CARTESIAN_POINT ( 'NONE',  ( 6.862500000000002487, 2.886751345948129099, -4.999999999999998224 ) ) ;
#41871=CARTESIAN_POINT ( 'NONE',  ( 19.38750000122903216, -4.330127018922194537, 2.499999999999995559 ) ) ;
#41872=CARTESIAN_POINT ( 'NONE',  ( 23.17500000122903359, 2.886751345948112668, -5.000000000000024869 ) ) ;
#41874=ORIENTED_EDGE ( 'NONE', *, *, #57289, .T. ) ;
#41875=CARTESIAN_POINT ( 'NONE',  ( 18.45000000000000284, -4.330127018922190985, -2.500000000000001332 ) ) ;
#41876=CARTESIAN_POINT ( 'NONE',  ( 18.67500000000000071, 4.330127018922191873, 2.499999999999999556 ) ) ;
#41877=CARTESIAN_POINT ( 'NONE',  ( 18.45937500061451431, 4.541064518000418104, -2.621784821874998173 ) ) ;
#41878=CARTESIAN_POINT ( 'NONE',  ( 13.82812500061451466, 6.421520780324663323E-16, -5.243569643749999010 ) ) ;
#41881=CARTESIAN_POINT ( 'NONE',  ( 1.071796769724491893, 18.44509619066136707, -26.00000000000000355 ) ) ;
#41882=CARTESIAN_POINT ( 'NONE',  ( 5.090625000614516615, -3.027376345333614438, 5.243569643749998122 ) ) ;
#41884=CARTESIAN_POINT ( 'NONE',  ( 12.41249999999999964, 2.886751345948126879, 4.999999999999999112 ) ) ;
#41886=CARTESIAN_POINT ( 'NONE',  ( 4.243569643749999898, 15.52812500061451750, 30.00000000000000000 ) ) ;
#41887=CARTESIAN_POINT ( 'NONE',  ( 26.80312500061451431, -4.541064518000417216, -2.621784821875001281 ) ) ;
#41889=AXIS2_PLACEMENT_3D ( 'NONE', #7604, #69669, #41593 ) ;
#41891=CARTESIAN_POINT ( 'NONE',  ( 23.93437500061451573, 4.541064518000418104, 2.621784821874999949 ) ) ;
#41893=CARTESIAN_POINT ( 'NONE',  ( 21.55312500061451431, 4.541064518000418104, -2.621784821874998173 ) ) ;
#41894=CARTESIAN_POINT ( 'NONE',  ( 24.08437500061451786, -4.541064518000419881, 2.621784821874995952 ) ) ;
#41895=CARTESIAN_POINT ( 'NONE',  ( 4.243569643749999898, 16.84062500061459389, -27.54997392385601529 ) ) ;
#41896=CARTESIAN_POINT ( 'NONE',  ( 7.228125000614517681, 4.541064518000418104, 2.621784821874999949 ) ) ;
#41898=CARTESIAN_POINT ( 'NONE',  ( 23.76562500061451289, 3.027376345333612662, -5.243569643749998122 ) ) ;
#41901=( BOUNDED_CURVE ( )  B_SPLINE_CURVE ( 2, ( #65831, #21852, #71008, #66564, #20753, #44041, #15944, #72467, #26310 ),
 .UNSPECIFIED., .F., .F. ) 
 B_SPLINE_CURVE_WITH_KNOTS ( ( 3, 2, 2, 2, 3 ),
 ( 0.8586956521739130821, 0.8623188405797101996, 0.8695652173913043237, 0.8768115942028985588, 0.8804347826086956763 ),
 .UNSPECIFIED. ) 
 CURVE ( )  GEOMETRIC_REPRESENTATION_ITEM ( )  RATIONAL_B_SPLINE_CURVE ( ( 0.9330127018922194093, 0.9330127018922194093, 1.000000000000000000, 0.8660254037844387076, 1.000000000000000000, 0.8660254037844387076, 1.000000000000000000, 0.9330127018922194093, 0.9330127018922194093 ) ) 
 REPRESENTATION_ITEM ( '' )  );
#41902=EDGE_CURVE ( 'NONE', #27313, #65915, #46689, .T. ) ;
#41903=CARTESIAN_POINT ( 'NONE',  ( 17.14687500061451786, 6.054752690667223547, 3.707466751127219781E-16 ) ) ;
#41904=CARTESIAN_POINT ( 'NONE',  ( 25.54687500061451644, -3.027376345333610441, -5.243569643749999898 ) ) ;
#41905=CARTESIAN_POINT ( 'NONE',  ( -4.243569643749999898, 14.90937500061451715, 30.00000000000000000 ) ) ;
#41906=CARTESIAN_POINT ( 'NONE',  ( 5.053125000614517859, 0.000000000000000000, 5.243569643749999010 ) ) ;
#41907=CARTESIAN_POINT ( 'NONE',  ( 29.31562500061451715, 3.027376345333611329, 5.243569643749999010 ) ) ;
#41908=CARTESIAN_POINT ( 'NONE',  ( 28.56562500061451715, -6.054752690667223547, -1.112240025338166033E-15 ) ) ;
#41909=CARTESIAN_POINT ( 'NONE',  ( 4.237500000000001599, 5.773502691896255534, 3.535250795749688401E-16 ) ) ;
#41910=CARTESIAN_POINT ( 'NONE',  ( 5.653125000614517504, -4.541064518000417216, -2.621784821875001281 ) ) ;
#41911=CARTESIAN_POINT ( 'NONE',  ( 10.13437500061451679, -4.541064518000419881, 2.621784821874995952 ) ) ;
#41913=CARTESIAN_POINT ( 'NONE',  ( 17.25000000122903288, -2.886751345948125991, -5.000000000000000000 ) ) ;
#41914=CARTESIAN_POINT ( 'NONE',  ( 29.69062500061451715, 6.054752690667223547, 3.707466751127219781E-16 ) ) ;
#41915=CARTESIAN_POINT ( 'NONE',  ( 6.103125000614515905, -4.541064518000417216, -2.621784821875001281 ) ) ;
#41918=CARTESIAN_POINT ( 'NONE',  ( 14.48437500061451821, 4.541064518000418104, 2.621784821874999949 ) ) ;
#41919=CARTESIAN_POINT ( 'NONE',  ( 7.320879633048903241E-15, 17.75000000122903288, 26.00000000000000355 ) ) ;
#41921=CARTESIAN_POINT ( 'NONE',  ( 21.10312500061451502, 4.541064518000418104, -2.621784821874998173 ) ) ;
#41922=CARTESIAN_POINT ( 'NONE',  ( 9.028125000614517504, 4.541064518000418104, 2.621784821874999949 ) ) ;
#41923=CARTESIAN_POINT ( 'NONE',  ( 24.87187500061451573, 3.027376345333611329, 5.243569643749999010 ) ) ;
#41924=CARTESIAN_POINT ( 'NONE',  ( 6.703125000614516438, 4.541064518000418104, -2.621784821874998173 ) ) ;
#41925=DIRECTION ( 'NONE',  ( -1.000000000000000000, -0.000000000000000000, -0.000000000000000000 ) ) ;
#41926=CARTESIAN_POINT ( 'NONE',  ( 11.40000000122903501, -2.886751345948125991, -5.000000000000000000 ) ) ;
#41927=CARTESIAN_POINT ( 'NONE',  ( 25.90312500061451573, -4.541064518000417216, -2.621784821875001281 ) ) ;
#41928=CARTESIAN_POINT ( 'NONE',  ( -2.121784821874996840, 9.978125000614518569, -26.32496088578401583 ) ) ;
#41929=CARTESIAN_POINT ( 'NONE',  ( 11.43750000122903465, 6.123233995736764310E-16, -4.999999999999998224 ) ) ;
#41930=CARTESIAN_POINT ( 'NONE',  ( 21.36562500061451431, -6.054752690667223547, -1.112240025338166033E-15 ) ) ;
#41931=CARTESIAN_POINT ( 'NONE',  ( 17.05312500061451786, 4.541064518000418104, -2.621784821874998173 ) ) ;
#41933=CARTESIAN_POINT ( 'NONE',  ( 18.22499999999999787, 4.330127018922191873, 2.499999999999999556 ) ) ;
#41934=CARTESIAN_POINT ( 'NONE',  ( 14.81250000122903288, 0.000000000000000000, 4.999999999999998224 ) ) ;
#41935=EDGE_CURVE ( 'NONE', #58014, #63961, #30720, .T. ) ;
#41936=CARTESIAN_POINT ( 'NONE',  ( 11.39062500061451644, -3.027376345333614438, 5.243569643749998122 ) ) ;
#41937=CARTESIAN_POINT ( 'NONE',  ( 13.22812500061451502, -4.541064518000419881, 2.621784821874995952 ) ) ;
#41939=CARTESIAN_POINT ( 'NONE',  ( 23.77500000122903145, 2.886751345948126879, 4.999999999999999112 ) ) ;
#41941=CARTESIAN_POINT ( 'NONE',  ( 22.20937500061451431, 0.000000000000000000, 5.243569643749999010 ) ) ;
#41942=CARTESIAN_POINT ( 'NONE',  ( 20.89687500061452141, -3.027376345333614438, 5.243569643749998122 ) ) ;
#41943=DIRECTION ( 'NONE',  ( 0.000000000000000000, 0.000000000000000000, 1.000000000000000000 ) ) ;
#41944=EDGE_CURVE ( 'NONE', #53042, #26808, #7630, .T. ) ;
#41945=CARTESIAN_POINT ( 'NONE',  ( 7.912500001229033408, 4.330127018922192761, -2.499999999999997780 ) ) ;
#41946=( BOUNDED_CURVE ( )  B_SPLINE_CURVE ( 2, ( #6335, #24403, #45864, #17048, #28866, #62126, #69130 ),
 .UNSPECIFIED., .F., .F. ) 
 B_SPLINE_CURVE_WITH_KNOTS ( ( 3, 2, 2, 3 ),
 ( 0.8333333333333334814, 0.8361111111111112493, 0.8388888888888890172, 0.8416666666666667851 ),
 .UNSPECIFIED. ) 
 CURVE ( )  GEOMETRIC_REPRESENTATION_ITEM ( )  RATIONAL_B_SPLINE_CURVE ( ( 0.9999999999999946709, 0.8660254037844440367, 1.000000000000000000, 0.8660254037844387076, 1.000000000000000000, 0.8660254037844333785, 1.000000000000005329 ) ) 
 REPRESENTATION_ITEM ( '' )  );
#41947=CARTESIAN_POINT ( 'NONE',  ( 6.496875000614517504, -3.027376345333614438, 5.243569643749998122 ) ) ;
#41948=CARTESIAN_POINT ( 'NONE',  ( 26.29687500061451644, -3.027376345333614438, 5.243569643749998122 ) ) ;
#41949=( BOUNDED_CURVE ( )  B_SPLINE_CURVE ( 2, ( #39348, #10896, #5361, #22697, #17156, #67428, #39714, #62232, #51150 ),
 .UNSPECIFIED., .F., .F. ) 
 B_SPLINE_CURVE_WITH_KNOTS ( ( 3, 2, 2, 2, 3 ),
 ( 0.6413043478260869179, 0.6449275362318840354, 0.6521739130434782705, 0.6594202898550725056, 0.6630434782608696231 ),
 .UNSPECIFIED. ) 
 CURVE ( )  GEOMETRIC_REPRESENTATION_ITEM ( )  RATIONAL_B_SPLINE_CURVE ( ( 0.9330127018922194093, 0.9330127018922194093, 1.000000000000000000, 0.8660254037844387076, 1.000000000000000000, 0.8660254037844387076, 1.000000000000000000, 0.9330127018922182991, 0.9330127018922192983 ) ) 
 REPRESENTATION_ITEM ( '' )  );
#41950=CARTESIAN_POINT ( 'NONE',  ( 4.256295036913345875, -2.623882848654998323, -4.373091964381822017 ) ) ;
#41951=CARTESIAN_POINT ( 'NONE',  ( 20.42812500061451431, -4.541064518000419881, 2.621784821874995952 ) ) ;
#41952=CARTESIAN_POINT ( 'NONE',  ( 23.55937500061451573, 0.000000000000000000, 5.243569643749999010 ) ) ;
#41954=CARTESIAN_POINT ( 'NONE',  ( 3.242103837493086330E-14, 13.13749999999999929, 26.00000000000000711 ) ) ;
#41955=CARTESIAN_POINT ( 'NONE',  ( 3.999999999999998668, 15.76250000000000107, 27.69059892324149530 ) ) ;
#41956=CARTESIAN_POINT ( 'NONE',  ( 5.446875000614518569, 6.054752690667223547, 3.707466751127219781E-16 ) ) ;
#41957=CARTESIAN_POINT ( 'NONE',  ( 17.27812500061451217, -4.541064518000419881, 2.621784821874995952 ) ) ;
#41959=CARTESIAN_POINT ( 'NONE',  ( 25.90312500061451573, -4.541064518000417216, -2.621784821875001281 ) ) ;
#41960=CARTESIAN_POINT ( 'NONE',  ( 2.934375000614518392, -4.541064518000419881, 2.621784821874995952 ) ) ;
#41961=CARTESIAN_POINT ( 'NONE',  ( 4.704389487731190478, 1.694379531550751272, 4.836684215720605806 ) ) ;
#41962=DIRECTION ( 'NONE',  ( -0.000000000000000000, -1.000000000000000000, -0.000000000000000000 ) ) ;
#41963=CARTESIAN_POINT ( 'NONE',  ( 14.55000000000000071, 4.330127018922192761, -2.499999999999997780 ) ) ;
#41964=CARTESIAN_POINT ( 'NONE',  ( 21.06562500061451715, 3.027376345333613106, -5.243569643749998122 ) ) ;
#41966=ORIENTED_EDGE ( 'NONE', *, *, #69513, .T. ) ;
#41967=CARTESIAN_POINT ( 'NONE',  ( 24.56250000000000000, 2.886751345948126879, 4.999999999999999112 ) ) ;
#41968=CARTESIAN_POINT ( 'NONE',  ( 25.99687500061451928, -3.027376345333610441, -5.243569643749999898 ) ) ;
#41972=CARTESIAN_POINT ( 'NONE',  ( 14.09062500061451750, -3.027376345333614438, 5.243569643749998122 ) ) ;
#41973=CARTESIAN_POINT ( 'NONE',  ( 25.12500000122902932, 2.886751345948143754, 4.999999999999969802 ) ) ;
#41975=CARTESIAN_POINT ( 'NONE',  ( 3.121875000614518836, 3.027376345333613106, -5.243569643749998122 ) ) ;
#41976=CARTESIAN_POINT ( 'NONE',  ( 12.07500000122903216, 2.886751345948126879, 4.999999999999999112 ) ) ;
#41977=CARTESIAN_POINT ( 'NONE',  ( 18.75000000000000000, 0.000000000000000000, 4.999999999999998224 ) ) ;
#41978=CARTESIAN_POINT ( 'NONE',  ( 27.00000000000000000, -4.330127018922190985, -2.500000000000001332 ) ) ;
#41979=CARTESIAN_POINT ( 'NONE',  ( 3.187500001229033764, -4.330127018922194537, 2.499999999999995559 ) ) ;
#41980=CARTESIAN_POINT ( 'NONE',  ( 7.509375000614517681, -4.541064518000417216, -2.621784821875001281 ) ) ;
#41981=CARTESIAN_POINT ( 'NONE',  ( 19.80937500061451573, 4.541064518000418104, -2.621784821874998173 ) ) ;
#41982=CARTESIAN_POINT ( 'NONE',  ( 19.98750000122903359, 6.123233995736764310E-16, -4.999999999999998224 ) ) ;
#41984=CARTESIAN_POINT ( 'NONE',  ( 27.81562500061452070, 3.027376345333613106, -5.243569643749998122 ) ) ;
#41985=CARTESIAN_POINT ( 'NONE',  ( 4.162499999999999645, 2.886751345948129099, -4.999999999999998224 ) ) ;
#41986=EDGE_CURVE ( 'NONE', #33272, #27910, #70853, .T. ) ;
#41987=CARTESIAN_POINT ( 'NONE',  ( 4.396875000614516971, -3.027376345333610441, -5.243569643749999898 ) ) ;
#41988=CARTESIAN_POINT ( 'NONE',  ( 15.15000000000000036, 0.000000000000000000, 4.999999999999998224 ) ) ;
#41989=CARTESIAN_POINT ( 'NONE',  ( 13.82812500061451466, 6.421520780324663323E-16, -5.243569643749999010 ) ) ;
#41993=CARTESIAN_POINT ( 'NONE',  ( 17.85000000122903430, 5.773502691896255534, 3.535250795749688894E-16 ) ) ;
#41996=CARTESIAN_POINT ( 'NONE',  ( 7.528125000614515727, 6.421520780324663323E-16, -5.243569643749999010 ) ) ;
#41997=CARTESIAN_POINT ( 'NONE',  ( 24.08437500061451786, -4.541064518000419881, 2.621784821874995952 ) ) ;
#41998=CARTESIAN_POINT ( 'NONE',  ( 27.00000000122903288, -2.886751345948096681, 5.000000000000054179 ) ) ;
#41999=CARTESIAN_POINT ( 'NONE',  ( 24.00937500061451502, 0.000000000000000000, 5.243569643749999010 ) ) ;
#42000=CARTESIAN_POINT ( 'NONE',  ( 6.150000000000003020, 0.000000000000000000, 4.999999999999998224 ) ) ;
#42001=CARTESIAN_POINT ( 'NONE',  ( -3.999999999999999556, 10.62500000122903643, 27.69059892324149530 ) ) ;
#42002=CARTESIAN_POINT ( 'NONE',  ( 15.62812500061451537, 6.421520780324663323E-16, -5.243569643749999010 ) ) ;
#42003=CARTESIAN_POINT ( 'NONE',  ( 4.387500001229033053, 4.330127018922191873, 2.499999999999999556 ) ) ;
#42004=CARTESIAN_POINT ( 'NONE',  ( 9.459375000614517859, 4.541064518000418104, -2.621784821874998173 ) ) ;
#42005=CARTESIAN_POINT ( 'NONE',  ( 3.807538167735159185, -3.240779705755961526, 4.122180188640082399 ) ) ;
#42006=EDGE_LOOP ( 'NONE', ( #51893, #17082, #48386, #16752, #71608, #48197, #28054, #72021, #31934, #62584, #27174, #53704, #37654, #5823, #42244, #63677, #45195, #58423, #3699, #60488, #58322, #36737, #52824, #59107, #23514, #8101, #5609, #7162, #46636, #67513, #66328, #60051, #62494, #70781, #9082, #12473, #32206, #14302, #55877, #72868, #14977, #69150, #49033, #51017, #41301, #26289, #71125 ) ) ;
#42007=CARTESIAN_POINT ( 'NONE',  ( 12.29062500061451857, -3.027376345333614438, 5.243569643749998122 ) ) ;
#42009=CARTESIAN_POINT ( 'NONE',  ( 23.36250000122903359, 0.000000000000000000, 4.999999999999998224 ) ) ;
#42010=CARTESIAN_POINT ( 'NONE',  ( 11.37187500061451750, 3.027376345333611329, 5.243569643749999010 ) ) ;
#42011=CARTESIAN_POINT ( 'NONE',  ( 11.91562500061451857, -6.054752690667223547, -1.112240025338166033E-15 ) ) ;
#42013=CARTESIAN_POINT ( 'NONE',  ( 24.64687500061451431, -3.027376345333610441, -5.243569643749999898 ) ) ;
#42014=DIRECTION ( 'NONE',  ( 0.000000000000000000, 0.000000000000000000, -1.000000000000000000 ) ) ;
#42015=CARTESIAN_POINT ( 'NONE',  ( -5.810221930991193690E-16, 10.10000000122903430, -34.00000000000000000 ) ) ;
#42016=CARTESIAN_POINT ( 'NONE',  ( 20.55000000122903359, 5.773502691896255534, 3.535250795749688401E-16 ) ) ;
#42017=CARTESIAN_POINT ( 'NONE',  ( 4.243569643749999898, 14.68437500061451750, -30.00000000000000000 ) ) ;
#42018=CARTESIAN_POINT ( 'NONE',  ( 16.92187500061451999, -6.054752690667223547, -1.112240025338166033E-15 ) ) ;
#42019=CARTESIAN_POINT ( 'NONE',  ( 16.83750000122903145, 6.123233995736764310E-16, -4.999999999999998224 ) ) ;
#42020=CARTESIAN_POINT ( 'NONE',  ( 11.93437500061451573, -4.541064518000419881, 2.621784821874995952 ) ) ;
#42021=CARTESIAN_POINT ( 'NONE',  ( -4.243569643749999898, 17.10312500061451502, -30.00000000000000000 ) ) ;
#42022=CARTESIAN_POINT ( 'NONE',  ( 20.17500000122903359, 2.886751345948126879, 4.999999999999999112 ) ) ;
#42023=CARTESIAN_POINT ( 'NONE',  ( 12.81562500061451537, -6.054752690667223547, -1.112240025338166033E-15 ) ) ;
#42024=ORIENTED_EDGE ( 'NONE', *, *, #20707, .T. ) ;
#42026=CARTESIAN_POINT ( 'NONE',  ( 15.26249999999999929, -5.773502691896255534, -1.060575238724906372E-15 ) ) ;
#42027=CARTESIAN_POINT ( 'NONE',  ( 18.07499999999999929, 6.123233995736764310E-16, -4.999999999999998224 ) ) ;
#42028=CARTESIAN_POINT ( 'NONE',  ( 11.85937500061451644, 0.000000000000000000, 5.243569643749999010 ) ) ;
#42029=CARTESIAN_POINT ( 'NONE',  ( 4.094832220624204489, 2.869363679410234624, 4.355156543258145163 ) ) ;
#42030=CARTESIAN_POINT ( 'NONE',  ( 11.85000000122903430, -2.886751345948125991, -5.000000000000000000 ) ) ;
#42031=CARTESIAN_POINT ( 'NONE',  ( 21.63750000122903572, -4.330127018922194537, 2.499999999999995559 ) ) ;
#42032=CARTESIAN_POINT ( 'NONE',  ( 17.39062500061451644, -3.027376345333610441, -5.243569643749999898 ) ) ;
#42033=CARTESIAN_POINT ( 'NONE',  ( 21.59062500061451928, 6.054752690667223547, 3.707466751127219781E-16 ) ) ;
#42034=CARTESIAN_POINT ( 'NONE',  ( 27.78750000122903074, 4.330127018922191873, 2.499999999999999556 ) ) ;
#42035=CARTESIAN_POINT ( 'NONE',  ( 25.80000000000000071, 4.330127018922192761, -2.499999999999997780 ) ) ;
#42037=AXIS2_PLACEMENT_3D ( 'NONE', #67318, #50324, #16677 ) ;
#42039=CARTESIAN_POINT ( 'NONE',  ( 28.95937500061451431, 0.000000000000000000, 5.243569643749999010 ) ) ;
#42040=CARTESIAN_POINT ( 'NONE',  ( 4.059357805649630002, -2.919411146374983446, -4.104029762320235086 ) ) ;
#42041=CARTESIAN_POINT ( 'NONE',  ( 4.243569643749999010, 13.82187500061451857, -32.45002607614398471 ) ) ;
#42042=CARTESIAN_POINT ( 'NONE',  ( 4.237500001229036251, 6.123233995736764310E-16, -4.999999999999998224 ) ) ;
#42043=CARTESIAN_POINT ( 'NONE',  ( 4.875000000000000888, -4.330127018922194537, 2.499999999999995559 ) ) ;
#42045=CARTESIAN_POINT ( 'NONE',  ( 7.771875000614516971, 3.027376345333611329, 5.243569643749999010 ) ) ;
#42046=CARTESIAN_POINT ( 'NONE',  ( 27.89062500061451289, 6.054752690667223547, 3.707466751127219781E-16 ) ) ;
#42048=CARTESIAN_POINT ( 'NONE',  ( 5.400000001229029678, -2.886751345948063374, 5.000000000000112799 ) ) ;
#42050=CARTESIAN_POINT ( 'NONE',  ( 6.084375000614518747, -4.541064518000419881, 2.621784821874995952 ) ) ;
#42051=CARTESIAN_POINT ( 'NONE',  ( 11.63437500061451857, 6.421520780324663323E-16, -5.243569643749999010 ) ) ;
#42052=EDGE_CURVE ( 'NONE', #19796, #59956, #53621, .T. ) ;
#42053=CARTESIAN_POINT ( 'NONE',  ( 4.875000000000000888, -4.330127018922194537, 2.499999999999995559 ) ) ;
#42054=CARTESIAN_POINT ( 'NONE',  ( 2.121784821874999061, 13.80312500061459602, 26.32496088578401583 ) ) ;
#42056=CARTESIAN_POINT ( 'NONE',  ( 6.899999999999999467, 4.330127018922192761, -2.499999999999997780 ) ) ;
#42058=CARTESIAN_POINT ( 'NONE',  ( 19.79062500061451502, 6.054752690667223547, 3.707466751127219781E-16 ) ) ;
#42059=CARTESIAN_POINT ( 'NONE',  ( 12.25312500061451537, 0.000000000000000000, 5.243569643749999010 ) ) ;
#42061=CARTESIAN_POINT ( 'NONE',  ( 9.046875000614518214, 6.054752690667223547, 3.707466751127219781E-16 ) ) ;
#42062=CARTESIAN_POINT ( 'NONE',  ( 26.09999999999999787, -4.330127018922190985, -2.500000000000001332 ) ) ;
#42063=CARTESIAN_POINT ( 'NONE',  ( 22.72500000122903430, 2.886751345948129099, -4.999999999999998224 ) ) ;
#42065=CARTESIAN_POINT ( 'NONE',  ( 9.796875000614519990, -3.027376345333610441, -5.243569643749999898 ) ) ;
#42066=CARTESIAN_POINT ( 'NONE',  ( 27.53437500061451360, 4.541064518000418104, 2.621784821874999949 ) ) ;
#42068=CARTESIAN_POINT ( 'NONE',  ( 8.737500001229033586, 6.123233995736764310E-16, -4.999999999999998224 ) ) ;
#42069=CARTESIAN_POINT ( 'NONE',  ( -3.999999999999999112, 12.87500000122903465, -32.30940107675850470 ) ) ;
#42070=ADVANCED_FACE ( 'NONE', ( #40454 ), #43033, .T. ) ;
#42071=CARTESIAN_POINT ( 'NONE',  ( 20.74687500061451573, 6.054752690667223547, 3.707466751127219781E-16 ) ) ;
#42072=CARTESIAN_POINT ( 'NONE',  ( 10.80937500061451928, 4.541064518000418104, -2.621784821874998173 ) ) ;
#42074=CARTESIAN_POINT ( 'NONE',  ( 24.56250000000000000, 2.886751345948126879, 4.999999999999999112 ) ) ;
#42076=CARTESIAN_POINT ( 'NONE',  ( 9.001249775931846008E-16, 12.77187500061451786, -25.09994784771203058 ) ) ;
#42078=CARTESIAN_POINT ( 'NONE',  ( 15.44062500061451537, -3.027376345333614438, 5.243569643749998122 ) ) ;
#42079=CARTESIAN_POINT ( 'NONE',  ( 4.612500000000002487, 2.886751345948129099, -4.999999999999998224 ) ) ;
#42082=CARTESIAN_POINT ( 'NONE',  ( 14.55000000000000071, 4.330127018922192761, -2.499999999999997780 ) ) ;
#42083=ADVANCED_FACE ( 'NONE', ( #66514 ), #55437, .F. ) ;
#42084=CARTESIAN_POINT ( 'NONE',  ( -2.000000000000000000, 17.33750000122903145, 26.53589838486224650 ) ) ;
#42085=CARTESIAN_POINT ( 'NONE',  ( 12.93750000122903465, 4.330127018922191873, 2.499999999999999556 ) ) ;
#42086=CARTESIAN_POINT ( 'NONE',  ( 24.72187500061451360, 3.027376345333613106, -5.243569643749998122 ) ) ;
#42087=CARTESIAN_POINT ( 'NONE',  ( 16.28437500061452070, 4.541064518000418104, 2.621784821874999949 ) ) ;
#42090=CARTESIAN_POINT ( 'NONE',  ( 19.22812500061451502, 6.421520780324663323E-16, -5.243569643749999010 ) ) ;
#42091=CARTESIAN_POINT ( 'NONE',  ( 3.140625000614516882, 6.054752690667223547, 3.707466751127219781E-16 ) ) ;
#42092=CARTESIAN_POINT ( 'NONE',  ( 18.79687500061451644, -3.027376345333610441, -5.243569643749999898 ) ) ;
#42093=CARTESIAN_POINT ( 'NONE',  ( 28.20937500061451786, -4.541064518000417216, -2.621784821875001281 ) ) ;
#42094=CARTESIAN_POINT ( 'NONE',  ( 4.978125000614518569, 4.541064518000418104, 2.621784821874999949 ) ) ;
#42095=CARTESIAN_POINT ( 'NONE',  ( 22.97812500061451857, 4.541064518000418104, 2.621784821874999949 ) ) ;
#42096=CARTESIAN_POINT ( 'NONE',  ( -4.243569643749999898, 15.71562500061451573, 27.54997392385601529 ) ) ;
#42097=CARTESIAN_POINT ( 'NONE',  ( 15.60000000122903607, 5.773502691896255534, 3.535250795749688894E-16 ) ) ;
#42099=CARTESIAN_POINT ( 'NONE',  ( 6.815625000614518925, 3.027376345333611329, 5.243569643749999010 ) ) ;
#42100=DIRECTION ( 'NONE',  ( -0.000000000000000000, -1.000000000000000000, -0.000000000000000000 ) ) ;
#42101=CARTESIAN_POINT ( 'NONE',  ( 28.71562500061451573, 3.027376345333613106, -5.243569643749998122 ) ) ;
#42102=CARTESIAN_POINT ( 'NONE',  ( 22.92187500061451644, 3.027376345333613106, -5.243569643749998122 ) ) ;
#42103=CARTESIAN_POINT ( 'NONE',  ( 15.06562500061451537, -6.054752690667223547, -1.112240025338166033E-15 ) ) ;
#42104=CARTESIAN_POINT ( 'NONE',  ( 23.70000000122903216, 5.773502691896255534, 3.535250795749688894E-16 ) ) ;
#42105=CARTESIAN_POINT ( 'NONE',  ( 24.32812500061451289, 4.541064518000418104, 2.621784821874999949 ) ) ;
#42106=CARTESIAN_POINT ( 'NONE',  ( 20.22187500061451715, 3.027376345333613106, -5.243569643749998122 ) ) ;
#42107=CARTESIAN_POINT ( 'NONE',  ( 13.64062500061451644, -3.027376345333614438, 5.243569643749998122 ) ) ;
#42108=CARTESIAN_POINT ( 'NONE',  ( 4.243569643749999898, 14.64687500061451964, 32.45002607614398471 ) ) ;
#42109=CARTESIAN_POINT ( 'NONE',  ( 19.49062500061451431, -3.027376345333614438, 5.243569643749998122 ) ) ;
#42110=CARTESIAN_POINT ( 'NONE',  ( 28.64062500061451289, -3.027376345333610441, -5.243569643749999898 ) ) ;
#42111=ORIENTED_EDGE ( 'NONE', *, *, #336, .F. ) ;
#42112=CARTESIAN_POINT ( 'NONE',  ( 26.21249999999999858, 2.886751345948129099, -4.999999999999998224 ) ) ;
#42113=CARTESIAN_POINT ( 'NONE',  ( -2.828200636599751609E-16, 10.88750000000000107, -34.61880215351700230 ) ) ;
#42114=CARTESIAN_POINT ( 'NONE',  ( 26.84062500061451573, -3.027376345333610441, -5.243569643749999898 ) ) ;
#42115=CARTESIAN_POINT ( 'NONE',  ( 8.353125000614518569, -4.541064518000417216, -2.621784821875001281 ) ) ;
#42116=CARTESIAN_POINT ( 'NONE',  ( 20.32500000122903572, -5.773502691896255534, -1.060575238724906372E-15 ) ) ;
#42117=CARTESIAN_POINT ( 'NONE',  ( 23.69062500061451004, -3.027376345333610441, -5.243569643749999898 ) ) ;
#42118=CARTESIAN_POINT ( 'NONE',  ( 25.98750000000000071, -2.886751345948129988, 4.999999999999997335 ) ) ;
#42119=CARTESIAN_POINT ( 'NONE',  ( 28.86562500061451786, 3.027376345333611329, 5.243569643749999010 ) ) ;
#42120=CARTESIAN_POINT ( 'NONE',  ( 7.753125000614518036, 0.000000000000000000, 5.243569643749999010 ) ) ;
#42122=CARTESIAN_POINT ( 'NONE',  ( 26.57812500061451644, 4.541064518000418104, 2.621784821874999949 ) ) ;
#42123=CARTESIAN_POINT ( 'NONE',  ( 5.803125000614517859, 4.541064518000418104, -2.621784821874998173 ) ) ;
#42125=CARTESIAN_POINT ( 'NONE',  ( 0.000000000000000000, 20.00000000000000000, 30.00000000000000000 ) ) ;
#42126=VECTOR ( 'NONE', #5667, 1000.000000000000000 ) ;
#42127=CARTESIAN_POINT ( 'NONE',  ( 13.91249999999999964, -5.773502691896255534, -1.060575238724906372E-15 ) ) ;
#42128=CARTESIAN_POINT ( 'NONE',  ( 14.18437500061451750, -4.541064518000419881, 2.621784821874995952 ) ) ;
#42129=CARTESIAN_POINT ( 'NONE',  ( 9.150000001229033231, -2.886751345948125991, -5.000000000000000000 ) ) ;
#42130=CARTESIAN_POINT ( 'NONE',  ( 17.22187500061451715, 3.027376345333611329, 5.243569643749999010 ) ) ;
#42132=CARTESIAN_POINT ( 'NONE',  ( 9.571875000614518569, 3.027376345333611329, 5.243569643749999010 ) ) ;
#42133=CARTESIAN_POINT ( 'NONE',  ( 9.001249775931846008E-16, 12.26562500061451644, -25.09994784771203058 ) ) ;
#42134=FACE_OUTER_BOUND ( 'NONE', #50171, .T. ) ;
#42136=ORIENTED_EDGE ( 'NONE', *, *, #50186, .F. ) ;
#42137=CARTESIAN_POINT ( 'NONE',  ( 25.00312500061451715, -4.541064518000417216, -2.621784821875001281 ) ) ;
#42138=CARTESIAN_POINT ( 'NONE',  ( 4.243569643749999010, 10.22187500061451892, 27.54997392385601174 ) ) ;
#42140=CARTESIAN_POINT ( 'NONE',  ( 26.48437500061451644, 6.421520780324663323E-16, -5.243569643749999010 ) ) ;
#42141=CARTESIAN_POINT ( 'NONE',  ( 27.94687500061451502, 6.054752690667223547, 3.707466751127219781E-16 ) ) ;
#42142=CARTESIAN_POINT ( 'NONE',  ( 3.590625000614518836, 6.054752690667223547, 3.707466751127219781E-16 ) ) ;
#42144=CARTESIAN_POINT ( 'NONE',  ( 16.28437500061452070, 4.541064518000418104, 2.621784821874999949 ) ) ;
#42146=CARTESIAN_POINT ( 'NONE',  ( 3.215625000614518836, 3.027376345333611329, 5.243569643749999010 ) ) ;
#42147=CARTESIAN_POINT ( 'NONE',  ( 7.096875000614517148, -3.027376345333610441, -5.243569643749999898 ) ) ;
#42148=CARTESIAN_POINT ( 'NONE',  ( 17.10937500061451999, 4.541064518000418104, -2.621784821874998173 ) ) ;
#42150=CARTESIAN_POINT ( 'NONE',  ( 26.58750000000000213, -2.886751345948125991, -5.000000000000000000 ) ) ;
#42151=CARTESIAN_POINT ( 'NONE',  ( 27.79687500061451999, -3.027376345333610441, -5.243569643749999898 ) ) ;
#42153=CARTESIAN_POINT ( 'NONE',  ( 29.84999999999999787, 4.330127018922192761, -2.499999999999997780 ) ) ;
#42154=ORIENTED_EDGE ( 'NONE', *, *, #38075, .F. ) ;
#42155=CARTESIAN_POINT ( 'NONE',  ( 8.212500000000000355, 2.886751345948129099, -4.999999999999998224 ) ) ;
#42157=CARTESIAN_POINT ( 'NONE',  ( 22.86562500061451431, 3.027376345333613106, -5.243569643749998122 ) ) ;
#42158=CARTESIAN_POINT ( 'NONE',  ( 12.41249999999999964, 2.886751345948126879, 4.999999999999999112 ) ) ;
#42159=CARTESIAN_POINT ( 'NONE',  ( 7.762500001229033053, -4.330127018922190985, -2.500000000000001332 ) ) ;
#42160=CARTESIAN_POINT ( 'NONE',  ( 6.890625000614516438, -3.027376345333614438, 5.243569643749998122 ) ) ;
#42161=CARTESIAN_POINT ( 'NONE',  ( 22.61250000000000071, 2.886751345948129099, -4.999999999999998224 ) ) ;
#42162=EDGE_CURVE ( 'NONE', #37978, #12333, #60930, .T. ) ;
#42163=CARTESIAN_POINT ( 'NONE',  ( 19.64062500061451644, -3.027376345333610441, -5.243569643749999898 ) ) ;
#42164=CARTESIAN_POINT ( 'NONE',  ( 14.81250000000000178, -5.773502691896255534, -1.060575238724906372E-15 ) ) ;
#42165=CARTESIAN_POINT ( 'NONE',  ( 25.16250000122903074, 0.000000000000000000, 4.999999999999998224 ) ) ;
#42167=CARTESIAN_POINT ( 'NONE',  ( 6.187500000000002665, -2.886751345948129988, 4.999999999999997335 ) ) ;
#42168=ORIENTED_EDGE ( 'NONE', *, *, #29620, .F. ) ;
#42169=CARTESIAN_POINT ( 'NONE',  ( 20.50312500061451715, -4.541064518000417216, -2.621784821875001281 ) ) ;
#42170=CARTESIAN_POINT ( 'NONE',  ( 25.67812500061451431, 4.541064518000418104, 2.621784821874999949 ) ) ;
#42171=CARTESIAN_POINT ( 'NONE',  ( 26.59687500061451360, 6.054752690667223547, 3.707466751127219781E-16 ) ) ;
#42172=CARTESIAN_POINT ( 'NONE',  ( 9.674999999999998934, 4.330127018922191873, 2.499999999999999556 ) ) ;
#42173=CARTESIAN_POINT ( 'NONE',  ( 10.82812500061451644, 4.541064518000418104, 2.621784821874999949 ) ) ;
#42174=CARTESIAN_POINT ( 'NONE',  ( 4.898587196589411843E-16, 20.00000000000000000, 33.99999999999999289 ) ) ;
#42175=CARTESIAN_POINT ( 'NONE',  ( 8.503125000614515372, 4.541064518000418104, -2.621784821874998173 ) ) ;
#42177=CARTESIAN_POINT ( 'NONE',  ( 9.001249775931846008E-16, 12.77187500061451786, 34.90005215228797653 ) ) ;
#42178=VECTOR ( 'NONE', #11294, 1000.000000000000000 ) ;
#42179=CARTESIAN_POINT ( 'NONE',  ( 24.78750000122903074, -4.330127018922194537, 2.499999999999995559 ) ) ;
#42181=CARTESIAN_POINT ( 'NONE',  ( 13.52812500061451750, 4.541064518000418104, 2.621784821874999949 ) ) ;
#42182=CARTESIAN_POINT ( 'NONE',  ( 11.03437500061451715, -4.541064518000419881, 2.621784821874995952 ) ) ;
#42183=CARTESIAN_POINT ( 'NONE',  ( 9.684375000614517504, -4.541064518000419881, 2.621784821874995952 ) ) ;
#42184=CARTESIAN_POINT ( 'NONE',  ( 17.10937500061451999, 4.541064518000418104, -2.621784821874998173 ) ) ;
#42185=EDGE_LOOP ( 'NONE', ( #43886, #20286, #1218, #42963, #30431, #58938, #64976 ) ) ;
#42186=CARTESIAN_POINT ( 'NONE',  ( 28.99687500061451573, -3.027376345333614438, 5.243569643749998122 ) ) ;
#42187=CARTESIAN_POINT ( 'NONE',  ( 21.02812500061451573, 6.421520780324663323E-16, -5.243569643749999010 ) ) ;
#42188=( BOUNDED_CURVE ( )  B_SPLINE_CURVE ( 2, ( #25447, #36529, #59049, #47990, #8454, #30989, #53522 ),
 .UNSPECIFIED., .F., .F. ) 
 B_SPLINE_CURVE_WITH_KNOTS ( ( 3, 2, 2, 3 ),
 ( 0.1583333333333333814, 0.1611111111111111771, 0.1638888888888889173, 0.1666666666666666852 ),
 .UNSPECIFIED. ) 
 CURVE ( )  GEOMETRIC_REPRESENTATION_ITEM ( )  RATIONAL_B_SPLINE_CURVE ( ( 0.9999999999999973355, 0.8660254037844413721, 1.000000000000000000, 0.8660254037844387076, 1.000000000000000000, 0.8660254037844373753, 1.000000000000001332 ) ) 
 REPRESENTATION_ITEM ( '' )  );
#42189=CARTESIAN_POINT ( 'NONE',  ( 15.72187500061451892, 3.027376345333613106, -5.243569643749998122 ) ) ;
#42190=CARTESIAN_POINT ( 'NONE',  ( 21.10312500061451502, 4.541064518000418104, -2.621784821874998173 ) ) ;
#42191=CARTESIAN_POINT ( 'NONE',  ( -3.999999999999999112, 13.25000000000000178, 30.00000000000000000 ) ) ;
#42192=CARTESIAN_POINT ( 'NONE',  ( 26.99062500061451431, 6.054752690667223547, 3.707466751127219781E-16 ) ) ;
#42193=CARTESIAN_POINT ( 'NONE',  ( 8.137500001229033941, -4.330127018922194537, 2.499999999999995559 ) ) ;
#42194=VERTEX_POINT ( 'NONE', #19318 ) ;
#42195=CARTESIAN_POINT ( 'NONE',  ( 4.425000001229032698, 2.886751345948126879, 4.999999999999999112 ) ) ;
#42196=CARTESIAN_POINT ( 'NONE',  ( 8.484601909799253346E-16, 17.41250000000000142, -25.38119784648299770 ) ) ;
#42197=CARTESIAN_POINT ( 'NONE',  ( 25.53750000122903074, 4.330127018922191873, 2.499999999999999556 ) ) ;
#42199=CARTESIAN_POINT ( 'NONE',  ( 7.396875000614519635, -3.027376345333614438, 5.243569643749998122 ) ) ;
#42200=CARTESIAN_POINT ( 'NONE',  ( 23.25000000000000000, 0.000000000000000000, 4.999999999999998224 ) ) ;
#42201=CARTESIAN_POINT ( 'NONE',  ( 15.29062500061451679, 6.054752690667223547, 3.707466751127219781E-16 ) ) ;
#42202=CARTESIAN_POINT ( 'NONE',  ( 9.234375000614518214, -4.541064518000419881, 2.621784821874995952 ) ) ;
#42203=CARTESIAN_POINT ( 'NONE',  ( 26.58750000122903145, -4.330127018922194537, 2.499999999999995559 ) ) ;
#42204=CARTESIAN_POINT ( 'NONE',  ( 18.15937500061451715, 0.000000000000000000, 5.243569643749999010 ) ) ;
#42205=CARTESIAN_POINT ( 'NONE',  ( 5.484375000614518214, 4.541064518000418104, 2.621784821874999949 ) ) ;
#42206=DIRECTION ( 'NONE',  ( -0.000000000000000000, -1.000000000000000000, -0.000000000000000000 ) ) ;
#42207=CARTESIAN_POINT ( 'NONE',  ( 5.465625000614517504, 3.027376345333611329, 5.243569643749999010 ) ) ;
#42208=CARTESIAN_POINT ( 'NONE',  ( 18.40312500061451573, 4.541064518000418104, -2.621784821874998173 ) ) ;
#42209=ORIENTED_EDGE ( 'NONE', *, *, #47090, .T. ) ;
#42210=CARTESIAN_POINT ( 'NONE',  ( 13.00312500061451537, 4.541064518000418104, -2.621784821874998173 ) ) ;
#42211=CARTESIAN_POINT ( 'NONE',  ( 4.837500001229035895, 4.330127018922191873, 2.499999999999999556 ) ) ;
#42212=CARTESIAN_POINT ( 'NONE',  ( 11.87812500061451537, -4.541064518000419881, 2.621784821874995952 ) ) ;
#42214=CARTESIAN_POINT ( 'NONE',  ( 10.05000000000000071, 4.330127018922192761, -2.499999999999997780 ) ) ;
#42215=CARTESIAN_POINT ( 'NONE',  ( 6.750000001229033764, -2.886751345948129988, 4.999999999999997335 ) ) ;
#42216=CARTESIAN_POINT ( 'NONE',  ( 19.79999999999999716, -4.330127018922190985, -2.500000000000001332 ) ) ;
#42217=CARTESIAN_POINT ( 'NONE',  ( 14.10937500061451644, 0.000000000000000000, 5.243569643749999010 ) ) ;
#42218=CARTESIAN_POINT ( 'NONE',  ( 15.67500000122903181, 2.886751345948126879, 4.999999999999999112 ) ) ;
#42220=CARTESIAN_POINT ( 'NONE',  ( -2.121784821874999949, 18.82812500061451644, -33.67503911421598417 ) ) ;
#42221=DIRECTION ( 'NONE',  ( -0.000000000000000000, -1.000000000000000000, -0.000000000000000000 ) ) ;
#42222=CARTESIAN_POINT ( 'NONE',  ( 1.999999999999998668, 15.01250000122903394, -33.46410161513775705 ) ) ;
#42223=CYLINDRICAL_SURFACE ( 'NONE', #71363, 3.999999999999996447 ) ;
#42224=CARTESIAN_POINT ( 'NONE',  ( 1.071796769724490339, 19.86740381056766225, 26.00000000000000355 ) ) ;
#42225=CARTESIAN_POINT ( 'NONE',  ( 4.809916128174254624, -1.365542690628744449, -5.062639209831853115 ) ) ;
#42226=CARTESIAN_POINT ( 'NONE',  ( 15.45937500061451608, 0.000000000000000000, 5.243569643749999010 ) ) ;
#42227=CARTESIAN_POINT ( 'NONE',  ( 28.08749999999999858, 5.773502691896255534, 3.535250795749688894E-16 ) ) ;
#42228=CARTESIAN_POINT ( 'NONE',  ( 10.90312500061451928, 0.000000000000000000, 5.243569643749999010 ) ) ;
#42230=CARTESIAN_POINT ( 'NONE',  ( 22.92187500061451644, 3.027376345333613106, -5.243569643749998122 ) ) ;
#42232=CARTESIAN_POINT ( 'NONE',  ( 9.403125000614517504, 4.541064518000418104, -2.621784821874998173 ) ) ;
#42233=CARTESIAN_POINT ( 'NONE',  ( 15.08437500061451786, -4.541064518000419881, 2.621784821874995952 ) ) ;
#42234=ORIENTED_EDGE ( 'NONE', *, *, #18001, .T. ) ;
#42235=CARTESIAN_POINT ( 'NONE',  ( 27.08437500061451786, 4.541064518000418104, 2.621784821874999949 ) ) ;
#42236=CARTESIAN_POINT ( 'NONE',  ( 26.95312500061451644, 4.541064518000418104, -2.621784821874998173 ) ) ;
#42237=CARTESIAN_POINT ( 'NONE',  ( 28.34062500061451928, 6.054752690667223547, 3.707466751127219781E-16 ) ) ;
#42238=EDGE_CURVE ( 'NONE', #63662, #23724, #53831, .T. ) ;
#42239=CYLINDRICAL_SURFACE ( 'NONE', #37236, 4.000000000000000000 ) ;
#42240=CARTESIAN_POINT ( 'NONE',  ( 7.950000000000001954, 0.000000000000000000, 4.999999999999998224 ) ) ;
#42241=CARTESIAN_POINT ( 'NONE',  ( 16.87500000122903288, 2.886751345948129099, -4.999999999999998224 ) ) ;
#42244=ORIENTED_EDGE ( 'NONE', *, *, #37713, .T. ) ;
#42245=CARTESIAN_POINT ( 'NONE',  ( 14.55000000000000071, 4.330127018922192761, -2.499999999999997780 ) ) ;
#42246=CARTESIAN_POINT ( 'NONE',  ( 19.42499999999999716, 6.123233995736764310E-16, -4.999999999999998224 ) ) ;
#42247=CARTESIAN_POINT ( 'NONE',  ( 13.49062500061451608, 6.054752690667223547, 3.707466751127219781E-16 ) ) ;
#42248=ORIENTED_EDGE ( 'NONE', *, *, #57822, .T. ) ;
#42249=CARTESIAN_POINT ( 'NONE',  ( -5.810221930991193690E-16, 18.65000000122903501, -34.00000000000000000 ) ) ;
#42250=CARTESIAN_POINT ( 'NONE',  ( 4.243569643749999898, 17.79687500061451999, -27.54997392385601529 ) ) ;
#42251=CARTESIAN_POINT ( 'NONE',  ( 5.578125000614518214, -4.541064518000419881, 2.621784821874995952 ) ) ;
#42253=CARTESIAN_POINT ( 'NONE',  ( 11.21250000000000036, -5.773502691896255534, -1.060575238724906372E-15 ) ) ;
#42256=CARTESIAN_POINT ( 'NONE',  ( 4.243569643749999898, 14.14062500061451644, 32.45002607614398471 ) ) ;
#42257=CARTESIAN_POINT ( 'NONE',  ( 25.60312500061451502, 4.541064518000418104, -2.621784821874998173 ) ) ;
#42260=CARTESIAN_POINT ( 'NONE',  ( 23.03437500061451715, 4.541064518000418104, 2.621784821874999949 ) ) ;
#42261=CARTESIAN_POINT ( 'NONE',  ( 22.19062500061451715, -3.027376345333614438, 5.243569643749998122 ) ) ;
#42262=CARTESIAN_POINT ( 'NONE',  ( 4.243569643749999898, 14.59062500061459744, -27.54997392385601529 ) ) ;
#42263=CARTESIAN_POINT ( 'NONE',  ( 22.42500000122903359, 2.886751345948126879, 4.999999999999999112 ) ) ;
#42264=CARTESIAN_POINT ( 'NONE',  ( 5.540625000614515905, -3.027376345333614438, 5.243569643749998122 ) ) ;
#42266=CARTESIAN_POINT ( 'NONE',  ( 24.02812500061451573, -4.541064518000419881, 2.621784821874995952 ) ) ;
#42269=CARTESIAN_POINT ( 'NONE',  ( 16.69687500061451502, 6.054752690667223547, 3.707466751127219781E-16 ) ) ;
#42270=CARTESIAN_POINT ( 'NONE',  ( 25.73437500061451644, 4.541064518000418104, 2.621784821874999949 ) ) ;
#42271=CARTESIAN_POINT ( 'NONE',  ( -2.121784821874999949, 14.38437500061451679, 26.32496088578401938 ) ) ;
#42272=CARTESIAN_POINT ( 'NONE',  ( 6.253125000614517148, 4.541064518000418104, -2.621784821874998173 ) ) ;
#42273=CARTESIAN_POINT ( 'NONE',  ( 29.05312500061451431, -4.541064518000417216, -2.621784821875001281 ) ) ;
#42274=CARTESIAN_POINT ( 'NONE',  ( 29.31562500061451715, 3.027376345333611329, 5.243569643749999010 ) ) ;
#42276=CARTESIAN_POINT ( 'NONE',  ( 3.286795329855858760, 3.767887532774327308, -3.286795329856085690 ) ) ;
#42277=CARTESIAN_POINT ( 'NONE',  ( 29.32500000122903216, -5.773502691896255534, -1.060575238724906372E-15 ) ) ;
#42278=CARTESIAN_POINT ( 'NONE',  ( 8.259375000614518569, 0.000000000000000000, 5.243569643749999010 ) ) ;
#42279=CARTESIAN_POINT ( 'NONE',  ( 14.47500000122903430, -5.773502691896255534, -1.060575238724906372E-15 ) ) ;
#42280=CARTESIAN_POINT ( 'NONE',  ( 2.971875000614517592, -6.054752690667223547, -1.112240025338166033E-15 ) ) ;
#42281=CARTESIAN_POINT ( 'NONE',  ( 12.37500000122903465, 2.886751345948129099, -4.999999999999998224 ) ) ;
#42282=CARTESIAN_POINT ( 'NONE',  ( 4.078125000614517326, 4.541064518000418104, 2.621784821874999949 ) ) ;
#42285=CARTESIAN_POINT ( 'NONE',  ( 15.42187500061451821, 3.027376345333611329, 5.243569643749999010 ) ) ;
#42286=CARTESIAN_POINT ( 'NONE',  ( 5.000000000000000000, 6.123233995736766282E-16, -50.00000000000000000 ) ) ;
#42287=ORIENTED_EDGE ( 'NONE', *, *, #7766, .F. ) ;
#42288=CARTESIAN_POINT ( 'NONE',  ( 22.07812500061451644, 4.541064518000418104, 2.621784821874999949 ) ) ;
#42289=CARTESIAN_POINT ( 'NONE',  ( 8.390625000614518214, -3.027376345333610441, -5.243569643749999898 ) ) ;
#42290=CARTESIAN_POINT ( 'NONE',  ( 24.57187500061451502, -6.054752690667223547, -1.112240025338166033E-15 ) ) ;
#42291=CARTESIAN_POINT ( 'NONE',  ( 7.640625000614517326, 6.054752690667223547, 3.707466751127219781E-16 ) ) ;
#42292=CARTESIAN_POINT ( 'NONE',  ( 30.00000000000000000, 0.000000000000000000, 0.000000000000000000 ) ) ;
#42293=CARTESIAN_POINT ( 'NONE',  ( 8.400000001229035007, 5.773502691896255534, 3.535250795749688894E-16 ) ) ;
#42294=CARTESIAN_POINT ( 'NONE',  ( 24.47812500061451502, -4.541064518000419881, 2.621784821874995952 ) ) ;
#42295=CARTESIAN_POINT ( 'NONE',  ( 2.000000000000001332, 19.36250000122903359, -26.53589838486224650 ) ) ;
#42296=CARTESIAN_POINT ( 'NONE',  ( 9.375000001229036428, 2.886751345948126879, 4.999999999999999112 ) ) ;
#42297=CARTESIAN_POINT ( 'NONE',  ( 18.66562500061451146, -6.054752690667223547, -1.112240025338166033E-15 ) ) ;
#42298=CARTESIAN_POINT ( 'NONE',  ( 17.84062500061451573, -3.027376345333610441, -5.243569643749999898 ) ) ;
#42300=CARTESIAN_POINT ( 'NONE',  ( 17.55000000000000071, -4.330127018922190985, -2.500000000000001332 ) ) ;
#42301=CARTESIAN_POINT ( 'NONE',  ( 13.65000000122903323, -2.886751345948125991, -5.000000000000000000 ) ) ;
#42302=CARTESIAN_POINT ( 'NONE',  ( 10.00312500061451715, 0.000000000000000000, 5.243569643749999010 ) ) ;
#42303=CARTESIAN_POINT ( 'NONE',  ( 13.75312500061451715, -4.541064518000417216, -2.621784821875001281 ) ) ;
#42304=EDGE_CURVE ( 'NONE', #12333, #72145, #27949, .T. ) ;
#42305=CARTESIAN_POINT ( 'NONE',  ( 23.21250000122903501, 4.330127018922192761, -2.499999999999997780 ) ) ;
#42306=CARTESIAN_POINT ( 'NONE',  ( 21.27187500061451786, 3.027376345333611329, 5.243569643749999010 ) ) ;
#42307=CARTESIAN_POINT ( 'NONE',  ( 21.23437500061451644, 4.541064518000418104, 2.621784821874999949 ) ) ;
#42310=CARTESIAN_POINT ( 'NONE',  ( 8.062500001229034652, 0.000000000000000000, 4.999999999999998224 ) ) ;
#42311=CARTESIAN_POINT ( 'NONE',  ( 7.659375000614518036, 4.541064518000418104, -2.621784821874998173 ) ) ;
#42312=CARTESIAN_POINT ( 'NONE',  ( 23.40937500061451715, 4.541064518000418104, -2.621784821874998173 ) ) ;
#42313=EDGE_CURVE ( 'NONE', #26824, #41179, #30788, .T. ) ;
#42315=CARTESIAN_POINT ( 'NONE',  ( 18.02812500061451573, 4.541064518000418104, 2.621784821874999949 ) ) ;
#42316=CARTESIAN_POINT ( 'NONE',  ( 24.53437500061451715, -4.541064518000419881, 2.621784821874995952 ) ) ;
#42320=CARTESIAN_POINT ( 'NONE',  ( 5.596875000614516260, -3.027376345333614438, 5.243569643749998122 ) ) ;
#42321=CARTESIAN_POINT ( 'NONE',  ( 18.36562500061451431, 3.027376345333613106, -5.243569643749998122 ) ) ;
#42322=VERTEX_POINT ( 'NONE', #23783 ) ;
#42323=CARTESIAN_POINT ( 'NONE',  ( 25.16250000000000142, -5.773502691896255534, -1.060575238724906372E-15 ) ) ;
#42324=CARTESIAN_POINT ( 'NONE',  ( 24.70312500061451644, 4.541064518000418104, -2.621784821874998173 ) ) ;
#42325=FACE_OUTER_BOUND ( 'NONE', #15658, .T. ) ;
#42327=CARTESIAN_POINT ( 'NONE',  ( 14.92500000000000071, 6.123233995736764310E-16, -4.999999999999998224 ) ) ;
#42328=CARTESIAN_POINT ( 'NONE',  ( 25.46250000122903501, 4.330127018922192761, -2.499999999999997780 ) ) ;
#42329=CARTESIAN_POINT ( 'NONE',  ( 20.12812500061451715, 6.421520780324663323E-16, -5.243569643749999010 ) ) ;
#42330=VERTEX_POINT ( 'NONE', #69235 ) ;
#42331=CARTESIAN_POINT ( 'NONE',  ( 22.53750000000000142, -2.886751345948125991, -5.000000000000000000 ) ) ;
#42333=CARTESIAN_POINT ( 'NONE',  ( 24.94687500061451502, -3.027376345333614438, 5.243569643749998122 ) ) ;
#42334=ORIENTED_EDGE ( 'NONE', *, *, #12948, .T. ) ;
#42335=B_SPLINE_CURVE_WITH_KNOTS ( 'NONE', 3,
 ( #9337, #3804, #64745, #31129, #65111, #59190, #26327, #8600, #20402, #53670 ),
 .UNSPECIFIED., .F., .F.,
 ( 4, 3, 3, 4 ),
 ( 0.000000000000000000, 2.812505701543726881E-05, 5.625011473905447835E-05, 9.076251227131168335E-05 ),
 .UNSPECIFIED. ) ;
#42337=CARTESIAN_POINT ( 'NONE',  ( 13.26562500061451644, -6.054752690667223547, -1.112240025338166033E-15 ) ) ;
#42338=CARTESIAN_POINT ( 'NONE',  ( 4.303125000614516971, -4.541064518000417216, -2.621784821875001281 ) ) ;
#42340=CARTESIAN_POINT ( 'NONE',  ( 3.346875000614518036, -3.027376345333614438, 5.243569643749998122 ) ) ;
#42341=CARTESIAN_POINT ( 'NONE',  ( 13.05000000122903536, -2.886751345948129988, 4.999999999999997335 ) ) ;
#42342=CARTESIAN_POINT ( 'NONE',  ( 18.52499999999999858, 6.123233995736764310E-16, -4.999999999999998224 ) ) ;
#42343=CARTESIAN_POINT ( 'NONE',  ( 27.89999999999999858, -4.330127018922190985, -2.500000000000001332 ) ) ;
#42345=CARTESIAN_POINT ( 'NONE',  ( 6.796875000614516438, 6.054752690667223547, 3.707466751127219781E-16 ) ) ;
#42346=CARTESIAN_POINT ( 'NONE',  ( 20.10937500061451289, -4.541064518000417216, -2.621784821875001281 ) ) ;
#42347=CARTESIAN_POINT ( 'NONE',  ( -2.000000000000000000, 13.73750000122903359, 26.53589838486224650 ) ) ;
#42348=ORIENTED_EDGE ( 'NONE', *, *, #33365, .T. ) ;
#42349=CARTESIAN_POINT ( 'NONE',  ( 29.39062500061451289, -3.027376345333614438, 5.243569643749998122 ) ) ;
#42350=CARTESIAN_POINT ( 'NONE',  ( 3.712499999999999911, 2.886751345948129099, -4.999999999999998224 ) ) ;
#42351=CARTESIAN_POINT ( 'NONE',  ( 4.509375000614518569, 4.541064518000418104, -2.621784821874998173 ) ) ;
#42352=ADVANCED_FACE ( 'NONE', ( #58118 ), #13412, .F. ) ;
#42353=CARTESIAN_POINT ( 'NONE',  ( 15.37500000000000000, 6.123233995736764310E-16, -4.999999999999998224 ) ) ;
#42354=CARTESIAN_POINT ( 'NONE',  ( 14.24062500061451608, -3.027376345333610441, -5.243569643749999898 ) ) ;
#42358=CARTESIAN_POINT ( 'NONE',  ( 17.51250000122903216, 0.000000000000000000, 4.999999999999998224 ) ) ;
#42359=DIRECTION ( 'NONE',  ( -0.000000000000000000, -1.000000000000000000, -0.000000000000000000 ) ) ;
#42361=CARTESIAN_POINT ( 'NONE',  ( 8.653125000614515727, 0.000000000000000000, 5.243569643749999010 ) ) ;
#42362=CARTESIAN_POINT ( 'NONE',  ( 23.48437500061451644, 4.541064518000418104, 2.621784821874999949 ) ) ;
#42363=CARTESIAN_POINT ( 'NONE',  ( -4.243569643749999898, 18.05937500061451928, 30.00000000000000000 ) ) ;
#42364=CARTESIAN_POINT ( 'NONE',  ( 23.29687500061451644, -3.027376345333610441, -5.243569643749999898 ) ) ;
#42365=CARTESIAN_POINT ( 'NONE',  ( 4.387500000000002842, -2.886751345948129988, 4.999999999999997335 ) ) ;
#42366=CARTESIAN_POINT ( 'NONE',  ( 3.999999999999998668, 10.02500000122903501, 27.69059892324149175 ) ) ;
#42367=CARTESIAN_POINT ( 'NONE',  ( 13.49062500061451608, 6.054752690667223547, 3.707466751127219781E-16 ) ) ;
#42368=CARTESIAN_POINT ( 'NONE',  ( 3.450000001229036162, 5.773502691896255534, 3.535250795749688894E-16 ) ) ;
#42369=CARTESIAN_POINT ( 'NONE',  ( 8.934375000614517504, 6.421520780324663323E-16, -5.243569643749999010 ) ) ;
#42372=CARTESIAN_POINT ( 'NONE',  ( 11.16562500061451679, 3.027376345333613106, -5.243569643749998122 ) ) ;
#42373=CARTESIAN_POINT ( 'NONE',  ( 15.57187500061451679, -6.054752690667223547, -1.112240025338166033E-15 ) ) ;
#42375=CARTESIAN_POINT ( 'NONE',  ( 24.67500000122903359, 2.886751345948126879, 4.999999999999999112 ) ) ;
#42376=CARTESIAN_POINT ( 'NONE',  ( 9.346875000614517148, -3.027376345333610441, -5.243569643749999898 ) ) ;
#42377=CARTESIAN_POINT ( 'NONE',  ( 11.12812500061451715, 6.421520780324663323E-16, -5.243569643749999010 ) ) ;
#42379=CARTESIAN_POINT ( 'NONE',  ( 21.90937500061451715, -4.541064518000417216, -2.621784821875001281 ) ) ;
#42381=CARTESIAN_POINT ( 'NONE',  ( 5.475000000000000533, 6.123233995736764310E-16, -4.999999999999998224 ) ) ;
#42383=CARTESIAN_POINT ( 'NONE',  ( 2.121784821875001281, 15.50937500061451857, -26.32496088578401938 ) ) ;
#42384=CARTESIAN_POINT ( 'NONE',  ( 15.90937500061451892, 0.000000000000000000, 5.243569643749999010 ) ) ;
#42385=CARTESIAN_POINT ( 'NONE',  ( 16.57500000122903216, 2.886751345948126879, 4.999999999999999112 ) ) ;
#42386=CARTESIAN_POINT ( 'NONE',  ( 11.22187500061451892, 3.027376345333613106, -5.243569643749998122 ) ) ;
#42387=CARTESIAN_POINT ( 'NONE',  ( 2.121784821875001281, 17.70312500061451644, -26.32496088578401938 ) ) ;
#42388=CARTESIAN_POINT ( 'NONE',  ( 16.72500000122903430, -5.773502691896255534, -1.060575238724906372E-15 ) ) ;
#42389=CARTESIAN_POINT ( 'NONE',  ( 11.84062500061451750, -3.027376345333614438, 5.243569643749998122 ) ) ;
#42391=CARTESIAN_POINT ( 'NONE',  ( 15.11249999999999893, 2.886751345948126879, 4.999999999999999112 ) ) ;
#42392=CARTESIAN_POINT ( 'NONE',  ( 5.062500001229035540, -4.330127018922190985, -2.500000000000001332 ) ) ;
#42393=CARTESIAN_POINT ( 'NONE',  ( 10.32187500061451679, 3.027376345333612662, -5.243569643749998122 ) ) ;
#42394=CARTESIAN_POINT ( 'NONE',  ( 4.060897850599462622, 2.917037649225213247, 4.254917590412954809 ) ) ;
#42395=CARTESIAN_POINT ( 'NONE',  ( 12.75000000122903643, -2.886751345948125991, -5.000000000000000000 ) ) ;
#42396=CARTESIAN_POINT ( 'NONE',  ( 21.75000000122903288, -2.886751345948125991, -5.000000000000000000 ) ) ;
#42397=CARTESIAN_POINT ( 'NONE',  ( 16.79062500061451857, -3.027376345333614438, 5.243569643749998122 ) ) ;
#42398=CARTESIAN_POINT ( 'NONE',  ( 20.20312500061451644, 4.541064518000418104, -2.621784821874998173 ) ) ;
#42399=CARTESIAN_POINT ( 'NONE',  ( 27.52500000122903145, -5.773502691896255534, -1.060575238724906372E-15 ) ) ;
#42401=CARTESIAN_POINT ( 'NONE',  ( 25.61250000000000071, -5.773502691896255534, -1.060575238724906372E-15 ) ) ;
#42402=DIRECTION ( 'NONE',  ( 0.000000000000000000, 0.000000000000000000, -1.000000000000000000 ) ) ;
#42404=CARTESIAN_POINT ( 'NONE',  ( 27.90937500061451715, 4.541064518000418104, -2.621784821874998173 ) ) ;
#42406=CARTESIAN_POINT ( 'NONE',  ( -3.000416591977282496E-16, 13.89687500061451786, -34.90005215228797653 ) ) ;
#42407=CARTESIAN_POINT ( 'NONE',  ( 4.762500001229033941, 4.330127018922192761, -2.499999999999997780 ) ) ;
#42408=CARTESIAN_POINT ( 'NONE',  ( 4.500000000000000888, -4.330127018922190985, -2.500000000000001332 ) ) ;
#42409=EDGE_CURVE ( 'NONE', #30305, #2861, #66115, .T. ) ;
#42411=CARTESIAN_POINT ( 'NONE',  ( 3.021917804904423743, -3.983467431823952687, -3.409840147052992432 ) ) ;
#42412=CARTESIAN_POINT ( 'NONE',  ( 6.534375000614517148, -4.541064518000419881, 2.621784821874995952 ) ) ;
#42413=CARTESIAN_POINT ( 'NONE',  ( 27.40312500061451573, 4.541064518000418104, -2.621784821874998173 ) ) ;
#42415=CARTESIAN_POINT ( 'NONE',  ( 5.625000000000001776, 4.330127018922191873, 2.499999999999999556 ) ) ;
#42416=LINE ( 'NONE', #63836, #17047 ) ;
#42417=CARTESIAN_POINT ( 'NONE',  ( 6.121875000614517504, -6.054752690667223547, -1.112240025338166033E-15 ) ) ;
#42418=CARTESIAN_POINT ( 'NONE',  ( 11.74687500061451573, 6.054752690667223547, 3.707466751127219781E-16 ) ) ;
#42419=CARTESIAN_POINT ( 'NONE',  ( 3.750000000000000000, 4.330127018922192761, -2.499999999999997780 ) ) ;
#42420=CARTESIAN_POINT ( 'NONE',  ( 9.001249775931846008E-16, 15.86562500061459602, 34.90005215228797653 ) ) ;
#42421=CARTESIAN_POINT ( 'NONE',  ( 1.626862140677534273E-15, 17.86250000000000071, 34.00000000000000000 ) ) ;
#42422=CARTESIAN_POINT ( 'NONE',  ( 5.924999999999999822, 6.123233995736764310E-16, -4.999999999999998224 ) ) ;
#42424=CARTESIAN_POINT ( 'NONE',  ( 20.80312500061451431, 0.000000000000000000, 5.243569643749999010 ) ) ;
#42425=CARTESIAN_POINT ( 'NONE',  ( 9.890625000614516438, 6.054752690667223547, 3.707466751127219781E-16 ) ) ;
#42427=CARTESIAN_POINT ( 'NONE',  ( 10.35937500061451644, 4.541064518000418104, -2.621784821874998173 ) ) ;
#42428=CARTESIAN_POINT ( 'NONE',  ( 26.02499999999999858, -4.330127018922194537, 2.499999999999995559 ) ) ;
#42429=CARTESIAN_POINT ( 'NONE',  ( 20.88750000122903572, 6.123233995736764310E-16, -4.999999999999998224 ) ) ;
#42430=CARTESIAN_POINT ( 'NONE',  ( 28.64062500061451289, -3.027376345333610441, -5.243569643749999898 ) ) ;
#42432=CARTESIAN_POINT ( 'NONE',  ( 10.39687500061451786, 6.054752690667223547, 3.707466751127219781E-16 ) ) ;
#42433=CARTESIAN_POINT ( 'NONE',  ( 15.04687500061451644, -3.027376345333614438, 5.243569643749998122 ) ) ;
#42434=CARTESIAN_POINT ( 'NONE',  ( 26.25937500061451857, 0.000000000000000000, 5.243569643749999010 ) ) ;
#42437=CARTESIAN_POINT ( 'NONE',  ( 19.09687500061451360, -3.027376345333614438, 5.243569643749998122 ) ) ;
#42438=CARTESIAN_POINT ( 'NONE',  ( 11.33437500061451608, 4.541064518000418104, 2.621784821874999949 ) ) ;
#42440=CARTESIAN_POINT ( 'NONE',  ( 23.25000000000000000, 0.000000000000000000, 4.999999999999998224 ) ) ;
#42442=CARTESIAN_POINT ( 'NONE',  ( -4.243569643749997233, 13.14687500061451786, -27.54997392385601174 ) ) ;
#42444=CARTESIAN_POINT ( 'NONE',  ( 13.97812500061451679, 4.541064518000418104, 2.621784821874999949 ) ) ;
#42445=CARTESIAN_POINT ( 'NONE',  ( 4.987500000000002487, -2.886751345948125991, -5.000000000000000000 ) ) ;
#42446=CARTESIAN_POINT ( 'NONE',  ( 1.626862140677534273E-15, 13.92500000122903181, -26.00000000000000355 ) ) ;
#42448=CARTESIAN_POINT ( 'NONE',  ( 12.86250000000000071, 2.886751345948126879, 4.999999999999999112 ) ) ;
#42449=CARTESIAN_POINT ( 'NONE',  ( -3.999999999999997335, 18.35000000122903430, 32.30940107675850470 ) ) ;
#42450=CARTESIAN_POINT ( 'NONE',  ( 12.67500000122903536, -5.773502691896255534, -1.060575238724906372E-15 ) ) ;
#42451=CARTESIAN_POINT ( 'NONE',  ( 22.77187500061451786, -6.054752690667223547, -1.112240025338166033E-15 ) ) ;
#42452=CARTESIAN_POINT ( 'NONE',  ( 15.57187500061451679, -6.054752690667223547, -1.112240025338166033E-15 ) ) ;
#42454=CARTESIAN_POINT ( 'NONE',  ( 18.47812500061451857, 4.541064518000418104, 2.621784821874999949 ) ) ;
#42455=CARTESIAN_POINT ( 'NONE',  ( 5.053125000614517859, 0.000000000000000000, 5.243569643749999010 ) ) ;
#42456=CARTESIAN_POINT ( 'NONE',  ( 16.54687500061451644, -3.027376345333610441, -5.243569643749999898 ) ) ;
#42457=CARTESIAN_POINT ( 'NONE',  ( 29.44687500061451857, -3.027376345333614438, 5.243569643749998122 ) ) ;
#42458=CARTESIAN_POINT ( 'NONE',  ( 4.903125000614516615, 4.541064518000418104, -2.621784821874998173 ) ) ;
#42459=CARTESIAN_POINT ( 'NONE',  ( 20.35312500061451502, 0.000000000000000000, 5.243569643749999010 ) ) ;
#42460=ADVANCED_FACE ( 'NONE', ( #47780 ), #12703, .T. ) ;
#42461=CARTESIAN_POINT ( 'NONE',  ( -3.000416591977282496E-16, 15.19062500061451715, 25.09994784771203058 ) ) ;
#42462=CARTESIAN_POINT ( 'NONE',  ( 16.53750000122903430, 4.330127018922191873, 2.499999999999999556 ) ) ;
#42464=CARTESIAN_POINT ( 'NONE',  ( 6.703125000614516438, 4.541064518000418104, -2.621784821874998173 ) ) ;
#42465=CARTESIAN_POINT ( 'NONE',  ( 29.20312500061451644, 4.541064518000418104, -2.621784821874998173 ) ) ;
#42466=DIRECTION ( 'NONE',  ( 0.000000000000000000, 0.000000000000000000, -1.000000000000000000 ) ) ;
#42467=CARTESIAN_POINT ( 'NONE',  ( 23.93437500061451573, 4.541064518000418104, 2.621784821874999949 ) ) ;
#42468=CARTESIAN_POINT ( 'NONE',  ( 15.44062500061451537, -3.027376345333614438, 5.243569643749998122 ) ) ;
#42469=CARTESIAN_POINT ( 'NONE',  ( 24.78750000122903074, -4.330127018922194537, 2.499999999999995559 ) ) ;
#42470=CARTESIAN_POINT ( 'NONE',  ( 22.49062500061451431, 6.054752690667223547, 3.707466751127219781E-16 ) ) ;
#42471=CARTESIAN_POINT ( 'NONE',  ( 20.25937500061451857, 4.541064518000418104, -2.621784821874998173 ) ) ;
#42472=CARTESIAN_POINT ( 'NONE',  ( 13.82812500061451466, 6.421520780324663323E-16, -5.243569643749999010 ) ) ;
#42473=CARTESIAN_POINT ( 'NONE',  ( -4.243569643749997233, 15.84687500061451715, 32.45002607614398471 ) ) ;
#42474=CARTESIAN_POINT ( 'NONE',  ( 20.24062500061451431, 6.054752690667223547, 3.707466751127219781E-16 ) ) ;
#42475=CARTESIAN_POINT ( 'NONE',  ( 28.82812500061451644, 4.541064518000418104, 2.621784821874999949 ) ) ;
#42477=EDGE_LOOP ( 'NONE', ( #8484, #41067, #62963, #59625, #48280, #7769, #46457 ) ) ;
#42478=CARTESIAN_POINT ( 'NONE',  ( 23.88749999999999929, -2.886751345948125991, -5.000000000000000000 ) ) ;
#42479=CARTESIAN_POINT ( 'NONE',  ( 4.243569643749999898, 19.59687500061452070, -27.54997392385601529 ) ) ;
#42480=FACE_OUTER_BOUND ( 'NONE', #43360, .T. ) ;
#42481=CARTESIAN_POINT ( 'NONE',  ( 27.10312500061451502, 0.000000000000000000, 5.243569643749999010 ) ) ;
#42482=CARTESIAN_POINT ( 'NONE',  ( 8.390625000614518214, -3.027376345333610441, -5.243569643749999898 ) ) ;
#42483=CARTESIAN_POINT ( 'NONE',  ( 19.38750000122903216, -4.330127018922194537, 2.499999999999995559 ) ) ;
#42484=CARTESIAN_POINT ( 'NONE',  ( 25.04062500061451502, -3.027376345333610441, -5.243569643749999898 ) ) ;
#42485=CARTESIAN_POINT ( 'NONE',  ( 26.06250000000000000, -5.773502691896255534, -1.060575238724906372E-15 ) ) ;
#42486=CARTESIAN_POINT ( 'NONE',  ( 27.21562500061451928, -6.054752690667223547, -1.112240025338166033E-15 ) ) ;
#42487=CARTESIAN_POINT ( 'NONE',  ( 8.915625000614515017, 3.027376345333613106, -5.243569643749998122 ) ) ;
#42488=ORIENTED_EDGE ( 'NONE', *, *, #50295, .T. ) ;
#42489=CARTESIAN_POINT ( 'NONE',  ( 22.45312500061451644, 4.541064518000418104, -2.621784821874998173 ) ) ;
#42490=CARTESIAN_POINT ( 'NONE',  ( 4.228125000614517681, -4.541064518000419881, 2.621784821874995952 ) ) ;
#42493=CARTESIAN_POINT ( 'NONE',  ( 1.999999999999998668, 13.10000000000000142, 26.53589838486224650 ) ) ;
#42495=CARTESIAN_POINT ( 'NONE',  ( 10.91250000000000320, 2.886751345948129099, -4.999999999999998224 ) ) ;
#42496=CARTESIAN_POINT ( 'NONE',  ( 11.18437500061451928, 6.421520780324663323E-16, -5.243569643749999010 ) ) ;
#42497=CARTESIAN_POINT ( 'NONE',  ( 8.137500001229033941, -4.330127018922194537, 2.499999999999995559 ) ) ;
#42498=CARTESIAN_POINT ( 'NONE',  ( 14.70937500061451786, -4.541064518000417216, -2.621784821875001281 ) ) ;
#42500=CARTESIAN_POINT ( 'NONE',  ( 8.446875000614518569, -3.027376345333610441, -5.243569643749999898 ) ) ;
#42502=CARTESIAN_POINT ( 'NONE',  ( 12.98437500061451821, 6.421520780324663323E-16, -5.243569643749999010 ) ) ;
#42503=DIRECTION ( 'NONE',  ( -1.000000000000000000, -0.000000000000000000, -0.000000000000000000 ) ) ;
#42504=CARTESIAN_POINT ( 'NONE',  ( 22.64062500061451644, -3.027376345333614438, 5.243569643749998122 ) ) ;
#42505=CARTESIAN_POINT ( 'NONE',  ( -2.121784821874996840, 10.03437500061451892, 33.67503911421598417 ) ) ;
#42507=CARTESIAN_POINT ( 'NONE',  ( 25.43437500061451573, -4.541064518000419881, 2.621784821874995952 ) ) ;
#42508=CARTESIAN_POINT ( 'NONE',  ( 5.578125000614518214, -4.541064518000419881, 2.621784821874995952 ) ) ;
#42510=CARTESIAN_POINT ( 'NONE',  ( 15.90937500061451892, 0.000000000000000000, 5.243569643749999010 ) ) ;
#42512=CARTESIAN_POINT ( 'NONE',  ( 28.38750000122903216, -4.330127018922194537, 2.499999999999995559 ) ) ;
#42513=CARTESIAN_POINT ( 'NONE',  ( 6.721875000614518925, 3.027376345333613106, -5.243569643749998122 ) ) ;
#42514=CARTESIAN_POINT ( 'NONE',  ( 16.47187500061452070, -6.054752690667223547, -1.112240025338166033E-15 ) ) ;
#42515=CARTESIAN_POINT ( 'NONE',  ( 21.63749999999999929, -2.886751345948126435, -5.000000000000000000 ) ) ;
#42516=CARTESIAN_POINT ( 'NONE',  ( 23.69999999999999929, 0.000000000000000000, 4.999999999999998224 ) ) ;
#42517=CARTESIAN_POINT ( 'NONE',  ( 27.08437500061451786, 4.541064518000418104, 2.621784821874999949 ) ) ;
#42519=CARTESIAN_POINT ( 'NONE',  ( 30.00000000000000000, 0.000000000000000000, 4.999999999999998224 ) ) ;
#42520=CARTESIAN_POINT ( 'NONE',  ( 7.800000000000001599, 4.330127018922192761, -2.499999999999997780 ) ) ;
#42522=CARTESIAN_POINT ( 'NONE',  ( 21.59062500061451928, 6.054752690667223547, 3.707466751127219781E-16 ) ) ;
#42523=CARTESIAN_POINT ( 'NONE',  ( 12.63749999999999929, -2.886751345948125991, -5.000000000000000000 ) ) ;
#42524=CARTESIAN_POINT ( 'NONE',  ( 7.753125000614518036, 0.000000000000000000, 5.243569643749999010 ) ) ;
#42525=CARTESIAN_POINT ( 'NONE',  ( 19.50000000000000000, 4.330127018922192761, -2.499999999999997780 ) ) ;
#42526=CARTESIAN_POINT ( 'NONE',  ( 18.59062500061451573, -3.027376345333614438, 5.243569643749998122 ) ) ;
#42527=CARTESIAN_POINT ( 'NONE',  ( 4.898587196589411843E-16, 20.00000000000000000, 33.99999999999999289 ) ) ;
#42528=CARTESIAN_POINT ( 'NONE',  ( 24.18750000122903288, 4.330127018922191873, 2.499999999999999556 ) ) ;
#42530=CARTESIAN_POINT ( 'NONE',  ( 6.075000000000000178, 4.330127018922191873, 2.499999999999999556 ) ) ;
#42531=ORIENTED_EDGE ( 'NONE', *, *, #20226, .T. ) ;
#42532=CARTESIAN_POINT ( 'NONE',  ( 19.94062500061451715, -3.027376345333614438, 5.243569643749998122 ) ) ;
#42533=CARTESIAN_POINT ( 'NONE',  ( 26.80312500061451431, -4.541064518000417216, -2.621784821875001281 ) ) ;
#42534=CARTESIAN_POINT ( 'NONE',  ( 24.23437500061451644, 6.421520780324663323E-16, -5.243569643749999010 ) ) ;
#42535=CARTESIAN_POINT ( 'NONE',  ( 9.562500000000001776, 2.886751345948129099, -4.999999999999998224 ) ) ;
#42536=CARTESIAN_POINT ( 'NONE',  ( 11.46562500061451573, -6.054752690667223547, -1.112240025338166033E-15 ) ) ;
#42537=CARTESIAN_POINT ( 'NONE',  ( 26.39062500061451644, -3.027376345333610441, -5.243569643749999898 ) ) ;
#42538=CARTESIAN_POINT ( 'NONE',  ( 15.90937500061451892, 0.000000000000000000, 5.243569643749999010 ) ) ;
#42539=CARTESIAN_POINT ( 'NONE',  ( 8.990625000614516082, 6.054752690667223547, 3.707466751127219781E-16 ) ) ;
#42541=CARTESIAN_POINT ( 'NONE',  ( 4.243569643749999898, 11.53437500061451892, 30.00000000000000000 ) ) ;
#42542=CARTESIAN_POINT ( 'NONE',  ( 23.32500000122903572, 2.886751345948126879, 4.999999999999999112 ) ) ;
#42544=CARTESIAN_POINT ( 'NONE',  ( 13.79062500061451502, -3.027376345333610441, -5.243569643749999898 ) ) ;
#42545=CARTESIAN_POINT ( 'NONE',  ( 10.24687500061451750, -3.027376345333610441, -5.243569643749999898 ) ) ;
#42546=CARTESIAN_POINT ( 'NONE',  ( 10.73437500061451644, 6.421520780324663323E-16, -5.243569643749999010 ) ) ;
#42547=VERTEX_POINT ( 'NONE', #58482 ) ;
#42548=CARTESIAN_POINT ( 'NONE',  ( -0.2030170140429748138, 10.00000000000000711, 36.00000000000002842 ) ) ;
#42549=CARTESIAN_POINT ( 'NONE',  ( 22.26562500061451644, -6.054752690667223547, -1.112240025338166033E-15 ) ) ;
#42550=CARTESIAN_POINT ( 'NONE',  ( 16.80937500061451573, 0.000000000000000000, 5.243569643749999010 ) ) ;
#42551=CARTESIAN_POINT ( 'NONE',  ( 22.00312500061451360, 4.541064518000418104, -2.621784821874998173 ) ) ;
#42552=CARTESIAN_POINT ( 'NONE',  ( 3.999999999999998668, 12.16250000000000142, 27.69059892324149175 ) ) ;
#42553=CARTESIAN_POINT ( 'NONE',  ( 26.84062500061451573, -3.027376345333610441, -5.243569643749999898 ) ) ;
#42554=CARTESIAN_POINT ( 'NONE',  ( 6.225000001229036073, 2.886751345948126879, 4.999999999999999112 ) ) ;
#42555=ORIENTED_EDGE ( 'NONE', *, *, #37818, .T. ) ;
#42556=CARTESIAN_POINT ( 'NONE',  ( 29.73750000000000071, -2.886751345948125991, -5.000000000000000000 ) ) ;
#42557=CARTESIAN_POINT ( 'NONE',  ( -1.999999999999997113, 18.72500000000000142, -26.53589838486224295 ) ) ;
#42558=CARTESIAN_POINT ( 'NONE',  ( 23.73750000122903359, 4.330127018922191873, 2.499999999999999556 ) ) ;
#42560=CARTESIAN_POINT ( 'NONE',  ( 7.921875000614517326, -6.054752690667223547, -1.112240025338166033E-15 ) ) ;
#42561=CARTESIAN_POINT ( 'NONE',  ( 12.75000000000000178, 4.330127018922192761, -2.499999999999997780 ) ) ;
#42562=CARTESIAN_POINT ( 'NONE',  ( 14.27812500061451573, 6.421520780324663323E-16, -5.243569643749999010 ) ) ;
#42563=CARTESIAN_POINT ( 'NONE',  ( 7.734375000614517326, 4.541064518000418104, 2.621784821874999949 ) ) ;
#42564=CARTESIAN_POINT ( 'NONE',  ( 26.02500000122903145, 2.886751345948126879, 4.999999999999999112 ) ) ;
#42565=CARTESIAN_POINT ( 'NONE',  ( 16.24687500061451573, 6.054752690667223547, 3.707466751127219781E-16 ) ) ;
#42566=CARTESIAN_POINT ( 'NONE',  ( 4.584375000614516971, 4.541064518000418104, 2.621784821874999949 ) ) ;
#42567=CARTESIAN_POINT ( 'NONE',  ( 4.924325218087134637, -0.8666147624583920850, 4.924325218087160394 ) ) ;
#42568=CARTESIAN_POINT ( 'NONE',  ( 4.565625000614516260, 3.027376345333611329, 5.243569643749999010 ) ) ;
#42569=CARTESIAN_POINT ( 'NONE',  ( 16.22812500061451857, 4.541064518000418104, 2.621784821874999949 ) ) ;
#42571=EDGE_CURVE ( 'NONE', #18997, #11892, #533, .T. ) ;
#42572=CARTESIAN_POINT ( 'NONE',  ( 13.11562500061451786, 3.027376345333611329, 5.243569643749999010 ) ) ;
#42573=CARTESIAN_POINT ( 'NONE',  ( 6.525000001229033231, 2.886751345948129099, -4.999999999999998224 ) ) ;
#42574=CARTESIAN_POINT ( 'NONE',  ( 9.628125000614517148, -4.541064518000419881, 2.621784821874995952 ) ) ;
#42576=CARTESIAN_POINT ( 'NONE',  ( 11.40000000000000036, 4.330127018922192761, -2.499999999999997780 ) ) ;
#42577=CARTESIAN_POINT ( 'NONE',  ( 4.837500001229035895, 4.330127018922191873, 2.499999999999999556 ) ) ;
#42578=EDGE_CURVE ( 'NONE', #100, #68026, #32619, .T. ) ;
#42579=CARTESIAN_POINT ( 'NONE',  ( 21.15000000000000213, -4.330127018922190985, -2.500000000000001332 ) ) ;
#42581=CARTESIAN_POINT ( 'NONE',  ( 15.83437500061451608, 4.541064518000418104, 2.621784821874999949 ) ) ;
#42582=CARTESIAN_POINT ( 'NONE',  ( 15.63750000122903216, 4.330127018922191873, 2.499999999999999556 ) ) ;
#42584=CARTESIAN_POINT ( 'NONE',  ( -3.000416591977282496E-16, 18.79062500061451857, -34.90005215228797653 ) ) ;
#42585=CARTESIAN_POINT ( 'NONE',  ( 30.00000000000000000, 6.123233995736764310E-16, -4.999999999999998224 ) ) ;
#42587=CARTESIAN_POINT ( 'NONE',  ( 29.09062500061451573, -3.027376345333610441, -5.243569643749999898 ) ) ;
#42588=CARTESIAN_POINT ( 'NONE',  ( 3.468651194388615799, -3.601174654424125432, 3.564426390351662199 ) ) ;
#42590=CARTESIAN_POINT ( 'NONE',  ( 14.85937500061451644, 4.541064518000418104, -2.621784821874998173 ) ) ;
#42591=EDGE_CURVE ( 'NONE', #41505, #33272, #20421, .T. ) ;
#42592=CARTESIAN_POINT ( 'NONE',  ( 29.96250000000000213, 2.886751345948126879, 4.999999999999999112 ) ) ;
#42593=CARTESIAN_POINT ( 'NONE',  ( 11.46562500061451573, -6.054752690667223547, -1.112240025338166033E-15 ) ) ;
#42595=CARTESIAN_POINT ( 'NONE',  ( 23.67187500061451999, -6.054752690667223547, -1.112240025338166033E-15 ) ) ;
#42597=CARTESIAN_POINT ( 'NONE',  ( 10.86562500061451431, 3.027376345333611329, 5.243569643749999010 ) ) ;
#42598=CARTESIAN_POINT ( 'NONE',  ( 14.29687500061451821, -3.027376345333610441, -5.243569643749999898 ) ) ;
#42599=ORIENTED_EDGE ( 'NONE', *, *, #33236, .F. ) ;
#42600=CARTESIAN_POINT ( 'NONE',  ( 23.93437500061451573, 4.541064518000418104, 2.621784821874999949 ) ) ;
#42601=CARTESIAN_POINT ( 'NONE',  ( 27.40312500061451573, 4.541064518000418104, -2.621784821874998173 ) ) ;
#42602=CARTESIAN_POINT ( 'NONE',  ( 0.000000000000000000, 20.00000000000000000, -30.00000000000000000 ) ) ;
#42603=CARTESIAN_POINT ( 'NONE',  ( 8.175000000000002487, 6.123233995736764310E-16, -4.999999999999998224 ) ) ;
#42604=CARTESIAN_POINT ( 'NONE',  ( 17.55000000122903359, -2.886751345948129988, 4.999999999999997335 ) ) ;
#42607=ORIENTED_EDGE ( 'NONE', *, *, #37730, .F. ) ;
#42608=CARTESIAN_POINT ( 'NONE',  ( 16.38749999999999929, 5.773502691896255534, 3.535250795749688894E-16 ) ) ;
#42609=CARTESIAN_POINT ( 'NONE',  ( 18.52499999999999858, 6.123233995736764310E-16, -4.999999999999998224 ) ) ;
#42610=CARTESIAN_POINT ( 'NONE',  ( 14.50312500061451537, 0.000000000000000000, 5.243569643749999010 ) ) ;
#42614=CARTESIAN_POINT ( 'NONE',  ( -4.243569643749999898, 18.02187500061452141, -32.45002607614398471 ) ) ;
#42615=CARTESIAN_POINT ( 'NONE',  ( 3.965625000614515727, 3.027376345333613106, -5.243569643749998122 ) ) ;
#42617=CARTESIAN_POINT ( 'NONE',  ( 11.62500000000000000, -4.330127018922194537, 2.499999999999995559 ) ) ;
#42619=EDGE_LOOP ( 'NONE', ( #61160, #29605, #20598, #10533 ) ) ;
#42620=CARTESIAN_POINT ( 'NONE',  ( 4.243569643749999898, 14.59062500061451750, 32.45002607614398471 ) ) ;
#42621=CARTESIAN_POINT ( 'NONE',  ( 26.57812500061451644, 4.541064518000418104, 2.621784821874999949 ) ) ;
#42622=DIRECTION ( 'NONE',  ( 0.000000000000000000, 0.000000000000000000, 1.000000000000000000 ) ) ;
#42624=CARTESIAN_POINT ( 'NONE',  ( 22.77187500061451786, -6.054752690667223547, -1.112240025338166033E-15 ) ) ;
#42625=CARTESIAN_POINT ( 'NONE',  ( 18.85312500061451502, 4.541064518000418104, -2.621784821874998173 ) ) ;
#42626=CARTESIAN_POINT ( 'NONE',  ( 4.243569643749999898, 13.69062500061459176, -27.54997392385601529 ) ) ;
#42627=CARTESIAN_POINT ( 'NONE',  ( 23.51250000122903216, -4.330127018922190985, -2.500000000000001332 ) ) ;
#42628=CARTESIAN_POINT ( 'NONE',  ( 2.915625000614516793, -6.054752690667223547, -1.112240025338166033E-15 ) ) ;
#42630=CARTESIAN_POINT ( 'NONE',  ( 21.85312500061451502, -4.541064518000417216, -2.621784821875001281 ) ) ;
#42633=CARTESIAN_POINT ( 'NONE',  ( 17.40937500061451715, -4.541064518000417216, -2.621784821875001281 ) ) ;
#42634=CARTESIAN_POINT ( 'NONE',  ( 17.63437500061451502, 4.541064518000418104, 2.621784821874999949 ) ) ;
#42635=CARTESIAN_POINT ( 'NONE',  ( 25.24687500061451573, 6.054752690667223547, 3.707466751127219781E-16 ) ) ;
#42636=CARTESIAN_POINT ( 'NONE',  ( -4.243569643749999898, 13.10937500061451821, 30.00000000000000000 ) ) ;
#42637=CARTESIAN_POINT ( 'NONE',  ( 5.728125000614515905, 6.421520780324663323E-16, -5.243569643749999010 ) ) ;
#42638=CARTESIAN_POINT ( 'NONE',  ( 28.56562500061451715, -6.054752690667223547, -1.112240025338166033E-15 ) ) ;
#42639=CARTESIAN_POINT ( 'NONE',  ( 29.80312500061451431, 0.000000000000000000, 5.243569643749999010 ) ) ;
#42640=CARTESIAN_POINT ( 'NONE',  ( 3.486133158594716510E-16, 19.55000000122903359, -34.00000000000000000 ) ) ;
#42641=CARTESIAN_POINT ( 'NONE',  ( -1.999999999999997113, 18.27499999999999858, 33.46410161513775705 ) ) ;
#42642=CARTESIAN_POINT ( 'NONE',  ( 3.740625000614516527, -3.027376345333614438, 5.243569643749998122 ) ) ;
#42643=CARTESIAN_POINT ( 'NONE',  ( 6.871875000614517504, 3.027376345333611329, 5.243569643749999010 ) ) ;
#42645=CARTESIAN_POINT ( 'NONE',  ( 13.31250000122903288, 4.330127018922192761, -2.499999999999997780 ) ) ;
#42646=CARTESIAN_POINT ( 'NONE',  ( 12.71250000122903145, -4.330127018922190985, -2.500000000000001332 ) ) ;
#42647=CARTESIAN_POINT ( 'NONE',  ( 5.353125000614515905, 4.541064518000418104, -2.621784821874998173 ) ) ;
#42650=CARTESIAN_POINT ( 'NONE',  ( 15.00937500061451679, 0.000000000000000000, 5.243569643749999010 ) ) ;
#42651=CARTESIAN_POINT ( 'NONE',  ( 1.592000809091587073E-14, 17.18750000000000355, -34.00000000000000000 ) ) ;
#42652=ORIENTED_EDGE ( 'NONE', *, *, #61749, .T. ) ;
#42653=CARTESIAN_POINT ( 'NONE',  ( 23.01562500061451644, 3.027376345333611329, 5.243569643749999010 ) ) ;
#42654=CARTESIAN_POINT ( 'NONE',  ( 7.603125000614517681, 4.541064518000418104, -2.621784821874998173 ) ) ;
#42655=CARTESIAN_POINT ( 'NONE',  ( 25.32187500061451857, 3.027376345333611329, 5.243569643749999010 ) ) ;
#42656=CARTESIAN_POINT ( 'NONE',  ( 7.565625000614518036, 3.027376345333613106, -5.243569643749998122 ) ) ;
#42657=CARTESIAN_POINT ( 'NONE',  ( 1.626862140677534273E-15, 10.32500000122903572, 34.00000000000000000 ) ) ;
#42658=CARTESIAN_POINT ( 'NONE',  ( 8.662500001229034297, -4.330127018922190985, -2.500000000000001332 ) ) ;
#42659=CARTESIAN_POINT ( 'NONE',  ( 22.07812500061451644, 4.541064518000418104, 2.621784821874999949 ) ) ;
#42660=CARTESIAN_POINT ( 'NONE',  ( -2.121784821874999949, 11.17812500061451786, -33.67503911421598417 ) ) ;
#42661=CARTESIAN_POINT ( 'NONE',  ( 9.975000001229034297, -5.773502691896255534, -1.060575238724906372E-15 ) ) ;
#42662=CARTESIAN_POINT ( 'NONE',  ( 19.56562500061451715, -6.054752690667223547, -1.112240025338166033E-15 ) ) ;
#42663=CARTESIAN_POINT ( 'NONE',  ( 18.47812500061451857, 4.541064518000418104, 2.621784821874999949 ) ) ;
#42666=CARTESIAN_POINT ( 'NONE',  ( 18.14999999999999858, 4.330127018922192761, -2.499999999999997780 ) ) ;
#42667=CARTESIAN_POINT ( 'NONE',  ( 12.75000000122903643, -2.886751345948125991, -5.000000000000000000 ) ) ;
#42668=CARTESIAN_POINT ( 'NONE',  ( 11.61562500061451608, 3.027376345333613106, -5.243569643749998122 ) ) ;
#42669=CARTESIAN_POINT ( 'NONE',  ( 12.47812500061451502, 6.421520780324663323E-16, -5.243569643749999010 ) ) ;
#42671=CARTESIAN_POINT ( 'NONE',  ( 23.36250000122903359, 0.000000000000000000, 4.999999999999998224 ) ) ;
#42672=CARTESIAN_POINT ( 'NONE',  ( 21.00937500061451857, -4.541064518000417216, -2.621784821875001281 ) ) ;
#42673=CARTESIAN_POINT ( 'NONE',  ( 20.37187500061451573, 3.027376345333611329, 5.243569643749999010 ) ) ;
#42674=CARTESIAN_POINT ( 'NONE',  ( 3.539158067892712811, 3.531921335771147863, -3.875648772243089457 ) ) ;
#42675=CARTESIAN_POINT ( 'NONE',  ( 8.812500001229034652, 4.330127018922192761, -2.499999999999997780 ) ) ;
#42676=CARTESIAN_POINT ( 'NONE',  ( 7.359375000614516438, 0.000000000000000000, 5.243569643749999010 ) ) ;
#42677=CARTESIAN_POINT ( 'NONE',  ( 22.58437500061451431, 4.541064518000418104, 2.621784821874999949 ) ) ;
#42678=CARTESIAN_POINT ( 'NONE',  ( 26.58750000122903145, -4.330127018922194537, 2.499999999999995559 ) ) ;
#42679=CARTESIAN_POINT ( 'NONE',  ( 19.67812500061451786, 6.421520780324663323E-16, -5.243569643749999010 ) ) ;
#42680=CARTESIAN_POINT ( 'NONE',  ( 24.72187500061451360, 3.027376345333613106, -5.243569643749998122 ) ) ;
#42682=CARTESIAN_POINT ( 'NONE',  ( -3.999999999999997335, 11.15000000122903501, -27.69059892324149530 ) ) ;
#42684=CARTESIAN_POINT ( 'NONE',  ( 6.159375000614517148, -4.541064518000417216, -2.621784821875001281 ) ) ;
#42685=CARTESIAN_POINT ( 'NONE',  ( 17.54062500061451502, 6.054752690667223547, 3.707466751127219781E-16 ) ) ;
#42686=CARTESIAN_POINT ( 'NONE',  ( 12.83437500061451786, -4.541064518000419881, 2.621784821874995952 ) ) ;
#42687=ORIENTED_EDGE ( 'NONE', *, *, #48920, .F. ) ;
#42689=CARTESIAN_POINT ( 'NONE',  ( 24.21562500061451573, 3.027376345333613106, -5.243569643749998122 ) ) ;
#42690=CARTESIAN_POINT ( 'NONE',  ( 3.531796677802674811, 3.539267187803308179, -3.868928841707397925 ) ) ;
#42691=LINE ( 'NONE', #24232, #17143 ) ;
#42692=CARTESIAN_POINT ( 'NONE',  ( 15.45000000000000107, 4.330127018922192761, -2.499999999999997780 ) ) ;
#42693=CARTESIAN_POINT ( 'NONE',  ( 24.93750000122903288, 6.123233995736764310E-16, -4.999999999999998224 ) ) ;
#42694=CARTESIAN_POINT ( 'NONE',  ( 17.80312500061451786, -4.541064518000417216, -2.621784821875001281 ) ) ;
#42696=CARTESIAN_POINT ( 'NONE',  ( 22.46250000000000213, -5.773502691896255534, -1.060575238724906372E-15 ) ) ;
#42697=CARTESIAN_POINT ( 'NONE',  ( 23.44687500061451502, 6.054752690667223547, 3.707466751127219781E-16 ) ) ;
#42700=CARTESIAN_POINT ( 'NONE',  ( 13.82812500061451466, 6.421520780324663323E-16, -5.243569643749999010 ) ) ;
#42701=CARTESIAN_POINT ( 'NONE',  ( 4.265625000614517326, -6.054752690667223547, -1.112240025338166033E-15 ) ) ;
#42703=CARTESIAN_POINT ( 'NONE',  ( 28.04062500061451502, -3.027376345333614438, 5.243569643749998122 ) ) ;
#42704=CARTESIAN_POINT ( 'NONE',  ( 11.81250000122903465, -4.330127018922190985, -2.500000000000001332 ) ) ;
#42705=CARTESIAN_POINT ( 'NONE',  ( 19.46249999999999858, 2.886751345948129099, -4.999999999999998224 ) ) ;
#42706=CARTESIAN_POINT ( 'NONE',  ( 27.56250000000000000, 2.886751345948129099, -4.999999999999998224 ) ) ;
#42708=CARTESIAN_POINT ( 'NONE',  ( 6.984375000614516438, -4.541064518000419881, 2.621784821874995952 ) ) ;
#42709=CARTESIAN_POINT ( 'NONE',  ( 18.04687500061451999, 6.054752690667223547, 3.707466751127219781E-16 ) ) ;
#42710=FACE_OUTER_BOUND ( 'NONE', #41812, .T. ) ;
#42712=CARTESIAN_POINT ( 'NONE',  ( 26.54062500061451146, 6.054752690667223547, 3.707466751127219781E-16 ) ) ;
#42713=CARTESIAN_POINT ( 'NONE',  ( 26.52187500061451431, 3.027376345333613106, -5.243569643749998122 ) ) ;
#42715=CARTESIAN_POINT ( 'NONE',  ( 16.19999999999999929, -4.330127018922190985, -2.500000000000001332 ) ) ;
#42716=CARTESIAN_POINT ( 'NONE',  ( 11.50312500061451892, -4.541064518000417216, -2.621784821875001281 ) ) ;
#42717=CARTESIAN_POINT ( 'NONE',  ( 30.00000000000000000, 6.123233995736764310E-16, -4.999999999999998224 ) ) ;
#42719=CARTESIAN_POINT ( 'NONE',  ( 28.90312500061451217, 0.000000000000000000, 5.243569643749999010 ) ) ;
#42720=CARTESIAN_POINT ( 'NONE',  ( 17.28750000122903430, 6.123233995736764310E-16, -4.999999999999998224 ) ) ;
#42721=CARTESIAN_POINT ( 'NONE',  ( 3.619842856578028734, -3.449164782042274169, -3.619842856578066481 ) ) ;
#42723=CARTESIAN_POINT ( 'NONE',  ( 5.803125000614517859, 4.541064518000418104, -2.621784821874998173 ) ) ;
#42724=CARTESIAN_POINT ( 'NONE',  ( 21.04687500061451644, -3.027376345333610441, -5.243569643749999898 ) ) ;
#42725=CARTESIAN_POINT ( 'NONE',  ( -4.243569643749997233, 16.29687500061451644, 32.45002607614398471 ) ) ;
#42726=CARTESIAN_POINT ( 'NONE',  ( 24.75937500061451502, 4.541064518000418104, -2.621784821874998173 ) ) ;
#42727=CARTESIAN_POINT ( 'NONE',  ( 4.050000000000001599, -4.330127018922190985, -2.500000000000001332 ) ) ;
#42728=CARTESIAN_POINT ( 'NONE',  ( 1.999999999999998668, 10.96250000122903501, 26.53589838486224650 ) ) ;
#42729=CARTESIAN_POINT ( 'NONE',  ( 11.46562500061451573, -6.054752690667223547, -1.112240025338166033E-15 ) ) ;
#42730=CARTESIAN_POINT ( 'NONE',  ( 5.100000001229034297, -2.886751345948125991, -5.000000000000000000 ) ) ;
#42731=EDGE_CURVE ( 'NONE', #3869, #13665, #8066, .T. ) ;
#42732=AXIS2_PLACEMENT_3D ( 'NONE', #58082, #41833, #8954 ) ;
#42733=CARTESIAN_POINT ( 'NONE',  ( 10.32187500061451679, 3.027376345333613106, -5.243569643749998122 ) ) ;
#42734=CARTESIAN_POINT ( 'NONE',  ( 3.849130445941352896, -3.191436642873679119, 4.069143491079585395 ) ) ;
#42735=CARTESIAN_POINT ( 'NONE',  ( 9.890625000614516438, 6.054752690667223547, 3.707466751127219781E-16 ) ) ;
#42736=CARTESIAN_POINT ( 'NONE',  ( 13.58437500061451786, 4.541064518000418104, 2.621784821874999949 ) ) ;
#42737=CYLINDRICAL_SURFACE ( 'NONE', #6067, 4.999999999999998224 ) ;
#42738=CARTESIAN_POINT ( 'NONE',  ( 21.37500000122902932, 2.886751345948129099, -4.999999999999998224 ) ) ;
#42739=CARTESIAN_POINT ( 'NONE',  ( 9.721875000614517148, -6.054752690667223547, -1.112240025338166033E-15 ) ) ;
#42740=CARTESIAN_POINT ( 'NONE',  ( 13.37812500061451715, 6.421520780324663323E-16, -5.243569643749999010 ) ) ;
#42742=CARTESIAN_POINT ( 'NONE',  ( 20.52187500061451786, -6.054752690667223547, -1.112240025338166033E-15 ) ) ;
#42743=CARTESIAN_POINT ( 'NONE',  ( 1.071796769724484344, 15.74509619066136956, 34.00000000000000000 ) ) ;
#42744=CARTESIAN_POINT ( 'NONE',  ( 1.626862140677534273E-15, 12.12500000122903465, -26.00000000000000355 ) ) ;
#42746=CARTESIAN_POINT ( 'NONE',  ( -2.121784821874999949, 15.28437500061451892, -33.67503911421598417 ) ) ;
#42747=CARTESIAN_POINT ( 'NONE',  ( 15.22500000122903252, 2.886751345948126879, 4.999999999999999112 ) ) ;
#42748=CARTESIAN_POINT ( 'NONE',  ( 13.05937500061451750, 4.541064518000418104, -2.621784821874998173 ) ) ;
#42749=CARTESIAN_POINT ( 'NONE',  ( -4.243569643749999898, 17.55312500061451786, -30.00000000000000000 ) ) ;
#42750=CARTESIAN_POINT ( 'NONE',  ( 18.56250000122903288, -4.330127018922190985, -2.500000000000001332 ) ) ;
#42751=CARTESIAN_POINT ( 'NONE',  ( 13.34062500061451750, -3.027376345333610441, -5.243569643749999898 ) ) ;
#42753=CARTESIAN_POINT ( 'NONE',  ( 15.67500000000000071, -4.330127018922194537, 2.499999999999995559 ) ) ;
#42754=CARTESIAN_POINT ( 'NONE',  ( -1.071796769724487453, 17.32009619066136707, -34.00000000000000000 ) ) ;
#42755=CARTESIAN_POINT ( 'NONE',  ( 9.909375000614517148, 4.541064518000418104, -2.621784821874998173 ) ) ;
#42757=CARTESIAN_POINT ( 'NONE',  ( -1.071796769724504328, 14.35490381179669939, 33.99999999999999289 ) ) ;
#42758=CARTESIAN_POINT ( 'NONE',  ( 11.58750000122903501, 4.330127018922191873, 2.499999999999999556 ) ) ;
#42759=CARTESIAN_POINT ( 'NONE',  ( 22.12500000122903288, -5.773502691896255534, -1.060575238724906372E-15 ) ) ;
#42760=CARTESIAN_POINT ( 'NONE',  ( 18.47812500061451857, 4.541064518000418104, 2.621784821874999949 ) ) ;
#42761=CARTESIAN_POINT ( 'NONE',  ( 21.06562500061451715, 3.027376345333613106, -5.243569643749998122 ) ) ;
#42762=CARTESIAN_POINT ( 'NONE',  ( 27.71250000122903145, 4.330127018922192761, -2.499999999999997780 ) ) ;
#42763=CARTESIAN_POINT ( 'NONE',  ( 3.403125000614518836, -4.541064518000417216, -2.621784821875001281 ) ) ;
#42764=CARTESIAN_POINT ( 'NONE',  ( 25.05000000000000071, 0.000000000000000000, 4.999999999999998224 ) ) ;
#42765=CARTESIAN_POINT ( 'NONE',  ( 28.23750000000000071, -2.886751345948137981, 4.999999999999982236 ) ) ;
#42767=CARTESIAN_POINT ( 'NONE',  ( 28.65937500061451715, -4.541064518000417216, -2.621784821875001281 ) ) ;
#42768=CARTESIAN_POINT ( 'NONE',  ( 2.000000000000001332, 17.44999999999999929, 33.46410161513774995 ) ) ;
#42769=CARTESIAN_POINT ( 'NONE',  ( 2.962500001229034119, 4.330127018922192761, -2.499999999999997780 ) ) ;
#42770=CARTESIAN_POINT ( 'NONE',  ( 4.462500000000001243, -5.773502691896255534, -1.060575238724906372E-15 ) ) ;
#42771=( BOUNDED_CURVE ( )  B_SPLINE_CURVE ( 2, ( #23186, #31185, #6207, #6577, #45740, #68275, #17637, #68999, #34635 ),
 .UNSPECIFIED., .F., .F. ) 
 B_SPLINE_CURVE_WITH_KNOTS ( ( 3, 2, 2, 2, 3 ),
 ( 0.6630434782608696231, 0.6666666666666666297, 0.6739130434782608647, 0.6811594202898550998, 0.6847826086956522174 ),
 .UNSPECIFIED. ) 
 CURVE ( )  GEOMETRIC_REPRESENTATION_ITEM ( )  RATIONAL_B_SPLINE_CURVE ( ( 0.9330127018922192983, 0.9330127018922202975, 1.000000000000000000, 0.8660254037844387076, 1.000000000000000000, 0.8660254037844387076, 1.000000000000000000, 0.9330127018922182991, 0.9330127018922192983 ) ) 
 REPRESENTATION_ITEM ( '' )  );
#42772=DIRECTION ( 'NONE',  ( 0.000000000000000000, -1.000000000000000000, 0.000000000000000000 ) ) ;
#42773=CARTESIAN_POINT ( 'NONE',  ( 8.034375000614518925, 6.421520780324663323E-16, -5.243569643749999010 ) ) ;
#42774=CARTESIAN_POINT ( 'NONE',  ( 26.12812500061451360, 4.541064518000418104, 2.621784821874999949 ) ) ;
#42777=CARTESIAN_POINT ( 'NONE',  ( 4.959375000614516971, 4.541064518000418104, -2.621784821874998173 ) ) ;
#42778=CARTESIAN_POINT ( 'NONE',  ( 9.234375000614518214, -4.541064518000419881, 2.621784821874995952 ) ) ;
#42779=CARTESIAN_POINT ( 'NONE',  ( 3.975000000000002753, -4.330127018922194537, 2.499999999999995559 ) ) ;
#42780=CARTESIAN_POINT ( 'NONE',  ( -2.121784821874999949, 12.07812500061459637, 26.32496088578401938 ) ) ;
#42781=CARTESIAN_POINT ( 'NONE',  ( 29.88749999999999929, 5.773502691896255534, 3.535250795749688894E-16 ) ) ;
#42782=CARTESIAN_POINT ( 'NONE',  ( 4.912499999999999645, -5.773502691896255534, -1.060575238724906372E-15 ) ) ;
#42784=ORIENTED_EDGE ( 'NONE', *, *, #11885, .T. ) ;
#42785=CARTESIAN_POINT ( 'NONE',  ( 19.37812500061451715, 4.541064518000418104, 2.621784821874999949 ) ) ;
#42786=CARTESIAN_POINT ( 'NONE',  ( 11.57812500061451644, 6.421520780324663323E-16, -5.243569643749999010 ) ) ;
#42788=CARTESIAN_POINT ( 'NONE',  ( 5.896875000614518747, 6.054752690667223547, 3.707466751127219781E-16 ) ) ;
#42789=CARTESIAN_POINT ( 'NONE',  ( 24.18750000000000355, -2.886751345948129988, 4.999999999999997335 ) ) ;
#42790=CARTESIAN_POINT ( 'NONE',  ( 21.33750000122903145, 6.123233995736764310E-16, -4.999999999999998224 ) ) ;
#42791=CARTESIAN_POINT ( 'NONE',  ( 28.07812500061451289, -4.541064518000419881, 2.621784821874995952 ) ) ;
#42793=CARTESIAN_POINT ( 'NONE',  ( 9.421875000614519990, 3.027376345333613106, -5.243569643749998122 ) ) ;
#42794=CARTESIAN_POINT ( 'NONE',  ( 14.97187500061451892, 3.027376345333611329, 5.243569643749999010 ) ) ;
#42795=CARTESIAN_POINT ( 'NONE',  ( 24.53437500061451715, -4.541064518000419881, 2.621784821874995952 ) ) ;
#42798=CARTESIAN_POINT ( 'NONE',  ( 20.22187500061451715, 3.027376345333613106, -5.243569643749998122 ) ) ;
#42799=CARTESIAN_POINT ( 'NONE',  ( 8.634375000614518569, 4.541064518000418104, 2.621784821874999949 ) ) ;
#42801=CARTESIAN_POINT ( 'NONE',  ( 22.76249999999999574, 2.886751345948126879, 4.999999999999999112 ) ) ;
#42803=CARTESIAN_POINT ( 'NONE',  ( 4.243569643749999010, 13.37187500061451750, -32.45002607614398471 ) ) ;
#42805=CARTESIAN_POINT ( 'NONE',  ( 15.14062500061451644, -3.027376345333610441, -5.243569643749999898 ) ) ;
#42806=CARTESIAN_POINT ( 'NONE',  ( 3.487500000000000711, -2.886751345948129988, 4.999999999999997335 ) ) ;
#42808=CARTESIAN_POINT ( 'NONE',  ( 15.93750000122903110, 6.123233995736764310E-16, -4.999999999999998224 ) ) ;
#42809=CARTESIAN_POINT ( 'NONE',  ( 12.07499999999999929, -4.330127018922194537, 2.499999999999995559 ) ) ;
#42810=CARTESIAN_POINT ( 'NONE',  ( 4.000000000000000000, 18.50000000122903288, 32.30940107675849049 ) ) ;
#42811=CARTESIAN_POINT ( 'NONE',  ( 11.88750000122903216, 6.123233995736764310E-16, -4.999999999999998224 ) ) ;
#42812=CARTESIAN_POINT ( 'NONE',  ( 22.09687500061451715, 6.054752690667223547, 3.707466751127219781E-16 ) ) ;
#42813=CARTESIAN_POINT ( 'NONE',  ( 16.80937500061451573, 0.000000000000000000, 5.243569643749999010 ) ) ;
#42815=ORIENTED_EDGE ( 'NONE', *, *, #46671, .F. ) ;
#42816=CARTESIAN_POINT ( 'NONE',  ( 17.72812500061451502, -4.541064518000419881, 2.621784821874995952 ) ) ;
#42817=CARTESIAN_POINT ( 'NONE',  ( 28.27500000122903145, 2.886751345948126879, 4.999999999999999112 ) ) ;
#42818=CARTESIAN_POINT ( 'NONE',  ( 16.47187500061452070, -6.054752690667223547, -1.112240025338166033E-15 ) ) ;
#42819=CARTESIAN_POINT ( 'NONE',  ( 28.80937500061451573, 4.541064518000418104, -2.621784821874998173 ) ) ;
#42820=CARTESIAN_POINT ( 'NONE',  ( 4.415625000614518569, 3.027376345333613106, -5.243569643749998122 ) ) ;
#42821=CARTESIAN_POINT ( 'NONE',  ( 18.59062500061451573, -3.027376345333614438, 5.243569643749998122 ) ) ;
#42822=CARTESIAN_POINT ( 'NONE',  ( 4.243569643749999898, 13.27812500061451750, 30.00000000000000000 ) ) ;
#42823=CARTESIAN_POINT ( 'NONE',  ( 16.05000000122903359, 5.773502691896255534, 3.535250795749688894E-16 ) ) ;
#42825=CARTESIAN_POINT ( 'NONE',  ( 7.715625000614515727, 3.027376345333611329, 5.243569643749999010 ) ) ;
#42826=CARTESIAN_POINT ( 'NONE',  ( 26.72812500061451502, -4.541064518000419881, 2.621784821874995952 ) ) ;
#42827=CARTESIAN_POINT ( 'NONE',  ( 1.071796769724490783, 19.07990381179670081, -34.00000000000000000 ) ) ;
#42829=CARTESIAN_POINT ( 'NONE',  ( 22.99687500061451573, 6.054752690667223547, 3.707466751127219781E-16 ) ) ;
#42830=CARTESIAN_POINT ( 'NONE',  ( 14.50312500061451537, 0.000000000000000000, 5.243569643749999010 ) ) ;
#42831=CARTESIAN_POINT ( 'NONE',  ( 21.75000000122903288, -2.886751345948125991, -5.000000000000000000 ) ) ;
#42832=( BOUNDED_CURVE ( )  B_SPLINE_CURVE ( 2, ( #15885, #66503, #55788, #26252, #9260, #10356, #37690 ),
 .UNSPECIFIED., .F., .F. ) 
 B_SPLINE_CURVE_WITH_KNOTS ( ( 3, 2, 2, 3 ),
 ( 0.1250000000000000000, 0.1277777777777777679, 0.1305555555555555358, 0.1333333333333333037 ),
 .UNSPECIFIED. ) 
 CURVE ( )  GEOMETRIC_REPRESENTATION_ITEM ( )  RATIONAL_B_SPLINE_CURVE ( ( 1.000000000000000000, 0.8660254037844387076, 1.000000000000000000, 0.8660254037844387076, 1.000000000000000000, 0.8660254037844400399, 0.9999999999999986677 ) ) 
 REPRESENTATION_ITEM ( '' )  );
#42833=CARTESIAN_POINT ( 'NONE',  ( 23.09062500061451573, -3.027376345333614438, 5.243569643749998122 ) ) ;
#42834=CARTESIAN_POINT ( 'NONE',  ( 18.68437500061451928, -4.541064518000419881, 2.621784821874995952 ) ) ;
#42835=CARTESIAN_POINT ( 'NONE',  ( 14.39062500061451821, 6.054752690667223547, 3.707466751127219781E-16 ) ) ;
#42836=CARTESIAN_POINT ( 'NONE',  ( 2.121784821874999061, 14.30937500061451750, 26.32496088578401583 ) ) ;
#42837=CARTESIAN_POINT ( 'NONE',  ( 18.77812500061451573, 6.421520780324663323E-16, -5.243569643749999010 ) ) ;
#42839=ORIENTED_EDGE ( 'NONE', *, *, #67858, .T. ) ;
#42840=ORIENTED_EDGE ( 'NONE', *, *, #34767, .T. ) ;
#42841=CARTESIAN_POINT ( 'NONE',  ( 22.38749999999999929, -2.886751345948129988, 4.999999999999997335 ) ) ;
#42842=CARTESIAN_POINT ( 'NONE',  ( -4.243569643749997233, 19.44687500061451502, -27.54997392385601174 ) ) ;
#42843=CARTESIAN_POINT ( 'NONE',  ( 13.12500000122903288, -5.773502691896255534, -1.060575238724906372E-15 ) ) ;
#42844=CARTESIAN_POINT ( 'NONE',  ( 26.16562500061451502, 3.027376345333611329, 5.243569643749999010 ) ) ;
#42845=CARTESIAN_POINT ( 'NONE',  ( 8.878125000614515372, 6.421520780324663323E-16, -5.243569643749999010 ) ) ;
#42846=CARTESIAN_POINT ( 'NONE',  ( 18.97500000122903074, -5.773502691896255534, -1.060575238724906372E-15 ) ) ;
#42847=CARTESIAN_POINT ( 'NONE',  ( 24.51562500061451289, -6.054752690667223547, -1.112240025338166033E-15 ) ) ;
#42848=CARTESIAN_POINT ( 'NONE',  ( 21.97500000000000142, -4.330127018922194537, 2.499999999999995559 ) ) ;
#42849=CARTESIAN_POINT ( 'NONE',  ( 28.97812500061451502, -4.541064518000419881, 2.621784821874995952 ) ) ;
#42850=CARTESIAN_POINT ( 'NONE',  ( 8.278125000614515727, -4.541064518000419881, 2.621784821874995952 ) ) ;
#42852=CARTESIAN_POINT ( 'NONE',  ( 23.46562500061451573, 3.027376345333611329, 5.243569643749999010 ) ) ;
#42853=CARTESIAN_POINT ( 'NONE',  ( 6.290625000614517681, 6.054752690667223547, 3.707466751127219781E-16 ) ) ;
#42855=CARTESIAN_POINT ( 'NONE',  ( 3.890625000614517326, -3.027376345333610441, -5.243569643749999898 ) ) ;
#42856=CARTESIAN_POINT ( 'NONE',  ( 8.484601909799253346E-16, 14.37500000122903288, -25.38119784648299770 ) ) ;
#42858=CARTESIAN_POINT ( 'NONE',  ( 11.81250000000000000, 2.886751345948129099, -4.999999999999998224 ) ) ;
#42859=CARTESIAN_POINT ( 'NONE',  ( 11.48437500061451644, -4.541064518000419881, 2.621784821874995952 ) ) ;
#42860=CARTESIAN_POINT ( 'NONE',  ( 8.775000001229033231, 2.886751345948129099, -4.999999999999998224 ) ) ;
#42861=CARTESIAN_POINT ( 'NONE',  ( 14.52187500061451608, 3.027376345333611329, 5.243569643749999010 ) ) ;
#42863=CARTESIAN_POINT ( 'NONE',  ( 5.896875000614518747, 6.054752690667223547, 3.707466751127219781E-16 ) ) ;
#42865=CARTESIAN_POINT ( 'NONE',  ( 3.727827348360245097, 3.332161949968362347, -3.727827348360304605 ) ) ;
#42866=CARTESIAN_POINT ( 'NONE',  ( 13.39687500061451608, -3.027376345333610441, -5.243569643749999898 ) ) ;
#42867=CARTESIAN_POINT ( 'NONE',  ( 3.673424073952555435, 3.392052302514600548, 3.998632574573837584 ) ) ;
#42869=CARTESIAN_POINT ( 'NONE',  ( 22.71562500061451573, -6.054752690667223547, -1.112240025338166033E-15 ) ) ;
#42870=CARTESIAN_POINT ( 'NONE',  ( -2.121784821874999949, 10.78437500061451715, 26.32496088578401938 ) ) ;
#42871=FACE_OUTER_BOUND ( 'NONE', #34816, .T. ) ;
#42872=CARTESIAN_POINT ( 'NONE',  ( 26.44687500061451502, -3.027376345333610441, -5.243569643749999898 ) ) ;
#42873=CARTESIAN_POINT ( 'NONE',  ( 29.66249999999999787, -5.773502691896255534, -1.060575238724906372E-15 ) ) ;
#42874=CARTESIAN_POINT ( 'NONE',  ( 3.965625000614515727, 3.027376345333613106, -5.243569643749998122 ) ) ;
#42876=CARTESIAN_POINT ( 'NONE',  ( 15.00937500061451679, 0.000000000000000000, 5.243569643749999010 ) ) ;
#42878=CARTESIAN_POINT ( 'NONE',  ( 27.75000000122903288, 5.773502691896255534, 3.535250795749688894E-16 ) ) ;
#42879=CARTESIAN_POINT ( 'NONE',  ( 5.184375000614516615, -4.541064518000419881, 2.621784821874995952 ) ) ;
#42880=CARTESIAN_POINT ( 'NONE',  ( 15.53437500061451715, -4.541064518000419881, 2.621784821874995952 ) ) ;
#42881=CARTESIAN_POINT ( 'NONE',  ( 3.286795329855858760, 3.767887532774327308, -3.286795329856085690 ) ) ;
#42882=CARTESIAN_POINT ( 'NONE',  ( 24.52499999999999858, 4.330127018922191873, 2.499999999999999556 ) ) ;
#42883=CARTESIAN_POINT ( 'NONE',  ( 3.562500001229033764, 0.000000000000000000, 4.999999999999998224 ) ) ;
#42884=CARTESIAN_POINT ( 'NONE',  ( 26.55937500061451573, 4.541064518000418104, -2.621784821874998173 ) ) ;
#42886=CARTESIAN_POINT ( 'NONE',  ( 14.21250000122903323, 4.330127018922192761, -2.499999999999997780 ) ) ;
#42887=CARTESIAN_POINT ( 'NONE',  ( 8.812500000000000000, 2.886751345948126879, 4.999999999999999112 ) ) ;
#42889=CARTESIAN_POINT ( 'NONE',  ( 22.37812500061451360, 6.421520780324663323E-16, -5.243569643749999010 ) ) ;
#42890=CARTESIAN_POINT ( 'NONE',  ( 11.70000000000000284, -4.330127018922190985, -2.500000000000001332 ) ) ;
#42891=CARTESIAN_POINT ( 'NONE',  ( 4.940625000614515372, 6.054752690667223547, 3.707466751127219781E-16 ) ) ;
#42892=CARTESIAN_POINT ( 'NONE',  ( 19.53749999999999432, 5.773502691896255534, 3.535250795749688894E-16 ) ) ;
#42893=CARTESIAN_POINT ( 'NONE',  ( 17.72812500061451502, -4.541064518000419881, 2.621784821874995952 ) ) ;
#42894=CARTESIAN_POINT ( 'NONE',  ( -3.999999999999997335, 18.80000000122903003, 32.30940107675850470 ) ) ;
#42895=CARTESIAN_POINT ( 'NONE',  ( 22.98750000122903003, -4.330127018922194537, 2.499999999999995559 ) ) ;
#42897=CARTESIAN_POINT ( 'NONE',  ( 29.85937500061451644, 0.000000000000000000, 5.243569643749999010 ) ) ;
#42898=VERTEX_POINT ( 'NONE', #9719 ) ;
#42899=CARTESIAN_POINT ( 'NONE',  ( 19.86562500061451786, 3.027376345333611329, 5.243569643749999010 ) ) ;
#42900=CARTESIAN_POINT ( 'NONE',  ( 24.17812500061451786, 6.421520780324663323E-16, -5.243569643749999010 ) ) ;
#42901=CARTESIAN_POINT ( 'NONE',  ( 24.64687500061451431, -3.027376345333610441, -5.243569643749999898 ) ) ;
#42902=CARTESIAN_POINT ( 'NONE',  ( 8.775000000000002132, 4.330127018922191873, 2.499999999999999556 ) ) ;
#42903=CARTESIAN_POINT ( 'NONE',  ( 12.25312500061451537, 0.000000000000000000, 5.243569643749999010 ) ) ;
#42904=CARTESIAN_POINT ( 'NONE',  ( 27.36562500061451786, 3.027376345333613106, -5.243569643749998122 ) ) ;
#42905=CARTESIAN_POINT ( 'NONE',  ( 17.29687500061451999, -3.027376345333614438, 5.243569643749998122 ) ) ;
#42906=CARTESIAN_POINT ( 'NONE',  ( 9.328125000614518214, 6.421520780324663323E-16, -5.243569643749999010 ) ) ;
#42907=CARTESIAN_POINT ( 'NONE',  ( 2.946926184779611990, -4.039365056661180731, 3.279941078183791880 ) ) ;
#42908=CARTESIAN_POINT ( 'NONE',  ( -4.243569643749999898, 9.921875000614519990, 27.54997392385601529 ) ) ;
#42910=CARTESIAN_POINT ( 'NONE',  ( 24.82500000122902861, -5.773502691896255534, -1.060575238724906372E-15 ) ) ;
#42912=CARTESIAN_POINT ( 'NONE',  ( 14.95312500061451644, 0.000000000000000000, 5.243569643749999010 ) ) ;
#42913=CARTESIAN_POINT ( 'NONE',  ( 8.596875000614518925, 6.054752690667223547, 3.707466751127219781E-16 ) ) ;
#42914=CARTESIAN_POINT ( 'NONE',  ( 6.421875000614519102, 3.027376345333611329, 5.243569643749999010 ) ) ;
#42915=ORIENTED_EDGE ( 'NONE', *, *, #5973, .F. ) ;
#42916=CARTESIAN_POINT ( 'NONE',  ( 29.63437500061451502, 6.421520780324663323E-16, -5.243569643749999010 ) ) ;
#42917=CARTESIAN_POINT ( 'NONE',  ( 20.69062500061451715, 6.054752690667223547, 3.707466751127219781E-16 ) ) ;
#42918=CARTESIAN_POINT ( 'NONE',  ( 15.94687500061451502, -3.027376345333614438, 5.243569643749998122 ) ) ;
#42919=CARTESIAN_POINT ( 'NONE',  ( 21.59062500061451928, 6.054752690667223547, 3.707466751127219781E-16 ) ) ;
#42920=CARTESIAN_POINT ( 'NONE',  ( 3.999999999999998668, 10.81250000000000178, 27.69059892324149175 ) ) ;
#42921=CARTESIAN_POINT ( 'NONE',  ( 27.96562500061451928, 3.027376345333611329, 5.243569643749999010 ) ) ;
#42922=CARTESIAN_POINT ( 'NONE',  ( 6.037500001229035185, 6.123233995736764310E-16, -4.999999999999998224 ) ) ;
#42924=CARTESIAN_POINT ( 'NONE',  ( 29.51249999999999929, 2.886751345948126879, 4.999999999999999112 ) ) ;
#42925=CARTESIAN_POINT ( 'NONE',  ( -3.999999999999999112, 18.19999999999999929, -30.00000000000000000 ) ) ;
#42926=CARTESIAN_POINT ( 'NONE',  ( 24.78750000122903074, -4.330127018922194537, 2.499999999999995559 ) ) ;
#42928=CARTESIAN_POINT ( 'NONE',  ( 8.296875000614516438, -3.027376345333614438, 5.243569643749998122 ) ) ;
#42929=CARTESIAN_POINT ( 'NONE',  ( 23.32499999999999929, -4.330127018922194537, 2.499999999999995559 ) ) ;
#42930=CARTESIAN_POINT ( 'NONE',  ( 14.80312500061451608, 4.541064518000418104, -2.621784821874998173 ) ) ;
#42931=CARTESIAN_POINT ( 'NONE',  ( 9.384375000614518569, 6.421520780324663323E-16, -5.243569643749999010 ) ) ;
#42932=CARTESIAN_POINT ( 'NONE',  ( 27.45000000122903572, -2.886751345948129988, 4.999999999999997335 ) ) ;
#42933=CARTESIAN_POINT ( 'NONE',  ( 18.27187500061451431, -6.054752690667223547, -1.112240025338166033E-15 ) ) ;
#42934=CARTESIAN_POINT ( 'NONE',  ( 4.471875000614518925, 3.027376345333613106, -5.243569643749998122 ) ) ;
#42935=CYLINDRICAL_SURFACE ( 'NONE', #20297, 9.999999999999998224 ) ;
#42936=CARTESIAN_POINT ( 'NONE',  ( 6.515625000614516438, -6.054752690667223547, -1.112240025338166033E-15 ) ) ;
#42937=CARTESIAN_POINT ( 'NONE',  ( 16.41562500061451857, -6.054752690667223547, -1.112240025338166033E-15 ) ) ;
#42939=CARTESIAN_POINT ( 'NONE',  ( 12.81562500061451537, -6.054752690667223547, -1.112240025338166033E-15 ) ) ;
#42940=CARTESIAN_POINT ( 'NONE',  ( 6.150000001229033231, 5.773502691896255534, 3.535250795749688894E-16 ) ) ;
#42941=CARTESIAN_POINT ( 'NONE',  ( 11.24062500061451608, 6.054752690667223547, 3.707466751127219781E-16 ) ) ;
#42943=CARTESIAN_POINT ( 'NONE',  ( 11.10000000000000142, 0.000000000000000000, 4.999999999999998224 ) ) ;
#42944=CARTESIAN_POINT ( 'NONE',  ( 5.362500001229033586, 0.000000000000000000, 4.999999999999998224 ) ) ;
#42945=CARTESIAN_POINT ( 'NONE',  ( 19.01249999999999929, 2.886751345948129099, -4.999999999999998224 ) ) ;
#42946=CARTESIAN_POINT ( 'NONE',  ( 17.59687500061451715, 6.054752690667223547, 3.707466751127219781E-16 ) ) ;
#42947=CARTESIAN_POINT ( 'NONE',  ( 16.80000000122903359, -2.886751345948125991, -5.000000000000000000 ) ) ;
#42949=CARTESIAN_POINT ( 'NONE',  ( -4.243569643749999898, 17.51562500061451644, -32.45002607614398471 ) ) ;
#42951=CARTESIAN_POINT ( 'NONE',  ( 2.735716306934586672, -4.261472593518762508, 2.618912952963186047 ) ) ;
#42952=LINE ( 'NONE', #14870, #12407 ) ;
#42953=CARTESIAN_POINT ( 'NONE',  ( 30.00000000000000000, 6.123233995736764310E-16, -4.999999999999998224 ) ) ;
#42954=CARTESIAN_POINT ( 'NONE',  ( 4.000000000000000000, 19.73749999999999716, 32.30940107675849760 ) ) ;
#42955=CARTESIAN_POINT ( 'NONE',  ( 16.28437500061452070, 4.541064518000418104, 2.621784821874999949 ) ) ;
#42956=CARTESIAN_POINT ( 'NONE',  ( 30.00000000000000000, 0.000000000000000000, 4.999999999999998224 ) ) ;
#42957=CARTESIAN_POINT ( 'NONE',  ( 11.16562500061451679, 3.027376345333613106, -5.243569643749998122 ) ) ;
#42959=CARTESIAN_POINT ( 'NONE',  ( 24.94687500061451502, -3.027376345333614438, 5.243569643749998122 ) ) ;
#42961=CARTESIAN_POINT ( 'NONE',  ( 6.778125000614518392, 4.541064518000418104, 2.621784821874999949 ) ) ;
#42962=CARTESIAN_POINT ( 'NONE',  ( 12.38437500061451857, -4.541064518000419881, 2.621784821874995952 ) ) ;
#42963=ORIENTED_EDGE ( 'NONE', *, *, #10153, .F. ) ;
#42964=CARTESIAN_POINT ( 'NONE',  ( 24.53437500061451715, -4.541064518000419881, 2.621784821874995952 ) ) ;
#42965=CARTESIAN_POINT ( 'NONE',  ( 27.85312500061451502, 4.541064518000418104, -2.621784821874998173 ) ) ;
#42967=CARTESIAN_POINT ( 'NONE',  ( 8.625000000000000000, 6.123233995736764310E-16, -4.999999999999998224 ) ) ;
#42968=CARTESIAN_POINT ( 'NONE',  ( 17.28750000122903430, 6.123233995736764310E-16, -4.999999999999998224 ) ) ;
#42969=CARTESIAN_POINT ( 'NONE',  ( 27.26250000122903216, 4.330127018922192761, -2.499999999999997780 ) ) ;
#42971=ORIENTED_EDGE ( 'NONE', *, *, #14959, .T. ) ;
#42972=CARTESIAN_POINT ( 'NONE',  ( 14.51250000000000107, 2.886751345948129099, -4.999999999999998224 ) ) ;
#42974=CARTESIAN_POINT ( 'NONE',  ( 18.11250000000000071, 2.886751345948129099, -4.999999999999998224 ) ) ;
#42975=CARTESIAN_POINT ( 'NONE',  ( 12.17812500061451608, 4.541064518000418104, 2.621784821874999949 ) ) ;
#42977=CARTESIAN_POINT ( 'NONE',  ( 30.00000000000000000, 0.000000000000000000, 4.999999999999998224 ) ) ;
#42978=CARTESIAN_POINT ( 'NONE',  ( 2.121784821874999061, 17.45937500061451786, -33.67503911421598417 ) ) ;
#42979=CARTESIAN_POINT ( 'NONE',  ( 3.253125000614518036, 0.000000000000000000, 5.243569643749999010 ) ) ;
#42981=CARTESIAN_POINT ( 'NONE',  ( 10.53750000000000320, 5.773502691896255534, 3.535250795749688894E-16 ) ) ;
#42984=CARTESIAN_POINT ( 'NONE',  ( -4.243569643749997233, 14.89062500061451644, 32.45002607614398471 ) ) ;
#42985=CARTESIAN_POINT ( 'NONE',  ( 25.94062500061451715, -3.027376345333610441, -5.243569643749999898 ) ) ;
#42988=CARTESIAN_POINT ( 'NONE',  ( 22.80937500061451573, -4.541064518000417216, -2.621784821875001281 ) ) ;
#42989=CARTESIAN_POINT ( 'NONE',  ( 18.81562500061452070, 3.027376345333613106, -5.243569643749998122 ) ) ;
#42990=EDGE_CURVE ( 'NONE', #46607, #21477, #71788, .T. ) ;
#42991=CARTESIAN_POINT ( 'NONE',  ( 4.243569643749999010, 13.76562500061459282, -32.45002607614398471 ) ) ;
#42992=CARTESIAN_POINT ( 'NONE',  ( 23.73750000122903359, 4.330127018922191873, 2.499999999999999556 ) ) ;
#42993=CARTESIAN_POINT ( 'NONE',  ( 3.628125000614518036, 4.541064518000418104, 2.621784821874999949 ) ) ;
#42995=CARTESIAN_POINT ( 'NONE',  ( 21.66562500061451502, 3.027376345333611329, 5.243569643749999010 ) ) ;
#42998=CARTESIAN_POINT ( 'NONE',  ( 17.07187500061451502, 3.027376345333613106, -5.243569643749998122 ) ) ;
#42999=CARTESIAN_POINT ( 'NONE',  ( 15.64687500061451608, -3.027376345333610441, -5.243569643749999898 ) ) ;
#43000=CARTESIAN_POINT ( 'NONE',  ( 25.95937500061451431, -4.541064518000417216, -2.621784821875001281 ) ) ;
#43001=CARTESIAN_POINT ( 'NONE',  ( 4.243569643749999898, 13.74687500061451750, 32.45002607614398471 ) ) ;
#43002=CARTESIAN_POINT ( 'NONE',  ( 4.565625000614516260, 3.027376345333611329, 5.243569643749999010 ) ) ;
#43003=CARTESIAN_POINT ( 'NONE',  ( 16.57500000122903216, 2.886751345948161074, 4.999999999999941380 ) ) ;
#43004=EDGE_CURVE ( 'NONE', #41088, #42194, #12807, .T. ) ;
#43006=CARTESIAN_POINT ( 'NONE',  ( 3.384375000614517237, -4.541064518000419881, 2.621784821874995952 ) ) ;
#43008=CARTESIAN_POINT ( 'NONE',  ( -1.999999999999997113, 18.72500000000000142, 33.46410161513775705 ) ) ;
#43009=CARTESIAN_POINT ( 'NONE',  ( 8.334375000614516082, -4.541064518000419881, 2.621784821874995952 ) ) ;
#43011=CARTESIAN_POINT ( 'NONE',  ( 15.30000000122903359, -2.886751345948129988, 4.999999999999997335 ) ) ;
#43012=CARTESIAN_POINT ( 'NONE',  ( 8.700000001229032165, -2.886751345948125991, -5.000000000000000000 ) ) ;
#43013=CARTESIAN_POINT ( 'NONE',  ( 5.615625000614517859, -6.054752690667223547, -1.112240025338166033E-15 ) ) ;
#43016=CARTESIAN_POINT ( 'NONE',  ( 15.34687500061451537, 6.054752690667223547, 3.707466751127219781E-16 ) ) ;
#43017=CARTESIAN_POINT ( 'NONE',  ( 21.15000000000000213, -4.330127018922190985, -2.500000000000001332 ) ) ;
#43018=ORIENTED_EDGE ( 'NONE', *, *, #9782, .F. ) ;
#43019=CARTESIAN_POINT ( 'NONE',  ( 21.59062500061451928, 6.054752690667223547, 3.707466751127219781E-16 ) ) ;
#43020=CARTESIAN_POINT ( 'NONE',  ( 6.440625000614517148, -3.027376345333614438, 5.243569643749998122 ) ) ;
#43021=CARTESIAN_POINT ( 'NONE',  ( 23.63437500061451502, -4.541064518000419881, 2.621784821874995952 ) ) ;
#43022=CARTESIAN_POINT ( 'NONE',  ( 7.415625000614516793, -6.054752690667223547, -1.112240025338166033E-15 ) ) ;
#43024=CARTESIAN_POINT ( 'NONE',  ( 7.425000001229034474, 2.886751345948129099, -4.999999999999998224 ) ) ;
#43025=CARTESIAN_POINT ( 'NONE',  ( 21.89062500061451289, -3.027376345333610441, -5.243569643749999898 ) ) ;
#43026=CARTESIAN_POINT ( 'NONE',  ( 4.243569643749999898, 10.12812500061451715, -30.00000000000000000 ) ) ;
#43027=CARTESIAN_POINT ( 'NONE',  ( 9.225000001229034297, 2.886751345948129099, -4.999999999999998224 ) ) ;
#43028=CARTESIAN_POINT ( 'NONE',  ( 19.30312500061451786, 4.541064518000418104, -2.621784821874998173 ) ) ;
#43029=CARTESIAN_POINT ( 'NONE',  ( 18.55312500061451431, 0.000000000000000000, 5.243569643749999010 ) ) ;
#43031=CARTESIAN_POINT ( 'NONE',  ( 17.02499999999999858, -4.330127018922194537, 2.499999999999995559 ) ) ;
#43032=CARTESIAN_POINT ( 'NONE',  ( 11.92500000122903181, 2.886751345948129099, -4.999999999999998224 ) ) ;
#43033=( BOUNDED_SURFACE ( )  B_SPLINE_SURFACE ( 1, 2, ( 
 ( #12010, #7825, #17182, #58412, #2647, #25166, #29005, #40100, #45996, #30360, #13723, #41801, #68175, #57063, #47707, #19246, #23450, #62613, #3012, #34170, #70246, #580, #64330, #62970, #23085, #58779, #36624, #17538, #34533, #6470, #19618, #2287, #47347, #25542, #64700, #51542, #11655, #68533, #67808, #24804, #14084, #17894, #36264, #12366, #6107, #34901, #69881, #8188, #59145, #8554, #31081, #62258, #36988, #43642, #10384, #32916, #55453, #26653, #15181, #4124, #15542, #32188, #53996, #65800, #4846, #42904, #48454, #49189, #71719, #21091, #54721, #44009, #8924, #38459, #54361, #43279, #65428, #48816, #37720, #31454, #48085, #70611, #19984, #59883, #66166, #3755, #55090, #60240, #9289, #27019, #60985, #42537, #65063, #49551, #38086, #71346, #3393, #60608, #25914, #10017, #20721, #14454, #4490, #59510, #31822, #14818, #70978, #20353, #26279, #9654, #37361, #32553, #72073, #21454, #66531, #15911, #50284, #72808, #67279, #22191, #16278, #28819, #11107, #57246, #27380, #61349, #16638, #12189, #38834, #33996, #10745, #61708, #43, #67991, #760, #39193, #45459, #11473, #51357, #33278, #55817, #44745, #23268, #33636, #56180, #5573, #67631, #28110, #50639, #22548, #21820, #68354, #11834, #56533, #45818, #17715, #28460, #45096, #40275, #17365, #5926, #5204, #49912, #44385, #16998, #39555, #27745, #62080, #50995, #393, #39922, #62436, #22900, #34352, #34716, #56885, #6290, #72436, #62796, #66910, #46907, #57967, #42095, #1487, #70160, #23993, #69446, #36179, #69800, #58696, #63523, #24723, #2564, #12552, #52807, #29906, #35443, #64617, #64247, #13635, #46178, #35086, #47266, #19166, #18803, #52446, #25084, #51722, #8107, #18077, #1851, #2208, #41367, #40638, #29188, #30635, #7375, #46540, #69082, #53167, #63157, #6659, #24359, #47627, #41720, #19537, #14003, #36542, #18443, #63877, #1123, #13268, #23632, #68717, #41008, #52082, #35806, #58328, #57612, #7015, #29546, #12910, #7739, #30274, #65344, #31372, #43925, #25460, #60525, #64982, #54633, #31739, #42459, #49104, #26938, #19907, #9569, #4040, #26564, #71633, #9931, #71997, #48004, #71257, #32470, #21371, #70896, #21006, #43558, #14373, #70532, #66451, #8467, #15828, #36908, #20637, #14734, #66080, #43194, #59428, #8836, #53913, #31002, #37276, #65714, #3306, #53535, #15458, #59798, #25833, #48370, #55003, #20269, #59062, #54277, #38003, #4409, #49463, #2931, #42821, #9204, #15100, #3671, #48734, #26194, #37636, #60159, #32101, #16556, #28029, #56456, #11393, #38749, #27660, #17282, #61993, #44665, #10663, #23187, #4764, #39843, #44297, #33913, #11027, #21736, #28378, #6208, #72355, #5846, #50915, #313, #22823, #62357, #51277, #27297, #50557, #11753, #680, #50199, #45375, #67911, #66825, #49831, #45741, #60897, #68276, #16198, #73085, #67195, #34270, #22466, #61269, #33193, #55732, #10301, #39108, #39470, #33549, #56803, #28736, #45016, #5126, #32833, #55371, #72724, #22107, #61624, #56099, #5490, #67552, #38372, #16915, #40931, #57537, #2480, #29468, #1405, #17638, #69719, #7298, #57889, #69000, #53085, #12478, #8023, #35006, #29828, #47187, #7655, #19087, #23914, #35728, #13549, #23552, #63799, #63446, #46462, #25005, #2130, #24641, #57165, #46100, #58250, #30194, #52363, #12832, #36096, #62719, #41642, #29109, #35366, #13189, #6937, #1767, #52004, #18361, #40558, #12113, #58616, #64161, #24281, #30559, #47547, #68637, #17999, #40198, #46829, #69366, #34636, #6578, #63076, #51643, #18724, #1044, #41288, #52724, #25749, #43105, #42740, #13925, #48286, #31285, #8752, #70810, #26479, #20924, #59341, #58979, #65631, #32380, #54920, #4327, #48650, #37190, #26111, #37556, #54192, #2846, #14649, #26852, #64899, #70449, #71175, #20547, #15018, #3589, #66000, #30915, #60441, #3220, #65259, #14289, #20185, #59714, #53456, #70076, #19451, #42011, #53827, #60078, #9121, #3956, #31658, #9489, #49019, #9851, #64531, #36463, #71550, #32018, #54554, #25375, #43476, #47920, #15381, #37923, #8385, #19825, #42377, #36826, #16113, #27214, #15744, #55648, #10944, #6125, #56723, #21654, #10583, #67113, #33110, #72277, #44211, #38665, #66743, #38283, #50835, #5044, #49384, #71915, #10219, #61188, #34189, #60811, #56013, #32752, #27580, #22024, #16836, #22743, #50112, #67473, #33466, #235, #55290, #4684, #72641, #45293, #44581, #16470, #43842, #39028, #61542, #49749, #5406, #27943, #50476, #39390, #61909, #73002, #22386, #21289, #44935, #11314, #66369, #28300, #33835, #56377, #5769, #11673, #67827, #39761, #17200, #62278, #58160, #18636, #7564, #12383, #46740, #24552, #34552, #1677, #51918, #57446, #13453, #13100, #35638, #68193, #57080, #69274, #41200, #18267, #1315, #47098, #598, #30100, #40117, #23824, #24186, #40840, #62633, #51195, #52635, #6850, #23469, #46015, #2041, #12027, #28656, #46375, #69630, #63708, #18992, #41554, #64071, #68552, #63358, #23103, #12742, #36001, #58520, #62988, #960, #29384, #35278, #45660, #17556, #29023, #17910, #6488, #52275, #34919, #40473, #51559, #68909, #57800, #7209, #29738, #53734, #64440, #71085, #48929, #41915, #31564, #26020, #3501, #48559, #9399, #20834, #47455, #20090, #31929, #43387, #19732, #20459, #43013, #13832, #19358, #65911, #30468, #15291, #58887, #42647, #36731, #65542, #65171, #36371, #8297, #69988, #52997, #14196, #9034, #3127, #54466, #14929, #14562, #30827, #2393, #37469, #59989, #70715, #31192, #26387, #24912, #3864, #53360, #25656, #71458, #37095, #2757, #25279, #37830, #59253, #47825, #70355, #7930, #42282, #64806, #48192, #8661, #59620, #54103, #28217, #33746, #4595, #72548, #9759, #50023, #22297, #44849, #21566, #32661, #38572, #21935, #5317, #33385, #60719, #49659, #39304, #10851, #66647, #55202, #45205, #26762, #61817, #66275, #55921, #33022, #43750, #50390, #50746 ),
 ( #44491, #16024, #67385, #67024, #21198, #15653, #49294, #32293, #61096, #61457, #55560, #11222, #72915, #16384, #38192, #54828, #4235, #27125, #72187, #10129, #10494, #44120, #38939, #16747, #27859, #4956, #27489, #67738, #56291, #5681, #60350, #149, #22655, #17111, #71827, #1958, #34465, #30009, #56993, #29296, #69189, #29651, #18549, #23378, #57717, #35552, #45573, #12657, #62900, #68458, #24465, #24101, #46649, #6037, #68104, #1591, #505, #51108, #47013, #62190, #69548, #17470, #51826, #17820, #41114, #23735, #23015, #40030, #28571, #11586, #45926, #40750, #12295, #63624, #52189, #46283, #62543, #34103, #56642, #11940, #6400, #28932, #40381, #51468, #1229, #13014, #7122, #34830, #871, #39670, #57356, #6762, #68824, #58071, #18181, #63265, #35192, #7481, #52552, #9311, #13746, #8575, #48475, #8945, #70999, #2670, #37010, #14842, #24825, #65085, #42197, #47730, #3776, #3415, #25935, #58436, #47372, #59533, #31477, #31103, #64721, #37383, #63987, #20375, #30383, #14105, #14476, #53643, #52912, #41468, #42926, #70269, #36287, #58801, #65450, #2310, #18907, #36645, #59906, #54019, #31845, #54381, #26301, #8211, #3035, #13369, #25566, #48838, #35911, #53272, #64355, #19641, #48107, #7847, #69903, #19269, #30740, #41823, #42558, #25187, #59167, #70630, #20005, #691, #4145, #67923, #45029, #54743, #62369, #40209, #32209, #22835, #17295, #39857, #11767, #23199, #12123, #37742, #11407, #45753, #34650, #10042, #34283, #26677, #56815, #67564, #65822, #6222, #43302, #32576, #38109, #49209, #60262, #5502, #33926, #29121, #6592, #43666, #55114, #16929, #28041, #21113, #66188, #60630, #15566, #9676, #68289, #50570, #71369, #20744, #71743, #73097, #57178, #22479, #5859, #39483, #62006, #56468, #28750, #17649, #28391, #51290, #50929, #62731, #326, #45387, #15204, #25016, #18376, #57901, #40944, #18735, #63458, #35378, #1419, #46112, #19464, #36107, #35741, #2492, #47558, #57547, #29481, #70087, #13201, #30205, #36473, #30570, #52018, #68649, #23925, #8397, #58260, #42022, #7310, #24652, #24292, #18013, #29840, #12845, #52375, #1781, #8035, #64543, #46840, #40570, #47198, #13936, #58991, #51655, #52736, #41299, #7666, #19098, #2141, #6949, #69380, #1057, #46475, #69013, #69729, #41653, #64174, #13562, #23567, #12491, #63090, #63809, #58628, #53096, #35018, #48660, #64910, #38293, #66378, #15754, #42750, #3967, #59724, #37932, #71185, #65271, #9860, #21299, #43853, #2858, #32390, #26489, #54202, #59352, #49031, #15029, #14300, #36838, #19836, #25388, #37201, #32028, #3599, #54930, #20935, #37566, #8763, #53467, #47932, #3233, #25760, #31297, #9132, #48296, #20558, #43486, #71560, #26121, #70822, #60822, #14658, #31669, #30926, #4337, #43116, #65641, #60090, #70461, #20196, #42388, #9499, #54564, #60452, #66010, #26862, #15390, #49393, #71924, #53838, #56391, #33477, #39040, #68209, #67842, #17214, #49760, #16124, #28312, #22756, #73015, #56026, #28671, #55299, #11688, #21664, #5418, #5781, #22399, #44221, #32762, #39776, #61554, #5054, #27591, #56738, #66754, #10228, #27957, #62292, #248, #45307, #51211, #6140, #50123, #44948, #4693, #67485, #34204, #611, #44594, #55658, #10956, #16848, #50848, #23118, #10593, #72654, #45673, #33847, #16483, #22035, #17570, #72286, #40132, #38677, #27223, #50489, #61198, #33121, #67125, #39404, #61921, #11327, #58174, #7579, #64086, #2406, #29039, #1691, #13468, #24927, #1329, #30114, #24567, #23483, #973, #47470, #12043, #70002, #40488, #24201, #18280, #47112, #52649, #2055, #36016, #19372, #51574, #46754, #58534, #62646, #23841, #69644, #19006, #46030, #68566, #34566, #57095, #6503, #63003, #69289, #40856, #41568, #18652, #17925, #12398, #34934, #57460, #68924, #63722, #35293, #7946, #30483, #41214, #6866, #29398, #51932, #46389, #63373, #12757, #57814, #7224, #52290, #53012, #29753, #13114, #35654, #26776, #53747, #25670, #41929, #20848, #31579, #9048, #20106, #4251, #36747, #32308, #59267, #54118, #71472, #31944, #43401, #48207, #60004, #37844, #47840, #14945, #65186, #70729, #49308, #26401, #48944, #8312, #70369, #9414, #54480, #3514, #14576, #60365, #13846, #65926, #53375, #37109, #37483, #26034, #2771, #64455, #15306, #42661, #8675, #31206, #9774, #25294, #36386, #59635, #54842, #3880, #71842, #58900, #30841, #3144, #48573, #19747, #71101, #42296, #64821, #20474, #14210, #43027, #65555, #39320, #67401, #21581, #10509, #164, #44865, #27504, #66662, #6051, #60735, #22669, #27141, #16762, #67040, #4611, #11238, #62204, #55216, #61833, #33760, #72204, #10144, #50037, #55937, #51123, #28586, #16039, #55577, #38954, #4970, #44135, #38587, #61113, #33037, #32677, #45220, #72563, #21213, #43766, #49675, #21949, #66290, #44506, #27873, #16400, #61472, #10867, #56305, #67753, #33400, #5694, #5332, #17125, #50406, #72930, #22312, #39685, #28230, #50760, #11600, #34117, #56657, #15669, #38207, #45586, #58086, #24115, #68838, #41129, #63639, #34480, #6415, #13028, #18195, #63280, #52565, #18563, #28947, #68119, #886, #24481, #40766, #35567, #12310, #57731, #6779, #17485, #34845, #17835, #40396, #57371, #69204, #7494, #68473, #40047, #7137, #1972, #30022, #520, #12672, #23750, #35209, #52203, #29667, #57010, #1245, #23031, #29311, #62915, #1604, #46664, #62559, #11955, #51486, #51842, #23393, #45942, #46299, #10729, #67261, #11089, #27363, #745, #28802, #51343, #5189, #39538, #22173, #376, #33617, #27727, #45442, #56870, #6274, #38441, #67975, #62063, #16619, #21802, #11457, #49894, #56517, #39174, #60967, #22884, #10367, #50265, #33261, #72790, #61690, #33978, #39907, #55799, #5910, #50621, #17348, #72419, #44366, #61331, #62420, #44726, #56161, #5556, #28093, #26, #22532, #16261, #32897, #34336, #50979, #45079, #11819, #23254, #66893 ) ),
 .UNSPECIFIED., .F., .F., .F. ) 
 B_SPLINE_SURFACE_WITH_KNOTS ( ( 2, 2 ),
 ( 3, 2, 2, 2, 2, 2, 2, 2, 2, 2, 2, 2, 2, 2, 2, 2, 2, 2, 2, 2, 2, 2, 2, 2, 2, 2, 2, 2, 2, 2, 2, 2, 2, 2, 2, 2, 2, 2, 2, 2, 2, 2, 2, 2, 2, 2, 2, 2, 2, 2, 2, 2, 2, 2, 2, 2, 2, 2, 2, 2, 2, 2, 2, 2, 2, 2, 2, 2, 2, 2, 2, 2, 2, 2, 2, 2, 2, 2, 2, 2, 2, 2, 2, 2, 2, 2, 2, 2, 2, 2, 2, 2, 2, 2, 2, 2, 2, 2, 2, 2, 2, 2, 2, 2, 2, 2, 2, 2, 2, 2, 2, 2, 2, 2, 2, 2, 2, 2, 2, 2, 2, 2, 2, 2, 2, 2, 2, 2, 2, 2, 2, 2, 2, 2, 2, 2, 2, 2, 2, 2, 2, 2, 2, 2, 2, 2, 2, 2, 2, 2, 2, 2, 2, 2, 2, 2, 2, 2, 2, 2, 2, 2, 2, 2, 2, 2, 2, 2, 2, 2, 2, 2, 2, 2, 2, 2, 2, 2, 2, 2, 2, 2, 2, 2, 2, 2, 2, 2, 2, 2, 2, 2, 2, 2, 2, 2, 2, 2, 2, 2, 2, 2, 2, 2, 2, 2, 2, 2, 2, 2, 2, 2, 2, 2, 2, 2, 2, 2, 2, 2, 2, 2, 2, 2, 2, 2, 2, 2, 2, 2, 2, 2, 2, 2, 2, 2, 2, 2, 2, 2, 2, 2, 2, 2, 2, 2, 2, 2, 2, 2, 2, 2, 2, 2, 2, 2, 2, 2, 2, 2, 2, 2, 2, 2, 2, 2, 2, 2, 2, 2, 2, 2, 2, 2, 2, 2, 2, 2, 2, 2, 2, 2, 2, 2, 2, 2, 2, 2, 2, 2, 2, 2, 2, 2, 2, 2, 2, 2, 2, 2, 2, 2, 2, 2, 2, 2, 2, 2, 2, 2, 2, 2, 2, 2, 2, 2, 2, 2, 2, 2, 2, 2, 2, 2, 2, 2, 2, 2, 2, 2, 2, 2, 2, 2, 2, 2, 2, 2, 2, 2, 2, 2, 2, 2, 2, 2, 2, 2, 2, 2, 2, 2, 2, 2, 2, 2, 2, 2, 2, 2, 3 ),
 ( 0.000000000000000000, 1.000000000000000000 ),
 ( 0.000000000000000000, 0.002777777777777777884, 0.005555555555555555768, 0.008333333333333333218, 0.01111111111111111154, 0.01388888888888888812, 0.01666666666666666644, 0.01944444444444444475, 0.02222222222222222307, 0.02500000000000000139, 0.02777777777777777624, 0.03055555555555555455, 0.03333333333333333287, 0.03611111111111110772, 0.03888888888888888951, 0.04166666666666666435, 0.04444444444444444614, 0.04722222222222222099, 0.05000000000000000278, 0.05277777777777777762, 0.05555555555555555247, 0.05833333333333333426, 0.06111111111111110911, 0.06388888888888888395, 0.06666666666666666574, 0.06944444444444444753, 0.07222222222222221544, 0.07499999999999999722, 0.07777777777777777901, 0.08055555555555556080, 0.08333333333333332871, 0.08611111111111111049, 0.08888888888888889228, 0.09166666666666666019, 0.09444444444444444198, 0.09722222222222222376, 0.1000000000000000056, 0.1027777777777777735, 0.1055555555555555552, 0.1083333333333333370, 0.1111111111111111049, 0.1138888888888888867, 0.1166666666666666685, 0.1194444444444444503, 0.1222222222222222182, 0.1250000000000000000, 0.1277777777777777679, 0.1305555555555555636, 0.1333333333333333315, 0.1361111111111110994, 0.1388888888888888951, 0.1416666666666666630, 0.1444444444444444309, 0.1472222222222222265, 0.1499999999999999944, 0.1527777777777777901, 0.1555555555555555580, 0.1583333333333333259, 0.1611111111111111216, 0.1638888888888888895, 0.1666666666666666574, 0.1694444444444444531, 0.1722222222222222210, 0.1749999999999999889, 0.1777777777777777846, 0.1805555555555555525, 0.1833333333333333204, 0.1861111111111111160, 0.1888888888888888840, 0.1916666666666666796, 0.1944444444444444475, 0.1972222222222222154, 0.2000000000000000111, 0.2027777777777777790, 0.2055555555555555469, 0.2083333333333333426, 0.2111111111111111105, 0.2138888888888888784, 0.2166666666666666741, 0.2194444444444444420, 0.2222222222222222099, 0.2250000000000000056, 0.2277777777777777735, 0.2305555555555555691, 0.2333333333333333370, 0.2361111111111111049, 0.2388888888888889006, 0.2416666666666666685, 0.2444444444444444364, 0.2472222222222222321, 0.2500000000000000000, 0.2527777777777777679, 0.2555555555555555358, 0.2583333333333333592, 0.2611111111111111271, 0.2638888888888888951, 0.2666666666666666630, 0.2694444444444444309, 0.2722222222222221988, 0.2750000000000000222, 0.2777777777777777901, 0.2805555555555555580, 0.2833333333333333259, 0.2861111111111110938, 0.2888888888888888618, 0.2916666666666666852, 0.2944444444444444531, 0.2972222222222222210, 0.2999999999999999889, 0.3027777777777777568, 0.3055555555555555802, 0.3083333333333333481, 0.3111111111111111160, 0.3138888888888888840, 0.3166666666666666519, 0.3194444444444444198, 0.3222222222222222432, 0.3250000000000000111, 0.3277777777777777790, 0.3305555555555555469, 0.3333333333333333148, 0.3361111111111111382, 0.3388888888888889062, 0.3416666666666666741, 0.3444444444444444420, 0.3472222222222222099, 0.3499999999999999778, 0.3527777777777778012, 0.3555555555555555691, 0.3583333333333333370, 0.3611111111111111049, 0.3638888888888888729, 0.3666666666666666408, 0.3694444444444444642, 0.3722222222222222321, 0.3750000000000000000, 0.3777777777777777679, 0.3805555555555555358, 0.3833333333333333592, 0.3861111111111111271, 0.3888888888888888951, 0.3916666666666666630, 0.3944444444444444309, 0.3972222222222221988, 0.4000000000000000222, 0.4027777777777777901, 0.4055555555555555580, 0.4083333333333333259, 0.4111111111111110938, 0.4138888888888888618, 0.4166666666666666852, 0.4194444444444444531, 0.4222222222222222210, 0.4249999999999999889, 0.4277777777777777568, 0.4305555555555555802, 0.4333333333333333481, 0.4361111111111111160, 0.4388888888888888840, 0.4416666666666666519, 0.4444444444444444198, 0.4472222222222222432, 0.4500000000000000111, 0.4527777777777777790, 0.4555555555555555469, 0.4583333333333333148, 0.4611111111111111382, 0.4638888888888889062, 0.4666666666666666741, 0.4694444444444444420, 0.4722222222222222099, 0.4749999999999999778, 0.4777777777777778012, 0.4805555555555555691, 0.4833333333333333370, 0.4861111111111111049, 0.4888888888888888729, 0.4916666666666666408, 0.4944444444444444642, 0.4972222222222222321, 0.5000000000000000000, 0.5027777777777777679, 0.5055555555555555358, 0.5083333333333333037, 0.5111111111111110716, 0.5138888888888888395, 0.5166666666666667185, 0.5194444444444444864, 0.5222222222222222543, 0.5250000000000000222, 0.5277777777777777901, 0.5305555555555555580, 0.5333333333333333259, 0.5361111111111110938, 0.5388888888888888618, 0.5416666666666666297, 0.5444444444444443976, 0.5472222222222222765, 0.5500000000000000444, 0.5527777777777778123, 0.5555555555555555802, 0.5583333333333333481, 0.5611111111111111160, 0.5638888888888888840, 0.5666666666666666519, 0.5694444444444444198, 0.5722222222222221877, 0.5749999999999999556, 0.5777777777777777235, 0.5805555555555556024, 0.5833333333333333703, 0.5861111111111111382, 0.5888888888888889062, 0.5916666666666666741, 0.5944444444444444420, 0.5972222222222222099, 0.5999999999999999778, 0.6027777777777777457, 0.6055555555555555136, 0.6083333333333332815, 0.6111111111111111605, 0.6138888888888889284, 0.6166666666666666963, 0.6194444444444444642, 0.6222222222222222321, 0.6250000000000000000, 0.6277777777777777679, 0.6305555555555555358, 0.6333333333333333037, 0.6361111111111110716, 0.6388888888888888395, 0.6416666666666667185, 0.6444444444444444864, 0.6472222222222222543, 0.6500000000000000222, 0.6527777777777777901, 0.6555555555555555580, 0.6583333333333333259, 0.6611111111111110938, 0.6638888888888888618, 0.6666666666666666297, 0.6694444444444443976, 0.6722222222222222765, 0.6750000000000000444, 0.6777777777777778123, 0.6805555555555555802, 0.6833333333333333481, 0.6861111111111111160, 0.6888888888888888840, 0.6916666666666666519, 0.6944444444444444198, 0.6972222222222221877, 0.6999999999999999556, 0.7027777777777777235, 0.7055555555555556024, 0.7083333333333333703, 0.7111111111111111382, 0.7138888888888889062, 0.7166666666666666741, 0.7194444444444444420, 0.7222222222222222099, 0.7249999999999999778, 0.7277777777777777457, 0.7305555555555555136, 0.7333333333333332815, 0.7361111111111111605, 0.7388888888888889284, 0.7416666666666666963, 0.7444444444444444642, 0.7472222222222222321, 0.7500000000000000000, 0.7527777777777777679, 0.7555555555555555358, 0.7583333333333333037, 0.7611111111111110716, 0.7638888888888888395, 0.7666666666666667185, 0.7694444444444444864, 0.7722222222222222543, 0.7750000000000000222, 0.7777777777777777901, 0.7805555555555555580, 0.7833333333333333259, 0.7861111111111110938, 0.7888888888888888618, 0.7916666666666666297, 0.7944444444444443976, 0.7972222222222222765, 0.8000000000000000444, 0.8027777777777778123, 0.8055555555555555802, 0.8083333333333333481, 0.8111111111111111160, 0.8138888888888888840, 0.8166666666666666519, 0.8194444444444444198, 0.8222222222222221877, 0.8249999999999999556, 0.8277777777777777235, 0.8305555555555556024, 0.8333333333333333703, 0.8361111111111111382, 0.8388888888888889062, 0.8416666666666666741, 0.8444444444444444420, 0.8472222222222222099, 0.8499999999999999778, 0.8527777777777777457, 0.8555555555555555136, 0.8583333333333332815, 0.8611111111111111605, 0.8638888888888889284, 0.8666666666666666963, 0.8694444444444444642, 0.8722222222222222321, 0.8750000000000000000, 0.8777777777777777679, 0.8805555555555555358, 0.8833333333333333037, 0.8861111111111110716, 0.8888888888888888395, 0.8916666666666667185, 0.8944444444444444864, 0.8972222222222222543, 0.9000000000000000222, 0.9027777777777777901, 0.9055555555555555580, 0.9083333333333333259, 0.9111111111111110938, 0.9138888888888888618, 0.9166666666666666297, 0.9194444444444443976, 0.9222222222222222765, 0.9250000000000000444, 0.9277777777777778123, 0.9305555555555555802, 0.9333333333333333481, 0.9361111111111111160, 0.9388888888888888840, 0.9416666666666666519, 0.9444444444444444198, 0.9472222222222221877, 0.9499999999999999556, 0.9527777777777777235, 0.9555555555555556024, 0.9583333333333333703, 0.9611111111111111382, 0.9638888888888889062, 0.9666666666666666741, 0.9694444444444444420, 0.9722222222222222099, 0.9749999999999999778, 0.9777777777777777457, 0.9805555555555555136, 0.9833333333333332815, 0.9861111111111111605, 0.9888888888888889284, 0.9916666666666666963, 0.9944444444444444642, 0.9972222222222222321, 1.000000000000000000 ),
 .UNSPECIFIED. ) 
 GEOMETRIC_REPRESENTATION_ITEM ( )  RATIONAL_B_SPLINE_SURFACE ( (
 ( 1.000000000000000000, 0.8660254037844387076, 1.000000000000000000, 0.8660254037844387076, 1.000000000000000000, 0.8660254037844387076, 1.000000000000000000, 0.8660254037844387076, 1.000000000000000000, 0.8660254037844387076, 1.000000000000000000, 0.8660254037844387076, 1.000000000000000000, 0.8660254037844387076, 1.000000000000000000, 0.8660254037844387076, 1.000000000000000000, 0.8660254037844387076, 1.000000000000000000, 0.8660254037844387076, 1.000000000000000000, 0.8660254037844387076, 1.000000000000000000, 0.8660254037844387076, 1.000000000000000000, 0.8660254037844387076, 1.000000000000000000, 0.8660254037844387076, 1.000000000000000000, 0.8660254037844387076, 1.000000000000000000, 0.8660254037844387076, 1.000000000000000000, 0.8660254037844387076, 1.000000000000000000, 0.8660254037844387076, 1.000000000000000000, 0.8660254037844387076, 1.000000000000000000, 0.8660254037844387076, 1.000000000000000000, 0.8660254037844387076, 1.000000000000000000, 0.8660254037844387076, 1.000000000000000000, 0.8660254037844387076, 1.000000000000000000, 0.8660254037844387076, 1.000000000000000000, 0.8660254037844387076, 1.000000000000000000, 0.8660254037844387076, 1.000000000000000000, 0.8660254037844387076, 1.000000000000000000, 0.8660254037844387076, 1.000000000000000000, 0.8660254037844387076, 1.000000000000000000, 0.8660254037844387076, 1.000000000000000000, 0.8660254037844387076, 1.000000000000000000, 0.8660254037844387076, 1.000000000000000000, 0.8660254037844387076, 1.000000000000000000, 0.8660254037844387076, 1.000000000000000000, 0.8660254037844387076, 1.000000000000000000, 0.8660254037844387076, 1.000000000000000000, 0.8660254037844387076, 1.000000000000000000, 0.8660254037844387076, 1.000000000000000000, 0.8660254037844387076, 1.000000000000000000, 0.8660254037844387076, 1.000000000000000000, 0.8660254037844387076, 1.000000000000000000, 0.8660254037844387076, 1.000000000000000000, 0.8660254037844387076, 1.000000000000000000, 0.8660254037844387076, 1.000000000000000000, 0.8660254037844387076, 1.000000000000000000, 0.8660254037844387076, 1.000000000000000000, 0.8660254037844387076, 1.000000000000000000, 0.8660254037844387076, 1.000000000000000000, 0.8660254037844387076, 1.000000000000000000, 0.8660254037844387076, 1.000000000000000000, 0.8660254037844387076, 1.000000000000000000, 0.8660254037844387076, 1.000000000000000000, 0.8660254037844387076, 1.000000000000000000, 0.8660254037844387076, 1.000000000000000000, 0.8660254037844387076, 1.000000000000000000, 0.8660254037844387076, 1.000000000000000000, 0.8660254037844387076, 1.000000000000000000, 0.8660254037844387076, 1.000000000000000000, 0.8660254037844387076, 1.000000000000000000, 0.8660254037844387076, 1.000000000000000000, 0.8660254037844387076, 1.000000000000000000, 0.8660254037844387076, 1.000000000000000000, 0.8660254037844387076, 1.000000000000000000, 0.8660254037844387076, 1.000000000000000000, 0.8660254037844387076, 1.000000000000000000, 0.8660254037844387076, 1.000000000000000000, 0.8660254037844387076, 1.000000000000000000, 0.8660254037844387076, 1.000000000000000000, 0.8660254037844387076, 1.000000000000000000, 0.8660254037844387076, 1.000000000000000000, 0.8660254037844387076, 1.000000000000000000, 0.8660254037844387076, 1.000000000000000000, 0.8660254037844387076, 1.000000000000000000, 0.8660254037844387076, 1.000000000000000000, 0.8660254037844387076, 1.000000000000000000, 0.8660254037844387076, 1.000000000000000000, 0.8660254037844387076, 1.000000000000000000, 0.8660254037844387076, 1.000000000000000000, 0.8660254037844387076, 1.000000000000000000, 0.8660254037844387076, 1.000000000000000000, 0.8660254037844387076, 1.000000000000000000, 0.8660254037844387076, 1.000000000000000000, 0.8660254037844387076, 1.000000000000000000, 0.8660254037844387076, 1.000000000000000000, 0.8660254037844387076, 1.000000000000000000, 0.8660254037844387076, 1.000000000000000000, 0.8660254037844387076, 1.000000000000000000, 0.8660254037844387076, 1.000000000000000000, 0.8660254037844387076, 1.000000000000000000, 0.8660254037844387076, 1.000000000000000000, 0.8660254037844387076, 1.000000000000000000, 0.8660254037844387076, 1.000000000000000000, 0.8660254037844387076, 1.000000000000000000, 0.8660254037844387076, 1.000000000000000000, 0.8660254037844387076, 1.000000000000000000, 0.8660254037844387076, 1.000000000000000000, 0.8660254037844387076, 1.000000000000000000, 0.8660254037844387076, 1.000000000000000000, 0.8660254037844387076, 1.000000000000000000, 0.8660254037844387076, 1.000000000000000000, 0.8660254037844387076, 1.000000000000000000, 0.8660254037844387076, 1.000000000000000000, 0.8660254037844387076, 1.000000000000000000, 0.8660254037844387076, 1.000000000000000000, 0.8660254037844387076, 1.000000000000000000, 0.8660254037844387076, 1.000000000000000000, 0.8660254037844387076, 1.000000000000000000, 0.8660254037844387076, 1.000000000000000000, 0.8660254037844387076, 1.000000000000000000, 0.8660254037844387076, 1.000000000000000000, 0.8660254037844387076, 1.000000000000000000, 0.8660254037844387076, 1.000000000000000000, 0.8660254037844387076, 1.000000000000000000, 0.8660254037844387076, 1.000000000000000000, 0.8660254037844387076, 1.000000000000000000, 0.8660254037844387076, 1.000000000000000000, 0.8660254037844387076, 1.000000000000000000, 0.8660254037844387076, 1.000000000000000000, 0.8660254037844387076, 1.000000000000000000, 0.8660254037844387076, 1.000000000000000000, 0.8660254037844387076, 1.000000000000000000, 0.8660254037844387076, 1.000000000000000000, 0.8660254037844387076, 1.000000000000000000, 0.8660254037844387076, 1.000000000000000000, 0.8660254037844387076, 1.000000000000000000, 0.8660254037844387076, 1.000000000000000000, 0.8660254037844387076, 1.000000000000000000, 0.8660254037844387076, 1.000000000000000000, 0.8660254037844387076, 1.000000000000000000, 0.8660254037844387076, 1.000000000000000000, 0.8660254037844387076, 1.000000000000000000, 0.8660254037844387076, 1.000000000000000000, 0.8660254037844387076, 1.000000000000000000, 0.8660254037844387076, 1.000000000000000000, 0.8660254037844387076, 1.000000000000000000, 0.8660254037844387076, 1.000000000000000000, 0.8660254037844387076, 1.000000000000000000, 0.8660254037844387076, 1.000000000000000000, 0.8660254037844387076, 1.000000000000000000, 0.8660254037844387076, 1.000000000000000000, 0.8660254037844387076, 1.000000000000000000, 0.8660254037844387076, 1.000000000000000000, 0.8660254037844387076, 1.000000000000000000, 0.8660254037844387076, 1.000000000000000000, 0.8660254037844387076, 1.000000000000000000, 0.8660254037844387076, 1.000000000000000000, 0.8660254037844387076, 1.000000000000000000, 0.8660254037844387076, 1.000000000000000000, 0.8660254037844387076, 1.000000000000000000, 0.8660254037844387076, 1.000000000000000000, 0.8660254037844387076, 1.000000000000000000, 0.8660254037844387076, 1.000000000000000000, 0.8660254037844387076, 1.000000000000000000, 0.8660254037844387076, 1.000000000000000000, 0.8660254037844387076, 1.000000000000000000, 0.8660254037844387076, 1.000000000000000000, 0.8660254037844387076, 1.000000000000000000, 0.8660254037844387076, 1.000000000000000000, 0.8660254037844387076, 1.000000000000000000, 0.8660254037844387076, 1.000000000000000000, 0.8660254037844387076, 1.000000000000000000, 0.8660254037844387076, 1.000000000000000000, 0.8660254037844387076, 1.000000000000000000, 0.8660254037844387076, 1.000000000000000000, 0.8660254037844387076, 1.000000000000000000, 0.8660254037844387076, 1.000000000000000000, 0.8660254037844387076, 1.000000000000000000, 0.8660254037844387076, 1.000000000000000000, 0.8660254037844387076, 1.000000000000000000, 0.8660254037844387076, 1.000000000000000000, 0.8660254037844387076, 1.000000000000000000, 0.8660254037844387076, 1.000000000000000000, 0.8660254037844387076, 1.000000000000000000, 0.8660254037844387076, 1.000000000000000000, 0.8660254037844387076, 1.000000000000000000, 0.8660254037844387076, 1.000000000000000000, 0.8660254037844387076, 1.000000000000000000, 0.8660254037844387076, 1.000000000000000000, 0.8660254037844387076, 1.000000000000000000, 0.8660254037844387076, 1.000000000000000000, 0.8660254037844387076, 1.000000000000000000, 0.8660254037844387076, 1.000000000000000000, 0.8660254037844387076, 1.000000000000000000, 0.8660254037844387076, 1.000000000000000000, 0.8660254037844387076, 1.000000000000000000, 0.8660254037844387076, 1.000000000000000000, 0.8660254037844387076, 1.000000000000000000, 0.8660254037844387076, 1.000000000000000000, 0.8660254037844387076, 1.000000000000000000, 0.8660254037844387076, 1.000000000000000000, 0.8660254037844387076, 1.000000000000000000, 0.8660254037844387076, 1.000000000000000000, 0.8660254037844387076, 1.000000000000000000, 0.8660254037844387076, 1.000000000000000000, 0.8660254037844387076, 1.000000000000000000, 0.8660254037844387076, 1.000000000000000000, 0.8660254037844387076, 1.000000000000000000, 0.8660254037844387076, 1.000000000000000000, 0.8660254037844387076, 1.000000000000000000, 0.8660254037844387076, 1.000000000000000000, 0.8660254037844387076, 1.000000000000000000, 0.8660254037844387076, 1.000000000000000000, 0.8660254037844387076, 1.000000000000000000, 0.8660254037844387076, 1.000000000000000000, 0.8660254037844387076, 1.000000000000000000, 0.8660254037844387076, 1.000000000000000000, 0.8660254037844387076, 1.000000000000000000, 0.8660254037844387076, 1.000000000000000000, 0.8660254037844387076, 1.000000000000000000, 0.8660254037844387076, 1.000000000000000000, 0.8660254037844387076, 1.000000000000000000, 0.8660254037844387076, 1.000000000000000000, 0.8660254037844387076, 1.000000000000000000, 0.8660254037844387076, 1.000000000000000000, 0.8660254037844387076, 1.000000000000000000, 0.8660254037844387076, 1.000000000000000000, 0.8660254037844387076, 1.000000000000000000, 0.8660254037844387076, 1.000000000000000000, 0.8660254037844387076, 1.000000000000000000, 0.8660254037844387076, 1.000000000000000000, 0.8660254037844387076, 1.000000000000000000, 0.8660254037844387076, 1.000000000000000000, 0.8660254037844387076, 1.000000000000000000, 0.8660254037844387076, 1.000000000000000000, 0.8660254037844387076, 1.000000000000000000, 0.8660254037844387076, 1.000000000000000000, 0.8660254037844387076, 1.000000000000000000, 0.8660254037844387076, 1.000000000000000000, 0.8660254037844387076, 1.000000000000000000, 0.8660254037844387076, 1.000000000000000000, 0.8660254037844387076, 1.000000000000000000, 0.8660254037844387076, 1.000000000000000000, 0.8660254037844387076, 1.000000000000000000, 0.8660254037844387076, 1.000000000000000000, 0.8660254037844387076, 1.000000000000000000, 0.8660254037844387076, 1.000000000000000000, 0.8660254037844387076, 1.000000000000000000, 0.8660254037844387076, 1.000000000000000000, 0.8660254037844387076, 1.000000000000000000, 0.8660254037844387076, 1.000000000000000000, 0.8660254037844387076, 1.000000000000000000, 0.8660254037844387076, 1.000000000000000000, 0.8660254037844387076, 1.000000000000000000, 0.8660254037844387076, 1.000000000000000000, 0.8660254037844387076, 1.000000000000000000, 0.8660254037844387076, 1.000000000000000000, 0.8660254037844387076, 1.000000000000000000, 0.8660254037844387076, 1.000000000000000000, 0.8660254037844387076, 1.000000000000000000, 0.8660254037844387076, 1.000000000000000000, 0.8660254037844387076, 1.000000000000000000, 0.8660254037844387076, 1.000000000000000000, 0.8660254037844387076, 1.000000000000000000, 0.8660254037844387076, 1.000000000000000000, 0.8660254037844387076, 1.000000000000000000, 0.8660254037844387076, 1.000000000000000000, 0.8660254037844387076, 1.000000000000000000, 0.8660254037844387076, 1.000000000000000000, 0.8660254037844387076, 1.000000000000000000, 0.8660254037844387076, 1.000000000000000000, 0.8660254037844387076, 1.000000000000000000, 0.8660254037844387076, 1.000000000000000000, 0.8660254037844387076, 1.000000000000000000, 0.8660254037844387076, 1.000000000000000000, 0.8660254037844387076, 1.000000000000000000, 0.8660254037844387076, 1.000000000000000000, 0.8660254037844387076, 1.000000000000000000, 0.8660254037844387076, 1.000000000000000000, 0.8660254037844387076, 1.000000000000000000, 0.8660254037844387076, 1.000000000000000000, 0.8660254037844387076, 1.000000000000000000, 0.8660254037844387076, 1.000000000000000000, 0.8660254037844387076, 1.000000000000000000, 0.8660254037844387076, 1.000000000000000000, 0.8660254037844387076, 1.000000000000000000, 0.8660254037844387076, 1.000000000000000000, 0.8660254037844387076, 1.000000000000000000, 0.8660254037844387076, 1.000000000000000000, 0.8660254037844387076, 1.000000000000000000, 0.8660254037844387076, 1.000000000000000000, 0.8660254037844387076, 1.000000000000000000, 0.8660254037844387076, 1.000000000000000000, 0.8660254037844387076, 1.000000000000000000, 0.8660254037844387076, 1.000000000000000000, 0.8660254037844387076, 1.000000000000000000, 0.8660254037844387076, 1.000000000000000000, 0.8660254037844387076, 1.000000000000000000, 0.8660254037844387076, 1.000000000000000000, 0.8660254037844387076, 1.000000000000000000, 0.8660254037844387076, 1.000000000000000000, 0.8660254037844387076, 1.000000000000000000, 0.8660254037844387076, 1.000000000000000000, 0.8660254037844387076, 1.000000000000000000, 0.8660254037844387076, 1.000000000000000000, 0.8660254037844387076, 1.000000000000000000, 0.8660254037844387076, 1.000000000000000000, 0.8660254037844387076, 1.000000000000000000, 0.8660254037844387076, 1.000000000000000000, 0.8660254037844387076, 1.000000000000000000, 0.8660254037844387076, 1.000000000000000000, 0.8660254037844387076, 1.000000000000000000, 0.8660254037844387076, 1.000000000000000000, 0.8660254037844387076, 1.000000000000000000, 0.8660254037844387076, 1.000000000000000000, 0.8660254037844387076, 1.000000000000000000, 0.8660254037844387076, 1.000000000000000000, 0.8660254037844387076, 1.000000000000000000, 0.8660254037844387076, 1.000000000000000000, 0.8660254037844387076, 1.000000000000000000, 0.8660254037844387076, 1.000000000000000000, 0.8660254037844387076, 1.000000000000000000, 0.8660254037844387076, 1.000000000000000000, 0.8660254037844387076, 1.000000000000000000, 0.8660254037844387076, 1.000000000000000000, 0.8660254037844387076, 1.000000000000000000, 0.8660254037844387076, 1.000000000000000000, 0.8660254037844387076, 1.000000000000000000, 0.8660254037844387076, 1.000000000000000000, 0.8660254037844387076, 1.000000000000000000, 0.8660254037844387076, 1.000000000000000000, 0.8660254037844387076, 1.000000000000000000, 0.8660254037844387076, 1.000000000000000000, 0.8660254037844387076, 1.000000000000000000, 0.8660254037844387076, 1.000000000000000000, 0.8660254037844387076, 1.000000000000000000, 0.8660254037844387076, 1.000000000000000000, 0.8660254037844387076, 1.000000000000000000, 0.8660254037844387076, 1.000000000000000000, 0.8660254037844387076, 1.000000000000000000, 0.8660254037844387076, 1.000000000000000000, 0.8660254037844387076, 1.000000000000000000, 0.8660254037844387076, 1.000000000000000000, 0.8660254037844387076, 1.000000000000000000, 0.8660254037844387076, 1.000000000000000000, 0.8660254037844387076, 1.000000000000000000, 0.8660254037844387076, 1.000000000000000000, 0.8660254037844387076, 1.000000000000000000, 0.8660254037844387076, 1.000000000000000000, 0.8660254037844387076, 1.000000000000000000, 0.8660254037844387076, 1.000000000000000000, 0.8660254037844387076, 1.000000000000000000, 0.8660254037844387076, 1.000000000000000000, 0.8660254037844387076, 1.000000000000000000, 0.8660254037844387076, 1.000000000000000000, 0.8660254037844387076, 1.000000000000000000, 0.8660254037844387076, 1.000000000000000000, 0.8660254037844387076, 1.000000000000000000, 0.8660254037844387076, 1.000000000000000000, 0.8660254037844387076, 1.000000000000000000, 0.8660254037844387076, 1.000000000000000000, 0.8660254037844387076, 1.000000000000000000, 0.8660254037844387076, 1.000000000000000000, 0.8660254037844387076, 1.000000000000000000, 0.8660254037844387076, 1.000000000000000000, 0.8660254037844387076, 1.000000000000000000, 0.8660254037844387076, 1.000000000000000000, 0.8660254037844387076, 1.000000000000000000, 0.8660254037844387076, 1.000000000000000000, 0.8660254037844387076, 1.000000000000000000, 0.8660254037844387076, 1.000000000000000000),
 ( 1.000000000000000000, 0.8660254037844387076, 1.000000000000000000, 0.8660254037844387076, 1.000000000000000000, 0.8660254037844387076, 1.000000000000000000, 0.8660254037844387076, 1.000000000000000000, 0.8660254037844387076, 1.000000000000000000, 0.8660254037844387076, 1.000000000000000000, 0.8660254037844387076, 1.000000000000000000, 0.8660254037844387076, 1.000000000000000000, 0.8660254037844387076, 1.000000000000000000, 0.8660254037844387076, 1.000000000000000000, 0.8660254037844387076, 1.000000000000000000, 0.8660254037844387076, 1.000000000000000000, 0.8660254037844387076, 1.000000000000000000, 0.8660254037844387076, 1.000000000000000000, 0.8660254037844387076, 1.000000000000000000, 0.8660254037844387076, 1.000000000000000000, 0.8660254037844387076, 1.000000000000000000, 0.8660254037844387076, 1.000000000000000000, 0.8660254037844387076, 1.000000000000000000, 0.8660254037844387076, 1.000000000000000000, 0.8660254037844387076, 1.000000000000000000, 0.8660254037844387076, 1.000000000000000000, 0.8660254037844387076, 1.000000000000000000, 0.8660254037844387076, 1.000000000000000000, 0.8660254037844387076, 1.000000000000000000, 0.8660254037844387076, 1.000000000000000000, 0.8660254037844387076, 1.000000000000000000, 0.8660254037844387076, 1.000000000000000000, 0.8660254037844387076, 1.000000000000000000, 0.8660254037844387076, 1.000000000000000000, 0.8660254037844387076, 1.000000000000000000, 0.8660254037844387076, 1.000000000000000000, 0.8660254037844387076, 1.000000000000000000, 0.8660254037844387076, 1.000000000000000000, 0.8660254037844387076, 1.000000000000000000, 0.8660254037844387076, 1.000000000000000000, 0.8660254037844387076, 1.000000000000000000, 0.8660254037844387076, 1.000000000000000000, 0.8660254037844387076, 1.000000000000000000, 0.8660254037844387076, 1.000000000000000000, 0.8660254037844387076, 1.000000000000000000, 0.8660254037844387076, 1.000000000000000000, 0.8660254037844387076, 1.000000000000000000, 0.8660254037844387076, 1.000000000000000000, 0.8660254037844387076, 1.000000000000000000, 0.8660254037844387076, 1.000000000000000000, 0.8660254037844387076, 1.000000000000000000, 0.8660254037844387076, 1.000000000000000000, 0.8660254037844387076, 1.000000000000000000, 0.8660254037844387076, 1.000000000000000000, 0.8660254037844387076, 1.000000000000000000, 0.8660254037844387076, 1.000000000000000000, 0.8660254037844387076, 1.000000000000000000, 0.8660254037844387076, 1.000000000000000000, 0.8660254037844387076, 1.000000000000000000, 0.8660254037844387076, 1.000000000000000000, 0.8660254037844387076, 1.000000000000000000, 0.8660254037844387076, 1.000000000000000000, 0.8660254037844387076, 1.000000000000000000, 0.8660254037844387076, 1.000000000000000000, 0.8660254037844387076, 1.000000000000000000, 0.8660254037844387076, 1.000000000000000000, 0.8660254037844387076, 1.000000000000000000, 0.8660254037844387076, 1.000000000000000000, 0.8660254037844387076, 1.000000000000000000, 0.8660254037844387076, 1.000000000000000000, 0.8660254037844387076, 1.000000000000000000, 0.8660254037844387076, 1.000000000000000000, 0.8660254037844387076, 1.000000000000000000, 0.8660254037844387076, 1.000000000000000000, 0.8660254037844387076, 1.000000000000000000, 0.8660254037844387076, 1.000000000000000000, 0.8660254037844387076, 1.000000000000000000, 0.8660254037844387076, 1.000000000000000000, 0.8660254037844387076, 1.000000000000000000, 0.8660254037844387076, 1.000000000000000000, 0.8660254037844387076, 1.000000000000000000, 0.8660254037844387076, 1.000000000000000000, 0.8660254037844387076, 1.000000000000000000, 0.8660254037844387076, 1.000000000000000000, 0.8660254037844387076, 1.000000000000000000, 0.8660254037844387076, 1.000000000000000000, 0.8660254037844387076, 1.000000000000000000, 0.8660254037844387076, 1.000000000000000000, 0.8660254037844387076, 1.000000000000000000, 0.8660254037844387076, 1.000000000000000000, 0.8660254037844387076, 1.000000000000000000, 0.8660254037844387076, 1.000000000000000000, 0.8660254037844387076, 1.000000000000000000, 0.8660254037844387076, 1.000000000000000000, 0.8660254037844387076, 1.000000000000000000, 0.8660254037844387076, 1.000000000000000000, 0.8660254037844387076, 1.000000000000000000, 0.8660254037844387076, 1.000000000000000000, 0.8660254037844387076, 1.000000000000000000, 0.8660254037844387076, 1.000000000000000000, 0.8660254037844387076, 1.000000000000000000, 0.8660254037844387076, 1.000000000000000000, 0.8660254037844387076, 1.000000000000000000, 0.8660254037844387076, 1.000000000000000000, 0.8660254037844387076, 1.000000000000000000, 0.8660254037844387076, 1.000000000000000000, 0.8660254037844387076, 1.000000000000000000, 0.8660254037844387076, 1.000000000000000000, 0.8660254037844387076, 1.000000000000000000, 0.8660254037844387076, 1.000000000000000000, 0.8660254037844387076, 1.000000000000000000, 0.8660254037844387076, 1.000000000000000000, 0.8660254037844387076, 1.000000000000000000, 0.8660254037844387076, 1.000000000000000000, 0.8660254037844387076, 1.000000000000000000, 0.8660254037844387076, 1.000000000000000000, 0.8660254037844387076, 1.000000000000000000, 0.8660254037844387076, 1.000000000000000000, 0.8660254037844387076, 1.000000000000000000, 0.8660254037844387076, 1.000000000000000000, 0.8660254037844387076, 1.000000000000000000, 0.8660254037844387076, 1.000000000000000000, 0.8660254037844387076, 1.000000000000000000, 0.8660254037844387076, 1.000000000000000000, 0.8660254037844387076, 1.000000000000000000, 0.8660254037844387076, 1.000000000000000000, 0.8660254037844387076, 1.000000000000000000, 0.8660254037844387076, 1.000000000000000000, 0.8660254037844387076, 1.000000000000000000, 0.8660254037844387076, 1.000000000000000000, 0.8660254037844387076, 1.000000000000000000, 0.8660254037844387076, 1.000000000000000000, 0.8660254037844387076, 1.000000000000000000, 0.8660254037844387076, 1.000000000000000000, 0.8660254037844387076, 1.000000000000000000, 0.8660254037844387076, 1.000000000000000000, 0.8660254037844387076, 1.000000000000000000, 0.8660254037844387076, 1.000000000000000000, 0.8660254037844387076, 1.000000000000000000, 0.8660254037844387076, 1.000000000000000000, 0.8660254037844387076, 1.000000000000000000, 0.8660254037844387076, 1.000000000000000000, 0.8660254037844387076, 1.000000000000000000, 0.8660254037844387076, 1.000000000000000000, 0.8660254037844387076, 1.000000000000000000, 0.8660254037844387076, 1.000000000000000000, 0.8660254037844387076, 1.000000000000000000, 0.8660254037844387076, 1.000000000000000000, 0.8660254037844387076, 1.000000000000000000, 0.8660254037844387076, 1.000000000000000000, 0.8660254037844387076, 1.000000000000000000, 0.8660254037844387076, 1.000000000000000000, 0.8660254037844387076, 1.000000000000000000, 0.8660254037844387076, 1.000000000000000000, 0.8660254037844387076, 1.000000000000000000, 0.8660254037844387076, 1.000000000000000000, 0.8660254037844387076, 1.000000000000000000, 0.8660254037844387076, 1.000000000000000000, 0.8660254037844387076, 1.000000000000000000, 0.8660254037844387076, 1.000000000000000000, 0.8660254037844387076, 1.000000000000000000, 0.8660254037844387076, 1.000000000000000000, 0.8660254037844387076, 1.000000000000000000, 0.8660254037844387076, 1.000000000000000000, 0.8660254037844387076, 1.000000000000000000, 0.8660254037844387076, 1.000000000000000000, 0.8660254037844387076, 1.000000000000000000, 0.8660254037844387076, 1.000000000000000000, 0.8660254037844387076, 1.000000000000000000, 0.8660254037844387076, 1.000000000000000000, 0.8660254037844387076, 1.000000000000000000, 0.8660254037844387076, 1.000000000000000000, 0.8660254037844387076, 1.000000000000000000, 0.8660254037844387076, 1.000000000000000000, 0.8660254037844387076, 1.000000000000000000, 0.8660254037844387076, 1.000000000000000000, 0.8660254037844387076, 1.000000000000000000, 0.8660254037844387076, 1.000000000000000000, 0.8660254037844387076, 1.000000000000000000, 0.8660254037844387076, 1.000000000000000000, 0.8660254037844387076, 1.000000000000000000, 0.8660254037844387076, 1.000000000000000000, 0.8660254037844387076, 1.000000000000000000, 0.8660254037844387076, 1.000000000000000000, 0.8660254037844387076, 1.000000000000000000, 0.8660254037844387076, 1.000000000000000000, 0.8660254037844387076, 1.000000000000000000, 0.8660254037844387076, 1.000000000000000000, 0.8660254037844387076, 1.000000000000000000, 0.8660254037844387076, 1.000000000000000000, 0.8660254037844387076, 1.000000000000000000, 0.8660254037844387076, 1.000000000000000000, 0.8660254037844387076, 1.000000000000000000, 0.8660254037844387076, 1.000000000000000000, 0.8660254037844387076, 1.000000000000000000, 0.8660254037844387076, 1.000000000000000000, 0.8660254037844387076, 1.000000000000000000, 0.8660254037844387076, 1.000000000000000000, 0.8660254037844387076, 1.000000000000000000, 0.8660254037844387076, 1.000000000000000000, 0.8660254037844387076, 1.000000000000000000, 0.8660254037844387076, 1.000000000000000000, 0.8660254037844387076, 1.000000000000000000, 0.8660254037844387076, 1.000000000000000000, 0.8660254037844387076, 1.000000000000000000, 0.8660254037844387076, 1.000000000000000000, 0.8660254037844387076, 1.000000000000000000, 0.8660254037844387076, 1.000000000000000000, 0.8660254037844387076, 1.000000000000000000, 0.8660254037844387076, 1.000000000000000000, 0.8660254037844387076, 1.000000000000000000, 0.8660254037844387076, 1.000000000000000000, 0.8660254037844387076, 1.000000000000000000, 0.8660254037844387076, 1.000000000000000000, 0.8660254037844387076, 1.000000000000000000, 0.8660254037844387076, 1.000000000000000000, 0.8660254037844387076, 1.000000000000000000, 0.8660254037844387076, 1.000000000000000000, 0.8660254037844387076, 1.000000000000000000, 0.8660254037844387076, 1.000000000000000000, 0.8660254037844387076, 1.000000000000000000, 0.8660254037844387076, 1.000000000000000000, 0.8660254037844387076, 1.000000000000000000, 0.8660254037844387076, 1.000000000000000000, 0.8660254037844387076, 1.000000000000000000, 0.8660254037844387076, 1.000000000000000000, 0.8660254037844387076, 1.000000000000000000, 0.8660254037844387076, 1.000000000000000000, 0.8660254037844387076, 1.000000000000000000, 0.8660254037844387076, 1.000000000000000000, 0.8660254037844387076, 1.000000000000000000, 0.8660254037844387076, 1.000000000000000000, 0.8660254037844387076, 1.000000000000000000, 0.8660254037844387076, 1.000000000000000000, 0.8660254037844387076, 1.000000000000000000, 0.8660254037844387076, 1.000000000000000000, 0.8660254037844387076, 1.000000000000000000, 0.8660254037844387076, 1.000000000000000000, 0.8660254037844387076, 1.000000000000000000, 0.8660254037844387076, 1.000000000000000000, 0.8660254037844387076, 1.000000000000000000, 0.8660254037844387076, 1.000000000000000000, 0.8660254037844387076, 1.000000000000000000, 0.8660254037844387076, 1.000000000000000000, 0.8660254037844387076, 1.000000000000000000, 0.8660254037844387076, 1.000000000000000000, 0.8660254037844387076, 1.000000000000000000, 0.8660254037844387076, 1.000000000000000000, 0.8660254037844387076, 1.000000000000000000, 0.8660254037844387076, 1.000000000000000000, 0.8660254037844387076, 1.000000000000000000, 0.8660254037844387076, 1.000000000000000000, 0.8660254037844387076, 1.000000000000000000, 0.8660254037844387076, 1.000000000000000000, 0.8660254037844387076, 1.000000000000000000, 0.8660254037844387076, 1.000000000000000000, 0.8660254037844387076, 1.000000000000000000, 0.8660254037844387076, 1.000000000000000000, 0.8660254037844387076, 1.000000000000000000, 0.8660254037844387076, 1.000000000000000000, 0.8660254037844387076, 1.000000000000000000, 0.8660254037844387076, 1.000000000000000000, 0.8660254037844387076, 1.000000000000000000, 0.8660254037844387076, 1.000000000000000000, 0.8660254037844387076, 1.000000000000000000, 0.8660254037844387076, 1.000000000000000000, 0.8660254037844387076, 1.000000000000000000, 0.8660254037844387076, 1.000000000000000000, 0.8660254037844387076, 1.000000000000000000, 0.8660254037844387076, 1.000000000000000000, 0.8660254037844387076, 1.000000000000000000, 0.8660254037844387076, 1.000000000000000000, 0.8660254037844387076, 1.000000000000000000, 0.8660254037844387076, 1.000000000000000000, 0.8660254037844387076, 1.000000000000000000, 0.8660254037844387076, 1.000000000000000000, 0.8660254037844387076, 1.000000000000000000, 0.8660254037844387076, 1.000000000000000000, 0.8660254037844387076, 1.000000000000000000, 0.8660254037844387076, 1.000000000000000000, 0.8660254037844387076, 1.000000000000000000, 0.8660254037844387076, 1.000000000000000000, 0.8660254037844387076, 1.000000000000000000, 0.8660254037844387076, 1.000000000000000000, 0.8660254037844387076, 1.000000000000000000, 0.8660254037844387076, 1.000000000000000000, 0.8660254037844387076, 1.000000000000000000, 0.8660254037844387076, 1.000000000000000000, 0.8660254037844387076, 1.000000000000000000, 0.8660254037844387076, 1.000000000000000000, 0.8660254037844387076, 1.000000000000000000, 0.8660254037844387076, 1.000000000000000000, 0.8660254037844387076, 1.000000000000000000, 0.8660254037844387076, 1.000000000000000000, 0.8660254037844387076, 1.000000000000000000, 0.8660254037844387076, 1.000000000000000000, 0.8660254037844387076, 1.000000000000000000, 0.8660254037844387076, 1.000000000000000000, 0.8660254037844387076, 1.000000000000000000, 0.8660254037844387076, 1.000000000000000000, 0.8660254037844387076, 1.000000000000000000, 0.8660254037844387076, 1.000000000000000000, 0.8660254037844387076, 1.000000000000000000, 0.8660254037844387076, 1.000000000000000000, 0.8660254037844387076, 1.000000000000000000, 0.8660254037844387076, 1.000000000000000000, 0.8660254037844387076, 1.000000000000000000, 0.8660254037844387076, 1.000000000000000000, 0.8660254037844387076, 1.000000000000000000, 0.8660254037844387076, 1.000000000000000000, 0.8660254037844387076, 1.000000000000000000, 0.8660254037844387076, 1.000000000000000000, 0.8660254037844387076, 1.000000000000000000, 0.8660254037844387076, 1.000000000000000000, 0.8660254037844387076, 1.000000000000000000, 0.8660254037844387076, 1.000000000000000000, 0.8660254037844387076, 1.000000000000000000, 0.8660254037844387076, 1.000000000000000000, 0.8660254037844387076, 1.000000000000000000, 0.8660254037844387076, 1.000000000000000000, 0.8660254037844387076, 1.000000000000000000, 0.8660254037844387076, 1.000000000000000000, 0.8660254037844387076, 1.000000000000000000, 0.8660254037844387076, 1.000000000000000000, 0.8660254037844387076, 1.000000000000000000, 0.8660254037844387076, 1.000000000000000000, 0.8660254037844387076, 1.000000000000000000, 0.8660254037844387076, 1.000000000000000000, 0.8660254037844387076, 1.000000000000000000, 0.8660254037844387076, 1.000000000000000000, 0.8660254037844387076, 1.000000000000000000, 0.8660254037844387076, 1.000000000000000000, 0.8660254037844387076, 1.000000000000000000, 0.8660254037844387076, 1.000000000000000000, 0.8660254037844387076, 1.000000000000000000, 0.8660254037844387076, 1.000000000000000000, 0.8660254037844387076, 1.000000000000000000, 0.8660254037844387076, 1.000000000000000000, 0.8660254037844387076, 1.000000000000000000, 0.8660254037844387076, 1.000000000000000000, 0.8660254037844387076, 1.000000000000000000, 0.8660254037844387076, 1.000000000000000000, 0.8660254037844387076, 1.000000000000000000, 0.8660254037844387076, 1.000000000000000000, 0.8660254037844387076, 1.000000000000000000, 0.8660254037844387076, 1.000000000000000000, 0.8660254037844387076, 1.000000000000000000, 0.8660254037844387076, 1.000000000000000000, 0.8660254037844387076, 1.000000000000000000, 0.8660254037844387076, 1.000000000000000000, 0.8660254037844387076, 1.000000000000000000, 0.8660254037844387076, 1.000000000000000000, 0.8660254037844387076, 1.000000000000000000, 0.8660254037844387076, 1.000000000000000000, 0.8660254037844387076, 1.000000000000000000, 0.8660254037844387076, 1.000000000000000000, 0.8660254037844387076, 1.000000000000000000, 0.8660254037844387076, 1.000000000000000000, 0.8660254037844387076, 1.000000000000000000, 0.8660254037844387076, 1.000000000000000000, 0.8660254037844387076, 1.000000000000000000, 0.8660254037844387076, 1.000000000000000000, 0.8660254037844387076, 1.000000000000000000, 0.8660254037844387076, 1.000000000000000000) ) ) 
 REPRESENTATION_ITEM ( '' )  SURFACE ( )  );
#43034=CARTESIAN_POINT ( 'NONE',  ( 8.390625000614518214, -3.027376345333610441, -5.243569643749999898 ) ) ;
#43035=CARTESIAN_POINT ( 'NONE',  ( 11.05312500061451608, -4.541064518000417216, -2.621784821875001281 ) ) ;
#43036=CARTESIAN_POINT ( 'NONE',  ( 24.33750000122903145, -4.330127018922194537, 2.499999999999995559 ) ) ;
#43038=CARTESIAN_POINT ( 'NONE',  ( 22.47187500061451715, 3.027376345333613106, -5.243569643749998122 ) ) ;
#43039=CARTESIAN_POINT ( 'NONE',  ( 3.570441056944901881, 3.500278654462113614, -3.904237691275162625 ) ) ;
#43040=CARTESIAN_POINT ( 'NONE',  ( 6.225000001229036073, 2.886751345948126879, 4.999999999999999112 ) ) ;
#43041=CARTESIAN_POINT ( 'NONE',  ( 6.009375000614519458, 0.000000000000000000, 5.243569643749999010 ) ) ;
#43042=CARTESIAN_POINT ( 'NONE',  ( 24.19687500061451857, -3.027376345333610441, -5.243569643749999898 ) ) ;
#43044=CARTESIAN_POINT ( 'NONE',  ( 4.531380608837685564, 2.113648287258761194, -4.671852478106539586 ) ) ;
#43045=CARTESIAN_POINT ( 'NONE',  ( 17.72812500061451502, -4.541064518000419881, 2.621784821874995952 ) ) ;
#43046=CARTESIAN_POINT ( 'NONE',  ( 24.23437500061451644, 6.421520780324663323E-16, -5.243569643749999010 ) ) ;
#43048=DIRECTION ( 'NONE',  ( -1.000000000000000000, -0.000000000000000000, -0.000000000000000000 ) ) ;
#43050=CARTESIAN_POINT ( 'NONE',  ( 4.996875000614516615, 6.054752690667223547, 3.707466751127219781E-16 ) ) ;
#43051=CARTESIAN_POINT ( 'NONE',  ( 13.67812500061451786, -4.541064518000419881, 2.621784821874995952 ) ) ;
#43052=VECTOR ( 'NONE', #25774, 1000.000000000000000 ) ;
#43053=CARTESIAN_POINT ( 'NONE',  ( 13.05937500061451750, 4.541064518000418104, -2.621784821874998173 ) ) ;
#43055=CARTESIAN_POINT ( 'NONE',  ( 22.35000000122903430, 5.773502691896255534, 3.535250795749688401E-16 ) ) ;
#43056=CARTESIAN_POINT ( 'NONE',  ( 25.07812500061451644, 6.421520780324663323E-16, -5.243569643749999010 ) ) ;
#43057=CARTESIAN_POINT ( 'NONE',  ( 3.461013385977631529, 3.608566055203085821, -3.626329471737537613 ) ) ;
#43059=CARTESIAN_POINT ( 'NONE',  ( 15.67500000000000071, -4.330127018922194537, 2.499999999999995559 ) ) ;
#43060=CARTESIAN_POINT ( 'NONE',  ( 25.23750000122903359, -4.330127018922194537, 2.499999999999995559 ) ) ;
#43061=CARTESIAN_POINT ( 'NONE',  ( 19.49062500061451431, -3.027376345333614438, 5.243569643749998122 ) ) ;
#43062=ORIENTED_EDGE ( 'NONE', *, *, #44217, .F. ) ;
#43063=CARTESIAN_POINT ( 'NONE',  ( 21.71249999999999858, 2.886751345948129099, -4.999999999999998224 ) ) ;
#43064=CARTESIAN_POINT ( 'NONE',  ( 23.18437500061451573, -4.541064518000419881, 2.621784821874995952 ) ) ;
#43065=ORIENTED_EDGE ( 'NONE', *, *, #55566, .F. ) ;
#43066=DIRECTION ( 'NONE',  ( 0.000000000000000000, 0.000000000000000000, 1.000000000000000000 ) ) ;
#43067=CARTESIAN_POINT ( 'NONE',  ( 11.05312500061451608, -4.541064518000417216, -2.621784821875001281 ) ) ;
#43068=CARTESIAN_POINT ( 'NONE',  ( 4.153125000614515727, 0.000000000000000000, 5.243569643749999010 ) ) ;
#43070=CARTESIAN_POINT ( 'NONE',  ( 27.10312500061451502, 0.000000000000000000, 5.243569643749999010 ) ) ;
#43072=CARTESIAN_POINT ( 'NONE',  ( 16.35000000000000142, 4.330127018922192761, -2.499999999999997780 ) ) ;
#43073=CARTESIAN_POINT ( 'NONE',  ( 27.26249999999999929, 2.886751345948126879, 4.999999999999999112 ) ) ;
#43075=CARTESIAN_POINT ( 'NONE',  ( 6.496875000614517504, -3.027376345333614438, 5.243569643749998122 ) ) ;
#43076=CARTESIAN_POINT ( 'NONE',  ( 17.14687500061451786, 6.054752690667223547, 3.707466751127219781E-16 ) ) ;
#43077=CARTESIAN_POINT ( 'NONE',  ( -5.810221930991193690E-16, 13.70000000122903394, 26.00000000000000355 ) ) ;
#43079=CARTESIAN_POINT ( 'NONE',  ( 25.60312500061451502, 4.541064518000418104, -2.621784821874998173 ) ) ;
#43080=CARTESIAN_POINT ( 'NONE',  ( 27.87187500061451573, 3.027376345333613106, -5.243569643749998122 ) ) ;
#43081=CARTESIAN_POINT ( 'NONE',  ( 3.234375000614516438, 4.541064518000418104, 2.621784821874999949 ) ) ;
#43082=CARTESIAN_POINT ( 'NONE',  ( 12.67499999999999893, 6.123233995736764310E-16, -4.999999999999998224 ) ) ;
#43083=CARTESIAN_POINT ( 'NONE',  ( 10.86562500061451431, 3.027376345333611329, 5.243569643749999010 ) ) ;
#43085=CARTESIAN_POINT ( 'NONE',  ( 15.41250000122903252, -4.330127018922190985, -2.500000000000001332 ) ) ;
#43086=CARTESIAN_POINT ( 'NONE',  ( 15.26250000122903216, 0.000000000000000000, 4.999999999999998224 ) ) ;
#43088=CARTESIAN_POINT ( 'NONE',  ( 4.528125000614516615, 4.541064518000418104, 2.621784821874999949 ) ) ;
#43089=CARTESIAN_POINT ( 'NONE',  ( 22.50937500061451857, 4.541064518000418104, -2.621784821874998173 ) ) ;
#43090=CARTESIAN_POINT ( 'NONE',  ( 4.243569643749999010, 16.97187500061451360, 27.54997392385601174 ) ) ;
#43091=CARTESIAN_POINT ( 'NONE',  ( 23.82187500061451502, 3.027376345333613106, -5.243569643749998122 ) ) ;
#43092=CARTESIAN_POINT ( 'NONE',  ( 5.400000000000002132, -4.330127018922190985, -2.500000000000001332 ) ) ;
#43093=CARTESIAN_POINT ( 'NONE',  ( -1.999999999999997113, 11.18750000122903288, 33.46410161513775705 ) ) ;
#43094=CARTESIAN_POINT ( 'NONE',  ( 12.92812500061451786, 6.421520780324663323E-16, -5.243569643749999010 ) ) ;
#43095=CARTESIAN_POINT ( 'NONE',  ( 4.275000001229035895, 2.886751345948129099, -4.999999999999998224 ) ) ;
#43097=CARTESIAN_POINT ( 'NONE',  ( 9.571875000614518569, 3.027376345333611329, 5.243569643749999010 ) ) ;
#43099=AXIS2_PLACEMENT_3D ( 'NONE', #63351, #12736, #23463 ) ;
#43100=CARTESIAN_POINT ( 'NONE',  ( 10.04062500061451502, -3.027376345333614438, 5.243569643749998122 ) ) ;
#43101=CARTESIAN_POINT ( 'NONE',  ( 15.53437500061451715, -4.541064518000419881, 2.621784821874995952 ) ) ;
#43103=CARTESIAN_POINT ( 'NONE',  ( 20.55000000122903359, 5.773502691896255534, 3.535250795749688894E-16 ) ) ;
#43104=CARTESIAN_POINT ( 'NONE',  ( 10.24687500061451750, -3.027376345333610441, -5.243569643749999898 ) ) ;
#43105=CARTESIAN_POINT ( 'NONE',  ( 13.41562500061451502, 3.027376345333613106, -5.243569643749998122 ) ) ;
#43107=CARTESIAN_POINT ( 'NONE',  ( 21.79687500061451644, -3.027376345333614438, 5.243569643749998122 ) ) ;
#43109=CARTESIAN_POINT ( 'NONE',  ( -2.065650683794914233, 4.559369103593684969, 33.43471409431110430 ) ) ;
#43110=CARTESIAN_POINT ( 'NONE',  ( 2.958716452545182118, -4.315365460520880880, -3.012707056649966741 ) ) ;
#43111=CARTESIAN_POINT ( 'NONE',  ( -4.243569643749999898, 13.55937500061451750, -30.00000000000000000 ) ) ;
#43112=CARTESIAN_POINT ( 'NONE',  ( 15.67500000122903181, 2.886751345948126879, 4.999999999999999112 ) ) ;
#43114=CARTESIAN_POINT ( 'NONE',  ( 9.271875000614516082, -6.054752690667223547, -1.112240025338166033E-15 ) ) ;
#43115=CARTESIAN_POINT ( 'NONE',  ( 2.121784821875001281, 18.60312500061451857, -26.32496088578401938 ) ) ;
#43116=CARTESIAN_POINT ( 'NONE',  ( 16.91250000122903430, 4.330127018922192761, -2.499999999999997780 ) ) ;
#43117=CARTESIAN_POINT ( 'NONE',  ( 9.590625000614517504, -3.027376345333614438, 5.243569643749998122 ) ) ;
#43119=AXIS2_PLACEMENT_3D ( 'NONE', #5035, #61179, #21646 ) ;
#43120=CARTESIAN_POINT ( 'NONE',  ( 16.16250000000000142, -5.773502691896255534, -1.060575238724906372E-15 ) ) ;
#43121=CARTESIAN_POINT ( 'NONE',  ( 10.50000000122903110, -2.886751345948193048, -4.999999999999883649 ) ) ;
#43122=CARTESIAN_POINT ( 'NONE',  ( 9.046875000614518214, 6.054752690667223547, 3.707466751127219781E-16 ) ) ;
#43124=CARTESIAN_POINT ( 'NONE',  ( 9.750000001229032875, 5.773502691896255534, 3.535250795749688894E-16 ) ) ;
#43125=CARTESIAN_POINT ( 'NONE',  ( 18.22500000122903430, 2.886751345948129099, -4.999999999999998224 ) ) ;
#43126=CARTESIAN_POINT ( 'NONE',  ( 16.30312500061451786, 0.000000000000000000, 5.243569643749999010 ) ) ;
#43127=CARTESIAN_POINT ( 'NONE',  ( 20.95312500061451999, -4.541064518000417216, -2.621784821875001281 ) ) ;
#43128=CARTESIAN_POINT ( 'NONE',  ( 27.48750000122903359, -4.330127018922194537, 2.499999999999995559 ) ) ;
#43129=CARTESIAN_POINT ( 'NONE',  ( 2.915625000614516793, -6.054752690667223547, -1.112240025338166033E-15 ) ) ;
#43130=CARTESIAN_POINT ( 'NONE',  ( 24.33749999999999858, -2.886751345948125991, -5.000000000000000000 ) ) ;
#43133=CARTESIAN_POINT ( 'NONE',  ( 28.99687500061451573, -3.027376345333614438, 5.243569643749998122 ) ) ;
#43134=CARTESIAN_POINT ( 'NONE',  ( 4.000000000000000000, 17.48750000000000071, 32.30940107675849760 ) ) ;
#43135=CARTESIAN_POINT ( 'NONE',  ( 12.07500000122903216, 2.886751345948126879, 4.999999999999999112 ) ) ;
#43136=CARTESIAN_POINT ( 'NONE',  ( 3.862500000000001155, 2.886751345948126879, 4.999999999999999112 ) ) ;
#43138=CARTESIAN_POINT ( 'NONE',  ( 22.72499999999999787, 4.330127018922191873, 2.499999999999999556 ) ) ;
#43139=CARTESIAN_POINT ( 'NONE',  ( 7.134375000614516793, 6.421520780324663323E-16, -5.243569643749999010 ) ) ;
#43140=CARTESIAN_POINT ( 'NONE',  ( 27.10312500061451502, 0.000000000000000000, 5.243569643749999010 ) ) ;
#43143=CARTESIAN_POINT ( 'NONE',  ( 14.40000000000000036, -4.330127018922190985, -2.500000000000001332 ) ) ;
#43144=AXIS2_PLACEMENT_3D ( 'NONE', #52007, #35369, #2133 ) ;
#43145=CARTESIAN_POINT ( 'NONE',  ( 30.00000000000000000, 6.123233995736764310E-16, -4.999999999999998224 ) ) ;
#43146=CARTESIAN_POINT ( 'NONE',  ( 5.371875000614516615, 3.027376345333613106, -5.243569643749998122 ) ) ;
#43147=CARTESIAN_POINT ( 'NONE',  ( 7.921875000614517326, -6.054752690667223547, -1.112240025338166033E-15 ) ) ;
#43148=CARTESIAN_POINT ( 'NONE',  ( 3.075000000000001510, -4.330127018922194537, 2.499999999999995559 ) ) ;
#43149=CARTESIAN_POINT ( 'NONE',  ( -3.000416591977282496E-16, 12.94062500061459353, 25.09994784771203058 ) ) ;
#43150=CARTESIAN_POINT ( 'NONE',  ( 22.46250000000000213, -5.773502691896255534, -1.060575238724906372E-15 ) ) ;
#43152=CARTESIAN_POINT ( 'NONE',  ( 28.98750000000000071, 5.773502691896255534, 3.535250795749688894E-16 ) ) ;
#43154=CARTESIAN_POINT ( 'NONE',  ( 3.525000000000000355, -4.330127018922194537, 2.499999999999995559 ) ) ;
#43157=ORIENTED_EDGE ( 'NONE', *, *, #51085, .T. ) ;
#43158=CARTESIAN_POINT ( 'NONE',  ( 17.42812500061451786, 6.421520780324663323E-16, -5.243569643749999010 ) ) ;
#43159=CARTESIAN_POINT ( 'NONE',  ( 11.35312500061451679, 0.000000000000000000, 5.243569643749999010 ) ) ;
#43161=CARTESIAN_POINT ( 'NONE',  ( 6.571875000614517681, -6.054752690667223547, -1.112240025338166033E-15 ) ) ;
#43162=CARTESIAN_POINT ( 'NONE',  ( 22.94999999999999929, -4.330127018922190985, -2.500000000000001332 ) ) ;
#43163=CARTESIAN_POINT ( 'NONE',  ( 20.32500000122903572, -5.773502691896255534, -1.060575238724906372E-15 ) ) ;
#43166=CARTESIAN_POINT ( 'NONE',  ( 8.259375000614518569, 0.000000000000000000, 5.243569643749999010 ) ) ;
#43167=CARTESIAN_POINT ( 'NONE',  ( 13.99687500061451928, 6.054752690667223547, 3.707466751127219781E-16 ) ) ;
#43168=CARTESIAN_POINT ( 'NONE',  ( 23.70937500061451786, -4.541064518000417216, -2.621784821875001281 ) ) ;
#43169=EDGE_CURVE ( 'NONE', #66704, #21346, #34422, .T. ) ;
#43172=CARTESIAN_POINT ( 'NONE',  ( 17.70937500061451431, 0.000000000000000000, 5.243569643749999010 ) ) ;
#43173=CARTESIAN_POINT ( 'NONE',  ( 10.28437500061451715, 6.421520780324663323E-16, -5.243569643749999010 ) ) ;
#43175=CARTESIAN_POINT ( 'NONE',  ( 23.09999999999999787, 4.330127018922192761, -2.499999999999997780 ) ) ;
#43177=CARTESIAN_POINT ( 'NONE',  ( -0.6945863667395647534, 9.663023495605401081, -33.93923213064925193 ) ) ;
#43179=CARTESIAN_POINT ( 'NONE',  ( 12.89062500061451821, -3.027376345333610441, -5.243569643749999898 ) ) ;
#43180=CARTESIAN_POINT ( 'NONE',  ( 29.70937500061451431, 4.541064518000418104, -2.621784821874998173 ) ) ;
#43182=DIRECTION ( 'NONE',  ( 0.000000000000000000, 0.000000000000000000, 1.000000000000000000 ) ) ;
#43183=CARTESIAN_POINT ( 'NONE',  ( 13.27500000000000213, 4.330127018922191873, 2.499999999999999556 ) ) ;
#43184=CARTESIAN_POINT ( 'NONE',  ( -2.000000000000000000, 19.13750000122903216, 26.53589838486224650 ) ) ;
#43185=CARTESIAN_POINT ( 'NONE',  ( 12.07500000122903216, 2.886751345948126879, 4.999999999999999112 ) ) ;
#43186=CARTESIAN_POINT ( 'NONE',  ( 21.53437500061451715, 6.421520780324663323E-16, -5.243569643749999010 ) ) ;
#43187=CARTESIAN_POINT ( 'NONE',  ( 17.14687500061451786, 6.054752690667223547, 3.707466751127219781E-16 ) ) ;
#43188=CARTESIAN_POINT ( 'NONE',  ( -1.999999999999997113, 16.47500000000000142, -26.53589838486224295 ) ) ;
#43190=CARTESIAN_POINT ( 'NONE',  ( 17.61562500061451786, 3.027376345333611329, 5.243569643749999010 ) ) ;
#43191=CARTESIAN_POINT ( 'NONE',  ( 28.01250000122903216, -4.330127018922190985, -2.500000000000001332 ) ) ;
#43192=CARTESIAN_POINT ( 'NONE',  ( 17.74687500061451928, -3.027376345333614438, 5.243569643749998122 ) ) ;
#43193=CARTESIAN_POINT ( 'NONE',  ( 5.540625000614515905, -3.027376345333614438, 5.243569643749998122 ) ) ;
#43194=CARTESIAN_POINT ( 'NONE',  ( 19.37812500061451715, 4.541064518000418104, 2.621784821874999949 ) ) ;
#43196=CARTESIAN_POINT ( 'NONE',  ( 27.87187500061451573, 3.027376345333613106, -5.243569643749998122 ) ) ;
#43197=CARTESIAN_POINT ( 'NONE',  ( 4.243569643749999010, 12.41562500061451857, 27.54997392385601174 ) ) ;
#43198=CARTESIAN_POINT ( 'NONE',  ( 17.10000000122903430, -2.886751345948129988, 4.999999999999997335 ) ) ;
#43200=CARTESIAN_POINT ( 'NONE',  ( 27.85312500061451502, 4.541064518000418104, -2.621784821874998173 ) ) ;
#43201=CARTESIAN_POINT ( 'NONE',  ( -3.999999999999997335, 9.800000001229033586, 32.30940107675850470 ) ) ;
#43202=CARTESIAN_POINT ( 'NONE',  ( 21.04687500061451644, -3.027376345333610441, -5.243569643749999898 ) ) ;
#43203=CARTESIAN_POINT ( 'NONE',  ( 22.98750000122903003, -4.330127018922194537, 2.499999999999995559 ) ) ;
#43204=CARTESIAN_POINT ( 'NONE',  ( 23.95312500061451289, 0.000000000000000000, 5.243569643749999010 ) ) ;
#43205=CARTESIAN_POINT ( 'NONE',  ( 16.24687500061451573, 6.054752690667223547, 3.707466751127219781E-16 ) ) ;
#43206=CARTESIAN_POINT ( 'NONE',  ( 11.57812500061451644, 6.421520780324663323E-16, -5.243569643749999010 ) ) ;
#43207=CARTESIAN_POINT ( 'NONE',  ( -2.121784821874999949, 13.93437500061451750, 26.32496088578401938 ) ) ;
#43209=CARTESIAN_POINT ( 'NONE',  ( 20.76562500061451644, 3.027376345333611329, 5.243569643749999010 ) ) ;
#43210=CARTESIAN_POINT ( 'NONE',  ( 9.975000000000001421, 6.123233995736764310E-16, -4.999999999999998224 ) ) ;
#43212=ORIENTED_EDGE ( 'NONE', *, *, #27586, .T. ) ;
#43213=CARTESIAN_POINT ( 'NONE',  ( 24.03750000000000142, 5.773502691896255534, 3.535250795749688894E-16 ) ) ;
#43214=CARTESIAN_POINT ( 'NONE',  ( -3.000416591977282496E-16, 18.39687500061451786, -34.90005215228797653 ) ) ;
#43215=CARTESIAN_POINT ( 'NONE',  ( 3.250662400336420177, 3.799104362746421604, 3.614115195980558859 ) ) ;
#43216=CARTESIAN_POINT ( 'NONE',  ( 24.44062500061451715, -3.027376345333614438, 5.243569643749998122 ) ) ;
#43217=CARTESIAN_POINT ( 'NONE',  ( 4.303125000614516971, -4.541064518000417216, -2.621784821875001281 ) ) ;
#43218=CARTESIAN_POINT ( 'NONE',  ( 20.62500000122903288, 2.886751345948126879, 4.999999999999999112 ) ) ;
#43219=CARTESIAN_POINT ( 'NONE',  ( 25.45312500061451644, -4.541064518000417216, -2.621784821875001281 ) ) ;
#43220=CARTESIAN_POINT ( 'NONE',  ( 21.89999999999999858, 0.000000000000000000, 4.999999999999998224 ) ) ;
#43221=( BOUNDED_CURVE ( )  B_SPLINE_CURVE ( 2, ( #48038, #19939, #42493, #62024, #10330, #32864, #50228, #27327, #55399 ),
 .UNSPECIFIED., .F., .F. ) 
 B_SPLINE_CURVE_WITH_KNOTS ( ( 3, 2, 2, 2, 3 ),
 ( 0.6630434782608696231, 0.6666666666666666297, 0.6739130434782608647, 0.6811594202898550998, 0.6847826086956522174 ),
 .UNSPECIFIED. ) 
 CURVE ( )  GEOMETRIC_REPRESENTATION_ITEM ( )  RATIONAL_B_SPLINE_CURVE ( ( 0.9330127018922192983, 0.9330127018922202975, 1.000000000000000000, 0.8660254037844387076, 1.000000000000000000, 0.8660254037844387076, 1.000000000000000000, 0.9330127018922182991, 0.9330127018922192983 ) ) 
 REPRESENTATION_ITEM ( '' )  );
#43222=CARTESIAN_POINT ( 'NONE',  ( 27.29062500061451502, -3.027376345333610441, -5.243569643749999898 ) ) ;
#43223=CARTESIAN_POINT ( 'NONE',  ( 8.878125000614515372, 6.421520780324663323E-16, -5.243569643749999010 ) ) ;
#43225=CARTESIAN_POINT ( 'NONE',  ( 24.47812500061451502, -4.541064518000419881, 2.621784821874995952 ) ) ;
#43226=CARTESIAN_POINT ( 'NONE',  ( 5.053125000614517859, 0.000000000000000000, 5.243569643749999010 ) ) ;
#43228=CARTESIAN_POINT ( 'NONE',  ( 3.815625000614518036, -6.054752690667223547, -1.112240025338166033E-15 ) ) ;
#43229=CARTESIAN_POINT ( 'NONE',  ( 1.999999999999998668, 12.76250000122903394, -33.46410161513775705 ) ) ;
#43230=CARTESIAN_POINT ( 'NONE',  ( 30.00000000000000000, 6.123233995736764310E-16, -4.999999999999998224 ) ) ;
#43231=CARTESIAN_POINT ( 'NONE',  ( 11.10000000000000142, 0.000000000000000000, 4.999999999999998224 ) ) ;
#43232=CARTESIAN_POINT ( 'NONE',  ( 10.84687500061451892, 6.054752690667223547, 3.707466751127219781E-16 ) ) ;
#43233=CARTESIAN_POINT ( 'NONE',  ( 5.812500001229035540, 0.000000000000000000, 4.999999999999998224 ) ) ;
#43234=CARTESIAN_POINT ( 'NONE',  ( 13.50937500061451679, 4.541064518000418104, -2.621784821874998173 ) ) ;
#43236=CARTESIAN_POINT ( 'NONE',  ( 5.559375000614517504, 0.000000000000000000, 5.243569643749999010 ) ) ;
#43237=CARTESIAN_POINT ( 'NONE',  ( 2.226602359779148887, 9.751272476441998904, -34.70164361699148259 ) ) ;
#43238=VECTOR ( 'NONE', #18792, 1000.000000000000000 ) ;
#43239=CARTESIAN_POINT ( 'NONE',  ( 11.52187500061451608, -6.054752690667223547, -1.112240025338166033E-15 ) ) ;
#43241=CARTESIAN_POINT ( 'NONE',  ( 5.000000000000000000, 6.123233995736766282E-16, 50.00000000000000000 ) ) ;
#43242=CARTESIAN_POINT ( 'NONE',  ( 22.00312500061451360, 4.541064518000418104, -2.621784821874998173 ) ) ;
#43243=CARTESIAN_POINT ( 'NONE',  ( 4.243569643749999898, 19.57812500061459460, 30.00000000000000000 ) ) ;
#43244=CARTESIAN_POINT ( 'NONE',  ( 24.57187500061451502, -6.054752690667223547, -1.112240025338166033E-15 ) ) ;
#43246=CARTESIAN_POINT ( 'NONE',  ( -1.071796769724488563, 13.90490381179670010, -26.00000000000000000 ) ) ;
#43247=CARTESIAN_POINT ( 'NONE',  ( 4.603125000614518569, 0.000000000000000000, 5.243569643749999010 ) ) ;
#43249=CARTESIAN_POINT ( 'NONE',  ( 18.02812500061451573, 4.541064518000418104, 2.621784821874999949 ) ) ;
#43250=CARTESIAN_POINT ( 'NONE',  ( 14.67187500061451821, -6.054752690667223547, -1.112240025338166033E-15 ) ) ;
#43251=VECTOR ( 'NONE', #44700, 1000.000000000000000 ) ;
#43252=CARTESIAN_POINT ( 'NONE',  ( 26.17500000122903359, -5.773502691896255534, -1.060575238724906372E-15 ) ) ;
#43253=CARTESIAN_POINT ( 'NONE',  ( 6.121875000614517504, -6.054752690667223547, -1.112240025338166033E-15 ) ) ;
#43254=CARTESIAN_POINT ( 'NONE',  ( 15.57187500061451679, -6.054752690667223547, -1.112240025338166033E-15 ) ) ;
#43255=CARTESIAN_POINT ( 'NONE',  ( 24.07499999999999929, 4.330127018922191873, 2.499999999999999556 ) ) ;
#43256=CARTESIAN_POINT ( 'NONE',  ( 4.050000001229035362, -2.886751345948129988, 4.999999999999997335 ) ) ;
#43257=CARTESIAN_POINT ( 'NONE',  ( 24.12187500061451217, -6.054752690667223547, -1.112240025338166033E-15 ) ) ;
#43258=CARTESIAN_POINT ( 'NONE',  ( 17.29687500061451999, -3.027376345333614438, 5.243569643749998122 ) ) ;
#43260=CARTESIAN_POINT ( 'NONE',  ( 29.69999999999999574, -4.330127018922190985, -2.500000000000001332 ) ) ;
#43261=CARTESIAN_POINT ( 'NONE',  ( 8.175000000000002487, 6.123233995736764310E-16, -4.999999999999998224 ) ) ;
#43263=CARTESIAN_POINT ( 'NONE',  ( 19.82812500061451644, 4.541064518000418104, 2.621784821874999949 ) ) ;
#43264=CARTESIAN_POINT ( 'NONE',  ( 10.23750000000000071, -2.886751345948129988, 4.999999999999997335 ) ) ;
#43265=CARTESIAN_POINT ( 'NONE',  ( 3.478125000614517237, 6.421520780324663323E-16, -5.243569643749999010 ) ) ;
#43267=CARTESIAN_POINT ( 'NONE',  ( 19.65000000000000213, 0.000000000000000000, 4.999999999999998224 ) ) ;
#43268=CARTESIAN_POINT ( 'NONE',  ( 17.50312500061451715, 4.541064518000418104, -2.621784821874998173 ) ) ;
#43270=CARTESIAN_POINT ( 'NONE',  ( 22.57500000122903572, -5.773502691896255534, -1.060575238724906372E-15 ) ) ;
#43271=CARTESIAN_POINT ( 'NONE',  ( 3.035296952380284186, 9.529902216964481809, 35.17929436357654538 ) ) ;
#43272=CARTESIAN_POINT ( 'NONE',  ( 29.07187500061451502, -6.054752690667223547, -1.112240025338166033E-15 ) ) ;
#43274=CARTESIAN_POINT ( 'NONE',  ( 16.67812500061451786, 4.541064518000418104, 2.621784821874999949 ) ) ;
#43275=CARTESIAN_POINT ( 'NONE',  ( 24.77812500061451217, 4.541064518000418104, 2.621784821874999949 ) ) ;
#43276=CARTESIAN_POINT ( 'NONE',  ( 25.62187500061451573, 3.027376345333613106, -5.243569643749998122 ) ) ;
#43277=CARTESIAN_POINT ( 'NONE',  ( 9.187500000000001776, 5.773502691896255534, 3.535250795749688894E-16 ) ) ;
#43278=CARTESIAN_POINT ( 'NONE',  ( 12.96562500061451750, 3.027376345333613106, -5.243569643749998122 ) ) ;
#43279=CARTESIAN_POINT ( 'NONE',  ( 26.99062500061451431, 6.054752690667223547, 3.707466751127219781E-16 ) ) ;
#43280=CARTESIAN_POINT ( 'NONE',  ( 16.73437500061451644, 4.541064518000418104, 2.621784821874999949 ) ) ;
#43281=CARTESIAN_POINT ( 'NONE',  ( 9.290625000614515017, -3.027376345333610441, -5.243569643749999898 ) ) ;
#43283=CARTESIAN_POINT ( 'NONE',  ( -2.121784821874996840, 19.42812500061451786, 33.67503911421598417 ) ) ;
#43285=CARTESIAN_POINT ( 'NONE',  ( 24.07500000122903216, 2.886751345948129099, -4.999999999999998224 ) ) ;
#43287=CARTESIAN_POINT ( 'NONE',  ( 14.35312500061451679, 4.541064518000418104, -2.621784821874998173 ) ) ;
#43288=CARTESIAN_POINT ( 'NONE',  ( 8.484375000614518214, 6.421520780324663323E-16, -5.243569643749999010 ) ) ;
#43289=CARTESIAN_POINT ( 'NONE',  ( 6.946875000614517681, -3.027376345333614438, 5.243569643749998122 ) ) ;
#43290=ORIENTED_EDGE ( 'NONE', *, *, #30129, .T. ) ;
#43291=CARTESIAN_POINT ( 'NONE',  ( -3.040073828171251158, 9.532700238123332781, 35.18707943735392973 ) ) ;
#43292=CARTESIAN_POINT ( 'NONE',  ( 20.27812500061451573, 4.541064518000418104, 2.621784821874999949 ) ) ;
#43293=CARTESIAN_POINT ( 'NONE',  ( 15.53437500061451715, -4.541064518000419881, 2.621784821874995952 ) ) ;
#43294=CARTESIAN_POINT ( 'NONE',  ( 19.04062500061451146, -3.027376345333614438, 5.243569643749998122 ) ) ;
#43295=CARTESIAN_POINT ( 'NONE',  ( -3.999999999999997335, 12.83750000000000213, 32.30940107675850470 ) ) ;
#43296=CARTESIAN_POINT ( 'NONE',  ( 26.80312500061451431, -4.541064518000417216, -2.621784821875001281 ) ) ;
#43297=CARTESIAN_POINT ( 'NONE',  ( 6.562500001229032875, 4.330127018922192761, -2.499999999999997780 ) ) ;
#43298=ORIENTED_EDGE ( 'NONE', *, *, #57235, .T. ) ;
#43299=CARTESIAN_POINT ( 'NONE',  ( 29.88749999999999929, 5.773502691896255534, 3.535250795749688894E-16 ) ) ;
#43300=CARTESIAN_POINT ( 'NONE',  ( -3.999999999999999556, 18.16250000000000497, -32.30940107675850470 ) ) ;
#43302=CARTESIAN_POINT ( 'NONE',  ( 22.61250000122903003, -4.330127018922190985, -2.500000000000001332 ) ) ;
#43304=CARTESIAN_POINT ( 'NONE',  ( 7.359375000614516438, 0.000000000000000000, 5.243569643749999010 ) ) ;
#43305=CARTESIAN_POINT ( 'NONE',  ( 12.47812500061451502, 6.421520780324663323E-16, -5.243569643749999010 ) ) ;
#43307=CARTESIAN_POINT ( 'NONE',  ( 7.509375000614517681, -4.541064518000417216, -2.621784821875001281 ) ) ;
#43308=CARTESIAN_POINT ( 'NONE',  ( 26.32500000122903216, 2.886751345948129099, -4.999999999999998224 ) ) ;
#43309=CARTESIAN_POINT ( 'NONE',  ( 16.43437500061451573, -4.541064518000419881, 2.621784821874995952 ) ) ;
#43310=CARTESIAN_POINT ( 'NONE',  ( 4.171875000614517326, 3.027376345333611329, 5.243569643749999010 ) ) ;
#43311=CARTESIAN_POINT ( 'NONE',  ( 29.58749999999999858, -2.886751345948129988, 4.999999999999997335 ) ) ;
#43312=CARTESIAN_POINT ( 'NONE',  ( 5.315625000614516260, 3.027376345333613106, -5.243569643749998122 ) ) ;
#43313=CARTESIAN_POINT ( 'NONE',  ( 16.11562500061451786, 3.027376345333613106, -5.243569643749998122 ) ) ;
#43314=ORIENTED_EDGE ( 'NONE', *, *, #37707, .T. ) ;
#43315=CARTESIAN_POINT ( 'NONE',  ( 11.50312500061451892, -4.541064518000417216, -2.621784821875001281 ) ) ;
#43316=CARTESIAN_POINT ( 'NONE',  ( 5.512500001229033941, -4.330127018922190985, -2.500000000000001332 ) ) ;
#43317=CARTESIAN_POINT ( 'NONE',  ( 8.878125000614515372, 6.421520780324663323E-16, -5.243569643749999010 ) ) ;
#43319=CARTESIAN_POINT ( 'NONE',  ( 7.800000000000001599, 4.330127018922192761, -2.499999999999997780 ) ) ;
#43320=CARTESIAN_POINT ( 'NONE',  ( 4.650000001229035895, -2.886751345948125991, -5.000000000000000000 ) ) ;
#43321=CARTESIAN_POINT ( 'NONE',  ( 16.83749999999999858, 5.773502691896255534, 3.535250795749688894E-16 ) ) ;
#43322=CARTESIAN_POINT ( 'NONE',  ( 18.98437500061451644, 4.541064518000418104, 2.621784821874999949 ) ) ;
#43323=CARTESIAN_POINT ( 'NONE',  ( 14.28750000122903430, 4.330127018922191873, 2.499999999999999556 ) ) ;
#43325=CARTESIAN_POINT ( 'NONE',  ( -3.000416591977282496E-16, 16.09062500061451573, -34.90005215228797653 ) ) ;
#43326=CARTESIAN_POINT ( 'NONE',  ( -1.071796769724483234, 15.97009619066136565, 25.99999999999999645 ) ) ;
#43329=CARTESIAN_POINT ( 'NONE',  ( 29.54062500061451502, -3.027376345333610441, -5.243569643749999898 ) ) ;
#43331=CARTESIAN_POINT ( 'NONE',  ( 15.75937500061451857, 4.541064518000418104, -2.621784821874998173 ) ) ;
#43332=EDGE_CURVE ( 'NONE', #16892, #10170, #44449, .T. ) ;
#43333=CARTESIAN_POINT ( 'NONE',  ( 27.86249999999999716, -5.773502691896255534, -1.060575238724906372E-15 ) ) ;
#43334=CARTESIAN_POINT ( 'NONE',  ( 11.42812500061451608, -4.541064518000419881, 2.621784821874995952 ) ) ;
#43336=CARTESIAN_POINT ( 'NONE',  ( 22.13437500061451502, 4.541064518000418104, 2.621784821874999949 ) ) ;
#43338=CARTESIAN_POINT ( 'NONE',  ( 7.115625000614516082, 3.027376345333613106, -5.243569643749998122 ) ) ;
#43339=CARTESIAN_POINT ( 'NONE',  ( 12.00937500061451857, -4.541064518000417216, -2.621784821875001281 ) ) ;
#43340=ORIENTED_EDGE ( 'NONE', *, *, #63166, .F. ) ;
#43341=CARTESIAN_POINT ( 'NONE',  ( 23.63437500061451502, -4.541064518000419881, 2.621784821874995952 ) ) ;
#43342=CARTESIAN_POINT ( 'NONE',  ( 4.000175247584507154, 2.999766337098573654, -29.86665409634473178 ) ) ;
#43343=CARTESIAN_POINT ( 'NONE',  ( 26.99062500061451431, 6.054752690667223547, 3.707466751127219781E-16 ) ) ;
#43345=CARTESIAN_POINT ( 'NONE',  ( 7.875000000000000000, 4.330127018922191873, 2.499999999999999556 ) ) ;
#43346=VECTOR ( 'NONE', #24943, 1000.000000000000000 ) ;
#43347=CARTESIAN_POINT ( 'NONE',  ( 17.13750000122903216, -4.330127018922194537, 2.499999999999995559 ) ) ;
#43350=VERTEX_POINT ( 'NONE', #56249 ) ;
#43351=CARTESIAN_POINT ( 'NONE',  ( 14.40000000000000036, -4.330127018922190985, -2.500000000000001332 ) ) ;
#43352=CARTESIAN_POINT ( 'NONE',  ( 17.88749999999999929, -2.886751345948129988, 4.999999999999997335 ) ) ;
#43353=CARTESIAN_POINT ( 'NONE',  ( 11.54062500061451857, -3.027376345333610441, -5.243569643749999898 ) ) ;
#43354=ORIENTED_EDGE ( 'NONE', *, *, #15041, .F. ) ;
#43355=CARTESIAN_POINT ( 'NONE',  ( 2.121784821875001281, 16.85937500061451999, -26.32496088578401938 ) ) ;
#43356=CARTESIAN_POINT ( 'NONE',  ( 2.953125000614516438, -4.541064518000417216, -2.621784821875001281 ) ) ;
#43358=CARTESIAN_POINT ( 'NONE',  ( 10.83750000000000036, -2.886751345948125991, -5.000000000000000000 ) ) ;
#43359=CARTESIAN_POINT ( 'NONE',  ( 3.950402052914877782, 3.833526817994171942, 3.360136779056243750 ) ) ;
#43360=EDGE_LOOP ( 'NONE', ( #1181, #17384, #47283, #26914, #5728 ) ) ;
#43361=CARTESIAN_POINT ( 'NONE',  ( 4.243569643749999898, 13.27812500061451750, 30.00000000000000000 ) ) ;
#43362=CARTESIAN_POINT ( 'NONE',  ( 27.55312500061451786, 0.000000000000000000, 5.243569643749999010 ) ) ;
#43363=CARTESIAN_POINT ( 'NONE',  ( -5.810221930991193690E-16, 13.58750000000000036, -34.00000000000000000 ) ) ;
#43365=CARTESIAN_POINT ( 'NONE',  ( 21.60937500061451644, 4.541064518000418104, -2.621784821874998173 ) ) ;
#43366=CARTESIAN_POINT ( 'NONE',  ( 19.75312500061451360, 4.541064518000418104, -2.621784821874998173 ) ) ;
#43367=CARTESIAN_POINT ( 'NONE',  ( 2.121784821874999061, 13.80312500061459424, -33.67503911421598417 ) ) ;
#43368=CARTESIAN_POINT ( 'NONE',  ( 22.27500000122903145, 2.886751345948129099, -4.999999999999998224 ) ) ;
#43369=CARTESIAN_POINT ( 'NONE',  ( 3.553125000614516082, 4.541064518000418104, -2.621784821874998173 ) ) ;
#43371=CARTESIAN_POINT ( 'NONE',  ( 21.06562500061451715, 3.027376345333612662, -5.243569643749998122 ) ) ;
#43374=CARTESIAN_POINT ( 'NONE',  ( 15.98437500061451821, -4.541064518000419881, 2.621784821874995952 ) ) ;
#43375=CARTESIAN_POINT ( 'NONE',  ( 13.69687500061451679, -3.027376345333614438, 5.243569643749998122 ) ) ;
#43376=CARTESIAN_POINT ( 'NONE',  ( 23.74687500061451573, -3.027376345333610441, -5.243569643749999898 ) ) ;
#43377=CARTESIAN_POINT ( 'NONE',  ( -3.000416591977282496E-16, 11.64687500061451786, 25.09994784771203058 ) ) ;
#43378=CARTESIAN_POINT ( 'NONE',  ( 4.228125000614517681, -4.541064518000419881, 2.621784821874995952 ) ) ;
#43379=CARTESIAN_POINT ( 'NONE',  ( 28.34062500061451928, 6.054752690667223547, 3.707466751127219781E-16 ) ) ;
#43380=CARTESIAN_POINT ( 'NONE',  ( 26.84062500061451573, -3.027376345333610441, -5.243569643749999898 ) ) ;
#43381=CARTESIAN_POINT ( 'NONE',  ( 8.400000001229035007, 5.773502691896255534, 3.535250795749688401E-16 ) ) ;
#43382=CARTESIAN_POINT ( 'NONE',  ( 8.484601909799253346E-16, 19.66249999999999787, 34.61880215351700230 ) ) ;
#43383=CARTESIAN_POINT ( 'NONE',  ( 8.221875000614518925, 3.027376345333611329, 5.243569643749999010 ) ) ;
#43385=CARTESIAN_POINT ( 'NONE',  ( 13.80000000122903181, 5.773502691896255534, 3.535250795749688894E-16 ) ) ;
#43386=CARTESIAN_POINT ( 'NONE',  ( 8.775000001229033231, 2.886751345948129099, -4.999999999999998224 ) ) ;
#43387=CARTESIAN_POINT ( 'NONE',  ( 5.728125000614515905, 6.421520780324663323E-16, -5.243569643749999010 ) ) ;
#43390=CARTESIAN_POINT ( 'NONE',  ( 14.40937500061451715, 4.541064518000418104, -2.621784821874998173 ) ) ;
#43393=EDGE_CURVE ( 'NONE', #58790, #22068, #50589, .T. ) ;
#43394=CARTESIAN_POINT ( 'NONE',  ( 21.21562500061451573, 3.027376345333611329, 5.243569643749999010 ) ) ;
#43395=CARTESIAN_POINT ( 'NONE',  ( 7.190625000614518036, 6.054752690667223547, 3.707466751127219781E-16 ) ) ;
#43396=CARTESIAN_POINT ( 'NONE',  ( 24.72187500061451360, 3.027376345333612662, -5.243569643749998122 ) ) ;
#43397=CARTESIAN_POINT ( 'NONE',  ( 8.278125000614515727, -4.541064518000419881, 2.621784821874995952 ) ) ;
#43398=CARTESIAN_POINT ( 'NONE',  ( 8.587500001229035007, -4.330127018922194537, 2.499999999999995559 ) ) ;
#43399=CARTESIAN_POINT ( 'NONE',  ( 23.46562500061451573, 3.027376345333611329, 5.243569643749999010 ) ) ;
#43400=CARTESIAN_POINT ( 'NONE',  ( -3.999999999999999556, 18.27500000122903501, -32.30940107675850470 ) ) ;
#43401=CARTESIAN_POINT ( 'NONE',  ( 10.98750000122903536, 6.123233995736764310E-16, -4.999999999999998224 ) ) ;
#43402=CARTESIAN_POINT ( 'NONE',  ( 20.84062500061451573, -3.027376345333614438, 5.243569643749998122 ) ) ;
#43403=CARTESIAN_POINT ( 'NONE',  ( 16.56562500061451715, 3.027376345333613106, -5.243569643749998122 ) ) ;
#43405=CARTESIAN_POINT ( 'NONE',  ( 14.73749999999999893, -2.886751345948129988, 4.999999999999997335 ) ) ;
#43406=CARTESIAN_POINT ( 'NONE',  ( 10.20000000122903572, 5.773502691896255534, 3.535250795749688894E-16 ) ) ;
#43407=AXIS2_PLACEMENT_3D ( 'NONE', #69005, #53460, #7302 ) ;
#43408=CARTESIAN_POINT ( 'NONE',  ( 8.053125000614516082, 4.541064518000418104, -2.621784821874998173 ) ) ;
#43409=CARTESIAN_POINT ( 'NONE',  ( 12.06562500061451537, 3.027376345333613106, -5.243569643749998122 ) ) ;
#43410=CARTESIAN_POINT ( 'NONE',  ( 22.08750000122903501, -4.330127018922194537, 2.499999999999995559 ) ) ;
#43411=CARTESIAN_POINT ( 'NONE',  ( 20.40937500061451715, 0.000000000000000000, 5.243569643749999010 ) ) ;
#43412=CARTESIAN_POINT ( 'NONE',  ( 4.715625000614516615, -6.054752690667223547, -1.112240025338166033E-15 ) ) ;
#43414=CARTESIAN_POINT ( 'NONE',  ( 5.025000001229035895, -5.773502691896255534, -1.060575238724906372E-15 ) ) ;
#43415=CARTESIAN_POINT ( 'NONE',  ( 3.571875000614517237, 3.027376345333613106, -5.243569643749998122 ) ) ;
#43416=CARTESIAN_POINT ( 'NONE',  ( 22.24687500061451217, -3.027376345333614438, 5.243569643749998122 ) ) ;
#43417=( BOUNDED_SURFACE ( )  B_SPLINE_SURFACE ( 1, 2, ( 
 ( #10327, #51302, #16582, #56480, #10689, #56124, #4791, #67221, #32861, #5517, #5152, #28404, #17310, #62381, #27324, #50941, #39497, #49858, #72382, #72750, #44691, #33937, #28055, #50583, #22493, #340, #22847, #28763, #45400, #11781, #34296, #56828, #704, #23212, #63103, #7681, #51667, #24665, #1796, #29853, #12857, #40583, #2506, #41312, #25029, #53109, #52389, #35390, #47572, #58641, #68663, #58274, #23580, #30217, #23938, #40955, #13215, #46125, #70102, #24306, #46853, #40222, #18026, #62744, #57915, #1432, #52751, #69394, #2154, #7322, #6605, #18748, #12137, #34662, #63822, #57191, #35753, #47211, #69743, #57559, #19111, #30583, #1072, #41667, #12503, #46487, #64189, #13576, #35031, #69026, #6962, #29134, #36121, #29493, #52029, #8049, #18388, #63470, #9874, #19850, #54216, #49407, #4351, #36485, #59737, #20210, #19477, #36849, #59004, #48311, #32408, #8409, #42035, #37216, #3613, #47944, #3245, #42401, #26878, #71574, #54946, #64559, #20948, #54577, #70835, #13948, #64923, #26134, #30938, #53479, #2871, #9146, #42764, #25402, #59365, #70473, #65284, #14313, #8776, #31311, #53853, #25773, #43501, #14672, #15404, #31682, #66026, #48675, #71199, #20574, #60465, #43130, #65653, #15043, #37580, #60103, #9512, #32045, #3981, #26505, #49046, #37946, #5069, #6151, #44608, #44236, #67496, #5790, #28322, #15769, #16859, #50500, #38311, #28680, #66767, #72299, #27970, #56747, #4707, #10967, #27238, #61211, #17225, #66392, #61935, #22047, #5430, #22411, #55672, #21679, #39414, #10243, #56400, #33490, #61565, #67138, #16140, #34213, #73027, #71939, #11697, #56038, #16496, #21315, #39785, #49775, #11340, #55313, #33856, #27604, #72668, #44958, #38692, #43868, #50859, #257, #60838, #10606, #32776, #39051, #33135, #22766, #45317, #67852, #62301, #50137, #68936, #37030, #59554, #35303, #68218, #57826, #53292, #70289, #68576, #36666, #42579, #62657, #7235, #12053, #12412, #622, #51220, #46040, #53664, #63014, #48126, #34577, #3056, #17936, #29049, #30760, #20024, #17580, #2691, #1340, #34945, #8965, #65106, #6877, #47754, #6516, #46400, #45685, #57472, #23129, #23852, #23493, #19661, #59185, #8595, #40141, #42216, #25206, #57105, #51585, #40498, #985, #64740, #29410, #51943, #63383, #18294, #40866, #70649, #12768, #14128, #31124, #25587, #14495, #15224, #54399, #72115, #42945, #15954, #66207, #21131, #4165, #31864, #66952, #32595, #16320, #44425, #43684, #26695, #38873, #49953, #59925, #49590, #14862, #21498, #37763, #32227, #4532, #37401, #61391, #15585, #38127, #31499, #9331, #54039, #49229, #65841, #44051, #60648, #66575, #71762, #71018, #10063, #3435, #25954, #55133, #48494, #27060, #38502, #61028, #48859, #10426, #21864, #65472, #32957, #3798, #60281, #55493, #4887, #26321, #9694, #71390, #20396, #27423, #20764, #43321, #72478, #54761, #39597, #1161, #11151, #45502, #40676, #68755, #27788, #51036, #11511, #10785, #28150, #50325, #62119, #23670, #72849, #34394, #67671, #33678, #51397, #22230, #68391, #68033, #433, #56570, #56221, #46216, #11871, #18113, #33318, #22941, #5967, #55857, #29227, #39235, #28858, #67319, #800, #17039, #34033, #56924, #16679, #5246, #17403, #39960, #44786, #61747, #5614, #28499, #45138, #23308, #62474, #45856, #6328, #50678, #17752, #82, #22587, #40311, #62834, #12227, #34755, #57291, #6696, #51762, #53570, #1524, #69836, #24030, #24396, #7777, #24758, #18481, #46945, #12947, #70566, #42127, #25495, #19941, #64653, #25118, #18840, #2967, #63560, #47300, #63196, #48041, #7056, #30312, #63918, #12592, #7413, #29584, #41402, #35125, #52122, #57649, #46579, #58005, #14037, #1891, #59098, #69123, #36578, #29941, #41047, #19201, #31034, #35484, #64283, #13303, #69482, #52481, #35840, #58365, #58731, #52844, #2242, #41755, #13672, #36216, #8143, #30669, #53202, #70194, #19571, #2598, #47661, #8505, #59464, #72387, #37313, #42858, #71668, #27332, #48408, #54671, #70934, #31777, #60931, #36944, #32504, #65751, #49140, #43595, #3346, #21405, #14769, #49864, #25868, #49499, #43231, #15135, #55040, #59837, #15862, #42495, #26970, #8873, #4442, #66483, #72029, #9968, #66116, #43962, #32138, #37673, #38037, #20304, #26601, #60195, #38409, #10335, #65380, #53949, #21043, #54316, #9242, #32867, #31409, #9606, #55403, #71295, #65018, #3707, #26234, #15495, #14407, #48771, #20674, #4074, #60561, #4798, #57198, #21768, #56130, #17316, #29141, #5158, #39877, #67228, #23220, #6613, #62388, #45050, #61657, #51674, #27693, #34670, #10695, #11056, #33227, #50232, #55766, #347, #39140, #68309, #5880, #11787, #56487, #62029, #44331, #66860, #45773, #72756, #16231, #11427, #45408, #22142, #16588, #28412, #34304, #44695, #50950, #51309, #5523, #56835, #6243, #22853, #38784, #12144, #17668, #33584, #28770, #61301, #28061, #713, #50591, #40229, #62751, #73117, #22501, #67943, #67585, #16951, #39504, #33945, #58281, #63477, #52396, #7688, #1439, #36492, #30225, #46494, #12865, #18395, #69033, #1803, #63829, #19118, #18755, #40962, #47579, #30945, #58648, #18034, #13583, #25036, #36129, #41673, #2161, #53116, #13221, #69400, #69750, #52036, #52758, #41319, #64196, #8056, #35038, #12510, #24672, #35396, #57566, #30591, #40590, #24313, #2514, #29860, #1079, #63111, #6969, #47218, #8415, #29500, #23945, #57922, #35760, #70109, #59012, #23587, #7329, #19485, #46132, #46861, #42043, #64566, #13954, #68670, #71579, #3619, #20216, #38316, #36856, #66398, #42408, #42770, #64930, #59372, #14321, #32051, #70841, #26883, #37587, #20953, #15049, #20581, #60843, #10248, #54951, #8783, #2878, #43136, #3987, #31317, #25780, #60109, #43506, #53861, #9519, #9879, #37222, #49052, #15409, #54583, #53486, #43873, #49412, #3252, #60471, #19857, #14678, #66031, #65290, #37952, #32414 ),
 ( #25409, #48318, #65660, #59744, #9152, #71943, #47952, #4357, #26140, #26512, #21320, #31687, #15775, #70480, #54222, #48681, #71205, #17587, #16145, #45690, #21685, #22053, #44242, #38697, #66772, #11343, #50144, #6155, #16863, #50863, #67500, #73031, #40146, #62662, #34217, #61216, #55318, #22415, #56404, #10611, #5074, #39418, #261, #33140, #61940, #62306, #16502, #28325, #67856, #33861, #32781, #23134, #28685, #55677, #39789, #72304, #67143, #22770, #72673, #45322, #11701, #27244, #17229, #5794, #56751, #51224, #628, #39056, #68224, #44613, #10972, #4712, #27609, #49780, #61569, #33494, #56043, #5435, #27974, #50504, #44962, #30132, #29769, #13129, #46046, #64100, #57477, #19387, #68581, #19023, #12773, #57831, #2071, #6882, #58552, #41948, #69658, #29054, #24580, #36034, #47127, #52664, #35668, #13485, #1705, #7240, #7594, #63019, #69304, #52304, #41583, #7962, #17941, #23498, #18666, #1347, #40504, #30498, #51590, #35308, #53026, #40871, #12059, #990, #12418, #63738, #34582, #34950, #29415, #23857, #24220, #46769, #47486, #57110, #46404, #2420, #6521, #51948, #24942, #68942, #41227, #18300, #63388, #70017, #58191, #14589, #26416, #20123, #64469, #53390, #47857, #43042, #71855, #2786, #70386, #3159, #31595, #3528, #26790, #13862, #25688, #60017, #21228, #19762, #9429, #36763, #65940, #49324, #31957, #37123, #31221, #36404, #42312, #4266, #25310, #53764, #64839, #14226, #59281, #65569, #8689, #37859, #48589, #54495, #26049, #54133, #58916, #8325, #15320, #48222, #30855, #71115, #14958, #70746, #42677, #20487, #3896, #65200, #37497, #20865, #59652, #48958, #71488, #43416, #9062, #54857, #60380, #9788, #32322, #10160, #4985, #11253, #61128, #61847, #22683, #38222, #33776, #67414, #50419, #67766, #28244, #27517, #27885, #16054, #39333, #50775, #178, #60751, #56319, #22326, #32694, #535, #38602, #44150, #72945, #28600, #49689, #55951, #72218, #33051, #62218, #55231, #5709, #67055, #44879, #16776, #50051, #66679, #45234, #4626, #17140, #5347, #33413, #16414, #10523, #6066, #39700, #51136, #56670, #11613, #38970, #43780, #34131, #21596, #66307, #27155, #15684, #55590, #61486, #72579, #10882, #21964, #44522, #7152, #40059, #29682, #24130, #41145, #40413, #7508, #13394, #34494, #52218, #57022, #57386, #40781, #57745, #51500, #6792, #45956, #30412, #1986, #58464, #52940, #24497, #58103, #51857, #35942, #23409, #1621, #23044, #7876, #62574, #63295, #23764, #45602, #62930, #11970, #1259, #68135, #6428, #17499, #28962, #17851, #47040, #34859, #18937, #901, #69575, #12323, #68488, #46680, #64017, #29327, #69219, #46317, #68853, #18210, #12687, #35224, #18579, #63653, #13044, #35582, #30039, #52578, #41495, #47764, #71030, #9343, #31875, #19302, #20407, #54050, #41855, #32237, #70300, #2702, #31510, #60292, #8241, #14506, #30771, #64750, #20775, #69932, #65484, #25598, #8977, #25964, #59195, #25217, #42955, #13775, #59936, #37040, #65116, #48135, #19672, #37773, #3445, #9703, #15236, #59564, #70660, #2337, #43331, #53302, #14873, #58831, #37413, #8605, #3068, #48504, #42226, #24855, #54410, #3810, #47400, #14140, #64383, #20034, #36676, #26332, #48870, #65853, #31134, #71401, #53675, #36316, #42590, #55503, #28778, #38137, #40598, #17325, #62397, #54771, #60659, #4176, #355, #15964, #723, #39884, #68317, #49965, #21142, #22862, #63120, #12516, #11795, #71772, #34312, #56845, #23229, #72128, #40236, #46141, #66217, #6251, #15594, #38514, #45417, #51319, #10074, #61038, #4541, #26705, #34678, #18041, #49239, #57207, #17677, #10436, #68680, #55143, #45782, #43695, #32605, #27069, #67953, #4899, #49601, #21507, #44060, #32966, #66587, #27434, #62759, #12151, #6622, #29150, #51684, #1088, #23595, #59021, #29867, #12873, #64204, #2886, #52044, #36138, #58290, #18763, #64938, #25416, #63838, #30598, #63485, #30234, #40970, #58657, #7697, #42418, #7338, #53125, #42051, #64574, #1448, #2524, #13591, #23953, #35047, #52404, #35405, #8064, #19865, #57931, #47227, #1812, #24320, #53494, #29509, #25045, #52766, #41681, #47588, #41329, #46868, #70117, #46503, #19494, #69759, #24680, #2169, #69408, #70488, #13963, #57575, #47960, #19127, #36500, #6978, #18403, #8422, #69041, #13229, #35768, #30958, #54593, #26522, #49788, #14329, #48689, #9888, #21694, #70851, #32423, #59753, #15784, #72313, #54960, #37596, #54230, #44251, #20224, #27255, #3260, #3627, #25789, #42778, #48326, #66039, #31695, #60854, #71588, #4365, #49060, #3995, #36864, #59382, #38326, #65298, #8793, #20961, #37960, #14688, #9160, #43516, #26894, #37230, #15417, #43882, #71213, #49420, #71953, #60480, #31326, #4721, #10258, #26149, #21329, #53869, #20590, #66408, #43147, #32790, #55327, #65669, #15058, #60117, #9527, #32059, #67866, #23143, #27618, #44622, #44970, #50871, #67152, #29064, #269, #39065, #56052, #10982, #61579, #67508, #56412, #11710, #11351, #17238, #50152, #45698, #33503, #1000, #72682, #636, #16873, #39427, #56759, #5444, #40154, #23507, #51232, #10620, #6164, #17595, #28693, #34226, #39798, #68231, #5803, #61947, #62314, #16512, #22779, #33869, #62673, #12068, #22064, #5083, #45330, #27984, #50514, #34591, #33150, #28333, #57119, #22423, #66782, #55687, #6531, #16154, #51600, #73040, #38706, #61226, #36046, #29780, #46781, #19037, #29424, #30867, #7606, #52675, #46056, #51959, #68590, #63751, #7251, #64113, #30144, #58567, #41239, #12428, #13140, #53405, #2797, #2083, #63029, #24592, #47140, #13499, #63398, #30510, #36414, #57489, #69671, #6893, #52316, #35679, #41595, #1359, #1719, #68953, #17952, #24955, #8337, #40514, #47498, #7974, #24231, #58929, #46416, #53037, #34962, #23868, #18311, #58202, #69316, #40882, #12783, #35320, #18677, #57842, #2432, #70029, #19401, #41960, #64482, #13875 ) ),
 .UNSPECIFIED., .F., .F., .F. ) 
 B_SPLINE_SURFACE_WITH_KNOTS ( ( 2, 2 ),
 ( 3, 2, 2, 2, 2, 2, 2, 2, 2, 2, 2, 2, 2, 2, 2, 2, 2, 2, 2, 2, 2, 2, 2, 2, 2, 2, 2, 2, 2, 2, 2, 2, 2, 2, 2, 2, 2, 2, 2, 2, 2, 2, 2, 2, 2, 2, 2, 2, 2, 2, 2, 2, 2, 2, 2, 2, 2, 2, 2, 2, 2, 2, 2, 2, 2, 2, 2, 2, 2, 2, 2, 2, 2, 2, 2, 2, 2, 2, 2, 2, 2, 2, 2, 2, 2, 2, 2, 2, 2, 2, 2, 2, 2, 2, 2, 2, 2, 2, 2, 2, 2, 2, 2, 2, 2, 2, 2, 2, 2, 2, 2, 2, 2, 2, 2, 2, 2, 2, 2, 2, 2, 2, 2, 2, 2, 2, 2, 2, 2, 2, 2, 2, 2, 2, 2, 2, 2, 2, 2, 2, 2, 2, 2, 2, 2, 2, 2, 2, 2, 2, 2, 2, 2, 2, 2, 2, 2, 2, 2, 2, 2, 2, 2, 2, 2, 2, 2, 2, 2, 2, 2, 2, 2, 2, 2, 2, 2, 2, 2, 2, 2, 2, 2, 2, 2, 2, 2, 2, 2, 2, 2, 2, 2, 2, 2, 2, 2, 2, 2, 2, 2, 2, 2, 2, 2, 2, 2, 2, 2, 2, 2, 2, 2, 2, 2, 2, 2, 2, 2, 2, 2, 2, 2, 2, 2, 2, 2, 2, 2, 2, 2, 2, 2, 2, 2, 2, 2, 2, 2, 2, 2, 2, 2, 2, 2, 2, 2, 2, 2, 2, 2, 2, 2, 2, 2, 2, 2, 2, 2, 2, 2, 2, 2, 2, 2, 2, 2, 2, 2, 2, 2, 2, 2, 2, 2, 2, 2, 2, 2, 2, 2, 2, 2, 2, 2, 2, 2, 2, 2, 2, 2, 2, 2, 2, 2, 2, 2, 2, 2, 2, 2, 2, 2, 2, 2, 2, 2, 2, 2, 2, 2, 2, 2, 2, 2, 2, 2, 2, 2, 2, 2, 2, 2, 2, 2, 2, 2, 2, 2, 2, 2, 2, 2, 2, 2, 2, 2, 2, 2, 2, 2, 2, 2, 2, 2, 2, 2, 2, 2, 2, 2, 2, 2, 2, 2, 2, 2, 2, 2, 2, 3 ),
 ( 0.000000000000000000, 1.000000000000000000 ),
 ( 0.000000000000000000, 0.002777777777777777884, 0.005555555555555555768, 0.008333333333333333218, 0.01111111111111111154, 0.01388888888888888812, 0.01666666666666666644, 0.01944444444444444475, 0.02222222222222222307, 0.02500000000000000139, 0.02777777777777777624, 0.03055555555555555455, 0.03333333333333333287, 0.03611111111111110772, 0.03888888888888888951, 0.04166666666666666435, 0.04444444444444444614, 0.04722222222222222099, 0.05000000000000000278, 0.05277777777777777762, 0.05555555555555555247, 0.05833333333333333426, 0.06111111111111110911, 0.06388888888888888395, 0.06666666666666666574, 0.06944444444444444753, 0.07222222222222221544, 0.07499999999999999722, 0.07777777777777777901, 0.08055555555555556080, 0.08333333333333332871, 0.08611111111111111049, 0.08888888888888889228, 0.09166666666666666019, 0.09444444444444444198, 0.09722222222222222376, 0.1000000000000000056, 0.1027777777777777735, 0.1055555555555555552, 0.1083333333333333370, 0.1111111111111111049, 0.1138888888888888867, 0.1166666666666666685, 0.1194444444444444503, 0.1222222222222222182, 0.1250000000000000000, 0.1277777777777777679, 0.1305555555555555636, 0.1333333333333333315, 0.1361111111111110994, 0.1388888888888888951, 0.1416666666666666630, 0.1444444444444444309, 0.1472222222222222265, 0.1499999999999999944, 0.1527777777777777901, 0.1555555555555555580, 0.1583333333333333259, 0.1611111111111111216, 0.1638888888888888895, 0.1666666666666666574, 0.1694444444444444531, 0.1722222222222222210, 0.1749999999999999889, 0.1777777777777777846, 0.1805555555555555525, 0.1833333333333333204, 0.1861111111111111160, 0.1888888888888888840, 0.1916666666666666796, 0.1944444444444444475, 0.1972222222222222154, 0.2000000000000000111, 0.2027777777777777790, 0.2055555555555555469, 0.2083333333333333426, 0.2111111111111111105, 0.2138888888888888784, 0.2166666666666666741, 0.2194444444444444420, 0.2222222222222222099, 0.2250000000000000056, 0.2277777777777777735, 0.2305555555555555691, 0.2333333333333333370, 0.2361111111111111049, 0.2388888888888889006, 0.2416666666666666685, 0.2444444444444444364, 0.2472222222222222321, 0.2500000000000000000, 0.2527777777777777679, 0.2555555555555555358, 0.2583333333333333592, 0.2611111111111111271, 0.2638888888888888951, 0.2666666666666666630, 0.2694444444444444309, 0.2722222222222221988, 0.2750000000000000222, 0.2777777777777777901, 0.2805555555555555580, 0.2833333333333333259, 0.2861111111111110938, 0.2888888888888888618, 0.2916666666666666852, 0.2944444444444444531, 0.2972222222222222210, 0.2999999999999999889, 0.3027777777777777568, 0.3055555555555555802, 0.3083333333333333481, 0.3111111111111111160, 0.3138888888888888840, 0.3166666666666666519, 0.3194444444444444198, 0.3222222222222222432, 0.3250000000000000111, 0.3277777777777777790, 0.3305555555555555469, 0.3333333333333333148, 0.3361111111111111382, 0.3388888888888889062, 0.3416666666666666741, 0.3444444444444444420, 0.3472222222222222099, 0.3499999999999999778, 0.3527777777777778012, 0.3555555555555555691, 0.3583333333333333370, 0.3611111111111111049, 0.3638888888888888729, 0.3666666666666666408, 0.3694444444444444642, 0.3722222222222222321, 0.3750000000000000000, 0.3777777777777777679, 0.3805555555555555358, 0.3833333333333333592, 0.3861111111111111271, 0.3888888888888888951, 0.3916666666666666630, 0.3944444444444444309, 0.3972222222222221988, 0.4000000000000000222, 0.4027777777777777901, 0.4055555555555555580, 0.4083333333333333259, 0.4111111111111110938, 0.4138888888888888618, 0.4166666666666666852, 0.4194444444444444531, 0.4222222222222222210, 0.4249999999999999889, 0.4277777777777777568, 0.4305555555555555802, 0.4333333333333333481, 0.4361111111111111160, 0.4388888888888888840, 0.4416666666666666519, 0.4444444444444444198, 0.4472222222222222432, 0.4500000000000000111, 0.4527777777777777790, 0.4555555555555555469, 0.4583333333333333148, 0.4611111111111111382, 0.4638888888888889062, 0.4666666666666666741, 0.4694444444444444420, 0.4722222222222222099, 0.4749999999999999778, 0.4777777777777778012, 0.4805555555555555691, 0.4833333333333333370, 0.4861111111111111049, 0.4888888888888888729, 0.4916666666666666408, 0.4944444444444444642, 0.4972222222222222321, 0.5000000000000000000, 0.5027777777777777679, 0.5055555555555555358, 0.5083333333333333037, 0.5111111111111110716, 0.5138888888888888395, 0.5166666666666667185, 0.5194444444444444864, 0.5222222222222222543, 0.5250000000000000222, 0.5277777777777777901, 0.5305555555555555580, 0.5333333333333333259, 0.5361111111111110938, 0.5388888888888888618, 0.5416666666666666297, 0.5444444444444443976, 0.5472222222222222765, 0.5500000000000000444, 0.5527777777777778123, 0.5555555555555555802, 0.5583333333333333481, 0.5611111111111111160, 0.5638888888888888840, 0.5666666666666666519, 0.5694444444444444198, 0.5722222222222221877, 0.5749999999999999556, 0.5777777777777777235, 0.5805555555555556024, 0.5833333333333333703, 0.5861111111111111382, 0.5888888888888889062, 0.5916666666666666741, 0.5944444444444444420, 0.5972222222222222099, 0.5999999999999999778, 0.6027777777777777457, 0.6055555555555555136, 0.6083333333333332815, 0.6111111111111111605, 0.6138888888888889284, 0.6166666666666666963, 0.6194444444444444642, 0.6222222222222222321, 0.6250000000000000000, 0.6277777777777777679, 0.6305555555555555358, 0.6333333333333333037, 0.6361111111111110716, 0.6388888888888888395, 0.6416666666666667185, 0.6444444444444444864, 0.6472222222222222543, 0.6500000000000000222, 0.6527777777777777901, 0.6555555555555555580, 0.6583333333333333259, 0.6611111111111110938, 0.6638888888888888618, 0.6666666666666666297, 0.6694444444444443976, 0.6722222222222222765, 0.6750000000000000444, 0.6777777777777778123, 0.6805555555555555802, 0.6833333333333333481, 0.6861111111111111160, 0.6888888888888888840, 0.6916666666666666519, 0.6944444444444444198, 0.6972222222222221877, 0.6999999999999999556, 0.7027777777777777235, 0.7055555555555556024, 0.7083333333333333703, 0.7111111111111111382, 0.7138888888888889062, 0.7166666666666666741, 0.7194444444444444420, 0.7222222222222222099, 0.7249999999999999778, 0.7277777777777777457, 0.7305555555555555136, 0.7333333333333332815, 0.7361111111111111605, 0.7388888888888889284, 0.7416666666666666963, 0.7444444444444444642, 0.7472222222222222321, 0.7500000000000000000, 0.7527777777777777679, 0.7555555555555555358, 0.7583333333333333037, 0.7611111111111110716, 0.7638888888888888395, 0.7666666666666667185, 0.7694444444444444864, 0.7722222222222222543, 0.7750000000000000222, 0.7777777777777777901, 0.7805555555555555580, 0.7833333333333333259, 0.7861111111111110938, 0.7888888888888888618, 0.7916666666666666297, 0.7944444444444443976, 0.7972222222222222765, 0.8000000000000000444, 0.8027777777777778123, 0.8055555555555555802, 0.8083333333333333481, 0.8111111111111111160, 0.8138888888888888840, 0.8166666666666666519, 0.8194444444444444198, 0.8222222222222221877, 0.8249999999999999556, 0.8277777777777777235, 0.8305555555555556024, 0.8333333333333333703, 0.8361111111111111382, 0.8388888888888889062, 0.8416666666666666741, 0.8444444444444444420, 0.8472222222222222099, 0.8499999999999999778, 0.8527777777777777457, 0.8555555555555555136, 0.8583333333333332815, 0.8611111111111111605, 0.8638888888888889284, 0.8666666666666666963, 0.8694444444444444642, 0.8722222222222222321, 0.8750000000000000000, 0.8777777777777777679, 0.8805555555555555358, 0.8833333333333333037, 0.8861111111111110716, 0.8888888888888888395, 0.8916666666666667185, 0.8944444444444444864, 0.8972222222222222543, 0.9000000000000000222, 0.9027777777777777901, 0.9055555555555555580, 0.9083333333333333259, 0.9111111111111110938, 0.9138888888888888618, 0.9166666666666666297, 0.9194444444444443976, 0.9222222222222222765, 0.9250000000000000444, 0.9277777777777778123, 0.9305555555555555802, 0.9333333333333333481, 0.9361111111111111160, 0.9388888888888888840, 0.9416666666666666519, 0.9444444444444444198, 0.9472222222222221877, 0.9499999999999999556, 0.9527777777777777235, 0.9555555555555556024, 0.9583333333333333703, 0.9611111111111111382, 0.9638888888888889062, 0.9666666666666666741, 0.9694444444444444420, 0.9722222222222222099, 0.9749999999999999778, 0.9777777777777777457, 0.9805555555555555136, 0.9833333333333332815, 0.9861111111111111605, 0.9888888888888889284, 0.9916666666666666963, 0.9944444444444444642, 0.9972222222222222321, 1.000000000000000000 ),
 .UNSPECIFIED. ) 
 GEOMETRIC_REPRESENTATION_ITEM ( )  RATIONAL_B_SPLINE_SURFACE ( (
 ( 1.000000000000000000, 0.8660254037844387076, 1.000000000000000000, 0.8660254037844387076, 1.000000000000000000, 0.8660254037844387076, 1.000000000000000000, 0.8660254037844387076, 1.000000000000000000, 0.8660254037844387076, 1.000000000000000000, 0.8660254037844387076, 1.000000000000000000, 0.8660254037844387076, 1.000000000000000000, 0.8660254037844387076, 1.000000000000000000, 0.8660254037844387076, 1.000000000000000000, 0.8660254037844387076, 1.000000000000000000, 0.8660254037844387076, 1.000000000000000000, 0.8660254037844387076, 1.000000000000000000, 0.8660254037844387076, 1.000000000000000000, 0.8660254037844387076, 1.000000000000000000, 0.8660254037844387076, 1.000000000000000000, 0.8660254037844387076, 1.000000000000000000, 0.8660254037844387076, 1.000000000000000000, 0.8660254037844387076, 1.000000000000000000, 0.8660254037844387076, 1.000000000000000000, 0.8660254037844387076, 1.000000000000000000, 0.8660254037844387076, 1.000000000000000000, 0.8660254037844387076, 1.000000000000000000, 0.8660254037844387076, 1.000000000000000000, 0.8660254037844387076, 1.000000000000000000, 0.8660254037844387076, 1.000000000000000000, 0.8660254037844387076, 1.000000000000000000, 0.8660254037844387076, 1.000000000000000000, 0.8660254037844387076, 1.000000000000000000, 0.8660254037844387076, 1.000000000000000000, 0.8660254037844387076, 1.000000000000000000, 0.8660254037844387076, 1.000000000000000000, 0.8660254037844387076, 1.000000000000000000, 0.8660254037844387076, 1.000000000000000000, 0.8660254037844387076, 1.000000000000000000, 0.8660254037844387076, 1.000000000000000000, 0.8660254037844387076, 1.000000000000000000, 0.8660254037844387076, 1.000000000000000000, 0.8660254037844387076, 1.000000000000000000, 0.8660254037844387076, 1.000000000000000000, 0.8660254037844387076, 1.000000000000000000, 0.8660254037844387076, 1.000000000000000000, 0.8660254037844387076, 1.000000000000000000, 0.8660254037844387076, 1.000000000000000000, 0.8660254037844387076, 1.000000000000000000, 0.8660254037844387076, 1.000000000000000000, 0.8660254037844387076, 1.000000000000000000, 0.8660254037844387076, 1.000000000000000000, 0.8660254037844387076, 1.000000000000000000, 0.8660254037844387076, 1.000000000000000000, 0.8660254037844387076, 1.000000000000000000, 0.8660254037844387076, 1.000000000000000000, 0.8660254037844387076, 1.000000000000000000, 0.8660254037844387076, 1.000000000000000000, 0.8660254037844387076, 1.000000000000000000, 0.8660254037844387076, 1.000000000000000000, 0.8660254037844387076, 1.000000000000000000, 0.8660254037844387076, 1.000000000000000000, 0.8660254037844387076, 1.000000000000000000, 0.8660254037844387076, 1.000000000000000000, 0.8660254037844387076, 1.000000000000000000, 0.8660254037844387076, 1.000000000000000000, 0.8660254037844387076, 1.000000000000000000, 0.8660254037844387076, 1.000000000000000000, 0.8660254037844387076, 1.000000000000000000, 0.8660254037844387076, 1.000000000000000000, 0.8660254037844387076, 1.000000000000000000, 0.8660254037844387076, 1.000000000000000000, 0.8660254037844387076, 1.000000000000000000, 0.8660254037844387076, 1.000000000000000000, 0.8660254037844387076, 1.000000000000000000, 0.8660254037844387076, 1.000000000000000000, 0.8660254037844387076, 1.000000000000000000, 0.8660254037844387076, 1.000000000000000000, 0.8660254037844387076, 1.000000000000000000, 0.8660254037844387076, 1.000000000000000000, 0.8660254037844387076, 1.000000000000000000, 0.8660254037844387076, 1.000000000000000000, 0.8660254037844387076, 1.000000000000000000, 0.8660254037844387076, 1.000000000000000000, 0.8660254037844387076, 1.000000000000000000, 0.8660254037844387076, 1.000000000000000000, 0.8660254037844387076, 1.000000000000000000, 0.8660254037844387076, 1.000000000000000000, 0.8660254037844387076, 1.000000000000000000, 0.8660254037844387076, 1.000000000000000000, 0.8660254037844387076, 1.000000000000000000, 0.8660254037844387076, 1.000000000000000000, 0.8660254037844387076, 1.000000000000000000, 0.8660254037844387076, 1.000000000000000000, 0.8660254037844387076, 1.000000000000000000, 0.8660254037844387076, 1.000000000000000000, 0.8660254037844387076, 1.000000000000000000, 0.8660254037844387076, 1.000000000000000000, 0.8660254037844387076, 1.000000000000000000, 0.8660254037844387076, 1.000000000000000000, 0.8660254037844387076, 1.000000000000000000, 0.8660254037844387076, 1.000000000000000000, 0.8660254037844387076, 1.000000000000000000, 0.8660254037844387076, 1.000000000000000000, 0.8660254037844387076, 1.000000000000000000, 0.8660254037844387076, 1.000000000000000000, 0.8660254037844387076, 1.000000000000000000, 0.8660254037844387076, 1.000000000000000000, 0.8660254037844387076, 1.000000000000000000, 0.8660254037844387076, 1.000000000000000000, 0.8660254037844387076, 1.000000000000000000, 0.8660254037844387076, 1.000000000000000000, 0.8660254037844387076, 1.000000000000000000, 0.8660254037844387076, 1.000000000000000000, 0.8660254037844387076, 1.000000000000000000, 0.8660254037844387076, 1.000000000000000000, 0.8660254037844387076, 1.000000000000000000, 0.8660254037844387076, 1.000000000000000000, 0.8660254037844387076, 1.000000000000000000, 0.8660254037844387076, 1.000000000000000000, 0.8660254037844387076, 1.000000000000000000, 0.8660254037844387076, 1.000000000000000000, 0.8660254037844387076, 1.000000000000000000, 0.8660254037844387076, 1.000000000000000000, 0.8660254037844387076, 1.000000000000000000, 0.8660254037844387076, 1.000000000000000000, 0.8660254037844387076, 1.000000000000000000, 0.8660254037844387076, 1.000000000000000000, 0.8660254037844387076, 1.000000000000000000, 0.8660254037844387076, 1.000000000000000000, 0.8660254037844387076, 1.000000000000000000, 0.8660254037844387076, 1.000000000000000000, 0.8660254037844387076, 1.000000000000000000, 0.8660254037844387076, 1.000000000000000000, 0.8660254037844387076, 1.000000000000000000, 0.8660254037844387076, 1.000000000000000000, 0.8660254037844387076, 1.000000000000000000, 0.8660254037844387076, 1.000000000000000000, 0.8660254037844387076, 1.000000000000000000, 0.8660254037844387076, 1.000000000000000000, 0.8660254037844387076, 1.000000000000000000, 0.8660254037844387076, 1.000000000000000000, 0.8660254037844387076, 1.000000000000000000, 0.8660254037844387076, 1.000000000000000000, 0.8660254037844387076, 1.000000000000000000, 0.8660254037844387076, 1.000000000000000000, 0.8660254037844387076, 1.000000000000000000, 0.8660254037844387076, 1.000000000000000000, 0.8660254037844387076, 1.000000000000000000, 0.8660254037844387076, 1.000000000000000000, 0.8660254037844387076, 1.000000000000000000, 0.8660254037844387076, 1.000000000000000000, 0.8660254037844387076, 1.000000000000000000, 0.8660254037844387076, 1.000000000000000000, 0.8660254037844387076, 1.000000000000000000, 0.8660254037844387076, 1.000000000000000000, 0.8660254037844387076, 1.000000000000000000, 0.8660254037844387076, 1.000000000000000000, 0.8660254037844387076, 1.000000000000000000, 0.8660254037844387076, 1.000000000000000000, 0.8660254037844387076, 1.000000000000000000, 0.8660254037844387076, 1.000000000000000000, 0.8660254037844387076, 1.000000000000000000, 0.8660254037844387076, 1.000000000000000000, 0.8660254037844387076, 1.000000000000000000, 0.8660254037844387076, 1.000000000000000000, 0.8660254037844387076, 1.000000000000000000, 0.8660254037844387076, 1.000000000000000000, 0.8660254037844387076, 1.000000000000000000, 0.8660254037844387076, 1.000000000000000000, 0.8660254037844387076, 1.000000000000000000, 0.8660254037844387076, 1.000000000000000000, 0.8660254037844387076, 1.000000000000000000, 0.8660254037844387076, 1.000000000000000000, 0.8660254037844387076, 1.000000000000000000, 0.8660254037844387076, 1.000000000000000000, 0.8660254037844387076, 1.000000000000000000, 0.8660254037844387076, 1.000000000000000000, 0.8660254037844387076, 1.000000000000000000, 0.8660254037844387076, 1.000000000000000000, 0.8660254037844387076, 1.000000000000000000, 0.8660254037844387076, 1.000000000000000000, 0.8660254037844387076, 1.000000000000000000, 0.8660254037844387076, 1.000000000000000000, 0.8660254037844387076, 1.000000000000000000, 0.8660254037844387076, 1.000000000000000000, 0.8660254037844387076, 1.000000000000000000, 0.8660254037844387076, 1.000000000000000000, 0.8660254037844387076, 1.000000000000000000, 0.8660254037844387076, 1.000000000000000000, 0.8660254037844387076, 1.000000000000000000, 0.8660254037844387076, 1.000000000000000000, 0.8660254037844387076, 1.000000000000000000, 0.8660254037844387076, 1.000000000000000000, 0.8660254037844387076, 1.000000000000000000, 0.8660254037844387076, 1.000000000000000000, 0.8660254037844387076, 1.000000000000000000, 0.8660254037844387076, 1.000000000000000000, 0.8660254037844387076, 1.000000000000000000, 0.8660254037844387076, 1.000000000000000000, 0.8660254037844387076, 1.000000000000000000, 0.8660254037844387076, 1.000000000000000000, 0.8660254037844387076, 1.000000000000000000, 0.8660254037844387076, 1.000000000000000000, 0.8660254037844387076, 1.000000000000000000, 0.8660254037844387076, 1.000000000000000000, 0.8660254037844387076, 1.000000000000000000, 0.8660254037844387076, 1.000000000000000000, 0.8660254037844387076, 1.000000000000000000, 0.8660254037844387076, 1.000000000000000000, 0.8660254037844387076, 1.000000000000000000, 0.8660254037844387076, 1.000000000000000000, 0.8660254037844387076, 1.000000000000000000, 0.8660254037844387076, 1.000000000000000000, 0.8660254037844387076, 1.000000000000000000, 0.8660254037844387076, 1.000000000000000000, 0.8660254037844387076, 1.000000000000000000, 0.8660254037844387076, 1.000000000000000000, 0.8660254037844387076, 1.000000000000000000, 0.8660254037844387076, 1.000000000000000000, 0.8660254037844387076, 1.000000000000000000, 0.8660254037844387076, 1.000000000000000000, 0.8660254037844387076, 1.000000000000000000, 0.8660254037844387076, 1.000000000000000000, 0.8660254037844387076, 1.000000000000000000, 0.8660254037844387076, 1.000000000000000000, 0.8660254037844387076, 1.000000000000000000, 0.8660254037844387076, 1.000000000000000000, 0.8660254037844387076, 1.000000000000000000, 0.8660254037844387076, 1.000000000000000000, 0.8660254037844387076, 1.000000000000000000, 0.8660254037844387076, 1.000000000000000000, 0.8660254037844387076, 1.000000000000000000, 0.8660254037844387076, 1.000000000000000000, 0.8660254037844387076, 1.000000000000000000, 0.8660254037844387076, 1.000000000000000000, 0.8660254037844387076, 1.000000000000000000, 0.8660254037844387076, 1.000000000000000000, 0.8660254037844387076, 1.000000000000000000, 0.8660254037844387076, 1.000000000000000000, 0.8660254037844387076, 1.000000000000000000, 0.8660254037844387076, 1.000000000000000000, 0.8660254037844387076, 1.000000000000000000, 0.8660254037844387076, 1.000000000000000000, 0.8660254037844387076, 1.000000000000000000, 0.8660254037844387076, 1.000000000000000000, 0.8660254037844387076, 1.000000000000000000, 0.8660254037844387076, 1.000000000000000000, 0.8660254037844387076, 1.000000000000000000, 0.8660254037844387076, 1.000000000000000000, 0.8660254037844387076, 1.000000000000000000, 0.8660254037844387076, 1.000000000000000000, 0.8660254037844387076, 1.000000000000000000, 0.8660254037844387076, 1.000000000000000000, 0.8660254037844387076, 1.000000000000000000, 0.8660254037844387076, 1.000000000000000000, 0.8660254037844387076, 1.000000000000000000, 0.8660254037844387076, 1.000000000000000000, 0.8660254037844387076, 1.000000000000000000, 0.8660254037844387076, 1.000000000000000000, 0.8660254037844387076, 1.000000000000000000, 0.8660254037844387076, 1.000000000000000000, 0.8660254037844387076, 1.000000000000000000, 0.8660254037844387076, 1.000000000000000000, 0.8660254037844387076, 1.000000000000000000, 0.8660254037844387076, 1.000000000000000000, 0.8660254037844387076, 1.000000000000000000, 0.8660254037844387076, 1.000000000000000000, 0.8660254037844387076, 1.000000000000000000, 0.8660254037844387076, 1.000000000000000000, 0.8660254037844387076, 1.000000000000000000, 0.8660254037844387076, 1.000000000000000000, 0.8660254037844387076, 1.000000000000000000, 0.8660254037844387076, 1.000000000000000000, 0.8660254037844387076, 1.000000000000000000, 0.8660254037844387076, 1.000000000000000000, 0.8660254037844387076, 1.000000000000000000, 0.8660254037844387076, 1.000000000000000000, 0.8660254037844387076, 1.000000000000000000, 0.8660254037844387076, 1.000000000000000000, 0.8660254037844387076, 1.000000000000000000, 0.8660254037844387076, 1.000000000000000000, 0.8660254037844387076, 1.000000000000000000, 0.8660254037844387076, 1.000000000000000000, 0.8660254037844387076, 1.000000000000000000, 0.8660254037844387076, 1.000000000000000000, 0.8660254037844387076, 1.000000000000000000, 0.8660254037844387076, 1.000000000000000000, 0.8660254037844387076, 1.000000000000000000, 0.8660254037844387076, 1.000000000000000000, 0.8660254037844387076, 1.000000000000000000, 0.8660254037844387076, 1.000000000000000000, 0.8660254037844387076, 1.000000000000000000, 0.8660254037844387076, 1.000000000000000000, 0.8660254037844387076, 1.000000000000000000, 0.8660254037844387076, 1.000000000000000000, 0.8660254037844387076, 1.000000000000000000, 0.8660254037844387076, 1.000000000000000000, 0.8660254037844387076, 1.000000000000000000, 0.8660254037844387076, 1.000000000000000000, 0.8660254037844387076, 1.000000000000000000, 0.8660254037844387076, 1.000000000000000000, 0.8660254037844387076, 1.000000000000000000, 0.8660254037844387076, 1.000000000000000000, 0.8660254037844387076, 1.000000000000000000, 0.8660254037844387076, 1.000000000000000000, 0.8660254037844387076, 1.000000000000000000, 0.8660254037844387076, 1.000000000000000000, 0.8660254037844387076, 1.000000000000000000, 0.8660254037844387076, 1.000000000000000000, 0.8660254037844387076, 1.000000000000000000, 0.8660254037844387076, 1.000000000000000000, 0.8660254037844387076, 1.000000000000000000, 0.8660254037844387076, 1.000000000000000000, 0.8660254037844387076, 1.000000000000000000, 0.8660254037844387076, 1.000000000000000000, 0.8660254037844387076, 1.000000000000000000, 0.8660254037844387076, 1.000000000000000000, 0.8660254037844387076, 1.000000000000000000, 0.8660254037844387076, 1.000000000000000000, 0.8660254037844387076, 1.000000000000000000, 0.8660254037844387076, 1.000000000000000000, 0.8660254037844387076, 1.000000000000000000, 0.8660254037844387076, 1.000000000000000000, 0.8660254037844387076, 1.000000000000000000, 0.8660254037844387076, 1.000000000000000000, 0.8660254037844387076, 1.000000000000000000, 0.8660254037844387076, 1.000000000000000000, 0.8660254037844387076, 1.000000000000000000, 0.8660254037844387076, 1.000000000000000000, 0.8660254037844387076, 1.000000000000000000, 0.8660254037844387076, 1.000000000000000000, 0.8660254037844387076, 1.000000000000000000, 0.8660254037844387076, 1.000000000000000000, 0.8660254037844387076, 1.000000000000000000, 0.8660254037844387076, 1.000000000000000000, 0.8660254037844387076, 1.000000000000000000, 0.8660254037844387076, 1.000000000000000000, 0.8660254037844387076, 1.000000000000000000, 0.8660254037844387076, 1.000000000000000000, 0.8660254037844387076, 1.000000000000000000, 0.8660254037844387076, 1.000000000000000000, 0.8660254037844387076, 1.000000000000000000, 0.8660254037844387076, 1.000000000000000000, 0.8660254037844387076, 1.000000000000000000, 0.8660254037844387076, 1.000000000000000000, 0.8660254037844387076, 1.000000000000000000, 0.8660254037844387076, 1.000000000000000000, 0.8660254037844387076, 1.000000000000000000, 0.8660254037844387076, 1.000000000000000000, 0.8660254037844387076, 1.000000000000000000, 0.8660254037844387076, 1.000000000000000000, 0.8660254037844387076, 1.000000000000000000, 0.8660254037844387076, 1.000000000000000000, 0.8660254037844387076, 1.000000000000000000, 0.8660254037844387076, 1.000000000000000000, 0.8660254037844387076, 1.000000000000000000, 0.8660254037844387076, 1.000000000000000000, 0.8660254037844387076, 1.000000000000000000, 0.8660254037844387076, 1.000000000000000000, 0.8660254037844387076, 1.000000000000000000, 0.8660254037844387076, 1.000000000000000000, 0.8660254037844387076, 1.000000000000000000, 0.8660254037844387076, 1.000000000000000000, 0.8660254037844387076, 1.000000000000000000),
 ( 1.000000000000000000, 0.8660254037844387076, 1.000000000000000000, 0.8660254037844387076, 1.000000000000000000, 0.8660254037844387076, 1.000000000000000000, 0.8660254037844387076, 1.000000000000000000, 0.8660254037844387076, 1.000000000000000000, 0.8660254037844387076, 1.000000000000000000, 0.8660254037844387076, 1.000000000000000000, 0.8660254037844387076, 1.000000000000000000, 0.8660254037844387076, 1.000000000000000000, 0.8660254037844387076, 1.000000000000000000, 0.8660254037844387076, 1.000000000000000000, 0.8660254037844387076, 1.000000000000000000, 0.8660254037844387076, 1.000000000000000000, 0.8660254037844387076, 1.000000000000000000, 0.8660254037844387076, 1.000000000000000000, 0.8660254037844387076, 1.000000000000000000, 0.8660254037844387076, 1.000000000000000000, 0.8660254037844387076, 1.000000000000000000, 0.8660254037844387076, 1.000000000000000000, 0.8660254037844387076, 1.000000000000000000, 0.8660254037844387076, 1.000000000000000000, 0.8660254037844387076, 1.000000000000000000, 0.8660254037844387076, 1.000000000000000000, 0.8660254037844387076, 1.000000000000000000, 0.8660254037844387076, 1.000000000000000000, 0.8660254037844387076, 1.000000000000000000, 0.8660254037844387076, 1.000000000000000000, 0.8660254037844387076, 1.000000000000000000, 0.8660254037844387076, 1.000000000000000000, 0.8660254037844387076, 1.000000000000000000, 0.8660254037844387076, 1.000000000000000000, 0.8660254037844387076, 1.000000000000000000, 0.8660254037844387076, 1.000000000000000000, 0.8660254037844387076, 1.000000000000000000, 0.8660254037844387076, 1.000000000000000000, 0.8660254037844387076, 1.000000000000000000, 0.8660254037844387076, 1.000000000000000000, 0.8660254037844387076, 1.000000000000000000, 0.8660254037844387076, 1.000000000000000000, 0.8660254037844387076, 1.000000000000000000, 0.8660254037844387076, 1.000000000000000000, 0.8660254037844387076, 1.000000000000000000, 0.8660254037844387076, 1.000000000000000000, 0.8660254037844387076, 1.000000000000000000, 0.8660254037844387076, 1.000000000000000000, 0.8660254037844387076, 1.000000000000000000, 0.8660254037844387076, 1.000000000000000000, 0.8660254037844387076, 1.000000000000000000, 0.8660254037844387076, 1.000000000000000000, 0.8660254037844387076, 1.000000000000000000, 0.8660254037844387076, 1.000000000000000000, 0.8660254037844387076, 1.000000000000000000, 0.8660254037844387076, 1.000000000000000000, 0.8660254037844387076, 1.000000000000000000, 0.8660254037844387076, 1.000000000000000000, 0.8660254037844387076, 1.000000000000000000, 0.8660254037844387076, 1.000000000000000000, 0.8660254037844387076, 1.000000000000000000, 0.8660254037844387076, 1.000000000000000000, 0.8660254037844387076, 1.000000000000000000, 0.8660254037844387076, 1.000000000000000000, 0.8660254037844387076, 1.000000000000000000, 0.8660254037844387076, 1.000000000000000000, 0.8660254037844387076, 1.000000000000000000, 0.8660254037844387076, 1.000000000000000000, 0.8660254037844387076, 1.000000000000000000, 0.8660254037844387076, 1.000000000000000000, 0.8660254037844387076, 1.000000000000000000, 0.8660254037844387076, 1.000000000000000000, 0.8660254037844387076, 1.000000000000000000, 0.8660254037844387076, 1.000000000000000000, 0.8660254037844387076, 1.000000000000000000, 0.8660254037844387076, 1.000000000000000000, 0.8660254037844387076, 1.000000000000000000, 0.8660254037844387076, 1.000000000000000000, 0.8660254037844387076, 1.000000000000000000, 0.8660254037844387076, 1.000000000000000000, 0.8660254037844387076, 1.000000000000000000, 0.8660254037844387076, 1.000000000000000000, 0.8660254037844387076, 1.000000000000000000, 0.8660254037844387076, 1.000000000000000000, 0.8660254037844387076, 1.000000000000000000, 0.8660254037844387076, 1.000000000000000000, 0.8660254037844387076, 1.000000000000000000, 0.8660254037844387076, 1.000000000000000000, 0.8660254037844387076, 1.000000000000000000, 0.8660254037844387076, 1.000000000000000000, 0.8660254037844387076, 1.000000000000000000, 0.8660254037844387076, 1.000000000000000000, 0.8660254037844387076, 1.000000000000000000, 0.8660254037844387076, 1.000000000000000000, 0.8660254037844387076, 1.000000000000000000, 0.8660254037844387076, 1.000000000000000000, 0.8660254037844387076, 1.000000000000000000, 0.8660254037844387076, 1.000000000000000000, 0.8660254037844387076, 1.000000000000000000, 0.8660254037844387076, 1.000000000000000000, 0.8660254037844387076, 1.000000000000000000, 0.8660254037844387076, 1.000000000000000000, 0.8660254037844387076, 1.000000000000000000, 0.8660254037844387076, 1.000000000000000000, 0.8660254037844387076, 1.000000000000000000, 0.8660254037844387076, 1.000000000000000000, 0.8660254037844387076, 1.000000000000000000, 0.8660254037844387076, 1.000000000000000000, 0.8660254037844387076, 1.000000000000000000, 0.8660254037844387076, 1.000000000000000000, 0.8660254037844387076, 1.000000000000000000, 0.8660254037844387076, 1.000000000000000000, 0.8660254037844387076, 1.000000000000000000, 0.8660254037844387076, 1.000000000000000000, 0.8660254037844387076, 1.000000000000000000, 0.8660254037844387076, 1.000000000000000000, 0.8660254037844387076, 1.000000000000000000, 0.8660254037844387076, 1.000000000000000000, 0.8660254037844387076, 1.000000000000000000, 0.8660254037844387076, 1.000000000000000000, 0.8660254037844387076, 1.000000000000000000, 0.8660254037844387076, 1.000000000000000000, 0.8660254037844387076, 1.000000000000000000, 0.8660254037844387076, 1.000000000000000000, 0.8660254037844387076, 1.000000000000000000, 0.8660254037844387076, 1.000000000000000000, 0.8660254037844387076, 1.000000000000000000, 0.8660254037844387076, 1.000000000000000000, 0.8660254037844387076, 1.000000000000000000, 0.8660254037844387076, 1.000000000000000000, 0.8660254037844387076, 1.000000000000000000, 0.8660254037844387076, 1.000000000000000000, 0.8660254037844387076, 1.000000000000000000, 0.8660254037844387076, 1.000000000000000000, 0.8660254037844387076, 1.000000000000000000, 0.8660254037844387076, 1.000000000000000000, 0.8660254037844387076, 1.000000000000000000, 0.8660254037844387076, 1.000000000000000000, 0.8660254037844387076, 1.000000000000000000, 0.8660254037844387076, 1.000000000000000000, 0.8660254037844387076, 1.000000000000000000, 0.8660254037844387076, 1.000000000000000000, 0.8660254037844387076, 1.000000000000000000, 0.8660254037844387076, 1.000000000000000000, 0.8660254037844387076, 1.000000000000000000, 0.8660254037844387076, 1.000000000000000000, 0.8660254037844387076, 1.000000000000000000, 0.8660254037844387076, 1.000000000000000000, 0.8660254037844387076, 1.000000000000000000, 0.8660254037844387076, 1.000000000000000000, 0.8660254037844387076, 1.000000000000000000, 0.8660254037844387076, 1.000000000000000000, 0.8660254037844387076, 1.000000000000000000, 0.8660254037844387076, 1.000000000000000000, 0.8660254037844387076, 1.000000000000000000, 0.8660254037844387076, 1.000000000000000000, 0.8660254037844387076, 1.000000000000000000, 0.8660254037844387076, 1.000000000000000000, 0.8660254037844387076, 1.000000000000000000, 0.8660254037844387076, 1.000000000000000000, 0.8660254037844387076, 1.000000000000000000, 0.8660254037844387076, 1.000000000000000000, 0.8660254037844387076, 1.000000000000000000, 0.8660254037844387076, 1.000000000000000000, 0.8660254037844387076, 1.000000000000000000, 0.8660254037844387076, 1.000000000000000000, 0.8660254037844387076, 1.000000000000000000, 0.8660254037844387076, 1.000000000000000000, 0.8660254037844387076, 1.000000000000000000, 0.8660254037844387076, 1.000000000000000000, 0.8660254037844387076, 1.000000000000000000, 0.8660254037844387076, 1.000000000000000000, 0.8660254037844387076, 1.000000000000000000, 0.8660254037844387076, 1.000000000000000000, 0.8660254037844387076, 1.000000000000000000, 0.8660254037844387076, 1.000000000000000000, 0.8660254037844387076, 1.000000000000000000, 0.8660254037844387076, 1.000000000000000000, 0.8660254037844387076, 1.000000000000000000, 0.8660254037844387076, 1.000000000000000000, 0.8660254037844387076, 1.000000000000000000, 0.8660254037844387076, 1.000000000000000000, 0.8660254037844387076, 1.000000000000000000, 0.8660254037844387076, 1.000000000000000000, 0.8660254037844387076, 1.000000000000000000, 0.8660254037844387076, 1.000000000000000000, 0.8660254037844387076, 1.000000000000000000, 0.8660254037844387076, 1.000000000000000000, 0.8660254037844387076, 1.000000000000000000, 0.8660254037844387076, 1.000000000000000000, 0.8660254037844387076, 1.000000000000000000, 0.8660254037844387076, 1.000000000000000000, 0.8660254037844387076, 1.000000000000000000, 0.8660254037844387076, 1.000000000000000000, 0.8660254037844387076, 1.000000000000000000, 0.8660254037844387076, 1.000000000000000000, 0.8660254037844387076, 1.000000000000000000, 0.8660254037844387076, 1.000000000000000000, 0.8660254037844387076, 1.000000000000000000, 0.8660254037844387076, 1.000000000000000000, 0.8660254037844387076, 1.000000000000000000, 0.8660254037844387076, 1.000000000000000000, 0.8660254037844387076, 1.000000000000000000, 0.8660254037844387076, 1.000000000000000000, 0.8660254037844387076, 1.000000000000000000, 0.8660254037844387076, 1.000000000000000000, 0.8660254037844387076, 1.000000000000000000, 0.8660254037844387076, 1.000000000000000000, 0.8660254037844387076, 1.000000000000000000, 0.8660254037844387076, 1.000000000000000000, 0.8660254037844387076, 1.000000000000000000, 0.8660254037844387076, 1.000000000000000000, 0.8660254037844387076, 1.000000000000000000, 0.8660254037844387076, 1.000000000000000000, 0.8660254037844387076, 1.000000000000000000, 0.8660254037844387076, 1.000000000000000000, 0.8660254037844387076, 1.000000000000000000, 0.8660254037844387076, 1.000000000000000000, 0.8660254037844387076, 1.000000000000000000, 0.8660254037844387076, 1.000000000000000000, 0.8660254037844387076, 1.000000000000000000, 0.8660254037844387076, 1.000000000000000000, 0.8660254037844387076, 1.000000000000000000, 0.8660254037844387076, 1.000000000000000000, 0.8660254037844387076, 1.000000000000000000, 0.8660254037844387076, 1.000000000000000000, 0.8660254037844387076, 1.000000000000000000, 0.8660254037844387076, 1.000000000000000000, 0.8660254037844387076, 1.000000000000000000, 0.8660254037844387076, 1.000000000000000000, 0.8660254037844387076, 1.000000000000000000, 0.8660254037844387076, 1.000000000000000000, 0.8660254037844387076, 1.000000000000000000, 0.8660254037844387076, 1.000000000000000000, 0.8660254037844387076, 1.000000000000000000, 0.8660254037844387076, 1.000000000000000000, 0.8660254037844387076, 1.000000000000000000, 0.8660254037844387076, 1.000000000000000000, 0.8660254037844387076, 1.000000000000000000, 0.8660254037844387076, 1.000000000000000000, 0.8660254037844387076, 1.000000000000000000, 0.8660254037844387076, 1.000000000000000000, 0.8660254037844387076, 1.000000000000000000, 0.8660254037844387076, 1.000000000000000000, 0.8660254037844387076, 1.000000000000000000, 0.8660254037844387076, 1.000000000000000000, 0.8660254037844387076, 1.000000000000000000, 0.8660254037844387076, 1.000000000000000000, 0.8660254037844387076, 1.000000000000000000, 0.8660254037844387076, 1.000000000000000000, 0.8660254037844387076, 1.000000000000000000, 0.8660254037844387076, 1.000000000000000000, 0.8660254037844387076, 1.000000000000000000, 0.8660254037844387076, 1.000000000000000000, 0.8660254037844387076, 1.000000000000000000, 0.8660254037844387076, 1.000000000000000000, 0.8660254037844387076, 1.000000000000000000, 0.8660254037844387076, 1.000000000000000000, 0.8660254037844387076, 1.000000000000000000, 0.8660254037844387076, 1.000000000000000000, 0.8660254037844387076, 1.000000000000000000, 0.8660254037844387076, 1.000000000000000000, 0.8660254037844387076, 1.000000000000000000, 0.8660254037844387076, 1.000000000000000000, 0.8660254037844387076, 1.000000000000000000, 0.8660254037844387076, 1.000000000000000000, 0.8660254037844387076, 1.000000000000000000, 0.8660254037844387076, 1.000000000000000000, 0.8660254037844387076, 1.000000000000000000, 0.8660254037844387076, 1.000000000000000000, 0.8660254037844387076, 1.000000000000000000, 0.8660254037844387076, 1.000000000000000000, 0.8660254037844387076, 1.000000000000000000, 0.8660254037844387076, 1.000000000000000000, 0.8660254037844387076, 1.000000000000000000, 0.8660254037844387076, 1.000000000000000000, 0.8660254037844387076, 1.000000000000000000, 0.8660254037844387076, 1.000000000000000000, 0.8660254037844387076, 1.000000000000000000, 0.8660254037844387076, 1.000000000000000000, 0.8660254037844387076, 1.000000000000000000, 0.8660254037844387076, 1.000000000000000000, 0.8660254037844387076, 1.000000000000000000, 0.8660254037844387076, 1.000000000000000000, 0.8660254037844387076, 1.000000000000000000, 0.8660254037844387076, 1.000000000000000000, 0.8660254037844387076, 1.000000000000000000, 0.8660254037844387076, 1.000000000000000000, 0.8660254037844387076, 1.000000000000000000, 0.8660254037844387076, 1.000000000000000000, 0.8660254037844387076, 1.000000000000000000, 0.8660254037844387076, 1.000000000000000000, 0.8660254037844387076, 1.000000000000000000, 0.8660254037844387076, 1.000000000000000000, 0.8660254037844387076, 1.000000000000000000, 0.8660254037844387076, 1.000000000000000000, 0.8660254037844387076, 1.000000000000000000, 0.8660254037844387076, 1.000000000000000000, 0.8660254037844387076, 1.000000000000000000, 0.8660254037844387076, 1.000000000000000000, 0.8660254037844387076, 1.000000000000000000, 0.8660254037844387076, 1.000000000000000000, 0.8660254037844387076, 1.000000000000000000, 0.8660254037844387076, 1.000000000000000000, 0.8660254037844387076, 1.000000000000000000, 0.8660254037844387076, 1.000000000000000000, 0.8660254037844387076, 1.000000000000000000, 0.8660254037844387076, 1.000000000000000000, 0.8660254037844387076, 1.000000000000000000, 0.8660254037844387076, 1.000000000000000000, 0.8660254037844387076, 1.000000000000000000, 0.8660254037844387076, 1.000000000000000000, 0.8660254037844387076, 1.000000000000000000, 0.8660254037844387076, 1.000000000000000000, 0.8660254037844387076, 1.000000000000000000, 0.8660254037844387076, 1.000000000000000000, 0.8660254037844387076, 1.000000000000000000, 0.8660254037844387076, 1.000000000000000000, 0.8660254037844387076, 1.000000000000000000, 0.8660254037844387076, 1.000000000000000000, 0.8660254037844387076, 1.000000000000000000, 0.8660254037844387076, 1.000000000000000000, 0.8660254037844387076, 1.000000000000000000, 0.8660254037844387076, 1.000000000000000000, 0.8660254037844387076, 1.000000000000000000, 0.8660254037844387076, 1.000000000000000000, 0.8660254037844387076, 1.000000000000000000, 0.8660254037844387076, 1.000000000000000000, 0.8660254037844387076, 1.000000000000000000, 0.8660254037844387076, 1.000000000000000000, 0.8660254037844387076, 1.000000000000000000, 0.8660254037844387076, 1.000000000000000000, 0.8660254037844387076, 1.000000000000000000, 0.8660254037844387076, 1.000000000000000000, 0.8660254037844387076, 1.000000000000000000, 0.8660254037844387076, 1.000000000000000000, 0.8660254037844387076, 1.000000000000000000, 0.8660254037844387076, 1.000000000000000000, 0.8660254037844387076, 1.000000000000000000, 0.8660254037844387076, 1.000000000000000000, 0.8660254037844387076, 1.000000000000000000, 0.8660254037844387076, 1.000000000000000000, 0.8660254037844387076, 1.000000000000000000, 0.8660254037844387076, 1.000000000000000000, 0.8660254037844387076, 1.000000000000000000, 0.8660254037844387076, 1.000000000000000000, 0.8660254037844387076, 1.000000000000000000, 0.8660254037844387076, 1.000000000000000000, 0.8660254037844387076, 1.000000000000000000, 0.8660254037844387076, 1.000000000000000000, 0.8660254037844387076, 1.000000000000000000, 0.8660254037844387076, 1.000000000000000000, 0.8660254037844387076, 1.000000000000000000, 0.8660254037844387076, 1.000000000000000000, 0.8660254037844387076, 1.000000000000000000, 0.8660254037844387076, 1.000000000000000000, 0.8660254037844387076, 1.000000000000000000, 0.8660254037844387076, 1.000000000000000000, 0.8660254037844387076, 1.000000000000000000, 0.8660254037844387076, 1.000000000000000000, 0.8660254037844387076, 1.000000000000000000, 0.8660254037844387076, 1.000000000000000000, 0.8660254037844387076, 1.000000000000000000) ) ) 
 REPRESENTATION_ITEM ( '' )  SURFACE ( )  );
#43419=CARTESIAN_POINT ( 'NONE',  ( 19.87500000000000000, 6.123233995736764310E-16, -4.999999999999998224 ) ) ;
#43420=CARTESIAN_POINT ( 'NONE',  ( 19.19062500061452070, -3.027376345333610441, -5.243569643749999898 ) ) ;
#43421=CARTESIAN_POINT ( 'NONE',  ( 24.19687500061451857, -3.027376345333610441, -5.243569643749999898 ) ) ;
#43424=CARTESIAN_POINT ( 'NONE',  ( 27.79687500061451999, -3.027376345333610441, -5.243569643749999898 ) ) ;
#43425=CARTESIAN_POINT ( 'NONE',  ( 5.484375000614518214, 4.541064518000418104, 2.621784821874999949 ) ) ;
#43426=CARTESIAN_POINT ( 'NONE',  ( 14.69062500061451537, -3.027376345333610441, -5.243569643749999898 ) ) ;
#43427=CARTESIAN_POINT ( 'NONE',  ( 12.57187500061451857, 3.027376345333613106, -5.243569643749998122 ) ) ;
#43429=CYLINDRICAL_SURFACE ( 'NONE', #33675, 4.999999999999998224 ) ;
#43430=CARTESIAN_POINT ( 'NONE',  ( 25.75312500061451715, 0.000000000000000000, 5.243569643749999010 ) ) ;
#43431=CARTESIAN_POINT ( 'NONE',  ( 3.474966266584414321, 3.595135176884375117, -3.675031694903898138 ) ) ;
#43432=CARTESIAN_POINT ( 'NONE',  ( 14.69999999999999929, 0.000000000000000000, 4.999999999999998224 ) ) ;
#43433=CARTESIAN_POINT ( 'NONE',  ( 14.06250000000000000, 2.886751345948129099, -4.999999999999998224 ) ) ;
#43434=CARTESIAN_POINT ( 'NONE',  ( 23.28750000122903430, 4.330127018922191873, 2.499999999999999556 ) ) ;
#43435=CARTESIAN_POINT ( 'NONE',  ( 18.55312500061451431, 0.000000000000000000, 5.243569643749999010 ) ) ;
#43436=ORIENTED_EDGE ( 'NONE', *, *, #23020, .F. ) ;
#43437=CARTESIAN_POINT ( 'NONE',  ( 22.16250000000000142, 2.886751345948129099, -4.999999999999998224 ) ) ;
#43438=CARTESIAN_POINT ( 'NONE',  ( 24.57187500061451502, -6.054752690667223547, -1.112240025338166033E-15 ) ) ;
#43440=CARTESIAN_POINT ( 'NONE',  ( 20.10000000000000142, 0.000000000000000000, 4.999999999999998224 ) ) ;
#43441=CARTESIAN_POINT ( 'NONE',  ( 11.76562500061451644, 3.027376345333611329, 5.243569643749999010 ) ) ;
#43442=CARTESIAN_POINT ( 'NONE',  ( 3.290625000614516793, -3.027376345333614438, 5.243569643749998122 ) ) ;
#43444=CARTESIAN_POINT ( 'NONE',  ( 26.31562500061451715, -6.054752690667223547, -1.112240025338166033E-15 ) ) ;
#43445=CARTESIAN_POINT ( 'NONE',  ( 16.72500000000000142, 6.123233995736764310E-16, -4.999999999999998224 ) ) ;
#43446=CARTESIAN_POINT ( 'NONE',  ( 25.01249999999999929, 2.886751345948126879, 4.999999999999999112 ) ) ;
#43447=CARTESIAN_POINT ( 'NONE',  ( -4.243569643749999898, 19.35312500061451857, 30.00000000000000000 ) ) ;
#43448=CARTESIAN_POINT ( 'NONE',  ( 7.096875000614517148, -3.027376345333610441, -5.243569643749999898 ) ) ;
#43449=CARTESIAN_POINT ( 'NONE',  ( 16.69687500061451502, 6.054752690667223547, 3.707466751127219781E-16 ) ) ;
#43450=CARTESIAN_POINT ( 'NONE',  ( 28.95937500061451431, 0.000000000000000000, 5.243569643749999010 ) ) ;
#43452=CARTESIAN_POINT ( 'NONE',  ( 27.17812500061451786, -4.541064518000419881, 2.621784821874995952 ) ) ;
#43453=CARTESIAN_POINT ( 'NONE',  ( 26.82187500061451857, -6.054752690667223547, -1.112240025338166033E-15 ) ) ;
#43455=CARTESIAN_POINT ( 'NONE',  ( 13.76250000000000107, 2.886751345948126879, 4.999999999999999112 ) ) ;
#43456=CARTESIAN_POINT ( 'NONE',  ( 12.29062500061451857, -3.027376345333614438, 5.243569643749998122 ) ) ;
#43458=CARTESIAN_POINT ( 'NONE',  ( 29.65312500061451573, 4.541064518000418104, -2.621784821874998173 ) ) ;
#43459=CARTESIAN_POINT ( 'NONE',  ( 17.13750000122903216, -4.330127018922194537, 2.499999999999995559 ) ) ;
#43461=CARTESIAN_POINT ( 'NONE',  ( 5.353125000614515905, 4.541064518000418104, -2.621784821874998173 ) ) ;
#43462=CARTESIAN_POINT ( 'NONE',  ( 20.78437500061451715, 4.541064518000418104, 2.621784821874999949 ) ) ;
#43463=CARTESIAN_POINT ( 'NONE',  ( -4.243569643749999898, 17.12187500061451573, 27.54997392385601529 ) ) ;
#43464=CARTESIAN_POINT ( 'NONE',  ( 20.70937500061451786, 4.541064518000418104, -2.621784821874998173 ) ) ;
#43465=CARTESIAN_POINT ( 'NONE',  ( 5.625000000000001776, 4.330127018922191873, 2.499999999999999556 ) ) ;
#43466=CARTESIAN_POINT ( 'NONE',  ( -3.999999999999999112, 9.762500001229033941, 30.00000000000000000 ) ) ;
#43467=CARTESIAN_POINT ( 'NONE',  ( 12.59062500061451573, 6.054752690667223547, 3.707466751127219781E-16 ) ) ;
#43468=CARTESIAN_POINT ( 'NONE',  ( 4.237500001229036251, 6.123233995736764310E-16, -4.999999999999998224 ) ) ;
#43469=CARTESIAN_POINT ( 'NONE',  ( 8.896875000614517859, -3.027376345333610441, -5.243569643749999898 ) ) ;
#43471=CARTESIAN_POINT ( 'NONE',  ( 9.215625000614515727, -6.054752690667223547, -1.112240025338166033E-15 ) ) ;
#43472=CARTESIAN_POINT ( 'NONE',  ( 15.49687500061451750, -3.027376345333614438, 5.243569643749998122 ) ) ;
#43473=CARTESIAN_POINT ( 'NONE',  ( 3.464268450295128865, -3.605406963609541382, -3.807383367585859268 ) ) ;
#43474=CARTESIAN_POINT ( 'NONE',  ( 21.22500000122903074, -5.773502691896255534, -1.060575238724906372E-15 ) ) ;
#43475=CARTESIAN_POINT ( 'NONE',  ( 9.684375000614517504, -4.541064518000419881, 2.621784821874995952 ) ) ;
#43476=CARTESIAN_POINT ( 'NONE',  ( 11.35312500061451679, 0.000000000000000000, 5.243569643749999010 ) ) ;
#43478=CARTESIAN_POINT ( 'NONE',  ( 22.13437500061451502, 4.541064518000418104, 2.621784821874999949 ) ) ;
#43481=CARTESIAN_POINT ( 'NONE',  ( -3.858979783667864982, 3.180598473748191157, 31.08663701263182233 ) ) ;
#43482=DIRECTION ( 'NONE',  ( -0.000000000000000000, -1.000000000000000000, -0.000000000000000000 ) ) ;
#43483=CARTESIAN_POINT ( 'NONE',  ( 2.121784821875001281, 11.90937500061451892, -26.32496088578401938 ) ) ;
#43484=CARTESIAN_POINT ( 'NONE',  ( 15.82500000122903216, -5.773502691896255534, -1.060575238724906372E-15 ) ) ;
#43485=CARTESIAN_POINT ( 'NONE',  ( 9.001249775931846008E-16, 17.21562500061451928, -25.09994784771203058 ) ) ;
#43486=CARTESIAN_POINT ( 'NONE',  ( 17.25000000122903288, -2.886751345948125991, -5.000000000000000000 ) ) ;
#43487=CARTESIAN_POINT ( 'NONE',  ( 9.290625000614515017, -3.027376345333610441, -5.243569643749999898 ) ) ;
#43488=ORIENTED_EDGE ( 'NONE', *, *, #47179, .T. ) ;
#43489=CARTESIAN_POINT ( 'NONE',  ( 16.23750000000000071, -2.886751345948125991, -5.000000000000000000 ) ) ;
#43490=CARTESIAN_POINT ( 'NONE',  ( 5.100000001229031632, -2.886751345948193048, -4.999999999999883649 ) ) ;
#43491=CARTESIAN_POINT ( 'NONE',  ( 10.43437500061451750, 4.541064518000418104, 2.621784821874999949 ) ) ;
#43492=CARTESIAN_POINT ( 'NONE',  ( -3.137519842735245283E-14, 14.37500000122903288, 34.00000000000000000 ) ) ;
#43493=CARTESIAN_POINT ( 'NONE',  ( 9.825000001229033941, 2.886751345948126879, 4.999999999999999112 ) ) ;
#43494=CARTESIAN_POINT ( 'NONE',  ( 19.38750000122903216, -4.330127018922194537, 2.499999999999995559 ) ) ;
#43495=CARTESIAN_POINT ( 'NONE',  ( 15.66562500061451857, 3.027376345333613106, -5.243569643749998122 ) ) ;
#43496=CARTESIAN_POINT ( 'NONE',  ( 19.15312500061451573, -4.541064518000417216, -2.621784821875001281 ) ) ;
#43497=CARTESIAN_POINT ( 'NONE',  ( 28.57500000122903572, 2.886751345948129099, -4.999999999999998224 ) ) ;
#43499=EDGE_CURVE ( 'NONE', #22787, #45851, #10448, .T. ) ;
#43500=CARTESIAN_POINT ( 'NONE',  ( 29.47500000122903430, 2.886751345948129099, -4.999999999999998224 ) ) ;
#43501=CARTESIAN_POINT ( 'NONE',  ( 24.67500000000000071, -4.330127018922194537, 2.499999999999995559 ) ) ;
#43503=CARTESIAN_POINT ( 'NONE',  ( 26.63437500061451857, 4.541064518000418104, 2.621784821874999949 ) ) ;
#43504=CARTESIAN_POINT ( 'NONE',  ( -3.999999999999999112, 15.91249999999999964, 27.69059892324149885 ) ) ;
#43505=CARTESIAN_POINT ( 'NONE',  ( 13.46250000122903323, 0.000000000000000000, 4.999999999999998224 ) ) ;
#43506=CARTESIAN_POINT ( 'NONE',  ( 3.675000000000001155, 6.123233995736764310E-16, -4.999999999999998224 ) ) ;
#43508=PLANE ( 'NONE',  #6607 ) ;
#43509=CARTESIAN_POINT ( 'NONE',  ( 7.021875000614518747, -6.054752690667223547, -1.112240025338166033E-15 ) ) ;
#43510=CARTESIAN_POINT ( 'NONE',  ( 27.06562500061451004, 3.027376345333611329, 5.243569643749999010 ) ) ;
#43512=CARTESIAN_POINT ( 'NONE',  ( 0.000000000000000000, 20.00000000000000000, -33.99999999999999289 ) ) ;
#43514=CARTESIAN_POINT ( 'NONE',  ( 3.693371437524641365, -3.370391871118413540, 3.876951387445791930 ) ) ;
#43515=CARTESIAN_POINT ( 'NONE',  ( 4.921875000614518214, 3.027376345333613106, -5.243569643749998122 ) ) ;
#43516=CARTESIAN_POINT ( 'NONE',  ( 8.559375000614515727, 4.541064518000418104, -2.621784821874998173 ) ) ;
#43517=CARTESIAN_POINT ( 'NONE',  ( 28.20937500061451786, -4.541064518000417216, -2.621784821875001281 ) ) ;
#43518=CARTESIAN_POINT ( 'NONE',  ( -4.243569643749999898, 13.01562500061459637, 27.54997392385601529 ) ) ;
#43519=CARTESIAN_POINT ( 'NONE',  ( 21.93750000000000000, -2.886751345948129988, 4.999999999999997335 ) ) ;
#43520=CARTESIAN_POINT ( 'NONE',  ( 20.81250000122903643, -4.330127018922190985, -2.500000000000001332 ) ) ;
#43522=CARTESIAN_POINT ( 'NONE',  ( 4.575000000000002842, 6.123233995736764310E-16, -4.999999999999998224 ) ) ;
#43523=EDGE_LOOP ( 'NONE', ( #13796, #18684, #68509, #41874 ) ) ;
#43524=CARTESIAN_POINT ( 'NONE',  ( 18.96562500061451573, 3.027376345333611329, 5.243569643749999010 ) ) ;
#43525=CARTESIAN_POINT ( 'NONE',  ( 10.49062500061451431, -3.027376345333614438, 5.243569643749998122 ) ) ;
#43527=CARTESIAN_POINT ( 'NONE',  ( 7.921875000614517326, -6.054752690667223547, -1.112240025338166033E-15 ) ) ;
#43528=CARTESIAN_POINT ( 'NONE',  ( 24.07499999999999929, 4.330127018922191873, 2.499999999999999556 ) ) ;
#43529=CARTESIAN_POINT ( 'NONE',  ( 21.30000000122903359, -2.886751345948125991, -5.000000000000000000 ) ) ;
#43530=CYLINDRICAL_SURFACE ( 'NONE', #2486, 3.999999999999996447 ) ;
#43531=CARTESIAN_POINT ( 'NONE',  ( 9.984375000614518214, 4.541064518000418104, 2.621784821874999949 ) ) ;
#43532=CARTESIAN_POINT ( 'NONE',  ( 13.43437500061451750, 6.421520780324663323E-16, -5.243569643749999010 ) ) ;
#43533=CARTESIAN_POINT ( 'NONE',  ( 25.20937500061451431, 4.541064518000418104, -2.621784821874998173 ) ) ;
#43534=CARTESIAN_POINT ( 'NONE',  ( 4.228125000614517681, -4.541064518000419881, 2.621784821874995952 ) ) ;
#43537=CARTESIAN_POINT ( 'NONE',  ( 18.53437500061451715, 4.541064518000418104, 2.621784821874999949 ) ) ;
#43538=CARTESIAN_POINT ( 'NONE',  ( 9.234375000614518214, -4.541064518000419881, 2.621784821874995952 ) ) ;
#43540=CARTESIAN_POINT ( 'NONE',  ( 20.69999999999999929, -4.330127018922190985, -2.500000000000001332 ) ) ;
#43542=CARTESIAN_POINT ( 'NONE',  ( -2.121784821874996840, 10.03437500061451892, -26.32496088578401583 ) ) ;
#43544=CARTESIAN_POINT ( 'NONE',  ( 11.91562500061451857, -6.054752690667223547, -1.112240025338166033E-15 ) ) ;
#43545=CARTESIAN_POINT ( 'NONE',  ( 28.20937500061451786, -4.541064518000417216, -2.621784821875001281 ) ) ;
#43546=DIRECTION ( 'NONE',  ( 1.000000000000000000, 0.000000000000000000, -0.000000000000000000 ) ) ;
#43547=CARTESIAN_POINT ( 'NONE',  ( 12.75000000000000178, 4.330127018922192761, -2.499999999999997780 ) ) ;
#43548=CARTESIAN_POINT ( 'NONE',  ( 1.999999999999998668, 19.06250000122903288, 26.53589838486224650 ) ) ;
#43549=CARTESIAN_POINT ( 'NONE',  ( 11.96250000122903501, 4.330127018922192761, -2.499999999999997780 ) ) ;
#43550=CARTESIAN_POINT ( 'NONE',  ( 22.88437500061451857, 6.421520780324663323E-16, -5.243569643749999010 ) ) ;
#43551=CARTESIAN_POINT ( 'NONE',  ( 17.25937500061451502, 0.000000000000000000, 5.243569643749999010 ) ) ;
#43552=CARTESIAN_POINT ( 'NONE',  ( 4.000000000000000000, 16.70000000122903216, 32.30940107675849760 ) ) ;
#43553=ORIENTED_EDGE ( 'NONE', *, *, #27246, .T. ) ;
#43554=CARTESIAN_POINT ( 'NONE',  ( 16.49062500061451786, -3.027376345333610441, -5.243569643749999898 ) ) ;
#43555=CARTESIAN_POINT ( 'NONE',  ( 29.51250000122903216, 4.330127018922192761, -2.499999999999997780 ) ) ;
#43556=CARTESIAN_POINT ( 'NONE',  ( 16.65937500061452070, 4.541064518000418104, -2.621784821874998173 ) ) ;
#43557=CARTESIAN_POINT ( 'NONE',  ( 5.690625000614516260, -3.027376345333610441, -5.243569643749999898 ) ) ;
#43558=CARTESIAN_POINT ( 'NONE',  ( 19.75312500061451360, 4.541064518000418104, -2.621784821874998173 ) ) ;
#43559=CARTESIAN_POINT ( 'NONE',  ( 3.999999999999998668, 18.46249999999999858, -32.30940107675850470 ) ) ;
#43560=CARTESIAN_POINT ( 'NONE',  ( 29.52187500061451431, -6.054752690667223547, -1.112240025338166033E-15 ) ) ;
#43561=CARTESIAN_POINT ( 'NONE',  ( 2.121784821874999061, 12.90312500061451750, 26.32496088578401583 ) ) ;
#43562=CARTESIAN_POINT ( 'NONE',  ( 16.92187500061451999, -6.054752690667223547, -1.112240025338166033E-15 ) ) ;
#43563=CARTESIAN_POINT ( 'NONE',  ( 17.47500000122903430, 2.886751345948126879, 4.999999999999999112 ) ) ;
#43565=CARTESIAN_POINT ( 'NONE',  ( 4.243569643749999898, 19.59687500061451360, -27.54997392385601529 ) ) ;
#43567=CARTESIAN_POINT ( 'NONE',  ( 20.44687500061451857, -3.027376345333614438, 5.243569643749998122 ) ) ;
#43568=CARTESIAN_POINT ( 'NONE',  ( 22.91250000122903430, 0.000000000000000000, 4.999999999999998224 ) ) ;
#43569=CARTESIAN_POINT ( 'NONE',  ( 23.35312500061451857, 4.541064518000418104, -2.621784821874998173 ) ) ;
#43570=CARTESIAN_POINT ( 'NONE',  ( 16.13437500061451502, 6.421520780324663323E-16, -5.243569643749999010 ) ) ;
#43571=CARTESIAN_POINT ( 'NONE',  ( 11.31562500061451892, 3.027376345333611329, 5.243569643749999010 ) ) ;
#43572=CARTESIAN_POINT ( 'NONE',  ( -4.243569643749997233, 13.59687500061451715, 32.45002607614398471 ) ) ;
#43573=CARTESIAN_POINT ( 'NONE',  ( 17.80312500061451786, -4.541064518000417216, -2.621784821875001281 ) ) ;
#43574=CARTESIAN_POINT ( 'NONE',  ( 26.12812500061451360, 4.541064518000418104, 2.621784821874999949 ) ) ;
#43575=VERTEX_POINT ( 'NONE', #41072 ) ;
#43577=CARTESIAN_POINT ( 'NONE',  ( 22.19999999999999574, 4.330127018922192761, -2.499999999999997780 ) ) ;
#43578=CARTESIAN_POINT ( 'NONE',  ( -2.121784821874999949, 19.33437500061451786, -33.67503911421598417 ) ) ;
#43579=CARTESIAN_POINT ( 'NONE',  ( 3.809532709742158296, -3.238520787748959240, -3.970891474530591658 ) ) ;
#43580=CARTESIAN_POINT ( 'NONE',  ( 24.96562500061451573, -6.054752690667223547, -1.112240025338166033E-15 ) ) ;
#43581=CARTESIAN_POINT ( 'NONE',  ( 5.240625000614516971, -3.027376345333610441, -5.243569643749999898 ) ) ;
#43582=CARTESIAN_POINT ( 'NONE',  ( 16.83750000122903145, 6.123233995736764310E-16, -4.999999999999998224 ) ) ;
#43583=CARTESIAN_POINT ( 'NONE',  ( 21.85312500061451502, -4.541064518000417216, -2.621784821875001281 ) ) ;
#43584=CARTESIAN_POINT ( 'NONE',  ( 23.47499999999999787, 6.123233995736764310E-16, -4.999999999999998224 ) ) ;
#43585=CARTESIAN_POINT ( 'NONE',  ( 25.49062500061451786, -3.027376345333610441, -5.243569643749999898 ) ) ;
#43586=CARTESIAN_POINT ( 'NONE',  ( 6.965625000614518392, -6.054752690667223547, -1.112240025338166033E-15 ) ) ;
#43588=CARTESIAN_POINT ( 'NONE',  ( 22.82812500061451644, 6.421520780324663323E-16, -5.243569643749999010 ) ) ;
#43591=CARTESIAN_POINT ( 'NONE',  ( 11.13750000122903216, 4.330127018922191873, 2.499999999999999556 ) ) ;
#43592=CARTESIAN_POINT ( 'NONE',  ( 3.999999999999998668, 14.52500000122903323, -32.30940107675850470 ) ) ;
#43593=ADVANCED_FACE ( 'NONE', ( #41781 ), #7804, .F. ) ;
#43594=CARTESIAN_POINT ( 'NONE',  ( -1.999999999999997113, 10.28750000122903430, 33.46410161513775705 ) ) ;
#43595=CARTESIAN_POINT ( 'NONE',  ( 11.36250000000000071, 2.886751345948129099, -4.999999999999998224 ) ) ;
#43596=CARTESIAN_POINT ( 'NONE',  ( 11.89687500061451608, -3.027376345333614438, 5.243569643749998122 ) ) ;
#43597=CARTESIAN_POINT ( 'NONE',  ( 5.587500001229033231, 6.123233995736764310E-16, -4.999999999999998224 ) ) ;
#43598=CARTESIAN_POINT ( 'NONE',  ( 13.84687500061451537, -3.027376345333610441, -5.243569643749999898 ) ) ;
#43599=CARTESIAN_POINT ( 'NONE',  ( 6.121875000614517504, -6.054752690667223547, -1.112240025338166033E-15 ) ) ;
#43600=CARTESIAN_POINT ( 'NONE',  ( 3.999999999999998668, 18.46249999999999858, 27.69059892324149530 ) ) ;
#43601=CYLINDRICAL_SURFACE ( 'NONE', #7602, 3.999999999999996447 ) ;
#43602=CARTESIAN_POINT ( 'NONE',  ( 11.40937500061451892, 0.000000000000000000, 5.243569643749999010 ) ) ;
#43603=DIRECTION ( 'NONE',  ( 0.000000000000000000, 0.000000000000000000, 1.000000000000000000 ) ) ;
#43604=CARTESIAN_POINT ( 'NONE',  ( 22.30312500061451431, -4.541064518000417216, -2.621784821875001281 ) ) ;
#43605=CARTESIAN_POINT ( 'NONE',  ( 4.243569643749999898, 10.59687500061451715, 32.45002607614398471 ) ) ;
#43607=CARTESIAN_POINT ( 'NONE',  ( 22.77187500061451786, -6.054752690667223547, -1.112240025338166033E-15 ) ) ;
#43608=CARTESIAN_POINT ( 'NONE',  ( 4.154761151537816666, 2.781809049394522670, -4.180738899374664364 ) ) ;
#43609=CARTESIAN_POINT ( 'NONE',  ( 28.53750000122903074, 6.123233995736764310E-16, -4.999999999999998224 ) ) ;
#43611=CARTESIAN_POINT ( 'NONE',  ( 25.34062500061451217, -3.027376345333614438, 5.243569643749998122 ) ) ;
#43612=CARTESIAN_POINT ( 'NONE',  ( 17.27812500061451217, -4.541064518000419881, 2.621784821874995952 ) ) ;
#43614=CARTESIAN_POINT ( 'NONE',  ( 14.40937500061451715, 4.541064518000418104, -2.621784821874998173 ) ) ;
#43616=CARTESIAN_POINT ( 'NONE',  ( 27.26250000122903216, 4.330127018922192761, -2.499999999999997780 ) ) ;
#43617=CARTESIAN_POINT ( 'NONE',  ( 5.821875000614519458, 3.027376345333613106, -5.243569643749998122 ) ) ;
#43618=CARTESIAN_POINT ( 'NONE',  ( 17.44687500061451857, -3.027376345333610441, -5.243569643749999898 ) ) ;
#43619=CARTESIAN_POINT ( 'NONE',  ( 4.854383007807864026, -1.197900502339936502, -5.104905189653401010 ) ) ;
#43620=CARTESIAN_POINT ( 'NONE',  ( 23.17500000000000071, 4.330127018922191873, 2.499999999999999556 ) ) ;
#43621=CARTESIAN_POINT ( 'NONE',  ( 3.300000001229034918, -2.886751345948125991, -5.000000000000000000 ) ) ;
#43622=CARTESIAN_POINT ( 'NONE',  ( 25.09687500061451715, -3.027376345333610441, -5.243569643749999898 ) ) ;
#43623=CARTESIAN_POINT ( 'NONE',  ( 16.13437500061451502, 6.421520780324663323E-16, -5.243569643749999010 ) ) ;
#43625=CARTESIAN_POINT ( 'NONE',  ( 29.02499999999999858, 4.330127018922191873, 2.499999999999999556 ) ) ;
#43626=CARTESIAN_POINT ( 'NONE',  ( 6.562500000000001776, 2.886751345948126879, 4.999999999999999112 ) ) ;
#43628=CARTESIAN_POINT ( 'NONE',  ( 20.46562500061451928, -6.054752690667223547, -1.112240025338166033E-15 ) ) ;
#43629=CARTESIAN_POINT ( 'NONE',  ( 9.449999999999999289, -4.330127018922190985, -2.500000000000001332 ) ) ;
#43630=CARTESIAN_POINT ( 'NONE',  ( 4.190625000614518925, -3.027376345333614438, 5.243569643749998122 ) ) ;
#43631=CARTESIAN_POINT ( 'NONE',  ( 20.02500000000000213, 4.330127018922191873, 2.499999999999999556 ) ) ;
#43632=DIRECTION ( 'NONE',  ( 0.000000000000000000, 0.000000000000000000, -1.000000000000000000 ) ) ;
#43633=CARTESIAN_POINT ( 'NONE',  ( 22.91250000122903430, 0.000000000000000000, 4.999999999999998224 ) ) ;
#43634=CARTESIAN_POINT ( 'NONE',  ( 2.516032931661821959, 9.680092174376738967, 35.45051723330771409 ) ) ;
#43635=CARTESIAN_POINT ( 'NONE',  ( 29.40937500061451715, 0.000000000000000000, 5.243569643749999010 ) ) ;
#43636=VERTEX_POINT ( 'NONE', #34784 ) ;
#43637=CARTESIAN_POINT ( 'NONE',  ( 16.37812500061451715, -4.541064518000419881, 2.621784821874995952 ) ) ;
#43638=CARTESIAN_POINT ( 'NONE',  ( 23.46562500061451573, 3.027376345333611329, 5.243569643749999010 ) ) ;
#43639=CARTESIAN_POINT ( 'NONE',  ( 25.99687500061451928, -3.027376345333610441, -5.243569643749999898 ) ) ;
#43640=CARTESIAN_POINT ( 'NONE',  ( 8.849999999999999645, 0.000000000000000000, 4.999999999999998224 ) ) ;
#43641=CARTESIAN_POINT ( 'NONE',  ( 12.44062500061451537, -3.027376345333610441, -5.243569643749999898 ) ) ;
#43642=CARTESIAN_POINT ( 'NONE',  ( 27.81562500061452070, 3.027376345333613106, -5.243569643749998122 ) ) ;
#43643=CARTESIAN_POINT ( 'NONE',  ( 14.44687500061451679, 6.054752690667223547, 3.707466751127219781E-16 ) ) ;
#43644=CARTESIAN_POINT ( 'NONE',  ( 19.05937500061451928, 0.000000000000000000, 5.243569643749999010 ) ) ;
#43646=CARTESIAN_POINT ( 'NONE',  ( -4.243569643749999898, 10.37187500061451750, 27.54997392385601529 ) ) ;
#43647=CARTESIAN_POINT ( 'NONE',  ( 24.45000000122903572, -2.886751345948125991, -5.000000000000000000 ) ) ;
#43649=CARTESIAN_POINT ( 'NONE',  ( 14.54062500061451679, -3.027376345333614438, 5.243569643749998122 ) ) ;
#43650=CARTESIAN_POINT ( 'NONE',  ( 6.984375000614516438, -4.541064518000419881, 2.621784821874995952 ) ) ;
#43651=CARTESIAN_POINT ( 'NONE',  ( 6.871875000614517504, 3.027376345333611329, 5.243569643749999010 ) ) ;
#43652=( BOUNDED_CURVE ( )  B_SPLINE_CURVE ( 2, ( #54315, #3705, #9604, #14406, #48770, #37672, #60194, #48039, #15494 ),
 .UNSPECIFIED., .F., .F. ) 
 B_SPLINE_CURVE_WITH_KNOTS ( ( 3, 2, 2, 2, 3 ),
 ( 0.9021739130434782705, 0.9057971014492753881, 0.9130434782608695121, 0.9202898550724637472, 0.9239130434782608647 ),
 .UNSPECIFIED. ) 
 CURVE ( )  GEOMETRIC_REPRESENTATION_ITEM ( )  RATIONAL_B_SPLINE_CURVE ( ( 0.9330127018922194093, 0.9330127018922194093, 1.000000000000000000, 0.8660254037844387076, 1.000000000000000000, 0.8660254037844387076, 1.000000000000000000, 0.9330127018922194093, 0.9330127018922194093 ) ) 
 REPRESENTATION_ITEM ( '' )  );
#43654=CARTESIAN_POINT ( 'NONE',  ( 28.39687500061452141, 6.054752690667223547, 3.707466751127219781E-16 ) ) ;
#43655=CARTESIAN_POINT ( 'NONE',  ( 19.41562500061451146, 3.027376345333611329, 5.243569643749999010 ) ) ;
#43657=CARTESIAN_POINT ( 'NONE',  ( 3.834375000614519635, -4.541064518000419881, 2.621784821874995952 ) ) ;
#43658=CARTESIAN_POINT ( 'NONE',  ( 25.09687500061451715, -3.027376345333610441, -5.243569643749999898 ) ) ;
#43659=CARTESIAN_POINT ( 'NONE',  ( 19.49062500061451431, -3.027376345333614438, 5.243569643749998122 ) ) ;
#43660=CARTESIAN_POINT ( 'NONE',  ( -3.999999999999997335, 11.03750000000000142, 32.30940107675850470 ) ) ;
#43661=CARTESIAN_POINT ( 'NONE',  ( 25.79062500061451502, -3.027376345333614438, 5.243569643749998122 ) ) ;
#43662=CARTESIAN_POINT ( 'NONE',  ( 7.425000001229034474, 2.886751345948129099, -4.999999999999998224 ) ) ;
#43663=EDGE_LOOP ( 'NONE', ( #38496, #47879, #63460, #51659 ) ) ;
#43664=CARTESIAN_POINT ( 'NONE',  ( 3.000000001229032875, 5.773502691896255534, 3.535250795749688894E-16 ) ) ;
#43665=CARTESIAN_POINT ( 'NONE',  ( 8.484601909799253346E-16, 14.26250000000000107, -25.38119784648299770 ) ) ;
#43666=CARTESIAN_POINT ( 'NONE',  ( 22.27500000122903145, 2.886751345948129099, -4.999999999999998224 ) ) ;
#43668=CARTESIAN_POINT ( 'NONE',  ( 3.609375000614516882, 4.541064518000418104, -2.621784821874998173 ) ) ;
#43669=CARTESIAN_POINT ( 'NONE',  ( 4.382503833126124348, 2.407183933188114189, -4.599998881930862815 ) ) ;
#43670=CARTESIAN_POINT ( 'NONE',  ( 13.60312500061451679, 0.000000000000000000, 5.243569643749999010 ) ) ;
#43671=CARTESIAN_POINT ( 'NONE',  ( 9.496875000614517504, 6.054752690667223547, 3.707466751127219781E-16 ) ) ;
#43672=CARTESIAN_POINT ( 'NONE',  ( 23.73750000122903359, 4.330127018922191873, 2.499999999999999556 ) ) ;
#43673=CARTESIAN_POINT ( 'NONE',  ( 14.37187500061451750, 3.027376345333612662, -5.243569643749998122 ) ) ;
#43674=CARTESIAN_POINT ( 'NONE',  ( 29.24062500061451431, 6.054752690667223547, 3.707466751127219781E-16 ) ) ;
#43675=CARTESIAN_POINT ( 'NONE',  ( 29.69999999999999574, -4.330127018922190985, -2.500000000000001332 ) ) ;
#43676=CARTESIAN_POINT ( 'NONE',  ( 5.353125000614515905, 4.541064518000418104, -2.621784821874998173 ) ) ;
#43677=CARTESIAN_POINT ( 'NONE',  ( 16.04062500061451857, -3.027376345333610441, -5.243569643749999898 ) ) ;
#43678=ORIENTED_EDGE ( 'NONE', *, *, #31941, .T. ) ;
#43679=CARTESIAN_POINT ( 'NONE',  ( 12.92812500061451786, 6.421520780324663323E-16, -5.243569643749999010 ) ) ;
#43680=CARTESIAN_POINT ( 'NONE',  ( 7.528125000614515727, 6.421520780324663323E-16, -5.243569643749999010 ) ) ;
#43682=CARTESIAN_POINT ( 'NONE',  ( 8.625000000000000000, 6.123233995736764310E-16, -4.999999999999998224 ) ) ;
#43683=CARTESIAN_POINT ( 'NONE',  ( 5.325000001229033941, 2.886751345948126879, 4.999999999999999112 ) ) ;
#43684=CARTESIAN_POINT ( 'NONE',  ( 18.63749999999999929, 5.773502691896255534, 3.535250795749688894E-16 ) ) ;
#43685=CARTESIAN_POINT ( 'NONE',  ( 18.27187500061451431, -6.054752690667223547, -1.112240025338166033E-15 ) ) ;
#43686=CARTESIAN_POINT ( 'NONE',  ( 14.21250000122903323, 4.330127018922192761, -2.499999999999997780 ) ) ;
#43688=CARTESIAN_POINT ( 'NONE',  ( -4.243569643749997233, 17.59062500061451928, -27.54997392385601174 ) ) ;
#43689=DIRECTION ( 'NONE',  ( -0.000000000000000000, -1.000000000000000000, -0.000000000000000000 ) ) ;
#43692=ADVANCED_FACE ( 'NONE', ( #19227 ), #64310, .F. ) ;
#43693=DIRECTION ( 'NONE',  ( 1.000000000000000000, 0.000000000000000000, 0.000000000000000000 ) ) ;
#43694=CARTESIAN_POINT ( 'NONE',  ( 24.29999999999999716, -4.330127018922190985, -2.500000000000001332 ) ) ;
#43695=CARTESIAN_POINT ( 'NONE',  ( 13.09687500061451892, 6.054752690667223547, 3.707466751127219781E-16 ) ) ;
#43696=( BOUNDED_CURVE ( )  B_SPLINE_CURVE ( 2, ( #32419, #70484, #25412, #32785, #54589, #3623, #59749 ),
 .UNSPECIFIED., .F., .F. ) 
 B_SPLINE_CURVE_WITH_KNOTS ( ( 3, 2, 2, 3 ),
 ( 0.9255912413769717961, 0.9277777777777778123, 0.9305555555555555802, 0.9324201688484926587 ),
 .UNSPECIFIED. ) 
 CURVE ( )  GEOMETRIC_REPRESENTATION_ITEM ( )  RATIONAL_B_SPLINE_CURVE ( ( 0.9551069630786563902, 0.8945414806928990714, 1.000000000000000000, 0.8660254037844387076, 1.000000000000000000, 0.9100681073130109100, 0.9408717204714907023 ) ) 
 REPRESENTATION_ITEM ( '' )  );
#43697=CARTESIAN_POINT ( 'NONE',  ( 26.81250000000000000, 2.886751345948126879, 4.999999999999999112 ) ) ;
#43698=CARTESIAN_POINT ( 'NONE',  ( 10.49062500061451431, -3.027376345333614438, 5.243569643749998122 ) ) ;
#43700=CARTESIAN_POINT ( 'NONE',  ( 22.35937500061451644, -4.541064518000417216, -2.621784821875001281 ) ) ;
#43702=CARTESIAN_POINT ( 'NONE',  ( 8.578125000614518214, 4.541064518000418104, 2.621784821874999949 ) ) ;
#43703=CARTESIAN_POINT ( 'NONE',  ( 13.35937500061451821, -4.541064518000417216, -2.621784821875001281 ) ) ;
#43704=ORIENTED_EDGE ( 'NONE', *, *, #45017, .T. ) ;
#43705=CARTESIAN_POINT ( 'NONE',  ( 24.34687500061451715, 6.054752690667223547, 3.707466751127219781E-16 ) ) ;
#43706=CARTESIAN_POINT ( 'NONE',  ( 0.5593513097472507800, 4.976037924071840202, -33.97015631813161463 ) ) ;
#43708=CARTESIAN_POINT ( 'NONE',  ( 4.650000000000001243, 4.330127018922192761, -2.499999999999997780 ) ) ;
#43709=CARTESIAN_POINT ( 'NONE',  ( 16.31250000122903288, -4.330127018922190985, -2.500000000000001332 ) ) ;
#43713=CARTESIAN_POINT ( 'NONE',  ( 15.29999999999999893, -4.330127018922190985, -2.500000000000001332 ) ) ;
#43714=CARTESIAN_POINT ( 'NONE',  ( 15.78749999999999964, -2.886751345948125991, -5.000000000000000000 ) ) ;
#43715=CARTESIAN_POINT ( 'NONE',  ( 11.80312500061451608, 0.000000000000000000, 5.243569643749999010 ) ) ;
#43716=VERTEX_POINT ( 'NONE', #36243 ) ;
#43717=CARTESIAN_POINT ( 'NONE',  ( 3.628170623289135754, -3.971039094590678165, 3.121958529326629428 ) ) ;
#43718=CARTESIAN_POINT ( 'NONE',  ( -4.243569643749999898, 17.57187500061451502, -32.45002607614398471 ) ) ;
#43719=CARTESIAN_POINT ( 'NONE',  ( 4.265625000614517326, -6.054752690667223547, -1.112240025338166033E-15 ) ) ;
#43721=CARTESIAN_POINT ( 'NONE',  ( 9.525000000000002132, 6.123233995736764310E-16, -4.999999999999998224 ) ) ;
#43722=CARTESIAN_POINT ( 'NONE',  ( 30.00000000000000000, 6.123233995736764310E-16, -4.999999999999998224 ) ) ;
#43724=CARTESIAN_POINT ( 'NONE',  ( 23.50312500061451360, 0.000000000000000000, 5.243569643749999010 ) ) ;
#43725=CARTESIAN_POINT ( 'NONE',  ( 4.229059543195655024, -2.667460491576031156, 4.514416570572414855 ) ) ;
#43727=CARTESIAN_POINT ( 'NONE',  ( 22.32187500061451502, -6.054752690667223547, -1.112240025338166033E-15 ) ) ;
#43728=CARTESIAN_POINT ( 'NONE',  ( 19.52812500061451573, -4.541064518000419881, 2.621784821874995952 ) ) ;
#43729=CARTESIAN_POINT ( 'NONE',  ( 9.001249775931846008E-16, 13.61562500061459424, -25.09994784771203058 ) ) ;
#43730=CARTESIAN_POINT ( 'NONE',  ( 24.45000000122903572, -2.886751345948125991, -5.000000000000000000 ) ) ;
#43731=CARTESIAN_POINT ( 'NONE',  ( 4.228125000614517681, -4.541064518000419881, 2.621784821874995952 ) ) ;
#43733=CARTESIAN_POINT ( 'NONE',  ( 22.22812500061451502, -4.541064518000419881, 2.621784821874995952 ) ) ;
#43736=CARTESIAN_POINT ( 'NONE',  ( 15.83437500061451608, 4.541064518000418104, 2.621784821874999949 ) ) ;
#43737=CARTESIAN_POINT ( 'NONE',  ( 15.60937500061451644, -4.541064518000417216, -2.621784821875001281 ) ) ;
#43738=CARTESIAN_POINT ( 'NONE',  ( 22.47187500061451715, 3.027376345333613106, -5.243569643749998122 ) ) ;
#43739=ORIENTED_EDGE ( 'NONE', *, *, #33984, .F. ) ;
#43740=CARTESIAN_POINT ( 'NONE',  ( 2.121784821874999061, 11.60937500061451821, 26.32496088578401583 ) ) ;
#43741=CARTESIAN_POINT ( 'NONE',  ( -1.999999999999997113, 14.78750000122903252, -26.53589838486224295 ) ) ;
#43742=CARTESIAN_POINT ( 'NONE',  ( 26.61562500061451786, 3.027376345333611329, 5.243569643749999010 ) ) ;
#43743=CARTESIAN_POINT ( 'NONE',  ( 27.66562500061451146, -6.054752690667223547, -1.112240025338166033E-15 ) ) ;
#43744=CARTESIAN_POINT ( 'NONE',  ( 8.512500001229033941, 0.000000000000000000, 4.999999999999998224 ) ) ;
#43745=CARTESIAN_POINT ( 'NONE',  ( 3.999999999999999112, 17.97500000000000142, 30.00000000000000000 ) ) ;
#43746=CARTESIAN_POINT ( 'NONE',  ( 7.171875000614517326, 3.027376345333613106, -5.243569643749998122 ) ) ;
#43748=CARTESIAN_POINT ( 'NONE',  ( 13.42500000122903536, 2.886751345948126879, 4.999999999999999112 ) ) ;
#43749=CARTESIAN_POINT ( 'NONE',  ( 10.01250000122903394, -4.330127018922190985, -2.500000000000001332 ) ) ;
#43750=CARTESIAN_POINT ( 'NONE',  ( 2.878125000614517592, -4.541064518000419881, 2.621784821874995952 ) ) ;
#43753=CARTESIAN_POINT ( 'NONE',  ( 13.05937500061451750, 4.541064518000418104, -2.621784821874998173 ) ) ;
#43754=CARTESIAN_POINT ( 'NONE',  ( 0.000000000000000000, 20.00000000000000000, 30.00000000000000000 ) ) ;
#43755=ORIENTED_EDGE ( 'NONE', *, *, #72282, .T. ) ;
#43756=CARTESIAN_POINT ( 'NONE',  ( 20.54062500061451502, -3.027376345333610441, -5.243569643749999898 ) ) ;
#43757=CARTESIAN_POINT ( 'NONE',  ( 15.04687500061451644, -3.027376345333614438, 5.243569643749998122 ) ) ;
#43758=CARTESIAN_POINT ( 'NONE',  ( 5.278125000614516615, 6.421520780324663323E-16, -5.243569643749999010 ) ) ;
#43759=CARTESIAN_POINT ( 'NONE',  ( 21.49687500061451573, -3.027376345333610441, -5.243569643749999898 ) ) ;
#43760=CARTESIAN_POINT ( 'NONE',  ( 4.903125000614516615, 4.541064518000418104, -2.621784821874998173 ) ) ;
#43761=FACE_OUTER_BOUND ( 'NONE', #65958, .T. ) ;
#43762=CARTESIAN_POINT ( 'NONE',  ( 6.975000001229032520, 2.886751345948129099, -4.999999999999998224 ) ) ;
#43764=CARTESIAN_POINT ( 'NONE',  ( 22.19062500061451715, -3.027376345333614438, 5.243569643749998122 ) ) ;
#43765=CARTESIAN_POINT ( 'NONE',  ( 4.000000000000000000, 17.15000000122903145, -27.69059892324149530 ) ) ;
#43766=CARTESIAN_POINT ( 'NONE',  ( 7.725000001229034297, -5.773502691896255534, -1.060575238724906372E-15 ) ) ;
#43767=CARTESIAN_POINT ( 'NONE',  ( 18.59062500061451573, -3.027376345333614438, 5.243569643749998122 ) ) ;
#43768=CARTESIAN_POINT ( 'NONE',  ( 15.89062500061451289, -3.027376345333614438, 5.243569643749998122 ) ) ;
#43770=CARTESIAN_POINT ( 'NONE',  ( 16.61250000000000426, -5.773502691896255534, -1.060575238724906372E-15 ) ) ;
#43771=CARTESIAN_POINT ( 'NONE',  ( 11.77500000122903501, -5.773502691896255534, -1.060575238724906372E-15 ) ) ;
#43772=CARTESIAN_POINT ( 'NONE',  ( 7.603125000614517681, 4.541064518000418104, -2.621784821874998173 ) ) ;
#43773=CARTESIAN_POINT ( 'NONE',  ( 12.02812500061451573, 6.421520780324663323E-16, -5.243569643749999010 ) ) ;
#43774=CARTESIAN_POINT ( 'NONE',  ( 21.60000000122903430, -2.886751345948129988, 4.999999999999997335 ) ) ;
#43775=CARTESIAN_POINT ( 'NONE',  ( 2.121784821874999061, 14.75937500061451679, -33.67503911421598417 ) ) ;
#43776=CARTESIAN_POINT ( 'NONE',  ( 18.27187500061451431, -6.054752690667223547, -1.112240025338166033E-15 ) ) ;
#43778=CARTESIAN_POINT ( 'NONE',  ( 5.250000001229035540, 5.773502691896255534, 3.535250795749688894E-16 ) ) ;
#43779=CARTESIAN_POINT ( 'NONE',  ( 3.759375000614517681, 0.000000000000000000, 5.243569643749999010 ) ) ;
#43780=CARTESIAN_POINT ( 'NONE',  ( 20.07187500061451857, -6.054752690667223547, -1.112240025338166033E-15 ) ) ;
#43781=CARTESIAN_POINT ( 'NONE',  ( -3.999999999999997335, 15.08750000000000036, 32.30940107675850470 ) ) ;
#43782=CARTESIAN_POINT ( 'NONE',  ( 18.66562500061451146, -6.054752690667223547, -1.112240025338166033E-15 ) ) ;
#43786=CARTESIAN_POINT ( 'NONE',  ( 27.68437500061451573, -4.541064518000419881, 2.621784821874995952 ) ) ;
#43788=CARTESIAN_POINT ( 'NONE',  ( 15.55312500061451608, -4.541064518000417216, -2.621784821875001281 ) ) ;
#43789=CARTESIAN_POINT ( 'NONE',  ( 13.95937500061451786, 4.541064518000418104, -2.621784821874998173 ) ) ;
#43790=ORIENTED_EDGE ( 'NONE', *, *, #15195, .F. ) ;
#43791=FACE_OUTER_BOUND ( 'NONE', #55527, .T. ) ;
#43792=CARTESIAN_POINT ( 'NONE',  ( 23.91562500061451502, 3.027376345333611329, 5.243569643749999010 ) ) ;
#43793=CYLINDRICAL_SURFACE ( 'NONE', #64008, 4.000000000000000000 ) ;
#43794=CARTESIAN_POINT ( 'NONE',  ( 28.53750000122903074, 6.123233995736764310E-16, -4.999999999999998224 ) ) ;
#43796=CARTESIAN_POINT ( 'NONE',  ( 11.81250000000000000, 2.886751345948129099, -4.999999999999998224 ) ) ;
#43798=CARTESIAN_POINT ( 'NONE',  ( 23.36250000122903359, 0.000000000000000000, 4.999999999999998224 ) ) ;
#43799=CARTESIAN_POINT ( 'NONE',  ( 17.99062500061451786, 6.054752690667223547, 3.707466751127219781E-16 ) ) ;
#43800=ORIENTED_EDGE ( 'NONE', *, *, #45083, .T. ) ;
#43801=CARTESIAN_POINT ( 'NONE',  ( 21.86250000000000071, 2.886751345948126879, 4.999999999999999112 ) ) ;
#43802=CARTESIAN_POINT ( 'NONE',  ( 23.74687500061451573, -3.027376345333610441, -5.243569643749999898 ) ) ;
#43803=VERTEX_POINT ( 'NONE', #3842 ) ;
#43805=CARTESIAN_POINT ( 'NONE',  ( 10.67812500061451608, 6.421520780324663323E-16, -5.243569643749999010 ) ) ;
#43808=CARTESIAN_POINT ( 'NONE',  ( 18.26249999999999929, 2.886751345948126879, 4.999999999999999112 ) ) ;
#43809=CARTESIAN_POINT ( 'NONE',  ( 24.82499999999999929, 6.123233995736764310E-16, -4.999999999999998224 ) ) ;
#43810=CARTESIAN_POINT ( 'NONE',  ( -2.121784821874996840, 18.97812500061451857, 33.67503911421598417 ) ) ;
#43811=CARTESIAN_POINT ( 'NONE',  ( 5.259375000614518569, -4.541064518000417216, -2.621784821875001281 ) ) ;
#43812=CARTESIAN_POINT ( 'NONE',  ( 16.43437500061451573, -4.541064518000419881, 2.621784821874995952 ) ) ;
#43813=CARTESIAN_POINT ( 'NONE',  ( 27.83437500061451786, 6.421520780324663323E-16, -5.243569643749999010 ) ) ;
#43816=CARTESIAN_POINT ( 'NONE',  ( 25.41562500061451146, -6.054752690667223547, -1.112240025338166033E-15 ) ) ;
#43817=CARTESIAN_POINT ( 'NONE',  ( 27.19687500061451857, -3.027376345333614438, 5.243569643749998122 ) ) ;
#43819=CARTESIAN_POINT ( 'NONE',  ( 14.77500000000000036, -4.330127018922194537, 2.499999999999995559 ) ) ;
#43820=CARTESIAN_POINT ( 'NONE',  ( 11.42812500061451608, -4.541064518000419881, 2.621784821874995952 ) ) ;
#43821=LINE ( 'NONE', #50457, #30409 ) ;
#43822=CARTESIAN_POINT ( 'NONE',  ( 1.999999999999998668, 19.40000000000000213, -33.46410161513775705 ) ) ;
#43823=CARTESIAN_POINT ( 'NONE',  ( 28.97812500061451502, -4.541064518000419881, 2.621784821874995952 ) ) ;
#43824=CARTESIAN_POINT ( 'NONE',  ( 15.86250000122903181, -4.330127018922190985, -2.500000000000001332 ) ) ;
#43825=LINE ( 'NONE', #64881, #40678 ) ;
#43827=CARTESIAN_POINT ( 'NONE',  ( 5.053125000614517859, 0.000000000000000000, 5.243569643749999010 ) ) ;
#43828=CARTESIAN_POINT ( 'NONE',  ( 21.98437500061451644, 6.421520780324663323E-16, -5.243569643749999010 ) ) ;
#43829=CARTESIAN_POINT ( 'NONE',  ( 2.121784821875001281, 16.85937500061451999, 33.67503911421598417 ) ) ;
#43830=CARTESIAN_POINT ( 'NONE',  ( 20.44687500061451857, -3.027376345333614438, 5.243569643749998122 ) ) ;
#43831=CARTESIAN_POINT ( 'NONE',  ( 28.84687500061452070, 6.054752690667223547, 3.707466751127219781E-16 ) ) ;
#43832=CARTESIAN_POINT ( 'NONE',  ( -3.000416591977282496E-16, 18.39687500061451786, 25.09994784771203058 ) ) ;
#43833=CARTESIAN_POINT ( 'NONE',  ( 11.65312500061451573, 4.541064518000418104, -2.621784821874998173 ) ) ;
#43834=CARTESIAN_POINT ( 'NONE',  ( 1.626862140677534273E-15, 15.27500000122903501, 34.00000000000000000 ) ) ;
#43835=CARTESIAN_POINT ( 'NONE',  ( 8.071875000614518569, 3.027376345333613106, -5.243569643749998122 ) ) ;
#43836=CARTESIAN_POINT ( 'NONE',  ( -5.810221930991193690E-16, 15.83749999999999680, -34.00000000000000000 ) ) ;
#43837=CARTESIAN_POINT ( 'NONE',  ( 8.915625000614515017, 3.027376345333613106, -5.243569643749998122 ) ) ;
#43838=CARTESIAN_POINT ( 'NONE',  ( 13.39687500061451608, -3.027376345333610441, -5.243569643749999898 ) ) ;
#43840=CARTESIAN_POINT ( 'NONE',  ( 21.63750000122903572, -4.330127018922194537, 2.499999999999995559 ) ) ;
#43841=CARTESIAN_POINT ( 'NONE',  ( 7.659375000614518036, 4.541064518000418104, -2.621784821874998173 ) ) ;
#43842=CARTESIAN_POINT ( 'NONE',  ( 9.553125000614517859, 0.000000000000000000, 5.243569643749999010 ) ) ;
#43844=CARTESIAN_POINT ( 'NONE',  ( 21.30937500061451573, 0.000000000000000000, 5.243569643749999010 ) ) ;
#43846=CARTESIAN_POINT ( 'NONE',  ( -1.839935159944502630, 4.656359355287978730, 33.56177517597544835 ) ) ;
#43847=DIRECTION ( 'NONE',  ( -1.000000000000000000, -0.000000000000000000, -0.000000000000000000 ) ) ;
#43848=ADVANCED_FACE ( 'NONE', ( #26363 ), #71433, .F. ) ;
#43849=CARTESIAN_POINT ( 'NONE',  ( 4.243569643749999898, 12.43437500061451750, -30.00000000000000000 ) ) ;
#43850=CARTESIAN_POINT ( 'NONE',  ( 14.32500000122903394, 2.886751345948126879, 4.999999999999999112 ) ) ;
#43851=B_SPLINE_CURVE_WITH_KNOTS ( 'NONE', 3,
 ( #29627, #11561, #29272, #57693, #34440, #56617, #51442, #50723, #28904, #24077 ),
 .UNSPECIFIED., .F., .F.,
 ( 4, 3, 3, 4 ),
 ( 0.000000000000000000, 0.0001572271610493928607, 0.0003144542605825271630, 0.0005320905539976019533 ),
 .UNSPECIFIED. ) ;
#43852=CARTESIAN_POINT ( 'NONE',  ( 9.001249775931846008E-16, 15.41562500061451679, -25.09994784771203058 ) ) ;
#43853=CARTESIAN_POINT ( 'NONE',  ( 18.26250000122903216, 4.330127018922192761, -2.499999999999997780 ) ) ;
#43854=CARTESIAN_POINT ( 'NONE',  ( 9.965625000614517504, 3.027376345333611329, 5.243569643749999010 ) ) ;
#43856=CARTESIAN_POINT ( 'NONE',  ( 14.02499999999999858, 6.123233995736764310E-16, -4.999999999999998224 ) ) ;
#43858=CARTESIAN_POINT ( 'NONE',  ( 22.79062500061451502, -3.027376345333610441, -5.243569643749999898 ) ) ;
#43859=CARTESIAN_POINT ( 'NONE',  ( 11.18437500061451928, 6.421520780324663323E-16, -5.243569643749999010 ) ) ;
#43860=CARTESIAN_POINT ( 'NONE',  ( -1.999999999999997113, 14.33750000122903323, 33.46410161513775705 ) ) ;
#43861=CARTESIAN_POINT ( 'NONE',  ( 9.075000001229033941, -5.773502691896255534, -1.060575238724906372E-15 ) ) ;
#43862=CARTESIAN_POINT ( 'NONE',  ( 18.75000000122903288, 5.773502691896255534, 3.535250795749688894E-16 ) ) ;
#43863=CARTESIAN_POINT ( 'NONE',  ( 15.70312500061451644, 4.541064518000418104, -2.621784821874998173 ) ) ;
#43865=CARTESIAN_POINT ( 'NONE',  ( 17.91562500061451502, 3.027376345333613106, -5.243569643749998122 ) ) ;
#43866=CARTESIAN_POINT ( 'NONE',  ( 25.53750000122903074, 4.330127018922191873, 2.499999999999999556 ) ) ;
#43867=CARTESIAN_POINT ( 'NONE',  ( 27.52500000122903145, -5.773502691896255534, -1.060575238724906372E-15 ) ) ;
#43868=CARTESIAN_POINT ( 'NONE',  ( 22.01249999999999574, -5.773502691896255534, -1.060575238724906372E-15 ) ) ;
#43870=CARTESIAN_POINT ( 'NONE',  ( 24.72187500061451360, 3.027376345333613106, -5.243569643749998122 ) ) ;
#43871=CARTESIAN_POINT ( 'NONE',  ( -3.999999999999997335, 15.98750000000000249, 32.30940107675850470 ) ) ;
#43872=CARTESIAN_POINT ( 'NONE',  ( 12.97500000122903252, 2.886751345948126879, 4.999999999999999112 ) ) ;
#43873=CARTESIAN_POINT ( 'NONE',  ( 3.337499999999999911, 5.773502691896255534, 3.535250795749688894E-16 ) ) ;
#43875=CARTESIAN_POINT ( 'NONE',  ( 5.859375000614519102, 4.541064518000418104, -2.621784821874998173 ) ) ;
#43876=CARTESIAN_POINT ( 'NONE',  ( 27.14062500061451644, -3.027376345333614438, 5.243569643749998122 ) ) ;
#43878=CARTESIAN_POINT ( 'NONE',  ( -5.810221930991193690E-16, 10.55000000122903359, 26.00000000000000355 ) ) ;
#43879=CARTESIAN_POINT ( 'NONE',  ( 10.88437500061451679, 4.541064518000418104, 2.621784821874999949 ) ) ;
#43880=CARTESIAN_POINT ( 'NONE',  ( 4.294292190751133553, -2.561165899037177507, 4.480540752805964644 ) ) ;
#43881=CARTESIAN_POINT ( 'NONE',  ( 28.82812500061451644, 4.541064518000418104, 2.621784821874999949 ) ) ;
#43882=CARTESIAN_POINT ( 'NONE',  ( 8.409375000614518925, -4.541064518000417216, -2.621784821875001281 ) ) ;
#43883=CARTESIAN_POINT ( 'NONE',  ( 29.25937500061451502, 4.541064518000418104, -2.621784821874998173 ) ) ;
#43884=CARTESIAN_POINT ( 'NONE',  ( -4.243569643749998122, 13.09062500061459389, 32.45002607614398471 ) ) ;
#43885=CARTESIAN_POINT ( 'NONE',  ( 23.02499999999999858, 6.123233995736764310E-16, -4.999999999999998224 ) ) ;
#43886=ORIENTED_EDGE ( 'NONE', *, *, #31085, .F. ) ;
#43887=CARTESIAN_POINT ( 'NONE',  ( 29.96250000000000213, 2.886751345948126879, 4.999999999999999112 ) ) ;
#43888=EDGE_CURVE ( 'NONE', #33565, #28698, #25547, .T. ) ;
#43889=CARTESIAN_POINT ( 'NONE',  ( 4.537500000000000533, -2.886751345948125991, -5.000000000000000000 ) ) ;
#43891=VECTOR ( 'NONE', #42206, 1000.000000000000000 ) ;
#43892=CARTESIAN_POINT ( 'NONE',  ( 17.76562500061451644, -6.054752690667223547, -1.112240025338166033E-15 ) ) ;
#43893=CARTESIAN_POINT ( 'NONE',  ( 11.80312500061451608, 0.000000000000000000, 5.243569643749999010 ) ) ;
#43895=CARTESIAN_POINT ( 'NONE',  ( 6.609375000614519102, -4.541064518000417216, -2.621784821875001281 ) ) ;
#43896=CARTESIAN_POINT ( 'NONE',  ( 19.27500000122903145, 2.886751345948126879, 4.999999999999999112 ) ) ;
#43897=CARTESIAN_POINT ( 'NONE',  ( 7.950000000000001954, 0.000000000000000000, 4.999999999999998224 ) ) ;
#43898=CARTESIAN_POINT ( 'NONE',  ( 6.271875000614517859, 3.027376345333613106, -5.243569643749998122 ) ) ;
#43899=CARTESIAN_POINT ( 'NONE',  ( 14.59687500061452070, -3.027376345333614438, 5.243569643749998122 ) ) ;
#43900=CARTESIAN_POINT ( 'NONE',  ( 24.87187500061451573, 3.027376345333611329, 5.243569643749999010 ) ) ;
#43901=CARTESIAN_POINT ( 'NONE',  ( 3.999999999999999112, 15.83750000122903501, -30.00000000000000000 ) ) ;
#43902=ORIENTED_EDGE ( 'NONE', *, *, #70232, .F. ) ;
#43904=CARTESIAN_POINT ( 'NONE',  ( 17.40937500061451715, -4.541064518000417216, -2.621784821875001281 ) ) ;
#43905=( BOUNDED_CURVE ( )  B_SPLINE_CURVE ( 2, ( #56410, #56757, #5801, #267, #39425, #10980, #57487, #998, #634 ),
 .UNSPECIFIED., .F., .F. ) 
 B_SPLINE_CURVE_WITH_KNOTS ( ( 3, 2, 2, 2, 3 ),
 ( 0.7065217391304348116, 0.7101449275362319291, 0.7173913043478260532, 0.7246376811594202882, 0.7282608695652174058 ),
 .UNSPECIFIED. ) 
 CURVE ( )  GEOMETRIC_REPRESENTATION_ITEM ( )  RATIONAL_B_SPLINE_CURVE ( ( 0.9330127018922194093, 0.9330127018922194093, 1.000000000000000000, 0.8660254037844387076, 1.000000000000000000, 0.8660254037844387076, 1.000000000000000000, 0.9330127018922194093, 0.9330127018922194093 ) ) 
 REPRESENTATION_ITEM ( '' )  );
#43906=CARTESIAN_POINT ( 'NONE',  ( 10.58437500061451964, -4.541064518000419881, 2.621784821874995952 ) ) ;
#43908=CARTESIAN_POINT ( 'NONE',  ( 20.92500000000000071, 4.330127018922191873, 2.499999999999999556 ) ) ;
#43911=CARTESIAN_POINT ( 'NONE',  ( 12.59062500061451573, 6.054752690667223547, 3.707466751127219781E-16 ) ) ;
#43912=CARTESIAN_POINT ( 'NONE',  ( 3.149999999999999911, -4.330127018922190985, -2.500000000000001332 ) ) ;
#43913=CARTESIAN_POINT ( 'NONE',  ( 28.88437500061451502, 4.541064518000418104, 2.621784821874999949 ) ) ;
#43914=CARTESIAN_POINT ( 'NONE',  ( 10.80000000000000071, -4.330127018922190985, -2.500000000000001332 ) ) ;
#43915=CARTESIAN_POINT ( 'NONE',  ( -3.999999999999997335, 15.65000000122903501, 32.30940107675850470 ) ) ;
#43916=CARTESIAN_POINT ( 'NONE',  ( 10.87500000122903288, -5.773502691896255534, -1.060575238724906372E-15 ) ) ;
#43917=CARTESIAN_POINT ( 'NONE',  ( 23.44687500061451502, 6.054752690667223547, 3.707466751127219781E-16 ) ) ;
#43918=CARTESIAN_POINT ( 'NONE',  ( 14.29687500061451821, -3.027376345333610441, -5.243569643749999898 ) ) ;
#43919=CYLINDRICAL_SURFACE ( 'NONE', #4182, 4.000000000000000000 ) ;
#43920=ORIENTED_EDGE ( 'NONE', *, *, #15421, .F. ) ;
#43921=CARTESIAN_POINT ( 'NONE',  ( 18.14062500061451644, -3.027376345333614438, 5.243569643749998122 ) ) ;
#43922=CARTESIAN_POINT ( 'NONE',  ( 28.61250000122903359, 4.330127018922192761, -2.499999999999997780 ) ) ;
#43923=CARTESIAN_POINT ( 'NONE',  ( 15.08437500061451786, -4.541064518000419881, 2.621784821874995952 ) ) ;
#43924=CARTESIAN_POINT ( 'NONE',  ( 2.803125000614518747, 0.000000000000000000, 5.243569643749999010 ) ) ;
#43925=CARTESIAN_POINT ( 'NONE',  ( 20.57812500061451644, 6.421520780324663323E-16, -5.243569643749999010 ) ) ;
#43926=CARTESIAN_POINT ( 'NONE',  ( 1.071796769724497445, 16.71740381056766367, -33.99999999999998579 ) ) ;
#43927=CARTESIAN_POINT ( 'NONE',  ( 29.37187500061451928, 3.027376345333611329, 5.243569643749999010 ) ) ;
#43928=CARTESIAN_POINT ( 'NONE',  ( -4.243569643749997233, 13.99062500061451786, 32.45002607614398471 ) ) ;
#43929=CARTESIAN_POINT ( 'NONE',  ( 16.50937500061451502, -4.541064518000417216, -2.621784821875001281 ) ) ;
#43930=CARTESIAN_POINT ( 'NONE',  ( 14.43750000122903288, -4.330127018922194537, 2.499999999999995559 ) ) ;
#43932=CARTESIAN_POINT ( 'NONE',  ( -4.243569643749999898, 19.85937500061451644, -30.00000000000000000 ) ) ;
#43933=CARTESIAN_POINT ( 'NONE',  ( 20.89687500061452141, -3.027376345333614438, 5.243569643749998122 ) ) ;
#43934=CARTESIAN_POINT ( 'NONE',  ( 23.62500000122902932, 2.886751345948129099, -4.999999999999998224 ) ) ;
#43935=EDGE_CURVE ( 'NONE', #36605, #33656, #11562, .T. ) ;
#43936=( BOUNDED_CURVE ( )  B_SPLINE_CURVE ( 2, ( #52880, #24433, #53239, #46982, #48073, #2278, #2636 ),
 .UNSPECIFIED., .F., .F. ) 
 B_SPLINE_CURVE_WITH_KNOTS ( ( 3, 2, 2, 3 ),
 ( 0.6583333333333334370, 0.6611111111111112049, 0.6638888888888888618, 0.6666666666666666297 ),
 .UNSPECIFIED. ) 
 CURVE ( )  GEOMETRIC_REPRESENTATION_ITEM ( )  RATIONAL_B_SPLINE_CURVE ( ( 0.9999999999999946709, 0.8660254037844440367, 1.000000000000000000, 0.8660254037844387076, 1.000000000000000000, 0.8660254037844387076, 1.000000000000000000 ) ) 
 REPRESENTATION_ITEM ( '' )  );
#43937=CARTESIAN_POINT ( 'NONE',  ( 17.18437500061451573, 4.541064518000418104, 2.621784821874999949 ) ) ;
#43938=CARTESIAN_POINT ( 'NONE',  ( 12.21562500061451573, 3.027376345333611329, 5.243569643749999010 ) ) ;
#43939=CARTESIAN_POINT ( 'NONE',  ( -2.121784821874996840, 11.83437500061451786, 33.67503911421598417 ) ) ;
#43940=CARTESIAN_POINT ( 'NONE',  ( 17.72812500061451502, -4.541064518000419881, 2.621784821874995952 ) ) ;
#43941=ORIENTED_EDGE ( 'NONE', *, *, #32035, .T. ) ;
#43943=CARTESIAN_POINT ( 'NONE',  ( 24.14999999999999858, 0.000000000000000000, 4.999999999999998224 ) ) ;
#43944=CARTESIAN_POINT ( 'NONE',  ( -4.243569643749999898, 18.95937500061451431, -30.00000000000000000 ) ) ;
#43946=CARTESIAN_POINT ( 'NONE',  ( 24.55312500061451786, -4.541064518000417216, -2.621784821875001281 ) ) ;
#43947=CARTESIAN_POINT ( 'NONE',  ( 6.140625000614516438, -3.027376345333610441, -5.243569643749999898 ) ) ;
#43948=CARTESIAN_POINT ( 'NONE',  ( 17.40000000122903145, 5.773502691896255534, 3.535250795749688894E-16 ) ) ;
#43949=CARTESIAN_POINT ( 'NONE',  ( 22.56562500061451715, 3.027376345333611329, 5.243569643749999010 ) ) ;
#43950=CARTESIAN_POINT ( 'NONE',  ( 22.80000000000000071, 0.000000000000000000, 4.999999999999998224 ) ) ;
#43951=CARTESIAN_POINT ( 'NONE',  ( 25.11562500061451431, 3.027376345333613106, -5.243569643749998122 ) ) ;
#43952=CARTESIAN_POINT ( 'NONE',  ( 6.440625000614517148, -3.027376345333614438, 5.243569643749998122 ) ) ;
#43953=VERTEX_POINT ( 'NONE', #17797 ) ;
#43954=VECTOR ( 'NONE', #9978, 1000.000000000000000 ) ;
#43955=CARTESIAN_POINT ( 'NONE',  ( 24.32812500061451289, 4.541064518000418104, 2.621784821874999949 ) ) ;
#43957=( BOUNDED_CURVE ( )  B_SPLINE_CURVE ( 2, ( #23202, #1059, #56817, #38112, #61010, #51657, #27045 ),
 .UNSPECIFIED., .F., .F. ) 
 B_SPLINE_CURVE_WITH_KNOTS ( ( 3, 2, 2, 3 ),
 ( 0.1666666666666666852, 0.1694444444444444808, 0.1722222222222222487, 0.1750000000000000167 ),
 .UNSPECIFIED. ) 
 CURVE ( )  GEOMETRIC_REPRESENTATION_ITEM ( )  RATIONAL_B_SPLINE_CURVE ( ( 0.9999999999999986677, 0.8660254037844400399, 1.000000000000000000, 0.8660254037844387076, 1.000000000000000000, 0.8660254037844373753, 1.000000000000001332 ) ) 
 REPRESENTATION_ITEM ( '' )  );
#43959=CARTESIAN_POINT ( 'NONE',  ( 30.00000000000000000, 0.000000000000000000, 0.000000000000000000 ) ) ;
#43960=CARTESIAN_POINT ( 'NONE',  ( 8.484601909799253346E-16, 14.82500000122903216, -25.38119784648299770 ) ) ;
#43961=CARTESIAN_POINT ( 'NONE',  ( 4.243569643749999010, 19.67187500061451644, -32.45002607614398471 ) ) ;
#43962=CARTESIAN_POINT ( 'NONE',  ( 10.61250000000000071, 2.886751345948126879, 4.999999999999999112 ) ) ;
#43963=CARTESIAN_POINT ( 'NONE',  ( 12.00937500061451857, -4.541064518000417216, -2.621784821875001281 ) ) ;
#43964=CARTESIAN_POINT ( 'NONE',  ( 7.200000001229035718, -2.886751345948129988, 4.999999999999997335 ) ) ;
#43965=CARTESIAN_POINT ( 'NONE',  ( 14.40937500061451715, 4.541064518000418104, -2.621784821874998173 ) ) ;
#43966=CARTESIAN_POINT ( 'NONE',  ( 5.784375000614517148, 6.421520780324663323E-16, -5.243569643749999010 ) ) ;
#43967=DIRECTION ( 'NONE',  ( -1.000000000000000000, -0.000000000000000000, -0.000000000000000000 ) ) ;
#43968=CARTESIAN_POINT ( 'NONE',  ( -2.000000000000000000, 10.58750000122903323, 26.53589838486224650 ) ) ;
#43969=CARTESIAN_POINT ( 'NONE',  ( 12.60937500061451821, 4.541064518000418104, -2.621784821874998173 ) ) ;
#43971=CARTESIAN_POINT ( 'NONE',  ( 22.79062500061451502, -3.027376345333610441, -5.243569643749999898 ) ) ;
#43973=CARTESIAN_POINT ( 'NONE',  ( 29.66250000122903074, 0.000000000000000000, 4.999999999999998224 ) ) ;
#43974=CARTESIAN_POINT ( 'NONE',  ( 24.83437500061451431, 4.541064518000418104, 2.621784821874999949 ) ) ;
#43975=CARTESIAN_POINT ( 'NONE',  ( 3.999999999999998668, 19.36249999999999716, 27.69059892324149530 ) ) ;
#43976=CARTESIAN_POINT ( 'NONE',  ( 29.36250000122903003, -4.330127018922190985, -2.500000000000001332 ) ) ;
#43978=CARTESIAN_POINT ( 'NONE',  ( 24.17812500061451786, 6.421520780324663323E-16, -5.243569643749999010 ) ) ;
#43979=CARTESIAN_POINT ( 'NONE',  ( 17.76562500061451644, -6.054752690667223547, -1.112240025338166033E-15 ) ) ;
#43981=CARTESIAN_POINT ( 'NONE',  ( 13.95937500061451786, 4.541064518000418104, -2.621784821874998173 ) ) ;
#43982=CARTESIAN_POINT ( 'NONE',  ( 16.76249999999999929, 2.886751345948129099, -4.999999999999997335 ) ) ;
#43983=CARTESIAN_POINT ( 'NONE',  ( 26.96250000122903145, 0.000000000000000000, 4.999999999999998224 ) ) ;
#43984=CARTESIAN_POINT ( 'NONE',  ( 4.629056002857023344, -1.889931353889065413, 4.891133006415133266 ) ) ;
#43985=CARTESIAN_POINT ( 'NONE',  ( 13.28437500061451715, -4.541064518000419881, 2.621784821874995952 ) ) ;
#43987=CARTESIAN_POINT ( 'NONE',  ( -2.000000000000000000, 11.37500000000000178, 26.53589838486224650 ) ) ;
#43988=CARTESIAN_POINT ( 'NONE',  ( 3.825000001229032609, 2.886751345948129099, -4.999999999999998224 ) ) ;
#43989=CARTESIAN_POINT ( 'NONE',  ( 25.28437500061451715, 4.541064518000418104, 2.621784821874999949 ) ) ;
#43990=CARTESIAN_POINT ( 'NONE',  ( 16.99687500061451573, -3.027376345333610441, -5.243569643749999898 ) ) ;
#43992=CARTESIAN_POINT ( 'NONE',  ( 28.49999999999999645, 4.330127018922192761, -2.499999999999997780 ) ) ;
#43993=CARTESIAN_POINT ( 'NONE',  ( 6.487499999999999822, 5.773502691896255534, 3.535250795749688894E-16 ) ) ;
#43995=CARTESIAN_POINT ( 'NONE',  ( 20.72812500061451502, 4.541064518000418104, 2.621784821874999949 ) ) ;
#43996=CARTESIAN_POINT ( 'NONE',  ( 9.412499999999999645, -5.773502691896255534, -1.060575238724906372E-15 ) ) ;
#43997=CARTESIAN_POINT ( 'NONE',  ( 4.490625000614516971, 6.054752690667223547, 3.707466751127219781E-16 ) ) ;
#43998=CARTESIAN_POINT ( 'NONE',  ( 20.36249999999999716, 2.886751345948129099, -4.999999999999998224 ) ) ;
#44000=CARTESIAN_POINT ( 'NONE',  ( 24.30000000122903359, -2.886751345948129988, 4.999999999999997335 ) ) ;
#44002=CARTESIAN_POINT ( 'NONE',  ( 3.825000000000001954, 4.330127018922191873, 2.499999999999999556 ) ) ;
#44004=CARTESIAN_POINT ( 'NONE',  ( 18.06562500061451715, 3.027376345333611329, 5.243569643749999010 ) ) ;
#44005=CARTESIAN_POINT ( 'NONE',  ( 24.66562500061451502, 3.027376345333613106, -5.243569643749998122 ) ) ;
#44006=CARTESIAN_POINT ( 'NONE',  ( 25.43437500061451573, -4.541064518000419881, 2.621784821874995952 ) ) ;
#44007=CARTESIAN_POINT ( 'NONE',  ( 7.650000000000000355, -4.330127018922190985, -2.500000000000001332 ) ) ;
#44008=CARTESIAN_POINT ( 'NONE',  ( 9.515625000614518214, 3.027376345333611329, 5.243569643749999010 ) ) ;
#44009=CARTESIAN_POINT ( 'NONE',  ( 27.14062500061451644, -3.027376345333614438, 5.243569643749998122 ) ) ;
#44010=CARTESIAN_POINT ( 'NONE',  ( 14.55937500061451573, 0.000000000000000000, 5.243569643749999010 ) ) ;
#44011=CARTESIAN_POINT ( 'NONE',  ( 18.79687500061451644, -3.027376345333610441, -5.243569643749999898 ) ) ;
#44012=CARTESIAN_POINT ( 'NONE',  ( 4.450256264752916024, 2.279367318176788615, -4.722266026914592629 ) ) ;
#44013=CARTESIAN_POINT ( 'NONE',  ( -2.121784821874996840, 10.03437500061451892, 33.67503911421598417 ) ) ;
#44014=CARTESIAN_POINT ( 'NONE',  ( 21.26250000122903572, -4.330127018922190985, -2.500000000000001332 ) ) ;
#44016=CARTESIAN_POINT ( 'NONE',  ( 11.31562500061451892, 3.027376345333611329, 5.243569643749999010 ) ) ;
#44017=CARTESIAN_POINT ( 'NONE',  ( 8.259375000614518569, 0.000000000000000000, 5.243569643749999010 ) ) ;
#44018=CARTESIAN_POINT ( 'NONE',  ( 7.696875000614516793, 6.054752690667223547, 3.707466751127219781E-16 ) ) ;
#44020=CARTESIAN_POINT ( 'NONE',  ( 26.67187500061451644, 3.027376345333611329, 5.243569643749999010 ) ) ;
#44021=CARTESIAN_POINT ( 'NONE',  ( 18.62812500061451715, -4.541064518000419881, 2.621784821874995952 ) ) ;
#44022=CARTESIAN_POINT ( 'NONE',  ( 28.76250000122903216, 0.000000000000000000, 4.999999999999998224 ) ) ;
#44023=ADVANCED_FACE ( 'NONE', ( #28548 ), #40357, .F. ) ;
#44024=CARTESIAN_POINT ( 'NONE',  ( 29.20312500061451644, 4.541064518000418104, -2.621784821874998173 ) ) ;
#44025=CARTESIAN_POINT ( 'NONE',  ( 23.48437500061451644, 4.541064518000418104, 2.621784821874999949 ) ) ;
#44026=CARTESIAN_POINT ( 'NONE',  ( 20.57812500061451644, 6.421520780324663323E-16, -5.243569643749999010 ) ) ;
#44027=CARTESIAN_POINT ( 'NONE',  ( 8.484601909799253346E-16, 12.91249999999999964, 34.61880215351700230 ) ) ;
#44028=CARTESIAN_POINT ( 'NONE',  ( 23.80312500061451786, 4.541064518000418104, -2.621784821874998173 ) ) ;
#44029=CARTESIAN_POINT ( 'NONE',  ( 4.687500001229034652, 6.123233995736764310E-16, -4.999999999999998224 ) ) ;
#44030=ORIENTED_EDGE ( 'NONE', *, *, #36869, .F. ) ;
#44031=CARTESIAN_POINT ( 'NONE',  ( 29.17500000000000071, -4.330127018922194537, 2.499999999999995559 ) ) ;
#44032=CARTESIAN_POINT ( 'NONE',  ( -3.999999999999999556, 15.01250000000000107, -32.30940107675850470 ) ) ;
#44034=CARTESIAN_POINT ( 'NONE',  ( 4.434375000614519280, 6.421520780324663323E-16, -5.243569643749999010 ) ) ;
#44035=CARTESIAN_POINT ( 'NONE',  ( 29.24062500061451431, 6.054752690667223547, 3.707466751127219781E-16 ) ) ;
#44036=CARTESIAN_POINT ( 'NONE',  ( 12.85312500061451502, -4.541064518000417216, -2.621784821875001281 ) ) ;
#44037=CARTESIAN_POINT ( 'NONE',  ( 5.596875000614516260, -3.027376345333614438, 5.243569643749998122 ) ) ;
#44038=CARTESIAN_POINT ( 'NONE',  ( 24.52500000122903145, 2.886751345948129099, -4.999999999999998224 ) ) ;
#44039=CARTESIAN_POINT ( 'NONE',  ( 15.98437500061451821, -4.541064518000419881, 2.621784821874995952 ) ) ;
#44040=CARTESIAN_POINT ( 'NONE',  ( 28.67812500061451431, 6.421520780324663323E-16, -5.243569643749999010 ) ) ;
#44041=CARTESIAN_POINT ( 'NONE',  ( -3.999999999999999112, 10.96250000000000213, 27.69059892324149885 ) ) ;
#44042=CARTESIAN_POINT ( 'NONE',  ( 26.97187500061451360, 3.027376345333613106, -5.243569643749998122 ) ) ;
#44043=CARTESIAN_POINT ( 'NONE',  ( 3.740625000614516527, -3.027376345333614438, 5.243569643749998122 ) ) ;
#44044=CARTESIAN_POINT ( 'NONE',  ( 13.15312500061451750, 0.000000000000000000, 5.243569643749999010 ) ) ;
#44045=VERTEX_POINT ( 'NONE', #16725 ) ;
#44046=CARTESIAN_POINT ( 'NONE',  ( 9.478125000614515017, 4.541064518000418104, 2.621784821874999949 ) ) ;
#44047=CARTESIAN_POINT ( 'NONE',  ( 7.640625000614517326, 6.054752690667223547, 3.707466751127219781E-16 ) ) ;
#44049=CARTESIAN_POINT ( 'NONE',  ( 9.562500000000001776, 2.886751345948129099, -4.999999999999998224 ) ) ;
#44050=CARTESIAN_POINT ( 'NONE',  ( 4.275000001229035895, 2.886751345948129099, -4.999999999999998224 ) ) ;
#44051=CARTESIAN_POINT ( 'NONE',  ( 17.88749999999999929, -2.886751345948129988, 4.999999999999997335 ) ) ;
#44052=CARTESIAN_POINT ( 'NONE',  ( 18.57187500061451857, 3.027376345333611329, 5.243569643749999010 ) ) ;
#44053=CARTESIAN_POINT ( 'NONE',  ( 13.53750000122903430, -4.330127018922194537, 2.499999999999995559 ) ) ;
#44055=CARTESIAN_POINT ( 'NONE',  ( -2.121784821874999949, 17.47812500061451502, -33.67503911421598417 ) ) ;
#44058=CARTESIAN_POINT ( 'NONE',  ( 28.49062500061451431, -3.027376345333614438, 5.243569643749998122 ) ) ;
#44059=DIRECTION ( 'NONE',  ( -1.000000000000000000, -0.000000000000000000, -0.000000000000000000 ) ) ;
#44060=CARTESIAN_POINT ( 'NONE',  ( 12.83437500061451786, -4.541064518000419881, 2.621784821874995952 ) ) ;
#44061=CARTESIAN_POINT ( 'NONE',  ( 26.39999999999999858, 0.000000000000000000, 4.999999999999998224 ) ) ;
#44063=CARTESIAN_POINT ( 'NONE',  ( 10.45312500061451644, 0.000000000000000000, 5.243569643749999010 ) ) ;
#44065=CARTESIAN_POINT ( 'NONE',  ( 21.94687500061451857, -3.027376345333610441, -5.243569643749999898 ) ) ;
#44067=ADVANCED_FACE ( 'NONE', ( #27836 ), #55765, .T. ) ;
#44068=CARTESIAN_POINT ( 'NONE',  ( 7.378125000614518036, -4.541064518000419881, 2.621784821874995952 ) ) ;
#44069=CARTESIAN_POINT ( 'NONE',  ( 12.79687500061451821, -3.027376345333614438, 5.243569643749998122 ) ) ;
#44070=ORIENTED_EDGE ( 'NONE', *, *, #16880, .T. ) ;
#44071=CARTESIAN_POINT ( 'NONE',  ( 24.49687500061451573, -3.027376345333614438, 5.243569643749998122 ) ) ;
#44072=CARTESIAN_POINT ( 'NONE',  ( 0.2791130135581331162, 5.000000000000003553, -34.00000000000001421 ) ) ;
#44073=CARTESIAN_POINT ( 'NONE',  ( 8.812500000000000000, 2.886751345948193936, 4.999999999999883649 ) ) ;
#44074=CARTESIAN_POINT ( 'NONE',  ( 4.462500000000001243, -5.773502691896255534, -1.060575238724906372E-15 ) ) ;
#44075=CARTESIAN_POINT ( 'NONE',  ( 14.25000000122903465, 5.773502691896255534, 3.535250795749688894E-16 ) ) ;
#44077=CARTESIAN_POINT ( 'NONE',  ( 17.28750000000000142, 5.773502691896255534, 3.535250795749688401E-16 ) ) ;
#44078=ORIENTED_EDGE ( 'NONE', *, *, #44436, .F. ) ;
#44079=CARTESIAN_POINT ( 'NONE',  ( 13.95000000000000107, -4.330127018922190985, -2.500000000000001332 ) ) ;
#44080=CARTESIAN_POINT ( 'NONE',  ( 15.56250000000000000, 2.886751345948126879, 4.999999999999999112 ) ) ;
#44081=ADVANCED_FACE ( 'NONE', ( #11094 ), #72795, .T. ) ;
#44082=CARTESIAN_POINT ( 'NONE',  ( 12.75000000122903643, -2.886751345948125991, -5.000000000000000000 ) ) ;
#44083=CARTESIAN_POINT ( 'NONE',  ( 12.47812500061451502, 6.421520780324663323E-16, -5.243569643749999010 ) ) ;
#44084=VERTEX_POINT ( 'NONE', #45446 ) ;
#44085=CARTESIAN_POINT ( 'NONE',  ( 8.437500000000000000, -2.886751345948129988, 4.999999999999997335 ) ) ;
#44086=CARTESIAN_POINT ( 'NONE',  ( -1.487416814333745711E-14, 15.72500000122903430, 34.00000000000000000 ) ) ;
#44087=CARTESIAN_POINT ( 'NONE',  ( 4.243569643749999898, 14.64687500061451964, -27.54997392385601529 ) ) ;
#44088=CARTESIAN_POINT ( 'NONE',  ( 3.628125000614518036, 4.541064518000418104, 2.621784821874999949 ) ) ;
#44090=CARTESIAN_POINT ( 'NONE',  ( 9.000000000000001776, -4.330127018922190985, -2.500000000000001332 ) ) ;
#44091=CARTESIAN_POINT ( 'NONE',  ( 3.837848076843223932, 3.204827942194517387, -3.837848076843223932 ) ) ;
#44092=ORIENTED_EDGE ( 'NONE', *, *, #10704, .F. ) ;
#44093=CARTESIAN_POINT ( 'NONE',  ( 25.19062500061451715, 6.054752690667223547, 3.707466751127219781E-16 ) ) ;
#44094=CARTESIAN_POINT ( 'NONE',  ( 29.43750000122903288, 6.123233995736764310E-16, -4.999999999999998224 ) ) ;
#44096=CARTESIAN_POINT ( 'NONE',  ( 22.09687500061451715, 6.054752690667223547, 3.707466751127219781E-16 ) ) ;
#44097=EDGE_CURVE ( 'NONE', #65143, #67926, #52938, .T. ) ;
#44098=CARTESIAN_POINT ( 'NONE',  ( 19.37812500061451715, 4.541064518000418104, 2.621784821874999949 ) ) ;
#44099=CARTESIAN_POINT ( 'NONE',  ( 4.243569643749999010, 11.06562500061459353, -32.45002607614398471 ) ) ;
#44100=CARTESIAN_POINT ( 'NONE',  ( 7.153125000614518392, 4.541064518000418104, -2.621784821874998173 ) ) ;
#44101=CARTESIAN_POINT ( 'NONE',  ( 3.365625000614516082, -6.054752690667223547, -1.112240025338166033E-15 ) ) ;
#44103=CARTESIAN_POINT ( 'NONE',  ( 20.57812500061451644, 6.421520780324663323E-16, -5.243569643749999010 ) ) ;
#44106=CARTESIAN_POINT ( 'NONE',  ( 16.24687500061451573, 6.054752690667223547, 3.707466751127219781E-16 ) ) ;
#44107=CARTESIAN_POINT ( 'NONE',  ( 14.25937500061451679, -4.541064518000417216, -2.621784821875001281 ) ) ;
#44108=CARTESIAN_POINT ( 'NONE',  ( 22.05937500061451573, 4.541064518000418104, -2.621784821874998173 ) ) ;
#44109=ORIENTED_EDGE ( 'NONE', *, *, #44978, .F. ) ;
#44110=CARTESIAN_POINT ( 'NONE',  ( 2.121784821874999061, 12.95937500061451786, 26.32496088578401583 ) ) ;
#44112=CARTESIAN_POINT ( 'NONE',  ( 26.01562500061451289, 3.027376345333613106, -5.243569643749998122 ) ) ;
#44113=CARTESIAN_POINT ( 'NONE',  ( 26.09062500061451573, 6.054752690667223547, 3.707466751127219781E-16 ) ) ;
#44115=CARTESIAN_POINT ( 'NONE',  ( 2.000000000000001332, 18.35000000000000142, 33.46410161513774995 ) ) ;
#44116=CARTESIAN_POINT ( 'NONE',  ( 5.859375000614519102, 4.541064518000418104, -2.621784821874998173 ) ) ;
#44118=CARTESIAN_POINT ( 'NONE',  ( 12.41250000122903430, 4.330127018922192761, -2.499999999999997780 ) ) ;
#44119=CARTESIAN_POINT ( 'NONE',  ( 9.412500001229034297, 0.000000000000000000, 4.999999999999998224 ) ) ;
#44120=CARTESIAN_POINT ( 'NONE',  ( 28.87500000122902932, -5.773502691896255534, -1.060575238724906372E-15 ) ) ;
#44123=CARTESIAN_POINT ( 'NONE',  ( 10.92187500061451644, 3.027376345333611329, 5.243569643749999010 ) ) ;
#44125=EDGE_LOOP ( 'NONE', ( #28004, #69892, #64312, #22082 ) ) ;
#44126=CARTESIAN_POINT ( 'NONE',  ( 18.66562500061451146, -6.054752690667223547, -1.112240025338166033E-15 ) ) ;
#44127=CARTESIAN_POINT ( 'NONE',  ( 12.68437500061451573, 4.541064518000418104, 2.621784821874999949 ) ) ;
#44128=CARTESIAN_POINT ( 'NONE',  ( 4.040625000614517681, 6.054752690667223547, 3.707466751127219781E-16 ) ) ;
#44129=CARTESIAN_POINT ( 'NONE',  ( 21.83437500061451786, -4.541064518000419881, 2.621784821874995952 ) ) ;
#44130=CARTESIAN_POINT ( 'NONE',  ( 6.065625000614516260, -6.054752690667223547, -1.112240025338166033E-15 ) ) ;
#44131=DIRECTION ( 'NONE',  ( -1.000000000000000000, -0.000000000000000000, -0.000000000000000000 ) ) ;
#44132=CARTESIAN_POINT ( 'NONE',  ( 6.787500001229032520, -4.330127018922194537, 2.499999999999995559 ) ) ;
#44133=CARTESIAN_POINT ( 'NONE',  ( 21.55312500061451431, 4.541064518000418104, -2.621784821874998173 ) ) ;
#44134=CARTESIAN_POINT ( 'NONE',  ( -3.999999999999999112, 16.96250000122903145, -30.00000000000000000 ) ) ;
#44135=CARTESIAN_POINT ( 'NONE',  ( 8.025000001229035007, 2.886751345948126879, 4.999999999999999112 ) ) ;
#44136=CARTESIAN_POINT ( 'NONE',  ( 16.45312500061451289, -4.541064518000417216, -2.621784821875001281 ) ) ;
#44137=CARTESIAN_POINT ( 'NONE',  ( 15.40312500061451573, 0.000000000000000000, 5.243569643749999010 ) ) ;
#44139=CARTESIAN_POINT ( 'NONE',  ( 15.71250000000000213, -5.773502691896255534, -1.060575238724906372E-15 ) ) ;
#44140=CARTESIAN_POINT ( 'NONE',  ( 12.52500000122903145, 2.886751345948126879, 4.999999999999999112 ) ) ;
#44141=CARTESIAN_POINT ( 'NONE',  ( 7.303125000614516082, 0.000000000000000000, 5.243569643749999010 ) ) ;
#44142=CARTESIAN_POINT ( 'NONE',  ( 10.45312500061451644, 0.000000000000000000, 5.243569643749999010 ) ) ;
#44144=CARTESIAN_POINT ( 'NONE',  ( 19.72500000122903074, 2.886751345948126879, 4.999999999999999112 ) ) ;
#44145=CARTESIAN_POINT ( 'NONE',  ( -4.243569643749997233, 12.69687500061451857, -27.54997392385601174 ) ) ;
#44146=CARTESIAN_POINT ( 'NONE',  ( 18.87187500061451573, 3.027376345333613106, -5.243569643749998122 ) ) ;
#44148=CARTESIAN_POINT ( 'NONE',  ( 5.812500001229035540, 0.000000000000000000, 4.999999999999998224 ) ) ;
#44149=CARTESIAN_POINT ( 'NONE',  ( 3.084375000614519191, 6.421520780324663323E-16, -5.243569643749999010 ) ) ;
#44150=CARTESIAN_POINT ( 'NONE',  ( 21.12187500061451573, 3.027376345333613106, -5.243569643749998122 ) ) ;
#44151=CARTESIAN_POINT ( 'NONE',  ( 12.33750000000000213, 5.773502691896255534, 3.535250795749688401E-16 ) ) ;
#44152=CARTESIAN_POINT ( 'NONE',  ( 15.89062500061451289, -3.027376345333614438, 5.243569643749998122 ) ) ;
#44154=CARTESIAN_POINT ( 'NONE',  ( -3.999999999999997335, 14.75000000122903288, 32.30940107675850470 ) ) ;
#44155=CARTESIAN_POINT ( 'NONE',  ( 4.462500000000001243, -5.773502691896255534, -1.060575238724906372E-15 ) ) ;
#44156=CARTESIAN_POINT ( 'NONE',  ( 29.03437500061451715, -4.541064518000419881, 2.621784821874995952 ) ) ;
#44159=CARTESIAN_POINT ( 'NONE',  ( 15.17812500061451608, 6.421520780324663323E-16, -5.243569643749999010 ) ) ;
#44160=CARTESIAN_POINT ( 'NONE',  ( 13.39687500061451608, -3.027376345333610441, -5.243569643749999898 ) ) ;
#44163=CARTESIAN_POINT ( 'NONE',  ( 23.09062500061451573, -3.027376345333614438, 5.243569643749998122 ) ) ;
#44164=FACE_OUTER_BOUND ( 'NONE', #49987, .T. ) ;
#44165=CARTESIAN_POINT ( 'NONE',  ( 28.76250000122903216, 0.000000000000000000, 4.999999999999998224 ) ) ;
#44166=CARTESIAN_POINT ( 'NONE',  ( 13.31250000000000178, 2.886751345948126879, 4.999999999999999112 ) ) ;
#44167=CARTESIAN_POINT ( 'NONE',  ( 24.00000000122902932, -2.886751345948125991, -5.000000000000000000 ) ) ;
#44168=CARTESIAN_POINT ( 'NONE',  ( 17.84062500061451573, -3.027376345333610441, -5.243569643749999898 ) ) ;
#44170=CARTESIAN_POINT ( 'NONE',  ( 19.94999999999999929, 4.330127018922192761, -2.499999999999997780 ) ) ;
#44172=CARTESIAN_POINT ( 'NONE',  ( 21.49687500061451573, -3.027376345333610441, -5.243569643749999898 ) ) ;
#44173=CARTESIAN_POINT ( 'NONE',  ( 28.22812500061451502, 6.421520780324663323E-16, -5.243569643749999010 ) ) ;
#44174=ORIENTED_EDGE ( 'NONE', *, *, #32854, .T. ) ;
#44175=CARTESIAN_POINT ( 'NONE',  ( 2.955228467731844333, 4.033190387708875946, -2.955228467731844333 ) ) ;
#44176=CARTESIAN_POINT ( 'NONE',  ( 11.84062500061451750, -3.027376345333614438, 5.243569643749998122 ) ) ;
#44177=CARTESIAN_POINT ( 'NONE',  ( 17.51250000122903216, 0.000000000000000000, 4.999999999999998224 ) ) ;
#44179=CARTESIAN_POINT ( 'NONE',  ( 15.93750000000000000, 5.773502691896255534, 3.535250795749688894E-16 ) ) ;
#44180=CARTESIAN_POINT ( 'NONE',  ( 23.96249999999999858, 2.886751345948129099, -4.999999999999998224 ) ) ;
#44181=CARTESIAN_POINT ( 'NONE',  ( -4.243569643749999898, 19.31562500061451715, 27.54997392385601529 ) ) ;
#44182=CARTESIAN_POINT ( 'NONE',  ( 3.684375000614518836, 4.541064518000418104, 2.621784821874999949 ) ) ;
#44183=CARTESIAN_POINT ( 'NONE',  ( 28.84687500061452070, 6.054752690667223547, 3.707466751127219781E-16 ) ) ;
#44184=VERTEX_POINT ( 'NONE', #44732 ) ;
#44185=CARTESIAN_POINT ( 'NONE',  ( 25.34062500061451217, -3.027376345333614438, 5.243569643749998122 ) ) ;
#44186=CARTESIAN_POINT ( 'NONE',  ( 27.68437500061451573, -4.541064518000419881, 2.621784821874995952 ) ) ;
#44188=CARTESIAN_POINT ( 'NONE',  ( 13.83749999999999858, -2.886751345948129988, 4.999999999999997335 ) ) ;
#44189=CARTESIAN_POINT ( 'NONE',  ( 11.57812500061451644, 6.421520780324663323E-16, -5.243569643749999010 ) ) ;
#44190=CARTESIAN_POINT ( 'NONE',  ( 3.748487153055565457, 3.308903755532668356, 3.979558567872137687 ) ) ;
#44191=DIRECTION ( 'NONE',  ( -0.000000000000000000, -1.000000000000000000, -0.000000000000000000 ) ) ;
#44192=CARTESIAN_POINT ( 'NONE',  ( 28.79062500061451502, 6.054752690667223547, 3.707466751127219781E-16 ) ) ;
#44193=CARTESIAN_POINT ( 'NONE',  ( 15.48750000122903359, 6.123233995736764310E-16, -4.999999999999998224 ) ) ;
#44196=CARTESIAN_POINT ( 'NONE',  ( 6.215625000614517504, 3.027376345333613106, -5.243569643749998122 ) ) ;
#44197=CARTESIAN_POINT ( 'NONE',  ( 22.77187500061451786, -6.054752690667223547, -1.112240025338166033E-15 ) ) ;
#44198=CARTESIAN_POINT ( 'NONE',  ( 4.243569643749999010, 14.27187500061451964, 27.54997392385601174 ) ) ;
#44199=CARTESIAN_POINT ( 'NONE',  ( 21.38437500061451502, -4.541064518000419881, 2.621784821874995952 ) ) ;
#44200=CARTESIAN_POINT ( 'NONE',  ( 28.80937500061451573, 4.541064518000418104, -2.621784821874998173 ) ) ;
#44201=CARTESIAN_POINT ( 'NONE',  ( -3.000416591977282496E-16, 17.94687500061451502, 25.09994784771203058 ) ) ;
#44202=CARTESIAN_POINT ( 'NONE',  ( 10.11562500061451608, -6.054752690667223547, -1.112240025338166033E-15 ) ) ;
#44203=CARTESIAN_POINT ( 'NONE',  ( 7.320879633048903241E-15, 17.30000000122903003, 26.00000000000000355 ) ) ;
#44204=CARTESIAN_POINT ( 'NONE',  ( 6.496875000614517504, -3.027376345333614438, 5.243569643749998122 ) ) ;
#44205=CARTESIAN_POINT ( 'NONE',  ( 3.972658874145789110, 3.036112888163414514, -4.275165627105516286 ) ) ;
#44206=CARTESIAN_POINT ( 'NONE',  ( 6.778125000614518392, 4.541064518000418104, 2.621784821874999949 ) ) ;
#44207=CARTESIAN_POINT ( 'NONE',  ( 12.75937500061451857, 0.000000000000000000, 5.243569643749999010 ) ) ;
#44209=CARTESIAN_POINT ( 'NONE',  ( 21.00000000122903288, 5.773502691896255534, 3.535250795749688894E-16 ) ) ;
#44210=CARTESIAN_POINT ( 'NONE',  ( 8.259375000614518569, 0.000000000000000000, 5.243569643749999010 ) ) ;
#44211=CARTESIAN_POINT ( 'NONE',  ( 10.60312500061451679, -4.541064518000417216, -2.621784821875001281 ) ) ;
#44212=CARTESIAN_POINT ( 'NONE',  ( 6.928125000614516082, -4.541064518000419881, 2.621784821874995952 ) ) ;
#44214=CARTESIAN_POINT ( 'NONE',  ( 20.18437500061451573, 6.421520780324663323E-16, -5.243569643749999010 ) ) ;
#44215=CARTESIAN_POINT ( 'NONE',  ( 18.18750000000000355, 5.773502691896255534, 3.535250795749688401E-16 ) ) ;
#44216=CARTESIAN_POINT ( 'NONE',  ( 11.57812500061451644, 6.421520780324663323E-16, -5.243569643749999010 ) ) ;
#44217=EDGE_CURVE ( 'NONE', #46571, #51638, #18405, .T. ) ;
#44218=CARTESIAN_POINT ( 'NONE',  ( 4.243569643749999898, 12.84687500061451715, -27.54997392385601529 ) ) ;
#44219=CARTESIAN_POINT ( 'NONE',  ( 14.17500000122903536, 2.886751345948129099, -4.999999999999998224 ) ) ;
#44220=CARTESIAN_POINT ( 'NONE',  ( -2.121784821874999949, 14.32812500061451644, -33.67503911421598417 ) ) ;
#44221=CARTESIAN_POINT ( 'NONE',  ( 15.63750000122903216, 4.330127018922191873, 2.499999999999999556 ) ) ;
#44222=CARTESIAN_POINT ( 'NONE',  ( 10.64062500061451644, -3.027376345333610441, -5.243569643749999898 ) ) ;
#44224=CARTESIAN_POINT ( 'NONE',  ( 13.57500000000000107, 6.123233995736764310E-16, -4.999999999999998224 ) ) ;
#44225=CARTESIAN_POINT ( 'NONE',  ( -0.6945881563830144101, 20.00000000000000000, 26.06076818491061076 ) ) ;
#44226=CARTESIAN_POINT ( 'NONE',  ( 23.84062500061451928, 6.054752690667223547, 3.707466751127219781E-16 ) ) ;
#44227=CARTESIAN_POINT ( 'NONE',  ( 7.059375000614518392, -4.541064518000417216, -2.621784821875001281 ) ) ;
#44228=ADVANCED_FACE ( 'NONE', ( #33622 ), #56874, .F. ) ;
#44229=CARTESIAN_POINT ( 'NONE',  ( 10.23750000122903359, 4.330127018922191873, 2.499999999999999556 ) ) ;
#44230=CARTESIAN_POINT ( 'NONE',  ( 19.35000000122903430, -2.886751345948129988, 4.999999999999997335 ) ) ;
#44231=CARTESIAN_POINT ( 'NONE',  ( 14.61562500061451608, -6.054752690667223547, -1.112240025338166033E-15 ) ) ;
#44232=CARTESIAN_POINT ( 'NONE',  ( 18.10312500061451502, 0.000000000000000000, 5.243569643749999010 ) ) ;
#44233=CARTESIAN_POINT ( 'NONE',  ( 25.98750000122903003, 4.330127018922191873, 2.499999999999999556 ) ) ;
#44234=CIRCLE ( 'NONE', #52438, 4.999999999999998224 ) ;
#44235=CARTESIAN_POINT ( 'NONE',  ( 27.33750000122903145, 4.330127018922191873, 2.499999999999999556 ) ) ;
#44236=CARTESIAN_POINT ( 'NONE',  ( 23.81250000000000000, -5.773502691896255534, -1.060575238724906372E-15 ) ) ;
#44239=CARTESIAN_POINT ( 'NONE',  ( 25.77187500061451075, 3.027376345333611329, 5.243569643749999010 ) ) ;
#44240=CARTESIAN_POINT ( 'NONE',  ( 4.898587196589411843E-16, 20.00000000000000000, 33.99999999999999289 ) ) ;
#44241=CARTESIAN_POINT ( 'NONE',  ( 13.68750000122903288, 6.123233995736764310E-16, -4.999999999999998224 ) ) ;
#44242=CARTESIAN_POINT ( 'NONE',  ( 29.03437500061451715, -4.541064518000419881, 2.621784821874995952 ) ) ;
#44244=CARTESIAN_POINT ( 'NONE',  ( 4.396875000614516971, -3.027376345333610441, -5.243569643749999898 ) ) ;
#44245=CARTESIAN_POINT ( 'NONE',  ( 25.79062500061451502, -3.027376345333614438, 5.243569643749998122 ) ) ;
#44248=CARTESIAN_POINT ( 'NONE',  ( 11.18437500061451928, 6.421520780324663323E-16, -5.243569643749999010 ) ) ;
#44249=CARTESIAN_POINT ( 'NONE',  ( 22.05000000122903003, -2.886751345948096681, 5.000000000000054179 ) ) ;
#44250=CARTESIAN_POINT ( 'NONE',  ( 29.76562500061451644, 3.027376345333611329, 5.243569643749999010 ) ) ;
#44251=CARTESIAN_POINT ( 'NONE',  ( 9.459375000614517859, 4.541064518000418104, -2.621784821874998173 ) ) ;
#44252=CARTESIAN_POINT ( 'NONE',  ( 27.87187500061451573, 3.027376345333613106, -5.243569643749998122 ) ) ;
#44254=CARTESIAN_POINT ( 'NONE',  ( 19.23749999999999716, -2.886751345948129988, 4.999999999999997335 ) ) ;
#44255=ORIENTED_EDGE ( 'NONE', *, *, #12948, .F. ) ;
#44256=CARTESIAN_POINT ( 'NONE',  ( 28.68749999999999645, -2.886751345948129988, 4.999999999999997335 ) ) ;
#44257=CARTESIAN_POINT ( 'NONE',  ( 3.600000000000002309, -4.330127018922190985, -2.500000000000001332 ) ) ;
#44258=VERTEX_POINT ( 'NONE', #50983 ) ;
#44259=CARTESIAN_POINT ( 'NONE',  ( 16.82812500061451644, -4.541064518000419881, 2.621784821874995952 ) ) ;
#44260=CARTESIAN_POINT ( 'NONE',  ( 8.015625000614518214, 3.027376345333613106, -5.243569643749998122 ) ) ;
#44262=CARTESIAN_POINT ( 'NONE',  ( 6.496875000614517504, -3.027376345333614438, 5.243569643749998122 ) ) ;
#44263=CARTESIAN_POINT ( 'NONE',  ( 18.30000000122903359, 5.773502691896255534, 3.535250795749688894E-16 ) ) ;
#44264=VECTOR ( 'NONE', #70889, 1000.000000000000000 ) ;
#44265=CARTESIAN_POINT ( 'NONE',  ( 15.67500000000000071, -4.330127018922194537, 2.499999999999995559 ) ) ;
#44266=CARTESIAN_POINT ( 'NONE',  ( 6.159375000614517148, -4.541064518000417216, -2.621784821875001281 ) ) ;
#44267=CARTESIAN_POINT ( 'NONE',  ( 11.55937500061451928, -4.541064518000417216, -2.621784821875001281 ) ) ;
#44268=CARTESIAN_POINT ( 'NONE',  ( 24.60937500061451644, -4.541064518000417216, -2.621784821875001281 ) ) ;
#44269=CARTESIAN_POINT ( 'NONE',  ( -3.999999999999999112, 16.36250000000000071, 27.69059892324149885 ) ) ;
#44272=CARTESIAN_POINT ( 'NONE',  ( 17.48437500061451999, 6.421520780324663323E-16, -5.243569643749999010 ) ) ;
#44273=VECTOR ( 'NONE', #71494, 1000.000000000000000 ) ;
#44274=CARTESIAN_POINT ( 'NONE',  ( 8.446875000614518569, -3.027376345333610441, -5.243569643749999898 ) ) ;
#44276=CARTESIAN_POINT ( 'NONE',  ( 19.79999999999999716, -4.330127018922190985, -2.500000000000001332 ) ) ;
#44278=CARTESIAN_POINT ( 'NONE',  ( 9.001249775931846008E-16, 10.97187500061451715, -25.09994784771203058 ) ) ;
#44280=CARTESIAN_POINT ( 'NONE',  ( 12.44062500061451537, -3.027376345333610441, -5.243569643749999898 ) ) ;
#44281=CARTESIAN_POINT ( 'NONE',  ( 28.43437500061451573, 4.541064518000418104, 2.621784821874999949 ) ) ;
#44282=CARTESIAN_POINT ( 'NONE',  ( 16.94999999999999929, 0.000000000000000000, 4.999999999999998224 ) ) ;
#44283=CARTESIAN_POINT ( 'NONE',  ( 28.17187500061451644, -6.054752690667223547, -1.112240025338166033E-15 ) ) ;
#44284=CARTESIAN_POINT ( 'NONE',  ( 10.57500000000000107, 4.330127018922191873, 2.499999999999999556 ) ) ;
#44285=CARTESIAN_POINT ( 'NONE',  ( -2.000000000000000000, 15.08750000122903501, 26.53589838486224650 ) ) ;
#44286=CARTESIAN_POINT ( 'NONE',  ( 9.825000001229033941, 2.886751345948126879, 4.999999999999999112 ) ) ;
#44287=AXIS2_PLACEMENT_3D ( 'NONE', #30199, #47192, #19092 ) ;
#44288=CARTESIAN_POINT ( 'NONE',  ( 19.69687500061451857, -3.027376345333610441, -5.243569643749999898 ) ) ;
#44289=CARTESIAN_POINT ( 'NONE',  ( 15.19687500061451857, -3.027376345333610441, -5.243569643749999898 ) ) ;
#44290=DIRECTION ( 'NONE',  ( -0.000000000000000000, -1.000000000000000000, -0.000000000000000000 ) ) ;
#44292=CARTESIAN_POINT ( 'NONE',  ( 17.99062500061451786, 6.054752690667223547, 3.707466751127219781E-16 ) ) ;
#44294=CARTESIAN_POINT ( 'NONE',  ( 2.953125000614516438, -4.541064518000417216, -2.621784821875001281 ) ) ;
#44295=CARTESIAN_POINT ( 'NONE',  ( 16.09687500061452070, -3.027376345333610441, -5.243569643749999898 ) ) ;
#44296=CARTESIAN_POINT ( 'NONE',  ( 5.603843221884248216, 8.282830004122001100, -27.84704757573690870 ) ) ;
#44297=CARTESIAN_POINT ( 'NONE',  ( 17.76562500061451644, -6.054752690667223547, -1.112240025338166033E-15 ) ) ;
#44298=CARTESIAN_POINT ( 'NONE',  ( 0.000000000000000000, 20.00000000000000000, 30.00000000000000000 ) ) ;
#44299=CARTESIAN_POINT ( 'NONE',  ( 25.28437500061451715, 4.541064518000418104, 2.621784821874999949 ) ) ;
#44300=CARTESIAN_POINT ( 'NONE',  ( -4.243569643749999898, 13.95312500061451821, 30.00000000000000000 ) ) ;
#44301=CARTESIAN_POINT ( 'NONE',  ( 14.59687500061452070, -3.027376345333614438, 5.243569643749998122 ) ) ;
#44302=CARTESIAN_POINT ( 'NONE',  ( 13.31250000122903288, 4.330127018922192761, -2.499999999999997780 ) ) ;
#44304=CARTESIAN_POINT ( 'NONE',  ( 4.243569643749999898, 19.63437500061451857, -30.00000000000000000 ) ) ;
#44306=CARTESIAN_POINT ( 'NONE',  ( 21.60937500061451644, 4.541064518000418104, -2.621784821874998173 ) ) ;
#44307=CARTESIAN_POINT ( 'NONE',  ( 22.83750000122903501, 4.330127018922191873, 2.499999999999999556 ) ) ;
#44308=CARTESIAN_POINT ( 'NONE',  ( 17.33437500061451431, -4.541064518000419881, 2.621784821874995952 ) ) ;
#44309=CARTESIAN_POINT ( 'NONE',  ( -4.243569643749999898, 13.10937500061451821, 30.00000000000000000 ) ) ;
#44310=CARTESIAN_POINT ( 'NONE',  ( 18.17812500061451786, -4.541064518000419881, 2.621784821874995952 ) ) ;
#44312=ORIENTED_EDGE ( 'NONE', *, *, #35309, .T. ) ;
#44313=CARTESIAN_POINT ( 'NONE',  ( 21.30000000000000071, 4.330127018922192761, -2.499999999999997780 ) ) ;
#44314=CARTESIAN_POINT ( 'NONE',  ( 17.39999999999999858, 0.000000000000000000, 4.999999999999998224 ) ) ;
#44315=CARTESIAN_POINT ( 'NONE',  ( 24.92812500061451431, -4.541064518000419881, 2.621784821874995952 ) ) ;
#44316=CARTESIAN_POINT ( 'NONE',  ( 4.753125000614515372, -4.541064518000417216, -2.621784821875001281 ) ) ;
#44317=CARTESIAN_POINT ( 'NONE',  ( 16.95000000122903216, 5.773502691896255534, 3.535250795749688894E-16 ) ) ;
#44318=CARTESIAN_POINT ( 'NONE',  ( 22.82812500061451644, 6.421520780324663323E-16, -5.243569643749999010 ) ) ;
#44319=CARTESIAN_POINT ( 'NONE',  ( 22.57499999999999929, 6.123233995736764310E-16, -4.999999999999998224 ) ) ;
#44320=CARTESIAN_POINT ( 'NONE',  ( 25.56562500061452070, 3.027376345333613106, -5.243569643749998122 ) ) ;
#44321=CARTESIAN_POINT ( 'NONE',  ( 6.778125000614518392, 4.541064518000418104, 2.621784821874999949 ) ) ;
#44322=ORIENTED_EDGE ( 'NONE', *, *, #4477, .F. ) ;
#44327=CARTESIAN_POINT ( 'NONE',  ( 3.999999999999999112, 18.87500000000000000, 30.00000000000000000 ) ) ;
#44328=CARTESIAN_POINT ( 'NONE',  ( -2.000000000000000000, 14.63750000122903394, -33.46410161513775705 ) ) ;
#44329=CARTESIAN_POINT ( 'NONE',  ( -3.000416591977282496E-16, 17.49687500061451573, -34.90005215228797653 ) ) ;
#44331=CARTESIAN_POINT ( 'NONE',  ( 8.474999999999999645, -4.330127018922194537, 2.499999999999995559 ) ) ;
#44333=CARTESIAN_POINT ( 'NONE',  ( 8.821875000614518569, -6.054752690667223547, -1.112240025338166033E-15 ) ) ;
#44334=CARTESIAN_POINT ( 'NONE',  ( 7.387500001229032165, 6.123233995736764310E-16, -4.999999999999998224 ) ) ;
#44335=CARTESIAN_POINT ( 'NONE',  ( 11.59687500061451892, -3.027376345333610441, -5.243569643749999898 ) ) ;
#44336=LINE ( 'NONE', #1084, #32690 ) ;
#44337=DIRECTION ( 'NONE',  ( -1.000000000000000000, -0.000000000000000000, -0.000000000000000000 ) ) ;
#44338=VECTOR ( 'NONE', #7170, 1000.000000000000000 ) ;
#44339=CARTESIAN_POINT ( 'NONE',  ( 19.68750000000000355, -2.886751345948163738, 4.999999999999939604 ) ) ;
#44340=CARTESIAN_POINT ( 'NONE',  ( 10.39687500061451786, 6.054752690667223547, 3.707466751127219781E-16 ) ) ;
#44341=CARTESIAN_POINT ( 'NONE',  ( 13.16250000000000142, 2.886751345948129099, -4.999999999999997335 ) ) ;
#44342=CARTESIAN_POINT ( 'NONE',  ( 20.54062500061451502, -3.027376345333610441, -5.243569643749999898 ) ) ;
#44344=( BOUNDED_CURVE ( )  B_SPLINE_CURVE ( 2, ( #13873, #3170, #19399, #25322, #63396, #47867, #24953 ),
 .UNSPECIFIED., .F., .F. ) 
 B_SPLINE_CURVE_WITH_KNOTS ( ( 3, 2, 2, 3 ),
 ( 0.6833333333333333481, 0.6861111111111111160, 0.6888888888888888840, 0.6916666666666666519 ),
 .UNSPECIFIED. ) 
 CURVE ( )  GEOMETRIC_REPRESENTATION_ITEM ( )  RATIONAL_B_SPLINE_CURVE ( ( 1.000000000000000000, 0.8660254037844387076, 1.000000000000000000, 0.8660254037844387076, 1.000000000000000000, 0.8660254037844387076, 1.000000000000000000 ) ) 
 REPRESENTATION_ITEM ( '' )  );
#44345=DIRECTION ( 'NONE',  ( -1.000000000000000000, -0.000000000000000000, -0.000000000000000000 ) ) ;
#44346=CARTESIAN_POINT ( 'NONE',  ( 23.25937500061451857, -4.541064518000417216, -2.621784821875001281 ) ) ;
#44349=EDGE_CURVE ( 'NONE', #30207, #8622, #5268, .T. ) ;
#44350=CARTESIAN_POINT ( 'NONE',  ( 28.83750000122903145, -4.330127018922194537, 2.499999999999995559 ) ) ;
#44352=CARTESIAN_POINT ( 'NONE',  ( 26.27812500061451573, -4.541064518000419881, 2.621784821874995952 ) ) ;
#44353=CARTESIAN_POINT ( 'NONE',  ( 15.21562500061451750, 3.027376345333613106, -5.243569643749998122 ) ) ;
#44355=CARTESIAN_POINT ( 'NONE',  ( 14.10937500061451644, 0.000000000000000000, 5.243569643749999010 ) ) ;
#44357=CARTESIAN_POINT ( 'NONE',  ( 24.00000000122902932, -2.886751345948125991, -5.000000000000000000 ) ) ;
#44358=CARTESIAN_POINT ( 'NONE',  ( 2.971875000614517592, -6.054752690667223547, -1.112240025338166033E-15 ) ) ;
#44359=CARTESIAN_POINT ( 'NONE',  ( 14.97187500061451892, 3.027376345333611329, 5.243569643749999010 ) ) ;
#44362=CARTESIAN_POINT ( 'NONE',  ( 23.59687500061451715, -3.027376345333614438, 5.243569643749998122 ) ) ;
#44363=CARTESIAN_POINT ( 'NONE',  ( 16.05937500061451573, -4.541064518000417216, -2.621784821875001281 ) ) ;
#44365=CARTESIAN_POINT ( 'NONE',  ( 27.37500000000000000, -4.330127018922194537, 2.499999999999995559 ) ) ;
#44366=CARTESIAN_POINT ( 'NONE',  ( 3.262500001229035718, -4.330127018922190985, -2.500000000000001332 ) ) ;
#44367=CARTESIAN_POINT ( 'NONE',  ( 4.650000000000001243, 4.330127018922192761, -2.499999999999997780 ) ) ;
#44369=CARTESIAN_POINT ( 'NONE',  ( 19.04062500061451146, -3.027376345333614438, 5.243569643749998122 ) ) ;
#44370=CARTESIAN_POINT ( 'NONE',  ( 10.20000000000000107, 0.000000000000000000, 4.999999999999998224 ) ) ;
#44371=CARTESIAN_POINT ( 'NONE',  ( 4.565625000614516260, 3.027376345333611329, 5.243569643749999010 ) ) ;
#44372=CARTESIAN_POINT ( 'NONE',  ( 17.36249999999999716, 2.886751345948126879, 4.999999999999999112 ) ) ;
#44373=( BOUNDED_CURVE ( )  B_SPLINE_CURVE ( 2, ( #47492, #14232, #30861, #41955, #19768, #65575, #8331, #53770, #64476 ),
 .UNSPECIFIED., .F., .T. ) 
 B_SPLINE_CURVE_WITH_KNOTS ( ( 3, 2, 2, 2, 3 ),
 ( 0.4021739130434782705, 0.4057971014492753881, 0.4130434782608695676, 0.4202898550724637472, 0.4239130434782608647 ),
 .UNSPECIFIED. ) 
 CURVE ( )  GEOMETRIC_REPRESENTATION_ITEM ( )  RATIONAL_B_SPLINE_CURVE ( ( 0.9330127018922194093, 0.9330127018922194093, 1.000000000000000000, 0.8660254037844387076, 1.000000000000000000, 0.8660254037844387076, 1.000000000000000000, 0.9330127018922194093, 0.9330127018922194093 ) ) 
 REPRESENTATION_ITEM ( '' )  );
#44375=CARTESIAN_POINT ( 'NONE',  ( 21.30000000122903359, -2.886751345948125991, -5.000000000000000000 ) ) ;
#44377=CARTESIAN_POINT ( 'NONE',  ( 25.99687500061451928, -3.027376345333610441, -5.243569643749999898 ) ) ;
#44379=EDGE_LOOP ( 'NONE', ( #13062, #10739, #476, #20063 ) ) ;
#44380=CARTESIAN_POINT ( 'NONE',  ( 16.19062500061451715, 6.054752690667223547, 3.707466751127219781E-16 ) ) ;
#44381=CARTESIAN_POINT ( 'NONE',  ( 24.29062500061451502, 6.054752690667223547, 3.707466751127219781E-16 ) ) ;
#44382=CARTESIAN_POINT ( 'NONE',  ( 21.34687500061451715, -3.027376345333614438, 5.243569643749998122 ) ) ;
#44383=CARTESIAN_POINT ( 'NONE',  ( 7.312500000000000000, 2.886751345948129099, -4.999999999999998224 ) ) ;
#44384=CARTESIAN_POINT ( 'NONE',  ( 10.04062500061451502, -3.027376345333614438, 5.243569643749998122 ) ) ;
#44385=CARTESIAN_POINT ( 'NONE',  ( 23.69062500061451004, -3.027376345333610441, -5.243569643749999898 ) ) ;
#44386=CARTESIAN_POINT ( 'NONE',  ( 15.45937500061451608, 0.000000000000000000, 5.243569643749999010 ) ) ;
#44387=CARTESIAN_POINT ( 'NONE',  ( 18.98437500061451644, 4.541064518000418104, 2.621784821874999949 ) ) ;
#44388=CARTESIAN_POINT ( 'NONE',  ( 19.38750000000000284, -2.886751345948193048, -4.999999999999883649 ) ) ;
#44389=CARTESIAN_POINT ( 'NONE',  ( 4.243569643749999898, 19.57812500061451644, 30.00000000000000000 ) ) ;
#44390=CARTESIAN_POINT ( 'NONE',  ( 21.67500000122903359, -5.773502691896255534, -1.060575238724906372E-15 ) ) ;
#44392=CARTESIAN_POINT ( 'NONE',  ( 12.10312500061451857, 4.541064518000418104, -2.621784821874998173 ) ) ;
#44393=CARTESIAN_POINT ( 'NONE',  ( 8.971875000614515372, 3.027376345333613106, -5.243569643749998122 ) ) ;
#44394=CARTESIAN_POINT ( 'NONE',  ( 6.759375000614516793, 4.541064518000418104, -2.621784821874998173 ) ) ;
#44396=CARTESIAN_POINT ( 'NONE',  ( 27.38437500061451857, 6.421520780324663323E-16, -5.243569643749999010 ) ) ;
#44397=CARTESIAN_POINT ( 'NONE',  ( 20.09062500061451573, -3.027376345333610441, -5.243569643749999898 ) ) ;
#44398=CARTESIAN_POINT ( 'NONE',  ( 28.61250000122903359, 4.330127018922192761, -2.499999999999997780 ) ) ;
#44399=CARTESIAN_POINT ( 'NONE',  ( 27.25312500061451360, -4.541064518000417216, -2.621784821875001281 ) ) ;
#44400=CARTESIAN_POINT ( 'NONE',  ( 23.93437500061451573, 4.541064518000418104, 2.621784821874999949 ) ) ;
#44401=CARTESIAN_POINT ( 'NONE',  ( 20.54062500061451502, -3.027376345333610441, -5.243569643749999898 ) ) ;
#44402=CARTESIAN_POINT ( 'NONE',  ( 2.121784821875001281, 18.65937500061451715, 33.67503911421598417 ) ) ;
#44403=CARTESIAN_POINT ( 'NONE',  ( 25.64062500061451644, 6.054752690667223547, 3.707466751127219781E-16 ) ) ;
#44404=CARTESIAN_POINT ( 'NONE',  ( 3.600000001229033408, -2.886751345948129988, 4.999999999999997335 ) ) ;
#44405=ORIENTED_EDGE ( 'NONE', *, *, #43499, .T. ) ;
#44406=CARTESIAN_POINT ( 'NONE',  ( 27.41250000000000142, -5.773502691896255534, -1.060575238724906372E-15 ) ) ;
#44407=CARTESIAN_POINT ( 'NONE',  ( -3.999999999999997335, 15.53749999999999964, -27.69059892324149175 ) ) ;
#44409=CARTESIAN_POINT ( 'NONE',  ( 5.671875000614519102, -6.054752690667223547, -1.112240025338166033E-15 ) ) ;
#44410=CARTESIAN_POINT ( 'NONE',  ( 13.15312500061451750, 0.000000000000000000, 5.243569643749999010 ) ) ;
#44411=CARTESIAN_POINT ( 'NONE',  ( 6.984375000614516438, -4.541064518000419881, 2.621784821874995952 ) ) ;
#44412=CARTESIAN_POINT ( 'NONE',  ( 25.53750000122903074, 4.330127018922191873, 2.499999999999999556 ) ) ;
#44413=CARTESIAN_POINT ( 'NONE',  ( 14.25937500061451679, -4.541064518000417216, -2.621784821875001281 ) ) ;
#44414=CARTESIAN_POINT ( 'NONE',  ( 3.496875000614518836, -3.027376345333610441, -5.243569643749999898 ) ) ;
#44415=CARTESIAN_POINT ( 'NONE',  ( 28.98750000000000071, 5.773502691896255534, 3.535250795749688894E-16 ) ) ;
#44416=CARTESIAN_POINT ( 'NONE',  ( 27.60937500061451644, 0.000000000000000000, 5.243569643749999010 ) ) ;
#44417=CARTESIAN_POINT ( 'NONE',  ( 3.628125000614518036, 4.541064518000418104, 2.621784821874999949 ) ) ;
#44418=CARTESIAN_POINT ( 'NONE',  ( 13.07812500061451821, 4.541064518000418104, 2.621784821874999949 ) ) ;
#44419=ORIENTED_EDGE ( 'NONE', *, *, #30054, .F. ) ;
#44420=CARTESIAN_POINT ( 'NONE',  ( 10.41562500061451679, 3.027376345333611329, 5.243569643749999010 ) ) ;
#44421=CARTESIAN_POINT ( 'NONE',  ( 7.453125000614516438, -4.541064518000417216, -2.621784821875001281 ) ) ;
#44423=CARTESIAN_POINT ( 'NONE',  ( 7.950000000000001954, 0.000000000000000000, 4.999999999999998224 ) ) ;
#44424=DIRECTION ( 'NONE',  ( -1.000000000000000000, -0.000000000000000000, -0.000000000000000000 ) ) ;
#44425=CARTESIAN_POINT ( 'NONE',  ( 18.67500000000000071, 4.330127018922191873, 2.499999999999999556 ) ) ;
#44426=CARTESIAN_POINT ( 'NONE',  ( 18.79687500061451644, -3.027376345333610441, -5.243569643749999898 ) ) ;
#44427=CARTESIAN_POINT ( 'NONE',  ( 14.02500000122903323, -5.773502691896255534, -1.060575238724906372E-15 ) ) ;
#44430=CARTESIAN_POINT ( 'NONE',  ( -2.121784821874996840, 15.37812500061451892, -26.32496088578401583 ) ) ;
#44434=CARTESIAN_POINT ( 'NONE',  ( 27.25312500061451360, -4.541064518000417216, -2.621784821875001281 ) ) ;
#44435=CARTESIAN_POINT ( 'NONE',  ( 27.41250000000000142, -5.773502691896255534, -1.060575238724906372E-15 ) ) ;
#44436=EDGE_CURVE ( 'NONE', #16881, #12792, #63292, .T. ) ;
#44437=CARTESIAN_POINT ( 'NONE',  ( 8.765625000614518214, -6.054752690667223547, -1.112240025338166033E-15 ) ) ;
#44439=CARTESIAN_POINT ( 'NONE',  ( 21.57187500061451502, 3.027376345333613106, -5.243569643749998122 ) ) ;
#44441=CARTESIAN_POINT ( 'NONE',  ( 6.890625000614516438, -3.027376345333614438, 5.243569643749998122 ) ) ;
#44442=CARTESIAN_POINT ( 'NONE',  ( 9.609375000614518214, 0.000000000000000000, 5.243569643749999010 ) ) ;
#44444=CARTESIAN_POINT ( 'NONE',  ( 21.49687500061451573, -3.027376345333610441, -5.243569643749999898 ) ) ;
#44446=CARTESIAN_POINT ( 'NONE',  ( 28.98750000000000071, 5.773502691896255534, 3.535250795749688894E-16 ) ) ;
#44447=CARTESIAN_POINT ( 'NONE',  ( 4.050000000000001599, -4.330127018922190985, -2.500000000000001332 ) ) ;
#44448=CARTESIAN_POINT ( 'NONE',  ( 14.02500000122903323, -5.773502691896255534, -1.060575238724906372E-15 ) ) ;
#44449=LINE ( 'NONE', #56599, #50240 ) ;
#44450=CARTESIAN_POINT ( 'NONE',  ( 3.807538167735159185, -3.240779705755961526, 4.122180188640082399 ) ) ;
#44451=VERTEX_POINT ( 'NONE', #57236 ) ;
#44452=CARTESIAN_POINT ( 'NONE',  ( 11.88749999999999751, 5.773502691896255534, 3.535250795749688894E-16 ) ) ;
#44453=CARTESIAN_POINT ( 'NONE',  ( 15.71250000000000213, -5.773502691896255534, -1.060575238724906372E-15 ) ) ;
#44454=CARTESIAN_POINT ( 'NONE',  ( 12.67500000122903536, -5.773502691896255534, -1.060575238724906372E-15 ) ) ;
#44455=CARTESIAN_POINT ( 'NONE',  ( 11.01562500061451821, -6.054752690667223547, -1.112240025338166033E-15 ) ) ;
#44456=ORIENTED_EDGE ( 'NONE', *, *, #40764, .F. ) ;
#44457=CARTESIAN_POINT ( 'NONE',  ( 10.01250000000000107, 2.886751345948129099, -4.999999999999998224 ) ) ;
#44458=CARTESIAN_POINT ( 'NONE',  ( 18.52500000122903145, -5.773502691896255534, -1.060575238724906372E-15 ) ) ;
#44459=CARTESIAN_POINT ( 'NONE',  ( -2.121784821874999949, 15.73437500061451644, -33.67503911421598417 ) ) ;
#44460=CARTESIAN_POINT ( 'NONE',  ( 28.87500000122902932, -5.773502691896255534, -1.060575238724906372E-15 ) ) ;
#44462=CARTESIAN_POINT ( 'NONE',  ( 10.57500000000000107, 4.330127018922191873, 2.499999999999999556 ) ) ;
#44463=CARTESIAN_POINT ( 'NONE',  ( 3.114784886354099669, 3.911322423985381658, 3.293568724887664168 ) ) ;
#44465=CARTESIAN_POINT ( 'NONE',  ( 25.15312500061451217, 4.541064518000418104, -2.621784821874998173 ) ) ;
#44467=VECTOR ( 'NONE', #28756, 1000.000000000000000 ) ;
#44468=CARTESIAN_POINT ( 'NONE',  ( 29.07187500061451502, -6.054752690667223547, -1.112240025338166033E-15 ) ) ;
#44469=CARTESIAN_POINT ( 'NONE',  ( 20.44687500061451857, -3.027376345333614438, 5.243569643749998122 ) ) ;
#44470=CARTESIAN_POINT ( 'NONE',  ( 17.91562500061451502, 3.027376345333613106, -5.243569643749998122 ) ) ;
#44471=CARTESIAN_POINT ( 'NONE',  ( -3.000416591977282496E-16, 11.14062500061459637, -34.90005215228797653 ) ) ;
#44472=CARTESIAN_POINT ( 'NONE',  ( 5.465625000614517504, 3.027376345333611329, 5.243569643749999010 ) ) ;
#44473=CARTESIAN_POINT ( 'NONE',  ( 28.65000000122903145, 5.773502691896255534, 3.535250795749688894E-16 ) ) ;
#44475=CARTESIAN_POINT ( 'NONE',  ( 20.20312500061451644, 4.541064518000418104, -2.621784821874998173 ) ) ;
#44478=CARTESIAN_POINT ( 'NONE',  ( 15.49687500061451750, -3.027376345333614438, 5.243569643749998122 ) ) ;
#44479=CARTESIAN_POINT ( 'NONE',  ( 15.42187500061451821, 3.027376345333611329, 5.243569643749999010 ) ) ;
#44480=CARTESIAN_POINT ( 'NONE',  ( 21.68437500061451573, 4.541064518000418104, 2.621784821874999949 ) ) ;
#44482=CARTESIAN_POINT ( 'NONE',  ( -3.000416591977282496E-16, 12.54687500061451999, 25.09994784771203058 ) ) ;
#44483=DIRECTION ( 'NONE',  ( -1.000000000000000000, -0.000000000000000000, -0.000000000000000000 ) ) ;
#44484=CARTESIAN_POINT ( 'NONE',  ( 26.05312500061451431, 4.541064518000418104, -2.621784821874998173 ) ) ;
#44485=CARTESIAN_POINT ( 'NONE',  ( 27.96562500061451928, 3.027376345333611329, 5.243569643749999010 ) ) ;
#44486=CARTESIAN_POINT ( 'NONE',  ( 4.000000000000000000, 16.13749999999999929, 32.30940107675849049 ) ) ;
#44488=CARTESIAN_POINT ( 'NONE',  ( 5.896875000614518747, 6.054752690667223547, 3.707466751127219781E-16 ) ) ;
#44489=CARTESIAN_POINT ( 'NONE',  ( 12.11250000122903181, 0.000000000000000000, 4.999999999999998224 ) ) ;
#44490=CARTESIAN_POINT ( 'NONE',  ( 6.712500001229034119, 0.000000000000000000, 4.999999999999998224 ) ) ;
#44491=CARTESIAN_POINT ( 'NONE',  ( 29.66250000122903074, 0.000000000000000000, 4.999999999999998224 ) ) ;
#44494=CARTESIAN_POINT ( 'NONE',  ( 12.00937500061451857, -4.541064518000417216, -2.621784821875001281 ) ) ;
#44497=CARTESIAN_POINT ( 'NONE',  ( 20.72812500061451502, 4.541064518000418104, 2.621784821874999949 ) ) ;
#44498=CARTESIAN_POINT ( 'NONE',  ( 14.40937500061451715, 4.541064518000418104, -2.621784821874998173 ) ) ;
#44499=CARTESIAN_POINT ( 'NONE',  ( 4.978125000614518569, 4.541064518000418104, 2.621784821874999949 ) ) ;
#44500=CARTESIAN_POINT ( 'NONE',  ( 21.15937500061451715, 4.541064518000418104, -2.621784821874998173 ) ) ;
#44501=CARTESIAN_POINT ( 'NONE',  ( 10.58437500061451964, -4.541064518000419881, 2.621784821874995952 ) ) ;
#44502=CARTESIAN_POINT ( 'NONE',  ( 5.615625000614517859, -6.054752690667223547, -1.112240025338166033E-15 ) ) ;
#44503=CARTESIAN_POINT ( 'NONE',  ( 10.98750000122903536, 6.123233995736764310E-16, -4.999999999999998224 ) ) ;
#44504=CARTESIAN_POINT ( 'NONE',  ( 5.512500001229033941, -4.330127018922190985, -2.500000000000001332 ) ) ;
#44505=CARTESIAN_POINT ( 'NONE',  ( 19.86562500061451786, 3.027376345333611329, 5.243569643749999010 ) ) ;
#44506=CARTESIAN_POINT ( 'NONE',  ( 7.575000001229033053, 2.886751345948126879, 4.999999999999999112 ) ) ;
#44507=CARTESIAN_POINT ( 'NONE',  ( 16.19062500061451715, 6.054752690667223547, 3.707466751127219781E-16 ) ) ;
#44508=CARTESIAN_POINT ( 'NONE',  ( 16.19062500061451715, 6.054752690667223547, 3.707466751127219781E-16 ) ) ;
#44510=CARTESIAN_POINT ( 'NONE',  ( 14.88750000000000107, -2.886751345948125991, -5.000000000000000000 ) ) ;
#44511=CARTESIAN_POINT ( 'NONE',  ( 10.42500000122903536, -5.773502691896255534, -1.060575238724906372E-15 ) ) ;
#44512=CARTESIAN_POINT ( 'NONE',  ( 8.990625000614516082, 6.054752690667223547, 3.707466751127219781E-16 ) ) ;
#44513=CARTESIAN_POINT ( 'NONE',  ( 11.24062500061451608, 6.054752690667223547, 3.707466751127219781E-16 ) ) ;
#44514=CARTESIAN_POINT ( 'NONE',  ( 22.05000000122903714, -2.886751345948129988, 4.999999999999997335 ) ) ;
#44516=CARTESIAN_POINT ( 'NONE',  ( 2.121784821874999061, 12.50937500061451857, -33.67503911421598417 ) ) ;
#44517=CARTESIAN_POINT ( 'NONE',  ( 0.000000000000000000, 20.00000000000000000, 30.00000000000000000 ) ) ;
#44518=EDGE_CURVE ( 'NONE', #52358, #35925, #48654, .T. ) ;
#44519=CARTESIAN_POINT ( 'NONE',  ( 3.300000001229034918, -2.886751345948125991, -5.000000000000000000 ) ) ;
#44520=VECTOR ( 'NONE', #41452, 1000.000000000000000 ) ;
#44521=CARTESIAN_POINT ( 'NONE',  ( 5.071875000614519458, 3.027376345333611329, 5.243569643749999010 ) ) ;
#44522=CARTESIAN_POINT ( 'NONE',  ( 19.65937500061451360, -4.541064518000417216, -2.621784821875001281 ) ) ;
#44524=CARTESIAN_POINT ( 'NONE',  ( 15.47812500061451679, -4.541064518000419881, 2.621784821874995952 ) ) ;
#44526=CARTESIAN_POINT ( 'NONE',  ( -1.071796769724483234, 15.40759618943233811, -34.00000000000000711 ) ) ;
#44527=CARTESIAN_POINT ( 'NONE',  ( 14.47499999999999964, 6.123233995736764310E-16, -4.999999999999998224 ) ) ;
#44528=CARTESIAN_POINT ( 'NONE',  ( 28.13437500061451502, -4.541064518000419881, 2.621784821874995952 ) ) ;
#44530=CARTESIAN_POINT ( 'NONE',  ( 14.09062500061451750, -3.027376345333614438, 5.243569643749998122 ) ) ;
#44531=CARTESIAN_POINT ( 'NONE',  ( 11.33437500061451608, 4.541064518000418104, 2.621784821874999949 ) ) ;
#44532=ORIENTED_EDGE ( 'NONE', *, *, #68656, .T. ) ;
#44533=B_SPLINE_CURVE_WITH_KNOTS ( 'NONE', 3,
 ( #15207, #70633, #43669, #14479, #71002, #2673, #8578, #25190, #20378, #47734 ),
 .UNSPECIFIED., .F., .F.,
 ( 4, 3, 3, 4 ),
 ( 1.830297688535119174E-16, 0.0001572358266159529683, 0.0003242863666395115214, 0.0004914386806651677500 ),
 .UNSPECIFIED. ) ;
#44534=CARTESIAN_POINT ( 'NONE',  ( 29.09062500061451573, -3.027376345333610441, -5.243569643749999898 ) ) ;
#44535=CARTESIAN_POINT ( 'NONE',  ( 22.82812500061451644, 6.421520780324663323E-16, -5.243569643749999010 ) ) ;
#44536=CYLINDRICAL_SURFACE ( 'NONE', #59265, 4.000000000000000000 ) ;
#44538=CARTESIAN_POINT ( 'NONE',  ( 11.70000000000000284, -4.330127018922190985, -2.500000000000001332 ) ) ;
#44539=CARTESIAN_POINT ( 'NONE',  ( 20.73750000122903359, -4.330127018922194537, 2.499999999999995559 ) ) ;
#44540=CARTESIAN_POINT ( 'NONE',  ( 16.71562500061451573, 3.027376345333611329, 5.243569643749999010 ) ) ;
#44543=CARTESIAN_POINT ( 'NONE',  ( 19.68750000000000355, -2.886751345948129988, 4.999999999999997335 ) ) ;
#44544=CARTESIAN_POINT ( 'NONE',  ( 21.34687500061451715, -3.027376345333614438, 5.243569643749998122 ) ) ;
#44545=CARTESIAN_POINT ( 'NONE',  ( 26.84062500061451573, -3.027376345333610441, -5.243569643749999898 ) ) ;
#44546=ORIENTED_EDGE ( 'NONE', *, *, #21079, .F. ) ;
#44548=CARTESIAN_POINT ( 'NONE',  ( 9.515625000614518214, 3.027376345333611329, 5.243569643749999010 ) ) ;
#44549=CARTESIAN_POINT ( 'NONE',  ( 6.262500000000000178, -5.773502691896255534, -1.060575238724906372E-15 ) ) ;
#44550=CARTESIAN_POINT ( 'NONE',  ( 16.98750000000000426, -2.886751345948129988, 4.999999999999997335 ) ) ;
#44551=CARTESIAN_POINT ( 'NONE',  ( 25.31250000000000000, 2.886751345948129099, -4.999999999999998224 ) ) ;
#44552=CARTESIAN_POINT ( 'NONE',  ( -4.243569643749997233, 18.94062500061451715, 32.45002607614398471 ) ) ;
#44553=CARTESIAN_POINT ( 'NONE',  ( 3.871875000614519280, -6.054752690667223547, -1.112240025338166033E-15 ) ) ;
#44554=CARTESIAN_POINT ( 'NONE',  ( 29.44687500061451857, -3.027376345333614438, 5.243569643749998122 ) ) ;
#44555=ORIENTED_EDGE ( 'NONE', *, *, #39198, .F. ) ;
#44556=CARTESIAN_POINT ( 'NONE',  ( 24.25312500061451715, 4.541064518000418104, -2.621784821874998173 ) ) ;
#44557=CARTESIAN_POINT ( 'NONE',  ( 24.49687500061451573, -3.027376345333614438, 5.243569643749998122 ) ) ;
#44558=CARTESIAN_POINT ( 'NONE',  ( -3.000416591977282496E-16, 19.24062500061459247, -34.90005215228797653 ) ) ;
#44559=CARTESIAN_POINT ( 'NONE',  ( 13.91249999999999964, -5.773502691896255534, -1.060575238724906372E-15 ) ) ;
#44560=CARTESIAN_POINT ( 'NONE',  ( 7.865625000614516971, -6.054752690667223547, -1.112240025338166033E-15 ) ) ;
#44561=CARTESIAN_POINT ( 'NONE',  ( 3.709174336338540989, 3.352913023424228811, 4.031500572517469294 ) ) ;
#44563=CARTESIAN_POINT ( 'NONE',  ( 25.45312500061451644, -4.541064518000417216, -2.621784821875001281 ) ) ;
#44564=CARTESIAN_POINT ( 'NONE',  ( 15.67500000122903181, 2.886751345948126879, 4.999999999999999112 ) ) ;
#44568=CARTESIAN_POINT ( 'NONE',  ( 19.99687500061451573, -3.027376345333614438, 5.243569643749998122 ) ) ;
#44569=CARTESIAN_POINT ( 'NONE',  ( -3.000416591977282496E-16, 13.89687500061451786, 25.09994784771203058 ) ) ;
#44570=CARTESIAN_POINT ( 'NONE',  ( 21.00937500061451857, -4.541064518000417216, -2.621784821875001281 ) ) ;
#44571=CARTESIAN_POINT ( 'NONE',  ( 29.59687500061451715, -3.027376345333610441, -5.243569643749999898 ) ) ;
#44572=CARTESIAN_POINT ( 'NONE',  ( -4.243569643749999898, 18.50937500061451857, 30.00000000000000000 ) ) ;
#44573=CARTESIAN_POINT ( 'NONE',  ( 10.90312500061451928, 0.000000000000000000, 5.243569643749999010 ) ) ;
#44574=CARTESIAN_POINT ( 'NONE',  ( 6.309375000614517504, 4.541064518000418104, -2.621784821874998173 ) ) ;
#44575=CARTESIAN_POINT ( 'NONE',  ( 7.425000001229032698, 2.886751345948062486, -5.000000000000113687 ) ) ;
#44576=CARTESIAN_POINT ( 'NONE',  ( 7.603125000614517681, 4.541064518000418104, -2.621784821874998173 ) ) ;
#44577=CARTESIAN_POINT ( 'NONE',  ( 11.93437500061451573, -4.541064518000419881, 2.621784821874995952 ) ) ;
#44578=SHAPE_REPRESENTATION_RELATIONSHIP ( 'NONE' , 'NONE' ,  #13196, #47954 ) ;
#44579=CARTESIAN_POINT ( 'NONE',  ( 19.53750000122903430, 6.123233995736764310E-16, -4.999999999999998224 ) ) ;
#44580=CARTESIAN_POINT ( 'NONE',  ( 8.109375000614518214, 4.541064518000418104, -2.621784821874998173 ) ) ;
#44581=CARTESIAN_POINT ( 'NONE',  ( 9.628125000614517148, -4.541064518000419881, 2.621784821874995952 ) ) ;
#44582=CARTESIAN_POINT ( 'NONE',  ( 6.178125000614518747, 6.421520780324663323E-16, -5.243569643749999010 ) ) ;
#44584=CARTESIAN_POINT ( 'NONE',  ( 18.79687500061451644, -3.027376345333610441, -5.243569643749999898 ) ) ;
#44586=CARTESIAN_POINT ( 'NONE',  ( 27.92812500061451431, 4.541064518000418104, 2.621784821874999949 ) ) ;
#44587=CARTESIAN_POINT ( 'NONE',  ( 11.35312500061451679, 0.000000000000000000, 5.243569643749999010 ) ) ;
#44588=CARTESIAN_POINT ( 'NONE',  ( 29.74687500061451573, 6.054752690667223547, 3.707466751127219781E-16 ) ) ;
#44589=CARTESIAN_POINT ( 'NONE',  ( 2.121784821874999061, 12.95937500061451786, -33.67503911421598417 ) ) ;
#44590=CARTESIAN_POINT ( 'NONE',  ( 13.23750000122903359, 6.123233995736764310E-16, -4.999999999999998224 ) ) ;
#44591=( BOUNDED_CURVE ( )  B_SPLINE_CURVE ( 2, ( #536, #7153, #62219, #57387, #6794, #17500, #63296, #51858, #34495 ),
 .UNSPECIFIED., .F., .F. ) 
 B_SPLINE_CURVE_WITH_KNOTS ( ( 3, 2, 2, 2, 3 ),
 ( 0.2934782608695652439, 0.2971014492753623060, 0.3043478260869565410, 0.3115942028985507206, 0.3152173913043478382 ),
 .UNSPECIFIED. ) 
 CURVE ( )  GEOMETRIC_REPRESENTATION_ITEM ( )  RATIONAL_B_SPLINE_CURVE ( ( 0.9330127018922194093, 0.9330127018922198534, 1.000000000000000000, 0.8660254037844387076, 1.000000000000000000, 0.8660254037844387076, 1.000000000000000000, 0.9330127018922188542, 0.9330127018922194093 ) ) 
 REPRESENTATION_ITEM ( '' )  );
#44593=CARTESIAN_POINT ( 'NONE',  ( 4.243569643749999010, 16.46562500061451573, -32.45002607614398471 ) ) ;
#44594=CARTESIAN_POINT ( 'NONE',  ( 14.85000000122903252, -2.886751345948129988, 4.999999999999997335 ) ) ;
#44595=CARTESIAN_POINT ( 'NONE',  ( 9.253125000614517148, -4.541064518000417216, -2.621784821875001281 ) ) ;
#44596=CARTESIAN_POINT ( 'NONE',  ( 14.17500000000000071, 4.330127018922191873, 2.499999999999999556 ) ) ;
#44598=CARTESIAN_POINT ( 'NONE',  ( 22.45312500061451644, 4.541064518000418104, -2.621784821874998173 ) ) ;
#44599=CARTESIAN_POINT ( 'NONE',  ( 8.709375000614517859, 0.000000000000000000, 5.243569643749999010 ) ) ;
#44601=CARTESIAN_POINT ( 'NONE',  ( 10.68750000122903288, 4.330127018922191873, 2.499999999999999556 ) ) ;
#44602=CARTESIAN_POINT ( 'NONE',  ( 17.43750000122903288, 4.330127018922191873, 2.499999999999999556 ) ) ;
#44603=CARTESIAN_POINT ( 'NONE',  ( 14.80312500061451608, 4.541064518000418104, -2.621784821874998173 ) ) ;
#44605=CARTESIAN_POINT ( 'NONE',  ( 19.37812500061451715, 4.541064518000418104, 2.621784821874999949 ) ) ;
#44606=CARTESIAN_POINT ( 'NONE',  ( 24.93750000122903288, 6.123233995736764310E-16, -4.999999999999998224 ) ) ;
#44607=CARTESIAN_POINT ( 'NONE',  ( 28.31250000122903288, 0.000000000000000000, 4.999999999999998224 ) ) ;
#44608=CARTESIAN_POINT ( 'NONE',  ( 23.85000000000000142, -4.330127018922190985, -2.500000000000001332 ) ) ;
#44610=CARTESIAN_POINT ( 'NONE',  ( 25.20937500061451431, 4.541064518000418104, -2.621784821874998173 ) ) ;
#44611=CARTESIAN_POINT ( 'NONE',  ( 30.00000000000000000, 0.000000000000000000, 4.999999999999998224 ) ) ;
#44612=CARTESIAN_POINT ( 'NONE',  ( 11.43750000122903465, 6.123233995736764310E-16, -4.999999999999998224 ) ) ;
#44613=CARTESIAN_POINT ( 'NONE',  ( 27.27187500061451431, -6.054752690667223547, -1.112240025338166033E-15 ) ) ;
#44614=DIRECTION ( 'NONE',  ( -1.000000000000000000, -0.000000000000000000, -0.000000000000000000 ) ) ;
#44615=CARTESIAN_POINT ( 'NONE',  ( 4.171875000614517326, 3.027376345333611329, 5.243569643749999010 ) ) ;
#44616=CARTESIAN_POINT ( 'NONE',  ( 24.44062500061451715, -3.027376345333614438, 5.243569643749998122 ) ) ;
#44619=CARTESIAN_POINT ( 'NONE',  ( 9.534375000614517148, 4.541064518000418104, 2.621784821874999949 ) ) ;
#44621=CARTESIAN_POINT ( 'NONE',  ( 29.46562500061451573, -6.054752690667223547, -1.112240025338166033E-15 ) ) ;
#44622=CARTESIAN_POINT ( 'NONE',  ( 7.509375000614517681, -4.541064518000417216, -2.621784821875001281 ) ) ;
#44623=CARTESIAN_POINT ( 'NONE',  ( 28.62187500061451573, -6.054752690667223547, -1.112240025338166033E-15 ) ) ;
#44625=CARTESIAN_POINT ( 'NONE',  ( 30.00000000000000000, 6.123233995736764310E-16, -4.999999999999998224 ) ) ;
#44626=CARTESIAN_POINT ( 'NONE',  ( 18.71249999999999858, 2.886751345948126879, 4.999999999999999112 ) ) ;
#44628=CARTESIAN_POINT ( 'NONE',  ( 27.00000000000000000, -4.330127018922190985, -2.500000000000001332 ) ) ;
#44629=CARTESIAN_POINT ( 'NONE',  ( 28.92187500061451644, 3.027376345333611329, 5.243569643749999010 ) ) ;
#44631=CARTESIAN_POINT ( 'NONE',  ( 18.02812500061451573, 4.541064518000418104, 2.621784821874999949 ) ) ;
#44632=CARTESIAN_POINT ( 'NONE',  ( 9.515625000614518214, 3.027376345333611329, 5.243569643749999010 ) ) ;
#44634=CARTESIAN_POINT ( 'NONE',  ( 4.621875000614516615, 3.027376345333611329, 5.243569643749999010 ) ) ;
#44635=CARTESIAN_POINT ( 'NONE',  ( 17.88750000122903216, 4.330127018922191873, 2.499999999999999556 ) ) ;
#44636=LINE ( 'NONE', #67165, #13790 ) ;
#44637=CARTESIAN_POINT ( 'NONE',  ( 8.071875000614518569, 3.027376345333613106, -5.243569643749998122 ) ) ;
#44638=CARTESIAN_POINT ( 'NONE',  ( 10.88437500061451679, 4.541064518000418104, 2.621784821874999949 ) ) ;
#44639=CARTESIAN_POINT ( 'NONE',  ( 22.28437500061451715, -4.541064518000419881, 2.621784821874995952 ) ) ;
#44640=CARTESIAN_POINT ( 'NONE',  ( 4.460096747122133110, -2.261369503107883983, 4.460096747122133110 ) ) ;
#44643=CARTESIAN_POINT ( 'NONE',  ( 8.184375000614515727, 4.541064518000418104, 2.621784821874999949 ) ) ;
#44645=CARTESIAN_POINT ( 'NONE',  ( 21.86250000000000071, 2.886751345948126879, 4.999999999999999112 ) ) ;
#44646=CARTESIAN_POINT ( 'NONE',  ( 19.45312500061451644, 0.000000000000000000, 5.243569643749999010 ) ) ;
#44650=CARTESIAN_POINT ( 'NONE',  ( 11.46562500061451573, -6.054752690667223547, -1.112240025338166033E-15 ) ) ;
#44651=CARTESIAN_POINT ( 'NONE',  ( 29.82187500061451502, 3.027376345333611329, 5.243569643749999010 ) ) ;
#44653=CARTESIAN_POINT ( 'NONE',  ( 28.95937500061451431, 0.000000000000000000, 5.243569643749999010 ) ) ;
#44654=CARTESIAN_POINT ( 'NONE',  ( 9.412499999999999645, -5.773502691896255534, -1.060575238724906372E-15 ) ) ;
#44655=CARTESIAN_POINT ( 'NONE',  ( 2.000000000000001332, 14.86250000122903536, 33.46410161513774995 ) ) ;
#44656=CARTESIAN_POINT ( 'NONE',  ( 9.675000001229035362, 2.886751345948129099, -4.999999999999998224 ) ) ;
#44657=CARTESIAN_POINT ( 'NONE',  ( 19.24687500061452283, -3.027376345333610441, -5.243569643749999898 ) ) ;
#44658=CARTESIAN_POINT ( 'NONE',  ( 13.13437500061451857, 4.541064518000418104, 2.621784821874999949 ) ) ;
#44659=CARTESIAN_POINT ( 'NONE',  ( 30.00000000000000000, 6.123233995736764310E-16, -4.999999999999998224 ) ) ;
#44660=ORIENTED_EDGE ( 'NONE', *, *, #4793, .T. ) ;
#44661=CARTESIAN_POINT ( 'NONE',  ( 14.91562500061451679, 3.027376345333611329, 5.243569643749999010 ) ) ;
#44662=CARTESIAN_POINT ( 'NONE',  ( 25.46250000122903501, 4.330127018922192761, -2.499999999999997780 ) ) ;
#44663=CARTESIAN_POINT ( 'NONE',  ( 15.79687500061451821, 6.054752690667223547, 3.707466751127219781E-16 ) ) ;
#44664=CARTESIAN_POINT ( 'NONE',  ( 3.253125000614518036, 0.000000000000000000, 5.243569643749999010 ) ) ;
#44665=CARTESIAN_POINT ( 'NONE',  ( 17.95312500061451644, 4.541064518000418104, -2.621784821874998173 ) ) ;
#44666=CARTESIAN_POINT ( 'NONE',  ( 28.76250000122903216, 0.000000000000000000, 4.999999999999998224 ) ) ;
#44667=CARTESIAN_POINT ( 'NONE',  ( 26.07187500061451857, 3.027376345333613106, -5.243569643749998122 ) ) ;
#44668=CARTESIAN_POINT ( 'NONE',  ( 2.121784821874999061, 11.55312500061451786, 26.32496088578401583 ) ) ;
#44669=CARTESIAN_POINT ( 'NONE',  ( 16.05937500061451573, -4.541064518000417216, -2.621784821875001281 ) ) ;
#44670=CARTESIAN_POINT ( 'NONE',  ( 13.16250000122903430, -4.330127018922190985, -2.500000000000001332 ) ) ;
#44672=CARTESIAN_POINT ( 'NONE',  ( -4.243569643749999898, 18.47187500061451715, -32.45002607614398471 ) ) ;
#44673=CARTESIAN_POINT ( 'NONE',  ( 21.27187500061451786, 3.027376345333611329, 5.243569643749999010 ) ) ;
#44674=CARTESIAN_POINT ( 'NONE',  ( 19.65000000122902790, 5.773502691896255534, 3.535250795749688894E-16 ) ) ;
#44675=CARTESIAN_POINT ( 'NONE',  ( 17.82187500061451502, -6.054752690667223547, -1.112240025338166033E-15 ) ) ;
#44676=CARTESIAN_POINT ( 'NONE',  ( 9.001249775931846008E-16, 13.22187500061451715, 34.90005215228797653 ) ) ;
#44677=CARTESIAN_POINT ( 'NONE',  ( 18.36562500061451431, 3.027376345333613106, -5.243569643749998122 ) ) ;
#44678=ORIENTED_EDGE ( 'NONE', *, *, #42571, .T. ) ;
#44679=ORIENTED_EDGE ( 'NONE', *, *, #57650, .F. ) ;
#44680=CARTESIAN_POINT ( 'NONE',  ( 21.26249999999999574, 2.886751345948129099, -4.999999999999998224 ) ) ;
#44681=CARTESIAN_POINT ( 'NONE',  ( -3.999999999999999112, 20.00000000000000000, -30.00000000000000000 ) ) ;
#44682=CARTESIAN_POINT ( 'NONE',  ( 23.95312500061451289, 0.000000000000000000, 5.243569643749999010 ) ) ;
#44683=CARTESIAN_POINT ( 'NONE',  ( 4.265625000614517326, -6.054752690667223547, -1.112240025338166033E-15 ) ) ;
#44684=CARTESIAN_POINT ( 'NONE',  ( 16.61250000122903359, 0.000000000000000000, 4.999999999999998224 ) ) ;
#44685=CARTESIAN_POINT ( 'NONE',  ( 22.49062500061451431, 6.054752690667223547, 3.707466751127219781E-16 ) ) ;
#44686=CARTESIAN_POINT ( 'NONE',  ( 20.58750000000000213, -2.886751345948129988, 4.999999999999997335 ) ) ;
#44687=EDGE_CURVE ( 'NONE', #45736, #10824, #25977, .T. ) ;
#44688=CARTESIAN_POINT ( 'NONE',  ( 25.00312500061451715, -4.541064518000417216, -2.621784821875001281 ) ) ;
#44689=CARTESIAN_POINT ( 'NONE',  ( 6.665625000614515905, 3.027376345333613106, -5.243569643749998122 ) ) ;
#44690=ORIENTED_EDGE ( 'NONE', *, *, #21542, .F. ) ;
#44691=CARTESIAN_POINT ( 'NONE',  ( 29.25000000000000000, -4.330127018922190985, -2.500000000000001332 ) ) ;
#44693=CARTESIAN_POINT ( 'NONE',  ( 4.000000000000000000, 11.30000000122903536, -27.69059892324149530 ) ) ;
#44694=CARTESIAN_POINT ( 'NONE',  ( 9.001249775931846008E-16, 19.52187500061451786, -25.09994784771203058 ) ) ;
#44695=CARTESIAN_POINT ( 'NONE',  ( 8.062500000000000000, -5.773502691896255534, -1.060575238724906372E-15 ) ) ;
#44696=CARTESIAN_POINT ( 'NONE',  ( 5.850000001229035185, -2.886751345948129988, 4.999999999999997335 ) ) ;
#44697=CARTESIAN_POINT ( 'NONE',  ( 12.45937500061451786, -4.541064518000417216, -2.621784821875001281 ) ) ;
#44698=FACE_OUTER_BOUND ( 'NONE', #70026, .T. ) ;
#44699=CARTESIAN_POINT ( 'NONE',  ( 4.059375000614519280, 4.541064518000418104, -2.621784821874998173 ) ) ;
#44700=DIRECTION ( 'NONE',  ( -0.000000000000000000, -1.000000000000000000, -0.000000000000000000 ) ) ;
#44702=CARTESIAN_POINT ( 'NONE',  ( 9.909375000614517148, 4.541064518000418104, -2.621784821874998173 ) ) ;
#44703=CARTESIAN_POINT ( 'NONE',  ( 3.507483327083503521, -3.563363679198468859, 3.507483327083555924 ) ) ;
#44704=CARTESIAN_POINT ( 'NONE',  ( 19.60312500061451502, -4.541064518000417216, -2.621784821875001281 ) ) ;
#44705=CARTESIAN_POINT ( 'NONE',  ( -3.999999999999999112, 12.46250000122903323, -30.00000000000000000 ) ) ;
#44706=CARTESIAN_POINT ( 'NONE',  ( 4.243569643749999010, 18.26562500061459460, 27.54997392385601174 ) ) ;
#44707=CARTESIAN_POINT ( 'NONE',  ( 23.48437500061451644, 4.541064518000418104, 2.621784821874999949 ) ) ;
#44708=CARTESIAN_POINT ( 'NONE',  ( 28.23750000122903359, 4.330127018922191873, 2.499999999999999556 ) ) ;
#44710=CARTESIAN_POINT ( 'NONE',  ( 24.59062500061451573, -3.027376345333610441, -5.243569643749999898 ) ) ;
#44711=CARTESIAN_POINT ( 'NONE',  ( 15.10312500061451502, -4.541064518000417216, -2.621784821875001281 ) ) ;
#44713=CARTESIAN_POINT ( 'NONE',  ( 11.22187500061451892, 3.027376345333613106, -5.243569643749998122 ) ) ;
#44715=CARTESIAN_POINT ( 'NONE',  ( 24.90000000122903145, -2.886751345948125991, -5.000000000000000000 ) ) ;
#44717=CARTESIAN_POINT ( 'NONE',  ( 15.30937500061451750, 4.541064518000418104, -2.621784821874998173 ) ) ;
#44718=CARTESIAN_POINT ( 'NONE',  ( -2.000000000000000000, 11.82500000000000107, 26.53589838486224650 ) ) ;
#44719=CARTESIAN_POINT ( 'NONE',  ( 3.310802318797580579, -3.746810377620464205, 3.668301323911666412 ) ) ;
#44720=EDGE_CURVE ( 'NONE', #65546, #22787, #58683, .T. ) ;
#44722=CARTESIAN_POINT ( 'NONE',  ( 25.92187500061451999, -6.054752690667223547, -1.112240025338166033E-15 ) ) ;
#44723=CARTESIAN_POINT ( 'NONE',  ( 17.48437500061451999, 6.421520780324663323E-16, -5.243569643749999010 ) ) ;
#44725=CARTESIAN_POINT ( 'NONE',  ( 28.12499999999999645, 4.330127018922191873, 2.499999999999999556 ) ) ;
#44726=CARTESIAN_POINT ( 'NONE',  ( 3.150000001229034119, -2.886751345948129988, 4.999999999999997335 ) ) ;
#44727=CARTESIAN_POINT ( 'NONE',  ( 4.425000000000001599, -4.330127018922194537, 2.499999999999995559 ) ) ;
#44729=CARTESIAN_POINT ( 'NONE',  ( 19.45312500061451644, 0.000000000000000000, 5.243569643749999010 ) ) ;
#44730=CARTESIAN_POINT ( 'NONE',  ( 9.337500000000000355, -2.886751345948129988, 4.999999999999997335 ) ) ;
#44731=( BOUNDED_CURVE ( )  B_SPLINE_CURVE ( 2, ( #4403, #38743, #67189, #71627, #15452, #27654, #72349, #21000, #32463 ),
 .UNSPECIFIED., .F., .F. ) 
 B_SPLINE_CURVE_WITH_KNOTS ( ( 3, 2, 2, 2, 3 ),
 ( 0.7282608695652174058, 0.7318840579710145233, 0.7391304347826086474, 0.7463768115942028825, 0.7500000000000000000 ),
 .UNSPECIFIED. ) 
 CURVE ( )  GEOMETRIC_REPRESENTATION_ITEM ( )  RATIONAL_B_SPLINE_CURVE ( ( 0.9330127018922194093, 0.9330127018922194093, 1.000000000000000000, 0.8660254037844387076, 1.000000000000000000, 0.8660254037844387076, 1.000000000000000000, 0.9330127018922194093, 0.9330127018922194093 ) ) 
 REPRESENTATION_ITEM ( '' )  );
#44732=CARTESIAN_POINT ( 'NONE',  ( 7.285825834671762338E-16, 10.00000000000000000, -24.00000000000000000 ) ) ;
#44733=CARTESIAN_POINT ( 'NONE',  ( 16.50000000000000000, 0.000000000000000000, 4.999999999999998224 ) ) ;
#44734=CARTESIAN_POINT ( 'NONE',  ( -4.243569643749999898, 11.70312500061451644, 30.00000000000000000 ) ) ;
#44736=CARTESIAN_POINT ( 'NONE',  ( 20.02500000122903145, 2.886751345948129099, -4.999999999999998224 ) ) ;
#44738=CARTESIAN_POINT ( 'NONE',  ( 27.83437500061451786, 6.421520780324663323E-16, -5.243569643749999010 ) ) ;
#44740=CARTESIAN_POINT ( 'NONE',  ( 16.11562500061451786, 3.027376345333613106, -5.243569643749998122 ) ) ;
#44741=CARTESIAN_POINT ( 'NONE',  ( 22.22812500061451502, -4.541064518000419881, 2.621784821874995952 ) ) ;
#44742=CARTESIAN_POINT ( 'NONE',  ( 22.65937500061451715, 0.000000000000000000, 5.243569643749999010 ) ) ;
#44743=CARTESIAN_POINT ( 'NONE',  ( 6.937499999999999112, 5.773502691896255534, 3.535250795749688894E-16 ) ) ;
#44744=CARTESIAN_POINT ( 'NONE',  ( 10.07812500061451644, -4.541064518000419881, 2.621784821874995952 ) ) ;
#44745=CARTESIAN_POINT ( 'NONE',  ( 24.51562500061451289, -6.054752690667223547, -1.112240025338166033E-15 ) ) ;
#44746=CARTESIAN_POINT ( 'NONE',  ( 14.97187500061451892, 3.027376345333611329, 5.243569643749999010 ) ) ;
#44747=CARTESIAN_POINT ( 'NONE',  ( 18.75937500061451857, -4.541064518000417216, -2.621784821875001281 ) ) ;
#44748=DIRECTION ( 'NONE',  ( -1.000000000000000000, -0.000000000000000000, -0.000000000000000000 ) ) ;
#44749=CARTESIAN_POINT ( 'NONE',  ( -2.121784821874996840, 18.07812500061451644, 33.67503911421598417 ) ) ;
#44750=CARTESIAN_POINT ( 'NONE',  ( 20.55000000122903359, 5.773502691896255534, 3.535250795749688894E-16 ) ) ;
#44752=CARTESIAN_POINT ( 'NONE',  ( 12.14062500061451821, 6.054752690667223547, 3.707466751127219781E-16 ) ) ;
#44753=CARTESIAN_POINT ( 'NONE',  ( 6.159375000614517148, -4.541064518000417216, -2.621784821875001281 ) ) ;
#44754=CARTESIAN_POINT ( 'NONE',  ( 5.559375000614517504, 0.000000000000000000, 5.243569643749999010 ) ) ;
#44756=CARTESIAN_POINT ( 'NONE',  ( 27.83437500061451786, 6.421520780324663323E-16, -5.243569643749999010 ) ) ;
#44757=CARTESIAN_POINT ( 'NONE',  ( 19.94062500061451715, -3.027376345333614438, 5.243569643749998122 ) ) ;
#44758=CARTESIAN_POINT ( 'NONE',  ( 3.290625000614516793, -3.027376345333614438, 5.243569643749998122 ) ) ;
#44759=CARTESIAN_POINT ( 'NONE',  ( 27.74062500061451431, -3.027376345333610441, -5.243569643749999898 ) ) ;
#44760=CARTESIAN_POINT ( 'NONE',  ( 23.40937500061451715, 4.541064518000418104, -2.621784821874998173 ) ) ;
#44761=CARTESIAN_POINT ( 'NONE',  ( 18.47812500061451857, 4.541064518000418104, 2.621784821874999949 ) ) ;
#44762=CARTESIAN_POINT ( 'NONE',  ( -3.999999999999999112, 10.55000000000000249, 30.00000000000000000 ) ) ;
#44763=CARTESIAN_POINT ( 'NONE',  ( 24.36562500061451786, 3.027376345333611329, 5.243569643749999010 ) ) ;
#44764=CARTESIAN_POINT ( 'NONE',  ( 4.950000001229033941, -2.886751345948129988, 4.999999999999997335 ) ) ;
#44766=CARTESIAN_POINT ( 'NONE',  ( 27.52500000000000213, 6.123233995736764310E-16, -4.999999999999998224 ) ) ;
#44767=CARTESIAN_POINT ( 'NONE',  ( -2.828200636599751609E-16, 14.93750000000000000, -34.61880215351700230 ) ) ;
#44769=CARTESIAN_POINT ( 'NONE',  ( 5.821875000614519458, 3.027376345333613106, -5.243569643749998122 ) ) ;
#44770=CARTESIAN_POINT ( 'NONE',  ( 12.02812500061451573, 6.421520780324663323E-16, -5.243569643749999010 ) ) ;
#44771=CARTESIAN_POINT ( 'NONE',  ( 7.209375000614519635, 4.541064518000418104, -2.621784821874998173 ) ) ;
#44772=CARTESIAN_POINT ( 'NONE',  ( 25.20000000122903216, -2.886751345948129988, 4.999999999999997335 ) ) ;
#44773=CARTESIAN_POINT ( 'NONE',  ( 13.88437500061451679, 6.421520780324663323E-16, -5.243569643749999010 ) ) ;
#44774=CARTESIAN_POINT ( 'NONE',  ( 29.80312500061451431, 0.000000000000000000, 5.243569643749999010 ) ) ;
#44775=CARTESIAN_POINT ( 'NONE',  ( 28.16249999999999787, 2.886751345948126879, 4.999999999999999112 ) ) ;
#44776=ADVANCED_FACE ( 'NONE', ( #25446 ), #24347, .F. ) ;
#44777=CARTESIAN_POINT ( 'NONE',  ( 27.23437500061451644, -4.541064518000419881, 2.621784821874995952 ) ) ;
#44778=CARTESIAN_POINT ( 'NONE',  ( 4.078125000614517326, 4.541064518000418104, 2.621784821874999949 ) ) ;
#44779=CARTESIAN_POINT ( 'NONE',  ( 13.52812500061451750, 4.541064518000418104, 2.621784821874999949 ) ) ;
#44781=EDGE_LOOP ( 'NONE', ( #77, #49584, #51294, #20002 ) ) ;
#44782=CARTESIAN_POINT ( 'NONE',  ( 9.740625000614516082, -3.027376345333610441, -5.243569643749999898 ) ) ;
#44783=CARTESIAN_POINT ( 'NONE',  ( 9.515625000614518214, 3.027376345333611329, 5.243569643749999010 ) ) ;
#44786=CARTESIAN_POINT ( 'NONE',  ( 15.07499999999999929, 4.330127018922191873, 2.499999999999999556 ) ) ;
#44787=( BOUNDED_CURVE ( )  B_SPLINE_CURVE ( 2, ( #66801, #60499, #4383, #45351, #43901, #50170, #56432, #15803, #61600 ),
 .UNSPECIFIED., .F., .F. ) 
 B_SPLINE_CURVE_WITH_KNOTS ( ( 3, 2, 2, 2, 3 ),
 ( 0.3586956521739130821, 0.3623188405797101441, 0.3695652173913043237, 0.3768115942028985588, 0.3804347826086956763 ),
 .UNSPECIFIED. ) 
 CURVE ( )  GEOMETRIC_REPRESENTATION_ITEM ( )  RATIONAL_B_SPLINE_CURVE ( ( 0.9330127018922194093, 0.9330127018922198534, 1.000000000000000000, 0.8660254037844387076, 1.000000000000000000, 0.8660254037844387076, 1.000000000000000000, 0.9330127018922188542, 0.9330127018922194093 ) ) 
 REPRESENTATION_ITEM ( '' )  );
#44788=CARTESIAN_POINT ( 'NONE',  ( 15.00937500061451679, 0.000000000000000000, 5.243569643749999010 ) ) ;
#44789=CARTESIAN_POINT ( 'NONE',  ( 12.60000000122903430, -2.886751345948129988, 4.999999999999997335 ) ) ;
#44791=CARTESIAN_POINT ( 'NONE',  ( 20.89687500061452141, -3.027376345333614438, 5.243569643749998122 ) ) ;
#44792=CARTESIAN_POINT ( 'NONE',  ( -2.121784821874999949, 14.32812500061451644, -33.67503911421598417 ) ) ;
#44795=CARTESIAN_POINT ( 'NONE',  ( 27.85312500061451502, 4.541064518000418104, -2.621784821874998173 ) ) ;
#44796=CARTESIAN_POINT ( 'NONE',  ( -3.999999999999999112, 19.55000000000000071, -30.00000000000000000 ) ) ;
#44797=CARTESIAN_POINT ( 'NONE',  ( 24.37500000000000000, 6.123233995736764310E-16, -4.999999999999998224 ) ) ;
#44798=CARTESIAN_POINT ( 'NONE',  ( 26.77499999999999858, 4.330127018922191873, 2.499999999999999556 ) ) ;
#44799=CARTESIAN_POINT ( 'NONE',  ( 9.628125000614517148, -4.541064518000419881, 2.621784821874995952 ) ) ;
#44801=CARTESIAN_POINT ( 'NONE',  ( 21.68437500061451573, 4.541064518000418104, 2.621784821874999949 ) ) ;
#44803=CARTESIAN_POINT ( 'NONE',  ( 4.340625000614515727, -3.027376345333610441, -5.243569643749999898 ) ) ;
#44804=CARTESIAN_POINT ( 'NONE',  ( 11.78437500061451892, 4.541064518000418104, 2.621784821874999949 ) ) ;
#44805=ORIENTED_EDGE ( 'NONE', *, *, #8112, .F. ) ;
#44806=CARTESIAN_POINT ( 'NONE',  ( 21.15937500061451715, 4.541064518000418104, -2.621784821874998173 ) ) ;
#44807=CARTESIAN_POINT ( 'NONE',  ( 3.578402880298067856, 3.495305883107370448, -31.80580486484916491 ) ) ;
#44808=CARTESIAN_POINT ( 'NONE',  ( 29.96250000000000213, 2.886751345948126879, 4.999999999999999112 ) ) ;
#44809=CARTESIAN_POINT ( 'NONE',  ( 4.949999999999999289, -4.330127018922190985, -2.500000000000001332 ) ) ;
#44810=CARTESIAN_POINT ( 'NONE',  ( 15.41250000122903252, -4.330127018922190985, -2.500000000000001332 ) ) ;
#44812=ORIENTED_EDGE ( 'NONE', *, *, #21977, .T. ) ;
#44813=CARTESIAN_POINT ( 'NONE',  ( 12.86250000000000071, 2.886751345948126879, 4.999999999999999112 ) ) ;
#44814=CARTESIAN_POINT ( 'NONE',  ( 27.85312500061451502, 4.541064518000418104, -2.621784821874998173 ) ) ;
#44815=CARTESIAN_POINT ( 'NONE',  ( 16.83749999999999858, 5.773502691896255534, 3.535250795749688894E-16 ) ) ;
#44816=CARTESIAN_POINT ( 'NONE',  ( 9.600000001229034297, -2.886751345948125991, -5.000000000000000000 ) ) ;
#44817=CARTESIAN_POINT ( 'NONE',  ( 9.065625000614517148, 3.027376345333611329, 5.243569643749999010 ) ) ;
#44818=CARTESIAN_POINT ( 'NONE',  ( 9.299999999999998934, 0.000000000000000000, 4.999999999999998224 ) ) ;
#44819=CARTESIAN_POINT ( 'NONE',  ( 2.121784821874999061, 15.65937500061451892, -33.67503911421598417 ) ) ;
#44820=CARTESIAN_POINT ( 'NONE',  ( 27.82500000122903572, 2.886751345948126879, 4.999999999999999112 ) ) ;
#44822=CARTESIAN_POINT ( 'NONE',  ( 6.299999999999999822, -4.330127018922190985, -2.500000000000001332 ) ) ;
#44823=CARTESIAN_POINT ( 'NONE',  ( -1.999999999999997113, 13.32499999999999929, -26.53589838486224295 ) ) ;
#44825=CARTESIAN_POINT ( 'NONE',  ( 25.22812500061451502, 4.541064518000418104, 2.621784821874999949 ) ) ;
#44826=CARTESIAN_POINT ( 'NONE',  ( 4.215355816196066030, -2.689023592745824143, 4.501582466356354395 ) ) ;
#44827=CARTESIAN_POINT ( 'NONE',  ( 28.95937500061451431, 0.000000000000000000, 5.243569643749999010 ) ) ;
#44828=CARTESIAN_POINT ( 'NONE',  ( 22.54687500061451999, 6.054752690667223547, 3.707466751127219781E-16 ) ) ;
#44829=CARTESIAN_POINT ( 'NONE',  ( 15.62812500061451537, 6.421520780324663323E-16, -5.243569643749999010 ) ) ;
#44830=CARTESIAN_POINT ( 'NONE',  ( 4.243569643749999898, 12.37812500061459353, -30.00000000000000000 ) ) ;
#44831=CARTESIAN_POINT ( 'NONE',  ( 6.778125000614518392, 4.541064518000418104, 2.621784821874999949 ) ) ;
#44832=CARTESIAN_POINT ( 'NONE',  ( 29.17500000122903714, 2.886751345948126879, 4.999999999999999112 ) ) ;
#44834=CARTESIAN_POINT ( 'NONE',  ( 18.51562500061451289, 3.027376345333611329, 5.243569643749999010 ) ) ;
#44835=CARTESIAN_POINT ( 'NONE',  ( 4.000000000000000000, 11.30000000122903536, -27.69059892324149885 ) ) ;
#44837=CARTESIAN_POINT ( 'NONE',  ( 15.00937500061451679, 0.000000000000000000, 5.243569643749999010 ) ) ;
#44838=CARTESIAN_POINT ( 'NONE',  ( 14.67187500061451821, -6.054752690667223547, -1.112240025338166033E-15 ) ) ;
#44839=CARTESIAN_POINT ( 'NONE',  ( 22.65937500061451715, 0.000000000000000000, 5.243569643749999010 ) ) ;
#44840=ORIENTED_EDGE ( 'NONE', *, *, #66601, .F. ) ;
#44841=CARTESIAN_POINT ( 'NONE',  ( 3.531796677802674811, 3.539267187803308179, -3.868928841707397925 ) ) ;
#44842=CARTESIAN_POINT ( 'NONE',  ( 25.86562500061451431, -6.054752690667223547, -1.112240025338166033E-15 ) ) ;
#44843=CARTESIAN_POINT ( 'NONE',  ( 26.54062500061451146, 6.054752690667223547, 3.707466751127219781E-16 ) ) ;
#44845=CARTESIAN_POINT ( 'NONE',  ( 3.999999999999999112, 16.62500000000000000, 30.00000000000000000 ) ) ;
#44846=CARTESIAN_POINT ( 'NONE',  ( 5.634375000614519458, -4.541064518000419881, 2.621784821874995952 ) ) ;
#44847=CARTESIAN_POINT ( 'NONE',  ( 12.15000000122903501, -2.886751345948129988, 4.999999999999997335 ) ) ;
#44848=CARTESIAN_POINT ( 'NONE',  ( 6.525000001229033231, 2.886751345948129099, -4.999999999999998224 ) ) ;
#44849=CARTESIAN_POINT ( 'NONE',  ( 3.590625000614518836, 6.054752690667223547, 3.707466751127219781E-16 ) ) ;
#44852=CARTESIAN_POINT ( 'NONE',  ( 10.80937500061451928, 4.541064518000418104, -2.621784821874998173 ) ) ;
#44855=CARTESIAN_POINT ( 'NONE',  ( 20.05312500061451431, -4.541064518000417216, -2.621784821875001281 ) ) ;
#44856=CARTESIAN_POINT ( 'NONE',  ( 13.99687500061451928, 6.054752690667223547, 3.707466751127219781E-16 ) ) ;
#44857=CARTESIAN_POINT ( 'NONE',  ( 4.340625000614515727, -3.027376345333610441, -5.243569643749999898 ) ) ;
#44858=CARTESIAN_POINT ( 'NONE',  ( 21.04687500061451644, -3.027376345333610441, -5.243569643749999898 ) ) ;
#44859=CARTESIAN_POINT ( 'NONE',  ( 10.24687500061451750, -3.027376345333610441, -5.243569643749999898 ) ) ;
#44860=CARTESIAN_POINT ( 'NONE',  ( 4.190625000614518925, -3.027376345333614438, 5.243569643749998122 ) ) ;
#44861=CARTESIAN_POINT ( 'NONE',  ( 11.73750000122903181, -4.330127018922194537, 2.499999999999995559 ) ) ;
#44862=CARTESIAN_POINT ( 'NONE',  ( 6.150000001229033231, 5.773502691896255534, 3.535250795749688894E-16 ) ) ;
#44863=CARTESIAN_POINT ( 'NONE',  ( 19.64062500061451644, -3.027376345333610441, -5.243569643749999898 ) ) ;
#44864=ADVANCED_FACE ( 'NONE', ( #57957 ), #2915, .F. ) ;
#44865=CARTESIAN_POINT ( 'NONE',  ( 8.962500001229033231, 0.000000000000000000, 4.999999999999998224 ) ) ;
#44866=CARTESIAN_POINT ( 'NONE',  ( 18.40312500061451573, 4.541064518000418104, -2.621784821874998173 ) ) ;
#44867=CARTESIAN_POINT ( 'NONE',  ( 15.51562500061451644, -6.054752690667223547, -1.112240025338166033E-15 ) ) ;
#44869=CARTESIAN_POINT ( 'NONE',  ( 16.72500000000000142, 6.123233995736764310E-16, -4.999999999999998224 ) ) ;
#44870=CARTESIAN_POINT ( 'NONE',  ( 9.037500001229034297, -4.330127018922194537, 2.499999999999995559 ) ) ;
#44871=CARTESIAN_POINT ( 'NONE',  ( 5.878125000614517148, 4.541064518000418104, 2.621784821874999949 ) ) ;
#44873=CARTESIAN_POINT ( 'NONE',  ( 21.41250000122903074, 4.330127018922192761, -2.499999999999997780 ) ) ;
#44875=CARTESIAN_POINT ( 'NONE',  ( 2.121784821875001281, 10.10937500061451821, -26.32496088578401938 ) ) ;
#44876=LINE ( 'NONE', #10877, #32392 ) ;
#44877=CARTESIAN_POINT ( 'NONE',  ( 2.662500001229036073, 0.000000000000000000, 4.999999999999998224 ) ) ;
#44878=CARTESIAN_POINT ( 'NONE',  ( 4.621875000614516615, 3.027376345333611329, 5.243569643749999010 ) ) ;
#44879=CARTESIAN_POINT ( 'NONE',  ( 20.70937500061451786, 4.541064518000418104, -2.621784821874998173 ) ) ;
#44880=CARTESIAN_POINT ( 'NONE',  ( -3.999999999999999112, 15.01250000000000107, 27.69059892324149885 ) ) ;
#44881=CARTESIAN_POINT ( 'NONE',  ( 15.85312500061451857, 0.000000000000000000, 5.243569643749999010 ) ) ;
#44883=CARTESIAN_POINT ( 'NONE',  ( 23.13749999999999929, 5.773502691896255534, 3.535250795749688401E-16 ) ) ;
#44884=CARTESIAN_POINT ( 'NONE',  ( 0.000000000000000000, 20.00000000000000000, 26.00000000000000000 ) ) ;
#44885=CARTESIAN_POINT ( 'NONE',  ( 28.05937500061451573, 0.000000000000000000, 5.243569643749999010 ) ) ;
#44887=CARTESIAN_POINT ( 'NONE',  ( 11.61562500061451608, 3.027376345333613106, -5.243569643749998122 ) ) ;
#44888=CARTESIAN_POINT ( 'NONE',  ( 11.25937500061451679, 4.541064518000418104, -2.621784821874998173 ) ) ;
#44890=CARTESIAN_POINT ( 'NONE',  ( 2.918837393651653400, -4.059695890482965197, -3.197878993417715865 ) ) ;
#44891=CARTESIAN_POINT ( 'NONE',  ( 22.04062500061451502, 6.054752690667223547, 3.707466751127219781E-16 ) ) ;
#44894=CARTESIAN_POINT ( 'NONE',  ( 12.11250000000000249, -5.773502691896255534, -1.060575238724906372E-15 ) ) ;
#44895=CARTESIAN_POINT ( 'NONE',  ( 22.01250000122903216, 0.000000000000000000, 4.999999999999998224 ) ) ;
#44896=CARTESIAN_POINT ( 'NONE',  ( 17.35312500061451502, -4.541064518000417216, -2.621784821875001281 ) ) ;
#44899=CARTESIAN_POINT ( 'NONE',  ( 19.20000000000000284, 0.000000000000000000, 4.999999999999998224 ) ) ;
#44900=CARTESIAN_POINT ( 'NONE',  ( 24.60000000000000142, 0.000000000000000000, 4.999999999999998224 ) ) ;
#44901=CARTESIAN_POINT ( 'NONE',  ( 21.68437500061451573, 4.541064518000418104, 2.621784821874999949 ) ) ;
#44902=CARTESIAN_POINT ( 'NONE',  ( 26.39062500061451644, -3.027376345333610441, -5.243569643749999898 ) ) ;
#44903=VERTEX_POINT ( 'NONE', #36165 ) ;
#44905=CARTESIAN_POINT ( 'NONE',  ( 8.953125000614518214, 4.541064518000418104, -2.621784821874998173 ) ) ;
#44907=CARTESIAN_POINT ( 'NONE',  ( 15.37500000000000000, 6.123233995736764310E-16, -4.999999999999998224 ) ) ;
#44908=CARTESIAN_POINT ( 'NONE',  ( 7.762500001229033053, -4.330127018922190985, -2.500000000000001332 ) ) ;
#44909=CARTESIAN_POINT ( 'NONE',  ( 5.484375000614518214, 4.541064518000418104, 2.621784821874999949 ) ) ;
#44910=CARTESIAN_POINT ( 'NONE',  ( 28.58437500061451786, -4.541064518000419881, 2.621784821874995952 ) ) ;
#44912=CARTESIAN_POINT ( 'NONE',  ( 24.44062500061451715, -3.027376345333614438, 5.243569643749998122 ) ) ;
#44913=CARTESIAN_POINT ( 'NONE',  ( 26.44687500061451502, -3.027376345333610441, -5.243569643749999898 ) ) ;
#44914=CARTESIAN_POINT ( 'NONE',  ( -2.121784821874999949, 18.82812500061459104, -33.67503911421598417 ) ) ;
#44915=CARTESIAN_POINT ( 'NONE',  ( 12.48750000000000249, -2.886751345948129988, 4.999999999999997335 ) ) ;
#44916=CARTESIAN_POINT ( 'NONE',  ( 10.04062500061451502, -3.027376345333614438, 5.243569643749998122 ) ) ;
#44919=CARTESIAN_POINT ( 'NONE',  ( 25.15312500061451217, 4.541064518000418104, -2.621784821874998173 ) ) ;
#44920=CARTESIAN_POINT ( 'NONE',  ( 12.78750000122903430, 6.123233995736764310E-16, -4.999999999999998224 ) ) ;
#44922=CARTESIAN_POINT ( 'NONE',  ( 3.815625000614518036, -6.054752690667223547, -1.112240025338166033E-15 ) ) ;
#44923=CARTESIAN_POINT ( 'NONE',  ( 20.22187500061451715, 3.027376345333613106, -5.243569643749998122 ) ) ;
#44924=CARTESIAN_POINT ( 'NONE',  ( -3.000416591977282496E-16, 14.34687500061451715, 25.09994784771203058 ) ) ;
#44925=CARTESIAN_POINT ( 'NONE',  ( 21.68437500061451573, 4.541064518000418104, 2.621784821874999949 ) ) ;
#44926=CARTESIAN_POINT ( 'NONE',  ( 3.112500000000000711, -5.773502691896255534, -1.060575238724906372E-15 ) ) ;
#44927=CARTESIAN_POINT ( 'NONE',  ( -4.243569643749999898, 18.92187500061451644, 27.54997392385601529 ) ) ;
#44928=CARTESIAN_POINT ( 'NONE',  ( 11.05312500061451608, -4.541064518000417216, -2.621784821875001281 ) ) ;
#44930=CARTESIAN_POINT ( 'NONE',  ( 6.796875000614516438, 6.054752690667223547, 3.707466751127219781E-16 ) ) ;
#44931=CARTESIAN_POINT ( 'NONE',  ( 6.815625000614517148, 3.027376345333611329, 5.243569643749999010 ) ) ;
#44932=CARTESIAN_POINT ( 'NONE',  ( 11.89687500061451608, -3.027376345333614438, 5.243569643749998122 ) ) ;
#44933=CARTESIAN_POINT ( 'NONE',  ( 18.56250000122903288, -4.330127018922190985, -2.500000000000001332 ) ) ;
#44934=CARTESIAN_POINT ( 'NONE',  ( 7.096875000614517148, -3.027376345333610441, -5.243569643749999898 ) ) ;
#44935=CARTESIAN_POINT ( 'NONE',  ( 9.103125000614515017, 0.000000000000000000, 5.243569643749999010 ) ) ;
#44938=CARTESIAN_POINT ( 'NONE',  ( 19.43437500061451928, 4.541064518000418104, 2.621784821874999949 ) ) ;
#44939=CARTESIAN_POINT ( 'NONE',  ( 4.471804083240662031, 2.236731597915199821, 4.552588781061169598 ) ) ;
#44940=CARTESIAN_POINT ( 'NONE',  ( 27.36562500061451786, 3.027376345333613106, -5.243569643749998122 ) ) ;
#44941=CARTESIAN_POINT ( 'NONE',  ( 12.81562500061451537, -6.054752690667223547, -1.112240025338166033E-15 ) ) ;
#44943=CARTESIAN_POINT ( 'NONE',  ( -4.243569643749999898, 11.72187500061451892, -32.45002607614398471 ) ) ;
#44944=CARTESIAN_POINT ( 'NONE',  ( 12.82500000122903394, 2.886751345948129099, -4.999999999999998224 ) ) ;
#44945=CARTESIAN_POINT ( 'NONE',  ( 27.21562500061451928, -6.054752690667223547, -1.112240025338166033E-15 ) ) ;
#44947=CARTESIAN_POINT ( 'NONE',  ( -4.243569643749999898, 15.26562500061451644, -32.45002607614398471 ) ) ;
#44948=CARTESIAN_POINT ( 'NONE',  ( 15.03750000122903252, 6.123233995736764310E-16, -4.999999999999998224 ) ) ;
#44949=CARTESIAN_POINT ( 'NONE',  ( 12.97499999999999964, -4.330127018922194537, 2.499999999999995559 ) ) ;
#44950=CARTESIAN_POINT ( 'NONE',  ( 21.96562500061451573, 3.027376345333613106, -5.243569643749998122 ) ) ;
#44951=CARTESIAN_POINT ( 'NONE',  ( 6.646875000614518747, -3.027376345333610441, -5.243569643749999898 ) ) ;
#44952=CARTESIAN_POINT ( 'NONE',  ( 8.475000001229034297, 2.886751345948126879, 4.999999999999999112 ) ) ;
#44953=CARTESIAN_POINT ( 'NONE',  ( 16.95000000122903216, 5.773502691896255534, 3.535250795749688894E-16 ) ) ;
#44954=CARTESIAN_POINT ( 'NONE',  ( 12.29062500061451857, -3.027376345333614438, 5.243569643749998122 ) ) ;
#44955=CARTESIAN_POINT ( 'NONE',  ( 17.27812500061451217, -4.541064518000419881, 2.621784821874995952 ) ) ;
#44956=CARTESIAN_POINT ( 'NONE',  ( 26.55000000122902648, -2.886751345948129988, 4.999999999999997335 ) ) ;
#44957=CARTESIAN_POINT ( 'NONE',  ( 28.42500000122904069, -5.773502691896255534, -1.060575238724906372E-15 ) ) ;
#44958=CARTESIAN_POINT ( 'NONE',  ( 22.08749999999999858, -2.886751345948125991, -5.000000000000000000 ) ) ;
#44959=CARTESIAN_POINT ( 'NONE',  ( 24.75937500061451502, 4.541064518000418104, -2.621784821874998173 ) ) ;
#44961=CARTESIAN_POINT ( 'NONE',  ( 10.61250000122903536, 4.330127018922192761, -2.499999999999997780 ) ) ;
#44962=CARTESIAN_POINT ( 'NONE',  ( 26.85937500061451644, -4.541064518000417216, -2.621784821875001281 ) ) ;
#44963=CARTESIAN_POINT ( 'NONE',  ( 5.746875000614517504, -3.027376345333610441, -5.243569643749999898 ) ) ;
#44964=CARTESIAN_POINT ( 'NONE',  ( 24.40312500061451573, 0.000000000000000000, 5.243569643749999010 ) ) ;
#44967=CARTESIAN_POINT ( 'NONE',  ( 10.73437500061451644, 6.421520780324663323E-16, -5.243569643749999010 ) ) ;
#44968=LINE ( 'NONE', #16871, #69056 ) ;
#44969=CARTESIAN_POINT ( 'NONE',  ( 3.871875000614519280, -6.054752690667223547, -1.112240025338166033E-15 ) ) ;
#44970=CARTESIAN_POINT ( 'NONE',  ( 7.471875000614519813, -6.054752690667223547, -1.112240025338166033E-15 ) ) ;
#44971=CARTESIAN_POINT ( 'NONE',  ( -10.00000000000000000, 0.000000000000000000, 50.00000000000000000 ) ) ;
#44972=CARTESIAN_POINT ( 'NONE',  ( 28.92187500061451644, 3.027376345333611329, 5.243569643749999010 ) ) ;
#44973=CARTESIAN_POINT ( 'NONE',  ( 3.849931240356728512, 3.190302406438068505, 3.849931240356827544 ) ) ;
#44974=CARTESIAN_POINT ( 'NONE',  ( 18.97499999999999787, 6.123233995736764310E-16, -4.999999999999998224 ) ) ;
#44975=ORIENTED_EDGE ( 'NONE', *, *, #47376, .F. ) ;
#44976=CARTESIAN_POINT ( 'NONE',  ( 26.13749999999999929, -2.886751345948125991, -5.000000000000000000 ) ) ;
#44977=CARTESIAN_POINT ( 'NONE',  ( 27.60937500061451644, 0.000000000000000000, 5.243569643749999010 ) ) ;
#44978=EDGE_CURVE ( 'NONE', #42322, #62090, #3345, .T. ) ;
#44979=ORIENTED_EDGE ( 'NONE', *, *, #61414, .T. ) ;
#44980=CARTESIAN_POINT ( 'NONE',  ( 16.41562500061451857, -6.054752690667223547, -1.112240025338166033E-15 ) ) ;
#44981=CARTESIAN_POINT ( 'NONE',  ( 7.265625000614516438, 3.027376345333611329, 5.243569643749999010 ) ) ;
#44983=CARTESIAN_POINT ( 'NONE',  ( 3.571875000614517237, 3.027376345333613106, -5.243569643749998122 ) ) ;
#44984=CARTESIAN_POINT ( 'NONE',  ( 18.56250000122903288, -4.330127018922190985, -2.500000000000001332 ) ) ;
#44985=CARTESIAN_POINT ( 'NONE',  ( 23.73749999999999716, -2.886751345948129988, 4.999999999999997335 ) ) ;
#44986=CARTESIAN_POINT ( 'NONE',  ( 23.92500000122903359, -5.773502691896255534, -1.060575238724906372E-15 ) ) ;
#44987=CARTESIAN_POINT ( 'NONE',  ( 7.134375000614516793, 6.421520780324663323E-16, -5.243569643749999010 ) ) ;
#44988=CARTESIAN_POINT ( 'NONE',  ( 12.30937500061451573, 0.000000000000000000, 5.243569643749999010 ) ) ;
#44989=CARTESIAN_POINT ( 'NONE',  ( 22.84687500061451715, -3.027376345333610441, -5.243569643749999898 ) ) ;
#44992=CARTESIAN_POINT ( 'NONE',  ( 4.509375000614518569, 4.541064518000418104, -2.621784821874998173 ) ) ;
#44994=CARTESIAN_POINT ( 'NONE',  ( 8.034375000614518925, 6.421520780324663323E-16, -5.243569643749999010 ) ) ;
#44995=CARTESIAN_POINT ( 'NONE',  ( 20.51249999999999929, 2.886751345948126879, 4.999999999999999112 ) ) ;
#44996=CARTESIAN_POINT ( 'NONE',  ( 15.85312500061451857, 0.000000000000000000, 5.243569643749999010 ) ) ;
#45000=CARTESIAN_POINT ( 'NONE',  ( 10.97812500061451679, -4.541064518000419881, 2.621784821874995952 ) ) ;
#45001=CARTESIAN_POINT ( 'NONE',  ( 25.92187500061451999, -6.054752690667223547, -1.112240025338166033E-15 ) ) ;
#45003=CARTESIAN_POINT ( 'NONE',  ( 4.167140676845648706, 2.763139261668956514, -4.167140676845877856 ) ) ;
#45004=CARTESIAN_POINT ( 'NONE',  ( 9.112500000000000711, 2.886751345948129099, -4.999999999999998224 ) ) ;
#45005=CARTESIAN_POINT ( 'NONE',  ( -2.828200636599751609E-16, 14.60000000122903430, 25.38119784648299770 ) ) ;
#45006=CARTESIAN_POINT ( 'NONE',  ( 8.550000001229031810, -2.886751345948129988, 4.999999999999997335 ) ) ;
#45007=( BOUNDED_CURVE ( )  B_SPLINE_CURVE ( 2, ( #27085, #67696, #67345, #49617, #39628, #16706, #39263, #15980, #62146 ),
 .UNSPECIFIED., .F., .F. ) 
 B_SPLINE_CURVE_WITH_KNOTS ( ( 3, 2, 2, 2, 3 ),
 ( 0.07608695652173913526, 0.07971014492753622505, 0.08695652173913043237, 0.09420289855072463969, 0.09782608695652174335 ),
 .UNSPECIFIED. ) 
 CURVE ( )  GEOMETRIC_REPRESENTATION_ITEM ( )  RATIONAL_B_SPLINE_CURVE ( ( 0.9330127018922192983, 0.9330127018922194093, 1.000000000000000000, 0.8660254037844387076, 1.000000000000000000, 0.8660254037844387076, 1.000000000000000000, 0.9330127018922194093, 0.9330127018922194093 ) ) 
 REPRESENTATION_ITEM ( '' )  );
#45008=CARTESIAN_POINT ( 'NONE',  ( 21.04687500061451644, -3.027376345333610441, -5.243569643749999898 ) ) ;
#45009=CARTESIAN_POINT ( 'NONE',  ( 13.43437500061451750, 6.421520780324663323E-16, -5.243569643749999010 ) ) ;
#45010=CARTESIAN_POINT ( 'NONE',  ( 3.998297483032399402, 3.002268681709985287, -4.299000508453080016 ) ) ;
#45012=CARTESIAN_POINT ( 'NONE',  ( 14.16562500061451679, -6.054752690667223547, -1.112240025338166033E-15 ) ) ;
#45013=CARTESIAN_POINT ( 'NONE',  ( 27.22500000122903430, 2.886751345948129099, -4.999999999999998224 ) ) ;
#45014=CARTESIAN_POINT ( 'NONE',  ( 15.42187500061451821, 3.027376345333611329, 5.243569643749999010 ) ) ;
#45015=CARTESIAN_POINT ( 'NONE',  ( 5.681944431425972830, 8.230953001180115081, -31.96676831340010239 ) ) ;
#45016=CARTESIAN_POINT ( 'NONE',  ( 16.30312500061451786, 0.000000000000000000, 5.243569643749999010 ) ) ;
#45017=EDGE_CURVE ( 'NONE', #755, #47001, #53899, .T. ) ;
#45019=CARTESIAN_POINT ( 'NONE',  ( 27.23437500061451644, -4.541064518000419881, 2.621784821874995952 ) ) ;
#45020=CARTESIAN_POINT ( 'NONE',  ( 2.121784821875001281, 10.05312500061451608, 33.67503911421598417 ) ) ;
#45021=CARTESIAN_POINT ( 'NONE',  ( 14.89687500061451786, 6.054752690667223547, 3.707466751127219781E-16 ) ) ;
#45022=CARTESIAN_POINT ( 'NONE',  ( 14.96250000122903323, -4.330127018922190985, -2.500000000000001332 ) ) ;
#45024=CARTESIAN_POINT ( 'NONE',  ( 4.243569643749999010, 18.77187500061451431, -32.45002607614398471 ) ) ;
#45025=CARTESIAN_POINT ( 'NONE',  ( 18.38437500061451857, 6.421520780324663323E-16, -5.243569643749999010 ) ) ;
#45026=CARTESIAN_POINT ( 'NONE',  ( 21.00000000122903288, 5.773502691896255534, 3.535250795749688894E-16 ) ) ;
#45027=CARTESIAN_POINT ( 'NONE',  ( 13.99687500061451928, 6.054752690667223547, 3.707466751127219781E-16 ) ) ;
#45028=CARTESIAN_POINT ( 'NONE',  ( -4.243569643749999898, 12.62187500061451928, 27.54997392385601529 ) ) ;
#45029=CARTESIAN_POINT ( 'NONE',  ( 23.43750000122902932, -4.330127018922194537, 2.499999999999995559 ) ) ;
#45030=CARTESIAN_POINT ( 'NONE',  ( 16.26562500061451289, 3.027376345333611329, 5.243569643749999010 ) ) ;
#45031=VERTEX_POINT ( 'NONE', #42446 ) ;
#45032=ORIENTED_EDGE ( 'NONE', *, *, #60829, .F. ) ;
#45033=CARTESIAN_POINT ( 'NONE',  ( 19.83750000000000213, -2.886751345948125991, -5.000000000000000000 ) ) ;
#45035=CARTESIAN_POINT ( 'NONE',  ( 22.22812500061451502, -4.541064518000419881, 2.621784821874995952 ) ) ;
#45036=CARTESIAN_POINT ( 'NONE',  ( 3.999818103236636890, 3.000242528463000991, 29.85633969779405206 ) ) ;
#45037=CARTESIAN_POINT ( 'NONE',  ( 14.81250000122903288, 0.000000000000000000, 4.999999999999998224 ) ) ;
#45038=CARTESIAN_POINT ( 'NONE',  ( 21.47812500061451502, 6.421520780324663323E-16, -5.243569643749999010 ) ) ;
#45039=CARTESIAN_POINT ( 'NONE',  ( 25.07812500061451644, 6.421520780324663323E-16, -5.243569643749999010 ) ) ;
#45041=CARTESIAN_POINT ( 'NONE',  ( 5.465625000614517504, 3.027376345333611329, 5.243569643749999010 ) ) ;
#45042=ORIENTED_EDGE ( 'NONE', *, *, #25641, .F. ) ;
#45043=LINE ( 'NONE', #22135, #7389 ) ;
#45044=CARTESIAN_POINT ( 'NONE',  ( -3.999999999999997335, 10.25000000122903643, -27.69059892324149530 ) ) ;
#45047=CARTESIAN_POINT ( 'NONE',  ( 4.000000000000000000, 10.40000000122903501, -27.69059892324149530 ) ) ;
#45048=CARTESIAN_POINT ( 'NONE',  ( 9.001249775931846008E-16, 18.62187500061451928, -25.09994784771203058 ) ) ;
#45049=CARTESIAN_POINT ( 'NONE',  ( 5.925000001229033586, -5.773502691896255534, -1.060575238724906372E-15 ) ) ;
#45050=CARTESIAN_POINT ( 'NONE',  ( 9.112500000000000711, 2.886751345948129099, -4.999999999999998224 ) ) ;
#45051=CARTESIAN_POINT ( 'NONE',  ( 4.012500001229033053, 0.000000000000000000, 4.999999999999998224 ) ) ;
#45052=CARTESIAN_POINT ( 'NONE',  ( 13.35937500061451821, -4.541064518000417216, -2.621784821875001281 ) ) ;
#45053=CARTESIAN_POINT ( 'NONE',  ( 30.00000000000000000, 0.000000000000000000, 0.000000000000000000 ) ) ;
#45054=CARTESIAN_POINT ( 'NONE',  ( 4.321875000614517681, -6.054752690667223547, -1.112240025338166033E-15 ) ) ;
#45056=CARTESIAN_POINT ( 'NONE',  ( 10.69687500061451679, -3.027376345333610441, -5.243569643749999898 ) ) ;
#45057=CARTESIAN_POINT ( 'NONE',  ( 1.071796769724493892, 17.27990381179670010, -34.00000000000000000 ) ) ;
#45058=CARTESIAN_POINT ( 'NONE',  ( 30.00000000000000000, 6.123233995736764310E-16, -4.999999999999998224 ) ) ;
#45059=CARTESIAN_POINT ( 'NONE',  ( -4.243569643749999898, 17.06562500061459176, 27.54997392385601529 ) ) ;
#45060=CARTESIAN_POINT ( 'NONE',  ( 21.00937500061451857, -4.541064518000417216, -2.621784821875001281 ) ) ;
#45062=CARTESIAN_POINT ( 'NONE',  ( 27.90000000122903145, -2.886751345948129988, 4.999999999999997335 ) ) ;
#45064=CARTESIAN_POINT ( 'NONE',  ( 25.97812500061451502, 6.421520780324663323E-16, -5.243569643749999010 ) ) ;
#45065=CARTESIAN_POINT ( 'NONE',  ( 14.42812500061451786, 4.541064518000418104, 2.621784821874999949 ) ) ;
#45067=CARTESIAN_POINT ( 'NONE',  ( 10.73437500061451644, 6.421520780324663323E-16, -5.243569643749999010 ) ) ;
#45068=CARTESIAN_POINT ( 'NONE',  ( 29.77499999999999858, 6.123233995736764310E-16, -4.999999999999998224 ) ) ;
#45069=CARTESIAN_POINT ( 'NONE',  ( 24.15000000122903145, 5.773502691896255534, 3.535250795749688894E-16 ) ) ;
#45070=CARTESIAN_POINT ( 'NONE',  ( 4.321875000614517681, -6.054752690667223547, -1.112240025338166033E-15 ) ) ;
#45071=CARTESIAN_POINT ( 'NONE',  ( 14.85937500061451644, 4.541064518000418104, -2.621784821874998173 ) ) ;
#45072=CARTESIAN_POINT ( 'NONE',  ( 29.10937500061451644, -4.541064518000417216, -2.621784821875001281 ) ) ;
#45073=CARTESIAN_POINT ( 'NONE',  ( -1.071796769724504328, 11.54240381056766829, 33.99999999999999289 ) ) ;
#45074=LINE ( 'NONE', #10724, #32505 ) ;
#45075=CARTESIAN_POINT ( 'NONE',  ( 22.24687500061451217, -3.027376345333614438, 5.243569643749998122 ) ) ;
#45076=CARTESIAN_POINT ( 'NONE',  ( 14.85937500061451644, 4.541064518000418104, -2.621784821874998173 ) ) ;
#45078=CARTESIAN_POINT ( 'NONE',  ( 27.86249999999999716, -5.773502691896255534, -1.060575238724906372E-15 ) ) ;
#45079=CARTESIAN_POINT ( 'NONE',  ( 2.775000001229033675, -5.773502691896255534, -1.060575238724906372E-15 ) ) ;
#45081=CARTESIAN_POINT ( 'NONE',  ( 17.20312500061451644, 0.000000000000000000, 5.243569643749999010 ) ) ;
#45082=CARTESIAN_POINT ( 'NONE',  ( 7.987500000000000711, -2.886751345948129988, 4.999999999999997335 ) ) ;
#45083=EDGE_CURVE ( 'NONE', #1870, #71251, #70881, .T. ) ;
#45084=DIRECTION ( 'NONE',  ( -0.000000000000000000, -1.000000000000000000, -0.000000000000000000 ) ) ;
#45085=CARTESIAN_POINT ( 'NONE',  ( 16.01249999999999929, 2.886751345948126879, 4.999999999999999112 ) ) ;
#45086=CARTESIAN_POINT ( 'NONE',  ( -2.121784821874996840, 13.57812500061451644, 33.67503911421598417 ) ) ;
#45088=CARTESIAN_POINT ( 'NONE',  ( 21.15000000122903145, -2.886751345948129988, 4.999999999999997335 ) ) ;
#45089=CARTESIAN_POINT ( 'NONE',  ( -3.999999999999999112, 13.36250000122903359, 30.00000000000000000 ) ) ;
#45090=CARTESIAN_POINT ( 'NONE',  ( 26.44687500061451502, -3.027376345333610441, -5.243569643749999898 ) ) ;
#45091=ORIENTED_EDGE ( 'NONE', *, *, #55867, .T. ) ;
#45092=CARTESIAN_POINT ( 'NONE',  ( 21.89062500061451289, -3.027376345333610441, -5.243569643749999898 ) ) ;
#45093=CARTESIAN_POINT ( 'NONE',  ( 22.43437500061451573, 6.421520780324663323E-16, -5.243569643749999010 ) ) ;
#45094=CARTESIAN_POINT ( 'NONE',  ( 6.562500000000001776, 2.886751345948126879, 4.999999999999999112 ) ) ;
#45095=CARTESIAN_POINT ( 'NONE',  ( 10.52812500061451750, -4.541064518000419881, 2.621784821874995952 ) ) ;
#45096=CARTESIAN_POINT ( 'NONE',  ( 23.91562500061451502, 3.027376345333611329, 5.243569643749999010 ) ) ;
#45097=CARTESIAN_POINT ( 'NONE',  ( 15.57187500061451679, -6.054752690667223547, -1.112240025338166033E-15 ) ) ;
#45098=CARTESIAN_POINT ( 'NONE',  ( 19.84687500061451360, 6.054752690667223547, 3.707466751127219781E-16 ) ) ;
#45100=CARTESIAN_POINT ( 'NONE',  ( 2.121784821875001281, 17.25312500061451715, 33.67503911421598417 ) ) ;
#45101=CARTESIAN_POINT ( 'NONE',  ( 22.16250000122903074, -4.330127018922190985, -2.500000000000001332 ) ) ;
#45103=CARTESIAN_POINT ( 'NONE',  ( 12.89062500061451821, -3.027376345333610441, -5.243569643749999898 ) ) ;
#45104=CARTESIAN_POINT ( 'NONE',  ( 5.821875000614519458, 3.027376345333613106, -5.243569643749998122 ) ) ;
#45105=CARTESIAN_POINT ( 'NONE',  ( 3.721875000614518036, 3.027376345333611329, 5.243569643749999010 ) ) ;
#45107=CARTESIAN_POINT ( 'NONE',  ( 28.47187500061451715, 3.027376345333611329, 5.243569643749999010 ) ) ;
#45108=CARTESIAN_POINT ( 'NONE',  ( 17.12812500061451715, 4.541064518000418104, 2.621784821874999949 ) ) ;
#45109=CARTESIAN_POINT ( 'NONE',  ( 27.97500000122903074, -5.773502691896255534, -1.060575238724906372E-15 ) ) ;
#45110=CARTESIAN_POINT ( 'NONE',  ( 27.55312500061451786, 0.000000000000000000, 5.243569643749999010 ) ) ;
#45112=CARTESIAN_POINT ( 'NONE',  ( 21.79687500061451644, -3.027376345333614438, 5.243569643749998122 ) ) ;
#45113=CARTESIAN_POINT ( 'NONE',  ( 17.80312500061451786, -4.541064518000417216, -2.621784821875001281 ) ) ;
#45114=CARTESIAN_POINT ( 'NONE',  ( -3.999999999999999556, 10.51250000000000107, 27.69059892324149530 ) ) ;
#45115=CARTESIAN_POINT ( 'NONE',  ( 24.10312500061451502, -4.541064518000417216, -2.621784821875001281 ) ) ;
#45116=CARTESIAN_POINT ( 'NONE',  ( 4.050000001229035362, -2.886751345948129988, 4.999999999999997335 ) ) ;
#45118=CARTESIAN_POINT ( 'NONE',  ( 27.93750000000000000, -2.886751345948125991, -5.000000000000000000 ) ) ;
#45119=CARTESIAN_POINT ( 'NONE',  ( 2.000000000000001332, 12.05000000000000249, -26.53589838486224650 ) ) ;
#45121=CARTESIAN_POINT ( 'NONE',  ( 4.246875000614519280, -3.027376345333614438, 5.243569643749998122 ) ) ;
#45122=CARTESIAN_POINT ( 'NONE',  ( 9.928125000614517859, 4.541064518000418104, 2.621784821874999949 ) ) ;
#45123=CARTESIAN_POINT ( 'NONE',  ( 7.059375000614518392, -4.541064518000417216, -2.621784821875001281 ) ) ;
#45124=CARTESIAN_POINT ( 'NONE',  ( 25.35000000122903074, -2.886751345948125991, -5.000000000000000000 ) ) ;
#45126=CARTESIAN_POINT ( 'NONE',  ( 13.80937500061451750, -4.541064518000417216, -2.621784821875001281 ) ) ;
#45127=CARTESIAN_POINT ( 'NONE',  ( 28.75312500061451715, 4.541064518000418104, -2.621784821874998173 ) ) ;
#45128=CARTESIAN_POINT ( 'NONE',  ( 27.82499999999999929, -4.330127018922194537, 2.499999999999995559 ) ) ;
#45130=CARTESIAN_POINT ( 'NONE',  ( 12.62812500061451537, 4.541064518000418104, 2.621784821874999949 ) ) ;
#45132=CARTESIAN_POINT ( 'NONE',  ( 9.253125000614517148, -4.541064518000417216, -2.621784821875001281 ) ) ;
#45133=CARTESIAN_POINT ( 'NONE',  ( 6.928125000614516082, -4.541064518000419881, 2.621784821874995952 ) ) ;
#45135=EDGE_CURVE ( 'NONE', #51427, #5506, #15815, .T. ) ;
#45137=EDGE_CURVE ( 'NONE', #7111, #29389, #3657, .T. ) ;
#45138=CARTESIAN_POINT ( 'NONE',  ( 14.92500000000000071, 6.123233995736764310E-16, -4.999999999999998224 ) ) ;
#45139=CARTESIAN_POINT ( 'NONE',  ( 17.10937500061451999, 4.541064518000418104, -2.621784821874998173 ) ) ;
#45140=CARTESIAN_POINT ( 'NONE',  ( 11.17500000122903536, 2.886751345948126879, 4.999999999999999112 ) ) ;
#45142=CARTESIAN_POINT ( 'NONE',  ( 21.00937500061451857, -4.541064518000417216, -2.621784821875001281 ) ) ;
#45143=CARTESIAN_POINT ( 'NONE',  ( -3.000416591977282496E-16, 14.29062500061451679, -34.90005215228797653 ) ) ;
#45146=DIRECTION ( 'NONE',  ( -1.000000000000000000, -0.000000000000000000, -0.000000000000000000 ) ) ;
#45147=CARTESIAN_POINT ( 'NONE',  ( 27.70312500061451289, -4.541064518000417216, -2.621784821875001281 ) ) ;
#45148=CARTESIAN_POINT ( 'NONE',  ( 17.21250000122903145, -4.330127018922190985, -2.500000000000001332 ) ) ;
#45149=CARTESIAN_POINT ( 'NONE',  ( 29.74687500061451217, 6.054752690667223547, 3.707466751127219781E-16 ) ) ;
#45151=CARTESIAN_POINT ( 'NONE',  ( 25.16249999999999432, -5.773502691896255534, -1.060575238724906372E-15 ) ) ;
#45152=CARTESIAN_POINT ( 'NONE',  ( 8.615625000614517859, 3.027376345333611329, 5.243569643749999010 ) ) ;
#45154=CARTESIAN_POINT ( 'NONE',  ( 18.15937500061451715, 0.000000000000000000, 5.243569643749999010 ) ) ;
#45156=CARTESIAN_POINT ( 'NONE',  ( 4.115625000614516082, 3.027376345333611329, 5.243569643749999010 ) ) ;
#45157=CARTESIAN_POINT ( 'NONE',  ( 9.909375000614517148, 4.541064518000418104, -2.621784821874998173 ) ) ;
#45159=CARTESIAN_POINT ( 'NONE',  ( 21.04687500061451644, -3.027376345333610441, -5.243569643749999898 ) ) ;
#45161=CARTESIAN_POINT ( 'NONE',  ( 28.35000000000000142, -4.330127018922190985, -2.500000000000001332 ) ) ;
#45162=CARTESIAN_POINT ( 'NONE',  ( 5.062500000000000888, 2.886751345948129099, -4.999999999999998224 ) ) ;
#45163=CARTESIAN_POINT ( 'NONE',  ( 14.32500000122903394, 2.886751345948126879, 4.999999999999999112 ) ) ;
#45164=CARTESIAN_POINT ( 'NONE',  ( 3.999999999999998668, 12.27500000122903501, 27.69059892324149530 ) ) ;
#45165=CARTESIAN_POINT ( 'NONE',  ( 19.12500000000000000, 4.330127018922191873, 2.499999999999999556 ) ) ;
#45167=CARTESIAN_POINT ( 'NONE',  ( 12.11250000000000249, -5.773502691896255534, -1.060575238724906372E-15 ) ) ;
#45168=CARTESIAN_POINT ( 'NONE',  ( 23.50312500061451360, 0.000000000000000000, 5.243569643749999010 ) ) ;
#45169=CARTESIAN_POINT ( 'NONE',  ( 17.77499999999999858, 4.330127018922191873, 2.499999999999999556 ) ) ;
#45170=CARTESIAN_POINT ( 'NONE',  ( 9.750000001229032875, 5.773502691896255534, 3.535250795749688894E-16 ) ) ;
#45171=CARTESIAN_POINT ( 'NONE',  ( 9.553125000614517859, 0.000000000000000000, 5.243569643749999010 ) ) ;
#45172=CARTESIAN_POINT ( 'NONE',  ( 9.375000000000001776, -4.330127018922194537, 2.499999999999995559 ) ) ;
#45173=CARTESIAN_POINT ( 'NONE',  ( 30.00000000000000000, 0.000000000000000000, 0.000000000000000000 ) ) ;
#45174=CARTESIAN_POINT ( 'NONE',  ( -4.243569643749999898, 14.00937500061451857, -30.00000000000000000 ) ) ;
#45175=CARTESIAN_POINT ( 'NONE',  ( 28.76250000122903216, 0.000000000000000000, 4.999999999999998224 ) ) ;
#45177=CARTESIAN_POINT ( 'NONE',  ( 8.099999999999999645, -4.330127018922190985, -2.500000000000001332 ) ) ;
#45180=CARTESIAN_POINT ( 'NONE',  ( 23.87812500061451715, 4.541064518000418104, 2.621784821874999949 ) ) ;
#45181=CARTESIAN_POINT ( 'NONE',  ( 14.25000000122903465, 5.773502691896255534, 3.535250795749688894E-16 ) ) ;
#45182=CARTESIAN_POINT ( 'NONE',  ( 29.54062500061451502, -3.027376345333610441, -5.243569643749999898 ) ) ;
#45183=CARTESIAN_POINT ( 'NONE',  ( 18.75937500061451857, -4.541064518000417216, -2.621784821875001281 ) ) ;
#45184=CARTESIAN_POINT ( 'NONE',  ( 17.76562500061451644, -6.054752690667223547, -1.112240025338166033E-15 ) ) ;
#45185=CARTESIAN_POINT ( 'NONE',  ( 4.243569643749999898, 12.34062500061459389, -27.54997392385601529 ) ) ;
#45186=CARTESIAN_POINT ( 'NONE',  ( 6.290625000614517681, 6.054752690667223547, 3.707466751127219781E-16 ) ) ;
#45187=CARTESIAN_POINT ( 'NONE',  ( 28.27500000122903145, 2.886751345948126879, 4.999999999999999112 ) ) ;
#45189=CARTESIAN_POINT ( 'NONE',  ( 20.01562500061451644, -6.054752690667223547, -1.112240025338166033E-15 ) ) ;
#45190=CYLINDRICAL_SURFACE ( 'NONE', #57468, 4.999999999999998224 ) ;
#45192=CARTESIAN_POINT ( 'NONE',  ( 13.43437500061451750, 6.421520780324663323E-16, -5.243569643749999010 ) ) ;
#45193=CARTESIAN_POINT ( 'NONE',  ( 12.12187500061451573, 3.027376345333613106, -5.243569643749998122 ) ) ;
#45194=CARTESIAN_POINT ( 'NONE',  ( 20.78437500061451715, 4.541064518000418104, 2.621784821874999949 ) ) ;
#45195=ORIENTED_EDGE ( 'NONE', *, *, #21528, .T. ) ;
#45197=CARTESIAN_POINT ( 'NONE',  ( 27.29062500061451502, -3.027376345333610441, -5.243569643749999898 ) ) ;
#45198=CARTESIAN_POINT ( 'NONE',  ( 23.69062500061451004, -3.027376345333610441, -5.243569643749999898 ) ) ;
#45199=LINE ( 'NONE', #12288, #36817 ) ;
#45200=CARTESIAN_POINT ( 'NONE',  ( 2.000000000000001332, 17.89999999999999858, 33.46410161513774995 ) ) ;
#45201=CARTESIAN_POINT ( 'NONE',  ( 3.909375000614518481, -4.541064518000417216, -2.621784821875001281 ) ) ;
#45202=CARTESIAN_POINT ( 'NONE',  ( 11.21250000122903501, 0.000000000000000000, 4.999999999999998224 ) ) ;
#45203=CARTESIAN_POINT ( 'NONE',  ( 6.600000001229032520, 5.773502691896255534, 3.535250795749688894E-16 ) ) ;
#45204=CARTESIAN_POINT ( 'NONE',  ( 21.75000000122903288, -2.886751345948159742, -4.999999999999942268 ) ) ;
#45205=CARTESIAN_POINT ( 'NONE',  ( 3.103125000614517237, 4.541064518000418104, -2.621784821874998173 ) ) ;
#45208=CARTESIAN_POINT ( 'NONE',  ( 12.53437500061451537, 6.421520780324663323E-16, -5.243569643749999010 ) ) ;
#45209=DIRECTION ( 'NONE',  ( 0.000000000000000000, 0.000000000000000000, -1.000000000000000000 ) ) ;
#45210=CARTESIAN_POINT ( 'NONE',  ( 16.75312500061451715, 0.000000000000000000, 5.243569643749999010 ) ) ;
#45211=CARTESIAN_POINT ( 'NONE',  ( 13.05937500061451750, 4.541064518000418104, -2.621784821874998173 ) ) ;
#45212=CARTESIAN_POINT ( 'NONE',  ( 5.353125000614515905, 4.541064518000418104, -2.621784821874998173 ) ) ;
#45213=CARTESIAN_POINT ( 'NONE',  ( 22.43437500061451573, 6.421520780324663323E-16, -5.243569643749999010 ) ) ;
#45214=CARTESIAN_POINT ( 'NONE',  ( 8.709375000614517859, 0.000000000000000000, 5.243569643749999010 ) ) ;
#45215=CARTESIAN_POINT ( 'NONE',  ( 5.165625000614518569, -6.054752690667223547, -1.112240025338166033E-15 ) ) ;
#45216=CARTESIAN_POINT ( 'NONE',  ( 11.81250000122903465, -4.330127018922190985, -2.500000000000001332 ) ) ;
#45217=CARTESIAN_POINT ( 'NONE',  ( 5.325000001229033941, 2.886751345948126879, 4.999999999999999112 ) ) ;
#45219=CARTESIAN_POINT ( 'NONE',  ( 20.69062500061451715, 6.054752690667223547, 3.707466751127219781E-16 ) ) ;
#45220=CARTESIAN_POINT ( 'NONE',  ( 7.837500001229035007, 6.123233995736764310E-16, -4.999999999999998224 ) ) ;
#45221=CARTESIAN_POINT ( 'NONE',  ( 17.80312500061451786, -4.541064518000417216, -2.621784821875001281 ) ) ;
#45222=CARTESIAN_POINT ( 'NONE',  ( 13.34062500061451750, -3.027376345333610441, -5.243569643749999898 ) ) ;
#45224=CARTESIAN_POINT ( 'NONE',  ( 13.23750000000000071, 5.773502691896255534, 3.535250795749688894E-16 ) ) ;
#45225=CARTESIAN_POINT ( 'NONE',  ( 8.850000001229034297, 5.773502691896255534, 3.535250795749688894E-16 ) ) ;
#45226=CARTESIAN_POINT ( 'NONE',  ( 5.840625000614516615, 6.054752690667223547, 3.707466751127219781E-16 ) ) ;
#45227=CARTESIAN_POINT ( 'NONE',  ( 20.85000000122903430, -2.886751345948125991, -5.000000000000000000 ) ) ;
#45229=CARTESIAN_POINT ( 'NONE',  ( 4.243569643749999010, 10.67187500061451644, -32.45002607614398471 ) ) ;
#45232=CARTESIAN_POINT ( 'NONE',  ( 1.626862140677534273E-15, 11.67500000122903181, -26.00000000000000355 ) ) ;
#45233=CARTESIAN_POINT ( 'NONE',  ( 9.562500001229032875, -4.330127018922190985, -2.500000000000001332 ) ) ;
#45234=CARTESIAN_POINT ( 'NONE',  ( 20.55937500061451573, -4.541064518000417216, -2.621784821875001281 ) ) ;
#45235=CARTESIAN_POINT ( 'NONE',  ( 4.000000000000000000, 18.50000000122903288, 32.30940107675849760 ) ) ;
#45236=CARTESIAN_POINT ( 'NONE',  ( 16.90312500061451573, -4.541064518000417216, -2.621784821875001281 ) ) ;
#45238=CARTESIAN_POINT ( 'NONE',  ( 1.592000809091587073E-14, 15.38750000000000284, -34.00000000000000000 ) ) ;
#45239=CARTESIAN_POINT ( 'NONE',  ( 4.406803030766965001, -3.629725346580264578, 3.713131282202427830 ) ) ;
#45240=CARTESIAN_POINT ( 'NONE',  ( 25.20937500061451431, 4.541064518000418104, -2.621784821874998173 ) ) ;
#45242=CARTESIAN_POINT ( 'NONE',  ( 11.46562500061451573, -6.054752690667223547, -1.112240025338166033E-15 ) ) ;
#45243=CARTESIAN_POINT ( 'NONE',  ( 9.909375000614517148, 4.541064518000418104, -2.621784821874998173 ) ) ;
#45245=CARTESIAN_POINT ( 'NONE',  ( 29.20312500061451644, 4.541064518000418104, -2.621784821874998173 ) ) ;
#45246=CARTESIAN_POINT ( 'NONE',  ( 23.61562500061451431, -6.054752690667223547, -1.112240025338166033E-15 ) ) ;
#45248=CARTESIAN_POINT ( 'NONE',  ( 1.071796769724489895, 15.47990381179670116, -34.00000000000000000 ) ) ;
#45249=EDGE_CURVE ( 'NONE', #66380, #47866, #56209, .T. ) ;
#45250=CARTESIAN_POINT ( 'NONE',  ( 12.37500000000000000, 4.330127018922191873, 2.499999999999999556 ) ) ;
#45251=CARTESIAN_POINT ( 'NONE',  ( 22.76250000122903216, 4.330127018922192761, -2.499999999999997780 ) ) ;
#45252=CARTESIAN_POINT ( 'NONE',  ( 17.16562500061451502, 3.027376345333611329, 5.243569643749999010 ) ) ;
#45255=CARTESIAN_POINT ( 'NONE',  ( 21.07499999999999929, -4.330127018922194537, 2.499999999999995559 ) ) ;
#45256=CARTESIAN_POINT ( 'NONE',  ( 23.77499999999999858, -4.330127018922194537, 2.499999999999995559 ) ) ;
#45257=CARTESIAN_POINT ( 'NONE',  ( 21.15937500061451715, 4.541064518000418104, -2.621784821874998173 ) ) ;
#45258=CARTESIAN_POINT ( 'NONE',  ( 25.90312500061451573, -4.541064518000417216, -2.621784821875001281 ) ) ;
#45259=ADVANCED_FACE ( 'NONE', ( #14720 ), #20255, .F. ) ;
#45260=ORIENTED_EDGE ( 'NONE', *, *, #1978, .F. ) ;
#45261=CARTESIAN_POINT ( 'NONE',  ( 0.000000000000000000, 20.00000000000000000, 30.00000000000000000 ) ) ;
#45262=CARTESIAN_POINT ( 'NONE',  ( 8.615625000614517859, 3.027376345333611329, 5.243569643749999010 ) ) ;
#45263=CARTESIAN_POINT ( 'NONE',  ( 23.92499999999999716, 6.123233995736764310E-16, -4.999999999999998224 ) ) ;
#45264=CARTESIAN_POINT ( 'NONE',  ( 15.59999999999999964, 0.000000000000000000, 4.999999999999998224 ) ) ;
#45265=CARTESIAN_POINT ( 'NONE',  ( -4.243569643749997233, 17.14062500061451644, 32.45002607614398471 ) ) ;
#45266=CARTESIAN_POINT ( 'NONE',  ( 5.596875000614516260, -3.027376345333614438, 5.243569643749998122 ) ) ;
#45267=CARTESIAN_POINT ( 'NONE',  ( 27.15937500061451360, 0.000000000000000000, 5.243569643749999010 ) ) ;
#45268=ORIENTED_EDGE ( 'NONE', *, *, #19563, .F. ) ;
#45269=CARTESIAN_POINT ( 'NONE',  ( 23.12812500061451360, -4.541064518000419881, 2.621784821874995952 ) ) ;
#45270=CARTESIAN_POINT ( 'NONE',  ( 24.94687500061451502, -3.027376345333614438, 5.243569643749998122 ) ) ;
#45271=CARTESIAN_POINT ( 'NONE',  ( -2.121784821874999949, 19.72812500061459318, -33.67503911421598417 ) ) ;
#45272=CARTESIAN_POINT ( 'NONE',  ( 12.26249999999999929, 2.886751345948129099, -4.999999999999998224 ) ) ;
#45273=CARTESIAN_POINT ( 'NONE',  ( 9.440625000614517148, 6.054752690667223547, 3.707466751127219781E-16 ) ) ;
#45274=LINE ( 'NONE', #32731, #42178 ) ;
#45275=DIRECTION ( 'NONE',  ( -0.000000000000000000, -1.000000000000000000, -0.000000000000000000 ) ) ;
#45276=CARTESIAN_POINT ( 'NONE',  ( 27.25312500061451360, -4.541064518000417216, -2.621784821875001281 ) ) ;
#45279=CARTESIAN_POINT ( 'NONE',  ( 2.878125000614517592, -4.541064518000419881, 2.621784821874995952 ) ) ;
#45280=CARTESIAN_POINT ( 'NONE',  ( 20.48437500061451289, -4.541064518000419881, 2.621784821874995952 ) ) ;
#45281=CARTESIAN_POINT ( 'NONE',  ( 2.121784821875001281, 14.15937500061451715, 33.67503911421598417 ) ) ;
#45282=CARTESIAN_POINT ( 'NONE',  ( 19.39687500061451786, 6.054752690667223547, 3.707466751127219781E-16 ) ) ;
#45283=CARTESIAN_POINT ( 'NONE',  ( 3.450000000000001510, 0.000000000000000000, 4.999999999999998224 ) ) ;
#45284=CARTESIAN_POINT ( 'NONE',  ( -2.121784821874999949, 18.43437500061451928, 26.32496088578401938 ) ) ;
#45285=CARTESIAN_POINT ( 'NONE',  ( 11.01562500061451821, -6.054752690667223547, -1.112240025338166033E-15 ) ) ;
#45287=CARTESIAN_POINT ( 'NONE',  ( 8.184375000614515727, 4.541064518000418104, 2.621784821874999949 ) ) ;
#45289=CARTESIAN_POINT ( 'NONE',  ( 8.203125000614518214, 0.000000000000000000, 5.243569643749999010 ) ) ;
#45290=CARTESIAN_POINT ( 'NONE',  ( 12.00937500061451857, -4.541064518000417216, -2.621784821875001281 ) ) ;
#45291=CARTESIAN_POINT ( 'NONE',  ( 19.27500000122903145, 2.886751345948126879, 4.999999999999999112 ) ) ;
#45292=CARTESIAN_POINT ( 'NONE',  ( 7.884375000614517681, -4.541064518000419881, 2.621784821874995952 ) ) ;
#45293=CARTESIAN_POINT ( 'NONE',  ( 9.665625000614515017, -6.054752690667223547, -1.112240025338166033E-15 ) ) ;
#45296=CARTESIAN_POINT ( 'NONE',  ( 19.69687500061451857, -3.027376345333610441, -5.243569643749999898 ) ) ;
#45297=CARTESIAN_POINT ( 'NONE',  ( -0.7368805616696194605, 9.859898480082234684, -34.17910162106521454 ) ) ;
#45299=CARTESIAN_POINT ( 'NONE',  ( 26.27812500061451573, -4.541064518000419881, 2.621784821874995952 ) ) ;
#45300=CARTESIAN_POINT ( 'NONE',  ( 12.96562500061451750, 3.027376345333613106, -5.243569643749998122 ) ) ;
#45301=CARTESIAN_POINT ( 'NONE',  ( 28.80937500061451573, 4.541064518000418104, -2.621784821874998173 ) ) ;
#45302=CARTESIAN_POINT ( 'NONE',  ( 12.47812500061451502, 6.421520780324663323E-16, -5.243569643749999010 ) ) ;
#45304=CARTESIAN_POINT ( 'NONE',  ( 13.65000000122903323, -2.886751345948125991, -5.000000000000000000 ) ) ;
#45305=CARTESIAN_POINT ( 'NONE',  ( 26.69062500061451715, -3.027376345333614438, 5.243569643749998122 ) ) ;
#45306=CARTESIAN_POINT ( 'NONE',  ( 4.243569643749999898, 14.62812500061451715, -30.00000000000000000 ) ) ;
#45307=CARTESIAN_POINT ( 'NONE',  ( 15.18750000122903465, 4.330127018922191873, 2.499999999999999556 ) ) ;
#45308=CARTESIAN_POINT ( 'NONE',  ( 12.44999999999999929, 0.000000000000000000, 4.999999999999998224 ) ) ;
#45309=B_SPLINE_CURVE_WITH_KNOTS ( 'NONE', 3,
 ( #52041, #36497, #8061, #64571, #29146, #53122, #13588, #52401, #7693, #24317, #19124, #51681, #1085, #46138, #69405, #46866, #18760, #18039, #63835, #40595, #35044, #63116, #46500, #12870, #35402, #41678, #36135, #13227, #30231, #47585, #52763, #19490, #70114, #2166, #24677, #58654, #2521, #26146, #25786, #26519, #60477, #37226, #3992, #36861, #3624, #2883 ),
 .UNSPECIFIED., .F., .F.,
 ( 4, 2, 2, 2, 2, 2, 2, 2, 2, 2, 2, 2, 2, 2, 2, 2, 2, 2, 2, 2, 2, 2, 4 ),
 ( 0.000000000000000000, 0.001203096460345616731, 0.002406192920691233462, 0.003609289381036850410, 0.004812385841382466924, 0.005413934071555267374, 0.006015482301728067825, 0.007218578762073687809, 0.008421675222419306925, 0.009023223452592120386, 0.009624771682764935582, 0.01082786814311056250, 0.01142941637328337770, 0.01203096460345619116, 0.01323406106380183023, 0.01443715752414746756, 0.01503870575432028275, 0.01564025398449309795, 0.01684335044483871446, 0.01744489867501152619, 0.01804644690518434139, 0.01864799513535714964, 0.01924954336552996484 ),
 .UNSPECIFIED. ) ;
#45310=CARTESIAN_POINT ( 'NONE',  ( 20.69062500061451715, 6.054752690667223547, 3.707466751127219781E-16 ) ) ;
#45311=CARTESIAN_POINT ( 'NONE',  ( 7.846875000614518036, -3.027376345333614438, 5.243569643749998122 ) ) ;
#45312=CARTESIAN_POINT ( 'NONE',  ( 7.350000001229033408, -2.886751345948125991, -5.000000000000000000 ) ) ;
#45313=CARTESIAN_POINT ( 'NONE',  ( 16.27500000122903501, -5.773502691896255534, -1.060575238724906372E-15 ) ) ;
#45314=CARTESIAN_POINT ( 'NONE',  ( 12.81562500061451537, -6.054752690667223547, -1.112240025338166033E-15 ) ) ;
#45315=CARTESIAN_POINT ( 'NONE',  ( 15.36562500061451608, 3.027376345333611329, 5.243569643749999010 ) ) ;
#45316=CARTESIAN_POINT ( 'NONE',  ( 29.13750000122903216, 4.330127018922191873, 2.499999999999999556 ) ) ;
#45317=CARTESIAN_POINT ( 'NONE',  ( 21.67500000000000071, 6.123233995736764310E-16, -4.999999999999998224 ) ) ;
#45318=AXIS2_PLACEMENT_3D ( 'NONE', #29856, #52392, #46856 ) ;
#45319=CARTESIAN_POINT ( 'NONE',  ( 24.12187500061451217, -6.054752690667223547, -1.112240025338166033E-15 ) ) ;
#45321=CARTESIAN_POINT ( 'NONE',  ( 10.01250000122903394, -4.330127018922190985, -2.500000000000001332 ) ) ;
#45322=CARTESIAN_POINT ( 'NONE',  ( 27.64687500061452141, -3.027376345333614438, 5.243569643749998122 ) ) ;
#45323=CARTESIAN_POINT ( 'NONE',  ( 5.446875000614518569, 6.054752690667223547, 3.707466751127219781E-16 ) ) ;
#45324=CARTESIAN_POINT ( 'NONE',  ( 23.20312500061451644, -4.541064518000417216, -2.621784821875001281 ) ) ;
#45326=CARTESIAN_POINT ( 'NONE',  ( 6.899999999999999467, 4.330127018922192761, -2.499999999999997780 ) ) ;
#45327=CARTESIAN_POINT ( 'NONE',  ( 11.25937500061451679, 4.541064518000418104, -2.621784821874998173 ) ) ;
#45329=CARTESIAN_POINT ( 'NONE',  ( 29.05312500061451431, -4.541064518000417216, -2.621784821875001281 ) ) ;
#45330=CARTESIAN_POINT ( 'NONE',  ( 5.821875000614519458, 3.027376345333613106, -5.243569643749998122 ) ) ;
#45332=CARTESIAN_POINT ( 'NONE',  ( -3.999999999999999112, 14.56250000000000000, 27.69059892324149885 ) ) ;
#45333=CARTESIAN_POINT ( 'NONE',  ( 26.44687500061451502, -3.027376345333610441, -5.243569643749999898 ) ) ;
#45334=CARTESIAN_POINT ( 'NONE',  ( 2.121784821875001281, 10.95312500061459460, 33.67503911421598417 ) ) ;
#45335=CARTESIAN_POINT ( 'NONE',  ( 18.48750000000000071, -2.886751345948125991, -5.000000000000000000 ) ) ;
#45336=ORIENTED_EDGE ( 'NONE', *, *, #52747, .T. ) ;
#45337=CARTESIAN_POINT ( 'NONE',  ( 27.52500000000000213, 6.123233995736764310E-16, -4.999999999999998224 ) ) ;
#45338=CARTESIAN_POINT ( 'NONE',  ( 28.47187500061451715, 3.027376345333611329, 5.243569643749999010 ) ) ;
#45340=VERTEX_POINT ( 'NONE', #44282 ) ;
#45341=CARTESIAN_POINT ( 'NONE',  ( 15.44062500061451537, -3.027376345333614438, 5.243569643749998122 ) ) ;
#45342=CARTESIAN_POINT ( 'NONE',  ( 8.128125000614515372, 4.541064518000418104, 2.621784821874999949 ) ) ;
#45344=CARTESIAN_POINT ( 'NONE',  ( 5.371875000614516615, 3.027376345333613106, -5.243569643749998122 ) ) ;
#45345=CARTESIAN_POINT ( 'NONE',  ( 18.60000000122903430, -2.886751345948125991, -5.000000000000000000 ) ) ;
#45346=CARTESIAN_POINT ( 'NONE',  ( 22.94999999999999929, -4.330127018922190985, -2.500000000000001332 ) ) ;
#45347=DIRECTION ( 'NONE',  ( 0.000000000000000000, 0.000000000000000000, 1.000000000000000000 ) ) ;
#45348=CARTESIAN_POINT ( 'NONE',  ( 7.209375000614519635, 4.541064518000418104, -2.621784821874998173 ) ) ;
#45349=CARTESIAN_POINT ( 'NONE',  ( 10.77187500061451786, 3.027376345333613106, -5.243569643749998122 ) ) ;
#45350=CARTESIAN_POINT ( 'NONE',  ( 21.49687500061451573, -3.027376345333610441, -5.243569643749999898 ) ) ;
#45351=CARTESIAN_POINT ( 'NONE',  ( 3.999999999999998668, 15.87500000122903465, -32.30940107675850470 ) ) ;
#45352=VERTEX_POINT ( 'NONE', #666 ) ;
#45353=CARTESIAN_POINT ( 'NONE',  ( 4.696875000614518569, -3.027376345333614438, 5.243569643749998122 ) ) ;
#45354=CARTESIAN_POINT ( 'NONE',  ( 7.771875000614516971, 3.027376345333611329, 5.243569643749999010 ) ) ;
#45355=CARTESIAN_POINT ( 'NONE',  ( 18.93750000000000000, -2.886751345948125991, -5.000000000000000000 ) ) ;
#45356=CARTESIAN_POINT ( 'NONE',  ( 16.56562500061451715, 3.027376345333613106, -5.243569643749998122 ) ) ;
#45360=CARTESIAN_POINT ( 'NONE',  ( 10.64062500061451644, -3.027376345333610441, -5.243569643749999898 ) ) ;
#45361=CARTESIAN_POINT ( 'NONE',  ( 25.84687500061451360, -3.027376345333614438, 5.243569643749998122 ) ) ;
#45362=CARTESIAN_POINT ( 'NONE',  ( 27.75937500061451502, -4.541064518000417216, -2.621784821875001281 ) ) ;
#45363=CARTESIAN_POINT ( 'NONE',  ( 10.91250000000000320, 2.886751345948129099, -4.999999999999998224 ) ) ;
#45364=CARTESIAN_POINT ( 'NONE',  ( 4.000000000000000000, 14.45000000122903572, 32.30940107675849049 ) ) ;
#45365=CARTESIAN_POINT ( 'NONE',  ( 8.400000001229035007, 5.773502691896255534, 3.535250795749688894E-16 ) ) ;
#45366=CARTESIAN_POINT ( 'NONE',  ( 20.74687500061451573, 6.054752690667223547, 3.707466751127219781E-16 ) ) ;
#45367=CARTESIAN_POINT ( 'NONE',  ( 14.85937500061451644, 4.541064518000418104, -2.621784821874998173 ) ) ;
#45368=CARTESIAN_POINT ( 'NONE',  ( -3.780580586577212632, 3.275490995243299341, -31.33113147093461492 ) ) ;
#45371=CARTESIAN_POINT ( 'NONE',  ( 15.14062500061451644, -3.027376345333610441, -5.243569643749999898 ) ) ;
#45372=CARTESIAN_POINT ( 'NONE',  ( 26.66250000122903430, -4.330127018922190985, -2.500000000000001332 ) ) ;
#45373=CARTESIAN_POINT ( 'NONE',  ( 15.83437500061451608, 4.541064518000418104, 2.621784821874999949 ) ) ;
#45374=CARTESIAN_POINT ( 'NONE',  ( 3.515625000614516882, 3.027376345333613106, -5.243569643749998122 ) ) ;
#45375=CARTESIAN_POINT ( 'NONE',  ( 17.09062500061451573, 6.054752690667223547, 3.707466751127219781E-16 ) ) ;
#45377=CARTESIAN_POINT ( 'NONE',  ( 25.80937500061451928, 0.000000000000000000, 5.243569643749999010 ) ) ;
#45378=CARTESIAN_POINT ( 'NONE',  ( -4.243569643749999898, 9.903125000614517504, 30.00000000000000000 ) ) ;
#45379=CARTESIAN_POINT ( 'NONE',  ( 15.53437500061451715, -4.541064518000419881, 2.621784821874995952 ) ) ;
#45380=CARTESIAN_POINT ( 'NONE',  ( 13.83750000122903323, 4.330127018922191873, 2.499999999999999556 ) ) ;
#45382=CARTESIAN_POINT ( 'NONE',  ( -2.121784821874999949, 16.18437500061451573, -33.67503911421598417 ) ) ;
#45383=CARTESIAN_POINT ( 'NONE',  ( 18.75937500061451857, -4.541064518000417216, -2.621784821875001281 ) ) ;
#45384=CARTESIAN_POINT ( 'NONE',  ( 19.68750000122903288, 4.330127018922191873, 2.499999999999999556 ) ) ;
#45385=CARTESIAN_POINT ( 'NONE',  ( 14.74687500061451573, -3.027376345333610441, -5.243569643749999898 ) ) ;
#45386=CARTESIAN_POINT ( 'NONE',  ( -4.243569643749999898, 11.27187500061451608, 27.54997392385601529 ) ) ;
#45387=CARTESIAN_POINT ( 'NONE',  ( 21.22500000122903074, -5.773502691896255534, -1.060575238724906372E-15 ) ) ;
#45388=CARTESIAN_POINT ( 'NONE',  ( 15.62812500061451537, 6.421520780324663323E-16, -5.243569643749999010 ) ) ;
#45389=CARTESIAN_POINT ( 'NONE',  ( 29.42812500061451431, -4.541064518000419881, 2.621784821874995952 ) ) ;
#45390=ORIENTED_EDGE ( 'NONE', *, *, #46996, .T. ) ;
#45391=VERTEX_POINT ( 'NONE', #55719 ) ;
#45392=CARTESIAN_POINT ( 'NONE',  ( 21.63749999999999929, -2.886751345948125991, -5.000000000000000000 ) ) ;
#45393=CARTESIAN_POINT ( 'NONE',  ( -3.999999999999999112, 17.86250000122903359, 30.00000000000000000 ) ) ;
#45394=CARTESIAN_POINT ( 'NONE',  ( 3.859048791629764885, 3.180512981247726856, 28.91364485973339526 ) ) ;
#45395=CARTESIAN_POINT ( 'NONE',  ( 15.41250000122903252, -4.330127018922190985, -2.500000000000001332 ) ) ;
#45396=CARTESIAN_POINT ( 'NONE',  ( 19.37812500061451715, 4.541064518000418104, 2.621784821874999949 ) ) ;
#45397=CARTESIAN_POINT ( 'NONE',  ( 22.49062500061451431, 6.054752690667223547, 3.707466751127219781E-16 ) ) ;
#45398=CARTESIAN_POINT ( 'NONE',  ( 4.603125000614518569, 0.000000000000000000, 5.243569643749999010 ) ) ;
#45400=CARTESIAN_POINT ( 'NONE',  ( 28.94999999999999929, 4.330127018922192761, -2.499999999999997780 ) ) ;
#45403=CARTESIAN_POINT ( 'NONE',  ( 29.74687500061451217, 6.054752690667223547, 3.707466751127219781E-16 ) ) ;
#45404=CARTESIAN_POINT ( 'NONE',  ( -3.999999999999999112, 10.66250000122903430, -30.00000000000000000 ) ) ;
#45405=CARTESIAN_POINT ( 'NONE',  ( 9.001249775931846008E-16, 17.27187500061451786, -25.09994784771203058 ) ) ;
#45406=( BOUNDED_CURVE ( )  B_SPLINE_CURVE ( 2, ( #61256, #23174, #5477, #5833, #10650 ),
 .UNSPECIFIED., .F., .F. ) 
 B_SPLINE_CURVE_WITH_KNOTS ( ( 3, 2, 3 ),
 ( 0.000000000000000000, 0.007246376811594202987, 0.01086956521739130578 ),
 .UNSPECIFIED. ) 
 CURVE ( )  GEOMETRIC_REPRESENTATION_ITEM ( )  RATIONAL_B_SPLINE_CURVE ( ( 1.000000000000000000, 0.8660254037844387076, 1.000000000000000000, 0.9330127018922192983, 0.9330127018922194093 ) ) 
 REPRESENTATION_ITEM ( '' )  );
#45407=CARTESIAN_POINT ( 'NONE',  ( 6.187500001229032875, 4.330127018922191873, 2.499999999999999556 ) ) ;
#45408=CARTESIAN_POINT ( 'NONE',  ( 8.250000000000000000, 4.330127018922192761, -2.499999999999997780 ) ) ;
#45409=CARTESIAN_POINT ( 'NONE',  ( 3.637500001229036162, -4.330127018922194537, 2.499999999999995559 ) ) ;
#45410=CARTESIAN_POINT ( 'NONE',  ( 11.25937500061451679, 4.541064518000418104, -2.621784821874998173 ) ) ;
#45411=CARTESIAN_POINT ( 'NONE',  ( 19.53750000122903430, 6.123233995736764310E-16, -4.999999999999998224 ) ) ;
#45412=CARTESIAN_POINT ( 'NONE',  ( 3.384375000614517237, -4.541064518000419881, 2.621784821874995952 ) ) ;
#45413=CARTESIAN_POINT ( 'NONE',  ( 12.78750000122903430, 6.123233995736764310E-16, -4.999999999999998224 ) ) ;
#45415=ADVANCED_FACE ( 'NONE', ( #39457 ), #5113, .F. ) ;
#45416=CARTESIAN_POINT ( 'NONE',  ( 9.234375000614518214, -4.541064518000419881, 2.621784821874995952 ) ) ;
#45417=CARTESIAN_POINT ( 'NONE',  ( 13.65937500061451715, 0.000000000000000000, 5.243569643749999010 ) ) ;
#45418=DIRECTION ( 'NONE',  ( 0.000000000000000000, -0.000000000000000000, -1.000000000000000000 ) ) ;
#45419=CARTESIAN_POINT ( 'NONE',  ( 7.387500000000001066, 5.773502691896255534, 3.535250795749688894E-16 ) ) ;
#45420=CARTESIAN_POINT ( 'NONE',  ( 4.243569643749999010, 16.46562500061459744, 27.54997392385601174 ) ) ;
#45421=CARTESIAN_POINT ( 'NONE',  ( 22.05937500061451573, 4.541064518000418104, -2.621784821874998173 ) ) ;
#45423=( BOUNDED_CURVE ( )  B_SPLINE_CURVE ( 2, ( #12812, #59320, #53437, #69345, #47168, #2827, #64512 ),
 .UNSPECIFIED., .F., .F. ) 
 B_SPLINE_CURVE_WITH_KNOTS ( ( 3, 2, 2, 3 ),
 ( 0.9599622389005039169, 0.9611111111111111382, 0.9638888888888889062, 0.9649218417165331685 ),
 .UNSPECIFIED. ) 
 CURVE ( )  GEOMETRIC_REPRESENTATION_ITEM ( )  RATIONAL_B_SPLINE_CURVE ( ( 0.9350132099087378190, 0.9445889114130223696, 1.000000000000000000, 0.8660254037844387076, 1.000000000000000000, 0.9501798023223894107, 0.9374121827714954058 ) ) 
 REPRESENTATION_ITEM ( '' )  );
#45424=CARTESIAN_POINT ( 'NONE',  ( 26.21250000122903501, -4.330127018922190985, -2.500000000000001332 ) ) ;
#45426=CARTESIAN_POINT ( 'NONE',  ( 23.31562500061451715, 3.027376345333613106, -5.243569643749998122 ) ) ;
#45427=CARTESIAN_POINT ( 'NONE',  ( 16.52812500061451573, 6.421520780324663323E-16, -5.243569643749999010 ) ) ;
#45429=CARTESIAN_POINT ( 'NONE',  ( 11.82187500061451679, 3.027376345333611329, 5.243569643749999010 ) ) ;
#45430=CARTESIAN_POINT ( 'NONE',  ( 27.75000000000000000, 0.000000000000000000, 4.999999999999998224 ) ) ;
#45431=CARTESIAN_POINT ( 'NONE',  ( 25.35000000122903074, -2.886751345948125991, -5.000000000000000000 ) ) ;
#45432=CARTESIAN_POINT ( 'NONE',  ( 3.421875000614516882, -6.054752690667223547, -1.112240025338166033E-15 ) ) ;
#45433=AXIS2_PLACEMENT_3D ( 'NONE', #59738, #9147, #31683 ) ;
#45434=CARTESIAN_POINT ( 'NONE',  ( 13.69687500061451679, -3.027376345333614438, 5.243569643749998122 ) ) ;
#45435=CARTESIAN_POINT ( 'NONE',  ( 28.43437500061451573, 4.541064518000418104, 2.621784821874999949 ) ) ;
#45436=CARTESIAN_POINT ( 'NONE',  ( 8.212500001229035007, -4.330127018922190985, -2.500000000000001332 ) ) ;
#45438=CARTESIAN_POINT ( 'NONE',  ( 23.44687500061451502, 6.054752690667223547, 3.707466751127219781E-16 ) ) ;
#45439=CARTESIAN_POINT ( 'NONE',  ( 14.52187500061451608, 3.027376345333611329, 5.243569643749999010 ) ) ;
#45441=CARTESIAN_POINT ( 'NONE',  ( 26.55000000000000071, -4.330127018922190985, -2.500000000000001332 ) ) ;
#45442=CARTESIAN_POINT ( 'NONE',  ( 4.237500001229036251, 6.123233995736764310E-16, -4.999999999999998224 ) ) ;
#45444=CARTESIAN_POINT ( 'NONE',  ( 17.91562500061451502, 3.027376345333613106, -5.243569643749998122 ) ) ;
#45445=CARTESIAN_POINT ( 'NONE',  ( 6.750000000000002665, -4.330127018922190985, -2.500000000000001332 ) ) ;
#45446=CARTESIAN_POINT ( 'NONE',  ( 26.06250000122903288, 0.000000000000000000, 4.999999999999998224 ) ) ;
#45447=CARTESIAN_POINT ( 'NONE',  ( 17.69999999999999929, 4.330127018922192761, -2.499999999999997780 ) ) ;
#45448=CARTESIAN_POINT ( 'NONE',  ( -4.243569643749999898, 13.46562500061451928, 27.54997392385601529 ) ) ;
#45449=LINE ( 'NONE', #35079, #37232 ) ;
#45450=CARTESIAN_POINT ( 'NONE',  ( 21.18750000122903288, -4.330127018922194537, 2.499999999999995559 ) ) ;
#45451=CARTESIAN_POINT ( 'NONE',  ( 3.975671559181609194, 9.180671356215654555, 25.48966973224918320 ) ) ;
#45452=( BOUNDED_SURFACE ( )  B_SPLINE_SURFACE ( 1, 2, ( 
 ( #50944, #39872, #22849, #45403, #11783, #56831, #45769, #708, #28766, #23216, #17664, #62747, #34665, #51670, #26137, #48678, #71202, #20578, #64192, #9149, #25405, #64926, #65287, #43133, #42039, #64562, #8779, #59007, #13951, #36488, #37219, #69746, #42767, #54218, #14675, #70837, #25032, #47214, #19114, #8411, #25776, #8052, #14316, #47948, #20213, #59741, #13579, #41669, #36852, #19481, #36125, #31685, #42404, #30941, #3616, #59368, #31314, #53482, #37584, #53857, #30221, #65657, #70476, #2157, #19853, #3248, #15046, #52754, #48314, #60106, #24668, #58644, #30586, #2874, #53112, #2509, #47575, #70105, #49409, #67497, #16143, #9876, #54948, #32411, #20950, #66028, #43503, #61213, #26880, #56040, #66769, #27606, #72301, #60840, #4709, #10246, #10968, #37948, #32048, #21681, #60467, #38694, #9515, #55315, #67140, #49049, #15406, #50140, #22050, #44239, #32778, #27971, #54580, #73028, #5431, #4354, #10608, #5071, #33137, #27240, #71941, #72670, #61566, #3984, #44610, #55674, #16498, #33491, #39053, #66394, #50501, #21317, #26509, #22412, #71576, #49777, #44959, #43870, #15771, #38313, #16860, #39415, #51586, #6878, #6517, #63015, #28681, #46765, #68577, #62302, #34214, #11698, #258, #45319, #22767, #40499, #6152, #35304, #46041, #29411, #986, #40142, #57106, #62658, #63384, #17226, #11341, #23494, #39786, #17937, #61937, #34578, #46401, #28323, #67853, #51944, #1341, #12414, #12054, #7236, #33857, #52300, #57827, #56748, #34946, #57473, #23853, #29050, #51221, #68937, #40867, #56401, #18296, #12769, #29763, #1701, #24215, #45686, #69300, #624, #5791, #18662, #50860, #23130, #68219, #17581, #36030, #64096, #41579, #2416, #64465, #47853, #19383, #30851, #30127, #59277, #70014, #36399, #64834, #48218, #58546, #7957, #53386, #53022, #30494, #24938, #14222, #58185, #19758, #8685, #42307, #70380, #13480, #35664, #7590, #47481, #36758, #47122, #58912, #41942, #31217, #53760, #52658, #2067, #8322, #13857, #24576, #3154, #2781, #25306, #25683, #70740, #20118, #42673, #65196, #41224, #63733, #13125, #69654, #19018, #1221, #46277, #69539, #34094, #23727, #41106, #63616, #13006, #40021, #40373, #7473, #29643, #52181, #57349, #68816, #62892, #69181, #18172, #40741, #6755, #41460, #63257, #56634, #58064, #51818, #6030, #12649, #35184, #18898, #28564, #57710, #35544, #29999, #52542, #62535, #12286, #1949, #1583, #24092, #29288, #863, #63979, #7114, #34457, #6391, #56985, #45565, #17462, #68097, #46640, #51460, #24456, #18542, #47004, #51100, #34821, #496, #23006, #11932, #28923, #23370, #45918, #68450, #17812, #13361, #59159, #70991, #52904, #19261, #31468, #25927, #3027, #36637, #31837, #35902, #3768, #9303, #69895, #19997, #8937, #48099, #31095, #30732, #54011, #65441, #7838, #3407, #37002, #42550, #37374, #20367, #70261, #70622, #2662, #58427, #26293, #30375, #8567, #65077, #58793, #25179, #53264, #8203, #64713, #25558, #48467, #53634, #14468, #47364, #14833, #59524, #42918, #59898, #48830, #47722, #19632, #54373, #42189, #14097, #71360, #20735, #2302, #43293, #24817, #41815, #64346, #13737, #36279, #2902, #48707, #54247, #66423, #4381, #14346, #4013, #42433, #49077, #42794, #59770, #32076, #64954, #20242, #25433, #15801, #53885, #59398, #15074, #43899, #36880, #71230, #8808, #59036, #54976, #26910, #49436, #71970, #31345, #21344, #8438, #14705, #26537, #20609, #3277, #43167, #65686, #31712, #25805, #71604, #48343, #30974, #47975, #37611, #3644, #53509, #70503, #70868, #20979, #65315, #43532, #37249, #9177, #54608, #26167, #60133, #9542, #66053, #19880, #15431, #37976, #60497, #9903, #32440, #16170, #32805, #4737, #27271, #56069, #23161, #45715, #50168, #288, #28351, #38342, #39080, #22439, #49804, #33166, #72329, #44988, #21709, #72697, #39444, #6182, #56430, #61965, #61242, #68249, #17255, #653, #60870, #39815, #22796, #67167, #67525, #61598, #5820, #10273, #55342, #44267, #5461, #10999, #16528, #51250, #33519, #66799, #38721, #10635, #62331, #73058, #16890, #55704, #11727, #5098, #27634, #34243, #22079, #44638, #28001, #50888, #45349, #50530, #11368, #33886, #67883, #28711, #56776, #13157, #46073, #12801, #12087, #23886, #24973, #63415, #17969, #18329, #57507, #58219, #34608, #35699, #69335, #41257, #24250, #41613, #2100, #1376, #1736, #6909, #17612, #30529, #57138, #35337, #46798, #63046, #29440, #34978, #12447, #68972, #7269, #7624, #57860, #18693, #51616, #69690, #29798, #52334, #52694, #7993, #51977, #46433, #63769, #40902, #30161, #24611, #47158, #6547, #19055, #64132, #13518, #36066, #2450, #58586, #53056, #47518, #40172, #68608, #62691, #29081, #1017, #23523, #40530, #8355, #54162, #59310, #53426, #54523, #9091, #25717, #31989, #3558, #31628, #20154, #4296, #26080, #70047, #20894, #14619, #41980, #37158, #48619, #32351, #19420, #59684, #3926, #26449, #48989, #2816, #3190, #43448, #65601, #14989, #42708, #36795, #54889, #71144, #70418, #42345, #19794, #30884, #25344, #47889, #20517, #14256, #65970, #43075, #37527, #60048, #48255, #65229, #70778, #71519, #64868, #64501, #9459, #8720, #15350, #13893, #37891, #60410, #36433, #31253, #9819, #26821, #58947, #53795, #67798, #49355, #39732, #45266, #32723, #55984, #44909, #10913, #67084, #66712, #67446, #28274, #43811, #39364, #4656, #5377, #71885, #21995, #33807, #15714, #55260, #16808, #61879, #39000, #72613, #17172, #21258, #62249, #11646, #27185, #27915, #11286, #33439, #16443, #16086, #56350, #50805, #66336, #5740, #72975, #50449, #208, #22713, #33081, #22357, #38634, #38252, #34161, #60781, #44553, #56698, #21624, #61158, #10553, #44182, #27550, #61515, #6098, #10188, #49719, #72247, #55620, #5016, #50082, #63684, #18968, #40443, #62959, #7183, #57418, #12354, #34889, #35613, #68166, #41175, #52611, #13074 ),
 ( #35252, #68882, #1287, #58133, #23440, #6460, #23076, #17529, #40091, #46348, #13427, #35976, #6822, #7539, #18610, #28629, #29356, #12716, #62605, #45986, #12001, #57773, #34524, #51889, #29711, #69607, #46713, #52249, #51532, #58496, #30072, #64047, #51167, #2017, #24528, #23797, #1652, #18239, #69248, #570, #45633, #57054, #40812, #63328, #28995, #47072, #24160, #41528, #932, #68522, #17883, #31164, #15266, #37071, #7905, #31904, #25628, #52972, #48165, #20065, #43362, #30443, #70690, #14903, #37444, #59964, #13808, #14171, #54441, #3475, #25995, #53706, #47798, #65885, #14536, #8272, #53335, #30802, #19333, #64415, #41887, #59594, #25250, #3840, #65145, #48534, #42621, #59227, #3099, #8635, #9372, #36347, #2368, #9007, #58862, #31539, #24886, #54079, #65516, #47431, #2733, #71061, #20436, #42985, #26361, #48901, #69962, #71430, #20807, #70328, #37804, #19704, #42257, #64780, #36705, #5288, #39278, #54801, #50365, #10825, #66996, #11195, #44825, #44093, #44465, #49632, #60324, #124, #4207, #32996, #16358, #32634, #72159, #4570, #55174, #38545, #49996, #27833, #4930, #61432, #21171, #61790, #55535, #21909, #22273, #50721, #21538, #66620, #38913, #15996, #61069, #10466, #67360, #26735, #72892, #33721, #16723, #56266, #45180, #27465, #72521, #5657, #55897, #38167, #33360, #28192, #22629, #67711, #43724, #71802, #17083, #9734, #32268, #49269, #66247, #15625, #60691, #10104, #27100, #17445, #23709, #57333, #7097, #1566, #477, #51080, #46260, #28903, #22986, #24076, #51801, #68432, #46622, #68799, #1204, #62874, #46987, #18155, #39644, #63601, #6737, #11559, #29271, #40723, #1933, #62162, #63239, #69165, #18524, #41089, #45546, #45901, #12991, #35168, #57692, #12270, #6371, #24438, #12633, #40002, #11914, #62516, #68076, #34439, #56967, #29626, #51441, #35527, #52163, #58048, #7456, #17795, #34801, #40355, #29983, #843, #34075, #52525, #23352, #69523, #56615, #6010, #28545, #58408, #24800, #36983, #31449, #8549, #42169, #37356, #18881, #9284, #14813, #2283, #25537, #14449, #53616, #36619, #36259, #59505, #70973, #13346, #8919, #42532, #48078, #42899, #3388, #2642, #3007, #8183, #41444, #31817, #35883, #64695, #70606, #64325, #30711, #58774, #13718, #70241, #31076, #53991, #59140, #19979, #52885, #20348, #14079, #65058, #25909, #54356, #53244, #25161, #48449, #47702, #19612, #65423, #59878, #7821, #3750, #26274, #48811, #47343, #63962, #30356, #69877, #19242, #41797, #32548, #38081, #49184, #37715, #4841, #38454, #44004, #5199, #66161, #71714, #65795, #60235, #9649, #15906, #56175, #5568, #10012, #33273, #61344, #71341, #72068, #55448, #32183, #15537, #54716, #27375, #4119, #55085, #72431, #39188, #16273, #21815, #21086, #28105, #50279, #33630, #20716, #72803, #55812, #27014, #49907, #21448, #38829, #43274, #15176, #26648, #60980, #66526, #49546, #11102, #10379, #43637, #60603, #4485, #22186, #32911, #44380, #66905, #44740, #10740, #27740, #67274, #16633, #61703, #40922, #69710, #64152, #29457, #1756, #35355, #8376, #42002, #7289, #47177, #6927, #46818, #46091, #57879, #58968, #24269, #51994, #52353, #18347, #19076, #68627, #41633, #30183, #17989, #50634, #46452, #1395, #7645, #36454, #57526, #63789, #23904, #38, #47539, #70068, #19441, #64522, #68990, #13915, #23541, #29818, #13539, #13179, #63434, #35718, #41278, #69356, #12821, #36087, #18713, #40548, #63064, #58240, #52714, #12467, #34997, #2120, #24632, #58607, #8014, #30549, #53076, #2471, #24995, #42367, #14277, #64889, #9481, #48276, #4317, #15010, #49009, #20538, #9112, #26102, #31650, #32371, #59330, #53447, #43094, #8741, #60069, #30905, #3579, #15372, #70439, #36815, #71540, #43467, #65622, #54183, #49376, #2837, #21279, #26842, #31274, #37547, #26470, #32010, #48640, #70800, #20915, #9842, #25366, #65991, #54545, #3947, #54909, #37914, #14639, #60431, #20175, #47910, #43833, #19814, #71165, #71906, #3210, #42729, #65250, #25739, #66358, #15735, #38274, #60802, #53817, #37180, #59705, #5397, #44928, #45285, #589, #22017, #44573, #61900, #39019, #67103, #16461, #17192, #49740, #22732, #34180, #67819, #50824, #68185, #61534, #27934, #11664, #5760, #61178, #67464, #50467, #227, #39752, #44202, #21645, #16827, #72633, #66733, #62269, #22376, #10932, #56715, #39381, #11305, #33458, #17548, #33826, #10208, #6116, #28293, #72267, #72995, #40109, #32743, #56003, #28647, #51185, #55280, #56369, #23094, #16104, #5034, #38654, #45651, #4675, #27205, #10573, #33101, #55640, #27571, #50103, #29729, #63347, #40831, #2384, #57791, #952, #68542, #40463, #13444, #24178, #41192, #47447, #41545, #62979, #46006, #35993, #57438, #12375, #51908, #7556, #2033, #34910, #12733, #46367, #19349, #52988, #18258, #58151, #17903, #7200, #57072, #68901, #69979, #35269, #6841, #52267, #29376, #30090, #6479, #52628, #63701, #29014, #62624, #1307, #23816, #18627, #12019, #1669, #46730, #69265, #34542, #58511, #7922, #30459, #24902, #13092, #51551, #23460, #35630, #24544, #47089, #69622, #18984, #64063, #14551, #42272, #54457, #64795, #26752, #58877, #31556, #37087, #49285, #60341, #70344, #59980, #25267, #31921, #25645, #42637, #14919, #47814, #3115, #8651, #19720, #8287, #48550, #9025, #59611, #48917, #64431, #54096, #30817, #37461, #53350, #3493, #71818, #41906, #53723, #3856, #26378, #13823, #65161, #26011, #2748, #36721, #14186, #71077, #59242, #48182, #43002, #9750, #9390, #65533, #31180, #36363, #20823, #4224, #70706, #43378, #71448, #65902, #15282, #20452, #37822, #32284, #20081, #54818, #10484, #21190, #34092, #38184, #67014, #27851, #66637, #33013, #38563, #16015, #72539, #10843, #39294, #38930, #22289, #55192, #140, #16375, #55913, #56284, #11577, #55552, #4948, #72907, #50015, #27482, #21927, #28209, #60708, #33738 ) ),
 .UNSPECIFIED., .F., .F., .F. ) 
 B_SPLINE_SURFACE_WITH_KNOTS ( ( 2, 2 ),
 ( 3, 2, 2, 2, 2, 2, 2, 2, 2, 2, 2, 2, 2, 2, 2, 2, 2, 2, 2, 2, 2, 2, 2, 2, 2, 2, 2, 2, 2, 2, 2, 2, 2, 2, 2, 2, 2, 2, 2, 2, 2, 2, 2, 2, 2, 2, 2, 2, 2, 2, 2, 2, 2, 2, 2, 2, 2, 2, 2, 2, 2, 2, 2, 2, 2, 2, 2, 2, 2, 2, 2, 2, 2, 2, 2, 2, 2, 2, 2, 2, 2, 2, 2, 2, 2, 2, 2, 2, 2, 2, 2, 2, 2, 2, 2, 2, 2, 2, 2, 2, 2, 2, 2, 2, 2, 2, 2, 2, 2, 2, 2, 2, 2, 2, 2, 2, 2, 2, 2, 2, 2, 2, 2, 2, 2, 2, 2, 2, 2, 2, 2, 2, 2, 2, 2, 2, 2, 2, 2, 2, 2, 2, 2, 2, 2, 2, 2, 2, 2, 2, 2, 2, 2, 2, 2, 2, 2, 2, 2, 2, 2, 2, 2, 2, 2, 2, 2, 2, 2, 2, 2, 2, 2, 2, 2, 2, 2, 2, 2, 2, 2, 2, 2, 2, 2, 2, 2, 2, 2, 2, 2, 2, 2, 2, 2, 2, 2, 2, 2, 2, 2, 2, 2, 2, 2, 2, 2, 2, 2, 2, 2, 2, 2, 2, 2, 2, 2, 2, 2, 2, 2, 2, 2, 2, 2, 2, 2, 2, 2, 2, 2, 2, 2, 2, 2, 2, 2, 2, 2, 2, 2, 2, 2, 2, 2, 2, 2, 2, 2, 2, 2, 2, 2, 2, 2, 2, 2, 2, 2, 2, 2, 2, 2, 2, 2, 2, 2, 2, 2, 2, 2, 2, 2, 2, 2, 2, 2, 2, 2, 2, 2, 2, 2, 2, 2, 2, 2, 2, 2, 2, 2, 2, 2, 2, 2, 2, 2, 2, 2, 2, 2, 2, 2, 2, 2, 2, 2, 2, 2, 2, 2, 2, 2, 2, 2, 2, 2, 2, 2, 2, 2, 2, 2, 2, 2, 2, 2, 2, 2, 2, 2, 2, 2, 2, 2, 2, 2, 2, 2, 2, 2, 2, 2, 2, 2, 2, 2, 2, 2, 2, 2, 2, 2, 2, 2, 2, 2, 2, 2, 2, 3 ),
 ( 0.000000000000000000, 1.000000000000000000 ),
 ( 0.000000000000000000, 0.002777777777777777884, 0.005555555555555555768, 0.008333333333333333218, 0.01111111111111111154, 0.01388888888888888812, 0.01666666666666666644, 0.01944444444444444475, 0.02222222222222222307, 0.02500000000000000139, 0.02777777777777777624, 0.03055555555555555455, 0.03333333333333333287, 0.03611111111111110772, 0.03888888888888888951, 0.04166666666666666435, 0.04444444444444444614, 0.04722222222222222099, 0.05000000000000000278, 0.05277777777777777762, 0.05555555555555555247, 0.05833333333333333426, 0.06111111111111110911, 0.06388888888888888395, 0.06666666666666666574, 0.06944444444444444753, 0.07222222222222221544, 0.07499999999999999722, 0.07777777777777777901, 0.08055555555555556080, 0.08333333333333332871, 0.08611111111111111049, 0.08888888888888889228, 0.09166666666666666019, 0.09444444444444444198, 0.09722222222222222376, 0.1000000000000000056, 0.1027777777777777735, 0.1055555555555555552, 0.1083333333333333370, 0.1111111111111111049, 0.1138888888888888867, 0.1166666666666666685, 0.1194444444444444503, 0.1222222222222222182, 0.1250000000000000000, 0.1277777777777777679, 0.1305555555555555636, 0.1333333333333333315, 0.1361111111111110994, 0.1388888888888888951, 0.1416666666666666630, 0.1444444444444444309, 0.1472222222222222265, 0.1499999999999999944, 0.1527777777777777901, 0.1555555555555555580, 0.1583333333333333259, 0.1611111111111111216, 0.1638888888888888895, 0.1666666666666666574, 0.1694444444444444531, 0.1722222222222222210, 0.1749999999999999889, 0.1777777777777777846, 0.1805555555555555525, 0.1833333333333333204, 0.1861111111111111160, 0.1888888888888888840, 0.1916666666666666796, 0.1944444444444444475, 0.1972222222222222154, 0.2000000000000000111, 0.2027777777777777790, 0.2055555555555555469, 0.2083333333333333426, 0.2111111111111111105, 0.2138888888888888784, 0.2166666666666666741, 0.2194444444444444420, 0.2222222222222222099, 0.2250000000000000056, 0.2277777777777777735, 0.2305555555555555691, 0.2333333333333333370, 0.2361111111111111049, 0.2388888888888889006, 0.2416666666666666685, 0.2444444444444444364, 0.2472222222222222321, 0.2500000000000000000, 0.2527777777777777679, 0.2555555555555555358, 0.2583333333333333592, 0.2611111111111111271, 0.2638888888888888951, 0.2666666666666666630, 0.2694444444444444309, 0.2722222222222221988, 0.2750000000000000222, 0.2777777777777777901, 0.2805555555555555580, 0.2833333333333333259, 0.2861111111111110938, 0.2888888888888888618, 0.2916666666666666852, 0.2944444444444444531, 0.2972222222222222210, 0.2999999999999999889, 0.3027777777777777568, 0.3055555555555555802, 0.3083333333333333481, 0.3111111111111111160, 0.3138888888888888840, 0.3166666666666666519, 0.3194444444444444198, 0.3222222222222222432, 0.3250000000000000111, 0.3277777777777777790, 0.3305555555555555469, 0.3333333333333333148, 0.3361111111111111382, 0.3388888888888889062, 0.3416666666666666741, 0.3444444444444444420, 0.3472222222222222099, 0.3499999999999999778, 0.3527777777777778012, 0.3555555555555555691, 0.3583333333333333370, 0.3611111111111111049, 0.3638888888888888729, 0.3666666666666666408, 0.3694444444444444642, 0.3722222222222222321, 0.3750000000000000000, 0.3777777777777777679, 0.3805555555555555358, 0.3833333333333333592, 0.3861111111111111271, 0.3888888888888888951, 0.3916666666666666630, 0.3944444444444444309, 0.3972222222222221988, 0.4000000000000000222, 0.4027777777777777901, 0.4055555555555555580, 0.4083333333333333259, 0.4111111111111110938, 0.4138888888888888618, 0.4166666666666666852, 0.4194444444444444531, 0.4222222222222222210, 0.4249999999999999889, 0.4277777777777777568, 0.4305555555555555802, 0.4333333333333333481, 0.4361111111111111160, 0.4388888888888888840, 0.4416666666666666519, 0.4444444444444444198, 0.4472222222222222432, 0.4500000000000000111, 0.4527777777777777790, 0.4555555555555555469, 0.4583333333333333148, 0.4611111111111111382, 0.4638888888888889062, 0.4666666666666666741, 0.4694444444444444420, 0.4722222222222222099, 0.4749999999999999778, 0.4777777777777778012, 0.4805555555555555691, 0.4833333333333333370, 0.4861111111111111049, 0.4888888888888888729, 0.4916666666666666408, 0.4944444444444444642, 0.4972222222222222321, 0.5000000000000000000, 0.5027777777777777679, 0.5055555555555555358, 0.5083333333333333037, 0.5111111111111110716, 0.5138888888888888395, 0.5166666666666667185, 0.5194444444444444864, 0.5222222222222222543, 0.5250000000000000222, 0.5277777777777777901, 0.5305555555555555580, 0.5333333333333333259, 0.5361111111111110938, 0.5388888888888888618, 0.5416666666666666297, 0.5444444444444443976, 0.5472222222222222765, 0.5500000000000000444, 0.5527777777777778123, 0.5555555555555555802, 0.5583333333333333481, 0.5611111111111111160, 0.5638888888888888840, 0.5666666666666666519, 0.5694444444444444198, 0.5722222222222221877, 0.5749999999999999556, 0.5777777777777777235, 0.5805555555555556024, 0.5833333333333333703, 0.5861111111111111382, 0.5888888888888889062, 0.5916666666666666741, 0.5944444444444444420, 0.5972222222222222099, 0.5999999999999999778, 0.6027777777777777457, 0.6055555555555555136, 0.6083333333333332815, 0.6111111111111111605, 0.6138888888888889284, 0.6166666666666666963, 0.6194444444444444642, 0.6222222222222222321, 0.6250000000000000000, 0.6277777777777777679, 0.6305555555555555358, 0.6333333333333333037, 0.6361111111111110716, 0.6388888888888888395, 0.6416666666666667185, 0.6444444444444444864, 0.6472222222222222543, 0.6500000000000000222, 0.6527777777777777901, 0.6555555555555555580, 0.6583333333333333259, 0.6611111111111110938, 0.6638888888888888618, 0.6666666666666666297, 0.6694444444444443976, 0.6722222222222222765, 0.6750000000000000444, 0.6777777777777778123, 0.6805555555555555802, 0.6833333333333333481, 0.6861111111111111160, 0.6888888888888888840, 0.6916666666666666519, 0.6944444444444444198, 0.6972222222222221877, 0.6999999999999999556, 0.7027777777777777235, 0.7055555555555556024, 0.7083333333333333703, 0.7111111111111111382, 0.7138888888888889062, 0.7166666666666666741, 0.7194444444444444420, 0.7222222222222222099, 0.7249999999999999778, 0.7277777777777777457, 0.7305555555555555136, 0.7333333333333332815, 0.7361111111111111605, 0.7388888888888889284, 0.7416666666666666963, 0.7444444444444444642, 0.7472222222222222321, 0.7500000000000000000, 0.7527777777777777679, 0.7555555555555555358, 0.7583333333333333037, 0.7611111111111110716, 0.7638888888888888395, 0.7666666666666667185, 0.7694444444444444864, 0.7722222222222222543, 0.7750000000000000222, 0.7777777777777777901, 0.7805555555555555580, 0.7833333333333333259, 0.7861111111111110938, 0.7888888888888888618, 0.7916666666666666297, 0.7944444444444443976, 0.7972222222222222765, 0.8000000000000000444, 0.8027777777777778123, 0.8055555555555555802, 0.8083333333333333481, 0.8111111111111111160, 0.8138888888888888840, 0.8166666666666666519, 0.8194444444444444198, 0.8222222222222221877, 0.8249999999999999556, 0.8277777777777777235, 0.8305555555555556024, 0.8333333333333333703, 0.8361111111111111382, 0.8388888888888889062, 0.8416666666666666741, 0.8444444444444444420, 0.8472222222222222099, 0.8499999999999999778, 0.8527777777777777457, 0.8555555555555555136, 0.8583333333333332815, 0.8611111111111111605, 0.8638888888888889284, 0.8666666666666666963, 0.8694444444444444642, 0.8722222222222222321, 0.8750000000000000000, 0.8777777777777777679, 0.8805555555555555358, 0.8833333333333333037, 0.8861111111111110716, 0.8888888888888888395, 0.8916666666666667185, 0.8944444444444444864, 0.8972222222222222543, 0.9000000000000000222, 0.9027777777777777901, 0.9055555555555555580, 0.9083333333333333259, 0.9111111111111110938, 0.9138888888888888618, 0.9166666666666666297, 0.9194444444444443976, 0.9222222222222222765, 0.9250000000000000444, 0.9277777777777778123, 0.9305555555555555802, 0.9333333333333333481, 0.9361111111111111160, 0.9388888888888888840, 0.9416666666666666519, 0.9444444444444444198, 0.9472222222222221877, 0.9499999999999999556, 0.9527777777777777235, 0.9555555555555556024, 0.9583333333333333703, 0.9611111111111111382, 0.9638888888888889062, 0.9666666666666666741, 0.9694444444444444420, 0.9722222222222222099, 0.9749999999999999778, 0.9777777777777777457, 0.9805555555555555136, 0.9833333333333332815, 0.9861111111111111605, 0.9888888888888889284, 0.9916666666666666963, 0.9944444444444444642, 0.9972222222222222321, 1.000000000000000000 ),
 .UNSPECIFIED. ) 
 GEOMETRIC_REPRESENTATION_ITEM ( )  RATIONAL_B_SPLINE_SURFACE ( (
 ( 1.000000000000000000, 0.8660254037844387076, 1.000000000000000000, 0.8660254037844387076, 1.000000000000000000, 0.8660254037844387076, 1.000000000000000000, 0.8660254037844387076, 1.000000000000000000, 0.8660254037844387076, 1.000000000000000000, 0.8660254037844387076, 1.000000000000000000, 0.8660254037844387076, 1.000000000000000000, 0.8660254037844387076, 1.000000000000000000, 0.8660254037844387076, 1.000000000000000000, 0.8660254037844387076, 1.000000000000000000, 0.8660254037844387076, 1.000000000000000000, 0.8660254037844387076, 1.000000000000000000, 0.8660254037844387076, 1.000000000000000000, 0.8660254037844387076, 1.000000000000000000, 0.8660254037844387076, 1.000000000000000000, 0.8660254037844387076, 1.000000000000000000, 0.8660254037844387076, 1.000000000000000000, 0.8660254037844387076, 1.000000000000000000, 0.8660254037844387076, 1.000000000000000000, 0.8660254037844387076, 1.000000000000000000, 0.8660254037844387076, 1.000000000000000000, 0.8660254037844387076, 1.000000000000000000, 0.8660254037844387076, 1.000000000000000000, 0.8660254037844387076, 1.000000000000000000, 0.8660254037844387076, 1.000000000000000000, 0.8660254037844387076, 1.000000000000000000, 0.8660254037844387076, 1.000000000000000000, 0.8660254037844387076, 1.000000000000000000, 0.8660254037844387076, 1.000000000000000000, 0.8660254037844387076, 1.000000000000000000, 0.8660254037844387076, 1.000000000000000000, 0.8660254037844387076, 1.000000000000000000, 0.8660254037844387076, 1.000000000000000000, 0.8660254037844387076, 1.000000000000000000, 0.8660254037844387076, 1.000000000000000000, 0.8660254037844387076, 1.000000000000000000, 0.8660254037844387076, 1.000000000000000000, 0.8660254037844387076, 1.000000000000000000, 0.8660254037844387076, 1.000000000000000000, 0.8660254037844387076, 1.000000000000000000, 0.8660254037844387076, 1.000000000000000000, 0.8660254037844387076, 1.000000000000000000, 0.8660254037844387076, 1.000000000000000000, 0.8660254037844387076, 1.000000000000000000, 0.8660254037844387076, 1.000000000000000000, 0.8660254037844387076, 1.000000000000000000, 0.8660254037844387076, 1.000000000000000000, 0.8660254037844387076, 1.000000000000000000, 0.8660254037844387076, 1.000000000000000000, 0.8660254037844387076, 1.000000000000000000, 0.8660254037844387076, 1.000000000000000000, 0.8660254037844387076, 1.000000000000000000, 0.8660254037844387076, 1.000000000000000000, 0.8660254037844387076, 1.000000000000000000, 0.8660254037844387076, 1.000000000000000000, 0.8660254037844387076, 1.000000000000000000, 0.8660254037844387076, 1.000000000000000000, 0.8660254037844387076, 1.000000000000000000, 0.8660254037844387076, 1.000000000000000000, 0.8660254037844387076, 1.000000000000000000, 0.8660254037844387076, 1.000000000000000000, 0.8660254037844387076, 1.000000000000000000, 0.8660254037844387076, 1.000000000000000000, 0.8660254037844387076, 1.000000000000000000, 0.8660254037844387076, 1.000000000000000000, 0.8660254037844387076, 1.000000000000000000, 0.8660254037844387076, 1.000000000000000000, 0.8660254037844387076, 1.000000000000000000, 0.8660254037844387076, 1.000000000000000000, 0.8660254037844387076, 1.000000000000000000, 0.8660254037844387076, 1.000000000000000000, 0.8660254037844387076, 1.000000000000000000, 0.8660254037844387076, 1.000000000000000000, 0.8660254037844387076, 1.000000000000000000, 0.8660254037844387076, 1.000000000000000000, 0.8660254037844387076, 1.000000000000000000, 0.8660254037844387076, 1.000000000000000000, 0.8660254037844387076, 1.000000000000000000, 0.8660254037844387076, 1.000000000000000000, 0.8660254037844387076, 1.000000000000000000, 0.8660254037844387076, 1.000000000000000000, 0.8660254037844387076, 1.000000000000000000, 0.8660254037844387076, 1.000000000000000000, 0.8660254037844387076, 1.000000000000000000, 0.8660254037844387076, 1.000000000000000000, 0.8660254037844387076, 1.000000000000000000, 0.8660254037844387076, 1.000000000000000000, 0.8660254037844387076, 1.000000000000000000, 0.8660254037844387076, 1.000000000000000000, 0.8660254037844387076, 1.000000000000000000, 0.8660254037844387076, 1.000000000000000000, 0.8660254037844387076, 1.000000000000000000, 0.8660254037844387076, 1.000000000000000000, 0.8660254037844387076, 1.000000000000000000, 0.8660254037844387076, 1.000000000000000000, 0.8660254037844387076, 1.000000000000000000, 0.8660254037844387076, 1.000000000000000000, 0.8660254037844387076, 1.000000000000000000, 0.8660254037844387076, 1.000000000000000000, 0.8660254037844387076, 1.000000000000000000, 0.8660254037844387076, 1.000000000000000000, 0.8660254037844387076, 1.000000000000000000, 0.8660254037844387076, 1.000000000000000000, 0.8660254037844387076, 1.000000000000000000, 0.8660254037844387076, 1.000000000000000000, 0.8660254037844387076, 1.000000000000000000, 0.8660254037844387076, 1.000000000000000000, 0.8660254037844387076, 1.000000000000000000, 0.8660254037844387076, 1.000000000000000000, 0.8660254037844387076, 1.000000000000000000, 0.8660254037844387076, 1.000000000000000000, 0.8660254037844387076, 1.000000000000000000, 0.8660254037844387076, 1.000000000000000000, 0.8660254037844387076, 1.000000000000000000, 0.8660254037844387076, 1.000000000000000000, 0.8660254037844387076, 1.000000000000000000, 0.8660254037844387076, 1.000000000000000000, 0.8660254037844387076, 1.000000000000000000, 0.8660254037844387076, 1.000000000000000000, 0.8660254037844387076, 1.000000000000000000, 0.8660254037844387076, 1.000000000000000000, 0.8660254037844387076, 1.000000000000000000, 0.8660254037844387076, 1.000000000000000000, 0.8660254037844387076, 1.000000000000000000, 0.8660254037844387076, 1.000000000000000000, 0.8660254037844387076, 1.000000000000000000, 0.8660254037844387076, 1.000000000000000000, 0.8660254037844387076, 1.000000000000000000, 0.8660254037844387076, 1.000000000000000000, 0.8660254037844387076, 1.000000000000000000, 0.8660254037844387076, 1.000000000000000000, 0.8660254037844387076, 1.000000000000000000, 0.8660254037844387076, 1.000000000000000000, 0.8660254037844387076, 1.000000000000000000, 0.8660254037844387076, 1.000000000000000000, 0.8660254037844387076, 1.000000000000000000, 0.8660254037844387076, 1.000000000000000000, 0.8660254037844387076, 1.000000000000000000, 0.8660254037844387076, 1.000000000000000000, 0.8660254037844387076, 1.000000000000000000, 0.8660254037844387076, 1.000000000000000000, 0.8660254037844387076, 1.000000000000000000, 0.8660254037844387076, 1.000000000000000000, 0.8660254037844387076, 1.000000000000000000, 0.8660254037844387076, 1.000000000000000000, 0.8660254037844387076, 1.000000000000000000, 0.8660254037844387076, 1.000000000000000000, 0.8660254037844387076, 1.000000000000000000, 0.8660254037844387076, 1.000000000000000000, 0.8660254037844387076, 1.000000000000000000, 0.8660254037844387076, 1.000000000000000000, 0.8660254037844387076, 1.000000000000000000, 0.8660254037844387076, 1.000000000000000000, 0.8660254037844387076, 1.000000000000000000, 0.8660254037844387076, 1.000000000000000000, 0.8660254037844387076, 1.000000000000000000, 0.8660254037844387076, 1.000000000000000000, 0.8660254037844387076, 1.000000000000000000, 0.8660254037844387076, 1.000000000000000000, 0.8660254037844387076, 1.000000000000000000, 0.8660254037844387076, 1.000000000000000000, 0.8660254037844387076, 1.000000000000000000, 0.8660254037844387076, 1.000000000000000000, 0.8660254037844387076, 1.000000000000000000, 0.8660254037844387076, 1.000000000000000000, 0.8660254037844387076, 1.000000000000000000, 0.8660254037844387076, 1.000000000000000000, 0.8660254037844387076, 1.000000000000000000, 0.8660254037844387076, 1.000000000000000000, 0.8660254037844387076, 1.000000000000000000, 0.8660254037844387076, 1.000000000000000000, 0.8660254037844387076, 1.000000000000000000, 0.8660254037844387076, 1.000000000000000000, 0.8660254037844387076, 1.000000000000000000, 0.8660254037844387076, 1.000000000000000000, 0.8660254037844387076, 1.000000000000000000, 0.8660254037844387076, 1.000000000000000000, 0.8660254037844387076, 1.000000000000000000, 0.8660254037844387076, 1.000000000000000000, 0.8660254037844387076, 1.000000000000000000, 0.8660254037844387076, 1.000000000000000000, 0.8660254037844387076, 1.000000000000000000, 0.8660254037844387076, 1.000000000000000000, 0.8660254037844387076, 1.000000000000000000, 0.8660254037844387076, 1.000000000000000000, 0.8660254037844387076, 1.000000000000000000, 0.8660254037844387076, 1.000000000000000000, 0.8660254037844387076, 1.000000000000000000, 0.8660254037844387076, 1.000000000000000000, 0.8660254037844387076, 1.000000000000000000, 0.8660254037844387076, 1.000000000000000000, 0.8660254037844387076, 1.000000000000000000, 0.8660254037844387076, 1.000000000000000000, 0.8660254037844387076, 1.000000000000000000, 0.8660254037844387076, 1.000000000000000000, 0.8660254037844387076, 1.000000000000000000, 0.8660254037844387076, 1.000000000000000000, 0.8660254037844387076, 1.000000000000000000, 0.8660254037844387076, 1.000000000000000000, 0.8660254037844387076, 1.000000000000000000, 0.8660254037844387076, 1.000000000000000000, 0.8660254037844387076, 1.000000000000000000, 0.8660254037844387076, 1.000000000000000000, 0.8660254037844387076, 1.000000000000000000, 0.8660254037844387076, 1.000000000000000000, 0.8660254037844387076, 1.000000000000000000, 0.8660254037844387076, 1.000000000000000000, 0.8660254037844387076, 1.000000000000000000, 0.8660254037844387076, 1.000000000000000000, 0.8660254037844387076, 1.000000000000000000, 0.8660254037844387076, 1.000000000000000000, 0.8660254037844387076, 1.000000000000000000, 0.8660254037844387076, 1.000000000000000000, 0.8660254037844387076, 1.000000000000000000, 0.8660254037844387076, 1.000000000000000000, 0.8660254037844387076, 1.000000000000000000, 0.8660254037844387076, 1.000000000000000000, 0.8660254037844387076, 1.000000000000000000, 0.8660254037844387076, 1.000000000000000000, 0.8660254037844387076, 1.000000000000000000, 0.8660254037844387076, 1.000000000000000000, 0.8660254037844387076, 1.000000000000000000, 0.8660254037844387076, 1.000000000000000000, 0.8660254037844387076, 1.000000000000000000, 0.8660254037844387076, 1.000000000000000000, 0.8660254037844387076, 1.000000000000000000, 0.8660254037844387076, 1.000000000000000000, 0.8660254037844387076, 1.000000000000000000, 0.8660254037844387076, 1.000000000000000000, 0.8660254037844387076, 1.000000000000000000, 0.8660254037844387076, 1.000000000000000000, 0.8660254037844387076, 1.000000000000000000, 0.8660254037844387076, 1.000000000000000000, 0.8660254037844387076, 1.000000000000000000, 0.8660254037844387076, 1.000000000000000000, 0.8660254037844387076, 1.000000000000000000, 0.8660254037844387076, 1.000000000000000000, 0.8660254037844387076, 1.000000000000000000, 0.8660254037844387076, 1.000000000000000000, 0.8660254037844387076, 1.000000000000000000, 0.8660254037844387076, 1.000000000000000000, 0.8660254037844387076, 1.000000000000000000, 0.8660254037844387076, 1.000000000000000000, 0.8660254037844387076, 1.000000000000000000, 0.8660254037844387076, 1.000000000000000000, 0.8660254037844387076, 1.000000000000000000, 0.8660254037844387076, 1.000000000000000000, 0.8660254037844387076, 1.000000000000000000, 0.8660254037844387076, 1.000000000000000000, 0.8660254037844387076, 1.000000000000000000, 0.8660254037844387076, 1.000000000000000000, 0.8660254037844387076, 1.000000000000000000, 0.8660254037844387076, 1.000000000000000000, 0.8660254037844387076, 1.000000000000000000, 0.8660254037844387076, 1.000000000000000000, 0.8660254037844387076, 1.000000000000000000, 0.8660254037844387076, 1.000000000000000000, 0.8660254037844387076, 1.000000000000000000, 0.8660254037844387076, 1.000000000000000000, 0.8660254037844387076, 1.000000000000000000, 0.8660254037844387076, 1.000000000000000000, 0.8660254037844387076, 1.000000000000000000, 0.8660254037844387076, 1.000000000000000000, 0.8660254037844387076, 1.000000000000000000, 0.8660254037844387076, 1.000000000000000000, 0.8660254037844387076, 1.000000000000000000, 0.8660254037844387076, 1.000000000000000000, 0.8660254037844387076, 1.000000000000000000, 0.8660254037844387076, 1.000000000000000000, 0.8660254037844387076, 1.000000000000000000, 0.8660254037844387076, 1.000000000000000000, 0.8660254037844387076, 1.000000000000000000, 0.8660254037844387076, 1.000000000000000000, 0.8660254037844387076, 1.000000000000000000, 0.8660254037844387076, 1.000000000000000000, 0.8660254037844387076, 1.000000000000000000, 0.8660254037844387076, 1.000000000000000000, 0.8660254037844387076, 1.000000000000000000, 0.8660254037844387076, 1.000000000000000000, 0.8660254037844387076, 1.000000000000000000, 0.8660254037844387076, 1.000000000000000000, 0.8660254037844387076, 1.000000000000000000, 0.8660254037844387076, 1.000000000000000000, 0.8660254037844387076, 1.000000000000000000, 0.8660254037844387076, 1.000000000000000000, 0.8660254037844387076, 1.000000000000000000, 0.8660254037844387076, 1.000000000000000000, 0.8660254037844387076, 1.000000000000000000, 0.8660254037844387076, 1.000000000000000000, 0.8660254037844387076, 1.000000000000000000, 0.8660254037844387076, 1.000000000000000000, 0.8660254037844387076, 1.000000000000000000, 0.8660254037844387076, 1.000000000000000000, 0.8660254037844387076, 1.000000000000000000, 0.8660254037844387076, 1.000000000000000000, 0.8660254037844387076, 1.000000000000000000, 0.8660254037844387076, 1.000000000000000000, 0.8660254037844387076, 1.000000000000000000, 0.8660254037844387076, 1.000000000000000000, 0.8660254037844387076, 1.000000000000000000, 0.8660254037844387076, 1.000000000000000000, 0.8660254037844387076, 1.000000000000000000, 0.8660254037844387076, 1.000000000000000000, 0.8660254037844387076, 1.000000000000000000, 0.8660254037844387076, 1.000000000000000000, 0.8660254037844387076, 1.000000000000000000, 0.8660254037844387076, 1.000000000000000000, 0.8660254037844387076, 1.000000000000000000, 0.8660254037844387076, 1.000000000000000000, 0.8660254037844387076, 1.000000000000000000, 0.8660254037844387076, 1.000000000000000000, 0.8660254037844387076, 1.000000000000000000, 0.8660254037844387076, 1.000000000000000000, 0.8660254037844387076, 1.000000000000000000, 0.8660254037844387076, 1.000000000000000000, 0.8660254037844387076, 1.000000000000000000, 0.8660254037844387076, 1.000000000000000000, 0.8660254037844387076, 1.000000000000000000, 0.8660254037844387076, 1.000000000000000000, 0.8660254037844387076, 1.000000000000000000, 0.8660254037844387076, 1.000000000000000000, 0.8660254037844387076, 1.000000000000000000, 0.8660254037844387076, 1.000000000000000000, 0.8660254037844387076, 1.000000000000000000, 0.8660254037844387076, 1.000000000000000000, 0.8660254037844387076, 1.000000000000000000, 0.8660254037844387076, 1.000000000000000000, 0.8660254037844387076, 1.000000000000000000, 0.8660254037844387076, 1.000000000000000000, 0.8660254037844387076, 1.000000000000000000, 0.8660254037844387076, 1.000000000000000000, 0.8660254037844387076, 1.000000000000000000, 0.8660254037844387076, 1.000000000000000000, 0.8660254037844387076, 1.000000000000000000, 0.8660254037844387076, 1.000000000000000000, 0.8660254037844387076, 1.000000000000000000, 0.8660254037844387076, 1.000000000000000000, 0.8660254037844387076, 1.000000000000000000, 0.8660254037844387076, 1.000000000000000000, 0.8660254037844387076, 1.000000000000000000, 0.8660254037844387076, 1.000000000000000000, 0.8660254037844387076, 1.000000000000000000, 0.8660254037844387076, 1.000000000000000000, 0.8660254037844387076, 1.000000000000000000, 0.8660254037844387076, 1.000000000000000000, 0.8660254037844387076, 1.000000000000000000, 0.8660254037844387076, 1.000000000000000000, 0.8660254037844387076, 1.000000000000000000, 0.8660254037844387076, 1.000000000000000000, 0.8660254037844387076, 1.000000000000000000, 0.8660254037844387076, 1.000000000000000000, 0.8660254037844387076, 1.000000000000000000, 0.8660254037844387076, 1.000000000000000000, 0.8660254037844387076, 1.000000000000000000, 0.8660254037844387076, 1.000000000000000000, 0.8660254037844387076, 1.000000000000000000, 0.8660254037844387076, 1.000000000000000000, 0.8660254037844387076, 1.000000000000000000, 0.8660254037844387076, 1.000000000000000000, 0.8660254037844387076, 1.000000000000000000),
 ( 1.000000000000000000, 0.8660254037844387076, 1.000000000000000000, 0.8660254037844387076, 1.000000000000000000, 0.8660254037844387076, 1.000000000000000000, 0.8660254037844387076, 1.000000000000000000, 0.8660254037844387076, 1.000000000000000000, 0.8660254037844387076, 1.000000000000000000, 0.8660254037844387076, 1.000000000000000000, 0.8660254037844387076, 1.000000000000000000, 0.8660254037844387076, 1.000000000000000000, 0.8660254037844387076, 1.000000000000000000, 0.8660254037844387076, 1.000000000000000000, 0.8660254037844387076, 1.000000000000000000, 0.8660254037844387076, 1.000000000000000000, 0.8660254037844387076, 1.000000000000000000, 0.8660254037844387076, 1.000000000000000000, 0.8660254037844387076, 1.000000000000000000, 0.8660254037844387076, 1.000000000000000000, 0.8660254037844387076, 1.000000000000000000, 0.8660254037844387076, 1.000000000000000000, 0.8660254037844387076, 1.000000000000000000, 0.8660254037844387076, 1.000000000000000000, 0.8660254037844387076, 1.000000000000000000, 0.8660254037844387076, 1.000000000000000000, 0.8660254037844387076, 1.000000000000000000, 0.8660254037844387076, 1.000000000000000000, 0.8660254037844387076, 1.000000000000000000, 0.8660254037844387076, 1.000000000000000000, 0.8660254037844387076, 1.000000000000000000, 0.8660254037844387076, 1.000000000000000000, 0.8660254037844387076, 1.000000000000000000, 0.8660254037844387076, 1.000000000000000000, 0.8660254037844387076, 1.000000000000000000, 0.8660254037844387076, 1.000000000000000000, 0.8660254037844387076, 1.000000000000000000, 0.8660254037844387076, 1.000000000000000000, 0.8660254037844387076, 1.000000000000000000, 0.8660254037844387076, 1.000000000000000000, 0.8660254037844387076, 1.000000000000000000, 0.8660254037844387076, 1.000000000000000000, 0.8660254037844387076, 1.000000000000000000, 0.8660254037844387076, 1.000000000000000000, 0.8660254037844387076, 1.000000000000000000, 0.8660254037844387076, 1.000000000000000000, 0.8660254037844387076, 1.000000000000000000, 0.8660254037844387076, 1.000000000000000000, 0.8660254037844387076, 1.000000000000000000, 0.8660254037844387076, 1.000000000000000000, 0.8660254037844387076, 1.000000000000000000, 0.8660254037844387076, 1.000000000000000000, 0.8660254037844387076, 1.000000000000000000, 0.8660254037844387076, 1.000000000000000000, 0.8660254037844387076, 1.000000000000000000, 0.8660254037844387076, 1.000000000000000000, 0.8660254037844387076, 1.000000000000000000, 0.8660254037844387076, 1.000000000000000000, 0.8660254037844387076, 1.000000000000000000, 0.8660254037844387076, 1.000000000000000000, 0.8660254037844387076, 1.000000000000000000, 0.8660254037844387076, 1.000000000000000000, 0.8660254037844387076, 1.000000000000000000, 0.8660254037844387076, 1.000000000000000000, 0.8660254037844387076, 1.000000000000000000, 0.8660254037844387076, 1.000000000000000000, 0.8660254037844387076, 1.000000000000000000, 0.8660254037844387076, 1.000000000000000000, 0.8660254037844387076, 1.000000000000000000, 0.8660254037844387076, 1.000000000000000000, 0.8660254037844387076, 1.000000000000000000, 0.8660254037844387076, 1.000000000000000000, 0.8660254037844387076, 1.000000000000000000, 0.8660254037844387076, 1.000000000000000000, 0.8660254037844387076, 1.000000000000000000, 0.8660254037844387076, 1.000000000000000000, 0.8660254037844387076, 1.000000000000000000, 0.8660254037844387076, 1.000000000000000000, 0.8660254037844387076, 1.000000000000000000, 0.8660254037844387076, 1.000000000000000000, 0.8660254037844387076, 1.000000000000000000, 0.8660254037844387076, 1.000000000000000000, 0.8660254037844387076, 1.000000000000000000, 0.8660254037844387076, 1.000000000000000000, 0.8660254037844387076, 1.000000000000000000, 0.8660254037844387076, 1.000000000000000000, 0.8660254037844387076, 1.000000000000000000, 0.8660254037844387076, 1.000000000000000000, 0.8660254037844387076, 1.000000000000000000, 0.8660254037844387076, 1.000000000000000000, 0.8660254037844387076, 1.000000000000000000, 0.8660254037844387076, 1.000000000000000000, 0.8660254037844387076, 1.000000000000000000, 0.8660254037844387076, 1.000000000000000000, 0.8660254037844387076, 1.000000000000000000, 0.8660254037844387076, 1.000000000000000000, 0.8660254037844387076, 1.000000000000000000, 0.8660254037844387076, 1.000000000000000000, 0.8660254037844387076, 1.000000000000000000, 0.8660254037844387076, 1.000000000000000000, 0.8660254037844387076, 1.000000000000000000, 0.8660254037844387076, 1.000000000000000000, 0.8660254037844387076, 1.000000000000000000, 0.8660254037844387076, 1.000000000000000000, 0.8660254037844387076, 1.000000000000000000, 0.8660254037844387076, 1.000000000000000000, 0.8660254037844387076, 1.000000000000000000, 0.8660254037844387076, 1.000000000000000000, 0.8660254037844387076, 1.000000000000000000, 0.8660254037844387076, 1.000000000000000000, 0.8660254037844387076, 1.000000000000000000, 0.8660254037844387076, 1.000000000000000000, 0.8660254037844387076, 1.000000000000000000, 0.8660254037844387076, 1.000000000000000000, 0.8660254037844387076, 1.000000000000000000, 0.8660254037844387076, 1.000000000000000000, 0.8660254037844387076, 1.000000000000000000, 0.8660254037844387076, 1.000000000000000000, 0.8660254037844387076, 1.000000000000000000, 0.8660254037844387076, 1.000000000000000000, 0.8660254037844387076, 1.000000000000000000, 0.8660254037844387076, 1.000000000000000000, 0.8660254037844387076, 1.000000000000000000, 0.8660254037844387076, 1.000000000000000000, 0.8660254037844387076, 1.000000000000000000, 0.8660254037844387076, 1.000000000000000000, 0.8660254037844387076, 1.000000000000000000, 0.8660254037844387076, 1.000000000000000000, 0.8660254037844387076, 1.000000000000000000, 0.8660254037844387076, 1.000000000000000000, 0.8660254037844387076, 1.000000000000000000, 0.8660254037844387076, 1.000000000000000000, 0.8660254037844387076, 1.000000000000000000, 0.8660254037844387076, 1.000000000000000000, 0.8660254037844387076, 1.000000000000000000, 0.8660254037844387076, 1.000000000000000000, 0.8660254037844387076, 1.000000000000000000, 0.8660254037844387076, 1.000000000000000000, 0.8660254037844387076, 1.000000000000000000, 0.8660254037844387076, 1.000000000000000000, 0.8660254037844387076, 1.000000000000000000, 0.8660254037844387076, 1.000000000000000000, 0.8660254037844387076, 1.000000000000000000, 0.8660254037844387076, 1.000000000000000000, 0.8660254037844387076, 1.000000000000000000, 0.8660254037844387076, 1.000000000000000000, 0.8660254037844387076, 1.000000000000000000, 0.8660254037844387076, 1.000000000000000000, 0.8660254037844387076, 1.000000000000000000, 0.8660254037844387076, 1.000000000000000000, 0.8660254037844387076, 1.000000000000000000, 0.8660254037844387076, 1.000000000000000000, 0.8660254037844387076, 1.000000000000000000, 0.8660254037844387076, 1.000000000000000000, 0.8660254037844387076, 1.000000000000000000, 0.8660254037844387076, 1.000000000000000000, 0.8660254037844387076, 1.000000000000000000, 0.8660254037844387076, 1.000000000000000000, 0.8660254037844387076, 1.000000000000000000, 0.8660254037844387076, 1.000000000000000000, 0.8660254037844387076, 1.000000000000000000, 0.8660254037844387076, 1.000000000000000000, 0.8660254037844387076, 1.000000000000000000, 0.8660254037844387076, 1.000000000000000000, 0.8660254037844387076, 1.000000000000000000, 0.8660254037844387076, 1.000000000000000000, 0.8660254037844387076, 1.000000000000000000, 0.8660254037844387076, 1.000000000000000000, 0.8660254037844387076, 1.000000000000000000, 0.8660254037844387076, 1.000000000000000000, 0.8660254037844387076, 1.000000000000000000, 0.8660254037844387076, 1.000000000000000000, 0.8660254037844387076, 1.000000000000000000, 0.8660254037844387076, 1.000000000000000000, 0.8660254037844387076, 1.000000000000000000, 0.8660254037844387076, 1.000000000000000000, 0.8660254037844387076, 1.000000000000000000, 0.8660254037844387076, 1.000000000000000000, 0.8660254037844387076, 1.000000000000000000, 0.8660254037844387076, 1.000000000000000000, 0.8660254037844387076, 1.000000000000000000, 0.8660254037844387076, 1.000000000000000000, 0.8660254037844387076, 1.000000000000000000, 0.8660254037844387076, 1.000000000000000000, 0.8660254037844387076, 1.000000000000000000, 0.8660254037844387076, 1.000000000000000000, 0.8660254037844387076, 1.000000000000000000, 0.8660254037844387076, 1.000000000000000000, 0.8660254037844387076, 1.000000000000000000, 0.8660254037844387076, 1.000000000000000000, 0.8660254037844387076, 1.000000000000000000, 0.8660254037844387076, 1.000000000000000000, 0.8660254037844387076, 1.000000000000000000, 0.8660254037844387076, 1.000000000000000000, 0.8660254037844387076, 1.000000000000000000, 0.8660254037844387076, 1.000000000000000000, 0.8660254037844387076, 1.000000000000000000, 0.8660254037844387076, 1.000000000000000000, 0.8660254037844387076, 1.000000000000000000, 0.8660254037844387076, 1.000000000000000000, 0.8660254037844387076, 1.000000000000000000, 0.8660254037844387076, 1.000000000000000000, 0.8660254037844387076, 1.000000000000000000, 0.8660254037844387076, 1.000000000000000000, 0.8660254037844387076, 1.000000000000000000, 0.8660254037844387076, 1.000000000000000000, 0.8660254037844387076, 1.000000000000000000, 0.8660254037844387076, 1.000000000000000000, 0.8660254037844387076, 1.000000000000000000, 0.8660254037844387076, 1.000000000000000000, 0.8660254037844387076, 1.000000000000000000, 0.8660254037844387076, 1.000000000000000000, 0.8660254037844387076, 1.000000000000000000, 0.8660254037844387076, 1.000000000000000000, 0.8660254037844387076, 1.000000000000000000, 0.8660254037844387076, 1.000000000000000000, 0.8660254037844387076, 1.000000000000000000, 0.8660254037844387076, 1.000000000000000000, 0.8660254037844387076, 1.000000000000000000, 0.8660254037844387076, 1.000000000000000000, 0.8660254037844387076, 1.000000000000000000, 0.8660254037844387076, 1.000000000000000000, 0.8660254037844387076, 1.000000000000000000, 0.8660254037844387076, 1.000000000000000000, 0.8660254037844387076, 1.000000000000000000, 0.8660254037844387076, 1.000000000000000000, 0.8660254037844387076, 1.000000000000000000, 0.8660254037844387076, 1.000000000000000000, 0.8660254037844387076, 1.000000000000000000, 0.8660254037844387076, 1.000000000000000000, 0.8660254037844387076, 1.000000000000000000, 0.8660254037844387076, 1.000000000000000000, 0.8660254037844387076, 1.000000000000000000, 0.8660254037844387076, 1.000000000000000000, 0.8660254037844387076, 1.000000000000000000, 0.8660254037844387076, 1.000000000000000000, 0.8660254037844387076, 1.000000000000000000, 0.8660254037844387076, 1.000000000000000000, 0.8660254037844387076, 1.000000000000000000, 0.8660254037844387076, 1.000000000000000000, 0.8660254037844387076, 1.000000000000000000, 0.8660254037844387076, 1.000000000000000000, 0.8660254037844387076, 1.000000000000000000, 0.8660254037844387076, 1.000000000000000000, 0.8660254037844387076, 1.000000000000000000, 0.8660254037844387076, 1.000000000000000000, 0.8660254037844387076, 1.000000000000000000, 0.8660254037844387076, 1.000000000000000000, 0.8660254037844387076, 1.000000000000000000, 0.8660254037844387076, 1.000000000000000000, 0.8660254037844387076, 1.000000000000000000, 0.8660254037844387076, 1.000000000000000000, 0.8660254037844387076, 1.000000000000000000, 0.8660254037844387076, 1.000000000000000000, 0.8660254037844387076, 1.000000000000000000, 0.8660254037844387076, 1.000000000000000000, 0.8660254037844387076, 1.000000000000000000, 0.8660254037844387076, 1.000000000000000000, 0.8660254037844387076, 1.000000000000000000, 0.8660254037844387076, 1.000000000000000000, 0.8660254037844387076, 1.000000000000000000, 0.8660254037844387076, 1.000000000000000000, 0.8660254037844387076, 1.000000000000000000, 0.8660254037844387076, 1.000000000000000000, 0.8660254037844387076, 1.000000000000000000, 0.8660254037844387076, 1.000000000000000000, 0.8660254037844387076, 1.000000000000000000, 0.8660254037844387076, 1.000000000000000000, 0.8660254037844387076, 1.000000000000000000, 0.8660254037844387076, 1.000000000000000000, 0.8660254037844387076, 1.000000000000000000, 0.8660254037844387076, 1.000000000000000000, 0.8660254037844387076, 1.000000000000000000, 0.8660254037844387076, 1.000000000000000000, 0.8660254037844387076, 1.000000000000000000, 0.8660254037844387076, 1.000000000000000000, 0.8660254037844387076, 1.000000000000000000, 0.8660254037844387076, 1.000000000000000000, 0.8660254037844387076, 1.000000000000000000, 0.8660254037844387076, 1.000000000000000000, 0.8660254037844387076, 1.000000000000000000, 0.8660254037844387076, 1.000000000000000000, 0.8660254037844387076, 1.000000000000000000, 0.8660254037844387076, 1.000000000000000000, 0.8660254037844387076, 1.000000000000000000, 0.8660254037844387076, 1.000000000000000000, 0.8660254037844387076, 1.000000000000000000, 0.8660254037844387076, 1.000000000000000000, 0.8660254037844387076, 1.000000000000000000, 0.8660254037844387076, 1.000000000000000000, 0.8660254037844387076, 1.000000000000000000, 0.8660254037844387076, 1.000000000000000000, 0.8660254037844387076, 1.000000000000000000, 0.8660254037844387076, 1.000000000000000000, 0.8660254037844387076, 1.000000000000000000, 0.8660254037844387076, 1.000000000000000000, 0.8660254037844387076, 1.000000000000000000, 0.8660254037844387076, 1.000000000000000000, 0.8660254037844387076, 1.000000000000000000, 0.8660254037844387076, 1.000000000000000000, 0.8660254037844387076, 1.000000000000000000, 0.8660254037844387076, 1.000000000000000000, 0.8660254037844387076, 1.000000000000000000, 0.8660254037844387076, 1.000000000000000000, 0.8660254037844387076, 1.000000000000000000, 0.8660254037844387076, 1.000000000000000000, 0.8660254037844387076, 1.000000000000000000, 0.8660254037844387076, 1.000000000000000000, 0.8660254037844387076, 1.000000000000000000, 0.8660254037844387076, 1.000000000000000000, 0.8660254037844387076, 1.000000000000000000, 0.8660254037844387076, 1.000000000000000000, 0.8660254037844387076, 1.000000000000000000, 0.8660254037844387076, 1.000000000000000000, 0.8660254037844387076, 1.000000000000000000, 0.8660254037844387076, 1.000000000000000000, 0.8660254037844387076, 1.000000000000000000, 0.8660254037844387076, 1.000000000000000000, 0.8660254037844387076, 1.000000000000000000, 0.8660254037844387076, 1.000000000000000000, 0.8660254037844387076, 1.000000000000000000, 0.8660254037844387076, 1.000000000000000000, 0.8660254037844387076, 1.000000000000000000, 0.8660254037844387076, 1.000000000000000000, 0.8660254037844387076, 1.000000000000000000, 0.8660254037844387076, 1.000000000000000000, 0.8660254037844387076, 1.000000000000000000, 0.8660254037844387076, 1.000000000000000000, 0.8660254037844387076, 1.000000000000000000, 0.8660254037844387076, 1.000000000000000000, 0.8660254037844387076, 1.000000000000000000, 0.8660254037844387076, 1.000000000000000000, 0.8660254037844387076, 1.000000000000000000, 0.8660254037844387076, 1.000000000000000000, 0.8660254037844387076, 1.000000000000000000, 0.8660254037844387076, 1.000000000000000000, 0.8660254037844387076, 1.000000000000000000, 0.8660254037844387076, 1.000000000000000000, 0.8660254037844387076, 1.000000000000000000, 0.8660254037844387076, 1.000000000000000000, 0.8660254037844387076, 1.000000000000000000, 0.8660254037844387076, 1.000000000000000000, 0.8660254037844387076, 1.000000000000000000, 0.8660254037844387076, 1.000000000000000000, 0.8660254037844387076, 1.000000000000000000, 0.8660254037844387076, 1.000000000000000000, 0.8660254037844387076, 1.000000000000000000, 0.8660254037844387076, 1.000000000000000000, 0.8660254037844387076, 1.000000000000000000, 0.8660254037844387076, 1.000000000000000000, 0.8660254037844387076, 1.000000000000000000, 0.8660254037844387076, 1.000000000000000000, 0.8660254037844387076, 1.000000000000000000, 0.8660254037844387076, 1.000000000000000000, 0.8660254037844387076, 1.000000000000000000, 0.8660254037844387076, 1.000000000000000000, 0.8660254037844387076, 1.000000000000000000, 0.8660254037844387076, 1.000000000000000000, 0.8660254037844387076, 1.000000000000000000, 0.8660254037844387076, 1.000000000000000000, 0.8660254037844387076, 1.000000000000000000, 0.8660254037844387076, 1.000000000000000000, 0.8660254037844387076, 1.000000000000000000) ) ) 
 REPRESENTATION_ITEM ( '' )  SURFACE ( )  );
#45453=CARTESIAN_POINT ( 'NONE',  ( 26.85937500061451644, -4.541064518000417216, -2.621784821875001281 ) ) ;
#45454=ORIENTED_EDGE ( 'NONE', *, *, #65842, .F. ) ;
#45455=CARTESIAN_POINT ( 'NONE',  ( 21.17812500061451431, 4.541064518000418104, 2.621784821874999949 ) ) ;
#45456=CARTESIAN_POINT ( 'NONE',  ( 21.60937500061451644, 4.541064518000418104, -2.621784821874998173 ) ) ;
#45457=CARTESIAN_POINT ( 'NONE',  ( 6.487499999999999822, 5.773502691896255534, 3.535250795749688894E-16 ) ) ;
#45458=CARTESIAN_POINT ( 'NONE',  ( 10.37812500061451715, 4.541064518000418104, 2.621784821874999949 ) ) ;
#45459=CARTESIAN_POINT ( 'NONE',  ( 24.70312500061451644, 4.541064518000418104, -2.621784821874998173 ) ) ;
#45460=CARTESIAN_POINT ( 'NONE',  ( 11.97187500061451892, -6.054752690667223547, -1.112240025338166033E-15 ) ) ;
#45461=CARTESIAN_POINT ( 'NONE',  ( 17.03437500061451715, 6.421520780324663323E-16, -5.243569643749999010 ) ) ;
#45462=FACE_OUTER_BOUND ( 'NONE', #62100, .T. ) ;
#45463=CARTESIAN_POINT ( 'NONE',  ( -3.000416591977282496E-16, 18.34062500061451928, 25.09994784771203058 ) ) ;
#45464=CARTESIAN_POINT ( 'NONE',  ( 20.73750000122903359, -4.330127018922194537, 2.499999999999995559 ) ) ;
#45466=CARTESIAN_POINT ( 'NONE',  ( 11.01562500061451644, -6.054752690667223547, -1.112240025338166033E-15 ) ) ;
#45467=CARTESIAN_POINT ( 'NONE',  ( 4.884375000614518569, 6.421520780324663323E-16, -5.243569643749999010 ) ) ;
#45468=CARTESIAN_POINT ( 'NONE',  ( 5.184375000614516615, -4.541064518000419881, 2.621784821874995952 ) ) ;
#45470=CARTESIAN_POINT ( 'NONE',  ( 26.48437500061451644, 6.421520780324663323E-16, -5.243569643749999010 ) ) ;
#45471=CARTESIAN_POINT ( 'NONE',  ( 16.07812500061451289, 6.421520780324663323E-16, -5.243569643749999010 ) ) ;
#45472=CARTESIAN_POINT ( 'NONE',  ( 28.16250000122903074, 4.330127018922192761, -2.499999999999997780 ) ) ;
#45473=CARTESIAN_POINT ( 'NONE',  ( 28.71562500061451573, 3.027376345333613106, -5.243569643749998122 ) ) ;
#45474=CARTESIAN_POINT ( 'NONE',  ( 22.58437500061451431, 4.541064518000418104, 2.621784821874999949 ) ) ;
#45475=CARTESIAN_POINT ( 'NONE',  ( 16.19062500061451715, 6.054752690667223547, 3.707466751127219781E-16 ) ) ;
#45476=CARTESIAN_POINT ( 'NONE',  ( -3.999999999999997335, 10.58750000000000213, 32.30940107675850470 ) ) ;
#45477=AXIS2_PLACEMENT_3D ( 'NONE', #28023, #9563, #10657 ) ;
#45478=CARTESIAN_POINT ( 'NONE',  ( 22.56562500061451715, 3.027376345333611329, 5.243569643749999010 ) ) ;
#45479=CARTESIAN_POINT ( 'NONE',  ( 4.575000001229033941, -5.773502691896255534, -1.060575238724906372E-15 ) ) ;
#45480=ORIENTED_EDGE ( 'NONE', *, *, #22055, .F. ) ;
#45481=CARTESIAN_POINT ( 'NONE',  ( 27.86249999999999716, -5.773502691896255534, -1.060575238724906372E-15 ) ) ;
#45482=CARTESIAN_POINT ( 'NONE',  ( 3.999999999999998668, 12.61250000000000071, -32.30940107675850470 ) ) ;
#45484=CARTESIAN_POINT ( 'NONE',  ( 28.79062500061451502, 6.054752690667223547, 3.707466751127219781E-16 ) ) ;
#45485=CARTESIAN_POINT ( 'NONE',  ( 11.09062500061451573, -3.027376345333610441, -5.243569643749999898 ) ) ;
#45486=CARTESIAN_POINT ( 'NONE',  ( 21.07500000122903572, 2.886751345948126879, 4.999999999999999112 ) ) ;
#45488=CARTESIAN_POINT ( 'NONE',  ( 13.73437500061451821, -4.541064518000419881, 2.621784821874995952 ) ) ;
#45489=CARTESIAN_POINT ( 'NONE',  ( 27.77812500061451573, 6.421520780324663323E-16, -5.243569643749999010 ) ) ;
#45490=CARTESIAN_POINT ( 'NONE',  ( 27.33750000000000213, -2.886751345948129988, 4.999999999999997335 ) ) ;
#45491=CARTESIAN_POINT ( 'NONE',  ( -1.999999999999997113, 19.28750000122903430, -26.53589838486224295 ) ) ;
#45492=CARTESIAN_POINT ( 'NONE',  ( 12.77812500061451750, -4.541064518000419881, 2.621784821874995952 ) ) ;
#45494=EDGE_CURVE ( 'NONE', #37790, #1400, #45406, .T. ) ;
#45495=VECTOR ( 'NONE', #52784, 1000.000000000000000 ) ;
#45496=CARTESIAN_POINT ( 'NONE',  ( 7.715625000614515727, 3.027376345333611329, 5.243569643749999010 ) ) ;
#45497=AXIS2_PLACEMENT_3D ( 'NONE', #72256, #45275, #15360 ) ;
#45498=CARTESIAN_POINT ( 'NONE',  ( 6.740625000614516082, 6.054752690667223547, 3.707466751127219781E-16 ) ) ;
#45500=EDGE_CURVE ( 'NONE', #52141, #11866, #50901, .T. ) ;
#45501=CARTESIAN_POINT ( 'NONE',  ( 2.700000001229035718, -2.886751345948129988, 4.999999999999997335 ) ) ;
#45502=CARTESIAN_POINT ( 'NONE',  ( 16.61250000000000426, -5.773502691896255534, -1.060575238724906372E-15 ) ) ;
#45504=CARTESIAN_POINT ( 'NONE',  ( 15.79687500061451821, 6.054752690667223547, 3.707466751127219781E-16 ) ) ;
#45505=CARTESIAN_POINT ( 'NONE',  ( 12.33750000122903145, 6.123233995736764310E-16, -4.999999999999998224 ) ) ;
#45506=CARTESIAN_POINT ( 'NONE',  ( 20.48437500061451289, -4.541064518000419881, 2.621784821874995952 ) ) ;
#45508=CARTESIAN_POINT ( 'NONE',  ( 19.92187500061451644, 3.027376345333611329, 5.243569643749999010 ) ) ;
#45509=CARTESIAN_POINT ( 'NONE',  ( 9.001249775931846008E-16, 14.96562500061451750, -25.09994784771203058 ) ) ;
#45512=CARTESIAN_POINT ( 'NONE',  ( 30.00000000000000000, 0.000000000000000000, 0.000000000000000000 ) ) ;
#45513=CARTESIAN_POINT ( 'NONE',  ( 26.57812500061451644, 4.541064518000418104, 2.621784821874999949 ) ) ;
#45514=CYLINDRICAL_SURFACE ( 'NONE', #19557, 4.999999999999998224 ) ;
#45515=CARTESIAN_POINT ( 'NONE',  ( 28.73437500061451644, 6.421520780324663323E-16, -5.243569643749999010 ) ) ;
#45516=CARTESIAN_POINT ( 'NONE',  ( 25.08749999999999858, -2.886751345948129988, 4.999999999999997335 ) ) ;
#45517=CARTESIAN_POINT ( 'NONE',  ( 9.890625000614516438, 6.054752690667223547, 3.707466751127219781E-16 ) ) ;
#45519=CARTESIAN_POINT ( 'NONE',  ( 18.75937500061451857, -4.541064518000417216, -2.621784821875001281 ) ) ;
#45522=CARTESIAN_POINT ( 'NONE',  ( 6.290625000614517681, 6.054752690667223547, 3.707466751127219781E-16 ) ) ;
#45523=CARTESIAN_POINT ( 'NONE',  ( 10.58437500061451964, -4.541064518000419881, 2.621784821874995952 ) ) ;
#45525=CARTESIAN_POINT ( 'NONE',  ( 21.79687500061451644, -3.027376345333614438, 5.243569643749998122 ) ) ;
#45527=CARTESIAN_POINT ( 'NONE',  ( 28.76249999999999929, -5.773502691896255534, -1.060575238724906372E-15 ) ) ;
#45528=CARTESIAN_POINT ( 'NONE',  ( 29.59687500061451715, -3.027376345333610441, -5.243569643749999898 ) ) ;
#45530=CARTESIAN_POINT ( 'NONE',  ( 14.81250000122903288, 0.000000000000000000, 4.999999999999998224 ) ) ;
#45533=ORIENTED_EDGE ( 'NONE', *, *, #16255, .T. ) ;
#45534=CARTESIAN_POINT ( 'NONE',  ( 12.97499999999999964, -4.330127018922194537, 2.499999999999995559 ) ) ;
#45536=CARTESIAN_POINT ( 'NONE',  ( 24.02812500061451573, -4.541064518000419881, 2.621784821874995952 ) ) ;
#45537=CARTESIAN_POINT ( 'NONE',  ( 14.55000000000000071, 4.330127018922192761, -2.499999999999997780 ) ) ;
#45538=CARTESIAN_POINT ( 'NONE',  ( 10.50000000122903465, -2.886751345948125991, -5.000000000000000000 ) ) ;
#45539=CARTESIAN_POINT ( 'NONE',  ( 9.365625000614519635, 3.027376345333613106, -5.243569643749998122 ) ) ;
#45540=CARTESIAN_POINT ( 'NONE',  ( 9.899999999999998579, -4.330127018922190985, -2.500000000000001332 ) ) ;
#45541=DIRECTION ( 'NONE',  ( 0.000000000000000000, 1.000000000000000000, 0.000000000000000000 ) ) ;
#45542=CARTESIAN_POINT ( 'NONE',  ( 27.67500000122903359, 2.886751345948129099, -4.999999999999998224 ) ) ;
#45544=CARTESIAN_POINT ( 'NONE',  ( 7.050000000000000711, 0.000000000000000000, 4.999999999999998224 ) ) ;
#45545=ORIENTED_EDGE ( 'NONE', *, *, #62566, .T. ) ;
#45546=CARTESIAN_POINT ( 'NONE',  ( 21.92812500061451431, 6.421520780324663323E-16, -5.243569643749999010 ) ) ;
#45547=CARTESIAN_POINT ( 'NONE',  ( 28.34062500061451928, 6.054752690667223547, 3.707466751127219781E-16 ) ) ;
#45549=CARTESIAN_POINT ( 'NONE',  ( 29.74687500061451217, 6.054752690667223547, 3.707466751127219781E-16 ) ) ;
#45550=CARTESIAN_POINT ( 'NONE',  ( 20.18437500061451573, 6.421520780324663323E-16, -5.243569643749999010 ) ) ;
#45551=CARTESIAN_POINT ( 'NONE',  ( 16.52812500061451573, 6.421520780324663323E-16, -5.243569643749999010 ) ) ;
#45552=CARTESIAN_POINT ( 'NONE',  ( 2.121784821874999061, 11.55312500061459424, -33.67503911421598417 ) ) ;
#45553=CARTESIAN_POINT ( 'NONE',  ( 5.728125000614515905, 6.421520780324663323E-16, -5.243569643749999010 ) ) ;
#45554=CARTESIAN_POINT ( 'NONE',  ( 2.803125000614518747, 0.000000000000000000, 5.243569643749999010 ) ) ;
#45556=CARTESIAN_POINT ( 'NONE',  ( 19.41562500061451502, 3.027376345333611329, 5.243569643749999010 ) ) ;
#45557=DIRECTION ( 'NONE',  ( 0.000000000000000000, 0.000000000000000000, 1.000000000000000000 ) ) ;
#45558=CARTESIAN_POINT ( 'NONE',  ( 3.187500001229033764, -4.330127018922194537, 2.499999999999995559 ) ) ;
#45559=CARTESIAN_POINT ( 'NONE',  ( 12.30937500061451573, 0.000000000000000000, 5.243569643749999010 ) ) ;
#45560=CARTESIAN_POINT ( 'NONE',  ( 11.40937500061451892, 0.000000000000000000, 5.243569643749999010 ) ) ;
#45561=CARTESIAN_POINT ( 'NONE',  ( 20.55937500061451573, -4.541064518000417216, -2.621784821875001281 ) ) ;
#45562=EDGE_LOOP ( 'NONE', ( #68813, #16357, #8830, #58850 ) ) ;
#45563=CARTESIAN_POINT ( 'NONE',  ( -4.757043123249223626, 8.797129135976163639, 26.33838535627023347 ) ) ;
#45564=CARTESIAN_POINT ( 'NONE',  ( 25.04062500061451502, -3.027376345333610441, -5.243569643749999898 ) ) ;
#45565=CARTESIAN_POINT ( 'NONE',  ( 18.38437500061451857, 6.421520780324663323E-16, -5.243569643749999010 ) ) ;
#45566=CARTESIAN_POINT ( 'NONE',  ( 25.45312500061451644, -4.541064518000417216, -2.621784821875001281 ) ) ;
#45568=CARTESIAN_POINT ( 'NONE',  ( 3.999999999999999112, 17.07499999999999929, 30.00000000000000000 ) ) ;
#45569=CARTESIAN_POINT ( 'NONE',  ( 4.996875000614516615, 6.054752690667223547, 3.707466751127219781E-16 ) ) ;
#45570=CARTESIAN_POINT ( 'NONE',  ( 10.91250000122903252, -4.330127018922190985, -2.500000000000001332 ) ) ;
#45571=CARTESIAN_POINT ( 'NONE',  ( 8.175000001229031810, -5.773502691896255534, -1.060575238724906372E-15 ) ) ;
#45572=CARTESIAN_POINT ( 'NONE',  ( 28.91250000122903074, -4.330127018922190985, -2.500000000000001332 ) ) ;
#45573=CARTESIAN_POINT ( 'NONE',  ( 27.93750000122903288, -4.330127018922194537, 2.499999999999995559 ) ) ;
#45576=CARTESIAN_POINT ( 'NONE',  ( 10.69687500061451679, -3.027376345333610441, -5.243569643749999898 ) ) ;
#45577=CARTESIAN_POINT ( 'NONE',  ( 17.84062500061451573, -3.027376345333610441, -5.243569643749999898 ) ) ;
#45578=CARTESIAN_POINT ( 'NONE',  ( 13.65937500061451715, 0.000000000000000000, 5.243569643749999010 ) ) ;
#45579=CARTESIAN_POINT ( 'NONE',  ( 29.02500000122903145, 2.886751345948129099, -4.999999999999998224 ) ) ;
#45580=CARTESIAN_POINT ( 'NONE',  ( 20.29687500061451289, 6.054752690667223547, 3.707466751127219781E-16 ) ) ;
#45581=CARTESIAN_POINT ( 'NONE',  ( 10.47187500061451715, 3.027376345333611329, 5.243569643749999010 ) ) ;
#45582=CARTESIAN_POINT ( 'NONE',  ( 3.093393010629925666, -3.928220930877811767, -3.281160880885886311 ) ) ;
#45584=CARTESIAN_POINT ( 'NONE',  ( 20.12812500061451715, 6.421520780324663323E-16, -5.243569643749999010 ) ) ;
#45585=ORIENTED_EDGE ( 'NONE', *, *, #12396, .F. ) ;
#45586=CARTESIAN_POINT ( 'NONE',  ( 6.750000001229033764, -2.886751345948129988, 4.999999999999997335 ) ) ;
#45587=CARTESIAN_POINT ( 'NONE',  ( 17.27812500061451217, -4.541064518000419881, 2.621784821874995952 ) ) ;
#45588=CARTESIAN_POINT ( 'NONE',  ( 12.51562500061451821, 3.027376345333613106, -5.243569643749998122 ) ) ;
#45590=CARTESIAN_POINT ( 'NONE',  ( 14.40000000000000036, -4.330127018922190985, -2.500000000000001332 ) ) ;
#45591=CARTESIAN_POINT ( 'NONE',  ( 9.375000001229036428, 2.886751345948126879, 4.999999999999999112 ) ) ;
#45593=CARTESIAN_POINT ( 'NONE',  ( 6.515625000614516438, -6.054752690667223547, -1.112240025338166033E-15 ) ) ;
#45594=( BOUNDED_CURVE ( )  B_SPLINE_CURVE ( 3, ( #350, #37964, #23224, #34673 ),
 .UNSPECIFIED., .F., .F. ) 
 B_SPLINE_CURVE_WITH_KNOTS ( ( 4, 4 ),
 ( 3.765666616430975555, 3.802312977632561708 ),
 .UNSPECIFIED. ) 
 CURVE ( )  GEOMETRIC_REPRESENTATION_ITEM ( )  RATIONAL_B_SPLINE_CURVE ( ( 1.000000000000000000, 0.9998880901486507655, 0.9998880901486507655, 1.000000000000000000 ) ) 
 REPRESENTATION_ITEM ( '' )  );
#45596=CARTESIAN_POINT ( 'NONE',  ( 18.78750000122903430, 4.330127018922191873, 2.499999999999999556 ) ) ;
#45598=CARTESIAN_POINT ( 'NONE',  ( -2.121784821874996840, 11.38437500061451679, -26.32496088578401583 ) ) ;
#45599=CARTESIAN_POINT ( 'NONE',  ( 4.494741915665277254, -2.190272839526016924, 4.494741915664858922 ) ) ;
#45600=CARTESIAN_POINT ( 'NONE',  ( 3.562500001229033764, 0.000000000000000000, 4.999999999999998224 ) ) ;
#45602=CARTESIAN_POINT ( 'NONE',  ( 18.42187500061451644, 3.027376345333613106, -5.243569643749998122 ) ) ;
#45603=CARTESIAN_POINT ( 'NONE',  ( 21.56250000122903288, 0.000000000000000000, 4.999999999999998224 ) ) ;
#45604=CARTESIAN_POINT ( 'NONE',  ( 16.37812500061451715, -4.541064518000419881, 2.621784821874995952 ) ) ;
#45606=CARTESIAN_POINT ( 'NONE',  ( 28.47187500061451715, 3.027376345333611329, 5.243569643749999010 ) ) ;
#45607=CARTESIAN_POINT ( 'NONE',  ( 26.29687500061451644, -3.027376345333614438, 5.243569643749998122 ) ) ;
#45609=CARTESIAN_POINT ( 'NONE',  ( 13.64062500061451644, -3.027376345333614438, 5.243569643749998122 ) ) ;
#45610=CARTESIAN_POINT ( 'NONE',  ( 10.09687500061451715, -3.027376345333614438, 5.243569643749998122 ) ) ;
#45611=VERTEX_POINT ( 'NONE', #40185 ) ;
#45613=CARTESIAN_POINT ( 'NONE',  ( 29.39062500061451289, -3.027376345333614438, 5.243569643749998122 ) ) ;
#45614=CARTESIAN_POINT ( 'NONE',  ( 20.27812500061451573, 4.541064518000418104, 2.621784821874999949 ) ) ;
#45616=CARTESIAN_POINT ( 'NONE',  ( 20.85000000000000142, 4.330127018922192761, -2.499999999999997780 ) ) ;
#45617=CARTESIAN_POINT ( 'NONE',  ( 10.83750000000000036, -2.886751345948125991, -5.000000000000000000 ) ) ;
#45618=CARTESIAN_POINT ( 'NONE',  ( 21.41250000122903074, 4.330127018922192761, -2.499999999999997780 ) ) ;
#45619=CARTESIAN_POINT ( 'NONE',  ( 16.75312500061451715, 0.000000000000000000, 5.243569643749999010 ) ) ;
#45621=ORIENTED_EDGE ( 'NONE', *, *, #39082, .T. ) ;
#45622=CARTESIAN_POINT ( 'NONE',  ( 19.16250000000000142, 2.886751345948126879, 4.999999999999999112 ) ) ;
#45623=CARTESIAN_POINT ( 'NONE',  ( 21.48750000000000071, -2.886751345948129988, 4.999999999999997335 ) ) ;
#45624=CARTESIAN_POINT ( 'NONE',  ( 20.25937500061451857, 4.541064518000418104, -2.621784821874998173 ) ) ;
#45625=CARTESIAN_POINT ( 'NONE',  ( 25.94062500061451715, -3.027376345333610441, -5.243569643749999898 ) ) ;
#45626=ORIENTED_EDGE ( 'NONE', *, *, #31751, .F. ) ;
#45627=CARTESIAN_POINT ( 'NONE',  ( 28.64999999999999858, 0.000000000000000000, 4.999999999999998224 ) ) ;
#45628=CARTESIAN_POINT ( 'NONE',  ( 9.028125000614517504, 4.541064518000418104, 2.621784821874999949 ) ) ;
#45629=CARTESIAN_POINT ( 'NONE',  ( 1.999999999999998668, 12.20000000000000107, 26.53589838486224650 ) ) ;
#45630=AXIS2_PLACEMENT_3D ( 'NONE', #10784, #62118, #22586 ) ;
#45631=CARTESIAN_POINT ( 'NONE',  ( 14.13750000000000107, 5.773502691896255534, 3.535250795749688894E-16 ) ) ;
#45632=CARTESIAN_POINT ( 'NONE',  ( 2.121784821874999061, 16.95312500061451999, 26.32496088578401583 ) ) ;
#45633=CARTESIAN_POINT ( 'NONE',  ( 28.30312500061451431, 4.541064518000418104, -2.621784821874998173 ) ) ;
#45634=CARTESIAN_POINT ( 'NONE',  ( 27.19687500061451857, -3.027376345333614438, 5.243569643749998122 ) ) ;
#45635=EDGE_LOOP ( 'NONE', ( #48697, #36536, #15948, #25226 ) ) ;
#45636=CARTESIAN_POINT ( 'NONE',  ( 24.40312500061451573, 0.000000000000000000, 5.243569643749999010 ) ) ;
#45637=CARTESIAN_POINT ( 'NONE',  ( 24.15937500061451715, -4.541064518000417216, -2.621784821875001281 ) ) ;
#45639=CARTESIAN_POINT ( 'NONE',  ( 9.001249775931846008E-16, 18.56562500061459886, -25.09994784771203058 ) ) ;
#45640=CARTESIAN_POINT ( 'NONE',  ( 12.22499999999999964, 6.123233995736764310E-16, -4.999999999999998224 ) ) ;
#45641=CARTESIAN_POINT ( 'NONE',  ( 8.878125000614515372, 6.421520780324663323E-16, -5.243569643749999010 ) ) ;
#45643=CARTESIAN_POINT ( 'NONE',  ( 26.84062500061451573, -3.027376345333610441, -5.243569643749999898 ) ) ;
#45646=CARTESIAN_POINT ( 'NONE',  ( 20.29687500061451644, 6.054752690667223547, 3.707466751127219781E-16 ) ) ;
#45647=CARTESIAN_POINT ( 'NONE',  ( -4.243569643749999898, 15.77187500061451608, 27.54997392385601529 ) ) ;
#45648=CARTESIAN_POINT ( 'NONE',  ( 19.50937500061451857, 0.000000000000000000, 5.243569643749999010 ) ) ;
#45649=CARTESIAN_POINT ( 'NONE',  ( 27.45937500061451786, 4.541064518000418104, -2.621784821874998173 ) ) ;
#45650=CARTESIAN_POINT ( 'NONE',  ( -4.243569643749999898, 17.15937500061451715, 30.00000000000000000 ) ) ;
#45651=CARTESIAN_POINT ( 'NONE',  ( 8.990625000614516082, 6.054752690667223547, 3.707466751127219781E-16 ) ) ;
#45653=( BOUNDED_CURVE ( )  B_SPLINE_CURVE ( 2, ( #10565, #6109, #67456, #22724, #67095, #5388, #61526, #51178, #582 ),
 .UNSPECIFIED., .F., .F. ) 
 B_SPLINE_CURVE_WITH_KNOTS ( ( 3, 2, 2, 2, 3 ),
 ( 0.1630434782608695676, 0.1666666666666666574, 0.1739130434782608647, 0.1811594202898550721, 0.1847826086956521896 ),
 .UNSPECIFIED. ) 
 CURVE ( )  GEOMETRIC_REPRESENTATION_ITEM ( )  RATIONAL_B_SPLINE_CURVE ( ( 0.9330127018922194093, 0.9330127018922196314, 1.000000000000000000, 0.8660254037844387076, 1.000000000000000000, 0.8660254037844387076, 1.000000000000000000, 0.9330127018922190762, 0.9330127018922194093 ) ) 
 REPRESENTATION_ITEM ( '' )  );
#45654=CARTESIAN_POINT ( 'NONE',  ( 4.621875000614516615, 3.027376345333611329, 5.243569643749999010 ) ) ;
#45656=CARTESIAN_POINT ( 'NONE',  ( 7.153125000614518392, 4.541064518000418104, -2.621784821874998173 ) ) ;
#45657=CARTESIAN_POINT ( 'NONE',  ( 10.92187500061451644, 3.027376345333611329, 5.243569643749999010 ) ) ;
#45658=CARTESIAN_POINT ( 'NONE',  ( 19.16250000122903430, 4.330127018922192761, -2.499999999999997780 ) ) ;
#45659=CARTESIAN_POINT ( 'NONE',  ( 6.646875000614518747, -3.027376345333610441, -5.243569643749999898 ) ) ;
#45660=CARTESIAN_POINT ( 'NONE',  ( 6.740625000614516082, 6.054752690667223547, 3.707466751127219781E-16 ) ) ;
#45661=CARTESIAN_POINT ( 'NONE',  ( 5.353125000614515905, 4.541064518000418104, -2.621784821874998173 ) ) ;
#45663=CARTESIAN_POINT ( 'NONE',  ( 19.80937500061451573, 4.541064518000418104, -2.621784821874998173 ) ) ;
#45664=CARTESIAN_POINT ( 'NONE',  ( 4.428044609675158227, 2.322158679919935409, 4.428044609675073850 ) ) ;
#45666=CARTESIAN_POINT ( 'NONE',  ( 23.69062500061451004, -3.027376345333610441, -5.243569643749999898 ) ) ;
#45667=CARTESIAN_POINT ( 'NONE',  ( 11.72812500061451857, 4.541064518000418104, 2.621784821874999949 ) ) ;
#45668=CARTESIAN_POINT ( 'NONE',  ( 25.77187500061451431, 3.027376345333611329, 5.243569643749999010 ) ) ;
#45669=CARTESIAN_POINT ( 'NONE',  ( 9.253125000614517148, -4.541064518000417216, -2.621784821875001281 ) ) ;
#45670=CARTESIAN_POINT ( 'NONE',  ( 12.67500000122903536, -5.773502691896255534, -1.060575238724906372E-15 ) ) ;
#45671=CARTESIAN_POINT ( 'NONE',  ( 26.24062500061451431, -3.027376345333614438, 5.243569643749998122 ) ) ;
#45672=CARTESIAN_POINT ( 'NONE',  ( -4.243569643749997233, 13.09062500061451750, -27.54997392385601174 ) ) ;
#45673=CARTESIAN_POINT ( 'NONE',  ( 14.55000000122903181, -2.886751345948125991, -5.000000000000000000 ) ) ;
#45674=CARTESIAN_POINT ( 'NONE',  ( 10.76250000000000107, -5.773502691896255534, -1.060575238724906372E-15 ) ) ;
#45675=CARTESIAN_POINT ( 'NONE',  ( 21.02812500061451573, 6.421520780324663323E-16, -5.243569643749999010 ) ) ;
#45676=CARTESIAN_POINT ( 'NONE',  ( 8.409375000614518925, -4.541064518000417216, -2.621784821875001281 ) ) ;
#45677=CARTESIAN_POINT ( 'NONE',  ( 7.875000001229034652, 2.886751345948129099, -4.999999999999998224 ) ) ;
#45678=EDGE_CURVE ( 'NONE', #65643, #46924, #63729, .T. ) ;
#45679=CARTESIAN_POINT ( 'NONE',  ( 17.10000000122903430, -2.886751345948129988, 4.999999999999997335 ) ) ;
#45680=AXIS2_PLACEMENT_3D ( 'NONE', #37055, #59580, #65500 ) ;
#45681=CARTESIAN_POINT ( 'NONE',  ( 13.79062500061451502, -3.027376345333610441, -5.243569643749999898 ) ) ;
#45682=CARTESIAN_POINT ( 'NONE',  ( 16.22812500061451857, 4.541064518000418104, 2.621784821874999949 ) ) ;
#45683=ADVANCED_FACE ( 'NONE', ( #52710 ), #24628, .F. ) ;
#45684=CARTESIAN_POINT ( 'NONE',  ( 26.51250000122903216, 0.000000000000000000, 4.999999999999998224 ) ) ;
#45685=CARTESIAN_POINT ( 'NONE',  ( 20.13749999999999929, -2.886751345948129988, 4.999999999999997335 ) ) ;
#45686=CARTESIAN_POINT ( 'NONE',  ( 22.47187500061451715, 3.027376345333613106, -5.243569643749998122 ) ) ;
#45688=CARTESIAN_POINT ( 'NONE',  ( 9.225000001229034297, 2.886751345948129099, -4.999999999999998224 ) ) ;
#45689=CARTESIAN_POINT ( 'NONE',  ( 8.259375000614518569, 0.000000000000000000, 5.243569643749999010 ) ) ;
#45690=CARTESIAN_POINT ( 'NONE',  ( 29.14687500061451075, -3.027376345333610441, -5.243569643749999898 ) ) ;
#45692=CARTESIAN_POINT ( 'NONE',  ( 24.55312500061451786, -4.541064518000417216, -2.621784821875001281 ) ) ;
#45695=CARTESIAN_POINT ( 'NONE',  ( 8.934375000614517504, 6.421520780324663323E-16, -5.243569643749999010 ) ) ;
#45696=CARTESIAN_POINT ( 'NONE',  ( 23.58750000122903145, 6.123233995736764310E-16, -4.999999999999998224 ) ) ;
#45697=CARTESIAN_POINT ( 'NONE',  ( 27.36562500061451786, 3.027376345333613106, -5.243569643749998122 ) ) ;
#45698=CARTESIAN_POINT ( 'NONE',  ( 6.909375000614518036, 0.000000000000000000, 5.243569643749999010 ) ) ;
#45700=CARTESIAN_POINT ( 'NONE',  ( 25.20937500061451431, 4.541064518000418104, -2.621784821874998173 ) ) ;
#45701=CARTESIAN_POINT ( 'NONE',  ( -4.243569643749999898, 11.21562500061459389, 27.54997392385601529 ) ) ;
#45702=CARTESIAN_POINT ( 'NONE',  ( 18.63749999999999929, 5.773502691896255534, 3.535250795749688894E-16 ) ) ;
#45704=CARTESIAN_POINT ( 'NONE',  ( 26.77499999999999858, 4.330127018922191873, 2.499999999999999556 ) ) ;
#45705=CARTESIAN_POINT ( 'NONE',  ( 27.79687500061451999, -3.027376345333610441, -5.243569643749999898 ) ) ;
#45706=ORIENTED_EDGE ( 'NONE', *, *, #10971, .T. ) ;
#45707=CARTESIAN_POINT ( 'NONE',  ( 14.42812500061451786, 4.541064518000418104, 2.621784821874999949 ) ) ;
#45708=CARTESIAN_POINT ( 'NONE',  ( 7.828125000614517326, -4.541064518000419881, 2.621784821874995952 ) ) ;
#45710=CARTESIAN_POINT ( 'NONE',  ( 5.746875000614517504, -3.027376345333610441, -5.243569643749999898 ) ) ;
#45711=CARTESIAN_POINT ( 'NONE',  ( 18.45000000122903216, -2.886751345948129988, 4.999999999999997335 ) ) ;
#45712=CARTESIAN_POINT ( 'NONE',  ( 22.83749999999999858, -2.886751345948129988, 4.999999999999997335 ) ) ;
#45713=CARTESIAN_POINT ( 'NONE',  ( 29.13749999999999929, -2.886751345948129988, 4.999999999999997335 ) ) ;
#45714=CARTESIAN_POINT ( 'NONE',  ( 4.246875000614519280, -3.027376345333614438, 5.243569643749998122 ) ) ;
#45715=CARTESIAN_POINT ( 'NONE',  ( 12.68437500061451573, 4.541064518000418104, 2.621784821874999949 ) ) ;
#45716=CARTESIAN_POINT ( 'NONE',  ( 22.47187500061451715, 3.027376345333613106, -5.243569643749998122 ) ) ;
#45717=DIRECTION ( 'NONE',  ( -0.000000000000000000, -1.000000000000000000, -0.000000000000000000 ) ) ;
#45719=CARTESIAN_POINT ( 'NONE',  ( 4.396875000614516971, -3.027376345333610441, -5.243569643749999898 ) ) ;
#45720=CARTESIAN_POINT ( 'NONE',  ( 8.071875000614518569, 3.027376345333613106, -5.243569643749998122 ) ) ;
#45721=CARTESIAN_POINT ( 'NONE',  ( 17.73750000000000071, 5.773502691896255534, 3.535250795749688894E-16 ) ) ;
#45722=CARTESIAN_POINT ( 'NONE',  ( 16.07812500061451289, 6.421520780324663323E-16, -5.243569643749999010 ) ) ;
#45726=CARTESIAN_POINT ( 'NONE',  ( 9.740625000614516082, -3.027376345333610441, -5.243569643749999898 ) ) ;
#45727=CARTESIAN_POINT ( 'NONE',  ( 25.58437500061451431, 6.421520780324663323E-16, -5.243569643749999010 ) ) ;
#45729=CARTESIAN_POINT ( 'NONE',  ( 25.47187500061451715, -6.054752690667223547, -1.112240025338166033E-15 ) ) ;
#45730=CARTESIAN_POINT ( 'NONE',  ( 6.337499999999998579, -2.886751345948125991, -5.000000000000000000 ) ) ;
#45731=CARTESIAN_POINT ( 'NONE',  ( 8.484601909799253346E-16, 12.57500000122903216, 34.61880215351700230 ) ) ;
#45732=CARTESIAN_POINT ( 'NONE',  ( 8.062500001229034652, 0.000000000000000000, 4.999999999999998224 ) ) ;
#45733=CARTESIAN_POINT ( 'NONE',  ( 20.89687500061452141, -3.027376345333614438, 5.243569643749998122 ) ) ;
#45734=CARTESIAN_POINT ( 'NONE',  ( 12.12187500061451573, 3.027376345333613106, -5.243569643749998122 ) ) ;
#45735=CARTESIAN_POINT ( 'NONE',  ( -3.462385672708551798, 3.612013013662439764, -32.01854131409610460 ) ) ;
#45736=VERTEX_POINT ( 'NONE', #68623 ) ;
#45737=CARTESIAN_POINT ( 'NONE',  ( 15.17812500061451608, 6.421520780324663323E-16, -5.243569643749999010 ) ) ;
#45738=CARTESIAN_POINT ( 'NONE',  ( 25.53750000122903074, 4.330127018922191873, 2.499999999999999556 ) ) ;
#45739=CARTESIAN_POINT ( 'NONE',  ( 12.87187500061451750, -6.054752690667223547, -1.112240025338166033E-15 ) ) ;
#45740=CARTESIAN_POINT ( 'NONE',  ( 3.999999999999999112, 12.68750000122903465, 30.00000000000000000 ) ) ;
#45741=CARTESIAN_POINT ( 'NONE',  ( 16.94062500061451715, -3.027376345333610441, -5.243569643749999898 ) ) ;
#45742=CARTESIAN_POINT ( 'NONE',  ( 26.40000000122903145, 5.773502691896255534, 3.535250795749688401E-16 ) ) ;
#45743=CARTESIAN_POINT ( 'NONE',  ( 27.15937500061451360, 0.000000000000000000, 5.243569643749999010 ) ) ;
#45744=CARTESIAN_POINT ( 'NONE',  ( 2.121784821875001281, 11.40312500061451750, 33.67503911421598417 ) ) ;
#45745=CARTESIAN_POINT ( 'NONE',  ( 10.68750000122903288, 4.330127018922191873, 2.499999999999999556 ) ) ;
#45747=CARTESIAN_POINT ( 'NONE',  ( -2.121784821874996840, 17.23437500061451999, -26.32496088578401583 ) ) ;
#45748=CARTESIAN_POINT ( 'NONE',  ( 17.18437500061451573, 4.541064518000418104, 2.621784821874999949 ) ) ;
#45749=CARTESIAN_POINT ( 'NONE',  ( 20.36250000122903359, -4.330127018922190985, -2.500000000000001332 ) ) ;
#45750=CARTESIAN_POINT ( 'NONE',  ( 14.82187500061451679, 3.027376345333613106, -5.243569643749998122 ) ) ;
#45751=EDGE_CURVE ( 'NONE', #13665, #69611, #71294, .T. ) ;
#45752=CARTESIAN_POINT ( 'NONE',  ( 4.243569643749999898, 19.57812500061451644, -30.00000000000000000 ) ) ;
#45753=CARTESIAN_POINT ( 'NONE',  ( 22.95000000122903216, -2.886751345948129988, 4.999999999999997335 ) ) ;
#45754=CARTESIAN_POINT ( 'NONE',  ( 14.69062500061451537, -3.027376345333610441, -5.243569643749999898 ) ) ;
#45755=CARTESIAN_POINT ( 'NONE',  ( 29.46562500061451573, -6.054752690667223547, -1.112240025338166033E-15 ) ) ;
#45756=ORIENTED_EDGE ( 'NONE', *, *, #48081, .T. ) ;
#45757=ORIENTED_EDGE ( 'NONE', *, *, #51752, .F. ) ;
#45758=CARTESIAN_POINT ( 'NONE',  ( 19.31250000000000000, -5.773502691896255534, -1.060575238724906372E-15 ) ) ;
#45759=CARTESIAN_POINT ( 'NONE',  ( -4.243569643749999898, 19.85937500061451644, 30.00000000000000000 ) ) ;
#45760=CARTESIAN_POINT ( 'NONE',  ( 3.628125000614518036, 4.541064518000418104, 2.621784821874999949 ) ) ;
#45761=CARTESIAN_POINT ( 'NONE',  ( 15.00000000122903465, -2.886751345948125991, -5.000000000000000000 ) ) ;
#45762=CARTESIAN_POINT ( 'NONE',  ( 20.24062500061451431, 6.054752690667223547, 3.707466751127219781E-16 ) ) ;
#45763=CARTESIAN_POINT ( 'NONE',  ( 23.87812500061451715, 4.541064518000418104, 2.621784821874999949 ) ) ;
#45764=CARTESIAN_POINT ( 'NONE',  ( 3.965625000614515727, 3.027376345333613106, -5.243569643749998122 ) ) ;
#45765=ADVANCED_FACE ( 'NONE', ( #47535 ), #18460, .T. ) ;
#45766=CARTESIAN_POINT ( 'NONE',  ( 1.592000809091587073E-14, 16.40000000122903501, 26.00000000000000000 ) ) ;
#45767=CARTESIAN_POINT ( 'NONE',  ( 23.02499999999999858, 6.123233995736764310E-16, -4.999999999999998224 ) ) ;
#45769=CARTESIAN_POINT ( 'NONE',  ( 29.63437500061451502, 6.421520780324663323E-16, -5.243569643749999010 ) ) ;
#45770=CARTESIAN_POINT ( 'NONE',  ( 2.000000000000001332, 10.36250000122903359, -26.53589838486224650 ) ) ;
#45771=CARTESIAN_POINT ( 'NONE',  ( -4.243569643749999898, 19.40937500061451715, -30.00000000000000000 ) ) ;
#45772=CARTESIAN_POINT ( 'NONE',  ( 6.000000001229033764, -2.886751345948125991, -5.000000000000000000 ) ) ;
#45773=CARTESIAN_POINT ( 'NONE',  ( 8.400000000000000355, 0.000000000000000000, 4.999999999999998224 ) ) ;
#45774=EDGE_CURVE ( 'NONE', #26212, #38561, #39302, .T. ) ;
#45775=CARTESIAN_POINT ( 'NONE',  ( 4.950000001229033941, -2.886751345948129988, 4.999999999999997335 ) ) ;
#45776=CARTESIAN_POINT ( 'NONE',  ( 12.30937500061451573, 0.000000000000000000, 5.243569643749999010 ) ) ;
#45777=CARTESIAN_POINT ( 'NONE',  ( 1.071796769724484344, 16.64509619066136992, -25.99999999999999645 ) ) ;
#45778=CARTESIAN_POINT ( 'NONE',  ( 2.934375000614518392, -4.541064518000419881, 2.621784821874995952 ) ) ;
#45779=CARTESIAN_POINT ( 'NONE',  ( 3.999999999999998668, 19.02500000122903501, 27.69059892324149530 ) ) ;
#45780=CARTESIAN_POINT ( 'NONE',  ( 1.999999999999998668, 19.51250000122903216, 26.53589838486224650 ) ) ;
#45781=CARTESIAN_POINT ( 'NONE',  ( 10.32187500061451679, 3.027376345333613106, -5.243569643749998122 ) ) ;
#45782=CARTESIAN_POINT ( 'NONE',  ( 13.13437500061451857, 4.541064518000418104, 2.621784821874999949 ) ) ;
#45783=CARTESIAN_POINT ( 'NONE',  ( 9.528763966825557376E-15, 17.07500000122903572, -26.00000000000000000 ) ) ;
#45784=CARTESIAN_POINT ( 'NONE',  ( 6.675000000000000711, -4.330127018922194537, 2.499999999999995559 ) ) ;
#45785=CARTESIAN_POINT ( 'NONE',  ( 9.001249775931846008E-16, 16.76562500061459815, 34.90005215228797653 ) ) ;
#45786=CARTESIAN_POINT ( 'NONE',  ( 21.30937500061451573, 0.000000000000000000, 5.243569643749999010 ) ) ;
#45787=CYLINDRICAL_SURFACE ( 'NONE', #68591, 3.999999999999996447 ) ;
#45788=CARTESIAN_POINT ( 'NONE',  ( 27.30000000122903359, 5.773502691896255534, 3.535250795749688894E-16 ) ) ;
#45790=CARTESIAN_POINT ( 'NONE',  ( 23.16562500061451502, -6.054752690667223547, -1.112240025338166033E-15 ) ) ;
#45791=CARTESIAN_POINT ( 'NONE',  ( 14.80312500061451608, 4.541064518000418104, -2.621784821874998173 ) ) ;
#45793=CARTESIAN_POINT ( 'NONE',  ( 11.93437500061451573, -4.541064518000419881, 2.621784821874995952 ) ) ;
#45794=CARTESIAN_POINT ( 'NONE',  ( 28.08749999999999858, 5.773502691896255534, 3.535250795749688894E-16 ) ) ;
#45795=CARTESIAN_POINT ( 'NONE',  ( 24.37500000122903288, -5.773502691896255534, -1.060575238724906372E-15 ) ) ;
#45797=CARTESIAN_POINT ( 'NONE',  ( 11.10937500061451644, -4.541064518000417216, -2.621784821875001281 ) ) ;
#45798=CARTESIAN_POINT ( 'NONE',  ( 28.65937500061451715, -4.541064518000417216, -2.621784821875001281 ) ) ;
#45799=CARTESIAN_POINT ( 'NONE',  ( 0.000000000000000000, 20.00000000000000000, 26.00000000000000000 ) ) ;
#45800=CARTESIAN_POINT ( 'NONE',  ( 22.65937500061451715, 0.000000000000000000, 5.243569643749999010 ) ) ;
#45801=CARTESIAN_POINT ( 'NONE',  ( 15.04687500061451644, -3.027376345333614438, 5.243569643749998122 ) ) ;
#45803=CARTESIAN_POINT ( 'NONE',  ( 25.72499999999999787, 6.123233995736764310E-16, -4.999999999999998224 ) ) ;
#45806=CARTESIAN_POINT ( 'NONE',  ( 18.21562500061451573, -6.054752690667223547, -1.112240025338166033E-15 ) ) ;
#45807=CARTESIAN_POINT ( 'NONE',  ( 7.875000000000000000, 4.330127018922191873, 2.499999999999999556 ) ) ;
#45808=CARTESIAN_POINT ( 'NONE',  ( 13.57500000122903572, -5.773502691896255534, -1.060575238724906372E-15 ) ) ;
#45809=CARTESIAN_POINT ( 'NONE',  ( 16.57499999999999929, -4.330127018922194537, 2.499999999999995559 ) ) ;
#45810=CARTESIAN_POINT ( 'NONE',  ( -4.243569643749997233, 12.19062500061451715, 32.45002607614398471 ) ) ;
#45812=CARTESIAN_POINT ( 'NONE',  ( 28.09687500061451360, -3.027376345333614438, 5.243569643749998122 ) ) ;
#45814=CARTESIAN_POINT ( 'NONE',  ( 22.11562500061451786, 3.027376345333611329, 5.243569643749999010 ) ) ;
#45815=CARTESIAN_POINT ( 'NONE',  ( 20.33437500061451786, 4.541064518000418104, 2.621784821874999949 ) ) ;
#45816=CARTESIAN_POINT ( 'NONE',  ( 4.875000000000000888, -4.330127018922194537, 2.499999999999995559 ) ) ;
#45817=CARTESIAN_POINT ( 'NONE',  ( 6.403125000614517504, 0.000000000000000000, 5.243569643749999010 ) ) ;
#45818=CARTESIAN_POINT ( 'NONE',  ( 24.02812500061451573, -4.541064518000419881, 2.621784821874995952 ) ) ;
#45819=CARTESIAN_POINT ( 'NONE',  ( 11.78437500061451892, 4.541064518000418104, 2.621784821874999949 ) ) ;
#45820=CARTESIAN_POINT ( 'NONE',  ( 17.29687500061451999, -3.027376345333614438, 5.243569643749998122 ) ) ;
#45821=CARTESIAN_POINT ( 'NONE',  ( 2.121784821875001281, 16.80312500061451786, 33.67503911421598417 ) ) ;
#45822=CARTESIAN_POINT ( 'NONE',  ( 18.07500000122903216, -5.773502691896255534, -1.060575238724906372E-15 ) ) ;
#45824=CARTESIAN_POINT ( 'NONE',  ( 10.60312500061451679, -4.541064518000417216, -2.621784821875001281 ) ) ;
#45825=CARTESIAN_POINT ( 'NONE',  ( 5.709375000614517859, -4.541064518000417216, -2.621784821875001281 ) ) ;
#45826=CARTESIAN_POINT ( 'NONE',  ( 4.134375000614517681, 4.541064518000418104, 2.621784821874999949 ) ) ;
#45828=CARTESIAN_POINT ( 'NONE',  ( 24.49687500061451573, -3.027376345333614438, 5.243569643749998122 ) ) ;
#45829=CARTESIAN_POINT ( 'NONE',  ( 17.20312500061451644, 0.000000000000000000, 5.243569643749999010 ) ) ;
#45830=CARTESIAN_POINT ( 'NONE',  ( 26.43750000122903288, 4.330127018922191873, 2.499999999999999556 ) ) ;
#45831=CARTESIAN_POINT ( 'NONE',  ( 28.15312500061451573, -4.541064518000417216, -2.621784821875001281 ) ) ;
#45832=CARTESIAN_POINT ( 'NONE',  ( 22.05937500061451573, 4.541064518000418104, -2.621784821874998173 ) ) ;
#45833=CARTESIAN_POINT ( 'NONE',  ( 17.69062500061451715, -3.027376345333614438, 5.243569643749998122 ) ) ;
#45834=CARTESIAN_POINT ( 'NONE',  ( -2.121784821874996840, 19.48437500061451644, 33.67503911421598417 ) ) ;
#45835=CARTESIAN_POINT ( 'NONE',  ( 21.81562500061451004, -6.054752690667223547, -1.112240025338166033E-15 ) ) ;
#45836=CARTESIAN_POINT ( 'NONE',  ( 2.812500001229033320, -4.330127018922190985, -2.500000000000001332 ) ) ;
#45838=CARTESIAN_POINT ( 'NONE',  ( 28.94999999999999929, 4.330127018922192761, -2.499999999999997780 ) ) ;
#45839=CARTESIAN_POINT ( 'NONE',  ( 3.999999999999999112, 13.02500000000000213, -30.00000000000000000 ) ) ;
#45841=ADVANCED_FACE ( 'NONE', ( #5129 ), #27663, .F. ) ;
#45842=CARTESIAN_POINT ( 'NONE',  ( 29.57812500061451644, 6.421520780324663323E-16, -5.243569643749999010 ) ) ;
#45843=CARTESIAN_POINT ( 'NONE',  ( 9.140625000614518214, -3.027376345333614438, 5.243569643749998122 ) ) ;
#45844=CARTESIAN_POINT ( 'NONE',  ( 21.30000000122903359, -2.886751345948125991, -5.000000000000000000 ) ) ;
#45846=CARTESIAN_POINT ( 'NONE',  ( 27.85312500061451502, 4.541064518000418104, -2.621784821874998173 ) ) ;
#45847=CARTESIAN_POINT ( 'NONE',  ( 27.71250000000000568, 2.886751345948126879, 4.999999999999999112 ) ) ;
#45848=CARTESIAN_POINT ( 'NONE',  ( -3.999999999999999112, 19.21250000122903501, -30.00000000000000000 ) ) ;
#45849=CARTESIAN_POINT ( 'NONE',  ( 22.57499999999999929, 6.123233995736764310E-16, -4.999999999999998224 ) ) ;
#45850=CARTESIAN_POINT ( 'NONE',  ( 10.37812500061451715, 4.541064518000418104, 2.621784821874999949 ) ) ;
#45851=VERTEX_POINT ( 'NONE', #6940 ) ;
#45852=CARTESIAN_POINT ( 'NONE',  ( 6.515625000614516438, -6.054752690667223547, -1.112240025338166033E-15 ) ) ;
#45853=CARTESIAN_POINT ( 'NONE',  ( 5.915625000614515905, 3.027376345333611329, 5.243569643749999010 ) ) ;
#45856=CARTESIAN_POINT ( 'NONE',  ( 14.81250000000000000, -5.773502691896255534, -1.060575238724906372E-15 ) ) ;
#45858=CARTESIAN_POINT ( 'NONE',  ( 15.30937500061451750, 4.541064518000418104, -2.621784821874998173 ) ) ;
#45859=CARTESIAN_POINT ( 'NONE',  ( 12.37500000122903465, 2.886751345948129099, -4.999999999999998224 ) ) ;
#45860=CARTESIAN_POINT ( 'NONE',  ( 19.50937500061451857, 0.000000000000000000, 5.243569643749999010 ) ) ;
#45862=CARTESIAN_POINT ( 'NONE',  ( 21.08437500061451786, 6.421520780324663323E-16, -5.243569643749999010 ) ) ;
#45863=CARTESIAN_POINT ( 'NONE',  ( 4.243569643749999010, 13.31562500061451537, -32.45002607614398471 ) ) ;
#45864=CARTESIAN_POINT ( 'NONE',  ( 7.425000000000000711, 4.330127018922191873, 2.499999999999999556 ) ) ;
#45866=CARTESIAN_POINT ( 'NONE',  ( -3.137519842735245283E-14, 11.56250000000000178, -26.00000000000000711 ) ) ;
#45867=PRODUCT_DEFINITION ( 'UNKNOWN', '', #19065, #14402 ) ;
#45868=CARTESIAN_POINT ( 'NONE',  ( 26.16562500061451502, 3.027376345333611329, 5.243569643749999010 ) ) ;
#45870=CARTESIAN_POINT ( 'NONE',  ( 27.90937500061451715, 4.541064518000418104, -2.621784821874998173 ) ) ;
#45871=CARTESIAN_POINT ( 'NONE',  ( 23.47499999999999787, 6.123233995736764310E-16, -4.999999999999998224 ) ) ;
#45872=CARTESIAN_POINT ( 'NONE',  ( 5.990625000614517859, -3.027376345333614438, 5.243569643749998122 ) ) ;
#45874=( BOUNDED_CURVE ( )  B_SPLINE_CURVE ( 2, ( #46862, #35761, #18757, #47581, #63831, #2162, #53487 ),
 .UNSPECIFIED., .F., .F. ) 
 B_SPLINE_CURVE_WITH_KNOTS ( ( 3, 2, 2, 3 ),
 ( 0.9684976324287967175, 0.9694444444444444420, 0.9722222222222222099, 0.9730832832466256299 ),
 .UNSPECIFIED. ) 
 CURVE ( )  GEOMETRIC_REPRESENTATION_ITEM ( )  RATIONAL_B_SPLINE_CURVE ( ( 0.9397993142837226532, 0.9543344473041595055, 1.000000000000000000, 0.8660254037844387076, 1.000000000000000000, 0.9584702908978937064, 0.9426875037768851495 ) ) 
 REPRESENTATION_ITEM ( '' )  );
#45875=CARTESIAN_POINT ( 'NONE',  ( 18.87187500061451573, 3.027376345333613106, -5.243569643749998122 ) ) ;
#45877=CARTESIAN_POINT ( 'NONE',  ( 5.878125000614517148, 4.541064518000418104, 2.621784821874999949 ) ) ;
#45878=CARTESIAN_POINT ( 'NONE',  ( 11.93437500061451573, -4.541064518000419881, 2.621784821874995952 ) ) ;
#45879=EDGE_LOOP ( 'NONE', ( #28342, #30753, #17161, #9324 ) ) ;
#45880=CARTESIAN_POINT ( 'NONE',  ( 21.38437500061451502, -4.541064518000419881, 2.621784821874995952 ) ) ;
#45881=CARTESIAN_POINT ( 'NONE',  ( 0.000000000000000000, 20.00000000000000000, -30.00000000000000000 ) ) ;
#45882=CARTESIAN_POINT ( 'NONE',  ( 28.83749999999999858, -2.886751345948125991, -5.000000000000000000 ) ) ;
#45883=CARTESIAN_POINT ( 'NONE',  ( 28.73437500061451644, 6.421520780324663323E-16, -5.243569643749999010 ) ) ;
#45887=CARTESIAN_POINT ( 'NONE',  ( 10.05000000000000071, 4.330127018922192761, -2.499999999999997780 ) ) ;
#45889=CARTESIAN_POINT ( 'NONE',  ( 23.31562500061451715, 3.027376345333613106, -5.243569643749998122 ) ) ;
#45890=CARTESIAN_POINT ( 'NONE',  ( 13.57500000000000107, 6.123233995736764310E-16, -4.999999999999998224 ) ) ;
#45891=CARTESIAN_POINT ( 'NONE',  ( 10.57500000122903572, 2.886751345948129099, -4.999999999999998224 ) ) ;
#45892=CARTESIAN_POINT ( 'NONE',  ( 9.778125000614517504, 6.421520780324663323E-16, -5.243569643749999010 ) ) ;
#45893=CARTESIAN_POINT ( 'NONE',  ( 23.73749999999999716, -2.886751345948129988, 4.999999999999997335 ) ) ;
#45895=CARTESIAN_POINT ( 'NONE',  ( 19.90312500061451573, 0.000000000000000000, 5.243569643749999010 ) ) ;
#45896=FACE_OUTER_BOUND ( 'NONE', #45635, .T. ) ;
#45897=CARTESIAN_POINT ( 'NONE',  ( 28.12500000122902932, 2.886751345948129099, -4.999999999999998224 ) ) ;
#45899=CARTESIAN_POINT ( 'NONE',  ( 6.712500000000000355, -5.773502691896255534, -1.060575238724906372E-15 ) ) ;
#45900=ORIENTED_EDGE ( 'NONE', *, *, #15195, .T. ) ;
#45901=CARTESIAN_POINT ( 'NONE',  ( 21.89062500061451289, -3.027376345333610441, -5.243569643749999898 ) ) ;
#45902=CARTESIAN_POINT ( 'NONE',  ( 29.42812500061451431, -4.541064518000419881, 2.621784821874995952 ) ) ;
#45903=CARTESIAN_POINT ( 'NONE',  ( 18.90000000122903145, -2.886751345948197045, 4.999999999999880096 ) ) ;
#45904=CARTESIAN_POINT ( 'NONE',  ( 18.27187500061451431, -6.054752690667223547, -1.112240025338166033E-15 ) ) ;
#45905=CARTESIAN_POINT ( 'NONE',  ( 15.92812500061451608, -4.541064518000419881, 2.621784821874995952 ) ) ;
#45906=CARTESIAN_POINT ( 'NONE',  ( -2.121784821874999949, 10.27812500061459566, -33.67503911421598417 ) ) ;
#45907=CARTESIAN_POINT ( 'NONE',  ( 27.45000000122903572, -2.886751345948129988, 4.999999999999997335 ) ) ;
#45909=CARTESIAN_POINT ( 'NONE',  ( 16.45312500061451289, -4.541064518000417216, -2.621784821875001281 ) ) ;
#45911=CARTESIAN_POINT ( 'NONE',  ( 4.012500001229033053, 0.000000000000000000, 4.999999999999998224 ) ) ;
#45912=CARTESIAN_POINT ( 'NONE',  ( 13.84687500061451537, -3.027376345333610441, -5.243569643749999898 ) ) ;
#45913=CARTESIAN_POINT ( 'NONE',  ( 12.19687500061451679, 6.054752690667223547, 3.707466751127219781E-16 ) ) ;
#45914=CARTESIAN_POINT ( 'NONE',  ( 19.50937500061451857, 0.000000000000000000, 5.243569643749999010 ) ) ;
#45916=CARTESIAN_POINT ( 'NONE',  ( -6.000139530219997575, 7.999895352344702282, 30.40432978294467858 ) ) ;
#45917=CARTESIAN_POINT ( 'NONE',  ( 24.47812500061451502, -4.541064518000419881, 2.621784821874995952 ) ) ;
#45918=CARTESIAN_POINT ( 'NONE',  ( 17.82187500061451502, -6.054752690667223547, -1.112240025338166033E-15 ) ) ;
#45919=CARTESIAN_POINT ( 'NONE',  ( 25.41562500061451146, -6.054752690667223547, -1.112240025338166033E-15 ) ) ;
#45920=CARTESIAN_POINT ( 'NONE',  ( 30.00000000000000000, 0.000000000000000000, 4.999999999999998224 ) ) ;
#45921=CARTESIAN_POINT ( 'NONE',  ( 4.000000000000000000, 15.68750000000000000, 32.30940107675849049 ) ) ;
#45922=CARTESIAN_POINT ( 'NONE',  ( 28.52812500061451573, -4.541064518000419881, 2.621784821874995952 ) ) ;
#45923=CARTESIAN_POINT ( 'NONE',  ( 9.862500001229033586, 0.000000000000000000, 4.999999999999998224 ) ) ;
#45924=CARTESIAN_POINT ( 'NONE',  ( 6.675000001229034474, 2.886751345948126879, 4.999999999999999112 ) ) ;
#45925=CARTESIAN_POINT ( 'NONE',  ( 28.95000000122903927, -2.886751345948095793, -5.000000000000054179 ) ) ;
#45926=CARTESIAN_POINT ( 'NONE',  ( 27.03750000122903430, -4.330127018922194537, 2.499999999999995559 ) ) ;
#45929=EDGE_CURVE ( 'NONE', #66635, #12333, #46466, .T. ) ;
#45930=CARTESIAN_POINT ( 'NONE',  ( 9.646875000614516082, -3.027376345333614438, 5.243569643749998122 ) ) ;
#45931=FACE_OUTER_BOUND ( 'NONE', #44125, .T. ) ;
#45932=CARTESIAN_POINT ( 'NONE',  ( 16.79062500061451857, -3.027376345333614438, 5.243569643749998122 ) ) ;
#45933=CARTESIAN_POINT ( 'NONE',  ( 11.89687500061451608, -3.027376345333614438, 5.243569643749998122 ) ) ;
#45934=CARTESIAN_POINT ( 'NONE',  ( 3.290625000614516793, -3.027376345333614438, 5.243569643749998122 ) ) ;
#45935=CARTESIAN_POINT ( 'NONE',  ( 19.50937500061451857, 0.000000000000000000, 5.243569643749999010 ) ) ;
#45936=CARTESIAN_POINT ( 'NONE',  ( 6.721875000614518925, 3.027376345333613106, -5.243569643749998122 ) ) ;
#45937=CARTESIAN_POINT ( 'NONE',  ( 3.365625000614516082, -6.054752690667223547, -1.112240025338166033E-15 ) ) ;
#45938=CARTESIAN_POINT ( 'NONE',  ( -3.999999999999997335, 17.78750000000000142, 32.30940107675850470 ) ) ;
#45939=CARTESIAN_POINT ( 'NONE',  ( 8.653125000614515727, 0.000000000000000000, 5.243569643749999010 ) ) ;
#45940=CARTESIAN_POINT ( 'NONE',  ( 19.26562500061451644, 3.027376345333613106, -5.243569643749998122 ) ) ;
#45942=CARTESIAN_POINT ( 'NONE',  ( 4.800000001229032698, 5.773502691896255534, 3.535250795749688894E-16 ) ) ;
#45943=CARTESIAN_POINT ( 'NONE',  ( 14.27812500061451573, 6.421520780324663323E-16, -5.243569643749999010 ) ) ;
#45944=CARTESIAN_POINT ( 'NONE',  ( 13.52812500061451750, 4.541064518000418104, 2.621784821874999949 ) ) ;
#45946=CARTESIAN_POINT ( 'NONE',  ( 13.83749999999999858, -2.886751345948129988, 4.999999999999997335 ) ) ;
#45947=CARTESIAN_POINT ( 'NONE',  ( 8.137500001229033941, -4.330127018922194537, 2.499999999999995559 ) ) ;
#45948=ADVANCED_FACE ( 'NONE', ( #23917 ), #70452, .F. ) ;
#45949=CARTESIAN_POINT ( 'NONE',  ( 5.990625000614517859, -3.027376345333614438, 5.243569643749998122 ) ) ;
#45950=CARTESIAN_POINT ( 'NONE',  ( 19.46250000122903145, -4.330127018922190985, -2.500000000000001332 ) ) ;
#45952=CARTESIAN_POINT ( 'NONE',  ( -4.243569643749999898, 11.75937500061451857, -30.00000000000000000 ) ) ;
#45953=CARTESIAN_POINT ( 'NONE',  ( 3.712500001229034563, -4.330127018922190985, -2.500000000000001332 ) ) ;
#45954=CARTESIAN_POINT ( 'NONE',  ( 3.242103837493086330E-14, 11.33750000000000213, -34.00000000000000000 ) ) ;
#45955=CARTESIAN_POINT ( 'NONE',  ( 30.00000000000000000, 0.000000000000000000, 0.000000000000000000 ) ) ;
#45956=CARTESIAN_POINT ( 'NONE',  ( 19.02187500061451786, 3.027376345333611329, 5.243569643749999010 ) ) ;
#45957=CARTESIAN_POINT ( 'NONE',  ( 10.61250000122903536, 4.330127018922192761, -2.499999999999997780 ) ) ;
#45958=CARTESIAN_POINT ( 'NONE',  ( 13.52812500061451750, 4.541064518000418104, 2.621784821874999949 ) ) ;
#45960=FACE_OUTER_BOUND ( 'NONE', #51241, .T. ) ;
#45961=CARTESIAN_POINT ( 'NONE',  ( 29.18437500061451573, 6.421520780324663323E-16, -5.243569643749999010 ) ) ;
#45962=CARTESIAN_POINT ( 'NONE',  ( 27.19687500061451857, -3.027376345333614438, 5.243569643749998122 ) ) ;
#45964=CARTESIAN_POINT ( 'NONE',  ( 13.07812500061451821, 4.541064518000418104, 2.621784821874999949 ) ) ;
#45965=CARTESIAN_POINT ( 'NONE',  ( 10.65937500061451715, -4.541064518000417216, -2.621784821875001281 ) ) ;
#45966=VERTEX_POINT ( 'NONE', #8026 ) ;
#45967=CARTESIAN_POINT ( 'NONE',  ( 29.54062500061451502, -3.027376345333610441, -5.243569643749999898 ) ) ;
#45968=CARTESIAN_POINT ( 'NONE',  ( 21.36562500061451431, -6.054752690667223547, -1.112240025338166033E-15 ) ) ;
#45969=CARTESIAN_POINT ( 'NONE',  ( 3.120664071082557278, 3.906599426175572543, -3.497650499216746312 ) ) ;
#45970=CARTESIAN_POINT ( 'NONE',  ( 3.999999999999998668, 14.86250000000000071, 27.69059892324149530 ) ) ;
#45971=CARTESIAN_POINT ( 'NONE',  ( 10.27499999999999858, -4.330127018922194537, 2.499999999999995559 ) ) ;
#45972=CARTESIAN_POINT ( 'NONE',  ( 21.48750000122903003, 4.330127018922191873, 2.499999999999999556 ) ) ;
#45973=CARTESIAN_POINT ( 'NONE',  ( 14.99062500061451786, -3.027376345333614438, 5.243569643749998122 ) ) ;
#45975=EDGE_LOOP ( 'NONE', ( #46342, #47182, #42154, #35242 ) ) ;
#45976=CARTESIAN_POINT ( 'NONE',  ( 17.69999999999999929, 4.330127018922192761, -2.499999999999997780 ) ) ;
#45977=CARTESIAN_POINT ( 'NONE',  ( 20.88749999999999929, 5.773502691896255534, 3.535250795749688894E-16 ) ) ;
#45978=CARTESIAN_POINT ( 'NONE',  ( 19.92187500061451644, 3.027376345333611329, 5.243569643749999010 ) ) ;
#45979=CARTESIAN_POINT ( 'NONE',  ( 26.24062500061451431, -3.027376345333614438, 5.243569643749998122 ) ) ;
#45980=ORIENTED_EDGE ( 'NONE', *, *, #30976, .F. ) ;
#45982=CARTESIAN_POINT ( 'NONE',  ( 8.465625000614515727, 3.027376345333613106, -5.243569643749998122 ) ) ;
#45984=CARTESIAN_POINT ( 'NONE',  ( 15.67500000000000071, -4.330127018922194537, 2.499999999999995559 ) ) ;
#45985=CARTESIAN_POINT ( 'NONE',  ( 2.121784821875001281, 18.15312500061451928, 33.67503911421598417 ) ) ;
#45986=CARTESIAN_POINT ( 'NONE',  ( 29.09062500061451573, -3.027376345333610441, -5.243569643749999898 ) ) ;
#45988=CARTESIAN_POINT ( 'NONE',  ( 26.03437500061451715, 6.421520780324663323E-16, -5.243569643749999010 ) ) ;
#45989=EDGE_LOOP ( 'NONE', ( #60859, #15244, #69228, #55207 ) ) ;
#45990=CARTESIAN_POINT ( 'NONE',  ( 23.80312500061451786, 4.541064518000418104, -2.621784821874998173 ) ) ;
#45991=CARTESIAN_POINT ( 'NONE',  ( 24.64687500061451431, -3.027376345333610441, -5.243569643749999898 ) ) ;
#45992=CARTESIAN_POINT ( 'NONE',  ( 4.243569643749999898, 18.22812500061459318, -30.00000000000000000 ) ) ;
#45993=CARTESIAN_POINT ( 'NONE',  ( 10.83750000000000036, -2.886751345948125991, -5.000000000000000000 ) ) ;
#45994=CARTESIAN_POINT ( 'NONE',  ( 9.328125000614518214, 6.421520780324663323E-16, -5.243569643749999010 ) ) ;
#45995=CARTESIAN_POINT ( 'NONE',  ( 3.836658989281606313, 3.881372312241275768, 3.277265952107013547 ) ) ;
#45996=CARTESIAN_POINT ( 'NONE',  ( 29.50312500061451360, -4.541064518000417216, -2.621784821875001281 ) ) ;
#45997=CARTESIAN_POINT ( 'NONE',  ( 27.17812500061451786, -4.541064518000419881, 2.621784821874995952 ) ) ;
#46000=CARTESIAN_POINT ( 'NONE',  ( 20.18437500061451573, 6.421520780324663323E-16, -5.243569643749999010 ) ) ;
#46001=CARTESIAN_POINT ( 'NONE',  ( 4.243569643749999010, 12.92187500061451644, 27.54997392385601174 ) ) ;
#46003=CARTESIAN_POINT ( 'NONE',  ( 18.42187500061451644, 3.027376345333613106, -5.243569643749998122 ) ) ;
#46004=CARTESIAN_POINT ( 'NONE',  ( 26.74687500061451573, -3.027376345333614438, 5.243569643749998122 ) ) ;
#46005=CARTESIAN_POINT ( 'NONE',  ( -3.000416591977282496E-16, 16.14687500061451786, 25.09994784771203058 ) ) ;
#46006=CARTESIAN_POINT ( 'NONE',  ( 8.165625000614516793, 3.027376345333611329, 5.243569643749999010 ) ) ;
#46007=CARTESIAN_POINT ( 'NONE',  ( 3.999999999999999112, 10.43750000122903465, -30.00000000000000000 ) ) ;
#46008=CARTESIAN_POINT ( 'NONE',  ( 3.571875000614517237, 3.027376345333613106, -5.243569643749998122 ) ) ;
#46010=CARTESIAN_POINT ( 'NONE',  ( 4.978125000614518569, 4.541064518000418104, 2.621784821874999949 ) ) ;
#46011=CARTESIAN_POINT ( 'NONE',  ( 9.984375000614518214, 4.541064518000418104, 2.621784821874999949 ) ) ;
#46012=DIRECTION ( 'NONE',  ( 1.000000000000000000, 0.000000000000000000, 0.000000000000000000 ) ) ;
#46013=CARTESIAN_POINT ( 'NONE',  ( 18.03750000122903430, -4.330127018922194537, 2.499999999999995559 ) ) ;
#46014=CARTESIAN_POINT ( 'NONE',  ( 6.046875000614519102, -3.027376345333614438, 5.243569643749998122 ) ) ;
#46015=CARTESIAN_POINT ( 'NONE',  ( 7.490625000614516082, -3.027376345333610441, -5.243569643749999898 ) ) ;
#46016=CARTESIAN_POINT ( 'NONE',  ( 5.728125000614515905, 6.421520780324663323E-16, -5.243569643749999010 ) ) ;
#46018=CARTESIAN_POINT ( 'NONE',  ( 17.48437500061451999, 6.421520780324663323E-16, -5.243569643749999010 ) ) ;
#46019=DIRECTION ( 'NONE',  ( -0.000000000000000000, -1.000000000000000000, -0.000000000000000000 ) ) ;
#46021=CARTESIAN_POINT ( 'NONE',  ( 23.95312500061451289, 0.000000000000000000, 5.243569643749999010 ) ) ;
#46022=CARTESIAN_POINT ( 'NONE',  ( 10.67812500061451608, 6.421520780324663323E-16, -5.243569643749999010 ) ) ;
#46023=CARTESIAN_POINT ( 'NONE',  ( 27.72187500061451715, -6.054752690667223547, -1.112240025338166033E-15 ) ) ;
#46024=CARTESIAN_POINT ( 'NONE',  ( 10.37812500061451715, 4.541064518000418104, 2.621784821874999949 ) ) ;
#46025=CARTESIAN_POINT ( 'NONE',  ( 4.400918202330496243, -2.373166445152071535, -4.675799785326651303 ) ) ;
#46026=( BOUNDED_CURVE ( )  B_SPLINE_CURVE ( 2, ( #69038, #69755, #68677, #29506, #1446, #42048, #59018 ),
 .UNSPECIFIED., .F., .F. ) 
 B_SPLINE_CURVE_WITH_KNOTS ( ( 3, 2, 2, 3 ),
 ( 0.8916666666666667185, 0.8944444444444444864, 0.8972222222222223653, 0.9000000000000001332 ),
 .UNSPECIFIED. ) 
 CURVE ( )  GEOMETRIC_REPRESENTATION_ITEM ( )  RATIONAL_B_SPLINE_CURVE ( ( 1.000000000000000000, 0.8660254037844387076, 1.000000000000000000, 0.8660254037844387076, 1.000000000000000000, 0.8660254037844333785, 1.000000000000005329 ) ) 
 REPRESENTATION_ITEM ( '' )  );
#46027=CARTESIAN_POINT ( 'NONE',  ( 13.87500000122903465, 2.886751345948126879, 4.999999999999999112 ) ) ;
#46028=CARTESIAN_POINT ( 'NONE',  ( 28.04062500061451502, -3.027376345333614438, 5.243569643749998122 ) ) ;
#46029=CARTESIAN_POINT ( 'NONE',  ( 4.243569643749999898, 11.89062500061451644, -27.54997392385601529 ) ) ;
#46030=CARTESIAN_POINT ( 'NONE',  ( 12.78750000122903430, 6.123233995736764310E-16, -4.999999999999998224 ) ) ;
#46031=CARTESIAN_POINT ( 'NONE',  ( 11.84999999999999964, 4.330127018922192761, -2.499999999999997780 ) ) ;
#46032=CARTESIAN_POINT ( 'NONE',  ( 21.25312500061451715, 0.000000000000000000, 5.243569643749999010 ) ) ;
#46033=CARTESIAN_POINT ( 'NONE',  ( 5.671875000614519102, -6.054752690667223547, -1.112240025338166033E-15 ) ) ;
#46034=CARTESIAN_POINT ( 'NONE',  ( 19.53749999999999432, 5.773502691896255534, 3.535250795749688894E-16 ) ) ;
#46035=CARTESIAN_POINT ( 'NONE',  ( 8.250000001229034652, -2.886751345948125991, -5.000000000000000000 ) ) ;
#46036=CARTESIAN_POINT ( 'NONE',  ( 16.65000000122903501, -2.886751345948129988, 4.999999999999997335 ) ) ;
#46037=CARTESIAN_POINT ( 'NONE',  ( 13.26562500061451644, -6.054752690667223547, -1.112240025338166033E-15 ) ) ;
#46038=CARTESIAN_POINT ( 'NONE',  ( 16.75312500061451715, 0.000000000000000000, 5.243569643749999010 ) ) ;
#46039=CARTESIAN_POINT ( 'NONE',  ( 24.97500000122903430, 2.886751345948129099, -4.999999999999998224 ) ) ;
#46040=CARTESIAN_POINT ( 'NONE',  ( 20.88749999999999929, 5.773502691896255534, 3.535250795749688894E-16 ) ) ;
#46041=CARTESIAN_POINT ( 'NONE',  ( 23.93437500061451573, 4.541064518000418104, 2.621784821874999949 ) ) ;
#46043=ADVANCED_FACE ( 'NONE', ( #1770 ), #19454, .F. ) ;
#46044=CARTESIAN_POINT ( 'NONE',  ( 10.05000000122903181, -2.886751345948125991, -5.000000000000000000 ) ) ;
#46045=CARTESIAN_POINT ( 'NONE',  ( 8.634375000614518569, 4.541064518000418104, 2.621784821874999949 ) ) ;
#46046=CARTESIAN_POINT ( 'NONE',  ( 26.70937500061451431, 0.000000000000000000, 5.243569643749999010 ) ) ;
#46048=CARTESIAN_POINT ( 'NONE',  ( 23.46562500061451573, 3.027376345333611329, 5.243569643749999010 ) ) ;
#46049=CARTESIAN_POINT ( 'NONE',  ( 26.18437500061451573, 4.541064518000418104, 2.621784821874999949 ) ) ;
#46051=CARTESIAN_POINT ( 'NONE',  ( 3.310802318797580579, -3.746810377620464205, 3.668301323911666412 ) ) ;
#46052=CARTESIAN_POINT ( 'NONE',  ( 8.521875000614516082, 3.027376345333613106, -5.243569643749998122 ) ) ;
#46053=CARTESIAN_POINT ( 'NONE',  ( 18.85312500061451502, 4.541064518000418104, -2.621784821874998173 ) ) ;
#46054=CARTESIAN_POINT ( 'NONE',  ( 30.00000000000000000, 6.123233995736764310E-16, -4.999999999999998224 ) ) ;
#46055=CARTESIAN_POINT ( 'NONE',  ( 28.19062500061451715, -3.027376345333610441, -5.243569643749999898 ) ) ;
#46056=CARTESIAN_POINT ( 'NONE',  ( 4.921875000614518214, 3.027376345333613106, -5.243569643749998122 ) ) ;
#46058=CARTESIAN_POINT ( 'NONE',  ( 4.003125000614518925, 4.541064518000418104, -2.621784821874998173 ) ) ;
#46059=CARTESIAN_POINT ( 'NONE',  ( 18.00000000000000355, -4.330127018922190985, -2.500000000000001332 ) ) ;
#46060=EDGE_LOOP ( 'NONE', ( #66264, #4549, #14599, #7048 ) ) ;
#46061=CARTESIAN_POINT ( 'NONE',  ( 27.75000000000000000, 0.000000000000000000, 4.999999999999998224 ) ) ;
#46062=( BOUNDED_CURVE ( )  B_SPLINE_CURVE ( 3, ( #4735, #72327, #54973, #286 ),
 .UNSPECIFIED., .F., .F. ) 
 B_SPLINE_CURVE_WITH_KNOTS ( ( 4, 4 ),
 ( 5.396747428351075015, 5.426701883967095519 ),
 .UNSPECIFIED. ) 
 CURVE ( )  GEOMETRIC_REPRESENTATION_ITEM ( )  RATIONAL_B_SPLINE_CURVE ( ( 1.000000000000000000, 0.9999252289467817079, 0.9999252289467817079, 1.000000000000000000 ) ) 
 REPRESENTATION_ITEM ( '' )  );
#46063=CARTESIAN_POINT ( 'NONE',  ( 27.00937500061451857, 4.541064518000418104, -2.621784821874998173 ) ) ;
#46065=CARTESIAN_POINT ( 'NONE',  ( 15.25312500061451715, 4.541064518000418104, -2.621784821874998173 ) ) ;
#46066=CARTESIAN_POINT ( 'NONE',  ( 7.040625000614517681, -3.027376345333610441, -5.243569643749999898 ) ) ;
#46068=CARTESIAN_POINT ( 'NONE',  ( 4.584375000614516971, 4.541064518000418104, 2.621784821874999949 ) ) ;
#46069=CARTESIAN_POINT ( 'NONE',  ( 16.50000000122903288, 5.773502691896255534, 3.535250795749688894E-16 ) ) ;
#46070=CARTESIAN_POINT ( 'NONE',  ( 21.22500000000000142, 6.123233995736764310E-16, -4.999999999999998224 ) ) ;
#46071=CARTESIAN_POINT ( 'NONE',  ( 29.77499999999999858, 6.123233995736764310E-16, -4.999999999999998224 ) ) ;
#46072=CARTESIAN_POINT ( 'NONE',  ( 4.059375000614519280, 4.541064518000418104, -2.621784821874998173 ) ) ;
#46073=CARTESIAN_POINT ( 'NONE',  ( 10.47187500061451715, 3.027376345333611329, 5.243569643749999010 ) ) ;
#46074=CARTESIAN_POINT ( 'NONE',  ( 21.83437500061451786, -4.541064518000419881, 2.621784821874995952 ) ) ;
#46075=CARTESIAN_POINT ( 'NONE',  ( 1.626862140677534273E-15, 15.27500000122903501, -26.00000000000000355 ) ) ;
#46077=CARTESIAN_POINT ( 'NONE',  ( 5.221875000614519813, -6.054752690667223547, -1.112240025338166033E-15 ) ) ;
#46078=CARTESIAN_POINT ( 'NONE',  ( 5.887500000000000178, -2.886751345948125991, -5.000000000000000000 ) ) ;
#46079=CARTESIAN_POINT ( 'NONE',  ( 6.271875000614517859, 3.027376345333613106, -5.243569643749998122 ) ) ;
#46080=CARTESIAN_POINT ( 'NONE',  ( 18.07499999999999929, 6.123233995736764310E-16, -4.999999999999998224 ) ) ;
#46081=CARTESIAN_POINT ( 'NONE',  ( 16.41562500061451857, -6.054752690667223547, -1.112240025338166033E-15 ) ) ;
#46083=CARTESIAN_POINT ( 'NONE',  ( 4.231215331025275361, 2.664084549475962405, 4.393375741670284107 ) ) ;
#46085=CARTESIAN_POINT ( 'NONE',  ( 10.79062500061451679, 6.054752690667223547, 3.707466751127219781E-16 ) ) ;
#46086=CARTESIAN_POINT ( 'NONE',  ( 27.19687500061451857, -3.027376345333614438, 5.243569643749998122 ) ) ;
#46087=CARTESIAN_POINT ( 'NONE',  ( 4.243569643749999898, 19.14687500061451431, 32.45002607614398471 ) ) ;
#46088=CARTESIAN_POINT ( 'NONE',  ( 26.03437500061451715, 6.421520780324663323E-16, -5.243569643749999010 ) ) ;
#46089=CARTESIAN_POINT ( 'NONE',  ( 7.687500000000000000, -2.886751345948125991, -5.000000000000000000 ) ) ;
#46090=CARTESIAN_POINT ( 'NONE',  ( 1.999999999999998668, 14.11250000122903359, 26.53589838486224650 ) ) ;
#46091=CARTESIAN_POINT ( 'NONE',  ( 15.44062500061451537, -3.027376345333614438, 5.243569643749998122 ) ) ;
#46092=CARTESIAN_POINT ( 'NONE',  ( 6.937500001229033764, 6.123233995736764310E-16, -4.999999999999998224 ) ) ;
#46093=CARTESIAN_POINT ( 'NONE',  ( 16.73437500061451644, 4.541064518000418104, 2.621784821874999949 ) ) ;
#46094=CARTESIAN_POINT ( 'NONE',  ( 12.04687500061451821, -3.027376345333610441, -5.243569643749999898 ) ) ;
#46095=CARTESIAN_POINT ( 'NONE',  ( 10.00000000000000000, 1.224646799147353256E-15, 10.00000000000000178 ) ) ;
#46097=CARTESIAN_POINT ( 'NONE',  ( 14.05312500061451431, 0.000000000000000000, 5.243569643749999010 ) ) ;
#46098=CARTESIAN_POINT ( 'NONE',  ( 25.42500000122903359, 2.886751345948129099, -4.999999999999998224 ) ) ;
#46099=CARTESIAN_POINT ( 'NONE',  ( 13.54687500061451999, 6.054752690667223547, 3.707466751127219781E-16 ) ) ;
#46100=CARTESIAN_POINT ( 'NONE',  ( 14.76562500061451821, 3.027376345333613106, -5.243569643749998122 ) ) ;
#46102=CARTESIAN_POINT ( 'NONE',  ( 23.63437500061451502, -4.541064518000419881, 2.621784821874995952 ) ) ;
#46103=CARTESIAN_POINT ( 'NONE',  ( 4.243569643749999010, 10.61562500061451786, 27.54997392385601174 ) ) ;
#46104=CARTESIAN_POINT ( 'NONE',  ( 10.72500000122903252, 2.886751345948126879, 4.999999999999999112 ) ) ;
#46105=CARTESIAN_POINT ( 'NONE',  ( 0.000000000000000000, 20.00000000000000000, 26.00000000000000000 ) ) ;
#46107=CARTESIAN_POINT ( 'NONE',  ( -4.243569643749999898, 16.25937500061451857, -30.00000000000000000 ) ) ;
#46108=CARTESIAN_POINT ( 'NONE',  ( 17.25937500061451502, 0.000000000000000000, 5.243569643749999010 ) ) ;
#46109=CARTESIAN_POINT ( 'NONE',  ( 20.77500000122903145, -5.773502691896255534, -1.060575238724906372E-15 ) ) ;
#46110=CARTESIAN_POINT ( 'NONE',  ( 14.37187500061451928, 3.027376345333613106, -5.243569643749998122 ) ) ;
#46111=CARTESIAN_POINT ( 'NONE',  ( 4.243569643749999010, 10.22187500061451892, 27.54997392385601174 ) ) ;
#46112=CARTESIAN_POINT ( 'NONE',  ( 20.85000000122903430, -2.886751345948125991, -5.000000000000000000 ) ) ;
#46113=CARTESIAN_POINT ( 'NONE',  ( 16.07812500061451289, 6.421520780324663323E-16, -5.243569643749999010 ) ) ;
#46114=CARTESIAN_POINT ( 'NONE',  ( 1.626862140677534273E-15, 12.46250000000000213, 34.00000000000000000 ) ) ;
#46115=ORIENTED_EDGE ( 'NONE', *, *, #52383, .T. ) ;
#46116=ORIENTED_EDGE ( 'NONE', *, *, #3889, .T. ) ;
#46117=CARTESIAN_POINT ( 'NONE',  ( 17.92500000000000071, -4.330127018922194537, 2.499999999999995559 ) ) ;
#46119=CARTESIAN_POINT ( 'NONE',  ( 3.964577175323932057, 3.046748717458611644, 30.54880584332639160 ) ) ;
#46120=CARTESIAN_POINT ( 'NONE',  ( 15.37500000122903465, -5.773502691896255534, -1.060575238724906372E-15 ) ) ;
#46121=CARTESIAN_POINT ( 'NONE',  ( 27.53437500061451360, 4.541064518000418104, 2.621784821874999949 ) ) ;
#46122=CARTESIAN_POINT ( 'NONE',  ( 19.67812500061451786, 6.421520780324663323E-16, -5.243569643749999010 ) ) ;
#46123=CARTESIAN_POINT ( 'NONE',  ( 23.27812500061451573, 6.421520780324663323E-16, -5.243569643749999010 ) ) ;
#46124=CARTESIAN_POINT ( 'NONE',  ( 29.62500000122903288, 2.886751345948126879, 4.999999999999999112 ) ) ;
#46125=CARTESIAN_POINT ( 'NONE',  ( 27.86249999999999716, -5.773502691896255534, -1.060575238724906372E-15 ) ) ;
#46126=CARTESIAN_POINT ( 'NONE',  ( 3.999999999999999112, 11.78750000122903430, 30.00000000000000000 ) ) ;
#46130=CARTESIAN_POINT ( 'NONE',  ( -2.121784821874996840, 16.33437500061451786, -26.32496088578401583 ) ) ;
#46131=CARTESIAN_POINT ( 'NONE',  ( 5.062500001229035540, -4.330127018922190985, -2.500000000000001332 ) ) ;
#46132=CARTESIAN_POINT ( 'NONE',  ( 4.949999999999999289, -4.330127018922190985, -2.500000000000001332 ) ) ;
#46134=CARTESIAN_POINT ( 'NONE',  ( 3.300000001229034918, -2.886751345948125991, -5.000000000000000000 ) ) ;
#46135=CARTESIAN_POINT ( 'NONE',  ( 9.046875000614518214, 6.054752690667223547, 3.707466751127219781E-16 ) ) ;
#46136=CYLINDRICAL_SURFACE ( 'NONE', #48953, 4.999999999999998224 ) ;
#46138=CARTESIAN_POINT ( 'NONE',  ( -5.193763058582908876, 8.549021686977599899, -33.02854916113439998 ) ) ;
#46139=DIRECTION ( 'NONE',  ( 0.000000000000000000, 0.000000000000000000, 1.000000000000000000 ) ) ;
#46140=CARTESIAN_POINT ( 'NONE',  ( 6.571875000614517681, -6.054752690667223547, -1.112240025338166033E-15 ) ) ;
#46141=CARTESIAN_POINT ( 'NONE',  ( 13.84687500061451537, -3.027376345333610441, -5.243569643749999898 ) ) ;
#46142=CARTESIAN_POINT ( 'NONE',  ( 5.549999999999998934, 4.330127018922192761, -2.499999999999997780 ) ) ;
#46143=CARTESIAN_POINT ( 'NONE',  ( 4.243569643749999898, 17.74062500061459602, 32.45002607614398471 ) ) ;
#46144=CARTESIAN_POINT ( 'NONE',  ( 21.27187500061451786, 3.027376345333611329, 5.243569643749999010 ) ) ;
#46145=CARTESIAN_POINT ( 'NONE',  ( 9.712500000000002132, 2.886751345948126879, 4.999999999999998224 ) ) ;
#46146=CARTESIAN_POINT ( 'NONE',  ( 26.25000000122903288, -2.886751345948125991, -5.000000000000000000 ) ) ;
#46148=CARTESIAN_POINT ( 'NONE',  ( 21.89062500061451289, -3.027376345333610441, -5.243569643749999898 ) ) ;
#46149=CARTESIAN_POINT ( 'NONE',  ( 13.37812500061451715, 6.421520780324663323E-16, -5.243569643749999010 ) ) ;
#46151=CARTESIAN_POINT ( 'NONE',  ( 11.14687500061451608, -3.027376345333610441, -5.243569643749999898 ) ) ;
#46152=CARTESIAN_POINT ( 'NONE',  ( 27.78749999999999787, -2.886751345948129988, 4.999999999999997335 ) ) ;
#46153=CARTESIAN_POINT ( 'NONE',  ( 21.48750000122903003, 4.330127018922191873, 2.499999999999999556 ) ) ;
#46155=CARTESIAN_POINT ( 'NONE',  ( 10.77187500061451786, 3.027376345333613106, -5.243569643749998122 ) ) ;
#46156=CARTESIAN_POINT ( 'NONE',  ( 28.80937500061451573, 4.541064518000418104, -2.621784821874998173 ) ) ;
#46157=CARTESIAN_POINT ( 'NONE',  ( 2.934375000614518392, -4.541064518000419881, 2.621784821874995952 ) ) ;
#46159=CARTESIAN_POINT ( 'NONE',  ( 22.39687500061451075, -3.027376345333610441, -5.243569643749999898 ) ) ;
#46160=CARTESIAN_POINT ( 'NONE',  ( 13.09687500061451892, 6.054752690667223547, 3.707466751127219781E-16 ) ) ;
#46162=CARTESIAN_POINT ( 'NONE',  ( 26.69999999999999929, 4.330127018922192761, -2.499999999999997780 ) ) ;
#46165=CARTESIAN_POINT ( 'NONE',  ( 17.72812500061451502, -4.541064518000419881, 2.621784821874995952 ) ) ;
#46166=CARTESIAN_POINT ( 'NONE',  ( 7.087499999999999467, -2.886751345948129988, 4.999999999999997335 ) ) ;
#46167=CARTESIAN_POINT ( 'NONE',  ( -0.6945863667395647534, 9.663023495605401081, 26.06076786935074097 ) ) ;
#46168=CARTESIAN_POINT ( 'NONE',  ( 14.51250000000000107, 2.886751345948129099, -4.999999999999998224 ) ) ;
#46170=CARTESIAN_POINT ( 'NONE',  ( -4.243569643749999898, 11.25312500061451892, 30.00000000000000000 ) ) ;
#46172=CARTESIAN_POINT ( 'NONE',  ( 25.84687500061451360, -3.027376345333614438, 5.243569643749998122 ) ) ;
#46174=CARTESIAN_POINT ( 'NONE',  ( 22.90312500061451573, 4.541064518000418104, -2.621784821874998173 ) ) ;
#46175=CARTESIAN_POINT ( 'NONE',  ( 19.13437500061451857, -4.541064518000419881, 2.621784821874995952 ) ) ;
#46176=CARTESIAN_POINT ( 'NONE',  ( 4.462500000000001243, -5.773502691896255534, -1.060575238724906372E-15 ) ) ;
#46177=CARTESIAN_POINT ( 'NONE',  ( 6.478125000614516793, -4.541064518000419881, 2.621784821874995952 ) ) ;
#46178=CARTESIAN_POINT ( 'NONE',  ( 22.30312500061451431, -4.541064518000417216, -2.621784821875001281 ) ) ;
#46179=CARTESIAN_POINT ( 'NONE',  ( 11.48437500061451644, -4.541064518000419881, 2.621784821874995952 ) ) ;
#46180=CARTESIAN_POINT ( 'NONE',  ( 16.43437500061451573, -4.541064518000419881, 2.621784821874995952 ) ) ;
#46181=CARTESIAN_POINT ( 'NONE',  ( -3.000416591977282496E-16, 16.99062500061451786, 25.09994784771203058 ) ) ;
#46182=CARTESIAN_POINT ( 'NONE',  ( 19.87500000122903288, -5.773502691896255534, -1.060575238724906372E-15 ) ) ;
#46184=CARTESIAN_POINT ( 'NONE',  ( 10.52812500061451750, -4.541064518000419881, 2.621784821874995952 ) ) ;
#46185=CARTESIAN_POINT ( 'NONE',  ( 4.509375000614518569, 4.541064518000418104, -2.621784821874998173 ) ) ;
#46186=CARTESIAN_POINT ( 'NONE',  ( 5.784375000614517148, 6.421520780324663323E-16, -5.243569643749999010 ) ) ;
#46187=CARTESIAN_POINT ( 'NONE',  ( 25.62187500061451573, 3.027376345333613106, -5.243569643749998122 ) ) ;
#46188=CARTESIAN_POINT ( 'NONE',  ( 17.61562500061451786, 3.027376345333611329, 5.243569643749999010 ) ) ;
#46189=CARTESIAN_POINT ( 'NONE',  ( 27.30000000122903359, 5.773502691896255534, 3.535250795749688894E-16 ) ) ;
#46190=CARTESIAN_POINT ( 'NONE',  ( 24.36562500061451786, 3.027376345333611329, 5.243569643749999010 ) ) ;
#46191=CARTESIAN_POINT ( 'NONE',  ( 23.03437500061451715, 4.541064518000418104, 2.621784821874999949 ) ) ;
#46192=CARTESIAN_POINT ( 'NONE',  ( 18.02812500061451573, 4.541064518000418104, 2.621784821874999949 ) ) ;
#46193=CARTESIAN_POINT ( 'NONE',  ( 4.243569643749999898, 17.79687500061451999, 32.45002607614398471 ) ) ;
#46194=CARTESIAN_POINT ( 'NONE',  ( 22.34062500061451573, -3.027376345333610441, -5.243569643749999898 ) ) ;
#46195=CARTESIAN_POINT ( 'NONE',  ( 15.37500000000000000, 6.123233995736764310E-16, -4.999999999999998224 ) ) ;
#46197=CARTESIAN_POINT ( 'NONE',  ( 26.55000000000000071, -4.330127018922190985, -2.500000000000001332 ) ) ;
#46198=CARTESIAN_POINT ( 'NONE',  ( -3.999999999999997335, 12.38750000000000107, -27.69059892324149175 ) ) ;
#46200=CARTESIAN_POINT ( 'NONE',  ( 29.69062500061451715, 6.054752690667223547, 3.707466751127219781E-16 ) ) ;
#46201=CARTESIAN_POINT ( 'NONE',  ( 11.01562500061451821, -6.054752690667223547, -1.112240025338166033E-15 ) ) ;
#46202=CARTESIAN_POINT ( 'NONE',  ( 22.31250000122903288, 4.330127018922192761, -2.499999999999997780 ) ) ;
#46203=CARTESIAN_POINT ( 'NONE',  ( 26.76562500061451644, -6.054752690667223547, -1.112240025338166033E-15 ) ) ;
#46205=CARTESIAN_POINT ( 'NONE',  ( 28.76249999999999929, -5.773502691896255534, -1.060575238724906372E-15 ) ) ;
#46206=CARTESIAN_POINT ( 'NONE',  ( -3.999999999999997335, 15.65000000122903501, -27.69059892324149175 ) ) ;
#46207=FACE_OUTER_BOUND ( 'NONE', #36419, .T. ) ;
#46208=CARTESIAN_POINT ( 'NONE',  ( 11.42812500061451608, -4.541064518000419881, 2.621784821874995952 ) ) ;
#46209=ORIENTED_EDGE ( 'NONE', *, *, #12441, .T. ) ;
#46210=CARTESIAN_POINT ( 'NONE',  ( 26.84062500061451573, -3.027376345333610441, -5.243569643749999898 ) ) ;
#46211=CARTESIAN_POINT ( 'NONE',  ( 7.415625000614516793, -6.054752690667223547, -1.112240025338166033E-15 ) ) ;
#46213=CARTESIAN_POINT ( 'NONE',  ( 4.903125000614516615, 4.541064518000418104, -2.621784821874998173 ) ) ;
#46215=CARTESIAN_POINT ( 'NONE',  ( 30.00000000000000000, 1.224646799147353059E-15, -9.999999999999998224 ) ) ;
#46216=CARTESIAN_POINT ( 'NONE',  ( 15.78749999999999964, -2.886751345948125991, -5.000000000000000000 ) ) ;
#46218=CARTESIAN_POINT ( 'NONE',  ( 16.99687500061451573, -3.027376345333610441, -5.243569643749999898 ) ) ;
#46219=CARTESIAN_POINT ( 'NONE',  ( 12.30000000122903181, -2.886751345948125991, -5.000000000000000000 ) ) ;
#46220=CARTESIAN_POINT ( 'NONE',  ( 18.15937500061451715, 0.000000000000000000, 5.243569643749999010 ) ) ;
#46222=CARTESIAN_POINT ( 'NONE',  ( 21.45937500061451786, -4.541064518000417216, -2.621784821875001281 ) ) ;
#46223=CARTESIAN_POINT ( 'NONE',  ( -4.243569643749999898, 14.85312500061451679, -30.00000000000000000 ) ) ;
#46224=CARTESIAN_POINT ( 'NONE',  ( -3.999999999999999112, 16.85000000000000142, 30.00000000000000000 ) ) ;
#46227=CARTESIAN_POINT ( 'NONE',  ( 25.07812500061451644, 6.421520780324663323E-16, -5.243569643749999010 ) ) ;
#46229=CARTESIAN_POINT ( 'NONE',  ( 28.47187500061451715, 3.027376345333611329, 5.243569643749999010 ) ) ;
#46230=CARTESIAN_POINT ( 'NONE',  ( 24.78750000000000497, -2.886751345948125991, -5.000000000000000000 ) ) ;
#46231=CARTESIAN_POINT ( 'NONE',  ( 6.328125000614515550, 4.541064518000418104, 2.621784821874999949 ) ) ;
#46233=CARTESIAN_POINT ( 'NONE',  ( 18.64687500061451786, -3.027376345333614438, 5.243569643749998122 ) ) ;
#46235=CARTESIAN_POINT ( 'NONE',  ( 4.903125000614516615, 4.541064518000418104, -2.621784821874998173 ) ) ;
#46236=CARTESIAN_POINT ( 'NONE',  ( 7.996875000614519280, -3.027376345333610441, -5.243569643749999898 ) ) ;
#46237=ORIENTED_EDGE ( 'NONE', *, *, #16958, .F. ) ;
#46238=CARTESIAN_POINT ( 'NONE',  ( 18.72187500061451360, -6.054752690667223547, -1.112240025338166033E-15 ) ) ;
#46240=CARTESIAN_POINT ( 'NONE',  ( 26.17500000000000071, 6.123233995736764310E-16, -4.999999999999998224 ) ) ;
#46241=CARTESIAN_POINT ( 'NONE',  ( 29.22187500061451715, 3.027376345333613106, -5.243569643749998122 ) ) ;
#46242=CARTESIAN_POINT ( 'NONE',  ( 1.626862140677534273E-15, 12.12500000122903465, 34.00000000000000000 ) ) ;
#46245=CARTESIAN_POINT ( 'NONE',  ( 10.27499999999999858, -4.330127018922194537, 2.499999999999995559 ) ) ;
#46247=CARTESIAN_POINT ( 'NONE',  ( 25.00312500061451715, -4.541064518000417216, -2.621784821875001281 ) ) ;
#46248=CARTESIAN_POINT ( 'NONE',  ( 13.64999999999999858, 4.330127018922192761, -2.499999999999997780 ) ) ;
#46249=CARTESIAN_POINT ( 'NONE',  ( 10.05000000122903181, -2.886751345948125991, -5.000000000000000000 ) ) ;
#46250=CARTESIAN_POINT ( 'NONE',  ( 9.178125000614517859, -4.541064518000419881, 2.621784821874995952 ) ) ;
#46251=CARTESIAN_POINT ( 'NONE',  ( 21.89999999999999858, 0.000000000000000000, 4.999999999999998224 ) ) ;
#46252=ADVANCED_FACE ( 'NONE', ( #13192 ), #35009, .F. ) ;
#46253=CARTESIAN_POINT ( 'NONE',  ( 21.21562500061451573, 3.027376345333611329, 5.243569643749999010 ) ) ;
#46254=CARTESIAN_POINT ( 'NONE',  ( 18.63750000122903216, 6.123233995736764310E-16, -4.999999999999998224 ) ) ;
#46255=AXIS2_PLACEMENT_3D ( 'NONE', #37643, #71264, #42466 ) ;
#46256=CARTESIAN_POINT ( 'NONE',  ( 26.06250000122903288, 0.000000000000000000, 4.999999999999998224 ) ) ;
#46258=CARTESIAN_POINT ( 'NONE',  ( 8.437500000000000000, -2.886751345948129988, 4.999999999999997335 ) ) ;
#46260=CARTESIAN_POINT ( 'NONE',  ( 22.82812500061451644, 6.421520780324663323E-16, -5.243569643749999010 ) ) ;
#46261=CARTESIAN_POINT ( 'NONE',  ( 26.82187500061451857, -6.054752690667223547, -1.112240025338166033E-15 ) ) ;
#46262=CARTESIAN_POINT ( 'NONE',  ( 17.89687500061451431, -3.027376345333610441, -5.243569643749999898 ) ) ;
#46263=CARTESIAN_POINT ( 'NONE',  ( 14.24062500061451608, -3.027376345333610441, -5.243569643749999898 ) ) ;
#46264=CARTESIAN_POINT ( 'NONE',  ( 4.243569643749999898, 10.12812500061459353, -30.00000000000000000 ) ) ;
#46265=( BOUNDED_CURVE ( )  B_SPLINE_CURVE ( 2, ( #57869, #7278, #24259, #69344, #52703, #18702, #41266, #30172, #2109 ),
 .UNSPECIFIED., .F., .F. ) 
 B_SPLINE_CURVE_WITH_KNOTS ( ( 3, 2, 2, 2, 3 ),
 ( 0.5326086956521739468, 0.5362318840579710644, 0.5434782608695651884, 0.5507246376811594235, 0.5543478260869565410 ),
 .UNSPECIFIED. ) 
 CURVE ( )  GEOMETRIC_REPRESENTATION_ITEM ( )  RATIONAL_B_SPLINE_CURVE ( ( 0.9330127018922194093, 0.9330127018922194093, 1.000000000000000000, 0.8660254037844387076, 1.000000000000000000, 0.8660254037844387076, 1.000000000000000000, 0.9330127018922194093, 0.9330127018922194093 ) ) 
 REPRESENTATION_ITEM ( '' )  );
#46266=CARTESIAN_POINT ( 'NONE',  ( 26.81250000122903288, 4.330127018922192761, -2.499999999999997780 ) ) ;
#46268=CARTESIAN_POINT ( 'NONE',  ( 15.62812500061451537, 6.421520780324663323E-16, -5.243569643749999010 ) ) ;
#46269=CARTESIAN_POINT ( 'NONE',  ( 13.53750000000000142, -2.886751345948126435, -5.000000000000000000 ) ) ;
#46270=CARTESIAN_POINT ( 'NONE',  ( 3.225000001229033408, -5.773502691896255534, -1.060575238724906372E-15 ) ) ;
#46271=CARTESIAN_POINT ( 'NONE',  ( 11.85937500061451644, 0.000000000000000000, 5.243569643749999010 ) ) ;
#46272=CARTESIAN_POINT ( 'NONE',  ( 12.57187500061451857, 3.027376345333613106, -5.243569643749998122 ) ) ;
#46273=CARTESIAN_POINT ( 'NONE',  ( 19.58437500061451786, -4.541064518000419881, 2.621784821874995952 ) ) ;
#46275=CARTESIAN_POINT ( 'NONE',  ( 29.39999999999999858, 4.330127018922192761, -2.499999999999997780 ) ) ;
#46276=CARTESIAN_POINT ( 'NONE',  ( 23.57812500061451289, -4.541064518000419881, 2.621784821874995952 ) ) ;
#46277=CARTESIAN_POINT ( 'NONE',  ( 20.07187500061451857, -6.054752690667223547, -1.112240025338166033E-15 ) ) ;
#46278=CARTESIAN_POINT ( 'NONE',  ( 23.42812500061451786, 4.541064518000418104, 2.621784821874999949 ) ) ;
#46279=CARTESIAN_POINT ( 'NONE',  ( 4.000000000000000000, 14.33750000000000213, 32.30940107675849049 ) ) ;
#46280=CARTESIAN_POINT ( 'NONE',  ( 28.30312500061451431, 4.541064518000418104, -2.621784821874998173 ) ) ;
#46281=CARTESIAN_POINT ( 'NONE',  ( 9.787500001229036073, 4.330127018922191873, 2.499999999999999556 ) ) ;
#46282=CARTESIAN_POINT ( 'NONE',  ( 3.787500001229033408, 6.123233995736764310E-16, -4.999999999999998224 ) ) ;
#46283=CARTESIAN_POINT ( 'NONE',  ( 26.85000000122903430, 5.773502691896255534, 3.535250795749688894E-16 ) ) ;
#46286=CARTESIAN_POINT ( 'NONE',  ( 8.446875000614518569, -3.027376345333610441, -5.243569643749999898 ) ) ;
#46287=CARTESIAN_POINT ( 'NONE',  ( 24.44999999999999929, 4.330127018922192761, -2.499999999999997780 ) ) ;
#46288=CARTESIAN_POINT ( 'NONE',  ( 18.47812500061451857, 4.541064518000418104, 2.621784821874999949 ) ) ;
#46289=CARTESIAN_POINT ( 'NONE',  ( 10.02187500061451964, 3.027376345333611329, 5.243569643749999010 ) ) ;
#46290=CARTESIAN_POINT ( 'NONE',  ( 29.36250000122903003, -4.330127018922190985, -2.500000000000001332 ) ) ;
#46291=CARTESIAN_POINT ( 'NONE',  ( 19.24687500061452283, -3.027376345333610441, -5.243569643749999898 ) ) ;
#46292=CARTESIAN_POINT ( 'NONE',  ( 7.771875000614516971, 3.027376345333611329, 5.243569643749999010 ) ) ;
#46293=CARTESIAN_POINT ( 'NONE',  ( 3.081468785175471403, -3.937611012629079976, -3.302521940835167591 ) ) ;
#46295=CARTESIAN_POINT ( 'NONE',  ( 8.015625000614518214, 3.027376345333613106, -5.243569643749998122 ) ) ;
#46296=CARTESIAN_POINT ( 'NONE',  ( 18.29062500061451502, -3.027376345333610441, -5.243569643749999898 ) ) ;
#46297=( BOUNDED_CURVE ( )  B_SPLINE_CURVE ( 2, ( #42027, #25764, #13941, #71564, #30930, #8040, #15033 ),
 .UNSPECIFIED., .F., .F. ) 
 B_SPLINE_CURVE_WITH_KNOTS ( ( 3, 2, 2, 3 ),
 ( 0.4416666666666666519, 0.4444444444444444753, 0.4472222222222222987, 0.4500000000000001221 ),
 .UNSPECIFIED. ) 
 CURVE ( )  GEOMETRIC_REPRESENTATION_ITEM ( )  RATIONAL_B_SPLINE_CURVE ( ( 1.000000000000000000, 0.8660254037844387076, 1.000000000000000000, 0.8660254037844387076, 1.000000000000000000, 0.8660254037844333785, 1.000000000000005329 ) ) 
 REPRESENTATION_ITEM ( '' )  );
#46299=CARTESIAN_POINT ( 'NONE',  ( 4.762500001229033941, 4.330127018922192761, -2.499999999999997780 ) ) ;
#46300=CARTESIAN_POINT ( 'NONE',  ( 14.20312500061451644, -4.541064518000417216, -2.621784821875001281 ) ) ;
#46301=CARTESIAN_POINT ( 'NONE',  ( 14.31562500061451537, 3.027376345333613106, -5.243569643749998122 ) ) ;
#46303=CARTESIAN_POINT ( 'NONE',  ( 13.91249999999999964, -5.773502691896255534, -1.060575238724906372E-15 ) ) ;
#46304=CARTESIAN_POINT ( 'NONE',  ( 7.012500001229035718, 4.330127018922192761, -2.499999999999997780 ) ) ;
#46305=CARTESIAN_POINT ( 'NONE',  ( 6.403125000614517504, 0.000000000000000000, 5.243569643749999010 ) ) ;
#46308=CARTESIAN_POINT ( 'NONE',  ( 17.73750000122903359, 6.123233995736764310E-16, -4.999999999999998224 ) ) ;
#46310=( BOUNDED_CURVE ( )  B_SPLINE_CURVE ( 2, ( #57996, #57639, #35116, #17745, #24750, #51753, #57279, #46936, #69473 ),
 .UNSPECIFIED., .F., .F. ) 
 B_SPLINE_CURVE_WITH_KNOTS ( ( 3, 2, 2, 2, 3 ),
 ( 0.6847826086956522174, 0.6884057971014492239, 0.6956521739130434590, 0.7028985507246376940, 0.7065217391304348116 ),
 .UNSPECIFIED. ) 
 CURVE ( )  GEOMETRIC_REPRESENTATION_ITEM ( )  RATIONAL_B_SPLINE_CURVE ( ( 0.9330127018922192983, 0.9330127018922202975, 1.000000000000000000, 0.8660254037844387076, 1.000000000000000000, 0.8660254037844387076, 1.000000000000000000, 0.9330127018922194093, 0.9330127018922194093 ) ) 
 REPRESENTATION_ITEM ( '' )  );
#46311=ADVANCED_FACE ( 'NONE', ( #19090 ), #41645, .F. ) ;
#46312=CARTESIAN_POINT ( 'NONE',  ( 2.121784821874999061, 10.70937500061451964, -33.67503911421598417 ) ) ;
#46314=CARTESIAN_POINT ( 'NONE',  ( 4.400918202330496243, -2.373166445152071535, -4.675799785326651303 ) ) ;
#46316=CARTESIAN_POINT ( 'NONE',  ( 13.87500000000000178, -4.330127018922194537, 2.499999999999995559 ) ) ;
#46317=CARTESIAN_POINT ( 'NONE',  ( 17.67187500061451644, 3.027376345333611329, 5.243569643749999010 ) ) ;
#46318=EDGE_CURVE ( 'NONE', #57370, #33074, #13282, .T. ) ;
#46320=CARTESIAN_POINT ( 'NONE',  ( 15.21562500061451750, 3.027376345333613106, -5.243569643749998122 ) ) ;
#46322=CARTESIAN_POINT ( 'NONE',  ( 15.71250000122903501, 0.000000000000000000, 4.999999999999998224 ) ) ;
#46323=CARTESIAN_POINT ( 'NONE',  ( 26.44687500061451502, -3.027376345333610441, -5.243569643749999898 ) ) ;
#46325=CARTESIAN_POINT ( 'NONE',  ( 11.95312500061451644, -4.541064518000417216, -2.621784821875001281 ) ) ;
#46326=CARTESIAN_POINT ( 'NONE',  ( 16.39687500061451786, -3.027376345333614438, 5.243569643749998122 ) ) ;
#46327=ORIENTED_EDGE ( 'NONE', *, *, #65368, .F. ) ;
#46328=CARTESIAN_POINT ( 'NONE',  ( 27.29062500061451502, -3.027376345333610441, -5.243569643749999898 ) ) ;
#46329=CARTESIAN_POINT ( 'NONE',  ( 20.72812500061451502, 4.541064518000418104, 2.621784821874999949 ) ) ;
#46330=DIRECTION ( 'NONE',  ( 0.000000000000000000, 0.000000000000000000, 1.000000000000000000 ) ) ;
#46332=CARTESIAN_POINT ( 'NONE',  ( 30.00000000000000000, 6.123233995736764310E-16, -4.999999999999998224 ) ) ;
#46333=CARTESIAN_POINT ( 'NONE',  ( 9.525000000000002132, 6.123233995736764310E-16, -4.999999999999998224 ) ) ;
#46334=CARTESIAN_POINT ( 'NONE',  ( 19.65000000122902790, 5.773502691896255534, 3.535250795749688894E-16 ) ) ;
#46337=EDGE_LOOP ( 'NONE', ( #30515, #13543, #19702, #37 ) ) ;
#46338=CARTESIAN_POINT ( 'NONE',  ( 17.17500000000000071, 6.123233995736764310E-16, -4.999999999999998224 ) ) ;
#46339=CARTESIAN_POINT ( 'NONE',  ( 20.21250000000000213, -5.773502691896255534, -1.060575238724906372E-15 ) ) ;
#46340=CARTESIAN_POINT ( 'NONE',  ( 18.57187500061451857, 3.027376345333611329, 5.243569643749999010 ) ) ;
#46341=CARTESIAN_POINT ( 'NONE',  ( 24.25312500061451715, 4.541064518000418104, -2.621784821874998173 ) ) ;
#46342=ORIENTED_EDGE ( 'NONE', *, *, #7032, .T. ) ;
#46343=DIRECTION ( 'NONE',  ( -0.000000000000000000, -1.000000000000000000, -0.000000000000000000 ) ) ;
#46344=CARTESIAN_POINT ( 'NONE',  ( 9.403125000614517504, 4.541064518000418104, -2.621784821874998173 ) ) ;
#46345=CARTESIAN_POINT ( 'NONE',  ( 3.152458665894561474, 4.261886542965685365, -3.105335258989349700 ) ) ;
#46346=CARTESIAN_POINT ( 'NONE',  ( 15.48749999999999893, 5.773502691896255534, 3.535250795749688894E-16 ) ) ;
#46347=CARTESIAN_POINT ( 'NONE',  ( -3.000416591977282496E-16, 18.79062500061451857, 25.09994784771203058 ) ) ;
#46348=CARTESIAN_POINT ( 'NONE',  ( 29.46562500061451573, -6.054752690667223547, -1.112240025338166033E-15 ) ) ;
#46351=CARTESIAN_POINT ( 'NONE',  ( 27.34687500061451360, -3.027376345333610441, -5.243569643749999898 ) ) ;
#46353=CARTESIAN_POINT ( 'NONE',  ( 22.26562500061451644, -6.054752690667223547, -1.112240025338166033E-15 ) ) ;
#46354=CARTESIAN_POINT ( 'NONE',  ( 22.99687500061451573, 6.054752690667223547, 3.707466751127219781E-16 ) ) ;
#46355=CARTESIAN_POINT ( 'NONE',  ( 4.243569643749999010, 16.01562500061459460, -32.45002607614398471 ) ) ;
#46356=CARTESIAN_POINT ( 'NONE',  ( 10.38750000000000107, -2.886751345948125991, -5.000000000000000000 ) ) ;
#46357=CARTESIAN_POINT ( 'NONE',  ( 5.353125000614515905, 4.541064518000418104, -2.621784821874998173 ) ) ;
#46359=CARTESIAN_POINT ( 'NONE',  ( 23.09062500061451573, -3.027376345333614438, 5.243569643749998122 ) ) ;
#46362=CARTESIAN_POINT ( 'NONE',  ( 16.84687500061451715, -3.027376345333614438, 5.243569643749998122 ) ) ;
#46363=CARTESIAN_POINT ( 'NONE',  ( -2.121784821874999949, 13.48437500061451821, 26.32496088578401938 ) ) ;
#46364=CARTESIAN_POINT ( 'NONE',  ( 18.19687500061451502, -3.027376345333614438, 5.243569643749998122 ) ) ;
#46365=CARTESIAN_POINT ( 'NONE',  ( 26.37187500061451217, -6.054752690667223547, -1.112240025338166033E-15 ) ) ;
#46366=CARTESIAN_POINT ( 'NONE',  ( -2.121784821874996840, 15.88437500061451857, 33.67503911421598417 ) ) ;
#46367=CARTESIAN_POINT ( 'NONE',  ( 7.828125000614517326, -4.541064518000419881, 2.621784821874995952 ) ) ;
#46369=CARTESIAN_POINT ( 'NONE',  ( 3.871875000614519280, -6.054752690667223547, -1.112240025338166033E-15 ) ) ;
#46371=CARTESIAN_POINT ( 'NONE',  ( 4.940625000614515372, 6.054752690667223547, 3.707466751127219781E-16 ) ) ;
#46372=CARTESIAN_POINT ( 'NONE',  ( 9.759375000614516793, -4.541064518000417216, -2.621784821875001281 ) ) ;
#46373=CARTESIAN_POINT ( 'NONE',  ( 16.76250000122903216, -4.330127018922190985, -2.500000000000001332 ) ) ;
#46374=CARTESIAN_POINT ( 'NONE',  ( 5.184375000614516615, -4.541064518000419881, 2.621784821874995952 ) ) ;
#46375=CARTESIAN_POINT ( 'NONE',  ( 7.340625000614518392, -3.027376345333614438, 5.243569643749998122 ) ) ;
#46376=CARTESIAN_POINT ( 'NONE',  ( 8.287500001229034297, 6.123233995736764310E-16, -4.999999999999998224 ) ) ;
#46378=CARTESIAN_POINT ( 'NONE',  ( 17.18437500061451573, 4.541064518000418104, 2.621784821874999949 ) ) ;
#46379=CARTESIAN_POINT ( 'NONE',  ( 27.75000000000000000, 0.000000000000000000, 4.999999999999998224 ) ) ;
#46381=CARTESIAN_POINT ( 'NONE',  ( 24.85312500061451502, 0.000000000000000000, 5.243569643749999010 ) ) ;
#46382=CARTESIAN_POINT ( 'NONE',  ( 9.890625000614516438, 6.054752690667223547, 3.707466751127219781E-16 ) ) ;
#46383=CARTESIAN_POINT ( 'NONE',  ( 26.33437500061451431, -4.541064518000419881, 2.621784821874995952 ) ) ;
#46384=CARTESIAN_POINT ( 'NONE',  ( 9.928125000614517859, 4.541064518000418104, 2.621784821874999949 ) ) ;
#46385=CARTESIAN_POINT ( 'NONE',  ( -1.394453263437886801E-15, 19.32500000122903216, -26.00000000000000000 ) ) ;
#46386=CARTESIAN_POINT ( 'NONE',  ( 10.08750000122903323, 6.123233995736764310E-16, -4.999999999999998224 ) ) ;
#46387=CARTESIAN_POINT ( 'NONE',  ( 25.34062500061451217, -3.027376345333614438, 5.243569643749998122 ) ) ;
#46388=CARTESIAN_POINT ( 'NONE',  ( -2.121784821874996840, 14.02812500061451750, -26.32496088578401583 ) ) ;
#46389=CARTESIAN_POINT ( 'NONE',  ( 11.92500000122903181, 2.886751345948129099, -4.999999999999998224 ) ) ;
#46390=CARTESIAN_POINT ( 'NONE',  ( 23.09062500061451573, -3.027376345333614438, 5.243569643749998122 ) ) ;
#46391=CARTESIAN_POINT ( 'NONE',  ( 11.66249999999999964, -5.773502691896255534, -1.060575238724906372E-15 ) ) ;
#46392=CARTESIAN_POINT ( 'NONE',  ( 19.60312500061451502, -4.541064518000417216, -2.621784821875001281 ) ) ;
#46393=CARTESIAN_POINT ( 'NONE',  ( 5.784375000614517148, 6.421520780324663323E-16, -5.243569643749999010 ) ) ;
#46394=CARTESIAN_POINT ( 'NONE',  ( 19.87500000000000000, 6.123233995736764310E-16, -4.999999999999998224 ) ) ;
#46395=CARTESIAN_POINT ( 'NONE',  ( 7.312500001229033764, -4.330127018922190985, -2.500000000000001332 ) ) ;
#46396=CARTESIAN_POINT ( 'NONE',  ( 16.38750000122903216, 6.123233995736764310E-16, -4.999999999999998224 ) ) ;
#46397=CARTESIAN_POINT ( 'NONE',  ( 11.80312500061451608, 0.000000000000000000, 5.243569643749999010 ) ) ;
#46398=CARTESIAN_POINT ( 'NONE',  ( 15.29062500061451679, 6.054752690667223547, 3.707466751127219781E-16 ) ) ;
#46399=CARTESIAN_POINT ( 'NONE',  ( 25.31250000122903288, -4.330127018922190985, -2.500000000000001332 ) ) ;
#46400=CARTESIAN_POINT ( 'NONE',  ( 20.17499999999999716, -4.330127018922194537, 2.499999999999995559 ) ) ;
#46401=CARTESIAN_POINT ( 'NONE',  ( 23.40937500061451715, 4.541064518000418104, -2.621784821874998173 ) ) ;
#46402=CARTESIAN_POINT ( 'NONE',  ( 10.68750000122903288, 4.330127018922191873, 2.499999999999999556 ) ) ;
#46403=CARTESIAN_POINT ( 'NONE',  ( 8.559375000614515727, 4.541064518000418104, -2.621784821874998173 ) ) ;
#46404=CARTESIAN_POINT ( 'NONE',  ( 24.83437500061451431, 4.541064518000418104, 2.621784821874999949 ) ) ;
#46406=CARTESIAN_POINT ( 'NONE',  ( 3.234375000614516438, 4.541064518000418104, 2.621784821874999949 ) ) ;
#46407=CARTESIAN_POINT ( 'NONE',  ( 21.62812500061451360, 4.541064518000418104, 2.621784821874999949 ) ) ;
#46408=CARTESIAN_POINT ( 'NONE',  ( 26.33437500061451431, -4.541064518000419881, 2.621784821874995952 ) ) ;
#46411=CARTESIAN_POINT ( 'NONE',  ( 6.721875000614518925, 3.027376345333613106, -5.243569643749998122 ) ) ;
#46412=CARTESIAN_POINT ( 'NONE',  ( 20.12812500061451715, 6.421520780324663323E-16, -5.243569643749999010 ) ) ;
#46414=CARTESIAN_POINT ( 'NONE',  ( 16.05000000000000071, 0.000000000000000000, 4.999999999999998224 ) ) ;
#46415=CARTESIAN_POINT ( 'NONE',  ( 27.89062500061451289, 6.054752690667223547, 3.707466751127219781E-16 ) ) ;
#46416=CARTESIAN_POINT ( 'NONE',  ( 3.496875000614518836, -3.027376345333610441, -5.243569643749999898 ) ) ;
#46417=CARTESIAN_POINT ( 'NONE',  ( 6.675000000000000711, -4.330127018922194537, 2.499999999999995559 ) ) ;
#46418=FACE_OUTER_BOUND ( 'NONE', #43523, .T. ) ;
#46419=CARTESIAN_POINT ( 'NONE',  ( 17.69999999999999929, 4.330127018922192761, -2.499999999999997780 ) ) ;
#46420=CARTESIAN_POINT ( 'NONE',  ( 20.91562500061451502, -6.054752690667223547, -1.112240025338166033E-15 ) ) ;
#46421=ORIENTED_EDGE ( 'NONE', *, *, #50590, .T. ) ;
#46422=CARTESIAN_POINT ( 'NONE',  ( 25.91250000000000142, 2.886751345948126879, 4.999999999999999112 ) ) ;
#46423=CARTESIAN_POINT ( 'NONE',  ( 26.67187500061451644, 3.027376345333611329, 5.243569643749999010 ) ) ;
#46424=ORIENTED_EDGE ( 'NONE', *, *, #68767, .T. ) ;
#46425=CARTESIAN_POINT ( 'NONE',  ( 16.11562500061451786, 3.027376345333613106, -5.243569643749998122 ) ) ;
#46426=CARTESIAN_POINT ( 'NONE',  ( 5.540625000614515905, -3.027376345333614438, 5.243569643749998122 ) ) ;
#46428=CARTESIAN_POINT ( 'NONE',  ( 28.07812500061451289, -4.541064518000419881, 2.621784821874995952 ) ) ;
#46429=CARTESIAN_POINT ( 'NONE',  ( 14.32500000122903394, 2.886751345948126879, 4.999999999999999112 ) ) ;
#46430=CARTESIAN_POINT ( 'NONE',  ( 21.11249999999999716, -5.773502691896255534, -1.060575238724906372E-15 ) ) ;
#46431=CARTESIAN_POINT ( 'NONE',  ( 28.23750000000000426, -2.886751345948129988, 4.999999999999997335 ) ) ;
#46432=CARTESIAN_POINT ( 'NONE',  ( 4.884375000614518569, 6.421520780324663323E-16, -5.243569643749999010 ) ) ;
#46433=CARTESIAN_POINT ( 'NONE',  ( 8.934375000614517504, 6.421520780324663323E-16, -5.243569643749999010 ) ) ;
#46434=CARTESIAN_POINT ( 'NONE',  ( 20.22187500061451715, 3.027376345333613106, -5.243569643749998122 ) ) ;
#46435=CARTESIAN_POINT ( 'NONE',  ( 10.01250000122903394, -4.330127018922190985, -2.500000000000001332 ) ) ;
#46436=ORIENTED_EDGE ( 'NONE', *, *, #39683, .F. ) ;
#46437=CARTESIAN_POINT ( 'NONE',  ( 29.42812500061451431, -4.541064518000419881, 2.621784821874995952 ) ) ;
#46438=CARTESIAN_POINT ( 'NONE',  ( 3.450000000000001510, 0.000000000000000000, 4.999999999999998224 ) ) ;
#46439=CARTESIAN_POINT ( 'NONE',  ( 5.409375000614516260, 4.541064518000418104, -2.621784821874998173 ) ) ;
#46441=CARTESIAN_POINT ( 'NONE',  ( 19.27500000000000213, -4.330127018922194537, 2.499999999999995559 ) ) ;
#46442=CARTESIAN_POINT ( 'NONE',  ( 16.97812500061451502, 6.421520780324663323E-16, -5.243569643749999010 ) ) ;
#46444=DIRECTION ( 'NONE',  ( -0.000000000000000000, -1.000000000000000000, -0.000000000000000000 ) ) ;
#46446=CARTESIAN_POINT ( 'NONE',  ( 7.453125000614516438, -4.541064518000417216, -2.621784821875001281 ) ) ;
#46447=CARTESIAN_POINT ( 'NONE',  ( 26.44687500061451502, -3.027376345333610441, -5.243569643749999898 ) ) ;
#46448=CARTESIAN_POINT ( 'NONE',  ( -4.243569643749999898, 18.50937500061451857, 30.00000000000000000 ) ) ;
#46449=CARTESIAN_POINT ( 'NONE',  ( 26.67187500061451644, 3.027376345333611329, 5.243569643749999010 ) ) ;
#46450=CARTESIAN_POINT ( 'NONE',  ( 6.975000000000002309, 4.330127018922191873, 2.499999999999999556 ) ) ;
#46451=CARTESIAN_POINT ( 'NONE',  ( -3.999999999999999556, 11.97500000122903252, 27.69059892324149530 ) ) ;
#46452=CARTESIAN_POINT ( 'NONE',  ( 14.95312500061451644, 0.000000000000000000, 5.243569643749999010 ) ) ;
#46453=CARTESIAN_POINT ( 'NONE',  ( 7.387500001229032165, 6.123233995736764310E-16, -4.999999999999998224 ) ) ;
#46454=CARTESIAN_POINT ( 'NONE',  ( 16.88437500061451502, -4.541064518000419881, 2.621784821874995952 ) ) ;
#46455=CARTESIAN_POINT ( 'NONE',  ( 12.75937500061451857, 0.000000000000000000, 5.243569643749999010 ) ) ;
#46456=CARTESIAN_POINT ( 'NONE',  ( 21.44999999999999929, 0.000000000000000000, 4.999999999999998224 ) ) ;
#46457=ORIENTED_EDGE ( 'NONE', *, *, #40712, .F. ) ;
#46458=CARTESIAN_POINT ( 'NONE',  ( 12.21562500061451573, 3.027376345333611329, 5.243569643749999010 ) ) ;
#46459=CARTESIAN_POINT ( 'NONE',  ( 24.63750000122903216, 4.330127018922191873, 2.499999999999999556 ) ) ;
#46460=CARTESIAN_POINT ( 'NONE',  ( 13.92187500061451644, 3.027376345333613106, -5.243569643749998122 ) ) ;
#46461=CARTESIAN_POINT ( 'NONE',  ( 4.044621064622349493, 3.945521627023633293, -3.653295367133241545 ) ) ;
#46462=CARTESIAN_POINT ( 'NONE',  ( 14.95312500061451644, 0.000000000000000000, 5.243569643749999010 ) ) ;
#46465=CARTESIAN_POINT ( 'NONE',  ( 24.94687500061451502, -3.027376345333614438, 5.243569643749998122 ) ) ;
#46466=LINE ( 'NONE', #47190, #10080 ) ;
#46467=CARTESIAN_POINT ( 'NONE',  ( 11.43750000122903465, 6.123233995736764310E-16, -4.999999999999998224 ) ) ;
#46468=FACE_OUTER_BOUND ( 'NONE', #21701, .T. ) ;
#46469=CARTESIAN_POINT ( 'NONE',  ( -1.071796769724490339, 19.64240381056766438, 34.00000000000000000 ) ) ;
#46470=CARTESIAN_POINT ( 'NONE',  ( 4.243569643749999898, 16.03437500061451715, -30.00000000000000000 ) ) ;
#46471=CARTESIAN_POINT ( 'NONE',  ( 17.22187500061451715, 3.027376345333611329, 5.243569643749999010 ) ) ;
#46472=CARTESIAN_POINT ( 'NONE',  ( 17.17500000122903359, -5.773502691896255534, -1.060575238724906372E-15 ) ) ;
#46473=CARTESIAN_POINT ( 'NONE',  ( 15.15937500061451715, -4.541064518000417216, -2.621784821875001281 ) ) ;
#46474=CARTESIAN_POINT ( 'NONE',  ( 4.243569643749999010, 10.67187500061451644, 27.54997392385601174 ) ) ;
#46475=CARTESIAN_POINT ( 'NONE',  ( 19.23750000122903714, 4.330127018922191873, 2.499999999999999556 ) ) ;
#46476=CARTESIAN_POINT ( 'NONE',  ( 14.09062500061451750, -3.027376345333614438, 5.243569643749998122 ) ) ;
#46477=ORIENTED_EDGE ( 'NONE', *, *, #60294, .F. ) ;
#46478=ORIENTED_EDGE ( 'NONE', *, *, #40515, .T. ) ;
#46479=CARTESIAN_POINT ( 'NONE',  ( 17.25000000000000000, 4.330127018922192761, -2.499999999999997780 ) ) ;
#46480=CARTESIAN_POINT ( 'NONE',  ( 6.375000000000001776, 6.123233995736764310E-16, -4.999999999999998224 ) ) ;
#46481=CARTESIAN_POINT ( 'NONE',  ( 0.2791130135581313398, 5.000000000000001776, 25.99999999999999645 ) ) ;
#46482=CARTESIAN_POINT ( 'NONE',  ( 14.21250000122903323, 4.330127018922192761, -2.499999999999997780 ) ) ;
#46483=CARTESIAN_POINT ( 'NONE',  ( 27.19687500061451857, -3.027376345333614438, 5.243569643749998122 ) ) ;
#46484=CARTESIAN_POINT ( 'NONE',  ( 19.56562500061451715, -6.054752690667223547, -1.112240025338166033E-15 ) ) ;
#46485=CARTESIAN_POINT ( 'NONE',  ( 22.22812500061451502, -4.541064518000419881, 2.621784821874995952 ) ) ;
#46486=CARTESIAN_POINT ( 'NONE',  ( 4.415625000614518569, 3.027376345333613106, -5.243569643749998122 ) ) ;
#46487=CARTESIAN_POINT ( 'NONE',  ( 26.81250000000000000, 2.886751345948126879, 4.999999999999999112 ) ) ;
#46490=CARTESIAN_POINT ( 'NONE',  ( 6.412500001229036073, -4.330127018922190985, -2.500000000000001332 ) ) ;
#46492=CARTESIAN_POINT ( 'NONE',  ( -2.121784821874999949, 16.18437500061451573, -33.67503911421598417 ) ) ;
#46493=CARTESIAN_POINT ( 'NONE',  ( 6.525000001229033231, 2.886751345948129099, -4.999999999999998224 ) ) ;
#46494=CARTESIAN_POINT ( 'NONE',  ( 6.862500000000002487, 2.886751345948129099, -4.999999999999998224 ) ) ;
#46495=( BOUNDED_CURVE ( )  B_SPLINE_CURVE ( 2, ( #33780, #56673, #62222, #4989, #15688, #34135, #6071 ),
 .UNSPECIFIED., .F., .F. ) 
 B_SPLINE_CURVE_WITH_KNOTS ( ( 3, 2, 2, 3 ),
 ( 0.6999999999999999556, 0.7027777777777777235, 0.7055555555555557135, 0.7083333333333334814 ),
 .UNSPECIFIED. ) 
 CURVE ( )  GEOMETRIC_REPRESENTATION_ITEM ( )  RATIONAL_B_SPLINE_CURVE ( ( 1.000000000000000000, 0.8660254037844387076, 1.000000000000000000, 0.8660254037844387076, 1.000000000000000000, 0.8660254037844333785, 1.000000000000005329 ) ) 
 REPRESENTATION_ITEM ( '' )  );
#46496=CARTESIAN_POINT ( 'NONE',  ( 4.162500001229033408, -4.330127018922190985, -2.500000000000001332 ) ) ;
#46497=CARTESIAN_POINT ( 'NONE',  ( 10.54687500061451644, -3.027376345333614438, 5.243569643749998122 ) ) ;
#46498=CARTESIAN_POINT ( 'NONE',  ( 28.90312500061451217, 0.000000000000000000, 5.243569643749999010 ) ) ;
#46499=CYLINDRICAL_SURFACE ( 'NONE', #848, 4.000000000000000000 ) ;
#46500=CARTESIAN_POINT ( 'NONE',  ( -5.959432963256016791, 8.030867404579453250, -29.19699834589561149 ) ) ;
#46502=CARTESIAN_POINT ( 'NONE',  ( 8.184375000614515727, 4.541064518000418104, 2.621784821874999949 ) ) ;
#46503=CARTESIAN_POINT ( 'NONE',  ( 10.73437500061451644, 6.421520780324663323E-16, -5.243569643749999010 ) ) ;
#46504=CARTESIAN_POINT ( 'NONE',  ( 6.637500000000001066, -2.886751345948129988, 4.999999999999997335 ) ) ;
#46505=CARTESIAN_POINT ( 'NONE',  ( -4.243569643749999898, 14.36562500061459424, 27.54997392385601529 ) ) ;
#46506=CARTESIAN_POINT ( 'NONE',  ( 7.320879633048903241E-15, 18.08749999999999858, 26.00000000000000355 ) ) ;
#46507=CARTESIAN_POINT ( 'NONE',  ( 6.787500000000001421, -2.886751345948125991, -5.000000000000000000 ) ) ;
#46508=CARTESIAN_POINT ( 'NONE',  ( 27.75000000122903288, 5.773502691896255534, 3.535250795749688894E-16 ) ) ;
#46510=CARTESIAN_POINT ( 'NONE',  ( 23.39062500061451289, 6.054752690667223547, 3.707466751127219781E-16 ) ) ;
#46511=CARTESIAN_POINT ( 'NONE',  ( 13.52812500061451750, 4.541064518000418104, 2.621784821874999949 ) ) ;
#46513=CARTESIAN_POINT ( 'NONE',  ( 8.934375000614517504, 6.421520780324663323E-16, -5.243569643749999010 ) ) ;
#46514=CARTESIAN_POINT ( 'NONE',  ( 28.53749999999999787, 5.773502691896255534, 3.535250795749688894E-16 ) ) ;
#46515=CARTESIAN_POINT ( 'NONE',  ( 22.27500000122903145, 2.886751345948129099, -4.999999999999998224 ) ) ;
#46516=CARTESIAN_POINT ( 'NONE',  ( 11.40000000122903501, -2.886751345948126435, -5.000000000000000000 ) ) ;
#46517=CARTESIAN_POINT ( 'NONE',  ( 11.85937500061451644, 0.000000000000000000, 5.243569643749999010 ) ) ;
#46518=CARTESIAN_POINT ( 'NONE',  ( 25.92187500061451999, -6.054752690667223547, -1.112240025338166033E-15 ) ) ;
#46519=CARTESIAN_POINT ( 'NONE',  ( 2.859375000614519546, 0.000000000000000000, 5.243569643749999010 ) ) ;
#46521=CARTESIAN_POINT ( 'NONE',  ( 22.80937500061451573, -4.541064518000417216, -2.621784821875001281 ) ) ;
#46522=CARTESIAN_POINT ( 'NONE',  ( 14.63437500061451679, -4.541064518000419881, 2.621784821874995952 ) ) ;
#46524=CARTESIAN_POINT ( 'NONE',  ( 26.21249999999999858, 2.886751345948129099, -4.999999999999998224 ) ) ;
#46526=CARTESIAN_POINT ( 'NONE',  ( -2.121784821874996840, 14.98437500061451644, -26.32496088578401583 ) ) ;
#46528=CARTESIAN_POINT ( 'NONE',  ( 17.46562500061451217, 3.027376345333613106, -5.243569643749998122 ) ) ;
#46529=CARTESIAN_POINT ( 'NONE',  ( 6.675000000000000711, -4.330127018922194537, 2.499999999999995559 ) ) ;
#46531=CARTESIAN_POINT ( 'NONE',  ( 14.47499999999999964, 6.123233995736764310E-16, -4.999999999999998224 ) ) ;
#46532=CARTESIAN_POINT ( 'NONE',  ( 1.999999999999998668, 19.51250000122903216, 26.53589838486224650 ) ) ;
#46533=CARTESIAN_POINT ( 'NONE',  ( 14.36250000122903359, 0.000000000000000000, 4.999999999999998224 ) ) ;
#46534=CARTESIAN_POINT ( 'NONE',  ( 24.38437500061451502, 4.541064518000418104, 2.621784821874999949 ) ) ;
#46535=VERTEX_POINT ( 'NONE', #21657 ) ;
#46536=CARTESIAN_POINT ( 'NONE',  ( 19.19062500061452070, -3.027376345333610441, -5.243569643749999898 ) ) ;
#46537=CARTESIAN_POINT ( 'NONE',  ( 20.03437500061451715, -4.541064518000419881, 2.621784821874995952 ) ) ;
#46538=CARTESIAN_POINT ( 'NONE',  ( 4.687500000000000000, 5.773502691896255534, 3.535250795749688894E-16 ) ) ;
#46539=CARTESIAN_POINT ( 'NONE',  ( 8.128125000614515372, 4.541064518000418104, 2.621784821874999949 ) ) ;
#46540=CARTESIAN_POINT ( 'NONE',  ( 21.66562500061451502, 3.027376345333611329, 5.243569643749999010 ) ) ;
#46541=CARTESIAN_POINT ( 'NONE',  ( 12.19687500061451679, 6.054752690667223547, 3.707466751127219781E-16 ) ) ;
#46542=EDGE_CURVE ( 'NONE', #49922, #19257, #10938, .T. ) ;
#46543=CARTESIAN_POINT ( 'NONE',  ( 16.20937500061451786, 4.541064518000418104, -2.621784821874998173 ) ) ;
#46544=CARTESIAN_POINT ( 'NONE',  ( 9.001249775931846008E-16, 15.41562500061451679, 34.90005215228797653 ) ) ;
#46545=CARTESIAN_POINT ( 'NONE',  ( 19.95000000122903572, -2.886751345948125991, -5.000000000000000000 ) ) ;
#46547=CARTESIAN_POINT ( 'NONE',  ( 10.45312500061451644, 0.000000000000000000, 5.243569643749999010 ) ) ;
#46548=CARTESIAN_POINT ( 'NONE',  ( 13.64999999999999858, 4.330127018922192761, -2.499999999999997780 ) ) ;
#46549=CARTESIAN_POINT ( 'NONE',  ( 29.24062500061451431, 6.054752690667223547, 3.707466751127219781E-16 ) ) ;
#46550=CARTESIAN_POINT ( 'NONE',  ( 25.05937500061451573, -4.541064518000417216, -2.621784821875001281 ) ) ;
#46551=CARTESIAN_POINT ( 'NONE',  ( 16.64062500061451289, 6.054752690667223547, 3.707466751127219781E-16 ) ) ;
#46552=CARTESIAN_POINT ( 'NONE',  ( 27.15000000122902790, -2.886751345948125991, -5.000000000000000000 ) ) ;
#46553=CARTESIAN_POINT ( 'NONE',  ( 25.37812500061451715, -4.541064518000419881, 2.621784821874995952 ) ) ;
#46554=CARTESIAN_POINT ( 'NONE',  ( 22.02187500061452141, 3.027376345333613106, -5.243569643749998122 ) ) ;
#46555=CARTESIAN_POINT ( 'NONE',  ( 16.75312500061451715, 0.000000000000000000, 5.243569643749999010 ) ) ;
#46556=CARTESIAN_POINT ( 'NONE',  ( 2.121784821875001281, 16.85937500061451999, 33.67503911421598417 ) ) ;
#46557=CARTESIAN_POINT ( 'NONE',  ( 23.39062500061451289, 6.054752690667223547, 3.707466751127219781E-16 ) ) ;
#46558=CARTESIAN_POINT ( 'NONE',  ( 3.000000001229032875, 5.773502691896255534, 3.535250795749688894E-16 ) ) ;
#46560=CARTESIAN_POINT ( 'NONE',  ( 25.27499999999999858, 6.123233995736764310E-16, -4.999999999999998224 ) ) ;
#46561=CARTESIAN_POINT ( 'NONE',  ( -3.999999999999999556, 12.76250000000000284, -32.30940107675850470 ) ) ;
#46563=CARTESIAN_POINT ( 'NONE',  ( 29.65312500061451573, 4.541064518000418104, -2.621784821874998173 ) ) ;
#46564=CARTESIAN_POINT ( 'NONE',  ( 9.440625000614517148, 6.054752690667223547, 3.707466751127219781E-16 ) ) ;
#46565=CARTESIAN_POINT ( 'NONE',  ( 21.78750000122903074, 6.123233995736764310E-16, -4.999999999999998224 ) ) ;
#46566=CARTESIAN_POINT ( 'NONE',  ( 27.81562500061452070, 3.027376345333613106, -5.243569643749998122 ) ) ;
#46567=CARTESIAN_POINT ( 'NONE',  ( 25.72499999999999787, 6.123233995736764310E-16, -4.999999999999998224 ) ) ;
#46568=CARTESIAN_POINT ( 'NONE',  ( -3.999999999999999556, 16.92500000122903359, -32.30940107675850470 ) ) ;
#46569=CARTESIAN_POINT ( 'NONE',  ( 29.24062500061451431, 6.054752690667223547, 3.707466751127219781E-16 ) ) ;
#46570=CARTESIAN_POINT ( 'NONE',  ( 9.403125000614517504, 4.541064518000418104, -2.621784821874998173 ) ) ;
#46571=VERTEX_POINT ( 'NONE', #48289 ) ;
#46572=CARTESIAN_POINT ( 'NONE',  ( 26.69062500061451715, -3.027376345333614438, 5.243569643749998122 ) ) ;
#46573=CARTESIAN_POINT ( 'NONE',  ( 8.390625000614518214, -3.027376345333610441, -5.243569643749999898 ) ) ;
#46575=CARTESIAN_POINT ( 'NONE',  ( 4.115625000614516082, 3.027376345333611329, 5.243569643749999010 ) ) ;
#46577=DIRECTION ( 'NONE',  ( -1.000000000000000000, -0.000000000000000000, -0.000000000000000000 ) ) ;
#46578=AXIS2_PLACEMENT_3D ( 'NONE', #1533, #35494, #70205 ) ;
#46579=CARTESIAN_POINT ( 'NONE',  ( 13.12500000000000178, 6.123233995736764310E-16, -4.999999999999998224 ) ) ;
#46581=CARTESIAN_POINT ( 'NONE',  ( 13.69687500061451679, -3.027376345333614438, 5.243569643749998122 ) ) ;
#46582=CARTESIAN_POINT ( 'NONE',  ( 10.50000000122903465, -2.886751345948125991, -5.000000000000000000 ) ) ;
#46583=CARTESIAN_POINT ( 'NONE',  ( 16.58437500061451786, 6.421520780324663323E-16, -5.243569643749999010 ) ) ;
#46585=B_SPLINE_CURVE_WITH_KNOTS ( 'NONE', 3,
 ( #3961, #26484, #4333, #30920, #65265, #15024, #20553, #9494, #53461, #3594 ),
 .UNSPECIFIED., .F., .F.,
 ( 4, 3, 3, 4 ),
 ( 1.332339343076284724E-16, 7.861290946297937144E-05, 0.0001572256709461994102, 0.0002973492893351208869 ),
 .UNSPECIFIED. ) ;
#46586=CARTESIAN_POINT ( 'NONE',  ( 7.959375000614516971, -4.541064518000417216, -2.621784821875001281 ) ) ;
#46587=CARTESIAN_POINT ( 'NONE',  ( -2.121784821874999949, 11.17812500061451786, -33.67503911421598417 ) ) ;
#46588=CARTESIAN_POINT ( 'NONE',  ( 1.626862140677534273E-15, 16.51249999999999929, 34.00000000000000000 ) ) ;
#46590=CARTESIAN_POINT ( 'NONE',  ( 30.00000000000000000, 0.000000000000000000, 0.000000000000000000 ) ) ;
#46591=CARTESIAN_POINT ( 'NONE',  ( 24.81562500061451715, 3.027376345333611329, 5.243569643749999010 ) ) ;
#46593=CARTESIAN_POINT ( 'NONE',  ( 28.35937500061451289, 4.541064518000418104, -2.621784821874998173 ) ) ;
#46594=CARTESIAN_POINT ( 'NONE',  ( 24.48749999999999716, 5.773502691896255534, 3.535250795749688894E-16 ) ) ;
#46595=CARTESIAN_POINT ( 'NONE',  ( 7.790625000614518569, -3.027376345333614438, 5.243569643749998122 ) ) ;
#46597=CARTESIAN_POINT ( 'NONE',  ( 19.02187500061451786, 3.027376345333611329, 5.243569643749999010 ) ) ;
#46599=CARTESIAN_POINT ( 'NONE',  ( 2.803125000614518747, 0.000000000000000000, 5.243569643749999010 ) ) ;
#46600=CARTESIAN_POINT ( 'NONE',  ( 9.309375000614517504, -4.541064518000417216, -2.621784821875001281 ) ) ;
#46601=ORIENTED_EDGE ( 'NONE', *, *, #27024, .F. ) ;
#46602=CARTESIAN_POINT ( 'NONE',  ( 18.08437500061451431, 4.541064518000418104, 2.621784821874999949 ) ) ;
#46603=CARTESIAN_POINT ( 'NONE',  ( 27.52500000000000213, 6.123233995736764310E-16, -4.999999999999998224 ) ) ;
#46604=CARTESIAN_POINT ( 'NONE',  ( 29.48437500061451644, -4.541064518000419881, 2.621784821874995952 ) ) ;
#46607=VERTEX_POINT ( 'NONE', #65634 ) ;
#46608=CARTESIAN_POINT ( 'NONE',  ( 10.95000000000000107, 4.330127018922192761, -2.499999999999997780 ) ) ;
#46610=CARTESIAN_POINT ( 'NONE',  ( 23.91562500061451502, 3.027376345333611329, 5.243569643749999010 ) ) ;
#46611=CARTESIAN_POINT ( 'NONE',  ( 14.51250000000000107, 2.886751345948129099, -4.999999999999998224 ) ) ;
#46612=CARTESIAN_POINT ( 'NONE',  ( 9.037500001229034297, -4.330127018922194537, 2.499999999999995559 ) ) ;
#46613=CARTESIAN_POINT ( 'NONE',  ( 6.215625000614517504, 3.027376345333613106, -5.243569643749998122 ) ) ;
#46614=CARTESIAN_POINT ( 'NONE',  ( 21.18749999999999645, -2.886751345948125991, -5.000000000000000000 ) ) ;
#46615=CARTESIAN_POINT ( 'NONE',  ( 19.71562500061451928, 3.027376345333613106, -5.243569643749998122 ) ) ;
#46617=CARTESIAN_POINT ( 'NONE',  ( 25.08750000122903145, 4.330127018922191873, 2.499999999999999556 ) ) ;
#46619=CARTESIAN_POINT ( 'NONE',  ( 5.512499999999999289, 2.886751345948129099, -4.999999999999998224 ) ) ;
#46621=ORIENTED_EDGE ( 'NONE', *, *, #793, .T. ) ;
#46622=CARTESIAN_POINT ( 'NONE',  ( 22.60312500061451857, 0.000000000000000000, 5.243569643749999010 ) ) ;
#46623=CARTESIAN_POINT ( 'NONE',  ( 25.60312500061451502, 4.541064518000418104, -2.621784821874998173 ) ) ;
#46624=CARTESIAN_POINT ( 'NONE',  ( 27.87187500061451573, 3.027376345333613106, -5.243569643749998122 ) ) ;
#46625=CARTESIAN_POINT ( 'NONE',  ( 15.29062500061451679, 6.054752690667223547, 3.707466751127219781E-16 ) ) ;
#46628=CARTESIAN_POINT ( 'NONE',  ( 26.73750000122903003, 6.123233995736764310E-16, -4.999999999999998224 ) ) ;
#46630=CARTESIAN_POINT ( 'NONE',  ( 15.55312500061451608, -4.541064518000417216, -2.621784821875001281 ) ) ;
#46631=CARTESIAN_POINT ( 'NONE',  ( -3.999999999999999112, 16.85000000000000142, -30.00000000000000000 ) ) ;
#46632=CARTESIAN_POINT ( 'NONE',  ( 4.237500001229036251, 6.123233995736764310E-16, -4.999999999999998224 ) ) ;
#46633=CARTESIAN_POINT ( 'NONE',  ( 9.234375000614518214, -4.541064518000419881, 2.621784821874995952 ) ) ;
#46634=CARTESIAN_POINT ( 'NONE',  ( 10.99687500061451750, -3.027376345333614438, 5.243569643749998122 ) ) ;
#46635=CARTESIAN_POINT ( 'NONE',  ( 20.89687500061452141, -3.027376345333614438, 5.243569643749998122 ) ) ;
#46636=ORIENTED_EDGE ( 'NONE', *, *, #18362, .T. ) ;
#46637=CARTESIAN_POINT ( 'NONE',  ( -0.4074127065224521504, 10.00000000000000178, 24.00000000000001066 ) ) ;
#46638=CARTESIAN_POINT ( 'NONE',  ( 23.20312500061451644, -4.541064518000417216, -2.621784821875001281 ) ) ;
#46640=CARTESIAN_POINT ( 'NONE',  ( 18.27187500061451431, -6.054752690667223547, -1.112240025338166033E-15 ) ) ;
#46641=CARTESIAN_POINT ( 'NONE',  ( 25.34062500061451217, -3.027376345333614438, 5.243569643749998122 ) ) ;
#46642=CARTESIAN_POINT ( 'NONE',  ( 9.712500001229033231, 4.330127018922192761, -2.499999999999997780 ) ) ;
#46643=CARTESIAN_POINT ( 'NONE',  ( -2.828200636599751609E-16, 14.48750000000000071, 25.38119784648299770 ) ) ;
#46644=CARTESIAN_POINT ( 'NONE',  ( 29.20312500061451644, 4.541064518000418104, -2.621784821874998173 ) ) ;
#46645=CARTESIAN_POINT ( 'NONE',  ( 8.887500001229033941, 4.330127018922191873, 2.499999999999999556 ) ) ;
#46646=VECTOR ( 'NONE', #34297, 1000.000000000000000 ) ;
#46647=CARTESIAN_POINT ( 'NONE',  ( 4.575000001229033941, -5.773502691896255534, -1.060575238724906372E-15 ) ) ;
#46648=CARTESIAN_POINT ( 'NONE',  ( 1.999999999999998668, 19.84999999999999787, -33.46410161513775705 ) ) ;
#46649=CARTESIAN_POINT ( 'NONE',  ( 27.71250000122903145, 4.330127018922192761, -2.499999999999997780 ) ) ;
#46651=CARTESIAN_POINT ( 'NONE',  ( 9.496875000614517504, 6.054752690667223547, 3.707466751127219781E-16 ) ) ;
#46652=CARTESIAN_POINT ( 'NONE',  ( 24.41250000000000142, 2.886751345948162850, -4.999999999999940492 ) ) ;
#46653=CARTESIAN_POINT ( 'NONE',  ( 16.71562500061451573, 3.027376345333611329, 5.243569643749999010 ) ) ;
#46654=CARTESIAN_POINT ( 'NONE',  ( 9.984375000614518214, 4.541064518000418104, 2.621784821874999949 ) ) ;
#46655=CARTESIAN_POINT ( 'NONE',  ( 29.55000000122903003, 5.773502691896255534, 3.535250795749688894E-16 ) ) ;
#46656=CARTESIAN_POINT ( 'NONE',  ( 18.79687500061451644, -3.027376345333610441, -5.243569643749999898 ) ) ;
#46657=CARTESIAN_POINT ( 'NONE',  ( 7.284375000614518036, 4.541064518000418104, 2.621784821874999949 ) ) ;
#46658=CARTESIAN_POINT ( 'NONE',  ( 3.033819321519781287, -3.974438763815245856, -3.388311280553572669 ) ) ;
#46659=LINE ( 'NONE', #69199, #39210 ) ;
#46660=( BOUNDED_CURVE ( )  B_SPLINE_CURVE ( 2, ( #40112, #29379, #51912, #1310, #40467, #67822, #23819 ),
 .UNSPECIFIED., .F., .F. ) 
 B_SPLINE_CURVE_WITH_KNOTS ( ( 3, 2, 2, 3 ),
 ( 0.1333333333333333037, 0.1361111111111110716, 0.1388888888888888673, 0.1416666666666666352 ),
 .UNSPECIFIED. ) 
 CURVE ( )  GEOMETRIC_REPRESENTATION_ITEM ( )  RATIONAL_B_SPLINE_CURVE ( ( 1.000000000000001332, 0.8660254037844373753, 1.000000000000000000, 0.8660254037844387076, 1.000000000000000000, 0.8660254037844400399, 0.9999999999999986677 ) ) 
 REPRESENTATION_ITEM ( '' )  );
#46661=CARTESIAN_POINT ( 'NONE',  ( 8.503125000614515372, 4.541064518000418104, -2.621784821874998173 ) ) ;
#46662=CARTESIAN_POINT ( 'NONE',  ( 17.20312500061451644, 0.000000000000000000, 5.243569643749999010 ) ) ;
#46663=ORIENTED_EDGE ( 'NONE', *, *, #64920, .T. ) ;
#46664=CARTESIAN_POINT ( 'NONE',  ( 5.025000001229035895, -5.773502691896255534, -1.060575238724906372E-15 ) ) ;
#46665=CARTESIAN_POINT ( 'NONE',  ( 15.59062500061451573, -3.027376345333610441, -5.243569643749999898 ) ) ;
#46666=CARTESIAN_POINT ( 'NONE',  ( 14.27812500061451573, 6.421520780324663323E-16, -5.243569643749999010 ) ) ;
#46668=CARTESIAN_POINT ( 'NONE',  ( 12.56250000000000178, -5.773502691896255534, -1.060575238724906372E-15 ) ) ;
#46669=CARTESIAN_POINT ( 'NONE',  ( 7.312500001229033764, -4.330127018922190985, -2.500000000000001332 ) ) ;
#46671=EDGE_CURVE ( 'NONE', #29206, #52162, #51054, .T. ) ;
#46672=CARTESIAN_POINT ( 'NONE',  ( 14.93437500061451750, 4.541064518000418104, 2.621784821874999949 ) ) ;
#46673=CARTESIAN_POINT ( 'NONE',  ( 18.41250000122903430, 0.000000000000000000, 4.999999999999998224 ) ) ;
#46675=CARTESIAN_POINT ( 'NONE',  ( -1.473776270879187500, 9.872922227264545825, -34.04916702557058983 ) ) ;
#46676=CYLINDRICAL_SURFACE ( 'NONE', #22937, 4.000000000000000000 ) ;
#46677=CARTESIAN_POINT ( 'NONE',  ( 4.267099419464107868, -3.843735374978448860, 3.829594327187515024 ) ) ;
#46678=CARTESIAN_POINT ( 'NONE',  ( 6.375000000000001776, 6.123233995736764310E-16, -4.999999999999998224 ) ) ;
#46680=CARTESIAN_POINT ( 'NONE',  ( 17.82187500061451502, -6.054752690667223547, -1.112240025338166033E-15 ) ) ;
#46681=CARTESIAN_POINT ( 'NONE',  ( 21.41250000122903074, 4.330127018922192761, -2.499999999999997780 ) ) ;
#46682=AXIS2_PLACEMENT_3D ( 'NONE', #52954, #30426, #13409 ) ;
#46683=CARTESIAN_POINT ( 'NONE',  ( 15.25312500061451715, 4.541064518000418104, -2.621784821874998173 ) ) ;
#46685=CARTESIAN_POINT ( 'NONE',  ( 22.53750000122903430, -4.330127018922194537, 2.499999999999995559 ) ) ;
#46686=CARTESIAN_POINT ( 'NONE',  ( 25.69687500061451502, 6.054752690667223547, 3.707466751127219781E-16 ) ) ;
#46688=CARTESIAN_POINT ( 'NONE',  ( 10.22812500061451679, 6.421520780324663323E-16, -5.243569643749999010 ) ) ;
#46689=CIRCLE ( 'NONE', #63192, 5.999999999999998224 ) ;
#46690=CARTESIAN_POINT ( 'NONE',  ( 16.54687500061451644, -3.027376345333610441, -5.243569643749999898 ) ) ;
#46692=CARTESIAN_POINT ( 'NONE',  ( 26.72812500061451502, -4.541064518000419881, 2.621784821874995952 ) ) ;
#46693=CARTESIAN_POINT ( 'NONE',  ( 20.95312500061451999, -4.541064518000417216, -2.621784821875001281 ) ) ;
#46694=CARTESIAN_POINT ( 'NONE',  ( 29.57812500061451644, 6.421520780324663323E-16, -5.243569643749999010 ) ) ;
#46695=CARTESIAN_POINT ( 'NONE',  ( 7.347880794884120722E-16, 20.00000000000000000, -24.00000000000000000 ) ) ;
#46696=( BOUNDED_SURFACE ( )  B_SPLINE_SURFACE ( 1, 2, ( 
 ( #11625, #28255, #12334, #67425, #40423, #39345, #34141, #45967, #17510, #68500, #50786, #45613, #34869, #33422, #68146, #22694, #45245, #57397, #27528, #44534, #67066, #55963, #40071, #62585, #38981, #61497, #10894, #5358, #27896, #72956, #30051, #2349, #18948, #40793, #29337, #24865, #14151, #30423, #64395, #51867, #36327, #35954, #8252, #13785, #69942, #19312, #47774, #53313, #24140, #41507, #1269, #69586, #41865, #58842, #41155, #52229, #58112, #64027, #47412, #52951, #7163, #69229, #30782, #2712, #13054, #1633, #64761, #46328, #25228, #12697, #52591, #47052, #70310, #68863, #19683, #23776, #42236, #36686, #13406, #6803, #63306, #35234, #46692, #18219, #18590, #35593, #63664, #58475, #7520, #1998, #29692, #57755, #24508, #7887, #44352, #11074, #33602, #66133, #38053, #56146, #21786, #38801, #45064, #39160, #60578, #4091, #32521, #16966, #66877, #5540, #15881, #33246, #32882, #61317, #49157, #66499, #49518, #9986, #27348, #43611, #50606, #71688, #55784, #22517, #67601, #59207, #10714, #49879, #16245, #27711, #5175, #15511, #4815, #8615, #55058, #4459, #50251, #72774, #22158, #44710, #28078, #21060, #10, #38426, #55422, #26989, #60949, #72404, #72043, #21421, #43978, #67246, #10352, #16604, #61675, #32156, #54689, #26620, #18411, #29875, #52411, #18048, #29159, #62405, #62767, #67960, #57583, #22868, #29517, #12158, #33963, #46510, #11443, #45426, #11804, #52052, #69049, #45790, #1095, #69414, #46875, #34321, #730, #57217, #23239, #56853, #6259, #28787, #51328, #28428, #40977, #68325, #39522, #62048, #361, #17685, #24326, #63492, #12880, #35413, #17333, #39892, #57938, #23603, #40606, #56502, #7345, #40246, #5895, #34686, #50965, #46148, #1819, #6630, #12523, #51691, #63127, #68688, #35056, #6986, #1456, #23962, #2175, #9168, #7706, #14337, #54238, #3635, #26159, #70494, #59027, #47966, #59389, #2892, #24688, #36507, #48698, #13599, #19133, #19871, #42424, #64945, #25423, #14696, #52773, #31703, #25051, #13969, #36145, #19501, #8429, #47232, #69765, #41687, #36871, #2531, #30965, #53500, #64581, #3268, #53132, #70859, #18769, #41335, #8799, #31335, #64210, #42058, #58664, #53876, #8072, #25796, #48334, #13236, #20233, #63845, #30604, #47594, #42785, #65306, #70123, #37240, #35774, #58297, #59761, #30240, #15794, #54968, #20971, #43524, #37968, #66046, #60125, #72690, #4374, #27993, #71221, #32068, #60489, #56060, #50160, #21337, #38334, #5091, #37603, #33159, #20599, #10991, #16163, #55335, #22072, #54600, #26528, #15424, #44631, #9895, #26903, #32431, #60863, #49429, #71963, #43892, #65678, #39073, #55697, #4730, #66416, #9534, #67160, #10266, #43158, #15066, #4005, #32799, #5453, #16521, #27264, #49797, #27627, #49068, #61590, #71596, #33511, #38715, #72322, #21702, #44259, #66792, #61235, #10629, #17247, #56769, #39807, #17604, #62323, #34235, #280, #44980, #18320, #34970, #34600, #1368, #23878, #56423, #28343, #46425, #12079, #29073, #35329, #29432, #50880, #67517, #22788, #7261, #57129, #68963, #6173, #23515, #23153, #51608, #39436, #28703, #11719, #45341, #40164, #33878, #40893, #61956, #46065, #12793, #57852, #50522, #1008, #62683, #6539, #17961, #68600, #5812, #68241, #73050, #67875, #51242, #40522, #63038, #12437, #57499, #63407, #11360, #22432, #645, #45707, #6901, #51969, #16882, #63760, #7616, #13149, #8347, #13510, #41972, #70039, #2442, #14248, #64124, #8713, #20146, #42700, #30876, #19412, #52686, #53048, #58211, #47881, #35691, #19786, #24965, #24241, #36787, #1728, #30152, #2092, #42337, #59302, #36057, #64493, #59676, #37151, #24602, #58577, #47510, #7985, #47150, #69682, #19047, #46790, #31245, #41249, #13885, #25336, #36425, #41605, #52326, #70410, #29790, #53417, #53786, #69326, #3182, #58940, #25709, #48246, #64860, #70770, #65222, #14612, #30521, #2808, #18685, #71879, #44176, #66706, #43441, #54516, #60403, #21252, #27179, #55254, #9452, #71511, #61152, #32717, #15343, #3919, #67079, #48612, #10547, #14982, #4650, #31621, #71137, #43067, #26442, #3551, #31982, #48982, #65963, #33076, #72608, #21989, #60775, #43805, #20887, #32344, #37520, #49713, #65593, #72241, #54882, #26073, #16079, #54155, #60041, #37883, #21619, #38628, #9812, #66330, #38995, #16438, #4288, #26814, #49348, #15708, #38246, #10182, #55614, #5010, #20510, #27544, #50076, #9084, #44548, #22353, #50801, #46344, #40439, #11642, #28625, #68518, #27912, #23436, #10908, #1283, #6456, #45628, #62955, #44905, #16804, #56346, #34885, #28270, #67794, #204, #51163, #22710, #45262, #11282, #55979, #29352, #45982, #68162, #12350, #57413, #67443, #39360, #6818, #23073, #40087, #68878, #51885, #61875, #5373, #33434, #18235, #33802, #50446, #72971, #5736, #23793, #17168, #39727, #62245, #34157, #56694, #62601, #6094, #61510, #51528, #17525, #566, #11997, #34520, #57050, #28991, #928, #17879, #35608, #30438, #30798, #63323, #70684, #19327, #41523, #30068, #14165, #2363, #58128, #52967, #7901, #18963, #3093, #7535, #31158, #52606, #24881, #70322, #53330, #19698, #24523, #58857, #36699, #46709, #13803, #64042, #69602, #25622, #25243, #47792, #7179, #69244, #8267, #2728, #47426, #13421, #59221, #12713, #42251, #52245, #35971, #36342, #69957, #1648, #35248, #64775, #48159, #64410, #8629, #57769, #53700, #41882, #40808, #29707, #24156, #18605, #41171, #63679, #2012, #13069, #47067, #58491, #55169, #4565, #54435, #65510, #71424, #9728, #38162, #66242, #20430, #9366, #72154, #43719, #26355, #14897, #4925, #59589, #21533, #25989, #15620, #42615, #9001, #54073, #37438, #3469, #60685, #10100, #32629, #27095, #44088, #32991, #31533, #21166, #48528, #49627, #38540, #66615, #15991, #71055, #42979, #27460, #59959, #3834, #37798, #48894, #31899, #20801, #43356, #65879, #15260, #61064, #60318 ),
 ( #32262, #10461, #55531, #49991, #54794, #20059, #65139, #4201, #14530, #26729, #49264, #37064, #71797, #56962, #38908, #5282, #17440, #11909, #62157, #22624, #17791, #44460, #839, #10820, #45175, #68071, #11554, #33355, #21904, #39997, #6733, #22980, #6366, #66991, #28898, #28540, #23348, #51437, #62511, #34434, #40351, #45897, #16718, #34070, #16353, #56610, #68428, #62870, #33716, #44820, #50716, #6005, #12266, #45542, #72887, #61785, #34796, #57329, #5652, #67355, #29267, #61427, #72515, #27828, #55893, #50360, #22268, #39273, #11189, #56261, #28187, #119, #67706, #17078, #39639, #51075, #472, #52881, #63235, #36255, #70235, #19238, #13713, #12629, #35164, #36615, #1200, #59136, #29622, #40718, #68795, #23705, #14076, #57688, #7093, #52159, #46256, #69873, #8544, #2279, #58770, #18151, #8179, #7817, #53240, #30707, #41793, #64321, #19608, #25157, #69161, #63958, #1562, #41440, #2638, #47698, #12987, #24072, #29979, #13342, #42165, #24796, #46617, #41085, #64691, #47339, #58044, #18520, #51797, #63597, #35523, #7452, #52520, #1929, #24434, #46983, #69519, #18877, #35879, #58404, #30352, #49180, #32543, #44000, #70602, #32179, #42528, #15533, #49542, #71710, #66156, #65054, #14445, #15902, #53612, #38449, #8914, #19975, #48074, #3003, #66523, #36979, #59501, #31445, #25532, #37352, #54712, #3745, #55081, #21082, #15172, #53986, #3383, #25905, #48445, #70969, #20344, #59874, #42895, #20711, #43633, #65419, #60975, #9645, #31813, #14808, #4481, #65791, #9279, #43270, #71336, #54352, #31072, #26270, #21444, #48807, #37710, #60599, #38077, #10008, #60231, #27010, #72064, #4115, #26643, #33626, #39184, #69346, #67983, #17358, #49903, #16269, #28452, #22892, #34, #56170, #28812, #55444, #11827, #21811, #5564, #5918, #22540, #44375, #38825, #50987, #45450, #45088, #28101, #51350, #4837, #34345, #66901, #50629, #385, #67623, #61340, #32907, #39915, #18704, #33988, #62429, #27371, #56878, #39547, #6282, #1748, #24260, #46809, #41268, #10375, #27736, #16989, #72427, #62071, #10736, #33269, #44736, #55807, #61699, #11465, #5195, #56525, #50275, #72799, #22182, #67270, #16629, #11098, #48631, #30174, #65241, #69701, #59321, #13169, #52705, #24622, #58598, #47169, #14268, #8731, #31265, #53807, #14630, #3570, #2111, #64880, #19067, #48267, #9103, #3201, #25729, #41624, #64143, #71156, #35709, #20528, #13530, #36077, #7636, #58231, #26093, #8005, #30540, #53067, #2462, #70058, #36806, #36445, #37170, #70791, #47902, #24985, #47530, #19432, #41993, #64513, #13906, #58959, #8367, #53438, #20166, #30895, #63780, #42358, #2828, #25356, #59696, #70430, #19805, #42720, #31641, #54173, #72624, #43459, #50093, #65982, #66348, #38645, #72258, #61169, #9833, #49731, #5025, #3938, #27196, #49367, #54900, #22008, #66724, #16096, #60060, #10199, #60793, #55631, #54536, #27562, #4308, #71897, #15362, #26833, #21270, #26461, #49000, #71531, #32734, #32363, #21635, #43824, #10564, #15726, #38265, #33092, #44564, #67094, #55271, #4666, #20906, #44193, #37904, #43085, #60422, #65612, #15001, #9471, #37538, #32001, #41359, #57960, #64235, #13259, #62163, #11560, #17084, #125, #35436, #30265, #1844, #53158, #19157, #35797, #6011, #50722, #22630, #1480, #23986, #34076, #7368, #46533, #18795, #41711, #45181, #59052, #7731, #29899, #18434, #2556, #63869, #69075, #58320, #69438, #52437, #64607, #41001, #19526, #63516, #52798, #58687, #13626, #8097, #12903, #47257, #25074, #56616, #2199, #24351, #46899, #13993, #36169, #30626, #67712, #28546, #69791, #47617, #24714, #70148, #42085, #39645, #36532, #52074, #28193, #4030, #20626, #42450, #30992, #26555, #15818, #32093, #66071, #53525, #37994, #37627, #9921, #15449, #71624, #20997, #49454, #54994, #25823, #43185, #2919, #71247, #43549, #60515, #42811, #53903, #59788, #65704, #49095, #54624, #32459, #15091, #60150, #66442, #4400, #59418, #25450, #3295, #38361, #9560, #26929, #37266, #71988, #54267, #21362, #70522, #14723, #70885, #31362, #48724, #64972, #43916, #19897, #8457, #47993, #14363, #36898, #8825, #48360, #20259, #65334, #9194, #31729, #26184, #3661, #55723, #61260, #16906, #61982, #39461, #67543, #56794, #21727, #51268, #67186, #56089, #5117, #61616, #5481, #44286, #38740, #66816, #11384, #44656, #33903, #16547, #67900, #28020, #22098, #39833, #670, #23178, #56447, #50548, #10654, #11018, #16189, #5837, #33184, #50905, #33539, #55361, #17272, #32823, #39099, #27651, #50188, #27288, #73076, #22457, #17629, #68267, #72715, #45006, #28369, #304, #22814, #45365, #62348, #11744, #49822, #34261, #6199, #60888, #10293, #28727, #45732, #4755, #72346, #63435, #7290, #47178, #6567, #2121, #62710, #53077, #58241, #24270, #41634, #23542, #68628, #34998, #13540, #6928, #46453, #29458, #29819, #51995, #23905, #63065, #34625, #8015, #24633, #46819, #64153, #36088, #46092, #17990, #68991, #69711, #69357, #1035, #40549, #29099, #12104, #18348, #41279, #12822, #58608, #30184, #18714, #12468, #57156, #51634, #57527, #1396, #40923, #35356, #57880, #52354, #52715, #1757, #70069, #63790, #13180, #35719, #30550, #7646, #19077, #2472, #24996, #47540, #40189, #14278, #9843, #36816, #9113, #49010, #9482, #71541, #3211, #37548, #15373, #25367, #65623, #42730, #48277, #4318, #3948, #26471, #58969, #47911, #60070, #32011, #31651, #65251, #37915, #64523, #20916, #30906, #14640, #15011, #54184, #53448, #42003, #54546, #26843, #43095, #43468, #13916, #65992, #48641, #60432, #32372, #54910, #49377, #19442, #36455, #59331, #3580, #8377, #26103, #2838, #70440, #53818, #64890, #70801, #71166, #19815, #42368, #8742, #31275, #25740, #20176, #37181, #59706, #20539, #38275, #228, #4676, #67465, #21280, #60803, #32744, #66734, #55281, #22377, #16828, #39382, #61901, #22733 ) ),
 .UNSPECIFIED., .F., .F., .F. ) 
 B_SPLINE_SURFACE_WITH_KNOTS ( ( 2, 2 ),
 ( 3, 2, 2, 2, 2, 2, 2, 2, 2, 2, 2, 2, 2, 2, 2, 2, 2, 2, 2, 2, 2, 2, 2, 2, 2, 2, 2, 2, 2, 2, 2, 2, 2, 2, 2, 2, 2, 2, 2, 2, 2, 2, 2, 2, 2, 2, 2, 2, 2, 2, 2, 2, 2, 2, 2, 2, 2, 2, 2, 2, 2, 2, 2, 2, 2, 2, 2, 2, 2, 2, 2, 2, 2, 2, 2, 2, 2, 2, 2, 2, 2, 2, 2, 2, 2, 2, 2, 2, 2, 2, 2, 2, 2, 2, 2, 2, 2, 2, 2, 2, 2, 2, 2, 2, 2, 2, 2, 2, 2, 2, 2, 2, 2, 2, 2, 2, 2, 2, 2, 2, 2, 2, 2, 2, 2, 2, 2, 2, 2, 2, 2, 2, 2, 2, 2, 2, 2, 2, 2, 2, 2, 2, 2, 2, 2, 2, 2, 2, 2, 2, 2, 2, 2, 2, 2, 2, 2, 2, 2, 2, 2, 2, 2, 2, 2, 2, 2, 2, 2, 2, 2, 2, 2, 2, 2, 2, 2, 2, 2, 2, 2, 2, 2, 2, 2, 2, 2, 2, 2, 2, 2, 2, 2, 2, 2, 2, 2, 2, 2, 2, 2, 2, 2, 2, 2, 2, 2, 2, 2, 2, 2, 2, 2, 2, 2, 2, 2, 2, 2, 2, 2, 2, 2, 2, 2, 2, 2, 2, 2, 2, 2, 2, 2, 2, 2, 2, 2, 2, 2, 2, 2, 2, 2, 2, 2, 2, 2, 2, 2, 2, 2, 2, 2, 2, 2, 2, 2, 2, 2, 2, 2, 2, 2, 2, 2, 2, 2, 2, 2, 2, 2, 2, 2, 2, 2, 2, 2, 2, 2, 2, 2, 2, 2, 2, 2, 2, 2, 2, 2, 2, 2, 2, 2, 2, 2, 2, 2, 2, 2, 2, 2, 2, 2, 2, 2, 2, 2, 2, 2, 2, 2, 2, 2, 2, 2, 2, 2, 2, 2, 2, 2, 2, 2, 2, 2, 2, 2, 2, 2, 2, 2, 2, 2, 2, 2, 2, 2, 2, 2, 2, 2, 2, 2, 2, 2, 2, 2, 2, 2, 2, 2, 2, 2, 2, 2, 2, 2, 2, 2, 2, 3 ),
 ( 0.000000000000000000, 1.000000000000000000 ),
 ( 0.000000000000000000, 0.002777777777777777884, 0.005555555555555555768, 0.008333333333333333218, 0.01111111111111111154, 0.01388888888888888812, 0.01666666666666666644, 0.01944444444444444475, 0.02222222222222222307, 0.02500000000000000139, 0.02777777777777777624, 0.03055555555555555455, 0.03333333333333333287, 0.03611111111111110772, 0.03888888888888888951, 0.04166666666666666435, 0.04444444444444444614, 0.04722222222222222099, 0.05000000000000000278, 0.05277777777777777762, 0.05555555555555555247, 0.05833333333333333426, 0.06111111111111110911, 0.06388888888888888395, 0.06666666666666666574, 0.06944444444444444753, 0.07222222222222221544, 0.07499999999999999722, 0.07777777777777777901, 0.08055555555555556080, 0.08333333333333332871, 0.08611111111111111049, 0.08888888888888889228, 0.09166666666666666019, 0.09444444444444444198, 0.09722222222222222376, 0.1000000000000000056, 0.1027777777777777735, 0.1055555555555555552, 0.1083333333333333370, 0.1111111111111111049, 0.1138888888888888867, 0.1166666666666666685, 0.1194444444444444503, 0.1222222222222222182, 0.1250000000000000000, 0.1277777777777777679, 0.1305555555555555636, 0.1333333333333333315, 0.1361111111111110994, 0.1388888888888888951, 0.1416666666666666630, 0.1444444444444444309, 0.1472222222222222265, 0.1499999999999999944, 0.1527777777777777901, 0.1555555555555555580, 0.1583333333333333259, 0.1611111111111111216, 0.1638888888888888895, 0.1666666666666666574, 0.1694444444444444531, 0.1722222222222222210, 0.1749999999999999889, 0.1777777777777777846, 0.1805555555555555525, 0.1833333333333333204, 0.1861111111111111160, 0.1888888888888888840, 0.1916666666666666796, 0.1944444444444444475, 0.1972222222222222154, 0.2000000000000000111, 0.2027777777777777790, 0.2055555555555555469, 0.2083333333333333426, 0.2111111111111111105, 0.2138888888888888784, 0.2166666666666666741, 0.2194444444444444420, 0.2222222222222222099, 0.2250000000000000056, 0.2277777777777777735, 0.2305555555555555691, 0.2333333333333333370, 0.2361111111111111049, 0.2388888888888889006, 0.2416666666666666685, 0.2444444444444444364, 0.2472222222222222321, 0.2500000000000000000, 0.2527777777777777679, 0.2555555555555555358, 0.2583333333333333592, 0.2611111111111111271, 0.2638888888888888951, 0.2666666666666666630, 0.2694444444444444309, 0.2722222222222221988, 0.2750000000000000222, 0.2777777777777777901, 0.2805555555555555580, 0.2833333333333333259, 0.2861111111111110938, 0.2888888888888888618, 0.2916666666666666852, 0.2944444444444444531, 0.2972222222222222210, 0.2999999999999999889, 0.3027777777777777568, 0.3055555555555555802, 0.3083333333333333481, 0.3111111111111111160, 0.3138888888888888840, 0.3166666666666666519, 0.3194444444444444198, 0.3222222222222222432, 0.3250000000000000111, 0.3277777777777777790, 0.3305555555555555469, 0.3333333333333333148, 0.3361111111111111382, 0.3388888888888889062, 0.3416666666666666741, 0.3444444444444444420, 0.3472222222222222099, 0.3499999999999999778, 0.3527777777777778012, 0.3555555555555555691, 0.3583333333333333370, 0.3611111111111111049, 0.3638888888888888729, 0.3666666666666666408, 0.3694444444444444642, 0.3722222222222222321, 0.3750000000000000000, 0.3777777777777777679, 0.3805555555555555358, 0.3833333333333333592, 0.3861111111111111271, 0.3888888888888888951, 0.3916666666666666630, 0.3944444444444444309, 0.3972222222222221988, 0.4000000000000000222, 0.4027777777777777901, 0.4055555555555555580, 0.4083333333333333259, 0.4111111111111110938, 0.4138888888888888618, 0.4166666666666666852, 0.4194444444444444531, 0.4222222222222222210, 0.4249999999999999889, 0.4277777777777777568, 0.4305555555555555802, 0.4333333333333333481, 0.4361111111111111160, 0.4388888888888888840, 0.4416666666666666519, 0.4444444444444444198, 0.4472222222222222432, 0.4500000000000000111, 0.4527777777777777790, 0.4555555555555555469, 0.4583333333333333148, 0.4611111111111111382, 0.4638888888888889062, 0.4666666666666666741, 0.4694444444444444420, 0.4722222222222222099, 0.4749999999999999778, 0.4777777777777778012, 0.4805555555555555691, 0.4833333333333333370, 0.4861111111111111049, 0.4888888888888888729, 0.4916666666666666408, 0.4944444444444444642, 0.4972222222222222321, 0.5000000000000000000, 0.5027777777777777679, 0.5055555555555555358, 0.5083333333333333037, 0.5111111111111110716, 0.5138888888888888395, 0.5166666666666667185, 0.5194444444444444864, 0.5222222222222222543, 0.5250000000000000222, 0.5277777777777777901, 0.5305555555555555580, 0.5333333333333333259, 0.5361111111111110938, 0.5388888888888888618, 0.5416666666666666297, 0.5444444444444443976, 0.5472222222222222765, 0.5500000000000000444, 0.5527777777777778123, 0.5555555555555555802, 0.5583333333333333481, 0.5611111111111111160, 0.5638888888888888840, 0.5666666666666666519, 0.5694444444444444198, 0.5722222222222221877, 0.5749999999999999556, 0.5777777777777777235, 0.5805555555555556024, 0.5833333333333333703, 0.5861111111111111382, 0.5888888888888889062, 0.5916666666666666741, 0.5944444444444444420, 0.5972222222222222099, 0.5999999999999999778, 0.6027777777777777457, 0.6055555555555555136, 0.6083333333333332815, 0.6111111111111111605, 0.6138888888888889284, 0.6166666666666666963, 0.6194444444444444642, 0.6222222222222222321, 0.6250000000000000000, 0.6277777777777777679, 0.6305555555555555358, 0.6333333333333333037, 0.6361111111111110716, 0.6388888888888888395, 0.6416666666666667185, 0.6444444444444444864, 0.6472222222222222543, 0.6500000000000000222, 0.6527777777777777901, 0.6555555555555555580, 0.6583333333333333259, 0.6611111111111110938, 0.6638888888888888618, 0.6666666666666666297, 0.6694444444444443976, 0.6722222222222222765, 0.6750000000000000444, 0.6777777777777778123, 0.6805555555555555802, 0.6833333333333333481, 0.6861111111111111160, 0.6888888888888888840, 0.6916666666666666519, 0.6944444444444444198, 0.6972222222222221877, 0.6999999999999999556, 0.7027777777777777235, 0.7055555555555556024, 0.7083333333333333703, 0.7111111111111111382, 0.7138888888888889062, 0.7166666666666666741, 0.7194444444444444420, 0.7222222222222222099, 0.7249999999999999778, 0.7277777777777777457, 0.7305555555555555136, 0.7333333333333332815, 0.7361111111111111605, 0.7388888888888889284, 0.7416666666666666963, 0.7444444444444444642, 0.7472222222222222321, 0.7500000000000000000, 0.7527777777777777679, 0.7555555555555555358, 0.7583333333333333037, 0.7611111111111110716, 0.7638888888888888395, 0.7666666666666667185, 0.7694444444444444864, 0.7722222222222222543, 0.7750000000000000222, 0.7777777777777777901, 0.7805555555555555580, 0.7833333333333333259, 0.7861111111111110938, 0.7888888888888888618, 0.7916666666666666297, 0.7944444444444443976, 0.7972222222222222765, 0.8000000000000000444, 0.8027777777777778123, 0.8055555555555555802, 0.8083333333333333481, 0.8111111111111111160, 0.8138888888888888840, 0.8166666666666666519, 0.8194444444444444198, 0.8222222222222221877, 0.8249999999999999556, 0.8277777777777777235, 0.8305555555555556024, 0.8333333333333333703, 0.8361111111111111382, 0.8388888888888889062, 0.8416666666666666741, 0.8444444444444444420, 0.8472222222222222099, 0.8499999999999999778, 0.8527777777777777457, 0.8555555555555555136, 0.8583333333333332815, 0.8611111111111111605, 0.8638888888888889284, 0.8666666666666666963, 0.8694444444444444642, 0.8722222222222222321, 0.8750000000000000000, 0.8777777777777777679, 0.8805555555555555358, 0.8833333333333333037, 0.8861111111111110716, 0.8888888888888888395, 0.8916666666666667185, 0.8944444444444444864, 0.8972222222222222543, 0.9000000000000000222, 0.9027777777777777901, 0.9055555555555555580, 0.9083333333333333259, 0.9111111111111110938, 0.9138888888888888618, 0.9166666666666666297, 0.9194444444444443976, 0.9222222222222222765, 0.9250000000000000444, 0.9277777777777778123, 0.9305555555555555802, 0.9333333333333333481, 0.9361111111111111160, 0.9388888888888888840, 0.9416666666666666519, 0.9444444444444444198, 0.9472222222222221877, 0.9499999999999999556, 0.9527777777777777235, 0.9555555555555556024, 0.9583333333333333703, 0.9611111111111111382, 0.9638888888888889062, 0.9666666666666666741, 0.9694444444444444420, 0.9722222222222222099, 0.9749999999999999778, 0.9777777777777777457, 0.9805555555555555136, 0.9833333333333332815, 0.9861111111111111605, 0.9888888888888889284, 0.9916666666666666963, 0.9944444444444444642, 0.9972222222222222321, 1.000000000000000000 ),
 .UNSPECIFIED. ) 
 GEOMETRIC_REPRESENTATION_ITEM ( )  RATIONAL_B_SPLINE_SURFACE ( (
 ( 1.000000000000000000, 0.8660254037844387076, 1.000000000000000000, 0.8660254037844387076, 1.000000000000000000, 0.8660254037844387076, 1.000000000000000000, 0.8660254037844387076, 1.000000000000000000, 0.8660254037844387076, 1.000000000000000000, 0.8660254037844387076, 1.000000000000000000, 0.8660254037844387076, 1.000000000000000000, 0.8660254037844387076, 1.000000000000000000, 0.8660254037844387076, 1.000000000000000000, 0.8660254037844387076, 1.000000000000000000, 0.8660254037844387076, 1.000000000000000000, 0.8660254037844387076, 1.000000000000000000, 0.8660254037844387076, 1.000000000000000000, 0.8660254037844387076, 1.000000000000000000, 0.8660254037844387076, 1.000000000000000000, 0.8660254037844387076, 1.000000000000000000, 0.8660254037844387076, 1.000000000000000000, 0.8660254037844387076, 1.000000000000000000, 0.8660254037844387076, 1.000000000000000000, 0.8660254037844387076, 1.000000000000000000, 0.8660254037844387076, 1.000000000000000000, 0.8660254037844387076, 1.000000000000000000, 0.8660254037844387076, 1.000000000000000000, 0.8660254037844387076, 1.000000000000000000, 0.8660254037844387076, 1.000000000000000000, 0.8660254037844387076, 1.000000000000000000, 0.8660254037844387076, 1.000000000000000000, 0.8660254037844387076, 1.000000000000000000, 0.8660254037844387076, 1.000000000000000000, 0.8660254037844387076, 1.000000000000000000, 0.8660254037844387076, 1.000000000000000000, 0.8660254037844387076, 1.000000000000000000, 0.8660254037844387076, 1.000000000000000000, 0.8660254037844387076, 1.000000000000000000, 0.8660254037844387076, 1.000000000000000000, 0.8660254037844387076, 1.000000000000000000, 0.8660254037844387076, 1.000000000000000000, 0.8660254037844387076, 1.000000000000000000, 0.8660254037844387076, 1.000000000000000000, 0.8660254037844387076, 1.000000000000000000, 0.8660254037844387076, 1.000000000000000000, 0.8660254037844387076, 1.000000000000000000, 0.8660254037844387076, 1.000000000000000000, 0.8660254037844387076, 1.000000000000000000, 0.8660254037844387076, 1.000000000000000000, 0.8660254037844387076, 1.000000000000000000, 0.8660254037844387076, 1.000000000000000000, 0.8660254037844387076, 1.000000000000000000, 0.8660254037844387076, 1.000000000000000000, 0.8660254037844387076, 1.000000000000000000, 0.8660254037844387076, 1.000000000000000000, 0.8660254037844387076, 1.000000000000000000, 0.8660254037844387076, 1.000000000000000000, 0.8660254037844387076, 1.000000000000000000, 0.8660254037844387076, 1.000000000000000000, 0.8660254037844387076, 1.000000000000000000, 0.8660254037844387076, 1.000000000000000000, 0.8660254037844387076, 1.000000000000000000, 0.8660254037844387076, 1.000000000000000000, 0.8660254037844387076, 1.000000000000000000, 0.8660254037844387076, 1.000000000000000000, 0.8660254037844387076, 1.000000000000000000, 0.8660254037844387076, 1.000000000000000000, 0.8660254037844387076, 1.000000000000000000, 0.8660254037844387076, 1.000000000000000000, 0.8660254037844387076, 1.000000000000000000, 0.8660254037844387076, 1.000000000000000000, 0.8660254037844387076, 1.000000000000000000, 0.8660254037844387076, 1.000000000000000000, 0.8660254037844387076, 1.000000000000000000, 0.8660254037844387076, 1.000000000000000000, 0.8660254037844387076, 1.000000000000000000, 0.8660254037844387076, 1.000000000000000000, 0.8660254037844387076, 1.000000000000000000, 0.8660254037844387076, 1.000000000000000000, 0.8660254037844387076, 1.000000000000000000, 0.8660254037844387076, 1.000000000000000000, 0.8660254037844387076, 1.000000000000000000, 0.8660254037844387076, 1.000000000000000000, 0.8660254037844387076, 1.000000000000000000, 0.8660254037844387076, 1.000000000000000000, 0.8660254037844387076, 1.000000000000000000, 0.8660254037844387076, 1.000000000000000000, 0.8660254037844387076, 1.000000000000000000, 0.8660254037844387076, 1.000000000000000000, 0.8660254037844387076, 1.000000000000000000, 0.8660254037844387076, 1.000000000000000000, 0.8660254037844387076, 1.000000000000000000, 0.8660254037844387076, 1.000000000000000000, 0.8660254037844387076, 1.000000000000000000, 0.8660254037844387076, 1.000000000000000000, 0.8660254037844387076, 1.000000000000000000, 0.8660254037844387076, 1.000000000000000000, 0.8660254037844387076, 1.000000000000000000, 0.8660254037844387076, 1.000000000000000000, 0.8660254037844387076, 1.000000000000000000, 0.8660254037844387076, 1.000000000000000000, 0.8660254037844387076, 1.000000000000000000, 0.8660254037844387076, 1.000000000000000000, 0.8660254037844387076, 1.000000000000000000, 0.8660254037844387076, 1.000000000000000000, 0.8660254037844387076, 1.000000000000000000, 0.8660254037844387076, 1.000000000000000000, 0.8660254037844387076, 1.000000000000000000, 0.8660254037844387076, 1.000000000000000000, 0.8660254037844387076, 1.000000000000000000, 0.8660254037844387076, 1.000000000000000000, 0.8660254037844387076, 1.000000000000000000, 0.8660254037844387076, 1.000000000000000000, 0.8660254037844387076, 1.000000000000000000, 0.8660254037844387076, 1.000000000000000000, 0.8660254037844387076, 1.000000000000000000, 0.8660254037844387076, 1.000000000000000000, 0.8660254037844387076, 1.000000000000000000, 0.8660254037844387076, 1.000000000000000000, 0.8660254037844387076, 1.000000000000000000, 0.8660254037844387076, 1.000000000000000000, 0.8660254037844387076, 1.000000000000000000, 0.8660254037844387076, 1.000000000000000000, 0.8660254037844387076, 1.000000000000000000, 0.8660254037844387076, 1.000000000000000000, 0.8660254037844387076, 1.000000000000000000, 0.8660254037844387076, 1.000000000000000000, 0.8660254037844387076, 1.000000000000000000, 0.8660254037844387076, 1.000000000000000000, 0.8660254037844387076, 1.000000000000000000, 0.8660254037844387076, 1.000000000000000000, 0.8660254037844387076, 1.000000000000000000, 0.8660254037844387076, 1.000000000000000000, 0.8660254037844387076, 1.000000000000000000, 0.8660254037844387076, 1.000000000000000000, 0.8660254037844387076, 1.000000000000000000, 0.8660254037844387076, 1.000000000000000000, 0.8660254037844387076, 1.000000000000000000, 0.8660254037844387076, 1.000000000000000000, 0.8660254037844387076, 1.000000000000000000, 0.8660254037844387076, 1.000000000000000000, 0.8660254037844387076, 1.000000000000000000, 0.8660254037844387076, 1.000000000000000000, 0.8660254037844387076, 1.000000000000000000, 0.8660254037844387076, 1.000000000000000000, 0.8660254037844387076, 1.000000000000000000, 0.8660254037844387076, 1.000000000000000000, 0.8660254037844387076, 1.000000000000000000, 0.8660254037844387076, 1.000000000000000000, 0.8660254037844387076, 1.000000000000000000, 0.8660254037844387076, 1.000000000000000000, 0.8660254037844387076, 1.000000000000000000, 0.8660254037844387076, 1.000000000000000000, 0.8660254037844387076, 1.000000000000000000, 0.8660254037844387076, 1.000000000000000000, 0.8660254037844387076, 1.000000000000000000, 0.8660254037844387076, 1.000000000000000000, 0.8660254037844387076, 1.000000000000000000, 0.8660254037844387076, 1.000000000000000000, 0.8660254037844387076, 1.000000000000000000, 0.8660254037844387076, 1.000000000000000000, 0.8660254037844387076, 1.000000000000000000, 0.8660254037844387076, 1.000000000000000000, 0.8660254037844387076, 1.000000000000000000, 0.8660254037844387076, 1.000000000000000000, 0.8660254037844387076, 1.000000000000000000, 0.8660254037844387076, 1.000000000000000000, 0.8660254037844387076, 1.000000000000000000, 0.8660254037844387076, 1.000000000000000000, 0.8660254037844387076, 1.000000000000000000, 0.8660254037844387076, 1.000000000000000000, 0.8660254037844387076, 1.000000000000000000, 0.8660254037844387076, 1.000000000000000000, 0.8660254037844387076, 1.000000000000000000, 0.8660254037844387076, 1.000000000000000000, 0.8660254037844387076, 1.000000000000000000, 0.8660254037844387076, 1.000000000000000000, 0.8660254037844387076, 1.000000000000000000, 0.8660254037844387076, 1.000000000000000000, 0.8660254037844387076, 1.000000000000000000, 0.8660254037844387076, 1.000000000000000000, 0.8660254037844387076, 1.000000000000000000, 0.8660254037844387076, 1.000000000000000000, 0.8660254037844387076, 1.000000000000000000, 0.8660254037844387076, 1.000000000000000000, 0.8660254037844387076, 1.000000000000000000, 0.8660254037844387076, 1.000000000000000000, 0.8660254037844387076, 1.000000000000000000, 0.8660254037844387076, 1.000000000000000000, 0.8660254037844387076, 1.000000000000000000, 0.8660254037844387076, 1.000000000000000000, 0.8660254037844387076, 1.000000000000000000, 0.8660254037844387076, 1.000000000000000000, 0.8660254037844387076, 1.000000000000000000, 0.8660254037844387076, 1.000000000000000000, 0.8660254037844387076, 1.000000000000000000, 0.8660254037844387076, 1.000000000000000000, 0.8660254037844387076, 1.000000000000000000, 0.8660254037844387076, 1.000000000000000000, 0.8660254037844387076, 1.000000000000000000, 0.8660254037844387076, 1.000000000000000000, 0.8660254037844387076, 1.000000000000000000, 0.8660254037844387076, 1.000000000000000000, 0.8660254037844387076, 1.000000000000000000, 0.8660254037844387076, 1.000000000000000000, 0.8660254037844387076, 1.000000000000000000, 0.8660254037844387076, 1.000000000000000000, 0.8660254037844387076, 1.000000000000000000, 0.8660254037844387076, 1.000000000000000000, 0.8660254037844387076, 1.000000000000000000, 0.8660254037844387076, 1.000000000000000000, 0.8660254037844387076, 1.000000000000000000, 0.8660254037844387076, 1.000000000000000000, 0.8660254037844387076, 1.000000000000000000, 0.8660254037844387076, 1.000000000000000000, 0.8660254037844387076, 1.000000000000000000, 0.8660254037844387076, 1.000000000000000000, 0.8660254037844387076, 1.000000000000000000, 0.8660254037844387076, 1.000000000000000000, 0.8660254037844387076, 1.000000000000000000, 0.8660254037844387076, 1.000000000000000000, 0.8660254037844387076, 1.000000000000000000, 0.8660254037844387076, 1.000000000000000000, 0.8660254037844387076, 1.000000000000000000, 0.8660254037844387076, 1.000000000000000000, 0.8660254037844387076, 1.000000000000000000, 0.8660254037844387076, 1.000000000000000000, 0.8660254037844387076, 1.000000000000000000, 0.8660254037844387076, 1.000000000000000000, 0.8660254037844387076, 1.000000000000000000, 0.8660254037844387076, 1.000000000000000000, 0.8660254037844387076, 1.000000000000000000, 0.8660254037844387076, 1.000000000000000000, 0.8660254037844387076, 1.000000000000000000, 0.8660254037844387076, 1.000000000000000000, 0.8660254037844387076, 1.000000000000000000, 0.8660254037844387076, 1.000000000000000000, 0.8660254037844387076, 1.000000000000000000, 0.8660254037844387076, 1.000000000000000000, 0.8660254037844387076, 1.000000000000000000, 0.8660254037844387076, 1.000000000000000000, 0.8660254037844387076, 1.000000000000000000, 0.8660254037844387076, 1.000000000000000000, 0.8660254037844387076, 1.000000000000000000, 0.8660254037844387076, 1.000000000000000000, 0.8660254037844387076, 1.000000000000000000, 0.8660254037844387076, 1.000000000000000000, 0.8660254037844387076, 1.000000000000000000, 0.8660254037844387076, 1.000000000000000000, 0.8660254037844387076, 1.000000000000000000, 0.8660254037844387076, 1.000000000000000000, 0.8660254037844387076, 1.000000000000000000, 0.8660254037844387076, 1.000000000000000000, 0.8660254037844387076, 1.000000000000000000, 0.8660254037844387076, 1.000000000000000000, 0.8660254037844387076, 1.000000000000000000, 0.8660254037844387076, 1.000000000000000000, 0.8660254037844387076, 1.000000000000000000, 0.8660254037844387076, 1.000000000000000000, 0.8660254037844387076, 1.000000000000000000, 0.8660254037844387076, 1.000000000000000000, 0.8660254037844387076, 1.000000000000000000, 0.8660254037844387076, 1.000000000000000000, 0.8660254037844387076, 1.000000000000000000, 0.8660254037844387076, 1.000000000000000000, 0.8660254037844387076, 1.000000000000000000, 0.8660254037844387076, 1.000000000000000000, 0.8660254037844387076, 1.000000000000000000, 0.8660254037844387076, 1.000000000000000000, 0.8660254037844387076, 1.000000000000000000, 0.8660254037844387076, 1.000000000000000000, 0.8660254037844387076, 1.000000000000000000, 0.8660254037844387076, 1.000000000000000000, 0.8660254037844387076, 1.000000000000000000, 0.8660254037844387076, 1.000000000000000000, 0.8660254037844387076, 1.000000000000000000, 0.8660254037844387076, 1.000000000000000000, 0.8660254037844387076, 1.000000000000000000, 0.8660254037844387076, 1.000000000000000000, 0.8660254037844387076, 1.000000000000000000, 0.8660254037844387076, 1.000000000000000000, 0.8660254037844387076, 1.000000000000000000, 0.8660254037844387076, 1.000000000000000000, 0.8660254037844387076, 1.000000000000000000, 0.8660254037844387076, 1.000000000000000000, 0.8660254037844387076, 1.000000000000000000, 0.8660254037844387076, 1.000000000000000000, 0.8660254037844387076, 1.000000000000000000, 0.8660254037844387076, 1.000000000000000000, 0.8660254037844387076, 1.000000000000000000, 0.8660254037844387076, 1.000000000000000000, 0.8660254037844387076, 1.000000000000000000, 0.8660254037844387076, 1.000000000000000000, 0.8660254037844387076, 1.000000000000000000, 0.8660254037844387076, 1.000000000000000000, 0.8660254037844387076, 1.000000000000000000, 0.8660254037844387076, 1.000000000000000000, 0.8660254037844387076, 1.000000000000000000, 0.8660254037844387076, 1.000000000000000000, 0.8660254037844387076, 1.000000000000000000, 0.8660254037844387076, 1.000000000000000000, 0.8660254037844387076, 1.000000000000000000, 0.8660254037844387076, 1.000000000000000000, 0.8660254037844387076, 1.000000000000000000, 0.8660254037844387076, 1.000000000000000000, 0.8660254037844387076, 1.000000000000000000, 0.8660254037844387076, 1.000000000000000000, 0.8660254037844387076, 1.000000000000000000, 0.8660254037844387076, 1.000000000000000000, 0.8660254037844387076, 1.000000000000000000, 0.8660254037844387076, 1.000000000000000000, 0.8660254037844387076, 1.000000000000000000, 0.8660254037844387076, 1.000000000000000000, 0.8660254037844387076, 1.000000000000000000, 0.8660254037844387076, 1.000000000000000000, 0.8660254037844387076, 1.000000000000000000, 0.8660254037844387076, 1.000000000000000000, 0.8660254037844387076, 1.000000000000000000, 0.8660254037844387076, 1.000000000000000000, 0.8660254037844387076, 1.000000000000000000, 0.8660254037844387076, 1.000000000000000000, 0.8660254037844387076, 1.000000000000000000, 0.8660254037844387076, 1.000000000000000000, 0.8660254037844387076, 1.000000000000000000, 0.8660254037844387076, 1.000000000000000000, 0.8660254037844387076, 1.000000000000000000, 0.8660254037844387076, 1.000000000000000000, 0.8660254037844387076, 1.000000000000000000, 0.8660254037844387076, 1.000000000000000000, 0.8660254037844387076, 1.000000000000000000, 0.8660254037844387076, 1.000000000000000000, 0.8660254037844387076, 1.000000000000000000, 0.8660254037844387076, 1.000000000000000000, 0.8660254037844387076, 1.000000000000000000, 0.8660254037844387076, 1.000000000000000000, 0.8660254037844387076, 1.000000000000000000, 0.8660254037844387076, 1.000000000000000000, 0.8660254037844387076, 1.000000000000000000, 0.8660254037844387076, 1.000000000000000000, 0.8660254037844387076, 1.000000000000000000, 0.8660254037844387076, 1.000000000000000000, 0.8660254037844387076, 1.000000000000000000, 0.8660254037844387076, 1.000000000000000000, 0.8660254037844387076, 1.000000000000000000, 0.8660254037844387076, 1.000000000000000000, 0.8660254037844387076, 1.000000000000000000, 0.8660254037844387076, 1.000000000000000000, 0.8660254037844387076, 1.000000000000000000, 0.8660254037844387076, 1.000000000000000000, 0.8660254037844387076, 1.000000000000000000, 0.8660254037844387076, 1.000000000000000000, 0.8660254037844387076, 1.000000000000000000, 0.8660254037844387076, 1.000000000000000000, 0.8660254037844387076, 1.000000000000000000, 0.8660254037844387076, 1.000000000000000000, 0.8660254037844387076, 1.000000000000000000, 0.8660254037844387076, 1.000000000000000000, 0.8660254037844387076, 1.000000000000000000, 0.8660254037844387076, 1.000000000000000000, 0.8660254037844387076, 1.000000000000000000, 0.8660254037844387076, 1.000000000000000000, 0.8660254037844387076, 1.000000000000000000, 0.8660254037844387076, 1.000000000000000000, 0.8660254037844387076, 1.000000000000000000),
 ( 1.000000000000000000, 0.8660254037844387076, 1.000000000000000000, 0.8660254037844387076, 1.000000000000000000, 0.8660254037844387076, 1.000000000000000000, 0.8660254037844387076, 1.000000000000000000, 0.8660254037844387076, 1.000000000000000000, 0.8660254037844387076, 1.000000000000000000, 0.8660254037844387076, 1.000000000000000000, 0.8660254037844387076, 1.000000000000000000, 0.8660254037844387076, 1.000000000000000000, 0.8660254037844387076, 1.000000000000000000, 0.8660254037844387076, 1.000000000000000000, 0.8660254037844387076, 1.000000000000000000, 0.8660254037844387076, 1.000000000000000000, 0.8660254037844387076, 1.000000000000000000, 0.8660254037844387076, 1.000000000000000000, 0.8660254037844387076, 1.000000000000000000, 0.8660254037844387076, 1.000000000000000000, 0.8660254037844387076, 1.000000000000000000, 0.8660254037844387076, 1.000000000000000000, 0.8660254037844387076, 1.000000000000000000, 0.8660254037844387076, 1.000000000000000000, 0.8660254037844387076, 1.000000000000000000, 0.8660254037844387076, 1.000000000000000000, 0.8660254037844387076, 1.000000000000000000, 0.8660254037844387076, 1.000000000000000000, 0.8660254037844387076, 1.000000000000000000, 0.8660254037844387076, 1.000000000000000000, 0.8660254037844387076, 1.000000000000000000, 0.8660254037844387076, 1.000000000000000000, 0.8660254037844387076, 1.000000000000000000, 0.8660254037844387076, 1.000000000000000000, 0.8660254037844387076, 1.000000000000000000, 0.8660254037844387076, 1.000000000000000000, 0.8660254037844387076, 1.000000000000000000, 0.8660254037844387076, 1.000000000000000000, 0.8660254037844387076, 1.000000000000000000, 0.8660254037844387076, 1.000000000000000000, 0.8660254037844387076, 1.000000000000000000, 0.8660254037844387076, 1.000000000000000000, 0.8660254037844387076, 1.000000000000000000, 0.8660254037844387076, 1.000000000000000000, 0.8660254037844387076, 1.000000000000000000, 0.8660254037844387076, 1.000000000000000000, 0.8660254037844387076, 1.000000000000000000, 0.8660254037844387076, 1.000000000000000000, 0.8660254037844387076, 1.000000000000000000, 0.8660254037844387076, 1.000000000000000000, 0.8660254037844387076, 1.000000000000000000, 0.8660254037844387076, 1.000000000000000000, 0.8660254037844387076, 1.000000000000000000, 0.8660254037844387076, 1.000000000000000000, 0.8660254037844387076, 1.000000000000000000, 0.8660254037844387076, 1.000000000000000000, 0.8660254037844387076, 1.000000000000000000, 0.8660254037844387076, 1.000000000000000000, 0.8660254037844387076, 1.000000000000000000, 0.8660254037844387076, 1.000000000000000000, 0.8660254037844387076, 1.000000000000000000, 0.8660254037844387076, 1.000000000000000000, 0.8660254037844387076, 1.000000000000000000, 0.8660254037844387076, 1.000000000000000000, 0.8660254037844387076, 1.000000000000000000, 0.8660254037844387076, 1.000000000000000000, 0.8660254037844387076, 1.000000000000000000, 0.8660254037844387076, 1.000000000000000000, 0.8660254037844387076, 1.000000000000000000, 0.8660254037844387076, 1.000000000000000000, 0.8660254037844387076, 1.000000000000000000, 0.8660254037844387076, 1.000000000000000000, 0.8660254037844387076, 1.000000000000000000, 0.8660254037844387076, 1.000000000000000000, 0.8660254037844387076, 1.000000000000000000, 0.8660254037844387076, 1.000000000000000000, 0.8660254037844387076, 1.000000000000000000, 0.8660254037844387076, 1.000000000000000000, 0.8660254037844387076, 1.000000000000000000, 0.8660254037844387076, 1.000000000000000000, 0.8660254037844387076, 1.000000000000000000, 0.8660254037844387076, 1.000000000000000000, 0.8660254037844387076, 1.000000000000000000, 0.8660254037844387076, 1.000000000000000000, 0.8660254037844387076, 1.000000000000000000, 0.8660254037844387076, 1.000000000000000000, 0.8660254037844387076, 1.000000000000000000, 0.8660254037844387076, 1.000000000000000000, 0.8660254037844387076, 1.000000000000000000, 0.8660254037844387076, 1.000000000000000000, 0.8660254037844387076, 1.000000000000000000, 0.8660254037844387076, 1.000000000000000000, 0.8660254037844387076, 1.000000000000000000, 0.8660254037844387076, 1.000000000000000000, 0.8660254037844387076, 1.000000000000000000, 0.8660254037844387076, 1.000000000000000000, 0.8660254037844387076, 1.000000000000000000, 0.8660254037844387076, 1.000000000000000000, 0.8660254037844387076, 1.000000000000000000, 0.8660254037844387076, 1.000000000000000000, 0.8660254037844387076, 1.000000000000000000, 0.8660254037844387076, 1.000000000000000000, 0.8660254037844387076, 1.000000000000000000, 0.8660254037844387076, 1.000000000000000000, 0.8660254037844387076, 1.000000000000000000, 0.8660254037844387076, 1.000000000000000000, 0.8660254037844387076, 1.000000000000000000, 0.8660254037844387076, 1.000000000000000000, 0.8660254037844387076, 1.000000000000000000, 0.8660254037844387076, 1.000000000000000000, 0.8660254037844387076, 1.000000000000000000, 0.8660254037844387076, 1.000000000000000000, 0.8660254037844387076, 1.000000000000000000, 0.8660254037844387076, 1.000000000000000000, 0.8660254037844387076, 1.000000000000000000, 0.8660254037844387076, 1.000000000000000000, 0.8660254037844387076, 1.000000000000000000, 0.8660254037844387076, 1.000000000000000000, 0.8660254037844387076, 1.000000000000000000, 0.8660254037844387076, 1.000000000000000000, 0.8660254037844387076, 1.000000000000000000, 0.8660254037844387076, 1.000000000000000000, 0.8660254037844387076, 1.000000000000000000, 0.8660254037844387076, 1.000000000000000000, 0.8660254037844387076, 1.000000000000000000, 0.8660254037844387076, 1.000000000000000000, 0.8660254037844387076, 1.000000000000000000, 0.8660254037844387076, 1.000000000000000000, 0.8660254037844387076, 1.000000000000000000, 0.8660254037844387076, 1.000000000000000000, 0.8660254037844387076, 1.000000000000000000, 0.8660254037844387076, 1.000000000000000000, 0.8660254037844387076, 1.000000000000000000, 0.8660254037844387076, 1.000000000000000000, 0.8660254037844387076, 1.000000000000000000, 0.8660254037844387076, 1.000000000000000000, 0.8660254037844387076, 1.000000000000000000, 0.8660254037844387076, 1.000000000000000000, 0.8660254037844387076, 1.000000000000000000, 0.8660254037844387076, 1.000000000000000000, 0.8660254037844387076, 1.000000000000000000, 0.8660254037844387076, 1.000000000000000000, 0.8660254037844387076, 1.000000000000000000, 0.8660254037844387076, 1.000000000000000000, 0.8660254037844387076, 1.000000000000000000, 0.8660254037844387076, 1.000000000000000000, 0.8660254037844387076, 1.000000000000000000, 0.8660254037844387076, 1.000000000000000000, 0.8660254037844387076, 1.000000000000000000, 0.8660254037844387076, 1.000000000000000000, 0.8660254037844387076, 1.000000000000000000, 0.8660254037844387076, 1.000000000000000000, 0.8660254037844387076, 1.000000000000000000, 0.8660254037844387076, 1.000000000000000000, 0.8660254037844387076, 1.000000000000000000, 0.8660254037844387076, 1.000000000000000000, 0.8660254037844387076, 1.000000000000000000, 0.8660254037844387076, 1.000000000000000000, 0.8660254037844387076, 1.000000000000000000, 0.8660254037844387076, 1.000000000000000000, 0.8660254037844387076, 1.000000000000000000, 0.8660254037844387076, 1.000000000000000000, 0.8660254037844387076, 1.000000000000000000, 0.8660254037844387076, 1.000000000000000000, 0.8660254037844387076, 1.000000000000000000, 0.8660254037844387076, 1.000000000000000000, 0.8660254037844387076, 1.000000000000000000, 0.8660254037844387076, 1.000000000000000000, 0.8660254037844387076, 1.000000000000000000, 0.8660254037844387076, 1.000000000000000000, 0.8660254037844387076, 1.000000000000000000, 0.8660254037844387076, 1.000000000000000000, 0.8660254037844387076, 1.000000000000000000, 0.8660254037844387076, 1.000000000000000000, 0.8660254037844387076, 1.000000000000000000, 0.8660254037844387076, 1.000000000000000000, 0.8660254037844387076, 1.000000000000000000, 0.8660254037844387076, 1.000000000000000000, 0.8660254037844387076, 1.000000000000000000, 0.8660254037844387076, 1.000000000000000000, 0.8660254037844387076, 1.000000000000000000, 0.8660254037844387076, 1.000000000000000000, 0.8660254037844387076, 1.000000000000000000, 0.8660254037844387076, 1.000000000000000000, 0.8660254037844387076, 1.000000000000000000, 0.8660254037844387076, 1.000000000000000000, 0.8660254037844387076, 1.000000000000000000, 0.8660254037844387076, 1.000000000000000000, 0.8660254037844387076, 1.000000000000000000, 0.8660254037844387076, 1.000000000000000000, 0.8660254037844387076, 1.000000000000000000, 0.8660254037844387076, 1.000000000000000000, 0.8660254037844387076, 1.000000000000000000, 0.8660254037844387076, 1.000000000000000000, 0.8660254037844387076, 1.000000000000000000, 0.8660254037844387076, 1.000000000000000000, 0.8660254037844387076, 1.000000000000000000, 0.8660254037844387076, 1.000000000000000000, 0.8660254037844387076, 1.000000000000000000, 0.8660254037844387076, 1.000000000000000000, 0.8660254037844387076, 1.000000000000000000, 0.8660254037844387076, 1.000000000000000000, 0.8660254037844387076, 1.000000000000000000, 0.8660254037844387076, 1.000000000000000000, 0.8660254037844387076, 1.000000000000000000, 0.8660254037844387076, 1.000000000000000000, 0.8660254037844387076, 1.000000000000000000, 0.8660254037844387076, 1.000000000000000000, 0.8660254037844387076, 1.000000000000000000, 0.8660254037844387076, 1.000000000000000000, 0.8660254037844387076, 1.000000000000000000, 0.8660254037844387076, 1.000000000000000000, 0.8660254037844387076, 1.000000000000000000, 0.8660254037844387076, 1.000000000000000000, 0.8660254037844387076, 1.000000000000000000, 0.8660254037844387076, 1.000000000000000000, 0.8660254037844387076, 1.000000000000000000, 0.8660254037844387076, 1.000000000000000000, 0.8660254037844387076, 1.000000000000000000, 0.8660254037844387076, 1.000000000000000000, 0.8660254037844387076, 1.000000000000000000, 0.8660254037844387076, 1.000000000000000000, 0.8660254037844387076, 1.000000000000000000, 0.8660254037844387076, 1.000000000000000000, 0.8660254037844387076, 1.000000000000000000, 0.8660254037844387076, 1.000000000000000000, 0.8660254037844387076, 1.000000000000000000, 0.8660254037844387076, 1.000000000000000000, 0.8660254037844387076, 1.000000000000000000, 0.8660254037844387076, 1.000000000000000000, 0.8660254037844387076, 1.000000000000000000, 0.8660254037844387076, 1.000000000000000000, 0.8660254037844387076, 1.000000000000000000, 0.8660254037844387076, 1.000000000000000000, 0.8660254037844387076, 1.000000000000000000, 0.8660254037844387076, 1.000000000000000000, 0.8660254037844387076, 1.000000000000000000, 0.8660254037844387076, 1.000000000000000000, 0.8660254037844387076, 1.000000000000000000, 0.8660254037844387076, 1.000000000000000000, 0.8660254037844387076, 1.000000000000000000, 0.8660254037844387076, 1.000000000000000000, 0.8660254037844387076, 1.000000000000000000, 0.8660254037844387076, 1.000000000000000000, 0.8660254037844387076, 1.000000000000000000, 0.8660254037844387076, 1.000000000000000000, 0.8660254037844387076, 1.000000000000000000, 0.8660254037844387076, 1.000000000000000000, 0.8660254037844387076, 1.000000000000000000, 0.8660254037844387076, 1.000000000000000000, 0.8660254037844387076, 1.000000000000000000, 0.8660254037844387076, 1.000000000000000000, 0.8660254037844387076, 1.000000000000000000, 0.8660254037844387076, 1.000000000000000000, 0.8660254037844387076, 1.000000000000000000, 0.8660254037844387076, 1.000000000000000000, 0.8660254037844387076, 1.000000000000000000, 0.8660254037844387076, 1.000000000000000000, 0.8660254037844387076, 1.000000000000000000, 0.8660254037844387076, 1.000000000000000000, 0.8660254037844387076, 1.000000000000000000, 0.8660254037844387076, 1.000000000000000000, 0.8660254037844387076, 1.000000000000000000, 0.8660254037844387076, 1.000000000000000000, 0.8660254037844387076, 1.000000000000000000, 0.8660254037844387076, 1.000000000000000000, 0.8660254037844387076, 1.000000000000000000, 0.8660254037844387076, 1.000000000000000000, 0.8660254037844387076, 1.000000000000000000, 0.8660254037844387076, 1.000000000000000000, 0.8660254037844387076, 1.000000000000000000, 0.8660254037844387076, 1.000000000000000000, 0.8660254037844387076, 1.000000000000000000, 0.8660254037844387076, 1.000000000000000000, 0.8660254037844387076, 1.000000000000000000, 0.8660254037844387076, 1.000000000000000000, 0.8660254037844387076, 1.000000000000000000, 0.8660254037844387076, 1.000000000000000000, 0.8660254037844387076, 1.000000000000000000, 0.8660254037844387076, 1.000000000000000000, 0.8660254037844387076, 1.000000000000000000, 0.8660254037844387076, 1.000000000000000000, 0.8660254037844387076, 1.000000000000000000, 0.8660254037844387076, 1.000000000000000000, 0.8660254037844387076, 1.000000000000000000, 0.8660254037844387076, 1.000000000000000000, 0.8660254037844387076, 1.000000000000000000, 0.8660254037844387076, 1.000000000000000000, 0.8660254037844387076, 1.000000000000000000, 0.8660254037844387076, 1.000000000000000000, 0.8660254037844387076, 1.000000000000000000, 0.8660254037844387076, 1.000000000000000000, 0.8660254037844387076, 1.000000000000000000, 0.8660254037844387076, 1.000000000000000000, 0.8660254037844387076, 1.000000000000000000, 0.8660254037844387076, 1.000000000000000000, 0.8660254037844387076, 1.000000000000000000, 0.8660254037844387076, 1.000000000000000000, 0.8660254037844387076, 1.000000000000000000, 0.8660254037844387076, 1.000000000000000000, 0.8660254037844387076, 1.000000000000000000, 0.8660254037844387076, 1.000000000000000000, 0.8660254037844387076, 1.000000000000000000, 0.8660254037844387076, 1.000000000000000000, 0.8660254037844387076, 1.000000000000000000, 0.8660254037844387076, 1.000000000000000000, 0.8660254037844387076, 1.000000000000000000, 0.8660254037844387076, 1.000000000000000000, 0.8660254037844387076, 1.000000000000000000, 0.8660254037844387076, 1.000000000000000000, 0.8660254037844387076, 1.000000000000000000, 0.8660254037844387076, 1.000000000000000000, 0.8660254037844387076, 1.000000000000000000, 0.8660254037844387076, 1.000000000000000000, 0.8660254037844387076, 1.000000000000000000, 0.8660254037844387076, 1.000000000000000000, 0.8660254037844387076, 1.000000000000000000, 0.8660254037844387076, 1.000000000000000000, 0.8660254037844387076, 1.000000000000000000, 0.8660254037844387076, 1.000000000000000000, 0.8660254037844387076, 1.000000000000000000, 0.8660254037844387076, 1.000000000000000000, 0.8660254037844387076, 1.000000000000000000, 0.8660254037844387076, 1.000000000000000000, 0.8660254037844387076, 1.000000000000000000, 0.8660254037844387076, 1.000000000000000000, 0.8660254037844387076, 1.000000000000000000, 0.8660254037844387076, 1.000000000000000000, 0.8660254037844387076, 1.000000000000000000, 0.8660254037844387076, 1.000000000000000000, 0.8660254037844387076, 1.000000000000000000, 0.8660254037844387076, 1.000000000000000000, 0.8660254037844387076, 1.000000000000000000, 0.8660254037844387076, 1.000000000000000000, 0.8660254037844387076, 1.000000000000000000, 0.8660254037844387076, 1.000000000000000000, 0.8660254037844387076, 1.000000000000000000, 0.8660254037844387076, 1.000000000000000000, 0.8660254037844387076, 1.000000000000000000, 0.8660254037844387076, 1.000000000000000000, 0.8660254037844387076, 1.000000000000000000, 0.8660254037844387076, 1.000000000000000000, 0.8660254037844387076, 1.000000000000000000, 0.8660254037844387076, 1.000000000000000000, 0.8660254037844387076, 1.000000000000000000, 0.8660254037844387076, 1.000000000000000000, 0.8660254037844387076, 1.000000000000000000, 0.8660254037844387076, 1.000000000000000000, 0.8660254037844387076, 1.000000000000000000, 0.8660254037844387076, 1.000000000000000000, 0.8660254037844387076, 1.000000000000000000, 0.8660254037844387076, 1.000000000000000000, 0.8660254037844387076, 1.000000000000000000, 0.8660254037844387076, 1.000000000000000000, 0.8660254037844387076, 1.000000000000000000, 0.8660254037844387076, 1.000000000000000000, 0.8660254037844387076, 1.000000000000000000, 0.8660254037844387076, 1.000000000000000000, 0.8660254037844387076, 1.000000000000000000, 0.8660254037844387076, 1.000000000000000000, 0.8660254037844387076, 1.000000000000000000, 0.8660254037844387076, 1.000000000000000000, 0.8660254037844387076, 1.000000000000000000) ) ) 
 REPRESENTATION_ITEM ( '' )  SURFACE ( )  );
#46697=CARTESIAN_POINT ( 'NONE',  ( 9.975000000000001421, 6.123233995736764310E-16, -4.999999999999998224 ) ) ;
#46698=CARTESIAN_POINT ( 'NONE',  ( 19.12500000122903288, 2.886751345948129099, -4.999999999999998224 ) ) ;
#46699=CARTESIAN_POINT ( 'NONE',  ( -3.999999999999999112, 18.76250000122903216, -30.00000000000000000 ) ) ;
#46701=VERTEX_POINT ( 'NONE', #60081 ) ;
#46702=CARTESIAN_POINT ( 'NONE',  ( 16.64999999999999858, -4.330127018922190985, -2.500000000000001332 ) ) ;
#46703=CARTESIAN_POINT ( 'NONE',  ( 21.89999999999999858, 0.000000000000000000, 4.999999999999998224 ) ) ;
#46704=( BOUNDED_CURVE ( )  B_SPLINE_CURVE ( 2, ( #17953, #35321, #12429, #34963, #68954, #29425, #51960 ),
 .UNSPECIFIED., .F., .F. ) 
 B_SPLINE_CURVE_WITH_KNOTS ( ( 3, 2, 2, 3 ),
 ( 0.2500000000000000000, 0.2527777777777777679, 0.2555555555555554803, 0.2583333333333333037 ),
 .UNSPECIFIED. ) 
 CURVE ( )  GEOMETRIC_REPRESENTATION_ITEM ( )  RATIONAL_B_SPLINE_CURVE ( ( 1.000000000000000000, 0.8660254037844387076, 1.000000000000000000, 0.8660254037844387076, 1.000000000000000000, 0.8660254037844413721, 0.9999999999999973355 ) ) 
 REPRESENTATION_ITEM ( '' )  );
#46705=CARTESIAN_POINT ( 'NONE',  ( 18.15937500061451715, 0.000000000000000000, 5.243569643749999010 ) ) ;
#46706=CARTESIAN_POINT ( 'NONE',  ( 25.04062500061451502, -3.027376345333610441, -5.243569643749999898 ) ) ;
#46707=VERTEX_POINT ( 'NONE', #27217 ) ;
#46708=CARTESIAN_POINT ( 'NONE',  ( 28.08750000122903145, 6.123233995736764310E-16, -4.999999999999998224 ) ) ;
#46709=CARTESIAN_POINT ( 'NONE',  ( 6.140625000614516438, -3.027376345333610441, -5.243569643749999898 ) ) ;
#46710=CARTESIAN_POINT ( 'NONE',  ( 3.999999999999999112, 15.38750000122903394, 30.00000000000000000 ) ) ;
#46711=CARTESIAN_POINT ( 'NONE',  ( 13.42499999999999893, -4.330127018922194537, 2.499999999999995559 ) ) ;
#46712=CARTESIAN_POINT ( 'NONE',  ( -4.243569643749999898, 16.61562500061451786, 27.54997392385601529 ) ) ;
#46713=CARTESIAN_POINT ( 'NONE',  ( 28.82812500061451644, 4.541064518000418104, 2.621784821874999949 ) ) ;
#46716=CARTESIAN_POINT ( 'NONE',  ( 25.13437500061451502, 6.421520780324663323E-16, -5.243569643749999010 ) ) ;
#46718=CARTESIAN_POINT ( 'NONE',  ( 21.44062500061452070, -3.027376345333610441, -5.243569643749999898 ) ) ;
#46719=CARTESIAN_POINT ( 'NONE',  ( 22.35937500061451644, -4.541064518000417216, -2.621784821875001281 ) ) ;
#46720=CARTESIAN_POINT ( 'NONE',  ( 9.001249775931846008E-16, 17.21562500061459744, -25.09994784771203058 ) ) ;
#46721=CARTESIAN_POINT ( 'NONE',  ( 5.878125000614517148, 4.541064518000418104, 2.621784821874999949 ) ) ;
#46723=CARTESIAN_POINT ( 'NONE',  ( 24.44062500061451715, -3.027376345333614438, 5.243569643749998122 ) ) ;
#46726=CARTESIAN_POINT ( 'NONE',  ( 16.77187500061451786, 3.027376345333611329, 5.243569643749999010 ) ) ;
#46727=CARTESIAN_POINT ( 'NONE',  ( 19.02187500061451786, 3.027376345333611329, 5.243569643749999010 ) ) ;
#46728=CARTESIAN_POINT ( 'NONE',  ( 28.20937500061451786, -4.541064518000417216, -2.621784821875001281 ) ) ;
#46729=CARTESIAN_POINT ( 'NONE',  ( 4.243569643749999898, 15.54687500061451644, 32.45002607614398471 ) ) ;
#46730=CARTESIAN_POINT ( 'NONE',  ( 6.890625000614516438, -3.027376345333614438, 5.243569643749998122 ) ) ;
#46731=CARTESIAN_POINT ( 'NONE',  ( 1.071796769724497445, 16.26740381056766438, 26.00000000000000355 ) ) ;
#46733=CARTESIAN_POINT ( 'NONE',  ( 5.034375000614519813, 4.541064518000418104, 2.621784821874999949 ) ) ;
#46735=CARTESIAN_POINT ( 'NONE',  ( 4.115625000614516082, 3.027376345333611329, 5.243569643749999010 ) ) ;
#46736=CARTESIAN_POINT ( 'NONE',  ( 9.721875000614517148, -6.054752690667223547, -1.112240025338166033E-15 ) ) ;
#46738=CARTESIAN_POINT ( 'NONE',  ( 16.68750000122903288, -4.330127018922194537, 2.499999999999995559 ) ) ;
#46739=CARTESIAN_POINT ( 'NONE',  ( 4.546875000614517326, 6.054752690667223547, 3.707466751127219781E-16 ) ) ;
#46740=CARTESIAN_POINT ( 'NONE',  ( 8.503125000614515372, 4.541064518000418104, -2.621784821874998173 ) ) ;
#46743=CARTESIAN_POINT ( 'NONE',  ( 17.55937500061451573, 4.541064518000418104, -2.621784821874998173 ) ) ;
#46744=CARTESIAN_POINT ( 'NONE',  ( 1.071796769724493892, 17.72990381179669583, 26.00000000000000711 ) ) ;
#46746=CARTESIAN_POINT ( 'NONE',  ( 25.52812500061451573, 6.421520780324663323E-16, -5.243569643749999010 ) ) ;
#46747=CARTESIAN_POINT ( 'NONE',  ( 10.07812500061451644, -4.541064518000419881, 2.621784821874995952 ) ) ;
#46748=CARTESIAN_POINT ( 'NONE',  ( 26.70937500061451431, 0.000000000000000000, 5.243569643749999010 ) ) ;
#46749=CARTESIAN_POINT ( 'NONE',  ( 10.97812500061451679, -4.541064518000419881, 2.621784821874995952 ) ) ;
#46751=CARTESIAN_POINT ( 'NONE',  ( 11.36250000122903536, -4.330127018922190985, -2.500000000000001332 ) ) ;
#46752=CARTESIAN_POINT ( 'NONE',  ( 24.96562500061451573, -6.054752690667223547, -1.112240025338166033E-15 ) ) ;
#46753=CARTESIAN_POINT ( 'NONE',  ( 4.243569643749999898, 14.17812500061451608, -30.00000000000000000 ) ) ;
#46754=CARTESIAN_POINT ( 'NONE',  ( 13.01250000122903394, 0.000000000000000000, 4.999999999999998224 ) ) ;
#46755=CARTESIAN_POINT ( 'NONE',  ( 21.81562500061451004, -6.054752690667223547, -1.112240025338166033E-15 ) ) ;
#46756=CARTESIAN_POINT ( 'NONE',  ( 10.35000000000000142, -4.330127018922190985, -2.500000000000001332 ) ) ;
#46757=CARTESIAN_POINT ( 'NONE',  ( 19.19062500061452070, -3.027376345333610441, -5.243569643749999898 ) ) ;
#46758=CARTESIAN_POINT ( 'NONE',  ( 5.409375000614516260, 4.541064518000418104, -2.621784821874998173 ) ) ;
#46760=CARTESIAN_POINT ( 'NONE',  ( 20.99999999999999645, 0.000000000000000000, 4.999999999999998224 ) ) ;
#46761=CARTESIAN_POINT ( 'NONE',  ( 14.66250000122903252, 4.330127018922192761, -2.499999999999997780 ) ) ;
#46762=CARTESIAN_POINT ( 'NONE',  ( 10.52812500061451750, -4.541064518000419881, 2.621784821874995952 ) ) ;
#46763=CARTESIAN_POINT ( 'NONE',  ( 15.66562500061451857, 3.027376345333613106, -5.243569643749998122 ) ) ;
#46764=CARTESIAN_POINT ( 'NONE',  ( 24.82500000122902861, -5.773502691896255534, -1.060575238724906372E-15 ) ) ;
#46765=CARTESIAN_POINT ( 'NONE',  ( 24.34687500061451715, 6.054752690667223547, 3.707466751127219781E-16 ) ) ;
#46766=FACE_OUTER_BOUND ( 'NONE', #32860, .T. ) ;
#46767=CARTESIAN_POINT ( 'NONE',  ( 8.250000001229034652, -2.886751345948125991, -5.000000000000000000 ) ) ;
#46768=CARTESIAN_POINT ( 'NONE',  ( 10.02187500061451964, 3.027376345333611329, 5.243569643749999010 ) ) ;
#46769=CARTESIAN_POINT ( 'NONE',  ( 24.94687500061451502, -3.027376345333614438, 5.243569643749998122 ) ) ;
#46770=CARTESIAN_POINT ( 'NONE',  ( 3.646875000614520079, 6.054752690667223547, 3.707466751127219781E-16 ) ) ;
#46771=CARTESIAN_POINT ( 'NONE',  ( 20.16562500061451146, 3.027376345333613106, -5.243569643749998122 ) ) ;
#46772=CARTESIAN_POINT ( 'NONE',  ( 25.47187500061451715, -6.054752690667223547, -1.112240025338166033E-15 ) ) ;
#46775=VECTOR ( 'NONE', #46577, 1000.000000000000000 ) ;
#46776=CARTESIAN_POINT ( 'NONE',  ( 8.259375000614518569, 0.000000000000000000, 5.243569643749999010 ) ) ;
#46777=CARTESIAN_POINT ( 'NONE',  ( 17.69062500061451715, -3.027376345333614438, 5.243569643749998122 ) ) ;
#46779=DIRECTION ( 'NONE',  ( -0.000000000000000000, -1.000000000000000000, -0.000000000000000000 ) ) ;
#46780=CARTESIAN_POINT ( 'NONE',  ( 26.87812500061451360, 6.421520780324663323E-16, -5.243569643749999010 ) ) ;
#46781=CARTESIAN_POINT ( 'NONE',  ( 5.146875000614517859, -3.027376345333614438, 5.243569643749998122 ) ) ;
#46783=DIRECTION ( 'NONE',  ( 0.000000000000000000, 0.000000000000000000, 1.000000000000000000 ) ) ;
#46784=CARTESIAN_POINT ( 'NONE',  ( 17.25000000000000000, 4.330127018922192761, -2.499999999999997780 ) ) ;
#46785=CARTESIAN_POINT ( 'NONE',  ( 20.76562500061451644, 3.027376345333611329, 5.243569643749999010 ) ) ;
#46787=CARTESIAN_POINT ( 'NONE',  ( 25.01249999999999929, 2.886751345948126879, 4.999999999999999112 ) ) ;
#46788=CARTESIAN_POINT ( 'NONE',  ( 27.30937500061451573, -4.541064518000417216, -2.621784821875001281 ) ) ;
#46790=CARTESIAN_POINT ( 'NONE',  ( 12.77812500061451750, -4.541064518000419881, 2.621784821874995952 ) ) ;
#46791=CARTESIAN_POINT ( 'NONE',  ( 5.203125000614518214, -4.541064518000417216, -2.621784821875001281 ) ) ;
#46793=CARTESIAN_POINT ( 'NONE',  ( 28.75312500061451715, 4.541064518000418104, -2.621784821874998173 ) ) ;
#46794=CARTESIAN_POINT ( 'NONE',  ( 15.90000000122903501, -2.886751345948125991, -5.000000000000000000 ) ) ;
#46795=CARTESIAN_POINT ( 'NONE',  ( 22.53750000000000142, -2.886751345948125991, -5.000000000000000000 ) ) ;
#46796=CARTESIAN_POINT ( 'NONE',  ( 29.69999999999999574, -4.330127018922190985, -2.500000000000001332 ) ) ;
#46797=CARTESIAN_POINT ( 'NONE',  ( 4.209375000614516971, 0.000000000000000000, 5.243569643749999010 ) ) ;
#46798=CARTESIAN_POINT ( 'NONE',  ( 9.571875000614518569, 3.027376345333611329, 5.243569643749999010 ) ) ;
#46799=CARTESIAN_POINT ( 'NONE',  ( 20.52187500061451786, -6.054752690667223547, -1.112240025338166033E-15 ) ) ;
#46800=CARTESIAN_POINT ( 'NONE',  ( 4.196151849995945149, -2.718880220196457476, -4.196151849995952254 ) ) ;
#46802=CARTESIAN_POINT ( 'NONE',  ( 29.65312500061451573, 4.541064518000418104, -2.621784821874998173 ) ) ;
#46803=CARTESIAN_POINT ( 'NONE',  ( 3.862500000000001155, 2.886751345948126879, 4.999999999999999112 ) ) ;
#46804=CARTESIAN_POINT ( 'NONE',  ( 5.259375000614518569, -4.541064518000417216, -2.621784821875001281 ) ) ;
#46805=CARTESIAN_POINT ( 'NONE',  ( 16.23750000000000071, -2.886751345948125991, -5.000000000000000000 ) ) ;
#46806=CARTESIAN_POINT ( 'NONE',  ( 13.41562500061451502, 3.027376345333613106, -5.243569643749998122 ) ) ;
#46809=CARTESIAN_POINT ( 'NONE',  ( 20.36250000122903359, -4.330127018922190985, -2.500000000000001332 ) ) ;
#46810=CARTESIAN_POINT ( 'NONE',  ( 0.8114860633430669434, 9.969066991719973458, 24.05167508342340454 ) ) ;
#46812=CARTESIAN_POINT ( 'NONE',  ( 6.778125000614518392, 4.541064518000418104, 2.621784821874999949 ) ) ;
#46813=CARTESIAN_POINT ( 'NONE',  ( 23.93437500061451573, 4.541064518000418104, 2.621784821874999949 ) ) ;
#46814=CARTESIAN_POINT ( 'NONE',  ( -4.243569643749997233, 19.44687500061451502, 32.45002607614398471 ) ) ;
#46815=CARTESIAN_POINT ( 'NONE',  ( 26.74687500061451573, -3.027376345333614438, 5.243569643749998122 ) ) ;
#46816=CARTESIAN_POINT ( 'NONE',  ( 6.487499999999999822, 5.773502691896255534, 3.535250795749688894E-16 ) ) ;
#46817=CARTESIAN_POINT ( 'NONE',  ( -3.999999999999999112, 14.26250000122903572, 30.00000000000000000 ) ) ;
#46818=CARTESIAN_POINT ( 'NONE',  ( 15.47812500061451679, -4.541064518000419881, 2.621784821874995952 ) ) ;
#46819=CARTESIAN_POINT ( 'NONE',  ( 7.050000001229036251, 5.773502691896255534, 3.535250795749688894E-16 ) ) ;
#46821=CARTESIAN_POINT ( 'NONE',  ( 18.08437500061451431, 4.541064518000418104, 2.621784821874999949 ) ) ;
#46822=CARTESIAN_POINT ( 'NONE',  ( 11.14687500061451608, -3.027376345333610441, -5.243569643749999898 ) ) ;
#46824=VERTEX_POINT ( 'NONE', #4331 ) ;
#46825=CARTESIAN_POINT ( 'NONE',  ( 11.87812500061451537, -4.541064518000419881, 2.621784821874995952 ) ) ;
#46826=CARTESIAN_POINT ( 'NONE',  ( 10.65000000000000036, 0.000000000000000000, 4.999999999999998224 ) ) ;
#46827=CARTESIAN_POINT ( 'NONE',  ( 24.48750000122903359, 6.123233995736764310E-16, -4.999999999999998224 ) ) ;
#46828=CARTESIAN_POINT ( 'NONE',  ( 13.09687500061451892, 6.054752690667223547, 3.707466751127219781E-16 ) ) ;
#46829=CARTESIAN_POINT ( 'NONE',  ( 13.82812500061451466, 6.421520780324663323E-16, -5.243569643749999010 ) ) ;
#46830=CARTESIAN_POINT ( 'NONE',  ( 1.071796769724491893, 18.78259618943233278, -26.00000000000000355 ) ) ;
#46831=CARTESIAN_POINT ( 'NONE',  ( 24.57187500061451502, -6.054752690667223547, -1.112240025338166033E-15 ) ) ;
#46832=CARTESIAN_POINT ( 'NONE',  ( 0.000000000000000000, 20.00000000000000000, 30.00000000000000000 ) ) ;
#46835=CARTESIAN_POINT ( 'NONE',  ( 9.001249775931846008E-16, 16.37187500061451573, -25.09994784771203058 ) ) ;
#46836=CARTESIAN_POINT ( 'NONE',  ( 15.49687500061451750, -3.027376345333614438, 5.243569643749998122 ) ) ;
#46837=CARTESIAN_POINT ( 'NONE',  ( 18.33750000122903501, 4.330127018922191873, 2.499999999999999556 ) ) ;
#46838=CARTESIAN_POINT ( 'NONE',  ( 13.20937500061451786, 0.000000000000000000, 5.243569643749999010 ) ) ;
#46839=CARTESIAN_POINT ( 'NONE',  ( -0.7368805616696193495, 9.859898480082234684, 25.82089837893477480 ) ) ;
#46840=CARTESIAN_POINT ( 'NONE',  ( 19.76250000122903216, 0.000000000000000000, 4.999999999999998224 ) ) ;
#46841=CARTESIAN_POINT ( 'NONE',  ( 15.44062500061451537, -3.027376345333614438, 5.243569643749998122 ) ) ;
#46843=VERTEX_POINT ( 'NONE', #66372 ) ;
#46844=CARTESIAN_POINT ( 'NONE',  ( 18.18750000000000000, 5.773502691896255534, 3.535250795749688894E-16 ) ) ;
#46845=CARTESIAN_POINT ( 'NONE',  ( -4.243569643749999898, 19.83125000061451715, 30.00000000000000000 ) ) ;
#46846=CARTESIAN_POINT ( 'NONE',  ( 13.09687500061451537, 6.054752690667223547, 3.707466751127219781E-16 ) ) ;
#46847=CARTESIAN_POINT ( 'NONE',  ( 3.022718161895720623, 3.982892879517589968, -3.221804244138950502 ) ) ;
#46848=CARTESIAN_POINT ( 'NONE',  ( 13.76250000122903394, 4.330127018922192761, -2.499999999999997780 ) ) ;
#46849=CARTESIAN_POINT ( 'NONE',  ( 19.80000000122903359, -2.886751345948129988, 4.999999999999997335 ) ) ;
#46850=CARTESIAN_POINT ( 'NONE',  ( 19.04062500061451146, -3.027376345333614438, 5.243569643749998122 ) ) ;
#46851=CARTESIAN_POINT ( 'NONE',  ( 23.61562500061451431, -6.054752690667223547, -1.112240025338166033E-15 ) ) ;
#46852=CARTESIAN_POINT ( 'NONE',  ( 3.740625000614516527, -3.027376345333614438, 5.243569643749998122 ) ) ;
#46853=CARTESIAN_POINT ( 'NONE',  ( 27.75000000000000000, 0.000000000000000000, 4.999999999999998224 ) ) ;
#46856=DIRECTION ( 'NONE',  ( 0.000000000000000000, 0.000000000000000000, -1.000000000000000000 ) ) ;
#46857=LINE ( 'NONE', #47215, #13425 ) ;
#46858=CARTESIAN_POINT ( 'NONE',  ( -3.000416591977282496E-16, 16.59687500061452070, -34.90005215228797653 ) ) ;
#46860=CARTESIAN_POINT ( 'NONE',  ( 2.775000001229033675, -5.773502691896255534, -1.060575238724906372E-15 ) ) ;
#46861=CARTESIAN_POINT ( 'NONE',  ( 4.912499999999999645, -5.773502691896255534, -1.060575238724906372E-15 ) ) ;
#46862=CARTESIAN_POINT ( 'NONE',  ( 3.709174336338540989, 3.352913023424228811, 4.031500572517469294 ) ) ;
#46863=CARTESIAN_POINT ( 'NONE',  ( 8.896875000614517859, -3.027376345333610441, -5.243569643749999898 ) ) ;
#46864=CARTESIAN_POINT ( 'NONE',  ( 28.19062500061451715, -3.027376345333610441, -5.243569643749999898 ) ) ;
#46865=FACE_OUTER_BOUND ( 'NONE', #54779, .T. ) ;
#46866=CARTESIAN_POINT ( 'NONE',  ( -5.678847837524354070, 8.233079231341507764, -31.97529239793390232 ) ) ;
#46867=CARTESIAN_POINT ( 'NONE',  ( 7.359375000614516438, 0.000000000000000000, 5.243569643749999010 ) ) ;
#46868=CARTESIAN_POINT ( 'NONE',  ( 10.80937500061451928, 4.541064518000418104, -2.621784821874998173 ) ) ;
#46869=CARTESIAN_POINT ( 'NONE',  ( 7.124999999999999112, -4.330127018922194537, 2.499999999999995559 ) ) ;
#46870=VECTOR ( 'NONE', #47042, 1000.000000000000000 ) ;
#46871=CARTESIAN_POINT ( 'NONE',  ( 4.243569643749999010, 15.56562500061459353, 27.54997392385601174 ) ) ;
#46872=CARTESIAN_POINT ( 'NONE',  ( 4.818692141996692158, -1.334243621178544226, 4.818692141997074074 ) ) ;
#46873=CARTESIAN_POINT ( 'NONE',  ( 6.187500000000002665, -2.886751345948129988, 4.999999999999997335 ) ) ;
#46875=CARTESIAN_POINT ( 'NONE',  ( 23.05312500061451431, 0.000000000000000000, 5.243569643749999010 ) ) ;
#46876=CARTESIAN_POINT ( 'NONE',  ( 13.94062500061451892, 6.054752690667223547, 3.707466751127219781E-16 ) ) ;
#46878=CARTESIAN_POINT ( 'NONE',  ( 8.559375000614515727, 4.541064518000418104, -2.621784821874998173 ) ) ;
#46879=CARTESIAN_POINT ( 'NONE',  ( 26.66250000000000142, 2.886751345948129099, -4.999999999999998224 ) ) ;
#46880=CARTESIAN_POINT ( 'NONE',  ( 22.80000000122903359, 5.773502691896255534, 3.535250795749688894E-16 ) ) ;
#46881=CARTESIAN_POINT ( 'NONE',  ( 11.36250000122903536, -4.330127018922190985, -2.500000000000001332 ) ) ;
#46882=CARTESIAN_POINT ( 'NONE',  ( 12.15937500061451892, 4.541064518000418104, -2.621784821874998173 ) ) ;
#46883=CARTESIAN_POINT ( 'NONE',  ( 27.08437500061451786, 4.541064518000418104, 2.621784821874999949 ) ) ;
#46884=CARTESIAN_POINT ( 'NONE',  ( 3.684375000614518836, 4.541064518000418104, 2.621784821874999949 ) ) ;
#46886=CARTESIAN_POINT ( 'NONE',  ( 18.94687500061451502, 6.054752690667223547, 3.707466751127219781E-16 ) ) ;
#46887=CARTESIAN_POINT ( 'NONE',  ( 11.55937500061451928, -4.541064518000417216, -2.621784821875001281 ) ) ;
#46889=CARTESIAN_POINT ( 'NONE',  ( 24.63749999999999574, -2.886751345948129988, 4.999999999999997335 ) ) ;
#46891=CARTESIAN_POINT ( 'NONE',  ( 2.121784821875001281, 12.35937500061451821, -26.32496088578401938 ) ) ;
#46893=CARTESIAN_POINT ( 'NONE',  ( 15.51562500061451644, -6.054752690667223547, -1.112240025338166033E-15 ) ) ;
#46894=CARTESIAN_POINT ( 'NONE',  ( 4.875000000000000888, -4.330127018922194537, 2.499999999999995559 ) ) ;
#46895=DIRECTION ( 'NONE',  ( 0.000000000000000000, 0.000000000000000000, -1.000000000000000000 ) ) ;
#46897=CARTESIAN_POINT ( 'NONE',  ( 13.83749999999999858, -2.886751345948129988, 4.999999999999997335 ) ) ;
#46898=CARTESIAN_POINT ( 'NONE',  ( 4.243569643749999898, 10.09062500061451928, 32.45002607614398471 ) ) ;
#46899=CARTESIAN_POINT ( 'NONE',  ( 13.31250000122903288, 4.330127018922192761, -2.499999999999997780 ) ) ;
#46900=CARTESIAN_POINT ( 'NONE',  ( 24.23437500061451644, 6.421520780324663323E-16, -5.243569643749999010 ) ) ;
#46901=ORIENTED_EDGE ( 'NONE', *, *, #40917, .F. ) ;
#46902=CARTESIAN_POINT ( 'NONE',  ( 18.89062500061451644, 6.054752690667223547, 3.707466751127219781E-16 ) ) ;
#46903=CARTESIAN_POINT ( 'NONE',  ( 4.453125000614517326, 4.541064518000418104, -2.621784821874998173 ) ) ;
#46904=CARTESIAN_POINT ( 'NONE',  ( 19.50937500061451857, 0.000000000000000000, 5.243569643749999010 ) ) ;
#46905=CARTESIAN_POINT ( 'NONE',  ( 5.325000000000000178, -4.330127018922194537, 2.499999999999995559 ) ) ;
#46906=CARTESIAN_POINT ( 'NONE',  ( 8.090625000614515727, 6.054752690667223547, 3.707466751127219781E-16 ) ) ;
#46907=CARTESIAN_POINT ( 'NONE',  ( 23.05312500061451431, 0.000000000000000000, 5.243569643749999010 ) ) ;
#46908=CARTESIAN_POINT ( 'NONE',  ( 4.243569643749999898, 15.97812500061451857, 30.00000000000000000 ) ) ;
#46909=CARTESIAN_POINT ( 'NONE',  ( 19.05000000122903359, -2.886751345948125991, -5.000000000000000000 ) ) ;
#46911=CARTESIAN_POINT ( 'NONE',  ( 10.04062500061451679, -3.027376345333614438, 5.243569643749998122 ) ) ;
#46912=CARTESIAN_POINT ( 'NONE',  ( 3.121875000614518836, 3.027376345333613106, -5.243569643749998122 ) ) ;
#46913=CARTESIAN_POINT ( 'NONE',  ( 28.26562500061451289, 3.027376345333613106, -5.243569643749998122 ) ) ;
#46914=ADVANCED_FACE ( 'NONE', ( #38286, #60814, #55293 ), #4687, .F. ) ;
#46915=CARTESIAN_POINT ( 'NONE',  ( 24.42187500061451999, 3.027376345333611329, 5.243569643749999010 ) ) ;
#46916=CARTESIAN_POINT ( 'NONE',  ( 15.29062500061451679, 6.054752690667223547, 3.707466751127219781E-16 ) ) ;
#46917=CARTESIAN_POINT ( 'NONE',  ( 25.76250000122903216, -4.330127018922190985, -2.500000000000001332 ) ) ;
#46918=CARTESIAN_POINT ( 'NONE',  ( 25.07812500061451644, 6.421520780324663323E-16, -5.243569643749999010 ) ) ;
#46919=CARTESIAN_POINT ( 'NONE',  ( 18.38437500061451857, 6.421520780324663323E-16, -5.243569643749999010 ) ) ;
#46920=CARTESIAN_POINT ( 'NONE',  ( 14.72812500061451679, 6.421520780324663323E-16, -5.243569643749999010 ) ) ;
#46921=CARTESIAN_POINT ( 'NONE',  ( -2.121784821874996840, 17.68437500061451928, 33.67503911421598417 ) ) ;
#46922=CARTESIAN_POINT ( 'NONE',  ( 23.16562500061451502, -6.054752690667223547, -1.112240025338166033E-15 ) ) ;
#46923=CARTESIAN_POINT ( 'NONE',  ( 2.662500001229036073, 0.000000000000000000, 4.999999999999998224 ) ) ;
#46924=VERTEX_POINT ( 'NONE', #12031 ) ;
#46925=CARTESIAN_POINT ( 'NONE',  ( 24.60000000000000142, 0.000000000000000000, 4.999999999999998224 ) ) ;
#46926=CARTESIAN_POINT ( 'NONE',  ( -3.999999999999999556, 10.96250000000000213, -32.30940107675850470 ) ) ;
#46928=CARTESIAN_POINT ( 'NONE',  ( 28.67812500061451431, 6.421520780324663323E-16, -5.243569643749999010 ) ) ;
#46929=CARTESIAN_POINT ( 'NONE',  ( 7.490625000614516082, -3.027376345333610441, -5.243569643749999898 ) ) ;
#46930=CARTESIAN_POINT ( 'NONE',  ( 22.50000000122903288, -2.886751345948129988, 4.999999999999997335 ) ) ;
#46932=CARTESIAN_POINT ( 'NONE',  ( 27.21562500061451928, -6.054752690667223547, -1.112240025338166033E-15 ) ) ;
#46933=CARTESIAN_POINT ( 'NONE',  ( 26.02499999999999858, -4.330127018922194537, 2.499999999999995559 ) ) ;
#46935=CARTESIAN_POINT ( 'NONE',  ( -2.828200636599751609E-16, 16.40000000122903501, -34.61880215351700230 ) ) ;
#46936=CARTESIAN_POINT ( 'NONE',  ( -1.071796769724491005, 12.37009619066136956, 26.00000000000000355 ) ) ;
#46937=CARTESIAN_POINT ( 'NONE',  ( 10.52812500061451750, -4.541064518000419881, 2.621784821874995952 ) ) ;
#46938=( BOUNDED_CURVE ( )  B_SPLINE_CURVE ( 3, ( #31359, #55358, #10651, #45003 ),
 .UNSPECIFIED., .F., .F. ) 
 B_SPLINE_CURVE_WITH_KNOTS ( ( 4, 4 ),
 ( 0.5446367559021773053, 0.5855140179436351122 ),
 .UNSPECIFIED. ) 
 CURVE ( )  GEOMETRIC_REPRESENTATION_ITEM ( )  RATIONAL_B_SPLINE_CURVE ( ( 1.000000000000000000, 0.9998607589679524565, 0.9998607589679524565, 1.000000000000000000 ) ) 
 REPRESENTATION_ITEM ( '' )  );
#46939=ORIENTED_EDGE ( 'NONE', *, *, #22648, .T. ) ;
#46940=CARTESIAN_POINT ( 'NONE',  ( 24.96562500061451573, -6.054752690667223547, -1.112240025338166033E-15 ) ) ;
#46941=CARTESIAN_POINT ( 'NONE',  ( 7.265625000614516438, 3.027376345333611329, 5.243569643749999010 ) ) ;
#46942=CARTESIAN_POINT ( 'NONE',  ( 3.103125000614517237, 4.541064518000418104, -2.621784821874998173 ) ) ;
#46944=CARTESIAN_POINT ( 'NONE',  ( 12.97499999999999964, -4.330127018922194537, 2.499999999999995559 ) ) ;
#46945=CARTESIAN_POINT ( 'NONE',  ( 14.02499999999999858, 6.123233995736764310E-16, -4.999999999999998224 ) ) ;
#46946=CARTESIAN_POINT ( 'NONE',  ( 12.75937500061451857, 0.000000000000000000, 5.243569643749999010 ) ) ;
#46947=CARTESIAN_POINT ( 'NONE',  ( 9.637500001229033941, 6.123233995736764310E-16, -4.999999999999998224 ) ) ;
#46948=CARTESIAN_POINT ( 'NONE',  ( 17.67187500061451644, 3.027376345333611329, 5.243569643749999010 ) ) ;
#46950=CARTESIAN_POINT ( 'NONE',  ( 8.821875000614518569, -6.054752690667223547, -1.112240025338166033E-15 ) ) ;
#46951=CARTESIAN_POINT ( 'NONE',  ( 4.243569643749999898, 10.54062500061451679, -27.54997392385601529 ) ) ;
#46952=DIRECTION ( 'NONE',  ( -1.000000000000000000, -0.000000000000000000, -0.000000000000000000 ) ) ;
#46955=EDGE_CURVE ( 'NONE', #41820, #68271, #62187, .T. ) ;
#46956=CARTESIAN_POINT ( 'NONE',  ( 23.57812500061451289, -4.541064518000419881, 2.621784821874995952 ) ) ;
#46958=CARTESIAN_POINT ( 'NONE',  ( 27.34687500061451360, -3.027376345333610441, -5.243569643749999898 ) ) ;
#46959=CARTESIAN_POINT ( 'NONE',  ( 20.96250000000000213, 2.886751345948126879, 4.999999999999999112 ) ) ;
#46960=CARTESIAN_POINT ( 'NONE',  ( 6.590625000614518392, -3.027376345333610441, -5.243569643749999898 ) ) ;
#46962=CARTESIAN_POINT ( 'NONE',  ( 16.39687500061451786, -3.027376345333614438, 5.243569643749998122 ) ) ;
#46964=CARTESIAN_POINT ( 'NONE',  ( 29.02500000122903145, 2.886751345948129099, -4.999999999999998224 ) ) ;
#46965=CARTESIAN_POINT ( 'NONE',  ( 7.509375000614517681, -4.541064518000417216, -2.621784821875001281 ) ) ;
#46967=CARTESIAN_POINT ( 'NONE',  ( 19.50937500061451857, 0.000000000000000000, 5.243569643749999010 ) ) ;
#46969=CARTESIAN_POINT ( 'NONE',  ( 26.21249999999999858, 2.886751345948129099, -4.999999999999998224 ) ) ;
#46970=CARTESIAN_POINT ( 'NONE',  ( 29.07187500061451502, -6.054752690667223547, -1.112240025338166033E-15 ) ) ;
#46973=EDGE_LOOP ( 'NONE', ( #27443, #56593, #33299, #39589 ) ) ;
#46974=CARTESIAN_POINT ( 'NONE',  ( 10.98750000000000071, 5.773502691896255534, 3.535250795749688894E-16 ) ) ;
#46976=CARTESIAN_POINT ( 'NONE',  ( 21.47812500061451502, 6.421520780324663323E-16, -5.243569643749999010 ) ) ;
#46977=CARTESIAN_POINT ( 'NONE',  ( 14.28750000000000142, -2.886751345948129988, 4.999999999999997335 ) ) ;
#46978=CARTESIAN_POINT ( 'NONE',  ( 8.550000001229031810, -2.886751345948129988, 4.999999999999997335 ) ) ;
#46979=CARTESIAN_POINT ( 'NONE',  ( 6.328125000614515550, 4.541064518000418104, 2.621784821874999949 ) ) ;
#46980=CARTESIAN_POINT ( 'NONE',  ( 20.77500000000000213, 6.123233995736764310E-16, -4.999999999999998224 ) ) ;
#46981=CARTESIAN_POINT ( 'NONE',  ( 21.81562500061451004, -6.054752690667223547, -1.112240025338166033E-15 ) ) ;
#46982=CARTESIAN_POINT ( 'NONE',  ( 12.11250000000000249, -5.773502691896255534, -1.060575238724906372E-15 ) ) ;
#46983=CARTESIAN_POINT ( 'NONE',  ( 24.60000000122903430, 5.773502691896255534, 3.535250795749688894E-16 ) ) ;
#46985=CARTESIAN_POINT ( 'NONE',  ( 5.962500000000002132, 2.886751345948129099, -4.999999999999998224 ) ) ;
#46986=ORIENTED_EDGE ( 'NONE', *, *, #60362, .F. ) ;
#46987=CARTESIAN_POINT ( 'NONE',  ( 22.45312500061451644, 4.541064518000418104, -2.621784821874998173 ) ) ;
#46988=CARTESIAN_POINT ( 'NONE',  ( 26.76562500061451644, -6.054752690667223547, -1.112240025338166033E-15 ) ) ;
#46989=CARTESIAN_POINT ( 'NONE',  ( 27.45937500061451786, 4.541064518000418104, -2.621784821874998173 ) ) ;
#46990=CARTESIAN_POINT ( 'NONE',  ( 14.80312500061451608, 4.541064518000418104, -2.621784821874998173 ) ) ;
#46992=CARTESIAN_POINT ( 'NONE',  ( 26.25000000122903288, -2.886751345948125991, -5.000000000000000000 ) ) ;
#46994=CARTESIAN_POINT ( 'NONE',  ( 16.07812500061451289, 6.421520780324663323E-16, -5.243569643749999010 ) ) ;
#46995=CARTESIAN_POINT ( 'NONE',  ( 4.000000000000000000, 14.45000000122903572, -27.69059892324149885 ) ) ;
#46996=EDGE_CURVE ( 'NONE', #48258, #39103, #30764, .T. ) ;
#46997=CARTESIAN_POINT ( 'NONE',  ( 3.900000001229034563, 5.773502691896255534, 3.535250795749688894E-16 ) ) ;
#46998=CARTESIAN_POINT ( 'NONE',  ( 10.88437500061451679, 4.541064518000418104, 2.621784821874999949 ) ) ;
#46999=CARTESIAN_POINT ( 'NONE',  ( 8.821875000614518569, -6.054752690667223547, -1.112240025338166033E-15 ) ) ;
#47000=CARTESIAN_POINT ( 'NONE',  ( 18.53437500061451715, 4.541064518000418104, 2.621784821874999949 ) ) ;
#47001=VERTEX_POINT ( 'NONE', #16840 ) ;
#47002=CARTESIAN_POINT ( 'NONE',  ( -4.872631645816655421, 8.733424155075979911, 26.49367970277769047 ) ) ;
#47003=CARTESIAN_POINT ( 'NONE',  ( 23.95312500061451289, 0.000000000000000000, 5.243569643749999010 ) ) ;
#47004=CARTESIAN_POINT ( 'NONE',  ( 18.12187500061451573, 3.027376345333611329, 5.243569643749999010 ) ) ;
#47005=CARTESIAN_POINT ( 'NONE',  ( 21.51562500061451644, 3.027376345333613106, -5.243569643749998122 ) ) ;
#47006=CARTESIAN_POINT ( 'NONE',  ( 30.00000000000000000, 6.123233995736764310E-16, -4.999999999999998224 ) ) ;
#47007=CARTESIAN_POINT ( 'NONE',  ( 3.999999999999999112, 13.92500000000000071, 30.00000000000000000 ) ) ;
#47008=CARTESIAN_POINT ( 'NONE',  ( 29.12812500061451715, 6.421520780324663323E-16, -5.243569643749999010 ) ) ;
#47009=CARTESIAN_POINT ( 'NONE',  ( 9.600000001229034297, -2.886751345948125991, -5.000000000000000000 ) ) ;
#47010=VERTEX_POINT ( 'NONE', #39765 ) ;
#47011=CARTESIAN_POINT ( 'NONE',  ( 5.512500001229033941, -4.330127018922190985, -2.500000000000001332 ) ) ;
#47012=CARTESIAN_POINT ( 'NONE',  ( -2.828200636599751609E-16, 19.43750000000000000, -34.61880215351700230 ) ) ;
#47013=CARTESIAN_POINT ( 'NONE',  ( 27.48750000122903359, -4.330127018922194537, 2.499999999999995559 ) ) ;
#47015=CARTESIAN_POINT ( 'NONE',  ( 9.946875000614516793, 6.054752690667223547, 3.707466751127219781E-16 ) ) ;
#47016=CARTESIAN_POINT ( 'NONE',  ( 1.626862140677534273E-15, 9.875000001229034652, 34.00000000000000000 ) ) ;
#47017=CARTESIAN_POINT ( 'NONE',  ( 14.05312500061451431, 0.000000000000000000, 5.243569643749999010 ) ) ;
#47018=CARTESIAN_POINT ( 'NONE',  ( 10.35937500061451644, 4.541064518000418104, -2.621784821874998173 ) ) ;
#47019=CARTESIAN_POINT ( 'NONE',  ( 29.25000000122903288, -2.886751345948129988, 4.999999999999997335 ) ) ;
#47020=CARTESIAN_POINT ( 'NONE',  ( 18.75937500061451857, -4.541064518000417216, -2.621784821875001281 ) ) ;
#47021=CARTESIAN_POINT ( 'NONE',  ( 7.546875000614517326, -3.027376345333610441, -5.243569643749999898 ) ) ;
#47022=DIRECTION ( 'NONE',  ( -1.000000000000000000, -0.000000000000000000, -0.000000000000000000 ) ) ;
#47023=CARTESIAN_POINT ( 'NONE',  ( 8.878125000614515372, 6.421520780324663323E-16, -5.243569643749999010 ) ) ;
#47024=CARTESIAN_POINT ( 'NONE',  ( 16.52812500061451573, 6.421520780324663323E-16, -5.243569643749999010 ) ) ;
#47025=ORIENTED_EDGE ( 'NONE', *, *, #561, .F. ) ;
#47026=CARTESIAN_POINT ( 'NONE',  ( 15.74062500061451608, 6.054752690667223547, 3.707466751127219781E-16 ) ) ;
#47027=CARTESIAN_POINT ( 'NONE',  ( 11.46562500061451573, -6.054752690667223547, -1.112240025338166033E-15 ) ) ;
#47029=CARTESIAN_POINT ( 'NONE',  ( 11.55000000000000071, 0.000000000000000000, 4.999999999999998224 ) ) ;
#47030=CARTESIAN_POINT ( 'NONE',  ( 7.275000001229035007, -5.773502691896255534, -1.060575238724906372E-15 ) ) ;
#47031=B_SPLINE_CURVE_WITH_KNOTS ( 'NONE', 3,
 ( #9657, #14086, #32191, #65066, #8927, #4127, #36626, #66169, #42907, #14821 ),
 .UNSPECIFIED., .F., .F.,
 ( 4, 3, 3, 4 ),
 ( 8.949075925690993792E-17, 7.861233265730306976E-05, 0.0001572246084809364789, 0.0003125746657383838330 ),
 .UNSPECIFIED. ) ;
#47032=CARTESIAN_POINT ( 'NONE',  ( 14.22187500061451537, -6.054752690667223547, -1.112240025338166033E-15 ) ) ;
#47033=CARTESIAN_POINT ( 'NONE',  ( 17.28750000122903430, 6.123233995736764310E-16, -4.999999999999998224 ) ) ;
#47035=CARTESIAN_POINT ( 'NONE',  ( 9.001249775931846008E-16, 19.01562500061451644, -25.09994784771203058 ) ) ;
#47037=FACE_OUTER_BOUND ( 'NONE', #9810, .T. ) ;
#47038=CARTESIAN_POINT ( 'NONE',  ( 1.999999999999998668, 10.96250000122903501, -33.46410161513775705 ) ) ;
#47039=CARTESIAN_POINT ( 'NONE',  ( 3.927649849665248105, 3.094731086393085917, 3.927649849665248105 ) ) ;
#47040=CARTESIAN_POINT ( 'NONE',  ( 18.08437500061451431, 4.541064518000418104, 2.621784821874999949 ) ) ;
#47041=EDGE_CURVE ( 'NONE', #45611, #66904, #55809, .T. ) ;
#47042=DIRECTION ( 'NONE',  ( -1.000000000000000000, -0.000000000000000000, -0.000000000000000000 ) ) ;
#47043=CARTESIAN_POINT ( 'NONE',  ( 15.17812500061451608, 6.421520780324663323E-16, -5.243569643749999010 ) ) ;
#47045=LINE ( 'NONE', #34498, #37744 ) ;
#47046=CARTESIAN_POINT ( 'NONE',  ( 24.90937500061451715, 0.000000000000000000, 5.243569643749999010 ) ) ;
#47048=CARTESIAN_POINT ( 'NONE',  ( 10.19062500061451892, -3.027376345333610441, -5.243569643749999898 ) ) ;
#47049=CARTESIAN_POINT ( 'NONE',  ( 14.59687500061452070, -3.027376345333614438, 5.243569643749998122 ) ) ;
#47051=CARTESIAN_POINT ( 'NONE',  ( 27.27187500061451431, -6.054752690667223547, -1.112240025338166033E-15 ) ) ;
#47052=CARTESIAN_POINT ( 'NONE',  ( 27.14062500061451644, -3.027376345333614438, 5.243569643749998122 ) ) ;
#47053=CARTESIAN_POINT ( 'NONE',  ( 20.42812500061451431, -4.541064518000419881, 2.621784821874995952 ) ) ;
#47054=CARTESIAN_POINT ( 'NONE',  ( 18.86249999999999716, -5.773502691896255534, -1.060575238724906372E-15 ) ) ;
#47056=CARTESIAN_POINT ( 'NONE',  ( 10.68750000000000000, -2.886751345948129988, 4.999999999999997335 ) ) ;
#47057=CARTESIAN_POINT ( 'NONE',  ( 19.53750000122903430, 6.123233995736764310E-16, -4.999999999999998224 ) ) ;
#47058=CARTESIAN_POINT ( 'NONE',  ( -3.999999999999999112, 10.10000000000000142, 30.00000000000000000 ) ) ;
#47060=ORIENTED_EDGE ( 'NONE', *, *, #42578, .F. ) ;
#47061=CARTESIAN_POINT ( 'NONE',  ( 18.67500000000000071, 4.330127018922191873, 2.499999999999999556 ) ) ;
#47062=CARTESIAN_POINT ( 'NONE',  ( 22.27499999999999858, 4.330127018922191873, 2.499999999999999556 ) ) ;
#47063=CARTESIAN_POINT ( 'NONE',  ( 18.30937500061451928, -4.541064518000417216, -2.621784821875001281 ) ) ;
#47064=CARTESIAN_POINT ( 'NONE',  ( 13.30312500061451786, -4.541064518000417216, -2.621784821875001281 ) ) ;
#47067=CARTESIAN_POINT ( 'NONE',  ( 4.753125000614515372, -4.541064518000417216, -2.621784821875001281 ) ) ;
#47068=CARTESIAN_POINT ( 'NONE',  ( 3.242103111326755549, 4.229119190475764789, 3.162089978331414031 ) ) ;
#47069=CARTESIAN_POINT ( 'NONE',  ( 13.35000000000000142, 0.000000000000000000, 4.999999999999998224 ) ) ;
#47071=CARTESIAN_POINT ( 'NONE',  ( 9.001249775931846008E-16, 15.86562500061451608, 34.90005215228797653 ) ) ;
#47072=CARTESIAN_POINT ( 'NONE',  ( 28.11562500061451431, -6.054752690667223547, -1.112240025338166033E-15 ) ) ;
#47075=CARTESIAN_POINT ( 'NONE',  ( 24.12187500061451217, -6.054752690667223547, -1.112240025338166033E-15 ) ) ;
#47076=VERTEX_POINT ( 'NONE', #28660 ) ;
#47077=CARTESIAN_POINT ( 'NONE',  ( 22.37812500061451360, 6.421520780324663323E-16, -5.243569643749999010 ) ) ;
#47078=CARTESIAN_POINT ( 'NONE',  ( 22.95937500061451431, 4.541064518000418104, -2.621784821874998173 ) ) ;
#47079=CARTESIAN_POINT ( 'NONE',  ( -4.243569643749999898, 15.75312500061459531, -30.00000000000000000 ) ) ;
#47080=CARTESIAN_POINT ( 'NONE',  ( 7.415625000614516793, -6.054752690667223547, -1.112240025338166033E-15 ) ) ;
#47081=CARTESIAN_POINT ( 'NONE',  ( 3.825000000000001954, 4.330127018922191873, 2.499999999999999556 ) ) ;
#47082=CARTESIAN_POINT ( 'NONE',  ( 24.81562500061451715, 3.027376345333611329, 5.243569643749999010 ) ) ;
#47085=( BOUNDED_CURVE ( )  B_SPLINE_CURVE ( 2, ( #57351, #11934, #51462, #34459, #51102, #18174, #40743 ),
 .UNSPECIFIED., .F., .F. ) 
 B_SPLINE_CURVE_WITH_KNOTS ( ( 3, 2, 2, 3 ),
 ( 0.1000000000000000611, 0.1027777777777778151, 0.1055555555555555969, 0.1083333333333333648 ),
 .UNSPECIFIED. ) 
 CURVE ( )  GEOMETRIC_REPRESENTATION_ITEM ( )  RATIONAL_B_SPLINE_CURVE ( ( 0.9999999999999973355, 0.8660254037844413721, 1.000000000000000000, 0.8660254037844387076, 1.000000000000000000, 0.8660254037844373753, 1.000000000000001332 ) ) 
 REPRESENTATION_ITEM ( '' )  );
#47086=CARTESIAN_POINT ( 'NONE',  ( 17.97187500061451715, 3.027376345333613106, -5.243569643749998122 ) ) ;
#47087=CARTESIAN_POINT ( 'NONE',  ( 26.03437500061451715, 6.421520780324663323E-16, -5.243569643749999010 ) ) ;
#47088=CARTESIAN_POINT ( 'NONE',  ( -2.121784821874996840, 17.68437500061451928, 33.67503911421598417 ) ) ;
#47089=CARTESIAN_POINT ( 'NONE',  ( 6.440625000614517148, -3.027376345333614438, 5.243569643749998122 ) ) ;
#47090=EDGE_CURVE ( 'NONE', #38159, #47076, #15670, .T. ) ;
#47091=CARTESIAN_POINT ( 'NONE',  ( 4.246875000614519280, -3.027376345333614438, 5.243569643749998122 ) ) ;
#47092=CARTESIAN_POINT ( 'NONE',  ( 4.184734259358962483, 3.742548387690015854, -3.517716042735904658 ) ) ;
#47093=CARTESIAN_POINT ( 'NONE',  ( 5.353125000614515905, 4.541064518000418104, -2.621784821874998173 ) ) ;
#47094=CARTESIAN_POINT ( 'NONE',  ( 9.571875000614518569, 3.027376345333611329, 5.243569643749999010 ) ) ;
#47096=CARTESIAN_POINT ( 'NONE',  ( 16.20000000122903216, -2.886751345948129988, 4.999999999999997335 ) ) ;
#47097=CARTESIAN_POINT ( 'NONE',  ( 3.421875000614516882, -6.054752690667223547, -1.112240025338166033E-15 ) ) ;
#47098=CARTESIAN_POINT ( 'NONE',  ( 7.940625000614518036, -3.027376345333610441, -5.243569643749999898 ) ) ;
#47101=CARTESIAN_POINT ( 'NONE',  ( 16.99687500061451573, -3.027376345333610441, -5.243569643749999898 ) ) ;
#47102=CARTESIAN_POINT ( 'NONE',  ( 1.999999999999998668, 17.71250000122903501, 26.53589838486224650 ) ) ;
#47103=ORIENTED_EDGE ( 'NONE', *, *, #798, .T. ) ;
#47104=CARTESIAN_POINT ( 'NONE',  ( 25.26562500061451289, 3.027376345333611329, 5.243569643749999010 ) ) ;
#47105=CARTESIAN_POINT ( 'NONE',  ( 9.965625000614517504, 3.027376345333611329, 5.243569643749999010 ) ) ;
#47106=CARTESIAN_POINT ( 'NONE',  ( 28.02187500061451431, 3.027376345333611329, 5.243569643749999010 ) ) ;
#47107=CARTESIAN_POINT ( 'NONE',  ( 11.09062500061451573, -3.027376345333610441, -5.243569643749999898 ) ) ;
#47108=CARTESIAN_POINT ( 'NONE',  ( 3.450000001229035718, 5.773502691896255534, 3.535250795749688401E-16 ) ) ;
#47109=CARTESIAN_POINT ( 'NONE',  ( 9.750000001229032875, 5.773502691896255534, 3.535250795749688894E-16 ) ) ;
#47110=CARTESIAN_POINT ( 'NONE',  ( 23.99062500061451786, -3.027376345333614438, 5.243569643749998122 ) ) ;
#47111=CARTESIAN_POINT ( 'NONE',  ( -2.121784821874996840, 13.12812500061451715, -26.32496088578401583 ) ) ;
#47112=CARTESIAN_POINT ( 'NONE',  ( 13.23750000122903359, 6.123233995736764310E-16, -4.999999999999998224 ) ) ;
#47113=CARTESIAN_POINT ( 'NONE',  ( 21.74062500061451431, -3.027376345333614438, 5.243569643749998122 ) ) ;
#47114=CARTESIAN_POINT ( 'NONE',  ( 17.95312500061451644, 4.541064518000418104, -2.621784821874998173 ) ) ;
#47116=CARTESIAN_POINT ( 'NONE',  ( 18.75000000000000000, 0.000000000000000000, 4.999999999999998224 ) ) ;
#47117=CARTESIAN_POINT ( 'NONE',  ( 14.10000000122903252, -2.886751345948125991, -5.000000000000000000 ) ) ;
#47118=CARTESIAN_POINT ( 'NONE',  ( 10.60312500061451679, -4.541064518000417216, -2.621784821875001281 ) ) ;
#47119=CARTESIAN_POINT ( 'NONE',  ( 14.39062500061451821, 6.054752690667223547, 3.707466751127219781E-16 ) ) ;
#47120=CARTESIAN_POINT ( 'NONE',  ( 25.38750000122903216, 6.123233995736764310E-16, -4.999999999999998224 ) ) ;
#47121=CARTESIAN_POINT ( 'NONE',  ( 21.94687500061451857, -3.027376345333610441, -5.243569643749999898 ) ) ;
#47122=CARTESIAN_POINT ( 'NONE',  ( 20.97187500061451715, -6.054752690667223547, -1.112240025338166033E-15 ) ) ;
#47124=CARTESIAN_POINT ( 'NONE',  ( 6.862500001229034474, -4.330127018922190985, -2.500000000000001332 ) ) ;
#47125=( BOUNDED_CURVE ( )  B_SPLINE_CURVE ( 2, ( #12700, #57758, #7166, #18594, #29695, #52233, #1637, #69232, #63667 ),
 .UNSPECIFIED., .F., .F. ) 
 B_SPLINE_CURVE_WITH_KNOTS ( ( 3, 2, 2, 2, 3 ),
 ( 0.5108695652173913526, 0.5144927536231883591, 0.5217391304347825942, 0.5289855072463768293, 0.5326086956521739468 ),
 .UNSPECIFIED. ) 
 CURVE ( )  GEOMETRIC_REPRESENTATION_ITEM ( )  RATIONAL_B_SPLINE_CURVE ( ( 0.9330127018922192983, 0.9330127018922202975, 1.000000000000000000, 0.8660254037844387076, 1.000000000000000000, 0.8660254037844387076, 1.000000000000000000, 0.9330127018922194093, 0.9330127018922194093 ) ) 
 REPRESENTATION_ITEM ( '' )  );
#47126=CARTESIAN_POINT ( 'NONE',  ( 6.309375000614517504, 4.541064518000418104, -2.621784821874998173 ) ) ;
#47127=CARTESIAN_POINT ( 'NONE',  ( 26.10937500061451644, 4.541064518000418104, -2.621784821874998173 ) ) ;
#47128=( BOUNDED_CURVE ( )  B_SPLINE_CURVE ( 2, ( #58588, #54525, #14621, #30531, #31630, #20156, #42347, #59312, #43077 ),
 .UNSPECIFIED., .F., .F. ) 
 B_SPLINE_CURVE_WITH_KNOTS ( ( 3, 2, 2, 2, 3 ),
 ( 0.5543478260869565410, 0.5579710144927536586, 0.5652173913043477826, 0.5724637681159420177, 0.5760869565217391353 ),
 .UNSPECIFIED. ) 
 CURVE ( )  GEOMETRIC_REPRESENTATION_ITEM ( )  RATIONAL_B_SPLINE_CURVE ( ( 0.9330127018922194093, 0.9330127018922194093, 1.000000000000000000, 0.8660254037844387076, 1.000000000000000000, 0.8660254037844387076, 1.000000000000000000, 0.9330127018922194093, 0.9330127018922194093 ) ) 
 REPRESENTATION_ITEM ( '' )  );
#47129=CARTESIAN_POINT ( 'NONE',  ( 15.33750000122903323, -4.330127018922194537, 2.499999999999995559 ) ) ;
#47130=CARTESIAN_POINT ( 'NONE',  ( 21.32812500061451644, -4.541064518000419881, 2.621784821874995952 ) ) ;
#47131=CARTESIAN_POINT ( 'NONE',  ( 25.84687500061451360, -3.027376345333614438, 5.243569643749998122 ) ) ;
#47134=DIRECTION ( 'NONE',  ( -0.000000000000000000, -1.000000000000000000, -0.000000000000000000 ) ) ;
#47135=CARTESIAN_POINT ( 'NONE',  ( 8.484375000614518214, 6.421520780324663323E-16, -5.243569643749999010 ) ) ;
#47136=CARTESIAN_POINT ( 'NONE',  ( 18.02812500061451573, 4.541064518000418104, 2.621784821874999949 ) ) ;
#47138=CYLINDRICAL_SURFACE ( 'NONE', #41889, 4.999999999999998224 ) ;
#47139=CARTESIAN_POINT ( 'NONE',  ( 26.65312500061451573, 0.000000000000000000, 5.243569643749999010 ) ) ;
#47140=CARTESIAN_POINT ( 'NONE',  ( 4.321875000614517681, -6.054752690667223547, -1.112240025338166033E-15 ) ) ;
#47142=CARTESIAN_POINT ( 'NONE',  ( 3.988952146040426694, 3.968976988887717994, -3.612669488674732587 ) ) ;
#47143=CARTESIAN_POINT ( 'NONE',  ( 17.92500000000000071, -4.330127018922194537, 2.499999999999995559 ) ) ;
#47144=CARTESIAN_POINT ( 'NONE',  ( 20.50312500061451715, -4.541064518000417216, -2.621784821875001281 ) ) ;
#47146=CARTESIAN_POINT ( 'NONE',  ( 25.87500000000000000, 4.330127018922191873, 2.499999999999999556 ) ) ;
#47147=CARTESIAN_POINT ( 'NONE',  ( 25.69687500061451502, 6.054752690667223547, 3.707466751127219781E-16 ) ) ;
#47148=( BOUNDED_CURVE ( )  B_SPLINE_CURVE ( 2, ( #72513, #61062, #60316, #21164, #66240, #37796, #27826 ),
 .UNSPECIFIED., .F., .F. ) 
 B_SPLINE_CURVE_WITH_KNOTS ( ( 3, 2, 2, 3 ),
 ( 0.1333333333333333037, 0.1361111111111110716, 0.1388888888888888673, 0.1416666666666666352 ),
 .UNSPECIFIED. ) 
 CURVE ( )  GEOMETRIC_REPRESENTATION_ITEM ( )  RATIONAL_B_SPLINE_CURVE ( ( 1.000000000000001332, 0.8660254037844373753, 1.000000000000000000, 0.8660254037844387076, 1.000000000000000000, 0.8660254037844400399, 0.9999999999999986677 ) ) 
 REPRESENTATION_ITEM ( '' )  );
#47149=EDGE_LOOP ( 'NONE', ( #47644, #35617, #5656, #4384 ) ) ;
#47150=CARTESIAN_POINT ( 'NONE',  ( 12.89062500061451821, -3.027376345333610441, -5.243569643749999898 ) ) ;
#47151=CARTESIAN_POINT ( 'NONE',  ( 4.828125000614518214, 6.421520780324663323E-16, -5.243569643749999010 ) ) ;
#47153=CARTESIAN_POINT ( 'NONE',  ( 29.80312500061451431, 0.000000000000000000, 5.243569643749999010 ) ) ;
#47154=CARTESIAN_POINT ( 'NONE',  ( 14.62500000122903288, 2.886751345948129099, -4.999999999999998224 ) ) ;
#47155=CARTESIAN_POINT ( 'NONE',  ( 19.27500000000000213, -4.330127018922194537, 2.499999999999995559 ) ) ;
#47156=CARTESIAN_POINT ( 'NONE',  ( 28.80000000000000071, -4.330127018922190985, -2.500000000000001332 ) ) ;
#47157=CARTESIAN_POINT ( 'NONE',  ( 4.284375000614518925, -4.541064518000419881, 2.621784821874995952 ) ) ;
#47158=CARTESIAN_POINT ( 'NONE',  ( 8.746875000614515727, -3.027376345333614438, 5.243569643749998122 ) ) ;
#47159=CARTESIAN_POINT ( 'NONE',  ( 19.84687500061451360, 6.054752690667223547, 3.707466751127219781E-16 ) ) ;
#47160=CARTESIAN_POINT ( 'NONE',  ( -3.999999999999999112, 17.30000000000000071, -30.00000000000000000 ) ) ;
#47161=ORIENTED_EDGE ( 'NONE', *, *, #65919, .T. ) ;
#47162=CARTESIAN_POINT ( 'NONE',  ( 28.34062500061451928, 6.054752690667223547, 3.707466751127219781E-16 ) ) ;
#47163=CARTESIAN_POINT ( 'NONE',  ( 29.14687500061451075, -3.027376345333610441, -5.243569643749999898 ) ) ;
#47164=CARTESIAN_POINT ( 'NONE',  ( 4.771875000614516971, -6.054752690667223547, -1.112240025338166033E-15 ) ) ;
#47165=CARTESIAN_POINT ( 'NONE',  ( 16.76249999999999929, 2.886751345948129099, -4.999999999999998224 ) ) ;
#47166=CARTESIAN_POINT ( 'NONE',  ( 12.81562500061451537, -6.054752690667223547, -1.112240025338166033E-15 ) ) ;
#47168=CARTESIAN_POINT ( 'NONE',  ( 3.975000000000002753, -4.330127018922194537, 2.499999999999995559 ) ) ;
#47169=CARTESIAN_POINT ( 'NONE',  ( 19.23750000122903714, 4.330127018922191873, 2.499999999999999556 ) ) ;
#47172=CARTESIAN_POINT ( 'NONE',  ( 6.965625000614518392, -6.054752690667223547, -1.112240025338166033E-15 ) ) ;
#47173=CARTESIAN_POINT ( 'NONE',  ( 24.00937500061451502, 0.000000000000000000, 5.243569643749999010 ) ) ;
#47174=CARTESIAN_POINT ( 'NONE',  ( 26.70937500061451431, 0.000000000000000000, 5.243569643749999010 ) ) ;
#47175=CARTESIAN_POINT ( 'NONE',  ( 7.350000000000002309, 4.330127018922192761, -2.499999999999997780 ) ) ;
#47176=CARTESIAN_POINT ( 'NONE',  ( -3.999999999999999112, 12.91250000122903430, 30.00000000000000000 ) ) ;
#47177=CARTESIAN_POINT ( 'NONE',  ( 15.55312500061451608, -4.541064518000417216, -2.621784821875001281 ) ) ;
#47178=CARTESIAN_POINT ( 'NONE',  ( 7.875000001229034652, 2.886751345948129099, -4.999999999999998224 ) ) ;
#47179=EDGE_CURVE ( 'NONE', #8722, #69635, #66158, .T. ) ;
#47180=CARTESIAN_POINT ( 'NONE',  ( 11.44687500061451857, -3.027376345333614438, 5.243569643749998122 ) ) ;
#47182=ORIENTED_EDGE ( 'NONE', *, *, #48691, .F. ) ;
#47183=CARTESIAN_POINT ( 'NONE',  ( 11.24062500061451608, 6.054752690667223547, 3.707466751127219781E-16 ) ) ;
#47185=CARTESIAN_POINT ( 'NONE',  ( 24.45000000122903572, -2.886751345948125991, -5.000000000000000000 ) ) ;
#47186=CARTESIAN_POINT ( 'NONE',  ( 11.85937500061451644, 0.000000000000000000, 5.243569643749999010 ) ) ;
#47187=CARTESIAN_POINT ( 'NONE',  ( 15.29062500061451679, 6.054752690667223547, 3.707466751127219781E-16 ) ) ;
#47189=CARTESIAN_POINT ( 'NONE',  ( 23.85937500061451644, 4.541064518000418104, -2.621784821874998173 ) ) ;
#47190=CARTESIAN_POINT ( 'NONE',  ( 4.898587196589411843E-16, 20.00000000000000000, 33.99999999999999289 ) ) ;
#47191=CARTESIAN_POINT ( 'NONE',  ( 5.287500000000000533, -2.886751345948130876, 4.999999999999996447 ) ) ;
#47192=DIRECTION ( 'NONE',  ( -0.000000000000000000, -1.000000000000000000, -0.000000000000000000 ) ) ;
#47193=CARTESIAN_POINT ( 'NONE',  ( -4.243569643749999898, 13.97187500061451715, -32.45002607614398471 ) ) ;
#47194=CARTESIAN_POINT ( 'NONE',  ( 16.24687500061451573, 6.054752690667223547, 3.707466751127219781E-16 ) ) ;
#47195=CARTESIAN_POINT ( 'NONE',  ( 17.06250000122903288, 0.000000000000000000, 4.999999999999998224 ) ) ;
#47196=CARTESIAN_POINT ( 'NONE',  ( 11.97187500061451892, -6.054752690667223547, -1.112240025338166033E-15 ) ) ;
#47197=CARTESIAN_POINT ( 'NONE',  ( -3.000416591977282496E-16, 19.69062500061451360, -34.90005215228797653 ) ) ;
#47198=CARTESIAN_POINT ( 'NONE',  ( 19.68750000122903288, 4.330127018922191873, 2.499999999999999556 ) ) ;
#47199=CARTESIAN_POINT ( 'NONE',  ( 11.91562500061451857, -6.054752690667223547, -1.112240025338166033E-15 ) ) ;
#47201=ORIENTED_EDGE ( 'NONE', *, *, #11270, .T. ) ;
#47202=CARTESIAN_POINT ( 'NONE',  ( 18.63749999999999929, 5.773502691896255534, 3.535250795749688894E-16 ) ) ;
#47204=CARTESIAN_POINT ( 'NONE',  ( 13.65937500061451715, 0.000000000000000000, 5.243569643749999010 ) ) ;
#47205=DIRECTION ( 'NONE',  ( 0.000000000000000000, 0.000000000000000000, 1.000000000000000000 ) ) ;
#47206=CARTESIAN_POINT ( 'NONE',  ( 11.62500000122903465, 2.886751345948126879, 4.999999999999999112 ) ) ;
#47207=CARTESIAN_POINT ( 'NONE',  ( 21.07500000122903572, 2.886751345948126879, 4.999999999999999112 ) ) ;
#47208=CARTESIAN_POINT ( 'NONE',  ( 17.50312500061451715, 4.541064518000418104, -2.621784821874998173 ) ) ;
#47209=CARTESIAN_POINT ( 'NONE',  ( 20.87812500061451715, -4.541064518000419881, 2.621784821874995952 ) ) ;
#47210=CARTESIAN_POINT ( 'NONE',  ( 2.953125000614516438, -4.541064518000417216, -2.621784821875001281 ) ) ;
#47211=CARTESIAN_POINT ( 'NONE',  ( 27.11249999999999716, 2.886751345948129099, -4.999999999999998224 ) ) ;
#47212=DIRECTION ( 'NONE',  ( -1.000000000000000000, -0.000000000000000000, -0.000000000000000000 ) ) ;
#47214=CARTESIAN_POINT ( 'NONE',  ( 28.47187500061451715, 3.027376345333611329, 5.243569643749999010 ) ) ;
#47215=CARTESIAN_POINT ( 'NONE',  ( 30.00000000000000000, 0.000000000000000000, 4.999999999999998224 ) ) ;
#47216=CARTESIAN_POINT ( 'NONE',  ( -2.121784821874999949, 14.83437500061451786, -33.67503911421598417 ) ) ;
#47217=CARTESIAN_POINT ( 'NONE',  ( 4.650000001229035895, -2.886751345948125991, -5.000000000000000000 ) ) ;
#47218=CARTESIAN_POINT ( 'NONE',  ( 5.362500000000003375, -5.773502691896255534, -1.060575238724906372E-15 ) ) ;
#47219=EDGE_CURVE ( 'NONE', #15128, #41505, #53865, .T. ) ;
#47221=CARTESIAN_POINT ( 'NONE',  ( 9.871875000614517504, 3.027376345333613106, -5.243569643749998122 ) ) ;
#47222=CARTESIAN_POINT ( 'NONE',  ( 28.45312500061451289, 0.000000000000000000, 5.243569643749999010 ) ) ;
#47224=CARTESIAN_POINT ( 'NONE',  ( 3.658875532774302997, -3.408200617373282171, -3.658875532774302997 ) ) ;
#47225=CARTESIAN_POINT ( 'NONE',  ( 8.324999999999999289, 4.330127018922191873, 2.499999999999999556 ) ) ;
#47226=CARTESIAN_POINT ( 'NONE',  ( 8.409375000614518925, -4.541064518000417216, -2.621784821875001281 ) ) ;
#47227=CARTESIAN_POINT ( 'NONE',  ( 11.18437500061451928, 6.421520780324663323E-16, -5.243569643749999010 ) ) ;
#47228=CARTESIAN_POINT ( 'NONE',  ( 4.687500000000000000, 5.773502691896255534, 3.535250795749688894E-16 ) ) ;
#47229=CARTESIAN_POINT ( 'NONE',  ( -4.243569643749999898, 15.26562500061459460, 27.54997392385601529 ) ) ;
#47230=CARTESIAN_POINT ( 'NONE',  ( 6.112499999999999822, 2.886751345948126879, 4.999999999999999112 ) ) ;
#47232=CARTESIAN_POINT ( 'NONE',  ( 20.39062500061451644, -3.027376345333614438, 5.243569643749998122 ) ) ;
#47233=CARTESIAN_POINT ( 'NONE',  ( 12.17812500061451608, 4.541064518000418104, 2.621784821874999949 ) ) ;
#47235=CARTESIAN_POINT ( 'NONE',  ( 9.796875000614519990, -3.027376345333610441, -5.243569643749999898 ) ) ;
#47236=CARTESIAN_POINT ( 'NONE',  ( 26.13749999999999929, -2.886751345948125991, -5.000000000000000000 ) ) ;
#47237=CARTESIAN_POINT ( 'NONE',  ( 23.55000000122903359, -2.886751345948125991, -5.000000000000000000 ) ) ;
#47238=CARTESIAN_POINT ( 'NONE',  ( 17.06250000000000000, -5.773502691896255534, -1.060575238724906372E-15 ) ) ;
#47239=CARTESIAN_POINT ( 'NONE',  ( 11.25937500061451679, 4.541064518000418104, -2.621784821874998173 ) ) ;
#47240=CARTESIAN_POINT ( 'NONE',  ( 27.34687500061451360, -3.027376345333610441, -5.243569643749999898 ) ) ;
#47242=CARTESIAN_POINT ( 'NONE',  ( 3.571875000614517237, 3.027376345333613106, -5.243569643749998122 ) ) ;
#47243=CARTESIAN_POINT ( 'NONE',  ( 24.33750000122903145, -4.330127018922194537, 2.499999999999995559 ) ) ;
#47244=CARTESIAN_POINT ( 'NONE',  ( 20.33437500061451786, 4.541064518000418104, 2.621784821874999949 ) ) ;
#47245=CARTESIAN_POINT ( 'NONE',  ( 11.70937500061451608, 4.541064518000418104, -2.621784821874998173 ) ) ;
#47247=CARTESIAN_POINT ( 'NONE',  ( 23.77499999999999858, -4.330127018922194537, 2.499999999999995559 ) ) ;
#47249=CARTESIAN_POINT ( 'NONE',  ( 9.001249775931846008E-16, 11.42187500061451999, -25.09994784771203058 ) ) ;
#47251=CARTESIAN_POINT ( 'NONE',  ( 14.09062500061451750, -3.027376345333614438, 5.243569643749998122 ) ) ;
#47252=CARTESIAN_POINT ( 'NONE',  ( 4.762499999999999289, 2.886751345948126879, 4.999999999999999112 ) ) ;
#47254=CARTESIAN_POINT ( 'NONE',  ( -3.137519842735245283E-14, 12.91250000000000142, 34.00000000000000000 ) ) ;
#47255=CARTESIAN_POINT ( 'NONE',  ( 14.36249999999999893, -5.773502691896255534, -1.060575238724906372E-15 ) ) ;
#47256=CARTESIAN_POINT ( 'NONE',  ( 4.243569643749999898, 10.99062500061451786, 32.45002607614398471 ) ) ;
#47257=CARTESIAN_POINT ( 'NONE',  ( 13.50000000122903288, -2.886751345948129988, 4.999999999999997335 ) ) ;
#47258=CARTESIAN_POINT ( 'NONE',  ( 23.63437500061451502, -4.541064518000419881, 2.621784821874995952 ) ) ;
#47259=CARTESIAN_POINT ( 'NONE',  ( 4.022770794281430362, 2.969407772832715953, -4.321770970117402300 ) ) ;
#47261=CARTESIAN_POINT ( 'NONE',  ( 20.35312500061451502, 0.000000000000000000, 5.243569643749999010 ) ) ;
#47262=CARTESIAN_POINT ( 'NONE',  ( 4.340625000614515727, -3.027376345333610441, -5.243569643749999898 ) ) ;
#47263=CARTESIAN_POINT ( 'NONE',  ( 20.40937500061451715, 0.000000000000000000, 5.243569643749999010 ) ) ;
#47264=CARTESIAN_POINT ( 'NONE',  ( 3.300000000000000711, 4.330127018922192761, -2.499999999999997780 ) ) ;
#47265=CARTESIAN_POINT ( 'NONE',  ( 6.028125000614517504, -4.541064518000419881, 2.621784821874995952 ) ) ;
#47266=CARTESIAN_POINT ( 'NONE',  ( 22.22812500061451502, -4.541064518000419881, 2.621784821874995952 ) ) ;
#47267=CARTESIAN_POINT ( 'NONE',  ( 2.121784821875001281, 14.10312500061451679, 33.67503911421598417 ) ) ;
#47268=CARTESIAN_POINT ( 'NONE',  ( 18.00000000122903288, -2.886751345948129988, 4.999999999999997335 ) ) ;
#47270=CARTESIAN_POINT ( 'NONE',  ( 9.703125000614514661, -4.541064518000417216, -2.621784821875001281 ) ) ;
#47271=CARTESIAN_POINT ( 'NONE',  ( 4.134375000614517681, 4.541064518000418104, 2.621784821874999949 ) ) ;
#47272=CARTESIAN_POINT ( 'NONE',  ( 3.384375000614517237, -4.541064518000419881, 2.621784821874995952 ) ) ;
#47273=CARTESIAN_POINT ( 'NONE',  ( 23.03437500061451715, 4.541064518000418104, 2.621784821874999949 ) ) ;
#47274=CARTESIAN_POINT ( 'NONE',  ( 15.21562500061451750, 3.027376345333613106, -5.243569643749998122 ) ) ;
#47276=CARTESIAN_POINT ( 'NONE',  ( 25.16250000122903074, 0.000000000000000000, 4.999999999999998224 ) ) ;
#47277=CARTESIAN_POINT ( 'NONE',  ( 24.70312500061451644, 4.541064518000418104, -2.621784821874998173 ) ) ;
#47278=CARTESIAN_POINT ( 'NONE',  ( 18.27187500061451431, -6.054752690667223547, -1.112240025338166033E-15 ) ) ;
#47279=CARTESIAN_POINT ( 'NONE',  ( 14.12812500061451715, -4.541064518000419881, 2.621784821874995952 ) ) ;
#47280=CARTESIAN_POINT ( 'NONE',  ( -3.000416591977282496E-16, 16.14687500061451431, 25.09994784771203058 ) ) ;
#47281=CARTESIAN_POINT ( 'NONE',  ( 20.54062500061451502, -3.027376345333610441, -5.243569643749999898 ) ) ;
#47283=ORIENTED_EDGE ( 'NONE', *, *, #42578, .T. ) ;
#47284=CARTESIAN_POINT ( 'NONE',  ( 24.26249999999999929, -5.773502691896255534, -1.060575238724906372E-15 ) ) ;
#47285=CARTESIAN_POINT ( 'NONE',  ( 2.000000000000001332, 10.70000000000000107, -26.53589838486224650 ) ) ;
#47287=CARTESIAN_POINT ( 'NONE',  ( 27.85312500061451502, 4.541064518000418104, -2.621784821874998173 ) ) ;
#47288=CARTESIAN_POINT ( 'NONE',  ( 7.828125000614517326, -4.541064518000419881, 2.621784821874995952 ) ) ;
#47289=CARTESIAN_POINT ( 'NONE',  ( 20.55000000122903359, 5.773502691896255534, 3.535250795749688894E-16 ) ) ;
#47290=CARTESIAN_POINT ( 'NONE',  ( 23.76562500061451644, 3.027376345333613106, -5.243569643749998122 ) ) ;
#47291=CARTESIAN_POINT ( 'NONE',  ( 26.39999999999999858, 0.000000000000000000, 4.999999999999998224 ) ) ;
#47292=CARTESIAN_POINT ( 'NONE',  ( 4.000000000000000000, 15.80000000122903359, -27.69059892324149530 ) ) ;
#47293=CARTESIAN_POINT ( 'NONE',  ( -5.810221930991193690E-16, 15.50000000122903465, -34.00000000000000000 ) ) ;
#47294=CARTESIAN_POINT ( 'NONE',  ( 11.24062500061451608, 6.054752690667223547, 3.707466751127219781E-16 ) ) ;
#47295=VERTEX_POINT ( 'NONE', #67117 ) ;
#47296=CARTESIAN_POINT ( 'NONE',  ( 25.49062500061451786, -3.027376345333610441, -5.243569643749999898 ) ) ;
#47297=CARTESIAN_POINT ( 'NONE',  ( 6.328125000614515550, 4.541064518000418104, 2.621784821874999949 ) ) ;
#47299=CARTESIAN_POINT ( 'NONE',  ( 4.646859583631838042, -1.845723709011792613, 4.907986002307686668 ) ) ;
#47300=CARTESIAN_POINT ( 'NONE',  ( 13.61250000000000071, 2.886751345948129099, -4.999999999999998224 ) ) ;
#47301=VECTOR ( 'NONE', #67523, 1000.000000000000000 ) ;
#47302=CARTESIAN_POINT ( 'NONE',  ( 14.48437500061451821, 4.541064518000418104, 2.621784821874999949 ) ) ;
#47303=CARTESIAN_POINT ( 'NONE',  ( 8.325000001229033941, 2.886751345948129099, -4.999999999999998224 ) ) ;
#47304=CARTESIAN_POINT ( 'NONE',  ( 16.69687500061451502, 6.054752690667223547, 3.707466751127219781E-16 ) ) ;
#47306=CARTESIAN_POINT ( 'NONE',  ( 8.184375000614515727, 4.541064518000418104, 2.621784821874999949 ) ) ;
#47307=CARTESIAN_POINT ( 'NONE',  ( -2.121784821874996840, 12.67812500061451786, -26.32496088578401583 ) ) ;
#47308=CARTESIAN_POINT ( 'NONE',  ( 20.88750000122903572, 6.123233995736764310E-16, -4.999999999999998224 ) ) ;
#47311=CARTESIAN_POINT ( 'NONE',  ( 23.31562500061451715, 3.027376345333613106, -5.243569643749998122 ) ) ;
#47312=CARTESIAN_POINT ( 'NONE',  ( -1.071796769724488563, 17.50490381179670152, 34.00000000000000000 ) ) ;
#47313=CARTESIAN_POINT ( 'NONE',  ( 26.07187500061451857, 3.027376345333613106, -5.243569643749998122 ) ) ;
#47315=CARTESIAN_POINT ( 'NONE',  ( 29.03437500061451715, -4.541064518000419881, 2.621784821874995952 ) ) ;
#47316=CARTESIAN_POINT ( 'NONE',  ( 20.92500000000000071, 4.330127018922191873, 2.499999999999999556 ) ) ;
#47317=CARTESIAN_POINT ( 'NONE',  ( 6.103125000614515905, -4.541064518000417216, -2.621784821875001281 ) ) ;
#47319=CARTESIAN_POINT ( 'NONE',  ( 17.55937500061451573, 4.541064518000418104, -2.621784821874998173 ) ) ;
#47321=CARTESIAN_POINT ( 'NONE',  ( 3.703125000614516882, 0.000000000000000000, 5.243569643749999010 ) ) ;
#47322=CARTESIAN_POINT ( 'NONE',  ( 9.121875000614517504, 3.027376345333611329, 5.243569643749999010 ) ) ;
#47323=CARTESIAN_POINT ( 'NONE',  ( 19.05937500061451928, 0.000000000000000000, 5.243569643749999010 ) ) ;
#47325=CARTESIAN_POINT ( 'NONE',  ( 26.88749999999999574, -2.886751345948129988, 4.999999999999997335 ) ) ;
#47326=CARTESIAN_POINT ( 'NONE',  ( 26.97187500061451360, 3.027376345333613106, -5.243569643749998122 ) ) ;
#47328=CARTESIAN_POINT ( 'NONE',  ( 21.71249999999999858, 2.886751345948129099, -4.999999999999997335 ) ) ;
#47329=ORIENTED_EDGE ( 'NONE', *, *, #40621, .F. ) ;
#47330=CARTESIAN_POINT ( 'NONE',  ( 11.55000000000000071, 0.000000000000000000, 4.999999999999998224 ) ) ;
#47332=CARTESIAN_POINT ( 'NONE',  ( 21.32812500061451644, -4.541064518000419881, 2.621784821874995952 ) ) ;
#47333=CARTESIAN_POINT ( 'NONE',  ( 12.18750000000000000, -2.886751345948125991, -5.000000000000000000 ) ) ;
#47334=CARTESIAN_POINT ( 'NONE',  ( 8.062500001229034652, 0.000000000000000000, 4.999999999999998224 ) ) ;
#47335=CARTESIAN_POINT ( 'NONE',  ( 6.178125000614518747, 6.421520780324663323E-16, -5.243569643749999010 ) ) ;
#47336=CARTESIAN_POINT ( 'NONE',  ( 21.93750000000000000, -2.886751345948129988, 4.999999999999997335 ) ) ;
#47337=CARTESIAN_POINT ( 'NONE',  ( 20.05312500061451431, -4.541064518000417216, -2.621784821875001281 ) ) ;
#47338=CARTESIAN_POINT ( 'NONE',  ( 14.69999999999999929, 0.000000000000000000, 4.999999999999998224 ) ) ;
#47339=CARTESIAN_POINT ( 'NONE',  ( 24.97500000122903430, 2.886751345948129099, -4.999999999999998224 ) ) ;
#47341=CARTESIAN_POINT ( 'NONE',  ( 6.112499999999999822, 2.886751345948126879, 4.999999999999999112 ) ) ;
#47342=ORIENTED_EDGE ( 'NONE', *, *, #72661, .F. ) ;
#47343=CARTESIAN_POINT ( 'NONE',  ( 18.51562500061451289, 3.027376345333611329, 5.243569643749999010 ) ) ;
#47344=CARTESIAN_POINT ( 'NONE',  ( 27.06562500061451004, 3.027376345333611329, 5.243569643749999010 ) ) ;
#47345=CARTESIAN_POINT ( 'NONE',  ( 26.29687500061451644, -3.027376345333614438, 5.243569643749998122 ) ) ;
#47346=CARTESIAN_POINT ( 'NONE',  ( 15.06562500061451537, -6.054752690667223547, -1.112240025338166033E-15 ) ) ;
#47347=CARTESIAN_POINT ( 'NONE',  ( 28.60312500061451502, -4.541064518000417216, -2.621784821875001281 ) ) ;
#47348=CARTESIAN_POINT ( 'NONE',  ( 8.353125000614518569, -4.541064518000417216, -2.621784821875001281 ) ) ;
#47350=ADVANCED_FACE ( 'NONE', ( #68913 ), #2045, .F. ) ;
#47351=CARTESIAN_POINT ( 'NONE',  ( 26.21250000122903501, -4.330127018922190985, -2.500000000000001332 ) ) ;
#47353=CARTESIAN_POINT ( 'NONE',  ( 16.34062500061451573, -3.027376345333614438, 5.243569643749998122 ) ) ;
#47354=CARTESIAN_POINT ( 'NONE',  ( 7.320879633048903241E-15, 18.53750000000000142, -34.00000000000000000 ) ) ;
#47355=CIRCLE ( 'NONE', #36754, 10.00000000000000000 ) ;
#47356=CARTESIAN_POINT ( 'NONE',  ( 29.03437500061451715, -4.541064518000419881, 2.621784821874995952 ) ) ;
#47357=CARTESIAN_POINT ( 'NONE',  ( 9.496875000614517504, 6.054752690667223547, 3.707466751127219781E-16 ) ) ;
#47358=CARTESIAN_POINT ( 'NONE',  ( 9.909375000614517148, 4.541064518000418104, -2.621784821874998173 ) ) ;
#47359=CARTESIAN_POINT ( 'NONE',  ( 17.82187500061451502, -6.054752690667223547, -1.112240025338166033E-15 ) ) ;
#47361=CARTESIAN_POINT ( 'NONE',  ( 29.07187500061451502, -6.054752690667223547, -1.112240025338166033E-15 ) ) ;
#47362=CARTESIAN_POINT ( 'NONE',  ( 22.86562500061451431, 3.027376345333613106, -5.243569643749998122 ) ) ;
#47363=( BOUNDED_SURFACE ( )  B_SPLINE_SURFACE ( 1, 2, ( 
 ( #42519, #3374, #8168, #25147, #42153, #9635, #64680, #65409, #43260, #14799, #37342, #48798, #14065, #54702, #59865, #65781, #24784, #16618, #71702, #49532, #72056, #10000, #4472, #32535, #33616, #21074, #43625, #55798, #72789, #56160, #60966, #11456, #66147, #39537, #60591, #66892, #25, #55071, #5188, #27002, #43992, #22172, #5555, #67260, #28092, #10365, #50620, #22531, #39173, #11088, #44725, #50264, #10728, #21435, #61689, #15525, #66513, #45078, #67614, #15894, #32896, #33260, #38067, #4828, #38440, #49893, #55436, #27362, #72418, #21801, #44365, #16260, #16980, #62062, #49171, #33977, #27726, #4107, #38815, #61330, #26634, #41349, #51342, #18784, #1470, #40260, #29531, #50978, #46162, #63859, #23253, #57951, #45441, #23976, #56516, #1109, #62781, #11818, #13249, #62419, #28801, #46524, #12894, #12537, #6273, #34335, #35071, #5909, #12173, #56869, #744, #68702, #28443, #375, #45803, #67974, #7359, #34701, #22883, #69066, #23616, #57230, #1833, #6645, #57597, #29172, #51706, #17347, #7000, #18062, #29888, #68339, #52066, #39906, #17699, #40623, #63142, #18425, #40991, #63507, #35427, #52427, #24341, #46889, #69427, #42074, #53893, #31352, #52788, #25812, #36888, #41701, #13614, #59778, #70511, #48350, #70138, #59042, #64596, #54255, #3651, #25440, #35787, #9184, #59407, #30255, #47247, #25065, #58310, #26174, #48715, #58677, #2909, #19147, #71237, #47983, #19516, #69780, #8815, #7721, #42440, #20617, #14353, #13983, #43175, #19887, #20249, #36522, #3284, #70875, #31719, #64225, #36159, #42801, #65323, #65694, #8087, #64962, #30617, #14714, #37256, #53515, #2189, #24703, #8446, #53147, #2546, #47608, #30982, #60878, #72704, #37983, #54614, #39089, #38730, #61606, #71978, #44645, #72337, #60505, #50537, #11007, #56078, #67175, #33528, #5469, #33174, #10283, #27279, #21351, #20987, #22087, #32813, #32449, #16536, #28009, #15809, #9911, #66431, #49812, #16179, #55712, #43908, #21717, #4020, #32083, #60140, #73065, #43540, #5106, #22446, #38351, #61250, #44995, #37618, #15081, #55351, #66807, #15439, #27640, #9549, #54984, #4390, #66061, #26919, #49444, #26545, #49086, #71614, #10644, #50176, #4745, #44276, #1744, #61971, #29806, #50894, #57144, #63422, #22803, #68615, #294, #34250, #12455, #23893, #57515, #46441, #51257, #68979, #12809, #6916, #1383, #34986, #40537, #1024, #45355, #51984, #33892, #67889, #29446, #63053, #6188, #659, #23530, #5827, #68256, #39823, #40178, #17261, #23167, #62337, #56436, #11733, #11373, #18336, #40909, #39450, #35344, #46080, #57867, #28358, #62698, #56782, #52341, #28717, #24257, #7276, #45721, #67532, #17618, #6556, #16895, #12093, #34614, #29088, #51624, #17978, #64508, #30536, #2107, #3565, #58594, #48262, #36440, #19062, #20161, #59317, #54168, #24618, #13901, #58227, #64139, #41264, #47165, #69697, #47897, #52701, #41620, #70786, #8362, #36802, #8001, #70054, #2457, #65236, #14626, #58954, #46805, #42715, #70425, #63776, #7632, #36073, #69342, #37165, #59691, #13526, #30891, #30170, #9098, #53433, #53063, #24980, #19800, #18700, #2823, #31636, #25351, #47525, #13164, #42353, #31260, #19427, #64875, #14263, #35705, #41988, #8726, #53802, #3197, #25725, #48996, #38260, #54531, #38640, #10559, #43819, #72253, #61521, #71892, #14996, #65608, #60788, #66343, #21265, #33087, #71526, #37533, #50088, #49726, #72619, #9828, #55626, #10194, #20901, #10919, #22003, #67090, #5022, #44559, #16449, #44188, #31996, #43455, #16092, #27557, #55266, #65977, #3933, #4661, #26088, #32358, #26456, #15357, #15721, #48626, #33446, #37899, #60055, #39006, #54896, #55990, #61164, #32729, #4303, #71151, #26828, #27191, #49362, #21630, #20523, #66719, #43082, #9466, #60417, #6467, #50455, #44915, #72981, #28635, #36262, #6104, #11652, #45272, #45640, #67805, #56356, #67452, #34167, #23447, #940, #22363, #68530, #17179, #16814, #6830, #62255, #5383, #17891, #23082, #56703, #23805, #51173, #29002, #577, #68172, #39370, #34530, #17535, #29365, #22719, #51539, #61887, #11292, #33813, #40097, #27921, #62611, #12007, #39738, #57060, #45993, #5746, #28280, #40451, #62967, #12363, #50812, #34897, #57426, #214, #51897, #1295, #46356, #68890, #18247, #40820, #63336, #13721, #4122, #48452, #58777, #9652, #9287, #53247, #70244, #48082, #8186, #26651, #71717, #8552, #25912, #42172, #49187, #70976, #42535, #19615, #31820, #30714, #65426, #21089, #37359, #19982, #66164, #20351, #43277, #14452, #59881, #3753, #32186, #64698, #59143, #48814, #54359, #43640, #31079, #42902, #14082, #71344, #65798, #3391, #26277, #15540, #31452, #47705, #25164, #14816, #20719, #53994, #15179, #53619, #36622, #54719, #37718, #2645, #65061, #60238, #3010, #25540, #70609, #36986, #59508, #8922, #33994, #28458, #56178, #44007, #10382, #28108, #67629, #67277, #60983, #15909, #16636, #38084, #44383, #38457, #32914, #27743, #60606, #22898, #72806, #39191, #5571, #66908, #44743, #27017, #55088, #10015, #391, #66529, #50637, #11471, #61347, #61706, #45094, #32551, #45457, #16276, #11105, #55451, #41, #4488, #4844, #27378, #49910, #72434, #21818, #16996, #49549, #72071, #33634, #22546, #39553, #38832, #67989, #21452, #10743, #33276, #50282, #56531, #55815, #62078, #5202, #22189, #5924, #50993, #7373, #46905, #1121, #18801, #13266, #29904, #24357, #35441, #63521, #23991, #23266, #1849, #56883, #45816, #57965, #12908, #29186, #23630, #46538, #28817, #18075, #62794, #63155, #40273, #46176, #17713, #6288, #12187, #11832, #52444, #69444, #62434, #41365, #69080, #63875, #51355, #12550, #34714, #2206, #57244, #52805, #35804, #68715, #58326, #34350, #7013, #24721, #6657, #7737, #758, #30272, #17363, #35084, #40636, #68352, #47264, #51720, #39920, #29544, #57610, #52080, #1485, #18441, #41006 ),
 ( #19905, #69798, #9202, #53911, #13633, #8105, #14001, #19164, #26192, #71255, #19535, #42457, #53165, #48732, #64980, #8465, #30633, #3304, #64245, #59426, #20635, #31370, #59060, #41718, #8834, #59796, #48002, #48368, #42819, #3669, #25082, #64615, #14732, #70894, #20267, #25458, #36540, #54275, #31000, #36177, #37274, #58694, #53533, #25831, #42093, #70530, #47625, #2929, #14371, #65342, #31737, #36906, #2562, #70158, #35312, #6885, #69662, #30501, #63391, #57481, #40874, #24223, #63743, #30136, #68945, #69308, #51594, #6525, #34585, #24946, #17945, #7597, #36037, #12776, #13132, #19027, #12062, #70020, #18303, #41231, #63022, #2074, #57113, #34953, #29418, #68584, #12421, #40507, #41586, #29057, #994, #35671, #58194, #64104, #46408, #19391, #23501, #47490, #46049, #52308, #58557, #51951, #52667, #1351, #23860, #24583, #13489, #47131, #7965, #57834, #53029, #2423, #62667, #7243, #29772, #1710, #18669, #46772, #26420, #8328, #47860, #60020, #37500, #53767, #25691, #48593, #71118, #70389, #48961, #30858, #19765, #9432, #31960, #3162, #48226, #20490, #53396, #42680, #14229, #14592, #64842, #70750, #42316, #2789, #36767, #36407, #54498, #3899, #13866, #71491, #43046, #43421, #25314, #37127, #59284, #26793, #8693, #4269, #20868, #20125, #14962, #58920, #31599, #49327, #31225, #65943, #65203, #15323, #41952, #59656, #9065, #54136, #65572, #3531, #26053, #37864, #60383, #9791, #32324, #71859, #54861, #64472, #30850, #59276, #14221, #19757, #31590, #70013, #13479, #71111, #70739, #20483, #53385, #3524, #31216, #19382, #9424, #43038, #14954, #26045, #65565, #37493, #65195, #53021, #41941, #37119, #48585, #3153, #64464, #24937, #25682, #47121, #2780, #47480, #13856, #36757, #69653, #31953, #36398, #36029, #60013, #25305, #3891, #59648, #64833, #47852, #54491, #70379, #48217, #42306, #8684, #41578, #20117, #53759, #19017, #58911, #42672, #64095, #58545, #7956, #14585, #30493, #9058, #54128, #8321, #2415, #66303, #4262, #65936, #32688, #45506, #22945, #43411, #49685, #57294, #27151, #55227, #15680, #66674, #38218, #26785, #15316, #4622, #68036, #17406, #37855, #39963, #28502, #32317, #49320, #51401, #62122, #62477, #60745, #72214, #21592, #45860, #68394, #17043, #26411, #804, #51040, #20859, #60376, #10156, #48954, #17755, #40315, #71851, #39601, #9784, #62838, #11514, #44146, #54853, #436, #71484, #34036, #12230, #5971, #56575, #34759, #11875, #34399, #56927, #6331, #28862, #23311, #21224, #43776, #69839, #7780, #46220, #29232, #30317, #63199, #19204, #64287, #24399, #52847, #57653, #12595, #58369, #63563, #18844, #46948, #52484, #13675, #29587, #68759, #30673, #2245, #53205, #12951, #36219, #63921, #52125, #42130, #2601, #47664, #58735, #25122, #70198, #24761, #35128, #1527, #41758, #8146, #35844, #24034, #7059, #47304, #6699, #35488, #46583, #69126, #69485, #51765, #64656, #18484, #18117, #19574, #58008, #36581, #14041, #41405, #7416, #1164, #29944, #23673, #1895, #13306, #40681, #41050, #65383, #9971, #3349, #60198, #31037, #25499, #53573, #48044, #2971, #70569, #21408, #14410, #4077, #32508, #9245, #9610, #66119, #8508, #66486, #14774, #37676, #59467, #71672, #19945, #31412, #53952, #65021, #8877, #36947, #15498, #42498, #25871, #32141, #54674, #38040, #42861, #15865, #48411, #43965, #70937, #48774, #55043, #20308, #26605, #37316, #59840, #49143, #60564, #21046, #4446, #31780, #26974, #49503, #43598, #72032, #59101, #54319, #65754, #3710, #26237, #71298, #20677, #43234, #15138, #50236, #22144, #45052, #49867, #39143, #10699, #11060, #61304, #67231, #38787, #27335, #33231, #32870, #50952, #5883, #10338, #67946, #67588, #39879, #4802, #33586, #55769, #23223, #5161, #716, #56489, #44697, #11429, #55407, #28063, #45776, #27696, #62391, #72391, #28414, #38413, #56132, #16590, #66863, #62033, #61660, #72758, #17319, #5525, #11789, #349, #68311, #60934, #21771, #44335, #50593, #16234, #48581, #22503, #16954, #39507, #33948, #22856, #45410, #34306, #56838, #6245, #28772, #51312, #12512, #69035, #52398, #18758, #58284, #23947, #24314, #8058, #69402, #52038, #25038, #7331, #2163, #46497, #41322, #35762, #41675, #51678, #18036, #7690, #63832, #57200, #40231, #13223, #1082, #30228, #24674, #35399, #52760, #68673, #23589, #47221, #1442, #29862, #57925, #63480, #69752, #40592, #6616, #64198, #19121, #13585, #18397, #36132, #1806, #63113, #53119, #58651, #30592, #2517, #47582, #17671, #62753, #46135, #35041, #12146, #34672, #46863, #57568, #6972, #29143, #29503, #40964, #12867, #47955, #59747, #19487, #54954, #59375, #59014, #71582, #53863, #26887, #9521, #14681, #3254, #15412, #25783, #71207, #20218, #42773, #64568, #26143, #48320, #20955, #14323, #20584, #42045, #36494, #13957, #65292, #70111, #70845, #37223, #36858, #9154, #8785, #70482, #8417, #31689, #15052, #65662, #30949, #60111, #43139, #2880, #19859, #43509, #54224, #32054, #31320, #3621, #48683, #37954, #60473, #37590, #53488, #66033, #54586, #25410, #42412, #3989, #64932, #9882, #32417, #26515, #49054, #4359, #39790, #16505, #33142, #60845, #73033, #71946, #56045, #49782, #55320, #5796, #43875, #66400, #27976, #44963, #28326, #55680, #56752, #15777, #11703, #32783, #39058, #45323, #4714, #50507, #27248, #16147, #67501, #50864, #39420, #262, #5077, #22771, #67859, #61941, #56405, #16865, #22416, #5437, #72306, #33862, #38319, #21688, #11345, #17230, #61218, #27610, #62307, #10252, #50146, #44244, #22057, #66775, #72674, #38699, #10613, #44615, #67145, #34219, #6157, #21322, #49414, #61572, #10975, #33496, #23858, #29055, #13486, #23499, #64102, #46770, #12419, #1707, #23136, #18301, #36035, #68582, #30134, #17588, #69306, #28686, #46406, #34951, #57111, #52306, #57479, #51592, #7595, #992, #2072, #41228, #58555 ) ),
 .UNSPECIFIED., .F., .F., .F. ) 
 B_SPLINE_SURFACE_WITH_KNOTS ( ( 2, 2 ),
 ( 3, 2, 2, 2, 2, 2, 2, 2, 2, 2, 2, 2, 2, 2, 2, 2, 2, 2, 2, 2, 2, 2, 2, 2, 2, 2, 2, 2, 2, 2, 2, 2, 2, 2, 2, 2, 2, 2, 2, 2, 2, 2, 2, 2, 2, 2, 2, 2, 2, 2, 2, 2, 2, 2, 2, 2, 2, 2, 2, 2, 2, 2, 2, 2, 2, 2, 2, 2, 2, 2, 2, 2, 2, 2, 2, 2, 2, 2, 2, 2, 2, 2, 2, 2, 2, 2, 2, 2, 2, 2, 2, 2, 2, 2, 2, 2, 2, 2, 2, 2, 2, 2, 2, 2, 2, 2, 2, 2, 2, 2, 2, 2, 2, 2, 2, 2, 2, 2, 2, 2, 2, 2, 2, 2, 2, 2, 2, 2, 2, 2, 2, 2, 2, 2, 2, 2, 2, 2, 2, 2, 2, 2, 2, 2, 2, 2, 2, 2, 2, 2, 2, 2, 2, 2, 2, 2, 2, 2, 2, 2, 2, 2, 2, 2, 2, 2, 2, 2, 2, 2, 2, 2, 2, 2, 2, 2, 2, 2, 2, 2, 2, 2, 2, 2, 2, 2, 2, 2, 2, 2, 2, 2, 2, 2, 2, 2, 2, 2, 2, 2, 2, 2, 2, 2, 2, 2, 2, 2, 2, 2, 2, 2, 2, 2, 2, 2, 2, 2, 2, 2, 2, 2, 2, 2, 2, 2, 2, 2, 2, 2, 2, 2, 2, 2, 2, 2, 2, 2, 2, 2, 2, 2, 2, 2, 2, 2, 2, 2, 2, 2, 2, 2, 2, 2, 2, 2, 2, 2, 2, 2, 2, 2, 2, 2, 2, 2, 2, 2, 2, 2, 2, 2, 2, 2, 2, 2, 2, 2, 2, 2, 2, 2, 2, 2, 2, 2, 2, 2, 2, 2, 2, 2, 2, 2, 2, 2, 2, 2, 2, 2, 2, 2, 2, 2, 2, 2, 2, 2, 2, 2, 2, 2, 2, 2, 2, 2, 2, 2, 2, 2, 2, 2, 2, 2, 2, 2, 2, 2, 2, 2, 2, 2, 2, 2, 2, 2, 2, 2, 2, 2, 2, 2, 2, 2, 2, 2, 2, 2, 2, 2, 2, 2, 2, 2, 2, 2, 2, 2, 2, 2, 3 ),
 ( 0.000000000000000000, 1.000000000000000000 ),
 ( 0.000000000000000000, 0.002777777777777777884, 0.005555555555555555768, 0.008333333333333333218, 0.01111111111111111154, 0.01388888888888888812, 0.01666666666666666644, 0.01944444444444444475, 0.02222222222222222307, 0.02500000000000000139, 0.02777777777777777624, 0.03055555555555555455, 0.03333333333333333287, 0.03611111111111110772, 0.03888888888888888951, 0.04166666666666666435, 0.04444444444444444614, 0.04722222222222222099, 0.05000000000000000278, 0.05277777777777777762, 0.05555555555555555247, 0.05833333333333333426, 0.06111111111111110911, 0.06388888888888888395, 0.06666666666666666574, 0.06944444444444444753, 0.07222222222222221544, 0.07499999999999999722, 0.07777777777777777901, 0.08055555555555556080, 0.08333333333333332871, 0.08611111111111111049, 0.08888888888888889228, 0.09166666666666666019, 0.09444444444444444198, 0.09722222222222222376, 0.1000000000000000056, 0.1027777777777777735, 0.1055555555555555552, 0.1083333333333333370, 0.1111111111111111049, 0.1138888888888888867, 0.1166666666666666685, 0.1194444444444444503, 0.1222222222222222182, 0.1250000000000000000, 0.1277777777777777679, 0.1305555555555555636, 0.1333333333333333315, 0.1361111111111110994, 0.1388888888888888951, 0.1416666666666666630, 0.1444444444444444309, 0.1472222222222222265, 0.1499999999999999944, 0.1527777777777777901, 0.1555555555555555580, 0.1583333333333333259, 0.1611111111111111216, 0.1638888888888888895, 0.1666666666666666574, 0.1694444444444444531, 0.1722222222222222210, 0.1749999999999999889, 0.1777777777777777846, 0.1805555555555555525, 0.1833333333333333204, 0.1861111111111111160, 0.1888888888888888840, 0.1916666666666666796, 0.1944444444444444475, 0.1972222222222222154, 0.2000000000000000111, 0.2027777777777777790, 0.2055555555555555469, 0.2083333333333333426, 0.2111111111111111105, 0.2138888888888888784, 0.2166666666666666741, 0.2194444444444444420, 0.2222222222222222099, 0.2250000000000000056, 0.2277777777777777735, 0.2305555555555555691, 0.2333333333333333370, 0.2361111111111111049, 0.2388888888888889006, 0.2416666666666666685, 0.2444444444444444364, 0.2472222222222222321, 0.2500000000000000000, 0.2527777777777777679, 0.2555555555555555358, 0.2583333333333333592, 0.2611111111111111271, 0.2638888888888888951, 0.2666666666666666630, 0.2694444444444444309, 0.2722222222222221988, 0.2750000000000000222, 0.2777777777777777901, 0.2805555555555555580, 0.2833333333333333259, 0.2861111111111110938, 0.2888888888888888618, 0.2916666666666666852, 0.2944444444444444531, 0.2972222222222222210, 0.2999999999999999889, 0.3027777777777777568, 0.3055555555555555802, 0.3083333333333333481, 0.3111111111111111160, 0.3138888888888888840, 0.3166666666666666519, 0.3194444444444444198, 0.3222222222222222432, 0.3250000000000000111, 0.3277777777777777790, 0.3305555555555555469, 0.3333333333333333148, 0.3361111111111111382, 0.3388888888888889062, 0.3416666666666666741, 0.3444444444444444420, 0.3472222222222222099, 0.3499999999999999778, 0.3527777777777778012, 0.3555555555555555691, 0.3583333333333333370, 0.3611111111111111049, 0.3638888888888888729, 0.3666666666666666408, 0.3694444444444444642, 0.3722222222222222321, 0.3750000000000000000, 0.3777777777777777679, 0.3805555555555555358, 0.3833333333333333592, 0.3861111111111111271, 0.3888888888888888951, 0.3916666666666666630, 0.3944444444444444309, 0.3972222222222221988, 0.4000000000000000222, 0.4027777777777777901, 0.4055555555555555580, 0.4083333333333333259, 0.4111111111111110938, 0.4138888888888888618, 0.4166666666666666852, 0.4194444444444444531, 0.4222222222222222210, 0.4249999999999999889, 0.4277777777777777568, 0.4305555555555555802, 0.4333333333333333481, 0.4361111111111111160, 0.4388888888888888840, 0.4416666666666666519, 0.4444444444444444198, 0.4472222222222222432, 0.4500000000000000111, 0.4527777777777777790, 0.4555555555555555469, 0.4583333333333333148, 0.4611111111111111382, 0.4638888888888889062, 0.4666666666666666741, 0.4694444444444444420, 0.4722222222222222099, 0.4749999999999999778, 0.4777777777777778012, 0.4805555555555555691, 0.4833333333333333370, 0.4861111111111111049, 0.4888888888888888729, 0.4916666666666666408, 0.4944444444444444642, 0.4972222222222222321, 0.5000000000000000000, 0.5027777777777777679, 0.5055555555555555358, 0.5083333333333333037, 0.5111111111111110716, 0.5138888888888888395, 0.5166666666666667185, 0.5194444444444444864, 0.5222222222222222543, 0.5250000000000000222, 0.5277777777777777901, 0.5305555555555555580, 0.5333333333333333259, 0.5361111111111110938, 0.5388888888888888618, 0.5416666666666666297, 0.5444444444444443976, 0.5472222222222222765, 0.5500000000000000444, 0.5527777777777778123, 0.5555555555555555802, 0.5583333333333333481, 0.5611111111111111160, 0.5638888888888888840, 0.5666666666666666519, 0.5694444444444444198, 0.5722222222222221877, 0.5749999999999999556, 0.5777777777777777235, 0.5805555555555556024, 0.5833333333333333703, 0.5861111111111111382, 0.5888888888888889062, 0.5916666666666666741, 0.5944444444444444420, 0.5972222222222222099, 0.5999999999999999778, 0.6027777777777777457, 0.6055555555555555136, 0.6083333333333332815, 0.6111111111111111605, 0.6138888888888889284, 0.6166666666666666963, 0.6194444444444444642, 0.6222222222222222321, 0.6250000000000000000, 0.6277777777777777679, 0.6305555555555555358, 0.6333333333333333037, 0.6361111111111110716, 0.6388888888888888395, 0.6416666666666667185, 0.6444444444444444864, 0.6472222222222222543, 0.6500000000000000222, 0.6527777777777777901, 0.6555555555555555580, 0.6583333333333333259, 0.6611111111111110938, 0.6638888888888888618, 0.6666666666666666297, 0.6694444444444443976, 0.6722222222222222765, 0.6750000000000000444, 0.6777777777777778123, 0.6805555555555555802, 0.6833333333333333481, 0.6861111111111111160, 0.6888888888888888840, 0.6916666666666666519, 0.6944444444444444198, 0.6972222222222221877, 0.6999999999999999556, 0.7027777777777777235, 0.7055555555555556024, 0.7083333333333333703, 0.7111111111111111382, 0.7138888888888889062, 0.7166666666666666741, 0.7194444444444444420, 0.7222222222222222099, 0.7249999999999999778, 0.7277777777777777457, 0.7305555555555555136, 0.7333333333333332815, 0.7361111111111111605, 0.7388888888888889284, 0.7416666666666666963, 0.7444444444444444642, 0.7472222222222222321, 0.7500000000000000000, 0.7527777777777777679, 0.7555555555555555358, 0.7583333333333333037, 0.7611111111111110716, 0.7638888888888888395, 0.7666666666666667185, 0.7694444444444444864, 0.7722222222222222543, 0.7750000000000000222, 0.7777777777777777901, 0.7805555555555555580, 0.7833333333333333259, 0.7861111111111110938, 0.7888888888888888618, 0.7916666666666666297, 0.7944444444444443976, 0.7972222222222222765, 0.8000000000000000444, 0.8027777777777778123, 0.8055555555555555802, 0.8083333333333333481, 0.8111111111111111160, 0.8138888888888888840, 0.8166666666666666519, 0.8194444444444444198, 0.8222222222222221877, 0.8249999999999999556, 0.8277777777777777235, 0.8305555555555556024, 0.8333333333333333703, 0.8361111111111111382, 0.8388888888888889062, 0.8416666666666666741, 0.8444444444444444420, 0.8472222222222222099, 0.8499999999999999778, 0.8527777777777777457, 0.8555555555555555136, 0.8583333333333332815, 0.8611111111111111605, 0.8638888888888889284, 0.8666666666666666963, 0.8694444444444444642, 0.8722222222222222321, 0.8750000000000000000, 0.8777777777777777679, 0.8805555555555555358, 0.8833333333333333037, 0.8861111111111110716, 0.8888888888888888395, 0.8916666666666667185, 0.8944444444444444864, 0.8972222222222222543, 0.9000000000000000222, 0.9027777777777777901, 0.9055555555555555580, 0.9083333333333333259, 0.9111111111111110938, 0.9138888888888888618, 0.9166666666666666297, 0.9194444444444443976, 0.9222222222222222765, 0.9250000000000000444, 0.9277777777777778123, 0.9305555555555555802, 0.9333333333333333481, 0.9361111111111111160, 0.9388888888888888840, 0.9416666666666666519, 0.9444444444444444198, 0.9472222222222221877, 0.9499999999999999556, 0.9527777777777777235, 0.9555555555555556024, 0.9583333333333333703, 0.9611111111111111382, 0.9638888888888889062, 0.9666666666666666741, 0.9694444444444444420, 0.9722222222222222099, 0.9749999999999999778, 0.9777777777777777457, 0.9805555555555555136, 0.9833333333333332815, 0.9861111111111111605, 0.9888888888888889284, 0.9916666666666666963, 0.9944444444444444642, 0.9972222222222222321, 1.000000000000000000 ),
 .UNSPECIFIED. ) 
 GEOMETRIC_REPRESENTATION_ITEM ( )  RATIONAL_B_SPLINE_SURFACE ( (
 ( 1.000000000000000000, 0.8660254037844387076, 1.000000000000000000, 0.8660254037844387076, 1.000000000000000000, 0.8660254037844387076, 1.000000000000000000, 0.8660254037844387076, 1.000000000000000000, 0.8660254037844387076, 1.000000000000000000, 0.8660254037844387076, 1.000000000000000000, 0.8660254037844387076, 1.000000000000000000, 0.8660254037844387076, 1.000000000000000000, 0.8660254037844387076, 1.000000000000000000, 0.8660254037844387076, 1.000000000000000000, 0.8660254037844387076, 1.000000000000000000, 0.8660254037844387076, 1.000000000000000000, 0.8660254037844387076, 1.000000000000000000, 0.8660254037844387076, 1.000000000000000000, 0.8660254037844387076, 1.000000000000000000, 0.8660254037844387076, 1.000000000000000000, 0.8660254037844387076, 1.000000000000000000, 0.8660254037844387076, 1.000000000000000000, 0.8660254037844387076, 1.000000000000000000, 0.8660254037844387076, 1.000000000000000000, 0.8660254037844387076, 1.000000000000000000, 0.8660254037844387076, 1.000000000000000000, 0.8660254037844387076, 1.000000000000000000, 0.8660254037844387076, 1.000000000000000000, 0.8660254037844387076, 1.000000000000000000, 0.8660254037844387076, 1.000000000000000000, 0.8660254037844387076, 1.000000000000000000, 0.8660254037844387076, 1.000000000000000000, 0.8660254037844387076, 1.000000000000000000, 0.8660254037844387076, 1.000000000000000000, 0.8660254037844387076, 1.000000000000000000, 0.8660254037844387076, 1.000000000000000000, 0.8660254037844387076, 1.000000000000000000, 0.8660254037844387076, 1.000000000000000000, 0.8660254037844387076, 1.000000000000000000, 0.8660254037844387076, 1.000000000000000000, 0.8660254037844387076, 1.000000000000000000, 0.8660254037844387076, 1.000000000000000000, 0.8660254037844387076, 1.000000000000000000, 0.8660254037844387076, 1.000000000000000000, 0.8660254037844387076, 1.000000000000000000, 0.8660254037844387076, 1.000000000000000000, 0.8660254037844387076, 1.000000000000000000, 0.8660254037844387076, 1.000000000000000000, 0.8660254037844387076, 1.000000000000000000, 0.8660254037844387076, 1.000000000000000000, 0.8660254037844387076, 1.000000000000000000, 0.8660254037844387076, 1.000000000000000000, 0.8660254037844387076, 1.000000000000000000, 0.8660254037844387076, 1.000000000000000000, 0.8660254037844387076, 1.000000000000000000, 0.8660254037844387076, 1.000000000000000000, 0.8660254037844387076, 1.000000000000000000, 0.8660254037844387076, 1.000000000000000000, 0.8660254037844387076, 1.000000000000000000, 0.8660254037844387076, 1.000000000000000000, 0.8660254037844387076, 1.000000000000000000, 0.8660254037844387076, 1.000000000000000000, 0.8660254037844387076, 1.000000000000000000, 0.8660254037844387076, 1.000000000000000000, 0.8660254037844387076, 1.000000000000000000, 0.8660254037844387076, 1.000000000000000000, 0.8660254037844387076, 1.000000000000000000, 0.8660254037844387076, 1.000000000000000000, 0.8660254037844387076, 1.000000000000000000, 0.8660254037844387076, 1.000000000000000000, 0.8660254037844387076, 1.000000000000000000, 0.8660254037844387076, 1.000000000000000000, 0.8660254037844387076, 1.000000000000000000, 0.8660254037844387076, 1.000000000000000000, 0.8660254037844387076, 1.000000000000000000, 0.8660254037844387076, 1.000000000000000000, 0.8660254037844387076, 1.000000000000000000, 0.8660254037844387076, 1.000000000000000000, 0.8660254037844387076, 1.000000000000000000, 0.8660254037844387076, 1.000000000000000000, 0.8660254037844387076, 1.000000000000000000, 0.8660254037844387076, 1.000000000000000000, 0.8660254037844387076, 1.000000000000000000, 0.8660254037844387076, 1.000000000000000000, 0.8660254037844387076, 1.000000000000000000, 0.8660254037844387076, 1.000000000000000000, 0.8660254037844387076, 1.000000000000000000, 0.8660254037844387076, 1.000000000000000000, 0.8660254037844387076, 1.000000000000000000, 0.8660254037844387076, 1.000000000000000000, 0.8660254037844387076, 1.000000000000000000, 0.8660254037844387076, 1.000000000000000000, 0.8660254037844387076, 1.000000000000000000, 0.8660254037844387076, 1.000000000000000000, 0.8660254037844387076, 1.000000000000000000, 0.8660254037844387076, 1.000000000000000000, 0.8660254037844387076, 1.000000000000000000, 0.8660254037844387076, 1.000000000000000000, 0.8660254037844387076, 1.000000000000000000, 0.8660254037844387076, 1.000000000000000000, 0.8660254037844387076, 1.000000000000000000, 0.8660254037844387076, 1.000000000000000000, 0.8660254037844387076, 1.000000000000000000, 0.8660254037844387076, 1.000000000000000000, 0.8660254037844387076, 1.000000000000000000, 0.8660254037844387076, 1.000000000000000000, 0.8660254037844387076, 1.000000000000000000, 0.8660254037844387076, 1.000000000000000000, 0.8660254037844387076, 1.000000000000000000, 0.8660254037844387076, 1.000000000000000000, 0.8660254037844387076, 1.000000000000000000, 0.8660254037844387076, 1.000000000000000000, 0.8660254037844387076, 1.000000000000000000, 0.8660254037844387076, 1.000000000000000000, 0.8660254037844387076, 1.000000000000000000, 0.8660254037844387076, 1.000000000000000000, 0.8660254037844387076, 1.000000000000000000, 0.8660254037844387076, 1.000000000000000000, 0.8660254037844387076, 1.000000000000000000, 0.8660254037844387076, 1.000000000000000000, 0.8660254037844387076, 1.000000000000000000, 0.8660254037844387076, 1.000000000000000000, 0.8660254037844387076, 1.000000000000000000, 0.8660254037844387076, 1.000000000000000000, 0.8660254037844387076, 1.000000000000000000, 0.8660254037844387076, 1.000000000000000000, 0.8660254037844387076, 1.000000000000000000, 0.8660254037844387076, 1.000000000000000000, 0.8660254037844387076, 1.000000000000000000, 0.8660254037844387076, 1.000000000000000000, 0.8660254037844387076, 1.000000000000000000, 0.8660254037844387076, 1.000000000000000000, 0.8660254037844387076, 1.000000000000000000, 0.8660254037844387076, 1.000000000000000000, 0.8660254037844387076, 1.000000000000000000, 0.8660254037844387076, 1.000000000000000000, 0.8660254037844387076, 1.000000000000000000, 0.8660254037844387076, 1.000000000000000000, 0.8660254037844387076, 1.000000000000000000, 0.8660254037844387076, 1.000000000000000000, 0.8660254037844387076, 1.000000000000000000, 0.8660254037844387076, 1.000000000000000000, 0.8660254037844387076, 1.000000000000000000, 0.8660254037844387076, 1.000000000000000000, 0.8660254037844387076, 1.000000000000000000, 0.8660254037844387076, 1.000000000000000000, 0.8660254037844387076, 1.000000000000000000, 0.8660254037844387076, 1.000000000000000000, 0.8660254037844387076, 1.000000000000000000, 0.8660254037844387076, 1.000000000000000000, 0.8660254037844387076, 1.000000000000000000, 0.8660254037844387076, 1.000000000000000000, 0.8660254037844387076, 1.000000000000000000, 0.8660254037844387076, 1.000000000000000000, 0.8660254037844387076, 1.000000000000000000, 0.8660254037844387076, 1.000000000000000000, 0.8660254037844387076, 1.000000000000000000, 0.8660254037844387076, 1.000000000000000000, 0.8660254037844387076, 1.000000000000000000, 0.8660254037844387076, 1.000000000000000000, 0.8660254037844387076, 1.000000000000000000, 0.8660254037844387076, 1.000000000000000000, 0.8660254037844387076, 1.000000000000000000, 0.8660254037844387076, 1.000000000000000000, 0.8660254037844387076, 1.000000000000000000, 0.8660254037844387076, 1.000000000000000000, 0.8660254037844387076, 1.000000000000000000, 0.8660254037844387076, 1.000000000000000000, 0.8660254037844387076, 1.000000000000000000, 0.8660254037844387076, 1.000000000000000000, 0.8660254037844387076, 1.000000000000000000, 0.8660254037844387076, 1.000000000000000000, 0.8660254037844387076, 1.000000000000000000, 0.8660254037844387076, 1.000000000000000000, 0.8660254037844387076, 1.000000000000000000, 0.8660254037844387076, 1.000000000000000000, 0.8660254037844387076, 1.000000000000000000, 0.8660254037844387076, 1.000000000000000000, 0.8660254037844387076, 1.000000000000000000, 0.8660254037844387076, 1.000000000000000000, 0.8660254037844387076, 1.000000000000000000, 0.8660254037844387076, 1.000000000000000000, 0.8660254037844387076, 1.000000000000000000, 0.8660254037844387076, 1.000000000000000000, 0.8660254037844387076, 1.000000000000000000, 0.8660254037844387076, 1.000000000000000000, 0.8660254037844387076, 1.000000000000000000, 0.8660254037844387076, 1.000000000000000000, 0.8660254037844387076, 1.000000000000000000, 0.8660254037844387076, 1.000000000000000000, 0.8660254037844387076, 1.000000000000000000, 0.8660254037844387076, 1.000000000000000000, 0.8660254037844387076, 1.000000000000000000, 0.8660254037844387076, 1.000000000000000000, 0.8660254037844387076, 1.000000000000000000, 0.8660254037844387076, 1.000000000000000000, 0.8660254037844387076, 1.000000000000000000, 0.8660254037844387076, 1.000000000000000000, 0.8660254037844387076, 1.000000000000000000, 0.8660254037844387076, 1.000000000000000000, 0.8660254037844387076, 1.000000000000000000, 0.8660254037844387076, 1.000000000000000000, 0.8660254037844387076, 1.000000000000000000, 0.8660254037844387076, 1.000000000000000000, 0.8660254037844387076, 1.000000000000000000, 0.8660254037844387076, 1.000000000000000000, 0.8660254037844387076, 1.000000000000000000, 0.8660254037844387076, 1.000000000000000000, 0.8660254037844387076, 1.000000000000000000, 0.8660254037844387076, 1.000000000000000000, 0.8660254037844387076, 1.000000000000000000, 0.8660254037844387076, 1.000000000000000000, 0.8660254037844387076, 1.000000000000000000, 0.8660254037844387076, 1.000000000000000000, 0.8660254037844387076, 1.000000000000000000, 0.8660254037844387076, 1.000000000000000000, 0.8660254037844387076, 1.000000000000000000, 0.8660254037844387076, 1.000000000000000000, 0.8660254037844387076, 1.000000000000000000, 0.8660254037844387076, 1.000000000000000000, 0.8660254037844387076, 1.000000000000000000, 0.8660254037844387076, 1.000000000000000000, 0.8660254037844387076, 1.000000000000000000, 0.8660254037844387076, 1.000000000000000000, 0.8660254037844387076, 1.000000000000000000, 0.8660254037844387076, 1.000000000000000000, 0.8660254037844387076, 1.000000000000000000, 0.8660254037844387076, 1.000000000000000000, 0.8660254037844387076, 1.000000000000000000, 0.8660254037844387076, 1.000000000000000000, 0.8660254037844387076, 1.000000000000000000, 0.8660254037844387076, 1.000000000000000000, 0.8660254037844387076, 1.000000000000000000, 0.8660254037844387076, 1.000000000000000000, 0.8660254037844387076, 1.000000000000000000, 0.8660254037844387076, 1.000000000000000000, 0.8660254037844387076, 1.000000000000000000, 0.8660254037844387076, 1.000000000000000000, 0.8660254037844387076, 1.000000000000000000, 0.8660254037844387076, 1.000000000000000000, 0.8660254037844387076, 1.000000000000000000, 0.8660254037844387076, 1.000000000000000000, 0.8660254037844387076, 1.000000000000000000, 0.8660254037844387076, 1.000000000000000000, 0.8660254037844387076, 1.000000000000000000, 0.8660254037844387076, 1.000000000000000000, 0.8660254037844387076, 1.000000000000000000, 0.8660254037844387076, 1.000000000000000000, 0.8660254037844387076, 1.000000000000000000, 0.8660254037844387076, 1.000000000000000000, 0.8660254037844387076, 1.000000000000000000, 0.8660254037844387076, 1.000000000000000000, 0.8660254037844387076, 1.000000000000000000, 0.8660254037844387076, 1.000000000000000000, 0.8660254037844387076, 1.000000000000000000, 0.8660254037844387076, 1.000000000000000000, 0.8660254037844387076, 1.000000000000000000, 0.8660254037844387076, 1.000000000000000000, 0.8660254037844387076, 1.000000000000000000, 0.8660254037844387076, 1.000000000000000000, 0.8660254037844387076, 1.000000000000000000, 0.8660254037844387076, 1.000000000000000000, 0.8660254037844387076, 1.000000000000000000, 0.8660254037844387076, 1.000000000000000000, 0.8660254037844387076, 1.000000000000000000, 0.8660254037844387076, 1.000000000000000000, 0.8660254037844387076, 1.000000000000000000, 0.8660254037844387076, 1.000000000000000000, 0.8660254037844387076, 1.000000000000000000, 0.8660254037844387076, 1.000000000000000000, 0.8660254037844387076, 1.000000000000000000, 0.8660254037844387076, 1.000000000000000000, 0.8660254037844387076, 1.000000000000000000, 0.8660254037844387076, 1.000000000000000000, 0.8660254037844387076, 1.000000000000000000, 0.8660254037844387076, 1.000000000000000000, 0.8660254037844387076, 1.000000000000000000, 0.8660254037844387076, 1.000000000000000000, 0.8660254037844387076, 1.000000000000000000, 0.8660254037844387076, 1.000000000000000000, 0.8660254037844387076, 1.000000000000000000, 0.8660254037844387076, 1.000000000000000000, 0.8660254037844387076, 1.000000000000000000, 0.8660254037844387076, 1.000000000000000000, 0.8660254037844387076, 1.000000000000000000, 0.8660254037844387076, 1.000000000000000000, 0.8660254037844387076, 1.000000000000000000, 0.8660254037844387076, 1.000000000000000000, 0.8660254037844387076, 1.000000000000000000, 0.8660254037844387076, 1.000000000000000000, 0.8660254037844387076, 1.000000000000000000, 0.8660254037844387076, 1.000000000000000000, 0.8660254037844387076, 1.000000000000000000, 0.8660254037844387076, 1.000000000000000000, 0.8660254037844387076, 1.000000000000000000, 0.8660254037844387076, 1.000000000000000000, 0.8660254037844387076, 1.000000000000000000, 0.8660254037844387076, 1.000000000000000000, 0.8660254037844387076, 1.000000000000000000, 0.8660254037844387076, 1.000000000000000000, 0.8660254037844387076, 1.000000000000000000, 0.8660254037844387076, 1.000000000000000000, 0.8660254037844387076, 1.000000000000000000, 0.8660254037844387076, 1.000000000000000000, 0.8660254037844387076, 1.000000000000000000, 0.8660254037844387076, 1.000000000000000000, 0.8660254037844387076, 1.000000000000000000, 0.8660254037844387076, 1.000000000000000000, 0.8660254037844387076, 1.000000000000000000, 0.8660254037844387076, 1.000000000000000000, 0.8660254037844387076, 1.000000000000000000, 0.8660254037844387076, 1.000000000000000000, 0.8660254037844387076, 1.000000000000000000, 0.8660254037844387076, 1.000000000000000000, 0.8660254037844387076, 1.000000000000000000, 0.8660254037844387076, 1.000000000000000000, 0.8660254037844387076, 1.000000000000000000, 0.8660254037844387076, 1.000000000000000000, 0.8660254037844387076, 1.000000000000000000, 0.8660254037844387076, 1.000000000000000000, 0.8660254037844387076, 1.000000000000000000, 0.8660254037844387076, 1.000000000000000000, 0.8660254037844387076, 1.000000000000000000, 0.8660254037844387076, 1.000000000000000000, 0.8660254037844387076, 1.000000000000000000, 0.8660254037844387076, 1.000000000000000000, 0.8660254037844387076, 1.000000000000000000, 0.8660254037844387076, 1.000000000000000000, 0.8660254037844387076, 1.000000000000000000, 0.8660254037844387076, 1.000000000000000000, 0.8660254037844387076, 1.000000000000000000, 0.8660254037844387076, 1.000000000000000000, 0.8660254037844387076, 1.000000000000000000, 0.8660254037844387076, 1.000000000000000000, 0.8660254037844387076, 1.000000000000000000, 0.8660254037844387076, 1.000000000000000000, 0.8660254037844387076, 1.000000000000000000, 0.8660254037844387076, 1.000000000000000000, 0.8660254037844387076, 1.000000000000000000, 0.8660254037844387076, 1.000000000000000000, 0.8660254037844387076, 1.000000000000000000, 0.8660254037844387076, 1.000000000000000000, 0.8660254037844387076, 1.000000000000000000, 0.8660254037844387076, 1.000000000000000000, 0.8660254037844387076, 1.000000000000000000, 0.8660254037844387076, 1.000000000000000000, 0.8660254037844387076, 1.000000000000000000, 0.8660254037844387076, 1.000000000000000000, 0.8660254037844387076, 1.000000000000000000, 0.8660254037844387076, 1.000000000000000000, 0.8660254037844387076, 1.000000000000000000, 0.8660254037844387076, 1.000000000000000000, 0.8660254037844387076, 1.000000000000000000, 0.8660254037844387076, 1.000000000000000000, 0.8660254037844387076, 1.000000000000000000, 0.8660254037844387076, 1.000000000000000000, 0.8660254037844387076, 1.000000000000000000, 0.8660254037844387076, 1.000000000000000000, 0.8660254037844387076, 1.000000000000000000, 0.8660254037844387076, 1.000000000000000000, 0.8660254037844387076, 1.000000000000000000, 0.8660254037844387076, 1.000000000000000000, 0.8660254037844387076, 1.000000000000000000, 0.8660254037844387076, 1.000000000000000000),
 ( 1.000000000000000000, 0.8660254037844387076, 1.000000000000000000, 0.8660254037844387076, 1.000000000000000000, 0.8660254037844387076, 1.000000000000000000, 0.8660254037844387076, 1.000000000000000000, 0.8660254037844387076, 1.000000000000000000, 0.8660254037844387076, 1.000000000000000000, 0.8660254037844387076, 1.000000000000000000, 0.8660254037844387076, 1.000000000000000000, 0.8660254037844387076, 1.000000000000000000, 0.8660254037844387076, 1.000000000000000000, 0.8660254037844387076, 1.000000000000000000, 0.8660254037844387076, 1.000000000000000000, 0.8660254037844387076, 1.000000000000000000, 0.8660254037844387076, 1.000000000000000000, 0.8660254037844387076, 1.000000000000000000, 0.8660254037844387076, 1.000000000000000000, 0.8660254037844387076, 1.000000000000000000, 0.8660254037844387076, 1.000000000000000000, 0.8660254037844387076, 1.000000000000000000, 0.8660254037844387076, 1.000000000000000000, 0.8660254037844387076, 1.000000000000000000, 0.8660254037844387076, 1.000000000000000000, 0.8660254037844387076, 1.000000000000000000, 0.8660254037844387076, 1.000000000000000000, 0.8660254037844387076, 1.000000000000000000, 0.8660254037844387076, 1.000000000000000000, 0.8660254037844387076, 1.000000000000000000, 0.8660254037844387076, 1.000000000000000000, 0.8660254037844387076, 1.000000000000000000, 0.8660254037844387076, 1.000000000000000000, 0.8660254037844387076, 1.000000000000000000, 0.8660254037844387076, 1.000000000000000000, 0.8660254037844387076, 1.000000000000000000, 0.8660254037844387076, 1.000000000000000000, 0.8660254037844387076, 1.000000000000000000, 0.8660254037844387076, 1.000000000000000000, 0.8660254037844387076, 1.000000000000000000, 0.8660254037844387076, 1.000000000000000000, 0.8660254037844387076, 1.000000000000000000, 0.8660254037844387076, 1.000000000000000000, 0.8660254037844387076, 1.000000000000000000, 0.8660254037844387076, 1.000000000000000000, 0.8660254037844387076, 1.000000000000000000, 0.8660254037844387076, 1.000000000000000000, 0.8660254037844387076, 1.000000000000000000, 0.8660254037844387076, 1.000000000000000000, 0.8660254037844387076, 1.000000000000000000, 0.8660254037844387076, 1.000000000000000000, 0.8660254037844387076, 1.000000000000000000, 0.8660254037844387076, 1.000000000000000000, 0.8660254037844387076, 1.000000000000000000, 0.8660254037844387076, 1.000000000000000000, 0.8660254037844387076, 1.000000000000000000, 0.8660254037844387076, 1.000000000000000000, 0.8660254037844387076, 1.000000000000000000, 0.8660254037844387076, 1.000000000000000000, 0.8660254037844387076, 1.000000000000000000, 0.8660254037844387076, 1.000000000000000000, 0.8660254037844387076, 1.000000000000000000, 0.8660254037844387076, 1.000000000000000000, 0.8660254037844387076, 1.000000000000000000, 0.8660254037844387076, 1.000000000000000000, 0.8660254037844387076, 1.000000000000000000, 0.8660254037844387076, 1.000000000000000000, 0.8660254037844387076, 1.000000000000000000, 0.8660254037844387076, 1.000000000000000000, 0.8660254037844387076, 1.000000000000000000, 0.8660254037844387076, 1.000000000000000000, 0.8660254037844387076, 1.000000000000000000, 0.8660254037844387076, 1.000000000000000000, 0.8660254037844387076, 1.000000000000000000, 0.8660254037844387076, 1.000000000000000000, 0.8660254037844387076, 1.000000000000000000, 0.8660254037844387076, 1.000000000000000000, 0.8660254037844387076, 1.000000000000000000, 0.8660254037844387076, 1.000000000000000000, 0.8660254037844387076, 1.000000000000000000, 0.8660254037844387076, 1.000000000000000000, 0.8660254037844387076, 1.000000000000000000, 0.8660254037844387076, 1.000000000000000000, 0.8660254037844387076, 1.000000000000000000, 0.8660254037844387076, 1.000000000000000000, 0.8660254037844387076, 1.000000000000000000, 0.8660254037844387076, 1.000000000000000000, 0.8660254037844387076, 1.000000000000000000, 0.8660254037844387076, 1.000000000000000000, 0.8660254037844387076, 1.000000000000000000, 0.8660254037844387076, 1.000000000000000000, 0.8660254037844387076, 1.000000000000000000, 0.8660254037844387076, 1.000000000000000000, 0.8660254037844387076, 1.000000000000000000, 0.8660254037844387076, 1.000000000000000000, 0.8660254037844387076, 1.000000000000000000, 0.8660254037844387076, 1.000000000000000000, 0.8660254037844387076, 1.000000000000000000, 0.8660254037844387076, 1.000000000000000000, 0.8660254037844387076, 1.000000000000000000, 0.8660254037844387076, 1.000000000000000000, 0.8660254037844387076, 1.000000000000000000, 0.8660254037844387076, 1.000000000000000000, 0.8660254037844387076, 1.000000000000000000, 0.8660254037844387076, 1.000000000000000000, 0.8660254037844387076, 1.000000000000000000, 0.8660254037844387076, 1.000000000000000000, 0.8660254037844387076, 1.000000000000000000, 0.8660254037844387076, 1.000000000000000000, 0.8660254037844387076, 1.000000000000000000, 0.8660254037844387076, 1.000000000000000000, 0.8660254037844387076, 1.000000000000000000, 0.8660254037844387076, 1.000000000000000000, 0.8660254037844387076, 1.000000000000000000, 0.8660254037844387076, 1.000000000000000000, 0.8660254037844387076, 1.000000000000000000, 0.8660254037844387076, 1.000000000000000000, 0.8660254037844387076, 1.000000000000000000, 0.8660254037844387076, 1.000000000000000000, 0.8660254037844387076, 1.000000000000000000, 0.8660254037844387076, 1.000000000000000000, 0.8660254037844387076, 1.000000000000000000, 0.8660254037844387076, 1.000000000000000000, 0.8660254037844387076, 1.000000000000000000, 0.8660254037844387076, 1.000000000000000000, 0.8660254037844387076, 1.000000000000000000, 0.8660254037844387076, 1.000000000000000000, 0.8660254037844387076, 1.000000000000000000, 0.8660254037844387076, 1.000000000000000000, 0.8660254037844387076, 1.000000000000000000, 0.8660254037844387076, 1.000000000000000000, 0.8660254037844387076, 1.000000000000000000, 0.8660254037844387076, 1.000000000000000000, 0.8660254037844387076, 1.000000000000000000, 0.8660254037844387076, 1.000000000000000000, 0.8660254037844387076, 1.000000000000000000, 0.8660254037844387076, 1.000000000000000000, 0.8660254037844387076, 1.000000000000000000, 0.8660254037844387076, 1.000000000000000000, 0.8660254037844387076, 1.000000000000000000, 0.8660254037844387076, 1.000000000000000000, 0.8660254037844387076, 1.000000000000000000, 0.8660254037844387076, 1.000000000000000000, 0.8660254037844387076, 1.000000000000000000, 0.8660254037844387076, 1.000000000000000000, 0.8660254037844387076, 1.000000000000000000, 0.8660254037844387076, 1.000000000000000000, 0.8660254037844387076, 1.000000000000000000, 0.8660254037844387076, 1.000000000000000000, 0.8660254037844387076, 1.000000000000000000, 0.8660254037844387076, 1.000000000000000000, 0.8660254037844387076, 1.000000000000000000, 0.8660254037844387076, 1.000000000000000000, 0.8660254037844387076, 1.000000000000000000, 0.8660254037844387076, 1.000000000000000000, 0.8660254037844387076, 1.000000000000000000, 0.8660254037844387076, 1.000000000000000000, 0.8660254037844387076, 1.000000000000000000, 0.8660254037844387076, 1.000000000000000000, 0.8660254037844387076, 1.000000000000000000, 0.8660254037844387076, 1.000000000000000000, 0.8660254037844387076, 1.000000000000000000, 0.8660254037844387076, 1.000000000000000000, 0.8660254037844387076, 1.000000000000000000, 0.8660254037844387076, 1.000000000000000000, 0.8660254037844387076, 1.000000000000000000, 0.8660254037844387076, 1.000000000000000000, 0.8660254037844387076, 1.000000000000000000, 0.8660254037844387076, 1.000000000000000000, 0.8660254037844387076, 1.000000000000000000, 0.8660254037844387076, 1.000000000000000000, 0.8660254037844387076, 1.000000000000000000, 0.8660254037844387076, 1.000000000000000000, 0.8660254037844387076, 1.000000000000000000, 0.8660254037844387076, 1.000000000000000000, 0.8660254037844387076, 1.000000000000000000, 0.8660254037844387076, 1.000000000000000000, 0.8660254037844387076, 1.000000000000000000, 0.8660254037844387076, 1.000000000000000000, 0.8660254037844387076, 1.000000000000000000, 0.8660254037844387076, 1.000000000000000000, 0.8660254037844387076, 1.000000000000000000, 0.8660254037844387076, 1.000000000000000000, 0.8660254037844387076, 1.000000000000000000, 0.8660254037844387076, 1.000000000000000000, 0.8660254037844387076, 1.000000000000000000, 0.8660254037844387076, 1.000000000000000000, 0.8660254037844387076, 1.000000000000000000, 0.8660254037844387076, 1.000000000000000000, 0.8660254037844387076, 1.000000000000000000, 0.8660254037844387076, 1.000000000000000000, 0.8660254037844387076, 1.000000000000000000, 0.8660254037844387076, 1.000000000000000000, 0.8660254037844387076, 1.000000000000000000, 0.8660254037844387076, 1.000000000000000000, 0.8660254037844387076, 1.000000000000000000, 0.8660254037844387076, 1.000000000000000000, 0.8660254037844387076, 1.000000000000000000, 0.8660254037844387076, 1.000000000000000000, 0.8660254037844387076, 1.000000000000000000, 0.8660254037844387076, 1.000000000000000000, 0.8660254037844387076, 1.000000000000000000, 0.8660254037844387076, 1.000000000000000000, 0.8660254037844387076, 1.000000000000000000, 0.8660254037844387076, 1.000000000000000000, 0.8660254037844387076, 1.000000000000000000, 0.8660254037844387076, 1.000000000000000000, 0.8660254037844387076, 1.000000000000000000, 0.8660254037844387076, 1.000000000000000000, 0.8660254037844387076, 1.000000000000000000, 0.8660254037844387076, 1.000000000000000000, 0.8660254037844387076, 1.000000000000000000, 0.8660254037844387076, 1.000000000000000000, 0.8660254037844387076, 1.000000000000000000, 0.8660254037844387076, 1.000000000000000000, 0.8660254037844387076, 1.000000000000000000, 0.8660254037844387076, 1.000000000000000000, 0.8660254037844387076, 1.000000000000000000, 0.8660254037844387076, 1.000000000000000000, 0.8660254037844387076, 1.000000000000000000, 0.8660254037844387076, 1.000000000000000000, 0.8660254037844387076, 1.000000000000000000, 0.8660254037844387076, 1.000000000000000000, 0.8660254037844387076, 1.000000000000000000, 0.8660254037844387076, 1.000000000000000000, 0.8660254037844387076, 1.000000000000000000, 0.8660254037844387076, 1.000000000000000000, 0.8660254037844387076, 1.000000000000000000, 0.8660254037844387076, 1.000000000000000000, 0.8660254037844387076, 1.000000000000000000, 0.8660254037844387076, 1.000000000000000000, 0.8660254037844387076, 1.000000000000000000, 0.8660254037844387076, 1.000000000000000000, 0.8660254037844387076, 1.000000000000000000, 0.8660254037844387076, 1.000000000000000000, 0.8660254037844387076, 1.000000000000000000, 0.8660254037844387076, 1.000000000000000000, 0.8660254037844387076, 1.000000000000000000, 0.8660254037844387076, 1.000000000000000000, 0.8660254037844387076, 1.000000000000000000, 0.8660254037844387076, 1.000000000000000000, 0.8660254037844387076, 1.000000000000000000, 0.8660254037844387076, 1.000000000000000000, 0.8660254037844387076, 1.000000000000000000, 0.8660254037844387076, 1.000000000000000000, 0.8660254037844387076, 1.000000000000000000, 0.8660254037844387076, 1.000000000000000000, 0.8660254037844387076, 1.000000000000000000, 0.8660254037844387076, 1.000000000000000000, 0.8660254037844387076, 1.000000000000000000, 0.8660254037844387076, 1.000000000000000000, 0.8660254037844387076, 1.000000000000000000, 0.8660254037844387076, 1.000000000000000000, 0.8660254037844387076, 1.000000000000000000, 0.8660254037844387076, 1.000000000000000000, 0.8660254037844387076, 1.000000000000000000, 0.8660254037844387076, 1.000000000000000000, 0.8660254037844387076, 1.000000000000000000, 0.8660254037844387076, 1.000000000000000000, 0.8660254037844387076, 1.000000000000000000, 0.8660254037844387076, 1.000000000000000000, 0.8660254037844387076, 1.000000000000000000, 0.8660254037844387076, 1.000000000000000000, 0.8660254037844387076, 1.000000000000000000, 0.8660254037844387076, 1.000000000000000000, 0.8660254037844387076, 1.000000000000000000, 0.8660254037844387076, 1.000000000000000000, 0.8660254037844387076, 1.000000000000000000, 0.8660254037844387076, 1.000000000000000000, 0.8660254037844387076, 1.000000000000000000, 0.8660254037844387076, 1.000000000000000000, 0.8660254037844387076, 1.000000000000000000, 0.8660254037844387076, 1.000000000000000000, 0.8660254037844387076, 1.000000000000000000, 0.8660254037844387076, 1.000000000000000000, 0.8660254037844387076, 1.000000000000000000, 0.8660254037844387076, 1.000000000000000000, 0.8660254037844387076, 1.000000000000000000, 0.8660254037844387076, 1.000000000000000000, 0.8660254037844387076, 1.000000000000000000, 0.8660254037844387076, 1.000000000000000000, 0.8660254037844387076, 1.000000000000000000, 0.8660254037844387076, 1.000000000000000000, 0.8660254037844387076, 1.000000000000000000, 0.8660254037844387076, 1.000000000000000000, 0.8660254037844387076, 1.000000000000000000, 0.8660254037844387076, 1.000000000000000000, 0.8660254037844387076, 1.000000000000000000, 0.8660254037844387076, 1.000000000000000000, 0.8660254037844387076, 1.000000000000000000, 0.8660254037844387076, 1.000000000000000000, 0.8660254037844387076, 1.000000000000000000, 0.8660254037844387076, 1.000000000000000000, 0.8660254037844387076, 1.000000000000000000, 0.8660254037844387076, 1.000000000000000000, 0.8660254037844387076, 1.000000000000000000, 0.8660254037844387076, 1.000000000000000000, 0.8660254037844387076, 1.000000000000000000, 0.8660254037844387076, 1.000000000000000000, 0.8660254037844387076, 1.000000000000000000, 0.8660254037844387076, 1.000000000000000000, 0.8660254037844387076, 1.000000000000000000, 0.8660254037844387076, 1.000000000000000000, 0.8660254037844387076, 1.000000000000000000, 0.8660254037844387076, 1.000000000000000000, 0.8660254037844387076, 1.000000000000000000, 0.8660254037844387076, 1.000000000000000000, 0.8660254037844387076, 1.000000000000000000, 0.8660254037844387076, 1.000000000000000000, 0.8660254037844387076, 1.000000000000000000, 0.8660254037844387076, 1.000000000000000000, 0.8660254037844387076, 1.000000000000000000, 0.8660254037844387076, 1.000000000000000000, 0.8660254037844387076, 1.000000000000000000, 0.8660254037844387076, 1.000000000000000000, 0.8660254037844387076, 1.000000000000000000, 0.8660254037844387076, 1.000000000000000000, 0.8660254037844387076, 1.000000000000000000, 0.8660254037844387076, 1.000000000000000000, 0.8660254037844387076, 1.000000000000000000, 0.8660254037844387076, 1.000000000000000000, 0.8660254037844387076, 1.000000000000000000, 0.8660254037844387076, 1.000000000000000000, 0.8660254037844387076, 1.000000000000000000, 0.8660254037844387076, 1.000000000000000000, 0.8660254037844387076, 1.000000000000000000, 0.8660254037844387076, 1.000000000000000000, 0.8660254037844387076, 1.000000000000000000, 0.8660254037844387076, 1.000000000000000000, 0.8660254037844387076, 1.000000000000000000, 0.8660254037844387076, 1.000000000000000000, 0.8660254037844387076, 1.000000000000000000, 0.8660254037844387076, 1.000000000000000000, 0.8660254037844387076, 1.000000000000000000, 0.8660254037844387076, 1.000000000000000000, 0.8660254037844387076, 1.000000000000000000, 0.8660254037844387076, 1.000000000000000000, 0.8660254037844387076, 1.000000000000000000, 0.8660254037844387076, 1.000000000000000000, 0.8660254037844387076, 1.000000000000000000, 0.8660254037844387076, 1.000000000000000000, 0.8660254037844387076, 1.000000000000000000, 0.8660254037844387076, 1.000000000000000000, 0.8660254037844387076, 1.000000000000000000, 0.8660254037844387076, 1.000000000000000000, 0.8660254037844387076, 1.000000000000000000, 0.8660254037844387076, 1.000000000000000000, 0.8660254037844387076, 1.000000000000000000, 0.8660254037844387076, 1.000000000000000000, 0.8660254037844387076, 1.000000000000000000, 0.8660254037844387076, 1.000000000000000000, 0.8660254037844387076, 1.000000000000000000, 0.8660254037844387076, 1.000000000000000000, 0.8660254037844387076, 1.000000000000000000, 0.8660254037844387076, 1.000000000000000000, 0.8660254037844387076, 1.000000000000000000, 0.8660254037844387076, 1.000000000000000000, 0.8660254037844387076, 1.000000000000000000, 0.8660254037844387076, 1.000000000000000000, 0.8660254037844387076, 1.000000000000000000, 0.8660254037844387076, 1.000000000000000000, 0.8660254037844387076, 1.000000000000000000, 0.8660254037844387076, 1.000000000000000000) ) ) 
 REPRESENTATION_ITEM ( '' )  SURFACE ( )  );
#47364=CARTESIAN_POINT ( 'NONE',  ( 16.05937500061451573, -4.541064518000417216, -2.621784821875001281 ) ) ;
#47365=CARTESIAN_POINT ( 'NONE',  ( 22.11562500061451786, 3.027376345333611329, 5.243569643749999010 ) ) ;
#47366=CARTESIAN_POINT ( 'NONE',  ( -3.999999999999999112, 15.05000000000000071, 30.00000000000000000 ) ) ;
#47367=CARTESIAN_POINT ( 'NONE',  ( 3.271875000614519635, 3.027376345333611329, 5.243569643749999010 ) ) ;
#47368=CARTESIAN_POINT ( 'NONE',  ( 9.075000001229033941, -5.773502691896255534, -1.060575238724906372E-15 ) ) ;
#47369=ORIENTED_EDGE ( 'NONE', *, *, #16702, .T. ) ;
#47370=CARTESIAN_POINT ( 'NONE',  ( 5.175000001229033586, 2.886751345948129099, -4.999999999999998224 ) ) ;
#47371=CARTESIAN_POINT ( 'NONE',  ( 1.999999999999998668, 18.95000000000000284, -33.46410161513775705 ) ) ;
#47372=CARTESIAN_POINT ( 'NONE',  ( 25.31250000122903288, -4.330127018922190985, -2.500000000000001332 ) ) ;
#47374=CARTESIAN_POINT ( 'NONE',  ( 8.146875000614516082, 6.054752690667223547, 3.707466751127219781E-16 ) ) ;
#47376=EDGE_CURVE ( 'NONE', #33433, #37978, #28836, .T. ) ;
#47377=CARTESIAN_POINT ( 'NONE',  ( 13.90312500061451750, 4.541064518000418104, -2.621784821874998173 ) ) ;
#47378=CARTESIAN_POINT ( 'NONE',  ( 10.95937500061451964, 0.000000000000000000, 5.243569643749999010 ) ) ;
#47379=CARTESIAN_POINT ( 'NONE',  ( 26.85000000122903430, 5.773502691896255534, 3.535250795749688894E-16 ) ) ;
#47380=CARTESIAN_POINT ( 'NONE',  ( 17.07187500061451502, 3.027376345333612662, -5.243569643749998122 ) ) ;
#47381=CARTESIAN_POINT ( 'NONE',  ( 6.009375000614519458, 0.000000000000000000, 5.243569643749999010 ) ) ;
#47382=CARTESIAN_POINT ( 'NONE',  ( 1.626862140677534273E-15, 16.17500000122903359, 34.00000000000000000 ) ) ;
#47383=CARTESIAN_POINT ( 'NONE',  ( 6.778125000614518392, 4.541064518000418104, 2.621784821874999949 ) ) ;
#47384=CARTESIAN_POINT ( 'NONE',  ( 17.69062500061451715, -3.027376345333614438, 5.243569643749998122 ) ) ;
#47386=CARTESIAN_POINT ( 'NONE',  ( 14.57812500061451644, -4.541064518000419881, 2.621784821874995952 ) ) ;
#47387=CARTESIAN_POINT ( 'NONE',  ( 10.56562500061451715, -6.054752690667223547, -1.112240025338166033E-15 ) ) ;
#47389=CARTESIAN_POINT ( 'NONE',  ( 12.15000000000000036, -4.330127018922190985, -2.500000000000001332 ) ) ;
#47390=CARTESIAN_POINT ( 'NONE',  ( 6.075000001229034829, 2.886751345948129099, -4.999999999999998224 ) ) ;
#47392=CARTESIAN_POINT ( 'NONE',  ( 13.77187500061451786, -6.054752690667223547, -1.112240025338166033E-15 ) ) ;
#47393=CARTESIAN_POINT ( 'NONE',  ( 15.78750000122903430, -4.330127018922194537, 2.499999999999995559 ) ) ;
#47395=CARTESIAN_POINT ( 'NONE',  ( -2.121784821874996840, 18.97812500061451857, -26.32496088578401583 ) ) ;
#47396=CARTESIAN_POINT ( 'NONE',  ( -3.999999999999999112, 16.02500000122903501, 27.69059892324149885 ) ) ;
#47397=FACE_OUTER_BOUND ( 'NONE', #23664, .T. ) ;
#47400=CARTESIAN_POINT ( 'NONE',  ( 15.30937500061451750, 4.541064518000418104, -2.621784821874998173 ) ) ;
#47402=CARTESIAN_POINT ( 'NONE',  ( 28.64999999999999858, 0.000000000000000000, 4.999999999999998224 ) ) ;
#47403=CARTESIAN_POINT ( 'NONE',  ( 13.04062500061451502, 6.054752690667223547, 3.707466751127219781E-16 ) ) ;
#47406=CARTESIAN_POINT ( 'NONE',  ( 24.30937500061451573, 4.541064518000418104, -2.621784821874998173 ) ) ;
#47408=CARTESIAN_POINT ( 'NONE',  ( 10.67812500061451608, 6.421520780324663323E-16, -5.243569643749999010 ) ) ;
#47409=CARTESIAN_POINT ( 'NONE',  ( 15.98437500061451821, -4.541064518000419881, 2.621784821874995952 ) ) ;
#47411=CARTESIAN_POINT ( 'NONE',  ( 26.74687500061451573, -3.027376345333614438, 5.243569643749998122 ) ) ;
#47412=CARTESIAN_POINT ( 'NONE',  ( 27.62812500061451360, -4.541064518000419881, 2.621784821874995952 ) ) ;
#47413=CARTESIAN_POINT ( 'NONE',  ( 17.42812500061451786, 6.421520780324663323E-16, -5.243569643749999010 ) ) ;
#47414=CARTESIAN_POINT ( 'NONE',  ( 1.626862140677534273E-15, 13.02500000122903323, -26.00000000000000355 ) ) ;
#47415=CARTESIAN_POINT ( 'NONE',  ( -1.487416814333745711E-14, 14.82500000122903572, -26.00000000000000000 ) ) ;
#47416=CARTESIAN_POINT ( 'NONE',  ( 8.025000000000000355, -4.330127018922194537, 2.499999999999995559 ) ) ;
#47417=CARTESIAN_POINT ( 'NONE',  ( 20.06250000122903643, 4.330127018922192761, -2.499999999999997780 ) ) ;
#47420=VERTEX_POINT ( 'NONE', #34923 ) ;
#47421=CARTESIAN_POINT ( 'NONE',  ( 16.61250000000000426, -5.773502691896255534, -1.060575238724906372E-15 ) ) ;
#47422=CARTESIAN_POINT ( 'NONE',  ( 18.93750000000000000, -2.886751345948125991, -5.000000000000000000 ) ) ;
#47423=CARTESIAN_POINT ( 'NONE',  ( 19.24687500061452283, -3.027376345333610441, -5.243569643749999898 ) ) ;
#47424=CARTESIAN_POINT ( 'NONE',  ( 14.09062500061451750, -3.027376345333614438, 5.243569643749998122 ) ) ;
#47425=ORIENTED_EDGE ( 'NONE', *, *, #40932, .F. ) ;
#47426=CARTESIAN_POINT ( 'NONE',  ( 5.728125000614515905, 6.421520780324663323E-16, -5.243569643749999010 ) ) ;
#47427=CARTESIAN_POINT ( 'NONE',  ( 0.000000000000000000, 10.00000000000000000, 0.000000000000000000 ) ) ;
#47428=CARTESIAN_POINT ( 'NONE',  ( 12.00000000000000000, 0.000000000000000000, 4.999999999999998224 ) ) ;
#47430=CARTESIAN_POINT ( 'NONE',  ( -3.000416591977282496E-16, 14.74062500061451786, 25.09994784771203058 ) ) ;
#47431=CARTESIAN_POINT ( 'NONE',  ( 26.09062500061451573, 6.054752690667223547, 3.707466751127219781E-16 ) ) ;
#47434=CARTESIAN_POINT ( 'NONE',  ( 24.27187500061452141, 3.027376345333613106, -5.243569643749998122 ) ) ;
#47436=CARTESIAN_POINT ( 'NONE',  ( 22.04062500061451502, 6.054752690667223547, 3.707466751127219781E-16 ) ) ;
#47437=CARTESIAN_POINT ( 'NONE',  ( 22.32187500061451502, -6.054752690667223547, -1.112240025338166033E-15 ) ) ;
#47438=CARTESIAN_POINT ( 'NONE',  ( -4.243569643749998122, 16.24062500061459247, -27.54997392385601174 ) ) ;
#47439=CARTESIAN_POINT ( 'NONE',  ( 7.378125000614518036, -4.541064518000419881, 2.621784821874995952 ) ) ;
#47441=CARTESIAN_POINT ( 'NONE',  ( 24.06562500061451715, -6.054752690667223547, -1.112240025338166033E-15 ) ) ;
#47444=CARTESIAN_POINT ( 'NONE',  ( 17.67187500061451644, 3.027376345333611329, 5.243569643749999010 ) ) ;
#47445=CARTESIAN_POINT ( 'NONE',  ( 24.60937500061451644, -4.541064518000417216, -2.621784821875001281 ) ) ;
#47446=CARTESIAN_POINT ( 'NONE',  ( -3.000416591977282496E-16, 14.79687500061451821, 25.09994784771203058 ) ) ;
#47447=CARTESIAN_POINT ( 'NONE',  ( 8.278125000614515727, -4.541064518000419881, 2.621784821874995952 ) ) ;
#47448=CARTESIAN_POINT ( 'NONE',  ( 27.96562500061451928, 3.027376345333611329, 5.243569643749999010 ) ) ;
#47449=CARTESIAN_POINT ( 'NONE',  ( 29.27812500061451573, 4.541064518000418104, 2.621784821874999949 ) ) ;
#47451=CARTESIAN_POINT ( 'NONE',  ( 5.015625000614518214, 3.027376345333611329, 5.243569643749999010 ) ) ;
#47452=CARTESIAN_POINT ( 'NONE',  ( 9.346875000614517148, -3.027376345333610441, -5.243569643749999898 ) ) ;
#47453=CARTESIAN_POINT ( 'NONE',  ( 15.67500000122903181, 2.886751345948126879, 4.999999999999999112 ) ) ;
#47454=CARTESIAN_POINT ( 'NONE',  ( 29.05312500061451431, -4.541064518000417216, -2.621784821875001281 ) ) ;
#47455=CARTESIAN_POINT ( 'NONE',  ( 5.840625000614516615, 6.054752690667223547, 3.707466751127219781E-16 ) ) ;
#47458=CARTESIAN_POINT ( 'NONE',  ( 16.65937500061452070, 4.541064518000418104, -2.621784821874998173 ) ) ;
#47459=CARTESIAN_POINT ( 'NONE',  ( 0.000000000000000000, 20.00000000000000000, 30.00000000000000000 ) ) ;
#47461=CARTESIAN_POINT ( 'NONE',  ( 21.14062500061451289, 6.054752690667223547, 3.707466751127219781E-16 ) ) ;
#47462=CARTESIAN_POINT ( 'NONE',  ( 9.065625000614517148, 3.027376345333611329, 5.243569643749999010 ) ) ;
#47463=CARTESIAN_POINT ( 'NONE',  ( 23.82187500061451502, 3.027376345333612662, -5.243569643749998122 ) ) ;
#47464=CARTESIAN_POINT ( 'NONE',  ( 7.753125000614518036, 0.000000000000000000, 5.243569643749999010 ) ) ;
#47465=CARTESIAN_POINT ( 'NONE',  ( 20.32499999999999929, 6.123233995736764310E-16, -4.999999999999998224 ) ) ;
#47466=CARTESIAN_POINT ( 'NONE',  ( 11.02500000122903501, 2.886751345948129099, -4.999999999999998224 ) ) ;
#47467=CARTESIAN_POINT ( 'NONE',  ( 23.80312500061451786, 4.541064518000418104, -2.621784821874998173 ) ) ;
#47468=AXIS2_PLACEMENT_3D ( 'NONE', #3758, #59886, #25168 ) ;
#47469=CARTESIAN_POINT ( 'NONE',  ( 4.243569643749999898, 11.02812500061451750, -30.00000000000000000 ) ) ;
#47470=CARTESIAN_POINT ( 'NONE',  ( 13.46250000122903323, 0.000000000000000000, 4.999999999999998224 ) ) ;
#47471=CARTESIAN_POINT ( 'NONE',  ( 22.52812500061451573, 4.541064518000418104, 2.621784821874999949 ) ) ;
#47472=CARTESIAN_POINT ( 'NONE',  ( 17.27812500061451217, -4.541064518000419881, 2.621784821874995952 ) ) ;
#47473=CARTESIAN_POINT ( 'NONE',  ( 5.221875000614519813, -6.054752690667223547, -1.112240025338166033E-15 ) ) ;
#47474=CARTESIAN_POINT ( 'NONE',  ( 18.82500000000000284, -4.330127018922194537, 2.499999999999995559 ) ) ;
#47476=CARTESIAN_POINT ( 'NONE',  ( 13.61250000122903359, -4.330127018922190985, -2.500000000000001332 ) ) ;
#47477=CARTESIAN_POINT ( 'NONE',  ( 11.05312500061451608, -4.541064518000417216, -2.621784821875001281 ) ) ;
#47478=CARTESIAN_POINT ( 'NONE',  ( 12.96562500061451750, 3.027376345333613106, -5.243569643749998122 ) ) ;
#47479=CARTESIAN_POINT ( 'NONE',  ( 24.37500000122903288, -5.773502691896255534, -1.060575238724906372E-15 ) ) ;
#47480=CARTESIAN_POINT ( 'NONE',  ( 21.87187500061451573, -6.054752690667223547, -1.112240025338166033E-15 ) ) ;
#47481=CARTESIAN_POINT ( 'NONE',  ( 21.04687500061451644, -3.027376345333610441, -5.243569643749999898 ) ) ;
#47482=CARTESIAN_POINT ( 'NONE',  ( 30.00000000000000000, 0.000000000000000000, 0.000000000000000000 ) ) ;
#47483=EDGE_CURVE ( 'NONE', #34653, #16314, #33144, .T. ) ;
#47484=CARTESIAN_POINT ( 'NONE',  ( 8.475000001229034297, 2.886751345948126879, 4.999999999999999112 ) ) ;
#47485=CARTESIAN_POINT ( 'NONE',  ( 6.346875000614517148, 6.054752690667223547, 3.707466751127219781E-16 ) ) ;
#47486=CARTESIAN_POINT ( 'NONE',  ( 24.90937500061451715, 0.000000000000000000, 5.243569643749999010 ) ) ;
#47487=ADVANCED_FACE ( 'NONE', ( #40844 ), #13104, .F. ) ;
#47488=CARTESIAN_POINT ( 'NONE',  ( 4.286481933758009788, -2.574115893188666959, -4.460274119859103159 ) ) ;
#47489=CARTESIAN_POINT ( 'NONE',  ( 22.19062500061451715, -3.027376345333614438, 5.243569643749998122 ) ) ;
#47490=CARTESIAN_POINT ( 'NONE',  ( 26.22187500061451715, 3.027376345333611329, 5.243569643749999010 ) ) ;
#47492=CARTESIAN_POINT ( 'NONE',  ( -5.810221930991193690E-16, 15.83749999999999680, 26.00000000000000355 ) ) ;
#47493=CARTESIAN_POINT ( 'NONE',  ( 6.646875000614518747, -3.027376345333610441, -5.243569643749999898 ) ) ;
#47494=CARTESIAN_POINT ( 'NONE',  ( 16.71562500061451573, 3.027376345333611329, 5.243569643749999010 ) ) ;
#47495=ORIENTED_EDGE ( 'NONE', *, *, #37141, .F. ) ;
#47496=CARTESIAN_POINT ( 'NONE',  ( 22.91250000000000142, -5.773502691896255534, -1.060575238724906372E-15 ) ) ;
#47497=CARTESIAN_POINT ( 'NONE',  ( 25.82812500061451644, -4.541064518000419881, 2.621784821874995952 ) ) ;
#47498=CARTESIAN_POINT ( 'NONE',  ( 3.646875000614520079, 6.054752690667223547, 3.707466751127219781E-16 ) ) ;
#47499=CARTESIAN_POINT ( 'NONE',  ( 10.27500000122903145, 2.886751345948193936, 4.999999999999883649 ) ) ;
#47500=CARTESIAN_POINT ( 'NONE',  ( 3.675409193445907441, 3.389947486076141381, -3.797828392354649640 ) ) ;
#47501=CARTESIAN_POINT ( 'NONE',  ( 16.38749999999999929, 5.773502691896255534, 3.535250795749688894E-16 ) ) ;
#47502=CARTESIAN_POINT ( 'NONE',  ( 19.94062500061451715, -3.027376345333614438, 5.243569643749998122 ) ) ;
#47503=ORIENTED_EDGE ( 'NONE', *, *, #31085, .T. ) ;
#47504=CARTESIAN_POINT ( 'NONE',  ( 25.23749999999999716, -2.886751345948125991, -5.000000000000000000 ) ) ;
#47506=CARTESIAN_POINT ( 'NONE',  ( 26.93437500061451573, 6.421520780324663323E-16, -5.243569643749999010 ) ) ;
#47509=CARTESIAN_POINT ( 'NONE',  ( 2.989682168262277173, -4.007725729151955463, -3.381303433842018258 ) ) ;
#47510=CARTESIAN_POINT ( 'NONE',  ( 12.96562500061451750, 3.027376345333613106, -5.243569643749998122 ) ) ;
#47511=CARTESIAN_POINT ( 'NONE',  ( 6.665625000614515905, 3.027376345333613106, -5.243569643749998122 ) ) ;
#47513=CARTESIAN_POINT ( 'NONE',  ( 2.896875000614518747, -3.027376345333614438, 5.243569643749998122 ) ) ;
#47514=CARTESIAN_POINT ( 'NONE',  ( 14.73750000122903359, 4.330127018922191873, 2.499999999999999556 ) ) ;
#47515=CARTESIAN_POINT ( 'NONE',  ( 19.38749999999999929, -2.886751345948125991, -5.000000000000000000 ) ) ;
#47516=CARTESIAN_POINT ( 'NONE',  ( 27.52500000000000213, 6.123233995736764310E-16, -4.999999999999998224 ) ) ;
#47517=LINE ( 'NONE', #64867, #61589 ) ;
#47518=CARTESIAN_POINT ( 'NONE',  ( 8.409375000614518925, -4.541064518000417216, -2.621784821875001281 ) ) ;
#47519=CARTESIAN_POINT ( 'NONE',  ( 18.68437500061451928, -4.541064518000419881, 2.621784821874995952 ) ) ;
#47520=CARTESIAN_POINT ( 'NONE',  ( 26.06250000000000000, -5.773502691896255534, -1.060575238724906372E-15 ) ) ;
#47521=ORIENTED_EDGE ( 'NONE', *, *, #36932, .T. ) ;
#47522=CARTESIAN_POINT ( 'NONE',  ( 27.89062500061451289, 6.054752690667223547, 3.707466751127219781E-16 ) ) ;
#47523=CARTESIAN_POINT ( 'NONE',  ( 3.787500000000002753, 5.773502691896255534, 3.535250795749688894E-16 ) ) ;
#47524=CARTESIAN_POINT ( 'NONE',  ( 4.246875000614519280, -3.027376345333614438, 5.243569643749998122 ) ) ;
#47525=CARTESIAN_POINT ( 'NONE',  ( 15.45000000000000107, 4.330127018922192761, -2.499999999999997780 ) ) ;
#47526=CARTESIAN_POINT ( 'NONE',  ( 14.69062500061451537, -3.027376345333610441, -5.243569643749999898 ) ) ;
#47529=CARTESIAN_POINT ( 'NONE',  ( 13.46250000122903323, 0.000000000000000000, 4.999999999999998224 ) ) ;
#47530=CARTESIAN_POINT ( 'NONE',  ( 17.92500000122903359, 2.886751345948126879, 4.999999999999999112 ) ) ;
#47531=CARTESIAN_POINT ( 'NONE',  ( -1.071796769724488563, 13.45490381179670081, 34.00000000000000000 ) ) ;
#47533=CARTESIAN_POINT ( 'NONE',  ( 8.690625000614515372, -3.027376345333614438, 5.243569643749998122 ) ) ;
#47534=CARTESIAN_POINT ( 'NONE',  ( 24.57187500061451502, -6.054752690667223547, -1.112240025338166033E-15 ) ) ;
#47535=FACE_OUTER_BOUND ( 'NONE', #25330, .T. ) ;
#47536=CARTESIAN_POINT ( 'NONE',  ( 22.92187500061451644, 3.027376345333613106, -5.243569643749998122 ) ) ;
#47537=CARTESIAN_POINT ( 'NONE',  ( 5.475000000000000533, 6.123233995736764310E-16, -4.999999999999998224 ) ) ;
#47538=CARTESIAN_POINT ( 'NONE',  ( 8.484601909799253346E-16, 11.22500000122903607, 34.61880215351700230 ) ) ;
#47539=CARTESIAN_POINT ( 'NONE',  ( 14.65312500061451573, -4.541064518000417216, -2.621784821875001281 ) ) ;
#47540=CARTESIAN_POINT ( 'NONE',  ( 5.625000001229036428, 2.886751345948129099, -4.999999999999998224 ) ) ;
#47541=CARTESIAN_POINT ( 'NONE',  ( 9.871875000614517504, 3.027376345333613106, -5.243569643749998122 ) ) ;
#47542=CARTESIAN_POINT ( 'NONE',  ( 1.999999999999998668, 15.01250000122903394, 26.53589838486224650 ) ) ;
#47544=CARTESIAN_POINT ( 'NONE',  ( 12.32812500061451821, -4.541064518000419881, 2.621784821874995952 ) ) ;
#47545=CARTESIAN_POINT ( 'NONE',  ( 24.30000000122903359, -2.886751345948129988, 4.999999999999997335 ) ) ;
#47546=CARTESIAN_POINT ( 'NONE',  ( 10.77187500061451786, 3.027376345333613106, -5.243569643749998122 ) ) ;
#47547=CARTESIAN_POINT ( 'NONE',  ( 13.97812500061451679, 4.541064518000418104, 2.621784821874999949 ) ) ;
#47549=CARTESIAN_POINT ( 'NONE',  ( 24.72187500061451360, 3.027376345333613106, -5.243569643749998122 ) ) ;
#47552=CARTESIAN_POINT ( 'NONE',  ( 20.51250000122903216, 4.330127018922192761, -2.499999999999997780 ) ) ;
#47553=CARTESIAN_POINT ( 'NONE',  ( 4.243569643749999010, 14.27187500061451786, -32.45002607614398471 ) ) ;
#47554=CARTESIAN_POINT ( 'NONE',  ( 15.45937500061451608, 0.000000000000000000, 5.243569643749999010 ) ) ;
#47555=CARTESIAN_POINT ( 'NONE',  ( 17.13750000122903216, -4.330127018922194537, 2.499999999999995559 ) ) ;
#47556=CARTESIAN_POINT ( 'NONE',  ( 12.45937500061451786, -4.541064518000417216, -2.621784821875001281 ) ) ;
#47557=CARTESIAN_POINT ( 'NONE',  ( -2.121784821874999949, 17.92812500061451786, -33.67503911421598417 ) ) ;
#47558=CARTESIAN_POINT ( 'NONE',  ( 20.66250000122903074, 0.000000000000000000, 4.999999999999998224 ) ) ;
#47559=CARTESIAN_POINT ( 'NONE',  ( 12.02812500061451573, 6.421520780324663323E-16, -5.243569643749999010 ) ) ;
#47561=ORIENTED_EDGE ( 'NONE', *, *, #48761, .T. ) ;
#47562=CARTESIAN_POINT ( 'NONE',  ( 15.71250000000000213, -5.773502691896255534, -1.060575238724906372E-15 ) ) ;
#47564=CARTESIAN_POINT ( 'NONE',  ( 13.39687500061451608, -3.027376345333610441, -5.243569643749999898 ) ) ;
#47566=CARTESIAN_POINT ( 'NONE',  ( 12.71250000122903145, -4.330127018922190985, -2.500000000000001332 ) ) ;
#47567=CARTESIAN_POINT ( 'NONE',  ( 20.32500000122903572, -5.773502691896255534, -1.060575238724906372E-15 ) ) ;
#47568=CARTESIAN_POINT ( 'NONE',  ( 17.76562500061451644, -6.054752690667223547, -1.112240025338166033E-15 ) ) ;
#47569=CARTESIAN_POINT ( 'NONE',  ( 20.80312500061451431, 0.000000000000000000, 5.243569643749999010 ) ) ;
#47570=CARTESIAN_POINT ( 'NONE',  ( 28.46250000122903145, -4.330127018922190985, -2.500000000000001332 ) ) ;
#47571=( BOUNDED_CURVE ( )  B_SPLINE_CURVE ( 2, ( #15975, #61048, #38147, #10446, #66974, #38894, #62141 ),
 .UNSPECIFIED., .F., .F. ) 
 B_SPLINE_CURVE_WITH_KNOTS ( ( 3, 2, 2, 3 ),
 ( 0.03333333333333339532, 0.03611111111111116323, 0.03888888888888894502, 0.04166666666666671293 ),
 .UNSPECIFIED. ) 
 CURVE ( )  GEOMETRIC_REPRESENTATION_ITEM ( )  RATIONAL_B_SPLINE_CURVE ( ( 0.9999999999999968914, 0.8660254037844417052, 1.000000000000000000, 0.8660254037844387076, 1.000000000000000000, 0.8660254037844363761, 1.000000000000002442 ) ) 
 REPRESENTATION_ITEM ( '' )  );
#47572=CARTESIAN_POINT ( 'NONE',  ( 28.19999999999999929, 0.000000000000000000, 4.999999999999998224 ) ) ;
#47573=CARTESIAN_POINT ( 'NONE',  ( 10.00000000000000000, 1.224646799147353256E-15, 10.00000000000000178 ) ) ;
#47575=CARTESIAN_POINT ( 'NONE',  ( 27.00937500061451857, 4.541064518000418104, -2.621784821874998173 ) ) ;
#47576=CARTESIAN_POINT ( 'NONE',  ( -0.6945863667395647534, 9.663023495605401081, -33.93923213064925903 ) ) ;
#47577=CARTESIAN_POINT ( 'NONE',  ( -2.121784821874999949, 13.48437500061451821, -33.67503911421598417 ) ) ;
#47578=CARTESIAN_POINT ( 'NONE',  ( 2.737500001229034474, -4.330127018922194537, 2.499999999999995559 ) ) ;
#47579=CARTESIAN_POINT ( 'NONE',  ( 6.524999999999999467, 4.330127018922191873, 2.499999999999999556 ) ) ;
#47580=ADVANCED_FACE ( 'NONE', ( #29742 ), #7568, .F. ) ;
#47581=CARTESIAN_POINT ( 'NONE',  ( 3.646875000614519635, 6.054752690667223547, 3.707466751127219781E-16 ) ) ;
#47582=CARTESIAN_POINT ( 'NONE',  ( 9.159375000614515372, 0.000000000000000000, 5.243569643749999010 ) ) ;
#47583=CARTESIAN_POINT ( 'NONE',  ( 28.97812500061451502, -4.541064518000419881, 2.621784821874995952 ) ) ;
#47584=CARTESIAN_POINT ( 'NONE',  ( -5.810221930991193690E-16, 10.88749999999999929, 26.00000000000000355 ) ) ;
#47585=CARTESIAN_POINT ( 'NONE',  ( -4.761366016028763859, 8.797204459235659968, -26.32883817404464821 ) ) ;
#47586=CARTESIAN_POINT ( 'NONE',  ( -2.000000000000000000, 19.13750000122903216, 26.53589838486224650 ) ) ;
#47587=CARTESIAN_POINT ( 'NONE',  ( 4.246875000614519280, -3.027376345333614438, 5.243569643749998122 ) ) ;
#47588=CARTESIAN_POINT ( 'NONE',  ( 10.88437500061451679, 4.541064518000418104, 2.621784821874999949 ) ) ;
#47589=CARTESIAN_POINT ( 'NONE',  ( 3.450000000000001510, 0.000000000000000000, 4.999999999999998224 ) ) ;
#47590=CARTESIAN_POINT ( 'NONE',  ( -2.121784821874999949, 13.87812500061459531, 26.32496088578401938 ) ) ;
#47591=CARTESIAN_POINT ( 'NONE',  ( 5.025000000000002132, 6.123233995736764310E-16, -4.999999999999998224 ) ) ;
#47592=CARTESIAN_POINT ( 'NONE',  ( 7.350000000000002309, 4.330127018922192761, -2.499999999999997780 ) ) ;
#47594=CARTESIAN_POINT ( 'NONE',  ( 19.41562500061451146, 3.027376345333611329, 5.243569643749999010 ) ) ;
#47595=CARTESIAN_POINT ( 'NONE',  ( 13.86562500061451431, 3.027376345333613106, -5.243569643749998122 ) ) ;
#47597=CARTESIAN_POINT ( 'NONE',  ( 9.496875000614517504, 6.054752690667223547, 3.707466751127219781E-16 ) ) ;
#47598=CARTESIAN_POINT ( 'NONE',  ( 25.27499999999999858, 6.123233995736764310E-16, -4.999999999999998224 ) ) ;
#47599=CARTESIAN_POINT ( 'NONE',  ( 21.78750000122903074, 6.123233995736764310E-16, -4.999999999999998224 ) ) ;
#47601=CARTESIAN_POINT ( 'NONE',  ( 9.721875000614517148, -6.054752690667223547, -1.112240025338166033E-15 ) ) ;
#47602=CARTESIAN_POINT ( 'NONE',  ( 26.85937500061451644, -4.541064518000417216, -2.621784821875001281 ) ) ;
#47605=CARTESIAN_POINT ( 'NONE',  ( 20.70937500061451786, 4.541064518000418104, -2.621784821874998173 ) ) ;
#47606=CARTESIAN_POINT ( 'NONE',  ( 12.75937500061451857, 0.000000000000000000, 5.243569643749999010 ) ) ;
#47608=CARTESIAN_POINT ( 'NONE',  ( 22.23750000000000071, 5.773502691896255534, 3.535250795749688894E-16 ) ) ;
#47610=CARTESIAN_POINT ( 'NONE',  ( 4.243569643749999898, 12.43437500061451750, -30.00000000000000000 ) ) ;
#47612=CARTESIAN_POINT ( 'NONE',  ( 15.74062500061451608, 6.054752690667223547, 3.707466751127219781E-16 ) ) ;
#47613=CARTESIAN_POINT ( 'NONE',  ( 4.012500000000001954, -5.773502691896255534, -1.060575238724906372E-15 ) ) ;
#47615=CARTESIAN_POINT ( 'NONE',  ( 15.22500000000000142, -4.330127018922194537, 2.499999999999995559 ) ) ;
#47616=CARTESIAN_POINT ( 'NONE',  ( -2.121784821874996840, 11.32812500061451644, 33.67503911421598417 ) ) ;
#47617=CARTESIAN_POINT ( 'NONE',  ( 13.05000000122903536, -2.886751345948129988, 4.999999999999997335 ) ) ;
#47618=CARTESIAN_POINT ( 'NONE',  ( 23.78437500061451360, 6.421520780324663323E-16, -5.243569643749999010 ) ) ;
#47619=CARTESIAN_POINT ( 'NONE',  ( 19.73437500061451644, 6.421520780324663323E-16, -5.243569643749999010 ) ) ;
#47622=CARTESIAN_POINT ( 'NONE',  ( 20.72812500061451502, 4.541064518000418104, 2.621784821874999949 ) ) ;
#47623=CARTESIAN_POINT ( 'NONE',  ( 4.265625000614517326, -6.054752690667223547, -1.112240025338166033E-15 ) ) ;
#47624=CARTESIAN_POINT ( 'NONE',  ( 17.22187500061451715, 3.027376345333611329, 5.243569643749999010 ) ) ;
#47625=CARTESIAN_POINT ( 'NONE',  ( 28.13437500061451502, -4.541064518000419881, 2.621784821874995952 ) ) ;
#47626=CARTESIAN_POINT ( 'NONE',  ( 4.378125000614518925, 6.421520780324663323E-16, -5.243569643749999010 ) ) ;
#47627=CARTESIAN_POINT ( 'NONE',  ( 21.44062500061452070, -3.027376345333610441, -5.243569643749999898 ) ) ;
#47628=CARTESIAN_POINT ( 'NONE',  ( -2.121784821874999949, 15.22812500061451679, 26.32496088578401938 ) ) ;
#47629=CARTESIAN_POINT ( 'NONE',  ( 16.46250000122903501, 4.330127018922192761, -2.499999999999997780 ) ) ;
#47631=CARTESIAN_POINT ( 'NONE',  ( 7.490625000614516082, -3.027376345333610441, -5.243569643749999898 ) ) ;
#47632=LINE ( 'NONE', #70165, #39635 ) ;
#47633=CARTESIAN_POINT ( 'NONE',  ( 28.94062500061452070, -3.027376345333614438, 5.243569643749998122 ) ) ;
#47634=CARTESIAN_POINT ( 'NONE',  ( 23.52187500061451786, 3.027376345333611329, 5.243569643749999010 ) ) ;
#47635=CARTESIAN_POINT ( 'NONE',  ( 14.09062500061451750, -3.027376345333614438, 5.243569643749998122 ) ) ;
#47636=CARTESIAN_POINT ( 'NONE',  ( 24.30000000122903359, -2.886751345948129988, 4.999999999999997335 ) ) ;
#47637=EDGE_CURVE ( 'NONE', #50074, #19796, #26035, .T. ) ;
#47638=CARTESIAN_POINT ( 'NONE',  ( 25.11562500061451431, 3.027376345333613106, -5.243569643749998122 ) ) ;
#47639=CARTESIAN_POINT ( 'NONE',  ( 18.83437500061451431, 6.421520780324663323E-16, -5.243569643749999010 ) ) ;
#47640=CARTESIAN_POINT ( 'NONE',  ( 13.90312500061451750, 4.541064518000418104, -2.621784821874998173 ) ) ;
#47641=CARTESIAN_POINT ( 'NONE',  ( -4.243569643749999898, 17.60937500061451999, 30.00000000000000000 ) ) ;
#47642=CARTESIAN_POINT ( 'NONE',  ( 19.04062500061451146, -3.027376345333614438, 5.243569643749998122 ) ) ;
#47644=ORIENTED_EDGE ( 'NONE', *, *, #69064, .T. ) ;
#47645=CARTESIAN_POINT ( 'NONE',  ( 25.50000000000000000, 0.000000000000000000, 4.999999999999998224 ) ) ;
#47646=CARTESIAN_POINT ( 'NONE',  ( -2.000000000000000000, 11.82500000000000107, -33.46410161513775705 ) ) ;
#47648=CARTESIAN_POINT ( 'NONE',  ( 26.72812500061451502, -4.541064518000419881, 2.621784821874995952 ) ) ;
#47649=CARTESIAN_POINT ( 'NONE',  ( 8.728125000614518569, -4.541064518000419881, 2.621784821874995952 ) ) ;
#47650=CARTESIAN_POINT ( 'NONE',  ( 21.00000000122903288, 5.773502691896255534, 3.535250795749688894E-16 ) ) ;
#47651=CARTESIAN_POINT ( 'NONE',  ( 24.10312500061451502, -4.541064518000417216, -2.621784821875001281 ) ) ;
#47652=CARTESIAN_POINT ( 'NONE',  ( 26.25000000000000000, 4.330127018922192761, -2.499999999999997780 ) ) ;
#47653=CARTESIAN_POINT ( 'NONE',  ( 27.14062500061451644, -3.027376345333614438, 5.243569643749998122 ) ) ;
#47654=CARTESIAN_POINT ( 'NONE',  ( 7.678125000614516082, 4.541064518000418104, 2.621784821874999949 ) ) ;
#47656=CARTESIAN_POINT ( 'NONE',  ( 24.89062500061451644, -3.027376345333614438, 5.243569643749998122 ) ) ;
#47657=CARTESIAN_POINT ( 'NONE',  ( 4.528125000614516615, 4.541064518000418104, 2.621784821874999949 ) ) ;
#47660=FACE_OUTER_BOUND ( 'NONE', #5742, .T. ) ;
#47661=CARTESIAN_POINT ( 'NONE',  ( 12.00000000000000000, 0.000000000000000000, 4.999999999999998224 ) ) ;
#47662=CARTESIAN_POINT ( 'NONE',  ( 13.20937500061451786, 0.000000000000000000, 5.243569643749999010 ) ) ;
#47663=CARTESIAN_POINT ( 'NONE',  ( 9.112500001229033586, -4.330127018922190985, -2.500000000000001332 ) ) ;
#47664=CARTESIAN_POINT ( 'NONE',  ( 17.14687500061451786, 6.054752690667223547, 3.707466751127219781E-16 ) ) ;
#47666=CARTESIAN_POINT ( 'NONE',  ( 7.284375000614518036, 4.541064518000418104, 2.621784821874999949 ) ) ;
#47667=CARTESIAN_POINT ( 'NONE',  ( 2.121784821875001281, 11.40312500061451750, -26.32496088578401938 ) ) ;
#47668=CARTESIAN_POINT ( 'NONE',  ( -5.810221930991193690E-16, 14.03750000000000142, -34.00000000000000000 ) ) ;
#47671=CARTESIAN_POINT ( 'NONE',  ( 25.19062500061451715, 6.054752690667223547, 3.707466751127219781E-16 ) ) ;
#47672=CARTESIAN_POINT ( 'NONE',  ( 4.243569643749999898, 10.18437500061451750, 30.00000000000000000 ) ) ;
#47673=DIRECTION ( 'NONE',  ( 0.000000000000000000, 0.000000000000000000, -1.000000000000000000 ) ) ;
#47674=CARTESIAN_POINT ( 'NONE',  ( 25.47187500061451715, -6.054752690667223547, -1.112240025338166033E-15 ) ) ;
#47675=CARTESIAN_POINT ( 'NONE',  ( 27.98437500061451289, 4.541064518000418104, 2.621784821874999949 ) ) ;
#47676=CARTESIAN_POINT ( 'NONE',  ( 4.528125000614516615, 4.541064518000418104, 2.621784821874999949 ) ) ;
#47678=CARTESIAN_POINT ( 'NONE',  ( 17.52187500061451431, 3.027376345333613106, -5.243569643749998122 ) ) ;
#47680=CARTESIAN_POINT ( 'NONE',  ( 3.328125000614516438, -4.541064518000419881, 2.621784821874995952 ) ) ;
#47681=CARTESIAN_POINT ( 'NONE',  ( 8.409375000614518925, -4.541064518000417216, -2.621784821875001281 ) ) ;
#47682=CARTESIAN_POINT ( 'NONE',  ( 17.52187500061451431, 3.027376345333613106, -5.243569643749998122 ) ) ;
#47683=CARTESIAN_POINT ( 'NONE',  ( 13.72500000122903074, 2.886751345948062486, -5.000000000000113687 ) ) ;
#47684=CARTESIAN_POINT ( 'NONE',  ( 27.29999999999999716, 0.000000000000000000, 4.999999999999998224 ) ) ;
#47685=CARTESIAN_POINT ( 'NONE',  ( 27.87187500061451573, 3.027376345333613106, -5.243569643749998122 ) ) ;
#47689=CARTESIAN_POINT ( 'NONE',  ( 7.124999999999999112, -4.330127018922194537, 2.499999999999995559 ) ) ;
#47691=CARTESIAN_POINT ( 'NONE',  ( 22.82812500061451644, 6.421520780324663323E-16, -5.243569643749999010 ) ) ;
#47692=CARTESIAN_POINT ( 'NONE',  ( 12.75000000000000178, 4.330127018922192761, -2.499999999999997780 ) ) ;
#47693=CARTESIAN_POINT ( 'NONE',  ( 7.912500001229033408, 4.330127018922192761, -2.499999999999997780 ) ) ;
#47694=CARTESIAN_POINT ( 'NONE',  ( 6.928125000614516082, -4.541064518000419881, 2.621784821874995952 ) ) ;
#47695=CARTESIAN_POINT ( 'NONE',  ( 22.50000000000000000, -4.330127018922190985, -2.500000000000001332 ) ) ;
#47696=CARTESIAN_POINT ( 'NONE',  ( 17.95312500061451644, 4.541064518000418104, -2.621784821874998173 ) ) ;
#47697=CARTESIAN_POINT ( 'NONE',  ( 4.087540598844761064, -2.879707068604791420, 4.153959617388856884 ) ) ;
#47698=CARTESIAN_POINT ( 'NONE',  ( 25.35000000122903074, -2.886751345948125991, -5.000000000000000000 ) ) ;
#47700=CARTESIAN_POINT ( 'NONE',  ( 4.650000000000001243, 4.330127018922192761, -2.499999999999997780 ) ) ;
#47701=ORIENTED_EDGE ( 'NONE', *, *, #54220, .T. ) ;
#47702=CARTESIAN_POINT ( 'NONE',  ( 18.81562500061452070, 3.027376345333613106, -5.243569643749998122 ) ) ;
#47703=CARTESIAN_POINT ( 'NONE',  ( 27.74062500061451431, -3.027376345333610441, -5.243569643749999898 ) ) ;
#47704=CARTESIAN_POINT ( 'NONE',  ( 26.97187500061451360, 3.027376345333613106, -5.243569643749998122 ) ) ;
#47705=CARTESIAN_POINT ( 'NONE',  ( 8.474999999999999645, -4.330127018922194537, 2.499999999999995559 ) ) ;
#47706=CARTESIAN_POINT ( 'NONE',  ( 10.90312500061451928, 0.000000000000000000, 5.243569643749999010 ) ) ;
#47707=CARTESIAN_POINT ( 'NONE',  ( 29.27812500061451573, 4.541064518000418104, 2.621784821874999949 ) ) ;
#47708=CARTESIAN_POINT ( 'NONE',  ( 8.203125000614518214, 0.000000000000000000, 5.243569643749999010 ) ) ;
#47710=CARTESIAN_POINT ( 'NONE',  ( -3.000416591977282496E-16, 13.44687500061451857, 25.09994784771203058 ) ) ;
#47711=CARTESIAN_POINT ( 'NONE',  ( 26.58750000122903145, -4.330127018922194537, 2.499999999999995559 ) ) ;
#47713=CARTESIAN_POINT ( 'NONE',  ( 13.64062500061451289, -3.027376345333614438, 5.243569643749998122 ) ) ;
#47715=CARTESIAN_POINT ( 'NONE',  ( 9.196875000614518569, -3.027376345333614438, 5.243569643749998122 ) ) ;
#47716=CARTESIAN_POINT ( 'NONE',  ( 9.271875000614516082, -6.054752690667223547, -1.112240025338166033E-15 ) ) ;
#47717=CARTESIAN_POINT ( 'NONE',  ( 17.18437500061451573, 4.541064518000418104, 2.621784821874999949 ) ) ;
#47719=CARTESIAN_POINT ( 'NONE',  ( 29.44687500061451857, -3.027376345333614438, 5.243569643749998122 ) ) ;
#47720=CARTESIAN_POINT ( 'NONE',  ( 22.19062500061451715, -3.027376345333614438, 5.243569643749998122 ) ) ;
#47721=ADVANCED_FACE ( 'NONE', ( #9403 ), #3505, .F. ) ;
#47722=CARTESIAN_POINT ( 'NONE',  ( 15.83437500061451608, 4.541064518000418104, 2.621784821874999949 ) ) ;
#47723=CARTESIAN_POINT ( 'NONE',  ( 22.04062500061451502, 6.054752690667223547, 3.707466751127219781E-16 ) ) ;
#47724=CARTESIAN_POINT ( 'NONE',  ( 8.484601909799253346E-16, 13.81250000000000000, 34.61880215351700230 ) ) ;
#47725=CARTESIAN_POINT ( 'NONE',  ( 27.62812500061451360, -4.541064518000419881, 2.621784821874995952 ) ) ;
#47726=CARTESIAN_POINT ( 'NONE',  ( 7.162500001229032520, 0.000000000000000000, 4.999999999999998224 ) ) ;
#47727=VERTEX_POINT ( 'NONE', #10133 ) ;
#47728=CARTESIAN_POINT ( 'NONE',  ( 5.775000001229033231, 2.886751345948126879, 4.999999999999999112 ) ) ;
#47729=CARTESIAN_POINT ( 'NONE',  ( -3.999999999999999112, 18.64999999999999858, -30.00000000000000000 ) ) ;
#47730=CARTESIAN_POINT ( 'NONE',  ( 25.50000000122903288, 5.773502691896255534, 3.535250795749688894E-16 ) ) ;
#47732=EDGE_CURVE ( 'NONE', #48333, #37161, #35501, .T. ) ;
#47733=CARTESIAN_POINT ( 'NONE',  ( 8.071875000614518569, 3.027376345333613106, -5.243569643749998122 ) ) ;
#47734=CARTESIAN_POINT ( 'NONE',  ( 4.276577733362700862, 2.590537181842085257, -4.276577733362700862 ) ) ;
#47735=CARTESIAN_POINT ( 'NONE',  ( 15.25312500061451715, 4.541064518000418104, -2.621784821874998173 ) ) ;
#47736=CARTESIAN_POINT ( 'NONE',  ( 8.221875000614518925, 3.027376345333611329, 5.243569643749999010 ) ) ;
#47737=CARTESIAN_POINT ( 'NONE',  ( 27.86250000122903359, 0.000000000000000000, 4.999999999999998224 ) ) ;
#47739=CARTESIAN_POINT ( 'NONE',  ( 17.85937500061451999, -4.541064518000417216, -2.621784821875001281 ) ) ;
#47740=CARTESIAN_POINT ( 'NONE',  ( 4.359375000614517326, -4.541064518000417216, -2.621784821875001281 ) ) ;
#47741=CARTESIAN_POINT ( 'NONE',  ( 1.071796769724491893, 16.19509619066136707, 33.99999999999999289 ) ) ;
#47742=EDGE_CURVE ( 'NONE', #25563, #66176, #28406, .T. ) ;
#47743=CARTESIAN_POINT ( 'NONE',  ( 6.065625000614516260, -6.054752690667223547, -1.112240025338166033E-15 ) ) ;
#47744=CARTESIAN_POINT ( 'NONE',  ( 16.86562500061451786, -6.054752690667223547, -1.112240025338166033E-15 ) ) ;
#47745=ORIENTED_EDGE ( 'NONE', *, *, #7942, .F. ) ;
#47746=AXIS2_PLACEMENT_3D ( 'NONE', #54781, #15606, #66599 ) ;
#47747=CARTESIAN_POINT ( 'NONE',  ( 12.62812500061451537, 4.541064518000418104, 2.621784821874999949 ) ) ;
#47748=CARTESIAN_POINT ( 'NONE',  ( 5.062500001229035540, -4.330127018922190985, -2.500000000000001332 ) ) ;
#47749=AXIS2_PLACEMENT_3D ( 'NONE', #35045, #62395, #46139 ) ;
#47750=CARTESIAN_POINT ( 'NONE',  ( 10.26562500061451644, 3.027376345333613106, -5.243569643749998122 ) ) ;
#47752=CARTESIAN_POINT ( 'NONE',  ( 12.00000000000000000, 0.000000000000000000, 4.999999999999998224 ) ) ;
#47753=CARTESIAN_POINT ( 'NONE',  ( 5.775000001229033231, 2.886751345948126879, 4.999999999999999112 ) ) ;
#47754=CARTESIAN_POINT ( 'NONE',  ( 20.24999999999999645, -4.330127018922190985, -2.500000000000001332 ) ) ;
#47755=CARTESIAN_POINT ( 'NONE',  ( 14.52187500061451608, 3.027376345333611329, 5.243569643749999010 ) ) ;
#47756=CARTESIAN_POINT ( 'NONE',  ( 16.35000000122903430, -2.886751345948125991, -5.000000000000000000 ) ) ;
#47758=CARTESIAN_POINT ( 'NONE',  ( 2.121784821874999061, 19.65312500061451573, -33.67503911421598417 ) ) ;
#47759=CARTESIAN_POINT ( 'NONE',  ( 11.92500000122902826, 2.886751345948062486, -5.000000000000113687 ) ) ;
#47760=CARTESIAN_POINT ( 'NONE',  ( 4.000000000000000000, 14.90000000122903323, -27.69059892324149885 ) ) ;
#47762=EDGE_CURVE ( 'NONE', #2667, #885, #61405, .T. ) ;
#47763=CARTESIAN_POINT ( 'NONE',  ( 3.912032792714240870, -3.113839981233385679, -4.218888856100475593 ) ) ;
#47764=CARTESIAN_POINT ( 'NONE',  ( 17.22187500061451715, 3.027376345333611329, 5.243569643749999010 ) ) ;
#47765=CARTESIAN_POINT ( 'NONE',  ( 29.09999999999999787, 0.000000000000000000, 4.999999999999998224 ) ) ;
#47766=CARTESIAN_POINT ( 'NONE',  ( 11.95312500061451644, -4.541064518000417216, -2.621784821875001281 ) ) ;
#47768=CARTESIAN_POINT ( 'NONE',  ( 24.19687500061451857, -3.027376345333610441, -5.243569643749999898 ) ) ;
#47770=CARTESIAN_POINT ( 'NONE',  ( 9.890625000614516438, 6.054752690667223547, 3.707466751127219781E-16 ) ) ;
#47771=CARTESIAN_POINT ( 'NONE',  ( 15.49687500061451750, -3.027376345333614438, 5.243569643749998122 ) ) ;
#47772=ORIENTED_EDGE ( 'NONE', *, *, #39082, .F. ) ;
#47773=CARTESIAN_POINT ( 'NONE',  ( 25.69687500061451502, 6.054752690667223547, 3.707466751127219781E-16 ) ) ;
#47774=CARTESIAN_POINT ( 'NONE',  ( 28.07812500061451289, -4.541064518000419881, 2.621784821874995952 ) ) ;
#47775=CARTESIAN_POINT ( 'NONE',  ( 18.29062500061451502, -3.027376345333610441, -5.243569643749999898 ) ) ;
#47776=CARTESIAN_POINT ( 'NONE',  ( 28.71562500061451573, 3.027376345333613106, -5.243569643749998122 ) ) ;
#47777=AXIS2_PLACEMENT_3D ( 'NONE', #19411, #7984, #43066 ) ;
#47778=CARTESIAN_POINT ( 'NONE',  ( 6.600000000000001421, 0.000000000000000000, 4.999999999999998224 ) ) ;
#47779=CARTESIAN_POINT ( 'NONE',  ( 20.43750000122903643, 6.123233995736764310E-16, -4.999999999999998224 ) ) ;
#47780=FACE_OUTER_BOUND ( 'NONE', #42477, .T. ) ;
#47783=CARTESIAN_POINT ( 'NONE',  ( 14.62500000000000000, 4.330127018922191873, 2.499999999999999556 ) ) ;
#47784=CARTESIAN_POINT ( 'NONE',  ( 19.53749999999999432, 5.773502691896255534, 3.535250795749688894E-16 ) ) ;
#47785=CARTESIAN_POINT ( 'NONE',  ( 16.80937500061451573, 0.000000000000000000, 5.243569643749999010 ) ) ;
#47786=CARTESIAN_POINT ( 'NONE',  ( 13.41562500061451502, 3.027376345333613106, -5.243569643749998122 ) ) ;
#47789=EDGE_LOOP ( 'NONE', ( #3032, #70547, #50156, #3506 ) ) ;
#47790=CARTESIAN_POINT ( 'NONE',  ( -0.7368805616696195715, 9.859898480082234684, -34.17910162106521454 ) ) ;
#47791=CARTESIAN_POINT ( 'NONE',  ( -4.243569643749997233, 16.74687500061451928, -27.54997392385601174 ) ) ;
#47792=CARTESIAN_POINT ( 'NONE',  ( 5.915625000614515905, 3.027376345333611329, 5.243569643749999010 ) ) ;
#47794=CARTESIAN_POINT ( 'NONE',  ( 11.58750000000000036, -2.886751345948129988, 4.999999999999997335 ) ) ;
#47796=VERTEX_POINT ( 'NONE', #48563 ) ;
#47797=CARTESIAN_POINT ( 'NONE',  ( 2.121784821875001281, 14.55312500061451786, 33.67503911421598417 ) ) ;
#47798=CARTESIAN_POINT ( 'NONE',  ( 27.10312500061451502, 0.000000000000000000, 5.243569643749999010 ) ) ;
#47800=AXIS2_PLACEMENT_3D ( 'NONE', #36486, #25030, #25403 ) ;
#47802=CARTESIAN_POINT ( 'NONE',  ( 23.14687500061451786, -3.027376345333614438, 5.243569643749998122 ) ) ;
#47803=CARTESIAN_POINT ( 'NONE',  ( 20.69062500061451715, 6.054752690667223547, 3.707466751127219781E-16 ) ) ;
#47804=CARTESIAN_POINT ( 'NONE',  ( -4.243569643749999898, 17.51562500061459104, -32.45002607614398471 ) ) ;
#47805=CARTESIAN_POINT ( 'NONE',  ( 23.25000000122903288, 5.773502691896255534, 3.535250795749688894E-16 ) ) ;
#47806=CARTESIAN_POINT ( 'NONE',  ( 6.178125000614518747, 6.421520780324663323E-16, -5.243569643749999010 ) ) ;
#47808=CARTESIAN_POINT ( 'NONE',  ( 23.39062500061451289, 6.054752690667223547, 3.707466751127219781E-16 ) ) ;
#47811=CARTESIAN_POINT ( 'NONE',  ( 17.52187500061451431, 3.027376345333613106, -5.243569643749998122 ) ) ;
#47812=CARTESIAN_POINT ( 'NONE',  ( 23.89687500061451786, 6.054752690667223547, 3.707466751127219781E-16 ) ) ;
#47813=CARTESIAN_POINT ( 'NONE',  ( 9.001249775931846008E-16, 13.67187500061451999, 34.90005215228797653 ) ) ;
#47814=CARTESIAN_POINT ( 'NONE',  ( 5.653125000614517504, -4.541064518000417216, -2.621784821875001281 ) ) ;
#47815=CARTESIAN_POINT ( 'NONE',  ( 28.82812500061451644, 4.541064518000418104, 2.621784821874999949 ) ) ;
#47816=CARTESIAN_POINT ( 'NONE',  ( 29.65312500061451573, 4.541064518000418104, -2.621784821874998173 ) ) ;
#47818=CARTESIAN_POINT ( 'NONE',  ( 3.374999999999999556, 4.330127018922191873, 2.499999999999999556 ) ) ;
#47819=CARTESIAN_POINT ( 'NONE',  ( 3.553125000614516082, 4.541064518000418104, -2.621784821874998173 ) ) ;
#47820=CARTESIAN_POINT ( 'NONE',  ( 7.959375000614516971, -4.541064518000417216, -2.621784821875001281 ) ) ;
#47822=CARTESIAN_POINT ( 'NONE',  ( 16.46250000122903501, 4.330127018922192761, -2.499999999999997780 ) ) ;
#47823=CARTESIAN_POINT ( 'NONE',  ( 4.021875000614516082, 3.027376345333613106, -5.243569643749998122 ) ) ;
#47824=CARTESIAN_POINT ( 'NONE',  ( 11.25000000122903288, -2.886751345948129988, 4.999999999999997335 ) ) ;
#47825=CARTESIAN_POINT ( 'NONE',  ( 4.190625000614518925, -3.027376345333614438, 5.243569643749998122 ) ) ;
#47828=CARTESIAN_POINT ( 'NONE',  ( 14.22187500061451537, -6.054752690667223547, -1.112240025338166033E-15 ) ) ;
#47831=CARTESIAN_POINT ( 'NONE',  ( 22.64062500061451644, -3.027376345333614438, 5.243569643749998122 ) ) ;
#47832=CARTESIAN_POINT ( 'NONE',  ( 8.165625000614516793, 3.027376345333611329, 5.243569643749999010 ) ) ;
#47833=CARTESIAN_POINT ( 'NONE',  ( 25.39687500061451431, -3.027376345333614438, 5.243569643749998122 ) ) ;
#47834=CARTESIAN_POINT ( 'NONE',  ( 8.690625000614515372, -3.027376345333614438, 5.243569643749998122 ) ) ;
#47835=DIRECTION ( 'NONE',  ( -0.000000000000000000, -1.000000000000000000, -0.000000000000000000 ) ) ;
#47836=CARTESIAN_POINT ( 'NONE',  ( 9.900000001229033231, -2.886751345948129988, 4.999999999999997335 ) ) ;
#47837=EDGE_CURVE ( 'NONE', #22971, #37048, #60354, .T. ) ;
#47838=CARTESIAN_POINT ( 'NONE',  ( 24.77812500061451217, 4.541064518000418104, 2.621784821874999949 ) ) ;
#47839=CARTESIAN_POINT ( 'NONE',  ( 4.243569643749999898, 10.99062500061451786, -27.54997392385601529 ) ) ;
#47840=CARTESIAN_POINT ( 'NONE',  ( 10.83750000122903501, -4.330127018922194537, 2.499999999999995559 ) ) ;
#47841=CARTESIAN_POINT ( 'NONE',  ( 20.27812500061451573, 4.541064518000418104, 2.621784821874999949 ) ) ;
#47843=CARTESIAN_POINT ( 'NONE',  ( 17.42812500061451786, 6.421520780324663323E-16, -5.243569643749999010 ) ) ;
#47845=CARTESIAN_POINT ( 'NONE',  ( 18.59999999999999787, 4.330127018922192761, -2.499999999999997780 ) ) ;
#47846=CARTESIAN_POINT ( 'NONE',  ( 14.06250000122903288, -4.330127018922190985, -2.500000000000001332 ) ) ;
#47848=CARTESIAN_POINT ( 'NONE',  ( 10.90312500061451928, 0.000000000000000000, 5.243569643749999010 ) ) ;
#47849=CARTESIAN_POINT ( 'NONE',  ( 14.46562500061451750, 3.027376345333611329, 5.243569643749999010 ) ) ;
#47850=AXIS2_PLACEMENT_3D ( 'NONE', #54197, #43482, #37928 ) ;
#47851=CARTESIAN_POINT ( 'NONE',  ( 23.51250000122903216, -4.330127018922190985, -2.500000000000001332 ) ) ;
#47852=CARTESIAN_POINT ( 'NONE',  ( 21.42187500061451644, -6.054752690667223547, -1.112240025338166033E-15 ) ) ;
#47853=CARTESIAN_POINT ( 'NONE',  ( 21.94687500061451857, -3.027376345333610441, -5.243569643749999898 ) ) ;
#47854=CARTESIAN_POINT ( 'NONE',  ( 7.320879633048903241E-15, 18.20000000122903216, 26.00000000000000355 ) ) ;
#47855=CARTESIAN_POINT ( 'NONE',  ( 8.325000001229033941, 2.886751345948129099, -4.999999999999998224 ) ) ;
#47856=CARTESIAN_POINT ( 'NONE',  ( 5.484375000614518214, 4.541064518000418104, 2.621784821874999949 ) ) ;
#47857=CARTESIAN_POINT ( 'NONE',  ( 24.23437500061451644, 6.421520780324663323E-16, -5.243569643749999010 ) ) ;
#47858=CARTESIAN_POINT ( 'NONE',  ( 26.62500000122902932, -5.773502691896255534, -1.060575238724906372E-15 ) ) ;
#47859=CARTESIAN_POINT ( 'NONE',  ( 21.25312500061451715, 0.000000000000000000, 5.243569643749999010 ) ) ;
#47860=CARTESIAN_POINT ( 'NONE',  ( 25.35937500061451644, 0.000000000000000000, 5.243569643749999010 ) ) ;
#47864=CARTESIAN_POINT ( 'NONE',  ( 4.921875000614518214, 3.027376345333613106, -5.243569643749998122 ) ) ;
#47865=CARTESIAN_POINT ( 'NONE',  ( 16.41562500061451857, -6.054752690667223547, -1.112240025338166033E-15 ) ) ;
#47866=VERTEX_POINT ( 'NONE', #9763 ) ;
#47867=CARTESIAN_POINT ( 'NONE',  ( 11.36250000000000071, 2.886751345948129099, -4.999999999999997335 ) ) ;
#47868=CARTESIAN_POINT ( 'NONE',  ( 26.12812500061451360, 4.541064518000418104, 2.621784821874999949 ) ) ;
#47869=DIRECTION ( 'NONE',  ( -0.000000000000000000, -1.000000000000000000, -0.000000000000000000 ) ) ;
#47872=CARTESIAN_POINT ( 'NONE',  ( 3.027206758929959385, 3.985217399322934284, -32.62660190005471605 ) ) ;
#47873=CARTESIAN_POINT ( 'NONE',  ( 14.96250000000000036, 2.886751345948129099, -4.999999999999998224 ) ) ;
#47874=CARTESIAN_POINT ( 'NONE',  ( 26.77500000122903145, 2.886751345948129099, -4.999999999999998224 ) ) ;
#47875=CARTESIAN_POINT ( 'NONE',  ( 21.02812500061451573, 6.421520780324663323E-16, -5.243569643749999010 ) ) ;
#47876=VERTEX_POINT ( 'NONE', #42286 ) ;
#47877=CARTESIAN_POINT ( 'NONE',  ( 22.19999999999999574, 4.330127018922192761, -2.499999999999997780 ) ) ;
#47878=CARTESIAN_POINT ( 'NONE',  ( 23.40937500061451715, 4.541064518000418104, -2.621784821874998173 ) ) ;
#47879=ORIENTED_EDGE ( 'NONE', *, *, #11716, .T. ) ;
#47880=LINE ( 'NONE', #25335, #25379 ) ;
#47881=CARTESIAN_POINT ( 'NONE',  ( 13.60312500061451679, 0.000000000000000000, 5.243569643749999010 ) ) ;
#47882=CARTESIAN_POINT ( 'NONE',  ( 30.00000000000000000, 6.123233995736764310E-16, -4.999999999999998224 ) ) ;
#47884=CARTESIAN_POINT ( 'NONE',  ( 28.41562500061451502, 3.027376345333611329, 5.243569643749999010 ) ) ;
#47885=CARTESIAN_POINT ( 'NONE',  ( 12.03750000122903430, 4.330127018922191873, 2.499999999999999556 ) ) ;
#47887=CARTESIAN_POINT ( 'NONE',  ( 18.78749999999999432, -2.886751345948129988, 4.999999999999997335 ) ) ;
#47888=CARTESIAN_POINT ( 'NONE',  ( 27.29999999999999716, 0.000000000000000000, 4.999999999999998224 ) ) ;
#47889=CARTESIAN_POINT ( 'NONE',  ( 6.646875000614518747, -3.027376345333610441, -5.243569643749999898 ) ) ;
#47890=CARTESIAN_POINT ( 'NONE',  ( 20.25937500061451857, 4.541064518000418104, -2.621784821874998173 ) ) ;
#47894=CARTESIAN_POINT ( 'NONE',  ( 27.62812500061451360, -4.541064518000419881, 2.621784821874995952 ) ) ;
#47895=CARTESIAN_POINT ( 'NONE',  ( 29.18437500061451573, 6.421520780324663323E-16, -5.243569643749999010 ) ) ;
#47896=CARTESIAN_POINT ( 'NONE',  ( 3.459375000614519635, -4.541064518000417216, -2.621784821875001281 ) ) ;
#47897=CARTESIAN_POINT ( 'NONE',  ( 16.68750000000000000, -2.886751345948125991, -5.000000000000000000 ) ) ;
#47898=CARTESIAN_POINT ( 'NONE',  ( 13.49062500061451608, 6.054752690667223547, 3.707466751127219781E-16 ) ) ;
#47899=DIRECTION ( 'NONE',  ( -0.000000000000000000, -1.000000000000000000, -0.000000000000000000 ) ) ;
#47901=CARTESIAN_POINT ( 'NONE',  ( 27.00000000000000000, -4.330127018922190985, -2.500000000000001332 ) ) ;
#47902=CARTESIAN_POINT ( 'NONE',  ( 18.00000000122903288, -2.886751345948129988, 4.999999999999997335 ) ) ;
#47904=CARTESIAN_POINT ( 'NONE',  ( 6.740625000614516082, 6.054752690667223547, 3.707466751127219781E-16 ) ) ;
#47905=CARTESIAN_POINT ( 'NONE',  ( 25.43437500061451573, -4.541064518000419881, 2.621784821874995952 ) ) ;
#47906=CARTESIAN_POINT ( 'NONE',  ( 2.121784821874999061, 17.00937500061451857, 26.32496088578401583 ) ) ;
#47907=CARTESIAN_POINT ( 'NONE',  ( 23.93437500061451573, 4.541064518000418104, 2.621784821874999949 ) ) ;
#47908=CARTESIAN_POINT ( 'NONE',  ( 4.500000000000000888, -4.330127018922190985, -2.500000000000001332 ) ) ;
#47909=CARTESIAN_POINT ( 'NONE',  ( 3.999999999999998668, 11.37500000122903288, 27.69059892324149175 ) ) ;
#47910=CARTESIAN_POINT ( 'NONE',  ( 11.69062500061451360, 6.054752690667223547, 3.707466751127219781E-16 ) ) ;
#47911=CARTESIAN_POINT ( 'NONE',  ( 4.875000001229034652, 2.886751345948126879, 4.999999999999999112 ) ) ;
#47912=CARTESIAN_POINT ( 'NONE',  ( 8.634375000614518569, 4.541064518000418104, 2.621784821874999949 ) ) ;
#47913=CARTESIAN_POINT ( 'NONE',  ( -0.1380872570243177055, 5.000000000000001776, -26.00000000000000000 ) ) ;
#47914=VERTEX_POINT ( 'NONE', #42651 ) ;
#47915=CARTESIAN_POINT ( 'NONE',  ( 8.803125000614517859, -4.541064518000417216, -2.621784821875001281 ) ) ;
#47916=CARTESIAN_POINT ( 'NONE',  ( 14.22187500061451537, -6.054752690667223547, -1.112240025338166033E-15 ) ) ;
#47918=CARTESIAN_POINT ( 'NONE',  ( 24.07500000122903216, 2.886751345948129099, -4.999999999999998224 ) ) ;
#47919=CARTESIAN_POINT ( 'NONE',  ( 9.384375000614518569, 6.421520780324663323E-16, -5.243569643749999010 ) ) ;
#47920=CARTESIAN_POINT ( 'NONE',  ( 11.31562500061451892, 3.027376345333611329, 5.243569643749999010 ) ) ;
#47922=CARTESIAN_POINT ( 'NONE',  ( 21.12187500061451573, 3.027376345333613106, -5.243569643749998122 ) ) ;
#47923=CARTESIAN_POINT ( 'NONE',  ( 0.000000000000000000, 20.00000000000000000, 30.00000000000000000 ) ) ;
#47924=CARTESIAN_POINT ( 'NONE',  ( 5.437500000000000888, -2.886751345948193048, -4.999999999999883649 ) ) ;
#47925=CARTESIAN_POINT ( 'NONE',  ( 15.15000000000000036, 0.000000000000000000, 4.999999999999998224 ) ) ;
#47926=CARTESIAN_POINT ( 'NONE',  ( 2.121784821874999061, 14.30937500061451750, -33.67503911421598417 ) ) ;
#47927=CARTESIAN_POINT ( 'NONE',  ( 15.23437500061451644, 6.421520780324663323E-16, -5.243569643749999010 ) ) ;
#47928=CARTESIAN_POINT ( 'NONE',  ( 16.68750000122903288, -4.330127018922194537, 2.499999999999995559 ) ) ;
#47929=ADVANCED_FACE ( 'NONE', ( #31568 ), #14566, .F. ) ;
#47930=CARTESIAN_POINT ( 'NONE',  ( 11.37187500061451750, 3.027376345333611329, 5.243569643749999010 ) ) ;
#47931=CARTESIAN_POINT ( 'NONE',  ( 4.243569643749999898, 17.74062500061451786, -27.54997392385601529 ) ) ;
#47932=CARTESIAN_POINT ( 'NONE',  ( 17.51250000122903216, 0.000000000000000000, 4.999999999999998224 ) ) ;
#47933=CARTESIAN_POINT ( 'NONE',  ( 11.95312500061451644, -4.541064518000417216, -2.621784821875001281 ) ) ;
#47934=ORIENTED_EDGE ( 'NONE', *, *, #38674, .T. ) ;
#47935=CARTESIAN_POINT ( 'NONE',  ( 16.80000000000000071, 4.330127018922192761, -2.499999999999997780 ) ) ;
#47936=CARTESIAN_POINT ( 'NONE',  ( 29.28749999999999787, -2.886751345948095793, -5.000000000000054179 ) ) ;
#47937=CARTESIAN_POINT ( 'NONE',  ( 9.796875000614518214, -3.027376345333610441, -5.243569643749999898 ) ) ;
#47939=CARTESIAN_POINT ( 'NONE',  ( 11.51250000122903216, 4.330127018922192761, -2.499999999999997780 ) ) ;
#47940=CARTESIAN_POINT ( 'NONE',  ( 20.02500000122903145, 2.886751345948129099, -4.999999999999998224 ) ) ;
#47941=CARTESIAN_POINT ( 'NONE',  ( 17.99062500061451786, 6.054752690667223547, 3.707466751127219781E-16 ) ) ;
#47942=CARTESIAN_POINT ( 'NONE',  ( 19.90312500061451573, 0.000000000000000000, 5.243569643749999010 ) ) ;
#47943=CARTESIAN_POINT ( 'NONE',  ( 27.33750000122903145, 4.330127018922191873, 2.499999999999999556 ) ) ;
#47944=CARTESIAN_POINT ( 'NONE',  ( 25.68750000000000000, -2.886751345948125991, -5.000000000000000000 ) ) ;
#47945=CARTESIAN_POINT ( 'NONE',  ( 12.67499999999999893, 6.123233995736764310E-16, -4.999999999999998224 ) ) ;
#47948=CARTESIAN_POINT ( 'NONE',  ( 28.24687500061451573, -3.027376345333610441, -5.243569643749999898 ) ) ;
#47950=CARTESIAN_POINT ( 'NONE',  ( 2.121784821874999061, 13.85937500061451821, -33.67503911421598417 ) ) ;
#47951=CARTESIAN_POINT ( 'NONE',  ( 4.162500001229033408, -4.330127018922190985, -2.500000000000001332 ) ) ;
#47952=CARTESIAN_POINT ( 'NONE',  ( 29.63437500061451502, 6.421520780324663323E-16, -5.243569643749999010 ) ) ;
#47954=ADVANCED_BREP_SHAPE_REPRESENTATION ( '', ( #22240, #23765 ), #56785 ) ;
#47955=CARTESIAN_POINT ( 'NONE',  ( 8.634375000614518569, 4.541064518000418104, 2.621784821874999949 ) ) ;
#47956=CARTESIAN_POINT ( 'NONE',  ( 27.47812500061451502, 4.541064518000418104, 2.621784821874999949 ) ) ;
#47958=CARTESIAN_POINT ( 'NONE',  ( -1.394453263437886604E-15, 19.32500000122903216, 33.99999999999999289 ) ) ;
#47959=CARTESIAN_POINT ( 'NONE',  ( 6.459375000614518747, 0.000000000000000000, 5.243569643749999010 ) ) ;
#47960=CARTESIAN_POINT ( 'NONE',  ( 10.39687500061451786, 6.054752690667223547, 3.707466751127219781E-16 ) ) ;
#47961=CARTESIAN_POINT ( 'NONE',  ( 4.162499999999999645, 2.886751345948129099, -4.999999999999998224 ) ) ;
#47962=CARTESIAN_POINT ( 'NONE',  ( -3.000416591977282496E-16, 13.84062500061459744, 25.09994784771203058 ) ) ;
#47964=CARTESIAN_POINT ( 'NONE',  ( 6.037500000000001421, 5.773502691896255534, 3.535250795749688894E-16 ) ) ;
#47966=CARTESIAN_POINT ( 'NONE',  ( 21.14062500061451289, 6.054752690667223547, 3.707466751127219781E-16 ) ) ;
#47967=CARTESIAN_POINT ( 'NONE',  ( 10.56562500061451715, -6.054752690667223547, -1.112240025338166033E-15 ) ) ;
#47969=CARTESIAN_POINT ( 'NONE',  ( 9.271875000614516082, -6.054752690667223547, -1.112240025338166033E-15 ) ) ;
#47970=CARTESIAN_POINT ( 'NONE',  ( 25.08749999999999858, -2.886751345948129988, 4.999999999999997335 ) ) ;
#47971=CARTESIAN_POINT ( 'NONE',  ( 21.11250000122903359, 0.000000000000000000, 4.999999999999998224 ) ) ;
#47972=CARTESIAN_POINT ( 'NONE',  ( 27.81562500061452070, 3.027376345333613106, -5.243569643749998122 ) ) ;
#47973=FACE_OUTER_BOUND ( 'NONE', #22185, .T. ) ;
#47974=CARTESIAN_POINT ( 'NONE',  ( 9.684375000614517504, -4.541064518000419881, 2.621784821874995952 ) ) ;
#47975=CARTESIAN_POINT ( 'NONE',  ( 13.73437500061451821, -4.541064518000419881, 2.621784821874995952 ) ) ;
#47976=CARTESIAN_POINT ( 'NONE',  ( 26.82187500061451857, -6.054752690667223547, -1.112240025338166033E-15 ) ) ;
#47978=DIRECTION ( 'NONE',  ( -0.000000000000000000, -1.000000000000000000, -0.000000000000000000 ) ) ;
#47980=CARTESIAN_POINT ( 'NONE',  ( 20.97187500061451715, -6.054752690667223547, -1.112240025338166033E-15 ) ) ;
#47981=CARTESIAN_POINT ( 'NONE',  ( 12.34687500061452070, -3.027376345333614438, 5.243569643749998122 ) ) ;
#47983=CARTESIAN_POINT ( 'NONE',  ( 23.43750000000000000, -2.886751345948125991, -5.000000000000000000 ) ) ;
#47985=CARTESIAN_POINT ( 'NONE',  ( 2.121784821875001281, 12.80937500061451928, -26.32496088578401938 ) ) ;
#47987=CARTESIAN_POINT ( 'NONE',  ( 14.24062500061451608, -3.027376345333610441, -5.243569643749999898 ) ) ;
#47988=CARTESIAN_POINT ( 'NONE',  ( 3.412500000000002309, 2.886751345948126879, 4.999999999999999112 ) ) ;
#47990=CARTESIAN_POINT ( 'NONE',  ( 25.61250000000000071, -5.773502691896255534, -1.060575238724906372E-15 ) ) ;
#47991=CARTESIAN_POINT ( 'NONE',  ( 13.04999999999999893, -4.330127018922190985, -2.500000000000001332 ) ) ;
#47992=CARTESIAN_POINT ( 'NONE',  ( -2.828200636599751609E-16, 17.75000000122903288, 25.38119784648299770 ) ) ;
#47993=CARTESIAN_POINT ( 'NONE',  ( 10.76250000122903572, 0.000000000000000000, 4.999999999999998224 ) ) ;
#47994=ADVANCED_FACE ( 'NONE', ( #25660 ), #71831, .F. ) ;
#47995=CARTESIAN_POINT ( 'NONE',  ( 22.20937500061451431, 0.000000000000000000, 5.243569643749999010 ) ) ;
#47996=CARTESIAN_POINT ( 'NONE',  ( 17.52187500061451431, 3.027376345333613106, -5.243569643749998122 ) ) ;
#47997=CARTESIAN_POINT ( 'NONE',  ( 20.32500000122903572, -5.773502691896255534, -1.060575238724906372E-15 ) ) ;
#47999=CARTESIAN_POINT ( 'NONE',  ( 18.92812500061451431, 4.541064518000418104, 2.621784821874999949 ) ) ;
#48000=CARTESIAN_POINT ( 'NONE',  ( 4.078125000614517326, 4.541064518000418104, 2.621784821874999949 ) ) ;
#48001=CARTESIAN_POINT ( 'NONE',  ( 16.84687500061451715, -3.027376345333614438, 5.243569643749998122 ) ) ;
#48002=CARTESIAN_POINT ( 'NONE',  ( 28.88437500061451502, 4.541064518000418104, 2.621784821874999949 ) ) ;
#48003=CARTESIAN_POINT ( 'NONE',  ( 3.890625000614517326, -3.027376345333610441, -5.243569643749999898 ) ) ;
#48004=CARTESIAN_POINT ( 'NONE',  ( 19.97812500061451502, -4.541064518000419881, 2.621784821874995952 ) ) ;
#48005=CARTESIAN_POINT ( 'NONE',  ( -2.121784821874996840, 16.27812500061451573, 33.67503911421598417 ) ) ;
#48006=CARTESIAN_POINT ( 'NONE',  ( 16.80000000122903359, -2.886751345948125991, -5.000000000000000000 ) ) ;
#48008=CARTESIAN_POINT ( 'NONE',  ( 7.528125000614515727, 6.421520780324663323E-16, -5.243569643749999010 ) ) ;
#48009=CARTESIAN_POINT ( 'NONE',  ( 29.42812500061451431, -4.541064518000419881, 2.621784821874995952 ) ) ;
#48010=CARTESIAN_POINT ( 'NONE',  ( 23.33437500061451786, 6.421520780324663323E-16, -5.243569643749999010 ) ) ;
#48011=CARTESIAN_POINT ( 'NONE',  ( 13.49062500061451608, 6.054752690667223547, 3.707466751127219781E-16 ) ) ;
#48012=CARTESIAN_POINT ( 'NONE',  ( 25.57500000122903216, 2.886751345948126879, 4.999999999999999112 ) ) ;
#48013=( BOUNDED_SURFACE ( )  B_SPLINE_SURFACE ( 1, 2, ( 
 ( #72047, #59856, #31795, #48789, #71316, #20692, #45068, #365, #5899, #34690, #56150, #29163, #40250, #67605, #16970, #63131, #734, #17689, #23966, #18052, #39526, #5544, #11447, #69053, #23243, #68692, #6634, #29521, #35060, #28432, #61679, #6990, #52056, #62052, #6263, #22521, #1460, #28082, #57221, #46514, #39164, #12162, #11078, #33967, #57587, #22872, #33606, #28791, #23607, #50610, #40610, #45794, #68329, #62771, #51695, #1099, #14, #56506, #50969, #46152, #45430, #67964, #39896, #56857, #17337, #62409, #12527, #11808, #34325, #51332, #13973, #40981, #57942, #52415, #13240, #12884, #18773, #41339, #64214, #36511, #19875, #31339, #7349, #19505, #29879, #2896, #36875, #24692, #35778, #46879, #59393, #3272, #63496, #25800, #69418, #1823, #35417, #24330, #53880, #63849, #59031, #64949, #41691, #47236, #42062, #13603, #42428, #8433, #2535, #58301, #7710, #30244, #52777, #2179, #69769, #19137, #36149, #8076, #30969, #58668, #48338, #70127, #30608, #53136, #18415, #25055, #47598, #64585, #53504, #14341, #25427, #47970, #70498, #8803, #16798, #28265, #61869, #50796, #54604, #199, #11637, #26532, #3639, #39355, #44900, #5368, #26163, #56341, #37244, #48702, #11277, #33797, #60493, #20975, #17163, #42789, #22704, #9172, #43528, #37607, #39722, #20603, #27907, #71225, #65310, #5730, #45256, #14700, #67789, #50441, #62240, #34152, #56689, #6089, #28620, #59765, #4009, #72966, #22348, #67436, #31707, #9899, #70863, #32435, #49072, #20237, #66050, #54242, #43162, #60129, #65682, #15070, #71600, #9538, #55974, #32072, #15428, #37972, #28985, #68157, #23431, #7896, #12707, #7530, #18601, #41518, #47062, #40433, #558, #18958, #64037, #923, #18229, #34515, #13416, #40082, #46703, #35965, #58487, #24150, #51157, #57044, #69596, #12344, #23068, #40803, #35603, #45623, #52601, #35244, #7174, #52240, #29702, #57765, #17520, #62596, #11992, #1644, #6450, #68512, #51879, #68873, #51523, #45977, #17874, #69239, #34879, #63316, #41165, #23788, #58122, #57408, #30063, #62950, #6813, #63674, #13064, #29347, #1278, #2007, #24518, #46339, #25617, #3088, #24875, #37432, #2358, #36338, #2722, #20425, #59954, #59583, #53323, #8262, #8996, #25238, #64770, #48154, #14160, #47784, #70318, #19693, #42246, #19322, #31894, #36694, #60313, #30433, #64405, #59216, #15255, #9361, #53694, #70679, #54430, #47422, #31528, #8624, #3829, #31153, #54068, #69952, #41876, #13798, #20054, #52961, #42609, #65134, #14525, #37059, #3464, #26350, #58852, #25984, #48523, #71050, #30793, #42974, #65504, #14892, #48889, #71419, #20796, #43352, #37792, #65874, #45169, #66236, #72507, #5645, #38156, #10815, #15614, #49620, #27820, #39267, #72880, #61779, #66608, #11183, #22618, #38533, #60679, #50353, #55887, #16347, #10093, #67349, #49259, #32623, #22262, #44815, #21896, #32984, #28181, #54789, #33707, #21161, #55524, #72147, #50709, #55163, #38902, #4560, #4195, #16711, #56254, #26724, #112, #61421, #67700, #17072, #39632, #9723, #32256, #71792, #15983, #33349, #5275, #43714, #27088, #44453, #21525, #66983, #61056, #44080, #4918, #10455, #27453, #49983, #41078, #12623, #68422, #62505, #63592, #28531, #12980, #68066, #57682, #11546, #51069, #22975, #56956, #56604, #11903, #34428, #34790, #7087, #35517, #1923, #467, #63229, #45537, #46611, #7446, #17784, #6360, #17434, #29972, #46977, #34063, #69512, #39992, #28892, #6000, #51431, #24428, #833, #29616, #58036, #12259, #40343, #35158, #57323, #52513, #52152, #46248, #23341, #45890, #62864, #6727, #29261, #51791, #1192, #23700, #68788, #1555, #18144, #18872, #40711, #62150, #24065, #69154, #18513, #20337, #64685, #8537, #48439, #35873, #70595, #47692, #65413, #58763, #42523, #13335, #7810, #58397, #14070, #71331, #42158, #70228, #8173, #31066, #30701, #14803, #47333, #2630, #53233, #36973, #30347, #31440, #65049, #69866, #19232, #37346, #2998, #19970, #26265, #42890, #41786, #52875, #13706, #41434, #25526, #70964, #8909, #31808, #59869, #25152, #63950, #9273, #54346, #64316, #53604, #24789, #3740, #2273, #59496, #48802, #36249, #14439, #19602, #36609, #59130, #48069, #53980, #3378, #25899, #39178, #22177, #55441, #49898, #21806, #72423, #27367, #16623, #60225, #43264, #44370, #4111, #38071, #21439, #38445, #54706, #71706, #26639, #66897, #4476, #32901, #60971, #66518, #5193, #55076, #72794, #11093, #33621, #16265, #10371, #43629, #43996, #50269, #44730, #21078, #15898, #4833, #15167, #27731, #65785, #49175, #66151, #10733, #67265, #38820, #15529, #60595, #61335, #10004, #27006, #33265, #49536, #32539, #72060, #55803, #61694, #9639, #56165, #5559, #50624, #28096, #20706, #32173, #37704, #18066, #12541, #62785, #23257, #18430, #45082, #1475, #11460, #45807, #39910, #40996, #22887, #6649, #379, #67618, #35075, #40627, #16984, #29535, #29176, #23981, #7004, #63146, #57601, #63512, #39541, #56873, #1113, #51710, #46166, #62066, #12177, #35432, #34705, #28805, #52070, #68343, #68706, #45445, #62423, #46529, #23620, #6277, #67978, #69071, #33981, #12899, #5913, #57956, #22535, #56520, #28447, #17351, #50982, #11822, #34339, #17703, #7364, #29893, #29, #51346, #748, #40264, #57234, #70880, #58682, #69785, #7726, #20254, #37261, #1838, #59783, #30260, #41354, #69432, #24346, #14719, #52793, #70516, #25817, #2551, #8092, #53520, #25070, #3289, #42445, #36527, #2194, #46894, #18789, #24708, #47252, #58315, #30622, #19152, #42079, #64967, #63864, #9189, #30987, #53152, #36164, #52432, #13254, #35792, #41706, #64601, #48355, #64230, #2914, #13619, #47613, #19892, #8820, #14358, #31357, #70143, #53898, #65328, #19521, #13988, #36893, #25445, #59047, #59412, #42806, #8451, #47988, #32818, #38356, #4750, #26179, #21356, #67181, #43912, #60510, #10649, #54989, #27284 ),
 ( #33179, #44651, #71242, #55356, #43180, #16184, #50182, #37988, #49091, #60145, #72710, #16542, #54260, #39095, #9554, #20622, #48720, #3656, #61612, #32088, #49817, #5112, #4395, #9916, #72341, #26924, #55717, #21722, #15814, #54619, #65699, #15086, #4025, #26550, #37623, #32454, #71619, #66436, #44281, #20992, #31724, #10288, #49449, #15444, #43545, #66066, #71983, #60883, #66812, #27646, #38735, #61255, #22093, #50900, #29094, #40543, #1030, #63059, #67895, #12461, #23899, #39829, #16901, #51630, #57150, #17625, #39456, #68622, #50543, #61977, #23536, #46086, #665, #34256, #29452, #56084, #34992, #22452, #56789, #300, #51989, #33898, #40184, #11379, #5476, #17984, #57521, #28015, #6922, #62705, #1390, #46447, #68985, #56442, #22809, #18342, #34620, #17267, #5832, #40916, #73071, #11013, #28364, #6562, #33534, #45001, #67538, #45361, #62344, #11739, #6194, #28722, #51263, #23173, #45727, #68262, #12099, #1751, #47905, #8735, #69705, #7640, #18708, #31269, #48271, #12816, #70795, #41272, #52348, #7284, #35350, #25733, #63784, #8371, #36810, #13534, #19071, #64517, #36081, #14272, #53441, #47534, #13173, #57874, #29813, #35713, #58235, #69350, #41627, #30178, #53071, #2832, #24264, #20170, #41997, #64147, #47173, #63429, #46813, #52709, #2115, #2466, #59325, #24626, #13910, #58602, #8009, #30899, #19809, #25360, #42362, #30544, #64884, #3205, #24989, #70062, #70434, #36449, #19436, #58963, #53811, #9107, #48635, #60797, #55275, #32366, #65986, #61173, #14634, #44197, #54177, #15366, #9475, #10568, #65616, #49371, #43089, #37174, #4670, #10202, #59700, #72262, #71901, #66728, #49735, #32738, #27200, #33096, #31645, #26465, #43828, #21274, #15730, #3574, #54904, #5028, #4312, #71535, #21639, #37908, #38269, #26097, #60426, #32005, #55635, #15005, #66352, #37542, #71160, #16099, #38649, #20532, #27566, #50097, #72628, #42724, #65245, #60064, #54540, #3942, #49004, #20910, #43462, #9837, #26837, #11659, #57432, #34174, #50819, #947, #45280, #68180, #22371, #11300, #23455, #45646, #28288, #44923, #46000, #61529, #68537, #27929, #17542, #44568, #10927, #55998, #16822, #16456, #67459, #39376, #67813, #40104, #17898, #34905, #33454, #23089, #5391, #6474, #40458, #222, #61895, #50462, #62974, #6836, #67098, #29371, #72989, #33820, #39014, #56364, #51903, #5754, #62617, #12370, #17187, #22727, #12014, #39747, #22012, #34537, #6111, #62263, #56710, #28642, #51180, #584, #57067, #29009, #51546, #65064, #65429, #23811, #32189, #53997, #3013, #58146, #9655, #68896, #37721, #57787, #14455, #71347, #29724, #3394, #7196, #41188, #20354, #31823, #14819, #54362, #7552, #3756, #15182, #30086, #52262, #42905, #48455, #8925, #1665, #59884, #40826, #24174, #37362, #9290, #36989, #25543, #20722, #46362, #26280, #46726, #43280, #35626, #1301, #59511, #48817, #65801, #60241, #31455, #25915, #70979, #18253, #63343, #12729, #35265, #69261, #18623, #63697, #13088, #48086, #19985, #52624, #70612, #42538, #33279, #38460, #66911, #21821, #27381, #39194, #15912, #33637, #45097, #67632, #55818, #44386, #4491, #4847, #11108, #5574, #32554, #49913, #72437, #49190, #61709, #26654, #60609, #27020, #44746, #56181, #10746, #49552, #55091, #5205, #72074, #60986, #16279, #10385, #21455, #44010, #66532, #32917, #43643, #28111, #55454, #11474, #54722, #15543, #38835, #39556, #50640, #61350, #27746, #44, #71720, #50285, #72809, #22549, #22192, #67280, #21092, #66167, #38087, #16639, #4125, #16999, #62081, #10018, #34717, #6291, #23994, #67992, #761, #18078, #40639, #68718, #51723, #17366, #57613, #50996, #39923, #63158, #35087, #57247, #40276, #69083, #5927, #52083, #394, #62797, #28820, #18444, #11835, #1124, #62437, #28461, #7016, #12553, #56534, #29547, #23633, #1488, #46541, #41009, #63524, #12911, #22901, #23269, #45460, #35444, #34353, #57968, #33997, #45819, #68355, #6660, #51358, #12190, #29189, #56886, #17716, #46179, #39794, #66405, #27981, #38323, #11349, #45327, #33147, #44248, #55324, #67863, #11707, #49417, #34223, #4718, #15781, #43879, #71950, #62311, #27252, #44967, #266, #50149, #55684, #50511, #72679, #50868, #16869, #10979, #49785, #21326, #60850, #72310, #21691, #32787, #5080, #66779, #16509, #39424, #10256, #56756, #5441, #27614, #10617, #26891, #16151, #38703, #61223, #39062, #22776, #22061, #73037, #44619, #67149, #67505, #56409, #61944, #5800, #61576, #33866, #17235, #33500, #22420, #28330, #56049, #12778, #12065, #63746, #45695, #34588, #24226, #18672, #68948, #29420, #24587, #51229, #7600, #17592, #51954, #46052, #47135, #29061, #35315, #6528, #633, #41234, #46776, #23140, #35674, #57837, #30139, #13135, #69311, #58197, #69666, #68229, #63025, #7246, #29775, #52311, #40151, #18306, #41590, #40878, #34957, #52670, #1354, #1713, #51597, #68586, #2078, #19032, #12424, #997, #64108, #13493, #62670, #36041, #57116, #6161, #28690, #57484, #23504, #17948, #40510, #6888, #23863, #46411, #63393, #47493, #2427, #30505, #20872, #13870, #3534, #31964, #8697, #64845, #59660, #31229, #9436, #48597, #42684, #36410, #7969, #53032, #30862, #53400, #64477, #14233, #2792, #48230, #71122, #24950, #15326, #37131, #59288, #42320, #65947, #70024, #43425, #41956, #70754, #54501, #58924, #9068, #8332, #25318, #26057, #14966, #20494, #37504, #36771, #43050, #3903, #47864, #31603, #65576, #54140, #65206, #70393, #60024, #19395, #19769, #26424, #48965, #20129, #53771, #71495, #3167, #58562, #25694, #14596, #57592, #1827, #1465, #18057, #51337, #69774, #41696, #51700, #69059, #12167, #19142, #17694, #24335, #64220, #13609, #46884, #36154, #34696, #47242, #63137, #58673, #18420, #13245, #28796, #30250, #63502, #57947, #29883, #7354, #35422, #24698, #68334, #739, #52421, #57225, #46157, #29526, #46519 ) ),
 .UNSPECIFIED., .F., .F., .F. ) 
 B_SPLINE_SURFACE_WITH_KNOTS ( ( 2, 2 ),
 ( 3, 2, 2, 2, 2, 2, 2, 2, 2, 2, 2, 2, 2, 2, 2, 2, 2, 2, 2, 2, 2, 2, 2, 2, 2, 2, 2, 2, 2, 2, 2, 2, 2, 2, 2, 2, 2, 2, 2, 2, 2, 2, 2, 2, 2, 2, 2, 2, 2, 2, 2, 2, 2, 2, 2, 2, 2, 2, 2, 2, 2, 2, 2, 2, 2, 2, 2, 2, 2, 2, 2, 2, 2, 2, 2, 2, 2, 2, 2, 2, 2, 2, 2, 2, 2, 2, 2, 2, 2, 2, 2, 2, 2, 2, 2, 2, 2, 2, 2, 2, 2, 2, 2, 2, 2, 2, 2, 2, 2, 2, 2, 2, 2, 2, 2, 2, 2, 2, 2, 2, 2, 2, 2, 2, 2, 2, 2, 2, 2, 2, 2, 2, 2, 2, 2, 2, 2, 2, 2, 2, 2, 2, 2, 2, 2, 2, 2, 2, 2, 2, 2, 2, 2, 2, 2, 2, 2, 2, 2, 2, 2, 2, 2, 2, 2, 2, 2, 2, 2, 2, 2, 2, 2, 2, 2, 2, 2, 2, 2, 2, 2, 2, 2, 2, 2, 2, 2, 2, 2, 2, 2, 2, 2, 2, 2, 2, 2, 2, 2, 2, 2, 2, 2, 2, 2, 2, 2, 2, 2, 2, 2, 2, 2, 2, 2, 2, 2, 2, 2, 2, 2, 2, 2, 2, 2, 2, 2, 2, 2, 2, 2, 2, 2, 2, 2, 2, 2, 2, 2, 2, 2, 2, 2, 2, 2, 2, 2, 2, 2, 2, 2, 2, 2, 2, 2, 2, 2, 2, 2, 2, 2, 2, 2, 2, 2, 2, 2, 2, 2, 2, 2, 2, 2, 2, 2, 2, 2, 2, 2, 2, 2, 2, 2, 2, 2, 2, 2, 2, 2, 2, 2, 2, 2, 2, 2, 2, 2, 2, 2, 2, 2, 2, 2, 2, 2, 2, 2, 2, 2, 2, 2, 2, 2, 2, 2, 2, 2, 2, 2, 2, 2, 2, 2, 2, 2, 2, 2, 2, 2, 2, 2, 2, 2, 2, 2, 2, 2, 2, 2, 2, 2, 2, 2, 2, 2, 2, 2, 2, 2, 2, 2, 2, 2, 2, 2, 2, 2, 2, 2, 2, 3 ),
 ( 0.000000000000000000, 1.000000000000000000 ),
 ( 0.000000000000000000, 0.002777777777777777884, 0.005555555555555555768, 0.008333333333333333218, 0.01111111111111111154, 0.01388888888888888812, 0.01666666666666666644, 0.01944444444444444475, 0.02222222222222222307, 0.02500000000000000139, 0.02777777777777777624, 0.03055555555555555455, 0.03333333333333333287, 0.03611111111111110772, 0.03888888888888888951, 0.04166666666666666435, 0.04444444444444444614, 0.04722222222222222099, 0.05000000000000000278, 0.05277777777777777762, 0.05555555555555555247, 0.05833333333333333426, 0.06111111111111110911, 0.06388888888888888395, 0.06666666666666666574, 0.06944444444444444753, 0.07222222222222221544, 0.07499999999999999722, 0.07777777777777777901, 0.08055555555555556080, 0.08333333333333332871, 0.08611111111111111049, 0.08888888888888889228, 0.09166666666666666019, 0.09444444444444444198, 0.09722222222222222376, 0.1000000000000000056, 0.1027777777777777735, 0.1055555555555555552, 0.1083333333333333370, 0.1111111111111111049, 0.1138888888888888867, 0.1166666666666666685, 0.1194444444444444503, 0.1222222222222222182, 0.1250000000000000000, 0.1277777777777777679, 0.1305555555555555636, 0.1333333333333333315, 0.1361111111111110994, 0.1388888888888888951, 0.1416666666666666630, 0.1444444444444444309, 0.1472222222222222265, 0.1499999999999999944, 0.1527777777777777901, 0.1555555555555555580, 0.1583333333333333259, 0.1611111111111111216, 0.1638888888888888895, 0.1666666666666666574, 0.1694444444444444531, 0.1722222222222222210, 0.1749999999999999889, 0.1777777777777777846, 0.1805555555555555525, 0.1833333333333333204, 0.1861111111111111160, 0.1888888888888888840, 0.1916666666666666796, 0.1944444444444444475, 0.1972222222222222154, 0.2000000000000000111, 0.2027777777777777790, 0.2055555555555555469, 0.2083333333333333426, 0.2111111111111111105, 0.2138888888888888784, 0.2166666666666666741, 0.2194444444444444420, 0.2222222222222222099, 0.2250000000000000056, 0.2277777777777777735, 0.2305555555555555691, 0.2333333333333333370, 0.2361111111111111049, 0.2388888888888889006, 0.2416666666666666685, 0.2444444444444444364, 0.2472222222222222321, 0.2500000000000000000, 0.2527777777777777679, 0.2555555555555555358, 0.2583333333333333592, 0.2611111111111111271, 0.2638888888888888951, 0.2666666666666666630, 0.2694444444444444309, 0.2722222222222221988, 0.2750000000000000222, 0.2777777777777777901, 0.2805555555555555580, 0.2833333333333333259, 0.2861111111111110938, 0.2888888888888888618, 0.2916666666666666852, 0.2944444444444444531, 0.2972222222222222210, 0.2999999999999999889, 0.3027777777777777568, 0.3055555555555555802, 0.3083333333333333481, 0.3111111111111111160, 0.3138888888888888840, 0.3166666666666666519, 0.3194444444444444198, 0.3222222222222222432, 0.3250000000000000111, 0.3277777777777777790, 0.3305555555555555469, 0.3333333333333333148, 0.3361111111111111382, 0.3388888888888889062, 0.3416666666666666741, 0.3444444444444444420, 0.3472222222222222099, 0.3499999999999999778, 0.3527777777777778012, 0.3555555555555555691, 0.3583333333333333370, 0.3611111111111111049, 0.3638888888888888729, 0.3666666666666666408, 0.3694444444444444642, 0.3722222222222222321, 0.3750000000000000000, 0.3777777777777777679, 0.3805555555555555358, 0.3833333333333333592, 0.3861111111111111271, 0.3888888888888888951, 0.3916666666666666630, 0.3944444444444444309, 0.3972222222222221988, 0.4000000000000000222, 0.4027777777777777901, 0.4055555555555555580, 0.4083333333333333259, 0.4111111111111110938, 0.4138888888888888618, 0.4166666666666666852, 0.4194444444444444531, 0.4222222222222222210, 0.4249999999999999889, 0.4277777777777777568, 0.4305555555555555802, 0.4333333333333333481, 0.4361111111111111160, 0.4388888888888888840, 0.4416666666666666519, 0.4444444444444444198, 0.4472222222222222432, 0.4500000000000000111, 0.4527777777777777790, 0.4555555555555555469, 0.4583333333333333148, 0.4611111111111111382, 0.4638888888888889062, 0.4666666666666666741, 0.4694444444444444420, 0.4722222222222222099, 0.4749999999999999778, 0.4777777777777778012, 0.4805555555555555691, 0.4833333333333333370, 0.4861111111111111049, 0.4888888888888888729, 0.4916666666666666408, 0.4944444444444444642, 0.4972222222222222321, 0.5000000000000000000, 0.5027777777777777679, 0.5055555555555555358, 0.5083333333333333037, 0.5111111111111110716, 0.5138888888888888395, 0.5166666666666667185, 0.5194444444444444864, 0.5222222222222222543, 0.5250000000000000222, 0.5277777777777777901, 0.5305555555555555580, 0.5333333333333333259, 0.5361111111111110938, 0.5388888888888888618, 0.5416666666666666297, 0.5444444444444443976, 0.5472222222222222765, 0.5500000000000000444, 0.5527777777777778123, 0.5555555555555555802, 0.5583333333333333481, 0.5611111111111111160, 0.5638888888888888840, 0.5666666666666666519, 0.5694444444444444198, 0.5722222222222221877, 0.5749999999999999556, 0.5777777777777777235, 0.5805555555555556024, 0.5833333333333333703, 0.5861111111111111382, 0.5888888888888889062, 0.5916666666666666741, 0.5944444444444444420, 0.5972222222222222099, 0.5999999999999999778, 0.6027777777777777457, 0.6055555555555555136, 0.6083333333333332815, 0.6111111111111111605, 0.6138888888888889284, 0.6166666666666666963, 0.6194444444444444642, 0.6222222222222222321, 0.6250000000000000000, 0.6277777777777777679, 0.6305555555555555358, 0.6333333333333333037, 0.6361111111111110716, 0.6388888888888888395, 0.6416666666666667185, 0.6444444444444444864, 0.6472222222222222543, 0.6500000000000000222, 0.6527777777777777901, 0.6555555555555555580, 0.6583333333333333259, 0.6611111111111110938, 0.6638888888888888618, 0.6666666666666666297, 0.6694444444444443976, 0.6722222222222222765, 0.6750000000000000444, 0.6777777777777778123, 0.6805555555555555802, 0.6833333333333333481, 0.6861111111111111160, 0.6888888888888888840, 0.6916666666666666519, 0.6944444444444444198, 0.6972222222222221877, 0.6999999999999999556, 0.7027777777777777235, 0.7055555555555556024, 0.7083333333333333703, 0.7111111111111111382, 0.7138888888888889062, 0.7166666666666666741, 0.7194444444444444420, 0.7222222222222222099, 0.7249999999999999778, 0.7277777777777777457, 0.7305555555555555136, 0.7333333333333332815, 0.7361111111111111605, 0.7388888888888889284, 0.7416666666666666963, 0.7444444444444444642, 0.7472222222222222321, 0.7500000000000000000, 0.7527777777777777679, 0.7555555555555555358, 0.7583333333333333037, 0.7611111111111110716, 0.7638888888888888395, 0.7666666666666667185, 0.7694444444444444864, 0.7722222222222222543, 0.7750000000000000222, 0.7777777777777777901, 0.7805555555555555580, 0.7833333333333333259, 0.7861111111111110938, 0.7888888888888888618, 0.7916666666666666297, 0.7944444444444443976, 0.7972222222222222765, 0.8000000000000000444, 0.8027777777777778123, 0.8055555555555555802, 0.8083333333333333481, 0.8111111111111111160, 0.8138888888888888840, 0.8166666666666666519, 0.8194444444444444198, 0.8222222222222221877, 0.8249999999999999556, 0.8277777777777777235, 0.8305555555555556024, 0.8333333333333333703, 0.8361111111111111382, 0.8388888888888889062, 0.8416666666666666741, 0.8444444444444444420, 0.8472222222222222099, 0.8499999999999999778, 0.8527777777777777457, 0.8555555555555555136, 0.8583333333333332815, 0.8611111111111111605, 0.8638888888888889284, 0.8666666666666666963, 0.8694444444444444642, 0.8722222222222222321, 0.8750000000000000000, 0.8777777777777777679, 0.8805555555555555358, 0.8833333333333333037, 0.8861111111111110716, 0.8888888888888888395, 0.8916666666666667185, 0.8944444444444444864, 0.8972222222222222543, 0.9000000000000000222, 0.9027777777777777901, 0.9055555555555555580, 0.9083333333333333259, 0.9111111111111110938, 0.9138888888888888618, 0.9166666666666666297, 0.9194444444444443976, 0.9222222222222222765, 0.9250000000000000444, 0.9277777777777778123, 0.9305555555555555802, 0.9333333333333333481, 0.9361111111111111160, 0.9388888888888888840, 0.9416666666666666519, 0.9444444444444444198, 0.9472222222222221877, 0.9499999999999999556, 0.9527777777777777235, 0.9555555555555556024, 0.9583333333333333703, 0.9611111111111111382, 0.9638888888888889062, 0.9666666666666666741, 0.9694444444444444420, 0.9722222222222222099, 0.9749999999999999778, 0.9777777777777777457, 0.9805555555555555136, 0.9833333333333332815, 0.9861111111111111605, 0.9888888888888889284, 0.9916666666666666963, 0.9944444444444444642, 0.9972222222222222321, 1.000000000000000000 ),
 .UNSPECIFIED. ) 
 GEOMETRIC_REPRESENTATION_ITEM ( )  RATIONAL_B_SPLINE_SURFACE ( (
 ( 1.000000000000000000, 0.8660254037844387076, 1.000000000000000000, 0.8660254037844387076, 1.000000000000000000, 0.8660254037844387076, 1.000000000000000000, 0.8660254037844387076, 1.000000000000000000, 0.8660254037844387076, 1.000000000000000000, 0.8660254037844387076, 1.000000000000000000, 0.8660254037844387076, 1.000000000000000000, 0.8660254037844387076, 1.000000000000000000, 0.8660254037844387076, 1.000000000000000000, 0.8660254037844387076, 1.000000000000000000, 0.8660254037844387076, 1.000000000000000000, 0.8660254037844387076, 1.000000000000000000, 0.8660254037844387076, 1.000000000000000000, 0.8660254037844387076, 1.000000000000000000, 0.8660254037844387076, 1.000000000000000000, 0.8660254037844387076, 1.000000000000000000, 0.8660254037844387076, 1.000000000000000000, 0.8660254037844387076, 1.000000000000000000, 0.8660254037844387076, 1.000000000000000000, 0.8660254037844387076, 1.000000000000000000, 0.8660254037844387076, 1.000000000000000000, 0.8660254037844387076, 1.000000000000000000, 0.8660254037844387076, 1.000000000000000000, 0.8660254037844387076, 1.000000000000000000, 0.8660254037844387076, 1.000000000000000000, 0.8660254037844387076, 1.000000000000000000, 0.8660254037844387076, 1.000000000000000000, 0.8660254037844387076, 1.000000000000000000, 0.8660254037844387076, 1.000000000000000000, 0.8660254037844387076, 1.000000000000000000, 0.8660254037844387076, 1.000000000000000000, 0.8660254037844387076, 1.000000000000000000, 0.8660254037844387076, 1.000000000000000000, 0.8660254037844387076, 1.000000000000000000, 0.8660254037844387076, 1.000000000000000000, 0.8660254037844387076, 1.000000000000000000, 0.8660254037844387076, 1.000000000000000000, 0.8660254037844387076, 1.000000000000000000, 0.8660254037844387076, 1.000000000000000000, 0.8660254037844387076, 1.000000000000000000, 0.8660254037844387076, 1.000000000000000000, 0.8660254037844387076, 1.000000000000000000, 0.8660254037844387076, 1.000000000000000000, 0.8660254037844387076, 1.000000000000000000, 0.8660254037844387076, 1.000000000000000000, 0.8660254037844387076, 1.000000000000000000, 0.8660254037844387076, 1.000000000000000000, 0.8660254037844387076, 1.000000000000000000, 0.8660254037844387076, 1.000000000000000000, 0.8660254037844387076, 1.000000000000000000, 0.8660254037844387076, 1.000000000000000000, 0.8660254037844387076, 1.000000000000000000, 0.8660254037844387076, 1.000000000000000000, 0.8660254037844387076, 1.000000000000000000, 0.8660254037844387076, 1.000000000000000000, 0.8660254037844387076, 1.000000000000000000, 0.8660254037844387076, 1.000000000000000000, 0.8660254037844387076, 1.000000000000000000, 0.8660254037844387076, 1.000000000000000000, 0.8660254037844387076, 1.000000000000000000, 0.8660254037844387076, 1.000000000000000000, 0.8660254037844387076, 1.000000000000000000, 0.8660254037844387076, 1.000000000000000000, 0.8660254037844387076, 1.000000000000000000, 0.8660254037844387076, 1.000000000000000000, 0.8660254037844387076, 1.000000000000000000, 0.8660254037844387076, 1.000000000000000000, 0.8660254037844387076, 1.000000000000000000, 0.8660254037844387076, 1.000000000000000000, 0.8660254037844387076, 1.000000000000000000, 0.8660254037844387076, 1.000000000000000000, 0.8660254037844387076, 1.000000000000000000, 0.8660254037844387076, 1.000000000000000000, 0.8660254037844387076, 1.000000000000000000, 0.8660254037844387076, 1.000000000000000000, 0.8660254037844387076, 1.000000000000000000, 0.8660254037844387076, 1.000000000000000000, 0.8660254037844387076, 1.000000000000000000, 0.8660254037844387076, 1.000000000000000000, 0.8660254037844387076, 1.000000000000000000, 0.8660254037844387076, 1.000000000000000000, 0.8660254037844387076, 1.000000000000000000, 0.8660254037844387076, 1.000000000000000000, 0.8660254037844387076, 1.000000000000000000, 0.8660254037844387076, 1.000000000000000000, 0.8660254037844387076, 1.000000000000000000, 0.8660254037844387076, 1.000000000000000000, 0.8660254037844387076, 1.000000000000000000, 0.8660254037844387076, 1.000000000000000000, 0.8660254037844387076, 1.000000000000000000, 0.8660254037844387076, 1.000000000000000000, 0.8660254037844387076, 1.000000000000000000, 0.8660254037844387076, 1.000000000000000000, 0.8660254037844387076, 1.000000000000000000, 0.8660254037844387076, 1.000000000000000000, 0.8660254037844387076, 1.000000000000000000, 0.8660254037844387076, 1.000000000000000000, 0.8660254037844387076, 1.000000000000000000, 0.8660254037844387076, 1.000000000000000000, 0.8660254037844387076, 1.000000000000000000, 0.8660254037844387076, 1.000000000000000000, 0.8660254037844387076, 1.000000000000000000, 0.8660254037844387076, 1.000000000000000000, 0.8660254037844387076, 1.000000000000000000, 0.8660254037844387076, 1.000000000000000000, 0.8660254037844387076, 1.000000000000000000, 0.8660254037844387076, 1.000000000000000000, 0.8660254037844387076, 1.000000000000000000, 0.8660254037844387076, 1.000000000000000000, 0.8660254037844387076, 1.000000000000000000, 0.8660254037844387076, 1.000000000000000000, 0.8660254037844387076, 1.000000000000000000, 0.8660254037844387076, 1.000000000000000000, 0.8660254037844387076, 1.000000000000000000, 0.8660254037844387076, 1.000000000000000000, 0.8660254037844387076, 1.000000000000000000, 0.8660254037844387076, 1.000000000000000000, 0.8660254037844387076, 1.000000000000000000, 0.8660254037844387076, 1.000000000000000000, 0.8660254037844387076, 1.000000000000000000, 0.8660254037844387076, 1.000000000000000000, 0.8660254037844387076, 1.000000000000000000, 0.8660254037844387076, 1.000000000000000000, 0.8660254037844387076, 1.000000000000000000, 0.8660254037844387076, 1.000000000000000000, 0.8660254037844387076, 1.000000000000000000, 0.8660254037844387076, 1.000000000000000000, 0.8660254037844387076, 1.000000000000000000, 0.8660254037844387076, 1.000000000000000000, 0.8660254037844387076, 1.000000000000000000, 0.8660254037844387076, 1.000000000000000000, 0.8660254037844387076, 1.000000000000000000, 0.8660254037844387076, 1.000000000000000000, 0.8660254037844387076, 1.000000000000000000, 0.8660254037844387076, 1.000000000000000000, 0.8660254037844387076, 1.000000000000000000, 0.8660254037844387076, 1.000000000000000000, 0.8660254037844387076, 1.000000000000000000, 0.8660254037844387076, 1.000000000000000000, 0.8660254037844387076, 1.000000000000000000, 0.8660254037844387076, 1.000000000000000000, 0.8660254037844387076, 1.000000000000000000, 0.8660254037844387076, 1.000000000000000000, 0.8660254037844387076, 1.000000000000000000, 0.8660254037844387076, 1.000000000000000000, 0.8660254037844387076, 1.000000000000000000, 0.8660254037844387076, 1.000000000000000000, 0.8660254037844387076, 1.000000000000000000, 0.8660254037844387076, 1.000000000000000000, 0.8660254037844387076, 1.000000000000000000, 0.8660254037844387076, 1.000000000000000000, 0.8660254037844387076, 1.000000000000000000, 0.8660254037844387076, 1.000000000000000000, 0.8660254037844387076, 1.000000000000000000, 0.8660254037844387076, 1.000000000000000000, 0.8660254037844387076, 1.000000000000000000, 0.8660254037844387076, 1.000000000000000000, 0.8660254037844387076, 1.000000000000000000, 0.8660254037844387076, 1.000000000000000000, 0.8660254037844387076, 1.000000000000000000, 0.8660254037844387076, 1.000000000000000000, 0.8660254037844387076, 1.000000000000000000, 0.8660254037844387076, 1.000000000000000000, 0.8660254037844387076, 1.000000000000000000, 0.8660254037844387076, 1.000000000000000000, 0.8660254037844387076, 1.000000000000000000, 0.8660254037844387076, 1.000000000000000000, 0.8660254037844387076, 1.000000000000000000, 0.8660254037844387076, 1.000000000000000000, 0.8660254037844387076, 1.000000000000000000, 0.8660254037844387076, 1.000000000000000000, 0.8660254037844387076, 1.000000000000000000, 0.8660254037844387076, 1.000000000000000000, 0.8660254037844387076, 1.000000000000000000, 0.8660254037844387076, 1.000000000000000000, 0.8660254037844387076, 1.000000000000000000, 0.8660254037844387076, 1.000000000000000000, 0.8660254037844387076, 1.000000000000000000, 0.8660254037844387076, 1.000000000000000000, 0.8660254037844387076, 1.000000000000000000, 0.8660254037844387076, 1.000000000000000000, 0.8660254037844387076, 1.000000000000000000, 0.8660254037844387076, 1.000000000000000000, 0.8660254037844387076, 1.000000000000000000, 0.8660254037844387076, 1.000000000000000000, 0.8660254037844387076, 1.000000000000000000, 0.8660254037844387076, 1.000000000000000000, 0.8660254037844387076, 1.000000000000000000, 0.8660254037844387076, 1.000000000000000000, 0.8660254037844387076, 1.000000000000000000, 0.8660254037844387076, 1.000000000000000000, 0.8660254037844387076, 1.000000000000000000, 0.8660254037844387076, 1.000000000000000000, 0.8660254037844387076, 1.000000000000000000, 0.8660254037844387076, 1.000000000000000000, 0.8660254037844387076, 1.000000000000000000, 0.8660254037844387076, 1.000000000000000000, 0.8660254037844387076, 1.000000000000000000, 0.8660254037844387076, 1.000000000000000000, 0.8660254037844387076, 1.000000000000000000, 0.8660254037844387076, 1.000000000000000000, 0.8660254037844387076, 1.000000000000000000, 0.8660254037844387076, 1.000000000000000000, 0.8660254037844387076, 1.000000000000000000, 0.8660254037844387076, 1.000000000000000000, 0.8660254037844387076, 1.000000000000000000, 0.8660254037844387076, 1.000000000000000000, 0.8660254037844387076, 1.000000000000000000, 0.8660254037844387076, 1.000000000000000000, 0.8660254037844387076, 1.000000000000000000, 0.8660254037844387076, 1.000000000000000000, 0.8660254037844387076, 1.000000000000000000, 0.8660254037844387076, 1.000000000000000000, 0.8660254037844387076, 1.000000000000000000, 0.8660254037844387076, 1.000000000000000000, 0.8660254037844387076, 1.000000000000000000, 0.8660254037844387076, 1.000000000000000000, 0.8660254037844387076, 1.000000000000000000, 0.8660254037844387076, 1.000000000000000000, 0.8660254037844387076, 1.000000000000000000, 0.8660254037844387076, 1.000000000000000000, 0.8660254037844387076, 1.000000000000000000, 0.8660254037844387076, 1.000000000000000000, 0.8660254037844387076, 1.000000000000000000, 0.8660254037844387076, 1.000000000000000000, 0.8660254037844387076, 1.000000000000000000, 0.8660254037844387076, 1.000000000000000000, 0.8660254037844387076, 1.000000000000000000, 0.8660254037844387076, 1.000000000000000000, 0.8660254037844387076, 1.000000000000000000, 0.8660254037844387076, 1.000000000000000000, 0.8660254037844387076, 1.000000000000000000, 0.8660254037844387076, 1.000000000000000000, 0.8660254037844387076, 1.000000000000000000, 0.8660254037844387076, 1.000000000000000000, 0.8660254037844387076, 1.000000000000000000, 0.8660254037844387076, 1.000000000000000000, 0.8660254037844387076, 1.000000000000000000, 0.8660254037844387076, 1.000000000000000000, 0.8660254037844387076, 1.000000000000000000, 0.8660254037844387076, 1.000000000000000000, 0.8660254037844387076, 1.000000000000000000, 0.8660254037844387076, 1.000000000000000000, 0.8660254037844387076, 1.000000000000000000, 0.8660254037844387076, 1.000000000000000000, 0.8660254037844387076, 1.000000000000000000, 0.8660254037844387076, 1.000000000000000000, 0.8660254037844387076, 1.000000000000000000, 0.8660254037844387076, 1.000000000000000000, 0.8660254037844387076, 1.000000000000000000, 0.8660254037844387076, 1.000000000000000000, 0.8660254037844387076, 1.000000000000000000, 0.8660254037844387076, 1.000000000000000000, 0.8660254037844387076, 1.000000000000000000, 0.8660254037844387076, 1.000000000000000000, 0.8660254037844387076, 1.000000000000000000, 0.8660254037844387076, 1.000000000000000000, 0.8660254037844387076, 1.000000000000000000, 0.8660254037844387076, 1.000000000000000000, 0.8660254037844387076, 1.000000000000000000, 0.8660254037844387076, 1.000000000000000000, 0.8660254037844387076, 1.000000000000000000, 0.8660254037844387076, 1.000000000000000000, 0.8660254037844387076, 1.000000000000000000, 0.8660254037844387076, 1.000000000000000000, 0.8660254037844387076, 1.000000000000000000, 0.8660254037844387076, 1.000000000000000000, 0.8660254037844387076, 1.000000000000000000, 0.8660254037844387076, 1.000000000000000000, 0.8660254037844387076, 1.000000000000000000, 0.8660254037844387076, 1.000000000000000000, 0.8660254037844387076, 1.000000000000000000, 0.8660254037844387076, 1.000000000000000000, 0.8660254037844387076, 1.000000000000000000, 0.8660254037844387076, 1.000000000000000000, 0.8660254037844387076, 1.000000000000000000, 0.8660254037844387076, 1.000000000000000000, 0.8660254037844387076, 1.000000000000000000, 0.8660254037844387076, 1.000000000000000000, 0.8660254037844387076, 1.000000000000000000, 0.8660254037844387076, 1.000000000000000000, 0.8660254037844387076, 1.000000000000000000, 0.8660254037844387076, 1.000000000000000000, 0.8660254037844387076, 1.000000000000000000, 0.8660254037844387076, 1.000000000000000000, 0.8660254037844387076, 1.000000000000000000, 0.8660254037844387076, 1.000000000000000000, 0.8660254037844387076, 1.000000000000000000, 0.8660254037844387076, 1.000000000000000000, 0.8660254037844387076, 1.000000000000000000, 0.8660254037844387076, 1.000000000000000000, 0.8660254037844387076, 1.000000000000000000, 0.8660254037844387076, 1.000000000000000000, 0.8660254037844387076, 1.000000000000000000, 0.8660254037844387076, 1.000000000000000000, 0.8660254037844387076, 1.000000000000000000, 0.8660254037844387076, 1.000000000000000000, 0.8660254037844387076, 1.000000000000000000, 0.8660254037844387076, 1.000000000000000000, 0.8660254037844387076, 1.000000000000000000, 0.8660254037844387076, 1.000000000000000000, 0.8660254037844387076, 1.000000000000000000, 0.8660254037844387076, 1.000000000000000000, 0.8660254037844387076, 1.000000000000000000, 0.8660254037844387076, 1.000000000000000000, 0.8660254037844387076, 1.000000000000000000, 0.8660254037844387076, 1.000000000000000000, 0.8660254037844387076, 1.000000000000000000, 0.8660254037844387076, 1.000000000000000000, 0.8660254037844387076, 1.000000000000000000, 0.8660254037844387076, 1.000000000000000000, 0.8660254037844387076, 1.000000000000000000, 0.8660254037844387076, 1.000000000000000000, 0.8660254037844387076, 1.000000000000000000, 0.8660254037844387076, 1.000000000000000000, 0.8660254037844387076, 1.000000000000000000, 0.8660254037844387076, 1.000000000000000000, 0.8660254037844387076, 1.000000000000000000, 0.8660254037844387076, 1.000000000000000000, 0.8660254037844387076, 1.000000000000000000, 0.8660254037844387076, 1.000000000000000000, 0.8660254037844387076, 1.000000000000000000, 0.8660254037844387076, 1.000000000000000000, 0.8660254037844387076, 1.000000000000000000, 0.8660254037844387076, 1.000000000000000000, 0.8660254037844387076, 1.000000000000000000, 0.8660254037844387076, 1.000000000000000000, 0.8660254037844387076, 1.000000000000000000, 0.8660254037844387076, 1.000000000000000000, 0.8660254037844387076, 1.000000000000000000, 0.8660254037844387076, 1.000000000000000000, 0.8660254037844387076, 1.000000000000000000, 0.8660254037844387076, 1.000000000000000000, 0.8660254037844387076, 1.000000000000000000, 0.8660254037844387076, 1.000000000000000000, 0.8660254037844387076, 1.000000000000000000, 0.8660254037844387076, 1.000000000000000000, 0.8660254037844387076, 1.000000000000000000, 0.8660254037844387076, 1.000000000000000000, 0.8660254037844387076, 1.000000000000000000, 0.8660254037844387076, 1.000000000000000000, 0.8660254037844387076, 1.000000000000000000, 0.8660254037844387076, 1.000000000000000000, 0.8660254037844387076, 1.000000000000000000, 0.8660254037844387076, 1.000000000000000000, 0.8660254037844387076, 1.000000000000000000, 0.8660254037844387076, 1.000000000000000000, 0.8660254037844387076, 1.000000000000000000, 0.8660254037844387076, 1.000000000000000000, 0.8660254037844387076, 1.000000000000000000, 0.8660254037844387076, 1.000000000000000000, 0.8660254037844387076, 1.000000000000000000, 0.8660254037844387076, 1.000000000000000000, 0.8660254037844387076, 1.000000000000000000, 0.8660254037844387076, 1.000000000000000000, 0.8660254037844387076, 1.000000000000000000, 0.8660254037844387076, 1.000000000000000000, 0.8660254037844387076, 1.000000000000000000, 0.8660254037844387076, 1.000000000000000000, 0.8660254037844387076, 1.000000000000000000),
 ( 1.000000000000000000, 0.8660254037844387076, 1.000000000000000000, 0.8660254037844387076, 1.000000000000000000, 0.8660254037844387076, 1.000000000000000000, 0.8660254037844387076, 1.000000000000000000, 0.8660254037844387076, 1.000000000000000000, 0.8660254037844387076, 1.000000000000000000, 0.8660254037844387076, 1.000000000000000000, 0.8660254037844387076, 1.000000000000000000, 0.8660254037844387076, 1.000000000000000000, 0.8660254037844387076, 1.000000000000000000, 0.8660254037844387076, 1.000000000000000000, 0.8660254037844387076, 1.000000000000000000, 0.8660254037844387076, 1.000000000000000000, 0.8660254037844387076, 1.000000000000000000, 0.8660254037844387076, 1.000000000000000000, 0.8660254037844387076, 1.000000000000000000, 0.8660254037844387076, 1.000000000000000000, 0.8660254037844387076, 1.000000000000000000, 0.8660254037844387076, 1.000000000000000000, 0.8660254037844387076, 1.000000000000000000, 0.8660254037844387076, 1.000000000000000000, 0.8660254037844387076, 1.000000000000000000, 0.8660254037844387076, 1.000000000000000000, 0.8660254037844387076, 1.000000000000000000, 0.8660254037844387076, 1.000000000000000000, 0.8660254037844387076, 1.000000000000000000, 0.8660254037844387076, 1.000000000000000000, 0.8660254037844387076, 1.000000000000000000, 0.8660254037844387076, 1.000000000000000000, 0.8660254037844387076, 1.000000000000000000, 0.8660254037844387076, 1.000000000000000000, 0.8660254037844387076, 1.000000000000000000, 0.8660254037844387076, 1.000000000000000000, 0.8660254037844387076, 1.000000000000000000, 0.8660254037844387076, 1.000000000000000000, 0.8660254037844387076, 1.000000000000000000, 0.8660254037844387076, 1.000000000000000000, 0.8660254037844387076, 1.000000000000000000, 0.8660254037844387076, 1.000000000000000000, 0.8660254037844387076, 1.000000000000000000, 0.8660254037844387076, 1.000000000000000000, 0.8660254037844387076, 1.000000000000000000, 0.8660254037844387076, 1.000000000000000000, 0.8660254037844387076, 1.000000000000000000, 0.8660254037844387076, 1.000000000000000000, 0.8660254037844387076, 1.000000000000000000, 0.8660254037844387076, 1.000000000000000000, 0.8660254037844387076, 1.000000000000000000, 0.8660254037844387076, 1.000000000000000000, 0.8660254037844387076, 1.000000000000000000, 0.8660254037844387076, 1.000000000000000000, 0.8660254037844387076, 1.000000000000000000, 0.8660254037844387076, 1.000000000000000000, 0.8660254037844387076, 1.000000000000000000, 0.8660254037844387076, 1.000000000000000000, 0.8660254037844387076, 1.000000000000000000, 0.8660254037844387076, 1.000000000000000000, 0.8660254037844387076, 1.000000000000000000, 0.8660254037844387076, 1.000000000000000000, 0.8660254037844387076, 1.000000000000000000, 0.8660254037844387076, 1.000000000000000000, 0.8660254037844387076, 1.000000000000000000, 0.8660254037844387076, 1.000000000000000000, 0.8660254037844387076, 1.000000000000000000, 0.8660254037844387076, 1.000000000000000000, 0.8660254037844387076, 1.000000000000000000, 0.8660254037844387076, 1.000000000000000000, 0.8660254037844387076, 1.000000000000000000, 0.8660254037844387076, 1.000000000000000000, 0.8660254037844387076, 1.000000000000000000, 0.8660254037844387076, 1.000000000000000000, 0.8660254037844387076, 1.000000000000000000, 0.8660254037844387076, 1.000000000000000000, 0.8660254037844387076, 1.000000000000000000, 0.8660254037844387076, 1.000000000000000000, 0.8660254037844387076, 1.000000000000000000, 0.8660254037844387076, 1.000000000000000000, 0.8660254037844387076, 1.000000000000000000, 0.8660254037844387076, 1.000000000000000000, 0.8660254037844387076, 1.000000000000000000, 0.8660254037844387076, 1.000000000000000000, 0.8660254037844387076, 1.000000000000000000, 0.8660254037844387076, 1.000000000000000000, 0.8660254037844387076, 1.000000000000000000, 0.8660254037844387076, 1.000000000000000000, 0.8660254037844387076, 1.000000000000000000, 0.8660254037844387076, 1.000000000000000000, 0.8660254037844387076, 1.000000000000000000, 0.8660254037844387076, 1.000000000000000000, 0.8660254037844387076, 1.000000000000000000, 0.8660254037844387076, 1.000000000000000000, 0.8660254037844387076, 1.000000000000000000, 0.8660254037844387076, 1.000000000000000000, 0.8660254037844387076, 1.000000000000000000, 0.8660254037844387076, 1.000000000000000000, 0.8660254037844387076, 1.000000000000000000, 0.8660254037844387076, 1.000000000000000000, 0.8660254037844387076, 1.000000000000000000, 0.8660254037844387076, 1.000000000000000000, 0.8660254037844387076, 1.000000000000000000, 0.8660254037844387076, 1.000000000000000000, 0.8660254037844387076, 1.000000000000000000, 0.8660254037844387076, 1.000000000000000000, 0.8660254037844387076, 1.000000000000000000, 0.8660254037844387076, 1.000000000000000000, 0.8660254037844387076, 1.000000000000000000, 0.8660254037844387076, 1.000000000000000000, 0.8660254037844387076, 1.000000000000000000, 0.8660254037844387076, 1.000000000000000000, 0.8660254037844387076, 1.000000000000000000, 0.8660254037844387076, 1.000000000000000000, 0.8660254037844387076, 1.000000000000000000, 0.8660254037844387076, 1.000000000000000000, 0.8660254037844387076, 1.000000000000000000, 0.8660254037844387076, 1.000000000000000000, 0.8660254037844387076, 1.000000000000000000, 0.8660254037844387076, 1.000000000000000000, 0.8660254037844387076, 1.000000000000000000, 0.8660254037844387076, 1.000000000000000000, 0.8660254037844387076, 1.000000000000000000, 0.8660254037844387076, 1.000000000000000000, 0.8660254037844387076, 1.000000000000000000, 0.8660254037844387076, 1.000000000000000000, 0.8660254037844387076, 1.000000000000000000, 0.8660254037844387076, 1.000000000000000000, 0.8660254037844387076, 1.000000000000000000, 0.8660254037844387076, 1.000000000000000000, 0.8660254037844387076, 1.000000000000000000, 0.8660254037844387076, 1.000000000000000000, 0.8660254037844387076, 1.000000000000000000, 0.8660254037844387076, 1.000000000000000000, 0.8660254037844387076, 1.000000000000000000, 0.8660254037844387076, 1.000000000000000000, 0.8660254037844387076, 1.000000000000000000, 0.8660254037844387076, 1.000000000000000000, 0.8660254037844387076, 1.000000000000000000, 0.8660254037844387076, 1.000000000000000000, 0.8660254037844387076, 1.000000000000000000, 0.8660254037844387076, 1.000000000000000000, 0.8660254037844387076, 1.000000000000000000, 0.8660254037844387076, 1.000000000000000000, 0.8660254037844387076, 1.000000000000000000, 0.8660254037844387076, 1.000000000000000000, 0.8660254037844387076, 1.000000000000000000, 0.8660254037844387076, 1.000000000000000000, 0.8660254037844387076, 1.000000000000000000, 0.8660254037844387076, 1.000000000000000000, 0.8660254037844387076, 1.000000000000000000, 0.8660254037844387076, 1.000000000000000000, 0.8660254037844387076, 1.000000000000000000, 0.8660254037844387076, 1.000000000000000000, 0.8660254037844387076, 1.000000000000000000, 0.8660254037844387076, 1.000000000000000000, 0.8660254037844387076, 1.000000000000000000, 0.8660254037844387076, 1.000000000000000000, 0.8660254037844387076, 1.000000000000000000, 0.8660254037844387076, 1.000000000000000000, 0.8660254037844387076, 1.000000000000000000, 0.8660254037844387076, 1.000000000000000000, 0.8660254037844387076, 1.000000000000000000, 0.8660254037844387076, 1.000000000000000000, 0.8660254037844387076, 1.000000000000000000, 0.8660254037844387076, 1.000000000000000000, 0.8660254037844387076, 1.000000000000000000, 0.8660254037844387076, 1.000000000000000000, 0.8660254037844387076, 1.000000000000000000, 0.8660254037844387076, 1.000000000000000000, 0.8660254037844387076, 1.000000000000000000, 0.8660254037844387076, 1.000000000000000000, 0.8660254037844387076, 1.000000000000000000, 0.8660254037844387076, 1.000000000000000000, 0.8660254037844387076, 1.000000000000000000, 0.8660254037844387076, 1.000000000000000000, 0.8660254037844387076, 1.000000000000000000, 0.8660254037844387076, 1.000000000000000000, 0.8660254037844387076, 1.000000000000000000, 0.8660254037844387076, 1.000000000000000000, 0.8660254037844387076, 1.000000000000000000, 0.8660254037844387076, 1.000000000000000000, 0.8660254037844387076, 1.000000000000000000, 0.8660254037844387076, 1.000000000000000000, 0.8660254037844387076, 1.000000000000000000, 0.8660254037844387076, 1.000000000000000000, 0.8660254037844387076, 1.000000000000000000, 0.8660254037844387076, 1.000000000000000000, 0.8660254037844387076, 1.000000000000000000, 0.8660254037844387076, 1.000000000000000000, 0.8660254037844387076, 1.000000000000000000, 0.8660254037844387076, 1.000000000000000000, 0.8660254037844387076, 1.000000000000000000, 0.8660254037844387076, 1.000000000000000000, 0.8660254037844387076, 1.000000000000000000, 0.8660254037844387076, 1.000000000000000000, 0.8660254037844387076, 1.000000000000000000, 0.8660254037844387076, 1.000000000000000000, 0.8660254037844387076, 1.000000000000000000, 0.8660254037844387076, 1.000000000000000000, 0.8660254037844387076, 1.000000000000000000, 0.8660254037844387076, 1.000000000000000000, 0.8660254037844387076, 1.000000000000000000, 0.8660254037844387076, 1.000000000000000000, 0.8660254037844387076, 1.000000000000000000, 0.8660254037844387076, 1.000000000000000000, 0.8660254037844387076, 1.000000000000000000, 0.8660254037844387076, 1.000000000000000000, 0.8660254037844387076, 1.000000000000000000, 0.8660254037844387076, 1.000000000000000000, 0.8660254037844387076, 1.000000000000000000, 0.8660254037844387076, 1.000000000000000000, 0.8660254037844387076, 1.000000000000000000, 0.8660254037844387076, 1.000000000000000000, 0.8660254037844387076, 1.000000000000000000, 0.8660254037844387076, 1.000000000000000000, 0.8660254037844387076, 1.000000000000000000, 0.8660254037844387076, 1.000000000000000000, 0.8660254037844387076, 1.000000000000000000, 0.8660254037844387076, 1.000000000000000000, 0.8660254037844387076, 1.000000000000000000, 0.8660254037844387076, 1.000000000000000000, 0.8660254037844387076, 1.000000000000000000, 0.8660254037844387076, 1.000000000000000000, 0.8660254037844387076, 1.000000000000000000, 0.8660254037844387076, 1.000000000000000000, 0.8660254037844387076, 1.000000000000000000, 0.8660254037844387076, 1.000000000000000000, 0.8660254037844387076, 1.000000000000000000, 0.8660254037844387076, 1.000000000000000000, 0.8660254037844387076, 1.000000000000000000, 0.8660254037844387076, 1.000000000000000000, 0.8660254037844387076, 1.000000000000000000, 0.8660254037844387076, 1.000000000000000000, 0.8660254037844387076, 1.000000000000000000, 0.8660254037844387076, 1.000000000000000000, 0.8660254037844387076, 1.000000000000000000, 0.8660254037844387076, 1.000000000000000000, 0.8660254037844387076, 1.000000000000000000, 0.8660254037844387076, 1.000000000000000000, 0.8660254037844387076, 1.000000000000000000, 0.8660254037844387076, 1.000000000000000000, 0.8660254037844387076, 1.000000000000000000, 0.8660254037844387076, 1.000000000000000000, 0.8660254037844387076, 1.000000000000000000, 0.8660254037844387076, 1.000000000000000000, 0.8660254037844387076, 1.000000000000000000, 0.8660254037844387076, 1.000000000000000000, 0.8660254037844387076, 1.000000000000000000, 0.8660254037844387076, 1.000000000000000000, 0.8660254037844387076, 1.000000000000000000, 0.8660254037844387076, 1.000000000000000000, 0.8660254037844387076, 1.000000000000000000, 0.8660254037844387076, 1.000000000000000000, 0.8660254037844387076, 1.000000000000000000, 0.8660254037844387076, 1.000000000000000000, 0.8660254037844387076, 1.000000000000000000, 0.8660254037844387076, 1.000000000000000000, 0.8660254037844387076, 1.000000000000000000, 0.8660254037844387076, 1.000000000000000000, 0.8660254037844387076, 1.000000000000000000, 0.8660254037844387076, 1.000000000000000000, 0.8660254037844387076, 1.000000000000000000, 0.8660254037844387076, 1.000000000000000000, 0.8660254037844387076, 1.000000000000000000, 0.8660254037844387076, 1.000000000000000000, 0.8660254037844387076, 1.000000000000000000, 0.8660254037844387076, 1.000000000000000000, 0.8660254037844387076, 1.000000000000000000, 0.8660254037844387076, 1.000000000000000000, 0.8660254037844387076, 1.000000000000000000, 0.8660254037844387076, 1.000000000000000000, 0.8660254037844387076, 1.000000000000000000, 0.8660254037844387076, 1.000000000000000000, 0.8660254037844387076, 1.000000000000000000, 0.8660254037844387076, 1.000000000000000000, 0.8660254037844387076, 1.000000000000000000, 0.8660254037844387076, 1.000000000000000000, 0.8660254037844387076, 1.000000000000000000, 0.8660254037844387076, 1.000000000000000000, 0.8660254037844387076, 1.000000000000000000, 0.8660254037844387076, 1.000000000000000000, 0.8660254037844387076, 1.000000000000000000, 0.8660254037844387076, 1.000000000000000000, 0.8660254037844387076, 1.000000000000000000, 0.8660254037844387076, 1.000000000000000000, 0.8660254037844387076, 1.000000000000000000, 0.8660254037844387076, 1.000000000000000000, 0.8660254037844387076, 1.000000000000000000, 0.8660254037844387076, 1.000000000000000000, 0.8660254037844387076, 1.000000000000000000, 0.8660254037844387076, 1.000000000000000000, 0.8660254037844387076, 1.000000000000000000, 0.8660254037844387076, 1.000000000000000000, 0.8660254037844387076, 1.000000000000000000, 0.8660254037844387076, 1.000000000000000000, 0.8660254037844387076, 1.000000000000000000, 0.8660254037844387076, 1.000000000000000000, 0.8660254037844387076, 1.000000000000000000, 0.8660254037844387076, 1.000000000000000000, 0.8660254037844387076, 1.000000000000000000, 0.8660254037844387076, 1.000000000000000000, 0.8660254037844387076, 1.000000000000000000, 0.8660254037844387076, 1.000000000000000000, 0.8660254037844387076, 1.000000000000000000, 0.8660254037844387076, 1.000000000000000000, 0.8660254037844387076, 1.000000000000000000, 0.8660254037844387076, 1.000000000000000000, 0.8660254037844387076, 1.000000000000000000, 0.8660254037844387076, 1.000000000000000000, 0.8660254037844387076, 1.000000000000000000, 0.8660254037844387076, 1.000000000000000000, 0.8660254037844387076, 1.000000000000000000, 0.8660254037844387076, 1.000000000000000000, 0.8660254037844387076, 1.000000000000000000, 0.8660254037844387076, 1.000000000000000000, 0.8660254037844387076, 1.000000000000000000, 0.8660254037844387076, 1.000000000000000000, 0.8660254037844387076, 1.000000000000000000, 0.8660254037844387076, 1.000000000000000000, 0.8660254037844387076, 1.000000000000000000, 0.8660254037844387076, 1.000000000000000000, 0.8660254037844387076, 1.000000000000000000, 0.8660254037844387076, 1.000000000000000000, 0.8660254037844387076, 1.000000000000000000, 0.8660254037844387076, 1.000000000000000000, 0.8660254037844387076, 1.000000000000000000, 0.8660254037844387076, 1.000000000000000000, 0.8660254037844387076, 1.000000000000000000, 0.8660254037844387076, 1.000000000000000000, 0.8660254037844387076, 1.000000000000000000, 0.8660254037844387076, 1.000000000000000000, 0.8660254037844387076, 1.000000000000000000, 0.8660254037844387076, 1.000000000000000000, 0.8660254037844387076, 1.000000000000000000, 0.8660254037844387076, 1.000000000000000000, 0.8660254037844387076, 1.000000000000000000, 0.8660254037844387076, 1.000000000000000000, 0.8660254037844387076, 1.000000000000000000, 0.8660254037844387076, 1.000000000000000000, 0.8660254037844387076, 1.000000000000000000, 0.8660254037844387076, 1.000000000000000000, 0.8660254037844387076, 1.000000000000000000, 0.8660254037844387076, 1.000000000000000000, 0.8660254037844387076, 1.000000000000000000, 0.8660254037844387076, 1.000000000000000000, 0.8660254037844387076, 1.000000000000000000, 0.8660254037844387076, 1.000000000000000000, 0.8660254037844387076, 1.000000000000000000, 0.8660254037844387076, 1.000000000000000000, 0.8660254037844387076, 1.000000000000000000, 0.8660254037844387076, 1.000000000000000000, 0.8660254037844387076, 1.000000000000000000, 0.8660254037844387076, 1.000000000000000000, 0.8660254037844387076, 1.000000000000000000, 0.8660254037844387076, 1.000000000000000000, 0.8660254037844387076, 1.000000000000000000, 0.8660254037844387076, 1.000000000000000000, 0.8660254037844387076, 1.000000000000000000, 0.8660254037844387076, 1.000000000000000000, 0.8660254037844387076, 1.000000000000000000, 0.8660254037844387076, 1.000000000000000000, 0.8660254037844387076, 1.000000000000000000) ) ) 
 REPRESENTATION_ITEM ( '' )  SURFACE ( )  );
#48015=CARTESIAN_POINT ( 'NONE',  ( 23.87812500061451715, 4.541064518000418104, 2.621784821874999949 ) ) ;
#48016=CARTESIAN_POINT ( 'NONE',  ( 18.87187500061451573, 3.027376345333613106, -5.243569643749998122 ) ) ;
#48017=CARTESIAN_POINT ( 'NONE',  ( 13.86562500061451431, 3.027376345333613106, -5.243569643749998122 ) ) ;
#48018=CARTESIAN_POINT ( 'NONE',  ( -3.000416591977282496E-16, 15.24687500061451928, 25.09994784771203058 ) ) ;
#48019=CARTESIAN_POINT ( 'NONE',  ( 19.67812500061451786, 6.421520780324663323E-16, -5.243569643749999010 ) ) ;
#48023=CARTESIAN_POINT ( 'NONE',  ( 23.06250000000000355, 2.886751345948129099, -4.999999999999998224 ) ) ;
#48024=CARTESIAN_POINT ( 'NONE',  ( -2.121784821874999949, 19.78437500061451715, -33.67503911421598417 ) ) ;
#48025=CARTESIAN_POINT ( 'NONE',  ( 3.749583905066019796, -3.307735353520828259, -3.782304699281895832 ) ) ;
#48026=CARTESIAN_POINT ( 'NONE',  ( 27.92812500061451431, 4.541064518000418104, 2.621784821874999949 ) ) ;
#48027=CARTESIAN_POINT ( 'NONE',  ( 8.653125000614515727, 0.000000000000000000, 5.243569643749999010 ) ) ;
#48028=CARTESIAN_POINT ( 'NONE',  ( 19.42500000122903714, -5.773502691896255534, -1.060575238724906372E-15 ) ) ;
#48029=CARTESIAN_POINT ( 'NONE',  ( 25.86562500061451431, -6.054752690667223547, -1.112240025338166033E-15 ) ) ;
#48030=CARTESIAN_POINT ( 'NONE',  ( 25.42500000000000071, 4.330127018922191873, 2.499999999999999556 ) ) ;
#48032=CARTESIAN_POINT ( 'NONE',  ( 28.94062500061452070, -3.027376345333614438, 5.243569643749998122 ) ) ;
#48033=CARTESIAN_POINT ( 'NONE',  ( 7.715625000614515727, 3.027376345333611329, 5.243569643749999010 ) ) ;
#48035=CARTESIAN_POINT ( 'NONE',  ( 22.94062500061451715, 6.054752690667223547, 3.707466751127219781E-16 ) ) ;
#48036=CARTESIAN_POINT ( 'NONE',  ( 6.478125000614516793, -4.541064518000419881, 2.621784821874995952 ) ) ;
#48038=CARTESIAN_POINT ( 'NONE',  ( 3.242103837493086330E-14, 13.13749999999999929, 26.00000000000000711 ) ) ;
#48039=CARTESIAN_POINT ( 'NONE',  ( -1.071796769724491005, 10.45759618943233527, -34.00000000000000000 ) ) ;
#48040=VECTOR ( 'NONE', #28030, 1000.000000000000000 ) ;
#48041=CARTESIAN_POINT ( 'NONE',  ( 13.53749999999999964, -2.886751345948125991, -5.000000000000000000 ) ) ;
#48042=CARTESIAN_POINT ( 'NONE',  ( 14.44687500061451679, 6.054752690667223547, 3.707466751127219781E-16 ) ) ;
#48043=CARTESIAN_POINT ( 'NONE',  ( 9.037500001229034297, -4.330127018922194537, 2.499999999999995559 ) ) ;
#48044=CARTESIAN_POINT ( 'NONE',  ( 15.57187500061451679, -6.054752690667223547, -1.112240025338166033E-15 ) ) ;
#48046=CARTESIAN_POINT ( 'NONE',  ( 9.159375000614515372, 0.000000000000000000, 5.243569643749999010 ) ) ;
#48047=CARTESIAN_POINT ( 'NONE',  ( -4.243569643749999898, 11.25312500061451892, -30.00000000000000000 ) ) ;
#48049=CARTESIAN_POINT ( 'NONE',  ( 12.79687500061451821, -3.027376345333614438, 5.243569643749998122 ) ) ;
#48050=ORIENTED_EDGE ( 'NONE', *, *, #2473, .T. ) ;
#48051=CARTESIAN_POINT ( 'NONE',  ( 21.10312500061451502, 4.541064518000418104, -2.621784821874998173 ) ) ;
#48052=CARTESIAN_POINT ( 'NONE',  ( 2.121784821874999061, 11.15937500061451715, 26.32496088578401583 ) ) ;
#48054=CARTESIAN_POINT ( 'NONE',  ( 25.77187500061451075, 3.027376345333611329, 5.243569643749999010 ) ) ;
#48055=CARTESIAN_POINT ( 'NONE',  ( 5.390625000614518214, 6.054752690667223547, 3.707466751127219781E-16 ) ) ;
#48057=CARTESIAN_POINT ( 'NONE',  ( 16.43437500061451573, -4.541064518000419881, 2.621784821874995952 ) ) ;
#48059=CARTESIAN_POINT ( 'NONE',  ( 27.30000000122903359, 5.773502691896255534, 3.535250795749688894E-16 ) ) ;
#48060=CARTESIAN_POINT ( 'NONE',  ( 6.684375000614518392, 6.421520780324663323E-16, -5.243569643749999010 ) ) ;
#48061=CARTESIAN_POINT ( 'NONE',  ( 16.69687500061451502, 6.054752690667223547, 3.707466751127219781E-16 ) ) ;
#48063=CARTESIAN_POINT ( 'NONE',  ( 24.33749999999999858, -2.886751345948125991, -5.000000000000000000 ) ) ;
#48064=CARTESIAN_POINT ( 'NONE',  ( 26.33437500061451431, -4.541064518000419881, 2.621784821874995952 ) ) ;
#48065=DIRECTION ( 'NONE',  ( -1.000000000000000000, -0.000000000000000000, -0.000000000000000000 ) ) ;
#48066=CARTESIAN_POINT ( 'NONE',  ( 8.324999999999999289, 4.330127018922191873, 2.499999999999999556 ) ) ;
#48068=CARTESIAN_POINT ( 'NONE',  ( 21.66562500061451502, 3.027376345333611329, 5.243569643749999010 ) ) ;
#48069=CARTESIAN_POINT ( 'NONE',  ( 10.72500000000000142, -4.330127018922194537, 2.499999999999995559 ) ) ;
#48070=CARTESIAN_POINT ( 'NONE',  ( 6.778125000614518392, 4.541064518000418104, 2.621784821874999949 ) ) ;
#48071=CARTESIAN_POINT ( 'NONE',  ( 19.01249999999999929, 2.886751345948129099, -4.999999999999998224 ) ) ;
#48072=CARTESIAN_POINT ( 'NONE',  ( 18.96562500061451573, 3.027376345333611329, 5.243569643749999010 ) ) ;
#48073=CARTESIAN_POINT ( 'NONE',  ( 12.07499999999999929, -4.330127018922194537, 2.499999999999995559 ) ) ;
#48074=CARTESIAN_POINT ( 'NONE',  ( 23.73750000122903359, 4.330127018922191873, 2.499999999999999556 ) ) ;
#48076=CARTESIAN_POINT ( 'NONE',  ( 4.349999999999999645, 0.000000000000000000, 4.999999999999998224 ) ) ;
#48077=ORIENTED_EDGE ( 'NONE', *, *, #61414, .F. ) ;
#48078=CARTESIAN_POINT ( 'NONE',  ( 19.90312500061451573, 0.000000000000000000, 5.243569643749999010 ) ) ;
#48079=CARTESIAN_POINT ( 'NONE',  ( 26.50312500061451360, 4.541064518000418104, -2.621784821874998173 ) ) ;
#48080=CARTESIAN_POINT ( 'NONE',  ( 24.87187500061451573, 3.027376345333611329, 5.243569643749999010 ) ) ;
#48081=EDGE_CURVE ( 'NONE', #1783, #48298, #35935, .T. ) ;
#48082=CARTESIAN_POINT ( 'NONE',  ( 9.899999999999998579, -4.330127018922190985, -2.500000000000001332 ) ) ;
#48084=CARTESIAN_POINT ( 'NONE',  ( 12.02812500061451573, 6.421520780324663323E-16, -5.243569643749999010 ) ) ;
#48085=CARTESIAN_POINT ( 'NONE',  ( 26.80312500061451431, -4.541064518000417216, -2.621784821875001281 ) ) ;
#48086=CARTESIAN_POINT ( 'NONE',  ( 16.05937500061451573, -4.541064518000417216, -2.621784821875001281 ) ) ;
#48087=CARTESIAN_POINT ( 'NONE',  ( 9.778125000614517504, 6.421520780324663323E-16, -5.243569643749999010 ) ) ;
#48089=CARTESIAN_POINT ( 'NONE',  ( 2.121784821874999061, 11.60937500061451821, 26.32496088578401583 ) ) ;
#48091=CARTESIAN_POINT ( 'NONE',  ( 23.73750000122903359, 4.330127018922191873, 2.499999999999999556 ) ) ;
#48093=CARTESIAN_POINT ( 'NONE',  ( 14.69062500061451537, -3.027376345333610441, -5.243569643749999898 ) ) ;
#48094=CARTESIAN_POINT ( 'NONE',  ( 11.14687500061451608, -3.027376345333610441, -5.243569643749999898 ) ) ;
#48095=CARTESIAN_POINT ( 'NONE',  ( 9.159375000614515372, 0.000000000000000000, 5.243569643749999010 ) ) ;
#48097=CARTESIAN_POINT ( 'NONE',  ( -3.968938398713111937, 9.180052406904112061, 34.50384684723260875 ) ) ;
#48098=CARTESIAN_POINT ( 'NONE',  ( 21.62812500061451360, 4.541064518000418104, 2.621784821874999949 ) ) ;
#48099=CARTESIAN_POINT ( 'NONE',  ( 17.10937500061451999, 4.541064518000418104, -2.621784821874998173 ) ) ;
#48100=CARTESIAN_POINT ( 'NONE',  ( 23.05312500061451431, 0.000000000000000000, 5.243569643749999010 ) ) ;
#48101=CARTESIAN_POINT ( 'NONE',  ( -3.999999999999999112, 11.45000000000000107, 30.00000000000000000 ) ) ;
#48102=CARTESIAN_POINT ( 'NONE',  ( 28.04062500061451502, -3.027376345333614438, 5.243569643749998122 ) ) ;
#48103=CARTESIAN_POINT ( 'NONE',  ( 7.912500001229033408, 4.330127018922192761, -2.499999999999997780 ) ) ;
#48104=VERTEX_POINT ( 'NONE', #5321 ) ;
#48105=CARTESIAN_POINT ( 'NONE',  ( 29.81250000000000000, 2.886751345948129099, -4.999999999999998224 ) ) ;
#48106=CARTESIAN_POINT ( 'NONE',  ( 3.999999999999998668, 18.46249999999999858, -32.30940107675850470 ) ) ;
#48107=CARTESIAN_POINT ( 'NONE',  ( 23.96250000122903145, -4.330127018922190985, -2.500000000000001332 ) ) ;
#48109=CARTESIAN_POINT ( 'NONE',  ( 6.571875000614517681, -6.054752690667223547, -1.112240025338166033E-15 ) ) ;
#48110=DIRECTION ( 'NONE',  ( -0.000000000000000000, -1.000000000000000000, -0.000000000000000000 ) ) ;
#48111=CARTESIAN_POINT ( 'NONE',  ( 14.35312500061451679, 4.541064518000418104, -2.621784821874998173 ) ) ;
#48112=CARTESIAN_POINT ( 'NONE',  ( 8.034375000614518925, 6.421520780324663323E-16, -5.243569643749999010 ) ) ;
#48113=CARTESIAN_POINT ( 'NONE',  ( 26.36250000122903003, 4.330127018922192761, -2.499999999999997780 ) ) ;
#48114=CARTESIAN_POINT ( 'NONE',  ( 16.58437500061451786, 6.421520780324663323E-16, -5.243569643749999010 ) ) ;
#48115=CARTESIAN_POINT ( 'NONE',  ( 5.596875000614516260, -3.027376345333614438, 5.243569643749998122 ) ) ;
#48116=CARTESIAN_POINT ( 'NONE',  ( 1.071796769724497445, 16.37990381179669797, 26.00000000000000355 ) ) ;
#48117=CARTESIAN_POINT ( 'NONE',  ( 4.678125000614516971, -4.541064518000419881, 2.621784821874995952 ) ) ;
#48118=CARTESIAN_POINT ( 'NONE',  ( 14.24062500061451608, -3.027376345333610441, -5.243569643749999898 ) ) ;
#48119=ORIENTED_EDGE ( 'NONE', *, *, #18934, .T. ) ;
#48120=CARTESIAN_POINT ( 'NONE',  ( 12.02812500061451573, 6.421520780324663323E-16, -5.243569643749999010 ) ) ;
#48121=CARTESIAN_POINT ( 'NONE',  ( 5.400000001229032343, -2.886751345948129988, 4.999999999999997335 ) ) ;
#48122=CARTESIAN_POINT ( 'NONE',  ( 10.90312500061451928, 0.000000000000000000, 5.243569643749999010 ) ) ;
#48124=CARTESIAN_POINT ( 'NONE',  ( 10.57500000000000107, 4.330127018922191873, 2.499999999999999556 ) ) ;
#48125=CARTESIAN_POINT ( 'NONE',  ( 4.912500001229034297, 0.000000000000000000, 4.999999999999998224 ) ) ;
#48126=CARTESIAN_POINT ( 'NONE',  ( 20.77500000000000213, 6.123233995736764310E-16, -4.999999999999998224 ) ) ;
#48127=CARTESIAN_POINT ( 'NONE',  ( 15.38437500061451679, 4.541064518000418104, 2.621784821874999949 ) ) ;
#48128=CARTESIAN_POINT ( 'NONE',  ( 15.26250000122903216, 0.000000000000000000, 4.999999999999998224 ) ) ;
#48130=CARTESIAN_POINT ( 'NONE',  ( 2.121784821875001281, 18.15312500061451928, -26.32496088578401938 ) ) ;
#48131=CARTESIAN_POINT ( 'NONE',  ( 0.000000000000000000, 20.00000000000000000, 26.00000000000000000 ) ) ;
#48133=CARTESIAN_POINT ( 'NONE',  ( 28.82812500061451644, 4.541064518000418104, 2.621784821874999949 ) ) ;
#48134=CARTESIAN_POINT ( 'NONE',  ( -5.810221930991193690E-16, 14.60000000122903252, 26.00000000000000355 ) ) ;
#48135=CARTESIAN_POINT ( 'NONE',  ( 16.09687500061452070, -3.027376345333610441, -5.243569643749999898 ) ) ;
#48138=CARTESIAN_POINT ( 'NONE',  ( 11.61562500061451608, 3.027376345333613106, -5.243569643749998122 ) ) ;
#48140=CARTESIAN_POINT ( 'NONE',  ( 24.38437500061451502, 4.541064518000418104, 2.621784821874999949 ) ) ;
#48142=CARTESIAN_POINT ( 'NONE',  ( 9.065625000614517148, 3.027376345333611329, 5.243569643749999010 ) ) ;
#48143=CARTESIAN_POINT ( 'NONE',  ( 14.14687500061451786, -3.027376345333614438, 5.243569643749998122 ) ) ;
#48144=VERTEX_POINT ( 'NONE', #72552 ) ;
#48145=CARTESIAN_POINT ( 'NONE',  ( 24.15937500061451715, -4.541064518000417216, -2.621784821875001281 ) ) ;
#48146=CARTESIAN_POINT ( 'NONE',  ( 28.45312500061451289, 0.000000000000000000, 5.243569643749999010 ) ) ;
#48147=CARTESIAN_POINT ( 'NONE',  ( 2.000000000000001332, 12.61250000122903536, -26.53589838486224650 ) ) ;
#48148=CARTESIAN_POINT ( 'NONE',  ( 6.299999999999999822, -4.330127018922190985, -2.500000000000001332 ) ) ;
#48149=CARTESIAN_POINT ( 'NONE',  ( 16.76250000122903216, -4.330127018922190985, -2.500000000000001332 ) ) ;
#48152=CARTESIAN_POINT ( 'NONE',  ( 14.36249999999999893, -5.773502691896255534, -1.060575238724906372E-15 ) ) ;
#48153=( BOUNDED_CURVE ( )  B_SPLINE_CURVE ( 2, ( #17001, #44388, #56183, #67634, #61711, #10020, #396 ),
 .UNSPECIFIED., .F., .F. ) 
 B_SPLINE_CURVE_WITH_KNOTS ( ( 3, 2, 2, 3 ),
 ( 0.3916666666666667740, 0.3944444444444444864, 0.3972222222222221433, 0.3999999999999999112 ),
 .UNSPECIFIED. ) 
 CURVE ( )  GEOMETRIC_REPRESENTATION_ITEM ( )  RATIONAL_B_SPLINE_CURVE ( ( 0.9999999999999946709, 0.8660254037844440367, 1.000000000000000000, 0.8660254037844387076, 1.000000000000000000, 0.8660254037844440367, 0.9999999999999946709 ) ) 
 REPRESENTATION_ITEM ( '' )  );
#48154=CARTESIAN_POINT ( 'NONE',  ( 19.61249999999999716, 2.886751345948126879, 4.999999999999999112 ) ) ;
#48155=CARTESIAN_POINT ( 'NONE',  ( 13.79062500061451502, -3.027376345333610441, -5.243569643749999898 ) ) ;
#48157=DIRECTION ( 'NONE',  ( -0.000000000000000000, -1.000000000000000000, -0.000000000000000000 ) ) ;
#48158=CARTESIAN_POINT ( 'NONE',  ( -4.243569643749999898, 15.80937500061451573, -30.00000000000000000 ) ) ;
#48159=CARTESIAN_POINT ( 'NONE',  ( 5.278125000614516615, 6.421520780324663323E-16, -5.243569643749999010 ) ) ;
#48161=CARTESIAN_POINT ( 'NONE',  ( 12.22499999999999964, 6.123233995736764310E-16, -4.999999999999998224 ) ) ;
#48164=CARTESIAN_POINT ( 'NONE',  ( 2.121784821874999061, 16.05312500061451786, 26.32496088578401583 ) ) ;
#48165=CARTESIAN_POINT ( 'NONE',  ( 27.62812500061451360, -4.541064518000419881, 2.621784821874995952 ) ) ;
#48168=CARTESIAN_POINT ( 'NONE',  ( 22.92187500061451644, 3.027376345333613106, -5.243569643749998122 ) ) ;
#48169=ADVANCED_FACE ( 'NONE', ( #28575 ), #39674, .F. ) ;
#48170=CARTESIAN_POINT ( 'NONE',  ( 19.79062500061451502, 6.054752690667223547, 3.707466751127219781E-16 ) ) ;
#48171=CARTESIAN_POINT ( 'NONE',  ( -3.000416591977282496E-16, 13.39062500061459460, -34.90005215228797653 ) ) ;
#48172=CARTESIAN_POINT ( 'NONE',  ( 23.70000000122903216, 5.773502691896255534, 3.535250795749688894E-16 ) ) ;
#48173=CARTESIAN_POINT ( 'NONE',  ( 2.990625000614519191, -3.027376345333610441, -5.243569643749999898 ) ) ;
#48175=CARTESIAN_POINT ( 'NONE',  ( 22.37812500061451360, 6.421520780324663323E-16, -5.243569643749999010 ) ) ;
#48178=CARTESIAN_POINT ( 'NONE',  ( 17.25937500061451502, 0.000000000000000000, 5.243569643749999010 ) ) ;
#48179=CARTESIAN_POINT ( 'NONE',  ( 15.87187500061451573, 3.027376345333611329, 5.243569643749999010 ) ) ;
#48180=CARTESIAN_POINT ( 'NONE',  ( 23.78437500061451360, 6.421520780324663323E-16, -5.243569643749999010 ) ) ;
#48181=CARTESIAN_POINT ( 'NONE',  ( 4.243569643749999010, 13.37187500061451750, 27.54997392385601174 ) ) ;
#48182=CARTESIAN_POINT ( 'NONE',  ( 4.603125000614518569, 0.000000000000000000, 5.243569643749999010 ) ) ;
#48183=CARTESIAN_POINT ( 'NONE',  ( 28.60312500061451502, -4.541064518000417216, -2.621784821875001281 ) ) ;
#48184=CARTESIAN_POINT ( 'NONE',  ( 28.49062500061451431, -3.027376345333614438, 5.243569643749998122 ) ) ;
#48186=LINE ( 'NONE', #57164, #20560 ) ;
#48187=CARTESIAN_POINT ( 'NONE',  ( 3.328125000614516438, -4.541064518000419881, 2.621784821874995952 ) ) ;
#48188=CARTESIAN_POINT ( 'NONE',  ( 8.296875000614516438, -3.027376345333614438, 5.243569643749998122 ) ) ;
#48189=CARTESIAN_POINT ( 'NONE',  ( 13.61250000122903359, -4.330127018922190985, -2.500000000000001332 ) ) ;
#48190=CARTESIAN_POINT ( 'NONE',  ( 29.42812500061451431, -4.541064518000419881, 2.621784821874995952 ) ) ;
#48191=CARTESIAN_POINT ( 'NONE',  ( 11.28750000122903252, -4.330127018922194537, 2.499999999999995559 ) ) ;
#48192=CARTESIAN_POINT ( 'NONE',  ( 4.003125000614518925, 4.541064518000418104, -2.621784821874998173 ) ) ;
#48195=CARTESIAN_POINT ( 'NONE',  ( 15.12187500061451750, -6.054752690667223547, -1.112240025338166033E-15 ) ) ;
#48197=ORIENTED_EDGE ( 'NONE', *, *, #52646, .T. ) ;
#48198=CARTESIAN_POINT ( 'NONE',  ( 21.81562500061451004, -6.054752690667223547, -1.112240025338166033E-15 ) ) ;
#48199=CARTESIAN_POINT ( 'NONE',  ( 7.265625000614516438, 3.027376345333611329, 5.243569643749999010 ) ) ;
#48201=CARTESIAN_POINT ( 'NONE',  ( 23.85937500061451644, 4.541064518000418104, -2.621784821874998173 ) ) ;
#48202=CARTESIAN_POINT ( 'NONE',  ( 6.928125000614516082, -4.541064518000419881, 2.621784821874995952 ) ) ;
#48203=CARTESIAN_POINT ( 'NONE',  ( 3.487500001229035362, 4.330127018922191873, 2.499999999999999556 ) ) ;
#48204=CARTESIAN_POINT ( 'NONE',  ( 8.325000001229033941, 2.886751345948129099, -4.999999999999998224 ) ) ;
#48205=CARTESIAN_POINT ( 'NONE',  ( 22.94062500061451715, 6.054752690667223547, 3.707466751127219781E-16 ) ) ;
#48206=CARTESIAN_POINT ( 'NONE',  ( 4.243569643749999898, 11.47812500061451679, -30.00000000000000000 ) ) ;
#48207=CARTESIAN_POINT ( 'NONE',  ( 10.95000000122903394, -2.886751345948125991, -5.000000000000000000 ) ) ;
#48208=CARTESIAN_POINT ( 'NONE',  ( 19.90312500061451573, 0.000000000000000000, 5.243569643749999010 ) ) ;
#48209=CARTESIAN_POINT ( 'NONE',  ( 17.09062500061451573, 6.054752690667223547, 3.707466751127219781E-16 ) ) ;
#48211=CARTESIAN_POINT ( 'NONE',  ( 17.84999999999999787, 0.000000000000000000, 4.999999999999998224 ) ) ;
#48212=CARTESIAN_POINT ( 'NONE',  ( 14.96250000122903323, -4.330127018922190985, -2.500000000000001332 ) ) ;
#48214=CARTESIAN_POINT ( 'NONE',  ( 9.553125000614517859, 0.000000000000000000, 5.243569643749999010 ) ) ;
#48215=CARTESIAN_POINT ( 'NONE',  ( 14.35312500061451679, 4.541064518000418104, -2.621784821874998173 ) ) ;
#48216=CARTESIAN_POINT ( 'NONE',  ( 24.00000000122902932, -2.886751345948125991, -5.000000000000000000 ) ) ;
#48217=CARTESIAN_POINT ( 'NONE',  ( 21.30937500061451573, 0.000000000000000000, 5.243569643749999010 ) ) ;
#48218=CARTESIAN_POINT ( 'NONE',  ( 21.64687500061451786, 6.054752690667223547, 3.707466751127219781E-16 ) ) ;
#48220=CARTESIAN_POINT ( 'NONE',  ( 7.500000001229034652, 5.773502691896255534, 3.535250795749688894E-16 ) ) ;
#48221=CARTESIAN_POINT ( 'NONE',  ( 6.796875000614516438, 6.054752690667223547, 3.707466751127219781E-16 ) ) ;
#48222=CARTESIAN_POINT ( 'NONE',  ( 22.77187500061451786, -6.054752690667223547, -1.112240025338166033E-15 ) ) ;
#48223=( BOUNDED_SURFACE ( )  B_SPLINE_SURFACE ( 1, 2, ( 
 ( #35551, #63986, #17469, #23377, #46648, #12294, #69188, #34829, #56992, #23014, #58070, #7480, #30008, #52551, #1957, #47012, #69547, #18906, #34102, #56641, #68103, #40029, #6399, #28931, #51467, #870, #25565, #53271, #47371, #54380, #36286, #13368, #20374, #3414, #42557, #13744, #47729, #7845, #58435, #71368, #25934, #48106, #30382, #65449, #19268, #48474, #26300, #59166, #42925, #43300, #69902, #2669, #37009, #25186, #31102, #70268, #58800, #2309, #14841, #19639, #53642, #70629, #65084, #3775, #36644, #48837, #3034, #20004, #8944, #42196, #20743, #14475, #70998, #35910, #59532, #64720, #37381, #30739, #52911, #31475, #54018, #59905, #9310, #31844, #24824, #41822, #64354, #8210, #14104, #8574, #4144, #27404, #21112, #22213, #27042, #55476, #66554, #72830, #10041, #61007, #4513, #38856, #28133, #61371, #10768, #54742, #55839, #66187, #32208, #38483, #5226, #65, #49573, #72459, #4868, #72095, #60629, #10406, #32575, #44407, #21844, #60261, #32938, #66933, #21479, #16302, #33301, #27768, #15934, #50308, #9675, #38108, #5596, #44032, #49934, #44767, #37741, #49208, #67302, #55113, #16660, #39218, #61730, #11131, #33658, #15565, #56203, #50661, #22571, #65821, #15203, #26676, #71742, #43665, #11496, #40296, #62818, #12210, #40658, #6312, #52465, #34739, #29566, #35465, #57268, #11855, #57631, #62457, #29925, #63179, #12573, #6680, #35107, #52103, #51744, #39579, #7037, #34018, #22924, #56907, #56555, #29208, #415, #1508, #28841, #1143, #45839, #24012, #34374, #23654, #51380, #18097, #7397, #46561, #69103, #5949, #18465, #45482, #28482, #17737, #41028, #1872, #782, #46198, #68739, #23291, #39944, #63544, #68376, #12930, #57987, #62102, #45119, #67654, #17020, #51019, #68014, #17386, #47646, #31019, #18822, #69819, #37296, #58715, #19555, #2583, #69464, #7758, #8486, #13654, #53553, #14390, #36197, #70178, #64266, #24741, #25478, #30654, #36927, #3326, #25852, #46926, #65002, #42113, #63897, #64636, #58347, #65363, #47285, #24378, #31392, #59448, #2950, #19185, #8127, #41385, #13287, #9224, #8855, #59082, #35824, #48389, #30294, #53931, #59819, #14022, #70917, #54298, #52826 ),
 ( #53186, #36562, #48024, #70550, #14753, #19925, #31761, #42479, #20288, #2228, #41738, #42842, #25102, #66099, #43578, #9950, #15477, #4426, #65734, #60179, #38021, #37656, #48754, #60544, #43944, #49123, #21025, #20655, #4057, #26954, #32487, #55022, #49481, #26583, #71652, #3690, #71278, #54654, #26215, #43214, #21388, #72013, #15119, #9588, #32120, #54072, #26728, #10099, #36698, #42614, #3833, #65138, #71054, #14529, #3092, #42250, #9727, #37063, #20429, #14896, #31898, #43718, #3468, #66241, #42978, #65509, #48893, #59588, #60684, #37437, #37797, #15619, #59958, #20058, #65878, #70683, #38161, #71423, #20800, #9365, #43355, #60317, #54434, #47791, #15259, #19697, #31157, #9000, #64774, #26354, #8628, #32261, #31532, #54793, #25988, #4200, #48527, #49263, #71796, #21165, #53329, #2727, #25242, #14164, #70321, #53699, #59220, #25621, #48158, #40993, #44459, #39272, #44819, #16352, #27459, #27827, #49990, #11188, #61784, #27094, #72886, #33715, #38907, #56260, #5651, #118, #55892, #28186, #49626, #4924, #46526, #66990, #50359, #10819, #51074, #1472, #67354, #50715, #22623, #44087, #23978, #6004, #72153, #67705, #61426, #5281, #69068, #33354, #16717, #72514, #21532, #18427, #32990, #63509, #66614, #22267, #45174, #17077, #39638, #32628, #21903, #55168, #62156, #11553, #34069, #56609, #28539, #4564, #15990, #38539, #61063, #10460, #55530, #42803, #19149, #58679, #36161, #53149, #70140, #42442, #2548, #25067, #7361, #13251, #31354, #2191, #64598, #19518, #47985, #42076, #14355, #63861, #52790, #8448, #7723, #29890, #13985, #20251, #47610, #36524, #46891, #8089, #36890, #59044, #64964, #30984, #30619, #53517, #35429, #52429, #69782, #70877, #12896, #70513, #41351, #2911, #24705, #25442, #57953, #41703, #59409, #19889, #8817, #53895, #3286, #47249, #64227, #13616, #25814, #18786, #48352, #1835, #35789, #24343, #69429, #58312, #30257, #44278, #72707, #32085, #65325, #38353, #59780, #54986, #27643, #15083, #66433, #61252, #4392, #10646, #60507, #54616, #31721, #21719, #71980, #21353, #55353, #71616, #37985, #49088, #22090, #16181, #43542, #26921, #4022, #54257, #55714, #65696, #5109 ) ),
 .UNSPECIFIED., .F., .F., .F. ) 
 B_SPLINE_SURFACE_WITH_KNOTS ( ( 2, 2 ),
 ( 3, 2, 2, 2, 2, 2, 2, 2, 2, 2, 2, 2, 2, 2, 2, 2, 2, 2, 2, 2, 2, 2, 2, 2, 2, 2, 2, 2, 2, 2, 2, 2, 2, 2, 2, 2, 2, 2, 2, 2, 2, 2, 2, 2, 2, 2, 2, 2, 2, 2, 2, 2, 2, 2, 2, 2, 2, 2, 2, 2, 2, 2, 2, 2, 2, 2, 2, 2, 2, 2, 2, 2, 2, 2, 2, 2, 2, 2, 2, 2, 2, 2, 2, 2, 2, 2, 2, 2, 2, 2, 2, 2, 2, 2, 2, 2, 2, 2, 2, 2, 2, 2, 2, 2, 2, 2, 2, 2, 2, 2, 2, 2, 2, 2, 2, 2, 2, 2, 2, 2, 2, 2, 2, 2, 2, 2, 2, 2, 2, 2, 2, 2, 2, 2, 3 ),
 ( 0.000000000000000000, 1.000000000000000000 ),
 ( 0.000000000000000000, 0.007246376811594202987, 0.01449275362318840597, 0.02173913043478260809, 0.02898550724637681195, 0.03623188405797101580, 0.04347826086956521618, 0.05072463768115942351, 0.05797101449275362389, 0.06521739130434782428, 0.07246376811594203160, 0.07971014492753622505, 0.08695652173913043237, 0.09420289855072463969, 0.1014492753623188470, 0.1086956521739130405, 0.1159420289855072478, 0.1231884057971014551, 0.1304347826086956486, 0.1376811594202898559, 0.1449275362318840632, 0.1521739130434782705, 0.1594202898550724501, 0.1666666666666666574, 0.1739130434782608647, 0.1811594202898550721, 0.1884057971014492794, 0.1956521739130434867, 0.2028985507246376940, 0.2101449275362318736, 0.2173913043478260809, 0.2246376811594202882, 0.2318840579710144956, 0.2391304347826087029, 0.2463768115942029102, 0.2536231884057971175, 0.2608695652173912971, 0.2681159420289855322, 0.2753623188405797118, 0.2826086956521738913, 0.2898550724637681264, 0.2971014492753623060, 0.3043478260869565410, 0.3115942028985507206, 0.3188405797101449002, 0.3260869565217391353, 0.3333333333333333148, 0.3405797101449275499, 0.3478260869565217295, 0.3550724637681159646, 0.3623188405797101441, 0.3695652173913043237, 0.3768115942028985588, 0.3840579710144927383, 0.3913043478260869734, 0.3985507246376811530, 0.4057971014492753881, 0.4130434782608695676, 0.4202898550724637472, 0.4275362318840579823, 0.4347826086956521618, 0.4420289855072463969, 0.4492753623188405765, 0.4565217391304347561, 0.4637681159420289911, 0.4710144927536231707, 0.4782608695652174058, 0.4855072463768115854, 0.4927536231884058204, 0.5000000000000000000, 0.5072463768115942351, 0.5144927536231883591, 0.5217391304347825942, 0.5289855072463768293, 0.5362318840579710644, 0.5434782608695651884, 0.5507246376811594235, 0.5579710144927536586, 0.5652173913043477826, 0.5724637681159420177, 0.5797101449275362528, 0.5869565217391304879, 0.5942028985507246119, 0.6014492753623188470, 0.6086956521739130821, 0.6159420289855072062, 0.6231884057971014412, 0.6304347826086956763, 0.6376811594202898004, 0.6449275362318840354, 0.6521739130434782705, 0.6594202898550725056, 0.6666666666666666297, 0.6739130434782608647, 0.6811594202898550998, 0.6884057971014492239, 0.6956521739130434590, 0.7028985507246376940, 0.7101449275362319291, 0.7173913043478260532, 0.7246376811594202882, 0.7318840579710145233, 0.7391304347826086474, 0.7463768115942028825, 0.7536231884057971175, 0.7608695652173913526, 0.7681159420289854767, 0.7753623188405797118, 0.7826086956521739468, 0.7898550724637680709, 0.7971014492753623060, 0.8043478260869565410, 0.8115942028985507761, 0.8188405797101449002, 0.8260869565217391353, 0.8333333333333333703, 0.8405797101449274944, 0.8478260869565217295, 0.8550724637681159646, 0.8623188405797101996, 0.8695652173913043237, 0.8768115942028985588, 0.8840579710144927938, 0.8913043478260869179, 0.8985507246376811530, 0.9057971014492753881, 0.9130434782608695121, 0.9202898550724637472, 0.9275362318840579823, 0.9347826086956522174, 0.9420289855072463414, 0.9492753623188405765, 0.9565217391304348116, 0.9637681159420289356, 0.9662083017040261623 ),
 .UNSPECIFIED. ) 
 GEOMETRIC_REPRESENTATION_ITEM ( )  RATIONAL_B_SPLINE_SURFACE ( (
 ( 1.000000000000000000, 0.8660254037844387076, 1.000000000000000000, 0.8660254037844387076, 1.000000000000000000, 0.8660254037844387076, 1.000000000000000000, 0.8660254037844387076, 1.000000000000000000, 0.8660254037844387076, 1.000000000000000000, 0.8660254037844387076, 1.000000000000000000, 0.8660254037844387076, 1.000000000000000000, 0.8660254037844387076, 1.000000000000000000, 0.8660254037844387076, 1.000000000000000000, 0.8660254037844387076, 1.000000000000000000, 0.8660254037844387076, 1.000000000000000000, 0.8660254037844387076, 1.000000000000000000, 0.8660254037844387076, 1.000000000000000000, 0.8660254037844387076, 1.000000000000000000, 0.8660254037844387076, 1.000000000000000000, 0.8660254037844387076, 1.000000000000000000, 0.8660254037844387076, 1.000000000000000000, 0.8660254037844387076, 1.000000000000000000, 0.8660254037844387076, 1.000000000000000000, 0.8660254037844387076, 1.000000000000000000, 0.8660254037844387076, 1.000000000000000000, 0.8660254037844387076, 1.000000000000000000, 0.8660254037844387076, 1.000000000000000000, 0.8660254037844387076, 1.000000000000000000, 0.8660254037844387076, 1.000000000000000000, 0.8660254037844387076, 1.000000000000000000, 0.8660254037844387076, 1.000000000000000000, 0.8660254037844387076, 1.000000000000000000, 0.8660254037844387076, 1.000000000000000000, 0.8660254037844387076, 1.000000000000000000, 0.8660254037844387076, 1.000000000000000000, 0.8660254037844387076, 1.000000000000000000, 0.8660254037844387076, 1.000000000000000000, 0.8660254037844387076, 1.000000000000000000, 0.8660254037844387076, 1.000000000000000000, 0.8660254037844387076, 1.000000000000000000, 0.8660254037844387076, 1.000000000000000000, 0.8660254037844387076, 1.000000000000000000, 0.8660254037844387076, 1.000000000000000000, 0.8660254037844387076, 1.000000000000000000, 0.8660254037844387076, 1.000000000000000000, 0.8660254037844387076, 1.000000000000000000, 0.8660254037844387076, 1.000000000000000000, 0.8660254037844387076, 1.000000000000000000, 0.8660254037844387076, 1.000000000000000000, 0.8660254037844387076, 1.000000000000000000, 0.8660254037844387076, 1.000000000000000000, 0.8660254037844387076, 1.000000000000000000, 0.8660254037844387076, 1.000000000000000000, 0.8660254037844387076, 1.000000000000000000, 0.8660254037844387076, 1.000000000000000000, 0.8660254037844387076, 1.000000000000000000, 0.8660254037844387076, 1.000000000000000000, 0.8660254037844387076, 1.000000000000000000, 0.8660254037844387076, 1.000000000000000000, 0.8660254037844387076, 1.000000000000000000, 0.8660254037844387076, 1.000000000000000000, 0.8660254037844387076, 1.000000000000000000, 0.8660254037844387076, 1.000000000000000000, 0.8660254037844387076, 1.000000000000000000, 0.8660254037844387076, 1.000000000000000000, 0.8660254037844387076, 1.000000000000000000, 0.8660254037844387076, 1.000000000000000000, 0.8660254037844387076, 1.000000000000000000, 0.8660254037844387076, 1.000000000000000000, 0.8660254037844387076, 1.000000000000000000, 0.8660254037844387076, 1.000000000000000000, 0.8660254037844387076, 1.000000000000000000, 0.8660254037844387076, 1.000000000000000000, 0.8660254037844387076, 1.000000000000000000, 0.8660254037844387076, 1.000000000000000000, 0.8660254037844387076, 1.000000000000000000, 0.8660254037844387076, 1.000000000000000000, 0.8660254037844387076, 1.000000000000000000, 0.8660254037844387076, 1.000000000000000000, 0.8660254037844387076, 1.000000000000000000, 0.8660254037844387076, 1.000000000000000000, 0.8660254037844387076, 1.000000000000000000, 0.8660254037844387076, 1.000000000000000000, 0.8660254037844387076, 1.000000000000000000, 0.8660254037844387076, 1.000000000000000000, 0.8660254037844387076, 1.000000000000000000, 0.8660254037844387076, 1.000000000000000000, 0.8660254037844387076, 1.000000000000000000, 0.8660254037844387076, 1.000000000000000000, 0.8660254037844387076, 1.000000000000000000, 0.8660254037844387076, 1.000000000000000000, 0.8660254037844387076, 1.000000000000000000, 0.8660254037844387076, 1.000000000000000000, 0.8660254037844387076, 1.000000000000000000, 0.8660254037844387076, 1.000000000000000000, 0.8660254037844387076, 1.000000000000000000, 0.8660254037844387076, 1.000000000000000000, 0.8660254037844387076, 1.000000000000000000, 0.8660254037844387076, 1.000000000000000000, 0.8660254037844387076, 1.000000000000000000, 0.8660254037844387076, 1.000000000000000000, 0.8660254037844387076, 1.000000000000000000, 0.8660254037844387076, 1.000000000000000000, 0.8660254037844387076, 1.000000000000000000, 0.8660254037844387076, 1.000000000000000000, 0.8660254037844387076, 1.000000000000000000, 0.8660254037844387076, 1.000000000000000000, 0.8660254037844387076, 1.000000000000000000, 0.8660254037844387076, 1.000000000000000000, 0.8660254037844387076, 1.000000000000000000, 0.8660254037844387076, 1.000000000000000000, 0.8660254037844387076, 1.000000000000000000, 0.8660254037844387076, 1.000000000000000000, 0.8660254037844387076, 1.000000000000000000, 0.8660254037844387076, 1.000000000000000000, 0.8660254037844387076, 1.000000000000000000, 0.8660254037844387076, 1.000000000000000000, 0.8660254037844387076, 1.000000000000000000, 0.8660254037844387076, 1.000000000000000000, 0.8660254037844387076, 1.000000000000000000, 0.8660254037844387076, 1.000000000000000000, 0.8660254037844387076, 1.000000000000000000, 0.8660254037844387076, 1.000000000000000000, 0.8660254037844387076, 1.000000000000000000, 0.8660254037844387076, 1.000000000000000000, 0.8660254037844387076, 1.000000000000000000, 0.8660254037844387076, 1.000000000000000000, 0.8660254037844387076, 1.000000000000000000, 0.8660254037844387076, 1.000000000000000000, 0.8660254037844387076, 1.000000000000000000, 0.8660254037844387076, 1.000000000000000000, 0.8660254037844387076, 1.000000000000000000, 0.8660254037844387076, 1.000000000000000000, 0.8660254037844387076, 1.000000000000000000, 0.8660254037844387076, 1.000000000000000000, 0.8660254037844387076, 1.000000000000000000, 0.8660254037844387076, 1.000000000000000000, 0.9548846395026737710, 0.9401540804572410259),
 ( 1.000000000000000000, 0.8660254037844387076, 1.000000000000000000, 0.8660254037844387076, 1.000000000000000000, 0.8660254037844387076, 1.000000000000000000, 0.8660254037844387076, 1.000000000000000000, 0.8660254037844387076, 1.000000000000000000, 0.8660254037844387076, 1.000000000000000000, 0.8660254037844387076, 1.000000000000000000, 0.8660254037844387076, 1.000000000000000000, 0.8660254037844387076, 1.000000000000000000, 0.8660254037844387076, 1.000000000000000000, 0.8660254037844387076, 1.000000000000000000, 0.8660254037844387076, 1.000000000000000000, 0.8660254037844387076, 1.000000000000000000, 0.8660254037844387076, 1.000000000000000000, 0.8660254037844387076, 1.000000000000000000, 0.8660254037844387076, 1.000000000000000000, 0.8660254037844387076, 1.000000000000000000, 0.8660254037844387076, 1.000000000000000000, 0.8660254037844387076, 1.000000000000000000, 0.8660254037844387076, 1.000000000000000000, 0.8660254037844387076, 1.000000000000000000, 0.8660254037844387076, 1.000000000000000000, 0.8660254037844387076, 1.000000000000000000, 0.8660254037844387076, 1.000000000000000000, 0.8660254037844387076, 1.000000000000000000, 0.8660254037844387076, 1.000000000000000000, 0.8660254037844387076, 1.000000000000000000, 0.8660254037844387076, 1.000000000000000000, 0.8660254037844387076, 1.000000000000000000, 0.8660254037844387076, 1.000000000000000000, 0.8660254037844387076, 1.000000000000000000, 0.8660254037844387076, 1.000000000000000000, 0.8660254037844387076, 1.000000000000000000, 0.8660254037844387076, 1.000000000000000000, 0.8660254037844387076, 1.000000000000000000, 0.8660254037844387076, 1.000000000000000000, 0.8660254037844387076, 1.000000000000000000, 0.8660254037844387076, 1.000000000000000000, 0.8660254037844387076, 1.000000000000000000, 0.8660254037844387076, 1.000000000000000000, 0.8660254037844387076, 1.000000000000000000, 0.8660254037844387076, 1.000000000000000000, 0.8660254037844387076, 1.000000000000000000, 0.8660254037844387076, 1.000000000000000000, 0.8660254037844387076, 1.000000000000000000, 0.8660254037844387076, 1.000000000000000000, 0.8660254037844387076, 1.000000000000000000, 0.8660254037844387076, 1.000000000000000000, 0.8660254037844387076, 1.000000000000000000, 0.8660254037844387076, 1.000000000000000000, 0.8660254037844387076, 1.000000000000000000, 0.8660254037844387076, 1.000000000000000000, 0.8660254037844387076, 1.000000000000000000, 0.8660254037844387076, 1.000000000000000000, 0.8660254037844387076, 1.000000000000000000, 0.8660254037844387076, 1.000000000000000000, 0.8660254037844387076, 1.000000000000000000, 0.8660254037844387076, 1.000000000000000000, 0.8660254037844387076, 1.000000000000000000, 0.8660254037844387076, 1.000000000000000000, 0.8660254037844387076, 1.000000000000000000, 0.8660254037844387076, 1.000000000000000000, 0.8660254037844387076, 1.000000000000000000, 0.8660254037844387076, 1.000000000000000000, 0.8660254037844387076, 1.000000000000000000, 0.8660254037844387076, 1.000000000000000000, 0.8660254037844387076, 1.000000000000000000, 0.8660254037844387076, 1.000000000000000000, 0.8660254037844387076, 1.000000000000000000, 0.8660254037844387076, 1.000000000000000000, 0.8660254037844387076, 1.000000000000000000, 0.8660254037844387076, 1.000000000000000000, 0.8660254037844387076, 1.000000000000000000, 0.8660254037844387076, 1.000000000000000000, 0.8660254037844387076, 1.000000000000000000, 0.8660254037844387076, 1.000000000000000000, 0.8660254037844387076, 1.000000000000000000, 0.8660254037844387076, 1.000000000000000000, 0.8660254037844387076, 1.000000000000000000, 0.8660254037844387076, 1.000000000000000000, 0.8660254037844387076, 1.000000000000000000, 0.8660254037844387076, 1.000000000000000000, 0.8660254037844387076, 1.000000000000000000, 0.8660254037844387076, 1.000000000000000000, 0.8660254037844387076, 1.000000000000000000, 0.8660254037844387076, 1.000000000000000000, 0.8660254037844387076, 1.000000000000000000, 0.8660254037844387076, 1.000000000000000000, 0.8660254037844387076, 1.000000000000000000, 0.8660254037844387076, 1.000000000000000000, 0.8660254037844387076, 1.000000000000000000, 0.8660254037844387076, 1.000000000000000000, 0.8660254037844387076, 1.000000000000000000, 0.8660254037844387076, 1.000000000000000000, 0.8660254037844387076, 1.000000000000000000, 0.8660254037844387076, 1.000000000000000000, 0.8660254037844387076, 1.000000000000000000, 0.8660254037844387076, 1.000000000000000000, 0.8660254037844387076, 1.000000000000000000, 0.8660254037844387076, 1.000000000000000000, 0.8660254037844387076, 1.000000000000000000, 0.8660254037844387076, 1.000000000000000000, 0.8660254037844387076, 1.000000000000000000, 0.8660254037844387076, 1.000000000000000000, 0.8660254037844387076, 1.000000000000000000, 0.8660254037844387076, 1.000000000000000000, 0.8660254037844387076, 1.000000000000000000, 0.8660254037844387076, 1.000000000000000000, 0.8660254037844387076, 1.000000000000000000, 0.8660254037844387076, 1.000000000000000000, 0.8660254037844387076, 1.000000000000000000, 0.8660254037844387076, 1.000000000000000000, 0.8660254037844387076, 1.000000000000000000, 0.8660254037844387076, 1.000000000000000000, 0.8660254037844387076, 1.000000000000000000, 0.8660254037844387076, 1.000000000000000000, 0.8660254037844387076, 1.000000000000000000, 0.8660254037844387076, 1.000000000000000000, 0.8660254037844387076, 1.000000000000000000, 0.8660254037844387076, 1.000000000000000000, 0.8660254037844387076, 1.000000000000000000, 0.8660254037844387076, 1.000000000000000000, 0.8660254037844387076, 1.000000000000000000, 0.8660254037844387076, 1.000000000000000000, 0.8660254037844387076, 1.000000000000000000, 0.8660254037844387076, 1.000000000000000000, 0.8660254037844387076, 1.000000000000000000, 0.8660254037844387076, 1.000000000000000000, 0.8660254037844387076, 1.000000000000000000, 0.8660254037844387076, 1.000000000000000000, 0.8660254037844387076, 1.000000000000000000, 0.8660254037844387076, 1.000000000000000000, 0.8660254037844387076, 1.000000000000000000, 0.9548846395026737710, 0.9401540804572410259) ) ) 
 REPRESENTATION_ITEM ( '' )  SURFACE ( )  );
#48224=CARTESIAN_POINT ( 'NONE',  ( 4.505505391250587799, 2.168045472173443233, -4.697296768249695553 ) ) ;
#48225=CARTESIAN_POINT ( 'NONE',  ( 18.17812500061451786, -4.541064518000419881, 2.621784821874995952 ) ) ;
#48226=CARTESIAN_POINT ( 'NONE',  ( 24.83437500061451431, 4.541064518000418104, 2.621784821874999949 ) ) ;
#48228=CARTESIAN_POINT ( 'NONE',  ( -1.071796769724475906, 11.02009619066136636, -34.00000000000000711 ) ) ;
#48230=CARTESIAN_POINT ( 'NONE',  ( 5.821875000614519458, 3.027376345333613106, -5.243569643749998122 ) ) ;
#48231=CARTESIAN_POINT ( 'NONE',  ( 16.79062500061451857, -3.027376345333614438, 5.243569643749998122 ) ) ;
#48234=CARTESIAN_POINT ( 'NONE',  ( 24.29062500061451502, 6.054752690667223547, 3.707466751127219781E-16 ) ) ;
#48235=CARTESIAN_POINT ( 'NONE',  ( -5.810221930991193690E-16, 10.55000000122903359, -34.00000000000000000 ) ) ;
#48236=CARTESIAN_POINT ( 'NONE',  ( 27.97500000000000142, 6.123233995736764310E-16, -4.999999999999998224 ) ) ;
#48237=CARTESIAN_POINT ( 'NONE',  ( 15.78749999999999964, -2.886751345948125991, -5.000000000000000000 ) ) ;
#48238=CARTESIAN_POINT ( 'NONE',  ( 24.15000000122903145, 5.773502691896255534, 3.535250795749688894E-16 ) ) ;
#48239=CARTESIAN_POINT ( 'NONE',  ( 19.60312500061451502, -4.541064518000417216, -2.621784821875001281 ) ) ;
#48240=VERTEX_POINT ( 'NONE', #17115 ) ;
#48241=CARTESIAN_POINT ( 'NONE',  ( 22.61250000000000071, 2.886751345948129099, -4.999999999999998224 ) ) ;
#48243=CARTESIAN_POINT ( 'NONE',  ( 24.30937500061451573, 4.541064518000418104, -2.621784821874998173 ) ) ;
#48244=ORIENTED_EDGE ( 'NONE', *, *, #20472, .F. ) ;
#48246=CARTESIAN_POINT ( 'NONE',  ( 12.17812500061451608, 4.541064518000418104, 2.621784821874999949 ) ) ;
#48247=CARTESIAN_POINT ( 'NONE',  ( 3.590625000614518836, 6.054752690667223547, 3.707466751127219781E-16 ) ) ;
#48249=CARTESIAN_POINT ( 'NONE',  ( 25.79062500061451502, -3.027376345333614438, 5.243569643749998122 ) ) ;
#48250=( BOUNDED_CURVE ( )  B_SPLINE_CURVE ( 2, ( #35941, #30038, #10974, #1985, #7151, #69574, #52217 ),
 .UNSPECIFIED., .F., .F. ) 
 B_SPLINE_CURVE_WITH_KNOTS ( ( 3, 2, 2, 3 ),
 ( 0.9343140676420280677, 0.9361111111111111160, 0.9388888888888888840, 0.9404862704844845211 ),
 .UNSPECIFIED. ) 
 CURVE ( )  GEOMETRIC_REPRESENTATION_ITEM ( )  RATIONAL_B_SPLINE_CURVE ( ( 0.9387977477080564626, 0.9133270576652030570, 1.000000000000000000, 0.8660254037844387076, 1.000000000000000000, 0.9229569204620456935, 0.9345222229958878302 ) ) 
 REPRESENTATION_ITEM ( '' )  );
#48251=CARTESIAN_POINT ( 'NONE',  ( 13.23750000122903359, 6.123233995736764310E-16, -4.999999999999998224 ) ) ;
#48252=CARTESIAN_POINT ( 'NONE',  ( 19.72499999999999787, -4.330127018922194537, 2.499999999999995559 ) ) ;
#48253=CARTESIAN_POINT ( 'NONE',  ( 27.03750000000000142, -2.886751345948125991, -5.000000000000000000 ) ) ;
#48254=CARTESIAN_POINT ( 'NONE',  ( 2.859375000614519546, 0.000000000000000000, 5.243569643749999010 ) ) ;
#48255=CARTESIAN_POINT ( 'NONE',  ( 6.384375000614516793, 4.541064518000418104, 2.621784821874999949 ) ) ;
#48256=CARTESIAN_POINT ( 'NONE',  ( 16.17187500061451644, 3.027376345333613106, -5.243569643749998122 ) ) ;
#48257=CARTESIAN_POINT ( 'NONE',  ( 29.82187500061451502, 3.027376345333611329, 5.243569643749999010 ) ) ;
#48258=VERTEX_POINT ( 'NONE', #5685 ) ;
#48259=CARTESIAN_POINT ( 'NONE',  ( 26.61562500061451786, 3.027376345333611329, 5.243569643749999010 ) ) ;
#48260=CARTESIAN_POINT ( 'NONE',  ( 28.84687500061452070, 6.054752690667223547, 3.707466751127219781E-16 ) ) ;
#48262=CARTESIAN_POINT ( 'NONE',  ( 17.17500000000000071, 6.123233995736764310E-16, -4.999999999999998224 ) ) ;
#48263=CARTESIAN_POINT ( 'NONE',  ( 14.39062500061451821, 6.054752690667223547, 3.707466751127219781E-16 ) ) ;
#48266=CARTESIAN_POINT ( 'NONE',  ( 29.01562500061451644, -6.054752690667223547, -1.112240025338166033E-15 ) ) ;
#48267=CARTESIAN_POINT ( 'NONE',  ( 18.86250000122903359, 0.000000000000000000, 4.999999999999998224 ) ) ;
#48268=CARTESIAN_POINT ( 'NONE',  ( 0.000000000000000000, 20.00000000000000000, 26.00000000000000000 ) ) ;
#48270=CARTESIAN_POINT ( 'NONE',  ( 5.315625000614516260, 3.027376345333613106, -5.243569643749998122 ) ) ;
#48271=CARTESIAN_POINT ( 'NONE',  ( 25.20937500061451431, 4.541064518000418104, -2.621784821874998173 ) ) ;
#48272=CARTESIAN_POINT ( 'NONE',  ( 2.121784821875001281, 16.40937500061452070, 33.67503911421598417 ) ) ;
#48273=CARTESIAN_POINT ( 'NONE',  ( 24.94687500061451502, -3.027376345333614438, 5.243569643749998122 ) ) ;
#48274=CARTESIAN_POINT ( 'NONE',  ( 5.924999999999999822, 6.123233995736764310E-16, -4.999999999999998224 ) ) ;
#48275=CARTESIAN_POINT ( 'NONE',  ( 3.999999999999999112, 11.78750000122903430, 30.00000000000000000 ) ) ;
#48276=CARTESIAN_POINT ( 'NONE',  ( 13.34062500061451750, -3.027376345333610441, -5.243569643749999898 ) ) ;
#48277=CARTESIAN_POINT ( 'NONE',  ( 5.062500001229035540, -4.330127018922190985, -2.500000000000001332 ) ) ;
#48278=CARTESIAN_POINT ( 'NONE',  ( 9.046875000614518214, 6.054752690667223547, 3.707466751127219781E-16 ) ) ;
#48279=CARTESIAN_POINT ( 'NONE',  ( -0.2761983717765570945, 4.994289515549795055, -26.00713100841934633 ) ) ;
#48280=ORIENTED_EDGE ( 'NONE', *, *, #47837, .F. ) ;
#48281=CARTESIAN_POINT ( 'NONE',  ( 11.12812500061451715, 6.421520780324663323E-16, -5.243569643749999010 ) ) ;
#48282=CARTESIAN_POINT ( 'NONE',  ( 13.54687500061451999, 6.054752690667223547, 3.707466751127219781E-16 ) ) ;
#48283=CARTESIAN_POINT ( 'NONE',  ( 3.999999999999999112, 12.23750000122903359, -30.00000000000000000 ) ) ;
#48284=CARTESIAN_POINT ( 'NONE',  ( 21.71250000122903501, -4.330127018922190985, -2.500000000000001332 ) ) ;
#48285=CARTESIAN_POINT ( 'NONE',  ( 10.65937500061451715, -4.541064518000417216, -2.621784821875001281 ) ) ;
#48286=CARTESIAN_POINT ( 'NONE',  ( 13.30312500061451786, -4.541064518000417216, -2.621784821875001281 ) ) ;
#48288=CARTESIAN_POINT ( 'NONE',  ( 21.19687500061451502, 6.054752690667223547, 3.707466751127219781E-16 ) ) ;
#48289=CARTESIAN_POINT ( 'NONE',  ( 15.59999999999999964, 0.000000000000000000, 4.999999999999998224 ) ) ;
#48290=CARTESIAN_POINT ( 'NONE',  ( -3.462385672708550910, 3.612013013662438432, 27.98145868590390606 ) ) ;
#48291=CARTESIAN_POINT ( 'NONE',  ( -3.000416591977282496E-16, 13.44687500061451679, -34.90005215228797653 ) ) ;
#48292=CARTESIAN_POINT ( 'NONE',  ( 16.54687500061451644, -3.027376345333610441, -5.243569643749999898 ) ) ;
#48293=CARTESIAN_POINT ( 'NONE',  ( 14.73750000122903359, 4.330127018922191873, 2.499999999999999556 ) ) ;
#48294=CARTESIAN_POINT ( 'NONE',  ( 12.72187500061451537, 3.027376345333611329, 5.243569643749999010 ) ) ;
#48295=CARTESIAN_POINT ( 'NONE',  ( -2.121784821874996840, 17.17812500061451786, -26.32496088578401583 ) ) ;
#48296=CARTESIAN_POINT ( 'NONE',  ( 17.32500000122903216, 2.886751345948129099, -4.999999999999998224 ) ) ;
#48297=CARTESIAN_POINT ( 'NONE',  ( 12.62812500061451537, 4.541064518000418104, 2.621784821874999949 ) ) ;
#48298=VERTEX_POINT ( 'NONE', #23382 ) ;
#48299=CARTESIAN_POINT ( 'NONE',  ( 16.94999999999999929, 0.000000000000000000, 4.999999999999998224 ) ) ;
#48300=CARTESIAN_POINT ( 'NONE',  ( -2.000000000000000000, 17.33750000122903145, -33.46410161513775705 ) ) ;
#48301=CARTESIAN_POINT ( 'NONE',  ( 10.69687500061451679, -3.027376345333610441, -5.243569643749999898 ) ) ;
#48304=CARTESIAN_POINT ( 'NONE',  ( 13.23750000122903359, 6.123233995736764310E-16, -4.999999999999998224 ) ) ;
#48305=CARTESIAN_POINT ( 'NONE',  ( 21.97500000122903074, 2.886751345948126879, 4.999999999999999112 ) ) ;
#48307=CARTESIAN_POINT ( 'NONE',  ( 18.59062500061451573, -3.027376345333614438, 5.243569643749998122 ) ) ;
#48308=CARTESIAN_POINT ( 'NONE',  ( 20.61562500061451431, 3.027376345333613106, -5.243569643749998122 ) ) ;
#48309=CARTESIAN_POINT ( 'NONE',  ( 26.77500000122903145, 2.886751345948129099, -4.999999999999998224 ) ) ;
#48310=CARTESIAN_POINT ( 'NONE',  ( 3.890625000614517326, -3.027376345333610441, -5.243569643749999898 ) ) ;
#48311=CARTESIAN_POINT ( 'NONE',  ( 25.91250000000000142, 2.886751345948126879, 4.999999999999999112 ) ) ;
#48314=CARTESIAN_POINT ( 'NONE',  ( 27.30937500061451573, -4.541064518000417216, -2.621784821875001281 ) ) ;
#48316=CARTESIAN_POINT ( 'NONE',  ( 2.121784821874999061, 14.30937500061451750, -33.67503911421598417 ) ) ;
#48317=CARTESIAN_POINT ( 'NONE',  ( 3.937500001229034208, 4.330127018922191873, 2.499999999999999556 ) ) ;
#48318=CARTESIAN_POINT ( 'NONE',  ( 29.82187500061451502, 3.027376345333611329, 5.243569643749999010 ) ) ;
#48319=CARTESIAN_POINT ( 'NONE',  ( 16.35000000000000142, 4.330127018922192761, -2.499999999999997780 ) ) ;
#48320=CARTESIAN_POINT ( 'NONE',  ( 7.921875000614517326, -6.054752690667223547, -1.112240025338166033E-15 ) ) ;
#48321=CARTESIAN_POINT ( 'NONE',  ( 26.16562500061451502, 3.027376345333611329, 5.243569643749999010 ) ) ;
#48323=CARTESIAN_POINT ( 'NONE',  ( 14.32500000000000107, -4.330127018922194537, 2.499999999999995559 ) ) ;
#48324=CARTESIAN_POINT ( 'NONE',  ( 4.000000000000000000, 17.60000000122903430, -27.69059892324149885 ) ) ;
#48325=CARTESIAN_POINT ( 'NONE',  ( 6.346875000614517148, 6.054752690667223547, 3.707466751127219781E-16 ) ) ;
#48326=CARTESIAN_POINT ( 'NONE',  ( 9.196875000614518569, -3.027376345333614438, 5.243569643749998122 ) ) ;
#48327=CARTESIAN_POINT ( 'NONE',  ( 3.300000000000000711, 4.330127018922192761, -2.499999999999997780 ) ) ;
#48328=ADVANCED_FACE ( 'NONE', ( #45931 ), #52555, .F. ) ;
#48329=CARTESIAN_POINT ( 'NONE',  ( 4.243569643749999898, 12.79062500061459495, 32.45002607614398471 ) ) ;
#48330=CARTESIAN_POINT ( 'NONE',  ( 28.53749999999999787, 5.773502691896255534, 3.535250795749688894E-16 ) ) ;
#48331=CARTESIAN_POINT ( 'NONE',  ( 3.075000000000001510, -4.330127018922194537, 2.499999999999995559 ) ) ;
#48333=VERTEX_POINT ( 'NONE', #41117 ) ;
#48334=CARTESIAN_POINT ( 'NONE',  ( 19.60312500061451502, -4.541064518000417216, -2.621784821875001281 ) ) ;
#48335=CARTESIAN_POINT ( 'NONE',  ( 11.12812500061451715, 6.421520780324663323E-16, -5.243569643749999010 ) ) ;
#48337=CARTESIAN_POINT ( 'NONE',  ( 7.846875000614518036, -3.027376345333614438, 5.243569643749998122 ) ) ;
#48338=CARTESIAN_POINT ( 'NONE',  ( 25.50000000000000000, 0.000000000000000000, 4.999999999999998224 ) ) ;
#48339=CARTESIAN_POINT ( 'NONE',  ( 20.28750000122903074, -4.330127018922194537, 2.499999999999995559 ) ) ;
#48340=CARTESIAN_POINT ( 'NONE',  ( 27.25312500061451360, -4.541064518000417216, -2.621784821875001281 ) ) ;
#48342=CARTESIAN_POINT ( 'NONE',  ( 9.084375000614517859, 4.541064518000418104, 2.621784821874999949 ) ) ;
#48343=CARTESIAN_POINT ( 'NONE',  ( 13.80937500061451750, -4.541064518000417216, -2.621784821875001281 ) ) ;
#48344=CARTESIAN_POINT ( 'NONE',  ( 25.17187500061451644, 3.027376345333613106, -5.243569643749998122 ) ) ;
#48345=CARTESIAN_POINT ( 'NONE',  ( 8.550000001229030033, -2.886751345948063374, 5.000000000000112799 ) ) ;
#48347=CARTESIAN_POINT ( 'NONE',  ( 20.48437500061451289, -4.541064518000419881, 2.621784821874995952 ) ) ;
#48348=CARTESIAN_POINT ( 'NONE',  ( 9.196875000614518569, -3.027376345333614438, 5.243569643749998122 ) ) ;
#48350=CARTESIAN_POINT ( 'NONE',  ( 24.18750000000000355, -2.886751345948129988, 4.999999999999997335 ) ) ;
#48352=CARTESIAN_POINT ( 'NONE',  ( -2.121784821874999949, 11.23437500061451821, -33.67503911421598417 ) ) ;
#48354=CARTESIAN_POINT ( 'NONE',  ( 13.82812500061451466, 6.421520780324663323E-16, -5.243569643749999010 ) ) ;
#48355=CARTESIAN_POINT ( 'NONE',  ( 4.162499999999999645, 2.886751345948129099, -4.999999999999998224 ) ) ;
#48356=CARTESIAN_POINT ( 'NONE',  ( 1.510657702057710734E-15, 19.10000000122903430, -33.99999999999999289 ) ) ;
#48358=CARTESIAN_POINT ( 'NONE',  ( 13.19999999999999929, 4.330127018922192761, -2.499999999999997780 ) ) ;
#48359=CARTESIAN_POINT ( 'NONE',  ( 4.000000000000000000, 17.60000000122903785, 32.30940107675849049 ) ) ;
#48360=CARTESIAN_POINT ( 'NONE',  ( 10.61250000122903536, 4.330127018922192761, -2.499999999999997780 ) ) ;
#48361=CARTESIAN_POINT ( 'NONE',  ( 23.10937500061451644, 0.000000000000000000, 5.243569643749999010 ) ) ;
#48362=CARTESIAN_POINT ( 'NONE',  ( 16.39687500061451786, -3.027376345333614438, 5.243569643749998122 ) ) ;
#48363=CARTESIAN_POINT ( 'NONE',  ( 20.36250000122903359, -4.330127018922190985, -2.500000000000001332 ) ) ;
#48364=ORIENTED_EDGE ( 'NONE', *, *, #26290, .F. ) ;
#48365=CARTESIAN_POINT ( 'NONE',  ( 18.32812500061451644, 6.421520780324663323E-16, -5.243569643749999010 ) ) ;
#48366=CARTESIAN_POINT ( 'NONE',  ( 5.390625000614518214, 6.054752690667223547, 3.707466751127219781E-16 ) ) ;
#48367=CARTESIAN_POINT ( 'NONE',  ( 17.03437500061451715, 6.421520780324663323E-16, -5.243569643749999010 ) ) ;
#48368=CARTESIAN_POINT ( 'NONE',  ( 28.84687500061452070, 6.054752690667223547, 3.707466751127219781E-16 ) ) ;
#48369=CARTESIAN_POINT ( 'NONE',  ( 5.465625000614517504, 3.027376345333611329, 5.243569643749999010 ) ) ;
#48370=CARTESIAN_POINT ( 'NONE',  ( 18.92812500061451431, 4.541064518000418104, 2.621784821874999949 ) ) ;
#48371=CARTESIAN_POINT ( 'NONE',  ( -2.121784821874999949, 13.87812500061451715, 26.32496088578401938 ) ) ;
#48372=CARTESIAN_POINT ( 'NONE',  ( 17.66250000122903430, -4.330127018922190985, -2.500000000000001332 ) ) ;
#48374=CARTESIAN_POINT ( 'NONE',  ( 7.828125000614517326, -4.541064518000419881, 2.621784821874995952 ) ) ;
#48375=CARTESIAN_POINT ( 'NONE',  ( 28.07812500061451289, -4.541064518000419881, 2.621784821874995952 ) ) ;
#48376=CARTESIAN_POINT ( 'NONE',  ( 9.862500001229033586, 0.000000000000000000, 4.999999999999998224 ) ) ;
#48377=CARTESIAN_POINT ( 'NONE',  ( 23.78437500061451360, 6.421520780324663323E-16, -5.243569643749999010 ) ) ;
#48378=CARTESIAN_POINT ( 'NONE',  ( 14.20312500061451644, -4.541064518000417216, -2.621784821875001281 ) ) ;
#48379=CARTESIAN_POINT ( 'NONE',  ( 24.22500000122903430, 2.886751345948126879, 4.999999999999999112 ) ) ;
#48380=CARTESIAN_POINT ( 'NONE',  ( 22.64062500061451644, -3.027376345333614438, 5.243569643749998122 ) ) ;
#48381=CARTESIAN_POINT ( 'NONE',  ( 19.58437500061451786, -4.541064518000419881, 2.621784821874995952 ) ) ;
#48382=CARTESIAN_POINT ( 'NONE',  ( 15.21562500061451750, 3.027376345333613106, -5.243569643749998122 ) ) ;
#48383=CARTESIAN_POINT ( 'NONE',  ( -4.243569643749999898, 13.97187500061451715, 27.54997392385601529 ) ) ;
#48384=CARTESIAN_POINT ( 'NONE',  ( 19.94062500061451715, -3.027376345333614438, 5.243569643749998122 ) ) ;
#48386=ORIENTED_EDGE ( 'NONE', *, *, #38051, .T. ) ;
#48388=CARTESIAN_POINT ( 'NONE',  ( 22.57499999999999929, 6.123233995736764310E-16, -4.999999999999998224 ) ) ;
#48389=CARTESIAN_POINT ( 'NONE',  ( 8.484601909799253346E-16, 10.21250000000000213, -25.38119784648299770 ) ) ;
#48390=CARTESIAN_POINT ( 'NONE',  ( 12.59999999999999964, -4.330127018922190985, -2.500000000000001332 ) ) ;
#48391=CARTESIAN_POINT ( 'NONE',  ( 26.54062500061451146, 6.054752690667223547, 3.707466751127219781E-16 ) ) ;
#48392=CARTESIAN_POINT ( 'NONE',  ( 7.115625000614516082, 3.027376345333613106, -5.243569643749998122 ) ) ;
#48393=CARTESIAN_POINT ( 'NONE',  ( 19.05000000122903359, -2.886751345948125991, -5.000000000000000000 ) ) ;
#48394=CARTESIAN_POINT ( 'NONE',  ( 24.40312500061451573, 0.000000000000000000, 5.243569643749999010 ) ) ;
#48395=CARTESIAN_POINT ( 'NONE',  ( 22.98749999999999716, -2.886751345948125991, -5.000000000000000000 ) ) ;
#48396=( BOUNDED_CURVE ( )  B_SPLINE_CURVE ( 2, ( #55236, #16781, #33416, #61851, #5713, #62223, #55595 ),
 .UNSPECIFIED., .F., .F. ) 
 B_SPLINE_CURVE_WITH_KNOTS ( ( 3, 2, 2, 3 ),
 ( 0.1166666666666666824, 0.1194444444444444642, 0.1222222222222222182, 0.1250000000000000000 ),
 .UNSPECIFIED. ) 
 CURVE ( )  GEOMETRIC_REPRESENTATION_ITEM ( )  RATIONAL_B_SPLINE_CURVE ( ( 0.9999999999999993339, 0.8660254037844393737, 1.000000000000000000, 0.8660254037844387076, 1.000000000000000000, 0.8660254037844387076, 1.000000000000000000 ) ) 
 REPRESENTATION_ITEM ( '' )  );
#48397=EDGE_CURVE ( 'NONE', #3838, #38197, #60977, .T. ) ;
#48398=CARTESIAN_POINT ( 'NONE',  ( 27.70312500061451289, -4.541064518000417216, -2.621784821875001281 ) ) ;
#48399=CARTESIAN_POINT ( 'NONE',  ( 8.840625000614515727, -3.027376345333610441, -5.243569643749999898 ) ) ;
#48401=CARTESIAN_POINT ( 'NONE',  ( 22.41562500061451502, 3.027376345333613106, -5.243569643749998122 ) ) ;
#48402=CARTESIAN_POINT ( 'NONE',  ( 6.215625000614517504, 3.027376345333613106, -5.243569643749998122 ) ) ;
#48404=CARTESIAN_POINT ( 'NONE',  ( 3.853125000614517681, -4.541064518000417216, -2.621784821875001281 ) ) ;
#48405=VECTOR ( 'NONE', #5712, 1000.000000000000000 ) ;
#48406=CARTESIAN_POINT ( 'NONE',  ( 8.484601909799253346E-16, 13.02500000122903501, -25.38119784648299770 ) ) ;
#48407=CARTESIAN_POINT ( 'NONE',  ( -1.999999999999997113, 13.77500000000000036, -26.53589838486224295 ) ) ;
#48408=CARTESIAN_POINT ( 'NONE',  ( 11.70000000000000284, -4.330127018922190985, -2.500000000000001332 ) ) ;
#48409=CARTESIAN_POINT ( 'NONE',  ( 10.20937500061451786, -4.541064518000417216, -2.621784821875001281 ) ) ;
#48410=CARTESIAN_POINT ( 'NONE',  ( 7.987500001229032698, 4.330127018922191873, 2.499999999999999556 ) ) ;
#48411=CARTESIAN_POINT ( 'NONE',  ( 14.44687500061451679, 6.054752690667223547, 3.707466751127219781E-16 ) ) ;
#48413=CARTESIAN_POINT ( 'NONE',  ( 5.709375000614517859, -4.541064518000417216, -2.621784821875001281 ) ) ;
#48414=CARTESIAN_POINT ( 'NONE',  ( 1.071796769724488119, 18.33259618943233704, 33.99999999999999289 ) ) ;
#48415=CARTESIAN_POINT ( 'NONE',  ( 12.15937500061451892, 4.541064518000418104, -2.621784821874998173 ) ) ;
#48417=CARTESIAN_POINT ( 'NONE',  ( 21.74062500061451431, -3.027376345333614438, 5.243569643749998122 ) ) ;
#48418=CARTESIAN_POINT ( 'NONE',  ( -4.243569643749999898, 9.921875000614516438, 27.54997392385601529 ) ) ;
#48419=FACE_OUTER_BOUND ( 'NONE', #51155, .T. ) ;
#48420=CARTESIAN_POINT ( 'NONE',  ( 25.80937500061451928, 0.000000000000000000, 5.243569643749999010 ) ) ;
#48421=CARTESIAN_POINT ( 'NONE',  ( 4.129838550988103485, 2.818587153659042777, -4.208548528382372034 ) ) ;
#48423=CARTESIAN_POINT ( 'NONE',  ( 5.503125000614516260, 0.000000000000000000, 5.243569643749999010 ) ) ;
#48425=CARTESIAN_POINT ( 'NONE',  ( 17.40937500061451715, -4.541064518000417216, -2.621784821875001281 ) ) ;
#48427=CARTESIAN_POINT ( 'NONE',  ( 27.97500000122903074, -5.773502691896255534, -1.060575238724906372E-15 ) ) ;
#48428=CARTESIAN_POINT ( 'NONE',  ( 5.859375000614519102, 4.541064518000418104, -2.621784821874998173 ) ) ;
#48429=CARTESIAN_POINT ( 'NONE',  ( 16.43437500061451573, -4.541064518000419881, 2.621784821874995952 ) ) ;
#48431=CARTESIAN_POINT ( 'NONE',  ( 24.86250000000000071, 2.886751345948129099, -4.999999999999998224 ) ) ;
#48432=CARTESIAN_POINT ( 'NONE',  ( 3.075000001229035718, 2.886751345948126879, 4.999999999999999112 ) ) ;
#48433=CARTESIAN_POINT ( 'NONE',  ( 26.18437500061451573, 4.541064518000418104, 2.621784821874999949 ) ) ;
#48435=CARTESIAN_POINT ( 'NONE',  ( 21.75000000000000000, 4.330127018922192761, -2.499999999999997780 ) ) ;
#48436=CARTESIAN_POINT ( 'NONE',  ( 7.575000000000001954, -4.330127018922194537, 2.499999999999995559 ) ) ;
#48438=CARTESIAN_POINT ( 'NONE',  ( 21.70312500061451644, 0.000000000000000000, 5.243569643749999010 ) ) ;
#48439=CARTESIAN_POINT ( 'NONE',  ( 12.86250000000000071, 2.886751345948126879, 4.999999999999999112 ) ) ;
#48440=CARTESIAN_POINT ( 'NONE',  ( 5.240625000614516971, -3.027376345333610441, -5.243569643749999898 ) ) ;
#48442=CARTESIAN_POINT ( 'NONE',  ( 19.91250000000000142, 2.886751345948129099, -4.999999999999998224 ) ) ;
#48443=CARTESIAN_POINT ( 'NONE',  ( 17.87812500061451715, 6.421520780324663323E-16, -5.243569643749999010 ) ) ;
#48444=CARTESIAN_POINT ( 'NONE',  ( 2.817472997146174052, -4.130598735093008678, -2.817472997146206026 ) ) ;
#48445=CARTESIAN_POINT ( 'NONE',  ( 23.13750000122903216, 6.123233995736764310E-16, -4.999999999999998224 ) ) ;
#48447=CARTESIAN_POINT ( 'NONE',  ( 3.149999999999999911, -4.330127018922190985, -2.500000000000001332 ) ) ;
#48449=CARTESIAN_POINT ( 'NONE',  ( 18.85312500061451502, 4.541064518000418104, -2.621784821874998173 ) ) ;
#48450=CARTESIAN_POINT ( 'NONE',  ( 25.56562500061452070, 3.027376345333613106, -5.243569643749998122 ) ) ;
#48451=CARTESIAN_POINT ( 'NONE',  ( 24.53437500061451715, -4.541064518000419881, 2.621784821874995952 ) ) ;
#48452=CARTESIAN_POINT ( 'NONE',  ( 10.12500000000000178, 4.330127018922191873, 2.499999999999999556 ) ) ;
#48453=CARTESIAN_POINT ( 'NONE',  ( 12.21562500061451573, 3.027376345333611329, 5.243569643749999010 ) ) ;
#48454=CARTESIAN_POINT ( 'NONE',  ( 27.32812500061451644, 6.421520780324663323E-16, -5.243569643749999010 ) ) ;
#48455=CARTESIAN_POINT ( 'NONE',  ( 17.25937500061451502, 0.000000000000000000, 5.243569643749999010 ) ) ;
#48456=CARTESIAN_POINT ( 'NONE',  ( 8.765625000614518214, -6.054752690667223547, -1.112240025338166033E-15 ) ) ;
#48457=FACE_OUTER_BOUND ( 'NONE', #55301, .T. ) ;
#48458=CARTESIAN_POINT ( 'NONE',  ( 2.121784821874999061, 12.05937500061451750, 26.32496088578401583 ) ) ;
#48459=CARTESIAN_POINT ( 'NONE',  ( 23.13750000122903216, 6.123233995736764310E-16, -4.999999999999998224 ) ) ;
#48461=CARTESIAN_POINT ( 'NONE',  ( 15.36562500061451608, 3.027376345333611329, 5.243569643749999010 ) ) ;
#48462=CARTESIAN_POINT ( 'NONE',  ( 8.746875000614515727, -3.027376345333614438, 5.243569643749998122 ) ) ;
#48463=CARTESIAN_POINT ( 'NONE',  ( 8.784375000614518925, -4.541064518000419881, 2.621784821874995952 ) ) ;
#48465=CARTESIAN_POINT ( 'NONE',  ( 29.55937500061451573, -4.541064518000417216, -2.621784821875001281 ) ) ;
#48466=CARTESIAN_POINT ( 'NONE',  ( 20.76562500061451644, 3.027376345333611329, 5.243569643749999010 ) ) ;
#48467=CARTESIAN_POINT ( 'NONE',  ( 16.17187500061451644, 3.027376345333613106, -5.243569643749998122 ) ) ;
#48468=CARTESIAN_POINT ( 'NONE',  ( 22.41562500061451502, 3.027376345333613106, -5.243569643749998122 ) ) ;
#48469=CARTESIAN_POINT ( 'NONE',  ( 8.484601909799253346E-16, 12.46250000000000213, 34.61880215351700230 ) ) ;
#48470=CARTESIAN_POINT ( 'NONE',  ( 26.65312500061451573, 0.000000000000000000, 5.243569643749999010 ) ) ;
#48471=CARTESIAN_POINT ( 'NONE',  ( 7.950000001229033053, 5.773502691896255534, 3.535250795749688894E-16 ) ) ;
#48474=CARTESIAN_POINT ( 'NONE',  ( 8.484601909799253346E-16, 18.31250000000000355, -25.38119784648299770 ) ) ;
#48475=CARTESIAN_POINT ( 'NONE',  ( 25.83750000122903501, 6.123233995736764310E-16, -4.999999999999998224 ) ) ;
#48477=CARTESIAN_POINT ( 'NONE',  ( 6.346875000614517148, 6.054752690667223547, 3.707466751127219781E-16 ) ) ;
#48479=CARTESIAN_POINT ( 'NONE',  ( 14.65312500061451573, -4.541064518000417216, -2.621784821875001281 ) ) ;
#48480=CARTESIAN_POINT ( 'NONE',  ( 8.746875000614515727, -3.027376345333614438, 5.243569643749998122 ) ) ;
#48481=CARTESIAN_POINT ( 'NONE',  ( 28.08750000122903145, 6.123233995736764310E-16, -4.999999999999998224 ) ) ;
#48482=CARTESIAN_POINT ( 'NONE',  ( 17.22187500061451715, 3.027376345333611329, 5.243569643749999010 ) ) ;
#48483=CARTESIAN_POINT ( 'NONE',  ( 5.296875000614518214, -3.027376345333610441, -5.243569643749999898 ) ) ;
#48484=CARTESIAN_POINT ( 'NONE',  ( 29.81250000000000000, 2.886751345948129099, -4.999999999999998224 ) ) ;
#48485=CARTESIAN_POINT ( 'NONE',  ( 5.128125000614516260, -4.541064518000419881, 2.621784821874995952 ) ) ;
#48486=CARTESIAN_POINT ( 'NONE',  ( 15.62812500061451537, 6.421520780324663323E-16, -5.243569643749999010 ) ) ;
#48487=ORIENTED_EDGE ( 'NONE', *, *, #8538, .F. ) ;
#48488=CARTESIAN_POINT ( 'NONE',  ( 11.65312500061451573, 4.541064518000418104, -2.621784821874998173 ) ) ;
#48489=CARTESIAN_POINT ( 'NONE',  ( 5.025000001229035895, -5.773502691896255534, -1.060575238724906372E-15 ) ) ;
#48490=CARTESIAN_POINT ( 'NONE',  ( 11.54062500061451857, -3.027376345333610441, -5.243569643749999898 ) ) ;
#48492=CARTESIAN_POINT ( 'NONE',  ( 11.25000000000000000, -4.330127018922190985, -2.500000000000001332 ) ) ;
#48493=CARTESIAN_POINT ( 'NONE',  ( 3.300000001229034918, -2.886751345948125991, -5.000000000000000000 ) ) ;
#48494=CARTESIAN_POINT ( 'NONE',  ( 17.55000000000000071, -4.330127018922190985, -2.500000000000001332 ) ) ;
#48495=CARTESIAN_POINT ( 'NONE',  ( 19.58437500061451786, -4.541064518000419881, 2.621784821874995952 ) ) ;
#48496=CARTESIAN_POINT ( 'NONE',  ( 16.87500000122903288, 2.886751345948129099, -4.999999999999998224 ) ) ;
#48498=CARTESIAN_POINT ( 'NONE',  ( 2.121784821875001281, 16.35312500061451857, -26.32496088578401938 ) ) ;
#48499=LINE ( 'NONE', #48131, #5286 ) ;
#48500=CARTESIAN_POINT ( 'NONE',  ( 7.320879633048903241E-15, 18.53750000000000142, 26.00000000000000355 ) ) ;
#48504=CARTESIAN_POINT ( 'NONE',  ( 15.49687500061451750, -3.027376345333614438, 5.243569643749998122 ) ) ;
#48506=EDGE_CURVE ( 'NONE', #13629, #55912, #8122, .T. ) ;
#48507=CARTESIAN_POINT ( 'NONE',  ( 10.97812500061451679, -4.541064518000419881, 2.621784821874995952 ) ) ;
#48509=CARTESIAN_POINT ( 'NONE',  ( 22.69687500061451857, -3.027376345333614438, 5.243569643749998122 ) ) ;
#48511=CARTESIAN_POINT ( 'NONE',  ( 7.715625000614515727, 3.027376345333611329, 5.243569643749999010 ) ) ;
#48512=CARTESIAN_POINT ( 'NONE',  ( 12.49687500061451573, -3.027376345333610441, -5.243569643749999898 ) ) ;
#48514=CARTESIAN_POINT ( 'NONE',  ( 23.25937500061451857, -4.541064518000417216, -2.621784821875001281 ) ) ;
#48515=CARTESIAN_POINT ( 'NONE',  ( 28.79062500061451502, 6.054752690667223547, 3.707466751127219781E-16 ) ) ;
#48517=CARTESIAN_POINT ( 'NONE',  ( 7.162500000000001421, -5.773502691896255534, -1.060575238724906372E-15 ) ) ;
#48518=CARTESIAN_POINT ( 'NONE',  ( 16.38750000122903216, 6.123233995736764310E-16, -4.999999999999998224 ) ) ;
#48519=CARTESIAN_POINT ( 'NONE',  ( 27.37500000122903998, 2.886751345948102454, 5.000000000000042633 ) ) ;
#48521=ORIENTED_EDGE ( 'NONE', *, *, #67203, .T. ) ;
#48522=CARTESIAN_POINT ( 'NONE',  ( 15.33750000000000036, -2.886751345948125991, -5.000000000000000000 ) ) ;
#48523=CARTESIAN_POINT ( 'NONE',  ( 18.22499999999999787, 4.330127018922191873, 2.499999999999999556 ) ) ;
#48524=CARTESIAN_POINT ( 'NONE',  ( 14.20312500061451644, -4.541064518000417216, -2.621784821875001281 ) ) ;
#48525=ORIENTED_EDGE ( 'NONE', *, *, #24878, .F. ) ;
#48526=CARTESIAN_POINT ( 'NONE',  ( 3.712500001229034563, -4.330127018922190985, -2.500000000000001332 ) ) ;
#48527=CARTESIAN_POINT ( 'NONE',  ( -4.243569643749999898, 16.25937500061451857, -30.00000000000000000 ) ) ;
#48528=CARTESIAN_POINT ( 'NONE',  ( 3.478125000614517237, 6.421520780324663323E-16, -5.243569643749999010 ) ) ;
#48529=CARTESIAN_POINT ( 'NONE',  ( 1.626862140677534273E-15, 12.01250000000000284, 34.00000000000000000 ) ) ;
#48530=CARTESIAN_POINT ( 'NONE',  ( 9.375000000000001776, -4.330127018922194537, 2.499999999999995559 ) ) ;
#48532=EDGE_LOOP ( 'NONE', ( #57998, #47201, #71522, #6951 ) ) ;
#48533=CARTESIAN_POINT ( 'NONE',  ( -4.243569643749997233, 14.44062500061451715, 32.45002607614398471 ) ) ;
#48534=CARTESIAN_POINT ( 'NONE',  ( 26.61562500061451786, 3.027376345333611329, 5.243569643749999010 ) ) ;
#48537=CARTESIAN_POINT ( 'NONE',  ( 23.07187500061451857, 3.027376345333611329, 5.243569643749999010 ) ) ;
#48538=CARTESIAN_POINT ( 'NONE',  ( 18.44062500061451715, 6.054752690667223547, 3.707466751127219781E-16 ) ) ;
#48539=CARTESIAN_POINT ( 'NONE',  ( -2.121784821874999949, 12.97812500061459318, -33.67503911421598417 ) ) ;
#48540=CARTESIAN_POINT ( 'NONE',  ( 23.17500000122903359, 2.886751345948129099, -4.999999999999998224 ) ) ;
#48541=CARTESIAN_POINT ( 'NONE',  ( 4.378125000614518925, 6.421520780324663323E-16, -5.243569643749999010 ) ) ;
#48543=CARTESIAN_POINT ( 'NONE',  ( 21.25312500061451715, 0.000000000000000000, 5.243569643749999010 ) ) ;
#48546=CARTESIAN_POINT ( 'NONE',  ( 17.82187500061451502, -6.054752690667223547, -1.112240025338166033E-15 ) ) ;
#48547=CARTESIAN_POINT ( 'NONE',  ( 16.54687500061451644, -3.027376345333610441, -5.243569643749999898 ) ) ;
#48548=CARTESIAN_POINT ( 'NONE',  ( 24.83437500061451431, 4.541064518000418104, 2.621784821874999949 ) ) ;
#48549=CARTESIAN_POINT ( 'NONE',  ( 2.121784821874999061, 15.20937500061451786, 26.32496088578401583 ) ) ;
#48550=CARTESIAN_POINT ( 'NONE',  ( 5.465625000614517504, 3.027376345333611329, 5.243569643749999010 ) ) ;
#48551=CARTESIAN_POINT ( 'NONE',  ( 29.01562500061451644, -6.054752690667223547, -1.112240025338166033E-15 ) ) ;
#48552=CARTESIAN_POINT ( 'NONE',  ( 28.19062500061451715, -3.027376345333610441, -5.243569643749999898 ) ) ;
#48553=CARTESIAN_POINT ( 'NONE',  ( 1.071796769724490783, 19.34509619066136565, -26.00000000000000000 ) ) ;
#48554=CARTESIAN_POINT ( 'NONE',  ( -3.999999999999999556, 19.06249999999999645, 27.69059892324149530 ) ) ;
#48555=CARTESIAN_POINT ( 'NONE',  ( 6.909375000614518036, 0.000000000000000000, 5.243569643749999010 ) ) ;
#48557=CARTESIAN_POINT ( 'NONE',  ( 13.16250000122903430, -4.330127018922190985, -2.500000000000001332 ) ) ;
#48558=CARTESIAN_POINT ( 'NONE',  ( 10.53750000122903252, 6.123233995736764310E-16, -4.999999999999998224 ) ) ;
#48559=CARTESIAN_POINT ( 'NONE',  ( 5.953125000614519102, 0.000000000000000000, 5.243569643749999010 ) ) ;
#48562=CARTESIAN_POINT ( 'NONE',  ( 15.27187500061451786, 3.027376345333613106, -5.243569643749998122 ) ) ;
#48563=CARTESIAN_POINT ( 'NONE',  ( 4.711411573247316298, 1.674097066322985938, -4.711411573247316298 ) ) ;
#48564=VERTEX_POINT ( 'NONE', #29300 ) ;
#48565=CARTESIAN_POINT ( 'NONE',  ( 22.04062500061451502, 6.054752690667223547, 3.707466751127219781E-16 ) ) ;
#48566=CARTESIAN_POINT ( 'NONE',  ( 8.240625000614516082, -3.027376345333614438, 5.243569643749998122 ) ) ;
#48567=CARTESIAN_POINT ( 'NONE',  ( 23.70937500061451786, -4.541064518000417216, -2.621784821875001281 ) ) ;
#48568=CARTESIAN_POINT ( 'NONE',  ( 7.715625000614515727, 3.027376345333611329, 5.243569643749999010 ) ) ;
#48569=CARTESIAN_POINT ( 'NONE',  ( 9.000000001229034652, -2.886751345948129988, 4.999999999999997335 ) ) ;
#48571=CARTESIAN_POINT ( 'NONE',  ( 22.30312500061451431, -4.541064518000417216, -2.621784821875001281 ) ) ;
#48572=CARTESIAN_POINT ( 'NONE',  ( -3.000416591977282496E-16, 11.14062500061451644, -34.90005215228797653 ) ) ;
#48573=CARTESIAN_POINT ( 'NONE',  ( 9.487500001229033586, -4.330127018922194537, 2.499999999999995559 ) ) ;
#48574=CARTESIAN_POINT ( 'NONE',  ( 20.16562500061451146, 3.027376345333613106, -5.243569643749998122 ) ) ;
#48576=CARTESIAN_POINT ( 'NONE',  ( 17.01562500061451644, 3.027376345333613106, -5.243569643749998122 ) ) ;
#48578=CARTESIAN_POINT ( 'NONE',  ( 18.97499999999999787, 6.123233995736764310E-16, -4.999999999999998224 ) ) ;
#48579=CARTESIAN_POINT ( 'NONE',  ( 10.38750000122903572, -4.330127018922194537, 2.499999999999995559 ) ) ;
#48580=CARTESIAN_POINT ( 'NONE',  ( 7.190625000614518036, 6.054752690667223547, 3.707466751127219781E-16 ) ) ;
#48581=CARTESIAN_POINT ( 'NONE',  ( 11.48437500061451644, -4.541064518000419881, 2.621784821874995952 ) ) ;
#48582=CARTESIAN_POINT ( 'NONE',  ( 12.25312500061451537, 0.000000000000000000, 5.243569643749999010 ) ) ;
#48583=EDGE_CURVE ( 'NONE', #13160, #30208, #40695, .T. ) ;
#48584=CARTESIAN_POINT ( 'NONE',  ( 24.22500000122903430, 2.886751345948126879, 4.999999999999999112 ) ) ;
#48585=CARTESIAN_POINT ( 'NONE',  ( 22.13437500061451502, 4.541064518000418104, 2.621784821874999949 ) ) ;
#48586=ADVANCED_FACE ( 'NONE', ( #59170 ), #31848, .F. ) ;
#48587=CARTESIAN_POINT ( 'NONE',  ( 5.662500001229035185, 4.330127018922192761, -2.499999999999997780 ) ) ;
#48588=CARTESIAN_POINT ( 'NONE',  ( 7.621875000614519280, 3.027376345333613106, -5.243569643749998122 ) ) ;
#48589=CARTESIAN_POINT ( 'NONE',  ( 23.03437500061451715, 4.541064518000418104, 2.621784821874999949 ) ) ;
#48590=( BOUNDED_SURFACE ( )  B_SPLINE_SURFACE ( 1, 2, ( 
 ( #18950, #7889, #13408, #52953, #7522, #64397, #46694, #24142, #52593, #34871, #41157, #69231, #12336, #57399, #6805, #29339, #63666, #18221, #63308, #35236, #18592, #13056, #30053, #2000, #36329, #25230, #70311, #48515, #60304, #47776, #19684, #3080, #59575, #31520, #15247, #58844, #48146, #65494, #8254, #42237, #37423, #8616, #71411, #25974, #31886, #8988, #64762, #54061, #30784, #53315, #20417, #14152, #42965, #14884, #9353, #25608, #48881, #2714, #70670, #54420, #20046, #3456, #59946, #3821, #42601, #71042, #65127, #36687, #59208, #31144, #53685, #14517, #37050, #26342, #20786, #43343, #65865, #37784, #14032, #46210, #69476, #29936, #59093, #46572, #68750, #58000, #42122, #18108, #51756, #29220, #24023, #30665, #41041, #25114, #12585, #53198, #69116, #7049, #58358, #70189, #40670, #30306, #52476, #12942, #1156, #19567, #7408, #24753, #57643, #24390, #35119, #52839, #1884, #36573, #1519, #47296, #36210, #58727, #63190, #69833, #7771, #29579, #23665, #18476, #52116, #2238, #63555, #35478, #41397, #46940, #18833, #47656, #63911, #19196, #13298, #35835, #41751, #64278, #13666, #8139, #2594, #64648, #43225, #71288, #54308, #8866, #43955, #9599, #66477, #21399, #20667, #3700, #15855, #26964, #36938, #26593, #65013, #71662, #65374, #9236, #54664, #14400, #38400, #65745, #15129, #8498, #59458, #31029, #26227, #42852, #49134, #19936, #66110, #37667, #60189, #48765, #31402, #53565, #32131, #2960, #25490, #4068, #21037, #48035, #49492, #53942, #43588, #3338, #15489, #14762, #31772, #38032, #25862, #70560, #60554, #9961, #42489, #48401, #70927, #32498, #37307, #55033, #4436, #72022, #20298, #59829, #18518, #52156, #18876, #63233, #24432, #36253, #12264, #46981, #1198, #30351, #13711, #69517, #1560, #68793, #58768, #34794, #41791, #17789, #18149, #40348, #57327, #62868, #7450, #46253, #2277, #12985, #41438, #63596, #69159, #28896, #51435, #52879, #6731, #837, #41083, #52518, #29265, #23704, #35521, #63955, #51795, #58041, #58402, #12627, #13340, #35877, #29977, #23346, #19236, #24794, #40716, #7815, #68426, #35162, #47337, #57686, #69870, #64320, #45895, #7091, #1927, #29621, #24070, #46615, #37708, #42163, #59134, #59499, #65418, #8542, #44646, #14806, #53609, #70600, #25530, #3001, #8912, #70967, #26268, #25903, #9277, #64689, #60229, #48072, #16537, #14074, #15170, #31443, #53984, #71334, #19973, #54710, #39090, #42526, #25156, #36977, #22088, #70233, #30705, #8177, #65052, #9643, #14442, #5107, #36613, #32176, #3381, #31070, #37350, #50177, #47696, #31811, #48443, #20340, #53238, #72705, #42893, #3743, #59872, #54350, #48805, #20710, #43268, #2635, #65789, #27641, #67176, #19606, #5470, #57145, #40179, #28010, #18337, #56437, #61972, #17619, #46442, #67533, #660, #16896, #50895, #6917, #56079, #51625, #11734, #68257, #12094, #45356, #11374, #29089, #73066, #46081, #23168, #51258, #34251, #33893, #23894, #62699, #68980, #1384, #45722, #56783, #61607, #29447, #39451, #6557, #44996, #1025, #67890, #62338, #34615, #5828, #11008, #23531, #68616, #33529, #28359, #50538, #6189, #22804, #17979, #40538, #63054, #28718, #12456, #34987, #57516, #295, #51985, #22447, #17262, #39824, #58955, #58228, #25352, #31261, #52342, #47526, #1745, #2108, #58595, #2458, #69343, #24619, #63777, #48263, #19801, #3198, #70787, #42354, #2824, #69698, #53803, #41265, #24981, #40910, #25726, #57868, #8002, #41621, #41989, #64876, #30537, #36074, #36441, #18701, #70055, #53064, #8363, #47898, #24258, #46806, #19428, #30171, #13165, #70426, #7277, #64140, #14264, #19063, #63423, #29807, #35706, #64509, #12810, #7633, #52702, #47166, #36803, #13902, #13527, #30892, #53434, #59318, #35345, #8727, #38261, #65609, #21631, #5023, #60789, #43456, #60056, #27558, #3566, #33088, #9099, #9467, #31637, #26089, #54169, #71893, #37534, #66720, #4304, #10195, #54897, #60418, #50089, #20162, #44189, #48627, #42716, #9829, #43820, #71152, #14997, #26829, #32730, #20524, #49363, #49727, #3934, #15722, #55267, #21266, #65237, #10560, #16093, #43083, #27192, #59692, #54532, #4662, #31997, #72254, #38641, #14627, #61165, #66344, #55627, #37166, #26457, #48997, #71527, #20902, #65978, #15358, #37900, #32359, #6105, #44916, #61888, #16815, #67453, #50813, #62256, #17536, #17180, #578, #33447, #51540, #39371, #6831, #55991, #6468, #215, #45273, #62612, #11293, #45994, #29366, #57061, #16450, #12008, #23448, #34531, #40098, #29003, #23083, #28636, #68531, #45641, #941, #5384, #50456, #22720, #56704, #72982, #34899, #51174, #33814, #56357, #5747, #28281, #67806, #11653, #17892, #39739, #68173, #27922, #40452, #34168, #72620, #22364, #62968, #12364, #57427, #22004, #44560, #67091, #39007, #61522, #10920, #64423, #2740, #13815, #19341, #52980, #30809, #41537, #47080, #47439, #29719, #35985, #69615, #41896, #36355, #12724, #63338, #58504, #41183, #35260, #58869, #18248, #2025, #8279, #7547, #51898, #40821, #57782, #30451, #59234, #7191, #52257, #63692, #53342, #64055, #24536, #25259, #13083, #69971, #8642, #1660, #47806, #24169, #70335, #36712, #19712, #18976, #18618, #1296, #46721, #64787, #69256, #35621, #58141, #30081, #52619, #2376, #13435, #42264, #7914, #14178, #24894, #23806, #46357, #68891, #32641, #59602, #53714, #20814, #54809, #9016, #3484, #15273, #71809, #37078, #37812, #60698, #14910, #26743, #66255, #65893, #31171, #21546, #27107, #14542, #38174, #70697, #65524, #21179, #48541, #49276, #10111, #25635, #43731, #4215, #60332, #55182, #32275, #4577, #65152, #31546, #9380, #9741, #54086, #66627, #15633, #26002, #20443, #71068, #42993, #31912, #43369, #49640, #48908, #72167, #37452, #44101, #59971, #38553, #54448, #16004, #3847, #26368, #61076, #71439, #3106, #48173, #20072, #42628, #22994, #34446, #45554 ),
 ( #39285, #10474, #72529, #67004, #62171, #17801, #21917, #16365, #22280, #62524, #132, #33729, #484, #44832, #6018, #40361, #38920, #28553, #55904, #11921, #68438, #51088, #56275, #50373, #33003, #61439, #23359, #44473, #72898, #10832, #33368, #5296, #11568, #27842, #56974, #67719, #68085, #45187, #50729, #55542, #4938, #6378, #67367, #27472, #22637, #34083, #16730, #61799, #17092, #17452, #11202, #39652, #40010, #5664, #28911, #51449, #56624, #50004, #852, #45907, #28200, #69884, #29277, #24081, #30364, #7103, #7828, #41804, #57339, #2652, #52530, #58053, #70250, #8193, #18161, #52893, #46266, #2290, #46628, #63606, #35891, #68805, #47711, #24444, #69528, #62880, #40730, #12276, #7462, #69170, #24806, #46992, #47351, #29988, #18887, #58415, #19249, #29632, #41449, #6744, #63967, #13350, #64335, #52170, #13727, #53253, #1210, #36269, #23716, #18530, #1938, #58783, #63245, #41095, #12639, #19622, #30721, #25170, #34808, #51807, #35174, #12996, #57698, #1572, #35532, #72077, #27025, #59149, #9294, #42910, #42179, #59516, #8558, #70983, #55096, #31086, #64704, #14088, #36993, #43647, #54002, #38090, #25548, #66171, #8929, #19989, #71352, #10022, #53625, #43285, #65433, #25919, #36628, #32558, #20359, #37725, #70615, #37366, #48091, #65805, #14824, #49556, #14460, #60245, #49193, #71726, #3017, #9659, #20726, #42542, #65068, #31459, #3398, #15187, #48459, #59889, #54365, #31827, #3760, #60613, #26284, #32193, #48821, #54726, #4129, #26659, #21096, #15547, #4496, #5931, #56185, #11112, #67284, #21825, #56889, #22553, #6294, #5578, #38464, #28115, #45101, #39560, #38839, #28465, #11838, #32921, #50644, #55459, #55821, #39199, #48, #49917, #5209, #44390, #28823, #398, #51362, #21459, #22906, #56538, #50289, #34357, #66915, #67637, #44014, #66536, #60990, #61713, #22196, #15916, #61354, #10389, #72813, #4851, #27385, #72441, #16284, #10751, #45464, #33282, #17369, #27750, #67996, #44750, #16643, #17003, #62440, #33641, #62085, #11478, #34001, #51000, #39926, #29550, #69448, #29192, #69086, #6664, #24362, #46545, #8109, #46182, #18805, #7741, #30277, #17719, #41369, #52449, #40279, #30637, #68721, #1127, #29909, #58699, #51726, #12914, #23636, #63161, #19168, #68358, #63879, #23997, #7378, #46909, #57616, #18081, #13270, #12193, #58330, #35447, #63527, #18447, #40642, #36181, #1855, #764, #13637, #57971, #41012, #23272, #41722, #12556, #35808, #57250, #52809, #7019, #1491, #2210, #35091, #45822, #24725, #47268, #62800, #52086, #34720, #69802, #64249, #71260, #37279, #65718, #48372, #9207, #48737, #60163, #19909, #43563, #8838, #20640, #8469, #70899, #59064, #3674, #25835, #60530, #25462, #43198, #9573, #32105, #70162, #15104, #31742, #19539, #9937, #48006, #53537, #54280, #38008, #31004, #65347, #2933, #42462, #71638, #47629, #37640, #3308, #59801, #26198, #36910, #70534, #54638, #64619, #4043, #14737, #42823, #20271, #64984, #15463, #26568, #53169, #66085, #49109, #21011, #2566, #25086, #14375, #42097, #36544, #14006, #59430, #53915, #31374, #15833, #17287, #67200, #39113, #32475, #38378, #55008, #50204, #66831, #50563, #16562, #45022, #27665, #61629, #28034, #39475, #72360, #11031, #49468, #33554, #56104, #73090, #49836, #16921, #22828, #43930, #5495, #66456, #16203, #72729, #22471, #60902, #38754, #55375, #39849, #11399, #67916, #62362, #33918, #67557, #61275, #45380, #32838, #61998, #4414, #26943, #72001, #22113, #33198, #21376, #21741, #10305, #10668, #4769, #27302, #44302, #55737, #5131, #56461, #44670, #28383, #5852, #50921, #319, #62724, #40936, #53733, #28742, #12836, #35010, #68641, #42646, #6941, #17642, #35370, #57540, #20089, #57170, #7301, #19731, #42281, #51282, #29832, #63450, #684, #11759, #6583, #12117, #57893, #70714, #40202, #23918, #34641, #1048, #31191, #6214, #1772, #29472, #18366, #52367, #18004, #29113, #25278, #23191, #70354, #46467, #1410, #52009, #51647, #48191, #47824, #34276, #25655, #69004, #64805, #56808, #3126, #23557, #14195, #68281, #36730, #40562, #12483, #59252, #46104, #45745, #8660, #63081, #65170, #48558, #14561, #9758, #26386, #10128, #49293, #4594, #60349, #21197, #60718, #72186, #31928, #71826, #9033, #43749, #66274, #32660, #9398, #49658, #55559, #3500, #15652, #26019, #48928, #32292, #26761, #20458, #71457, #14928, #72547, #44119, #27488, #21934, #66646, #27124, #20833, #4955, #65541, #38191, #37094, #50022, #31563, #54827, #65910, #59619, #54465, #54102, #43386, #71084, #43012, #37468, #59988, #3863, #16023, #15290, #61095, #37829, #38571, #4234, #55201, #21565, #33021, #10493, #45571, #67736, #28216, #1227, #34828, #148, #40028, #72914, #67023, #62188, #5680, #62541, #28570, #56991, #39668, #503, #11938, #51466, #11221, #51106, #61456, #23013, #68102, #34463, #61816, #28930, #57355, #55920, #17468, #5316, #50745, #11584, #6036, #22296, #22654, #67384, #51824, #23376, #6760, #44490, #45924, #6398, #45203, #29294, #44848, #869, #16383, #38938, #10850, #34101, #17109, #33384, #33745, #27858, #56640, #50389, #16746, #39303, #56290, #68456, #17818, #40379, #62898, #12293, #47728, #18547, #1589, #52910, #64719, #40748, #24823, #47011, #7479, #53641, #14103, #52550, #19267, #52187, #18905, #29649, #47370, #69546, #31101, #69187, #41821, #30738, #53270, #63263, #64353, #2308, #12655, #23733, #41112, #24099, #69901, #8573, #46647, #35909, #63622, #13012, #42195, #18179, #13743, #41466, #30381, #36285, #30007, #35550, #58799, #35190, #8209, #58434, #13367, #63985, #58069, #59165, #2668, #46282, #36643, #7844, #25185, #68822, #57715, #1956, #70267, #7120, #19638, #24463, #3774, #49207, #59531, #61006, #37740, #9674, #3033, #8943, #27041, #15564, #43664, #4143, #55112, #65820, #71367, #71741, #54017, #60260, #20742, #66186 ) ),
 .UNSPECIFIED., .F., .F., .F. ) 
 B_SPLINE_SURFACE_WITH_KNOTS ( ( 2, 2 ),
 ( 3, 2, 2, 2, 2, 2, 2, 2, 2, 2, 2, 2, 2, 2, 2, 2, 2, 2, 2, 2, 2, 2, 2, 2, 2, 2, 2, 2, 2, 2, 2, 2, 2, 2, 2, 2, 2, 2, 2, 2, 2, 2, 2, 2, 2, 2, 2, 2, 2, 2, 2, 2, 2, 2, 2, 2, 2, 2, 2, 2, 2, 2, 2, 2, 2, 2, 2, 2, 2, 2, 2, 2, 2, 2, 2, 2, 2, 2, 2, 2, 2, 2, 2, 2, 2, 2, 2, 2, 2, 2, 2, 2, 2, 2, 2, 2, 2, 2, 2, 2, 2, 2, 2, 2, 2, 2, 2, 2, 2, 2, 2, 2, 2, 2, 2, 2, 2, 2, 2, 2, 2, 2, 2, 2, 2, 2, 2, 2, 2, 2, 2, 2, 2, 2, 2, 2, 2, 2, 2, 2, 2, 2, 2, 2, 2, 2, 2, 2, 2, 2, 2, 2, 2, 2, 2, 2, 2, 2, 2, 2, 2, 2, 2, 2, 2, 2, 2, 2, 2, 2, 2, 2, 2, 2, 2, 2, 2, 2, 2, 2, 2, 2, 2, 2, 2, 2, 2, 2, 2, 2, 2, 2, 2, 2, 2, 2, 2, 2, 2, 2, 2, 2, 2, 2, 2, 2, 2, 2, 2, 2, 2, 2, 2, 2, 2, 2, 2, 2, 2, 2, 2, 2, 2, 2, 2, 2, 2, 2, 2, 2, 2, 2, 2, 2, 2, 2, 2, 2, 2, 2, 2, 2, 2, 2, 2, 2, 2, 2, 2, 2, 2, 2, 2, 2, 2, 2, 2, 2, 2, 2, 2, 2, 2, 2, 2, 2, 2, 2, 2, 2, 2, 2, 2, 2, 2, 2, 2, 2, 2, 2, 2, 2, 2, 2, 2, 2, 2, 2, 2, 2, 2, 2, 2, 2, 2, 2, 2, 2, 2, 2, 2, 2, 2, 2, 2, 2, 2, 2, 2, 2, 2, 2, 2, 2, 2, 2, 2, 2, 2, 2, 2, 2, 2, 2, 2, 2, 2, 2, 2, 2, 2, 2, 2, 2, 2, 2, 2, 2, 2, 2, 2, 2, 2, 2, 2, 2, 2, 2, 2, 2, 2, 2, 2, 2, 2, 2, 2, 2, 2, 2, 3 ),
 ( 0.000000000000000000, 1.000000000000000000 ),
 ( 0.000000000000000000, 0.002777777777777777884, 0.005555555555555555768, 0.008333333333333333218, 0.01111111111111111154, 0.01388888888888888812, 0.01666666666666666644, 0.01944444444444444475, 0.02222222222222222307, 0.02500000000000000139, 0.02777777777777777624, 0.03055555555555555455, 0.03333333333333333287, 0.03611111111111110772, 0.03888888888888888951, 0.04166666666666666435, 0.04444444444444444614, 0.04722222222222222099, 0.05000000000000000278, 0.05277777777777777762, 0.05555555555555555247, 0.05833333333333333426, 0.06111111111111110911, 0.06388888888888888395, 0.06666666666666666574, 0.06944444444444444753, 0.07222222222222221544, 0.07499999999999999722, 0.07777777777777777901, 0.08055555555555556080, 0.08333333333333332871, 0.08611111111111111049, 0.08888888888888889228, 0.09166666666666666019, 0.09444444444444444198, 0.09722222222222222376, 0.1000000000000000056, 0.1027777777777777735, 0.1055555555555555552, 0.1083333333333333370, 0.1111111111111111049, 0.1138888888888888867, 0.1166666666666666685, 0.1194444444444444503, 0.1222222222222222182, 0.1250000000000000000, 0.1277777777777777679, 0.1305555555555555636, 0.1333333333333333315, 0.1361111111111110994, 0.1388888888888888951, 0.1416666666666666630, 0.1444444444444444309, 0.1472222222222222265, 0.1499999999999999944, 0.1527777777777777901, 0.1555555555555555580, 0.1583333333333333259, 0.1611111111111111216, 0.1638888888888888895, 0.1666666666666666574, 0.1694444444444444531, 0.1722222222222222210, 0.1749999999999999889, 0.1777777777777777846, 0.1805555555555555525, 0.1833333333333333204, 0.1861111111111111160, 0.1888888888888888840, 0.1916666666666666796, 0.1944444444444444475, 0.1972222222222222154, 0.2000000000000000111, 0.2027777777777777790, 0.2055555555555555469, 0.2083333333333333426, 0.2111111111111111105, 0.2138888888888888784, 0.2166666666666666741, 0.2194444444444444420, 0.2222222222222222099, 0.2250000000000000056, 0.2277777777777777735, 0.2305555555555555691, 0.2333333333333333370, 0.2361111111111111049, 0.2388888888888889006, 0.2416666666666666685, 0.2444444444444444364, 0.2472222222222222321, 0.2500000000000000000, 0.2527777777777777679, 0.2555555555555555358, 0.2583333333333333592, 0.2611111111111111271, 0.2638888888888888951, 0.2666666666666666630, 0.2694444444444444309, 0.2722222222222221988, 0.2750000000000000222, 0.2777777777777777901, 0.2805555555555555580, 0.2833333333333333259, 0.2861111111111110938, 0.2888888888888888618, 0.2916666666666666852, 0.2944444444444444531, 0.2972222222222222210, 0.2999999999999999889, 0.3027777777777777568, 0.3055555555555555802, 0.3083333333333333481, 0.3111111111111111160, 0.3138888888888888840, 0.3166666666666666519, 0.3194444444444444198, 0.3222222222222222432, 0.3250000000000000111, 0.3277777777777777790, 0.3305555555555555469, 0.3333333333333333148, 0.3361111111111111382, 0.3388888888888889062, 0.3416666666666666741, 0.3444444444444444420, 0.3472222222222222099, 0.3499999999999999778, 0.3527777777777778012, 0.3555555555555555691, 0.3583333333333333370, 0.3611111111111111049, 0.3638888888888888729, 0.3666666666666666408, 0.3694444444444444642, 0.3722222222222222321, 0.3750000000000000000, 0.3777777777777777679, 0.3805555555555555358, 0.3833333333333333592, 0.3861111111111111271, 0.3888888888888888951, 0.3916666666666666630, 0.3944444444444444309, 0.3972222222222221988, 0.4000000000000000222, 0.4027777777777777901, 0.4055555555555555580, 0.4083333333333333259, 0.4111111111111110938, 0.4138888888888888618, 0.4166666666666666852, 0.4194444444444444531, 0.4222222222222222210, 0.4249999999999999889, 0.4277777777777777568, 0.4305555555555555802, 0.4333333333333333481, 0.4361111111111111160, 0.4388888888888888840, 0.4416666666666666519, 0.4444444444444444198, 0.4472222222222222432, 0.4500000000000000111, 0.4527777777777777790, 0.4555555555555555469, 0.4583333333333333148, 0.4611111111111111382, 0.4638888888888889062, 0.4666666666666666741, 0.4694444444444444420, 0.4722222222222222099, 0.4749999999999999778, 0.4777777777777778012, 0.4805555555555555691, 0.4833333333333333370, 0.4861111111111111049, 0.4888888888888888729, 0.4916666666666666408, 0.4944444444444444642, 0.4972222222222222321, 0.5000000000000000000, 0.5027777777777777679, 0.5055555555555555358, 0.5083333333333333037, 0.5111111111111110716, 0.5138888888888888395, 0.5166666666666667185, 0.5194444444444444864, 0.5222222222222222543, 0.5250000000000000222, 0.5277777777777777901, 0.5305555555555555580, 0.5333333333333333259, 0.5361111111111110938, 0.5388888888888888618, 0.5416666666666666297, 0.5444444444444443976, 0.5472222222222222765, 0.5500000000000000444, 0.5527777777777778123, 0.5555555555555555802, 0.5583333333333333481, 0.5611111111111111160, 0.5638888888888888840, 0.5666666666666666519, 0.5694444444444444198, 0.5722222222222221877, 0.5749999999999999556, 0.5777777777777777235, 0.5805555555555556024, 0.5833333333333333703, 0.5861111111111111382, 0.5888888888888889062, 0.5916666666666666741, 0.5944444444444444420, 0.5972222222222222099, 0.5999999999999999778, 0.6027777777777777457, 0.6055555555555555136, 0.6083333333333332815, 0.6111111111111111605, 0.6138888888888889284, 0.6166666666666666963, 0.6194444444444444642, 0.6222222222222222321, 0.6250000000000000000, 0.6277777777777777679, 0.6305555555555555358, 0.6333333333333333037, 0.6361111111111110716, 0.6388888888888888395, 0.6416666666666667185, 0.6444444444444444864, 0.6472222222222222543, 0.6500000000000000222, 0.6527777777777777901, 0.6555555555555555580, 0.6583333333333333259, 0.6611111111111110938, 0.6638888888888888618, 0.6666666666666666297, 0.6694444444444443976, 0.6722222222222222765, 0.6750000000000000444, 0.6777777777777778123, 0.6805555555555555802, 0.6833333333333333481, 0.6861111111111111160, 0.6888888888888888840, 0.6916666666666666519, 0.6944444444444444198, 0.6972222222222221877, 0.6999999999999999556, 0.7027777777777777235, 0.7055555555555556024, 0.7083333333333333703, 0.7111111111111111382, 0.7138888888888889062, 0.7166666666666666741, 0.7194444444444444420, 0.7222222222222222099, 0.7249999999999999778, 0.7277777777777777457, 0.7305555555555555136, 0.7333333333333332815, 0.7361111111111111605, 0.7388888888888889284, 0.7416666666666666963, 0.7444444444444444642, 0.7472222222222222321, 0.7500000000000000000, 0.7527777777777777679, 0.7555555555555555358, 0.7583333333333333037, 0.7611111111111110716, 0.7638888888888888395, 0.7666666666666667185, 0.7694444444444444864, 0.7722222222222222543, 0.7750000000000000222, 0.7777777777777777901, 0.7805555555555555580, 0.7833333333333333259, 0.7861111111111110938, 0.7888888888888888618, 0.7916666666666666297, 0.7944444444444443976, 0.7972222222222222765, 0.8000000000000000444, 0.8027777777777778123, 0.8055555555555555802, 0.8083333333333333481, 0.8111111111111111160, 0.8138888888888888840, 0.8166666666666666519, 0.8194444444444444198, 0.8222222222222221877, 0.8249999999999999556, 0.8277777777777777235, 0.8305555555555556024, 0.8333333333333333703, 0.8361111111111111382, 0.8388888888888889062, 0.8416666666666666741, 0.8444444444444444420, 0.8472222222222222099, 0.8499999999999999778, 0.8527777777777777457, 0.8555555555555555136, 0.8583333333333332815, 0.8611111111111111605, 0.8638888888888889284, 0.8666666666666666963, 0.8694444444444444642, 0.8722222222222222321, 0.8750000000000000000, 0.8777777777777777679, 0.8805555555555555358, 0.8833333333333333037, 0.8861111111111110716, 0.8888888888888888395, 0.8916666666666667185, 0.8944444444444444864, 0.8972222222222222543, 0.9000000000000000222, 0.9027777777777777901, 0.9055555555555555580, 0.9083333333333333259, 0.9111111111111110938, 0.9138888888888888618, 0.9166666666666666297, 0.9194444444444443976, 0.9222222222222222765, 0.9250000000000000444, 0.9277777777777778123, 0.9305555555555555802, 0.9333333333333333481, 0.9361111111111111160, 0.9388888888888888840, 0.9416666666666666519, 0.9444444444444444198, 0.9472222222222221877, 0.9499999999999999556, 0.9527777777777777235, 0.9555555555555556024, 0.9583333333333333703, 0.9611111111111111382, 0.9638888888888889062, 0.9666666666666666741, 0.9694444444444444420, 0.9722222222222222099, 0.9749999999999999778, 0.9777777777777777457, 0.9805555555555555136, 0.9833333333333332815, 0.9861111111111111605, 0.9888888888888889284, 0.9916666666666666963, 0.9944444444444444642, 0.9972222222222222321, 1.000000000000000000 ),
 .UNSPECIFIED. ) 
 GEOMETRIC_REPRESENTATION_ITEM ( )  RATIONAL_B_SPLINE_SURFACE ( (
 ( 1.000000000000000000, 0.8660254037844387076, 1.000000000000000000, 0.8660254037844387076, 1.000000000000000000, 0.8660254037844387076, 1.000000000000000000, 0.8660254037844387076, 1.000000000000000000, 0.8660254037844387076, 1.000000000000000000, 0.8660254037844387076, 1.000000000000000000, 0.8660254037844387076, 1.000000000000000000, 0.8660254037844387076, 1.000000000000000000, 0.8660254037844387076, 1.000000000000000000, 0.8660254037844387076, 1.000000000000000000, 0.8660254037844387076, 1.000000000000000000, 0.8660254037844387076, 1.000000000000000000, 0.8660254037844387076, 1.000000000000000000, 0.8660254037844387076, 1.000000000000000000, 0.8660254037844387076, 1.000000000000000000, 0.8660254037844387076, 1.000000000000000000, 0.8660254037844387076, 1.000000000000000000, 0.8660254037844387076, 1.000000000000000000, 0.8660254037844387076, 1.000000000000000000, 0.8660254037844387076, 1.000000000000000000, 0.8660254037844387076, 1.000000000000000000, 0.8660254037844387076, 1.000000000000000000, 0.8660254037844387076, 1.000000000000000000, 0.8660254037844387076, 1.000000000000000000, 0.8660254037844387076, 1.000000000000000000, 0.8660254037844387076, 1.000000000000000000, 0.8660254037844387076, 1.000000000000000000, 0.8660254037844387076, 1.000000000000000000, 0.8660254037844387076, 1.000000000000000000, 0.8660254037844387076, 1.000000000000000000, 0.8660254037844387076, 1.000000000000000000, 0.8660254037844387076, 1.000000000000000000, 0.8660254037844387076, 1.000000000000000000, 0.8660254037844387076, 1.000000000000000000, 0.8660254037844387076, 1.000000000000000000, 0.8660254037844387076, 1.000000000000000000, 0.8660254037844387076, 1.000000000000000000, 0.8660254037844387076, 1.000000000000000000, 0.8660254037844387076, 1.000000000000000000, 0.8660254037844387076, 1.000000000000000000, 0.8660254037844387076, 1.000000000000000000, 0.8660254037844387076, 1.000000000000000000, 0.8660254037844387076, 1.000000000000000000, 0.8660254037844387076, 1.000000000000000000, 0.8660254037844387076, 1.000000000000000000, 0.8660254037844387076, 1.000000000000000000, 0.8660254037844387076, 1.000000000000000000, 0.8660254037844387076, 1.000000000000000000, 0.8660254037844387076, 1.000000000000000000, 0.8660254037844387076, 1.000000000000000000, 0.8660254037844387076, 1.000000000000000000, 0.8660254037844387076, 1.000000000000000000, 0.8660254037844387076, 1.000000000000000000, 0.8660254037844387076, 1.000000000000000000, 0.8660254037844387076, 1.000000000000000000, 0.8660254037844387076, 1.000000000000000000, 0.8660254037844387076, 1.000000000000000000, 0.8660254037844387076, 1.000000000000000000, 0.8660254037844387076, 1.000000000000000000, 0.8660254037844387076, 1.000000000000000000, 0.8660254037844387076, 1.000000000000000000, 0.8660254037844387076, 1.000000000000000000, 0.8660254037844387076, 1.000000000000000000, 0.8660254037844387076, 1.000000000000000000, 0.8660254037844387076, 1.000000000000000000, 0.8660254037844387076, 1.000000000000000000, 0.8660254037844387076, 1.000000000000000000, 0.8660254037844387076, 1.000000000000000000, 0.8660254037844387076, 1.000000000000000000, 0.8660254037844387076, 1.000000000000000000, 0.8660254037844387076, 1.000000000000000000, 0.8660254037844387076, 1.000000000000000000, 0.8660254037844387076, 1.000000000000000000, 0.8660254037844387076, 1.000000000000000000, 0.8660254037844387076, 1.000000000000000000, 0.8660254037844387076, 1.000000000000000000, 0.8660254037844387076, 1.000000000000000000, 0.8660254037844387076, 1.000000000000000000, 0.8660254037844387076, 1.000000000000000000, 0.8660254037844387076, 1.000000000000000000, 0.8660254037844387076, 1.000000000000000000, 0.8660254037844387076, 1.000000000000000000, 0.8660254037844387076, 1.000000000000000000, 0.8660254037844387076, 1.000000000000000000, 0.8660254037844387076, 1.000000000000000000, 0.8660254037844387076, 1.000000000000000000, 0.8660254037844387076, 1.000000000000000000, 0.8660254037844387076, 1.000000000000000000, 0.8660254037844387076, 1.000000000000000000, 0.8660254037844387076, 1.000000000000000000, 0.8660254037844387076, 1.000000000000000000, 0.8660254037844387076, 1.000000000000000000, 0.8660254037844387076, 1.000000000000000000, 0.8660254037844387076, 1.000000000000000000, 0.8660254037844387076, 1.000000000000000000, 0.8660254037844387076, 1.000000000000000000, 0.8660254037844387076, 1.000000000000000000, 0.8660254037844387076, 1.000000000000000000, 0.8660254037844387076, 1.000000000000000000, 0.8660254037844387076, 1.000000000000000000, 0.8660254037844387076, 1.000000000000000000, 0.8660254037844387076, 1.000000000000000000, 0.8660254037844387076, 1.000000000000000000, 0.8660254037844387076, 1.000000000000000000, 0.8660254037844387076, 1.000000000000000000, 0.8660254037844387076, 1.000000000000000000, 0.8660254037844387076, 1.000000000000000000, 0.8660254037844387076, 1.000000000000000000, 0.8660254037844387076, 1.000000000000000000, 0.8660254037844387076, 1.000000000000000000, 0.8660254037844387076, 1.000000000000000000, 0.8660254037844387076, 1.000000000000000000, 0.8660254037844387076, 1.000000000000000000, 0.8660254037844387076, 1.000000000000000000, 0.8660254037844387076, 1.000000000000000000, 0.8660254037844387076, 1.000000000000000000, 0.8660254037844387076, 1.000000000000000000, 0.8660254037844387076, 1.000000000000000000, 0.8660254037844387076, 1.000000000000000000, 0.8660254037844387076, 1.000000000000000000, 0.8660254037844387076, 1.000000000000000000, 0.8660254037844387076, 1.000000000000000000, 0.8660254037844387076, 1.000000000000000000, 0.8660254037844387076, 1.000000000000000000, 0.8660254037844387076, 1.000000000000000000, 0.8660254037844387076, 1.000000000000000000, 0.8660254037844387076, 1.000000000000000000, 0.8660254037844387076, 1.000000000000000000, 0.8660254037844387076, 1.000000000000000000, 0.8660254037844387076, 1.000000000000000000, 0.8660254037844387076, 1.000000000000000000, 0.8660254037844387076, 1.000000000000000000, 0.8660254037844387076, 1.000000000000000000, 0.8660254037844387076, 1.000000000000000000, 0.8660254037844387076, 1.000000000000000000, 0.8660254037844387076, 1.000000000000000000, 0.8660254037844387076, 1.000000000000000000, 0.8660254037844387076, 1.000000000000000000, 0.8660254037844387076, 1.000000000000000000, 0.8660254037844387076, 1.000000000000000000, 0.8660254037844387076, 1.000000000000000000, 0.8660254037844387076, 1.000000000000000000, 0.8660254037844387076, 1.000000000000000000, 0.8660254037844387076, 1.000000000000000000, 0.8660254037844387076, 1.000000000000000000, 0.8660254037844387076, 1.000000000000000000, 0.8660254037844387076, 1.000000000000000000, 0.8660254037844387076, 1.000000000000000000, 0.8660254037844387076, 1.000000000000000000, 0.8660254037844387076, 1.000000000000000000, 0.8660254037844387076, 1.000000000000000000, 0.8660254037844387076, 1.000000000000000000, 0.8660254037844387076, 1.000000000000000000, 0.8660254037844387076, 1.000000000000000000, 0.8660254037844387076, 1.000000000000000000, 0.8660254037844387076, 1.000000000000000000, 0.8660254037844387076, 1.000000000000000000, 0.8660254037844387076, 1.000000000000000000, 0.8660254037844387076, 1.000000000000000000, 0.8660254037844387076, 1.000000000000000000, 0.8660254037844387076, 1.000000000000000000, 0.8660254037844387076, 1.000000000000000000, 0.8660254037844387076, 1.000000000000000000, 0.8660254037844387076, 1.000000000000000000, 0.8660254037844387076, 1.000000000000000000, 0.8660254037844387076, 1.000000000000000000, 0.8660254037844387076, 1.000000000000000000, 0.8660254037844387076, 1.000000000000000000, 0.8660254037844387076, 1.000000000000000000, 0.8660254037844387076, 1.000000000000000000, 0.8660254037844387076, 1.000000000000000000, 0.8660254037844387076, 1.000000000000000000, 0.8660254037844387076, 1.000000000000000000, 0.8660254037844387076, 1.000000000000000000, 0.8660254037844387076, 1.000000000000000000, 0.8660254037844387076, 1.000000000000000000, 0.8660254037844387076, 1.000000000000000000, 0.8660254037844387076, 1.000000000000000000, 0.8660254037844387076, 1.000000000000000000, 0.8660254037844387076, 1.000000000000000000, 0.8660254037844387076, 1.000000000000000000, 0.8660254037844387076, 1.000000000000000000, 0.8660254037844387076, 1.000000000000000000, 0.8660254037844387076, 1.000000000000000000, 0.8660254037844387076, 1.000000000000000000, 0.8660254037844387076, 1.000000000000000000, 0.8660254037844387076, 1.000000000000000000, 0.8660254037844387076, 1.000000000000000000, 0.8660254037844387076, 1.000000000000000000, 0.8660254037844387076, 1.000000000000000000, 0.8660254037844387076, 1.000000000000000000, 0.8660254037844387076, 1.000000000000000000, 0.8660254037844387076, 1.000000000000000000, 0.8660254037844387076, 1.000000000000000000, 0.8660254037844387076, 1.000000000000000000, 0.8660254037844387076, 1.000000000000000000, 0.8660254037844387076, 1.000000000000000000, 0.8660254037844387076, 1.000000000000000000, 0.8660254037844387076, 1.000000000000000000, 0.8660254037844387076, 1.000000000000000000, 0.8660254037844387076, 1.000000000000000000, 0.8660254037844387076, 1.000000000000000000, 0.8660254037844387076, 1.000000000000000000, 0.8660254037844387076, 1.000000000000000000, 0.8660254037844387076, 1.000000000000000000, 0.8660254037844387076, 1.000000000000000000, 0.8660254037844387076, 1.000000000000000000, 0.8660254037844387076, 1.000000000000000000, 0.8660254037844387076, 1.000000000000000000, 0.8660254037844387076, 1.000000000000000000, 0.8660254037844387076, 1.000000000000000000, 0.8660254037844387076, 1.000000000000000000, 0.8660254037844387076, 1.000000000000000000, 0.8660254037844387076, 1.000000000000000000, 0.8660254037844387076, 1.000000000000000000, 0.8660254037844387076, 1.000000000000000000, 0.8660254037844387076, 1.000000000000000000, 0.8660254037844387076, 1.000000000000000000, 0.8660254037844387076, 1.000000000000000000, 0.8660254037844387076, 1.000000000000000000, 0.8660254037844387076, 1.000000000000000000, 0.8660254037844387076, 1.000000000000000000, 0.8660254037844387076, 1.000000000000000000, 0.8660254037844387076, 1.000000000000000000, 0.8660254037844387076, 1.000000000000000000, 0.8660254037844387076, 1.000000000000000000, 0.8660254037844387076, 1.000000000000000000, 0.8660254037844387076, 1.000000000000000000, 0.8660254037844387076, 1.000000000000000000, 0.8660254037844387076, 1.000000000000000000, 0.8660254037844387076, 1.000000000000000000, 0.8660254037844387076, 1.000000000000000000, 0.8660254037844387076, 1.000000000000000000, 0.8660254037844387076, 1.000000000000000000, 0.8660254037844387076, 1.000000000000000000, 0.8660254037844387076, 1.000000000000000000, 0.8660254037844387076, 1.000000000000000000, 0.8660254037844387076, 1.000000000000000000, 0.8660254037844387076, 1.000000000000000000, 0.8660254037844387076, 1.000000000000000000, 0.8660254037844387076, 1.000000000000000000, 0.8660254037844387076, 1.000000000000000000, 0.8660254037844387076, 1.000000000000000000, 0.8660254037844387076, 1.000000000000000000, 0.8660254037844387076, 1.000000000000000000, 0.8660254037844387076, 1.000000000000000000, 0.8660254037844387076, 1.000000000000000000, 0.8660254037844387076, 1.000000000000000000, 0.8660254037844387076, 1.000000000000000000, 0.8660254037844387076, 1.000000000000000000, 0.8660254037844387076, 1.000000000000000000, 0.8660254037844387076, 1.000000000000000000, 0.8660254037844387076, 1.000000000000000000, 0.8660254037844387076, 1.000000000000000000, 0.8660254037844387076, 1.000000000000000000, 0.8660254037844387076, 1.000000000000000000, 0.8660254037844387076, 1.000000000000000000, 0.8660254037844387076, 1.000000000000000000, 0.8660254037844387076, 1.000000000000000000, 0.8660254037844387076, 1.000000000000000000, 0.8660254037844387076, 1.000000000000000000, 0.8660254037844387076, 1.000000000000000000, 0.8660254037844387076, 1.000000000000000000, 0.8660254037844387076, 1.000000000000000000, 0.8660254037844387076, 1.000000000000000000, 0.8660254037844387076, 1.000000000000000000, 0.8660254037844387076, 1.000000000000000000, 0.8660254037844387076, 1.000000000000000000, 0.8660254037844387076, 1.000000000000000000, 0.8660254037844387076, 1.000000000000000000, 0.8660254037844387076, 1.000000000000000000, 0.8660254037844387076, 1.000000000000000000, 0.8660254037844387076, 1.000000000000000000, 0.8660254037844387076, 1.000000000000000000, 0.8660254037844387076, 1.000000000000000000, 0.8660254037844387076, 1.000000000000000000, 0.8660254037844387076, 1.000000000000000000, 0.8660254037844387076, 1.000000000000000000, 0.8660254037844387076, 1.000000000000000000, 0.8660254037844387076, 1.000000000000000000, 0.8660254037844387076, 1.000000000000000000, 0.8660254037844387076, 1.000000000000000000, 0.8660254037844387076, 1.000000000000000000, 0.8660254037844387076, 1.000000000000000000, 0.8660254037844387076, 1.000000000000000000, 0.8660254037844387076, 1.000000000000000000, 0.8660254037844387076, 1.000000000000000000, 0.8660254037844387076, 1.000000000000000000, 0.8660254037844387076, 1.000000000000000000, 0.8660254037844387076, 1.000000000000000000, 0.8660254037844387076, 1.000000000000000000, 0.8660254037844387076, 1.000000000000000000, 0.8660254037844387076, 1.000000000000000000, 0.8660254037844387076, 1.000000000000000000, 0.8660254037844387076, 1.000000000000000000, 0.8660254037844387076, 1.000000000000000000, 0.8660254037844387076, 1.000000000000000000, 0.8660254037844387076, 1.000000000000000000, 0.8660254037844387076, 1.000000000000000000, 0.8660254037844387076, 1.000000000000000000, 0.8660254037844387076, 1.000000000000000000, 0.8660254037844387076, 1.000000000000000000, 0.8660254037844387076, 1.000000000000000000, 0.8660254037844387076, 1.000000000000000000, 0.8660254037844387076, 1.000000000000000000, 0.8660254037844387076, 1.000000000000000000, 0.8660254037844387076, 1.000000000000000000, 0.8660254037844387076, 1.000000000000000000, 0.8660254037844387076, 1.000000000000000000, 0.8660254037844387076, 1.000000000000000000, 0.8660254037844387076, 1.000000000000000000, 0.8660254037844387076, 1.000000000000000000, 0.8660254037844387076, 1.000000000000000000, 0.8660254037844387076, 1.000000000000000000, 0.8660254037844387076, 1.000000000000000000, 0.8660254037844387076, 1.000000000000000000, 0.8660254037844387076, 1.000000000000000000, 0.8660254037844387076, 1.000000000000000000, 0.8660254037844387076, 1.000000000000000000, 0.8660254037844387076, 1.000000000000000000, 0.8660254037844387076, 1.000000000000000000, 0.8660254037844387076, 1.000000000000000000, 0.8660254037844387076, 1.000000000000000000, 0.8660254037844387076, 1.000000000000000000, 0.8660254037844387076, 1.000000000000000000, 0.8660254037844387076, 1.000000000000000000, 0.8660254037844387076, 1.000000000000000000, 0.8660254037844387076, 1.000000000000000000, 0.8660254037844387076, 1.000000000000000000, 0.8660254037844387076, 1.000000000000000000, 0.8660254037844387076, 1.000000000000000000, 0.8660254037844387076, 1.000000000000000000, 0.8660254037844387076, 1.000000000000000000, 0.8660254037844387076, 1.000000000000000000, 0.8660254037844387076, 1.000000000000000000, 0.8660254037844387076, 1.000000000000000000, 0.8660254037844387076, 1.000000000000000000, 0.8660254037844387076, 1.000000000000000000, 0.8660254037844387076, 1.000000000000000000, 0.8660254037844387076, 1.000000000000000000, 0.8660254037844387076, 1.000000000000000000, 0.8660254037844387076, 1.000000000000000000, 0.8660254037844387076, 1.000000000000000000, 0.8660254037844387076, 1.000000000000000000, 0.8660254037844387076, 1.000000000000000000, 0.8660254037844387076, 1.000000000000000000, 0.8660254037844387076, 1.000000000000000000, 0.8660254037844387076, 1.000000000000000000, 0.8660254037844387076, 1.000000000000000000, 0.8660254037844387076, 1.000000000000000000, 0.8660254037844387076, 1.000000000000000000, 0.8660254037844387076, 1.000000000000000000, 0.8660254037844387076, 1.000000000000000000, 0.8660254037844387076, 1.000000000000000000, 0.8660254037844387076, 1.000000000000000000, 0.8660254037844387076, 1.000000000000000000, 0.8660254037844387076, 1.000000000000000000, 0.8660254037844387076, 1.000000000000000000, 0.8660254037844387076, 1.000000000000000000, 0.8660254037844387076, 1.000000000000000000),
 ( 1.000000000000000000, 0.8660254037844387076, 1.000000000000000000, 0.8660254037844387076, 1.000000000000000000, 0.8660254037844387076, 1.000000000000000000, 0.8660254037844387076, 1.000000000000000000, 0.8660254037844387076, 1.000000000000000000, 0.8660254037844387076, 1.000000000000000000, 0.8660254037844387076, 1.000000000000000000, 0.8660254037844387076, 1.000000000000000000, 0.8660254037844387076, 1.000000000000000000, 0.8660254037844387076, 1.000000000000000000, 0.8660254037844387076, 1.000000000000000000, 0.8660254037844387076, 1.000000000000000000, 0.8660254037844387076, 1.000000000000000000, 0.8660254037844387076, 1.000000000000000000, 0.8660254037844387076, 1.000000000000000000, 0.8660254037844387076, 1.000000000000000000, 0.8660254037844387076, 1.000000000000000000, 0.8660254037844387076, 1.000000000000000000, 0.8660254037844387076, 1.000000000000000000, 0.8660254037844387076, 1.000000000000000000, 0.8660254037844387076, 1.000000000000000000, 0.8660254037844387076, 1.000000000000000000, 0.8660254037844387076, 1.000000000000000000, 0.8660254037844387076, 1.000000000000000000, 0.8660254037844387076, 1.000000000000000000, 0.8660254037844387076, 1.000000000000000000, 0.8660254037844387076, 1.000000000000000000, 0.8660254037844387076, 1.000000000000000000, 0.8660254037844387076, 1.000000000000000000, 0.8660254037844387076, 1.000000000000000000, 0.8660254037844387076, 1.000000000000000000, 0.8660254037844387076, 1.000000000000000000, 0.8660254037844387076, 1.000000000000000000, 0.8660254037844387076, 1.000000000000000000, 0.8660254037844387076, 1.000000000000000000, 0.8660254037844387076, 1.000000000000000000, 0.8660254037844387076, 1.000000000000000000, 0.8660254037844387076, 1.000000000000000000, 0.8660254037844387076, 1.000000000000000000, 0.8660254037844387076, 1.000000000000000000, 0.8660254037844387076, 1.000000000000000000, 0.8660254037844387076, 1.000000000000000000, 0.8660254037844387076, 1.000000000000000000, 0.8660254037844387076, 1.000000000000000000, 0.8660254037844387076, 1.000000000000000000, 0.8660254037844387076, 1.000000000000000000, 0.8660254037844387076, 1.000000000000000000, 0.8660254037844387076, 1.000000000000000000, 0.8660254037844387076, 1.000000000000000000, 0.8660254037844387076, 1.000000000000000000, 0.8660254037844387076, 1.000000000000000000, 0.8660254037844387076, 1.000000000000000000, 0.8660254037844387076, 1.000000000000000000, 0.8660254037844387076, 1.000000000000000000, 0.8660254037844387076, 1.000000000000000000, 0.8660254037844387076, 1.000000000000000000, 0.8660254037844387076, 1.000000000000000000, 0.8660254037844387076, 1.000000000000000000, 0.8660254037844387076, 1.000000000000000000, 0.8660254037844387076, 1.000000000000000000, 0.8660254037844387076, 1.000000000000000000, 0.8660254037844387076, 1.000000000000000000, 0.8660254037844387076, 1.000000000000000000, 0.8660254037844387076, 1.000000000000000000, 0.8660254037844387076, 1.000000000000000000, 0.8660254037844387076, 1.000000000000000000, 0.8660254037844387076, 1.000000000000000000, 0.8660254037844387076, 1.000000000000000000, 0.8660254037844387076, 1.000000000000000000, 0.8660254037844387076, 1.000000000000000000, 0.8660254037844387076, 1.000000000000000000, 0.8660254037844387076, 1.000000000000000000, 0.8660254037844387076, 1.000000000000000000, 0.8660254037844387076, 1.000000000000000000, 0.8660254037844387076, 1.000000000000000000, 0.8660254037844387076, 1.000000000000000000, 0.8660254037844387076, 1.000000000000000000, 0.8660254037844387076, 1.000000000000000000, 0.8660254037844387076, 1.000000000000000000, 0.8660254037844387076, 1.000000000000000000, 0.8660254037844387076, 1.000000000000000000, 0.8660254037844387076, 1.000000000000000000, 0.8660254037844387076, 1.000000000000000000, 0.8660254037844387076, 1.000000000000000000, 0.8660254037844387076, 1.000000000000000000, 0.8660254037844387076, 1.000000000000000000, 0.8660254037844387076, 1.000000000000000000, 0.8660254037844387076, 1.000000000000000000, 0.8660254037844387076, 1.000000000000000000, 0.8660254037844387076, 1.000000000000000000, 0.8660254037844387076, 1.000000000000000000, 0.8660254037844387076, 1.000000000000000000, 0.8660254037844387076, 1.000000000000000000, 0.8660254037844387076, 1.000000000000000000, 0.8660254037844387076, 1.000000000000000000, 0.8660254037844387076, 1.000000000000000000, 0.8660254037844387076, 1.000000000000000000, 0.8660254037844387076, 1.000000000000000000, 0.8660254037844387076, 1.000000000000000000, 0.8660254037844387076, 1.000000000000000000, 0.8660254037844387076, 1.000000000000000000, 0.8660254037844387076, 1.000000000000000000, 0.8660254037844387076, 1.000000000000000000, 0.8660254037844387076, 1.000000000000000000, 0.8660254037844387076, 1.000000000000000000, 0.8660254037844387076, 1.000000000000000000, 0.8660254037844387076, 1.000000000000000000, 0.8660254037844387076, 1.000000000000000000, 0.8660254037844387076, 1.000000000000000000, 0.8660254037844387076, 1.000000000000000000, 0.8660254037844387076, 1.000000000000000000, 0.8660254037844387076, 1.000000000000000000, 0.8660254037844387076, 1.000000000000000000, 0.8660254037844387076, 1.000000000000000000, 0.8660254037844387076, 1.000000000000000000, 0.8660254037844387076, 1.000000000000000000, 0.8660254037844387076, 1.000000000000000000, 0.8660254037844387076, 1.000000000000000000, 0.8660254037844387076, 1.000000000000000000, 0.8660254037844387076, 1.000000000000000000, 0.8660254037844387076, 1.000000000000000000, 0.8660254037844387076, 1.000000000000000000, 0.8660254037844387076, 1.000000000000000000, 0.8660254037844387076, 1.000000000000000000, 0.8660254037844387076, 1.000000000000000000, 0.8660254037844387076, 1.000000000000000000, 0.8660254037844387076, 1.000000000000000000, 0.8660254037844387076, 1.000000000000000000, 0.8660254037844387076, 1.000000000000000000, 0.8660254037844387076, 1.000000000000000000, 0.8660254037844387076, 1.000000000000000000, 0.8660254037844387076, 1.000000000000000000, 0.8660254037844387076, 1.000000000000000000, 0.8660254037844387076, 1.000000000000000000, 0.8660254037844387076, 1.000000000000000000, 0.8660254037844387076, 1.000000000000000000, 0.8660254037844387076, 1.000000000000000000, 0.8660254037844387076, 1.000000000000000000, 0.8660254037844387076, 1.000000000000000000, 0.8660254037844387076, 1.000000000000000000, 0.8660254037844387076, 1.000000000000000000, 0.8660254037844387076, 1.000000000000000000, 0.8660254037844387076, 1.000000000000000000, 0.8660254037844387076, 1.000000000000000000, 0.8660254037844387076, 1.000000000000000000, 0.8660254037844387076, 1.000000000000000000, 0.8660254037844387076, 1.000000000000000000, 0.8660254037844387076, 1.000000000000000000, 0.8660254037844387076, 1.000000000000000000, 0.8660254037844387076, 1.000000000000000000, 0.8660254037844387076, 1.000000000000000000, 0.8660254037844387076, 1.000000000000000000, 0.8660254037844387076, 1.000000000000000000, 0.8660254037844387076, 1.000000000000000000, 0.8660254037844387076, 1.000000000000000000, 0.8660254037844387076, 1.000000000000000000, 0.8660254037844387076, 1.000000000000000000, 0.8660254037844387076, 1.000000000000000000, 0.8660254037844387076, 1.000000000000000000, 0.8660254037844387076, 1.000000000000000000, 0.8660254037844387076, 1.000000000000000000, 0.8660254037844387076, 1.000000000000000000, 0.8660254037844387076, 1.000000000000000000, 0.8660254037844387076, 1.000000000000000000, 0.8660254037844387076, 1.000000000000000000, 0.8660254037844387076, 1.000000000000000000, 0.8660254037844387076, 1.000000000000000000, 0.8660254037844387076, 1.000000000000000000, 0.8660254037844387076, 1.000000000000000000, 0.8660254037844387076, 1.000000000000000000, 0.8660254037844387076, 1.000000000000000000, 0.8660254037844387076, 1.000000000000000000, 0.8660254037844387076, 1.000000000000000000, 0.8660254037844387076, 1.000000000000000000, 0.8660254037844387076, 1.000000000000000000, 0.8660254037844387076, 1.000000000000000000, 0.8660254037844387076, 1.000000000000000000, 0.8660254037844387076, 1.000000000000000000, 0.8660254037844387076, 1.000000000000000000, 0.8660254037844387076, 1.000000000000000000, 0.8660254037844387076, 1.000000000000000000, 0.8660254037844387076, 1.000000000000000000, 0.8660254037844387076, 1.000000000000000000, 0.8660254037844387076, 1.000000000000000000, 0.8660254037844387076, 1.000000000000000000, 0.8660254037844387076, 1.000000000000000000, 0.8660254037844387076, 1.000000000000000000, 0.8660254037844387076, 1.000000000000000000, 0.8660254037844387076, 1.000000000000000000, 0.8660254037844387076, 1.000000000000000000, 0.8660254037844387076, 1.000000000000000000, 0.8660254037844387076, 1.000000000000000000, 0.8660254037844387076, 1.000000000000000000, 0.8660254037844387076, 1.000000000000000000, 0.8660254037844387076, 1.000000000000000000, 0.8660254037844387076, 1.000000000000000000, 0.8660254037844387076, 1.000000000000000000, 0.8660254037844387076, 1.000000000000000000, 0.8660254037844387076, 1.000000000000000000, 0.8660254037844387076, 1.000000000000000000, 0.8660254037844387076, 1.000000000000000000, 0.8660254037844387076, 1.000000000000000000, 0.8660254037844387076, 1.000000000000000000, 0.8660254037844387076, 1.000000000000000000, 0.8660254037844387076, 1.000000000000000000, 0.8660254037844387076, 1.000000000000000000, 0.8660254037844387076, 1.000000000000000000, 0.8660254037844387076, 1.000000000000000000, 0.8660254037844387076, 1.000000000000000000, 0.8660254037844387076, 1.000000000000000000, 0.8660254037844387076, 1.000000000000000000, 0.8660254037844387076, 1.000000000000000000, 0.8660254037844387076, 1.000000000000000000, 0.8660254037844387076, 1.000000000000000000, 0.8660254037844387076, 1.000000000000000000, 0.8660254037844387076, 1.000000000000000000, 0.8660254037844387076, 1.000000000000000000, 0.8660254037844387076, 1.000000000000000000, 0.8660254037844387076, 1.000000000000000000, 0.8660254037844387076, 1.000000000000000000, 0.8660254037844387076, 1.000000000000000000, 0.8660254037844387076, 1.000000000000000000, 0.8660254037844387076, 1.000000000000000000, 0.8660254037844387076, 1.000000000000000000, 0.8660254037844387076, 1.000000000000000000, 0.8660254037844387076, 1.000000000000000000, 0.8660254037844387076, 1.000000000000000000, 0.8660254037844387076, 1.000000000000000000, 0.8660254037844387076, 1.000000000000000000, 0.8660254037844387076, 1.000000000000000000, 0.8660254037844387076, 1.000000000000000000, 0.8660254037844387076, 1.000000000000000000, 0.8660254037844387076, 1.000000000000000000, 0.8660254037844387076, 1.000000000000000000, 0.8660254037844387076, 1.000000000000000000, 0.8660254037844387076, 1.000000000000000000, 0.8660254037844387076, 1.000000000000000000, 0.8660254037844387076, 1.000000000000000000, 0.8660254037844387076, 1.000000000000000000, 0.8660254037844387076, 1.000000000000000000, 0.8660254037844387076, 1.000000000000000000, 0.8660254037844387076, 1.000000000000000000, 0.8660254037844387076, 1.000000000000000000, 0.8660254037844387076, 1.000000000000000000, 0.8660254037844387076, 1.000000000000000000, 0.8660254037844387076, 1.000000000000000000, 0.8660254037844387076, 1.000000000000000000, 0.8660254037844387076, 1.000000000000000000, 0.8660254037844387076, 1.000000000000000000, 0.8660254037844387076, 1.000000000000000000, 0.8660254037844387076, 1.000000000000000000, 0.8660254037844387076, 1.000000000000000000, 0.8660254037844387076, 1.000000000000000000, 0.8660254037844387076, 1.000000000000000000, 0.8660254037844387076, 1.000000000000000000, 0.8660254037844387076, 1.000000000000000000, 0.8660254037844387076, 1.000000000000000000, 0.8660254037844387076, 1.000000000000000000, 0.8660254037844387076, 1.000000000000000000, 0.8660254037844387076, 1.000000000000000000, 0.8660254037844387076, 1.000000000000000000, 0.8660254037844387076, 1.000000000000000000, 0.8660254037844387076, 1.000000000000000000, 0.8660254037844387076, 1.000000000000000000, 0.8660254037844387076, 1.000000000000000000, 0.8660254037844387076, 1.000000000000000000, 0.8660254037844387076, 1.000000000000000000, 0.8660254037844387076, 1.000000000000000000, 0.8660254037844387076, 1.000000000000000000, 0.8660254037844387076, 1.000000000000000000, 0.8660254037844387076, 1.000000000000000000, 0.8660254037844387076, 1.000000000000000000, 0.8660254037844387076, 1.000000000000000000, 0.8660254037844387076, 1.000000000000000000, 0.8660254037844387076, 1.000000000000000000, 0.8660254037844387076, 1.000000000000000000, 0.8660254037844387076, 1.000000000000000000, 0.8660254037844387076, 1.000000000000000000, 0.8660254037844387076, 1.000000000000000000, 0.8660254037844387076, 1.000000000000000000, 0.8660254037844387076, 1.000000000000000000, 0.8660254037844387076, 1.000000000000000000, 0.8660254037844387076, 1.000000000000000000, 0.8660254037844387076, 1.000000000000000000, 0.8660254037844387076, 1.000000000000000000, 0.8660254037844387076, 1.000000000000000000, 0.8660254037844387076, 1.000000000000000000, 0.8660254037844387076, 1.000000000000000000, 0.8660254037844387076, 1.000000000000000000, 0.8660254037844387076, 1.000000000000000000, 0.8660254037844387076, 1.000000000000000000, 0.8660254037844387076, 1.000000000000000000, 0.8660254037844387076, 1.000000000000000000, 0.8660254037844387076, 1.000000000000000000, 0.8660254037844387076, 1.000000000000000000, 0.8660254037844387076, 1.000000000000000000, 0.8660254037844387076, 1.000000000000000000, 0.8660254037844387076, 1.000000000000000000, 0.8660254037844387076, 1.000000000000000000, 0.8660254037844387076, 1.000000000000000000, 0.8660254037844387076, 1.000000000000000000, 0.8660254037844387076, 1.000000000000000000, 0.8660254037844387076, 1.000000000000000000, 0.8660254037844387076, 1.000000000000000000, 0.8660254037844387076, 1.000000000000000000, 0.8660254037844387076, 1.000000000000000000, 0.8660254037844387076, 1.000000000000000000, 0.8660254037844387076, 1.000000000000000000, 0.8660254037844387076, 1.000000000000000000, 0.8660254037844387076, 1.000000000000000000, 0.8660254037844387076, 1.000000000000000000, 0.8660254037844387076, 1.000000000000000000, 0.8660254037844387076, 1.000000000000000000, 0.8660254037844387076, 1.000000000000000000, 0.8660254037844387076, 1.000000000000000000, 0.8660254037844387076, 1.000000000000000000, 0.8660254037844387076, 1.000000000000000000, 0.8660254037844387076, 1.000000000000000000, 0.8660254037844387076, 1.000000000000000000, 0.8660254037844387076, 1.000000000000000000, 0.8660254037844387076, 1.000000000000000000, 0.8660254037844387076, 1.000000000000000000, 0.8660254037844387076, 1.000000000000000000, 0.8660254037844387076, 1.000000000000000000, 0.8660254037844387076, 1.000000000000000000, 0.8660254037844387076, 1.000000000000000000, 0.8660254037844387076, 1.000000000000000000, 0.8660254037844387076, 1.000000000000000000, 0.8660254037844387076, 1.000000000000000000, 0.8660254037844387076, 1.000000000000000000, 0.8660254037844387076, 1.000000000000000000, 0.8660254037844387076, 1.000000000000000000, 0.8660254037844387076, 1.000000000000000000, 0.8660254037844387076, 1.000000000000000000, 0.8660254037844387076, 1.000000000000000000, 0.8660254037844387076, 1.000000000000000000, 0.8660254037844387076, 1.000000000000000000, 0.8660254037844387076, 1.000000000000000000, 0.8660254037844387076, 1.000000000000000000, 0.8660254037844387076, 1.000000000000000000, 0.8660254037844387076, 1.000000000000000000, 0.8660254037844387076, 1.000000000000000000, 0.8660254037844387076, 1.000000000000000000, 0.8660254037844387076, 1.000000000000000000, 0.8660254037844387076, 1.000000000000000000, 0.8660254037844387076, 1.000000000000000000, 0.8660254037844387076, 1.000000000000000000, 0.8660254037844387076, 1.000000000000000000, 0.8660254037844387076, 1.000000000000000000, 0.8660254037844387076, 1.000000000000000000, 0.8660254037844387076, 1.000000000000000000, 0.8660254037844387076, 1.000000000000000000, 0.8660254037844387076, 1.000000000000000000, 0.8660254037844387076, 1.000000000000000000, 0.8660254037844387076, 1.000000000000000000, 0.8660254037844387076, 1.000000000000000000, 0.8660254037844387076, 1.000000000000000000, 0.8660254037844387076, 1.000000000000000000, 0.8660254037844387076, 1.000000000000000000, 0.8660254037844387076, 1.000000000000000000) ) ) 
 REPRESENTATION_ITEM ( '' )  SURFACE ( )  );
#48591=CARTESIAN_POINT ( 'NONE',  ( 4.805076099715074989, -1.383418685542648907, 4.830700292553183672 ) ) ;
#48592=CARTESIAN_POINT ( 'NONE',  ( 19.86562500061451786, 3.027376345333611329, 5.243569643749999010 ) ) ;
#48593=CARTESIAN_POINT ( 'NONE',  ( 25.17187500061451644, 3.027376345333613106, -5.243569643749998122 ) ) ;
#48595=CARTESIAN_POINT ( 'NONE',  ( 3.366080804335946919, -3.697228694398128290, 3.718268762498968094 ) ) ;
#48596=FACE_OUTER_BOUND ( 'NONE', #26899, .T. ) ;
#48597=CARTESIAN_POINT ( 'NONE',  ( 6.196875000614515905, -3.027376345333610441, -5.243569643749999898 ) ) ;
#48598=CARTESIAN_POINT ( 'NONE',  ( 15.36562500061451608, 3.027376345333611329, 5.243569643749999010 ) ) ;
#48599=CARTESIAN_POINT ( 'NONE',  ( 13.17187500061451999, 3.027376345333611329, 5.243569643749999010 ) ) ;
#48600=EDGE_LOOP ( 'NONE', ( #1913, #1682, #43488, #63713 ) ) ;
#48601=CARTESIAN_POINT ( 'NONE',  ( 24.74062500061451786, 6.054752690667223547, 3.707466751127219781E-16 ) ) ;
#48602=DIRECTION ( 'NONE',  ( -1.000000000000000000, -0.000000000000000000, -0.000000000000000000 ) ) ;
#48603=CARTESIAN_POINT ( 'NONE',  ( -2.000000000000000000, 11.48750000122903359, -33.46410161513775705 ) ) ;
#48604=CARTESIAN_POINT ( 'NONE',  ( 13.83749999999999858, -2.886751345948129988, 4.999999999999997335 ) ) ;
#48605=CARTESIAN_POINT ( 'NONE',  ( 23.58750000122903145, 6.123233995736764310E-16, -4.999999999999998224 ) ) ;
#48606=CARTESIAN_POINT ( 'NONE',  ( 18.40312500061451573, 4.541064518000418104, -2.621784821874998173 ) ) ;
#48607=VERTEX_POINT ( 'NONE', #49212 ) ;
#48608=CARTESIAN_POINT ( 'NONE',  ( 22.12500000000000000, 6.123233995736764310E-16, -4.999999999999998224 ) ) ;
#48609=CARTESIAN_POINT ( 'NONE',  ( 24.45937500061451786, 0.000000000000000000, 5.243569643749999010 ) ) ;
#48612=CARTESIAN_POINT ( 'NONE',  ( 11.27812500061451573, 4.541064518000418104, 2.621784821874999949 ) ) ;
#48613=CARTESIAN_POINT ( 'NONE',  ( 3.778125000614519280, -4.541064518000419881, 2.621784821874995952 ) ) ;
#48615=CARTESIAN_POINT ( 'NONE',  ( 27.25312500061451360, -4.541064518000417216, -2.621784821875001281 ) ) ;
#48616=CARTESIAN_POINT ( 'NONE',  ( 18.41250000000000142, -5.773502691896255534, -1.060575238724906372E-15 ) ) ;
#48617=CARTESIAN_POINT ( 'NONE',  ( 26.25000000000000000, 4.330127018922192761, -2.499999999999997780 ) ) ;
#48618=CARTESIAN_POINT ( 'NONE',  ( 3.176339285701963888, -3.861459405730729433, 3.176339285701963888 ) ) ;
#48619=CARTESIAN_POINT ( 'NONE',  ( 7.434375000614519280, -4.541064518000419881, 2.621784821874995952 ) ) ;
#48620=CARTESIAN_POINT ( 'NONE',  ( 17.59687500061451715, 6.054752690667223547, 3.707466751127219781E-16 ) ) ;
#48622=ORIENTED_EDGE ( 'NONE', *, *, #19782, .T. ) ;
#48623=CARTESIAN_POINT ( 'NONE',  ( 27.02812500061451573, 4.541064518000418104, 2.621784821874999949 ) ) ;
#48624=CARTESIAN_POINT ( 'NONE',  ( 28.43437500061451573, 4.541064518000418104, 2.621784821874999949 ) ) ;
#48626=CARTESIAN_POINT ( 'NONE',  ( 13.31250000000000178, 2.886751345948126879, 4.999999999999999112 ) ) ;
#48627=CARTESIAN_POINT ( 'NONE',  ( 11.54062500061451857, -3.027376345333610441, -5.243569643749999898 ) ) ;
#48630=CARTESIAN_POINT ( 'NONE',  ( 27.96562500061451573, 3.027376345333611329, 5.243569643749999010 ) ) ;
#48631=CARTESIAN_POINT ( 'NONE',  ( 19.57500000122903216, 2.886751345948129099, -4.999999999999998224 ) ) ;
#48634=CARTESIAN_POINT ( 'NONE',  ( 5.165625000614518569, -6.054752690667223547, -1.112240025338166033E-15 ) ) ;
#48635=CARTESIAN_POINT ( 'NONE',  ( 23.03437500061451715, 4.541064518000418104, 2.621784821874999949 ) ) ;
#48636=CARTESIAN_POINT ( 'NONE',  ( 4.243569643749999898, 16.93437500061451573, 30.00000000000000000 ) ) ;
#48637=CARTESIAN_POINT ( 'NONE',  ( 23.63437500061451502, -4.541064518000419881, 2.621784821874995952 ) ) ;
#48638=CARTESIAN_POINT ( 'NONE',  ( 4.650000000000001243, 4.330127018922192761, -2.499999999999997780 ) ) ;
#48639=CARTESIAN_POINT ( 'NONE',  ( 3.999999999999998668, 11.82500000122903572, 27.69059892324149175 ) ) ;
#48640=CARTESIAN_POINT ( 'NONE',  ( 12.17812500061451608, 4.541064518000418104, 2.621784821874999949 ) ) ;
#48641=CARTESIAN_POINT ( 'NONE',  ( 4.125000001229034652, -5.773502691896255534, -1.060575238724906372E-15 ) ) ;
#48643=CARTESIAN_POINT ( 'NONE',  ( 10.05937500061451750, 0.000000000000000000, 5.243569643749999010 ) ) ;
#48645=CARTESIAN_POINT ( 'NONE',  ( 9.628125000614517148, -4.541064518000419881, 2.621784821874995952 ) ) ;
#48646=CARTESIAN_POINT ( 'NONE',  ( 14.55937500061451573, 0.000000000000000000, 5.243569643749999010 ) ) ;
#48648=CARTESIAN_POINT ( 'NONE',  ( 21.93750000122903288, 4.330127018922191873, 2.499999999999999556 ) ) ;
#48649=CARTESIAN_POINT ( 'NONE',  ( 10.99687500061451750, -3.027376345333614438, 5.243569643749998122 ) ) ;
#48650=CARTESIAN_POINT ( 'NONE',  ( 12.85312500061451502, -4.541064518000417216, -2.621784821875001281 ) ) ;
#48652=CARTESIAN_POINT ( 'NONE',  ( 20.44687500061451857, -3.027376345333614438, 5.243569643749998122 ) ) ;
#48654=( BOUNDED_CURVE ( )  B_SPLINE_CURVE ( 1, ( #46167, #68707 ),
 .UNSPECIFIED., .F., .F. ) 
 B_SPLINE_CURVE_WITH_KNOTS ( ( 2, 2 ),
 ( 0.000000000000000000, 1.000000000000000000 ),
 .UNSPECIFIED. ) 
 CURVE ( )  GEOMETRIC_REPRESENTATION_ITEM ( )  RATIONAL_B_SPLINE_CURVE ( ( 0.9401540970596797830, 0.9401540970596797830 ) ) 
 REPRESENTATION_ITEM ( '' )  );
#48655=CARTESIAN_POINT ( 'NONE',  ( -1.351880753582008765, 4.820610340066097343, 26.22604083275753695 ) ) ;
#48656=CARTESIAN_POINT ( 'NONE',  ( 2.121784821875001281, 14.15937500061451715, -26.32496088578401938 ) ) ;
#48657=CARTESIAN_POINT ( 'NONE',  ( 16.20000000122903216, -2.886751345948129988, 4.999999999999997335 ) ) ;
#48658=CARTESIAN_POINT ( 'NONE',  ( 10.28437500061451715, 6.421520780324663323E-16, -5.243569643749999010 ) ) ;
#48659=CARTESIAN_POINT ( 'NONE',  ( 4.243569643749999898, 18.64062500061451644, -27.54997392385601529 ) ) ;
#48660=CARTESIAN_POINT ( 'NONE',  ( 18.75000000122903288, 5.773502691896255534, 3.535250795749688894E-16 ) ) ;
#48661=CARTESIAN_POINT ( 'NONE',  ( 13.75312500061451715, -4.541064518000417216, -2.621784821875001281 ) ) ;
#48662=VERTEX_POINT ( 'NONE', #54384 ) ;
#48663=CARTESIAN_POINT ( 'NONE',  ( 16.87500000000000000, 4.330127018922191873, 2.499999999999999556 ) ) ;
#48664=CARTESIAN_POINT ( 'NONE',  ( 29.32499999999999929, 6.123233995736764310E-16, -4.999999999999998224 ) ) ;
#48665=CARTESIAN_POINT ( 'NONE',  ( 9.084375000614517859, 4.541064518000418104, 2.621784821874999949 ) ) ;
#48667=CARTESIAN_POINT ( 'NONE',  ( 11.40000000122903501, -2.886751345948125991, -5.000000000000000000 ) ) ;
#48668=CARTESIAN_POINT ( 'NONE',  ( 17.70000000122903216, -2.886751345948125991, -5.000000000000000000 ) ) ;
#48669=CARTESIAN_POINT ( 'NONE',  ( 15.96562500061451573, -6.054752690667223547, -1.112240025338166033E-15 ) ) ;
#48671=CARTESIAN_POINT ( 'NONE',  ( 19.56562500061451715, -6.054752690667223547, -1.112240025338166033E-15 ) ) ;
#48672=CARTESIAN_POINT ( 'NONE',  ( 27.86250000122903359, 0.000000000000000000, 4.999999999999998224 ) ) ;
#48673=( BOUNDED_CURVE ( )  B_SPLINE_CURVE ( 2, ( #15758, #50491, #38298, #49764, #73017, #60826, #16128, #22401, #16850 ),
 .UNSPECIFIED., .F., .F. ) 
 B_SPLINE_CURVE_WITH_KNOTS ( ( 3, 2, 2, 2, 3 ),
 ( 0.5978260869565217295, 0.6014492753623188470, 0.6086956521739130821, 0.6159420289855072062, 0.6195652173913043237 ),
 .UNSPECIFIED. ) 
 CURVE ( )  GEOMETRIC_REPRESENTATION_ITEM ( )  RATIONAL_B_SPLINE_CURVE ( ( 0.9330127018922194093, 0.9330127018922194093, 1.000000000000000000, 0.8660254037844387076, 1.000000000000000000, 0.8660254037844387076, 1.000000000000000000, 0.9330127018922194093, 0.9330127018922194093 ) ) 
 REPRESENTATION_ITEM ( '' )  );
#48674=CARTESIAN_POINT ( 'NONE',  ( 3.703125000614516882, 0.000000000000000000, 5.243569643749999010 ) ) ;
#48675=CARTESIAN_POINT ( 'NONE',  ( 24.48749999999999716, 5.773502691896255534, 3.535250795749688894E-16 ) ) ;
#48678=CARTESIAN_POINT ( 'NONE',  ( 29.29687500061451644, 6.054752690667223547, 3.707466751127219781E-16 ) ) ;
#48679=CARTESIAN_POINT ( 'NONE',  ( 0.000000000000000000, 20.00000000000000000, 26.00000000000000000 ) ) ;
#48680=CARTESIAN_POINT ( 'NONE',  ( 12.18750000122903465, -4.330127018922194537, 2.499999999999995559 ) ) ;
#48681=CARTESIAN_POINT ( 'NONE',  ( 29.29687500061451644, 6.054752690667223547, 3.707466751127219781E-16 ) ) ;
#48682=CARTESIAN_POINT ( 'NONE',  ( 30.00000000000000000, 0.000000000000000000, 0.000000000000000000 ) ) ;
#48683=CARTESIAN_POINT ( 'NONE',  ( 6.834375000614518747, 4.541064518000418104, 2.621784821874999949 ) ) ;
#48684=CARTESIAN_POINT ( 'NONE',  ( 27.02812500061451573, 4.541064518000418104, 2.621784821874999949 ) ) ;
#48687=CARTESIAN_POINT ( 'NONE',  ( 4.363395578908656702, -2.441916286472800124, 4.408370384982540635 ) ) ;
#48688=CARTESIAN_POINT ( 'NONE',  ( 5.784375000614517148, 6.421520780324663323E-16, -5.243569643749999010 ) ) ;
#48689=CARTESIAN_POINT ( 'NONE',  ( 9.871875000614517504, 3.027376345333613106, -5.243569643749998122 ) ) ;
#48690=CARTESIAN_POINT ( 'NONE',  ( 4.425000000000001599, -4.330127018922194537, 2.499999999999995559 ) ) ;
#48691=EDGE_CURVE ( 'NONE', #54526, #427, #44533, .T. ) ;
#48692=CARTESIAN_POINT ( 'NONE',  ( -2.121784821874996840, 13.57812500061459282, 33.67503911421598417 ) ) ;
#48693=CARTESIAN_POINT ( 'NONE',  ( 21.86250000000000071, 2.886751345948126879, 4.999999999999999112 ) ) ;
#48694=CARTESIAN_POINT ( 'NONE',  ( 29.17500000000000071, -4.330127018922194537, 2.499999999999995559 ) ) ;
#48695=CARTESIAN_POINT ( 'NONE',  ( 4.125000000000000000, 6.123233995736764310E-16, -4.999999999999998224 ) ) ;
#48697=ORIENTED_EDGE ( 'NONE', *, *, #62265, .F. ) ;
#48698=CARTESIAN_POINT ( 'NONE',  ( 20.95312500061451999, -4.541064518000417216, -2.621784821875001281 ) ) ;
#48699=CARTESIAN_POINT ( 'NONE',  ( 9.628125000614517148, -4.541064518000419881, 2.621784821874995952 ) ) ;
#48701=CARTESIAN_POINT ( 'NONE',  ( 7.396875000614519635, -3.027376345333614438, 5.243569643749998122 ) ) ;
#48702=CARTESIAN_POINT ( 'NONE',  ( 24.41250000000000142, 2.886751345948129099, -4.999999999999998224 ) ) ;
#48703=CARTESIAN_POINT ( 'NONE',  ( 19.87500000122903288, -5.773502691896255534, -1.060575238724906372E-15 ) ) ;
#48704=CARTESIAN_POINT ( 'NONE',  ( 27.06562500061451004, 3.027376345333611329, 5.243569643749999010 ) ) ;
#48705=CARTESIAN_POINT ( 'NONE',  ( 3.242103837493086330E-14, 11.00000000122903288, 26.00000000000000711 ) ) ;
#48706=CARTESIAN_POINT ( 'NONE',  ( 9.384375000614518569, 6.421520780324663323E-16, -5.243569643749999010 ) ) ;
#48707=CARTESIAN_POINT ( 'NONE',  ( 15.27187500061451786, 3.027376345333613106, -5.243569643749998122 ) ) ;
#48708=CARTESIAN_POINT ( 'NONE',  ( 24.94687500061451502, -3.027376345333614438, 5.243569643749998122 ) ) ;
#48709=LINE ( 'NONE', #3279, #31223 ) ;
#48710=EDGE_CURVE ( 'NONE', #2558, #49922, #3779, .T. ) ;
#48712=CARTESIAN_POINT ( 'NONE',  ( 17.67187500061451644, 3.027376345333611329, 5.243569643749999010 ) ) ;
#48713=CARTESIAN_POINT ( 'NONE',  ( 10.24687500061451750, -3.027376345333610441, -5.243569643749999898 ) ) ;
#48715=CARTESIAN_POINT ( 'NONE',  ( 23.62500000000000000, 4.330127018922191873, 2.499999999999999556 ) ) ;
#48717=CARTESIAN_POINT ( 'NONE',  ( -2.000000000000000000, 9.687500001229034652, -33.46410161513775705 ) ) ;
#48719=CARTESIAN_POINT ( 'NONE',  ( 11.84062500061451750, -3.027376345333614438, 5.243569643749998122 ) ) ;
#48720=CARTESIAN_POINT ( 'NONE',  ( 29.25937500061451502, 4.541064518000418104, -2.621784821874998173 ) ) ;
#48721=CARTESIAN_POINT ( 'NONE',  ( -5.810221930991193690E-16, 10.10000000122903430, -34.00000000000000000 ) ) ;
#48722=CARTESIAN_POINT ( 'NONE',  ( 11.25000000000000000, -4.330127018922190985, -2.500000000000001332 ) ) ;
#48723=CARTESIAN_POINT ( 'NONE',  ( -1.999999999999997113, 18.83750000122903501, 33.46410161513775705 ) ) ;
#48724=CARTESIAN_POINT ( 'NONE',  ( 10.95000000122903394, -2.886751345948125991, -5.000000000000000000 ) ) ;
#48725=CARTESIAN_POINT ( 'NONE',  ( 22.92187500061451644, 3.027376345333613106, -5.243569643749998122 ) ) ;
#48726=CARTESIAN_POINT ( 'NONE',  ( 17.07187500061451502, 3.027376345333613106, -5.243569643749998122 ) ) ;
#48727=DIRECTION ( 'NONE',  ( 0.000000000000000000, 0.000000000000000000, 1.000000000000000000 ) ) ;
#48728=ORIENTED_EDGE ( 'NONE', *, *, #57133, .T. ) ;
#48729=CARTESIAN_POINT ( 'NONE',  ( 16.79062500061451857, -3.027376345333614438, 5.243569643749998122 ) ) ;
#48730=CARTESIAN_POINT ( 'NONE',  ( 28.46250000122903145, -4.330127018922190985, -2.500000000000001332 ) ) ;
#48731=CARTESIAN_POINT ( 'NONE',  ( 17.78437500061451715, -4.541064518000419881, 2.621784821874995952 ) ) ;
#48732=CARTESIAN_POINT ( 'NONE',  ( 29.37187500061451928, 3.027376345333611329, 5.243569643749999010 ) ) ;
#48733=CARTESIAN_POINT ( 'NONE',  ( 4.940625000614515372, 6.054752690667223547, 3.707466751127219781E-16 ) ) ;
#48734=CARTESIAN_POINT ( 'NONE',  ( 18.44062500061451715, 6.054752690667223547, 3.707466751127219781E-16 ) ) ;
#48735=CARTESIAN_POINT ( 'NONE',  ( 28.77187500061451431, 3.027376345333613106, -5.243569643749998122 ) ) ;
#48736=CARTESIAN_POINT ( 'NONE',  ( 2.121784821874999061, 13.80312500061451786, 26.32496088578401583 ) ) ;
#48737=CARTESIAN_POINT ( 'NONE',  ( 17.58750000122903145, -4.330127018922194537, 2.499999999999995559 ) ) ;
#48739=CARTESIAN_POINT ( 'NONE',  ( 8.015625000614516438, 3.027376345333612662, -5.243569643749998122 ) ) ;
#48740=CARTESIAN_POINT ( 'NONE',  ( 26.76562500061451644, -6.054752690667223547, -1.112240025338166033E-15 ) ) ;
#48741=CARTESIAN_POINT ( 'NONE',  ( -1.389182545231912203, 9.676047173952133207, 26.18324276292616304 ) ) ;
#48742=CARTESIAN_POINT ( 'NONE',  ( 23.55937500061451573, 0.000000000000000000, 5.243569643749999010 ) ) ;
#48743=CARTESIAN_POINT ( 'NONE',  ( 11.46562500061451573, -6.054752690667223547, -1.112240025338166033E-15 ) ) ;
#48744=CARTESIAN_POINT ( 'NONE',  ( 22.35000000122903074, 5.773502691896255534, 3.535250795749688894E-16 ) ) ;
#48745=CARTESIAN_POINT ( 'NONE',  ( 23.20312500061451644, -4.541064518000417216, -2.621784821875001281 ) ) ;
#48746=CARTESIAN_POINT ( 'NONE',  ( 16.62187500061451573, 3.027376345333613106, -5.243569643749998122 ) ) ;
#48747=CARTESIAN_POINT ( 'NONE',  ( 12.14062500061451821, 6.054752690667223547, 3.707466751127219781E-16 ) ) ;
#48748=CARTESIAN_POINT ( 'NONE',  ( -4.243569643749999898, 14.45937500061451964, 30.00000000000000000 ) ) ;
#48749=CARTESIAN_POINT ( 'NONE',  ( 19.41562500061451146, 3.027376345333611329, 5.243569643749999010 ) ) ;
#48750=CARTESIAN_POINT ( 'NONE',  ( 29.72812500061451502, 4.541064518000418104, 2.621784821874999949 ) ) ;
#48752=ORIENTED_EDGE ( 'NONE', *, *, #66261, .F. ) ;
#48753=CARTESIAN_POINT ( 'NONE',  ( 23.40000000000000213, -4.330127018922190985, -2.500000000000001332 ) ) ;
#48754=CARTESIAN_POINT ( 'NONE',  ( -2.121784821874996840, 19.03437500061451715, -26.32496088578401583 ) ) ;
#48755=CARTESIAN_POINT ( 'NONE',  ( -6.275039685470489619E-15, 17.97500000122903074, 33.99999999999999289 ) ) ;
#48756=CARTESIAN_POINT ( 'NONE',  ( 26.20312500061451644, 0.000000000000000000, 5.243569643749999010 ) ) ;
#48757=CARTESIAN_POINT ( 'NONE',  ( 4.903125000614516615, 4.541064518000418104, -2.621784821874998173 ) ) ;
#48758=CARTESIAN_POINT ( 'NONE',  ( 18.78750000122903430, 4.330127018922191873, 2.499999999999999556 ) ) ;
#48759=CARTESIAN_POINT ( 'NONE',  ( 24.17812500061451786, 6.421520780324663323E-16, -5.243569643749999010 ) ) ;
#48760=CARTESIAN_POINT ( 'NONE',  ( 24.03750000000000142, 5.773502691896255534, 3.535250795749688894E-16 ) ) ;
#48761=EDGE_CURVE ( 'NONE', #54869, #54799, #20768, .T. ) ;
#48762=CARTESIAN_POINT ( 'NONE',  ( 28.00312500061451715, 0.000000000000000000, 5.243569643749999010 ) ) ;
#48763=CARTESIAN_POINT ( 'NONE',  ( 7.153125000614518392, 4.541064518000418104, -2.621784821874998173 ) ) ;
#48765=CARTESIAN_POINT ( 'NONE',  ( 23.24062500061451786, -3.027376345333610441, -5.243569643749999898 ) ) ;
#48766=CARTESIAN_POINT ( 'NONE',  ( 5.278125000614516615, 6.421520780324663323E-16, -5.243569643749999010 ) ) ;
#48768=CARTESIAN_POINT ( 'NONE',  ( 4.898587196589411843E-16, 20.00000000000000000, 33.99999999999999289 ) ) ;
#48769=CARTESIAN_POINT ( 'NONE',  ( 3.999999999999999112, 13.13750000122903394, -30.00000000000000000 ) ) ;
#48770=CARTESIAN_POINT ( 'NONE',  ( -3.999999999999999112, 10.55000000000000249, -30.00000000000000000 ) ) ;
#48771=CARTESIAN_POINT ( 'NONE',  ( 9.712500000000002132, 2.886751345948126879, 4.999999999999999112 ) ) ;
#48772=CARTESIAN_POINT ( 'NONE',  ( 11.25937500061451679, 4.541064518000418104, -2.621784821874998173 ) ) ;
#48773=CARTESIAN_POINT ( 'NONE',  ( 5.662500001229035185, 4.330127018922192761, -2.499999999999997780 ) ) ;
#48774=CARTESIAN_POINT ( 'NONE',  ( 14.33437500061451786, 6.421520780324663323E-16, -5.243569643749999010 ) ) ;
#48776=CARTESIAN_POINT ( 'NONE',  ( 7.171875000614517326, 3.027376345333613106, -5.243569643749998122 ) ) ;
#48777=CARTESIAN_POINT ( 'NONE',  ( 4.000000000000000000, 18.38750000000000284, 32.30940107675849760 ) ) ;
#48779=CARTESIAN_POINT ( 'NONE',  ( 11.78437500061451892, 4.541064518000418104, 2.621784821874999949 ) ) ;
#48780=CARTESIAN_POINT ( 'NONE',  ( 3.692551571010786127, 3.371233518040734012, 4.016210762354105235 ) ) ;
#48781=CARTESIAN_POINT ( 'NONE',  ( 21.36562500061451431, -6.054752690667223547, -1.112240025338166033E-15 ) ) ;
#48782=CARTESIAN_POINT ( 'NONE',  ( 9.001249775931846008E-16, 10.07187500061451857, 34.90005215228797653 ) ) ;
#48783=CARTESIAN_POINT ( 'NONE',  ( 2.121784821874999061, 19.65312500061459389, 26.32496088578401583 ) ) ;
#48784=CARTESIAN_POINT ( 'NONE',  ( 24.90937500061451715, 0.000000000000000000, 5.243569643749999010 ) ) ;
#48785=CARTESIAN_POINT ( 'NONE',  ( 4.352316639481299987, 2.462457182806187639, 4.352316639481299987 ) ) ;
#48786=CARTESIAN_POINT ( 'NONE',  ( 5.090625000614516615, -3.027376345333614438, 5.243569643749998122 ) ) ;
#48788=CARTESIAN_POINT ( 'NONE',  ( 14.78437500061451715, 6.421520780324663323E-16, -5.243569643749999010 ) ) ;
#48789=CARTESIAN_POINT ( 'NONE',  ( 29.88749999999999929, 5.773502691896255534, 3.535250795749688894E-16 ) ) ;
#48790=CARTESIAN_POINT ( 'NONE',  ( 27.71250000122903145, 4.330127018922192761, -2.499999999999997780 ) ) ;
#48791=CARTESIAN_POINT ( 'NONE',  ( 5.259375000614518569, -4.541064518000417216, -2.621784821875001281 ) ) ;
#48792=CARTESIAN_POINT ( 'NONE',  ( 16.62187500061451573, 3.027376345333613106, -5.243569643749998122 ) ) ;
#48793=CARTESIAN_POINT ( 'NONE',  ( 24.26249999999999929, -5.773502691896255534, -1.060575238724906372E-15 ) ) ;
#48794=EDGE_CURVE ( 'NONE', #54869, #61146, #71372, .T. ) ;
#48795=CARTESIAN_POINT ( 'NONE',  ( 4.125000001229034652, -5.773502691896255534, -1.060575238724906372E-15 ) ) ;
#48796=CARTESIAN_POINT ( 'NONE',  ( 26.40937500061451715, -4.541064518000417216, -2.621784821875001281 ) ) ;
#48798=CARTESIAN_POINT ( 'NONE',  ( 29.58749999999999858, -2.886751345948129988, 4.999999999999997335 ) ) ;
#48799=CARTESIAN_POINT ( 'NONE',  ( 8.587500000000002132, -2.886751345948125991, -5.000000000000000000 ) ) ;
#48801=CARTESIAN_POINT ( 'NONE',  ( 18.77812500061451573, 6.421520780324663323E-16, -5.243569643749999010 ) ) ;
#48802=CARTESIAN_POINT ( 'NONE',  ( 10.95000000000000107, 4.330127018922192761, -2.499999999999997780 ) ) ;
#48803=CARTESIAN_POINT ( 'NONE',  ( 5.278125000614516615, 6.421520780324663323E-16, -5.243569643749999010 ) ) ;
#48804=CARTESIAN_POINT ( 'NONE',  ( 18.71249999999999858, 2.886751345948126879, 4.999999999999999112 ) ) ;
#48805=CARTESIAN_POINT ( 'NONE',  ( 17.57812500061451644, 4.541064518000418104, 2.621784821874999949 ) ) ;
#48806=CARTESIAN_POINT ( 'NONE',  ( -5.810221930991193690E-16, 18.65000000122903501, 26.00000000000000355 ) ) ;
#48807=CARTESIAN_POINT ( 'NONE',  ( 22.35000000122903074, 5.773502691896255534, 3.535250795749688894E-16 ) ) ;
#48809=CARTESIAN_POINT ( 'NONE',  ( 29.33437500061451431, 4.541064518000418104, 2.621784821874999949 ) ) ;
#48811=CARTESIAN_POINT ( 'NONE',  ( 18.55312500061451431, 0.000000000000000000, 5.243569643749999010 ) ) ;
#48812=CARTESIAN_POINT ( 'NONE',  ( 24.59062500061451573, -3.027376345333610441, -5.243569643749999898 ) ) ;
#48813=CARTESIAN_POINT ( 'NONE',  ( 24.57187500061451502, -6.054752690667223547, -1.112240025338166033E-15 ) ) ;
#48814=CARTESIAN_POINT ( 'NONE',  ( 8.925000000000002487, -4.330127018922194537, 2.499999999999995559 ) ) ;
#48815=CARTESIAN_POINT ( 'NONE',  ( 11.27812500061451573, 4.541064518000418104, 2.621784821874999949 ) ) ;
#48816=CARTESIAN_POINT ( 'NONE',  ( 26.91562500061451146, 3.027376345333613106, -5.243569643749998122 ) ) ;
#48817=CARTESIAN_POINT ( 'NONE',  ( 16.58437500061451786, 6.421520780324663323E-16, -5.243569643749999010 ) ) ;
#48818=CARTESIAN_POINT ( 'NONE',  ( 10.11562500061451608, -6.054752690667223547, -1.112240025338166033E-15 ) ) ;
#48820=CARTESIAN_POINT ( 'NONE',  ( 4.243569643749999898, 19.54062500061451857, 32.45002607614398471 ) ) ;
#48821=CARTESIAN_POINT ( 'NONE',  ( 22.83750000122903501, 4.330127018922191873, 2.499999999999999556 ) ) ;
#48823=CARTESIAN_POINT ( 'NONE',  ( 14.57812500061451644, -4.541064518000419881, 2.621784821874995952 ) ) ;
#48824=CARTESIAN_POINT ( 'NONE',  ( 7.584375000614516082, 6.421520780324663323E-16, -5.243569643749999010 ) ) ;
#48825=CARTESIAN_POINT ( 'NONE',  ( 6.121875000614517504, -6.054752690667223547, -1.112240025338166033E-15 ) ) ;
#48828=CARTESIAN_POINT ( 'NONE',  ( 1.999999999999998668, 13.55000000000000071, 26.53589838486224650 ) ) ;
#48829=CARTESIAN_POINT ( 'NONE',  ( 21.85312500061451502, -4.541064518000417216, -2.621784821875001281 ) ) ;
#48830=CARTESIAN_POINT ( 'NONE',  ( 15.87187500061451573, 3.027376345333611329, 5.243569643749999010 ) ) ;
#48831=CARTESIAN_POINT ( 'NONE',  ( 20.27812500061451573, 4.541064518000418104, 2.621784821874999949 ) ) ;
#48832=CARTESIAN_POINT ( 'NONE',  ( 4.000000000000000000, 12.98749999999999893, 32.30940107675849049 ) ) ;
#48833=CARTESIAN_POINT ( 'NONE',  ( 26.16562500061451502, 3.027376345333611329, 5.243569643749999010 ) ) ;
#48834=CARTESIAN_POINT ( 'NONE',  ( 7.875000001229034652, 2.886751345948129099, -4.999999999999998224 ) ) ;
#48835=ORIENTED_EDGE ( 'NONE', *, *, #67839, .T. ) ;
#48836=FACE_OUTER_BOUND ( 'NONE', #63672, .T. ) ;
#48837=CARTESIAN_POINT ( 'NONE',  ( 3.999999999999998668, 17.56250000000000000, -32.30940107675850470 ) ) ;
#48838=CARTESIAN_POINT ( 'NONE',  ( 24.15000000122903145, 5.773502691896255534, 3.535250795749688894E-16 ) ) ;
#48840=CARTESIAN_POINT ( 'NONE',  ( 7.059375000614518392, -4.541064518000417216, -2.621784821875001281 ) ) ;
#48841=CARTESIAN_POINT ( 'NONE',  ( 0.000000000000000000, 20.00000000000000000, -30.00000000000000000 ) ) ;
#48842=CARTESIAN_POINT ( 'NONE',  ( 12.70312500061451821, 0.000000000000000000, 5.243569643749999010 ) ) ;
#48843=EDGE_CURVE ( 'NONE', #64135, #56329, #21283, .T. ) ;
#48844=CARTESIAN_POINT ( 'NONE',  ( 7.621875000614519280, 3.027376345333613106, -5.243569643749998122 ) ) ;
#48845=CARTESIAN_POINT ( 'NONE',  ( 26.66250000122903430, -4.330127018922190985, -2.500000000000001332 ) ) ;
#48846=CARTESIAN_POINT ( 'NONE',  ( 16.65937500061452070, 4.541064518000418104, -2.621784821874998173 ) ) ;
#48847=CARTESIAN_POINT ( 'NONE',  ( 4.959375000614516971, 4.541064518000418104, -2.621784821874998173 ) ) ;
#48848=CARTESIAN_POINT ( 'NONE',  ( 29.73750000000000071, -2.886751345948125991, -5.000000000000000000 ) ) ;
#48849=CARTESIAN_POINT ( 'NONE',  ( 5.615625000614517859, -6.054752690667223547, -1.112240025338166033E-15 ) ) ;
#48850=CARTESIAN_POINT ( 'NONE',  ( 15.85312500061451857, 0.000000000000000000, 5.243569643749999010 ) ) ;
#48851=EDGE_CURVE ( 'NONE', #9450, #63279, #23214, .T. ) ;
#48852=VERTEX_POINT ( 'NONE', #31106 ) ;
#48853=CARTESIAN_POINT ( 'NONE',  ( 11.57812500061451644, 6.421520780324663323E-16, -5.243569643749999010 ) ) ;
#48854=CARTESIAN_POINT ( 'NONE',  ( 5.700000001229033941, 5.773502691896255534, 3.535250795749688894E-16 ) ) ;
#48855=CARTESIAN_POINT ( 'NONE',  ( 7.753125000614518036, 0.000000000000000000, 5.243569643749999010 ) ) ;
#48857=CARTESIAN_POINT ( 'NONE',  ( 7.875000000000000000, 4.330127018922191873, 2.499999999999999556 ) ) ;
#48858=CARTESIAN_POINT ( 'NONE',  ( 3.075000001229035718, 2.886751345948126879, 4.999999999999999112 ) ) ;
#48859=CARTESIAN_POINT ( 'NONE',  ( 17.39999999999999858, 0.000000000000000000, 4.999999999999998224 ) ) ;
#48860=CARTESIAN_POINT ( 'NONE',  ( 17.44687500061451857, -3.027376345333610441, -5.243569643749999898 ) ) ;
#48861=CARTESIAN_POINT ( 'NONE',  ( 13.01250000122903394, 0.000000000000000000, 4.999999999999998224 ) ) ;
#48863=CARTESIAN_POINT ( 'NONE',  ( -4.243569643749999898, 17.55312500061451786, -30.00000000000000000 ) ) ;
#48864=CARTESIAN_POINT ( 'NONE',  ( 11.96250000122903501, 4.330127018922192761, -2.499999999999997780 ) ) ;
#48867=CARTESIAN_POINT ( 'NONE',  ( 29.16562500061451502, 3.027376345333613106, -5.243569643749998122 ) ) ;
#48868=DIRECTION ( 'NONE',  ( 0.000000000000000000, 0.000000000000000000, 1.000000000000000000 ) ) ;
#48870=CARTESIAN_POINT ( 'NONE',  ( 15.08437500061451786, -4.541064518000419881, 2.621784821874995952 ) ) ;
#48871=( BOUNDED_CURVE ( )  B_SPLINE_CURVE ( 2, ( #35043, #57570, #18399, #40966, #63482, #12869, #35401 ),
 .UNSPECIFIED., .F., .F. ) 
 B_SPLINE_CURVE_WITH_KNOTS ( ( 3, 2, 2, 3 ),
 ( 0.07499999999999996947, 0.07777777777777775126, 0.08055555555555551916, 0.08333333333333328707 ),
 .UNSPECIFIED. ) 
 CURVE ( )  GEOMETRIC_REPRESENTATION_ITEM ( )  RATIONAL_B_SPLINE_CURVE ( ( 1.000000000000001332, 0.8660254037844373753, 1.000000000000000000, 0.8660254037844387076, 1.000000000000000000, 0.8660254037844407060, 0.9999999999999980016 ) ) 
 REPRESENTATION_ITEM ( '' )  );
#48872=CARTESIAN_POINT ( 'NONE',  ( 28.35000000000000142, -4.330127018922190985, -2.500000000000001332 ) ) ;
#48873=CARTESIAN_POINT ( 'NONE',  ( 12.17812500061451608, 4.541064518000418104, 2.621784821874999949 ) ) ;
#48875=CARTESIAN_POINT ( 'NONE',  ( 20.37187500061451573, 3.027376345333611329, 5.243569643749999010 ) ) ;
#48877=CARTESIAN_POINT ( 'NONE',  ( 8.128125000614515372, 4.541064518000418104, 2.621784821874999949 ) ) ;
#48878=CARTESIAN_POINT ( 'NONE',  ( 13.65937500061451715, 0.000000000000000000, 5.243569643749999010 ) ) ;
#48880=CARTESIAN_POINT ( 'NONE',  ( 23.89687500061451786, 6.054752690667223547, 3.707466751127219781E-16 ) ) ;
#48881=CARTESIAN_POINT ( 'NONE',  ( 27.70312500061451289, -4.541064518000417216, -2.621784821875001281 ) ) ;
#48883=CARTESIAN_POINT ( 'NONE',  ( 7.087499999999999467, -2.886751345948129988, 4.999999999999997335 ) ) ;
#48884=CARTESIAN_POINT ( 'NONE',  ( 17.85000000122903430, 5.773502691896255534, 3.535250795749688894E-16 ) ) ;
#48885=CARTESIAN_POINT ( 'NONE',  ( 27.22500000122903785, 2.886751345948162850, -4.999999999999940492 ) ) ;
#48887=ORIENTED_EDGE ( 'NONE', *, *, #60961, .T. ) ;
#48888=CARTESIAN_POINT ( 'NONE',  ( 15.67500000000000071, -4.330127018922194537, 2.499999999999995559 ) ) ;
#48889=CARTESIAN_POINT ( 'NONE',  ( 18.00000000000000355, -4.330127018922190985, -2.500000000000001332 ) ) ;
#48890=CARTESIAN_POINT ( 'NONE',  ( 11.65312500061451573, 4.541064518000418104, -2.621784821874998173 ) ) ;
#48891=VERTEX_POINT ( 'NONE', #53646 ) ;
#48892=CARTESIAN_POINT ( 'NONE',  ( -1.071796769724491005, 10.90759618943233455, -34.00000000000000000 ) ) ;
#48893=CARTESIAN_POINT ( 'NONE',  ( 4.243569643749999898, 17.38437500061451502, -30.00000000000000000 ) ) ;
#48894=CARTESIAN_POINT ( 'NONE',  ( 3.065625000614517592, 3.027376345333613106, -5.243569643749998122 ) ) ;
#48895=CARTESIAN_POINT ( 'NONE',  ( 10.20000000000000107, 0.000000000000000000, 4.999999999999998224 ) ) ;
#48896=CARTESIAN_POINT ( 'NONE',  ( 10.05000000000000071, 4.330127018922192761, -2.499999999999997780 ) ) ;
#48897=CARTESIAN_POINT ( 'NONE',  ( 3.128911089188104011, 3.899989153312591661, 3.342749051770597557 ) ) ;
#48898=VECTOR ( 'NONE', #16861, 1000.000000000000000 ) ;
#48899=ORIENTED_EDGE ( 'NONE', *, *, #40501, .T. ) ;
#48900=CARTESIAN_POINT ( 'NONE',  ( 4.243569643749999010, 12.41562500061451857, 27.54997392385601174 ) ) ;
#48901=CARTESIAN_POINT ( 'NONE',  ( 25.86562500061451431, -6.054752690667223547, -1.112240025338166033E-15 ) ) ;
#48903=CARTESIAN_POINT ( 'NONE',  ( 21.87187500061451573, -6.054752690667223547, -1.112240025338166033E-15 ) ) ;
#48904=CARTESIAN_POINT ( 'NONE',  ( 19.60312500061451502, -4.541064518000417216, -2.621784821875001281 ) ) ;
#48905=CARTESIAN_POINT ( 'NONE',  ( -4.243569643749999898, 13.46562500061459744, -32.45002607614398471 ) ) ;
#48906=CARTESIAN_POINT ( 'NONE',  ( 22.98750000122903003, -4.330127018922194537, 2.499999999999995559 ) ) ;
#48908=CARTESIAN_POINT ( 'NONE',  ( 3.478125000614517237, 6.421520780324663323E-16, -5.243569643749999010 ) ) ;
#48910=CARTESIAN_POINT ( 'NONE',  ( 21.74062500061451431, -3.027376345333614438, 5.243569643749998122 ) ) ;
#48913=CARTESIAN_POINT ( 'NONE',  ( 14.37187500061451928, 3.027376345333613106, -5.243569643749998122 ) ) ;
#48914=CARTESIAN_POINT ( 'NONE',  ( 15.04687500061451644, -3.027376345333614438, 5.243569643749998122 ) ) ;
#48915=CARTESIAN_POINT ( 'NONE',  ( 24.42187500061451999, 3.027376345333611329, 5.243569643749999010 ) ) ;
#48916=CARTESIAN_POINT ( 'NONE',  ( -4.243569643749998122, 14.49687500061451750, 32.45002607614398471 ) ) ;
#48917=CARTESIAN_POINT ( 'NONE',  ( 5.353125000614515905, 4.541064518000418104, -2.621784821874998173 ) ) ;
#48918=CARTESIAN_POINT ( 'NONE',  ( 16.46250000122903501, 4.330127018922192761, -2.499999999999997780 ) ) ;
#48919=VECTOR ( 'NONE', #7078, 1000.000000000000000 ) ;
#48920=EDGE_CURVE ( 'NONE', #15201, #40801, #38321, .T. ) ;
#48921=CARTESIAN_POINT ( 'NONE',  ( 29.01562500061451644, -6.054752690667223547, -1.112240025338166033E-15 ) ) ;
#48923=CARTESIAN_POINT ( 'NONE',  ( 4.000000000000000000, 19.73749999999999716, 32.30940107675849049 ) ) ;
#48924=CARTESIAN_POINT ( 'NONE',  ( 7.696875000614516793, 6.054752690667223547, 3.707466751127219781E-16 ) ) ;
#48926=CARTESIAN_POINT ( 'NONE',  ( 14.10000000122903252, -2.886751345948125991, -5.000000000000000000 ) ) ;
#48927=CIRCLE ( 'NONE', #33566, 4.000000000000000000 ) ;
#48928=CARTESIAN_POINT ( 'NONE',  ( 9.675000001229035362, 2.886751345948129099, -4.999999999999998224 ) ) ;
#48929=CARTESIAN_POINT ( 'NONE',  ( 6.140625000614516438, -3.027376345333610441, -5.243569643749999898 ) ) ;
#48932=CARTESIAN_POINT ( 'NONE',  ( 14.67187500061451821, -6.054752690667223547, -1.112240025338166033E-15 ) ) ;
#48933=DIRECTION ( 'NONE',  ( -0.000000000000000000, -1.000000000000000000, -0.000000000000000000 ) ) ;
#48934=EDGE_LOOP ( 'NONE', ( #63, #6453, #21983, #22715 ) ) ;
#48935=CARTESIAN_POINT ( 'NONE',  ( 21.66562500061451502, 3.027376345333611329, 5.243569643749999010 ) ) ;
#48936=CARTESIAN_POINT ( 'NONE',  ( 6.815625000614517148, 3.027376345333611329, 5.243569643749999010 ) ) ;
#48937=CARTESIAN_POINT ( 'NONE',  ( 25.09687500061451715, -3.027376345333610441, -5.243569643749999898 ) ) ;
#48938=CARTESIAN_POINT ( 'NONE',  ( 6.853125000614516793, 0.000000000000000000, 5.243569643749999010 ) ) ;
#48939=CARTESIAN_POINT ( 'NONE',  ( 6.525000001229035007, 2.886751345948129099, -4.999999999999997335 ) ) ;
#48940=CARTESIAN_POINT ( 'NONE',  ( 8.625000001229034652, -5.773502691896255534, -1.060575238724906372E-15 ) ) ;
#48941=CARTESIAN_POINT ( 'NONE',  ( 23.24062500061451786, -3.027376345333610441, -5.243569643749999898 ) ) ;
#48943=CARTESIAN_POINT ( 'NONE',  ( 2.121784821874999061, 11.55312500061451786, -33.67503911421598417 ) ) ;
#48944=CARTESIAN_POINT ( 'NONE',  ( 10.61250000122903536, 4.330127018922192761, -2.499999999999997780 ) ) ;
#48945=CARTESIAN_POINT ( 'NONE',  ( 18.77812500061451573, 6.421520780324663323E-16, -5.243569643749999010 ) ) ;
#48946=CARTESIAN_POINT ( 'NONE',  ( 15.74062500061451608, 6.054752690667223547, 3.707466751127219781E-16 ) ) ;
#48948=CARTESIAN_POINT ( 'NONE',  ( 15.11249999999999893, 2.886751345948126879, 4.999999999999999112 ) ) ;
#48949=CARTESIAN_POINT ( 'NONE',  ( 10.31250000122903288, 0.000000000000000000, 4.999999999999998224 ) ) ;
#48950=CARTESIAN_POINT ( 'NONE',  ( 8.240625000614516082, -3.027376345333614438, 5.243569643749998122 ) ) ;
#48951=CARTESIAN_POINT ( 'NONE',  ( 11.91562500061451857, -6.054752690667223547, -1.112240025338166033E-15 ) ) ;
#48952=CARTESIAN_POINT ( 'NONE',  ( 22.12500000122903288, -5.773502691896255534, -1.060575238724906372E-15 ) ) ;
#48953=AXIS2_PLACEMENT_3D ( 'NONE', #45053, #68312, #17672 ) ;
#48954=CARTESIAN_POINT ( 'NONE',  ( 19.17187500061451999, -6.054752690667223547, -1.112240025338166033E-15 ) ) ;
#48955=CARTESIAN_POINT ( 'NONE',  ( 5.137500001229033941, 6.123233995736764310E-16, -4.999999999999998224 ) ) ;
#48957=CARTESIAN_POINT ( 'NONE',  ( 4.359375000614517326, -4.541064518000417216, -2.621784821875001281 ) ) ;
#48958=CARTESIAN_POINT ( 'NONE',  ( 22.32187500061451502, -6.054752690667223547, -1.112240025338166033E-15 ) ) ;
#48959=CARTESIAN_POINT ( 'NONE',  ( 10.65000000000000036, 0.000000000000000000, 4.999999999999998224 ) ) ;
#48960=CARTESIAN_POINT ( 'NONE',  ( 18.14062500061451644, -3.027376345333614438, 5.243569643749998122 ) ) ;
#48961=CARTESIAN_POINT ( 'NONE',  ( 25.05937500061451573, -4.541064518000417216, -2.621784821875001281 ) ) ;
#48964=CARTESIAN_POINT ( 'NONE',  ( 0.000000000000000000, 20.00000000000000000, -33.99999999999999289 ) ) ;
#48965=CARTESIAN_POINT ( 'NONE',  ( 4.546875000614517326, 6.054752690667223547, 3.707466751127219781E-16 ) ) ;
#48966=CARTESIAN_POINT ( 'NONE',  ( 14.87812500061451537, 4.541064518000418104, 2.621784821874999949 ) ) ;
#48967=VECTOR ( 'NONE', #35318, 1000.000000000000000 ) ;
#48968=CARTESIAN_POINT ( 'NONE',  ( 13.20937500061451786, 0.000000000000000000, 5.243569643749999010 ) ) ;
#48969=VERTEX_POINT ( 'NONE', #46114 ) ;
#48970=CARTESIAN_POINT ( 'NONE',  ( 22.38750000122903216, 4.330127018922191873, 2.499999999999999556 ) ) ;
#48971=CARTESIAN_POINT ( 'NONE',  ( 26.20312500061451644, 0.000000000000000000, 5.243569643749999010 ) ) ;
#48972=CARTESIAN_POINT ( 'NONE',  ( 1.071796769724476572, 12.93259618943233313, -25.99999999999999289 ) ) ;
#48973=CARTESIAN_POINT ( 'NONE',  ( 30.00000000000000000, 0.000000000000000000, 4.999999999999998224 ) ) ;
#48974=CARTESIAN_POINT ( 'NONE',  ( 13.95000000000000107, -4.330127018922190985, -2.500000000000001332 ) ) ;
#48975=CARTESIAN_POINT ( 'NONE',  ( 25.35000000122903074, -2.886751345948125991, -5.000000000000000000 ) ) ;
#48976=CARTESIAN_POINT ( 'NONE',  ( 18.89062500061451644, 6.054752690667223547, 3.707466751127219781E-16 ) ) ;
#48978=CARTESIAN_POINT ( 'NONE',  ( 23.28750000000000142, -2.886751345948129988, 4.999999999999997335 ) ) ;
#48979=CARTESIAN_POINT ( 'NONE',  ( 24.60937500061451644, -4.541064518000417216, -2.621784821875001281 ) ) ;
#48980=ORIENTED_EDGE ( 'NONE', *, *, #531, .T. ) ;
#48982=CARTESIAN_POINT ( 'NONE',  ( 10.90312500061451928, 0.000000000000000000, 5.243569643749999010 ) ) ;
#48983=CARTESIAN_POINT ( 'NONE',  ( 3.815625000614518036, -6.054752690667223547, -1.112240025338166033E-15 ) ) ;
#48985=CARTESIAN_POINT ( 'NONE',  ( 26.80312500061451431, -4.541064518000417216, -2.621784821875001281 ) ) ;
#48986=CARTESIAN_POINT ( 'NONE',  ( 17.55000000000000071, -4.330127018922190985, -2.500000000000001332 ) ) ;
#48987=CARTESIAN_POINT ( 'NONE',  ( 27.82499999999999929, -4.330127018922194537, 2.499999999999995559 ) ) ;
#48988=CARTESIAN_POINT ( 'NONE',  ( 7.837499999999999467, 5.773502691896255534, 3.535250795749688401E-16 ) ) ;
#48989=CARTESIAN_POINT ( 'NONE',  ( 7.209375000614519635, 4.541064518000418104, -2.621784821874998173 ) ) ;
#48990=CARTESIAN_POINT ( 'NONE',  ( 17.18437500061451573, 4.541064518000418104, 2.621784821874999949 ) ) ;
#48991=CARTESIAN_POINT ( 'NONE',  ( 19.76250000122903216, 0.000000000000000000, 4.999999999999998224 ) ) ;
#48992=ORIENTED_EDGE ( 'NONE', *, *, #7054, .F. ) ;
#48993=CARTESIAN_POINT ( 'NONE',  ( 26.69062500061451715, -3.027376345333614438, 5.243569643749998122 ) ) ;
#48994=CARTESIAN_POINT ( 'NONE',  ( 27.98437500061451289, 4.541064518000418104, 2.621784821874999949 ) ) ;
#48996=CARTESIAN_POINT ( 'NONE',  ( 14.96250000000000036, 2.886751345948129099, -4.999999999999998224 ) ) ;
#48997=CARTESIAN_POINT ( 'NONE',  ( 10.34062500061451750, 6.054752690667223547, 3.707466751127219781E-16 ) ) ;
#48999=CARTESIAN_POINT ( 'NONE',  ( 29.54062500061451502, -3.027376345333610441, -5.243569643749999898 ) ) ;
#49000=CARTESIAN_POINT ( 'NONE',  ( 16.05000000122903359, 5.773502691896255534, 3.535250795749688894E-16 ) ) ;
#49003=CARTESIAN_POINT ( 'NONE',  ( 5.578125000614518214, -4.541064518000419881, 2.621784821874995952 ) ) ;
#49004=CARTESIAN_POINT ( 'NONE',  ( 20.85937500061451644, 0.000000000000000000, 5.243569643749999010 ) ) ;
#49005=CARTESIAN_POINT ( 'NONE',  ( 9.001249775931846008E-16, 17.27187500061451786, 34.90005215228797653 ) ) ;
#49006=CARTESIAN_POINT ( 'NONE',  ( 22.99687500061451573, 6.054752690667223547, 3.707466751127219781E-16 ) ) ;
#49007=CARTESIAN_POINT ( 'NONE',  ( 6.299999999999999822, -4.330127018922190985, -2.500000000000001332 ) ) ;
#49008=CARTESIAN_POINT ( 'NONE',  ( 3.999999999999998668, 10.47500000122903430, 27.69059892324149175 ) ) ;
#49009=CARTESIAN_POINT ( 'NONE',  ( 13.22812500061451502, -4.541064518000419881, 2.621784821874995952 ) ) ;
#49010=CARTESIAN_POINT ( 'NONE',  ( 5.400000001229032343, -2.886751345948129988, 4.999999999999997335 ) ) ;
#49011=CARTESIAN_POINT ( 'NONE',  ( 9.009375000614518569, 4.541064518000418104, -2.621784821874998173 ) ) ;
#49012=DIRECTION ( 'NONE',  ( -1.000000000000000000, -0.000000000000000000, -0.000000000000000000 ) ) ;
#49014=CARTESIAN_POINT ( 'NONE',  ( 10.86562500061451431, 3.027376345333611329, 5.243569643749999010 ) ) ;
#49015=CARTESIAN_POINT ( 'NONE',  ( 13.95937500061451786, 4.541064518000418104, -2.621784821874998173 ) ) ;
#49016=DIRECTION ( 'NONE',  ( 0.000000000000000000, 0.000000000000000000, 1.000000000000000000 ) ) ;
#49017=CARTESIAN_POINT ( 'NONE',  ( 21.18750000122903288, -4.330127018922194537, 2.499999999999995559 ) ) ;
#49018=CARTESIAN_POINT ( 'NONE',  ( 10.09687500061451715, -3.027376345333614438, 5.243569643749998122 ) ) ;
#49019=CARTESIAN_POINT ( 'NONE',  ( 11.65312500061451573, 4.541064518000418104, -2.621784821874998173 ) ) ;
#49020=ADVANCED_FACE ( 'NONE', ( #72098 ), #328, .F. ) ;
#49022=CARTESIAN_POINT ( 'NONE',  ( 22.58437500061451431, 4.541064518000418104, 2.621784821874999949 ) ) ;
#49023=CARTESIAN_POINT ( 'NONE',  ( 25.38750000122903216, 6.123233995736764310E-16, -4.999999999999998224 ) ) ;
#49024=CARTESIAN_POINT ( 'NONE',  ( -2.081578678577454156, 4.574985540471383061, 26.54335022361717478 ) ) ;
#49025=CARTESIAN_POINT ( 'NONE',  ( 3.486133158594716510E-16, 19.88749999999999929, -34.00000000000000000 ) ) ;
#49026=CARTESIAN_POINT ( 'NONE',  ( -4.243569643749998122, 11.34687500061451892, -27.54997392385601174 ) ) ;
#49027=CARTESIAN_POINT ( 'NONE',  ( 15.07500000122903394, 2.886751345948129099, -4.999999999999998224 ) ) ;
#49028=VECTOR ( 'NONE', #10467, 1000.000000000000000 ) ;
#49029=CARTESIAN_POINT ( 'NONE',  ( 10.17187500061451999, -6.054752690667223547, -1.112240025338166033E-15 ) ) ;
#49030=CARTESIAN_POINT ( 'NONE',  ( 2.121784821874999061, 17.40312500061451573, -33.67503911421598417 ) ) ;
#49031=CARTESIAN_POINT ( 'NONE',  ( 18.03750000122903430, -4.330127018922194537, 2.499999999999995559 ) ) ;
#49032=CARTESIAN_POINT ( 'NONE',  ( 10.49062500061451431, -3.027376345333614438, 5.243569643749998122 ) ) ;
#49033=ORIENTED_EDGE ( 'NONE', *, *, #24479, .T. ) ;
#49035=CARTESIAN_POINT ( 'NONE',  ( 14.96250000000000036, 2.886751345948129099, -4.999999999999998224 ) ) ;
#49036=CARTESIAN_POINT ( 'NONE',  ( -1.071796769724488563, 17.50490381179670152, -26.00000000000000000 ) ) ;
#49037=CARTESIAN_POINT ( 'NONE',  ( 9.534375000614517148, 4.541064518000418104, 2.621784821874999949 ) ) ;
#49038=CARTESIAN_POINT ( 'NONE',  ( 4.373597137442938099, -2.423175050767027550, -4.650093653908929703 ) ) ;
#49039=CARTESIAN_POINT ( 'NONE',  ( 10.35000000122903074, -2.886751345948129988, 4.999999999999997335 ) ) ;
#49040=CARTESIAN_POINT ( 'NONE',  ( 18.18750000122903288, 6.123233995736764310E-16, -4.999999999999998224 ) ) ;
#49041=CARTESIAN_POINT ( 'NONE',  ( 14.09062500061451750, -3.027376345333614438, 5.243569643749998122 ) ) ;
#49043=CARTESIAN_POINT ( 'NONE',  ( 17.42812500061451786, 6.421520780324663323E-16, -5.243569643749999010 ) ) ;
#49044=CARTESIAN_POINT ( 'NONE',  ( 27.03750000122903430, -4.330127018922194537, 2.499999999999995559 ) ) ;
#49045=CARTESIAN_POINT ( 'NONE',  ( 4.003125000614518925, 4.541064518000418104, -2.621784821874998173 ) ) ;
#49046=CARTESIAN_POINT ( 'NONE',  ( 24.00000000000000000, 4.330127018922192761, -2.499999999999997780 ) ) ;
#49049=CARTESIAN_POINT ( 'NONE',  ( 25.92187500061451999, -6.054752690667223547, -1.112240025338166033E-15 ) ) ;
#49050=CARTESIAN_POINT ( 'NONE',  ( 1.071796769724489895, 12.66740381056766651, -34.00000000000000000 ) ) ;
#49051=CARTESIAN_POINT ( 'NONE',  ( 13.72500000122903074, 2.886751345948129099, -4.999999999999998224 ) ) ;
#49052=CARTESIAN_POINT ( 'NONE',  ( 3.487500000000000711, -2.886751345948129988, 4.999999999999997335 ) ) ;
#49054=CARTESIAN_POINT ( 'NONE',  ( 6.309375000614517504, 4.541064518000418104, -2.621784821874998173 ) ) ;
#49055=CARTESIAN_POINT ( 'NONE',  ( 26.61562500061451786, 3.027376345333611329, 5.243569643749999010 ) ) ;
#49057=CARTESIAN_POINT ( 'NONE',  ( 11.55000000122903181, 5.773502691896255534, 3.535250795749688401E-16 ) ) ;
#49059=CARTESIAN_POINT ( 'NONE',  ( 5.896875000614518747, 6.054752690667223547, 3.707466751127219781E-16 ) ) ;
#49060=CARTESIAN_POINT ( 'NONE',  ( 8.971875000614515372, 3.027376345333613106, -5.243569643749998122 ) ) ;
#49061=CARTESIAN_POINT ( 'NONE',  ( 29.33437500061451431, 4.541064518000418104, 2.621784821874999949 ) ) ;
#49062=CARTESIAN_POINT ( 'NONE',  ( 9.001249775931846008E-16, 11.81562500061459353, 34.90005215228797653 ) ) ;
#49063=CARTESIAN_POINT ( 'NONE',  ( 22.31250000000000000, 2.886751345948126879, 4.999999999999999112 ) ) ;
#49064=CARTESIAN_POINT ( 'NONE',  ( 29.51249999999999929, 2.886751345948126879, 4.999999999999999112 ) ) ;
#49065=CARTESIAN_POINT ( 'NONE',  ( 5.100000000000000533, 4.330127018922192761, -2.499999999999997780 ) ) ;
#49068=CARTESIAN_POINT ( 'NONE',  ( 17.09062500061451573, 6.054752690667223547, 3.707466751127219781E-16 ) ) ;
#49069=CARTESIAN_POINT ( 'NONE',  ( 10.75312500061451715, 4.541064518000418104, -2.621784821874998173 ) ) ;
#49071=CARTESIAN_POINT ( 'NONE',  ( 7.134375000614516793, 6.421520780324663323E-16, -5.243569643749999010 ) ) ;
#49072=CARTESIAN_POINT ( 'NONE',  ( 23.09999999999999787, 4.330127018922192761, -2.499999999999997780 ) ) ;
#49073=CARTESIAN_POINT ( 'NONE',  ( 20.55000000122903359, 5.773502691896255534, 3.535250795749688894E-16 ) ) ;
#49075=VECTOR ( 'NONE', #26815, 1000.000000000000000 ) ;
#49076=CARTESIAN_POINT ( 'NONE',  ( 8.559375000614515727, 4.541064518000418104, -2.621784821874998173 ) ) ;
#49077=CARTESIAN_POINT ( 'NONE',  ( 15.00937500061451679, 0.000000000000000000, 5.243569643749999010 ) ) ;
#49078=CARTESIAN_POINT ( 'NONE',  ( 24.00937500061451502, 0.000000000000000000, 5.243569643749999010 ) ) ;
#49082=CARTESIAN_POINT ( 'NONE',  ( 18.42187500061451644, 3.027376345333613106, -5.243569643749998122 ) ) ;
#49083=( BOUNDED_CURVE ( )  B_SPLINE_CURVE ( 2, ( #43834, #66359, #56004, #67104, #15736, #16462, #33459, #5398, #50468 ),
 .UNSPECIFIED., .F., .F. ) 
 B_SPLINE_CURVE_WITH_KNOTS ( ( 3, 2, 2, 2, 3 ),
 ( 0.4239130434782608647, 0.4275362318840579823, 0.4347826086956521618, 0.4420289855072463969, 0.4456521739130435145 ),
 .UNSPECIFIED. ) 
 CURVE ( )  GEOMETRIC_REPRESENTATION_ITEM ( )  RATIONAL_B_SPLINE_CURVE ( ( 0.9330127018922194093, 0.9330127018922194093, 1.000000000000000000, 0.8660254037844387076, 1.000000000000000000, 0.8660254037844387076, 1.000000000000000000, 0.9330127018922188542, 0.9330127018922194093 ) ) 
 REPRESENTATION_ITEM ( '' )  );
#49084=CARTESIAN_POINT ( 'NONE',  ( 8.934375000614517504, 6.421520780324663323E-16, -5.243569643749999010 ) ) ;
#49086=CARTESIAN_POINT ( 'NONE',  ( 19.98749999999999716, 5.773502691896255534, 3.535250795749688894E-16 ) ) ;
#49088=CARTESIAN_POINT ( 'NONE',  ( 4.243569643749999898, 10.14687500061451786, -27.54997392385601529 ) ) ;
#49090=CARTESIAN_POINT ( 'NONE',  ( 12.21562500061451573, 3.027376345333611329, 5.243569643749999010 ) ) ;
#49091=CARTESIAN_POINT ( 'NONE',  ( 29.55937500061451573, -4.541064518000417216, -2.621784821875001281 ) ) ;
#49092=CYLINDRICAL_SURFACE ( 'NONE', #27959, 4.999999999999998224 ) ;
#49093=CARTESIAN_POINT ( 'NONE',  ( 12.30000000000000249, 4.330127018922192761, -2.499999999999997780 ) ) ;
#49094=CARTESIAN_POINT ( 'NONE',  ( -3.999999999999999112, 17.41250000122903430, 30.00000000000000000 ) ) ;
#49095=CARTESIAN_POINT ( 'NONE',  ( 11.73750000122903181, -4.330127018922194537, 2.499999999999995559 ) ) ;
#49096=CARTESIAN_POINT ( 'NONE',  ( 21.23437500061451644, 4.541064518000418104, 2.621784821874999949 ) ) ;
#49097=CARTESIAN_POINT ( 'NONE',  ( 16.43437500061451573, -4.541064518000419881, 2.621784821874995952 ) ) ;
#49100=CARTESIAN_POINT ( 'NONE',  ( 16.67812500061451786, 4.541064518000418104, 2.621784821874999949 ) ) ;
#49101=CARTESIAN_POINT ( 'NONE',  ( 27.67500000122903359, 2.886751345948129099, -4.999999999999998224 ) ) ;
#49102=CARTESIAN_POINT ( 'NONE',  ( 18.27187500061451431, -6.054752690667223547, -1.112240025338166033E-15 ) ) ;
#49103=CARTESIAN_POINT ( 'NONE',  ( 5.803125000614517859, 4.541064518000418104, -2.621784821874998173 ) ) ;
#49104=CARTESIAN_POINT ( 'NONE',  ( 20.31562500061451715, 3.027376345333611329, 5.243569643749999010 ) ) ;
#49105=CARTESIAN_POINT ( 'NONE',  ( -3.999999999999997335, 16.88749999999999929, -27.69059892324149530 ) ) ;
#49106=CARTESIAN_POINT ( 'NONE',  ( 27.75937500061451502, -4.541064518000417216, -2.621784821875001281 ) ) ;
#49107=CARTESIAN_POINT ( 'NONE',  ( -4.243569643749997233, 13.54062500061451679, 32.45002607614398471 ) ) ;
#49108=CARTESIAN_POINT ( 'NONE',  ( 16.80937500061451573, 0.000000000000000000, 5.243569643749999010 ) ) ;
#49109=CARTESIAN_POINT ( 'NONE',  ( 15.78750000122903430, -4.330127018922194537, 2.499999999999995559 ) ) ;
#49111=CARTESIAN_POINT ( 'NONE',  ( 2.000000000000001332, 18.91250000122903430, -26.53589838486224650 ) ) ;
#49112=CARTESIAN_POINT ( 'NONE',  ( 20.70937500061451786, 4.541064518000418104, -2.621784821874998173 ) ) ;
#49113=CARTESIAN_POINT ( 'NONE',  ( 21.78750000122903074, 6.123233995736764310E-16, -4.999999999999998224 ) ) ;
#49115=CARTESIAN_POINT ( 'NONE',  ( 23.65312500061451573, -4.541064518000417216, -2.621784821875001281 ) ) ;
#49116=CARTESIAN_POINT ( 'NONE',  ( 16.54687500061451644, -3.027376345333610441, -5.243569643749999898 ) ) ;
#49117=CARTESIAN_POINT ( 'NONE',  ( 12.29062500061451857, -3.027376345333614438, 5.243569643749998122 ) ) ;
#49118=CARTESIAN_POINT ( 'NONE',  ( 2.121784821875001281, 14.15937500061451715, 33.67503911421598417 ) ) ;
#49119=CARTESIAN_POINT ( 'NONE',  ( 18.40312500061451573, 4.541064518000418104, -2.621784821874998173 ) ) ;
#49120=CARTESIAN_POINT ( 'NONE',  ( 28.71562500061451573, 3.027376345333613106, -5.243569643749998122 ) ) ;
#49121=ORIENTED_EDGE ( 'NONE', *, *, #26290, .T. ) ;
#49122=CARTESIAN_POINT ( 'NONE',  ( 22.31250000000000000, 2.886751345948126879, 4.999999999999999112 ) ) ;
#49123=CARTESIAN_POINT ( 'NONE',  ( -4.243569643749999898, 18.92187500061451644, -32.45002607614398471 ) ) ;
#49124=CARTESIAN_POINT ( 'NONE',  ( 3.734827092922140768, -3.324314453528163682, -3.734827092927292203 ) ) ;
#49125=CARTESIAN_POINT ( 'NONE',  ( 25.11562500061451431, 3.027376345333613106, -5.243569643749998122 ) ) ;
#49126=CARTESIAN_POINT ( 'NONE',  ( 5.765625000614519102, 3.027376345333613106, -5.243569643749998122 ) ) ;
#49127=CARTESIAN_POINT ( 'NONE',  ( 17.81250000122903288, 4.330127018922192761, -2.499999999999997780 ) ) ;
#49128=ADVANCED_FACE ( 'NONE', ( #68651 ), #38486, .F. ) ;
#49129=CARTESIAN_POINT ( 'NONE',  ( 22.19062500061451715, -3.027376345333614438, 5.243569643749998122 ) ) ;
#49130=CARTESIAN_POINT ( 'NONE',  ( 21.78750000000000142, 5.773502691896255534, 3.535250795749688894E-16 ) ) ;
#49131=CARTESIAN_POINT ( 'NONE',  ( 27.96562500061451928, 3.027376345333611329, 5.243569643749999010 ) ) ;
#49132=CARTESIAN_POINT ( 'NONE',  ( 7.228125000614517681, 4.541064518000418104, 2.621784821874999949 ) ) ;
#49133=ORIENTED_EDGE ( 'NONE', *, *, #47219, .F. ) ;
#49134=CARTESIAN_POINT ( 'NONE',  ( 23.42812500061451786, 4.541064518000418104, 2.621784821874999949 ) ) ;
#49135=CARTESIAN_POINT ( 'NONE',  ( 3.778125000614519280, -4.541064518000419881, 2.621784821874995952 ) ) ;
#49138=CARTESIAN_POINT ( 'NONE',  ( -1.999999999999997113, 13.88750000122903394, -26.53589838486224295 ) ) ;
#49139=DIRECTION ( 'NONE',  ( -1.000000000000000000, -0.000000000000000000, -0.000000000000000000 ) ) ;
#49140=CARTESIAN_POINT ( 'NONE',  ( 11.40000000000000036, 4.330127018922192761, -2.499999999999997780 ) ) ;
#49141=CARTESIAN_POINT ( 'NONE',  ( 11.52187500061451608, -6.054752690667223547, -1.112240025338166033E-15 ) ) ;
#49142=CARTESIAN_POINT ( 'NONE',  ( 5.437500001229035540, -4.330127018922194537, 2.499999999999995559 ) ) ;
#49143=CARTESIAN_POINT ( 'NONE',  ( 14.10937500061451644, 0.000000000000000000, 5.243569643749999010 ) ) ;
#49144=CARTESIAN_POINT ( 'NONE',  ( 4.884375000614518569, 6.421520780324663323E-16, -5.243569643749999010 ) ) ;
#49146=AXIS2_PLACEMENT_3D ( 'NONE', #53900, #9191, #19523 ) ;
#49147=CARTESIAN_POINT ( 'NONE',  ( -5.810221930991193690E-16, 10.55000000122903359, 26.00000000000000355 ) ) ;
#49148=CARTESIAN_POINT ( 'NONE',  ( 12.00937500061451857, -4.541064518000417216, -2.621784821875001281 ) ) ;
#49149=CARTESIAN_POINT ( 'NONE',  ( 6.225000001229035185, 2.886751345948126879, 4.999999999999998224 ) ) ;
#49150=CARTESIAN_POINT ( 'NONE',  ( 22.37812500061451360, 6.421520780324663323E-16, -5.243569643749999010 ) ) ;
#49151=DIRECTION ( 'NONE',  ( -0.000000000000000000, -1.000000000000000000, -0.000000000000000000 ) ) ;
#49152=CARTESIAN_POINT ( 'NONE',  ( -4.243569643749998122, 18.49062500061459247, 32.45002607614398471 ) ) ;
#49153=CARTESIAN_POINT ( 'NONE',  ( 24.08437500061451786, -4.541064518000419881, 2.621784821874995952 ) ) ;
#49154=CARTESIAN_POINT ( 'NONE',  ( -2.000000000000000000, 13.73750000122903359, -33.46410161513775705 ) ) ;
#49155=CARTESIAN_POINT ( 'NONE',  ( 4.265625000614517326, -6.054752690667223547, -1.112240025338166033E-15 ) ) ;
#49157=CARTESIAN_POINT ( 'NONE',  ( 25.52812500061451573, 6.421520780324663323E-16, -5.243569643749999010 ) ) ;
#49158=CARTESIAN_POINT ( 'NONE',  ( 17.35312500061451502, -4.541064518000417216, -2.621784821875001281 ) ) ;
#49160=CARTESIAN_POINT ( 'NONE',  ( 14.89687500061451786, 6.054752690667223547, 3.707466751127219781E-16 ) ) ;
#49162=CARTESIAN_POINT ( 'NONE',  ( 27.56250000122902932, -4.330127018922190985, -2.500000000000001332 ) ) ;
#49163=CARTESIAN_POINT ( 'NONE',  ( 6.646875000614518747, -3.027376345333610441, -5.243569643749999898 ) ) ;
#49164=CARTESIAN_POINT ( 'NONE',  ( 17.14687500061451786, 6.054752690667223547, 3.707466751127219781E-16 ) ) ;
#49165=FACE_OUTER_BOUND ( 'NONE', #13997, .T. ) ;
#49166=CARTESIAN_POINT ( 'NONE',  ( 24.03750000000000142, 5.773502691896255534, 3.535250795749688894E-16 ) ) ;
#49167=CARTESIAN_POINT ( 'NONE',  ( 2.925000001229034918, 2.886751345948129099, -4.999999999999998224 ) ) ;
#49168=CARTESIAN_POINT ( 'NONE',  ( 25.65937500061451715, 4.541064518000418104, -2.621784821874998173 ) ) ;
#49169=CARTESIAN_POINT ( 'NONE',  ( 15.83437500061451608, 4.541064518000418104, 2.621784821874999949 ) ) ;
#49171=CARTESIAN_POINT ( 'NONE',  ( 27.22499999999999787, 4.330127018922191873, 2.499999999999999556 ) ) ;
#49172=CARTESIAN_POINT ( 'NONE',  ( 4.949999999999999289, -4.330127018922190985, -2.500000000000001332 ) ) ;
#49174=CARTESIAN_POINT ( 'NONE',  ( 18.55312500061451431, 0.000000000000000000, 5.243569643749999010 ) ) ;
#49175=CARTESIAN_POINT ( 'NONE',  ( 9.074999999999999289, 6.123233995736764310E-16, -4.999999999999998224 ) ) ;
#49176=EDGE_CURVE ( 'NONE', #72969, #24589, #43957, .T. ) ;
#49177=CARTESIAN_POINT ( 'NONE',  ( 3.103125000614517237, 4.541064518000418104, -2.621784821874998173 ) ) ;
#49178=CARTESIAN_POINT ( 'NONE',  ( 20.28750000000000142, -2.886751345948125991, -5.000000000000000000 ) ) ;
#49180=CARTESIAN_POINT ( 'NONE',  ( 24.37500000122903288, -5.773502691896255534, -1.060575238724906372E-15 ) ) ;
#49181=CARTESIAN_POINT ( 'NONE',  ( 1.968632615237263517, 9.806224642577900497, 35.67136274582625788 ) ) ;
#49182=CARTESIAN_POINT ( 'NONE',  ( 28.54687500061451644, -3.027376345333614438, 5.243569643749998122 ) ) ;
#49184=CARTESIAN_POINT ( 'NONE',  ( 18.21562500061451573, -6.054752690667223547, -1.112240025338166033E-15 ) ) ;
#49185=CARTESIAN_POINT ( 'NONE',  ( 23.69062500061451004, -3.027376345333610441, -5.243569643749999898 ) ) ;
#49186=CARTESIAN_POINT ( 'NONE',  ( 24.12187500061451217, -6.054752690667223547, -1.112240025338166033E-15 ) ) ;
#49187=CARTESIAN_POINT ( 'NONE',  ( 9.637499999999999289, 5.773502691896255534, 3.535250795749688894E-16 ) ) ;
#49188=CARTESIAN_POINT ( 'NONE',  ( 12.17812500061451608, 4.541064518000418104, 2.621784821874999949 ) ) ;
#49189=CARTESIAN_POINT ( 'NONE',  ( 27.29062500061451502, -3.027376345333610441, -5.243569643749999898 ) ) ;
#49190=CARTESIAN_POINT ( 'NONE',  ( 15.15937500061451715, -4.541064518000417216, -2.621784821875001281 ) ) ;
#49191=CARTESIAN_POINT ( 'NONE',  ( 19.73437500061451644, 6.421520780324663323E-16, -5.243569643749999010 ) ) ;
#49192=CARTESIAN_POINT ( 'NONE',  ( 9.001249775931846008E-16, 19.01562500061451644, 34.90005215228797653 ) ) ;
#49193=CARTESIAN_POINT ( 'NONE',  ( 23.51250000122903216, -4.330127018922190985, -2.500000000000001332 ) ) ;
#49195=CARTESIAN_POINT ( 'NONE',  ( 14.09062500061451750, -3.027376345333614438, 5.243569643749998122 ) ) ;
#49196=CARTESIAN_POINT ( 'NONE',  ( 7.734375000614517326, 4.541064518000418104, 2.621784821874999949 ) ) ;
#49197=CARTESIAN_POINT ( 'NONE',  ( 7.734375000614517326, 4.541064518000418104, 2.621784821874999949 ) ) ;
#49198=ORIENTED_EDGE ( 'NONE', *, *, #36389, .T. ) ;
#49199=CARTESIAN_POINT ( 'NONE',  ( 28.62187500061451573, -6.054752690667223547, -1.112240025338166033E-15 ) ) ;
#49200=CARTESIAN_POINT ( 'NONE',  ( 19.79062500061451502, 6.054752690667223547, 3.707466751127219781E-16 ) ) ;
#49201=CARTESIAN_POINT ( 'NONE',  ( 24.30937500061451573, 4.541064518000418104, -2.621784821874998173 ) ) ;
#49202=CARTESIAN_POINT ( 'NONE',  ( 20.72812500061451502, 4.541064518000418104, 2.621784821874999949 ) ) ;
#49203=CARTESIAN_POINT ( 'NONE',  ( -1.999999999999997113, 11.97500000000000142, 33.46410161513775705 ) ) ;
#49204=CARTESIAN_POINT ( 'NONE',  ( 25.34062500061451217, -3.027376345333614438, 5.243569643749998122 ) ) ;
#49205=CARTESIAN_POINT ( 'NONE',  ( 8.250000001229034652, -2.886751345948125991, -5.000000000000000000 ) ) ;
#49207=CARTESIAN_POINT ( 'NONE',  ( 3.337500001229034563, 6.123233995736764310E-16, -4.999999999999998224 ) ) ;
#49208=CARTESIAN_POINT ( 'NONE',  ( 3.999999999999998668, 14.86250000000000071, -32.30940107675850470 ) ) ;
#49209=CARTESIAN_POINT ( 'NONE',  ( 22.50000000122903288, -2.886751345948129988, 4.999999999999997335 ) ) ;
#49211=CARTESIAN_POINT ( 'NONE',  ( 3.721875000614518036, 3.027376345333611329, 5.243569643749999010 ) ) ;
#49212=CARTESIAN_POINT ( 'NONE',  ( 20.21250000122903145, 0.000000000000000000, 4.999999999999998224 ) ) ;
#49213=CARTESIAN_POINT ( 'NONE',  ( 13.00312500061451537, 4.541064518000418104, -2.621784821874998173 ) ) ;
#49214=AXIS2_PLACEMENT_3D ( 'NONE', #4379, #45347, #66421 ) ;
#49215=CARTESIAN_POINT ( 'NONE',  ( 8.971875000614515372, 3.027376345333613106, -5.243569643749998122 ) ) ;
#49216=CARTESIAN_POINT ( 'NONE',  ( 24.41250000122903430, -4.330127018922190985, -2.500000000000001332 ) ) ;
#49217=CARTESIAN_POINT ( 'NONE',  ( 15.49687500061451750, -3.027376345333614438, 5.243569643749998122 ) ) ;
#49218=CARTESIAN_POINT ( 'NONE',  ( 29.69062500061451715, 6.054752690667223547, 3.707466751127219781E-16 ) ) ;
#49219=CARTESIAN_POINT ( 'NONE',  ( 29.51249999999999929, 2.886751345948126879, 4.999999999999999112 ) ) ;
#49220=CARTESIAN_POINT ( 'NONE',  ( 4.978125000614518569, 4.541064518000418104, 2.621784821874999949 ) ) ;
#49221=CARTESIAN_POINT ( 'NONE',  ( 14.20312500061451644, -4.541064518000417216, -2.621784821875001281 ) ) ;
#49223=CARTESIAN_POINT ( 'NONE',  ( 12.29062500061451857, -3.027376345333614438, 5.243569643749998122 ) ) ;
#49224=CARTESIAN_POINT ( 'NONE',  ( 8.578125000614518214, 4.541064518000418104, 2.621784821874999949 ) ) ;
#49226=CARTESIAN_POINT ( 'NONE',  ( 7.987500000000000711, -2.886751345948129988, 4.999999999999997335 ) ) ;
#49227=ADVANCED_FACE ( 'NONE', ( #49576 ), #51495, .T. ) ;
#49228=CARTESIAN_POINT ( 'NONE',  ( 3.000000001229032875, 5.773502691896255534, 3.535250795749688894E-16 ) ) ;
#49229=CARTESIAN_POINT ( 'NONE',  ( 17.96250000000000213, -5.773502691896255534, -1.060575238724906372E-15 ) ) ;
#49230=CARTESIAN_POINT ( 'NONE',  ( 19.09687500061451360, -3.027376345333614438, 5.243569643749998122 ) ) ;
#49231=CARTESIAN_POINT ( 'NONE',  ( 13.16250000122903430, -4.330127018922190985, -2.500000000000001332 ) ) ;
#49233=CARTESIAN_POINT ( 'NONE',  ( 2.121784821874999061, 16.50312500061451715, -33.67503911421598417 ) ) ;
#49234=CARTESIAN_POINT ( 'NONE',  ( 22.12500000000000000, 6.123233995736764310E-16, -4.999999999999998224 ) ) ;
#49236=CARTESIAN_POINT ( 'NONE',  ( 28.60312500061451502, -4.541064518000417216, -2.621784821875001281 ) ) ;
#49238=CARTESIAN_POINT ( 'NONE',  ( 0.000000000000000000, 0.000000000000000000, -50.00000000000000000 ) ) ;
#49239=CARTESIAN_POINT ( 'NONE',  ( 13.35937500061451821, -4.541064518000417216, -2.621784821875001281 ) ) ;
#49240=CARTESIAN_POINT ( 'NONE',  ( 25.72499999999999787, 6.123233995736764310E-16, -4.999999999999998224 ) ) ;
#49241=CARTESIAN_POINT ( 'NONE',  ( 10.60312500061451679, -4.541064518000417216, -2.621784821875001281 ) ) ;
#49243=CARTESIAN_POINT ( 'NONE',  ( 21.53437500061451715, 6.421520780324663323E-16, -5.243569643749999010 ) ) ;
#49245=CARTESIAN_POINT ( 'NONE',  ( 7.753125000614518036, 0.000000000000000000, 5.243569643749999010 ) ) ;
#49246=CARTESIAN_POINT ( 'NONE',  ( 13.05937500061451750, 4.541064518000418104, -2.621784821874998173 ) ) ;
#49247=ORIENTED_EDGE ( 'NONE', *, *, #45494, .T. ) ;
#49248=CARTESIAN_POINT ( 'NONE',  ( 22.92187500061451644, 3.027376345333613106, -5.243569643749998122 ) ) ;
#49249=CARTESIAN_POINT ( 'NONE',  ( 3.482548389542084344, 3.599757532507413149, -27.96763060114582444 ) ) ;
#49250=CARTESIAN_POINT ( 'NONE',  ( 8.737500000000002487, 5.773502691896255534, 3.535250795749688401E-16 ) ) ;
#49251=CARTESIAN_POINT ( 'NONE',  ( 4.687500000000000000, 5.773502691896255534, 3.535250795749688894E-16 ) ) ;
#49253=CARTESIAN_POINT ( 'NONE',  ( 17.77500000122903145, 2.886751345948129099, -4.999999999999998224 ) ) ;
#49256=EDGE_LOOP ( 'NONE', ( #62283, #7669, #27166, #53990 ) ) ;
#49258=CARTESIAN_POINT ( 'NONE',  ( 15.59999999999999964, 0.000000000000000000, 4.999999999999998224 ) ) ;
#49259=CARTESIAN_POINT ( 'NONE',  ( 16.94999999999999929, 0.000000000000000000, 4.999999999999998224 ) ) ;
#49260=CARTESIAN_POINT ( 'NONE',  ( 11.42812500061451608, -4.541064518000419881, 2.621784821874995952 ) ) ;
#49263=CARTESIAN_POINT ( 'NONE',  ( -4.243569643749999898, 16.22187500061452070, -32.45002607614398471 ) ) ;
#49264=CARTESIAN_POINT ( 'NONE',  ( 29.28750000122903074, -4.330127018922194537, 2.499999999999995559 ) ) ;
#49266=CARTESIAN_POINT ( 'NONE',  ( 9.412499999999999645, -5.773502691896255534, -1.060575238724906372E-15 ) ) ;
#49267=CARTESIAN_POINT ( 'NONE',  ( 30.00000000000000000, 0.000000000000000000, 0.000000000000000000 ) ) ;
#49269=CARTESIAN_POINT ( 'NONE',  ( 23.31562500061451715, 3.027376345333613106, -5.243569643749998122 ) ) ;
#49270=CARTESIAN_POINT ( 'NONE',  ( 4.201576942248188118, -2.710502447772806800, 4.488682300801404956 ) ) ;
#49272=CARTESIAN_POINT ( 'NONE',  ( 20.55937500061451573, -4.541064518000417216, -2.621784821875001281 ) ) ;
#49273=CARTESIAN_POINT ( 'NONE',  ( 20.27812500061451573, 4.541064518000418104, 2.621784821874999949 ) ) ;
#49274=CARTESIAN_POINT ( 'NONE',  ( 2.121784821874999061, 14.25312500061459353, -33.67503911421598417 ) ) ;
#49275=CARTESIAN_POINT ( 'NONE',  ( 23.43750000122902932, -4.330127018922194537, 2.499999999999995559 ) ) ;
#49276=CARTESIAN_POINT ( 'NONE',  ( 4.340625000614515727, -3.027376345333610441, -5.243569643749999898 ) ) ;
#49278=CARTESIAN_POINT ( 'NONE',  ( 21.89062500061451644, -3.027376345333610441, -5.243569643749999898 ) ) ;
#49281=CARTESIAN_POINT ( 'NONE',  ( 14.78437500061451715, 6.421520780324663323E-16, -5.243569643749999010 ) ) ;
#49282=CARTESIAN_POINT ( 'NONE',  ( 15.12187500061451750, -6.054752690667223547, -1.112240025338166033E-15 ) ) ;
#49283=CARTESIAN_POINT ( 'NONE',  ( 22.84687500061451715, -3.027376345333610441, -5.243569643749999898 ) ) ;
#49284=CARTESIAN_POINT ( 'NONE',  ( 9.001249775931846008E-16, 12.32187500061451857, 34.90005215228797653 ) ) ;
#49285=CARTESIAN_POINT ( 'NONE',  ( 5.990625000614517859, -3.027376345333614438, 5.243569643749998122 ) ) ;
#49286=CARTESIAN_POINT ( 'NONE',  ( 25.34062500061451217, -3.027376345333614438, 5.243569643749998122 ) ) ;
#49287=CARTESIAN_POINT ( 'NONE',  ( 27.92812500061451431, 4.541064518000418104, 2.621784821874999949 ) ) ;
#49289=CARTESIAN_POINT ( 'NONE',  ( 1.999999999999998668, 19.40000000000000213, 26.53589838486224650 ) ) ;
#49290=CARTESIAN_POINT ( 'NONE',  ( 7.659375000614518036, 4.541064518000418104, -2.621784821874998173 ) ) ;
#49292=CARTESIAN_POINT ( 'NONE',  ( 13.65000000122903323, -2.886751345948125991, -5.000000000000000000 ) ) ;
#49293=CARTESIAN_POINT ( 'NONE',  ( 10.35000000122903074, -2.886751345948129988, 4.999999999999997335 ) ) ;
#49294=CARTESIAN_POINT ( 'NONE',  ( 29.43750000122903288, 6.123233995736764310E-16, -4.999999999999998224 ) ) ;
#49297=CARTESIAN_POINT ( 'NONE',  ( 14.89687500061451786, 6.054752690667223547, 3.707466751127219781E-16 ) ) ;
#49298=CARTESIAN_POINT ( 'NONE',  ( 11.96250000000000213, 2.886751345948126879, 4.999999999999998224 ) ) ;
#49300=CARTESIAN_POINT ( 'NONE',  ( 18.77812500061451573, 6.421520780324663323E-16, -5.243569643749999010 ) ) ;
#49301=CARTESIAN_POINT ( 'NONE',  ( 8.503125000614515372, 4.541064518000418104, -2.621784821874998173 ) ) ;
#49302=CARTESIAN_POINT ( 'NONE',  ( 21.45937500061451786, -4.541064518000417216, -2.621784821875001281 ) ) ;
#49303=CARTESIAN_POINT ( 'NONE',  ( 5.053125000614517859, 0.000000000000000000, 5.243569643749999010 ) ) ;
#49304=FACE_OUTER_BOUND ( 'NONE', #5862, .T. ) ;
#49305=CARTESIAN_POINT ( 'NONE',  ( 7.050000001229036251, 5.773502691896255534, 3.535250795749688894E-16 ) ) ;
#49306=CARTESIAN_POINT ( 'NONE',  ( 23.16562500061451502, -6.054752690667223547, -1.112240025338166033E-15 ) ) ;
#49307=CARTESIAN_POINT ( 'NONE',  ( 3.999999999999998668, 17.22500000122903785, -32.30940107675850470 ) ) ;
#49308=CARTESIAN_POINT ( 'NONE',  ( 10.68750000122903288, 4.330127018922191873, 2.499999999999999556 ) ) ;
#49309=CARTESIAN_POINT ( 'NONE',  ( 18.89062500061451644, 6.054752690667223547, 3.707466751127219781E-16 ) ) ;
#49310=CARTESIAN_POINT ( 'NONE',  ( 16.45312500061451289, -4.541064518000417216, -2.621784821875001281 ) ) ;
#49312=CARTESIAN_POINT ( 'NONE',  ( 16.46249999999999503, 2.886751345948126879, 4.999999999999999112 ) ) ;
#49313=CARTESIAN_POINT ( 'NONE',  ( 11.85000000122903430, -2.886751345948125991, -5.000000000000000000 ) ) ;
#49315=CARTESIAN_POINT ( 'NONE',  ( 7.828125000614517326, -4.541064518000419881, 2.621784821874995952 ) ) ;
#49316=CARTESIAN_POINT ( 'NONE',  ( 11.61562500061451608, 3.027376345333613106, -5.243569643749998122 ) ) ;
#49317=EDGE_CURVE ( 'NONE', #43350, #26212, #13715, .T. ) ;
#49319=CARTESIAN_POINT ( 'NONE',  ( 21.63750000122903572, -4.330127018922194537, 2.499999999999995559 ) ) ;
#49320=CARTESIAN_POINT ( 'NONE',  ( 19.77187500061451786, 3.027376345333613106, -5.243569643749998122 ) ) ;
#49322=CARTESIAN_POINT ( 'NONE',  ( 5.550000001229032698, -2.886751345948125991, -5.000000000000000000 ) ) ;
#49323=CARTESIAN_POINT ( 'NONE',  ( 4.771875000614516971, -6.054752690667223547, -1.112240025338166033E-15 ) ) ;
#49324=CARTESIAN_POINT ( 'NONE',  ( 23.59687500061451715, -3.027376345333614438, 5.243569643749998122 ) ) ;
#49326=CARTESIAN_POINT ( 'NONE',  ( 19.30312500061451786, 4.541064518000418104, -2.621784821874998173 ) ) ;
#49327=CARTESIAN_POINT ( 'NONE',  ( 23.74687500061451573, -3.027376345333610441, -5.243569643749999898 ) ) ;
#49329=CARTESIAN_POINT ( 'NONE',  ( -3.999999999999999112, 11.07500000122903394, -32.30940107675850470 ) ) ;
#49330=CARTESIAN_POINT ( 'NONE',  ( 29.74687500061451217, 6.054752690667223547, 3.707466751127219781E-16 ) ) ;
#49332=CARTESIAN_POINT ( 'NONE',  ( 13.94062500061451892, 6.054752690667223547, 3.707466751127219781E-16 ) ) ;
#49333=CARTESIAN_POINT ( 'NONE',  ( 12.19687500061451679, 6.054752690667223547, 3.707466751127219781E-16 ) ) ;
#49335=CARTESIAN_POINT ( 'NONE',  ( 29.09999999999999787, 0.000000000000000000, 4.999999999999998224 ) ) ;
#49336=CARTESIAN_POINT ( 'NONE',  ( 22.45312500061451644, 4.541064518000418104, -2.621784821874998173 ) ) ;
#49338=CARTESIAN_POINT ( 'NONE',  ( 28.68750000122903288, 4.330127018922191873, 2.499999999999999556 ) ) ;
#49339=CARTESIAN_POINT ( 'NONE',  ( 13.64999999999999858, 4.330127018922192761, -2.499999999999997780 ) ) ;
#49340=CARTESIAN_POINT ( 'NONE',  ( 23.40000000122903145, -2.886751345948129988, 4.999999999999997335 ) ) ;
#49341=CARTESIAN_POINT ( 'NONE',  ( 18.66562500061451146, -6.054752690667223547, -1.112240025338166033E-15 ) ) ;
#49343=CARTESIAN_POINT ( 'NONE',  ( 21.56250000000000000, -5.773502691896255534, -1.060575238724906372E-15 ) ) ;
#49344=CARTESIAN_POINT ( 'NONE',  ( 22.88437500061451857, 6.421520780324663323E-16, -5.243569643749999010 ) ) ;
#49345=EDGE_CURVE ( 'NONE', #40707, #5936, #45874, .T. ) ;
#49347=CARTESIAN_POINT ( 'NONE',  ( 20.06250000000000000, 2.886751345948126879, 4.999999999999998224 ) ) ;
#49348=CARTESIAN_POINT ( 'NONE',  ( 9.890625000614516438, 6.054752690667223547, 3.707466751127219781E-16 ) ) ;
#49349=CARTESIAN_POINT ( 'NONE',  ( 3.215625000614518836, 3.027376345333611329, 5.243569643749999010 ) ) ;
#49351=CARTESIAN_POINT ( 'NONE',  ( 26.76562500061451644, -6.054752690667223547, -1.112240025338166033E-15 ) ) ;
#49352=CARTESIAN_POINT ( 'NONE',  ( 17.66249999999999787, 2.886751345948129099, -4.999999999999998224 ) ) ;
#49353=CARTESIAN_POINT ( 'NONE',  ( 25.34999999999999787, 4.330127018922192761, -2.499999999999997780 ) ) ;
#49354=CARTESIAN_POINT ( 'NONE',  ( 3.531447089546592366, -3.539662852346280975, -3.745757099853723293 ) ) ;
#49355=CARTESIAN_POINT ( 'NONE',  ( 5.671875000614519102, -6.054752690667223547, -1.112240025338166033E-15 ) ) ;
#49356=CARTESIAN_POINT ( 'NONE',  ( 16.84687500061451715, -3.027376345333614438, 5.243569643749998122 ) ) ;
#49357=CARTESIAN_POINT ( 'NONE',  ( 29.18437500061451573, 6.421520780324663323E-16, -5.243569643749999010 ) ) ;
#49359=CARTESIAN_POINT ( 'NONE',  ( 25.71562500061451573, 3.027376345333611329, 5.243569643749999010 ) ) ;
#49360=CARTESIAN_POINT ( 'NONE',  ( 27.64687500061452141, -3.027376345333614438, 5.243569643749998122 ) ) ;
#49362=CARTESIAN_POINT ( 'NONE',  ( 12.82499999999999929, 4.330127018922191873, 2.499999999999999556 ) ) ;
#49363=CARTESIAN_POINT ( 'NONE',  ( 11.20312500061451644, 4.541064518000418104, -2.621784821874998173 ) ) ;
#49364=CARTESIAN_POINT ( 'NONE',  ( 3.808519521103546523, 3.239781818325435658, 3.901918515728798997 ) ) ;
#49366=CARTESIAN_POINT ( 'NONE',  ( 28.04062500061451502, -3.027376345333614438, 5.243569643749998122 ) ) ;
#49367=CARTESIAN_POINT ( 'NONE',  ( 16.68750000122903288, -4.330127018922194537, 2.499999999999995559 ) ) ;
#49368=CARTESIAN_POINT ( 'NONE',  ( 3.853125000614517681, -4.541064518000417216, -2.621784821875001281 ) ) ;
#49370=CARTESIAN_POINT ( 'NONE',  ( 5.428125000614517859, 4.541064518000418104, 2.621784821874999949 ) ) ;
#49371=CARTESIAN_POINT ( 'NONE',  ( 22.54687500061451999, 6.054752690667223547, 3.707466751127219781E-16 ) ) ;
#49372=CARTESIAN_POINT ( 'NONE',  ( 9.001249775931846008E-16, 18.17187500061451999, 34.90005215228797653 ) ) ;
#49373=CARTESIAN_POINT ( 'NONE',  ( 20.52187500061451786, -6.054752690667223547, -1.112240025338166033E-15 ) ) ;
#49374=CARTESIAN_POINT ( 'NONE',  ( 29.70937500061451431, 4.541064518000418104, -2.621784821874998173 ) ) ;
#49375=CARTESIAN_POINT ( 'NONE',  ( -4.243569643749999898, 18.95937500061451431, 30.00000000000000000 ) ) ;
#49376=CARTESIAN_POINT ( 'NONE',  ( 12.47812500061451502, 6.421520780324663323E-16, -5.243569643749999010 ) ) ;
#49377=CARTESIAN_POINT ( 'NONE',  ( 3.975000001229033852, 2.886751345948126879, 4.999999999999999112 ) ) ;
#49378=CARTESIAN_POINT ( 'NONE',  ( 7.621875000614519280, 3.027376345333613106, -5.243569643749998122 ) ) ;
#49380=CARTESIAN_POINT ( 'NONE',  ( 10.97812500061451679, -4.541064518000419881, 2.621784821874995952 ) ) ;
#49381=CARTESIAN_POINT ( 'NONE',  ( 13.80937500061451750, -4.541064518000417216, -2.621784821875001281 ) ) ;
#49382=CARTESIAN_POINT ( 'NONE',  ( 22.50000000122903288, -2.886751345948129988, 4.999999999999997335 ) ) ;
#49383=CARTESIAN_POINT ( 'NONE',  ( 9.046875000614518214, 6.054752690667223547, 3.707466751127219781E-16 ) ) ;
#49384=CARTESIAN_POINT ( 'NONE',  ( 10.37812500061451715, 4.541064518000418104, 2.621784821874999949 ) ) ;
#49386=CARTESIAN_POINT ( 'NONE',  ( 22.02187500061452141, 3.027376345333613106, -5.243569643749998122 ) ) ;
#49388=CARTESIAN_POINT ( 'NONE',  ( -3.999828644916960663, 3.000228472979582506, 30.14345285717328693 ) ) ;
#49389=CARTESIAN_POINT ( 'NONE',  ( 2.915625000614516793, -6.054752690667223547, -1.112240025338166033E-15 ) ) ;
#49390=CARTESIAN_POINT ( 'NONE',  ( 2.121784821874999061, 11.15937500061451715, -33.67503911421598417 ) ) ;
#49391=CARTESIAN_POINT ( 'NONE',  ( 14.40000000122903323, -2.886751345948129988, 4.999999999999997335 ) ) ;
#49392=CARTESIAN_POINT ( 'NONE',  ( -2.121784821874996840, 14.92812500061451608, -26.32496088578401583 ) ) ;
#49393=CARTESIAN_POINT ( 'NONE',  ( 16.46250000122903501, 4.330127018922192761, -2.499999999999997780 ) ) ;
#49394=CARTESIAN_POINT ( 'NONE',  ( 9.778125000614517504, 6.421520780324663323E-16, -5.243569643749999010 ) ) ;
#49395=ORIENTED_EDGE ( 'NONE', *, *, #45137, .T. ) ;
#49396=CARTESIAN_POINT ( 'NONE',  ( 13.83749999999999858, -2.886751345948129988, 4.999999999999997335 ) ) ;
#49398=CARTESIAN_POINT ( 'NONE',  ( 23.01562500061451644, 3.027376345333611329, 5.243569643749999010 ) ) ;
#49399=CARTESIAN_POINT ( 'NONE',  ( 10.73437500061451644, 6.421520780324663323E-16, -5.243569643749999010 ) ) ;
#49400=LINE ( 'NONE', #70828, #65688 ) ;
#49401=CARTESIAN_POINT ( 'NONE',  ( 9.600000001229034297, -2.886751345948125991, -5.000000000000000000 ) ) ;
#49402=CARTESIAN_POINT ( 'NONE',  ( 19.31250000122903288, 0.000000000000000000, 4.999999999999998224 ) ) ;
#49403=CARTESIAN_POINT ( 'NONE',  ( 15.02812500061451750, -4.541064518000419881, 2.621784821874995952 ) ) ;
#49404=CARTESIAN_POINT ( 'NONE',  ( 18.92812500061451431, 4.541064518000418104, 2.621784821874999949 ) ) ;
#49405=CARTESIAN_POINT ( 'NONE',  ( 25.87500000122903288, 2.886751345948129099, -4.999999999999998224 ) ) ;
#49406=CARTESIAN_POINT ( 'NONE',  ( 26.88750000122903216, 4.330127018922191873, 2.499999999999999556 ) ) ;
#49407=CARTESIAN_POINT ( 'NONE',  ( 26.21249999999999858, 2.886751345948129099, -4.999999999999998224 ) ) ;
#49409=CARTESIAN_POINT ( 'NONE',  ( 26.93437500061451573, 6.421520780324663323E-16, -5.243569643749999010 ) ) ;
#49410=DIRECTION ( 'NONE',  ( -0.000000000000000000, -1.000000000000000000, -0.000000000000000000 ) ) ;
#49411=CARTESIAN_POINT ( 'NONE',  ( 12.93750000122903465, 4.330127018922191873, 2.499999999999999556 ) ) ;
#49412=CARTESIAN_POINT ( 'NONE',  ( 3.300000000000000711, 4.330127018922192761, -2.499999999999997780 ) ) ;
#49414=CARTESIAN_POINT ( 'NONE',  ( 3.984375000614517326, 6.421520780324663323E-16, -5.243569643749999010 ) ) ;
#49415=CARTESIAN_POINT ( 'NONE',  ( 25.64062500061451644, 6.054752690667223547, 3.707466751127219781E-16 ) ) ;
#49417=CARTESIAN_POINT ( 'NONE',  ( 11.03437500061451715, -4.541064518000419881, 2.621784821874995952 ) ) ;
#49419=CARTESIAN_POINT ( 'NONE',  ( 29.72812500061451502, 4.541064518000418104, 2.621784821874999949 ) ) ;
#49420=CARTESIAN_POINT ( 'NONE',  ( 8.334375000614516082, -4.541064518000419881, 2.621784821874995952 ) ) ;
#49421=CARTESIAN_POINT ( 'NONE',  ( 28.58437500061451786, -4.541064518000419881, 2.621784821874995952 ) ) ;
#49422=CARTESIAN_POINT ( 'NONE',  ( 4.243569643749999898, 11.92812500061459247, 30.00000000000000000 ) ) ;
#49423=CARTESIAN_POINT ( 'NONE',  ( 21.11249999999999716, -5.773502691896255534, -1.060575238724906372E-15 ) ) ;
#49425=CARTESIAN_POINT ( 'NONE',  ( 20.70000000122903216, -2.886751345948096681, 5.000000000000054179 ) ) ;
#49426=CARTESIAN_POINT ( 'NONE',  ( 4.425000000000001599, -4.330127018922194537, 2.499999999999995559 ) ) ;
#49428=ORIENTED_EDGE ( 'NONE', *, *, #57151, .F. ) ;
#49429=CARTESIAN_POINT ( 'NONE',  ( 17.84062500061451573, -3.027376345333610441, -5.243569643749999898 ) ) ;
#49430=CARTESIAN_POINT ( 'NONE',  ( 11.42812500061451608, -4.541064518000419881, 2.621784821874995952 ) ) ;
#49432=CARTESIAN_POINT ( 'NONE',  ( 7.434375000614519280, -4.541064518000419881, 2.621784821874995952 ) ) ;
#49433=CARTESIAN_POINT ( 'NONE',  ( 20.96250000122903145, 4.330127018922192761, -2.499999999999997780 ) ) ;
#49434=CARTESIAN_POINT ( 'NONE',  ( 24.00000000122903288, -2.886751345948092684, -5.000000000000057732 ) ) ;
#49435=CARTESIAN_POINT ( 'NONE',  ( 6.234375000614519102, 6.421520780324663323E-16, -5.243569643749999010 ) ) ;
#49436=CARTESIAN_POINT ( 'NONE',  ( 14.33437500061451786, 6.421520780324663323E-16, -5.243569643749999010 ) ) ;
#49437=CARTESIAN_POINT ( 'NONE',  ( 24.42187500061451999, 3.027376345333611329, 5.243569643749999010 ) ) ;
#49438=DIRECTION ( 'NONE',  ( -0.000000000000000000, -1.000000000000000000, -0.000000000000000000 ) ) ;
#49441=CARTESIAN_POINT ( 'NONE',  ( 17.89687500061451431, -3.027376345333610441, -5.243569643749999898 ) ) ;
#49442=CARTESIAN_POINT ( 'NONE',  ( 9.384375000614518569, 6.421520780324663323E-16, -5.243569643749999010 ) ) ;
#49444=CARTESIAN_POINT ( 'NONE',  ( 20.06250000000000000, 2.886751345948126879, 4.999999999999999112 ) ) ;
#49446=CARTESIAN_POINT ( 'NONE',  ( 29.84999999999999787, 4.330127018922192761, -2.499999999999997780 ) ) ;
#49448=CARTESIAN_POINT ( 'NONE',  ( 11.69062500061451360, 6.054752690667223547, 3.707466751127219781E-16 ) ) ;
#49449=CARTESIAN_POINT ( 'NONE',  ( 28.28437500061451715, 6.421520780324663323E-16, -5.243569643749999010 ) ) ;
#49450=DIRECTION ( 'NONE',  ( -1.000000000000000000, -0.000000000000000000, -0.000000000000000000 ) ) ;
#49451=CARTESIAN_POINT ( 'NONE',  ( 28.54687500061451644, -3.027376345333614438, 5.243569643749998122 ) ) ;
#49452=CARTESIAN_POINT ( 'NONE',  ( 11.28749999999999787, -2.886751345948125991, -5.000000000000000000 ) ) ;
#49453=CARTESIAN_POINT ( 'NONE',  ( -3.999999999999999556, 17.82500000122903572, 27.69059892324149530 ) ) ;
#49454=CARTESIAN_POINT ( 'NONE',  ( 12.18750000122903465, -4.330127018922194537, 2.499999999999995559 ) ) ;
#49455=CARTESIAN_POINT ( 'NONE',  ( 21.87187500061451573, -6.054752690667223547, -1.112240025338166033E-15 ) ) ;
#49456=CARTESIAN_POINT ( 'NONE',  ( 17.40937500061451715, -4.541064518000417216, -2.621784821875001281 ) ) ;
#49457=CARTESIAN_POINT ( 'NONE',  ( 1.071796769724497445, 16.82990381179670081, 26.00000000000000355 ) ) ;
#49458=VERTEX_POINT ( 'NONE', #58650 ) ;
#49459=CARTESIAN_POINT ( 'NONE',  ( 17.05312500061451786, 4.541064518000418104, -2.621784821874998173 ) ) ;
#49460=CARTESIAN_POINT ( 'NONE',  ( 28.16250000122903074, 4.330127018922192761, -2.499999999999997780 ) ) ;
#49461=CARTESIAN_POINT ( 'NONE',  ( 14.82187500061451679, 3.027376345333613106, -5.243569643749998122 ) ) ;
#49462=CARTESIAN_POINT ( 'NONE',  ( 2.840625000614518392, -3.027376345333614438, 5.243569643749998122 ) ) ;
#49463=CARTESIAN_POINT ( 'NONE',  ( 18.66562500061451146, -6.054752690667223547, -1.112240025338166033E-15 ) ) ;
#49464=DIRECTION ( 'NONE',  ( -1.000000000000000000, -0.000000000000000000, -0.000000000000000000 ) ) ;
#49465=CARTESIAN_POINT ( 'NONE',  ( 28.47187500061451715, 3.027376345333611329, 5.243569643749999010 ) ) ;
#49466=CARTESIAN_POINT ( 'NONE',  ( 9.001249775931846008E-16, 13.61562500061451786, 34.90005215228797653 ) ) ;
#49467=CARTESIAN_POINT ( 'NONE',  ( 16.54687500061451644, -3.027376345333610441, -5.243569643749999898 ) ) ;
#49468=CARTESIAN_POINT ( 'NONE',  ( 14.70000000122903394, 5.773502691896255534, 3.535250795749688894E-16 ) ) ;
#49470=CARTESIAN_POINT ( 'NONE',  ( -2.121784821874996840, 19.03437500061451715, -26.32496088578401583 ) ) ;
#49471=( BOUNDED_CURVE ( )  B_SPLINE_CURVE ( 2, ( #9211, #42827, #3678, #59434, #29645, #31378, #49111, #71640, #1951 ),
 .UNSPECIFIED., .F., .F. ) 
 B_SPLINE_CURVE_WITH_KNOTS ( ( 3, 2, 2, 2, 3 ),
 ( 0.05434782608695652717, 0.05797101449275362389, 0.06521739130434782428, 0.07246376811594203160, 0.07608695652173913526 ),
 .UNSPECIFIED. ) 
 CURVE ( )  GEOMETRIC_REPRESENTATION_ITEM ( )  RATIONAL_B_SPLINE_CURVE ( ( 0.9330127018922194093, 0.9330127018922194093, 1.000000000000000000, 0.8660254037844387076, 1.000000000000000000, 0.8660254037844387076, 1.000000000000000000, 0.9330127018922191873, 0.9330127018922192983 ) ) 
 REPRESENTATION_ITEM ( '' )  );
#49472=CARTESIAN_POINT ( 'NONE',  ( 19.77187500061451786, 3.027376345333613106, -5.243569643749998122 ) ) ;
#49473=CARTESIAN_POINT ( 'NONE',  ( 22.23750000122903003, 6.123233995736764310E-16, -4.999999999999998224 ) ) ;
#49474=CARTESIAN_POINT ( 'NONE',  ( 16.35937500061451644, 0.000000000000000000, 5.243569643749999010 ) ) ;
#49475=CARTESIAN_POINT ( 'NONE',  ( 12.02812500061451573, 6.421520780324663323E-16, -5.243569643749999010 ) ) ;
#49476=CARTESIAN_POINT ( 'NONE',  ( -4.243569643749999898, 14.42187500061451644, 27.54997392385601529 ) ) ;
#49477=CARTESIAN_POINT ( 'NONE',  ( 17.54062500061451502, 6.054752690667223547, 3.707466751127219781E-16 ) ) ;
#49478=ORIENTED_EDGE ( 'NONE', *, *, #39698, .F. ) ;
#49479=ORIENTED_EDGE ( 'NONE', *, *, #34377, .T. ) ;
#49480=CARTESIAN_POINT ( 'NONE',  ( 23.25000000000000000, 0.000000000000000000, 4.999999999999998224 ) ) ;
#49481=CARTESIAN_POINT ( 'NONE',  ( 2.121784821875001281, 18.65937500061451715, -26.32496088578401938 ) ) ;
#49482=DIRECTION ( 'NONE',  ( -1.000000000000000000, 0.000000000000000000, 0.000000000000000000 ) ) ;
#49483=CARTESIAN_POINT ( 'NONE',  ( 24.66562500061451502, 3.027376345333613106, -5.243569643749998122 ) ) ;
#49484=CARTESIAN_POINT ( 'NONE',  ( 5.015625000614518214, 3.027376345333611329, 5.243569643749999010 ) ) ;
#49485=CARTESIAN_POINT ( 'NONE',  ( 18.37500000122903288, 2.886751345948126879, 4.999999999999999112 ) ) ;
#49486=CARTESIAN_POINT ( 'NONE',  ( 22.71562500061451573, -6.054752690667223547, -1.112240025338166033E-15 ) ) ;
#49487=CARTESIAN_POINT ( 'NONE',  ( 22.46250000000000213, -5.773502691896255534, -1.060575238724906372E-15 ) ) ;
#49488=CARTESIAN_POINT ( 'NONE',  ( 25.19062500061451715, 6.054752690667223547, 3.707466751127219781E-16 ) ) ;
#49489=CARTESIAN_POINT ( 'NONE',  ( 5.915625000614515905, 3.027376345333611329, 5.243569643749999010 ) ) ;
#49492=CARTESIAN_POINT ( 'NONE',  ( 22.90312500061451573, 4.541064518000418104, -2.621784821874998173 ) ) ;
#49497=CARTESIAN_POINT ( 'NONE',  ( -2.000000000000000000, 13.73750000122903359, -33.46410161513775705 ) ) ;
#49498=CARTESIAN_POINT ( 'NONE',  ( -3.999999999999999112, 13.70000000000000107, -30.00000000000000000 ) ) ;
#49499=CARTESIAN_POINT ( 'NONE',  ( 11.13750000000000284, -2.886751345948129988, 4.999999999999997335 ) ) ;
#49501=CARTESIAN_POINT ( 'NONE',  ( 11.55937500061451928, -4.541064518000417216, -2.621784821875001281 ) ) ;
#49502=CARTESIAN_POINT ( 'NONE',  ( 7.312500001229033764, -4.330127018922190985, -2.500000000000001332 ) ) ;
#49503=CARTESIAN_POINT ( 'NONE',  ( 13.88437500061451679, 6.421520780324663323E-16, -5.243569643749999010 ) ) ;
#49504=CARTESIAN_POINT ( 'NONE',  ( 7.096875000614517148, -3.027376345333610441, -5.243569643749999898 ) ) ;
#49505=CARTESIAN_POINT ( 'NONE',  ( 2.121784821874999061, 10.20312500061451821, -33.67503911421598417 ) ) ;
#49506=LINE ( 'NONE', #4080, #20576 ) ;
#49507=EDGE_CURVE ( 'NONE', #18523, #54370, #41139, .T. ) ;
#49508=CARTESIAN_POINT ( 'NONE',  ( 11.63437500061451857, 6.421520780324663323E-16, -5.243569643749999010 ) ) ;
#49509=CARTESIAN_POINT ( 'NONE',  ( 13.31250000000000178, 2.886751345948126879, 4.999999999999998224 ) ) ;
#49510=CARTESIAN_POINT ( 'NONE',  ( 20.87812500061451715, -4.541064518000419881, 2.621784821874995952 ) ) ;
#49512=CARTESIAN_POINT ( 'NONE',  ( 2.121784821875001281, 18.60312500061459673, 33.67503911421598417 ) ) ;
#49513=CARTESIAN_POINT ( 'NONE',  ( 22.50937500061451857, 4.541064518000418104, -2.621784821874998173 ) ) ;
#49514=CARTESIAN_POINT ( 'NONE',  ( 1.999999999999998668, 19.40000000000000213, 26.53589838486224650 ) ) ;
#49516=CARTESIAN_POINT ( 'NONE',  ( 29.40000000122903145, -2.886751345948125991, -5.000000000000000000 ) ) ;
#49518=CARTESIAN_POINT ( 'NONE',  ( 25.45312500061451644, -4.541064518000417216, -2.621784821875001281 ) ) ;
#49519=CARTESIAN_POINT ( 'NONE',  ( 18.51562500061451289, 3.027376345333611329, 5.243569643749999010 ) ) ;
#49521=CARTESIAN_POINT ( 'NONE',  ( 14.14687500061451786, -3.027376345333614438, 5.243569643749998122 ) ) ;
#49523=CARTESIAN_POINT ( 'NONE',  ( 27.48750000122903359, -4.330127018922194537, 2.499999999999995559 ) ) ;
#49524=CARTESIAN_POINT ( 'NONE',  ( 6.534375000614517148, -4.541064518000419881, 2.621784821874995952 ) ) ;
#49525=CARTESIAN_POINT ( 'NONE',  ( 14.59687500061452070, -3.027376345333614438, 5.243569643749998122 ) ) ;
#49526=CARTESIAN_POINT ( 'NONE',  ( 16.05000000000000071, 0.000000000000000000, 4.999999999999998224 ) ) ;
#49527=CARTESIAN_POINT ( 'NONE',  ( 8.137500001229033941, -4.330127018922194537, 2.499999999999995559 ) ) ;
#49528=CARTESIAN_POINT ( 'NONE',  ( 4.200000001229033053, -2.886751345948125991, -5.000000000000000000 ) ) ;
#49529=CARTESIAN_POINT ( 'NONE',  ( 25.39687500061451431, -3.027376345333614438, 5.243569643749998122 ) ) ;
#49530=CARTESIAN_POINT ( 'NONE',  ( 17.55937500061451573, 4.541064518000418104, -2.621784821874998173 ) ) ;
#49532=CARTESIAN_POINT ( 'NONE',  ( 29.28749999999999787, -2.886751345948125991, -5.000000000000000000 ) ) ;
#49533=CARTESIAN_POINT ( 'NONE',  ( 6.637500000000001066, -2.886751345948129988, 4.999999999999997335 ) ) ;
#49535=CARTESIAN_POINT ( 'NONE',  ( 20.65312500061451573, 4.541064518000418104, -2.621784821874998173 ) ) ;
#49536=CARTESIAN_POINT ( 'NONE',  ( 8.662499999999999645, 2.886751345948129099, -4.999999999999998224 ) ) ;
#49538=CARTESIAN_POINT ( 'NONE',  ( 4.828125000614518214, 6.421520780324663323E-16, -5.243569643749999010 ) ) ;
#49539=CARTESIAN_POINT ( 'NONE',  ( 20.21250000000000213, -5.773502691896255534, -1.060575238724906372E-15 ) ) ;
#49540=( BOUNDED_CURVE ( )  B_SPLINE_CURVE ( 1, ( #47790, #13420 ),
 .UNSPECIFIED., .F., .F. ) 
 B_SPLINE_CURVE_WITH_KNOTS ( ( 2, 2 ),
 ( 0.000000000000000000, 1.000000000000000000 ),
 .UNSPECIFIED. ) 
 CURVE ( )  GEOMETRIC_REPRESENTATION_ITEM ( )  RATIONAL_B_SPLINE_CURVE ( ( 0.9401540804572410259, 0.9401540804572410259 ) ) 
 REPRESENTATION_ITEM ( '' )  );
#49541=CARTESIAN_POINT ( 'NONE',  ( 1.592000809091587073E-14, 17.18750000000000355, 26.00000000000000000 ) ) ;
#49542=CARTESIAN_POINT ( 'NONE',  ( 24.11250000122903359, 4.330127018922192761, -2.499999999999997780 ) ) ;
#49543=CARTESIAN_POINT ( 'NONE',  ( 5.948646956027291210, 8.038298999021536773, 30.80897801260831770 ) ) ;
#49544=CARTESIAN_POINT ( 'NONE',  ( 3.112500000000000711, -5.773502691896255534, -1.060575238724906372E-15 ) ) ;
#49546=CARTESIAN_POINT ( 'NONE',  ( 16.49062500061451786, -3.027376345333610441, -5.243569643749999898 ) ) ;
#49547=CARTESIAN_POINT ( 'NONE',  ( 24.47812500061451502, -4.541064518000419881, 2.621784821874995952 ) ) ;
#49548=CARTESIAN_POINT ( 'NONE',  ( 25.80937500061451928, 0.000000000000000000, 5.243569643749999010 ) ) ;
#49549=CARTESIAN_POINT ( 'NONE',  ( 6.037500000000001421, 5.773502691896255534, 3.535250795749688894E-16 ) ) ;
#49550=CARTESIAN_POINT ( 'NONE',  ( 10.34062500061451750, 6.054752690667223547, 3.707466751127219781E-16 ) ) ;
#49551=CARTESIAN_POINT ( 'NONE',  ( 26.31562500061451715, -6.054752690667223547, -1.112240025338166033E-15 ) ) ;
#49552=CARTESIAN_POINT ( 'NONE',  ( 14.85937500061451644, 4.541064518000418104, -2.621784821874998173 ) ) ;
#49553=CARTESIAN_POINT ( 'NONE',  ( 18.68437500061451928, -4.541064518000419881, 2.621784821874995952 ) ) ;
#49554=CARTESIAN_POINT ( 'NONE',  ( 30.00000000000000000, 6.123233995736764310E-16, -4.999999999999998224 ) ) ;
#49555=CARTESIAN_POINT ( 'NONE',  ( 2.121784821875001281, 10.10937500061451821, 33.67503911421598417 ) ) ;
#49556=CARTESIAN_POINT ( 'NONE',  ( 23.62500000122902932, 2.886751345948129099, -4.999999999999998224 ) ) ;
#49558=CARTESIAN_POINT ( 'NONE',  ( 12.40312500061451573, -4.541064518000417216, -2.621784821875001281 ) ) ;
#49559=CARTESIAN_POINT ( 'NONE',  ( 6.796875000614516438, 6.054752690667223547, 3.707466751127219781E-16 ) ) ;
#49560=CARTESIAN_POINT ( 'NONE',  ( 7.884375000614517681, -4.541064518000419881, 2.621784821874995952 ) ) ;
#49562=CARTESIAN_POINT ( 'NONE',  ( 27.00937500061451857, 4.541064518000418104, -2.621784821874998173 ) ) ;
#49563=CARTESIAN_POINT ( 'NONE',  ( 19.34062500061451573, 6.054752690667223547, 3.707466751127219781E-16 ) ) ;
#49564=CARTESIAN_POINT ( 'NONE',  ( 29.66250000122903074, 0.000000000000000000, 4.999999999999998224 ) ) ;
#49565=CARTESIAN_POINT ( 'NONE',  ( 3.046875000614519990, -3.027376345333610441, -5.243569643749999898 ) ) ;
#49566=CARTESIAN_POINT ( 'NONE',  ( 24.23437500061451644, 6.421520780324663323E-16, -5.243569643749999010 ) ) ;
#49567=CARTESIAN_POINT ( 'NONE',  ( 18.92812500061451431, 4.541064518000418104, 2.621784821874999949 ) ) ;
#49568=CARTESIAN_POINT ( 'NONE',  ( 8.484601909799253346E-16, 11.11250000000000071, 34.61880215351700230 ) ) ;
#49569=CARTESIAN_POINT ( 'NONE',  ( 24.77812500061451217, 4.541064518000418104, 2.621784821874999949 ) ) ;
#49570=CARTESIAN_POINT ( 'NONE',  ( 5.437500001229035540, -4.330127018922194537, 2.499999999999995559 ) ) ;
#49571=ORIENTED_EDGE ( 'NONE', *, *, #35816, .F. ) ;
#49572=LINE ( 'NONE', #15933, #41604 ) ;
#49573=CARTESIAN_POINT ( 'NONE',  ( 1.999999999999998668, 15.80000000000000071, -33.46410161513775705 ) ) ;
#49575=CARTESIAN_POINT ( 'NONE',  ( 5.709375000614517859, -4.541064518000417216, -2.621784821875001281 ) ) ;
#49576=FACE_OUTER_BOUND ( 'NONE', #27464, .T. ) ;
#49577=CARTESIAN_POINT ( 'NONE',  ( 12.89062500061451821, -3.027376345333610441, -5.243569643749999898 ) ) ;
#49578=CARTESIAN_POINT ( 'NONE',  ( 5.671875000614519102, -6.054752690667223547, -1.112240025338166033E-15 ) ) ;
#49579=CARTESIAN_POINT ( 'NONE',  ( 25.38750000122903216, 6.123233995736764310E-16, -4.999999999999998224 ) ) ;
#49580=CARTESIAN_POINT ( 'NONE',  ( 15.15937500061451715, -4.541064518000417216, -2.621784821875001281 ) ) ;
#49581=CARTESIAN_POINT ( 'NONE',  ( 29.72812500061451502, 4.541064518000418104, 2.621784821874999949 ) ) ;
#49582=CARTESIAN_POINT ( 'NONE',  ( 14.62500000122903288, 2.886751345948129099, -4.999999999999997335 ) ) ;
#49583=CARTESIAN_POINT ( 'NONE',  ( 16.07812500061451289, 6.421520780324663323E-16, -5.243569643749999010 ) ) ;
#49584=ORIENTED_EDGE ( 'NONE', *, *, #64257, .F. ) ;
#49585=CARTESIAN_POINT ( 'NONE',  ( 10.45312500061451644, 0.000000000000000000, 5.243569643749999010 ) ) ;
#49586=CARTESIAN_POINT ( 'NONE',  ( 8.690625000614515372, -3.027376345333614438, 5.243569643749998122 ) ) ;
#49588=CARTESIAN_POINT ( 'NONE',  ( 8.512499999999999289, -5.773502691896255534, -1.060575238724906372E-15 ) ) ;
#49589=CARTESIAN_POINT ( 'NONE',  ( 3.787500001229033408, 6.123233995736764310E-16, -4.999999999999998224 ) ) ;
#49590=CARTESIAN_POINT ( 'NONE',  ( 18.45000000000000284, -4.330127018922190985, -2.500000000000001332 ) ) ;
#49592=CARTESIAN_POINT ( 'NONE',  ( 18.75937500061451857, -4.541064518000417216, -2.621784821875001281 ) ) ;
#49593=CARTESIAN_POINT ( 'NONE',  ( 13.35000000122903430, 5.773502691896255534, 3.535250795749688894E-16 ) ) ;
#49595=CARTESIAN_POINT ( 'NONE',  ( -4.243569643749999898, 16.16562500061451857, -32.45002607614398471 ) ) ;
#49598=CARTESIAN_POINT ( 'NONE',  ( 29.69062500061451715, 6.054752690667223547, 3.707466751127219781E-16 ) ) ;
#49599=CARTESIAN_POINT ( 'NONE',  ( 0.000000000000000000, 0.000000000000000000, -50.00000000000000000 ) ) ;
#49600=CARTESIAN_POINT ( 'NONE',  ( 1.071796769724497445, 16.26740381056766438, -33.99999999999998579 ) ) ;
#49601=CARTESIAN_POINT ( 'NONE',  ( 12.90937500061451537, -4.541064518000417216, -2.621784821875001281 ) ) ;
#49602=CARTESIAN_POINT ( 'NONE',  ( 26.32499999999999929, 4.330127018922191873, 2.499999999999999556 ) ) ;
#49603=CARTESIAN_POINT ( 'NONE',  ( 9.965625000614517504, 3.027376345333611329, 5.243569643749999010 ) ) ;
#49605=CARTESIAN_POINT ( 'NONE',  ( 22.39687500061451075, -3.027376345333610441, -5.243569643749999898 ) ) ;
#49607=CARTESIAN_POINT ( 'NONE',  ( 7.303125000614516082, 0.000000000000000000, 5.243569643749999010 ) ) ;
#49608=CARTESIAN_POINT ( 'NONE',  ( 13.13437500061451857, 4.541064518000418104, 2.621784821874999949 ) ) ;
#49609=ORIENTED_EDGE ( 'NONE', *, *, #6300, .T. ) ;
#49610=CARTESIAN_POINT ( 'NONE',  ( 24.60937500061451644, -4.541064518000417216, -2.621784821875001281 ) ) ;
#49611=CARTESIAN_POINT ( 'NONE',  ( 1.091159441285790788, 4.887044806266472641, -26.14197170220922573 ) ) ;
#49613=CARTESIAN_POINT ( 'NONE',  ( 5.287500000000000533, -2.886751345948129988, 4.999999999999997335 ) ) ;
#49614=ADVANCED_FACE ( 'NONE', ( #71945 ), #3988, .F. ) ;
#49615=CARTESIAN_POINT ( 'NONE',  ( 16.12500000122903288, 2.886751345948126879, 4.999999999999999112 ) ) ;
#49617=CARTESIAN_POINT ( 'NONE',  ( -3.999999999999997335, 19.13750000000000284, -27.69059892324149530 ) ) ;
#49619=CARTESIAN_POINT ( 'NONE',  ( 12.30000000000000249, 4.330127018922192761, -2.499999999999997780 ) ) ;
#49620=CARTESIAN_POINT ( 'NONE',  ( 17.51249999999999929, -5.773502691896255534, -1.060575238724906372E-15 ) ) ;
#49621=CARTESIAN_POINT ( 'NONE',  ( 13.20000000122903394, -2.886751345948125991, -5.000000000000000000 ) ) ;
#49622=CARTESIAN_POINT ( 'NONE',  ( 10.60312500061451679, -4.541064518000417216, -2.621784821875001281 ) ) ;
#49623=ORIENTED_EDGE ( 'NONE', *, *, #10028, .F. ) ;
#49624=CARTESIAN_POINT ( 'NONE',  ( 10.05000000000000071, 4.330127018922192761, -2.499999999999997780 ) ) ;
#49625=CARTESIAN_POINT ( 'NONE',  ( -1.999999999999997113, 17.03750000122903430, -26.53589838486224295 ) ) ;
#49626=CARTESIAN_POINT ( 'NONE',  ( 2.121784821875001281, 15.05937500061451928, -26.32496088578401938 ) ) ;
#49627=CARTESIAN_POINT ( 'NONE',  ( 3.440625000614518036, -3.027376345333610441, -5.243569643749999898 ) ) ;
#49629=CARTESIAN_POINT ( 'NONE',  ( 10.49999999999999822, 4.330127018922192761, -2.499999999999997780 ) ) ;
#49630=CARTESIAN_POINT ( 'NONE',  ( 3.059722729795383067, 3.954539355547352919, 3.095961626413553436 ) ) ;
#49632=CARTESIAN_POINT ( 'NONE',  ( 25.11562500061451431, 3.027376345333613106, -5.243569643749998122 ) ) ;
#49635=CARTESIAN_POINT ( 'NONE',  ( 21.38437500061451502, -4.541064518000419881, 2.621784821874995952 ) ) ;
#49636=CARTESIAN_POINT ( 'NONE',  ( 18.51562500061451289, 3.027376345333611329, 5.243569643749999010 ) ) ;
#49637=ADVANCED_FACE ( 'NONE', ( #37589, #38318 ), #43508, .F. ) ;
#49638=CARTESIAN_POINT ( 'NONE',  ( 9.001249775931846008E-16, 11.81562500061459531, -25.09994784771203058 ) ) ;
#49639=CARTESIAN_POINT ( 'NONE',  ( 6.853125000614516793, 0.000000000000000000, 5.243569643749999010 ) ) ;
#49640=CARTESIAN_POINT ( 'NONE',  ( 3.515625000614516882, 3.027376345333613106, -5.243569643749998122 ) ) ;
#49642=CARTESIAN_POINT ( 'NONE',  ( 20.76562500061451999, 3.027376345333611329, 5.243569643749999010 ) ) ;
#49645=CARTESIAN_POINT ( 'NONE',  ( 15.27187500061451786, 3.027376345333613106, -5.243569643749998122 ) ) ;
#49646=CARTESIAN_POINT ( 'NONE',  ( 14.59687500061452070, -3.027376345333614438, 5.243569643749998122 ) ) ;
#49647=CARTESIAN_POINT ( 'NONE',  ( 23.22187500061451715, -6.054752690667223547, -1.112240025338166033E-15 ) ) ;
#49648=ORIENTED_EDGE ( 'NONE', *, *, #46542, .T. ) ;
#49649=CARTESIAN_POINT ( 'NONE',  ( -4.243569643749999898, 12.65937500061451715, 30.00000000000000000 ) ) ;
#49651=CARTESIAN_POINT ( 'NONE',  ( 25.79062500061451502, -3.027376345333614438, 5.243569643749998122 ) ) ;
#49652=CARTESIAN_POINT ( 'NONE',  ( 25.67812500061451431, 4.541064518000418104, 2.621784821874999949 ) ) ;
#49653=CARTESIAN_POINT ( 'NONE',  ( 1.626862140677534273E-15, 13.36250000000000071, -26.00000000000000355 ) ) ;
#49654=CARTESIAN_POINT ( 'NONE',  ( -3.999999999999999556, 18.61250000000000426, 27.69059892324149530 ) ) ;
#49655=CARTESIAN_POINT ( 'NONE',  ( 5.221875000614519813, -6.054752690667223547, -1.112240025338166033E-15 ) ) ;
#49657=CARTESIAN_POINT ( 'NONE',  ( 13.68750000122903288, 6.123233995736764310E-16, -4.999999999999998224 ) ) ;
#49658=CARTESIAN_POINT ( 'NONE',  ( 9.862500001229033586, 0.000000000000000000, 4.999999999999998224 ) ) ;
#49659=CARTESIAN_POINT ( 'NONE',  ( 3.290625000614516793, -3.027376345333614438, 5.243569643749998122 ) ) ;
#49662=CARTESIAN_POINT ( 'NONE',  ( 11.22187500061451892, 3.027376345333613106, -5.243569643749998122 ) ) ;
#49664=ORIENTED_EDGE ( 'NONE', *, *, #55830, .T. ) ;
#49665=CARTESIAN_POINT ( 'NONE',  ( 19.82812500061451644, 4.541064518000418104, 2.621784821874999949 ) ) ;
#49666=CARTESIAN_POINT ( 'NONE',  ( 12.27187500061451786, 3.027376345333611329, 5.243569643749999010 ) ) ;
#49667=CARTESIAN_POINT ( 'NONE',  ( 4.678125000614516971, -4.541064518000419881, 2.621784821874995952 ) ) ;
#49668=CARTESIAN_POINT ( 'NONE',  ( 23.14687500061451786, -3.027376345333614438, 5.243569643749998122 ) ) ;
#49670=CARTESIAN_POINT ( 'NONE',  ( 6.290625000614517681, 6.054752690667223547, 3.707466751127219781E-16 ) ) ;
#49671=CARTESIAN_POINT ( 'NONE',  ( 6.712500001229034119, 0.000000000000000000, 4.999999999999998224 ) ) ;
#49672=CARTESIAN_POINT ( 'NONE',  ( 8.737500001229033586, 6.123233995736764310E-16, -4.999999999999998224 ) ) ;
#49673=CARTESIAN_POINT ( 'NONE',  ( 21.59062500061451928, 6.054752690667223547, 3.707466751127219781E-16 ) ) ;
#49674=CARTESIAN_POINT ( 'NONE',  ( 2.000000000000001332, 17.11250000122903359, -26.53589838486224650 ) ) ;
#49675=CARTESIAN_POINT ( 'NONE',  ( 7.687500001229033764, -4.330127018922194537, 2.499999999999995559 ) ) ;
#49676=CARTESIAN_POINT ( 'NONE',  ( 16.60312500061451857, 4.541064518000418104, -2.621784821874998173 ) ) ;
#49677=CARTESIAN_POINT ( 'NONE',  ( 14.42812500061451786, 4.541064518000418104, 2.621784821874999949 ) ) ;
#49679=CARTESIAN_POINT ( 'NONE',  ( 14.58750000000000036, 5.773502691896255534, 3.535250795749688894E-16 ) ) ;
#49680=CARTESIAN_POINT ( 'NONE',  ( 11.02500000122903501, 2.886751345948129099, -4.999999999999998224 ) ) ;
#49681=CARTESIAN_POINT ( 'NONE',  ( 7.528125000614515727, 6.421520780324663323E-16, -5.243569643749999010 ) ) ;
#49682=CARTESIAN_POINT ( 'NONE',  ( 10.49062500061451431, -3.027376345333614438, 5.243569643749998122 ) ) ;
#49683=CARTESIAN_POINT ( 'NONE',  ( 19.91250000122903074, -4.330127018922190985, -2.500000000000001332 ) ) ;
#49684=CARTESIAN_POINT ( 'NONE',  ( -2.121784821874996840, 12.73437500061451821, -26.32496088578401583 ) ) ;
#49685=CARTESIAN_POINT ( 'NONE',  ( 20.37187500061451573, 3.027376345333611329, 5.243569643749999010 ) ) ;
#49686=CYLINDRICAL_SURFACE ( 'NONE', #53637, 4.999999999999998224 ) ;
#49687=CARTESIAN_POINT ( 'NONE',  ( 6.075000001229034829, 2.886751345948129099, -4.999999999999998224 ) ) ;
#49688=CARTESIAN_POINT ( 'NONE',  ( 3.684375000614518836, 4.541064518000418104, 2.621784821874999949 ) ) ;
#49689=CARTESIAN_POINT ( 'NONE',  ( 21.00937500061451857, -4.541064518000417216, -2.621784821875001281 ) ) ;
#49691=LINE ( 'NONE', #39335, #61014 ) ;
#49692=CARTESIAN_POINT ( 'NONE',  ( 17.20312500061451644, 0.000000000000000000, 5.243569643749999010 ) ) ;
#49696=CARTESIAN_POINT ( 'NONE',  ( 27.53437500061451360, 4.541064518000418104, 2.621784821874999949 ) ) ;
#49698=CARTESIAN_POINT ( 'NONE',  ( 14.50312500061451537, 0.000000000000000000, 5.243569643749999010 ) ) ;
#49699=CARTESIAN_POINT ( 'NONE',  ( 13.02187500061451608, 3.027376345333613106, -5.243569643749998122 ) ) ;
#49700=ORIENTED_EDGE ( 'NONE', *, *, #59478, .T. ) ;
#49702=CARTESIAN_POINT ( 'NONE',  ( 22.56562500061451715, 3.027376345333611329, 5.243569643749999010 ) ) ;
#49703=CARTESIAN_POINT ( 'NONE',  ( 17.66250000122903430, -4.330127018922190985, -2.500000000000001332 ) ) ;
#49705=CARTESIAN_POINT ( 'NONE',  ( 12.15000000000000036, -4.330127018922190985, -2.500000000000001332 ) ) ;
#49706=CARTESIAN_POINT ( 'NONE',  ( 23.02500000122903145, -5.773502691896255534, -1.060575238724906372E-15 ) ) ;
#49707=CARTESIAN_POINT ( 'NONE',  ( 17.61562500061451786, 3.027376345333611329, 5.243569643749999010 ) ) ;
#49709=CARTESIAN_POINT ( 'NONE',  ( 19.46249999999999858, 2.886751345948129099, -4.999999999999998224 ) ) ;
#49710=CARTESIAN_POINT ( 'NONE',  ( 20.67187500061451289, 3.027376345333613106, -5.243569643749998122 ) ) ;
#49713=CARTESIAN_POINT ( 'NONE',  ( 10.52812500061451750, -4.541064518000419881, 2.621784821874995952 ) ) ;
#49714=CARTESIAN_POINT ( 'NONE',  ( 3.325761423091350366, 3.733538664146505592, 3.492540098399592452 ) ) ;
#49716=CARTESIAN_POINT ( 'NONE',  ( 16.01249999999999929, 2.886751345948126879, 4.999999999999999112 ) ) ;
#49717=CARTESIAN_POINT ( 'NONE',  ( 24.67500000000000071, -4.330127018922194537, 2.499999999999995559 ) ) ;
#49718=CARTESIAN_POINT ( 'NONE',  ( -2.121784821874999949, 18.82812500061451644, 26.32496088578401938 ) ) ;
#49719=CARTESIAN_POINT ( 'NONE',  ( 3.496875000614518836, -3.027376345333610441, -5.243569643749999898 ) ) ;
#49720=CARTESIAN_POINT ( 'NONE',  ( 27.57187500061451857, 3.027376345333611329, 5.243569643749999010 ) ) ;
#49723=CARTESIAN_POINT ( 'NONE',  ( 26.24062500061451431, -3.027376345333614438, 5.243569643749998122 ) ) ;
#49724=CARTESIAN_POINT ( 'NONE',  ( 28.39687500061452141, 6.054752690667223547, 3.707466751127219781E-16 ) ) ;
#49725=CARTESIAN_POINT ( 'NONE',  ( 3.159375000614518036, 4.541064518000418104, -2.621784821874998173 ) ) ;
#49726=CARTESIAN_POINT ( 'NONE',  ( 14.28750000000000142, -2.886751345948129988, 4.999999999999997335 ) ) ;
#49727=CARTESIAN_POINT ( 'NONE',  ( 11.16562500061451679, 3.027376345333613106, -5.243569643749998122 ) ) ;
#49728=CARTESIAN_POINT ( 'NONE',  ( 6.075000000000000178, 4.330127018922191873, 2.499999999999999556 ) ) ;
#49729=FACE_OUTER_BOUND ( 'NONE', #71048, .T. ) ;
#49730=CARTESIAN_POINT ( 'NONE',  ( 27.77812500061451573, 6.421520780324663323E-16, -5.243569643749999010 ) ) ;
#49731=CARTESIAN_POINT ( 'NONE',  ( 16.83750000122903145, 6.123233995736764310E-16, -4.999999999999998224 ) ) ;
#49734=CARTESIAN_POINT ( 'NONE',  ( 5.540625000614515905, -3.027376345333614438, 5.243569643749998122 ) ) ;
#49735=CARTESIAN_POINT ( 'NONE',  ( 22.20937500061451431, 0.000000000000000000, 5.243569643749999010 ) ) ;
#49736=CARTESIAN_POINT ( 'NONE',  ( -4.243569643749999898, 14.45937500061451964, 30.00000000000000000 ) ) ;
#49737=CARTESIAN_POINT ( 'NONE',  ( 21.42187500061451644, -6.054752690667223547, -1.112240025338166033E-15 ) ) ;
#49738=CARTESIAN_POINT ( 'NONE',  ( 3.000000000000002665, 0.000000000000000000, 4.999999999999998224 ) ) ;
#49739=CARTESIAN_POINT ( 'NONE',  ( 4.243569643749999010, 19.67187500061451644, 27.54997392385601174 ) ) ;
#49740=CARTESIAN_POINT ( 'NONE',  ( 10.67812500061451608, 6.421520780324663323E-16, -5.243569643749999010 ) ) ;
#49741=CYLINDRICAL_SURFACE ( 'NONE', #43119, 4.999999999999998224 ) ;
#49742=CARTESIAN_POINT ( 'NONE',  ( 7.921875000614517326, -6.054752690667223547, -1.112240025338166033E-15 ) ) ;
#49744=CARTESIAN_POINT ( 'NONE',  ( 7.715625000614515727, 3.027376345333611329, 5.243569643749999010 ) ) ;
#49745=CARTESIAN_POINT ( 'NONE',  ( 11.82187500061451679, 3.027376345333611329, 5.243569643749999010 ) ) ;
#49747=CARTESIAN_POINT ( 'NONE',  ( 21.48750000122903003, 4.330127018922191873, 2.499999999999999556 ) ) ;
#49748=CARTESIAN_POINT ( 'NONE',  ( 7.509375000614517681, -4.541064518000417216, -2.621784821875001281 ) ) ;
#49749=CARTESIAN_POINT ( 'NONE',  ( 9.440625000614517148, 6.054752690667223547, 3.707466751127219781E-16 ) ) ;
#49751=CARTESIAN_POINT ( 'NONE',  ( 19.92187500061451644, 3.027376345333611329, 5.243569643749999010 ) ) ;
#49753=CARTESIAN_POINT ( 'NONE',  ( 21.71250000122903501, -4.330127018922190985, -2.500000000000001332 ) ) ;
#49754=CARTESIAN_POINT ( 'NONE',  ( 29.40937500061451715, 0.000000000000000000, 5.243569643749999010 ) ) ;
#49756=CARTESIAN_POINT ( 'NONE',  ( 2.121784821875001281, 12.80937500061451928, -26.32496088578401938 ) ) ;
#49757=CARTESIAN_POINT ( 'NONE',  ( 14.62500000122903288, 2.886751345948129099, -4.999999999999998224 ) ) ;
#49759=CARTESIAN_POINT ( 'NONE',  ( -2.121784821874999949, 15.67812500061451608, -33.67503911421598417 ) ) ;
#49760=CARTESIAN_POINT ( 'NONE',  ( 16.12500000122903288, 2.886751345948126879, 4.999999999999999112 ) ) ;
#49761=CARTESIAN_POINT ( 'NONE',  ( 9.553125000614517859, 0.000000000000000000, 5.243569643749999010 ) ) ;
#49762=ORIENTED_EDGE ( 'NONE', *, *, #32239, .T. ) ;
#49763=CARTESIAN_POINT ( 'NONE',  ( 13.01249999999999929, -5.773502691896255534, -1.060575238724906372E-15 ) ) ;
#49764=CARTESIAN_POINT ( 'NONE',  ( -3.999999999999997335, 13.73749999999999893, 32.30940107675850470 ) ) ;
#49765=CARTESIAN_POINT ( 'NONE',  ( 22.34062500061451573, -3.027376345333610441, -5.243569643749999898 ) ) ;
#49766=CARTESIAN_POINT ( 'NONE',  ( 7.809375000614519280, 0.000000000000000000, 5.243569643749999010 ) ) ;
#49768=CARTESIAN_POINT ( 'NONE',  ( 10.05000000122903181, -2.886751345948125991, -5.000000000000000000 ) ) ;
#49769=CARTESIAN_POINT ( 'NONE',  ( 17.55000000122903359, -2.886751345948129988, 4.999999999999997335 ) ) ;
#49770=CARTESIAN_POINT ( 'NONE',  ( 15.47812500061451679, -4.541064518000419881, 2.621784821874995952 ) ) ;
#49771=CARTESIAN_POINT ( 'NONE',  ( 18.96562500061451573, 3.027376345333611329, 5.243569643749999010 ) ) ;
#49772=CARTESIAN_POINT ( 'NONE',  ( 25.95000000122903216, 5.773502691896255534, 3.535250795749688894E-16 ) ) ;
#49773=ADVANCED_FACE ( 'NONE', ( #9881 ), #38698, .F. ) ;
#49774=CARTESIAN_POINT ( 'NONE',  ( 27.82500000122903572, 2.886751345948126879, 4.999999999999999112 ) ) ;
#49775=CARTESIAN_POINT ( 'NONE',  ( 22.31250000000000000, 2.886751345948126879, 4.999999999999999112 ) ) ;
#49777=CARTESIAN_POINT ( 'NONE',  ( 24.79687500061451999, 6.054752690667223547, 3.707466751127219781E-16 ) ) ;
#49779=CARTESIAN_POINT ( 'NONE',  ( 13.65000000122903323, -2.886751345948125991, -5.000000000000000000 ) ) ;
#49780=CARTESIAN_POINT ( 'NONE',  ( 27.12187500061451573, 3.027376345333611329, 5.243569643749999010 ) ) ;
#49782=CARTESIAN_POINT ( 'NONE',  ( 5.971875000614516260, 3.027376345333611329, 5.243569643749999010 ) ) ;
#49783=CARTESIAN_POINT ( 'NONE',  ( 25.45312500061451644, -4.541064518000417216, -2.621784821875001281 ) ) ;
#49785=CARTESIAN_POINT ( 'NONE',  ( 10.39687500061451786, 6.054752690667223547, 3.707466751127219781E-16 ) ) ;
#49787=CARTESIAN_POINT ( 'NONE',  ( 3.309375000614518836, 0.000000000000000000, 5.243569643749999010 ) ) ;
#49788=CARTESIAN_POINT ( 'NONE',  ( 9.946875000614516793, 6.054752690667223547, 3.707466751127219781E-16 ) ) ;
#49789=CARTESIAN_POINT ( 'NONE',  ( 28.39687500061452141, 6.054752690667223547, 3.707466751127219781E-16 ) ) ;
#49790=CARTESIAN_POINT ( 'NONE',  ( -4.243569643749999898, 13.46562500061459744, 27.54997392385601529 ) ) ;
#49791=CARTESIAN_POINT ( 'NONE',  ( 19.57500000000000284, 4.330127018922191873, 2.499999999999999556 ) ) ;
#49792=ORIENTED_EDGE ( 'NONE', *, *, #42731, .F. ) ;
#49793=CARTESIAN_POINT ( 'NONE',  ( 29.55000000000000071, 0.000000000000000000, 4.999999999999998224 ) ) ;
#49794=CARTESIAN_POINT ( 'NONE',  ( 3.187500000000002220, -2.886751345948125991, -5.000000000000000000 ) ) ;
#49795=EDGE_LOOP ( 'NONE', ( #27494, #61637, #41558, #45757 ) ) ;
#49797=CARTESIAN_POINT ( 'NONE',  ( 17.16562500061451502, 3.027376345333611329, 5.243569643749999010 ) ) ;
#49798=CARTESIAN_POINT ( 'NONE',  ( 8.240625000614516082, -3.027376345333614438, 5.243569643749998122 ) ) ;
#49800=CARTESIAN_POINT ( 'NONE',  ( 6.796875000614516438, 6.054752690667223547, 3.707466751127219781E-16 ) ) ;
#49801=CARTESIAN_POINT ( 'NONE',  ( 18.86250000122903359, 0.000000000000000000, 4.999999999999998224 ) ) ;
#49802=CARTESIAN_POINT ( 'NONE',  ( -0.6945863667395647534, 9.663023495605401081, -33.93923213064925903 ) ) ;
#49803=CARTESIAN_POINT ( 'NONE',  ( 7.621875000614519280, 3.027376345333613106, -5.243569643749998122 ) ) ;
#49804=CARTESIAN_POINT ( 'NONE',  ( 12.42187500061451821, -6.054752690667223547, -1.112240025338166033E-15 ) ) ;
#49805=CARTESIAN_POINT ( 'NONE',  ( 23.85937500061451644, 4.541064518000418104, -2.621784821874998173 ) ) ;
#49806=CARTESIAN_POINT ( 'NONE',  ( -3.999999999999999112, 14.56250000000000000, -32.30940107675850470 ) ) ;
#49809=CARTESIAN_POINT ( 'NONE',  ( 17.37187500061451573, -6.054752690667223547, -1.112240025338166033E-15 ) ) ;
#49810=CARTESIAN_POINT ( 'NONE',  ( 8.784375000614518925, -4.541064518000419881, 2.621784821874995952 ) ) ;
#49812=CARTESIAN_POINT ( 'NONE',  ( 21.03750000000000142, -2.886751345948129988, 4.999999999999997335 ) ) ;
#49816=CARTESIAN_POINT ( 'NONE',  ( 13.07812500061451821, 4.541064518000418104, 2.621784821874999949 ) ) ;
#49817=CARTESIAN_POINT ( 'NONE',  ( 29.10937500061451644, -4.541064518000417216, -2.621784821875001281 ) ) ;
#49818=DIRECTION ( 'NONE',  ( -0.000000000000000000, -1.000000000000000000, -0.000000000000000000 ) ) ;
#49819=CARTESIAN_POINT ( 'NONE',  ( 29.18437500061451573, 6.421520780324663323E-16, -5.243569643749999010 ) ) ;
#49820=CARTESIAN_POINT ( 'NONE',  ( 9.975000000000001421, 6.123233995736764310E-16, -4.999999999999998224 ) ) ;
#49821=CARTESIAN_POINT ( 'NONE',  ( -3.999999999999997335, 15.20000000122903572, 32.30940107675850470 ) ) ;
#49822=CARTESIAN_POINT ( 'NONE',  ( 8.287500001229034297, 6.123233995736764310E-16, -4.999999999999998224 ) ) ;
#49823=CARTESIAN_POINT ( 'NONE',  ( 21.15937500061451715, 4.541064518000418104, -2.621784821874998173 ) ) ;
#49824=CARTESIAN_POINT ( 'NONE',  ( 13.80937500061451750, -4.541064518000417216, -2.621784821875001281 ) ) ;
#49826=ORIENTED_EDGE ( 'NONE', *, *, #48710, .F. ) ;
#49827=CARTESIAN_POINT ( 'NONE',  ( 16.00312500061451715, -4.541064518000417216, -2.621784821875001281 ) ) ;
#49828=CARTESIAN_POINT ( 'NONE',  ( 27.75000000122903288, 5.773502691896255534, 3.535250795749688894E-16 ) ) ;
#49829=CARTESIAN_POINT ( 'NONE',  ( 16.39687500061451786, -3.027376345333614438, 5.243569643749998122 ) ) ;
#49830=CARTESIAN_POINT ( 'NONE',  ( 5.959992197959416593, 8.030459126529553515, -30.80005261327864829 ) ) ;
#49831=CARTESIAN_POINT ( 'NONE',  ( 16.97812500061451502, 6.421520780324663323E-16, -5.243569643749999010 ) ) ;
#49833=CARTESIAN_POINT ( 'NONE',  ( 28.88437500061451502, 4.541064518000418104, 2.621784821874999949 ) ) ;
#49834=CARTESIAN_POINT ( 'NONE',  ( -4.243569643749999898, 11.70312500061451644, 30.00000000000000000 ) ) ;
#49835=CARTESIAN_POINT ( 'NONE',  ( 16.24687500061451573, 6.054752690667223547, 3.707466751127219781E-16 ) ) ;
#49836=CARTESIAN_POINT ( 'NONE',  ( 14.55000000122903181, -2.886751345948125991, -5.000000000000000000 ) ) ;
#49838=CARTESIAN_POINT ( 'NONE',  ( -4.243569643749999898, 18.50937500061451857, -30.00000000000000000 ) ) ;
#49839=CARTESIAN_POINT ( 'NONE',  ( 21.72187500061451715, 3.027376345333611329, 5.243569643749999010 ) ) ;
#49840=CARTESIAN_POINT ( 'NONE',  ( 23.51250000122903216, -4.330127018922190985, -2.500000000000001332 ) ) ;
#49841=CARTESIAN_POINT ( 'NONE',  ( 16.80937500061451573, 0.000000000000000000, 5.243569643749999010 ) ) ;
#49842=CARTESIAN_POINT ( 'NONE',  ( 13.37812500061451715, 6.421520780324663323E-16, -5.243569643749999010 ) ) ;
#49843=CARTESIAN_POINT ( 'NONE',  ( 4.243569643749999010, 12.47187500061451715, 27.54997392385601174 ) ) ;
#49844=CARTESIAN_POINT ( 'NONE',  ( 18.02812500061451573, 4.541064518000418104, 2.621784821874999949 ) ) ;
#49846=EDGE_LOOP ( 'NONE', ( #25199, #24354, #67434, #51511 ) ) ;
#49847=CARTESIAN_POINT ( 'NONE',  ( 20.73750000000000071, -2.886751345948125991, -5.000000000000000000 ) ) ;
#49848=CARTESIAN_POINT ( 'NONE',  ( 24.81562500061451715, 3.027376345333611329, 5.243569643749999010 ) ) ;
#49849=CARTESIAN_POINT ( 'NONE',  ( 5.203125000614518214, -4.541064518000417216, -2.621784821875001281 ) ) ;
#49850=CARTESIAN_POINT ( 'NONE',  ( 17.55000000122903359, -2.886751345948129988, 4.999999999999997335 ) ) ;
#49851=CARTESIAN_POINT ( 'NONE',  ( 22.00312500061451360, 4.541064518000418104, -2.621784821874998173 ) ) ;
#49852=CARTESIAN_POINT ( 'NONE',  ( 23.40000000000000213, -4.330127018922190985, -2.500000000000001332 ) ) ;
#49853=CARTESIAN_POINT ( 'NONE',  ( 24.70312500061451644, 4.541064518000418104, -2.621784821874998173 ) ) ;
#49854=CARTESIAN_POINT ( 'NONE',  ( 6.253125000614517148, 4.541064518000418104, -2.621784821874998173 ) ) ;
#49857=AXIS2_PLACEMENT_3D ( 'NONE', #53623, #26282, #15184 ) ;
#49858=CARTESIAN_POINT ( 'NONE',  ( 29.36250000000000071, 2.886751345948129099, -4.999999999999998224 ) ) ;
#49859=CARTESIAN_POINT ( 'NONE',  ( 3.665625000614517681, 3.027376345333611329, 5.243569643749999010 ) ) ;
#49862=CARTESIAN_POINT ( 'NONE',  ( 2.000000000000001332, 12.61250000122903536, -26.53589838486224650 ) ) ;
#49863=CARTESIAN_POINT ( 'NONE',  ( 4.243569643749999898, 19.14687500061451431, -27.54997392385601529 ) ) ;
#49864=CARTESIAN_POINT ( 'NONE',  ( 11.21250000000000036, -5.773502691896255534, -1.060575238724906372E-15 ) ) ;
#49865=CARTESIAN_POINT ( 'NONE',  ( 12.12187500061451573, 3.027376345333613106, -5.243569643749998122 ) ) ;
#49866=CARTESIAN_POINT ( 'NONE',  ( 6.150000001229033231, 5.773502691896255534, 3.535250795749688894E-16 ) ) ;
#49867=CARTESIAN_POINT ( 'NONE',  ( 13.32187500061451502, -6.054752690667223547, -1.112240025338166033E-15 ) ) ;
#49868=CARTESIAN_POINT ( 'NONE',  ( 5.446875000614518569, 6.054752690667223547, 3.707466751127219781E-16 ) ) ;
#49869=DIRECTION ( 'NONE',  ( 0.000000000000000000, 0.000000000000000000, -1.000000000000000000 ) ) ;
#49870=CARTESIAN_POINT ( 'NONE',  ( 9.159375000614515372, 0.000000000000000000, 5.243569643749999010 ) ) ;
#49872=CARTESIAN_POINT ( 'NONE',  ( 20.84062500061451573, -3.027376345333614438, 5.243569643749998122 ) ) ;
#49875=CARTESIAN_POINT ( 'NONE',  ( 23.93437500061451573, 4.541064518000418104, 2.621784821874999949 ) ) ;
#49876=CARTESIAN_POINT ( 'NONE',  ( -1.999999999999997113, 13.88750000122903394, -26.53589838486224295 ) ) ;
#49877=CARTESIAN_POINT ( 'NONE',  ( 28.16250000122903074, 4.330127018922192761, -2.499999999999997780 ) ) ;
#49879=CARTESIAN_POINT ( 'NONE',  ( 25.04062500061451502, -3.027376345333610441, -5.243569643749999898 ) ) ;
#49880=CARTESIAN_POINT ( 'NONE',  ( 15.25312500061451715, 4.541064518000418104, -2.621784821874998173 ) ) ;
#49882=CARTESIAN_POINT ( 'NONE',  ( 13.58437500061451786, 4.541064518000418104, 2.621784821874999949 ) ) ;
#49883=CARTESIAN_POINT ( 'NONE',  ( 16.80000000000000071, 4.330127018922192761, -2.499999999999997780 ) ) ;
#49884=CARTESIAN_POINT ( 'NONE',  ( 24.63750000122903216, 4.330127018922191873, 2.499999999999999556 ) ) ;
#49885=CARTESIAN_POINT ( 'NONE',  ( 3.684375000614518836, 4.541064518000418104, 2.621784821874999949 ) ) ;
#49886=CARTESIAN_POINT ( 'NONE',  ( 14.14687500061451786, -3.027376345333614438, 5.243569643749998122 ) ) ;
#49887=CARTESIAN_POINT ( 'NONE',  ( 16.23749999999999716, -2.886751345948193048, -4.999999999999883649 ) ) ;
#49888=CARTESIAN_POINT ( 'NONE',  ( -3.999999999999999112, 11.41250000000000142, 27.69059892324149885 ) ) ;
#49889=CARTESIAN_POINT ( 'NONE',  ( 2.887500001229035274, 6.123233995736764310E-16, -4.999999999999998224 ) ) ;
#49890=CARTESIAN_POINT ( 'NONE',  ( 25.69687500061451502, 6.054752690667223547, 3.707466751127219781E-16 ) ) ;
#49891=CARTESIAN_POINT ( 'NONE',  ( 16.24687500061451573, 6.054752690667223547, 3.707466751127219781E-16 ) ) ;
#49893=CARTESIAN_POINT ( 'NONE',  ( 27.56250000000000000, 2.886751345948129099, -4.999999999999998224 ) ) ;
#49894=CARTESIAN_POINT ( 'NONE',  ( 3.900000001229034563, 5.773502691896255534, 3.535250795749688894E-16 ) ) ;
#49895=CARTESIAN_POINT ( 'NONE',  ( 6.150000000000003020, 0.000000000000000000, 4.999999999999998224 ) ) ;
#49897=CARTESIAN_POINT ( 'NONE',  ( 20.24062500061451431, 6.054752690667223547, 3.707466751127219781E-16 ) ) ;
#49898=CARTESIAN_POINT ( 'NONE',  ( 10.46249999999999858, 2.886751345948129099, -4.999999999999998224 ) ) ;
#49900=CARTESIAN_POINT ( 'NONE',  ( 4.978125000614518569, 4.541064518000418104, 2.621784821874999949 ) ) ;
#49901=CARTESIAN_POINT ( 'NONE',  ( 18.22499999999999787, 4.330127018922191873, 2.499999999999999556 ) ) ;
#49902=CARTESIAN_POINT ( 'NONE',  ( 10.00000000000000000, 1.224646799147353256E-15, 50.00000000000000000 ) ) ;
#49903=CARTESIAN_POINT ( 'NONE',  ( 21.78750000122903074, 6.123233995736764310E-16, -4.999999999999998224 ) ) ;
#49904=CARTESIAN_POINT ( 'NONE',  ( -1.389181105737270716, 10.01354714573257532, -33.81675806816645036 ) ) ;
#49905=CARTESIAN_POINT ( 'NONE',  ( 28.58437500061451786, -4.541064518000419881, 2.621784821874995952 ) ) ;
#49906=ORIENTED_EDGE ( 'NONE', *, *, #43332, .F. ) ;
#49907=CARTESIAN_POINT ( 'NONE',  ( 16.79062500061451857, -3.027376345333614438, 5.243569643749998122 ) ) ;
#49908=CARTESIAN_POINT ( 'NONE',  ( 24.51562500061451289, -6.054752690667223547, -1.112240025338166033E-15 ) ) ;
#49909=CARTESIAN_POINT ( 'NONE',  ( 22.95937500061451431, 4.541064518000418104, -2.621784821874998173 ) ) ;
#49910=CARTESIAN_POINT ( 'NONE',  ( 6.187500000000002665, -2.886751345948129988, 4.999999999999997335 ) ) ;
#49911=CARTESIAN_POINT ( 'NONE',  ( 8.390625000614518214, -3.027376345333610441, -5.243569643749999898 ) ) ;
#49912=CARTESIAN_POINT ( 'NONE',  ( 23.72812500061451502, 6.421520780324663323E-16, -5.243569643749999010 ) ) ;
#49913=CARTESIAN_POINT ( 'NONE',  ( 15.23437500061451644, 6.421520780324663323E-16, -5.243569643749999010 ) ) ;
#49914=CARTESIAN_POINT ( 'NONE',  ( 18.23437500061451999, -4.541064518000419881, 2.621784821874995952 ) ) ;
#49915=CARTESIAN_POINT ( 'NONE',  ( 17.73750000122903359, 6.123233995736764310E-16, -4.999999999999998224 ) ) ;
#49916=CARTESIAN_POINT ( 'NONE',  ( -4.243569643749999898, 19.76562500061451644, 27.54997392385601529 ) ) ;
#49917=CARTESIAN_POINT ( 'NONE',  ( 21.75000000122903288, -2.886751345948125991, -5.000000000000000000 ) ) ;
#49919=CARTESIAN_POINT ( 'NONE',  ( 13.00312500061451537, 4.541064518000418104, -2.621784821874998173 ) ) ;
#49920=CARTESIAN_POINT ( 'NONE',  ( 7.621875000614519280, 3.027376345333613106, -5.243569643749998122 ) ) ;
#49921=CARTESIAN_POINT ( 'NONE',  ( 6.909375000614518036, 0.000000000000000000, 5.243569643749999010 ) ) ;
#49922=VERTEX_POINT ( 'NONE', #10251 ) ;
#49923=CARTESIAN_POINT ( 'NONE',  ( 27.60937500061451644, 0.000000000000000000, 5.243569643749999010 ) ) ;
#49924=CARTESIAN_POINT ( 'NONE',  ( 18.29062500061451502, -3.027376345333610441, -5.243569643749999898 ) ) ;
#49925=CARTESIAN_POINT ( 'NONE',  ( 28.91250000122903074, -4.330127018922190985, -2.500000000000001332 ) ) ;
#49926=CARTESIAN_POINT ( 'NONE',  ( 27.85312500061451502, 4.541064518000418104, -2.621784821874998173 ) ) ;
#49927=CARTESIAN_POINT ( 'NONE',  ( 24.83437500061451431, 4.541064518000418104, 2.621784821874999949 ) ) ;
#49928=CARTESIAN_POINT ( 'NONE',  ( 18.77812500061451573, 6.421520780324663323E-16, -5.243569643749999010 ) ) ;
#49929=CARTESIAN_POINT ( 'NONE',  ( -4.243569643749999898, 19.85937500061451644, 30.00000000000000000 ) ) ;
#49930=CARTESIAN_POINT ( 'NONE',  ( 25.60312500061451502, 4.541064518000418104, -2.621784821874998173 ) ) ;
#49931=CARTESIAN_POINT ( 'NONE',  ( 4.200000001229033053, -2.886751345948125991, -5.000000000000000000 ) ) ;
#49933=CARTESIAN_POINT ( 'NONE',  ( 26.58750000000000213, -2.886751345948125991, -5.000000000000000000 ) ) ;
#49934=CARTESIAN_POINT ( 'NONE',  ( -2.000000000000000000, 14.97499999999999964, -33.46410161513775705 ) ) ;
#49937=CARTESIAN_POINT ( 'NONE',  ( 4.021875000614516082, 3.027376345333613106, -5.243569643749998122 ) ) ;
#49938=CARTESIAN_POINT ( 'NONE',  ( 12.66562500061451502, 3.027376345333611329, 5.243569643749999010 ) ) ;
#49939=CARTESIAN_POINT ( 'NONE',  ( 5.409375000614516260, 4.541064518000418104, -2.621784821874998173 ) ) ;
#49940=CARTESIAN_POINT ( 'NONE',  ( 23.70000000122903216, 5.773502691896255534, 3.535250795749688894E-16 ) ) ;
#49941=CARTESIAN_POINT ( 'NONE',  ( 14.97187500061451892, 3.027376345333611329, 5.243569643749999010 ) ) ;
#49942=CARTESIAN_POINT ( 'NONE',  ( 3.796875000614517326, -3.027376345333614438, 5.243569643749998122 ) ) ;
#49943=CARTESIAN_POINT ( 'NONE',  ( 29.02499999999999858, 4.330127018922191873, 2.499999999999999556 ) ) ;
#49944=CARTESIAN_POINT ( 'NONE',  ( 26.82187500061451857, -6.054752690667223547, -1.112240025338166033E-15 ) ) ;
#49945=CARTESIAN_POINT ( 'NONE',  ( 3.553125000614516082, 4.541064518000418104, -2.621784821874998173 ) ) ;
#49946=CARTESIAN_POINT ( 'NONE',  ( 13.45312500061451466, 4.541064518000418104, -2.621784821874998173 ) ) ;
#49948=CARTESIAN_POINT ( 'NONE',  ( 11.01562500061451821, -6.054752690667223547, -1.112240025338166033E-15 ) ) ;
#49949=CARTESIAN_POINT ( 'NONE',  ( 7.865625000614516971, -6.054752690667223547, -1.112240025338166033E-15 ) ) ;
#49951=CARTESIAN_POINT ( 'NONE',  ( 8.887499999999999289, -2.886751345948129988, 4.999999999999997335 ) ) ;
#49952=CARTESIAN_POINT ( 'NONE',  ( 2.850000001229036073, -2.886751345948125991, -5.000000000000000000 ) ) ;
#49953=CARTESIAN_POINT ( 'NONE',  ( 18.52499999999999858, 6.123233995736764310E-16, -4.999999999999998224 ) ) ;
#49954=( BOUNDED_CURVE ( )  B_SPLINE_CURVE ( 2, ( #17614, #58221, #24613, #11729, #47160, #62693, #655, #56778, #34245 ),
 .UNSPECIFIED., .F., .F. ) 
 B_SPLINE_CURVE_WITH_KNOTS ( ( 3, 2, 2, 2, 3 ),
 ( 0.2500000000000000000, 0.2536231884057971175, 0.2608695652173912971, 0.2681159420289855322, 0.2717391304347826497 ),
 .UNSPECIFIED. ) 
 CURVE ( )  GEOMETRIC_REPRESENTATION_ITEM ( )  RATIONAL_B_SPLINE_CURVE ( ( 0.9330127018922194093, 0.9330127018922190762, 1.000000000000000000, 0.8660254037844387076, 1.000000000000000000, 0.8660254037844387076, 1.000000000000000000, 0.9330127018922188542, 0.9330127018922194093 ) ) 
 REPRESENTATION_ITEM ( '' )  );
#49955=CARTESIAN_POINT ( 'NONE',  ( 17.74687500061451928, -3.027376345333614438, 5.243569643749998122 ) ) ;
#49956=CARTESIAN_POINT ( 'NONE',  ( 14.55000000122903181, -2.886751345948125991, -5.000000000000000000 ) ) ;
#49958=CARTESIAN_POINT ( 'NONE',  ( 9.001249775931846008E-16, 15.41562500061451679, -25.09994784771203058 ) ) ;
#49962=CARTESIAN_POINT ( 'NONE',  ( 25.86562500061451431, -6.054752690667223547, -1.112240025338166033E-15 ) ) ;
#49963=CARTESIAN_POINT ( 'NONE',  ( 20.17500000122903003, 2.886751345948161074, 4.999999999999941380 ) ) ;
#49964=CARTESIAN_POINT ( 'NONE',  ( 30.00000000000000000, 0.000000000000000000, 0.000000000000000000 ) ) ;
#49965=CARTESIAN_POINT ( 'NONE',  ( 14.29687500061451821, -3.027376345333610441, -5.243569643749999898 ) ) ;
#49966=CARTESIAN_POINT ( 'NONE',  ( 25.80000000000000071, 4.330127018922192761, -2.499999999999997780 ) ) ;
#49967=CARTESIAN_POINT ( 'NONE',  ( 9.403125000614517504, 4.541064518000418104, -2.621784821874998173 ) ) ;
#49969=CARTESIAN_POINT ( 'NONE',  ( 21.34687500061451715, -3.027376345333614438, 5.243569643749998122 ) ) ;
#49971=CARTESIAN_POINT ( 'NONE',  ( 6.928125000614516082, -4.541064518000419881, 2.621784821874995952 ) ) ;
#49972=CARTESIAN_POINT ( 'NONE',  ( 11.52187500061451608, -6.054752690667223547, -1.112240025338166033E-15 ) ) ;
#49973=ORIENTED_EDGE ( 'NONE', *, *, #14935, .F. ) ;
#49974=CARTESIAN_POINT ( 'NONE',  ( 21.64687500061451786, 6.054752690667223547, 3.707466751127219781E-16 ) ) ;
#49975=DIRECTION ( 'NONE',  ( -0.000000000000000000, -1.000000000000000000, -0.000000000000000000 ) ) ;
#49977=CARTESIAN_POINT ( 'NONE',  ( 4.125000000000000000, 6.123233995736764310E-16, -4.999999999999998224 ) ) ;
#49978=CARTESIAN_POINT ( 'NONE',  ( 14.58750000122903323, 6.123233995736764310E-16, -4.999999999999998224 ) ) ;
#49979=CARTESIAN_POINT ( 'NONE',  ( 4.000000000000000000, 15.23750000000000071, -27.69059892324149885 ) ) ;
#49980=CARTESIAN_POINT ( 'NONE',  ( -5.810221930991193690E-16, 11.90000000122903323, -34.00000000000000000 ) ) ;
#49981=VERTEX_POINT ( 'NONE', #9520 ) ;
#49982=CARTESIAN_POINT ( 'NONE',  ( 11.73750000000000249, -2.886751345948125991, -5.000000000000000000 ) ) ;
#49983=CARTESIAN_POINT ( 'NONE',  ( 15.41250000000000142, 2.886751345948129099, -4.999999999999998224 ) ) ;
#49984=CARTESIAN_POINT ( 'NONE',  ( 14.02500000122903323, -5.773502691896255534, -1.060575238724906372E-15 ) ) ;
#49985=CARTESIAN_POINT ( 'NONE',  ( 12.29062500061451857, -3.027376345333614438, 5.243569643749998122 ) ) ;
#49987=EDGE_LOOP ( 'NONE', ( #34800, #7312, #61005, #39069 ) ) ;
#49988=CARTESIAN_POINT ( 'NONE',  ( 8.625000000000000000, 6.123233995736764310E-16, -4.999999999999998224 ) ) ;
#49989=CARTESIAN_POINT ( 'NONE',  ( 27.41250000122903430, 0.000000000000000000, 4.999999999999998224 ) ) ;
#49990=CARTESIAN_POINT ( 'NONE',  ( 2.121784821875001281, 15.50937500061451857, -26.32496088578401938 ) ) ;
#49991=CARTESIAN_POINT ( 'NONE',  ( 29.55000000122903003, 5.773502691896255534, 3.535250795749688894E-16 ) ) ;
#49993=CARTESIAN_POINT ( 'NONE',  ( 9.825000000000001066, -4.330127018922194537, 2.499999999999995559 ) ) ;
#49994=LINE ( 'NONE', #43722, #13745 ) ;
#49995=VERTEX_POINT ( 'NONE', #61217 ) ;
#49996=CARTESIAN_POINT ( 'NONE',  ( 24.70312500061451644, 4.541064518000418104, -2.621784821874998173 ) ) ;
#49997=CARTESIAN_POINT ( 'NONE',  ( 3.999999999999998668, 13.51250000000000107, -32.30940107675850470 ) ) ;
#49998=CARTESIAN_POINT ( 'NONE',  ( 18.93750000122903288, -4.330127018922194537, 2.499999999999995559 ) ) ;
#49999=CARTESIAN_POINT ( 'NONE',  ( 21.12187500061451573, 3.027376345333613106, -5.243569643749998122 ) ) ;
#50001=CARTESIAN_POINT ( 'NONE',  ( 15.96562500061451573, -6.054752690667223547, -1.112240025338166033E-15 ) ) ;
#50002=CARTESIAN_POINT ( 'NONE',  ( -2.121784821874996840, 11.77812500061459566, -26.32496088578401583 ) ) ;
#50003=CARTESIAN_POINT ( 'NONE',  ( 5.540625000614515905, -3.027376345333614438, 5.243569643749998122 ) ) ;
#50004=CARTESIAN_POINT ( 'NONE',  ( 27.52500000122903145, -5.773502691896255534, -1.060575238724906372E-15 ) ) ;
#50006=CARTESIAN_POINT ( 'NONE',  ( 19.15312500061451573, -4.541064518000417216, -2.621784821875001281 ) ) ;
#50009=CARTESIAN_POINT ( 'NONE',  ( 14.03437500061451715, 4.541064518000418104, 2.621784821874999949 ) ) ;
#50010=EDGE_CURVE ( 'NONE', #8864, #51420, #70911, .T. ) ;
#50011=CARTESIAN_POINT ( 'NONE',  ( 13.65937500061451715, 0.000000000000000000, 5.243569643749999010 ) ) ;
#50012=CARTESIAN_POINT ( 'NONE',  ( 21.72187500061451715, 3.027376345333611329, 5.243569643749999010 ) ) ;
#50013=ORIENTED_EDGE ( 'NONE', *, *, #27534, .T. ) ;
#50014=CARTESIAN_POINT ( 'NONE',  ( 4.243569643749999898, 11.94687500061451857, 32.45002607614398471 ) ) ;
#50015=CARTESIAN_POINT ( 'NONE',  ( 2.990625000614519191, -3.027376345333610441, -5.243569643749999898 ) ) ;
#50016=CARTESIAN_POINT ( 'NONE',  ( 27.47812500061451502, 4.541064518000418104, 2.621784821874999949 ) ) ;
#50017=CARTESIAN_POINT ( 'NONE',  ( 26.50312500061451360, 4.541064518000418104, -2.621784821874998173 ) ) ;
#50019=CARTESIAN_POINT ( 'NONE',  ( -2.000000000000000000, 16.77500000000000213, 26.53589838486224650 ) ) ;
#50020=CARTESIAN_POINT ( 'NONE',  ( 4.321875000614517681, -6.054752690667223547, -1.112240025338166033E-15 ) ) ;
#50021=CARTESIAN_POINT ( 'NONE',  ( 13.08750000122903323, -4.330127018922194537, 2.499999999999995559 ) ) ;
#50022=CARTESIAN_POINT ( 'NONE',  ( 9.037500001229034297, -4.330127018922194537, 2.499999999999995559 ) ) ;
#50023=CARTESIAN_POINT ( 'NONE',  ( 3.665625000614517681, 3.027376345333611329, 5.243569643749999010 ) ) ;
#50026=CARTESIAN_POINT ( 'NONE',  ( 12.90937500061451537, -4.541064518000417216, -2.621784821875001281 ) ) ;
#50027=CARTESIAN_POINT ( 'NONE',  ( 2.000000000000001332, 14.75000000000000178, -26.53589838486224650 ) ) ;
#50028=VERTEX_POINT ( 'NONE', #56044 ) ;
#50029=CARTESIAN_POINT ( 'NONE',  ( 19.37812500061451715, 4.541064518000418104, 2.621784821874999949 ) ) ;
#50030=CARTESIAN_POINT ( 'NONE',  ( 14.07187500061451679, 3.027376345333611329, 5.243569643749999010 ) ) ;
#50031=CARTESIAN_POINT ( 'NONE',  ( 5.840625000614516615, 6.054752690667223547, 3.707466751127219781E-16 ) ) ;
#50032=CARTESIAN_POINT ( 'NONE',  ( 22.54687500061451644, 6.054752690667223547, 3.707466751127219781E-16 ) ) ;
#50033=CARTESIAN_POINT ( 'NONE',  ( 4.715625000614516615, -6.054752690667223547, -1.112240025338166033E-15 ) ) ;
#50034=CYLINDRICAL_SURFACE ( 'NONE', #1443, 4.000000000000000000 ) ;
#50035=CARTESIAN_POINT ( 'NONE',  ( 6.712500001229034119, 0.000000000000000000, 4.999999999999998224 ) ) ;
#50036=CARTESIAN_POINT ( 'NONE',  ( 19.52812500061451573, -4.541064518000419881, 2.621784821874995952 ) ) ;
#50037=CARTESIAN_POINT ( 'NONE',  ( 8.325000001229033941, 2.886751345948129099, -4.999999999999998224 ) ) ;
#50038=CARTESIAN_POINT ( 'NONE',  ( 17.31562500061451715, -6.054752690667223547, -1.112240025338166033E-15 ) ) ;
#50039=CARTESIAN_POINT ( 'NONE',  ( 15.55312500061451608, -4.541064518000417216, -2.621784821875001281 ) ) ;
#50041=CARTESIAN_POINT ( 'NONE',  ( 15.97499999999999964, 4.330127018922191873, 2.499999999999999556 ) ) ;
#50042=CARTESIAN_POINT ( 'NONE',  ( 12.37500000122903465, 2.886751345948129099, -4.999999999999998224 ) ) ;
#50043=ADVANCED_FACE ( 'NONE', ( #69218 ), #5436, .F. ) ;
#50044=CARTESIAN_POINT ( 'NONE',  ( 7.978125000614517681, 6.421520780324663323E-16, -5.243569643749999010 ) ) ;
#50045=CARTESIAN_POINT ( 'NONE',  ( 11.54062500061451857, -3.027376345333610441, -5.243569643749999898 ) ) ;
#50046=CARTESIAN_POINT ( 'NONE',  ( 20.28750000122903074, -4.330127018922194537, 2.499999999999995559 ) ) ;
#50047=CARTESIAN_POINT ( 'NONE',  ( 4.243569643749999010, 12.92187500061451644, -32.45002607614398471 ) ) ;
#50048=B_SPLINE_CURVE_WITH_KNOTS ( 'NONE', 1,
 ( #13159, #1378 ),
 .UNSPECIFIED., .F., .F.,
 ( 2, 2 ),
 ( 0.000000000000000000, 1.000000000000000000 ),
 .UNSPECIFIED. ) ;
#50049=CARTESIAN_POINT ( 'NONE',  ( 6.450000001229034829, -2.886751345948125991, -5.000000000000000000 ) ) ;
#50050=CARTESIAN_POINT ( 'NONE',  ( 4.696875000614518569, -3.027376345333614438, 5.243569643749998122 ) ) ;
#50051=CARTESIAN_POINT ( 'NONE',  ( 20.63437500061451857, 6.421520780324663323E-16, -5.243569643749999010 ) ) ;
#50052=CARTESIAN_POINT ( 'NONE',  ( -2.000000000000000000, 14.97499999999999964, 26.53589838486224650 ) ) ;
#50053=CARTESIAN_POINT ( 'NONE',  ( 15.96562500061451573, -6.054752690667223547, -1.112240025338166033E-15 ) ) ;
#50056=CARTESIAN_POINT ( 'NONE',  ( 28.69687500061451502, -3.027376345333610441, -5.243569643749999898 ) ) ;
#50059=CARTESIAN_POINT ( 'NONE',  ( 14.42812500061451786, 4.541064518000418104, 2.621784821874999949 ) ) ;
#50060=CARTESIAN_POINT ( 'NONE',  ( 10.84687500061451892, 6.054752690667223547, 3.707466751127219781E-16 ) ) ;
#50062=CARTESIAN_POINT ( 'NONE',  ( 3.479729569495786379, -3.590471016896914946, -3.821457900550485398 ) ) ;
#50063=CARTESIAN_POINT ( 'NONE',  ( 21.62812500061451360, 4.541064518000418104, 2.621784821874999949 ) ) ;
#50065=CARTESIAN_POINT ( 'NONE',  ( 28.72500000122903074, 2.886751345948164182, 4.999999999999933387 ) ) ;
#50066=CARTESIAN_POINT ( 'NONE',  ( 13.27500000000000213, 4.330127018922191873, 2.499999999999999556 ) ) ;
#50067=CARTESIAN_POINT ( 'NONE',  ( 21.90000000122903145, 5.773502691896255534, 3.535250795749688894E-16 ) ) ;
#50068=CARTESIAN_POINT ( 'NONE',  ( 17.24062500061451786, -3.027376345333614438, 5.243569643749998122 ) ) ;
#50070=ORIENTED_EDGE ( 'NONE', *, *, #31407, .F. ) ;
#50071=CARTESIAN_POINT ( 'NONE',  ( 20.66250000000000142, -5.773502691896255534, -1.060575238724906372E-15 ) ) ;
#50072=CARTESIAN_POINT ( 'NONE',  ( 20.93437500061451573, -4.541064518000419881, 2.621784821874995952 ) ) ;
#50073=CARTESIAN_POINT ( 'NONE',  ( 28.60312500061451502, -4.541064518000417216, -2.621784821875001281 ) ) ;
#50074=VERTEX_POINT ( 'NONE', #23763 ) ;
#50075=CARTESIAN_POINT ( 'NONE',  ( 0.000000000000000000, 20.00000000000000000, -33.99999999999999289 ) ) ;
#50076=CARTESIAN_POINT ( 'NONE',  ( 9.590625000614517504, -3.027376345333614438, 5.243569643749998122 ) ) ;
#50077=CARTESIAN_POINT ( 'NONE',  ( 6.299999999999999822, -4.330127018922190985, -2.500000000000001332 ) ) ;
#50079=CARTESIAN_POINT ( 'NONE',  ( 16.61250000000000426, -5.773502691896255534, -1.060575238724906372E-15 ) ) ;
#50080=CARTESIAN_POINT ( 'NONE',  ( 23.81250000000000000, -5.773502691896255534, -1.060575238724906372E-15 ) ) ;
#50081=CARTESIAN_POINT ( 'NONE',  ( 3.557364438369462256, -3.513567738442655131, -3.708418381339127379 ) ) ;
#50082=CARTESIAN_POINT ( 'NONE',  ( 3.346875000614518036, -3.027376345333614438, 5.243569643749998122 ) ) ;
#50083=CARTESIAN_POINT ( 'NONE',  ( 28.09687500061451360, -3.027376345333614438, 5.243569643749998122 ) ) ;
#50085=CARTESIAN_POINT ( 'NONE',  ( 23.65312500061451573, -4.541064518000417216, -2.621784821875001281 ) ) ;
#50086=CARTESIAN_POINT ( 'NONE',  ( 25.43437500061451573, -4.541064518000419881, 2.621784821874995952 ) ) ;
#50087=CARTESIAN_POINT ( 'NONE',  ( -4.243569643749999898, 19.76562500061459104, -32.45002607614398471 ) ) ;
#50088=CARTESIAN_POINT ( 'NONE',  ( 14.32500000000000107, -4.330127018922194537, 2.499999999999995559 ) ) ;
#50089=CARTESIAN_POINT ( 'NONE',  ( 11.65312500061451573, 4.541064518000418104, -2.621784821874998173 ) ) ;
#50090=CARTESIAN_POINT ( 'NONE',  ( 3.787803386340530043, 3.263823755417472050, 3.928545305590518399 ) ) ;
#50091=CARTESIAN_POINT ( 'NONE',  ( 7.050000000000000711, 0.000000000000000000, 4.999999999999998224 ) ) ;
#50092=CARTESIAN_POINT ( 'NONE',  ( 25.67812500061451431, 4.541064518000418104, 2.621784821874999949 ) ) ;
#50093=CARTESIAN_POINT ( 'NONE',  ( 17.10000000122903430, -2.886751345948129988, 4.999999999999997335 ) ) ;
#50097=CARTESIAN_POINT ( 'NONE',  ( 21.12187500061451573, 3.027376345333613106, -5.243569643749998122 ) ) ;
#50098=CARTESIAN_POINT ( 'NONE',  ( 2.121784821874999061, 14.75937500061451679, 26.32496088578401583 ) ) ;
#50100=CARTESIAN_POINT ( 'NONE',  ( 21.27187500061451786, 3.027376345333611329, 5.243569643749999010 ) ) ;
#50101=CARTESIAN_POINT ( 'NONE',  ( 28.65937500061451715, -4.541064518000417216, -2.621784821875001281 ) ) ;
#50102=CARTESIAN_POINT ( 'NONE',  ( 2.121784821875001281, 18.65937500061451715, 33.67503911421598417 ) ) ;
#50103=CARTESIAN_POINT ( 'NONE',  ( 8.728125000614518569, -4.541064518000419881, 2.621784821874995952 ) ) ;
#50105=CARTESIAN_POINT ( 'NONE',  ( 6.384375000614516793, 4.541064518000418104, 2.621784821874999949 ) ) ;
#50106=CARTESIAN_POINT ( 'NONE',  ( 3.837848076843224376, 3.204827942194517831, -3.837848076843224376 ) ) ;
#50107=CARTESIAN_POINT ( 'NONE',  ( 7.940625000614518036, -3.027376345333610441, -5.243569643749999898 ) ) ;
#50108=CARTESIAN_POINT ( 'NONE',  ( 12.23437500061451821, 4.541064518000418104, 2.621784821874999949 ) ) ;
#50110=CARTESIAN_POINT ( 'NONE',  ( 20.17500000122903359, 2.886751345948126879, 4.999999999999999112 ) ) ;
#50111=CARTESIAN_POINT ( 'NONE',  ( 8.296875000614516438, -3.027376345333614438, 5.243569643749998122 ) ) ;
#50112=CARTESIAN_POINT ( 'NONE',  ( 9.928125000614517859, 4.541064518000418104, 2.621784821874999949 ) ) ;
#50113=CARTESIAN_POINT ( 'NONE',  ( 6.215625000614517504, 3.027376345333612662, -5.243569643749998122 ) ) ;
#50115=CARTESIAN_POINT ( 'NONE',  ( 18.75937500061451857, -4.541064518000417216, -2.621784821875001281 ) ) ;
#50116=CARTESIAN_POINT ( 'NONE',  ( -2.000000000000000000, 11.48750000122903359, 26.53589838486224650 ) ) ;
#50117=CARTESIAN_POINT ( 'NONE',  ( 27.55312500061451786, 0.000000000000000000, 5.243569643749999010 ) ) ;
#50118=CARTESIAN_POINT ( 'NONE',  ( 12.85312500061451502, -4.541064518000417216, -2.621784821875001281 ) ) ;
#50119=CARTESIAN_POINT ( 'NONE',  ( 28.92187500061451644, 3.027376345333611329, 5.243569643749999010 ) ) ;
#50120=CARTESIAN_POINT ( 'NONE',  ( 9.001249775931846008E-16, 12.77187500061451786, -25.09994784771203058 ) ) ;
#50121=CARTESIAN_POINT ( 'NONE',  ( 13.16250000122903430, -4.330127018922190985, -2.500000000000001332 ) ) ;
#50122=CARTESIAN_POINT ( 'NONE',  ( 4.243569643749999898, 15.49062500061451786, -27.54997392385601529 ) ) ;
#50123=CARTESIAN_POINT ( 'NONE',  ( 15.07500000122903394, 2.886751345948129099, -4.999999999999998224 ) ) ;
#50124=CARTESIAN_POINT ( 'NONE',  ( 9.403125000614517504, 4.541064518000418104, -2.621784821874998173 ) ) ;
#50125=VECTOR ( 'NONE', #57828, 1000.000000000000000 ) ;
#50126=CARTESIAN_POINT ( 'NONE',  ( 12.78749999999999964, 5.773502691896255534, 3.535250795749688894E-16 ) ) ;
#50128=CARTESIAN_POINT ( 'NONE',  ( 22.75312500061451360, -4.541064518000417216, -2.621784821875001281 ) ) ;
#50129=CARTESIAN_POINT ( 'NONE',  ( 7.621875000614519280, 3.027376345333612662, -5.243569643749998122 ) ) ;
#50130=CARTESIAN_POINT ( 'NONE',  ( 10.65000000122903323, 5.773502691896255534, 3.535250795749688894E-16 ) ) ;
#50131=CARTESIAN_POINT ( 'NONE',  ( 17.85000000122903430, 5.773502691896255534, 3.535250795749688894E-16 ) ) ;
#50132=CARTESIAN_POINT ( 'NONE',  ( 15.40312500061451573, 0.000000000000000000, 5.243569643749999010 ) ) ;
#50133=CARTESIAN_POINT ( 'NONE',  ( 19.41562500061451146, 3.027376345333611329, 5.243569643749999010 ) ) ;
#50134=CARTESIAN_POINT ( 'NONE',  ( 25.16250000122903074, 0.000000000000000000, 4.999999999999998224 ) ) ;
#50136=CARTESIAN_POINT ( 'NONE',  ( 27.18750000122903288, 6.123233995736764310E-16, -4.999999999999998224 ) ) ;
#50137=CARTESIAN_POINT ( 'NONE',  ( 21.56250000000000000, -5.773502691896255534, -1.060575238724906372E-15 ) ) ;
#50139=VECTOR ( 'NONE', #12149, 1000.000000000000000 ) ;
#50140=CARTESIAN_POINT ( 'NONE',  ( 25.84687500061451360, -3.027376345333614438, 5.243569643749998122 ) ) ;
#50141=CARTESIAN_POINT ( 'NONE',  ( 18.18750000122903288, 6.123233995736764310E-16, -4.999999999999998224 ) ) ;
#50142=EDGE_CURVE ( 'NONE', #19257, #59354, #20400, .T. ) ;
#50143=CARTESIAN_POINT ( 'NONE',  ( 11.51250000122903216, 4.330127018922192761, -2.499999999999997780 ) ) ;
#50144=CARTESIAN_POINT ( 'NONE',  ( 28.88437500061451502, 4.541064518000418104, 2.621784821874999949 ) ) ;
#50145=FACE_OUTER_BOUND ( 'NONE', #8852, .T. ) ;
#50146=CARTESIAN_POINT ( 'NONE',  ( 4.434375000614519280, 6.421520780324663323E-16, -5.243569643749999010 ) ) ;
#50147=CARTESIAN_POINT ( 'NONE',  ( 23.99062500061451786, -3.027376345333614438, 5.243569643749998122 ) ) ;
#50149=CARTESIAN_POINT ( 'NONE',  ( 10.65937500061451715, -4.541064518000417216, -2.621784821875001281 ) ) ;
#50151=CARTESIAN_POINT ( 'NONE',  ( 29.57812500061451644, 6.421520780324663323E-16, -5.243569643749999010 ) ) ;
#50152=CARTESIAN_POINT ( 'NONE',  ( 6.946875000614517681, -3.027376345333614438, 5.243569643749998122 ) ) ;
#50153=CARTESIAN_POINT ( 'NONE',  ( 29.67187500061451644, 3.027376345333613106, -5.243569643749998122 ) ) ;
#50155=CARTESIAN_POINT ( 'NONE',  ( 19.34999999999999787, -4.330127018922190985, -2.500000000000001332 ) ) ;
#50156=ORIENTED_EDGE ( 'NONE', *, *, #7027, .T. ) ;
#50157=CARTESIAN_POINT ( 'NONE',  ( 27.48749999999999716, -2.886751345948125991, -5.000000000000000000 ) ) ;
#50158=CARTESIAN_POINT ( 'NONE',  ( 29.29687500061451644, 6.054752690667223547, 3.707466751127219781E-16 ) ) ;
#50159=ORIENTED_EDGE ( 'NONE', *, *, #50272, .F. ) ;
#50160=CARTESIAN_POINT ( 'NONE',  ( 18.55312500061451431, 0.000000000000000000, 5.243569643749999010 ) ) ;
#50161=CARTESIAN_POINT ( 'NONE',  ( 9.028125000614517504, 4.541064518000418104, 2.621784821874999949 ) ) ;
#50163=CARTESIAN_POINT ( 'NONE',  ( 5.596875000614516260, -3.027376345333614438, 5.243569643749998122 ) ) ;
#50164=CARTESIAN_POINT ( 'NONE',  ( 17.51250000122903216, 0.000000000000000000, 4.999999999999998224 ) ) ;
#50166=CARTESIAN_POINT ( 'NONE',  ( 2.000000000000001332, 13.85000000000000142, -26.53589838486224650 ) ) ;
#50167=CARTESIAN_POINT ( 'NONE',  ( 6.571875000614517681, -6.054752690667223547, -1.112240025338166033E-15 ) ) ;
#50168=CARTESIAN_POINT ( 'NONE',  ( 12.64687500061451608, 6.054752690667223547, 3.707466751127219781E-16 ) ) ;
#50169=CARTESIAN_POINT ( 'NONE',  ( 21.72187500061451715, 3.027376345333611329, 5.243569643749999010 ) ) ;
#50170=CARTESIAN_POINT ( 'NONE',  ( 4.000000000000000000, 15.80000000122903181, -27.69059892324149885 ) ) ;
#50171=EDGE_LOOP ( 'NONE', ( #5056, #50785, #15995, #44840 ) ) ;
#50173=AXIS2_PLACEMENT_3D ( 'NONE', #22508, #19031, #45418 ) ;
#50174=CARTESIAN_POINT ( 'NONE',  ( 6.196875000614515905, -3.027376345333610441, -5.243569643749999898 ) ) ;
#50176=CARTESIAN_POINT ( 'NONE',  ( 19.87500000000000000, 6.123233995736764310E-16, -4.999999999999998224 ) ) ;
#50177=CARTESIAN_POINT ( 'NONE',  ( 17.99062500061451786, 6.054752690667223547, 3.707466751127219781E-16 ) ) ;
#50179=ADVANCED_FACE ( 'NONE', ( #50145 ), #64016, .F. ) ;
#50181=CARTESIAN_POINT ( 'NONE',  ( 13.37812500061451715, 6.421520780324663323E-16, -5.243569643749999010 ) ) ;
#50182=CARTESIAN_POINT ( 'NONE',  ( 29.63437500061451502, 6.421520780324663323E-16, -5.243569643749999010 ) ) ;
#50184=CARTESIAN_POINT ( 'NONE',  ( 29.74687500061451217, 6.054752690667223547, 3.707466751127219781E-16 ) ) ;
#50185=CARTESIAN_POINT ( 'NONE',  ( 10.61250000000000071, 2.886751345948126879, 4.999999999999999112 ) ) ;
#50186=EDGE_CURVE ( 'NONE', #14890, #23263, #61571, .T. ) ;
#50187=CARTESIAN_POINT ( 'NONE',  ( -2.000000000000000000, 15.53750000122903430, 26.53589838486224650 ) ) ;
#50188=CARTESIAN_POINT ( 'NONE',  ( 8.812500001229034652, 4.330127018922192761, -2.499999999999997780 ) ) ;
#50189=( BOUNDED_CURVE ( )  B_SPLINE_CURVE ( 2, ( #9369, #54438, #44823, #30262, #56264, #7728, #6008, #39642, #2196 ),
 .UNSPECIFIED., .F., .F. ) 
 B_SPLINE_CURVE_WITH_KNOTS ( ( 3, 2, 2, 2, 3 ),
 ( 0.6413043478260869179, 0.6449275362318840354, 0.6521739130434782705, 0.6594202898550725056, 0.6630434782608696231 ),
 .UNSPECIFIED. ) 
 CURVE ( )  GEOMETRIC_REPRESENTATION_ITEM ( )  RATIONAL_B_SPLINE_CURVE ( ( 0.9330127018922194093, 0.9330127018922194093, 1.000000000000000000, 0.8660254037844387076, 1.000000000000000000, 0.8660254037844387076, 1.000000000000000000, 0.9330127018922182991, 0.9330127018922192983 ) ) 
 REPRESENTATION_ITEM ( '' )  );
#50190=VECTOR ( 'NONE', #7252, 1000.000000000000000 ) ;
#50191=CARTESIAN_POINT ( 'NONE',  ( 20.93437500061451573, -4.541064518000419881, 2.621784821874995952 ) ) ;
#50192=CARTESIAN_POINT ( 'NONE',  ( 14.44687500061451679, 6.054752690667223547, 3.707466751127219781E-16 ) ) ;
#50194=CARTESIAN_POINT ( 'NONE',  ( 15.44062500061451537, -3.027376345333614438, 5.243569643749998122 ) ) ;
#50195=AXIS2_PLACEMENT_3D ( 'NONE', #6480, #68902, #7923 ) ;
#50196=CARTESIAN_POINT ( 'NONE',  ( 25.83750000122903501, 6.123233995736764310E-16, -4.999999999999998224 ) ) ;
#50197=CARTESIAN_POINT ( 'NONE',  ( 15.15937500061451715, -4.541064518000417216, -2.621784821875001281 ) ) ;
#50198=CARTESIAN_POINT ( 'NONE',  ( 2.692168354449048895, 9.632460402479562589, -24.63433627171737328 ) ) ;
#50199=CARTESIAN_POINT ( 'NONE',  ( 17.12812500061451715, 4.541064518000418104, 2.621784821874999949 ) ) ;
#50200=CARTESIAN_POINT ( 'NONE',  ( 18.00000000122903288, -2.886751345948130876, 4.999999999999996447 ) ) ;
#50201=CARTESIAN_POINT ( 'NONE',  ( 26.33437500061451431, -4.541064518000419881, 2.621784821874995952 ) ) ;
#50202=CARTESIAN_POINT ( 'NONE',  ( -4.243569643749999898, 10.76562500061451644, 27.54997392385601529 ) ) ;
#50203=CARTESIAN_POINT ( 'NONE',  ( 15.68437500061451573, 6.421520780324663323E-16, -5.243569643749999010 ) ) ;
#50204=CARTESIAN_POINT ( 'NONE',  ( 15.11250000122903359, 4.330127018922192761, -2.499999999999997780 ) ) ;
#50206=CARTESIAN_POINT ( 'NONE',  ( 3.348770750331622637, -3.712914550824308879, 3.702605588924299695 ) ) ;
#50207=CARTESIAN_POINT ( 'NONE',  ( 19.47187500061451360, 3.027376345333611329, 5.243569643749999010 ) ) ;
#50208=CARTESIAN_POINT ( 'NONE',  ( 19.31250000122903288, 0.000000000000000000, 4.999999999999998224 ) ) ;
#50209=CARTESIAN_POINT ( 'NONE',  ( 18.04687500061451999, 6.054752690667223547, 3.707466751127219781E-16 ) ) ;
#50210=CARTESIAN_POINT ( 'NONE',  ( 9.001249775931846008E-16, 11.42187500061451999, 34.90005215228797653 ) ) ;
#50211=CARTESIAN_POINT ( 'NONE',  ( 18.25312500061451715, -4.541064518000417216, -2.621784821875001281 ) ) ;
#50212=ORIENTED_EDGE ( 'NONE', *, *, #68849, .T. ) ;
#50213=ORIENTED_EDGE ( 'NONE', *, *, #6144, .T. ) ;
#50214=CARTESIAN_POINT ( 'NONE',  ( 19.57500000000000284, 4.330127018922191873, 2.499999999999999556 ) ) ;
#50215=CARTESIAN_POINT ( 'NONE',  ( 28.12500000122902932, 2.886751345948125103, -5.000000000000004441 ) ) ;
#50216=CARTESIAN_POINT ( 'NONE',  ( 24.21562500061451573, 3.027376345333613106, -5.243569643749998122 ) ) ;
#50217=CARTESIAN_POINT ( 'NONE',  ( 4.340625000614515727, -3.027376345333610441, -5.243569643749999898 ) ) ;
#50218=CARTESIAN_POINT ( 'NONE',  ( 16.98750000122903359, 4.330127018922191873, 2.499999999999999556 ) ) ;
#50219=CARTESIAN_POINT ( 'NONE',  ( 22.41562500061451502, 3.027376345333613106, -5.243569643749998122 ) ) ;
#50220=CARTESIAN_POINT ( 'NONE',  ( 21.33749999999999858, 5.773502691896255534, 3.535250795749688894E-16 ) ) ;
#50221=CARTESIAN_POINT ( 'NONE',  ( 25.60312500061451502, 4.541064518000418104, -2.621784821874998173 ) ) ;
#50222=CARTESIAN_POINT ( 'NONE',  ( 5.878125000614517148, 4.541064518000418104, 2.621784821874999949 ) ) ;
#50225=CARTESIAN_POINT ( 'NONE',  ( 26.81250000122903288, 4.330127018922192761, -2.499999999999997780 ) ) ;
#50226=VECTOR ( 'NONE', #54620, 1000.000000000000000 ) ;
#50228=CARTESIAN_POINT ( 'NONE',  ( 2.000000000000001332, 12.95000000000000107, 33.46410161513774995 ) ) ;
#50229=CARTESIAN_POINT ( 'NONE',  ( 8.484601909799253346E-16, 11.22500000122903607, -25.38119784648299770 ) ) ;
#50230=CARTESIAN_POINT ( 'NONE',  ( 2.121784821875001281, 19.10937500061451644, -26.32496088578401938 ) ) ;
#50231=AXIS2_PLACEMENT_3D ( 'NONE', #40717, #63234, #61783 ) ;
#50232=CARTESIAN_POINT ( 'NONE',  ( 8.812500000000000000, 2.886751345948126879, 4.999999999999999112 ) ) ;
#50234=CARTESIAN_POINT ( 'NONE',  ( 9.684375000614517504, -4.541064518000419881, 2.621784821874995952 ) ) ;
#50235=CARTESIAN_POINT ( 'NONE',  ( 6.037500001229035185, 6.123233995736764310E-16, -4.999999999999998224 ) ) ;
#50236=CARTESIAN_POINT ( 'NONE',  ( 13.43437500061451750, 6.421520780324663323E-16, -5.243569643749999010 ) ) ;
#50237=CARTESIAN_POINT ( 'NONE',  ( 30.00000000000000000, 6.123233995736764310E-16, -4.999999999999998224 ) ) ;
#50238=CARTESIAN_POINT ( 'NONE',  ( 4.696875000614518569, -3.027376345333614438, 5.243569643749998122 ) ) ;
#50239=CARTESIAN_POINT ( 'NONE',  ( 0.000000000000000000, 20.00000000000000000, -36.00000000000000000 ) ) ;
#50240=VECTOR ( 'NONE', #66979, 1000.000000000000000 ) ;
#50241=CARTESIAN_POINT ( 'NONE',  ( 3.504965621013899746, 3.565840152826760256, 3.504965621013765631 ) ) ;
#50242=CARTESIAN_POINT ( 'NONE',  ( 10.95937500061451964, 0.000000000000000000, 5.243569643749999010 ) ) ;
#50244=CARTESIAN_POINT ( 'NONE',  ( 20.76562500061451644, 3.027376345333611329, 5.243569643749999010 ) ) ;
#50245=CARTESIAN_POINT ( 'NONE',  ( 4.661467738957716378, -1.808512791952580301, -4.661467738957749241 ) ) ;
#50246=CARTESIAN_POINT ( 'NONE',  ( -4.243569643749999898, 16.65312500061459744, 30.00000000000000000 ) ) ;
#50247=CARTESIAN_POINT ( 'NONE',  ( 24.68437500061451573, 6.421520780324663323E-16, -5.243569643749999010 ) ) ;
#50248=CARTESIAN_POINT ( 'NONE',  ( 2.854733137546939137, -4.104967572847192159, 3.224293301434809411 ) ) ;
#50249=CARTESIAN_POINT ( 'NONE',  ( 28.87500000122902932, -5.773502691896255534, -1.060575238724906372E-15 ) ) ;
#50251=CARTESIAN_POINT ( 'NONE',  ( 24.70312500061451644, 4.541064518000418104, -2.621784821874998173 ) ) ;
#50252=CARTESIAN_POINT ( 'NONE',  ( 15.62812500061451537, 6.421520780324663323E-16, -5.243569643749999010 ) ) ;
#50254=CARTESIAN_POINT ( 'NONE',  ( 13.99687500061451928, 6.054752690667223547, 3.707466751127219781E-16 ) ) ;
#50256=CARTESIAN_POINT ( 'NONE',  ( 24.22500000122903430, 2.886751345948126879, 4.999999999999999112 ) ) ;
#50257=DIRECTION ( 'NONE',  ( 0.000000000000000000, 0.000000000000000000, -1.000000000000000000 ) ) ;
#50258=CARTESIAN_POINT ( 'NONE',  ( 13.13437500061451857, 4.541064518000418104, 2.621784821874999949 ) ) ;
#50259=CARTESIAN_POINT ( 'NONE',  ( 4.843974908776027988, -1.239501918800440361, -5.095008608840551290 ) ) ;
#50261=CARTESIAN_POINT ( 'NONE',  ( 25.80937500061451928, 0.000000000000000000, 5.243569643749999010 ) ) ;
#50262=CARTESIAN_POINT ( 'NONE',  ( 17.59687500061451715, 6.054752690667223547, 3.707466751127219781E-16 ) ) ;
#50264=CARTESIAN_POINT ( 'NONE',  ( 28.08749999999999858, 5.773502691896255534, 3.535250795749688894E-16 ) ) ;
#50265=CARTESIAN_POINT ( 'NONE',  ( 3.675000001229035362, -5.773502691896255534, -1.060575238724906372E-15 ) ) ;
#50266=CARTESIAN_POINT ( 'NONE',  ( 6.187500000000002665, -2.886751345948129988, 4.999999999999997335 ) ) ;
#50268=CARTESIAN_POINT ( 'NONE',  ( 19.49062500061451431, -3.027376345333614438, 5.243569643749998122 ) ) ;
#50269=CARTESIAN_POINT ( 'NONE',  ( 9.375000000000001776, -4.330127018922194537, 2.499999999999995559 ) ) ;
#50270=CARTESIAN_POINT ( 'NONE',  ( 15.45000000000000107, 4.330127018922192761, -2.499999999999997780 ) ) ;
#50271=CARTESIAN_POINT ( 'NONE',  ( 16.94999999999999929, 0.000000000000000000, 4.999999999999998224 ) ) ;
#50272=EDGE_CURVE ( 'NONE', #19034, #70765, #48250, .T. ) ;
#50273=CARTESIAN_POINT ( 'NONE',  ( 4.243569643749999010, 13.31562500061451537, 27.54997392385601174 ) ) ;
#50274=DIRECTION ( 'NONE',  ( -0.000000000000000000, -1.000000000000000000, -0.000000000000000000 ) ) ;
#50275=CARTESIAN_POINT ( 'NONE',  ( 19.80000000122903359, -2.886751345948129988, 4.999999999999997335 ) ) ;
#50276=CARTESIAN_POINT ( 'NONE',  ( 5.999957575222543582, 8.000031818581996745, 30.20273605092067726 ) ) ;
#50277=CARTESIAN_POINT ( 'NONE',  ( 28.35937500061451289, 4.541064518000418104, -2.621784821874998173 ) ) ;
#50279=CARTESIAN_POINT ( 'NONE',  ( 17.01562500061451644, 3.027376345333613106, -5.243569643749998122 ) ) ;
#50280=CARTESIAN_POINT ( 'NONE',  ( 21.29062500061451502, -3.027376345333614438, 5.243569643749998122 ) ) ;
#50281=CARTESIAN_POINT ( 'NONE',  ( 23.52187500061451786, 3.027376345333611329, 5.243569643749999010 ) ) ;
#50282=CARTESIAN_POINT ( 'NONE',  ( 5.662500000000000533, 2.886751345948126879, 4.999999999999999112 ) ) ;
#50283=CARTESIAN_POINT ( 'NONE',  ( 10.41562500061451679, 3.027376345333611329, 5.243569643749999010 ) ) ;
#50284=CARTESIAN_POINT ( 'NONE',  ( 25.45312500061451644, -4.541064518000417216, -2.621784821875001281 ) ) ;
#50285=CARTESIAN_POINT ( 'NONE',  ( 13.95937500061451786, 4.541064518000418104, -2.621784821874998173 ) ) ;
#50286=CARTESIAN_POINT ( 'NONE',  ( 19.13437500061451857, -4.541064518000419881, 2.621784821874995952 ) ) ;
#50287=CARTESIAN_POINT ( 'NONE',  ( 1.071796769724489895, 12.32990381179670081, -34.00000000000000000 ) ) ;
#50288=CARTESIAN_POINT ( 'NONE',  ( -4.243569643749999898, 18.90312500061451573, 30.00000000000000000 ) ) ;
#50289=CARTESIAN_POINT ( 'NONE',  ( 21.41250000122903074, 4.330127018922192761, -2.499999999999997780 ) ) ;
#50291=CARTESIAN_POINT ( 'NONE',  ( 12.55312500061451786, 4.541064518000418104, -2.621784821874998173 ) ) ;
#50293=CARTESIAN_POINT ( 'NONE',  ( 5.221875000614519813, -6.054752690667223547, -1.112240025338166033E-15 ) ) ;
#50294=CARTESIAN_POINT ( 'NONE',  ( 8.221875000614518925, 3.027376345333611329, 5.243569643749999010 ) ) ;
#50295=EDGE_CURVE ( 'NONE', #23277, #32974, #66592, .T. ) ;
#50297=CARTESIAN_POINT ( 'NONE',  ( 27.87187500061451573, 3.027376345333613106, -5.243569643749998122 ) ) ;
#50298=CARTESIAN_POINT ( 'NONE',  ( 18.92812500061451431, 4.541064518000418104, 2.621784821874999949 ) ) ;
#50299=CARTESIAN_POINT ( 'NONE',  ( 28.83750000122903145, -4.330127018922194537, 2.499999999999995559 ) ) ;
#50300=CARTESIAN_POINT ( 'NONE',  ( 26.80312500061451431, -4.541064518000417216, -2.621784821875001281 ) ) ;
#50301=CARTESIAN_POINT ( 'NONE',  ( 23.22187500061451715, -6.054752690667223547, -1.112240025338166033E-15 ) ) ;
#50302=CARTESIAN_POINT ( 'NONE',  ( 20.12812500061451715, 6.421520780324663323E-16, -5.243569643749999010 ) ) ;
#50303=CARTESIAN_POINT ( 'NONE',  ( -2.000000000000000000, 10.47500000000000142, 26.53589838486224650 ) ) ;
#50304=CARTESIAN_POINT ( 'NONE',  ( 24.40312500061451573, 0.000000000000000000, 5.243569643749999010 ) ) ;
#50305=CARTESIAN_POINT ( 'NONE',  ( 4.912500001229034297, 0.000000000000000000, 4.999999999999998224 ) ) ;
#50306=ORIENTED_EDGE ( 'NONE', *, *, #46542, .F. ) ;
#50307=CARTESIAN_POINT ( 'NONE',  ( 28.27499999999999858, -4.330127018922194537, 2.499999999999995559 ) ) ;
#50308=CARTESIAN_POINT ( 'NONE',  ( 8.484601909799253346E-16, 15.16250000000000142, -25.38119784648299770 ) ) ;
#50310=CARTESIAN_POINT ( 'NONE',  ( 5.334375000614517859, 6.421520780324663323E-16, -5.243569643749999010 ) ) ;
#50311=CARTESIAN_POINT ( 'NONE',  ( 12.32812500061451821, -4.541064518000419881, 2.621784821874995952 ) ) ;
#50312=CARTESIAN_POINT ( 'NONE',  ( 6.009375000614519458, 0.000000000000000000, 5.243569643749999010 ) ) ;
#50313=CARTESIAN_POINT ( 'NONE',  ( 23.66250000122903430, 4.330127018922192761, -2.499999999999997780 ) ) ;
#50314=CARTESIAN_POINT ( 'NONE',  ( 13.92187500061451289, 3.027376345333612662, -5.243569643749998122 ) ) ;
#50315=CARTESIAN_POINT ( 'NONE',  ( 29.76562500061451644, 3.027376345333611329, 5.243569643749999010 ) ) ;
#50316=CARTESIAN_POINT ( 'NONE',  ( 28.57499999999999929, 4.330127018922191873, 2.499999999999999556 ) ) ;
#50317=CARTESIAN_POINT ( 'NONE',  ( 25.50937500061451502, -4.541064518000417216, -2.621784821875001281 ) ) ;
#50318=CARTESIAN_POINT ( 'NONE',  ( 3.290625000614516793, -3.027376345333614438, 5.243569643749998122 ) ) ;
#50319=CARTESIAN_POINT ( 'NONE',  ( 13.26562500061451644, -6.054752690667223547, -1.112240025338166033E-15 ) ) ;
#50320=ORIENTED_EDGE ( 'NONE', *, *, #58832, .T. ) ;
#50321=CARTESIAN_POINT ( 'NONE',  ( 10.19062500061451892, -3.027376345333610441, -5.243569643749999898 ) ) ;
#50322=CARTESIAN_POINT ( 'NONE',  ( 9.478125000614515017, 4.541064518000418104, 2.621784821874999949 ) ) ;
#50324=DIRECTION ( 'NONE',  ( -0.000000000000000000, -1.000000000000000000, -0.000000000000000000 ) ) ;
#50325=CARTESIAN_POINT ( 'NONE',  ( 16.31250000000000000, 2.886751345948129099, -4.999999999999998224 ) ) ;
#50326=CARTESIAN_POINT ( 'NONE',  ( 16.92187500061451999, -6.054752690667223547, -1.112240025338166033E-15 ) ) ;
#50327=CARTESIAN_POINT ( 'NONE',  ( 13.23750000122903359, 6.123233995736764310E-16, -4.999999999999998224 ) ) ;
#50329=CARTESIAN_POINT ( 'NONE',  ( 20.55937500061451573, -4.541064518000417216, -2.621784821875001281 ) ) ;
#50330=CARTESIAN_POINT ( 'NONE',  ( -4.243569643749999898, 15.26562500061451644, -32.45002607614398471 ) ) ;
#50334=CARTESIAN_POINT ( 'NONE',  ( 27.77812500061451573, 6.421520780324663323E-16, -5.243569643749999010 ) ) ;
#50336=( BOUNDED_CURVE ( )  B_SPLINE_CURVE ( 2, ( #55228, #22323, #55948, #61483, #22680, #38219, #5344 ),
 .UNSPECIFIED., .F., .F. ) 
 B_SPLINE_CURVE_WITH_KNOTS ( ( 3, 2, 2, 3 ),
 ( 0.3166666666666666519, 0.3194444444444444198, 0.3222222222222222432, 0.3250000000000000111 ),
 .UNSPECIFIED. ) 
 CURVE ( )  GEOMETRIC_REPRESENTATION_ITEM ( )  RATIONAL_B_SPLINE_CURVE ( ( 1.000000000000000000, 0.8660254037844387076, 1.000000000000000000, 0.8660254037844387076, 1.000000000000000000, 0.8660254037844387076, 1.000000000000000000 ) ) 
 REPRESENTATION_ITEM ( '' )  );
#50337=CARTESIAN_POINT ( 'NONE',  ( 26.84999999999999787, 0.000000000000000000, 4.999999999999998224 ) ) ;
#50338=CARTESIAN_POINT ( 'NONE',  ( 10.07812500061451644, -4.541064518000419881, 2.621784821874995952 ) ) ;
#50340=CARTESIAN_POINT ( 'NONE',  ( 20.63437500061451857, 6.421520780324663323E-16, -5.243569643749999010 ) ) ;
#50342=CARTESIAN_POINT ( 'NONE',  ( 5.315625000614516260, 3.027376345333613106, -5.243569643749998122 ) ) ;
#50343=CARTESIAN_POINT ( 'NONE',  ( 10.77187500061451786, 3.027376345333613106, -5.243569643749998122 ) ) ;
#50345=CARTESIAN_POINT ( 'NONE',  ( 22.35937500061451644, -4.541064518000417216, -2.621784821875001281 ) ) ;
#50346=CARTESIAN_POINT ( 'NONE',  ( 0.1378111602261695712, 5.000000000000000000, -26.00000000000000000 ) ) ;
#50347=CARTESIAN_POINT ( 'NONE',  ( 28.87499999999999645, 6.123233995736764310E-16, -4.999999999999998224 ) ) ;
#50348=CARTESIAN_POINT ( 'NONE',  ( 5.737499999999998934, -2.886751345948129988, 4.999999999999997335 ) ) ;
#50349=CARTESIAN_POINT ( 'NONE',  ( 15.52500000122903323, 2.886751345948129099, -4.999999999999998224 ) ) ;
#50350=CARTESIAN_POINT ( 'NONE',  ( 17.25000000000000000, 4.330127018922192761, -2.499999999999997780 ) ) ;
#50351=ORIENTED_EDGE ( 'NONE', *, *, #16407, .F. ) ;
#50352=CARTESIAN_POINT ( 'NONE',  ( 12.67499999999999893, 6.123233995736764310E-16, -4.999999999999998224 ) ) ;
#50353=CARTESIAN_POINT ( 'NONE',  ( 17.13749999999999929, -2.886751345948125991, -5.000000000000000000 ) ) ;
#50354=CARTESIAN_POINT ( 'NONE',  ( 10.87500000122903288, -5.773502691896255534, -1.060575238724906372E-15 ) ) ;
#50355=CARTESIAN_POINT ( 'NONE',  ( 9.403125000614517504, 4.541064518000418104, -2.621784821874998173 ) ) ;
#50356=EDGE_CURVE ( 'NONE', #13938, #55464, #18028, .T. ) ;
#50357=CARTESIAN_POINT ( 'NONE',  ( 8.062500000000000000, -5.773502691896255534, -1.060575238724906372E-15 ) ) ;
#50358=CARTESIAN_POINT ( 'NONE',  ( 3.617702362022032325, -3.451409801779584008, 3.617702362022032325 ) ) ;
#50359=CARTESIAN_POINT ( 'NONE',  ( -4.243569643749999898, 14.90937500061451715, -30.00000000000000000 ) ) ;
#50360=CARTESIAN_POINT ( 'NONE',  ( 27.22500000122903430, 2.886751345948129099, -4.999999999999998224 ) ) ;
#50362=CARTESIAN_POINT ( 'NONE',  ( 6.337499999999998579, -2.886751345948125991, -5.000000000000000000 ) ) ;
#50365=CARTESIAN_POINT ( 'NONE',  ( 25.37812500061451715, -4.541064518000419881, 2.621784821874995952 ) ) ;
#50366=CARTESIAN_POINT ( 'NONE',  ( 1.626862140677534273E-15, 13.36250000000000071, -26.00000000000000355 ) ) ;
#50367=VECTOR ( 'NONE', #22627, 1000.000000000000000 ) ;
#50368=CARTESIAN_POINT ( 'NONE',  ( 28.99687500061451573, -3.027376345333614438, 5.243569643749998122 ) ) ;
#50369=CARTESIAN_POINT ( 'NONE',  ( 22.17187500061451644, 3.027376345333611329, 5.243569643749999010 ) ) ;
#50370=CARTESIAN_POINT ( 'NONE',  ( 15.70312500061451644, 4.541064518000418104, -2.621784821874998173 ) ) ;
#50371=CARTESIAN_POINT ( 'NONE',  ( -3.000416591977282496E-16, 12.04062500061459495, -34.90005215228797653 ) ) ;
#50372=CARTESIAN_POINT ( 'NONE',  ( 7.415625000614516793, -6.054752690667223547, -1.112240025338166033E-15 ) ) ;
#50373=CARTESIAN_POINT ( 'NONE',  ( 28.80000000122903003, -2.886751345948129988, 4.999999999999997335 ) ) ;
#50375=CARTESIAN_POINT ( 'NONE',  ( 18.77812500061451573, 6.421520780324663323E-16, -5.243569643749999010 ) ) ;
#50376=CARTESIAN_POINT ( 'NONE',  ( -3.137519842735245283E-14, 11.22500000122903430, -26.00000000000000711 ) ) ;
#50378=CARTESIAN_POINT ( 'NONE',  ( 14.67187500061451821, -6.054752690667223547, -1.112240025338166033E-15 ) ) ;
#50379=CARTESIAN_POINT ( 'NONE',  ( 15.53437500061451715, -4.541064518000419881, 2.621784821874995952 ) ) ;
#50380=CARTESIAN_POINT ( 'NONE',  ( 23.14687500061451786, -3.027376345333614438, 5.243569643749998122 ) ) ;
#50381=ORIENTED_EDGE ( 'NONE', *, *, #42162, .F. ) ;
#50382=CARTESIAN_POINT ( 'NONE',  ( -5.810221930991193690E-16, 14.60000000122903252, -34.00000000000000000 ) ) ;
#50383=CARTESIAN_POINT ( 'NONE',  ( 27.06562500061451004, 3.027376345333611329, 5.243569643749999010 ) ) ;
#50384=CARTESIAN_POINT ( 'NONE',  ( 25.79062500061451502, -3.027376345333614438, 5.243569643749998122 ) ) ;
#50386=CARTESIAN_POINT ( 'NONE',  ( 8.484601909799253346E-16, 16.51249999999999929, 34.61880215351700230 ) ) ;
#50387=CARTESIAN_POINT ( 'NONE',  ( 4.584375000614516971, 4.541064518000418104, 2.621784821874999949 ) ) ;
#50388=CARTESIAN_POINT ( 'NONE',  ( 11.92500000122903181, 2.886751345948129099, -4.999999999999998224 ) ) ;
#50389=CARTESIAN_POINT ( 'NONE',  ( 6.112500001229034474, 4.330127018922192761, -2.499999999999997780 ) ) ;
#50390=CARTESIAN_POINT ( 'NONE',  ( 2.840625000614518392, -3.027376345333614438, 5.243569643749998122 ) ) ;
#50393=CARTESIAN_POINT ( 'NONE',  ( 11.48437500061451644, -4.541064518000419881, 2.621784821874995952 ) ) ;
#50396=CARTESIAN_POINT ( 'NONE',  ( 19.71562500061451928, 3.027376345333613106, -5.243569643749998122 ) ) ;
#50397=CARTESIAN_POINT ( 'NONE',  ( 13.77187500061451786, -6.054752690667223547, -1.112240025338166033E-15 ) ) ;
#50398=CARTESIAN_POINT ( 'NONE',  ( 5.053125000614517859, 0.000000000000000000, 5.243569643749999010 ) ) ;
#50399=CARTESIAN_POINT ( 'NONE',  ( 23.25937500061451857, -4.541064518000417216, -2.621784821875001281 ) ) ;
#50400=CARTESIAN_POINT ( 'NONE',  ( 9.309375000614517504, -4.541064518000417216, -2.621784821875001281 ) ) ;
#50401=CARTESIAN_POINT ( 'NONE',  ( 4.265625000614517326, -6.054752690667223547, -1.112240025338166033E-15 ) ) ;
#50402=DIRECTION ( 'NONE',  ( 0.000000000000000000, 0.000000000000000000, 1.000000000000000000 ) ) ;
#50403=CARTESIAN_POINT ( 'NONE',  ( 5.025000001229035895, -5.773502691896255534, -1.060575238724906372E-15 ) ) ;
#50405=CARTESIAN_POINT ( 'NONE',  ( 21.02812500061451573, 6.421520780324663323E-16, -5.243569643749999010 ) ) ;
#50406=CARTESIAN_POINT ( 'NONE',  ( 7.162500001229032520, 0.000000000000000000, 4.999999999999998224 ) ) ;
#50407=CARTESIAN_POINT ( 'NONE',  ( 17.72812500061451502, -4.541064518000419881, 2.621784821874995952 ) ) ;
#50408=CARTESIAN_POINT ( 'NONE',  ( 16.41562500061451857, -6.054752690667223547, -1.112240025338166033E-15 ) ) ;
#50410=CARTESIAN_POINT ( 'NONE',  ( 15.63749999999999751, -2.886751345948129988, 4.999999999999997335 ) ) ;
#50411=CARTESIAN_POINT ( 'NONE',  ( 9.900000001229033231, -2.886751345948129988, 4.999999999999997335 ) ) ;
#50412=CARTESIAN_POINT ( 'NONE',  ( 6.815625000614517148, 3.027376345333611329, 5.243569643749999010 ) ) ;
#50413=ADVANCED_FACE ( 'NONE', ( #1620 ), #24129, .F. ) ;
#50414=CARTESIAN_POINT ( 'NONE',  ( 20.47500000122903074, 2.886751345948129099, -4.999999999999998224 ) ) ;
#50416=CARTESIAN_POINT ( 'NONE',  ( -4.243569643749999898, 10.82187500061451857, -32.45002607614398471 ) ) ;
#50418=CARTESIAN_POINT ( 'NONE',  ( 3.421875000614516882, -6.054752690667223547, -1.112240025338166033E-15 ) ) ;
#50419=CARTESIAN_POINT ( 'NONE',  ( 21.68437500061451573, 4.541064518000418104, 2.621784821874999949 ) ) ;
#50420=CARTESIAN_POINT ( 'NONE',  ( 5.100000000000000533, 4.330127018922192761, -2.499999999999997780 ) ) ;
#50421=CARTESIAN_POINT ( 'NONE',  ( 15.29062500061451679, 6.054752690667223547, 3.707466751127219781E-16 ) ) ;
#50423=CARTESIAN_POINT ( 'NONE',  ( 23.09999999999999787, 4.330127018922192761, -2.499999999999997780 ) ) ;
#50425=CARTESIAN_POINT ( 'NONE',  ( 29.70937500061451431, 4.541064518000418104, -2.621784821874998173 ) ) ;
#50427=CARTESIAN_POINT ( 'NONE',  ( 11.76562500061451644, 3.027376345333611329, 5.243569643749999010 ) ) ;
#50428=CARTESIAN_POINT ( 'NONE',  ( 11.40937500061451892, 0.000000000000000000, 5.243569643749999010 ) ) ;
#50429=ORIENTED_EDGE ( 'NONE', *, *, #52646, .F. ) ;
#50430=CARTESIAN_POINT ( 'NONE',  ( -1.071796769724491005, 14.05759618943233669, -34.00000000000000000 ) ) ;
#50431=CARTESIAN_POINT ( 'NONE',  ( 22.64062500061451644, -3.027376345333614438, 5.243569643749998122 ) ) ;
#50432=CARTESIAN_POINT ( 'NONE',  ( 1.999999999999998668, 13.21250000122903501, -33.46410161513775705 ) ) ;
#50435=CARTESIAN_POINT ( 'NONE',  ( 12.93750000000000178, -2.886751345948129988, 4.999999999999997335 ) ) ;
#50436=CARTESIAN_POINT ( 'NONE',  ( 21.97500000122903074, 2.886751345948126879, 4.999999999999999112 ) ) ;
#50437=CARTESIAN_POINT ( 'NONE',  ( 17.31562500061451715, -6.054752690667223547, -1.112240025338166033E-15 ) ) ;
#50439=VERTEX_POINT ( 'NONE', #70299 ) ;
#50440=CARTESIAN_POINT ( 'NONE',  ( 19.27500000000000213, -4.330127018922194537, 2.499999999999995559 ) ) ;
#50441=CARTESIAN_POINT ( 'NONE',  ( 23.66250000000000142, 2.886751345948126879, 4.999999999999999112 ) ) ;
#50442=CARTESIAN_POINT ( 'NONE',  ( 20.44687500061451857, -3.027376345333614438, 5.243569643749998122 ) ) ;
#50443=CARTESIAN_POINT ( 'NONE',  ( 26.50312500061451360, 4.541064518000418104, -2.621784821874998173 ) ) ;
#50444=ORIENTED_EDGE ( 'NONE', *, *, #23135, .F. ) ;
#50446=CARTESIAN_POINT ( 'NONE',  ( 7.865625000614516971, -6.054752690667223547, -1.112240025338166033E-15 ) ) ;
#50447=CARTESIAN_POINT ( 'NONE',  ( 17.36250000122903359, 4.330127018922192761, -2.499999999999997780 ) ) ;
#50448=CARTESIAN_POINT ( 'NONE',  ( 18.18750000000000000, 5.773502691896255534, 3.535250795749688894E-16 ) ) ;
#50449=CARTESIAN_POINT ( 'NONE',  ( 4.209375000614516971, 0.000000000000000000, 5.243569643749999010 ) ) ;
#50450=CARTESIAN_POINT ( 'NONE',  ( 29.63437500061451502, 6.421520780324663323E-16, -5.243569643749999010 ) ) ;
#50452=CARTESIAN_POINT ( 'NONE',  ( 23.95312500061451289, 0.000000000000000000, 5.243569643749999010 ) ) ;
#50453=CARTESIAN_POINT ( 'NONE',  ( 25.65937500061451715, 4.541064518000418104, -2.621784821874998173 ) ) ;
#50454=CARTESIAN_POINT ( 'NONE',  ( -2.121784821874996840, 18.52812500061459389, -26.32496088578401583 ) ) ;
#50455=CARTESIAN_POINT ( 'NONE',  ( 12.52500000000000213, -4.330127018922194537, 2.499999999999995559 ) ) ;
#50456=CARTESIAN_POINT ( 'NONE',  ( 8.765625000614518214, -6.054752690667223547, -1.112240025338166033E-15 ) ) ;
#50457=CARTESIAN_POINT ( 'NONE',  ( 30.00000000000000000, 0.000000000000000000, 4.999999999999998224 ) ) ;
#50458=CARTESIAN_POINT ( 'NONE',  ( 25.52812500061451573, 6.421520780324663323E-16, -5.243569643749999010 ) ) ;
#50461=CARTESIAN_POINT ( 'NONE',  ( 3.965625000614515727, 3.027376345333613106, -5.243569643749998122 ) ) ;
#50462=CARTESIAN_POINT ( 'NONE',  ( 19.32187500061451857, 3.027376345333613106, -5.243569643749998122 ) ) ;
#50463=CARTESIAN_POINT ( 'NONE',  ( 4.243569643749999010, 15.62187500061451928, 27.54997392385601174 ) ) ;
#50464=CARTESIAN_POINT ( 'NONE',  ( 22.13437500061451502, 4.541064518000418104, 2.621784821874999949 ) ) ;
#50465=CARTESIAN_POINT ( 'NONE',  ( 3.374999999999999556, 4.330127018922191873, 2.499999999999999556 ) ) ;
#50466=EDGE_CURVE ( 'NONE', #23337, #59218, #62038, .T. ) ;
#50467=CARTESIAN_POINT ( 'NONE',  ( 10.22812500061451679, 6.421520780324663323E-16, -5.243569643749999010 ) ) ;
#50468=CARTESIAN_POINT ( 'NONE',  ( 1.592000809091587073E-14, 15.05000000122903714, 26.00000000000000000 ) ) ;
#50469=CARTESIAN_POINT ( 'NONE',  ( 7.471875000614519813, -6.054752690667223547, -1.112240025338166033E-15 ) ) ;
#50470=CARTESIAN_POINT ( 'NONE',  ( 7.462500001229035007, 4.330127018922192761, -2.499999999999997780 ) ) ;
#50471=CARTESIAN_POINT ( 'NONE',  ( 7.003125000614518036, -4.541064518000417216, -2.621784821875001281 ) ) ;
#50472=CARTESIAN_POINT ( 'NONE',  ( 12.90937500061451537, -4.541064518000417216, -2.621784821875001281 ) ) ;
#50474=CARTESIAN_POINT ( 'NONE',  ( 19.01250000122903216, -4.330127018922190985, -2.500000000000001332 ) ) ;
#50475=CARTESIAN_POINT ( 'NONE',  ( 8.559375000614515727, 4.541064518000418104, -2.621784821874998173 ) ) ;
#50476=CARTESIAN_POINT ( 'NONE',  ( 9.328125000614518214, 6.421520780324663323E-16, -5.243569643749999010 ) ) ;
#50477=CARTESIAN_POINT ( 'NONE',  ( 4.978125000614518569, 4.541064518000418104, 2.621784821874999949 ) ) ;
#50479=CARTESIAN_POINT ( 'NONE',  ( 18.19687500061451502, -3.027376345333614438, 5.243569643749998122 ) ) ;
#50481=CARTESIAN_POINT ( 'NONE',  ( 27.40312500061451573, 4.541064518000418104, -2.621784821874998173 ) ) ;
#50482=CARTESIAN_POINT ( 'NONE',  ( 11.09062500061451573, -3.027376345333610441, -5.243569643749999898 ) ) ;
#50483=AXIS2_PLACEMENT_3D ( 'NONE', #5472, #12458, #67535 ) ;
#50484=CARTESIAN_POINT ( 'NONE',  ( 28.88437500061451502, 4.541064518000418104, 2.621784821874999949 ) ) ;
#50485=CARTESIAN_POINT ( 'NONE',  ( 2.121784821875001281, 12.35937500061451821, -26.32496088578401938 ) ) ;
#50486=CARTESIAN_POINT ( 'NONE',  ( 13.46250000122903323, 0.000000000000000000, 4.999999999999998224 ) ) ;
#50487=CARTESIAN_POINT ( 'NONE',  ( 27.55312500061451786, 0.000000000000000000, 5.243569643749999010 ) ) ;
#50488=CARTESIAN_POINT ( 'NONE',  ( 4.243569643749999898, 15.52812500061451750, -30.00000000000000000 ) ) ;
#50489=CARTESIAN_POINT ( 'NONE',  ( 14.21250000122903323, 4.330127018922192761, -2.499999999999997780 ) ) ;
#50490=CARTESIAN_POINT ( 'NONE',  ( 12.48750000000000249, -2.886751345948129988, 4.999999999999997335 ) ) ;
#50491=CARTESIAN_POINT ( 'NONE',  ( -1.071796769724488563, 13.79240381056766829, 34.00000000000000000 ) ) ;
#50492=CARTESIAN_POINT ( 'NONE',  ( 22.94062500061451715, 6.054752690667223547, 3.707466751127219781E-16 ) ) ;
#50493=CARTESIAN_POINT ( 'NONE',  ( 7.284375000614518036, 4.541064518000418104, 2.621784821874999949 ) ) ;
#50494=CARTESIAN_POINT ( 'NONE',  ( 8.137500001229033941, -4.330127018922194537, 2.499999999999995559 ) ) ;
#50495=CARTESIAN_POINT ( 'NONE',  ( 15.00000000122903465, -2.886751345948125991, -5.000000000000000000 ) ) ;
#50496=CARTESIAN_POINT ( 'NONE',  ( 13.60312500061451679, 0.000000000000000000, 5.243569643749999010 ) ) ;
#50497=CARTESIAN_POINT ( 'NONE',  ( 19.26562500061451644, 3.027376345333613106, -5.243569643749998122 ) ) ;
#50498=CARTESIAN_POINT ( 'NONE',  ( 25.27500000122903145, -5.773502691896255534, -1.060575238724906372E-15 ) ) ;
#50499=CARTESIAN_POINT ( 'NONE',  ( 28.05000000122903359, -2.886751345948125991, -5.000000000000000000 ) ) ;
#50500=CARTESIAN_POINT ( 'NONE',  ( 23.58749999999999858, 5.773502691896255534, 3.535250795749688894E-16 ) ) ;
#50501=CARTESIAN_POINT ( 'NONE',  ( 24.98437500061451644, -4.541064518000419881, 2.621784821874995952 ) ) ;
#50503=CARTESIAN_POINT ( 'NONE',  ( 10.83750000122903501, -4.330127018922194537, 2.499999999999995559 ) ) ;
#50504=CARTESIAN_POINT ( 'NONE',  ( 26.89687500061451431, -3.027376345333610441, -5.243569643749999898 ) ) ;
#50506=CARTESIAN_POINT ( 'NONE',  ( 13.91250000000000142, -5.773502691896255534, -1.060575238724906372E-15 ) ) ;
#50507=CARTESIAN_POINT ( 'NONE',  ( 5.371875000614516615, 3.027376345333613106, -5.243569643749998122 ) ) ;
#50508=CARTESIAN_POINT ( 'NONE',  ( 22.97812500061451857, 4.541064518000418104, 2.621784821874999949 ) ) ;
#50511=CARTESIAN_POINT ( 'NONE',  ( 10.58437500061451964, -4.541064518000419881, 2.621784821874995952 ) ) ;
#50512=LINE ( 'NONE', #46054, #72589 ) ;
#50513=CARTESIAN_POINT ( 'NONE',  ( 29.80312500061451431, 0.000000000000000000, 5.243569643749999010 ) ) ;
#50514=CARTESIAN_POINT ( 'NONE',  ( 5.746875000614517504, -3.027376345333610441, -5.243569643749999898 ) ) ;
#50515=CARTESIAN_POINT ( 'NONE',  ( 27.57187500061451857, 3.027376345333611329, 5.243569643749999010 ) ) ;
#50516=CARTESIAN_POINT ( 'NONE',  ( 4.243569643749999010, 10.16562500061459495, 27.54997392385601174 ) ) ;
#50517=CARTESIAN_POINT ( 'NONE',  ( 19.42499999999999716, 6.123233995736764310E-16, -4.999999999999998224 ) ) ;
#50519=CARTESIAN_POINT ( 'NONE',  ( 27.78749999999999787, -2.886751345948129988, 4.999999999999997335 ) ) ;
#50520=CARTESIAN_POINT ( 'NONE',  ( 29.22187500061451715, 3.027376345333613106, -5.243569643749998122 ) ) ;
#50522=CARTESIAN_POINT ( 'NONE',  ( 15.14062500061451644, -3.027376345333610441, -5.243569643749999898 ) ) ;
#50523=CARTESIAN_POINT ( 'NONE',  ( 9.328125000614518214, 6.421520780324663323E-16, -5.243569643749999010 ) ) ;
#50525=CARTESIAN_POINT ( 'NONE',  ( 3.609375000614516882, 4.541064518000418104, -2.621784821874998173 ) ) ;
#50526=CARTESIAN_POINT ( 'NONE',  ( 18.67500000122903714, 2.886751345948129099, -4.999999999999998224 ) ) ;
#50527=CARTESIAN_POINT ( 'NONE',  ( 24.14999999999999858, 0.000000000000000000, 4.999999999999998224 ) ) ;
#50529=CARTESIAN_POINT ( 'NONE',  ( 7.021875000614518747, -6.054752690667223547, -1.112240025338166033E-15 ) ) ;
#50530=CARTESIAN_POINT ( 'NONE',  ( 10.73437500061451644, 6.421520780324663323E-16, -5.243569643749999010 ) ) ;
#50531=CARTESIAN_POINT ( 'NONE',  ( 21.94687500061451857, -3.027376345333610441, -5.243569643749999898 ) ) ;
#50532=CARTESIAN_POINT ( 'NONE',  ( 1.626862140677534273E-15, 11.11250000000000071, 34.00000000000000000 ) ) ;
#50533=ORIENTED_EDGE ( 'NONE', *, *, #64551, .F. ) ;
#50534=CARTESIAN_POINT ( 'NONE',  ( 4.246875000614519280, -3.027376345333614438, 5.243569643749998122 ) ) ;
#50536=CARTESIAN_POINT ( 'NONE',  ( 6.721875000614518925, 3.027376345333613106, -5.243569643749998122 ) ) ;
#50537=CARTESIAN_POINT ( 'NONE',  ( 21.75000000000000000, 4.330127018922192761, -2.499999999999997780 ) ) ;
#50538=CARTESIAN_POINT ( 'NONE',  ( 15.44062500061451537, -3.027376345333614438, 5.243569643749998122 ) ) ;
#50540=CARTESIAN_POINT ( 'NONE',  ( -3.999999999999999112, 19.96250000000000213, 27.69059892324149885 ) ) ;
#50542=CARTESIAN_POINT ( 'NONE',  ( 8.878125000614515372, 6.421520780324663323E-16, -5.243569643749999010 ) ) ;
#50543=CARTESIAN_POINT ( 'NONE',  ( 27.30937500061451573, -4.541064518000417216, -2.621784821875001281 ) ) ;
#50545=CARTESIAN_POINT ( 'NONE',  ( 28.62187500061451573, -6.054752690667223547, -1.112240025338166033E-15 ) ) ;
#50546=CARTESIAN_POINT ( 'NONE',  ( 9.074999999999999289, 6.123233995736764310E-16, -4.999999999999998224 ) ) ;
#50547=CARTESIAN_POINT ( 'NONE',  ( -3.999999999999999556, 14.67500000122903536, 27.69059892324149530 ) ) ;
#50548=CARTESIAN_POINT ( 'NONE',  ( 9.300000001229035362, 5.773502691896255534, 3.535250795749688894E-16 ) ) ;
#50549=CARTESIAN_POINT ( 'NONE',  ( 19.02187500061451786, 3.027376345333611329, 5.243569643749999010 ) ) ;
#50550=CARTESIAN_POINT ( 'NONE',  ( 13.47187500061451537, 3.027376345333613106, -5.243569643749998122 ) ) ;
#50551=CARTESIAN_POINT ( 'NONE',  ( 9.262500001229033941, 4.330127018922192761, -2.499999999999997780 ) ) ;
#50553=CARTESIAN_POINT ( 'NONE',  ( 13.82812500061451466, 6.421520780324663323E-16, -5.243569643749999010 ) ) ;
#50554=CARTESIAN_POINT ( 'NONE',  ( 25.68750000122903288, -4.330127018922194537, 2.499999999999995559 ) ) ;
#50555=CARTESIAN_POINT ( 'NONE',  ( 15.30937500061451750, 4.541064518000418104, -2.621784821874998173 ) ) ;
#50556=CARTESIAN_POINT ( 'NONE',  ( 2.154264117376507581, 9.766972526336937577, -24.39663440989477294 ) ) ;
#50557=CARTESIAN_POINT ( 'NONE',  ( 17.24062500061451786, -3.027376345333614438, 5.243569643749998122 ) ) ;
#50559=EDGE_CURVE ( 'NONE', #53550, #33928, #33911, .T. ) ;
#50560=CARTESIAN_POINT ( 'NONE',  ( 26.63437500061451857, 4.541064518000418104, 2.621784821874999949 ) ) ;
#50561=CARTESIAN_POINT ( 'NONE',  ( -3.000416591977282496E-16, 11.14062500061451644, 25.09994784771203058 ) ) ;
#50562=CARTESIAN_POINT ( 'NONE',  ( 14.67187500061451821, -6.054752690667223547, -1.112240025338166033E-15 ) ) ;
#50563=CARTESIAN_POINT ( 'NONE',  ( 15.03750000122903252, 6.123233995736764310E-16, -4.999999999999998224 ) ) ;
#50565=CARTESIAN_POINT ( 'NONE',  ( 4.243569643749999010, 19.22187500061452070, -32.45002607614398471 ) ) ;
#50566=CARTESIAN_POINT ( 'NONE',  ( 21.42187500061451644, -6.054752690667223547, -1.112240025338166033E-15 ) ) ;
#50567=CARTESIAN_POINT ( 'NONE',  ( 21.26250000122903572, -4.330127018922190985, -2.500000000000001332 ) ) ;
#50568=CARTESIAN_POINT ( 'NONE',  ( 13.73437500061451821, -4.541064518000419881, 2.621784821874995952 ) ) ;
#50569=CARTESIAN_POINT ( 'NONE',  ( -4.243569643749999898, 11.75937500061451857, 30.00000000000000000 ) ) ;
#50570=CARTESIAN_POINT ( 'NONE',  ( 21.90000000122903145, 5.773502691896255534, 3.535250795749688894E-16 ) ) ;
#50571=CARTESIAN_POINT ( 'NONE',  ( 16.34062500061451573, -3.027376345333614438, 5.243569643749998122 ) ) ;
#50574=CARTESIAN_POINT ( 'NONE',  ( 21.22500000000000142, 6.123233995736764310E-16, -4.999999999999998224 ) ) ;
#50576=CARTESIAN_POINT ( 'NONE',  ( 25.34062500061451217, -3.027376345333614438, 5.243569643749998122 ) ) ;
#50577=CARTESIAN_POINT ( 'NONE',  ( 2.679675080847534030, 4.226630133448147753, 32.98013821123856104 ) ) ;
#50578=CARTESIAN_POINT ( 'NONE',  ( 17.92500000122903359, 2.886751345948126879, 4.999999999999999112 ) ) ;
#50579=CARTESIAN_POINT ( 'NONE',  ( 23.42812500061451786, 4.541064518000418104, 2.621784821874999949 ) ) ;
#50580=CARTESIAN_POINT ( 'NONE',  ( 24.51562500061451289, -6.054752690667223547, -1.112240025338166033E-15 ) ) ;
#50581=CARTESIAN_POINT ( 'NONE',  ( 5.840625000614516615, 6.054752690667223547, 3.707466751127219781E-16 ) ) ;
#50582=EDGE_LOOP ( 'NONE', ( #49133, #1276, #644, #34246 ) ) ;
#50583=CARTESIAN_POINT ( 'NONE',  ( 29.13749999999999929, -2.886751345948129988, 4.999999999999997335 ) ) ;
#50584=CARTESIAN_POINT ( 'NONE',  ( 2.878125000614517592, -4.541064518000419881, 2.621784821874995952 ) ) ;
#50586=DIRECTION ( 'NONE',  ( 0.000000000000000000, 0.000000000000000000, -1.000000000000000000 ) ) ;
#50587=CARTESIAN_POINT ( 'NONE',  ( -3.999999999999997335, 11.15000000122903323, -27.69059892324149175 ) ) ;
#50588=CARTESIAN_POINT ( 'NONE',  ( -4.243569643749999898, 18.05937500061451928, -30.00000000000000000 ) ) ;
#50589=( BOUNDED_CURVE ( )  B_SPLINE_CURVE ( 2, ( #15979, #5641, #107, #45164, #67695, #5995, #28525, #35152, #46242 ),
 .UNSPECIFIED., .F., .F. ) 
 B_SPLINE_CURVE_WITH_KNOTS ( ( 3, 2, 2, 2, 3 ),
 ( 0.7065217391304348116, 0.7101449275362319291, 0.7173913043478260532, 0.7246376811594202882, 0.7282608695652174058 ),
 .UNSPECIFIED. ) 
 CURVE ( )  GEOMETRIC_REPRESENTATION_ITEM ( )  RATIONAL_B_SPLINE_CURVE ( ( 0.9330127018922194093, 0.9330127018922194093, 1.000000000000000000, 0.8660254037844387076, 1.000000000000000000, 0.8660254037844387076, 1.000000000000000000, 0.9330127018922194093, 0.9330127018922194093 ) ) 
 REPRESENTATION_ITEM ( '' )  );
#50590=EDGE_CURVE ( 'NONE', #40294, #10190, #23649, .T. ) ;
#50591=CARTESIAN_POINT ( 'NONE',  ( 7.500000000000000000, 0.000000000000000000, 4.999999999999998224 ) ) ;
#50592=CARTESIAN_POINT ( 'NONE',  ( 4.800000001229032698, 5.773502691896255534, 3.535250795749688894E-16 ) ) ;
#50593=CARTESIAN_POINT ( 'NONE',  ( 11.55937500061451928, -4.541064518000417216, -2.621784821875001281 ) ) ;
#50594=CARTESIAN_POINT ( 'NONE',  ( 23.77500000122902790, 2.886751345948161074, 4.999999999999941380 ) ) ;
#50595=CARTESIAN_POINT ( 'NONE',  ( 3.796875000614517326, -3.027376345333614438, 5.243569643749998122 ) ) ;
#50596=CARTESIAN_POINT ( 'NONE',  ( 29.58750000122903501, 4.330127018922191873, 2.499999999999999556 ) ) ;
#50597=CARTESIAN_POINT ( 'NONE',  ( 10.73437500061451644, 6.421520780324663323E-16, -5.243569643749999010 ) ) ;
#50599=CARTESIAN_POINT ( 'NONE',  ( 19.34062500061451573, 6.054752690667223547, 3.707466751127219781E-16 ) ) ;
#50600=CARTESIAN_POINT ( 'NONE',  ( -2.121784821874996840, 17.62812500061459176, 33.67503911421598417 ) ) ;
#50601=CARTESIAN_POINT ( 'NONE',  ( 22.47187500061451715, 3.027376345333613106, -5.243569643749998122 ) ) ;
#50604=CARTESIAN_POINT ( 'NONE',  ( 28.35000000122903430, -2.886751345948129988, 4.999999999999997335 ) ) ;
#50606=CARTESIAN_POINT ( 'NONE',  ( 25.30312500061451431, 0.000000000000000000, 5.243569643749999010 ) ) ;
#50607=CARTESIAN_POINT ( 'NONE',  ( 14.76562500061451821, 3.027376345333613106, -5.243569643749998122 ) ) ;
#50609=CARTESIAN_POINT ( 'NONE',  ( 12.30937500061451573, 0.000000000000000000, 5.243569643749999010 ) ) ;
#50610=CARTESIAN_POINT ( 'NONE',  ( 28.16249999999999787, 2.886751345948126879, 4.999999999999999112 ) ) ;
#50611=CARTESIAN_POINT ( 'NONE',  ( 26.06250000122903288, 0.000000000000000000, 4.999999999999998224 ) ) ;
#50612=CYLINDRICAL_SURFACE ( 'NONE', #8392, 4.000000000000000000 ) ;
#50613=CARTESIAN_POINT ( 'NONE',  ( 14.52187500061451608, 3.027376345333611329, 5.243569643749999010 ) ) ;
#50614=CARTESIAN_POINT ( 'NONE',  ( 28.73437500061451644, 6.421520780324663323E-16, -5.243569643749999010 ) ) ;
#50615=DIRECTION ( 'NONE',  ( -1.000000000000000000, -0.000000000000000000, -0.000000000000000000 ) ) ;
#50617=CARTESIAN_POINT ( 'NONE',  ( 24.30937500061451573, 4.541064518000418104, -2.621784821874998173 ) ) ;
#50618=CARTESIAN_POINT ( 'NONE',  ( 15.00937500061451679, 0.000000000000000000, 5.243569643749999010 ) ) ;
#50620=CARTESIAN_POINT ( 'NONE',  ( 28.27499999999999858, -4.330127018922194537, 2.499999999999995559 ) ) ;
#50621=CARTESIAN_POINT ( 'NONE',  ( 3.375000001229033320, 2.886751345948129099, -4.999999999999998224 ) ) ;
#50623=CARTESIAN_POINT ( 'NONE',  ( 18.36562500061451431, 3.027376345333613106, -5.243569643749998122 ) ) ;
#50624=CARTESIAN_POINT ( 'NONE',  ( 8.362500000000002487, 2.886751345948126879, 4.999999999999999112 ) ) ;
#50625=CARTESIAN_POINT ( 'NONE',  ( 0.000000000000000000, 20.00000000000000000, -30.00000000000000000 ) ) ;
#50626=CARTESIAN_POINT ( 'NONE',  ( 16.12500000000000000, -4.330127018922194537, 2.499999999999995559 ) ) ;
#50627=CARTESIAN_POINT ( 'NONE',  ( 4.243569643749999898, 13.72812500061451679, 30.00000000000000000 ) ) ;
#50628=B_SPLINE_CURVE_WITH_KNOTS ( 'NONE', 3,
 ( #56118, #39864, #5510, #23207, #68296, #57186, #50936, #28048, #17656, #23574, #50577, #40216, #332, #29129, #22842, #73104, #46119, #63096, #12497, #45036, #67571, #16936, #39491, #45394, #67930, #62376, #70467, #25023, #2865, #70095, #69736, #64182, #69019, #40949, #30211, #31304, #46481, #8403 ),
 .UNSPECIFIED., .F., .F.,
 ( 4, 2, 2, 2, 2, 2, 2, 2, 2, 2, 2, 2, 2, 2, 2, 2, 2, 2, 4 ),
 ( 0.01305910913008846361, 0.01347211191627388852, 0.01388511470245931169, 0.01471112027483015630, 0.01553712584720099918, 0.01636313141957184206, 0.01801514256431353128, 0.01884114813668436722, 0.01925415092286978519, 0.01966715370905520316, 0.02008015649524062113, 0.02049315928142603910, 0.02131916485379688891, 0.02214517042616773179, 0.02297117599853857467, 0.02379718157090942449, 0.02462318714328026736, 0.02544919271565111371, 0.02627519828802195659 ),
 .UNSPECIFIED. ) ;
#50629=CARTESIAN_POINT ( 'NONE',  ( 20.92500000122903714, 2.886751345948129099, -4.999999999999998224 ) ) ;
#50630=CARTESIAN_POINT ( 'NONE',  ( 5.789369777004291784, 8.154036291478783838, 31.58818119731339635 ) ) ;
#50631=( BOUNDED_CURVE ( )  B_SPLINE_CURVE ( 2, ( #5875, #28408, #43591, #66113, #38404, #15492, #55036 ),
 .UNSPECIFIED., .F., .F. ) 
 B_SPLINE_CURVE_WITH_KNOTS ( ( 3, 2, 2, 3 ),
 ( 0.6833333333333333481, 0.6861111111111111160, 0.6888888888888888840, 0.6916666666666666519 ),
 .UNSPECIFIED. ) 
 CURVE ( )  GEOMETRIC_REPRESENTATION_ITEM ( )  RATIONAL_B_SPLINE_CURVE ( ( 1.000000000000000000, 0.8660254037844387076, 1.000000000000000000, 0.8660254037844387076, 1.000000000000000000, 0.8660254037844387076, 1.000000000000000000 ) ) 
 REPRESENTATION_ITEM ( '' )  );
#50632=CARTESIAN_POINT ( 'NONE',  ( 27.57187500061451857, 3.027376345333611329, 5.243569643749999010 ) ) ;
#50633=ORIENTED_EDGE ( 'NONE', *, *, #16791, .T. ) ;
#50634=CARTESIAN_POINT ( 'NONE',  ( 14.99062500061451786, -3.027376345333614438, 5.243569643749998122 ) ) ;
#50635=CARTESIAN_POINT ( 'NONE',  ( 22.67812500061451431, -4.541064518000419881, 2.621784821874995952 ) ) ;
#50636=CARTESIAN_POINT ( 'NONE',  ( 21.83437500061451786, -4.541064518000419881, 2.621784821874995952 ) ) ;
#50637=CARTESIAN_POINT ( 'NONE',  ( 6.712500000000000355, -5.773502691896255534, -1.060575238724906372E-15 ) ) ;
#50638=CARTESIAN_POINT ( 'NONE',  ( 9.853125000614516793, 4.541064518000418104, -2.621784821874998173 ) ) ;
#50639=CARTESIAN_POINT ( 'NONE',  ( 24.25312500061451715, 4.541064518000418104, -2.621784821874998173 ) ) ;
#50640=CARTESIAN_POINT ( 'NONE',  ( 14.14687500061451786, -3.027376345333614438, 5.243569643749998122 ) ) ;
#50641=CARTESIAN_POINT ( 'NONE',  ( 18.15937500061451715, 0.000000000000000000, 5.243569643749999010 ) ) ;
#50642=CARTESIAN_POINT ( 'NONE',  ( 15.48750000122903359, 6.123233995736764310E-16, -4.999999999999998224 ) ) ;
#50643=CARTESIAN_POINT ( 'NONE',  ( 9.001249775931846008E-16, 18.56562500061451715, 34.90005215228797653 ) ) ;
#50644=CARTESIAN_POINT ( 'NONE',  ( 21.93750000122903288, 4.330127018922191873, 2.499999999999999556 ) ) ;
#50646=CARTESIAN_POINT ( 'NONE',  ( 12.81562500061451537, -6.054752690667223547, -1.112240025338166033E-15 ) ) ;
#50647=CARTESIAN_POINT ( 'NONE',  ( 6.609375000614519102, -4.541064518000417216, -2.621784821875001281 ) ) ;
#50648=CARTESIAN_POINT ( 'NONE',  ( 5.634375000614519458, -4.541064518000419881, 2.621784821874995952 ) ) ;
#50650=CARTESIAN_POINT ( 'NONE',  ( 26.93437500061451573, 6.421520780324663323E-16, -5.243569643749999010 ) ) ;
#50651=CARTESIAN_POINT ( 'NONE',  ( 19.45312500061451644, 0.000000000000000000, 5.243569643749999010 ) ) ;
#50652=CARTESIAN_POINT ( 'NONE',  ( 27.48750000122903359, -4.330127018922194537, 2.499999999999995559 ) ) ;
#50653=CARTESIAN_POINT ( 'NONE',  ( 28.19062500061451715, -3.027376345333610441, -5.243569643749999898 ) ) ;
#50654=CARTESIAN_POINT ( 'NONE',  ( 25.43437500061451573, -4.541064518000419881, 2.621784821874995952 ) ) ;
#50655=CARTESIAN_POINT ( 'NONE',  ( 17.42812500061451786, 6.421520780324663323E-16, -5.243569643749999010 ) ) ;
#50656=CARTESIAN_POINT ( 'NONE',  ( -3.999999999999999556, 10.06250000000000178, 27.69059892324149530 ) ) ;
#50657=CARTESIAN_POINT ( 'NONE',  ( 25.56562500061452070, 3.027376345333613106, -5.243569643749998122 ) ) ;
#50658=CARTESIAN_POINT ( 'NONE',  ( 4.837500001229035895, 4.330127018922191873, 2.499999999999999556 ) ) ;
#50660=CARTESIAN_POINT ( 'NONE',  ( 28.80000000000000071, -4.330127018922190985, -2.500000000000001332 ) ) ;
#50661=CARTESIAN_POINT ( 'NONE',  ( -2.828200636599751609E-16, 14.48750000000000071, -34.61880215351700230 ) ) ;
#50663=CARTESIAN_POINT ( 'NONE',  ( 4.546875000614517326, 6.054752690667223547, 3.707466751127219781E-16 ) ) ;
#50664=CARTESIAN_POINT ( 'NONE',  ( 10.11562500061451608, -6.054752690667223547, -1.112240025338166033E-15 ) ) ;
#50665=CARTESIAN_POINT ( 'NONE',  ( 5.971875000614516260, 3.027376345333611329, 5.243569643749999010 ) ) ;
#50666=CARTESIAN_POINT ( 'NONE',  ( 25.05000000122903714, 5.773502691896255534, 3.535250795749688894E-16 ) ) ;
#50667=CARTESIAN_POINT ( 'NONE',  ( 14.44687500061451679, 6.054752690667223547, 3.707466751127219781E-16 ) ) ;
#50668=CARTESIAN_POINT ( 'NONE',  ( 28.90312500061451217, 0.000000000000000000, 5.243569643749999010 ) ) ;
#50669=CARTESIAN_POINT ( 'NONE',  ( 28.08749999999999858, 5.773502691896255534, 3.535250795749688894E-16 ) ) ;
#50670=CARTESIAN_POINT ( 'NONE',  ( 26.70937500061451431, 0.000000000000000000, 5.243569643749999010 ) ) ;
#50671=CARTESIAN_POINT ( 'NONE',  ( 3.515625000614516882, 3.027376345333613106, -5.243569643749998122 ) ) ;
#50672=CARTESIAN_POINT ( 'NONE',  ( 12.96562500061451750, 3.027376345333613106, -5.243569643749998122 ) ) ;
#50674=CARTESIAN_POINT ( 'NONE',  ( 9.628125000614517148, -4.541064518000419881, 2.621784821874995952 ) ) ;
#50675=CARTESIAN_POINT ( 'NONE',  ( 5.240625000614516971, -3.027376345333610441, -5.243569643749999898 ) ) ;
#50677=CARTESIAN_POINT ( 'NONE',  ( 13.91250000122903252, 0.000000000000000000, 4.999999999999998224 ) ) ;
#50678=CARTESIAN_POINT ( 'NONE',  ( 14.73749999999999893, -2.886751345948129988, 4.999999999999997335 ) ) ;
#50680=CARTESIAN_POINT ( 'NONE',  ( 16.95937500061451786, -4.541064518000417216, -2.621784821875001281 ) ) ;
#50681=CARTESIAN_POINT ( 'NONE',  ( 10.42500000122903536, -5.773502691896255534, -1.060575238724906372E-15 ) ) ;
#50683=CARTESIAN_POINT ( 'NONE',  ( 20.59687500061451360, -3.027376345333610441, -5.243569643749999898 ) ) ;
#50684=CARTESIAN_POINT ( 'NONE',  ( 4.243569643749999898, 13.72812500061451679, -30.00000000000000000 ) ) ;
#50687=CARTESIAN_POINT ( 'NONE',  ( 20.62499999999999645, -4.330127018922194537, 2.499999999999995559 ) ) ;
#50688=CARTESIAN_POINT ( 'NONE',  ( 25.67812500061451431, 4.541064518000418104, 2.621784821874999949 ) ) ;
#50689=CARTESIAN_POINT ( 'NONE',  ( 5.362500001229033586, 0.000000000000000000, 4.999999999999998224 ) ) ;
#50690=CARTESIAN_POINT ( 'NONE',  ( 29.85937500061451644, 0.000000000000000000, 5.243569643749999010 ) ) ;
#50691=CARTESIAN_POINT ( 'NONE',  ( 23.32499999999999929, -4.330127018922194537, 2.499999999999995559 ) ) ;
#50692=CARTESIAN_POINT ( 'NONE',  ( 9.740625000614516082, -3.027376345333610441, -5.243569643749999898 ) ) ;
#50694=CARTESIAN_POINT ( 'NONE',  ( 20.07187500061451857, -6.054752690667223547, -1.112240025338166033E-15 ) ) ;
#50696=CARTESIAN_POINT ( 'NONE',  ( 4.190625000614518925, -3.027376345333614438, 5.243569643749998122 ) ) ;
#50697=CARTESIAN_POINT ( 'NONE',  ( 11.67187500061451821, 3.027376345333613106, -5.243569643749998122 ) ) ;
#50699=CARTESIAN_POINT ( 'NONE',  ( 21.53437500061451715, 6.421520780324663323E-16, -5.243569643749999010 ) ) ;
#50700=CARTESIAN_POINT ( 'NONE',  ( 0.000000000000000000, 20.00000000000000000, 26.00000000000000000 ) ) ;
#50701=CARTESIAN_POINT ( 'NONE',  ( 28.57499999999999929, 4.330127018922191873, 2.499999999999999556 ) ) ;
#50702=CARTESIAN_POINT ( 'NONE',  ( 5.812500000000001776, -5.773502691896255534, -1.060575238724906372E-15 ) ) ;
#50703=CARTESIAN_POINT ( 'NONE',  ( 14.92500000122903181, -5.773502691896255534, -1.060575238724906372E-15 ) ) ;
#50704=CARTESIAN_POINT ( 'NONE',  ( 3.999999999999999112, 15.27500000000000036, -30.00000000000000000 ) ) ;
#50705=DIRECTION ( 'NONE',  ( -1.000000000000000000, -0.000000000000000000, -0.000000000000000000 ) ) ;
#50707=CARTESIAN_POINT ( 'NONE',  ( 12.37500000000000000, 4.330127018922191873, 2.499999999999999556 ) ) ;
#50708=CARTESIAN_POINT ( 'NONE',  ( 26.54062500061451146, 6.054752690667223547, 3.707466751127219781E-16 ) ) ;
#50709=CARTESIAN_POINT ( 'NONE',  ( 16.50000000000000000, 0.000000000000000000, 4.999999999999998224 ) ) ;
#50710=CARTESIAN_POINT ( 'NONE',  ( 10.23750000122903359, 4.330127018922191873, 2.499999999999999556 ) ) ;
#50711=CARTESIAN_POINT ( 'NONE',  ( 8.690625000614515372, -3.027376345333614438, 5.243569643749998122 ) ) ;
#50712=B_SPLINE_CURVE_WITH_KNOTS ( 'NONE', 3,
 ( #1271, #914, #12699, #69944, #45969, #28977, #51515, #23778, #58477, #68865 ),
 .UNSPECIFIED., .F., .F.,
 ( 4, 3, 3, 4 ),
 ( 1.663831787158942381E-16, 2.812505563865755982E-05, 5.721718141143529657E-05, 8.630979428994332348E-05 ),
 .UNSPECIFIED. ) ;
#50713=CARTESIAN_POINT ( 'NONE',  ( 9.600000000000001421, 4.330127018922192761, -2.499999999999997780 ) ) ;
#50715=CARTESIAN_POINT ( 'NONE',  ( 4.243569643749999010, 14.72187500061451715, -32.45002607614398471 ) ) ;
#50716=CARTESIAN_POINT ( 'NONE',  ( 27.78750000122903074, 4.330127018922191873, 2.499999999999999556 ) ) ;
#50718=CARTESIAN_POINT ( 'NONE',  ( 7.350000000000002309, 4.330127018922192761, -2.499999999999997780 ) ) ;
#50719=LINE ( 'NONE', #28543, #50367 ) ;
#50721=CARTESIAN_POINT ( 'NONE',  ( 24.36562500061451786, 3.027376345333611329, 5.243569643749999010 ) ) ;
#50722=CARTESIAN_POINT ( 'NONE',  ( 14.58750000122903323, 6.123233995736764310E-16, -4.999999999999998224 ) ) ;
#50723=CARTESIAN_POINT ( 'NONE',  ( 3.381234057738627730, -3.683476499272080318, -3.635624298366154861 ) ) ;
#50724=CARTESIAN_POINT ( 'NONE',  ( 28.65937500061451715, -4.541064518000417216, -2.621784821875001281 ) ) ;
#50725=CARTESIAN_POINT ( 'NONE',  ( 19.99687500061451573, -3.027376345333614438, 5.243569643749998122 ) ) ;
#50726=CARTESIAN_POINT ( 'NONE',  ( 17.12812500061451715, 4.541064518000418104, 2.621784821874999949 ) ) ;
#50727=CARTESIAN_POINT ( 'NONE',  ( -3.000416591977282496E-16, 12.49062500061459424, -34.90005215228797653 ) ) ;
#50728=CARTESIAN_POINT ( 'NONE',  ( 7.078125000614516438, 6.421520780324663323E-16, -5.243569643749999010 ) ) ;
#50729=CARTESIAN_POINT ( 'NONE',  ( 28.23750000122903359, 4.330127018922191873, 2.499999999999999556 ) ) ;
#50731=CARTESIAN_POINT ( 'NONE',  ( 19.82812500061451644, 4.541064518000418104, 2.621784821874999949 ) ) ;
#50732=CYLINDRICAL_SURFACE ( 'NONE', #24443, 4.000000000000000000 ) ;
#50734=CARTESIAN_POINT ( 'NONE',  ( 13.62187500061451750, 3.027376345333611329, 5.243569643749999010 ) ) ;
#50735=CARTESIAN_POINT ( 'NONE',  ( 11.78437500061451892, 4.541064518000418104, 2.621784821874999949 ) ) ;
#50736=CARTESIAN_POINT ( 'NONE',  ( 21.30937500061451573, 0.000000000000000000, 5.243569643749999010 ) ) ;
#50738=CARTESIAN_POINT ( 'NONE',  ( -1.487416814333745711E-14, 14.82500000122903572, -26.00000000000000000 ) ) ;
#50739=CARTESIAN_POINT ( 'NONE',  ( 25.49062500061451786, -3.027376345333610441, -5.243569643749999898 ) ) ;
#50740=CARTESIAN_POINT ( 'NONE',  ( 26.91562500061451146, 3.027376345333613106, -5.243569643749998122 ) ) ;
#50742=CARTESIAN_POINT ( 'NONE',  ( 1.999999999999998668, 17.60000000000000142, 26.53589838486224650 ) ) ;
#50743=CARTESIAN_POINT ( 'NONE',  ( 4.659375000614518925, 0.000000000000000000, 5.243569643749999010 ) ) ;
#50744=CARTESIAN_POINT ( 'NONE',  ( 11.66250000122903430, 0.000000000000000000, 4.999999999999998224 ) ) ;
#50745=CARTESIAN_POINT ( 'NONE',  ( 7.050000001229036251, 5.773502691896255534, 3.535250795749688894E-16 ) ) ;
#50746=CARTESIAN_POINT ( 'NONE',  ( 2.803125000614518747, 0.000000000000000000, 5.243569643749999010 ) ) ;
#50749=CARTESIAN_POINT ( 'NONE',  ( 11.44687500061451857, -3.027376345333614438, 5.243569643749998122 ) ) ;
#50751=CARTESIAN_POINT ( 'NONE',  ( 19.79062500061451502, 6.054752690667223547, 3.707466751127219781E-16 ) ) ;
#50752=CARTESIAN_POINT ( 'NONE',  ( 12.60937500061451821, 4.541064518000418104, -2.621784821874998173 ) ) ;
#50753=CARTESIAN_POINT ( 'NONE',  ( 6.065625000614516260, -6.054752690667223547, -1.112240025338166033E-15 ) ) ;
#50754=CARTESIAN_POINT ( 'NONE',  ( 22.65937500061451715, 0.000000000000000000, 5.243569643749999010 ) ) ;
#50755=CARTESIAN_POINT ( 'NONE',  ( 9.759375000614516793, -4.541064518000417216, -2.621784821875001281 ) ) ;
#50756=CARTESIAN_POINT ( 'NONE',  ( 4.753125000614515372, -4.541064518000417216, -2.621784821875001281 ) ) ;
#50757=CARTESIAN_POINT ( 'NONE',  ( 5.887500000000000178, -2.886751345948126435, -5.000000000000000000 ) ) ;
#50758=CARTESIAN_POINT ( 'NONE',  ( 5.925000001229033586, -5.773502691896255534, -1.060575238724906372E-15 ) ) ;
#50759=CARTESIAN_POINT ( 'NONE',  ( 20.01562500061451644, -6.054752690667223547, -1.112240025338166033E-15 ) ) ;
#50760=CARTESIAN_POINT ( 'NONE',  ( 6.975000001229032520, 2.886751345948129099, -4.999999999999998224 ) ) ;
#50761=CARTESIAN_POINT ( 'NONE',  ( 18.14062500061451644, -3.027376345333614438, 5.243569643749998122 ) ) ;
#50762=CARTESIAN_POINT ( 'NONE',  ( 14.20312500061451644, -4.541064518000417216, -2.621784821875001281 ) ) ;
#50764=CARTESIAN_POINT ( 'NONE',  ( 13.12500000000000178, 6.123233995736764310E-16, -4.999999999999998224 ) ) ;
#50765=CARTESIAN_POINT ( 'NONE',  ( 9.637500001229033941, 6.123233995736764310E-16, -4.999999999999998224 ) ) ;
#50766=CARTESIAN_POINT ( 'NONE',  ( 4.828125000614518214, 6.421520780324663323E-16, -5.243569643749999010 ) ) ;
#50767=( BOUNDED_CURVE ( )  B_SPLINE_CURVE ( 2, ( #3257, #59750, #71210, #49057, #21325, #71585, #70485 ),
 .UNSPECIFIED., .F., .F. ) 
 B_SPLINE_CURVE_WITH_KNOTS ( ( 3, 2, 2, 3 ),
 ( 0.6666666666666666297, 0.6694444444444443976, 0.6722222222222222765, 0.6750000000000000444 ),
 .UNSPECIFIED. ) 
 CURVE ( )  GEOMETRIC_REPRESENTATION_ITEM ( )  RATIONAL_B_SPLINE_CURVE ( ( 1.000000000000000000, 0.8660254037844387076, 1.000000000000000000, 0.8660254037844387076, 1.000000000000000000, 0.8660254037844387076, 1.000000000000000000 ) ) 
 REPRESENTATION_ITEM ( '' )  );
#50769=CARTESIAN_POINT ( 'NONE',  ( 21.71250000122903501, -4.330127018922190985, -2.500000000000001332 ) ) ;
#50771=CARTESIAN_POINT ( 'NONE',  ( -2.121784821874999949, 11.68437500061451750, -33.67503911421598417 ) ) ;
#50772=CYLINDRICAL_SURFACE ( 'NONE', #59527, 4.000000000000000000 ) ;
#50773=CARTESIAN_POINT ( 'NONE',  ( 2.812500001229033320, -4.330127018922190985, -2.500000000000001332 ) ) ;
#50775=CARTESIAN_POINT ( 'NONE',  ( 21.42187500061451644, -6.054752690667223547, -1.112240025338166033E-15 ) ) ;
#50776=CARTESIAN_POINT ( 'NONE',  ( -5.810221930991193690E-16, 14.15000000122903145, -34.00000000000000000 ) ) ;
#50777=CARTESIAN_POINT ( 'NONE',  ( 16.45312500061451289, -4.541064518000417216, -2.621784821875001281 ) ) ;
#50780=CARTESIAN_POINT ( 'NONE',  ( -1.071796769724488563, 15.59240381056766722, 34.00000000000000000 ) ) ;
#50781=CARTESIAN_POINT ( 'NONE',  ( 28.99687500061451573, -3.027376345333614438, 5.243569643749998122 ) ) ;
#50783=CARTESIAN_POINT ( 'NONE',  ( 11.57812500061451644, 6.421520780324663323E-16, -5.243569643749999010 ) ) ;
#50784=CARTESIAN_POINT ( 'NONE',  ( 10.92187500061451644, 3.027376345333611329, 5.243569643749999010 ) ) ;
#50785=ORIENTED_EDGE ( 'NONE', *, *, #68132, .T. ) ;
#50786=CARTESIAN_POINT ( 'NONE',  ( 29.42812500061451431, -4.541064518000419881, 2.621784821874995952 ) ) ;
#50787=CARTESIAN_POINT ( 'NONE',  ( 23.01562500061451644, 3.027376345333611329, 5.243569643749999010 ) ) ;
#50789=CARTESIAN_POINT ( 'NONE',  ( 3.242103837493086330E-14, 11.33750000000000213, 26.00000000000000711 ) ) ;
#50790=CARTESIAN_POINT ( 'NONE',  ( 12.97499999999999964, -4.330127018922194537, 2.499999999999995559 ) ) ;
#50791=CARTESIAN_POINT ( 'NONE',  ( 21.82500000122903572, 2.886751345948129099, -4.999999999999998224 ) ) ;
#50792=CARTESIAN_POINT ( 'NONE',  ( 15.74062500061451608, 6.054752690667223547, 3.707466751127219781E-16 ) ) ;
#50794=VERTEX_POINT ( 'NONE', #36315 ) ;
#50795=CARTESIAN_POINT ( 'NONE',  ( 19.76250000000000639, -5.773502691896255534, -1.060575238724906372E-15 ) ) ;
#50796=CARTESIAN_POINT ( 'NONE',  ( 24.86250000000000071, 2.886751345948129099, -4.999999999999998224 ) ) ;
#50797=CARTESIAN_POINT ( 'NONE',  ( 21.98437500061451644, 6.421520780324663323E-16, -5.243569643749999010 ) ) ;
#50798=CARTESIAN_POINT ( 'NONE',  ( 26.27812500061451573, -4.541064518000419881, 2.621784821874995952 ) ) ;
#50801=CARTESIAN_POINT ( 'NONE',  ( 9.440625000614517148, 6.054752690667223547, 3.707466751127219781E-16 ) ) ;
#50802=DIRECTION ( 'NONE',  ( -0.000000000000000000, -1.000000000000000000, -0.000000000000000000 ) ) ;
#50803=CARTESIAN_POINT ( 'NONE',  ( 14.77500000000000036, -4.330127018922194537, 2.499999999999995559 ) ) ;
#50804=CARTESIAN_POINT ( 'NONE',  ( -2.121784821874996840, 18.52812500061451928, 33.67503911421598417 ) ) ;
#50805=CARTESIAN_POINT ( 'NONE',  ( 4.359375000614517326, -4.541064518000417216, -2.621784821875001281 ) ) ;
#50806=B_SPLINE_CURVE_WITH_KNOTS ( 'NONE', 3,
 ( #6606, #6236, #67936, #1073, #18027, #13216, #63823, #705, #40584, #63104 ),
 .UNSPECIFIED., .F., .F.,
 ( 4, 3, 3, 4 ),
 ( 0.000000000000000000, 5.625111044264893015E-05, 0.0001079408190112657892, 0.0001596376222420049817 ),
 .UNSPECIFIED. ) ;
#50807=CARTESIAN_POINT ( 'NONE',  ( 25.02187500061451431, -6.054752690667223547, -1.112240025338166033E-15 ) ) ;
#50809=CARTESIAN_POINT ( 'NONE',  ( 24.55312500061451786, -4.541064518000417216, -2.621784821875001281 ) ) ;
#50810=CARTESIAN_POINT ( 'NONE',  ( 25.69687500061451502, 6.054752690667223547, 3.707466751127219781E-16 ) ) ;
#50811=CARTESIAN_POINT ( 'NONE',  ( -3.000416591977282496E-16, 17.89062500061459104, -34.90005215228797653 ) ) ;
#50812=CARTESIAN_POINT ( 'NONE',  ( 10.61250000000000071, 2.886751345948126879, 4.999999999999999112 ) ) ;
#50813=CARTESIAN_POINT ( 'NONE',  ( 9.890625000614516438, 6.054752690667223547, 3.707466751127219781E-16 ) ) ;
#50814=DIRECTION ( 'NONE',  ( -1.000000000000000000, -0.000000000000000000, -0.000000000000000000 ) ) ;
#50816=CARTESIAN_POINT ( 'NONE',  ( 26.12812500061451360, 4.541064518000418104, 2.621784821874999949 ) ) ;
#50818=CARTESIAN_POINT ( 'NONE',  ( 3.928125000614516527, 6.421520780324663323E-16, -5.243569643749999010 ) ) ;
#50819=CARTESIAN_POINT ( 'NONE',  ( 20.55937500061451573, -4.541064518000417216, -2.621784821875001281 ) ) ;
#50820=CARTESIAN_POINT ( 'NONE',  ( 4.243569643749999898, 15.54687500061451644, 32.45002607614398471 ) ) ;
#50821=CARTESIAN_POINT ( 'NONE',  ( 20.82187500061451857, 3.027376345333611329, 5.243569643749999010 ) ) ;
#50822=CARTESIAN_POINT ( 'NONE',  ( 3.300000000000000711, 4.330127018922192761, -2.499999999999997780 ) ) ;
#50823=CARTESIAN_POINT ( 'NONE',  ( -2.121784821874999949, 19.33437500061451786, 26.32496088578401938 ) ) ;
#50824=CARTESIAN_POINT ( 'NONE',  ( 10.52812500061451750, -4.541064518000419881, 2.621784821874995952 ) ) ;
#50827=ADVANCED_FACE ( 'NONE', ( #58830 ), #25963, .F. ) ;
#50828=CARTESIAN_POINT ( 'NONE',  ( 7.996875000614519280, -3.027376345333610441, -5.243569643749999898 ) ) ;
#50829=CARTESIAN_POINT ( 'NONE',  ( -3.999999999999999112, 16.02500000122903501, -32.30940107675850470 ) ) ;
#50830=ADVANCED_FACE ( 'NONE', ( #2336 ), #65852, .F. ) ;
#50831=CARTESIAN_POINT ( 'NONE',  ( 8.015625000614518214, 3.027376345333613106, -5.243569643749998122 ) ) ;
#50832=CARTESIAN_POINT ( 'NONE',  ( 11.37187500061451750, 3.027376345333611329, 5.243569643749999010 ) ) ;
#50833=CARTESIAN_POINT ( 'NONE',  ( 18.11250000122903359, -4.330127018922190985, -2.500000000000001332 ) ) ;
#50834=CARTESIAN_POINT ( 'NONE',  ( 8.671875000614518214, 3.027376345333611329, 5.243569643749999010 ) ) ;
#50835=CARTESIAN_POINT ( 'NONE',  ( 10.45312500061451644, 0.000000000000000000, 5.243569643749999010 ) ) ;
#50836=CARTESIAN_POINT ( 'NONE',  ( 5.915625000614515905, 3.027376345333611329, 5.243569643749999010 ) ) ;
#50838=CARTESIAN_POINT ( 'NONE',  ( 20.03437500061451715, -4.541064518000419881, 2.621784821874995952 ) ) ;
#50839=CARTESIAN_POINT ( 'NONE',  ( 4.555452590171750415, 2.061616698417762628, 4.786020548300175648 ) ) ;
#50840=CARTESIAN_POINT ( 'NONE',  ( 26.46562500061451573, 3.027376345333613106, -5.243569643749998122 ) ) ;
#50841=CARTESIAN_POINT ( 'NONE',  ( 12.47812500061451502, 6.421520780324663323E-16, -5.243569643749999010 ) ) ;
#50842=CARTESIAN_POINT ( 'NONE',  ( 29.07187500061451502, -6.054752690667223547, -1.112240025338166033E-15 ) ) ;
#50843=CARTESIAN_POINT ( 'NONE',  ( -4.243569643749999898, 9.959375000614517859, -30.00000000000000000 ) ) ;
#50844=EDGE_CURVE ( 'NONE', #38197, #29431, #25591, .T. ) ;
#50845=CARTESIAN_POINT ( 'NONE',  ( 12.75000000122903643, -2.886751345948125991, -5.000000000000000000 ) ) ;
#50846=CARTESIAN_POINT ( 'NONE',  ( 27.32812500061451644, 6.421520780324663323E-16, -5.243569643749999010 ) ) ;
#50847=CARTESIAN_POINT ( 'NONE',  ( -2.121784821874999949, 14.77812500061451750, -33.67503911421598417 ) ) ;
#50848=CARTESIAN_POINT ( 'NONE',  ( 14.70000000122903394, 5.773502691896255534, 3.535250795749688894E-16 ) ) ;
#50849=CARTESIAN_POINT ( 'NONE',  ( 12.18750000000000000, -2.886751345948125991, -5.000000000000000000 ) ) ;
#50850=CARTESIAN_POINT ( 'NONE',  ( 21.66562500061451502, 3.027376345333611329, 5.243569643749999010 ) ) ;
#50851=CARTESIAN_POINT ( 'NONE',  ( 8.221875000614518925, 3.027376345333611329, 5.243569643749999010 ) ) ;
#50853=CARTESIAN_POINT ( 'NONE',  ( 8.025000001229035007, 2.886751345948126879, 4.999999999999999112 ) ) ;
#50854=CARTESIAN_POINT ( 'NONE',  ( 17.17500000122903359, -5.773502691896255534, -1.060575238724906372E-15 ) ) ;
#50855=CARTESIAN_POINT ( 'NONE',  ( 13.00312500061451537, 4.541064518000418104, -2.621784821874998173 ) ) ;
#50857=CARTESIAN_POINT ( 'NONE',  ( 16.26562500061451289, 3.027376345333611329, 5.243569643749999010 ) ) ;
#50858=CARTESIAN_POINT ( 'NONE',  ( 28.65000000122903145, 5.773502691896255534, 3.535250795749688894E-16 ) ) ;
#50859=CARTESIAN_POINT ( 'NONE',  ( 21.97500000000000142, -4.330127018922194537, 2.499999999999995559 ) ) ;
#50860=CARTESIAN_POINT ( 'NONE',  ( 22.28437500061451715, -4.541064518000419881, 2.621784821874995952 ) ) ;
#50862=CARTESIAN_POINT ( 'NONE',  ( 10.20000000122903572, 5.773502691896255534, 3.535250795749688894E-16 ) ) ;
#50863=CARTESIAN_POINT ( 'NONE',  ( 28.77187500061451431, 3.027376345333613106, -5.243569643749998122 ) ) ;
#50864=CARTESIAN_POINT ( 'NONE',  ( 5.221875000614519813, -6.054752690667223547, -1.112240025338166033E-15 ) ) ;
#50865=CARTESIAN_POINT ( 'NONE',  ( 24.70312500061451644, 4.541064518000418104, -2.621784821874998173 ) ) ;
#50868=CARTESIAN_POINT ( 'NONE',  ( 10.50937500061451679, 0.000000000000000000, 5.243569643749999010 ) ) ;
#50869=CARTESIAN_POINT ( 'NONE',  ( 0.000000000000000000, 20.00000000000000000, -30.00000000000000000 ) ) ;
#50870=CARTESIAN_POINT ( 'NONE',  ( 29.24062500061451431, 6.054752690667223547, 3.707466751127219781E-16 ) ) ;
#50871=CARTESIAN_POINT ( 'NONE',  ( 7.434375000614519280, -4.541064518000419881, 2.621784821874995952 ) ) ;
#50873=CARTESIAN_POINT ( 'NONE',  ( 25.32187500061451857, 3.027376345333611329, 5.243569643749999010 ) ) ;
#50874=CARTESIAN_POINT ( 'NONE',  ( 9.001249775931846008E-16, 10.91562500061459495, 34.90005215228797653 ) ) ;
#50875=CARTESIAN_POINT ( 'NONE',  ( 18.59999999999999787, 4.330127018922192761, -2.499999999999997780 ) ) ;
#50876=ORIENTED_EDGE ( 'NONE', *, *, #420, .F. ) ;
#50877=CARTESIAN_POINT ( 'NONE',  ( 27.56250000000000000, 2.886751345948129099, -4.999999999999998224 ) ) ;
#50878=CARTESIAN_POINT ( 'NONE',  ( 29.03437500061451715, -4.541064518000419881, 2.621784821874995952 ) ) ;
#50879=VERTEX_POINT ( 'NONE', #38884 ) ;
#50880=CARTESIAN_POINT ( 'NONE',  ( 15.92812500061451608, -4.541064518000419881, 2.621784821874995952 ) ) ;
#50881=CARTESIAN_POINT ( 'NONE',  ( 7.790625000614518569, -3.027376345333614438, 5.243569643749998122 ) ) ;
#50883=CARTESIAN_POINT ( 'NONE',  ( 4.396875000614516971, -3.027376345333610441, -5.243569643749999898 ) ) ;
#50884=CARTESIAN_POINT ( 'NONE',  ( 17.17500000122903359, -5.773502691896255534, -1.060575238724906372E-15 ) ) ;
#50885=CARTESIAN_POINT ( 'NONE',  ( 22.08749999999999858, -2.886751345948125991, -5.000000000000000000 ) ) ;
#50886=CARTESIAN_POINT ( 'NONE',  ( 15.78749999999999964, -2.886751345948126435, -5.000000000000000000 ) ) ;
#50887=CARTESIAN_POINT ( 'NONE',  ( 6.346875000614517148, 6.054752690667223547, 3.707466751127219781E-16 ) ) ;
#50888=CARTESIAN_POINT ( 'NONE',  ( 10.80937500061451928, 4.541064518000418104, -2.621784821874998173 ) ) ;
#50889=CARTESIAN_POINT ( 'NONE',  ( 21.90937500061451715, -4.541064518000417216, -2.621784821875001281 ) ) ;
#50890=LINE ( 'NONE', #5463, #51326 ) ;
#50891=ORIENTED_EDGE ( 'NONE', *, *, #20037, .F. ) ;
#50892=CARTESIAN_POINT ( 'NONE',  ( 5.334375000614517859, 6.421520780324663323E-16, -5.243569643749999010 ) ) ;
#50893=CARTESIAN_POINT ( 'NONE',  ( 6.871875000614517504, 3.027376345333611329, 5.243569643749999010 ) ) ;
#50894=CARTESIAN_POINT ( 'NONE',  ( 19.65000000000000213, 0.000000000000000000, 4.999999999999998224 ) ) ;
#50895=CARTESIAN_POINT ( 'NONE',  ( 16.82812500061451644, -4.541064518000419881, 2.621784821874995952 ) ) ;
#50899=CARTESIAN_POINT ( 'NONE',  ( 11.01562500061451821, -6.054752690667223547, -1.112240025338166033E-15 ) ) ;
#50900=CARTESIAN_POINT ( 'NONE',  ( 27.87187500061451573, 3.027376345333613106, -5.243569643749998122 ) ) ;
#50901=LINE ( 'NONE', #11740, #18325 ) ;
#50902=CARTESIAN_POINT ( 'NONE',  ( 28.05937500061451573, 0.000000000000000000, 5.243569643749999010 ) ) ;
#50903=CARTESIAN_POINT ( 'NONE',  ( 9.825000000000001066, -4.330127018922194537, 2.499999999999995559 ) ) ;
#50904=CARTESIAN_POINT ( 'NONE',  ( 8.484601909799253346E-16, 16.17500000122903003, 34.61880215351700230 ) ) ;
#50905=CARTESIAN_POINT ( 'NONE',  ( 9.075000001229033941, -5.773502691896255534, -1.060575238724906372E-15 ) ) ;
#50907=CARTESIAN_POINT ( 'NONE',  ( 19.88437500061451857, 4.541064518000418104, 2.621784821874999949 ) ) ;
#50908=CARTESIAN_POINT ( 'NONE',  ( 13.02187500061451608, 3.027376345333613106, -5.243569643749998122 ) ) ;
#50909=CARTESIAN_POINT ( 'NONE',  ( -0.6909613911670684505, 4.953869264242466208, -33.94222170460632526 ) ) ;
#50910=ORIENTED_EDGE ( 'NONE', *, *, #39400, .F. ) ;
#50911=CARTESIAN_POINT ( 'NONE',  ( 14.54062500061451679, -3.027376345333614438, 5.243569643749998122 ) ) ;
#50912=CARTESIAN_POINT ( 'NONE',  ( 26.77500000122903145, 2.886751345948129099, -4.999999999999998224 ) ) ;
#50913=CARTESIAN_POINT ( 'NONE',  ( 14.52187500061451608, 3.027376345333611329, 5.243569643749999010 ) ) ;
#50914=CARTESIAN_POINT ( 'NONE',  ( 2.915625000614516793, -6.054752690667223547, -1.112240025338166033E-15 ) ) ;
#50915=CARTESIAN_POINT ( 'NONE',  ( 17.46562500061451217, 3.027376345333613106, -5.243569643749998122 ) ) ;
#50918=CARTESIAN_POINT ( 'NONE',  ( 26.18437500061451573, 4.541064518000418104, 2.621784821874999949 ) ) ;
#50919=CARTESIAN_POINT ( 'NONE',  ( 4.243569643749999898, 10.57812500061451821, 30.00000000000000000 ) ) ;
#50920=CARTESIAN_POINT ( 'NONE',  ( 14.55937500061451573, 0.000000000000000000, 5.243569643749999010 ) ) ;
#50921=CARTESIAN_POINT ( 'NONE',  ( 13.05000000122903536, -2.886751345948129988, 4.999999999999997335 ) ) ;
#50923=CARTESIAN_POINT ( 'NONE',  ( -4.243569643749998122, 18.54687500061451644, -27.54997392385601174 ) ) ;
#50925=CARTESIAN_POINT ( 'NONE',  ( 19.09687500061451360, -3.027376345333614438, 5.243569643749998122 ) ) ;
#50926=CARTESIAN_POINT ( 'NONE',  ( 20.55000000122903359, 5.773502691896255534, 3.535250795749688894E-16 ) ) ;
#50927=CARTESIAN_POINT ( 'NONE',  ( 15.57187500061451679, -6.054752690667223547, -1.112240025338166033E-15 ) ) ;
#50928=CARTESIAN_POINT ( 'NONE',  ( 2.121784821875001281, 11.45937500061451786, 33.67503911421598417 ) ) ;
#50929=CARTESIAN_POINT ( 'NONE',  ( 21.33750000122903145, 6.123233995736764310E-16, -4.999999999999998224 ) ) ;
#50930=CARTESIAN_POINT ( 'NONE',  ( 15.66562500061451857, 3.027376345333613106, -5.243569643749998122 ) ) ;
#50931=CARTESIAN_POINT ( 'NONE',  ( 28.79062500061451502, 6.054752690667223547, 3.707466751127219781E-16 ) ) ;
#50933=ORIENTED_EDGE ( 'NONE', *, *, #53086, .F. ) ;
#50934=CARTESIAN_POINT ( 'NONE',  ( 20.28750000000000142, -2.886751345948125991, -5.000000000000000000 ) ) ;
#50935=CYLINDRICAL_SURFACE ( 'NONE', #3156, 4.999999999999998224 ) ;
#50936=CARTESIAN_POINT ( 'NONE',  ( 1.347985686992487997, 4.821799686897913162, 33.77548493594544965 ) ) ;
#50937=CARTESIAN_POINT ( 'NONE',  ( 15.56250000122903465, 4.330127018922192761, -2.499999999999997780 ) ) ;
#50938=CARTESIAN_POINT ( 'NONE',  ( 20.57812500061451644, 6.421520780324663323E-16, -5.243569643749999010 ) ) ;
#50939=CARTESIAN_POINT ( 'NONE',  ( 26.57812500061451644, 4.541064518000418104, 2.621784821874999949 ) ) ;
#50940=CARTESIAN_POINT ( 'NONE',  ( 6.028125000614517504, -4.541064518000419881, 2.621784821874995952 ) ) ;
#50941=CARTESIAN_POINT ( 'NONE',  ( 29.43750000000000000, 5.773502691896255534, 3.535250795749688894E-16 ) ) ;
#50942=CARTESIAN_POINT ( 'NONE',  ( 11.43750000122903465, 6.123233995736764310E-16, -4.999999999999998224 ) ) ;
#50944=CARTESIAN_POINT ( 'NONE',  ( 29.85937500061451644, 0.000000000000000000, 5.243569643749999010 ) ) ;
#50945=CARTESIAN_POINT ( 'NONE',  ( -2.828200636599751609E-16, 11.45000000122903394, -34.61880215351700230 ) ) ;
#50946=CARTESIAN_POINT ( 'NONE',  ( 4.243569643749999898, 18.69687500061451857, -27.54997392385601529 ) ) ;
#50947=EDGE_CURVE ( 'NONE', #60892, #13717, #5333, .T. ) ;
#50948=CARTESIAN_POINT ( 'NONE',  ( 6.675000001229034474, 2.886751345948126879, 4.999999999999999112 ) ) ;
#50950=CARTESIAN_POINT ( 'NONE',  ( 8.025000000000000355, -4.330127018922194537, 2.499999999999995559 ) ) ;
#50951=CARTESIAN_POINT ( 'NONE',  ( 3.075000001229035718, 2.886751345948126879, 4.999999999999999112 ) ) ;
#50952=CARTESIAN_POINT ( 'NONE',  ( 12.94687500061451857, -3.027376345333610441, -5.243569643749999898 ) ) ;
#50953=CARTESIAN_POINT ( 'NONE',  ( 4.734375000614518214, -4.541064518000419881, 2.621784821874995952 ) ) ;
#50956=CARTESIAN_POINT ( 'NONE',  ( 9.421875000614519990, 3.027376345333613106, -5.243569643749998122 ) ) ;
#50957=PLANE ( 'NONE',  #50173 ) ;
#50958=CARTESIAN_POINT ( 'NONE',  ( 4.537500001229034297, -4.330127018922194537, 2.499999999999995559 ) ) ;
#50959=CARTESIAN_POINT ( 'NONE',  ( 4.243569643749999898, 16.87812500061459176, 30.00000000000000000 ) ) ;
#50960=CARTESIAN_POINT ( 'NONE',  ( 21.38437500061451502, -4.541064518000419881, 2.621784821874995952 ) ) ;
#50962=CARTESIAN_POINT ( 'NONE',  ( 2.733878782416514941, -4.186395442746991158, 2.733878782416514941 ) ) ;
#50963=CARTESIAN_POINT ( 'NONE',  ( 27.18750000122903288, 6.123233995736764310E-16, -4.999999999999998224 ) ) ;
#50965=CARTESIAN_POINT ( 'NONE',  ( 21.92812500061451431, 6.421520780324663323E-16, -5.243569643749999010 ) ) ;
#50966=CARTESIAN_POINT ( 'NONE',  ( 15.96562500061451573, -6.054752690667223547, -1.112240025338166033E-15 ) ) ;
#50968=CARTESIAN_POINT ( 'NONE',  ( 11.33437500061451608, 4.541064518000418104, 2.621784821874999949 ) ) ;
#50969=CARTESIAN_POINT ( 'NONE',  ( 27.82499999999999929, -4.330127018922194537, 2.499999999999995559 ) ) ;
#50970=CARTESIAN_POINT ( 'NONE',  ( 24.82500000122902861, -5.773502691896255534, -1.060575238724906372E-15 ) ) ;
#50971=CARTESIAN_POINT ( 'NONE',  ( 3.496875000614518836, -3.027376345333610441, -5.243569643749999898 ) ) ;
#50972=CARTESIAN_POINT ( 'NONE',  ( 13.73437500061451821, -4.541064518000419881, 2.621784821874995952 ) ) ;
#50973=CARTESIAN_POINT ( 'NONE',  ( 28.58437500061451786, -4.541064518000419881, 2.621784821874995952 ) ) ;
#50975=CARTESIAN_POINT ( 'NONE',  ( 22.88437500061451857, 6.421520780324663323E-16, -5.243569643749999010 ) ) ;
#50976=CARTESIAN_POINT ( 'NONE',  ( 14.97187500061451892, 3.027376345333611329, 5.243569643749999010 ) ) ;
#50978=CARTESIAN_POINT ( 'NONE',  ( 26.73749999999999716, 5.773502691896255534, 3.535250795749688894E-16 ) ) ;
#50979=CARTESIAN_POINT ( 'NONE',  ( 2.812500001229033320, -4.330127018922190985, -2.500000000000001332 ) ) ;
#50981=CARTESIAN_POINT ( 'NONE',  ( 16.30312500061451786, 0.000000000000000000, 5.243569643749999010 ) ) ;
#50982=CARTESIAN_POINT ( 'NONE',  ( 6.187500000000002665, -2.886751345948129988, 4.999999999999997335 ) ) ;
#50983=CARTESIAN_POINT ( 'NONE',  ( -5.810221930991193690E-16, 11.78749999999999964, -34.00000000000000000 ) ) ;
#50984=CARTESIAN_POINT ( 'NONE',  ( 18.07499999999999929, 6.123233995736764310E-16, -4.999999999999998224 ) ) ;
#50985=CARTESIAN_POINT ( 'NONE',  ( -4.243569643749999898, 13.50312500061451715, 30.00000000000000000 ) ) ;
#50987=CARTESIAN_POINT ( 'NONE',  ( 21.22500000122903074, -5.773502691896255534, -1.060575238724906372E-15 ) ) ;
#50988=CARTESIAN_POINT ( 'NONE',  ( 2.516621263038625322, 9.679961675009989719, 24.54971018585778353 ) ) ;
#50989=CARTESIAN_POINT ( 'NONE',  ( 26.22187500061451715, 3.027376345333611329, 5.243569643749999010 ) ) ;
#50991=CARTESIAN_POINT ( 'NONE',  ( 21.81562500061451004, -6.054752690667223547, -1.112240025338166033E-15 ) ) ;
#50992=CARTESIAN_POINT ( 'NONE',  ( 21.38437500061451502, -4.541064518000419881, 2.621784821874995952 ) ) ;
#50993=CARTESIAN_POINT ( 'NONE',  ( 5.400000000000002132, -4.330127018922190985, -2.500000000000001332 ) ) ;
#50994=CARTESIAN_POINT ( 'NONE',  ( 9.778125000614517504, 6.421520780324663323E-16, -5.243569643749999010 ) ) ;
#50995=CARTESIAN_POINT ( 'NONE',  ( 23.50312500061451360, 0.000000000000000000, 5.243569643749999010 ) ) ;
#50996=CARTESIAN_POINT ( 'NONE',  ( 13.05937500061451750, 4.541064518000418104, -2.621784821874998173 ) ) ;
#50997=CARTESIAN_POINT ( 'NONE',  ( 15.72187500061451892, 3.027376345333613106, -5.243569643749998122 ) ) ;
#50998=CARTESIAN_POINT ( 'NONE',  ( 20.66250000122903074, 0.000000000000000000, 4.999999999999998224 ) ) ;
#50999=CARTESIAN_POINT ( 'NONE',  ( 4.243569643749999898, 16.42812500061451786, 30.00000000000000000 ) ) ;
#51000=CARTESIAN_POINT ( 'NONE',  ( 20.25000000122903288, -2.886751345948129988, 4.999999999999997335 ) ) ;
#51002=CARTESIAN_POINT ( 'NONE',  ( 11.50312500061451892, -4.541064518000417216, -2.621784821875001281 ) ) ;
#51003=CARTESIAN_POINT ( 'NONE',  ( 5.746875000614517504, -3.027376345333610441, -5.243569643749999898 ) ) ;
#51004=CARTESIAN_POINT ( 'NONE',  ( 5.859375000614519102, 4.541064518000418104, -2.621784821874998173 ) ) ;
#51005=ORIENTED_EDGE ( 'NONE', *, *, #14215, .T. ) ;
#51007=CARTESIAN_POINT ( 'NONE',  ( 25.77187500061451075, 3.027376345333611329, 5.243569643749999010 ) ) ;
#51008=CARTESIAN_POINT ( 'NONE',  ( 16.19062500061451715, 6.054752690667223547, 3.707466751127219781E-16 ) ) ;
#51009=CARTESIAN_POINT ( 'NONE',  ( 26.92500000122903359, 2.886751345948126879, 4.999999999999999112 ) ) ;
#51010=CARTESIAN_POINT ( 'NONE',  ( 26.69062500061451715, -3.027376345333614438, 5.243569643749998122 ) ) ;
#51011=AXIS2_PLACEMENT_3D ( 'NONE', #59262, #8671, #58530 ) ;
#51012=CARTESIAN_POINT ( 'NONE',  ( 21.64687500061451786, 6.054752690667223547, 3.707466751127219781E-16 ) ) ;
#51013=CARTESIAN_POINT ( 'NONE',  ( 16.26562500061451289, 3.027376345333611329, 5.243569643749999010 ) ) ;
#51014=CARTESIAN_POINT ( 'NONE',  ( 4.000000000000000000, 10.73750000000000071, 32.30940107675849049 ) ) ;
#51015=CARTESIAN_POINT ( 'NONE',  ( 21.02812500061451573, 6.421520780324663323E-16, -5.243569643749999010 ) ) ;
#51016=CARTESIAN_POINT ( 'NONE',  ( 3.862500001229035362, 4.330127018922192761, -2.499999999999997780 ) ) ;
#51017=ORIENTED_EDGE ( 'NONE', *, *, #40621, .T. ) ;
#51018=CARTESIAN_POINT ( 'NONE',  ( 28.87499999999999645, 6.123233995736764310E-16, -4.999999999999998224 ) ) ;
#51019=CARTESIAN_POINT ( 'NONE',  ( -3.999999999999997335, 11.93750000000000355, -27.69059892324149175 ) ) ;
#51021=CARTESIAN_POINT ( 'NONE',  ( 3.121875000614518836, 3.027376345333613106, -5.243569643749998122 ) ) ;
#51022=CARTESIAN_POINT ( 'NONE',  ( 10.19062500061451892, -3.027376345333610441, -5.243569643749999898 ) ) ;
#51023=CARTESIAN_POINT ( 'NONE',  ( 21.11250000122903359, 0.000000000000000000, 4.999999999999998224 ) ) ;
#51025=CARTESIAN_POINT ( 'NONE',  ( 13.69687500061451679, -3.027376345333614438, 5.243569643749998122 ) ) ;
#51026=CARTESIAN_POINT ( 'NONE',  ( 27.10312500061451502, 0.000000000000000000, 5.243569643749999010 ) ) ;
#51027=CARTESIAN_POINT ( 'NONE',  ( 28.61249999999999716, 2.886751345948126879, 4.999999999999999112 ) ) ;
#51028=CARTESIAN_POINT ( 'NONE',  ( 8.484601909799253346E-16, 18.87500000122903643, -25.38119784648299770 ) ) ;
#51030=CARTESIAN_POINT ( 'NONE',  ( 12.17812500061451608, 4.541064518000418104, 2.621784821874999949 ) ) ;
#51032=CARTESIAN_POINT ( 'NONE',  ( 10.56562500061451715, -6.054752690667223547, -1.112240025338166033E-15 ) ) ;
#51033=CARTESIAN_POINT ( 'NONE',  ( 6.853125000614516793, 0.000000000000000000, 5.243569643749999010 ) ) ;
#51036=CARTESIAN_POINT ( 'NONE',  ( 16.46249999999999503, 2.886751345948126879, 4.999999999999999112 ) ) ;
#51037=( BOUNDED_CURVE ( )  B_SPLINE_CURVE ( 2, ( #42381, #47924, #24285, #70453, #52729, #47191, #14293 ),
 .UNSPECIFIED., .F., .F. ) 
 B_SPLINE_CURVE_WITH_KNOTS ( ( 3, 2, 2, 3 ),
 ( 0.9083333333333334370, 0.9111111111111112049, 0.9138888888888888618, 0.9166666666666666297 ),
 .UNSPECIFIED. ) 
 CURVE ( )  GEOMETRIC_REPRESENTATION_ITEM ( )  RATIONAL_B_SPLINE_CURVE ( ( 0.9999999999999946709, 0.8660254037844440367, 1.000000000000000000, 0.8660254037844387076, 1.000000000000000000, 0.8660254037844387076, 1.000000000000000000 ) ) 
 REPRESENTATION_ITEM ( '' )  );
#51038=CARTESIAN_POINT ( 'NONE',  ( 17.07187500061451502, 3.027376345333613106, -5.243569643749998122 ) ) ;
#51039=CARTESIAN_POINT ( 'NONE',  ( 10.91250000122903252, -4.330127018922190985, -2.500000000000001332 ) ) ;
#51040=CARTESIAN_POINT ( 'NONE',  ( 19.32187500061451857, 3.027376345333613106, -5.243569643749998122 ) ) ;
#51042=CARTESIAN_POINT ( 'NONE',  ( 19.77187500061451786, 3.027376345333613106, -5.243569643749998122 ) ) ;
#51043=CARTESIAN_POINT ( 'NONE',  ( 4.243569643749999898, 15.07812500061451644, -30.00000000000000000 ) ) ;
#51044=CARTESIAN_POINT ( 'NONE',  ( 0.000000000000000000, 20.00000000000000000, 30.00000000000000000 ) ) ;
#51046=CARTESIAN_POINT ( 'NONE',  ( 4.155299848256742479, 2.780943907573066198, 4.445394570867353679 ) ) ;
#51047=ADVANCED_FACE ( 'NONE', ( #27433 ), #11163, .F. ) ;
#51048=CARTESIAN_POINT ( 'NONE',  ( 26.72812500061451502, -4.541064518000419881, 2.621784821874995952 ) ) ;
#51049=CARTESIAN_POINT ( 'NONE',  ( 29.37187500061451928, 3.027376345333611329, 5.243569643749999010 ) ) ;
#51050=CARTESIAN_POINT ( 'NONE',  ( 25.23749999999999716, -2.886751345948125991, -5.000000000000000000 ) ) ;
#51051=CARTESIAN_POINT ( 'NONE',  ( 8.278125000614515727, -4.541064518000419881, 2.621784821874995952 ) ) ;
#51054=( BOUNDED_CURVE ( )  B_SPLINE_CURVE ( 2, ( #15021, #37926, #32756, #26482, #37559, #71918, #49023 ),
 .UNSPECIFIED., .F., .F. ) 
 B_SPLINE_CURVE_WITH_KNOTS ( ( 3, 2, 2, 3 ),
 ( 0.1499999999999999389, 0.1527777777777777624, 0.1555555555555555858, 0.1583333333333333814 ),
 .UNSPECIFIED. ) 
 CURVE ( )  GEOMETRIC_REPRESENTATION_ITEM ( )  RATIONAL_B_SPLINE_CURVE ( ( 1.000000000000002665, 0.8660254037844360431, 1.000000000000000000, 0.8660254037844387076, 1.000000000000000000, 0.8660254037844360431, 1.000000000000002665 ) ) 
 REPRESENTATION_ITEM ( '' )  );
#51055=CARTESIAN_POINT ( 'NONE',  ( 19.35937500061451644, 4.541064518000418104, -2.621784821874998173 ) ) ;
#51057=CARTESIAN_POINT ( 'NONE',  ( 6.403125000614517504, 0.000000000000000000, 5.243569643749999010 ) ) ;
#51058=CARTESIAN_POINT ( 'NONE',  ( 10.17187500061451999, -6.054752690667223547, -1.112240025338166033E-15 ) ) ;
#51060=CARTESIAN_POINT ( 'NONE',  ( 21.98437500061451644, 6.421520780324663323E-16, -5.243569643749999010 ) ) ;
#51062=CARTESIAN_POINT ( 'NONE',  ( 3.149999999999999911, -4.330127018922190985, -2.500000000000001332 ) ) ;
#51063=CARTESIAN_POINT ( 'NONE',  ( 15.30000000122903359, -2.886751345948129988, 4.999999999999997335 ) ) ;
#51066=ORIENTED_EDGE ( 'NONE', *, *, #33488, .F. ) ;
#51067=CARTESIAN_POINT ( 'NONE',  ( 13.27500000000000213, 4.330127018922191873, 2.499999999999999556 ) ) ;
#51068=CARTESIAN_POINT ( 'NONE',  ( 23.61562500061451431, -6.054752690667223547, -1.112240025338166033E-15 ) ) ;
#51069=CARTESIAN_POINT ( 'NONE',  ( 15.00000000000000000, 4.330127018922192761, -2.499999999999997780 ) ) ;
#51070=CARTESIAN_POINT ( 'NONE',  ( 9.412500001229034297, 0.000000000000000000, 4.999999999999998224 ) ) ;
#51071=CARTESIAN_POINT ( 'NONE',  ( 7.865625000614516971, -6.054752690667223547, -1.112240025338166033E-15 ) ) ;
#51072=CARTESIAN_POINT ( 'NONE',  ( 9.975000000000001421, 6.123233995736764310E-16, -4.999999999999998224 ) ) ;
#51073=DIRECTION ( 'NONE',  ( 0.000000000000000000, 0.000000000000000000, 1.000000000000000000 ) ) ;
#51074=CARTESIAN_POINT ( 'NONE',  ( -2.121784821874999949, 14.83437500061451786, -33.67503911421598417 ) ) ;
#51075=CARTESIAN_POINT ( 'NONE',  ( 26.85000000122903430, 5.773502691896255534, 3.535250795749688894E-16 ) ) ;
#51077=CARTESIAN_POINT ( 'NONE',  ( 7.275000000000000355, 6.123233995736764310E-16, -4.999999999999998224 ) ) ;
#51078=LINE ( 'NONE', #9556, #62116 ) ;
#51079=ORIENTED_EDGE ( 'NONE', *, *, #56586, .T. ) ;
#51080=CARTESIAN_POINT ( 'NONE',  ( 22.86562500061451431, 3.027376345333613106, -5.243569643749998122 ) ) ;
#51081=CARTESIAN_POINT ( 'NONE',  ( 28.41562500061451502, 3.027376345333611329, 5.243569643749999010 ) ) ;
#51082=CARTESIAN_POINT ( 'NONE',  ( 29.85937500061451644, 0.000000000000000000, 5.243569643749999010 ) ) ;
#51083=CARTESIAN_POINT ( 'NONE',  ( 19.77187500061451786, 3.027376345333613106, -5.243569643749998122 ) ) ;
#51084=CARTESIAN_POINT ( 'NONE',  ( 16.56562500061451715, 3.027376345333613106, -5.243569643749998122 ) ) ;
#51085=EDGE_CURVE ( 'NONE', #19994, #47876, #39729, .T. ) ;
#51086=CARTESIAN_POINT ( 'NONE',  ( 2.121784821874999061, 12.45312500061459460, -33.67503911421598417 ) ) ;
#51087=CARTESIAN_POINT ( 'NONE',  ( 6.140625000614516438, -3.027376345333610441, -5.243569643749999898 ) ) ;
#51088=CARTESIAN_POINT ( 'NONE',  ( 28.87500000122902932, -5.773502691896255534, -1.060575238724906372E-15 ) ) ;
#51090=CARTESIAN_POINT ( 'NONE',  ( 18.66562500061451502, -6.054752690667223547, -1.112240025338166033E-15 ) ) ;
#51092=CARTESIAN_POINT ( 'NONE',  ( 3.262500001229035718, -4.330127018922190985, -2.500000000000001332 ) ) ;
#51093=CARTESIAN_POINT ( 'NONE',  ( 12.38437500061451857, -4.541064518000419881, 2.621784821874995952 ) ) ;
#51094=CARTESIAN_POINT ( 'NONE',  ( 12.42187500061451821, -6.054752690667223547, -1.112240025338166033E-15 ) ) ;
#51095=CARTESIAN_POINT ( 'NONE',  ( 19.95937500061451786, 0.000000000000000000, 5.243569643749999010 ) ) ;
#51096=ORIENTED_EDGE ( 'NONE', *, *, #13387, .T. ) ;
#51098=CARTESIAN_POINT ( 'NONE',  ( 24.21562500061451573, 3.027376345333613106, -5.243569643749998122 ) ) ;
#51099=EDGE_CURVE ( 'NONE', #54799, #49995, #57373, .T. ) ;
#51100=CARTESIAN_POINT ( 'NONE',  ( 18.08437500061451431, 4.541064518000418104, 2.621784821874999949 ) ) ;
#51101=CARTESIAN_POINT ( 'NONE',  ( 24.47812500061451502, -4.541064518000419881, 2.621784821874995952 ) ) ;
#51102=CARTESIAN_POINT ( 'NONE',  ( 27.15000000000000213, 4.330127018922192761, -2.499999999999997780 ) ) ;
#51103=CARTESIAN_POINT ( 'NONE',  ( -3.999999999999997335, 15.98750000000000249, 32.30940107675850470 ) ) ;
#51104=CARTESIAN_POINT ( 'NONE',  ( 5.296875000614518214, -3.027376345333610441, -5.243569643749999898 ) ) ;
#51105=CARTESIAN_POINT ( 'NONE',  ( 11.43750000122903465, 6.123233995736764310E-16, -4.999999999999998224 ) ) ;
#51106=CARTESIAN_POINT ( 'NONE',  ( 7.462500001229035007, 4.330127018922192761, -2.499999999999997780 ) ) ;
#51108=CARTESIAN_POINT ( 'NONE',  ( 27.52500000122903145, -5.773502691896255534, -1.060575238724906372E-15 ) ) ;
#51111=CARTESIAN_POINT ( 'NONE',  ( 11.93437500061451573, -4.541064518000419881, 2.621784821874995952 ) ) ;
#51113=CARTESIAN_POINT ( 'NONE',  ( 16.41562500061451857, -6.054752690667223547, -1.112240025338166033E-15 ) ) ;
#51114=CARTESIAN_POINT ( 'NONE',  ( 13.28437500061451715, -4.541064518000419881, 2.621784821874995952 ) ) ;
#51115=CARTESIAN_POINT ( 'NONE',  ( 5.728125000614515905, 6.421520780324663323E-16, -5.243569643749999010 ) ) ;
#51116=CARTESIAN_POINT ( 'NONE',  ( 19.58437500061451786, -4.541064518000419881, 2.621784821874995952 ) ) ;
#51117=CARTESIAN_POINT ( 'NONE',  ( 9.871875000614517504, 3.027376345333613106, -5.243569643749998122 ) ) ;
#51118=CARTESIAN_POINT ( 'NONE',  ( 3.853125000614517681, -4.541064518000417216, -2.621784821875001281 ) ) ;
#51120=CARTESIAN_POINT ( 'NONE',  ( 5.175000001229033586, 2.886751345948129099, -4.999999999999998224 ) ) ;
#51121=CARTESIAN_POINT ( 'NONE',  ( 21.29062500061451502, -3.027376345333614438, 5.243569643749998122 ) ) ;
#51123=CARTESIAN_POINT ( 'NONE',  ( 8.250000001229034652, -2.886751345948125991, -5.000000000000000000 ) ) ;
#51124=CARTESIAN_POINT ( 'NONE',  ( 16.97812500061451502, 6.421520780324663323E-16, -5.243569643749999010 ) ) ;
#51125=CARTESIAN_POINT ( 'NONE',  ( 14.12812500061451715, -4.541064518000419881, 2.621784821874995952 ) ) ;
#51127=CARTESIAN_POINT ( 'NONE',  ( 13.50000000000000178, -4.330127018922190985, -2.500000000000001332 ) ) ;
#51128=CARTESIAN_POINT ( 'NONE',  ( 9.862500001229033586, 0.000000000000000000, 4.999999999999998224 ) ) ;
#51129=CARTESIAN_POINT ( 'NONE',  ( 6.628125000614517148, 6.421520780324663323E-16, -5.243569643749999010 ) ) ;
#51130=CARTESIAN_POINT ( 'NONE',  ( 19.35000000122903430, -2.886751345948129988, 4.999999999999997335 ) ) ;
#51132=CARTESIAN_POINT ( 'NONE',  ( -3.000416591977282496E-16, 11.64687500061451786, -34.90005215228797653 ) ) ;
#51133=CARTESIAN_POINT ( 'NONE',  ( 4.512434258951183885, -2.153965711245202197, 4.548138340231743904 ) ) ;
#51134=DIRECTION ( 'NONE',  ( -1.000000000000000000, -0.000000000000000000, -0.000000000000000000 ) ) ;
#51136=CARTESIAN_POINT ( 'NONE',  ( 20.22187500061451715, 3.027376345333613106, -5.243569643749998122 ) ) ;
#51137=DIRECTION ( 'NONE',  ( 0.000000000000000000, 0.000000000000000000, 1.000000000000000000 ) ) ;
#51138=CARTESIAN_POINT ( 'NONE',  ( 16.11562500061451786, 3.027376345333613106, -5.243569643749998122 ) ) ;
#51141=CARTESIAN_POINT ( 'NONE',  ( 28.58437500061451786, -4.541064518000419881, 2.621784821874995952 ) ) ;
#51142=CARTESIAN_POINT ( 'NONE',  ( 26.78437500061451360, -4.541064518000419881, 2.621784821874995952 ) ) ;
#51144=CARTESIAN_POINT ( 'NONE',  ( 12.14062500061451821, 6.054752690667223547, 3.707466751127219781E-16 ) ) ;
#51145=CARTESIAN_POINT ( 'NONE',  ( 11.63437500061451857, 6.421520780324663323E-16, -5.243569643749999010 ) ) ;
#51147=CARTESIAN_POINT ( 'NONE',  ( 9.525000000000002132, 6.123233995736764310E-16, -4.999999999999998224 ) ) ;
#51148=CARTESIAN_POINT ( 'NONE',  ( 19.15312500061451573, -4.541064518000417216, -2.621784821875001281 ) ) ;
#51150=CARTESIAN_POINT ( 'NONE',  ( 3.242103837493086330E-14, 12.80000000122903536, 26.00000000000000711 ) ) ;
#51151=CARTESIAN_POINT ( 'NONE',  ( 11.84999999999999964, 4.330127018922192761, -2.499999999999997780 ) ) ;
#51152=CARTESIAN_POINT ( 'NONE',  ( 21.52500000122903145, 2.886751345948126879, 4.999999999999999112 ) ) ;
#51153=CARTESIAN_POINT ( 'NONE',  ( 15.40312500061451573, 0.000000000000000000, 5.243569643749999010 ) ) ;
#51155=EDGE_LOOP ( 'NONE', ( #49973, #13148, #65438, #49826 ) ) ;
#51156=CARTESIAN_POINT ( 'NONE',  ( 19.65000000000000213, 0.000000000000000000, 4.999999999999998224 ) ) ;
#51157=CARTESIAN_POINT ( 'NONE',  ( 21.75000000000000000, 4.330127018922192761, -2.499999999999997780 ) ) ;
#51158=CARTESIAN_POINT ( 'NONE',  ( 20.48437500061451289, -4.541064518000419881, 2.621784821874995952 ) ) ;
#51159=CARTESIAN_POINT ( 'NONE',  ( 24.77812500061451217, 4.541064518000418104, 2.621784821874999949 ) ) ;
#51161=ADVANCED_FACE ( 'NONE', ( #28161 ), #71777, .T. ) ;
#51163=CARTESIAN_POINT ( 'NONE',  ( 8.690625000614515372, -3.027376345333614438, 5.243569643749998122 ) ) ;
#51164=CARTESIAN_POINT ( 'NONE',  ( -5.810221930991193690E-16, 12.23750000000000071, 26.00000000000000355 ) ) ;
#51165=CARTESIAN_POINT ( 'NONE',  ( 14.51250000000000107, 2.886751345948129099, -4.999999999999998224 ) ) ;
#51166=CARTESIAN_POINT ( 'NONE',  ( -2.121784821874996840, 17.62812500061451715, 33.67503911421598417 ) ) ;
#51167=CARTESIAN_POINT ( 'NONE',  ( 28.60312500061451502, -4.541064518000417216, -2.621784821875001281 ) ) ;
#51168=CARTESIAN_POINT ( 'NONE',  ( 27.12187500061451573, 3.027376345333611329, 5.243569643749999010 ) ) ;
#51169=ORIENTED_EDGE ( 'NONE', *, *, #5968, .T. ) ;
#51170=CARTESIAN_POINT ( 'NONE',  ( 22.86562500061451431, 3.027376345333613106, -5.243569643749998122 ) ) ;
#51171=CARTESIAN_POINT ( 'NONE',  ( 25.39687500061451431, -3.027376345333614438, 5.243569643749998122 ) ) ;
#51172=CARTESIAN_POINT ( 'NONE',  ( -3.000416591977282496E-16, 18.34062500061459389, -34.90005215228797653 ) ) ;
#51173=CARTESIAN_POINT ( 'NONE',  ( 11.55000000000000071, 0.000000000000000000, 4.999999999999998224 ) ) ;
#51174=CARTESIAN_POINT ( 'NONE',  ( 8.578125000614518214, 4.541064518000418104, 2.621784821874999949 ) ) ;
#51176=CARTESIAN_POINT ( 'NONE',  ( 4.000000000000000000, 11.18750000000000178, 32.30940107675849760 ) ) ;
#51177=CARTESIAN_POINT ( 'NONE',  ( 27.36562500061451786, 3.027376345333612662, -5.243569643749998122 ) ) ;
#51178=CARTESIAN_POINT ( 'NONE',  ( -1.071796769724487453, 18.10759618943233207, 26.00000000000000000 ) ) ;
#51180=CARTESIAN_POINT ( 'NONE',  ( 18.45937500061451431, 4.541064518000418104, -2.621784821874998173 ) ) ;
#51181=CARTESIAN_POINT ( 'NONE',  ( -4.243569643749999898, 13.55937500061451750, 30.00000000000000000 ) ) ;
#51182=CARTESIAN_POINT ( 'NONE',  ( 18.30937500061451928, -4.541064518000417216, -2.621784821875001281 ) ) ;
#51183=CARTESIAN_POINT ( 'NONE',  ( 27.72187500061451715, -6.054752690667223547, -1.112240025338166033E-15 ) ) ;
#51184=CARTESIAN_POINT ( 'NONE',  ( -2.121784821874999949, 17.08437500061451786, 26.32496088578401938 ) ) ;
#51185=CARTESIAN_POINT ( 'NONE',  ( 9.253125000614517148, -4.541064518000417216, -2.621784821875001281 ) ) ;
#51188=CARTESIAN_POINT ( 'NONE',  ( 5.109375000614518214, 0.000000000000000000, 5.243569643749999010 ) ) ;
#51190=CARTESIAN_POINT ( 'NONE',  ( 8.503125000614515372, 4.541064518000418104, -2.621784821874998173 ) ) ;
#51191=CARTESIAN_POINT ( 'NONE',  ( 12.42187500061451821, -6.054752690667223547, -1.112240025338166033E-15 ) ) ;
#51193=CARTESIAN_POINT ( 'NONE',  ( 19.87500000122903288, -5.773502691896255534, -1.060575238724906372E-15 ) ) ;
#51194=CARTESIAN_POINT ( 'NONE',  ( 5.746875000614517504, -3.027376345333610441, -5.243569643749999898 ) ) ;
#51195=CARTESIAN_POINT ( 'NONE',  ( 7.640625000614517326, 6.054752690667223547, 3.707466751127219781E-16 ) ) ;
#51196=CARTESIAN_POINT ( 'NONE',  ( 4.162500001229033408, -4.330127018922190985, -2.500000000000001332 ) ) ;
#51198=CARTESIAN_POINT ( 'NONE',  ( 20.22187500061451715, 3.027376345333613106, -5.243569643749998122 ) ) ;
#51199=CARTESIAN_POINT ( 'NONE',  ( -1.999999999999997113, 11.63750000122903394, 33.46410161513775705 ) ) ;
#51200=ORIENTED_EDGE ( 'NONE', *, *, #19674, .T. ) ;
#51201=CARTESIAN_POINT ( 'NONE',  ( 24.44062500061451715, -3.027376345333614438, 5.243569643749998122 ) ) ;
#51202=CARTESIAN_POINT ( 'NONE',  ( 11.80312500061451608, 0.000000000000000000, 5.243569643749999010 ) ) ;
#51203=CARTESIAN_POINT ( 'NONE',  ( 29.37187500061451928, 3.027376345333611329, 5.243569643749999010 ) ) ;
#51204=CARTESIAN_POINT ( 'NONE',  ( 11.87812500061451537, -4.541064518000419881, 2.621784821874995952 ) ) ;
#51205=CARTESIAN_POINT ( 'NONE',  ( 4.492182058117979437, -2.195518243313848039, -4.590536574672159809 ) ) ;
#51206=ADVANCED_FACE ( 'NONE', ( #56214 ), #28143, .F. ) ;
#51207=( BOUNDED_CURVE ( )  B_SPLINE_CURVE ( 2, ( #68032, #81, #39595, #17402, #4886, #68390, #50677 ),
 .UNSPECIFIED., .F., .F. ) 
 B_SPLINE_CURVE_WITH_KNOTS ( ( 3, 2, 2, 3 ),
 ( 0.5749999999999999556, 0.5777777777777777235, 0.5805555555555557135, 0.5833333333333334814 ),
 .UNSPECIFIED. ) 
 CURVE ( )  GEOMETRIC_REPRESENTATION_ITEM ( )  RATIONAL_B_SPLINE_CURVE ( ( 1.000000000000000000, 0.8660254037844387076, 1.000000000000000000, 0.8660254037844387076, 1.000000000000000000, 0.8660254037844333785, 1.000000000000005329 ) ) 
 REPRESENTATION_ITEM ( '' )  );
#51208=CARTESIAN_POINT ( 'NONE',  ( 11.96250000122903501, 4.330127018922192761, -2.499999999999997780 ) ) ;
#51209=CARTESIAN_POINT ( 'NONE',  ( 27.25312500061451360, -4.541064518000417216, -2.621784821875001281 ) ) ;
#51210=CARTESIAN_POINT ( 'NONE',  ( -4.243569643749999898, 13.01562500061451999, -32.45002607614398471 ) ) ;
#51211=CARTESIAN_POINT ( 'NONE',  ( 15.15000000122903323, 5.773502691896255534, 3.535250795749688894E-16 ) ) ;
#51212=CARTESIAN_POINT ( 'NONE',  ( 10.80000000000000071, -4.330127018922190985, -2.500000000000001332 ) ) ;
#51213=CARTESIAN_POINT ( 'NONE',  ( 21.06562500061451715, 3.027376345333613106, -5.243569643749998122 ) ) ;
#51214=CARTESIAN_POINT ( 'NONE',  ( 8.371875000614515727, -6.054752690667223547, -1.112240025338166033E-15 ) ) ;
#51215=CARTESIAN_POINT ( 'NONE',  ( 7.087500001229034119, 4.330127018922191873, 2.499999999999999556 ) ) ;
#51216=CARTESIAN_POINT ( 'NONE',  ( 17.21250000122903145, -4.330127018922190985, -2.500000000000001332 ) ) ;
#51217=CARTESIAN_POINT ( 'NONE',  ( 13.97812500061451679, 4.541064518000418104, 2.621784821874999949 ) ) ;
#51218=CARTESIAN_POINT ( 'NONE',  ( 15.81562500061451537, 3.027376345333611329, 5.243569643749999010 ) ) ;
#51219=CARTESIAN_POINT ( 'NONE',  ( 25.05000000122903714, 5.773502691896255534, 3.535250795749688894E-16 ) ) ;
#51220=CARTESIAN_POINT ( 'NONE',  ( 20.92500000000000071, 4.330127018922191873, 2.499999999999999556 ) ) ;
#51221=CARTESIAN_POINT ( 'NONE',  ( 22.80937500061451573, -4.541064518000417216, -2.621784821875001281 ) ) ;
#51222=FACE_OUTER_BOUND ( 'NONE', #67159, .T. ) ;
#51223=CARTESIAN_POINT ( 'NONE',  ( 9.712500001229033231, 4.330127018922192761, -2.499999999999997780 ) ) ;
#51224=CARTESIAN_POINT ( 'NONE',  ( 27.42187500061451644, 3.027376345333613106, -5.243569643749998122 ) ) ;
#51226=CARTESIAN_POINT ( 'NONE',  ( 23.61562500061451431, -6.054752690667223547, -1.112240025338166033E-15 ) ) ;
#51229=CARTESIAN_POINT ( 'NONE',  ( 8.671875000614518214, 3.027376345333611329, 5.243569643749999010 ) ) ;
#51230=CARTESIAN_POINT ( 'NONE',  ( 16.01250000000000284, 2.886751345948060266, 5.000000000000114575 ) ) ;
#51231=CARTESIAN_POINT ( 'NONE',  ( 27.40312500061451573, 4.541064518000418104, -2.621784821874998173 ) ) ;
#51232=CARTESIAN_POINT ( 'NONE',  ( 6.496875000614517504, -3.027376345333614438, 5.243569643749998122 ) ) ;
#51233=CARTESIAN_POINT ( 'NONE',  ( -1.487416814333745711E-14, 16.62500000122903288, -26.00000000000000000 ) ) ;
#51234=CARTESIAN_POINT ( 'NONE',  ( 25.43437500061451573, -4.541064518000419881, 2.621784821874995952 ) ) ;
#51235=CARTESIAN_POINT ( 'NONE',  ( -2.121784821874999949, 11.17812500061459602, 26.32496088578401938 ) ) ;
#51236=CARTESIAN_POINT ( 'NONE',  ( 19.08750000000000213, 5.773502691896255534, 3.535250795749688894E-16 ) ) ;
#51237=ORIENTED_EDGE ( 'NONE', *, *, #55966, .F. ) ;
#51238=CARTESIAN_POINT ( 'NONE',  ( 26.36249999999999716, 2.886751345948126879, 4.999999999999999112 ) ) ;
#51239=( BOUNDED_CURVE ( )  B_SPLINE_CURVE ( 3, ( #33243, #48785, #15877, #72401 ),
 .UNSPECIFIED., .F., .F. ) 
 B_SPLINE_CURVE_WITH_KNOTS ( ( 4, 4 ),
 ( 2.610771512460038579, 2.658599815149916612 ),
 .UNSPECIFIED. ) 
 CURVE ( )  GEOMETRIC_REPRESENTATION_ITEM ( )  RATIONAL_B_SPLINE_CURVE ( ( 1.000000000000000000, 0.9998093802064862423, 0.9998093802064862423, 1.000000000000000000 ) ) 
 REPRESENTATION_ITEM ( '' )  );
#51240=CARTESIAN_POINT ( 'NONE',  ( 28.24687500061451573, -3.027376345333610441, -5.243569643749999898 ) ) ;
#51241=EDGE_LOOP ( 'NONE', ( #38145, #36925, #27527, #21925 ) ) ;
#51242=CARTESIAN_POINT ( 'NONE',  ( 14.76562500061451821, 3.027376345333613106, -5.243569643749998122 ) ) ;
#51243=CARTESIAN_POINT ( 'NONE',  ( 7.865625000614516971, -6.054752690667223547, -1.112240025338166033E-15 ) ) ;
#51245=CARTESIAN_POINT ( 'NONE',  ( 4.659375000614518925, 0.000000000000000000, 5.243569643749999010 ) ) ;
#51246=CARTESIAN_POINT ( 'NONE',  ( 17.58750000122903145, -4.330127018922194537, 2.499999999999995559 ) ) ;
#51247=CARTESIAN_POINT ( 'NONE',  ( 21.86250000000000071, 2.886751345948126879, 4.999999999999999112 ) ) ;
#51248=CARTESIAN_POINT ( 'NONE',  ( 29.39999999999999858, 4.330127018922192761, -2.499999999999997780 ) ) ;
#51249=CARTESIAN_POINT ( 'NONE',  ( 4.396875000614516971, -3.027376345333610441, -5.243569643749999898 ) ) ;
#51250=CARTESIAN_POINT ( 'NONE',  ( 11.40937500061451892, 0.000000000000000000, 5.243569643749999010 ) ) ;
#51251=CARTESIAN_POINT ( 'NONE',  ( 22.43437500061451573, 6.421520780324663323E-16, -5.243569643749999010 ) ) ;
#51252=EDGE_CURVE ( 'NONE', #55622, #44045, #38778, .T. ) ;
#51253=FACE_OUTER_BOUND ( 'NONE', #14812, .T. ) ;
#51255=CARTESIAN_POINT ( 'NONE',  ( 3.534375000614518036, 6.421520780324663323E-16, -5.243569643749999010 ) ) ;
#51256=CARTESIAN_POINT ( 'NONE',  ( 7.209375000614519635, 4.541064518000418104, -2.621784821874998173 ) ) ;
#51257=CARTESIAN_POINT ( 'NONE',  ( 19.23749999999999716, -2.886751345948129988, 4.999999999999997335 ) ) ;
#51258=CARTESIAN_POINT ( 'NONE',  ( 16.34062500061451573, -3.027376345333614438, 5.243569643749998122 ) ) ;
#51262=CARTESIAN_POINT ( 'NONE',  ( 9.853125000614516793, 4.541064518000418104, -2.621784821874998173 ) ) ;
#51263=CARTESIAN_POINT ( 'NONE',  ( 25.65937500061451715, 4.541064518000418104, -2.621784821874998173 ) ) ;
#51264=DIRECTION ( 'NONE',  ( -0.000000000000000000, -1.000000000000000000, -0.000000000000000000 ) ) ;
#51265=CARTESIAN_POINT ( 'NONE',  ( 27.30937500061451573, -4.541064518000417216, -2.621784821875001281 ) ) ;
#51266=CARTESIAN_POINT ( 'NONE',  ( 10.38750000000000107, -2.886751345948125991, -5.000000000000000000 ) ) ;
#51267=CARTESIAN_POINT ( 'NONE',  ( 3.999999999999998668, 13.62500000122903288, 27.69059892324149175 ) ) ;
#51268=CARTESIAN_POINT ( 'NONE',  ( 10.05000000122903181, -2.886751345948125991, -5.000000000000000000 ) ) ;
#51269=CARTESIAN_POINT ( 'NONE',  ( 21.00937500061451857, -4.541064518000417216, -2.621784821875001281 ) ) ;
#51270=CARTESIAN_POINT ( 'NONE',  ( 14.55937500061451573, 0.000000000000000000, 5.243569643749999010 ) ) ;
#51271=CARTESIAN_POINT ( 'NONE',  ( -0.5556303621801368386, 4.970948098741851062, -33.96363479047759881 ) ) ;
#51272=ORIENTED_EDGE ( 'NONE', *, *, #29804, .F. ) ;
#51273=CARTESIAN_POINT ( 'NONE',  ( 15.29062500061451679, 6.054752690667223547, 3.707466751127219781E-16 ) ) ;
#51274=CARTESIAN_POINT ( 'NONE',  ( 25.87500000122903288, 2.886751345948129099, -4.999999999999998224 ) ) ;
#51275=CARTESIAN_POINT ( 'NONE',  ( 12.53437500061451537, 6.421520780324663323E-16, -5.243569643749999010 ) ) ;
#51276=CARTESIAN_POINT ( 'NONE',  ( 3.680627977383744920, 9.304151242747316530, -34.75401982126012967 ) ) ;
#51277=CARTESIAN_POINT ( 'NONE',  ( 17.31562500061451715, -6.054752690667223547, -1.112240025338166033E-15 ) ) ;
#51278=CARTESIAN_POINT ( 'NONE',  ( 3.999999999999999112, 18.87500000000000000, -30.00000000000000000 ) ) ;
#51279=CARTESIAN_POINT ( 'NONE',  ( 26.10937500061451644, 4.541064518000418104, -2.621784821874998173 ) ) ;
#51280=CARTESIAN_POINT ( 'NONE',  ( 9.001249775931846008E-16, 10.01562500061451644, 34.90005215228797653 ) ) ;
#51281=AXIS2_PLACEMENT_3D ( 'NONE', #1901, #42503, #7786 ) ;
#51282=CARTESIAN_POINT ( 'NONE',  ( 12.33750000122903145, 6.123233995736764310E-16, -4.999999999999998224 ) ) ;
#51283=DIRECTION ( 'NONE',  ( -1.000000000000000000, -0.000000000000000000, -0.000000000000000000 ) ) ;
#51284=CARTESIAN_POINT ( 'NONE',  ( 4.243569643749999010, 17.87187500061451928, -32.45002607614398471 ) ) ;
#51285=CARTESIAN_POINT ( 'NONE',  ( 17.44687500061451857, -3.027376345333610441, -5.243569643749999898 ) ) ;
#51286=CARTESIAN_POINT ( 'NONE',  ( 21.22500000122903074, -5.773502691896255534, -1.060575238724906372E-15 ) ) ;
#51288=CARTESIAN_POINT ( 'NONE',  ( 14.67187500061451821, -6.054752690667223547, -1.112240025338166033E-15 ) ) ;
#51289=CARTESIAN_POINT ( 'NONE',  ( -4.243569643749999898, 9.921875000614519990, 27.54997392385601529 ) ) ;
#51290=CARTESIAN_POINT ( 'NONE',  ( 21.37500000122902932, 2.886751345948129099, -4.999999999999998224 ) ) ;
#51291=CARTESIAN_POINT ( 'NONE',  ( 14.16562500061451679, -6.054752690667223547, -1.112240025338166033E-15 ) ) ;
#51294=ORIENTED_EDGE ( 'NONE', *, *, #23299, .F. ) ;
#51295=CARTESIAN_POINT ( 'NONE',  ( 19.91250000000000142, 2.886751345948129099, -4.999999999999998224 ) ) ;
#51297=CARTESIAN_POINT ( 'NONE',  ( 3.778125000614519280, -4.541064518000419881, 2.621784821874995952 ) ) ;
#51298=CARTESIAN_POINT ( 'NONE',  ( 16.16250000122903430, 0.000000000000000000, 4.999999999999998224 ) ) ;
#51299=CARTESIAN_POINT ( 'NONE',  ( 20.31562500061451715, 3.027376345333611329, 5.243569643749999010 ) ) ;
#51300=CARTESIAN_POINT ( 'NONE',  ( 22.11562500061451786, 3.027376345333611329, 5.243569643749999010 ) ) ;
#51301=CARTESIAN_POINT ( 'NONE',  ( 3.103125000614517237, 4.541064518000418104, -2.621784821874998173 ) ) ;
#51302=CARTESIAN_POINT ( 'NONE',  ( 29.96250000000000213, 2.886751345948126879, 4.999999999999999112 ) ) ;
#51303=CARTESIAN_POINT ( 'NONE',  ( 1.626862140677534273E-15, 11.67500000122903181, 34.00000000000000000 ) ) ;
#51306=CARTESIAN_POINT ( 'NONE',  ( 3.999999999999999112, 11.78750000122903430, -30.00000000000000000 ) ) ;
#51307=CARTESIAN_POINT ( 'NONE',  ( 2.121784821874999061, 18.80937500061451928, -33.67503911421598417 ) ) ;
#51308=CARTESIAN_POINT ( 'NONE',  ( 7.087500001229034119, 4.330127018922191873, 2.499999999999999556 ) ) ;
#51309=CARTESIAN_POINT ( 'NONE',  ( 7.987500000000000711, -2.886751345948129988, 4.999999999999997335 ) ) ;
#51310=EDGE_CURVE ( 'NONE', #15563, #58630, #33579, .T. ) ;
#51311=CARTESIAN_POINT ( 'NONE',  ( 4.237500001229036251, 6.123233995736764310E-16, -4.999999999999998224 ) ) ;
#51312=CARTESIAN_POINT ( 'NONE',  ( 11.07187500061451679, -6.054752690667223547, -1.112240025338166033E-15 ) ) ;
#51313=CARTESIAN_POINT ( 'NONE',  ( 19.50000000122903288, -2.886751345948126435, -5.000000000000000000 ) ) ;
#51314=CARTESIAN_POINT ( 'NONE',  ( 3.721875000614518036, 3.027376345333611329, 5.243569643749999010 ) ) ;
#51315=CARTESIAN_POINT ( 'NONE',  ( 1.999999999999998668, 19.06250000122903288, 26.53589838486224650 ) ) ;
#51317=CARTESIAN_POINT ( 'NONE',  ( -2.000000000000000000, 19.58750000122903501, -33.46410161513775705 ) ) ;
#51318=CARTESIAN_POINT ( 'NONE',  ( 11.18437500061451928, 6.421520780324663323E-16, -5.243569643749999010 ) ) ;
#51319=CARTESIAN_POINT ( 'NONE',  ( 13.62187500061451750, 3.027376345333611329, 5.243569643749999010 ) ) ;
#51320=CARTESIAN_POINT ( 'NONE',  ( 4.898587196589411843E-16, 20.00000000000000000, 33.99999999999999289 ) ) ;
#51321=CARTESIAN_POINT ( 'NONE',  ( 7.575000000000001954, -4.330127018922194537, 2.499999999999995559 ) ) ;
#51322=CARTESIAN_POINT ( 'NONE',  ( 4.243569643749999010, 17.81562500061459531, 27.54997392385601174 ) ) ;
#51323=CARTESIAN_POINT ( 'NONE',  ( 20.93437500061451573, -4.541064518000419881, 2.621784821874995952 ) ) ;
#51325=CARTESIAN_POINT ( 'NONE',  ( 27.26250000122903216, 4.330127018922192761, -2.499999999999997780 ) ) ;
#51326=VECTOR ( 'NONE', #21711, 1000.000000000000000 ) ;
#51328=CARTESIAN_POINT ( 'NONE',  ( 22.75312500061451360, -4.541064518000417216, -2.621784821875001281 ) ) ;
#51329=CARTESIAN_POINT ( 'NONE',  ( 16.07812500061451289, 6.421520780324663323E-16, -5.243569643749999010 ) ) ;
#51331=CARTESIAN_POINT ( 'NONE',  ( 12.00937500061451857, -4.541064518000417216, -2.621784821875001281 ) ) ;
#51332=CARTESIAN_POINT ( 'NONE',  ( 27.41250000000000142, -5.773502691896255534, -1.060575238724906372E-15 ) ) ;
#51333=CARTESIAN_POINT ( 'NONE',  ( 24.03750000122903430, 6.123233995736764310E-16, -4.999999999999998224 ) ) ;
#51334=FACE_OUTER_BOUND ( 'NONE', #60500, .T. ) ;
#51335=CARTESIAN_POINT ( 'NONE',  ( 10.88437500061451679, 4.541064518000418104, 2.621784821874999949 ) ) ;
#51336=CARTESIAN_POINT ( 'NONE',  ( 29.14687500061451075, -3.027376345333610441, -5.243569643749999898 ) ) ;
#51337=CARTESIAN_POINT ( 'NONE',  ( 4.096875000614518925, 6.054752690667223547, 3.707466751127219781E-16 ) ) ;
#51338=CARTESIAN_POINT ( 'NONE',  ( -1.071796769724488563, 12.44240381056766864, -26.00000000000000000 ) ) ;
#51339=CARTESIAN_POINT ( 'NONE',  ( 22.62187500061451573, 3.027376345333611329, 5.243569643749999010 ) ) ;
#51340=CARTESIAN_POINT ( 'NONE',  ( 14.89687500061451786, 6.054752690667223547, 3.707466751127219781E-16 ) ) ;
#51342=CARTESIAN_POINT ( 'NONE',  ( 26.92499999999999716, -4.330127018922194537, 2.499999999999995559 ) ) ;
#51343=CARTESIAN_POINT ( 'NONE',  ( 4.500000001229034652, -2.886751345948129988, 4.999999999999997335 ) ) ;
#51345=CARTESIAN_POINT ( 'NONE',  ( 17.95312500061451644, 4.541064518000418104, -2.621784821874998173 ) ) ;
#51346=CARTESIAN_POINT ( 'NONE',  ( 5.924999999999999822, 6.123233995736764310E-16, -4.999999999999998224 ) ) ;
#51347=CARTESIAN_POINT ( 'NONE',  ( 16.19999999999999929, -4.330127018922190985, -2.500000000000001332 ) ) ;
#51348=CARTESIAN_POINT ( 'NONE',  ( 4.243569643749999898, 12.34062500061451750, 32.45002607614398471 ) ) ;
#51350=CARTESIAN_POINT ( 'NONE',  ( 21.07500000122903572, 2.886751345948126879, 4.999999999999999112 ) ) ;
#51351=CARTESIAN_POINT ( 'NONE',  ( 26.67187500061451644, 3.027376345333611329, 5.243569643749999010 ) ) ;
#51353=CARTESIAN_POINT ( 'NONE',  ( 22.52812500061451573, 4.541064518000418104, 2.621784821874999949 ) ) ;
#51354=CARTESIAN_POINT ( 'NONE',  ( 23.07187500061451857, 3.027376345333611329, 5.243569643749999010 ) ) ;
#51355=CARTESIAN_POINT ( 'NONE',  ( 4.050000000000001599, -4.330127018922190985, -2.500000000000001332 ) ) ;
#51356=CARTESIAN_POINT ( 'NONE',  ( 6.253125000614517148, 4.541064518000418104, -2.621784821874998173 ) ) ;
#51357=CARTESIAN_POINT ( 'NONE',  ( 24.62812500061451715, 6.421520780324663323E-16, -5.243569643749999010 ) ) ;
#51358=CARTESIAN_POINT ( 'NONE',  ( 11.67187500061451821, 3.027376345333613106, -5.243569643749998122 ) ) ;
#51359=CARTESIAN_POINT ( 'NONE',  ( 17.52187500061451431, 3.027376345333613106, -5.243569643749998122 ) ) ;
#51360=CARTESIAN_POINT ( 'NONE',  ( -3.000416591977282496E-16, 17.44062500061451360, 25.09994784771203058 ) ) ;
#51361=ADVANCED_FACE ( 'NONE', ( #41393 ), #34385, .F. ) ;
#51362=CARTESIAN_POINT ( 'NONE',  ( 21.56250000122903288, 0.000000000000000000, 4.999999999999998224 ) ) ;
#51364=CARTESIAN_POINT ( 'NONE',  ( 10.37812500061451715, 4.541064518000418104, 2.621784821874999949 ) ) ;
#51365=CARTESIAN_POINT ( 'NONE',  ( 6.459375000614518747, 0.000000000000000000, 5.243569643749999010 ) ) ;
#51366=CARTESIAN_POINT ( 'NONE',  ( 4.434375000614519280, 6.421520780324663323E-16, -5.243569643749999010 ) ) ;
#51367=ORIENTED_EDGE ( 'NONE', *, *, #42313, .T. ) ;
#51368=CARTESIAN_POINT ( 'NONE',  ( 25.20937500061451431, 4.541064518000418104, -2.621784821874998173 ) ) ;
#51369=CARTESIAN_POINT ( 'NONE',  ( 18.10312500061451502, 0.000000000000000000, 5.243569643749999010 ) ) ;
#51370=CARTESIAN_POINT ( 'NONE',  ( 26.51250000122903216, 0.000000000000000000, 4.999999999999998224 ) ) ;
#51371=CARTESIAN_POINT ( 'NONE',  ( 27.81562500061452070, 3.027376345333613106, -5.243569643749998122 ) ) ;
#51372=CARTESIAN_POINT ( 'NONE',  ( 20.70937500061451786, 4.541064518000418104, -2.621784821874998173 ) ) ;
#51373=CARTESIAN_POINT ( 'NONE',  ( 16.04062500061451857, -3.027376345333610441, -5.243569643749999898 ) ) ;
#51374=CARTESIAN_POINT ( 'NONE',  ( -3.000416591977282496E-16, 18.84687500061452070, 25.09994784771203058 ) ) ;
#51376=CARTESIAN_POINT ( 'NONE',  ( 22.07812500061451644, 4.541064518000418104, 2.621784821874999949 ) ) ;
#51377=CARTESIAN_POINT ( 'NONE',  ( 3.150000001229034119, -2.886751345948129988, 4.999999999999997335 ) ) ;
#51378=ORIENTED_EDGE ( 'NONE', *, *, #44687, .F. ) ;
#51379=CARTESIAN_POINT ( 'NONE',  ( 27.07499999999999929, 6.123233995736764310E-16, -4.999999999999998224 ) ) ;
#51380=CARTESIAN_POINT ( 'NONE',  ( -1.999999999999997113, 12.87500000000000178, -26.53589838486224295 ) ) ;
#51382=CARTESIAN_POINT ( 'NONE',  ( 28.34062500061451928, 6.054752690667223547, 3.707466751127219781E-16 ) ) ;
#51383=CARTESIAN_POINT ( 'NONE',  ( 11.27812500061451573, 4.541064518000418104, 2.621784821874999949 ) ) ;
#51384=CARTESIAN_POINT ( 'NONE',  ( 22.38750000122903216, 4.330127018922191873, 2.499999999999999556 ) ) ;
#51385=CARTESIAN_POINT ( 'NONE',  ( 27.70312500061451289, -4.541064518000417216, -2.621784821875001281 ) ) ;
#51386=CARTESIAN_POINT ( 'NONE',  ( 28.68749999999999645, -2.886751345948129988, 4.999999999999997335 ) ) ;
#51387=CARTESIAN_POINT ( 'NONE',  ( -3.999999999999997335, 17.90000000122903501, -27.69059892324149175 ) ) ;
#51388=DIRECTION ( 'NONE',  ( -1.000000000000000000, -0.000000000000000000, -0.000000000000000000 ) ) ;
#51389=CARTESIAN_POINT ( 'NONE',  ( 13.79062500061451502, -3.027376345333610441, -5.243569643749999898 ) ) ;
#51390=ORIENTED_EDGE ( 'NONE', *, *, #24843, .T. ) ;
#51391=VECTOR ( 'NONE', #68866, 1000.000000000000000 ) ;
#51392=CARTESIAN_POINT ( 'NONE',  ( 8.128125000614515372, 4.541064518000418104, 2.621784821874999949 ) ) ;
#51394=CARTESIAN_POINT ( 'NONE',  ( 5.615625000614517859, -6.054752690667223547, -1.112240025338166033E-15 ) ) ;
#51397=CARTESIAN_POINT ( 'NONE',  ( 16.05000000000000071, 0.000000000000000000, 4.999999999999998224 ) ) ;
#51399=CARTESIAN_POINT ( 'NONE',  ( 15.64687500061451608, -3.027376345333610441, -5.243569643749999898 ) ) ;
#51400=CARTESIAN_POINT ( 'NONE',  ( 10.68750000122903288, 4.330127018922191873, 2.499999999999999556 ) ) ;
#51401=CARTESIAN_POINT ( 'NONE',  ( 19.73437500061451644, 6.421520780324663323E-16, -5.243569643749999010 ) ) ;
#51403=CARTESIAN_POINT ( 'NONE',  ( 21.68437500061451573, 4.541064518000418104, 2.621784821874999949 ) ) ;
#51404=CARTESIAN_POINT ( 'NONE',  ( 9.001249775931846008E-16, 13.61562500061451786, -25.09994784771203058 ) ) ;
#51405=DIRECTION ( 'NONE',  ( 0.000000000000000000, 0.000000000000000000, -1.000000000000000000 ) ) ;
#51407=CARTESIAN_POINT ( 'NONE',  ( 1.626862140677534273E-15, 13.02500000122903501, -26.00000000000000355 ) ) ;
#51408=CARTESIAN_POINT ( 'NONE',  ( 26.27812500061451573, -4.541064518000419881, 2.621784821874995952 ) ) ;
#51409=( LENGTH_UNIT ( ) NAMED_UNIT ( * ) SI_UNIT ( .MILLI., .METRE. ) );
#51410=CARTESIAN_POINT ( 'NONE',  ( 28.20937500061451786, -4.541064518000417216, -2.621784821875001281 ) ) ;
#51411=EDGE_CURVE ( 'NONE', #52162, #56056, #56237, .T. ) ;
#51412=CARTESIAN_POINT ( 'NONE',  ( 23.69999999999999929, 0.000000000000000000, 4.999999999999998224 ) ) ;
#51413=CARTESIAN_POINT ( 'NONE',  ( 6.928125000614516082, -4.541064518000419881, 2.621784821874995952 ) ) ;
#51415=CARTESIAN_POINT ( 'NONE',  ( 19.84687500061451360, 6.054752690667223547, 3.707466751127219781E-16 ) ) ;
#51418=CARTESIAN_POINT ( 'NONE',  ( 4.790625000614518569, -3.027376345333610441, -5.243569643749999898 ) ) ;
#51419=CARTESIAN_POINT ( 'NONE',  ( 10.20937500061451786, -4.541064518000417216, -2.621784821875001281 ) ) ;
#51420=VERTEX_POINT ( 'NONE', #45849 ) ;
#51421=CARTESIAN_POINT ( 'NONE',  ( 21.30937500061451573, 0.000000000000000000, 5.243569643749999010 ) ) ;
#51422=CARTESIAN_POINT ( 'NONE',  ( 3.193447721043152665, 3.847322660365763536, 3.562742055761627835 ) ) ;
#51423=CARTESIAN_POINT ( 'NONE',  ( 29.36250000000000071, 2.886751345948129099, -4.999999999999998224 ) ) ;
#51424=CARTESIAN_POINT ( 'NONE',  ( 29.18437500061451573, 6.421520780324663323E-16, -5.243569643749999010 ) ) ;
#51426=CARTESIAN_POINT ( 'NONE',  ( 27.86249999999999716, -5.773502691896255534, -1.060575238724906372E-15 ) ) ;
#51427=VERTEX_POINT ( 'NONE', #1516 ) ;
#51428=CARTESIAN_POINT ( 'NONE',  ( 9.337500000000000355, -2.886751345948129988, 4.999999999999997335 ) ) ;
#51430=CARTESIAN_POINT ( 'NONE',  ( 24.17812500061451786, 6.421520780324663323E-16, -5.243569643749999010 ) ) ;
#51431=CARTESIAN_POINT ( 'NONE',  ( 14.06250000000000000, 2.886751345948129099, -4.999999999999998224 ) ) ;
#51432=CARTESIAN_POINT ( 'NONE',  ( 10.95000000122903394, -2.886751345948125991, -5.000000000000000000 ) ) ;
#51433=CARTESIAN_POINT ( 'NONE',  ( 8.503125000614515372, 4.541064518000418104, -2.621784821874998173 ) ) ;
#51434=CARTESIAN_POINT ( 'NONE',  ( 23.88749999999999929, -2.886751345948125991, -5.000000000000000000 ) ) ;
#51435=CARTESIAN_POINT ( 'NONE',  ( 20.95312500061451999, -4.541064518000417216, -2.621784821875001281 ) ) ;
#51436=CARTESIAN_POINT ( 'NONE',  ( 18.75000000122903288, 5.773502691896255534, 3.535250795749688401E-16 ) ) ;
#51437=CARTESIAN_POINT ( 'NONE',  ( 28.27500000122903145, 2.886751345948126879, 4.999999999999999112 ) ) ;
#51439=CARTESIAN_POINT ( 'NONE',  ( 7.425000000000000711, 4.330127018922191873, 2.499999999999999556 ) ) ;
#51441=CARTESIAN_POINT ( 'NONE',  ( 21.32812500061451644, -4.541064518000419881, 2.621784821874995952 ) ) ;
#51442=CARTESIAN_POINT ( 'NONE',  ( 3.361055028349045237, -3.701798089632991839, -3.568395224226307061 ) ) ;
#51443=CARTESIAN_POINT ( 'NONE',  ( 28.47187500061451715, 3.027376345333611329, 5.243569643749999010 ) ) ;
#51444=CARTESIAN_POINT ( 'NONE',  ( 19.02187500061451786, 3.027376345333611329, 5.243569643749999010 ) ) ;
#51445=CARTESIAN_POINT ( 'NONE',  ( 16.30312500061451786, 0.000000000000000000, 5.243569643749999010 ) ) ;
#51446=CARTESIAN_POINT ( 'NONE',  ( 4.243569643749999898, 10.09062500061459566, -27.54997392385601529 ) ) ;
#51447=CARTESIAN_POINT ( 'NONE',  ( 5.278125000614516615, 6.421520780324663323E-16, -5.243569643749999010 ) ) ;
#51448=( BOUNDED_CURVE ( )  B_SPLINE_CURVE ( 2, ( #13497, #52673, #18675, #41237, #35677, #63749, #57840, #70396, #2081 ),
 .UNSPECIFIED., .F., .F. ) 
 B_SPLINE_CURVE_WITH_KNOTS ( ( 3, 2, 2, 2, 3 ),
 ( 0.6847826086956522174, 0.6884057971014492239, 0.6956521739130434590, 0.7028985507246376940, 0.7065217391304348116 ),
 .UNSPECIFIED. ) 
 CURVE ( )  GEOMETRIC_REPRESENTATION_ITEM ( )  RATIONAL_B_SPLINE_CURVE ( ( 0.9330127018922192983, 0.9330127018922202975, 1.000000000000000000, 0.8660254037844387076, 1.000000000000000000, 0.8660254037844387076, 1.000000000000000000, 0.9330127018922194093, 0.9330127018922194093 ) ) 
 REPRESENTATION_ITEM ( '' )  );
#51449=CARTESIAN_POINT ( 'NONE',  ( 27.60000000122903430, -2.886751345948125991, -5.000000000000000000 ) ) ;
#51451=CARTESIAN_POINT ( 'NONE',  ( 18.74062500061451431, -3.027376345333610441, -5.243569643749999898 ) ) ;
#51452=CARTESIAN_POINT ( 'NONE',  ( 27.18750000122903288, 6.123233995736764310E-16, -4.999999999999998224 ) ) ;
#51453=CARTESIAN_POINT ( 'NONE',  ( 3.337500001229034563, 6.123233995736764310E-16, -4.999999999999998224 ) ) ;
#51454=CARTESIAN_POINT ( 'NONE',  ( 12.94687500061451857, -3.027376345333610441, -5.243569643749999898 ) ) ;
#51455=CARTESIAN_POINT ( 'NONE',  ( 12.98437500061451821, 6.421520780324663323E-16, -5.243569643749999010 ) ) ;
#51456=CARTESIAN_POINT ( 'NONE',  ( 20.70937500061451786, 4.541064518000418104, -2.621784821874998173 ) ) ;
#51457=VERTEX_POINT ( 'NONE', #62826 ) ;
#51458=CARTESIAN_POINT ( 'NONE',  ( 24.22500000122903430, 2.886751345948093572, 5.000000000000056843 ) ) ;
#51459=CARTESIAN_POINT ( 'NONE',  ( 24.29062500061451502, 6.054752690667223547, 3.707466751127219781E-16 ) ) ;
#51460=CARTESIAN_POINT ( 'NONE',  ( 18.23437500061451999, -4.541064518000419881, 2.621784821874995952 ) ) ;
#51461=CARTESIAN_POINT ( 'NONE',  ( 23.65312500061451573, -4.541064518000417216, -2.621784821875001281 ) ) ;
#51462=CARTESIAN_POINT ( 'NONE',  ( 27.22499999999999787, 4.330127018922191873, 2.499999999999999556 ) ) ;
#51463=CARTESIAN_POINT ( 'NONE',  ( 2.000000000000001332, 16.10000000000000142, 33.46410161513774995 ) ) ;
#51464=CARTESIAN_POINT ( 'NONE',  ( 29.01562500061451644, -6.054752690667223547, -1.112240025338166033E-15 ) ) ;
#51465=CARTESIAN_POINT ( 'NONE',  ( 8.587500001229035007, -4.330127018922194537, 2.499999999999995559 ) ) ;
#51466=CARTESIAN_POINT ( 'NONE',  ( 7.537500001229033408, 4.330127018922191873, 2.499999999999999556 ) ) ;
#51467=CARTESIAN_POINT ( 'NONE',  ( -3.999999999999999112, 19.09999999999999787, -30.00000000000000000 ) ) ;
#51468=CARTESIAN_POINT ( 'NONE',  ( 26.55000000122902648, -2.886751345948129988, 4.999999999999997335 ) ) ;
#51471=CARTESIAN_POINT ( 'NONE',  ( 8.821875000614518569, -6.054752690667223547, -1.112240025338166033E-15 ) ) ;
#51472=CARTESIAN_POINT ( 'NONE',  ( 17.62500000000000000, 6.123233995736764310E-16, -4.999999999999998224 ) ) ;
#51473=EDGE_CURVE ( 'NONE', #16300, #39486, #6321, .T. ) ;
#51474=CARTESIAN_POINT ( 'NONE',  ( 18.06562500061451715, 3.027376345333611329, 5.243569643749999010 ) ) ;
#51475=CARTESIAN_POINT ( 'NONE',  ( 11.10937500061451644, -4.541064518000417216, -2.621784821875001281 ) ) ;
#51476=CARTESIAN_POINT ( 'NONE',  ( 29.21250000122903145, 0.000000000000000000, 4.999999999999998224 ) ) ;
#51477=ADVANCED_FACE ( 'NONE', ( #30303 ), #12219, .T. ) ;
#51478=CARTESIAN_POINT ( 'NONE',  ( 19.84687500061451360, 6.054752690667223547, 3.707466751127219781E-16 ) ) ;
#51479=CARTESIAN_POINT ( 'NONE',  ( 6.534375000614517148, -4.541064518000419881, 2.621784821874995952 ) ) ;
#51481=CARTESIAN_POINT ( 'NONE',  ( 5.850000000000001421, -4.330127018922190985, -2.500000000000001332 ) ) ;
#51482=CARTESIAN_POINT ( 'NONE',  ( 8.540625000614518569, 6.054752690667223547, 3.707466751127219781E-16 ) ) ;
#51483=CARTESIAN_POINT ( 'NONE',  ( 21.06562500061451715, 3.027376345333613106, -5.243569643749998122 ) ) ;
#51484=( BOUNDED_CURVE ( )  B_SPLINE_CURVE ( 2, ( #69518, #19974, #41792, #13341, #53611, #35878, #8543 ),
 .UNSPECIFIED., .F., .F. ) 
 B_SPLINE_CURVE_WITH_KNOTS ( ( 3, 2, 2, 3 ),
 ( 0.2333333333333333648, 0.2361111111111111327, 0.2388888888888889284, 0.2416666666666666963 ),
 .UNSPECIFIED. ) 
 CURVE ( )  GEOMETRIC_REPRESENTATION_ITEM ( )  RATIONAL_B_SPLINE_CURVE ( ( 0.9999999999999986677, 0.8660254037844400399, 1.000000000000000000, 0.8660254037844387076, 1.000000000000000000, 0.8660254037844373753, 1.000000000000001332 ) ) 
 REPRESENTATION_ITEM ( '' )  );
#51486=CARTESIAN_POINT ( 'NONE',  ( 4.912500001229034297, 0.000000000000000000, 4.999999999999998224 ) ) ;
#51487=CARTESIAN_POINT ( 'NONE',  ( 14.39062500061451821, 6.054752690667223547, 3.707466751127219781E-16 ) ) ;
#51488=CARTESIAN_POINT ( 'NONE',  ( 13.22812500061451502, -4.541064518000419881, 2.621784821874995952 ) ) ;
#51490=CARTESIAN_POINT ( 'NONE',  ( 12.26249999999999929, 2.886751345948129099, -4.999999999999998224 ) ) ;
#51491=CARTESIAN_POINT ( 'NONE',  ( 8.062500001229034652, 0.000000000000000000, 4.999999999999998224 ) ) ;
#51492=CARTESIAN_POINT ( 'NONE',  ( 4.865625000614517859, 3.027376345333613106, -5.243569643749998122 ) ) ;
#51493=CARTESIAN_POINT ( 'NONE',  ( 17.47500000122903430, 2.886751345948126879, 4.999999999999999112 ) ) ;
#51495=( BOUNDED_SURFACE ( )  B_SPLINE_SURFACE ( 1, 2, ( 
 ( #6224, #21483, #6594, #28752, #29124, #62371, #23569, #60633, #22837, #45755, #45389, #67925, #18015, #66192, #11410, #44035, #62733, #12125, #15570, #34652, #40211, #5861, #32579, #28393, #68291, #17651, #10045, #50931, #5370, #14343, #5007, #42430, #50073, #38625, #20606, #31341, #70500, #20239, #25802, #36877, #25429, #65312, #44173, #16800, #67439, #53882, #42791, #3641, #14702, #66703, #26165, #59033, #16075, #47972, #61507, #37246, #8435, #59767, #61149, #19877, #3274, #64951, #10544, #59395, #9174, #72605, #33072, #55611, #48340, #8805, #31709, #70865, #54244, #48704, #71227, #27541, #30971, #53506, #21986, #44545, #67076, #16435, #38992, #10904, #2899, #33432, #55976, #27909, #50443, #72968, #22350, #44902, #28267, #34154, #50798, #45979, #201, #560, #51882, #6091, #6815, #11994, #28622, #45625, #45258, #56691, #6452, #17522, #34881, #17165, #68514, #62598, #29349, #69241, #24152, #56343, #28987, #40084, #34517, #52242, #57047, #22706, #67791, #39724, #63318, #925, #17876, #46706, #18231, #62243, #5732, #11639, #39357, #23433, #51159, #57410, #1280, #23070, #51525, #68159, #61871, #29704, #40435, #68875, #12709, #62952, #12346, #23790, #46341, #7176, #40805, #35246, #33799, #57767, #1646, #11279, #9865, #66383, #38299, #44226, #55663, #10959, #5783, #61557, #54936, #33480, #72659, #11331, #67129, #32767, #4342, #22758, #56030, #37937, #26867, #66015, #66759, #16130, #39043, #33849, #16851, #49398, #33126, #50492, #67488, #5059, #5422, #43858, #50128, #10598, #27960, #73018, #71929, #22039, #27596, #15395, #44598, #21304, #39407, #49765, #60456, #38682, #16486, #15759, #60827, #10233, #22402, #55304, #27228, #44950, #4698, #61925, #61203, #72291, #21669, #56393, #28314, #50850, #250, #32396, #23121, #51935, #68568, #12760, #2057, #30117, #62294, #12402, #46032, #23485, #58177, #40490, #56740, #51213, #45675, #69292, #6869, #23844, #52651, #24205, #68211, #11690, #17572, #45310, #29401, #34568, #63376, #57817, #40134, #17927, #29041, #67845, #35657, #63005, #1694, #18655, #57097, #34206, #6506, #34937, #13117, #6142, #7227, #39778, #57463, #28673, #51576, #1332, #41217, #17217, #62648, #12045, #46392, #613, #63725, #68927, #7582, #18284, #975, #40859, #35296, #29756, #52293, #46757, #54482, #60006, #64457, #13470, #9050, #31581, #37485, #14578, #65188, #19008, #69646, #36390, #70731, #14212, #19749, #31946, #43029, #53014, #42663, #7948, #37111, #3146, #59269, #70004, #36019, #58902, #13848, #2408, #64088, #30843, #8677, #24569, #47114, #19374, #8314, #42298, #53377, #53749, #41570, #70371, #54120, #58536, #30485, #59638, #3516, #36749, #47843, #65558, #24929, #26037, #47472, #64824, #31209, #20109, #25672, #48209, #41931, #48576, #71103, #2773, #20476, #25296, #14947, #9416, #39322, #10869, #55579, #60737, #21951, #43403, #4972, #65928, #49310, #50408, #20851, #4253, #71844, #55218, #66664, #44508, #16764, #72565, #15308, #67042, #10512, #22314, #27506, #43768, #37846, #33763, #16402, #48946, #60367, #3883, #4613, #27143, #50039, #44867, #27875, #9776, #44137, #61474, #5335, #16041, #38956, #54844, #61115, #21583, #33402, #55939, #32310, #26778, #38589, #21215, #72932, #67403, #33039, #32679, #61835, #11240, #66292, #15672, #38209, #71475, #10147, #26403, #49677, #72206, #167, #46301, #46666, #34847, #50762, #28588, #51125, #62206, #11602, #62561, #29669, #51844, #1247, #6417, #23033, #41131, #23752, #12674, #1606, #522, #5696, #18565, #45944, #40049, #28949, #29313, #22671, #45222, #68475, #34482, #51488, #57012, #57733, #34119, #28232, #17837, #56659, #11957, #40398, #888, #13030, #62917, #67755, #7139, #23395, #56307, #12312, #57374, #17127, #45588, #39688, #6781, #6053, #17487, #68840, #68122, #18197, #40768, #63282, #35211, #52205, #24117, #69207, #63641, #31120, #13383, #42212, #58817, #3052, #65467, #20392, #52567, #2686, #36303, #13761, #48490, #30756, #47027, #41483, #35928, #59550, #70285, #14124, #42941, #14491, #58450, #1974, #7862, #35569, #19657, #24839, #53660, #48122, #30398, #8228, #19287, #58088, #25950, #53287, #65102, #8961, #47387, #24483, #69917, #25202, #3430, #69562, #70645, #30024, #47750, #18923, #41841, #64736, #31495, #7496, #52927, #2324, #36662, #64003, #54035, #59181, #71014, #8590, #64370, #25583, #20020, #42574, #37025, #60644, #44783, #50322, #54757, #3794, #72474, #21860, #27785, #4883, #55489, #9327, #59921, #26691, #61024, #4527, #10059, #22227, #33315, #43317, #32952, #71386, #27418, #66571, #49586, #60277, #26316, #49224, #4161, #65837, #54395, #21127, #72110, #14858, #37397, #9690, #71758, #32591, #20759, #32223, #55129, #66203, #10421, #15220, #21494, #38123, #49949, #31860, #72846, #48855, #27056, #15581, #44047, #37759, #15950, #43680, #38498, #44421, #38869, #66948, #16316, #61386, #10782, #55853, #5243, #39592, #24026, #28854, #56567, #12224, #6692, #45133, #17400, #51033, #67316, #57645, #45498, #23667, #18110, #5963, #33676, #28497, #56921, #35122, #28147, #29222, #61744, #11868, #5611, #429, #39957, #40673, #16674, #62115, #67668, #23304, #22584, #63193, #45853, #12587, #6325, #29581, #11146, #62471, #62830, #34389, #51394, #39232, #52119, #34030, #56218, #51758, #1158, #7052, #57287, #34752, #50675, #79, #22938, #40308, #795, #68388, #1521, #17035, #11508, #46213, #68028, #68752, #17749, #9145, #18836, #58002, #7775, #13300, #24392, #12944, #53852, #31681, #4350, #54945, #41399, #31310, #65283, #3244, #54215, #14671, #46575, #3612, #35480, #49045, #25772, #69120, #48310, #26133, #7410, #63914, #29938, #48674, #52478, #70834, #60102, #35837, #15042, #20209, #58361, #42763, #18478, #37215, #1888, #71198, #41043, #59736, #32044, #46942, #69478, #65652, #9511, #20573, #43129, #66025, #63557, #71573 ),
 ( #37579, #54576, #20947, #3980, #26504, #43500, #15403, #37945, #60464, #9873, #32407, #15768, #22410, #33489, #45316, #27969, #66766, #38310, #56746, #67495, #71938, #60837, #26877, #5068, #27603, #73026, #67851, #50858, #10242, #67137, #11339, #28321, #16495, #44957, #4706, #10966, #44607, #16858, #61934, #32775, #55312, #39050, #27237, #50499, #17224, #61564, #55671, #33855, #56037, #49774, #72298, #21678, #21314, #33134, #39413, #72667, #256, #43867, #56399, #39784, #5429, #66391, #44235, #16139, #38691, #61210, #50136, #22765, #5789, #62300, #22046, #10605, #11696, #34212, #49406, #24575, #23492, #28679, #41577, #68935, #63013, #51942, #52299, #621, #45684, #18293, #57471, #1339, #6876, #7588, #34576, #57825, #64094, #58184, #57104, #23128, #51584, #36027, #40865, #68575, #24213, #18661, #6515, #29409, #12411, #6150, #69652, #23851, #35663, #30125, #17935, #68217, #40497, #63382, #47120, #29048, #46399, #7234, #34944, #17579, #12767, #35302, #52657, #51219, #984, #46039, #29762, #1700, #2066, #46764, #19016, #69299, #13477, #40140, #41223, #63732, #13124, #62656, #12052, #20858, #25303, #47479, #43036, #65564, #71483, #48584, #26044, #53020, #30492, #70378, #31589, #48216, #53757, #65935, #3890, #13855, #3523, #41939, #71110, #37117, #20116, #30849, #70012, #19756, #47851, #36397, #24936, #64832, #42671, #15315, #58544, #53384, #42305, #3152, #14220, #65194, #25681, #7955, #14584, #19380, #60012, #36756, #2414, #59275, #59646, #64463, #2779, #58910, #9057, #8320, #8683, #20482, #31215, #14953, #70738, #54127, #37492, #9423, #31952, #54490, #26410, #48952, #43410, #44514, #61123, #5341, #67760, #22677, #54851, #4980, #38596, #16047, #50769, #33046, #49319, #43774, #15678, #61841, #72571, #172, #44873, #16408, #21590, #4260, #71850, #21958, #26784, #10154, #11245, #21222, #38216, #32686, #10518, #27512, #55945, #45227, #33407, #66301, #27880, #67049, #56312, #38963, #4620, #60743, #37854, #50414, #9783, #55225, #60375, #55585, #50046, #10874, #5702, #33770, #27149, #61480, #22320, #39327, #72938, #67408, #49683, #16770, #28237, #32316, #72212, #44144, #66671, #29320, #527, #18204, #58095, #51849, #45950, #52211, #1253, #51130, #23038, #6060, #62212, #23401, #40773, #62923, #41137, #34125, #7144, #7501, #68845, #11607, #62567, #11963, #45596, #68127, #68480, #63646, #12680, #35217, #40405, #57017, #1980, #57738, #46673, #35574, #34488, #39693, #52572, #6786, #894, #12317, #63287, #56664, #28594, #23757, #17843, #34852, #57379, #18571, #17493, #40054, #46308, #6422, #29675, #17133, #1613, #24123, #28954, #51493, #69213, #13037, #30031, #24489, #47033, #41489, #71021, #7868, #19664, #3058, #65108, #31126, #14132, #13767, #14498, #48496, #64009, #42947, #30404, #69568, #64742, #52932, #53667, #58456, #41848, #65475, #13389, #69924, #64375, #47756, #59187, #37032, #9334, #59556, #2329, #8969, #25589, #14864, #70652, #36308, #24847, #26324, #31501, #35933, #47393, #18929, #70292, #42218, #42582, #37404, #20398, #19293, #36668, #54041, #59927, #8597, #3437, #58823, #48128, #20026, #25956, #31866, #8233, #30762, #54401, #53294, #3801, #2694, #25209, #4534, #10787, #32959, #9696, #32229, #37765, #20766, #55136, #49956, #21500, #72851, #65844, #38875, #39237, #27425, #43323, #21134, #43686, #54764, #4168, #27062, #22233, #44427, #66956, #72118, #15587, #33680, #16322, #5248, #67321, #66209, #71392, #11153, #38505, #32597, #44053, #21866, #15226, #60284, #61030, #49593, #66579, #15956, #50327, #26697, #49231, #10428, #71764, #4890, #48861, #55495, #33321, #38129, #60651, #61394, #55859, #72480, #27790, #16681, #10066, #44789, #61751, #56224, #5617, #23672, #62837, #45859, #45505, #46219, #7058, #22589, #1526, #39600, #28152, #23310, #63562, #35127, #6698, #11873, #67673, #62121, #11513, #40313, #34035, #29231, #69125, #12229, #56926, #63198, #34758, #56573, #5970, #17042, #84, #34398, #51764, #803, #52124, #45140, #18116, #18483, #1163, #28501, #435, #22944, #51039, #68035, #6330, #24033, #68757, #40680, #51400, #17405, #12950, #12594, #57652, #46582, #39962, #50681, #35487, #17754, #28861, #68393, #29586, #62476, #57293, #41049, #58007, #2600, #8145, #8876, #35843, #29943, #70197, #58368, #36580, #7415, #53204, #65020, #46947, #13305, #25498, #19944, #19573, #30672, #25870, #52483, #31411, #18843, #25121, #14040, #2970, #42129, #47663, #24760, #48043, #59466, #1894, #53951, #41404, #24398, #64655, #42860, #14409, #59100, #64286, #69484, #63920, #8507, #7779, #52846, #3348, #30316, #2244, #47303, #58734, #31036, #70568, #20307, #42497, #69838, #36946, #53572, #48410, #70936, #19203, #41757, #37315, #65382, #13674, #36218, #14773, #38039, #60563, #32869, #5160, #10698, #71297, #26973, #44334, #61303, #49502, #55406, #37675, #43964, #4445, #27334, #21770, #72031, #9970, #55042, #32507, #33230, #15137, #9244, #21407, #60197, #15864, #59839, #66485, #66862, #26236, #65753, #4801, #72390, #38412, #60933, #27695, #31779, #55768, #20676, #10337, #49866, #16233, #38786, #50235, #4076, #72757, #22143, #54318, #44696, #43233, #3709, #67230, #16589, #48773, #9609, #43597, #32140, #54673, #26604, #49142, #71671, #21045, #66118, #15497, #11428, #17318, #28771, #57199, #52037, #34671, #28062, #6615, #45775, #57567, #40230, #5882, #50592, #69034, #29142, #11059, #57993, #39142, #39878, #62390, #12145, #6971, #63112, #22502, #6244, #62752, #34305, #51311, #56837, #46496, #29502, #67587, #51677, #45051, #1081, #17670, #715, #33947, #16953, #348, #28413, #39506, #5524, #45409, #23222, #61659, #33585, #56488, #22855, #68310, #67945, #23588, #46134, #56131, #68672, #62032, #40591, #11788, #50951, #18035, #12511, #35040, #1441, #23946, #25037, #52397, #52759, #30948, #58283, #59013 ) ),
 .UNSPECIFIED., .F., .F., .F. ) 
 B_SPLINE_SURFACE_WITH_KNOTS ( ( 2, 2 ),
 ( 3, 2, 2, 2, 2, 2, 2, 2, 2, 2, 2, 2, 2, 2, 2, 2, 2, 2, 2, 2, 2, 2, 2, 2, 2, 2, 2, 2, 2, 2, 2, 2, 2, 2, 2, 2, 2, 2, 2, 2, 2, 2, 2, 2, 2, 2, 2, 2, 2, 2, 2, 2, 2, 2, 2, 2, 2, 2, 2, 2, 2, 2, 2, 2, 2, 2, 2, 2, 2, 2, 2, 2, 2, 2, 2, 2, 2, 2, 2, 2, 2, 2, 2, 2, 2, 2, 2, 2, 2, 2, 2, 2, 2, 2, 2, 2, 2, 2, 2, 2, 2, 2, 2, 2, 2, 2, 2, 2, 2, 2, 2, 2, 2, 2, 2, 2, 2, 2, 2, 2, 2, 2, 2, 2, 2, 2, 2, 2, 2, 2, 2, 2, 2, 2, 2, 2, 2, 2, 2, 2, 2, 2, 2, 2, 2, 2, 2, 2, 2, 2, 2, 2, 2, 2, 2, 2, 2, 2, 2, 2, 2, 2, 2, 2, 2, 2, 2, 2, 2, 2, 2, 2, 2, 2, 2, 2, 2, 2, 2, 2, 2, 2, 2, 2, 2, 2, 2, 2, 2, 2, 2, 2, 2, 2, 2, 2, 2, 2, 2, 2, 2, 2, 2, 2, 2, 2, 2, 2, 2, 2, 2, 2, 2, 2, 2, 2, 2, 2, 2, 2, 2, 2, 2, 2, 2, 2, 2, 2, 2, 2, 2, 2, 2, 2, 2, 2, 2, 2, 2, 2, 2, 2, 2, 2, 2, 2, 2, 2, 2, 2, 2, 2, 2, 2, 2, 2, 2, 2, 2, 2, 2, 2, 2, 2, 2, 2, 2, 2, 2, 2, 2, 2, 2, 2, 2, 2, 2, 2, 2, 2, 2, 2, 2, 2, 2, 2, 2, 2, 2, 2, 2, 2, 2, 2, 2, 2, 2, 2, 2, 2, 2, 2, 2, 2, 2, 2, 2, 2, 2, 2, 2, 2, 2, 2, 2, 2, 2, 2, 2, 2, 2, 2, 2, 2, 2, 2, 2, 2, 2, 2, 2, 2, 2, 2, 2, 2, 2, 2, 2, 2, 2, 2, 2, 2, 2, 2, 2, 2, 2, 2, 2, 2, 2, 2, 2, 2, 2, 2, 2, 2, 3 ),
 ( 0.000000000000000000, 1.000000000000000000 ),
 ( 0.000000000000000000, 0.002777777777777777884, 0.005555555555555555768, 0.008333333333333333218, 0.01111111111111111154, 0.01388888888888888812, 0.01666666666666666644, 0.01944444444444444475, 0.02222222222222222307, 0.02500000000000000139, 0.02777777777777777624, 0.03055555555555555455, 0.03333333333333333287, 0.03611111111111110772, 0.03888888888888888951, 0.04166666666666666435, 0.04444444444444444614, 0.04722222222222222099, 0.05000000000000000278, 0.05277777777777777762, 0.05555555555555555247, 0.05833333333333333426, 0.06111111111111110911, 0.06388888888888888395, 0.06666666666666666574, 0.06944444444444444753, 0.07222222222222221544, 0.07499999999999999722, 0.07777777777777777901, 0.08055555555555556080, 0.08333333333333332871, 0.08611111111111111049, 0.08888888888888889228, 0.09166666666666666019, 0.09444444444444444198, 0.09722222222222222376, 0.1000000000000000056, 0.1027777777777777735, 0.1055555555555555552, 0.1083333333333333370, 0.1111111111111111049, 0.1138888888888888867, 0.1166666666666666685, 0.1194444444444444503, 0.1222222222222222182, 0.1250000000000000000, 0.1277777777777777679, 0.1305555555555555636, 0.1333333333333333315, 0.1361111111111110994, 0.1388888888888888951, 0.1416666666666666630, 0.1444444444444444309, 0.1472222222222222265, 0.1499999999999999944, 0.1527777777777777901, 0.1555555555555555580, 0.1583333333333333259, 0.1611111111111111216, 0.1638888888888888895, 0.1666666666666666574, 0.1694444444444444531, 0.1722222222222222210, 0.1749999999999999889, 0.1777777777777777846, 0.1805555555555555525, 0.1833333333333333204, 0.1861111111111111160, 0.1888888888888888840, 0.1916666666666666796, 0.1944444444444444475, 0.1972222222222222154, 0.2000000000000000111, 0.2027777777777777790, 0.2055555555555555469, 0.2083333333333333426, 0.2111111111111111105, 0.2138888888888888784, 0.2166666666666666741, 0.2194444444444444420, 0.2222222222222222099, 0.2250000000000000056, 0.2277777777777777735, 0.2305555555555555691, 0.2333333333333333370, 0.2361111111111111049, 0.2388888888888889006, 0.2416666666666666685, 0.2444444444444444364, 0.2472222222222222321, 0.2500000000000000000, 0.2527777777777777679, 0.2555555555555555358, 0.2583333333333333592, 0.2611111111111111271, 0.2638888888888888951, 0.2666666666666666630, 0.2694444444444444309, 0.2722222222222221988, 0.2750000000000000222, 0.2777777777777777901, 0.2805555555555555580, 0.2833333333333333259, 0.2861111111111110938, 0.2888888888888888618, 0.2916666666666666852, 0.2944444444444444531, 0.2972222222222222210, 0.2999999999999999889, 0.3027777777777777568, 0.3055555555555555802, 0.3083333333333333481, 0.3111111111111111160, 0.3138888888888888840, 0.3166666666666666519, 0.3194444444444444198, 0.3222222222222222432, 0.3250000000000000111, 0.3277777777777777790, 0.3305555555555555469, 0.3333333333333333148, 0.3361111111111111382, 0.3388888888888889062, 0.3416666666666666741, 0.3444444444444444420, 0.3472222222222222099, 0.3499999999999999778, 0.3527777777777778012, 0.3555555555555555691, 0.3583333333333333370, 0.3611111111111111049, 0.3638888888888888729, 0.3666666666666666408, 0.3694444444444444642, 0.3722222222222222321, 0.3750000000000000000, 0.3777777777777777679, 0.3805555555555555358, 0.3833333333333333592, 0.3861111111111111271, 0.3888888888888888951, 0.3916666666666666630, 0.3944444444444444309, 0.3972222222222221988, 0.4000000000000000222, 0.4027777777777777901, 0.4055555555555555580, 0.4083333333333333259, 0.4111111111111110938, 0.4138888888888888618, 0.4166666666666666852, 0.4194444444444444531, 0.4222222222222222210, 0.4249999999999999889, 0.4277777777777777568, 0.4305555555555555802, 0.4333333333333333481, 0.4361111111111111160, 0.4388888888888888840, 0.4416666666666666519, 0.4444444444444444198, 0.4472222222222222432, 0.4500000000000000111, 0.4527777777777777790, 0.4555555555555555469, 0.4583333333333333148, 0.4611111111111111382, 0.4638888888888889062, 0.4666666666666666741, 0.4694444444444444420, 0.4722222222222222099, 0.4749999999999999778, 0.4777777777777778012, 0.4805555555555555691, 0.4833333333333333370, 0.4861111111111111049, 0.4888888888888888729, 0.4916666666666666408, 0.4944444444444444642, 0.4972222222222222321, 0.5000000000000000000, 0.5027777777777777679, 0.5055555555555555358, 0.5083333333333333037, 0.5111111111111110716, 0.5138888888888888395, 0.5166666666666667185, 0.5194444444444444864, 0.5222222222222222543, 0.5250000000000000222, 0.5277777777777777901, 0.5305555555555555580, 0.5333333333333333259, 0.5361111111111110938, 0.5388888888888888618, 0.5416666666666666297, 0.5444444444444443976, 0.5472222222222222765, 0.5500000000000000444, 0.5527777777777778123, 0.5555555555555555802, 0.5583333333333333481, 0.5611111111111111160, 0.5638888888888888840, 0.5666666666666666519, 0.5694444444444444198, 0.5722222222222221877, 0.5749999999999999556, 0.5777777777777777235, 0.5805555555555556024, 0.5833333333333333703, 0.5861111111111111382, 0.5888888888888889062, 0.5916666666666666741, 0.5944444444444444420, 0.5972222222222222099, 0.5999999999999999778, 0.6027777777777777457, 0.6055555555555555136, 0.6083333333333332815, 0.6111111111111111605, 0.6138888888888889284, 0.6166666666666666963, 0.6194444444444444642, 0.6222222222222222321, 0.6250000000000000000, 0.6277777777777777679, 0.6305555555555555358, 0.6333333333333333037, 0.6361111111111110716, 0.6388888888888888395, 0.6416666666666667185, 0.6444444444444444864, 0.6472222222222222543, 0.6500000000000000222, 0.6527777777777777901, 0.6555555555555555580, 0.6583333333333333259, 0.6611111111111110938, 0.6638888888888888618, 0.6666666666666666297, 0.6694444444444443976, 0.6722222222222222765, 0.6750000000000000444, 0.6777777777777778123, 0.6805555555555555802, 0.6833333333333333481, 0.6861111111111111160, 0.6888888888888888840, 0.6916666666666666519, 0.6944444444444444198, 0.6972222222222221877, 0.6999999999999999556, 0.7027777777777777235, 0.7055555555555556024, 0.7083333333333333703, 0.7111111111111111382, 0.7138888888888889062, 0.7166666666666666741, 0.7194444444444444420, 0.7222222222222222099, 0.7249999999999999778, 0.7277777777777777457, 0.7305555555555555136, 0.7333333333333332815, 0.7361111111111111605, 0.7388888888888889284, 0.7416666666666666963, 0.7444444444444444642, 0.7472222222222222321, 0.7500000000000000000, 0.7527777777777777679, 0.7555555555555555358, 0.7583333333333333037, 0.7611111111111110716, 0.7638888888888888395, 0.7666666666666667185, 0.7694444444444444864, 0.7722222222222222543, 0.7750000000000000222, 0.7777777777777777901, 0.7805555555555555580, 0.7833333333333333259, 0.7861111111111110938, 0.7888888888888888618, 0.7916666666666666297, 0.7944444444444443976, 0.7972222222222222765, 0.8000000000000000444, 0.8027777777777778123, 0.8055555555555555802, 0.8083333333333333481, 0.8111111111111111160, 0.8138888888888888840, 0.8166666666666666519, 0.8194444444444444198, 0.8222222222222221877, 0.8249999999999999556, 0.8277777777777777235, 0.8305555555555556024, 0.8333333333333333703, 0.8361111111111111382, 0.8388888888888889062, 0.8416666666666666741, 0.8444444444444444420, 0.8472222222222222099, 0.8499999999999999778, 0.8527777777777777457, 0.8555555555555555136, 0.8583333333333332815, 0.8611111111111111605, 0.8638888888888889284, 0.8666666666666666963, 0.8694444444444444642, 0.8722222222222222321, 0.8750000000000000000, 0.8777777777777777679, 0.8805555555555555358, 0.8833333333333333037, 0.8861111111111110716, 0.8888888888888888395, 0.8916666666666667185, 0.8944444444444444864, 0.8972222222222222543, 0.9000000000000000222, 0.9027777777777777901, 0.9055555555555555580, 0.9083333333333333259, 0.9111111111111110938, 0.9138888888888888618, 0.9166666666666666297, 0.9194444444444443976, 0.9222222222222222765, 0.9250000000000000444, 0.9277777777777778123, 0.9305555555555555802, 0.9333333333333333481, 0.9361111111111111160, 0.9388888888888888840, 0.9416666666666666519, 0.9444444444444444198, 0.9472222222222221877, 0.9499999999999999556, 0.9527777777777777235, 0.9555555555555556024, 0.9583333333333333703, 0.9611111111111111382, 0.9638888888888889062, 0.9666666666666666741, 0.9694444444444444420, 0.9722222222222222099, 0.9749999999999999778, 0.9777777777777777457, 0.9805555555555555136, 0.9833333333333332815, 0.9861111111111111605, 0.9888888888888889284, 0.9916666666666666963, 0.9944444444444444642, 0.9972222222222222321, 1.000000000000000000 ),
 .UNSPECIFIED. ) 
 GEOMETRIC_REPRESENTATION_ITEM ( )  RATIONAL_B_SPLINE_SURFACE ( (
 ( 1.000000000000000000, 0.8660254037844387076, 1.000000000000000000, 0.8660254037844387076, 1.000000000000000000, 0.8660254037844387076, 1.000000000000000000, 0.8660254037844387076, 1.000000000000000000, 0.8660254037844387076, 1.000000000000000000, 0.8660254037844387076, 1.000000000000000000, 0.8660254037844387076, 1.000000000000000000, 0.8660254037844387076, 1.000000000000000000, 0.8660254037844387076, 1.000000000000000000, 0.8660254037844387076, 1.000000000000000000, 0.8660254037844387076, 1.000000000000000000, 0.8660254037844387076, 1.000000000000000000, 0.8660254037844387076, 1.000000000000000000, 0.8660254037844387076, 1.000000000000000000, 0.8660254037844387076, 1.000000000000000000, 0.8660254037844387076, 1.000000000000000000, 0.8660254037844387076, 1.000000000000000000, 0.8660254037844387076, 1.000000000000000000, 0.8660254037844387076, 1.000000000000000000, 0.8660254037844387076, 1.000000000000000000, 0.8660254037844387076, 1.000000000000000000, 0.8660254037844387076, 1.000000000000000000, 0.8660254037844387076, 1.000000000000000000, 0.8660254037844387076, 1.000000000000000000, 0.8660254037844387076, 1.000000000000000000, 0.8660254037844387076, 1.000000000000000000, 0.8660254037844387076, 1.000000000000000000, 0.8660254037844387076, 1.000000000000000000, 0.8660254037844387076, 1.000000000000000000, 0.8660254037844387076, 1.000000000000000000, 0.8660254037844387076, 1.000000000000000000, 0.8660254037844387076, 1.000000000000000000, 0.8660254037844387076, 1.000000000000000000, 0.8660254037844387076, 1.000000000000000000, 0.8660254037844387076, 1.000000000000000000, 0.8660254037844387076, 1.000000000000000000, 0.8660254037844387076, 1.000000000000000000, 0.8660254037844387076, 1.000000000000000000, 0.8660254037844387076, 1.000000000000000000, 0.8660254037844387076, 1.000000000000000000, 0.8660254037844387076, 1.000000000000000000, 0.8660254037844387076, 1.000000000000000000, 0.8660254037844387076, 1.000000000000000000, 0.8660254037844387076, 1.000000000000000000, 0.8660254037844387076, 1.000000000000000000, 0.8660254037844387076, 1.000000000000000000, 0.8660254037844387076, 1.000000000000000000, 0.8660254037844387076, 1.000000000000000000, 0.8660254037844387076, 1.000000000000000000, 0.8660254037844387076, 1.000000000000000000, 0.8660254037844387076, 1.000000000000000000, 0.8660254037844387076, 1.000000000000000000, 0.8660254037844387076, 1.000000000000000000, 0.8660254037844387076, 1.000000000000000000, 0.8660254037844387076, 1.000000000000000000, 0.8660254037844387076, 1.000000000000000000, 0.8660254037844387076, 1.000000000000000000, 0.8660254037844387076, 1.000000000000000000, 0.8660254037844387076, 1.000000000000000000, 0.8660254037844387076, 1.000000000000000000, 0.8660254037844387076, 1.000000000000000000, 0.8660254037844387076, 1.000000000000000000, 0.8660254037844387076, 1.000000000000000000, 0.8660254037844387076, 1.000000000000000000, 0.8660254037844387076, 1.000000000000000000, 0.8660254037844387076, 1.000000000000000000, 0.8660254037844387076, 1.000000000000000000, 0.8660254037844387076, 1.000000000000000000, 0.8660254037844387076, 1.000000000000000000, 0.8660254037844387076, 1.000000000000000000, 0.8660254037844387076, 1.000000000000000000, 0.8660254037844387076, 1.000000000000000000, 0.8660254037844387076, 1.000000000000000000, 0.8660254037844387076, 1.000000000000000000, 0.8660254037844387076, 1.000000000000000000, 0.8660254037844387076, 1.000000000000000000, 0.8660254037844387076, 1.000000000000000000, 0.8660254037844387076, 1.000000000000000000, 0.8660254037844387076, 1.000000000000000000, 0.8660254037844387076, 1.000000000000000000, 0.8660254037844387076, 1.000000000000000000, 0.8660254037844387076, 1.000000000000000000, 0.8660254037844387076, 1.000000000000000000, 0.8660254037844387076, 1.000000000000000000, 0.8660254037844387076, 1.000000000000000000, 0.8660254037844387076, 1.000000000000000000, 0.8660254037844387076, 1.000000000000000000, 0.8660254037844387076, 1.000000000000000000, 0.8660254037844387076, 1.000000000000000000, 0.8660254037844387076, 1.000000000000000000, 0.8660254037844387076, 1.000000000000000000, 0.8660254037844387076, 1.000000000000000000, 0.8660254037844387076, 1.000000000000000000, 0.8660254037844387076, 1.000000000000000000, 0.8660254037844387076, 1.000000000000000000, 0.8660254037844387076, 1.000000000000000000, 0.8660254037844387076, 1.000000000000000000, 0.8660254037844387076, 1.000000000000000000, 0.8660254037844387076, 1.000000000000000000, 0.8660254037844387076, 1.000000000000000000, 0.8660254037844387076, 1.000000000000000000, 0.8660254037844387076, 1.000000000000000000, 0.8660254037844387076, 1.000000000000000000, 0.8660254037844387076, 1.000000000000000000, 0.8660254037844387076, 1.000000000000000000, 0.8660254037844387076, 1.000000000000000000, 0.8660254037844387076, 1.000000000000000000, 0.8660254037844387076, 1.000000000000000000, 0.8660254037844387076, 1.000000000000000000, 0.8660254037844387076, 1.000000000000000000, 0.8660254037844387076, 1.000000000000000000, 0.8660254037844387076, 1.000000000000000000, 0.8660254037844387076, 1.000000000000000000, 0.8660254037844387076, 1.000000000000000000, 0.8660254037844387076, 1.000000000000000000, 0.8660254037844387076, 1.000000000000000000, 0.8660254037844387076, 1.000000000000000000, 0.8660254037844387076, 1.000000000000000000, 0.8660254037844387076, 1.000000000000000000, 0.8660254037844387076, 1.000000000000000000, 0.8660254037844387076, 1.000000000000000000, 0.8660254037844387076, 1.000000000000000000, 0.8660254037844387076, 1.000000000000000000, 0.8660254037844387076, 1.000000000000000000, 0.8660254037844387076, 1.000000000000000000, 0.8660254037844387076, 1.000000000000000000, 0.8660254037844387076, 1.000000000000000000, 0.8660254037844387076, 1.000000000000000000, 0.8660254037844387076, 1.000000000000000000, 0.8660254037844387076, 1.000000000000000000, 0.8660254037844387076, 1.000000000000000000, 0.8660254037844387076, 1.000000000000000000, 0.8660254037844387076, 1.000000000000000000, 0.8660254037844387076, 1.000000000000000000, 0.8660254037844387076, 1.000000000000000000, 0.8660254037844387076, 1.000000000000000000, 0.8660254037844387076, 1.000000000000000000, 0.8660254037844387076, 1.000000000000000000, 0.8660254037844387076, 1.000000000000000000, 0.8660254037844387076, 1.000000000000000000, 0.8660254037844387076, 1.000000000000000000, 0.8660254037844387076, 1.000000000000000000, 0.8660254037844387076, 1.000000000000000000, 0.8660254037844387076, 1.000000000000000000, 0.8660254037844387076, 1.000000000000000000, 0.8660254037844387076, 1.000000000000000000, 0.8660254037844387076, 1.000000000000000000, 0.8660254037844387076, 1.000000000000000000, 0.8660254037844387076, 1.000000000000000000, 0.8660254037844387076, 1.000000000000000000, 0.8660254037844387076, 1.000000000000000000, 0.8660254037844387076, 1.000000000000000000, 0.8660254037844387076, 1.000000000000000000, 0.8660254037844387076, 1.000000000000000000, 0.8660254037844387076, 1.000000000000000000, 0.8660254037844387076, 1.000000000000000000, 0.8660254037844387076, 1.000000000000000000, 0.8660254037844387076, 1.000000000000000000, 0.8660254037844387076, 1.000000000000000000, 0.8660254037844387076, 1.000000000000000000, 0.8660254037844387076, 1.000000000000000000, 0.8660254037844387076, 1.000000000000000000, 0.8660254037844387076, 1.000000000000000000, 0.8660254037844387076, 1.000000000000000000, 0.8660254037844387076, 1.000000000000000000, 0.8660254037844387076, 1.000000000000000000, 0.8660254037844387076, 1.000000000000000000, 0.8660254037844387076, 1.000000000000000000, 0.8660254037844387076, 1.000000000000000000, 0.8660254037844387076, 1.000000000000000000, 0.8660254037844387076, 1.000000000000000000, 0.8660254037844387076, 1.000000000000000000, 0.8660254037844387076, 1.000000000000000000, 0.8660254037844387076, 1.000000000000000000, 0.8660254037844387076, 1.000000000000000000, 0.8660254037844387076, 1.000000000000000000, 0.8660254037844387076, 1.000000000000000000, 0.8660254037844387076, 1.000000000000000000, 0.8660254037844387076, 1.000000000000000000, 0.8660254037844387076, 1.000000000000000000, 0.8660254037844387076, 1.000000000000000000, 0.8660254037844387076, 1.000000000000000000, 0.8660254037844387076, 1.000000000000000000, 0.8660254037844387076, 1.000000000000000000, 0.8660254037844387076, 1.000000000000000000, 0.8660254037844387076, 1.000000000000000000, 0.8660254037844387076, 1.000000000000000000, 0.8660254037844387076, 1.000000000000000000, 0.8660254037844387076, 1.000000000000000000, 0.8660254037844387076, 1.000000000000000000, 0.8660254037844387076, 1.000000000000000000, 0.8660254037844387076, 1.000000000000000000, 0.8660254037844387076, 1.000000000000000000, 0.8660254037844387076, 1.000000000000000000, 0.8660254037844387076, 1.000000000000000000, 0.8660254037844387076, 1.000000000000000000, 0.8660254037844387076, 1.000000000000000000, 0.8660254037844387076, 1.000000000000000000, 0.8660254037844387076, 1.000000000000000000, 0.8660254037844387076, 1.000000000000000000, 0.8660254037844387076, 1.000000000000000000, 0.8660254037844387076, 1.000000000000000000, 0.8660254037844387076, 1.000000000000000000, 0.8660254037844387076, 1.000000000000000000, 0.8660254037844387076, 1.000000000000000000, 0.8660254037844387076, 1.000000000000000000, 0.8660254037844387076, 1.000000000000000000, 0.8660254037844387076, 1.000000000000000000, 0.8660254037844387076, 1.000000000000000000, 0.8660254037844387076, 1.000000000000000000, 0.8660254037844387076, 1.000000000000000000, 0.8660254037844387076, 1.000000000000000000, 0.8660254037844387076, 1.000000000000000000, 0.8660254037844387076, 1.000000000000000000, 0.8660254037844387076, 1.000000000000000000, 0.8660254037844387076, 1.000000000000000000, 0.8660254037844387076, 1.000000000000000000, 0.8660254037844387076, 1.000000000000000000, 0.8660254037844387076, 1.000000000000000000, 0.8660254037844387076, 1.000000000000000000, 0.8660254037844387076, 1.000000000000000000, 0.8660254037844387076, 1.000000000000000000, 0.8660254037844387076, 1.000000000000000000, 0.8660254037844387076, 1.000000000000000000, 0.8660254037844387076, 1.000000000000000000, 0.8660254037844387076, 1.000000000000000000, 0.8660254037844387076, 1.000000000000000000, 0.8660254037844387076, 1.000000000000000000, 0.8660254037844387076, 1.000000000000000000, 0.8660254037844387076, 1.000000000000000000, 0.8660254037844387076, 1.000000000000000000, 0.8660254037844387076, 1.000000000000000000, 0.8660254037844387076, 1.000000000000000000, 0.8660254037844387076, 1.000000000000000000, 0.8660254037844387076, 1.000000000000000000, 0.8660254037844387076, 1.000000000000000000, 0.8660254037844387076, 1.000000000000000000, 0.8660254037844387076, 1.000000000000000000, 0.8660254037844387076, 1.000000000000000000, 0.8660254037844387076, 1.000000000000000000, 0.8660254037844387076, 1.000000000000000000, 0.8660254037844387076, 1.000000000000000000, 0.8660254037844387076, 1.000000000000000000, 0.8660254037844387076, 1.000000000000000000, 0.8660254037844387076, 1.000000000000000000, 0.8660254037844387076, 1.000000000000000000, 0.8660254037844387076, 1.000000000000000000, 0.8660254037844387076, 1.000000000000000000, 0.8660254037844387076, 1.000000000000000000, 0.8660254037844387076, 1.000000000000000000, 0.8660254037844387076, 1.000000000000000000, 0.8660254037844387076, 1.000000000000000000, 0.8660254037844387076, 1.000000000000000000, 0.8660254037844387076, 1.000000000000000000, 0.8660254037844387076, 1.000000000000000000, 0.8660254037844387076, 1.000000000000000000, 0.8660254037844387076, 1.000000000000000000, 0.8660254037844387076, 1.000000000000000000, 0.8660254037844387076, 1.000000000000000000, 0.8660254037844387076, 1.000000000000000000, 0.8660254037844387076, 1.000000000000000000, 0.8660254037844387076, 1.000000000000000000, 0.8660254037844387076, 1.000000000000000000, 0.8660254037844387076, 1.000000000000000000, 0.8660254037844387076, 1.000000000000000000, 0.8660254037844387076, 1.000000000000000000, 0.8660254037844387076, 1.000000000000000000, 0.8660254037844387076, 1.000000000000000000, 0.8660254037844387076, 1.000000000000000000, 0.8660254037844387076, 1.000000000000000000, 0.8660254037844387076, 1.000000000000000000, 0.8660254037844387076, 1.000000000000000000, 0.8660254037844387076, 1.000000000000000000, 0.8660254037844387076, 1.000000000000000000, 0.8660254037844387076, 1.000000000000000000, 0.8660254037844387076, 1.000000000000000000, 0.8660254037844387076, 1.000000000000000000, 0.8660254037844387076, 1.000000000000000000, 0.8660254037844387076, 1.000000000000000000, 0.8660254037844387076, 1.000000000000000000, 0.8660254037844387076, 1.000000000000000000, 0.8660254037844387076, 1.000000000000000000, 0.8660254037844387076, 1.000000000000000000, 0.8660254037844387076, 1.000000000000000000, 0.8660254037844387076, 1.000000000000000000, 0.8660254037844387076, 1.000000000000000000, 0.8660254037844387076, 1.000000000000000000, 0.8660254037844387076, 1.000000000000000000, 0.8660254037844387076, 1.000000000000000000, 0.8660254037844387076, 1.000000000000000000, 0.8660254037844387076, 1.000000000000000000, 0.8660254037844387076, 1.000000000000000000, 0.8660254037844387076, 1.000000000000000000, 0.8660254037844387076, 1.000000000000000000, 0.8660254037844387076, 1.000000000000000000, 0.8660254037844387076, 1.000000000000000000, 0.8660254037844387076, 1.000000000000000000, 0.8660254037844387076, 1.000000000000000000, 0.8660254037844387076, 1.000000000000000000, 0.8660254037844387076, 1.000000000000000000, 0.8660254037844387076, 1.000000000000000000, 0.8660254037844387076, 1.000000000000000000, 0.8660254037844387076, 1.000000000000000000, 0.8660254037844387076, 1.000000000000000000, 0.8660254037844387076, 1.000000000000000000, 0.8660254037844387076, 1.000000000000000000, 0.8660254037844387076, 1.000000000000000000, 0.8660254037844387076, 1.000000000000000000, 0.8660254037844387076, 1.000000000000000000, 0.8660254037844387076, 1.000000000000000000, 0.8660254037844387076, 1.000000000000000000, 0.8660254037844387076, 1.000000000000000000, 0.8660254037844387076, 1.000000000000000000, 0.8660254037844387076, 1.000000000000000000, 0.8660254037844387076, 1.000000000000000000, 0.8660254037844387076, 1.000000000000000000, 0.8660254037844387076, 1.000000000000000000, 0.8660254037844387076, 1.000000000000000000, 0.8660254037844387076, 1.000000000000000000, 0.8660254037844387076, 1.000000000000000000, 0.8660254037844387076, 1.000000000000000000, 0.8660254037844387076, 1.000000000000000000, 0.8660254037844387076, 1.000000000000000000, 0.8660254037844387076, 1.000000000000000000, 0.8660254037844387076, 1.000000000000000000, 0.8660254037844387076, 1.000000000000000000, 0.8660254037844387076, 1.000000000000000000, 0.8660254037844387076, 1.000000000000000000, 0.8660254037844387076, 1.000000000000000000, 0.8660254037844387076, 1.000000000000000000, 0.8660254037844387076, 1.000000000000000000, 0.8660254037844387076, 1.000000000000000000, 0.8660254037844387076, 1.000000000000000000, 0.8660254037844387076, 1.000000000000000000, 0.8660254037844387076, 1.000000000000000000, 0.8660254037844387076, 1.000000000000000000, 0.8660254037844387076, 1.000000000000000000, 0.8660254037844387076, 1.000000000000000000, 0.8660254037844387076, 1.000000000000000000, 0.8660254037844387076, 1.000000000000000000, 0.8660254037844387076, 1.000000000000000000, 0.8660254037844387076, 1.000000000000000000, 0.8660254037844387076, 1.000000000000000000, 0.8660254037844387076, 1.000000000000000000, 0.8660254037844387076, 1.000000000000000000, 0.8660254037844387076, 1.000000000000000000, 0.8660254037844387076, 1.000000000000000000, 0.8660254037844387076, 1.000000000000000000, 0.8660254037844387076, 1.000000000000000000, 0.8660254037844387076, 1.000000000000000000, 0.8660254037844387076, 1.000000000000000000, 0.8660254037844387076, 1.000000000000000000, 0.8660254037844387076, 1.000000000000000000, 0.8660254037844387076, 1.000000000000000000, 0.8660254037844387076, 1.000000000000000000, 0.8660254037844387076, 1.000000000000000000, 0.8660254037844387076, 1.000000000000000000, 0.8660254037844387076, 1.000000000000000000, 0.8660254037844387076, 1.000000000000000000, 0.8660254037844387076, 1.000000000000000000),
 ( 1.000000000000000000, 0.8660254037844387076, 1.000000000000000000, 0.8660254037844387076, 1.000000000000000000, 0.8660254037844387076, 1.000000000000000000, 0.8660254037844387076, 1.000000000000000000, 0.8660254037844387076, 1.000000000000000000, 0.8660254037844387076, 1.000000000000000000, 0.8660254037844387076, 1.000000000000000000, 0.8660254037844387076, 1.000000000000000000, 0.8660254037844387076, 1.000000000000000000, 0.8660254037844387076, 1.000000000000000000, 0.8660254037844387076, 1.000000000000000000, 0.8660254037844387076, 1.000000000000000000, 0.8660254037844387076, 1.000000000000000000, 0.8660254037844387076, 1.000000000000000000, 0.8660254037844387076, 1.000000000000000000, 0.8660254037844387076, 1.000000000000000000, 0.8660254037844387076, 1.000000000000000000, 0.8660254037844387076, 1.000000000000000000, 0.8660254037844387076, 1.000000000000000000, 0.8660254037844387076, 1.000000000000000000, 0.8660254037844387076, 1.000000000000000000, 0.8660254037844387076, 1.000000000000000000, 0.8660254037844387076, 1.000000000000000000, 0.8660254037844387076, 1.000000000000000000, 0.8660254037844387076, 1.000000000000000000, 0.8660254037844387076, 1.000000000000000000, 0.8660254037844387076, 1.000000000000000000, 0.8660254037844387076, 1.000000000000000000, 0.8660254037844387076, 1.000000000000000000, 0.8660254037844387076, 1.000000000000000000, 0.8660254037844387076, 1.000000000000000000, 0.8660254037844387076, 1.000000000000000000, 0.8660254037844387076, 1.000000000000000000, 0.8660254037844387076, 1.000000000000000000, 0.8660254037844387076, 1.000000000000000000, 0.8660254037844387076, 1.000000000000000000, 0.8660254037844387076, 1.000000000000000000, 0.8660254037844387076, 1.000000000000000000, 0.8660254037844387076, 1.000000000000000000, 0.8660254037844387076, 1.000000000000000000, 0.8660254037844387076, 1.000000000000000000, 0.8660254037844387076, 1.000000000000000000, 0.8660254037844387076, 1.000000000000000000, 0.8660254037844387076, 1.000000000000000000, 0.8660254037844387076, 1.000000000000000000, 0.8660254037844387076, 1.000000000000000000, 0.8660254037844387076, 1.000000000000000000, 0.8660254037844387076, 1.000000000000000000, 0.8660254037844387076, 1.000000000000000000, 0.8660254037844387076, 1.000000000000000000, 0.8660254037844387076, 1.000000000000000000, 0.8660254037844387076, 1.000000000000000000, 0.8660254037844387076, 1.000000000000000000, 0.8660254037844387076, 1.000000000000000000, 0.8660254037844387076, 1.000000000000000000, 0.8660254037844387076, 1.000000000000000000, 0.8660254037844387076, 1.000000000000000000, 0.8660254037844387076, 1.000000000000000000, 0.8660254037844387076, 1.000000000000000000, 0.8660254037844387076, 1.000000000000000000, 0.8660254037844387076, 1.000000000000000000, 0.8660254037844387076, 1.000000000000000000, 0.8660254037844387076, 1.000000000000000000, 0.8660254037844387076, 1.000000000000000000, 0.8660254037844387076, 1.000000000000000000, 0.8660254037844387076, 1.000000000000000000, 0.8660254037844387076, 1.000000000000000000, 0.8660254037844387076, 1.000000000000000000, 0.8660254037844387076, 1.000000000000000000, 0.8660254037844387076, 1.000000000000000000, 0.8660254037844387076, 1.000000000000000000, 0.8660254037844387076, 1.000000000000000000, 0.8660254037844387076, 1.000000000000000000, 0.8660254037844387076, 1.000000000000000000, 0.8660254037844387076, 1.000000000000000000, 0.8660254037844387076, 1.000000000000000000, 0.8660254037844387076, 1.000000000000000000, 0.8660254037844387076, 1.000000000000000000, 0.8660254037844387076, 1.000000000000000000, 0.8660254037844387076, 1.000000000000000000, 0.8660254037844387076, 1.000000000000000000, 0.8660254037844387076, 1.000000000000000000, 0.8660254037844387076, 1.000000000000000000, 0.8660254037844387076, 1.000000000000000000, 0.8660254037844387076, 1.000000000000000000, 0.8660254037844387076, 1.000000000000000000, 0.8660254037844387076, 1.000000000000000000, 0.8660254037844387076, 1.000000000000000000, 0.8660254037844387076, 1.000000000000000000, 0.8660254037844387076, 1.000000000000000000, 0.8660254037844387076, 1.000000000000000000, 0.8660254037844387076, 1.000000000000000000, 0.8660254037844387076, 1.000000000000000000, 0.8660254037844387076, 1.000000000000000000, 0.8660254037844387076, 1.000000000000000000, 0.8660254037844387076, 1.000000000000000000, 0.8660254037844387076, 1.000000000000000000, 0.8660254037844387076, 1.000000000000000000, 0.8660254037844387076, 1.000000000000000000, 0.8660254037844387076, 1.000000000000000000, 0.8660254037844387076, 1.000000000000000000, 0.8660254037844387076, 1.000000000000000000, 0.8660254037844387076, 1.000000000000000000, 0.8660254037844387076, 1.000000000000000000, 0.8660254037844387076, 1.000000000000000000, 0.8660254037844387076, 1.000000000000000000, 0.8660254037844387076, 1.000000000000000000, 0.8660254037844387076, 1.000000000000000000, 0.8660254037844387076, 1.000000000000000000, 0.8660254037844387076, 1.000000000000000000, 0.8660254037844387076, 1.000000000000000000, 0.8660254037844387076, 1.000000000000000000, 0.8660254037844387076, 1.000000000000000000, 0.8660254037844387076, 1.000000000000000000, 0.8660254037844387076, 1.000000000000000000, 0.8660254037844387076, 1.000000000000000000, 0.8660254037844387076, 1.000000000000000000, 0.8660254037844387076, 1.000000000000000000, 0.8660254037844387076, 1.000000000000000000, 0.8660254037844387076, 1.000000000000000000, 0.8660254037844387076, 1.000000000000000000, 0.8660254037844387076, 1.000000000000000000, 0.8660254037844387076, 1.000000000000000000, 0.8660254037844387076, 1.000000000000000000, 0.8660254037844387076, 1.000000000000000000, 0.8660254037844387076, 1.000000000000000000, 0.8660254037844387076, 1.000000000000000000, 0.8660254037844387076, 1.000000000000000000, 0.8660254037844387076, 1.000000000000000000, 0.8660254037844387076, 1.000000000000000000, 0.8660254037844387076, 1.000000000000000000, 0.8660254037844387076, 1.000000000000000000, 0.8660254037844387076, 1.000000000000000000, 0.8660254037844387076, 1.000000000000000000, 0.8660254037844387076, 1.000000000000000000, 0.8660254037844387076, 1.000000000000000000, 0.8660254037844387076, 1.000000000000000000, 0.8660254037844387076, 1.000000000000000000, 0.8660254037844387076, 1.000000000000000000, 0.8660254037844387076, 1.000000000000000000, 0.8660254037844387076, 1.000000000000000000, 0.8660254037844387076, 1.000000000000000000, 0.8660254037844387076, 1.000000000000000000, 0.8660254037844387076, 1.000000000000000000, 0.8660254037844387076, 1.000000000000000000, 0.8660254037844387076, 1.000000000000000000, 0.8660254037844387076, 1.000000000000000000, 0.8660254037844387076, 1.000000000000000000, 0.8660254037844387076, 1.000000000000000000, 0.8660254037844387076, 1.000000000000000000, 0.8660254037844387076, 1.000000000000000000, 0.8660254037844387076, 1.000000000000000000, 0.8660254037844387076, 1.000000000000000000, 0.8660254037844387076, 1.000000000000000000, 0.8660254037844387076, 1.000000000000000000, 0.8660254037844387076, 1.000000000000000000, 0.8660254037844387076, 1.000000000000000000, 0.8660254037844387076, 1.000000000000000000, 0.8660254037844387076, 1.000000000000000000, 0.8660254037844387076, 1.000000000000000000, 0.8660254037844387076, 1.000000000000000000, 0.8660254037844387076, 1.000000000000000000, 0.8660254037844387076, 1.000000000000000000, 0.8660254037844387076, 1.000000000000000000, 0.8660254037844387076, 1.000000000000000000, 0.8660254037844387076, 1.000000000000000000, 0.8660254037844387076, 1.000000000000000000, 0.8660254037844387076, 1.000000000000000000, 0.8660254037844387076, 1.000000000000000000, 0.8660254037844387076, 1.000000000000000000, 0.8660254037844387076, 1.000000000000000000, 0.8660254037844387076, 1.000000000000000000, 0.8660254037844387076, 1.000000000000000000, 0.8660254037844387076, 1.000000000000000000, 0.8660254037844387076, 1.000000000000000000, 0.8660254037844387076, 1.000000000000000000, 0.8660254037844387076, 1.000000000000000000, 0.8660254037844387076, 1.000000000000000000, 0.8660254037844387076, 1.000000000000000000, 0.8660254037844387076, 1.000000000000000000, 0.8660254037844387076, 1.000000000000000000, 0.8660254037844387076, 1.000000000000000000, 0.8660254037844387076, 1.000000000000000000, 0.8660254037844387076, 1.000000000000000000, 0.8660254037844387076, 1.000000000000000000, 0.8660254037844387076, 1.000000000000000000, 0.8660254037844387076, 1.000000000000000000, 0.8660254037844387076, 1.000000000000000000, 0.8660254037844387076, 1.000000000000000000, 0.8660254037844387076, 1.000000000000000000, 0.8660254037844387076, 1.000000000000000000, 0.8660254037844387076, 1.000000000000000000, 0.8660254037844387076, 1.000000000000000000, 0.8660254037844387076, 1.000000000000000000, 0.8660254037844387076, 1.000000000000000000, 0.8660254037844387076, 1.000000000000000000, 0.8660254037844387076, 1.000000000000000000, 0.8660254037844387076, 1.000000000000000000, 0.8660254037844387076, 1.000000000000000000, 0.8660254037844387076, 1.000000000000000000, 0.8660254037844387076, 1.000000000000000000, 0.8660254037844387076, 1.000000000000000000, 0.8660254037844387076, 1.000000000000000000, 0.8660254037844387076, 1.000000000000000000, 0.8660254037844387076, 1.000000000000000000, 0.8660254037844387076, 1.000000000000000000, 0.8660254037844387076, 1.000000000000000000, 0.8660254037844387076, 1.000000000000000000, 0.8660254037844387076, 1.000000000000000000, 0.8660254037844387076, 1.000000000000000000, 0.8660254037844387076, 1.000000000000000000, 0.8660254037844387076, 1.000000000000000000, 0.8660254037844387076, 1.000000000000000000, 0.8660254037844387076, 1.000000000000000000, 0.8660254037844387076, 1.000000000000000000, 0.8660254037844387076, 1.000000000000000000, 0.8660254037844387076, 1.000000000000000000, 0.8660254037844387076, 1.000000000000000000, 0.8660254037844387076, 1.000000000000000000, 0.8660254037844387076, 1.000000000000000000, 0.8660254037844387076, 1.000000000000000000, 0.8660254037844387076, 1.000000000000000000, 0.8660254037844387076, 1.000000000000000000, 0.8660254037844387076, 1.000000000000000000, 0.8660254037844387076, 1.000000000000000000, 0.8660254037844387076, 1.000000000000000000, 0.8660254037844387076, 1.000000000000000000, 0.8660254037844387076, 1.000000000000000000, 0.8660254037844387076, 1.000000000000000000, 0.8660254037844387076, 1.000000000000000000, 0.8660254037844387076, 1.000000000000000000, 0.8660254037844387076, 1.000000000000000000, 0.8660254037844387076, 1.000000000000000000, 0.8660254037844387076, 1.000000000000000000, 0.8660254037844387076, 1.000000000000000000, 0.8660254037844387076, 1.000000000000000000, 0.8660254037844387076, 1.000000000000000000, 0.8660254037844387076, 1.000000000000000000, 0.8660254037844387076, 1.000000000000000000, 0.8660254037844387076, 1.000000000000000000, 0.8660254037844387076, 1.000000000000000000, 0.8660254037844387076, 1.000000000000000000, 0.8660254037844387076, 1.000000000000000000, 0.8660254037844387076, 1.000000000000000000, 0.8660254037844387076, 1.000000000000000000, 0.8660254037844387076, 1.000000000000000000, 0.8660254037844387076, 1.000000000000000000, 0.8660254037844387076, 1.000000000000000000, 0.8660254037844387076, 1.000000000000000000, 0.8660254037844387076, 1.000000000000000000, 0.8660254037844387076, 1.000000000000000000, 0.8660254037844387076, 1.000000000000000000, 0.8660254037844387076, 1.000000000000000000, 0.8660254037844387076, 1.000000000000000000, 0.8660254037844387076, 1.000000000000000000, 0.8660254037844387076, 1.000000000000000000, 0.8660254037844387076, 1.000000000000000000, 0.8660254037844387076, 1.000000000000000000, 0.8660254037844387076, 1.000000000000000000, 0.8660254037844387076, 1.000000000000000000, 0.8660254037844387076, 1.000000000000000000, 0.8660254037844387076, 1.000000000000000000, 0.8660254037844387076, 1.000000000000000000, 0.8660254037844387076, 1.000000000000000000, 0.8660254037844387076, 1.000000000000000000, 0.8660254037844387076, 1.000000000000000000, 0.8660254037844387076, 1.000000000000000000, 0.8660254037844387076, 1.000000000000000000, 0.8660254037844387076, 1.000000000000000000, 0.8660254037844387076, 1.000000000000000000, 0.8660254037844387076, 1.000000000000000000, 0.8660254037844387076, 1.000000000000000000, 0.8660254037844387076, 1.000000000000000000, 0.8660254037844387076, 1.000000000000000000, 0.8660254037844387076, 1.000000000000000000, 0.8660254037844387076, 1.000000000000000000, 0.8660254037844387076, 1.000000000000000000, 0.8660254037844387076, 1.000000000000000000, 0.8660254037844387076, 1.000000000000000000, 0.8660254037844387076, 1.000000000000000000, 0.8660254037844387076, 1.000000000000000000, 0.8660254037844387076, 1.000000000000000000, 0.8660254037844387076, 1.000000000000000000, 0.8660254037844387076, 1.000000000000000000, 0.8660254037844387076, 1.000000000000000000, 0.8660254037844387076, 1.000000000000000000, 0.8660254037844387076, 1.000000000000000000, 0.8660254037844387076, 1.000000000000000000, 0.8660254037844387076, 1.000000000000000000, 0.8660254037844387076, 1.000000000000000000, 0.8660254037844387076, 1.000000000000000000, 0.8660254037844387076, 1.000000000000000000, 0.8660254037844387076, 1.000000000000000000, 0.8660254037844387076, 1.000000000000000000, 0.8660254037844387076, 1.000000000000000000, 0.8660254037844387076, 1.000000000000000000, 0.8660254037844387076, 1.000000000000000000, 0.8660254037844387076, 1.000000000000000000, 0.8660254037844387076, 1.000000000000000000, 0.8660254037844387076, 1.000000000000000000, 0.8660254037844387076, 1.000000000000000000, 0.8660254037844387076, 1.000000000000000000, 0.8660254037844387076, 1.000000000000000000, 0.8660254037844387076, 1.000000000000000000, 0.8660254037844387076, 1.000000000000000000, 0.8660254037844387076, 1.000000000000000000, 0.8660254037844387076, 1.000000000000000000, 0.8660254037844387076, 1.000000000000000000, 0.8660254037844387076, 1.000000000000000000, 0.8660254037844387076, 1.000000000000000000, 0.8660254037844387076, 1.000000000000000000, 0.8660254037844387076, 1.000000000000000000, 0.8660254037844387076, 1.000000000000000000, 0.8660254037844387076, 1.000000000000000000, 0.8660254037844387076, 1.000000000000000000, 0.8660254037844387076, 1.000000000000000000, 0.8660254037844387076, 1.000000000000000000, 0.8660254037844387076, 1.000000000000000000, 0.8660254037844387076, 1.000000000000000000, 0.8660254037844387076, 1.000000000000000000, 0.8660254037844387076, 1.000000000000000000, 0.8660254037844387076, 1.000000000000000000, 0.8660254037844387076, 1.000000000000000000, 0.8660254037844387076, 1.000000000000000000, 0.8660254037844387076, 1.000000000000000000, 0.8660254037844387076, 1.000000000000000000, 0.8660254037844387076, 1.000000000000000000, 0.8660254037844387076, 1.000000000000000000, 0.8660254037844387076, 1.000000000000000000, 0.8660254037844387076, 1.000000000000000000, 0.8660254037844387076, 1.000000000000000000, 0.8660254037844387076, 1.000000000000000000, 0.8660254037844387076, 1.000000000000000000, 0.8660254037844387076, 1.000000000000000000, 0.8660254037844387076, 1.000000000000000000, 0.8660254037844387076, 1.000000000000000000, 0.8660254037844387076, 1.000000000000000000, 0.8660254037844387076, 1.000000000000000000, 0.8660254037844387076, 1.000000000000000000, 0.8660254037844387076, 1.000000000000000000, 0.8660254037844387076, 1.000000000000000000, 0.8660254037844387076, 1.000000000000000000, 0.8660254037844387076, 1.000000000000000000, 0.8660254037844387076, 1.000000000000000000, 0.8660254037844387076, 1.000000000000000000, 0.8660254037844387076, 1.000000000000000000, 0.8660254037844387076, 1.000000000000000000, 0.8660254037844387076, 1.000000000000000000, 0.8660254037844387076, 1.000000000000000000, 0.8660254037844387076, 1.000000000000000000, 0.8660254037844387076, 1.000000000000000000, 0.8660254037844387076, 1.000000000000000000, 0.8660254037844387076, 1.000000000000000000, 0.8660254037844387076, 1.000000000000000000, 0.8660254037844387076, 1.000000000000000000, 0.8660254037844387076, 1.000000000000000000, 0.8660254037844387076, 1.000000000000000000, 0.8660254037844387076, 1.000000000000000000, 0.8660254037844387076, 1.000000000000000000, 0.8660254037844387076, 1.000000000000000000) ) ) 
 REPRESENTATION_ITEM ( '' )  SURFACE ( )  );
#51496=CARTESIAN_POINT ( 'NONE',  ( 4.243569643749999010, 10.22187500061451892, -32.45002607614398471 ) ) ;
#51497=CYLINDRICAL_SURFACE ( 'NONE', #1762, 4.000000000000000000 ) ;
#51498=CARTESIAN_POINT ( 'NONE',  ( 3.075000001229035718, 2.886751345948126879, 4.999999999999999112 ) ) ;
#51500=CARTESIAN_POINT ( 'NONE',  ( 19.09687500061451360, -3.027376345333614438, 5.243569643749998122 ) ) ;
#51501=EDGE_CURVE ( 'NONE', #8342, #58790, #46310, .T. ) ;
#51502=LINE ( 'NONE', #57746, #58659 ) ;
#51503=CARTESIAN_POINT ( 'NONE',  ( 13.56562500061451892, 3.027376345333611329, 5.243569643749999010 ) ) ;
#51505=CARTESIAN_POINT ( 'NONE',  ( 30.00000000000000000, 0.000000000000000000, 0.000000000000000000 ) ) ;
#51506=CARTESIAN_POINT ( 'NONE',  ( 29.52187500061451431, -6.054752690667223547, -1.112240025338166033E-15 ) ) ;
#51507=CARTESIAN_POINT ( 'NONE',  ( 27.15937500061451360, 0.000000000000000000, 5.243569643749999010 ) ) ;
#51509=CARTESIAN_POINT ( 'NONE',  ( 13.56562500061451892, 3.027376345333611329, 5.243569643749999010 ) ) ;
#51510=CARTESIAN_POINT ( 'NONE',  ( 10.35937500061451644, 4.541064518000418104, -2.621784821874998173 ) ) ;
#51511=ORIENTED_EDGE ( 'NONE', *, *, #11164, .F. ) ;
#51514=CARTESIAN_POINT ( 'NONE',  ( 20.01562500061451644, -6.054752690667223547, -1.112240025338166033E-15 ) ) ;
#51515=CARTESIAN_POINT ( 'NONE',  ( 3.108217618452874476, 3.916501402570781387, -3.486551214670091881 ) ) ;
#51516=CARTESIAN_POINT ( 'NONE',  ( 20.77500000000000213, 6.123233995736764310E-16, -4.999999999999998224 ) ) ;
#51517=CARTESIAN_POINT ( 'NONE',  ( 10.12500000000000178, 4.330127018922191873, 2.499999999999999556 ) ) ;
#51518=CARTESIAN_POINT ( 'NONE',  ( 20.70000000122903216, -2.886751345948129988, 4.999999999999997335 ) ) ;
#51519=CARTESIAN_POINT ( 'NONE',  ( 15.25312500061451715, 4.541064518000418104, -2.621784821874998173 ) ) ;
#51522=CARTESIAN_POINT ( 'NONE',  ( 18.48750000000000071, -2.886751345948125991, -5.000000000000000000 ) ) ;
#51523=CARTESIAN_POINT ( 'NONE',  ( 20.92500000000000071, 4.330127018922191873, 2.499999999999999556 ) ) ;
#51524=CARTESIAN_POINT ( 'NONE',  ( 18.60937500061451644, 0.000000000000000000, 5.243569643749999010 ) ) ;
#51525=CARTESIAN_POINT ( 'NONE',  ( 24.62812500061451715, 6.421520780324663323E-16, -5.243569643749999010 ) ) ;
#51526=ORIENTED_EDGE ( 'NONE', *, *, #16255, .F. ) ;
#51528=CARTESIAN_POINT ( 'NONE',  ( 7.415625000614516793, -6.054752690667223547, -1.112240025338166033E-15 ) ) ;
#51529=CARTESIAN_POINT ( 'NONE',  ( 4.898587196589411843E-16, 20.00000000000000000, 33.99999999999999289 ) ) ;
#51530=CARTESIAN_POINT ( 'NONE',  ( 13.53749999999999964, -2.886751345948125991, -5.000000000000000000 ) ) ;
#51531=CARTESIAN_POINT ( 'NONE',  ( -4.243569643749999898, 17.06562500061451360, 27.54997392385601529 ) ) ;
#51532=CARTESIAN_POINT ( 'NONE',  ( 28.75312500061451715, 4.541064518000418104, -2.621784821874998173 ) ) ;
#51534=CARTESIAN_POINT ( 'NONE',  ( 25.69687500061451502, 6.054752690667223547, 3.707466751127219781E-16 ) ) ;
#51536=CARTESIAN_POINT ( 'NONE',  ( 22.75312500061451360, -4.541064518000417216, -2.621784821875001281 ) ) ;
#51537=CARTESIAN_POINT ( 'NONE',  ( 24.98437500061451644, -4.541064518000419881, 2.621784821874995952 ) ) ;
#51538=CARTESIAN_POINT ( 'NONE',  ( -4.243569643749999898, 18.00312500061459176, -30.00000000000000000 ) ) ;
#51539=CARTESIAN_POINT ( 'NONE',  ( 11.21250000000000036, -5.773502691896255534, -1.060575238724906372E-15 ) ) ;
#51540=CARTESIAN_POINT ( 'NONE',  ( 9.665625000614515017, -6.054752690667223547, -1.112240025338166033E-15 ) ) ;
#51542=CARTESIAN_POINT ( 'NONE',  ( 28.49062500061451431, -3.027376345333614438, 5.243569643749998122 ) ) ;
#51543=CARTESIAN_POINT ( 'NONE',  ( 26.01562500061451289, 3.027376345333612662, -5.243569643749998122 ) ) ;
#51546=CARTESIAN_POINT ( 'NONE',  ( 18.30937500061451928, -4.541064518000417216, -2.621784821875001281 ) ) ;
#51547=CARTESIAN_POINT ( 'NONE',  ( 4.243569643749999898, 13.29687500061451644, 32.45002607614398471 ) ) ;
#51548=CARTESIAN_POINT ( 'NONE',  ( 18.83437500061451431, 6.421520780324663323E-16, -5.243569643749999010 ) ) ;
#51549=CARTESIAN_POINT ( 'NONE',  ( 26.93437500061451573, 6.421520780324663323E-16, -5.243569643749999010 ) ) ;
#51550=CARTESIAN_POINT ( 'NONE',  ( -3.000416591977282496E-16, 17.04687500061451999, 25.09994784771203058 ) ) ;
#51551=CARTESIAN_POINT ( 'NONE',  ( 6.590625000614518392, -3.027376345333610441, -5.243569643749999898 ) ) ;
#51552=CARTESIAN_POINT ( 'NONE',  ( -3.999999999999999112, 19.06250000000000000, 27.69059892324149885 ) ) ;
#51553=CARTESIAN_POINT ( 'NONE',  ( 5.671875000614519102, -6.054752690667223547, -1.112240025338166033E-15 ) ) ;
#51554=CARTESIAN_POINT ( 'NONE',  ( 5.915625000614515905, 3.027376345333611329, 5.243569643749999010 ) ) ;
#51555=CARTESIAN_POINT ( 'NONE',  ( 10.73437500061451644, 6.421520780324663323E-16, -5.243569643749999010 ) ) ;
#51556=( NAMED_UNIT ( * ) PLANE_ANGLE_UNIT ( ) SI_UNIT ( $, .RADIAN. ) );
#51557=CARTESIAN_POINT ( 'NONE',  ( 18.52500000122903145, -5.773502691896255534, -1.060575238724906372E-15 ) ) ;
#51558=CARTESIAN_POINT ( 'NONE',  ( 6.384375000614516793, 4.541064518000418104, 2.621784821874999949 ) ) ;
#51559=CARTESIAN_POINT ( 'NONE',  ( 6.440625000614517148, -3.027376345333614438, 5.243569643749998122 ) ) ;
#51560=CARTESIAN_POINT ( 'NONE',  ( 5.390625000614518214, 6.054752690667223547, 3.707466751127219781E-16 ) ) ;
#51562=CARTESIAN_POINT ( 'NONE',  ( 16.20937500061451786, 4.541064518000418104, -2.621784821874998173 ) ) ;
#51563=DIRECTION ( 'NONE',  ( -0.000000000000000000, -0.000000000000000000, -1.000000000000000000 ) ) ;
#51565=CARTESIAN_POINT ( 'NONE',  ( 24.74062500061451786, 6.054752690667223547, 3.707466751127219781E-16 ) ) ;
#51566=CARTESIAN_POINT ( 'NONE',  ( 9.403125000614517504, 4.541064518000418104, -2.621784821874998173 ) ) ;
#51567=CARTESIAN_POINT ( 'NONE',  ( 27.98437500061451289, 4.541064518000418104, 2.621784821874999949 ) ) ;
#51568=CARTESIAN_POINT ( 'NONE',  ( 9.665625000614515017, -6.054752690667223547, -1.112240025338166033E-15 ) ) ;
#51569=CARTESIAN_POINT ( 'NONE',  ( -3.000416591977282496E-16, 10.29687500061451644, -34.90005215228797653 ) ) ;
#51570=CARTESIAN_POINT ( 'NONE',  ( 13.20000000122903394, -2.886751345948125991, -5.000000000000000000 ) ) ;
#51571=ADVANCED_FACE ( 'NONE', ( #46207 ), #63764, .T. ) ;
#51572=CARTESIAN_POINT ( 'NONE',  ( 27.06562500061451004, 3.027376345333611329, 5.243569643749999010 ) ) ;
#51573=CARTESIAN_POINT ( 'NONE',  ( -2.121784821874999949, 12.97812500061451679, -33.67503911421598417 ) ) ;
#51574=CARTESIAN_POINT ( 'NONE',  ( 13.05000000122903536, -2.886751345948129988, 4.999999999999997335 ) ) ;
#51575=CARTESIAN_POINT ( 'NONE',  ( 11.55000000000000071, 0.000000000000000000, 4.999999999999998224 ) ) ;
#51576=CARTESIAN_POINT ( 'NONE',  ( 19.82812500061451644, 4.541064518000418104, 2.621784821874999949 ) ) ;
#51577=CARTESIAN_POINT ( 'NONE',  ( 6.046875000614519102, -3.027376345333614438, 5.243569643749998122 ) ) ;
#51578=CARTESIAN_POINT ( 'NONE',  ( 20.51249999999999929, 2.886751345948126879, 4.999999999999999112 ) ) ;
#51579=CARTESIAN_POINT ( 'NONE',  ( 6.675000001229034474, 2.886751345948126879, 4.999999999999999112 ) ) ;
#51580=CARTESIAN_POINT ( 'NONE',  ( 16.98750000122903359, 4.330127018922191873, 2.499999999999999556 ) ) ;
#51582=CARTESIAN_POINT ( 'NONE',  ( 12.40312500061451573, -4.541064518000417216, -2.621784821875001281 ) ) ;
#51583=CARTESIAN_POINT ( 'NONE',  ( 15.10312500061451502, -4.541064518000417216, -2.621784821875001281 ) ) ;
#51584=CARTESIAN_POINT ( 'NONE',  ( 26.06250000122903288, 0.000000000000000000, 4.999999999999998224 ) ) ;
#51585=CARTESIAN_POINT ( 'NONE',  ( 19.68750000000000355, -2.886751345948129988, 4.999999999999997335 ) ) ;
#51586=CARTESIAN_POINT ( 'NONE',  ( 24.53437500061451715, -4.541064518000419881, 2.621784821874995952 ) ) ;
#51588=CARTESIAN_POINT ( 'NONE',  ( 10.08750000122903323, 6.123233995736764310E-16, -4.999999999999998224 ) ) ;
#51589=CARTESIAN_POINT ( 'NONE',  ( 8.596875000614518925, 6.054752690667223547, 3.707466751127219781E-16 ) ) ;
#51590=CARTESIAN_POINT ( 'NONE',  ( 25.43437500061451573, -4.541064518000419881, 2.621784821874995952 ) ) ;
#51592=CARTESIAN_POINT ( 'NONE',  ( 3.046875000614519990, -3.027376345333610441, -5.243569643749999898 ) ) ;
#51593=CARTESIAN_POINT ( 'NONE',  ( 24.10312500061451502, -4.541064518000417216, -2.621784821875001281 ) ) ;
#51594=CARTESIAN_POINT ( 'NONE',  ( 27.38437500061451857, 6.421520780324663323E-16, -5.243569643749999010 ) ) ;
#51597=CARTESIAN_POINT ( 'NONE',  ( 7.434375000614519280, -4.541064518000419881, 2.621784821874995952 ) ) ;
#51599=CARTESIAN_POINT ( 'NONE',  ( 28.64062500061451289, -3.027376345333610441, -5.243569643749999898 ) ) ;
#51600=CARTESIAN_POINT ( 'NONE',  ( 5.371875000614516615, 3.027376345333613106, -5.243569643749998122 ) ) ;
#51603=CARTESIAN_POINT ( 'NONE',  ( 17.47499999999999787, -4.330127018922194537, 2.499999999999995559 ) ) ;
#51605=CARTESIAN_POINT ( 'NONE',  ( 28.01249999999999574, 2.886751345948129099, -4.999999999999998224 ) ) ;
#51606=CARTESIAN_POINT ( 'NONE',  ( 29.59687500061451715, -3.027376345333610441, -5.243569643749999898 ) ) ;
#51608=CARTESIAN_POINT ( 'NONE',  ( 15.59062500061451573, -3.027376345333610441, -5.243569643749999898 ) ) ;
#51609=CARTESIAN_POINT ( 'NONE',  ( 5.690625000614516260, -3.027376345333610441, -5.243569643749999898 ) ) ;
#51611=CARTESIAN_POINT ( 'NONE',  ( 5.334375000614517859, 6.421520780324663323E-16, -5.243569643749999010 ) ) ;
#51612=CARTESIAN_POINT ( 'NONE',  ( 15.15000000122903323, 5.773502691896255534, 3.535250795749688894E-16 ) ) ;
#51613=CARTESIAN_POINT ( 'NONE',  ( 21.30000000000000071, 4.330127018922192761, -2.499999999999997780 ) ) ;
#51614=CARTESIAN_POINT ( 'NONE',  ( 28.83749999999999858, -2.886751345948125991, -5.000000000000000000 ) ) ;
#51615=CARTESIAN_POINT ( 'NONE',  ( 4.696875000614518569, -3.027376345333614438, 5.243569643749998122 ) ) ;
#51616=CARTESIAN_POINT ( 'NONE',  ( 9.196875000614518569, -3.027376345333614438, 5.243569643749998122 ) ) ;
#51617=CARTESIAN_POINT ( 'NONE',  ( 21.42187500061451644, -6.054752690667223547, -1.112240025338166033E-15 ) ) ;
#51618=DIRECTION ( 'NONE',  ( -0.000000000000000000, -1.000000000000000000, -0.000000000000000000 ) ) ;
#51620=CARTESIAN_POINT ( 'NONE',  ( 3.046875000614519990, -3.027376345333610441, -5.243569643749999898 ) ) ;
#51621=CARTESIAN_POINT ( 'NONE',  ( 5.587500000000003020, 5.773502691896255534, 3.535250795749688894E-16 ) ) ;
#51622=CARTESIAN_POINT ( 'NONE',  ( 6.571875000614517681, -6.054752690667223547, -1.112240025338166033E-15 ) ) ;
#51623=VECTOR ( 'NONE', #13554, 1000.000000000000000 ) ;
#51624=CARTESIAN_POINT ( 'NONE',  ( 17.43750000000000355, -2.886751345948129988, 4.999999999999997335 ) ) ;
#51625=CARTESIAN_POINT ( 'NONE',  ( 16.71562500061451573, 3.027376345333611329, 5.243569643749999010 ) ) ;
#51629=CARTESIAN_POINT ( 'NONE',  ( 9.703125000614514661, -4.541064518000417216, -2.621784821875001281 ) ) ;
#51630=CARTESIAN_POINT ( 'NONE',  ( 27.49687500061451217, 6.054752690667223547, 3.707466751127219781E-16 ) ) ;
#51631=CARTESIAN_POINT ( 'NONE',  ( 27.45937500061451786, 4.541064518000418104, -2.621784821874998173 ) ) ;
#51632=CARTESIAN_POINT ( 'NONE',  ( 8.175000000000002487, 6.123233995736764310E-16, -4.999999999999998224 ) ) ;
#51633=CARTESIAN_POINT ( 'NONE',  ( 3.999999999999998668, 14.07500000122903572, 27.69059892324149175 ) ) ;
#51634=CARTESIAN_POINT ( 'NONE',  ( 6.300000001229033586, -2.886751345948129988, 4.999999999999997335 ) ) ;
#51635=CARTESIAN_POINT ( 'NONE',  ( 17.44687500061451857, -3.027376345333610441, -5.243569643749999898 ) ) ;
#51636=CARTESIAN_POINT ( 'NONE',  ( 12.98437500061451821, 6.421520780324663323E-16, -5.243569643749999010 ) ) ;
#51637=CARTESIAN_POINT ( 'NONE',  ( -3.964499721297434665, 3.046849790701494420, -30.54937706598502700 ) ) ;
#51638=VERTEX_POINT ( 'NONE', #46195 ) ;
#51639=CARTESIAN_POINT ( 'NONE',  ( 14.35312500061451679, 4.541064518000418104, -2.621784821874998173 ) ) ;
#51640=CARTESIAN_POINT ( 'NONE',  ( 27.15000000122902790, -2.886751345948125991, -5.000000000000000000 ) ) ;
#51641=CARTESIAN_POINT ( 'NONE',  ( 12.45937500061451786, -4.541064518000417216, -2.621784821875001281 ) ) ;
#51642=LINE ( 'NONE', #23913, #52417 ) ;
#51643=CARTESIAN_POINT ( 'NONE',  ( 13.64062500061451644, -3.027376345333614438, 5.243569643749998122 ) ) ;
#51645=CARTESIAN_POINT ( 'NONE',  ( 23.97187500061451360, 3.027376345333611329, 5.243569643749999010 ) ) ;
#51646=CARTESIAN_POINT ( 'NONE',  ( 2.880239685073342937, -4.087086472263080417, 3.284934485538541171 ) ) ;
#51647=CARTESIAN_POINT ( 'NONE',  ( 11.32500000122903394, -5.773502691896255534, -1.060575238724906372E-15 ) ) ;
#51648=DIRECTION ( 'NONE',  ( -1.000000000000000000, -0.000000000000000000, -0.000000000000000000 ) ) ;
#51650=CARTESIAN_POINT ( 'NONE',  ( -4.243569643749999898, 16.22187500061452070, -32.45002607614398471 ) ) ;
#51651=CARTESIAN_POINT ( 'NONE',  ( 19.24687500061452283, -3.027376345333610441, -5.243569643749999898 ) ) ;
#51652=CARTESIAN_POINT ( 'NONE',  ( 19.42500000122903714, -5.773502691896255534, -1.060575238724906372E-15 ) ) ;
#51653=CARTESIAN_POINT ( 'NONE',  ( 13.92187500061451644, 3.027376345333613106, -5.243569643749998122 ) ) ;
#51654=CARTESIAN_POINT ( 'NONE',  ( 2.121784821875001281, 11.00937500061451857, 33.67503911421598417 ) ) ;
#51655=CARTESIAN_POINT ( 'NONE',  ( 19.57500000122903216, 2.886751345948129099, -4.999999999999998224 ) ) ;
#51656=CARTESIAN_POINT ( 'NONE',  ( 14.61562500061451608, -6.054752690667223547, -1.112240025338166033E-15 ) ) ;
#51657=CARTESIAN_POINT ( 'NONE',  ( 25.31249999999999645, 2.886751345948112668, -5.000000000000024869 ) ) ;
#51658=ORIENTED_EDGE ( 'NONE', *, *, #37910, .T. ) ;
#51659=ORIENTED_EDGE ( 'NONE', *, *, #25362, .F. ) ;
#51660=CARTESIAN_POINT ( 'NONE',  ( 18.75000000000000000, 0.000000000000000000, 4.999999999999998224 ) ) ;
#51662=CARTESIAN_POINT ( 'NONE',  ( 3.253125000614518036, 0.000000000000000000, 5.243569643749999010 ) ) ;
#51663=CARTESIAN_POINT ( 'NONE',  ( 15.26250000122903216, 0.000000000000000000, 4.999999999999998224 ) ) ;
#51664=CARTESIAN_POINT ( 'NONE',  ( 20.91562500061451502, -6.054752690667223547, -1.112240025338166033E-15 ) ) ;
#51665=CARTESIAN_POINT ( 'NONE',  ( 22.30312500061451431, -4.541064518000417216, -2.621784821875001281 ) ) ;
#51666=CARTESIAN_POINT ( 'NONE',  ( 3.478125000614517237, 6.421520780324663323E-16, -5.243569643749999010 ) ) ;
#51667=CARTESIAN_POINT ( 'NONE',  ( 28.64999999999999858, 0.000000000000000000, 4.999999999999998224 ) ) ;
#51670=CARTESIAN_POINT ( 'NONE',  ( 29.37187500061451928, 3.027376345333611329, 5.243569643749999010 ) ) ;
#51671=CARTESIAN_POINT ( 'NONE',  ( -2.828200636599751609E-16, 12.35000000122903430, -34.61880215351700230 ) ) ;
#51672=CARTESIAN_POINT ( 'NONE',  ( 4.243569643749999898, 15.13437500061451679, -30.00000000000000000 ) ) ;
#51673=CARTESIAN_POINT ( 'NONE',  ( 5.137500001229033941, 6.123233995736764310E-16, -4.999999999999998224 ) ) ;
#51674=CARTESIAN_POINT ( 'NONE',  ( 9.037499999999999645, -2.886751345948125991, -5.000000000000000000 ) ) ;
#51675=( BOUNDED_CURVE ( )  B_SPLINE_CURVE ( 2, ( #68851, #28961, #57384, #62217, #67765, #62928, #68134, #23407, #45954 ),
 .UNSPECIFIED., .F., .F. ) 
 B_SPLINE_CURVE_WITH_KNOTS ( ( 3, 2, 2, 2, 3 ),
 ( 0.8152173913043478937, 0.8188405797101449002, 0.8260869565217391353, 0.8333333333333333703, 0.8369565217391304879 ),
 .UNSPECIFIED. ) 
 CURVE ( )  GEOMETRIC_REPRESENTATION_ITEM ( )  RATIONAL_B_SPLINE_CURVE ( ( 0.9330127018922192983, 0.9330127018922202975, 1.000000000000000000, 0.8660254037844387076, 1.000000000000000000, 0.8660254037844387076, 1.000000000000000000, 0.9330127018922182991, 0.9330127018922192983 ) ) 
 REPRESENTATION_ITEM ( '' )  );
#51677=CARTESIAN_POINT ( 'NONE',  ( 4.050000001229035362, -2.886751345948129988, 4.999999999999997335 ) ) ;
#51678=CARTESIAN_POINT ( 'NONE',  ( 10.39687500061451786, 6.054752690667223547, 3.707466751127219781E-16 ) ) ;
#51679=CARTESIAN_POINT ( 'NONE',  ( 30.00000000000000000, 6.123233995736764310E-16, -4.999999999999998224 ) ) ;
#51680=CARTESIAN_POINT ( 'NONE',  ( 3.534375000614518036, 6.421520780324663323E-16, -5.243569643749999010 ) ) ;
#51681=CARTESIAN_POINT ( 'NONE',  ( -4.757043123249222738, 8.797129135976163639, -33.66161464372975587 ) ) ;
#51682=CARTESIAN_POINT ( 'NONE',  ( 16.98750000122903359, 4.330127018922191873, 2.499999999999999556 ) ) ;
#51683=CARTESIAN_POINT ( 'NONE',  ( 6.946875000614517681, -3.027376345333614438, 5.243569643749998122 ) ) ;
#51684=CARTESIAN_POINT ( 'NONE',  ( 12.53437500061451537, 6.421520780324663323E-16, -5.243569643749999010 ) ) ;
#51685=CARTESIAN_POINT ( 'NONE',  ( 5.924999999999999822, 6.123233995736764310E-16, -4.999999999999998224 ) ) ;
#51686=CARTESIAN_POINT ( 'NONE',  ( -4.243569643749999898, 17.55312500061459602, 30.00000000000000000 ) ) ;
#51687=CARTESIAN_POINT ( 'NONE',  ( 21.94687500061451857, -3.027376345333610441, -5.243569643749999898 ) ) ;
#51688=CARTESIAN_POINT ( 'NONE',  ( 2.803505685599422037, -4.140118174855662581, 3.024073416196122466 ) ) ;
#51689=CARTESIAN_POINT ( 'NONE',  ( 25.95000000122903216, 5.773502691896255534, 3.535250795749688894E-16 ) ) ;
#51691=CARTESIAN_POINT ( 'NONE',  ( 21.74062500061451431, -3.027376345333614438, 5.243569643749998122 ) ) ;
#51692=CARTESIAN_POINT ( 'NONE',  ( 12.36562500061451608, -6.054752690667223547, -1.112240025338166033E-15 ) ) ;
#51694=CARTESIAN_POINT ( 'NONE',  ( 11.85937500061451644, 0.000000000000000000, 5.243569643749999010 ) ) ;
#51695=CARTESIAN_POINT ( 'NONE',  ( 27.97500000000000142, 6.123233995736764310E-16, -4.999999999999998224 ) ) ;
#51696=CARTESIAN_POINT ( 'NONE',  ( 21.63750000122903572, -4.330127018922194537, 2.499999999999995559 ) ) ;
#51698=CARTESIAN_POINT ( 'NONE',  ( 13.02187500061451608, 3.027376345333613106, -5.243569643749998122 ) ) ;
#51699=CARTESIAN_POINT ( 'NONE',  ( 28.09687500061451360, -3.027376345333614438, 5.243569643749998122 ) ) ;
#51700=CARTESIAN_POINT ( 'NONE',  ( 3.984375000614517326, 6.421520780324663323E-16, -5.243569643749999010 ) ) ;
#51701=CARTESIAN_POINT ( 'NONE',  ( -3.999999999999999112, 12.31250000000000000, -32.30940107675850470 ) ) ;
#51702=VECTOR ( 'NONE', #60290, 1000.000000000000000 ) ;
#51703=CARTESIAN_POINT ( 'NONE',  ( 21.60937500061451644, 4.541064518000418104, -2.621784821874998173 ) ) ;
#51704=CARTESIAN_POINT ( 'NONE',  ( 14.55937500061451573, 0.000000000000000000, 5.243569643749999010 ) ) ;
#51706=CARTESIAN_POINT ( 'NONE',  ( 25.27499999999999858, 6.123233995736764310E-16, -4.999999999999998224 ) ) ;
#51709=CARTESIAN_POINT ( 'NONE',  ( 18.32812500061451644, 6.421520780324663323E-16, -5.243569643749999010 ) ) ;
#51710=CARTESIAN_POINT ( 'NONE',  ( 7.124999999999999112, -4.330127018922194537, 2.499999999999995559 ) ) ;
#51711=CARTESIAN_POINT ( 'NONE',  ( 2.803125000614518747, 0.000000000000000000, 5.243569643749999010 ) ) ;
#51712=CARTESIAN_POINT ( 'NONE',  ( 15.41250000000000142, 2.886751345948129099, -4.999999999999998224 ) ) ;
#51713=CARTESIAN_POINT ( 'NONE',  ( -4.243569643749997233, 11.29062500061451857, 32.45002607614398471 ) ) ;
#51714=DIRECTION ( 'NONE',  ( -1.000000000000000000, -0.000000000000000000, -0.000000000000000000 ) ) ;
#51715=CARTESIAN_POINT ( 'NONE',  ( 26.48437500061451644, 6.421520780324663323E-16, -5.243569643749999010 ) ) ;
#51716=ORIENTED_EDGE ( 'NONE', *, *, #1232, .T. ) ;
#51717=CARTESIAN_POINT ( 'NONE',  ( 22.19062500061451715, -3.027376345333614438, 5.243569643749998122 ) ) ;
#51718=CARTESIAN_POINT ( 'NONE',  ( 19.32187500061451857, 3.027376345333613106, -5.243569643749998122 ) ) ;
#51719=B_SPLINE_CURVE_WITH_KNOTS ( 'NONE', 3,
 ( #25354, #30894, #24983, #9469 ),
 .UNSPECIFIED., .F., .F.,
 ( 4, 4 ),
 ( 0.001150238639792624086, 0.002170813345905252094 ),
 .UNSPECIFIED. ) ;
#51720=CARTESIAN_POINT ( 'NONE',  ( 3.262500000000001510, 2.886751345948129099, -4.999999999999998224 ) ) ;
#51721=CARTESIAN_POINT ( 'NONE',  ( 6.553125000614518747, -4.541064518000417216, -2.621784821875001281 ) ) ;
#51722=CARTESIAN_POINT ( 'NONE',  ( 22.04062500061451502, 6.054752690667223547, 3.707466751127219781E-16 ) ) ;
#51723=CARTESIAN_POINT ( 'NONE',  ( 13.17187500061451999, 3.027376345333611329, 5.243569643749999010 ) ) ;
#51724=CARTESIAN_POINT ( 'NONE',  ( 16.69687500061451502, 6.054752690667223547, 3.707466751127219781E-16 ) ) ;
#51725=CARTESIAN_POINT ( 'NONE',  ( 4.243569643749999898, 18.19062500061451360, 32.45002607614398471 ) ) ;
#51726=CARTESIAN_POINT ( 'NONE',  ( 19.38750000122903216, -4.330127018922194537, 2.499999999999995559 ) ) ;
#51728=CARTESIAN_POINT ( 'NONE',  ( 9.515625000614518214, 3.027376345333611329, 5.243569643749999010 ) ) ;
#51729=CARTESIAN_POINT ( 'NONE',  ( 5.671875000614519102, -6.054752690667223547, -1.112240025338166033E-15 ) ) ;
#51730=CARTESIAN_POINT ( 'NONE',  ( 5.896875000614518747, 6.054752690667223547, 3.707466751127219781E-16 ) ) ;
#51731=CARTESIAN_POINT ( 'NONE',  ( 24.64687500061451431, -3.027376345333610441, -5.243569643749999898 ) ) ;
#51732=CARTESIAN_POINT ( 'NONE',  ( 15.89062500061451289, -3.027376345333614438, 5.243569643749998122 ) ) ;
#51733=CARTESIAN_POINT ( 'NONE',  ( 26.32500000122903216, 2.886751345948129099, -4.999999999999998224 ) ) ;
#51735=CARTESIAN_POINT ( 'NONE',  ( 26.09062500061451573, 6.054752690667223547, 3.707466751127219781E-16 ) ) ;
#51736=CARTESIAN_POINT ( 'NONE',  ( 22.62187500061451573, 3.027376345333611329, 5.243569643749999010 ) ) ;
#51737=CARTESIAN_POINT ( 'NONE',  ( 18.32812500061451644, 6.421520780324663323E-16, -5.243569643749999010 ) ) ;
#51738=CARTESIAN_POINT ( 'NONE',  ( 4.243569643749999898, 17.83437500061451786, 30.00000000000000000 ) ) ;
#51740=CARTESIAN_POINT ( 'NONE',  ( 21.36562500061451431, -6.054752690667223547, -1.112240025338166033E-15 ) ) ;
#51741=CARTESIAN_POINT ( 'NONE',  ( 2.737500001229034474, -4.330127018922194537, 2.499999999999995559 ) ) ;
#51743=CARTESIAN_POINT ( 'NONE',  ( 25.76249999999999929, 2.886751345948129099, -4.999999999999998224 ) ) ;
#51744=CARTESIAN_POINT ( 'NONE',  ( 3.999999999999999112, 13.47500000000000142, -30.00000000000000000 ) ) ;
#51745=CARTESIAN_POINT ( 'NONE',  ( 1.071796769724493892, 18.17990381179669868, 26.00000000000000711 ) ) ;
#51746=CARTESIAN_POINT ( 'NONE',  ( 28.22812500061451502, 6.421520780324663323E-16, -5.243569643749999010 ) ) ;
#51747=CARTESIAN_POINT ( 'NONE',  ( 9.065625000614517148, 3.027376345333611329, 5.243569643749999010 ) ) ;
#51748=CARTESIAN_POINT ( 'NONE',  ( 22.87500000122903288, 2.886751345948126879, 4.999999999999999112 ) ) ;
#51749=CARTESIAN_POINT ( 'NONE',  ( 27.96562500061451928, 3.027376345333611329, 5.243569643749999010 ) ) ;
#51750=CARTESIAN_POINT ( 'NONE',  ( 27.56250000000000000, 2.886751345948129099, -4.999999999999998224 ) ) ;
#51751=CARTESIAN_POINT ( 'NONE',  ( 3.999999999999999112, 18.08750000122903501, -30.00000000000000000 ) ) ;
#51752=EDGE_CURVE ( 'NONE', #29206, #72969, #29563, .T. ) ;
#51753=CARTESIAN_POINT ( 'NONE',  ( -3.999999999999999112, 12.42500000122903536, 27.69059892324149885 ) ) ;
#51754=CARTESIAN_POINT ( 'NONE',  ( 11.35312500061451679, 0.000000000000000000, 5.243569643749999010 ) ) ;
#51756=CARTESIAN_POINT ( 'NONE',  ( 26.50312500061451360, 4.541064518000418104, -2.621784821874998173 ) ) ;
#51757=CARTESIAN_POINT ( 'NONE',  ( 8.803125000614517859, -4.541064518000417216, -2.621784821875001281 ) ) ;
#51758=CARTESIAN_POINT ( 'NONE',  ( 5.428125000614517859, 4.541064518000418104, 2.621784821874999949 ) ) ;
#51760=EDGE_CURVE ( 'NONE', #3193, #18895, #58344, .T. ) ;
#51761=DIRECTION ( 'NONE',  ( -0.000000000000000000, -1.000000000000000000, -0.000000000000000000 ) ) ;
#51762=CARTESIAN_POINT ( 'NONE',  ( 14.36249999999999893, -5.773502691896255534, -1.060575238724906372E-15 ) ) ;
#51763=CARTESIAN_POINT ( 'NONE',  ( 15.23437500061451644, 6.421520780324663323E-16, -5.243569643749999010 ) ) ;
#51764=CARTESIAN_POINT ( 'NONE',  ( 11.28750000122903252, -4.330127018922194537, 2.499999999999995559 ) ) ;
#51765=CARTESIAN_POINT ( 'NONE',  ( 16.47187500061452070, -6.054752690667223547, -1.112240025338166033E-15 ) ) ;
#51767=CARTESIAN_POINT ( 'NONE',  ( 20.29687500061451644, 6.054752690667223547, 3.707466751127219781E-16 ) ) ;
#51768=CARTESIAN_POINT ( 'NONE',  ( 9.001249775931846008E-16, 13.16562500061451857, -25.09994784771203058 ) ) ;
#51769=CARTESIAN_POINT ( 'NONE',  ( 21.07500000122903572, 2.886751345948126879, 4.999999999999998224 ) ) ;
#51771=CARTESIAN_POINT ( 'NONE',  ( -5.810221930991193690E-16, 14.93750000000000000, -34.00000000000000000 ) ) ;
#51772=CARTESIAN_POINT ( 'NONE',  ( 23.80312500061451786, 4.541064518000418104, -2.621784821874998173 ) ) ;
#51773=CARTESIAN_POINT ( 'NONE',  ( 29.52187500061451431, -6.054752690667223547, -1.112240025338166033E-15 ) ) ;
#51774=CARTESIAN_POINT ( 'NONE',  ( 25.46249999999999858, 2.886751345948126879, 4.999999999999999112 ) ) ;
#51775=CARTESIAN_POINT ( 'NONE',  ( 7.340625000614518392, -3.027376345333614438, 5.243569643749998122 ) ) ;
#51777=CARTESIAN_POINT ( 'NONE',  ( 19.65937500061451360, -4.541064518000417216, -2.621784821875001281 ) ) ;
#51779=CARTESIAN_POINT ( 'NONE',  ( 6.028125000614517504, -4.541064518000419881, 2.621784821874995952 ) ) ;
#51780=CARTESIAN_POINT ( 'NONE',  ( 8.334375000614516082, -4.541064518000419881, 2.621784821874995952 ) ) ;
#51782=CARTESIAN_POINT ( 'NONE',  ( 19.54687500061451644, -3.027376345333614438, 5.243569643749998122 ) ) ;
#51783=FACE_OUTER_BOUND ( 'NONE', #25334, .T. ) ;
#51784=CARTESIAN_POINT ( 'NONE',  ( 25.83749999999999858, 5.773502691896255534, 3.535250795749688894E-16 ) ) ;
#51785=CARTESIAN_POINT ( 'NONE',  ( 29.82187500061451502, 3.027376345333611329, 5.243569643749999010 ) ) ;
#51788=CARTESIAN_POINT ( 'NONE',  ( 10.76250000000000107, -5.773502691896255534, -1.060575238724906372E-15 ) ) ;
#51790=CARTESIAN_POINT ( 'NONE',  ( 24.96562500061451573, -6.054752690667223547, -1.112240025338166033E-15 ) ) ;
#51791=CARTESIAN_POINT ( 'NONE',  ( 13.42499999999999893, -4.330127018922194537, 2.499999999999995559 ) ) ;
#51792=CARTESIAN_POINT ( 'NONE',  ( 10.72500000122903252, 2.886751345948126879, 4.999999999999999112 ) ) ;
#51793=CARTESIAN_POINT ( 'NONE',  ( 9.890625000614516438, 6.054752690667223547, 3.707466751127219781E-16 ) ) ;
#51794=CARTESIAN_POINT ( 'NONE',  ( 24.41250000000000142, 2.886751345948129099, -4.999999999999998224 ) ) ;
#51795=CARTESIAN_POINT ( 'NONE',  ( 20.57812500061451644, 6.421520780324663323E-16, -5.243569643749999010 ) ) ;
#51797=CARTESIAN_POINT ( 'NONE',  ( 24.86250000122903359, -4.330127018922190985, -2.500000000000001332 ) ) ;
#51799=CARTESIAN_POINT ( 'NONE',  ( 6.375000000000001776, 6.123233995736764310E-16, -4.999999999999998224 ) ) ;
#51800=ORIENTED_EDGE ( 'NONE', *, *, #50590, .F. ) ;
#51801=CARTESIAN_POINT ( 'NONE',  ( 22.67812500061451431, -4.541064518000419881, 2.621784821874995952 ) ) ;
#51802=CARTESIAN_POINT ( 'NONE',  ( 28.45312500061451289, 0.000000000000000000, 5.243569643749999010 ) ) ;
#51803=CARTESIAN_POINT ( 'NONE',  ( 27.00937500061451857, 4.541064518000418104, -2.621784821874998173 ) ) ;
#51804=CARTESIAN_POINT ( 'NONE',  ( 18.72187500061451360, -6.054752690667223547, -1.112240025338166033E-15 ) ) ;
#51805=CARTESIAN_POINT ( 'NONE',  ( 14.05312500061451431, 0.000000000000000000, 5.243569643749999010 ) ) ;
#51807=CARTESIAN_POINT ( 'NONE',  ( 25.20000000122903216, -2.886751345948129988, 4.999999999999997335 ) ) ;
#51809=CARTESIAN_POINT ( 'NONE',  ( 15.77812500061451573, 4.541064518000418104, 2.621784821874999949 ) ) ;
#51811=CARTESIAN_POINT ( 'NONE',  ( 2.775000001229033675, -5.773502691896255534, -1.060575238724906372E-15 ) ) ;
#51812=CARTESIAN_POINT ( 'NONE',  ( 11.82187500061451679, 3.027376345333611329, 5.243569643749999010 ) ) ;
#51813=CARTESIAN_POINT ( 'NONE',  ( 11.89687500061451608, -3.027376345333614438, 5.243569643749998122 ) ) ;
#51814=CARTESIAN_POINT ( 'NONE',  ( 19.47187500061451360, 3.027376345333611329, 5.243569643749999010 ) ) ;
#51816=CARTESIAN_POINT ( 'NONE',  ( 9.899999999999998579, -4.330127018922190985, -2.500000000000001332 ) ) ;
#51817=CARTESIAN_POINT ( 'NONE',  ( 25.22812500061451502, 4.541064518000418104, 2.621784821874999949 ) ) ;
#51818=CARTESIAN_POINT ( 'NONE',  ( 19.20937500061451786, -4.541064518000417216, -2.621784821875001281 ) ) ;
#51819=CARTESIAN_POINT ( 'NONE',  ( 24.92812500061451431, -4.541064518000419881, 2.621784821874995952 ) ) ;
#51821=CARTESIAN_POINT ( 'NONE',  ( -2.828200636599751609E-16, 14.03750000000000142, 25.38119784648299770 ) ) ;
#51822=CARTESIAN_POINT ( 'NONE',  ( 28.34062500061451928, 6.054752690667223547, 3.707466751127219781E-16 ) ) ;
#51823=CARTESIAN_POINT ( 'NONE',  ( 9.750000001229032875, 5.773502691896255534, 3.535250795749688894E-16 ) ) ;
#51824=CARTESIAN_POINT ( 'NONE',  ( 6.825000001229034829, -5.773502691896255534, -1.060575238724906372E-15 ) ) ;
#51826=CARTESIAN_POINT ( 'NONE',  ( 27.33750000122903145, 4.330127018922191873, 2.499999999999999556 ) ) ;
#51829=CARTESIAN_POINT ( 'NONE',  ( 9.609375000614518214, 0.000000000000000000, 5.243569643749999010 ) ) ;
#51830=DIRECTION ( 'NONE',  ( 0.000000000000000000, 0.000000000000000000, 1.000000000000000000 ) ) ;
#51831=CARTESIAN_POINT ( 'NONE',  ( 18.17812500061451786, -4.541064518000419881, 2.621784821874995952 ) ) ;
#51832=CARTESIAN_POINT ( 'NONE',  ( 10.47187500061451715, 3.027376345333611329, 5.243569643749999010 ) ) ;
#51833=CARTESIAN_POINT ( 'NONE',  ( 3.553125000614516082, 4.541064518000418104, -2.621784821874998173 ) ) ;
#51834=CARTESIAN_POINT ( 'NONE',  ( 19.28437500061451360, 6.421520780324663323E-16, -5.243569643749999010 ) ) ;
#51835=CARTESIAN_POINT ( 'NONE',  ( 8.596875000614518925, 6.054752690667223547, 3.707466751127219781E-16 ) ) ;
#51836=CARTESIAN_POINT ( 'NONE',  ( 14.92500000122903359, -5.773502691896255534, -1.060575238724906372E-15 ) ) ;
#51837=( BOUNDED_CURVE ( )  B_SPLINE_CURVE ( 2, ( #38118, #26686, #10776, #32585, #33309, #14852, #59915 ),
 .UNSPECIFIED., .F., .F. ) 
 B_SPLINE_CURVE_WITH_KNOTS ( ( 3, 2, 2, 3 ),
 ( 0.8000000000000000444, 0.8027777777777778123, 0.8055555555555555802, 0.8083333333333333481 ),
 .UNSPECIFIED. ) 
 CURVE ( )  GEOMETRIC_REPRESENTATION_ITEM ( )  RATIONAL_B_SPLINE_CURVE ( ( 1.000000000000000000, 0.8660254037844387076, 1.000000000000000000, 0.8660254037844387076, 1.000000000000000000, 0.8660254037844387076, 1.000000000000000000 ) ) 
 REPRESENTATION_ITEM ( '' )  );
#51838=ADVANCED_FACE ( 'NONE', ( #18462 ), #41382, .F. ) ;
#51839=CARTESIAN_POINT ( 'NONE',  ( 7.153125000614518392, 4.541064518000418104, -2.621784821874998173 ) ) ;
#51840=CARTESIAN_POINT ( 'NONE',  ( 16.94062500061451715, -3.027376345333610441, -5.243569643749999898 ) ) ;
#51841=ORIENTED_EDGE ( 'NONE', *, *, #31751, .T. ) ;
#51842=CARTESIAN_POINT ( 'NONE',  ( 4.875000001229034652, 2.886751345948126879, 4.999999999999999112 ) ) ;
#51843=CARTESIAN_POINT ( 'NONE',  ( 15.62812500061451537, 6.421520780324663323E-16, -5.243569643749999010 ) ) ;
#51844=CARTESIAN_POINT ( 'NONE',  ( 13.94062500061451892, 6.054752690667223547, 3.707466751127219781E-16 ) ) ;
#51846=CARTESIAN_POINT ( 'NONE',  ( 12.63749999999999929, -2.886751345948125991, -5.000000000000000000 ) ) ;
#51847=CARTESIAN_POINT ( 'NONE',  ( 8.662500001229034297, -4.330127018922190985, -2.500000000000001332 ) ) ;
#51848=CARTESIAN_POINT ( 'NONE',  ( 4.565625000614516260, 3.027376345333611329, 5.243569643749999010 ) ) ;
#51849=CARTESIAN_POINT ( 'NONE',  ( 19.50000000122903288, -2.886751345948125991, -5.000000000000000000 ) ) ;
#51851=CARTESIAN_POINT ( 'NONE',  ( -4.243569643749999898, 12.17187500061451999, -32.45002607614398471 ) ) ;
#51853=CARTESIAN_POINT ( 'NONE',  ( 2.850000001229036073, -2.886751345948125991, -5.000000000000000000 ) ) ;
#51855=CARTESIAN_POINT ( 'NONE',  ( 2.958964567276093582, 4.194048102626701358, -2.735695596862700807 ) ) ;
#51857=CARTESIAN_POINT ( 'NONE',  ( 18.75937500061451857, -4.541064518000417216, -2.621784821875001281 ) ) ;
#51858=CARTESIAN_POINT ( 'NONE',  ( -1.071796769724483234, 16.42009619066137205, 25.99999999999999645 ) ) ;
#51859=CARTESIAN_POINT ( 'NONE',  ( 14.01562500061451644, 3.027376345333611329, 5.243569643749999010 ) ) ;
#51861=CARTESIAN_POINT ( 'NONE',  ( 18.63750000122903216, 6.123233995736764310E-16, -4.999999999999998224 ) ) ;
#51862=CARTESIAN_POINT ( 'NONE',  ( 25.84687500061451360, -3.027376345333614438, 5.243569643749998122 ) ) ;
#51864=CARTESIAN_POINT ( 'NONE',  ( 13.34062500061451750, -3.027376345333610441, -5.243569643749999898 ) ) ;
#51865=CARTESIAN_POINT ( 'NONE',  ( 15.15937500061451715, -4.541064518000417216, -2.621784821875001281 ) ) ;
#51866=ORIENTED_EDGE ( 'NONE', *, *, #54850, .F. ) ;
#51867=CARTESIAN_POINT ( 'NONE',  ( 28.34062500061451928, 6.054752690667223547, 3.707466751127219781E-16 ) ) ;
#51868=CARTESIAN_POINT ( 'NONE',  ( 20.16562500061451146, 3.027376345333613106, -5.243569643749998122 ) ) ;
#51869=CARTESIAN_POINT ( 'NONE',  ( 18.82500000000000284, -4.330127018922194537, 2.499999999999995559 ) ) ;
#51870=CARTESIAN_POINT ( 'NONE',  ( 30.00000000000000000, 6.123233995736764310E-16, -4.999999999999998224 ) ) ;
#51873=CARTESIAN_POINT ( 'NONE',  ( 9.674999999999998934, 4.330127018922191873, 2.499999999999999556 ) ) ;
#51874=CARTESIAN_POINT ( 'NONE',  ( 18.41250000122903430, 0.000000000000000000, 4.999999999999998224 ) ) ;
#51878=CARTESIAN_POINT ( 'NONE',  ( 17.92500000000000071, -4.330127018922194537, 2.499999999999995559 ) ) ;
#51879=CARTESIAN_POINT ( 'NONE',  ( 20.99999999999999645, 0.000000000000000000, 4.999999999999998224 ) ) ;
#51881=CARTESIAN_POINT ( 'NONE',  ( 19.80937500061451573, 4.541064518000418104, -2.621784821874998173 ) ) ;
#51882=CARTESIAN_POINT ( 'NONE',  ( 26.12812500061451360, 4.541064518000418104, 2.621784821874999949 ) ) ;
#51883=ORIENTED_EDGE ( 'NONE', *, *, #2540, .F. ) ;
#51884=FACE_OUTER_BOUND ( 'NONE', #10595, .T. ) ;
#51885=CARTESIAN_POINT ( 'NONE',  ( 8.090625000614515727, 6.054752690667223547, 3.707466751127219781E-16 ) ) ;
#51887=CARTESIAN_POINT ( 'NONE',  ( 13.72500000000000142, 4.330127018922191873, 2.499999999999999556 ) ) ;
#51888=CARTESIAN_POINT ( 'NONE',  ( -4.243569643749999898, 18.45312500061451644, 30.00000000000000000 ) ) ;
#51889=CARTESIAN_POINT ( 'NONE',  ( 28.94062500061452070, -3.027376345333614438, 5.243569643749998122 ) ) ;
#51892=CARTESIAN_POINT ( 'NONE',  ( 26.85937500061451644, -4.541064518000417216, -2.621784821875001281 ) ) ;
#51893=ORIENTED_EDGE ( 'NONE', *, *, #66002, .T. ) ;
#51894=CARTESIAN_POINT ( 'NONE',  ( 20.42812500061451431, -4.541064518000419881, 2.621784821874995952 ) ) ;
#51895=CARTESIAN_POINT ( 'NONE',  ( 23.55937500061451573, 0.000000000000000000, 5.243569643749999010 ) ) ;
#51896=CARTESIAN_POINT ( 'NONE',  ( -4.243569643749999898, 16.20312500061459460, -30.00000000000000000 ) ) ;
#51897=CARTESIAN_POINT ( 'NONE',  ( 10.46249999999999858, 2.886751345948129099, -4.999999999999998224 ) ) ;
#51898=CARTESIAN_POINT ( 'NONE',  ( 6.778125000614518392, 4.541064518000418104, 2.621784821874999949 ) ) ;
#51900=CARTESIAN_POINT ( 'NONE',  ( 23.20312500061451644, -4.541064518000417216, -2.621784821875001281 ) ) ;
#51903=CARTESIAN_POINT ( 'NONE',  ( 18.98437500061451644, 4.541064518000418104, 2.621784821874999949 ) ) ;
#51904=CARTESIAN_POINT ( 'NONE',  ( -4.243569643749999898, 12.62187500061451928, 27.54997392385601529 ) ) ;
#51905=CARTESIAN_POINT ( 'NONE',  ( 19.54687500061451644, -3.027376345333614438, 5.243569643749998122 ) ) ;
#51906=CARTESIAN_POINT ( 'NONE',  ( 26.55937500061451573, 4.541064518000418104, -2.621784821874998173 ) ) ;
#51907=CARTESIAN_POINT ( 'NONE',  ( 4.243569643749999898, 15.99687500061451573, 32.45002607614398471 ) ) ;
#51908=CARTESIAN_POINT ( 'NONE',  ( 8.015625000614518214, 3.027376345333613106, -5.243569643749998122 ) ) ;
#51909=CARTESIAN_POINT ( 'NONE',  ( -1.071796769724490783, 19.19240381056767220, 34.00000000000000000 ) ) ;
#51911=CARTESIAN_POINT ( 'NONE',  ( 3.421875000614516882, -6.054752690667223547, -1.112240025338166033E-15 ) ) ;
#51912=CARTESIAN_POINT ( 'NONE',  ( 25.98750000122903003, 4.330127018922191873, 2.499999999999999556 ) ) ;
#51913=CARTESIAN_POINT ( 'NONE',  ( 6.178125000614518747, 6.421520780324663323E-16, -5.243569643749999010 ) ) ;
#51914=CARTESIAN_POINT ( 'NONE',  ( 9.834375000614517859, 6.421520780324663323E-16, -5.243569643749999010 ) ) ;
#51916=CARTESIAN_POINT ( 'NONE',  ( 15.60000000122903607, 5.773502691896255534, 3.535250795749688894E-16 ) ) ;
#51917=CARTESIAN_POINT ( 'NONE',  ( 5.221875000614519813, -6.054752690667223547, -1.112240025338166033E-15 ) ) ;
#51918=CARTESIAN_POINT ( 'NONE',  ( 8.353125000614518569, -4.541064518000417216, -2.621784821875001281 ) ) ;
#51919=CARTESIAN_POINT ( 'NONE',  ( 4.073549908004127751, -3.793187680347479329, 3.430006214993830405 ) ) ;
#51921=CARTESIAN_POINT ( 'NONE',  ( 17.33437500061451431, -4.541064518000419881, 2.621784821874995952 ) ) ;
#51922=CARTESIAN_POINT ( 'NONE',  ( 1.626862140677534273E-15, 10.66249999999999964, 34.00000000000000000 ) ) ;
#51924=CARTESIAN_POINT ( 'NONE',  ( 25.15312500061451217, 4.541064518000418104, -2.621784821874998173 ) ) ;
#51925=CARTESIAN_POINT ( 'NONE',  ( 9.140625000614518214, -3.027376345333614438, 5.243569643749998122 ) ) ;
#51926=CARTESIAN_POINT ( 'NONE',  ( 26.89687500061451431, -3.027376345333610441, -5.243569643749999898 ) ) ;
#51927=CARTESIAN_POINT ( 'NONE',  ( 10.82812500061451644, 4.541064518000418104, 2.621784821874999949 ) ) ;
#51928=CARTESIAN_POINT ( 'NONE',  ( -4.243569643749998122, 10.89687500061451786, -27.54997392385601174 ) ) ;
#51929=CARTESIAN_POINT ( 'NONE',  ( 9.787500001229036073, 4.330127018922191873, 2.499999999999999556 ) ) ;
#51930=CARTESIAN_POINT ( 'NONE',  ( 28.37812500061451715, 4.541064518000418104, 2.621784821874999949 ) ) ;
#51931=CARTESIAN_POINT ( 'NONE',  ( 4.243569643749999898, 13.72812500061451679, -30.00000000000000000 ) ) ;
#51932=CARTESIAN_POINT ( 'NONE',  ( 11.96250000122903501, 4.330127018922192761, -2.499999999999997780 ) ) ;
#51933=CARTESIAN_POINT ( 'NONE',  ( 21.29062500061451502, -3.027376345333614438, 5.243569643749998122 ) ) ;
#51934=CARTESIAN_POINT ( 'NONE',  ( 10.42500000000000071, 6.123233995736764310E-16, -4.999999999999998224 ) ) ;
#51935=CARTESIAN_POINT ( 'NONE',  ( 21.51562500061451644, 3.027376345333613106, -5.243569643749998122 ) ) ;
#51936=CARTESIAN_POINT ( 'NONE',  ( 6.309375000614517504, 4.541064518000418104, -2.621784821874998173 ) ) ;
#51937=CARTESIAN_POINT ( 'NONE',  ( 20.13749999999999929, -2.886751345948129988, 4.999999999999997335 ) ) ;
#51938=CARTESIAN_POINT ( 'NONE',  ( 7.012500001229035718, 4.330127018922192761, -2.499999999999997780 ) ) ;
#51939=CARTESIAN_POINT ( 'NONE',  ( 15.11250000122903359, 4.330127018922192761, -2.499999999999997780 ) ) ;
#51940=CARTESIAN_POINT ( 'NONE',  ( 13.82812500061451466, 6.421520780324663323E-16, -5.243569643749999010 ) ) ;
#51941=CARTESIAN_POINT ( 'NONE',  ( 15.70312500061451644, 4.541064518000418104, -2.621784821874998173 ) ) ;
#51942=CARTESIAN_POINT ( 'NONE',  ( 26.62500000122903288, -5.773502691896255534, -1.060575238724906372E-15 ) ) ;
#51943=CARTESIAN_POINT ( 'NONE',  ( 19.50000000000000000, 4.330127018922192761, -2.499999999999997780 ) ) ;
#51944=CARTESIAN_POINT ( 'NONE',  ( 23.29687500061451644, -3.027376345333610441, -5.243569643749999898 ) ) ;
#51946=CARTESIAN_POINT ( 'NONE',  ( 9.000000001229034652, -2.886751345948129988, 4.999999999999997335 ) ) ;
#51947=CARTESIAN_POINT ( 'NONE',  ( 8.409375000614518925, -4.541064518000417216, -2.621784821875001281 ) ) ;
#51948=CARTESIAN_POINT ( 'NONE',  ( 24.72187500061451360, 3.027376345333613106, -5.243569643749998122 ) ) ;
#51949=CARTESIAN_POINT ( 'NONE',  ( 23.69999999999999929, 0.000000000000000000, 4.999999999999998224 ) ) ;
#51950=CARTESIAN_POINT ( 'NONE',  ( 21.59062500061451928, 6.054752690667223547, 3.707466751127219781E-16 ) ) ;
#51951=CARTESIAN_POINT ( 'NONE',  ( 26.07187500061451857, 3.027376345333613106, -5.243569643749998122 ) ) ;
#51954=CARTESIAN_POINT ( 'NONE',  ( 8.559375000614515727, 4.541064518000418104, -2.621784821874998173 ) ) ;
#51955=CARTESIAN_POINT ( 'NONE',  ( 18.92812500061451431, 4.541064518000418104, 2.621784821874999949 ) ) ;
#51958=CARTESIAN_POINT ( 'NONE',  ( 27.47812500061451502, 4.541064518000418104, 2.621784821874999949 ) ) ;
#51959=CARTESIAN_POINT ( 'NONE',  ( 4.884375000614518569, 6.421520780324663323E-16, -5.243569643749999010 ) ) ;
#51960=CARTESIAN_POINT ( 'NONE',  ( 22.68750000122903288, 6.123233995736764310E-16, -4.999999999999998224 ) ) ;
#51963=CARTESIAN_POINT ( 'NONE',  ( 16.53750000000000142, -2.886751345948129988, 4.999999999999997335 ) ) ;
#51964=CARTESIAN_POINT ( 'NONE',  ( 21.40312500061451573, -4.541064518000417216, -2.621784821875001281 ) ) ;
#51965=ORIENTED_EDGE ( 'NONE', *, *, #20707, .F. ) ;
#51966=CARTESIAN_POINT ( 'NONE',  ( 24.00000000000000000, 4.330127018922192761, -2.499999999999997780 ) ) ;
#51967=CARTESIAN_POINT ( 'NONE',  ( 26.25937500061451857, 0.000000000000000000, 5.243569643749999010 ) ) ;
#51969=CARTESIAN_POINT ( 'NONE',  ( 14.35312500061451679, 4.541064518000418104, -2.621784821874998173 ) ) ;
#51970=CARTESIAN_POINT ( 'NONE',  ( 5.653125000614517504, -4.541064518000417216, -2.621784821875001281 ) ) ;
#51972=CARTESIAN_POINT ( 'NONE',  ( 28.60312500061451502, -4.541064518000417216, -2.621784821875001281 ) ) ;
#51973=CARTESIAN_POINT ( 'NONE',  ( 14.28750000122903430, 4.330127018922191873, 2.499999999999999556 ) ) ;
#51974=CARTESIAN_POINT ( 'NONE',  ( 20.77500000000000213, 6.123233995736764310E-16, -4.999999999999998224 ) ) ;
#51976=CARTESIAN_POINT ( 'NONE',  ( 4.546875000614517326, 6.054752690667223547, 3.707466751127219781E-16 ) ) ;
#51977=CARTESIAN_POINT ( 'NONE',  ( 8.971875000614515372, 3.027376345333613106, -5.243569643749998122 ) ) ;
#51978=CARTESIAN_POINT ( 'NONE',  ( 19.43437500061451928, 4.541064518000418104, 2.621784821874999949 ) ) ;
#51979=CARTESIAN_POINT ( 'NONE',  ( 10.08750000122903323, 6.123233995736764310E-16, -4.999999999999998224 ) ) ;
#51981=CARTESIAN_POINT ( 'NONE',  ( 4.846875000614519813, -3.027376345333610441, -5.243569643749999898 ) ) ;
#51982=CARTESIAN_POINT ( 'NONE',  ( 4.087500000000001243, -2.886751345948125991, -5.000000000000000000 ) ) ;
#51983=CARTESIAN_POINT ( 'NONE',  ( 4.471875000614518925, 3.027376345333613106, -5.243569643749998122 ) ) ;
#51984=CARTESIAN_POINT ( 'NONE',  ( 18.89999999999999858, -4.330127018922190985, -2.500000000000001332 ) ) ;
#51985=CARTESIAN_POINT ( 'NONE',  ( 15.02812500061451750, -4.541064518000419881, 2.621784821874995952 ) ) ;
#51988=CARTESIAN_POINT ( 'NONE',  ( 9.478125000614515017, 4.541064518000418104, 2.621784821874999949 ) ) ;
#51989=CARTESIAN_POINT ( 'NONE',  ( 26.85937500061451644, -4.541064518000417216, -2.621784821875001281 ) ) ;
#51990=CARTESIAN_POINT ( 'NONE',  ( 4.243569643749999898, 18.69687500061451857, 32.45002607614398471 ) ) ;
#51991=CARTESIAN_POINT ( 'NONE',  ( 26.93437500061451573, 6.421520780324663323E-16, -5.243569643749999010 ) ) ;
#51992=CARTESIAN_POINT ( 'NONE',  ( 8.362500000000002487, 2.886751345948126879, 4.999999999999999112 ) ) ;
#51993=CARTESIAN_POINT ( 'NONE',  ( -1.999999999999997113, 12.08750000122903501, 33.46410161513775705 ) ) ;
#51994=CARTESIAN_POINT ( 'NONE',  ( 15.29062500061451679, 6.054752690667223547, 3.707466751127219781E-16 ) ) ;
#51995=CARTESIAN_POINT ( 'NONE',  ( 7.275000001229035007, -5.773502691896255534, -1.060575238724906372E-15 ) ) ;
#51996=CARTESIAN_POINT ( 'NONE',  ( 17.29687500061451999, -3.027376345333614438, 5.243569643749998122 ) ) ;
#51997=CARTESIAN_POINT ( 'NONE',  ( 11.55937500061451928, -4.541064518000417216, -2.621784821875001281 ) ) ;
#51998=CARTESIAN_POINT ( 'NONE',  ( -3.027546007007308138, 3.984809627175307067, -32.62591084855416312 ) ) ;
#51999=ORIENTED_EDGE ( 'NONE', *, *, #11236, .T. ) ;
#52000=CARTESIAN_POINT ( 'NONE',  ( 12.17812500061451608, 4.541064518000418104, 2.621784821874999949 ) ) ;
#52001=CARTESIAN_POINT ( 'NONE',  ( 24.71250000122903145, 0.000000000000000000, 4.999999999999998224 ) ) ;
#52002=CARTESIAN_POINT ( 'NONE',  ( 12.72187500061451537, 3.027376345333611329, 5.243569643749999010 ) ) ;
#52003=CARTESIAN_POINT ( 'NONE',  ( 2.695452854360172346, 9.631537354464013490, -35.36400652783709830 ) ) ;
#52004=CARTESIAN_POINT ( 'NONE',  ( 14.27812500061451573, 6.421520780324663323E-16, -5.243569643749999010 ) ) ;
#52006=CARTESIAN_POINT ( 'NONE',  ( 24.90937500061451715, 0.000000000000000000, 5.243569643749999010 ) ) ;
#52007=CARTESIAN_POINT ( 'NONE',  ( 30.00000000000000000, 0.000000000000000000, 0.000000000000000000 ) ) ;
#52008=EDGE_CURVE ( 'NONE', #7649, #6802, #52992, .T. ) ;
#52009=CARTESIAN_POINT ( 'NONE',  ( 11.36250000122903536, -4.330127018922190985, -2.500000000000001332 ) ) ;
#52011=CARTESIAN_POINT ( 'NONE',  ( 3.185410902401353272, 4.246968961681812260, 3.131173267699055796 ) ) ;
#52012=CARTESIAN_POINT ( 'NONE',  ( -4.243569643749999898, 18.02187500061451786, -32.45002607614398471 ) ) ;
#52013=CARTESIAN_POINT ( 'NONE',  ( 17.40937500061451715, -4.541064518000417216, -2.621784821875001281 ) ) ;
#52014=CARTESIAN_POINT ( 'NONE',  ( 17.51250000122903216, 0.000000000000000000, 4.999999999999998224 ) ) ;
#52015=ADVANCED_FACE ( 'NONE', ( #19921 ), #66299, .T. ) ;
#52016=CARTESIAN_POINT ( 'NONE',  ( 15.27187500061451786, 3.027376345333613106, -5.243569643749998122 ) ) ;
#52017=CARTESIAN_POINT ( 'NONE',  ( -2.121784821874999949, 10.78437500061451715, 26.32496088578401938 ) ) ;
#52018=CARTESIAN_POINT ( 'NONE',  ( 20.36250000122903359, -4.330127018922190985, -2.500000000000001332 ) ) ;
#52019=CARTESIAN_POINT ( 'NONE',  ( 14.31562500061451537, 3.027376345333613106, -5.243569643749998122 ) ) ;
#52020=VERTEX_POINT ( 'NONE', #72477 ) ;
#52021=VERTEX_POINT ( 'NONE', #61746 ) ;
#52022=CARTESIAN_POINT ( 'NONE',  ( 17.32499999999999929, 4.330127018922191873, 2.499999999999999556 ) ) ;
#52023=CARTESIAN_POINT ( 'NONE',  ( 3.515625000614516882, 3.027376345333613106, -5.243569643749998122 ) ) ;
#52024=CARTESIAN_POINT ( 'NONE',  ( 14.28750000122903430, 4.330127018922191873, 2.499999999999999556 ) ) ;
#52025=CARTESIAN_POINT ( 'NONE',  ( 26.10937500061451644, 4.541064518000418104, -2.621784821874998173 ) ) ;
#52026=CARTESIAN_POINT ( 'NONE',  ( 20.42812500061451431, -4.541064518000419881, 2.621784821874995952 ) ) ;
#52027=CARTESIAN_POINT ( 'NONE',  ( 23.57812500061451289, -4.541064518000419881, 2.621784821874995952 ) ) ;
#52028=CARTESIAN_POINT ( 'NONE',  ( 4.303125000614516971, -4.541064518000417216, -2.621784821875001281 ) ) ;
#52029=CARTESIAN_POINT ( 'NONE',  ( 26.47499999999999787, -4.330127018922194537, 2.499999999999995559 ) ) ;
#52033=CARTESIAN_POINT ( 'NONE',  ( 3.952052806804493112, -3.062959721132712865, -4.228389990733410819 ) ) ;
#52034=CARTESIAN_POINT ( 'NONE',  ( -4.243569643749999898, 15.80937500061451573, -30.00000000000000000 ) ) ;
#52035=CARTESIAN_POINT ( 'NONE',  ( 5.437500001229035540, -4.330127018922194537, 2.499999999999995559 ) ) ;
#52036=CARTESIAN_POINT ( 'NONE',  ( 6.037500000000001421, 5.773502691896255534, 3.535250795749688894E-16 ) ) ;
#52037=CARTESIAN_POINT ( 'NONE',  ( 5.100000001229034297, -2.886751345948125991, -5.000000000000000000 ) ) ;
#52038=CARTESIAN_POINT ( 'NONE',  ( 10.69687500061451679, -3.027376345333610441, -5.243569643749999898 ) ) ;
#52039=CARTESIAN_POINT ( 'NONE',  ( 28.37812500061451715, 4.541064518000418104, 2.621784821874999949 ) ) ;
#52041=CARTESIAN_POINT ( 'NONE',  ( 0.000000000000000000, 10.00000000000000000, -36.00000000000000000 ) ) ;
#52043=CARTESIAN_POINT ( 'NONE',  ( 8.896875000614517859, -3.027376345333610441, -5.243569643749999898 ) ) ;
#52044=CARTESIAN_POINT ( 'NONE',  ( 12.23437500061451821, 4.541064518000418104, 2.621784821874999949 ) ) ;
#52045=CARTESIAN_POINT ( 'NONE',  ( 6.375000000000001776, 6.123233995736764310E-16, -4.999999999999998224 ) ) ;
#52046=CARTESIAN_POINT ( 'NONE',  ( 4.243569643749999898, 15.97812500061459495, 30.00000000000000000 ) ) ;
#52047=CARTESIAN_POINT ( 'NONE',  ( 20.97187500061451715, -6.054752690667223547, -1.112240025338166033E-15 ) ) ;
#52049=CARTESIAN_POINT ( 'NONE',  ( 7.387500000000001066, 5.773502691896255534, 3.535250795749688894E-16 ) ) ;
#52050=CARTESIAN_POINT ( 'NONE',  ( 25.65000000122903145, -2.886751345948129988, 4.999999999999997335 ) ) ;
#52052=CARTESIAN_POINT ( 'NONE',  ( 23.24062500061451786, -3.027376345333610441, -5.243569643749999898 ) ) ;
#52053=CARTESIAN_POINT ( 'NONE',  ( 14.27812500061451573, 6.421520780324663323E-16, -5.243569643749999010 ) ) ;
#52055=CARTESIAN_POINT ( 'NONE',  ( 10.88437500061451679, 4.541064518000418104, 2.621784821874999949 ) ) ;
#52056=CARTESIAN_POINT ( 'NONE',  ( 28.80000000000000071, -4.330127018922190985, -2.500000000000001332 ) ) ;
#52057=CARTESIAN_POINT ( 'NONE',  ( 22.01250000122903216, 0.000000000000000000, 4.999999999999998224 ) ) ;
#52058=CARTESIAN_POINT ( 'NONE',  ( 11.43750000122903465, 6.123233995736764310E-16, -4.999999999999998224 ) ) ;
#52059=CARTESIAN_POINT ( 'NONE',  ( 12.53437500061451537, 6.421520780324663323E-16, -5.243569643749999010 ) ) ;
#52060=CARTESIAN_POINT ( 'NONE',  ( 28.47187500061451715, 3.027376345333611329, 5.243569643749999010 ) ) ;
#52061=CARTESIAN_POINT ( 'NONE',  ( 1.071796769724493892, 18.17990381179669868, -34.00000000000000000 ) ) ;
#52062=CARTESIAN_POINT ( 'NONE',  ( 24.41250000122903430, -4.330127018922190985, -2.500000000000001332 ) ) ;
#52063=CARTESIAN_POINT ( 'NONE',  ( 21.57187500061451502, 3.027376345333613106, -5.243569643749998122 ) ) ;
#52064=CARTESIAN_POINT ( 'NONE',  ( 14.67187500061451821, -6.054752690667223547, -1.112240025338166033E-15 ) ) ;
#52066=CARTESIAN_POINT ( 'NONE',  ( 25.05000000000000071, 0.000000000000000000, 4.999999999999998224 ) ) ;
#52069=CARTESIAN_POINT ( 'NONE',  ( 18.06562500061451715, 3.027376345333611329, 5.243569643749999010 ) ) ;
#52070=CARTESIAN_POINT ( 'NONE',  ( 6.862500000000002487, 2.886751345948129099, -4.999999999999998224 ) ) ;
#52072=CARTESIAN_POINT ( 'NONE',  ( 14.96250000000000036, 2.886751345948129099, -4.999999999999998224 ) ) ;
#52073=CARTESIAN_POINT ( 'NONE',  ( -4.243569643749999898, 11.21562500061451750, 27.54997392385601529 ) ) ;
#52074=CARTESIAN_POINT ( 'NONE',  ( 12.82500000122903394, 2.886751345948129099, -4.999999999999998224 ) ) ;
#52076=CARTESIAN_POINT ( 'NONE',  ( 25.09687500061451715, -3.027376345333610441, -5.243569643749999898 ) ) ;
#52078=CARTESIAN_POINT ( 'NONE',  ( 20.57812500061451644, 6.421520780324663323E-16, -5.243569643749999010 ) ) ;
#52079=CARTESIAN_POINT ( 'NONE',  ( 20.89687500061452141, -3.027376345333614438, 5.243569643749998122 ) ) ;
#52080=CARTESIAN_POINT ( 'NONE',  ( 3.112500000000000711, -5.773502691896255534, -1.060575238724906372E-15 ) ) ;
#52081=CARTESIAN_POINT ( 'NONE',  ( 7.003125000614518036, -4.541064518000417216, -2.621784821875001281 ) ) ;
#52082=CARTESIAN_POINT ( 'NONE',  ( 20.99062500061451431, -3.027376345333610441, -5.243569643749999898 ) ) ;
#52083=CARTESIAN_POINT ( 'NONE',  ( 12.75937500061451857, 0.000000000000000000, 5.243569643749999010 ) ) ;
#52084=CARTESIAN_POINT ( 'NONE',  ( 16.88437500061451502, -4.541064518000419881, 2.621784821874995952 ) ) ;
#52085=CARTESIAN_POINT ( 'NONE',  ( 4.243569643749999010, 16.46562500061451573, 27.54997392385601174 ) ) ;
#52086=CARTESIAN_POINT ( 'NONE',  ( 17.92500000122903359, 2.886751345948126879, 4.999999999999999112 ) ) ;
#52088=CARTESIAN_POINT ( 'NONE',  ( 9.778125000614517504, 6.421520780324663323E-16, -5.243569643749999010 ) ) ;
#52089=CARTESIAN_POINT ( 'NONE',  ( 3.984375000614517326, 6.421520780324663323E-16, -5.243569643749999010 ) ) ;
#52090=CARTESIAN_POINT ( 'NONE',  ( 5.709375000614517859, -4.541064518000417216, -2.621784821875001281 ) ) ;
#52091=CARTESIAN_POINT ( 'NONE',  ( 25.69687500061451502, 6.054752690667223547, 3.707466751127219781E-16 ) ) ;
#52092=CARTESIAN_POINT ( 'NONE',  ( 17.80312500061451786, -4.541064518000417216, -2.621784821875001281 ) ) ;
#52093=CARTESIAN_POINT ( 'NONE',  ( 27.52500000122903145, -5.773502691896255534, -1.060575238724906372E-15 ) ) ;
#52094=EDGE_CURVE ( 'NONE', #15128, #69237, #11149, .T. ) ;
#52095=CARTESIAN_POINT ( 'NONE',  ( 25.71562500061451573, 3.027376345333611329, 5.243569643749999010 ) ) ;
#52096=CARTESIAN_POINT ( 'NONE',  ( 21.19687500061451502, 6.054752690667223547, 3.707466751127219781E-16 ) ) ;
#52097=CARTESIAN_POINT ( 'NONE',  ( 17.91562500061451502, 3.027376345333613106, -5.243569643749998122 ) ) ;
#52098=CARTESIAN_POINT ( 'NONE',  ( -4.243569643749999898, 16.67187500061451644, 27.54997392385601529 ) ) ;
#52099=CARTESIAN_POINT ( 'NONE',  ( 21.66562500061451502, 3.027376345333611329, 5.243569643749999010 ) ) ;
#52101=ORIENTED_EDGE ( 'NONE', *, *, #2520, .F. ) ;
#52102=CARTESIAN_POINT ( 'NONE',  ( 25.61250000000000071, -5.773502691896255534, -1.060575238724906372E-15 ) ) ;
#52103=CARTESIAN_POINT ( 'NONE',  ( 3.999999999999998668, 13.51250000000000107, -32.30940107675850470 ) ) ;
#52105=CARTESIAN_POINT ( 'NONE',  ( 3.046875000614519990, -3.027376345333610441, -5.243569643749999898 ) ) ;
#52106=CARTESIAN_POINT ( 'NONE',  ( 9.665625000614515017, -6.054752690667223547, -1.112240025338166033E-15 ) ) ;
#52107=CARTESIAN_POINT ( 'NONE',  ( 22.16250000122903074, -4.330127018922190985, -2.500000000000001332 ) ) ;
#52108=CARTESIAN_POINT ( 'NONE',  ( 26.57812500061451644, 4.541064518000418104, 2.621784821874999949 ) ) ;
#52110=CARTESIAN_POINT ( 'NONE',  ( 24.78750000000000497, -2.886751345948125991, -5.000000000000000000 ) ) ;
#52111=CARTESIAN_POINT ( 'NONE',  ( 1.999999999999998668, 15.91250000122903430, -33.46410161513775705 ) ) ;
#52112=CARTESIAN_POINT ( 'NONE',  ( 29.35312500061451502, 0.000000000000000000, 5.243569643749999010 ) ) ;
#52113=CARTESIAN_POINT ( 'NONE',  ( 9.590625000614517504, -3.027376345333614438, 5.243569643749998122 ) ) ;
#52115=ORIENTED_EDGE ( 'NONE', *, *, #4793, .F. ) ;
#52116=CARTESIAN_POINT ( 'NONE',  ( 25.15312500061451217, 4.541064518000418104, -2.621784821874998173 ) ) ;
#52117=CARTESIAN_POINT ( 'NONE',  ( 7.378125000614518036, -4.541064518000419881, 2.621784821874995952 ) ) ;
#52119=CARTESIAN_POINT ( 'NONE',  ( 5.540625000614515905, -3.027376345333614438, 5.243569643749998122 ) ) ;
#52121=CARTESIAN_POINT ( 'NONE',  ( 4.629056002857023344, -1.889931353889065413, 4.891133006415133266 ) ) ;
#52122=CARTESIAN_POINT ( 'NONE',  ( 13.19999999999999929, 4.330127018922192761, -2.499999999999997780 ) ) ;
#52123=CARTESIAN_POINT ( 'NONE',  ( 13.62187500061451750, 3.027376345333611329, 5.243569643749999010 ) ) ;
#52124=CARTESIAN_POINT ( 'NONE',  ( 11.21250000122903501, 0.000000000000000000, 4.999999999999998224 ) ) ;
#52125=CARTESIAN_POINT ( 'NONE',  ( 17.25937500061451502, 0.000000000000000000, 5.243569643749999010 ) ) ;
#52127=CARTESIAN_POINT ( 'NONE',  ( 8.559375000614515727, 4.541064518000418104, -2.621784821874998173 ) ) ;
#52128=CARTESIAN_POINT ( 'NONE',  ( -2.121784821874999949, 10.72812500061451679, -33.67503911421598417 ) ) ;
#52131=CARTESIAN_POINT ( 'NONE',  ( 23.76562500061451644, 3.027376345333613106, -5.243569643749998122 ) ) ;
#52133=CARTESIAN_POINT ( 'NONE',  ( 29.07187500061451502, -6.054752690667223547, -1.112240025338166033E-15 ) ) ;
#52134=CARTESIAN_POINT ( 'NONE',  ( 24.26249999999999929, -5.773502691896255534, -1.060575238724906372E-15 ) ) ;
#52135=CARTESIAN_POINT ( 'NONE',  ( 6.965625000614518392, -6.054752690667223547, -1.112240025338166033E-15 ) ) ;
#52137=CARTESIAN_POINT ( 'NONE',  ( 20.18437500061451573, 6.421520780324663323E-16, -5.243569643749999010 ) ) ;
#52139=CARTESIAN_POINT ( 'NONE',  ( 2.990625000614519191, -3.027376345333610441, -5.243569643749999898 ) ) ;
#52140=CARTESIAN_POINT ( 'NONE',  ( 7.659375000614518036, 4.541064518000418104, -2.621784821874998173 ) ) ;
#52141=VERTEX_POINT ( 'NONE', #56569 ) ;
#52142=CARTESIAN_POINT ( 'NONE',  ( 20.03437500061451715, -4.541064518000419881, 2.621784821874995952 ) ) ;
#52143=CARTESIAN_POINT ( 'NONE',  ( 30.00000000000000000, 0.000000000000000000, 0.000000000000000000 ) ) ;
#52144=CARTESIAN_POINT ( 'NONE',  ( 27.78749999999999787, -2.886751345948129988, 4.999999999999997335 ) ) ;
#52145=CARTESIAN_POINT ( 'NONE',  ( 29.44687500061451857, -3.027376345333614438, 5.243569643749998122 ) ) ;
#52146=CARTESIAN_POINT ( 'NONE',  ( 3.999999999999998668, 10.36250000000000426, -32.30940107675850470 ) ) ;
#52147=CARTESIAN_POINT ( 'NONE',  ( 3.422429900546629877, -3.645130117820770455, -3.769356580772429410 ) ) ;
#52149=CARTESIAN_POINT ( 'NONE',  ( 9.262499999999999289, 2.886751345948126879, 4.999999999999999112 ) ) ;
#52151=CARTESIAN_POINT ( 'NONE',  ( 25.41562500061451146, -6.054752690667223547, -1.112240025338166033E-15 ) ) ;
#52152=CARTESIAN_POINT ( 'NONE',  ( 13.68750000000000178, 5.773502691896255534, 3.535250795749688894E-16 ) ) ;
#52153=CARTESIAN_POINT ( 'NONE',  ( 7.987500001229032698, 4.330127018922191873, 2.499999999999999556 ) ) ;
#52154=CARTESIAN_POINT ( 'NONE',  ( 7.490625000614516082, -3.027376345333610441, -5.243569643749999898 ) ) ;
#52155=CARTESIAN_POINT ( 'NONE',  ( 22.91249999999999432, -5.773502691896255534, -1.060575238724906372E-15 ) ) ;
#52156=CARTESIAN_POINT ( 'NONE',  ( 22.04062500061451502, 6.054752690667223547, 3.707466751127219781E-16 ) ) ;
#52159=CARTESIAN_POINT ( 'NONE',  ( 26.10000000122903430, -2.886751345948129988, 4.999999999999997335 ) ) ;
#52161=CARTESIAN_POINT ( 'NONE',  ( 4.987500000000002487, -2.886751345948125991, -5.000000000000000000 ) ) ;
#52162=VERTEX_POINT ( 'NONE', #67670 ) ;
#52163=CARTESIAN_POINT ( 'NONE',  ( 21.25312500061451715, 0.000000000000000000, 5.243569643749999010 ) ) ;
#52164=CARTESIAN_POINT ( 'NONE',  ( 29.39062500061451289, -3.027376345333614438, 5.243569643749998122 ) ) ;
#52165=CARTESIAN_POINT ( 'NONE',  ( 28.13437500061451502, -4.541064518000419881, 2.621784821874995952 ) ) ;
#52166=CARTESIAN_POINT ( 'NONE',  ( 17.97187500061451715, 3.027376345333613106, -5.243569643749998122 ) ) ;
#52167=EDGE_CURVE ( 'NONE', #55474, #11533, #22940, .T. ) ;
#52168=CARTESIAN_POINT ( 'NONE',  ( 14.39062500061451821, 6.054752690667223547, 3.707466751127219781E-16 ) ) ;
#52170=CARTESIAN_POINT ( 'NONE',  ( 25.80000000122903714, -2.886751345948125991, -5.000000000000000000 ) ) ;
#52172=CARTESIAN_POINT ( 'NONE',  ( 16.11562500061451786, 3.027376345333612662, -5.243569643749998122 ) ) ;
#52173=CARTESIAN_POINT ( 'NONE',  ( 1.071796769724493892, 18.51740381056766793, -34.00000000000000000 ) ) ;
#52174=CARTESIAN_POINT ( 'NONE',  ( 2.962500001229034119, 4.330127018922192761, -2.499999999999997780 ) ) ;
#52175=CARTESIAN_POINT ( 'NONE',  ( 12.27187500061451786, 3.027376345333611329, 5.243569643749999010 ) ) ;
#52176=CARTESIAN_POINT ( 'NONE',  ( 11.29687500061451644, 6.054752690667223547, 3.707466751127219781E-16 ) ) ;
#52177=CARTESIAN_POINT ( 'NONE',  ( 19.80937500061451573, 4.541064518000418104, -2.621784821874998173 ) ) ;
#52178=EDGE_LOOP ( 'NONE', ( #23526, #16698, #43704, #45900 ) ) ;
#52179=CARTESIAN_POINT ( 'NONE',  ( 1.111888759404800586, 4.999999999999998224, 1.111888759404800586 ) ) ;
#52180=CARTESIAN_POINT ( 'NONE',  ( 25.00312500061451715, -4.541064518000417216, -2.621784821875001281 ) ) ;
#52181=CARTESIAN_POINT ( 'NONE',  ( 19.65937500061451360, -4.541064518000417216, -2.621784821875001281 ) ) ;
#52182=CARTESIAN_POINT ( 'NONE',  ( 25.37812500061451715, -4.541064518000419881, 2.621784821874995952 ) ) ;
#52183=LINE ( 'NONE', #47006, #12041 ) ;
#52184=CARTESIAN_POINT ( 'NONE',  ( -1.999999999999997113, 15.12500000000000000, 33.46410161513775705 ) ) ;
#52185=CARTESIAN_POINT ( 'NONE',  ( 29.54062500061451502, -3.027376345333610441, -5.243569643749999898 ) ) ;
#52186=CARTESIAN_POINT ( 'NONE',  ( 8.850000001229034297, 5.773502691896255534, 3.535250795749688894E-16 ) ) ;
#52187=CARTESIAN_POINT ( 'NONE',  ( 5.287500001229035185, 4.330127018922191873, 2.499999999999999556 ) ) ;
#52189=CARTESIAN_POINT ( 'NONE',  ( 26.88750000122903216, 4.330127018922191873, 2.499999999999999556 ) ) ;
#52191=CARTESIAN_POINT ( 'NONE',  ( 8.746875000614515727, -3.027376345333614438, 5.243569643749998122 ) ) ;
#52193=CARTESIAN_POINT ( 'NONE',  ( 17.91562500061451502, 3.027376345333613106, -5.243569643749998122 ) ) ;
#52194=CARTESIAN_POINT ( 'NONE',  ( 10.24687500061451750, -3.027376345333610441, -5.243569643749999898 ) ) ;
#52195=CARTESIAN_POINT ( 'NONE',  ( 2.878125000614517592, -4.541064518000419881, 2.621784821874995952 ) ) ;
#52196=CARTESIAN_POINT ( 'NONE',  ( 18.68437500061451928, -4.541064518000419881, 2.621784821874995952 ) ) ;
#52197=CARTESIAN_POINT ( 'NONE',  ( 8.184375000614515727, 4.541064518000418104, 2.621784821874999949 ) ) ;
#52198=CARTESIAN_POINT ( 'NONE',  ( 3.478125000614517237, 6.421520780324663323E-16, -5.243569643749999010 ) ) ;
#52200=CARTESIAN_POINT ( 'NONE',  ( 7.340625000614518392, -3.027376345333614438, 5.243569643749998122 ) ) ;
#52201=CARTESIAN_POINT ( 'NONE',  ( 18.47812500061451857, 4.541064518000418104, 2.621784821874999949 ) ) ;
#52202=ORIENTED_EDGE ( 'NONE', *, *, #58814, .T. ) ;
#52203=CARTESIAN_POINT ( 'NONE',  ( 5.325000001229033941, 2.886751345948126879, 4.999999999999999112 ) ) ;
#52204=CARTESIAN_POINT ( 'NONE',  ( 13.82812500061451466, 6.421520780324663323E-16, -5.243569643749999010 ) ) ;
#52205=CARTESIAN_POINT ( 'NONE',  ( 12.10312500061451857, 4.541064518000418104, -2.621784821874998173 ) ) ;
#52207=CARTESIAN_POINT ( 'NONE',  ( 13.98750000000000249, -2.886751345948125991, -5.000000000000000000 ) ) ;
#52208=CARTESIAN_POINT ( 'NONE',  ( 5.887500001229034829, -4.330127018922194537, 2.499999999999995559 ) ) ;
#52209=CARTESIAN_POINT ( 'NONE',  ( 3.103125000614517237, 4.541064518000418104, -2.621784821874998173 ) ) ;
#52210=CARTESIAN_POINT ( 'NONE',  ( 15.90937500061451892, 0.000000000000000000, 5.243569643749999010 ) ) ;
#52211=CARTESIAN_POINT ( 'NONE',  ( 19.42500000122903714, -5.773502691896255534, -1.060575238724906372E-15 ) ) ;
#52213=CARTESIAN_POINT ( 'NONE',  ( 4.243569643749999898, 17.77812500061451928, -30.00000000000000000 ) ) ;
#52214=FACE_OUTER_BOUND ( 'NONE', #12613, .T. ) ;
#52215=CARTESIAN_POINT ( 'NONE',  ( 22.98750000122903003, -4.330127018922194537, 2.499999999999995559 ) ) ;
#52216=CARTESIAN_POINT ( 'NONE',  ( 3.041778030301053981, 4.165465603166717656, 2.785201938134701738 ) ) ;
#52217=CARTESIAN_POINT ( 'NONE',  ( 4.465851277537014496, 2.248593419656079284, -4.736966354317482697 ) ) ;
#52218=CARTESIAN_POINT ( 'NONE',  ( 19.28437500061451360, 6.421520780324663323E-16, -5.243569643749999010 ) ) ;
#52219=CARTESIAN_POINT ( 'NONE',  ( 10.53750000122903252, 6.123233995736764310E-16, -4.999999999999998224 ) ) ;
#52221=CARTESIAN_POINT ( 'NONE',  ( 13.67812500061451786, -4.541064518000419881, 2.621784821874995952 ) ) ;
#52223=CYLINDRICAL_SURFACE ( 'NONE', #63663, 4.999999999999998224 ) ;
#52224=CARTESIAN_POINT ( 'NONE',  ( 25.39687500061451431, -3.027376345333614438, 5.243569643749998122 ) ) ;
#52226=CARTESIAN_POINT ( 'NONE',  ( 9.628125000614517148, -4.541064518000419881, 2.621784821874995952 ) ) ;
#52227=CARTESIAN_POINT ( 'NONE',  ( 15.04687500061451644, -3.027376345333614438, 5.243569643749998122 ) ) ;
#52229=CARTESIAN_POINT ( 'NONE',  ( 27.74062500061451431, -3.027376345333610441, -5.243569643749999898 ) ) ;
#52230=CARTESIAN_POINT ( 'NONE',  ( 19.52812500061451573, -4.541064518000419881, 2.621784821874995952 ) ) ;
#52231=FACE_OUTER_BOUND ( 'NONE', #54164, .T. ) ;
#52233=CARTESIAN_POINT ( 'NONE',  ( -3.999999999999999112, 14.22500000122903430, -32.30940107675850470 ) ) ;
#52234=CARTESIAN_POINT ( 'NONE',  ( 10.42500000000000071, 6.123233995736764310E-16, -4.999999999999998224 ) ) ;
#52235=CARTESIAN_POINT ( 'NONE',  ( 19.05000000122903359, -2.886751345948125991, -5.000000000000000000 ) ) ;
#52238=CARTESIAN_POINT ( 'NONE',  ( 18.18750000000000000, 5.773502691896255534, 3.535250795749688894E-16 ) ) ;
#52239=ADVANCED_FACE ( 'NONE', ( #56220 ), #17038, .F. ) ;
#52240=CARTESIAN_POINT ( 'NONE',  ( 21.33749999999999858, 5.773502691896255534, 3.535250795749688894E-16 ) ) ;
#52241=CARTESIAN_POINT ( 'NONE',  ( 19.09687500061451360, -3.027376345333614438, 5.243569643749998122 ) ) ;
#52242=CARTESIAN_POINT ( 'NONE',  ( 25.34062500061451217, -3.027376345333614438, 5.243569643749998122 ) ) ;
#52244=CARTESIAN_POINT ( 'NONE',  ( 8.887500001229033941, 4.330127018922191873, 2.499999999999999556 ) ) ;
#52245=CARTESIAN_POINT ( 'NONE',  ( 5.540625000614515905, -3.027376345333614438, 5.243569643749998122 ) ) ;
#52246=CARTESIAN_POINT ( 'NONE',  ( 1.071796769724491893, 15.29509619066137027, 33.99999999999999289 ) ) ;
#52247=CARTESIAN_POINT ( 'NONE',  ( 13.68750000000000178, 5.773502691896255534, 3.535250795749688894E-16 ) ) ;
#52248=CARTESIAN_POINT ( 'NONE',  ( 4.243569643749999898, 17.32812500061451644, 30.00000000000000000 ) ) ;
#52249=CARTESIAN_POINT ( 'NONE',  ( 28.79062500061451502, 6.054752690667223547, 3.707466751127219781E-16 ) ) ;
#52252=CARTESIAN_POINT ( 'NONE',  ( 26.97187500061451360, 3.027376345333613106, -5.243569643749998122 ) ) ;
#52254=CARTESIAN_POINT ( 'NONE',  ( 21.85312500061451502, -4.541064518000417216, -2.621784821875001281 ) ) ;
#52255=CARTESIAN_POINT ( 'NONE',  ( 22.84687500061451715, -3.027376345333610441, -5.243569643749999898 ) ) ;
#52256=CARTESIAN_POINT ( 'NONE',  ( -4.243569643749999898, 16.65312500061459389, -30.00000000000000000 ) ) ;
#52257=CARTESIAN_POINT ( 'NONE',  ( 6.553125000614518747, -4.541064518000417216, -2.621784821875001281 ) ) ;
#52258=DIRECTION ( 'NONE',  ( 0.000000000000000000, 0.000000000000000000, 1.000000000000000000 ) ) ;
#52259=CARTESIAN_POINT ( 'NONE',  ( 22.75312500061451360, -4.541064518000417216, -2.621784821875001281 ) ) ;
#52262=CARTESIAN_POINT ( 'NONE',  ( 17.33437500061451431, -4.541064518000419881, 2.621784821874995952 ) ) ;
#52263=( BOUNDED_CURVE ( )  B_SPLINE_CURVE ( 2, ( #72718, #49457, #4758, #4033, #15821, #43552, #55365, #66445, #22101 ),
 .UNSPECIFIED., .F., .F. ) 
 B_SPLINE_CURVE_WITH_KNOTS ( ( 3, 2, 2, 2, 3 ),
 ( 0.2717391304347826497, 0.2753623188405797118, 0.2826086956521738913, 0.2898550724637681264, 0.2934782608695652439 ),
 .UNSPECIFIED. ) 
 CURVE ( )  GEOMETRIC_REPRESENTATION_ITEM ( )  RATIONAL_B_SPLINE_CURVE ( ( 0.9330127018922194093, 0.9330127018922198534, 1.000000000000000000, 0.8660254037844387076, 1.000000000000000000, 0.8660254037844387076, 1.000000000000000000, 0.9330127018922188542, 0.9330127018922194093 ) ) 
 REPRESENTATION_ITEM ( '' )  );
#52264=CARTESIAN_POINT ( 'NONE',  ( 20.03437500061451715, -4.541064518000419881, 2.621784821874995952 ) ) ;
#52265=CARTESIAN_POINT ( 'NONE',  ( 27.27187500061451431, -6.054752690667223547, -1.112240025338166033E-15 ) ) ;
#52266=CARTESIAN_POINT ( 'NONE',  ( -2.121784821874999949, 15.73437500061451644, 26.32496088578401938 ) ) ;
#52267=CARTESIAN_POINT ( 'NONE',  ( 7.378125000614518036, -4.541064518000419881, 2.621784821874995952 ) ) ;
#52269=CARTESIAN_POINT ( 'NONE',  ( 5.446875000614518569, 6.054752690667223547, 3.707466751127219781E-16 ) ) ;
#52270=CARTESIAN_POINT ( 'NONE',  ( 26.55000000000000071, -4.330127018922190985, -2.500000000000001332 ) ) ;
#52271=CARTESIAN_POINT ( 'NONE',  ( 4.490625000614516971, 6.054752690667223547, 3.707466751127219781E-16 ) ) ;
#52272=CARTESIAN_POINT ( 'NONE',  ( 10.62187500061451928, -6.054752690667223547, -1.112240025338166033E-15 ) ) ;
#52273=CARTESIAN_POINT ( 'NONE',  ( 16.31250000122903288, -4.330127018922190985, -2.500000000000001332 ) ) ;
#52274=CARTESIAN_POINT ( 'NONE',  ( 4.621875000614516615, 3.027376345333611329, 5.243569643749999010 ) ) ;
#52275=CARTESIAN_POINT ( 'NONE',  ( 6.553125000614518747, -4.541064518000417216, -2.621784821875001281 ) ) ;
#52278=CARTESIAN_POINT ( 'NONE',  ( 16.05937500061451573, -4.541064518000417216, -2.621784821875001281 ) ) ;
#52279=DIRECTION ( 'NONE',  ( 0.000000000000000000, 0.000000000000000000, -1.000000000000000000 ) ) ;
#52281=CARTESIAN_POINT ( 'NONE',  ( 24.66562500061451502, 3.027376345333613106, -5.243569643749998122 ) ) ;
#52282=CARTESIAN_POINT ( 'NONE',  ( 8.615625000614517859, 3.027376345333611329, 5.243569643749999010 ) ) ;
#52284=CARTESIAN_POINT ( 'NONE',  ( 26.29687500061451644, -3.027376345333614438, 5.243569643749998122 ) ) ;
#52285=CARTESIAN_POINT ( 'NONE',  ( 9.028125000614517504, 4.541064518000418104, 2.621784821874999949 ) ) ;
#52287=CARTESIAN_POINT ( 'NONE',  ( 10.61250000122903536, 4.330127018922192761, -2.499999999999997780 ) ) ;
#52288=CARTESIAN_POINT ( 'NONE',  ( 26.01562500061451289, 3.027376345333613106, -5.243569643749998122 ) ) ;
#52289=CARTESIAN_POINT ( 'NONE',  ( -4.243569643749997233, 12.64062500061451999, -27.54997392385601174 ) ) ;
#52290=CARTESIAN_POINT ( 'NONE',  ( 11.73750000122903181, -4.330127018922194537, 2.499999999999995559 ) ) ;
#52291=CARTESIAN_POINT ( 'NONE',  ( 22.07812500061451644, 4.541064518000418104, 2.621784821874999949 ) ) ;
#52292=CARTESIAN_POINT ( 'NONE',  ( 11.58750000000000036, -2.886751345948129988, 4.999999999999997335 ) ) ;
#52293=CARTESIAN_POINT ( 'NONE',  ( 19.22812500061451502, 6.421520780324663323E-16, -5.243569643749999010 ) ) ;
#52295=CARTESIAN_POINT ( 'NONE',  ( 21.75000000000000000, 4.330127018922192761, -2.499999999999997780 ) ) ;
#52296=CARTESIAN_POINT ( 'NONE',  ( 14.17500000122903536, 2.886751345948129099, -4.999999999999998224 ) ) ;
#52297=CARTESIAN_POINT ( 'NONE',  ( 9.403125000614517504, 4.541064518000418104, -2.621784821874998173 ) ) ;
#52298=CARTESIAN_POINT ( 'NONE',  ( 16.15312500061451573, 4.541064518000418104, -2.621784821874998173 ) ) ;
#52299=CARTESIAN_POINT ( 'NONE',  ( 26.58750000122903145, -4.330127018922194537, 2.499999999999995559 ) ) ;
#52300=CARTESIAN_POINT ( 'NONE',  ( 23.07187500061451857, 3.027376345333611329, 5.243569643749999010 ) ) ;
#52302=CARTESIAN_POINT ( 'NONE',  ( 6.562500001229032875, 4.330127018922192761, -2.499999999999997780 ) ) ;
#52303=CARTESIAN_POINT ( 'NONE',  ( 8.071875000614518569, 3.027376345333613106, -5.243569643749998122 ) ) ;
#52304=CARTESIAN_POINT ( 'NONE',  ( 25.77187500061451075, 3.027376345333611329, 5.243569643749999010 ) ) ;
#52306=CARTESIAN_POINT ( 'NONE',  ( 3.121875000614518836, 3.027376345333613106, -5.243569643749998122 ) ) ;
#52307=CARTESIAN_POINT ( 'NONE',  ( 20.24062500061451431, 6.054752690667223547, 3.707466751127219781E-16 ) ) ;
#52308=CARTESIAN_POINT ( 'NONE',  ( 26.14687500061451431, 6.054752690667223547, 3.707466751127219781E-16 ) ) ;
#52310=CARTESIAN_POINT ( 'NONE',  ( 18.75000000000000000, 0.000000000000000000, 4.999999999999998224 ) ) ;
#52311=CARTESIAN_POINT ( 'NONE',  ( 7.771875000614516971, 3.027376345333611329, 5.243569643749999010 ) ) ;
#52312=CARTESIAN_POINT ( 'NONE',  ( 19.75312500061451360, 4.541064518000418104, -2.621784821874998173 ) ) ;
#52313=ORIENTED_EDGE ( 'NONE', *, *, #31488, .T. ) ;
#52314=DIRECTION ( 'NONE',  ( 0.000000000000000000, 1.000000000000000000, -0.000000000000000000 ) ) ;
#52315=CARTESIAN_POINT ( 'NONE',  ( 27.06562500061451004, 3.027376345333611329, 5.243569643749999010 ) ) ;
#52316=CARTESIAN_POINT ( 'NONE',  ( 4.021875000614516082, 3.027376345333613106, -5.243569643749998122 ) ) ;
#52317=DIRECTION ( 'NONE',  ( -0.000000000000000000, -1.000000000000000000, -0.000000000000000000 ) ) ;
#52318=DIRECTION ( 'NONE',  ( 0.000000000000000000, 0.000000000000000000, -1.000000000000000000 ) ) ;
#52319=CARTESIAN_POINT ( 'NONE',  ( 16.46249999999999503, 2.886751345948126879, 4.999999999999999112 ) ) ;
#52320=CARTESIAN_POINT ( 'NONE',  ( 20.80312500061451431, 0.000000000000000000, 5.243569643749999010 ) ) ;
#52321=ORIENTED_EDGE ( 'NONE', *, *, #26600, .F. ) ;
#52322=CARTESIAN_POINT ( 'NONE',  ( 25.72499999999999787, 6.123233995736764310E-16, -4.999999999999998224 ) ) ;
#52323=ADVANCED_FACE ( 'NONE', ( #28149 ), #28857, .F. ) ;
#52324=CARTESIAN_POINT ( 'NONE',  ( 25.73437500061451644, 4.541064518000418104, 2.621784821874999949 ) ) ;
#52325=EDGE_LOOP ( 'NONE', ( #3634, #6690, #15175, #36773 ) ) ;
#52326=CARTESIAN_POINT ( 'NONE',  ( 12.51562500061451821, 3.027376345333613106, -5.243569643749998122 ) ) ;
#52327=CARTESIAN_POINT ( 'NONE',  ( 5.503125000614516260, 0.000000000000000000, 5.243569643749999010 ) ) ;
#52329=CARTESIAN_POINT ( 'NONE',  ( 29.46562500061451573, -6.054752690667223547, -1.112240025338166033E-15 ) ) ;
#52330=CARTESIAN_POINT ( 'NONE',  ( 16.20000000122903216, -2.886751345948129988, 4.999999999999997335 ) ) ;
#52331=CARTESIAN_POINT ( 'NONE',  ( 20.96250000000000213, 2.886751345948126879, 4.999999999999999112 ) ) ;
#52332=CARTESIAN_POINT ( 'NONE',  ( 29.02499999999999858, 4.330127018922191873, 2.499999999999999556 ) ) ;
#52333=CARTESIAN_POINT ( 'NONE',  ( 3.871875000614519280, -6.054752690667223547, -1.112240025338166033E-15 ) ) ;
#52334=CARTESIAN_POINT ( 'NONE',  ( 9.084375000614517859, 4.541064518000418104, 2.621784821874999949 ) ) ;
#52335=CARTESIAN_POINT ( 'NONE',  ( 18.75937500061451857, -4.541064518000417216, -2.621784821875001281 ) ) ;
#52336=CARTESIAN_POINT ( 'NONE',  ( 9.862500001229033586, 0.000000000000000000, 4.999999999999998224 ) ) ;
#52337=ORIENTED_EDGE ( 'NONE', *, *, #22115, .T. ) ;
#52338=CARTESIAN_POINT ( 'NONE',  ( 29.54062500061451502, -3.027376345333610441, -5.243569643749999898 ) ) ;
#52339=CARTESIAN_POINT ( 'NONE',  ( 3.900000000000000799, 0.000000000000000000, 4.999999999999998224 ) ) ;
#52340=CARTESIAN_POINT ( 'NONE',  ( 4.021875000614516082, 3.027376345333613106, -5.243569643749998122 ) ) ;
#52341=CARTESIAN_POINT ( 'NONE',  ( 17.88749999999999929, -2.886751345948129988, 4.999999999999997335 ) ) ;
#52342=CARTESIAN_POINT ( 'NONE',  ( 14.72812500061451679, 6.421520780324663323E-16, -5.243569643749999010 ) ) ;
#52344=CARTESIAN_POINT ( 'NONE',  ( 26.96249999999999858, -5.773502691896255534, -1.060575238724906372E-15 ) ) ;
#52345=CARTESIAN_POINT ( 'NONE',  ( 1.626862140677534273E-15, 13.47500000122903252, 34.00000000000000000 ) ) ;
#52347=CARTESIAN_POINT ( 'NONE',  ( 7.115625000614516082, 3.027376345333613106, -5.243569643749998122 ) ) ;
#52348=CARTESIAN_POINT ( 'NONE',  ( 25.05937500061451573, -4.541064518000417216, -2.621784821875001281 ) ) ;
#52349=CARTESIAN_POINT ( 'NONE',  ( 19.61250000122903359, 4.330127018922192761, -2.499999999999997780 ) ) ;
#52350=CARTESIAN_POINT ( 'NONE',  ( 26.37187500061451217, -6.054752690667223547, -1.112240025338166033E-15 ) ) ;
#52351=CARTESIAN_POINT ( 'NONE',  ( 7.875000000000000000, 4.330127018922191873, 2.499999999999999556 ) ) ;
#52352=CARTESIAN_POINT ( 'NONE',  ( -3.999999999999999112, 12.46250000122903323, 30.00000000000000000 ) ) ;
#52353=CARTESIAN_POINT ( 'NONE',  ( 15.25312500061451715, 4.541064518000418104, -2.621784821874998173 ) ) ;
#52354=CARTESIAN_POINT ( 'NONE',  ( 6.075000001229034829, 2.886751345948129099, -4.999999999999998224 ) ) ;
#52355=CARTESIAN_POINT ( 'NONE',  ( 16.95937500061451786, -4.541064518000417216, -2.621784821875001281 ) ) ;
#52356=CARTESIAN_POINT ( 'NONE',  ( 12.90937500061451537, -4.541064518000417216, -2.621784821875001281 ) ) ;
#52357=CARTESIAN_POINT ( 'NONE',  ( 30.00000000000000000, 0.000000000000000000, 4.999999999999998224 ) ) ;
#52358=VERTEX_POINT ( 'NONE', #39234 ) ;
#52359=CARTESIAN_POINT ( 'NONE',  ( 13.30312500061451786, -4.541064518000417216, -2.621784821875001281 ) ) ;
#52360=CARTESIAN_POINT ( 'NONE',  ( 29.10000000122903074, 5.773502691896255534, 3.535250795749688401E-16 ) ) ;
#52361=CARTESIAN_POINT ( 'NONE',  ( 23.13750000122903216, 6.123233995736764310E-16, -4.999999999999998224 ) ) ;
#52362=CARTESIAN_POINT ( 'NONE',  ( 13.20937500061451786, 0.000000000000000000, 5.243569643749999010 ) ) ;
#52363=CARTESIAN_POINT ( 'NONE',  ( 14.65312500061451573, -4.541064518000417216, -2.621784821875001281 ) ) ;
#52364=CARTESIAN_POINT ( 'NONE',  ( 30.00000000000000000, 0.000000000000000000, 0.000000000000000000 ) ) ;
#52365=CARTESIAN_POINT ( 'NONE',  ( 24.49687500061451573, -3.027376345333614438, 5.243569643749998122 ) ) ;
#52367=CARTESIAN_POINT ( 'NONE',  ( 11.66250000122903430, 0.000000000000000000, 4.999999999999998224 ) ) ;
#52368=DIRECTION ( 'NONE',  ( 0.000000000000000000, 0.000000000000000000, 1.000000000000000000 ) ) ;
#52370=CARTESIAN_POINT ( 'NONE',  ( 2.121784821874999061, 16.55937500061451573, -33.67503911421598417 ) ) ;
#52371=CARTESIAN_POINT ( 'NONE',  ( 19.35937500061451644, 4.541064518000418104, -2.621784821874998173 ) ) ;
#52372=CARTESIAN_POINT ( 'NONE',  ( 17.43750000122903288, 4.330127018922191873, 2.499999999999999556 ) ) ;
#52373=CARTESIAN_POINT ( 'NONE',  ( 11.55937500061451928, -4.541064518000417216, -2.621784821875001281 ) ) ;
#52374=CARTESIAN_POINT ( 'NONE',  ( 2.121784821875001281, 19.50312500061451360, -26.32496088578401938 ) ) ;
#52375=CARTESIAN_POINT ( 'NONE',  ( 19.91250000122903074, -4.330127018922190985, -2.500000000000001332 ) ) ;
#52376=CARTESIAN_POINT ( 'NONE',  ( 15.74062500061451608, 6.054752690667223547, 3.707466751127219781E-16 ) ) ;
#52377=ORIENTED_EDGE ( 'NONE', *, *, #62265, .T. ) ;
#52378=VERTEX_POINT ( 'NONE', #799 ) ;
#52379=CARTESIAN_POINT ( 'NONE',  ( 17.10000000000000142, -4.330127018922190985, -2.500000000000001332 ) ) ;
#52380=CARTESIAN_POINT ( 'NONE',  ( 27.33749999999999858, -2.886751345948096681, 5.000000000000054179 ) ) ;
#52381=CARTESIAN_POINT ( 'NONE',  ( 13.62187500061451750, 3.027376345333611329, 5.243569643749999010 ) ) ;
#52382=CARTESIAN_POINT ( 'NONE',  ( 7.320879633048903241E-15, 17.30000000122903003, -34.00000000000000000 ) ) ;
#52383=EDGE_CURVE ( 'NONE', #64110, #63984, #51207, .T. ) ;
#52384=CARTESIAN_POINT ( 'NONE',  ( 15.78750000122903430, -4.330127018922194537, 2.499999999999995559 ) ) ;
#52385=CARTESIAN_POINT ( 'NONE',  ( 25.92187500061451999, -6.054752690667223547, -1.112240025338166033E-15 ) ) ;
#52386=CARTESIAN_POINT ( 'NONE',  ( 19.15312500061451573, -4.541064518000417216, -2.621784821875001281 ) ) ;
#52387=CARTESIAN_POINT ( 'NONE',  ( 21.92812500061451431, 6.421520780324663323E-16, -5.243569643749999010 ) ) ;
#52388=CARTESIAN_POINT ( 'NONE',  ( 29.28750000122903074, -4.330127018922194537, 2.499999999999995559 ) ) ;
#52389=CARTESIAN_POINT ( 'NONE',  ( 28.27499999999999858, -4.330127018922194537, 2.499999999999995559 ) ) ;
#52390=LINE ( 'NONE', #40956, #46646 ) ;
#52392=DIRECTION ( 'NONE',  ( -0.000000000000000000, -1.000000000000000000, -0.000000000000000000 ) ) ;
#52394=CARTESIAN_POINT ( 'NONE',  ( 2.121784821875001281, 15.05937500061451928, -26.32496088578401938 ) ) ;
#52395=CARTESIAN_POINT ( 'NONE',  ( 7.200000001229035718, -2.886751345948129988, 4.999999999999997335 ) ) ;
#52396=CARTESIAN_POINT ( 'NONE',  ( 7.050000000000000711, 0.000000000000000000, 4.999999999999998224 ) ) ;
#52397=CARTESIAN_POINT ( 'NONE',  ( 2.812500001229033320, -4.330127018922190985, -2.500000000000001332 ) ) ;
#52398=CARTESIAN_POINT ( 'NONE',  ( 10.95937500061451964, 0.000000000000000000, 5.243569643749999010 ) ) ;
#52399=CARTESIAN_POINT ( 'NONE',  ( 29.16562500061451502, 3.027376345333613106, -5.243569643749998122 ) ) ;
#52400=DIRECTION ( 'NONE',  ( 0.000000000000000000, 0.000000000000000000, -1.000000000000000000 ) ) ;
#52401=CARTESIAN_POINT ( 'NONE',  ( -3.685099084293383509, 9.302545652542773880, -34.75097178947568466 ) ) ;
#52402=DIRECTION ( 'NONE',  ( -1.000000000000000000, -0.000000000000000000, -0.000000000000000000 ) ) ;
#52403=CARTESIAN_POINT ( 'NONE',  ( 7.096875000614517148, -3.027376345333610441, -5.243569643749999898 ) ) ;
#52404=CARTESIAN_POINT ( 'NONE',  ( 11.37187500061451750, 3.027376345333611329, 5.243569643749999010 ) ) ;
#52405=CARTESIAN_POINT ( 'NONE',  ( 7.312500000000000000, 2.886751345948129099, -4.999999999999998224 ) ) ;
#52406=CARTESIAN_POINT ( 'NONE',  ( -4.243569643749999898, 15.75312500061459531, 30.00000000000000000 ) ) ;
#52409=CARTESIAN_POINT ( 'NONE',  ( 5.549999999999998934, 4.330127018922192761, -2.499999999999997780 ) ) ;
#52411=CARTESIAN_POINT ( 'NONE',  ( 23.80312500061451786, 4.541064518000418104, -2.621784821874998173 ) ) ;
#52412=CARTESIAN_POINT ( 'NONE',  ( 13.79062500061451502, -3.027376345333610441, -5.243569643749999898 ) ) ;
#52414=CARTESIAN_POINT ( 'NONE',  ( 10.39687500061451786, 6.054752690667223547, 3.707466751127219781E-16 ) ) ;
#52415=CARTESIAN_POINT ( 'NONE',  ( 27.26249999999999929, 2.886751345948126879, 4.999999999999999112 ) ) ;
#52416=CARTESIAN_POINT ( 'NONE',  ( 22.95000000122903216, -2.886751345948129988, 4.999999999999997335 ) ) ;
#52417=VECTOR ( 'NONE', #11752, 1000.000000000000000 ) ;
#52418=CARTESIAN_POINT ( 'NONE',  ( 11.28750000122903252, -4.330127018922194537, 2.499999999999995559 ) ) ;
#52419=CARTESIAN_POINT ( 'NONE',  ( 11.52187500061451608, -6.054752690667223547, -1.112240025338166033E-15 ) ) ;
#52420=CARTESIAN_POINT ( 'NONE',  ( 27.72187500061451715, -6.054752690667223547, -1.112240025338166033E-15 ) ) ;
#52421=CARTESIAN_POINT ( 'NONE',  ( 3.009375000614516793, -4.541064518000417216, -2.621784821875001281 ) ) ;
#52422=LINE ( 'NONE', #24337, #45495 ) ;
#52423=CARTESIAN_POINT ( 'NONE',  ( 21.64687500061451786, 6.054752690667223547, 3.707466751127219781E-16 ) ) ;
#52424=AXIS2_PLACEMENT_3D ( 'NONE', #25877, #54325, #21777 ) ;
#52425=CARTESIAN_POINT ( 'NONE',  ( 11.63437500061451857, 6.421520780324663323E-16, -5.243569643749999010 ) ) ;
#52427=CARTESIAN_POINT ( 'NONE',  ( 24.71250000000000213, -5.773502691896255534, -1.060575238724906372E-15 ) ) ;
#52429=CARTESIAN_POINT ( 'NONE',  ( 4.243569643749999010, 12.02187500061451786, -32.45002607614398471 ) ) ;
#52431=CARTESIAN_POINT ( 'NONE',  ( 15.21562500061451750, 3.027376345333613106, -5.243569643749998122 ) ) ;
#52432=CARTESIAN_POINT ( 'NONE',  ( 4.349999999999999645, 0.000000000000000000, 4.999999999999998224 ) ) ;
#52434=CARTESIAN_POINT ( 'NONE',  ( 30.00000000000000000, 0.000000000000000000, 0.000000000000000000 ) ) ;
#52435=CARTESIAN_POINT ( 'NONE',  ( 13.98750000000000249, -2.886751345948125991, -5.000000000000000000 ) ) ;
#52436=CARTESIAN_POINT ( 'NONE',  ( -3.000416591977282496E-16, 11.14062500061451644, 25.09994784771203058 ) ) ;
#52437=CARTESIAN_POINT ( 'NONE',  ( 13.87500000122903465, 2.886751345948126879, 4.999999999999999112 ) ) ;
#52438=AXIS2_PLACEMENT_3D ( 'NONE', #61581, #10984, #5446 ) ;
#52439=CARTESIAN_POINT ( 'NONE',  ( 25.65937500061451715, 4.541064518000418104, -2.621784821874998173 ) ) ;
#52441=CARTESIAN_POINT ( 'NONE',  ( 20.50312500061451715, -4.541064518000417216, -2.621784821875001281 ) ) ;
#52442=AXIS2_PLACEMENT_3D ( 'NONE', #14779, #59844, #36223 ) ;
#52443=CARTESIAN_POINT ( 'NONE',  ( 20.10937500061451289, -4.541064518000417216, -2.621784821875001281 ) ) ;
#52444=CARTESIAN_POINT ( 'NONE',  ( 4.275000000000001243, 4.330127018922191873, 2.499999999999999556 ) ) ;
#52445=CARTESIAN_POINT ( 'NONE',  ( 7.303125000614516082, 0.000000000000000000, 5.243569643749999010 ) ) ;
#52446=CARTESIAN_POINT ( 'NONE',  ( 22.11562500061451786, 3.027376345333611329, 5.243569643749999010 ) ) ;
#52447=CARTESIAN_POINT ( 'NONE',  ( 17.82187500061451502, -6.054752690667223547, -1.112240025338166033E-15 ) ) ;
#52448=CARTESIAN_POINT ( 'NONE',  ( -4.243569643749997233, 14.89062500061451644, 32.45002607614398471 ) ) ;
#52449=CARTESIAN_POINT ( 'NONE',  ( 19.65000000122902790, 5.773502691896255534, 3.535250795749688894E-16 ) ) ;
#52451=CARTESIAN_POINT ( 'NONE',  ( 8.390625000614518214, -3.027376345333610441, -5.243569643749999898 ) ) ;
#52452=CARTESIAN_POINT ( 'NONE',  ( 13.68750000000000000, 5.773502691896255534, 3.535250795749688401E-16 ) ) ;
#52453=CARTESIAN_POINT ( 'NONE',  ( 28.34062500061451928, 6.054752690667223547, 3.707466751127219781E-16 ) ) ;
#52454=CARTESIAN_POINT ( 'NONE',  ( 24.60937500061451644, -4.541064518000417216, -2.621784821875001281 ) ) ;
#52455=CARTESIAN_POINT ( 'NONE',  ( 14.76562500061451821, 3.027376345333613106, -5.243569643749998122 ) ) ;
#52456=CARTESIAN_POINT ( 'NONE',  ( 24.60000000122903430, 5.773502691896255534, 3.535250795749688894E-16 ) ) ;
#52457=CARTESIAN_POINT ( 'NONE',  ( 26.46562500061451573, 3.027376345333613106, -5.243569643749998122 ) ) ;
#52458=CARTESIAN_POINT ( 'NONE',  ( 22.84687500061451715, -3.027376345333610441, -5.243569643749999898 ) ) ;
#52459=CARTESIAN_POINT ( 'NONE',  ( 15.81562500061451537, 3.027376345333611329, 5.243569643749999010 ) ) ;
#52460=CARTESIAN_POINT ( 'NONE',  ( 9.001249775931846008E-16, 16.37187500061451573, 34.90005215228797653 ) ) ;
#52461=CARTESIAN_POINT ( 'NONE',  ( 22.67812500061451431, -4.541064518000419881, 2.621784821874995952 ) ) ;
#52463=EDGE_LOOP ( 'NONE', ( #55031, #57181, #58611, #72802 ) ) ;
#52464=CARTESIAN_POINT ( 'NONE',  ( 26.39999999999999858, 0.000000000000000000, 4.999999999999998224 ) ) ;
#52465=CARTESIAN_POINT ( 'NONE',  ( 1.999999999999998668, 14.00000000000000178, -33.46410161513775705 ) ) ;
#52467=CARTESIAN_POINT ( 'NONE',  ( 28.82812500061451644, 4.541064518000418104, 2.621784821874999949 ) ) ;
#52468=CARTESIAN_POINT ( 'NONE',  ( 8.128125000614515372, 4.541064518000418104, 2.621784821874999949 ) ) ;
#52469=CARTESIAN_POINT ( 'NONE',  ( 21.15000000122903145, -2.886751345948129988, 4.999999999999997335 ) ) ;
#52470=CARTESIAN_POINT ( 'NONE',  ( 26.09062500061451573, 6.054752690667223547, 3.707466751127219781E-16 ) ) ;
#52471=CARTESIAN_POINT ( 'NONE',  ( 25.83749999999999858, 5.773502691896255534, 3.535250795749688894E-16 ) ) ;
#52472=CARTESIAN_POINT ( 'NONE',  ( 8.484601909799253346E-16, 15.72500000122903252, -25.38119784648299770 ) ) ;
#52473=CARTESIAN_POINT ( 'NONE',  ( 25.20000000122902861, -2.886751345948114000, 5.000000000000024869 ) ) ;
#52474=CARTESIAN_POINT ( 'NONE',  ( 11.39062500061451644, -3.027376345333614438, 5.243569643749998122 ) ) ;
#52475=VERTEX_POINT ( 'NONE', #6327 ) ;
#52476=CARTESIAN_POINT ( 'NONE',  ( 25.97812500061451502, 6.421520780324663323E-16, -5.243569643749999010 ) ) ;
#52477=CARTESIAN_POINT ( 'NONE',  ( 6.890625000614516438, -3.027376345333614438, 5.243569643749998122 ) ) ;
#52478=CARTESIAN_POINT ( 'NONE',  ( 3.665625000614517681, 3.027376345333611329, 5.243569643749999010 ) ) ;
#52480=CARTESIAN_POINT ( 'NONE',  ( 13.08750000000000213, -2.886751345948126435, -5.000000000000000000 ) ) ;
#52481=CARTESIAN_POINT ( 'NONE',  ( 12.56250000000000178, -5.773502691896255534, -1.060575238724906372E-15 ) ) ;
#52482=CARTESIAN_POINT ( 'NONE',  ( 12.79687500061451821, -3.027376345333614438, 5.243569643749998122 ) ) ;
#52483=CARTESIAN_POINT ( 'NONE',  ( 9.375000001229036428, 2.886751345948126879, 4.999999999999999112 ) ) ;
#52484=CARTESIAN_POINT ( 'NONE',  ( 17.63437500061451502, 4.541064518000418104, 2.621784821874999949 ) ) ;
#52486=CARTESIAN_POINT ( 'NONE',  ( 8.109375000614518214, 4.541064518000418104, -2.621784821874998173 ) ) ;
#52487=CARTESIAN_POINT ( 'NONE',  ( -2.121784821874996840, 10.87812500061451715, -26.32496088578401583 ) ) ;
#52488=CARTESIAN_POINT ( 'NONE',  ( 2.000000000000001332, 16.55000000000000071, 33.46410161513774995 ) ) ;
#52491=CARTESIAN_POINT ( 'NONE',  ( 24.92812500061451431, -4.541064518000419881, 2.621784821874995952 ) ) ;
#52492=CARTESIAN_POINT ( 'NONE',  ( 21.33750000122903145, 6.123233995736764310E-16, -4.999999999999998224 ) ) ;
#52493=CARTESIAN_POINT ( 'NONE',  ( 27.57187500061451857, 3.027376345333611329, 5.243569643749999010 ) ) ;
#52494=CARTESIAN_POINT ( 'NONE',  ( 22.68750000000000000, 5.773502691896255534, 3.535250795749688894E-16 ) ) ;
#52495=EDGE_CURVE ( 'NONE', #8533, #72227, #28120, .T. ) ;
#52496=CARTESIAN_POINT ( 'NONE',  ( 6.515625000614516438, -6.054752690667223547, -1.112240025338166033E-15 ) ) ;
#52498=CARTESIAN_POINT ( 'NONE',  ( 15.79687500061451821, 6.054752690667223547, 3.707466751127219781E-16 ) ) ;
#52500=CARTESIAN_POINT ( 'NONE',  ( 29.13750000122903216, 4.330127018922191873, 2.499999999999999556 ) ) ;
#52501=CARTESIAN_POINT ( 'NONE',  ( 8.071875000614518569, 3.027376345333613106, -5.243569643749998122 ) ) ;
#52503=CARTESIAN_POINT ( 'NONE',  ( 18.34687500061451715, -3.027376345333610441, -5.243569643749999898 ) ) ;
#52505=CARTESIAN_POINT ( 'NONE',  ( 27.07499999999999929, 6.123233995736764310E-16, -4.999999999999998224 ) ) ;
#52506=CARTESIAN_POINT ( 'NONE',  ( 28.47187500061451715, 3.027376345333611329, 5.243569643749999010 ) ) ;
#52507=DIRECTION ( 'NONE',  ( -1.000000000000000000, -0.000000000000000000, -0.000000000000000000 ) ) ;
#52510=CARTESIAN_POINT ( 'NONE',  ( 10.16249999999999964, 2.886751345948126879, 4.999999999999999112 ) ) ;
#52512=CARTESIAN_POINT ( 'NONE',  ( 25.30312500061451431, 0.000000000000000000, 5.243569643749999010 ) ) ;
#52513=CARTESIAN_POINT ( 'NONE',  ( 13.72500000000000142, 4.330127018922191873, 2.499999999999999556 ) ) ;
#52514=ADVANCED_FACE ( 'NONE', ( #40675, #13670 ), #36213, .T. ) ;
#52515=CARTESIAN_POINT ( 'NONE',  ( 7.387500001229032165, 6.123233995736764310E-16, -4.999999999999998224 ) ) ;
#52516=CARTESIAN_POINT ( 'NONE',  ( 6.515625000614516438, -6.054752690667223547, -1.112240025338166033E-15 ) ) ;
#52517=CARTESIAN_POINT ( 'NONE',  ( 21.60000000000000142, -4.330127018922190985, -2.500000000000001332 ) ) ;
#52518=CARTESIAN_POINT ( 'NONE',  ( 20.76562500061451644, 3.027376345333611329, 5.243569643749999010 ) ) ;
#52520=CARTESIAN_POINT ( 'NONE',  ( 24.71250000122903145, 0.000000000000000000, 4.999999999999998224 ) ) ;
#52522=CARTESIAN_POINT ( 'NONE',  ( 5.775000000000002132, -4.330127018922194537, 2.499999999999995559 ) ) ;
#52524=ORIENTED_EDGE ( 'NONE', *, *, #57647, .T. ) ;
#52525=CARTESIAN_POINT ( 'NONE',  ( 20.91562500061451502, -6.054752690667223547, -1.112240025338166033E-15 ) ) ;
#52526=CARTESIAN_POINT ( 'NONE',  ( 27.36562500061451786, 3.027376345333613106, -5.243569643749998122 ) ) ;
#52527=CARTESIAN_POINT ( 'NONE',  ( 27.12187500061451573, 3.027376345333611329, 5.243569643749999010 ) ) ;
#52528=CARTESIAN_POINT ( 'NONE',  ( 14.20312500061451644, -4.541064518000417216, -2.621784821875001281 ) ) ;
#52530=CARTESIAN_POINT ( 'NONE',  ( 27.03750000122903430, -4.330127018922194537, 2.499999999999995559 ) ) ;
#52532=CARTESIAN_POINT ( 'NONE',  ( 17.12812500061451715, 4.541064518000418104, 2.621784821874999949 ) ) ;
#52533=FACE_OUTER_BOUND ( 'NONE', #6027, .T. ) ;
#52534=CARTESIAN_POINT ( 'NONE',  ( 11.40937500061451892, 0.000000000000000000, 5.243569643749999010 ) ) ;
#52535=CARTESIAN_POINT ( 'NONE',  ( 9.046875000614518214, 6.054752690667223547, 3.707466751127219781E-16 ) ) ;
#52536=CARTESIAN_POINT ( 'NONE',  ( 20.37187500061451573, 3.027376345333611329, 5.243569643749999010 ) ) ;
#52538=CARTESIAN_POINT ( 'NONE',  ( -3.685099084293382177, 9.302545652542775656, 25.24902821052430824 ) ) ;
#52539=CARTESIAN_POINT ( 'NONE',  ( 22.97812500061451857, 4.541064518000418104, 2.621784821874999949 ) ) ;
#52540=( BOUNDED_CURVE ( )  B_SPLINE_CURVE ( 2, ( #47354, #52173, #71634, #43559, #9570, #13730, #21007, #29635, #69887 ),
 .UNSPECIFIED., .F., .F. ) 
 B_SPLINE_CURVE_WITH_KNOTS ( ( 3, 2, 2, 2, 3 ),
 ( 0.1413043478260869734, 0.1449275362318840632, 0.1521739130434782705, 0.1594202898550724501, 0.1630434782608695676 ),
 .UNSPECIFIED. ) 
 CURVE ( )  GEOMETRIC_REPRESENTATION_ITEM ( )  RATIONAL_B_SPLINE_CURVE ( ( 0.9330127018922194093, 0.9330127018922196314, 1.000000000000000000, 0.8660254037844387076, 1.000000000000000000, 0.8660254037844387076, 1.000000000000000000, 0.9330127018922190762, 0.9330127018922194093 ) ) 
 REPRESENTATION_ITEM ( '' )  );
#52541=CIRCLE ( 'NONE', #70260, 10.00000000000000000 ) ;
#52542=CARTESIAN_POINT ( 'NONE',  ( 18.87187500061451573, 3.027376345333613106, -5.243569643749998122 ) ) ;
#52543=CARTESIAN_POINT ( 'NONE',  ( 23.31562500061451715, 3.027376345333613106, -5.243569643749998122 ) ) ;
#52545=CARTESIAN_POINT ( 'NONE',  ( -2.828200636599751609E-16, 14.93750000000000000, 25.38119784648299770 ) ) ;
#52546=CARTESIAN_POINT ( 'NONE',  ( 28.94062500061452070, -3.027376345333614438, 5.243569643749998122 ) ) ;
#52547=CARTESIAN_POINT ( 'NONE',  ( 8.700000001229032165, -2.886751345948125991, -5.000000000000000000 ) ) ;
#52548=AXIS2_PLACEMENT_3D ( 'NONE', #20809, #23354, #68434 ) ;
#52549=ORIENTED_EDGE ( 'NONE', *, *, #37707, .F. ) ;
#52550=CARTESIAN_POINT ( 'NONE',  ( 5.362500001229033586, 0.000000000000000000, 4.999999999999998224 ) ) ;
#52551=CARTESIAN_POINT ( 'NONE',  ( -3.999999999999999556, 19.51250000000000284, -32.30940107675850470 ) ) ;
#52552=CARTESIAN_POINT ( 'NONE',  ( 25.98750000122903003, 4.330127018922191873, 2.499999999999999556 ) ) ;
#52554=CARTESIAN_POINT ( 'NONE',  ( 9.721875000614517148, -6.054752690667223547, -1.112240025338166033E-15 ) ) ;
#52555=CYLINDRICAL_SURFACE ( 'NONE', #34914, 4.999999999999998224 ) ;
#52556=CARTESIAN_POINT ( 'NONE',  ( 16.56562500061451715, 3.027376345333613106, -5.243569643749998122 ) ) ;
#52557=CARTESIAN_POINT ( 'NONE',  ( 11.67187500061451821, 3.027376345333613106, -5.243569643749998122 ) ) ;
#52558=CARTESIAN_POINT ( 'NONE',  ( 28.87500000122902932, -5.773502691896255534, -1.060575238724906372E-15 ) ) ;
#52559=CARTESIAN_POINT ( 'NONE',  ( 19.05937500061451928, 0.000000000000000000, 5.243569643749999010 ) ) ;
#52560=CARTESIAN_POINT ( 'NONE',  ( 8.259375000614518569, 0.000000000000000000, 5.243569643749999010 ) ) ;
#52562=CARTESIAN_POINT ( 'NONE',  ( 7.715625000614515727, 3.027376345333611329, 5.243569643749999010 ) ) ;
#52563=CARTESIAN_POINT ( 'NONE',  ( 16.67812500061451786, 4.541064518000418104, 2.621784821874999949 ) ) ;
#52565=CARTESIAN_POINT ( 'NONE',  ( 6.337500001229033231, -4.330127018922194537, 2.499999999999995559 ) ) ;
#52566=CARTESIAN_POINT ( 'NONE',  ( 15.25312500061451715, 4.541064518000418104, -2.621784821874998173 ) ) ;
#52567=CARTESIAN_POINT ( 'NONE',  ( 11.69062500061451360, 6.054752690667223547, 3.707466751127219781E-16 ) ) ;
#52569=CARTESIAN_POINT ( 'NONE',  ( 10.72500000000000142, -4.330127018922194537, 2.499999999999995559 ) ) ;
#52570=CARTESIAN_POINT ( 'NONE',  ( 5.437500001229035540, -4.330127018922194537, 2.499999999999995559 ) ) ;
#52571=CARTESIAN_POINT ( 'NONE',  ( 15.79687500061451821, 6.054752690667223547, 3.707466751127219781E-16 ) ) ;
#52572=CARTESIAN_POINT ( 'NONE',  ( 18.26250000122903216, 4.330127018922192761, -2.499999999999997780 ) ) ;
#52574=CARTESIAN_POINT ( 'NONE',  ( 4.243569643749999898, 19.09062500061451573, -27.54997392385601529 ) ) ;
#52576=CARTESIAN_POINT ( 'NONE',  ( 23.06250000122903288, -4.330127018922190985, -2.500000000000001332 ) ) ;
#52577=CARTESIAN_POINT ( 'NONE',  ( 3.999999999999999112, 10.88750000122903394, -30.00000000000000000 ) ) ;
#52578=CARTESIAN_POINT ( 'NONE',  ( 17.29687500061451999, -3.027376345333614438, 5.243569643749998122 ) ) ;
#52581=ADVANCED_FACE ( 'NONE', ( #18480 ), #64652, .F. ) ;
#52582=CARTESIAN_POINT ( 'NONE',  ( 15.02812500061451750, -4.541064518000419881, 2.621784821874995952 ) ) ;
#52585=CARTESIAN_POINT ( 'NONE',  ( 24.42187500061451999, 3.027376345333611329, 5.243569643749999010 ) ) ;
#52587=CARTESIAN_POINT ( 'NONE',  ( 9.665625000614515017, -6.054752690667223547, -1.112240025338166033E-15 ) ) ;
#52588=CARTESIAN_POINT ( 'NONE',  ( 16.35937500061451644, 0.000000000000000000, 5.243569643749999010 ) ) ;
#52589=ORIENTED_EDGE ( 'NONE', *, *, #41229, .T. ) ;
#52590=CARTESIAN_POINT ( 'NONE',  ( 26.97187500061451360, 3.027376345333613106, -5.243569643749998122 ) ) ;
#52591=CARTESIAN_POINT ( 'NONE',  ( 27.17812500061451786, -4.541064518000419881, 2.621784821874995952 ) ) ;
#52592=CARTESIAN_POINT ( 'NONE',  ( 21.44062500061452070, -3.027376345333610441, -5.243569643749999898 ) ) ;
#52593=CARTESIAN_POINT ( 'NONE',  ( 29.50312500061451360, -4.541064518000417216, -2.621784821875001281 ) ) ;
#52595=CARTESIAN_POINT ( 'NONE',  ( 9.899999999999998579, -4.330127018922190985, -2.500000000000001332 ) ) ;
#52596=CARTESIAN_POINT ( 'NONE',  ( 20.25000000122903288, -2.886751345948129988, 4.999999999999997335 ) ) ;
#52597=CARTESIAN_POINT ( 'NONE',  ( -1.071796769724491005, 18.67009619066136494, -34.00000000000000000 ) ) ;
#52600=CARTESIAN_POINT ( 'NONE',  ( 17.58749999999999858, -2.886751345948125991, -5.000000000000000000 ) ) ;
#52601=CARTESIAN_POINT ( 'NONE',  ( 21.44999999999999929, 0.000000000000000000, 4.999999999999998224 ) ) ;
#52602=CARTESIAN_POINT ( 'NONE',  ( 19.17187500061451999, -6.054752690667223547, -1.112240025338166033E-15 ) ) ;
#52603=CARTESIAN_POINT ( 'NONE',  ( 12.89062500061451821, -3.027376345333610441, -5.243569643749999898 ) ) ;
#52604=EDGE_LOOP ( 'NONE', ( #22124, #27092, #36341, #2710 ) ) ;
#52605=CARTESIAN_POINT ( 'NONE',  ( 28.57499999999999929, 4.330127018922191873, 2.499999999999999556 ) ) ;
#52606=CARTESIAN_POINT ( 'NONE',  ( 6.440625000614517148, -3.027376345333614438, 5.243569643749998122 ) ) ;
#52608=CARTESIAN_POINT ( 'NONE',  ( 11.43750000000000000, 5.773502691896255534, 3.535250795749688894E-16 ) ) ;
#52610=CARTESIAN_POINT ( 'NONE',  ( 2.121784821875001281, 14.10312500061451679, 33.67503911421598417 ) ) ;
#52611=CARTESIAN_POINT ( 'NONE',  ( 2.896875000614518747, -3.027376345333614438, 5.243569643749998122 ) ) ;
#52614=CARTESIAN_POINT ( 'NONE',  ( 24.04687500061451644, -3.027376345333614438, 5.243569643749998122 ) ) ;
#52616=CARTESIAN_POINT ( 'NONE',  ( 21.29062500061451502, -3.027376345333614438, 5.243569643749998122 ) ) ;
#52617=CARTESIAN_POINT ( 'NONE',  ( 23.70937500061451786, -4.541064518000417216, -2.621784821875001281 ) ) ;
#52618=CARTESIAN_POINT ( 'NONE',  ( -4.243569643749999898, 15.30312500061459247, -30.00000000000000000 ) ) ;
#52619=CARTESIAN_POINT ( 'NONE',  ( 5.653125000614517504, -4.541064518000417216, -2.621784821875001281 ) ) ;
#52621=CARTESIAN_POINT ( 'NONE',  ( 24.10312500061451502, -4.541064518000417216, -2.621784821875001281 ) ) ;
#52624=CARTESIAN_POINT ( 'NONE',  ( 15.98437500061451821, -4.541064518000419881, 2.621784821874995952 ) ) ;
#52625=CARTESIAN_POINT ( 'NONE',  ( 17.85937500061451999, -4.541064518000417216, -2.621784821875001281 ) ) ;
#52626=CARTESIAN_POINT ( 'NONE',  ( 26.10937500061451644, 4.541064518000418104, -2.621784821874998173 ) ) ;
#52627=CARTESIAN_POINT ( 'NONE',  ( -4.243569643749998122, 16.74687500061451573, 32.45002607614398471 ) ) ;
#52628=CARTESIAN_POINT ( 'NONE',  ( 7.228125000614517681, 4.541064518000418104, 2.621784821874999949 ) ) ;
#52629=CYLINDRICAL_SURFACE ( 'NONE', #27784, 4.999999999999998224 ) ;
#52630=CARTESIAN_POINT ( 'NONE',  ( 4.434375000614519280, 6.421520780324663323E-16, -5.243569643749999010 ) ) ;
#52631=CARTESIAN_POINT ( 'NONE',  ( 5.053125000614517859, 0.000000000000000000, 5.243569643749999010 ) ) ;
#52632=CARTESIAN_POINT ( 'NONE',  ( 8.934375000614517504, 6.421520780324663323E-16, -5.243569643749999010 ) ) ;
#52633=CARTESIAN_POINT ( 'NONE',  ( 17.40000000122903145, 5.773502691896255534, 3.535250795749688894E-16 ) ) ;
#52634=CARTESIAN_POINT ( 'NONE',  ( 5.859375000614519102, 4.541064518000418104, -2.621784821874998173 ) ) ;
#52635=CARTESIAN_POINT ( 'NONE',  ( 7.603125000614517681, 4.541064518000418104, -2.621784821874998173 ) ) ;
#52638=CARTESIAN_POINT ( 'NONE',  ( 15.75937500061451857, 4.541064518000418104, -2.621784821874998173 ) ) ;
#52639=ORIENTED_EDGE ( 'NONE', *, *, #62566, .F. ) ;
#52640=CARTESIAN_POINT ( 'NONE',  ( 23.76562500061451644, 3.027376345333613106, -5.243569643749998122 ) ) ;
#52641=CARTESIAN_POINT ( 'NONE',  ( 9.740625000614516082, -3.027376345333610441, -5.243569643749999898 ) ) ;
#52642=CARTESIAN_POINT ( 'NONE',  ( 27.30937500061451573, -4.541064518000417216, -2.621784821875001281 ) ) ;
#52643=CARTESIAN_POINT ( 'NONE',  ( 8.840625000614515727, -3.027376345333610441, -5.243569643749999898 ) ) ;
#52645=CARTESIAN_POINT ( 'NONE',  ( 10.23750000122903359, 4.330127018922191873, 2.499999999999999556 ) ) ;
#52646=EDGE_CURVE ( 'NONE', #47727, #17166, #66368, .T. ) ;
#52647=CARTESIAN_POINT ( 'NONE',  ( 24.25312500061451715, 4.541064518000418104, -2.621784821874998173 ) ) ;
#52648=CARTESIAN_POINT ( 'NONE',  ( -2.121784821874999949, 12.07812500061451821, -33.67503911421598417 ) ) ;
#52649=CARTESIAN_POINT ( 'NONE',  ( 13.20000000122903394, -2.886751345948125991, -5.000000000000000000 ) ) ;
#52650=CARTESIAN_POINT ( 'NONE',  ( 22.56562500061451715, 3.027376345333611329, 5.243569643749999010 ) ) ;
#52651=CARTESIAN_POINT ( 'NONE',  ( 20.87812500061451715, -4.541064518000419881, 2.621784821874995952 ) ) ;
#52653=CARTESIAN_POINT ( 'NONE',  ( 19.98749999999999716, 5.773502691896255534, 3.535250795749688894E-16 ) ) ;
#52654=CARTESIAN_POINT ( 'NONE',  ( 13.42500000122903536, 2.886751345948126879, 4.999999999999999112 ) ) ;
#52655=CARTESIAN_POINT ( 'NONE',  ( 10.30312500061451431, 4.541064518000418104, -2.621784821874998173 ) ) ;
#52656=CARTESIAN_POINT ( 'NONE',  ( 14.09062500061451750, -3.027376345333614438, 5.243569643749998122 ) ) ;
#52657=CARTESIAN_POINT ( 'NONE',  ( 25.08750000122903145, 4.330127018922191873, 2.499999999999999556 ) ) ;
#52658=CARTESIAN_POINT ( 'NONE',  ( 20.78437500061451715, 4.541064518000418104, 2.621784821874999949 ) ) ;
#52661=ADVANCED_FACE ( 'NONE', ( #41046 ), #29225, .F. ) ;
#52662=CARTESIAN_POINT ( 'NONE',  ( 8.850000001229034297, 5.773502691896255534, 3.535250795749688894E-16 ) ) ;
#52663=CARTESIAN_POINT ( 'NONE',  ( 5.746875000614517504, -3.027376345333610441, -5.243569643749999898 ) ) ;
#52664=CARTESIAN_POINT ( 'NONE',  ( 26.07187500061451857, 3.027376345333613106, -5.243569643749998122 ) ) ;
#52665=LINE ( 'NONE', #35310, #64536 ) ;
#52666=CARTESIAN_POINT ( 'NONE',  ( 22.26562500061451644, -6.054752690667223547, -1.112240025338166033E-15 ) ) ;
#52667=CARTESIAN_POINT ( 'NONE',  ( 26.03437500061451715, 6.421520780324663323E-16, -5.243569643749999010 ) ) ;
#52669=VECTOR ( 'NONE', #18819, 1000.000000000000000 ) ;
#52670=CARTESIAN_POINT ( 'NONE',  ( 7.546875000614517326, -3.027376345333610441, -5.243569643749999898 ) ) ;
#52671=CARTESIAN_POINT ( 'NONE',  ( 17.91562500061451502, 3.027376345333613106, -5.243569643749998122 ) ) ;
#52673=CARTESIAN_POINT ( 'NONE',  ( -1.071796769724504328, 12.89240381056766616, -26.00000000000001066 ) ) ;
#52674=CARTESIAN_POINT ( 'NONE',  ( 27.02812500061451573, 4.541064518000418104, 2.621784821874999949 ) ) ;
#52675=CARTESIAN_POINT ( 'NONE',  ( 4.959375000614516971, 4.541064518000418104, -2.621784821874998173 ) ) ;
#52676=CARTESIAN_POINT ( 'NONE',  ( -5.810221930991193690E-16, 15.83749999999999680, -34.00000000000000000 ) ) ;
#52677=CARTESIAN_POINT ( 'NONE',  ( 4.111889464957033447, 2.844708250062874200, 4.404844785106587501 ) ) ;
#52678=CARTESIAN_POINT ( 'NONE',  ( 18.18750000000000000, 5.773502691896255534, 3.535250795749688894E-16 ) ) ;
#52679=CARTESIAN_POINT ( 'NONE',  ( 20.61562500061451431, 3.027376345333613106, -5.243569643749998122 ) ) ;
#52680=ORIENTED_EDGE ( 'NONE', *, *, #29219, .F. ) ;
#52681=CARTESIAN_POINT ( 'NONE',  ( 24.44999999999999929, 4.330127018922192761, -2.499999999999997780 ) ) ;
#52683=ADVANCED_FACE ( 'NONE', ( #24395 ), #7412, .F. ) ;
#52684=CARTESIAN_POINT ( 'NONE',  ( 25.50937500061451502, -4.541064518000417216, -2.621784821875001281 ) ) ;
#52685=ORIENTED_EDGE ( 'NONE', *, *, #28856, .T. ) ;
#52686=CARTESIAN_POINT ( 'NONE',  ( 13.71562500061451750, -6.054752690667223547, -1.112240025338166033E-15 ) ) ;
#52687=CARTESIAN_POINT ( 'NONE',  ( 4.903125000614516615, 4.541064518000418104, -2.621784821874998173 ) ) ;
#52689=CARTESIAN_POINT ( 'NONE',  ( 3.196875000614516793, 6.054752690667223547, 3.707466751127219781E-16 ) ) ;
#52690=CARTESIAN_POINT ( 'NONE',  ( 14.88750000122903394, -4.330127018922194537, 2.499999999999995559 ) ) ;
#52691=CARTESIAN_POINT ( 'NONE',  ( 19.61249999999999716, 2.886751345948126879, 4.999999999999999112 ) ) ;
#52692=CARTESIAN_POINT ( 'NONE',  ( 28.01249999999999574, 2.886751345948129099, -4.999999999999998224 ) ) ;
#52693=CARTESIAN_POINT ( 'NONE',  ( 5.521875000614517859, 3.027376345333611329, 5.243569643749999010 ) ) ;
#52694=CARTESIAN_POINT ( 'NONE',  ( 9.046875000614518214, 6.054752690667223547, 3.707466751127219781E-16 ) ) ;
#52695=CARTESIAN_POINT ( 'NONE',  ( 18.27187500061451431, -6.054752690667223547, -1.112240025338166033E-15 ) ) ;
#52698=CARTESIAN_POINT ( 'NONE',  ( 28.22812500061451502, 6.421520780324663323E-16, -5.243569643749999010 ) ) ;
#52699=CARTESIAN_POINT ( 'NONE',  ( 29.40937500061451715, 0.000000000000000000, 5.243569643749999010 ) ) ;
#52700=CARTESIAN_POINT ( 'NONE',  ( 3.796875000614517326, -3.027376345333614438, 5.243569643749998122 ) ) ;
#52701=CARTESIAN_POINT ( 'NONE',  ( 16.64999999999999858, -4.330127018922190985, -2.500000000000001332 ) ) ;
#52702=CARTESIAN_POINT ( 'NONE',  ( 12.85312500061451502, -4.541064518000417216, -2.621784821875001281 ) ) ;
#52703=CARTESIAN_POINT ( 'NONE',  ( 3.999999999999999112, 14.03750000122903430, 30.00000000000000000 ) ) ;
#52704=CARTESIAN_POINT ( 'NONE',  ( 27.03750000000000142, -2.886751345948142422, -4.999999999999970690 ) ) ;
#52705=CARTESIAN_POINT ( 'NONE',  ( 19.35000000122903430, -2.886751345948129988, 4.999999999999997335 ) ) ;
#52706=CARTESIAN_POINT ( 'NONE',  ( 1.970565482296614990, 9.811066920826819526, 24.31906361249631843 ) ) ;
#52708=CARTESIAN_POINT ( 'NONE',  ( 8.278125000614515727, -4.541064518000419881, 2.621784821874995952 ) ) ;
#52709=CARTESIAN_POINT ( 'NONE',  ( 23.89687500061451786, 6.054752690667223547, 3.707466751127219781E-16 ) ) ;
#52710=FACE_OUTER_BOUND ( 'NONE', #17780, .T. ) ;
#52711=CARTESIAN_POINT ( 'NONE',  ( 27.08437500061451786, 4.541064518000418104, 2.621784821874999949 ) ) ;
#52712=CARTESIAN_POINT ( 'NONE',  ( 8.587500000000002132, -2.886751345948125991, -5.000000000000000000 ) ) ;
#52713=CARTESIAN_POINT ( 'NONE',  ( 3.999999999999999112, 13.58750000122903323, 30.00000000000000000 ) ) ;
#52714=CARTESIAN_POINT ( 'NONE',  ( 13.90312500061451750, 4.541064518000418104, -2.621784821874998173 ) ) ;
#52715=CARTESIAN_POINT ( 'NONE',  ( 6.037500001229035185, 6.123233995736764310E-16, -4.999999999999998224 ) ) ;
#52716=CARTESIAN_POINT ( 'NONE',  ( 12.64687500061451608, 6.054752690667223547, 3.707466751127219781E-16 ) ) ;
#52717=CARTESIAN_POINT ( 'NONE',  ( -2.482458701038962712, 4.346511033910189781, -26.85332358594694924 ) ) ;
#52718=EDGE_LOOP ( 'NONE', ( #42915, #53402, #30372, #27781 ) ) ;
#52719=CARTESIAN_POINT ( 'NONE',  ( 11.31562500061451892, 3.027376345333611329, 5.243569643749999010 ) ) ;
#52721=CARTESIAN_POINT ( 'NONE',  ( 23.70000000122903216, 5.773502691896255534, 3.535250795749688894E-16 ) ) ;
#52722=CARTESIAN_POINT ( 'NONE',  ( 11.82187500061451679, 3.027376345333611329, 5.243569643749999010 ) ) ;
#52723=AXIS2_PLACEMENT_3D ( 'NONE', #64916, #30577, #35747 ) ;
#52724=CARTESIAN_POINT ( 'NONE',  ( 13.49062500061451608, 6.054752690667223547, 3.707466751127219781E-16 ) ) ;
#52726=CARTESIAN_POINT ( 'NONE',  ( 24.83437500061451431, 4.541064518000418104, 2.621784821874999949 ) ) ;
#52729=CARTESIAN_POINT ( 'NONE',  ( 5.325000000000000178, -4.330127018922194537, 2.499999999999995559 ) ) ;
#52730=CARTESIAN_POINT ( 'NONE',  ( 8.062500001229034652, 0.000000000000000000, 4.999999999999998224 ) ) ;
#52731=CARTESIAN_POINT ( 'NONE',  ( -2.121784821874996840, 16.33437500061451786, -26.32496088578401583 ) ) ;
#52732=CARTESIAN_POINT ( 'NONE',  ( 15.57187500061451679, -6.054752690667223547, -1.112240025338166033E-15 ) ) ;
#52733=CARTESIAN_POINT ( 'NONE',  ( 18.60000000122903430, -2.886751345948125991, -5.000000000000000000 ) ) ;
#52734=CARTESIAN_POINT ( 'NONE',  ( 12.64687500061451608, 6.054752690667223547, 3.707466751127219781E-16 ) ) ;
#52735=CARTESIAN_POINT ( 'NONE',  ( -4.243569643749999898, 19.80312500061451786, -30.00000000000000000 ) ) ;
#52736=CARTESIAN_POINT ( 'NONE',  ( 19.53750000122903430, 6.123233995736764310E-16, -4.999999999999998224 ) ) ;
#52737=CARTESIAN_POINT ( 'NONE',  ( 12.21562500061451573, 3.027376345333611329, 5.243569643749999010 ) ) ;
#52739=ORIENTED_EDGE ( 'NONE', *, *, #72113, .T. ) ;
#52740=CARTESIAN_POINT ( 'NONE',  ( 17.62500000000000000, 6.123233995736764310E-16, -4.999999999999998224 ) ) ;
#52741=PLANE ( 'NONE',  #53887 ) ;
#52742=CARTESIAN_POINT ( 'NONE',  ( 11.89687500061451608, -3.027376345333614438, 5.243569643749998122 ) ) ;
#52743=CARTESIAN_POINT ( 'NONE',  ( 22.46250000000000213, -5.773502691896255534, -1.060575238724906372E-15 ) ) ;
#52744=CARTESIAN_POINT ( 'NONE',  ( 11.92500000122903181, 2.886751345948129099, -4.999999999999998224 ) ) ;
#52745=CARTESIAN_POINT ( 'NONE',  ( 21.15000000122903145, -2.886751345948129988, 4.999999999999997335 ) ) ;
#52746=CARTESIAN_POINT ( 'NONE',  ( 18.06562500061451715, 3.027376345333611329, 5.243569643749999010 ) ) ;
#52747=EDGE_CURVE ( 'NONE', #32704, #22971, #12946, .T. ) ;
#52748=CARTESIAN_POINT ( 'NONE',  ( 19.60312500061451502, -4.541064518000417216, -2.621784821875001281 ) ) ;
#52749=CARTESIAN_POINT ( 'NONE',  ( 29.10000000122903074, 5.773502691896255534, 3.535250795749688894E-16 ) ) ;
#52750=( BOUNDED_CURVE ( )  B_SPLINE_CURVE ( 2, ( #4015, #71607, #14348, #8441, #43534, #70133, #15433 ),
 .UNSPECIFIED., .F., .F. ) 
 B_SPLINE_CURVE_WITH_KNOTS ( ( 3, 2, 2, 3 ),
 ( 0.9429739840102342452, 0.9444444444444444198, 0.9472222222222221877, 0.9485519436316427466 ),
 .UNSPECIFIED. ) 
 CURVE ( )  GEOMETRIC_REPRESENTATION_ITEM ( )  RATIONAL_B_SPLINE_CURVE ( ( 0.9332437672470215162, 0.9290784365472635198, 1.000000000000000000, 0.8660254037844387076, 1.000000000000000000, 0.9358663999937293365, 0.9331342711013768110 ) ) 
 REPRESENTATION_ITEM ( '' )  );
#52751=CARTESIAN_POINT ( 'NONE',  ( 27.52500000000000213, 6.123233995736764310E-16, -4.999999999999998224 ) ) ;
#52754=CARTESIAN_POINT ( 'NONE',  ( 27.34687500061451360, -3.027376345333610441, -5.243569643749999898 ) ) ;
#52755=CARTESIAN_POINT ( 'NONE',  ( 1.999999999999998668, 10.06250000122903465, -33.46410161513775705 ) ) ;
#52756=CARTESIAN_POINT ( 'NONE',  ( -4.243569643749999898, 14.87187500061451928, -32.45002607614398471 ) ) ;
#52757=CARTESIAN_POINT ( 'NONE',  ( 3.450000001229036162, 5.773502691896255534, 3.535250795749688894E-16 ) ) ;
#52758=CARTESIAN_POINT ( 'NONE',  ( 6.000000000000001776, 4.330127018922192761, -2.499999999999997780 ) ) ;
#52759=CARTESIAN_POINT ( 'NONE',  ( 2.775000001229033675, -5.773502691896255534, -1.060575238724906372E-15 ) ) ;
#52760=CARTESIAN_POINT ( 'NONE',  ( 9.984375000614518214, 4.541064518000418104, 2.621784821874999949 ) ) ;
#52761=CARTESIAN_POINT ( 'NONE',  ( 29.20312500061451644, 4.541064518000418104, -2.621784821874998173 ) ) ;
#52763=CARTESIAN_POINT ( 'NONE',  ( -4.518949595698578570, 8.925733855591198918, -26.03435065765658152 ) ) ;
#52765=CARTESIAN_POINT ( 'NONE',  ( 7.209375000614519635, 4.541064518000418104, -2.621784821874998173 ) ) ;
#52766=CARTESIAN_POINT ( 'NONE',  ( 10.95937500061451964, 0.000000000000000000, 5.243569643749999010 ) ) ;
#52767=CARTESIAN_POINT ( 'NONE',  ( 7.650000000000000355, -4.330127018922190985, -2.500000000000001332 ) ) ;
#52768=ADVANCED_FACE ( 'NONE', ( #58363 ), #63195, .F. ) ;
#52769=CARTESIAN_POINT ( 'NONE',  ( -4.243569643749999898, 15.71562500061459744, 27.54997392385601529 ) ) ;
#52771=CARTESIAN_POINT ( 'NONE',  ( 6.937499999999999112, 5.773502691896255534, 3.535250795749688894E-16 ) ) ;
#52773=CARTESIAN_POINT ( 'NONE',  ( 20.65312500061451573, 4.541064518000418104, -2.621784821874998173 ) ) ;
#52774=CARTESIAN_POINT ( 'NONE',  ( 12.81562500061451537, -6.054752690667223547, -1.112240025338166033E-15 ) ) ;
#52776=CARTESIAN_POINT ( 'NONE',  ( 10.05937500061451750, 0.000000000000000000, 5.243569643749999010 ) ) ;
#52777=CARTESIAN_POINT ( 'NONE',  ( 25.80000000000000071, 4.330127018922192761, -2.499999999999997780 ) ) ;
#52778=CARTESIAN_POINT ( 'NONE',  ( 22.65000000122903856, -2.886751345948125991, -5.000000000000000000 ) ) ;
#52779=CARTESIAN_POINT ( 'NONE',  ( 17.10000000000000142, -4.330127018922190985, -2.500000000000001332 ) ) ;
#52780=CARTESIAN_POINT ( 'NONE',  ( 12.42187500061451821, -6.054752690667223547, -1.112240025338166033E-15 ) ) ;
#52781=CARTESIAN_POINT ( 'NONE',  ( 26.59687500061451360, 6.054752690667223547, 3.707466751127219781E-16 ) ) ;
#52783=EDGE_CURVE ( 'NONE', #55608, #15201, #8242, .T. ) ;
#52784=DIRECTION ( 'NONE',  ( -0.000000000000000000, -1.000000000000000000, -0.000000000000000000 ) ) ;
#52785=CARTESIAN_POINT ( 'NONE',  ( 20.93437500061451573, -4.541064518000419881, 2.621784821874995952 ) ) ;
#52786=CARTESIAN_POINT ( 'NONE',  ( 12.45937500061451786, -4.541064518000417216, -2.621784821875001281 ) ) ;
#52788=CARTESIAN_POINT ( 'NONE',  ( 24.44999999999999929, 4.330127018922192761, -2.499999999999997780 ) ) ;
#52790=CARTESIAN_POINT ( 'NONE',  ( -4.243569643749999898, 12.65937500061451715, -30.00000000000000000 ) ) ;
#52792=CARTESIAN_POINT ( 'NONE',  ( 13.94062500061451892, 6.054752690667223547, 3.707466751127219781E-16 ) ) ;
#52793=CARTESIAN_POINT ( 'NONE',  ( 5.287500000000000533, -2.886751345948129988, 4.999999999999997335 ) ) ;
#52795=LINE ( 'NONE', #67709, #43238 ) ;
#52796=CARTESIAN_POINT ( 'NONE',  ( 15.59999999999999964, 0.000000000000000000, 4.999999999999998224 ) ) ;
#52797=CARTESIAN_POINT ( 'NONE',  ( 2.000000000000001332, 19.36250000122903359, 33.46410161513774995 ) ) ;
#52798=CARTESIAN_POINT ( 'NONE',  ( 13.68750000122903288, 6.123233995736764310E-16, -4.999999999999998224 ) ) ;
#52799=CARTESIAN_POINT ( 'NONE',  ( 23.97187500061451360, 3.027376345333611329, 5.243569643749999010 ) ) ;
#52800=CARTESIAN_POINT ( 'NONE',  ( 3.422429900546629877, -3.645130117820770455, -3.769356580772429410 ) ) ;
#52802=CARTESIAN_POINT ( 'NONE',  ( 18.66562500061451146, -6.054752690667223547, -1.112240025338166033E-15 ) ) ;
#52803=CARTESIAN_POINT ( 'NONE',  ( 3.740625000614516527, -3.027376345333614438, 5.243569643749998122 ) ) ;
#52804=CARTESIAN_POINT ( 'NONE',  ( 21.12187500061451573, 3.027376345333613106, -5.243569643749998122 ) ) ;
#52805=CARTESIAN_POINT ( 'NONE',  ( 3.862500000000001155, 2.886751345948126879, 4.999999999999999112 ) ) ;
#52806=CARTESIAN_POINT ( 'NONE',  ( 6.365625000614518747, 3.027376345333611329, 5.243569643749999010 ) ) ;
#52807=CARTESIAN_POINT ( 'NONE',  ( 22.52812500061451573, 4.541064518000418104, 2.621784821874999949 ) ) ;
#52808=CARTESIAN_POINT ( 'NONE',  ( 4.243569643749999898, 15.94062500061451537, 32.45002607614398471 ) ) ;
#52809=CARTESIAN_POINT ( 'NONE',  ( 18.26250000122903216, 4.330127018922192761, -2.499999999999997780 ) ) ;
#52811=CARTESIAN_POINT ( 'NONE',  ( 8.990625000614517859, 6.054752690667223547, 3.707466751127219781E-16 ) ) ;
#52812=ADVANCED_FACE ( 'NONE', ( #2241 ), #64282, .F. ) ;
#52813=CARTESIAN_POINT ( 'NONE',  ( 3.684375000614518836, 4.541064518000418104, 2.621784821874999949 ) ) ;
#52814=CARTESIAN_POINT ( 'NONE',  ( 28.67812500061451431, 6.421520780324663323E-16, -5.243569643749999010 ) ) ;
#52815=CARTESIAN_POINT ( 'NONE',  ( 22.28437500061451715, -4.541064518000419881, 2.621784821874995952 ) ) ;
#52816=CARTESIAN_POINT ( 'NONE',  ( 13.86562500061451431, 3.027376345333613106, -5.243569643749998122 ) ) ;
#52817=CARTESIAN_POINT ( 'NONE',  ( 23.96250000122903145, -4.330127018922190985, -2.500000000000001332 ) ) ;
#52818=CARTESIAN_POINT ( 'NONE',  ( 24.59062500061451573, -3.027376345333610441, -5.243569643749999898 ) ) ;
#52819=CARTESIAN_POINT ( 'NONE',  ( 18.94687500061451502, 6.054752690667223547, 3.707466751127219781E-16 ) ) ;
#52820=CARTESIAN_POINT ( 'NONE',  ( 14.54062500061451679, -3.027376345333614438, 5.243569643749998122 ) ) ;
#52821=CARTESIAN_POINT ( 'NONE',  ( 9.001249775931846008E-16, 17.27187500061451786, 34.90005215228797653 ) ) ;
#52822=CARTESIAN_POINT ( 'NONE',  ( 20.27812500061451573, 4.541064518000418104, 2.621784821874999949 ) ) ;
#52824=ORIENTED_EDGE ( 'NONE', *, *, #20472, .T. ) ;
#52825=CARTESIAN_POINT ( 'NONE',  ( 24.44999999999999929, 4.330127018922192761, -2.499999999999997780 ) ) ;
#52826=CARTESIAN_POINT ( 'NONE',  ( -0.6945855716117766976, 10.00052347946771825, -33.93923227085034000 ) ) ;
#52828=CARTESIAN_POINT ( 'NONE',  ( 27.81562500061452070, 3.027376345333613106, -5.243569643749998122 ) ) ;
#52829=CARTESIAN_POINT ( 'NONE',  ( 8.615625000614517859, 3.027376345333611329, 5.243569643749999010 ) ) ;
#52830=CARTESIAN_POINT ( 'NONE',  ( 18.67500000122903714, 2.886751345948129099, -4.999999999999998224 ) ) ;
#52831=ADVANCED_FACE ( 'NONE', ( #47660 ), #19570, .F. ) ;
#52833=CARTESIAN_POINT ( 'NONE',  ( 24.21562500061451573, 3.027376345333613106, -5.243569643749998122 ) ) ;
#52834=CARTESIAN_POINT ( 'NONE',  ( 26.21249999999999858, 2.886751345948129099, -4.999999999999998224 ) ) ;
#52835=CARTESIAN_POINT ( 'NONE',  ( 3.999999999999999112, 15.83750000122903501, -30.00000000000000000 ) ) ;
#52836=CARTESIAN_POINT ( 'NONE',  ( 30.00000000000000000, 6.123233995736764310E-16, -4.999999999999998224 ) ) ;
#52837=CARTESIAN_POINT ( 'NONE',  ( 9.628125000614517148, -4.541064518000419881, 2.621784821874995952 ) ) ;
#52838=ORIENTED_EDGE ( 'NONE', *, *, #3226, .F. ) ;
#52839=CARTESIAN_POINT ( 'NONE',  ( 25.64062500061451644, 6.054752690667223547, 3.707466751127219781E-16 ) ) ;
#52840=CARTESIAN_POINT ( 'NONE',  ( 8.428125000614517859, 6.421520780324663323E-16, -5.243569643749999010 ) ) ;
#52843=CARTESIAN_POINT ( 'NONE',  ( 17.96250000122903501, 0.000000000000000000, 4.999999999999998224 ) ) ;
#52844=CARTESIAN_POINT ( 'NONE',  ( 12.41249999999999964, 2.886751345948126879, 4.999999999999999112 ) ) ;
#52845=CARTESIAN_POINT ( 'NONE',  ( 13.73437500061451821, -4.541064518000419881, 2.621784821874995952 ) ) ;
#52846=CARTESIAN_POINT ( 'NONE',  ( 8.475000001229034297, 2.886751345948126879, 4.999999999999999112 ) ) ;
#52847=CARTESIAN_POINT ( 'NONE',  ( 17.89687500061451431, -3.027376345333610441, -5.243569643749999898 ) ) ;
#52849=CARTESIAN_POINT ( 'NONE',  ( 9.234375000614518214, -4.541064518000419881, 2.621784821874995952 ) ) ;
#52850=CARTESIAN_POINT ( 'NONE',  ( -4.243569643749999898, 12.60312500061451679, -30.00000000000000000 ) ) ;
#52851=CARTESIAN_POINT ( 'NONE',  ( -3.999999999999999112, 11.86249999999999893, -32.30940107675850470 ) ) ;
#52854=CARTESIAN_POINT ( 'NONE',  ( 25.37812500061451715, -4.541064518000419881, 2.621784821874995952 ) ) ;
#52855=CYLINDRICAL_SURFACE ( 'NONE', #40366, 4.000000000000000000 ) ;
#52856=CARTESIAN_POINT ( 'NONE',  ( 25.54687500061451644, -3.027376345333610441, -5.243569643749999898 ) ) ;
#52857=CARTESIAN_POINT ( 'NONE',  ( 29.63437500061451502, 6.421520780324663323E-16, -5.243569643749999010 ) ) ;
#52858=CARTESIAN_POINT ( 'NONE',  ( 22.98749999999999716, -2.886751345948125991, -5.000000000000000000 ) ) ;
#52859=CARTESIAN_POINT ( 'NONE',  ( 6.140625000614516438, -3.027376345333610441, -5.243569643749999898 ) ) ;
#52861=CARTESIAN_POINT ( 'NONE',  ( 15.60937500061451644, -4.541064518000417216, -2.621784821875001281 ) ) ;
#52863=CARTESIAN_POINT ( 'NONE',  ( 3.928125000614516527, 6.421520780324663323E-16, -5.243569643749999010 ) ) ;
#52864=CARTESIAN_POINT ( 'NONE',  ( 9.384375000614518569, 6.421520780324663323E-16, -5.243569643749999010 ) ) ;
#52865=CARTESIAN_POINT ( 'NONE',  ( 17.97187500061451715, 3.027376345333613106, -5.243569643749998122 ) ) ;
#52866=CARTESIAN_POINT ( 'NONE',  ( 21.67500000000000071, 6.123233995736764310E-16, -4.999999999999998224 ) ) ;
#52867=CARTESIAN_POINT ( 'NONE',  ( 27.75000000000000000, 0.000000000000000000, 4.999999999999998224 ) ) ;
#52868=CARTESIAN_POINT ( 'NONE',  ( 27.57187500061451857, 3.027376345333611329, 5.243569643749999010 ) ) ;
#52871=ORIENTED_EDGE ( 'NONE', *, *, #57914, .T. ) ;
#52872=CARTESIAN_POINT ( 'NONE',  ( 11.36250000000000071, 2.886751345948129099, -4.999999999999998224 ) ) ;
#52874=CARTESIAN_POINT ( 'NONE',  ( 21.25312500061451715, 0.000000000000000000, 5.243569643749999010 ) ) ;
#52875=CARTESIAN_POINT ( 'NONE',  ( 11.62500000000000000, -4.330127018922194537, 2.499999999999995559 ) ) ;
#52876=CARTESIAN_POINT ( 'NONE',  ( 9.262500001229033941, 4.330127018922192761, -2.499999999999997780 ) ) ;
#52877=CARTESIAN_POINT ( 'NONE',  ( 6.815625000614517148, 3.027376345333611329, 5.243569643749999010 ) ) ;
#52878=CARTESIAN_POINT ( 'NONE',  ( 21.78750000000000142, 5.773502691896255534, 3.535250795749688894E-16 ) ) ;
#52879=CARTESIAN_POINT ( 'NONE',  ( 20.91562500061451502, -6.054752690667223547, -1.112240025338166033E-15 ) ) ;
#52880=CARTESIAN_POINT ( 'NONE',  ( 12.22499999999999964, 6.123233995736764310E-16, -4.999999999999998224 ) ) ;
#52881=CARTESIAN_POINT ( 'NONE',  ( 26.77500000122903145, 2.886751345948129099, -4.999999999999998224 ) ) ;
#52883=CARTESIAN_POINT ( 'NONE',  ( 5.325000000000000178, -4.330127018922194537, 2.499999999999995559 ) ) ;
#52884=ORIENTED_EDGE ( 'NONE', *, *, #66833, .T. ) ;
#52885=CARTESIAN_POINT ( 'NONE',  ( 19.15312500061451573, -4.541064518000417216, -2.621784821875001281 ) ) ;
#52886=CARTESIAN_POINT ( 'NONE',  ( 27.77812500061451573, 6.421520780324663323E-16, -5.243569643749999010 ) ) ;
#52887=CARTESIAN_POINT ( 'NONE',  ( 28.02187500061451431, 3.027376345333611329, 5.243569643749999010 ) ) ;
#52888=CARTESIAN_POINT ( 'NONE',  ( 14.65312500061451573, -4.541064518000417216, -2.621784821875001281 ) ) ;
#52889=CARTESIAN_POINT ( 'NONE',  ( 3.999999999999998668, 11.26250000000000107, 27.69059892324149530 ) ) ;
#52891=CARTESIAN_POINT ( 'NONE',  ( 7.865625000614516971, -6.054752690667223547, -1.112240025338166033E-15 ) ) ;
#52892=CARTESIAN_POINT ( 'NONE',  ( 4.758977648302459507, 1.540231855627056223, -4.851099530879135813 ) ) ;
#52893=CARTESIAN_POINT ( 'NONE',  ( 26.85000000122903430, 5.773502691896255534, 3.535250795749688894E-16 ) ) ;
#52895=CARTESIAN_POINT ( 'NONE',  ( 17.16562500061451502, 3.027376345333611329, 5.243569643749999010 ) ) ;
#52896=CARTESIAN_POINT ( 'NONE',  ( 29.55937500061451573, -4.541064518000417216, -2.621784821875001281 ) ) ;
#52897=( BOUNDED_CURVE ( )  B_SPLINE_CURVE ( 2, ( #64029, #57757, #29694, #47054, #51869, #30425, #6442 ),
 .UNSPECIFIED., .F., .F. ) 
 B_SPLINE_CURVE_WITH_KNOTS ( ( 3, 2, 2, 3 ),
 ( 0.4083333333333333814, 0.4111111111111111494, 0.4138888888888889173, 0.4166666666666667407 ),
 .UNSPECIFIED. ) 
 CURVE ( )  GEOMETRIC_REPRESENTATION_ITEM ( )  RATIONAL_B_SPLINE_CURVE ( ( 0.9999999999999973355, 0.8660254037844413721, 1.000000000000000000, 0.8660254037844387076, 1.000000000000000000, 0.8660254037844360431, 1.000000000000002665 ) ) 
 REPRESENTATION_ITEM ( '' )  );
#52898=CARTESIAN_POINT ( 'NONE',  ( 10.17187500061451999, -6.054752690667223547, -1.112240025338166033E-15 ) ) ;
#52899=CARTESIAN_POINT ( 'NONE',  ( 10.20937500061451786, -4.541064518000417216, -2.621784821875001281 ) ) ;
#52900=CARTESIAN_POINT ( 'NONE',  ( 18.64687500061451786, -3.027376345333614438, 5.243569643749998122 ) ) ;
#52901=ORIENTED_EDGE ( 'NONE', *, *, #65368, .T. ) ;
#52902=CARTESIAN_POINT ( 'NONE',  ( 29.74687500061451217, 6.054752690667223547, 3.707466751127219781E-16 ) ) ;
#52903=CARTESIAN_POINT ( 'NONE',  ( 21.96562500061451573, 3.027376345333613106, -5.243569643749998122 ) ) ;
#52904=CARTESIAN_POINT ( 'NONE',  ( 17.59687500061451715, 6.054752690667223547, 3.707466751127219781E-16 ) ) ;
#52905=CARTESIAN_POINT ( 'NONE',  ( 21.44062500061452070, -3.027376345333610441, -5.243569643749999898 ) ) ;
#52906=CARTESIAN_POINT ( 'NONE',  ( 2.000000000000001332, 13.40000000000000213, 33.46410161513774995 ) ) ;
#52907=CARTESIAN_POINT ( 'NONE',  ( 3.496875000614518836, -3.027376345333610441, -5.243569643749999898 ) ) ;
#52908=CARTESIAN_POINT ( 'NONE',  ( 8.812500001229034652, 4.330127018922192761, -2.499999999999997780 ) ) ;
#52909=ORIENTED_EDGE ( 'NONE', *, *, #31467, .T. ) ;
#52910=CARTESIAN_POINT ( 'NONE',  ( 5.662500001229035185, 4.330127018922192761, -2.499999999999997780 ) ) ;
#52911=CARTESIAN_POINT ( 'NONE',  ( 3.999999999999999112, 17.07499999999999929, -30.00000000000000000 ) ) ;
#52912=CARTESIAN_POINT ( 'NONE',  ( 24.86250000122903359, -4.330127018922190985, -2.500000000000001332 ) ) ;
#52914=CARTESIAN_POINT ( 'NONE',  ( 7.621875000614519280, 3.027376345333613106, -5.243569643749998122 ) ) ;
#52915=DIRECTION ( 'NONE',  ( -1.000000000000000000, -0.000000000000000000, -0.000000000000000000 ) ) ;
#52916=CARTESIAN_POINT ( 'NONE',  ( 13.94062500061451892, 6.054752690667223547, 3.707466751127219781E-16 ) ) ;
#52917=CARTESIAN_POINT ( 'NONE',  ( 9.796875000614519990, -3.027376345333610441, -5.243569643749999898 ) ) ;
#52918=CARTESIAN_POINT ( 'NONE',  ( 3.665625000614517681, 3.027376345333611329, 5.243569643749999010 ) ) ;
#52919=CARTESIAN_POINT ( 'NONE',  ( 17.44687500061451502, -3.027376345333610441, -5.243569643749999898 ) ) ;
#52920=CARTESIAN_POINT ( 'NONE',  ( 6.571875000614517681, -6.054752690667223547, -1.112240025338166033E-15 ) ) ;
#52921=CARTESIAN_POINT ( 'NONE',  ( 3.999999999999998668, 17.56250000000000000, -32.30940107675850470 ) ) ;
#52922=CARTESIAN_POINT ( 'NONE',  ( 6.815625000614517148, 3.027376345333611329, 5.243569643749999010 ) ) ;
#52923=CARTESIAN_POINT ( 'NONE',  ( 18.62812500061451715, -4.541064518000419881, 2.621784821874995952 ) ) ;
#52924=EDGE_CURVE ( 'NONE', #13105, #4055, #25867, .T. ) ;
#52926=CARTESIAN_POINT ( 'NONE',  ( 14.69062500061451537, -3.027376345333610441, -5.243569643749999898 ) ) ;
#52927=CARTESIAN_POINT ( 'NONE',  ( 10.04062500061451502, -3.027376345333614438, 5.243569643749998122 ) ) ;
#52929=CARTESIAN_POINT ( 'NONE',  ( 11.77500000000000036, 6.123233995736764310E-16, -4.999999999999998224 ) ) ;
#52930=CARTESIAN_POINT ( 'NONE',  ( 6.112500001229034474, 4.330127018922192761, -2.499999999999997780 ) ) ;
#52931=CARTESIAN_POINT ( 'NONE',  ( 14.03437500061451715, 4.541064518000418104, 2.621784821874999949 ) ) ;
#52932=CARTESIAN_POINT ( 'NONE',  ( 16.65000000122903501, -2.886751345948129988, 4.999999999999997335 ) ) ;
#52934=CARTESIAN_POINT ( 'NONE',  ( -4.243569643749999898, 9.921875000614519990, -32.45002607614398471 ) ) ;
#52936=LINE ( 'NONE', #2333, #18350 ) ;
#52938=( BOUNDED_CURVE ( )  B_SPLINE_CURVE ( 2, ( #67266, #5914, #18067, #5560, #61695, #17353, #62424, #39911, #67979 ),
 .UNSPECIFIED., .F., .F. ) 
 B_SPLINE_CURVE_WITH_KNOTS ( ( 3, 2, 2, 2, 3 ),
 ( 0.5543478260869565410, 0.5579710144927536586, 0.5652173913043477826, 0.5724637681159420177, 0.5760869565217391353 ),
 .UNSPECIFIED. ) 
 CURVE ( )  GEOMETRIC_REPRESENTATION_ITEM ( )  RATIONAL_B_SPLINE_CURVE ( ( 0.9330127018922194093, 0.9330127018922194093, 1.000000000000000000, 0.8660254037844387076, 1.000000000000000000, 0.8660254037844387076, 1.000000000000000000, 0.9330127018922194093, 0.9330127018922194093 ) ) 
 REPRESENTATION_ITEM ( '' )  );
#52939=CARTESIAN_POINT ( 'NONE',  ( 30.00000000000000000, 0.000000000000000000, 0.000000000000000000 ) ) ;
#52940=CARTESIAN_POINT ( 'NONE',  ( 18.87187500061451573, 3.027376345333613106, -5.243569643749998122 ) ) ;
#52941=CARTESIAN_POINT ( 'NONE',  ( 29.47499999999999787, 4.330127018922191873, 2.499999999999999556 ) ) ;
#52942=B_SPLINE_CURVE_WITH_KNOTS ( 'NONE', 3,
 ( #60945, #43608, #9620, #48421, #20319, #71685, #66129, #55419, #65395, #4456 ),
 .UNSPECIFIED., .F., .F.,
 ( 4, 3, 3, 4 ),
 ( 1.859757873009560816E-16, 7.861633092733088819E-05, 0.0001572323307352020715, 0.0002910318696070817368 ),
 .UNSPECIFIED. ) ;
#52943=CARTESIAN_POINT ( 'NONE',  ( 14.95312500061451644, 0.000000000000000000, 5.243569643749999010 ) ) ;
#52945=CARTESIAN_POINT ( 'NONE',  ( 23.78437500061451360, 6.421520780324663323E-16, -5.243569643749999010 ) ) ;
#52947=CARTESIAN_POINT ( 'NONE',  ( 8.990625000614516082, 6.054752690667223547, 3.707466751127219781E-16 ) ) ;
#52948=CARTESIAN_POINT ( 'NONE',  ( 15.83437500061451608, 4.541064518000418104, 2.621784821874999949 ) ) ;
#52949=ORIENTED_EDGE ( 'NONE', *, *, #62426, .T. ) ;
#52950=CARTESIAN_POINT ( 'NONE',  ( 25.05937500061451573, -4.541064518000417216, -2.621784821875001281 ) ) ;
#52951=CARTESIAN_POINT ( 'NONE',  ( 27.59062500061451573, -3.027376345333614438, 5.243569643749998122 ) ) ;
#52952=CARTESIAN_POINT ( 'NONE',  ( 16.79062500061451857, -3.027376345333614438, 5.243569643749998122 ) ) ;
#52953=CARTESIAN_POINT ( 'NONE',  ( 29.69062500061451715, 6.054752690667223547, 3.707466751127219781E-16 ) ) ;
#52954=CARTESIAN_POINT ( 'NONE',  ( 30.00000000000000000, 0.000000000000000000, 0.000000000000000000 ) ) ;
#52955=CARTESIAN_POINT ( 'NONE',  ( 8.137500000000002842, -2.886751345948125991, -5.000000000000000000 ) ) ;
#52956=CARTESIAN_POINT ( 'NONE',  ( 19.42500000122903714, -5.773502691896255534, -1.060575238724906372E-15 ) ) ;
#52957=CARTESIAN_POINT ( 'NONE',  ( -3.999999999999997335, 10.13750000000000284, 32.30940107675850470 ) ) ;
#52959=ORIENTED_EDGE ( 'NONE', *, *, #1978, .T. ) ;
#52960=CARTESIAN_POINT ( 'NONE',  ( 18.33749999999999858, -2.886751345948129988, 4.999999999999997335 ) ) ;
#52961=CARTESIAN_POINT ( 'NONE',  ( 18.56250000000000000, 2.886751345948129099, -4.999999999999998224 ) ) ;
#52962=CARTESIAN_POINT ( 'NONE',  ( 19.69687500061451857, -3.027376345333610441, -5.243569643749999898 ) ) ;
#52963=CARTESIAN_POINT ( 'NONE',  ( 13.90312500061451750, 4.541064518000418104, -2.621784821874998173 ) ) ;
#52964=( BOUNDED_CURVE ( )  B_SPLINE_CURVE ( 2, ( #69734, #2146, #17655, #7672, #12850, #52380, #19103 ),
 .UNSPECIFIED., .F., .F. ) 
 B_SPLINE_CURVE_WITH_KNOTS ( ( 3, 2, 2, 3 ),
 ( 0.09166666666666660468, 0.09444444444444442810, 0.09722222222222223764, 0.1000000000000000611 ),
 .UNSPECIFIED. ) 
 CURVE ( )  GEOMETRIC_REPRESENTATION_ITEM ( )  RATIONAL_B_SPLINE_CURVE ( ( 1.000000000000002665, 0.8660254037844360431, 1.000000000000000000, 0.8660254037844387076, 1.000000000000000000, 0.8660254037844360431, 1.000000000000002665 ) ) 
 REPRESENTATION_ITEM ( '' )  );
#52967=CARTESIAN_POINT ( 'NONE',  ( 6.665625000614515905, 3.027376345333613106, -5.243569643749998122 ) ) ;
#52968=CARTESIAN_POINT ( 'NONE',  ( 10.35000000000000142, -4.330127018922190985, -2.500000000000001332 ) ) ;
#52969=CARTESIAN_POINT ( 'NONE',  ( 12.26249999999999929, 2.886751345948129099, -4.999999999999998224 ) ) ;
#52971=CARTESIAN_POINT ( 'NONE',  ( -2.121784821874999949, 16.12812500061451715, 26.32496088578401938 ) ) ;
#52972=CARTESIAN_POINT ( 'NONE',  ( 27.66562500061451146, -6.054752690667223547, -1.112240025338166033E-15 ) ) ;
#52975=CARTESIAN_POINT ( 'NONE',  ( 24.98437500061451644, -4.541064518000419881, 2.621784821874995952 ) ) ;
#52976=ORIENTED_EDGE ( 'NONE', *, *, #36421, .F. ) ;
#52977=CARTESIAN_POINT ( 'NONE',  ( 22.30312500061451431, -4.541064518000417216, -2.621784821875001281 ) ) ;
#52978=CARTESIAN_POINT ( 'NONE',  ( 22.73437500061451644, -4.541064518000419881, 2.621784821874995952 ) ) ;
#52979=CARTESIAN_POINT ( 'NONE',  ( -2.121784821874996840, 15.37812500061459531, -26.32496088578401583 ) ) ;
#52980=CARTESIAN_POINT ( 'NONE',  ( 7.528125000614515727, 6.421520780324663323E-16, -5.243569643749999010 ) ) ;
#52982=CARTESIAN_POINT ( 'NONE',  ( 24.29062500061452212, 6.054752690667223547, 3.707466751127219781E-16 ) ) ;
#52985=CARTESIAN_POINT ( 'NONE',  ( 17.37187500061451573, -6.054752690667223547, -1.112240025338166033E-15 ) ) ;
#52986=CARTESIAN_POINT ( 'NONE',  ( 25.47187500061451715, -6.054752690667223547, -1.112240025338166033E-15 ) ) ;
#52987=CARTESIAN_POINT ( 'NONE',  ( 4.243569643749999010, 14.27187500061451786, 27.54997392385601174 ) ) ;
#52988=CARTESIAN_POINT ( 'NONE',  ( 7.753125000614518036, 0.000000000000000000, 5.243569643749999010 ) ) ;
#52989=CARTESIAN_POINT ( 'NONE',  ( 28.07812500061451289, -4.541064518000419881, 2.621784821874995952 ) ) ;
#52990=CARTESIAN_POINT ( 'NONE',  ( 3.159375000614518036, 4.541064518000418104, -2.621784821874998173 ) ) ;
#52991=CARTESIAN_POINT ( 'NONE',  ( 26.39999999999999858, 0.000000000000000000, 4.999999999999998224 ) ) ;
#52992=( BOUNDED_CURVE ( )  B_SPLINE_CURVE ( 2, ( #3687, #26211, #31388, #64998, #9584, #13651, #43210 ),
 .UNSPECIFIED., .F., .F. ) 
 B_SPLINE_CURVE_WITH_KNOTS ( ( 3, 2, 2, 3 ),
 ( 0.7333333333333332815, 0.7361111111111111605, 0.7388888888888889284, 0.7416666666666666963 ),
 .UNSPECIFIED. ) 
 CURVE ( )  GEOMETRIC_REPRESENTATION_ITEM ( )  RATIONAL_B_SPLINE_CURVE ( ( 1.000000000000000000, 0.8660254037844387076, 1.000000000000000000, 0.8660254037844387076, 1.000000000000000000, 0.8660254037844387076, 1.000000000000000000 ) ) 
 REPRESENTATION_ITEM ( '' )  );
#52993=CARTESIAN_POINT ( 'NONE',  ( 4.415625000614518569, 3.027376345333613106, -5.243569643749998122 ) ) ;
#52994=CARTESIAN_POINT ( 'NONE',  ( 10.28437500061451715, 6.421520780324663323E-16, -5.243569643749999010 ) ) ;
#52995=CARTESIAN_POINT ( 'NONE',  ( 16.57500000122903216, 2.886751345948126879, 4.999999999999999112 ) ) ;
#52996=CARTESIAN_POINT ( 'NONE',  ( 3.496875000614518836, -3.027376345333610441, -5.243569643749999898 ) ) ;
#52997=CARTESIAN_POINT ( 'NONE',  ( 5.090625000614516615, -3.027376345333614438, 5.243569643749998122 ) ) ;
#53000=CARTESIAN_POINT ( 'NONE',  ( 16.77187500061451786, 3.027376345333611329, 5.243569643749999010 ) ) ;
#53001=CARTESIAN_POINT ( 'NONE',  ( 27.67499999999999716, 4.330127018922191873, 2.499999999999999556 ) ) ;
#53003=CARTESIAN_POINT ( 'NONE',  ( 21.92812500061451431, 6.421520780324663323E-16, -5.243569643749999010 ) ) ;
#53004=CARTESIAN_POINT ( 'NONE',  ( 10.19062500061451892, -3.027376345333610441, -5.243569643749999898 ) ) ;
#53005=CARTESIAN_POINT ( 'NONE',  ( 25.80937500061451928, 0.000000000000000000, 5.243569643749999010 ) ) ;
#53006=CARTESIAN_POINT ( 'NONE',  ( 10.60312500061451679, -4.541064518000417216, -2.621784821875001281 ) ) ;
#53008=CARTESIAN_POINT ( 'NONE',  ( 9.375000001229036428, 2.886751345948126879, 4.999999999999999112 ) ) ;
#53009=CARTESIAN_POINT ( 'NONE',  ( 25.04062500061451502, -3.027376345333610441, -5.243569643749999898 ) ) ;
#53010=EDGE_CURVE ( 'NONE', #19466, #10804, #7811, .T. ) ;
#53011=CARTESIAN_POINT ( 'NONE',  ( 4.243569643749999898, 10.57812500061451821, -30.00000000000000000 ) ) ;
#53012=CARTESIAN_POINT ( 'NONE',  ( 11.70000000122903216, -2.886751345948129988, 4.999999999999997335 ) ) ;
#53013=CARTESIAN_POINT ( 'NONE',  ( 22.60312500061451857, 0.000000000000000000, 5.243569643749999010 ) ) ;
#53014=CARTESIAN_POINT ( 'NONE',  ( 18.51562500061451289, 3.027376345333611329, 5.243569643749999010 ) ) ;
#53015=CARTESIAN_POINT ( 'NONE',  ( 5.821875000614519458, 3.027376345333612662, -5.243569643749998122 ) ) ;
#53016=CARTESIAN_POINT ( 'NONE',  ( 17.69999999999999929, 4.330127018922192761, -2.499999999999997780 ) ) ;
#53017=CARTESIAN_POINT ( 'NONE',  ( 13.95000000122903572, -2.886751345948129988, 4.999999999999997335 ) ) ;
#53018=CARTESIAN_POINT ( 'NONE',  ( 11.31562500061451892, 3.027376345333611329, 5.243569643749999010 ) ) ;
#53019=CARTESIAN_POINT ( 'NONE',  ( 14.42812500061451786, 4.541064518000418104, 2.621784821874999949 ) ) ;
#53020=CARTESIAN_POINT ( 'NONE',  ( 24.15000000122903145, 5.773502691896255534, 3.535250795749688894E-16 ) ) ;
#53021=CARTESIAN_POINT ( 'NONE',  ( 22.24687500061451217, -3.027376345333614438, 5.243569643749998122 ) ) ;
#53022=CARTESIAN_POINT ( 'NONE',  ( 21.49687500061451573, -3.027376345333610441, -5.243569643749999898 ) ) ;
#53024=CARTESIAN_POINT ( 'NONE',  ( 7.575000001229033053, 2.886751345948126879, 4.999999999999999112 ) ) ;
#53025=CARTESIAN_POINT ( 'NONE',  ( 6.871875000614517504, 3.027376345333611329, 5.243569643749999010 ) ) ;
#53026=CARTESIAN_POINT ( 'NONE',  ( 25.35937500061451644, 0.000000000000000000, 5.243569643749999010 ) ) ;
#53027=CARTESIAN_POINT ( 'NONE',  ( 5.000000000000000000, 6.123233995736766282E-16, 50.00000000000000000 ) ) ;
#53028=CARTESIAN_POINT ( 'NONE',  ( 20.46562500061451928, -6.054752690667223547, -1.112240025338166033E-15 ) ) ;
#53029=CARTESIAN_POINT ( 'NONE',  ( 25.73437500061451644, 4.541064518000418104, 2.621784821874999949 ) ) ;
#53031=CARTESIAN_POINT ( 'NONE',  ( -0.7368881354385758975, 9.803648613939513368, 25.82089971438751519 ) ) ;
#53032=CARTESIAN_POINT ( 'NONE',  ( 6.046875000614519102, -3.027376345333614438, 5.243569643749998122 ) ) ;
#53033=CARTESIAN_POINT ( 'NONE',  ( 16.64062500061451289, 6.054752690667223547, 3.707466751127219781E-16 ) ) ;
#53034=ORIENTED_EDGE ( 'NONE', *, *, #39683, .T. ) ;
#53036=CARTESIAN_POINT ( 'NONE',  ( 25.45312500061451644, -4.541064518000417216, -2.621784821875001281 ) ) ;
#53037=CARTESIAN_POINT ( 'NONE',  ( 3.459375000614519635, -4.541064518000417216, -2.621784821875001281 ) ) ;
#53039=CARTESIAN_POINT ( 'NONE',  ( 0.000000000000000000, 20.00000000000000000, 30.00000000000000000 ) ) ;
#53040=CARTESIAN_POINT ( 'NONE',  ( 16.98750000000000426, -2.886751345948129988, 4.999999999999997335 ) ) ;
#53041=CARTESIAN_POINT ( 'NONE',  ( 20.09062500061451573, -3.027376345333610441, -5.243569643749999898 ) ) ;
#53042=VERTEX_POINT ( 'NONE', #26232 ) ;
#53043=CARTESIAN_POINT ( 'NONE',  ( 23.77499999999999858, -4.330127018922194537, 2.499999999999995559 ) ) ;
#53044=CARTESIAN_POINT ( 'NONE',  ( 25.13437500061451502, 6.421520780324663323E-16, -5.243569643749999010 ) ) ;
#53047=DIRECTION ( 'NONE',  ( -0.000000000000000000, -1.000000000000000000, -0.000000000000000000 ) ) ;
#53048=CARTESIAN_POINT ( 'NONE',  ( 13.67812500061451786, -4.541064518000419881, 2.621784821874995952 ) ) ;
#53049=CARTESIAN_POINT ( 'NONE',  ( 6.065625000614516260, -6.054752690667223547, -1.112240025338166033E-15 ) ) ;
#53051=CARTESIAN_POINT ( 'NONE',  ( 28.56562500061451715, -6.054752690667223547, -1.112240025338166033E-15 ) ) ;
#53052=CARTESIAN_POINT ( 'NONE',  ( 15.56250000122903465, 4.330127018922192761, -2.499999999999997780 ) ) ;
#53053=CARTESIAN_POINT ( 'NONE',  ( 19.12500000000000000, 4.330127018922191873, 2.499999999999999556 ) ) ;
#53054=CARTESIAN_POINT ( 'NONE',  ( 26.66250000000000142, 2.886751345948129099, -4.999999999999998224 ) ) ;
#53055=CARTESIAN_POINT ( 'NONE',  ( 3.196875000614516793, 6.054752690667223547, 3.707466751127219781E-16 ) ) ;
#53056=CARTESIAN_POINT ( 'NONE',  ( 8.446875000614518569, -3.027376345333610441, -5.243569643749999898 ) ) ;
#53057=CARTESIAN_POINT ( 'NONE',  ( 20.18437500061451573, 6.421520780324663323E-16, -5.243569643749999010 ) ) ;
#53060=CARTESIAN_POINT ( 'NONE',  ( 28.07812500061451289, -4.541064518000419881, 2.621784821874995952 ) ) ;
#53061=CARTESIAN_POINT ( 'NONE',  ( 4.387500000000002842, -2.886751345948129988, 4.999999999999997335 ) ) ;
#53062=CARTESIAN_POINT ( 'NONE',  ( 4.734375000614518214, -4.541064518000419881, 2.621784821874995952 ) ) ;
#53063=CARTESIAN_POINT ( 'NONE',  ( 15.71250000000000213, -5.773502691896255534, -1.060575238724906372E-15 ) ) ;
#53064=CARTESIAN_POINT ( 'NONE',  ( 13.56562500061451892, 3.027376345333611329, 5.243569643749999010 ) ) ;
#53065=LINE ( 'NONE', #13904, #28929 ) ;
#53067=CARTESIAN_POINT ( 'NONE',  ( 18.26250000122903216, 4.330127018922192761, -2.499999999999997780 ) ) ;
#53070=CARTESIAN_POINT ( 'NONE',  ( 8.390625000614518214, -3.027376345333610441, -5.243569643749999898 ) ) ;
#53071=CARTESIAN_POINT ( 'NONE',  ( 24.23437500061451644, 6.421520780324663323E-16, -5.243569643749999010 ) ) ;
#53072=CARTESIAN_POINT ( 'NONE',  ( 19.72500000122903074, 2.886751345948126879, 4.999999999999998224 ) ) ;
#53073=CARTESIAN_POINT ( 'NONE',  ( 23.22187500061451715, -6.054752690667223547, -1.112240025338166033E-15 ) ) ;
#53074=CARTESIAN_POINT ( 'NONE',  ( 6.375000000000001776, 6.123233995736764310E-16, -4.999999999999998224 ) ) ;
#53075=CARTESIAN_POINT ( 'NONE',  ( -2.000000000000000000, 10.13750000122903572, 26.53589838486224650 ) ) ;
#53076=CARTESIAN_POINT ( 'NONE',  ( 13.60312500061451679, 0.000000000000000000, 5.243569643749999010 ) ) ;
#53077=CARTESIAN_POINT ( 'NONE',  ( 7.725000001229034297, -5.773502691896255534, -1.060575238724906372E-15 ) ) ;
#53078=CARTESIAN_POINT ( 'NONE',  ( 8.221875000614518925, 3.027376345333611329, 5.243569643749999010 ) ) ;
#53079=CARTESIAN_POINT ( 'NONE',  ( 3.882888313307707229, -3.150174730667082201, 4.026983590546891811 ) ) ;
#53080=ORIENTED_EDGE ( 'NONE', *, *, #21079, .T. ) ;
#53081=CARTESIAN_POINT ( 'NONE',  ( 13.26562500061451644, -6.054752690667223547, -1.112240025338166033E-15 ) ) ;
#53082=CARTESIAN_POINT ( 'NONE',  ( 3.439498972087754236, -3.629028357702141161, -3.784861396121385724 ) ) ;
#53083=CARTESIAN_POINT ( 'NONE',  ( 22.87500000122903288, 2.886751345948126879, 4.999999999999999112 ) ) ;
#53084=CARTESIAN_POINT ( 'NONE',  ( 9.984375000614518214, 4.541064518000418104, 2.621784821874999949 ) ) ;
#53085=CARTESIAN_POINT ( 'NONE',  ( 15.47812500061451679, -4.541064518000419881, 2.621784821874995952 ) ) ;
#53086=EDGE_CURVE ( 'NONE', #66635, #13629, #60539, .T. ) ;
#53088=CARTESIAN_POINT ( 'NONE',  ( 23.89687500061451786, 6.054752690667223547, 3.707466751127219781E-16 ) ) ;
#53089=DIRECTION ( 'NONE',  ( 0.000000000000000000, 0.000000000000000000, -1.000000000000000000 ) ) ;
#53090=CARTESIAN_POINT ( 'NONE',  ( 19.20000000000000284, 0.000000000000000000, 4.999999999999998224 ) ) ;
#53091=CARTESIAN_POINT ( 'NONE',  ( -4.243569643749998122, 14.49687500061451750, -27.54997392385601174 ) ) ;
#53092=CARTESIAN_POINT ( 'NONE',  ( 15.83437500061451608, 4.541064518000418104, 2.621784821874999949 ) ) ;
#53093=CARTESIAN_POINT ( 'NONE',  ( 17.70000000122903216, -2.886751345948125991, -5.000000000000000000 ) ) ;
#53094=CARTESIAN_POINT ( 'NONE',  ( 11.85937500061451644, 0.000000000000000000, 5.243569643749999010 ) ) ;
#53095=CARTESIAN_POINT ( 'NONE',  ( -2.121784821874996840, 17.62812500061451715, -26.32496088578401583 ) ) ;
#53096=CARTESIAN_POINT ( 'NONE',  ( 18.82500000122903216, 2.886751345948126879, 4.999999999999999112 ) ) ;
#53097=CARTESIAN_POINT ( 'NONE',  ( 12.47812500061451502, 6.421520780324663323E-16, -5.243569643749999010 ) ) ;
#53098=ORIENTED_EDGE ( 'NONE', *, *, #47219, .T. ) ;
#53099=ORIENTED_EDGE ( 'NONE', *, *, #25113, .T. ) ;
#53100=CARTESIAN_POINT ( 'NONE',  ( 18.78749999999999432, -2.886751345948129988, 4.999999999999997335 ) ) ;
#53101=CARTESIAN_POINT ( 'NONE',  ( -5.000000000000000000, 0.000000000000000000, 50.00000000000000000 ) ) ;
#53102=CARTESIAN_POINT ( 'NONE',  ( 13.47187500061451537, 3.027376345333612662, -5.243569643749998122 ) ) ;
#53103=CARTESIAN_POINT ( 'NONE',  ( 22.57499999999999929, 6.123233995736764310E-16, -4.999999999999998224 ) ) ;
#53104=CARTESIAN_POINT ( 'NONE',  ( 13.61250000122903359, -4.330127018922190985, -2.500000000000001332 ) ) ;
#53105=CARTESIAN_POINT ( 'NONE',  ( 21.26250000122903572, -4.330127018922190985, -2.500000000000001332 ) ) ;
#53106=CARTESIAN_POINT ( 'NONE',  ( 16.49062500061451786, -3.027376345333610441, -5.243569643749999898 ) ) ;
#53107=CARTESIAN_POINT ( 'NONE',  ( 20.76562500061451644, 3.027376345333611329, 5.243569643749999010 ) ) ;
#53108=CARTESIAN_POINT ( 'NONE',  ( 27.11250000122903359, -4.330127018922190985, -2.500000000000001332 ) ) ;
#53109=CARTESIAN_POINT ( 'NONE',  ( 28.31250000000000000, -5.773502691896255534, -1.060575238724906372E-15 ) ) ;
#53112=CARTESIAN_POINT ( 'NONE',  ( 27.08437500061451786, 4.541064518000418104, 2.621784821874999949 ) ) ;
#53114=CARTESIAN_POINT ( 'NONE',  ( -4.243569643749999898, 16.25937500061451857, -30.00000000000000000 ) ) ;
#53115=CARTESIAN_POINT ( 'NONE',  ( 4.500000001229034652, -2.886751345948129988, 4.999999999999997335 ) ) ;
#53116=CARTESIAN_POINT ( 'NONE',  ( 6.187500000000002665, -2.886751345948129988, 4.999999999999997335 ) ) ;
#53117=( BOUNDED_SURFACE ( )  B_SPLINE_SURFACE ( 1, 2, ( 
 ( #27485, #61091, #26382, #15648, #26015, #15286, #65165, #48923, #4952, #43382, #71081, #71454, #37465, #60713, #37091, #32656, #49289, #59615, #70710, #65537, #20455, #26757, #55556, #3497, #32288, #48554, #20084, #66642, #16019, #38567, #14923, #55197, #4591, #10490, #43008, #27120, #9029, #49654, #54822, #59984, #72182, #21561, #33017, #9395, #44115, #31560, #42641, #4230, #60345, #37826, #31925, #20828, #71822, #21194, #43745, #39665, #45200, #57352, #68453, #5312, #68099, #33381, #40024, #33742, #50742, #23009, #55917, #11216, #16743, #27854, #16380, #56637, #17105, #22651, #56988, #72543, #62184, #67019, #45568, #38935, #67731, #34824, #6757, #61813, #11935, #62538, #50019, #145, #34097, #61453, #44845, #10847, #6033, #50386, #56287, #11581, #28567, #72911, #5677, #22293, #21931, #28926, #12289, #44486, #51463, #34460, #28213, #51103, #499, #17465, #67381, #39298, #6394, #866, #23373, #45921, #62895, #17815, #40376, #35187, #7117, #53266, #63981, #7840, #14099, #8205, #29646, #12652, #2664, #24095, #52184, #18544, #47366, #41817, #1586, #52545, #13009, #59161, #19634, #58066, #24819, #57712, #24459, #23730, #35547, #36639, #1952, #46643, #30002, #69184, #69897, #46279, #19263, #30377, #68819, #29291, #41109, #63619, #58429, #51821, #7476, #41462, #47007, #1224, #25181, #47724, #70263, #64348, #13739, #63260, #40744, #13363, #69542, #18901, #36281, #35904, #52906, #58795, #2304, #30734, #42191, #18175, #64715, #65816, #25560, #37376, #71362, #48832, #20737, #44027, #8569, #43295, #15560, #38103, #60625, #14470, #14835, #55108, #4139, #26670, #31839, #48469, #66549, #65079, #21474, #70624, #70993, #19999, #37004, #42552, #60256, #25929, #4508, #15198, #49203, #37736, #59900, #3770, #9305, #10035, #59526, #31097, #9670, #8939, #32203, #53636, #54375, #66182, #48101, #31470, #71737, #21107, #54737, #26295, #27037, #3029, #72090, #49568, #54013, #43660, #32570, #15928, #38478, #20369, #3409, #42920, #65443, #51014, #11491, #67649, #11850, #45476, #44762, #45114, #50303, #61002, #777, #4863, #33653, #17015, #33296, #72825, #5221, #55834, #39213, #50656, #5944, #5591, #62097 ),
 ( #49929, #72454, #34369, #17732, #68009, #27399, #410, #56902, #22919, #28477, #45834, #67297, #28128, #62452, #56550, #38851, #39573, #60, #23285, #10401, #22566, #17381, #39939, #6307, #66928, #16655, #28835, #51374, #68371, #11126, #27763, #32933, #44402, #55471, #21838, #22208, #16297, #61366, #10763, #34013, #61725, #56198, #24373, #58342, #40653, #1867, #70174, #25097, #57262, #7392, #41023, #18459, #53181, #35459, #51738, #46193, #18092, #64261, #46921, #18817, #47641, #19180, #63173, #23648, #13648, #35102, #12568, #29561, #7752, #52821, #57627, #63539, #24008, #40291, #30649, #69097, #35820, #68734, #57982, #34733, #46556, #62813, #12925, #7031, #29920, #52098, #30289, #6675, #2223, #41380, #29203, #12205, #1503, #52460, #69459, #1138, #63891, #13281, #24736, #47280, #36192, #58710, #8121, #69814, #41733, #2578, #15472, #42473, #60173, #31014, #4052, #54292, #9218, #65358, #19919, #32114, #64996, #4421, #36556, #31755, #14748, #26950, #38016, #48018, #37650, #2943, #9582, #3320, #20282, #65727, #25472, #53925, #59442, #70544, #59076, #26209, #59813, #37290, #26578, #42108, #3685, #8480, #15113, #53547, #48748, #49476, #71272, #14386, #42836, #8849, #54648, #36921, #49118, #20650, #31385, #19551, #25846, #48383, #43207, #64631, #70910, #71646, #21019, #14017, #60538, #9945, #32483, #43572, #66093, #55016, #67922, #21748, #39482, #10313, #56467, #33562, #61635, #44676, #72368, #11406, #44309, #56814, #15840, #11037, #67207, #6221, #17294, #27310, #16928, #55382, #62005, #55743, #72734, #45028, #4776, #33204, #38762, #49843, #38386, #5501, #39120, #16568, #5858, #21383, #56111, #60909, #67563, #32845, #28040, #28749, #72008, #10674, #33925, #28390, #43939, #22121, #50569, #66838, #16209, #61281, #73096, #5137, #27672, #22478, #50928, #50210, #325, #22834, #66463, #45386, #34282, #39856, #62368, #11766, #6948, #41652, #51654, #12844, #8034, #36106, #68288, #18375, #52017, #29480, #64173, #46474, #62730, #57177, #29120, #2140, #35377, #29839, #58627, #30204, #1056, #34649, #24651, #46111, #23566, #40569, #69379, #63808, #68648, #1418, #35017, #51289, #13561, #23924, #46839 ) ),
 .UNSPECIFIED., .F., .F., .F. ) 
 B_SPLINE_SURFACE_WITH_KNOTS ( ( 2, 2 ),
 ( 3, 2, 2, 2, 2, 2, 2, 2, 2, 2, 2, 2, 2, 2, 2, 2, 2, 2, 2, 2, 2, 2, 2, 2, 2, 2, 2, 2, 2, 2, 2, 2, 2, 2, 2, 2, 2, 2, 2, 2, 2, 2, 2, 2, 2, 2, 2, 2, 2, 2, 2, 2, 2, 2, 2, 2, 2, 2, 2, 2, 2, 2, 2, 2, 2, 2, 2, 2, 2, 2, 2, 2, 2, 2, 2, 2, 2, 2, 2, 2, 2, 2, 2, 2, 2, 2, 2, 2, 2, 2, 2, 2, 2, 2, 2, 2, 2, 2, 2, 2, 2, 2, 2, 2, 2, 2, 2, 2, 2, 2, 2, 2, 2, 2, 2, 2, 2, 2, 2, 2, 2, 2, 2, 2, 2, 2, 2, 2, 2, 2, 2, 2, 2, 2, 3 ),
 ( 0.000000000000000000, 1.000000000000000000 ),
 ( 0.000000000000000000, 0.007246376811594202987, 0.01449275362318840597, 0.02173913043478260809, 0.02898550724637681195, 0.03623188405797101580, 0.04347826086956521618, 0.05072463768115942351, 0.05797101449275362389, 0.06521739130434782428, 0.07246376811594203160, 0.07971014492753622505, 0.08695652173913043237, 0.09420289855072463969, 0.1014492753623188470, 0.1086956521739130405, 0.1159420289855072478, 0.1231884057971014551, 0.1304347826086956486, 0.1376811594202898559, 0.1449275362318840632, 0.1521739130434782705, 0.1594202898550724501, 0.1666666666666666574, 0.1739130434782608647, 0.1811594202898550721, 0.1884057971014492794, 0.1956521739130434867, 0.2028985507246376940, 0.2101449275362318736, 0.2173913043478260809, 0.2246376811594202882, 0.2318840579710144956, 0.2391304347826087029, 0.2463768115942029102, 0.2536231884057971175, 0.2608695652173912971, 0.2681159420289855322, 0.2753623188405797118, 0.2826086956521738913, 0.2898550724637681264, 0.2971014492753623060, 0.3043478260869565410, 0.3115942028985507206, 0.3188405797101449002, 0.3260869565217391353, 0.3333333333333333148, 0.3405797101449275499, 0.3478260869565217295, 0.3550724637681159646, 0.3623188405797101441, 0.3695652173913043237, 0.3768115942028985588, 0.3840579710144927383, 0.3913043478260869734, 0.3985507246376811530, 0.4057971014492753881, 0.4130434782608695676, 0.4202898550724637472, 0.4275362318840579823, 0.4347826086956521618, 0.4420289855072463969, 0.4492753623188405765, 0.4565217391304347561, 0.4637681159420289911, 0.4710144927536231707, 0.4782608695652174058, 0.4855072463768115854, 0.4927536231884058204, 0.5000000000000000000, 0.5072463768115942351, 0.5144927536231883591, 0.5217391304347825942, 0.5289855072463768293, 0.5362318840579710644, 0.5434782608695651884, 0.5507246376811594235, 0.5579710144927536586, 0.5652173913043477826, 0.5724637681159420177, 0.5797101449275362528, 0.5869565217391304879, 0.5942028985507246119, 0.6014492753623188470, 0.6086956521739130821, 0.6159420289855072062, 0.6231884057971014412, 0.6304347826086956763, 0.6376811594202898004, 0.6449275362318840354, 0.6521739130434782705, 0.6594202898550725056, 0.6666666666666666297, 0.6739130434782608647, 0.6811594202898550998, 0.6884057971014492239, 0.6956521739130434590, 0.7028985507246376940, 0.7101449275362319291, 0.7173913043478260532, 0.7246376811594202882, 0.7318840579710145233, 0.7391304347826086474, 0.7463768115942028825, 0.7536231884057971175, 0.7608695652173913526, 0.7681159420289854767, 0.7753623188405797118, 0.7826086956521739468, 0.7898550724637680709, 0.7971014492753623060, 0.8043478260869565410, 0.8115942028985507761, 0.8188405797101449002, 0.8260869565217391353, 0.8333333333333333703, 0.8405797101449274944, 0.8478260869565217295, 0.8550724637681159646, 0.8623188405797101996, 0.8695652173913043237, 0.8768115942028985588, 0.8840579710144927938, 0.8913043478260869179, 0.8985507246376811530, 0.9057971014492753881, 0.9130434782608695121, 0.9202898550724637472, 0.9275362318840579823, 0.9347826086956522174, 0.9420289855072463414, 0.9492753623188405765, 0.9565217391304348116, 0.9637681159420289356, 0.9662083017040261623 ),
 .UNSPECIFIED. ) 
 GEOMETRIC_REPRESENTATION_ITEM ( )  RATIONAL_B_SPLINE_SURFACE ( (
 ( 1.000000000000000000, 0.8660254037844387076, 1.000000000000000000, 0.8660254037844387076, 1.000000000000000000, 0.8660254037844387076, 1.000000000000000000, 0.8660254037844387076, 1.000000000000000000, 0.8660254037844387076, 1.000000000000000000, 0.8660254037844387076, 1.000000000000000000, 0.8660254037844387076, 1.000000000000000000, 0.8660254037844387076, 1.000000000000000000, 0.8660254037844387076, 1.000000000000000000, 0.8660254037844387076, 1.000000000000000000, 0.8660254037844387076, 1.000000000000000000, 0.8660254037844387076, 1.000000000000000000, 0.8660254037844387076, 1.000000000000000000, 0.8660254037844387076, 1.000000000000000000, 0.8660254037844387076, 1.000000000000000000, 0.8660254037844387076, 1.000000000000000000, 0.8660254037844387076, 1.000000000000000000, 0.8660254037844387076, 1.000000000000000000, 0.8660254037844387076, 1.000000000000000000, 0.8660254037844387076, 1.000000000000000000, 0.8660254037844387076, 1.000000000000000000, 0.8660254037844387076, 1.000000000000000000, 0.8660254037844387076, 1.000000000000000000, 0.8660254037844387076, 1.000000000000000000, 0.8660254037844387076, 1.000000000000000000, 0.8660254037844387076, 1.000000000000000000, 0.8660254037844387076, 1.000000000000000000, 0.8660254037844387076, 1.000000000000000000, 0.8660254037844387076, 1.000000000000000000, 0.8660254037844387076, 1.000000000000000000, 0.8660254037844387076, 1.000000000000000000, 0.8660254037844387076, 1.000000000000000000, 0.8660254037844387076, 1.000000000000000000, 0.8660254037844387076, 1.000000000000000000, 0.8660254037844387076, 1.000000000000000000, 0.8660254037844387076, 1.000000000000000000, 0.8660254037844387076, 1.000000000000000000, 0.8660254037844387076, 1.000000000000000000, 0.8660254037844387076, 1.000000000000000000, 0.8660254037844387076, 1.000000000000000000, 0.8660254037844387076, 1.000000000000000000, 0.8660254037844387076, 1.000000000000000000, 0.8660254037844387076, 1.000000000000000000, 0.8660254037844387076, 1.000000000000000000, 0.8660254037844387076, 1.000000000000000000, 0.8660254037844387076, 1.000000000000000000, 0.8660254037844387076, 1.000000000000000000, 0.8660254037844387076, 1.000000000000000000, 0.8660254037844387076, 1.000000000000000000, 0.8660254037844387076, 1.000000000000000000, 0.8660254037844387076, 1.000000000000000000, 0.8660254037844387076, 1.000000000000000000, 0.8660254037844387076, 1.000000000000000000, 0.8660254037844387076, 1.000000000000000000, 0.8660254037844387076, 1.000000000000000000, 0.8660254037844387076, 1.000000000000000000, 0.8660254037844387076, 1.000000000000000000, 0.8660254037844387076, 1.000000000000000000, 0.8660254037844387076, 1.000000000000000000, 0.8660254037844387076, 1.000000000000000000, 0.8660254037844387076, 1.000000000000000000, 0.8660254037844387076, 1.000000000000000000, 0.8660254037844387076, 1.000000000000000000, 0.8660254037844387076, 1.000000000000000000, 0.8660254037844387076, 1.000000000000000000, 0.8660254037844387076, 1.000000000000000000, 0.8660254037844387076, 1.000000000000000000, 0.8660254037844387076, 1.000000000000000000, 0.8660254037844387076, 1.000000000000000000, 0.8660254037844387076, 1.000000000000000000, 0.8660254037844387076, 1.000000000000000000, 0.8660254037844387076, 1.000000000000000000, 0.8660254037844387076, 1.000000000000000000, 0.8660254037844387076, 1.000000000000000000, 0.8660254037844387076, 1.000000000000000000, 0.8660254037844387076, 1.000000000000000000, 0.8660254037844387076, 1.000000000000000000, 0.8660254037844387076, 1.000000000000000000, 0.8660254037844387076, 1.000000000000000000, 0.8660254037844387076, 1.000000000000000000, 0.8660254037844387076, 1.000000000000000000, 0.8660254037844387076, 1.000000000000000000, 0.8660254037844387076, 1.000000000000000000, 0.8660254037844387076, 1.000000000000000000, 0.8660254037844387076, 1.000000000000000000, 0.8660254037844387076, 1.000000000000000000, 0.8660254037844387076, 1.000000000000000000, 0.8660254037844387076, 1.000000000000000000, 0.8660254037844387076, 1.000000000000000000, 0.8660254037844387076, 1.000000000000000000, 0.8660254037844387076, 1.000000000000000000, 0.8660254037844387076, 1.000000000000000000, 0.8660254037844387076, 1.000000000000000000, 0.8660254037844387076, 1.000000000000000000, 0.8660254037844387076, 1.000000000000000000, 0.8660254037844387076, 1.000000000000000000, 0.8660254037844387076, 1.000000000000000000, 0.8660254037844387076, 1.000000000000000000, 0.8660254037844387076, 1.000000000000000000, 0.8660254037844387076, 1.000000000000000000, 0.8660254037844387076, 1.000000000000000000, 0.8660254037844387076, 1.000000000000000000, 0.8660254037844387076, 1.000000000000000000, 0.8660254037844387076, 1.000000000000000000, 0.8660254037844387076, 1.000000000000000000, 0.8660254037844387076, 1.000000000000000000, 0.8660254037844387076, 1.000000000000000000, 0.8660254037844387076, 1.000000000000000000, 0.8660254037844387076, 1.000000000000000000, 0.8660254037844387076, 1.000000000000000000, 0.8660254037844387076, 1.000000000000000000, 0.8660254037844387076, 1.000000000000000000, 0.8660254037844387076, 1.000000000000000000, 0.8660254037844387076, 1.000000000000000000, 0.8660254037844387076, 1.000000000000000000, 0.8660254037844387076, 1.000000000000000000, 0.8660254037844387076, 1.000000000000000000, 0.8660254037844387076, 1.000000000000000000, 0.8660254037844387076, 1.000000000000000000, 0.8660254037844387076, 1.000000000000000000, 0.8660254037844387076, 1.000000000000000000, 0.8660254037844387076, 1.000000000000000000, 0.8660254037844387076, 1.000000000000000000, 0.8660254037844387076, 1.000000000000000000, 0.8660254037844387076, 1.000000000000000000, 0.8660254037844387076, 1.000000000000000000, 0.8660254037844387076, 1.000000000000000000, 0.8660254037844387076, 1.000000000000000000, 0.8660254037844387076, 1.000000000000000000, 0.8660254037844387076, 1.000000000000000000, 0.8660254037844387076, 1.000000000000000000, 0.8660254037844387076, 1.000000000000000000, 0.8660254037844387076, 1.000000000000000000, 0.9548846395026737710, 0.9401540804572410259),
 ( 1.000000000000000000, 0.8660254037844387076, 1.000000000000000000, 0.8660254037844387076, 1.000000000000000000, 0.8660254037844387076, 1.000000000000000000, 0.8660254037844387076, 1.000000000000000000, 0.8660254037844387076, 1.000000000000000000, 0.8660254037844387076, 1.000000000000000000, 0.8660254037844387076, 1.000000000000000000, 0.8660254037844387076, 1.000000000000000000, 0.8660254037844387076, 1.000000000000000000, 0.8660254037844387076, 1.000000000000000000, 0.8660254037844387076, 1.000000000000000000, 0.8660254037844387076, 1.000000000000000000, 0.8660254037844387076, 1.000000000000000000, 0.8660254037844387076, 1.000000000000000000, 0.8660254037844387076, 1.000000000000000000, 0.8660254037844387076, 1.000000000000000000, 0.8660254037844387076, 1.000000000000000000, 0.8660254037844387076, 1.000000000000000000, 0.8660254037844387076, 1.000000000000000000, 0.8660254037844387076, 1.000000000000000000, 0.8660254037844387076, 1.000000000000000000, 0.8660254037844387076, 1.000000000000000000, 0.8660254037844387076, 1.000000000000000000, 0.8660254037844387076, 1.000000000000000000, 0.8660254037844387076, 1.000000000000000000, 0.8660254037844387076, 1.000000000000000000, 0.8660254037844387076, 1.000000000000000000, 0.8660254037844387076, 1.000000000000000000, 0.8660254037844387076, 1.000000000000000000, 0.8660254037844387076, 1.000000000000000000, 0.8660254037844387076, 1.000000000000000000, 0.8660254037844387076, 1.000000000000000000, 0.8660254037844387076, 1.000000000000000000, 0.8660254037844387076, 1.000000000000000000, 0.8660254037844387076, 1.000000000000000000, 0.8660254037844387076, 1.000000000000000000, 0.8660254037844387076, 1.000000000000000000, 0.8660254037844387076, 1.000000000000000000, 0.8660254037844387076, 1.000000000000000000, 0.8660254037844387076, 1.000000000000000000, 0.8660254037844387076, 1.000000000000000000, 0.8660254037844387076, 1.000000000000000000, 0.8660254037844387076, 1.000000000000000000, 0.8660254037844387076, 1.000000000000000000, 0.8660254037844387076, 1.000000000000000000, 0.8660254037844387076, 1.000000000000000000, 0.8660254037844387076, 1.000000000000000000, 0.8660254037844387076, 1.000000000000000000, 0.8660254037844387076, 1.000000000000000000, 0.8660254037844387076, 1.000000000000000000, 0.8660254037844387076, 1.000000000000000000, 0.8660254037844387076, 1.000000000000000000, 0.8660254037844387076, 1.000000000000000000, 0.8660254037844387076, 1.000000000000000000, 0.8660254037844387076, 1.000000000000000000, 0.8660254037844387076, 1.000000000000000000, 0.8660254037844387076, 1.000000000000000000, 0.8660254037844387076, 1.000000000000000000, 0.8660254037844387076, 1.000000000000000000, 0.8660254037844387076, 1.000000000000000000, 0.8660254037844387076, 1.000000000000000000, 0.8660254037844387076, 1.000000000000000000, 0.8660254037844387076, 1.000000000000000000, 0.8660254037844387076, 1.000000000000000000, 0.8660254037844387076, 1.000000000000000000, 0.8660254037844387076, 1.000000000000000000, 0.8660254037844387076, 1.000000000000000000, 0.8660254037844387076, 1.000000000000000000, 0.8660254037844387076, 1.000000000000000000, 0.8660254037844387076, 1.000000000000000000, 0.8660254037844387076, 1.000000000000000000, 0.8660254037844387076, 1.000000000000000000, 0.8660254037844387076, 1.000000000000000000, 0.8660254037844387076, 1.000000000000000000, 0.8660254037844387076, 1.000000000000000000, 0.8660254037844387076, 1.000000000000000000, 0.8660254037844387076, 1.000000000000000000, 0.8660254037844387076, 1.000000000000000000, 0.8660254037844387076, 1.000000000000000000, 0.8660254037844387076, 1.000000000000000000, 0.8660254037844387076, 1.000000000000000000, 0.8660254037844387076, 1.000000000000000000, 0.8660254037844387076, 1.000000000000000000, 0.8660254037844387076, 1.000000000000000000, 0.8660254037844387076, 1.000000000000000000, 0.8660254037844387076, 1.000000000000000000, 0.8660254037844387076, 1.000000000000000000, 0.8660254037844387076, 1.000000000000000000, 0.8660254037844387076, 1.000000000000000000, 0.8660254037844387076, 1.000000000000000000, 0.8660254037844387076, 1.000000000000000000, 0.8660254037844387076, 1.000000000000000000, 0.8660254037844387076, 1.000000000000000000, 0.8660254037844387076, 1.000000000000000000, 0.8660254037844387076, 1.000000000000000000, 0.8660254037844387076, 1.000000000000000000, 0.8660254037844387076, 1.000000000000000000, 0.8660254037844387076, 1.000000000000000000, 0.8660254037844387076, 1.000000000000000000, 0.8660254037844387076, 1.000000000000000000, 0.8660254037844387076, 1.000000000000000000, 0.8660254037844387076, 1.000000000000000000, 0.8660254037844387076, 1.000000000000000000, 0.8660254037844387076, 1.000000000000000000, 0.8660254037844387076, 1.000000000000000000, 0.8660254037844387076, 1.000000000000000000, 0.8660254037844387076, 1.000000000000000000, 0.8660254037844387076, 1.000000000000000000, 0.8660254037844387076, 1.000000000000000000, 0.8660254037844387076, 1.000000000000000000, 0.8660254037844387076, 1.000000000000000000, 0.8660254037844387076, 1.000000000000000000, 0.8660254037844387076, 1.000000000000000000, 0.8660254037844387076, 1.000000000000000000, 0.8660254037844387076, 1.000000000000000000, 0.8660254037844387076, 1.000000000000000000, 0.8660254037844387076, 1.000000000000000000, 0.8660254037844387076, 1.000000000000000000, 0.8660254037844387076, 1.000000000000000000, 0.8660254037844387076, 1.000000000000000000, 0.8660254037844387076, 1.000000000000000000, 0.8660254037844387076, 1.000000000000000000, 0.8660254037844387076, 1.000000000000000000, 0.8660254037844387076, 1.000000000000000000, 0.8660254037844387076, 1.000000000000000000, 0.8660254037844387076, 1.000000000000000000, 0.8660254037844387076, 1.000000000000000000, 0.8660254037844387076, 1.000000000000000000, 0.8660254037844387076, 1.000000000000000000, 0.8660254037844387076, 1.000000000000000000, 0.8660254037844387076, 1.000000000000000000, 0.8660254037844387076, 1.000000000000000000, 0.8660254037844387076, 1.000000000000000000, 0.9548846395026737710, 0.9401540804572410259) ) ) 
 REPRESENTATION_ITEM ( '' )  SURFACE ( )  );
#53119=CARTESIAN_POINT ( 'NONE',  ( 9.309375000614517504, -4.541064518000417216, -2.621784821875001281 ) ) ;
#53120=CARTESIAN_POINT ( 'NONE',  ( 27.59062500061451573, -3.027376345333614438, 5.243569643749998122 ) ) ;
#53122=CARTESIAN_POINT ( 'NONE',  ( -2.698377630233219193, 9.636255672932172445, -35.37338662132845712 ) ) ;
#53124=CARTESIAN_POINT ( 'NONE',  ( 6.759375000614516793, 4.541064518000418104, -2.621784821874998173 ) ) ;
#53125=CARTESIAN_POINT ( 'NONE',  ( 11.67187500061451821, 3.027376345333613106, -5.243569643749998122 ) ) ;
#53126=CARTESIAN_POINT ( 'NONE',  ( 3.937500000000000444, -2.886751345948129988, 4.999999999999997335 ) ) ;
#53127=CARTESIAN_POINT ( 'NONE',  ( 9.001249775931846008E-16, 14.06562500061459886, 34.90005215228797653 ) ) ;
#53128=CARTESIAN_POINT ( 'NONE',  ( 1.592000809091587073E-14, 16.73750000000000071, -34.00000000000000000 ) ) ;
#53129=CARTESIAN_POINT ( 'NONE',  ( 5.962500000000002132, 2.886751345948129099, -4.999999999999998224 ) ) ;
#53132=CARTESIAN_POINT ( 'NONE',  ( 20.05312500061451431, -4.541064518000417216, -2.621784821875001281 ) ) ;
#53133=CARTESIAN_POINT ( 'NONE',  ( 13.56562500061451892, 3.027376345333611329, 5.243569643749999010 ) ) ;
#53135=CARTESIAN_POINT ( 'NONE',  ( 9.909375000614517148, 4.541064518000418104, -2.621784821874998173 ) ) ;
#53136=CARTESIAN_POINT ( 'NONE',  ( 25.38749999999999929, 5.773502691896255534, 3.535250795749688894E-16 ) ) ;
#53137=CARTESIAN_POINT ( 'NONE',  ( 22.42500000122903359, 2.886751345948126879, 4.999999999999999112 ) ) ;
#53139=CARTESIAN_POINT ( 'NONE',  ( 9.121875000614517504, 3.027376345333611329, 5.243569643749999010 ) ) ;
#53140=CARTESIAN_POINT ( 'NONE',  ( 27.75937500061451502, -4.541064518000417216, -2.621784821875001281 ) ) ;
#53141=EDGE_CURVE ( 'NONE', #41179, #22787, #43652, .T. ) ;
#53142=DIRECTION ( 'NONE',  ( -1.000000000000000000, -0.000000000000000000, -0.000000000000000000 ) ) ;
#53143=LINE ( 'NONE', #69423, #34860 ) ;
#53144=CARTESIAN_POINT ( 'NONE',  ( 19.35937500061451644, 4.541064518000418104, -2.621784821874998173 ) ) ;
#53145=CARTESIAN_POINT ( 'NONE',  ( 10.92187500061451644, 3.027376345333611329, 5.243569643749999010 ) ) ;
#53147=CARTESIAN_POINT ( 'NONE',  ( 22.31250000000000000, 2.886751345948126879, 4.999999999999999112 ) ) ;
#53149=CARTESIAN_POINT ( 'NONE',  ( 9.001249775931846008E-16, 13.22187500061451715, -25.09994784771203058 ) ) ;
#53151=CARTESIAN_POINT ( 'NONE',  ( 14.80312500061451608, 4.541064518000418104, -2.621784821874998173 ) ) ;
#53152=CARTESIAN_POINT ( 'NONE',  ( 4.425000000000001599, -4.330127018922194537, 2.499999999999995559 ) ) ;
#53153=ADVANCED_FACE ( 'NONE', ( #60560 ), #15791, .T. ) ;
#53156=CARTESIAN_POINT ( 'NONE',  ( 13.61250000000000071, 2.886751345948129099, -4.999999999999998224 ) ) ;
#53157=CARTESIAN_POINT ( 'NONE',  ( 4.243569643749999898, 10.54062500061451679, 32.45002607614398471 ) ) ;
#53158=CARTESIAN_POINT ( 'NONE',  ( 14.73750000122903359, 4.330127018922191873, 2.499999999999999556 ) ) ;
#53159=CARTESIAN_POINT ( 'NONE',  ( 24.90937500061451715, 0.000000000000000000, 5.243569643749999010 ) ) ;
#53161=ORIENTED_EDGE ( 'NONE', *, *, #61105, .T. ) ;
#53162=CARTESIAN_POINT ( 'NONE',  ( 18.85312500061451502, 4.541064518000418104, -2.621784821874998173 ) ) ;
#53163=CARTESIAN_POINT ( 'NONE',  ( 3.178125000614515638, 4.541064518000418104, 2.621784821874999949 ) ) ;
#53164=CARTESIAN_POINT ( 'NONE',  ( 20.78437500061451715, 4.541064518000418104, 2.621784821874999949 ) ) ;
#53165=CARTESIAN_POINT ( 'NONE',  ( 29.40937500061451715, 0.000000000000000000, 5.243569643749999010 ) ) ;
#53166=CARTESIAN_POINT ( 'NONE',  ( 4.040625000614517681, 6.054752690667223547, 3.707466751127219781E-16 ) ) ;
#53167=CARTESIAN_POINT ( 'NONE',  ( 21.59062500061451928, 6.054752690667223547, 3.707466751127219781E-16 ) ) ;
#53168=CARTESIAN_POINT ( 'NONE',  ( 2.121784821875001281, 16.35312500061451857, 33.67503911421598417 ) ) ;
#53169=CARTESIAN_POINT ( 'NONE',  ( 15.86250000122903181, -4.330127018922190985, -2.500000000000001332 ) ) ;
#53171=CARTESIAN_POINT ( 'NONE',  ( 7.678125000614516082, 4.541064518000418104, 2.621784821874999949 ) ) ;
#53172=CARTESIAN_POINT ( 'NONE',  ( 3.159375000614518036, 4.541064518000418104, -2.621784821874998173 ) ) ;
#53173=CARTESIAN_POINT ( 'NONE',  ( 2.971875000614517592, -6.054752690667223547, -1.112240025338166033E-15 ) ) ;
#53174=CARTESIAN_POINT ( 'NONE',  ( 23.07187500061451857, 3.027376345333611329, 5.243569643749999010 ) ) ;
#53175=CARTESIAN_POINT ( 'NONE',  ( 14.27812500061451573, 6.421520780324663323E-16, -5.243569643749999010 ) ) ;
#53176=CARTESIAN_POINT ( 'NONE',  ( 25.72500000122903074, -5.773502691896255534, -1.060575238724906372E-15 ) ) ;
#53177=( BOUNDED_CURVE ( )  B_SPLINE_CURVE ( 2, ( #15157, #60217, #60586, #32890, #61324, #27720, #54337 ),
 .UNSPECIFIED., .F., .F. ) 
 B_SPLINE_CURVE_WITH_KNOTS ( ( 3, 2, 2, 3 ),
 ( 0.5500000000000000444, 0.5527777777777778123, 0.5555555555555555802, 0.5583333333333333481 ),
 .UNSPECIFIED. ) 
 CURVE ( )  GEOMETRIC_REPRESENTATION_ITEM ( )  RATIONAL_B_SPLINE_CURVE ( ( 1.000000000000000000, 0.8660254037844387076, 1.000000000000000000, 0.8660254037844387076, 1.000000000000000000, 0.8660254037844387076, 1.000000000000000000 ) ) 
 REPRESENTATION_ITEM ( '' )  );
#53178=CARTESIAN_POINT ( 'NONE',  ( 24.77812500061451217, 4.541064518000418104, 2.621784821874999949 ) ) ;
#53179=CARTESIAN_POINT ( 'NONE',  ( 19.80937500061451573, 4.541064518000418104, -2.621784821874998173 ) ) ;
#53180=CARTESIAN_POINT ( 'NONE',  ( 13.94062500061451892, 6.054752690667223547, 3.707466751127219781E-16 ) ) ;
#53181=CARTESIAN_POINT ( 'NONE',  ( 2.121784821874999061, 17.90937500061451715, 26.32496088578401583 ) ) ;
#53182=CARTESIAN_POINT ( 'NONE',  ( 19.19062500061452070, -3.027376345333610441, -5.243569643749999898 ) ) ;
#53184=EDGE_LOOP ( 'NONE', ( #38928, #12990, #18227, #32848 ) ) ;
#53185=CARTESIAN_POINT ( 'NONE',  ( 24.18750000000000355, -2.886751345948129988, 4.999999999999997335 ) ) ;
#53186=CARTESIAN_POINT ( 'NONE',  ( -4.243569643749999898, 19.85937500061451644, -30.00000000000000000 ) ) ;
#53188=CARTESIAN_POINT ( 'NONE',  ( 26.87812500061451360, 6.421520780324663323E-16, -5.243569643749999010 ) ) ;
#53189=CARTESIAN_POINT ( 'NONE',  ( 8.990625000614516082, 6.054752690667223547, 3.707466751127219781E-16 ) ) ;
#53190=CARTESIAN_POINT ( 'NONE',  ( 20.81250000122903643, -4.330127018922190985, -2.500000000000001332 ) ) ;
#53191=EDGE_CURVE ( 'NONE', #2372, #16272, #60566, .T. ) ;
#53192=CARTESIAN_POINT ( 'NONE',  ( 24.44062500061451715, -3.027376345333614438, 5.243569643749998122 ) ) ;
#53193=CARTESIAN_POINT ( 'NONE',  ( 26.32499999999999929, 4.330127018922191873, 2.499999999999999556 ) ) ;
#53194=CARTESIAN_POINT ( 'NONE',  ( -2.000000000000000000, 16.88750000122903572, -33.46410161513775705 ) ) ;
#53195=CARTESIAN_POINT ( 'NONE',  ( 26.99062500061451431, 6.054752690667223547, 3.707466751127219781E-16 ) ) ;
#53196=CARTESIAN_POINT ( 'NONE',  ( 11.50312500061451892, -4.541064518000417216, -2.621784821875001281 ) ) ;
#53198=CARTESIAN_POINT ( 'NONE',  ( 26.24062500061451431, -3.027376345333614438, 5.243569643749998122 ) ) ;
#53199=CARTESIAN_POINT ( 'NONE',  ( 4.790625000614518569, -3.027376345333610441, -5.243569643749999898 ) ) ;
#53201=CARTESIAN_POINT ( 'NONE',  ( 30.00000000000000000, 0.000000000000000000, 0.000000000000000000 ) ) ;
#53202=CARTESIAN_POINT ( 'NONE',  ( 12.15000000000000036, -4.330127018922190985, -2.500000000000001332 ) ) ;
#53203=CARTESIAN_POINT ( 'NONE',  ( 13.09687500061451892, 6.054752690667223547, 3.707466751127219781E-16 ) ) ;
#53204=CARTESIAN_POINT ( 'NONE',  ( 9.712500001229033231, 4.330127018922192761, -2.499999999999997780 ) ) ;
#53205=CARTESIAN_POINT ( 'NONE',  ( 17.40937500061451715, -4.541064518000417216, -2.621784821875001281 ) ) ;
#53207=CARTESIAN_POINT ( 'NONE',  ( 9.534375000614517148, 4.541064518000418104, 2.621784821874999949 ) ) ;
#53208=CARTESIAN_POINT ( 'NONE',  ( 2.121784821874999061, 11.55312500061451786, -33.67503911421598417 ) ) ;
#53209=CARTESIAN_POINT ( 'NONE',  ( 20.17499999999999716, -4.330127018922194537, 2.499999999999995559 ) ) ;
#53212=CARTESIAN_POINT ( 'NONE',  ( 23.39062500061451289, 6.054752690667223547, 3.707466751127219781E-16 ) ) ;
#53213=CARTESIAN_POINT ( 'NONE',  ( 9.001249775931846008E-16, 10.97187500061451715, 34.90005215228797653 ) ) ;
#53215=CARTESIAN_POINT ( 'NONE',  ( 25.05937500061451573, -4.541064518000417216, -2.621784821875001281 ) ) ;
#53216=CARTESIAN_POINT ( 'NONE',  ( 28.02187500061451431, 3.027376345333611329, 5.243569643749999010 ) ) ;
#53217=CARTESIAN_POINT ( 'NONE',  ( 4.003125000614518925, 4.541064518000418104, -2.621784821874998173 ) ) ;
#53219=CARTESIAN_POINT ( 'NONE',  ( 16.62187500061451573, 3.027376345333613106, -5.243569643749998122 ) ) ;
#53221=CARTESIAN_POINT ( 'NONE',  ( 29.25000000122903288, -2.886751345948129988, 4.999999999999997335 ) ) ;
#53222=CARTESIAN_POINT ( 'NONE',  ( 7.209375000614519635, 4.541064518000418104, -2.621784821874998173 ) ) ;
#53223=CARTESIAN_POINT ( 'NONE',  ( 18.90937500061451360, 4.541064518000418104, -2.621784821874998173 ) ) ;
#53225=CARTESIAN_POINT ( 'NONE',  ( 25.94999999999999929, 0.000000000000000000, 4.999999999999998224 ) ) ;
#53226=CARTESIAN_POINT ( 'NONE',  ( 26.89687500061451431, -3.027376345333610441, -5.243569643749999898 ) ) ;
#53228=CARTESIAN_POINT ( 'NONE',  ( 14.25000000122903288, 5.773502691896255534, 3.535250795749688401E-16 ) ) ;
#53230=CARTESIAN_POINT ( 'NONE',  ( 7.350000000000002309, 4.330127018922192761, -2.499999999999997780 ) ) ;
#53232=CARTESIAN_POINT ( 'NONE',  ( 20.87812500061451715, -4.541064518000419881, 2.621784821874995952 ) ) ;
#53233=CARTESIAN_POINT ( 'NONE',  ( 12.11250000000000249, -5.773502691896255534, -1.060575238724906372E-15 ) ) ;
#53234=ADVANCED_FACE ( 'NONE', ( #20680 ), #21048, .F. ) ;
#53235=CARTESIAN_POINT ( 'NONE',  ( 8.175000001229031810, -5.773502691896255534, -1.060575238724906372E-15 ) ) ;
#53236=CARTESIAN_POINT ( 'NONE',  ( 5.390625000614518214, 6.054752690667223547, 3.707466751127219781E-16 ) ) ;
#53237=CARTESIAN_POINT ( 'NONE',  ( 21.15000000000000213, -4.330127018922190985, -2.500000000000001332 ) ) ;
#53238=CARTESIAN_POINT ( 'NONE',  ( 17.80312500061451786, -4.541064518000417216, -2.621784821875001281 ) ) ;
#53239=CARTESIAN_POINT ( 'NONE',  ( 12.15000000000000036, -4.330127018922190985, -2.500000000000001332 ) ) ;
#53240=CARTESIAN_POINT ( 'NONE',  ( 25.76250000122903216, -4.330127018922190985, -2.500000000000001332 ) ) ;
#53242=CARTESIAN_POINT ( 'NONE',  ( 4.875000000000000888, -4.330127018922194537, 2.499999999999995559 ) ) ;
#53244=CARTESIAN_POINT ( 'NONE',  ( 18.92812500061451431, 4.541064518000418104, 2.621784821874999949 ) ) ;
#53245=CARTESIAN_POINT ( 'NONE',  ( 26.65312500061451573, 0.000000000000000000, 5.243569643749999010 ) ) ;
#53246=CARTESIAN_POINT ( 'NONE',  ( 26.10937500061451644, 4.541064518000418104, -2.621784821874998173 ) ) ;
#53247=CARTESIAN_POINT ( 'NONE',  ( 9.975000000000001421, 6.123233995736764310E-16, -4.999999999999998224 ) ) ;
#53248=CARTESIAN_POINT ( 'NONE',  ( 14.42812500061451786, 4.541064518000418104, 2.621784821874999949 ) ) ;
#53249=DIRECTION ( 'NONE',  ( -0.000000000000000000, -1.000000000000000000, -0.000000000000000000 ) ) ;
#53250=CARTESIAN_POINT ( 'NONE',  ( 8.315625000614515372, -6.054752690667223547, -1.112240025338166033E-15 ) ) ;
#53251=DIRECTION ( 'NONE',  ( 0.000000000000000000, 0.000000000000000000, 1.000000000000000000 ) ) ;
#53252=CARTESIAN_POINT ( 'NONE',  ( 4.243569643749999898, 11.98437500061451821, 30.00000000000000000 ) ) ;
#53253=CARTESIAN_POINT ( 'NONE',  ( 25.72500000122903074, -5.773502691896255534, -1.060575238724906372E-15 ) ) ;
#53255=CARTESIAN_POINT ( 'NONE',  ( 17.65312500061451573, 0.000000000000000000, 5.243569643749999010 ) ) ;
#53256=CARTESIAN_POINT ( 'NONE',  ( 1.626862140677534273E-15, 13.36250000000000071, 34.00000000000000000 ) ) ;
#53257=VECTOR ( 'NONE', #64158, 1000.000000000000000 ) ;
#53258=CARTESIAN_POINT ( 'NONE',  ( 9.309375000614517504, -4.541064518000417216, -2.621784821875001281 ) ) ;
#53259=CARTESIAN_POINT ( 'NONE',  ( 10.50937500061451679, 0.000000000000000000, 5.243569643749999010 ) ) ;
#53260=CARTESIAN_POINT ( 'NONE',  ( 17.33437500061451431, -4.541064518000419881, 2.621784821874995952 ) ) ;
#53261=ORIENTED_EDGE ( 'NONE', *, *, #42409, .T. ) ;
#53262=CARTESIAN_POINT ( 'NONE',  ( 15.18750000000000000, -2.886751345948130876, 4.999999999999996447 ) ) ;
#53263=CARTESIAN_POINT ( 'NONE',  ( 20.95312500061451999, -4.541064518000417216, -2.621784821875001281 ) ) ;
#53264=CARTESIAN_POINT ( 'NONE',  ( 16.32187500061451502, 3.027376345333611329, 5.243569643749999010 ) ) ;
#53265=CARTESIAN_POINT ( 'NONE',  ( 21.70312500061451644, 0.000000000000000000, 5.243569643749999010 ) ) ;
#53266=CARTESIAN_POINT ( 'NONE',  ( -3.999999999999999556, 15.46250000000000036, 27.69059892324149530 ) ) ;
#53267=CARTESIAN_POINT ( 'NONE',  ( 27.44062500061451715, 6.054752690667223547, 3.707466751127219781E-16 ) ) ;
#53268=CARTESIAN_POINT ( 'NONE',  ( 7.462500001229035007, 4.330127018922192761, -2.499999999999997780 ) ) ;
#53269=EDGE_LOOP ( 'NONE', ( #13053, #23889, #31896, #1727, #48992, #36276, #16931, #15579, #60355, #16516, #30151, #51866, #72553, #70257, #32464, #3078, #28044, #9198, #18017, #4725, #65834, #47772, #24822, #51965, #39230, #60677, #27312, #18904, #43920, #35882, #68950, #6596, #69676, #68737, #69732, #53773, #2495, #42687, #35154, #16910, #26674, #68236, #37714, #50306, #9283, #38233, #62860, #38844, #2819, #43062, #9462, #62805, #24654, #9806, #25018, #65220, #37355, #43790, #463, #18016, #28268, #62469, #388, #54514, #28373, #12940, #60036, #61718, #5584, #9862, #33809, #35118, #45260, #51066, #23108, #28519, #16337, #25019, #70240, #44555, #33704, #33696, #33441, #56201, #13496, #15192, #17994, #14607, #3549, #37568, #62714, #41749, #53563, #53875, #34194, #57312, #1141, #1291, #9947, #64294, #48487, #69252, #59257, #23419, #18797, #13458, #47425, #52838, #6448, #72749, #36325, #64076, #50891, #4484, #40478, #30652, #1244, #47329 ) ) ;
#53270=CARTESIAN_POINT ( 'NONE',  ( 4.950000001229033941, -2.886751345948129988, 4.999999999999997335 ) ) ;
#53271=CARTESIAN_POINT ( 'NONE',  ( -2.828200636599751609E-16, 18.98749999999999716, -34.61880215351700230 ) ) ;
#53272=CARTESIAN_POINT ( 'NONE',  ( 24.07500000122903216, 2.886751345948129099, -4.999999999999998224 ) ) ;
#53274=CARTESIAN_POINT ( 'NONE',  ( 6.721875000614518925, 3.027376345333613106, -5.243569643749998122 ) ) ;
#53276=CARTESIAN_POINT ( 'NONE',  ( 13.82812500061451466, 6.421520780324663323E-16, -5.243569643749999010 ) ) ;
#53277=CARTESIAN_POINT ( 'NONE',  ( 9.534375000614517148, 4.541064518000418104, 2.621784821874999949 ) ) ;
#53278=CARTESIAN_POINT ( 'NONE',  ( 26.96250000122903145, 0.000000000000000000, 4.999999999999998224 ) ) ;
#53279=CARTESIAN_POINT ( 'NONE',  ( 18.08437500061451431, 4.541064518000418104, 2.621784821874999949 ) ) ;
#53280=CARTESIAN_POINT ( 'NONE',  ( 4.659375000614518925, 0.000000000000000000, 5.243569643749999010 ) ) ;
#53281=DIRECTION ( 'NONE',  ( -1.000000000000000000, -0.000000000000000000, -0.000000000000000000 ) ) ;
#53282=CARTESIAN_POINT ( 'NONE',  ( 4.378125000614518925, 6.421520780324663323E-16, -5.243569643749999010 ) ) ;
#53283=CARTESIAN_POINT ( 'NONE',  ( 18.10312500061451502, 0.000000000000000000, 5.243569643749999010 ) ) ;
#53284=ORIENTED_EDGE ( 'NONE', *, *, #10988, .T. ) ;
#53285=CARTESIAN_POINT ( 'NONE',  ( 11.54062500061451857, -3.027376345333610441, -5.243569643749999898 ) ) ;
#53286=CARTESIAN_POINT ( 'NONE',  ( 5.212500001229032343, 4.330127018922192761, -2.499999999999997780 ) ) ;
#53287=CARTESIAN_POINT ( 'NONE',  ( 10.67812500061451608, 6.421520780324663323E-16, -5.243569643749999010 ) ) ;
#53289=CARTESIAN_POINT ( 'NONE',  ( 10.16249999999999964, 2.886751345948126879, 4.999999999999999112 ) ) ;
#53290=EDGE_CURVE ( 'NONE', #16431, #21477, #714, .T. ) ;
#53291=CARTESIAN_POINT ( 'NONE',  ( 6.262500001229034829, 0.000000000000000000, 4.999999999999998224 ) ) ;
#53292=CARTESIAN_POINT ( 'NONE',  ( 21.30000000000000071, 4.330127018922192761, -2.499999999999997780 ) ) ;
#53293=CARTESIAN_POINT ( 'NONE',  ( 14.82187500061451679, 3.027376345333613106, -5.243569643749998122 ) ) ;
#53294=CARTESIAN_POINT ( 'NONE',  ( 15.00000000122903465, -2.886751345948125991, -5.000000000000000000 ) ) ;
#53296=CARTESIAN_POINT ( 'NONE',  ( 2.121784821874999061, 18.30312500061451431, -33.67503911421598417 ) ) ;
#53297=CARTESIAN_POINT ( 'NONE',  ( -5.810221930991193690E-16, 14.93750000000000000, 26.00000000000000355 ) ) ;
#53298=CARTESIAN_POINT ( 'NONE',  ( -1.999999999999997113, 18.72500000000000142, 33.46410161513775705 ) ) ;
#53299=CARTESIAN_POINT ( 'NONE',  ( 4.321875000614518569, -6.054752690667223547, -1.112240025338166033E-15 ) ) ;
#53300=CYLINDRICAL_SURFACE ( 'NONE', #25680, 4.000000000000000000 ) ;
#53301=CARTESIAN_POINT ( 'NONE',  ( 30.00000000000000000, 0.000000000000000000, 0.000000000000000000 ) ) ;
#53302=CARTESIAN_POINT ( 'NONE',  ( 15.72187500061451892, 3.027376345333613106, -5.243569643749998122 ) ) ;
#53303=CARTESIAN_POINT ( 'NONE',  ( 29.25000000000000000, -4.330127018922190985, -2.500000000000001332 ) ) ;
#53304=CARTESIAN_POINT ( 'NONE',  ( 10.94062500061451537, -3.027376345333614438, 5.243569643749998122 ) ) ;
#53305=CIRCLE ( 'NONE', #27396, 5.999999999999998224 ) ;
#53307=CARTESIAN_POINT ( 'NONE',  ( 24.53437500061451715, -4.541064518000419881, 2.621784821874995952 ) ) ;
#53309=CARTESIAN_POINT ( 'NONE',  ( 10.49062500061451431, -3.027376345333614438, 5.243569643749998122 ) ) ;
#53310=CARTESIAN_POINT ( 'NONE',  ( 16.58437500061451786, 6.421520780324663323E-16, -5.243569643749999010 ) ) ;
#53312=CARTESIAN_POINT ( 'NONE',  ( 25.28437500061451715, 4.541064518000418104, 2.621784821874999949 ) ) ;
#53313=CARTESIAN_POINT ( 'NONE',  ( 28.04062500061451502, -3.027376345333614438, 5.243569643749998122 ) ) ;
#53314=CARTESIAN_POINT ( 'NONE',  ( 19.00312500061451715, 0.000000000000000000, 5.243569643749999010 ) ) ;
#53315=CARTESIAN_POINT ( 'NONE',  ( 27.96562500061451928, 3.027376345333611329, 5.243569643749999010 ) ) ;
#53316=CARTESIAN_POINT ( 'NONE',  ( 4.864635650123212862, 1.155751203253316817, -5.114655441610994835 ) ) ;
#53317=CARTESIAN_POINT ( 'NONE',  ( 7.012500000000001066, 2.886751345948126879, 4.999999999999999112 ) ) ;
#53318=CARTESIAN_POINT ( 'NONE',  ( 19.72500000122903074, 2.886751345948126879, 4.999999999999999112 ) ) ;
#53319=DIRECTION ( 'NONE',  ( -0.000000000000000000, -1.000000000000000000, -0.000000000000000000 ) ) ;
#53321=ORIENTED_EDGE ( 'NONE', *, *, #643, .F. ) ;
#53322=CARTESIAN_POINT ( 'NONE',  ( 15.97499999999999964, 4.330127018922191873, 2.499999999999999556 ) ) ;
#53323=CARTESIAN_POINT ( 'NONE',  ( 19.79999999999999716, -4.330127018922190985, -2.500000000000001332 ) ) ;
#53324=CARTESIAN_POINT ( 'NONE',  ( 15.87187500061451573, 3.027376345333611329, 5.243569643749999010 ) ) ;
#53325=CARTESIAN_POINT ( 'NONE',  ( 14.46562500061451750, 3.027376345333611329, 5.243569643749999010 ) ) ;
#53327=ORIENTED_EDGE ( 'NONE', *, *, #33228, .F. ) ;
#53328=LINE ( 'NONE', #42977, #72577 ) ;
#53329=CARTESIAN_POINT ( 'NONE',  ( 2.121784821874999061, 16.10937500061451644, -33.67503911421598417 ) ) ;
#53330=CARTESIAN_POINT ( 'NONE',  ( 6.328125000614515550, 4.541064518000418104, 2.621784821874999949 ) ) ;
#53332=CARTESIAN_POINT ( 'NONE',  ( 11.73750000000000249, -2.886751345948125991, -5.000000000000000000 ) ) ;
#53334=CARTESIAN_POINT ( 'NONE',  ( 2.121784821874999061, 14.25312500061451715, 26.32496088578401583 ) ) ;
#53335=CARTESIAN_POINT ( 'NONE',  ( 26.95312500061451644, 4.541064518000418104, -2.621784821874998173 ) ) ;
#53338=CARTESIAN_POINT ( 'NONE',  ( 24.53437500061451715, -4.541064518000419881, 2.621784821874995952 ) ) ;
#53339=CARTESIAN_POINT ( 'NONE',  ( 20.61562500061451431, 3.027376345333613106, -5.243569643749998122 ) ) ;
#53340=CARTESIAN_POINT ( 'NONE',  ( -3.000416591977282496E-16, 15.19062500061459353, -34.90005215228797653 ) ) ;
#53341=CARTESIAN_POINT ( 'NONE',  ( 22.46250000122903501, 0.000000000000000000, 4.999999999999998224 ) ) ;
#53342=CARTESIAN_POINT ( 'NONE',  ( 6.478125000614516793, -4.541064518000419881, 2.621784821874995952 ) ) ;
#53344=CARTESIAN_POINT ( 'NONE',  ( 24.70312500061451644, 4.541064518000418104, -2.621784821874998173 ) ) ;
#53347=CARTESIAN_POINT ( 'NONE',  ( 15.68437500061451573, 6.421520780324663323E-16, -5.243569643749999010 ) ) ;
#53348=CARTESIAN_POINT ( 'NONE',  ( 24.45937500061451786, 0.000000000000000000, 5.243569643749999010 ) ) ;
#53349=CARTESIAN_POINT ( 'NONE',  ( -4.243569643749999898, 14.00937500061451857, 30.00000000000000000 ) ) ;
#53350=CARTESIAN_POINT ( 'NONE',  ( 5.165625000614518569, -6.054752690667223547, -1.112240025338166033E-15 ) ) ;
#53351=CARTESIAN_POINT ( 'NONE',  ( 29.76562500061451644, 3.027376345333611329, 5.243569643749999010 ) ) ;
#53352=CARTESIAN_POINT ( 'NONE',  ( 29.54062500061451502, -3.027376345333610441, -5.243569643749999898 ) ) ;
#53354=CARTESIAN_POINT ( 'NONE',  ( 2.516621263038615997, 9.679961675009989719, -35.45028981414222358 ) ) ;
#53355=CARTESIAN_POINT ( 'NONE',  ( 3.103125000614517237, 4.541064518000418104, -2.621784821874998173 ) ) ;
#53356=CARTESIAN_POINT ( 'NONE',  ( 7.584375000614516082, 6.421520780324663323E-16, -5.243569643749999010 ) ) ;
#53358=CARTESIAN_POINT ( 'NONE',  ( 16.08750000122903501, 4.330127018922191873, 2.499999999999999556 ) ) ;
#53359=CARTESIAN_POINT ( 'NONE',  ( 29.31562500061451715, 3.027376345333611329, 5.243569643749999010 ) ) ;
#53360=CARTESIAN_POINT ( 'NONE',  ( 4.490625000614516971, 6.054752690667223547, 3.707466751127219781E-16 ) ) ;
#53363=CARTESIAN_POINT ( 'NONE',  ( 13.24687500061451750, -3.027376345333614438, 5.243569643749998122 ) ) ;
#53364=CARTESIAN_POINT ( 'NONE',  ( 27.56250000000000000, 2.886751345948162850, -4.999999999999940492 ) ) ;
#53366=CARTESIAN_POINT ( 'NONE',  ( 22.22812500061451502, -4.541064518000419881, 2.621784821874995952 ) ) ;
#53367=CARTESIAN_POINT ( 'NONE',  ( 8.128125000614515372, 4.541064518000418104, 2.621784821874999949 ) ) ;
#53368=CARTESIAN_POINT ( 'NONE',  ( 23.97187500061451715, 3.027376345333611329, 5.243569643749999010 ) ) ;
#53369=CARTESIAN_POINT ( 'NONE',  ( 7.678125000614516082, 4.541064518000418104, 2.621784821874999949 ) ) ;
#53370=CARTESIAN_POINT ( 'NONE',  ( 29.77499999999999858, 6.123233995736764310E-16, -4.999999999999998224 ) ) ;
#53371=CARTESIAN_POINT ( 'NONE',  ( 10.01250000122903394, -4.330127018922190985, -2.500000000000001332 ) ) ;
#53372=CARTESIAN_POINT ( 'NONE',  ( 24.70312500061451644, 4.541064518000418104, -2.621784821874998173 ) ) ;
#53374=CARTESIAN_POINT ( 'NONE',  ( 3.999999999999998668, 19.47500000122903430, -32.30940107675850470 ) ) ;
#53375=CARTESIAN_POINT ( 'NONE',  ( 10.23750000122903359, 4.330127018922191873, 2.499999999999999556 ) ) ;
#53376=CARTESIAN_POINT ( 'NONE',  ( 22.82812500061451644, 6.421520780324663323E-16, -5.243569643749999010 ) ) ;
#53377=CARTESIAN_POINT ( 'NONE',  ( 17.80312500061451786, -4.541064518000417216, -2.621784821875001281 ) ) ;
#53379=CARTESIAN_POINT ( 'NONE',  ( 17.77499999999999858, 4.330127018922191873, 2.499999999999999556 ) ) ;
#53380=CARTESIAN_POINT ( 'NONE',  ( 14.85000000122903252, -2.886751345948129988, 4.999999999999997335 ) ) ;
#53382=CARTESIAN_POINT ( 'NONE',  ( 10.71562500061451928, 3.027376345333613106, -5.243569643749998122 ) ) ;
#53383=CARTESIAN_POINT ( 'NONE',  ( 12.51562500061451821, 3.027376345333613106, -5.243569643749998122 ) ) ;
#53384=CARTESIAN_POINT ( 'NONE',  ( 23.25000000122903288, 5.773502691896255534, 3.535250795749688894E-16 ) ) ;
#53385=CARTESIAN_POINT ( 'NONE',  ( 22.65937500061451715, 0.000000000000000000, 5.243569643749999010 ) ) ;
#53386=CARTESIAN_POINT ( 'NONE',  ( 21.53437500061451715, 6.421520780324663323E-16, -5.243569643749999010 ) ) ;
#53388=CARTESIAN_POINT ( 'NONE',  ( 8.737500001229033586, 6.123233995736764310E-16, -4.999999999999998224 ) ) ;
#53389=CARTESIAN_POINT ( 'NONE',  ( 6.609375000614519102, -4.541064518000417216, -2.621784821875001281 ) ) ;
#53390=CARTESIAN_POINT ( 'NONE',  ( 24.27187500061452141, 3.027376345333613106, -5.243569643749998122 ) ) ;
#53392=( BOUNDED_CURVE ( )  B_SPLINE_CURVE ( 2, ( #60790, #27923, #49728, #16816, #10196, #66345, #22005 ),
 .UNSPECIFIED., .F., .F. ) 
 B_SPLINE_CURVE_WITH_KNOTS ( ( 3, 2, 2, 3 ),
 ( 0.8833333333333333037, 0.8861111111111110716, 0.8888888888888888395, 0.8916666666666667185 ),
 .UNSPECIFIED. ) 
 CURVE ( )  GEOMETRIC_REPRESENTATION_ITEM ( )  RATIONAL_B_SPLINE_CURVE ( ( 1.000000000000000000, 0.8660254037844387076, 1.000000000000000000, 0.8660254037844387076, 1.000000000000000000, 0.8660254037844387076, 1.000000000000000000 ) ) 
 REPRESENTATION_ITEM ( '' )  );
#53393=CARTESIAN_POINT ( 'NONE',  ( 4.699789363897854955, -1.707107682658927095, 4.926740801328898911 ) ) ;
#53394=EDGE_CURVE ( 'NONE', #71040, #58014, #71674, .T. ) ;
#53395=CARTESIAN_POINT ( 'NONE',  ( 22.34062500061451573, -3.027376345333610441, -5.243569643749999898 ) ) ;
#53396=CARTESIAN_POINT ( 'NONE',  ( 24.75937500061451502, 4.541064518000418104, -2.621784821874998173 ) ) ;
#53398=CARTESIAN_POINT ( 'NONE',  ( 3.375730161298836407, -4.192115423953711506, 3.226182382019024519 ) ) ;
#53399=CARTESIAN_POINT ( 'NONE',  ( 27.63750000122903216, 6.123233995736764310E-16, -4.999999999999998224 ) ) ;
#53400=CARTESIAN_POINT ( 'NONE',  ( 5.971875000614516260, 3.027376345333611329, 5.243569643749999010 ) ) ;
#53401=CARTESIAN_POINT ( 'NONE',  ( 16.45312500061451289, -4.541064518000417216, -2.621784821875001281 ) ) ;
#53402=ORIENTED_EDGE ( 'NONE', *, *, #63906, .F. ) ;
#53404=CARTESIAN_POINT ( 'NONE',  ( 25.49062500061451786, -3.027376345333610441, -5.243569643749999898 ) ) ;
#53405=CARTESIAN_POINT ( 'NONE',  ( 4.509375000614518569, 4.541064518000418104, -2.621784821874998173 ) ) ;
#53406=CARTESIAN_POINT ( 'NONE',  ( 4.750580614020113224, 1.560202551697607465, 4.800619732442354071 ) ) ;
#53408=CARTESIAN_POINT ( 'NONE',  ( 15.07499999999999929, 4.330127018922191873, 2.499999999999999556 ) ) ;
#53409=CARTESIAN_POINT ( 'NONE',  ( 26.02500000122903145, 2.886751345948126879, 4.999999999999999112 ) ) ;
#53410=CARTESIAN_POINT ( 'NONE',  ( 22.11562500061451786, 3.027376345333611329, 5.243569643749999010 ) ) ;
#53412=CARTESIAN_POINT ( 'NONE',  ( 25.61250000000000071, -5.773502691896255534, -1.060575238724906372E-15 ) ) ;
#53413=CARTESIAN_POINT ( 'NONE',  ( 26.85937500061451644, -4.541064518000417216, -2.621784821875001281 ) ) ;
#53415=ORIENTED_EDGE ( 'NONE', *, *, #12441, .F. ) ;
#53416=CARTESIAN_POINT ( 'NONE',  ( 30.00000000000000000, 0.000000000000000000, 0.000000000000000000 ) ) ;
#53417=CARTESIAN_POINT ( 'NONE',  ( 12.40312500061451573, -4.541064518000417216, -2.621784821875001281 ) ) ;
#53418=CARTESIAN_POINT ( 'NONE',  ( 24.97500000122903074, 2.886751345948112668, -5.000000000000024869 ) ) ;
#53420=CARTESIAN_POINT ( 'NONE',  ( 28.30312500061451431, 4.541064518000418104, -2.621784821874998173 ) ) ;
#53422=CARTESIAN_POINT ( 'NONE',  ( 13.87500000122903465, 2.886751345948126879, 4.999999999999999112 ) ) ;
#53423=CARTESIAN_POINT ( 'NONE',  ( 20.51249999999999929, 2.886751345948126879, 4.999999999999999112 ) ) ;
#53424=CARTESIAN_POINT ( 'NONE',  ( 26.77499999999999858, 4.330127018922191873, 2.499999999999999556 ) ) ;
#53426=CARTESIAN_POINT ( 'NONE',  ( 7.996875000614519280, -3.027376345333610441, -5.243569643749999898 ) ) ;
#53427=CARTESIAN_POINT ( 'NONE',  ( 20.55937500061451573, -4.541064518000417216, -2.621784821875001281 ) ) ;
#53429=EDGE_LOOP ( 'NONE', ( #18832, #51169, #68145, #42287 ) ) ;
#53430=CARTESIAN_POINT ( 'NONE',  ( 27.96562500061451928, 3.027376345333611329, 5.243569643749999010 ) ) ;
#53431=CARTESIAN_POINT ( 'NONE',  ( 29.25937500061451502, 4.541064518000418104, -2.621784821874998173 ) ) ;
#53432=CARTESIAN_POINT ( 'NONE',  ( 3.534375000614518036, 6.421520780324663323E-16, -5.243569643749999010 ) ) ;
#53433=CARTESIAN_POINT ( 'NONE',  ( 15.75000000000000000, -4.330127018922190985, -2.500000000000001332 ) ) ;
#53434=CARTESIAN_POINT ( 'NONE',  ( 12.62812500061451537, 4.541064518000418104, 2.621784821874999949 ) ) ;
#53435=FACE_OUTER_BOUND ( 'NONE', #7493, .T. ) ;
#53437=CARTESIAN_POINT ( 'NONE',  ( 4.050000000000001599, -4.330127018922190985, -2.500000000000001332 ) ) ;
#53438=CARTESIAN_POINT ( 'NONE',  ( 17.66250000122903430, -4.330127018922190985, -2.500000000000001332 ) ) ;
#53440=CARTESIAN_POINT ( 'NONE',  ( 6.890625000614516438, -3.027376345333614438, 5.243569643749998122 ) ) ;
#53441=CARTESIAN_POINT ( 'NONE',  ( 24.60937500061451644, -4.541064518000417216, -2.621784821875001281 ) ) ;
#53443=CARTESIAN_POINT ( 'NONE',  ( -2.121784821874999949, 17.08437500061451786, 26.32496088578401938 ) ) ;
#53444=CARTESIAN_POINT ( 'NONE',  ( 24.12187500061451217, -6.054752690667223547, -1.112240025338166033E-15 ) ) ;
#53445=CARTESIAN_POINT ( 'NONE',  ( 4.537500000000000533, -2.886751345948125991, -5.000000000000000000 ) ) ;
#53446=CARTESIAN_POINT ( 'NONE',  ( -2.828200636599751609E-16, 10.10000000122903430, 25.38119784648299770 ) ) ;
#53447=CARTESIAN_POINT ( 'NONE',  ( 12.96562500061451750, 3.027376345333613106, -5.243569643749998122 ) ) ;
#53448=CARTESIAN_POINT ( 'NONE',  ( 4.425000001229032698, 2.886751345948126879, 4.999999999999999112 ) ) ;
#53449=CARTESIAN_POINT ( 'NONE',  ( 9.909375000614517148, 4.541064518000418104, -2.621784821874998173 ) ) ;
#53450=CARTESIAN_POINT ( 'NONE',  ( -0.6906555412606095734, 4.953935347589260019, -26.05769473322559548 ) ) ;
#53452=CARTESIAN_POINT ( 'NONE',  ( 12.02812500061451573, 6.421520780324663323E-16, -5.243569643749999010 ) ) ;
#53454=CARTESIAN_POINT ( 'NONE',  ( 23.58750000122903145, 6.123233995736764310E-16, -4.999999999999998224 ) ) ;
#53455=CARTESIAN_POINT ( 'NONE',  ( 10.43437500061451750, 4.541064518000418104, 2.621784821874999949 ) ) ;
#53456=CARTESIAN_POINT ( 'NONE',  ( 12.02812500061451573, 6.421520780324663323E-16, -5.243569643749999010 ) ) ;
#53458=CARTESIAN_POINT ( 'NONE',  ( 21.72187500061451715, 3.027376345333611329, 5.243569643749999010 ) ) ;
#53459=CARTESIAN_POINT ( 'NONE',  ( 2.000000000000001332, 15.76250000122903216, 33.46410161513774995 ) ) ;
#53460=DIRECTION ( 'NONE',  ( -1.000000000000000000, -0.000000000000000000, -0.000000000000000000 ) ) ;
#53461=CARTESIAN_POINT ( 'NONE',  ( 3.167073630078104607, 3.869168037755827960, -3.482309847224001054 ) ) ;
#53462=CARTESIAN_POINT ( 'NONE',  ( -2.121784821874996840, 13.63437500061451857, -26.32496088578401583 ) ) ;
#53463=CARTESIAN_POINT ( 'NONE',  ( 16.05937500061451573, -4.541064518000417216, -2.621784821875001281 ) ) ;
#53464=CARTESIAN_POINT ( 'NONE',  ( 18.37500000122903288, 2.886751345948126879, 4.999999999999999112 ) ) ;
#53465=CARTESIAN_POINT ( 'NONE',  ( 12.04687500061451821, -3.027376345333610441, -5.243569643749999898 ) ) ;
#53466=CARTESIAN_POINT ( 'NONE',  ( 9.001249775931846008E-16, 18.56562500061451715, -25.09994784771203058 ) ) ;
#53467=CARTESIAN_POINT ( 'NONE',  ( 17.55000000122903359, -2.886751345948129988, 4.999999999999997335 ) ) ;
#53468=CARTESIAN_POINT ( 'NONE',  ( 13.30312500061451786, -4.541064518000417216, -2.621784821875001281 ) ) ;
#53469=VERTEX_POINT ( 'NONE', #13167 ) ;
#53470=CARTESIAN_POINT ( 'NONE',  ( 16.19999999999999929, -4.330127018922190985, -2.500000000000001332 ) ) ;
#53472=CARTESIAN_POINT ( 'NONE',  ( 12.98437500061451821, 6.421520780324663323E-16, -5.243569643749999010 ) ) ;
#53474=CARTESIAN_POINT ( 'NONE',  ( 12.18750000122903465, -4.330127018922194537, 2.499999999999995559 ) ) ;
#53475=CARTESIAN_POINT ( 'NONE',  ( 21.18750000122903288, -4.330127018922194537, 2.499999999999995559 ) ) ;
#53476=CARTESIAN_POINT ( 'NONE',  ( 17.87812500061451715, 6.421520780324663323E-16, -5.243569643749999010 ) ) ;
#53477=CARTESIAN_POINT ( 'NONE',  ( 19.86562500061451786, 3.027376345333611329, 5.243569643749999010 ) ) ;
#53478=CARTESIAN_POINT ( 'NONE',  ( 28.65000000122903145, 5.773502691896255534, 3.535250795749688894E-16 ) ) ;
#53479=CARTESIAN_POINT ( 'NONE',  ( 25.16249999999999432, -5.773502691896255534, -1.060575238724906372E-15 ) ) ;
#53482=CARTESIAN_POINT ( 'NONE',  ( 27.72187500061451715, -6.054752690667223547, -1.112240025338166033E-15 ) ) ;
#53483=CARTESIAN_POINT ( 'NONE',  ( -3.999999999999999112, 9.762500001229033941, -30.00000000000000000 ) ) ;
#53484=CARTESIAN_POINT ( 'NONE',  ( 4.243569643749999898, 14.23437500061451821, -30.00000000000000000 ) ) ;
#53485=CARTESIAN_POINT ( 'NONE',  ( 3.037500001229032964, 4.330127018922191873, 2.499999999999999556 ) ) ;
#53486=CARTESIAN_POINT ( 'NONE',  ( 3.374999999999999556, 4.330127018922191873, 2.499999999999999556 ) ) ;
#53487=CARTESIAN_POINT ( 'NONE',  ( 3.586992791275801729, 3.483314903268937446, -3.919380039434936513 ) ) ;
#53488=CARTESIAN_POINT ( 'NONE',  ( 6.684375000614518392, 6.421520780324663323E-16, -5.243569643749999010 ) ) ;
#53489=CARTESIAN_POINT ( 'NONE',  ( 28.60312500061451502, -4.541064518000417216, -2.621784821875001281 ) ) ;
#53490=FACE_OUTER_BOUND ( 'NONE', #37442, .T. ) ;
#53491=CARTESIAN_POINT ( 'NONE',  ( 1.071796769724491893, 17.54509619066136850, -26.00000000000000355 ) ) ;
#53492=EDGE_CURVE ( 'NONE', #46701, #65074, #62394, .T. ) ;
#53493=CARTESIAN_POINT ( 'NONE',  ( 5.296875000614518214, -3.027376345333610441, -5.243569643749999898 ) ) ;
#53494=CARTESIAN_POINT ( 'NONE',  ( 11.07187500061451679, -6.054752690667223547, -1.112240025338166033E-15 ) ) ;
#53495=CARTESIAN_POINT ( 'NONE',  ( 5.250000000000000888, 0.000000000000000000, 4.999999999999998224 ) ) ;
#53496=CARTESIAN_POINT ( 'NONE',  ( 4.243569643749999898, 15.04062500061459495, 32.45002607614398471 ) ) ;
#53498=CARTESIAN_POINT ( 'NONE',  ( 6.524999999999999467, 4.330127018922191873, 2.499999999999999556 ) ) ;
#53500=CARTESIAN_POINT ( 'NONE',  ( 20.16562500061451146, 3.027376345333613106, -5.243569643749998122 ) ) ;
#53501=CARTESIAN_POINT ( 'NONE',  ( 10.04062500061451502, -3.027376345333614438, 5.243569643749998122 ) ) ;
#53503=CARTESIAN_POINT ( 'NONE',  ( 10.20937500061451786, -4.541064518000417216, -2.621784821875001281 ) ) ;
#53504=CARTESIAN_POINT ( 'NONE',  ( 25.19999999999999929, -4.330127018922190985, -2.500000000000001332 ) ) ;
#53505=CARTESIAN_POINT ( 'NONE',  ( 20.58750000122903145, 4.330127018922191873, 2.499999999999999556 ) ) ;
#53506=CARTESIAN_POINT ( 'NONE',  ( 26.91562500061451146, 3.027376345333613106, -5.243569643749998122 ) ) ;
#53507=DIRECTION ( 'NONE',  ( -0.000000000000000000, -1.000000000000000000, -0.000000000000000000 ) ) ;
#53508=CARTESIAN_POINT ( 'NONE',  ( 9.009375000614518569, 4.541064518000418104, -2.621784821874998173 ) ) ;
#53509=CARTESIAN_POINT ( 'NONE',  ( 13.62187500061451750, 3.027376345333611329, 5.243569643749999010 ) ) ;
#53510=CARTESIAN_POINT ( 'NONE',  ( 26.78437500061451360, -4.541064518000419881, 2.621784821874995952 ) ) ;
#53511=CARTESIAN_POINT ( 'NONE',  ( -5.810221930991193690E-16, 13.70000000122903394, -34.00000000000000000 ) ) ;
#53512=CARTESIAN_POINT ( 'NONE',  ( 20.85937500061451644, 0.000000000000000000, 5.243569643749999010 ) ) ;
#53513=CARTESIAN_POINT ( 'NONE',  ( 10.69687500061451679, -3.027376345333610441, -5.243569643749999898 ) ) ;
#53515=CARTESIAN_POINT ( 'NONE',  ( 22.46250000000000213, -5.773502691896255534, -1.060575238724906372E-15 ) ) ;
#53517=CARTESIAN_POINT ( 'NONE',  ( -3.000416591977282496E-16, 12.09687500061451715, -34.90005215228797653 ) ) ;
#53519=CARTESIAN_POINT ( 'NONE',  ( 14.61562500061451608, -6.054752690667223547, -1.112240025338166033E-15 ) ) ;
#53520=CARTESIAN_POINT ( 'NONE',  ( 5.100000000000000533, 4.330127018922192761, -2.499999999999997780 ) ) ;
#53522=CARTESIAN_POINT ( 'NONE',  ( 25.50000000000000000, 0.000000000000000000, 4.999999999999998224 ) ) ;
#53523=CARTESIAN_POINT ( 'NONE',  ( 11.73750000000000249, -2.886751345948125991, -5.000000000000000000 ) ) ;
#53524=CARTESIAN_POINT ( 'NONE',  ( 1.999999999999998668, 16.81250000122903643, 26.53589838486224650 ) ) ;
#53525=CARTESIAN_POINT ( 'NONE',  ( 12.45000000122903394, 5.773502691896255534, 3.535250795749688894E-16 ) ) ;
#53526=CARTESIAN_POINT ( 'NONE',  ( 25.47187500061451715, -6.054752690667223547, -1.112240025338166033E-15 ) ) ;
#53527=CARTESIAN_POINT ( 'NONE',  ( 15.60937500061451644, -4.541064518000417216, -2.621784821875001281 ) ) ;
#53528=CARTESIAN_POINT ( 'NONE',  ( 7.320879633048903241E-15, 18.08749999999999858, 26.00000000000000355 ) ) ;
#53530=CARTESIAN_POINT ( 'NONE',  ( 19.90312500061451573, 0.000000000000000000, 5.243569643749999010 ) ) ;
#53531=CARTESIAN_POINT ( 'NONE',  ( 4.640625000614518214, -3.027376345333614438, 5.243569643749998122 ) ) ;
#53532=CARTESIAN_POINT ( 'NONE',  ( 16.92187500061451999, -6.054752690667223547, -1.112240025338166033E-15 ) ) ;
#53533=CARTESIAN_POINT ( 'NONE',  ( 28.28437500061451715, 6.421520780324663323E-16, -5.243569643749999010 ) ) ;
#53534=CARTESIAN_POINT ( 'NONE',  ( 4.678125000614516971, -4.541064518000419881, 2.621784821874995952 ) ) ;
#53535=CARTESIAN_POINT ( 'NONE',  ( 19.07812500061451644, -4.541064518000419881, 2.621784821874995952 ) ) ;
#53536=CARTESIAN_POINT ( 'NONE',  ( -2.121784821874999949, 14.77812500061451750, 26.32496088578401938 ) ) ;
#53537=CARTESIAN_POINT ( 'NONE',  ( 16.76250000122903216, -4.330127018922190985, -2.500000000000001332 ) ) ;
#53539=CARTESIAN_POINT ( 'NONE',  ( 7.978125000614517681, 6.421520780324663323E-16, -5.243569643749999010 ) ) ;
#53540=CARTESIAN_POINT ( 'NONE',  ( 29.65312500061451573, 4.541064518000418104, -2.621784821874998173 ) ) ;
#53541=CARTESIAN_POINT ( 'NONE',  ( 22.47187500061451715, 3.027376345333613106, -5.243569643749998122 ) ) ;
#53542=CARTESIAN_POINT ( 'NONE',  ( 15.55312500061451608, -4.541064518000417216, -2.621784821875001281 ) ) ;
#53543=CARTESIAN_POINT ( 'NONE',  ( 24.97500000122903430, 2.886751345948129099, -4.999999999999998224 ) ) ;
#53544=CARTESIAN_POINT ( 'NONE',  ( 23.24062500061451786, -3.027376345333610441, -5.243569643749999898 ) ) ;
#53545=CARTESIAN_POINT ( 'NONE',  ( 19.02187500061451786, 3.027376345333611329, 5.243569643749999010 ) ) ;
#53546=CARTESIAN_POINT ( 'NONE',  ( 15.14062500061451644, -3.027376345333610441, -5.243569643749999898 ) ) ;
#53547=CARTESIAN_POINT ( 'NONE',  ( -4.243569643749997233, 14.49687500061451928, 32.45002607614398471 ) ) ;
#53548=CARTESIAN_POINT ( 'NONE',  ( 20.65312500061451573, 4.541064518000418104, -2.621784821874998173 ) ) ;
#53549=CARTESIAN_POINT ( 'NONE',  ( 28.94062500061452070, -3.027376345333614438, 5.243569643749998122 ) ) ;
#53550=VERTEX_POINT ( 'NONE', #16957 ) ;
#53552=CARTESIAN_POINT ( 'NONE',  ( 21.82499999999999574, 4.330127018922191873, 2.499999999999999556 ) ) ;
#53553=CARTESIAN_POINT ( 'NONE',  ( -2.000000000000000000, 11.37500000000000178, -33.46410161513775705 ) ) ;
#53554=CARTESIAN_POINT ( 'NONE',  ( 1.592000809091587073E-14, 15.38750000000000284, 26.00000000000000000 ) ) ;
#53555=CARTESIAN_POINT ( 'NONE',  ( 26.05312500061451431, 4.541064518000418104, -2.621784821874998173 ) ) ;
#53556=CARTESIAN_POINT ( 'NONE',  ( 8.540625000614518569, 6.054752690667223547, 3.707466751127219781E-16 ) ) ;
#53557=CARTESIAN_POINT ( 'NONE',  ( 19.76250000122903216, 0.000000000000000000, 4.999999999999998224 ) ) ;
#53558=CARTESIAN_POINT ( 'NONE',  ( 24.89062500061451644, -3.027376345333614438, 5.243569643749998122 ) ) ;
#53559=CARTESIAN_POINT ( 'NONE',  ( 24.56250000000000000, 2.886751345948126879, 4.999999999999999112 ) ) ;
#53560=( BOUNDED_CURVE ( )  B_SPLINE_CURVE ( 2, ( #43878, #8420, #65666, #9885, #37593, #32420, #14326, #14685, #4362 ),
 .UNSPECIFIED., .F., .F. ) 
 B_SPLINE_CURVE_WITH_KNOTS ( ( 3, 2, 2, 2, 3 ),
 ( 0.8804347826086956763, 0.8840579710144927938, 0.8913043478260869179, 0.8985507246376811530, 0.9021739130434782705 ),
 .UNSPECIFIED. ) 
 CURVE ( )  GEOMETRIC_REPRESENTATION_ITEM ( )  RATIONAL_B_SPLINE_CURVE ( ( 0.9330127018922194093, 0.9330127018922194093, 1.000000000000000000, 0.8660254037844387076, 1.000000000000000000, 0.8660254037844387076, 1.000000000000000000, 0.9330127018922194093, 0.9330127018922194093 ) ) 
 REPRESENTATION_ITEM ( '' )  );
#53561=CARTESIAN_POINT ( 'NONE',  ( 26.76562500061451644, -6.054752690667223547, -1.112240025338166033E-15 ) ) ;
#53562=CARTESIAN_POINT ( 'NONE',  ( 8.015625000614518214, 3.027376345333613106, -5.243569643749998122 ) ) ;
#53563=ORIENTED_EDGE ( 'NONE', *, *, #38471, .F. ) ;
#53565=CARTESIAN_POINT ( 'NONE',  ( 23.16562500061451502, -6.054752690667223547, -1.112240025338166033E-15 ) ) ;
#53566=CARTESIAN_POINT ( 'NONE',  ( 4.340625000614515727, -3.027376345333610441, -5.243569643749999898 ) ) ;
#53568=CARTESIAN_POINT ( 'NONE',  ( 2.840625000614518392, -3.027376345333614438, 5.243569643749998122 ) ) ;
#53569=CARTESIAN_POINT ( 'NONE',  ( -3.999999999999999112, 13.66250000000000142, -32.30940107675850470 ) ) ;
#53570=CARTESIAN_POINT ( 'NONE',  ( 14.32500000000000107, -4.330127018922194537, 2.499999999999995559 ) ) ;
#53571=CARTESIAN_POINT ( 'NONE',  ( 14.85937500061451644, 4.541064518000418104, -2.621784821874998173 ) ) ;
#53572=CARTESIAN_POINT ( 'NONE',  ( 8.025000001229035007, 2.886751345948126879, 4.999999999999999112 ) ) ;
#53573=CARTESIAN_POINT ( 'NONE',  ( 15.60937500061451644, -4.541064518000417216, -2.621784821875001281 ) ) ;
#53575=CARTESIAN_POINT ( 'NONE',  ( 9.346875000614517148, -3.027376345333610441, -5.243569643749999898 ) ) ;
#53576=CARTESIAN_POINT ( 'NONE',  ( 2.121784821875001281, 11.85312500061451857, -26.32496088578401938 ) ) ;
#53577=VECTOR ( 'NONE', #27161, 1000.000000000000000 ) ;
#53578=CARTESIAN_POINT ( 'NONE',  ( 20.28750000000000142, -2.886751345948159742, -4.999999999999942268 ) ) ;
#53580=CARTESIAN_POINT ( 'NONE',  ( 13.65937500061451715, 0.000000000000000000, 5.243569643749999010 ) ) ;
#53581=VERTEX_POINT ( 'NONE', #6248 ) ;
#53582=CARTESIAN_POINT ( 'NONE',  ( 22.15312500061451573, 0.000000000000000000, 5.243569643749999010 ) ) ;
#53583=CARTESIAN_POINT ( 'NONE',  ( -2.121784821874996840, 10.48437500061451821, 33.67503911421598417 ) ) ;
#53585=CARTESIAN_POINT ( 'NONE',  ( 26.59687500061451360, 6.054752690667223547, 3.707466751127219781E-16 ) ) ;
#53586=CARTESIAN_POINT ( 'NONE',  ( 29.29687500061451644, 6.054752690667223547, 3.707466751127219781E-16 ) ) ;
#53587=CARTESIAN_POINT ( 'NONE',  ( 3.403125000614518836, -4.541064518000417216, -2.621784821875001281 ) ) ;
#53589=CARTESIAN_POINT ( 'NONE',  ( 16.13437500061451502, 6.421520780324663323E-16, -5.243569643749999010 ) ) ;
#53591=CARTESIAN_POINT ( 'NONE',  ( 3.028125000614518392, 6.421520780324663323E-16, -5.243569643749999010 ) ) ;
#53592=CARTESIAN_POINT ( 'NONE',  ( 4.959375000614516971, 4.541064518000418104, -2.621784821874998173 ) ) ;
#53593=CARTESIAN_POINT ( 'NONE',  ( 17.78437500061451715, -4.541064518000419881, 2.621784821874995952 ) ) ;
#53595=CARTESIAN_POINT ( 'NONE',  ( 23.55000000000000071, 4.330127018922192761, -2.499999999999997780 ) ) ;
#53596=CARTESIAN_POINT ( 'NONE',  ( 26.37187500061451217, -6.054752690667223547, -1.112240025338166033E-15 ) ) ;
#53597=ADVANCED_FACE ( 'NONE', ( #61306 ), #39510, .F. ) ;
#53601=CARTESIAN_POINT ( 'NONE',  ( 8.849999999999999645, 0.000000000000000000, 4.999999999999998224 ) ) ;
#53603=CARTESIAN_POINT ( 'NONE',  ( 21.92812500061451431, 6.421520780324663323E-16, -5.243569643749999010 ) ) ;
#53604=CARTESIAN_POINT ( 'NONE',  ( 11.13750000000000284, -2.886751345948129988, 4.999999999999997335 ) ) ;
#53605=CARTESIAN_POINT ( 'NONE',  ( 8.137500001229033941, -4.330127018922194537, 2.499999999999995559 ) ) ;
#53606=CARTESIAN_POINT ( 'NONE',  ( 6.065625000614516260, -6.054752690667223547, -1.112240025338166033E-15 ) ) ;
#53607=( BOUNDED_CURVE ( )  B_SPLINE_CURVE ( 2, ( #52058, #46516, #46881, #69055, #52418, #41693, #18775 ),
 .UNSPECIFIED., .F., .F. ) 
 B_SPLINE_CURVE_WITH_KNOTS ( ( 3, 2, 2, 3 ),
 ( 0.6750000000000000444, 0.6777777777777778123, 0.6805555555555555802, 0.6833333333333333481 ),
 .UNSPECIFIED. ) 
 CURVE ( )  GEOMETRIC_REPRESENTATION_ITEM ( )  RATIONAL_B_SPLINE_CURVE ( ( 1.000000000000000000, 0.8660254037844387076, 1.000000000000000000, 0.8660254037844387076, 1.000000000000000000, 0.8660254037844387076, 1.000000000000000000 ) ) 
 REPRESENTATION_ITEM ( '' )  );
#53608=CARTESIAN_POINT ( 'NONE',  ( 19.79999999999999716, -4.330127018922190985, -2.500000000000001332 ) ) ;
#53609=CARTESIAN_POINT ( 'NONE',  ( 19.37812500061451715, 4.541064518000418104, 2.621784821874999949 ) ) ;
#53610=AXIS2_PLACEMENT_3D ( 'NONE', #7365, #2195, #29894 ) ;
#53611=CARTESIAN_POINT ( 'NONE',  ( 23.55000000000000071, 4.330127018922192761, -2.499999999999997780 ) ) ;
#53612=CARTESIAN_POINT ( 'NONE',  ( 23.88750000122903216, -4.330127018922194537, 2.499999999999995559 ) ) ;
#53614=CARTESIAN_POINT ( 'NONE',  ( 4.575000000000002842, 6.123233995736764310E-16, -4.999999999999998224 ) ) ;
#53616=CARTESIAN_POINT ( 'NONE',  ( 20.20312500061451644, 4.541064518000418104, -2.621784821874998173 ) ) ;
#53617=CARTESIAN_POINT ( 'NONE',  ( 26.01562500061451289, 3.027376345333613106, -5.243569643749998122 ) ) ;
#53618=CARTESIAN_POINT ( 'NONE',  ( 24.38437500061451502, 4.541064518000418104, 2.621784821874999949 ) ) ;
#53619=CARTESIAN_POINT ( 'NONE',  ( 8.250000000000000000, 4.330127018922192761, -2.499999999999997780 ) ) ;
#53620=CARTESIAN_POINT ( 'NONE',  ( 13.07812500061451821, 4.541064518000418104, 2.621784821874999949 ) ) ;
#53621=LINE ( 'NONE', #42174, #58432 ) ;
#53622=CARTESIAN_POINT ( 'NONE',  ( 9.590625000614517504, -3.027376345333614438, 5.243569643749998122 ) ) ;
#53623=CARTESIAN_POINT ( 'NONE',  ( 0.000000000000000000, 20.00000000000000000, -30.00000000000000000 ) ) ;
#53624=CARTESIAN_POINT ( 'NONE',  ( -2.121784821874999949, 12.13437500061451857, 26.32496088578401938 ) ) ;
#53625=CARTESIAN_POINT ( 'NONE',  ( 24.11250000122903359, 4.330127018922192761, -2.499999999999997780 ) ) ;
#53627=CARTESIAN_POINT ( 'NONE',  ( 14.01562500061451644, 3.027376345333611329, 5.243569643749999010 ) ) ;
#53628=CARTESIAN_POINT ( 'NONE',  ( 10.58437500061451964, -4.541064518000419881, 2.621784821874995952 ) ) ;
#53629=CARTESIAN_POINT ( 'NONE',  ( 10.02187500061451964, 3.027376345333611329, 5.243569643749999010 ) ) ;
#53630=CARTESIAN_POINT ( 'NONE',  ( 16.73437500061451644, 4.541064518000418104, 2.621784821874999949 ) ) ;
#53631=ORIENTED_EDGE ( 'NONE', *, *, #27951, .F. ) ;
#53632=CARTESIAN_POINT ( 'NONE',  ( 15.37500000000000000, 6.123233995736764310E-16, -4.999999999999998224 ) ) ;
#53633=CARTESIAN_POINT ( 'NONE',  ( 20.99062500061451431, -3.027376345333610441, -5.243569643749999898 ) ) ;
#53634=CARTESIAN_POINT ( 'NONE',  ( 16.13437500061451502, 6.421520780324663323E-16, -5.243569643749999010 ) ) ;
#53635=CARTESIAN_POINT ( 'NONE',  ( 20.84062500061451573, -3.027376345333614438, 5.243569643749998122 ) ) ;
#53636=CARTESIAN_POINT ( 'NONE',  ( 8.484601909799253346E-16, 11.56250000000000000, 34.61880215351700230 ) ) ;
#53637=AXIS2_PLACEMENT_3D ( 'NONE', #21593, #66675, #39696 ) ;
#53638=CARTESIAN_POINT ( 'NONE',  ( 26.50312500061451360, 4.541064518000418104, -2.621784821874998173 ) ) ;
#53639=CARTESIAN_POINT ( 'NONE',  ( 6.675000001229034474, 2.886751345948126879, 4.999999999999999112 ) ) ;
#53641=CARTESIAN_POINT ( 'NONE',  ( 5.437500001229035540, -4.330127018922194537, 2.499999999999995559 ) ) ;
#53642=CARTESIAN_POINT ( 'NONE',  ( -3.999999999999999112, 17.75000000000000355, -30.00000000000000000 ) ) ;
#53643=CARTESIAN_POINT ( 'NONE',  ( 24.90000000122903145, -2.886751345948125991, -5.000000000000000000 ) ) ;
#53645=CARTESIAN_POINT ( 'NONE',  ( 6.909375000614518036, 0.000000000000000000, 5.243569643749999010 ) ) ;
#53646=CARTESIAN_POINT ( 'NONE',  ( -10.00000000000000000, 0.000000000000000000, -50.00000000000000000 ) ) ;
#53647=CARTESIAN_POINT ( 'NONE',  ( 14.69062500061451537, -3.027376345333610441, -5.243569643749999898 ) ) ;
#53648=CARTESIAN_POINT ( 'NONE',  ( 9.721875000614517148, -6.054752690667223547, -1.112240025338166033E-15 ) ) ;
#53649=CARTESIAN_POINT ( 'NONE',  ( 28.20000000122903216, 5.773502691896255534, 3.535250795749688894E-16 ) ) ;
#53650=CARTESIAN_POINT ( 'NONE',  ( 16.32187500061451502, 3.027376345333611329, 5.243569643749999010 ) ) ;
#53651=CARTESIAN_POINT ( 'NONE',  ( 3.871875000614519280, -6.054752690667223547, -1.112240025338166033E-15 ) ) ;
#53653=CARTESIAN_POINT ( 'NONE',  ( 4.865625000614517859, 3.027376345333613106, -5.243569643749998122 ) ) ;
#53654=CARTESIAN_POINT ( 'NONE',  ( 15.06562500061451537, -6.054752690667223547, -1.112240025338166033E-15 ) ) ;
#53657=CARTESIAN_POINT ( 'NONE',  ( 12.89062500061451821, -3.027376345333610441, -5.243569643749999898 ) ) ;
#53658=CARTESIAN_POINT ( 'NONE',  ( 4.987500001229032698, -4.330127018922194537, 2.499999999999995559 ) ) ;
#53659=AXIS2_PLACEMENT_3D ( 'NONE', #7784, #46952, #18848 ) ;
#53660=CARTESIAN_POINT ( 'NONE',  ( 10.94062500061451537, -3.027376345333614438, 5.243569643749998122 ) ) ;
#53662=CARTESIAN_POINT ( 'NONE',  ( 10.53750000000000320, 5.773502691896255534, 3.535250795749688894E-16 ) ) ;
#53663=CARTESIAN_POINT ( 'NONE',  ( 5.700000001229033941, 5.773502691896255534, 3.535250795749688894E-16 ) ) ;
#53664=CARTESIAN_POINT ( 'NONE',  ( 20.85000000000000142, 4.330127018922192761, -2.499999999999997780 ) ) ;
#53666=CARTESIAN_POINT ( 'NONE',  ( 13.88437500061451679, 6.421520780324663323E-16, -5.243569643749999010 ) ) ;
#53667=CARTESIAN_POINT ( 'NONE',  ( 16.61250000122903359, 0.000000000000000000, 4.999999999999998224 ) ) ;
#53669=CARTESIAN_POINT ( 'NONE',  ( 4.243569643749999898, 18.19062500061451360, -27.54997392385601529 ) ) ;
#53670=CARTESIAN_POINT ( 'NONE',  ( 3.250662400336420177, 3.799104362746421604, 3.614115195980558859 ) ) ;
#53672=CARTESIAN_POINT ( 'NONE',  ( 23.13750000122903216, 6.123233995736764310E-16, -4.999999999999998224 ) ) ;
#53673=CARTESIAN_POINT ( 'NONE',  ( 9.412500001229034297, 0.000000000000000000, 4.999999999999998224 ) ) ;
#53675=CARTESIAN_POINT ( 'NONE',  ( 14.93437500061451750, 4.541064518000418104, 2.621784821874999949 ) ) ;
#53676=CARTESIAN_POINT ( 'NONE',  ( 29.17500000000000071, -4.330127018922194537, 2.499999999999995559 ) ) ;
#53677=CARTESIAN_POINT ( 'NONE',  ( 12.21562500061451573, 3.027376345333611329, 5.243569643749999010 ) ) ;
#53679=CARTESIAN_POINT ( 'NONE',  ( 23.74687500061451573, -3.027376345333610441, -5.243569643749999898 ) ) ;
#53681=CARTESIAN_POINT ( 'NONE',  ( 10.52812500061451750, -4.541064518000419881, 2.621784821874995952 ) ) ;
#53682=CARTESIAN_POINT ( 'NONE',  ( 12.19687500061451679, 6.054752690667223547, 3.707466751127219781E-16 ) ) ;
#53683=VERTEX_POINT ( 'NONE', #67949 ) ;
#53684=CARTESIAN_POINT ( 'NONE',  ( 24.87187500061451573, 3.027376345333611329, 5.243569643749999010 ) ) ;
#53685=CARTESIAN_POINT ( 'NONE',  ( 27.17812500061451786, -4.541064518000419881, 2.621784821874995952 ) ) ;
#53688=CARTESIAN_POINT ( 'NONE',  ( 6.487499999999999822, 5.773502691896255534, 3.535250795749688894E-16 ) ) ;
#53689=CARTESIAN_POINT ( 'NONE',  ( 18.15000000122903501, -2.886751345948125991, -5.000000000000000000 ) ) ;
#53690=CARTESIAN_POINT ( 'NONE',  ( 4.898587196589411843E-16, 20.00000000000000000, 33.99999999999999289 ) ) ;
#53691=CARTESIAN_POINT ( 'NONE',  ( 29.21250000122903145, 0.000000000000000000, 4.999999999999998224 ) ) ;
#53692=ORIENTED_EDGE ( 'NONE', *, *, #55194, .T. ) ;
#53693=CARTESIAN_POINT ( 'NONE',  ( 15.56250000000000000, 2.886751345948126879, 4.999999999999999112 ) ) ;
#53694=CARTESIAN_POINT ( 'NONE',  ( 19.04999999999999716, 4.330127018922192761, -2.499999999999997780 ) ) ;
#53695=CARTESIAN_POINT ( 'NONE',  ( 13.00312500061451537, 4.541064518000418104, -2.621784821874998173 ) ) ;
#53696=VECTOR ( 'NONE', #2184, 1000.000000000000000 ) ;
#53697=ORIENTED_EDGE ( 'NONE', *, *, #22115, .F. ) ;
#53699=CARTESIAN_POINT ( 'NONE',  ( 9.001249775931846008E-16, 15.92187500061451821, -25.09994784771203058 ) ) ;
#53700=CARTESIAN_POINT ( 'NONE',  ( 5.128125000614516260, -4.541064518000419881, 2.621784821874995952 ) ) ;
#53702=CARTESIAN_POINT ( 'NONE',  ( 12.48750000000000249, -2.886751345948129988, 4.999999999999997335 ) ) ;
#53704=ORIENTED_EDGE ( 'NONE', *, *, #61290, .T. ) ;
#53705=CARTESIAN_POINT ( 'NONE',  ( -4.243569643749999898, 15.26562500061451644, 27.54997392385601529 ) ) ;
#53706=CARTESIAN_POINT ( 'NONE',  ( 27.14062500061451644, -3.027376345333614438, 5.243569643749998122 ) ) ;
#53707=CYLINDRICAL_SURFACE ( 'NONE', #30124, 4.000000000000000000 ) ;
#53709=CARTESIAN_POINT ( 'NONE',  ( 23.55937500061451573, 0.000000000000000000, 5.243569643749999010 ) ) ;
#53710=CARTESIAN_POINT ( 'NONE',  ( 19.26562500061451644, 3.027376345333613106, -5.243569643749998122 ) ) ;
#53711=EDGE_CURVE ( 'NONE', #58137, #58126, #28532, .T. ) ;
#53712=CARTESIAN_POINT ( 'NONE',  ( -3.000416591977282496E-16, 14.29062500061459140, -34.90005215228797653 ) ) ;
#53713=CARTESIAN_POINT ( 'NONE',  ( 23.10000000122903074, -2.886751345948125991, -5.000000000000000000 ) ) ;
#53714=CARTESIAN_POINT ( 'NONE',  ( 5.203125000614518214, -4.541064518000417216, -2.621784821875001281 ) ) ;
#53716=CARTESIAN_POINT ( 'NONE',  ( 22.45312500061451644, 4.541064518000418104, -2.621784821874998173 ) ) ;
#53719=CARTESIAN_POINT ( 'NONE',  ( 17.59687500061451715, 6.054752690667223547, 3.707466751127219781E-16 ) ) ;
#53720=CARTESIAN_POINT ( 'NONE',  ( 17.07187500061451502, 3.027376345333613106, -5.243569643749998122 ) ) ;
#53721=CARTESIAN_POINT ( 'NONE',  ( 23.93437500061451573, 4.541064518000418104, 2.621784821874999949 ) ) ;
#53722=CARTESIAN_POINT ( 'NONE',  ( 2.121784821874999061, 14.75937500061451679, 26.32496088578401583 ) ) ;
#53723=CARTESIAN_POINT ( 'NONE',  ( 5.015625000614518214, 3.027376345333611329, 5.243569643749999010 ) ) ;
#53724=CARTESIAN_POINT ( 'NONE',  ( 16.50000000122903288, 5.773502691896255534, 3.535250795749688401E-16 ) ) ;
#53725=CARTESIAN_POINT ( 'NONE',  ( 28.75312500061451715, 4.541064518000418104, -2.621784821874998173 ) ) ;
#53727=CARTESIAN_POINT ( 'NONE',  ( 4.134375000614517681, 4.541064518000418104, 2.621784821874999949 ) ) ;
#53728=CARTESIAN_POINT ( 'NONE',  ( 3.665625000614517681, 3.027376345333611329, 5.243569643749999010 ) ) ;
#53729=CARTESIAN_POINT ( 'NONE',  ( 7.509375000614517681, -4.541064518000417216, -2.621784821875001281 ) ) ;
#53731=CARTESIAN_POINT ( 'NONE',  ( 14.73750000122903359, 4.330127018922191873, 2.499999999999999556 ) ) ;
#53732=CARTESIAN_POINT ( 'NONE',  ( 29.54062500061451502, -3.027376345333610441, -5.243569643749999898 ) ) ;
#53733=CARTESIAN_POINT ( 'NONE',  ( 12.90000000122903145, 5.773502691896255534, 3.535250795749688894E-16 ) ) ;
#53734=CARTESIAN_POINT ( 'NONE',  ( 6.253125000614517148, 4.541064518000418104, -2.621784821874998173 ) ) ;
#53737=CARTESIAN_POINT ( 'NONE',  ( 14.78437500061451715, 6.421520780324663323E-16, -5.243569643749999010 ) ) ;
#53738=CARTESIAN_POINT ( 'NONE',  ( 7.612500000000000711, -5.773502691896255534, -1.060575238724906372E-15 ) ) ;
#53739=EDGE_LOOP ( 'NONE', ( #59586, #67529, #17972, #35081 ) ) ;
#53740=CARTESIAN_POINT ( 'NONE',  ( 23.05312500061451431, 0.000000000000000000, 5.243569643749999010 ) ) ;
#53741=CARTESIAN_POINT ( 'NONE',  ( 7.003125000614518036, -4.541064518000417216, -2.621784821875001281 ) ) ;
#53742=CARTESIAN_POINT ( 'NONE',  ( 24.68437500061451573, 6.421520780324663323E-16, -5.243569643749999010 ) ) ;
#53743=CARTESIAN_POINT ( 'NONE',  ( 6.440625000614517148, -3.027376345333614438, 5.243569643749998122 ) ) ;
#53744=CARTESIAN_POINT ( 'NONE',  ( 8.212500001229035007, -4.330127018922190985, -2.500000000000001332 ) ) ;
#53745=CARTESIAN_POINT ( 'NONE',  ( 22.82812500061451644, 6.421520780324663323E-16, -5.243569643749999010 ) ) ;
#53746=CARTESIAN_POINT ( 'NONE',  ( -2.121784821874996840, 11.77812500061451750, -26.32496088578401583 ) ) ;
#53747=CARTESIAN_POINT ( 'NONE',  ( 11.51250000122903216, 4.330127018922192761, -2.499999999999997780 ) ) ;
#53748=CARTESIAN_POINT ( 'NONE',  ( 20.57812500061451644, 6.421520780324663323E-16, -5.243569643749999010 ) ) ;
#53749=CARTESIAN_POINT ( 'NONE',  ( 17.76562500061451644, -6.054752690667223547, -1.112240025338166033E-15 ) ) ;
#53751=CARTESIAN_POINT ( 'NONE',  ( 17.39999999999999858, 0.000000000000000000, 4.999999999999998224 ) ) ;
#53752=CARTESIAN_POINT ( 'NONE',  ( 14.77500000122903501, 2.886751345948126879, 4.999999999999999112 ) ) ;
#53753=AXIS2_PLACEMENT_3D ( 'NONE', #28185, #17076, #39637 ) ;
#53754=CARTESIAN_POINT ( 'NONE',  ( 9.440625000614517148, 6.054752690667223547, 3.707466751127219781E-16 ) ) ;
#53755=CARTESIAN_POINT ( 'NONE',  ( 13.90312500061451750, 4.541064518000418104, -2.621784821874998173 ) ) ;
#53757=CARTESIAN_POINT ( 'NONE',  ( 23.96250000122903145, -4.330127018922190985, -2.500000000000001332 ) ) ;
#53759=CARTESIAN_POINT ( 'NONE',  ( 21.12187500061451573, 3.027376345333613106, -5.243569643749998122 ) ) ;
#53760=CARTESIAN_POINT ( 'NONE',  ( 20.82187500061451857, 3.027376345333611329, 5.243569643749999010 ) ) ;
#53761=CARTESIAN_POINT ( 'NONE',  ( 3.564913708944925208, 3.505916797073983293, -3.899182909318817725 ) ) ;
#53762=CARTESIAN_POINT ( 'NONE',  ( 7.162500001229032520, 0.000000000000000000, 4.999999999999998224 ) ) ;
#53763=CARTESIAN_POINT ( 'NONE',  ( 7.546875000614517326, -3.027376345333610441, -5.243569643749999898 ) ) ;
#53764=CARTESIAN_POINT ( 'NONE',  ( 23.29687500061451644, -3.027376345333610441, -5.243569643749999898 ) ) ;
#53765=CARTESIAN_POINT ( 'NONE',  ( 4.683223236373093457, -1.751405183929441556, 4.942428804804532838 ) ) ;
#53766=CARTESIAN_POINT ( 'NONE',  ( 19.04062500061451146, -3.027376345333614438, 5.243569643749998122 ) ) ;
#53767=CARTESIAN_POINT ( 'NONE',  ( 25.24687500061451573, 6.054752690667223547, 3.707466751127219781E-16 ) ) ;
#53770=CARTESIAN_POINT ( 'NONE',  ( 1.071796769724491893, 15.63259618943233598, 33.99999999999999289 ) ) ;
#53771=CARTESIAN_POINT ( 'NONE',  ( 4.471875000614518925, 3.027376345333613106, -5.243569643749998122 ) ) ;
#53772=CARTESIAN_POINT ( 'NONE',  ( 18.32812500061451644, 6.421520780324663323E-16, -5.243569643749999010 ) ) ;
#53773=ORIENTED_EDGE ( 'NONE', *, *, #16481, .F. ) ;
#53775=CARTESIAN_POINT ( 'NONE',  ( 24.40312500061451573, 0.000000000000000000, 5.243569643749999010 ) ) ;
#53776=CARTESIAN_POINT ( 'NONE',  ( 4.342984975361706468, -2.477595912125914790, -4.621313785610477787 ) ) ;
#53778=CARTESIAN_POINT ( 'NONE',  ( 14.28750000000000142, -2.886751345948129988, 4.999999999999997335 ) ) ;
#53779=CARTESIAN_POINT ( 'NONE',  ( 24.48750000122903359, 6.123233995736764310E-16, -4.999999999999998224 ) ) ;
#53780=CARTESIAN_POINT ( 'NONE',  ( 18.25312500061451715, -4.541064518000417216, -2.621784821875001281 ) ) ;
#53782=CARTESIAN_POINT ( 'NONE',  ( 22.42500000000000071, -4.330127018922194537, 2.499999999999995559 ) ) ;
#53783=CARTESIAN_POINT ( 'NONE',  ( 24.64687500061451431, -3.027376345333610441, -5.243569643749999898 ) ) ;
#53786=CARTESIAN_POINT ( 'NONE',  ( 12.36562500061451608, -6.054752690667223547, -1.112240025338166033E-15 ) ) ;
#53787=CARTESIAN_POINT ( 'NONE',  ( 4.528125000614516615, 4.541064518000418104, 2.621784821874999949 ) ) ;
#53789=CARTESIAN_POINT ( 'NONE',  ( 27.32812500061451644, 6.421520780324663323E-16, -5.243569643749999010 ) ) ;
#53790=CARTESIAN_POINT ( 'NONE',  ( 13.35000000122903430, 5.773502691896255534, 3.535250795749688894E-16 ) ) ;
#53792=CARTESIAN_POINT ( 'NONE',  ( 19.76250000000000639, -5.773502691896255534, -1.060575238724906372E-15 ) ) ;
#53793=CARTESIAN_POINT ( 'NONE',  ( 25.80000000000000071, 4.330127018922192761, -2.499999999999997780 ) ) ;
#53794=CARTESIAN_POINT ( 'NONE',  ( 3.271875000614519635, 3.027376345333611329, 5.243569643749999010 ) ) ;
#53795=CARTESIAN_POINT ( 'NONE',  ( 5.746875000614517504, -3.027376345333610441, -5.243569643749999898 ) ) ;
#53796=CARTESIAN_POINT ( 'NONE',  ( 16.65937500061452070, 4.541064518000418104, -2.621784821874998173 ) ) ;
#53799=CARTESIAN_POINT ( 'NONE',  ( 29.16562500061451502, 3.027376345333613106, -5.243569643749998122 ) ) ;
#53800=CARTESIAN_POINT ( 'NONE',  ( 26.59687500061451360, 6.054752690667223547, 3.707466751127219781E-16 ) ) ;
#53802=CARTESIAN_POINT ( 'NONE',  ( 15.07499999999999929, 4.330127018922191873, 2.499999999999999556 ) ) ;
#53803=CARTESIAN_POINT ( 'NONE',  ( 14.12812500061451715, -4.541064518000419881, 2.621784821874995952 ) ) ;
#53805=DIRECTION ( 'NONE',  ( -0.000000000000000000, -1.000000000000000000, -0.000000000000000000 ) ) ;
#53807=CARTESIAN_POINT ( 'NONE',  ( 19.08750000122903145, 6.123233995736764310E-16, -4.999999999999998224 ) ) ;
#53810=CARTESIAN_POINT ( 'NONE',  ( 7.640625000614517326, 6.054752690667223547, 3.707466751127219781E-16 ) ) ;
#53811=CARTESIAN_POINT ( 'NONE',  ( 23.10937500061451644, 0.000000000000000000, 5.243569643749999010 ) ) ;
#53812=CARTESIAN_POINT ( 'NONE',  ( -4.243569643749999898, 16.70937500061451786, 30.00000000000000000 ) ) ;
#53813=EDGE_CURVE ( 'NONE', #67359, #63939, #38469, .T. ) ;
#53814=CARTESIAN_POINT ( 'NONE',  ( 25.09687500061451715, -3.027376345333610441, -5.243569643749999898 ) ) ;
#53815=CARTESIAN_POINT ( 'NONE',  ( 4.687500000000000000, 5.773502691896255534, 3.535250795749688894E-16 ) ) ;
#53816=CARTESIAN_POINT ( 'NONE',  ( 4.000000000000000000, 10.40000000122903501, 32.30940107675849049 ) ) ;
#53817=CARTESIAN_POINT ( 'NONE',  ( 11.20312500061451644, 4.541064518000418104, -2.621784821874998173 ) ) ;
#53818=CARTESIAN_POINT ( 'NONE',  ( 3.637500001229036162, -4.330127018922194537, 2.499999999999995559 ) ) ;
#53819=CARTESIAN_POINT ( 'NONE',  ( 8.371875000614515727, -6.054752690667223547, -1.112240025338166033E-15 ) ) ;
#53821=ORIENTED_EDGE ( 'NONE', *, *, #62622, .F. ) ;
#53822=CARTESIAN_POINT ( 'NONE',  ( 10.22812500061451679, 6.421520780324663323E-16, -5.243569643749999010 ) ) ;
#53823=CARTESIAN_POINT ( 'NONE',  ( 14.48437500061451821, 4.541064518000418104, 2.621784821874999949 ) ) ;
#53825=CARTESIAN_POINT ( 'NONE',  ( 22.65000000122903856, -2.886751345948125991, -5.000000000000000000 ) ) ;
#53826=CARTESIAN_POINT ( 'NONE',  ( 10.28437500061451715, 6.421520780324663323E-16, -5.243569643749999010 ) ) ;
#53827=CARTESIAN_POINT ( 'NONE',  ( 11.87812500061451537, -4.541064518000419881, 2.621784821874995952 ) ) ;
#53829=CARTESIAN_POINT ( 'NONE',  ( 20.67187500061451289, 3.027376345333613106, -5.243569643749998122 ) ) ;
#53830=CARTESIAN_POINT ( 'NONE',  ( 14.24999999999999822, 0.000000000000000000, 4.999999999999998224 ) ) ;
#53831=( BOUNDED_CURVE ( )  B_SPLINE_CURVE ( 2, ( #6809, #41161, #24146, #1640, #63670, #41872, #13794 ),
 .UNSPECIFIED., .F., .F. ) 
 B_SPLINE_CURVE_WITH_KNOTS ( ( 3, 2, 2, 3 ),
 ( 0.2333333333333333648, 0.2361111111111111327, 0.2388888888888889284, 0.2416666666666666963 ),
 .UNSPECIFIED. ) 
 CURVE ( )  GEOMETRIC_REPRESENTATION_ITEM ( )  RATIONAL_B_SPLINE_CURVE ( ( 0.9999999999999986677, 0.8660254037844400399, 1.000000000000000000, 0.8660254037844387076, 1.000000000000000000, 0.8660254037844373753, 1.000000000000001332 ) ) 
 REPRESENTATION_ITEM ( '' )  );
#53832=CARTESIAN_POINT ( 'NONE',  ( -5.810221930991193690E-16, 12.68750000000000000, 26.00000000000000355 ) ) ;
#53833=CARTESIAN_POINT ( 'NONE',  ( -4.243569643749998122, 14.04687500061451999, -27.54997392385601174 ) ) ;
#53834=CARTESIAN_POINT ( 'NONE',  ( 16.65937500061452070, 4.541064518000418104, -2.621784821874998173 ) ) ;
#53835=CARTESIAN_POINT ( 'NONE',  ( 16.05000000122903359, 5.773502691896255534, 3.535250795749688894E-16 ) ) ;
#53836=CARTESIAN_POINT ( 'NONE',  ( 12.30937500061451573, 0.000000000000000000, 5.243569643749999010 ) ) ;
#53837=CARTESIAN_POINT ( 'NONE',  ( -2.121784821874996840, 18.52812500061451928, -26.32496088578401583 ) ) ;
#53838=CARTESIAN_POINT ( 'NONE',  ( 16.38750000122903216, 6.123233995736764310E-16, -4.999999999999998224 ) ) ;
#53839=CARTESIAN_POINT ( 'NONE',  ( 11.54062500061451857, -3.027376345333610441, -5.243569643749999898 ) ) ;
#53841=CARTESIAN_POINT ( 'NONE',  ( 14.88750000000000107, -2.886751345948125991, -5.000000000000000000 ) ) ;
#53842=CARTESIAN_POINT ( 'NONE',  ( 4.711411573247316298, 1.674097066322985938, -4.711411573247316298 ) ) ;
#53843=CARTESIAN_POINT ( 'NONE',  ( 11.14687500061451608, -3.027376345333610441, -5.243569643749999898 ) ) ;
#53844=CARTESIAN_POINT ( 'NONE',  ( 3.049098432412538973, 3.962700941209165606, -3.321219890071966496 ) ) ;
#53845=CARTESIAN_POINT ( 'NONE',  ( 12.15000000122903501, -2.886751345948129988, 4.999999999999997335 ) ) ;
#53846=CARTESIAN_POINT ( 'NONE',  ( 21.00000000122903288, 5.773502691896255534, 3.535250795749688894E-16 ) ) ;
#53847=CARTESIAN_POINT ( 'NONE',  ( 17.35312500061451502, -4.541064518000417216, -2.621784821875001281 ) ) ;
#53848=CARTESIAN_POINT ( 'NONE',  ( 19.67812500061451786, 6.421520780324663323E-16, -5.243569643749999010 ) ) ;
#53849=CARTESIAN_POINT ( 'NONE',  ( 26.81250000122903288, 4.330127018922192761, -2.499999999999997780 ) ) ;
#53850=EDGE_CURVE ( 'NONE', #27675, #32725, #165, .T. ) ;
#53851=( BOUNDED_CURVE ( )  B_SPLINE_CURVE ( 2, ( #3603, #43490, #42392, #26125, #71189, #66014, #14304 ),
 .UNSPECIFIED., .F., .F. ) 
 B_SPLINE_CURVE_WITH_KNOTS ( ( 3, 2, 2, 3 ),
 ( 0.9083333333333334370, 0.9111111111111112049, 0.9138888888888888618, 0.9161926342374220322 ),
 .UNSPECIFIED. ) 
 CURVE ( )  GEOMETRIC_REPRESENTATION_ITEM ( )  RATIONAL_B_SPLINE_CURVE ( ( 0.9999999999999946709, 0.8660254037844440367, 1.000000000000000000, 0.8660254037844387076, 1.000000000000000000, 0.8888883929728443878, 0.9620772364026252133 ) ) 
 REPRESENTATION_ITEM ( '' )  );
#53852=CARTESIAN_POINT ( 'NONE',  ( 4.490625000614516971, 6.054752690667223547, 3.707466751127219781E-16 ) ) ;
#53853=CARTESIAN_POINT ( 'NONE',  ( 24.75000000000000000, -4.330127018922190985, -2.500000000000001332 ) ) ;
#53855=AXIS2_PLACEMENT_3D ( 'NONE', #53201, #2597, #25117 ) ;
#53857=CARTESIAN_POINT ( 'NONE',  ( 27.64687500061452141, -3.027376345333614438, 5.243569643749998122 ) ) ;
#53858=CARTESIAN_POINT ( 'NONE',  ( -3.999999999999999112, 15.94999999999999929, 30.00000000000000000 ) ) ;
#53859=CARTESIAN_POINT ( 'NONE',  ( -2.121784821874996840, 13.18437500061451750, -26.32496088578401583 ) ) ;
#53860=CARTESIAN_POINT ( 'NONE',  ( 4.275000001229035895, 2.886751345948129099, -4.999999999999998224 ) ) ;
#53861=CARTESIAN_POINT ( 'NONE',  ( 3.637500000000001954, -2.886751345948125991, -5.000000000000000000 ) ) ;
#53862=CARTESIAN_POINT ( 'NONE',  ( 16.42500000000000071, 4.330127018922191873, 2.499999999999999556 ) ) ;
#53863=CARTESIAN_POINT ( 'NONE',  ( 8.371875000614515727, -6.054752690667223547, -1.112240025338166033E-15 ) ) ;
#53864=CARTESIAN_POINT ( 'NONE',  ( 25.07812500061451644, 6.421520780324663323E-16, -5.243569643749999010 ) ) ;
#53865=( BOUNDED_CURVE ( )  B_SPLINE_CURVE ( 2, ( #39394, #6492, #51199, #67831, #17204, #56727, #50116, #68197, #72645 ),
 .UNSPECIFIED., .F., .F. ) 
 B_SPLINE_CURVE_WITH_KNOTS ( ( 3, 2, 2, 2, 3 ),
 ( 0.7717391304347825942, 0.7753623188405797118, 0.7826086956521739468, 0.7898550724637680709, 0.7934782608695651884 ),
 .UNSPECIFIED. ) 
 CURVE ( )  GEOMETRIC_REPRESENTATION_ITEM ( )  RATIONAL_B_SPLINE_CURVE ( ( 0.9330127018922194093, 0.9330127018922194093, 1.000000000000000000, 0.8660254037844387076, 1.000000000000000000, 0.8660254037844387076, 1.000000000000000000, 0.9330127018922194093, 0.9330127018922194093 ) ) 
 REPRESENTATION_ITEM ( '' )  );
#53866=CARTESIAN_POINT ( 'NONE',  ( 0.000000000000000000, 20.00000000000000000, 30.00000000000000000 ) ) ;
#53868=CARTESIAN_POINT ( 'NONE',  ( 6.496875000614517504, -3.027376345333614438, 5.243569643749998122 ) ) ;
#53869=CARTESIAN_POINT ( 'NONE',  ( 8.034375000614518925, 6.421520780324663323E-16, -5.243569643749999010 ) ) ;
#53870=CARTESIAN_POINT ( 'NONE',  ( 4.312500000000000000, 2.886751345948126879, 4.999999999999999112 ) ) ;
#53871=CARTESIAN_POINT ( 'NONE',  ( -3.000416591977282496E-16, 13.39062500061459460, 25.09994784771203058 ) ) ;
#53872=CARTESIAN_POINT ( 'NONE',  ( -3.999999999999999112, 17.71249999999999858, -32.30940107675850470 ) ) ;
#53873=CARTESIAN_POINT ( 'NONE',  ( 4.162499999999999645, 2.886751345948129099, -4.999999999999998224 ) ) ;
#53875=ORIENTED_EDGE ( 'NONE', *, *, #49176, .F. ) ;
#53876=CARTESIAN_POINT ( 'NONE',  ( 19.71562500061451928, 3.027376345333613106, -5.243569643749998122 ) ) ;
#53877=CARTESIAN_POINT ( 'NONE',  ( 10.22812500061451679, 6.421520780324663323E-16, -5.243569643749999010 ) ) ;
#53879=CARTESIAN_POINT ( 'NONE',  ( 6.309375000614517504, 4.541064518000418104, -2.621784821874998173 ) ) ;
#53880=CARTESIAN_POINT ( 'NONE',  ( 26.32499999999999929, 4.330127018922191873, 2.499999999999999556 ) ) ;
#53881=CARTESIAN_POINT ( 'NONE',  ( 19.95000000122903572, -2.886751345948125991, -5.000000000000000000 ) ) ;
#53882=CARTESIAN_POINT ( 'NONE',  ( 28.11562500061451431, -6.054752690667223547, -1.112240025338166033E-15 ) ) ;
#53884=CARTESIAN_POINT ( 'NONE',  ( 8.371875000614515727, -6.054752690667223547, -1.112240025338166033E-15 ) ) ;
#53885=CARTESIAN_POINT ( 'NONE',  ( 14.70937500061451786, -4.541064518000417216, -2.621784821875001281 ) ) ;
#53886=CARTESIAN_POINT ( 'NONE',  ( 25.99687500061451928, -3.027376345333610441, -5.243569643749999898 ) ) ;
#53887=AXIS2_PLACEMENT_3D ( 'NONE', #46845, #57552, #24297 ) ;
#53888=LINE ( 'NONE', #30612, #24153 ) ;
#53890=CARTESIAN_POINT ( 'NONE',  ( 20.18437500061451573, 6.421520780324663323E-16, -5.243569643749999010 ) ) ;
#53891=CARTESIAN_POINT ( 'NONE',  ( 12.53437500061451537, 6.421520780324663323E-16, -5.243569643749999010 ) ) ;
#53893=CARTESIAN_POINT ( 'NONE',  ( 24.52499999999999858, 4.330127018922191873, 2.499999999999999556 ) ) ;
#53895=CARTESIAN_POINT ( 'NONE',  ( 4.243569643749999898, 11.49687500061451928, -27.54997392385601529 ) ) ;
#53897=CARTESIAN_POINT ( 'NONE',  ( 15.62812500061451537, 6.421520780324663323E-16, -5.243569643749999010 ) ) ;
#53898=CARTESIAN_POINT ( 'NONE',  ( 3.787500000000002753, 5.773502691896255534, 3.535250795749688894E-16 ) ) ;
#53899=LINE ( 'NONE', #65700, #32500 ) ;
#53900=CARTESIAN_POINT ( 'NONE',  ( 0.000000000000000000, 20.00000000000000000, 30.00000000000000000 ) ) ;
#53901=CARTESIAN_POINT ( 'NONE',  ( 11.84999999999999964, 4.330127018922192761, -2.499999999999997780 ) ) ;
#53902=CARTESIAN_POINT ( 'NONE',  ( 3.999999999999999112, 17.18750000122903288, 30.00000000000000000 ) ) ;
#53903=CARTESIAN_POINT ( 'NONE',  ( 11.85000000122903430, -2.886751345948125991, -5.000000000000000000 ) ) ;
#53904=CARTESIAN_POINT ( 'NONE',  ( 22.32187500061451502, -6.054752690667223547, -1.112240025338166033E-15 ) ) ;
#53905=CARTESIAN_POINT ( 'NONE',  ( 15.45937500061451608, 0.000000000000000000, 5.243569643749999010 ) ) ;
#53906=AXIS2_PLACEMENT_3D ( 'NONE', #71120, #59658, #65205 ) ;
#53907=EDGE_LOOP ( 'NONE', ( #23434, #67300, #49700, #7395 ) ) ;
#53908=CARTESIAN_POINT ( 'NONE',  ( 17.87812500061451715, 6.421520780324663323E-16, -5.243569643749999010 ) ) ;
#53909=CARTESIAN_POINT ( 'NONE',  ( 3.215625000614518836, 3.027376345333611329, 5.243569643749999010 ) ) ;
#53910=CARTESIAN_POINT ( 'NONE',  ( 18.60937500061451644, 0.000000000000000000, 5.243569643749999010 ) ) ;
#53911=CARTESIAN_POINT ( 'NONE',  ( 29.74687500061451217, 6.054752690667223547, 3.707466751127219781E-16 ) ) ;
#53912=CARTESIAN_POINT ( 'NONE',  ( 5.165625000614518569, -6.054752690667223547, -1.112240025338166033E-15 ) ) ;
#53913=CARTESIAN_POINT ( 'NONE',  ( 19.26562500061451644, 3.027376345333613106, -5.243569643749998122 ) ) ;
#53914=CARTESIAN_POINT ( 'NONE',  ( -2.121784821874996840, 12.22812500061451857, 33.67503911421598417 ) ) ;
#53915=CARTESIAN_POINT ( 'NONE',  ( 15.45000000122903216, -2.886751345948125991, -5.000000000000000000 ) ) ;
#53917=CARTESIAN_POINT ( 'NONE',  ( 5.990625000614517859, -3.027376345333614438, 5.243569643749998122 ) ) ;
#53918=CARTESIAN_POINT ( 'NONE',  ( 26.09062500061451573, 6.054752690667223547, 3.707466751127219781E-16 ) ) ;
#53919=CARTESIAN_POINT ( 'NONE',  ( 23.25937500061451857, -4.541064518000417216, -2.621784821875001281 ) ) ;
#53920=CARTESIAN_POINT ( 'NONE',  ( 14.31562500061451537, 3.027376345333613106, -5.243569643749998122 ) ) ;
#53921=CARTESIAN_POINT ( 'NONE',  ( 25.91250000122903074, 4.330127018922192761, -2.499999999999997780 ) ) ;
#53922=CARTESIAN_POINT ( 'NONE',  ( 22.22812500061451502, -4.541064518000419881, 2.621784821874995952 ) ) ;
#53923=CARTESIAN_POINT ( 'NONE',  ( 19.13437500061451857, -4.541064518000419881, 2.621784821874995952 ) ) ;
#53924=CARTESIAN_POINT ( 'NONE',  ( 15.51562500061451644, -6.054752690667223547, -1.112240025338166033E-15 ) ) ;
#53925=CARTESIAN_POINT ( 'NONE',  ( -4.243569643749997233, 14.94687500061451679, 32.45002607614398471 ) ) ;
#53926=CARTESIAN_POINT ( 'NONE',  ( 20.61562500061451431, 3.027376345333613106, -5.243569643749998122 ) ) ;
#53927=CARTESIAN_POINT ( 'NONE',  ( 29.05312500061451431, -4.541064518000417216, -2.621784821875001281 ) ) ;
#53928=ORIENTED_EDGE ( 'NONE', *, *, #71265, .F. ) ;
#53930=CARTESIAN_POINT ( 'NONE',  ( 22.91249999999999432, -5.773502691896255534, -1.060575238724906372E-15 ) ) ;
#53931=CARTESIAN_POINT ( 'NONE',  ( -3.999999999999997335, 10.13750000000000284, -27.69059892324149175 ) ) ;
#53932=CARTESIAN_POINT ( 'NONE',  ( 2.733878782416514941, -4.186395442746991158, 2.733878782416514941 ) ) ;
#53933=CARTESIAN_POINT ( 'NONE',  ( 27.59062500061451573, -3.027376345333614438, 5.243569643749998122 ) ) ;
#53934=CARTESIAN_POINT ( 'NONE',  ( 7.265625000614516438, 3.027376345333611329, 5.243569643749999010 ) ) ;
#53935=CARTESIAN_POINT ( 'NONE',  ( 20.25000000122903288, -2.886751345948129988, 4.999999999999997335 ) ) ;
#53936=CARTESIAN_POINT ( 'NONE',  ( 25.60312500061451502, 4.541064518000418104, -2.621784821874998173 ) ) ;
#53937=CARTESIAN_POINT ( 'NONE',  ( 24.07499999999999929, 4.330127018922191873, 2.499999999999999556 ) ) ;
#53938=CARTESIAN_POINT ( 'NONE',  ( 28.45312500061451289, 0.000000000000000000, 5.243569643749999010 ) ) ;
#53939=CARTESIAN_POINT ( 'NONE',  ( 8.203125000614518214, 0.000000000000000000, 5.243569643749999010 ) ) ;
#53940=ORIENTED_EDGE ( 'NONE', *, *, #44720, .F. ) ;
#53941=EDGE_CURVE ( 'NONE', #41163, #49458, #21773, .T. ) ;
#53942=CARTESIAN_POINT ( 'NONE',  ( 22.86562500061451431, 3.027376345333613106, -5.243569643749998122 ) ) ;
#53943=CARTESIAN_POINT ( 'NONE',  ( 6.065625000614516260, -6.054752690667223547, -1.112240025338166033E-15 ) ) ;
#53945=CARTESIAN_POINT ( 'NONE',  ( 4.153125000614515727, 0.000000000000000000, 5.243569643749999010 ) ) ;
#53946=CARTESIAN_POINT ( 'NONE',  ( -3.999999999999999556, 14.67500000122903536, -32.30940107675850470 ) ) ;
#53947=CARTESIAN_POINT ( 'NONE',  ( -5.810221930991193690E-16, 10.10000000122903430, 26.00000000000000355 ) ) ;
#53949=CARTESIAN_POINT ( 'NONE',  ( 10.23750000000000071, -2.886751345948129988, 4.999999999999997335 ) ) ;
#53950=CARTESIAN_POINT ( 'NONE',  ( 10.32187500061451679, 3.027376345333613106, -5.243569643749998122 ) ) ;
#53951=CARTESIAN_POINT ( 'NONE',  ( 8.925000001229033586, 2.886751345948126879, 4.999999999999999112 ) ) ;
#53952=CARTESIAN_POINT ( 'NONE',  ( 14.89687500061451786, 6.054752690667223547, 3.707466751127219781E-16 ) ) ;
#53954=CARTESIAN_POINT ( 'NONE',  ( 6.609375000614519102, -4.541064518000417216, -2.621784821875001281 ) ) ;
#53955=CARTESIAN_POINT ( 'NONE',  ( -4.243569643749999898, 9.903125000614517504, -30.00000000000000000 ) ) ;
#53957=CARTESIAN_POINT ( 'NONE',  ( 12.38437500061451857, -4.541064518000419881, 2.621784821874995952 ) ) ;
#53959=CARTESIAN_POINT ( 'NONE',  ( 21.85312500061451502, -4.541064518000417216, -2.621784821875001281 ) ) ;
#53960=CARTESIAN_POINT ( 'NONE',  ( -2.121784821874996840, 10.93437500061451928, 33.67503911421598417 ) ) ;
#53961=CARTESIAN_POINT ( 'NONE',  ( -4.243569643749999898, 18.90312500061459033, 30.00000000000000000 ) ) ;
#53962=CARTESIAN_POINT ( 'NONE',  ( 25.99687500061451928, -3.027376345333610441, -5.243569643749999898 ) ) ;
#53963=FACE_OUTER_BOUND ( 'NONE', #66225, .T. ) ;
#53964=CARTESIAN_POINT ( 'NONE',  ( 5.615625000614517859, -6.054752690667223547, -1.112240025338166033E-15 ) ) ;
#53966=CARTESIAN_POINT ( 'NONE',  ( 17.63437500061451502, 4.541064518000418104, 2.621784821874999949 ) ) ;
#53968=CARTESIAN_POINT ( 'NONE',  ( 26.47500000122903074, 2.886751345948126879, 4.999999999999999112 ) ) ;
#53969=CARTESIAN_POINT ( 'NONE',  ( 5.334375000614517859, 6.421520780324663323E-16, -5.243569643749999010 ) ) ;
#53970=CARTESIAN_POINT ( 'NONE',  ( 16.17187500061451644, 3.027376345333613106, -5.243569643749998122 ) ) ;
#53971=CARTESIAN_POINT ( 'NONE',  ( 4.829389079492484527, -1.295504259766551813, -5.081142917896463551 ) ) ;
#53972=CARTESIAN_POINT ( 'NONE',  ( 24.37500000000000000, 6.123233995736764310E-16, -4.999999999999998224 ) ) ;
#53973=CARTESIAN_POINT ( 'NONE',  ( 4.350000001229033408, 5.773502691896255534, 3.535250795749688894E-16 ) ) ;
#53974=CARTESIAN_POINT ( 'NONE',  ( 26.22187500061451715, 3.027376345333611329, 5.243569643749999010 ) ) ;
#53976=CARTESIAN_POINT ( 'NONE',  ( 5.587500001229033231, 6.123233995736764310E-16, -4.999999999999998224 ) ) ;
#53977=CARTESIAN_POINT ( 'NONE',  ( 7.612500000000000711, -5.773502691896255534, -1.060575238724906372E-15 ) ) ;
#53979=CARTESIAN_POINT ( 'NONE',  ( 22.56562500061451715, 3.027376345333611329, 5.243569643749999010 ) ) ;
#53980=CARTESIAN_POINT ( 'NONE',  ( 10.68750000000000000, -2.886751345948129988, 4.999999999999997335 ) ) ;
#53981=CARTESIAN_POINT ( 'NONE',  ( 3.928125000614516527, 6.421520780324663323E-16, -5.243569643749999010 ) ) ;
#53982=CARTESIAN_POINT ( 'NONE',  ( 19.72499999999999787, -4.330127018922194537, 2.499999999999995559 ) ) ;
#53983=EDGE_CURVE ( 'NONE', #9370, #63581, #39146, .T. ) ;
#53984=CARTESIAN_POINT ( 'NONE',  ( 18.77812500061451573, 6.421520780324663323E-16, -5.243569643749999010 ) ) ;
#53985=CARTESIAN_POINT ( 'NONE',  ( 4.738577610423850395, 3.409353767520035383, -4.094826053678926492 ) ) ;
#53986=CARTESIAN_POINT ( 'NONE',  ( 23.25000000122903288, 5.773502691896255534, 3.535250795749688894E-16 ) ) ;
#53988=CARTESIAN_POINT ( 'NONE',  ( 3.600000000000002309, -4.330127018922190985, -2.500000000000001332 ) ) ;
#53989=EDGE_CURVE ( 'NONE', #60188, #4158, #46026, .T. ) ;
#53990=ORIENTED_EDGE ( 'NONE', *, *, #68150, .T. ) ;
#53991=CARTESIAN_POINT ( 'NONE',  ( 19.26562500061451644, 3.027376345333613106, -5.243569643749998122 ) ) ;
#53992=CARTESIAN_POINT ( 'NONE',  ( 26.99062500061451431, 6.054752690667223547, 3.707466751127219781E-16 ) ) ;
#53993=CARTESIAN_POINT ( 'NONE',  ( 23.89687500061451786, 6.054752690667223547, 3.707466751127219781E-16 ) ) ;
#53994=CARTESIAN_POINT ( 'NONE',  ( 8.324999999999999289, 4.330127018922191873, 2.499999999999999556 ) ) ;
#53995=CARTESIAN_POINT ( 'NONE',  ( 13.04062500061451502, 6.054752690667223547, 3.707466751127219781E-16 ) ) ;
#53996=CARTESIAN_POINT ( 'NONE',  ( 27.47812500061451502, 4.541064518000418104, 2.621784821874999949 ) ) ;
#53997=CARTESIAN_POINT ( 'NONE',  ( 18.12187500061451573, 3.027376345333611329, 5.243569643749999010 ) ) ;
#53998=CARTESIAN_POINT ( 'NONE',  ( 8.840625000614515727, -3.027376345333610441, -5.243569643749999898 ) ) ;
#53999=CARTESIAN_POINT ( 'NONE',  ( -5.810221930991193690E-16, 18.65000000122903501, 26.00000000000000355 ) ) ;
#54000=CARTESIAN_POINT ( 'NONE',  ( -3.000416591977282496E-16, 11.19687500061451679, 25.09994784771203058 ) ) ;
#54002=CARTESIAN_POINT ( 'NONE',  ( 24.41250000122903430, -4.330127018922190985, -2.500000000000001332 ) ) ;
#54004=CARTESIAN_POINT ( 'NONE',  ( 14.24062500061451608, -3.027376345333610441, -5.243569643749999898 ) ) ;
#54005=CARTESIAN_POINT ( 'NONE',  ( 9.646875000614516082, -3.027376345333614438, 5.243569643749998122 ) ) ;
#54006=CARTESIAN_POINT ( 'NONE',  ( 9.346875000614517148, -3.027376345333610441, -5.243569643749999898 ) ) ;
#54008=VERTEX_POINT ( 'NONE', #13960 ) ;
#54010=CARTESIAN_POINT ( 'NONE',  ( 21.32812500061451644, -4.541064518000419881, 2.621784821874995952 ) ) ;
#54011=CARTESIAN_POINT ( 'NONE',  ( 16.99687500061451573, -3.027376345333610441, -5.243569643749999898 ) ) ;
#54012=CARTESIAN_POINT ( 'NONE',  ( 22.82812500061451644, 6.421520780324663323E-16, -5.243569643749999010 ) ) ;
#54013=CARTESIAN_POINT ( 'NONE',  ( -1.999999999999997113, 11.07500000000000107, 33.46410161513775705 ) ) ;
#54014=CARTESIAN_POINT ( 'NONE',  ( 27.59062500061451573, -3.027376345333614438, 5.243569643749998122 ) ) ;
#54015=CARTESIAN_POINT ( 'NONE',  ( 8.287500001229034297, 6.123233995736764310E-16, -4.999999999999998224 ) ) ;
#54017=CARTESIAN_POINT ( 'NONE',  ( 2.775000001229033675, -5.773502691896255534, -1.060575238724906372E-15 ) ) ;
#54018=CARTESIAN_POINT ( 'NONE',  ( 2.000000000000001332, 17.00000000000000000, -26.53589838486224650 ) ) ;
#54019=CARTESIAN_POINT ( 'NONE',  ( 24.45000000122903572, -2.886751345948125991, -5.000000000000000000 ) ) ;
#54021=EDGE_CURVE ( 'NONE', #26767, #27538, #3522, .T. ) ;
#54022=CARTESIAN_POINT ( 'NONE',  ( 5.934375000614517504, 4.541064518000418104, 2.621784821874999949 ) ) ;
#54023=CARTESIAN_POINT ( 'NONE',  ( 23.47499999999999787, 6.123233995736764310E-16, -4.999999999999998224 ) ) ;
#54024=CARTESIAN_POINT ( 'NONE',  ( 15.32812500061451644, 4.541064518000418104, 2.621784821874999949 ) ) ;
#54025=CARTESIAN_POINT ( 'NONE',  ( 7.809375000614519280, 0.000000000000000000, 5.243569643749999010 ) ) ;
#54026=CARTESIAN_POINT ( 'NONE',  ( 25.91250000122903074, 4.330127018922192761, -2.499999999999997780 ) ) ;
#54027=CARTESIAN_POINT ( 'NONE',  ( 17.63437500061451502, 4.541064518000418104, 2.621784821874999949 ) ) ;
#54028=CARTESIAN_POINT ( 'NONE',  ( 5.559375000614517504, 0.000000000000000000, 5.243569643749999010 ) ) ;
#54030=CARTESIAN_POINT ( 'NONE',  ( 4.490625000614516971, 6.054752690667223547, 3.707466751127219781E-16 ) ) ;
#54031=CARTESIAN_POINT ( 'NONE',  ( 15.81562500061451537, 3.027376345333611329, 5.243569643749999010 ) ) ;
#54033=CARTESIAN_POINT ( 'NONE',  ( 12.40312500061451573, -4.541064518000417216, -2.621784821875001281 ) ) ;
#54034=CARTESIAN_POINT ( 'NONE',  ( 4.612500001229032698, -4.330127018922190985, -2.500000000000001332 ) ) ;
#54035=CARTESIAN_POINT ( 'NONE',  ( 9.890625000614516438, 6.054752690667223547, 3.707466751127219781E-16 ) ) ;
#54037=CARTESIAN_POINT ( 'NONE',  ( 10.46249999999999858, 2.886751345948129099, -4.999999999999998224 ) ) ;
#54038=CARTESIAN_POINT ( 'NONE',  ( 3.637500001229036162, -4.330127018922194537, 2.499999999999995559 ) ) ;
#54039=CARTESIAN_POINT ( 'NONE',  ( 18.00000000000000355, -4.330127018922190985, -2.500000000000001332 ) ) ;
#54040=CARTESIAN_POINT ( 'NONE',  ( 17.93437500061451928, 6.421520780324663323E-16, -5.243569643749999010 ) ) ;
#54041=CARTESIAN_POINT ( 'NONE',  ( 15.45000000122903216, -2.886751345948125991, -5.000000000000000000 ) ) ;
#54043=CARTESIAN_POINT ( 'NONE',  ( -4.243569643749997233, 15.34062500061451750, -27.54997392385601174 ) ) ;
#54045=CARTESIAN_POINT ( 'NONE',  ( -1.071796769724487453, 18.55759618943233491, 26.00000000000000000 ) ) ;
#54046=CARTESIAN_POINT ( 'NONE',  ( 29.27812500061451573, 4.541064518000418104, 2.621784821874999949 ) ) ;
#54048=CARTESIAN_POINT ( 'NONE',  ( -6.275039685470489619E-15, 18.31250000000000000, 33.99999999999999289 ) ) ;
#54050=CARTESIAN_POINT ( 'NONE',  ( 16.99687500061451573, -3.027376345333610441, -5.243569643749999898 ) ) ;
#54051=( BOUNDED_CURVE ( )  B_SPLINE_CURVE ( 2, ( #4726, #59757, #43520, #37234, #31330, #49425, #26900 ),
 .UNSPECIFIED., .F., .F. ) 
 B_SPLINE_CURVE_WITH_KNOTS ( ( 3, 2, 2, 3 ),
 ( 0.3250000000000000111, 0.3277777777777777790, 0.3305555555555556024, 0.3333333333333333703 ),
 .UNSPECIFIED. ) 
 CURVE ( )  GEOMETRIC_REPRESENTATION_ITEM ( )  RATIONAL_B_SPLINE_CURVE ( ( 1.000000000000000000, 0.8660254037844387076, 1.000000000000000000, 0.8660254037844387076, 1.000000000000000000, 0.8660254037844360431, 1.000000000000002665 ) ) 
 REPRESENTATION_ITEM ( '' )  );
#54052=CARTESIAN_POINT ( 'NONE',  ( 28.68749999999999645, -2.886751345948129988, 4.999999999999997335 ) ) ;
#54053=CARTESIAN_POINT ( 'NONE',  ( 12.25312500061451537, 0.000000000000000000, 5.243569643749999010 ) ) ;
#54055=CARTESIAN_POINT ( 'NONE',  ( 23.59687500061451715, -3.027376345333614438, 5.243569643749998122 ) ) ;
#54057=CARTESIAN_POINT ( 'NONE',  ( 7.340625000614518392, -3.027376345333614438, 5.243569643749998122 ) ) ;
#54058=CARTESIAN_POINT ( 'NONE',  ( 12.87187500061451750, -6.054752690667223547, -1.112240025338166033E-15 ) ) ;
#54060=CARTESIAN_POINT ( 'NONE',  ( 24.72187500061451360, 3.027376345333613106, -5.243569643749998122 ) ) ;
#54061=CARTESIAN_POINT ( 'NONE',  ( 28.04062500061451502, -3.027376345333614438, 5.243569643749998122 ) ) ;
#54062=CARTESIAN_POINT ( 'NONE',  ( 8.587500000000002132, -2.886751345948125991, -5.000000000000000000 ) ) ;
#54063=CARTESIAN_POINT ( 'NONE',  ( 17.40000000122903145, 5.773502691896255534, 3.535250795749688894E-16 ) ) ;
#54064=CARTESIAN_POINT ( 'NONE',  ( 27.30000000122903359, 5.773502691896255534, 3.535250795749688401E-16 ) ) ;
#54066=EDGE_LOOP ( 'NONE', ( #46477, #22922, #49609, #38241 ) ) ;
#54067=CARTESIAN_POINT ( 'NONE',  ( 14.96250000000000036, 2.886751345948129099, -4.999999999999998224 ) ) ;
#54068=CARTESIAN_POINT ( 'NONE',  ( 18.75000000000000000, 0.000000000000000000, 4.999999999999998224 ) ) ;
#54069=CARTESIAN_POINT ( 'NONE',  ( 13.60312500061451679, 0.000000000000000000, 5.243569643749999010 ) ) ;
#54070=VERTEX_POINT ( 'NONE', #6975 ) ;
#54072=CARTESIAN_POINT ( 'NONE',  ( 9.001249775931846008E-16, 18.17187500061451999, -25.09994784771203058 ) ) ;
#54073=CARTESIAN_POINT ( 'NONE',  ( 3.890625000614517326, -3.027376345333610441, -5.243569643749999898 ) ) ;
#54075=CARTESIAN_POINT ( 'NONE',  ( 10.08749999999999858, 5.773502691896255534, 3.535250795749688894E-16 ) ) ;
#54077=EDGE_LOOP ( 'NONE', ( #65501, #70890, #39860, #32254 ) ) ;
#54078=CARTESIAN_POINT ( 'NONE',  ( -3.000416591977282496E-16, 15.19062500061451715, 25.09994784771203058 ) ) ;
#54079=CARTESIAN_POINT ( 'NONE',  ( 26.16562500061451502, 3.027376345333611329, 5.243569643749999010 ) ) ;
#54082=CARTESIAN_POINT ( 'NONE',  ( 24.30937500061451573, 4.541064518000418104, -2.621784821874998173 ) ) ;
#54083=CARTESIAN_POINT ( 'NONE',  ( 18.25312500061451715, -4.541064518000417216, -2.621784821875001281 ) ) ;
#54084=CARTESIAN_POINT ( 'NONE',  ( -4.243569643749999898, 13.05312500061459424, -30.00000000000000000 ) ) ;
#54085=CARTESIAN_POINT ( 'NONE',  ( 24.22500000122903430, 2.886751345948126879, 4.999999999999999112 ) ) ;
#54086=CARTESIAN_POINT ( 'NONE',  ( 3.853125000614517681, -4.541064518000417216, -2.621784821875001281 ) ) ;
#54088=CARTESIAN_POINT ( 'NONE',  ( 21.77812500061451928, -4.541064518000419881, 2.621784821874995952 ) ) ;
#54091=CARTESIAN_POINT ( 'NONE',  ( 16.50937500061451502, -4.541064518000417216, -2.621784821875001281 ) ) ;
#54093=CARTESIAN_POINT ( 'NONE',  ( 17.55937500061451573, 4.541064518000418104, -2.621784821874998173 ) ) ;
#54094=CARTESIAN_POINT ( 'NONE',  ( 25.65937500061451715, 4.541064518000418104, -2.621784821874998173 ) ) ;
#54095=CARTESIAN_POINT ( 'NONE',  ( -2.121784821874996840, 13.63437500061451857, 33.67503911421598417 ) ) ;
#54096=CARTESIAN_POINT ( 'NONE',  ( 5.278125000614516615, 6.421520780324663323E-16, -5.243569643749999010 ) ) ;
#54097=CARTESIAN_POINT ( 'NONE',  ( 28.00312500061451715, 0.000000000000000000, 5.243569643749999010 ) ) ;
#54098=CARTESIAN_POINT ( 'NONE',  ( 28.30312500061451431, 4.541064518000418104, -2.621784821874998173 ) ) ;
#54099=CARTESIAN_POINT ( 'NONE',  ( 3.999999999999998668, 16.32500000122903216, -32.30940107675850470 ) ) ;
#54100=CARTESIAN_POINT ( 'NONE',  ( 6.834375000614518747, 4.541064518000418104, 2.621784821874999949 ) ) ;
#54101=CARTESIAN_POINT ( 'NONE',  ( 13.23750000122903359, 6.123233995736764310E-16, -4.999999999999998224 ) ) ;
#54102=CARTESIAN_POINT ( 'NONE',  ( 8.812500001229034652, 4.330127018922192761, -2.499999999999997780 ) ) ;
#54103=CARTESIAN_POINT ( 'NONE',  ( 3.890625000614517326, -3.027376345333610441, -5.243569643749999898 ) ) ;
#54106=CARTESIAN_POINT ( 'NONE',  ( 13.39687500061451608, -3.027376345333610441, -5.243569643749999898 ) ) ;
#54108=ORIENTED_EDGE ( 'NONE', *, *, #29492, .T. ) ;
#54109=CARTESIAN_POINT ( 'NONE',  ( 22.86562500061451431, 3.027376345333613106, -5.243569643749998122 ) ) ;
#54110=CARTESIAN_POINT ( 'NONE',  ( 7.528125000614515727, 6.421520780324663323E-16, -5.243569643749999010 ) ) ;
#54111=CARTESIAN_POINT ( 'NONE',  ( 24.34687500061451715, 6.054752690667223547, 3.707466751127219781E-16 ) ) ;
#54112=CARTESIAN_POINT ( 'NONE',  ( 7.978125000614517681, 6.421520780324663323E-16, -5.243569643749999010 ) ) ;
#54113=CARTESIAN_POINT ( 'NONE',  ( 20.51249999999999929, 2.886751345948161074, 4.999999999999941380 ) ) ;
#54114=CARTESIAN_POINT ( 'NONE',  ( 8.062500001229034652, 0.000000000000000000, 4.999999999999998224 ) ) ;
#54115=CARTESIAN_POINT ( 'NONE',  ( 21.66562500061451502, 3.027376345333611329, 5.243569643749999010 ) ) ;
#54117=CARTESIAN_POINT ( 'NONE',  ( -3.000416591977282496E-16, 10.24062500061451608, -34.90005215228797653 ) ) ;
#54118=CARTESIAN_POINT ( 'NONE',  ( 11.10000000122903252, 5.773502691896255534, 3.535250795749688894E-16 ) ) ;
#54119=CARTESIAN_POINT ( 'NONE',  ( 19.79062500061451502, 6.054752690667223547, 3.707466751127219781E-16 ) ) ;
#54120=CARTESIAN_POINT ( 'NONE',  ( 17.65312500061451573, 0.000000000000000000, 5.243569643749999010 ) ) ;
#54122=CARTESIAN_POINT ( 'NONE',  ( 17.28750000000000142, 5.773502691896255534, 3.535250795749688894E-16 ) ) ;
#54123=CARTESIAN_POINT ( 'NONE',  ( 11.62500000122903465, 2.886751345948126879, 4.999999999999999112 ) ) ;
#54124=EDGE_CURVE ( 'NONE', #8958, #57550, #23950, .T. ) ;
#54125=CARTESIAN_POINT ( 'NONE',  ( 7.790625000614518569, -3.027376345333614438, 5.243569643749998122 ) ) ;
#54126=CARTESIAN_POINT ( 'NONE',  ( 13.79062500061451502, -3.027376345333610441, -5.243569643749999898 ) ) ;
#54127=CARTESIAN_POINT ( 'NONE',  ( 22.35000000122903074, 5.773502691896255534, 3.535250795749688894E-16 ) ) ;
#54128=CARTESIAN_POINT ( 'NONE',  ( 20.74687500061451573, 6.054752690667223547, 3.707466751127219781E-16 ) ) ;
#54129=CARTESIAN_POINT ( 'NONE',  ( 9.637500001229033941, 6.123233995736764310E-16, -4.999999999999998224 ) ) ;
#54130=EDGE_CURVE ( 'NONE', #65074, #44184, #45309, .T. ) ;
#54131=CARTESIAN_POINT ( 'NONE',  ( 5.887500001229034829, -4.330127018922194537, 2.499999999999995559 ) ) ;
#54132=CARTESIAN_POINT ( 'NONE',  ( 7.246875000614518392, 6.054752690667223547, 3.707466751127219781E-16 ) ) ;
#54133=CARTESIAN_POINT ( 'NONE',  ( 22.92187500061451644, 3.027376345333613106, -5.243569643749998122 ) ) ;
#54134=CARTESIAN_POINT ( 'NONE',  ( 4.564313923822768793, 2.041911324548167261, -4.640016024762649849 ) ) ;
#54135=CARTESIAN_POINT ( 'NONE',  ( 19.97812500061451502, -4.541064518000419881, 2.621784821874995952 ) ) ;
#54136=CARTESIAN_POINT ( 'NONE',  ( 23.44687500061451502, 6.054752690667223547, 3.707466751127219781E-16 ) ) ;
#54138=CARTESIAN_POINT ( 'NONE',  ( 12.56250000122903465, 0.000000000000000000, 4.999999999999998224 ) ) ;
#54139=CARTESIAN_POINT ( 'NONE',  ( 1.626862140677534273E-15, 13.47500000122903252, -26.00000000000000355 ) ) ;
#54140=CARTESIAN_POINT ( 'NONE',  ( 4.809375000614516615, -4.541064518000417216, -2.621784821875001281 ) ) ;
#54141=CARTESIAN_POINT ( 'NONE',  ( 17.12812500061451715, 4.541064518000418104, 2.621784821874999949 ) ) ;
#54142=CARTESIAN_POINT ( 'NONE',  ( 12.75937500061451857, 0.000000000000000000, 5.243569643749999010 ) ) ;
#54144=CARTESIAN_POINT ( 'NONE',  ( 1.071796769724484344, 16.98259618943233562, -25.99999999999999645 ) ) ;
#54145=CARTESIAN_POINT ( 'NONE',  ( 25.79062500061451502, -3.027376345333614438, 5.243569643749998122 ) ) ;
#54146=CARTESIAN_POINT ( 'NONE',  ( 1.626862140677534273E-15, 10.77500000122903323, -26.00000000000000355 ) ) ;
#54147=CARTESIAN_POINT ( 'NONE',  ( -3.999999999999999112, 11.52500000122903501, -32.30940107675850470 ) ) ;
#54148=CARTESIAN_POINT ( 'NONE',  ( 14.47499999999999964, 6.123233995736764310E-16, -4.999999999999998224 ) ) ;
#54149=CARTESIAN_POINT ( 'NONE',  ( 24.63750000122903216, 4.330127018922191873, 2.499999999999999556 ) ) ;
#54150=CARTESIAN_POINT ( 'NONE',  ( 17.46562500061451217, 3.027376345333613106, -5.243569643749998122 ) ) ;
#54151=VERTEX_POINT ( 'NONE', #54957 ) ;
#54152=CARTESIAN_POINT ( 'NONE',  ( 23.21250000000000213, 2.886751345948126879, 4.999999999999999112 ) ) ;
#54153=CARTESIAN_POINT ( 'NONE',  ( 22.84687500061451715, -3.027376345333610441, -5.243569643749999898 ) ) ;
#54154=ORIENTED_EDGE ( 'NONE', *, *, #44687, .T. ) ;
#54155=CARTESIAN_POINT ( 'NONE',  ( 10.30312500061451431, 4.541064518000418104, -2.621784821874998173 ) ) ;
#54156=CARTESIAN_POINT ( 'NONE',  ( 3.253125000614518036, 0.000000000000000000, 5.243569643749999010 ) ) ;
#54158=CARTESIAN_POINT ( 'NONE',  ( 27.47812500061451502, 4.541064518000418104, 2.621784821874999949 ) ) ;
#54159=CARTESIAN_POINT ( 'NONE',  ( 19.57500000000000284, 4.330127018922191873, 2.499999999999999556 ) ) ;
#54160=CARTESIAN_POINT ( 'NONE',  ( 26.84999999999999787, 0.000000000000000000, 4.999999999999998224 ) ) ;
#54161=CARTESIAN_POINT ( 'NONE',  ( 3.159375000614518036, 4.541064518000418104, -2.621784821874998173 ) ) ;
#54162=CARTESIAN_POINT ( 'NONE',  ( 8.071875000614518569, 3.027376345333613106, -5.243569643749998122 ) ) ;
#54163=CARTESIAN_POINT ( 'NONE',  ( 17.07187500061451502, 3.027376345333613106, -5.243569643749998122 ) ) ;
#54164=EDGE_LOOP ( 'NONE', ( #19320, #19410, #52321, #64324 ) ) ;
#54165=CARTESIAN_POINT ( 'NONE',  ( 27.10312500061451502, 0.000000000000000000, 5.243569643749999010 ) ) ;
#54166=CARTESIAN_POINT ( 'NONE',  ( 28.50937500061451502, 0.000000000000000000, 5.243569643749999010 ) ) ;
#54168=CARTESIAN_POINT ( 'NONE',  ( 16.98750000000000426, -2.886751345948129988, 4.999999999999997335 ) ) ;
#54169=CARTESIAN_POINT ( 'NONE',  ( 11.95312500061451644, -4.541064518000417216, -2.621784821875001281 ) ) ;
#54172=CARTESIAN_POINT ( 'NONE',  ( 29.12812500061451715, 6.421520780324663323E-16, -5.243569643749999010 ) ) ;
#54173=CARTESIAN_POINT ( 'NONE',  ( 17.21250000122903145, -4.330127018922190985, -2.500000000000001332 ) ) ;
#54174=CARTESIAN_POINT ( 'NONE',  ( 8.400000000000000355, 0.000000000000000000, 4.999999999999998224 ) ) ;
#54176=CARTESIAN_POINT ( 'NONE',  ( 5.090625000614516615, -3.027376345333614438, 5.243569643749998122 ) ) ;
#54177=CARTESIAN_POINT ( 'NONE',  ( 22.73437500061451644, -4.541064518000419881, 2.621784821874995952 ) ) ;
#54178=CARTESIAN_POINT ( 'NONE',  ( 2.121784821875001281, 17.30937500061451573, 33.67503911421598417 ) ) ;
#54179=EDGE_CURVE ( 'NONE', #14728, #40395, #50767, .T. ) ;
#54180=CARTESIAN_POINT ( 'NONE',  ( 25.17187500061451644, 3.027376345333613106, -5.243569643749998122 ) ) ;
#54181=CARTESIAN_POINT ( 'NONE',  ( 4.875000000000000888, -4.330127018922194537, 2.499999999999995559 ) ) ;
#54182=CARTESIAN_POINT ( 'NONE',  ( -2.000000000000000000, 11.03750000122903430, 26.53589838486224650 ) ) ;
#54183=CARTESIAN_POINT ( 'NONE',  ( 12.51562500061451821, 3.027376345333613106, -5.243569643749998122 ) ) ;
#54184=CARTESIAN_POINT ( 'NONE',  ( 4.462500001229035007, 0.000000000000000000, 4.999999999999998224 ) ) ;
#54185=CARTESIAN_POINT ( 'NONE',  ( 9.384375000614518569, 6.421520780324663323E-16, -5.243569643749999010 ) ) ;
#54187=CARTESIAN_POINT ( 'NONE',  ( 10.11562500061451608, -6.054752690667223547, -1.112240025338166033E-15 ) ) ;
#54188=CARTESIAN_POINT ( 'NONE',  ( 14.29687500061451821, -3.027376345333610441, -5.243569643749999898 ) ) ;
#54189=( LENGTH_UNIT ( ) NAMED_UNIT ( * ) SI_UNIT ( .MILLI., .METRE. ) );
#54190=CARTESIAN_POINT ( 'NONE',  ( 22.27500000122903145, 2.886751345948129099, -4.999999999999998224 ) ) ;
#54191=CARTESIAN_POINT ( 'NONE',  ( 11.44687500061451857, -3.027376345333614438, 5.243569643749998122 ) ) ;
#54192=CARTESIAN_POINT ( 'NONE',  ( 12.70312500061451821, 0.000000000000000000, 5.243569643749999010 ) ) ;
#54194=CARTESIAN_POINT ( 'NONE',  ( 22.43437500061451573, 6.421520780324663323E-16, -5.243569643749999010 ) ) ;
#54195=CARTESIAN_POINT ( 'NONE',  ( 14.06249999999999645, 2.886751345948062486, -5.000000000000113687 ) ) ;
#54196=CARTESIAN_POINT ( 'NONE',  ( -2.674018119152297590, 4.230323444454995752, 32.98541807432768280 ) ) ;
#54197=CARTESIAN_POINT ( 'NONE',  ( 0.000000000000000000, 20.00000000000000000, -30.00000000000000000 ) ) ;
#54198=CARTESIAN_POINT ( 'NONE',  ( 9.001249775931846008E-16, 15.02187500061451608, -25.09994784771203058 ) ) ;
#54199=CARTESIAN_POINT ( 'NONE',  ( 15.97500000122903430, 2.886751345948129099, -4.999999999999998224 ) ) ;
#54200=CARTESIAN_POINT ( 'NONE',  ( 10.77187500061451786, 3.027376345333613106, -5.243569643749998122 ) ) ;
#54201=CARTESIAN_POINT ( 'NONE',  ( 9.001249775931846008E-16, 16.76562500061451999, -25.09994784771203058 ) ) ;
#54202=CARTESIAN_POINT ( 'NONE',  ( 18.11250000122903359, -4.330127018922190985, -2.500000000000001332 ) ) ;
#54203=CARTESIAN_POINT ( 'NONE',  ( 12.10312500061451857, 4.541064518000418104, -2.621784821874998173 ) ) ;
#54205=CARTESIAN_POINT ( 'NONE',  ( 15.82499999999999929, 6.123233995736764310E-16, -4.999999999999998224 ) ) ;
#54206=FACE_OUTER_BOUND ( 'NONE', #69950, .T. ) ;
#54207=CARTESIAN_POINT ( 'NONE',  ( 9.646875000614519635, -3.027376345333614438, 5.243569643749998122 ) ) ;
#54208=DIRECTION ( 'NONE',  ( -1.000000000000000000, -0.000000000000000000, -0.000000000000000000 ) ) ;
#54209=CARTESIAN_POINT ( 'NONE',  ( 12.63750000122903394, -4.330127018922194537, 2.499999999999995559 ) ) ;
#54210=CARTESIAN_POINT ( 'NONE',  ( 20.25000000122903288, -2.886751345948129988, 4.999999999999997335 ) ) ;
#54211=CARTESIAN_POINT ( 'NONE',  ( 18.29062500061451502, -3.027376345333610441, -5.243569643749999898 ) ) ;
#54212=( BOUNDED_SURFACE ( )  B_SPLINE_SURFACE ( 1, 2, ( 
 ( #16085, #5015, #56349, #20893, #27549, #72974, #22356, #67445, #16442, #21257, #16807, #5739, #43447, #44181, #15713, #65969, #26820, #37890, #60409, #38251, #9818, #71884, #43810, #44552, #55259, #4655, #49718, #46347, #62958, #68521, #13073, #35612, #29710, #56697, #50804, #17882, #51888, #6097, #569, #12353, #68881, #34160, #34888, #57772, #45985, #67797, #28628, #7182, #28273, #18609, #63327, #57053, #207, #17171, #11645, #6821, #58132, #39731, #51166, #40090, #40442, #57417, #63683, #22712, #29355, #35251, #52248, #1651, #18238, #23075, #24159, #45265, #40811, #51531, #68165, #62248, #45632, #41174, #17528, #62604, #12000, #34523, #6459, #1286, #28994, #46712, #23796, #12715, #69247, #931, #23439, #65515, #9006, #35975, #30071, #70327, #31163, #58495, #52971, #64779, #48164, #13426, #14170, #37070, #25249, #47071, #7904, #59593, #7538, #71060, #3474, #64046, #14535, #69606, #41886, #70689, #24885, #25627, #31538, #2016, #20064, #53705, #36704, #54078, #65144, #64414, #59226, #69961, #58861, #8634, #30442, #42984, #3098, #2367, #19332, #47430, #13807, #8271, #19703, #42620, #47797, #25994, #41527, #48533, #36346, #14902, #30801, #20435, #53334, #2732, #37443, #42256, #52610, #24527, #18967, #3839, #383, #11825, #22890, #28450, #62069, #39913, #50627, #56168, #56523, #37803, #45086, #5563, #50985, #45448, #20806, #71429, #67621, #50273, #43361, #67981, #26360, #11096, #32267, #39181, #32, #5916, #28099, #11463, #65884, #62427, #54800, #68346, #15265, #17356, #61697, #33624, #34343, #4206, #56876, #17707, #6280, #48900, #28809, #51348, #751, #23260, #33985, #45810, #22538, #16987, #59963, #60323, #39545, #9371, #31903, #54440, #9733, #26734, #72797, #22180, #44734, #67268, #16627, #63515, #2198, #69074, #40267, #29180, #23623, #18794, #47616, #51713, #46170, #52073, #7367, #52436, #2555, #62788, #29898, #47256, #69790, #19156, #58319, #12544, #41710, #25073, #7730, #12902, #7008, #70147, #68709, #53157, #1116, #29538, #18069, #40630, #63149, #41358, #57604, #13625, #24350, #30264, #1843, #46898, #12181, #34708, #64234, #35078, #57238, #69437, #63868, #1479, #23985 ),
 ( #36168, #6651, #30625, #58686, #46532, #8096, #18433, #41000, #52797, #35435, #24713, #57959, #13258, #35796, #43184, #26183, #43548, #4029, #3294, #3660, #8824, #70884, #48723, #19896, #54993, #71246, #64971, #31361, #36897, #13992, #9559, #42810, #20625, #65703, #25822, #42449, #60149, #30991, #26554, #54266, #9193, #65333, #14362, #4399, #15090, #26928, #32458, #31728, #14722, #49453, #37993, #47992, #37626, #2918, #32092, #48359, #20258, #54623, #25449, #19525, #49094, #71623, #42084, #70521, #64606, #37265, #53902, #20996, #66070, #15448, #59787, #59051, #60514, #36531, #8456, #9920, #53524, #59417, #71987, #16905, #16188, #56446, #62347, #10292, #5480, #32822, #33183, #16546, #33538, #27287, #55722, #21726, #6198, #50904, #34260, #28726, #303, #33902, #27650, #11743, #72345, #56088, #21361, #56793, #15817, #39098, #72714, #43915, #38739, #38360, #50187, #66441, #60887, #55360, #4754, #61259, #66815, #61981, #67542, #49821, #22813, #10653, #44285, #28019, #39832, #5116, #73075, #22097, #44655, #67185, #61615, #11017, #39460, #50547, #22456, #45005, #11383, #5836, #28368, #45364, #67899, #17271, #7644, #68266, #46817, #29817, #17628, #8013, #46090, #51633, #7288, #36086, #57155, #63433, #6566, #40547, #69709, #69355, #12820, #18346, #58606, #51267, #52713, #29098, #669, #40921, #1755, #1034, #23540, #35354, #18712, #68626, #57878, #30182, #68989, #40188, #17988, #2119, #23177, #41632, #47176, #34624, #58239, #62709, #12466, #41277, #63063, #63788, #24631, #45731, #13178, #24268, #52352, #19075, #35717, #34996, #64151, #57525, #29456, #13538, #6926, #12103, #51993, #1394, #23903, #46451, #2836, #8740, #20174, #48639, #48275, #31649, #64521, #9480, #25365, #37913, #13914, #37546, #31273, #3209, #20537, #47909, #3946, #60430, #15009, #47538, #43093, #54544, #65621, #71164, #54182, #32009, #42728, #25738, #26101, #8375, #14638, #70799, #60068, #26469, #36453, #42001, #37179, #19813, #58967, #49008, #70067, #53816, #71539, #59329, #30548, #19440, #30904, #9111, #53075, #53446, #70438, #42366, #65249, #59704, #65990, #2470, #3578, #20914, #43466, #15371, #24994, #64888, #14276 ) ),
 .UNSPECIFIED., .F., .F., .F. ) 
 B_SPLINE_SURFACE_WITH_KNOTS ( ( 2, 2 ),
 ( 3, 2, 2, 2, 2, 2, 2, 2, 2, 2, 2, 2, 2, 2, 2, 2, 2, 2, 2, 2, 2, 2, 2, 2, 2, 2, 2, 2, 2, 2, 2, 2, 2, 2, 2, 2, 2, 2, 2, 2, 2, 2, 2, 2, 2, 2, 2, 2, 2, 2, 2, 2, 2, 2, 2, 2, 2, 2, 2, 2, 2, 2, 2, 2, 2, 2, 2, 2, 2, 2, 2, 2, 2, 2, 2, 2, 2, 2, 2, 2, 2, 2, 2, 2, 2, 2, 2, 2, 2, 2, 2, 2, 2, 2, 2, 2, 2, 2, 2, 2, 2, 2, 2, 2, 2, 2, 2, 2, 2, 2, 2, 2, 2, 2, 2, 2, 2, 2, 2, 2, 2, 2, 2, 2, 2, 2, 2, 2, 2, 2, 2, 2, 2, 2, 3 ),
 ( 0.000000000000000000, 1.000000000000000000 ),
 ( 0.000000000000000000, 0.007246376811594202987, 0.01449275362318840597, 0.02173913043478260809, 0.02898550724637681195, 0.03623188405797101580, 0.04347826086956521618, 0.05072463768115942351, 0.05797101449275362389, 0.06521739130434782428, 0.07246376811594203160, 0.07971014492753622505, 0.08695652173913043237, 0.09420289855072463969, 0.1014492753623188470, 0.1086956521739130405, 0.1159420289855072478, 0.1231884057971014551, 0.1304347826086956486, 0.1376811594202898559, 0.1449275362318840632, 0.1521739130434782705, 0.1594202898550724501, 0.1666666666666666574, 0.1739130434782608647, 0.1811594202898550721, 0.1884057971014492794, 0.1956521739130434867, 0.2028985507246376940, 0.2101449275362318736, 0.2173913043478260809, 0.2246376811594202882, 0.2318840579710144956, 0.2391304347826087029, 0.2463768115942029102, 0.2536231884057971175, 0.2608695652173912971, 0.2681159420289855322, 0.2753623188405797118, 0.2826086956521738913, 0.2898550724637681264, 0.2971014492753623060, 0.3043478260869565410, 0.3115942028985507206, 0.3188405797101449002, 0.3260869565217391353, 0.3333333333333333148, 0.3405797101449275499, 0.3478260869565217295, 0.3550724637681159646, 0.3623188405797101441, 0.3695652173913043237, 0.3768115942028985588, 0.3840579710144927383, 0.3913043478260869734, 0.3985507246376811530, 0.4057971014492753881, 0.4130434782608695676, 0.4202898550724637472, 0.4275362318840579823, 0.4347826086956521618, 0.4420289855072463969, 0.4492753623188405765, 0.4565217391304347561, 0.4637681159420289911, 0.4710144927536231707, 0.4782608695652174058, 0.4855072463768115854, 0.4927536231884058204, 0.5000000000000000000, 0.5072463768115942351, 0.5144927536231883591, 0.5217391304347825942, 0.5289855072463768293, 0.5362318840579710644, 0.5434782608695651884, 0.5507246376811594235, 0.5579710144927536586, 0.5652173913043477826, 0.5724637681159420177, 0.5797101449275362528, 0.5869565217391304879, 0.5942028985507246119, 0.6014492753623188470, 0.6086956521739130821, 0.6159420289855072062, 0.6231884057971014412, 0.6304347826086956763, 0.6376811594202898004, 0.6449275362318840354, 0.6521739130434782705, 0.6594202898550725056, 0.6666666666666666297, 0.6739130434782608647, 0.6811594202898550998, 0.6884057971014492239, 0.6956521739130434590, 0.7028985507246376940, 0.7101449275362319291, 0.7173913043478260532, 0.7246376811594202882, 0.7318840579710145233, 0.7391304347826086474, 0.7463768115942028825, 0.7536231884057971175, 0.7608695652173913526, 0.7681159420289854767, 0.7753623188405797118, 0.7826086956521739468, 0.7898550724637680709, 0.7971014492753623060, 0.8043478260869565410, 0.8115942028985507761, 0.8188405797101449002, 0.8260869565217391353, 0.8333333333333333703, 0.8405797101449274944, 0.8478260869565217295, 0.8550724637681159646, 0.8623188405797101996, 0.8695652173913043237, 0.8768115942028985588, 0.8840579710144927938, 0.8913043478260869179, 0.8985507246376811530, 0.9057971014492753881, 0.9130434782608695121, 0.9202898550724637472, 0.9275362318840579823, 0.9347826086956522174, 0.9420289855072463414, 0.9492753623188405765, 0.9565217391304348116, 0.9637681159420289356, 0.9662083003288912675 ),
 .UNSPECIFIED. ) 
 GEOMETRIC_REPRESENTATION_ITEM ( )  RATIONAL_B_SPLINE_SURFACE ( (
 ( 1.000000000000000000, 0.8660254037844387076, 1.000000000000000000, 0.8660254037844387076, 1.000000000000000000, 0.8660254037844387076, 1.000000000000000000, 0.8660254037844387076, 1.000000000000000000, 0.8660254037844387076, 1.000000000000000000, 0.8660254037844387076, 1.000000000000000000, 0.8660254037844387076, 1.000000000000000000, 0.8660254037844387076, 1.000000000000000000, 0.8660254037844387076, 1.000000000000000000, 0.8660254037844387076, 1.000000000000000000, 0.8660254037844387076, 1.000000000000000000, 0.8660254037844387076, 1.000000000000000000, 0.8660254037844387076, 1.000000000000000000, 0.8660254037844387076, 1.000000000000000000, 0.8660254037844387076, 1.000000000000000000, 0.8660254037844387076, 1.000000000000000000, 0.8660254037844387076, 1.000000000000000000, 0.8660254037844387076, 1.000000000000000000, 0.8660254037844387076, 1.000000000000000000, 0.8660254037844387076, 1.000000000000000000, 0.8660254037844387076, 1.000000000000000000, 0.8660254037844387076, 1.000000000000000000, 0.8660254037844387076, 1.000000000000000000, 0.8660254037844387076, 1.000000000000000000, 0.8660254037844387076, 1.000000000000000000, 0.8660254037844387076, 1.000000000000000000, 0.8660254037844387076, 1.000000000000000000, 0.8660254037844387076, 1.000000000000000000, 0.8660254037844387076, 1.000000000000000000, 0.8660254037844387076, 1.000000000000000000, 0.8660254037844387076, 1.000000000000000000, 0.8660254037844387076, 1.000000000000000000, 0.8660254037844387076, 1.000000000000000000, 0.8660254037844387076, 1.000000000000000000, 0.8660254037844387076, 1.000000000000000000, 0.8660254037844387076, 1.000000000000000000, 0.8660254037844387076, 1.000000000000000000, 0.8660254037844387076, 1.000000000000000000, 0.8660254037844387076, 1.000000000000000000, 0.8660254037844387076, 1.000000000000000000, 0.8660254037844387076, 1.000000000000000000, 0.8660254037844387076, 1.000000000000000000, 0.8660254037844387076, 1.000000000000000000, 0.8660254037844387076, 1.000000000000000000, 0.8660254037844387076, 1.000000000000000000, 0.8660254037844387076, 1.000000000000000000, 0.8660254037844387076, 1.000000000000000000, 0.8660254037844387076, 1.000000000000000000, 0.8660254037844387076, 1.000000000000000000, 0.8660254037844387076, 1.000000000000000000, 0.8660254037844387076, 1.000000000000000000, 0.8660254037844387076, 1.000000000000000000, 0.8660254037844387076, 1.000000000000000000, 0.8660254037844387076, 1.000000000000000000, 0.8660254037844387076, 1.000000000000000000, 0.8660254037844387076, 1.000000000000000000, 0.8660254037844387076, 1.000000000000000000, 0.8660254037844387076, 1.000000000000000000, 0.8660254037844387076, 1.000000000000000000, 0.8660254037844387076, 1.000000000000000000, 0.8660254037844387076, 1.000000000000000000, 0.8660254037844387076, 1.000000000000000000, 0.8660254037844387076, 1.000000000000000000, 0.8660254037844387076, 1.000000000000000000, 0.8660254037844387076, 1.000000000000000000, 0.8660254037844387076, 1.000000000000000000, 0.8660254037844387076, 1.000000000000000000, 0.8660254037844387076, 1.000000000000000000, 0.8660254037844387076, 1.000000000000000000, 0.8660254037844387076, 1.000000000000000000, 0.8660254037844387076, 1.000000000000000000, 0.8660254037844387076, 1.000000000000000000, 0.8660254037844387076, 1.000000000000000000, 0.8660254037844387076, 1.000000000000000000, 0.8660254037844387076, 1.000000000000000000, 0.8660254037844387076, 1.000000000000000000, 0.8660254037844387076, 1.000000000000000000, 0.8660254037844387076, 1.000000000000000000, 0.8660254037844387076, 1.000000000000000000, 0.8660254037844387076, 1.000000000000000000, 0.8660254037844387076, 1.000000000000000000, 0.8660254037844387076, 1.000000000000000000, 0.8660254037844387076, 1.000000000000000000, 0.8660254037844387076, 1.000000000000000000, 0.8660254037844387076, 1.000000000000000000, 0.8660254037844387076, 1.000000000000000000, 0.8660254037844387076, 1.000000000000000000, 0.8660254037844387076, 1.000000000000000000, 0.8660254037844387076, 1.000000000000000000, 0.8660254037844387076, 1.000000000000000000, 0.8660254037844387076, 1.000000000000000000, 0.8660254037844387076, 1.000000000000000000, 0.8660254037844387076, 1.000000000000000000, 0.8660254037844387076, 1.000000000000000000, 0.8660254037844387076, 1.000000000000000000, 0.8660254037844387076, 1.000000000000000000, 0.8660254037844387076, 1.000000000000000000, 0.8660254037844387076, 1.000000000000000000, 0.8660254037844387076, 1.000000000000000000, 0.8660254037844387076, 1.000000000000000000, 0.8660254037844387076, 1.000000000000000000, 0.8660254037844387076, 1.000000000000000000, 0.8660254037844387076, 1.000000000000000000, 0.8660254037844387076, 1.000000000000000000, 0.8660254037844387076, 1.000000000000000000, 0.8660254037844387076, 1.000000000000000000, 0.8660254037844387076, 1.000000000000000000, 0.8660254037844387076, 1.000000000000000000, 0.8660254037844387076, 1.000000000000000000, 0.8660254037844387076, 1.000000000000000000, 0.8660254037844387076, 1.000000000000000000, 0.8660254037844387076, 1.000000000000000000, 0.8660254037844387076, 1.000000000000000000, 0.8660254037844387076, 1.000000000000000000, 0.8660254037844387076, 1.000000000000000000, 0.8660254037844387076, 1.000000000000000000, 0.8660254037844387076, 1.000000000000000000, 0.8660254037844387076, 1.000000000000000000, 0.8660254037844387076, 1.000000000000000000, 0.8660254037844387076, 1.000000000000000000, 0.8660254037844387076, 1.000000000000000000, 0.8660254037844387076, 1.000000000000000000, 0.8660254037844387076, 1.000000000000000000, 0.8660254037844387076, 1.000000000000000000, 0.8660254037844387076, 1.000000000000000000, 0.8660254037844387076, 1.000000000000000000, 0.8660254037844387076, 1.000000000000000000, 0.8660254037844387076, 1.000000000000000000, 0.8660254037844387076, 1.000000000000000000, 0.8660254037844387076, 1.000000000000000000, 0.8660254037844387076, 1.000000000000000000, 0.8660254037844387076, 1.000000000000000000, 0.8660254037844387076, 1.000000000000000000, 0.9548846649268474263, 0.9401540970596797830),
 ( 1.000000000000000000, 0.8660254037844387076, 1.000000000000000000, 0.8660254037844387076, 1.000000000000000000, 0.8660254037844387076, 1.000000000000000000, 0.8660254037844387076, 1.000000000000000000, 0.8660254037844387076, 1.000000000000000000, 0.8660254037844387076, 1.000000000000000000, 0.8660254037844387076, 1.000000000000000000, 0.8660254037844387076, 1.000000000000000000, 0.8660254037844387076, 1.000000000000000000, 0.8660254037844387076, 1.000000000000000000, 0.8660254037844387076, 1.000000000000000000, 0.8660254037844387076, 1.000000000000000000, 0.8660254037844387076, 1.000000000000000000, 0.8660254037844387076, 1.000000000000000000, 0.8660254037844387076, 1.000000000000000000, 0.8660254037844387076, 1.000000000000000000, 0.8660254037844387076, 1.000000000000000000, 0.8660254037844387076, 1.000000000000000000, 0.8660254037844387076, 1.000000000000000000, 0.8660254037844387076, 1.000000000000000000, 0.8660254037844387076, 1.000000000000000000, 0.8660254037844387076, 1.000000000000000000, 0.8660254037844387076, 1.000000000000000000, 0.8660254037844387076, 1.000000000000000000, 0.8660254037844387076, 1.000000000000000000, 0.8660254037844387076, 1.000000000000000000, 0.8660254037844387076, 1.000000000000000000, 0.8660254037844387076, 1.000000000000000000, 0.8660254037844387076, 1.000000000000000000, 0.8660254037844387076, 1.000000000000000000, 0.8660254037844387076, 1.000000000000000000, 0.8660254037844387076, 1.000000000000000000, 0.8660254037844387076, 1.000000000000000000, 0.8660254037844387076, 1.000000000000000000, 0.8660254037844387076, 1.000000000000000000, 0.8660254037844387076, 1.000000000000000000, 0.8660254037844387076, 1.000000000000000000, 0.8660254037844387076, 1.000000000000000000, 0.8660254037844387076, 1.000000000000000000, 0.8660254037844387076, 1.000000000000000000, 0.8660254037844387076, 1.000000000000000000, 0.8660254037844387076, 1.000000000000000000, 0.8660254037844387076, 1.000000000000000000, 0.8660254037844387076, 1.000000000000000000, 0.8660254037844387076, 1.000000000000000000, 0.8660254037844387076, 1.000000000000000000, 0.8660254037844387076, 1.000000000000000000, 0.8660254037844387076, 1.000000000000000000, 0.8660254037844387076, 1.000000000000000000, 0.8660254037844387076, 1.000000000000000000, 0.8660254037844387076, 1.000000000000000000, 0.8660254037844387076, 1.000000000000000000, 0.8660254037844387076, 1.000000000000000000, 0.8660254037844387076, 1.000000000000000000, 0.8660254037844387076, 1.000000000000000000, 0.8660254037844387076, 1.000000000000000000, 0.8660254037844387076, 1.000000000000000000, 0.8660254037844387076, 1.000000000000000000, 0.8660254037844387076, 1.000000000000000000, 0.8660254037844387076, 1.000000000000000000, 0.8660254037844387076, 1.000000000000000000, 0.8660254037844387076, 1.000000000000000000, 0.8660254037844387076, 1.000000000000000000, 0.8660254037844387076, 1.000000000000000000, 0.8660254037844387076, 1.000000000000000000, 0.8660254037844387076, 1.000000000000000000, 0.8660254037844387076, 1.000000000000000000, 0.8660254037844387076, 1.000000000000000000, 0.8660254037844387076, 1.000000000000000000, 0.8660254037844387076, 1.000000000000000000, 0.8660254037844387076, 1.000000000000000000, 0.8660254037844387076, 1.000000000000000000, 0.8660254037844387076, 1.000000000000000000, 0.8660254037844387076, 1.000000000000000000, 0.8660254037844387076, 1.000000000000000000, 0.8660254037844387076, 1.000000000000000000, 0.8660254037844387076, 1.000000000000000000, 0.8660254037844387076, 1.000000000000000000, 0.8660254037844387076, 1.000000000000000000, 0.8660254037844387076, 1.000000000000000000, 0.8660254037844387076, 1.000000000000000000, 0.8660254037844387076, 1.000000000000000000, 0.8660254037844387076, 1.000000000000000000, 0.8660254037844387076, 1.000000000000000000, 0.8660254037844387076, 1.000000000000000000, 0.8660254037844387076, 1.000000000000000000, 0.8660254037844387076, 1.000000000000000000, 0.8660254037844387076, 1.000000000000000000, 0.8660254037844387076, 1.000000000000000000, 0.8660254037844387076, 1.000000000000000000, 0.8660254037844387076, 1.000000000000000000, 0.8660254037844387076, 1.000000000000000000, 0.8660254037844387076, 1.000000000000000000, 0.8660254037844387076, 1.000000000000000000, 0.8660254037844387076, 1.000000000000000000, 0.8660254037844387076, 1.000000000000000000, 0.8660254037844387076, 1.000000000000000000, 0.8660254037844387076, 1.000000000000000000, 0.8660254037844387076, 1.000000000000000000, 0.8660254037844387076, 1.000000000000000000, 0.8660254037844387076, 1.000000000000000000, 0.8660254037844387076, 1.000000000000000000, 0.8660254037844387076, 1.000000000000000000, 0.8660254037844387076, 1.000000000000000000, 0.8660254037844387076, 1.000000000000000000, 0.8660254037844387076, 1.000000000000000000, 0.8660254037844387076, 1.000000000000000000, 0.8660254037844387076, 1.000000000000000000, 0.8660254037844387076, 1.000000000000000000, 0.8660254037844387076, 1.000000000000000000, 0.8660254037844387076, 1.000000000000000000, 0.8660254037844387076, 1.000000000000000000, 0.8660254037844387076, 1.000000000000000000, 0.8660254037844387076, 1.000000000000000000, 0.8660254037844387076, 1.000000000000000000, 0.8660254037844387076, 1.000000000000000000, 0.8660254037844387076, 1.000000000000000000, 0.8660254037844387076, 1.000000000000000000, 0.8660254037844387076, 1.000000000000000000, 0.8660254037844387076, 1.000000000000000000, 0.8660254037844387076, 1.000000000000000000, 0.8660254037844387076, 1.000000000000000000, 0.8660254037844387076, 1.000000000000000000, 0.8660254037844387076, 1.000000000000000000, 0.8660254037844387076, 1.000000000000000000, 0.8660254037844387076, 1.000000000000000000, 0.8660254037844387076, 1.000000000000000000, 0.8660254037844387076, 1.000000000000000000, 0.8660254037844387076, 1.000000000000000000, 0.8660254037844387076, 1.000000000000000000, 0.8660254037844387076, 1.000000000000000000, 0.8660254037844387076, 1.000000000000000000, 0.8660254037844387076, 1.000000000000000000, 0.9548846649268474263, 0.9401540970596797830) ) ) 
 REPRESENTATION_ITEM ( '' )  SURFACE ( )  );
#54213=CARTESIAN_POINT ( 'NONE',  ( 20.39062500061451644, -3.027376345333614438, 5.243569643749998122 ) ) ;
#54214=CARTESIAN_POINT ( 'NONE',  ( 28.80000000122903003, -2.886751345948129988, 4.999999999999997335 ) ) ;
#54215=CARTESIAN_POINT ( 'NONE',  ( 4.190625000614518925, -3.027376345333614438, 5.243569643749998122 ) ) ;
#54216=CARTESIAN_POINT ( 'NONE',  ( 26.25000000000000000, 4.330127018922192761, -2.499999999999997780 ) ) ;
#54218=CARTESIAN_POINT ( 'NONE',  ( 28.62187500061451573, -6.054752690667223547, -1.112240025338166033E-15 ) ) ;
#54220=EDGE_CURVE ( 'NONE', #26952, #66635, #53560, .T. ) ;
#54221=CARTESIAN_POINT ( 'NONE',  ( 12.11250000122903181, 0.000000000000000000, 4.999999999999998224 ) ) ;
#54222=CARTESIAN_POINT ( 'NONE',  ( 29.33437500061451431, 4.541064518000418104, 2.621784821874999949 ) ) ;
#54223=DIRECTION ( 'NONE',  ( 0.000000000000000000, 0.000000000000000000, 1.000000000000000000 ) ) ;
#54224=CARTESIAN_POINT ( 'NONE',  ( 6.984375000614516438, -4.541064518000419881, 2.621784821874995952 ) ) ;
#54225=CARTESIAN_POINT ( 'NONE',  ( 26.69062500061451715, -3.027376345333614438, 5.243569643749998122 ) ) ;
#54227=CARTESIAN_POINT ( 'NONE',  ( 14.28749999999999964, -2.886751345948063374, 5.000000000000112799 ) ) ;
#54229=CARTESIAN_POINT ( 'NONE',  ( 4.434375000614519280, 6.421520780324663323E-16, -5.243569643749999010 ) ) ;
#54230=CARTESIAN_POINT ( 'NONE',  ( 9.496875000614517504, 6.054752690667223547, 3.707466751127219781E-16 ) ) ;
#54231=CARTESIAN_POINT ( 'NONE',  ( 3.600000000000002309, -4.330127018922190985, -2.500000000000001332 ) ) ;
#54232=CARTESIAN_POINT ( 'NONE',  ( -2.121784821874999949, 13.42812500061459602, 26.32496088578401938 ) ) ;
#54233=CARTESIAN_POINT ( 'NONE',  ( 20.73750000000000071, -2.886751345948125991, -5.000000000000000000 ) ) ;
#54234=CARTESIAN_POINT ( 'NONE',  ( -3.999999999999999112, 17.75000000000000355, -30.00000000000000000 ) ) ;
#54235=CARTESIAN_POINT ( 'NONE',  ( 3.450000000000001510, 0.000000000000000000, 4.999999999999998224 ) ) ;
#54237=EDGE_LOOP ( 'NONE', ( #44109, #38679, #15921, #45268 ) ) ;
#54238=CARTESIAN_POINT ( 'NONE',  ( 21.32812500061451644, -4.541064518000419881, 2.621784821874995952 ) ) ;
#54239=CARTESIAN_POINT ( 'NONE',  ( 10.19062500061451892, -3.027376345333610441, -5.243569643749999898 ) ) ;
#54241=CARTESIAN_POINT ( 'NONE',  ( 7.809375000614519280, 0.000000000000000000, 5.243569643749999010 ) ) ;
#54242=CARTESIAN_POINT ( 'NONE',  ( 22.98749999999999716, -2.886751345948125991, -5.000000000000000000 ) ) ;
#54243=CARTESIAN_POINT ( 'NONE',  ( 18.97500000122903074, -5.773502691896255534, -1.060575238724906372E-15 ) ) ;
#54244=CARTESIAN_POINT ( 'NONE',  ( 27.10312500061451502, 0.000000000000000000, 5.243569643749999010 ) ) ;
#54245=CARTESIAN_POINT ( 'NONE',  ( 1.626862140677534273E-15, 10.77500000122903323, 34.00000000000000000 ) ) ;
#54246=CARTESIAN_POINT ( 'NONE',  ( 8.296875000614516438, -3.027376345333614438, 5.243569643749998122 ) ) ;
#54247=CARTESIAN_POINT ( 'NONE',  ( 15.23437500061451644, 6.421520780324663323E-16, -5.243569643749999010 ) ) ;
#54248=CARTESIAN_POINT ( 'NONE',  ( 24.19687500061451857, -3.027376345333610441, -5.243569643749999898 ) ) ;
#54249=CARTESIAN_POINT ( 'NONE',  ( 3.999999999999998668, 18.12500000122903288, -32.30940107675850470 ) ) ;
#54251=CARTESIAN_POINT ( 'NONE',  ( 16.77187500061451786, 3.027376345333611329, 5.243569643749999010 ) ) ;
#54252=( BOUNDED_CURVE ( )  B_SPLINE_CURVE ( 2, ( #66228, #3457, #60305, #9716, #32249, #25976, #54782 ),
 .UNSPECIFIED., .F., .F. ) 
 B_SPLINE_CURVE_WITH_KNOTS ( ( 3, 2, 2, 3 ),
 ( 0.1916666666666666519, 0.1944444444444444198, 0.1972222222222221599, 0.1999999999999999556 ),
 .UNSPECIFIED. ) 
 CURVE ( )  GEOMETRIC_REPRESENTATION_ITEM ( )  RATIONAL_B_SPLINE_CURVE ( ( 1.000000000000001332, 0.8660254037844373753, 1.000000000000000000, 0.8660254037844387076, 1.000000000000000000, 0.8660254037844413721, 0.9999999999999973355 ) ) 
 REPRESENTATION_ITEM ( '' )  );
#54253=CARTESIAN_POINT ( 'NONE',  ( 10.13437500061451679, -4.541064518000419881, 2.621784821874995952 ) ) ;
#54255=CARTESIAN_POINT ( 'NONE',  ( 24.03750000000000142, 5.773502691896255534, 3.535250795749688894E-16 ) ) ;
#54257=CARTESIAN_POINT ( 'NONE',  ( -4.243569643749999898, 9.921875000614519990, -32.45002607614398471 ) ) ;
#54259=CARTESIAN_POINT ( 'NONE',  ( 13.52812500061451750, 4.541064518000418104, 2.621784821874999949 ) ) ;
#54260=CARTESIAN_POINT ( 'NONE',  ( 29.40937500061451715, 0.000000000000000000, 5.243569643749999010 ) ) ;
#54262=FACE_OUTER_BOUND ( 'NONE', #28989, .T. ) ;
#54263=( BOUNDED_CURVE ( )  B_SPLINE_CURVE ( 2, ( #6047, #881, #57366, #51836, #23745, #28581, #4823 ),
 .UNSPECIFIED., .F., .F. ) 
 B_SPLINE_CURVE_WITH_KNOTS ( ( 3, 2, 2, 3 ),
 ( 0.5416666666666666297, 0.5444444444444443976, 0.5472222222222222765, 0.5500000000000000444 ),
 .UNSPECIFIED. ) 
 CURVE ( )  GEOMETRIC_REPRESENTATION_ITEM ( )  RATIONAL_B_SPLINE_CURVE ( ( 1.000000000000000000, 0.8660254037844387076, 1.000000000000000000, 0.8660254037844387076, 1.000000000000000000, 0.8660254037844387076, 1.000000000000000000 ) ) 
 REPRESENTATION_ITEM ( '' )  );
#54264=CARTESIAN_POINT ( 'NONE',  ( 13.01249999999999929, -5.773502691896255534, -1.060575238724906372E-15 ) ) ;
#54266=CARTESIAN_POINT ( 'NONE',  ( -2.828200636599751609E-16, 18.20000000122903216, 25.38119784648299770 ) ) ;
#54267=CARTESIAN_POINT ( 'NONE',  ( 11.17500000122903536, 2.886751345948126879, 4.999999999999999112 ) ) ;
#54268=CARTESIAN_POINT ( 'NONE',  ( 23.07187500061451857, 3.027376345333611329, 5.243569643749999010 ) ) ;
#54269=CARTESIAN_POINT ( 'NONE',  ( 16.54687500061451644, -3.027376345333610441, -5.243569643749999898 ) ) ;
#54271=ORIENTED_EDGE ( 'NONE', *, *, #6454, .F. ) ;
#54272=CARTESIAN_POINT ( 'NONE',  ( 17.20312500061451644, 0.000000000000000000, 5.243569643749999010 ) ) ;
#54273=CARTESIAN_POINT ( 'NONE',  ( 28.76250000122903216, 0.000000000000000000, 4.999999999999998224 ) ) ;
#54274=CARTESIAN_POINT ( 'NONE',  ( 17.93437500061451928, 6.421520780324663323E-16, -5.243569643749999010 ) ) ;
#54275=CARTESIAN_POINT ( 'NONE',  ( 28.47187500061451715, 3.027376345333611329, 5.243569643749999010 ) ) ;
#54276=CARTESIAN_POINT ( 'NONE',  ( 4.340625000614515727, -3.027376345333610441, -5.243569643749999898 ) ) ;
#54277=CARTESIAN_POINT ( 'NONE',  ( 18.77812500061451573, 6.421520780324663323E-16, -5.243569643749999010 ) ) ;
#54278=CARTESIAN_POINT ( 'NONE',  ( 28.28437500061451715, 6.421520780324663323E-16, -5.243569643749999010 ) ) ;
#54279=CARTESIAN_POINT ( 'NONE',  ( 4.243569643749999898, 12.37812500061451715, 30.00000000000000000 ) ) ;
#54280=CARTESIAN_POINT ( 'NONE',  ( 16.72500000122903430, -5.773502691896255534, -1.060575238724906372E-15 ) ) ;
#54282=CARTESIAN_POINT ( 'NONE',  ( 7.790625000614516793, -3.027376345333614438, 5.243569643749998122 ) ) ;
#54283=CARTESIAN_POINT ( 'NONE',  ( 26.87812500061451360, 6.421520780324663323E-16, -5.243569643749999010 ) ) ;
#54284=CARTESIAN_POINT ( 'NONE',  ( 0.000000000000000000, 0.000000000000000000, 50.00000000000000000 ) ) ;
#54285=CARTESIAN_POINT ( 'NONE',  ( 24.04687500061451644, -3.027376345333614438, 5.243569643749998122 ) ) ;
#54286=CARTESIAN_POINT ( 'NONE',  ( 12.77812500061451750, -4.541064518000419881, 2.621784821874995952 ) ) ;
#54287=CARTESIAN_POINT ( 'NONE',  ( 22.68750000122903288, 6.123233995736764310E-16, -4.999999999999998224 ) ) ;
#54288=( BOUNDED_CURVE ( )  B_SPLINE_CURVE ( 2, ( #17878, #927, #28269, #6455, #23435, #62954, #12349, #34884, #29706 ),
 .UNSPECIFIED., .F., .F. ) 
 B_SPLINE_CURVE_WITH_KNOTS ( ( 3, 2, 2, 2, 3 ),
 ( 0.2500000000000000000, 0.2536231884057971175, 0.2608695652173912971, 0.2681159420289855322, 0.2717391304347826497 ),
 .UNSPECIFIED. ) 
 CURVE ( )  GEOMETRIC_REPRESENTATION_ITEM ( )  RATIONAL_B_SPLINE_CURVE ( ( 0.9330127018922194093, 0.9330127018922190762, 1.000000000000000000, 0.8660254037844387076, 1.000000000000000000, 0.8660254037844387076, 1.000000000000000000, 0.9330127018922188542, 0.9330127018922194093 ) ) 
 REPRESENTATION_ITEM ( '' )  );
#54289=CARTESIAN_POINT ( 'NONE',  ( 22.41562500061451502, 3.027376345333613106, -5.243569643749998122 ) ) ;
#54290=CARTESIAN_POINT ( 'NONE',  ( 18.42187500061451644, 3.027376345333613106, -5.243569643749998122 ) ) ;
#54291=CARTESIAN_POINT ( 'NONE',  ( 12.32812500061451821, -4.541064518000419881, 2.621784821874995952 ) ) ;
#54292=CARTESIAN_POINT ( 'NONE',  ( -3.000416591977282496E-16, 15.69687500061451857, 25.09994784771203058 ) ) ;
#54293=CARTESIAN_POINT ( 'NONE',  ( 18.89062500061451644, 6.054752690667223547, 3.707466751127219781E-16 ) ) ;
#54295=ORIENTED_EDGE ( 'NONE', *, *, #38095, .F. ) ;
#54296=ORIENTED_EDGE ( 'NONE', *, *, #24479, .F. ) ;
#54297=CARTESIAN_POINT ( 'NONE',  ( 22.72499999999999787, 4.330127018922191873, 2.499999999999999556 ) ) ;
#54298=CARTESIAN_POINT ( 'NONE',  ( -1.389182184750238802, 10.01354716596406824, -33.81675744519802151 ) ) ;
#54300=CARTESIAN_POINT ( 'NONE',  ( 26.42812500061451431, 6.421520780324663323E-16, -5.243569643749999010 ) ) ;
#54301=CARTESIAN_POINT ( 'NONE',  ( 4.978125000614518569, 4.541064518000418104, 2.621784821874999949 ) ) ;
#54302=CARTESIAN_POINT ( 'NONE',  ( 18.86250000122903359, 0.000000000000000000, 4.999999999999998224 ) ) ;
#54303=CARTESIAN_POINT ( 'NONE',  ( 25.07812500061451644, 6.421520780324663323E-16, -5.243569643749999010 ) ) ;
#54304=CARTESIAN_POINT ( 'NONE',  ( 23.25000000000000000, 0.000000000000000000, 4.999999999999998224 ) ) ;
#54305=CARTESIAN_POINT ( 'NONE',  ( 27.59062500061451573, -3.027376345333614438, 5.243569643749998122 ) ) ;
#54306=CARTESIAN_POINT ( 'NONE',  ( 7.903125000614515727, -4.541064518000417216, -2.621784821875001281 ) ) ;
#54308=CARTESIAN_POINT ( 'NONE',  ( 24.40312500061451573, 0.000000000000000000, 5.243569643749999010 ) ) ;
#54309=CARTESIAN_POINT ( 'NONE',  ( 6.103125000614515905, -4.541064518000417216, -2.621784821875001281 ) ) ;
#54312=CARTESIAN_POINT ( 'NONE',  ( 2.953125000614516438, -4.541064518000417216, -2.621784821875001281 ) ) ;
#54314=CARTESIAN_POINT ( 'NONE',  ( -2.828200636599751609E-16, 13.70000000122903572, -34.61880215351700230 ) ) ;
#54315=CARTESIAN_POINT ( 'NONE',  ( 1.626862140677534273E-15, 10.66249999999999964, -26.00000000000000355 ) ) ;
#54316=CARTESIAN_POINT ( 'NONE',  ( 10.16249999999999964, 2.886751345948126879, 4.999999999999999112 ) ) ;
#54317=CARTESIAN_POINT ( 'NONE',  ( 12.27187500061451786, 3.027376345333611329, 5.243569643749999010 ) ) ;
#54318=CARTESIAN_POINT ( 'NONE',  ( 5.887500001229034829, -4.330127018922194537, 2.499999999999995559 ) ) ;
#54319=CARTESIAN_POINT ( 'NONE',  ( 13.73437500061451821, -4.541064518000419881, 2.621784821874995952 ) ) ;
#54321=CARTESIAN_POINT ( 'NONE',  ( 5.521875000614517859, 3.027376345333611329, 5.243569643749999010 ) ) ;
#54322=CARTESIAN_POINT ( 'NONE',  ( 1.071796769724493892, 18.51740381056766793, 26.00000000000000711 ) ) ;
#54324=CARTESIAN_POINT ( 'NONE',  ( 11.59687500061451892, -3.027376345333610441, -5.243569643749999898 ) ) ;
#54325=DIRECTION ( 'NONE',  ( -1.000000000000000000, -0.000000000000000000, -0.000000000000000000 ) ) ;
#54326=CARTESIAN_POINT ( 'NONE',  ( 21.25312500061451715, 0.000000000000000000, 5.243569643749999010 ) ) ;
#54327=CARTESIAN_POINT ( 'NONE',  ( 2.121784821874999061, 10.70937500061451964, 26.32496088578401583 ) ) ;
#54328=CARTESIAN_POINT ( 'NONE',  ( 24.94687500061451502, -3.027376345333614438, 5.243569643749998122 ) ) ;
#54329=CARTESIAN_POINT ( 'NONE',  ( 29.55000000000000071, 0.000000000000000000, 4.999999999999998224 ) ) ;
#54330=CARTESIAN_POINT ( 'NONE',  ( 3.778125000614519280, -4.541064518000419881, 2.621784821874995952 ) ) ;
#54333=CARTESIAN_POINT ( 'NONE',  ( 14.33437500061451786, 6.421520780324663323E-16, -5.243569643749999010 ) ) ;
#54334=CARTESIAN_POINT ( 'NONE',  ( 26.81250000122903288, 4.330127018922192761, -2.499999999999997780 ) ) ;
#54335=CARTESIAN_POINT ( 'NONE',  ( 4.921875000614518214, 3.027376345333613106, -5.243569643749998122 ) ) ;
#54336=CARTESIAN_POINT ( 'NONE',  ( 16.99687500061451573, -3.027376345333610441, -5.243569643749999898 ) ) ;
#54337=CARTESIAN_POINT ( 'NONE',  ( 14.92500000000000071, 6.123233995736764310E-16, -4.999999999999998224 ) ) ;
#54338=CARTESIAN_POINT ( 'NONE',  ( 25.12499999999999645, -4.330127018922194537, 2.499999999999995559 ) ) ;
#54339=CARTESIAN_POINT ( 'NONE',  ( 3.862500001229035362, 4.330127018922192761, -2.499999999999997780 ) ) ;
#54340=CARTESIAN_POINT ( 'NONE',  ( 26.03437500061451715, 6.421520780324663323E-16, -5.243569643749999010 ) ) ;
#54343=CARTESIAN_POINT ( 'NONE',  ( 7.275000000000000355, 6.123233995736764310E-16, -4.999999999999998224 ) ) ;
#54345=CARTESIAN_POINT ( 'NONE',  ( 22.79062500061451502, -3.027376345333610441, -5.243569643749999898 ) ) ;
#54346=CARTESIAN_POINT ( 'NONE',  ( 11.21250000000000036, -5.773502691896255534, -1.060575238724906372E-15 ) ) ;
#54347=CARTESIAN_POINT ( 'NONE',  ( 3.965625000614515727, 3.027376345333613106, -5.243569643749998122 ) ) ;
#54348=CARTESIAN_POINT ( 'NONE',  ( 18.93750000000000000, -2.886751345948125991, -5.000000000000000000 ) ) ;
#54349=EDGE_CURVE ( 'NONE', #8399, #29691, #7683, .T. ) ;
#54350=CARTESIAN_POINT ( 'NONE',  ( 17.61562500061451786, 3.027376345333611329, 5.243569643749999010 ) ) ;
#54351=CARTESIAN_POINT ( 'NONE',  ( 15.60000000122903607, 5.773502691896255534, 3.535250795749688401E-16 ) ) ;
#54352=CARTESIAN_POINT ( 'NONE',  ( 22.50000000122903288, -2.886751345948129988, 4.999999999999997335 ) ) ;
#54354=CARTESIAN_POINT ( 'NONE',  ( 29.59687500061451715, -3.027376345333610441, -5.243569643749999898 ) ) ;
#54356=CARTESIAN_POINT ( 'NONE',  ( 18.96562500061451573, 3.027376345333611329, 5.243569643749999010 ) ) ;
#54357=CARTESIAN_POINT ( 'NONE',  ( 24.25312500061451715, 4.541064518000418104, -2.621784821874998173 ) ) ;
#54358=CARTESIAN_POINT ( 'NONE',  ( 25.65937500061451715, 4.541064518000418104, -2.621784821874998173 ) ) ;
#54359=CARTESIAN_POINT ( 'NONE',  ( 8.887499999999999289, -2.886751345948129988, 4.999999999999997335 ) ) ;
#54360=CARTESIAN_POINT ( 'NONE',  ( 11.24062500061451608, 6.054752690667223547, 3.707466751127219781E-16 ) ) ;
#54361=CARTESIAN_POINT ( 'NONE',  ( 27.02812500061451573, 4.541064518000418104, 2.621784821874999949 ) ) ;
#54362=CARTESIAN_POINT ( 'NONE',  ( 17.52187500061451431, 3.027376345333613106, -5.243569643749998122 ) ) ;
#54363=CARTESIAN_POINT ( 'NONE',  ( 8.915625000614515017, 3.027376345333613106, -5.243569643749998122 ) ) ;
#54364=CARTESIAN_POINT ( 'NONE',  ( 4.243569643749999898, 10.18437500061451750, 30.00000000000000000 ) ) ;
#54365=CARTESIAN_POINT ( 'NONE',  ( 23.06250000122903288, -4.330127018922190985, -2.500000000000001332 ) ) ;
#54367=CARTESIAN_POINT ( 'NONE',  ( 14.76562500061451644, 3.027376345333612662, -5.243569643749998122 ) ) ;
#54368=CARTESIAN_POINT ( 'NONE',  ( 7.921875000614517326, -6.054752690667223547, -1.112240025338166033E-15 ) ) ;
#54369=CARTESIAN_POINT ( 'NONE',  ( 6.159375000614517148, -4.541064518000417216, -2.621784821875001281 ) ) ;
#54370=VERTEX_POINT ( 'NONE', #71949 ) ;
#54371=CARTESIAN_POINT ( 'NONE',  ( 15.33750000000000036, -2.886751345948126435, -5.000000000000000000 ) ) ;
#54372=CARTESIAN_POINT ( 'NONE',  ( 21.17812500061451431, 4.541064518000418104, 2.621784821874999949 ) ) ;
#54373=CARTESIAN_POINT ( 'NONE',  ( 15.75937500061451857, 4.541064518000418104, -2.621784821874998173 ) ) ;
#54374=CARTESIAN_POINT ( 'NONE',  ( 19.19062500061452070, -3.027376345333610441, -5.243569643749999898 ) ) ;
#54375=CARTESIAN_POINT ( 'NONE',  ( -1.999999999999997113, 11.52500000000000036, 33.46410161513775705 ) ) ;
#54376=CARTESIAN_POINT ( 'NONE',  ( 27.25312500061451360, -4.541064518000417216, -2.621784821875001281 ) ) ;
#54377=CARTESIAN_POINT ( 'NONE',  ( 5.962500001229033231, -4.330127018922190985, -2.500000000000001332 ) ) ;
#54379=CARTESIAN_POINT ( 'NONE',  ( 29.69999999999999574, -4.330127018922190985, -2.500000000000001332 ) ) ;
#54380=CARTESIAN_POINT ( 'NONE',  ( 3.999999999999998668, 18.91249999999999787, -32.30940107675850470 ) ) ;
#54381=CARTESIAN_POINT ( 'NONE',  ( 24.37500000122903288, -5.773502691896255534, -1.060575238724906372E-15 ) ) ;
#54383=CARTESIAN_POINT ( 'NONE',  ( 7.171875000614517326, 3.027376345333613106, -5.243569643749998122 ) ) ;
#54384=CARTESIAN_POINT ( 'NONE',  ( 4.869423765992945796, -1.135214599616954256, -5.119209941160161037 ) ) ;
#54385=CARTESIAN_POINT ( 'NONE',  ( 15.21562500061451750, 3.027376345333613106, -5.243569643749998122 ) ) ;
#54386=CARTESIAN_POINT ( 'NONE',  ( 9.684375000614517504, -4.541064518000419881, 2.621784821874995952 ) ) ;
#54387=CARTESIAN_POINT ( 'NONE',  ( 27.97500000122903074, -5.773502691896255534, -1.060575238724906372E-15 ) ) ;
#54388=CARTESIAN_POINT ( 'NONE',  ( 17.48437500061451999, 6.421520780324663323E-16, -5.243569643749999010 ) ) ;
#54389=CARTESIAN_POINT ( 'NONE',  ( 4.921875000614518214, 3.027376345333613106, -5.243569643749998122 ) ) ;
#54390=CARTESIAN_POINT ( 'NONE',  ( 5.165625000614518569, -6.054752690667223547, -1.112240025338166033E-15 ) ) ;
#54391=CARTESIAN_POINT ( 'NONE',  ( 15.29062500061451679, 6.054752690667223547, 3.707466751127219781E-16 ) ) ;
#54393=CARTESIAN_POINT ( 'NONE',  ( 11.69062500061451360, 6.054752690667223547, 3.707466751127219781E-16 ) ) ;
#54394=CARTESIAN_POINT ( 'NONE',  ( 6.412500001229036073, -4.330127018922190985, -2.500000000000001332 ) ) ;
#54395=CARTESIAN_POINT ( 'NONE',  ( 8.465625000614515727, 3.027376345333613106, -5.243569643749998122 ) ) ;
#54397=CARTESIAN_POINT ( 'NONE',  ( 9.487500000000000711, -2.886751345948125991, -5.000000000000000000 ) ) ;
#54398=CARTESIAN_POINT ( 'NONE',  ( 3.225000001229033408, -5.773502691896255534, -1.060575238724906372E-15 ) ) ;
#54399=CARTESIAN_POINT ( 'NONE',  ( 19.08750000000000213, 5.773502691896255534, 3.535250795749688894E-16 ) ) ;
#54400=CARTESIAN_POINT ( 'NONE',  ( 17.55937500061451573, 4.541064518000418104, -2.621784821874998173 ) ) ;
#54401=CARTESIAN_POINT ( 'NONE',  ( 15.03750000122903252, 6.123233995736764310E-16, -4.999999999999998224 ) ) ;
#54403=CARTESIAN_POINT ( 'NONE',  ( -2.121784821874999949, 16.57812500061451644, -33.67503911421598417 ) ) ;
#54404=DIRECTION ( 'NONE',  ( -1.000000000000000000, -0.000000000000000000, -0.000000000000000000 ) ) ;
#54405=CARTESIAN_POINT ( 'NONE',  ( 1.626862140677534273E-15, 18.76250000000000284, 34.00000000000000000 ) ) ;
#54408=DIRECTION ( 'NONE',  ( 0.000000000000000000, 0.000000000000000000, 1.000000000000000000 ) ) ;
#54409=CARTESIAN_POINT ( 'NONE',  ( 4.661467738957717266, -1.808512791952580301, -4.661467738957749241 ) ) ;
#54410=CARTESIAN_POINT ( 'NONE',  ( 15.38437500061451679, 4.541064518000418104, 2.621784821874999949 ) ) ;
#54411=CARTESIAN_POINT ( 'NONE',  ( 29.32499999999999929, 6.123233995736764310E-16, -4.999999999999998224 ) ) ;
#54412=CARTESIAN_POINT ( 'NONE',  ( 10.56562500061451715, -6.054752690667223547, -1.112240025338166033E-15 ) ) ;
#54414=CARTESIAN_POINT ( 'NONE',  ( 20.44687500061451857, -3.027376345333614438, 5.243569643749998122 ) ) ;
#54416=CARTESIAN_POINT ( 'NONE',  ( 8.803125000614517859, -4.541064518000417216, -2.621784821875001281 ) ) ;
#54417=CARTESIAN_POINT ( 'NONE',  ( 13.62187500061451750, 3.027376345333611329, 5.243569643749999010 ) ) ;
#54419=CARTESIAN_POINT ( 'NONE',  ( 23.03437500061451715, 4.541064518000418104, 2.621784821874999949 ) ) ;
#54420=CARTESIAN_POINT ( 'NONE',  ( 27.59062500061451573, -3.027376345333614438, 5.243569643749998122 ) ) ;
#54421=EDGE_CURVE ( 'NONE', #55550, #49922, #61122, .T. ) ;
#54423=CARTESIAN_POINT ( 'NONE',  ( 6.637500000000001066, -2.886751345948129988, 4.999999999999997335 ) ) ;
#54424=CARTESIAN_POINT ( 'NONE',  ( 16.35000000122903430, -2.886751345948125991, -5.000000000000000000 ) ) ;
#54429=CARTESIAN_POINT ( 'NONE',  ( 14.43750000000000000, -2.886751345948125991, -5.000000000000000000 ) ) ;
#54430=CARTESIAN_POINT ( 'NONE',  ( 18.97499999999999787, 6.123233995736764310E-16, -4.999999999999998224 ) ) ;
#54431=CARTESIAN_POINT ( 'NONE',  ( 10.19062500061451892, -3.027376345333610441, -5.243569643749999898 ) ) ;
#54433=CARTESIAN_POINT ( 'NONE',  ( -3.999999999999999112, 11.00000000000000178, -30.00000000000000000 ) ) ;
#54434=CARTESIAN_POINT ( 'NONE',  ( -2.121784821874996840, 16.78437500061452070, -26.32496088578401583 ) ) ;
#54435=CARTESIAN_POINT ( 'NONE',  ( 4.603125000614518569, 0.000000000000000000, 5.243569643749999010 ) ) ;
#54437=CARTESIAN_POINT ( 'NONE',  ( 10.31250000000000355, -5.773502691896255534, -1.060575238724906372E-15 ) ) ;
#54438=CARTESIAN_POINT ( 'NONE',  ( -1.071796769724488563, 13.34240381056766545, -26.00000000000000000 ) ) ;
#54440=CARTESIAN_POINT ( 'NONE',  ( 4.243569643749999898, 11.89062500061451644, 32.45002607614398471 ) ) ;
#54441=CARTESIAN_POINT ( 'NONE',  ( 27.25312500061451360, -4.541064518000417216, -2.621784821875001281 ) ) ;
#54442=CARTESIAN_POINT ( 'NONE',  ( 3.548580288327752630, 3.522439202781492806, 3.649653710620935243 ) ) ;
#54444=CARTESIAN_POINT ( 'NONE',  ( 20.63437500061451857, 6.421520780324663323E-16, -5.243569643749999010 ) ) ;
#54445=CARTESIAN_POINT ( 'NONE',  ( 20.12812500061451715, 6.421520780324663323E-16, -5.243569643749999010 ) ) ;
#54446=CARTESIAN_POINT ( 'NONE',  ( 4.243569643749999898, 12.79062500061459495, -27.54997392385601529 ) ) ;
#54447=CARTESIAN_POINT ( 'NONE',  ( 22.35000000122903074, 5.773502691896255534, 3.535250795749688894E-16 ) ) ;
#54448=CARTESIAN_POINT ( 'NONE',  ( 3.253125000614518036, 0.000000000000000000, 5.243569643749999010 ) ) ;
#54450=CARTESIAN_POINT ( 'NONE',  ( 22.11562500061451431, 3.027376345333611329, 5.243569643749999010 ) ) ;
#54453=CARTESIAN_POINT ( 'NONE',  ( 16.02187500061451786, -6.054752690667223547, -1.112240025338166033E-15 ) ) ;
#54454=CARTESIAN_POINT ( 'NONE',  ( 13.43437500061451750, 6.421520780324663323E-16, -5.243569643749999010 ) ) ;
#54455=CARTESIAN_POINT ( 'NONE',  ( 24.12187500061451217, -6.054752690667223547, -1.112240025338166033E-15 ) ) ;
#54456=CARTESIAN_POINT ( 'NONE',  ( 4.243569643749999898, 14.19687500061452035, 32.45002607614398471 ) ) ;
#54457=CARTESIAN_POINT ( 'NONE',  ( 6.215625000614517504, 3.027376345333613106, -5.243569643749998122 ) ) ;
#54458=CARTESIAN_POINT ( 'NONE',  ( 29.57812500061451644, 6.421520780324663323E-16, -5.243569643749999010 ) ) ;
#54459=CARTESIAN_POINT ( 'NONE',  ( 28.11562500061451431, -6.054752690667223547, -1.112240025338166033E-15 ) ) ;
#54462=CARTESIAN_POINT ( 'NONE',  ( 7.321875000614516793, 3.027376345333611329, 5.243569643749999010 ) ) ;
#54464=CARTESIAN_POINT ( 'NONE',  ( 15.00000000122903465, -2.886751345948125991, -5.000000000000000000 ) ) ;
#54465=CARTESIAN_POINT ( 'NONE',  ( 8.850000001229034297, 5.773502691896255534, 3.535250795749688894E-16 ) ) ;
#54466=CARTESIAN_POINT ( 'NONE',  ( 4.940625000614515372, 6.054752690667223547, 3.707466751127219781E-16 ) ) ;
#54469=CARTESIAN_POINT ( 'NONE',  ( 13.77187500061451786, -6.054752690667223547, -1.112240025338166033E-15 ) ) ;
#54470=CARTESIAN_POINT ( 'NONE',  ( 7.500000000000000000, 0.000000000000000000, 4.999999999999998224 ) ) ;
#54472=CARTESIAN_POINT ( 'NONE',  ( 21.29062500061451502, -3.027376345333614438, 5.243569643749998122 ) ) ;
#54473=CARTESIAN_POINT ( 'NONE',  ( 7.903125000614515727, -4.541064518000417216, -2.621784821875001281 ) ) ;
#54474=CARTESIAN_POINT ( 'NONE',  ( 25.28437500061451715, 4.541064518000418104, 2.621784821874999949 ) ) ;
#54475=CARTESIAN_POINT ( 'NONE',  ( 6.890625000614516438, -3.027376345333614438, 5.243569643749998122 ) ) ;
#54476=DIRECTION ( 'NONE',  ( -0.000000000000000000, -1.000000000000000000, -0.000000000000000000 ) ) ;
#54477=CARTESIAN_POINT ( 'NONE',  ( 8.775000001229033231, 2.886751345948129099, -4.999999999999998224 ) ) ;
#54478=CARTESIAN_POINT ( 'NONE',  ( 21.62812500061451360, 4.541064518000418104, 2.621784821874999949 ) ) ;
#54479=CARTESIAN_POINT ( 'NONE',  ( -3.000416591977282496E-16, 10.69062500061451715, -34.90005215228797653 ) ) ;
#54480=CARTESIAN_POINT ( 'NONE',  ( 10.46250000122903323, -4.330127018922190985, -2.500000000000001332 ) ) ;
#54481=CARTESIAN_POINT ( 'NONE',  ( 18.74062500061451431, -3.027376345333610441, -5.243569643749999898 ) ) ;
#54482=CARTESIAN_POINT ( 'NONE',  ( 19.15312500061451573, -4.541064518000417216, -2.621784821875001281 ) ) ;
#54484=CARTESIAN_POINT ( 'NONE',  ( 19.12500000000000000, 4.330127018922191873, 2.499999999999999556 ) ) ;
#54485=CARTESIAN_POINT ( 'NONE',  ( 12.26250000122903394, -4.330127018922190985, -2.500000000000001332 ) ) ;
#54486=CARTESIAN_POINT ( 'NONE',  ( 8.315625000614515372, -6.054752690667223547, -1.112240025338166033E-15 ) ) ;
#54487=CARTESIAN_POINT ( 'NONE',  ( 10.52812500061451750, -4.541064518000419881, 2.621784821874995952 ) ) ;
#54488=( BOUNDED_CURVE ( )  B_SPLINE_CURVE ( 2, ( #6747, #855, #487, #68088, #72901, #44835, #34086, #35177, #50376 ),
 .UNSPECIFIED., .F., .F. ) 
 B_SPLINE_CURVE_WITH_KNOTS ( ( 3, 2, 2, 2, 3 ),
 ( 0.7934782608695651884, 0.7971014492753623060, 0.8043478260869565410, 0.8115942028985507761, 0.8152173913043478937 ),
 .UNSPECIFIED. ) 
 CURVE ( )  GEOMETRIC_REPRESENTATION_ITEM ( )  RATIONAL_B_SPLINE_CURVE ( ( 0.9330127018922194093, 0.9330127018922194093, 1.000000000000000000, 0.8660254037844387076, 1.000000000000000000, 0.8660254037844387076, 1.000000000000000000, 0.9330127018922182991, 0.9330127018922192983 ) ) 
 REPRESENTATION_ITEM ( '' )  );
#54490=CARTESIAN_POINT ( 'NONE',  ( 22.20000000122903216, -2.886751345948125991, -5.000000000000000000 ) ) ;
#54491=CARTESIAN_POINT ( 'NONE',  ( 21.38437500061451502, -4.541064518000419881, 2.621784821874995952 ) ) ;
#54493=CARTESIAN_POINT ( 'NONE',  ( 5.062500001229035540, -4.330127018922190985, -2.500000000000001332 ) ) ;
#54494=CARTESIAN_POINT ( 'NONE',  ( 4.996875000614516615, 6.054752690667223547, 3.707466751127219781E-16 ) ) ;
#54495=CARTESIAN_POINT ( 'NONE',  ( 22.99687500061451573, 6.054752690667223547, 3.707466751127219781E-16 ) ) ;
#54496=CARTESIAN_POINT ( 'NONE',  ( 4.342984975361706468, -2.477595912125914790, -4.621313785610477787 ) ) ;
#54497=CARTESIAN_POINT ( 'NONE',  ( 19.94062500061451715, -3.027376345333614438, 5.243569643749998122 ) ) ;
#54498=CARTESIAN_POINT ( 'NONE',  ( 24.38437500061451502, 4.541064518000418104, 2.621784821874999949 ) ) ;
#54501=CARTESIAN_POINT ( 'NONE',  ( 5.371875000614516615, 3.027376345333613106, -5.243569643749998122 ) ) ;
#54502=CARTESIAN_POINT ( 'NONE',  ( 15.47812500061451679, -4.541064518000419881, 2.621784821874995952 ) ) ;
#54503=CARTESIAN_POINT ( 'NONE',  ( 13.99687500061451928, 6.054752690667223547, 3.707466751127219781E-16 ) ) ;
#54506=CARTESIAN_POINT ( 'NONE',  ( 26.16562500061451502, 3.027376345333611329, 5.243569643749999010 ) ) ;
#54508=CARTESIAN_POINT ( 'NONE',  ( 14.81250000000000000, -5.773502691896255534, -1.060575238724906372E-15 ) ) ;
#54509=CARTESIAN_POINT ( 'NONE',  ( 24.07500000122903216, 2.886751345948129099, -4.999999999999998224 ) ) ;
#54510=CARTESIAN_POINT ( 'NONE',  ( 18.36562500061451431, 3.027376345333613106, -5.243569643749998122 ) ) ;
#54511=ORIENTED_EDGE ( 'NONE', *, *, #64554, .T. ) ;
#54512=CARTESIAN_POINT ( 'NONE',  ( 23.51249999999999574, 2.886751345948129099, -4.999999999999998224 ) ) ;
#54513=CARTESIAN_POINT ( 'NONE',  ( 24.79687500061451999, 6.054752690667223547, 3.707466751127219781E-16 ) ) ;
#54514=ORIENTED_EDGE ( 'NONE', *, *, #55072, .F. ) ;
#54516=CARTESIAN_POINT ( 'NONE',  ( 11.72812500061451857, 4.541064518000418104, 2.621784821874999949 ) ) ;
#54517=CARTESIAN_POINT ( 'NONE',  ( 2.840625000614518392, -3.027376345333614438, 5.243569643749998122 ) ) ;
#54519=CARTESIAN_POINT ( 'NONE',  ( 27.21562500061451928, -6.054752690667223547, -1.112240025338166033E-15 ) ) ;
#54520=CARTESIAN_POINT ( 'NONE',  ( 16.94999999999999929, 0.000000000000000000, 4.999999999999998224 ) ) ;
#54521=CARTESIAN_POINT ( 'NONE',  ( 27.22499999999999787, 4.330127018922191873, 2.499999999999999556 ) ) ;
#54522=CARTESIAN_POINT ( 'NONE',  ( 3.999999999999999112, 10.77500000000000213, -30.00000000000000000 ) ) ;
#54523=CARTESIAN_POINT ( 'NONE',  ( 7.959375000614516971, -4.541064518000417216, -2.621784821875001281 ) ) ;
#54524=CARTESIAN_POINT ( 'NONE',  ( 16.77187500061451786, 3.027376345333611329, 5.243569643749999010 ) ) ;
#54525=CARTESIAN_POINT ( 'NONE',  ( -1.071796769724488563, 13.90490381179670010, 34.00000000000000000 ) ) ;
#54526=VERTEX_POINT ( 'NONE', #28689 ) ;
#54527=CARTESIAN_POINT ( 'NONE',  ( 26.76562500061451644, -6.054752690667223547, -1.112240025338166033E-15 ) ) ;
#54528=CARTESIAN_POINT ( 'NONE',  ( 28.47187500061451715, 3.027376345333611329, 5.243569643749999010 ) ) ;
#54529=CARTESIAN_POINT ( 'NONE',  ( 3.009375000614516793, -4.541064518000417216, -2.621784821875001281 ) ) ;
#54530=EDGE_CURVE ( 'NONE', #23877, #55608, #33499, .T. ) ;
#54531=CARTESIAN_POINT ( 'NONE',  ( 14.88750000000000107, -2.886751345948125991, -5.000000000000000000 ) ) ;
#54532=CARTESIAN_POINT ( 'NONE',  ( 10.75312500061451715, 4.541064518000418104, -2.621784821874998173 ) ) ;
#54534=DIRECTION ( 'NONE',  ( -1.000000000000000000, -0.000000000000000000, -0.000000000000000000 ) ) ;
#54535=CARTESIAN_POINT ( 'NONE',  ( 27.89062500061451289, 6.054752690667223547, 3.707466751127219781E-16 ) ) ;
#54536=CARTESIAN_POINT ( 'NONE',  ( 16.35000000122903430, -2.886751345948125991, -5.000000000000000000 ) ) ;
#54537=CARTESIAN_POINT ( 'NONE',  ( 21.33750000122903145, 6.123233995736764310E-16, -4.999999999999998224 ) ) ;
#54539=CARTESIAN_POINT ( 'NONE',  ( 4.603125000614518569, 0.000000000000000000, 5.243569643749999010 ) ) ;
#54540=CARTESIAN_POINT ( 'NONE',  ( 20.93437500061451573, -4.541064518000419881, 2.621784821874995952 ) ) ;
#54541=CARTESIAN_POINT ( 'NONE',  ( -3.000416591977282496E-16, 16.59687500061452070, 25.09994784771203058 ) ) ;
#54542=CARTESIAN_POINT ( 'NONE',  ( 24.49687500061451573, -3.027376345333614438, 5.243569643749998122 ) ) ;
#54543=CARTESIAN_POINT ( 'NONE',  ( 4.312500000000000000, 2.886751345948126879, 4.999999999999999112 ) ) ;
#54544=CARTESIAN_POINT ( 'NONE',  ( -3.999999999999997335, 11.15000000122903323, 32.30940107675850470 ) ) ;
#54545=CARTESIAN_POINT ( 'NONE',  ( 11.95312500061451644, -4.541064518000417216, -2.621784821875001281 ) ) ;
#54546=CARTESIAN_POINT ( 'NONE',  ( 4.350000001229033408, 5.773502691896255534, 3.535250795749688894E-16 ) ) ;
#54547=CARTESIAN_POINT ( 'NONE',  ( 10.17187500061451999, -6.054752690667223547, -1.112240025338166033E-15 ) ) ;
#54549=CARTESIAN_POINT ( 'NONE',  ( 9.178125000614517859, -4.541064518000419881, 2.621784821874995952 ) ) ;
#54550=CARTESIAN_POINT ( 'NONE',  ( 14.25937500061451679, -4.541064518000417216, -2.621784821875001281 ) ) ;
#54551=CARTESIAN_POINT ( 'NONE',  ( 3.479729569495786379, -3.590471016896914946, -3.821457900550485398 ) ) ;
#54552=CARTESIAN_POINT ( 'NONE',  ( 21.78750000122903074, 6.123233995736764310E-16, -4.999999999999998224 ) ) ;
#54553=CARTESIAN_POINT ( 'NONE',  ( 10.88437500061451679, 4.541064518000418104, 2.621784821874999949 ) ) ;
#54554=CARTESIAN_POINT ( 'NONE',  ( 11.42812500061451608, -4.541064518000419881, 2.621784821874995952 ) ) ;
#54556=CARTESIAN_POINT ( 'NONE',  ( 21.60937500061451644, 4.541064518000418104, -2.621784821874998173 ) ) ;
#54559=CARTESIAN_POINT ( 'NONE',  ( -1.071796769724490561, 19.90759618943233278, -34.00000000000000000 ) ) ;
#54560=CARTESIAN_POINT ( 'NONE',  ( -3.000416591977282496E-16, 11.64687500061451786, -34.90005215228797653 ) ) ;
#54561=CARTESIAN_POINT ( 'NONE',  ( 16.16250000122903430, 0.000000000000000000, 4.999999999999998224 ) ) ;
#54562=CARTESIAN_POINT ( 'NONE',  ( 9.046875000614518214, 6.054752690667223547, 3.707466751127219781E-16 ) ) ;
#54563=CARTESIAN_POINT ( 'NONE',  ( -3.000416591977282496E-16, 18.79062500061451857, -34.90005215228797653 ) ) ;
#54564=CARTESIAN_POINT ( 'NONE',  ( 16.65000000122903501, -2.886751345948129988, 4.999999999999997335 ) ) ;
#54565=CARTESIAN_POINT ( 'NONE',  ( 10.79062500061451679, 6.054752690667223547, 3.707466751127219781E-16 ) ) ;
#54567=CARTESIAN_POINT ( 'NONE',  ( 15.18750000000000000, -2.886751345948129988, 4.999999999999997335 ) ) ;
#54568=CARTESIAN_POINT ( 'NONE',  ( 29.21249999999999858, -5.773502691896255534, -1.060575238724906372E-15 ) ) ;
#54569=CARTESIAN_POINT ( 'NONE',  ( 9.571875000614518569, 3.027376345333611329, 5.243569643749999010 ) ) ;
#54571=CARTESIAN_POINT ( 'NONE',  ( 9.375000001229036428, 2.886751345948126879, 4.999999999999999112 ) ) ;
#54572=CARTESIAN_POINT ( 'NONE',  ( 18.48750000122903359, -4.330127018922194537, 2.499999999999995559 ) ) ;
#54573=CARTESIAN_POINT ( 'NONE',  ( 14.35312500061451679, 4.541064518000418104, -2.621784821874998173 ) ) ;
#54574=CARTESIAN_POINT ( 'NONE',  ( 17.09062500061451573, 6.054752690667223547, 3.707466751127219781E-16 ) ) ;
#54575=CARTESIAN_POINT ( 'NONE',  ( 28.27500000122903145, 2.886751345948126879, 4.999999999999999112 ) ) ;
#54576=CARTESIAN_POINT ( 'NONE',  ( 29.62500000122903288, 2.886751345948126879, 4.999999999999999112 ) ) ;
#54577=CARTESIAN_POINT ( 'NONE',  ( 25.38749999999999929, 5.773502691896255534, 3.535250795749688894E-16 ) ) ;
#54580=CARTESIAN_POINT ( 'NONE',  ( 25.65937500061451715, 4.541064518000418104, -2.621784821874998173 ) ) ;
#54582=CARTESIAN_POINT ( 'NONE',  ( 13.35000000122903430, 5.773502691896255534, 3.535250795749688894E-16 ) ) ;
#54583=CARTESIAN_POINT ( 'NONE',  ( 3.412500000000002309, 2.886751345948126879, 4.999999999999999112 ) ) ;
#54584=EDGE_CURVE ( 'NONE', #11143, #61146, #10626, .T. ) ;
#54586=CARTESIAN_POINT ( 'NONE',  ( 6.609375000614519102, -4.541064518000417216, -2.621784821875001281 ) ) ;
#54587=AXIS2_PLACEMENT_3D ( 'NONE', #20900, #37898, #10918 ) ;
#54588=CARTESIAN_POINT ( 'NONE',  ( 24.89062500061451644, -3.027376345333614438, 5.243569643749998122 ) ) ;
#54589=CARTESIAN_POINT ( 'NONE',  ( 4.734375000614518214, -4.541064518000419881, 2.621784821874995952 ) ) ;
#54592=CARTESIAN_POINT ( 'NONE',  ( 4.171875000614517326, 3.027376345333611329, 5.243569643749999010 ) ) ;
#54593=CARTESIAN_POINT ( 'NONE',  ( 10.02187500061451964, 3.027376345333611329, 5.243569643749999010 ) ) ;
#54594=CARTESIAN_POINT ( 'NONE',  ( 5.100000000000000533, 4.330127018922192761, -2.499999999999997780 ) ) ;
#54595=CARTESIAN_POINT ( 'NONE',  ( -4.243569643749998122, 13.54062500061459140, 32.45002607614398471 ) ) ;
#54596=CARTESIAN_POINT ( 'NONE',  ( 22.72499999999999787, 4.330127018922191873, 2.499999999999999556 ) ) ;
#54597=CARTESIAN_POINT ( 'NONE',  ( 28.72500000000000142, -4.330127018922194537, 2.499999999999995559 ) ) ;
#54598=CARTESIAN_POINT ( 'NONE',  ( 5.062500000000000888, 2.886751345948129099, -4.999999999999998224 ) ) ;
#54599=ORIENTED_EDGE ( 'NONE', *, *, #34645, .F. ) ;
#54600=CARTESIAN_POINT ( 'NONE',  ( 18.14062500061451644, -3.027376345333614438, 5.243569643749998122 ) ) ;
#54601=CARTESIAN_POINT ( 'NONE',  ( 11.72812500061451857, 4.541064518000418104, 2.621784821874999949 ) ) ;
#54603=CARTESIAN_POINT ( 'NONE',  ( 8.221875000614518925, 3.027376345333611329, 5.243569643749999010 ) ) ;
#54604=CARTESIAN_POINT ( 'NONE',  ( 24.82499999999999929, 6.123233995736764310E-16, -4.999999999999998224 ) ) ;
#54605=CARTESIAN_POINT ( 'NONE',  ( 20.81250000122903643, -4.330127018922190985, -2.500000000000001332 ) ) ;
#54606=CARTESIAN_POINT ( 'NONE',  ( 1.071796769724505438, 10.97990381179670116, 26.00000000000001421 ) ) ;
#54607=CARTESIAN_POINT ( 'NONE',  ( 8.784375000614518925, -4.541064518000419881, 2.621784821874995952 ) ) ;
#54608=CARTESIAN_POINT ( 'NONE',  ( 13.32187500061451502, -6.054752690667223547, -1.112240025338166033E-15 ) ) ;
#54609=CARTESIAN_POINT ( 'NONE',  ( 25.24687500061451573, 6.054752690667223547, 3.707466751127219781E-16 ) ) ;
#54611=CARTESIAN_POINT ( 'NONE',  ( 17.97187500061451715, 3.027376345333613106, -5.243569643749998122 ) ) ;
#54612=CARTESIAN_POINT ( 'NONE',  ( 8.971875000614515372, 3.027376345333613106, -5.243569643749998122 ) ) ;
#54614=CARTESIAN_POINT ( 'NONE',  ( 22.05000000000000071, -4.330127018922190985, -2.500000000000001332 ) ) ;
#54616=CARTESIAN_POINT ( 'NONE',  ( -4.243569643749997233, 10.44687500061451857, -27.54997392385601174 ) ) ;
#54618=CARTESIAN_POINT ( 'NONE',  ( 11.87812500061451537, -4.541064518000419881, 2.621784821874995952 ) ) ;
#54619=CARTESIAN_POINT ( 'NONE',  ( 28.77187500061451431, 3.027376345333613106, -5.243569643749998122 ) ) ;
#54620=DIRECTION ( 'NONE',  ( -0.000000000000000000, -1.000000000000000000, -0.000000000000000000 ) ) ;
#54621=CARTESIAN_POINT ( 'NONE',  ( 3.999999999999999112, 9.987500001229033586, -30.00000000000000000 ) ) ;
#54622=CARTESIAN_POINT ( 'NONE',  ( 12.71250000000000036, 2.886751345948129099, -4.999999999999998224 ) ) ;
#54623=CARTESIAN_POINT ( 'NONE',  ( 8.484601909799253346E-16, 17.52500000122903501, 34.61880215351700230 ) ) ;
#54624=CARTESIAN_POINT ( 'NONE',  ( 11.70000000122903216, -2.886751345948129988, 4.999999999999997335 ) ) ;
#54625=CARTESIAN_POINT ( 'NONE',  ( 21.30937500061451573, 0.000000000000000000, 5.243569643749999010 ) ) ;
#54626=CARTESIAN_POINT ( 'NONE',  ( 15.79687500061451821, 6.054752690667223547, 3.707466751127219781E-16 ) ) ;
#54629=CARTESIAN_POINT ( 'NONE',  ( 16.60312500061451857, 4.541064518000418104, -2.621784821874998173 ) ) ;
#54630=CARTESIAN_POINT ( 'NONE',  ( 28.68750000122903288, 4.330127018922191873, 2.499999999999999556 ) ) ;
#54631=CARTESIAN_POINT ( 'NONE',  ( 18.30937500061451928, -4.541064518000417216, -2.621784821875001281 ) ) ;
#54632=CARTESIAN_POINT ( 'NONE',  ( 5.915625000614515905, 3.027376345333611329, 5.243569643749999010 ) ) ;
#54633=CARTESIAN_POINT ( 'NONE',  ( 20.42812500061451431, -4.541064518000419881, 2.621784821874995952 ) ) ;
#54636=CARTESIAN_POINT ( 'NONE',  ( 28.80937500061451573, 4.541064518000418104, -2.621784821874998173 ) ) ;
#54637=CARTESIAN_POINT ( 'NONE',  ( -3.000416591977282496E-16, 12.04062500061451857, 25.09994784771203058 ) ) ;
#54638=CARTESIAN_POINT ( 'NONE',  ( 16.20000000122903216, -2.886751345948129988, 4.999999999999997335 ) ) ;
#54640=CARTESIAN_POINT ( 'NONE',  ( 27.66562500061451146, -6.054752690667223547, -1.112240025338166033E-15 ) ) ;
#54642=( BOUNDED_CURVE ( )  B_SPLINE_CURVE ( 2, ( #69541, #13008, #21013, #43201, #26571, #63259, #65721, #48741, #18900 ),
 .UNSPECIFIED., .F., .F. ) 
 B_SPLINE_CURVE_WITH_KNOTS ( ( 3, 2, 2, 2, 3 ),
 ( 0.9456521739130434590, 0.9492753623188405765, 0.9565217391304348116, 0.9637681159420289356, 0.9662083003288912675 ),
 .UNSPECIFIED. ) 
 CURVE ( )  GEOMETRIC_REPRESENTATION_ITEM ( )  RATIONAL_B_SPLINE_CURVE ( ( 0.9330127018922194093, 0.9330127018922194093, 1.000000000000000000, 0.8660254037844387076, 1.000000000000000000, 0.8660254037844387076, 1.000000000000000000, 0.9548846649268474263, 0.9401540970596797830 ) ) 
 REPRESENTATION_ITEM ( '' )  );
#54643=CARTESIAN_POINT ( 'NONE',  ( 21.75937500061451502, 0.000000000000000000, 5.243569643749999010 ) ) ;
#54644=CARTESIAN_POINT ( 'NONE',  ( 22.05000000122903714, -2.886751345948129988, 4.999999999999997335 ) ) ;
#54645=CARTESIAN_POINT ( 'NONE',  ( 23.80312500061451786, 4.541064518000418104, -2.621784821874998173 ) ) ;
#54646=CARTESIAN_POINT ( 'NONE',  ( 16.92187500061451999, -6.054752690667223547, -1.112240025338166033E-15 ) ) ;
#54647=CARTESIAN_POINT ( 'NONE',  ( 11.80312500061451608, 0.000000000000000000, 5.243569643749999010 ) ) ;
#54648=CARTESIAN_POINT ( 'NONE',  ( 4.243569643749999898, 14.23437500061451821, 30.00000000000000000 ) ) ;
#54649=CARTESIAN_POINT ( 'NONE',  ( 16.86562500061451786, -6.054752690667223547, -1.112240025338166033E-15 ) ) ;
#54652=ORIENTED_EDGE ( 'NONE', *, *, #6970, .F. ) ;
#54653=CARTESIAN_POINT ( 'NONE',  ( 23.51249999999999574, 2.886751345948129099, -4.999999999999998224 ) ) ;
#54654=CARTESIAN_POINT ( 'NONE',  ( -4.243569643749999898, 18.47187500061451715, -32.45002607614398471 ) ) ;
#54655=CARTESIAN_POINT ( 'NONE',  ( 3.764462467596158657, -3.290797220303479875, -3.829620922746740153 ) ) ;
#54656=CARTESIAN_POINT ( 'NONE',  ( 23.65312500061451573, -4.541064518000417216, -2.621784821875001281 ) ) ;
#54657=CARTESIAN_POINT ( 'NONE',  ( 5.353125000614515905, 4.541064518000418104, -2.621784821874998173 ) ) ;
#54658=CARTESIAN_POINT ( 'NONE',  ( 18.18750000122903288, 6.123233995736764310E-16, -4.999999999999998224 ) ) ;
#54659=CARTESIAN_POINT ( 'NONE',  ( 23.39062500061451289, 6.054752690667223547, 3.707466751127219781E-16 ) ) ;
#54660=CARTESIAN_POINT ( 'NONE',  ( 22.05000000000000071, -4.330127018922190985, -2.500000000000001332 ) ) ;
#54661=CARTESIAN_POINT ( 'NONE',  ( 28.79062500061451502, 6.054752690667223547, 3.707466751127219781E-16 ) ) ;
#54662=CARTESIAN_POINT ( 'NONE',  ( 7.828125000614517326, -4.541064518000419881, 2.621784821874995952 ) ) ;
#54663=ORIENTED_EDGE ( 'NONE', *, *, #8736, .F. ) ;
#54664=CARTESIAN_POINT ( 'NONE',  ( 23.80312500061451786, 4.541064518000418104, -2.621784821874998173 ) ) ;
#54665=CARTESIAN_POINT ( 'NONE',  ( 4.753125000614515372, -4.541064518000417216, -2.621784821875001281 ) ) ;
#54667=CARTESIAN_POINT ( 'NONE',  ( 2.915625000614516793, -6.054752690667223547, -1.112240025338166033E-15 ) ) ;
#54668=CARTESIAN_POINT ( 'NONE',  ( -3.999999999999997335, 12.95000000122903572, -27.69059892324149175 ) ) ;
#54670=EDGE_CURVE ( 'NONE', #54755, #23337, #63907, .T. ) ;
#54671=CARTESIAN_POINT ( 'NONE',  ( 11.66249999999999964, -5.773502691896255534, -1.060575238724906372E-15 ) ) ;
#54672=CARTESIAN_POINT ( 'NONE',  ( 10.88437500061451679, 4.541064518000418104, 2.621784821874999949 ) ) ;
#54673=CARTESIAN_POINT ( 'NONE',  ( 5.512500001229033941, -4.330127018922190985, -2.500000000000001332 ) ) ;
#54674=CARTESIAN_POINT ( 'NONE',  ( 14.59687500061452070, -3.027376345333614438, 5.243569643749998122 ) ) ;
#54675=CARTESIAN_POINT ( 'NONE',  ( 5.371875000614516615, 3.027376345333613106, -5.243569643749998122 ) ) ;
#54676=CARTESIAN_POINT ( 'NONE',  ( 4.243569643749999898, 10.09062500061451928, -27.54997392385601529 ) ) ;
#54678=CARTESIAN_POINT ( 'NONE',  ( 13.50937500061451679, 4.541064518000418104, -2.621784821874998173 ) ) ;
#54679=CARTESIAN_POINT ( 'NONE',  ( 3.662614727433532558, 3.403720994510690101, 3.988704636966998063 ) ) ;
#54680=CARTESIAN_POINT ( 'NONE',  ( 22.67812500061451431, -4.541064518000419881, 2.621784821874995952 ) ) ;
#54683=CARTESIAN_POINT ( 'NONE',  ( -3.000416591977282496E-16, 19.69062500061459176, 25.09994784771203058 ) ) ;
#54684=CARTESIAN_POINT ( 'NONE',  ( 23.10937500061451644, 0.000000000000000000, 5.243569643749999010 ) ) ;
#54685=CARTESIAN_POINT ( 'NONE',  ( 29.77499999999999858, 6.123233995736764310E-16, -4.999999999999998224 ) ) ;
#54686=( BOUNDED_CURVE ( )  B_SPLINE_CURVE ( 2, ( #51979, #23888, #46435, #68974, #18331, #63417, #52336 ),
 .UNSPECIFIED., .F., .F. ) 
 B_SPLINE_CURVE_WITH_KNOTS ( ( 3, 2, 2, 3 ),
 ( 0.7249999999999999778, 0.7277777777777777457, 0.7305555555555555136, 0.7333333333333332815 ),
 .UNSPECIFIED. ) 
 CURVE ( )  GEOMETRIC_REPRESENTATION_ITEM ( )  RATIONAL_B_SPLINE_CURVE ( ( 1.000000000000000000, 0.8660254037844387076, 1.000000000000000000, 0.8660254037844387076, 1.000000000000000000, 0.8660254037844387076, 1.000000000000000000 ) ) 
 REPRESENTATION_ITEM ( '' )  );
#54687=CARTESIAN_POINT ( 'NONE',  ( 5.240625000614516971, -3.027376345333610441, -5.243569643749999898 ) ) ;
#54689=CARTESIAN_POINT ( 'NONE',  ( 23.95312500061451289, 0.000000000000000000, 5.243569643749999010 ) ) ;
#54690=CARTESIAN_POINT ( 'NONE',  ( 17.69062500061451715, -3.027376345333614438, 5.243569643749998122 ) ) ;
#54691=CARTESIAN_POINT ( 'NONE',  ( 14.93437500061451750, 4.541064518000418104, 2.621784821874999949 ) ) ;
#54693=CARTESIAN_POINT ( 'NONE',  ( 28.27500000122903145, 2.886751345948126879, 4.999999999999999112 ) ) ;
#54694=CARTESIAN_POINT ( 'NONE',  ( 5.746875000614517504, -3.027376345333610441, -5.243569643749999898 ) ) ;
#54695=CARTESIAN_POINT ( 'NONE',  ( 17.37187500061451573, -6.054752690667223547, -1.112240025338166033E-15 ) ) ;
#54696=CARTESIAN_POINT ( 'NONE',  ( -1.071796769724491005, 11.80759618943233669, 26.00000000000000355 ) ) ;
#54697=CARTESIAN_POINT ( 'NONE',  ( 23.85000000000000142, -4.330127018922190985, -2.500000000000001332 ) ) ;
#54698=CARTESIAN_POINT ( 'NONE',  ( 4.012500001229033053, 0.000000000000000000, 4.999999999999998224 ) ) ;
#54699=CARTESIAN_POINT ( 'NONE',  ( 25.32187500061451857, 3.027376345333611329, 5.243569643749999010 ) ) ;
#54700=CARTESIAN_POINT ( 'NONE',  ( 16.20937500061451786, 4.541064518000418104, -2.621784821874998173 ) ) ;
#54702=CARTESIAN_POINT ( 'NONE',  ( 29.51249999999999929, 2.886751345948126879, 4.999999999999999112 ) ) ;
#54703=CARTESIAN_POINT ( 'NONE',  ( 8.699999999999999289, 4.330127018922192761, -2.499999999999997780 ) ) ;
#54705=CARTESIAN_POINT ( 'NONE',  ( 20.39062500061451644, -3.027376345333614438, 5.243569643749998122 ) ) ;
#54706=CARTESIAN_POINT ( 'NONE',  ( 10.01250000000000107, 2.886751345948129099, -4.999999999999998224 ) ) ;
#54707=CARTESIAN_POINT ( 'NONE',  ( 5.090625000614516615, -3.027376345333614438, 5.243569643749998122 ) ) ;
#54708=CARTESIAN_POINT ( 'NONE',  ( 18.41250000000000142, -5.773502691896255534, -1.060575238724906372E-15 ) ) ;
#54710=CARTESIAN_POINT ( 'NONE',  ( 18.66562500061451146, -6.054752690667223547, -1.112240025338166033E-15 ) ) ;
#54711=CARTESIAN_POINT ( 'NONE',  ( -1.999999999999997113, 17.37500000000000000, 33.46410161513775705 ) ) ;
#54712=CARTESIAN_POINT ( 'NONE',  ( 23.43750000122902932, -4.330127018922194537, 2.499999999999995559 ) ) ;
#54714=CARTESIAN_POINT ( 'NONE',  ( 29.55937500061451573, -4.541064518000417216, -2.621784821875001281 ) ) ;
#54716=CARTESIAN_POINT ( 'NONE',  ( 17.39062500061451644, -3.027376345333610441, -5.243569643749999898 ) ) ;
#54717=CARTESIAN_POINT ( 'NONE',  ( 23.99062500061451786, -3.027376345333614438, 5.243569643749998122 ) ) ;
#54718=CARTESIAN_POINT ( 'NONE',  ( 25.58437500061451431, 6.421520780324663323E-16, -5.243569643749999010 ) ) ;
#54719=CARTESIAN_POINT ( 'NONE',  ( 8.175000000000002487, 6.123233995736764310E-16, -4.999999999999998224 ) ) ;
#54720=CARTESIAN_POINT ( 'NONE',  ( 13.11562500061451786, 3.027376345333611329, 5.243569643749999010 ) ) ;
#54721=CARTESIAN_POINT ( 'NONE',  ( 27.17812500061451786, -4.541064518000419881, 2.621784821874995952 ) ) ;
#54722=CARTESIAN_POINT ( 'NONE',  ( 14.29687500061451821, -3.027376345333610441, -5.243569643749999898 ) ) ;
#54723=CARTESIAN_POINT ( 'NONE',  ( 18.38437500061451857, 6.421520780324663323E-16, -5.243569643749999010 ) ) ;
#54725=CARTESIAN_POINT ( 'NONE',  ( 4.243569643749999898, 19.09062500061451573, 32.45002607614398471 ) ) ;
#54726=CARTESIAN_POINT ( 'NONE',  ( 22.80000000122903359, 5.773502691896255534, 3.535250795749688894E-16 ) ) ;
#54728=CARTESIAN_POINT ( 'NONE',  ( 15.25312500061451715, 4.541064518000418104, -2.621784821874998173 ) ) ;
#54729=CARTESIAN_POINT ( 'NONE',  ( 7.209375000614519635, 4.541064518000418104, -2.621784821874998173 ) ) ;
#54730=CARTESIAN_POINT ( 'NONE',  ( 8.184375000614515727, 4.541064518000418104, 2.621784821874999949 ) ) ;
#54733=CARTESIAN_POINT ( 'NONE',  ( 27.68437500061451573, -4.541064518000419881, 2.621784821874995952 ) ) ;
#54734=CARTESIAN_POINT ( 'NONE',  ( 20.20312500061451644, 4.541064518000418104, -2.621784821874998173 ) ) ;
#54735=CARTESIAN_POINT ( 'NONE',  ( 23.67187500061451999, -6.054752690667223547, -1.112240025338166033E-15 ) ) ;
#54736=CARTESIAN_POINT ( 'NONE',  ( 19.60312500061451502, -4.541064518000417216, -2.621784821875001281 ) ) ;
#54737=CARTESIAN_POINT ( 'NONE',  ( 1.999999999999998668, 11.30000000000000071, 26.53589838486224650 ) ) ;
#54738=CARTESIAN_POINT ( 'NONE',  ( 26.20312500061451644, 0.000000000000000000, 5.243569643749999010 ) ) ;
#54739=CARTESIAN_POINT ( 'NONE',  ( 6.375000001229031987, -5.773502691896255534, -1.060575238724906372E-15 ) ) ;
#54741=CARTESIAN_POINT ( 'NONE',  ( 29.21249999999999858, -5.773502691896255534, -1.060575238724906372E-15 ) ) ;
#54742=CARTESIAN_POINT ( 'NONE',  ( 8.484601909799253346E-16, 16.06250000000000000, -25.38119784648299770 ) ) ;
#54743=CARTESIAN_POINT ( 'NONE',  ( 23.40000000122903145, -2.886751345948129988, 4.999999999999997335 ) ) ;
#54745=CARTESIAN_POINT ( 'NONE',  ( 5.634375000614519458, -4.541064518000419881, 2.621784821874995952 ) ) ;
#54746=CARTESIAN_POINT ( 'NONE',  ( 12.67499999999999893, 6.123233995736764310E-16, -4.999999999999998224 ) ) ;
#54747=CARTESIAN_POINT ( 'NONE',  ( 13.34062500061451750, -3.027376345333610441, -5.243569643749999898 ) ) ;
#54748=CARTESIAN_POINT ( 'NONE',  ( 9.084375000614517859, 4.541064518000418104, 2.621784821874999949 ) ) ;
#54749=CARTESIAN_POINT ( 'NONE',  ( 25.61250000122903359, 0.000000000000000000, 4.999999999999998224 ) ) ;
#54750=CARTESIAN_POINT ( 'NONE',  ( 14.03437500061451715, 4.541064518000418104, 2.621784821874999949 ) ) ;
#54751=CARTESIAN_POINT ( 'NONE',  ( 6.084375000614518747, -4.541064518000419881, 2.621784821874995952 ) ) ;
#54752=CARTESIAN_POINT ( 'NONE',  ( 29.96250000000000213, 2.886751345948126879, 4.999999999999999112 ) ) ;
#54753=CARTESIAN_POINT ( 'NONE',  ( 6.103125000614515905, -4.541064518000417216, -2.621784821875001281 ) ) ;
#54754=CARTESIAN_POINT ( 'NONE',  ( 14.39062500061451821, 6.054752690667223547, 3.707466751127219781E-16 ) ) ;
#54755=VERTEX_POINT ( 'NONE', #22419 ) ;
#54756=CARTESIAN_POINT ( 'NONE',  ( 11.31562500061451892, 3.027376345333611329, 5.243569643749999010 ) ) ;
#54757=CARTESIAN_POINT ( 'NONE',  ( 9.440625000614517148, 6.054752690667223547, 3.707466751127219781E-16 ) ) ;
#54759=CARTESIAN_POINT ( 'NONE',  ( 8.587500000000002132, -2.886751345948125991, -5.000000000000000000 ) ) ;
#54760=CARTESIAN_POINT ( 'NONE',  ( 3.262500001229035718, -4.330127018922190985, -2.500000000000001332 ) ) ;
#54761=CARTESIAN_POINT ( 'NONE',  ( 16.76249999999999929, 2.886751345948129099, -4.999999999999998224 ) ) ;
#54763=CARTESIAN_POINT ( 'NONE',  ( 19.05937500061451928, 0.000000000000000000, 5.243569643749999010 ) ) ;
#54764=CARTESIAN_POINT ( 'NONE',  ( 14.17500000122903536, 2.886751345948129099, -4.999999999999998224 ) ) ;
#54766=CARTESIAN_POINT ( 'NONE',  ( -4.243569643749999898, 16.61562500061451786, -32.45002607614398471 ) ) ;
#54767=CARTESIAN_POINT ( 'NONE',  ( 22.05000000000000071, -4.330127018922190985, -2.500000000000001332 ) ) ;
#54768=CARTESIAN_POINT ( 'NONE',  ( 29.76562500061451644, 3.027376345333611329, 5.243569643749999010 ) ) ;
#54770=CARTESIAN_POINT ( 'NONE',  ( 24.18750000000000000, -2.886751345948096681, 5.000000000000054179 ) ) ;
#54771=CARTESIAN_POINT ( 'NONE',  ( 14.59687500061452070, -3.027376345333614438, 5.243569643749998122 ) ) ;
#54772=CARTESIAN_POINT ( 'NONE',  ( 25.76249999999999929, 2.886751345948129099, -4.999999999999998224 ) ) ;
#54773=CARTESIAN_POINT ( 'NONE',  ( 10.67812500061451608, 6.421520780324663323E-16, -5.243569643749999010 ) ) ;
#54775=CARTESIAN_POINT ( 'NONE',  ( 22.32187500061451502, -6.054752690667223547, -1.112240025338166033E-15 ) ) ;
#54777=CARTESIAN_POINT ( 'NONE',  ( 8.840625000614515727, -3.027376345333610441, -5.243569643749999898 ) ) ;
#54778=CARTESIAN_POINT ( 'NONE',  ( 13.88437500061451679, 6.421520780324663323E-16, -5.243569643749999010 ) ) ;
#54779=EDGE_LOOP ( 'NONE', ( #3006, #60402, #57486, #65232 ) ) ;
#54780=CARTESIAN_POINT ( 'NONE',  ( 24.23437500061451644, 6.421520780324663323E-16, -5.243569643749999010 ) ) ;
#54781=CARTESIAN_POINT ( 'NONE',  ( 30.00000000000000000, 0.000000000000000000, 0.000000000000000000 ) ) ;
#54782=CARTESIAN_POINT ( 'NONE',  ( 24.60000000000000142, 0.000000000000000000, 4.999999999999998224 ) ) ;
#54783=CARTESIAN_POINT ( 'NONE',  ( 5.212500000000002132, 2.886751345948126879, 4.999999999999999112 ) ) ;
#54784=CARTESIAN_POINT ( 'NONE',  ( 16.57500000122903216, 2.886751345948126879, 4.999999999999999112 ) ) ;
#54787=ORIENTED_EDGE ( 'NONE', *, *, #63337, .T. ) ;
#54788=CARTESIAN_POINT ( 'NONE',  ( 14.32500000000000107, -4.330127018922194537, 2.499999999999995559 ) ) ;
#54789=CARTESIAN_POINT ( 'NONE',  ( 16.68750000000000000, -2.886751345948125991, -5.000000000000000000 ) ) ;
#54790=CARTESIAN_POINT ( 'NONE',  ( 11.12812500061451715, 6.421520780324663323E-16, -5.243569643749999010 ) ) ;
#54792=CARTESIAN_POINT ( 'NONE',  ( 18.63750000122903216, 6.123233995736764310E-16, -4.999999999999998224 ) ) ;
#54793=CARTESIAN_POINT ( 'NONE',  ( 9.001249775931846008E-16, 16.37187500061451573, -25.09994784771203058 ) ) ;
#54794=CARTESIAN_POINT ( 'NONE',  ( 29.51250000122903216, 4.330127018922192761, -2.499999999999997780 ) ) ;
#54796=CARTESIAN_POINT ( 'NONE',  ( 9.487500000000000711, -2.886751345948125991, -5.000000000000000000 ) ) ;
#54799=VERTEX_POINT ( 'NONE', #39423 ) ;
#54800=CARTESIAN_POINT ( 'NONE',  ( 4.243569643749999898, 12.82812500061451821, 30.00000000000000000 ) ) ;
#54801=CARTESIAN_POINT ( 'NONE',  ( 25.41562500061451146, -6.054752690667223547, -1.112240025338166033E-15 ) ) ;
#54802=CARTESIAN_POINT ( 'NONE',  ( 3.504965621013899746, 3.565840152826760256, 3.504965621013765631 ) ) ;
#54804=CARTESIAN_POINT ( 'NONE',  ( 20.82187500061451857, 3.027376345333611329, 5.243569643749999010 ) ) ;
#54805=CARTESIAN_POINT ( 'NONE',  ( 19.00312500061451715, 0.000000000000000000, 5.243569643749999010 ) ) ;
#54806=CARTESIAN_POINT ( 'NONE',  ( -4.243569643749999898, 13.50312500061459531, -30.00000000000000000 ) ) ;
#54807=CARTESIAN_POINT ( 'NONE',  ( 22.61250000122903003, -4.330127018922190985, -2.500000000000001332 ) ) ;
#54808=AXIS2_PLACEMENT_3D ( 'NONE', #3716, #26243, #20682 ) ;
#54809=CARTESIAN_POINT ( 'NONE',  ( 5.128125000614516260, -4.541064518000419881, 2.621784821874995952 ) ) ;
#54811=CARTESIAN_POINT ( 'NONE',  ( 22.52812500061451573, 4.541064518000418104, 2.621784821874999949 ) ) ;
#54814=CARTESIAN_POINT ( 'NONE',  ( 15.87187500061451573, 3.027376345333611329, 5.243569643749999010 ) ) ;
#54815=CARTESIAN_POINT ( 'NONE',  ( 13.24687500061451750, -3.027376345333614438, 5.243569643749998122 ) ) ;
#54816=CARTESIAN_POINT ( 'NONE',  ( 22.24687500061451217, -3.027376345333614438, 5.243569643749998122 ) ) ;
#54817=CARTESIAN_POINT ( 'NONE',  ( -4.243569643749999898, 12.62187500061451750, 27.54997392385601529 ) ) ;
#54818=CARTESIAN_POINT ( 'NONE',  ( 3.928125000614516527, 6.421520780324663323E-16, -5.243569643749999010 ) ) ;
#54819=CARTESIAN_POINT ( 'NONE',  ( 25.45312500061451644, -4.541064518000417216, -2.621784821875001281 ) ) ;
#54820=CARTESIAN_POINT ( 'NONE',  ( 26.24062500061451431, -3.027376345333614438, 5.243569643749998122 ) ) ;
#54822=CARTESIAN_POINT ( 'NONE',  ( -2.000000000000000000, 18.57500000000000284, 26.53589838486224650 ) ) ;
#54823=CARTESIAN_POINT ( 'NONE',  ( 6.159375000614517148, -4.541064518000417216, -2.621784821875001281 ) ) ;
#54825=CARTESIAN_POINT ( 'NONE',  ( 13.98750000122903359, -4.330127018922194537, 2.499999999999995559 ) ) ;
#54826=AXIS2_PLACEMENT_3D ( 'NONE', #66122, #55410, #15501 ) ;
#54827=CARTESIAN_POINT ( 'NONE',  ( 8.962500001229033231, 0.000000000000000000, 4.999999999999998224 ) ) ;
#54828=CARTESIAN_POINT ( 'NONE',  ( 29.10000000122903074, 5.773502691896255534, 3.535250795749688894E-16 ) ) ;
#54831=CARTESIAN_POINT ( 'NONE',  ( 14.52187500061451608, 3.027376345333611329, 5.243569643749999010 ) ) ;
#54832=DIRECTION ( 'NONE',  ( -0.000000000000000000, -1.000000000000000000, -0.000000000000000000 ) ) ;
#54834=CARTESIAN_POINT ( 'NONE',  ( 19.22812500061451502, 6.421520780324663323E-16, -5.243569643749999010 ) ) ;
#54835=CARTESIAN_POINT ( 'NONE',  ( 6.965625000614518392, -6.054752690667223547, -1.112240025338166033E-15 ) ) ;
#54836=CARTESIAN_POINT ( 'NONE',  ( 24.79687500061452354, 6.054752690667223547, 3.707466751127219781E-16 ) ) ;
#54837=CARTESIAN_POINT ( 'NONE',  ( 8.203125000614518214, 0.000000000000000000, 5.243569643749999010 ) ) ;
#54839=CARTESIAN_POINT ( 'NONE',  ( 7.087500001229034119, 4.330127018922191873, 2.499999999999999556 ) ) ;
#54840=CARTESIAN_POINT ( 'NONE',  ( 22.22812500061451502, -4.541064518000419881, 2.621784821874995952 ) ) ;
#54841=CARTESIAN_POINT ( 'NONE',  ( 4.000000000000000000, 18.50000000122903288, -27.69059892324149530 ) ) ;
#54842=CARTESIAN_POINT ( 'NONE',  ( 9.712500001229033231, 4.330127018922192761, -2.499999999999997780 ) ) ;
#54843=CARTESIAN_POINT ( 'NONE',  ( 19.37812500061451715, 4.541064518000418104, 2.621784821874999949 ) ) ;
#54844=CARTESIAN_POINT ( 'NONE',  ( 15.21562500061451750, 3.027376345333613106, -5.243569643749998122 ) ) ;
#54846=CARTESIAN_POINT ( 'NONE',  ( 16.80000000000000071, 4.330127018922192761, -2.499999999999997780 ) ) ;
#54847=CARTESIAN_POINT ( 'NONE',  ( 10.80000000122903536, -2.886751345948129988, 4.999999999999997335 ) ) ;
#54848=CARTESIAN_POINT ( 'NONE',  ( 8.765625000614518214, -6.054752690667223547, -1.112240025338166033E-15 ) ) ;
#54849=CARTESIAN_POINT ( 'NONE',  ( 10.79062500061451679, 6.054752690667223547, 3.707466751127219781E-16 ) ) ;
#54850=EDGE_CURVE ( 'NONE', #63961, #62008, #18145, .T. ) ;
#54851=CARTESIAN_POINT ( 'NONE',  ( 21.86250000122903003, 4.330127018922192761, -2.499999999999997780 ) ) ;
#54853=CARTESIAN_POINT ( 'NONE',  ( 18.83437500061451431, 6.421520780324663323E-16, -5.243569643749999010 ) ) ;
#54855=CARTESIAN_POINT ( 'NONE',  ( 6.262500001229034829, 0.000000000000000000, 4.999999999999998224 ) ) ;
#54856=CARTESIAN_POINT ( 'NONE',  ( 4.809375000614516615, -4.541064518000417216, -2.621784821875001281 ) ) ;
#54857=CARTESIAN_POINT ( 'NONE',  ( 22.17187500061451644, 3.027376345333611329, 5.243569643749999010 ) ) ;
#54858=CARTESIAN_POINT ( 'NONE',  ( 3.999999999999998668, 18.57500000122903216, 27.69059892324149530 ) ) ;
#54859=AXIS2_PLACEMENT_3D ( 'NONE', #27721, #56862, #56155 ) ;
#54860=CARTESIAN_POINT ( 'NONE',  ( 20.01562500061451644, -6.054752690667223547, -1.112240025338166033E-15 ) ) ;
#54861=CARTESIAN_POINT ( 'NONE',  ( 23.10937500061451644, 0.000000000000000000, 5.243569643749999010 ) ) ;
#54864=CARTESIAN_POINT ( 'NONE',  ( 28.47187500061451715, 3.027376345333611329, 5.243569643749999010 ) ) ;
#54866=CARTESIAN_POINT ( 'NONE',  ( 13.97812500061451679, 4.541064518000418104, 2.621784821874999949 ) ) ;
#54868=CARTESIAN_POINT ( 'NONE',  ( 12.34687500061452070, -3.027376345333614438, 5.243569643749998122 ) ) ;
#54869=VERTEX_POINT ( 'NONE', #39793 ) ;
#54870=CARTESIAN_POINT ( 'NONE',  ( 18.07499999999999929, 6.123233995736764310E-16, -4.999999999999998224 ) ) ;
#54871=CARTESIAN_POINT ( 'NONE',  ( 23.57812500061451289, -4.541064518000419881, 2.621784821874995952 ) ) ;
#54872=CARTESIAN_POINT ( 'NONE',  ( -1.071796769724491005, 10.57009619066136707, -34.00000000000000000 ) ) ;
#54873=DIRECTION ( 'NONE',  ( -1.000000000000000000, -0.000000000000000000, -0.000000000000000000 ) ) ;
#54874=CARTESIAN_POINT ( 'NONE',  ( 13.91249999999999964, -5.773502691896255534, -1.060575238724906372E-15 ) ) ;
#54875=CARTESIAN_POINT ( 'NONE',  ( 23.25000000122903288, 5.773502691896255534, 3.535250795749688894E-16 ) ) ;
#54876=CARTESIAN_POINT ( 'NONE',  ( 18.70312500061451644, -4.541064518000417216, -2.621784821875001281 ) ) ;
#54878=CARTESIAN_POINT ( 'NONE',  ( 21.33749999999999858, 5.773502691896255534, 3.535250795749688894E-16 ) ) ;
#54879=CARTESIAN_POINT ( 'NONE',  ( 23.33437500061451786, 6.421520780324663323E-16, -5.243569643749999010 ) ) ;
#54882=CARTESIAN_POINT ( 'NONE',  ( 10.41562500061451679, 3.027376345333611329, 5.243569643749999010 ) ) ;
#54883=CARTESIAN_POINT ( 'NONE',  ( 4.190625000614518925, -3.027376345333614438, 5.243569643749998122 ) ) ;
#54885=CARTESIAN_POINT ( 'NONE',  ( 26.39062500061451644, -3.027376345333610441, -5.243569643749999898 ) ) ;
#54886=CARTESIAN_POINT ( 'NONE',  ( 16.23750000000000071, -2.886751345948125991, -5.000000000000000000 ) ) ;
#54887=CARTESIAN_POINT ( 'NONE',  ( 24.93750000000000355, 5.773502691896255534, 3.535250795749688894E-16 ) ) ;
#54888=CARTESIAN_POINT ( 'NONE',  ( 7.725000001229034297, -5.773502691896255534, -1.060575238724906372E-15 ) ) ;
#54889=CARTESIAN_POINT ( 'NONE',  ( 6.909375000614518036, 0.000000000000000000, 5.243569643749999010 ) ) ;
#54890=CARTESIAN_POINT ( 'NONE',  ( 17.37187500061451573, -6.054752690667223547, -1.112240025338166033E-15 ) ) ;
#54891=CARTESIAN_POINT ( 'NONE',  ( 28.02187500061451431, 3.027376345333611329, 5.243569643749999010 ) ) ;
#54892=VERTEX_POINT ( 'NONE', #11706 ) ;
#54893=CARTESIAN_POINT ( 'NONE',  ( 26.72812500061451502, -4.541064518000419881, 2.621784821874995952 ) ) ;
#54894=CARTESIAN_POINT ( 'NONE',  ( 28.20937500061451786, -4.541064518000417216, -2.621784821875001281 ) ) ;
#54895=CARTESIAN_POINT ( 'NONE',  ( 3.084375000614519191, 6.421520780324663323E-16, -5.243569643749999010 ) ) ;
#54896=CARTESIAN_POINT ( 'NONE',  ( 13.12500000000000178, 6.123233995736764310E-16, -4.999999999999998224 ) ) ;
#54897=CARTESIAN_POINT ( 'NONE',  ( 11.72812500061451857, 4.541064518000418104, 2.621784821874999949 ) ) ;
#54898=DIRECTION ( 'NONE',  ( -1.000000000000000000, -0.000000000000000000, -0.000000000000000000 ) ) ;
#54899=CARTESIAN_POINT ( 'NONE',  ( 29.46562500061451928, -6.054752690667223547, -1.112240025338166033E-15 ) ) ;
#54900=CARTESIAN_POINT ( 'NONE',  ( 16.65000000122903501, -2.886751345948129988, 4.999999999999997335 ) ) ;
#54903=CARTESIAN_POINT ( 'NONE',  ( 5.765625000614519102, 3.027376345333613106, -5.243569643749998122 ) ) ;
#54904=CARTESIAN_POINT ( 'NONE',  ( 21.83437500061451786, -4.541064518000419881, 2.621784821874995952 ) ) ;
#54905=CARTESIAN_POINT ( 'NONE',  ( -2.121784821874996840, 17.68437500061451928, 33.67503911421598417 ) ) ;
#54906=CARTESIAN_POINT ( 'NONE',  ( 20.63437500061451857, 6.421520780324663323E-16, -5.243569643749999010 ) ) ;
#54907=CARTESIAN_POINT ( 'NONE',  ( 29.14687500061451075, -3.027376345333610441, -5.243569643749999898 ) ) ;
#54908=CARTESIAN_POINT ( 'NONE',  ( 9.001249775931846008E-16, 18.17187500061451999, 34.90005215228797653 ) ) ;
#54909=CARTESIAN_POINT ( 'NONE',  ( 11.87812500061451537, -4.541064518000419881, 2.621784821874995952 ) ) ;
#54910=CARTESIAN_POINT ( 'NONE',  ( 4.012500001229033053, 0.000000000000000000, 4.999999999999998224 ) ) ;
#54911=ADVANCED_FACE ( 'NONE', ( #34222 ), #56755, .F. ) ;
#54912=CARTESIAN_POINT ( 'NONE',  ( 7.771875000614516971, 3.027376345333611329, 5.243569643749999010 ) ) ;
#54915=CARTESIAN_POINT ( 'NONE',  ( 10.64062500061451644, -3.027376345333610441, -5.243569643749999898 ) ) ;
#54916=CARTESIAN_POINT ( 'NONE',  ( 15.19687500061451857, -3.027376345333610441, -5.243569643749999898 ) ) ;
#54918=CARTESIAN_POINT ( 'NONE',  ( 20.32500000122903572, -5.773502691896255534, -1.060575238724906372E-15 ) ) ;
#54919=CARTESIAN_POINT ( 'NONE',  ( 8.784375000614518925, -4.541064518000419881, 2.621784821874995952 ) ) ;
#54920=CARTESIAN_POINT ( 'NONE',  ( 12.92812500061451786, 6.421520780324663323E-16, -5.243569643749999010 ) ) ;
#54922=CARTESIAN_POINT ( 'NONE',  ( 21.49687500061451573, -3.027376345333610441, -5.243569643749999898 ) ) ;
#54923=CARTESIAN_POINT ( 'NONE',  ( -3.780580586577210855, 3.275490995243301562, 28.66886852906538863 ) ) ;
#54924=DIRECTION ( 'NONE',  ( 0.000000000000000000, 0.000000000000000000, 1.000000000000000000 ) ) ;
#54925=CARTESIAN_POINT ( 'NONE',  ( -2.121784821874996840, 12.28437500061451892, -26.32496088578401583 ) ) ;
#54926=CARTESIAN_POINT ( 'NONE',  ( 14.51250000122903394, -4.330127018922190985, -2.500000000000001332 ) ) ;
#54928=VECTOR ( 'NONE', #71502, 1000.000000000000000 ) ;
#54929=CARTESIAN_POINT ( 'NONE',  ( 9.001249775931846008E-16, 14.51562500061451466, -25.09994784771203058 ) ) ;
#54930=CARTESIAN_POINT ( 'NONE',  ( 17.70000000122903216, -2.886751345948125991, -5.000000000000000000 ) ) ;
#54931=CARTESIAN_POINT ( 'NONE',  ( 10.71562500061451928, 3.027376345333613106, -5.243569643749998122 ) ) ;
#54932=ORIENTED_EDGE ( 'NONE', *, *, #21442, .F. ) ;
#54933=AXIS2_PLACEMENT_3D ( 'NONE', #18597, #13060, #41514 ) ;
#54934=CARTESIAN_POINT ( 'NONE',  ( 15.90000000000000036, 4.330127018922192761, -2.499999999999997780 ) ) ;
#54936=CARTESIAN_POINT ( 'NONE',  ( 23.65312500061451573, -4.541064518000417216, -2.621784821875001281 ) ) ;
#54937=CARTESIAN_POINT ( 'NONE',  ( 11.03437500061451715, -4.541064518000419881, 2.621784821874995952 ) ) ;
#54940=CARTESIAN_POINT ( 'NONE',  ( 10.31250000122903288, 0.000000000000000000, 4.999999999999998224 ) ) ;
#54941=CARTESIAN_POINT ( 'NONE',  ( 18.67500000122903714, 2.886751345948129099, -4.999999999999998224 ) ) ;
#54942=CARTESIAN_POINT ( 'NONE',  ( 15.06562500061451537, -6.054752690667223547, -1.112240025338166033E-15 ) ) ;
#54943=CARTESIAN_POINT ( 'NONE',  ( 17.12812500061451715, 4.541064518000418104, 2.621784821874999949 ) ) ;
#54944=CARTESIAN_POINT ( 'NONE',  ( 24.60000000122903430, 5.773502691896255534, 3.535250795749688894E-16 ) ) ;
#54945=CARTESIAN_POINT ( 'NONE',  ( 4.378125000614518925, 6.421520780324663323E-16, -5.243569643749999010 ) ) ;
#54946=CARTESIAN_POINT ( 'NONE',  ( 25.50000000000000000, 0.000000000000000000, 4.999999999999998224 ) ) ;
#54948=CARTESIAN_POINT ( 'NONE',  ( 26.78437500061451360, -4.541064518000419881, 2.621784821874995952 ) ) ;
#54949=CYLINDRICAL_SURFACE ( 'NONE', #7589, 4.000000000000000000 ) ;
#54950=CARTESIAN_POINT ( 'NONE',  ( 12.63750000122903394, -4.330127018922194537, 2.499999999999995559 ) ) ;
#54951=CARTESIAN_POINT ( 'NONE',  ( 3.975000000000002753, -4.330127018922194537, 2.499999999999995559 ) ) ;
#54952=EDGE_CURVE ( 'NONE', #35925, #52021, #33708, .T. ) ;
#54953=CARTESIAN_POINT ( 'NONE',  ( 0.000000000000000000, 20.00000000000000000, -30.00000000000000000 ) ) ;
#54954=CARTESIAN_POINT ( 'NONE',  ( 8.521875000614516082, 3.027376345333613106, -5.243569643749998122 ) ) ;
#54955=CARTESIAN_POINT ( 'NONE',  ( 26.20312500061451644, 0.000000000000000000, 5.243569643749999010 ) ) ;
#54957=CARTESIAN_POINT ( 'NONE',  ( 1.626862140677534273E-15, 13.92500000122903181, 34.00000000000000000 ) ) ;
#54958=CARTESIAN_POINT ( 'NONE',  ( 4.385796401931335353, -2.400997692794667682, 4.385796401931427724 ) ) ;
#54959=CARTESIAN_POINT ( 'NONE',  ( 5.634375000614519458, -4.541064518000419881, 2.621784821874995952 ) ) ;
#54960=CARTESIAN_POINT ( 'NONE',  ( 9.571875000614518569, 3.027376345333611329, 5.243569643749999010 ) ) ;
#54961=CARTESIAN_POINT ( 'NONE',  ( 29.10937500061451644, -4.541064518000417216, -2.621784821875001281 ) ) ;
#54962=CARTESIAN_POINT ( 'NONE',  ( 2.121784821874999061, 12.45312500061459637, 26.32496088578401583 ) ) ;
#54963=CARTESIAN_POINT ( 'NONE',  ( 22.27499999999999858, 4.330127018922191873, 2.499999999999999556 ) ) ;
#54965=CARTESIAN_POINT ( 'NONE',  ( 28.42499999999999716, 6.123233995736764310E-16, -4.999999999999998224 ) ) ;
#54966=CARTESIAN_POINT ( 'NONE',  ( 4.650000000000001243, 4.330127018922192761, -2.499999999999997780 ) ) ;
#54967=EDGE_LOOP ( 'NONE', ( #36684, #55395, #28544, #2397 ) ) ;
#54968=CARTESIAN_POINT ( 'NONE',  ( 19.04062500061451146, -3.027376345333614438, 5.243569643749998122 ) ) ;
#54969=CARTESIAN_POINT ( 'NONE',  ( 10.45312500061451644, 0.000000000000000000, 5.243569643749999010 ) ) ;
#54971=CARTESIAN_POINT ( 'NONE',  ( 7.059375000614518392, -4.541064518000417216, -2.621784821875001281 ) ) ;
#54972=CARTESIAN_POINT ( 'NONE',  ( 20.92500000122903714, 2.886751345948129099, -4.999999999999998224 ) ) ;
#54973=CARTESIAN_POINT ( 'NONE',  ( 3.237770964828680764, -3.810424094601559286, -3.237770964828680764 ) ) ;
#54974=VECTOR ( 'NONE', #71880, 1000.000000000000000 ) ;
#54975=CARTESIAN_POINT ( 'NONE',  ( 6.834375000614518747, 4.541064518000418104, 2.621784821874999949 ) ) ;
#54976=CARTESIAN_POINT ( 'NONE',  ( 14.40937500061451715, 4.541064518000418104, -2.621784821874998173 ) ) ;
#54977=CARTESIAN_POINT ( 'NONE',  ( 23.25937500061451857, -4.541064518000417216, -2.621784821875001281 ) ) ;
#54978=CARTESIAN_POINT ( 'NONE',  ( -1.071796769724483234, 16.30759618943233491, 25.99999999999999645 ) ) ;
#54981=CARTESIAN_POINT ( 'NONE',  ( 18.45937500061451431, 4.541064518000418104, -2.621784821874998173 ) ) ;
#54982=CARTESIAN_POINT ( 'NONE',  ( 9.834375000614517859, 6.421520780324663323E-16, -5.243569643749999010 ) ) ;
#54984=CARTESIAN_POINT ( 'NONE',  ( 20.21250000000000213, -5.773502691896255534, -1.060575238724906372E-15 ) ) ;
#54986=CARTESIAN_POINT ( 'NONE',  ( -3.000416591977282496E-16, 10.74687500061451928, -34.90005215228797653 ) ) ;
#54988=CARTESIAN_POINT ( 'NONE',  ( 13.56562500061451892, 3.027376345333611329, 5.243569643749999010 ) ) ;
#54989=CARTESIAN_POINT ( 'NONE',  ( 3.037500000000002309, -2.886751345948129988, 4.999999999999997335 ) ) ;
#54990=CARTESIAN_POINT ( 'NONE',  ( 4.898587196589411843E-16, 20.00000000000000000, -26.00000000000000000 ) ) ;
#54991=CARTESIAN_POINT ( 'NONE',  ( 27.72187500061451715, -6.054752690667223547, -1.112240025338166033E-15 ) ) ;
#54992=CARTESIAN_POINT ( 'NONE',  ( 11.13750000000000284, -2.886751345948129988, 4.999999999999997335 ) ) ;
#54993=CARTESIAN_POINT ( 'NONE',  ( -3.999999999999999112, 18.76250000122903216, 30.00000000000000000 ) ) ;
#54994=CARTESIAN_POINT ( 'NONE',  ( 12.15000000122903501, -2.886751345948129988, 4.999999999999997335 ) ) ;
#54995=CARTESIAN_POINT ( 'NONE',  ( 22.54687500061451999, 6.054752690667223547, 3.707466751127219781E-16 ) ) ;
#54996=CARTESIAN_POINT ( 'NONE',  ( 17.55937500061451573, 4.541064518000418104, -2.621784821874998173 ) ) ;
#54997=CARTESIAN_POINT ( 'NONE',  ( 3.981242275647779216, 3.024881775420318331, -4.283141675081658661 ) ) ;
#54999=CARTESIAN_POINT ( 'NONE',  ( 16.26562500061451289, 3.027376345333611329, 5.243569643749999010 ) ) ;
#55000=CARTESIAN_POINT ( 'NONE',  ( 29.13750000122903216, 4.330127018922191873, 2.499999999999999556 ) ) ;
#55001=CARTESIAN_POINT ( 'NONE',  ( 18.72187500061451360, -6.054752690667223547, -1.112240025338166033E-15 ) ) ;
#55002=CARTESIAN_POINT ( 'NONE',  ( 3.065625000614517592, 3.027376345333613106, -5.243569643749998122 ) ) ;
#55003=CARTESIAN_POINT ( 'NONE',  ( 18.89062500061451644, 6.054752690667223547, 3.707466751127219781E-16 ) ) ;
#55004=CARTESIAN_POINT ( 'NONE',  ( 30.00000000000000000, 0.000000000000000000, 4.999999999999998224 ) ) ;
#55005=CARTESIAN_POINT ( 'NONE',  ( 29.10937500061451644, -4.541064518000417216, -2.621784821875001281 ) ) ;
#55006=CARTESIAN_POINT ( 'NONE',  ( -4.243569643749999898, 12.60312500061451679, 30.00000000000000000 ) ) ;
#55007=CARTESIAN_POINT ( 'NONE',  ( 18.60937500061451644, 0.000000000000000000, 5.243569643749999010 ) ) ;
#55008=CARTESIAN_POINT ( 'NONE',  ( 15.15000000122903323, 5.773502691896255534, 3.535250795749688894E-16 ) ) ;
#55010=CARTESIAN_POINT ( 'NONE',  ( -2.121784821874999949, 19.33437500061451786, -33.67503911421598417 ) ) ;
#55011=EDGE_CURVE ( 'NONE', #29428, #13883, #11672, .T. ) ;
#55012=CARTESIAN_POINT ( 'NONE',  ( 19.65937500061451360, -4.541064518000417216, -2.621784821875001281 ) ) ;
#55013=CARTESIAN_POINT ( 'NONE',  ( 21.97500000122903074, 2.886751345948126879, 4.999999999999999112 ) ) ;
#55014=CARTESIAN_POINT ( 'NONE',  ( 17.10937500061451999, 4.541064518000418104, -2.621784821874998173 ) ) ;
#55015=CARTESIAN_POINT ( 'NONE',  ( 13.19062500061451537, -3.027376345333614438, 5.243569643749998122 ) ) ;
#55016=CARTESIAN_POINT ( 'NONE',  ( -4.243569643749999898, 13.52187500061451786, 27.54997392385601529 ) ) ;
#55017=VECTOR ( 'NONE', #3418, 1000.000000000000000 ) ;
#55018=CARTESIAN_POINT ( 'NONE',  ( 16.71562500061451573, 3.027376345333611329, 5.243569643749999010 ) ) ;
#55021=CARTESIAN_POINT ( 'NONE',  ( 21.93750000000000000, -2.886751345948129988, 4.999999999999997335 ) ) ;
#55022=CARTESIAN_POINT ( 'NONE',  ( 4.243569643749999898, 18.69687500061451857, -27.54997392385601529 ) ) ;
#55024=CARTESIAN_POINT ( 'NONE',  ( 24.32812500061451289, 4.541064518000418104, 2.621784821874999949 ) ) ;
#55025=CARTESIAN_POINT ( 'NONE',  ( 6.178125000614518747, 6.421520780324663323E-16, -5.243569643749999010 ) ) ;
#55026=CARTESIAN_POINT ( 'NONE',  ( 17.96250000122903501, 0.000000000000000000, 4.999999999999998224 ) ) ;
#55027=CARTESIAN_POINT ( 'NONE',  ( 23.24062500061451786, -3.027376345333610441, -5.243569643749999898 ) ) ;
#55028=CARTESIAN_POINT ( 'NONE',  ( 24.00000000000000000, 4.330127018922192761, -2.499999999999997780 ) ) ;
#55029=CARTESIAN_POINT ( 'NONE',  ( 26.20312500061451644, 0.000000000000000000, 5.243569643749999010 ) ) ;
#55030=CARTESIAN_POINT ( 'NONE',  ( 5.728125000614515905, 6.421520780324663323E-16, -5.243569643749999010 ) ) ;
#55031=ORIENTED_EDGE ( 'NONE', *, *, #10471, .F. ) ;
#55032=B_SPLINE_CURVE_WITH_KNOTS ( 'NONE', 3,
 ( #64528, #58613, #30556, #53082, #13922, #72274, #9848, #43473, #10216, #54551 ),
 .UNSPECIFIED., .F., .F.,
 ( 4, 3, 3, 4 ),
 ( 0.000000000000000000, 2.812506322124666422E-05, 5.625012732888523369E-05, 9.479223614486993082E-05 ),
 .UNSPECIFIED. ) ;
#55033=CARTESIAN_POINT ( 'NONE',  ( 22.26562500061451644, -6.054752690667223547, -1.112240025338166033E-15 ) ) ;
#55034=CARTESIAN_POINT ( 'NONE',  ( 4.078125000614517326, 4.541064518000418104, 2.621784821874999949 ) ) ;
#55036=CARTESIAN_POINT ( 'NONE',  ( 10.98750000122903536, 6.123233995736764310E-16, -4.999999999999998224 ) ) ;
#55037=CARTESIAN_POINT ( 'NONE',  ( -2.828200636599751609E-16, 14.15000000122903501, -34.61880215351700230 ) ) ;
#55039=ADVANCED_FACE ( 'NONE', ( #69310 ), #41233, .F. ) ;
#55040=CARTESIAN_POINT ( 'NONE',  ( 11.02500000000000036, 4.330127018922191873, 2.499999999999999556 ) ) ;
#55041=CARTESIAN_POINT ( 'NONE',  ( 10.28437500061451715, 6.421520780324663323E-16, -5.243569643749999010 ) ) ;
#55042=CARTESIAN_POINT ( 'NONE',  ( 6.975000001229032520, 2.886751345948129099, -4.999999999999998224 ) ) ;
#55043=CARTESIAN_POINT ( 'NONE',  ( 14.29687500061451821, -3.027376345333610441, -5.243569643749999898 ) ) ;
#55044=CARTESIAN_POINT ( 'NONE',  ( 5.146875000614517859, -3.027376345333614438, 5.243569643749998122 ) ) ;
#55045=CARTESIAN_POINT ( 'NONE',  ( 7.320879633048903241E-15, 18.53750000000000142, 26.00000000000000355 ) ) ;
#55048=CARTESIAN_POINT ( 'NONE',  ( 12.08437500061451608, 6.421520780324663323E-16, -5.243569643749999010 ) ) ;
#55049=CARTESIAN_POINT ( 'NONE',  ( 6.150000001229033231, 5.773502691896255534, 3.535250795749688401E-16 ) ) ;
#55051=CARTESIAN_POINT ( 'NONE',  ( 21.21562500061451573, 3.027376345333611329, 5.243569643749999010 ) ) ;
#55053=DIRECTION ( 'NONE',  ( 0.000000000000000000, 0.000000000000000000, -1.000000000000000000 ) ) ;
#55054=CARTESIAN_POINT ( 'NONE',  ( 22.54687500061451999, 6.054752690667223547, 3.707466751127219781E-16 ) ) ;
#55055=CARTESIAN_POINT ( 'NONE',  ( 29.73749999999999716, -2.886751345948115777, -5.000000000000017764 ) ) ;
#55056=CARTESIAN_POINT ( 'NONE',  ( 2.915625000614516793, -6.054752690667223547, -1.112240025338166033E-15 ) ) ;
#55058=CARTESIAN_POINT ( 'NONE',  ( 24.77812500061451217, 4.541064518000418104, 2.621784821874999949 ) ) ;
#55059=CARTESIAN_POINT ( 'NONE',  ( 17.09062500061451573, 6.054752690667223547, 3.707466751127219781E-16 ) ) ;
#55061=CARTESIAN_POINT ( 'NONE',  ( 14.25937500061451679, -4.541064518000417216, -2.621784821875001281 ) ) ;
#55062=CARTESIAN_POINT ( 'NONE',  ( 7.162500001229032520, 0.000000000000000000, 4.999999999999998224 ) ) ;
#55063=CARTESIAN_POINT ( 'NONE',  ( 27.07500000122903216, -5.773502691896255534, -1.060575238724906372E-15 ) ) ;
#55064=CARTESIAN_POINT ( 'NONE',  ( 6.309375000614517504, 4.541064518000418104, -2.621784821874998173 ) ) ;
#55065=CARTESIAN_POINT ( 'NONE',  ( 16.13437500061451502, 6.421520780324663323E-16, -5.243569643749999010 ) ) ;
#55066=CARTESIAN_POINT ( 'NONE',  ( -5.810221930991193690E-16, 11.78749999999999964, 26.00000000000000355 ) ) ;
#55067=CARTESIAN_POINT ( 'NONE',  ( 4.500000001229034652, -2.886751345948129988, 4.999999999999997335 ) ) ;
#55068=CARTESIAN_POINT ( 'NONE',  ( 25.43437500061451573, -4.541064518000419881, 2.621784821874995952 ) ) ;
#55069=CARTESIAN_POINT ( 'NONE',  ( 16.65937500061452070, 4.541064518000418104, -2.621784821874998173 ) ) ;
#55071=CARTESIAN_POINT ( 'NONE',  ( 28.61249999999999716, 2.886751345948126879, 4.999999999999999112 ) ) ;
#55072=EDGE_CURVE ( 'NONE', #53581, #30832, #13395, .T. ) ;
#55073=CARTESIAN_POINT ( 'NONE',  ( 6.450000000000001066, 4.330127018922192761, -2.499999999999997780 ) ) ;
#55075=CARTESIAN_POINT ( 'NONE',  ( 20.54062500061451502, -3.027376345333610441, -5.243569643749999898 ) ) ;
#55076=CARTESIAN_POINT ( 'NONE',  ( 9.674999999999998934, 4.330127018922191873, 2.499999999999999556 ) ) ;
#55077=( BOUNDED_CURVE ( )  B_SPLINE_CURVE ( 2, ( #58062, #57707, #51816, #35542, #7112, #29641, #1581 ),
 .UNSPECIFIED., .F., .F. ) 
 B_SPLINE_CURVE_WITH_KNOTS ( ( 3, 2, 2, 3 ),
 ( 0.7416666666666666963, 0.7444444444444444642, 0.7472222222222222321, 0.7500000000000000000 ),
 .UNSPECIFIED. ) 
 CURVE ( )  GEOMETRIC_REPRESENTATION_ITEM ( )  RATIONAL_B_SPLINE_CURVE ( ( 1.000000000000000000, 0.8660254037844387076, 1.000000000000000000, 0.8660254037844387076, 1.000000000000000000, 0.8660254037844387076, 1.000000000000000000 ) ) 
 REPRESENTATION_ITEM ( '' )  );
#55078=CARTESIAN_POINT ( 'NONE',  ( 3.853125000614517681, -4.541064518000417216, -2.621784821875001281 ) ) ;
#55079=CARTESIAN_POINT ( 'NONE',  ( 19.98749999999999716, 5.773502691896255534, 3.535250795749688894E-16 ) ) ;
#55081=CARTESIAN_POINT ( 'NONE',  ( 23.36250000122903359, 0.000000000000000000, 4.999999999999998224 ) ) ;
#55082=CARTESIAN_POINT ( 'NONE',  ( 5.838630383562665394, 8.118670948950970967, 31.39639828276943945 ) ) ;
#55083=CARTESIAN_POINT ( 'NONE',  ( 29.52187500061451431, -6.054752690667223547, -1.112240025338166033E-15 ) ) ;
#55085=CARTESIAN_POINT ( 'NONE',  ( 17.27812500061451217, -4.541064518000419881, 2.621784821874995952 ) ) ;
#55086=CARTESIAN_POINT ( 'NONE',  ( 25.30312500061451431, 0.000000000000000000, 5.243569643749999010 ) ) ;
#55087=CARTESIAN_POINT ( 'NONE',  ( 23.63437500061451502, -4.541064518000419881, 2.621784821874995952 ) ) ;
#55088=CARTESIAN_POINT ( 'NONE',  ( 6.862500000000002487, 2.886751345948129099, -4.999999999999998224 ) ) ;
#55089=CARTESIAN_POINT ( 'NONE',  ( 11.57812500061451644, 6.421520780324663323E-16, -5.243569643749999010 ) ) ;
#55090=CARTESIAN_POINT ( 'NONE',  ( 26.57812500061451644, 4.541064518000418104, 2.621784821874999949 ) ) ;
#55091=CARTESIAN_POINT ( 'NONE',  ( 14.82187500061451679, 3.027376345333613106, -5.243569643749998122 ) ) ;
#55092=CARTESIAN_POINT ( 'NONE',  ( 19.92187500061451644, 3.027376345333611329, 5.243569643749999010 ) ) ;
#55093=CARTESIAN_POINT ( 'NONE',  ( 1.071796769724489895, 11.87990381179669974, -34.00000000000000000 ) ) ;
#55094=CARTESIAN_POINT ( 'NONE',  ( 4.243569643749999898, 10.63437500061451857, 30.00000000000000000 ) ) ;
#55096=CARTESIAN_POINT ( 'NONE',  ( 24.63750000122903216, 4.330127018922191873, 2.499999999999999556 ) ) ;
#55098=CARTESIAN_POINT ( 'NONE',  ( 15.47812500061451679, -4.541064518000419881, 2.621784821874995952 ) ) ;
#55099=CARTESIAN_POINT ( 'NONE',  ( 7.134375000614516793, 6.421520780324663323E-16, -5.243569643749999010 ) ) ;
#55100=CARTESIAN_POINT ( 'NONE',  ( 8.034375000614518925, 6.421520780324663323E-16, -5.243569643749999010 ) ) ;
#55101=ORIENTED_EDGE ( 'NONE', *, *, #5758, .F. ) ;
#55102=CARTESIAN_POINT ( 'NONE',  ( 27.94687500061451502, 6.054752690667223547, 3.707466751127219781E-16 ) ) ;
#55103=CARTESIAN_POINT ( 'NONE',  ( 18.77812500061451573, 6.421520780324663323E-16, -5.243569643749999010 ) ) ;
#55104=CARTESIAN_POINT ( 'NONE',  ( 29.43750000122903288, 6.123233995736764310E-16, -4.999999999999998224 ) ) ;
#55105=CARTESIAN_POINT ( 'NONE',  ( 3.309375000614518836, 0.000000000000000000, 5.243569643749999010 ) ) ;
#55106=CARTESIAN_POINT ( 'NONE',  ( 23.78437500061451360, 6.421520780324663323E-16, -5.243569643749999010 ) ) ;
#55107=CARTESIAN_POINT ( 'NONE',  ( 20.39062500061451644, -3.027376345333614438, 5.243569643749998122 ) ) ;
#55108=CARTESIAN_POINT ( 'NONE',  ( 3.999999999999998668, 12.61250000000000071, 27.69059892324149175 ) ) ;
#55109=CARTESIAN_POINT ( 'NONE',  ( 25.19062500061451715, 6.054752690667223547, 3.707466751127219781E-16 ) ) ;
#55110=CARTESIAN_POINT ( 'NONE',  ( 5.175000001229033586, 2.886751345948129099, -4.999999999999998224 ) ) ;
#55111=ORIENTED_EDGE ( 'NONE', *, *, #25529, .T. ) ;
#55112=CARTESIAN_POINT ( 'NONE',  ( 2.925000001229034918, 2.886751345948129099, -4.999999999999998224 ) ) ;
#55113=CARTESIAN_POINT ( 'NONE',  ( 4.000000000000000000, 14.78750000000000320, -27.69059892324149530 ) ) ;
#55114=CARTESIAN_POINT ( 'NONE',  ( 22.23750000122903003, 6.123233995736764310E-16, -4.999999999999998224 ) ) ;
#55116=CARTESIAN_POINT ( 'NONE',  ( 3.534375000614518036, 6.421520780324663323E-16, -5.243569643749999010 ) ) ;
#55117=CARTESIAN_POINT ( 'NONE',  ( 30.00000000000000000, 0.000000000000000000, 0.000000000000000000 ) ) ;
#55118=CARTESIAN_POINT ( 'NONE',  ( 11.46562500061451573, -6.054752690667223547, -1.112240025338166033E-15 ) ) ;
#55119=CARTESIAN_POINT ( 'NONE',  ( 6.684375000614518392, 6.421520780324663323E-16, -5.243569643749999010 ) ) ;
#55120=CARTESIAN_POINT ( 'NONE',  ( 24.15000000122903145, 5.773502691896255534, 3.535250795749688894E-16 ) ) ;
#55122=CARTESIAN_POINT ( 'NONE',  ( 14.59687500061452070, -3.027376345333614438, 5.243569643749998122 ) ) ;
#55123=CARTESIAN_POINT ( 'NONE',  ( 28.97812500061451502, -4.541064518000419881, 2.621784821874995952 ) ) ;
#55124=DIRECTION ( 'NONE',  ( -1.000000000000000000, -0.000000000000000000, -0.000000000000000000 ) ) ;
#55126=CARTESIAN_POINT ( 'NONE',  ( 15.55312500061451608, -4.541064518000417216, -2.621784821875001281 ) ) ;
#55128=CARTESIAN_POINT ( 'NONE',  ( 10.82812500061451644, 4.541064518000418104, 2.621784821874999949 ) ) ;
#55129=CARTESIAN_POINT ( 'NONE',  ( 8.090625000614515727, 6.054752690667223547, 3.707466751127219781E-16 ) ) ;
#55131=CARTESIAN_POINT ( 'NONE',  ( 8.400000000000000355, 0.000000000000000000, 4.999999999999998224 ) ) ;
#55132=CARTESIAN_POINT ( 'NONE',  ( 3.412500001229032964, 4.330127018922192761, -2.499999999999997780 ) ) ;
#55133=CARTESIAN_POINT ( 'NONE',  ( 17.58749999999999858, -2.886751345948125991, -5.000000000000000000 ) ) ;
#55135=CARTESIAN_POINT ( 'NONE',  ( 19.32187500061451857, 3.027376345333613106, -5.243569643749998122 ) ) ;
#55136=CARTESIAN_POINT ( 'NONE',  ( 14.58750000122903323, 6.123233995736764310E-16, -4.999999999999998224 ) ) ;
#55138=CARTESIAN_POINT ( 'NONE',  ( 4.243569643749999898, 16.39062500061451999, -27.54997392385601529 ) ) ;
#55140=CARTESIAN_POINT ( 'NONE',  ( 29.01562500061451644, -6.054752690667223547, -1.112240025338166033E-15 ) ) ;
#55143=CARTESIAN_POINT ( 'NONE',  ( 13.17187500061451999, 3.027376345333611329, 5.243569643749999010 ) ) ;
#55144=CARTESIAN_POINT ( 'NONE',  ( 27.44999999999999929, -4.330127018922190985, -2.500000000000001332 ) ) ;
#55145=CARTESIAN_POINT ( 'NONE',  ( 8.840625000614515727, -3.027376345333610441, -5.243569643749999898 ) ) ;
#55147=CARTESIAN_POINT ( 'NONE',  ( 20.89687500061452141, -3.027376345333614438, 5.243569643749998122 ) ) ;
#55149=CARTESIAN_POINT ( 'NONE',  ( 8.765625000614518214, -6.054752690667223547, -1.112240025338166033E-15 ) ) ;
#55150=CARTESIAN_POINT ( 'NONE',  ( 13.47187500061451537, 3.027376345333613106, -5.243569643749998122 ) ) ;
#55151=EDGE_LOOP ( 'NONE', ( #56905, #66056, #19598, #61136 ) ) ;
#55152=CARTESIAN_POINT ( 'NONE',  ( 23.78437500061451360, 6.421520780324663323E-16, -5.243569643749999010 ) ) ;
#55153=CARTESIAN_POINT ( 'NONE',  ( 3.779877903161416253, 3.276378095916669508, -31.33357467763542914 ) ) ;
#55156=CARTESIAN_POINT ( 'NONE',  ( 5.512499999999999289, 2.886751345948129099, -4.999999999999998224 ) ) ;
#55157=AXIS2_PLACEMENT_3D ( 'NONE', #320, #51283, #57171 ) ;
#55158=CARTESIAN_POINT ( 'NONE',  ( 16.20000000122903216, -2.886751345948129988, 4.999999999999997335 ) ) ;
#55159=CARTESIAN_POINT ( 'NONE',  ( 27.41250000122903430, 0.000000000000000000, 4.999999999999998224 ) ) ;
#55160=CARTESIAN_POINT ( 'NONE',  ( -0.6945831915928805111, 10.00052343484236950, -33.93923269050669944 ) ) ;
#55162=CARTESIAN_POINT ( 'NONE',  ( 12.71250000000000036, 2.886751345948129099, -4.999999999999998224 ) ) ;
#55163=CARTESIAN_POINT ( 'NONE',  ( 16.46249999999999503, 2.886751345948126879, 4.999999999999999112 ) ) ;
#55164=CARTESIAN_POINT ( 'NONE',  ( 13.31250000122903288, 4.330127018922192761, -2.499999999999997780 ) ) ;
#55165=CARTESIAN_POINT ( 'NONE',  ( 11.69062500061451360, 6.054752690667223547, 3.707466751127219781E-16 ) ) ;
#55167=CARTESIAN_POINT ( 'NONE',  ( -3.999999999999999112, 16.96250000122903145, -30.00000000000000000 ) ) ;
#55168=CARTESIAN_POINT ( 'NONE',  ( 4.243569643749999010, 13.82187500061451857, -32.45002607614398471 ) ) ;
#55169=CARTESIAN_POINT ( 'NONE',  ( 4.678125000614516971, -4.541064518000419881, 2.621784821874995952 ) ) ;
#55171=CARTESIAN_POINT ( 'NONE',  ( 10.27499999999999858, -4.330127018922194537, 2.499999999999995559 ) ) ;
#55172=CARTESIAN_POINT ( 'NONE',  ( 9.074999999999999289, 6.123233995736764310E-16, -4.999999999999998224 ) ) ;
#55173=ORIENTED_EDGE ( 'NONE', *, *, #65759, .T. ) ;
#55174=CARTESIAN_POINT ( 'NONE',  ( 24.77812500061451217, 4.541064518000418104, 2.621784821874999949 ) ) ;
#55177=CARTESIAN_POINT ( 'NONE',  ( 21.34687500061451715, -3.027376345333614438, 5.243569643749998122 ) ) ;
#55178=CARTESIAN_POINT ( 'NONE',  ( 18.74062500061451431, -3.027376345333610441, -5.243569643749999898 ) ) ;
#55180=CARTESIAN_POINT ( 'NONE',  ( -2.121784821874996840, 14.92812500061459424, -26.32496088578401583 ) ) ;
#55181=CARTESIAN_POINT ( 'NONE',  ( 6.403125000614517504, 0.000000000000000000, 5.243569643749999010 ) ) ;
#55182=CARTESIAN_POINT ( 'NONE',  ( 4.115625000614516082, 3.027376345333611329, 5.243569643749999010 ) ) ;
#55184=CARTESIAN_POINT ( 'NONE',  ( 22.34062500061451573, -3.027376345333610441, -5.243569643749999898 ) ) ;
#55187=CARTESIAN_POINT ( 'NONE',  ( 16.35937500061451644, 0.000000000000000000, 5.243569643749999010 ) ) ;
#55188=CARTESIAN_POINT ( 'NONE',  ( 14.55937500061451573, 0.000000000000000000, 5.243569643749999010 ) ) ;
#55189=CARTESIAN_POINT ( 'NONE',  ( 22.20937500061451431, 0.000000000000000000, 5.243569643749999010 ) ) ;
#55190=ORIENTED_EDGE ( 'NONE', *, *, #30133, .T. ) ;
#55191=CARTESIAN_POINT ( 'NONE',  ( 2.121784821875001281, 11.45937500061451786, 33.67503911421598417 ) ) ;
#55192=CARTESIAN_POINT ( 'NONE',  ( 3.328125000614516438, -4.541064518000419881, 2.621784821874995952 ) ) ;
#55193=CARTESIAN_POINT ( 'NONE',  ( 26.27812500061451573, -4.541064518000419881, 2.621784821874995952 ) ) ;
#55194=EDGE_CURVE ( 'NONE', #3917, #70308, #63478, .T. ) ;
#55195=CARTESIAN_POINT ( 'NONE',  ( 25.94062500061451715, -3.027376345333610441, -5.243569643749999898 ) ) ;
#55196=CARTESIAN_POINT ( 'NONE',  ( 8.362500001229031810, 4.330127018922192761, -2.499999999999997780 ) ) ;
#55197=CARTESIAN_POINT ( 'NONE',  ( 4.000000000000000000, 18.83749999999999858, 32.30940107675849049 ) ) ;
#55198=CARTESIAN_POINT ( 'NONE',  ( 5.446875000614518569, 6.054752690667223547, 3.707466751127219781E-16 ) ) ;
#55200=CARTESIAN_POINT ( 'NONE',  ( 14.62500000122903288, 2.886751345948129099, -4.999999999999998224 ) ) ;
#55201=CARTESIAN_POINT ( 'NONE',  ( 8.325000001229033941, 2.886751345948129099, -4.999999999999998224 ) ) ;
#55202=CARTESIAN_POINT ( 'NONE',  ( 3.140625000614516882, 6.054752690667223547, 3.707466751127219781E-16 ) ) ;
#55205=CARTESIAN_POINT ( 'NONE',  ( 12.79687500061451821, -3.027376345333614438, 5.243569643749998122 ) ) ;
#55207=ORIENTED_EDGE ( 'NONE', *, *, #37992, .T. ) ;
#55208=CARTESIAN_POINT ( 'NONE',  ( 20.76562500061451644, 3.027376345333611329, 5.243569643749999010 ) ) ;
#55209=CARTESIAN_POINT ( 'NONE',  ( 14.37187500061451928, 3.027376345333613106, -5.243569643749998122 ) ) ;
#55210=CARTESIAN_POINT ( 'NONE',  ( 5.090625000614516615, -3.027376345333614438, 5.243569643749998122 ) ) ;
#55211=CARTESIAN_POINT ( 'NONE',  ( 23.07187500061452212, 3.027376345333611329, 5.243569643749999010 ) ) ;
#55212=CARTESIAN_POINT ( 'NONE',  ( 6.365625000614518747, 3.027376345333611329, 5.243569643749999010 ) ) ;
#55213=CARTESIAN_POINT ( 'NONE',  ( 9.112500001229033586, -4.330127018922190985, -2.500000000000001332 ) ) ;
#55214=CARTESIAN_POINT ( 'NONE',  ( 23.31562500061451715, 3.027376345333613106, -5.243569643749998122 ) ) ;
#55215=CARTESIAN_POINT ( 'NONE',  ( -1.999999999999997113, 17.03750000122903430, -26.53589838486224295 ) ) ;
#55216=CARTESIAN_POINT ( 'NONE',  ( 8.512500001229033941, 0.000000000000000000, 4.999999999999998224 ) ) ;
#55217=CARTESIAN_POINT ( 'NONE',  ( 17.54062500061451502, 6.054752690667223547, 3.707466751127219781E-16 ) ) ;
#55218=CARTESIAN_POINT ( 'NONE',  ( 16.26562500061451289, 3.027376345333611329, 5.243569643749999010 ) ) ;
#55220=CARTESIAN_POINT ( 'NONE',  ( 15.00000000000000000, 4.330127018922192761, -2.499999999999997780 ) ) ;
#55221=CARTESIAN_POINT ( 'NONE',  ( 12.15000000122903501, -2.886751345948129988, 4.999999999999997335 ) ) ;
#55223=CARTESIAN_POINT ( 'NONE',  ( 7.903125000614515727, -4.541064518000417216, -2.621784821875001281 ) ) ;
#55224=CARTESIAN_POINT ( 'NONE',  ( 10.82812500061451644, 4.541064518000418104, 2.621784821874999949 ) ) ;
#55225=CARTESIAN_POINT ( 'NONE',  ( 20.40000000122903145, -2.886751345948125991, -5.000000000000000000 ) ) ;
#55226=CARTESIAN_POINT ( 'NONE',  ( -4.243569643749997233, 14.04687500061451999, -27.54997392385601174 ) ) ;
#55227=CARTESIAN_POINT ( 'NONE',  ( 20.25937500061451857, 4.541064518000418104, -2.621784821874998173 ) ) ;
#55228=CARTESIAN_POINT ( 'NONE',  ( 21.44999999999999929, 0.000000000000000000, 4.999999999999998224 ) ) ;
#55229=CARTESIAN_POINT ( 'NONE',  ( 5.325000001229033941, 2.886751345948126879, 4.999999999999999112 ) ) ;
#55230=CARTESIAN_POINT ( 'NONE',  ( 3.234375000614516438, 4.541064518000418104, 2.621784821874999949 ) ) ;
#55231=CARTESIAN_POINT ( 'NONE',  ( 20.82187500061451857, 3.027376345333611329, 5.243569643749999010 ) ) ;
#55232=CARTESIAN_POINT ( 'NONE',  ( 7.320879633048903241E-15, 18.53750000000000142, 26.00000000000000355 ) ) ;
#55233=CARTESIAN_POINT ( 'NONE',  ( 18.36562500061451431, 3.027376345333613106, -5.243569643749998122 ) ) ;
#55236=CARTESIAN_POINT ( 'NONE',  ( 26.84999999999999787, 0.000000000000000000, 4.999999999999998224 ) ) ;
#55237=CARTESIAN_POINT ( 'NONE',  ( 29.67187500061451644, 3.027376345333613106, -5.243569643749998122 ) ) ;
#55239=CARTESIAN_POINT ( 'NONE',  ( 15.40312500061451573, 0.000000000000000000, 5.243569643749999010 ) ) ;
#55240=CARTESIAN_POINT ( 'NONE',  ( 12.42187500061451821, -6.054752690667223547, -1.112240025338166033E-15 ) ) ;
#55242=CARTESIAN_POINT ( 'NONE',  ( 4.000000000000000000, 17.03750000000000142, -27.69059892324149885 ) ) ;
#55243=CARTESIAN_POINT ( 'NONE',  ( 22.22812500061451502, -4.541064518000419881, 2.621784821874995952 ) ) ;
#55244=LINE ( 'NONE', #26063, #20342 ) ;
#55246=CARTESIAN_POINT ( 'NONE',  ( 12.33750000000000036, 5.773502691896255534, 3.535250795749688894E-16 ) ) ;
#55247=CARTESIAN_POINT ( 'NONE',  ( 23.81250000122903288, 0.000000000000000000, 4.999999999999998224 ) ) ;
#55248=CARTESIAN_POINT ( 'NONE',  ( 19.37812500061451715, 4.541064518000418104, 2.621784821874999949 ) ) ;
#55249=ORIENTED_EDGE ( 'NONE', *, *, #64836, .T. ) ;
#55250=CARTESIAN_POINT ( 'NONE',  ( 23.43750000000000000, -2.886751345948125991, -5.000000000000000000 ) ) ;
#55251=CARTESIAN_POINT ( 'NONE',  ( 24.90937500061451715, 0.000000000000000000, 5.243569643749999010 ) ) ;
#55253=CARTESIAN_POINT ( 'NONE',  ( 7.320879633048903241E-15, 18.08749999999999858, -34.00000000000000000 ) ) ;
#55254=CARTESIAN_POINT ( 'NONE',  ( 11.57812500061451644, 6.421520780324663323E-16, -5.243569643749999010 ) ) ;
#55255=CARTESIAN_POINT ( 'NONE',  ( 3.288170700621412479, 3.766687330211323737, 3.553104967622100929 ) ) ;
#55257=CARTESIAN_POINT ( 'NONE',  ( 17.81250000000000355, 2.886751345948126879, 4.999999999999999112 ) ) ;
#55258=CARTESIAN_POINT ( 'NONE',  ( 24.33749999999999858, -2.886751345948125991, -5.000000000000000000 ) ) ;
#55259=CARTESIAN_POINT ( 'NONE',  ( -4.243569643749999898, 18.90312500061451573, 30.00000000000000000 ) ) ;
#55260=CARTESIAN_POINT ( 'NONE',  ( 4.959375000614516971, 4.541064518000418104, -2.621784821874998173 ) ) ;
#55261=CARTESIAN_POINT ( 'NONE',  ( 29.59687500061451715, -3.027376345333610441, -5.243569643749999898 ) ) ;
#55262=EDGE_LOOP ( 'NONE', ( #12432, #55111, #14246, #32621 ) ) ;
#55263=CARTESIAN_POINT ( 'NONE',  ( 25.19062500061451715, 6.054752690667223547, 3.707466751127219781E-16 ) ) ;
#55264=CARTESIAN_POINT ( 'NONE',  ( 27.00937500061451857, 4.541064518000418104, -2.621784821874998173 ) ) ;
#55265=DIRECTION ( 'NONE',  ( -1.000000000000000000, -0.000000000000000000, -0.000000000000000000 ) ) ;
#55266=CARTESIAN_POINT ( 'NONE',  ( 13.64999999999999858, 4.330127018922192761, -2.499999999999997780 ) ) ;
#55267=CARTESIAN_POINT ( 'NONE',  ( 11.05312500061451608, -4.541064518000417216, -2.621784821875001281 ) ) ;
#55268=FACE_OUTER_BOUND ( 'NONE', #19935, .T. ) ;
#55269=CARTESIAN_POINT ( 'NONE',  ( 4.000000000000000000, 19.28749999999999787, -27.69059892324149885 ) ) ;
#55270=CARTESIAN_POINT ( 'NONE',  ( 28.07812500061451289, -4.541064518000419881, 2.621784821874995952 ) ) ;
#55271=CARTESIAN_POINT ( 'NONE',  ( 15.60000000122903607, 5.773502691896255534, 3.535250795749688894E-16 ) ) ;
#55274=CARTESIAN_POINT ( 'NONE',  ( 6.403125000614517504, 0.000000000000000000, 5.243569643749999010 ) ) ;
#55275=CARTESIAN_POINT ( 'NONE',  ( 22.95937500061451431, 4.541064518000418104, -2.621784821874998173 ) ) ;
#55276=CARTESIAN_POINT ( 'NONE',  ( -3.000416591977282496E-16, 14.79687500061451821, 25.09994784771203058 ) ) ;
#55277=CARTESIAN_POINT ( 'NONE',  ( 22.09687500061451715, 6.054752690667223547, 3.707466751127219781E-16 ) ) ;
#55278=CARTESIAN_POINT ( 'NONE',  ( 29.07187500061451502, -6.054752690667223547, -1.112240025338166033E-15 ) ) ;
#55279=CARTESIAN_POINT ( 'NONE',  ( -4.243569643749999898, 18.05937500061451928, 30.00000000000000000 ) ) ;
#55280=CARTESIAN_POINT ( 'NONE',  ( 9.215625000614515727, -6.054752690667223547, -1.112240025338166033E-15 ) ) ;
#55281=CARTESIAN_POINT ( 'NONE',  ( 2.850000001229036073, -2.886751345948125991, -5.000000000000000000 ) ) ;
#55282=EDGE_CURVE ( 'NONE', #39309, #11494, #15228, .T. ) ;
#55283=CARTESIAN_POINT ( 'NONE',  ( 7.134375000614516793, 6.421520780324663323E-16, -5.243569643749999010 ) ) ;
#55284=CARTESIAN_POINT ( 'NONE',  ( 7.575000001229033053, 2.886751345948126879, 4.999999999999998224 ) ) ;
#55285=CARTESIAN_POINT ( 'NONE',  ( 10.49062500061451431, -3.027376345333614438, 5.243569643749998122 ) ) ;
#55286=CARTESIAN_POINT ( 'NONE',  ( 14.82187500061451679, 3.027376345333613106, -5.243569643749998122 ) ) ;
#55287=DIRECTION ( 'NONE',  ( -1.000000000000000000, -0.000000000000000000, -0.000000000000000000 ) ) ;
#55288=CARTESIAN_POINT ( 'NONE',  ( 22.08750000122903501, -4.330127018922194537, 2.499999999999995559 ) ) ;
#55289=CARTESIAN_POINT ( 'NONE',  ( 6.946875000614517681, -3.027376345333614438, 5.243569643749998122 ) ) ;
#55290=CARTESIAN_POINT ( 'NONE',  ( 9.778125000614517504, 6.421520780324663323E-16, -5.243569643749999010 ) ) ;
#55292=CARTESIAN_POINT ( 'NONE',  ( 19.17187500061451999, -6.054752690667223547, -1.112240025338166033E-15 ) ) ;
#55293=FACE_BOUND ( 'NONE', #55756, .T. ) ;
#55294=CARTESIAN_POINT ( 'NONE',  ( -0.5524690355592152269, 4.971316854763021986, 33.96409715941054230 ) ) ;
#55295=CARTESIAN_POINT ( 'NONE',  ( 29.33437500061451431, 4.541064518000418104, 2.621784821874999949 ) ) ;
#55296=CARTESIAN_POINT ( 'NONE',  ( -2.121784821874996840, 10.93437500061451928, -26.32496088578401583 ) ) ;
#55297=CARTESIAN_POINT ( 'NONE',  ( 16.23750000122903359, -4.330127018922194537, 2.499999999999995559 ) ) ;
#55298=CARTESIAN_POINT ( 'NONE',  ( -4.243569643749999898, 15.75312500061451537, -30.00000000000000000 ) ) ;
#55299=CARTESIAN_POINT ( 'NONE',  ( 15.86250000122903181, -4.330127018922190985, -2.500000000000001332 ) ) ;
#55300=CARTESIAN_POINT ( 'NONE',  ( 11.16562500061451679, 3.027376345333613106, -5.243569643749998122 ) ) ;
#55301=EDGE_LOOP ( 'NONE', ( #26664, #47561, #42784, #38828 ) ) ;
#55302=CARTESIAN_POINT ( 'NONE',  ( 12.93750000000000178, -2.886751345948129988, 4.999999999999997335 ) ) ;
#55304=CARTESIAN_POINT ( 'NONE',  ( 22.04062500061451502, 6.054752690667223547, 3.707466751127219781E-16 ) ) ;
#55305=CARTESIAN_POINT ( 'NONE',  ( 9.871875000614517504, 3.027376345333612662, -5.243569643749998122 ) ) ;
#55307=CARTESIAN_POINT ( 'NONE',  ( 9.037500001229034297, -4.330127018922194537, 2.499999999999995559 ) ) ;
#55308=CARTESIAN_POINT ( 'NONE',  ( 18.37500000122903288, 2.886751345948126879, 4.999999999999999112 ) ) ;
#55309=CARTESIAN_POINT ( 'NONE',  ( 16.19062500061451715, 6.054752690667223547, 3.707466751127219781E-16 ) ) ;
#55310=CARTESIAN_POINT ( 'NONE',  ( 19.30312500061451786, 4.541064518000418104, -2.621784821874998173 ) ) ;
#55311=CARTESIAN_POINT ( 'NONE',  ( 25.01250000122903216, 4.330127018922192761, -2.499999999999997780 ) ) ;
#55312=CARTESIAN_POINT ( 'NONE',  ( 28.16250000122903074, 4.330127018922192761, -2.499999999999997780 ) ) ;
#55313=CARTESIAN_POINT ( 'NONE',  ( 22.23750000000000071, 5.773502691896255534, 3.535250795749688894E-16 ) ) ;
#55315=CARTESIAN_POINT ( 'NONE',  ( 25.99687500061451928, -3.027376345333610441, -5.243569643749999898 ) ) ;
#55316=CARTESIAN_POINT ( 'NONE',  ( 1.999999999999998668, 12.65000000000000213, -33.46410161513775705 ) ) ;
#55317=CARTESIAN_POINT ( 'NONE',  ( 11.58750000122903501, 4.330127018922191873, 2.499999999999999556 ) ) ;
#55318=CARTESIAN_POINT ( 'NONE',  ( 28.50937500061451502, 0.000000000000000000, 5.243569643749999010 ) ) ;
#55320=CARTESIAN_POINT ( 'NONE',  ( 5.934375000614517504, 4.541064518000418104, 2.621784821874999949 ) ) ;
#55321=CARTESIAN_POINT ( 'NONE',  ( 25.90312500061451573, -4.541064518000417216, -2.621784821875001281 ) ) ;
#55323=CARTESIAN_POINT ( 'NONE',  ( 4.661467738957717266, -1.808512791952580301, -4.661467738957749241 ) ) ;
#55324=CARTESIAN_POINT ( 'NONE',  ( 11.14687500061451608, -3.027376345333610441, -5.243569643749999898 ) ) ;
#55325=CARTESIAN_POINT ( 'NONE',  ( 22.12500000122903288, -5.773502691896255534, -1.060575238724906372E-15 ) ) ;
#55326=CARTESIAN_POINT ( 'NONE',  ( 4.021875000614516082, 3.027376345333613106, -5.243569643749998122 ) ) ;
#55327=CARTESIAN_POINT ( 'NONE',  ( 7.846875000614518036, -3.027376345333614438, 5.243569643749998122 ) ) ;
#55328=CARTESIAN_POINT ( 'NONE',  ( 28.47187500061451715, 3.027376345333611329, 5.243569643749999010 ) ) ;
#55329=CARTESIAN_POINT ( 'NONE',  ( -2.121784821874996840, 11.77812500061459566, 33.67503911421598417 ) ) ;
#55330=CARTESIAN_POINT ( 'NONE',  ( 19.61249999999999716, 2.886751345948126879, 4.999999999999999112 ) ) ;
#55331=ORIENTED_EDGE ( 'NONE', *, *, #51411, .T. ) ;
#55332=CARTESIAN_POINT ( 'NONE',  ( 29.58749999999999858, -2.886751345948129988, 4.999999999999997335 ) ) ;
#55333=CARTESIAN_POINT ( 'NONE',  ( 3.787500000000002753, 5.773502691896255534, 3.535250795749688894E-16 ) ) ;
#55334=VERTEX_POINT ( 'NONE', #37866 ) ;
#55335=CARTESIAN_POINT ( 'NONE',  ( 18.21562500061451573, -6.054752690667223547, -1.112240025338166033E-15 ) ) ;
#55336=CARTESIAN_POINT ( 'NONE',  ( 9.365625000614519635, 3.027376345333613106, -5.243569643749998122 ) ) ;
#55338=CARTESIAN_POINT ( 'NONE',  ( 7.546875000614517326, -3.027376345333610441, -5.243569643749999898 ) ) ;
#55339=CARTESIAN_POINT ( 'NONE',  ( 16.72500000122903430, -5.773502691896255534, -1.060575238724906372E-15 ) ) ;
#55341=CARTESIAN_POINT ( 'NONE',  ( 7.584375000614516082, 6.421520780324663323E-16, -5.243569643749999010 ) ) ;
#55342=CARTESIAN_POINT ( 'NONE',  ( 11.59687500061451892, -3.027376345333610441, -5.243569643749999898 ) ) ;
#55343=CARTESIAN_POINT ( 'NONE',  ( 25.32187500061451857, 3.027376345333611329, 5.243569643749999010 ) ) ;
#55344=ADVANCED_FACE ( 'NONE', ( #60385 ), #58922, .F. ) ;
#55346=EDGE_LOOP ( 'NONE', ( #14488, #26726, #37379 ) ) ;
#55348=CARTESIAN_POINT ( 'NONE',  ( 17.52187500061451431, 3.027376345333613106, -5.243569643749998122 ) ) ;
#55349=CARTESIAN_POINT ( 'NONE',  ( 10.54687500061451644, -3.027376345333614438, 5.243569643749998122 ) ) ;
#55351=CARTESIAN_POINT ( 'NONE',  ( 20.40000000000000213, 4.330127018922192761, -2.499999999999997780 ) ) ;
#55353=CARTESIAN_POINT ( 'NONE',  ( 2.121784821874999061, 10.25937500061451857, -33.67503911421598417 ) ) ;
#55355=CARTESIAN_POINT ( 'NONE',  ( 13.26562500061451644, -6.054752690667223547, -1.112240025338166033E-15 ) ) ;
#55356=CARTESIAN_POINT ( 'NONE',  ( 29.74687500061451217, 6.054752690667223547, 3.707466751127219781E-16 ) ) ;
#55357=CARTESIAN_POINT ( 'NONE',  ( -2.000000000000000000, 19.13750000122903216, -33.46410161513775705 ) ) ;
#55358=CARTESIAN_POINT ( 'NONE',  ( 4.241277253184729368, 2.648812835464926518, -4.241277253184729368 ) ) ;
#55359=CARTESIAN_POINT ( 'NONE',  ( 9.487500000000000711, -2.886751345948125991, -5.000000000000000000 ) ) ;
#55360=CARTESIAN_POINT ( 'NONE',  ( 3.999999999999998668, 15.42500000122903359, 27.69059892324149175 ) ) ;
#55361=CARTESIAN_POINT ( 'NONE',  ( 9.000000001229034652, -2.886751345948129988, 4.999999999999997335 ) ) ;
#55363=CARTESIAN_POINT ( 'NONE',  ( 19.32187500061451857, 3.027376345333613106, -5.243569643749998122 ) ) ;
#55364=CARTESIAN_POINT ( 'NONE',  ( 13.58437500061451786, 4.541064518000418104, 2.621784821874999949 ) ) ;
#55365=CARTESIAN_POINT ( 'NONE',  ( 2.000000000000001332, 16.66250000122903430, 33.46410161513774995 ) ) ;
#55367=CARTESIAN_POINT ( 'NONE',  ( 18.25312500061451715, -4.541064518000417216, -2.621784821875001281 ) ) ;
#55368=CARTESIAN_POINT ( 'NONE',  ( 29.32500000122903216, -5.773502691896255534, -1.060575238724906372E-15 ) ) ;
#55369=CARTESIAN_POINT ( 'NONE',  ( 15.27187500061451786, 3.027376345333613106, -5.243569643749998122 ) ) ;
#55370=CARTESIAN_POINT ( 'NONE',  ( 0.8036833610285047946, 9.975469519845873378, -24.04062768261224647 ) ) ;
#55371=CARTESIAN_POINT ( 'NONE',  ( 16.19062500061451715, 6.054752690667223547, 3.707466751127219781E-16 ) ) ;
#55373=CARTESIAN_POINT ( 'NONE',  ( 9.001249775931846008E-16, 11.81562500061451715, 34.90005215228797653 ) ) ;
#55374=CARTESIAN_POINT ( 'NONE',  ( 18.49687500061452283, 6.054752690667223547, 3.707466751127219781E-16 ) ) ;
#55375=CARTESIAN_POINT ( 'NONE',  ( 14.13750000122903394, 6.123233995736764310E-16, -4.999999999999998224 ) ) ;
#55377=CARTESIAN_POINT ( 'NONE',  ( -3.000416591977282496E-16, 18.84687500061451360, -34.90005215228797653 ) ) ;
#55378=CARTESIAN_POINT ( 'NONE',  ( 19.69687500061451857, -3.027376345333610441, -5.243569643749999898 ) ) ;
#55379=CARTESIAN_POINT ( 'NONE',  ( 21.30000000122903359, -2.886751345948125991, -5.000000000000000000 ) ) ;
#55380=CARTESIAN_POINT ( 'NONE',  ( 17.40937500061451715, -4.541064518000417216, -2.621784821875001281 ) ) ;
#55381=CARTESIAN_POINT ( 'NONE',  ( 12.92812500061451786, 6.421520780324663323E-16, -5.243569643749999010 ) ) ;
#55382=CARTESIAN_POINT ( 'NONE',  ( 9.001249775931846008E-16, 12.77187500061451786, 34.90005215228797653 ) ) ;
#55383=CARTESIAN_POINT ( 'NONE',  ( 18.59062500061451573, -3.027376345333614438, 5.243569643749998122 ) ) ;
#55384=ORIENTED_EDGE ( 'NONE', *, *, #4790, .T. ) ;
#55386=CARTESIAN_POINT ( 'NONE',  ( 19.46249999999999858, 2.886751345948129099, -4.999999999999998224 ) ) ;
#55388=CARTESIAN_POINT ( 'NONE',  ( 24.51562500061451289, -6.054752690667223547, -1.112240025338166033E-15 ) ) ;
#55389=CARTESIAN_POINT ( 'NONE',  ( 5.990625000614517859, -3.027376345333614438, 5.243569643749998122 ) ) ;
#55390=CARTESIAN_POINT ( 'NONE',  ( 17.17500000122903359, -5.773502691896255534, -1.060575238724906372E-15 ) ) ;
#55391=CARTESIAN_POINT ( 'NONE',  ( 23.01562500061451644, 3.027376345333611329, 5.243569643749999010 ) ) ;
#55392=CARTESIAN_POINT ( 'NONE',  ( 22.38749999999999929, -2.886751345948129988, 4.999999999999997335 ) ) ;
#55393=CARTESIAN_POINT ( 'NONE',  ( 26.09062500061451573, 6.054752690667223547, 3.707466751127219781E-16 ) ) ;
#55394=CARTESIAN_POINT ( 'NONE',  ( 6.590625000614518392, -3.027376345333610441, -5.243569643749999898 ) ) ;
#55395=ORIENTED_EDGE ( 'NONE', *, *, #71031, .T. ) ;
#55396=CARTESIAN_POINT ( 'NONE',  ( 26.73750000122903003, 6.123233995736764310E-16, -4.999999999999998224 ) ) ;
#55397=CARTESIAN_POINT ( 'NONE',  ( 3.253125000614518036, 0.000000000000000000, 5.243569643749999010 ) ) ;
#55399=CARTESIAN_POINT ( 'NONE',  ( -3.137519842735245283E-14, 12.91250000000000142, 34.00000000000000000 ) ) ;
#55400=B_SPLINE_CURVE_WITH_KNOTS ( 'NONE', 3,
 ( #54958, #48687, #4363, #71951, #60852, #43880, #10618, #72311, #66406, #15782 ),
 .UNSPECIFIED., .F., .F.,
 ( 4, 3, 3, 4 ),
 ( 9.758590510124697839E-17, 0.0001554715923351995962, 0.0002333273007130473695, 0.0003112188215848752607 ),
 .UNSPECIFIED. ) ;
#55401=CARTESIAN_POINT ( 'NONE',  ( -3.999999999999999556, 14.22500000122903430, -32.30940107675850470 ) ) ;
#55402=CARTESIAN_POINT ( 'NONE',  ( 4.243569643749999898, 17.83437500061451786, -30.00000000000000000 ) ) ;
#55403=CARTESIAN_POINT ( 'NONE',  ( 9.975000000000001421, 6.123233995736764310E-16, -4.999999999999998224 ) ) ;
#55405=CARTESIAN_POINT ( 'NONE',  ( 12.08437500061451608, 6.421520780324663323E-16, -5.243569643749999010 ) ) ;
#55406=CARTESIAN_POINT ( 'NONE',  ( 7.275000001229035007, -5.773502691896255534, -1.060575238724906372E-15 ) ) ;
#55407=CARTESIAN_POINT ( 'NONE',  ( 12.38437500061451857, -4.541064518000419881, 2.621784821874995952 ) ) ;
#55408=CARTESIAN_POINT ( 'NONE',  ( 4.809375000614516615, -4.541064518000417216, -2.621784821875001281 ) ) ;
#55409=CARTESIAN_POINT ( 'NONE',  ( -4.243569643749999898, 10.35312500061451857, -30.00000000000000000 ) ) ;
#55410=DIRECTION ( 'NONE',  ( -0.000000000000000000, -1.000000000000000000, -0.000000000000000000 ) ) ;
#55411=CARTESIAN_POINT ( 'NONE',  ( 10.50937500061451679, 0.000000000000000000, 5.243569643749999010 ) ) ;
#55413=CARTESIAN_POINT ( 'NONE',  ( 0.000000000000000000, 20.00000000000000000, 26.00000000000000000 ) ) ;
#55414=CARTESIAN_POINT ( 'NONE',  ( 18.55312500061451431, 0.000000000000000000, 5.243569643749999010 ) ) ;
#55415=CARTESIAN_POINT ( 'NONE',  ( 16.50000000000000000, 0.000000000000000000, 4.999999999999998224 ) ) ;
#55416=CARTESIAN_POINT ( 'NONE',  ( 4.243569643749999010, 19.16562500061459673, 27.54997392385601174 ) ) ;
#55417=CARTESIAN_POINT ( 'NONE',  ( 24.00937500061451502, 0.000000000000000000, 5.243569643749999010 ) ) ;
#55418=EDGE_CURVE ( 'NONE', #8622, #38892, #70752, .T. ) ;
#55419=CARTESIAN_POINT ( 'NONE',  ( 4.070823519296731696, 2.903409097154723284, -4.275654497055423775 ) ) ;
#55420=CARTESIAN_POINT ( 'NONE',  ( 28.38750000122903216, -4.330127018922194537, 2.499999999999995559 ) ) ;
#55422=CARTESIAN_POINT ( 'NONE',  ( 24.40312500061451573, 0.000000000000000000, 5.243569643749999010 ) ) ;
#55423=CARTESIAN_POINT ( 'NONE',  ( 16.90312500061451573, -4.541064518000417216, -2.621784821875001281 ) ) ;
#55425=CARTESIAN_POINT ( 'NONE',  ( 13.77187500061451786, -6.054752690667223547, -1.112240025338166033E-15 ) ) ;
#55427=CARTESIAN_POINT ( 'NONE',  ( 26.58750000122903145, -4.330127018922194537, 2.499999999999995559 ) ) ;
#55428=CARTESIAN_POINT ( 'NONE',  ( 3.796875000614517326, -3.027376345333614438, 5.243569643749998122 ) ) ;
#55429=CARTESIAN_POINT ( 'NONE',  ( 14.63437500061451679, -4.541064518000419881, 2.621784821874995952 ) ) ;
#55430=CARTESIAN_POINT ( 'NONE',  ( 1.626862140677534273E-15, 12.01250000000000284, 34.00000000000000000 ) ) ;
#55431=CARTESIAN_POINT ( 'NONE',  ( -3.999999999999997335, 11.48750000000000071, 32.30940107675850470 ) ) ;
#55432=CARTESIAN_POINT ( 'NONE',  ( 4.312500001229034652, 4.330127018922192761, -2.499999999999997780 ) ) ;
#55433=CARTESIAN_POINT ( 'NONE',  ( 23.82187500061451502, 3.027376345333613106, -5.243569643749998122 ) ) ;
#55434=CARTESIAN_POINT ( 'NONE',  ( 17.37187500061451573, -6.054752690667223547, -1.112240025338166033E-15 ) ) ;
#55436=CARTESIAN_POINT ( 'NONE',  ( 27.52500000000000213, 6.123233995736764310E-16, -4.999999999999998224 ) ) ;
#55437=CYLINDRICAL_SURFACE ( 'NONE', #13606, 4.000000000000000000 ) ;
#55438=CARTESIAN_POINT ( 'NONE',  ( 6.712500000000000355, -5.773502691896255534, -1.060575238724906372E-15 ) ) ;
#55440=CARTESIAN_POINT ( 'NONE',  ( 19.34062500061451573, 6.054752690667223547, 3.707466751127219781E-16 ) ) ;
#55441=CARTESIAN_POINT ( 'NONE',  ( 10.49999999999999822, 4.330127018922192761, -2.499999999999997780 ) ) ;
#55442=CARTESIAN_POINT ( 'NONE',  ( 4.603125000614518569, 0.000000000000000000, 5.243569643749999010 ) ) ;
#55443=CARTESIAN_POINT ( 'NONE',  ( 17.88749999999999929, -2.886751345948129988, 4.999999999999997335 ) ) ;
#55444=CARTESIAN_POINT ( 'NONE',  ( 21.52500000122903145, 2.886751345948126879, 4.999999999999999112 ) ) ;
#55445=CARTESIAN_POINT ( 'NONE',  ( -2.000000000000000000, 10.02500000000000036, -33.46410161513775705 ) ) ;
#55446=CARTESIAN_POINT ( 'NONE',  ( 28.99687500061451573, -3.027376345333614438, 5.243569643749998122 ) ) ;
#55448=CARTESIAN_POINT ( 'NONE',  ( 17.50312500061451715, 4.541064518000418104, -2.621784821874998173 ) ) ;
#55449=CARTESIAN_POINT ( 'NONE',  ( 25.34062500061451217, -3.027376345333614438, 5.243569643749998122 ) ) ;
#55450=CARTESIAN_POINT ( 'NONE',  ( 23.33437500061451786, 6.421520780324663323E-16, -5.243569643749999010 ) ) ;
#55451=CARTESIAN_POINT ( 'NONE',  ( 6.375000000000001776, 6.123233995736764310E-16, -4.999999999999998224 ) ) ;
#55452=CARTESIAN_POINT ( 'NONE',  ( 8.503125000614515372, 4.541064518000418104, -2.621784821874998173 ) ) ;
#55453=CARTESIAN_POINT ( 'NONE',  ( 27.70312500061451289, -4.541064518000417216, -2.621784821875001281 ) ) ;
#55454=CARTESIAN_POINT ( 'NONE',  ( 14.37187500061451928, 3.027376345333613106, -5.243569643749998122 ) ) ;
#55455=CARTESIAN_POINT ( 'NONE',  ( 18.45937500061451431, 4.541064518000418104, -2.621784821874998173 ) ) ;
#55456=LINE ( 'NONE', #38837, #14444 ) ;
#55457=CARTESIAN_POINT ( 'NONE',  ( -2.121784821874999949, 9.884375000614518569, 26.32496088578401938 ) ) ;
#55458=EDGE_CURVE ( 'NONE', #44903, #22838, #31227, .T. ) ;
#55459=CARTESIAN_POINT ( 'NONE',  ( 21.90000000122903145, 5.773502691896255534, 3.535250795749688894E-16 ) ) ;
#55461=CARTESIAN_POINT ( 'NONE',  ( 10.86562500061451608, 3.027376345333611329, 5.243569643749999010 ) ) ;
#55462=CARTESIAN_POINT ( 'NONE',  ( 8.409375000614518925, -4.541064518000417216, -2.621784821875001281 ) ) ;
#55463=CARTESIAN_POINT ( 'NONE',  ( 8.259375000614518569, 0.000000000000000000, 5.243569643749999010 ) ) ;
#55464=VERTEX_POINT ( 'NONE', #41954 ) ;
#55465=CARTESIAN_POINT ( 'NONE',  ( 28.77187500061451431, 3.027376345333613106, -5.243569643749998122 ) ) ;
#55466=CARTESIAN_POINT ( 'NONE',  ( 18.32812500061451644, 6.421520780324663323E-16, -5.243569643749999010 ) ) ;
#55467=CARTESIAN_POINT ( 'NONE',  ( 29.40000000122903145, -2.886751345948125991, -5.000000000000000000 ) ) ;
#55468=CARTESIAN_POINT ( 'NONE',  ( 3.721875000614518036, 3.027376345333611329, 5.243569643749999010 ) ) ;
#55469=CARTESIAN_POINT ( 'NONE',  ( 24.79687500061451999, 6.054752690667223547, 3.707466751127219781E-16 ) ) ;
#55470=CARTESIAN_POINT ( 'NONE',  ( 20.05312500061451431, -4.541064518000417216, -2.621784821875001281 ) ) ;
#55471=CARTESIAN_POINT ( 'NONE',  ( 9.001249775931846008E-16, 18.62187500061451928, 34.90005215228797653 ) ) ;
#55472=CARTESIAN_POINT ( 'NONE',  ( 23.50312500061451360, 0.000000000000000000, 5.243569643749999010 ) ) ;
#55473=CARTESIAN_POINT ( 'NONE',  ( 4.275000001229035895, 2.886751345948129099, -4.999999999999998224 ) ) ;
#55474=VERTEX_POINT ( 'NONE', #37129 ) ;
#55475=CARTESIAN_POINT ( 'NONE',  ( 27.26249999999999929, 2.886751345948126879, 4.999999999999999112 ) ) ;
#55476=CARTESIAN_POINT ( 'NONE',  ( -3.999999999999997335, 16.43750000000000000, -27.69059892324149175 ) ) ;
#55478=CARTESIAN_POINT ( 'NONE',  ( 4.171875000614517326, 3.027376345333611329, 5.243569643749999010 ) ) ;
#55479=CARTESIAN_POINT ( 'NONE',  ( 11.84062500061451750, -3.027376345333614438, 5.243569643749998122 ) ) ;
#55480=CARTESIAN_POINT ( 'NONE',  ( 5.446875000614518569, 6.054752690667223547, 3.707466751127219781E-16 ) ) ;
#55481=CARTESIAN_POINT ( 'NONE',  ( 24.48750000122903359, 6.123233995736764310E-16, -4.999999999999998224 ) ) ;
#55482=CARTESIAN_POINT ( 'NONE',  ( 15.27187500061451786, 3.027376345333612662, -5.243569643749998122 ) ) ;
#55483=CARTESIAN_POINT ( 'NONE',  ( 3.646875000614520079, 6.054752690667223547, 3.707466751127219781E-16 ) ) ;
#55485=CARTESIAN_POINT ( 'NONE',  ( 25.65937500061451715, 4.541064518000418104, -2.621784821874998173 ) ) ;
#55486=CARTESIAN_POINT ( 'NONE',  ( 12.59062500061451573, 6.054752690667223547, 3.707466751127219781E-16 ) ) ;
#55488=CARTESIAN_POINT ( 'NONE',  ( 10.60312500061451679, -4.541064518000417216, -2.621784821875001281 ) ) ;
#55489=CARTESIAN_POINT ( 'NONE',  ( 9.215625000614515727, -6.054752690667223547, -1.112240025338166033E-15 ) ) ;
#55491=CARTESIAN_POINT ( 'NONE',  ( 8.737500000000002487, 5.773502691896255534, 3.535250795749688894E-16 ) ) ;
#55492=CARTESIAN_POINT ( 'NONE',  ( 4.125000001229034652, -5.773502691896255534, -1.060575238724906372E-15 ) ) ;
#55493=CARTESIAN_POINT ( 'NONE',  ( 17.13749999999999929, -2.886751345948125991, -5.000000000000000000 ) ) ;
#55494=CARTESIAN_POINT ( 'NONE',  ( 18.08437500061451431, 4.541064518000418104, 2.621784821874999949 ) ) ;
#55495=CARTESIAN_POINT ( 'NONE',  ( 12.97500000122903252, 2.886751345948126879, 4.999999999999999112 ) ) ;
#55497=CARTESIAN_POINT ( 'NONE',  ( 2.121784821875001281, 15.45312500061451644, -26.32496088578401938 ) ) ;
#55500=CARTESIAN_POINT ( 'NONE',  ( 27.32812500061451644, 6.421520780324663323E-16, -5.243569643749999010 ) ) ;
#55501=DIRECTION ( 'NONE',  ( 1.000000000000000000, 0.000000000000000000, -0.000000000000000000 ) ) ;
#55503=CARTESIAN_POINT ( 'NONE',  ( 14.82187500061451679, 3.027376345333613106, -5.243569643749998122 ) ) ;
#55504=( BOUNDED_CURVE ( )  B_SPLINE_CURVE ( 2, ( #15772, #26138, #19854, #60841, #64927, #14317, #59369 ),
 .UNSPECIFIED., .F., .F. ) 
 B_SPLINE_CURVE_WITH_KNOTS ( ( 3, 2, 2, 3 ),
 ( 0.6750000000000000444, 0.6777777777777778123, 0.6805555555555555802, 0.6833333333333333481 ),
 .UNSPECIFIED. ) 
 CURVE ( )  GEOMETRIC_REPRESENTATION_ITEM ( )  RATIONAL_B_SPLINE_CURVE ( ( 1.000000000000000000, 0.8660254037844387076, 1.000000000000000000, 0.8660254037844387076, 1.000000000000000000, 0.8660254037844387076, 1.000000000000000000 ) ) 
 REPRESENTATION_ITEM ( '' )  );
#55505=EDGE_CURVE ( 'NONE', #56216, #45736, #35649, .T. ) ;
#55507=CARTESIAN_POINT ( 'NONE',  ( 25.94999999999999929, 0.000000000000000000, 4.999999999999998224 ) ) ;
#55508=CARTESIAN_POINT ( 'NONE',  ( 9.553125000614517859, 0.000000000000000000, 5.243569643749999010 ) ) ;
#55510=CARTESIAN_POINT ( 'NONE',  ( 20.82187500061451857, 3.027376345333611329, 5.243569643749999010 ) ) ;
#55512=CARTESIAN_POINT ( 'NONE',  ( 7.640625000614517326, 6.054752690667223547, 3.707466751127219781E-16 ) ) ;
#55513=CARTESIAN_POINT ( 'NONE',  ( 11.70937500061451608, 4.541064518000418104, -2.621784821874998173 ) ) ;
#55515=CARTESIAN_POINT ( 'NONE',  ( 22.17187500061451644, 3.027376345333611329, 5.243569643749999010 ) ) ;
#55516=CARTESIAN_POINT ( 'NONE',  ( 2.064291216241248783, 4.560108959200712242, -26.56427412444418579 ) ) ;
#55518=CARTESIAN_POINT ( 'NONE',  ( 4.275000000000001243, 4.330127018922191873, 2.499999999999999556 ) ) ;
#55519=CARTESIAN_POINT ( 'NONE',  ( 15.45000000122903216, -2.886751345948125991, -5.000000000000000000 ) ) ;
#55521=CARTESIAN_POINT ( 'NONE',  ( 1.626862140677534273E-15, 11.67500000122903181, 34.00000000000000000 ) ) ;
#55522=ORIENTED_EDGE ( 'NONE', *, *, #9642, .T. ) ;
#55523=CARTESIAN_POINT ( 'NONE',  ( 11.96250000000000213, 2.886751345948126879, 4.999999999999999112 ) ) ;
#55524=CARTESIAN_POINT ( 'NONE',  ( 16.57499999999999929, -4.330127018922194537, 2.499999999999995559 ) ) ;
#55525=CARTESIAN_POINT ( 'NONE',  ( 13.38750000122903394, 4.330127018922191873, 2.499999999999999556 ) ) ;
#55526=CARTESIAN_POINT ( 'NONE',  ( 10.41562500061451679, 3.027376345333611329, 5.243569643749999010 ) ) ;
#55527=EDGE_LOOP ( 'NONE', ( #50444, #63794, #64156, #8699 ) ) ;
#55528=CARTESIAN_POINT ( 'NONE',  ( 9.262499999999999289, 2.886751345948126879, 4.999999999999999112 ) ) ;
#55529=CARTESIAN_POINT ( 'NONE',  ( -1.071796769724496556, 15.70490381179669903, 33.99999999999998579 ) ) ;
#55530=CARTESIAN_POINT ( 'NONE',  ( 2.121784821874999061, 13.40937500061451892, -33.67503911421598417 ) ) ;
#55531=CARTESIAN_POINT ( 'NONE',  ( 29.58750000122903501, 4.330127018922191873, 2.499999999999999556 ) ) ;
#55533=CARTESIAN_POINT ( 'NONE',  ( 8.699999999999999289, 4.330127018922192761, -2.499999999999997780 ) ) ;
#55534=VERTEX_POINT ( 'NONE', #67060 ) ;
#55535=CARTESIAN_POINT ( 'NONE',  ( 24.47812500061451502, -4.541064518000419881, 2.621784821874995952 ) ) ;
#55536=CARTESIAN_POINT ( 'NONE',  ( 1.999999999999998668, 13.55000000000000071, -33.46410161513775705 ) ) ;
#55537=CARTESIAN_POINT ( 'NONE',  ( 29.70937500061451431, 4.541064518000418104, -2.621784821874998173 ) ) ;
#55538=CARTESIAN_POINT ( 'NONE',  ( 22.47187500061451715, 3.027376345333613106, -5.243569643749998122 ) ) ;
#55539=CARTESIAN_POINT ( 'NONE',  ( 17.61562500061451786, 3.027376345333611329, 5.243569643749999010 ) ) ;
#55540=CARTESIAN_POINT ( 'NONE',  ( 4.243569643749999010, 11.96562500061459389, -32.45002607614398471 ) ) ;
#55541=CARTESIAN_POINT ( 'NONE',  ( 6.628125000614517148, 6.421520780324663323E-16, -5.243569643749999010 ) ) ;
#55542=CARTESIAN_POINT ( 'NONE',  ( 28.20000000122903216, 5.773502691896255534, 3.535250795749688894E-16 ) ) ;
#55544=CARTESIAN_POINT ( 'NONE',  ( 18.32812500061451644, 6.421520780324663323E-16, -5.243569643749999010 ) ) ;
#55547=CARTESIAN_POINT ( 'NONE',  ( 14.14687500061451786, -3.027376345333614438, 5.243569643749998122 ) ) ;
#55548=CARTESIAN_POINT ( 'NONE',  ( 13.92187500061451644, 3.027376345333613106, -5.243569643749998122 ) ) ;
#55549=CARTESIAN_POINT ( 'NONE',  ( 22.99687500061451573, 6.054752690667223547, 3.707466751127219781E-16 ) ) ;
#55550=VERTEX_POINT ( 'NONE', #44527 ) ;
#55551=CARTESIAN_POINT ( 'NONE',  ( -2.121784821874999949, 12.13437500061451857, 26.32496088578401938 ) ) ;
#55552=CARTESIAN_POINT ( 'NONE',  ( 3.103125000614517237, 4.541064518000418104, -2.621784821874998173 ) ) ;
#55553=CARTESIAN_POINT ( 'NONE',  ( 27.70312500061451289, -4.541064518000417216, -2.621784821875001281 ) ) ;
#55554=CARTESIAN_POINT ( 'NONE',  ( 25.82812500061451644, -4.541064518000419881, 2.621784821874995952 ) ) ;
#55555=CARTESIAN_POINT ( 'NONE',  ( 30.00000000000000000, 0.000000000000000000, 4.999999999999998224 ) ) ;
#55556=CARTESIAN_POINT ( 'NONE',  ( -1.999999999999997113, 19.17500000000000071, 33.46410161513775705 ) ) ;
#55557=CARTESIAN_POINT ( 'NONE',  ( 4.621875000614516615, 3.027376345333611329, 5.243569643749999010 ) ) ;
#55558=CARTESIAN_POINT ( 'NONE',  ( 12.75000000122903643, -2.886751345948125991, -5.000000000000000000 ) ) ;
#55559=CARTESIAN_POINT ( 'NONE',  ( 9.825000001229033941, 2.886751345948126879, 4.999999999999999112 ) ) ;
#55560=CARTESIAN_POINT ( 'NONE',  ( 29.28750000122903074, -4.330127018922194537, 2.499999999999995559 ) ) ;
#55563=CARTESIAN_POINT ( 'NONE',  ( 11.52187500061451608, -6.054752690667223547, -1.112240025338166033E-15 ) ) ;
#55565=ORIENTED_EDGE ( 'NONE', *, *, #33711, .F. ) ;
#55566=EDGE_CURVE ( 'NONE', #17652, #9450, #65728, .T. ) ;
#55567=CARTESIAN_POINT ( 'NONE',  ( 20.27812500061451573, 4.541064518000418104, 2.621784821874999949 ) ) ;
#55568=CARTESIAN_POINT ( 'NONE',  ( 12.23437500061451821, 4.541064518000418104, 2.621784821874999949 ) ) ;
#55569=CARTESIAN_POINT ( 'NONE',  ( 5.165625000614518569, -6.054752690667223547, -1.112240025338166033E-15 ) ) ;
#55570=CARTESIAN_POINT ( 'NONE',  ( 21.72187500061451715, 3.027376345333611329, 5.243569643749999010 ) ) ;
#55571=CARTESIAN_POINT ( 'NONE',  ( 5.278125000614516615, 6.421520780324663323E-16, -5.243569643749999010 ) ) ;
#55572=FACE_OUTER_BOUND ( 'NONE', #54077, .T. ) ;
#55573=CARTESIAN_POINT ( 'NONE',  ( 6.075000001229034829, 2.886751345948129099, -4.999999999999998224 ) ) ;
#55574=( BOUNDED_CURVE ( )  B_SPLINE_CURVE ( 2, ( #52677, #2085, #19404, #63031, #46058, #47142, #6895 ),
 .UNSPECIFIED., .F., .F. ) 
 B_SPLINE_CURVE_WITH_KNOTS ( ( 3, 2, 2, 3 ),
 ( 0.9515180543127474966, 0.9527777777777777235, 0.9555555555555556024, 0.9567008448923609576 ),
 .UNSPECIFIED. ) 
 CURVE ( )  GEOMETRIC_REPRESENTATION_ITEM ( )  RATIONAL_B_SPLINE_CURVE ( ( 0.9335920638844523722, 0.9392424606745505278, 1.000000000000000000, 0.8660254037844387076, 1.000000000000000000, 0.9447617164785451216, 0.9350733812694886904 ) ) 
 REPRESENTATION_ITEM ( '' )  );
#55575=CARTESIAN_POINT ( 'NONE',  ( 20.99062500061451431, -3.027376345333610441, -5.243569643749999898 ) ) ;
#55576=CARTESIAN_POINT ( 'NONE',  ( -1.999999999999997113, 18.38750000122903572, -26.53589838486224295 ) ) ;
#55577=CARTESIAN_POINT ( 'NONE',  ( 8.137500001229033941, -4.330127018922194537, 2.499999999999995559 ) ) ;
#55578=CARTESIAN_POINT ( 'NONE',  ( 16.34062500061451573, -3.027376345333614438, 5.243569643749998122 ) ) ;
#55579=CARTESIAN_POINT ( 'NONE',  ( 16.67812500061451786, 4.541064518000418104, 2.621784821874999949 ) ) ;
#55581=CARTESIAN_POINT ( 'NONE',  ( 16.94999999999999929, 0.000000000000000000, 4.999999999999998224 ) ) ;
#55582=CARTESIAN_POINT ( 'NONE',  ( 11.40000000122903501, -2.886751345948125991, -5.000000000000000000 ) ) ;
#55583=CARTESIAN_POINT ( 'NONE',  ( 7.340625000614518392, -3.027376345333614438, 5.243569643749998122 ) ) ;
#55584=CARTESIAN_POINT ( 'NONE',  ( 10.30312500061451431, 4.541064518000418104, -2.621784821874998173 ) ) ;
#55585=CARTESIAN_POINT ( 'NONE',  ( 20.32500000122903572, -5.773502691896255534, -1.060575238724906372E-15 ) ) ;
#55586=CARTESIAN_POINT ( 'NONE',  ( -2.121784821874999949, 13.93437500061451750, -33.67503911421598417 ) ) ;
#55587=CARTESIAN_POINT ( 'NONE',  ( 30.00000000000000000, 0.000000000000000000, 0.000000000000000000 ) ) ;
#55588=CARTESIAN_POINT ( 'NONE',  ( 5.737500001229033586, 4.330127018922191873, 2.499999999999999556 ) ) ;
#55589=CARTESIAN_POINT ( 'NONE',  ( 2.971875000614517592, -6.054752690667223547, -1.112240025338166033E-15 ) ) ;
#55590=CARTESIAN_POINT ( 'NONE',  ( 19.84687500061451360, 6.054752690667223547, 3.707466751127219781E-16 ) ) ;
#55591=CARTESIAN_POINT ( 'NONE',  ( 1.071796769724489895, 18.62990381179669797, 26.00000000000000355 ) ) ;
#55592=CARTESIAN_POINT ( 'NONE',  ( 17.01562500061451644, 3.027376345333613106, -5.243569643749998122 ) ) ;
#55595=CARTESIAN_POINT ( 'NONE',  ( 26.62500000000000000, 6.123233995736764310E-16, -4.999999999999998224 ) ) ;
#55596=CARTESIAN_POINT ( 'NONE',  ( 29.78437500061451715, 4.541064518000418104, 2.621784821874999949 ) ) ;
#55598=CARTESIAN_POINT ( 'NONE',  ( 14.31562500061451537, 3.027376345333613106, -5.243569643749998122 ) ) ;
#55599=CARTESIAN_POINT ( 'NONE',  ( 14.14687500061451786, -3.027376345333614438, 5.243569643749998122 ) ) ;
#55601=CARTESIAN_POINT ( 'NONE',  ( 21.70312500061451644, 0.000000000000000000, 5.243569643749999010 ) ) ;
#55602=CARTESIAN_POINT ( 'NONE',  ( 1.071796769724491893, 11.13259618943233420, -26.00000000000000355 ) ) ;
#55603=CARTESIAN_POINT ( 'NONE',  ( 22.34999999999999787, 0.000000000000000000, 4.999999999999998224 ) ) ;
#55604=CARTESIAN_POINT ( 'NONE',  ( 11.96250000000000213, 2.886751345948126879, 4.999999999999999112 ) ) ;
#55605=CARTESIAN_POINT ( 'NONE',  ( 20.62500000122903288, 2.886751345948126879, 4.999999999999999112 ) ) ;
#55606=CARTESIAN_POINT ( 'NONE',  ( 16.22812500061451857, 4.541064518000418104, 2.621784821874999949 ) ) ;
#55608=VERTEX_POINT ( 'NONE', #32699 ) ;
#55609=CARTESIAN_POINT ( 'NONE',  ( 19.04999999999999716, 4.330127018922192761, -2.499999999999997780 ) ) ;
#55610=CARTESIAN_POINT ( 'NONE',  ( 21.57187500061451502, 3.027376345333613106, -5.243569643749998122 ) ) ;
#55611=CARTESIAN_POINT ( 'NONE',  ( 27.29062500061451502, -3.027376345333610441, -5.243569643749999898 ) ) ;
#55613=LINE ( 'NONE', #50075, #70193 ) ;
#55614=CARTESIAN_POINT ( 'NONE',  ( 9.740625000614516082, -3.027376345333610441, -5.243569643749999898 ) ) ;
#55617=CARTESIAN_POINT ( 'NONE',  ( 17.17500000000000071, 6.123233995736764310E-16, -4.999999999999998224 ) ) ;
#55618=CARTESIAN_POINT ( 'NONE',  ( 23.77499999999999858, -4.330127018922194537, 2.499999999999995559 ) ) ;
#55620=CARTESIAN_POINT ( 'NONE',  ( 3.421875000614516882, -6.054752690667223547, -1.112240025338166033E-15 ) ) ;
#55621=CARTESIAN_POINT ( 'NONE',  ( 27.90937500061451715, 4.541064518000418104, -2.621784821874998173 ) ) ;
#55622=VERTEX_POINT ( 'NONE', #17147 ) ;
#55623=CARTESIAN_POINT ( 'NONE',  ( 26.87812500061451360, 6.421520780324663323E-16, -5.243569643749999010 ) ) ;
#55624=CARTESIAN_POINT ( 'NONE',  ( 26.22187500061451715, 3.027376345333611329, 5.243569643749999010 ) ) ;
#55625=CARTESIAN_POINT ( 'NONE',  ( -4.243569643749999898, 18.45312500061459104, -30.00000000000000000 ) ) ;
#55626=CARTESIAN_POINT ( 'NONE',  ( 14.17500000000000071, 4.330127018922191873, 2.499999999999999556 ) ) ;
#55627=CARTESIAN_POINT ( 'NONE',  ( 10.45312500061451644, 0.000000000000000000, 5.243569643749999010 ) ) ;
#55629=CARTESIAN_POINT ( 'NONE',  ( -2.556497649636125342E-15, 19.21250000000000213, -26.00000000000000000 ) ) ;
#55630=CARTESIAN_POINT ( 'NONE',  ( 26.09062500061451573, 6.054752690667223547, 3.707466751127219781E-16 ) ) ;
#55631=CARTESIAN_POINT ( 'NONE',  ( 16.38750000122903216, 6.123233995736764310E-16, -4.999999999999998224 ) ) ;
#55634=CARTESIAN_POINT ( 'NONE',  ( 4.115625000614516082, 3.027376345333611329, 5.243569643749999010 ) ) ;
#55635=CARTESIAN_POINT ( 'NONE',  ( 21.45937500061451786, -4.541064518000417216, -2.621784821875001281 ) ) ;
#55636=CARTESIAN_POINT ( 'NONE',  ( -4.243569643749999898, 13.97187500061451715, 27.54997392385601529 ) ) ;
#55637=CARTESIAN_POINT ( 'NONE',  ( 22.17187500061451644, 3.027376345333611329, 5.243569643749999010 ) ) ;
#55638=CARTESIAN_POINT ( 'NONE',  ( 29.82187500061451502, 3.027376345333611329, 5.243569643749999010 ) ) ;
#55639=CARTESIAN_POINT ( 'NONE',  ( 4.243569643749999898, 17.83437500061451786, 30.00000000000000000 ) ) ;
#55640=CARTESIAN_POINT ( 'NONE',  ( 8.803125000614517859, -4.541064518000417216, -2.621784821875001281 ) ) ;
#55642=CARTESIAN_POINT ( 'NONE',  ( 7.396875000614519635, -3.027376345333614438, 5.243569643749998122 ) ) ;
#55643=FACE_OUTER_BOUND ( 'NONE', #29310, .T. ) ;
#55644=CARTESIAN_POINT ( 'NONE',  ( 8.465625000614515727, 3.027376345333613106, -5.243569643749998122 ) ) ;
#55645=CARTESIAN_POINT ( 'NONE',  ( 12.49687500061451573, -3.027376345333610441, -5.243569643749999898 ) ) ;
#55646=CARTESIAN_POINT ( 'NONE',  ( 18.63750000122903216, 6.123233995736764310E-16, -4.999999999999998224 ) ) ;
#55647=CARTESIAN_POINT ( 'NONE',  ( 7.359375000614516438, 0.000000000000000000, 5.243569643749999010 ) ) ;
#55648=CARTESIAN_POINT ( 'NONE',  ( 10.94062500061451537, -3.027376345333614438, 5.243569643749998122 ) ) ;
#55649=CARTESIAN_POINT ( 'NONE',  ( 7.265625000614516438, 3.027376345333611329, 5.243569643749999010 ) ) ;
#55651=CARTESIAN_POINT ( 'NONE',  ( 18.68437500061451928, -4.541064518000419881, 2.621784821874995952 ) ) ;
#55652=CARTESIAN_POINT ( 'NONE',  ( 4.535435261965744758, 2.105238004946854868, 4.730754414875756986 ) ) ;
#55653=CARTESIAN_POINT ( 'NONE',  ( 11.39062500061451644, -3.027376345333614438, 5.243569643749998122 ) ) ;
#55655=CARTESIAN_POINT ( 'NONE',  ( -4.243569643749999898, 13.07187500061452035, -32.45002607614398471 ) ) ;
#55656=CARTESIAN_POINT ( 'NONE',  ( 12.15000000122903501, -2.886751345948129988, 4.999999999999997335 ) ) ;
#55657=CARTESIAN_POINT ( 'NONE',  ( -2.121784821874996840, 15.82812500061451644, -26.32496088578401583 ) ) ;
#55658=CARTESIAN_POINT ( 'NONE',  ( 14.81250000122903288, 0.000000000000000000, 4.999999999999998224 ) ) ;
#55659=CARTESIAN_POINT ( 'NONE',  ( 11.35312500061451679, 0.000000000000000000, 5.243569643749999010 ) ) ;
#55661=CARTESIAN_POINT ( 'NONE',  ( 13.98750000000000249, -2.886751345948125991, -5.000000000000000000 ) ) ;
#55663=CARTESIAN_POINT ( 'NONE',  ( 23.80312500061451786, 4.541064518000418104, -2.621784821874998173 ) ) ;
#55664=CARTESIAN_POINT ( 'NONE',  ( 7.396875000614519635, -3.027376345333614438, 5.243569643749998122 ) ) ;
#55665=CARTESIAN_POINT ( 'NONE',  ( 10.42500000122903536, -5.773502691896255534, -1.060575238724906372E-15 ) ) ;
#55666=CARTESIAN_POINT ( 'NONE',  ( 18.30000000122903359, 5.773502691896255534, 3.535250795749688894E-16 ) ) ;
#55667=CARTESIAN_POINT ( 'NONE',  ( 14.99062500061451786, -3.027376345333614438, 5.243569643749998122 ) ) ;
#55668=CARTESIAN_POINT ( 'NONE',  ( 17.76562500061451644, -6.054752690667223547, -1.112240025338166033E-15 ) ) ;
#55669=CARTESIAN_POINT ( 'NONE',  ( 25.65000000122903145, -2.886751345948129988, 4.999999999999997335 ) ) ;
#55671=CARTESIAN_POINT ( 'NONE',  ( 27.93750000122903288, -4.330127018922194537, 2.499999999999995559 ) ) ;
#55672=CARTESIAN_POINT ( 'NONE',  ( 22.94999999999999929, -4.330127018922190985, -2.500000000000001332 ) ) ;
#55674=CARTESIAN_POINT ( 'NONE',  ( 25.17187500061451644, 3.027376345333613106, -5.243569643749998122 ) ) ;
#55675=CARTESIAN_POINT ( 'NONE',  ( 18.41250000122903430, 0.000000000000000000, 4.999999999999998224 ) ) ;
#55676=CARTESIAN_POINT ( 'NONE',  ( 11.85000000122903430, -2.886751345948125991, -5.000000000000000000 ) ) ;
#55677=CARTESIAN_POINT ( 'NONE',  ( 27.87187500061451573, 3.027376345333613106, -5.243569643749998122 ) ) ;
#55679=CARTESIAN_POINT ( 'NONE',  ( 22.61250000000000426, 2.886751345948095793, -5.000000000000055067 ) ) ;
#55680=CARTESIAN_POINT ( 'NONE',  ( 5.671875000614519102, -6.054752690667223547, -1.112240025338166033E-15 ) ) ;
#55681=CARTESIAN_POINT ( 'NONE',  ( 24.85312500061451502, 0.000000000000000000, 5.243569643749999010 ) ) ;
#55683=CARTESIAN_POINT ( 'NONE',  ( 1.071796769724490783, 19.68259618943233491, -26.00000000000000000 ) ) ;
#55684=CARTESIAN_POINT ( 'NONE',  ( 10.62187500061451928, -6.054752690667223547, -1.112240025338166033E-15 ) ) ;
#55685=LINE ( 'NONE', #72680, #34763 ) ;
#55686=CARTESIAN_POINT ( 'NONE',  ( 3.609375000614516882, 4.541064518000418104, -2.621784821874998173 ) ) ;
#55687=CARTESIAN_POINT ( 'NONE',  ( 5.484375000614518214, 4.541064518000418104, 2.621784821874999949 ) ) ;
#55688=CARTESIAN_POINT ( 'NONE',  ( 28.13437500061451502, -4.541064518000419881, 2.621784821874995952 ) ) ;
#55690=CARTESIAN_POINT ( 'NONE',  ( 19.01249999999999929, 2.886751345948129099, -4.999999999999998224 ) ) ;
#55692=CARTESIAN_POINT ( 'NONE',  ( 27.33750000000000213, -2.886751345948129988, 4.999999999999997335 ) ) ;
#55694=CARTESIAN_POINT ( 'NONE',  ( 27.75937500061451502, -4.541064518000417216, -2.621784821875001281 ) ) ;
#55697=CARTESIAN_POINT ( 'NONE',  ( 17.65312500061451573, 0.000000000000000000, 5.243569643749999010 ) ) ;
#55698=CARTESIAN_POINT ( 'NONE',  ( 8.540625000614518569, 6.054752690667223547, 3.707466751127219781E-16 ) ) ;
#55700=CARTESIAN_POINT ( 'NONE',  ( 4.134375000614517681, 4.541064518000418104, 2.621784821874999949 ) ) ;
#55701=CARTESIAN_POINT ( 'NONE',  ( 17.32500000122903216, 2.886751345948129099, -4.999999999999998224 ) ) ;
#55702=CARTESIAN_POINT ( 'NONE',  ( 3.999999999999999112, 13.92500000000000071, -30.00000000000000000 ) ) ;
#55703=CARTESIAN_POINT ( 'NONE',  ( 7.396875000614519635, -3.027376345333614438, 5.243569643749998122 ) ) ;
#55704=CARTESIAN_POINT ( 'NONE',  ( 11.10937500061451644, -4.541064518000417216, -2.621784821875001281 ) ) ;
#55705=CARTESIAN_POINT ( 'NONE',  ( 23.33437500061451786, 6.421520780324663323E-16, -5.243569643749999010 ) ) ;
#55707=ORIENTED_EDGE ( 'NONE', *, *, #14692, .F. ) ;
#55709=CARTESIAN_POINT ( 'NONE',  ( 17.29687500061451999, -3.027376345333614438, 5.243569643749998122 ) ) ;
#55710=CARTESIAN_POINT ( 'NONE',  ( 9.346875000614517148, -3.027376345333610441, -5.243569643749999898 ) ) ;
#55712=CARTESIAN_POINT ( 'NONE',  ( 20.96250000000000213, 2.886751345948126879, 4.999999999999999112 ) ) ;
#55714=CARTESIAN_POINT ( 'NONE',  ( -2.121784821874999949, 9.884375000614518569, -33.67503911421598417 ) ) ;
#55716=CARTESIAN_POINT ( 'NONE',  ( 12.96562500061451750, 3.027376345333613106, -5.243569643749998122 ) ) ;
#55717=CARTESIAN_POINT ( 'NONE',  ( 28.88437500061451502, 4.541064518000418104, 2.621784821874999949 ) ) ;
#55718=( BOUNDED_CURVE ( )  B_SPLINE_CURVE ( 2, ( #60925, #16225, #73111, #38776, #50225, #6235, #55396 ),
 .UNSPECIFIED., .F., .F. ) 
 B_SPLINE_CURVE_WITH_KNOTS ( ( 3, 2, 2, 3 ),
 ( 0.1000000000000000611, 0.1027777777777778151, 0.1055555555555555969, 0.1083333333333333648 ),
 .UNSPECIFIED. ) 
 CURVE ( )  GEOMETRIC_REPRESENTATION_ITEM ( )  RATIONAL_B_SPLINE_CURVE ( ( 0.9999999999999973355, 0.8660254037844413721, 1.000000000000000000, 0.8660254037844387076, 1.000000000000000000, 0.8660254037844373753, 1.000000000000001332 ) ) 
 REPRESENTATION_ITEM ( '' )  );
#55719=CARTESIAN_POINT ( 'NONE',  ( 10.08750000122903323, 6.123233995736764310E-16, -4.999999999999998224 ) ) ;
#55720=CARTESIAN_POINT ( 'NONE',  ( 29.82187500061451502, 3.027376345333611329, 5.243569643749999010 ) ) ;
#55721=CARTESIAN_POINT ( 'NONE',  ( 9.562500000000001776, 2.886751345948129099, -4.999999999999998224 ) ) ;
#55722=CARTESIAN_POINT ( 'NONE',  ( 3.999999999999999112, 16.28750000122903430, 30.00000000000000000 ) ) ;
#55723=CARTESIAN_POINT ( 'NONE',  ( 10.35000000122903074, -2.886751345948129988, 4.999999999999997335 ) ) ;
#55724=CARTESIAN_POINT ( 'NONE',  ( 19.73437500061451644, 6.421520780324663323E-16, -5.243569643749999010 ) ) ;
#55725=CARTESIAN_POINT ( 'NONE',  ( 13.73437500061451821, -4.541064518000419881, 2.621784821874995952 ) ) ;
#55726=CYLINDRICAL_SURFACE ( 'NONE', #45477, 3.999999999999996447 ) ;
#55727=ORIENTED_EDGE ( 'NONE', *, *, #21809, .F. ) ;
#55728=CARTESIAN_POINT ( 'NONE',  ( 15.92812500061451608, -4.541064518000419881, 2.621784821874995952 ) ) ;
#55729=CARTESIAN_POINT ( 'NONE',  ( 29.43750000122903288, 6.123233995736764310E-16, -4.999999999999998224 ) ) ;
#55730=CARTESIAN_POINT ( 'NONE',  ( 15.45937500061451608, 0.000000000000000000, 5.243569643749999010 ) ) ;
#55732=CARTESIAN_POINT ( 'NONE',  ( 16.56562500061451715, 3.027376345333613106, -5.243569643749998122 ) ) ;
#55733=CARTESIAN_POINT ( 'NONE',  ( 18.07500000122903216, -5.773502691896255534, -1.060575238724906372E-15 ) ) ;
#55734=CARTESIAN_POINT ( 'NONE',  ( 27.30937500061451573, -4.541064518000417216, -2.621784821875001281 ) ) ;
#55735=CARTESIAN_POINT ( 'NONE',  ( -2.121784821874999949, 9.828125000614516438, 26.32496088578401938 ) ) ;
#55736=CARTESIAN_POINT ( 'NONE',  ( 15.72187500061451892, 3.027376345333613106, -5.243569643749998122 ) ) ;
#55737=CARTESIAN_POINT ( 'NONE',  ( 13.27500000122903323, 2.886751345948129099, -4.999999999999998224 ) ) ;
#55739=CARTESIAN_POINT ( 'NONE',  ( -2.121784821874996840, 18.13437500061451502, -26.32496088578401583 ) ) ;
#55740=CARTESIAN_POINT ( 'NONE',  ( 20.18437500061451573, 6.421520780324663323E-16, -5.243569643749999010 ) ) ;
#55741=CARTESIAN_POINT ( 'NONE',  ( 22.20000000122903216, -2.886751345948125991, -5.000000000000000000 ) ) ;
#55742=CARTESIAN_POINT ( 'NONE',  ( 17.63437500061451502, 4.541064518000418104, 2.621784821874999949 ) ) ;
#55743=CARTESIAN_POINT ( 'NONE',  ( -4.243569643749997233, 12.69687500061451857, 32.45002607614398471 ) ) ;
#55744=CARTESIAN_POINT ( 'NONE',  ( 16.82812500061451644, -4.541064518000419881, 2.621784821874995952 ) ) ;
#55745=VERTEX_POINT ( 'NONE', #56674 ) ;
#55746=ORIENTED_EDGE ( 'NONE', *, *, #12056, .T. ) ;
#55747=CARTESIAN_POINT ( 'NONE',  ( 21.03750000000000142, -2.886751345948129988, 4.999999999999997335 ) ) ;
#55748=CARTESIAN_POINT ( 'NONE',  ( 3.972658874145789110, 3.036112888163414514, -4.275165627105516286 ) ) ;
#55749=CARTESIAN_POINT ( 'NONE',  ( 23.80312500061451786, 4.541064518000418104, -2.621784821874998173 ) ) ;
#55750=CARTESIAN_POINT ( 'NONE',  ( 4.865625000614517859, 3.027376345333613106, -5.243569643749998122 ) ) ;
#55751=CARTESIAN_POINT ( 'NONE',  ( 16.42500000122903359, 2.886751345948129099, -4.999999999999998224 ) ) ;
#55752=CARTESIAN_POINT ( 'NONE',  ( 23.05312500061451431, 0.000000000000000000, 5.243569643749999010 ) ) ;
#55753=CARTESIAN_POINT ( 'NONE',  ( 20.24999999999999645, -4.330127018922190985, -2.500000000000001332 ) ) ;
#55754=CARTESIAN_POINT ( 'NONE',  ( 26.54062500061451146, 6.054752690667223547, 3.707466751127219781E-16 ) ) ;
#55755=CARTESIAN_POINT ( 'NONE',  ( 6.553125000614518747, -4.541064518000417216, -2.621784821875001281 ) ) ;
#55756=EDGE_LOOP ( 'NONE', ( #12126, #23865 ) ) ;
#55757=VECTOR ( 'NONE', #70577, 1000.000000000000000 ) ;
#55758=FACE_OUTER_BOUND ( 'NONE', #66652, .T. ) ;
#55759=CARTESIAN_POINT ( 'NONE',  ( 2.803125000614518747, 0.000000000000000000, 5.243569643749999010 ) ) ;
#55762=CARTESIAN_POINT ( 'NONE',  ( -3.999999999999999556, 10.62500000122903643, -32.30940107675850470 ) ) ;
#55763=EDGE_CURVE ( 'NONE', #13629, #20263, #21233, .T. ) ;
#55764=CARTESIAN_POINT ( 'NONE',  ( -2.121784821874996840, 19.03437500061451715, -26.32496088578401583 ) ) ;
#55765=( BOUNDED_SURFACE ( )  B_SPLINE_SURFACE ( 1, 2, ( 
 ( #51082, #28195, #38914, #45549, #55537, #61434, #6013, #22988, #68078, #17447, #56969, #4932, #21912, #67714, #6373, #27467, #67362, #40004, #62518, #10827, #33362, #44468, #55899, #50368, #44827, #17086, #11197, #11916, #39647, #61792, #56269, #5659, #50724, #127, #56618, #34441, #28905, #51443, #845, #12635, #57335, #29273, #7099, #29628, #40725, #63603, #52165, #24440, #24802, #52887, #58050, #1568, #19614, #46624, #18526, #34803, #13720, #41091, #2644, #1935, #68801, #24078, #25163, #69167, #46989, #64327, #63241, #12993, #8185, #35529, #7458, #29985, #69525, #52527, #18883, #57694, #51803, #47704, #41446, #70243, #63964, #46261, #35170, #13348, #58776, #35885, #58410, #42171, #36261, #7823, #1206, #30358, #64697, #2285, #30713, #47345, #69879, #19244, #23711, #41799, #53246, #6739, #18157, #43639, #38083, #3390, #3009, #9651, #49548, #72070, #21450, #65797, #54358, #43276, #54718, #71343, #19981, #31819, #44006, #8921, #14451, #15178, #37717, #60237, #20718, #10014, #26276, #14081, #8551, #9286, #31451, #14815, #3752, #48080, #36621, #59142, #31078, #25911, #32185, #42901, #21088, #48813, #48451, #66163, #4487, #27016, #53618, #15539, #4121, #37358, #42534, #26650, #70608, #49186, #59880, #25539, #60605, #65060, #70975, #53993, #36985, #59507, #20350, #71716, #65425, #32550, #55087, #27742, #11104, #50281, #16275, #38831, #33275, #61346, #55450, #67988, #72805, #23265, #66528, #27377, #55814, #51354, #4843, #40, #49909, #22188, #39190, #33993, #39919, #5201, #33633, #15908, #44742, #22545, #56177, #38456, #10742, #66907, #45093, #67628, #16994, #39552, #62433, #5570, #28816, #60982, #61705, #67276, #16635, #28107, #72433, #757, #10381, #32913, #50636, #62077, #11470, #390, #56530, #5923, #45456, #56882, #6287, #21817, #17362, #28457, #50992, #44382, #22897, #11831, #34349, #18440, #40272, #52804, #17712, #7012, #12549, #23629, #12186, #52079, #7372, #2561, #53164, #18074, #29543, #63520, #1484, #68714, #40635, #35083, #63154, #34713, #47263, #23990, #45815, #68351, #6656, #57609, #30632, #57243, #52443, #29185, #46537, #41005, #13265, #19163, #69079, #12907, #62793, #35440, #1848, #1120, #57964, #41717, #29903, #24356, #46904, #69443, #18800, #41364, #63874, #51718, #13632, #35803, #58693, #58325, #46175, #7736, #30271, #69797, #2205, #24720, #64244, #36176, #8104, #42092, #70529, #55001, #59795, #71631, #53910, #71254, #70893, #64614, #3303, #59425, #36905, #25830, #54631, #49102, #14370, #14000, #20634, #60523, #9929, #32468, #3668, #65341, #54274, #65712, #9201, #30999, #48731, #43192, #15098, #37634, #26562, #38001, #36539, #37273, #21004, #25081, #8833, #60157, #9567, #59059, #8464, #47624, #70157, #19534, #2928, #31736, #48367, #32099, #26191, #53532, #25457, #48001, #19904, #31369, #4038, #20266, #43556, #66078, #15456, #42456, #64979, #42818, #14731, #49829, #10300, #33191, #72353, #67193, #67550, #22464, #27658, #44295, #62355, #16196, #61267, #4407, #56454, #10661, #45373, #44663, #38370, #21734, #67909, #66823, #16554, #33910, #16913, #5844, #55730, #45014, #311, #32831, #50555, #55369, #33547, #26936, #50197, #61991, #43923, #4762, #39468, #11391, #39106, #72722, #22821, #49461, #28376, #15826, #22105, #73083, #61622, #60895, #71995, #50913, #5124, #38747, #11025, #17279, #27295, #21369, #56097, #39841, #11751, #34268, #66449, #5488, #28027, #68998, #6206, #46460, #18723, #41287, #17997, #29106, #35005, #18359, #1766, #29827, #57163, #46099, #35727, #63444, #2129, #57888, #23549, #23185, #58249, #62717, #52362, #29466, #40196, #46828, #24640, #17636, #40930, #12111, #34634, #45739, #28734, #63074, #7297, #52002, #7654, #69365, #12830, #6576, #51275, #679, #51641, #1042, #68635, #12476, #40556, #35364, #63798, #24280, #6935, #57535, #41641, #1403, #23912, #56801, #30193, #13188, #47186, #52722, #69718, #19086, #64160, #13548, #68274, #65630, #26110, #15017, #19824, #54191, #32017, #42010, #9120, #64530, #65258, #36095, #8751, #20546, #2479, #13924, #3588, #48649, #25748, #59340, #54553, #8022, #37555, #47546, #31284, #31657, #48285, #70075, #58615, #60077, #64898, #30914, #53455, #9488, #19450, #30558, #53826, #43104, #71174, #3955, #26478, #49018, #2845, #70809, #53084, #20184, #71549, #20923, #70448, #8384, #14288, #42739, #43475, #65999, #36462, #25374, #25004, #14648, #58977, #37189, #47919, #42376, #36825, #3219, #59713, #61187, #71914, #5405, #56376, #49383, #39027, #33465, #10943, #56012, #16835, #28299, #54919, #27579, #39389, #50834, #27213, #27942, #50475, #21288, #26851, #234, #37922, #22742, #66367, #50111, #44210, #73001, #10218, #15743, #44580, #16468, #67112, #22023, #11313, #72640, #45292, #9850, #10582, #32751, #16112, #33109, #43841, #15380, #60440, #32379, #49748, #61541, #66742, #22385, #55647, #72276, #67472, #5768, #4326, #38282, #61908, #44934, #38664, #60810, #33834, #55289, #4683, #5043, #21653, #1676, #39760, #29022, #34551, #45659, #34188, #959, #29383, #24551, #2040, #40116, #51558, #12382, #23468, #17555, #62632, #57079, #12026, #56722, #69273, #46014, #67826, #17199, #28655, #6487, #52634, #6124, #1314, #51194, #68551, #40472, #35277, #41199, #17909, #34918, #62277, #62987, #23823, #23102, #57445, #63707, #6849, #51917, #46374, #68908, #18266, #40839, #63357, #11671, #35637, #12741, #7563, #57799, #597, #68192, #7208, #18635, #29737, #52274, #24185, #46739, #13099, #58159, #30099, #4860, #8659, #21470, #2756, #21104, #19730, #64070, #25276, #8296, #58886, #47823, #4505, #72087, #36370, #36000, #43657, #10398, #32930, #55468, #25654, #14194, #3125, #15557, #31190, #52996, #64804, #47097, #66179, #70353, #55105, #36729, #30826, #27034, #38475, #60999, #18991, #49565, #38100, #42280, #2392, #60622, #30467 ),
 ( #69629, #41553, #19357, #41914, #24911, #59251, #64439, #53732, #10032, #32567, #48190, #13831, #13452, #53359, #71734, #58519, #44024, #66546, #15925, #7929, #47454, #69987, #17729, #22205, #17012, #56898, #17378, #6304, #11123, #45473, #23282, #33292, #407, #55831, #56547, #27395, #57, #11847, #66925, #5218, #68006, #39936, #39570, #50653, #45831, #72451, #28832, #38848, #22563, #22916, #62094, #61363, #49926, #51371, #56195, #44759, #67294, #774, #10760, #21835, #45110, #34366, #62449, #68368, #40288, #62809, #16652, #11488, #44399, #34010, #12202, #34730, #61722, #72822, #5588, #5941, #57259, #16294, #27760, #39209, #50300, #28474, #33650, #51010, #28125, #67646, #8118, #12565, #2220, #52457, #63170, #69811, #18814, #35456, #41730, #63888, #40650, #35099, #68730, #51735, #12922, #7749, #1864, #30646, #19176, #13278, #57624, #29200, #1135, #52095, #1499, #7028, #57979, #24005, #69456, #64258, #24733, #29917, #46553, #64628, #18456, #63536, #6672, #58707, #7388, #47638, #46918, #29558, #69094, #70171, #41020, #41377, #36189, #13645, #53178, #24370, #47277, #2575, #35817, #52818, #58339, #30286, #23645, #25094, #19548, #46190, #42105, #14014, #36553, #18089, #65355, #21016, #31011, #4049, #25469, #14745, #43204, #9215, #48015, #8477, #54645, #70907, #59439, #8846, #49115, #70541, #59073, #31752, #26575, #32111, #71643, #38013, #43569, #3317, #26206, #53544, #48745, #66090, #15469, #42833, #25843, #37287, #71269, #9579, #37647, #31382, #20279, #60535, #20647, #9942, #15110, #48380, #19916, #2940, #59810, #42470, #65724, #54289, #64993, #14383, #3682, #36918, #53922, #60170, #70033, #53410, #64854, #18315, #64118, #2802, #14242, #63755, #19406, #13879, #12787, #63402, #36780, #1363, #59296, #29784, #40886, #25329, #35684, #8706, #51964, #35324, #41243, #23872, #57846, #58571, #7256, #13144, #24596, #41964, #47875, #18680, #69675, #46420, #58206, #7978, #52320, #46785, #70403, #7610, #30147, #52679, #19041, #2087, #47144, #1723, #68958, #19779, #41599, #24235, #13503, #69320, #36050, #30514, #42329, #53041, #2436, #24958, #30870, #47502, #64486, #36418, #58934, #8341, #4643, #60035, #4281, #3913, #48239, #9446, #65586, #43061, #31974, #60769, #55248, #20504, #20139, #26807, #66698, #16070, #38620, #9805, #71505, #60397, #71873, #15337, #37143, #48976, #61144, #26067, #31614, #32338, #54876, #49341, #37877, #27173, #43435, #31239, #25703, #26435, #48606, #54510, #20881, #65216, #53780, #3176, #70764, #14976, #21245, #65957, #38240, #43799, #37514, #10176, #21613, #44168, #42694, #32711, #66324, #15701, #59670, #49707, #14606, #72235, #9078, #54150, #3544, #71131, #44896, #50437, #61502, #50068, #16794, #45252, #40429, #17870, #55970, #67432, #28261, #39351, #33427, #5364, #72962, #27902, #45619, #44540, #21981, #68507, #33067, #10539, #10899, #22700, #61865, #68153, #67785, #67071, #16429, #72598, #55606, #11272, #11632, #56336, #34511, #554, #17159, #22344, #5002, #27536, #33793, #5726, #38987, #50792, #195, #39718, #23064, #28616, #62236, #34148, #56685, #6084, #51153, #17516, #62592, #40077, #51519, #11988, #57040, #6446, #918, #28981, #23427, #45973, #41167, #19694, #2360, #41520, #13066, #59584, #69954, #31529, #13800, #30065, #24520, #69598, #42610, #53325, #70319, #3465, #70680, #18960, #35605, #64039, #48524, #2724, #65135, #47424, #64771, #64407, #58124, #19324, #52963, #30435, #41878, #48155, #14526, #7898, #7532, #14161, #54069, #25985, #18603, #42247, #58854, #47786, #59217, #25240, #47064, #36340, #63676, #13418, #35967, #36695, #8625, #31154, #53695, #37060, #30795, #52603, #2009, #8264, #58489, #3089, #25618, #24877, #20055, #8997, #55889, #9724, #44083, #26725, #4920, #38158, #32257, #49985, #61423, #10817, #42975, #72510, #66610, #21162, #26351, #15985, #59955, #65505, #4196, #72149, #43715, #21898, #61058, #55165, #48890, #20426, #14893, #43353, #65875, #3830, #49260, #15256, #60681, #10457, #38535, #66237, #37793, #5277, #54790, #71793, #71051, #44455, #15616, #38904, #10095, #31895, #60314, #33351, #32625, #4562, #66985, #27090, #49622, #71420, #32986, #16349, #20797, #55526, #21527, #27455, #37433, #27823, #9362, #54431, #56257, #68424, #62866, #39994, #469, #68791, #22264, #51793, #61781, #22977, #45892, #62507, #11185, #72882, #6729, #6002, #45171, #67702, #23702, #33710, #50355, #45539, #57325, #40346, #12262, #18147, #46250, #17074, #11906, #44817, #34430, #34792, #29263, #11549, #22620, #28535, #56959, #17786, #23344, #50711, #39634, #1194, #6362, #40714, #51433, #62152, #16713, #63231, #5647, #12625, #68068, #28183, #35160, #57684, #115, #835, #7089, #67351, #39269, #34065, #56606, #51071, #28894, #17436, #42524, #41436, #70230, #64687, #63594, #41081, #14440, #52154, #36975, #7448, #41788, #58399, #14072, #13708, #12983, #35519, #58765, #29618, #2275, #36611, #69156, #58038, #47694, #42160, #19234, #52877, #48070, #1557, #31068, #29974, #24792, #25154, #64318, #52516, #24068, #59132, #7813, #24430, #46979, #2999, #1925, #46613, #47335, #8540, #19604, #53606, #70597, #25527, #69515, #36251, #18515, #8175, #19971, #65050, #63952, #18874, #30349, #30703, #59497, #2633, #13337, #35875, #69868, #53236, #27368, #10005, #48803, #48440, #10372, #14804, #4478, #54707, #65416, #72061, #49900, #42891, #32540, #27007, #49538, #21440, #32903, #21807, #70965, #21080, #55442, #44371, #20708, #43997, #66519, #37348, #20338, #66898, #31441, #16266, #59870, #43630, #37705, #15899, #66152, #9274, #31809, #54347, #53981, #15168, #55078, #4112, #4834, #38446, #15530, #3741, #3379, #25900, #26266, #71332, #43265, #60227, #65787, #71707, #60972, #72424, #32174, #9640, #38821, #26640, #49177, #8910, #38072, #60596, #29178, #28448, #22178, #56166, #51711 ) ),
 .UNSPECIFIED., .F., .F., .F. ) 
 B_SPLINE_SURFACE_WITH_KNOTS ( ( 2, 2 ),
 ( 3, 2, 2, 2, 2, 2, 2, 2, 2, 2, 2, 2, 2, 2, 2, 2, 2, 2, 2, 2, 2, 2, 2, 2, 2, 2, 2, 2, 2, 2, 2, 2, 2, 2, 2, 2, 2, 2, 2, 2, 2, 2, 2, 2, 2, 2, 2, 2, 2, 2, 2, 2, 2, 2, 2, 2, 2, 2, 2, 2, 2, 2, 2, 2, 2, 2, 2, 2, 2, 2, 2, 2, 2, 2, 2, 2, 2, 2, 2, 2, 2, 2, 2, 2, 2, 2, 2, 2, 2, 2, 2, 2, 2, 2, 2, 2, 2, 2, 2, 2, 2, 2, 2, 2, 2, 2, 2, 2, 2, 2, 2, 2, 2, 2, 2, 2, 2, 2, 2, 2, 2, 2, 2, 2, 2, 2, 2, 2, 2, 2, 2, 2, 2, 2, 2, 2, 2, 2, 2, 2, 2, 2, 2, 2, 2, 2, 2, 2, 2, 2, 2, 2, 2, 2, 2, 2, 2, 2, 2, 2, 2, 2, 2, 2, 2, 2, 2, 2, 2, 2, 2, 2, 2, 2, 2, 2, 2, 2, 2, 2, 2, 2, 2, 2, 2, 2, 2, 2, 2, 2, 2, 2, 2, 2, 2, 2, 2, 2, 2, 2, 2, 2, 2, 2, 2, 2, 2, 2, 2, 2, 2, 2, 2, 2, 2, 2, 2, 2, 2, 2, 2, 2, 2, 2, 2, 2, 2, 2, 2, 2, 2, 2, 2, 2, 2, 2, 2, 2, 2, 2, 2, 2, 2, 2, 2, 2, 2, 2, 2, 2, 2, 2, 2, 2, 2, 2, 2, 2, 2, 2, 2, 2, 2, 2, 2, 2, 2, 2, 2, 2, 2, 2, 2, 2, 2, 2, 2, 2, 2, 2, 2, 2, 2, 2, 2, 2, 2, 2, 2, 2, 2, 2, 2, 2, 2, 2, 2, 2, 2, 2, 2, 2, 2, 2, 2, 2, 2, 2, 2, 2, 2, 2, 2, 2, 2, 2, 2, 2, 2, 2, 2, 2, 2, 2, 2, 2, 2, 2, 2, 2, 2, 2, 2, 2, 2, 2, 2, 2, 2, 2, 2, 2, 2, 2, 2, 2, 2, 2, 2, 2, 2, 2, 2, 2, 2, 2, 2, 2, 2, 2, 3 ),
 ( 0.000000000000000000, 1.000000000000000000 ),
 ( 0.000000000000000000, 0.002777777777777777884, 0.005555555555555555768, 0.008333333333333333218, 0.01111111111111111154, 0.01388888888888888812, 0.01666666666666666644, 0.01944444444444444475, 0.02222222222222222307, 0.02500000000000000139, 0.02777777777777777624, 0.03055555555555555455, 0.03333333333333333287, 0.03611111111111110772, 0.03888888888888888951, 0.04166666666666666435, 0.04444444444444444614, 0.04722222222222222099, 0.05000000000000000278, 0.05277777777777777762, 0.05555555555555555247, 0.05833333333333333426, 0.06111111111111110911, 0.06388888888888888395, 0.06666666666666666574, 0.06944444444444444753, 0.07222222222222221544, 0.07499999999999999722, 0.07777777777777777901, 0.08055555555555556080, 0.08333333333333332871, 0.08611111111111111049, 0.08888888888888889228, 0.09166666666666666019, 0.09444444444444444198, 0.09722222222222222376, 0.1000000000000000056, 0.1027777777777777735, 0.1055555555555555552, 0.1083333333333333370, 0.1111111111111111049, 0.1138888888888888867, 0.1166666666666666685, 0.1194444444444444503, 0.1222222222222222182, 0.1250000000000000000, 0.1277777777777777679, 0.1305555555555555636, 0.1333333333333333315, 0.1361111111111110994, 0.1388888888888888951, 0.1416666666666666630, 0.1444444444444444309, 0.1472222222222222265, 0.1499999999999999944, 0.1527777777777777901, 0.1555555555555555580, 0.1583333333333333259, 0.1611111111111111216, 0.1638888888888888895, 0.1666666666666666574, 0.1694444444444444531, 0.1722222222222222210, 0.1749999999999999889, 0.1777777777777777846, 0.1805555555555555525, 0.1833333333333333204, 0.1861111111111111160, 0.1888888888888888840, 0.1916666666666666796, 0.1944444444444444475, 0.1972222222222222154, 0.2000000000000000111, 0.2027777777777777790, 0.2055555555555555469, 0.2083333333333333426, 0.2111111111111111105, 0.2138888888888888784, 0.2166666666666666741, 0.2194444444444444420, 0.2222222222222222099, 0.2250000000000000056, 0.2277777777777777735, 0.2305555555555555691, 0.2333333333333333370, 0.2361111111111111049, 0.2388888888888889006, 0.2416666666666666685, 0.2444444444444444364, 0.2472222222222222321, 0.2500000000000000000, 0.2527777777777777679, 0.2555555555555555358, 0.2583333333333333592, 0.2611111111111111271, 0.2638888888888888951, 0.2666666666666666630, 0.2694444444444444309, 0.2722222222222221988, 0.2750000000000000222, 0.2777777777777777901, 0.2805555555555555580, 0.2833333333333333259, 0.2861111111111110938, 0.2888888888888888618, 0.2916666666666666852, 0.2944444444444444531, 0.2972222222222222210, 0.2999999999999999889, 0.3027777777777777568, 0.3055555555555555802, 0.3083333333333333481, 0.3111111111111111160, 0.3138888888888888840, 0.3166666666666666519, 0.3194444444444444198, 0.3222222222222222432, 0.3250000000000000111, 0.3277777777777777790, 0.3305555555555555469, 0.3333333333333333148, 0.3361111111111111382, 0.3388888888888889062, 0.3416666666666666741, 0.3444444444444444420, 0.3472222222222222099, 0.3499999999999999778, 0.3527777777777778012, 0.3555555555555555691, 0.3583333333333333370, 0.3611111111111111049, 0.3638888888888888729, 0.3666666666666666408, 0.3694444444444444642, 0.3722222222222222321, 0.3750000000000000000, 0.3777777777777777679, 0.3805555555555555358, 0.3833333333333333592, 0.3861111111111111271, 0.3888888888888888951, 0.3916666666666666630, 0.3944444444444444309, 0.3972222222222221988, 0.4000000000000000222, 0.4027777777777777901, 0.4055555555555555580, 0.4083333333333333259, 0.4111111111111110938, 0.4138888888888888618, 0.4166666666666666852, 0.4194444444444444531, 0.4222222222222222210, 0.4249999999999999889, 0.4277777777777777568, 0.4305555555555555802, 0.4333333333333333481, 0.4361111111111111160, 0.4388888888888888840, 0.4416666666666666519, 0.4444444444444444198, 0.4472222222222222432, 0.4500000000000000111, 0.4527777777777777790, 0.4555555555555555469, 0.4583333333333333148, 0.4611111111111111382, 0.4638888888888889062, 0.4666666666666666741, 0.4694444444444444420, 0.4722222222222222099, 0.4749999999999999778, 0.4777777777777778012, 0.4805555555555555691, 0.4833333333333333370, 0.4861111111111111049, 0.4888888888888888729, 0.4916666666666666408, 0.4944444444444444642, 0.4972222222222222321, 0.5000000000000000000, 0.5027777777777777679, 0.5055555555555555358, 0.5083333333333333037, 0.5111111111111110716, 0.5138888888888888395, 0.5166666666666667185, 0.5194444444444444864, 0.5222222222222222543, 0.5250000000000000222, 0.5277777777777777901, 0.5305555555555555580, 0.5333333333333333259, 0.5361111111111110938, 0.5388888888888888618, 0.5416666666666666297, 0.5444444444444443976, 0.5472222222222222765, 0.5500000000000000444, 0.5527777777777778123, 0.5555555555555555802, 0.5583333333333333481, 0.5611111111111111160, 0.5638888888888888840, 0.5666666666666666519, 0.5694444444444444198, 0.5722222222222221877, 0.5749999999999999556, 0.5777777777777777235, 0.5805555555555556024, 0.5833333333333333703, 0.5861111111111111382, 0.5888888888888889062, 0.5916666666666666741, 0.5944444444444444420, 0.5972222222222222099, 0.5999999999999999778, 0.6027777777777777457, 0.6055555555555555136, 0.6083333333333332815, 0.6111111111111111605, 0.6138888888888889284, 0.6166666666666666963, 0.6194444444444444642, 0.6222222222222222321, 0.6250000000000000000, 0.6277777777777777679, 0.6305555555555555358, 0.6333333333333333037, 0.6361111111111110716, 0.6388888888888888395, 0.6416666666666667185, 0.6444444444444444864, 0.6472222222222222543, 0.6500000000000000222, 0.6527777777777777901, 0.6555555555555555580, 0.6583333333333333259, 0.6611111111111110938, 0.6638888888888888618, 0.6666666666666666297, 0.6694444444444443976, 0.6722222222222222765, 0.6750000000000000444, 0.6777777777777778123, 0.6805555555555555802, 0.6833333333333333481, 0.6861111111111111160, 0.6888888888888888840, 0.6916666666666666519, 0.6944444444444444198, 0.6972222222222221877, 0.6999999999999999556, 0.7027777777777777235, 0.7055555555555556024, 0.7083333333333333703, 0.7111111111111111382, 0.7138888888888889062, 0.7166666666666666741, 0.7194444444444444420, 0.7222222222222222099, 0.7249999999999999778, 0.7277777777777777457, 0.7305555555555555136, 0.7333333333333332815, 0.7361111111111111605, 0.7388888888888889284, 0.7416666666666666963, 0.7444444444444444642, 0.7472222222222222321, 0.7500000000000000000, 0.7527777777777777679, 0.7555555555555555358, 0.7583333333333333037, 0.7611111111111110716, 0.7638888888888888395, 0.7666666666666667185, 0.7694444444444444864, 0.7722222222222222543, 0.7750000000000000222, 0.7777777777777777901, 0.7805555555555555580, 0.7833333333333333259, 0.7861111111111110938, 0.7888888888888888618, 0.7916666666666666297, 0.7944444444444443976, 0.7972222222222222765, 0.8000000000000000444, 0.8027777777777778123, 0.8055555555555555802, 0.8083333333333333481, 0.8111111111111111160, 0.8138888888888888840, 0.8166666666666666519, 0.8194444444444444198, 0.8222222222222221877, 0.8249999999999999556, 0.8277777777777777235, 0.8305555555555556024, 0.8333333333333333703, 0.8361111111111111382, 0.8388888888888889062, 0.8416666666666666741, 0.8444444444444444420, 0.8472222222222222099, 0.8499999999999999778, 0.8527777777777777457, 0.8555555555555555136, 0.8583333333333332815, 0.8611111111111111605, 0.8638888888888889284, 0.8666666666666666963, 0.8694444444444444642, 0.8722222222222222321, 0.8750000000000000000, 0.8777777777777777679, 0.8805555555555555358, 0.8833333333333333037, 0.8861111111111110716, 0.8888888888888888395, 0.8916666666666667185, 0.8944444444444444864, 0.8972222222222222543, 0.9000000000000000222, 0.9027777777777777901, 0.9055555555555555580, 0.9083333333333333259, 0.9111111111111110938, 0.9138888888888888618, 0.9166666666666666297, 0.9194444444444443976, 0.9222222222222222765, 0.9250000000000000444, 0.9277777777777778123, 0.9305555555555555802, 0.9333333333333333481, 0.9361111111111111160, 0.9388888888888888840, 0.9416666666666666519, 0.9444444444444444198, 0.9472222222222221877, 0.9499999999999999556, 0.9527777777777777235, 0.9555555555555556024, 0.9583333333333333703, 0.9611111111111111382, 0.9638888888888889062, 0.9666666666666666741, 0.9694444444444444420, 0.9722222222222222099, 0.9749999999999999778, 0.9777777777777777457, 0.9805555555555555136, 0.9833333333333332815, 0.9861111111111111605, 0.9888888888888889284, 0.9916666666666666963, 0.9944444444444444642, 0.9972222222222222321, 1.000000000000000000 ),
 .UNSPECIFIED. ) 
 GEOMETRIC_REPRESENTATION_ITEM ( )  RATIONAL_B_SPLINE_SURFACE ( (
 ( 1.000000000000000000, 0.8660254037844387076, 1.000000000000000000, 0.8660254037844387076, 1.000000000000000000, 0.8660254037844387076, 1.000000000000000000, 0.8660254037844387076, 1.000000000000000000, 0.8660254037844387076, 1.000000000000000000, 0.8660254037844387076, 1.000000000000000000, 0.8660254037844387076, 1.000000000000000000, 0.8660254037844387076, 1.000000000000000000, 0.8660254037844387076, 1.000000000000000000, 0.8660254037844387076, 1.000000000000000000, 0.8660254037844387076, 1.000000000000000000, 0.8660254037844387076, 1.000000000000000000, 0.8660254037844387076, 1.000000000000000000, 0.8660254037844387076, 1.000000000000000000, 0.8660254037844387076, 1.000000000000000000, 0.8660254037844387076, 1.000000000000000000, 0.8660254037844387076, 1.000000000000000000, 0.8660254037844387076, 1.000000000000000000, 0.8660254037844387076, 1.000000000000000000, 0.8660254037844387076, 1.000000000000000000, 0.8660254037844387076, 1.000000000000000000, 0.8660254037844387076, 1.000000000000000000, 0.8660254037844387076, 1.000000000000000000, 0.8660254037844387076, 1.000000000000000000, 0.8660254037844387076, 1.000000000000000000, 0.8660254037844387076, 1.000000000000000000, 0.8660254037844387076, 1.000000000000000000, 0.8660254037844387076, 1.000000000000000000, 0.8660254037844387076, 1.000000000000000000, 0.8660254037844387076, 1.000000000000000000, 0.8660254037844387076, 1.000000000000000000, 0.8660254037844387076, 1.000000000000000000, 0.8660254037844387076, 1.000000000000000000, 0.8660254037844387076, 1.000000000000000000, 0.8660254037844387076, 1.000000000000000000, 0.8660254037844387076, 1.000000000000000000, 0.8660254037844387076, 1.000000000000000000, 0.8660254037844387076, 1.000000000000000000, 0.8660254037844387076, 1.000000000000000000, 0.8660254037844387076, 1.000000000000000000, 0.8660254037844387076, 1.000000000000000000, 0.8660254037844387076, 1.000000000000000000, 0.8660254037844387076, 1.000000000000000000, 0.8660254037844387076, 1.000000000000000000, 0.8660254037844387076, 1.000000000000000000, 0.8660254037844387076, 1.000000000000000000, 0.8660254037844387076, 1.000000000000000000, 0.8660254037844387076, 1.000000000000000000, 0.8660254037844387076, 1.000000000000000000, 0.8660254037844387076, 1.000000000000000000, 0.8660254037844387076, 1.000000000000000000, 0.8660254037844387076, 1.000000000000000000, 0.8660254037844387076, 1.000000000000000000, 0.8660254037844387076, 1.000000000000000000, 0.8660254037844387076, 1.000000000000000000, 0.8660254037844387076, 1.000000000000000000, 0.8660254037844387076, 1.000000000000000000, 0.8660254037844387076, 1.000000000000000000, 0.8660254037844387076, 1.000000000000000000, 0.8660254037844387076, 1.000000000000000000, 0.8660254037844387076, 1.000000000000000000, 0.8660254037844387076, 1.000000000000000000, 0.8660254037844387076, 1.000000000000000000, 0.8660254037844387076, 1.000000000000000000, 0.8660254037844387076, 1.000000000000000000, 0.8660254037844387076, 1.000000000000000000, 0.8660254037844387076, 1.000000000000000000, 0.8660254037844387076, 1.000000000000000000, 0.8660254037844387076, 1.000000000000000000, 0.8660254037844387076, 1.000000000000000000, 0.8660254037844387076, 1.000000000000000000, 0.8660254037844387076, 1.000000000000000000, 0.8660254037844387076, 1.000000000000000000, 0.8660254037844387076, 1.000000000000000000, 0.8660254037844387076, 1.000000000000000000, 0.8660254037844387076, 1.000000000000000000, 0.8660254037844387076, 1.000000000000000000, 0.8660254037844387076, 1.000000000000000000, 0.8660254037844387076, 1.000000000000000000, 0.8660254037844387076, 1.000000000000000000, 0.8660254037844387076, 1.000000000000000000, 0.8660254037844387076, 1.000000000000000000, 0.8660254037844387076, 1.000000000000000000, 0.8660254037844387076, 1.000000000000000000, 0.8660254037844387076, 1.000000000000000000, 0.8660254037844387076, 1.000000000000000000, 0.8660254037844387076, 1.000000000000000000, 0.8660254037844387076, 1.000000000000000000, 0.8660254037844387076, 1.000000000000000000, 0.8660254037844387076, 1.000000000000000000, 0.8660254037844387076, 1.000000000000000000, 0.8660254037844387076, 1.000000000000000000, 0.8660254037844387076, 1.000000000000000000, 0.8660254037844387076, 1.000000000000000000, 0.8660254037844387076, 1.000000000000000000, 0.8660254037844387076, 1.000000000000000000, 0.8660254037844387076, 1.000000000000000000, 0.8660254037844387076, 1.000000000000000000, 0.8660254037844387076, 1.000000000000000000, 0.8660254037844387076, 1.000000000000000000, 0.8660254037844387076, 1.000000000000000000, 0.8660254037844387076, 1.000000000000000000, 0.8660254037844387076, 1.000000000000000000, 0.8660254037844387076, 1.000000000000000000, 0.8660254037844387076, 1.000000000000000000, 0.8660254037844387076, 1.000000000000000000, 0.8660254037844387076, 1.000000000000000000, 0.8660254037844387076, 1.000000000000000000, 0.8660254037844387076, 1.000000000000000000, 0.8660254037844387076, 1.000000000000000000, 0.8660254037844387076, 1.000000000000000000, 0.8660254037844387076, 1.000000000000000000, 0.8660254037844387076, 1.000000000000000000, 0.8660254037844387076, 1.000000000000000000, 0.8660254037844387076, 1.000000000000000000, 0.8660254037844387076, 1.000000000000000000, 0.8660254037844387076, 1.000000000000000000, 0.8660254037844387076, 1.000000000000000000, 0.8660254037844387076, 1.000000000000000000, 0.8660254037844387076, 1.000000000000000000, 0.8660254037844387076, 1.000000000000000000, 0.8660254037844387076, 1.000000000000000000, 0.8660254037844387076, 1.000000000000000000, 0.8660254037844387076, 1.000000000000000000, 0.8660254037844387076, 1.000000000000000000, 0.8660254037844387076, 1.000000000000000000, 0.8660254037844387076, 1.000000000000000000, 0.8660254037844387076, 1.000000000000000000, 0.8660254037844387076, 1.000000000000000000, 0.8660254037844387076, 1.000000000000000000, 0.8660254037844387076, 1.000000000000000000, 0.8660254037844387076, 1.000000000000000000, 0.8660254037844387076, 1.000000000000000000, 0.8660254037844387076, 1.000000000000000000, 0.8660254037844387076, 1.000000000000000000, 0.8660254037844387076, 1.000000000000000000, 0.8660254037844387076, 1.000000000000000000, 0.8660254037844387076, 1.000000000000000000, 0.8660254037844387076, 1.000000000000000000, 0.8660254037844387076, 1.000000000000000000, 0.8660254037844387076, 1.000000000000000000, 0.8660254037844387076, 1.000000000000000000, 0.8660254037844387076, 1.000000000000000000, 0.8660254037844387076, 1.000000000000000000, 0.8660254037844387076, 1.000000000000000000, 0.8660254037844387076, 1.000000000000000000, 0.8660254037844387076, 1.000000000000000000, 0.8660254037844387076, 1.000000000000000000, 0.8660254037844387076, 1.000000000000000000, 0.8660254037844387076, 1.000000000000000000, 0.8660254037844387076, 1.000000000000000000, 0.8660254037844387076, 1.000000000000000000, 0.8660254037844387076, 1.000000000000000000, 0.8660254037844387076, 1.000000000000000000, 0.8660254037844387076, 1.000000000000000000, 0.8660254037844387076, 1.000000000000000000, 0.8660254037844387076, 1.000000000000000000, 0.8660254037844387076, 1.000000000000000000, 0.8660254037844387076, 1.000000000000000000, 0.8660254037844387076, 1.000000000000000000, 0.8660254037844387076, 1.000000000000000000, 0.8660254037844387076, 1.000000000000000000, 0.8660254037844387076, 1.000000000000000000, 0.8660254037844387076, 1.000000000000000000, 0.8660254037844387076, 1.000000000000000000, 0.8660254037844387076, 1.000000000000000000, 0.8660254037844387076, 1.000000000000000000, 0.8660254037844387076, 1.000000000000000000, 0.8660254037844387076, 1.000000000000000000, 0.8660254037844387076, 1.000000000000000000, 0.8660254037844387076, 1.000000000000000000, 0.8660254037844387076, 1.000000000000000000, 0.8660254037844387076, 1.000000000000000000, 0.8660254037844387076, 1.000000000000000000, 0.8660254037844387076, 1.000000000000000000, 0.8660254037844387076, 1.000000000000000000, 0.8660254037844387076, 1.000000000000000000, 0.8660254037844387076, 1.000000000000000000, 0.8660254037844387076, 1.000000000000000000, 0.8660254037844387076, 1.000000000000000000, 0.8660254037844387076, 1.000000000000000000, 0.8660254037844387076, 1.000000000000000000, 0.8660254037844387076, 1.000000000000000000, 0.8660254037844387076, 1.000000000000000000, 0.8660254037844387076, 1.000000000000000000, 0.8660254037844387076, 1.000000000000000000, 0.8660254037844387076, 1.000000000000000000, 0.8660254037844387076, 1.000000000000000000, 0.8660254037844387076, 1.000000000000000000, 0.8660254037844387076, 1.000000000000000000, 0.8660254037844387076, 1.000000000000000000, 0.8660254037844387076, 1.000000000000000000, 0.8660254037844387076, 1.000000000000000000, 0.8660254037844387076, 1.000000000000000000, 0.8660254037844387076, 1.000000000000000000, 0.8660254037844387076, 1.000000000000000000, 0.8660254037844387076, 1.000000000000000000, 0.8660254037844387076, 1.000000000000000000, 0.8660254037844387076, 1.000000000000000000, 0.8660254037844387076, 1.000000000000000000, 0.8660254037844387076, 1.000000000000000000, 0.8660254037844387076, 1.000000000000000000, 0.8660254037844387076, 1.000000000000000000, 0.8660254037844387076, 1.000000000000000000, 0.8660254037844387076, 1.000000000000000000, 0.8660254037844387076, 1.000000000000000000, 0.8660254037844387076, 1.000000000000000000, 0.8660254037844387076, 1.000000000000000000, 0.8660254037844387076, 1.000000000000000000, 0.8660254037844387076, 1.000000000000000000, 0.8660254037844387076, 1.000000000000000000, 0.8660254037844387076, 1.000000000000000000, 0.8660254037844387076, 1.000000000000000000, 0.8660254037844387076, 1.000000000000000000, 0.8660254037844387076, 1.000000000000000000, 0.8660254037844387076, 1.000000000000000000, 0.8660254037844387076, 1.000000000000000000, 0.8660254037844387076, 1.000000000000000000, 0.8660254037844387076, 1.000000000000000000, 0.8660254037844387076, 1.000000000000000000, 0.8660254037844387076, 1.000000000000000000, 0.8660254037844387076, 1.000000000000000000, 0.8660254037844387076, 1.000000000000000000, 0.8660254037844387076, 1.000000000000000000, 0.8660254037844387076, 1.000000000000000000, 0.8660254037844387076, 1.000000000000000000, 0.8660254037844387076, 1.000000000000000000, 0.8660254037844387076, 1.000000000000000000, 0.8660254037844387076, 1.000000000000000000, 0.8660254037844387076, 1.000000000000000000, 0.8660254037844387076, 1.000000000000000000, 0.8660254037844387076, 1.000000000000000000, 0.8660254037844387076, 1.000000000000000000, 0.8660254037844387076, 1.000000000000000000, 0.8660254037844387076, 1.000000000000000000, 0.8660254037844387076, 1.000000000000000000, 0.8660254037844387076, 1.000000000000000000, 0.8660254037844387076, 1.000000000000000000, 0.8660254037844387076, 1.000000000000000000, 0.8660254037844387076, 1.000000000000000000, 0.8660254037844387076, 1.000000000000000000, 0.8660254037844387076, 1.000000000000000000, 0.8660254037844387076, 1.000000000000000000, 0.8660254037844387076, 1.000000000000000000, 0.8660254037844387076, 1.000000000000000000, 0.8660254037844387076, 1.000000000000000000, 0.8660254037844387076, 1.000000000000000000, 0.8660254037844387076, 1.000000000000000000, 0.8660254037844387076, 1.000000000000000000, 0.8660254037844387076, 1.000000000000000000, 0.8660254037844387076, 1.000000000000000000, 0.8660254037844387076, 1.000000000000000000, 0.8660254037844387076, 1.000000000000000000, 0.8660254037844387076, 1.000000000000000000, 0.8660254037844387076, 1.000000000000000000, 0.8660254037844387076, 1.000000000000000000, 0.8660254037844387076, 1.000000000000000000, 0.8660254037844387076, 1.000000000000000000, 0.8660254037844387076, 1.000000000000000000, 0.8660254037844387076, 1.000000000000000000, 0.8660254037844387076, 1.000000000000000000, 0.8660254037844387076, 1.000000000000000000, 0.8660254037844387076, 1.000000000000000000, 0.8660254037844387076, 1.000000000000000000, 0.8660254037844387076, 1.000000000000000000, 0.8660254037844387076, 1.000000000000000000, 0.8660254037844387076, 1.000000000000000000, 0.8660254037844387076, 1.000000000000000000, 0.8660254037844387076, 1.000000000000000000, 0.8660254037844387076, 1.000000000000000000, 0.8660254037844387076, 1.000000000000000000, 0.8660254037844387076, 1.000000000000000000, 0.8660254037844387076, 1.000000000000000000, 0.8660254037844387076, 1.000000000000000000, 0.8660254037844387076, 1.000000000000000000, 0.8660254037844387076, 1.000000000000000000, 0.8660254037844387076, 1.000000000000000000, 0.8660254037844387076, 1.000000000000000000, 0.8660254037844387076, 1.000000000000000000, 0.8660254037844387076, 1.000000000000000000, 0.8660254037844387076, 1.000000000000000000, 0.8660254037844387076, 1.000000000000000000, 0.8660254037844387076, 1.000000000000000000, 0.8660254037844387076, 1.000000000000000000, 0.8660254037844387076, 1.000000000000000000, 0.8660254037844387076, 1.000000000000000000, 0.8660254037844387076, 1.000000000000000000, 0.8660254037844387076, 1.000000000000000000, 0.8660254037844387076, 1.000000000000000000, 0.8660254037844387076, 1.000000000000000000, 0.8660254037844387076, 1.000000000000000000, 0.8660254037844387076, 1.000000000000000000, 0.8660254037844387076, 1.000000000000000000, 0.8660254037844387076, 1.000000000000000000, 0.8660254037844387076, 1.000000000000000000, 0.8660254037844387076, 1.000000000000000000, 0.8660254037844387076, 1.000000000000000000, 0.8660254037844387076, 1.000000000000000000, 0.8660254037844387076, 1.000000000000000000, 0.8660254037844387076, 1.000000000000000000, 0.8660254037844387076, 1.000000000000000000, 0.8660254037844387076, 1.000000000000000000, 0.8660254037844387076, 1.000000000000000000, 0.8660254037844387076, 1.000000000000000000, 0.8660254037844387076, 1.000000000000000000, 0.8660254037844387076, 1.000000000000000000, 0.8660254037844387076, 1.000000000000000000, 0.8660254037844387076, 1.000000000000000000, 0.8660254037844387076, 1.000000000000000000, 0.8660254037844387076, 1.000000000000000000, 0.8660254037844387076, 1.000000000000000000, 0.8660254037844387076, 1.000000000000000000, 0.8660254037844387076, 1.000000000000000000, 0.8660254037844387076, 1.000000000000000000, 0.8660254037844387076, 1.000000000000000000, 0.8660254037844387076, 1.000000000000000000, 0.8660254037844387076, 1.000000000000000000, 0.8660254037844387076, 1.000000000000000000, 0.8660254037844387076, 1.000000000000000000, 0.8660254037844387076, 1.000000000000000000, 0.8660254037844387076, 1.000000000000000000, 0.8660254037844387076, 1.000000000000000000, 0.8660254037844387076, 1.000000000000000000, 0.8660254037844387076, 1.000000000000000000, 0.8660254037844387076, 1.000000000000000000, 0.8660254037844387076, 1.000000000000000000, 0.8660254037844387076, 1.000000000000000000, 0.8660254037844387076, 1.000000000000000000, 0.8660254037844387076, 1.000000000000000000, 0.8660254037844387076, 1.000000000000000000, 0.8660254037844387076, 1.000000000000000000, 0.8660254037844387076, 1.000000000000000000, 0.8660254037844387076, 1.000000000000000000, 0.8660254037844387076, 1.000000000000000000, 0.8660254037844387076, 1.000000000000000000, 0.8660254037844387076, 1.000000000000000000, 0.8660254037844387076, 1.000000000000000000, 0.8660254037844387076, 1.000000000000000000, 0.8660254037844387076, 1.000000000000000000, 0.8660254037844387076, 1.000000000000000000, 0.8660254037844387076, 1.000000000000000000, 0.8660254037844387076, 1.000000000000000000, 0.8660254037844387076, 1.000000000000000000, 0.8660254037844387076, 1.000000000000000000, 0.8660254037844387076, 1.000000000000000000, 0.8660254037844387076, 1.000000000000000000, 0.8660254037844387076, 1.000000000000000000, 0.8660254037844387076, 1.000000000000000000, 0.8660254037844387076, 1.000000000000000000, 0.8660254037844387076, 1.000000000000000000, 0.8660254037844387076, 1.000000000000000000, 0.8660254037844387076, 1.000000000000000000, 0.8660254037844387076, 1.000000000000000000, 0.8660254037844387076, 1.000000000000000000, 0.8660254037844387076, 1.000000000000000000, 0.8660254037844387076, 1.000000000000000000, 0.8660254037844387076, 1.000000000000000000, 0.8660254037844387076, 1.000000000000000000, 0.8660254037844387076, 1.000000000000000000, 0.8660254037844387076, 1.000000000000000000),
 ( 1.000000000000000000, 0.8660254037844387076, 1.000000000000000000, 0.8660254037844387076, 1.000000000000000000, 0.8660254037844387076, 1.000000000000000000, 0.8660254037844387076, 1.000000000000000000, 0.8660254037844387076, 1.000000000000000000, 0.8660254037844387076, 1.000000000000000000, 0.8660254037844387076, 1.000000000000000000, 0.8660254037844387076, 1.000000000000000000, 0.8660254037844387076, 1.000000000000000000, 0.8660254037844387076, 1.000000000000000000, 0.8660254037844387076, 1.000000000000000000, 0.8660254037844387076, 1.000000000000000000, 0.8660254037844387076, 1.000000000000000000, 0.8660254037844387076, 1.000000000000000000, 0.8660254037844387076, 1.000000000000000000, 0.8660254037844387076, 1.000000000000000000, 0.8660254037844387076, 1.000000000000000000, 0.8660254037844387076, 1.000000000000000000, 0.8660254037844387076, 1.000000000000000000, 0.8660254037844387076, 1.000000000000000000, 0.8660254037844387076, 1.000000000000000000, 0.8660254037844387076, 1.000000000000000000, 0.8660254037844387076, 1.000000000000000000, 0.8660254037844387076, 1.000000000000000000, 0.8660254037844387076, 1.000000000000000000, 0.8660254037844387076, 1.000000000000000000, 0.8660254037844387076, 1.000000000000000000, 0.8660254037844387076, 1.000000000000000000, 0.8660254037844387076, 1.000000000000000000, 0.8660254037844387076, 1.000000000000000000, 0.8660254037844387076, 1.000000000000000000, 0.8660254037844387076, 1.000000000000000000, 0.8660254037844387076, 1.000000000000000000, 0.8660254037844387076, 1.000000000000000000, 0.8660254037844387076, 1.000000000000000000, 0.8660254037844387076, 1.000000000000000000, 0.8660254037844387076, 1.000000000000000000, 0.8660254037844387076, 1.000000000000000000, 0.8660254037844387076, 1.000000000000000000, 0.8660254037844387076, 1.000000000000000000, 0.8660254037844387076, 1.000000000000000000, 0.8660254037844387076, 1.000000000000000000, 0.8660254037844387076, 1.000000000000000000, 0.8660254037844387076, 1.000000000000000000, 0.8660254037844387076, 1.000000000000000000, 0.8660254037844387076, 1.000000000000000000, 0.8660254037844387076, 1.000000000000000000, 0.8660254037844387076, 1.000000000000000000, 0.8660254037844387076, 1.000000000000000000, 0.8660254037844387076, 1.000000000000000000, 0.8660254037844387076, 1.000000000000000000, 0.8660254037844387076, 1.000000000000000000, 0.8660254037844387076, 1.000000000000000000, 0.8660254037844387076, 1.000000000000000000, 0.8660254037844387076, 1.000000000000000000, 0.8660254037844387076, 1.000000000000000000, 0.8660254037844387076, 1.000000000000000000, 0.8660254037844387076, 1.000000000000000000, 0.8660254037844387076, 1.000000000000000000, 0.8660254037844387076, 1.000000000000000000, 0.8660254037844387076, 1.000000000000000000, 0.8660254037844387076, 1.000000000000000000, 0.8660254037844387076, 1.000000000000000000, 0.8660254037844387076, 1.000000000000000000, 0.8660254037844387076, 1.000000000000000000, 0.8660254037844387076, 1.000000000000000000, 0.8660254037844387076, 1.000000000000000000, 0.8660254037844387076, 1.000000000000000000, 0.8660254037844387076, 1.000000000000000000, 0.8660254037844387076, 1.000000000000000000, 0.8660254037844387076, 1.000000000000000000, 0.8660254037844387076, 1.000000000000000000, 0.8660254037844387076, 1.000000000000000000, 0.8660254037844387076, 1.000000000000000000, 0.8660254037844387076, 1.000000000000000000, 0.8660254037844387076, 1.000000000000000000, 0.8660254037844387076, 1.000000000000000000, 0.8660254037844387076, 1.000000000000000000, 0.8660254037844387076, 1.000000000000000000, 0.8660254037844387076, 1.000000000000000000, 0.8660254037844387076, 1.000000000000000000, 0.8660254037844387076, 1.000000000000000000, 0.8660254037844387076, 1.000000000000000000, 0.8660254037844387076, 1.000000000000000000, 0.8660254037844387076, 1.000000000000000000, 0.8660254037844387076, 1.000000000000000000, 0.8660254037844387076, 1.000000000000000000, 0.8660254037844387076, 1.000000000000000000, 0.8660254037844387076, 1.000000000000000000, 0.8660254037844387076, 1.000000000000000000, 0.8660254037844387076, 1.000000000000000000, 0.8660254037844387076, 1.000000000000000000, 0.8660254037844387076, 1.000000000000000000, 0.8660254037844387076, 1.000000000000000000, 0.8660254037844387076, 1.000000000000000000, 0.8660254037844387076, 1.000000000000000000, 0.8660254037844387076, 1.000000000000000000, 0.8660254037844387076, 1.000000000000000000, 0.8660254037844387076, 1.000000000000000000, 0.8660254037844387076, 1.000000000000000000, 0.8660254037844387076, 1.000000000000000000, 0.8660254037844387076, 1.000000000000000000, 0.8660254037844387076, 1.000000000000000000, 0.8660254037844387076, 1.000000000000000000, 0.8660254037844387076, 1.000000000000000000, 0.8660254037844387076, 1.000000000000000000, 0.8660254037844387076, 1.000000000000000000, 0.8660254037844387076, 1.000000000000000000, 0.8660254037844387076, 1.000000000000000000, 0.8660254037844387076, 1.000000000000000000, 0.8660254037844387076, 1.000000000000000000, 0.8660254037844387076, 1.000000000000000000, 0.8660254037844387076, 1.000000000000000000, 0.8660254037844387076, 1.000000000000000000, 0.8660254037844387076, 1.000000000000000000, 0.8660254037844387076, 1.000000000000000000, 0.8660254037844387076, 1.000000000000000000, 0.8660254037844387076, 1.000000000000000000, 0.8660254037844387076, 1.000000000000000000, 0.8660254037844387076, 1.000000000000000000, 0.8660254037844387076, 1.000000000000000000, 0.8660254037844387076, 1.000000000000000000, 0.8660254037844387076, 1.000000000000000000, 0.8660254037844387076, 1.000000000000000000, 0.8660254037844387076, 1.000000000000000000, 0.8660254037844387076, 1.000000000000000000, 0.8660254037844387076, 1.000000000000000000, 0.8660254037844387076, 1.000000000000000000, 0.8660254037844387076, 1.000000000000000000, 0.8660254037844387076, 1.000000000000000000, 0.8660254037844387076, 1.000000000000000000, 0.8660254037844387076, 1.000000000000000000, 0.8660254037844387076, 1.000000000000000000, 0.8660254037844387076, 1.000000000000000000, 0.8660254037844387076, 1.000000000000000000, 0.8660254037844387076, 1.000000000000000000, 0.8660254037844387076, 1.000000000000000000, 0.8660254037844387076, 1.000000000000000000, 0.8660254037844387076, 1.000000000000000000, 0.8660254037844387076, 1.000000000000000000, 0.8660254037844387076, 1.000000000000000000, 0.8660254037844387076, 1.000000000000000000, 0.8660254037844387076, 1.000000000000000000, 0.8660254037844387076, 1.000000000000000000, 0.8660254037844387076, 1.000000000000000000, 0.8660254037844387076, 1.000000000000000000, 0.8660254037844387076, 1.000000000000000000, 0.8660254037844387076, 1.000000000000000000, 0.8660254037844387076, 1.000000000000000000, 0.8660254037844387076, 1.000000000000000000, 0.8660254037844387076, 1.000000000000000000, 0.8660254037844387076, 1.000000000000000000, 0.8660254037844387076, 1.000000000000000000, 0.8660254037844387076, 1.000000000000000000, 0.8660254037844387076, 1.000000000000000000, 0.8660254037844387076, 1.000000000000000000, 0.8660254037844387076, 1.000000000000000000, 0.8660254037844387076, 1.000000000000000000, 0.8660254037844387076, 1.000000000000000000, 0.8660254037844387076, 1.000000000000000000, 0.8660254037844387076, 1.000000000000000000, 0.8660254037844387076, 1.000000000000000000, 0.8660254037844387076, 1.000000000000000000, 0.8660254037844387076, 1.000000000000000000, 0.8660254037844387076, 1.000000000000000000, 0.8660254037844387076, 1.000000000000000000, 0.8660254037844387076, 1.000000000000000000, 0.8660254037844387076, 1.000000000000000000, 0.8660254037844387076, 1.000000000000000000, 0.8660254037844387076, 1.000000000000000000, 0.8660254037844387076, 1.000000000000000000, 0.8660254037844387076, 1.000000000000000000, 0.8660254037844387076, 1.000000000000000000, 0.8660254037844387076, 1.000000000000000000, 0.8660254037844387076, 1.000000000000000000, 0.8660254037844387076, 1.000000000000000000, 0.8660254037844387076, 1.000000000000000000, 0.8660254037844387076, 1.000000000000000000, 0.8660254037844387076, 1.000000000000000000, 0.8660254037844387076, 1.000000000000000000, 0.8660254037844387076, 1.000000000000000000, 0.8660254037844387076, 1.000000000000000000, 0.8660254037844387076, 1.000000000000000000, 0.8660254037844387076, 1.000000000000000000, 0.8660254037844387076, 1.000000000000000000, 0.8660254037844387076, 1.000000000000000000, 0.8660254037844387076, 1.000000000000000000, 0.8660254037844387076, 1.000000000000000000, 0.8660254037844387076, 1.000000000000000000, 0.8660254037844387076, 1.000000000000000000, 0.8660254037844387076, 1.000000000000000000, 0.8660254037844387076, 1.000000000000000000, 0.8660254037844387076, 1.000000000000000000, 0.8660254037844387076, 1.000000000000000000, 0.8660254037844387076, 1.000000000000000000, 0.8660254037844387076, 1.000000000000000000, 0.8660254037844387076, 1.000000000000000000, 0.8660254037844387076, 1.000000000000000000, 0.8660254037844387076, 1.000000000000000000, 0.8660254037844387076, 1.000000000000000000, 0.8660254037844387076, 1.000000000000000000, 0.8660254037844387076, 1.000000000000000000, 0.8660254037844387076, 1.000000000000000000, 0.8660254037844387076, 1.000000000000000000, 0.8660254037844387076, 1.000000000000000000, 0.8660254037844387076, 1.000000000000000000, 0.8660254037844387076, 1.000000000000000000, 0.8660254037844387076, 1.000000000000000000, 0.8660254037844387076, 1.000000000000000000, 0.8660254037844387076, 1.000000000000000000, 0.8660254037844387076, 1.000000000000000000, 0.8660254037844387076, 1.000000000000000000, 0.8660254037844387076, 1.000000000000000000, 0.8660254037844387076, 1.000000000000000000, 0.8660254037844387076, 1.000000000000000000, 0.8660254037844387076, 1.000000000000000000, 0.8660254037844387076, 1.000000000000000000, 0.8660254037844387076, 1.000000000000000000, 0.8660254037844387076, 1.000000000000000000, 0.8660254037844387076, 1.000000000000000000, 0.8660254037844387076, 1.000000000000000000, 0.8660254037844387076, 1.000000000000000000, 0.8660254037844387076, 1.000000000000000000, 0.8660254037844387076, 1.000000000000000000, 0.8660254037844387076, 1.000000000000000000, 0.8660254037844387076, 1.000000000000000000, 0.8660254037844387076, 1.000000000000000000, 0.8660254037844387076, 1.000000000000000000, 0.8660254037844387076, 1.000000000000000000, 0.8660254037844387076, 1.000000000000000000, 0.8660254037844387076, 1.000000000000000000, 0.8660254037844387076, 1.000000000000000000, 0.8660254037844387076, 1.000000000000000000, 0.8660254037844387076, 1.000000000000000000, 0.8660254037844387076, 1.000000000000000000, 0.8660254037844387076, 1.000000000000000000, 0.8660254037844387076, 1.000000000000000000, 0.8660254037844387076, 1.000000000000000000, 0.8660254037844387076, 1.000000000000000000, 0.8660254037844387076, 1.000000000000000000, 0.8660254037844387076, 1.000000000000000000, 0.8660254037844387076, 1.000000000000000000, 0.8660254037844387076, 1.000000000000000000, 0.8660254037844387076, 1.000000000000000000, 0.8660254037844387076, 1.000000000000000000, 0.8660254037844387076, 1.000000000000000000, 0.8660254037844387076, 1.000000000000000000, 0.8660254037844387076, 1.000000000000000000, 0.8660254037844387076, 1.000000000000000000, 0.8660254037844387076, 1.000000000000000000, 0.8660254037844387076, 1.000000000000000000, 0.8660254037844387076, 1.000000000000000000, 0.8660254037844387076, 1.000000000000000000, 0.8660254037844387076, 1.000000000000000000, 0.8660254037844387076, 1.000000000000000000, 0.8660254037844387076, 1.000000000000000000, 0.8660254037844387076, 1.000000000000000000, 0.8660254037844387076, 1.000000000000000000, 0.8660254037844387076, 1.000000000000000000, 0.8660254037844387076, 1.000000000000000000, 0.8660254037844387076, 1.000000000000000000, 0.8660254037844387076, 1.000000000000000000, 0.8660254037844387076, 1.000000000000000000, 0.8660254037844387076, 1.000000000000000000, 0.8660254037844387076, 1.000000000000000000, 0.8660254037844387076, 1.000000000000000000, 0.8660254037844387076, 1.000000000000000000, 0.8660254037844387076, 1.000000000000000000, 0.8660254037844387076, 1.000000000000000000, 0.8660254037844387076, 1.000000000000000000, 0.8660254037844387076, 1.000000000000000000, 0.8660254037844387076, 1.000000000000000000, 0.8660254037844387076, 1.000000000000000000, 0.8660254037844387076, 1.000000000000000000, 0.8660254037844387076, 1.000000000000000000, 0.8660254037844387076, 1.000000000000000000, 0.8660254037844387076, 1.000000000000000000, 0.8660254037844387076, 1.000000000000000000, 0.8660254037844387076, 1.000000000000000000, 0.8660254037844387076, 1.000000000000000000, 0.8660254037844387076, 1.000000000000000000, 0.8660254037844387076, 1.000000000000000000, 0.8660254037844387076, 1.000000000000000000, 0.8660254037844387076, 1.000000000000000000, 0.8660254037844387076, 1.000000000000000000, 0.8660254037844387076, 1.000000000000000000, 0.8660254037844387076, 1.000000000000000000, 0.8660254037844387076, 1.000000000000000000, 0.8660254037844387076, 1.000000000000000000, 0.8660254037844387076, 1.000000000000000000, 0.8660254037844387076, 1.000000000000000000, 0.8660254037844387076, 1.000000000000000000, 0.8660254037844387076, 1.000000000000000000, 0.8660254037844387076, 1.000000000000000000, 0.8660254037844387076, 1.000000000000000000, 0.8660254037844387076, 1.000000000000000000, 0.8660254037844387076, 1.000000000000000000, 0.8660254037844387076, 1.000000000000000000, 0.8660254037844387076, 1.000000000000000000, 0.8660254037844387076, 1.000000000000000000, 0.8660254037844387076, 1.000000000000000000, 0.8660254037844387076, 1.000000000000000000, 0.8660254037844387076, 1.000000000000000000, 0.8660254037844387076, 1.000000000000000000, 0.8660254037844387076, 1.000000000000000000, 0.8660254037844387076, 1.000000000000000000, 0.8660254037844387076, 1.000000000000000000, 0.8660254037844387076, 1.000000000000000000, 0.8660254037844387076, 1.000000000000000000, 0.8660254037844387076, 1.000000000000000000, 0.8660254037844387076, 1.000000000000000000, 0.8660254037844387076, 1.000000000000000000, 0.8660254037844387076, 1.000000000000000000, 0.8660254037844387076, 1.000000000000000000, 0.8660254037844387076, 1.000000000000000000, 0.8660254037844387076, 1.000000000000000000, 0.8660254037844387076, 1.000000000000000000, 0.8660254037844387076, 1.000000000000000000, 0.8660254037844387076, 1.000000000000000000, 0.8660254037844387076, 1.000000000000000000, 0.8660254037844387076, 1.000000000000000000, 0.8660254037844387076, 1.000000000000000000, 0.8660254037844387076, 1.000000000000000000, 0.8660254037844387076, 1.000000000000000000, 0.8660254037844387076, 1.000000000000000000, 0.8660254037844387076, 1.000000000000000000, 0.8660254037844387076, 1.000000000000000000, 0.8660254037844387076, 1.000000000000000000, 0.8660254037844387076, 1.000000000000000000, 0.8660254037844387076, 1.000000000000000000, 0.8660254037844387076, 1.000000000000000000, 0.8660254037844387076, 1.000000000000000000, 0.8660254037844387076, 1.000000000000000000, 0.8660254037844387076, 1.000000000000000000, 0.8660254037844387076, 1.000000000000000000, 0.8660254037844387076, 1.000000000000000000, 0.8660254037844387076, 1.000000000000000000, 0.8660254037844387076, 1.000000000000000000, 0.8660254037844387076, 1.000000000000000000, 0.8660254037844387076, 1.000000000000000000, 0.8660254037844387076, 1.000000000000000000, 0.8660254037844387076, 1.000000000000000000, 0.8660254037844387076, 1.000000000000000000, 0.8660254037844387076, 1.000000000000000000, 0.8660254037844387076, 1.000000000000000000, 0.8660254037844387076, 1.000000000000000000, 0.8660254037844387076, 1.000000000000000000, 0.8660254037844387076, 1.000000000000000000, 0.8660254037844387076, 1.000000000000000000, 0.8660254037844387076, 1.000000000000000000, 0.8660254037844387076, 1.000000000000000000, 0.8660254037844387076, 1.000000000000000000, 0.8660254037844387076, 1.000000000000000000, 0.8660254037844387076, 1.000000000000000000, 0.8660254037844387076, 1.000000000000000000, 0.8660254037844387076, 1.000000000000000000, 0.8660254037844387076, 1.000000000000000000, 0.8660254037844387076, 1.000000000000000000, 0.8660254037844387076, 1.000000000000000000, 0.8660254037844387076, 1.000000000000000000) ) ) 
 REPRESENTATION_ITEM ( '' )  SURFACE ( )  );
#55766=CARTESIAN_POINT ( 'NONE',  ( 8.775000000000002132, 4.330127018922191873, 2.499999999999999556 ) ) ;
#55767=CARTESIAN_POINT ( 'NONE',  ( 7.771875000614516971, 3.027376345333611329, 5.243569643749999010 ) ) ;
#55768=CARTESIAN_POINT ( 'NONE',  ( 6.262500001229034829, 0.000000000000000000, 4.999999999999998224 ) ) ;
#55769=CARTESIAN_POINT ( 'NONE',  ( 12.64687500061451608, 6.054752690667223547, 3.707466751127219781E-16 ) ) ;
#55770=CARTESIAN_POINT ( 'NONE',  ( 12.03750000122903430, 4.330127018922191873, 2.499999999999999556 ) ) ;
#55771=CARTESIAN_POINT ( 'NONE',  ( 4.359375000614517326, -4.541064518000417216, -2.621784821875001281 ) ) ;
#55772=CARTESIAN_POINT ( 'NONE',  ( 28.19999999999999929, 0.000000000000000000, 4.999999999999998224 ) ) ;
#55774=CARTESIAN_POINT ( 'NONE',  ( 9.121875000614517504, 3.027376345333611329, 5.243569643749999010 ) ) ;
#55775=CARTESIAN_POINT ( 'NONE',  ( 3.600000000000002309, -4.330127018922190985, -2.500000000000001332 ) ) ;
#55776=CARTESIAN_POINT ( 'NONE',  ( 19.30312500061451786, 4.541064518000418104, -2.621784821874998173 ) ) ;
#55778=CARTESIAN_POINT ( 'NONE',  ( -2.121784821874999949, 18.37812500061459531, 26.32496088578401938 ) ) ;
#55779=CARTESIAN_POINT ( 'NONE',  ( 22.95937500061451431, 4.541064518000418104, -2.621784821874998173 ) ) ;
#55780=CARTESIAN_POINT ( 'NONE',  ( -5.810221930991193690E-16, 13.70000000122903394, -34.00000000000000000 ) ) ;
#55782=CARTESIAN_POINT ( 'NONE',  ( 28.91250000122903074, -4.330127018922190985, -2.500000000000001332 ) ) ;
#55784=CARTESIAN_POINT ( 'NONE',  ( 25.22812500061451502, 4.541064518000418104, 2.621784821874999949 ) ) ;
#55785=CARTESIAN_POINT ( 'NONE',  ( 16.34062500061451573, -3.027376345333614438, 5.243569643749998122 ) ) ;
#55787=CARTESIAN_POINT ( 'NONE',  ( 13.88437500061451679, 6.421520780324663323E-16, -5.243569643749999010 ) ) ;
#55788=CARTESIAN_POINT ( 'NONE',  ( 26.21250000122903501, -4.330127018922190985, -2.500000000000001332 ) ) ;
#55789=CARTESIAN_POINT ( 'NONE',  ( 25.50000000122903288, 5.773502691896255534, 3.535250795749688894E-16 ) ) ;
#55790=CARTESIAN_POINT ( 'NONE',  ( 4.359375000614517326, -4.541064518000417216, -2.621784821875001281 ) ) ;
#55791=CARTESIAN_POINT ( 'NONE',  ( 13.20937500061451786, 0.000000000000000000, 5.243569643749999010 ) ) ;
#55792=CARTESIAN_POINT ( 'NONE',  ( -3.999999999999999112, 11.86249999999999893, 27.69059892324149885 ) ) ;
#55793=CARTESIAN_POINT ( 'NONE',  ( 29.85937500061451644, 0.000000000000000000, 5.243569643749999010 ) ) ;
#55794=DIRECTION ( 'NONE',  ( -1.000000000000000000, -0.000000000000000000, -0.000000000000000000 ) ) ;
#55795=CARTESIAN_POINT ( 'NONE',  ( 24.94687500061451502, -3.027376345333614438, 5.243569643749998122 ) ) ;
#55796=CARTESIAN_POINT ( 'NONE',  ( 17.44687500061451857, -3.027376345333610441, -5.243569643749999898 ) ) ;
#55798=CARTESIAN_POINT ( 'NONE',  ( 28.98750000000000071, 5.773502691896255534, 3.535250795749688894E-16 ) ) ;
#55799=CARTESIAN_POINT ( 'NONE',  ( 3.450000001229036162, 5.773502691896255534, 3.535250795749688894E-16 ) ) ;
#55800=CARTESIAN_POINT ( 'NONE',  ( 4.462500000000001243, -5.773502691896255534, -1.060575238724906372E-15 ) ) ;
#55802=CARTESIAN_POINT ( 'NONE',  ( 18.66562500061451146, -6.054752690667223547, -1.112240025338166033E-15 ) ) ;
#55803=CARTESIAN_POINT ( 'NONE',  ( 8.550000000000002487, -4.330127018922190985, -2.500000000000001332 ) ) ;
#55804=CARTESIAN_POINT ( 'NONE',  ( 15.41250000000000142, 2.886751345948129099, -4.999999999999997335 ) ) ;
#55805=CARTESIAN_POINT ( 'NONE',  ( 17.51249999999999929, -5.773502691896255534, -1.060575238724906372E-15 ) ) ;
#55806=CARTESIAN_POINT ( 'NONE',  ( 25.05000000000000071, 0.000000000000000000, 4.999999999999998224 ) ) ;
#55807=CARTESIAN_POINT ( 'NONE',  ( 19.98750000122903359, 6.123233995736764310E-16, -4.999999999999998224 ) ) ;
#55808=CARTESIAN_POINT ( 'NONE',  ( 5.603843221884249104, 8.282830004121999323, 32.15295242426309130 ) ) ;
#55809=( BOUNDED_CURVE ( )  B_SPLINE_CURVE ( 2, ( #239, #61913, #61546, #62282, #23107, #38669, #17560, #27584, #16117 ),
 .UNSPECIFIED., .F., .F. ) 
 B_SPLINE_CURVE_WITH_KNOTS ( ( 3, 2, 2, 2, 3 ),
 ( 0.6195652173913043237, 0.6231884057971014412, 0.6304347826086956763, 0.6376811594202898004, 0.6413043478260869179 ),
 .UNSPECIFIED. ) 
 CURVE ( )  GEOMETRIC_REPRESENTATION_ITEM ( )  RATIONAL_B_SPLINE_CURVE ( ( 0.9330127018922194093, 0.9330127018922194093, 1.000000000000000000, 0.8660254037844387076, 1.000000000000000000, 0.8660254037844387076, 1.000000000000000000, 0.9330127018922194093, 0.9330127018922194093 ) ) 
 REPRESENTATION_ITEM ( '' )  );
#55810=CARTESIAN_POINT ( 'NONE',  ( 28.05937500061451573, 0.000000000000000000, 5.243569643749999010 ) ) ;
#55812=CARTESIAN_POINT ( 'NONE',  ( 16.86562500061451786, -6.054752690667223547, -1.112240025338166033E-15 ) ) ;
#55813=CARTESIAN_POINT ( 'NONE',  ( 23.65312500061451573, -4.541064518000417216, -2.621784821875001281 ) ) ;
#55814=CARTESIAN_POINT ( 'NONE',  ( 23.10937500061451644, 0.000000000000000000, 5.243569643749999010 ) ) ;
#55815=CARTESIAN_POINT ( 'NONE',  ( 5.587500000000003020, 5.773502691896255534, 3.535250795749688894E-16 ) ) ;
#55816=CARTESIAN_POINT ( 'NONE',  ( 8.728125000614518569, -4.541064518000419881, 2.621784821874995952 ) ) ;
#55817=CARTESIAN_POINT ( 'NONE',  ( 24.55312500061451786, -4.541064518000417216, -2.621784821875001281 ) ) ;
#55818=CARTESIAN_POINT ( 'NONE',  ( 15.49687500061451750, -3.027376345333614438, 5.243569643749998122 ) ) ;
#55819=CARTESIAN_POINT ( 'NONE',  ( 20.07187500061451857, -6.054752690667223547, -1.112240025338166033E-15 ) ) ;
#55820=CARTESIAN_POINT ( 'NONE',  ( 2.121784821874999061, 10.25937500061451857, 26.32496088578401583 ) ) ;
#55821=CARTESIAN_POINT ( 'NONE',  ( 21.86250000122903003, 4.330127018922192761, -2.499999999999997780 ) ) ;
#55823=CARTESIAN_POINT ( 'NONE',  ( 12.44062500061451537, -3.027376345333610441, -5.243569643749999898 ) ) ;
#55824=CARTESIAN_POINT ( 'NONE',  ( 7.246875000614518392, 6.054752690667223547, 3.707466751127219781E-16 ) ) ;
#55825=CARTESIAN_POINT ( 'NONE',  ( 7.434375000614519280, -4.541064518000419881, 2.621784821874995952 ) ) ;
#55826=EDGE_LOOP ( 'NONE', ( #19445, #12359, #62953, #52101 ) ) ;
#55827=CARTESIAN_POINT ( 'NONE',  ( 27.27187500061451431, -6.054752690667223547, -1.112240025338166033E-15 ) ) ;
#55828=CARTESIAN_POINT ( 'NONE',  ( 19.64062500061451644, -3.027376345333610441, -5.243569643749999898 ) ) ;
#55829=CARTESIAN_POINT ( 'NONE',  ( 28.98750000122903359, 6.123233995736764310E-16, -4.999999999999998224 ) ) ;
#55830=EDGE_CURVE ( 'NONE', #30395, #33359, #48396, .T. ) ;
#55831=CARTESIAN_POINT ( 'NONE',  ( 28.56562500061451715, -6.054752690667223547, -1.112240025338166033E-15 ) ) ;
#55832=CARTESIAN_POINT ( 'NONE',  ( 24.27187500061452141, 3.027376345333613106, -5.243569643749998122 ) ) ;
#55833=CARTESIAN_POINT ( 'NONE',  ( 18.62812500061451715, -4.541064518000419881, 2.621784821874995952 ) ) ;
#55834=CARTESIAN_POINT ( 'NONE',  ( -3.999999999999997335, 10.13750000000000284, 32.30940107675850470 ) ) ;
#55835=CARTESIAN_POINT ( 'NONE',  ( 24.81562500061451715, 3.027376345333611329, 5.243569643749999010 ) ) ;
#55836=CARTESIAN_POINT ( 'NONE',  ( 5.512500001229033941, -4.330127018922190985, -2.500000000000001332 ) ) ;
#55838=CARTESIAN_POINT ( 'NONE',  ( 28.23750000000000426, -2.886751345948129988, 4.999999999999997335 ) ) ;
#55839=CARTESIAN_POINT ( 'NONE',  ( -1.999999999999997113, 16.02500000000000213, -26.53589838486224295 ) ) ;
#55841=CARTESIAN_POINT ( 'NONE',  ( 5.146875000614517859, -3.027376345333614438, 5.243569643749998122 ) ) ;
#55842=CARTESIAN_POINT ( 'NONE',  ( 12.81562500061451537, -6.054752690667223547, -1.112240025338166033E-15 ) ) ;
#55843=CARTESIAN_POINT ( 'NONE',  ( 6.309375000614517504, 4.541064518000418104, -2.621784821874998173 ) ) ;
#55844=CARTESIAN_POINT ( 'NONE',  ( 23.77500000122903145, 2.886751345948126879, 4.999999999999999112 ) ) ;
#55845=CARTESIAN_POINT ( 'NONE',  ( 13.95937500061451786, 4.541064518000418104, -2.621784821874998173 ) ) ;
#55846=CARTESIAN_POINT ( 'NONE',  ( 3.046875000614519990, -3.027376345333610441, -5.243569643749999898 ) ) ;
#55847=CARTESIAN_POINT ( 'NONE',  ( 28.12499999999999645, 4.330127018922191873, 2.499999999999999556 ) ) ;
#55848=CARTESIAN_POINT ( 'NONE',  ( 25.62187500061451573, 3.027376345333613106, -5.243569643749998122 ) ) ;
#55849=CARTESIAN_POINT ( 'NONE',  ( 3.478125000614517237, 6.421520780324663323E-16, -5.243569643749999010 ) ) ;
#55850=CARTESIAN_POINT ( 'NONE',  ( 12.21562500061451573, 3.027376345333611329, 5.243569643749999010 ) ) ;
#55851=VERTEX_POINT ( 'NONE', #21601 ) ;
#55852=CARTESIAN_POINT ( 'NONE',  ( 9.853125000614516793, 4.541064518000418104, -2.621784821874998173 ) ) ;
#55853=CARTESIAN_POINT ( 'NONE',  ( 7.228125000614517681, 4.541064518000418104, 2.621784821874999949 ) ) ;
#55857=CARTESIAN_POINT ( 'NONE',  ( 15.56250000000000000, 2.886751345948126879, 4.999999999999999112 ) ) ;
#55858=CARTESIAN_POINT ( 'NONE',  ( 16.47187500061452070, -6.054752690667223547, -1.112240025338166033E-15 ) ) ;
#55859=CARTESIAN_POINT ( 'NONE',  ( 12.78750000122903430, 6.123233995736764310E-16, -4.999999999999998224 ) ) ;
#55861=CARTESIAN_POINT ( 'NONE',  ( 20.07187500061451857, -6.054752690667223547, -1.112240025338166033E-15 ) ) ;
#55862=CARTESIAN_POINT ( 'NONE',  ( 2.121784821875001281, 13.20312500061451821, -26.32496088578401938 ) ) ;
#55863=CARTESIAN_POINT ( 'NONE',  ( 21.89999999999999858, 0.000000000000000000, 4.999999999999998224 ) ) ;
#55866=CARTESIAN_POINT ( 'NONE',  ( 28.00312500061451715, 0.000000000000000000, 5.243569643749999010 ) ) ;
#55867=EDGE_CURVE ( 'NONE', #54755, #55534, #55944, .T. ) ;
#55868=PLANE ( 'NONE',  #31588 ) ;
#55869=DIRECTION ( 'NONE',  ( 0.000000000000000000, 0.000000000000000000, 1.000000000000000000 ) ) ;
#55870=CARTESIAN_POINT ( 'NONE',  ( 26.25000000000000000, 4.330127018922192761, -2.499999999999997780 ) ) ;
#55871=CARTESIAN_POINT ( 'NONE',  ( 8.653125000614515727, 0.000000000000000000, 5.243569643749999010 ) ) ;
#55873=CARTESIAN_POINT ( 'NONE',  ( 20.93437500061451573, -4.541064518000419881, 2.621784821874995952 ) ) ;
#55875=CARTESIAN_POINT ( 'NONE',  ( 4.378125000614518925, 6.421520780324663323E-16, -5.243569643749999010 ) ) ;
#55876=CARTESIAN_POINT ( 'NONE',  ( 11.89687500061451608, -3.027376345333614438, 5.243569643749998122 ) ) ;
#55877=ORIENTED_EDGE ( 'NONE', *, *, #13034, .T. ) ;
#55878=CARTESIAN_POINT ( 'NONE',  ( 20.78437500061451715, 4.541064518000418104, 2.621784821874999949 ) ) ;
#55879=CARTESIAN_POINT ( 'NONE',  ( 3.992981257374419890, 3.009426956198102854, -29.72584546141768769 ) ) ;
#55880=CARTESIAN_POINT ( 'NONE',  ( 28.53749999999999787, 5.773502691896255534, 3.535250795749688894E-16 ) ) ;
#55881=CARTESIAN_POINT ( 'NONE',  ( 6.187500000000002665, -2.886751345948129988, 4.999999999999997335 ) ) ;
#55882=CARTESIAN_POINT ( 'NONE',  ( 13.80000000122903181, 5.773502691896255534, 3.535250795749688894E-16 ) ) ;
#55883=CARTESIAN_POINT ( 'NONE',  ( -1.487416814333745711E-14, 15.16250000000000142, -26.00000000000000000 ) ) ;
#55884=DIRECTION ( 'NONE',  ( -0.000000000000000000, -1.000000000000000000, -0.000000000000000000 ) ) ;
#55885=VERTEX_POINT ( 'NONE', #39705 ) ;
#55886=CARTESIAN_POINT ( 'NONE',  ( 12.07499999999999929, -4.330127018922194537, 2.499999999999995559 ) ) ;
#55887=CARTESIAN_POINT ( 'NONE',  ( 17.10000000000000142, -4.330127018922190985, -2.500000000000001332 ) ) ;
#55888=CARTESIAN_POINT ( 'NONE',  ( 12.15000000122903501, -2.886751345948129988, 4.999999999999997335 ) ) ;
#55889=CARTESIAN_POINT ( 'NONE',  ( 12.55312500061451786, 4.541064518000418104, -2.621784821874998173 ) ) ;
#55890=CARTESIAN_POINT ( 'NONE',  ( 8.812500000000000000, 2.886751345948126879, 4.999999999999999112 ) ) ;
#55891=CARTESIAN_POINT ( 'NONE',  ( -2.000000000000000000, 15.53750000122903430, 26.53589838486224650 ) ) ;
#55892=CARTESIAN_POINT ( 'NONE',  ( 4.243569643749999898, 15.13437500061451679, -30.00000000000000000 ) ) ;
#55893=CARTESIAN_POINT ( 'NONE',  ( 27.26250000122903216, 4.330127018922192761, -2.499999999999997780 ) ) ;
#55895=CARTESIAN_POINT ( 'NONE',  ( 8.512499999999999289, -5.773502691896255534, -1.060575238724906372E-15 ) ) ;
#55897=CARTESIAN_POINT ( 'NONE',  ( 23.72812500061451502, 6.421520780324663323E-16, -5.243569643749999010 ) ) ;
#55899=CARTESIAN_POINT ( 'NONE',  ( 29.03437500061451715, -4.541064518000419881, 2.621784821874995952 ) ) ;
#55900=CARTESIAN_POINT ( 'NONE',  ( 20.85937500061451644, 0.000000000000000000, 5.243569643749999010 ) ) ;
#55901=CARTESIAN_POINT ( 'NONE',  ( 16.07812500061451289, 6.421520780324663323E-16, -5.243569643749999010 ) ) ;
#55902=CARTESIAN_POINT ( 'NONE',  ( -4.243569643749999898, 11.66562500061459495, -32.45002607614398471 ) ) ;
#55903=CARTESIAN_POINT ( 'NONE',  ( 6.815625000614517148, 3.027376345333611329, 5.243569643749999010 ) ) ;
#55904=CARTESIAN_POINT ( 'NONE',  ( 28.98750000122903359, 6.123233995736764310E-16, -4.999999999999998224 ) ) ;
#55906=CARTESIAN_POINT ( 'NONE',  ( 19.79062500061451502, 6.054752690667223547, 3.707466751127219781E-16 ) ) ;
#55909=CARTESIAN_POINT ( 'NONE',  ( 15.57187500061451679, -6.054752690667223547, -1.112240025338166033E-15 ) ) ;
#55910=CARTESIAN_POINT ( 'NONE',  ( 13.95937500061451786, 4.541064518000418104, -2.621784821874998173 ) ) ;
#55911=CARTESIAN_POINT ( 'NONE',  ( 22.69687500061451857, -3.027376345333614438, 5.243569643749998122 ) ) ;
#55912=VERTEX_POINT ( 'NONE', #21968 ) ;
#55913=CARTESIAN_POINT ( 'NONE',  ( 3.215625000614518836, 3.027376345333611329, 5.243569643749999010 ) ) ;
#55914=CARTESIAN_POINT ( 'NONE',  ( 26.76562500061451644, -6.054752690667223547, -1.112240025338166033E-15 ) ) ;
#55915=CARTESIAN_POINT ( 'NONE',  ( 26.20312500061451644, 0.000000000000000000, 5.243569643749999010 ) ) ;
#55917=CARTESIAN_POINT ( 'NONE',  ( 3.999999999999999112, 17.52499999999999858, 30.00000000000000000 ) ) ;
#55918=CARTESIAN_POINT ( 'NONE',  ( 5.259375000614518569, -4.541064518000417216, -2.621784821875001281 ) ) ;
#55919=CARTESIAN_POINT ( 'NONE',  ( 11.10000000122903252, 5.773502691896255534, 3.535250795749688894E-16 ) ) ;
#55920=CARTESIAN_POINT ( 'NONE',  ( 7.162500001229032520, 0.000000000000000000, 4.999999999999998224 ) ) ;
#55921=CARTESIAN_POINT ( 'NONE',  ( 2.953125000614516438, -4.541064518000417216, -2.621784821875001281 ) ) ;
#55924=CARTESIAN_POINT ( 'NONE',  ( 11.74687500061451573, 6.054752690667223547, 3.707466751127219781E-16 ) ) ;
#55925=CARTESIAN_POINT ( 'NONE',  ( 3.999999999999998668, 14.86250000000000071, -32.30940107675850470 ) ) ;
#55927=CARTESIAN_POINT ( 'NONE',  ( 19.52812500061451573, -4.541064518000419881, 2.621784821874995952 ) ) ;
#55928=CARTESIAN_POINT ( 'NONE',  ( 13.13437500061451857, 4.541064518000418104, 2.621784821874999949 ) ) ;
#55929=CARTESIAN_POINT ( 'NONE',  ( 4.453125000614517326, 4.541064518000418104, -2.621784821874998173 ) ) ;
#55930=CARTESIAN_POINT ( 'NONE',  ( 22.95937500061451431, 4.541064518000418104, -2.621784821874998173 ) ) ;
#55931=CARTESIAN_POINT ( 'NONE',  ( 10.99687500061451750, -3.027376345333614438, 5.243569643749998122 ) ) ;
#55932=CARTESIAN_POINT ( 'NONE',  ( 6.328125000614515550, 4.541064518000418104, 2.621784821874999949 ) ) ;
#55934=CARTESIAN_POINT ( 'NONE',  ( 6.375000001229031987, -5.773502691896255534, -1.060575238724906372E-15 ) ) ;
#55935=ADVANCED_FACE ( 'NONE', ( #38608 ), #71032, .T. ) ;
#55936=CARTESIAN_POINT ( 'NONE',  ( 19.07812500061451644, -4.541064518000419881, 2.621784821874995952 ) ) ;
#55937=CARTESIAN_POINT ( 'NONE',  ( 8.287500001229034297, 6.123233995736764310E-16, -4.999999999999998224 ) ) ;
#55938=CARTESIAN_POINT ( 'NONE',  ( 16.11562500061451786, 3.027376345333613106, -5.243569643749998122 ) ) ;
#55939=CARTESIAN_POINT ( 'NONE',  ( 15.06562500061451537, -6.054752690667223547, -1.112240025338166033E-15 ) ) ;
#55941=CARTESIAN_POINT ( 'NONE',  ( 16.01249999999999929, 2.886751345948126879, 4.999999999999999112 ) ) ;
#55942=CARTESIAN_POINT ( 'NONE',  ( 9.712500001229033231, 4.330127018922192761, -2.499999999999997780 ) ) ;
#55943=CARTESIAN_POINT ( 'NONE',  ( 4.753125000614515372, -4.541064518000417216, -2.621784821875001281 ) ) ;
#55944=( BOUNDED_CURVE ( )  B_SPLINE_CURVE ( 2, ( #38227, #11259, #28249, #44155, #16059, #45239, #67772 ),
 .UNSPECIFIED., .F., .F. ) 
 B_SPLINE_CURVE_WITH_KNOTS ( ( 3, 2, 2, 3 ),
 ( 0.9428132104952601233, 0.9444444444444444198, 0.9472222222222221877, 0.9486699882857303479 ),
 .UNSPECIFIED. ) 
 CURVE ( )  GEOMETRIC_REPRESENTATION_ITEM ( )  RATIONAL_B_SPLINE_CURVE ( ( 0.9350522116989212762, 0.9213241925169703972, 1.000000000000000000, 0.8660254037844387076, 1.000000000000000000, 0.9301730054416843529, 0.9331330810709438373 ) ) 
 REPRESENTATION_ITEM ( '' )  );
#55945=CARTESIAN_POINT ( 'NONE',  ( 20.88750000122903572, 6.123233995736764310E-16, -4.999999999999998224 ) ) ;
#55947=CARTESIAN_POINT ( 'NONE',  ( 9.001249775931846008E-16, 14.57187500061451679, -25.09994784771203058 ) ) ;
#55948=CARTESIAN_POINT ( 'NONE',  ( 21.37499999999999645, 4.330127018922191873, 2.499999999999999556 ) ) ;
#55949=CARTESIAN_POINT ( 'NONE',  ( 3.412500001229032964, 4.330127018922192761, -2.499999999999997780 ) ) ;
#55950=CARTESIAN_POINT ( 'NONE',  ( 4.209375000614516971, 0.000000000000000000, 5.243569643749999010 ) ) ;
#55951=CARTESIAN_POINT ( 'NONE',  ( 20.97187500061451715, -6.054752690667223547, -1.112240025338166033E-15 ) ) ;
#55952=CARTESIAN_POINT ( 'NONE',  ( -1.999999999999997113, 15.12500000000000000, 33.46410161513775705 ) ) ;
#55953=CARTESIAN_POINT ( 'NONE',  ( 16.97812500061451502, 6.421520780324663323E-16, -5.243569643749999010 ) ) ;
#55955=CARTESIAN_POINT ( 'NONE',  ( -3.999999999999999112, 15.50000000000000000, -30.00000000000000000 ) ) ;
#55956=CARTESIAN_POINT ( 'NONE',  ( -3.999999999999999112, 15.50000000000000000, 30.00000000000000000 ) ) ;
#55957=CARTESIAN_POINT ( 'NONE',  ( 28.54687500061451644, -3.027376345333614438, 5.243569643749998122 ) ) ;
#55960=CARTESIAN_POINT ( 'NONE',  ( 13.71562500061451750, -6.054752690667223547, -1.112240025338166033E-15 ) ) ;
#55961=CARTESIAN_POINT ( 'NONE',  ( 11.22187500061451892, 3.027376345333613106, -5.243569643749998122 ) ) ;
#55962=EDGE_LOOP ( 'NONE', ( #2046, #9501, #54511, #21618 ) ) ;
#55963=CARTESIAN_POINT ( 'NONE',  ( 29.01562500061451644, -6.054752690667223547, -1.112240025338166033E-15 ) ) ;
#55964=CARTESIAN_POINT ( 'NONE',  ( 23.24062500061451786, -3.027376345333610441, -5.243569643749999898 ) ) ;
#55965=CARTESIAN_POINT ( 'NONE',  ( 3.999999999999998668, 15.42500000122903359, -32.30940107675850470 ) ) ;
#55966=EDGE_CURVE ( 'NONE', #66904, #18961, #26230, .T. ) ;
#55967=CARTESIAN_POINT ( 'NONE',  ( 11.55000000000000071, 0.000000000000000000, 4.999999999999998224 ) ) ;
#55969=CARTESIAN_POINT ( 'NONE',  ( 22.83750000122903501, 4.330127018922191873, 2.499999999999999556 ) ) ;
#55970=CARTESIAN_POINT ( 'NONE',  ( 17.05312500061451786, 4.541064518000418104, -2.621784821874998173 ) ) ;
#55972=ORIENTED_EDGE ( 'NONE', *, *, #41790, .T. ) ;
#55973=CARTESIAN_POINT ( 'NONE',  ( 19.79999999999999716, -4.330127018922190985, -2.500000000000001332 ) ) ;
#55974=CARTESIAN_POINT ( 'NONE',  ( 22.72499999999999787, 4.330127018922191873, 2.499999999999999556 ) ) ;
#55975=CARTESIAN_POINT ( 'NONE',  ( 20.89687500061452141, -3.027376345333614438, 5.243569643749998122 ) ) ;
#55976=CARTESIAN_POINT ( 'NONE',  ( 26.57812500061451644, 4.541064518000418104, 2.621784821874999949 ) ) ;
#55978=FACE_OUTER_BOUND ( 'NONE', #49846, .T. ) ;
#55979=CARTESIAN_POINT ( 'NONE',  ( 8.540625000614518569, 6.054752690667223547, 3.707466751127219781E-16 ) ) ;
#55981=CARTESIAN_POINT ( 'NONE',  ( 17.06250000000000000, -5.773502691896255534, -1.060575238724906372E-15 ) ) ;
#55982=CARTESIAN_POINT ( 'NONE',  ( 24.14999999999999858, 0.000000000000000000, 4.999999999999998224 ) ) ;
#55983=CARTESIAN_POINT ( 'NONE',  ( 7.724999999999999645, 6.123233995736764310E-16, -4.999999999999998224 ) ) ;
#55984=CARTESIAN_POINT ( 'NONE',  ( 5.521875000614517859, 3.027376345333611329, 5.243569643749999010 ) ) ;
#55985=CARTESIAN_POINT ( 'NONE',  ( 29.25937500061451502, 4.541064518000418104, -2.621784821874998173 ) ) ;
#55987=CARTESIAN_POINT ( 'NONE',  ( 25.00312500061451715, -4.541064518000417216, -2.621784821875001281 ) ) ;
#55988=CARTESIAN_POINT ( 'NONE',  ( 24.27187500061452141, 3.027376345333613106, -5.243569643749998122 ) ) ;
#55989=CARTESIAN_POINT ( 'NONE',  ( -4.243569643749998122, 18.94062500061459531, -27.54997392385601174 ) ) ;
#55990=CARTESIAN_POINT ( 'NONE',  ( 13.08750000000000036, -2.886751345948125991, -5.000000000000000000 ) ) ;
#55991=CARTESIAN_POINT ( 'NONE',  ( 9.553125000614517859, 0.000000000000000000, 5.243569643749999010 ) ) ;
#55992=CARTESIAN_POINT ( 'NONE',  ( 1.626862140677534273E-15, 13.47500000122903252, -26.00000000000000355 ) ) ;
#55994=CARTESIAN_POINT ( 'NONE',  ( 25.22812500061451502, 4.541064518000418104, 2.621784821874999949 ) ) ;
#55997=CARTESIAN_POINT ( 'NONE',  ( 3.628125000614518036, 4.541064518000418104, 2.621784821874999949 ) ) ;
#55998=CARTESIAN_POINT ( 'NONE',  ( 19.92187500061451644, 3.027376345333611329, 5.243569643749999010 ) ) ;
#55999=CARTESIAN_POINT ( 'NONE',  ( -4.243569643749999898, 14.87187500061451928, 27.54997392385601529 ) ) ;
#56000=CARTESIAN_POINT ( 'NONE',  ( 21.75937500061451502, 0.000000000000000000, 5.243569643749999010 ) ) ;
#56001=CARTESIAN_POINT ( 'NONE',  ( 29.48437500061451644, -4.541064518000419881, 2.621784821874995952 ) ) ;
#56002=CARTESIAN_POINT ( 'NONE',  ( 4.243569643749999898, 19.14687500061451431, 32.45002607614398471 ) ) ;
#56003=CARTESIAN_POINT ( 'NONE',  ( 9.328125000614518214, 6.421520780324663323E-16, -5.243569643749999010 ) ) ;
#56004=CARTESIAN_POINT ( 'NONE',  ( -1.999999999999997113, 15.23750000122903536, 33.46410161513775705 ) ) ;
#56006=CARTESIAN_POINT ( 'NONE',  ( 7.321875000614516793, 3.027376345333611329, 5.243569643749999010 ) ) ;
#56007=CARTESIAN_POINT ( 'NONE',  ( 3.957880893006796352, 3.055449414859130464, -4.228749118501266224 ) ) ;
#56008=CARTESIAN_POINT ( 'NONE',  ( 7.115625000614516082, 3.027376345333613106, -5.243569643749998122 ) ) ;
#56009=CARTESIAN_POINT ( 'NONE',  ( 11.29687500061451644, 6.054752690667223547, 3.707466751127219781E-16 ) ) ;
#56010=SURFACE_STYLE_USAGE ( .BOTH. , #34186 ) ;
#56011=CARTESIAN_POINT ( 'NONE',  ( 19.50000000122903288, -2.886751345948125991, -5.000000000000000000 ) ) ;
#56012=CARTESIAN_POINT ( 'NONE',  ( 8.896875000614517859, -3.027376345333610441, -5.243569643749999898 ) ) ;
#56013=CARTESIAN_POINT ( 'NONE',  ( 10.15312500061451750, -4.541064518000417216, -2.621784821875001281 ) ) ;
#56016=CARTESIAN_POINT ( 'NONE',  ( 19.05937500061451928, 0.000000000000000000, 5.243569643749999010 ) ) ;
#56018=CARTESIAN_POINT ( 'NONE',  ( 26.42812500061451431, 6.421520780324663323E-16, -5.243569643749999010 ) ) ;
#56019=CARTESIAN_POINT ( 'NONE',  ( 11.20312500061451644, 4.541064518000418104, -2.621784821874998173 ) ) ;
#56022=CARTESIAN_POINT ( 'NONE',  ( -2.121784821874999949, 12.58437500061451786, -33.67503911421598417 ) ) ;
#56023=CARTESIAN_POINT ( 'NONE',  ( 12.93750000122903465, 4.330127018922191873, 2.499999999999999556 ) ) ;
#56024=CARTESIAN_POINT ( 'NONE',  ( 28.26562500061451289, 3.027376345333613106, -5.243569643749998122 ) ) ;
#56025=CARTESIAN_POINT ( 'NONE',  ( -4.243569643749999898, 15.30312500061451608, -30.00000000000000000 ) ) ;
#56026=CARTESIAN_POINT ( 'NONE',  ( 15.93750000122903110, 6.123233995736764310E-16, -4.999999999999998224 ) ) ;
#56027=CIRCLE ( 'NONE', #67775, 4.999999999999998224 ) ;
#56028=CARTESIAN_POINT ( 'NONE',  ( 12.56250000000000178, -5.773502691896255534, -1.060575238724906372E-15 ) ) ;
#56030=CARTESIAN_POINT ( 'NONE',  ( 23.35312500061451857, 4.541064518000418104, -2.621784821874998173 ) ) ;
#56031=CARTESIAN_POINT ( 'NONE',  ( 6.796875000614516438, 6.054752690667223547, 3.707466751127219781E-16 ) ) ;
#56032=CARTESIAN_POINT ( 'NONE',  ( 7.575000001229033053, 2.886751345948126879, 4.999999999999999112 ) ) ;
#56033=CARTESIAN_POINT ( 'NONE',  ( 15.41250000122903252, -4.330127018922190985, -2.500000000000001332 ) ) ;
#56034=CARTESIAN_POINT ( 'NONE',  ( 14.27812500061451573, 6.421520780324663323E-16, -5.243569643749999010 ) ) ;
#56035=CARTESIAN_POINT ( 'NONE',  ( 17.54062500061451502, 6.054752690667223547, 3.707466751127219781E-16 ) ) ;
#56036=CARTESIAN_POINT ( 'NONE',  ( 25.46250000122903501, 4.330127018922192761, -2.499999999999997780 ) ) ;
#56037=CARTESIAN_POINT ( 'NONE',  ( 27.86250000122903359, 0.000000000000000000, 4.999999999999998224 ) ) ;
#56038=CARTESIAN_POINT ( 'NONE',  ( 22.46250000000000213, -5.773502691896255534, -1.060575238724906372E-15 ) ) ;
#56040=CARTESIAN_POINT ( 'NONE',  ( 26.52187500061451431, 3.027376345333613106, -5.243569643749998122 ) ) ;
#56042=CARTESIAN_POINT ( 'NONE',  ( 9.900000001229033231, -2.886751345948129988, 4.999999999999997335 ) ) ;
#56043=CARTESIAN_POINT ( 'NONE',  ( 27.00937500061451857, 4.541064518000418104, -2.621784821874998173 ) ) ;
#56044=CARTESIAN_POINT ( 'NONE',  ( 10.31250000122903288, 0.000000000000000000, 4.999999999999998224 ) ) ;
#56045=CARTESIAN_POINT ( 'NONE',  ( 6.009375000614519458, 0.000000000000000000, 5.243569643749999010 ) ) ;
#56046=CARTESIAN_POINT ( 'NONE',  ( 22.94062500061451715, 6.054752690667223547, 3.707466751127219781E-16 ) ) ;
#56049=CARTESIAN_POINT ( 'NONE',  ( 9.084375000614517859, 4.541064518000418104, 2.621784821874999949 ) ) ;
#56050=CARTESIAN_POINT ( 'NONE',  ( 9.187500001229034652, 6.123233995736764310E-16, -4.999999999999998224 ) ) ;
#56051=CARTESIAN_POINT ( 'NONE',  ( 3.121875000614518836, 3.027376345333613106, -5.243569643749998122 ) ) ;
#56052=CARTESIAN_POINT ( 'NONE',  ( 7.246875000614518392, 6.054752690667223547, 3.707466751127219781E-16 ) ) ;
#56053=CARTESIAN_POINT ( 'NONE',  ( 28.17187500061451644, -6.054752690667223547, -1.112240025338166033E-15 ) ) ;
#56054=CARTESIAN_POINT ( 'NONE',  ( 21.89999999999999858, 0.000000000000000000, 4.999999999999998224 ) ) ;
#56055=CARTESIAN_POINT ( 'NONE',  ( 19.87500000000000000, 6.123233995736764310E-16, -4.999999999999998224 ) ) ;
#56056=VERTEX_POINT ( 'NONE', #69211 ) ;
#56057=CARTESIAN_POINT ( 'NONE',  ( 26.21249999999999858, 2.886751345948129099, -4.999999999999998224 ) ) ;
#56058=CARTESIAN_POINT ( 'NONE',  ( 27.72187500061451715, -6.054752690667223547, -1.112240025338166033E-15 ) ) ;
#56059=ORIENTED_EDGE ( 'NONE', *, *, #71580, .F. ) ;
#56060=CARTESIAN_POINT ( 'NONE',  ( 18.59062500061451573, -3.027376345333614438, 5.243569643749998122 ) ) ;
#56061=CARTESIAN_POINT ( 'NONE',  ( 7.490625000614516082, -3.027376345333610441, -5.243569643749999898 ) ) ;
#56063=CARTESIAN_POINT ( 'NONE',  ( 5.484375000614518214, 4.541064518000418104, 2.621784821874999949 ) ) ;
#56064=CARTESIAN_POINT ( 'NONE',  ( 16.57500000122903216, 2.886751345948126879, 4.999999999999999112 ) ) ;
#56065=VECTOR ( 'NONE', #17194, 1000.000000000000000 ) ;
#56066=CARTESIAN_POINT ( 'NONE',  ( 24.89999999999999858, 4.330127018922192761, -2.499999999999997780 ) ) ;
#56067=CARTESIAN_POINT ( 'NONE',  ( 15.82499999999999929, 6.123233995736764310E-16, -4.999999999999998224 ) ) ;
#56068=CARTESIAN_POINT ( 'NONE',  ( 7.434375000614519280, -4.541064518000419881, 2.621784821874995952 ) ) ;
#56069=CARTESIAN_POINT ( 'NONE',  ( 12.75937500061451857, 0.000000000000000000, 5.243569643749999010 ) ) ;
#56070=CARTESIAN_POINT ( 'NONE',  ( 22.35937500061451644, -4.541064518000417216, -2.621784821875001281 ) ) ;
#56071=CARTESIAN_POINT ( 'NONE',  ( -3.999999999999997335, 14.63750000000000107, -27.69059892324149530 ) ) ;
#56072=ORIENTED_EDGE ( 'NONE', *, *, #67743, .T. ) ;
#56073=CARTESIAN_POINT ( 'NONE',  ( 3.459375000614519635, -4.541064518000417216, -2.621784821875001281 ) ) ;
#56076=CARTESIAN_POINT ( 'NONE',  ( 7.059375000614518392, -4.541064518000417216, -2.621784821875001281 ) ) ;
#56078=CARTESIAN_POINT ( 'NONE',  ( 21.67500000000000071, 6.123233995736764310E-16, -4.999999999999998224 ) ) ;
#56079=CARTESIAN_POINT ( 'NONE',  ( 16.75312500061451715, 0.000000000000000000, 5.243569643749999010 ) ) ;
#56083=CARTESIAN_POINT ( 'NONE',  ( 10.26562500061451644, 3.027376345333613106, -5.243569643749998122 ) ) ;
#56084=CARTESIAN_POINT ( 'NONE',  ( 27.04687500061451644, 6.054752690667223547, 3.707466751127219781E-16 ) ) ;
#56086=CARTESIAN_POINT ( 'NONE',  ( 28.77187500061451431, 3.027376345333613106, -5.243569643749998122 ) ) ;
#56087=CARTESIAN_POINT ( 'NONE',  ( 10.05000000000000071, 4.330127018922192761, -2.499999999999997780 ) ) ;
#56088=CARTESIAN_POINT ( 'NONE',  ( 3.999999999999998668, 15.87500000122903465, 27.69059892324149175 ) ) ;
#56089=CARTESIAN_POINT ( 'NONE',  ( 9.975000001229034297, -5.773502691896255534, -1.060575238724906372E-15 ) ) ;
#56091=CARTESIAN_POINT ( 'NONE',  ( 19.05937500061451928, 0.000000000000000000, 5.243569643749999010 ) ) ;
#56092=CARTESIAN_POINT ( 'NONE',  ( 14.82187500061451679, 3.027376345333613106, -5.243569643749998122 ) ) ;
#56093=CARTESIAN_POINT ( 'NONE',  ( 9.300000001229031810, 5.773502691896255534, 3.535250795749688401E-16 ) ) ;
#56094=ORIENTED_EDGE ( 'NONE', *, *, #703, .F. ) ;
#56095=CARTESIAN_POINT ( 'NONE',  ( 14.01562500061451644, 3.027376345333611329, 5.243569643749999010 ) ) ;
#56096=CARTESIAN_POINT ( 'NONE',  ( 27.26250000122903216, 4.330127018922192761, -2.499999999999997780 ) ) ;
#56097=CARTESIAN_POINT ( 'NONE',  ( 14.25937500061451679, -4.541064518000417216, -2.621784821875001281 ) ) ;
#56099=CARTESIAN_POINT ( 'NONE',  ( 16.04062500061451857, -3.027376345333610441, -5.243569643749999898 ) ) ;
#56101=CARTESIAN_POINT ( 'NONE',  ( 26.74687500061451573, -3.027376345333614438, 5.243569643749998122 ) ) ;
#56102=CARTESIAN_POINT ( 'NONE',  ( -3.000416591977282496E-16, 10.24062500061451608, 25.09994784771203058 ) ) ;
#56103=CARTESIAN_POINT ( 'NONE',  ( 14.74687500061451573, -3.027376345333610441, -5.243569643749999898 ) ) ;
#56104=CARTESIAN_POINT ( 'NONE',  ( 14.62500000122903288, 2.886751345948129099, -4.999999999999998224 ) ) ;
#56105=CARTESIAN_POINT ( 'NONE',  ( 30.00000000000000000, 0.000000000000000000, 4.999999999999998224 ) ) ;
#56106=CYLINDRICAL_SURFACE ( 'NONE', #23839, 4.000000000000000000 ) ;
#56107=CARTESIAN_POINT ( 'NONE',  ( 20.82187500061451857, 3.027376345333611329, 5.243569643749999010 ) ) ;
#56108=CARTESIAN_POINT ( 'NONE',  ( 20.62500000122903288, 2.886751345948126879, 4.999999999999999112 ) ) ;
#56109=EDGE_CURVE ( 'NONE', #55464, #18961, #43221, .T. ) ;
#56110=CARTESIAN_POINT ( 'NONE',  ( 15.30937500061451750, 4.541064518000418104, -2.621784821874998173 ) ) ;
#56111=CARTESIAN_POINT ( 'NONE',  ( -4.243569643749999898, 12.20937500061451608, 30.00000000000000000 ) ) ;
#56112=CARTESIAN_POINT ( 'NONE',  ( 16.41562500061451857, -6.054752690667223547, -1.112240025338166033E-15 ) ) ;
#56114=EDGE_LOOP ( 'NONE', ( #4185, #11040, #14094, #2299 ) ) ;
#56115=CARTESIAN_POINT ( 'NONE',  ( 20.88749999999999929, 5.773502691896255534, 3.535250795749688894E-16 ) ) ;
#56117=CARTESIAN_POINT ( 'NONE',  ( 24.70312500061451644, 4.541064518000418104, -2.621784821874998173 ) ) ;
#56118=CARTESIAN_POINT ( 'NONE',  ( 4.907911205059083602E-16, 5.000000000000000000, 33.99999999999999289 ) ) ;
#56119=CARTESIAN_POINT ( 'NONE',  ( 16.87500000122903288, 2.886751345948129099, -4.999999999999998224 ) ) ;
#56120=CARTESIAN_POINT ( 'NONE',  ( 21.62812500061451360, 4.541064518000418104, 2.621784821874999949 ) ) ;
#56121=CARTESIAN_POINT ( 'NONE',  ( 24.62812500061451715, 6.421520780324663323E-16, -5.243569643749999010 ) ) ;
#56122=CARTESIAN_POINT ( 'NONE',  ( 5.203125000614518214, -4.541064518000417216, -2.621784821875001281 ) ) ;
#56123=ORIENTED_EDGE ( 'NONE', *, *, #49317, .T. ) ;
#56124=CARTESIAN_POINT ( 'NONE',  ( 29.81250000000000000, 2.886751345948129099, -4.999999999999998224 ) ) ;
#56125=CARTESIAN_POINT ( 'NONE',  ( 1.626862140677534273E-15, 10.32500000122903572, -26.00000000000000355 ) ) ;
#56128=CARTESIAN_POINT ( 'NONE',  ( -2.000000000000000000, 11.03750000122903430, -33.46410161513775705 ) ) ;
#56129=CARTESIAN_POINT ( 'NONE',  ( -3.000416591977282496E-16, 18.39687500061451786, -34.90005215228797653 ) ) ;
#56130=CARTESIAN_POINT ( 'NONE',  ( 9.449999999999999289, -4.330127018922190985, -2.500000000000001332 ) ) ;
#56131=CARTESIAN_POINT ( 'NONE',  ( 3.262500001229035718, -4.330127018922190985, -2.500000000000001332 ) ) ;
#56132=CARTESIAN_POINT ( 'NONE',  ( 12.08437500061451608, 6.421520780324663323E-16, -5.243569643749999010 ) ) ;
#56133=CARTESIAN_POINT ( 'NONE',  ( 4.471875000614518925, 3.027376345333613106, -5.243569643749998122 ) ) ;
#56136=CARTESIAN_POINT ( 'NONE',  ( -1.999999999999997113, 10.73750000122903536, 33.46410161513775705 ) ) ;
#56137=CARTESIAN_POINT ( 'NONE',  ( 10.02187500061451964, 3.027376345333611329, 5.243569643749999010 ) ) ;
#56139=CARTESIAN_POINT ( 'NONE',  ( 19.67812500061451786, 6.421520780324663323E-16, -5.243569643749999010 ) ) ;
#56141=CARTESIAN_POINT ( 'NONE',  ( -3.000416591977282496E-16, 17.89062500061459104, 25.09994784771203058 ) ) ;
#56142=CARTESIAN_POINT ( 'NONE',  ( 24.53437500061451715, -4.541064518000419881, 2.621784821874995952 ) ) ;
#56143=CARTESIAN_POINT ( 'NONE',  ( 2.828911952606729230, -4.122772994526751056, 3.124276913337163286 ) ) ;
#56144=CARTESIAN_POINT ( 'NONE',  ( 28.95000000122903572, -2.886751345948125991, -5.000000000000000000 ) ) ;
#56146=CARTESIAN_POINT ( 'NONE',  ( 26.09062500061451573, 6.054752690667223547, 3.707466751127219781E-16 ) ) ;
#56147=CARTESIAN_POINT ( 'NONE',  ( 15.51562500061451644, -6.054752690667223547, -1.112240025338166033E-15 ) ) ;
#56149=CARTESIAN_POINT ( 'NONE',  ( 11.25937500061451679, 4.541064518000418104, -2.621784821874998173 ) ) ;
#56150=CARTESIAN_POINT ( 'NONE',  ( 29.62500000000000000, -4.330127018922194537, 2.499999999999995559 ) ) ;
#56151=CARTESIAN_POINT ( 'NONE',  ( 23.85000000122903430, -2.886751345948129988, 4.999999999999997335 ) ) ;
#56153=CARTESIAN_POINT ( 'NONE',  ( 14.89687500061451786, 6.054752690667223547, 3.707466751127219781E-16 ) ) ;
#56154=CARTESIAN_POINT ( 'NONE',  ( 29.63437500061451502, 6.421520780324663323E-16, -5.243569643749999010 ) ) ;
#56155=DIRECTION ( 'NONE',  ( 0.000000000000000000, 0.000000000000000000, 1.000000000000000000 ) ) ;
#56156=CARTESIAN_POINT ( 'NONE',  ( 18.37500000000000355, -4.330127018922194537, 2.499999999999995559 ) ) ;
#56157=CARTESIAN_POINT ( 'NONE',  ( 23.78437500061451360, 6.421520780324663323E-16, -5.243569643749999010 ) ) ;
#56158=CARTESIAN_POINT ( 'NONE',  ( 14.29687500061451821, -3.027376345333610441, -5.243569643749999898 ) ) ;
#56160=CARTESIAN_POINT ( 'NONE',  ( 28.91250000000000497, 2.886751345948129099, -4.999999999999998224 ) ) ;
#56161=CARTESIAN_POINT ( 'NONE',  ( 3.112500001229034918, 0.000000000000000000, 4.999999999999998224 ) ) ;
#56162=CARTESIAN_POINT ( 'NONE',  ( 5.137500000000000178, 5.773502691896255534, 3.535250795749688894E-16 ) ) ;
#56164=CARTESIAN_POINT ( 'NONE',  ( 16.86562500061451786, -6.054752690667223547, -1.112240025338166033E-15 ) ) ;
#56165=CARTESIAN_POINT ( 'NONE',  ( 8.437500000000000000, -2.886751345948129988, 4.999999999999997335 ) ) ;
#56166=CARTESIAN_POINT ( 'NONE',  ( 2.840625000614518392, -3.027376345333614438, 5.243569643749998122 ) ) ;
#56167=CARTESIAN_POINT ( 'NONE',  ( 18.00000000000000355, -4.330127018922190985, -2.500000000000001332 ) ) ;
#56168=CARTESIAN_POINT ( 'NONE',  ( 4.243569643749999898, 13.69062500061451537, 32.45002607614398471 ) ) ;
#56170=CARTESIAN_POINT ( 'NONE',  ( 21.60000000122903430, -2.886751345948129988, 4.999999999999997335 ) ) ;
#56171=CARTESIAN_POINT ( 'NONE',  ( 2.154264117376507137, 9.766972526336937577, 35.60336559010523416 ) ) ;
#56172=CARTESIAN_POINT ( 'NONE',  ( 26.89687500061451431, -3.027376345333610441, -5.243569643749999898 ) ) ;
#56175=CARTESIAN_POINT ( 'NONE',  ( 17.76562500061451644, -6.054752690667223547, -1.112240025338166033E-15 ) ) ;
#56176=CARTESIAN_POINT ( 'NONE',  ( 22.15312500061451573, 0.000000000000000000, 5.243569643749999010 ) ) ;
#56177=CARTESIAN_POINT ( 'NONE',  ( 22.58437500061451431, 4.541064518000418104, 2.621784821874999949 ) ) ;
#56178=CARTESIAN_POINT ( 'NONE',  ( 7.687500000000000000, -2.886751345948125991, -5.000000000000000000 ) ) ;
#56179=CARTESIAN_POINT ( 'NONE',  ( 9.815625000614518925, 3.027376345333613106, -5.243569643749998122 ) ) ;
#56180=CARTESIAN_POINT ( 'NONE',  ( 24.40312500061451573, 0.000000000000000000, 5.243569643749999010 ) ) ;
#56181=CARTESIAN_POINT ( 'NONE',  ( 14.93437500061451750, 4.541064518000418104, 2.621784821874999949 ) ) ;
#56182=CARTESIAN_POINT ( 'NONE',  ( 19.54687500061451644, -3.027376345333614438, 5.243569643749998122 ) ) ;
#56183=CARTESIAN_POINT ( 'NONE',  ( 19.34999999999999787, -4.330127018922190985, -2.500000000000001332 ) ) ;
#56184=CARTESIAN_POINT ( 'NONE',  ( 2.121784821874999061, 16.95312500061451999, 26.32496088578401583 ) ) ;
#56185=CARTESIAN_POINT ( 'NONE',  ( 22.53750000122903430, -4.330127018922194537, 2.499999999999995559 ) ) ;
#56187=CARTESIAN_POINT ( 'NONE',  ( 11.54062500061451857, -3.027376345333610441, -5.243569643749999898 ) ) ;
#56188=CARTESIAN_POINT ( 'NONE',  ( 5.334375000614517859, 6.421520780324663323E-16, -5.243569643749999010 ) ) ;
#56189=CARTESIAN_POINT ( 'NONE',  ( 3.909375000614518481, -4.541064518000417216, -2.621784821875001281 ) ) ;
#56190=ORIENTED_EDGE ( 'NONE', *, *, #13900, .F. ) ;
#56191=CARTESIAN_POINT ( 'NONE',  ( 28.28437500061451715, 6.421520780324663323E-16, -5.243569643749999010 ) ) ;
#56192=CARTESIAN_POINT ( 'NONE',  ( 18.14062500061451644, -3.027376345333614438, 5.243569643749998122 ) ) ;
#56193=CARTESIAN_POINT ( 'NONE',  ( 27.03750000122903430, -4.330127018922194537, 2.499999999999995559 ) ) ;
#56195=CARTESIAN_POINT ( 'NONE',  ( 27.77812500061451573, 6.421520780324663323E-16, -5.243569643749999010 ) ) ;
#56196=CARTESIAN_POINT ( 'NONE',  ( 25.13437500061451502, 6.421520780324663323E-16, -5.243569643749999010 ) ) ;
#56197=CARTESIAN_POINT ( 'NONE',  ( 17.61562500061451786, 3.027376345333611329, 5.243569643749999010 ) ) ;
#56198=CARTESIAN_POINT ( 'NONE',  ( 4.243569643749999010, 18.32187500061451502, 27.54997392385601174 ) ) ;
#56199=CARTESIAN_POINT ( 'NONE',  ( 23.99062500061451786, -3.027376345333614438, 5.243569643749998122 ) ) ;
#56200=CARTESIAN_POINT ( 'NONE',  ( 4.162500001229033408, -4.330127018922190985, -2.500000000000001332 ) ) ;
#56201=ORIENTED_EDGE ( 'NONE', *, *, #19460, .F. ) ;
#56202=CARTESIAN_POINT ( 'NONE',  ( 26.81250000000000000, 2.886751345948126879, 4.999999999999999112 ) ) ;
#56203=CARTESIAN_POINT ( 'NONE',  ( -2.000000000000000000, 14.52500000000000036, -33.46410161513775705 ) ) ;
#56205=CARTESIAN_POINT ( 'NONE',  ( 4.621875000614516615, 3.027376345333611329, 5.243569643749999010 ) ) ;
#56206=CARTESIAN_POINT ( 'NONE',  ( 10.34062500061451750, 6.054752690667223547, 3.707466751127219781E-16 ) ) ;
#56207=CARTESIAN_POINT ( 'NONE',  ( 7.359375000614516438, 0.000000000000000000, 5.243569643749999010 ) ) ;
#56208=CARTESIAN_POINT ( 'NONE',  ( 25.16250000122903074, 0.000000000000000000, 4.999999999999998224 ) ) ;
#56209=( BOUNDED_CURVE ( )  B_SPLINE_CURVE ( 2, ( #8821, #4026, #38357, #32819, #31725, #60511, #55357, #3291, #48356 ),
 .UNSPECIFIED., .F., .F. ) 
 B_SPLINE_CURVE_WITH_KNOTS ( ( 3, 2, 2, 2, 3 ),
 ( 0.03260869565217391908, 0.03623188405797101580, 0.04347826086956521618, 0.05072463768115942351, 0.05434782608695652717 ),
 .UNSPECIFIED. ) 
 CURVE ( )  GEOMETRIC_REPRESENTATION_ITEM ( )  RATIONAL_B_SPLINE_CURVE ( ( 0.9330127018922192983, 0.9330127018922194093, 1.000000000000000000, 0.8660254037844387076, 1.000000000000000000, 0.8660254037844387076, 1.000000000000000000, 0.9330127018922192983, 0.9330127018922194093 ) ) 
 REPRESENTATION_ITEM ( '' )  );
#56210=CARTESIAN_POINT ( 'NONE',  ( 13.84687500061451537, -3.027376345333610441, -5.243569643749999898 ) ) ;
#56211=CARTESIAN_POINT ( 'NONE',  ( 29.50312500061451360, -4.541064518000417216, -2.621784821875001281 ) ) ;
#56212=CARTESIAN_POINT ( 'NONE',  ( 28.04999999999999716, 4.330127018922192761, -2.499999999999997780 ) ) ;
#56213=CARTESIAN_POINT ( 'NONE',  ( 27.08437500061451786, 4.541064518000418104, 2.621784821874999949 ) ) ;
#56214=FACE_OUTER_BOUND ( 'NONE', #63418, .T. ) ;
#56215=CARTESIAN_POINT ( 'NONE',  ( 13.04062500061451502, 6.054752690667223547, 3.707466751127219781E-16 ) ) ;
#56216=VERTEX_POINT ( 'NONE', #11053 ) ;
#56217=CARTESIAN_POINT ( 'NONE',  ( 9.140625000614518214, -3.027376345333614438, 5.243569643749998122 ) ) ;
#56218=CARTESIAN_POINT ( 'NONE',  ( 5.465625000614517504, 3.027376345333611329, 5.243569643749999010 ) ) ;
#56220=FACE_OUTER_BOUND ( 'NONE', #54967, .T. ) ;
#56221=CARTESIAN_POINT ( 'NONE',  ( 15.82499999999999929, 6.123233995736764310E-16, -4.999999999999998224 ) ) ;
#56223=CARTESIAN_POINT ( 'NONE',  ( 14.89687500061451786, 6.054752690667223547, 3.707466751127219781E-16 ) ) ;
#56224=CARTESIAN_POINT ( 'NONE',  ( 12.52500000122903145, 2.886751345948126879, 4.999999999999999112 ) ) ;
#56226=CARTESIAN_POINT ( 'NONE',  ( 21.12187500061451573, 3.027376345333613106, -5.243569643749998122 ) ) ;
#56227=CARTESIAN_POINT ( 'NONE',  ( -4.243569643749999898, 13.91562500061451679, -32.45002607614398471 ) ) ;
#56228=CARTESIAN_POINT ( 'NONE',  ( -1.487416814333745711E-14, 16.96250000000000213, 34.00000000000000000 ) ) ;
#56230=CARTESIAN_POINT ( 'NONE',  ( 25.71562500061451573, 3.027376345333611329, 5.243569643749999010 ) ) ;
#56231=CARTESIAN_POINT ( 'NONE',  ( -2.000000000000000000, 19.47499999999999787, -33.46410161513775705 ) ) ;
#56233=CARTESIAN_POINT ( 'NONE',  ( 27.59999999999999787, 4.330127018922192761, -2.499999999999997780 ) ) ;
#56234=ADVANCED_FACE ( 'NONE', ( #39136 ), #38780, .F. ) ;
#56235=CARTESIAN_POINT ( 'NONE',  ( 10.00312500061451715, 0.000000000000000000, 5.243569643749999010 ) ) ;
#56237=( BOUNDED_CURVE ( )  B_SPLINE_CURVE ( 2, ( #7767, #63552, #29216, #790, #11864, #52473, #56917 ),
 .UNSPECIFIED., .F., .F. ) 
 B_SPLINE_CURVE_WITH_KNOTS ( ( 3, 2, 2, 3 ),
 ( 0.1583333333333333814, 0.1611111111111111771, 0.1638888888888889173, 0.1666666666666666852 ),
 .UNSPECIFIED. ) 
 CURVE ( )  GEOMETRIC_REPRESENTATION_ITEM ( )  RATIONAL_B_SPLINE_CURVE ( ( 0.9999999999999973355, 0.8660254037844413721, 1.000000000000000000, 0.8660254037844387076, 1.000000000000000000, 0.8660254037844373753, 1.000000000000001332 ) ) 
 REPRESENTATION_ITEM ( '' )  );
#56238=CARTESIAN_POINT ( 'NONE',  ( 18.08437500061451431, 4.541064518000418104, 2.621784821874999949 ) ) ;
#56241=CARTESIAN_POINT ( 'NONE',  ( 4.265625000614517326, -6.054752690667223547, -1.112240025338166033E-15 ) ) ;
#56242=CARTESIAN_POINT ( 'NONE',  ( 10.54687500061451644, -3.027376345333614438, 5.243569643749998122 ) ) ;
#56243=ORIENTED_EDGE ( 'NONE', *, *, #16399, .T. ) ;
#56244=CARTESIAN_POINT ( 'NONE',  ( 22.13437500061451502, 4.541064518000418104, 2.621784821874999949 ) ) ;
#56246=CARTESIAN_POINT ( 'NONE',  ( 29.84999999999999787, 4.330127018922192761, -2.499999999999997780 ) ) ;
#56247=CARTESIAN_POINT ( 'NONE',  ( 6.225000000000001421, -4.330127018922194537, 2.499999999999995559 ) ) ;
#56248=CARTESIAN_POINT ( 'NONE',  ( 14.51250000122903394, -4.330127018922190985, -2.500000000000001332 ) ) ;
#56249=CARTESIAN_POINT ( 'NONE',  ( 3.021917804904423743, -3.983467431823952687, -3.409840147052992432 ) ) ;
#56250=CARTESIAN_POINT ( 'NONE',  ( 3.797099728130578278, -3.253013707837530522, 4.112539957277816072 ) ) ;
#56252=CARTESIAN_POINT ( 'NONE',  ( 12.03749999999999964, -2.886751345948129988, 4.999999999999997335 ) ) ;
#56253=CARTESIAN_POINT ( 'NONE',  ( 27.62812500061451360, -4.541064518000419881, 2.621784821874995952 ) ) ;
#56254=CARTESIAN_POINT ( 'NONE',  ( 16.27499999999999858, 6.123233995736764310E-16, -4.999999999999998224 ) ) ;
#56256=CARTESIAN_POINT ( 'NONE',  ( 11.06250000122903288, 4.330127018922192761, -2.499999999999997780 ) ) ;
#56257=CARTESIAN_POINT ( 'NONE',  ( 10.15312500061451750, -4.541064518000417216, -2.621784821875001281 ) ) ;
#56258=CARTESIAN_POINT ( 'NONE',  ( 7.800000000000001599, 4.330127018922192761, -2.499999999999997780 ) ) ;
#56259=CYLINDRICAL_SURFACE ( 'NONE', #53753, 4.999999999999998224 ) ;
#56260=CARTESIAN_POINT ( 'NONE',  ( -3.000416591977282496E-16, 15.24687500061451928, -34.90005215228797653 ) ) ;
#56261=CARTESIAN_POINT ( 'NONE',  ( 27.07500000122903216, -5.773502691896255534, -1.060575238724906372E-15 ) ) ;
#56263=CARTESIAN_POINT ( 'NONE',  ( 8.400000000000000355, 0.000000000000000000, 4.999999999999998224 ) ) ;
#56264=CARTESIAN_POINT ( 'NONE',  ( -3.999999999999999112, 13.25000000000000178, -30.00000000000000000 ) ) ;
#56265=ORIENTED_EDGE ( 'NONE', *, *, #7253, .F. ) ;
#56266=CARTESIAN_POINT ( 'NONE',  ( 23.91562500061451502, 3.027376345333611329, 5.243569643749999010 ) ) ;
#56267=CARTESIAN_POINT ( 'NONE',  ( 28.71562500061451573, 3.027376345333613106, -5.243569643749998122 ) ) ;
#56268=VECTOR ( 'NONE', #29847, 1000.000000000000000 ) ;
#56269=CARTESIAN_POINT ( 'NONE',  ( 28.73437500061451644, 6.421520780324663323E-16, -5.243569643749999010 ) ) ;
#56270=CARTESIAN_POINT ( 'NONE',  ( 19.54687500061451644, -3.027376345333614438, 5.243569643749998122 ) ) ;
#56271=EDGE_CURVE ( 'NONE', #4004, #68252, #58282, .T. ) ;
#56272=CARTESIAN_POINT ( 'NONE',  ( 16.45312500061451289, -4.541064518000417216, -2.621784821875001281 ) ) ;
#56273=CARTESIAN_POINT ( 'NONE',  ( 2.121784821875001281, 11.85312500061459673, -26.32496088578401938 ) ) ;
#56274=CARTESIAN_POINT ( 'NONE',  ( 7.715625000614515727, 3.027376345333611329, 5.243569643749999010 ) ) ;
#56275=CARTESIAN_POINT ( 'NONE',  ( 28.83750000122903145, -4.330127018922194537, 2.499999999999995559 ) ) ;
#56277=CARTESIAN_POINT ( 'NONE',  ( 18.25312500061451715, -4.541064518000417216, -2.621784821875001281 ) ) ;
#56278=DIRECTION ( 'NONE',  ( -1.000000000000000000, -0.000000000000000000, -0.000000000000000000 ) ) ;
#56280=CARTESIAN_POINT ( 'NONE',  ( 13.20937500061451786, 0.000000000000000000, 5.243569643749999010 ) ) ;
#56281=CARTESIAN_POINT ( 'NONE',  ( 11.22187500061451892, 3.027376345333613106, -5.243569643749998122 ) ) ;
#56282=CARTESIAN_POINT ( 'NONE',  ( 21.38437500061451502, -4.541064518000419881, 2.621784821874995952 ) ) ;
#56284=CARTESIAN_POINT ( 'NONE',  ( 3.178125000614515638, 4.541064518000418104, 2.621784821874999949 ) ) ;
#56285=CARTESIAN_POINT ( 'NONE',  ( 25.56562500061452070, 3.027376345333613106, -5.243569643749998122 ) ) ;
#56286=CARTESIAN_POINT ( 'NONE',  ( 27.21562500061451928, -6.054752690667223547, -1.112240025338166033E-15 ) ) ;
#56287=CARTESIAN_POINT ( 'NONE',  ( -1.999999999999997113, 16.47500000000000142, 33.46410161513775705 ) ) ;
#56288=CARTESIAN_POINT ( 'NONE',  ( 4.696875000614518569, -3.027376345333614438, 5.243569643749998122 ) ) ;
#56289=CARTESIAN_POINT ( 'NONE',  ( 13.05000000122903536, -2.886751345948129988, 4.999999999999997335 ) ) ;
#56290=CARTESIAN_POINT ( 'NONE',  ( 6.000000001229033764, -2.886751345948125991, -5.000000000000000000 ) ) ;
#56291=CARTESIAN_POINT ( 'NONE',  ( 28.61250000122903359, 4.330127018922192761, -2.499999999999997780 ) ) ;
#56294=CARTESIAN_POINT ( 'NONE',  ( 12.87187500061451750, -6.054752690667223547, -1.112240025338166033E-15 ) ) ;
#56296=CARTESIAN_POINT ( 'NONE',  ( 18.89062500061451644, 6.054752690667223547, 3.707466751127219781E-16 ) ) ;
#56297=CARTESIAN_POINT ( 'NONE',  ( 13.88437500061451679, 6.421520780324663323E-16, -5.243569643749999010 ) ) ;
#56298=CARTESIAN_POINT ( 'NONE',  ( 3.890625000614517326, -3.027376345333610441, -5.243569643749999898 ) ) ;
#56299=CARTESIAN_POINT ( 'NONE',  ( 22.88437500061451857, 6.421520780324663323E-16, -5.243569643749999010 ) ) ;
#56300=CARTESIAN_POINT ( 'NONE',  ( 9.609375000614518214, 0.000000000000000000, 5.243569643749999010 ) ) ;
#56301=CARTESIAN_POINT ( 'NONE',  ( 5.690625000614516260, -3.027376345333610441, -5.243569643749999898 ) ) ;
#56303=CARTESIAN_POINT ( 'NONE',  ( 5.625000001229036428, 2.886751345948129099, -4.999999999999998224 ) ) ;
#56304=CARTESIAN_POINT ( 'NONE',  ( 21.25312500061451715, 0.000000000000000000, 5.243569643749999010 ) ) ;
#56305=CARTESIAN_POINT ( 'NONE',  ( 7.387500001229032165, 6.123233995736764310E-16, -4.999999999999998224 ) ) ;
#56306=CARTESIAN_POINT ( 'NONE',  ( 16.30312500061451786, 0.000000000000000000, 5.243569643749999010 ) ) ;
#56307=CARTESIAN_POINT ( 'NONE',  ( 12.66562500061451502, 3.027376345333611329, 5.243569643749999010 ) ) ;
#56309=CARTESIAN_POINT ( 'NONE',  ( 15.07499999999999929, 4.330127018922191873, 2.499999999999999556 ) ) ;
#56310=CARTESIAN_POINT ( 'NONE',  ( 9.112500001229033586, -4.330127018922190985, -2.500000000000001332 ) ) ;
#56311=CARTESIAN_POINT ( 'NONE',  ( 5.278125000614516615, 6.421520780324663323E-16, -5.243569643749999010 ) ) ;
#56312=CARTESIAN_POINT ( 'NONE',  ( 20.66250000122903074, 0.000000000000000000, 4.999999999999998224 ) ) ;
#56314=CARTESIAN_POINT ( 'NONE',  ( 9.001249775931846008E-16, 11.42187500061451999, -25.09994784771203058 ) ) ;
#56315=DIRECTION ( 'NONE',  ( -1.000000000000000000, -0.000000000000000000, -0.000000000000000000 ) ) ;
#56316=CYLINDRICAL_SURFACE ( 'NONE', #40672, 3.999999999999996447 ) ;
#56318=CARTESIAN_POINT ( 'NONE',  ( 28.31250000122903288, 0.000000000000000000, 4.999999999999998224 ) ) ;
#56319=CARTESIAN_POINT ( 'NONE',  ( 21.30937500061451573, 0.000000000000000000, 5.243569643749999010 ) ) ;
#56320=CARTESIAN_POINT ( 'NONE',  ( 12.37500000000000000, 4.330127018922191873, 2.499999999999999556 ) ) ;
#56321=CARTESIAN_POINT ( 'NONE',  ( 17.46562500061451217, 3.027376345333613106, -5.243569643749998122 ) ) ;
#56325=CARTESIAN_POINT ( 'NONE',  ( 29.37187500061451928, 3.027376345333611329, 5.243569643749999010 ) ) ;
#56327=CARTESIAN_POINT ( 'NONE',  ( 12.85312500061451502, -4.541064518000417216, -2.621784821875001281 ) ) ;
#56328=CARTESIAN_POINT ( 'NONE',  ( 11.48437500061451644, -4.541064518000419881, 2.621784821874995952 ) ) ;
#56329=VERTEX_POINT ( 'NONE', #72753 ) ;
#56330=CARTESIAN_POINT ( 'NONE',  ( 1.626862140677534273E-15, 14.26250000000000107, -26.00000000000000355 ) ) ;
#56331=CARTESIAN_POINT ( 'NONE',  ( 21.92812500061451431, 6.421520780324663323E-16, -5.243569643749999010 ) ) ;
#56332=CARTESIAN_POINT ( 'NONE',  ( -5.810221930991193690E-16, 13.25000000122903465, -34.00000000000000000 ) ) ;
#56333=EDGE_CURVE ( 'NONE', #27416, #18316, #58155, .T. ) ;
#56334=CARTESIAN_POINT ( 'NONE',  ( 11.88749999999999751, 5.773502691896255534, 3.535250795749688894E-16 ) ) ;
#56335=CARTESIAN_POINT ( 'NONE',  ( 22.87500000122903288, 2.886751345948126879, 4.999999999999999112 ) ) ;
#56336=CARTESIAN_POINT ( 'NONE',  ( 16.11562500061451786, 3.027376345333613106, -5.243569643749998122 ) ) ;
#56338=EDGE_LOOP ( 'NONE', ( #6736, #51800, #25986, #27054 ) ) ;
#56339=CARTESIAN_POINT ( 'NONE',  ( 20.62499999999999645, -4.330127018922194537, 2.499999999999995559 ) ) ;
#56341=CARTESIAN_POINT ( 'NONE',  ( 24.48749999999999716, 5.773502691896255534, 3.535250795749688894E-16 ) ) ;
#56342=CARTESIAN_POINT ( 'NONE',  ( 21.45937500061451786, -4.541064518000417216, -2.621784821875001281 ) ) ;
#56343=CARTESIAN_POINT ( 'NONE',  ( 25.49062500061451786, -3.027376345333610441, -5.243569643749999898 ) ) ;
#56344=ORIENTED_EDGE ( 'NONE', *, *, #23135, .T. ) ;
#56346=CARTESIAN_POINT ( 'NONE',  ( 8.878125000614515372, 6.421520780324663323E-16, -5.243569643749999010 ) ) ;
#56348=CARTESIAN_POINT ( 'NONE',  ( 15.29999999999999893, -4.330127018922190985, -2.500000000000001332 ) ) ;
#56349=CARTESIAN_POINT ( 'NONE',  ( -2.121784821874999949, 19.72812500061451857, 26.32496088578401938 ) ) ;
#56350=CARTESIAN_POINT ( 'NONE',  ( 4.396875000614516971, -3.027376345333610441, -5.243569643749999898 ) ) ;
#56351=CARTESIAN_POINT ( 'NONE',  ( 28.32187500061451502, 3.027376345333613106, -5.243569643749998122 ) ) ;
#56352=ORIENTED_EDGE ( 'NONE', *, *, #62588, .T. ) ;
#56353=CARTESIAN_POINT ( 'NONE',  ( 23.27812500061451573, 6.421520780324663323E-16, -5.243569643749999010 ) ) ;
#56354=CARTESIAN_POINT ( 'NONE',  ( 25.09687500061451715, -3.027376345333610441, -5.243569643749999898 ) ) ;
#56355=CARTESIAN_POINT ( 'NONE',  ( 4.243569643749999010, 19.61562500061459602, -32.45002607614398471 ) ) ;
#56356=CARTESIAN_POINT ( 'NONE',  ( 12.15000000000000036, -4.330127018922190985, -2.500000000000001332 ) ) ;
#56357=CARTESIAN_POINT ( 'NONE',  ( 8.503125000614515372, 4.541064518000418104, -2.621784821874998173 ) ) ;
#56358=DIRECTION ( 'NONE',  ( -0.000000000000000000, -1.000000000000000000, -0.000000000000000000 ) ) ;
#56360=CARTESIAN_POINT ( 'NONE',  ( 25.75312500061451715, 0.000000000000000000, 5.243569643749999010 ) ) ;
#56363=CARTESIAN_POINT ( 'NONE',  ( 3.028125000614518392, 6.421520780324663323E-16, -5.243569643749999010 ) ) ;
#56364=CARTESIAN_POINT ( 'NONE',  ( 19.02187500061451786, 3.027376345333611329, 5.243569643749999010 ) ) ;
#56365=CARTESIAN_POINT ( 'NONE',  ( -2.121784821874999949, 14.38437500061451679, 26.32496088578401938 ) ) ;
#56366=CARTESIAN_POINT ( 'NONE',  ( 21.79687500061451644, -3.027376345333614438, 5.243569643749998122 ) ) ;
#56367=CARTESIAN_POINT ( 'NONE',  ( 3.075000000000001510, -4.330127018922194537, 2.499999999999995559 ) ) ;
#56368=CARTESIAN_POINT ( 'NONE',  ( 9.001249775931846008E-16, 19.07187500061451857, 34.90005215228797653 ) ) ;
#56369=CARTESIAN_POINT ( 'NONE',  ( 9.178125000614517859, -4.541064518000419881, 2.621784821874995952 ) ) ;
#56371=CARTESIAN_POINT ( 'NONE',  ( 7.246875000614518392, 6.054752690667223547, 3.707466751127219781E-16 ) ) ;
#56373=CARTESIAN_POINT ( 'NONE',  ( 6.515625000614516438, -6.054752690667223547, -1.112240025338166033E-15 ) ) ;
#56374=CARTESIAN_POINT ( 'NONE',  ( 11.52187500061451608, -6.054752690667223547, -1.112240025338166033E-15 ) ) ;
#56375=CARTESIAN_POINT ( 'NONE',  ( 18.18750000122903288, 6.123233995736764310E-16, -4.999999999999998224 ) ) ;
#56376=CARTESIAN_POINT ( 'NONE',  ( 9.084375000614517859, 4.541064518000418104, 2.621784821874999949 ) ) ;
#56377=CARTESIAN_POINT ( 'NONE',  ( 8.915625000614515017, 3.027376345333613106, -5.243569643749998122 ) ) ;
#56378=CARTESIAN_POINT ( 'NONE',  ( 5.240625000614517859, -3.027376345333610441, -5.243569643749999898 ) ) ;
#56380=CARTESIAN_POINT ( 'NONE',  ( 18.04687500061451999, 6.054752690667223547, 3.707466751127219781E-16 ) ) ;
#56381=CARTESIAN_POINT ( 'NONE',  ( 26.99062500061451431, 6.054752690667223547, 3.707466751127219781E-16 ) ) ;
#56382=CARTESIAN_POINT ( 'NONE',  ( 13.26562500061451644, -6.054752690667223547, -1.112240025338166033E-15 ) ) ;
#56383=EDGE_CURVE ( 'NONE', #64264, #15264, #50631, .T. ) ;
#56385=CARTESIAN_POINT ( 'NONE',  ( 29.29687500061450933, 6.054752690667223547, 3.707466751127219781E-16 ) ) ;
#56386=CARTESIAN_POINT ( 'NONE',  ( 4.243569643749999010, 10.67187500061451644, -32.45002607614398471 ) ) ;
#56388=CARTESIAN_POINT ( 'NONE',  ( 12.71250000122903145, -4.330127018922190985, -2.500000000000001332 ) ) ;
#56389=CARTESIAN_POINT ( 'NONE',  ( 27.02812500061451573, 4.541064518000418104, 2.621784821874999949 ) ) ;
#56390=CARTESIAN_POINT ( 'NONE',  ( 4.243569643749999898, 15.04062500061451679, -27.54997392385601529 ) ) ;
#56391=CARTESIAN_POINT ( 'NONE',  ( 16.35000000122903430, -2.886751345948125991, -5.000000000000000000 ) ) ;
#56392=CARTESIAN_POINT ( 'NONE',  ( 12.22499999999999964, 6.123233995736764310E-16, -4.999999999999998224 ) ) ;
#56393=CARTESIAN_POINT ( 'NONE',  ( 21.74062500061451431, -3.027376345333614438, 5.243569643749998122 ) ) ;
#56394=CARTESIAN_POINT ( 'NONE',  ( 8.896875000614517859, -3.027376345333610441, -5.243569643749999898 ) ) ;
#56395=CARTESIAN_POINT ( 'NONE',  ( 8.175000001229031810, -5.773502691896255534, -1.060575238724906372E-15 ) ) ;
#56396=CARTESIAN_POINT ( 'NONE',  ( 15.86250000122903181, -4.330127018922190985, -2.500000000000001332 ) ) ;
#56397=CARTESIAN_POINT ( 'NONE',  ( 12.47812500061451502, 6.421520780324663323E-16, -5.243569643749999010 ) ) ;
#56398=CARTESIAN_POINT ( 'NONE',  ( 15.32812500061451644, 4.541064518000418104, 2.621784821874999949 ) ) ;
#56399=CARTESIAN_POINT ( 'NONE',  ( 27.48750000122903359, -4.330127018922194537, 2.499999999999995559 ) ) ;
#56400=CARTESIAN_POINT ( 'NONE',  ( 22.80000000000000071, 0.000000000000000000, 4.999999999999998224 ) ) ;
#56401=CARTESIAN_POINT ( 'NONE',  ( 22.69687500061451857, -3.027376345333614438, 5.243569643749998122 ) ) ;
#56403=CARTESIAN_POINT ( 'NONE',  ( 11.32500000122903394, -5.773502691896255534, -1.060575238724906372E-15 ) ) ;
#56404=CARTESIAN_POINT ( 'NONE',  ( 28.43437500061451573, 4.541064518000418104, 2.621784821874999949 ) ) ;
#56405=CARTESIAN_POINT ( 'NONE',  ( 4.959375000614516971, 4.541064518000418104, -2.621784821874998173 ) ) ;
#56406=CARTESIAN_POINT ( 'NONE',  ( 23.39062500061451289, 6.054752690667223547, 3.707466751127219781E-16 ) ) ;
#56408=CARTESIAN_POINT ( 'NONE',  ( 7.012500000000001954, 2.886751345948126879, 4.999999999999998224 ) ) ;
#56409=CARTESIAN_POINT ( 'NONE',  ( 9.421875000614519990, 3.027376345333613106, -5.243569643749998122 ) ) ;
#56410=CARTESIAN_POINT ( 'NONE',  ( -5.810221930991193690E-16, 12.68750000000000000, 26.00000000000000355 ) ) ;
#56411=CARTESIAN_POINT ( 'NONE',  ( 3.834375000614519635, -4.541064518000419881, 2.621784821874995952 ) ) ;
#56412=CARTESIAN_POINT ( 'NONE',  ( 7.096875000614517148, -3.027376345333610441, -5.243569643749999898 ) ) ;
#56414=CARTESIAN_POINT ( 'NONE',  ( 25.99687500061451928, -3.027376345333610441, -5.243569643749999898 ) ) ;
#56416=CARTESIAN_POINT ( 'NONE',  ( 19.27500000000000213, -4.330127018922194537, 2.499999999999995559 ) ) ;
#56417=ORIENTED_EDGE ( 'NONE', *, *, #43935, .F. ) ;
#56418=CARTESIAN_POINT ( 'NONE',  ( 28.19999999999999929, 0.000000000000000000, 4.999999999999998224 ) ) ;
#56419=ADVANCED_FACE ( 'NONE', ( #4439 ), #21402, .F. ) ;
#56420=( BOUNDED_CURVE ( )  B_SPLINE_CURVE ( 2, ( #48705, #54606, #64587, #2900, #20607, #31710, #70130, #2537, #54245 ),
 .UNSPECIFIED., .F., .F. ) 
 B_SPLINE_CURVE_WITH_KNOTS ( ( 3, 2, 2, 2, 3 ),
 ( 0.8369565217391304879, 0.8405797101449274944, 0.8478260869565217295, 0.8550724637681159646, 0.8586956521739130821 ),
 .UNSPECIFIED. ) 
 CURVE ( )  GEOMETRIC_REPRESENTATION_ITEM ( )  RATIONAL_B_SPLINE_CURVE ( ( 0.9330127018922192983, 0.9330127018922202975, 1.000000000000000000, 0.8660254037844387076, 1.000000000000000000, 0.8660254037844387076, 1.000000000000000000, 0.9330127018922194093, 0.9330127018922194093 ) ) 
 REPRESENTATION_ITEM ( '' )  );
#56421=CARTESIAN_POINT ( 'NONE',  ( 29.78437500061451715, 4.541064518000418104, 2.621784821874999949 ) ) ;
#56423=CARTESIAN_POINT ( 'NONE',  ( 16.19062500061451715, 6.054752690667223547, 3.707466751127219781E-16 ) ) ;
#56424=CARTESIAN_POINT ( 'NONE',  ( 9.103125000614515017, 0.000000000000000000, 5.243569643749999010 ) ) ;
#56426=CARTESIAN_POINT ( 'NONE',  ( 3.496875000614518836, -3.027376345333610441, -5.243569643749999898 ) ) ;
#56427=CARTESIAN_POINT ( 'NONE',  ( 17.77500000122903145, 2.886751345948129099, -4.999999999999998224 ) ) ;
#56428=CARTESIAN_POINT ( 'NONE',  ( 22.57499999999999929, 6.123233995736764310E-16, -4.999999999999998224 ) ) ;
#56429=CARTESIAN_POINT ( 'NONE',  ( 6.721875000614518925, 3.027376345333613106, -5.243569643749998122 ) ) ;
#56430=CARTESIAN_POINT ( 'NONE',  ( 12.12187500061451573, 3.027376345333613106, -5.243569643749998122 ) ) ;
#56431=CARTESIAN_POINT ( 'NONE',  ( 21.57187500061451502, 3.027376345333613106, -5.243569643749998122 ) ) ;
#56432=CARTESIAN_POINT ( 'NONE',  ( 2.000000000000001332, 15.76250000122903216, -26.53589838486224650 ) ) ;
#56433=ORIENTED_EDGE ( 'NONE', *, *, #44720, .T. ) ;
#56434=CARTESIAN_POINT ( 'NONE',  ( 4.096875000614518925, 6.054752690667223547, 3.707466751127219781E-16 ) ) ;
#56435=CARTESIAN_POINT ( 'NONE',  ( 5.896875000614518747, 6.054752690667223547, 3.707466751127219781E-16 ) ) ;
#56436=CARTESIAN_POINT ( 'NONE',  ( 18.33749999999999858, -2.886751345948129988, 4.999999999999997335 ) ) ;
#56437=CARTESIAN_POINT ( 'NONE',  ( 17.09062500061451573, 6.054752690667223547, 3.707466751127219781E-16 ) ) ;
#56441=CARTESIAN_POINT ( 'NONE',  ( 10.41562500061451679, 3.027376345333611329, 5.243569643749999010 ) ) ;
#56442=CARTESIAN_POINT ( 'NONE',  ( 26.37187500061451217, -6.054752690667223547, -1.112240025338166033E-15 ) ) ;
#56443=DIRECTION ( 'NONE',  ( 0.000000000000000000, 0.000000000000000000, -1.000000000000000000 ) ) ;
#56444=CARTESIAN_POINT ( 'NONE',  ( 28.13437500061451502, -4.541064518000419881, 2.621784821874995952 ) ) ;
#56445=CARTESIAN_POINT ( 'NONE',  ( 10.42500000000000071, 6.123233995736764310E-16, -4.999999999999998224 ) ) ;
#56446=CARTESIAN_POINT ( 'NONE',  ( 8.484601909799253346E-16, 16.62500000122903288, 34.61880215351700230 ) ) ;
#56447=CARTESIAN_POINT ( 'NONE',  ( 9.337500001229033231, 4.330127018922191873, 2.499999999999999556 ) ) ;
#56448=CARTESIAN_POINT ( 'NONE',  ( 18.83437500061451431, 6.421520780324663323E-16, -5.243569643749999010 ) ) ;
#56449=CARTESIAN_POINT ( 'NONE',  ( 13.35937500061451821, -4.541064518000417216, -2.621784821875001281 ) ) ;
#56451=ORIENTED_EDGE ( 'NONE', *, *, #61270, .T. ) ;
#56452=CARTESIAN_POINT ( 'NONE',  ( 13.64062500061451644, -3.027376345333614438, 5.243569643749998122 ) ) ;
#56453=CARTESIAN_POINT ( 'NONE',  ( 27.30000000122903359, 5.773502691896255534, 3.535250795749688894E-16 ) ) ;
#56454=CARTESIAN_POINT ( 'NONE',  ( 15.90937500061451892, 0.000000000000000000, 5.243569643749999010 ) ) ;
#56455=CARTESIAN_POINT ( 'NONE',  ( 4.520916466877470619, 8.924797207603102578, -33.96362936841865121 ) ) ;
#56456=CARTESIAN_POINT ( 'NONE',  ( 18.17812500061451786, -4.541064518000419881, 2.621784821874995952 ) ) ;
#56458=CARTESIAN_POINT ( 'NONE',  ( 27.04687500061451644, 6.054752690667223547, 3.707466751127219781E-16 ) ) ;
#56459=CARTESIAN_POINT ( 'NONE',  ( 9.001249775931846008E-16, 10.91562500061451857, 34.90005215228797653 ) ) ;
#56460=CARTESIAN_POINT ( 'NONE',  ( 15.30937500061451750, 4.541064518000418104, -2.621784821874998173 ) ) ;
#56461=CARTESIAN_POINT ( 'NONE',  ( 13.20000000122903394, -2.886751345948125991, -5.000000000000000000 ) ) ;
#56463=CARTESIAN_POINT ( 'NONE',  ( -4.243569643749998122, 19.44687500061451857, -27.54997392385601174 ) ) ;
#56464=CARTESIAN_POINT ( 'NONE',  ( 17.59687500061451715, 6.054752690667223547, 3.707466751127219781E-16 ) ) ;
#56465=CARTESIAN_POINT ( 'NONE',  ( 19.53750000122903430, 6.123233995736764310E-16, -4.999999999999998224 ) ) ;
#56466=CARTESIAN_POINT ( 'NONE',  ( 15.72187500061451892, 3.027376345333613106, -5.243569643749998122 ) ) ;
#56467=CARTESIAN_POINT ( 'NONE',  ( 4.243569643749999898, 13.33437500061451786, 30.00000000000000000 ) ) ;
#56468=CARTESIAN_POINT ( 'NONE',  ( 21.52500000122903145, 2.886751345948126879, 4.999999999999999112 ) ) ;
#56469=CARTESIAN_POINT ( 'NONE',  ( 15.89062500061451289, -3.027376345333614438, 5.243569643749998122 ) ) ;
#56471=ORIENTED_EDGE ( 'NONE', *, *, #37141, .T. ) ;
#56472=CARTESIAN_POINT ( 'NONE',  ( 21.56250000000000000, -5.773502691896255534, -1.060575238724906372E-15 ) ) ;
#56473=CARTESIAN_POINT ( 'NONE',  ( 17.62500000000000000, 6.123233995736764310E-16, -4.999999999999998224 ) ) ;
#56474=CARTESIAN_POINT ( 'NONE',  ( 4.190625000614518925, -3.027376345333614438, 5.243569643749998122 ) ) ;
#56476=CARTESIAN_POINT ( 'NONE',  ( 15.93750000122903110, 6.123233995736764310E-16, -4.999999999999998224 ) ) ;
#56477=CARTESIAN_POINT ( 'NONE',  ( 20.09062500061451573, -3.027376345333610441, -5.243569643749999898 ) ) ;
#56478=CARTESIAN_POINT ( 'NONE',  ( 24.25312500061451715, 4.541064518000418104, -2.621784821874998173 ) ) ;
#56479=CARTESIAN_POINT ( 'NONE',  ( 4.640625000614518214, -3.027376345333614438, 5.243569643749998122 ) ) ;
#56480=CARTESIAN_POINT ( 'NONE',  ( 29.88749999999999929, 5.773502691896255534, 3.535250795749688894E-16 ) ) ;
#56481=CARTESIAN_POINT ( 'NONE',  ( 1.999999999999998668, 11.86250000122903359, 26.53589838486224650 ) ) ;
#56484=CARTESIAN_POINT ( 'NONE',  ( 2.000000000000001332, 11.71250000122903501, -26.53589838486224650 ) ) ;
#56485=CARTESIAN_POINT ( 'NONE',  ( -4.243569643749997233, 18.99687500061451928, -27.54997392385601174 ) ) ;
#56486=CARTESIAN_POINT ( 'NONE',  ( 5.250000001229035540, 5.773502691896255534, 3.535250795749688894E-16 ) ) ;
#56487=CARTESIAN_POINT ( 'NONE',  ( 8.550000000000002487, -4.330127018922190985, -2.500000000000001332 ) ) ;
#56488=CARTESIAN_POINT ( 'NONE',  ( 3.487500001229035362, 4.330127018922191873, 2.499999999999999556 ) ) ;
#56489=CARTESIAN_POINT ( 'NONE',  ( 12.49687500061451573, -3.027376345333610441, -5.243569643749999898 ) ) ;
#56490=CARTESIAN_POINT ( 'NONE',  ( 24.52500000122903501, 2.886751345948146419, -4.999999999999968914 ) ) ;
#56491=CARTESIAN_POINT ( 'NONE',  ( 3.834375000614519635, -4.541064518000419881, 2.621784821874995952 ) ) ;
#56494=CARTESIAN_POINT ( 'NONE',  ( 9.759375000614516793, -4.541064518000417216, -2.621784821875001281 ) ) ;
#56495=CARTESIAN_POINT ( 'NONE',  ( 2.000000000000001332, 14.30000000000000071, 33.46410161513774995 ) ) ;
#56496=CARTESIAN_POINT ( 'NONE',  ( -2.121784821874999949, 16.57812500061459815, 26.32496088578401938 ) ) ;
#56497=CARTESIAN_POINT ( 'NONE',  ( 21.53437500061451715, 6.421520780324663323E-16, -5.243569643749999010 ) ) ;
#56499=EDGE_CURVE ( 'NONE', #26952, #37978, #6609, .T. ) ;
#56500=CARTESIAN_POINT ( 'NONE',  ( 29.51250000122903216, 4.330127018922192761, -2.499999999999997780 ) ) ;
#56502=CARTESIAN_POINT ( 'NONE',  ( 22.11562500061451786, 3.027376345333611329, 5.243569643749999010 ) ) ;
#56503=CARTESIAN_POINT ( 'NONE',  ( 15.14062500061451644, -3.027376345333610441, -5.243569643749999898 ) ) ;
#56505=CARTESIAN_POINT ( 'NONE',  ( 11.63437500061451857, 6.421520780324663323E-16, -5.243569643749999010 ) ) ;
#56506=CARTESIAN_POINT ( 'NONE',  ( 27.86249999999999716, -5.773502691896255534, -1.060575238724906372E-15 ) ) ;
#56507=CARTESIAN_POINT ( 'NONE',  ( 25.98750000122903003, 4.330127018922191873, 2.499999999999999556 ) ) ;
#56508=CARTESIAN_POINT ( 'NONE',  ( 3.196875000614516793, 6.054752690667223547, 3.707466751127219781E-16 ) ) ;
#56509=CARTESIAN_POINT ( 'NONE',  ( 14.25937500061451679, -4.541064518000417216, -2.621784821875001281 ) ) ;
#56510=CARTESIAN_POINT ( 'NONE',  ( 28.84687500061452070, 6.054752690667223547, 3.707466751127219781E-16 ) ) ;
#56511=CARTESIAN_POINT ( 'NONE',  ( 8.250000001229034652, -2.886751345948126435, -5.000000000000000000 ) ) ;
#56513=CARTESIAN_POINT ( 'NONE',  ( 21.90937500061451715, -4.541064518000417216, -2.621784821875001281 ) ) ;
#56514=CARTESIAN_POINT ( 'NONE',  ( 15.42187500061451821, 3.027376345333611329, 5.243569643749999010 ) ) ;
#56516=CARTESIAN_POINT ( 'NONE',  ( 26.47499999999999787, -4.330127018922194537, 2.499999999999995559 ) ) ;
#56517=CARTESIAN_POINT ( 'NONE',  ( 3.862500001229035362, 4.330127018922192761, -2.499999999999997780 ) ) ;
#56519=CARTESIAN_POINT ( 'NONE',  ( 16.49062500061451786, -3.027376345333610441, -5.243569643749999898 ) ) ;
#56520=CARTESIAN_POINT ( 'NONE',  ( 6.299999999999999822, -4.330127018922190985, -2.500000000000001332 ) ) ;
#56521=DIRECTION ( 'NONE',  ( -0.9848080501874550974, 0.000000000000000000, 0.1736464922939214839 ) ) ;
#56522=CARTESIAN_POINT ( 'NONE',  ( 17.28750000000000142, 5.773502691896255534, 3.535250795749688894E-16 ) ) ;
#56523=CARTESIAN_POINT ( 'NONE',  ( 2.121784821875001281, 13.65312500061451750, 33.67503911421598417 ) ) ;
#56525=CARTESIAN_POINT ( 'NONE',  ( 19.83750000122903145, -4.330127018922194537, 2.499999999999995559 ) ) ;
#56526=DIRECTION ( 'NONE',  ( -0.000000000000000000, -1.000000000000000000, -0.000000000000000000 ) ) ;
#56527=CARTESIAN_POINT ( 'NONE',  ( 27.94687500061451502, 6.054752690667223547, 3.707466751127219781E-16 ) ) ;
#56529=CARTESIAN_POINT ( 'NONE',  ( 22.64062500061451644, -3.027376345333614438, 5.243569643749998122 ) ) ;
#56530=CARTESIAN_POINT ( 'NONE',  ( 21.68437500061451573, 4.541064518000418104, 2.621784821874999949 ) ) ;
#56531=CARTESIAN_POINT ( 'NONE',  ( 5.625000000000001776, 4.330127018922191873, 2.499999999999999556 ) ) ;
#56532=CARTESIAN_POINT ( 'NONE',  ( 8.953125000614518214, 4.541064518000418104, -2.621784821874998173 ) ) ;
#56533=CARTESIAN_POINT ( 'NONE',  ( 24.06562500061451715, -6.054752690667223547, -1.112240025338166033E-15 ) ) ;
#56534=CARTESIAN_POINT ( 'NONE',  ( 12.34687500061452070, -3.027376345333614438, 5.243569643749998122 ) ) ;
#56535=CARTESIAN_POINT ( 'NONE',  ( 16.84687500061451715, -3.027376345333614438, 5.243569643749998122 ) ) ;
#56536=CARTESIAN_POINT ( 'NONE',  ( 0.000000000000000000, 20.00000000000000000, -33.99999999999999289 ) ) ;
#56537=CARTESIAN_POINT ( 'NONE',  ( 2.121784821874999061, 16.50312500061451715, 26.32496088578401583 ) ) ;
#56538=CARTESIAN_POINT ( 'NONE',  ( 21.45000000122903216, 5.773502691896255534, 3.535250795749688894E-16 ) ) ;
#56540=CARTESIAN_POINT ( 'NONE',  ( 11.91562500061451857, -6.054752690667223547, -1.112240025338166033E-15 ) ) ;
#56541=CARTESIAN_POINT ( 'NONE',  ( 6.571875000614517681, -6.054752690667223547, -1.112240025338166033E-15 ) ) ;
#56542=CARTESIAN_POINT ( 'NONE',  ( 5.371875000614516615, 3.027376345333613106, -5.243569643749998122 ) ) ;
#56543=ORIENTED_EDGE ( 'NONE', *, *, #30819, .T. ) ;
#56544=CARTESIAN_POINT ( 'NONE',  ( 25.50937500061451502, -4.541064518000417216, -2.621784821875001281 ) ) ;
#56545=CARTESIAN_POINT ( 'NONE',  ( 16.26562500061451289, 3.027376345333611329, 5.243569643749999010 ) ) ;
#56546=CARTESIAN_POINT ( 'NONE',  ( 27.67500000122903359, 2.886751345948129099, -4.999999999999998224 ) ) ;
#56547=CARTESIAN_POINT ( 'NONE',  ( 28.52812500061451573, -4.541064518000419881, 2.621784821874995952 ) ) ;
#56548=CARTESIAN_POINT ( 'NONE',  ( 22.47187500061451715, 3.027376345333613106, -5.243569643749998122 ) ) ;
#56549=CARTESIAN_POINT ( 'NONE',  ( 16.64062500061451289, 6.054752690667223547, 3.707466751127219781E-16 ) ) ;
#56550=CARTESIAN_POINT ( 'NONE',  ( -2.121784821874999949, 19.33437500061451786, 26.32496088578401938 ) ) ;
#56551=CARTESIAN_POINT ( 'NONE',  ( 23.54062500061451146, -3.027376345333614438, 5.243569643749998122 ) ) ;
#56552=CARTESIAN_POINT ( 'NONE',  ( 4.725000001229034297, 2.886751345948129099, -4.999999999999998224 ) ) ;
#56553=ORIENTED_EDGE ( 'NONE', *, *, #7032, .F. ) ;
#56554=CARTESIAN_POINT ( 'NONE',  ( 28.01249999999999574, 2.886751345948129099, -4.999999999999998224 ) ) ;
#56555=CARTESIAN_POINT ( 'NONE',  ( -3.999999999999999112, 13.25000000000000178, -30.00000000000000000 ) ) ;
#56557=CARTESIAN_POINT ( 'NONE',  ( 2.859375000614519546, 0.000000000000000000, 5.243569643749999010 ) ) ;
#56558=CARTESIAN_POINT ( 'NONE',  ( 10.86562500061451431, 3.027376345333611329, 5.243569643749999010 ) ) ;
#56559=CARTESIAN_POINT ( 'NONE',  ( 21.82500000122903572, 2.886751345948129099, -4.999999999999998224 ) ) ;
#56560=CARTESIAN_POINT ( 'NONE',  ( 12.83437500061451786, -4.541064518000419881, 2.621784821874995952 ) ) ;
#56561=CARTESIAN_POINT ( 'NONE',  ( 3.721875000614518036, 3.027376345333611329, 5.243569643749999010 ) ) ;
#56562=CARTESIAN_POINT ( 'NONE',  ( 26.73749999999999716, 5.773502691896255534, 3.535250795749688894E-16 ) ) ;
#56563=CARTESIAN_POINT ( 'NONE',  ( 14.70000000122903216, 5.773502691896255534, 3.535250795749688401E-16 ) ) ;
#56564=CARTESIAN_POINT ( 'NONE',  ( 13.60312500061451679, 0.000000000000000000, 5.243569643749999010 ) ) ;
#56565=ORIENTED_EDGE ( 'NONE', *, *, #55072, .T. ) ;
#56566=CARTESIAN_POINT ( 'NONE',  ( 9.515625000614518214, 3.027376345333611329, 5.243569643749999010 ) ) ;
#56567=CARTESIAN_POINT ( 'NONE',  ( 7.040625000614517681, -3.027376345333610441, -5.243569643749999898 ) ) ;
#56569=CARTESIAN_POINT ( 'NONE',  ( 9.528763966825557376E-15, 17.07500000122903572, -26.00000000000000000 ) ) ;
#56570=CARTESIAN_POINT ( 'NONE',  ( 15.86250000000000249, 2.886751345948129099, -4.999999999999998224 ) ) ;
#56572=CARTESIAN_POINT ( 'NONE',  ( 16.02187500061451786, -6.054752690667223547, -1.112240025338166033E-15 ) ) ;
#56573=CARTESIAN_POINT ( 'NONE',  ( 11.47500000122903252, 2.886751345948129099, -4.999999999999998224 ) ) ;
#56574=EDGE_CURVE ( 'NONE', #16892, #45352, #22773, .T. ) ;
#56575=CARTESIAN_POINT ( 'NONE',  ( 18.60937500061451644, 0.000000000000000000, 5.243569643749999010 ) ) ;
#56577=CARTESIAN_POINT ( 'NONE',  ( 19.88437500061451857, 4.541064518000418104, 2.621784821874999949 ) ) ;
#56578=CARTESIAN_POINT ( 'NONE',  ( 2.121784821874999061, 14.70312500061451644, -33.67503911421598417 ) ) ;
#56579=CARTESIAN_POINT ( 'NONE',  ( 3.999999999999998668, 16.66250000000000142, 27.69059892324149530 ) ) ;
#56582=CARTESIAN_POINT ( 'NONE',  ( 27.59062500061451573, -3.027376345333614438, 5.243569643749998122 ) ) ;
#56583=CARTESIAN_POINT ( 'NONE',  ( 25.01249999999999929, 2.886751345948126879, 4.999999999999998224 ) ) ;
#56584=CARTESIAN_POINT ( 'NONE',  ( 27.83437500061451786, 6.421520780324663323E-16, -5.243569643749999010 ) ) ;
#56585=CARTESIAN_POINT ( 'NONE',  ( 25.05000000000000071, 0.000000000000000000, 4.999999999999998224 ) ) ;
#56586=EDGE_CURVE ( 'NONE', #18379, #8722, #30332, .T. ) ;
#56587=CARTESIAN_POINT ( 'NONE',  ( 8.240625000614516082, -3.027376345333614438, 5.243569643749998122 ) ) ;
#56589=CARTESIAN_POINT ( 'NONE',  ( 17.97187500061451715, 3.027376345333613106, -5.243569643749998122 ) ) ;
#56591=CARTESIAN_POINT ( 'NONE',  ( 6.103125000614515905, -4.541064518000417216, -2.621784821875001281 ) ) ;
#56592=CARTESIAN_POINT ( 'NONE',  ( 9.721875000614517148, -6.054752690667223547, -1.112240025338166033E-15 ) ) ;
#56593=ORIENTED_EDGE ( 'NONE', *, *, #5758, .T. ) ;
#56594=CARTESIAN_POINT ( 'NONE',  ( 22.32187500061451502, -6.054752690667223547, -1.112240025338166033E-15 ) ) ;
#56596=CARTESIAN_POINT ( 'NONE',  ( 28.49999999999999645, 4.330127018922192761, -2.499999999999997780 ) ) ;
#56597=CARTESIAN_POINT ( 'NONE',  ( 3.187500000000002220, -2.886751345948125991, -5.000000000000000000 ) ) ;
#56598=CARTESIAN_POINT ( 'NONE',  ( 15.00000000122903465, -2.886751345948125991, -5.000000000000000000 ) ) ;
#56599=CARTESIAN_POINT ( 'NONE',  ( 30.00000000000000000, 6.123233995736764310E-16, -4.999999999999998224 ) ) ;
#56600=CARTESIAN_POINT ( 'NONE',  ( 3.768252779319924972, -3.286398503110366409, 4.085920018314769919 ) ) ;
#56602=CARTESIAN_POINT ( 'NONE',  ( 13.64999999999999858, 4.330127018922192761, -2.499999999999997780 ) ) ;
#56603=CARTESIAN_POINT ( 'NONE',  ( 23.69062500061451004, -3.027376345333610441, -5.243569643749999898 ) ) ;
#56604=CARTESIAN_POINT ( 'NONE',  ( 14.88750000000000107, -2.886751345948125991, -5.000000000000000000 ) ) ;
#56605=CARTESIAN_POINT ( 'NONE',  ( 10.65000000122903323, 5.773502691896255534, 3.535250795749688894E-16 ) ) ;
#56606=CARTESIAN_POINT ( 'NONE',  ( 7.903125000614515727, -4.541064518000417216, -2.621784821875001281 ) ) ;
#56607=CARTESIAN_POINT ( 'NONE',  ( 9.037499999999999645, -2.886751345948125991, -5.000000000000000000 ) ) ;
#56608=CARTESIAN_POINT ( 'NONE',  ( 19.31250000122903288, 0.000000000000000000, 4.999999999999998224 ) ) ;
#56609=CARTESIAN_POINT ( 'NONE',  ( 9.001249775931846008E-16, 13.67187500061451999, -25.09994784771203058 ) ) ;
#56610=CARTESIAN_POINT ( 'NONE',  ( 27.97500000122903074, -5.773502691896255534, -1.060575238724906372E-15 ) ) ;
#56612=CARTESIAN_POINT ( 'NONE',  ( 6.675000000000000711, -4.330127018922194537, 2.499999999999995559 ) ) ;
#56614=ORIENTED_EDGE ( 'NONE', *, *, #58189, .F. ) ;
#56615=CARTESIAN_POINT ( 'NONE',  ( 20.80312500061451431, 0.000000000000000000, 5.243569643749999010 ) ) ;
#56616=CARTESIAN_POINT ( 'NONE',  ( 13.42500000122903536, 2.886751345948126879, 4.999999999999999112 ) ) ;
#56617=CARTESIAN_POINT ( 'NONE',  ( 3.346476778685950837, -3.715034440765132562, -3.519825879858566431 ) ) ;
#56618=CARTESIAN_POINT ( 'NONE',  ( 28.58437500061451786, -4.541064518000419881, 2.621784821874995952 ) ) ;
#56619=CARTESIAN_POINT ( 'NONE',  ( 20.03437500061451715, -4.541064518000419881, 2.621784821874995952 ) ) ;
#56620=CARTESIAN_POINT ( 'NONE',  ( 17.01562500061451644, 3.027376345333613106, -5.243569643749998122 ) ) ;
#56621=CARTESIAN_POINT ( 'NONE',  ( -2.121784821874999949, 11.17812500061459424, -33.67503911421598417 ) ) ;
#56622=CARTESIAN_POINT ( 'NONE',  ( 6.965625000614518392, -6.054752690667223547, -1.112240025338166033E-15 ) ) ;
#56623=( BOUNDED_CURVE ( )  B_SPLINE_CURVE ( 2, ( #40832, #18259, #29377, #13445, #46007, #41546, #68543, #63348, #7557 ),
 .UNSPECIFIED., .F., .F. ) 
 B_SPLINE_CURVE_WITH_KNOTS ( ( 3, 2, 2, 2, 3 ),
 ( 0.8804347826086956763, 0.8840579710144927938, 0.8913043478260869179, 0.8985507246376811530, 0.9021739130434782705 ),
 .UNSPECIFIED. ) 
 CURVE ( )  GEOMETRIC_REPRESENTATION_ITEM ( )  RATIONAL_B_SPLINE_CURVE ( ( 0.9330127018922194093, 0.9330127018922194093, 1.000000000000000000, 0.8660254037844387076, 1.000000000000000000, 0.8660254037844387076, 1.000000000000000000, 0.9330127018922194093, 0.9330127018922194093 ) ) 
 REPRESENTATION_ITEM ( '' )  );
#56624=CARTESIAN_POINT ( 'NONE',  ( 27.56250000122902932, -4.330127018922190985, -2.500000000000001332 ) ) ;
#56626=CARTESIAN_POINT ( 'NONE',  ( 19.71562500061451928, 3.027376345333612662, -5.243569643749998122 ) ) ;
#56627=CARTESIAN_POINT ( 'NONE',  ( 30.00000000000000000, 0.000000000000000000, 0.000000000000000000 ) ) ;
#56629=CARTESIAN_POINT ( 'NONE',  ( 12.72187500061451537, 3.027376345333611329, 5.243569643749999010 ) ) ;
#56630=CARTESIAN_POINT ( 'NONE',  ( 11.18437500061451928, 6.421520780324663323E-16, -5.243569643749999010 ) ) ;
#56631=CARTESIAN_POINT ( 'NONE',  ( 19.69687500061451857, -3.027376345333610441, -5.243569643749999898 ) ) ;
#56632=ORIENTED_EDGE ( 'NONE', *, *, #10028, .T. ) ;
#56633=CARTESIAN_POINT ( 'NONE',  ( 24.92812500061451431, -4.541064518000419881, 2.621784821874995952 ) ) ;
#56634=CARTESIAN_POINT ( 'NONE',  ( 19.28437500061451360, 6.421520780324663323E-16, -5.243569643749999010 ) ) ;
#56635=CARTESIAN_POINT ( 'NONE',  ( 23.72812500061451502, 6.421520780324663323E-16, -5.243569643749999010 ) ) ;
#56637=CARTESIAN_POINT ( 'NONE',  ( -3.999999999999997335, 17.33749999999999858, 32.30940107675850470 ) ) ;
#56638=CARTESIAN_POINT ( 'NONE',  ( 3.721875000614518036, 3.027376345333611329, 5.243569643749999010 ) ) ;
#56639=CARTESIAN_POINT ( 'NONE',  ( 12.71250000122903145, -4.330127018922190985, -2.500000000000001332 ) ) ;
#56640=CARTESIAN_POINT ( 'NONE',  ( 6.150000001229033231, 5.773502691896255534, 3.535250795749688894E-16 ) ) ;
#56641=CARTESIAN_POINT ( 'NONE',  ( 4.000000000000000000, 19.28750000000000142, -27.69059892324149530 ) ) ;
#56642=CARTESIAN_POINT ( 'NONE',  ( 26.73750000122903003, 6.123233995736764310E-16, -4.999999999999998224 ) ) ;
#56645=CARTESIAN_POINT ( 'NONE',  ( 11.63437500061451857, 6.421520780324663323E-16, -5.243569643749999010 ) ) ;
#56647=CARTESIAN_POINT ( 'NONE',  ( 17.69062500061451715, -3.027376345333614438, 5.243569643749998122 ) ) ;
#56648=CARTESIAN_POINT ( 'NONE',  ( 12.98437500061451821, 6.421520780324663323E-16, -5.243569643749999010 ) ) ;
#56649=CARTESIAN_POINT ( 'NONE',  ( 3.965625000614515727, 3.027376345333613106, -5.243569643749998122 ) ) ;
#56650=CARTESIAN_POINT ( 'NONE',  ( 19.62187500061451573, -6.054752690667223547, -1.112240025338166033E-15 ) ) ;
#56651=CARTESIAN_POINT ( 'NONE',  ( 10.09687500061451715, -3.027376345333614438, 5.243569643749998122 ) ) ;
#56654=CARTESIAN_POINT ( 'NONE',  ( 5.700000001229033941, 5.773502691896255534, 3.535250795749688894E-16 ) ) ;
#56655=CARTESIAN_POINT ( 'NONE',  ( 19.67812500061451786, 6.421520780324663323E-16, -5.243569643749999010 ) ) ;
#56656=( BOUNDED_CURVE ( )  B_SPLINE_CURVE ( 2, ( #45627, #40086, #52605, #64041, #64773, #69956, #36697 ),
 .UNSPECIFIED., .F., .F. ) 
 B_SPLINE_CURVE_WITH_KNOTS ( ( 3, 2, 2, 3 ),
 ( 0.05000000000000003053, 0.05277777777777779844, 0.05555555555555556635, 0.05833333333333334120 ),
 .UNSPECIFIED. ) 
 CURVE ( )  GEOMETRIC_REPRESENTATION_ITEM ( )  RATIONAL_B_SPLINE_CURVE ( ( 0.9999999999999986677, 0.8660254037844400399, 1.000000000000000000, 0.8660254037844387076, 1.000000000000000000, 0.8660254037844383745, 1.000000000000000222 ) ) 
 REPRESENTATION_ITEM ( '' )  );
#56657=CARTESIAN_POINT ( 'NONE',  ( 6.862500001229034474, -4.330127018922190985, -2.500000000000001332 ) ) ;
#56658=CARTESIAN_POINT ( 'NONE',  ( 18.25312500061451715, -4.541064518000417216, -2.621784821875001281 ) ) ;
#56659=CARTESIAN_POINT ( 'NONE',  ( 13.00312500061451537, 4.541064518000418104, -2.621784821874998173 ) ) ;
#56661=CARTESIAN_POINT ( 'NONE',  ( 13.53749999999999964, -2.886751345948125991, -5.000000000000000000 ) ) ;
#56662=CARTESIAN_POINT ( 'NONE',  ( 8.512500001229033941, 0.000000000000000000, 4.999999999999998224 ) ) ;
#56663=CARTESIAN_POINT ( 'NONE',  ( 6.253125000614517148, 4.541064518000418104, -2.621784821874998173 ) ) ;
#56664=CARTESIAN_POINT ( 'NONE',  ( 18.07500000122903216, -5.773502691896255534, -1.060575238724906372E-15 ) ) ;
#56666=CARTESIAN_POINT ( 'NONE',  ( 4.243569643749999898, 11.49687500061451928, -27.54997392385601529 ) ) ;
#56667=CARTESIAN_POINT ( 'NONE',  ( 4.561349860989134974, -2.048213574975756401, 4.693545306252407734 ) ) ;
#56669=CARTESIAN_POINT ( 'NONE',  ( 2.775000001229033675, -5.773502691896255534, -1.060575238724906372E-15 ) ) ;
#56670=CARTESIAN_POINT ( 'NONE',  ( 20.18437500061451573, 6.421520780324663323E-16, -5.243569643749999010 ) ) ;
#56671=CARTESIAN_POINT ( 'NONE',  ( 17.12812500061451715, 4.541064518000418104, 2.621784821874999949 ) ) ;
#56673=CARTESIAN_POINT ( 'NONE',  ( 11.06250000000000178, 2.886751345948126879, 4.999999999999998224 ) ) ;
#56674=CARTESIAN_POINT ( 'NONE',  ( -5.810221930991193690E-16, 14.15000000122903145, 26.00000000000000355 ) ) ;
#56675=CARTESIAN_POINT ( 'NONE',  ( 27.08437500061451786, 4.541064518000418104, 2.621784821874999949 ) ) ;
#56677=CARTESIAN_POINT ( 'NONE',  ( 11.31562500061451892, 3.027376345333611329, 5.243569643749999010 ) ) ;
#56678=CARTESIAN_POINT ( 'NONE',  ( 11.97187500061451892, -6.054752690667223547, -1.112240025338166033E-15 ) ) ;
#56680=CARTESIAN_POINT ( 'NONE',  ( 9.375000000000001776, -4.330127018922194537, 2.499999999999995559 ) ) ;
#56681=CARTESIAN_POINT ( 'NONE',  ( 20.76562500061451644, 3.027376345333611329, 5.243569643749999010 ) ) ;
#56682=DIRECTION ( 'NONE',  ( -0.000000000000000000, -1.000000000000000000, -0.000000000000000000 ) ) ;
#56683=CARTESIAN_POINT ( 'NONE',  ( 12.67499999999999893, 6.123233995736764310E-16, -4.999999999999998224 ) ) ;
#56684=CARTESIAN_POINT ( 'NONE',  ( 22.08750000122903501, -4.330127018922194537, 2.499999999999995559 ) ) ;
#56685=CARTESIAN_POINT ( 'NONE',  ( 15.47812500061451679, -4.541064518000419881, 2.621784821874995952 ) ) ;
#56688=CARTESIAN_POINT ( 'NONE',  ( 20.40000000000000213, 4.330127018922192761, -2.499999999999997780 ) ) ;
#56689=CARTESIAN_POINT ( 'NONE',  ( 23.55000000000000071, 4.330127018922192761, -2.499999999999997780 ) ) ;
#56690=CARTESIAN_POINT ( 'NONE',  ( 22.13437500061451502, 4.541064518000418104, 2.621784821874999949 ) ) ;
#56691=CARTESIAN_POINT ( 'NONE',  ( 25.86562500061451431, -6.054752690667223547, -1.112240025338166033E-15 ) ) ;
#56692=ORIENTED_EDGE ( 'NONE', *, *, #23221, .T. ) ;
#56693=CARTESIAN_POINT ( 'NONE',  ( 8.962500001229033231, 0.000000000000000000, 4.999999999999998224 ) ) ;
#56694=CARTESIAN_POINT ( 'NONE',  ( 7.565625000614518036, 3.027376345333613106, -5.243569643749998122 ) ) ;
#56696=CARTESIAN_POINT ( 'NONE',  ( 14.66249999999999964, 2.886751345948126879, 4.999999999999999112 ) ) ;
#56697=CARTESIAN_POINT ( 'NONE',  ( 9.001249775931846008E-16, 18.56562500061451715, 34.90005215228797653 ) ) ;
#56698=CARTESIAN_POINT ( 'NONE',  ( 3.834375000614519635, -4.541064518000419881, 2.621784821874995952 ) ) ;
#56699=CARTESIAN_POINT ( 'NONE',  ( 27.38437500061451857, 6.421520780324663323E-16, -5.243569643749999010 ) ) ;
#56701=CARTESIAN_POINT ( 'NONE',  ( 24.29062500061451502, 6.054752690667223547, 3.707466751127219781E-16 ) ) ;
#56702=CARTESIAN_POINT ( 'NONE',  ( 25.47187500061451715, -6.054752690667223547, -1.112240025338166033E-15 ) ) ;
#56703=CARTESIAN_POINT ( 'NONE',  ( 11.62500000000000000, -4.330127018922194537, 2.499999999999995559 ) ) ;
#56704=CARTESIAN_POINT ( 'NONE',  ( 8.690625000614515372, -3.027376345333614438, 5.243569643749998122 ) ) ;
#56705=CARTESIAN_POINT ( 'NONE',  ( 3.849931240356728512, 3.190302406438068505, 3.849931240356827544 ) ) ;
#56706=CARTESIAN_POINT ( 'NONE',  ( 2.000000000000001332, 11.15000000000000213, 33.46410161513774995 ) ) ;
#56707=CARTESIAN_POINT ( 'NONE',  ( 25.60312500061451502, 4.541064518000418104, -2.621784821874998173 ) ) ;
#56710=CARTESIAN_POINT ( 'NONE',  ( 18.53437500061451715, 4.541064518000418104, 2.621784821874999949 ) ) ;
#56711=CARTESIAN_POINT ( 'NONE',  ( 2.121784821874999061, 15.20937500061451786, 26.32496088578401583 ) ) ;
#56712=CARTESIAN_POINT ( 'NONE',  ( 18.68437500061451928, -4.541064518000419881, 2.621784821874995952 ) ) ;
#56713=CARTESIAN_POINT ( 'NONE',  ( 27.64687500061452141, -3.027376345333614438, 5.243569643749998122 ) ) ;
#56714=CARTESIAN_POINT ( 'NONE',  ( 4.243569643749999898, 16.44687500061451857, 32.45002607614398471 ) ) ;
#56715=CARTESIAN_POINT ( 'NONE',  ( 9.815625000614518925, 3.027376345333613106, -5.243569643749998122 ) ) ;
#56716=CARTESIAN_POINT ( 'NONE',  ( 3.999999999999999112, 17.18750000122903288, 30.00000000000000000 ) ) ;
#56717=CARTESIAN_POINT ( 'NONE',  ( 4.846875000614519813, -3.027376345333610441, -5.243569643749999898 ) ) ;
#56718=CARTESIAN_POINT ( 'NONE',  ( 30.00000000000000000, 0.000000000000000000, 0.000000000000000000 ) ) ;
#56719=CARTESIAN_POINT ( 'NONE',  ( 7.040625000614517681, -3.027376345333610441, -5.243569643749999898 ) ) ;
#56720=CARTESIAN_POINT ( 'NONE',  ( 11.70937500061451608, 4.541064518000418104, -2.621784821874998173 ) ) ;
#56721=CARTESIAN_POINT ( 'NONE',  ( 20.21250000122903145, 0.000000000000000000, 4.999999999999998224 ) ) ;
#56722=CARTESIAN_POINT ( 'NONE',  ( 6.121875000614517504, -6.054752690667223547, -1.112240025338166033E-15 ) ) ;
#56723=CARTESIAN_POINT ( 'NONE',  ( 10.82812500061451644, 4.541064518000418104, 2.621784821874999949 ) ) ;
#56724=CARTESIAN_POINT ( 'NONE',  ( 5.690625000614515372, -3.027376345333610441, -5.243569643749999898 ) ) ;
#56726=CARTESIAN_POINT ( 'NONE',  ( 19.02187500061451786, 3.027376345333611329, 5.243569643749999010 ) ) ;
#56727=CARTESIAN_POINT ( 'NONE',  ( -3.999999999999999112, 11.52500000122903501, 27.69059892324149885 ) ) ;
#56728=ORIENTED_EDGE ( 'NONE', *, *, #47742, .T. ) ;
#56729=CARTESIAN_POINT ( 'NONE',  ( 24.70312500061451644, 4.541064518000418104, -2.621784821874998173 ) ) ;
#56730=CARTESIAN_POINT ( 'NONE',  ( 12.32812500061451821, -4.541064518000419881, 2.621784821874995952 ) ) ;
#56732=CARTESIAN_POINT ( 'NONE',  ( 12.17812500061451608, 4.541064518000418104, 2.621784821874999949 ) ) ;
#56733=CARTESIAN_POINT ( 'NONE',  ( 9.001249775931846008E-16, 10.07187500061451857, -25.09994784771203058 ) ) ;
#56734=CARTESIAN_POINT ( 'NONE',  ( 13.12500000122903288, -5.773502691896255534, -1.060575238724906372E-15 ) ) ;
#56735=ADVANCED_FACE ( 'NONE', ( #62384 ), #67939, .F. ) ;
#56736=CARTESIAN_POINT ( 'NONE',  ( 26.39062500061451644, -3.027376345333610441, -5.243569643749999898 ) ) ;
#56737=CARTESIAN_POINT ( 'NONE',  ( 9.001249775931846008E-16, 12.26562500061451644, -25.09994784771203058 ) ) ;
#56738=CARTESIAN_POINT ( 'NONE',  ( 15.41250000122903252, -4.330127018922190985, -2.500000000000001332 ) ) ;
#56739=CARTESIAN_POINT ( 'NONE',  ( 12.00000000000000000, 0.000000000000000000, 4.999999999999998224 ) ) ;
#56740=CARTESIAN_POINT ( 'NONE',  ( 21.10312500061451502, 4.541064518000418104, -2.621784821874998173 ) ) ;
#56741=CARTESIAN_POINT ( 'NONE',  ( 8.934375000614517504, 6.421520780324663323E-16, -5.243569643749999010 ) ) ;
#56742=CARTESIAN_POINT ( 'NONE',  ( 7.425000001229034474, 2.886751345948129099, -4.999999999999998224 ) ) ;
#56743=CARTESIAN_POINT ( 'NONE',  ( 15.26250000122903216, 0.000000000000000000, 4.999999999999998224 ) ) ;
#56744=CARTESIAN_POINT ( 'NONE',  ( 11.65312500061451573, 4.541064518000418104, -2.621784821874998173 ) ) ;
#56745=CARTESIAN_POINT ( 'NONE',  ( 16.82812500061451644, -4.541064518000419881, 2.621784821874995952 ) ) ;
#56746=CARTESIAN_POINT ( 'NONE',  ( 28.98750000122903359, 6.123233995736764310E-16, -4.999999999999998224 ) ) ;
#56747=CARTESIAN_POINT ( 'NONE',  ( 23.36250000000000071, -5.773502691896255534, -1.060575238724906372E-15 ) ) ;
#56748=CARTESIAN_POINT ( 'NONE',  ( 22.99687500061451573, 6.054752690667223547, 3.707466751127219781E-16 ) ) ;
#56749=CARTESIAN_POINT ( 'NONE',  ( 30.00000000000000000, 0.000000000000000000, 0.000000000000000000 ) ) ;
#56750=CARTESIAN_POINT ( 'NONE',  ( 9.975000001229034297, -5.773502691896255534, -1.060575238724906372E-15 ) ) ;
#56751=CARTESIAN_POINT ( 'NONE',  ( 27.45937500061451786, 4.541064518000418104, -2.621784821874998173 ) ) ;
#56752=CARTESIAN_POINT ( 'NONE',  ( 5.634375000614519458, -4.541064518000419881, 2.621784821874995952 ) ) ;
#56753=CARTESIAN_POINT ( 'NONE',  ( 24.29062500061451502, 6.054752690667223547, 3.707466751127219781E-16 ) ) ;
#56755=CYLINDRICAL_SURFACE ( 'NONE', #16142, 4.000000000000000000 ) ;
#56756=CARTESIAN_POINT ( 'NONE',  ( 9.984375000614518214, 4.541064518000418104, 2.621784821874999949 ) ) ;
#56757=CARTESIAN_POINT ( 'NONE',  ( 1.071796769724489895, 12.66740381056766651, 26.00000000000000355 ) ) ;
#56758=CARTESIAN_POINT ( 'NONE',  ( 29.69062500061451715, 6.054752690667223547, 3.707466751127219781E-16 ) ) ;
#56759=CARTESIAN_POINT ( 'NONE',  ( 6.646875000614518747, -3.027376345333610441, -5.243569643749999898 ) ) ;
#56760=CARTESIAN_POINT ( 'NONE',  ( -5.810221930991193690E-16, 14.48749999999999893, 26.00000000000000355 ) ) ;
#56761=CARTESIAN_POINT ( 'NONE',  ( 27.19687500061451857, -3.027376345333614438, 5.243569643749998122 ) ) ;
#56763=CARTESIAN_POINT ( 'NONE',  ( 2.121784821874999061, 11.10312500061459495, 26.32496088578401583 ) ) ;
#56764=CARTESIAN_POINT ( 'NONE',  ( 19.31250000000000000, -5.773502691896255534, -1.060575238724906372E-15 ) ) ;
#56765=ORIENTED_EDGE ( 'NONE', *, *, #27624, .T. ) ;
#56766=CARTESIAN_POINT ( 'NONE',  ( 26.51249999999999929, -5.773502691896255534, -1.060575238724906372E-15 ) ) ;
#56767=CARTESIAN_POINT ( 'NONE',  ( 29.25937500061451502, 4.541064518000418104, -2.621784821874998173 ) ) ;
#56768=ORIENTED_EDGE ( 'NONE', *, *, #4430, .T. ) ;
#56769=CARTESIAN_POINT ( 'NONE',  ( 16.64062500061451289, 6.054752690667223547, 3.707466751127219781E-16 ) ) ;
#56770=CARTESIAN_POINT ( 'NONE',  ( 7.903125000614515727, -4.541064518000417216, -2.621784821875001281 ) ) ;
#56772=CARTESIAN_POINT ( 'NONE',  ( 4.546875000614517326, 6.054752690667223547, 3.707466751127219781E-16 ) ) ;
#56773=CARTESIAN_POINT ( 'NONE',  ( 17.02500000122903145, 2.886751345948126879, 4.999999999999999112 ) ) ;
#56774=CARTESIAN_POINT ( 'NONE',  ( 22.01249999999999574, -5.773502691896255534, -1.060575238724906372E-15 ) ) ;
#56775=CARTESIAN_POINT ( 'NONE',  ( 3.571875000614517237, 3.027376345333613106, -5.243569643749998122 ) ) ;
#56776=CARTESIAN_POINT ( 'NONE',  ( 10.54687500061451644, -3.027376345333614438, 5.243569643749998122 ) ) ;
#56777=CARTESIAN_POINT ( 'NONE',  ( 20.93437500061451573, -4.541064518000419881, 2.621784821874995952 ) ) ;
#56778=CARTESIAN_POINT ( 'NONE',  ( -1.071796769724483234, 17.20759618943233704, -34.00000000000000711 ) ) ;
#56780=CARTESIAN_POINT ( 'NONE',  ( 3.684375000614518836, 4.541064518000418104, 2.621784821874999949 ) ) ;
#56781=CARTESIAN_POINT ( 'NONE',  ( 7.884375000614517681, -4.541064518000419881, 2.621784821874995952 ) ) ;
#56782=CARTESIAN_POINT ( 'NONE',  ( 17.92500000000000071, -4.330127018922194537, 2.499999999999995559 ) ) ;
#56783=CARTESIAN_POINT ( 'NONE',  ( 16.04062500061451857, -3.027376345333610441, -5.243569643749999898 ) ) ;
#56785=( GEOMETRIC_REPRESENTATION_CONTEXT ( 3 ) GLOBAL_UNCERTAINTY_ASSIGNED_CONTEXT ( ( #70562 ) ) GLOBAL_UNIT_ASSIGNED_CONTEXT ( ( #54189, #23466, #6847 ) ) REPRESENTATION_CONTEXT ( 'NONE', 'WORKASPACE' ) );
#56788=CARTESIAN_POINT ( 'NONE',  ( 10.15312500061451750, -4.541064518000417216, -2.621784821875001281 ) ) ;
#56789=CARTESIAN_POINT ( 'NONE',  ( 26.93437500061451573, 6.421520780324663323E-16, -5.243569643749999010 ) ) ;
#56791=CARTESIAN_POINT ( 'NONE',  ( 26.25937500061451857, 0.000000000000000000, 5.243569643749999010 ) ) ;
#56792=CARTESIAN_POINT ( 'NONE',  ( 8.737500000000002487, 5.773502691896255534, 3.535250795749688894E-16 ) ) ;
#56793=CARTESIAN_POINT ( 'NONE',  ( 4.000000000000000000, 15.80000000122903359, 32.30940107675849049 ) ) ;
#56794=CARTESIAN_POINT ( 'NONE',  ( 10.12500000122903465, 2.886751345948129099, -4.999999999999998224 ) ) ;
#56795=CARTESIAN_POINT ( 'NONE',  ( 19.99687500061451573, -3.027376345333614438, 5.243569643749998122 ) ) ;
#56796=CARTESIAN_POINT ( 'NONE',  ( 14.07187500061451679, 3.027376345333611329, 5.243569643749999010 ) ) ;
#56797=CARTESIAN_POINT ( 'NONE',  ( -3.305247878049081707E-15, 5.000000000000034639, -34.00000000000004263 ) ) ;
#56799=CARTESIAN_POINT ( 'NONE',  ( 15.25312500061451715, 4.541064518000418104, -2.621784821874998173 ) ) ;
#56800=CARTESIAN_POINT ( 'NONE',  ( 27.03750000122903430, -4.330127018922194537, 2.499999999999995559 ) ) ;
#56801=CARTESIAN_POINT ( 'NONE',  ( 11.97187500061451892, -6.054752690667223547, -1.112240025338166033E-15 ) ) ;
#56802=CARTESIAN_POINT ( 'NONE',  ( 3.337500000000000355, 5.773502691896255534, 3.535250795749688401E-16 ) ) ;
#56803=CARTESIAN_POINT ( 'NONE',  ( 16.37812500061451715, -4.541064518000419881, 2.621784821874995952 ) ) ;
#56805=CARTESIAN_POINT ( 'NONE',  ( 26.48437500061451644, 6.421520780324663323E-16, -5.243569643749999010 ) ) ;
#56806=CARTESIAN_POINT ( 'NONE',  ( 2.923357432354301455, -4.056350739605543154, 3.322806236625610588 ) ) ;
#56807=CARTESIAN_POINT ( 'NONE',  ( 15.42187500061451821, 3.027376345333611329, 5.243569643749999010 ) ) ;
#56808=CARTESIAN_POINT ( 'NONE',  ( 11.06250000122903288, 4.330127018922192761, -2.499999999999997780 ) ) ;
#56810=CARTESIAN_POINT ( 'NONE',  ( -2.121784821874999949, 15.73437500061451644, -33.67503911421598417 ) ) ;
#56811=CARTESIAN_POINT ( 'NONE',  ( 17.55937500061451573, 4.541064518000418104, -2.621784821874998173 ) ) ;
#56812=CARTESIAN_POINT ( 'NONE',  ( 20.81250000122903643, -4.330127018922190985, -2.500000000000001332 ) ) ;
#56813=CARTESIAN_POINT ( 'NONE',  ( 14.22187500061451537, -6.054752690667223547, -1.112240025338166033E-15 ) ) ;
#56814=CARTESIAN_POINT ( 'NONE',  ( -4.243569643749999898, 13.07187500061452035, 27.54997392385601529 ) ) ;
#56815=CARTESIAN_POINT ( 'NONE',  ( 22.76250000122903216, 4.330127018922192761, -2.499999999999997780 ) ) ;
#56816=CARTESIAN_POINT ( 'NONE',  ( 14.50312500061451537, 0.000000000000000000, 5.243569643749999010 ) ) ;
#56817=CARTESIAN_POINT ( 'NONE',  ( 25.42500000000000071, 4.330127018922191873, 2.499999999999999556 ) ) ;
#56818=EDGE_LOOP ( 'NONE', ( #27086, #44660, #70266, #63033, #23203, #33672 ) ) ;
#56820=CARTESIAN_POINT ( 'NONE',  ( 20.10000000000000142, 0.000000000000000000, 4.999999999999998224 ) ) ;
#56821=CARTESIAN_POINT ( 'NONE',  ( -6.275039685470489619E-15, 17.97500000122903074, 33.99999999999999289 ) ) ;
#56822=CARTESIAN_POINT ( 'NONE',  ( 3.290625000614516793, -3.027376345333614438, 5.243569643749998122 ) ) ;
#56823=CARTESIAN_POINT ( 'NONE',  ( 14.40000000122903323, -2.886751345948129988, 4.999999999999997335 ) ) ;
#56824=CARTESIAN_POINT ( 'NONE',  ( 19.90312500061451573, 0.000000000000000000, 5.243569643749999010 ) ) ;
#56825=ADVANCED_FACE ( 'NONE', ( #57918 ), #7325, .F. ) ;
#56826=CARTESIAN_POINT ( 'NONE',  ( 22.37812500061451360, 6.421520780324663323E-16, -5.243569643749999010 ) ) ;
#56827=CARTESIAN_POINT ( 'NONE',  ( 3.178125000614515638, 4.541064518000418104, 2.621784821874999949 ) ) ;
#56828=CARTESIAN_POINT ( 'NONE',  ( 28.83749999999999858, -2.886751345948125991, -5.000000000000000000 ) ) ;
#56829=CARTESIAN_POINT ( 'NONE',  ( 4.628252511229727695, 3.493065785874447826, -3.949832584684945580 ) ) ;
#56831=CARTESIAN_POINT ( 'NONE',  ( 29.67187500061451644, 3.027376345333613106, -5.243569643749998122 ) ) ;
#56832=CARTESIAN_POINT ( 'NONE',  ( -3.999999999999999556, 11.97500000122903252, -32.30940107675850470 ) ) ;
#56833=CARTESIAN_POINT ( 'NONE',  ( -4.243569643749997233, 17.19687500061451502, -27.54997392385601174 ) ) ;
#56834=CARTESIAN_POINT ( 'NONE',  ( 6.037500001229035185, 6.123233995736764310E-16, -4.999999999999998224 ) ) ;
#56835=CARTESIAN_POINT ( 'NONE',  ( 7.912499999999999645, 2.886751345948126879, 4.999999999999999112 ) ) ;
#56836=( BOUNDED_CURVE ( )  B_SPLINE_CURVE ( 2, ( #35136, #22242, #62485, #34407, #44796, #16689, #56231, #56935, #5625 ),
 .UNSPECIFIED., .F., .F. ) 
 B_SPLINE_CURVE_WITH_KNOTS ( ( 3, 2, 2, 2, 3 ),
 ( 0.03260869565217391908, 0.03623188405797101580, 0.04347826086956521618, 0.05072463768115942351, 0.05434782608695652717 ),
 .UNSPECIFIED. ) 
 CURVE ( )  GEOMETRIC_REPRESENTATION_ITEM ( )  RATIONAL_B_SPLINE_CURVE ( ( 0.9330127018922192983, 0.9330127018922194093, 1.000000000000000000, 0.8660254037844387076, 1.000000000000000000, 0.8660254037844387076, 1.000000000000000000, 0.9330127018922192983, 0.9330127018922194093 ) ) 
 REPRESENTATION_ITEM ( '' )  );
#56837=CARTESIAN_POINT ( 'NONE',  ( 4.200000001229033053, -2.886751345948125991, -5.000000000000000000 ) ) ;
#56838=CARTESIAN_POINT ( 'NONE',  ( 11.18437500061451928, 6.421520780324663323E-16, -5.243569643749999010 ) ) ;
#56839=AXIS2_PLACEMENT_3D ( 'NONE', #23372, #17104, #11580 ) ;
#56840=CARTESIAN_POINT ( 'NONE',  ( -1.487416814333745711E-14, 16.62500000122903288, -26.00000000000000000 ) ) ;
#56841=CARTESIAN_POINT ( 'NONE',  ( 3.984375000614517326, 6.421520780324663323E-16, -5.243569643749999010 ) ) ;
#56843=CARTESIAN_POINT ( 'NONE',  ( 3.999999999999998668, 19.47500000122903430, 27.69059892324149530 ) ) ;
#56844=CARTESIAN_POINT ( 'NONE',  ( 10.80937500061451928, 4.541064518000418104, -2.621784821874998173 ) ) ;
#56845=CARTESIAN_POINT ( 'NONE',  ( 13.99687500061451928, 6.054752690667223547, 3.707466751127219781E-16 ) ) ;
#56846=CARTESIAN_POINT ( 'NONE',  ( -3.999999999999999112, 18.61250000000000426, -32.30940107675850470 ) ) ;
#56847=CARTESIAN_POINT ( 'NONE',  ( 7.612500000000000711, -5.773502691896255534, -1.060575238724906372E-15 ) ) ;
#56848=CARTESIAN_POINT ( 'NONE',  ( -3.000416591977282496E-16, 18.34062500061459744, 25.09994784771203058 ) ) ;
#56849=CARTESIAN_POINT ( 'NONE',  ( 20.74687500061451573, 6.054752690667223547, 3.707466751127219781E-16 ) ) ;
#56850=CARTESIAN_POINT ( 'NONE',  ( -3.137519842735245283E-14, 14.37500000122903288, -26.00000000000000711 ) ) ;
#56851=CARTESIAN_POINT ( 'NONE',  ( 27.15000000122902790, -2.886751345948125991, -5.000000000000000000 ) ) ;
#56853=CARTESIAN_POINT ( 'NONE',  ( 22.86562500061451431, 3.027376345333613106, -5.243569643749998122 ) ) ;
#56854=CARTESIAN_POINT ( 'NONE',  ( 15.36562500061451608, 3.027376345333611329, 5.243569643749999010 ) ) ;
#56856=CARTESIAN_POINT ( 'NONE',  ( 11.10937500061451644, -4.541064518000417216, -2.621784821875001281 ) ) ;
#56857=CARTESIAN_POINT ( 'NONE',  ( 27.63749999999999929, 5.773502691896255534, 3.535250795749688894E-16 ) ) ;
#56858=CARTESIAN_POINT ( 'NONE',  ( 25.57500000122903216, 2.886751345948126879, 4.999999999999999112 ) ) ;
#56859=CARTESIAN_POINT ( 'NONE',  ( 4.509375000614518569, 4.541064518000418104, -2.621784821874998173 ) ) ;
#56860=CARTESIAN_POINT ( 'NONE',  ( 13.47187500061451537, 3.027376345333613106, -5.243569643749998122 ) ) ;
#56861=CARTESIAN_POINT ( 'NONE',  ( 28.39687500061452141, 6.054752690667223547, 3.707466751127219781E-16 ) ) ;
#56862=DIRECTION ( 'NONE',  ( -1.000000000000000000, -0.000000000000000000, -0.000000000000000000 ) ) ;
#56864=CARTESIAN_POINT ( 'NONE',  ( -1.999999999999997113, 12.08750000122903501, 33.46410161513775705 ) ) ;
#56865=CARTESIAN_POINT ( 'NONE',  ( 22.69687500061451857, -3.027376345333614438, 5.243569643749998122 ) ) ;
#56866=CARTESIAN_POINT ( 'NONE',  ( 14.25937500061451679, -4.541064518000417216, -2.621784821875001281 ) ) ;
#56867=ADVANCED_FACE ( 'NONE', ( #35756 ), #45452, .T. ) ;
#56869=CARTESIAN_POINT ( 'NONE',  ( 25.91250000000000142, 2.886751345948126879, 4.999999999999999112 ) ) ;
#56870=CARTESIAN_POINT ( 'NONE',  ( 4.200000001229033053, -2.886751345948125991, -5.000000000000000000 ) ) ;
#56872=CARTESIAN_POINT ( 'NONE',  ( 16.37812500061451715, -4.541064518000419881, 2.621784821874995952 ) ) ;
#56873=CARTESIAN_POINT ( 'NONE',  ( 7.200000000000001954, -4.330127018922190985, -2.500000000000001332 ) ) ;
#56874=CYLINDRICAL_SURFACE ( 'NONE', #25431, 3.999999999999996447 ) ;
#56875=CARTESIAN_POINT ( 'NONE',  ( 16.61250000000000426, -5.773502691896255534, -1.060575238724906372E-15 ) ) ;
#56876=CARTESIAN_POINT ( 'NONE',  ( -2.121784821874999949, 12.52812500061451573, 26.32496088578401938 ) ) ;
#56877=CARTESIAN_POINT ( 'NONE',  ( 30.00000000000000000, 0.000000000000000000, 0.000000000000000000 ) ) ;
#56878=CARTESIAN_POINT ( 'NONE',  ( 20.55000000122903359, 5.773502691896255534, 3.535250795749688894E-16 ) ) ;
#56879=CARTESIAN_POINT ( 'NONE',  ( 28.28437500061451715, 6.421520780324663323E-16, -5.243569643749999010 ) ) ;
#56880=ORIENTED_EDGE ( 'NONE', *, *, #47376, .T. ) ;
#56881=CARTESIAN_POINT ( 'NONE',  ( 20.87812500061451715, -4.541064518000419881, 2.621784821874995952 ) ) ;
#56882=CARTESIAN_POINT ( 'NONE',  ( 21.57187500061451502, 3.027376345333613106, -5.243569643749998122 ) ) ;
#56883=CARTESIAN_POINT ( 'NONE',  ( 4.912499999999999645, -5.773502691896255534, -1.060575238724906372E-15 ) ) ;
#56884=CARTESIAN_POINT ( 'NONE',  ( 8.653125000614515727, 0.000000000000000000, 5.243569643749999010 ) ) ;
#56885=CARTESIAN_POINT ( 'NONE',  ( 23.24062500061451786, -3.027376345333610441, -5.243569643749999898 ) ) ;
#56886=CARTESIAN_POINT ( 'NONE',  ( 11.55937500061451928, -4.541064518000417216, -2.621784821875001281 ) ) ;
#56887=CARTESIAN_POINT ( 'NONE',  ( 16.28437500061452070, 4.541064518000418104, 2.621784821874999949 ) ) ;
#56888=CARTESIAN_POINT ( 'NONE',  ( -4.243569643749999898, 17.51562500061451644, 27.54997392385601529 ) ) ;
#56889=CARTESIAN_POINT ( 'NONE',  ( 22.38750000122903216, 4.330127018922191873, 2.499999999999999556 ) ) ;
#56891=CARTESIAN_POINT ( 'NONE',  ( 9.628125000614517148, -4.541064518000419881, 2.621784821874995952 ) ) ;
#56892=CARTESIAN_POINT ( 'NONE',  ( 4.546875000614517326, 6.054752690667223547, 3.707466751127219781E-16 ) ) ;
#56893=CARTESIAN_POINT ( 'NONE',  ( 5.296875000614518214, -3.027376345333610441, -5.243569643749999898 ) ) ;
#56895=CARTESIAN_POINT ( 'NONE',  ( 24.57187500061451502, -6.054752690667223547, -1.112240025338166033E-15 ) ) ;
#56896=CARTESIAN_POINT ( 'NONE',  ( 17.76562500061451644, -6.054752690667223547, -1.112240025338166033E-15 ) ) ;
#56897=CARTESIAN_POINT ( 'NONE',  ( 26.70000000122903572, -2.886751345948125991, -5.000000000000000000 ) ) ;
#56898=CARTESIAN_POINT ( 'NONE',  ( 28.86562500061451786, 3.027376345333611329, 5.243569643749999010 ) ) ;
#56899=AXIS2_PLACEMENT_3D ( 'NONE', #19620, #30718, #53251 ) ;
#56900=CARTESIAN_POINT ( 'NONE',  ( 21.12187500061451573, 3.027376345333613106, -5.243569643749998122 ) ) ;
#56901=CARTESIAN_POINT ( 'NONE',  ( 17.95312500061451644, 4.541064518000418104, -2.621784821874998173 ) ) ;
#56902=CARTESIAN_POINT ( 'NONE',  ( 4.243569643749999898, 19.59687500061452070, 32.45002607614398471 ) ) ;
#56903=CARTESIAN_POINT ( 'NONE',  ( 22.22812500061451502, -4.541064518000419881, 2.621784821874995952 ) ) ;
#56905=ORIENTED_EDGE ( 'NONE', *, *, #51310, .F. ) ;
#56906=CARTESIAN_POINT ( 'NONE',  ( 27.33750000000000213, -2.886751345948129988, 4.999999999999997335 ) ) ;
#56907=CARTESIAN_POINT ( 'NONE',  ( -3.999999999999997335, 13.28749999999999964, -27.69059892324149175 ) ) ;
#56909=CARTESIAN_POINT ( 'NONE',  ( 29.54062500061451502, -3.027376345333610441, -5.243569643749999898 ) ) ;
#56910=CARTESIAN_POINT ( 'NONE',  ( 9.740625000614516082, -3.027376345333610441, -5.243569643749999898 ) ) ;
#56911=CARTESIAN_POINT ( 'NONE',  ( 22.20000000122903216, -2.886751345948125991, -5.000000000000000000 ) ) ;
#56912=CARTESIAN_POINT ( 'NONE',  ( 12.30937500061451573, 0.000000000000000000, 5.243569643749999010 ) ) ;
#56913=CARTESIAN_POINT ( 'NONE',  ( 28.41562500061451502, 3.027376345333611329, 5.243569643749999010 ) ) ;
#56914=CARTESIAN_POINT ( 'NONE',  ( 28.91250000000000497, 2.886751345948129099, -4.999999999999998224 ) ) ;
#56915=EDGE_CURVE ( 'NONE', #44045, #55550, #5673, .T. ) ;
#56916=CARTESIAN_POINT ( 'NONE',  ( -3.999999999999997335, 18.35000000122903430, -27.69059892324149175 ) ) ;
#56917=CARTESIAN_POINT ( 'NONE',  ( 25.16250000122903074, 0.000000000000000000, 4.999999999999998224 ) ) ;
#56918=CARTESIAN_POINT ( 'NONE',  ( 11.80312500061451608, 0.000000000000000000, 5.243569643749999010 ) ) ;
#56919=ORIENTED_EDGE ( 'NONE', *, *, #9235, .T. ) ;
#56920=CARTESIAN_POINT ( 'NONE',  ( 8.578125000614518214, 4.541064518000418104, 2.621784821874999949 ) ) ;
#56921=CARTESIAN_POINT ( 'NONE',  ( 6.515625000614516438, -6.054752690667223547, -1.112240025338166033E-15 ) ) ;
#56924=CARTESIAN_POINT ( 'NONE',  ( 15.26249999999999929, -5.773502691896255534, -1.060575238724906372E-15 ) ) ;
#56925=CARTESIAN_POINT ( 'NONE',  ( 15.72187500061451892, 3.027376345333613106, -5.243569643749998122 ) ) ;
#56926=CARTESIAN_POINT ( 'NONE',  ( 11.58750000122903501, 4.330127018922191873, 2.499999999999999556 ) ) ;
#56927=CARTESIAN_POINT ( 'NONE',  ( 18.45937500061451431, 4.541064518000418104, -2.621784821874998173 ) ) ;
#56929=CARTESIAN_POINT ( 'NONE',  ( 20.37187500061451573, 3.027376345333611329, 5.243569643749999010 ) ) ;
#56930=CARTESIAN_POINT ( 'NONE',  ( 4.243569643749999898, 14.17812500061451608, -30.00000000000000000 ) ) ;
#56934=CARTESIAN_POINT ( 'NONE',  ( 26.76562500061451644, -6.054752690667223547, -1.112240025338166033E-15 ) ) ;
#56935=CARTESIAN_POINT ( 'NONE',  ( -1.071796769724490117, 19.45759618943232994, -34.00000000000000000 ) ) ;
#56936=CARTESIAN_POINT ( 'NONE',  ( 28.69687500061451502, -3.027376345333610441, -5.243569643749999898 ) ) ;
#56937=CARTESIAN_POINT ( 'NONE',  ( 25.31250000000000000, 2.886751345948129099, -4.999999999999998224 ) ) ;
#56938=CARTESIAN_POINT ( 'NONE',  ( 6.553125000614518747, -4.541064518000417216, -2.621784821875001281 ) ) ;
#56939=VECTOR ( 'NONE', #20544, 1000.000000000000000 ) ;
#56941=CARTESIAN_POINT ( 'NONE',  ( 19.54687500061451644, -3.027376345333614438, 5.243569643749998122 ) ) ;
#56943=CARTESIAN_POINT ( 'NONE',  ( 5.240625000614516971, -3.027376345333610441, -5.243569643749999898 ) ) ;
#56944=CARTESIAN_POINT ( 'NONE',  ( 10.24687500061451750, -3.027376345333610441, -5.243569643749999898 ) ) ;
#56946=CARTESIAN_POINT ( 'NONE',  ( 20.25937500061451857, 4.541064518000418104, -2.621784821874998173 ) ) ;
#56947=LINE ( 'NONE', #50700, #13487 ) ;
#56948=CARTESIAN_POINT ( 'NONE',  ( 27.97500000000000142, 6.123233995736764310E-16, -4.999999999999998224 ) ) ;
#56949=CARTESIAN_POINT ( 'NONE',  ( 29.78437500061451715, 4.541064518000418104, 2.621784821874999949 ) ) ;
#56951=CARTESIAN_POINT ( 'NONE',  ( 3.412230204620315011, -4.173532794979288418, -3.258368439540926698 ) ) ;
#56952=ORIENTED_EDGE ( 'NONE', *, *, #66019, .F. ) ;
#56953=CARTESIAN_POINT ( 'NONE',  ( 9.975000000000001421, 6.123233995736764310E-16, -4.999999999999998224 ) ) ;
#56955=CARTESIAN_POINT ( 'NONE',  ( 25.26562500061451289, 3.027376345333611329, 5.243569643749999010 ) ) ;
#56956=CARTESIAN_POINT ( 'NONE',  ( 14.92500000000000071, 6.123233995736764310E-16, -4.999999999999998224 ) ) ;
#56957=EDGE_CURVE ( 'NONE', #33991, #6203, #68120, .T. ) ;
#56958=CARTESIAN_POINT ( 'NONE',  ( 11.32500000122903394, -5.773502691896255534, -1.060575238724906372E-15 ) ) ;
#56959=CARTESIAN_POINT ( 'NONE',  ( 8.803125000614517859, -4.541064518000417216, -2.621784821875001281 ) ) ;
#56960=CARTESIAN_POINT ( 'NONE',  ( 9.150000000000002132, 4.330127018922192761, -2.499999999999997780 ) ) ;
#56961=CARTESIAN_POINT ( 'NONE',  ( 18.82500000122903572, 2.886751345948060266, 5.000000000000114575 ) ) ;
#56962=CARTESIAN_POINT ( 'NONE',  ( 29.17500000122903714, 2.886751345948126879, 4.999999999999999112 ) ) ;
#56964=CARTESIAN_POINT ( 'NONE',  ( 7.650000000000000355, -4.330127018922190985, -2.500000000000001332 ) ) ;
#56965=LINE ( 'NONE', #16721, #71565 ) ;
#56966=ORIENTED_EDGE ( 'NONE', *, *, #70256, .T. ) ;
#56967=CARTESIAN_POINT ( 'NONE',  ( 21.40312500061451573, -4.541064518000417216, -2.621784821875001281 ) ) ;
#56968=CARTESIAN_POINT ( 'NONE',  ( 28.79062500061451502, 6.054752690667223547, 3.707466751127219781E-16 ) ) ;
#56969=CARTESIAN_POINT ( 'NONE',  ( 29.48437500061451644, -4.541064518000419881, 2.621784821874995952 ) ) ;
#56970=CARTESIAN_POINT ( 'NONE',  ( 18.94687500061451502, 6.054752690667223547, 3.707466751127219781E-16 ) ) ;
#56971=CARTESIAN_POINT ( 'NONE',  ( 16.41562500061451857, -6.054752690667223547, -1.112240025338166033E-15 ) ) ;
#56972=CARTESIAN_POINT ( 'NONE',  ( -2.121784821874999949, 11.62812500061459353, -33.67503911421598417 ) ) ;
#56973=CARTESIAN_POINT ( 'NONE',  ( 3.928125000614516527, 6.421520780324663323E-16, -5.243569643749999010 ) ) ;
#56974=CARTESIAN_POINT ( 'NONE',  ( 28.38750000122903216, -4.330127018922194537, 2.499999999999995559 ) ) ;
#56976=CARTESIAN_POINT ( 'NONE',  ( 18.14062500061451644, -3.027376345333614438, 5.243569643749998122 ) ) ;
#56977=CARTESIAN_POINT ( 'NONE',  ( 1.071796769724489895, 14.01740381056766793, 26.00000000000000355 ) ) ;
#56978=CARTESIAN_POINT ( 'NONE',  ( 3.600000001229033408, -2.886751345948129988, 4.999999999999997335 ) ) ;
#56979=CARTESIAN_POINT ( 'NONE',  ( 12.60937500061451821, 4.541064518000418104, -2.621784821874998173 ) ) ;
#56980=CARTESIAN_POINT ( 'NONE',  ( 13.05937500061451750, 4.541064518000418104, -2.621784821874998173 ) ) ;
#56981=CARTESIAN_POINT ( 'NONE',  ( 19.35937500061451644, 4.541064518000418104, -2.621784821874998173 ) ) ;
#56983=CARTESIAN_POINT ( 'NONE',  ( -5.999929701724457942, 8.000052723701786661, 29.79473720932466918 ) ) ;
#56984=CARTESIAN_POINT ( 'NONE',  ( 24.36562500061451786, 3.027376345333611329, 5.243569643749999010 ) ) ;
#56985=CARTESIAN_POINT ( 'NONE',  ( 18.42187500061451644, 3.027376345333613106, -5.243569643749998122 ) ) ;
#56986=CARTESIAN_POINT ( 'NONE',  ( 24.74062500061451786, 6.054752690667223547, 3.707466751127219781E-16 ) ) ;
#56987=CARTESIAN_POINT ( 'NONE',  ( 1.592000809091587073E-14, 15.95000000122903394, -34.00000000000000000 ) ) ;
#56988=CARTESIAN_POINT ( 'NONE',  ( -2.000000000000000000, 17.22500000000000142, 26.53589838486224650 ) ) ;
#56989=CARTESIAN_POINT ( 'NONE',  ( 29.35312500061451502, 0.000000000000000000, 5.243569643749999010 ) ) ;
#56990=CARTESIAN_POINT ( 'NONE',  ( 10.80000000122903536, -2.886751345948129988, 4.999999999999997335 ) ) ;
#56991=CARTESIAN_POINT ( 'NONE',  ( 7.687500001229033764, -4.330127018922194537, 2.499999999999995559 ) ) ;
#56992=CARTESIAN_POINT ( 'NONE',  ( 2.000000000000001332, 19.69999999999999929, -26.53589838486224650 ) ) ;
#56993=CARTESIAN_POINT ( 'NONE',  ( 28.23750000122903359, 4.330127018922191873, 2.499999999999999556 ) ) ;
#56996=CARTESIAN_POINT ( 'NONE',  ( 8.971875000614515372, 3.027376345333613106, -5.243569643749998122 ) ) ;
#56998=CARTESIAN_POINT ( 'NONE',  ( 17.50312500061451715, 4.541064518000418104, -2.621784821874998173 ) ) ;
#56999=CARTESIAN_POINT ( 'NONE',  ( 11.18437500061451928, 6.421520780324663323E-16, -5.243569643749999010 ) ) ;
#57000=CARTESIAN_POINT ( 'NONE',  ( 29.66250000122903074, 0.000000000000000000, 4.999999999999998224 ) ) ;
#57001=CARTESIAN_POINT ( 'NONE',  ( 19.54687500061451289, -3.027376345333614438, 5.243569643749998122 ) ) ;
#57002=CARTESIAN_POINT ( 'NONE',  ( 6.871875000614517504, 3.027376345333611329, 5.243569643749999010 ) ) ;
#57003=CARTESIAN_POINT ( 'NONE',  ( 25.61250000122903359, 0.000000000000000000, 4.999999999999998224 ) ) ;
#57006=CARTESIAN_POINT ( 'NONE',  ( 10.30312500061451431, 4.541064518000418104, -2.621784821874998173 ) ) ;
#57007=CARTESIAN_POINT ( 'NONE',  ( 19.90312500061451573, 0.000000000000000000, 5.243569643749999010 ) ) ;
#57010=CARTESIAN_POINT ( 'NONE',  ( 5.250000001229035540, 5.773502691896255534, 3.535250795749688894E-16 ) ) ;
#57011=CARTESIAN_POINT ( 'NONE',  ( 15.55312500061451608, -4.541064518000417216, -2.621784821875001281 ) ) ;
#57012=CARTESIAN_POINT ( 'NONE',  ( 13.19062500061451537, -3.027376345333614438, 5.243569643749998122 ) ) ;
#57014=CARTESIAN_POINT ( 'NONE',  ( 12.37500000000000000, 4.330127018922191873, 2.499999999999999556 ) ) ;
#57015=CARTESIAN_POINT ( 'NONE',  ( 8.737500001229033586, 6.123233995736764310E-16, -4.999999999999998224 ) ) ;
#57016=CARTESIAN_POINT ( 'NONE',  ( 5.728125000614515905, 6.421520780324663323E-16, -5.243569643749999010 ) ) ;
#57017=CARTESIAN_POINT ( 'NONE',  ( 18.52500000122903145, -5.773502691896255534, -1.060575238724906372E-15 ) ) ;
#57019=CARTESIAN_POINT ( 'NONE',  ( 2.121784821874999061, 11.15937500061451715, -33.67503911421598417 ) ) ;
#57020=CARTESIAN_POINT ( 'NONE',  ( 8.550000000000002487, -4.330127018922190985, -2.500000000000001332 ) ) ;
#57021=CARTESIAN_POINT ( 'NONE',  ( 3.975000001229033852, 2.886751345948126879, 4.999999999999999112 ) ) ;
#57022=CARTESIAN_POINT ( 'NONE',  ( 19.24687500061452283, -3.027376345333610441, -5.243569643749999898 ) ) ;
#57023=CARTESIAN_POINT ( 'NONE',  ( 21.45000000122903216, 5.773502691896255534, 3.535250795749688401E-16 ) ) ;
#57024=CARTESIAN_POINT ( 'NONE',  ( 17.54062500061451502, 6.054752690667223547, 3.707466751127219781E-16 ) ) ;
#57026=CARTESIAN_POINT ( 'NONE',  ( 22.50000000122903288, -2.886751345948163738, 4.999999999999939604 ) ) ;
#57027=CARTESIAN_POINT ( 'NONE',  ( 29.74687500061451217, 6.054752690667223547, 3.707466751127219781E-16 ) ) ;
#57028=CARTESIAN_POINT ( 'NONE',  ( 27.34687500061451360, -3.027376345333610441, -5.243569643749999898 ) ) ;
#57030=CARTESIAN_POINT ( 'NONE',  ( 12.17812500061451608, 4.541064518000418104, 2.621784821874999949 ) ) ;
#57031=CARTESIAN_POINT ( 'NONE',  ( 11.59687500061451892, -3.027376345333610441, -5.243569643749999898 ) ) ;
#57032=VERTEX_POINT ( 'NONE', #44841 ) ;
#57033=CARTESIAN_POINT ( 'NONE',  ( 9.412499999999999645, -5.773502691896255534, -1.060575238724906372E-15 ) ) ;
#57034=CARTESIAN_POINT ( 'NONE',  ( 19.22812500061451502, 6.421520780324663323E-16, -5.243569643749999010 ) ) ;
#57037=( BOUNDED_CURVE ( )  B_SPLINE_CURVE ( 2, ( #54405, #69928, #53298, #14136, #20403, #19297, #13771, #54045, #48500 ),
 .UNSPECIFIED., .F., .F. ) 
 B_SPLINE_CURVE_WITH_KNOTS ( ( 3, 2, 2, 2, 3 ),
 ( 0.1195652173913043514, 0.1231884057971014551, 0.1304347826086956486, 0.1376811594202898559, 0.1413043478260869734 ),
 .UNSPECIFIED. ) 
 CURVE ( )  GEOMETRIC_REPRESENTATION_ITEM ( )  RATIONAL_B_SPLINE_CURVE ( ( 0.9330127018922194093, 0.9330127018922194093, 1.000000000000000000, 0.8660254037844387076, 1.000000000000000000, 0.8660254037844387076, 1.000000000000000000, 0.9330127018922190762, 0.9330127018922194093 ) ) 
 REPRESENTATION_ITEM ( '' )  );
#57038=CARTESIAN_POINT ( 'NONE',  ( 9.449999999999999289, -4.330127018922190985, -2.500000000000001332 ) ) ;
#57039=CARTESIAN_POINT ( 'NONE',  ( 21.18750000122903288, -4.330127018922194537, 2.499999999999995559 ) ) ;
#57040=CARTESIAN_POINT ( 'NONE',  ( 15.17812500061451608, 6.421520780324663323E-16, -5.243569643749999010 ) ) ;
#57043=CARTESIAN_POINT ( 'NONE',  ( 19.08750000000000213, 5.773502691896255534, 3.535250795749688894E-16 ) ) ;
#57044=CARTESIAN_POINT ( 'NONE',  ( 21.71249999999999858, 2.886751345948129099, -4.999999999999998224 ) ) ;
#57045=( BOUNDED_CURVE ( )  B_SPLINE_CURVE ( 2, ( #61861, #6443, #28978, #45970, #41158, #41868, #30055, #24868, #24143 ),
 .UNSPECIFIED., .F., .F. ) 
 B_SPLINE_CURVE_WITH_KNOTS ( ( 3, 2, 2, 2, 3 ),
 ( 0.4891304347826087029, 0.4927536231884058204, 0.5000000000000000000, 0.5072463768115942351, 0.5108695652173913526 ),
 .UNSPECIFIED. ) 
 CURVE ( )  GEOMETRIC_REPRESENTATION_ITEM ( )  RATIONAL_B_SPLINE_CURVE ( ( 0.9330127018922194093, 0.9330127018922194093, 1.000000000000000000, 0.8660254037844387076, 1.000000000000000000, 0.8660254037844387076, 1.000000000000000000, 0.9330127018922182991, 0.9330127018922192983 ) ) 
 REPRESENTATION_ITEM ( '' )  );
#57046=CARTESIAN_POINT ( 'NONE',  ( 19.84687500061451360, 6.054752690667223547, 3.707466751127219781E-16 ) ) ;
#57047=CARTESIAN_POINT ( 'NONE',  ( 25.30312500061451431, 0.000000000000000000, 5.243569643749999010 ) ) ;
#57049=CARTESIAN_POINT ( 'NONE',  ( 8.925000001229033586, 2.886751345948193936, 4.999999999999883649 ) ) ;
#57050=CARTESIAN_POINT ( 'NONE',  ( 7.228125000614517681, 4.541064518000418104, 2.621784821874999949 ) ) ;
#57051=CARTESIAN_POINT ( 'NONE',  ( 1.071796769724489895, 15.47990381179670116, 26.00000000000000355 ) ) ;
#57052=CARTESIAN_POINT ( 'NONE',  ( 13.76250000000000107, 2.886751345948126879, 4.999999999999999112 ) ) ;
#57053=CARTESIAN_POINT ( 'NONE',  ( -3.000416591977282496E-16, 17.89062500061451644, 25.09994784771203058 ) ) ;
#57054=CARTESIAN_POINT ( 'NONE',  ( 28.26562500061451289, 3.027376345333613106, -5.243569643749998122 ) ) ;
#57055=CARTESIAN_POINT ( 'NONE',  ( 26.70937500061451431, 0.000000000000000000, 5.243569643749999010 ) ) ;
#57057=CARTESIAN_POINT ( 'NONE',  ( 22.90312500061451573, 4.541064518000418104, -2.621784821874998173 ) ) ;
#57058=CARTESIAN_POINT ( 'NONE',  ( 25.24687500061451573, 6.054752690667223547, 3.707466751127219781E-16 ) ) ;
#57059=CARTESIAN_POINT ( 'NONE',  ( 4.243569643749999898, 17.74062500061459602, -27.54997392385601529 ) ) ;
#57060=CARTESIAN_POINT ( 'NONE',  ( 10.87500000000000000, 6.123233995736764310E-16, -4.999999999999998224 ) ) ;
#57061=CARTESIAN_POINT ( 'NONE',  ( 9.253125000614517148, -4.541064518000417216, -2.621784821875001281 ) ) ;
#57063=CARTESIAN_POINT ( 'NONE',  ( 29.31562500061451715, 3.027376345333611329, 5.243569643749999010 ) ) ;
#57064=CARTESIAN_POINT ( 'NONE',  ( 25.90312500061451573, -4.541064518000417216, -2.621784821875001281 ) ) ;
#57067=CARTESIAN_POINT ( 'NONE',  ( 18.38437500061451857, 6.421520780324663323E-16, -5.243569643749999010 ) ) ;
#57068=CARTESIAN_POINT ( 'NONE',  ( 4.243569643749999010, 11.12187500061451928, 27.54997392385601174 ) ) ;
#57069=CARTESIAN_POINT ( 'NONE',  ( 19.05937500061451928, 0.000000000000000000, 5.243569643749999010 ) ) ;
#57070=CARTESIAN_POINT ( 'NONE',  ( 28.28437500061451715, 6.421520780324663323E-16, -5.243569643749999010 ) ) ;
#57071=CARTESIAN_POINT ( 'NONE',  ( -2.121784821874999949, 16.18437500061451573, 26.32496088578401938 ) ) ;
#57072=CARTESIAN_POINT ( 'NONE',  ( 7.565625000614518036, 3.027376345333613106, -5.243569643749998122 ) ) ;
#57073=( BOUNDED_CURVE ( )  B_SPLINE_CURVE ( 3, ( #59135, #41084, #36614, #48444 ),
 .UNSPECIFIED., .F., .F. ) 
 B_SPLINE_CURVE_WITH_KNOTS ( ( 4, 4 ),
 ( 4.712388980384689674, 5.310998844378103989 ),
 .UNSPECIFIED. ) 
 CURVE ( )  GEOMETRIC_REPRESENTATION_ITEM ( )  RATIONAL_B_SPLINE_CURVE ( ( 1.000000000000000000, 0.9703611099854635436, 0.9703611099854635436, 1.000000000000000000 ) ) 
 REPRESENTATION_ITEM ( '' )  );
#57074=CARTESIAN_POINT ( 'NONE',  ( 3.909375000614518481, -4.541064518000417216, -2.621784821875001281 ) ) ;
#57075=CARTESIAN_POINT ( 'NONE',  ( 2.000000000000001332, 15.65000000000000036, -26.53589838486224650 ) ) ;
#57076=CARTESIAN_POINT ( 'NONE',  ( 6.478125000614516793, -4.541064518000419881, 2.621784821874995952 ) ) ;
#57077=CARTESIAN_POINT ( 'NONE',  ( 12.83437500061451786, -4.541064518000419881, 2.621784821874995952 ) ) ;
#57078=CARTESIAN_POINT ( 'NONE',  ( 18.07500000122903216, -5.773502691896255534, -1.060575238724906372E-15 ) ) ;
#57079=CARTESIAN_POINT ( 'NONE',  ( 6.196875000614515905, -3.027376345333610441, -5.243569643749999898 ) ) ;
#57080=CARTESIAN_POINT ( 'NONE',  ( 8.128125000614515372, 4.541064518000418104, 2.621784821874999949 ) ) ;
#57081=CARTESIAN_POINT ( 'NONE',  ( 4.057522967627288146, -2.921730200955767298, 4.057522967627288146 ) ) ;
#57083=CARTESIAN_POINT ( 'NONE',  ( 17.07187500061451502, 3.027376345333613106, -5.243569643749998122 ) ) ;
#57085=EDGE_LOOP ( 'NONE', ( #8260, #72686, #5863, #12804 ) ) ;
#57086=CARTESIAN_POINT ( 'NONE',  ( 23.54062500061451146, -3.027376345333614438, 5.243569643749998122 ) ) ;
#57087=CARTESIAN_POINT ( 'NONE',  ( 10.90312500061451928, 0.000000000000000000, 5.243569643749999010 ) ) ;
#57088=CARTESIAN_POINT ( 'NONE',  ( 26.82187500061451857, -6.054752690667223547, -1.112240025338166033E-15 ) ) ;
#57089=CARTESIAN_POINT ( 'NONE',  ( 10.94062500061451537, -3.027376345333614438, 5.243569643749998122 ) ) ;
#57090=CARTESIAN_POINT ( 'NONE',  ( -2.121784821874999949, 9.884375000614518569, -33.67503911421598417 ) ) ;
#57091=CARTESIAN_POINT ( 'NONE',  ( 12.26250000122903394, -4.330127018922190985, -2.500000000000001332 ) ) ;
#57092=CARTESIAN_POINT ( 'NONE',  ( 27.62812500061451360, -4.541064518000419881, 2.621784821874995952 ) ) ;
#57094=CARTESIAN_POINT ( 'NONE',  ( 2.121784821874999061, 12.00312500061451715, -33.67503911421598417 ) ) ;
#57095=CARTESIAN_POINT ( 'NONE',  ( 12.67500000122903536, -5.773502691896255534, -1.060575238724906372E-15 ) ) ;
#57096=CARTESIAN_POINT ( 'NONE',  ( 10.91250000000000320, 2.886751345948129099, -4.999999999999998224 ) ) ;
#57097=CARTESIAN_POINT ( 'NONE',  ( 20.20312500061451644, 4.541064518000418104, -2.621784821874998173 ) ) ;
#57098=CARTESIAN_POINT ( 'NONE',  ( 7.021875000614519635, -6.054752690667223547, -1.112240025338166033E-15 ) ) ;
#57099=CARTESIAN_POINT ( 'NONE',  ( 19.61249999999999716, 2.886751345948126879, 4.999999999999999112 ) ) ;
#57100=CARTESIAN_POINT ( 'NONE',  ( 8.362500001229031810, 4.330127018922192761, -2.499999999999997780 ) ) ;
#57101=CARTESIAN_POINT ( 'NONE',  ( 16.80000000122903359, -2.886751345948125991, -5.000000000000000000 ) ) ;
#57102=CARTESIAN_POINT ( 'NONE',  ( 13.90312500061451750, 4.541064518000418104, -2.621784821874998173 ) ) ;
#57103=CARTESIAN_POINT ( 'NONE',  ( 16.00312500061451715, -4.541064518000417216, -2.621784821875001281 ) ) ;
#57104=CARTESIAN_POINT ( 'NONE',  ( 26.13750000122903216, -4.330127018922194537, 2.499999999999995559 ) ) ;
#57105=CARTESIAN_POINT ( 'NONE',  ( 19.72499999999999787, -4.330127018922194537, 2.499999999999995559 ) ) ;
#57106=CARTESIAN_POINT ( 'NONE',  ( 23.78437500061451360, 6.421520780324663323E-16, -5.243569643749999010 ) ) ;
#57108=CARTESIAN_POINT ( 'NONE',  ( 9.075000001229033941, -5.773502691896255534, -1.060575238724906372E-15 ) ) ;
#57109=CARTESIAN_POINT ( 'NONE',  ( 9.534375000614517148, 4.541064518000418104, 2.621784821874999949 ) ) ;
#57110=CARTESIAN_POINT ( 'NONE',  ( 24.87187500061451573, 3.027376345333611329, 5.243569643749999010 ) ) ;
#57111=CARTESIAN_POINT ( 'NONE',  ( 3.159375000614518036, 4.541064518000418104, -2.621784821874998173 ) ) ;
#57112=CARTESIAN_POINT ( 'NONE',  ( 23.16562500061451502, -6.054752690667223547, -1.112240025338166033E-15 ) ) ;
#57113=CARTESIAN_POINT ( 'NONE',  ( 26.78437500061451360, -4.541064518000419881, 2.621784821874995952 ) ) ;
#57115=CARTESIAN_POINT ( 'NONE',  ( -0.7368805616696194605, 9.859898480082234684, 25.82089837893477480 ) ) ;
#57116=CARTESIAN_POINT ( 'NONE',  ( 7.059375000614518392, -4.541064518000417216, -2.621784821875001281 ) ) ;
#57118=CARTESIAN_POINT ( 'NONE',  ( 28.45312500061451289, 0.000000000000000000, 5.243569643749999010 ) ) ;
#57119=CARTESIAN_POINT ( 'NONE',  ( 5.596875000614516260, -3.027376345333614438, 5.243569643749998122 ) ) ;
#57120=CARTESIAN_POINT ( 'NONE',  ( 25.83749999999999503, 5.773502691896255534, 3.535250795749688401E-16 ) ) ;
#57121=CARTESIAN_POINT ( 'NONE',  ( 26.67187500061451644, 3.027376345333611329, 5.243569643749999010 ) ) ;
#57122=CARTESIAN_POINT ( 'NONE',  ( -4.243569643749999898, 9.865625000614596019, 27.54997392385601529 ) ) ;
#57123=CARTESIAN_POINT ( 'NONE',  ( 16.05000000000000071, 0.000000000000000000, 4.999999999999998224 ) ) ;
#57124=ORIENTED_EDGE ( 'NONE', *, *, #41575, .T. ) ;
#57125=CARTESIAN_POINT ( 'NONE',  ( 28.31250000000000000, -5.773502691896255534, -1.060575238724906372E-15 ) ) ;
#57126=CARTESIAN_POINT ( 'NONE',  ( 28.20937500061451786, -4.541064518000417216, -2.621784821875001281 ) ) ;
#57127=ADVANCED_FACE ( 'NONE', ( #39661 ), #66266, .F. ) ;
#57128=ORIENTED_EDGE ( 'NONE', *, *, #69433, .F. ) ;
#57129=CARTESIAN_POINT ( 'NONE',  ( 15.77812500061451573, 4.541064518000418104, 2.621784821874999949 ) ) ;
#57130=CARTESIAN_POINT ( 'NONE',  ( 6.628125000614517148, 6.421520780324663323E-16, -5.243569643749999010 ) ) ;
#57132=CARTESIAN_POINT ( 'NONE',  ( 4.846875000614519813, -3.027376345333610441, -5.243569643749999898 ) ) ;
#57133=EDGE_CURVE ( 'NONE', #52162, #24589, #63255, .T. ) ;
#57134=CARTESIAN_POINT ( 'NONE',  ( 16.53750000122903430, 4.330127018922191873, 2.499999999999999556 ) ) ;
#57135=CARTESIAN_POINT ( 'NONE',  ( 22.27499999999999858, 4.330127018922191873, 2.499999999999999556 ) ) ;
#57136=CARTESIAN_POINT ( 'NONE',  ( 30.00000000000000000, 0.000000000000000000, 4.999999999999998224 ) ) ;
#57137=CARTESIAN_POINT ( 'NONE',  ( 4.659375000614518925, 0.000000000000000000, 5.243569643749999010 ) ) ;
#57138=CARTESIAN_POINT ( 'NONE',  ( 9.646875000614516082, -3.027376345333614438, 5.243569643749998122 ) ) ;
#57139=CARTESIAN_POINT ( 'NONE',  ( 22.69687500061451857, -3.027376345333614438, 5.243569643749998122 ) ) ;
#57140=CYLINDRICAL_SURFACE ( 'NONE', #33600, 3.999999999999996447 ) ;
#57141=ORIENTED_EDGE ( 'NONE', *, *, #38471, .T. ) ;
#57142=CARTESIAN_POINT ( 'NONE',  ( 3.084375000614519191, 6.421520780324663323E-16, -5.243569643749999010 ) ) ;
#57143=CARTESIAN_POINT ( 'NONE',  ( 7.509375000614517681, -4.541064518000417216, -2.621784821875001281 ) ) ;
#57144=CARTESIAN_POINT ( 'NONE',  ( 19.61249999999999716, 2.886751345948126879, 4.999999999999999112 ) ) ;
#57145=CARTESIAN_POINT ( 'NONE',  ( 17.24062500061451786, -3.027376345333614438, 5.243569643749998122 ) ) ;
#57147=CARTESIAN_POINT ( 'NONE',  ( 3.486133158594716510E-16, 19.88749999999999929, 26.00000000000000355 ) ) ;
#57149=CARTESIAN_POINT ( 'NONE',  ( 11.16562500061451679, 3.027376345333613106, -5.243569643749998122 ) ) ;
#57150=CARTESIAN_POINT ( 'NONE',  ( 27.45937500061451786, 4.541064518000418104, -2.621784821874998173 ) ) ;
#57151=EDGE_CURVE ( 'NONE', #25696, #63910, #71481, .T. ) ;
#57153=CARTESIAN_POINT ( 'NONE',  ( 25.24687500061451573, 6.054752690667223547, 3.707466751127219781E-16 ) ) ;
#57154=CARTESIAN_POINT ( 'NONE',  ( 7.237500000000000711, -2.886751345948125991, -5.000000000000000000 ) ) ;
#57155=CARTESIAN_POINT ( 'NONE',  ( 2.000000000000001332, 13.96250000122903323, 33.46410161513774995 ) ) ;
#57156=CARTESIAN_POINT ( 'NONE',  ( 6.337500001229033231, -4.330127018922194537, 2.499999999999995559 ) ) ;
#57157=CARTESIAN_POINT ( 'NONE',  ( 18.38437500061451857, 6.421520780324663323E-16, -5.243569643749999010 ) ) ;
#57158=CARTESIAN_POINT ( 'NONE',  ( 12.94687500061451857, -3.027376345333610441, -5.243569643749999898 ) ) ;
#57161=CARTESIAN_POINT ( 'NONE',  ( 14.95312500061451644, 0.000000000000000000, 5.243569643749999010 ) ) ;
#57162=CARTESIAN_POINT ( 'NONE',  ( 25.65000000122903145, -2.886751345948129988, 4.999999999999997335 ) ) ;
#57163=CARTESIAN_POINT ( 'NONE',  ( 13.58437500061451786, 4.541064518000418104, 2.621784821874999949 ) ) ;
#57164=CARTESIAN_POINT ( 'NONE',  ( 30.00000000000000000, 6.123233995736764310E-16, -4.999999999999998224 ) ) ;
#57165=CARTESIAN_POINT ( 'NONE',  ( 14.80312500061451608, 4.541064518000418104, -2.621784821874998173 ) ) ;
#57166=EDGE_CURVE ( 'NONE', #24963, #42547, #72990, .T. ) ;
#57167=CARTESIAN_POINT ( 'NONE',  ( 26.51250000122903216, 0.000000000000000000, 4.999999999999998224 ) ) ;
#57168=CARTESIAN_POINT ( 'NONE',  ( 27.42187500061451644, 3.027376345333613106, -5.243569643749998122 ) ) ;
#57169=CARTESIAN_POINT ( 'NONE',  ( -2.121784821874996840, 10.42812500061451786, 33.67503911421598417 ) ) ;
#57170=CARTESIAN_POINT ( 'NONE',  ( 12.48750000122903359, 4.330127018922191873, 2.499999999999999556 ) ) ;
#57171=DIRECTION ( 'NONE',  ( 0.000000000000000000, 0.000000000000000000, 1.000000000000000000 ) ) ;
#57173=CARTESIAN_POINT ( 'NONE',  ( -4.243569643749998122, 17.19687500061451502, -27.54997392385601174 ) ) ;
#57174=CARTESIAN_POINT ( 'NONE',  ( 18.60937500061451644, 0.000000000000000000, 5.243569643749999010 ) ) ;
#57175=CARTESIAN_POINT ( 'NONE',  ( 19.80000000122903359, -2.886751345948129988, 4.999999999999997335 ) ) ;
#57176=CARTESIAN_POINT ( 'NONE',  ( 13.95937500061451786, 4.541064518000418104, -2.621784821874998173 ) ) ;
#57177=CARTESIAN_POINT ( 'NONE',  ( 4.243569643749999898, 10.59687500061451715, 32.45002607614398471 ) ) ;
#57178=CARTESIAN_POINT ( 'NONE',  ( 21.71250000122903501, -4.330127018922190985, -2.500000000000001332 ) ) ;
#57179=CARTESIAN_POINT ( 'NONE',  ( 14.99062500061451786, -3.027376345333614438, 5.243569643749998122 ) ) ;
#57181=ORIENTED_EDGE ( 'NONE', *, *, #13482, .T. ) ;
#57184=CARTESIAN_POINT ( 'NONE',  ( 17.43750000000000355, -2.886751345948129988, 4.999999999999997335 ) ) ;
#57186=CARTESIAN_POINT ( 'NONE',  ( 1.091159441285789677, 4.887044806266474417, 33.85802829779076717 ) ) ;
#57187=CARTESIAN_POINT ( 'NONE',  ( 14.73750000122903359, 4.330127018922191873, 2.499999999999999556 ) ) ;
#57188=CARTESIAN_POINT ( 'NONE',  ( 20.50312500061451715, -4.541064518000417216, -2.621784821875001281 ) ) ;
#57189=CARTESIAN_POINT ( 'NONE',  ( 22.04062500061451502, 6.054752690667223547, 3.707466751127219781E-16 ) ) ;
#57190=CARTESIAN_POINT ( 'NONE',  ( 2.840625000614518392, -3.027376345333614438, 5.243569643749998122 ) ) ;
#57191=CARTESIAN_POINT ( 'NONE',  ( 27.18750000000000000, 5.773502691896255534, 3.535250795749688894E-16 ) ) ;
#57192=CARTESIAN_POINT ( 'NONE',  ( 4.750527263192109828, 3.347582200546265430, 4.201817546140637738 ) ) ;
#57195=CARTESIAN_POINT ( 'NONE',  ( -2.000000000000000000, 11.93750000122903465, -33.46410161513775705 ) ) ;
#57196=CARTESIAN_POINT ( 'NONE',  ( 4.243569643749999010, 16.52187500061451786, -32.45002607614398471 ) ) ;
#57197=CARTESIAN_POINT ( 'NONE',  ( 6.975000001229032520, 2.886751345948129099, -4.999999999999998224 ) ) ;
#57198=CARTESIAN_POINT ( 'NONE',  ( 9.525000000000002132, 6.123233995736764310E-16, -4.999999999999998224 ) ) ;
#57199=CARTESIAN_POINT ( 'NONE',  ( 5.137500001229033941, 6.123233995736764310E-16, -4.999999999999998224 ) ) ;
#57200=CARTESIAN_POINT ( 'NONE',  ( 10.24687500061451750, -3.027376345333610441, -5.243569643749999898 ) ) ;
#57201=CARTESIAN_POINT ( 'NONE',  ( 23.66250000122903430, 4.330127018922192761, -2.499999999999997780 ) ) ;
#57202=CARTESIAN_POINT ( 'NONE',  ( 3.531796677802674367, 3.539267187803308179, -3.868928841707397925 ) ) ;
#57203=CARTESIAN_POINT ( 'NONE',  ( 28.04999999999999716, 4.330127018922192761, -2.499999999999997780 ) ) ;
#57206=CARTESIAN_POINT ( 'NONE',  ( 8.709375000614517859, 0.000000000000000000, 5.243569643749999010 ) ) ;
#57207=CARTESIAN_POINT ( 'NONE',  ( 13.32187500061451502, -6.054752690667223547, -1.112240025338166033E-15 ) ) ;
#57209=CARTESIAN_POINT ( 'NONE',  ( 7.537500000000002309, -2.886751345948129988, 4.999999999999997335 ) ) ;
#57210=AXIS2_PLACEMENT_3D ( 'NONE', #45512, #28508, #22239 ) ;
#57211=CARTESIAN_POINT ( 'NONE',  ( 4.243569643749999898, 16.42812500061459247, 30.00000000000000000 ) ) ;
#57212=CARTESIAN_POINT ( 'NONE',  ( 22.28437500061451715, -4.541064518000419881, 2.621784821874995952 ) ) ;
#57214=CARTESIAN_POINT ( 'NONE',  ( 25.87500000122903288, 2.886751345948129099, -4.999999999999998224 ) ) ;
#57215=VECTOR ( 'NONE', #62776, 1000.000000000000000 ) ;
#57217=CARTESIAN_POINT ( 'NONE',  ( 22.94062500061451715, 6.054752690667223547, 3.707466751127219781E-16 ) ) ;
#57218=CARTESIAN_POINT ( 'NONE',  ( 16.22812500061451857, 4.541064518000418104, 2.621784821874999949 ) ) ;
#57220=CARTESIAN_POINT ( 'NONE',  ( 12.49687500061451573, -3.027376345333610441, -5.243569643749999898 ) ) ;
#57221=CARTESIAN_POINT ( 'NONE',  ( 28.57499999999999929, 4.330127018922191873, 2.499999999999999556 ) ) ;
#57222=CARTESIAN_POINT ( 'NONE',  ( 24.67500000122903359, 2.886751345948126879, 4.999999999999999112 ) ) ;
#57223=CARTESIAN_POINT ( 'NONE',  ( 11.93437500061451573, -4.541064518000419881, 2.621784821874995952 ) ) ;
#57224=CARTESIAN_POINT ( 'NONE',  ( 29.44687500061451857, -3.027376345333614438, 5.243569643749998122 ) ) ;
#57225=CARTESIAN_POINT ( 'NONE',  ( 2.971875000614517592, -6.054752690667223547, -1.112240025338166033E-15 ) ) ;
#57226=CARTESIAN_POINT ( 'NONE',  ( 16.61250000122903359, 0.000000000000000000, 4.999999999999998224 ) ) ;
#57227=CARTESIAN_POINT ( 'NONE',  ( 22.77187500061451786, -6.054752690667223547, -1.112240025338166033E-15 ) ) ;
#57228=CARTESIAN_POINT ( 'NONE',  ( 13.24687500061451750, -3.027376345333614438, 5.243569643749998122 ) ) ;
#57230=CARTESIAN_POINT ( 'NONE',  ( 25.46249999999999858, 2.886751345948126879, 4.999999999999999112 ) ) ;
#57233=CARTESIAN_POINT ( 'NONE',  ( 18.10312500061451502, 0.000000000000000000, 5.243569643749999010 ) ) ;
#57234=CARTESIAN_POINT ( 'NONE',  ( 5.812500000000001776, -5.773502691896255534, -1.060575238724906372E-15 ) ) ;
#57235=EDGE_CURVE ( 'NONE', #45966, #31631, #17724, .T. ) ;
#57236=CARTESIAN_POINT ( 'NONE',  ( 4.169580978743460342, 2.759455464706926708, 4.458747374224691029 ) ) ;
#57237=CARTESIAN_POINT ( 'NONE',  ( 15.56250000000000000, 2.886751345948126879, 4.999999999999999112 ) ) ;
#57238=CARTESIAN_POINT ( 'NONE',  ( -4.243569643749999898, 9.903125000614517504, 30.00000000000000000 ) ) ;
#57239=CARTESIAN_POINT ( 'NONE',  ( 3.275492200589926739, -3.777717676570560901, -3.275492200590059078 ) ) ;
#57240=CARTESIAN_POINT ( 'NONE',  ( 26.93437500061451573, 6.421520780324663323E-16, -5.243569643749999010 ) ) ;
#57242=CARTESIAN_POINT ( 'NONE',  ( 22.41562500061451502, 3.027376345333613106, -5.243569643749998122 ) ) ;
#57243=CARTESIAN_POINT ( 'NONE',  ( 20.14687500061451786, -3.027376345333610441, -5.243569643749999898 ) ) ;
#57244=CARTESIAN_POINT ( 'NONE',  ( 3.900000000000000799, 0.000000000000000000, 4.999999999999998224 ) ) ;
#57245=CARTESIAN_POINT ( 'NONE',  ( 8.203125000614518214, 0.000000000000000000, 5.243569643749999010 ) ) ;
#57246=CARTESIAN_POINT ( 'NONE',  ( 25.19062500061451715, 6.054752690667223547, 3.707466751127219781E-16 ) ) ;
#57247=CARTESIAN_POINT ( 'NONE',  ( 12.90937500061451537, -4.541064518000417216, -2.621784821875001281 ) ) ;
#57248=CARTESIAN_POINT ( 'NONE',  ( 17.55937500061451573, 4.541064518000418104, -2.621784821874998173 ) ) ;
#57249=CARTESIAN_POINT ( 'NONE',  ( -2.121784821874996840, 17.17812500061451786, 33.67503911421598417 ) ) ;
#57250=CARTESIAN_POINT ( 'NONE',  ( 18.30000000122903359, 5.773502691896255534, 3.535250795749688894E-16 ) ) ;
#57252=CARTESIAN_POINT ( 'NONE',  ( 10.34062500061451750, 6.054752690667223547, 3.707466751127219781E-16 ) ) ;
#57253=CARTESIAN_POINT ( 'NONE',  ( 6.346875000614517148, 6.054752690667223547, 3.707466751127219781E-16 ) ) ;
#57254=CARTESIAN_POINT ( 'NONE',  ( 4.359375000614517326, -4.541064518000417216, -2.621784821875001281 ) ) ;
#57255=ORIENTED_EDGE ( 'NONE', *, *, #60575, .F. ) ;
#57256=CARTESIAN_POINT ( 'NONE',  ( 25.84687500061451360, -3.027376345333614438, 5.243569643749998122 ) ) ;
#57257=CARTESIAN_POINT ( 'NONE',  ( 16.30312500061451786, 0.000000000000000000, 5.243569643749999010 ) ) ;
#57258=CARTESIAN_POINT ( 'NONE',  ( 28.38750000122903216, -4.330127018922194537, 2.499999999999995559 ) ) ;
#57259=CARTESIAN_POINT ( 'NONE',  ( 26.95312500061451644, 4.541064518000418104, -2.621784821874998173 ) ) ;
#57260=CARTESIAN_POINT ( 'NONE',  ( 21.90937500061451715, -4.541064518000417216, -2.621784821875001281 ) ) ;
#57261=CARTESIAN_POINT ( 'NONE',  ( 16.52812500061451573, 6.421520780324663323E-16, -5.243569643749999010 ) ) ;
#57262=CARTESIAN_POINT ( 'NONE',  ( -4.243569643749999898, 18.05937500061451928, 30.00000000000000000 ) ) ;
#57264=CARTESIAN_POINT ( 'NONE',  ( 21.96562500061451573, 3.027376345333613106, -5.243569643749998122 ) ) ;
#57265=CARTESIAN_POINT ( 'NONE',  ( 3.225000001229033408, -5.773502691896255534, -1.060575238724906372E-15 ) ) ;
#57266=VERTEX_POINT ( 'NONE', #11930 ) ;
#57267=CARTESIAN_POINT ( 'NONE',  ( 25.64999999999999858, -4.330127018922190985, -2.500000000000001332 ) ) ;
#57268=CARTESIAN_POINT ( 'NONE',  ( 2.000000000000001332, 13.85000000000000142, -26.53589838486224650 ) ) ;
#57271=CARTESIAN_POINT ( 'NONE',  ( 2.934375000614518392, -4.541064518000419881, 2.621784821874995952 ) ) ;
#57272=CARTESIAN_POINT ( 'NONE',  ( 10.82812500061451644, 4.541064518000418104, 2.621784821874999949 ) ) ;
#57273=CARTESIAN_POINT ( 'NONE',  ( 21.67500000122903359, -5.773502691896255534, -1.060575238724906372E-15 ) ) ;
#57275=EDGE_CURVE ( 'NONE', #6802, #3090, #55077, .T. ) ;
#57276=CARTESIAN_POINT ( 'NONE',  ( 27.02812500061451573, 4.541064518000418104, 2.621784821874999949 ) ) ;
#57277=CARTESIAN_POINT ( 'NONE',  ( 26.88749999999999574, -2.886751345948129988, 4.999999999999997335 ) ) ;
#57278=CARTESIAN_POINT ( 'NONE',  ( -3.999999999999999112, 17.41250000122903430, -30.00000000000000000 ) ) ;
#57279=CARTESIAN_POINT ( 'NONE',  ( -2.000000000000000000, 12.38750000122903394, 26.53589838486224650 ) ) ;
#57280=CARTESIAN_POINT ( 'NONE',  ( 9.703125000614514661, -4.541064518000417216, -2.621784821875001281 ) ) ;
#57281=( BOUNDED_CURVE ( )  B_SPLINE_CURVE ( 2, ( #68417, #57677, #23336, #58031, #29967, #63224, #18508 ),
 .UNSPECIFIED., .F., .F. ) 
 B_SPLINE_CURVE_WITH_KNOTS ( ( 3, 2, 2, 3 ),
 ( 0.7083333333333334814, 0.7111111111111112493, 0.7138888888888890172, 0.7166666666666667851 ),
 .UNSPECIFIED. ) 
 CURVE ( )  GEOMETRIC_REPRESENTATION_ITEM ( )  RATIONAL_B_SPLINE_CURVE ( ( 0.9999999999999946709, 0.8660254037844440367, 1.000000000000000000, 0.8660254037844387076, 1.000000000000000000, 0.8660254037844333785, 1.000000000000005329 ) ) 
 REPRESENTATION_ITEM ( '' )  );
#57283=VECTOR ( 'NONE', #43847, 1000.000000000000000 ) ;
#57284=CARTESIAN_POINT ( 'NONE',  ( 7.790625000614518569, -3.027376345333614438, 5.243569643749998122 ) ) ;
#57286=VECTOR ( 'NONE', #22969, 1000.000000000000000 ) ;
#57287=CARTESIAN_POINT ( 'NONE',  ( 5.315625000614516260, 3.027376345333613106, -5.243569643749998122 ) ) ;
#57289=EDGE_CURVE ( 'NONE', #50879, #30796, #33632, .T. ) ;
#57290=DIRECTION ( 'NONE',  ( -0.000000000000000000, -1.000000000000000000, -0.000000000000000000 ) ) ;
#57291=CARTESIAN_POINT ( 'NONE',  ( 14.43750000000000000, -2.886751345948125991, -5.000000000000000000 ) ) ;
#57292=CARTESIAN_POINT ( 'NONE',  ( 15.49687500061451750, -3.027376345333614438, 5.243569643749998122 ) ) ;
#57293=CARTESIAN_POINT ( 'NONE',  ( 10.16250000122903252, 4.330127018922192761, -2.499999999999997780 ) ) ;
#57294=CARTESIAN_POINT ( 'NONE',  ( 20.33437500061451786, 4.541064518000418104, 2.621784821874999949 ) ) ;
#57296=CARTESIAN_POINT ( 'NONE',  ( 20.40937500061451715, 0.000000000000000000, 5.243569643749999010 ) ) ;
#57297=CARTESIAN_POINT ( 'NONE',  ( -4.243569643749999898, 13.95312500061451821, -30.00000000000000000 ) ) ;
#57298=CARTESIAN_POINT ( 'NONE',  ( -3.999999999999999112, 16.81250000000000000, 27.69059892324149885 ) ) ;
#57301=CARTESIAN_POINT ( 'NONE',  ( 24.70312500061451644, 4.541064518000418104, -2.621784821874998173 ) ) ;
#57302=CARTESIAN_POINT ( 'NONE',  ( 24.82499999999999929, 6.123233995736764310E-16, -4.999999999999998224 ) ) ;
#57303=CARTESIAN_POINT ( 'NONE',  ( 27.72187500061451715, -6.054752690667223547, -1.112240025338166033E-15 ) ) ;
#57304=CARTESIAN_POINT ( 'NONE',  ( 23.13749999999999929, 5.773502691896255534, 3.535250795749688894E-16 ) ) ;
#57305=CARTESIAN_POINT ( 'NONE',  ( 8.015625000614518214, 3.027376345333613106, -5.243569643749998122 ) ) ;
#57307=CARTESIAN_POINT ( 'NONE',  ( 19.58437500061451786, -4.541064518000419881, 2.621784821874995952 ) ) ;
#57309=VECTOR ( 'NONE', #20094, 1000.000000000000000 ) ;
#57310=CARTESIAN_POINT ( 'NONE',  ( 4.565625000614516260, 3.027376345333611329, 5.243569643749999010 ) ) ;
#57311=CARTESIAN_POINT ( 'NONE',  ( 8.784375000614518925, -4.541064518000419881, 2.621784821874995952 ) ) ;
#57312=ORIENTED_EDGE ( 'NONE', *, *, #32388, .F. ) ;
#57313=CARTESIAN_POINT ( 'NONE',  ( 19.58437500061451786, -4.541064518000419881, 2.621784821874995952 ) ) ;
#57314=CARTESIAN_POINT ( 'NONE',  ( 13.83750000122903323, 4.330127018922191873, 2.499999999999999556 ) ) ;
#57315=CARTESIAN_POINT ( 'NONE',  ( 29.39999999999999858, 4.330127018922192761, -2.499999999999997780 ) ) ;
#57316=CARTESIAN_POINT ( 'NONE',  ( 3.450000000000001510, 0.000000000000000000, 4.999999999999998224 ) ) ;
#57318=CARTESIAN_POINT ( 'NONE',  ( 27.82499999999999929, -4.330127018922194537, 2.499999999999995559 ) ) ;
#57319=ORIENTED_EDGE ( 'NONE', *, *, #55505, .T. ) ;
#57320=CARTESIAN_POINT ( 'NONE',  ( 9.562500000000001776, 2.886751345948129099, -4.999999999999998224 ) ) ;
#57322=CARTESIAN_POINT ( 'NONE',  ( 23.65312500061451573, -4.541064518000417216, -2.621784821875001281 ) ) ;
#57323=CARTESIAN_POINT ( 'NONE',  ( 13.76250000000000107, 2.886751345948126879, 4.999999999999999112 ) ) ;
#57324=CARTESIAN_POINT ( 'NONE',  ( 11.36250000122903536, -4.330127018922190985, -2.500000000000001332 ) ) ;
#57325=CARTESIAN_POINT ( 'NONE',  ( 9.328125000614518214, 6.421520780324663323E-16, -5.243569643749999010 ) ) ;
#57326=CARTESIAN_POINT ( 'NONE',  ( 23.17500000000000071, 4.330127018922191873, 2.499999999999999556 ) ) ;
#57327=CARTESIAN_POINT ( 'NONE',  ( 21.32812500061451644, -4.541064518000419881, 2.621784821874995952 ) ) ;
#57328=CARTESIAN_POINT ( 'NONE',  ( 18.78750000122903430, 4.330127018922191873, 2.499999999999999556 ) ) ;
#57329=CARTESIAN_POINT ( 'NONE',  ( 27.52500000122903145, -5.773502691896255534, -1.060575238724906372E-15 ) ) ;
#57331=CARTESIAN_POINT ( 'NONE',  ( 6.487499999999999822, 5.773502691896255534, 3.535250795749688894E-16 ) ) ;
#57332=ORIENTED_EDGE ( 'NONE', *, *, #32403, .T. ) ;
#57333=CARTESIAN_POINT ( 'NONE',  ( 23.01562500061451644, 3.027376345333611329, 5.243569643749999010 ) ) ;
#57334=CARTESIAN_POINT ( 'NONE',  ( 28.04062500061451502, -3.027376345333614438, 5.243569643749998122 ) ) ;
#57335=CARTESIAN_POINT ( 'NONE',  ( 28.35937500061451289, 4.541064518000418104, -2.621784821874998173 ) ) ;
#57336=CARTESIAN_POINT ( 'NONE',  ( 18.79687500061451644, -3.027376345333610441, -5.243569643749999898 ) ) ;
#57337=CARTESIAN_POINT ( 'NONE',  ( 13.30312500061451786, -4.541064518000417216, -2.621784821875001281 ) ) ;
#57338=CARTESIAN_POINT ( 'NONE',  ( 4.111889464957033447, 2.844708250062874644, 4.404844785106587501 ) ) ;
#57339=CARTESIAN_POINT ( 'NONE',  ( 27.11250000122903359, -4.330127018922190985, -2.500000000000001332 ) ) ;
#57341=CARTESIAN_POINT ( 'NONE',  ( 16.71562500061451573, 3.027376345333611329, 5.243569643749999010 ) ) ;
#57342=CARTESIAN_POINT ( 'NONE',  ( 3.787500001229033408, 6.123233995736764310E-16, -4.999999999999998224 ) ) ;
#57343=CARTESIAN_POINT ( 'NONE',  ( 12.98437500061451821, 6.421520780324663323E-16, -5.243569643749999010 ) ) ;
#57344=CARTESIAN_POINT ( 'NONE',  ( 12.00937500061451857, -4.541064518000417216, -2.621784821875001281 ) ) ;
#57345=CARTESIAN_POINT ( 'NONE',  ( 20.03437500061451715, -4.541064518000419881, 2.621784821874995952 ) ) ;
#57347=CARTESIAN_POINT ( 'NONE',  ( -4.761366016028759418, 8.797204459235659968, 33.67116182595535889 ) ) ;
#57348=CARTESIAN_POINT ( 'NONE',  ( 23.80312500061451786, 4.541064518000418104, -2.621784821874998173 ) ) ;
#57349=CARTESIAN_POINT ( 'NONE',  ( 19.62187500061451573, -6.054752690667223547, -1.112240025338166033E-15 ) ) ;
#57350=CARTESIAN_POINT ( 'NONE',  ( 23.84062500061451928, 6.054752690667223547, 3.707466751127219781E-16 ) ) ;
#57351=CARTESIAN_POINT ( 'NONE',  ( 27.29999999999999716, 0.000000000000000000, 4.999999999999998224 ) ) ;
#57352=CARTESIAN_POINT ( 'NONE',  ( 8.484601909799253346E-16, 17.86250000000000071, 34.61880215351700230 ) ) ;
#57353=CARTESIAN_POINT ( 'NONE',  ( 3.196875000614516793, 6.054752690667223547, 3.707466751127219781E-16 ) ) ;
#57354=CARTESIAN_POINT ( 'NONE',  ( 10.31250000122903288, 0.000000000000000000, 4.999999999999998224 ) ) ;
#57355=CARTESIAN_POINT ( 'NONE',  ( 7.200000001229035718, -2.886751345948129988, 4.999999999999997335 ) ) ;
#57356=CARTESIAN_POINT ( 'NONE',  ( 26.28750000122903430, 6.123233995736764310E-16, -4.999999999999998224 ) ) ;
#57359=CARTESIAN_POINT ( 'NONE',  ( 8.559375000614515727, 4.541064518000418104, -2.621784821874998173 ) ) ;
#57361=CARTESIAN_POINT ( 'NONE',  ( 18.40312500061451573, 4.541064518000418104, -2.621784821874998173 ) ) ;
#57362=CARTESIAN_POINT ( 'NONE',  ( 11.59687500061451892, -3.027376345333610441, -5.243569643749999898 ) ) ;
#57363=CARTESIAN_POINT ( 'NONE',  ( 28.38750000122903216, -4.330127018922194537, 2.499999999999995559 ) ) ;
#57364=CARTESIAN_POINT ( 'NONE',  ( 19.65937500061451360, -4.541064518000417216, -2.621784821875001281 ) ) ;
#57365=CARTESIAN_POINT ( 'NONE',  ( 8.146875000614516082, 6.054752690667223547, 3.707466751127219781E-16 ) ) ;
#57366=CARTESIAN_POINT ( 'NONE',  ( 14.96250000122903323, -4.330127018922190985, -2.500000000000001332 ) ) ;
#57368=CARTESIAN_POINT ( 'NONE',  ( 7.790625000614518569, -3.027376345333614438, 5.243569643749998122 ) ) ;
#57369=CARTESIAN_POINT ( 'NONE',  ( 18.32812500061451644, 6.421520780324663323E-16, -5.243569643749999010 ) ) ;
#57370=VERTEX_POINT ( 'NONE', #19258 ) ;
#57371=CARTESIAN_POINT ( 'NONE',  ( 5.775000001229033231, 2.886751345948126879, 4.999999999999999112 ) ) ;
#57372=CARTESIAN_POINT ( 'NONE',  ( 14.12812500061451715, -4.541064518000419881, 2.621784821874995952 ) ) ;
#57373=CIRCLE ( 'NONE', #37333, 4.000000000000000000 ) ;
#57374=CARTESIAN_POINT ( 'NONE',  ( 12.59062500061451573, 6.054752690667223547, 3.707466751127219781E-16 ) ) ;
#57376=CARTESIAN_POINT ( 'NONE',  ( 14.06250000000000000, 2.886751345948129099, -4.999999999999998224 ) ) ;
#57377=CARTESIAN_POINT ( 'NONE',  ( 7.987500001229032698, 4.330127018922191873, 2.499999999999999556 ) ) ;
#57378=CARTESIAN_POINT ( 'NONE',  ( 4.790625000614518569, -3.027376345333610441, -5.243569643749999898 ) ) ;
#57379=CARTESIAN_POINT ( 'NONE',  ( 17.88750000122903216, 4.330127018922191873, 2.499999999999999556 ) ) ;
#57381=CARTESIAN_POINT ( 'NONE',  ( -3.000416591977282496E-16, 10.74687500061451928, -34.90005215228797653 ) ) ;
#57382=DIRECTION ( 'NONE',  ( -1.000000000000000000, -0.000000000000000000, -0.000000000000000000 ) ) ;
#57383=CARTESIAN_POINT ( 'NONE',  ( 2.737500001229034474, -4.330127018922194537, 2.499999999999995559 ) ) ;
#57384=CARTESIAN_POINT ( 'NONE',  ( -1.999999999999997113, 11.52500000000000036, -26.53589838486224295 ) ) ;
#57385=CARTESIAN_POINT ( 'NONE',  ( -1.071796769724488563, 13.34240381056766545, 34.00000000000000000 ) ) ;
#57386=CARTESIAN_POINT ( 'NONE',  ( 19.20937500061451786, -4.541064518000417216, -2.621784821875001281 ) ) ;
#57387=CARTESIAN_POINT ( 'NONE',  ( -3.999999999999997335, 16.55000000122903359, 32.30940107675850470 ) ) ;
#57388=CARTESIAN_POINT ( 'NONE',  ( 14.09062500061451750, -3.027376345333614438, 5.243569643749998122 ) ) ;
#57391=CARTESIAN_POINT ( 'NONE',  ( 27.27187500061451431, -6.054752690667223547, -1.112240025338166033E-15 ) ) ;
#57393=CARTESIAN_POINT ( 'NONE',  ( 12.36562500061451608, -6.054752690667223547, -1.112240025338166033E-15 ) ) ;
#57394=CARTESIAN_POINT ( 'NONE',  ( 11.52187500061451608, -6.054752690667223547, -1.112240025338166033E-15 ) ) ;
#57395=ORIENTED_EDGE ( 'NONE', *, *, #21641, .T. ) ;
#57396=AXIS2_PLACEMENT_3D ( 'NONE', #49267, #32632, #66994 ) ;
#57397=CARTESIAN_POINT ( 'NONE',  ( 29.16562500061451502, 3.027376345333613106, -5.243569643749998122 ) ) ;
#57398=CARTESIAN_POINT ( 'NONE',  ( 20.12812500061451715, 6.421520780324663323E-16, -5.243569643749999010 ) ) ;
#57399=CARTESIAN_POINT ( 'NONE',  ( 29.31562500061451715, 3.027376345333611329, 5.243569643749999010 ) ) ;
#57401=EDGE_CURVE ( 'NONE', #51638, #30066, #70596, .T. ) ;
#57402=CARTESIAN_POINT ( 'NONE',  ( 9.862500000000000711, -5.773502691896255534, -1.060575238724906372E-15 ) ) ;
#57403=CARTESIAN_POINT ( 'NONE',  ( 19.35000000122903430, -2.886751345948129988, 4.999999999999997335 ) ) ;
#57404=CARTESIAN_POINT ( 'NONE',  ( -1.389181105737270716, 10.01354714573257532, 26.18324193183354964 ) ) ;
#57407=CARTESIAN_POINT ( 'NONE',  ( 17.77499999999999858, 4.330127018922191873, 2.499999999999999556 ) ) ;
#57408=CARTESIAN_POINT ( 'NONE',  ( 20.58750000000000213, -2.886751345948129988, 4.999999999999997335 ) ) ;
#57409=CARTESIAN_POINT ( 'NONE',  ( 18.64687500061451786, -3.027376345333614438, 5.243569643749998122 ) ) ;
#57410=CARTESIAN_POINT ( 'NONE',  ( 24.74062500061451786, 6.054752690667223547, 3.707466751127219781E-16 ) ) ;
#57411=EDGE_CURVE ( 'NONE', #46843, #13938, #39973, .T. ) ;
#57413=CARTESIAN_POINT ( 'NONE',  ( 8.353125000614518569, -4.541064518000417216, -2.621784821875001281 ) ) ;
#57415=VECTOR ( 'NONE', #44337, 1000.000000000000000 ) ;
#57416=CARTESIAN_POINT ( 'NONE',  ( 13.79999999999999893, 0.000000000000000000, 4.999999999999998224 ) ) ;
#57417=CARTESIAN_POINT ( 'NONE',  ( -4.243569643749999898, 17.51562500061451644, 27.54997392385601529 ) ) ;
#57418=CARTESIAN_POINT ( 'NONE',  ( 3.121875000614518836, 3.027376345333613106, -5.243569643749998122 ) ) ;
#57421=CARTESIAN_POINT ( 'NONE',  ( 25.43437500061451573, -4.541064518000419881, 2.621784821874995952 ) ) ;
#57422=VERTEX_POINT ( 'NONE', #37372 ) ;
#57423=CARTESIAN_POINT ( 'NONE',  ( 22.00312500061451360, 4.541064518000418104, -2.621784821874998173 ) ) ;
#57424=CARTESIAN_POINT ( 'NONE',  ( 23.67187500061451999, -6.054752690667223547, -1.112240025338166033E-15 ) ) ;
#57425=CARTESIAN_POINT ( 'NONE',  ( 2.121784821875001281, 17.25312500061459176, -26.32496088578401938 ) ) ;
#57426=CARTESIAN_POINT ( 'NONE',  ( 10.53750000000000320, 5.773502691896255534, 3.535250795749688894E-16 ) ) ;
#57427=CARTESIAN_POINT ( 'NONE',  ( 7.940625000614518036, -3.027376345333610441, -5.243569643749999898 ) ) ;
#57429=CARTESIAN_POINT ( 'NONE',  ( 23.35312500061451857, 4.541064518000418104, -2.621784821874998173 ) ) ;
#57432=CARTESIAN_POINT ( 'NONE',  ( 20.63437500061451857, 6.421520780324663323E-16, -5.243569643749999010 ) ) ;
#57434=CARTESIAN_POINT ( 'NONE',  ( -2.121784821874999949, 13.03437500061451715, 26.32496088578401938 ) ) ;
#57435=CARTESIAN_POINT ( 'NONE',  ( 18.53437500061451715, 4.541064518000418104, 2.621784821874999949 ) ) ;
#57436=CARTESIAN_POINT ( 'NONE',  ( 27.19687500061451857, -3.027376345333614438, 5.243569643749998122 ) ) ;
#57437=CARTESIAN_POINT ( 'NONE',  ( 4.243569643749999898, 17.79687500061451999, 32.45002607614398471 ) ) ;
#57438=CARTESIAN_POINT ( 'NONE',  ( 8.090625000614515727, 6.054752690667223547, 3.707466751127219781E-16 ) ) ;
#57440=CARTESIAN_POINT ( 'NONE',  ( 4.734375000614518214, -4.541064518000419881, 2.621784821874995952 ) ) ;
#57441=FACE_OUTER_BOUND ( 'NONE', #36696, .T. ) ;
#57442=CARTESIAN_POINT ( 'NONE',  ( 6.290625000614517681, 6.054752690667223547, 3.707466751127219781E-16 ) ) ;
#57443=CARTESIAN_POINT ( 'NONE',  ( 9.084375000614517859, 4.541064518000418104, 2.621784821874999949 ) ) ;
#57444=CARTESIAN_POINT ( 'NONE',  ( 16.27500000122903501, -5.773502691896255534, -1.060575238724906372E-15 ) ) ;
#57445=CARTESIAN_POINT ( 'NONE',  ( 5.334375000614517859, 6.421520780324663323E-16, -5.243569643749999010 ) ) ;
#57446=CARTESIAN_POINT ( 'NONE',  ( 8.315625000614515372, -6.054752690667223547, -1.112240025338166033E-15 ) ) ;
#57447=CARTESIAN_POINT ( 'NONE',  ( 4.940625000614516260, 6.054752690667223547, 3.707466751127219781E-16 ) ) ;
#57449=CARTESIAN_POINT ( 'NONE',  ( 17.40937500061451715, -4.541064518000417216, -2.621784821875001281 ) ) ;
#57452=CARTESIAN_POINT ( 'NONE',  ( 25.71562500061451573, 3.027376345333611329, 5.243569643749999010 ) ) ;
#57453=CARTESIAN_POINT ( 'NONE',  ( 9.853125000614516793, 4.541064518000418104, -2.621784821874998173 ) ) ;
#57454=CARTESIAN_POINT ( 'NONE',  ( 26.48437500061451644, 6.421520780324663323E-16, -5.243569643749999010 ) ) ;
#57455=CARTESIAN_POINT ( 'NONE',  ( 9.778125000614517504, 6.421520780324663323E-16, -5.243569643749999010 ) ) ;
#57456=CARTESIAN_POINT ( 'NONE',  ( 4.243569643749999898, 10.59687500061451715, -27.54997392385601529 ) ) ;
#57457=CARTESIAN_POINT ( 'NONE',  ( 10.31250000122903288, 0.000000000000000000, 4.999999999999998224 ) ) ;
#57458=CARTESIAN_POINT ( 'NONE',  ( 26.20312500061451644, 0.000000000000000000, 5.243569643749999010 ) ) ;
#57459=CARTESIAN_POINT ( 'NONE',  ( -2.121784821874996840, 12.22812500061451857, -26.32496088578401583 ) ) ;
#57460=CARTESIAN_POINT ( 'NONE',  ( 12.30000000122903181, -2.886751345948125991, -5.000000000000000000 ) ) ;
#57461=CARTESIAN_POINT ( 'NONE',  ( 22.75312500061451360, -4.541064518000417216, -2.621784821875001281 ) ) ;
#57462=CARTESIAN_POINT ( 'NONE',  ( 11.88749999999999751, 5.773502691896255534, 3.535250795749688894E-16 ) ) ;
#57463=CARTESIAN_POINT ( 'NONE',  ( 19.90312500061451573, 0.000000000000000000, 5.243569643749999010 ) ) ;
#57464=CARTESIAN_POINT ( 'NONE',  ( 6.421875000614519102, 3.027376345333611329, 5.243569643749999010 ) ) ;
#57465=CARTESIAN_POINT ( 'NONE',  ( 21.11249999999999716, -5.773502691896255534, -1.060575238724906372E-15 ) ) ;
#57466=CARTESIAN_POINT ( 'NONE',  ( 7.125000001229033764, 2.886751345948126879, 4.999999999999999112 ) ) ;
#57467=CARTESIAN_POINT ( 'NONE',  ( 15.22500000122903252, 2.886751345948126879, 4.999999999999999112 ) ) ;
#57468=AXIS2_PLACEMENT_3D ( 'NONE', #62883, #56278, #40733 ) ;
#57469=CARTESIAN_POINT ( 'NONE',  ( 13.49062500061451608, 6.054752690667223547, 3.707466751127219781E-16 ) ) ;
#57470=CARTESIAN_POINT ( 'NONE',  ( 15.06562500061451537, -6.054752690667223547, -1.112240025338166033E-15 ) ) ;
#57471=CARTESIAN_POINT ( 'NONE',  ( 26.43750000122903288, 4.330127018922191873, 2.499999999999999556 ) ) ;
#57472=CARTESIAN_POINT ( 'NONE',  ( 20.10000000000000142, 0.000000000000000000, 4.999999999999998224 ) ) ;
#57473=CARTESIAN_POINT ( 'NONE',  ( 22.92187500061451644, 3.027376345333613106, -5.243569643749998122 ) ) ;
#57475=CARTESIAN_POINT ( 'NONE',  ( 10.50000000122903465, -2.886751345948125991, -5.000000000000000000 ) ) ;
#57476=CARTESIAN_POINT ( 'NONE',  ( 7.846875000614518036, -3.027376345333614438, 5.243569643749998122 ) ) ;
#57477=CARTESIAN_POINT ( 'NONE',  ( 26.63437500061451857, 4.541064518000418104, 2.621784821874999949 ) ) ;
#57478=( BOUNDED_CURVE ( )  B_SPLINE_CURVE ( 2, ( #43363, #32997, #55536, #49997, #72522, #21910, #5289, #27834, #50366 ),
 .UNSPECIFIED., .F., .F. ) 
 B_SPLINE_CURVE_WITH_KNOTS ( ( 3, 2, 2, 2, 3 ),
 ( 0.6195652173913043237, 0.6231884057971014412, 0.6304347826086956763, 0.6376811594202898004, 0.6413043478260869179 ),
 .UNSPECIFIED. ) 
 CURVE ( )  GEOMETRIC_REPRESENTATION_ITEM ( )  RATIONAL_B_SPLINE_CURVE ( ( 0.9330127018922194093, 0.9330127018922194093, 1.000000000000000000, 0.8660254037844387076, 1.000000000000000000, 0.8660254037844387076, 1.000000000000000000, 0.9330127018922194093, 0.9330127018922194093 ) ) 
 REPRESENTATION_ITEM ( '' )  );
#57479=CARTESIAN_POINT ( 'NONE',  ( 3.084375000614519191, 6.421520780324663323E-16, -5.243569643749999010 ) ) ;
#57480=CARTESIAN_POINT ( 'NONE',  ( 20.87812500061451715, -4.541064518000419881, 2.621784821874995952 ) ) ;
#57481=CARTESIAN_POINT ( 'NONE',  ( 27.64687500061452141, -3.027376345333614438, 5.243569643749998122 ) ) ;
#57484=CARTESIAN_POINT ( 'NONE',  ( 6.946875000614517681, -3.027376345333614438, 5.243569643749998122 ) ) ;
#57485=CARTESIAN_POINT ( 'NONE',  ( 20.80312500061451431, 0.000000000000000000, 5.243569643749999010 ) ) ;
#57486=ORIENTED_EDGE ( 'NONE', *, *, #31877, .T. ) ;
#57487=CARTESIAN_POINT ( 'NONE',  ( 2.000000000000001332, 12.50000000000000000, 33.46410161513774995 ) ) ;
#57488=CARTESIAN_POINT ( 'NONE',  ( 27.85312500061451502, 4.541064518000418104, -2.621784821874998173 ) ) ;
#57489=CARTESIAN_POINT ( 'NONE',  ( 4.134375000614517681, 4.541064518000418104, 2.621784821874999949 ) ) ;
#57490=CARTESIAN_POINT ( 'NONE',  ( 6.712500000000000355, -5.773502691896255534, -1.060575238724906372E-15 ) ) ;
#57492=CARTESIAN_POINT ( 'NONE',  ( 16.87500000000000000, 4.330127018922191873, 2.499999999999999556 ) ) ;
#57493=ORIENTED_EDGE ( 'NONE', *, *, #60829, .T. ) ;
#57494=CARTESIAN_POINT ( 'NONE',  ( 25.53750000000000142, -2.886751345948129988, 4.999999999999997335 ) ) ;
#57495=CARTESIAN_POINT ( 'NONE',  ( 26.52187500061451431, 3.027376345333613106, -5.243569643749998122 ) ) ;
#57496=ADVANCED_FACE ( 'NONE', ( #3404 ), #40403, .T. ) ;
#57497=VERTEX_POINT ( 'NONE', #22465 ) ;
#57498=B_SPLINE_CURVE_WITH_KNOTS ( 'NONE', 3,
 ( #44561, #38262, #39372, #44190, #72621, #10561, #50090, #49364, #22365, #21632 ),
 .UNSPECIFIED., .F., .F.,
 ( 4, 3, 3, 4 ),
 ( 3.004629197474318463E-18, 7.861478909946387531E-05, 0.0001572300094823956738, 0.0002815188877693150082 ),
 .UNSPECIFIED. ) ;
#57499=CARTESIAN_POINT ( 'NONE',  ( 14.61562500061451608, -6.054752690667223547, -1.112240025338166033E-15 ) ) ;
#57500=CARTESIAN_POINT ( 'NONE',  ( 6.028125000614517504, -4.541064518000419881, 2.621784821874995952 ) ) ;
#57502=CARTESIAN_POINT ( 'NONE',  ( 28.15312500061451573, -4.541064518000417216, -2.621784821875001281 ) ) ;
#57503=CARTESIAN_POINT ( 'NONE',  ( 15.41250000122903252, -4.330127018922190985, -2.500000000000001332 ) ) ;
#57504=CARTESIAN_POINT ( 'NONE',  ( 20.88749999999999929, 5.773502691896255534, 3.535250795749688894E-16 ) ) ;
#57505=CARTESIAN_POINT ( 'NONE',  ( 29.66249999999999432, -5.773502691896255534, -1.060575238724906372E-15 ) ) ;
#57506=CARTESIAN_POINT ( 'NONE',  ( 5.596875000614516260, -3.027376345333614438, 5.243569643749998122 ) ) ;
#57507=CARTESIAN_POINT ( 'NONE',  ( 10.17187500061451999, -6.054752690667223547, -1.112240025338166033E-15 ) ) ;
#57508=CARTESIAN_POINT ( 'NONE',  ( 19.77187500061451786, 3.027376345333613106, -5.243569643749998122 ) ) ;
#57510=ORIENTED_EDGE ( 'NONE', *, *, #55763, .F. ) ;
#57511=CARTESIAN_POINT ( 'NONE',  ( 3.834375000614519635, -4.541064518000419881, 2.621784821874995952 ) ) ;
#57512=CARTESIAN_POINT ( 'NONE',  ( 6.075000000000000178, 4.330127018922191873, 2.499999999999999556 ) ) ;
#57513=CARTESIAN_POINT ( 'NONE',  ( 7.321875000614516793, 3.027376345333611329, 5.243569643749999010 ) ) ;
#57515=CARTESIAN_POINT ( 'NONE',  ( 19.31250000000000000, -5.773502691896255534, -1.060575238724906372E-15 ) ) ;
#57516=CARTESIAN_POINT ( 'NONE',  ( 15.10312500061451502, -4.541064518000417216, -2.621784821875001281 ) ) ;
#57518=CARTESIAN_POINT ( 'NONE',  ( 24.82500000122902861, -5.773502691896255534, -1.060575238724906372E-15 ) ) ;
#57520=CARTESIAN_POINT ( 'NONE',  ( 10.56562500061451715, -6.054752690667223547, -1.112240025338166033E-15 ) ) ;
#57521=CARTESIAN_POINT ( 'NONE',  ( 26.63437500061451857, 4.541064518000418104, 2.621784821874999949 ) ) ;
#57522=CARTESIAN_POINT ( 'NONE',  ( -2.121784821874999949, 19.78437500061451715, 26.32496088578401938 ) ) ;
#57523=CARTESIAN_POINT ( 'NONE',  ( 25.73437500061451644, 4.541064518000418104, 2.621784821874999949 ) ) ;
#57524=CARTESIAN_POINT ( 'NONE',  ( 6.787500000000001421, -2.886751345948125991, -5.000000000000000000 ) ) ;
#57525=CARTESIAN_POINT ( 'NONE',  ( 3.999999999999998668, 12.27500000122903501, 27.69059892324149175 ) ) ;
#57526=CARTESIAN_POINT ( 'NONE',  ( 14.80312500061451608, 4.541064518000418104, -2.621784821874998173 ) ) ;
#57527=CARTESIAN_POINT ( 'NONE',  ( 6.262500001229034829, 0.000000000000000000, 4.999999999999998224 ) ) ;
#57529=CARTESIAN_POINT ( 'NONE',  ( 18.19687500061451502, -3.027376345333614438, 5.243569643749998122 ) ) ;
#57530=CARTESIAN_POINT ( 'NONE',  ( 12.87187500061451750, -6.054752690667223547, -1.112240025338166033E-15 ) ) ;
#57533=CARTESIAN_POINT ( 'NONE',  ( 12.51562500061451821, 3.027376345333613106, -5.243569643749998122 ) ) ;
#57534=CARTESIAN_POINT ( 'NONE',  ( 27.18750000122903288, 6.123233995736764310E-16, -4.999999999999998224 ) ) ;
#57535=CARTESIAN_POINT ( 'NONE',  ( 12.12187500061451573, 3.027376345333613106, -5.243569643749998122 ) ) ;
#57536=CARTESIAN_POINT ( 'NONE',  ( 3.939080010846523372, -3.079553322829319928, -4.243980907203444453 ) ) ;
#57537=CARTESIAN_POINT ( 'NONE',  ( 15.81562500061451537, 3.027376345333611329, 5.243569643749999010 ) ) ;
#57538=CARTESIAN_POINT ( 'NONE',  ( 25.05937500061451573, -4.541064518000417216, -2.621784821875001281 ) ) ;
#57540=CARTESIAN_POINT ( 'NONE',  ( 12.56250000122903465, 0.000000000000000000, 4.999999999999998224 ) ) ;
#57542=CARTESIAN_POINT ( 'NONE',  ( -4.243569643749998122, 16.74687500061451573, -27.54997392385601174 ) ) ;
#57543=CARTESIAN_POINT ( 'NONE',  ( 17.67187500061451644, 3.027376345333611329, 5.243569643749999010 ) ) ;
#57544=CARTESIAN_POINT ( 'NONE',  ( 19.27500000122903145, 2.886751345948126879, 4.999999999999999112 ) ) ;
#57545=CARTESIAN_POINT ( 'NONE',  ( 13.54687500061451999, 6.054752690667223547, 3.707466751127219781E-16 ) ) ;
#57546=CARTESIAN_POINT ( 'NONE',  ( -3.000416591977282496E-16, 19.24062500061451431, -34.90005215228797653 ) ) ;
#57547=CARTESIAN_POINT ( 'NONE',  ( 20.62500000122903288, 2.886751345948126879, 4.999999999999999112 ) ) ;
#57548=CARTESIAN_POINT ( 'NONE',  ( 14.42812500061451786, 4.541064518000418104, 2.621784821874999949 ) ) ;
#57549=ORIENTED_EDGE ( 'NONE', *, *, #71167, .T. ) ;
#57550=VERTEX_POINT ( 'NONE', #67194 ) ;
#57551=CARTESIAN_POINT ( 'NONE',  ( 17.36249999999999716, 2.886751345948126879, 4.999999999999999112 ) ) ;
#57552=DIRECTION ( 'NONE',  ( 0.000000000000000000, 0.000000000000000000, 1.000000000000000000 ) ) ;
#57553=CARTESIAN_POINT ( 'NONE',  ( 3.740625000614516527, -3.027376345333614438, 5.243569643749998122 ) ) ;
#57554=CARTESIAN_POINT ( 'NONE',  ( 14.47500000122903430, -5.773502691896255534, -1.060575238724906372E-15 ) ) ;
#57555=CARTESIAN_POINT ( 'NONE',  ( 26.74687500061451573, -3.027376345333614438, 5.243569643749998122 ) ) ;
#57556=CARTESIAN_POINT ( 'NONE',  ( 19.94062500061451715, -3.027376345333614438, 5.243569643749998122 ) ) ;
#57557=CARTESIAN_POINT ( 'NONE',  ( 22.90312500061451573, 4.541064518000418104, -2.621784821874998173 ) ) ;
#57558=CARTESIAN_POINT ( 'NONE',  ( 3.253125000614518036, 0.000000000000000000, 5.243569643749999010 ) ) ;
#57559=CARTESIAN_POINT ( 'NONE',  ( 27.03750000000000142, -2.886751345948125991, -5.000000000000000000 ) ) ;
#57562=CARTESIAN_POINT ( 'NONE',  ( 6.450000001229034829, -2.886751345948126435, -5.000000000000000000 ) ) ;
#57563=CARTESIAN_POINT ( 'NONE',  ( -2.828200636599751609E-16, 10.10000000122903430, -34.61880215351700230 ) ) ;
#57564=CARTESIAN_POINT ( 'NONE',  ( 4.243569643749999898, 16.48437500061451644, -30.00000000000000000 ) ) ;
#57565=CARTESIAN_POINT ( 'NONE',  ( 7.125000001229033764, 2.886751345948126879, 4.999999999999999112 ) ) ;
#57566=CARTESIAN_POINT ( 'NONE',  ( 5.700000000000000178, 0.000000000000000000, 4.999999999999998224 ) ) ;
#57567=CARTESIAN_POINT ( 'NONE',  ( 4.912500001229034297, 0.000000000000000000, 4.999999999999998224 ) ) ;
#57568=CARTESIAN_POINT ( 'NONE',  ( 8.859375000614518214, -4.541064518000417216, -2.621784821875001281 ) ) ;
#57570=CARTESIAN_POINT ( 'NONE',  ( 27.60000000122903430, -2.886751345948109559, -5.000000000000028422 ) ) ;
#57571=CARTESIAN_POINT ( 'NONE',  ( 3.734827092922140768, -3.324314453528163682, -3.734827092927292203 ) ) ;
#57574=CARTESIAN_POINT ( 'NONE',  ( 7.771875000614516971, 3.027376345333611329, 5.243569643749999010 ) ) ;
#57575=CARTESIAN_POINT ( 'NONE',  ( 10.43437500061451750, 4.541064518000418104, 2.621784821874999949 ) ) ;
#57576=CARTESIAN_POINT ( 'NONE',  ( 7.462500000000001243, 2.886751345948126879, 4.999999999999999112 ) ) ;
#57577=CARTESIAN_POINT ( 'NONE',  ( 4.243569643749999010, 16.01562500061459460, 27.54997392385601174 ) ) ;
#57578=CARTESIAN_POINT ( 'NONE',  ( 21.64687500061451786, 6.054752690667223547, 3.707466751127219781E-16 ) ) ;
#57580=CARTESIAN_POINT ( 'NONE',  ( 5.775000000000002132, -4.330127018922194537, 2.499999999999995559 ) ) ;
#57581=CARTESIAN_POINT ( 'NONE',  ( 25.68750000122903288, -4.330127018922194537, 2.499999999999995559 ) ) ;
#57583=CARTESIAN_POINT ( 'NONE',  ( 23.57812500061451289, -4.541064518000419881, 2.621784821874995952 ) ) ;
#57584=CARTESIAN_POINT ( 'NONE',  ( 12.77812500061451750, -4.541064518000419881, 2.621784821874995952 ) ) ;
#57586=CARTESIAN_POINT ( 'NONE',  ( 12.79687500061451821, -3.027376345333614438, 5.243569643749998122 ) ) ;
#57587=CARTESIAN_POINT ( 'NONE',  ( 28.35000000000000142, -4.330127018922190985, -2.500000000000001332 ) ) ;
#57588=CARTESIAN_POINT ( 'NONE',  ( 23.66250000122903430, 4.330127018922192761, -2.499999999999997780 ) ) ;
#57590=CARTESIAN_POINT ( 'NONE',  ( 12.98437500061451821, 6.421520780324663323E-16, -5.243569643749999010 ) ) ;
#57591=CARTESIAN_POINT ( 'NONE',  ( 27.83437500061451786, 6.421520780324663323E-16, -5.243569643749999010 ) ) ;
#57592=CARTESIAN_POINT ( 'NONE',  ( 4.246875000614519280, -3.027376345333614438, 5.243569643749998122 ) ) ;
#57593=CARTESIAN_POINT ( 'NONE',  ( -2.000000000000000000, 12.83750000122903501, -33.46410161513775705 ) ) ;
#57594=CARTESIAN_POINT ( 'NONE',  ( 21.30937500061451573, 0.000000000000000000, 5.243569643749999010 ) ) ;
#57595=CARTESIAN_POINT ( 'NONE',  ( 13.54687500061451999, 6.054752690667223547, 3.707466751127219781E-16 ) ) ;
#57597=CARTESIAN_POINT ( 'NONE',  ( 25.34999999999999787, 4.330127018922192761, -2.499999999999997780 ) ) ;
#57600=CARTESIAN_POINT ( 'NONE',  ( 16.34062500061451573, -3.027376345333614438, 5.243569643749998122 ) ) ;
#57601=CARTESIAN_POINT ( 'NONE',  ( 7.312500000000000000, 2.886751345948129099, -4.999999999999998224 ) ) ;
#57603=CARTESIAN_POINT ( 'NONE',  ( 15.71250000000000213, -5.773502691896255534, -1.060575238724906372E-15 ) ) ;
#57604=CARTESIAN_POINT ( 'NONE',  ( -2.121784821874999949, 10.27812500061451750, 26.32496088578401938 ) ) ;
#57606=CARTESIAN_POINT ( 'NONE',  ( 24.08437500061451786, -4.541064518000419881, 2.621784821874995952 ) ) ;
#57607=ORIENTED_EDGE ( 'NONE', *, *, #52924, .F. ) ;
#57608=CARTESIAN_POINT ( 'NONE',  ( 18.44062500061451715, 6.054752690667223547, 3.707466751127219781E-16 ) ) ;
#57609=CARTESIAN_POINT ( 'NONE',  ( 20.22187500061451715, 3.027376345333613106, -5.243569643749998122 ) ) ;
#57610=CARTESIAN_POINT ( 'NONE',  ( 3.149999999999999911, -4.330127018922190985, -2.500000000000001332 ) ) ;
#57611=CARTESIAN_POINT ( 'NONE',  ( 7.415625000614516793, -6.054752690667223547, -1.112240025338166033E-15 ) ) ;
#57612=CARTESIAN_POINT ( 'NONE',  ( 20.87812500061451715, -4.541064518000419881, 2.621784821874995952 ) ) ;
#57613=CARTESIAN_POINT ( 'NONE',  ( 13.09687500061451892, 6.054752690667223547, 3.707466751127219781E-16 ) ) ;
#57614=CARTESIAN_POINT ( 'NONE',  ( 16.77187500061451786, 3.027376345333611329, 5.243569643749999010 ) ) ;
#57615=CARTESIAN_POINT ( 'NONE',  ( -4.243569643749997233, 18.04062500061451857, 32.45002607614398471 ) ) ;
#57616=CARTESIAN_POINT ( 'NONE',  ( 19.01250000122903216, -4.330127018922190985, -2.500000000000001332 ) ) ;
#57618=CARTESIAN_POINT ( 'NONE',  ( 9.065625000614515372, 3.027376345333611329, 5.243569643749999010 ) ) ;
#57619=CARTESIAN_POINT ( 'NONE',  ( 3.046875000614519990, -3.027376345333610441, -5.243569643749999898 ) ) ;
#57620=CARTESIAN_POINT ( 'NONE',  ( 5.146875000614517859, -3.027376345333614438, 5.243569643749998122 ) ) ;
#57621=CARTESIAN_POINT ( 'NONE',  ( 24.98437500061451644, -4.541064518000419881, 2.621784821874995952 ) ) ;
#57622=CARTESIAN_POINT ( 'NONE',  ( 17.46562500061451217, 3.027376345333613106, -5.243569643749998122 ) ) ;
#57623=CARTESIAN_POINT ( 'NONE',  ( 27.41250000122903430, 0.000000000000000000, 4.999999999999998224 ) ) ;
#57624=CARTESIAN_POINT ( 'NONE',  ( 25.82812500061451644, -4.541064518000419881, 2.621784821874995952 ) ) ;
#57625=CARTESIAN_POINT ( 'NONE',  ( 21.60937500061451644, 4.541064518000418104, -2.621784821874998173 ) ) ;
#57626=CARTESIAN_POINT ( 'NONE',  ( 17.31562500061451715, -6.054752690667223547, -1.112240025338166033E-15 ) ) ;
#57627=CARTESIAN_POINT ( 'NONE',  ( -2.121784821874996840, 17.23437500061451999, 33.67503911421598417 ) ) ;
#57628=CARTESIAN_POINT ( 'NONE',  ( 22.15312500061451573, 0.000000000000000000, 5.243569643749999010 ) ) ;
#57629=ORIENTED_EDGE ( 'NONE', *, *, #32239, .F. ) ;
#57630=CARTESIAN_POINT ( 'NONE',  ( 26.25000000000000000, 4.330127018922192761, -2.499999999999997780 ) ) ;
#57631=CARTESIAN_POINT ( 'NONE',  ( -1.999999999999997113, 13.77500000000000036, -26.53589838486224295 ) ) ;
#57633=CARTESIAN_POINT ( 'NONE',  ( 3.346875000614518036, -3.027376345333614438, 5.243569643749998122 ) ) ;
#57634=CARTESIAN_POINT ( 'NONE',  ( 10.67812500061451608, 6.421520780324663323E-16, -5.243569643749999010 ) ) ;
#57635=CARTESIAN_POINT ( 'NONE',  ( 22.68750000122903288, 6.123233995736764310E-16, -4.999999999999998224 ) ) ;
#57636=CARTESIAN_POINT ( 'NONE',  ( 26.69062500061451715, -3.027376345333614438, 5.243569643749998122 ) ) ;
#57637=CARTESIAN_POINT ( 'NONE',  ( 25.50000000000000000, 0.000000000000000000, 4.999999999999998224 ) ) ;
#57638=CARTESIAN_POINT ( 'NONE',  ( 8.484601909799253346E-16, 16.62500000122903288, -25.38119784648299770 ) ) ;
#57639=CARTESIAN_POINT ( 'NONE',  ( -1.071796769724504328, 12.55490381179670045, 33.99999999999999289 ) ) ;
#57640=CARTESIAN_POINT ( 'NONE',  ( 10.00312500061451715, 0.000000000000000000, 5.243569643749999010 ) ) ;
#57642=EDGE_CURVE ( 'NONE', #44184, #65074, #16870, .T. ) ;
#57643=CARTESIAN_POINT ( 'NONE',  ( 25.75312500061451715, 0.000000000000000000, 5.243569643749999010 ) ) ;
#57644=CARTESIAN_POINT ( 'NONE',  ( 8.015625000614518214, 3.027376345333613106, -5.243569643749998122 ) ) ;
#57645=CARTESIAN_POINT ( 'NONE',  ( 6.778125000614518392, 4.541064518000418104, 2.621784821874999949 ) ) ;
#57647=EDGE_CURVE ( 'NONE', #68293, #8342, #42771, .T. ) ;
#57648=CARTESIAN_POINT ( 'NONE',  ( 0.000000000000000000, 0.000000000000000000, 50.00000000000000000 ) ) ;
#57649=CARTESIAN_POINT ( 'NONE',  ( 13.16249999999999964, 2.886751345948129099, -4.999999999999998224 ) ) ;
#57650=EDGE_CURVE ( 'NONE', #33928, #4907, #7383, .T. ) ;
#57651=CARTESIAN_POINT ( 'NONE',  ( 13.54687500061451999, 6.054752690667223547, 3.707466751127219781E-16 ) ) ;
#57652=CARTESIAN_POINT ( 'NONE',  ( 10.53750000122903252, 6.123233995736764310E-16, -4.999999999999998224 ) ) ;
#57653=CARTESIAN_POINT ( 'NONE',  ( 17.85937500061451999, -4.541064518000417216, -2.621784821875001281 ) ) ;
#57655=CARTESIAN_POINT ( 'NONE',  ( 8.971875000614515372, 3.027376345333613106, -5.243569643749998122 ) ) ;
#57656=CARTESIAN_POINT ( 'NONE',  ( 4.243569643749999010, 11.06562500061451715, -32.45002607614398471 ) ) ;
#57660=CARTESIAN_POINT ( 'NONE',  ( 24.21562500061451573, 3.027376345333613106, -5.243569643749998122 ) ) ;
#57662=CARTESIAN_POINT ( 'NONE',  ( 29.40937500061451715, 0.000000000000000000, 5.243569643749999010 ) ) ;
#57663=CARTESIAN_POINT ( 'NONE',  ( 25.42500000000000071, 4.330127018922191873, 2.499999999999999556 ) ) ;
#57664=CARTESIAN_POINT ( 'NONE',  ( 8.053125000614516082, 4.541064518000418104, -2.621784821874998173 ) ) ;
#57666=CARTESIAN_POINT ( 'NONE',  ( 18.38437500061451857, 6.421520780324663323E-16, -5.243569643749999010 ) ) ;
#57668=CARTESIAN_POINT ( 'NONE',  ( 2.915625000614516793, -6.054752690667223547, -1.112240025338166033E-15 ) ) ;
#57669=CARTESIAN_POINT ( 'NONE',  ( 8.934375000614517504, 6.421520780324663323E-16, -5.243569643749999010 ) ) ;
#57670=ORIENTED_EDGE ( 'NONE', *, *, #69599, .T. ) ;
#57671=CARTESIAN_POINT ( 'NONE',  ( 18.60937500061451644, 0.000000000000000000, 5.243569643749999010 ) ) ;
#57672=DIRECTION ( 'NONE',  ( 0.000000000000000000, 0.000000000000000000, -1.000000000000000000 ) ) ;
#57673=CARTESIAN_POINT ( 'NONE',  ( 27.15000000000000213, 4.330127018922192761, -2.499999999999997780 ) ) ;
#57674=CARTESIAN_POINT ( 'NONE',  ( 28.95937500061451431, 0.000000000000000000, 5.243569643749999010 ) ) ;
#57675=EDGE_CURVE ( 'NONE', #64110, #19257, #48186, .T. ) ;
#57677=CARTESIAN_POINT ( 'NONE',  ( 10.83750000000000036, -2.886751345948193048, -4.999999999999883649 ) ) ;
#57679=CARTESIAN_POINT ( 'NONE',  ( 10.31250000000000355, -5.773502691896255534, -1.060575238724906372E-15 ) ) ;
#57681=CARTESIAN_POINT ( 'NONE',  ( 25.49062500061451786, -3.027376345333610441, -5.243569643749999898 ) ) ;
#57682=CARTESIAN_POINT ( 'NONE',  ( 15.07499999999999929, 4.330127018922191873, 2.499999999999999556 ) ) ;
#57683=CARTESIAN_POINT ( 'NONE',  ( 11.21250000122903501, 0.000000000000000000, 4.999999999999998224 ) ) ;
#57684=CARTESIAN_POINT ( 'NONE',  ( 8.165625000614516793, 3.027376345333611329, 5.243569643749999010 ) ) ;
#57685=CARTESIAN_POINT ( 'NONE',  ( 22.12500000000000000, 6.123233995736764310E-16, -4.999999999999998224 ) ) ;
#57686=CARTESIAN_POINT ( 'NONE',  ( 20.01562500061451644, -6.054752690667223547, -1.112240025338166033E-15 ) ) ;
#57687=CARTESIAN_POINT ( 'NONE',  ( 16.08750000122903501, 4.330127018922191873, 2.499999999999999556 ) ) ;
#57688=CARTESIAN_POINT ( 'NONE',  ( 26.17500000122903359, -5.773502691896255534, -1.060575238724906372E-15 ) ) ;
#57690=CARTESIAN_POINT ( 'NONE',  ( 5.025000000000002132, 6.123233995736764310E-16, -4.999999999999998224 ) ) ;
#57691=ORIENTED_EDGE ( 'NONE', *, *, #5473, .F. ) ;
#57692=CARTESIAN_POINT ( 'NONE',  ( 21.77812500061451928, -4.541064518000419881, 2.621784821874995952 ) ) ;
#57693=CARTESIAN_POINT ( 'NONE',  ( 3.317784727594947913, -3.740628891154329061, -3.422312309320198143 ) ) ;
#57694=CARTESIAN_POINT ( 'NONE',  ( 27.04687500061451644, 6.054752690667223547, 3.707466751127219781E-16 ) ) ;
#57695=CARTESIAN_POINT ( 'NONE',  ( 18.42187500061451644, 3.027376345333613106, -5.243569643749998122 ) ) ;
#57696=CARTESIAN_POINT ( 'NONE',  ( 15.40312500061451573, 0.000000000000000000, 5.243569643749999010 ) ) ;
#57697=CARTESIAN_POINT ( 'NONE',  ( 30.00000000000000000, 0.000000000000000000, 0.000000000000000000 ) ) ;
#57698=CARTESIAN_POINT ( 'NONE',  ( 25.08750000122903145, 4.330127018922191873, 2.499999999999999556 ) ) ;
#57700=CARTESIAN_POINT ( 'NONE',  ( 16.52812500061451573, 6.421520780324663323E-16, -5.243569643749999010 ) ) ;
#57701=CARTESIAN_POINT ( 'NONE',  ( 4.000000000000000000, 13.88750000000000107, 32.30940107675849760 ) ) ;
#57702=CARTESIAN_POINT ( 'NONE',  ( 4.425000001229032698, 2.886751345948126879, 4.999999999999999112 ) ) ;
#57703=CARTESIAN_POINT ( 'NONE',  ( 12.04687500061451821, -3.027376345333610441, -5.243569643749999898 ) ) ;
#57704=CARTESIAN_POINT ( 'NONE',  ( 11.37187500061451750, 3.027376345333611329, 5.243569643749999010 ) ) ;
#57705=CARTESIAN_POINT ( 'NONE',  ( 20.40937500061451715, 0.000000000000000000, 5.243569643749999010 ) ) ;
#57707=CARTESIAN_POINT ( 'NONE',  ( 9.937500000000001776, -2.886751345948126435, -5.000000000000000000 ) ) ;
#57708=CARTESIAN_POINT ( 'NONE',  ( 23.27812500061451573, 6.421520780324663323E-16, -5.243569643749999010 ) ) ;
#57709=( BOUNDED_CURVE ( )  B_SPLINE_CURVE ( 2, ( #40872, #63389, #12774, #57832, #47129, #19025, #41584 ),
 .UNSPECIFIED., .F., .F. ) 
 B_SPLINE_CURVE_WITH_KNOTS ( ( 3, 2, 2, 3 ),
 ( 0.5250000000000000222, 0.5277777777777777901, 0.5305555555555556690, 0.5333333333333334370 ),
 .UNSPECIFIED. ) 
 CURVE ( )  GEOMETRIC_REPRESENTATION_ITEM ( )  RATIONAL_B_SPLINE_CURVE ( ( 1.000000000000000000, 0.8660254037844387076, 1.000000000000000000, 0.8660254037844387076, 1.000000000000000000, 0.8660254037844333785, 1.000000000000005329 ) ) 
 REPRESENTATION_ITEM ( '' )  );
#57710=CARTESIAN_POINT ( 'NONE',  ( 18.98437500061451644, 4.541064518000418104, 2.621784821874999949 ) ) ;
#57711=CARTESIAN_POINT ( 'NONE',  ( 24.10312500061451502, -4.541064518000417216, -2.621784821875001281 ) ) ;
#57712=CARTESIAN_POINT ( 'NONE',  ( 8.484601909799253346E-16, 14.71250000000000036, 34.61880215351700230 ) ) ;
#57713=CARTESIAN_POINT ( 'NONE',  ( 2.896875000614518747, -3.027376345333614438, 5.243569643749998122 ) ) ;
#57714=CARTESIAN_POINT ( 'NONE',  ( 9.675000001229035362, 2.886751345948129099, -4.999999999999998224 ) ) ;
#57715=CARTESIAN_POINT ( 'NONE',  ( 3.600000001229033408, -2.886751345948129988, 4.999999999999997335 ) ) ;
#57717=CARTESIAN_POINT ( 'NONE',  ( 28.01250000122903216, -4.330127018922190985, -2.500000000000001332 ) ) ;
#57719=CARTESIAN_POINT ( 'NONE',  ( 9.571875000614518569, 3.027376345333611329, 5.243569643749999010 ) ) ;
#57721=CARTESIAN_POINT ( 'NONE',  ( 17.31562500061451715, -6.054752690667223547, -1.112240025338166033E-15 ) ) ;
#57722=CARTESIAN_POINT ( 'NONE',  ( 11.25937500061451679, 4.541064518000418104, -2.621784821874998173 ) ) ;
#57723=CARTESIAN_POINT ( 'NONE',  ( 3.628125000614518036, 4.541064518000418104, 2.621784821874999949 ) ) ;
#57724=CARTESIAN_POINT ( 'NONE',  ( 20.74687500061452283, 6.054752690667223547, 3.707466751127219781E-16 ) ) ;
#57725=CARTESIAN_POINT ( 'NONE',  ( 7.734375000614517326, 4.541064518000418104, 2.621784821874999949 ) ) ;
#57726=CARTESIAN_POINT ( 'NONE',  ( 3.178125000614515638, 4.541064518000418104, 2.621784821874999949 ) ) ;
#57727=CARTESIAN_POINT ( 'NONE',  ( 1.510657702057710734E-15, 19.10000000122903430, 26.00000000000000000 ) ) ;
#57728=CARTESIAN_POINT ( 'NONE',  ( 6.928125000614516082, -4.541064518000419881, 2.621784821874995952 ) ) ;
#57729=CARTESIAN_POINT ( 'NONE',  ( 18.89062500061451644, 6.054752690667223547, 3.707466751127219781E-16 ) ) ;
#57731=CARTESIAN_POINT ( 'NONE',  ( 6.000000001229033764, -2.886751345948125991, -5.000000000000000000 ) ) ;
#57732=CARTESIAN_POINT ( 'NONE',  ( 13.94062500061451892, 6.054752690667223547, 3.707466751127219781E-16 ) ) ;
#57733=CARTESIAN_POINT ( 'NONE',  ( 13.15312500061451750, 0.000000000000000000, 5.243569643749999010 ) ) ;
#57735=CARTESIAN_POINT ( 'NONE',  ( 13.16249999999999964, 2.886751345948129099, -4.999999999999998224 ) ) ;
#57736=CARTESIAN_POINT ( 'NONE',  ( 5.925000001229033586, -5.773502691896255534, -1.060575238724906372E-15 ) ) ;
#57737=EDGE_CURVE ( 'NONE', #3869, #4423, #51642, .T. ) ;
#57738=CARTESIAN_POINT ( 'NONE',  ( 18.45000000122903216, -2.886751345948129988, 4.999999999999997335 ) ) ;
#57740=CARTESIAN_POINT ( 'NONE',  ( 2.121784821875001281, 11.90937500061451892, -26.32496088578401938 ) ) ;
#57743=CARTESIAN_POINT ( 'NONE',  ( 6.450000000000001066, 4.330127018922192761, -2.499999999999997780 ) ) ;
#57745=CARTESIAN_POINT ( 'NONE',  ( 19.13437500061451857, -4.541064518000419881, 2.621784821874995952 ) ) ;
#57746=CARTESIAN_POINT ( 'NONE',  ( 4.898587196589411843E-16, 20.00000000000000000, -26.00000000000000000 ) ) ;
#57747=CARTESIAN_POINT ( 'NONE',  ( 13.75312500061451715, -4.541064518000417216, -2.621784821875001281 ) ) ;
#57749=DIRECTION ( 'NONE',  ( 0.000000000000000000, 0.000000000000000000, -1.000000000000000000 ) ) ;
#57750=CARTESIAN_POINT ( 'NONE',  ( 25.54687500061451644, -3.027376345333610441, -5.243569643749999898 ) ) ;
#57752=CARTESIAN_POINT ( 'NONE',  ( 9.778125000614517504, 6.421520780324663323E-16, -5.243569643749999010 ) ) ;
#57753=CARTESIAN_POINT ( 'NONE',  ( 14.97187500061451892, 3.027376345333611329, 5.243569643749999010 ) ) ;
#57755=CARTESIAN_POINT ( 'NONE',  ( 26.39062500061451644, -3.027376345333610441, -5.243569643749999898 ) ) ;
#57756=CARTESIAN_POINT ( 'NONE',  ( 19.71562500061451928, 3.027376345333613106, -5.243569643749998122 ) ) ;
#57757=CARTESIAN_POINT ( 'NONE',  ( 18.93750000000000000, -2.886751345948159742, -4.999999999999942268 ) ) ;
#57758=CARTESIAN_POINT ( 'NONE',  ( -1.071796769724504328, 14.35490381179669939, -26.00000000000001066 ) ) ;
#57759=CARTESIAN_POINT ( 'NONE',  ( 8.925000000000002487, -4.330127018922194537, 2.499999999999995559 ) ) ;
#57760=CARTESIAN_POINT ( 'NONE',  ( 18.71250000122903145, 4.330127018922192761, -2.499999999999997780 ) ) ;
#57761=CARTESIAN_POINT ( 'NONE',  ( 1.071796769724491893, 10.23259618943233384, 33.99999999999999289 ) ) ;
#57763=ORIENTED_EDGE ( 'NONE', *, *, #70520, .T. ) ;
#57764=CARTESIAN_POINT ( 'NONE',  ( 18.11250000000000071, 2.886751345948129099, -4.999999999999998224 ) ) ;
#57765=CARTESIAN_POINT ( 'NONE',  ( 21.26249999999999574, 2.886751345948129099, -4.999999999999998224 ) ) ;
#57766=CARTESIAN_POINT ( 'NONE',  ( 20.14687500061451786, -3.027376345333610441, -5.243569643749999898 ) ) ;
#57767=CARTESIAN_POINT ( 'NONE',  ( 24.06562500061451715, -6.054752690667223547, -1.112240025338166033E-15 ) ) ;
#57769=CARTESIAN_POINT ( 'NONE',  ( 5.165625000614518569, -6.054752690667223547, -1.112240025338166033E-15 ) ) ;
#57770=DIRECTION ( 'NONE',  ( -0.000000000000000000, -1.000000000000000000, -0.000000000000000000 ) ) ;
#57771=CARTESIAN_POINT ( 'NONE',  ( 13.87500000000000178, -4.330127018922194537, 2.499999999999995559 ) ) ;
#57772=CARTESIAN_POINT ( 'NONE',  ( 4.243569643749999898, 18.19062500061451360, 32.45002607614398471 ) ) ;
#57773=CARTESIAN_POINT ( 'NONE',  ( 29.01562500061451644, -6.054752690667223547, -1.112240025338166033E-15 ) ) ;
#57776=CARTESIAN_POINT ( 'NONE',  ( 25.54687500061451644, -3.027376345333610441, -5.243569643749999898 ) ) ;
#57778=CARTESIAN_POINT ( 'NONE',  ( 20.39062500061451644, -3.027376345333614438, 5.243569643749998122 ) ) ;
#57779=CARTESIAN_POINT ( 'NONE',  ( 22.39687500061451075, -3.027376345333610441, -5.243569643749999898 ) ) ;
#57781=CARTESIAN_POINT ( 'NONE',  ( 2.121784821875001281, 16.80312500061459247, -26.32496088578401938 ) ) ;
#57782=CARTESIAN_POINT ( 'NONE',  ( 6.703125000614516438, 4.541064518000418104, -2.621784821874998173 ) ) ;
#57784=CARTESIAN_POINT ( 'NONE',  ( 22.79062500061451502, -3.027376345333610441, -5.243569643749999898 ) ) ;
#57787=CARTESIAN_POINT ( 'NONE',  ( 17.89687500061451431, -3.027376345333610441, -5.243569643749999898 ) ) ;
#57788=CARTESIAN_POINT ( 'NONE',  ( 19.32187500061451857, 3.027376345333613106, -5.243569643749998122 ) ) ;
#57789=CARTESIAN_POINT ( 'NONE',  ( 27.15937500061451360, 0.000000000000000000, 5.243569643749999010 ) ) ;
#57790=CARTESIAN_POINT ( 'NONE',  ( 9.001249775931846008E-16, 15.47187500061451892, 34.90005215228797653 ) ) ;
#57791=CARTESIAN_POINT ( 'NONE',  ( 8.540625000614518569, 6.054752690667223547, 3.707466751127219781E-16 ) ) ;
#57792=CARTESIAN_POINT ( 'NONE',  ( -3.999999999999999112, 18.19999999999999929, -30.00000000000000000 ) ) ;
#57793=CARTESIAN_POINT ( 'NONE',  ( 5.334375000614517859, 6.421520780324663323E-16, -5.243569643749999010 ) ) ;
#57795=CARTESIAN_POINT ( 'NONE',  ( 4.903125000614516615, 4.541064518000418104, -2.621784821874998173 ) ) ;
#57796=CARTESIAN_POINT ( 'NONE',  ( 9.646875000614516082, -3.027376345333614438, 5.243569643749998122 ) ) ;
#57798=CARTESIAN_POINT ( 'NONE',  ( 17.73750000122903359, 6.123233995736764310E-16, -4.999999999999998224 ) ) ;
#57799=CARTESIAN_POINT ( 'NONE',  ( 4.846875000614519813, -3.027376345333610441, -5.243569643749999898 ) ) ;
#57800=CARTESIAN_POINT ( 'NONE',  ( 6.365625000614518747, 3.027376345333611329, 5.243569643749999010 ) ) ;
#57803=CARTESIAN_POINT ( 'NONE',  ( 16.28437500061452070, 4.541064518000418104, 2.621784821874999949 ) ) ;
#57806=CARTESIAN_POINT ( 'NONE',  ( 24.06562500061451715, -6.054752690667223547, -1.112240025338166033E-15 ) ) ;
#57807=CARTESIAN_POINT ( 'NONE',  ( 8.728125000614518569, -4.541064518000419881, 2.621784821874995952 ) ) ;
#57808=CARTESIAN_POINT ( 'NONE',  ( 26.67187500061451644, 3.027376345333611329, 5.243569643749999010 ) ) ;
#57809=CARTESIAN_POINT ( 'NONE',  ( 9.103125000614515017, 0.000000000000000000, 5.243569643749999010 ) ) ;
#57810=CARTESIAN_POINT ( 'NONE',  ( 4.474433822073803135, -2.231832360841083496, -4.606514653318270369 ) ) ;
#57811=CARTESIAN_POINT ( 'NONE',  ( 10.83750000122903501, -4.330127018922194537, 2.499999999999995559 ) ) ;
#57812=CARTESIAN_POINT ( 'NONE',  ( 25.67812500061451431, 4.541064518000418104, 2.621784821874999949 ) ) ;
#57813=CARTESIAN_POINT ( 'NONE',  ( 4.243569643749999898, 13.27812500061451750, -30.00000000000000000 ) ) ;
#57814=CARTESIAN_POINT ( 'NONE',  ( 11.81250000122903465, -4.330127018922190985, -2.500000000000001332 ) ) ;
#57815=CARTESIAN_POINT ( 'NONE',  ( 23.20312500061451644, -4.541064518000417216, -2.621784821875001281 ) ) ;
#57816=CARTESIAN_POINT ( 'NONE',  ( 10.57500000000000107, 4.330127018922191873, 2.499999999999999556 ) ) ;
#57817=CARTESIAN_POINT ( 'NONE',  ( 20.54062500061451502, -3.027376345333610441, -5.243569643749999898 ) ) ;
#57818=CARTESIAN_POINT ( 'NONE',  ( 5.334375000614517859, 6.421520780324663323E-16, -5.243569643749999010 ) ) ;
#57819=CARTESIAN_POINT ( 'NONE',  ( 20.62499999999999645, -4.330127018922194537, 2.499999999999995559 ) ) ;
#57820=CARTESIAN_POINT ( 'NONE',  ( 12.60000000122903430, -2.886751345948129988, 4.999999999999997335 ) ) ;
#57821=CARTESIAN_POINT ( 'NONE',  ( 12.14062500061451821, 6.054752690667223547, 3.707466751127219781E-16 ) ) ;
#57822=EDGE_CURVE ( 'NONE', #44451, #72067, #62618, .T. ) ;
#57823=CARTESIAN_POINT ( 'NONE',  ( 14.99062500061451786, -3.027376345333614438, 5.243569643749998122 ) ) ;
#57825=CARTESIAN_POINT ( 'NONE',  ( 26.25000000122903288, -2.886751345948125991, -5.000000000000000000 ) ) ;
#57826=CARTESIAN_POINT ( 'NONE',  ( 21.33749999999999858, 5.773502691896255534, 3.535250795749688894E-16 ) ) ;
#57827=CARTESIAN_POINT ( 'NONE',  ( 23.03437500061451715, 4.541064518000418104, 2.621784821874999949 ) ) ;
#57828=DIRECTION ( 'NONE',  ( -0.000000000000000000, -1.000000000000000000, -0.000000000000000000 ) ) ;
#57829=CARTESIAN_POINT ( 'NONE',  ( 6.675000001229034474, 2.886751345948126879, 4.999999999999999112 ) ) ;
#57830=CARTESIAN_POINT ( 'NONE',  ( 8.334375000614516082, -4.541064518000419881, 2.621784821874995952 ) ) ;
#57831=CARTESIAN_POINT ( 'NONE',  ( 26.44687500061451502, -3.027376345333610441, -5.243569643749999898 ) ) ;
#57832=CARTESIAN_POINT ( 'NONE',  ( 15.37500000122903465, -5.773502691896255534, -1.060575238724906372E-15 ) ) ;
#57833=CARTESIAN_POINT ( 'NONE',  ( 21.89062500061451289, -3.027376345333610441, -5.243569643749999898 ) ) ;
#57834=CARTESIAN_POINT ( 'NONE',  ( 25.77187500061451075, 3.027376345333611329, 5.243569643749999010 ) ) ;
#57836=DIRECTION ( 'NONE',  ( 0.000000000000000000, 0.000000000000000000, -1.000000000000000000 ) ) ;
#57837=CARTESIAN_POINT ( 'NONE',  ( 8.146875000614516082, 6.054752690667223547, 3.707466751127219781E-16 ) ) ;
#57838=CARTESIAN_POINT ( 'NONE',  ( 19.90312500061451573, 0.000000000000000000, 5.243569643749999010 ) ) ;
#57839=ORIENTED_EDGE ( 'NONE', *, *, #12677, .T. ) ;
#57840=CARTESIAN_POINT ( 'NONE',  ( -2.000000000000000000, 12.72499999999999964, -33.46410161513775705 ) ) ;
#57841=CARTESIAN_POINT ( 'NONE',  ( 28.41562500061451502, 3.027376345333611329, 5.243569643749999010 ) ) ;
#57842=CARTESIAN_POINT ( 'NONE',  ( 3.084375000614519191, 6.421520780324663323E-16, -5.243569643749999010 ) ) ;
#57844=CARTESIAN_POINT ( 'NONE',  ( 3.688512509775060177, 3.375629639820296735, -3.780221722430626485 ) ) ;
#57845=CARTESIAN_POINT ( 'NONE',  ( 15.93750000000000000, 5.773502691896255534, 3.535250795749688894E-16 ) ) ;
#57846=CARTESIAN_POINT ( 'NONE',  ( 21.25312500061451715, 0.000000000000000000, 5.243569643749999010 ) ) ;
#57848=CARTESIAN_POINT ( 'NONE',  ( 25.57499999999999929, -4.330127018922194537, 2.499999999999995559 ) ) ;
#57849=( BOUNDED_CURVE ( )  B_SPLINE_CURVE ( 2, ( #62571, #59930, #37035, #70655, #65847, #47396, #37768, #43326, #30766 ),
 .UNSPECIFIED., .F., .F. ) 
 B_SPLINE_CURVE_WITH_KNOTS ( ( 3, 2, 2, 2, 3 ),
 ( 0.3369565217391304324, 0.3405797101449275499, 0.3478260869565217295, 0.3550724637681159646, 0.3586956521739130821 ),
 .UNSPECIFIED. ) 
 CURVE ( )  GEOMETRIC_REPRESENTATION_ITEM ( )  RATIONAL_B_SPLINE_CURVE ( ( 0.9330127018922194093, 0.9330127018922194093, 1.000000000000000000, 0.8660254037844387076, 1.000000000000000000, 0.8660254037844387076, 1.000000000000000000, 0.9330127018922188542, 0.9330127018922194093 ) ) 
 REPRESENTATION_ITEM ( '' )  );
#57850=CARTESIAN_POINT ( 'NONE',  ( 26.03437500061451715, 6.421520780324663323E-16, -5.243569643749999010 ) ) ;
#57852=CARTESIAN_POINT ( 'NONE',  ( 15.17812500061451608, 6.421520780324663323E-16, -5.243569643749999010 ) ) ;
#57853=CARTESIAN_POINT ( 'NONE',  ( 4.978125000614518569, 4.541064518000418104, 2.621784821874999949 ) ) ;
#57855=CARTESIAN_POINT ( 'NONE',  ( 28.97812500061451502, -4.541064518000419881, 2.621784821874995952 ) ) ;
#57856=CARTESIAN_POINT ( 'NONE',  ( 15.22500000122903252, 2.886751345948126879, 4.999999999999999112 ) ) ;
#57857=CARTESIAN_POINT ( 'NONE',  ( 20.69999999999999929, -4.330127018922190985, -2.500000000000001332 ) ) ;
#57858=CARTESIAN_POINT ( 'NONE',  ( 28.16249999999999787, 2.886751345948126879, 4.999999999999999112 ) ) ;
#57859=CARTESIAN_POINT ( 'NONE',  ( 4.509375000614518569, 4.541064518000418104, -2.621784821874998173 ) ) ;
#57860=CARTESIAN_POINT ( 'NONE',  ( 9.271875000614516082, -6.054752690667223547, -1.112240025338166033E-15 ) ) ;
#57861=CARTESIAN_POINT ( 'NONE',  ( 19.17187500061451999, -6.054752690667223547, -1.112240025338166033E-15 ) ) ;
#57863=ORIENTED_EDGE ( 'NONE', *, *, #20206, .T. ) ;
#57864=CARTESIAN_POINT ( 'NONE',  ( 29.05312500061451431, -4.541064518000417216, -2.621784821875001281 ) ) ;
#57865=CARTESIAN_POINT ( 'NONE',  ( 3.037500000000002309, -2.886751345948129988, 4.999999999999997335 ) ) ;
#57866=CARTESIAN_POINT ( 'NONE',  ( 4.134375000614517681, 4.541064518000418104, 2.621784821874999949 ) ) ;
#57867=CARTESIAN_POINT ( 'NONE',  ( 18.03749999999999787, -2.886751345948125991, -5.000000000000000000 ) ) ;
#57868=CARTESIAN_POINT ( 'NONE',  ( 13.94062500061451892, 6.054752690667223547, 3.707466751127219781E-16 ) ) ;
#57869=CARTESIAN_POINT ( 'NONE',  ( -5.810221930991193690E-16, 14.15000000122903145, 26.00000000000000355 ) ) ;
#57873=CARTESIAN_POINT ( 'NONE',  ( 7.903125000614515727, -4.541064518000417216, -2.621784821875001281 ) ) ;
#57874=CARTESIAN_POINT ( 'NONE',  ( 24.49687500061451573, -3.027376345333614438, 5.243569643749998122 ) ) ;
#57875=CARTESIAN_POINT ( 'NONE',  ( 2.121784821874999061, 18.35937500061451644, 26.32496088578401583 ) ) ;
#57876=CARTESIAN_POINT ( 'NONE',  ( 26.89687500061451431, -3.027376345333610441, -5.243569643749999898 ) ) ;
#57877=CARTESIAN_POINT ( 'NONE',  ( 6.524999999999999467, 4.330127018922191873, 2.499999999999999556 ) ) ;
#57878=CARTESIAN_POINT ( 'NONE',  ( 1.999999999999998668, 13.21250000122903501, 26.53589838486224650 ) ) ;
#57879=CARTESIAN_POINT ( 'NONE',  ( 15.40312500061451573, 0.000000000000000000, 5.243569643749999010 ) ) ;
#57880=CARTESIAN_POINT ( 'NONE',  ( 6.112500001229034474, 4.330127018922192761, -2.499999999999997780 ) ) ;
#57881=CARTESIAN_POINT ( 'NONE',  ( 17.67187500061451644, 3.027376345333611329, 5.243569643749999010 ) ) ;
#57882=CARTESIAN_POINT ( 'NONE',  ( 11.40937500061451892, 0.000000000000000000, 5.243569643749999010 ) ) ;
#57884=VERTEX_POINT ( 'NONE', #18360 ) ;
#57885=CARTESIAN_POINT ( 'NONE',  ( 11.69062500061451360, 6.054752690667223547, 3.707466751127219781E-16 ) ) ;
#57887=CARTESIAN_POINT ( 'NONE',  ( 23.47500000122903430, -5.773502691896255534, -1.060575238724906372E-15 ) ) ;
#57888=CARTESIAN_POINT ( 'NONE',  ( 13.39687500061451608, -3.027376345333610441, -5.243569643749999898 ) ) ;
#57889=CARTESIAN_POINT ( 'NONE',  ( 15.55312500061451608, -4.541064518000417216, -2.621784821875001281 ) ) ;
#57890=CARTESIAN_POINT ( 'NONE',  ( 4.000000000000000000, 16.58750000000000213, -27.69059892324149885 ) ) ;
#57891=CARTESIAN_POINT ( 'NONE',  ( 24.60937500061451644, -4.541064518000417216, -2.621784821875001281 ) ) ;
#57892=DIRECTION ( 'NONE',  ( -0.000000000000000000, -1.000000000000000000, -0.000000000000000000 ) ) ;
#57893=CARTESIAN_POINT ( 'NONE',  ( 12.07500000122903216, 2.886751345948126879, 4.999999999999999112 ) ) ;
#57894=CARTESIAN_POINT ( 'NONE',  ( 4.406325135406961024, 3.605547266578323029, 3.755008945195253300 ) ) ;
#57896=CARTESIAN_POINT ( 'NONE',  ( 4.243569643749999898, 16.44687500061451857, -27.54997392385601529 ) ) ;
#57897=CARTESIAN_POINT ( 'NONE',  ( 18.83437500061451431, 6.421520780324663323E-16, -5.243569643749999010 ) ) ;
#57898=CARTESIAN_POINT ( 'NONE',  ( 16.95000000122903216, 5.773502691896255534, 3.535250795749688894E-16 ) ) ;
#57899=CARTESIAN_POINT ( 'NONE',  ( 12.38437500061451857, -4.541064518000419881, 2.621784821874995952 ) ) ;
#57901=CARTESIAN_POINT ( 'NONE',  ( 21.07500000122903572, 2.886751345948126879, 4.999999999999999112 ) ) ;
#57902=CARTESIAN_POINT ( 'NONE',  ( 13.94062500061451892, 6.054752690667223547, 3.707466751127219781E-16 ) ) ;
#57903=ORIENTED_EDGE ( 'NONE', *, *, #53191, .T. ) ;
#57904=ORIENTED_EDGE ( 'NONE', *, *, #38881, .F. ) ;
#57905=CARTESIAN_POINT ( 'NONE',  ( 17.21249999999999858, 2.886751345948129099, -4.999999999999998224 ) ) ;
#57907=LINE ( 'NONE', #36843, #56268 ) ;
#57908=CARTESIAN_POINT ( 'NONE',  ( 15.15000000122903323, 5.773502691896255534, 3.535250795749688894E-16 ) ) ;
#57909=CARTESIAN_POINT ( 'NONE',  ( 26.03437500061451715, 6.421520780324663323E-16, -5.243569643749999010 ) ) ;
#57910=CARTESIAN_POINT ( 'NONE',  ( 19.19062500061452070, -3.027376345333610441, -5.243569643749999898 ) ) ;
#57911=CARTESIAN_POINT ( 'NONE',  ( 23.09062500061451573, -3.027376345333614438, 5.243569643749998122 ) ) ;
#57912=CARTESIAN_POINT ( 'NONE',  ( 29.43750000122903288, 6.123233995736764310E-16, -4.999999999999998224 ) ) ;
#57913=( BOUNDED_CURVE ( )  B_SPLINE_CURVE ( 2, ( #19413, #41973, #19787, #64494, #30877, #53418, #2809 ),
 .UNSPECIFIED., .F., .F. ) 
 B_SPLINE_CURVE_WITH_KNOTS ( ( 3, 2, 2, 3 ),
 ( 0.1666666666666666852, 0.1694444444444444808, 0.1722222222222222487, 0.1750000000000000167 ),
 .UNSPECIFIED. ) 
 CURVE ( )  GEOMETRIC_REPRESENTATION_ITEM ( )  RATIONAL_B_SPLINE_CURVE ( ( 0.9999999999999986677, 0.8660254037844400399, 1.000000000000000000, 0.8660254037844387076, 1.000000000000000000, 0.8660254037844373753, 1.000000000000001332 ) ) 
 REPRESENTATION_ITEM ( '' )  );
#57914=EDGE_CURVE ( 'NONE', #69502, #14839, #60226, .T. ) ;
#57915=CARTESIAN_POINT ( 'NONE',  ( 27.59999999999999787, 4.330127018922192761, -2.499999999999997780 ) ) ;
#57918=FACE_OUTER_BOUND ( 'NONE', #4286, .T. ) ;
#57920=CARTESIAN_POINT ( 'NONE',  ( 4.243569643749999898, 15.54687500061451644, -27.54997392385601529 ) ) ;
#57921=CARTESIAN_POINT ( 'NONE',  ( 7.237500001229035362, -4.330127018922194537, 2.499999999999995559 ) ) ;
#57922=CARTESIAN_POINT ( 'NONE',  ( 5.212500000000002132, 2.886751345948126879, 4.999999999999999112 ) ) ;
#57923=ADVANCED_FACE ( 'NONE', ( #3119 ), #64799, .F. ) ;
#57925=CARTESIAN_POINT ( 'NONE',  ( 9.759375000614516793, -4.541064518000417216, -2.621784821875001281 ) ) ;
#57926=CARTESIAN_POINT ( 'NONE',  ( 29.65312500061451573, 4.541064518000418104, -2.621784821874998173 ) ) ;
#57927=CARTESIAN_POINT ( 'NONE',  ( -3.137519842735245283E-14, 12.91250000000000142, 34.00000000000000000 ) ) ;
#57929=CYLINDRICAL_SURFACE ( 'NONE', #37133, 4.999999999999998224 ) ;
#57930=CARTESIAN_POINT ( 'NONE',  ( 8.334375000614516082, -4.541064518000419881, 2.621784821874995952 ) ) ;
#57931=CARTESIAN_POINT ( 'NONE',  ( 11.22187500061451892, 3.027376345333613106, -5.243569643749998122 ) ) ;
#57932=CARTESIAN_POINT ( 'NONE',  ( 6.337499999999998579, -2.886751345948125991, -5.000000000000000000 ) ) ;
#57933=CARTESIAN_POINT ( 'NONE',  ( 4.243569643749999010, 14.21562500061459744, 27.54997392385601174 ) ) ;
#57935=CARTESIAN_POINT ( 'NONE',  ( 5.587500000000003020, 5.773502691896255534, 3.535250795749688894E-16 ) ) ;
#57936=CARTESIAN_POINT ( 'NONE',  ( 27.56250000122902932, -4.330127018922190985, -2.500000000000001332 ) ) ;
#57938=CARTESIAN_POINT ( 'NONE',  ( 22.22812500061451502, -4.541064518000419881, 2.621784821874995952 ) ) ;
#57939=CARTESIAN_POINT ( 'NONE',  ( 13.90312500061451750, 4.541064518000418104, -2.621784821874998173 ) ) ;
#57941=CARTESIAN_POINT ( 'NONE',  ( 8.671875000614518214, 3.027376345333611329, 5.243569643749999010 ) ) ;
#57942=CARTESIAN_POINT ( 'NONE',  ( 27.29999999999999716, 0.000000000000000000, 4.999999999999998224 ) ) ;
#57943=CARTESIAN_POINT ( 'NONE',  ( 21.41250000122903074, 4.330127018922192761, -2.499999999999997780 ) ) ;
#57944=CARTESIAN_POINT ( 'NONE',  ( 22.68750000122903288, 6.123233995736764310E-16, -4.999999999999998224 ) ) ;
#57945=CARTESIAN_POINT ( 'NONE',  ( 11.14687500061451608, -3.027376345333610441, -5.243569643749999898 ) ) ;
#57946=CARTESIAN_POINT ( 'NONE',  ( 27.38437500061451857, 6.421520780324663323E-16, -5.243569643749999010 ) ) ;
#57947=CARTESIAN_POINT ( 'NONE',  ( 3.271875000614519635, 3.027376345333611329, 5.243569643749999010 ) ) ;
#57948=CARTESIAN_POINT ( 'NONE',  ( 22.17187500061451644, 3.027376345333611329, 5.243569643749999010 ) ) ;
#57949=CARTESIAN_POINT ( 'NONE',  ( 11.93437500061451573, -4.541064518000419881, 2.621784821874995952 ) ) ;
#57951=CARTESIAN_POINT ( 'NONE',  ( 26.58750000000000213, -2.886751345948125991, -5.000000000000000000 ) ) ;
#57953=CARTESIAN_POINT ( 'NONE',  ( -2.121784821874999949, 11.68437500061451750, -33.67503911421598417 ) ) ;
#57955=CARTESIAN_POINT ( 'NONE',  ( 14.72812500061451679, 6.421520780324663323E-16, -5.243569643749999010 ) ) ;
#57956=CARTESIAN_POINT ( 'NONE',  ( 6.375000000000001776, 6.123233995736764310E-16, -4.999999999999998224 ) ) ;
#57957=FACE_OUTER_BOUND ( 'NONE', #49256, .T. ) ;
#57958=CARTESIAN_POINT ( 'NONE',  ( 15.90000000000000036, 4.330127018922192761, -2.499999999999997780 ) ) ;
#57959=CARTESIAN_POINT ( 'NONE',  ( -3.999999999999997335, 19.25000000122903288, 32.30940107675850470 ) ) ;
#57960=CARTESIAN_POINT ( 'NONE',  ( 15.11250000122903359, 4.330127018922192761, -2.499999999999997780 ) ) ;
#57961=CARTESIAN_POINT ( 'NONE',  ( 23.93437500061451573, 4.541064518000418104, 2.621784821874999949 ) ) ;
#57963=CARTESIAN_POINT ( 'NONE',  ( 19.45312500061451644, 0.000000000000000000, 5.243569643749999010 ) ) ;
#57964=CARTESIAN_POINT ( 'NONE',  ( 19.65937500061451360, -4.541064518000417216, -2.621784821875001281 ) ) ;
#57965=CARTESIAN_POINT ( 'NONE',  ( 4.837500000000001243, -2.886751345948129988, 4.999999999999997335 ) ) ;
#57966=CARTESIAN_POINT ( 'NONE',  ( 7.528125000614515727, 6.421520780324663323E-16, -5.243569643749999010 ) ) ;
#57967=CARTESIAN_POINT ( 'NONE',  ( 23.01562500061451644, 3.027376345333611329, 5.243569643749999010 ) ) ;
#57968=CARTESIAN_POINT ( 'NONE',  ( 11.85937500061451644, 0.000000000000000000, 5.243569643749999010 ) ) ;
#57969=CARTESIAN_POINT ( 'NONE',  ( 15.83437500061451608, 4.541064518000418104, 2.621784821874999949 ) ) ;
#57970=CARTESIAN_POINT ( 'NONE',  ( 4.243569643749999010, 15.11562500061451608, 27.54997392385601174 ) ) ;
#57971=CARTESIAN_POINT ( 'NONE',  ( 18.52500000122903145, -5.773502691896255534, -1.060575238724906372E-15 ) ) ;
#57973=CARTESIAN_POINT ( 'NONE',  ( 10.11562500061451608, -6.054752690667223547, -1.112240025338166033E-15 ) ) ;
#57974=CARTESIAN_POINT ( 'NONE',  ( 4.321875000614517681, -6.054752690667223547, -1.112240025338166033E-15 ) ) ;
#57975=CARTESIAN_POINT ( 'NONE',  ( 28.41562500061451502, 3.027376345333611329, 5.243569643749999010 ) ) ;
#57976=CARTESIAN_POINT ( 'NONE',  ( 26.37187500061451217, -6.054752690667223547, -1.112240025338166033E-15 ) ) ;
#57977=CARTESIAN_POINT ( 'NONE',  ( 17.50312500061451715, 4.541064518000418104, -2.621784821874998173 ) ) ;
#57978=CARTESIAN_POINT ( 'NONE',  ( 25.08750000122903145, 4.330127018922191873, 2.499999999999999556 ) ) ;
#57979=CARTESIAN_POINT ( 'NONE',  ( 25.60312500061451502, 4.541064518000418104, -2.621784821874998173 ) ) ;
#57980=CARTESIAN_POINT ( 'NONE',  ( 20.97187500061451715, -6.054752690667223547, -1.112240025338166033E-15 ) ) ;
#57981=CARTESIAN_POINT ( 'NONE',  ( 15.25312500061451715, 4.541064518000418104, -2.621784821874998173 ) ) ;
#57982=CARTESIAN_POINT ( 'NONE',  ( 4.243569643749999898, 16.93437500061451573, 30.00000000000000000 ) ) ;
#57983=CARTESIAN_POINT ( 'NONE',  ( 21.92812500061451431, 6.421520780324663323E-16, -5.243569643749999010 ) ) ;
#57984=CARTESIAN_POINT ( 'NONE',  ( 3.075000001229035718, 2.886751345948126879, 4.999999999999999112 ) ) ;
#57986=CARTESIAN_POINT ( 'NONE',  ( 24.89999999999999858, 4.330127018922192761, -2.499999999999997780 ) ) ;
#57987=CARTESIAN_POINT ( 'NONE',  ( 3.999999999999999112, 12.12500000000000000, -30.00000000000000000 ) ) ;
#57989=CARTESIAN_POINT ( 'NONE',  ( 28.86562500061451786, 3.027376345333611329, 5.243569643749999010 ) ) ;
#57990=CARTESIAN_POINT ( 'NONE',  ( 6.890625000614516438, -3.027376345333614438, 5.243569643749998122 ) ) ;
#57991=CARTESIAN_POINT ( 'NONE',  ( 21.26250000122903572, -4.330127018922190985, -2.500000000000001332 ) ) ;
#57992=CARTESIAN_POINT ( 'NONE',  ( 26.27812500061451573, -4.541064518000419881, 2.621784821874995952 ) ) ;
#57993=CARTESIAN_POINT ( 'NONE',  ( 4.650000001229035895, -2.886751345948125991, -5.000000000000000000 ) ) ;
#57994=CARTESIAN_POINT ( 'NONE',  ( 24.67500000000000071, -4.330127018922194537, 2.499999999999995559 ) ) ;
#57995=CARTESIAN_POINT ( 'NONE',  ( -3.999999999999999556, 15.12500000122903288, -32.30940107675850470 ) ) ;
#57996=CARTESIAN_POINT ( 'NONE',  ( -3.137519842735245283E-14, 12.57500000122903572, 34.00000000000000000 ) ) ;
#57997=CARTESIAN_POINT ( 'NONE',  ( 10.45312500061451644, 0.000000000000000000, 5.243569643749999010 ) ) ;
#57998=ORIENTED_EDGE ( 'NONE', *, *, #44349, .F. ) ;
#58000=CARTESIAN_POINT ( 'NONE',  ( 26.61562500061451786, 3.027376345333611329, 5.243569643749999010 ) ) ;
#58001=CARTESIAN_POINT ( 'NONE',  ( 7.303125000614516082, 0.000000000000000000, 5.243569643749999010 ) ) ;
#58002=CARTESIAN_POINT ( 'NONE',  ( 4.678125000614516971, -4.541064518000419881, 2.621784821874995952 ) ) ;
#58004=CARTESIAN_POINT ( 'NONE',  ( 4.658538704007320064, -1.816114365443275425, 4.919044833179992082 ) ) ;
#58005=CARTESIAN_POINT ( 'NONE',  ( 13.08750000000000036, -2.886751345948125991, -5.000000000000000000 ) ) ;
#58006=CARTESIAN_POINT ( 'NONE',  ( 12.90937500061451537, -4.541064518000417216, -2.621784821875001281 ) ) ;
#58007=CARTESIAN_POINT ( 'NONE',  ( 10.08750000122903323, 6.123233995736764310E-16, -4.999999999999998224 ) ) ;
#58008=CARTESIAN_POINT ( 'NONE',  ( 16.28437500061452070, 4.541064518000418104, 2.621784821874999949 ) ) ;
#58010=CARTESIAN_POINT ( 'NONE',  ( 7.734375000614517326, 4.541064518000418104, 2.621784821874999949 ) ) ;
#58011=CARTESIAN_POINT ( 'NONE',  ( -4.243569643749997233, 10.84062500061451395, -27.54997392385601174 ) ) ;
#58012=CARTESIAN_POINT ( 'NONE',  ( 1.999999999999998668, 16.69999999999999929, 26.53589838486224650 ) ) ;
#58014=VERTEX_POINT ( 'NONE', #9754 ) ;
#58015=CARTESIAN_POINT ( 'NONE',  ( 25.34062500061451217, -3.027376345333614438, 5.243569643749998122 ) ) ;
#58016=CARTESIAN_POINT ( 'NONE',  ( 11.10000000000000142, 0.000000000000000000, 4.999999999999998224 ) ) ;
#58017=CARTESIAN_POINT ( 'NONE',  ( 27.42187500061451644, 3.027376345333613106, -5.243569643749998122 ) ) ;
#58018=CARTESIAN_POINT ( 'NONE',  ( 25.34999999999999787, 4.330127018922192761, -2.499999999999997780 ) ) ;
#58019=CARTESIAN_POINT ( 'NONE',  ( 7.978125000614517681, 6.421520780324663323E-16, -5.243569643749999010 ) ) ;
#58021=CARTESIAN_POINT ( 'NONE',  ( 17.59687500061451715, 6.054752690667223547, 3.707466751127219781E-16 ) ) ;
#58023=CARTESIAN_POINT ( 'NONE',  ( 2.878125000614517592, -4.541064518000419881, 2.621784821874995952 ) ) ;
#58024=CARTESIAN_POINT ( 'NONE',  ( 9.346875000614517148, -3.027376345333610441, -5.243569643749999898 ) ) ;
#58025=ORIENTED_EDGE ( 'NONE', *, *, #21219, .F. ) ;
#58026=CARTESIAN_POINT ( 'NONE',  ( 19.17187500061451999, -6.054752690667223547, -1.112240025338166033E-15 ) ) ;
#58027=CARTESIAN_POINT ( 'NONE',  ( 3.360876423103621669, 3.702290849829691588, -3.360876423103621669 ) ) ;
#58028=CARTESIAN_POINT ( 'NONE',  ( 26.25000000000000000, 4.330127018922192761, -2.499999999999997780 ) ) ;
#58029=CARTESIAN_POINT ( 'NONE',  ( 29.29687500061451644, 6.054752690667223547, 3.707466751127219781E-16 ) ) ;
#58030=CARTESIAN_POINT ( 'NONE',  ( 30.00000000000000000, 0.000000000000000000, 0.000000000000000000 ) ) ;
#58031=CARTESIAN_POINT ( 'NONE',  ( 10.76250000000000107, -5.773502691896255534, -1.060575238724906372E-15 ) ) ;
#58032=ORIENTED_EDGE ( 'NONE', *, *, #32425, .F. ) ;
#58033=CARTESIAN_POINT ( 'NONE',  ( 11.47499999999999964, 4.330127018922191873, 2.499999999999999556 ) ) ;
#58035=CARTESIAN_POINT ( 'NONE',  ( 24.51562500061451289, -6.054752690667223547, -1.112240025338166033E-15 ) ) ;
#58036=CARTESIAN_POINT ( 'NONE',  ( 13.91249999999999964, -5.773502691896255534, -1.060575238724906372E-15 ) ) ;
#58037=CARTESIAN_POINT ( 'NONE',  ( 9.187500001229034652, 6.123233995736764310E-16, -4.999999999999998224 ) ) ;
#58038=CARTESIAN_POINT ( 'NONE',  ( 6.965625000614518392, -6.054752690667223547, -1.112240025338166033E-15 ) ) ;
#58039=CARTESIAN_POINT ( 'NONE',  ( 22.01249999999999574, -5.773502691896255534, -1.060575238724906372E-15 ) ) ;
#58040=ADVANCED_FACE ( 'NONE', ( #3859 ), #53117, .T. ) ;
#58041=CARTESIAN_POINT ( 'NONE',  ( 20.54062500061451502, -3.027376345333610441, -5.243569643749999898 ) ) ;
#58043=VECTOR ( 'NONE', #4295, 1000.000000000000000 ) ;
#58044=CARTESIAN_POINT ( 'NONE',  ( 24.93750000122903288, 6.123233995736764310E-16, -4.999999999999998224 ) ) ;
#58046=CARTESIAN_POINT ( 'NONE',  ( 6.262500000000000178, -5.773502691896255534, -1.060575238724906372E-15 ) ) ;
#58047=ORIENTED_EDGE ( 'NONE', *, *, #3893, .T. ) ;
#58048=CARTESIAN_POINT ( 'NONE',  ( 21.21562500061451573, 3.027376345333611329, 5.243569643749999010 ) ) ;
#58049=CARTESIAN_POINT ( 'NONE',  ( 26.24062500061451431, -3.027376345333614438, 5.243569643749998122 ) ) ;
#58050=CARTESIAN_POINT ( 'NONE',  ( 27.98437500061451289, 4.541064518000418104, 2.621784821874999949 ) ) ;
#58051=CARTESIAN_POINT ( 'NONE',  ( 15.25312500061451715, 4.541064518000418104, -2.621784821874998173 ) ) ;
#58053=CARTESIAN_POINT ( 'NONE',  ( 27.00000000122903288, -2.886751345948129988, 4.999999999999997335 ) ) ;
#58055=CARTESIAN_POINT ( 'NONE',  ( 17.50312500061451715, 4.541064518000418104, -2.621784821874998173 ) ) ;
#58056=CARTESIAN_POINT ( 'NONE',  ( 1.999999999999998668, 14.56250000122903288, -33.46410161513775705 ) ) ;
#58057=CARTESIAN_POINT ( 'NONE',  ( 2.737500001229034474, -4.330127018922194537, 2.499999999999995559 ) ) ;
#58058=CARTESIAN_POINT ( 'NONE',  ( 11.10937500061451644, -4.541064518000417216, -2.621784821875001281 ) ) ;
#58059=CARTESIAN_POINT ( 'NONE',  ( 10.54687500061451644, -3.027376345333614438, 5.243569643749998122 ) ) ;
#58060=CARTESIAN_POINT ( 'NONE',  ( 18.83437500061451431, 6.421520780324663323E-16, -5.243569643749999010 ) ) ;
#58061=ORIENTED_EDGE ( 'NONE', *, *, #50010, .T. ) ;
#58062=CARTESIAN_POINT ( 'NONE',  ( 9.975000000000001421, 6.123233995736764310E-16, -4.999999999999998224 ) ) ;
#58063=CARTESIAN_POINT ( 'NONE',  ( 23.39062500061451289, 6.054752690667223547, 3.707466751127219781E-16 ) ) ;
#58064=CARTESIAN_POINT ( 'NONE',  ( 19.24687500061452283, -3.027376345333610441, -5.243569643749999898 ) ) ;
#58065=CARTESIAN_POINT ( 'NONE',  ( 23.46562500061451573, 3.027376345333611329, 5.243569643749999010 ) ) ;
#58066=CARTESIAN_POINT ( 'NONE',  ( 4.000000000000000000, 14.78750000000000320, 32.30940107675849049 ) ) ;
#58067=CARTESIAN_POINT ( 'NONE',  ( 2.971875000614517592, -6.054752690667223547, -1.112240025338166033E-15 ) ) ;
#58068=CARTESIAN_POINT ( 'NONE',  ( 10.35000000122903074, -2.886751345948129988, 4.999999999999997335 ) ) ;
#58069=CARTESIAN_POINT ( 'NONE',  ( 3.900000001229034563, 5.773502691896255534, 3.535250795749688894E-16 ) ) ;
#58070=CARTESIAN_POINT ( 'NONE',  ( -1.999999999999997113, 19.62500000000000000, -26.53589838486224295 ) ) ;
#58071=CARTESIAN_POINT ( 'NONE',  ( 26.17500000122903359, -5.773502691896255534, -1.060575238724906372E-15 ) ) ;
#58074=CARTESIAN_POINT ( 'NONE',  ( 10.28437500061451715, 6.421520780324663323E-16, -5.243569643749999010 ) ) ;
#58075=CARTESIAN_POINT ( 'NONE',  ( 17.81250000000000355, 2.886751345948193936, 4.999999999999883649 ) ) ;
#58076=CARTESIAN_POINT ( 'NONE',  ( 17.24062500061451786, -3.027376345333614438, 5.243569643749998122 ) ) ;
#58077=CARTESIAN_POINT ( 'NONE',  ( 11.63437500061451857, 6.421520780324663323E-16, -5.243569643749999010 ) ) ;
#58078=CARTESIAN_POINT ( 'NONE',  ( 29.13750000122903216, 4.330127018922191873, 2.499999999999999556 ) ) ;
#58079=CARTESIAN_POINT ( 'NONE',  ( 19.69687500061451857, -3.027376345333610441, -5.243569643749999898 ) ) ;
#58080=CARTESIAN_POINT ( 'NONE',  ( 6.796875000614516438, 6.054752690667223547, 3.707466751127219781E-16 ) ) ;
#58081=CARTESIAN_POINT ( 'NONE',  ( 3.890625000614517326, -3.027376345333610441, -5.243569643749999898 ) ) ;
#58082=CARTESIAN_POINT ( 'NONE',  ( 30.00000000000000000, 0.000000000000000000, 0.000000000000000000 ) ) ;
#58083=CARTESIAN_POINT ( 'NONE',  ( 8.915625000614515017, 3.027376345333613106, -5.243569643749998122 ) ) ;
#58084=CARTESIAN_POINT ( 'NONE',  ( 16.79062500061451857, -3.027376345333614438, 5.243569643749998122 ) ) ;
#58086=CARTESIAN_POINT ( 'NONE',  ( 6.712500001229034119, 0.000000000000000000, 4.999999999999998224 ) ) ;
#58087=CARTESIAN_POINT ( 'NONE',  ( 16.04062500061451857, -3.027376345333610441, -5.243569643749999898 ) ) ;
#58088=CARTESIAN_POINT ( 'NONE',  ( 10.75312500061451715, 4.541064518000418104, -2.621784821874998173 ) ) ;
#58090=CARTESIAN_POINT ( 'NONE',  ( 11.62500000000000000, -4.330127018922194537, 2.499999999999995559 ) ) ;
#58091=CARTESIAN_POINT ( 'NONE',  ( 7.425000001229034474, 2.886751345948129099, -4.999999999999998224 ) ) ;
#58092=ADVANCED_FACE ( 'NONE', ( #6591 ), #19662, .T. ) ;
#58093=CARTESIAN_POINT ( 'NONE',  ( 14.78437500061451715, 6.421520780324663323E-16, -5.243569643749999010 ) ) ;
#58094=AXIS2_PLACEMENT_3D ( 'NONE', #66553, #3413, #32207 ) ;
#58095=CARTESIAN_POINT ( 'NONE',  ( 19.53750000122903430, 6.123233995736764310E-16, -4.999999999999998224 ) ) ;
#58097=CARTESIAN_POINT ( 'NONE',  ( 2.121784821874999061, 17.85312500061451502, -33.67503911421598417 ) ) ;
#58098=DIRECTION ( 'NONE',  ( -0.000000000000000000, -1.000000000000000000, -0.000000000000000000 ) ) ;
#58099=DIRECTION ( 'NONE',  ( 0.000000000000000000, 0.000000000000000000, -1.000000000000000000 ) ) ;
#58102=DIRECTION ( 'NONE',  ( 0.000000000000000000, 0.000000000000000000, 1.000000000000000000 ) ) ;
#58103=CARTESIAN_POINT ( 'NONE',  ( 18.79687500061451644, -3.027376345333610441, -5.243569643749999898 ) ) ;
#58104=CARTESIAN_POINT ( 'NONE',  ( 14.72812500061451679, 6.421520780324663323E-16, -5.243569643749999010 ) ) ;
#58106=CARTESIAN_POINT ( 'NONE',  ( 22.57500000122903572, -5.773502691896255534, -1.060575238724906372E-15 ) ) ;
#58107=CARTESIAN_POINT ( 'NONE',  ( 25.43437500061451573, -4.541064518000419881, 2.621784821874995952 ) ) ;
#58109=CARTESIAN_POINT ( 'NONE',  ( 10.15312500061451750, -4.541064518000417216, -2.621784821875001281 ) ) ;
#58110=CARTESIAN_POINT ( 'NONE',  ( 16.24687500061451573, 6.054752690667223547, 3.707466751127219781E-16 ) ) ;
#58112=CARTESIAN_POINT ( 'NONE',  ( 27.70312500061451289, -4.541064518000417216, -2.621784821875001281 ) ) ;
#58113=CARTESIAN_POINT ( 'NONE',  ( 19.49062500061451431, -3.027376345333614438, 5.243569643749998122 ) ) ;
#58114=CARTESIAN_POINT ( 'NONE',  ( 3.999999999999999112, 13.13750000122903394, -30.00000000000000000 ) ) ;
#58116=CARTESIAN_POINT ( 'NONE',  ( 8.887499999999999289, -2.886751345948129988, 4.999999999999997335 ) ) ;
#58117=CARTESIAN_POINT ( 'NONE',  ( 18.18750000122903288, 6.123233995736764310E-16, -4.999999999999998224 ) ) ;
#58118=FACE_OUTER_BOUND ( 'NONE', #1946, .T. ) ;
#58121=CARTESIAN_POINT ( 'NONE',  ( 18.07499999999999929, 6.123233995736764310E-16, -4.999999999999998224 ) ) ;
#58122=CARTESIAN_POINT ( 'NONE',  ( 20.62499999999999645, -4.330127018922194537, 2.499999999999995559 ) ) ;
#58123=CARTESIAN_POINT ( 'NONE',  ( 19.39687500061451786, 6.054752690667223547, 3.707466751127219781E-16 ) ) ;
#58124=CARTESIAN_POINT ( 'NONE',  ( 13.97812500061451679, 4.541064518000418104, 2.621784821874999949 ) ) ;
#58126=VERTEX_POINT ( 'NONE', #35393 ) ;
#58128=CARTESIAN_POINT ( 'NONE',  ( 6.703125000614516438, 4.541064518000418104, -2.621784821874998173 ) ) ;
#58129=DIRECTION ( 'NONE',  ( -1.000000000000000000, -0.000000000000000000, -0.000000000000000000 ) ) ;
#58130=CARTESIAN_POINT ( 'NONE',  ( 11.25000000000000000, -4.330127018922190985, -2.500000000000001332 ) ) ;
#58132=CARTESIAN_POINT ( 'NONE',  ( 2.121784821875001281, 17.70312500061451644, 33.67503911421598417 ) ) ;
#58133=CARTESIAN_POINT ( 'NONE',  ( 29.69062500061451715, 6.054752690667223547, 3.707466751127219781E-16 ) ) ;
#58136=CARTESIAN_POINT ( 'NONE',  ( 26.48437500061451644, 6.421520780324663323E-16, -5.243569643749999010 ) ) ;
#58137=VERTEX_POINT ( 'NONE', #41670 ) ;
#58138=CARTESIAN_POINT ( 'NONE',  ( 21.96562500061451573, 3.027376345333613106, -5.243569643749998122 ) ) ;
#58139=CARTESIAN_POINT ( 'NONE',  ( 22.13437500061451502, 4.541064518000418104, 2.621784821874999949 ) ) ;
#58140=CARTESIAN_POINT ( 'NONE',  ( -4.243569643749999898, 17.55312500061459602, -30.00000000000000000 ) ) ;
#58141=CARTESIAN_POINT ( 'NONE',  ( 5.728125000614515905, 6.421520780324663323E-16, -5.243569643749999010 ) ) ;
#58143=CARTESIAN_POINT ( 'NONE',  ( 25.00312500061451715, -4.541064518000417216, -2.621784821875001281 ) ) ;
#58146=CARTESIAN_POINT ( 'NONE',  ( 18.04687500061451999, 6.054752690667223547, 3.707466751127219781E-16 ) ) ;
#58148=CARTESIAN_POINT ( 'NONE',  ( 19.35937500061451644, 4.541064518000418104, -2.621784821874998173 ) ) ;
#58149=CARTESIAN_POINT ( 'NONE',  ( 26.14687500061451431, 6.054752690667223547, 3.707466751127219781E-16 ) ) ;
#58150=CARTESIAN_POINT ( 'NONE',  ( 9.001249775931846008E-16, 15.92187500061451821, 34.90005215228797653 ) ) ;
#58151=CARTESIAN_POINT ( 'NONE',  ( 7.678125000614516082, 4.541064518000418104, 2.621784821874999949 ) ) ;
#58152=CARTESIAN_POINT ( 'NONE',  ( -1.487416814333745711E-14, 16.06250000000000000, 34.00000000000000000 ) ) ;
#58153=CARTESIAN_POINT ( 'NONE',  ( 4.471875000614518925, 3.027376345333613106, -5.243569643749998122 ) ) ;
#58155=( BOUNDED_CURVE ( )  B_SPLINE_CURVE ( 2, ( #21040, #21765, #67224, #60557, #15858, #9964, #16585, #32502, #4795 ),
 .UNSPECIFIED., .F., .F. ) 
 B_SPLINE_CURVE_WITH_KNOTS ( ( 3, 2, 2, 2, 3 ),
 ( 0.8152173913043478937, 0.8188405797101449002, 0.8260869565217391353, 0.8333333333333333703, 0.8369565217391304879 ),
 .UNSPECIFIED. ) 
 CURVE ( )  GEOMETRIC_REPRESENTATION_ITEM ( )  RATIONAL_B_SPLINE_CURVE ( ( 0.9330127018922192983, 0.9330127018922202975, 1.000000000000000000, 0.8660254037844387076, 1.000000000000000000, 0.8660254037844387076, 1.000000000000000000, 0.9330127018922182991, 0.9330127018922192983 ) ) 
 REPRESENTATION_ITEM ( '' )  );
#58156=CARTESIAN_POINT ( 'NONE',  ( 5.840625000614516615, 6.054752690667223547, 3.707466751127219781E-16 ) ) ;
#58157=CARTESIAN_POINT ( 'NONE',  ( 10.05937500061451750, 0.000000000000000000, 5.243569643749999010 ) ) ;
#58158=CARTESIAN_POINT ( 'NONE',  ( 15.90000000122903501, -2.886751345948125991, -5.000000000000000000 ) ) ;
#58159=CARTESIAN_POINT ( 'NONE',  ( 4.471875000614518925, 3.027376345333613106, -5.243569643749998122 ) ) ;
#58160=CARTESIAN_POINT ( 'NONE',  ( 8.653125000614515727, 0.000000000000000000, 5.243569643749999010 ) ) ;
#58163=CARTESIAN_POINT ( 'NONE',  ( 15.90937500061451892, 0.000000000000000000, 5.243569643749999010 ) ) ;
#58164=CARTESIAN_POINT ( 'NONE',  ( -3.999999999999997335, 10.58750000000000213, 32.30940107675850470 ) ) ;
#58166=CARTESIAN_POINT ( 'NONE',  ( 24.14062500061451289, -3.027376345333610441, -5.243569643749999898 ) ) ;
#58167=CARTESIAN_POINT ( 'NONE',  ( 9.703125000614514661, -4.541064518000417216, -2.621784821875001281 ) ) ;
#58168=CARTESIAN_POINT ( 'NONE',  ( 26.59687500061451360, 6.054752690667223547, 3.707466751127219781E-16 ) ) ;
#58169=CARTESIAN_POINT ( 'NONE',  ( 8.915625000614515017, 3.027376345333613106, -5.243569643749998122 ) ) ;
#58171=CARTESIAN_POINT ( 'NONE',  ( 11.66250000122903430, 0.000000000000000000, 4.999999999999998224 ) ) ;
#58172=CARTESIAN_POINT ( 'NONE',  ( 24.29062500061451502, 6.054752690667223547, 3.707466751127219781E-16 ) ) ;
#58173=CARTESIAN_POINT ( 'NONE',  ( 2.121784821875001281, 12.75312500061451715, -26.32496088578401938 ) ) ;
#58174=CARTESIAN_POINT ( 'NONE',  ( 13.95000000122903572, -2.886751345948129988, 4.999999999999997335 ) ) ;
#58175=CARTESIAN_POINT ( 'NONE',  ( 21.96562500061451573, 3.027376345333613106, -5.243569643749998122 ) ) ;
#58176=CARTESIAN_POINT ( 'NONE',  ( 10.53750000000000320, 5.773502691896255534, 3.535250795749688894E-16 ) ) ;
#58177=CARTESIAN_POINT ( 'NONE',  ( 21.17812500061451431, 4.541064518000418104, 2.621784821874999949 ) ) ;
#58178=CARTESIAN_POINT ( 'NONE',  ( 5.971875000614517148, 3.027376345333611329, 5.243569643749999010 ) ) ;
#58179=CARTESIAN_POINT ( 'NONE',  ( 20.06250000000000000, 2.886751345948126879, 4.999999999999999112 ) ) ;
#58180=CARTESIAN_POINT ( 'NONE',  ( 13.68750000122903288, 6.123233995736764310E-16, -4.999999999999998224 ) ) ;
#58182=CARTESIAN_POINT ( 'NONE',  ( 10.94062500061451537, -3.027376345333614438, 5.243569643749998122 ) ) ;
#58183=CARTESIAN_POINT ( 'NONE',  ( 13.71562500061451750, -6.054752690667223547, -1.112240025338166033E-15 ) ) ;
#58184=CARTESIAN_POINT ( 'NONE',  ( 26.17500000122903359, -5.773502691896255534, -1.060575238724906372E-15 ) ) ;
#58185=CARTESIAN_POINT ( 'NONE',  ( 21.34687500061451715, -3.027376345333614438, 5.243569643749998122 ) ) ;
#58187=EDGE_CURVE ( 'NONE', #33928, #31017, #6286, .T. ) ;
#58188=CARTESIAN_POINT ( 'NONE',  ( 8.925000001229033586, 2.886751345948126879, 4.999999999999999112 ) ) ;
#58189=EDGE_CURVE ( 'NONE', #18641, #3838, #46857, .T. ) ;
#58190=CARTESIAN_POINT ( 'NONE',  ( 8.484375000614518214, 6.421520780324663323E-16, -5.243569643749999010 ) ) ;
#58191=CARTESIAN_POINT ( 'NONE',  ( 24.45937500061451786, 0.000000000000000000, 5.243569643749999010 ) ) ;
#58192=CARTESIAN_POINT ( 'NONE',  ( 4.494741915665277254, -2.190272839526016924, 4.494741915664858922 ) ) ;
#58193=CARTESIAN_POINT ( 'NONE',  ( 22.41562500061451502, 3.027376345333613106, -5.243569643749998122 ) ) ;
#58194=CARTESIAN_POINT ( 'NONE',  ( 26.40937500061451715, -4.541064518000417216, -2.621784821875001281 ) ) ;
#58197=CARTESIAN_POINT ( 'NONE',  ( 7.996875000614519280, -3.027376345333610441, -5.243569643749999898 ) ) ;
#58198=CARTESIAN_POINT ( 'NONE',  ( 17.42812500061451786, 6.421520780324663323E-16, -5.243569643749999010 ) ) ;
#58201=CARTESIAN_POINT ( 'NONE',  ( 27.77812500061451573, 6.421520780324663323E-16, -5.243569643749999010 ) ) ;
#58202=CARTESIAN_POINT ( 'NONE',  ( 3.309375000614518836, 0.000000000000000000, 5.243569643749999010 ) ) ;
#58203=CARTESIAN_POINT ( 'NONE',  ( 4.633613603196540254, 1.878729617659674167, 4.895446622381335544 ) ) ;
#58204=CARTESIAN_POINT ( 'NONE',  ( 0.000000000000000000, 20.00000000000000000, 26.00000000000000000 ) ) ;
#58205=CARTESIAN_POINT ( 'NONE',  ( 17.39999999999999858, 0.000000000000000000, 4.999999999999998224 ) ) ;
#58206=CARTESIAN_POINT ( 'NONE',  ( 20.87812500061451715, -4.541064518000419881, 2.621784821874995952 ) ) ;
#58208=CARTESIAN_POINT ( 'NONE',  ( 25.68750000000000000, -2.886751345948125991, -5.000000000000000000 ) ) ;
#58209=CARTESIAN_POINT ( 'NONE',  ( 25.58437500061451431, 6.421520780324663323E-16, -5.243569643749999010 ) ) ;
#58210=ORIENTED_EDGE ( 'NONE', *, *, #25488, .T. ) ;
#58211=CARTESIAN_POINT ( 'NONE',  ( 13.64062500061451644, -3.027376345333614438, 5.243569643749998122 ) ) ;
#58212=CARTESIAN_POINT ( 'NONE',  ( 5.240625000614516971, -3.027376345333610441, -5.243569643749999898 ) ) ;
#58214=CARTESIAN_POINT ( 'NONE',  ( 3.271875000614519635, 3.027376345333611329, 5.243569643749999010 ) ) ;
#58215=CARTESIAN_POINT ( 'NONE',  ( 15.26250000122903216, 0.000000000000000000, 4.999999999999998224 ) ) ;
#58216=CARTESIAN_POINT ( 'NONE',  ( 20.06250000000000000, 2.886751345948126879, 4.999999999999999112 ) ) ;
#58217=CARTESIAN_POINT ( 'NONE',  ( 28.68749999999999645, -2.886751345948129988, 4.999999999999997335 ) ) ;
#58218=CARTESIAN_POINT ( 'NONE',  ( 3.796875000614517326, -3.027376345333614438, 5.243569643749998122 ) ) ;
#58219=CARTESIAN_POINT ( 'NONE',  ( 10.13437500061451679, -4.541064518000419881, 2.621784821874995952 ) ) ;
#58220=CARTESIAN_POINT ( 'NONE',  ( 18.34687500061451715, -3.027376345333610441, -5.243569643749999898 ) ) ;
#58221=CARTESIAN_POINT ( 'NONE',  ( -1.071796769724485010, 17.39240381056766083, -25.99999999999999289 ) ) ;
#58222=ORIENTED_EDGE ( 'NONE', *, *, #28401, .T. ) ;
#58223=CARTESIAN_POINT ( 'NONE',  ( 28.52812500061451573, -4.541064518000419881, 2.621784821874995952 ) ) ;
#58224=CARTESIAN_POINT ( 'NONE',  ( 3.262500000000001510, 2.886751345948129099, -4.999999999999998224 ) ) ;
#58225=EDGE_CURVE ( 'NONE', #30519, #29484, #64563, .T. ) ;
#58226=CARTESIAN_POINT ( 'NONE',  ( 3.909375000614518481, -4.541064518000417216, -2.621784821875001281 ) ) ;
#58227=CARTESIAN_POINT ( 'NONE',  ( 16.87500000000000000, 4.330127018922191873, 2.499999999999999556 ) ) ;
#58228=CARTESIAN_POINT ( 'NONE',  ( 14.84062500061451750, 6.054752690667223547, 3.707466751127219781E-16 ) ) ;
#58231=CARTESIAN_POINT ( 'NONE',  ( 18.41250000122903430, 0.000000000000000000, 4.999999999999998224 ) ) ;
#58232=CARTESIAN_POINT ( 'NONE',  ( 0.000000000000000000, 10.00000000000000000, 24.00000000000000000 ) ) ;
#58234=CARTESIAN_POINT ( 'NONE',  ( 6.515625000614516438, -6.054752690667223547, -1.112240025338166033E-15 ) ) ;
#58235=CARTESIAN_POINT ( 'NONE',  ( 24.38437500061451502, 4.541064518000418104, 2.621784821874999949 ) ) ;
#58236=CARTESIAN_POINT ( 'NONE',  ( -4.243569643749999898, 19.40937500061451715, 30.00000000000000000 ) ) ;
#58237=CARTESIAN_POINT ( 'NONE',  ( 25.58437500061451431, 6.421520780324663323E-16, -5.243569643749999010 ) ) ;
#58238=CARTESIAN_POINT ( 'NONE',  ( 7.462500000000001243, 2.886751345948126879, 4.999999999999999112 ) ) ;
#58239=CARTESIAN_POINT ( 'NONE',  ( -2.000000000000000000, 12.83750000122903501, 26.53589838486224650 ) ) ;
#58240=CARTESIAN_POINT ( 'NONE',  ( 13.94062500061451892, 6.054752690667223547, 3.707466751127219781E-16 ) ) ;
#58241=CARTESIAN_POINT ( 'NONE',  ( 7.687500001229033764, -4.330127018922194537, 2.499999999999995559 ) ) ;
#58242=CARTESIAN_POINT ( 'NONE',  ( 18.68437500061451928, -4.541064518000419881, 2.621784821874995952 ) ) ;
#58243=CARTESIAN_POINT ( 'NONE',  ( 12.72187500061451537, 3.027376345333611329, 5.243569643749999010 ) ) ;
#58245=EDGE_LOOP ( 'NONE', ( #4695, #71340, #66339, #8766 ) ) ;
#58246=CARTESIAN_POINT ( 'NONE',  ( 13.07812500061451821, 4.541064518000418104, 2.621784821874999949 ) ) ;
#58248=CARTESIAN_POINT ( 'NONE',  ( 22.98750000122903003, -4.330127018922194537, 2.499999999999995559 ) ) ;
#58249=CARTESIAN_POINT ( 'NONE',  ( 13.28437500061451715, -4.541064518000419881, 2.621784821874995952 ) ) ;
#58250=CARTESIAN_POINT ( 'NONE',  ( 14.72812500061451679, 6.421520780324663323E-16, -5.243569643749999010 ) ) ;
#58251=CARTESIAN_POINT ( 'NONE',  ( 24.75937500061451502, 4.541064518000418104, -2.621784821874998173 ) ) ;
#58252=DIRECTION ( 'NONE',  ( -0.000000000000000000, -1.000000000000000000, -0.000000000000000000 ) ) ;
#58255=CARTESIAN_POINT ( 'NONE',  ( -4.243569643749999898, 16.67187500061451644, -32.45002607614398471 ) ) ;
#58256=CARTESIAN_POINT ( 'NONE',  ( 16.13437500061451502, 6.421520780324663323E-16, -5.243569643749999010 ) ) ;
#58257=CARTESIAN_POINT ( 'NONE',  ( 18.03750000122903430, -4.330127018922194537, 2.499999999999995559 ) ) ;
#58258=CARTESIAN_POINT ( 'NONE',  ( 12.79687500061451821, -3.027376345333614438, 5.243569643749998122 ) ) ;
#58259=CARTESIAN_POINT ( 'NONE',  ( 4.243569643749999898, 19.12812500061451715, -30.00000000000000000 ) ) ;
#58260=CARTESIAN_POINT ( 'NONE',  ( 20.21250000122903145, 0.000000000000000000, 4.999999999999998224 ) ) ;
#58261=CARTESIAN_POINT ( 'NONE',  ( 13.11562500061451786, 3.027376345333611329, 5.243569643749999010 ) ) ;
#58262=AXIS2_PLACEMENT_3D ( 'NONE', #62180, #15643, #63614 ) ;
#58264=ORIENTED_EDGE ( 'NONE', *, *, #10064, .T. ) ;
#58265=CARTESIAN_POINT ( 'NONE',  ( 17.96250000000000213, -5.773502691896255534, -1.060575238724906372E-15 ) ) ;
#58267=CARTESIAN_POINT ( 'NONE',  ( 12.04687500061451821, -3.027376345333610441, -5.243569643749999898 ) ) ;
#58269=CARTESIAN_POINT ( 'NONE',  ( 13.50000000122903288, -2.886751345948129988, 4.999999999999997335 ) ) ;
#58270=CARTESIAN_POINT ( 'NONE',  ( 21.52500000122903145, 2.886751345948126879, 4.999999999999999112 ) ) ;
#58271=CARTESIAN_POINT ( 'NONE',  ( 16.56562500061451715, 3.027376345333613106, -5.243569643749998122 ) ) ;
#58272=CARTESIAN_POINT ( 'NONE',  ( 23.20312500061451644, -4.541064518000417216, -2.621784821875001281 ) ) ;
#58273=CARTESIAN_POINT ( 'NONE',  ( 3.403125000614518836, -4.541064518000417216, -2.621784821875001281 ) ) ;
#58274=CARTESIAN_POINT ( 'NONE',  ( 28.08749999999999858, 5.773502691896255534, 3.535250795749688894E-16 ) ) ;
#58275=FACE_OUTER_BOUND ( 'NONE', #9533, .T. ) ;
#58278=CARTESIAN_POINT ( 'NONE',  ( 1.071796769724489895, 14.46740381056766545, -34.00000000000000000 ) ) ;
#58279=CARTESIAN_POINT ( 'NONE',  ( -2.121784821874996840, 15.88437500061451857, -26.32496088578401583 ) ) ;
#58280=CARTESIAN_POINT ( 'NONE',  ( 4.012500001229033053, 0.000000000000000000, 4.999999999999998224 ) ) ;
#58281=CARTESIAN_POINT ( 'NONE',  ( 7.124999999999999112, -4.330127018922194537, 2.499999999999995559 ) ) ;
#58282=( BOUNDED_CURVE ( )  B_SPLINE_CURVE ( 2, ( #10692, #26967, #33223, #5155, #44327, #72025, #27690, #66856, #22138 ),
 .UNSPECIFIED., .F., .F. ) 
 B_SPLINE_CURVE_WITH_KNOTS ( ( 3, 2, 2, 2, 3 ),
 ( 0.09782608695652174335, 0.1014492753623188470, 0.1086956521739130405, 0.1159420289855072478, 0.1195652173913043514 ),
 .UNSPECIFIED. ) 
 CURVE ( )  GEOMETRIC_REPRESENTATION_ITEM ( )  RATIONAL_B_SPLINE_CURVE ( ( 0.9330127018922194093, 0.9330127018922194093, 1.000000000000000000, 0.8660254037844387076, 1.000000000000000000, 0.8660254037844387076, 1.000000000000000000, 0.9330127018922194093, 0.9330127018922194093 ) ) 
 REPRESENTATION_ITEM ( '' )  );
#58283=CARTESIAN_POINT ( 'NONE',  ( 2.700000001229035718, -2.886751345948129988, 4.999999999999997335 ) ) ;
#58284=CARTESIAN_POINT ( 'NONE',  ( 10.88437500061451679, 4.541064518000418104, 2.621784821874999949 ) ) ;
#58285=CARTESIAN_POINT ( 'NONE',  ( 27.32812500061451644, 6.421520780324663323E-16, -5.243569643749999010 ) ) ;
#58288=FACE_OUTER_BOUND ( 'NONE', #41714, .T. ) ;
#58289=CARTESIAN_POINT ( 'NONE',  ( 7.434375000614519280, -4.541064518000419881, 2.621784821874995952 ) ) ;
#58290=CARTESIAN_POINT ( 'NONE',  ( 12.15937500061451892, 4.541064518000418104, -2.621784821874998173 ) ) ;
#58291=EDGE_CURVE ( 'NONE', #69560, #11634, #25290, .T. ) ;
#58292=CARTESIAN_POINT ( 'NONE',  ( 6.862500000000002487, 2.886751345948129099, -4.999999999999998224 ) ) ;
#58293=CARTESIAN_POINT ( 'NONE',  ( 2.121784821874999061, 15.15312500061459566, 26.32496088578401583 ) ) ;
#58294=CARTESIAN_POINT ( 'NONE',  ( 3.999999999999999112, 17.97500000000000142, 30.00000000000000000 ) ) ;
#58295=CARTESIAN_POINT ( 'NONE',  ( 6.562500000000001776, 2.886751345948126879, 4.999999999999999112 ) ) ;
#58297=CARTESIAN_POINT ( 'NONE',  ( 19.19062500061452070, -3.027376345333610441, -5.243569643749999898 ) ) ;
#58298=CARTESIAN_POINT ( 'NONE',  ( 13.64062500061451644, -3.027376345333614438, 5.243569643749998122 ) ) ;
#58300=CARTESIAN_POINT ( 'NONE',  ( 10.43437500061451750, 4.541064518000418104, 2.621784821874999949 ) ) ;
#58301=CARTESIAN_POINT ( 'NONE',  ( 25.91250000000000142, 2.886751345948126879, 4.999999999999999112 ) ) ;
#58302=CARTESIAN_POINT ( 'NONE',  ( 22.98750000122903003, -4.330127018922194537, 2.499999999999995559 ) ) ;
#58304=CARTESIAN_POINT ( 'NONE',  ( 12.75937500061451857, 0.000000000000000000, 5.243569643749999010 ) ) ;
#58305=CARTESIAN_POINT ( 'NONE',  ( 27.49687500061451217, 6.054752690667223547, 3.707466751127219781E-16 ) ) ;
#58307=CARTESIAN_POINT ( 'NONE',  ( 21.12187500061451573, 3.027376345333613106, -5.243569643749998122 ) ) ;
#58308=CARTESIAN_POINT ( 'NONE',  ( 11.52187500061451608, -6.054752690667223547, -1.112240025338166033E-15 ) ) ;
#58310=CARTESIAN_POINT ( 'NONE',  ( 23.69999999999999929, 0.000000000000000000, 4.999999999999998224 ) ) ;
#58312=CARTESIAN_POINT ( 'NONE',  ( 4.243569643749999898, 11.04687500061451999, -27.54997392385601529 ) ) ;
#58314=CARTESIAN_POINT ( 'NONE',  ( 14.57812500061451644, -4.541064518000419881, 2.621784821874995952 ) ) ;
#58315=CARTESIAN_POINT ( 'NONE',  ( 4.724999999999999645, 4.330127018922191873, 2.499999999999999556 ) ) ;
#58317=CARTESIAN_POINT ( 'NONE',  ( 15.11249999999999893, 2.886751345948126879, 4.999999999999999112 ) ) ;
#58318=EDGE_CURVE ( 'NONE', #57884, #34155, #60660, .T. ) ;
#58319=CARTESIAN_POINT ( 'NONE',  ( -2.121784821874996840, 10.87812500061451715, 33.67503911421598417 ) ) ;
#58320=CARTESIAN_POINT ( 'NONE',  ( 13.95000000122903572, -2.886751345948129988, 4.999999999999997335 ) ) ;
#58321=CARTESIAN_POINT ( 'NONE',  ( 24.94687500061451502, -3.027376345333614438, 5.243569643749998122 ) ) ;
#58322=ORIENTED_EDGE ( 'NONE', *, *, #71773, .T. ) ;
#58323=CARTESIAN_POINT ( 'NONE',  ( 20.16562500061451146, 3.027376345333613106, -5.243569643749998122 ) ) ;
#58324=CARTESIAN_POINT ( 'NONE',  ( 3.778125000614519280, -4.541064518000419881, 2.621784821874995952 ) ) ;
#58325=CARTESIAN_POINT ( 'NONE',  ( 19.17187500061451999, -6.054752690667223547, -1.112240025338166033E-15 ) ) ;
#58326=CARTESIAN_POINT ( 'NONE',  ( 3.750000000000000000, 4.330127018922192761, -2.499999999999997780 ) ) ;
#58327=CARTESIAN_POINT ( 'NONE',  ( 6.515625000614516438, -6.054752690667223547, -1.112240025338166033E-15 ) ) ;
#58328=CARTESIAN_POINT ( 'NONE',  ( 20.91562500061451502, -6.054752690667223547, -1.112240025338166033E-15 ) ) ;
#58329=CARTESIAN_POINT ( 'NONE',  ( 9.001249775931846008E-16, 16.31562500061451715, 34.90005215228797653 ) ) ;
#58330=CARTESIAN_POINT ( 'NONE',  ( 18.86250000122903359, 0.000000000000000000, 4.999999999999998224 ) ) ;
#58332=CARTESIAN_POINT ( 'NONE',  ( 9.965625000614517504, 3.027376345333611329, 5.243569643749999010 ) ) ;
#58333=CARTESIAN_POINT ( 'NONE',  ( 2.859375000614519546, 0.000000000000000000, 5.243569643749999010 ) ) ;
#58334=CARTESIAN_POINT ( 'NONE',  ( 29.05312500061451431, -4.541064518000417216, -2.621784821875001281 ) ) ;
#58335=CARTESIAN_POINT ( 'NONE',  ( 21.98437500061451644, 6.421520780324663323E-16, -5.243569643749999010 ) ) ;
#58336=CARTESIAN_POINT ( 'NONE',  ( 15.17812500061451608, 6.421520780324663323E-16, -5.243569643749999010 ) ) ;
#58337=CARTESIAN_POINT ( 'NONE',  ( 24.07500000122903216, 2.886751345948129099, -4.999999999999998224 ) ) ;
#58338=( BOUNDED_CURVE ( )  B_SPLINE_CURVE ( 2, ( #52345, #47531, #24261, #69702, #45089, #39548, #62072, #69347, #30896 ),
 .UNSPECIFIED., .F., .F. ) 
 B_SPLINE_CURVE_WITH_KNOTS ( ( 3, 2, 2, 2, 3 ),
 ( 0.5978260869565217295, 0.6014492753623188470, 0.6086956521739130821, 0.6159420289855072062, 0.6195652173913043237 ),
 .UNSPECIFIED. ) 
 CURVE ( )  GEOMETRIC_REPRESENTATION_ITEM ( )  RATIONAL_B_SPLINE_CURVE ( ( 0.9330127018922194093, 0.9330127018922194093, 1.000000000000000000, 0.8660254037844387076, 1.000000000000000000, 0.8660254037844387076, 1.000000000000000000, 0.9330127018922194093, 0.9330127018922194093 ) ) 
 REPRESENTATION_ITEM ( '' )  );
#58339=CARTESIAN_POINT ( 'NONE',  ( 24.55312500061451786, -4.541064518000417216, -2.621784821875001281 ) ) ;
#58340=CARTESIAN_POINT ( 'NONE',  ( 20.14687500061451786, -3.027376345333610441, -5.243569643749999898 ) ) ;
#58341=CARTESIAN_POINT ( 'NONE',  ( 14.69062500061451537, -3.027376345333610441, -5.243569643749999898 ) ) ;
#58342=CARTESIAN_POINT ( 'NONE',  ( 4.243569643749999898, 18.24687500061451928, 32.45002607614398471 ) ) ;
#58343=CARTESIAN_POINT ( 'NONE',  ( 23.01562500061451644, 3.027376345333611329, 5.243569643749999010 ) ) ;
#58344=LINE ( 'NONE', #6677, #29060 ) ;
#58345=ORIENTED_EDGE ( 'NONE', *, *, #39744, .F. ) ;
#58346=CARTESIAN_POINT ( 'NONE',  ( 24.56250000000000000, 2.886751345948126879, 4.999999999999999112 ) ) ;
#58347=CARTESIAN_POINT ( 'NONE',  ( 3.999999999999999112, 10.77500000000000213, -30.00000000000000000 ) ) ;
#58349=CARTESIAN_POINT ( 'NONE',  ( 26.61562500061451786, 3.027376345333611329, 5.243569643749999010 ) ) ;
#58350=CARTESIAN_POINT ( 'NONE',  ( 6.703125000614516438, 4.541064518000418104, -2.621784821874998173 ) ) ;
#58351=CARTESIAN_POINT ( 'NONE',  ( 18.82500000122903216, 2.886751345948126879, 4.999999999999999112 ) ) ;
#58352=CARTESIAN_POINT ( 'NONE',  ( 25.90312500061451573, -4.541064518000417216, -2.621784821875001281 ) ) ;
#58353=CARTESIAN_POINT ( 'NONE',  ( 25.57499999999999929, -4.330127018922194537, 2.499999999999995559 ) ) ;
#58354=CARTESIAN_POINT ( 'NONE',  ( 4.000000000000000000, 15.35000000122903252, -27.69059892324149530 ) ) ;
#58355=CARTESIAN_POINT ( 'NONE',  ( 29.05312500061451431, -4.541064518000417216, -2.621784821875001281 ) ) ;
#58356=CARTESIAN_POINT ( 'NONE',  ( 10.19062500061451892, -3.027376345333610441, -5.243569643749999898 ) ) ;
#58358=CARTESIAN_POINT ( 'NONE',  ( 26.12812500061451360, 4.541064518000418104, 2.621784821874999949 ) ) ;
#58359=CARTESIAN_POINT ( 'NONE',  ( 7.453125000614516438, -4.541064518000417216, -2.621784821875001281 ) ) ;
#58360=VECTOR ( 'NONE', #61035, 1000.000000000000000 ) ;
#58361=CARTESIAN_POINT ( 'NONE',  ( 3.440625000614518036, -3.027376345333610441, -5.243569643749999898 ) ) ;
#58363=FACE_OUTER_BOUND ( 'NONE', #68349, .T. ) ;
#58364=VECTOR ( 'NONE', #37409, 1000.000000000000000 ) ;
#58365=CARTESIAN_POINT ( 'NONE',  ( 12.48750000000000249, -2.886751345948129988, 4.999999999999997335 ) ) ;
#58367=CARTESIAN_POINT ( 'NONE',  ( 12.64687500061451608, 6.054752690667223547, 3.707466751127219781E-16 ) ) ;
#58368=CARTESIAN_POINT ( 'NONE',  ( 9.825000001229033941, 2.886751345948126879, 4.999999999999999112 ) ) ;
#58369=CARTESIAN_POINT ( 'NONE',  ( 17.78437500061451715, -4.541064518000419881, 2.621784821874995952 ) ) ;
#58371=CARTESIAN_POINT ( 'NONE',  ( 7.396875000614519635, -3.027376345333614438, 5.243569643749998122 ) ) ;
#58372=CARTESIAN_POINT ( 'NONE',  ( -4.243569643749999898, 11.66562500061451679, -32.45002607614398471 ) ) ;
#58374=ORIENTED_EDGE ( 'NONE', *, *, #33319, .T. ) ;
#58375=CARTESIAN_POINT ( 'NONE',  ( 23.46562500061451573, 3.027376345333611329, 5.243569643749999010 ) ) ;
#58377=CARTESIAN_POINT ( 'NONE',  ( 25.84687500061451360, -3.027376345333614438, 5.243569643749998122 ) ) ;
#58378=CARTESIAN_POINT ( 'NONE',  ( 28.39687500061452141, 6.054752690667223547, 3.707466751127219781E-16 ) ) ;
#58379=CARTESIAN_POINT ( 'NONE',  ( 21.75000000000000000, 4.330127018922192761, -2.499999999999997780 ) ) ;
#58380=CARTESIAN_POINT ( 'NONE',  ( 6.853125000614516793, 0.000000000000000000, 5.243569643749999010 ) ) ;
#58382=CARTESIAN_POINT ( 'NONE',  ( 16.09687500061452070, -3.027376345333610441, -5.243569643749999898 ) ) ;
#58384=CARTESIAN_POINT ( 'NONE',  ( 3.628125000614518036, 4.541064518000418104, 2.621784821874999949 ) ) ;
#58385=CARTESIAN_POINT ( 'NONE',  ( 7.321875000614516793, 3.027376345333611329, 5.243569643749999010 ) ) ;
#58387=CARTESIAN_POINT ( 'NONE',  ( 18.87187500061451573, 3.027376345333613106, -5.243569643749998122 ) ) ;
#58389=CARTESIAN_POINT ( 'NONE',  ( 27.33750000000000213, -2.886751345948129988, 4.999999999999997335 ) ) ;
#58390=CARTESIAN_POINT ( 'NONE',  ( 28.05937500061451573, 0.000000000000000000, 5.243569643749999010 ) ) ;
#58393=EDGE_LOOP ( 'NONE', ( #21856, #15822, #29625, #67210 ) ) ;
#58394=CARTESIAN_POINT ( 'NONE',  ( 9.862500000000000711, -5.773502691896255534, -1.060575238724906372E-15 ) ) ;
#58396=CARTESIAN_POINT ( 'NONE',  ( 21.77812500061451928, -4.541064518000419881, 2.621784821874995952 ) ) ;
#58397=CARTESIAN_POINT ( 'NONE',  ( 12.52500000000000213, -4.330127018922194537, 2.499999999999995559 ) ) ;
#58398=CARTESIAN_POINT ( 'NONE',  ( 8.962500001229033231, 0.000000000000000000, 4.999999999999998224 ) ) ;
#58399=CARTESIAN_POINT ( 'NONE',  ( 7.340625000614518392, -3.027376345333614438, 5.243569643749998122 ) ) ;
#58400=CARTESIAN_POINT ( 'NONE',  ( 21.67500000000000071, 6.123233995736764310E-16, -4.999999999999998224 ) ) ;
#58401=EDGE_CURVE ( 'NONE', #27655, #53683, #70167, .T. ) ;
#58402=CARTESIAN_POINT ( 'NONE',  ( 20.50312500061451715, -4.541064518000417216, -2.621784821875001281 ) ) ;
#58403=CARTESIAN_POINT ( 'NONE',  ( 14.77500000000000036, -4.330127018922194537, 2.499999999999995559 ) ) ;
#58404=CARTESIAN_POINT ( 'NONE',  ( 24.45000000122903572, -2.886751345948125991, -5.000000000000000000 ) ) ;
#58406=CARTESIAN_POINT ( 'NONE',  ( 4.312500000000000000, 2.886751345948126879, 4.999999999999999112 ) ) ;
#58408=CARTESIAN_POINT ( 'NONE',  ( 20.69062500061451715, 6.054752690667223547, 3.707466751127219781E-16 ) ) ;
#58409=CARTESIAN_POINT ( 'NONE',  ( 26.05312500061451431, 4.541064518000418104, -2.621784821874998173 ) ) ;
#58410=CARTESIAN_POINT ( 'NONE',  ( 26.63437500061451857, 4.541064518000418104, 2.621784821874999949 ) ) ;
#58411=CARTESIAN_POINT ( 'NONE',  ( 14.12812500061451715, -4.541064518000419881, 2.621784821874995952 ) ) ;
#58412=CARTESIAN_POINT ( 'NONE',  ( 29.69062500061451715, 6.054752690667223547, 3.707466751127219781E-16 ) ) ;
#58413=CARTESIAN_POINT ( 'NONE',  ( 8.953125000614518214, 4.541064518000418104, -2.621784821874998173 ) ) ;
#58414=CARTESIAN_POINT ( 'NONE',  ( -2.121784821874999949, 9.828125000614592821, -33.67503911421598417 ) ) ;
#58415=CARTESIAN_POINT ( 'NONE',  ( 26.10000000122903430, -2.886751345948129988, 4.999999999999997335 ) ) ;
#58417=CARTESIAN_POINT ( 'NONE',  ( 17.42812500061451786, 6.421520780324663323E-16, -5.243569643749999010 ) ) ;
#58419=CARTESIAN_POINT ( 'NONE',  ( 29.85937500061451644, 0.000000000000000000, 5.243569643749999010 ) ) ;
#58420=CARTESIAN_POINT ( 'NONE',  ( 9.609375000614518214, 0.000000000000000000, 5.243569643749999010 ) ) ;
#58421=CARTESIAN_POINT ( 'NONE',  ( 9.196875000614518569, -3.027376345333614438, 5.243569643749998122 ) ) ;
#58422=CARTESIAN_POINT ( 'NONE',  ( 17.93437500061451928, 6.421520780324663323E-16, -5.243569643749999010 ) ) ;
#58423=ORIENTED_EDGE ( 'NONE', *, *, #66261, .T. ) ;
#58424=CARTESIAN_POINT ( 'NONE',  ( 24.15000000122903145, 5.773502691896255534, 3.535250795749688401E-16 ) ) ;
#58425=CARTESIAN_POINT ( 'NONE',  ( 22.56562500061451715, 3.027376345333611329, 5.243569643749999010 ) ) ;
#58426=VECTOR ( 'NONE', #60447, 1000.000000000000000 ) ;
#58427=CARTESIAN_POINT ( 'NONE',  ( 16.58437500061451786, 6.421520780324663323E-16, -5.243569643749999010 ) ) ;
#58428=CARTESIAN_POINT ( 'NONE',  ( 21.81562500061451004, -6.054752690667223547, -1.112240025338166033E-15 ) ) ;
#58429=CARTESIAN_POINT ( 'NONE',  ( -2.000000000000000000, 14.07500000000000107, 26.53589838486224650 ) ) ;
#58430=CARTESIAN_POINT ( 'NONE',  ( 28.64062500061451289, -3.027376345333610441, -5.243569643749999898 ) ) ;
#58431=CARTESIAN_POINT ( 'NONE',  ( 10.16250000122903252, 4.330127018922192761, -2.499999999999997780 ) ) ;
#58432=VECTOR ( 'NONE', #53249, 1000.000000000000000 ) ;
#58433=VERTEX_POINT ( 'NONE', #38314 ) ;
#58434=CARTESIAN_POINT ( 'NONE',  ( 4.012500001229033053, 0.000000000000000000, 4.999999999999998224 ) ) ;
#58435=CARTESIAN_POINT ( 'NONE',  ( -2.000000000000000000, 18.57500000000000284, -33.46410161513775705 ) ) ;
#58436=CARTESIAN_POINT ( 'NONE',  ( 25.35000000122903074, -2.886751345948125991, -5.000000000000000000 ) ) ;
#58438=CARTESIAN_POINT ( 'NONE',  ( 9.121875000614517504, 3.027376345333611329, 5.243569643749999010 ) ) ;
#58439=CARTESIAN_POINT ( 'NONE',  ( 24.60000000000000142, 0.000000000000000000, 4.999999999999998224 ) ) ;
#58440=CARTESIAN_POINT ( 'NONE',  ( 14.20312500061451644, -4.541064518000417216, -2.621784821875001281 ) ) ;
#58441=CARTESIAN_POINT ( 'NONE',  ( 10.77187500061451786, 3.027376345333613106, -5.243569643749998122 ) ) ;
#58442=CARTESIAN_POINT ( 'NONE',  ( 3.065625000614517592, 3.027376345333613106, -5.243569643749998122 ) ) ;
#58443=CARTESIAN_POINT ( 'NONE',  ( 16.73437500061451644, 4.541064518000418104, 2.621784821874999949 ) ) ;
#58444=CARTESIAN_POINT ( 'NONE',  ( 8.521875000614516082, 3.027376345333613106, -5.243569643749998122 ) ) ;
#58445=CARTESIAN_POINT ( 'NONE',  ( 1.071796769724493892, 17.61740381056766580, -34.00000000000000000 ) ) ;
#58446=CARTESIAN_POINT ( 'NONE',  ( 8.428125000614517859, 6.421520780324663323E-16, -5.243569643749999010 ) ) ;
#58447=CARTESIAN_POINT ( 'NONE',  ( 18.14062500061451644, -3.027376345333614438, 5.243569643749998122 ) ) ;
#58448=ORIENTED_EDGE ( 'NONE', *, *, #71031, .F. ) ;
#58449=CARTESIAN_POINT ( 'NONE',  ( 15.10312500061451502, -4.541064518000417216, -2.621784821875001281 ) ) ;
#58450=CARTESIAN_POINT ( 'NONE',  ( 11.16562500061451679, 3.027376345333613106, -5.243569643749998122 ) ) ;
#58452=CARTESIAN_POINT ( 'NONE',  ( 11.21250000000000036, -5.773502691896255534, -1.060575238724906372E-15 ) ) ;
#58453=CARTESIAN_POINT ( 'NONE',  ( 6.712500001229034119, 0.000000000000000000, 4.999999999999998224 ) ) ;
#58455=CARTESIAN_POINT ( 'NONE',  ( 14.29687500061451821, -3.027376345333610441, -5.243569643749999898 ) ) ;
#58456=CARTESIAN_POINT ( 'NONE',  ( 16.57500000122903216, 2.886751345948126879, 4.999999999999999112 ) ) ;
#58459=CARTESIAN_POINT ( 'NONE',  ( -4.243569643749999898, 18.90312500061451573, -30.00000000000000000 ) ) ;
#58460=CARTESIAN_POINT ( 'NONE',  ( 16.23750000122903359, -4.330127018922194537, 2.499999999999995559 ) ) ;
#58461=DIRECTION ( 'NONE',  ( 0.000000000000000000, 0.000000000000000000, 1.000000000000000000 ) ) ;
#58462=CARTESIAN_POINT ( 'NONE',  ( 4.898734551532200499, 1.001199177798645534, 4.898734551532190729 ) ) ;
#58463=CARTESIAN_POINT ( 'NONE',  ( 30.00000000000000000, 0.000000000000000000, 0.000000000000000000 ) ) ;
#58464=CARTESIAN_POINT ( 'NONE',  ( 18.90937500061451360, 4.541064518000418104, -2.621784821874998173 ) ) ;
#58465=CARTESIAN_POINT ( 'NONE',  ( 28.57499999999999929, 4.330127018922191873, 2.499999999999999556 ) ) ;
#58466=CARTESIAN_POINT ( 'NONE',  ( 13.11562500061451786, 3.027376345333611329, 5.243569643749999010 ) ) ;
#58468=CARTESIAN_POINT ( 'NONE',  ( 23.37187500061451573, 3.027376345333613106, -5.243569643749998122 ) ) ;
#58470=CARTESIAN_POINT ( 'NONE',  ( 9.103125000614515017, 0.000000000000000000, 5.243569643749999010 ) ) ;
#58472=CARTESIAN_POINT ( 'NONE',  ( 16.65937500061452070, 4.541064518000418104, -2.621784821874998173 ) ) ;
#58474=CARTESIAN_POINT ( 'NONE',  ( 27.12187500061451573, 3.027376345333611329, 5.243569643749999010 ) ) ;
#58475=CARTESIAN_POINT ( 'NONE',  ( 26.54062500061451146, 6.054752690667223547, 3.707466751127219781E-16 ) ) ;
#58476=CARTESIAN_POINT ( 'NONE',  ( 18.81562500061452070, 3.027376345333613106, -5.243569643749998122 ) ) ;
#58477=CARTESIAN_POINT ( 'NONE',  ( 3.095752589150487122, 3.926369699671143909, -3.475442218917008663 ) ) ;
#58479=CARTESIAN_POINT ( 'NONE',  ( 4.897546610576117843, 1.006994139586731674, -5.145967878999484491 ) ) ;
#58480=CARTESIAN_POINT ( 'NONE',  ( 9.750000000000001776, 0.000000000000000000, 4.999999999999998224 ) ) ;
#58481=CARTESIAN_POINT ( 'NONE',  ( 19.57500000122903216, 2.886751345948129099, -4.999999999999998224 ) ) ;
#58482=CARTESIAN_POINT ( 'NONE',  ( 29.32499999999999929, 6.123233995736764310E-16, -4.999999999999998224 ) ) ;
#58484=ORIENTED_EDGE ( 'NONE', *, *, #69660, .T. ) ;
#58485=CARTESIAN_POINT ( 'NONE',  ( 17.06250000000000000, -5.773502691896255534, -1.060575238724906372E-15 ) ) ;
#58486=( BOUNDED_CURVE ( )  B_SPLINE_CURVE ( 2, ( #27748, #50287, #72811, #36460, #48283, #24278, #58975, #13186, #3217 ),
 .UNSPECIFIED., .F., .F. ) 
 B_SPLINE_CURVE_WITH_KNOTS ( ( 3, 2, 2, 2, 3 ),
 ( 0.7065217391304348116, 0.7101449275362319291, 0.7173913043478260532, 0.7246376811594202882, 0.7282608695652174058 ),
 .UNSPECIFIED. ) 
 CURVE ( )  GEOMETRIC_REPRESENTATION_ITEM ( )  RATIONAL_B_SPLINE_CURVE ( ( 0.9330127018922194093, 0.9330127018922194093, 1.000000000000000000, 0.8660254037844387076, 1.000000000000000000, 0.8660254037844387076, 1.000000000000000000, 0.9330127018922194093, 0.9330127018922194093 ) ) 
 REPRESENTATION_ITEM ( '' )  );
#58487=CARTESIAN_POINT ( 'NONE',  ( 21.82499999999999574, 4.330127018922191873, 2.499999999999999556 ) ) ;
#58488=CARTESIAN_POINT ( 'NONE',  ( 19.77187500061451786, 3.027376345333613106, -5.243569643749998122 ) ) ;
#58489=CARTESIAN_POINT ( 'NONE',  ( 12.77812500061451750, -4.541064518000419881, 2.621784821874995952 ) ) ;
#58490=ORIENTED_EDGE ( 'NONE', *, *, #21207, .T. ) ;
#58491=CARTESIAN_POINT ( 'NONE',  ( 4.715625000614516615, -6.054752690667223547, -1.112240025338166033E-15 ) ) ;
#58492=CYLINDRICAL_SURFACE ( 'NONE', #20572, 4.999999999999998224 ) ;
#58493=CARTESIAN_POINT ( 'NONE',  ( 12.97499999999999964, -4.330127018922194537, 2.499999999999995559 ) ) ;
#58495=CARTESIAN_POINT ( 'NONE',  ( -4.243569643749999898, 16.16562500061451857, 27.54997392385601529 ) ) ;
#58496=CARTESIAN_POINT ( 'NONE',  ( 28.71562500061451573, 3.027376345333613106, -5.243569643749998122 ) ) ;
#58499=CARTESIAN_POINT ( 'NONE',  ( 23.22187500061451715, -6.054752690667223547, -1.112240025338166033E-15 ) ) ;
#58500=ORIENTED_EDGE ( 'NONE', *, *, #57737, .F. ) ;
#58501=CARTESIAN_POINT ( 'NONE',  ( 21.25312500061451715, 0.000000000000000000, 5.243569643749999010 ) ) ;
#58502=CARTESIAN_POINT ( 'NONE',  ( 22.65937500061451715, 0.000000000000000000, 5.243569643749999010 ) ) ;
#58503=CARTESIAN_POINT ( 'NONE',  ( -4.243569643749999898, 16.61562500061459602, -32.45002607614398471 ) ) ;
#58504=CARTESIAN_POINT ( 'NONE',  ( 7.078125000614516438, 6.421520780324663323E-16, -5.243569643749999010 ) ) ;
#58506=CARTESIAN_POINT ( 'NONE',  ( 23.80312500061451786, 4.541064518000418104, -2.621784821874998173 ) ) ;
#58508=CARTESIAN_POINT ( 'NONE',  ( 17.22187500061451715, 3.027376345333611329, 5.243569643749999010 ) ) ;
#58509=CARTESIAN_POINT ( 'NONE',  ( 24.75937500061451502, 4.541064518000418104, -2.621784821874998173 ) ) ;
#58510=CARTESIAN_POINT ( 'NONE',  ( 4.243569643749999898, 15.13437500061451679, 30.00000000000000000 ) ) ;
#58511=CARTESIAN_POINT ( 'NONE',  ( 6.778125000614518392, 4.541064518000418104, 2.621784821874999949 ) ) ;
#58512=CARTESIAN_POINT ( 'NONE',  ( -1.999999999999997113, 18.27499999999999858, -26.53589838486224295 ) ) ;
#58513=CARTESIAN_POINT ( 'NONE',  ( 3.046875000614519990, -3.027376345333610441, -5.243569643749999898 ) ) ;
#58515=AXIS2_PLACEMENT_3D ( 'NONE', #45955, #18209, #29326 ) ;
#58516=CARTESIAN_POINT ( 'NONE',  ( 5.428125000614517859, 4.541064518000418104, 2.621784821874999949 ) ) ;
#58517=CARTESIAN_POINT ( 'NONE',  ( 10.35937500061451644, 4.541064518000418104, -2.621784821874998173 ) ) ;
#58518=CARTESIAN_POINT ( 'NONE',  ( 17.85000000122903430, 5.773502691896255534, 3.535250795749688894E-16 ) ) ;
#58519=CARTESIAN_POINT ( 'NONE',  ( 29.24062500061451431, 6.054752690667223547, 3.707466751127219781E-16 ) ) ;
#58520=CARTESIAN_POINT ( 'NONE',  ( 6.928125000614516082, -4.541064518000419881, 2.621784821874995952 ) ) ;
#58523=CARTESIAN_POINT ( 'NONE',  ( 17.37187500061451573, -6.054752690667223547, -1.112240025338166033E-15 ) ) ;
#58525=ORIENTED_EDGE ( 'NONE', *, *, #15234, .T. ) ;
#58526=CARTESIAN_POINT ( 'NONE',  ( 22.52812500061451573, 4.541064518000418104, 2.621784821874999949 ) ) ;
#58527=CARTESIAN_POINT ( 'NONE',  ( 10.15312500061451750, -4.541064518000417216, -2.621784821875001281 ) ) ;
#58528=CARTESIAN_POINT ( 'NONE',  ( 27.53437500061451360, 4.541064518000418104, 2.621784821874999949 ) ) ;
#58529=CARTESIAN_POINT ( 'NONE',  ( 11.05312500061451608, -4.541064518000417216, -2.621784821875001281 ) ) ;
#58530=DIRECTION ( 'NONE',  ( 0.000000000000000000, 0.000000000000000000, 1.000000000000000000 ) ) ;
#58531=CARTESIAN_POINT ( 'NONE',  ( 9.525000001229033231, -5.773502691896255534, -1.060575238724906372E-15 ) ) ;
#58532=CARTESIAN_POINT ( 'NONE',  ( 25.97812500061451502, 6.421520780324663323E-16, -5.243569643749999010 ) ) ;
#58533=CARTESIAN_POINT ( 'NONE',  ( 4.243569643749999898, 11.44062500061451715, -27.54997392385601529 ) ) ;
#58534=CARTESIAN_POINT ( 'NONE',  ( 12.97500000122903252, 2.886751345948126879, 4.999999999999999112 ) ) ;
#58535=CARTESIAN_POINT ( 'NONE',  ( 22.15312500061451573, 0.000000000000000000, 5.243569643749999010 ) ) ;
#58536=CARTESIAN_POINT ( 'NONE',  ( 17.61562500061451786, 3.027376345333611329, 5.243569643749999010 ) ) ;
#58537=CARTESIAN_POINT ( 'NONE',  ( 1.626862140677534273E-15, 18.76250000000000284, -26.00000000000000355 ) ) ;
#58538=CARTESIAN_POINT ( 'NONE',  ( 17.88749999999999929, -2.886751345948129988, 4.999999999999997335 ) ) ;
#58539=CARTESIAN_POINT ( 'NONE',  ( 12.93750000122903465, 4.330127018922191873, 2.499999999999999556 ) ) ;
#58540=( BOUNDED_CURVE ( )  B_SPLINE_CURVE ( 2, ( #61890, #71895, #43822, #10197, #11295, #55269, #21633, #27194, #55629 ),
 .UNSPECIFIED., .F., .F. ) 
 B_SPLINE_CURVE_WITH_KNOTS ( ( 3, 2, 2, 2, 3 ),
 ( 0.05434782608695652717, 0.05797101449275362389, 0.06521739130434782428, 0.07246376811594203160, 0.07608695652173913526 ),
 .UNSPECIFIED. ) 
 CURVE ( )  GEOMETRIC_REPRESENTATION_ITEM ( )  RATIONAL_B_SPLINE_CURVE ( ( 0.9330127018922194093, 0.9330127018922194093, 1.000000000000000000, 0.8660254037844387076, 1.000000000000000000, 0.8660254037844387076, 1.000000000000000000, 0.9330127018922191873, 0.9330127018922192983 ) ) 
 REPRESENTATION_ITEM ( '' )  );
#58541=CARTESIAN_POINT ( 'NONE',  ( 9.628125000614517148, -4.541064518000419881, 2.621784821874995952 ) ) ;
#58542=CARTESIAN_POINT ( 'NONE',  ( 13.64062500061451644, -3.027376345333614438, 5.243569643749998122 ) ) ;
#58543=EDGE_CURVE ( 'NONE', #20630, #59956, #4607, .T. ) ;
#58544=CARTESIAN_POINT ( 'NONE',  ( 23.28750000122903430, 4.330127018922191873, 2.499999999999999556 ) ) ;
#58545=CARTESIAN_POINT ( 'NONE',  ( 20.93437500061451573, -4.541064518000419881, 2.621784821874995952 ) ) ;
#58546=CARTESIAN_POINT ( 'NONE',  ( 21.60937500061451644, 4.541064518000418104, -2.621784821874998173 ) ) ;
#58547=CYLINDRICAL_SURFACE ( 'NONE', #13478, 4.999999999999998224 ) ;
#58550=CARTESIAN_POINT ( 'NONE',  ( 7.725000001229034297, -5.773502691896255534, -1.060575238724906372E-15 ) ) ;
#58551=CARTESIAN_POINT ( 'NONE',  ( 7.134375000614516793, 6.421520780324663323E-16, -5.243569643749999010 ) ) ;
#58552=CARTESIAN_POINT ( 'NONE',  ( 26.33437500061451431, -4.541064518000419881, 2.621784821874995952 ) ) ;
#58553=EDGE_CURVE ( 'NONE', #20715, #17509, #37588, .T. ) ;
#58554=( BOUNDED_CURVE ( )  B_SPLINE_CURVE ( 2, ( #15441, #66809, #9551, #38732, #3653, #26176, #48717, #71239, #43177 ),
 .UNSPECIFIED., .F., .F. ) 
 B_SPLINE_CURVE_WITH_KNOTS ( ( 3, 2, 2, 2, 3 ),
 ( 0.9456521739130434590, 0.9492753623188405765, 0.9565217391304348116, 0.9637681159420289356, 0.9662083003288912675 ),
 .UNSPECIFIED. ) 
 CURVE ( )  GEOMETRIC_REPRESENTATION_ITEM ( )  RATIONAL_B_SPLINE_CURVE ( ( 0.9330127018922194093, 0.9330127018922194093, 1.000000000000000000, 0.8660254037844387076, 1.000000000000000000, 0.8660254037844387076, 1.000000000000000000, 0.9548846649268474263, 0.9401540970596797830 ) ) 
 REPRESENTATION_ITEM ( '' )  );
#58555=CARTESIAN_POINT ( 'NONE',  ( 2.859375000614519546, 0.000000000000000000, 5.243569643749999010 ) ) ;
#58556=CARTESIAN_POINT ( 'NONE',  ( 21.40312500061451573, -4.541064518000417216, -2.621784821875001281 ) ) ;
#58557=CARTESIAN_POINT ( 'NONE',  ( 26.10937500061451644, 4.541064518000418104, -2.621784821874998173 ) ) ;
#58561=CARTESIAN_POINT ( 'NONE',  ( -3.999999999999999112, 13.32500000122903216, -32.30940107675850470 ) ) ;
#58562=CARTESIAN_POINT ( 'NONE',  ( 4.359375000614517326, -4.541064518000417216, -2.621784821875001281 ) ) ;
#58563=CARTESIAN_POINT ( 'NONE',  ( 17.24062500061451786, -3.027376345333614438, 5.243569643749998122 ) ) ;
#58564=VERTEX_POINT ( 'NONE', #48679 ) ;
#58565=LINE ( 'NONE', #64848, #48967 ) ;
#58566=CARTESIAN_POINT ( 'NONE',  ( 26.31562500061451715, -6.054752690667223547, -1.112240025338166033E-15 ) ) ;
#58567=CARTESIAN_POINT ( 'NONE',  ( 4.659375000614518925, 0.000000000000000000, 5.243569643749999010 ) ) ;
#58568=CARTESIAN_POINT ( 'NONE',  ( 7.320879633048903241E-15, 17.63749999999999574, -34.00000000000000000 ) ) ;
#58570=CARTESIAN_POINT ( 'NONE',  ( 17.13749999999999929, -2.886751345948125991, -5.000000000000000000 ) ) ;
#58571=CARTESIAN_POINT ( 'NONE',  ( 21.21562500061451573, 3.027376345333611329, 5.243569643749999010 ) ) ;
#58572=ORIENTED_EDGE ( 'NONE', *, *, #4888, .F. ) ;
#58573=CARTESIAN_POINT ( 'NONE',  ( 23.81250000000000000, -5.773502691896255534, -1.060575238724906372E-15 ) ) ;
#58574=CARTESIAN_POINT ( 'NONE',  ( 25.20937500061451431, 4.541064518000418104, -2.621784821874998173 ) ) ;
#58575=EDGE_LOOP ( 'NONE', ( #33390, #49623, #29350, #22431 ) ) ;
#58576=CARTESIAN_POINT ( 'NONE',  ( 13.46250000122903323, 0.000000000000000000, 4.999999999999998224 ) ) ;
#58577=CARTESIAN_POINT ( 'NONE',  ( 13.00312500061451537, 4.541064518000418104, -2.621784821874998173 ) ) ;
#58578=CARTESIAN_POINT ( 'NONE',  ( 6.215625000614517504, 3.027376345333613106, -5.243569643749998122 ) ) ;
#58580=CARTESIAN_POINT ( 'NONE',  ( 28.82812500061451644, 4.541064518000418104, 2.621784821874999949 ) ) ;
#58582=CARTESIAN_POINT ( 'NONE',  ( 14.77500000122903501, 2.886751345948126879, 4.999999999999999112 ) ) ;
#58583=CARTESIAN_POINT ( 'NONE',  ( 19.42499999999999716, 6.123233995736764310E-16, -4.999999999999998224 ) ) ;
#58584=CARTESIAN_POINT ( 'NONE',  ( 26.32499999999999929, 4.330127018922191873, 2.499999999999999556 ) ) ;
#58585=CARTESIAN_POINT ( 'NONE',  ( 2.934375000614518392, -4.541064518000419881, 2.621784821874995952 ) ) ;
#58586=CARTESIAN_POINT ( 'NONE',  ( 8.484375000614518214, 6.421520780324663323E-16, -5.243569643749999010 ) ) ;
#58587=CARTESIAN_POINT ( 'NONE',  ( 19.62187500061451573, -6.054752690667223547, -1.112240025338166033E-15 ) ) ;
#58588=CARTESIAN_POINT ( 'NONE',  ( 1.626862140677534273E-15, 13.92500000122903181, 34.00000000000000000 ) ) ;
#58589=ORIENTED_EDGE ( 'NONE', *, *, #15386, .F. ) ;
#58590=CARTESIAN_POINT ( 'NONE',  ( 29.50312500061451360, -4.541064518000417216, -2.621784821875001281 ) ) ;
#58591=CARTESIAN_POINT ( 'NONE',  ( 3.600000000000002309, -4.330127018922190985, -2.500000000000001332 ) ) ;
#58592=CARTESIAN_POINT ( 'NONE',  ( 5.146875000614517859, -3.027376345333614438, 5.243569643749998122 ) ) ;
#58593=ADVANCED_FACE ( 'NONE', ( #36853 ), #54949, .F. ) ;
#58594=CARTESIAN_POINT ( 'NONE',  ( 17.21249999999999858, 2.886751345948129099, -4.999999999999998224 ) ) ;
#58595=CARTESIAN_POINT ( 'NONE',  ( 14.57812500061451644, -4.541064518000419881, 2.621784821874995952 ) ) ;
#58597=CARTESIAN_POINT ( 'NONE',  ( 17.96250000122903501, 0.000000000000000000, 4.999999999999998224 ) ) ;
#58598=CARTESIAN_POINT ( 'NONE',  ( 19.27500000122903145, 2.886751345948126879, 4.999999999999999112 ) ) ;
#58601=CARTESIAN_POINT ( 'NONE',  ( 8.615625000614517859, 3.027376345333611329, 5.243569643749999010 ) ) ;
#58602=CARTESIAN_POINT ( 'NONE',  ( 23.67187500061451999, -6.054752690667223547, -1.112240025338166033E-15 ) ) ;
#58603=CARTESIAN_POINT ( 'NONE',  ( -4.243569643749999898, 18.95937500061451431, 30.00000000000000000 ) ) ;
#58604=CARTESIAN_POINT ( 'NONE',  ( 24.57187500061451502, -6.054752690667223547, -1.112240025338166033E-15 ) ) ;
#58605=CARTESIAN_POINT ( 'NONE',  ( 7.050000000000000711, 0.000000000000000000, 4.999999999999998224 ) ) ;
#58606=CARTESIAN_POINT ( 'NONE',  ( 1.999999999999998668, 13.66250000122903607, 26.53589838486224650 ) ) ;
#58607=CARTESIAN_POINT ( 'NONE',  ( 13.71562500061451750, -6.054752690667223547, -1.112240025338166033E-15 ) ) ;
#58608=CARTESIAN_POINT ( 'NONE',  ( 6.487500001229034474, 6.123233995736764310E-16, -4.999999999999998224 ) ) ;
#58609=CARTESIAN_POINT ( 'NONE',  ( 10.80937500061451928, 4.541064518000418104, -2.621784821874998173 ) ) ;
#58611=ORIENTED_EDGE ( 'NONE', *, *, #28491, .T. ) ;
#58612=CARTESIAN_POINT ( 'NONE',  ( 12.55312500061451786, 4.541064518000418104, -2.621784821874998173 ) ) ;
#58613=CARTESIAN_POINT ( 'NONE',  ( 3.428129095426660555, -3.639779116804093828, -3.774531229163594848 ) ) ;
#58614=CARTESIAN_POINT ( 'NONE',  ( 23.06250000122903288, -4.330127018922190985, -2.500000000000001332 ) ) ;
#58615=CARTESIAN_POINT ( 'NONE',  ( 10.58437500061451964, -4.541064518000419881, 2.621784821874995952 ) ) ;
#58616=CARTESIAN_POINT ( 'NONE',  ( 14.12812500061451715, -4.541064518000419881, 2.621784821874995952 ) ) ;
#58618=CARTESIAN_POINT ( 'NONE',  ( 24.15937500061451715, -4.541064518000417216, -2.621784821875001281 ) ) ;
#58619=CARTESIAN_POINT ( 'NONE',  ( 4.000000000000000000, 15.80000000122903181, 32.30940107675849760 ) ) ;
#58621=CARTESIAN_POINT ( 'NONE',  ( 0.000000000000000000, 20.00000000000000000, 26.00000000000000000 ) ) ;
#58623=CARTESIAN_POINT ( 'NONE',  ( -4.243569643749999898, 14.87187500061451928, -32.45002607614398471 ) ) ;
#58624=CARTESIAN_POINT ( 'NONE',  ( 14.63437500061451679, -4.541064518000419881, 2.621784821874995952 ) ) ;
#58625=CARTESIAN_POINT ( 'NONE',  ( 18.45000000122903216, -2.886751345948129988, 4.999999999999997335 ) ) ;
#58626=CARTESIAN_POINT ( 'NONE',  ( 12.94687500061451857, -3.027376345333610441, -5.243569643749999898 ) ) ;
#58627=CARTESIAN_POINT ( 'NONE',  ( -4.243569643749999898, 10.40937500061451892, 30.00000000000000000 ) ) ;
#58628=CARTESIAN_POINT ( 'NONE',  ( 18.86250000122903359, 0.000000000000000000, 4.999999999999998224 ) ) ;
#58629=CARTESIAN_POINT ( 'NONE',  ( 12.14062500061451821, 6.054752690667223547, 3.707466751127219781E-16 ) ) ;
#58630=VERTEX_POINT ( 'NONE', #59742 ) ;
#58631=ORIENTED_EDGE ( 'NONE', *, *, #63906, .T. ) ;
#58632=CARTESIAN_POINT ( 'NONE',  ( 18.03749999999999787, -2.886751345948125991, -5.000000000000000000 ) ) ;
#58634=CARTESIAN_POINT ( 'NONE',  ( 11.52187500061451608, -6.054752690667223547, -1.112240025338166033E-15 ) ) ;
#58635=CYLINDRICAL_SURFACE ( 'NONE', #52723, 4.999999999999998224 ) ;
#58636=CARTESIAN_POINT ( 'NONE',  ( 12.22500000122903430, -5.773502691896255534, -1.060575238724906372E-15 ) ) ;
#58637=CARTESIAN_POINT ( 'NONE',  ( 20.58750000122903145, 4.330127018922191873, 2.499999999999999556 ) ) ;
#58638=CARTESIAN_POINT ( 'NONE',  ( 16.94062500061451715, -3.027376345333610441, -5.243569643749999898 ) ) ;
#58639=CARTESIAN_POINT ( 'NONE',  ( 21.32812500061451644, -4.541064518000419881, 2.621784821874995952 ) ) ;
#58640=CARTESIAN_POINT ( 'NONE',  ( 28.50000000122903288, -2.886751345948125991, -5.000000000000000000 ) ) ;
#58641=CARTESIAN_POINT ( 'NONE',  ( 28.16249999999999787, 2.886751345948126879, 4.999999999999999112 ) ) ;
#58642=CARTESIAN_POINT ( 'NONE',  ( 28.27499999999999858, -4.330127018922194537, 2.499999999999995559 ) ) ;
#58644=CARTESIAN_POINT ( 'NONE',  ( 27.19687500061451857, -3.027376345333614438, 5.243569643749998122 ) ) ;
#58646=CARTESIAN_POINT ( 'NONE',  ( -3.000416591977282496E-16, 15.24687500061451928, -34.90005215228797653 ) ) ;
#58647=CARTESIAN_POINT ( 'NONE',  ( 3.600000001229033408, -2.886751345948129988, 4.999999999999997335 ) ) ;
#58648=CARTESIAN_POINT ( 'NONE',  ( 6.450000000000001066, 4.330127018922192761, -2.499999999999997780 ) ) ;
#58649=EDGE_CURVE ( 'NONE', #66176, #69731, #55504, .T. ) ;
#58650=CARTESIAN_POINT ( 'NONE',  ( 25.72499999999999787, 6.123233995736764310E-16, -4.999999999999998224 ) ) ;
#58651=CARTESIAN_POINT ( 'NONE',  ( 9.271875000614516082, -6.054752690667223547, -1.112240025338166033E-15 ) ) ;
#58652=CARTESIAN_POINT ( 'NONE',  ( 28.94062500061452070, -3.027376345333614438, 5.243569643749998122 ) ) ;
#58653=DIRECTION ( 'NONE',  ( 0.000000000000000000, 0.000000000000000000, 1.000000000000000000 ) ) ;
#58654=CARTESIAN_POINT ( 'NONE',  ( -3.040073828171254267, 9.532700238123338110, -24.81292056264607737 ) ) ;
#58656=CARTESIAN_POINT ( 'NONE',  ( 7.171875000614517326, 3.027376345333613106, -5.243569643749998122 ) ) ;
#58657=CARTESIAN_POINT ( 'NONE',  ( 11.82187500061451679, 3.027376345333611329, 5.243569643749999010 ) ) ;
#58658=CARTESIAN_POINT ( 'NONE',  ( 3.862500000000001155, 2.886751345948126879, 4.999999999999999112 ) ) ;
#58659=VECTOR ( 'NONE', #40782, 1000.000000000000000 ) ;
#58660=CARTESIAN_POINT ( 'NONE',  ( 2.121784821875001281, 14.10312500061459495, 33.67503911421598417 ) ) ;
#58662=CARTESIAN_POINT ( 'NONE',  ( 5.400000000000002132, -4.330127018922190985, -2.500000000000001332 ) ) ;
#58664=CARTESIAN_POINT ( 'NONE',  ( 19.75312500061451360, 4.541064518000418104, -2.621784821874998173 ) ) ;
#58665=CARTESIAN_POINT ( 'NONE',  ( 12.32812500061451821, -4.541064518000419881, 2.621784821874995952 ) ) ;
#58667=CARTESIAN_POINT ( 'NONE',  ( 9.121875000614517504, 3.027376345333611329, 5.243569643749999010 ) ) ;
#58668=CARTESIAN_POINT ( 'NONE',  ( 25.53750000000000142, -2.886751345948129988, 4.999999999999997335 ) ) ;
#58669=CARTESIAN_POINT ( 'NONE',  ( 22.57500000122903572, -5.773502691896255534, -1.060575238724906372E-15 ) ) ;
#58671=CARTESIAN_POINT ( 'NONE',  ( 9.834375000614517859, 6.421520780324663323E-16, -5.243569643749999010 ) ) ;
#58672=CARTESIAN_POINT ( 'NONE',  ( 25.77187500061451075, 3.027376345333611329, 5.243569643749999010 ) ) ;
#58673=CARTESIAN_POINT ( 'NONE',  ( 3.496875000614518836, -3.027376345333610441, -5.243569643749999898 ) ) ;
#58674=CARTESIAN_POINT ( 'NONE',  ( 20.82187500061451857, 3.027376345333611329, 5.243569643749999010 ) ) ;
#58675=CARTESIAN_POINT ( 'NONE',  ( 10.99687500061451750, -3.027376345333614438, 5.243569643749998122 ) ) ;
#58677=CARTESIAN_POINT ( 'NONE',  ( 23.58749999999999858, 5.773502691896255534, 3.535250795749688894E-16 ) ) ;
#58679=CARTESIAN_POINT ( 'NONE',  ( 4.243569643749999898, 13.29687500061451644, -27.54997392385601529 ) ) ;
#58681=CARTESIAN_POINT ( 'NONE',  ( 15.92812500061451608, -4.541064518000419881, 2.621784821874995952 ) ) ;
#58682=CARTESIAN_POINT ( 'NONE',  ( 5.737499999999998934, -2.886751345948129988, 4.999999999999997335 ) ) ;
#58683=LINE ( 'NONE', #12900, #30126 ) ;
#58685=CARTESIAN_POINT ( 'NONE',  ( 14.02499999999999858, 6.123233995736764310E-16, -4.999999999999998224 ) ) ;
#58686=CARTESIAN_POINT ( 'NONE',  ( -2.828200636599751609E-16, 19.55000000122903359, 25.38119784648299770 ) ) ;
#58687=CARTESIAN_POINT ( 'NONE',  ( 13.65000000122903323, -2.886751345948125991, -5.000000000000000000 ) ) ;
#58688=CARTESIAN_POINT ( 'NONE',  ( 24.87187500061451573, 3.027376345333611329, 5.243569643749999010 ) ) ;
#58689=CARTESIAN_POINT ( 'NONE',  ( 20.25000000122903288, -2.886751345948096681, 5.000000000000054179 ) ) ;
#58690=ORIENTED_EDGE ( 'NONE', *, *, #27502, .F. ) ;
#58691=CARTESIAN_POINT ( 'NONE',  ( 18.55312500061451431, 0.000000000000000000, 5.243569643749999010 ) ) ;
#58692=CARTESIAN_POINT ( 'NONE',  ( 3.290625000614516793, -3.027376345333614438, 5.243569643749998122 ) ) ;
#58693=CARTESIAN_POINT ( 'NONE',  ( 19.20937500061451786, -4.541064518000417216, -2.621784821875001281 ) ) ;
#58694=CARTESIAN_POINT ( 'NONE',  ( 28.32187500061451502, 3.027376345333613106, -5.243569643749998122 ) ) ;
#58695=CARTESIAN_POINT ( 'NONE',  ( 4.228125000614517681, -4.541064518000419881, 2.621784821874995952 ) ) ;
#58696=CARTESIAN_POINT ( 'NONE',  ( 22.71562500061451573, -6.054752690667223547, -1.112240025338166033E-15 ) ) ;
#58698=CARTESIAN_POINT ( 'NONE',  ( 9.001249775931846008E-16, 14.96562500061451750, 34.90005215228797653 ) ) ;
#58699=CARTESIAN_POINT ( 'NONE',  ( 19.42500000122903714, -5.773502691896255534, -1.060575238724906372E-15 ) ) ;
#58701=CARTESIAN_POINT ( 'NONE',  ( 6.065625000614517148, -6.054752690667223547, -1.112240025338166033E-15 ) ) ;
#58702=CARTESIAN_POINT ( 'NONE',  ( 3.196875000614516793, 6.054752690667223547, 3.707466751127219781E-16 ) ) ;
#58703=CARTESIAN_POINT ( 'NONE',  ( 3.271875000614519635, 3.027376345333611329, 5.243569643749999010 ) ) ;
#58704=CARTESIAN_POINT ( 'NONE',  ( 21.83437500061451786, -4.541064518000419881, 2.621784821874995952 ) ) ;
#58705=CARTESIAN_POINT ( 'NONE',  ( 15.59062500061451573, -3.027376345333610441, -5.243569643749999898 ) ) ;
#58706=CARTESIAN_POINT ( 'NONE',  ( 23.81250000122903288, 0.000000000000000000, 4.999999999999998224 ) ) ;
#58707=CARTESIAN_POINT ( 'NONE',  ( 25.19062500061451715, 6.054752690667223547, 3.707466751127219781E-16 ) ) ;
#58708=CARTESIAN_POINT ( 'NONE',  ( 19.88437500061451857, 4.541064518000418104, 2.621784821874999949 ) ) ;
#58709=CARTESIAN_POINT ( 'NONE',  ( 15.96562500061451573, -6.054752690667223547, -1.112240025338166033E-15 ) ) ;
#58710=CARTESIAN_POINT ( 'NONE',  ( 4.243569643749999010, 16.07187500061451857, 27.54997392385601174 ) ) ;
#58711=CARTESIAN_POINT ( 'NONE',  ( 20.20312500061451644, 4.541064518000418104, -2.621784821874998173 ) ) ;
#58712=CARTESIAN_POINT ( 'NONE',  ( 29.09062500061451573, -3.027376345333610441, -5.243569643749999898 ) ) ;
#58714=CARTESIAN_POINT ( 'NONE',  ( 25.31250000000000000, 2.886751345948129099, -4.999999999999998224 ) ) ;
#58715=CARTESIAN_POINT ( 'NONE',  ( 4.000000000000000000, 11.63750000000000284, -27.69059892324149530 ) ) ;
#58717=CARTESIAN_POINT ( 'NONE',  ( 26.95312500061451644, 4.541064518000418104, -2.621784821874998173 ) ) ;
#58718=CARTESIAN_POINT ( 'NONE',  ( 7.153125000614518392, 4.541064518000418104, -2.621784821874998173 ) ) ;
#58719=CARTESIAN_POINT ( 'NONE',  ( 20.85000000122903430, -2.886751345948125991, -5.000000000000000000 ) ) ;
#58720=CARTESIAN_POINT ( 'NONE',  ( 25.37812500061451715, -4.541064518000419881, 2.621784821874995952 ) ) ;
#58721=CARTESIAN_POINT ( 'NONE',  ( 24.71250000000000213, -5.773502691896255534, -1.060575238724906372E-15 ) ) ;
#58722=CARTESIAN_POINT ( 'NONE',  ( -2.828200636599751609E-16, 15.50000000122903465, -34.61880215351700230 ) ) ;
#58724=CARTESIAN_POINT ( 'NONE',  ( 26.84062500061451573, -3.027376345333610441, -5.243569643749999898 ) ) ;
#58725=CARTESIAN_POINT ( 'NONE',  ( 11.16562500061451679, 3.027376345333613106, -5.243569643749998122 ) ) ;
#58726=ORIENTED_EDGE ( 'NONE', *, *, #66521, .T. ) ;
#58727=CARTESIAN_POINT ( 'NONE',  ( 25.41562500061451146, -6.054752690667223547, -1.112240025338166033E-15 ) ) ;
#58728=CARTESIAN_POINT ( 'NONE',  ( 6.365625000614518747, 3.027376345333611329, 5.243569643749999010 ) ) ;
#58730=CARTESIAN_POINT ( 'NONE',  ( 30.00000000000000000, 0.000000000000000000, 0.000000000000000000 ) ) ;
#58731=CARTESIAN_POINT ( 'NONE',  ( 12.44999999999999929, 0.000000000000000000, 4.999999999999998224 ) ) ;
#58732=EDGE_CURVE ( 'NONE', #41163, #29206, #27245, .T. ) ;
#58733=CARTESIAN_POINT ( 'NONE',  ( 13.58437500061451786, 4.541064518000418104, 2.621784821874999949 ) ) ;
#58734=CARTESIAN_POINT ( 'NONE',  ( 8.287500001229034297, 6.123233995736764310E-16, -4.999999999999998224 ) ) ;
#58735=CARTESIAN_POINT ( 'NONE',  ( 17.10937500061451999, 4.541064518000418104, -2.621784821874998173 ) ) ;
#58737=CARTESIAN_POINT ( 'NONE',  ( 8.259375000614518569, 0.000000000000000000, 5.243569643749999010 ) ) ;
#58738=CARTESIAN_POINT ( 'NONE',  ( 4.243569643749999010, 11.51562500061451644, -32.45002607614398471 ) ) ;
#58741=ORIENTED_EDGE ( 'NONE', *, *, #18853, .F. ) ;
#58742=CARTESIAN_POINT ( 'NONE',  ( 24.02812500061451573, -4.541064518000419881, 2.621784821874995952 ) ) ;
#58744=CARTESIAN_POINT ( 'NONE',  ( -3.999999999999997335, 17.45000000122903572, 32.30940107675850470 ) ) ;
#58745=CARTESIAN_POINT ( 'NONE',  ( 26.93437500061451573, 6.421520780324663323E-16, -5.243569643749999010 ) ) ;
#58746=CARTESIAN_POINT ( 'NONE',  ( 28.69687500061451502, -3.027376345333610441, -5.243569643749999898 ) ) ;
#58747=CARTESIAN_POINT ( 'NONE',  ( 3.515625000614516882, 3.027376345333613106, -5.243569643749998122 ) ) ;
#58749=CARTESIAN_POINT ( 'NONE',  ( 16.77187500061451786, 3.027376345333611329, 5.243569643749999010 ) ) ;
#58751=CARTESIAN_POINT ( 'NONE',  ( 29.55000000122903003, 5.773502691896255534, 3.535250795749688894E-16 ) ) ;
#58752=CARTESIAN_POINT ( 'NONE',  ( 9.271875000614516082, -6.054752690667223547, -1.112240025338166033E-15 ) ) ;
#58753=CARTESIAN_POINT ( 'NONE',  ( 19.95937500061451786, 0.000000000000000000, 5.243569643749999010 ) ) ;
#58755=CARTESIAN_POINT ( 'NONE',  ( 26.32499999999999929, 4.330127018922191873, 2.499999999999999556 ) ) ;
#58756=CARTESIAN_POINT ( 'NONE',  ( 28.09687500061451360, -3.027376345333614438, 5.243569643749998122 ) ) ;
#58758=CARTESIAN_POINT ( 'NONE',  ( 5.700000001229034829, 5.773502691896255534, 3.535250795749688401E-16 ) ) ;
#58759=ORIENTED_EDGE ( 'NONE', *, *, #1232, .F. ) ;
#58760=CARTESIAN_POINT ( 'NONE',  ( 7.650000000000000355, -4.330127018922190985, -2.500000000000001332 ) ) ;
#58762=CARTESIAN_POINT ( 'NONE',  ( 20.91562500061451502, -6.054752690667223547, -1.112240025338166033E-15 ) ) ;
#58763=CARTESIAN_POINT ( 'NONE',  ( 12.67499999999999893, 6.123233995736764310E-16, -4.999999999999998224 ) ) ;
#58764=CARTESIAN_POINT ( 'NONE',  ( 7.800000001229035362, -2.886751345948125991, -5.000000000000000000 ) ) ;
#58765=CARTESIAN_POINT ( 'NONE',  ( 7.153125000614518392, 4.541064518000418104, -2.621784821874998173 ) ) ;
#58766=( BOUNDED_CURVE ( )  B_SPLINE_CURVE ( 2, ( #16888, #50886, #17253, #26908, #44265, #32438, #33517 ),
 .UNSPECIFIED., .F., .F. ) 
 B_SPLINE_CURVE_WITH_KNOTS ( ( 3, 2, 2, 3 ),
 ( 0.5250000000000000222, 0.5277777777777777901, 0.5305555555555556690, 0.5333333333333334370 ),
 .UNSPECIFIED. ) 
 CURVE ( )  GEOMETRIC_REPRESENTATION_ITEM ( )  RATIONAL_B_SPLINE_CURVE ( ( 1.000000000000000000, 0.8660254037844387076, 1.000000000000000000, 0.8660254037844387076, 1.000000000000000000, 0.8660254037844333785, 1.000000000000005329 ) ) 
 REPRESENTATION_ITEM ( '' )  );
#58767=CARTESIAN_POINT ( 'NONE',  ( 21.63749999999999929, -2.886751345948125991, -5.000000000000000000 ) ) ;
#58768=CARTESIAN_POINT ( 'NONE',  ( 21.55312500061451431, 4.541064518000418104, -2.621784821874998173 ) ) ;
#58769=CARTESIAN_POINT ( 'NONE',  ( 14.84999999999999964, -4.330127018922190985, -2.500000000000001332 ) ) ;
#58770=CARTESIAN_POINT ( 'NONE',  ( 25.91250000122903074, 4.330127018922192761, -2.499999999999997780 ) ) ;
#58772=CARTESIAN_POINT ( 'NONE',  ( 4.087500000000001243, -2.886751345948125991, -5.000000000000000000 ) ) ;
#58773=ORIENTED_EDGE ( 'NONE', *, *, #65919, .F. ) ;
#58774=CARTESIAN_POINT ( 'NONE',  ( 19.41562500061451146, 3.027376345333611329, 5.243569643749999010 ) ) ;
#58775=CARTESIAN_POINT ( 'NONE',  ( 26.84062500061451573, -3.027376345333610441, -5.243569643749999898 ) ) ;
#58776=CARTESIAN_POINT ( 'NONE',  ( 26.70937500061451431, 0.000000000000000000, 5.243569643749999010 ) ) ;
#58777=CARTESIAN_POINT ( 'NONE',  ( 10.08749999999999858, 5.773502691896255534, 3.535250795749688894E-16 ) ) ;
#58778=CARTESIAN_POINT ( 'NONE',  ( 14.91562500061451679, 3.027376345333611329, 5.243569643749999010 ) ) ;
#58779=CARTESIAN_POINT ( 'NONE',  ( 28.86562500061451786, 3.027376345333611329, 5.243569643749999010 ) ) ;
#58780=CARTESIAN_POINT ( 'NONE',  ( 10.00312500061451715, 0.000000000000000000, 5.243569643749999010 ) ) ;
#58781=CARTESIAN_POINT ( 'NONE',  ( -4.243569643749999898, 10.35312500061459673, -30.00000000000000000 ) ) ;
#58782=CARTESIAN_POINT ( 'NONE',  ( -4.243569643749999898, 12.17187500061451999, 27.54997392385601529 ) ) ;
#58783=CARTESIAN_POINT ( 'NONE',  ( 25.50000000122903288, 5.773502691896255534, 3.535250795749688894E-16 ) ) ;
#58785=CARTESIAN_POINT ( 'NONE',  ( 17.91562500061451502, 3.027376345333612662, -5.243569643749998122 ) ) ;
#58786=CARTESIAN_POINT ( 'NONE',  ( 8.175000000000002487, 6.123233995736764310E-16, -4.999999999999998224 ) ) ;
#58787=CARTESIAN_POINT ( 'NONE',  ( 10.99687500061451750, -3.027376345333614438, 5.243569643749998122 ) ) ;
#58788=CARTESIAN_POINT ( 'NONE',  ( 10.24687500061451750, -3.027376345333610441, -5.243569643749999898 ) ) ;
#58789=CARTESIAN_POINT ( 'NONE',  ( 17.37187500061451573, -6.054752690667223547, -1.112240025338166033E-15 ) ) ;
#58790=VERTEX_POINT ( 'NONE', #22768 ) ;
#58791=CARTESIAN_POINT ( 'NONE',  ( 1.071796769724489895, 13.56740381056766687, 26.00000000000000355 ) ) ;
#58792=CARTESIAN_POINT ( 'NONE',  ( 21.44062500061452070, -3.027376345333610441, -5.243569643749999898 ) ) ;
#58793=CARTESIAN_POINT ( 'NONE',  ( 16.39687500061451786, -3.027376345333614438, 5.243569643749998122 ) ) ;
#58794=CARTESIAN_POINT ( 'NONE',  ( 23.16562500061451502, -6.054752690667223547, -1.112240025338166033E-15 ) ) ;
#58795=CARTESIAN_POINT ( 'NONE',  ( 8.484601909799253346E-16, 13.36250000000000071, 34.61880215351700230 ) ) ;
#58796=CARTESIAN_POINT ( 'NONE',  ( 27.74062500061451431, -3.027376345333610441, -5.243569643749999898 ) ) ;
#58797=CARTESIAN_POINT ( 'NONE',  ( 8.362500001229031810, 4.330127018922192761, -2.499999999999997780 ) ) ;
#58798=ORIENTED_EDGE ( 'NONE', *, *, #53989, .T. ) ;
#58799=CARTESIAN_POINT ( 'NONE',  ( 4.125000001229034652, -5.773502691896255534, -1.060575238724906372E-15 ) ) ;
#58800=CARTESIAN_POINT ( 'NONE',  ( 2.000000000000001332, 17.89999999999999858, -26.53589838486224650 ) ) ;
#58801=CARTESIAN_POINT ( 'NONE',  ( 24.67500000122903359, 2.886751345948126879, 4.999999999999999112 ) ) ;
#58803=CARTESIAN_POINT ( 'NONE',  ( 8.034375000614518925, 6.421520780324663323E-16, -5.243569643749999010 ) ) ;
#58804=CARTESIAN_POINT ( 'NONE',  ( 4.000000000000000000, 15.23750000000000071, 32.30940107675849760 ) ) ;
#58805=CARTESIAN_POINT ( 'NONE',  ( 13.86562500061451431, 3.027376345333613106, -5.243569643749998122 ) ) ;
#58806=CARTESIAN_POINT ( 'NONE',  ( 8.371875000614515727, -6.054752690667223547, -1.112240025338166033E-15 ) ) ;
#58807=CARTESIAN_POINT ( 'NONE',  ( 27.48750000122903359, -4.330127018922194537, 2.499999999999995559 ) ) ;
#58808=CARTESIAN_POINT ( 'NONE',  ( 16.62187500061451573, 3.027376345333612662, -5.243569643749998122 ) ) ;
#58809=CARTESIAN_POINT ( 'NONE',  ( 5.446875000614518569, 6.054752690667223547, 3.707466751127219781E-16 ) ) ;
#58811=CARTESIAN_POINT ( 'NONE',  ( 6.628125000614517148, 6.421520780324663323E-16, -5.243569643749999010 ) ) ;
#58812=CARTESIAN_POINT ( 'NONE',  ( 16.90312500061451573, -4.541064518000417216, -2.621784821875001281 ) ) ;
#58814=EDGE_CURVE ( 'NONE', #10190, #65143, #40143, .T. ) ;
#58815=CARTESIAN_POINT ( 'NONE',  ( 13.60312500061451679, 0.000000000000000000, 5.243569643749999010 ) ) ;
#58816=CARTESIAN_POINT ( 'NONE',  ( 6.187500001229032875, 4.330127018922191873, 2.499999999999999556 ) ) ;
#58817=CARTESIAN_POINT ( 'NONE',  ( 11.84062500061451750, -3.027376345333614438, 5.243569643749998122 ) ) ;
#58819=CARTESIAN_POINT ( 'NONE',  ( 10.98750000000000071, 5.773502691896255534, 3.535250795749688894E-16 ) ) ;
#58820=CARTESIAN_POINT ( 'NONE',  ( 6.412500001229036073, -4.330127018922190985, -2.500000000000001332 ) ) ;
#58822=CARTESIAN_POINT ( 'NONE',  ( 15.08437500061451786, -4.541064518000419881, 2.621784821874995952 ) ) ;
#58823=CARTESIAN_POINT ( 'NONE',  ( 15.30000000122903359, -2.886751345948129988, 4.999999999999997335 ) ) ;
#58825=CARTESIAN_POINT ( 'NONE',  ( -2.121784821874996840, 18.52812500061451928, -26.32496088578401583 ) ) ;
#58826=CARTESIAN_POINT ( 'NONE',  ( 30.00000000000000000, 0.000000000000000000, 0.000000000000000000 ) ) ;
#58827=CARTESIAN_POINT ( 'NONE',  ( 1.071796769724484344, 14.84509619066137098, -25.99999999999999645 ) ) ;
#58830=FACE_OUTER_BOUND ( 'NONE', #38389, .T. ) ;
#58831=CARTESIAN_POINT ( 'NONE',  ( 15.64687500061451608, -3.027376345333610441, -5.243569643749999898 ) ) ;
#58832=EDGE_CURVE ( 'NONE', #54070, #2091, #63035, .T. ) ;
#58833=CARTESIAN_POINT ( 'NONE',  ( 28.16249999999999787, 2.886751345948126879, 4.999999999999999112 ) ) ;
#58834=CARTESIAN_POINT ( 'NONE',  ( 13.86562500061451431, 3.027376345333613106, -5.243569643749998122 ) ) ;
#58836=CARTESIAN_POINT ( 'NONE',  ( 23.93437500061451573, 4.541064518000418104, 2.621784821874999949 ) ) ;
#58838=CARTESIAN_POINT ( 'NONE',  ( 10.04062500061451502, -3.027376345333614438, 5.243569643749998122 ) ) ;
#58839=CARTESIAN_POINT ( 'NONE',  ( 14.44687500061451679, 6.054752690667223547, 3.707466751127219781E-16 ) ) ;
#58841=CARTESIAN_POINT ( 'NONE',  ( 25.88437500061451502, -4.541064518000419881, 2.621784821874995952 ) ) ;
#58842=CARTESIAN_POINT ( 'NONE',  ( 27.81562500061452070, 3.027376345333613106, -5.243569643749998122 ) ) ;
#58843=CARTESIAN_POINT ( 'NONE',  ( 18.21562500061451573, -6.054752690667223547, -1.112240025338166033E-15 ) ) ;
#58844=CARTESIAN_POINT ( 'NONE',  ( 28.49062500061451431, -3.027376345333614438, 5.243569643749998122 ) ) ;
#58845=CARTESIAN_POINT ( 'NONE',  ( 4.849693137238607399, 1.216928655869232712, -5.100445426819982586 ) ) ;
#58846=CARTESIAN_POINT ( 'NONE',  ( 8.550000000000002487, -4.330127018922190985, -2.500000000000001332 ) ) ;
#58847=CARTESIAN_POINT ( 'NONE',  ( 19.68750000122903288, 4.330127018922191873, 2.499999999999999556 ) ) ;
#58848=CARTESIAN_POINT ( 'NONE',  ( -1.999999999999997113, 10.17500000000000249, 33.46410161513775705 ) ) ;
#58850=ORIENTED_EDGE ( 'NONE', *, *, #54130, .T. ) ;
#58851=CARTESIAN_POINT ( 'NONE',  ( 15.11249999999999893, 2.886751345948126879, 4.999999999999999112 ) ) ;
#58852=CARTESIAN_POINT ( 'NONE',  ( 18.30000000000000071, 0.000000000000000000, 4.999999999999998224 ) ) ;
#58853=CARTESIAN_POINT ( 'NONE',  ( 16.47187500061452070, -6.054752690667223547, -1.112240025338166033E-15 ) ) ;
#58854=CARTESIAN_POINT ( 'NONE',  ( 13.45312500061451466, 4.541064518000418104, -2.621784821874998173 ) ) ;
#58856=DIRECTION ( 'NONE',  ( -1.000000000000000000, -0.000000000000000000, -0.000000000000000000 ) ) ;
#58857=CARTESIAN_POINT ( 'NONE',  ( 6.215625000614517504, 3.027376345333613106, -5.243569643749998122 ) ) ;
#58858=CARTESIAN_POINT ( 'NONE',  ( 1.071796769724491893, 12.03259618943233455, 33.99999999999999289 ) ) ;
#58859=CARTESIAN_POINT ( 'NONE',  ( 11.81250000000000000, 2.886751345948129099, -4.999999999999998224 ) ) ;
#58861=CARTESIAN_POINT ( 'NONE',  ( 2.121784821875001281, 15.00312500061451715, 33.67503911421598417 ) ) ;
#58862=CARTESIAN_POINT ( 'NONE',  ( 26.27812500061451573, -4.541064518000419881, 2.621784821874995952 ) ) ;
#58865=CARTESIAN_POINT ( 'NONE',  ( 23.97187500061451360, 3.027376345333611329, 5.243569643749999010 ) ) ;
#58866=CARTESIAN_POINT ( 'NONE',  ( 20.72812500061451502, 4.541064518000418104, 2.621784821874999949 ) ) ;
#58867=CARTESIAN_POINT ( 'NONE',  ( -4.243569643749999898, 15.26562500061459282, -32.45002607614398471 ) ) ;
#58868=CARTESIAN_POINT ( 'NONE',  ( 23.77500000122903145, 2.886751345948126879, 4.999999999999999112 ) ) ;
#58869=CARTESIAN_POINT ( 'NONE',  ( 6.965625000614518392, -6.054752690667223547, -1.112240025338166033E-15 ) ) ;
#58871=CARTESIAN_POINT ( 'NONE',  ( 24.25312500061451715, 4.541064518000418104, -2.621784821874998173 ) ) ;
#58874=CARTESIAN_POINT ( 'NONE',  ( 16.17187500061451644, 3.027376345333613106, -5.243569643749998122 ) ) ;
#58875=CARTESIAN_POINT ( 'NONE',  ( 25.13437500061451502, 6.421520780324663323E-16, -5.243569643749999010 ) ) ;
#58876=CARTESIAN_POINT ( 'NONE',  ( 2.121784821874999061, 14.30937500061451750, 26.32496088578401583 ) ) ;
#58877=CARTESIAN_POINT ( 'NONE',  ( 6.103125000614515905, -4.541064518000417216, -2.621784821875001281 ) ) ;
#58878=CARTESIAN_POINT ( 'NONE',  ( 28.86562500061451786, 3.027376345333611329, 5.243569643749999010 ) ) ;
#58879=CARTESIAN_POINT ( 'NONE',  ( 3.084375000614519191, 6.421520780324663323E-16, -5.243569643749999010 ) ) ;
#58880=CARTESIAN_POINT ( 'NONE',  ( 26.58749999999999858, -2.886751345948126435, -5.000000000000000000 ) ) ;
#58881=CARTESIAN_POINT ( 'NONE',  ( 0.2033016277077263623, 10.00000000000000355, -36.00000000000001421 ) ) ;
#58882=CARTESIAN_POINT ( 'NONE',  ( 3.440625000614518036, -3.027376345333610441, -5.243569643749999898 ) ) ;
#58883=CARTESIAN_POINT ( 'NONE',  ( 6.421875000614519102, 3.027376345333611329, 5.243569643749999010 ) ) ;
#58885=CARTESIAN_POINT ( 'NONE',  ( 17.77500000122903145, 2.886751345948129099, -4.999999999999998224 ) ) ;
#58886=CARTESIAN_POINT ( 'NONE',  ( 4.059375000614519280, 4.541064518000418104, -2.621784821874998173 ) ) ;
#58887=CARTESIAN_POINT ( 'NONE',  ( 5.390625000614518214, 6.054752690667223547, 3.707466751127219781E-16 ) ) ;
#58890=CARTESIAN_POINT ( 'NONE',  ( 13.32187500061451502, -6.054752690667223547, -1.112240025338166033E-15 ) ) ;
#58891=DIRECTION ( 'NONE',  ( 0.000000000000000000, 0.000000000000000000, -1.000000000000000000 ) ) ;
#58892=ORIENTED_EDGE ( 'NONE', *, *, #18647, .T. ) ;
#58893=CARTESIAN_POINT ( 'NONE',  ( 23.31562500061451715, 3.027376345333613106, -5.243569643749998122 ) ) ;
#58894=CARTESIAN_POINT ( 'NONE',  ( 7.790625000614518569, -3.027376345333614438, 5.243569643749998122 ) ) ;
#58895=CARTESIAN_POINT ( 'NONE',  ( 23.52187500061451786, 3.027376345333611329, 5.243569643749999010 ) ) ;
#58896=CARTESIAN_POINT ( 'NONE',  ( 7.528125000614515727, 6.421520780324663323E-16, -5.243569643749999010 ) ) ;
#58897=CARTESIAN_POINT ( 'NONE',  ( 10.16250000122903252, 4.330127018922192761, -2.499999999999997780 ) ) ;
#58898=CARTESIAN_POINT ( 'NONE',  ( 25.64062500061451644, 6.054752690667223547, 3.707466751127219781E-16 ) ) ;
#58899=CARTESIAN_POINT ( 'NONE',  ( -2.121784821874996840, 10.42812500061451786, -26.32496088578401583 ) ) ;
#58900=CARTESIAN_POINT ( 'NONE',  ( 9.600000001229034297, -2.886751345948125991, -5.000000000000000000 ) ) ;
#58901=CARTESIAN_POINT ( 'NONE',  ( 21.17812500061451431, 4.541064518000418104, 2.621784821874999949 ) ) ;
#58902=CARTESIAN_POINT ( 'NONE',  ( 18.21562500061451573, -6.054752690667223547, -1.112240025338166033E-15 ) ) ;
#58903=B_SPLINE_CURVE_WITH_KNOTS ( 'NONE', 3,
 ( #71211, #20588, #26147, #9158, #43514, #38324, #9886, #61224, #27253, #21327 ),
 .UNSPECIFIED., .F., .F.,
 ( 4, 3, 3, 4 ),
 ( 0.000000000000000000, 0.0001572280391461213552, 0.0003263780256893500592, 0.0004955716359015445178 ),
 .UNSPECIFIED. ) ;
#58905=EDGE_CURVE ( 'NONE', #44084, #38296, #22051, .T. ) ;
#58906=CARTESIAN_POINT ( 'NONE',  ( 17.51249999999999929, -5.773502691896255534, -1.060575238724906372E-15 ) ) ;
#58907=CARTESIAN_POINT ( 'NONE',  ( 13.05000000122903536, -2.886751345948129988, 4.999999999999997335 ) ) ;
#58908=CARTESIAN_POINT ( 'NONE',  ( 10.45312500061451644, 0.000000000000000000, 5.243569643749999010 ) ) ;
#58909=CARTESIAN_POINT ( 'NONE',  ( 12.62812500061451537, 4.541064518000418104, 2.621784821874999949 ) ) ;
#58910=CARTESIAN_POINT ( 'NONE',  ( 22.65000000122903856, -2.886751345948125991, -5.000000000000000000 ) ) ;
#58911=CARTESIAN_POINT ( 'NONE',  ( 21.04687500061451644, -3.027376345333610441, -5.243569643749999898 ) ) ;
#58912=CARTESIAN_POINT ( 'NONE',  ( 20.93437500061451573, -4.541064518000419881, 2.621784821874995952 ) ) ;
#58913=CARTESIAN_POINT ( 'NONE',  ( 3.559376264448871563, 3.511538523441492199, -3.894120815303806271 ) ) ;
#58914=CARTESIAN_POINT ( 'NONE',  ( 7.612500001229035362, 0.000000000000000000, 4.999999999999998224 ) ) ;
#58915=CARTESIAN_POINT ( 'NONE',  ( 6.721875000614518925, 3.027376345333613106, -5.243569643749998122 ) ) ;
#58916=CARTESIAN_POINT ( 'NONE',  ( 22.88437500061451857, 6.421520780324663323E-16, -5.243569643749999010 ) ) ;
#58918=CARTESIAN_POINT ( 'NONE',  ( 4.479244028039631509, 2.221994555042201114, -4.723416822329412845 ) ) ;
#58919=CARTESIAN_POINT ( 'NONE',  ( 20.54062500061451502, -3.027376345333610441, -5.243569643749999898 ) ) ;
#58920=CARTESIAN_POINT ( 'NONE',  ( 23.82187500061451502, 3.027376345333613106, -5.243569643749998122 ) ) ;
#58922=CYLINDRICAL_SURFACE ( 'NONE', #53906, 4.999999999999998224 ) ;
#58923=CARTESIAN_POINT ( 'NONE',  ( -1.071796769724491005, 13.27009619066136636, -34.00000000000000000 ) ) ;
#58924=CARTESIAN_POINT ( 'NONE',  ( 5.334375000614517859, 6.421520780324663323E-16, -5.243569643749999010 ) ) ;
#58925=CARTESIAN_POINT ( 'NONE',  ( 17.87812500061451715, 6.421520780324663323E-16, -5.243569643749999010 ) ) ;
#58927=CARTESIAN_POINT ( 'NONE',  ( 25.27499999999999858, 6.123233995736764310E-16, -4.999999999999998224 ) ) ;
#58928=CARTESIAN_POINT ( 'NONE',  ( 25.41562500061451146, -6.054752690667223547, -1.112240025338166033E-15 ) ) ;
#58929=CARTESIAN_POINT ( 'NONE',  ( 3.534375000614518036, 6.421520780324663323E-16, -5.243569643749999010 ) ) ;
#58931=CARTESIAN_POINT ( 'NONE',  ( 4.765225409100392717, 1.514895174305637138, 4.789578167053410773 ) ) ;
#58932=CARTESIAN_POINT ( 'NONE',  ( 1.592000809091587073E-14, 16.40000000122903501, -34.00000000000000000 ) ) ;
#58933=CARTESIAN_POINT ( 'NONE',  ( 15.56250000000000000, 2.886751345948126879, 4.999999999999999112 ) ) ;
#58934=CARTESIAN_POINT ( 'NONE',  ( 19.82812500061451644, 4.541064518000418104, 2.621784821874999949 ) ) ;
#58935=EDGE_LOOP ( 'NONE', ( #10394, #17877, #70224, #39710 ) ) ;
#58936=CARTESIAN_POINT ( 'NONE',  ( 23.69999999999999929, 0.000000000000000000, 4.999999999999998224 ) ) ;
#58937=CARTESIAN_POINT ( 'NONE',  ( 27.12187500061451573, 3.027376345333611329, 5.243569643749999010 ) ) ;
#58938=ORIENTED_EDGE ( 'NONE', *, *, #73107, .T. ) ;
#58939=CYLINDRICAL_SURFACE ( 'NONE', #47777, 4.999999999999998224 ) ;
#58940=CARTESIAN_POINT ( 'NONE',  ( 12.25312500061451537, 0.000000000000000000, 5.243569643749999010 ) ) ;
#58942=CARTESIAN_POINT ( 'NONE',  ( 28.37812500061451715, 4.541064518000418104, 2.621784821874999949 ) ) ;
#58943=CARTESIAN_POINT ( 'NONE',  ( 12.41250000122903430, 4.330127018922192761, -2.499999999999997780 ) ) ;
#58944=CARTESIAN_POINT ( 'NONE',  ( 18.89999999999999858, -4.330127018922190985, -2.500000000000001332 ) ) ;
#58945=CARTESIAN_POINT ( 'NONE',  ( 26.43750000000000000, -2.886751345948129988, 4.999999999999997335 ) ) ;
#58946=CARTESIAN_POINT ( 'NONE',  ( 3.234375000614516438, 4.541064518000418104, 2.621784821874999949 ) ) ;
#58947=CARTESIAN_POINT ( 'NONE',  ( 5.784375000614517148, 6.421520780324663323E-16, -5.243569643749999010 ) ) ;
#58948=CARTESIAN_POINT ( 'NONE',  ( 19.73437500061451644, 6.421520780324663323E-16, -5.243569643749999010 ) ) ;
#58949=CARTESIAN_POINT ( 'NONE',  ( 19.95000000122903216, -2.886751345948159742, -4.999999999999942268 ) ) ;
#58950=ORIENTED_EDGE ( 'NONE', *, *, #22378, .T. ) ;
#58951=CARTESIAN_POINT ( 'NONE',  ( 28.82812500061451644, 4.541064518000418104, 2.621784821874999949 ) ) ;
#58952=CARTESIAN_POINT ( 'NONE',  ( 29.33437500061451431, 4.541064518000418104, 2.621784821874999949 ) ) ;
#58953=CARTESIAN_POINT ( 'NONE',  ( 4.546875000614517326, 6.054752690667223547, 3.707466751127219781E-16 ) ) ;
#58954=CARTESIAN_POINT ( 'NONE',  ( 16.27499999999999858, 6.123233995736764310E-16, -4.999999999999998224 ) ) ;
#58955=CARTESIAN_POINT ( 'NONE',  ( 14.87812500061451537, 4.541064518000418104, 2.621784821874999949 ) ) ;
#58956=CARTESIAN_POINT ( 'NONE',  ( -1.487416814333745711E-14, 15.16250000000000142, -26.00000000000000000 ) ) ;
#58957=LINE ( 'NONE', #31263, #12413 ) ;
#58958=CARTESIAN_POINT ( 'NONE',  ( -3.137519842735245283E-14, 12.57500000122903572, 34.00000000000000000 ) ) ;
#58959=CARTESIAN_POINT ( 'NONE',  ( 17.73750000122903359, 6.123233995736764310E-16, -4.999999999999998224 ) ) ;
#58960=CYLINDRICAL_SURFACE ( 'NONE', #19461, 3.999999999999996447 ) ;
#58962=CARTESIAN_POINT ( 'NONE',  ( 7.228125000614517681, 4.541064518000418104, 2.621784821874999949 ) ) ;
#58963=CARTESIAN_POINT ( 'NONE',  ( 23.14687500061451786, -3.027376345333614438, 5.243569643749998122 ) ) ;
#58964=CARTESIAN_POINT ( 'NONE',  ( 30.00000000000000000, 0.000000000000000000, 0.000000000000000000 ) ) ;
#58965=CARTESIAN_POINT ( 'NONE',  ( 24.53437500061451715, -4.541064518000419881, 2.621784821874995952 ) ) ;
#58966=CARTESIAN_POINT ( 'NONE',  ( 5.212500000000002132, 2.886751345948126879, 4.999999999999999112 ) ) ;
#58967=CARTESIAN_POINT ( 'NONE',  ( 1.999999999999998668, 10.51250000122903572, 26.53589838486224650 ) ) ;
#58968=CARTESIAN_POINT ( 'NONE',  ( 15.36562500061451608, 3.027376345333611329, 5.243569643749999010 ) ) ;
#58969=CARTESIAN_POINT ( 'NONE',  ( 4.912500001229034297, 0.000000000000000000, 4.999999999999998224 ) ) ;
#58971=CARTESIAN_POINT ( 'NONE',  ( 10.54687500061451644, -3.027376345333614438, 5.243569643749998122 ) ) ;
#58972=CARTESIAN_POINT ( 'NONE',  ( -3.457895701286862522, 3.616202803579613434, -27.97416577253550685 ) ) ;
#58974=CARTESIAN_POINT ( 'NONE',  ( 12.25312500061451537, 0.000000000000000000, 5.243569643749999010 ) ) ;
#58975=CARTESIAN_POINT ( 'NONE',  ( 2.000000000000001332, 12.16250000122903430, -26.53589838486224650 ) ) ;
#58976=CARTESIAN_POINT ( 'NONE',  ( 22.95000000122903216, -2.886751345948129988, 4.999999999999997335 ) ) ;
#58977=CARTESIAN_POINT ( 'NONE',  ( 9.459375000614517859, 4.541064518000418104, -2.621784821874998173 ) ) ;
#58978=AXIS2_PLACEMENT_3D ( 'NONE', #53866, #65665, #19861 ) ;
#58979=CARTESIAN_POINT ( 'NONE',  ( 13.04062500061451502, 6.054752690667223547, 3.707466751127219781E-16 ) ) ;
#58981=CARTESIAN_POINT ( 'NONE',  ( 24.38437500061451502, 4.541064518000418104, 2.621784821874999949 ) ) ;
#58984=CARTESIAN_POINT ( 'NONE',  ( 4.350000001229034297, 5.773502691896255534, 3.535250795749688401E-16 ) ) ;
#58985=FACE_OUTER_BOUND ( 'NONE', #52463, .T. ) ;
#58986=CARTESIAN_POINT ( 'NONE',  ( 9.001249775931846008E-16, 13.67187500061451999, -25.09994784771203058 ) ) ;
#58987=CARTESIAN_POINT ( 'NONE',  ( 15.94687500061451502, -3.027376345333614438, 5.243569643749998122 ) ) ;
#58988=CARTESIAN_POINT ( 'NONE',  ( 16.72500000122903430, -5.773502691896255534, -1.060575238724906372E-15 ) ) ;
#58989=CARTESIAN_POINT ( 'NONE',  ( 11.70937500061451608, 4.541064518000418104, -2.621784821874998173 ) ) ;
#58990=CARTESIAN_POINT ( 'NONE',  ( 2.121784821874999061, 18.30312500061451431, -33.67503911421598417 ) ) ;
#58991=CARTESIAN_POINT ( 'NONE',  ( 19.61250000122903359, 4.330127018922192761, -2.499999999999997780 ) ) ;
#58992=CARTESIAN_POINT ( 'NONE',  ( 13.64062500061451644, -3.027376345333614438, 5.243569643749998122 ) ) ;
#58993=ORIENTED_EDGE ( 'NONE', *, *, #70507, .T. ) ;
#58994=CARTESIAN_POINT ( 'NONE',  ( 15.00000000000000000, 4.330127018922192761, -2.499999999999997780 ) ) ;
#58995=CARTESIAN_POINT ( 'NONE',  ( 13.35937500061451821, -4.541064518000417216, -2.621784821875001281 ) ) ;
#58998=CARTESIAN_POINT ( 'NONE',  ( 12.45000000122903394, 5.773502691896255534, 3.535250795749688894E-16 ) ) ;
#58999=CARTESIAN_POINT ( 'NONE',  ( 20.28750000122903074, -4.330127018922194537, 2.499999999999995559 ) ) ;
#59000=CARTESIAN_POINT ( 'NONE',  ( 17.80312500061451786, -4.541064518000417216, -2.621784821875001281 ) ) ;
#59001=CARTESIAN_POINT ( 'NONE',  ( 20.69062500061451715, 6.054752690667223547, 3.707466751127219781E-16 ) ) ;
#59002=CARTESIAN_POINT ( 'NONE',  ( 27.41250000122903430, 0.000000000000000000, 4.999999999999998224 ) ) ;
#59003=( BOUNDED_CURVE ( )  B_SPLINE_CURVE ( 2, ( #19607, #70601, #58769, #42164, #58403, #24795, #47338 ),
 .UNSPECIFIED., .F., .F. ) 
 B_SPLINE_CURVE_WITH_KNOTS ( ( 3, 2, 2, 3 ),
 ( 0.5583333333333333481, 0.5611111111111111160, 0.5638888888888889950, 0.5666666666666667629 ),
 .UNSPECIFIED. ) 
 CURVE ( )  GEOMETRIC_REPRESENTATION_ITEM ( )  RATIONAL_B_SPLINE_CURVE ( ( 1.000000000000000000, 0.8660254037844387076, 1.000000000000000000, 0.8660254037844387076, 1.000000000000000000, 0.8660254037844333785, 1.000000000000005329 ) ) 
 REPRESENTATION_ITEM ( '' )  );
#59004=CARTESIAN_POINT ( 'NONE',  ( 25.94999999999999929, 0.000000000000000000, 4.999999999999998224 ) ) ;
#59005=CARTESIAN_POINT ( 'NONE',  ( 3.709174336338540989, 3.352913023424228811, 4.031500572517469294 ) ) ;
#59007=CARTESIAN_POINT ( 'NONE',  ( 28.84687500061452070, 6.054752690667223547, 3.707466751127219781E-16 ) ) ;
#59008=CARTESIAN_POINT ( 'NONE',  ( 28.83750000000000213, -2.886751345948155745, -4.999999999999948486 ) ) ;
#59009=CARTESIAN_POINT ( 'NONE',  ( 4.243569643749999898, 13.74687500061451750, -27.54997392385601529 ) ) ;
#59011=CARTESIAN_POINT ( 'NONE',  ( 3.412500001229032964, 4.330127018922192761, -2.499999999999997780 ) ) ;
#59012=CARTESIAN_POINT ( 'NONE',  ( 5.100000000000000533, 4.330127018922192761, -2.499999999999997780 ) ) ;
#59013=CARTESIAN_POINT ( 'NONE',  ( 2.662500001229036073, 0.000000000000000000, 4.999999999999998224 ) ) ;
#59014=CARTESIAN_POINT ( 'NONE',  ( 8.446875000614518569, -3.027376345333610441, -5.243569643749999898 ) ) ;
#59015=CARTESIAN_POINT ( 'NONE',  ( 27.55312500061451786, 0.000000000000000000, 5.243569643749999010 ) ) ;
#59017=CARTESIAN_POINT ( 'NONE',  ( 30.00000000000000000, 0.000000000000000000, 0.000000000000000000 ) ) ;
#59018=CARTESIAN_POINT ( 'NONE',  ( 5.362500001229033586, 0.000000000000000000, 4.999999999999998224 ) ) ;
#59019=CARTESIAN_POINT ( 'NONE',  ( 16.91250000122903430, 4.330127018922192761, -2.499999999999997780 ) ) ;
#59020=CARTESIAN_POINT ( 'NONE',  ( 5.746875000614517504, -3.027376345333610441, -5.243569643749999898 ) ) ;
#59021=CARTESIAN_POINT ( 'NONE',  ( 12.42187500061451821, -6.054752690667223547, -1.112240025338166033E-15 ) ) ;
#59022=CARTESIAN_POINT ( 'NONE',  ( 3.374999999999999556, 4.330127018922191873, 2.499999999999999556 ) ) ;
#59023=CARTESIAN_POINT ( 'NONE',  ( -3.000416591977282496E-16, 15.64062500061459282, 25.09994784771203058 ) ) ;
#59025=CARTESIAN_POINT ( 'NONE',  ( 7.687500000000000000, -2.886751345948125991, -5.000000000000000000 ) ) ;
#59027=CARTESIAN_POINT ( 'NONE',  ( 21.17812500061451431, 4.541064518000418104, 2.621784821874999949 ) ) ;
#59028=CARTESIAN_POINT ( 'NONE',  ( 14.01562500061451644, 3.027376345333611329, 5.243569643749999010 ) ) ;
#59030=CARTESIAN_POINT ( 'NONE',  ( 8.784375000614518925, -4.541064518000419881, 2.621784821874995952 ) ) ;
#59031=CARTESIAN_POINT ( 'NONE',  ( 26.25000000000000000, 4.330127018922192761, -2.499999999999997780 ) ) ;
#59032=CARTESIAN_POINT ( 'NONE',  ( 21.00000000122903288, 5.773502691896255534, 3.535250795749688894E-16 ) ) ;
#59033=CARTESIAN_POINT ( 'NONE',  ( 27.89062500061451289, 6.054752690667223547, 3.707466751127219781E-16 ) ) ;
#59034=CARTESIAN_POINT ( 'NONE',  ( 9.528763966825557376E-15, 17.07500000122903572, 34.00000000000000000 ) ) ;
#59035=CARTESIAN_POINT ( 'NONE',  ( 9.159375000614515372, 0.000000000000000000, 5.243569643749999010 ) ) ;
#59036=CARTESIAN_POINT ( 'NONE',  ( 14.44687500061451679, 6.054752690667223547, 3.707466751127219781E-16 ) ) ;
#59037=CARTESIAN_POINT ( 'NONE',  ( 27.00937500061451857, 4.541064518000418104, -2.621784821874998173 ) ) ;
#59039=CARTESIAN_POINT ( 'NONE',  ( 20.37187500061451573, 3.027376345333611329, 5.243569643749999010 ) ) ;
#59040=CARTESIAN_POINT ( 'NONE',  ( 10.77187500061451786, 3.027376345333613106, -5.243569643749998122 ) ) ;
#59042=CARTESIAN_POINT ( 'NONE',  ( 24.11249999999999716, 2.886751345948126879, 4.999999999999999112 ) ) ;
#59044=CARTESIAN_POINT ( 'NONE',  ( -4.243569643749997233, 12.24687500061451928, -27.54997392385601174 ) ) ;
#59046=CARTESIAN_POINT ( 'NONE',  ( 14.84062500061451750, 6.054752690667223547, 3.707466751127219781E-16 ) ) ;
#59047=CARTESIAN_POINT ( 'NONE',  ( 3.562500000000000444, -5.773502691896255534, -1.060575238724906372E-15 ) ) ;
#59049=CARTESIAN_POINT ( 'NONE',  ( 25.64999999999999858, -4.330127018922190985, -2.500000000000001332 ) ) ;
#59050=CARTESIAN_POINT ( 'NONE',  ( 13.38750000000000107, -2.886751345948129988, 4.999999999999997335 ) ) ;
#59051=CARTESIAN_POINT ( 'NONE',  ( -3.999999999999997335, 17.00000000122903288, 32.30940107675850470 ) ) ;
#59052=CARTESIAN_POINT ( 'NONE',  ( 14.21250000122903323, 4.330127018922192761, -2.499999999999997780 ) ) ;
#59053=CARTESIAN_POINT ( 'NONE',  ( 25.24687500061451573, 6.054752690667223547, 3.707466751127219781E-16 ) ) ;
#59054=CARTESIAN_POINT ( 'NONE',  ( 15.72187500061451892, 3.027376345333613106, -5.243569643749998122 ) ) ;
#59056=ORIENTED_EDGE ( 'NONE', *, *, #45249, .T. ) ;
#59057=CARTESIAN_POINT ( 'NONE',  ( 19.60312500061451502, -4.541064518000417216, -2.621784821875001281 ) ) ;
#59058=CARTESIAN_POINT ( 'NONE',  ( 5.353125000614515905, 4.541064518000418104, -2.621784821874998173 ) ) ;
#59059=CARTESIAN_POINT ( 'NONE',  ( 17.29687500061451999, -3.027376345333614438, 5.243569643749998122 ) ) ;
#59060=CARTESIAN_POINT ( 'NONE',  ( 29.03437500061451715, -4.541064518000419881, 2.621784821874995952 ) ) ;
#59061=CARTESIAN_POINT ( 'NONE',  ( 5.390625000614518214, 6.054752690667223547, 3.707466751127219781E-16 ) ) ;
#59062=CARTESIAN_POINT ( 'NONE',  ( 18.81562500061452070, 3.027376345333613106, -5.243569643749998122 ) ) ;
#59063=CARTESIAN_POINT ( 'NONE',  ( 2.121784821874999061, 16.05312500061451786, 26.32496088578401583 ) ) ;
#59064=CARTESIAN_POINT ( 'NONE',  ( 17.28750000122903430, 6.123233995736764310E-16, -4.999999999999998224 ) ) ;
#59066=CARTESIAN_POINT ( 'NONE',  ( 8.090625000614515727, 6.054752690667223547, 3.707466751127219781E-16 ) ) ;
#59067=CARTESIAN_POINT ( 'NONE',  ( 4.021875000614516082, 3.027376345333613106, -5.243569643749998122 ) ) ;
#59068=CARTESIAN_POINT ( 'NONE',  ( 28.56562500061451715, -6.054752690667223547, -1.112240025338166033E-15 ) ) ;
#59069=ADVANCED_FACE ( 'NONE', ( #51222 ), #34215, .F. ) ;
#59070=CARTESIAN_POINT ( 'NONE',  ( 24.15937500061451715, -4.541064518000417216, -2.621784821875001281 ) ) ;
#59071=CARTESIAN_POINT ( 'NONE',  ( 13.75312500061451715, -4.541064518000417216, -2.621784821875001281 ) ) ;
#59072=CARTESIAN_POINT ( 'NONE',  ( 25.61250000122903359, 0.000000000000000000, 4.999999999999998224 ) ) ;
#59073=CARTESIAN_POINT ( 'NONE',  ( 23.57812500061451289, -4.541064518000419881, 2.621784821874995952 ) ) ;
#59074=CARTESIAN_POINT ( 'NONE',  ( 20.48437500061451289, -4.541064518000419881, 2.621784821874995952 ) ) ;
#59075=CARTESIAN_POINT ( 'NONE',  ( 13.97812500061451679, 4.541064518000418104, 2.621784821874999949 ) ) ;
#59076=CARTESIAN_POINT ( 'NONE',  ( -2.121784821874999949, 14.83437500061451786, 26.32496088578401938 ) ) ;
#59077=CARTESIAN_POINT ( 'NONE',  ( 20.46562500061451928, -6.054752690667223547, -1.112240025338166033E-15 ) ) ;
#59078=CARTESIAN_POINT ( 'NONE',  ( 29.61562500061451431, 3.027376345333613106, -5.243569643749998122 ) ) ;
#59079=EDGE_LOOP ( 'NONE', ( #59903, #47025, #63569, #50213 ) ) ;
#59080=ORIENTED_EDGE ( 'NONE', *, *, #9880, .T. ) ;
#59081=CARTESIAN_POINT ( 'NONE',  ( 22.01249999999999574, -5.773502691896255534, -1.060575238724906372E-15 ) ) ;
#59082=CARTESIAN_POINT ( 'NONE',  ( 4.000000000000000000, 10.28750000000000142, -27.69059892324149530 ) ) ;
#59084=CARTESIAN_POINT ( 'NONE',  ( 27.29062500061451502, -3.027376345333610441, -5.243569643749999898 ) ) ;
#59085=CARTESIAN_POINT ( 'NONE',  ( 7.415625000614516793, -6.054752690667223547, -1.112240025338166033E-15 ) ) ;
#59086=CARTESIAN_POINT ( 'NONE',  ( 20.28750000122903074, -4.330127018922194537, 2.499999999999995559 ) ) ;
#59087=CARTESIAN_POINT ( 'NONE',  ( 24.85312500061451502, 0.000000000000000000, 5.243569643749999010 ) ) ;
#59088=CARTESIAN_POINT ( 'NONE',  ( 25.05000000000000071, 0.000000000000000000, 4.999999999999998224 ) ) ;
#59089=CARTESIAN_POINT ( 'NONE',  ( 27.02812500061451573, 4.541064518000418104, 2.621784821874999949 ) ) ;
#59090=CARTESIAN_POINT ( 'NONE',  ( 8.090625000614515727, 6.054752690667223547, 3.707466751127219781E-16 ) ) ;
#59091=ORIENTED_EDGE ( 'NONE', *, *, #57675, .F. ) ;
#59092=B_SPLINE_CURVE_WITH_KNOTS ( 'NONE', 3,
 ( #63753, #69318, #7976, #57844, #47500, #13877, #36416, #24594, #13142, #68956 ),
 .UNSPECIFIED., .F., .F.,
 ( 4, 3, 3, 4 ),
 ( 8.113426134873485606E-18, 7.861467438249196448E-05, 0.0001572289795642654289, 0.0002817739516380214507 ),
 .UNSPECIFIED. ) ;
#59093=CARTESIAN_POINT ( 'NONE',  ( 26.72812500061451502, -4.541064518000419881, 2.621784821874995952 ) ) ;
#59094=CARTESIAN_POINT ( 'NONE',  ( 5.578125000614518214, -4.541064518000419881, 2.621784821874995952 ) ) ;
#59096=CARTESIAN_POINT ( 'NONE',  ( 3.403125000614518836, -4.541064518000417216, -2.621784821875001281 ) ) ;
#59097=CARTESIAN_POINT ( 'NONE',  ( 4.243569643749999898, 19.63437500061451857, -30.00000000000000000 ) ) ;
#59098=CARTESIAN_POINT ( 'NONE',  ( 12.97499999999999964, -4.330127018922194537, 2.499999999999995559 ) ) ;
#59099=CARTESIAN_POINT ( 'NONE',  ( 14.22187500061451537, -6.054752690667223547, -1.112240025338166033E-15 ) ) ;
#59100=CARTESIAN_POINT ( 'NONE',  ( 8.700000001229032165, -2.886751345948125991, -5.000000000000000000 ) ) ;
#59101=CARTESIAN_POINT ( 'NONE',  ( 13.77187500061451786, -6.054752690667223547, -1.112240025338166033E-15 ) ) ;
#59103=CARTESIAN_POINT ( 'NONE',  ( 7.621875000614519280, 3.027376345333613106, -5.243569643749998122 ) ) ;
#59104=CARTESIAN_POINT ( 'NONE',  ( 2.121784821875001281, 12.75312500061451715, -26.32496088578401938 ) ) ;
#59106=CARTESIAN_POINT ( 'NONE',  ( 13.13437500061451857, 4.541064518000418104, 2.621784821874999949 ) ) ;
#59107=ORIENTED_EDGE ( 'NONE', *, *, #9276, .T. ) ;
#59109=CARTESIAN_POINT ( 'NONE',  ( 21.14062500061451289, 6.054752690667223547, 3.707466751127219781E-16 ) ) ;
#59110=CARTESIAN_POINT ( 'NONE',  ( 4.243569643749999010, 10.67187500061451644, 27.54997392385601174 ) ) ;
#59111=DIRECTION ( 'NONE',  ( -0.000000000000000000, -1.000000000000000000, -0.000000000000000000 ) ) ;
#59112=CARTESIAN_POINT ( 'NONE',  ( 26.18437500061451573, 4.541064518000418104, 2.621784821874999949 ) ) ;
#59113=CARTESIAN_POINT ( 'NONE',  ( 27.87187500061451573, 3.027376345333613106, -5.243569643749998122 ) ) ;
#59114=CARTESIAN_POINT ( 'NONE',  ( 4.790625000614518569, -3.027376345333610441, -5.243569643749999898 ) ) ;
#59116=CARTESIAN_POINT ( 'NONE',  ( 17.07187500061451502, 3.027376345333613106, -5.243569643749998122 ) ) ;
#59118=CARTESIAN_POINT ( 'NONE',  ( 29.06250000122903288, 4.330127018922192761, -2.499999999999997780 ) ) ;
#59119=CARTESIAN_POINT ( 'NONE',  ( 6.346875000614517148, 6.054752690667223547, 3.707466751127219781E-16 ) ) ;
#59120=CARTESIAN_POINT ( 'NONE',  ( 15.64687500061451608, -3.027376345333610441, -5.243569643749999898 ) ) ;
#59122=CARTESIAN_POINT ( 'NONE',  ( 25.80000000000000071, 4.330127018922192761, -2.499999999999997780 ) ) ;
#59123=CARTESIAN_POINT ( 'NONE',  ( 26.67187500061451644, 3.027376345333611329, 5.243569643749999010 ) ) ;
#59126=EDGE_LOOP ( 'NONE', ( #24389, #62179 ) ) ;
#59127=CARTESIAN_POINT ( 'NONE',  ( 7.087499999999999467, -2.886751345948129988, 4.999999999999997335 ) ) ;
#59129=CARTESIAN_POINT ( 'NONE',  ( 21.85312500061451502, -4.541064518000417216, -2.621784821875001281 ) ) ;
#59130=CARTESIAN_POINT ( 'NONE',  ( 10.76250000000000107, -5.773502691896255534, -1.060575238724906372E-15 ) ) ;
#59131=CARTESIAN_POINT ( 'NONE',  ( 7.462500001229035007, 4.330127018922192761, -2.499999999999997780 ) ) ;
#59132=CARTESIAN_POINT ( 'NONE',  ( 6.440625000614517148, -3.027376345333614438, 5.243569643749998122 ) ) ;
#59133=CARTESIAN_POINT ( 'NONE',  ( 21.82499999999999574, 4.330127018922191873, 2.499999999999999556 ) ) ;
#59134=CARTESIAN_POINT ( 'NONE',  ( 19.60312500061451502, -4.541064518000417216, -2.621784821875001281 ) ) ;
#59135=CARTESIAN_POINT ( 'NONE',  ( 0.000000000000000000, -4.999999999999998224, 0.000000000000000000 ) ) ;
#59136=CARTESIAN_POINT ( 'NONE',  ( 26.40000000122902790, 5.773502691896255534, 3.535250795749688894E-16 ) ) ;
#59138=CARTESIAN_POINT ( 'NONE',  ( 4.800000000000002487, 0.000000000000000000, 4.999999999999998224 ) ) ;
#59140=CARTESIAN_POINT ( 'NONE',  ( 19.22812500061451502, 6.421520780324663323E-16, -5.243569643749999010 ) ) ;
#59141=CARTESIAN_POINT ( 'NONE',  ( 27.21562500061451928, -6.054752690667223547, -1.112240025338166033E-15 ) ) ;
#59142=CARTESIAN_POINT ( 'NONE',  ( 24.79687500061451999, 6.054752690667223547, 3.707466751127219781E-16 ) ) ;
#59143=CARTESIAN_POINT ( 'NONE',  ( 8.962500000000002132, -5.773502691896255534, -1.060575238724906372E-15 ) ) ;
#59144=CARTESIAN_POINT ( 'NONE',  ( 12.62812500061451537, 4.541064518000418104, 2.621784821874999949 ) ) ;
#59145=CARTESIAN_POINT ( 'NONE',  ( 28.00312500061451715, 0.000000000000000000, 5.243569643749999010 ) ) ;
#59146=CARTESIAN_POINT ( 'NONE',  ( 8.428125000614517859, 6.421520780324663323E-16, -5.243569643749999010 ) ) ;
#59148=CARTESIAN_POINT ( 'NONE',  ( -2.121784821874996840, 12.28437500061451892, 33.67503911421598417 ) ) ;
#59149=CARTESIAN_POINT ( 'NONE',  ( 24.90000000122903145, -2.886751345948125991, -5.000000000000000000 ) ) ;
#59151=CARTESIAN_POINT ( 'NONE',  ( 13.41562500061451502, 3.027376345333612662, -5.243569643749998122 ) ) ;
#59152=( GEOMETRIC_REPRESENTATION_CONTEXT ( 3 ) GLOBAL_UNCERTAINTY_ASSIGNED_CONTEXT ( ( #7051 ) ) GLOBAL_UNIT_ASSIGNED_CONTEXT ( ( #33832, #51556, #27940 ) ) REPRESENTATION_CONTEXT ( 'NONE', 'WORKASPACE' ) );
#59153=CARTESIAN_POINT ( 'NONE',  ( 11.33437500061451608, 4.541064518000418104, 2.621784821874999949 ) ) ;
#59154=CARTESIAN_POINT ( 'NONE',  ( 9.646875000614516082, -3.027376345333614438, 5.243569643749998122 ) ) ;
#59155=CARTESIAN_POINT ( 'NONE',  ( 16.95937500061451786, -4.541064518000417216, -2.621784821875001281 ) ) ;
#59157=CARTESIAN_POINT ( 'NONE',  ( 29.70937500061451431, 4.541064518000418104, -2.621784821874998173 ) ) ;
#59158=CARTESIAN_POINT ( 'NONE',  ( 21.55312500061451431, 4.541064518000418104, -2.621784821874998173 ) ) ;
#59159=CARTESIAN_POINT ( 'NONE',  ( 17.67187500061451644, 3.027376345333611329, 5.243569643749999010 ) ) ;
#59160=CARTESIAN_POINT ( 'NONE',  ( 20.91562500061451502, -6.054752690667223547, -1.112240025338166033E-15 ) ) ;
#59161=CARTESIAN_POINT ( 'NONE',  ( 3.999999999999998668, 14.86250000000000071, 27.69059892324149175 ) ) ;
#59162=CARTESIAN_POINT ( 'NONE',  ( 27.32812500061451644, 6.421520780324663323E-16, -5.243569643749999010 ) ) ;
#59163=CARTESIAN_POINT ( 'NONE',  ( 7.087500001229034119, 4.330127018922191873, 2.499999999999999556 ) ) ;
#59164=ORIENTED_EDGE ( 'NONE', *, *, #49176, .T. ) ;
#59165=CARTESIAN_POINT ( 'NONE',  ( 3.862500001229035362, 4.330127018922192761, -2.499999999999997780 ) ) ;
#59166=CARTESIAN_POINT ( 'NONE',  ( -3.999999999999997335, 18.23750000000000071, -27.69059892324149175 ) ) ;
#59167=CARTESIAN_POINT ( 'NONE',  ( 23.66250000122903430, 4.330127018922192761, -2.499999999999997780 ) ) ;
#59169=CARTESIAN_POINT ( 'NONE',  ( 7.134375000614516793, 6.421520780324663323E-16, -5.243569643749999010 ) ) ;
#59170=FACE_OUTER_BOUND ( 'NONE', #61867, .T. ) ;
#59171=CARTESIAN_POINT ( 'NONE',  ( 16.15312500061451573, 4.541064518000418104, -2.621784821874998173 ) ) ;
#59172=CARTESIAN_POINT ( 'NONE',  ( 8.634375000614518569, 4.541064518000418104, 2.621784821874999949 ) ) ;
#59173=CARTESIAN_POINT ( 'NONE',  ( 26.21250000122903501, -4.330127018922190985, -2.500000000000001332 ) ) ;
#59174=CARTESIAN_POINT ( 'NONE',  ( 18.34687500061451715, -3.027376345333610441, -5.243569643749999898 ) ) ;
#59175=CARTESIAN_POINT ( 'NONE',  ( 3.984375000614517326, 6.421520780324663323E-16, -5.243569643749999010 ) ) ;
#59176=CARTESIAN_POINT ( 'NONE',  ( 5.803125000614517859, 4.541064518000418104, -2.621784821874998173 ) ) ;
#59177=CARTESIAN_POINT ( 'NONE',  ( 14.54062500061451679, -3.027376345333614438, 5.243569643749998122 ) ) ;
#59179=CARTESIAN_POINT ( 'NONE',  ( 13.22812500061451502, -4.541064518000419881, 2.621784821874995952 ) ) ;
#59180=CARTESIAN_POINT ( 'NONE',  ( 5.662500001229035185, 4.330127018922192761, -2.499999999999997780 ) ) ;
#59181=CARTESIAN_POINT ( 'NONE',  ( 9.853125000614516793, 4.541064518000418104, -2.621784821874998173 ) ) ;
#59183=CARTESIAN_POINT ( 'NONE',  ( 11.88749999999999751, 5.773502691896255534, 3.535250795749688894E-16 ) ) ;
#59184=CARTESIAN_POINT ( 'NONE',  ( 7.050000001229036251, 5.773502691896255534, 3.535250795749688894E-16 ) ) ;
#59185=CARTESIAN_POINT ( 'NONE',  ( 19.91250000000000142, 2.886751345948129099, -4.999999999999998224 ) ) ;
#59186=CARTESIAN_POINT ( 'NONE',  ( 16.09687500061452070, -3.027376345333610441, -5.243569643749999898 ) ) ;
#59187=CARTESIAN_POINT ( 'NONE',  ( 16.31250000122903288, -4.330127018922190985, -2.500000000000001332 ) ) ;
#59189=CARTESIAN_POINT ( 'NONE',  ( 4.243569643749999010, 19.61562500061451431, -32.45002607614398471 ) ) ;
#59190=CARTESIAN_POINT ( 'NONE',  ( 3.223068828554207066, 3.822549816615882445, 3.589315889418955408 ) ) ;
#59192=DIRECTION ( 'NONE',  ( 0.000000000000000000, 0.000000000000000000, 1.000000000000000000 ) ) ;
#59193=CARTESIAN_POINT ( 'NONE',  ( 9.487500001229033586, -4.330127018922194537, 2.499999999999995559 ) ) ;
#59195=CARTESIAN_POINT ( 'NONE',  ( 16.35937500061451644, 0.000000000000000000, 5.243569643749999010 ) ) ;
#59198=CARTESIAN_POINT ( 'NONE',  ( 12.85312500061451502, -4.541064518000417216, -2.621784821875001281 ) ) ;
#59199=AXIS2_PLACEMENT_3D ( 'NONE', #54284, #14741, #20275 ) ;
#59201=CARTESIAN_POINT ( 'NONE',  ( 24.04687500061451644, -3.027376345333614438, 5.243569643749998122 ) ) ;
#59203=CARTESIAN_POINT ( 'NONE',  ( 10.79062500061451679, 6.054752690667223547, 3.707466751127219781E-16 ) ) ;
#59204=CARTESIAN_POINT ( 'NONE',  ( 16.32187500061451502, 3.027376345333611329, 5.243569643749999010 ) ) ;
#59205=ORIENTED_EDGE ( 'NONE', *, *, #21176, .T. ) ;
#59206=CARTESIAN_POINT ( 'NONE',  ( 24.12187500061451217, -6.054752690667223547, -1.112240025338166033E-15 ) ) ;
#59207=CARTESIAN_POINT ( 'NONE',  ( 25.11562500061451431, 3.027376345333613106, -5.243569643749998122 ) ) ;
#59208=CARTESIAN_POINT ( 'NONE',  ( 27.25312500061451360, -4.541064518000417216, -2.621784821875001281 ) ) ;
#59209=CARTESIAN_POINT ( 'NONE',  ( 30.00000000000000000, 0.000000000000000000, 4.999999999999998224 ) ) ;
#59210=CARTESIAN_POINT ( 'NONE',  ( 7.350000000000002309, 4.330127018922192761, -2.499999999999997780 ) ) ;
#59211=CARTESIAN_POINT ( 'NONE',  ( 18.00000000122903288, -2.886751345948129988, 4.999999999999997335 ) ) ;
#59215=CARTESIAN_POINT ( 'NONE',  ( 16.01249999999999929, 2.886751345948126879, 4.999999999999999112 ) ) ;
#59216=CARTESIAN_POINT ( 'NONE',  ( 19.16250000000000142, 2.886751345948126879, 4.999999999999999112 ) ) ;
#59217=CARTESIAN_POINT ( 'NONE',  ( 13.37812500061451715, 6.421520780324663323E-16, -5.243569643749999010 ) ) ;
#59218=VERTEX_POINT ( 'NONE', #64097 ) ;
#59219=CARTESIAN_POINT ( 'NONE',  ( 4.000000000000000000, 18.50000000122903288, -27.69059892324149885 ) ) ;
#59220=CARTESIAN_POINT ( 'NONE',  ( -2.121784821874996840, 15.88437500061451857, -26.32496088578401583 ) ) ;
#59221=CARTESIAN_POINT ( 'NONE',  ( 5.653125000614517504, -4.541064518000417216, -2.621784821875001281 ) ) ;
#59222=CARTESIAN_POINT ( 'NONE',  ( 0.000000000000000000, 4.999999999999998224, 0.000000000000000000 ) ) ;
#59223=CARTESIAN_POINT ( 'NONE',  ( 11.10000000000000142, 0.000000000000000000, 4.999999999999998224 ) ) ;
#59226=CARTESIAN_POINT ( 'NONE',  ( 4.243569643749999898, 15.07812500061451644, 30.00000000000000000 ) ) ;
#59227=CARTESIAN_POINT ( 'NONE',  ( 26.54062500061451146, 6.054752690667223547, 3.707466751127219781E-16 ) ) ;
#59228=FACE_OUTER_BOUND ( 'NONE', #30447, .T. ) ;
#59230=CARTESIAN_POINT ( 'NONE',  ( 24.38437500061451502, 4.541064518000418104, 2.621784821874999949 ) ) ;
#59231=CARTESIAN_POINT ( 'NONE',  ( 18.21562500061451573, -6.054752690667223547, -1.112240025338166033E-15 ) ) ;
#59232=CARTESIAN_POINT ( 'NONE',  ( 4.243569643749999010, 14.66562500061459495, -32.45002607614398471 ) ) ;
#59233=CARTESIAN_POINT ( 'NONE',  ( 23.88750000122903216, -4.330127018922194537, 2.499999999999995559 ) ) ;
#59234=CARTESIAN_POINT ( 'NONE',  ( 6.628125000614517148, 6.421520780324663323E-16, -5.243569643749999010 ) ) ;
#59236=CARTESIAN_POINT ( 'NONE',  ( 22.07812500061451644, 4.541064518000418104, 2.621784821874999949 ) ) ;
#59239=CARTESIAN_POINT ( 'NONE',  ( 16.28437500061452070, 4.541064518000418104, 2.621784821874999949 ) ) ;
#59240=CARTESIAN_POINT ( 'NONE',  ( 25.09687500061451715, -3.027376345333610441, -5.243569643749999898 ) ) ;
#59241=CARTESIAN_POINT ( 'NONE',  ( -2.121784821874996840, 13.18437500061451750, 33.67503911421598417 ) ) ;
#59242=CARTESIAN_POINT ( 'NONE',  ( 4.640625000614518214, -3.027376345333614438, 5.243569643749998122 ) ) ;
#59243=CARTESIAN_POINT ( 'NONE',  ( 28.75312500061451715, 4.541064518000418104, -2.621784821874998173 ) ) ;
#59245=CARTESIAN_POINT ( 'NONE',  ( 28.94062500061452070, -3.027376345333614438, 5.243569643749998122 ) ) ;
#59247=CARTESIAN_POINT ( 'NONE',  ( 0.000000000000000000, 20.00000000000000000, -30.00000000000000000 ) ) ;
#59248=CARTESIAN_POINT ( 'NONE',  ( 29.25000000122903288, -2.886751345948129988, 4.999999999999997335 ) ) ;
#59249=CARTESIAN_POINT ( 'NONE',  ( 7.434375000614519280, -4.541064518000419881, 2.621784821874995952 ) ) ;
#59250=CARTESIAN_POINT ( 'NONE',  ( 15.48750000122903359, 6.123233995736764310E-16, -4.999999999999998224 ) ) ;
#59251=CARTESIAN_POINT ( 'NONE',  ( 29.61562500061451431, 3.027376345333613106, -5.243569643749998122 ) ) ;
#59252=CARTESIAN_POINT ( 'NONE',  ( 10.76250000122903572, 0.000000000000000000, 4.999999999999998224 ) ) ;
#59253=CARTESIAN_POINT ( 'NONE',  ( 4.228125000614517681, -4.541064518000419881, 2.621784821874995952 ) ) ;
#59256=CARTESIAN_POINT ( 'NONE',  ( 15.04687500061451644, -3.027376345333614438, 5.243569643749998122 ) ) ;
#59257=ORIENTED_EDGE ( 'NONE', *, *, #10249, .F. ) ;
#59258=CARTESIAN_POINT ( 'NONE',  ( 22.82812500061451644, 6.421520780324663323E-16, -5.243569643749999010 ) ) ;
#59259=CARTESIAN_POINT ( 'NONE',  ( 7.678125000614516082, 4.541064518000418104, 2.621784821874999949 ) ) ;
#59260=CARTESIAN_POINT ( 'NONE',  ( 24.12187500061451573, -6.054752690667223547, -1.112240025338166033E-15 ) ) ;
#59261=CARTESIAN_POINT ( 'NONE',  ( 8.240625000614516082, -3.027376345333614438, 5.243569643749998122 ) ) ;
#59262=CARTESIAN_POINT ( 'NONE',  ( 30.00000000000000000, 0.000000000000000000, 0.000000000000000000 ) ) ;
#59263=CARTESIAN_POINT ( 'NONE',  ( 8.437500001229034652, 4.330127018922191873, 2.499999999999999556 ) ) ;
#59264=CARTESIAN_POINT ( 'NONE',  ( 24.59062500061451573, -3.027376345333610441, -5.243569643749999898 ) ) ;
#59265=AXIS2_PLACEMENT_3D ( 'NONE', #22696, #56682, #72230 ) ;
#59266=CARTESIAN_POINT ( 'NONE',  ( 1.999999999999998668, 19.51250000122903216, -33.46410161513775705 ) ) ;
#59267=CARTESIAN_POINT ( 'NONE',  ( 11.13750000122903216, 4.330127018922191873, 2.499999999999999556 ) ) ;
#59268=CARTESIAN_POINT ( 'NONE',  ( 20.39062500061451644, -3.027376345333614438, 5.243569643749998122 ) ) ;
#59269=CARTESIAN_POINT ( 'NONE',  ( 18.32812500061451644, 6.421520780324663323E-16, -5.243569643749999010 ) ) ;
#59271=CARTESIAN_POINT ( 'NONE',  ( 17.43750000000000355, -2.886751345948129988, 4.999999999999997335 ) ) ;
#59272=CARTESIAN_POINT ( 'NONE',  ( 14.28750000122903430, 4.330127018922191873, 2.499999999999999556 ) ) ;
#59273=CARTESIAN_POINT ( 'NONE',  ( 9.590625000614517504, -3.027376345333614438, 5.243569643749998122 ) ) ;
#59274=CARTESIAN_POINT ( 'NONE',  ( 13.45312500061451466, 4.541064518000418104, -2.621784821874998173 ) ) ;
#59275=CARTESIAN_POINT ( 'NONE',  ( 22.80000000122903359, 5.773502691896255534, 3.535250795749688894E-16 ) ) ;
#59276=CARTESIAN_POINT ( 'NONE',  ( 22.99687500061451573, 6.054752690667223547, 3.707466751127219781E-16 ) ) ;
#59277=CARTESIAN_POINT ( 'NONE',  ( 21.79687500061451644, -3.027376345333614438, 5.243569643749998122 ) ) ;
#59279=CARTESIAN_POINT ( 'NONE',  ( 7.312500001229033764, -4.330127018922190985, -2.500000000000001332 ) ) ;
#59280=CARTESIAN_POINT ( 'NONE',  ( 7.021875000614518747, -6.054752690667223547, -1.112240025338166033E-15 ) ) ;
#59281=CARTESIAN_POINT ( 'NONE',  ( 23.18437500061451573, -4.541064518000419881, 2.621784821874995952 ) ) ;
#59282=CARTESIAN_POINT ( 'NONE',  ( 10.57500000000000107, 4.330127018922191873, 2.499999999999999556 ) ) ;
#59283=CARTESIAN_POINT ( 'NONE',  ( 18.74062500061451431, -3.027376345333610441, -5.243569643749999898 ) ) ;
#59284=CARTESIAN_POINT ( 'NONE',  ( 24.08437500061451786, -4.541064518000419881, 2.621784821874995952 ) ) ;
#59287=DIRECTION ( 'NONE',  ( -1.000000000000000000, -0.000000000000000000, -0.000000000000000000 ) ) ;
#59288=CARTESIAN_POINT ( 'NONE',  ( 5.634375000614519458, -4.541064518000419881, 2.621784821874995952 ) ) ;
#59289=CARTESIAN_POINT ( 'NONE',  ( 17.46562500061451217, 3.027376345333613106, -5.243569643749998122 ) ) ;
#59290=EDGE_LOOP ( 'NONE', ( #42607, #34711, #27636, #45621 ) ) ;
#59291=CARTESIAN_POINT ( 'NONE',  ( 24.55312500061451786, -4.541064518000417216, -2.621784821875001281 ) ) ;
#59292=CARTESIAN_POINT ( 'NONE',  ( 3.430292791878407410, 3.637806684167773863, -3.517583096594174119 ) ) ;
#59294=CARTESIAN_POINT ( 'NONE',  ( 15.71250000000000213, -5.773502691896255534, -1.060575238724906372E-15 ) ) ;
#59295=CARTESIAN_POINT ( 'NONE',  ( 27.60000000122903430, -2.886751345948125991, -5.000000000000000000 ) ) ;
#59296=CARTESIAN_POINT ( 'NONE',  ( 21.62812500061451360, 4.541064518000418104, 2.621784821874999949 ) ) ;
#59297=ORIENTED_EDGE ( 'NONE', *, *, #61121, .F. ) ;
#59298=CARTESIAN_POINT ( 'NONE',  ( 22.27499999999999858, 4.330127018922191873, 2.499999999999999556 ) ) ;
#59299=CARTESIAN_POINT ( 'NONE',  ( 22.77187500061451786, -6.054752690667223547, -1.112240025338166033E-15 ) ) ;
#59300=VERTEX_POINT ( 'NONE', #35665 ) ;
#59301=CARTESIAN_POINT ( 'NONE',  ( 13.42500000122903536, 2.886751345948126879, 4.999999999999998224 ) ) ;
#59302=CARTESIAN_POINT ( 'NONE',  ( 13.22812500061451502, -4.541064518000419881, 2.621784821874995952 ) ) ;
#59303=CARTESIAN_POINT ( 'NONE',  ( 3.478125000614517237, 6.421520780324663323E-16, -5.243569643749999010 ) ) ;
#59305=CARTESIAN_POINT ( 'NONE',  ( 27.89062500061451289, 6.054752690667223547, 3.707466751127219781E-16 ) ) ;
#59306=CARTESIAN_POINT ( 'NONE',  ( 13.27500000122903323, 2.886751345948129099, -4.999999999999998224 ) ) ;
#59307=CARTESIAN_POINT ( 'NONE',  ( 20.24999999999999645, -4.330127018922190985, -2.500000000000001332 ) ) ;
#59308=CARTESIAN_POINT ( 'NONE',  ( 26.02499999999999858, -4.330127018922194537, 2.499999999999995559 ) ) ;
#59310=CARTESIAN_POINT ( 'NONE',  ( 8.034375000614518925, 6.421520780324663323E-16, -5.243569643749999010 ) ) ;
#59311=CARTESIAN_POINT ( 'NONE',  ( 16.99687500061451573, -3.027376345333610441, -5.243569643749999898 ) ) ;
#59312=CARTESIAN_POINT ( 'NONE',  ( -1.071796769724491005, 13.72009619066136921, 26.00000000000000355 ) ) ;
#59313=ORIENTED_EDGE ( 'NONE', *, *, #64489, .T. ) ;
#59314=CARTESIAN_POINT ( 'NONE',  ( 28.56562500061451715, -6.054752690667223547, -1.112240025338166033E-15 ) ) ;
#59315=CARTESIAN_POINT ( 'NONE',  ( 3.525000000000000355, -4.330127018922194537, 2.499999999999995559 ) ) ;
#59317=CARTESIAN_POINT ( 'NONE',  ( 17.02499999999999858, -4.330127018922194537, 2.499999999999995559 ) ) ;
#59318=CARTESIAN_POINT ( 'NONE',  ( 12.59062500061451573, 6.054752690667223547, 3.707466751127219781E-16 ) ) ;
#59319=CARTESIAN_POINT ( 'NONE',  ( -5.810221930991193690E-16, 11.45000000122903216, 26.00000000000000355 ) ) ;
#59320=CARTESIAN_POINT ( 'NONE',  ( 4.064219793244338241, -3.782806921759631624, -3.447986216289088635 ) ) ;
#59321=CARTESIAN_POINT ( 'NONE',  ( 19.42500000122903714, -5.773502691896255534, -1.060575238724906372E-15 ) ) ;
#59322=CARTESIAN_POINT ( 'NONE',  ( 3.752440054025286909, -3.304420318444254878, 4.071342403668507082 ) ) ;
#59324=CARTESIAN_POINT ( 'NONE',  ( 7.865625000614516971, -6.054752690667223547, -1.112240025338166033E-15 ) ) ;
#59325=CARTESIAN_POINT ( 'NONE',  ( 23.78437500061451360, 6.421520780324663323E-16, -5.243569643749999010 ) ) ;
#59326=CARTESIAN_POINT ( 'NONE',  ( -2.121784821874996840, 16.78437500061452070, 33.67503911421598417 ) ) ;
#59327=CARTESIAN_POINT ( 'NONE',  ( 24.42187500061451999, 3.027376345333611329, 5.243569643749999010 ) ) ;
#59328=CARTESIAN_POINT ( 'NONE',  ( 5.850000000000001421, -4.330127018922190985, -2.500000000000001332 ) ) ;
#59329=CARTESIAN_POINT ( 'NONE',  ( 8.484601909799253346E-16, 10.32500000122903572, 34.61880215351700230 ) ) ;
#59330=CARTESIAN_POINT ( 'NONE',  ( 13.00312500061451537, 4.541064518000418104, -2.621784821874998173 ) ) ;
#59331=CARTESIAN_POINT ( 'NONE',  ( 3.862500001229035362, 4.330127018922192761, -2.499999999999997780 ) ) ;
#59333=CARTESIAN_POINT ( 'NONE',  ( 8.821875000614518569, -6.054752690667223547, -1.112240025338166033E-15 ) ) ;
#59336=CARTESIAN_POINT ( 'NONE',  ( 10.82812500061451644, 4.541064518000418104, 2.621784821874999949 ) ) ;
#59337=CARTESIAN_POINT ( 'NONE',  ( 13.84687500061451537, -3.027376345333610441, -5.243569643749999898 ) ) ;
#59339=CARTESIAN_POINT ( 'NONE',  ( 23.92500000122903359, -5.773502691896255534, -1.060575238724906372E-15 ) ) ;
#59340=CARTESIAN_POINT ( 'NONE',  ( 10.92187500061451644, 3.027376345333611329, 5.243569643749999010 ) ) ;
#59341=CARTESIAN_POINT ( 'NONE',  ( 13.07812500061451821, 4.541064518000418104, 2.621784821874999949 ) ) ;
#59343=CARTESIAN_POINT ( 'NONE',  ( 22.20937500061451431, 0.000000000000000000, 5.243569643749999010 ) ) ;
#59345=CARTESIAN_POINT ( 'NONE',  ( 4.387500001229033053, 4.330127018922191873, 2.499999999999999556 ) ) ;
#59346=CARTESIAN_POINT ( 'NONE',  ( 13.68750000122903288, 6.123233995736764310E-16, -4.999999999999998224 ) ) ;
#59347=CARTESIAN_POINT ( 'NONE',  ( -4.243569643749999898, 15.32187500061451502, -32.45002607614398471 ) ) ;
#59348=CARTESIAN_POINT ( 'NONE',  ( 15.42187500061451821, 3.027376345333611329, 5.243569643749999010 ) ) ;
#59349=CARTESIAN_POINT ( 'NONE',  ( 18.82500000122903216, 2.886751345948126879, 4.999999999999999112 ) ) ;
#59350=CARTESIAN_POINT ( 'NONE',  ( 11.10937500061451644, -4.541064518000417216, -2.621784821875001281 ) ) ;
#59351=CARTESIAN_POINT ( 'NONE',  ( -2.121784821874999949, 18.37812500061451715, -33.67503911421598417 ) ) ;
#59352=CARTESIAN_POINT ( 'NONE',  ( 18.07500000122903216, -5.773502691896255534, -1.060575238724906372E-15 ) ) ;
#59353=CARTESIAN_POINT ( 'NONE',  ( 13.79062500061451502, -3.027376345333610441, -5.243569643749999898 ) ) ;
#59354=VERTEX_POINT ( 'NONE', #69655 ) ;
#59355=CARTESIAN_POINT ( 'NONE',  ( 15.63749999999999751, -2.886751345948129988, 4.999999999999997335 ) ) ;
#59356=CARTESIAN_POINT ( 'NONE',  ( 4.642109779777202405, 1.860292132678681210, -4.642109779777202405 ) ) ;
#59357=CARTESIAN_POINT ( 'NONE',  ( 9.384375000614518569, 6.421520780324663323E-16, -5.243569643749999010 ) ) ;
#59358=CARTESIAN_POINT ( 'NONE',  ( 3.089506346739232967, 3.931278485869285522, -3.469880700456108968 ) ) ;
#59359=CARTESIAN_POINT ( 'NONE',  ( 13.57500000122903572, -5.773502691896255534, -1.060575238724906372E-15 ) ) ;
#59360=CARTESIAN_POINT ( 'NONE',  ( 21.56250000122903288, 0.000000000000000000, 4.999999999999998224 ) ) ;
#59361=CARTESIAN_POINT ( 'NONE',  ( 17.24062500061451786, -3.027376345333614438, 5.243569643749998122 ) ) ;
#59363=CARTESIAN_POINT ( 'NONE',  ( 21.36562500061451431, -6.054752690667223547, -1.112240025338166033E-15 ) ) ;
#59364=CARTESIAN_POINT ( 'NONE',  ( 26.88750000122903216, 4.330127018922191873, 2.499999999999999556 ) ) ;
#59365=CARTESIAN_POINT ( 'NONE',  ( 24.97499999999999787, 4.330127018922191873, 2.499999999999999556 ) ) ;
#59366=CARTESIAN_POINT ( 'NONE',  ( 28.31249999999999645, -5.773502691896255534, -1.060575238724906372E-15 ) ) ;
#59368=CARTESIAN_POINT ( 'NONE',  ( 27.79687500061451999, -3.027376345333610441, -5.243569643749999898 ) ) ;
#59369=CARTESIAN_POINT ( 'NONE',  ( 11.55000000000000071, 0.000000000000000000, 4.999999999999998224 ) ) ;
#59370=CARTESIAN_POINT ( 'NONE',  ( -4.243569643749999898, 13.55937500061451750, -30.00000000000000000 ) ) ;
#59371=CARTESIAN_POINT ( 'NONE',  ( 3.862500001229035362, 4.330127018922192761, -2.499999999999997780 ) ) ;
#59372=CARTESIAN_POINT ( 'NONE',  ( 4.387500000000002842, -2.886751345948129988, 4.999999999999997335 ) ) ;
#59373=EDGE_CURVE ( 'NONE', #15563, #46535, #19019, .T. ) ;
#59374=CARTESIAN_POINT ( 'NONE',  ( 16.50000000000000000, 0.000000000000000000, 4.999999999999998224 ) ) ;
#59375=CARTESIAN_POINT ( 'NONE',  ( 8.484375000614518214, 6.421520780324663323E-16, -5.243569643749999010 ) ) ;
#59376=CARTESIAN_POINT ( 'NONE',  ( 26.24062500061451431, -3.027376345333614438, 5.243569643749998122 ) ) ;
#59377=FACE_OUTER_BOUND ( 'NONE', #12388, .T. ) ;
#59378=ADVANCED_FACE ( 'NONE', ( #46766 ), #58547, .F. ) ;
#59380=CARTESIAN_POINT ( 'NONE',  ( 8.212500000000000355, 2.886751345948129099, -4.999999999999997335 ) ) ;
#59381=CARTESIAN_POINT ( 'NONE',  ( 4.696875000614518569, -3.027376345333614438, 5.243569643749998122 ) ) ;
#59382=CARTESIAN_POINT ( 'NONE',  ( 8.859375000614518214, -4.541064518000417216, -2.621784821875001281 ) ) ;
#59383=CARTESIAN_POINT ( 'NONE',  ( 5.137500000000000178, 5.773502691896255534, 3.535250795749688894E-16 ) ) ;
#59384=CARTESIAN_POINT ( 'NONE',  ( 4.243569643749999010, 12.86562500061459247, 27.54997392385601174 ) ) ;
#59385=CARTESIAN_POINT ( 'NONE',  ( 28.57499999999999929, 4.330127018922191873, 2.499999999999999556 ) ) ;
#59387=CARTESIAN_POINT ( 'NONE',  ( 3.262500000000001510, 2.886751345948129099, -4.999999999999998224 ) ) ;
#59389=CARTESIAN_POINT ( 'NONE',  ( 21.10312500061451502, 4.541064518000418104, -2.621784821874998173 ) ) ;
#59390=CARTESIAN_POINT ( 'NONE',  ( 10.64062500061451644, -3.027376345333610441, -5.243569643749999898 ) ) ;
#59392=CARTESIAN_POINT ( 'NONE',  ( 9.309375000614517504, -4.541064518000417216, -2.621784821875001281 ) ) ;
#59393=CARTESIAN_POINT ( 'NONE',  ( 26.62500000000000000, 6.123233995736764310E-16, -4.999999999999998224 ) ) ;
#59394=CARTESIAN_POINT ( 'NONE',  ( 20.17500000122903359, 2.886751345948126879, 4.999999999999999112 ) ) ;
#59395=CARTESIAN_POINT ( 'NONE',  ( 27.44062500061451715, 6.054752690667223547, 3.707466751127219781E-16 ) ) ;
#59397=CARTESIAN_POINT ( 'NONE',  ( 8.446875000614518569, -3.027376345333610441, -5.243569643749999898 ) ) ;
#59398=CARTESIAN_POINT ( 'NONE',  ( 14.67187500061451821, -6.054752690667223547, -1.112240025338166033E-15 ) ) ;
#59399=CARTESIAN_POINT ( 'NONE',  ( 26.18437500061451573, 4.541064518000418104, 2.621784821874999949 ) ) ;
#59403=CARTESIAN_POINT ( 'NONE',  ( 21.04687500061451644, -3.027376345333610441, -5.243569643749999898 ) ) ;
#59404=( BOUNDED_CURVE ( )  B_SPLINE_CURVE ( 3, ( #27700, #67235, #61308, #22148 ),
 .UNSPECIFIED., .F., .F. ) 
 B_SPLINE_CURVE_WITH_KNOTS ( ( 4, 4 ),
 ( 4.712388980384689674, 6.283185307179586232 ),
 .UNSPECIFIED. ) 
 CURVE ( )  GEOMETRIC_REPRESENTATION_ITEM ( )  RATIONAL_B_SPLINE_CURVE ( ( 1.000000000000000000, 0.8047378541243649375, 0.8047378541243649375, 1.000000000000000000 ) ) 
 REPRESENTATION_ITEM ( '' )  );
#59405=CARTESIAN_POINT ( 'NONE',  ( 12.12187500061451573, 3.027376345333613106, -5.243569643749998122 ) ) ;
#59407=CARTESIAN_POINT ( 'NONE',  ( 23.85000000000000142, -4.330127018922190985, -2.500000000000001332 ) ) ;
#59409=CARTESIAN_POINT ( 'NONE',  ( 2.121784821874999061, 11.60937500061451821, -33.67503911421598417 ) ) ;
#59411=CARTESIAN_POINT ( 'NONE',  ( 14.95312500061451644, 0.000000000000000000, 5.243569643749999010 ) ) ;
#59412=CARTESIAN_POINT ( 'NONE',  ( 3.525000000000000355, -4.330127018922194537, 2.499999999999995559 ) ) ;
#59414=FACE_OUTER_BOUND ( 'NONE', #40339, .T. ) ;
#59415=( BOUNDED_CURVE ( )  B_SPLINE_CURVE ( 2, ( #23111, #27952, #62286, #44588, #33842, #39035, #5050, #15750, #34197, #28664, #16119, #33472, #49754, #51203, #55295, #56385, #66374, #38289, #10589, #28307, #32758, #50842, #72281, #242, #61194, #50119, #50484, #67120, #45301, #61549, #22751, #66749, #27587, #67835, #16843, #72650, #38672, #17208, #4689, #11682, #21660, #33117, #10951, #67480, #73009, #27219, #12751, #18274, #12035, #47106, #51567, #41208, #68203, #34560, #6496, #40481, #40126, #46023, #68560, #40848, #63716, #36010, #58528, #24194, #35286, #17918, #68917, #62996, #52642, #19000, #12391, #63366, #62640, #2049, #17564, #967, #34927, #35646, #24560, #51926, #7217, #57088, #29031, #1323, #46748, #57808, #69638, #58168, #29746, #23477, #57454, #6859, #29392, #23833, #46383, #52284, #1685, #69282, #7573, #18644, #2400, #41561, #13108, #30108, #64079, #13461, #7938, #30476, #53005, #45668, #2765, #26395, #36740, #71466, #31200, #64814, #65179, #14204, #8669, #47833, #19365, #42655, #54474, #31937, #20842, #30835, #25287, #48937, #59629, #3509, #9767, #3872, #70363, #41923, #19741, #54836, #9042, #43396, #53742, #71093, #70723, #42290, #64449, #37477, #65549, #69996, #65918, #54111, #15299, #37838, #14938, #59997, #60358, #59260, #32301, #3135, #9407, #53368, #24921, #25664, #48201, #47463, #31572, #26028, #48567, #20467, #43021, #13840, #36379, #58895, #8305, #20098, #14570, #37103, #157, #10138, #50399, #22663, #71836, #49668, #61106, #55211, #28224, #38948, #55930, #62198, #56299, #4604, #21206, #72196, #34111, #61466, #50754, #33031, #72924, #50032, #66656, #26770, #45213, #17119, #27135, #33754, #33394, #5689, #11231, #67394, #16756, #67747, #21575, #39678, #16033, #61826, #32670, #39314, #44129, #10503, #67033, #55570, #11594, #27498, #22306, #10861, #4243, #43759, #49302, #27867, #60727, #38581, #4965, #21945, #38201, #72557, #44500, #5326, #16393, #44858, #66284, #15662, #41121, #17828, #35559, #69555, #23024, #57724, #68112, #63633, #1965, #17478, #34838, #13021, #40389, #41475, #6045, #63995, #34473, #45580, #513, #28579, #18916, #40038, #62552, #13376, #28940, #62908, #1238, #12302, #6408, #51478, #23386, #879, #11948, #58079, #57364, #56650, #51116, #57001, #45935, #68466, #7487, #6772, #23743, #29304, #51834, #46291, #68832, #18188, #40758, #63273, #52559, #12665, #35202, #30016, #7129, #24108, #24474, #46656, #47020, #29659, #52196, #1597, #69196, #18556, #35919, #69910, #25194, #20751, #14850, #59174, #3043, #42933, #30390, #65093, #42204, #59913, #53279, #37017, #7854, #2317, #13752, #37389, #47739, #3422, #65458, #25942, #9319, #19648, #54027, #31852, #41831, #8952, #54388, #52919, #8219, #64728, #20382, #24832, #64362, #48482, #71006, #25574, #8582, #47380, #30747, #65829, #70637, #3784, #14114, #31485, #31111, #70277, #58443, #26308, #48846, #58808, #48114, #19278, #71376, #36294, #43309, #2678, #36653, #53650, #20012, #42565, #14483, #59541, #27775, #10050, #72102, #4874, #44039, #67308, #38490, #61378, #15574, #4520, #16666, #38862, #21487, #38116, #39224, #15942, #32944, #49217, #66196, #71751, #66940, #66562, #27410, #55482, #61015, #72837, #49580, #61736, #5603, #28139, #16308, #49941, #60637, #10412, #32583, #72465, #22219, #21850, #71, #37751, #22577, #55122, #4152, #32216, #60269, #50667, #21120, #43673, #26684, #9683, #44413, #10774, #33307, #11137, #5233, #33666, #54750, #27049, #55845, #50314, #44773, #56210, #45126, #15211, #45488, #51025, #47204, #52381, #7673, #35746, #41305, #53102, #29846, #47564, #58995, #34023, #69735, #5955, #2498, #13942, #28487, #46846, #25022, #1788, #53472, #17026, #2864, #68019, #56560, #11501, #39584, #30931, #421, #22929, #17392, #39949, #24298, #13207, #69386, #62462, #11860, #34380, #56912, #6317, #70094, #18741, #25394, #67660, #63815, #58267, #62108, #19470, #30210, #52742, #42028, #2147, #24658, #19104, #41659, #64181, #13569, #64549, #36113, #58634, #36477, #8041, #30576, #8402, #37938, #4343, #31674, #66016, #43859, #53843, #20940, #26868, #54937, #21305, #3237, #25765, #71930, #9504, #26494, #32768, #49399, #48301, #64915, #20201, #4699, #32033, #66384, #3604, #43491, #20564, #37207, #42393, #60457, #15396, #19841, #15760, #3971, #38300, #60828, #9866, #32397, #10234, #42755, #55305, #59729, #47937, #70827, #70466, #65276, #54207, #37571, #54569, #49037, #71566, #14305, #36842, #59357, #8769, #71190, #31303, #60095, #14664, #9137, #26126, #48665, #43122, #65646, #15034, #56741, #56394, #28674, #22759, #62649, #12046, #44599, #62295, #17573, #67489, #16487, #11332, #10599, #61926, #45676, #51214, #33850, #5784, #28315, #50851, #251, #23122, #66760, #33481, #27597, #6143, #16131, #614, #33127, #45311, #49766, #38683, #61204, #22040, #21670, #50129, #72660, #73019, #67846, #68212, #40135, #55664, #17218, #67130, #50493, #39044, #34207, #34569, #61558, #22403, #44227, #57098, #72292, #5060, #10960, #39779, #27229, #56031, #11691, #5423, #27961, #44951, #16852, #39408, #30486, #69647, #63726, #57464, #29042, #976, #51936, #1333, #12403, #35297, #23845, #69293, #19009, #51577, #36391, #58178, #7228, #63377, #13849, #53015, #46393, #7583, #23486, #46033, #6870, #7949, #18285, #2409, #12761, #68928, #46758, #40860, #57818, #29402, #68569, #47473, #24206, #36020, #13471, #29757, #64089, #17928, #34938, #24570, #41571 ),
 .UNSPECIFIED., .F., .F. ) 
 B_SPLINE_CURVE_WITH_KNOTS ( ( 3, 2, 2, 2, 2, 2, 2, 2, 2, 2, 2, 2, 2, 2, 2, 2, 2, 2, 2, 2, 2, 2, 2, 2, 2, 2, 2, 2, 2, 2, 2, 2, 2, 2, 2, 2, 2, 2, 2, 2, 2, 2, 2, 2, 2, 2, 2, 2, 2, 2, 2, 2, 2, 2, 2, 2, 2, 2, 2, 2, 2, 2, 2, 2, 2, 2, 2, 2, 2, 2, 2, 2, 2, 2, 2, 2, 2, 2, 2, 2, 2, 2, 2, 2, 2, 2, 2, 2, 2, 2, 2, 2, 2, 2, 2, 2, 2, 2, 2, 2, 2, 2, 2, 2, 2, 2, 2, 2, 2, 2, 2, 2, 2, 2, 2, 2, 2, 2, 2, 2, 2, 2, 2, 2, 2, 2, 2, 2, 2, 2, 2, 2, 2, 2, 2, 2, 2, 2, 2, 2, 2, 2, 2, 2, 2, 2, 2, 2, 2, 2, 2, 2, 2, 2, 2, 2, 2, 2, 2, 2, 2, 2, 2, 2, 2, 2, 2, 2, 2, 2, 2, 2, 2, 2, 2, 2, 2, 2, 2, 2, 2, 2, 2, 2, 2, 2, 2, 2, 2, 2, 2, 2, 2, 2, 2, 2, 2, 2, 2, 2, 2, 2, 2, 2, 2, 2, 2, 2, 2, 2, 2, 2, 2, 2, 2, 2, 2, 2, 2, 2, 2, 2, 2, 2, 2, 2, 2, 2, 2, 2, 2, 2, 2, 2, 2, 2, 2, 2, 2, 2, 2, 2, 2, 2, 2, 2, 2, 2, 2, 2, 2, 2, 2, 2, 2, 2, 2, 2, 2, 2, 2, 2, 2, 2, 2, 2, 2, 2, 2, 2, 2, 2, 2, 2, 2, 2, 2, 2, 2, 2, 2, 2, 2, 2, 2, 2, 2, 2, 2, 2, 2, 2, 2, 2, 2, 2, 2, 2, 2, 2, 2, 2, 2, 2, 2, 2, 2, 2, 2, 2, 2, 2, 2, 2, 2, 2, 2, 2, 2, 2, 2, 2, 2, 2, 2, 2, 2, 2, 2, 2, 2, 2, 2, 3 ),
 ( 0.000000000000000000, 0.002777777777777777884, 0.005555555555555555768, 0.008333333333333333218, 0.01111111111111111154, 0.01388888888888888812, 0.01666666666666666644, 0.01944444444444444475, 0.02222222222222222307, 0.02500000000000000139, 0.02777777777777777624, 0.03055555555555555455, 0.03333333333333333287, 0.03611111111111110772, 0.03888888888888888951, 0.04166666666666666435, 0.04444444444444444614, 0.04722222222222222099, 0.05000000000000000278, 0.05277777777777777762, 0.05555555555555555247, 0.05833333333333333426, 0.06111111111111110911, 0.06388888888888888395, 0.06666666666666666574, 0.06944444444444444753, 0.07222222222222221544, 0.07499999999999999722, 0.07777777777777777901, 0.08055555555555556080, 0.08333333333333332871, 0.08611111111111111049, 0.08888888888888889228, 0.09166666666666666019, 0.09444444444444444198, 0.09722222222222222376, 0.1000000000000000056, 0.1027777777777777873, 0.1055555555555555552, 0.1083333333333333370, 0.1111111111111111049, 0.1138888888888888867, 0.1166666666666666685, 0.1194444444444444503, 0.1222222222222222182, 0.1250000000000000000, 0.1277777777777777679, 0.1305555555555555636, 0.1333333333333333315, 0.1361111111111110994, 0.1388888888888888951, 0.1416666666666666630, 0.1444444444444444309, 0.1472222222222222265, 0.1499999999999999944, 0.1527777777777777901, 0.1555555555555555580, 0.1583333333333333259, 0.1611111111111111216, 0.1638888888888888895, 0.1666666666666666574, 0.1694444444444444253, 0.1722222222222222210, 0.1749999999999999889, 0.1777777777777777846, 0.1805555555555555525, 0.1833333333333333204, 0.1861111111111111160, 0.1888888888888888840, 0.1916666666666666796, 0.1944444444444444475, 0.1972222222222222154, 0.2000000000000000111, 0.2027777777777777790, 0.2055555555555555747, 0.2083333333333333426, 0.2111111111111111105, 0.2138888888888888784, 0.2166666666666666741, 0.2194444444444444420, 0.2222222222222222099, 0.2250000000000000056, 0.2277777777777777735, 0.2305555555555555691, 0.2333333333333333370, 0.2361111111111111049, 0.2388888888888889006, 0.2416666666666666685, 0.2444444444444444364, 0.2472222222222222321, 0.2500000000000000000, 0.2527777777777777679, 0.2555555555555555358, 0.2583333333333333592, 0.2611111111111111271, 0.2638888888888888951, 0.2666666666666666630, 0.2694444444444444309, 0.2722222222222221988, 0.2750000000000000222, 0.2777777777777777901, 0.2805555555555555580, 0.2833333333333333259, 0.2861111111111111494, 0.2888888888888888618, 0.2916666666666666852, 0.2944444444444444531, 0.2972222222222222210, 0.2999999999999999889, 0.3027777777777777568, 0.3055555555555555802, 0.3083333333333333481, 0.3111111111111111160, 0.3138888888888888840, 0.3166666666666666519, 0.3194444444444444198, 0.3222222222222222432, 0.3250000000000000111, 0.3277777777777777790, 0.3305555555555555469, 0.3333333333333333148, 0.3361111111111111382, 0.3388888888888888506, 0.3416666666666666741, 0.3444444444444444420, 0.3472222222222222099, 0.3499999999999999778, 0.3527777777777778012, 0.3555555555555555691, 0.3583333333333333370, 0.3611111111111111049, 0.3638888888888888729, 0.3666666666666666408, 0.3694444444444444642, 0.3722222222222222321, 0.3750000000000000000, 0.3777777777777777679, 0.3805555555555555358, 0.3833333333333333592, 0.3861111111111111271, 0.3888888888888888951, 0.3916666666666666630, 0.3944444444444444309, 0.3972222222222221988, 0.4000000000000000222, 0.4027777777777777901, 0.4055555555555555580, 0.4083333333333333259, 0.4111111111111111494, 0.4138888888888888618, 0.4166666666666666852, 0.4194444444444444531, 0.4222222222222222210, 0.4249999999999999889, 0.4277777777777777568, 0.4305555555555555802, 0.4333333333333333481, 0.4361111111111111160, 0.4388888888888888840, 0.4416666666666666519, 0.4444444444444444198, 0.4472222222222222432, 0.4500000000000000111, 0.4527777777777777790, 0.4555555555555555469, 0.4583333333333333148, 0.4611111111111111382, 0.4638888888888888506, 0.4666666666666666741, 0.4694444444444444420, 0.4722222222222222099, 0.4749999999999999778, 0.4777777777777778012, 0.4805555555555555691, 0.4833333333333333370, 0.4861111111111111049, 0.4888888888888888729, 0.4916666666666666408, 0.4944444444444444642, 0.4972222222222222321, 0.5000000000000000000, 0.5027777777777777679, 0.5055555555555555358, 0.5083333333333333037, 0.5111111111111110716, 0.5138888888888888395, 0.5166666666666667185, 0.5194444444444444864, 0.5222222222222222543, 0.5250000000000000222, 0.5277777777777777901, 0.5305555555555555580, 0.5333333333333333259, 0.5361111111111110938, 0.5388888888888888618, 0.5416666666666666297, 0.5444444444444443976, 0.5472222222222222765, 0.5500000000000000444, 0.5527777777777778123, 0.5555555555555555802, 0.5583333333333333481, 0.5611111111111111160, 0.5638888888888888840, 0.5666666666666666519, 0.5694444444444444198, 0.5722222222222222987, 0.5749999999999999556, 0.5777777777777777235, 0.5805555555555556024, 0.5833333333333333703, 0.5861111111111112493, 0.5888888888888889062, 0.5916666666666666741, 0.5944444444444444420, 0.5972222222222222099, 0.5999999999999999778, 0.6027777777777777457, 0.6055555555555555136, 0.6083333333333332815, 0.6111111111111111605, 0.6138888888888889284, 0.6166666666666666963, 0.6194444444444444642, 0.6222222222222222321, 0.6249999999999998890, 0.6277777777777777679, 0.6305555555555555358, 0.6333333333333333037, 0.6361111111111110716, 0.6388888888888888395, 0.6416666666666667185, 0.6444444444444444864, 0.6472222222222222543, 0.6500000000000000222, 0.6527777777777777901, 0.6555555555555555580, 0.6583333333333333259, 0.6611111111111110938, 0.6638888888888887507, 0.6666666666666666297, 0.6694444444444443976, 0.6722222222222222765, 0.6750000000000000444, 0.6777777777777777013, 0.6805555555555555802, 0.6833333333333333481, 0.6861111111111111160, 0.6888888888888888840, 0.6916666666666666519, 0.6944444444444444198, 0.6972222222222221877, 0.6999999999999999556, 0.7027777777777777235, 0.7055555555555556024, 0.7083333333333333703, 0.7111111111111111382, 0.7138888888888889062, 0.7166666666666666741, 0.7194444444444444420, 0.7222222222222222099, 0.7249999999999999778, 0.7277777777777777457, 0.7305555555555555136, 0.7333333333333332815, 0.7361111111111111605, 0.7388888888888889284, 0.7416666666666666963, 0.7444444444444444642, 0.7472222222222222321, 0.7500000000000000000, 0.7527777777777777679, 0.7555555555555555358, 0.7583333333333333037, 0.7611111111111110716, 0.7638888888888888395, 0.7666666666666667185, 0.7694444444444444864, 0.7722222222222222543, 0.7750000000000000222, 0.7777777777777777901, 0.7805555555555555580, 0.7833333333333333259, 0.7861111111111110938, 0.7888888888888888618, 0.7916666666666666297, 0.7944444444444443976, 0.7972222222222222765, 0.8000000000000000444, 0.8027777777777778123, 0.8055555555555555802, 0.8083333333333333481, 0.8111111111111111160, 0.8138888888888888840, 0.8166666666666666519, 0.8194444444444444198, 0.8222222222222222987, 0.8249999999999999556, 0.8277777777777777235, 0.8305555555555556024, 0.8333333333333333703, 0.8361111111111112493, 0.8388888888888889062, 0.8416666666666666741, 0.8444444444444444420, 0.8472222222222222099, 0.8499999999999999778, 0.8527777777777777457, 0.8555555555555555136, 0.8583333333333332815, 0.8611111111111111605, 0.8638888888888889284, 0.8666666666666666963, 0.8694444444444444642, 0.8722222222222222321, 0.8750000000000001110, 0.8777777777777777679, 0.8805555555555555358, 0.8833333333333333037, 0.8861111111111110716, 0.8888888888888888395, 0.8916666666666667185, 0.8944444444444444864, 0.8972222222222222543, 0.9000000000000000222, 0.9027777777777777901, 0.9055555555555555580, 0.9083333333333333259, 0.9111111111111110938, 0.9138888888888887507, 0.9166666666666666297, 0.9194444444444443976, 0.9222222222222222765, 0.9244751644120873246 ),
 .UNSPECIFIED. ) 
 CURVE ( )  GEOMETRIC_REPRESENTATION_ITEM ( )  RATIONAL_B_SPLINE_CURVE ( ( 1.000000000000000000, 0.8660254037844387076, 1.000000000000000000, 0.8660254037844387076, 1.000000000000000000, 0.8660254037844387076, 1.000000000000000000, 0.8660254037844387076, 1.000000000000000000, 0.8660254037844387076, 1.000000000000000000, 0.8660254037844387076, 1.000000000000000000, 0.8660254037844387076, 1.000000000000000000, 0.8660254037844387076, 1.000000000000000000, 0.8660254037844387076, 1.000000000000000000, 0.8660254037844387076, 1.000000000000000000, 0.8660254037844387076, 1.000000000000000000, 0.8660254037844387076, 1.000000000000000000, 0.8660254037844387076, 1.000000000000000000, 0.8660254037844387076, 1.000000000000000000, 0.8660254037844387076, 1.000000000000000000, 0.8660254037844387076, 1.000000000000000000, 0.8660254037844387076, 1.000000000000000000, 0.8660254037844387076, 1.000000000000000000, 0.8660254037844387076, 1.000000000000000000, 0.8660254037844387076, 1.000000000000000000, 0.8660254037844387076, 1.000000000000000000, 0.8660254037844387076, 1.000000000000000000, 0.8660254037844387076, 1.000000000000000000, 0.8660254037844387076, 1.000000000000000000, 0.8660254037844387076, 1.000000000000000000, 0.8660254037844387076, 1.000000000000000000, 0.8660254037844387076, 1.000000000000000000, 0.8660254037844387076, 1.000000000000000000, 0.8660254037844387076, 1.000000000000000000, 0.8660254037844387076, 1.000000000000000000, 0.8660254037844387076, 1.000000000000000000, 0.8660254037844387076, 1.000000000000000000, 0.8660254037844387076, 1.000000000000000000, 0.8660254037844387076, 1.000000000000000000, 0.8660254037844387076, 1.000000000000000000, 0.8660254037844387076, 1.000000000000000000, 0.8660254037844387076, 1.000000000000000000, 0.8660254037844387076, 1.000000000000000000, 0.8660254037844387076, 1.000000000000000000, 0.8660254037844387076, 1.000000000000000000, 0.8660254037844387076, 1.000000000000000000, 0.8660254037844387076, 1.000000000000000000, 0.8660254037844387076, 1.000000000000000000, 0.8660254037844387076, 1.000000000000000000, 0.8660254037844387076, 1.000000000000000000, 0.8660254037844387076, 1.000000000000000000, 0.8660254037844387076, 1.000000000000000000, 0.8660254037844387076, 1.000000000000000000, 0.8660254037844387076, 1.000000000000000000, 0.8660254037844387076, 1.000000000000000000, 0.8660254037844387076, 1.000000000000000000, 0.8660254037844387076, 1.000000000000000000, 0.8660254037844387076, 1.000000000000000000, 0.8660254037844387076, 1.000000000000000000, 0.8660254037844387076, 1.000000000000000000, 0.8660254037844387076, 1.000000000000000000, 0.8660254037844387076, 1.000000000000000000, 0.8660254037844387076, 1.000000000000000000, 0.8660254037844387076, 1.000000000000000000, 0.8660254037844387076, 1.000000000000000000, 0.8660254037844387076, 1.000000000000000000, 0.8660254037844387076, 1.000000000000000000, 0.8660254037844387076, 1.000000000000000000, 0.8660254037844387076, 1.000000000000000000, 0.8660254037844387076, 1.000000000000000000, 0.8660254037844387076, 1.000000000000000000, 0.8660254037844387076, 1.000000000000000000, 0.8660254037844387076, 1.000000000000000000, 0.8660254037844387076, 1.000000000000000000, 0.8660254037844387076, 1.000000000000000000, 0.8660254037844387076, 1.000000000000000000, 0.8660254037844387076, 1.000000000000000000, 0.8660254037844387076, 1.000000000000000000, 0.8660254037844387076, 1.000000000000000000, 0.8660254037844387076, 1.000000000000000000, 0.8660254037844387076, 1.000000000000000000, 0.8660254037844387076, 1.000000000000000000, 0.8660254037844387076, 1.000000000000000000, 0.8660254037844387076, 1.000000000000000000, 0.8660254037844387076, 1.000000000000000000, 0.8660254037844387076, 1.000000000000000000, 0.8660254037844387076, 1.000000000000000000, 0.8660254037844387076, 1.000000000000000000, 0.8660254037844387076, 1.000000000000000000, 0.8660254037844387076, 1.000000000000000000, 0.8660254037844387076, 1.000000000000000000, 0.8660254037844387076, 1.000000000000000000, 0.8660254037844387076, 1.000000000000000000, 0.8660254037844387076, 1.000000000000000000, 0.8660254037844387076, 1.000000000000000000, 0.8660254037844387076, 1.000000000000000000, 0.8660254037844387076, 1.000000000000000000, 0.8660254037844387076, 1.000000000000000000, 0.8660254037844387076, 1.000000000000000000, 0.8660254037844387076, 1.000000000000000000, 0.8660254037844387076, 1.000000000000000000, 0.8660254037844387076, 1.000000000000000000, 0.8660254037844387076, 1.000000000000000000, 0.8660254037844387076, 1.000000000000000000, 0.8660254037844387076, 1.000000000000000000, 0.8660254037844387076, 1.000000000000000000, 0.8660254037844387076, 1.000000000000000000, 0.8660254037844387076, 1.000000000000000000, 0.8660254037844387076, 1.000000000000000000, 0.8660254037844387076, 1.000000000000000000, 0.8660254037844387076, 1.000000000000000000, 0.8660254037844387076, 1.000000000000000000, 0.8660254037844387076, 1.000000000000000000, 0.8660254037844387076, 1.000000000000000000, 0.8660254037844387076, 1.000000000000000000, 0.8660254037844387076, 1.000000000000000000, 0.8660254037844387076, 1.000000000000000000, 0.8660254037844387076, 1.000000000000000000, 0.8660254037844387076, 1.000000000000000000, 0.8660254037844387076, 1.000000000000000000, 0.8660254037844387076, 1.000000000000000000, 0.8660254037844387076, 1.000000000000000000, 0.8660254037844387076, 1.000000000000000000, 0.8660254037844387076, 1.000000000000000000, 0.8660254037844387076, 1.000000000000000000, 0.8660254037844387076, 1.000000000000000000, 0.8660254037844387076, 1.000000000000000000, 0.8660254037844387076, 1.000000000000000000, 0.8660254037844387076, 1.000000000000000000, 0.8660254037844387076, 1.000000000000000000, 0.8660254037844387076, 1.000000000000000000, 0.8660254037844387076, 1.000000000000000000, 0.8660254037844387076, 1.000000000000000000, 0.8660254037844387076, 1.000000000000000000, 0.8660254037844387076, 1.000000000000000000, 0.8660254037844387076, 1.000000000000000000, 0.8660254037844387076, 1.000000000000000000, 0.8660254037844387076, 1.000000000000000000, 0.8660254037844387076, 1.000000000000000000, 0.8660254037844387076, 1.000000000000000000, 0.8660254037844387076, 1.000000000000000000, 0.8660254037844387076, 1.000000000000000000, 0.8660254037844387076, 1.000000000000000000, 0.8660254037844387076, 1.000000000000000000, 0.8660254037844387076, 1.000000000000000000, 0.8660254037844387076, 1.000000000000000000, 0.8660254037844387076, 1.000000000000000000, 0.8660254037844387076, 1.000000000000000000, 0.8660254037844387076, 1.000000000000000000, 0.8660254037844387076, 1.000000000000000000, 0.8660254037844387076, 1.000000000000000000, 0.8660254037844387076, 1.000000000000000000, 0.8660254037844387076, 1.000000000000000000, 0.8660254037844387076, 1.000000000000000000, 0.8660254037844387076, 1.000000000000000000, 0.8660254037844387076, 1.000000000000000000, 0.8660254037844387076, 1.000000000000000000, 0.8660254037844387076, 1.000000000000000000, 0.8660254037844387076, 1.000000000000000000, 0.8660254037844387076, 1.000000000000000000, 0.8660254037844387076, 1.000000000000000000, 0.8660254037844387076, 1.000000000000000000, 0.8660254037844387076, 1.000000000000000000, 0.8660254037844387076, 1.000000000000000000, 0.8660254037844387076, 1.000000000000000000, 0.8660254037844387076, 1.000000000000000000, 0.8660254037844387076, 1.000000000000000000, 0.8660254037844387076, 1.000000000000000000, 0.8660254037844387076, 1.000000000000000000, 0.8660254037844387076, 1.000000000000000000, 0.8660254037844387076, 1.000000000000000000, 0.8660254037844387076, 1.000000000000000000, 0.8660254037844387076, 1.000000000000000000, 0.8660254037844387076, 1.000000000000000000, 0.8660254037844387076, 1.000000000000000000, 0.8660254037844387076, 1.000000000000000000, 0.8660254037844387076, 1.000000000000000000, 0.8660254037844387076, 1.000000000000000000, 0.8660254037844387076, 1.000000000000000000, 0.8660254037844387076, 1.000000000000000000, 0.8660254037844387076, 1.000000000000000000, 0.8660254037844387076, 1.000000000000000000, 0.8660254037844387076, 1.000000000000000000, 0.8660254037844387076, 1.000000000000000000, 0.8660254037844387076, 1.000000000000000000, 0.8660254037844387076, 1.000000000000000000, 0.8660254037844387076, 1.000000000000000000, 0.8660254037844387076, 1.000000000000000000, 0.8660254037844387076, 1.000000000000000000, 0.8660254037844387076, 1.000000000000000000, 0.8660254037844387076, 1.000000000000000000, 0.8660254037844387076, 1.000000000000000000, 0.8660254037844387076, 1.000000000000000000, 0.8660254037844387076, 1.000000000000000000, 0.8660254037844387076, 1.000000000000000000, 0.8660254037844387076, 1.000000000000000000, 0.8660254037844387076, 1.000000000000000000, 0.8660254037844387076, 1.000000000000000000, 0.8660254037844387076, 1.000000000000000000, 0.8660254037844387076, 1.000000000000000000, 0.8660254037844387076, 1.000000000000000000, 0.8660254037844387076, 1.000000000000000000, 0.8660254037844387076, 1.000000000000000000, 0.8660254037844387076, 1.000000000000000000, 0.8660254037844387076, 1.000000000000000000, 0.8660254037844387076, 1.000000000000000000, 0.8660254037844387076, 1.000000000000000000, 0.8660254037844387076, 1.000000000000000000, 0.8660254037844387076, 1.000000000000000000, 0.8660254037844387076, 1.000000000000000000, 0.8660254037844387076, 1.000000000000000000, 0.8660254037844387076, 1.000000000000000000, 0.8660254037844387076, 1.000000000000000000, 0.8660254037844387076, 1.000000000000000000, 0.8660254037844387076, 1.000000000000000000, 0.8660254037844387076, 1.000000000000000000, 0.8660254037844387076, 1.000000000000000000, 0.8660254037844387076, 1.000000000000000000, 0.8660254037844387076, 1.000000000000000000, 0.8660254037844387076, 1.000000000000000000, 0.8660254037844387076, 1.000000000000000000, 0.8660254037844387076, 1.000000000000000000, 0.8660254037844387076, 1.000000000000000000, 0.8660254037844387076, 1.000000000000000000, 0.8660254037844387076, 1.000000000000000000, 0.8660254037844387076, 1.000000000000000000, 0.8660254037844387076, 1.000000000000000000, 0.8660254037844387076, 1.000000000000000000, 0.8660254037844387076, 1.000000000000000000, 0.8660254037844387076, 1.000000000000000000, 0.8660254037844387076, 1.000000000000000000, 0.8660254037844387076, 1.000000000000000000, 0.8660254037844387076, 1.000000000000000000, 0.8660254037844387076, 1.000000000000000000, 0.8660254037844387076, 1.000000000000000000, 0.8660254037844387076, 1.000000000000000000, 0.8660254037844387076, 1.000000000000000000, 0.8660254037844387076, 1.000000000000000000, 0.8660254037844387076, 1.000000000000000000, 0.8660254037844387076, 1.000000000000000000, 0.8660254037844387076, 1.000000000000000000, 0.8660254037844387076, 1.000000000000000000, 0.8660254037844387076, 1.000000000000000000, 0.8660254037844387076, 1.000000000000000000, 0.8660254037844387076, 1.000000000000000000, 0.8660254037844387076, 1.000000000000000000, 0.8660254037844387076, 1.000000000000000000, 0.8660254037844387076, 1.000000000000000000, 0.8660254037844387076, 1.000000000000000000, 0.8660254037844387076, 1.000000000000000000, 0.8660254037844387076, 1.000000000000000000, 0.8660254037844387076, 1.000000000000000000, 0.8660254037844387076, 1.000000000000000000, 0.8660254037844387076, 1.000000000000000000, 0.8660254037844387076, 1.000000000000000000, 0.8660254037844387076, 1.000000000000000000, 0.8660254037844387076, 1.000000000000000000, 0.8660254037844387076, 1.000000000000000000, 0.8660254037844387076, 1.000000000000000000, 0.8660254037844387076, 1.000000000000000000, 0.8660254037844387076, 1.000000000000000000, 0.8660254037844387076, 1.000000000000000000, 0.8660254037844387076, 1.000000000000000000, 0.8660254037844387076, 1.000000000000000000, 0.8660254037844387076, 1.000000000000000000, 0.8660254037844387076, 1.000000000000000000, 0.8660254037844387076, 1.000000000000000000, 0.8660254037844387076, 1.000000000000000000, 0.8660254037844387076, 1.000000000000000000, 0.8660254037844387076, 1.000000000000000000, 0.8660254037844387076, 1.000000000000000000, 0.8660254037844387076, 1.000000000000000000, 0.8660254037844387076, 1.000000000000000000, 0.8660254037844387076, 1.000000000000000000, 0.8660254037844387076, 1.000000000000000000, 0.8660254037844387076, 1.000000000000000000, 0.8660254037844387076, 1.000000000000000000, 0.8660254037844387076, 1.000000000000000000, 0.8660254037844387076, 1.000000000000000000, 0.8660254037844387076, 1.000000000000000000, 0.8660254037844387076, 1.000000000000000000, 0.8660254037844387076, 1.000000000000000000, 0.8660254037844387076, 1.000000000000000000, 0.8660254037844387076, 1.000000000000000000, 0.8660254037844387076, 1.000000000000000000, 0.8660254037844387076, 1.000000000000000000, 0.8660254037844387076, 1.000000000000000000, 0.8660254037844387076, 1.000000000000000000, 0.8660254037844387076, 1.000000000000000000, 0.8660254037844387076, 1.000000000000000000, 0.8660254037844387076, 1.000000000000000000, 0.8660254037844387076, 1.000000000000000000, 0.8660254037844387076, 1.000000000000000000, 0.8660254037844387076, 1.000000000000000000, 0.8660254037844387076, 1.000000000000000000, 0.8660254037844387076, 1.000000000000000000, 0.8660254037844387076, 1.000000000000000000, 0.8660254037844387076, 1.000000000000000000, 0.8660254037844387076, 1.000000000000000000, 0.8660254037844387076, 1.000000000000000000, 0.8660254037844387076, 1.000000000000000000, 0.8660254037844387076, 1.000000000000000000, 0.8660254037844387076, 1.000000000000000000, 0.8660254037844387076, 1.000000000000000000, 0.8660254037844387076, 1.000000000000000000, 0.8660254037844387076, 1.000000000000000000, 0.8660254037844387076, 1.000000000000000000, 0.8660254037844387076, 1.000000000000000000, 0.8660254037844387076, 1.000000000000000000, 0.8660254037844387076, 1.000000000000000000, 0.8660254037844387076, 1.000000000000000000, 0.8660254037844387076, 1.000000000000000000, 0.8660254037844387076, 1.000000000000000000, 0.8660254037844387076, 1.000000000000000000, 0.8660254037844387076, 1.000000000000000000, 0.8660254037844387076, 1.000000000000000000, 0.8660254037844387076, 1.000000000000000000, 0.8660254037844387076, 1.000000000000000000, 0.8660254037844387076, 1.000000000000000000, 0.8660254037844387076, 1.000000000000000000, 0.8660254037844387076, 1.000000000000000000, 0.8660254037844387076, 1.000000000000000000, 0.8660254037844387076, 1.000000000000000000, 0.8660254037844387076, 1.000000000000000000, 0.8660254037844387076, 1.000000000000000000, 0.8660254037844387076, 1.000000000000000000, 0.8660254037844387076, 1.000000000000000000, 0.8660254037844387076, 1.000000000000000000, 0.8660254037844387076, 1.000000000000000000, 0.8660254037844387076, 1.000000000000000000, 0.8660254037844387076, 1.000000000000000000, 0.8660254037844387076, 1.000000000000000000, 0.8660254037844387076, 1.000000000000000000, 0.8660254037844387076, 1.000000000000000000, 0.8660254037844387076, 1.000000000000000000, 0.8660254037844387076, 1.000000000000000000, 0.8660254037844387076, 1.000000000000000000, 0.8913386727337029303, 0.9589388812629791037 ) ) 
 REPRESENTATION_ITEM ( '' )  );
#59416=CARTESIAN_POINT ( 'NONE',  ( 12.22499999999999964, 6.123233995736764310E-16, -4.999999999999998224 ) ) ;
#59417=CARTESIAN_POINT ( 'NONE',  ( 3.999999999999998668, 16.77500000122903145, 27.69059892324149175 ) ) ;
#59418=CARTESIAN_POINT ( 'NONE',  ( 11.47500000122903252, 2.886751345948129099, -4.999999999999998224 ) ) ;
#59419=CARTESIAN_POINT ( 'NONE',  ( 22.47187500061451715, 3.027376345333613106, -5.243569643749998122 ) ) ;
#59420=CARTESIAN_POINT ( 'NONE',  ( 16.84687500061451715, -3.027376345333614438, 5.243569643749998122 ) ) ;
#59422=ORIENTED_EDGE ( 'NONE', *, *, #10971, .F. ) ;
#59423=CARTESIAN_POINT ( 'NONE',  ( 18.02812500061451573, 4.541064518000418104, 2.621784821874999949 ) ) ;
#59424=CARTESIAN_POINT ( 'NONE',  ( 4.003125000614518925, 4.541064518000418104, -2.621784821874998173 ) ) ;
#59425=CARTESIAN_POINT ( 'NONE',  ( 18.42187500061451644, 3.027376345333613106, -5.243569643749998122 ) ) ;
#59426=CARTESIAN_POINT ( 'NONE',  ( 29.14687500061451075, -3.027376345333610441, -5.243569643749999898 ) ) ;
#59427=CARTESIAN_POINT ( 'NONE',  ( 4.865625000614517859, 3.027376345333613106, -5.243569643749998122 ) ) ;
#59428=CARTESIAN_POINT ( 'NONE',  ( 19.34062500061451573, 6.054752690667223547, 3.707466751127219781E-16 ) ) ;
#59429=CARTESIAN_POINT ( 'NONE',  ( -2.121784821874996840, 14.47812500061451679, 33.67503911421598417 ) ) ;
#59430=CARTESIAN_POINT ( 'NONE',  ( 15.48750000122903359, 6.123233995736764310E-16, -4.999999999999998224 ) ) ;
#59432=CARTESIAN_POINT ( 'NONE',  ( 6.103125000614515905, -4.541064518000417216, -2.621784821875001281 ) ) ;
#59433=CARTESIAN_POINT ( 'NONE',  ( 29.80312500061451431, 0.000000000000000000, 5.243569643749999010 ) ) ;
#59434=CARTESIAN_POINT ( 'NONE',  ( 3.999999999999998668, 19.02500000122903501, -32.30940107675850470 ) ) ;
#59435=CARTESIAN_POINT ( 'NONE',  ( 23.40937500061451715, 4.541064518000418104, -2.621784821874998173 ) ) ;
#59436=CARTESIAN_POINT ( 'NONE',  ( 13.94062500061451892, 6.054752690667223547, 3.707466751127219781E-16 ) ) ;
#59437=CARTESIAN_POINT ( 'NONE',  ( 25.27500000122903145, -5.773502691896255534, -1.060575238724906372E-15 ) ) ;
#59438=( BOUNDED_CURVE ( )  B_SPLINE_CURVE ( 2, ( #68318, #16596, #6252, #2, #16960, #72765, #69665, #39885, #5167 ),
 .UNSPECIFIED., .F., .T. ) 
 B_SPLINE_CURVE_WITH_KNOTS ( ( 3, 2, 2, 2, 3 ),
 ( 0.5326086956521739468, 0.5362318840579710644, 0.5434782608695651884, 0.5507246376811594235, 0.5543478260869565410 ),
 .UNSPECIFIED. ) 
 CURVE ( )  GEOMETRIC_REPRESENTATION_ITEM ( )  RATIONAL_B_SPLINE_CURVE ( ( 0.9330127018922194093, 0.9330127018922194093, 1.000000000000000000, 0.8660254037844387076, 1.000000000000000000, 0.8660254037844387076, 1.000000000000000000, 0.9330127018922194093, 0.9330127018922194093 ) ) 
 REPRESENTATION_ITEM ( '' )  );
#59439=CARTESIAN_POINT ( 'NONE',  ( 23.72812500061451502, 6.421520780324663323E-16, -5.243569643749999010 ) ) ;
#59440=CARTESIAN_POINT ( 'NONE',  ( 19.99687500061451573, -3.027376345333614438, 5.243569643749998122 ) ) ;
#59441=CARTESIAN_POINT ( 'NONE',  ( 15.10312500061451502, -4.541064518000417216, -2.621784821875001281 ) ) ;
#59442=CARTESIAN_POINT ( 'NONE',  ( -4.243569643749999898, 14.90937500061451715, 30.00000000000000000 ) ) ;
#59443=CARTESIAN_POINT ( 'NONE',  ( 19.00312500061451715, 0.000000000000000000, 5.243569643749999010 ) ) ;
#59444=CARTESIAN_POINT ( 'NONE',  ( 29.65312500061451573, 4.541064518000418104, -2.621784821874998173 ) ) ;
#59446=ORIENTED_EDGE ( 'NONE', *, *, #32425, .T. ) ;
#59447=CARTESIAN_POINT ( 'NONE',  ( 23.28750000000000142, -2.886751345948129988, 4.999999999999997335 ) ) ;
#59448=CARTESIAN_POINT ( 'NONE',  ( -3.999999999999997335, 10.58750000000000213, -27.69059892324149175 ) ) ;
#59449=CARTESIAN_POINT ( 'NONE',  ( 4.000000000000000000, 18.05000000122903359, 32.30940107675849760 ) ) ;
#59450=CARTESIAN_POINT ( 'NONE',  ( 25.97812500061451502, 6.421520780324663323E-16, -5.243569643749999010 ) ) ;
#59451=CARTESIAN_POINT ( 'NONE',  ( 7.640625000614517326, 6.054752690667223547, 3.707466751127219781E-16 ) ) ;
#59452=CARTESIAN_POINT ( 'NONE',  ( 19.53750000122903430, 6.123233995736764310E-16, -4.999999999999998224 ) ) ;
#59453=CARTESIAN_POINT ( 'NONE',  ( 24.62812500061451715, 6.421520780324663323E-16, -5.243569643749999010 ) ) ;
#59454=CARTESIAN_POINT ( 'NONE',  ( 22.01249999999999574, -5.773502691896255534, -1.060575238724906372E-15 ) ) ;
#59455=CARTESIAN_POINT ( 'NONE',  ( 29.01562500061451644, -6.054752690667223547, -1.112240025338166033E-15 ) ) ;
#59456=CARTESIAN_POINT ( 'NONE',  ( 7.415625000614516793, -6.054752690667223547, -1.112240025338166033E-15 ) ) ;
#59458=CARTESIAN_POINT ( 'NONE',  ( 23.57812500061451289, -4.541064518000419881, 2.621784821874995952 ) ) ;
#59459=CARTESIAN_POINT ( 'NONE',  ( 5.765625000614519102, 3.027376345333613106, -5.243569643749998122 ) ) ;
#59461=CARTESIAN_POINT ( 'NONE',  ( 3.178125000614515638, 4.541064518000418104, 2.621784821874999949 ) ) ;
#59462=CARTESIAN_POINT ( 'NONE',  ( -2.000000000000000000, 12.83750000122903501, -33.46410161513775705 ) ) ;
#59463=CARTESIAN_POINT ( 'NONE',  ( -3.999999999999999112, 10.21250000122903501, 30.00000000000000000 ) ) ;
#59464=CARTESIAN_POINT ( 'NONE',  ( 11.92500000000000071, 4.330127018922191873, 2.499999999999999556 ) ) ;
#59465=CARTESIAN_POINT ( 'NONE',  ( 10.39687500061451786, 6.054752690667223547, 3.707466751127219781E-16 ) ) ;
#59466=CARTESIAN_POINT ( 'NONE',  ( 9.000000001229034652, -2.886751345948129988, 4.999999999999997335 ) ) ;
#59467=CARTESIAN_POINT ( 'NONE',  ( 15.04687500061451644, -3.027376345333614438, 5.243569643749998122 ) ) ;
#59469=CARTESIAN_POINT ( 'NONE',  ( 6.234375000614519102, 6.421520780324663323E-16, -5.243569643749999010 ) ) ;
#59470=CARTESIAN_POINT ( 'NONE',  ( -2.121784821874996840, 10.42812500061451786, -26.32496088578401583 ) ) ;
#59471=DIRECTION ( 'NONE',  ( -1.000000000000000000, -0.000000000000000000, -0.000000000000000000 ) ) ;
#59472=CARTESIAN_POINT ( 'NONE',  ( 12.90937500061451537, -4.541064518000417216, -2.621784821875001281 ) ) ;
#59474=CARTESIAN_POINT ( 'NONE',  ( 22.41562500061451502, 3.027376345333613106, -5.243569643749998122 ) ) ;
#59475=LINE ( 'NONE', #71307, #16829 ) ;
#59476=CARTESIAN_POINT ( 'NONE',  ( -3.999999999999999112, 17.41250000122903430, 30.00000000000000000 ) ) ;
#59477=CARTESIAN_POINT ( 'NONE',  ( 27.19687500061451857, -3.027376345333614438, 5.243569643749998122 ) ) ;
#59478=EDGE_CURVE ( 'NONE', #55622, #49981, #6879, .T. ) ;
#59480=CARTESIAN_POINT ( 'NONE',  ( 5.315625000614516260, 3.027376345333613106, -5.243569643749998122 ) ) ;
#59482=CARTESIAN_POINT ( 'NONE',  ( 16.32187500061451502, 3.027376345333611329, 5.243569643749999010 ) ) ;
#59484=CARTESIAN_POINT ( 'NONE',  ( 27.41250000122903430, 0.000000000000000000, 4.999999999999998224 ) ) ;
#59485=CARTESIAN_POINT ( 'NONE',  ( 6.046875000614519102, -3.027376345333614438, 5.243569643749998122 ) ) ;
#59486=CARTESIAN_POINT ( 'NONE',  ( 16.54687500061451644, -3.027376345333610441, -5.243569643749999898 ) ) ;
#59488=CARTESIAN_POINT ( 'NONE',  ( 24.71250000000000213, -5.773502691896255534, -1.060575238724906372E-15 ) ) ;
#59489=CARTESIAN_POINT ( 'NONE',  ( 4.800000001229032698, 5.773502691896255534, 3.535250795749688894E-16 ) ) ;
#59490=CARTESIAN_POINT ( 'NONE',  ( 26.59687500061451360, 6.054752690667223547, 3.707466751127219781E-16 ) ) ;
#59493=CARTESIAN_POINT ( 'NONE',  ( 8.737500000000002487, 5.773502691896255534, 3.535250795749688894E-16 ) ) ;
#59495=CARTESIAN_POINT ( 'NONE',  ( 23.09062500061451573, -3.027376345333614438, 5.243569643749998122 ) ) ;
#59496=CARTESIAN_POINT ( 'NONE',  ( 10.98750000000000071, 5.773502691896255534, 3.535250795749688894E-16 ) ) ;
#59497=CARTESIAN_POINT ( 'NONE',  ( 5.578125000614518214, -4.541064518000419881, 2.621784821874995952 ) ) ;
#59498=CARTESIAN_POINT ( 'NONE',  ( 20.10000000000000142, 0.000000000000000000, 4.999999999999998224 ) ) ;
#59499=CARTESIAN_POINT ( 'NONE',  ( 19.56562500061451715, -6.054752690667223547, -1.112240025338166033E-15 ) ) ;
#59500=CARTESIAN_POINT ( 'NONE',  ( 4.177602232894093603, -2.747429830345227142, 4.435137505375752909 ) ) ;
#59501=CARTESIAN_POINT ( 'NONE',  ( 23.58750000122903145, 6.123233995736764310E-16, -4.999999999999998224 ) ) ;
#59503=CARTESIAN_POINT ( 'NONE',  ( 3.487500000000000711, -2.886751345948129988, 4.999999999999997335 ) ) ;
#59505=CARTESIAN_POINT ( 'NONE',  ( 20.09062500061451573, -3.027376345333610441, -5.243569643749999898 ) ) ;
#59506=CARTESIAN_POINT ( 'NONE',  ( 25.79062500061451502, -3.027376345333614438, 5.243569643749998122 ) ) ;
#59507=CARTESIAN_POINT ( 'NONE',  ( 23.82187500061451502, 3.027376345333613106, -5.243569643749998122 ) ) ;
#59508=CARTESIAN_POINT ( 'NONE',  ( 7.837499999999999467, 5.773502691896255534, 3.535250795749688894E-16 ) ) ;
#59509=CARTESIAN_POINT ( 'NONE',  ( 11.61562500061451608, 3.027376345333613106, -5.243569643749998122 ) ) ;
#59510=CARTESIAN_POINT ( 'NONE',  ( 25.94062500061451715, -3.027376345333610441, -5.243569643749999898 ) ) ;
#59511=CARTESIAN_POINT ( 'NONE',  ( 16.62187500061451573, 3.027376345333613106, -5.243569643749998122 ) ) ;
#59512=CARTESIAN_POINT ( 'NONE',  ( 9.103125000614515017, 0.000000000000000000, 5.243569643749999010 ) ) ;
#59514=CARTESIAN_POINT ( 'NONE',  ( -4.243569643749999898, 11.30937500061451928, 30.00000000000000000 ) ) ;
#59516=CARTESIAN_POINT ( 'NONE',  ( 24.75000000122902932, -2.886751345948129988, 4.999999999999997335 ) ) ;
#59518=CARTESIAN_POINT ( 'NONE',  ( 14.84062500061451750, 6.054752690667223547, 3.707466751127219781E-16 ) ) ;
#59519=CARTESIAN_POINT ( 'NONE',  ( 10.02187500061451964, 3.027376345333611329, 5.243569643749999010 ) ) ;
#59520=CARTESIAN_POINT ( 'NONE',  ( 10.35937500061451644, 4.541064518000418104, -2.621784821874998173 ) ) ;
#59521=ORIENTED_EDGE ( 'NONE', *, *, #16132, .T. ) ;
#59522=CARTESIAN_POINT ( 'NONE',  ( 15.22500000000000142, -4.330127018922194537, 2.499999999999995559 ) ) ;
#59523=CARTESIAN_POINT ( 'NONE',  ( 21.40312500061451573, -4.541064518000417216, -2.621784821875001281 ) ) ;
#59524=CARTESIAN_POINT ( 'NONE',  ( 15.98437500061451821, -4.541064518000419881, 2.621784821874995952 ) ) ;
#59525=CARTESIAN_POINT ( 'NONE',  ( 21.77812500061451928, -4.541064518000419881, 2.621784821874995952 ) ) ;
#59526=CARTESIAN_POINT ( 'NONE',  ( 1.999999999999998668, 11.75000000000000178, 26.53589838486224650 ) ) ;
#59527=AXIS2_PLACEMENT_3D ( 'NONE', #44517, #6063, #38598 ) ;
#59528=CARTESIAN_POINT ( 'NONE',  ( 26.24062500061451431, -3.027376345333614438, 5.243569643749998122 ) ) ;
#59529=CARTESIAN_POINT ( 'NONE',  ( 7.387500001229032165, 6.123233995736764310E-16, -4.999999999999998224 ) ) ;
#59531=CARTESIAN_POINT ( 'NONE',  ( 3.300000001229034918, -2.886751345948125991, -5.000000000000000000 ) ) ;
#59532=CARTESIAN_POINT ( 'NONE',  ( -2.000000000000000000, 17.22500000000000142, -33.46410161513775705 ) ) ;
#59533=CARTESIAN_POINT ( 'NONE',  ( 25.27500000122903145, -5.773502691896255534, -1.060575238724906372E-15 ) ) ;
#59535=CARTESIAN_POINT ( 'NONE',  ( 6.609375000614519102, -4.541064518000417216, -2.621784821875001281 ) ) ;
#59536=DIRECTION ( 'NONE',  ( 0.000000000000000000, 0.000000000000000000, 1.000000000000000000 ) ) ;
#59538=CARTESIAN_POINT ( 'NONE',  ( 16.04062500061451857, -3.027376345333610441, -5.243569643749999898 ) ) ;
#59539=CARTESIAN_POINT ( 'NONE',  ( 8.671875000614518214, 3.027376345333611329, 5.243569643749999010 ) ) ;
#59540=CARTESIAN_POINT ( 'NONE',  ( 26.62500000122903288, -5.773502691896255534, -1.060575238724906372E-15 ) ) ;
#59541=CARTESIAN_POINT ( 'NONE',  ( 16.17187500061451644, 3.027376345333612662, -5.243569643749998122 ) ) ;
#59542=CARTESIAN_POINT ( 'NONE',  ( 5.821875000614519458, 3.027376345333613106, -5.243569643749998122 ) ) ;
#59543=CARTESIAN_POINT ( 'NONE',  ( 4.861368277861656928, -1.180116475822727162, 4.861368277861656928 ) ) ;
#59544=CARTESIAN_POINT ( 'NONE',  ( 6.478125000614516793, -4.541064518000419881, 2.621784821874995952 ) ) ;
#59545=CARTESIAN_POINT ( 'NONE',  ( 15.21562500061451750, 3.027376345333613106, -5.243569643749998122 ) ) ;
#59546=ORIENTED_EDGE ( 'NONE', *, *, #28336, .T. ) ;
#59547=CARTESIAN_POINT ( 'NONE',  ( 13.49062500061451608, 6.054752690667223547, 3.707466751127219781E-16 ) ) ;
#59548=CARTESIAN_POINT ( 'NONE',  ( 6.562500001229032875, 4.330127018922192761, -2.499999999999997780 ) ) ;
#59550=CARTESIAN_POINT ( 'NONE',  ( 11.35312500061451679, 0.000000000000000000, 5.243569643749999010 ) ) ;
#59552=CARTESIAN_POINT ( 'NONE',  ( 9.825000000000001066, -4.330127018922194537, 2.499999999999995559 ) ) ;
#59553=CARTESIAN_POINT ( 'NONE',  ( 4.162500001229033408, -4.330127018922190985, -2.500000000000001332 ) ) ;
#59554=CARTESIAN_POINT ( 'NONE',  ( 21.44999999999999929, 0.000000000000000000, 4.999999999999998224 ) ) ;
#59555=CARTESIAN_POINT ( 'NONE',  ( 15.45937500061451608, 0.000000000000000000, 5.243569643749999010 ) ) ;
#59556=CARTESIAN_POINT ( 'NONE',  ( 16.20000000122903216, -2.886751345948129988, 4.999999999999997335 ) ) ;
#59558=CARTESIAN_POINT ( 'NONE',  ( -4.243569643749997233, 17.14062500061451644, -27.54997392385601174 ) ) ;
#59559=CARTESIAN_POINT ( 'NONE',  ( 12.07500000122903039, 2.886751345948193936, 4.999999999999883649 ) ) ;
#59561=DIRECTION ( 'NONE',  ( -0.000000000000000000, -1.000000000000000000, -0.000000000000000000 ) ) ;
#59562=CARTESIAN_POINT ( 'NONE',  ( 3.455719506257207918, -3.613630455596491320, 3.583513068947109748 ) ) ;
#59564=CARTESIAN_POINT ( 'NONE',  ( 15.87187500061451573, 3.027376345333611329, 5.243569643749999010 ) ) ;
#59565=CARTESIAN_POINT ( 'NONE',  ( 28.76249999999999929, -5.773502691896255534, -1.060575238724906372E-15 ) ) ;
#59566=CARTESIAN_POINT ( 'NONE',  ( 11.31562500061451892, 3.027376345333611329, 5.243569643749999010 ) ) ;
#59568=CARTESIAN_POINT ( 'NONE',  ( 23.22187500061451715, -6.054752690667223547, -1.112240025338166033E-15 ) ) ;
#59571=CARTESIAN_POINT ( 'NONE',  ( 6.853125000614516793, 0.000000000000000000, 5.243569643749999010 ) ) ;
#59572=CARTESIAN_POINT ( 'NONE',  ( 13.84687500061451537, -3.027376345333610441, -5.243569643749999898 ) ) ;
#59574=CARTESIAN_POINT ( 'NONE',  ( 24.04687500061451644, -3.027376345333614438, 5.243569643749998122 ) ) ;
#59575=CARTESIAN_POINT ( 'NONE',  ( 28.60312500061451502, -4.541064518000417216, -2.621784821875001281 ) ) ;
#59576=CARTESIAN_POINT ( 'NONE',  ( 8.625000000000000000, 6.123233995736764310E-16, -4.999999999999998224 ) ) ;
#59577=CARTESIAN_POINT ( 'NONE',  ( 7.462500000000001243, 2.886751345948126879, 4.999999999999999112 ) ) ;
#59578=CARTESIAN_POINT ( 'NONE',  ( 17.36250000122903359, 4.330127018922192761, -2.499999999999997780 ) ) ;
#59580=DIRECTION ( 'NONE',  ( -0.000000000000000000, -1.000000000000000000, -0.000000000000000000 ) ) ;
#59581=ORIENTED_EDGE ( 'NONE', *, *, #57650, .T. ) ;
#59582=CARTESIAN_POINT ( 'NONE',  ( 16.27499999999999858, 6.123233995736764310E-16, -4.999999999999998224 ) ) ;
#59583=CARTESIAN_POINT ( 'NONE',  ( 19.83750000000000213, -2.886751345948125991, -5.000000000000000000 ) ) ;
#59584=CARTESIAN_POINT ( 'NONE',  ( 14.76562500061451821, 3.027376345333613106, -5.243569643749998122 ) ) ;
#59585=VECTOR ( 'NONE', #54873, 1000.000000000000000 ) ;
#59586=ORIENTED_EDGE ( 'NONE', *, *, #19616, .F. ) ;
#59588=CARTESIAN_POINT ( 'NONE',  ( 4.243569643749999898, 17.34687500061451715, -27.54997392385601529 ) ) ;
#59589=CARTESIAN_POINT ( 'NONE',  ( 4.115625000614516082, 3.027376345333611329, 5.243569643749999010 ) ) ;
#59590=CARTESIAN_POINT ( 'NONE',  ( 12.52500000000000213, -4.330127018922194537, 2.499999999999995559 ) ) ;
#59593=CARTESIAN_POINT ( 'NONE',  ( -4.243569643749997233, 15.79062500061451857, 32.45002607614398471 ) ) ;
#59594=CARTESIAN_POINT ( 'NONE',  ( 26.76562500061451644, -6.054752690667223547, -1.112240025338166033E-15 ) ) ;
#59598=CARTESIAN_POINT ( 'NONE',  ( 22.62187500061451573, 3.027376345333611329, 5.243569643749999010 ) ) ;
#59599=CARTESIAN_POINT ( 'NONE',  ( 18.36562500061451431, 3.027376345333613106, -5.243569643749998122 ) ) ;
#59600=CARTESIAN_POINT ( 'NONE',  ( 2.121784821875001281, 13.20312500061459460, -26.32496088578401938 ) ) ;
#59601=CARTESIAN_POINT ( 'NONE',  ( 24.33750000122903145, -4.330127018922194537, 2.499999999999995559 ) ) ;
#59602=CARTESIAN_POINT ( 'NONE',  ( 5.240625000614516971, -3.027376345333610441, -5.243569643749999898 ) ) ;
#59604=CARTESIAN_POINT ( 'NONE',  ( 21.36562500061451075, -6.054752690667223547, -1.112240025338166033E-15 ) ) ;
#59607=CARTESIAN_POINT ( 'NONE',  ( 18.49687500061452283, 6.054752690667223547, 3.707466751127219781E-16 ) ) ;
#59608=CARTESIAN_POINT ( 'NONE',  ( 16.02187500061451786, -6.054752690667223547, -1.112240025338166033E-15 ) ) ;
#59609=CARTESIAN_POINT ( 'NONE',  ( 25.62187500061451573, 3.027376345333613106, -5.243569643749998122 ) ) ;
#59610=CARTESIAN_POINT ( 'NONE',  ( 4.243569643749999898, 15.09687500061451715, 32.45002607614398471 ) ) ;
#59611=CARTESIAN_POINT ( 'NONE',  ( 5.390625000614518214, 6.054752690667223547, 3.707466751127219781E-16 ) ) ;
#59612=CARTESIAN_POINT ( 'NONE',  ( 28.37812500061451715, 4.541064518000418104, 2.621784821874999949 ) ) ;
#59613=CARTESIAN_POINT ( 'NONE',  ( 3.234375000614516438, 4.541064518000418104, 2.621784821874999949 ) ) ;
#59615=CARTESIAN_POINT ( 'NONE',  ( 3.999999999999998668, 19.36250000000000426, 27.69059892324149175 ) ) ;
#59616=CARTESIAN_POINT ( 'NONE',  ( 6.646875000614518747, -3.027376345333610441, -5.243569643749999898 ) ) ;
#59618=CARTESIAN_POINT ( 'NONE',  ( 14.25000000122903465, 5.773502691896255534, 3.535250795749688894E-16 ) ) ;
#59619=CARTESIAN_POINT ( 'NONE',  ( 8.887500001229033941, 4.330127018922191873, 2.499999999999999556 ) ) ;
#59620=CARTESIAN_POINT ( 'NONE',  ( 3.928125000614516527, 6.421520780324663323E-16, -5.243569643749999010 ) ) ;
#59623=CARTESIAN_POINT ( 'NONE',  ( 14.97187500061451892, 3.027376345333611329, 5.243569643749999010 ) ) ;
#59624=CARTESIAN_POINT ( 'NONE',  ( 21.11250000000000071, -5.773502691896255534, -1.060575238724906372E-15 ) ) ;
#59625=ORIENTED_EDGE ( 'NONE', *, *, #21830, .T. ) ;
#59627=CARTESIAN_POINT ( 'NONE',  ( 22.79062500061451502, -3.027376345333610441, -5.243569643749999898 ) ) ;
#59628=CARTESIAN_POINT ( 'NONE',  ( 6.740625000614516082, 6.054752690667223547, 3.707466751127219781E-16 ) ) ;
#59629=CARTESIAN_POINT ( 'NONE',  ( 25.05937500061451573, -4.541064518000417216, -2.621784821875001281 ) ) ;
#59630=CARTESIAN_POINT ( 'NONE',  ( 8.015625000614518214, 3.027376345333613106, -5.243569643749998122 ) ) ;
#59632=CARTESIAN_POINT ( 'NONE',  ( 8.175000001229031810, -5.773502691896255534, -1.060575238724906372E-15 ) ) ;
#59633=CARTESIAN_POINT ( 'NONE',  ( 23.57812500061451289, -4.541064518000419881, 2.621784821874995952 ) ) ;
#59634=CARTESIAN_POINT ( 'NONE',  ( -2.121784821874996840, 10.87812500061451715, -26.32496088578401583 ) ) ;
#59635=CARTESIAN_POINT ( 'NONE',  ( 9.750000001229032875, 5.773502691896255534, 3.535250795749688894E-16 ) ) ;
#59636=CARTESIAN_POINT ( 'NONE',  ( 19.45312500061451644, 0.000000000000000000, 5.243569643749999010 ) ) ;
#59638=CARTESIAN_POINT ( 'NONE',  ( 17.54062500061451502, 6.054752690667223547, 3.707466751127219781E-16 ) ) ;
#59640=CARTESIAN_POINT ( 'NONE',  ( 17.17500000000000071, 6.123233995736764310E-16, -4.999999999999998224 ) ) ;
#59641=CARTESIAN_POINT ( 'NONE',  ( 11.88750000122903216, 6.123233995736764310E-16, -4.999999999999998224 ) ) ;
#59642=CARTESIAN_POINT ( 'NONE',  ( 8.015625000614518214, 3.027376345333613106, -5.243569643749998122 ) ) ;
#59643=CARTESIAN_POINT ( 'NONE',  ( 12.40312500061451573, -4.541064518000417216, -2.621784821875001281 ) ) ;
#59644=( BOUNDED_CURVE ( )  B_SPLINE_CURVE ( 2, ( #24498, #28963, #28601, #41146, #45957, #39701, #52219 ),
 .UNSPECIFIED., .F., .F. ) 
 B_SPLINE_CURVE_WITH_KNOTS ( ( 3, 2, 2, 3 ),
 ( 0.6999999999999999556, 0.7027777777777777235, 0.7055555555555557135, 0.7083333333333334814 ),
 .UNSPECIFIED. ) 
 CURVE ( )  GEOMETRIC_REPRESENTATION_ITEM ( )  RATIONAL_B_SPLINE_CURVE ( ( 1.000000000000000000, 0.8660254037844387076, 1.000000000000000000, 0.8660254037844387076, 1.000000000000000000, 0.8660254037844333785, 1.000000000000005329 ) ) 
 REPRESENTATION_ITEM ( '' )  );
#59646=CARTESIAN_POINT ( 'NONE',  ( 22.76250000122903216, 4.330127018922192761, -2.499999999999997780 ) ) ;
#59647=AXIS2_PLACEMENT_3D ( 'NONE', #66998, #62166, #16360 ) ;
#59648=CARTESIAN_POINT ( 'NONE',  ( 21.49687500061451573, -3.027376345333610441, -5.243569643749999898 ) ) ;
#59650=CARTESIAN_POINT ( 'NONE',  ( 5.362500001229033586, 0.000000000000000000, 4.999999999999998224 ) ) ;
#59651=CARTESIAN_POINT ( 'NONE',  ( 6.234375000614519102, 6.421520780324663323E-16, -5.243569643749999010 ) ) ;
#59652=CARTESIAN_POINT ( 'NONE',  ( 22.35937500061451644, -4.541064518000417216, -2.621784821875001281 ) ) ;
#59653=ADVANCED_FACE ( 'NONE', ( #35305 ), #24939, .F. ) ;
#59655=CARTESIAN_POINT ( 'NONE',  ( 19.90312500061451573, 0.000000000000000000, 5.243569643749999010 ) ) ;
#59656=CARTESIAN_POINT ( 'NONE',  ( 23.52187500061451786, 3.027376345333611329, 5.243569643749999010 ) ) ;
#59658=DIRECTION ( 'NONE',  ( -1.000000000000000000, -0.000000000000000000, -0.000000000000000000 ) ) ;
#59659=CARTESIAN_POINT ( 'NONE',  ( 27.78750000122903074, 4.330127018922191873, 2.499999999999999556 ) ) ;
#59660=CARTESIAN_POINT ( 'NONE',  ( 6.309375000614517504, 4.541064518000418104, -2.621784821874998173 ) ) ;
#59661=CARTESIAN_POINT ( 'NONE',  ( 16.11562500061451786, 3.027376345333613106, -5.243569643749998122 ) ) ;
#59662=CARTESIAN_POINT ( 'NONE',  ( 13.73437500061451821, -4.541064518000419881, 2.621784821874995952 ) ) ;
#59665=CARTESIAN_POINT ( 'NONE',  ( 25.15312500061451217, 4.541064518000418104, -2.621784821874998173 ) ) ;
#59666=CARTESIAN_POINT ( 'NONE',  ( 3.242103837493086330E-14, 13.13749999999999929, -34.00000000000000000 ) ) ;
#59667=CYLINDRICAL_SURFACE ( 'NONE', #27782, 3.999999999999996447 ) ;
#59668=CARTESIAN_POINT ( 'NONE',  ( 13.57500000000000107, 6.123233995736764310E-16, -4.999999999999998224 ) ) ;
#59669=CARTESIAN_POINT ( 'NONE',  ( 24.71250000122903145, 0.000000000000000000, 4.999999999999998224 ) ) ;
#59670=CARTESIAN_POINT ( 'NONE',  ( 17.65312500061451573, 0.000000000000000000, 5.243569643749999010 ) ) ;
#59671=ORIENTED_EDGE ( 'NONE', *, *, #13387, .F. ) ;
#59672=CARTESIAN_POINT ( 'NONE',  ( 21.75000000000000000, 4.330127018922192761, -2.499999999999997780 ) ) ;
#59673=CARTESIAN_POINT ( 'NONE',  ( 23.14687500061451786, -3.027376345333614438, 5.243569643749998122 ) ) ;
#59674=ORIENTED_EDGE ( 'NONE', *, *, #16952, .T. ) ;
#59675=CARTESIAN_POINT ( 'NONE',  ( 1.626862140677534273E-15, 17.52500000122903145, -26.00000000000000355 ) ) ;
#59676=CARTESIAN_POINT ( 'NONE',  ( 13.11562500061451786, 3.027376345333611329, 5.243569643749999010 ) ) ;
#59677=CARTESIAN_POINT ( 'NONE',  ( 4.640625000614518214, -3.027376345333614438, 5.243569643749998122 ) ) ;
#59679=CARTESIAN_POINT ( 'NONE',  ( 26.01562500061451289, 3.027376345333613106, -5.243569643749998122 ) ) ;
#59680=VECTOR ( 'NONE', #48110, 1000.000000000000000 ) ;
#59681=CARTESIAN_POINT ( 'NONE',  ( 18.86249999999999716, -5.773502691896255534, -1.060575238724906372E-15 ) ) ;
#59682=CARTESIAN_POINT ( 'NONE',  ( 27.44999999999999929, -4.330127018922190985, -2.500000000000001332 ) ) ;
#59684=CARTESIAN_POINT ( 'NONE',  ( 7.321875000614516793, 3.027376345333611329, 5.243569643749999010 ) ) ;
#59685=CARTESIAN_POINT ( 'NONE',  ( 17.82187500061451502, -6.054752690667223547, -1.112240025338166033E-15 ) ) ;
#59688=CARTESIAN_POINT ( 'NONE',  ( 27.25312500061451360, -4.541064518000417216, -2.621784821875001281 ) ) ;
#59689=CARTESIAN_POINT ( 'NONE',  ( 28.17187500061451644, -6.054752690667223547, -1.112240025338166033E-15 ) ) ;
#59691=CARTESIAN_POINT ( 'NONE',  ( 15.93750000000000000, 5.773502691896255534, 3.535250795749688894E-16 ) ) ;
#59692=CARTESIAN_POINT ( 'NONE',  ( 10.79062500061451679, 6.054752690667223547, 3.707466751127219781E-16 ) ) ;
#59695=CARTESIAN_POINT ( 'NONE',  ( 28.82812500061451644, 4.541064518000418104, 2.621784821874999949 ) ) ;
#59696=CARTESIAN_POINT ( 'NONE',  ( 17.40000000122903145, 5.773502691896255534, 3.535250795749688894E-16 ) ) ;
#59699=CARTESIAN_POINT ( 'NONE',  ( 5.615625000614517859, -6.054752690667223547, -1.112240025338166033E-15 ) ) ;
#59700=CARTESIAN_POINT ( 'NONE',  ( 22.35937500061451644, -4.541064518000417216, -2.621784821875001281 ) ) ;
#59701=CARTESIAN_POINT ( 'NONE',  ( 4.243569643749999010, 16.07187500061451857, 27.54997392385601174 ) ) ;
#59702=CARTESIAN_POINT ( 'NONE',  ( 23.97187500061451360, 3.027376345333611329, 5.243569643749999010 ) ) ;
#59703=CARTESIAN_POINT ( 'NONE',  ( 3.937500000000000444, -2.886751345948129988, 4.999999999999997335 ) ) ;
#59704=CARTESIAN_POINT ( 'NONE',  ( 4.000000000000000000, 9.950000001229035718, 32.30940107675849049 ) ) ;
#59705=CARTESIAN_POINT ( 'NONE',  ( 11.12812500061451715, 6.421520780324663323E-16, -5.243569643749999010 ) ) ;
#59706=CARTESIAN_POINT ( 'NONE',  ( 3.225000001229033408, -5.773502691896255534, -1.060575238724906372E-15 ) ) ;
#59707=CARTESIAN_POINT ( 'NONE',  ( 10.58437500061451964, -4.541064518000419881, 2.621784821874995952 ) ) ;
#59708=CARTESIAN_POINT ( 'NONE',  ( -2.556497649636125342E-15, 18.87500000122903288, 34.00000000000000000 ) ) ;
#59709=CARTESIAN_POINT ( 'NONE',  ( 9.740625000614516082, -3.027376345333610441, -5.243569643749999898 ) ) ;
#59710=CARTESIAN_POINT ( 'NONE',  ( 13.35937500061451821, -4.541064518000417216, -2.621784821875001281 ) ) ;
#59712=CARTESIAN_POINT ( 'NONE',  ( 22.16250000122903074, -4.330127018922190985, -2.500000000000001332 ) ) ;
#59713=CARTESIAN_POINT ( 'NONE',  ( 9.234375000614518214, -4.541064518000419881, 2.621784821874995952 ) ) ;
#59714=CARTESIAN_POINT ( 'NONE',  ( 12.06562500061451537, 3.027376345333613106, -5.243569643749998122 ) ) ;
#59716=CARTESIAN_POINT ( 'NONE',  ( 22.39687500061451075, -3.027376345333610441, -5.243569643749999898 ) ) ;
#59718=CARTESIAN_POINT ( 'NONE',  ( -3.999999999999999112, 11.97500000122903430, -32.30940107675850470 ) ) ;
#59720=CARTESIAN_POINT ( 'NONE',  ( 2.121784821874999061, 13.40937500061451892, -33.67503911421598417 ) ) ;
#59721=CARTESIAN_POINT ( 'NONE',  ( 14.66250000122903252, 4.330127018922192761, -2.499999999999997780 ) ) ;
#59722=CARTESIAN_POINT ( 'NONE',  ( 9.571875000614518569, 3.027376345333611329, 5.243569643749999010 ) ) ;
#59723=CARTESIAN_POINT ( 'NONE',  ( 9.001249775931846008E-16, 17.66562500061451502, -25.09994784771203058 ) ) ;
#59724=CARTESIAN_POINT ( 'NONE',  ( 18.48750000122903359, -4.330127018922194537, 2.499999999999995559 ) ) ;
#59725=CARTESIAN_POINT ( 'NONE',  ( 12.40312500061451573, -4.541064518000417216, -2.621784821875001281 ) ) ;
#59726=VERTEX_POINT ( 'NONE', #54129 ) ;
#59727=CARTESIAN_POINT ( 'NONE',  ( 16.64999999999999858, -4.330127018922190985, -2.500000000000001332 ) ) ;
#59728=CARTESIAN_POINT ( 'NONE',  ( 7.320879633048903241E-15, 17.30000000122903003, -34.00000000000000000 ) ) ;
#59729=CARTESIAN_POINT ( 'NONE',  ( 9.834375000614517859, 6.421520780324663323E-16, -5.243569643749999010 ) ) ;
#59730=CARTESIAN_POINT ( 'NONE',  ( -3.999999999999997335, 14.30000000122903359, 32.30940107675850470 ) ) ;
#59731=CARTESIAN_POINT ( 'NONE',  ( 12.33750000122903145, 6.123233995736764310E-16, -4.999999999999998224 ) ) ;
#59732=CARTESIAN_POINT ( 'NONE',  ( 19.87500000122903288, -5.773502691896255534, -1.060575238724906372E-15 ) ) ;
#59733=CARTESIAN_POINT ( 'NONE',  ( 17.01562500061451644, 3.027376345333613106, -5.243569643749998122 ) ) ;
#59734=CARTESIAN_POINT ( 'NONE',  ( 21.40312500061451573, -4.541064518000417216, -2.621784821875001281 ) ) ;
#59735=CARTESIAN_POINT ( 'NONE',  ( 28.31250000122903288, 0.000000000000000000, 4.999999999999998224 ) ) ;
#59736=CARTESIAN_POINT ( 'NONE',  ( 3.178125000614515638, 4.541064518000418104, 2.621784821874999949 ) ) ;
#59737=CARTESIAN_POINT ( 'NONE',  ( 26.09999999999999787, -4.330127018922190985, -2.500000000000001332 ) ) ;
#59738=CARTESIAN_POINT ( 'NONE',  ( 30.00000000000000000, 0.000000000000000000, 0.000000000000000000 ) ) ;
#59741=CARTESIAN_POINT ( 'NONE',  ( 28.17187500061451644, -6.054752690667223547, -1.112240025338166033E-15 ) ) ;
#59742=CARTESIAN_POINT ( 'NONE',  ( -5.810221930991193690E-16, 15.50000000122903465, -34.00000000000000000 ) ) ;
#59743=CARTESIAN_POINT ( 'NONE',  ( 3.637500001229036162, -4.330127018922194537, 2.499999999999995559 ) ) ;
#59744=CARTESIAN_POINT ( 'NONE',  ( 29.74687500061451217, 6.054752690667223547, 3.707466751127219781E-16 ) ) ;
#59747=CARTESIAN_POINT ( 'NONE',  ( 8.596875000614518925, 6.054752690667223547, 3.707466751127219781E-16 ) ) ;
#59748=CARTESIAN_POINT ( 'NONE',  ( 26.91562500061451146, 3.027376345333613106, -5.243569643749998122 ) ) ;
#59749=CARTESIAN_POINT ( 'NONE',  ( 4.683223236373093457, -1.751405183929441556, 4.942428804804532838 ) ) ;
#59750=CARTESIAN_POINT ( 'NONE',  ( 11.62500000122903465, 2.886751345948126879, 4.999999999999998224 ) ) ;
#59752=CARTESIAN_POINT ( 'NONE',  ( 4.546875000614517326, 6.054752690667223547, 3.707466751127219781E-16 ) ) ;
#59753=CARTESIAN_POINT ( 'NONE',  ( 9.684375000614517504, -4.541064518000419881, 2.621784821874995952 ) ) ;
#59754=CARTESIAN_POINT ( 'NONE',  ( 5.287500000000000533, -2.886751345948129988, 4.999999999999997335 ) ) ;
#59755=CARTESIAN_POINT ( 'NONE',  ( -2.121784821874996840, 11.32812500061459282, 33.67503911421598417 ) ) ;
#59756=CARTESIAN_POINT ( 'NONE',  ( 22.38749999999999929, -2.886751345948129988, 4.999999999999997335 ) ) ;
#59757=CARTESIAN_POINT ( 'NONE',  ( 20.85000000122903430, -2.886751345948126435, -5.000000000000000000 ) ) ;
#59758=CARTESIAN_POINT ( 'NONE',  ( 4.724999999999999645, 4.330127018922191873, 2.499999999999999556 ) ) ;
#59761=CARTESIAN_POINT ( 'NONE',  ( 19.15312500061451573, -4.541064518000417216, -2.621784821875001281 ) ) ;
#59762=CARTESIAN_POINT ( 'NONE',  ( 9.778125000614517504, 6.421520780324663323E-16, -5.243569643749999010 ) ) ;
#59764=CARTESIAN_POINT ( 'NONE',  ( 6.271875000614517859, 3.027376345333613106, -5.243569643749998122 ) ) ;
#59765=CARTESIAN_POINT ( 'NONE',  ( 23.43750000000000000, -2.886751345948125991, -5.000000000000000000 ) ) ;
#59766=CARTESIAN_POINT ( 'NONE',  ( 19.91250000122903074, -4.330127018922190985, -2.500000000000001332 ) ) ;
#59767=CARTESIAN_POINT ( 'NONE',  ( 27.66562500061451146, -6.054752690667223547, -1.112240025338166033E-15 ) ) ;
#59768=CARTESIAN_POINT ( 'NONE',  ( 30.00000000000000000, 0.000000000000000000, 0.000000000000000000 ) ) ;
#59769=CARTESIAN_POINT ( 'NONE',  ( 8.934375000614517504, 6.421520780324663323E-16, -5.243569643749999010 ) ) ;
#59770=CARTESIAN_POINT ( 'NONE',  ( 14.93437500061451750, 4.541064518000418104, 2.621784821874999949 ) ) ;
#59771=CARTESIAN_POINT ( 'NONE',  ( 25.09687500061451715, -3.027376345333610441, -5.243569643749999898 ) ) ;
#59775=CARTESIAN_POINT ( 'NONE',  ( 19.50937500061451857, 0.000000000000000000, 5.243569643749999010 ) ) ;
#59776=CARTESIAN_POINT ( 'NONE',  ( 9.646875000614516082, -3.027376345333614438, 5.243569643749998122 ) ) ;
#59778=CARTESIAN_POINT ( 'NONE',  ( 24.26249999999999929, -5.773502691896255534, -1.060575238724906372E-15 ) ) ;
#59780=CARTESIAN_POINT ( 'NONE',  ( -2.121784821874999949, 10.78437500061451715, -33.67503911421598417 ) ) ;
#59782=CARTESIAN_POINT ( 'NONE',  ( 12.10312500061451857, 4.541064518000418104, -2.621784821874998173 ) ) ;
#59783=CARTESIAN_POINT ( 'NONE',  ( 5.512499999999999289, 2.886751345948129099, -4.999999999999998224 ) ) ;
#59786=CARTESIAN_POINT ( 'NONE',  ( 11.81250000000000000, 2.886751345948129099, -4.999999999999998224 ) ) ;
#59787=CARTESIAN_POINT ( 'NONE',  ( -1.999999999999997113, 17.03750000122903430, 33.46410161513775705 ) ) ;
#59788=CARTESIAN_POINT ( 'NONE',  ( 11.81250000122903465, -4.330127018922190985, -2.500000000000001332 ) ) ;
#59789=CARTESIAN_POINT ( 'NONE',  ( 23.14687500061451786, -3.027376345333614438, 5.243569643749998122 ) ) ;
#59790=CARTESIAN_POINT ( 'NONE',  ( 16.77187500061451786, 3.027376345333611329, 5.243569643749999010 ) ) ;
#59792=ORIENTED_EDGE ( 'NONE', *, *, #55458, .T. ) ;
#59793=CARTESIAN_POINT ( 'NONE',  ( 17.31562500061451715, -6.054752690667223547, -1.112240025338166033E-15 ) ) ;
#59794=CARTESIAN_POINT ( 'NONE',  ( 29.36250000122903003, -4.330127018922190985, -2.500000000000001332 ) ) ;
#59795=CARTESIAN_POINT ( 'NONE',  ( 18.68437500061451928, -4.541064518000419881, 2.621784821874995952 ) ) ;
#59796=CARTESIAN_POINT ( 'NONE',  ( 28.92187500061451644, 3.027376345333611329, 5.243569643749999010 ) ) ;
#59797=CARTESIAN_POINT ( 'NONE',  ( 3.815625000614518036, -6.054752690667223547, -1.112240025338166033E-15 ) ) ;
#59798=CARTESIAN_POINT ( 'NONE',  ( 19.00312500061451715, 0.000000000000000000, 5.243569643749999010 ) ) ;
#59799=CARTESIAN_POINT ( 'NONE',  ( 28.24687500061451573, -3.027376345333610441, -5.243569643749999898 ) ) ;
#59800=CARTESIAN_POINT ( 'NONE',  ( 4.243569643749999010, 13.76562500061451644, 27.54997392385601174 ) ) ;
#59801=CARTESIAN_POINT ( 'NONE',  ( 16.35000000122903430, -2.886751345948125991, -5.000000000000000000 ) ) ;
#59803=CARTESIAN_POINT ( 'NONE',  ( 6.440625000614517148, -3.027376345333614438, 5.243569643749998122 ) ) ;
#59804=CARTESIAN_POINT ( 'NONE',  ( 25.86562500061451431, -6.054752690667223547, -1.112240025338166033E-15 ) ) ;
#59805=CARTESIAN_POINT ( 'NONE',  ( 8.887499999999997513, -2.886751345948063374, 5.000000000000112799 ) ) ;
#59806=( BOUNDED_CURVE ( )  B_SPLINE_CURVE ( 2, ( #38653, #22731, #71905, #32370, #9841, #49739, #4674, #22375, #27933, #66357, #33825, #27204, #10207, #39018, #50823, #26841, #10931, #33100, #16460, #56002, #66732, #56368, #39751, #67463, #49375, #44927, #5759, #16826, #39380, #61899, #11304, #22016, #50102, #28292, #32742, #61533, #44572, #226, #45284, #43832, #21278, #10572, #67818, #15734, #17191, #54908, #4316, #38273, #55279, #72266, #21644, #44201, #16103, #61177, #55639, #57437, #28646, #6840, #47088, #69621, #951, #69264, #18626, #41191, #7199, #34541, #63700, #18983, #29728, #12374, #29013, #62268, #45650, #2032, #51184, #51550, #588, #68184, #23093, #40830, #6478, #24177, #17902, #52627, #62623, #23815, #11663, #34179, #6115, #29375, #62978, #56714, #23459, #17547, #40462, #24543, #40108, #12018, #57071, #46005, #68541, #34909, #13091, #51907, #1306, #58150, #46366, #35629, #68900, #18257, #52266, #63346, #1668, #7555, #12732, #46729, #35268, #57790, #30089, #26010, #25266, #14185, #13822, #37086, #48549, #71076, #58510, #59610, #20080, #7921, #71447, #36362, #41905, #70705, #26377, #47446, #53722, #69978, #30816, #59979, #35992, #20451, #41544, #48916, #30458, #8650, #42271, #64062, #58876, #52987, #70343, #54456, #2383, #13443, #24901, #8286, #53349, #31555, #9024, #19348, #65532, #37460, #64430, #43001, #2747, #47813, #54095, #19719, #3492, #14918, #64794, #9389, #65160, #48181, #31920, #3855, #36720, #25644, #59241, #31179, #42636, #3114, #14550, #38562, #44110, #15281, #10842, #71817, #4223, #66636, #38929, #32283, #49649, #54817, #21189, #44482, #65901, #10483, #10120, #72176, #16014, #49284, #72538, #20822, #27481, #37821, #55551, #21926, #4947, #33012, #61085, #50014, #21556, #4586, #67013, #26751, #16374, #27116, #61448, #43377, #43740, #32650, #60340, #9749, #55191, #66265, #15642, #38183, #60707, #70207, #36227, #31420, #48052, #31788, #70945, #26245, #8887, #53213, #53960, #71680, #21054, #20316, #42870, #25879, #54327, #59110, #15145, #43605, #3718, #36954, #53583, #13683, #19582, #26614, #2609, #2979, #25131, #42138, #47672, #65392, #31045, #48782, #42505, #4084, #14049, #48418, #37325, #64664, #8516 ),
 .UNSPECIFIED., .F., .F. ) 
 B_SPLINE_CURVE_WITH_KNOTS ( ( 3, 2, 2, 2, 2, 2, 2, 2, 2, 2, 2, 2, 2, 2, 2, 2, 2, 2, 2, 2, 2, 2, 2, 2, 2, 2, 2, 2, 2, 2, 2, 2, 2, 2, 2, 2, 2, 2, 2, 2, 2, 2, 2, 2, 2, 2, 2, 2, 2, 2, 2, 2, 2, 2, 2, 2, 2, 2, 2, 2, 2, 2, 2, 2, 2, 2, 2, 2, 2, 2, 2, 2, 2, 2, 2, 2, 2, 2, 2, 2, 2, 2, 2, 2, 2, 2, 2, 2, 2, 2, 2, 2, 2, 2, 2, 2, 2, 2, 2, 2, 2, 2, 2, 2, 2, 2, 2, 2, 2, 2, 2, 2, 2, 2, 2, 2, 2, 2, 2, 2, 2, 2, 2, 2, 2, 2, 2, 2, 2, 2, 2, 2, 2, 2, 3 ),
 ( 0.000000000000000000, 0.007499808062934601276, 0.01499961612586920255, 0.02249942418880380296, 0.02999923225173840510, 0.03749904031467300725, 0.04499884837760760592, 0.05249865644054221153, 0.05999846450347681021, 0.06749827256641140194, 0.07499808062934601449, 0.08249788869228059929, 0.08999769675521521184, 0.09749750481814981051, 0.1049973128810844231, 0.1124971209440190079, 0.1199969290069536204, 0.1274967370698882330, 0.1349965451328228039, 0.1424963531957574303, 0.1499961612586920290, 0.1574959693216266277, 0.1649957773845611986, 0.1724955854474958250, 0.1799953935104304237, 0.1874952015733650224, 0.1949950096362996210, 0.2024948176992342197, 0.2099946257621688461, 0.2174944338251034170, 0.2249942418880380157, 0.2324940499509726144, 0.2399938580139072408, 0.2474936660768418395, 0.2549934741397764659, 0.2624932822027110646, 0.2699930902656456078, 0.2774928983285802619, 0.2849927063915148606, 0.2924925144544494038, 0.2999923225173840580, 0.3074921305803186011, 0.3149919386432532553, 0.3224917467061878540, 0.3299915547691223972, 0.3374913628320570513, 0.3449911708949916500, 0.3524909789579262487, 0.3599907870208608474, 0.3674905950837954460, 0.3749904031467300447, 0.3824902112096646434, 0.3899900192725992421, 0.3974898273355338407, 0.4049896353984684394, 0.4124894434614030381, 0.4199892515243376923, 0.4274890595872722354, 0.4349888676502068341, 0.4424886757131414883, 0.4499884837760760314, 0.4574882918390106856, 0.4649880999019452288, 0.4724879079648798275, 0.4799877160278144816, 0.4874875240907490248, 0.4949873321536836790, 0.5024871402166182222, 0.5099869482795529319, 0.5174867563424874195, 0.5249865644054221292, 0.5324863724683566168, 0.5399861805312912155, 0.5474859885942259252, 0.5549857966571605239, 0.5624856047200950115, 0.5699854127830297212, 0.5774852208459643199, 0.5849850289088988076, 0.5924848369718334062, 0.5999846450347681159, 0.6074844530977027146, 0.6149842611606372023, 0.6224840692235719120, 0.6299838772865065106, 0.6374836853494409983, 0.6449834934123757080, 0.6524833014753103066, 0.6599831095382447943, 0.6674829176011795040, 0.6749827256641141027, 0.6824825337270487013, 0.6899823417899833000, 0.6974821498529178987, 0.7049819579158524974, 0.7124817659787869850, 0.7199815740417216947, 0.7274813821046562934, 0.7349811901675908921, 0.7424809982305254907, 0.7499808062934600894, 0.7574806143563946881, 0.7649804224193292868, 0.7724802304822638854, 0.7799800385451984841, 0.7874798466081331938, 0.7949796546710676814, 0.8024794627340022801, 0.8099792707969368788, 0.8174790788598714775, 0.8249788869228060761, 0.8324786949857406748, 0.8399785030486753845, 0.8474783111116098722, 0.8549781191745444708, 0.8624779272374791805, 0.8699777353004136682, 0.8774775433633482669, 0.8849773514262829766, 0.8924771594892175752, 0.8999769675521520629, 0.9074767756150867726, 0.9149765836780213712, 0.9224763917409558589, 0.9299761998038904576, 0.9374760078668251673, 0.9449758159297596549, 0.9524756239926942536, 0.9599754320556289633, 0.9674752401185635620, 0.9749750481814980496, 0.9824748562444327593, 0.9899746643073673580, 0.9974744723703018456, 1.000000000000000000 ),
 .UNSPECIFIED. ) 
 CURVE ( )  GEOMETRIC_REPRESENTATION_ITEM ( )  RATIONAL_B_SPLINE_CURVE ( ( 1.000000000000000000, 0.8660254037844387076, 1.000000000000000000, 0.8660254037844387076, 1.000000000000000000, 0.8660254037844387076, 1.000000000000000000, 0.8660254037844387076, 1.000000000000000000, 0.8660254037844387076, 1.000000000000000000, 0.8660254037844387076, 1.000000000000000000, 0.8660254037844387076, 1.000000000000000000, 0.8660254037844387076, 1.000000000000000000, 0.8660254037844387076, 1.000000000000000000, 0.8660254037844387076, 1.000000000000000000, 0.8660254037844387076, 1.000000000000000000, 0.8660254037844387076, 1.000000000000000000, 0.8660254037844387076, 1.000000000000000000, 0.8660254037844387076, 1.000000000000000000, 0.8660254037844387076, 1.000000000000000000, 0.8660254037844387076, 1.000000000000000000, 0.8660254037844387076, 1.000000000000000000, 0.8660254037844387076, 1.000000000000000000, 0.8660254037844387076, 1.000000000000000000, 0.8660254037844387076, 1.000000000000000000, 0.8660254037844387076, 1.000000000000000000, 0.8660254037844387076, 1.000000000000000000, 0.8660254037844387076, 1.000000000000000000, 0.8660254037844387076, 1.000000000000000000, 0.8660254037844387076, 1.000000000000000000, 0.8660254037844387076, 1.000000000000000000, 0.8660254037844387076, 1.000000000000000000, 0.8660254037844387076, 1.000000000000000000, 0.8660254037844387076, 1.000000000000000000, 0.8660254037844387076, 1.000000000000000000, 0.8660254037844387076, 1.000000000000000000, 0.8660254037844387076, 1.000000000000000000, 0.8660254037844387076, 1.000000000000000000, 0.8660254037844387076, 1.000000000000000000, 0.8660254037844387076, 1.000000000000000000, 0.8660254037844387076, 1.000000000000000000, 0.8660254037844387076, 1.000000000000000000, 0.8660254037844387076, 1.000000000000000000, 0.8660254037844387076, 1.000000000000000000, 0.8660254037844387076, 1.000000000000000000, 0.8660254037844387076, 1.000000000000000000, 0.8660254037844387076, 1.000000000000000000, 0.8660254037844387076, 1.000000000000000000, 0.8660254037844387076, 1.000000000000000000, 0.8660254037844387076, 1.000000000000000000, 0.8660254037844387076, 1.000000000000000000, 0.8660254037844387076, 1.000000000000000000, 0.8660254037844387076, 1.000000000000000000, 0.8660254037844387076, 1.000000000000000000, 0.8660254037844387076, 1.000000000000000000, 0.8660254037844387076, 1.000000000000000000, 0.8660254037844387076, 1.000000000000000000, 0.8660254037844387076, 1.000000000000000000, 0.8660254037844387076, 1.000000000000000000, 0.8660254037844387076, 1.000000000000000000, 0.8660254037844387076, 1.000000000000000000, 0.8660254037844387076, 1.000000000000000000, 0.8660254037844387076, 1.000000000000000000, 0.8660254037844387076, 1.000000000000000000, 0.8660254037844387076, 1.000000000000000000, 0.8660254037844387076, 1.000000000000000000, 0.8660254037844387076, 1.000000000000000000, 0.8660254037844387076, 1.000000000000000000, 0.8660254037844387076, 1.000000000000000000, 0.8660254037844387076, 1.000000000000000000, 0.8660254037844387076, 1.000000000000000000, 0.8660254037844387076, 1.000000000000000000, 0.8660254037844387076, 1.000000000000000000, 0.8660254037844387076, 1.000000000000000000, 0.8660254037844387076, 1.000000000000000000, 0.8660254037844387076, 1.000000000000000000, 0.8660254037844387076, 1.000000000000000000, 0.8660254037844387076, 1.000000000000000000, 0.8660254037844387076, 1.000000000000000000, 0.8660254037844387076, 1.000000000000000000, 0.8660254037844387076, 1.000000000000000000, 0.8660254037844387076, 1.000000000000000000, 0.8660254037844387076, 1.000000000000000000, 0.8660254037844387076, 1.000000000000000000, 0.8660254037844387076, 1.000000000000000000, 0.8660254037844387076, 1.000000000000000000, 0.8660254037844387076, 1.000000000000000000, 0.8660254037844387076, 1.000000000000000000, 0.8660254037844387076, 1.000000000000000000, 0.8660254037844387076, 1.000000000000000000, 0.8660254037844387076, 1.000000000000000000, 0.8660254037844387076, 1.000000000000000000, 0.8660254037844387076, 1.000000000000000000, 0.8660254037844387076, 1.000000000000000000, 0.8660254037844387076, 1.000000000000000000, 0.8660254037844387076, 1.000000000000000000, 0.8660254037844387076, 1.000000000000000000, 0.8660254037844387076, 1.000000000000000000, 0.8660254037844387076, 1.000000000000000000, 0.8660254037844387076, 1.000000000000000000, 0.8660254037844387076, 1.000000000000000000, 0.8660254037844387076, 1.000000000000000000, 0.8660254037844387076, 1.000000000000000000, 0.8660254037844387076, 1.000000000000000000, 0.8660254037844387076, 1.000000000000000000, 0.8660254037844387076, 1.000000000000000000, 0.8660254037844387076, 1.000000000000000000, 0.8660254037844387076, 1.000000000000000000, 0.8660254037844387076, 1.000000000000000000, 0.8660254037844387076, 1.000000000000000000, 0.8660254037844387076, 1.000000000000000000, 0.8660254037844387076, 1.000000000000000000, 0.8660254037844387076, 1.000000000000000000, 0.8660254037844387076, 1.000000000000000000, 0.8660254037844387076, 1.000000000000000000, 0.8660254037844387076, 1.000000000000000000, 0.8660254037844387076, 1.000000000000000000, 0.8660254037844387076, 1.000000000000000000, 0.8660254037844387076, 1.000000000000000000, 0.8660254037844387076, 1.000000000000000000, 0.8660254037844387076, 1.000000000000000000, 0.8660254037844387076, 1.000000000000000000, 0.8660254037844387076, 1.000000000000000000, 0.8660254037844387076, 1.000000000000000000, 0.8660254037844387076, 1.000000000000000000, 0.8660254037844387076, 1.000000000000000000, 0.8660254037844387076, 1.000000000000000000, 0.8660254037844387076, 1.000000000000000000, 0.8660254037844387076, 1.000000000000000000, 0.8660254037844387076, 1.000000000000000000, 0.8660254037844387076, 1.000000000000000000, 0.8660254037844387076, 1.000000000000000000, 0.8660254037844387076, 1.000000000000000000, 0.8660254037844387076, 1.000000000000000000, 0.8660254037844387076, 1.000000000000000000, 0.8660254037844387076, 1.000000000000000000, 0.8660254037844387076, 1.000000000000000000, 0.8660254037844387076, 1.000000000000000000, 0.9548846395026737710, 0.9401540804572410259 ) ) 
 REPRESENTATION_ITEM ( '' )  );
#59807=CARTESIAN_POINT ( 'NONE',  ( 22.88437500061451857, 6.421520780324663323E-16, -5.243569643749999010 ) ) ;
#59808=CARTESIAN_POINT ( 'NONE',  ( 14.01562500061451644, 3.027376345333611329, 5.243569643749999010 ) ) ;
#59809=CARTESIAN_POINT ( 'NONE',  ( 23.13750000122903216, 6.123233995736764310E-16, -4.999999999999998224 ) ) ;
#59810=CARTESIAN_POINT ( 'NONE',  ( 22.52812500061451573, 4.541064518000418104, 2.621784821874999949 ) ) ;
#59811=CARTESIAN_POINT ( 'NONE',  ( 18.53437500061451715, 4.541064518000418104, 2.621784821874999949 ) ) ;
#59812=CARTESIAN_POINT ( 'NONE',  ( 12.74062500061451786, -3.027376345333614438, 5.243569643749998122 ) ) ;
#59813=CARTESIAN_POINT ( 'NONE',  ( 2.121784821874999061, 14.75937500061451679, 26.32496088578401583 ) ) ;
#59814=CARTESIAN_POINT ( 'NONE',  ( 19.64062500061451644, -3.027376345333610441, -5.243569643749999898 ) ) ;
#59818=CARTESIAN_POINT ( 'NONE',  ( 23.32499999999999929, -4.330127018922194537, 2.499999999999995559 ) ) ;
#59819=CARTESIAN_POINT ( 'NONE',  ( -3.999999999999999112, 10.10000000000000142, -30.00000000000000000 ) ) ;
#59821=CARTESIAN_POINT ( 'NONE',  ( 26.91562500061451146, 3.027376345333613106, -5.243569643749998122 ) ) ;
#59822=CARTESIAN_POINT ( 'NONE',  ( 5.653125000614517504, -4.541064518000417216, -2.621784821875001281 ) ) ;
#59823=CARTESIAN_POINT ( 'NONE',  ( 20.21250000122903145, 0.000000000000000000, 4.999999999999998224 ) ) ;
#59824=CARTESIAN_POINT ( 'NONE',  ( 24.81562500061451715, 3.027376345333611329, 5.243569643749999010 ) ) ;
#59825=CARTESIAN_POINT ( 'NONE',  ( 23.32499999999999929, -4.330127018922194537, 2.499999999999995559 ) ) ;
#59826=CARTESIAN_POINT ( 'NONE',  ( 27.62812500061451360, -4.541064518000419881, 2.621784821874995952 ) ) ;
#59827=CARTESIAN_POINT ( 'NONE',  ( 9.215625000614515727, -6.054752690667223547, -1.112240025338166033E-15 ) ) ;
#59828=ORIENTED_EDGE ( 'NONE', *, *, #23424, .T. ) ;
#59829=CARTESIAN_POINT ( 'NONE',  ( 22.11562500061451786, 3.027376345333611329, 5.243569643749999010 ) ) ;
#59830=CARTESIAN_POINT ( 'NONE',  ( 5.653125000614517504, -4.541064518000417216, -2.621784821875001281 ) ) ;
#59832=CARTESIAN_POINT ( 'NONE',  ( 3.215625000614518836, 3.027376345333611329, 5.243569643749999010 ) ) ;
#59833=CARTESIAN_POINT ( 'NONE',  ( -3.999999999999999556, 13.77500000122903678, -32.30940107675850470 ) ) ;
#59835=CARTESIAN_POINT ( 'NONE',  ( 1.626862140677534273E-15, 10.32500000122903572, 34.00000000000000000 ) ) ;
#59837=CARTESIAN_POINT ( 'NONE',  ( 10.98750000000000071, 5.773502691896255534, 3.535250795749688894E-16 ) ) ;
#59838=CARTESIAN_POINT ( 'NONE',  ( 10.13437500061451679, -4.541064518000419881, 2.621784821874995952 ) ) ;
#59839=CARTESIAN_POINT ( 'NONE',  ( 6.675000001229034474, 2.886751345948126879, 4.999999999999999112 ) ) ;
#59840=CARTESIAN_POINT ( 'NONE',  ( 14.14687500061451786, -3.027376345333614438, 5.243569643749998122 ) ) ;
#59842=CARTESIAN_POINT ( 'NONE',  ( 5.934375000614517504, 4.541064518000418104, 2.621784821874999949 ) ) ;
#59843=CARTESIAN_POINT ( 'NONE',  ( 2.000000000000001332, 18.35000000000000142, 33.46410161513774995 ) ) ;
#59844=DIRECTION ( 'NONE',  ( 0.000000000000000000, 1.000000000000000000, 0.000000000000000000 ) ) ;
#59845=CARTESIAN_POINT ( 'NONE',  ( 13.43437500061451750, 6.421520780324663323E-16, -5.243569643749999010 ) ) ;
#59846=CARTESIAN_POINT ( 'NONE',  ( 11.32500000000000107, 6.123233995736764310E-16, -4.999999999999998224 ) ) ;
#59847=CARTESIAN_POINT ( 'NONE',  ( 22.45312500061451644, 4.541064518000418104, -2.621784821874998173 ) ) ;
#59848=CARTESIAN_POINT ( 'NONE',  ( -3.137519842735245283E-14, 11.56250000000000178, 34.00000000000000000 ) ) ;
#59849=CARTESIAN_POINT ( 'NONE',  ( -4.243569643749998122, 18.94062500061459531, 32.45002607614398471 ) ) ;
#59850=CARTESIAN_POINT ( 'NONE',  ( 26.97187500061451360, 3.027376345333613106, -5.243569643749998122 ) ) ;
#59851=CARTESIAN_POINT ( 'NONE',  ( -3.305248395036964552E-15, 5.000000000000034639, 25.99999999999995737 ) ) ;
#59853=CARTESIAN_POINT ( 'NONE',  ( 4.415625000614518569, 3.027376345333613106, -5.243569643749998122 ) ) ;
#59855=CARTESIAN_POINT ( 'NONE',  ( 13.09687500061451892, 6.054752690667223547, 3.707466751127219781E-16 ) ) ;
#59856=CARTESIAN_POINT ( 'NONE',  ( 29.96250000000000213, 2.886751345948126879, 4.999999999999999112 ) ) ;
#59857=CARTESIAN_POINT ( 'NONE',  ( 27.82500000122903572, 2.886751345948126879, 4.999999999999999112 ) ) ;
#59858=CARTESIAN_POINT ( 'NONE',  ( 5.034375000614519813, 4.541064518000418104, 2.621784821874999949 ) ) ;
#59859=CARTESIAN_POINT ( 'NONE',  ( 15.49687500061451750, -3.027376345333614438, 5.243569643749998122 ) ) ;
#59861=CARTESIAN_POINT ( 'NONE',  ( 24.56250000000000000, 2.886751345948126879, 4.999999999999999112 ) ) ;
#59862=CARTESIAN_POINT ( 'NONE',  ( 4.162500001229033408, -4.330127018922190985, -2.500000000000001332 ) ) ;
#59863=CARTESIAN_POINT ( 'NONE',  ( 27.34687500061451360, -3.027376345333610441, -5.243569643749999898 ) ) ;
#59865=CARTESIAN_POINT ( 'NONE',  ( 29.47499999999999787, 4.330127018922191873, 2.499999999999999556 ) ) ;
#59866=CARTESIAN_POINT ( 'NONE',  ( 9.074999999999999289, 6.123233995736764310E-16, -4.999999999999998224 ) ) ;
#59868=CARTESIAN_POINT ( 'NONE',  ( 23.24062500061451786, -3.027376345333610441, -5.243569643749999898 ) ) ;
#59869=CARTESIAN_POINT ( 'NONE',  ( 11.36250000000000071, 2.886751345948129099, -4.999999999999998224 ) ) ;
#59870=CARTESIAN_POINT ( 'NONE',  ( 4.228125000614517681, -4.541064518000419881, 2.621784821874995952 ) ) ;
#59871=CARTESIAN_POINT ( 'NONE',  ( 19.76250000000000639, -5.773502691896255534, -1.060575238724906372E-15 ) ) ;
#59872=CARTESIAN_POINT ( 'NONE',  ( 17.65312500061451573, 0.000000000000000000, 5.243569643749999010 ) ) ;
#59873=CARTESIAN_POINT ( 'NONE',  ( -3.999999999999999112, 18.76250000122903216, 30.00000000000000000 ) ) ;
#59874=CARTESIAN_POINT ( 'NONE',  ( 23.02500000122903145, -5.773502691896255534, -1.060575238724906372E-15 ) ) ;
#59876=CARTESIAN_POINT ( 'NONE',  ( 3.525000000000000355, -4.330127018922194537, 2.499999999999995559 ) ) ;
#59878=CARTESIAN_POINT ( 'NONE',  ( 18.70312500061451644, -4.541064518000417216, -2.621784821875001281 ) ) ;
#59879=CARTESIAN_POINT ( 'NONE',  ( 24.10312500061451502, -4.541064518000417216, -2.621784821875001281 ) ) ;
#59880=CARTESIAN_POINT ( 'NONE',  ( 24.08437500061451786, -4.541064518000419881, 2.621784821874995952 ) ) ;
#59881=CARTESIAN_POINT ( 'NONE',  ( 9.112500000000000711, 2.886751345948129099, -4.999999999999998224 ) ) ;
#59882=CARTESIAN_POINT ( 'NONE',  ( 12.06562500061451537, 3.027376345333613106, -5.243569643749998122 ) ) ;
#59883=CARTESIAN_POINT ( 'NONE',  ( 26.69062500061451715, -3.027376345333614438, 5.243569643749998122 ) ) ;
#59884=CARTESIAN_POINT ( 'NONE',  ( 17.14687500061451786, 6.054752690667223547, 3.707466751127219781E-16 ) ) ;
#59885=CARTESIAN_POINT ( 'NONE',  ( 9.815625000614518925, 3.027376345333613106, -5.243569643749998122 ) ) ;
#59886=DIRECTION ( 'NONE',  ( -0.000000000000000000, -1.000000000000000000, -0.000000000000000000 ) ) ;
#59887=CARTESIAN_POINT ( 'NONE',  ( 2.121784821875001281, 19.05312500061451431, 33.67503911421598417 ) ) ;
#59888=AXIS2_PLACEMENT_3D ( 'NONE', #32360, #54898, #52258 ) ;
#59889=CARTESIAN_POINT ( 'NONE',  ( 23.10000000122903074, -2.886751345948125991, -5.000000000000000000 ) ) ;
#59891=CARTESIAN_POINT ( 'NONE',  ( 15.14062500061451644, -3.027376345333610441, -5.243569643749999898 ) ) ;
#59892=CARTESIAN_POINT ( 'NONE',  ( 8.859375000614518214, -4.541064518000417216, -2.621784821875001281 ) ) ;
#59893=CARTESIAN_POINT ( 'NONE',  ( 7.509375000614517681, -4.541064518000417216, -2.621784821875001281 ) ) ;
#59894=ORIENTED_EDGE ( 'NONE', *, *, #16132, .F. ) ;
#59895=CARTESIAN_POINT ( 'NONE',  ( 29.67187500061451644, 3.027376345333613106, -5.243569643749998122 ) ) ;
#59896=CARTESIAN_POINT ( 'NONE',  ( 21.25312500061451715, 0.000000000000000000, 5.243569643749999010 ) ) ;
#59898=CARTESIAN_POINT ( 'NONE',  ( 15.90937500061451892, 0.000000000000000000, 5.243569643749999010 ) ) ;
#59899=CARTESIAN_POINT ( 'NONE',  ( 21.55312500061451431, 4.541064518000418104, -2.621784821874998173 ) ) ;
#59900=CARTESIAN_POINT ( 'NONE',  ( -3.999999999999999112, 11.90000000000000036, 30.00000000000000000 ) ) ;
#59901=CARTESIAN_POINT ( 'NONE',  ( 27.51562500061451644, 3.027376345333611329, 5.243569643749999010 ) ) ;
#59902=CARTESIAN_POINT ( 'NONE',  ( 6.000000001229033764, -2.886751345948125991, -5.000000000000000000 ) ) ;
#59903=ORIENTED_EDGE ( 'NONE', *, *, #41229, .F. ) ;
#59904=CARTESIAN_POINT ( 'NONE',  ( 29.02499999999999858, 4.330127018922191873, 2.499999999999999556 ) ) ;
#59905=CARTESIAN_POINT ( 'NONE',  ( 8.484601909799253346E-16, 16.96250000000000213, -25.38119784648299770 ) ) ;
#59906=CARTESIAN_POINT ( 'NONE',  ( 24.48750000122903359, 6.123233995736764310E-16, -4.999999999999998224 ) ) ;
#59908=CARTESIAN_POINT ( 'NONE',  ( 6.796875000614516438, 6.054752690667223547, 3.707466751127219781E-16 ) ) ;
#59909=CARTESIAN_POINT ( 'NONE',  ( 3.999999999999998668, 15.31250000000000000, 27.69059892324149530 ) ) ;
#59910=CARTESIAN_POINT ( 'NONE',  ( 15.66562500061451857, 3.027376345333613106, -5.243569643749998122 ) ) ;
#59911=CARTESIAN_POINT ( 'NONE',  ( 7.659375000614518036, 4.541064518000418104, -2.621784821874998173 ) ) ;
#59912=CARTESIAN_POINT ( 'NONE',  ( 27.11250000122903359, -4.330127018922190985, -2.500000000000001332 ) ) ;
#59913=CARTESIAN_POINT ( 'NONE',  ( 18.12187500061451928, 3.027376345333611329, 5.243569643749999010 ) ) ;
#59914=CARTESIAN_POINT ( 'NONE',  ( 4.284375000614518925, -4.541064518000419881, 2.621784821874995952 ) ) ;
#59915=CARTESIAN_POINT ( 'NONE',  ( 7.837500001229035007, 6.123233995736764310E-16, -4.999999999999998224 ) ) ;
#59916=CARTESIAN_POINT ( 'NONE',  ( 4.340625000614515727, -3.027376345333610441, -5.243569643749999898 ) ) ;
#59917=CARTESIAN_POINT ( 'NONE',  ( 16.34062500061451573, -3.027376345333614438, 5.243569643749998122 ) ) ;
#59918=ORIENTED_EDGE ( 'NONE', *, *, #35474, .F. ) ;
#59919=CARTESIAN_POINT ( 'NONE',  ( 12.70312500061451821, 0.000000000000000000, 5.243569643749999010 ) ) ;
#59920=CARTESIAN_POINT ( 'NONE',  ( 6.037500001229035185, 6.123233995736764310E-16, -4.999999999999998224 ) ) ;
#59921=CARTESIAN_POINT ( 'NONE',  ( 9.140625000614518214, -3.027376345333614438, 5.243569643749998122 ) ) ;
#59923=CARTESIAN_POINT ( 'NONE',  ( 8.324999999999999289, 4.330127018922191873, 2.499999999999999556 ) ) ;
#59924=CARTESIAN_POINT ( 'NONE',  ( 3.600000001229033408, -2.886751345948129988, 4.999999999999997335 ) ) ;
#59925=CARTESIAN_POINT ( 'NONE',  ( 18.48750000000000071, -2.886751345948125991, -5.000000000000000000 ) ) ;
#59926=CARTESIAN_POINT ( 'NONE',  ( 19.28437500061451360, 6.421520780324663323E-16, -5.243569643749999010 ) ) ;
#59927=CARTESIAN_POINT ( 'NONE',  ( 15.41250000122903252, -4.330127018922190985, -2.500000000000001332 ) ) ;
#59929=CARTESIAN_POINT ( 'NONE',  ( 4.243569643749999898, 15.49062500061451786, -27.54997392385601529 ) ) ;
#59930=CARTESIAN_POINT ( 'NONE',  ( -1.071796769724488563, 16.15490381179669654, 34.00000000000000000 ) ) ;
#59932=CARTESIAN_POINT ( 'NONE',  ( 28.26562500061451289, 3.027376345333613106, -5.243569643749998122 ) ) ;
#59933=EDGE_CURVE ( 'NONE', #5936, #57032, #19479, .T. ) ;
#59936=CARTESIAN_POINT ( 'NONE',  ( 16.20937500061451786, 4.541064518000418104, -2.621784821874998173 ) ) ;
#59937=CARTESIAN_POINT ( 'NONE',  ( 29.77499999999999858, 6.123233995736764310E-16, -4.999999999999998224 ) ) ;
#59938=CARTESIAN_POINT ( 'NONE',  ( 11.99062500061451608, -3.027376345333610441, -5.243569643749999898 ) ) ;
#59940=CARTESIAN_POINT ( 'NONE',  ( 24.75937500061451502, 4.541064518000418104, -2.621784821874998173 ) ) ;
#59942=CARTESIAN_POINT ( 'NONE',  ( 6.628125000614517148, 6.421520780324663323E-16, -5.243569643749999010 ) ) ;
#59943=CARTESIAN_POINT ( 'NONE',  ( 12.45937500061451786, -4.541064518000417216, -2.621784821875001281 ) ) ;
#59944=EDGE_LOOP ( 'NONE', ( #46901, #45336, #10465, #37270, #47060 ) ) ;
#59945=CARTESIAN_POINT ( 'NONE',  ( 23.67187500061451999, -6.054752690667223547, -1.112240025338166033E-15 ) ) ;
#59946=CARTESIAN_POINT ( 'NONE',  ( 27.47812500061451502, 4.541064518000418104, 2.621784821874999949 ) ) ;
#59948=CARTESIAN_POINT ( 'NONE',  ( 6.825000000000001066, 6.123233995736764310E-16, -4.999999999999998224 ) ) ;
#59949=CARTESIAN_POINT ( 'NONE',  ( 17.17500000122903359, -5.773502691896255534, -1.060575238724906372E-15 ) ) ;
#59952=VERTEX_POINT ( 'NONE', #47854 ) ;
#59953=CARTESIAN_POINT ( 'NONE',  ( 14.81250000000000000, -5.773502691896255534, -1.060575238724906372E-15 ) ) ;
#59954=CARTESIAN_POINT ( 'NONE',  ( 19.87500000000000000, 6.123233995736764310E-16, -4.999999999999998224 ) ) ;
#59955=CARTESIAN_POINT ( 'NONE',  ( 11.95312500061451644, -4.541064518000417216, -2.621784821875001281 ) ) ;
#59956=VERTEX_POINT ( 'NONE', #3892 ) ;
#59957=CARTESIAN_POINT ( 'NONE',  ( 18.48750000122903359, -4.330127018922194537, 2.499999999999995559 ) ) ;
#59958=CARTESIAN_POINT ( 'NONE',  ( -4.243569643749999898, 17.15937500061451715, -30.00000000000000000 ) ) ;
#59959=CARTESIAN_POINT ( 'NONE',  ( 3.178125000614515638, 4.541064518000418104, 2.621784821874999949 ) ) ;
#59961=CARTESIAN_POINT ( 'NONE',  ( 10.16249999999999964, 2.886751345948126879, 4.999999999999999112 ) ) ;
#59963=CARTESIAN_POINT ( 'NONE',  ( -2.121784821874999949, 12.07812500061451821, 26.32496088578401938 ) ) ;
#59964=CARTESIAN_POINT ( 'NONE',  ( 27.36562500061451786, 3.027376345333613106, -5.243569643749998122 ) ) ;
#59965=CARTESIAN_POINT ( 'NONE',  ( 3.533900615097678610, 3.537227818301726501, 3.601564948538577671 ) ) ;
#59967=CARTESIAN_POINT ( 'NONE',  ( 24.75937500061451502, 4.541064518000418104, -2.621784821874998173 ) ) ;
#59968=CARTESIAN_POINT ( 'NONE',  ( 19.41562500061451146, 3.027376345333611329, 5.243569643749999010 ) ) ;
#59969=CARTESIAN_POINT ( 'NONE',  ( -4.243569643749999898, 14.85312500061459495, -30.00000000000000000 ) ) ;
#59970=CARTESIAN_POINT ( 'NONE',  ( 22.57500000122903572, -5.773502691896255534, -1.060575238724906372E-15 ) ) ;
#59971=CARTESIAN_POINT ( 'NONE',  ( 3.328125000614516438, -4.541064518000419881, 2.621784821874995952 ) ) ;
#59973=CARTESIAN_POINT ( 'NONE',  ( 21.55312500061451431, 4.541064518000418104, -2.621784821874998173 ) ) ;
#59976=CARTESIAN_POINT ( 'NONE',  ( 16.05937500061451573, -4.541064518000417216, -2.621784821875001281 ) ) ;
#59977=CARTESIAN_POINT ( 'NONE',  ( 16.88437500061451502, -4.541064518000419881, 2.621784821874995952 ) ) ;
#59978=CARTESIAN_POINT ( 'NONE',  ( 24.64687500061451431, -3.027376345333610441, -5.243569643749999898 ) ) ;
#59979=CARTESIAN_POINT ( 'NONE',  ( 4.243569643749999898, 14.64687500061451964, 32.45002607614398471 ) ) ;
#59980=CARTESIAN_POINT ( 'NONE',  ( 5.878125000614517148, 4.541064518000418104, 2.621784821874999949 ) ) ;
#59981=CARTESIAN_POINT ( 'NONE',  ( 27.74062500061451431, -3.027376345333610441, -5.243569643749999898 ) ) ;
#59982=CARTESIAN_POINT ( 'NONE',  ( 29.24062500061451431, 6.054752690667223547, 3.707466751127219781E-16 ) ) ;
#59984=CARTESIAN_POINT ( 'NONE',  ( -2.828200636599751609E-16, 18.53750000000000142, 25.38119784648299770 ) ) ;
#59985=CARTESIAN_POINT ( 'NONE',  ( 7.846875000614518036, -3.027376345333614438, 5.243569643749998122 ) ) ;
#59987=CARTESIAN_POINT ( 'NONE',  ( 14.36250000122903359, 0.000000000000000000, 4.999999999999998224 ) ) ;
#59988=CARTESIAN_POINT ( 'NONE',  ( 8.625000001229034652, -5.773502691896255534, -1.060575238724906372E-15 ) ) ;
#59989=CARTESIAN_POINT ( 'NONE',  ( 4.715625000614516615, -6.054752690667223547, -1.112240025338166033E-15 ) ) ;
#59992=CARTESIAN_POINT ( 'NONE',  ( 14.25937500061451679, -4.541064518000417216, -2.621784821875001281 ) ) ;
#59993=CARTESIAN_POINT ( 'NONE',  ( 7.537500000000000533, -2.886751345948063374, 5.000000000000112799 ) ) ;
#59994=EDGE_LOOP ( 'NONE', ( #3086, #7909, #27863, #59056, #1020, #53261, #37756, #25606, #50013, #44678, #15423, #34286, #46621, #46116, #44979, #12127, #6284, #33874, #10262, #60682, #58374, #58222, #35899, #31117, #65082, #5087, #47103, #57863, #12696, #51716, #66097, #51841, #32995, #14473, #43755, #23429, #13508, #29705, #51096, #53692, #57395, #60315, #37294, #656, #55746, #5150, #51079, #53928 ) ) ;
#59995=CARTESIAN_POINT ( 'NONE',  ( 21.47812500061451502, 6.421520780324663323E-16, -5.243569643749999010 ) ) ;
#59996=CARTESIAN_POINT ( 'NONE',  ( 6.328125000614515550, 4.541064518000418104, 2.621784821874999949 ) ) ;
#59997=CARTESIAN_POINT ( 'NONE',  ( 24.19687500061451502, -3.027376345333610441, -5.243569643749999898 ) ) ;
#59998=CARTESIAN_POINT ( 'NONE',  ( 6.515625000614516438, -6.054752690667223547, -1.112240025338166033E-15 ) ) ;
#60000=CARTESIAN_POINT ( 'NONE',  ( 7.275000001229035007, -5.773502691896255534, -1.060575238724906372E-15 ) ) ;
#60002=CARTESIAN_POINT ( 'NONE',  ( 21.40312500061451573, -4.541064518000417216, -2.621784821875001281 ) ) ;
#60003=CARTESIAN_POINT ( 'NONE',  ( -2.121784821874999949, 9.828125000614516438, -33.67503911421598417 ) ) ;
#60004=CARTESIAN_POINT ( 'NONE',  ( 10.91250000122903252, -4.330127018922190985, -2.500000000000001332 ) ) ;
#60005=CARTESIAN_POINT ( 'NONE',  ( 20.42812500061451431, -4.541064518000419881, 2.621784821874995952 ) ) ;
#60006=CARTESIAN_POINT ( 'NONE',  ( 19.11562500061451431, -6.054752690667223547, -1.112240025338166033E-15 ) ) ;
#60008=CARTESIAN_POINT ( 'NONE',  ( 18.41250000000000142, -5.773502691896255534, -1.060575238724906372E-15 ) ) ;
#60009=CARTESIAN_POINT ( 'NONE',  ( 10.35000000122903074, -2.886751345948129988, 4.999999999999997335 ) ) ;
#60010=CARTESIAN_POINT ( 'NONE',  ( 8.428125000614517859, 6.421520780324663323E-16, -5.243569643749999010 ) ) ;
#60011=CARTESIAN_POINT ( 'NONE',  ( 11.12812500061451715, 6.421520780324663323E-16, -5.243569643749999010 ) ) ;
#60012=CARTESIAN_POINT ( 'NONE',  ( 22.91250000122903430, 0.000000000000000000, 4.999999999999998224 ) ) ;
#60013=CARTESIAN_POINT ( 'NONE',  ( 21.60937500061451644, 4.541064518000418104, -2.621784821874998173 ) ) ;
#60014=CARTESIAN_POINT ( 'NONE',  ( 4.779965814201476704, -3.457634596098181579, -4.498340493050051236 ) ) ;
#60015=CARTESIAN_POINT ( 'NONE',  ( 4.725000001229034297, 2.886751345948129099, -4.999999999999998224 ) ) ;
#60016=CARTESIAN_POINT ( 'NONE',  ( 5.859375000614519102, 4.541064518000418104, -2.621784821874998173 ) ) ;
#60017=CARTESIAN_POINT ( 'NONE',  ( 23.82187500061451502, 3.027376345333613106, -5.243569643749998122 ) ) ;
#60018=CARTESIAN_POINT ( 'NONE',  ( 27.52500000000000213, 6.123233995736764310E-16, -4.999999999999998224 ) ) ;
#60019=CARTESIAN_POINT ( 'NONE',  ( 19.49062500061451431, -3.027376345333614438, 5.243569643749998122 ) ) ;
#60020=CARTESIAN_POINT ( 'NONE',  ( 25.32187500061451857, 3.027376345333611329, 5.243569643749999010 ) ) ;
#60022=CARTESIAN_POINT ( 'NONE',  ( 12.48750000122903359, 4.330127018922191873, 2.499999999999999556 ) ) ;
#60023=CARTESIAN_POINT ( 'NONE',  ( -5.810221930991193690E-16, 13.25000000122903465, -34.00000000000000000 ) ) ;
#60024=CARTESIAN_POINT ( 'NONE',  ( 4.696875000614518569, -3.027376345333614438, 5.243569643749998122 ) ) ;
#60025=CARTESIAN_POINT ( 'NONE',  ( 15.62812500061451537, 6.421520780324663323E-16, -5.243569643749999010 ) ) ;
#60026=CARTESIAN_POINT ( 'NONE',  ( 12.72187500061451537, 3.027376345333611329, 5.243569643749999010 ) ) ;
#60028=CARTESIAN_POINT ( 'NONE',  ( 9.112499999999997158, 2.886751345948062486, -5.000000000000113687 ) ) ;
#60029=CARTESIAN_POINT ( 'NONE',  ( 25.26562500061451289, 3.027376345333611329, 5.243569643749999010 ) ) ;
#60030=CARTESIAN_POINT ( 'NONE',  ( -3.999999999999999112, 10.62500000122903643, -32.30940107675850470 ) ) ;
#60033=CARTESIAN_POINT ( 'NONE',  ( 15.15000000000000036, 0.000000000000000000, 4.999999999999998224 ) ) ;
#60034=CARTESIAN_POINT ( 'NONE',  ( 24.37500000122903288, -5.773502691896255534, -1.060575238724906372E-15 ) ) ;
#60035=CARTESIAN_POINT ( 'NONE',  ( 19.71562500061451928, 3.027376345333613106, -5.243569643749998122 ) ) ;
#60036=ORIENTED_EDGE ( 'NONE', *, *, #72113, .F. ) ;
#60037=CARTESIAN_POINT ( 'NONE',  ( 21.37499999999999645, 4.330127018922191873, 2.499999999999999556 ) ) ;
#60038=CARTESIAN_POINT ( 'NONE',  ( 24.15937500061451715, -4.541064518000417216, -2.621784821875001281 ) ) ;
#60040=CARTESIAN_POINT ( 'NONE',  ( 2.970930829860112254, -4.021644987030126295, -3.364735388248410786 ) ) ;
#60041=CARTESIAN_POINT ( 'NONE',  ( 10.26562500061451644, 3.027376345333613106, -5.243569643749998122 ) ) ;
#60042=CARTESIAN_POINT ( 'NONE',  ( 2.953125000614516438, -4.541064518000417216, -2.621784821875001281 ) ) ;
#60044=CARTESIAN_POINT ( 'NONE',  ( 26.91562500061451146, 3.027376345333613106, -5.243569643749998122 ) ) ;
#60045=CARTESIAN_POINT ( 'NONE',  ( 17.43750000000000355, -2.886751345948129988, 4.999999999999997335 ) ) ;
#60046=CARTESIAN_POINT ( 'NONE',  ( 25.83749999999999858, 5.773502691896255534, 3.535250795749688894E-16 ) ) ;
#60047=CARTESIAN_POINT ( 'NONE',  ( -5.810221930991193690E-16, 10.88749999999999929, -34.00000000000000000 ) ) ;
#60048=CARTESIAN_POINT ( 'NONE',  ( 6.421875000614519102, 3.027376345333611329, 5.243569643749999010 ) ) ;
#60049=CARTESIAN_POINT ( 'NONE',  ( 17.29687500061451999, -3.027376345333614438, 5.243569643749998122 ) ) ;
#60050=CARTESIAN_POINT ( 'NONE',  ( 26.17500000000000071, 6.123233995736764310E-16, -4.999999999999998224 ) ) ;
#60051=ORIENTED_EDGE ( 'NONE', *, *, #68597, .T. ) ;
#60052=CARTESIAN_POINT ( 'NONE',  ( 27.21562500061451928, -6.054752690667223547, -1.112240025338166033E-15 ) ) ;
#60053=CARTESIAN_POINT ( 'NONE',  ( 27.57187500061451857, 3.027376345333611329, 5.243569643749999010 ) ) ;
#60055=CARTESIAN_POINT ( 'NONE',  ( 13.19999999999999929, 4.330127018922192761, -2.499999999999997780 ) ) ;
#60056=CARTESIAN_POINT ( 'NONE',  ( 12.25312500061451537, 0.000000000000000000, 5.243569643749999010 ) ) ;
#60057=CARTESIAN_POINT ( 'NONE',  ( -1.071796769724496556, 15.14240381056766616, -26.00000000000000355 ) ) ;
#60059=CARTESIAN_POINT ( 'NONE',  ( 29.20312500061451644, 4.541064518000418104, -2.621784821874998173 ) ) ;
#60060=CARTESIAN_POINT ( 'NONE',  ( 16.50000000122903288, 5.773502691896255534, 3.535250795749688894E-16 ) ) ;
#60061=CARTESIAN_POINT ( 'NONE',  ( 3.866371165286906830, -4.006382843392613857, -3.547880648171726214 ) ) ;
#60063=CARTESIAN_POINT ( 'NONE',  ( 4.453125000614517326, 4.541064518000418104, -2.621784821874998173 ) ) ;
#60064=CARTESIAN_POINT ( 'NONE',  ( 20.97187500061451715, -6.054752690667223547, -1.112240025338166033E-15 ) ) ;
#60065=CARTESIAN_POINT ( 'NONE',  ( -4.243569643749997233, 17.19687500061451502, 32.45002607614398471 ) ) ;
#60066=CARTESIAN_POINT ( 'NONE',  ( 23.10937500061451644, 0.000000000000000000, 5.243569643749999010 ) ) ;
#60067=CARTESIAN_POINT ( 'NONE',  ( 5.775000000000002132, -4.330127018922194537, 2.499999999999995559 ) ) ;
#60068=CARTESIAN_POINT ( 'NONE',  ( -1.999999999999997113, 10.73750000122903536, 33.46410161513775705 ) ) ;
#60069=CARTESIAN_POINT ( 'NONE',  ( 12.85312500061451502, -4.541064518000417216, -2.621784821875001281 ) ) ;
#60070=CARTESIAN_POINT ( 'NONE',  ( 4.837500001229035895, 4.330127018922191873, 2.499999999999999556 ) ) ;
#60071=CARTESIAN_POINT ( 'NONE',  ( 9.609375000614518214, 0.000000000000000000, 5.243569643749999010 ) ) ;
#60073=CARTESIAN_POINT ( 'NONE',  ( 9.290625000614515017, -3.027376345333610441, -5.243569643749999898 ) ) ;
#60074=CARTESIAN_POINT ( 'NONE',  ( 14.89687500061451786, 6.054752690667223547, 3.707466751127219781E-16 ) ) ;
#60076=CARTESIAN_POINT ( 'NONE',  ( 20.40000000122903145, -2.886751345948125991, -5.000000000000000000 ) ) ;
#60077=CARTESIAN_POINT ( 'NONE',  ( 10.54687500061451644, -3.027376345333614438, 5.243569643749998122 ) ) ;
#60078=CARTESIAN_POINT ( 'NONE',  ( 11.84062500061451750, -3.027376345333614438, 5.243569643749998122 ) ) ;
#60080=CARTESIAN_POINT ( 'NONE',  ( 21.45937500061451786, -4.541064518000417216, -2.621784821875001281 ) ) ;
#60081=CARTESIAN_POINT ( 'NONE',  ( 0.000000000000000000, 20.00000000000000000, -36.00000000000000000 ) ) ;
#60082=CARTESIAN_POINT ( 'NONE',  ( -3.861264241427936117, 3.177798304702606824, 28.92162313090120662 ) ) ;
#60084=EDGE_CURVE ( 'NONE', #59218, #17166, #30028, .T. ) ;
#60085=CARTESIAN_POINT ( 'NONE',  ( 4.243569643749999898, 15.58437500061451786, -30.00000000000000000 ) ) ;
#60086=CARTESIAN_POINT ( 'NONE',  ( 15.45000000122903216, -2.886751345948125991, -5.000000000000000000 ) ) ;
#60088=CARTESIAN_POINT ( 'NONE',  ( 9.196875000614518569, -3.027376345333614438, 5.243569643749998122 ) ) ;
#60089=CARTESIAN_POINT ( 'NONE',  ( -4.243569643749999898, 17.06562500061451360, -32.45002607614398471 ) ) ;
#60090=CARTESIAN_POINT ( 'NONE',  ( 16.83750000122903145, 6.123233995736764310E-16, -4.999999999999998224 ) ) ;
#60091=CARTESIAN_POINT ( 'NONE',  ( 11.39062500061451644, -3.027376345333614438, 5.243569643749998122 ) ) ;
#60092=ORIENTED_EDGE ( 'NONE', *, *, #63628, .T. ) ;
#60093=CARTESIAN_POINT ( 'NONE',  ( 15.22500000000000142, -4.330127018922194537, 2.499999999999995559 ) ) ;
#60094=CYLINDRICAL_SURFACE ( 'NONE', #31476, 4.999999999999998224 ) ;
#60095=CARTESIAN_POINT ( 'NONE',  ( 9.234375000614518214, -4.541064518000419881, 2.621784821874995952 ) ) ;
#60097=CARTESIAN_POINT ( 'NONE',  ( 9.562500001229032875, -4.330127018922190985, -2.500000000000001332 ) ) ;
#60098=CARTESIAN_POINT ( 'NONE',  ( 18.56250000122903288, -4.330127018922190985, -2.500000000000001332 ) ) ;
#60099=CARTESIAN_POINT ( 'NONE',  ( 14.69062500061451537, -3.027376345333610441, -5.243569643749999898 ) ) ;
#60100=CARTESIAN_POINT ( 'NONE',  ( 19.49062500061451431, -3.027376345333614438, 5.243569643749998122 ) ) ;
#60101=CARTESIAN_POINT ( 'NONE',  ( 27.07500000122903216, -5.773502691896255534, -1.060575238724906372E-15 ) ) ;
#60102=CARTESIAN_POINT ( 'NONE',  ( 3.590625000614518836, 6.054752690667223547, 3.707466751127219781E-16 ) ) ;
#60103=CARTESIAN_POINT ( 'NONE',  ( 24.18750000000000355, -2.886751345948129988, 4.999999999999997335 ) ) ;
#60106=CARTESIAN_POINT ( 'NONE',  ( 27.27187500061451431, -6.054752690667223547, -1.112240025338166033E-15 ) ) ;
#60107=CARTESIAN_POINT ( 'NONE',  ( 3.999999999999999112, 17.52499999999999858, 30.00000000000000000 ) ) ;
#60108=CARTESIAN_POINT ( 'NONE',  ( 12.75000000122903643, -2.886751345948125991, -5.000000000000000000 ) ) ;
#60109=CARTESIAN_POINT ( 'NONE',  ( 3.712499999999999911, 2.886751345948129099, -4.999999999999998224 ) ) ;
#60111=CARTESIAN_POINT ( 'NONE',  ( 7.171875000614517326, 3.027376345333613106, -5.243569643749998122 ) ) ;
#60112=CARTESIAN_POINT ( 'NONE',  ( 26.65312500061451573, 0.000000000000000000, 5.243569643749999010 ) ) ;
#60115=DIRECTION ( 'NONE',  ( -1.000000000000000000, -0.000000000000000000, -0.000000000000000000 ) ) ;
#60116=CARTESIAN_POINT ( 'NONE',  ( 4.284375000614518925, -4.541064518000419881, 2.621784821874995952 ) ) ;
#60117=CARTESIAN_POINT ( 'NONE',  ( 7.734375000614517326, 4.541064518000418104, 2.621784821874999949 ) ) ;
#60118=CARTESIAN_POINT ( 'NONE',  ( 4.050000000000001599, -4.330127018922190985, -2.500000000000001332 ) ) ;
#60119=CARTESIAN_POINT ( 'NONE',  ( 2.121784821875001281, 11.85312500061459673, 33.67503911421598417 ) ) ;
#60120=CARTESIAN_POINT ( 'NONE',  ( 21.22500000000000142, 6.123233995736764310E-16, -4.999999999999998224 ) ) ;
#60121=CARTESIAN_POINT ( 'NONE',  ( 29.66249999999999432, -5.773502691896255534, -1.060575238724906372E-15 ) ) ;
#60123=CARTESIAN_POINT ( 'NONE',  ( 3.300000000000000711, 4.330127018922192761, -2.499999999999997780 ) ) ;
#60125=CARTESIAN_POINT ( 'NONE',  ( 18.85312500061451502, 4.541064518000418104, -2.621784821874998173 ) ) ;
#60126=CARTESIAN_POINT ( 'NONE',  ( 11.24062500061451608, 6.054752690667223547, 3.707466751127219781E-16 ) ) ;
#60128=CARTESIAN_POINT ( 'NONE',  ( 8.146875000614516082, 6.054752690667223547, 3.707466751127219781E-16 ) ) ;
#60129=CARTESIAN_POINT ( 'NONE',  ( 22.91249999999999432, -5.773502691896255534, -1.060575238724906372E-15 ) ) ;
#60130=CARTESIAN_POINT ( 'NONE',  ( 20.10000000122903074, 5.773502691896255534, 3.535250795749688894E-16 ) ) ;
#60131=CYLINDRICAL_SURFACE ( 'NONE', #6024, 4.999999999999998224 ) ;
#60132=CARTESIAN_POINT ( 'NONE',  ( 10.02187500061451964, 3.027376345333611329, 5.243569643749999010 ) ) ;
#60133=CARTESIAN_POINT ( 'NONE',  ( 13.24687500061451750, -3.027376345333614438, 5.243569643749998122 ) ) ;
#60134=CARTESIAN_POINT ( 'NONE',  ( 24.49687500061451573, -3.027376345333614438, 5.243569643749998122 ) ) ;
#60135=CARTESIAN_POINT ( 'NONE',  ( 8.625000001229034652, -5.773502691896255534, -1.060575238724906372E-15 ) ) ;
#60137=CARTESIAN_POINT ( 'NONE',  ( 18.38437500061451857, 6.421520780324663323E-16, -5.243569643749999010 ) ) ;
#60138=CARTESIAN_POINT ( 'NONE',  ( 8.671875000614518214, 3.027376345333611329, 5.243569643749999010 ) ) ;
#60140=CARTESIAN_POINT ( 'NONE',  ( 20.77500000000000213, 6.123233995736764310E-16, -4.999999999999998224 ) ) ;
#60144=CARTESIAN_POINT ( 'NONE',  ( 12.29062500061451857, -3.027376345333614438, 5.243569643749998122 ) ) ;
#60145=CARTESIAN_POINT ( 'NONE',  ( 29.52187500061451431, -6.054752690667223547, -1.112240025338166033E-15 ) ) ;
#60148=CARTESIAN_POINT ( 'NONE',  ( 12.15000000000000036, -4.330127018922190985, -2.500000000000001332 ) ) ;
#60149=CARTESIAN_POINT ( 'NONE',  ( -3.999999999999999112, 18.31250000122903288, 30.00000000000000000 ) ) ;
#60150=CARTESIAN_POINT ( 'NONE',  ( 11.58750000122903501, 4.330127018922191873, 2.499999999999999556 ) ) ;
#60151=CARTESIAN_POINT ( 'NONE',  ( 21.79687500061451644, -3.027376345333614438, 5.243569643749998122 ) ) ;
#60152=CARTESIAN_POINT ( 'NONE',  ( 16.62187500061451573, 3.027376345333613106, -5.243569643749998122 ) ) ;
#60153=CARTESIAN_POINT ( 'NONE',  ( -1.071796769724488563, 16.49240381056766580, -26.00000000000000000 ) ) ;
#60155=CARTESIAN_POINT ( 'NONE',  ( 16.75312500061451715, 0.000000000000000000, 5.243569643749999010 ) ) ;
#60156=CARTESIAN_POINT ( 'NONE',  ( 28.50000000122903288, -2.886751345948125991, -5.000000000000000000 ) ) ;
#60157=CARTESIAN_POINT ( 'NONE',  ( 17.37187500061451573, -6.054752690667223547, -1.112240025338166033E-15 ) ) ;
#60158=CARTESIAN_POINT ( 'NONE',  ( 3.628125000614518036, 4.541064518000418104, 2.621784821874999949 ) ) ;
#60159=CARTESIAN_POINT ( 'NONE',  ( 18.32812500061451644, 6.421520780324663323E-16, -5.243569643749999010 ) ) ;
#60160=CARTESIAN_POINT ( 'NONE',  ( 3.176339285701963888, -3.861459405730729433, 3.176339285701963888 ) ) ;
#60161=CARTESIAN_POINT ( 'NONE',  ( 27.83437500061451786, 6.421520780324663323E-16, -5.243569643749999010 ) ) ;
#60162=CARTESIAN_POINT ( 'NONE',  ( 4.243569643749999898, 13.69062500061451537, 32.45002607614398471 ) ) ;
#60163=CARTESIAN_POINT ( 'NONE',  ( 17.55000000122903359, -2.886751345948129988, 4.999999999999997335 ) ) ;
#60165=CARTESIAN_POINT ( 'NONE',  ( 27.06562500061451004, 3.027376345333611329, 5.243569643749999010 ) ) ;
#60167=CARTESIAN_POINT ( 'NONE',  ( 20.97187500061451715, -6.054752690667223547, -1.112240025338166033E-15 ) ) ;
#60168=CARTESIAN_POINT ( 'NONE',  ( 23.55000000122903359, -2.886751345948125991, -5.000000000000000000 ) ) ;
#60169=ADVANCED_FACE ( 'NONE', ( #16049 ), #50772, .F. ) ;
#60170=CARTESIAN_POINT ( 'NONE',  ( 22.19062500061451715, -3.027376345333614438, 5.243569643749998122 ) ) ;
#60171=CARTESIAN_POINT ( 'NONE',  ( 16.65937500061452070, 4.541064518000418104, -2.621784821874998173 ) ) ;
#60172=CARTESIAN_POINT ( 'NONE',  ( 11.50312500061451892, -4.541064518000417216, -2.621784821875001281 ) ) ;
#60173=CARTESIAN_POINT ( 'NONE',  ( -4.243569643749999898, 15.80937500061451573, 30.00000000000000000 ) ) ;
#60174=CARTESIAN_POINT ( 'NONE',  ( 17.35312500061451502, -4.541064518000417216, -2.621784821875001281 ) ) ;
#60176=ORIENTED_EDGE ( 'NONE', *, *, #51752, .T. ) ;
#60177=EDGE_LOOP ( 'NONE', ( #18308, #57903, #49198, #40159 ) ) ;
#60178=CARTESIAN_POINT ( 'NONE',  ( 22.50000000000000000, -4.330127018922190985, -2.500000000000001332 ) ) ;
#60179=CARTESIAN_POINT ( 'NONE',  ( 4.243569643749999898, 19.14687500061451431, -27.54997392385601529 ) ) ;
#60181=CARTESIAN_POINT ( 'NONE',  ( 24.02812500061451573, -4.541064518000419881, 2.621784821874995952 ) ) ;
#60182=CARTESIAN_POINT ( 'NONE',  ( 6.440625000614517148, -3.027376345333614438, 5.243569643749998122 ) ) ;
#60183=CARTESIAN_POINT ( 'NONE',  ( 17.06250000122903288, 0.000000000000000000, 4.999999999999998224 ) ) ;
#60184=CARTESIAN_POINT ( 'NONE',  ( 21.36562500061451431, -6.054752690667223547, -1.112240025338166033E-15 ) ) ;
#60185=CARTESIAN_POINT ( 'NONE',  ( 21.82499999999999574, 4.330127018922191873, 2.499999999999999556 ) ) ;
#60186=CARTESIAN_POINT ( 'NONE',  ( 27.44062500061451715, 6.054752690667223547, 3.707466751127219781E-16 ) ) ;
#60187=CARTESIAN_POINT ( 'NONE',  ( 7.528125000614515727, 6.421520780324663323E-16, -5.243569643749999010 ) ) ;
#60188=VERTEX_POINT ( 'NONE', #175 ) ;
#60189=CARTESIAN_POINT ( 'NONE',  ( 23.27812500061451573, 6.421520780324663323E-16, -5.243569643749999010 ) ) ;
#60190=CARTESIAN_POINT ( 'NONE',  ( 4.828125000614518214, 6.421520780324663323E-16, -5.243569643749999010 ) ) ;
#60193=CARTESIAN_POINT ( 'NONE',  ( -3.999999999999999112, 13.81250000122903465, -30.00000000000000000 ) ) ;
#60194=CARTESIAN_POINT ( 'NONE',  ( -2.000000000000000000, 10.47500000000000142, -33.46410161513775705 ) ) ;
#60195=CARTESIAN_POINT ( 'NONE',  ( 10.38750000000000107, -2.886751345948125991, -5.000000000000000000 ) ) ;
#60196=CARTESIAN_POINT ( 'NONE',  ( 12.38437500061451857, -4.541064518000419881, 2.621784821874995952 ) ) ;
#60197=CARTESIAN_POINT ( 'NONE',  ( 6.750000001229033764, -2.886751345948129988, 4.999999999999997335 ) ) ;
#60198=CARTESIAN_POINT ( 'NONE',  ( 15.72187500061451892, 3.027376345333613106, -5.243569643749998122 ) ) ;
#60199=CARTESIAN_POINT ( 'NONE',  ( 5.409375000614516260, 4.541064518000418104, -2.621784821874998173 ) ) ;
#60200=DIRECTION ( 'NONE',  ( -1.000000000000000000, -0.000000000000000000, -0.000000000000000000 ) ) ;
#60201=CARTESIAN_POINT ( 'NONE',  ( -5.000000000000000000, 0.000000000000000000, 50.00000000000000000 ) ) ;
#60202=CARTESIAN_POINT ( 'NONE',  ( 12.34687500061452070, -3.027376345333614438, 5.243569643749998122 ) ) ;
#60204=CARTESIAN_POINT ( 'NONE',  ( 20.91562500061451502, -6.054752690667223547, -1.112240025338166033E-15 ) ) ;
#60205=CARTESIAN_POINT ( 'NONE',  ( 3.999999999999998668, 11.71250000000000036, 27.69059892324149530 ) ) ;
#60207=CARTESIAN_POINT ( 'NONE',  ( 24.30937500061451573, 4.541064518000418104, -2.621784821874998173 ) ) ;
#60208=CARTESIAN_POINT ( 'NONE',  ( -3.999999999999999112, 13.77500000122903678, -32.30940107675850470 ) ) ;
#60209=CARTESIAN_POINT ( 'NONE',  ( 3.890625000614517326, -3.027376345333610441, -5.243569643749999898 ) ) ;
#60211=CARTESIAN_POINT ( 'NONE',  ( 18.44062500061451715, 6.054752690667223547, 3.707466751127219781E-16 ) ) ;
#60212=CARTESIAN_POINT ( 'NONE',  ( 13.73437500061451821, -4.541064518000419881, 2.621784821874995952 ) ) ;
#60213=CARTESIAN_POINT ( 'NONE',  ( 16.72500000000000142, 6.123233995736764310E-16, -4.999999999999998224 ) ) ;
#60214=CARTESIAN_POINT ( 'NONE',  ( 27.45000000122903572, -2.886751345948129988, 4.999999999999997335 ) ) ;
#60215=CARTESIAN_POINT ( 'NONE',  ( 5.671875000614519102, -6.054752690667223547, -1.112240025338166033E-15 ) ) ;
#60216=CARTESIAN_POINT ( 'NONE',  ( 17.07187500061451502, 3.027376345333613106, -5.243569643749998122 ) ) ;
#60217=CARTESIAN_POINT ( 'NONE',  ( 15.11249999999999893, 2.886751345948126879, 4.999999999999998224 ) ) ;
#60218=CARTESIAN_POINT ( 'NONE',  ( 24.97499999999999787, 4.330127018922191873, 2.499999999999999556 ) ) ;
#60219=CARTESIAN_POINT ( 'NONE',  ( 24.38437500061451502, 4.541064518000418104, 2.621784821874999949 ) ) ;
#60220=CARTESIAN_POINT ( 'NONE',  ( 16.88437500061451502, -4.541064518000419881, 2.621784821874995952 ) ) ;
#60222=CARTESIAN_POINT ( 'NONE',  ( 6.825000000000001066, 6.123233995736764310E-16, -4.999999999999998224 ) ) ;
#60224=CARTESIAN_POINT ( 'NONE',  ( 18.70312500061451644, -4.541064518000417216, -2.621784821875001281 ) ) ;
#60225=CARTESIAN_POINT ( 'NONE',  ( 10.27499999999999858, -4.330127018922194537, 2.499999999999995559 ) ) ;
#60226=( BOUNDED_CURVE ( )  B_SPLINE_CURVE ( 2, ( #63445, #25271, #47818, #56802, #12831, #19725, #42276 ),
 .UNSPECIFIED., .F., .F. ) 
 B_SPLINE_CURVE_WITH_KNOTS ( ( 3, 2, 2, 3 ),
 ( 0.9855112084356887348, 0.9861111111111111605, 0.9888888888888889284, 0.9894149656234122459 ),
 .UNSPECIFIED. ) 
 CURVE ( )  GEOMETRIC_REPRESENTATION_ITEM ( )  RATIONAL_B_SPLINE_CURVE ( ( 0.9546297447238953904, 0.9710661812649934443, 1.000000000000000000, 0.8660254037844387076, 1.000000000000000000, 0.9746268694889814732, 0.9588644528015497492 ) ) 
 REPRESENTATION_ITEM ( '' )  );
#60227=CARTESIAN_POINT ( 'NONE',  ( 3.440625000614518036, -3.027376345333610441, -5.243569643749999898 ) ) ;
#60228=CARTESIAN_POINT ( 'NONE',  ( 18.45000000000000284, -4.330127018922190985, -2.500000000000001332 ) ) ;
#60229=CARTESIAN_POINT ( 'NONE',  ( 19.00312500061451715, 0.000000000000000000, 5.243569643749999010 ) ) ;
#60231=CARTESIAN_POINT ( 'NONE',  ( 22.16250000122903074, -4.330127018922190985, -2.500000000000001332 ) ) ;
#60233=CARTESIAN_POINT ( 'NONE',  ( 28.95937500061451431, 0.000000000000000000, 5.243569643749999010 ) ) ;
#60235=CARTESIAN_POINT ( 'NONE',  ( 17.87812500061451715, 6.421520780324663323E-16, -5.243569643749999010 ) ) ;
#60236=CARTESIAN_POINT ( 'NONE',  ( 24.06562500061451715, -6.054752690667223547, -1.112240025338166033E-15 ) ) ;
#60237=CARTESIAN_POINT ( 'NONE',  ( 25.24687500061451573, 6.054752690667223547, 3.707466751127219781E-16 ) ) ;
#60238=CARTESIAN_POINT ( 'NONE',  ( 8.025000000000000355, -4.330127018922194537, 2.499999999999995559 ) ) ;
#60239=CARTESIAN_POINT ( 'NONE',  ( 11.69062500061451360, 6.054752690667223547, 3.707466751127219781E-16 ) ) ;
#60240=CARTESIAN_POINT ( 'NONE',  ( 26.54062500061451146, 6.054752690667223547, 3.707466751127219781E-16 ) ) ;
#60241=CARTESIAN_POINT ( 'NONE',  ( 16.50937500061451502, -4.541064518000417216, -2.621784821875001281 ) ) ;
#60242=CARTESIAN_POINT ( 'NONE',  ( 19.77187500061451786, 3.027376345333613106, -5.243569643749998122 ) ) ;
#60243=CARTESIAN_POINT ( 'NONE',  ( 7.050000001229036251, 5.773502691896255534, 3.535250795749688401E-16 ) ) ;
#60244=CARTESIAN_POINT ( 'NONE',  ( 4.243569643749999010, 10.67187500061451644, 27.54997392385601174 ) ) ;
#60245=CARTESIAN_POINT ( 'NONE',  ( 23.55000000122903359, -2.886751345948125991, -5.000000000000000000 ) ) ;
#60247=CARTESIAN_POINT ( 'NONE',  ( 13.90312500061451750, 4.541064518000418104, -2.621784821874998173 ) ) ;
#60248=CARTESIAN_POINT ( 'NONE',  ( 7.321875000614516793, 3.027376345333611329, 5.243569643749999010 ) ) ;
#60249=CARTESIAN_POINT ( 'NONE',  ( 7.471875000614519813, -6.054752690667223547, -1.112240025338166033E-15 ) ) ;
#60251=CARTESIAN_POINT ( 'NONE',  ( 1.071796769724491893, 13.38259618943233598, 33.99999999999999289 ) ) ;
#60252=CARTESIAN_POINT ( 'NONE',  ( 20.42812500061451431, -4.541064518000419881, 2.621784821874995952 ) ) ;
#60253=EDGE_CURVE ( 'NONE', #63581, #2667, #50336, .T. ) ;
#60254=CARTESIAN_POINT ( 'NONE',  ( 23.70937500061451786, -4.541064518000417216, -2.621784821875001281 ) ) ;
#60255=CARTESIAN_POINT ( 'NONE',  ( 20.69062500061451715, 6.054752690667223547, 3.707466751127219781E-16 ) ) ;
#60256=CARTESIAN_POINT ( 'NONE',  ( 3.999999999999999112, 12.12500000000000000, 30.00000000000000000 ) ) ;
#60257=CARTESIAN_POINT ( 'NONE',  ( 26.69062500061451715, -3.027376345333614438, 5.243569643749998122 ) ) ;
#60258=CARTESIAN_POINT ( 'NONE',  ( 6.525000001229033231, 2.886751345948129099, -4.999999999999998224 ) ) ;
#60260=CARTESIAN_POINT ( 'NONE',  ( 2.737500001229034474, -4.330127018922194537, 2.499999999999995559 ) ) ;
#60261=CARTESIAN_POINT ( 'NONE',  ( -3.999999999999999556, 15.46250000000000036, -32.30940107675850470 ) ) ;
#60262=CARTESIAN_POINT ( 'NONE',  ( 22.46250000122903501, 0.000000000000000000, 4.999999999999998224 ) ) ;
#60264=CARTESIAN_POINT ( 'NONE',  ( 6.871875000614517504, 3.027376345333611329, 5.243569643749999010 ) ) ;
#60265=CARTESIAN_POINT ( 'NONE',  ( 12.90000000000000213, 0.000000000000000000, 4.999999999999998224 ) ) ;
#60266=CARTESIAN_POINT ( 'NONE',  ( 11.54062500061451857, -3.027376345333610441, -5.243569643749999898 ) ) ;
#60267=CARTESIAN_POINT ( 'NONE',  ( 7.396875000614519635, -3.027376345333614438, 5.243569643749998122 ) ) ;
#60268=CARTESIAN_POINT ( 'NONE',  ( 27.82500000122903572, 2.886751345948126879, 4.999999999999999112 ) ) ;
#60269=CARTESIAN_POINT ( 'NONE',  ( 14.48437500061451821, 4.541064518000418104, 2.621784821874999949 ) ) ;
#60270=CARTESIAN_POINT ( 'NONE',  ( 4.509375000614518569, 4.541064518000418104, -2.621784821874998173 ) ) ;
#60271=CARTESIAN_POINT ( 'NONE',  ( 29.43750000000000000, 5.773502691896255534, 3.535250795749688894E-16 ) ) ;
#60272=CARTESIAN_POINT ( 'NONE',  ( 5.390625000614518214, 6.054752690667223547, 3.707466751127219781E-16 ) ) ;
#60273=CARTESIAN_POINT ( 'NONE',  ( 14.46562500061451750, 3.027376345333611329, 5.243569643749999010 ) ) ;
#60275=CARTESIAN_POINT ( 'NONE',  ( 11.39062500061451644, -3.027376345333614438, 5.243569643749998122 ) ) ;
#60276=CARTESIAN_POINT ( 'NONE',  ( 5.137500001229033941, 6.123233995736764310E-16, -4.999999999999998224 ) ) ;
#60277=CARTESIAN_POINT ( 'NONE',  ( 8.653125000614515727, 0.000000000000000000, 5.243569643749999010 ) ) ;
#60279=CARTESIAN_POINT ( 'NONE',  ( 9.412499999999999645, -5.773502691896255534, -1.060575238724906372E-15 ) ) ;
#60280=CARTESIAN_POINT ( 'NONE',  ( 4.725000001229034297, 2.886751345948129099, -4.999999999999998224 ) ) ;
#60281=CARTESIAN_POINT ( 'NONE',  ( 17.17500000000000071, 6.123233995736764310E-16, -4.999999999999998224 ) ) ;
#60283=CARTESIAN_POINT ( 'NONE',  ( 18.68437500061451928, -4.541064518000419881, 2.621784821874995952 ) ) ;
#60284=CARTESIAN_POINT ( 'NONE',  ( 13.42500000122903536, 2.886751345948126879, 4.999999999999999112 ) ) ;
#60286=CARTESIAN_POINT ( 'NONE',  ( 4.243569643749999010, 16.01562500061451644, -32.45002607614398471 ) ) ;
#60290=DIRECTION ( 'NONE',  ( -1.000000000000000000, -0.000000000000000000, -0.000000000000000000 ) ) ;
#60292=CARTESIAN_POINT ( 'NONE',  ( 16.77187500061451786, 3.027376345333611329, 5.243569643749999010 ) ) ;
#60293=CARTESIAN_POINT ( 'NONE',  ( 27.18750000000000000, 5.773502691896255534, 3.535250795749688894E-16 ) ) ;
#60294=EDGE_CURVE ( 'NONE', #9597, #37881, #44876, .T. ) ;
#60295=CARTESIAN_POINT ( 'NONE',  ( 11.27812500061451573, 4.541064518000418104, 2.621784821874999949 ) ) ;
#60297=CARTESIAN_POINT ( 'NONE',  ( 22.47187500061451715, 3.027376345333613106, -5.243569643749998122 ) ) ;
#60299=CARTESIAN_POINT ( 'NONE',  ( 6.553125000614518747, -4.541064518000417216, -2.621784821875001281 ) ) ;
#60300=CARTESIAN_POINT ( 'NONE',  ( 13.77187500061451786, -6.054752690667223547, -1.112240025338166033E-15 ) ) ;
#60302=CARTESIAN_POINT ( 'NONE',  ( 23.59687500061451715, -3.027376345333614438, 5.243569643749998122 ) ) ;
#60303=CYLINDRICAL_SURFACE ( 'NONE', #47746, 4.999999999999998224 ) ;
#60304=CARTESIAN_POINT ( 'NONE',  ( 28.75312500061451715, 4.541064518000418104, -2.621784821874998173 ) ) ;
#60305=CARTESIAN_POINT ( 'NONE',  ( 24.75000000000000000, -4.330127018922190985, -2.500000000000001332 ) ) ;
#60306=CARTESIAN_POINT ( 'NONE',  ( 7.312500000000000000, 2.886751345948129099, -4.999999999999998224 ) ) ;
#60307=CARTESIAN_POINT ( 'NONE',  ( 17.21250000122903145, -4.330127018922190985, -2.500000000000001332 ) ) ;
#60312=CARTESIAN_POINT ( 'NONE',  ( 15.75000000000000000, -4.330127018922190985, -2.500000000000001332 ) ) ;
#60313=CARTESIAN_POINT ( 'NONE',  ( 19.27500000000000213, -4.330127018922194537, 2.499999999999995559 ) ) ;
#60314=CARTESIAN_POINT ( 'NONE',  ( 10.82812500061451644, 4.541064518000418104, 2.621784821874999949 ) ) ;
#60315=ORIENTED_EDGE ( 'NONE', *, *, #69831, .T. ) ;
#60316=CARTESIAN_POINT ( 'NONE',  ( 26.32499999999999929, 4.330127018922191873, 2.499999999999999556 ) ) ;
#60317=CARTESIAN_POINT ( 'NONE',  ( 9.001249775931846008E-16, 16.82187500061451857, -25.09994784771203058 ) ) ;
#60318=CARTESIAN_POINT ( 'NONE',  ( 2.803125000614518747, 0.000000000000000000, 5.243569643749999010 ) ) ;
#60320=CARTESIAN_POINT ( 'NONE',  ( 9.600000000000001421, 4.330127018922192761, -2.499999999999997780 ) ) ;
#60321=CARTESIAN_POINT ( 'NONE',  ( 3.727827348360245097, 3.332161949968362347, -3.727827348360304605 ) ) ;
#60322=VERTEX_POINT ( 'NONE', #5705 ) ;
#60323=CARTESIAN_POINT ( 'NONE',  ( -3.000416591977282496E-16, 12.04062500061451857, 25.09994784771203058 ) ) ;
#60324=CARTESIAN_POINT ( 'NONE',  ( 25.07812500061451644, 6.421520780324663323E-16, -5.243569643749999010 ) ) ;
#60325=CARTESIAN_POINT ( 'NONE',  ( 4.206174892561018730, -2.703348437251418268, 4.492986738870575536 ) ) ;
#60327=CARTESIAN_POINT ( 'NONE',  ( 21.57187500061451502, 3.027376345333613106, -5.243569643749998122 ) ) ;
#60328=EDGE_CURVE ( 'NONE', #58564, #43716, #67411, .T. ) ;
#60329=CARTESIAN_POINT ( 'NONE',  ( 19.15312500061451573, -4.541064518000417216, -2.621784821875001281 ) ) ;
#60330=CARTESIAN_POINT ( 'NONE',  ( -4.243569643749999898, 13.95312500061459282, -30.00000000000000000 ) ) ;
#60331=CARTESIAN_POINT ( 'NONE',  ( 22.20000000122903216, -2.886751345948125991, -5.000000000000000000 ) ) ;
#60332=CARTESIAN_POINT ( 'NONE',  ( 4.153125000614515727, 0.000000000000000000, 5.243569643749999010 ) ) ;
#60334=CARTESIAN_POINT ( 'NONE',  ( 20.99062500061451431, -3.027376345333610441, -5.243569643749999898 ) ) ;
#60337=CARTESIAN_POINT ( 'NONE',  ( 15.04687500061451644, -3.027376345333614438, 5.243569643749998122 ) ) ;
#60338=CARTESIAN_POINT ( 'NONE',  ( 13.28437500061451715, -4.541064518000419881, 2.621784821874995952 ) ) ;
#60339=CARTESIAN_POINT ( 'NONE',  ( 23.40937500061451715, 4.541064518000418104, -2.621784821874998173 ) ) ;
#60340=CARTESIAN_POINT ( 'NONE',  ( 4.243569643749999898, 11.53437500061451892, 30.00000000000000000 ) ) ;
#60341=CARTESIAN_POINT ( 'NONE',  ( 5.953125000614519102, 0.000000000000000000, 5.243569643749999010 ) ) ;
#60342=CARTESIAN_POINT ( 'NONE',  ( 29.50312500061451360, -4.541064518000417216, -2.621784821875001281 ) ) ;
#60343=CARTESIAN_POINT ( 'NONE',  ( 27.62812500061451360, -4.541064518000419881, 2.621784821874995952 ) ) ;
#60344=CARTESIAN_POINT ( 'NONE',  ( 1.071796769724490339, 19.52990381179669654, -34.00000000000000000 ) ) ;
#60345=CARTESIAN_POINT ( 'NONE',  ( -3.999999999999999112, 18.19999999999999929, 30.00000000000000000 ) ) ;
#60346=CARTESIAN_POINT ( 'NONE',  ( 6.496875000614517504, -3.027376345333614438, 5.243569643749998122 ) ) ;
#60348=CARTESIAN_POINT ( 'NONE',  ( 14.88750000122903394, -4.330127018922194537, 2.499999999999995559 ) ) ;
#60349=CARTESIAN_POINT ( 'NONE',  ( 10.27500000122903323, 2.886751345948126879, 4.999999999999999112 ) ) ;
#60350=CARTESIAN_POINT ( 'NONE',  ( 28.53750000122903074, 6.123233995736764310E-16, -4.999999999999998224 ) ) ;
#60353=CARTESIAN_POINT ( 'NONE',  ( 13.35937500061451821, -4.541064518000417216, -2.621784821875001281 ) ) ;
#60354=LINE ( 'NONE', #9038, #57309 ) ;
#60355=ORIENTED_EDGE ( 'NONE', *, *, #25207, .F. ) ;
#60356=CARTESIAN_POINT ( 'NONE',  ( 20.87812500061451715, -4.541064518000419881, 2.621784821874995952 ) ) ;
#60357=CARTESIAN_POINT ( 'NONE',  ( 6.665625000614515905, 3.027376345333613106, -5.243569643749998122 ) ) ;
#60358=CARTESIAN_POINT ( 'NONE',  ( 24.15937500061451715, -4.541064518000417216, -2.621784821875001281 ) ) ;
#60359=CARTESIAN_POINT ( 'NONE',  ( 8.465625000614515727, 3.027376345333613106, -5.243569643749998122 ) ) ;
#60361=CARTESIAN_POINT ( 'NONE',  ( 7.837500001229035007, 6.123233995736764310E-16, -4.999999999999998224 ) ) ;
#60362=EDGE_CURVE ( 'NONE', #50794, #31197, #39795, .T. ) ;
#60363=CARTESIAN_POINT ( 'NONE',  ( 23.20312500061451644, -4.541064518000417216, -2.621784821875001281 ) ) ;
#60364=CARTESIAN_POINT ( 'NONE',  ( 2.000000000000001332, 18.01250000122903572, -26.53589838486224650 ) ) ;
#60365=CARTESIAN_POINT ( 'NONE',  ( 10.35000000122903074, -2.886751345948129988, 4.999999999999997335 ) ) ;
#60366=CARTESIAN_POINT ( 'NONE',  ( 20.46562500061451928, -6.054752690667223547, -1.112240025338166033E-15 ) ) ;
#60367=CARTESIAN_POINT ( 'NONE',  ( 15.70312500061451644, 4.541064518000418104, -2.621784821874998173 ) ) ;
#60369=CARTESIAN_POINT ( 'NONE',  ( 15.59999999999999964, 0.000000000000000000, 4.999999999999998224 ) ) ;
#60370=CARTESIAN_POINT ( 'NONE',  ( 11.70000000122903216, -2.886751345948129988, 4.999999999999997335 ) ) ;
#60371=CARTESIAN_POINT ( 'NONE',  ( 8.878125000614515372, 6.421520780324663323E-16, -5.243569643749999010 ) ) ;
#60373=CARTESIAN_POINT ( 'NONE',  ( 10.97812500061451679, -4.541064518000419881, 2.621784821874995952 ) ) ;
#60375=CARTESIAN_POINT ( 'NONE',  ( 20.36250000122903359, -4.330127018922190985, -2.500000000000001332 ) ) ;
#60376=CARTESIAN_POINT ( 'NONE',  ( 19.24687500061452283, -3.027376345333610441, -5.243569643749999898 ) ) ;
#60378=CARTESIAN_POINT ( 'NONE',  ( 4.162500001229033408, -4.330127018922190985, -2.500000000000001332 ) ) ;
#60379=CARTESIAN_POINT ( 'NONE',  ( 3.346875000614518036, -3.027376345333614438, 5.243569643749998122 ) ) ;
#60380=CARTESIAN_POINT ( 'NONE',  ( 22.13437500061451502, 4.541064518000418104, 2.621784821874999949 ) ) ;
#60382=CARTESIAN_POINT ( 'NONE',  ( 18.40312500061451573, 4.541064518000418104, -2.621784821874998173 ) ) ;
#60383=CARTESIAN_POINT ( 'NONE',  ( 23.25937500061451857, -4.541064518000417216, -2.621784821875001281 ) ) ;
#60385=FACE_OUTER_BOUND ( 'NONE', #73110, .T. ) ;
#60386=CARTESIAN_POINT ( 'NONE',  ( 29.52187500061451431, -6.054752690667223547, -1.112240025338166033E-15 ) ) ;
#60388=CARTESIAN_POINT ( 'NONE',  ( 15.59062500061451573, -3.027376345333610441, -5.243569643749999898 ) ) ;
#60389=CARTESIAN_POINT ( 'NONE',  ( 13.88437500061451679, 6.421520780324663323E-16, -5.243569643749999010 ) ) ;
#60391=CARTESIAN_POINT ( 'NONE',  ( 9.074999999999999289, 6.123233995736764310E-16, -4.999999999999998224 ) ) ;
#60392=CARTESIAN_POINT ( 'NONE',  ( 23.80312500061451786, 4.541064518000418104, -2.621784821874998173 ) ) ;
#60393=CARTESIAN_POINT ( 'NONE',  ( 1.592000809091587073E-14, 17.18750000000000355, 26.00000000000000000 ) ) ;
#60395=CARTESIAN_POINT ( 'NONE',  ( 14.66249999999999964, 2.886751345948126879, 4.999999999999999112 ) ) ;
#60396=CARTESIAN_POINT ( 'NONE',  ( 24.26250000122903216, 0.000000000000000000, 4.999999999999998224 ) ) ;
#60397=CARTESIAN_POINT ( 'NONE',  ( 19.04062500061451146, -3.027376345333614438, 5.243569643749998122 ) ) ;
#60399=CARTESIAN_POINT ( 'NONE',  ( 22.57499999999999929, 6.123233995736764310E-16, -4.999999999999998224 ) ) ;
#60400=ADVANCED_FACE ( 'NONE', ( #67052 ), #49686, .F. ) ;
#60401=CARTESIAN_POINT ( 'NONE',  ( 23.48437500061451644, 4.541064518000418104, 2.621784821874999949 ) ) ;
#60402=ORIENTED_EDGE ( 'NONE', *, *, #36932, .F. ) ;
#60403=CARTESIAN_POINT ( 'NONE',  ( 11.69062500061451360, 6.054752690667223547, 3.707466751127219781E-16 ) ) ;
#60404=CARTESIAN_POINT ( 'NONE',  ( 2.803125000614518747, 0.000000000000000000, 5.243569643749999010 ) ) ;
#60406=CARTESIAN_POINT ( 'NONE',  ( 26.50312500061451360, 4.541064518000418104, -2.621784821874998173 ) ) ;
#60407=CARTESIAN_POINT ( 'NONE',  ( 17.84999999999999787, 0.000000000000000000, 4.999999999999998224 ) ) ;
#60408=CARTESIAN_POINT ( 'NONE',  ( 24.97499999999999787, 4.330127018922191873, 2.499999999999999556 ) ) ;
#60409=CARTESIAN_POINT ( 'NONE',  ( 4.243569643749999898, 19.12812500061451715, 30.00000000000000000 ) ) ;
#60410=CARTESIAN_POINT ( 'NONE',  ( 5.971875000614516260, 3.027376345333611329, 5.243569643749999010 ) ) ;
#60411=CARTESIAN_POINT ( 'NONE',  ( 16.50937500061451502, -4.541064518000417216, -2.621784821875001281 ) ) ;
#60412=CARTESIAN_POINT ( 'NONE',  ( 28.20937500061451786, -4.541064518000417216, -2.621784821875001281 ) ) ;
#60414=CARTESIAN_POINT ( 'NONE',  ( 27.14062500061451644, -3.027376345333614438, 5.243569643749998122 ) ) ;
#60415=CARTESIAN_POINT ( 'NONE',  ( 28.09687500061451360, -3.027376345333614438, 5.243569643749998122 ) ) ;
#60416=CARTESIAN_POINT ( 'NONE',  ( 3.309375000614518836, 0.000000000000000000, 5.243569643749999010 ) ) ;
#60417=CARTESIAN_POINT ( 'NONE',  ( 12.59999999999999964, -4.330127018922190985, -2.500000000000001332 ) ) ;
#60418=CARTESIAN_POINT ( 'NONE',  ( 11.69062500061451360, 6.054752690667223547, 3.707466751127219781E-16 ) ) ;
#60420=CARTESIAN_POINT ( 'NONE',  ( 19.57500000000000284, 4.330127018922191873, 2.499999999999999556 ) ) ;
#60421=CARTESIAN_POINT ( 'NONE',  ( 28.34062500061451928, 6.054752690667223547, 3.707466751127219781E-16 ) ) ;
#60422=CARTESIAN_POINT ( 'NONE',  ( 15.37500000122903465, -5.773502691896255534, -1.060575238724906372E-15 ) ) ;
#60423=DIRECTION ( 'NONE',  ( 1.000000000000000000, 0.000000000000000000, 0.000000000000000000 ) ) ;
#60425=CARTESIAN_POINT ( 'NONE',  ( 5.653125000614517504, -4.541064518000417216, -2.621784821875001281 ) ) ;
#60426=CARTESIAN_POINT ( 'NONE',  ( 21.53437500061451715, 6.421520780324663323E-16, -5.243569643749999010 ) ) ;
#60427=CARTESIAN_POINT ( 'NONE',  ( -3.000416591977282496E-16, 16.14687500061451431, 25.09994784771203058 ) ) ;
#60428=CARTESIAN_POINT ( 'NONE',  ( 22.35937500061451644, -4.541064518000417216, -2.621784821875001281 ) ) ;
#60429=CARTESIAN_POINT ( 'NONE',  ( 4.012500000000001954, -5.773502691896255534, -1.060575238724906372E-15 ) ) ;
#60430=CARTESIAN_POINT ( 'NONE',  ( 4.000000000000000000, 11.30000000122903536, 32.30940107675849049 ) ) ;
#60431=CARTESIAN_POINT ( 'NONE',  ( 11.76562500061451644, 3.027376345333611329, 5.243569643749999010 ) ) ;
#60432=CARTESIAN_POINT ( 'NONE',  ( 4.087500001229035007, -4.330127018922194537, 2.499999999999995559 ) ) ;
#60434=CARTESIAN_POINT ( 'NONE',  ( 8.596875000614518925, 6.054752690667223547, 3.707466751127219781E-16 ) ) ;
#60436=CARTESIAN_POINT ( 'NONE',  ( 9.553125000614517859, 0.000000000000000000, 5.243569643749999010 ) ) ;
#60437=CARTESIAN_POINT ( 'NONE',  ( 14.63437500061451679, -4.541064518000419881, 2.621784821874995952 ) ) ;
#60439=CARTESIAN_POINT ( 'NONE',  ( 22.35000000122903074, 5.773502691896255534, 3.535250795749688894E-16 ) ) ;
#60440=CARTESIAN_POINT ( 'NONE',  ( 7.584375000614516082, 6.421520780324663323E-16, -5.243569643749999010 ) ) ;
#60441=CARTESIAN_POINT ( 'NONE',  ( 12.25312500061451537, 0.000000000000000000, 5.243569643749999010 ) ) ;
#60443=CARTESIAN_POINT ( 'NONE',  ( 22.65937500061451715, 0.000000000000000000, 5.243569643749999010 ) ) ;
#60444=CARTESIAN_POINT ( 'NONE',  ( 14.21249999999999858, 2.886751345948193936, 4.999999999999883649 ) ) ;
#60446=CARTESIAN_POINT ( 'NONE',  ( -0.5556303621801399473, 4.970948098741851950, 26.03636520952240474 ) ) ;
#60447=DIRECTION ( 'NONE',  ( -0.000000000000000000, -1.000000000000000000, -0.000000000000000000 ) ) ;
#60448=CARTESIAN_POINT ( 'NONE',  ( -4.243569643749999898, 11.30937500061451928, -30.00000000000000000 ) ) ;
#60449=( BOUNDED_CURVE ( )  B_SPLINE_CURVE ( 2, ( #66871, #39151, #10346, #32515, #44705, #67240, #4810, #27342, #21779 ),
 .UNSPECIFIED., .F., .F. ) 
 B_SPLINE_CURVE_WITH_KNOTS ( ( 3, 2, 2, 2, 3 ),
 ( 0.6847826086956522174, 0.6884057971014492239, 0.6956521739130434590, 0.7028985507246376940, 0.7065217391304348116 ),
 .UNSPECIFIED. ) 
 CURVE ( )  GEOMETRIC_REPRESENTATION_ITEM ( )  RATIONAL_B_SPLINE_CURVE ( ( 0.9330127018922192983, 0.9330127018922202975, 1.000000000000000000, 0.8660254037844387076, 1.000000000000000000, 0.8660254037844387076, 1.000000000000000000, 0.9330127018922194093, 0.9330127018922194093 ) ) 
 REPRESENTATION_ITEM ( '' )  );
#60450=CARTESIAN_POINT ( 'NONE',  ( 16.46250000122903501, 4.330127018922192761, -2.499999999999997780 ) ) ;
#60451=CARTESIAN_POINT ( 'NONE',  ( -4.243569643749999898, 18.45312500061451644, -30.00000000000000000 ) ) ;
#60452=CARTESIAN_POINT ( 'NONE',  ( 16.61250000122903359, 0.000000000000000000, 4.999999999999998224 ) ) ;
#60453=CARTESIAN_POINT ( 'NONE',  ( 10.34062500061451750, 6.054752690667223547, 3.707466751127219781E-16 ) ) ;
#60454=VERTEX_POINT ( 'NONE', #67763 ) ;
#60455=CARTESIAN_POINT ( 'NONE',  ( 16.50000000000000000, 0.000000000000000000, 4.999999999999998224 ) ) ;
#60456=CARTESIAN_POINT ( 'NONE',  ( 22.30312500061451431, -4.541064518000417216, -2.621784821875001281 ) ) ;
#60457=CARTESIAN_POINT ( 'NONE',  ( 10.28437500061451715, 6.421520780324663323E-16, -5.243569643749999010 ) ) ;
#60458=ADVANCED_FACE ( 'NONE', ( #10520 ), #4623, .F. ) ;
#60459=CARTESIAN_POINT ( 'NONE',  ( 9.262500001229033941, 4.330127018922192761, -2.499999999999997780 ) ) ;
#60460=CARTESIAN_POINT ( 'NONE',  ( 17.73750000122903359, 6.123233995736764310E-16, -4.999999999999998224 ) ) ;
#60461=CARTESIAN_POINT ( 'NONE',  ( 15.21562500061451750, 3.027376345333613106, -5.243569643749998122 ) ) ;
#60462=CARTESIAN_POINT ( 'NONE',  ( 17.20312500061451644, 0.000000000000000000, 5.243569643749999010 ) ) ;
#60463=CARTESIAN_POINT ( 'NONE',  ( 24.75000000122902932, -2.886751345948129988, 4.999999999999997335 ) ) ;
#60464=CARTESIAN_POINT ( 'NONE',  ( 29.36250000122903003, -4.330127018922190985, -2.500000000000001332 ) ) ;
#60465=CARTESIAN_POINT ( 'NONE',  ( 24.37500000000000000, 6.123233995736764310E-16, -4.999999999999998224 ) ) ;
#60467=CARTESIAN_POINT ( 'NONE',  ( 26.10937500061451644, 4.541064518000418104, -2.621784821874998173 ) ) ;
#60468=CARTESIAN_POINT ( 'NONE',  ( 1.071796769724491893, 12.48259618943233384, -26.00000000000000355 ) ) ;
#60469=CARTESIAN_POINT ( 'NONE',  ( 12.67500000122903536, -5.773502691896255534, -1.060575238724906372E-15 ) ) ;
#60470=EDGE_CURVE ( 'NONE', #17166, #16088, #66212, .T. ) ;
#60471=CARTESIAN_POINT ( 'NONE',  ( 3.225000000000002309, 6.123233995736764310E-16, -4.999999999999998224 ) ) ;
#60472=DIRECTION ( 'NONE',  ( -0.000000000000000000, -1.000000000000000000, -0.000000000000000000 ) ) ;
#60473=CARTESIAN_POINT ( 'NONE',  ( 6.759375000614516793, 4.541064518000418104, -2.621784821874998173 ) ) ;
#60475=CARTESIAN_POINT ( 'NONE',  ( 26.50312500061451360, 4.541064518000418104, -2.621784821874998173 ) ) ;
#60477=CARTESIAN_POINT ( 'NONE',  ( -1.393485112971538653, 9.904374691868481406, -24.16067974760139236 ) ) ;
#60479=CARTESIAN_POINT ( 'NONE',  ( 5.859375000614519102, 4.541064518000418104, -2.621784821874998173 ) ) ;
#60480=CARTESIAN_POINT ( 'NONE',  ( 8.259375000614518569, 0.000000000000000000, 5.243569643749999010 ) ) ;
#60481=CARTESIAN_POINT ( 'NONE',  ( 29.82187500061451502, 3.027376345333611329, 5.243569643749999010 ) ) ;
#60484=CARTESIAN_POINT ( 'NONE',  ( -2.121784821874996840, 12.22812500061459673, 33.67503911421598417 ) ) ;
#60485=CARTESIAN_POINT ( 'NONE',  ( 21.52499999999999858, -4.330127018922194537, 2.499999999999995559 ) ) ;
#60486=CARTESIAN_POINT ( 'NONE',  ( 29.02499999999999858, 4.330127018922191873, 2.499999999999999556 ) ) ;
#60487=CARTESIAN_POINT ( 'NONE',  ( 3.825000000000001954, 4.330127018922191873, 2.499999999999999556 ) ) ;
#60488=ORIENTED_EDGE ( 'NONE', *, *, #26844, .T. ) ;
#60489=CARTESIAN_POINT ( 'NONE',  ( 18.62812500061451715, -4.541064518000419881, 2.621784821874995952 ) ) ;
#60490=CARTESIAN_POINT ( 'NONE',  ( 10.97812500061451679, -4.541064518000419881, 2.621784821874995952 ) ) ;
#60492=CARTESIAN_POINT ( 'NONE',  ( 7.584375000614516082, 6.421520780324663323E-16, -5.243569643749999010 ) ) ;
#60493=CARTESIAN_POINT ( 'NONE',  ( 24.29999999999999716, -4.330127018922190985, -2.500000000000001332 ) ) ;
#60494=CARTESIAN_POINT ( 'NONE',  ( 20.62500000122903288, 2.886751345948126879, 4.999999999999999112 ) ) ;
#60496=CARTESIAN_POINT ( 'NONE',  ( 6.084375000614518747, -4.541064518000419881, 2.621784821874995952 ) ) ;
#60497=CARTESIAN_POINT ( 'NONE',  ( 13.02187500061451608, 3.027376345333613106, -5.243569643749998122 ) ) ;
#60498=CARTESIAN_POINT ( 'NONE',  ( 23.37187500061451573, 3.027376345333613106, -5.243569643749998122 ) ) ;
#60499=CARTESIAN_POINT ( 'NONE',  ( 1.071796769724497445, 15.92990381179669868, -33.99999999999998579 ) ) ;
#60500=EDGE_LOOP ( 'NONE', ( #27259, #37435, #45706, #9725 ) ) ;
#60502=CARTESIAN_POINT ( 'NONE',  ( 18.57187500061451857, 3.027376345333611329, 5.243569643749999010 ) ) ;
#60503=CARTESIAN_POINT ( 'NONE',  ( 10.09687500061451715, -3.027376345333614438, 5.243569643749998122 ) ) ;
#60505=CARTESIAN_POINT ( 'NONE',  ( 21.78750000000000142, 5.773502691896255534, 3.535250795749688894E-16 ) ) ;
#60507=CARTESIAN_POINT ( 'NONE',  ( -2.121784821874996840, 10.48437500061451821, -26.32496088578401583 ) ) ;
#60509=CARTESIAN_POINT ( 'NONE',  ( 13.11562500061451786, 3.027376345333611329, 5.243569643749999010 ) ) ;
#60510=CARTESIAN_POINT ( 'NONE',  ( 3.112500000000000711, -5.773502691896255534, -1.060575238724906372E-15 ) ) ;
#60511=CARTESIAN_POINT ( 'NONE',  ( -3.999999999999999112, 19.17500000122903359, -32.30940107675850470 ) ) ;
#60513=CARTESIAN_POINT ( 'NONE',  ( 12.97499999999999964, -4.330127018922194537, 2.499999999999995559 ) ) ;
#60514=CARTESIAN_POINT ( 'NONE',  ( -3.999999999999999112, 16.96250000122903145, 30.00000000000000000 ) ) ;
#60515=CARTESIAN_POINT ( 'NONE',  ( 11.92500000122903181, 2.886751345948129099, -4.999999999999998224 ) ) ;
#60516=( BOUNDED_CURVE ( )  B_SPLINE_CURVE ( 2, ( #42744, #25753, #65264, #14652, #37195, #59718, #9125, #3593, #12656 ),
 .UNSPECIFIED., .F., .F. ) 
 B_SPLINE_CURVE_WITH_KNOTS ( ( 3, 2, 2, 2, 3 ),
 ( 0.7282608695652174058, 0.7318840579710145233, 0.7391304347826086474, 0.7463768115942028825, 0.7500000000000000000 ),
 .UNSPECIFIED. ) 
 CURVE ( )  GEOMETRIC_REPRESENTATION_ITEM ( )  RATIONAL_B_SPLINE_CURVE ( ( 0.9330127018922194093, 0.9330127018922194093, 1.000000000000000000, 0.8660254037844387076, 1.000000000000000000, 0.8660254037844387076, 1.000000000000000000, 0.9330127018922194093, 0.9330127018922194093 ) ) 
 REPRESENTATION_ITEM ( '' )  );
#60517=CARTESIAN_POINT ( 'NONE',  ( 22.65937500061451715, 0.000000000000000000, 5.243569643749999010 ) ) ;
#60518=CARTESIAN_POINT ( 'NONE',  ( 17.48437500061451999, 6.421520780324663323E-16, -5.243569643749999010 ) ) ;
#60520=ORIENTED_EDGE ( 'NONE', *, *, #66521, .F. ) ;
#60521=CARTESIAN_POINT ( 'NONE',  ( 17.57812500061451644, 4.541064518000418104, 2.621784821874999949 ) ) ;
#60522=CARTESIAN_POINT ( 'NONE',  ( 29.10000000122903074, 5.773502691896255534, 3.535250795749688894E-16 ) ) ;
#60523=CARTESIAN_POINT ( 'NONE',  ( 18.12187500061451573, 3.027376345333611329, 5.243569643749999010 ) ) ;
#60524=CARTESIAN_POINT ( 'NONE',  ( 3.203040009831849222, 9.474684130322206244, -24.92277861900284819 ) ) ;
#60525=CARTESIAN_POINT ( 'NONE',  ( 20.50312500061451715, -4.541064518000417216, -2.621784821875001281 ) ) ;
#60526=CARTESIAN_POINT ( 'NONE',  ( 7.950000000000001954, 0.000000000000000000, 4.999999999999998224 ) ) ;
#60527=CARTESIAN_POINT ( 'NONE',  ( 29.44687500061451857, -3.027376345333614438, 5.243569643749998122 ) ) ;
#60528=CARTESIAN_POINT ( 'NONE',  ( 2.121784821874999061, 12.00312500061451715, 26.32496088578401583 ) ) ;
#60529=CARTESIAN_POINT ( 'NONE',  ( 16.58437500061451786, 6.421520780324663323E-16, -5.243569643749999010 ) ) ;
#60530=CARTESIAN_POINT ( 'NONE',  ( 17.17500000122903359, -5.773502691896255534, -1.060575238724906372E-15 ) ) ;
#60532=CARTESIAN_POINT ( 'NONE',  ( 2.121784821874999061, 19.70937500061451786, -33.67503911421598417 ) ) ;
#60533=CARTESIAN_POINT ( 'NONE',  ( 20.14687500061451786, -3.027376345333610441, -5.243569643749999898 ) ) ;
#60534=CARTESIAN_POINT ( 'NONE',  ( 21.52500000122903145, 2.886751345948126879, 4.999999999999999112 ) ) ;
#60535=CARTESIAN_POINT ( 'NONE',  ( 22.79062500061451502, -3.027376345333610441, -5.243569643749999898 ) ) ;
#60536=CARTESIAN_POINT ( 'NONE',  ( 16.32187500061451502, 3.027376345333611329, 5.243569643749999010 ) ) ;
#60537=CARTESIAN_POINT ( 'NONE',  ( 11.91562500061451857, -6.054752690667223547, -1.112240025338166033E-15 ) ) ;
#60538=CARTESIAN_POINT ( 'NONE',  ( 2.121784821875001281, 13.70937500061451786, 33.67503911421598417 ) ) ;
#60539=( BOUNDED_CURVE ( )  B_SPLINE_CURVE ( 2, ( #59835, #3344, #43594, #2965, #59463, #31408, #72028, #66482, #53947 ),
 .UNSPECIFIED., .F., .F. ) 
 B_SPLINE_CURVE_WITH_KNOTS ( ( 3, 2, 2, 2, 3 ),
 ( 0.9021739130434782705, 0.9057971014492753881, 0.9130434782608695121, 0.9202898550724637472, 0.9239130434782608647 ),
 .UNSPECIFIED. ) 
 CURVE ( )  GEOMETRIC_REPRESENTATION_ITEM ( )  RATIONAL_B_SPLINE_CURVE ( ( 0.9330127018922194093, 0.9330127018922194093, 1.000000000000000000, 0.8660254037844387076, 1.000000000000000000, 0.8660254037844387076, 1.000000000000000000, 0.9330127018922194093, 0.9330127018922194093 ) ) 
 REPRESENTATION_ITEM ( '' )  );
#60540=CARTESIAN_POINT ( 'NONE',  ( 16.67812500061451786, 4.541064518000418104, 2.621784821874999949 ) ) ;
#60542=ORIENTED_EDGE ( 'NONE', *, *, #13034, .F. ) ;
#60543=CARTESIAN_POINT ( 'NONE',  ( 22.87500000000000000, -4.330127018922194537, 2.499999999999995559 ) ) ;
#60544=CARTESIAN_POINT ( 'NONE',  ( -4.243569643749997233, 18.99687500061451928, -27.54997392385601174 ) ) ;
#60545=DIRECTION ( 'NONE',  ( 0.000000000000000000, 0.000000000000000000, 1.000000000000000000 ) ) ;
#60546=CARTESIAN_POINT ( 'NONE',  ( 24.59062500061451573, -3.027376345333610441, -5.243569643749999898 ) ) ;
#60547=CARTESIAN_POINT ( 'NONE',  ( 5.953125000614519102, 0.000000000000000000, 5.243569643749999010 ) ) ;
#60548=CARTESIAN_POINT ( 'NONE',  ( 18.30000000122903359, 5.773502691896255534, 3.535250795749688894E-16 ) ) ;
#60549=CARTESIAN_POINT ( 'NONE',  ( 21.25312500061451715, 0.000000000000000000, 5.243569643749999010 ) ) ;
#60550=CARTESIAN_POINT ( 'NONE',  ( 22.72499999999999787, 4.330127018922191873, 2.499999999999999556 ) ) ;
#60551=CARTESIAN_POINT ( 'NONE',  ( 24.85312500061451502, 0.000000000000000000, 5.243569643749999010 ) ) ;
#60552=CARTESIAN_POINT ( 'NONE',  ( 8.353125000614518569, -4.541064518000417216, -2.621784821875001281 ) ) ;
#60553=EDGE_LOOP ( 'NONE', ( #4193, #65136, #52909, #45032 ) ) ;
#60554=CARTESIAN_POINT ( 'NONE',  ( 22.52812500061451573, 4.541064518000418104, 2.621784821874999949 ) ) ;
#60555=CARTESIAN_POINT ( 'NONE',  ( 3.853125000614517681, -4.541064518000417216, -2.621784821875001281 ) ) ;
#60557=CARTESIAN_POINT ( 'NONE',  ( -3.999999999999997335, 11.15000000122903501, 32.30940107675850470 ) ) ;
#60558=CARTESIAN_POINT ( 'NONE',  ( 1.999999999999998668, 13.21250000122903501, -33.46410161513775705 ) ) ;
#60560=FACE_OUTER_BOUND ( 'NONE', #48600, .T. ) ;
#60561=CARTESIAN_POINT ( 'NONE',  ( 9.600000000000001421, 4.330127018922192761, -2.499999999999997780 ) ) ;
#60562=CARTESIAN_POINT ( 'NONE',  ( 12.04687500061451821, -3.027376345333610441, -5.243569643749999898 ) ) ;
#60563=CARTESIAN_POINT ( 'NONE',  ( 7.612500001229035362, 0.000000000000000000, 4.999999999999998224 ) ) ;
#60564=CARTESIAN_POINT ( 'NONE',  ( 14.07187500061451679, 3.027376345333611329, 5.243569643749999010 ) ) ;
#60565=CARTESIAN_POINT ( 'NONE',  ( 5.259375000614518569, -4.541064518000417216, -2.621784821875001281 ) ) ;
#60566=LINE ( 'NONE', #65757, #34956 ) ;
#60567=CARTESIAN_POINT ( 'NONE',  ( -3.999999999999999112, 10.62500000122903643, 27.69059892324149885 ) ) ;
#60568=CARTESIAN_POINT ( 'NONE',  ( 13.28437500061451715, -4.541064518000419881, 2.621784821874995952 ) ) ;
#60570=CARTESIAN_POINT ( 'NONE',  ( 21.47812500061451502, 6.421520780324663323E-16, -5.243569643749999010 ) ) ;
#60572=CARTESIAN_POINT ( 'NONE',  ( 9.001249775931846008E-16, 19.46562500061459033, 34.90005215228797653 ) ) ;
#60573=CARTESIAN_POINT ( 'NONE',  ( 24.79687500061451999, 6.054752690667223547, 3.707466751127219781E-16 ) ) ;
#60575=EDGE_CURVE ( 'NONE', #31017, #28731, #12561, .T. ) ;
#60576=CARTESIAN_POINT ( 'NONE',  ( 29.32500000122903216, -5.773502691896255534, -1.060575238724906372E-15 ) ) ;
#60578=CARTESIAN_POINT ( 'NONE',  ( 25.90312500061451573, -4.541064518000417216, -2.621784821875001281 ) ) ;
#60579=CARTESIAN_POINT ( 'NONE',  ( 17.54062500061451502, 6.054752690667223547, 3.707466751127219781E-16 ) ) ;
#60581=CARTESIAN_POINT ( 'NONE',  ( 14.59687500061452070, -3.027376345333614438, 5.243569643749998122 ) ) ;
#60582=CARTESIAN_POINT ( 'NONE',  ( 7.387500001229032165, 6.123233995736764310E-16, -4.999999999999998224 ) ) ;
#60583=CARTESIAN_POINT ( 'NONE',  ( 27.00000000122903288, -2.886751345948129988, 4.999999999999997335 ) ) ;
#60584=CARTESIAN_POINT ( 'NONE',  ( 5.409375000614516260, 4.541064518000418104, -2.621784821874998173 ) ) ;
#60585=CARTESIAN_POINT ( 'NONE',  ( 15.87187500061451573, 3.027376345333611329, 5.243569643749999010 ) ) ;
#60586=CARTESIAN_POINT ( 'NONE',  ( 15.07499999999999929, 4.330127018922191873, 2.499999999999999556 ) ) ;
#60587=CARTESIAN_POINT ( 'NONE',  ( 3.525000001229034119, 2.886751345948126879, 4.999999999999999112 ) ) ;
#60588=CARTESIAN_POINT ( 'NONE',  ( 24.64687500061451431, -3.027376345333610441, -5.243569643749999898 ) ) ;
#60589=CARTESIAN_POINT ( 'NONE',  ( 17.03437500061451715, 6.421520780324663323E-16, -5.243569643749999010 ) ) ;
#60591=CARTESIAN_POINT ( 'NONE',  ( 28.72500000000000142, -4.330127018922194537, 2.499999999999995559 ) ) ;
#60592=CARTESIAN_POINT ( 'NONE',  ( 4.800000000000002487, 0.000000000000000000, 4.999999999999998224 ) ) ;
#60594=CARTESIAN_POINT ( 'NONE',  ( 20.80312500061451431, 0.000000000000000000, 5.243569643749999010 ) ) ;
#60595=CARTESIAN_POINT ( 'NONE',  ( 8.849999999999999645, 0.000000000000000000, 4.999999999999998224 ) ) ;
#60596=CARTESIAN_POINT ( 'NONE',  ( 2.990625000614519191, -3.027376345333610441, -5.243569643749999898 ) ) ;
#60597=CARTESIAN_POINT ( 'NONE',  ( 18.63749999999999929, 5.773502691896255534, 3.535250795749688894E-16 ) ) ;
#60598=CARTESIAN_POINT ( 'NONE',  ( 15.56250000122903465, 4.330127018922192761, -2.499999999999997780 ) ) ;
#60599=CARTESIAN_POINT ( 'NONE',  ( 22.27500000122903145, 2.886751345948129099, -4.999999999999998224 ) ) ;
#60600=CARTESIAN_POINT ( 'NONE',  ( 4.519730000842645978, 8.925305311771492001, 33.96464799308335358 ) ) ;
#60601=CARTESIAN_POINT ( 'NONE',  ( 3.675000000000001155, 6.123233995736764310E-16, -4.999999999999998224 ) ) ;
#60602=ORIENTED_EDGE ( 'NONE', *, *, #38674, .F. ) ;
#60603=CARTESIAN_POINT ( 'NONE',  ( 16.34062500061451573, -3.027376345333614438, 5.243569643749998122 ) ) ;
#60604=CARTESIAN_POINT ( 'NONE',  ( 23.61562500061451431, -6.054752690667223547, -1.112240025338166033E-15 ) ) ;
#60605=CARTESIAN_POINT ( 'NONE',  ( 24.00937500061451502, 0.000000000000000000, 5.243569643749999010 ) ) ;
#60606=CARTESIAN_POINT ( 'NONE',  ( 7.162500000000001421, -5.773502691896255534, -1.060575238724906372E-15 ) ) ;
#60607=CARTESIAN_POINT ( 'NONE',  ( 12.74062500061451786, -3.027376345333614438, 5.243569643749998122 ) ) ;
#60608=CARTESIAN_POINT ( 'NONE',  ( 26.16562500061451502, 3.027376345333611329, 5.243569643749999010 ) ) ;
#60609=CARTESIAN_POINT ( 'NONE',  ( 15.04687500061451644, -3.027376345333614438, 5.243569643749998122 ) ) ;
#60610=CARTESIAN_POINT ( 'NONE',  ( 20.33437500061451786, 4.541064518000418104, 2.621784821874999949 ) ) ;
#60611=DIRECTION ( 'NONE',  ( -0.000000000000000000, -1.000000000000000000, -0.000000000000000000 ) ) ;
#60612=CARTESIAN_POINT ( 'NONE',  ( 2.121784821874999061, 19.65312500061451573, 26.32496088578401583 ) ) ;
#60613=CARTESIAN_POINT ( 'NONE',  ( 22.95000000122903216, -2.886751345948129988, 4.999999999999997335 ) ) ;
#60615=CARTESIAN_POINT ( 'NONE',  ( 14.72812500061451679, 6.421520780324663323E-16, -5.243569643749999010 ) ) ;
#60616=CARTESIAN_POINT ( 'NONE',  ( 7.471875000614519813, -6.054752690667223547, -1.112240025338166033E-15 ) ) ;
#60617=CARTESIAN_POINT ( 'NONE',  ( 7.584375000614516082, 6.421520780324663323E-16, -5.243569643749999010 ) ) ;
#60618=ORIENTED_EDGE ( 'NONE', *, *, #18452, .T. ) ;
#60619=CARTESIAN_POINT ( 'NONE',  ( 27.53437500061451360, 4.541064518000418104, 2.621784821874999949 ) ) ;
#60620=CARTESIAN_POINT ( 'NONE',  ( 19.19062500061452070, -3.027376345333610441, -5.243569643749999898 ) ) ;
#60621=CARTESIAN_POINT ( 'NONE',  ( 28.80000000122903003, -2.886751345948129988, 4.999999999999997335 ) ) ;
#60622=CARTESIAN_POINT ( 'NONE',  ( 2.896875000614518747, -3.027376345333614438, 5.243569643749998122 ) ) ;
#60623=CARTESIAN_POINT ( 'NONE',  ( 24.12187500061451217, -6.054752690667223547, -1.112240025338166033E-15 ) ) ;
#60624=CARTESIAN_POINT ( 'NONE',  ( 19.07812500061451644, -4.541064518000419881, 2.621784821874995952 ) ) ;
#60625=CARTESIAN_POINT ( 'NONE',  ( -2.000000000000000000, 12.72499999999999964, 26.53589838486224650 ) ) ;
#60626=CARTESIAN_POINT ( 'NONE',  ( 24.89062500061451644, -3.027376345333614438, 5.243569643749998122 ) ) ;
#60627=CARTESIAN_POINT ( 'NONE',  ( 6.300000001229033586, -2.886751345948129988, 4.999999999999997335 ) ) ;
#60629=CARTESIAN_POINT ( 'NONE',  ( 2.000000000000001332, 15.65000000000000036, -26.53589838486224650 ) ) ;
#60630=CARTESIAN_POINT ( 'NONE',  ( 22.05000000122903714, -2.886751345948129988, 4.999999999999997335 ) ) ;
#60632=CARTESIAN_POINT ( 'NONE',  ( 4.396875000614516971, -3.027376345333610441, -5.243569643749999898 ) ) ;
#60633=CARTESIAN_POINT ( 'NONE',  ( 29.54062500061451502, -3.027376345333610441, -5.243569643749999898 ) ) ;
#60634=CARTESIAN_POINT ( 'NONE',  ( 12.29062500061451857, -3.027376345333614438, 5.243569643749998122 ) ) ;
#60635=CARTESIAN_POINT ( 'NONE',  ( 7.246875000614518392, 6.054752690667223547, 3.707466751127219781E-16 ) ) ;
#60636=CARTESIAN_POINT ( 'NONE',  ( 25.01250000122903216, 4.330127018922192761, -2.499999999999997780 ) ) ;
#60637=CARTESIAN_POINT ( 'NONE',  ( 14.93437500061451750, 4.541064518000418104, 2.621784821874999949 ) ) ;
#60638=CARTESIAN_POINT ( 'NONE',  ( 3.384375000614517237, -4.541064518000419881, 2.621784821874995952 ) ) ;
#60639=CARTESIAN_POINT ( 'NONE',  ( 29.84999999999999787, 4.330127018922192761, -2.499999999999997780 ) ) ;
#60640=CARTESIAN_POINT ( 'NONE',  ( 5.578125000614518214, -4.541064518000419881, 2.621784821874995952 ) ) ;
#60641=CARTESIAN_POINT ( 'NONE',  ( 14.72812500061451679, 6.421520780324663323E-16, -5.243569643749999010 ) ) ;
#60642=VERTEX_POINT ( 'NONE', #897 ) ;
#60643=CARTESIAN_POINT ( 'NONE',  ( 9.703125000614514661, -4.541064518000417216, -2.621784821875001281 ) ) ;
#60644=CARTESIAN_POINT ( 'NONE',  ( 9.553125000614517859, 0.000000000000000000, 5.243569643749999010 ) ) ;
#60646=CARTESIAN_POINT ( 'NONE',  ( 8.662499999999999645, 2.886751345948129099, -4.999999999999998224 ) ) ;
#60647=CARTESIAN_POINT ( 'NONE',  ( 3.862500001229035362, 4.330127018922192761, -2.499999999999997780 ) ) ;
#60648=CARTESIAN_POINT ( 'NONE',  ( 17.84999999999999787, 0.000000000000000000, 4.999999999999998224 ) ) ;
#60650=CARTESIAN_POINT ( 'NONE',  ( 19.20937500061451786, -4.541064518000417216, -2.621784821875001281 ) ) ;
#60651=CARTESIAN_POINT ( 'NONE',  ( 12.86250000122903359, 4.330127018922192761, -2.499999999999997780 ) ) ;
#60653=CARTESIAN_POINT ( 'NONE',  ( 4.243569643749999898, 16.84062500061451573, -27.54997392385601529 ) ) ;
#60654=CYLINDRICAL_SURFACE ( 'NONE', #72546, 3.999999999999996447 ) ;
#60656=DIRECTION ( 'NONE',  ( 0.000000000000000000, 0.000000000000000000, -1.000000000000000000 ) ) ;
#60657=CARTESIAN_POINT ( 'NONE',  ( 19.98750000122903359, 6.123233995736764310E-16, -4.999999999999998224 ) ) ;
#60659=CARTESIAN_POINT ( 'NONE',  ( 14.55937500061451573, 0.000000000000000000, 5.243569643749999010 ) ) ;
#60660=( BOUNDED_CURVE ( )  B_SPLINE_CURVE ( 2, ( #36489, #59008, #68667, #18031, #40587, #63107, #3249 ),
 .UNSPECIFIED., .F., .F. ) 
 B_SPLINE_CURVE_WITH_KNOTS ( ( 3, 2, 2, 3 ),
 ( 0.04166666666666671293, 0.04444444444444448777, 0.04722222222222225568, 0.05000000000000003053 ),
 .UNSPECIFIED. ) 
 CURVE ( )  GEOMETRIC_REPRESENTATION_ITEM ( )  RATIONAL_B_SPLINE_CURVE ( ( 0.9999999999999976685, 0.8660254037844410391, 1.000000000000000000, 0.8660254037844387076, 1.000000000000000000, 0.8660254037844373753, 1.000000000000001332 ) ) 
 REPRESENTATION_ITEM ( '' )  );
#60661=CARTESIAN_POINT ( 'NONE',  ( 26.47499999999999787, -4.330127018922194537, 2.499999999999995559 ) ) ;
#60662=ADVANCED_FACE ( 'NONE', ( #52214 ), #51497, .F. ) ;
#60663=CARTESIAN_POINT ( 'NONE',  ( 9.703125000614514661, -4.541064518000417216, -2.621784821875001281 ) ) ;
#60665=CARTESIAN_POINT ( 'NONE',  ( 22.65937500061451715, 0.000000000000000000, 5.243569643749999010 ) ) ;
#60667=CARTESIAN_POINT ( 'NONE',  ( 8.615625000614517859, 3.027376345333611329, 5.243569643749999010 ) ) ;
#60668=CARTESIAN_POINT ( 'NONE',  ( 13.32187500061451502, -6.054752690667223547, -1.112240025338166033E-15 ) ) ;
#60670=CARTESIAN_POINT ( 'NONE',  ( 22.77187500061451786, -6.054752690667223547, -1.112240025338166033E-15 ) ) ;
#60671=CARTESIAN_POINT ( 'NONE',  ( 30.00000000000000000, 6.123233995736764310E-16, -4.999999999999998224 ) ) ;
#60673=CARTESIAN_POINT ( 'NONE',  ( 4.537500000000000533, -2.886751345948125991, -5.000000000000000000 ) ) ;
#60674=CARTESIAN_POINT ( 'NONE',  ( 16.91250000122903430, 4.330127018922192761, -2.499999999999997780 ) ) ;
#60676=CARTESIAN_POINT ( 'NONE',  ( 30.00000000000000000, 6.123233995736764310E-16, -4.999999999999998224 ) ) ;
#60677=ORIENTED_EDGE ( 'NONE', *, *, #52008, .F. ) ;
#60678=CARTESIAN_POINT ( 'NONE',  ( 13.31250000000000178, 2.886751345948126879, 4.999999999999999112 ) ) ;
#60679=CARTESIAN_POINT ( 'NONE',  ( 17.17500000000000071, 6.123233995736764310E-16, -4.999999999999998224 ) ) ;
#60680=CARTESIAN_POINT ( 'NONE',  ( 12.86250000122903359, 4.330127018922192761, -2.499999999999997780 ) ) ;
#60681=CARTESIAN_POINT ( 'NONE',  ( 11.35312500061451679, 0.000000000000000000, 5.243569643749999010 ) ) ;
#60682=ORIENTED_EDGE ( 'NONE', *, *, #51310, .T. ) ;
#60683=CARTESIAN_POINT ( 'NONE',  ( -1.071796769724483234, 16.87009619066137134, -34.00000000000000711 ) ) ;
#60684=CARTESIAN_POINT ( 'NONE',  ( 2.121784821875001281, 17.30937500061451573, -26.32496088578401938 ) ) ;
#60685=CARTESIAN_POINT ( 'NONE',  ( 3.778125000614519280, -4.541064518000419881, 2.621784821874995952 ) ) ;
#60687=CARTESIAN_POINT ( 'NONE',  ( 10.12500000000000178, 4.330127018922191873, 2.499999999999999556 ) ) ;
#60688=FACE_OUTER_BOUND ( 'NONE', #10628, .T. ) ;
#60691=CARTESIAN_POINT ( 'NONE',  ( 23.20312500061451644, -4.541064518000417216, -2.621784821875001281 ) ) ;
#60694=CARTESIAN_POINT ( 'NONE',  ( 20.25937500061451857, 4.541064518000418104, -2.621784821874998173 ) ) ;
#60695=CARTESIAN_POINT ( 'NONE',  ( 20.31562500061451715, 3.027376345333611329, 5.243569643749999010 ) ) ;
#60696=CARTESIAN_POINT ( 'NONE',  ( -4.243569643749999898, 14.36562500061459424, -32.45002607614398471 ) ) ;
#60697=CARTESIAN_POINT ( 'NONE',  ( 7.453125000614516438, -4.541064518000417216, -2.621784821875001281 ) ) ;
#60698=CARTESIAN_POINT ( 'NONE',  ( 4.865625000614517859, 3.027376345333613106, -5.243569643749998122 ) ) ;
#60700=CARTESIAN_POINT ( 'NONE',  ( 21.29062500061451502, -3.027376345333614438, 5.243569643749998122 ) ) ;
#60703=CARTESIAN_POINT ( 'NONE',  ( 14.82187500061451679, 3.027376345333613106, -5.243569643749998122 ) ) ;
#60704=CARTESIAN_POINT ( 'NONE',  ( 13.50937500061451679, 4.541064518000418104, -2.621784821874998173 ) ) ;
#60705=CARTESIAN_POINT ( 'NONE',  ( 23.44687500061451502, 6.054752690667223547, 3.707466751127219781E-16 ) ) ;
#60706=ORIENTED_EDGE ( 'NONE', *, *, #62922, .F. ) ;
#60707=CARTESIAN_POINT ( 'NONE',  ( -4.243569643749999898, 11.30937500061451928, 30.00000000000000000 ) ) ;
#60708=CARTESIAN_POINT ( 'NONE',  ( 2.840625000614518392, -3.027376345333614438, 5.243569643749998122 ) ) ;
#60709=CARTESIAN_POINT ( 'NONE',  ( 26.31562500061451715, -6.054752690667223547, -1.112240025338166033E-15 ) ) ;
#60710=VECTOR ( 'NONE', #19068, 1000.000000000000000 ) ;
#60711=CARTESIAN_POINT ( 'NONE',  ( 26.12812500061451360, 4.541064518000418104, 2.621784821874999949 ) ) ;
#60713=CARTESIAN_POINT ( 'NONE',  ( -3.999999999999999556, 19.51250000000000284, 27.69059892324149530 ) ) ;
#60714=CARTESIAN_POINT ( 'NONE',  ( 4.509375000614518569, 4.541064518000418104, -2.621784821874998173 ) ) ;
#60716=CARTESIAN_POINT ( 'NONE',  ( 13.83750000122903323, 4.330127018922191873, 2.499999999999999556 ) ) ;
#60718=CARTESIAN_POINT ( 'NONE',  ( 10.20000000122903572, 5.773502691896255534, 3.535250795749688894E-16 ) ) ;
#60719=CARTESIAN_POINT ( 'NONE',  ( 3.328125000614516438, -4.541064518000419881, 2.621784821874995952 ) ) ;
#60722=CARTESIAN_POINT ( 'NONE',  ( 11.07187500061451679, -6.054752690667223547, -1.112240025338166033E-15 ) ) ;
#60723=ORIENTED_EDGE ( 'NONE', *, *, #2879, .T. ) ;
#60724=CARTESIAN_POINT ( 'NONE',  ( 20.42812500061451431, -4.541064518000419881, 2.621784821874995952 ) ) ;
#60725=CARTESIAN_POINT ( 'NONE',  ( 16.35937500061451644, 0.000000000000000000, 5.243569643749999010 ) ) ;
#60726=CARTESIAN_POINT ( 'NONE',  ( 4.265625000614517326, -6.054752690667223547, -1.112240025338166033E-15 ) ) ;
#60727=CARTESIAN_POINT ( 'NONE',  ( 21.38437500061451502, -4.541064518000419881, 2.621784821874995952 ) ) ;
#60728=CARTESIAN_POINT ( 'NONE',  ( 4.978125000614518569, 4.541064518000418104, 2.621784821874999949 ) ) ;
#60730=CARTESIAN_POINT ( 'NONE',  ( 6.900000001229035007, -2.886751345948125991, -5.000000000000000000 ) ) ;
#60732=EDGE_CURVE ( 'NONE', #24253, #26902, #22489, .T. ) ;
#60733=CARTESIAN_POINT ( 'NONE',  ( 22.71562500061451573, -6.054752690667223547, -1.112240025338166033E-15 ) ) ;
#60734=CARTESIAN_POINT ( 'NONE',  ( 8.484601909799253346E-16, 17.07500000122903572, -25.38119784648299770 ) ) ;
#60735=CARTESIAN_POINT ( 'NONE',  ( 8.812500001229034652, 4.330127018922192761, -2.499999999999997780 ) ) ;
#60736=CARTESIAN_POINT ( 'NONE',  ( 20.69062500061451715, 6.054752690667223547, 3.707466751127219781E-16 ) ) ;
#60737=CARTESIAN_POINT ( 'NONE',  ( 16.64062500061451289, 6.054752690667223547, 3.707466751127219781E-16 ) ) ;
#60739=CARTESIAN_POINT ( 'NONE',  ( 15.18750000000000000, -2.886751345948129988, 4.999999999999997335 ) ) ;
#60740=CARTESIAN_POINT ( 'NONE',  ( 10.76250000122903572, 0.000000000000000000, 4.999999999999998224 ) ) ;
#60741=CARTESIAN_POINT ( 'NONE',  ( 7.115625000614516082, 3.027376345333613106, -5.243569643749998122 ) ) ;
#60742=CARTESIAN_POINT ( 'NONE',  ( 11.87812500061451537, -4.541064518000419881, 2.621784821874995952 ) ) ;
#60743=CARTESIAN_POINT ( 'NONE',  ( 20.55000000122903359, 5.773502691896255534, 3.535250795749688894E-16 ) ) ;
#60744=CARTESIAN_POINT ( 'NONE',  ( -4.243569643749999898, 14.00937500061451857, -30.00000000000000000 ) ) ;
#60745=CARTESIAN_POINT ( 'NONE',  ( 19.62187500061451573, -6.054752690667223547, -1.112240025338166033E-15 ) ) ;
#60748=CARTESIAN_POINT ( 'NONE',  ( 5.587500001229033231, 6.123233995736764310E-16, -4.999999999999998224 ) ) ;
#60750=CARTESIAN_POINT ( 'NONE',  ( 3.646875000614520079, 6.054752690667223547, 3.707466751127219781E-16 ) ) ;
#60751=CARTESIAN_POINT ( 'NONE',  ( 21.34687500061451715, -3.027376345333614438, 5.243569643749998122 ) ) ;
#60752=CARTESIAN_POINT ( 'NONE',  ( -5.810221930991193690E-16, 14.93750000000000000, 26.00000000000000355 ) ) ;
#60753=AXIS2_PLACEMENT_3D ( 'NONE', #32442, #49438, #38344 ) ;
#60754=CARTESIAN_POINT ( 'NONE',  ( 18.25312500061451715, -4.541064518000417216, -2.621784821875001281 ) ) ;
#60756=CARTESIAN_POINT ( 'NONE',  ( 23.25000000000000000, 0.000000000000000000, 4.999999999999998224 ) ) ;
#60757=CARTESIAN_POINT ( 'NONE',  ( -3.999999999999999112, 15.46250000000000036, 27.69059892324149885 ) ) ;
#60758=CARTESIAN_POINT ( 'NONE',  ( 28.28437500061451715, 6.421520780324663323E-16, -5.243569643749999010 ) ) ;
#60760=CARTESIAN_POINT ( 'NONE',  ( 15.51562500061451644, -6.054752690667223547, -1.112240025338166033E-15 ) ) ;
#60761=AXIS2_PLACEMENT_3D ( 'NONE', #50869, #68588, #6891 ) ;
#60762=CARTESIAN_POINT ( 'NONE',  ( 13.32187500061451502, -6.054752690667223547, -1.112240025338166033E-15 ) ) ;
#60765=CARTESIAN_POINT ( 'NONE',  ( 22.79062500061451502, -3.027376345333610441, -5.243569643749999898 ) ) ;
#60766=CARTESIAN_POINT ( 'NONE',  ( -3.999999999999997335, 10.70000000122903394, -27.69059892324149530 ) ) ;
#60767=CARTESIAN_POINT ( 'NONE',  ( 12.86250000000000071, 2.886751345948126879, 4.999999999999999112 ) ) ;
#60768=CARTESIAN_POINT ( 'NONE',  ( 23.06250000122903288, -4.330127018922190985, -2.500000000000001332 ) ) ;
#60769=CARTESIAN_POINT ( 'NONE',  ( 19.41562500061451146, 3.027376345333611329, 5.243569643749999010 ) ) ;
#60771=CARTESIAN_POINT ( 'NONE',  ( 21.44999999999999929, 0.000000000000000000, 4.999999999999998224 ) ) ;
#60772=CARTESIAN_POINT ( 'NONE',  ( 24.00937500061451502, 0.000000000000000000, 5.243569643749999010 ) ) ;
#60773=ORIENTED_EDGE ( 'NONE', *, *, #12396, .T. ) ;
#60774=CARTESIAN_POINT ( 'NONE',  ( 2.090614718769495450, 4.666716435056564194, -2.090614718769495450 ) ) ;
#60775=CARTESIAN_POINT ( 'NONE',  ( 10.71562500061451928, 3.027376345333613106, -5.243569643749998122 ) ) ;
#60778=CARTESIAN_POINT ( 'NONE',  ( 16.08749999999999503, -2.886751345948129988, 4.999999999999997335 ) ) ;
#60779=CARTESIAN_POINT ( 'NONE',  ( 24.52499999999999858, 4.330127018922191873, 2.499999999999999556 ) ) ;
#60780=CARTESIAN_POINT ( 'NONE',  ( 7.950000000000001954, 0.000000000000000000, 4.999999999999998224 ) ) ;
#60781=CARTESIAN_POINT ( 'NONE',  ( 3.909375000614518481, -4.541064518000417216, -2.621784821875001281 ) ) ;
#60782=CARTESIAN_POINT ( 'NONE',  ( 17.55937500061451573, 4.541064518000418104, -2.621784821874998173 ) ) ;
#60783=CARTESIAN_POINT ( 'NONE',  ( 27.68437500061451573, -4.541064518000419881, 2.621784821874995952 ) ) ;
#60785=CARTESIAN_POINT ( 'NONE',  ( 26.80312500061451431, -4.541064518000417216, -2.621784821875001281 ) ) ;
#60786=CARTESIAN_POINT ( 'NONE',  ( 27.83437500061451786, 6.421520780324663323E-16, -5.243569643749999010 ) ) ;
#60787=LINE ( 'NONE', #4302, #67577 ) ;
#60788=CARTESIAN_POINT ( 'NONE',  ( 14.55000000000000071, 4.330127018922192761, -2.499999999999997780 ) ) ;
#60789=CARTESIAN_POINT ( 'NONE',  ( 12.32812500061451821, -4.541064518000419881, 2.621784821874995952 ) ) ;
#60790=CARTESIAN_POINT ( 'NONE',  ( 6.150000000000003020, 0.000000000000000000, 4.999999999999998224 ) ) ;
#60791=CARTESIAN_POINT ( 'NONE',  ( 1.071796769724505438, 11.31740381056766864, 26.00000000000001421 ) ) ;
#60792=CARTESIAN_POINT ( 'NONE',  ( 27.81562500061452070, 3.027376345333612662, -5.243569643749998122 ) ) ;
#60793=CARTESIAN_POINT ( 'NONE',  ( 16.42500000122903359, 2.886751345948129099, -4.999999999999998224 ) ) ;
#60796=CARTESIAN_POINT ( 'NONE',  ( 6.178125000614518747, 6.421520780324663323E-16, -5.243569643749999010 ) ) ;
#60797=CARTESIAN_POINT ( 'NONE',  ( 22.99687500061451573, 6.054752690667223547, 3.707466751127219781E-16 ) ) ;
#60798=CARTESIAN_POINT ( 'NONE',  ( -4.243569643749999898, 18.02187500061452141, 27.54997392385601529 ) ) ;
#60799=CARTESIAN_POINT ( 'NONE',  ( 22.80937500061451573, -4.541064518000417216, -2.621784821875001281 ) ) ;
#60800=CARTESIAN_POINT ( 'NONE',  ( 3.187500000000002220, -2.886751345948125991, -5.000000000000000000 ) ) ;
#60802=CARTESIAN_POINT ( 'NONE',  ( 11.24062500061451608, 6.054752690667223547, 3.707466751127219781E-16 ) ) ;
#60803=CARTESIAN_POINT ( 'NONE',  ( 2.962500001229034119, 4.330127018922192761, -2.499999999999997780 ) ) ;
#60804=CARTESIAN_POINT ( 'NONE',  ( 7.884375000614517681, -4.541064518000419881, 2.621784821874995952 ) ) ;
#60805=CARTESIAN_POINT ( 'NONE',  ( 7.537500001229033408, 4.330127018922191873, 2.499999999999999556 ) ) ;
#60806=CARTESIAN_POINT ( 'NONE',  ( 10.94062500061451537, -3.027376345333614438, 5.243569643749998122 ) ) ;
#60807=CARTESIAN_POINT ( 'NONE',  ( 15.15937500061451715, -4.541064518000417216, -2.621784821875001281 ) ) ;
#60809=CARTESIAN_POINT ( 'NONE',  ( 21.60000000122903430, -2.886751345948129988, 4.999999999999997335 ) ) ;
#60810=CARTESIAN_POINT ( 'NONE',  ( 7.021875000614518747, -6.054752690667223547, -1.112240025338166033E-15 ) ) ;
#60811=CARTESIAN_POINT ( 'NONE',  ( 10.19062500061451892, -3.027376345333610441, -5.243569643749999898 ) ) ;
#60813=CARTESIAN_POINT ( 'NONE',  ( 21.23437500061451644, 4.541064518000418104, 2.621784821874999949 ) ) ;
#60814=FACE_BOUND ( 'NONE', #72891, .T. ) ;
#60815=CARTESIAN_POINT ( 'NONE',  ( 4.907911205059083602E-16, 5.000000000000000000, 33.99999999999999289 ) ) ;
#60817=CARTESIAN_POINT ( 'NONE',  ( 4.243569643749999898, 11.08437500061451786, -30.00000000000000000 ) ) ;
#60818=CARTESIAN_POINT ( 'NONE',  ( 15.90000000122903501, -2.886751345948125991, -5.000000000000000000 ) ) ;
#60819=ADVANCED_FACE ( 'NONE', ( #17847 ), #46676, .F. ) ;
#60820=AXIS2_PLACEMENT_3D ( 'NONE', #36832, #8390, #54924 ) ;
#60821=CARTESIAN_POINT ( 'NONE',  ( 2.121784821875001281, 14.55312500061451786, -26.32496088578401938 ) ) ;
#60822=CARTESIAN_POINT ( 'NONE',  ( 17.10000000122903430, -2.886751345948129988, 4.999999999999997335 ) ) ;
#60823=CARTESIAN_POINT ( 'NONE',  ( 11.01562500061451821, -6.054752690667223547, -1.112240025338166033E-15 ) ) ;
#60824=ORIENTED_EDGE ( 'NONE', *, *, #55867, .F. ) ;
#60825=CARTESIAN_POINT ( 'NONE',  ( 13.64999999999999858, 4.330127018922192761, -2.499999999999997780 ) ) ;
#60826=CARTESIAN_POINT ( 'NONE',  ( -3.999999999999999112, 13.66250000000000142, 27.69059892324149885 ) ) ;
#60827=CARTESIAN_POINT ( 'NONE',  ( 22.15312500061451573, 0.000000000000000000, 5.243569643749999010 ) ) ;
#60828=CARTESIAN_POINT ( 'NONE',  ( 10.05937500061451750, 0.000000000000000000, 5.243569643749999010 ) ) ;
#60829=EDGE_CURVE ( 'NONE', #54070, #48258, #40777, .T. ) ;
#60830=CARTESIAN_POINT ( 'NONE',  ( 4.395499815916704911, -2.383214571124957271, -4.670699935784250911 ) ) ;
#60831=CARTESIAN_POINT ( 'NONE',  ( 10.27500000122903323, 2.886751345948126879, 4.999999999999999112 ) ) ;
#60832=CARTESIAN_POINT ( 'NONE',  ( 19.68750000122903288, 4.330127018922191873, 2.499999999999999556 ) ) ;
#60833=CARTESIAN_POINT ( 'NONE',  ( 14.65312500061451573, -4.541064518000417216, -2.621784821875001281 ) ) ;
#60835=CARTESIAN_POINT ( 'NONE',  ( 17.05312500061451786, 4.541064518000418104, -2.621784821874998173 ) ) ;
#60836=CARTESIAN_POINT ( 'NONE',  ( 26.21250000122903501, -4.330127018922190985, -2.500000000000001332 ) ) ;
#60837=CARTESIAN_POINT ( 'NONE',  ( 28.87500000122902932, -5.773502691896255534, -1.060575238724906372E-15 ) ) ;
#60838=CARTESIAN_POINT ( 'NONE',  ( 21.89999999999999858, 0.000000000000000000, 4.999999999999998224 ) ) ;
#60840=CARTESIAN_POINT ( 'NONE',  ( 26.37187500061451217, -6.054752690667223547, -1.112240025338166033E-15 ) ) ;
#60841=CARTESIAN_POINT ( 'NONE',  ( 11.66249999999999964, -5.773502691896255534, -1.060575238724906372E-15 ) ) ;
#60842=CARTESIAN_POINT ( 'NONE',  ( 12.37500000122903465, 2.886751345948129099, -4.999999999999998224 ) ) ;
#60843=CARTESIAN_POINT ( 'NONE',  ( 4.050000000000001599, -4.330127018922190985, -2.500000000000001332 ) ) ;
#60844=DIRECTION ( 'NONE',  ( -1.000000000000000000, -0.000000000000000000, -0.000000000000000000 ) ) ;
#60845=CARTESIAN_POINT ( 'NONE',  ( 6.121875000614517504, -6.054752690667223547, -1.112240025338166033E-15 ) ) ;
#60846=CARTESIAN_POINT ( 'NONE',  ( 25.67812500061451431, 4.541064518000418104, 2.621784821874999949 ) ) ;
#60848=DIRECTION ( 'NONE',  ( -1.000000000000000000, -0.000000000000000000, -0.000000000000000000 ) ) ;
#60850=CARTESIAN_POINT ( 'NONE',  ( 10.32187500061451679, 3.027376345333613106, -5.243569643749998122 ) ) ;
#60852=CARTESIAN_POINT ( 'NONE',  ( 4.305944032607977867, -2.541529510831473271, 4.468189746291087339 ) ) ;
#60853=CARTESIAN_POINT ( 'NONE',  ( 28.75312500061451715, 4.541064518000418104, -2.621784821874998173 ) ) ;
#60854=CARTESIAN_POINT ( 'NONE',  ( 9.084375000614517859, 4.541064518000418104, 2.621784821874999949 ) ) ;
#60855=CARTESIAN_POINT ( 'NONE',  ( 29.74687500061451217, 6.054752690667223547, 3.707466751127219781E-16 ) ) ;
#60856=EDGE_CURVE ( 'NONE', #66791, #64403, #9770, .T. ) ;
#60857=CARTESIAN_POINT ( 'NONE',  ( 9.001249775931846008E-16, 12.71562500061459389, 34.90005215228797653 ) ) ;
#60858=CARTESIAN_POINT ( 'NONE',  ( 21.07499999999999929, -4.330127018922194537, 2.499999999999995559 ) ) ;
#60859=ORIENTED_EDGE ( 'NONE', *, *, #34767, .F. ) ;
#60860=CARTESIAN_POINT ( 'NONE',  ( 29.81250000000000000, 2.886751345948129099, -4.999999999999998224 ) ) ;
#60861=CARTESIAN_POINT ( 'NONE',  ( 5.212500000000002132, 2.886751345948126879, 4.999999999999999112 ) ) ;
#60863=CARTESIAN_POINT ( 'NONE',  ( 17.87812500061451715, 6.421520780324663323E-16, -5.243569643749999010 ) ) ;
#60864=CARTESIAN_POINT ( 'NONE',  ( 7.340625000614518392, -3.027376345333614438, 5.243569643749998122 ) ) ;
#60866=CARTESIAN_POINT ( 'NONE',  ( 6.384375000614516793, 4.541064518000418104, 2.621784821874999949 ) ) ;
#60867=CARTESIAN_POINT ( 'NONE',  ( 17.06250000122903288, 0.000000000000000000, 4.999999999999998224 ) ) ;
#60869=CARTESIAN_POINT ( 'NONE',  ( 5.859375000614519102, 4.541064518000418104, -2.621784821874998173 ) ) ;
#60870=CARTESIAN_POINT ( 'NONE',  ( 11.89687500061451608, -3.027376345333614438, 5.243569643749998122 ) ) ;
#60871=CARTESIAN_POINT ( 'NONE',  ( 23.14687500061451786, -3.027376345333614438, 5.243569643749998122 ) ) ;
#60873=VERTEX_POINT ( 'NONE', #24850 ) ;
#60875=CARTESIAN_POINT ( 'NONE',  ( 18.27187500061451431, -6.054752690667223547, -1.112240025338166033E-15 ) ) ;
#60876=CARTESIAN_POINT ( 'NONE',  ( 9.084375000614517859, 4.541064518000418104, 2.621784821874999949 ) ) ;
#60878=CARTESIAN_POINT ( 'NONE',  ( 22.16250000000000142, 2.886751345948129099, -4.999999999999998224 ) ) ;
#60882=CARTESIAN_POINT ( 'NONE',  ( 13.41562500061451502, 3.027376345333613106, -5.243569643749998122 ) ) ;
#60883=CARTESIAN_POINT ( 'NONE',  ( 28.09687500061451360, -3.027376345333614438, 5.243569643749998122 ) ) ;
#60884=CARTESIAN_POINT ( 'NONE',  ( 6.787500001229032520, -4.330127018922194537, 2.499999999999995559 ) ) ;
#60885=CARTESIAN_POINT ( 'NONE',  ( 29.22187500061451715, 3.027376345333613106, -5.243569643749998122 ) ) ;
#60886=CARTESIAN_POINT ( 'NONE',  ( 10.20000000000000107, 0.000000000000000000, 4.999999999999998224 ) ) ;
#60887=CARTESIAN_POINT ( 'NONE',  ( 1.999999999999998668, 15.46250000122903501, 26.53589838486224650 ) ) ;
#60888=CARTESIAN_POINT ( 'NONE',  ( 8.175000001229031810, -5.773502691896255534, -1.060575238724906372E-15 ) ) ;
#60889=CARTESIAN_POINT ( 'NONE',  ( 22.43437500061451573, 6.421520780324663323E-16, -5.243569643749999010 ) ) ;
#60890=CARTESIAN_POINT ( 'NONE',  ( 14.63437500061451679, -4.541064518000419881, 2.621784821874995952 ) ) ;
#60891=CARTESIAN_POINT ( 'NONE',  ( 4.013004193198248970, 2.982582328347916700, -4.312681910770049143 ) ) ;
#60892=VERTEX_POINT ( 'NONE', #68130 ) ;
#60893=CARTESIAN_POINT ( 'NONE',  ( 17.50312500061451715, 4.541064518000418104, -2.621784821874998173 ) ) ;
#60894=CARTESIAN_POINT ( 'NONE',  ( 29.21250000122903145, 0.000000000000000000, 4.999999999999998224 ) ) ;
#60895=CARTESIAN_POINT ( 'NONE',  ( 14.59687500061452070, -3.027376345333614438, 5.243569643749998122 ) ) ;
#60896=CARTESIAN_POINT ( 'NONE',  ( 5.838630383562667170, 8.118670948950970967, -28.60360171723054634 ) ) ;
#60897=CARTESIAN_POINT ( 'NONE',  ( 16.90312500061451573, -4.541064518000417216, -2.621784821875001281 ) ) ;
#60898=CYLINDRICAL_SURFACE ( 'NONE', #26788, 10.00000000000000000 ) ;
#60899=CARTESIAN_POINT ( 'NONE',  ( 29.59687500061451715, -3.027376345333610441, -5.243569643749999898 ) ) ;
#60900=CARTESIAN_POINT ( 'NONE',  ( 2.121784821875001281, 13.20312500061451821, 33.67503911421598417 ) ) ;
#60901=CARTESIAN_POINT ( 'NONE',  ( 18.27187500061451431, -6.054752690667223547, -1.112240025338166033E-15 ) ) ;
#60902=CARTESIAN_POINT ( 'NONE',  ( 14.21250000122903323, 4.330127018922192761, -2.499999999999997780 ) ) ;
#60904=CARTESIAN_POINT ( 'NONE',  ( 2.121784821875001281, 19.55937500061451573, -26.32496088578401938 ) ) ;
#60905=CARTESIAN_POINT ( 'NONE',  ( 19.95937500061451786, 0.000000000000000000, 5.243569643749999010 ) ) ;
#60906=CARTESIAN_POINT ( 'NONE',  ( 21.86250000122903003, 4.330127018922192761, -2.499999999999997780 ) ) ;
#60907=CARTESIAN_POINT ( 'NONE',  ( 15.94687500061451502, -3.027376345333614438, 5.243569643749998122 ) ) ;
#60908=CARTESIAN_POINT ( 'NONE',  ( 13.49062500061451608, 6.054752690667223547, 3.707466751127219781E-16 ) ) ;
#60909=CARTESIAN_POINT ( 'NONE',  ( -4.243569643749999898, 12.17187500061451999, 27.54997392385601529 ) ) ;
#60910=AXIS2_PLACEMENT_3D ( 'NONE', #37678, #60200, #9612 ) ;
#60911=CARTESIAN_POINT ( 'NONE',  ( 17.69062500061451715, -3.027376345333614438, 5.243569643749998122 ) ) ;
#60914=CARTESIAN_POINT ( 'NONE',  ( 21.60000000000000142, -4.330127018922190985, -2.500000000000001332 ) ) ;
#60916=CARTESIAN_POINT ( 'NONE',  ( 25.07812500061451644, 6.421520780324663323E-16, -5.243569643749999010 ) ) ;
#60917=CARTESIAN_POINT ( 'NONE',  ( 5.915625000614515905, 3.027376345333611329, 5.243569643749999010 ) ) ;
#60918=CARTESIAN_POINT ( 'NONE',  ( 17.25000000122903288, -2.886751345948125991, -5.000000000000000000 ) ) ;
#60919=CARTESIAN_POINT ( 'NONE',  ( 22.15312500061451573, 0.000000000000000000, 5.243569643749999010 ) ) ;
#60920=CARTESIAN_POINT ( 'NONE',  ( 22.61250000000000071, 2.886751345948129099, -4.999999999999998224 ) ) ;
#60921=EDGE_CURVE ( 'NONE', #43636, #57370, #57849, .T. ) ;
#60922=CARTESIAN_POINT ( 'NONE',  ( 26.01562500061451289, 3.027376345333613106, -5.243569643749998122 ) ) ;
#60923=CARTESIAN_POINT ( 'NONE',  ( 4.828125000614518214, 6.421520780324663323E-16, -5.243569643749999010 ) ) ;
#60925=CARTESIAN_POINT ( 'NONE',  ( 26.96250000122903145, 0.000000000000000000, 4.999999999999998224 ) ) ;
#60927=DIRECTION ( 'NONE',  ( -1.000000000000000000, -0.000000000000000000, -0.000000000000000000 ) ) ;
#60928=CARTESIAN_POINT ( 'NONE',  ( 3.999999999999998668, 12.72500000122903430, -32.30940107675850470 ) ) ;
#60929=CARTESIAN_POINT ( 'NONE',  ( -4.243569643749999898, 18.47187500061451715, -32.45002607614398471 ) ) ;
#60930=( BOUNDED_CURVE ( )  B_SPLINE_CURVE ( 2, ( #4829, #38816, #7526, #62946, #29698, #18954, #18225, #57761, #36334 ),
 .UNSPECIFIED., .F., .F. ) 
 B_SPLINE_CURVE_WITH_KNOTS ( ( 3, 2, 2, 2, 3 ),
 ( 0.9239130434782608647, 0.9275362318840579823, 0.9347826086956522174, 0.9420289855072463414, 0.9456521739130434590 ),
 .UNSPECIFIED. ) 
 CURVE ( )  GEOMETRIC_REPRESENTATION_ITEM ( )  RATIONAL_B_SPLINE_CURVE ( ( 0.9330127018922194093, 0.9330127018922194093, 1.000000000000000000, 0.8660254037844387076, 1.000000000000000000, 0.8660254037844387076, 1.000000000000000000, 0.9330127018922194093, 0.9330127018922194093 ) ) 
 REPRESENTATION_ITEM ( '' )  );
#60931=CARTESIAN_POINT ( 'NONE',  ( 11.55000000000000071, 0.000000000000000000, 4.999999999999998224 ) ) ;
#60932=CARTESIAN_POINT ( 'NONE',  ( 10.77187500061451786, 3.027376345333613106, -5.243569643749998122 ) ) ;
#60933=CARTESIAN_POINT ( 'NONE',  ( 6.375000001229031987, -5.773502691896255534, -1.060575238724906372E-15 ) ) ;
#60934=CARTESIAN_POINT ( 'NONE',  ( 11.67187500061451821, 3.027376345333613106, -5.243569643749998122 ) ) ;
#60935=CARTESIAN_POINT ( 'NONE',  ( 5.334375000614517859, 6.421520780324663323E-16, -5.243569643749999010 ) ) ;
#60938=CARTESIAN_POINT ( 'NONE',  ( -1.071796769724488563, 10.75490381179670152, 34.00000000000000000 ) ) ;
#60939=CARTESIAN_POINT ( 'NONE',  ( 10.35937500061451644, 4.541064518000418104, -2.621784821874998173 ) ) ;
#60940=CARTESIAN_POINT ( 'NONE',  ( 13.35000000000000142, 0.000000000000000000, 4.999999999999998224 ) ) ;
#60941=CARTESIAN_POINT ( 'NONE',  ( 20.27812500061451573, 4.541064518000418104, 2.621784821874999949 ) ) ;
#60943=CARTESIAN_POINT ( 'NONE',  ( -4.243569643749999898, 19.31562500061459176, 27.54997392385601529 ) ) ;
#60944=CARTESIAN_POINT ( 'NONE',  ( 23.59687500061451715, -3.027376345333614438, 5.243569643749998122 ) ) ;
#60945=CARTESIAN_POINT ( 'NONE',  ( 4.167140676845648706, 2.763139261668956514, -4.167140676845877856 ) ) ;
#60946=( BOUNDED_CURVE ( )  B_SPLINE_CURVE ( 2, ( #34740, #51745, #1144, #12931, #26584, #59449, #37297, #31762, #48755 ),
 .UNSPECIFIED., .F., .F. ) 
 B_SPLINE_CURVE_WITH_KNOTS ( ( 3, 2, 2, 2, 3 ),
 ( 0.1413043478260869734, 0.1449275362318840632, 0.1521739130434782705, 0.1594202898550724501, 0.1630434782608695676 ),
 .UNSPECIFIED. ) 
 CURVE ( )  GEOMETRIC_REPRESENTATION_ITEM ( )  RATIONAL_B_SPLINE_CURVE ( ( 0.9330127018922194093, 0.9330127018922196314, 1.000000000000000000, 0.8660254037844387076, 1.000000000000000000, 0.8660254037844387076, 1.000000000000000000, 0.9330127018922190762, 0.9330127018922194093 ) ) 
 REPRESENTATION_ITEM ( '' )  );
#60947=CARTESIAN_POINT ( 'NONE',  ( 28.80000000122903003, -2.886751345948129988, 4.999999999999997335 ) ) ;
#60949=CARTESIAN_POINT ( 'NONE',  ( 24.32812500061451289, 4.541064518000418104, 2.621784821874999949 ) ) ;
#60950=CARTESIAN_POINT ( 'NONE',  ( 17.12812500061451715, 4.541064518000418104, 2.621784821874999949 ) ) ;
#60952=CARTESIAN_POINT ( 'NONE',  ( 15.30937500061451750, 4.541064518000418104, -2.621784821874998173 ) ) ;
#60953=CARTESIAN_POINT ( 'NONE',  ( 16.91250000000000142, 2.886751345948161074, 4.999999999999941380 ) ) ;
#60954=VECTOR ( 'NONE', #40967, 1000.000000000000000 ) ;
#60955=CARTESIAN_POINT ( 'NONE',  ( 26.62500000122903288, -5.773502691896255534, -1.060575238724906372E-15 ) ) ;
#60956=CARTESIAN_POINT ( 'NONE',  ( 4.096875000614518925, 6.054752690667223547, 3.707466751127219781E-16 ) ) ;
#60957=CARTESIAN_POINT ( 'NONE',  ( 15.19687500061451857, -3.027376345333610441, -5.243569643749999898 ) ) ;
#60958=CARTESIAN_POINT ( 'NONE',  ( 4.869423765992945796, -1.135214599616954256, -5.119209941160161037 ) ) ;
#60959=B_SPLINE_CURVE_WITH_KNOTS ( 'NONE', 1,
 ( #15022, #32757 ),
 .UNSPECIFIED., .F., .F.,
 ( 2, 2 ),
 ( 0.000000000000000000, 1.000000000000000000 ),
 .UNSPECIFIED. ) ;
#60961=EDGE_CURVE ( 'NONE', #30519, #48240, #56027, .T. ) ;
#60962=CARTESIAN_POINT ( 'NONE',  ( 3.600000001229033408, -2.886751345948129988, 4.999999999999997335 ) ) ;
#60963=CARTESIAN_POINT ( 'NONE',  ( 24.08437500061451786, -4.541064518000419881, 2.621784821874995952 ) ) ;
#60964=CARTESIAN_POINT ( 'NONE',  ( 17.18437500061451573, 4.541064518000418104, 2.621784821874999949 ) ) ;
#60966=CARTESIAN_POINT ( 'NONE',  ( 28.87499999999999645, 6.123233995736764310E-16, -4.999999999999998224 ) ) ;
#60967=CARTESIAN_POINT ( 'NONE',  ( 3.787500001229033408, 6.123233995736764310E-16, -4.999999999999998224 ) ) ;
#60968=CARTESIAN_POINT ( 'NONE',  ( 4.987500000000002487, -2.886751345948125991, -5.000000000000000000 ) ) ;
#60970=CARTESIAN_POINT ( 'NONE',  ( 19.37812500061451715, 4.541064518000418104, 2.621784821874999949 ) ) ;
#60971=CARTESIAN_POINT ( 'NONE',  ( 9.787499999999999645, -2.886751345948129988, 4.999999999999997335 ) ) ;
#60972=CARTESIAN_POINT ( 'NONE',  ( 3.328125000614516438, -4.541064518000419881, 2.621784821874995952 ) ) ;
#60973=CARTESIAN_POINT ( 'NONE',  ( 19.20000000000000284, 0.000000000000000000, 4.999999999999998224 ) ) ;
#60975=CARTESIAN_POINT ( 'NONE',  ( 22.83750000122903501, 4.330127018922191873, 2.499999999999999556 ) ) ;
#60976=CARTESIAN_POINT ( 'NONE',  ( 5.800002967315413649, 8.146762937617078038, 28.41205895484640820 ) ) ;
#60977=( BOUNDED_CURVE ( )  B_SPLINE_CURVE ( 2, ( #58439, #7850, #23739, #875, #46287, #46652, #2313 ),
 .UNSPECIFIED., .F., .F. ) 
 B_SPLINE_CURVE_WITH_KNOTS ( ( 3, 2, 2, 3 ),
 ( 0.1999999999999999556, 0.2027777777777777235, 0.2055555555555554914, 0.2083333333333332871 ),
 .UNSPECIFIED. ) 
 CURVE ( )  GEOMETRIC_REPRESENTATION_ITEM ( )  RATIONAL_B_SPLINE_CURVE ( ( 1.000000000000002665, 0.8660254037844360431, 1.000000000000000000, 0.8660254037844387076, 1.000000000000000000, 0.8660254037844413721, 0.9999999999999973355 ) ) 
 REPRESENTATION_ITEM ( '' )  );
#60978=CARTESIAN_POINT ( 'NONE',  ( 29.10937500061451644, -4.541064518000417216, -2.621784821875001281 ) ) ;
#60980=CARTESIAN_POINT ( 'NONE',  ( 16.56562500061451715, 3.027376345333613106, -5.243569643749998122 ) ) ;
#60981=CARTESIAN_POINT ( 'NONE',  ( 25.15312500061451217, 4.541064518000418104, -2.621784821874998173 ) ) ;
#60982=CARTESIAN_POINT ( 'NONE',  ( 22.17187500061451644, 3.027376345333611329, 5.243569643749999010 ) ) ;
#60983=CARTESIAN_POINT ( 'NONE',  ( 7.462500000000001243, 2.886751345948126879, 4.999999999999999112 ) ) ;
#60984=CARTESIAN_POINT ( 'NONE',  ( 9.065625000614517148, 3.027376345333611329, 5.243569643749999010 ) ) ;
#60985=CARTESIAN_POINT ( 'NONE',  ( 26.42812500061451431, 6.421520780324663323E-16, -5.243569643749999010 ) ) ;
#60986=CARTESIAN_POINT ( 'NONE',  ( 14.70937500061451786, -4.541064518000417216, -2.621784821875001281 ) ) ;
#60987=CARTESIAN_POINT ( 'NONE',  ( 20.37187500061451573, 3.027376345333611329, 5.243569643749999010 ) ) ;
#60988=CARTESIAN_POINT ( 'NONE',  ( 3.999999999999999112, 11.78750000122903430, -30.00000000000000000 ) ) ;
#60989=CARTESIAN_POINT ( 'NONE',  ( -3.000416591977282496E-16, 10.29687500061451644, 25.09994784771203058 ) ) ;
#60990=CARTESIAN_POINT ( 'NONE',  ( 21.18750000122903288, -4.330127018922194537, 2.499999999999995559 ) ) ;
#60992=CARTESIAN_POINT ( 'NONE',  ( 12.36562500061451786, -6.054752690667223547, -1.112240025338166033E-15 ) ) ;
#60993=CARTESIAN_POINT ( 'NONE',  ( 8.896875000614517859, -3.027376345333610441, -5.243569643749999898 ) ) ;
#60994=CARTESIAN_POINT ( 'NONE',  ( 8.409375000614518925, -4.541064518000417216, -2.621784821875001281 ) ) ;
#60995=VERTEX_POINT ( 'NONE', #53297 ) ;
#60996=CARTESIAN_POINT ( 'NONE',  ( 28.84687500061452070, 6.054752690667223547, 3.707466751127219781E-16 ) ) ;
#60997=CARTESIAN_POINT ( 'NONE',  ( 18.40312500061451573, 4.541064518000418104, -2.621784821874998173 ) ) ;
#60998=CARTESIAN_POINT ( 'NONE',  ( 2.915625000614516793, -6.054752690667223547, -1.112240025338166033E-15 ) ) ;
#60999=CARTESIAN_POINT ( 'NONE',  ( 3.121875000614518836, 3.027376345333613106, -5.243569643749998122 ) ) ;
#61000=CARTESIAN_POINT ( 'NONE',  ( 24.64687500061451431, -3.027376345333610441, -5.243569643749999898 ) ) ;
#61001=CARTESIAN_POINT ( 'NONE',  ( 18.89062500061451644, 6.054752690667223547, 3.707466751127219781E-16 ) ) ;
#61002=CARTESIAN_POINT ( 'NONE',  ( -2.828200636599751609E-16, 10.43750000000000178, 25.38119784648299770 ) ) ;
#61003=CARTESIAN_POINT ( 'NONE',  ( 23.65312500061451573, -4.541064518000417216, -2.621784821875001281 ) ) ;
#61004=CARTESIAN_POINT ( 'NONE',  ( 5.625000001229036428, 2.886751345948129099, -4.999999999999998224 ) ) ;
#61005=ORIENTED_EDGE ( 'NONE', *, *, #68031, .T. ) ;
#61006=CARTESIAN_POINT ( 'NONE',  ( 3.262500001229035718, -4.330127018922190985, -2.500000000000001332 ) ) ;
#61007=CARTESIAN_POINT ( 'NONE',  ( -2.828200636599751609E-16, 16.28749999999999787, -34.61880215351700230 ) ) ;
#61009=CARTESIAN_POINT ( 'NONE',  ( 4.359375000614517326, -4.541064518000417216, -2.621784821875001281 ) ) ;
#61010=CARTESIAN_POINT ( 'NONE',  ( 25.34999999999999787, 4.330127018922192761, -2.499999999999997780 ) ) ;
#61011=CARTESIAN_POINT ( 'NONE',  ( 11.91562500061451857, -6.054752690667223547, -1.112240025338166033E-15 ) ) ;
#61012=CARTESIAN_POINT ( 'NONE',  ( 6.571875000614517681, -6.054752690667223547, -1.112240025338166033E-15 ) ) ;
#61013=CARTESIAN_POINT ( 'NONE',  ( 25.12500000122903288, 2.886751345948126879, 4.999999999999999112 ) ) ;
#61014=VECTOR ( 'NONE', #61848, 1000.000000000000000 ) ;
#61015=CARTESIAN_POINT ( 'NONE',  ( 15.23437500061451644, 6.421520780324663323E-16, -5.243569643749999010 ) ) ;
#61016=CARTESIAN_POINT ( 'NONE',  ( 28.52812500061451573, -4.541064518000419881, 2.621784821874995952 ) ) ;
#61017=CARTESIAN_POINT ( 'NONE',  ( 29.25000000000000000, -4.330127018922190985, -2.500000000000001332 ) ) ;
#61018=CARTESIAN_POINT ( 'NONE',  ( 25.84687500061451360, -3.027376345333614438, 5.243569643749998122 ) ) ;
#61019=CARTESIAN_POINT ( 'NONE',  ( 3.178125000614515638, 4.541064518000418104, 2.621784821874999949 ) ) ;
#61020=CARTESIAN_POINT ( 'NONE',  ( 12.06562500061451537, 3.027376345333613106, -5.243569643749998122 ) ) ;
#61023=CARTESIAN_POINT ( 'NONE',  ( 10.94062500061451537, -3.027376345333614438, 5.243569643749998122 ) ) ;
#61024=CARTESIAN_POINT ( 'NONE',  ( 9.065625000614517148, 3.027376345333611329, 5.243569643749999010 ) ) ;
#61026=CARTESIAN_POINT ( 'NONE',  ( 8.812500000000000000, 2.886751345948126879, 4.999999999999999112 ) ) ;
#61027=CARTESIAN_POINT ( 'NONE',  ( 5.062500001229035540, -4.330127018922190985, -2.500000000000001332 ) ) ;
#61028=CARTESIAN_POINT ( 'NONE',  ( 17.43750000000000355, -2.886751345948129988, 4.999999999999997335 ) ) ;
#61029=CARTESIAN_POINT ( 'NONE',  ( 18.94687500061451502, 6.054752690667223547, 3.707466751127219781E-16 ) ) ;
#61030=CARTESIAN_POINT ( 'NONE',  ( 13.38750000122903394, 4.330127018922191873, 2.499999999999999556 ) ) ;
#61032=CARTESIAN_POINT ( 'NONE',  ( 4.243569643749999898, 15.52812500061451750, -30.00000000000000000 ) ) ;
#61033=CARTESIAN_POINT ( 'NONE',  ( 21.97500000000000142, -4.330127018922194537, 2.499999999999995559 ) ) ;
#61035=DIRECTION ( 'NONE',  ( -0.000000000000000000, -1.000000000000000000, -0.000000000000000000 ) ) ;
#61036=FACE_BOUND ( 'NONE', #21614, .T. ) ;
#61037=CARTESIAN_POINT ( 'NONE',  ( 4.000000000000000000, 16.13749999999999929, -27.69059892324149885 ) ) ;
#61038=CARTESIAN_POINT ( 'NONE',  ( 13.54687500061451999, 6.054752690667223547, 3.707466751127219781E-16 ) ) ;
#61039=CARTESIAN_POINT ( 'NONE',  ( 27.33750000000000213, -2.886751345948129988, 4.999999999999997335 ) ) ;
#61040=CARTESIAN_POINT ( 'NONE',  ( 9.328125000614518214, 6.421520780324663323E-16, -5.243569643749999010 ) ) ;
#61042=CARTESIAN_POINT ( 'NONE',  ( 21.27187500061451786, 3.027376345333611329, 5.243569643749999010 ) ) ;
#61044=CARTESIAN_POINT ( 'NONE',  ( 8.540625000614518569, 6.054752690667223547, 3.707466751127219781E-16 ) ) ;
#61045=CARTESIAN_POINT ( 'NONE',  ( 11.44687500061451857, -3.027376345333614438, 5.243569643749998122 ) ) ;
#61046=EDGE_LOOP ( 'NONE', ( #37878, #51526, #26158, #17258 ) ) ;
#61047=CARTESIAN_POINT ( 'NONE',  ( 21.27187500061451786, 3.027376345333611329, 5.243569643749999010 ) ) ;
#61048=CARTESIAN_POINT ( 'NONE',  ( 29.06249999999999645, 2.886751345948164182, 4.999999999999933387 ) ) ;
#61049=CARTESIAN_POINT ( 'NONE',  ( 5.025000000000002132, 6.123233995736764310E-16, -4.999999999999998224 ) ) ;
#61051=CARTESIAN_POINT ( 'NONE',  ( 13.91250000122903252, 0.000000000000000000, 4.999999999999998224 ) ) ;
#61052=CARTESIAN_POINT ( 'NONE',  ( 30.00000000000000000, 6.123233995736764310E-16, -4.999999999999998224 ) ) ;
#61053=CARTESIAN_POINT ( 'NONE',  ( 3.802324603042571027, -3.246905036188573845, 4.117364570290419579 ) ) ;
#61054=VERTEX_POINT ( 'NONE', #14868 ) ;
#61055=CARTESIAN_POINT ( 'NONE',  ( 13.19999999999999929, 4.330127018922192761, -2.499999999999997780 ) ) ;
#61056=CARTESIAN_POINT ( 'NONE',  ( 15.59999999999999964, 0.000000000000000000, 4.999999999999998224 ) ) ;
#61057=CARTESIAN_POINT ( 'NONE',  ( 13.53750000122903430, -4.330127018922194537, 2.499999999999995559 ) ) ;
#61058=CARTESIAN_POINT ( 'NONE',  ( 11.72812500061451857, 4.541064518000418104, 2.621784821874999949 ) ) ;
#61061=CARTESIAN_POINT ( 'NONE',  ( 8.849999999999999645, 0.000000000000000000, 4.999999999999998224 ) ) ;
#61062=CARTESIAN_POINT ( 'NONE',  ( 26.36250000000000071, 2.886751345948110892, 5.000000000000026645 ) ) ;
#61063=CARTESIAN_POINT ( 'NONE',  ( -2.121784821874999949, 13.48437500061451821, -33.67503911421598417 ) ) ;
#61064=CARTESIAN_POINT ( 'NONE',  ( 2.840625000614518392, -3.027376345333614438, 5.243569643749998122 ) ) ;
#61066=CARTESIAN_POINT ( 'NONE',  ( 9.225000000000001421, 4.330127018922191873, 2.499999999999999556 ) ) ;
#61067=CARTESIAN_POINT ( 'NONE',  ( 3.171572016300020724, 3.865480461419896763, 3.489665696640699810 ) ) ;
#61069=CARTESIAN_POINT ( 'NONE',  ( 24.17812500061451786, 6.421520780324663323E-16, -5.243569643749999010 ) ) ;
#61070=CARTESIAN_POINT ( 'NONE',  ( 30.00000000000000000, 6.123233995736764310E-16, -4.999999999999998224 ) ) ;
#61072=CARTESIAN_POINT ( 'NONE',  ( 21.98437500061451644, 6.421520780324663323E-16, -5.243569643749999010 ) ) ;
#61073=CARTESIAN_POINT ( 'NONE',  ( 17.35312500061451502, -4.541064518000417216, -2.621784821875001281 ) ) ;
#61074=CARTESIAN_POINT ( 'NONE',  ( -2.121784821874999949, 10.72812500061459318, -33.67503911421598417 ) ) ;
#61075=CARTESIAN_POINT ( 'NONE',  ( 5.615625000614517859, -6.054752690667223547, -1.112240025338166033E-15 ) ) ;
#61076=CARTESIAN_POINT ( 'NONE',  ( 3.103125000614517237, 4.541064518000418104, -2.621784821874998173 ) ) ;
#61078=CARTESIAN_POINT ( 'NONE',  ( 20.31562500061451715, 3.027376345333611329, 5.243569643749999010 ) ) ;
#61081=CARTESIAN_POINT ( 'NONE',  ( 14.85937500061451644, 4.541064518000418104, -2.621784821874998173 ) ) ;
#61082=CARTESIAN_POINT ( 'NONE',  ( 14.22187500061451537, -6.054752690667223547, -1.112240025338166033E-15 ) ) ;
#61083=CARTESIAN_POINT ( 'NONE',  ( 23.10937500061451644, 0.000000000000000000, 5.243569643749999010 ) ) ;
#61084=ORIENTED_EDGE ( 'NONE', *, *, #62019, .T. ) ;
#61085=CARTESIAN_POINT ( 'NONE',  ( 4.243569643749999898, 11.98437500061451821, 30.00000000000000000 ) ) ;
#61086=CARTESIAN_POINT ( 'NONE',  ( -2.000000000000000000, 14.63750000122903394, -33.46410161513775705 ) ) ;
#61087=CARTESIAN_POINT ( 'NONE',  ( 26.12812500061451360, 4.541064518000418104, 2.621784821874999949 ) ) ;
#61089=CARTESIAN_POINT ( 'NONE',  ( 26.05312500061451431, 4.541064518000418104, -2.621784821874998173 ) ) ;
#61090=CARTESIAN_POINT ( 'NONE',  ( 8.287500001229034297, 6.123233995736764310E-16, -4.999999999999998224 ) ) ;
#61091=CARTESIAN_POINT ( 'NONE',  ( -3.999999999999999556, 19.96250000000000213, 27.69059892324149530 ) ) ;
#61092=CARTESIAN_POINT ( 'NONE',  ( 4.921875000614518214, 3.027376345333613106, -5.243569643749998122 ) ) ;
#61094=CARTESIAN_POINT ( 'NONE',  ( 12.45000000122903394, 5.773502691896255534, 3.535250795749688894E-16 ) ) ;
#61095=CARTESIAN_POINT ( 'NONE',  ( 8.475000001229034297, 2.886751345948126879, 4.999999999999999112 ) ) ;
#61096=CARTESIAN_POINT ( 'NONE',  ( 29.36250000122903003, -4.330127018922190985, -2.500000000000001332 ) ) ;
#61099=CARTESIAN_POINT ( 'NONE',  ( 11.97187500061451892, -6.054752690667223547, -1.112240025338166033E-15 ) ) ;
#61102=CARTESIAN_POINT ( 'NONE',  ( 19.41562500061451146, 3.027376345333611329, 5.243569643749999010 ) ) ;
#61103=CARTESIAN_POINT ( 'NONE',  ( 12.83437500061451786, -4.541064518000419881, 2.621784821874995952 ) ) ;
#61104=CARTESIAN_POINT ( 'NONE',  ( 5.428125000614517859, 4.541064518000418104, 2.621784821874999949 ) ) ;
#61105=EDGE_CURVE ( 'NONE', #14078, #34155, #5162, .T. ) ;
#61106=CARTESIAN_POINT ( 'NONE',  ( 23.10937500061451644, 0.000000000000000000, 5.243569643749999010 ) ) ;
#61107=CARTESIAN_POINT ( 'NONE',  ( 6.178125000614518747, 6.421520780324663323E-16, -5.243569643749999010 ) ) ;
#61109=CARTESIAN_POINT ( 'NONE',  ( 5.400000001229032343, -2.886751345948129988, 4.999999999999997335 ) ) ;
#61110=CARTESIAN_POINT ( 'NONE',  ( 21.36562500061451431, -6.054752690667223547, -1.112240025338166033E-15 ) ) ;
#61111=EDGE_CURVE ( 'NONE', #30507, #12269, #14501, .T. ) ;
#61112=CARTESIAN_POINT ( 'NONE',  ( -2.828200636599751609E-16, 17.75000000122903288, -34.61880215351700230 ) ) ;
#61113=CARTESIAN_POINT ( 'NONE',  ( 7.950000001229033053, 5.773502691896255534, 3.535250795749688894E-16 ) ) ;
#61114=CARTESIAN_POINT ( 'NONE',  ( 16.94062500061451715, -3.027376345333610441, -5.243569643749999898 ) ) ;
#61115=CARTESIAN_POINT ( 'NONE',  ( 15.17812500061451608, 6.421520780324663323E-16, -5.243569643749999010 ) ) ;
#61117=CARTESIAN_POINT ( 'NONE',  ( 16.31250000000000000, 2.886751345948129099, -4.999999999999998224 ) ) ;
#61118=CARTESIAN_POINT ( 'NONE',  ( 12.22500000122903430, -5.773502691896255534, -1.060575238724906372E-15 ) ) ;
#61119=CARTESIAN_POINT ( 'NONE',  ( 6.965625000614518392, -6.054752690667223547, -1.112240025338166033E-15 ) ) ;
#61120=CARTESIAN_POINT ( 'NONE',  ( 11.20312500061451644, 4.541064518000418104, -2.621784821874998173 ) ) ;
#61121=EDGE_CURVE ( 'NONE', #10824, #31619, #34771, .T. ) ;
#61122=( BOUNDED_CURVE ( )  B_SPLINE_CURVE ( 2, ( #8788, #31322, #43143, #25413, #48323, #54227, #20221 ),
 .UNSPECIFIED., .F., .F. ) 
 B_SPLINE_CURVE_WITH_KNOTS ( ( 3, 2, 2, 3 ),
 ( 0.5749999999999999556, 0.5777777777777777235, 0.5805555555555557135, 0.5833333333333334814 ),
 .UNSPECIFIED. ) 
 CURVE ( )  GEOMETRIC_REPRESENTATION_ITEM ( )  RATIONAL_B_SPLINE_CURVE ( ( 1.000000000000000000, 0.8660254037844387076, 1.000000000000000000, 0.8660254037844387076, 1.000000000000000000, 0.8660254037844333785, 1.000000000000005329 ) ) 
 REPRESENTATION_ITEM ( '' )  );
#61123=CARTESIAN_POINT ( 'NONE',  ( 22.01250000122903216, 0.000000000000000000, 4.999999999999998224 ) ) ;
#61124=CARTESIAN_POINT ( 'NONE',  ( -4.243569643749997233, 13.14687500061451786, -27.54997392385601174 ) ) ;
#61125=CARTESIAN_POINT ( 'NONE',  ( 4.929940333177246004, 0.8485134343999930495, 4.980930601228622301 ) ) ;
#61126=CARTESIAN_POINT ( 'NONE',  ( 5.700000001229033941, 5.773502691896255534, 3.535250795749688894E-16 ) ) ;
#61127=CARTESIAN_POINT ( 'NONE',  ( 4.509375000614518569, 4.541064518000418104, -2.621784821874998173 ) ) ;
#61128=CARTESIAN_POINT ( 'NONE',  ( 21.90937500061451715, -4.541064518000417216, -2.621784821875001281 ) ) ;
#61130=CARTESIAN_POINT ( 'NONE',  ( 16.56562500061451715, 3.027376345333613106, -5.243569643749998122 ) ) ;
#61132=CARTESIAN_POINT ( 'NONE',  ( 29.55937500061451573, -4.541064518000417216, -2.621784821875001281 ) ) ;
#61134=CARTESIAN_POINT ( 'NONE',  ( 15.96562500061451573, -6.054752690667223547, -1.112240025338166033E-15 ) ) ;
#61135=CARTESIAN_POINT ( 'NONE',  ( 12.04687500061451821, -3.027376345333610441, -5.243569643749999898 ) ) ;
#61136=ORIENTED_EDGE ( 'NONE', *, *, #19011, .F. ) ;
#61137=CARTESIAN_POINT ( 'NONE',  ( 22.23750000000000071, 5.773502691896255534, 3.535250795749688401E-16 ) ) ;
#61138=CARTESIAN_POINT ( 'NONE',  ( 22.41562500061451502, 3.027376345333613106, -5.243569643749998122 ) ) ;
#61139=CARTESIAN_POINT ( 'NONE',  ( 3.999999999999999112, 11.22500000000000142, -30.00000000000000000 ) ) ;
#61140=CARTESIAN_POINT ( 'NONE',  ( -1.999999999999997113, 18.38750000122903572, 33.46410161513775705 ) ) ;
#61142=CARTESIAN_POINT ( 'NONE',  ( 12.71250000000000036, 2.886751345948129099, -4.999999999999998224 ) ) ;
#61143=CARTESIAN_POINT ( 'NONE',  ( 24.60000000122903430, 5.773502691896255534, 3.535250795749688894E-16 ) ) ;
#61144=CARTESIAN_POINT ( 'NONE',  ( 18.85312500061451502, 4.541064518000418104, -2.621784821874998173 ) ) ;
#61146=VERTEX_POINT ( 'NONE', #37407 ) ;
#61147=CARTESIAN_POINT ( 'NONE',  ( 19.38749999999999929, -2.886751345948125991, -5.000000000000000000 ) ) ;
#61148=CARTESIAN_POINT ( 'NONE',  ( 21.94687500061451857, -3.027376345333610441, -5.243569643749999898 ) ) ;
#61149=CARTESIAN_POINT ( 'NONE',  ( 27.62812500061451360, -4.541064518000419881, 2.621784821874995952 ) ) ;
#61150=ORIENTED_EDGE ( 'NONE', *, *, #33221, .F. ) ;
#61151=CARTESIAN_POINT ( 'NONE',  ( 2.000000000000001332, 17.89999999999999858, -26.53589838486224650 ) ) ;
#61152=CARTESIAN_POINT ( 'NONE',  ( 11.46562500061451573, -6.054752690667223547, -1.112240025338166033E-15 ) ) ;
#61155=CARTESIAN_POINT ( 'NONE',  ( 17.62500000000000000, 6.123233995736764310E-16, -4.999999999999998224 ) ) ;
#61156=CARTESIAN_POINT ( 'NONE',  ( 24.11249999999999716, 2.886751345948126879, 4.999999999999999112 ) ) ;
#61157=CARTESIAN_POINT ( 'NONE',  ( 3.619842856578028734, -3.449164782042274169, -3.619842856578066481 ) ) ;
#61158=CARTESIAN_POINT ( 'NONE',  ( 3.759375000614517681, 0.000000000000000000, 5.243569643749999010 ) ) ;
#61159=CARTESIAN_POINT ( 'NONE',  ( 29.07187500061451502, -6.054752690667223547, -1.112240025338166033E-15 ) ) ;
#61160=ORIENTED_EDGE ( 'NONE', *, *, #10710, .F. ) ;
#61161=CARTESIAN_POINT ( 'NONE',  ( 26.91562500061451146, 3.027376345333613106, -5.243569643749998122 ) ) ;
#61162=CARTESIAN_POINT ( 'NONE',  ( 24.90937500061451715, 0.000000000000000000, 5.243569643749999010 ) ) ;
#61163=CARTESIAN_POINT ( 'NONE',  ( -4.243569643749999898, 18.90312500061459389, -30.00000000000000000 ) ) ;
#61164=CARTESIAN_POINT ( 'NONE',  ( 13.04999999999999893, -4.330127018922190985, -2.500000000000001332 ) ) ;
#61165=CARTESIAN_POINT ( 'NONE',  ( 10.52812500061451750, -4.541064518000419881, 2.621784821874995952 ) ) ;
#61167=CARTESIAN_POINT ( 'NONE',  ( 4.428044609675158227, 2.322158679919935409, 4.428044609675073850 ) ) ;
#61168=CARTESIAN_POINT ( 'NONE',  ( 28.41562500061451502, 3.027376345333611329, 5.243569643749999010 ) ) ;
#61169=CARTESIAN_POINT ( 'NONE',  ( 16.91250000122903430, 4.330127018922192761, -2.499999999999997780 ) ) ;
#61172=CARTESIAN_POINT ( 'NONE',  ( 4.228125000614517681, -4.541064518000419881, 2.621784821874995952 ) ) ;
#61173=CARTESIAN_POINT ( 'NONE',  ( 22.84687500061451715, -3.027376345333610441, -5.243569643749999898 ) ) ;
#61174=CARTESIAN_POINT ( 'NONE',  ( 4.243569643749999898, 14.19687500061451857, 32.45002607614398471 ) ) ;
#61175=CARTESIAN_POINT ( 'NONE',  ( 21.04687500061451644, -3.027376345333610441, -5.243569643749999898 ) ) ;
#61176=CARTESIAN_POINT ( 'NONE',  ( 29.78437500061451715, 4.541064518000418104, 2.621784821874999949 ) ) ;
#61177=CARTESIAN_POINT ( 'NONE',  ( 4.243569643749999010, 17.87187500061451928, 27.54997392385601174 ) ) ;
#61178=CARTESIAN_POINT ( 'NONE',  ( 10.30312500061451431, 4.541064518000418104, -2.621784821874998173 ) ) ;
#61179=DIRECTION ( 'NONE',  ( -1.000000000000000000, -0.000000000000000000, -0.000000000000000000 ) ) ;
#61181=CARTESIAN_POINT ( 'NONE',  ( 7.359375000614516438, 0.000000000000000000, 5.243569643749999010 ) ) ;
#61182=CARTESIAN_POINT ( 'NONE',  ( 7.612500001229035362, 0.000000000000000000, 4.999999999999998224 ) ) ;
#61183=CARTESIAN_POINT ( 'NONE',  ( 7.640625000614517326, 6.054752690667223547, 3.707466751127219781E-16 ) ) ;
#61184=CARTESIAN_POINT ( 'NONE',  ( 10.99687500061451750, -3.027376345333614438, 5.243569643749998122 ) ) ;
#61185=CARTESIAN_POINT ( 'NONE',  ( 0.000000000000000000, 0.000000000000000000, -50.00000000000000000 ) ) ;
#61186=CARTESIAN_POINT ( 'NONE',  ( 19.76250000122903216, 0.000000000000000000, 4.999999999999998224 ) ) ;
#61187=CARTESIAN_POINT ( 'NONE',  ( 9.196875000614518569, -3.027376345333614438, 5.243569643749998122 ) ) ;
#61188=CARTESIAN_POINT ( 'NONE',  ( 10.26562500061451644, 3.027376345333613106, -5.243569643749998122 ) ) ;
#61189=CARTESIAN_POINT ( 'NONE',  ( 6.403125000614517504, 0.000000000000000000, 5.243569643749999010 ) ) ;
#61192=CARTESIAN_POINT ( 'NONE',  ( 19.47187500061451360, 3.027376345333611329, 5.243569643749999010 ) ) ;
#61193=CARTESIAN_POINT ( 'NONE',  ( 11.50312500061451892, -4.541064518000417216, -2.621784821875001281 ) ) ;
#61194=CARTESIAN_POINT ( 'NONE',  ( 28.95937500061451431, 0.000000000000000000, 5.243569643749999010 ) ) ;
#61195=CARTESIAN_POINT ( 'NONE',  ( 4.243569643749999010, 12.47187500061451715, -32.45002607614398471 ) ) ;
#61196=CARTESIAN_POINT ( 'NONE',  ( 12.52500000122903145, 2.886751345948126879, 4.999999999999999112 ) ) ;
#61197=CARTESIAN_POINT ( 'NONE',  ( 2.121784821874999061, 15.60312500061451857, -33.67503911421598417 ) ) ;
#61198=CARTESIAN_POINT ( 'NONE',  ( 14.17500000122903536, 2.886751345948129099, -4.999999999999998224 ) ) ;
#61199=CARTESIAN_POINT ( 'NONE',  ( 11.24062500061451608, 6.054752690667223547, 3.707466751127219781E-16 ) ) ;
#61200=ORIENTED_EDGE ( 'NONE', *, *, #380, .T. ) ;
#61201=CARTESIAN_POINT ( 'NONE',  ( 13.04999999999999893, -4.330127018922190985, -2.500000000000001332 ) ) ;
#61203=CARTESIAN_POINT ( 'NONE',  ( 21.85312500061451502, -4.541064518000417216, -2.621784821875001281 ) ) ;
#61204=CARTESIAN_POINT ( 'NONE',  ( 7.734375000614517326, 4.541064518000418104, 2.621784821874999949 ) ) ;
#61205=CARTESIAN_POINT ( 'NONE',  ( 10.98750000122903536, 6.123233995736764310E-16, -4.999999999999998224 ) ) ;
#61206=CARTESIAN_POINT ( 'NONE',  ( 17.51250000122903216, 0.000000000000000000, 4.999999999999998224 ) ) ;
#61207=CARTESIAN_POINT ( 'NONE',  ( 14.91562500061451679, 3.027376345333611329, 5.243569643749999010 ) ) ;
#61208=CARTESIAN_POINT ( 'NONE',  ( 18.29062500061451502, -3.027376345333610441, -5.243569643749999898 ) ) ;
#61209=CARTESIAN_POINT ( 'NONE',  ( 26.13750000122903216, -4.330127018922194537, 2.499999999999995559 ) ) ;
#61210=CARTESIAN_POINT ( 'NONE',  ( 27.22500000122903430, 2.886751345948129099, -4.999999999999998224 ) ) ;
#61211=CARTESIAN_POINT ( 'NONE',  ( 23.21250000000000213, 2.886751345948126879, 4.999999999999999112 ) ) ;
#61213=CARTESIAN_POINT ( 'NONE',  ( 26.59687500061451360, 6.054752690667223547, 3.707466751127219781E-16 ) ) ;
#61214=DIRECTION ( 'NONE',  ( -0.000000000000000000, -1.000000000000000000, -0.000000000000000000 ) ) ;
#61215=CARTESIAN_POINT ( 'NONE',  ( 12.26250000122903394, -4.330127018922190985, -2.500000000000001332 ) ) ;
#61216=CARTESIAN_POINT ( 'NONE',  ( 28.54687500061451644, -3.027376345333614438, 5.243569643749998122 ) ) ;
#61217=CARTESIAN_POINT ( 'NONE',  ( -3.999999999999999112, 20.00000000000000000, -30.00000000000000000 ) ) ;
#61218=CARTESIAN_POINT ( 'NONE',  ( 4.584375000614516971, 4.541064518000418104, 2.621784821874999949 ) ) ;
#61219=B_SPLINE_CURVE_WITH_KNOTS ( 'NONE', 1,
 ( #45759, #63814 ),
 .UNSPECIFIED., .F., .F.,
 ( 2, 2 ),
 ( 0.000000000000000000, 1.000000000000000000 ),
 .UNSPECIFIED. ) ;
#61220=CARTESIAN_POINT ( 'NONE',  ( 22.79062500061451502, -3.027376345333610441, -5.243569643749999898 ) ) ;
#61222=CARTESIAN_POINT ( 'NONE',  ( 3.999999999999998668, 19.81250000000000000, -32.30940107675850470 ) ) ;
#61223=CARTESIAN_POINT ( 'NONE',  ( 9.721875000614517148, -6.054752690667223547, -1.112240025338166033E-15 ) ) ;
#61224=CARTESIAN_POINT ( 'NONE',  ( 3.647618174410700131, -3.419850926247963940, 3.721781544883157711 ) ) ;
#61225=CARTESIAN_POINT ( 'NONE',  ( 29.61562500061451431, 3.027376345333613106, -5.243569643749998122 ) ) ;
#61226=CARTESIAN_POINT ( 'NONE',  ( 5.259375000614518569, -4.541064518000417216, -2.621784821875001281 ) ) ;
#61227=CARTESIAN_POINT ( 'NONE',  ( 27.68437500061451573, -4.541064518000419881, 2.621784821874995952 ) ) ;
#61228=CARTESIAN_POINT ( 'NONE',  ( 4.243569643749999898, 11.02812500061459566, 30.00000000000000000 ) ) ;
#61229=CARTESIAN_POINT ( 'NONE',  ( 20.66250000000000142, -5.773502691896255534, -1.060575238724906372E-15 ) ) ;
#61230=ORIENTED_EDGE ( 'NONE', *, *, #16557, .F. ) ;
#61231=CARTESIAN_POINT ( 'NONE',  ( 27.93750000000000000, -2.886751345948125991, -5.000000000000000000 ) ) ;
#61232=CARTESIAN_POINT ( 'NONE',  ( 27.83437500061451786, 6.421520780324663323E-16, -5.243569643749999010 ) ) ;
#61233=EDGE_CURVE ( 'NONE', #23988, #5357, #48499, .T. ) ;
#61235=CARTESIAN_POINT ( 'NONE',  ( 16.75312500061451715, 0.000000000000000000, 5.243569643749999010 ) ) ;
#61236=CARTESIAN_POINT ( 'NONE',  ( 9.065625000614517148, 3.027376345333611329, 5.243569643749999010 ) ) ;
#61238=CARTESIAN_POINT ( 'NONE',  ( 7.284375000614518036, 4.541064518000418104, 2.621784821874999949 ) ) ;
#61239=CARTESIAN_POINT ( 'NONE',  ( 17.43750000122903288, 4.330127018922191873, 2.499999999999999556 ) ) ;
#61240=CARTESIAN_POINT ( 'NONE',  ( 23.81250000122903288, 0.000000000000000000, 4.999999999999998224 ) ) ;
#61241=CARTESIAN_POINT ( 'NONE',  ( 7.096875000614517148, -3.027376345333610441, -5.243569643749999898 ) ) ;
#61242=CARTESIAN_POINT ( 'NONE',  ( 12.04687500061451821, -3.027376345333610441, -5.243569643749999898 ) ) ;
#61243=CARTESIAN_POINT ( 'NONE',  ( 24.15937500061451715, -4.541064518000417216, -2.621784821875001281 ) ) ;
#61244=CARTESIAN_POINT ( 'NONE',  ( -3.999999999999999112, 16.40000000000000213, 30.00000000000000000 ) ) ;
#61247=CARTESIAN_POINT ( 'NONE',  ( 16.84687500061451715, -3.027376345333614438, 5.243569643749998122 ) ) ;
#61248=CARTESIAN_POINT ( 'NONE',  ( 9.309375000614517504, -4.541064518000417216, -2.621784821875001281 ) ) ;
#61250=CARTESIAN_POINT ( 'NONE',  ( 20.54999999999999716, 0.000000000000000000, 4.999999999999998224 ) ) ;
#61252=CARTESIAN_POINT ( 'NONE',  ( 4.243569643749999898, 10.59687500061451715, -27.54997392385601529 ) ) ;
#61254=CARTESIAN_POINT ( 'NONE',  ( 11.65312500061451573, 4.541064518000418104, -2.621784821874998173 ) ) ;
#61255=CARTESIAN_POINT ( 'NONE',  ( 27.94687500061451502, 6.054752690667223547, 3.707466751127219781E-16 ) ) ;
#61256=CARTESIAN_POINT ( 'NONE',  ( -3.999999999999999112, 19.66250000122903430, 30.00000000000000000 ) ) ;
#61257=CARTESIAN_POINT ( 'NONE',  ( 27.79687500061451999, -3.027376345333610441, -5.243569643749999898 ) ) ;
#61258=CARTESIAN_POINT ( 'NONE',  ( 10.12500000000000178, 4.330127018922191873, 2.499999999999999556 ) ) ;
#61259=CARTESIAN_POINT ( 'NONE',  ( 4.000000000000000000, 15.35000000122903252, 32.30940107675849049 ) ) ;
#61260=CARTESIAN_POINT ( 'NONE',  ( 10.31250000122903288, 0.000000000000000000, 4.999999999999998224 ) ) ;
#61261=CARTESIAN_POINT ( 'NONE',  ( 20.55937500061451573, -4.541064518000417216, -2.621784821875001281 ) ) ;
#61262=CARTESIAN_POINT ( 'NONE',  ( 15.34687500061451537, 6.054752690667223547, 3.707466751127219781E-16 ) ) ;
#61264=ORIENTED_EDGE ( 'NONE', *, *, #41845, .T. ) ;
#61265=CARTESIAN_POINT ( 'NONE',  ( 15.66562500061451857, 3.027376345333613106, -5.243569643749998122 ) ) ;
#61266=CARTESIAN_POINT ( 'NONE',  ( 27.52500000122903145, -5.773502691896255534, -1.060575238724906372E-15 ) ) ;
#61267=CARTESIAN_POINT ( 'NONE',  ( 15.98437500061451821, -4.541064518000419881, 2.621784821874995952 ) ) ;
#61268=CARTESIAN_POINT ( 'NONE',  ( 3.215625000614518836, 3.027376345333611329, 5.243569643749999010 ) ) ;
#61269=CARTESIAN_POINT ( 'NONE',  ( 16.64062500061451289, 6.054752690667223547, 3.707466751127219781E-16 ) ) ;
#61270=EDGE_CURVE ( 'NONE', #24148, #9351, #42335, .T. ) ;
#61271=DIRECTION ( 'NONE',  ( 0.000000000000000000, 0.000000000000000000, -1.000000000000000000 ) ) ;
#61272=CARTESIAN_POINT ( 'NONE',  ( 25.69687500061451502, 6.054752690667223547, 3.707466751127219781E-16 ) ) ;
#61273=CARTESIAN_POINT ( 'NONE',  ( 4.243569643749999898, 12.82812500061451821, 30.00000000000000000 ) ) ;
#61274=CARTESIAN_POINT ( 'NONE',  ( 16.32187500061451502, 3.027376345333611329, 5.243569643749999010 ) ) ;
#61275=CARTESIAN_POINT ( 'NONE',  ( 13.87500000122903465, 2.886751345948126879, 4.999999999999999112 ) ) ;
#61277=CARTESIAN_POINT ( 'NONE',  ( 2.121784821875001281, 18.20937500061451786, -26.32496088578401938 ) ) ;
#61278=CARTESIAN_POINT ( 'NONE',  ( 21.53437500061451715, 6.421520780324663323E-16, -5.243569643749999010 ) ) ;
#61279=CARTESIAN_POINT ( 'NONE',  ( 22.16250000122903074, -4.330127018922190985, -2.500000000000001332 ) ) ;
#61280=CARTESIAN_POINT ( 'NONE',  ( 16.17187500061451644, 3.027376345333613106, -5.243569643749998122 ) ) ;
#61281=CARTESIAN_POINT ( 'NONE',  ( -3.000416591977282496E-16, 11.64687500061451786, 25.09994784771203058 ) ) ;
#61282=CARTESIAN_POINT ( 'NONE',  ( 17.01562500061451644, 3.027376345333613106, -5.243569643749998122 ) ) ;
#61285=CARTESIAN_POINT ( 'NONE',  ( 20.96250000000000213, 2.886751345948126879, 4.999999999999999112 ) ) ;
#61286=DIRECTION ( 'NONE',  ( -1.000000000000000000, -0.000000000000000000, -0.000000000000000000 ) ) ;
#61287=CARTESIAN_POINT ( 'NONE',  ( 24.29062500061451502, 6.054752690667223547, 3.707466751127219781E-16 ) ) ;
#61288=CARTESIAN_POINT ( 'NONE',  ( 4.678125000614516971, -4.541064518000419881, 2.621784821874995952 ) ) ;
#61289=CARTESIAN_POINT ( 'NONE',  ( 16.50000000122903288, 5.773502691896255534, 3.535250795749688894E-16 ) ) ;
#61290=EDGE_CURVE ( 'NONE', #66075, #60322, #45594, .T. ) ;
#61291=CARTESIAN_POINT ( 'NONE',  ( 21.81562500061451004, -6.054752690667223547, -1.112240025338166033E-15 ) ) ;
#61292=CARTESIAN_POINT ( 'NONE',  ( 19.79999999999999716, -4.330127018922190985, -2.500000000000001332 ) ) ;
#61293=CARTESIAN_POINT ( 'NONE',  ( 25.75312500061451715, 0.000000000000000000, 5.243569643749999010 ) ) ;
#61294=CARTESIAN_POINT ( 'NONE',  ( 4.790625000614518569, -3.027376345333610441, -5.243569643749999898 ) ) ;
#61295=ORIENTED_EDGE ( 'NONE', *, *, #51760, .F. ) ;
#61296=CARTESIAN_POINT ( 'NONE',  ( 3.928125000614516527, 6.421520780324663323E-16, -5.243569643749999010 ) ) ;
#61299=CARTESIAN_POINT ( 'NONE',  ( 3.999999999999998668, 10.47500000122903430, -32.30940107675850470 ) ) ;
#61300=CARTESIAN_POINT ( 'NONE',  ( -4.243569643749999898, 17.60937500061451999, -30.00000000000000000 ) ) ;
#61301=CARTESIAN_POINT ( 'NONE',  ( 7.612500000000000711, -5.773502691896255534, -1.060575238724906372E-15 ) ) ;
#61302=CARTESIAN_POINT ( 'NONE',  ( 8.896875000614517859, -3.027376345333610441, -5.243569643749999898 ) ) ;
#61303=CARTESIAN_POINT ( 'NONE',  ( 7.350000001229033408, -2.886751345948125991, -5.000000000000000000 ) ) ;
#61304=CARTESIAN_POINT ( 'NONE',  ( 13.17187500061451999, 3.027376345333611329, 5.243569643749999010 ) ) ;
#61305=CARTESIAN_POINT ( 'NONE',  ( 3.496875000614518836, -3.027376345333610441, -5.243569643749999898 ) ) ;
#61306=FACE_OUTER_BOUND ( 'NONE', #64119, .T. ) ;
#61308=CARTESIAN_POINT ( 'NONE',  ( 9.999999999999992895, -5.857864376269048101, -9.999999999999992895 ) ) ;
#61309=CARTESIAN_POINT ( 'NONE',  ( 9.684375000614517504, -4.541064518000419881, 2.621784821874995952 ) ) ;
#61310=CARTESIAN_POINT ( 'NONE',  ( 26.73750000122903003, 6.123233995736764310E-16, -4.999999999999998224 ) ) ;
#61311=CARTESIAN_POINT ( 'NONE',  ( 19.26562500061451644, 3.027376345333613106, -5.243569643749998122 ) ) ;
#61312=CARTESIAN_POINT ( 'NONE',  ( 2.121784821875001281, 19.05312500061459602, 33.67503911421598417 ) ) ;
#61313=CARTESIAN_POINT ( 'NONE',  ( 23.70937500061451786, -4.541064518000417216, -2.621784821875001281 ) ) ;
#61314=CARTESIAN_POINT ( 'NONE',  ( 29.58749999999999858, -2.886751345948150860, 4.999999999999960920 ) ) ;
#61315=CARTESIAN_POINT ( 'NONE',  ( 3.140625000614516882, 6.054752690667223547, 3.707466751127219781E-16 ) ) ;
#61317=CARTESIAN_POINT ( 'NONE',  ( 25.56562500061452070, 3.027376345333613106, -5.243569643749998122 ) ) ;
#61318=CARTESIAN_POINT ( 'NONE',  ( 14.46562500061451750, 3.027376345333611329, 5.243569643749999010 ) ) ;
#61320=CARTESIAN_POINT ( 'NONE',  ( 13.39687500061451608, -3.027376345333610441, -5.243569643749999898 ) ) ;
#61321=CARTESIAN_POINT ( 'NONE',  ( 24.97500000122903430, 2.886751345948129099, -4.999999999999998224 ) ) ;
#61322=CARTESIAN_POINT ( 'NONE',  ( 3.571875000614517237, 3.027376345333613106, -5.243569643749998122 ) ) ;
#61323=CARTESIAN_POINT ( 'NONE',  ( 13.84687500061451537, -3.027376345333610441, -5.243569643749999898 ) ) ;
#61324=CARTESIAN_POINT ( 'NONE',  ( 15.00000000000000000, 4.330127018922192761, -2.499999999999997780 ) ) ;
#61325=CYLINDRICAL_SURFACE ( 'NONE', #70195, 4.999999999999998224 ) ;
#61326=CARTESIAN_POINT ( 'NONE',  ( -5.810221930991193690E-16, 12.23750000000000071, -34.00000000000000000 ) ) ;
#61327=CARTESIAN_POINT ( 'NONE',  ( 25.77187500061451075, 3.027376345333611329, 5.243569643749999010 ) ) ;
#61328=CARTESIAN_POINT ( 'NONE',  ( 15.53437500061451715, -4.541064518000419881, 2.621784821874995952 ) ) ;
#61330=CARTESIAN_POINT ( 'NONE',  ( 27.03750000000000142, -2.886751345948125991, -5.000000000000000000 ) ) ;
#61331=CARTESIAN_POINT ( 'NONE',  ( 3.225000001229033408, -5.773502691896255534, -1.060575238724906372E-15 ) ) ;
#61332=CARTESIAN_POINT ( 'NONE',  ( 4.762499999999999289, 2.886751345948126879, 4.999999999999999112 ) ) ;
#61334=CARTESIAN_POINT ( 'NONE',  ( 18.89062500061451644, 6.054752690667223547, 3.707466751127219781E-16 ) ) ;
#61335=CARTESIAN_POINT ( 'NONE',  ( 8.812500000000000000, 2.886751345948126879, 4.999999999999999112 ) ) ;
#61336=ADVANCED_FACE ( 'NONE', ( #62392 ), #46136, .F. ) ;
#61337=CARTESIAN_POINT ( 'NONE',  ( -0.7157356635157281488, 9.902086024390941432, 25.94083351194041143 ) ) ;
#61338=CARTESIAN_POINT ( 'NONE',  ( 18.11250000000000071, 2.886751345948129099, -4.999999999999998224 ) ) ;
#61340=CARTESIAN_POINT ( 'NONE',  ( 20.81250000122903643, -4.330127018922190985, -2.500000000000001332 ) ) ;
#61342=CARTESIAN_POINT ( 'NONE',  ( 27.30937500061451573, -4.541064518000417216, -2.621784821875001281 ) ) ;
#61344=CARTESIAN_POINT ( 'NONE',  ( 17.61562500061451786, 3.027376345333611329, 5.243569643749999010 ) ) ;
#61345=CARTESIAN_POINT ( 'NONE',  ( 23.80312500061451786, 4.541064518000418104, -2.621784821874998173 ) ) ;
#61346=CARTESIAN_POINT ( 'NONE',  ( 23.37187500061451573, 3.027376345333613106, -5.243569643749998122 ) ) ;
#61347=CARTESIAN_POINT ( 'NONE',  ( 6.637500000000001066, -2.886751345948129988, 4.999999999999997335 ) ) ;
#61348=CARTESIAN_POINT ( 'NONE',  ( 8.840625000614515727, -3.027376345333610441, -5.243569643749999898 ) ) ;
#61349=CARTESIAN_POINT ( 'NONE',  ( 25.11562500061451431, 3.027376345333613106, -5.243569643749998122 ) ) ;
#61350=CARTESIAN_POINT ( 'NONE',  ( 14.10937500061451644, 0.000000000000000000, 5.243569643749999010 ) ) ;
#61351=CARTESIAN_POINT ( 'NONE',  ( 19.58437500061451786, -4.541064518000419881, 2.621784821874995952 ) ) ;
#61352=CARTESIAN_POINT ( 'NONE',  ( 1.626862140677534273E-15, 11.67500000122903181, -26.00000000000000355 ) ) ;
#61353=CARTESIAN_POINT ( 'NONE',  ( 9.001249775931846008E-16, 10.07187500061451857, 34.90005215228797653 ) ) ;
#61354=CARTESIAN_POINT ( 'NONE',  ( 21.03750000122903074, 4.330127018922191873, 2.499999999999999556 ) ) ;
#61356=CARTESIAN_POINT ( 'NONE',  ( 11.27812500061451573, 4.541064518000418104, 2.621784821874999949 ) ) ;
#61357=CARTESIAN_POINT ( 'NONE',  ( 7.696875000614516793, 6.054752690667223547, 3.707466751127219781E-16 ) ) ;
#61358=CARTESIAN_POINT ( 'NONE',  ( 6.384375000614516793, 4.541064518000418104, 2.621784821874999949 ) ) ;
#61360=CARTESIAN_POINT ( 'NONE',  ( 27.34687500061451360, -3.027376345333610441, -5.243569643749999898 ) ) ;
#61361=CARTESIAN_POINT ( 'NONE',  ( 20.01562500061451644, -6.054752690667223547, -1.112240025338166033E-15 ) ) ;
#61362=CARTESIAN_POINT ( 'NONE',  ( 3.515625000614516882, 3.027376345333613106, -5.243569643749998122 ) ) ;
#61363=CARTESIAN_POINT ( 'NONE',  ( 27.89062500061451289, 6.054752690667223547, 3.707466751127219781E-16 ) ) ;
#61364=CARTESIAN_POINT ( 'NONE',  ( 23.85937500061451644, 4.541064518000418104, -2.621784821874998173 ) ) ;
#61365=CARTESIAN_POINT ( 'NONE',  ( 18.59062500061451573, -3.027376345333614438, 5.243569643749998122 ) ) ;
#61366=CARTESIAN_POINT ( 'NONE',  ( -4.243569643749999898, 18.47187500061451715, 27.54997392385601529 ) ) ;
#61367=CARTESIAN_POINT ( 'NONE',  ( 25.45312500061451644, -4.541064518000417216, -2.621784821875001281 ) ) ;
#61368=CARTESIAN_POINT ( 'NONE',  ( 5.887500001229034829, -4.330127018922194537, 2.499999999999995559 ) ) ;
#61370=CARTESIAN_POINT ( 'NONE',  ( 28.76249999999999929, -5.773502691896255534, -1.060575238724906372E-15 ) ) ;
#61371=CARTESIAN_POINT ( 'NONE',  ( 4.000000000000000000, 16.13749999999999929, -27.69059892324149530 ) ) ;
#61373=CARTESIAN_POINT ( 'NONE',  ( 3.834375000614519635, -4.541064518000419881, 2.621784821874995952 ) ) ;
#61374=CARTESIAN_POINT ( 'NONE',  ( 13.11562500061451786, 3.027376345333611329, 5.243569643749999010 ) ) ;
#61375=CARTESIAN_POINT ( 'NONE',  ( 6.609375000614519102, -4.541064518000417216, -2.621784821875001281 ) ) ;
#61376=CARTESIAN_POINT ( 'NONE',  ( 24.30000000122903359, -2.886751345948129988, 4.999999999999997335 ) ) ;
#61378=CARTESIAN_POINT ( 'NONE',  ( 15.87187500061451573, 3.027376345333611329, 5.243569643749999010 ) ) ;
#61379=CARTESIAN_POINT ( 'NONE',  ( 3.009375000614516793, -4.541064518000417216, -2.621784821875001281 ) ) ;
#61380=CARTESIAN_POINT ( 'NONE',  ( 29.77499999999999858, 6.123233995736764310E-16, -4.999999999999998224 ) ) ;
#61381=CARTESIAN_POINT ( 'NONE',  ( 27.49687500061451217, 6.054752690667223547, 3.707466751127219781E-16 ) ) ;
#61382=CARTESIAN_POINT ( 'NONE',  ( 3.253125000614518036, 0.000000000000000000, 5.243569643749999010 ) ) ;
#61383=CARTESIAN_POINT ( 'NONE',  ( 12.14062500061451821, 6.054752690667223547, 3.707466751127219781E-16 ) ) ;
#61385=CARTESIAN_POINT ( 'NONE',  ( 9.928125000614517859, 4.541064518000418104, 2.621784821874999949 ) ) ;
#61386=CARTESIAN_POINT ( 'NONE',  ( 7.303125000614516082, 0.000000000000000000, 5.243569643749999010 ) ) ;
#61388=CARTESIAN_POINT ( 'NONE',  ( 9.449999999999999289, -4.330127018922190985, -2.500000000000001332 ) ) ;
#61389=EDGE_CURVE ( 'NONE', #15981, #38080, #15367, .T. ) ;
#61390=CARTESIAN_POINT ( 'NONE',  ( 2.925000001229034918, 2.886751345948129099, -4.999999999999998224 ) ) ;
#61391=CARTESIAN_POINT ( 'NONE',  ( 18.18750000000000000, 5.773502691896255534, 3.535250795749688894E-16 ) ) ;
#61392=( BOUNDED_CURVE ( )  B_SPLINE_CURVE ( 2, ( #48664, #47936, #8768, #54568, #32032, #37936, #8401 ),
 .UNSPECIFIED., .F., .F. ) 
 B_SPLINE_CURVE_WITH_KNOTS ( ( 3, 2, 2, 3 ),
 ( 0.02499999999999994935, 0.02777777777777776236, 0.03055555555555557884, 0.03333333333333339532 ),
 .UNSPECIFIED. ) 
 CURVE ( )  GEOMETRIC_REPRESENTATION_ITEM ( )  RATIONAL_B_SPLINE_CURVE ( ( 1.000000000000002442, 0.8660254037844360431, 1.000000000000000000, 0.8660254037844387076, 1.000000000000000000, 0.8660254037844357100, 1.000000000000003109 ) ) 
 REPRESENTATION_ITEM ( '' )  );
#61393=CARTESIAN_POINT ( 'NONE',  ( 16.09687500061452070, -3.027376345333610441, -5.243569643749999898 ) ) ;
#61394=CARTESIAN_POINT ( 'NONE',  ( 12.82500000122903394, 2.886751345948129099, -4.999999999999998224 ) ) ;
#61396=CARTESIAN_POINT ( 'NONE',  ( 9.001249775931846008E-16, 14.51562500061451466, -25.09994784771203058 ) ) ;
#61399=CARTESIAN_POINT ( 'NONE',  ( 26.50312500061451360, 4.541064518000418104, -2.621784821874998173 ) ) ;
#61400=CARTESIAN_POINT ( 'NONE',  ( 1.999999999999998668, 19.84999999999999787, 26.53589838486224650 ) ) ;
#61402=CARTESIAN_POINT ( 'NONE',  ( 25.87500000000000000, 4.330127018922191873, 2.499999999999999556 ) ) ;
#61403=CARTESIAN_POINT ( 'NONE',  ( 9.665625000614515017, -6.054752690667223547, -1.112240025338166033E-15 ) ) ;
#61405=( BOUNDED_CURVE ( )  B_SPLINE_CURVE ( 2, ( #70719, #37099, #43017, #59624, #31933, #26391, #2761 ),
 .UNSPECIFIED., .F., .F. ) 
 B_SPLINE_CURVE_WITH_KNOTS ( ( 3, 2, 2, 3 ),
 ( 0.3250000000000000111, 0.3277777777777777790, 0.3305555555555556024, 0.3333333333333333703 ),
 .UNSPECIFIED. ) 
 CURVE ( )  GEOMETRIC_REPRESENTATION_ITEM ( )  RATIONAL_B_SPLINE_CURVE ( ( 1.000000000000000000, 0.8660254037844387076, 1.000000000000000000, 0.8660254037844387076, 1.000000000000000000, 0.8660254037844360431, 1.000000000000002665 ) ) 
 REPRESENTATION_ITEM ( '' )  );
#61406=CARTESIAN_POINT ( 'NONE',  ( 22.24687500061451217, -3.027376345333614438, 5.243569643749998122 ) ) ;
#61408=CARTESIAN_POINT ( 'NONE',  ( 4.640625000614518214, -3.027376345333614438, 5.243569643749998122 ) ) ;
#61409=CARTESIAN_POINT ( 'NONE',  ( 11.22187500061451892, 3.027376345333613106, -5.243569643749998122 ) ) ;
#61411=CARTESIAN_POINT ( 'NONE',  ( 21.42187500061451644, -6.054752690667223547, -1.112240025338166033E-15 ) ) ;
#61412=CYLINDRICAL_SURFACE ( 'NONE', #20740, 4.999999999999998224 ) ;
#61413=CARTESIAN_POINT ( 'NONE',  ( 29.66249999999999432, -5.773502691896255534, -1.060575238724906372E-15 ) ) ;
#61414=EDGE_CURVE ( 'NONE', #43575, #61054, #14941, .T. ) ;
#61415=CARTESIAN_POINT ( 'NONE',  ( 5.549999999999998934, 4.330127018922192761, -2.499999999999997780 ) ) ;
#61416=CARTESIAN_POINT ( 'NONE',  ( 13.87500000122903465, 2.886751345948126879, 4.999999999999999112 ) ) ;
#61417=CARTESIAN_POINT ( 'NONE',  ( 1.592000809091587073E-14, 15.38750000000000284, -34.00000000000000000 ) ) ;
#61420=CARTESIAN_POINT ( 'NONE',  ( 13.72500000000000142, 4.330127018922191873, 2.499999999999999556 ) ) ;
#61421=CARTESIAN_POINT ( 'NONE',  ( 16.16250000000000142, -5.773502691896255534, -1.060575238724906372E-15 ) ) ;
#61422=CARTESIAN_POINT ( 'NONE',  ( 13.95000000122903572, -2.886751345948129988, 4.999999999999997335 ) ) ;
#61423=CARTESIAN_POINT ( 'NONE',  ( 12.25312500061451537, 0.000000000000000000, 5.243569643749999010 ) ) ;
#61424=CARTESIAN_POINT ( 'NONE',  ( 9.937500000000001776, -2.886751345948125991, -5.000000000000000000 ) ) ;
#61425=CARTESIAN_POINT ( 'NONE',  ( -3.999999999999999112, 15.61250000122903359, 30.00000000000000000 ) ) ;
#61426=CARTESIAN_POINT ( 'NONE',  ( -4.243569643749999898, 14.45937500061451964, -30.00000000000000000 ) ) ;
#61427=CARTESIAN_POINT ( 'NONE',  ( 27.37500000122903288, 2.886751345948126879, 4.999999999999999112 ) ) ;
#61429=CARTESIAN_POINT ( 'NONE',  ( 9.337500000000000355, -2.886751345948129988, 4.999999999999997335 ) ) ;
#61431=ORIENTED_EDGE ( 'NONE', *, *, #35197, .T. ) ;
#61432=CARTESIAN_POINT ( 'NONE',  ( 24.59062500061451573, -3.027376345333610441, -5.243569643749999898 ) ) ;
#61433=CARTESIAN_POINT ( 'NONE',  ( 3.612401643004526264, 3.457069727864729991, 3.855493425756290282 ) ) ;
#61434=CARTESIAN_POINT ( 'NONE',  ( 29.67187500061451644, 3.027376345333613106, -5.243569643749998122 ) ) ;
#61435=CARTESIAN_POINT ( 'NONE',  ( 21.23437500061451644, 4.541064518000418104, 2.621784821874999949 ) ) ;
#61436=CARTESIAN_POINT ( 'NONE',  ( 15.89062500061451289, -3.027376345333614438, 5.243569643749998122 ) ) ;
#61437=CARTESIAN_POINT ( 'NONE',  ( -4.243569643749999898, 10.76562500061459637, -32.45002607614398471 ) ) ;
#61438=CARTESIAN_POINT ( 'NONE',  ( 7.003125000614518036, -4.541064518000417216, -2.621784821875001281 ) ) ;
#61439=CARTESIAN_POINT ( 'NONE',  ( 28.72500000122903074, 2.886751345948126879, 4.999999999999999112 ) ) ;
#61441=CARTESIAN_POINT ( 'NONE',  ( 17.99062500061451786, 6.054752690667223547, 3.707466751127219781E-16 ) ) ;
#61444=CARTESIAN_POINT ( 'NONE',  ( 15.90937500061451892, 0.000000000000000000, 5.243569643749999010 ) ) ;
#61445=CARTESIAN_POINT ( 'NONE',  ( 14.63437500061451679, -4.541064518000419881, 2.621784821874995952 ) ) ;
#61446=CARTESIAN_POINT ( 'NONE',  ( 22.13437500061451502, 4.541064518000418104, 2.621784821874999949 ) ) ;
#61447=EDGE_LOOP ( 'NONE', ( #291, #13681, #1268, #72192 ) ) ;
#61448=CARTESIAN_POINT ( 'NONE',  ( -2.121784821874999949, 11.68437500061451750, 26.32496088578401938 ) ) ;
#61449=CARTESIAN_POINT ( 'NONE',  ( -3.999999999999997335, 14.75000000122903288, -27.69059892324149530 ) ) ;
#61450=CARTESIAN_POINT ( 'NONE',  ( 27.66562500061451146, -6.054752690667223547, -1.112240025338166033E-15 ) ) ;
#61451=CARTESIAN_POINT ( 'NONE',  ( 26.87812500061451360, 6.421520780324663323E-16, -5.243569643749999010 ) ) ;
#61452=CARTESIAN_POINT ( 'NONE',  ( 4.000000000000000000, 19.40000000122903856, -27.69059892324149885 ) ) ;
#61453=CARTESIAN_POINT ( 'NONE',  ( 3.999999999999998668, 16.66249999999999787, 27.69059892324149175 ) ) ;
#61454=CARTESIAN_POINT ( 'NONE',  ( 5.596875000614516260, -3.027376345333614438, 5.243569643749998122 ) ) ;
#61455=CARTESIAN_POINT ( 'NONE',  ( 12.78750000122903430, 6.123233995736764310E-16, -4.999999999999998224 ) ) ;
#61456=CARTESIAN_POINT ( 'NONE',  ( 7.425000001229034474, 2.886751345948129099, -4.999999999999998224 ) ) ;
#61457=CARTESIAN_POINT ( 'NONE',  ( 29.32500000122903216, -5.773502691896255534, -1.060575238724906372E-15 ) ) ;
#61460=CARTESIAN_POINT ( 'NONE',  ( 11.70937500061451608, 4.541064518000418104, -2.621784821874998173 ) ) ;
#61463=CARTESIAN_POINT ( 'NONE',  ( 20.46562500061451928, -6.054752690667223547, -1.112240025338166033E-15 ) ) ;
#61464=CARTESIAN_POINT ( 'NONE',  ( 13.58437500061451786, 4.541064518000418104, 2.621784821874999949 ) ) ;
#61465=CARTESIAN_POINT ( 'NONE',  ( 5.615625000614517859, -6.054752690667223547, -1.112240025338166033E-15 ) ) ;
#61466=CARTESIAN_POINT ( 'NONE',  ( 22.69687500061451857, -3.027376345333614438, 5.243569643749998122 ) ) ;
#61467=CARTESIAN_POINT ( 'NONE',  ( 10.95937500061451964, 0.000000000000000000, 5.243569643749999010 ) ) ;
#61468=CARTESIAN_POINT ( 'NONE',  ( 4.490625000614516971, 6.054752690667223547, 3.707466751127219781E-16 ) ) ;
#61469=CARTESIAN_POINT ( 'NONE',  ( 10.83750000122903501, -4.330127018922194537, 2.499999999999995559 ) ) ;
#61470=CARTESIAN_POINT ( 'NONE',  ( 5.775000001229033231, 2.886751345948126879, 4.999999999999999112 ) ) ;
#61471=CARTESIAN_POINT ( 'NONE',  ( 20.50312500061451715, -4.541064518000417216, -2.621784821875001281 ) ) ;
#61472=CARTESIAN_POINT ( 'NONE',  ( 7.462500001229035007, 4.330127018922192761, -2.499999999999997780 ) ) ;
#61473=CARTESIAN_POINT ( 'NONE',  ( 17.05312500061451786, 4.541064518000418104, -2.621784821874998173 ) ) ;
#61474=CARTESIAN_POINT ( 'NONE',  ( 15.36562500061451608, 3.027376345333611329, 5.243569643749999010 ) ) ;
#61476=CARTESIAN_POINT ( 'NONE',  ( 16.42500000000000071, 4.330127018922191873, 2.499999999999999556 ) ) ;
#61477=CARTESIAN_POINT ( 'NONE',  ( 10.01250000122903394, -4.330127018922190985, -2.500000000000001332 ) ) ;
#61478=CARTESIAN_POINT ( 'NONE',  ( 6.065625000614516260, -6.054752690667223547, -1.112240025338166033E-15 ) ) ;
#61480=CARTESIAN_POINT ( 'NONE',  ( 20.10000000122903074, 5.773502691896255534, 3.535250795749688894E-16 ) ) ;
#61482=CARTESIAN_POINT ( 'NONE',  ( 4.243569643749999898, 12.39687500061451608, -27.54997392385601529 ) ) ;
#61483=CARTESIAN_POINT ( 'NONE',  ( 21.33749999999999858, 5.773502691896255534, 3.535250795749688401E-16 ) ) ;
#61484=CARTESIAN_POINT ( 'NONE',  ( 4.012500001229033053, 0.000000000000000000, 4.999999999999998224 ) ) ;
#61485=CARTESIAN_POINT ( 'NONE',  ( 3.946875000614517681, -3.027376345333610441, -5.243569643749999898 ) ) ;
#61486=CARTESIAN_POINT ( 'NONE',  ( 19.80937500061451573, 4.541064518000418104, -2.621784821874998173 ) ) ;
#61488=CARTESIAN_POINT ( 'NONE',  ( 15.44062500061451537, -3.027376345333614438, 5.243569643749998122 ) ) ;
#61490=CARTESIAN_POINT ( 'NONE',  ( -1.999999999999997113, 15.57500000000000284, -26.53589838486224295 ) ) ;
#61492=CARTESIAN_POINT ( 'NONE',  ( 29.25937500061451502, 4.541064518000418104, -2.621784821874998173 ) ) ;
#61494=CARTESIAN_POINT ( 'NONE',  ( 14.12812500061451715, -4.541064518000419881, 2.621784821874995952 ) ) ;
#61495=CARTESIAN_POINT ( 'NONE',  ( 11.03437500061451715, -4.541064518000419881, 2.621784821874995952 ) ) ;
#61496=VERTEX_POINT ( 'NONE', #22857 ) ;
#61497=CARTESIAN_POINT ( 'NONE',  ( 28.86562500061451786, 3.027376345333611329, 5.243569643749999010 ) ) ;
#61498=CARTESIAN_POINT ( 'NONE',  ( 22.19062500061451715, -3.027376345333614438, 5.243569643749998122 ) ) ;
#61499=DIRECTION ( 'NONE',  ( -1.000000000000000000, -0.000000000000000000, -0.000000000000000000 ) ) ;
#61500=CARTESIAN_POINT ( 'NONE',  ( 11.62500000000000000, -4.330127018922194537, 2.499999999999995559 ) ) ;
#61501=CARTESIAN_POINT ( 'NONE',  ( 21.93750000122903288, 4.330127018922191873, 2.499999999999999556 ) ) ;
#61502=CARTESIAN_POINT ( 'NONE',  ( 17.27812500061451217, -4.541064518000419881, 2.621784821874995952 ) ) ;
#61504=ORIENTED_EDGE ( 'NONE', *, *, #22002, .F. ) ;
#61505=CARTESIAN_POINT ( 'NONE',  ( 19.34999999999999787, -4.330127018922190985, -2.500000000000001332 ) ) ;
#61506=CARTESIAN_POINT ( 'NONE',  ( 22.24687500061451217, -3.027376345333614438, 5.243569643749998122 ) ) ;
#61507=CARTESIAN_POINT ( 'NONE',  ( 27.77812500061451573, 6.421520780324663323E-16, -5.243569643749999010 ) ) ;
#61508=EDGE_CURVE ( 'NONE', #46924, #4424, #24845, .T. ) ;
#61510=CARTESIAN_POINT ( 'NONE',  ( 7.453125000614516438, -4.541064518000417216, -2.621784821875001281 ) ) ;
#61511=CARTESIAN_POINT ( 'NONE',  ( 3.300686927427837425, 3.755761153797071206, 3.532840975251721805 ) ) ;
#61512=CARTESIAN_POINT ( 'NONE',  ( 17.58749999999999858, -2.886751345948125991, -5.000000000000000000 ) ) ;
#61513=CARTESIAN_POINT ( 'NONE',  ( 25.50000000000000000, 0.000000000000000000, 4.999999999999998224 ) ) ;
#61514=CARTESIAN_POINT ( 'NONE',  ( 5.924999999999999822, 6.123233995736764310E-16, -4.999999999999998224 ) ) ;
#61515=CARTESIAN_POINT ( 'NONE',  ( 3.609375000614516882, 4.541064518000418104, -2.621784821874998173 ) ) ;
#61516=CARTESIAN_POINT ( 'NONE',  ( 29.67187500061451644, 3.027376345333613106, -5.243569643749998122 ) ) ;
#61518=CARTESIAN_POINT ( 'NONE',  ( 23.09062500061451573, -3.027376345333614438, 5.243569643749998122 ) ) ;
#61519=CARTESIAN_POINT ( 'NONE',  ( 24.34687500061451715, 6.054752690667223547, 3.707466751127219781E-16 ) ) ;
#61520=CARTESIAN_POINT ( 'NONE',  ( 4.243569643749999898, 19.12812500061459531, -30.00000000000000000 ) ) ;
#61521=CARTESIAN_POINT ( 'NONE',  ( 14.69999999999999929, 0.000000000000000000, 4.999999999999998224 ) ) ;
#61522=CARTESIAN_POINT ( 'NONE',  ( 7.753125000614518036, 0.000000000000000000, 5.243569643749999010 ) ) ;
#61525=CARTESIAN_POINT ( 'NONE',  ( 25.34062500061451573, -3.027376345333614438, 5.243569643749998122 ) ) ;
#61526=CARTESIAN_POINT ( 'NONE',  ( -2.000000000000000000, 18.12500000000000355, 26.53589838486224650 ) ) ;
#61528=CARTESIAN_POINT ( 'NONE',  ( 2.953125000614516438, -4.541064518000417216, -2.621784821875001281 ) ) ;
#61529=CARTESIAN_POINT ( 'NONE',  ( 20.14687500061451786, -3.027376345333610441, -5.243569643749999898 ) ) ;
#61530=CARTESIAN_POINT ( 'NONE',  ( 9.001249775931846008E-16, 13.67187500061451999, 34.90005215228797653 ) ) ;
#61531=CARTESIAN_POINT ( 'NONE',  ( 22.62187500061451573, 3.027376345333611329, 5.243569643749999010 ) ) ;
#61532=CARTESIAN_POINT ( 'NONE',  ( 28.95937500061451431, 0.000000000000000000, 5.243569643749999010 ) ) ;
#61533=CARTESIAN_POINT ( 'NONE',  ( -4.243569643749998122, 18.54687500061451644, 32.45002607614398471 ) ) ;
#61534=CARTESIAN_POINT ( 'NONE',  ( 10.45312500061451644, 0.000000000000000000, 5.243569643749999010 ) ) ;
#61535=DIRECTION ( 'NONE',  ( -0.000000000000000000, -0.000000000000000000, -1.000000000000000000 ) ) ;
#61536=CARTESIAN_POINT ( 'NONE',  ( 6.159375000614517148, -4.541064518000417216, -2.621784821875001281 ) ) ;
#61538=CARTESIAN_POINT ( 'NONE',  ( 7.228125000614517681, 4.541064518000418104, 2.621784821874999949 ) ) ;
#61539=CARTESIAN_POINT ( 'NONE',  ( 11.55937500061451928, -4.541064518000417216, -2.621784821875001281 ) ) ;
#61540=CARTESIAN_POINT ( 'NONE',  ( 19.08750000122903145, 6.123233995736764310E-16, -4.999999999999998224 ) ) ;
#61541=CARTESIAN_POINT ( 'NONE',  ( 7.471875000614519813, -6.054752690667223547, -1.112240025338166033E-15 ) ) ;
#61542=CARTESIAN_POINT ( 'NONE',  ( 9.478125000614515017, 4.541064518000418104, 2.621784821874999949 ) ) ;
#61545=CARTESIAN_POINT ( 'NONE',  ( 18.64687500061451786, -3.027376345333614438, 5.243569643749998122 ) ) ;
#61546=CARTESIAN_POINT ( 'NONE',  ( 1.999999999999998668, 13.21250000122903501, 26.53589838486224650 ) ) ;
#61547=CARTESIAN_POINT ( 'NONE',  ( 28.11562500061451431, -6.054752690667223547, -1.112240025338166033E-15 ) ) ;
#61548=CARTESIAN_POINT ( 'NONE',  ( 11.31562500061451892, 3.027376345333611329, 5.243569643749999010 ) ) ;
#61549=CARTESIAN_POINT ( 'NONE',  ( 28.77187500061451431, 3.027376345333612662, -5.243569643749998122 ) ) ;
#61550=CARTESIAN_POINT ( 'NONE',  ( -3.000416591977282496E-16, 12.99687500061451750, -34.90005215228797653 ) ) ;
#61551=CARTESIAN_POINT ( 'NONE',  ( 13.80000000122903181, 5.773502691896255534, 3.535250795749688894E-16 ) ) ;
#61552=CARTESIAN_POINT ( 'NONE',  ( 26.91562500061451146, 3.027376345333613106, -5.243569643749998122 ) ) ;
#61553=CARTESIAN_POINT ( 'NONE',  ( -4.243569643749997233, 15.79062500061451857, -27.54997392385601174 ) ) ;
#61554=CARTESIAN_POINT ( 'NONE',  ( 15.52500000122903323, 2.886751345948129099, -4.999999999999998224 ) ) ;
#61555=CARTESIAN_POINT ( 'NONE',  ( 12.86250000000000071, 2.886751345948126879, 4.999999999999999112 ) ) ;
#61557=CARTESIAN_POINT ( 'NONE',  ( 23.69062500061451004, -3.027376345333610441, -5.243569643749999898 ) ) ;
#61558=CARTESIAN_POINT ( 'NONE',  ( 7.134375000614516793, 6.421520780324663323E-16, -5.243569643749999010 ) ) ;
#61559=CARTESIAN_POINT ( 'NONE',  ( 9.787500001229036073, 4.330127018922191873, 2.499999999999999556 ) ) ;
#61560=CARTESIAN_POINT ( 'NONE',  ( 18.82500000122903216, 2.886751345948126879, 4.999999999999999112 ) ) ;
#61561=CARTESIAN_POINT ( 'NONE',  ( 15.92812500061451608, -4.541064518000419881, 2.621784821874995952 ) ) ;
#61562=CARTESIAN_POINT ( 'NONE',  ( 17.57812500061451644, 4.541064518000418104, 2.621784821874999949 ) ) ;
#61563=CARTESIAN_POINT ( 'NONE',  ( 26.47500000122903074, 2.886751345948126879, 4.999999999999999112 ) ) ;
#61564=CARTESIAN_POINT ( 'NONE',  ( 27.97500000122903074, -5.773502691896255534, -1.060575238724906372E-15 ) ) ;
#61565=CARTESIAN_POINT ( 'NONE',  ( 22.72499999999999787, 4.330127018922191873, 2.499999999999999556 ) ) ;
#61566=CARTESIAN_POINT ( 'NONE',  ( 25.28437500061451715, 4.541064518000418104, 2.621784821874999949 ) ) ;
#61567=CARTESIAN_POINT ( 'NONE',  ( 25.68750000122903288, -4.330127018922194537, 2.499999999999995559 ) ) ;
#61568=CARTESIAN_POINT ( 'NONE',  ( 12.90000000122903145, 5.773502691896255534, 3.535250795749688894E-16 ) ) ;
#61569=CARTESIAN_POINT ( 'NONE',  ( 27.08437500061451786, 4.541064518000418104, 2.621784821874999949 ) ) ;
#61570=B_SPLINE_CURVE_WITH_KNOTS ( 'NONE', 3,
 ( #67271, #10737, #27011, #21083, #11099, #49181, #56171, #43634, #33270, #43271, #66157, #15534, #38078, #60600, #10009, #32544, #15903, #55808, #5565, #50630, #55082, #4838, #49543, #38450, #50276, #20712, #72065, #60976, #21445, #27372, #70059, #35347, #5919, #45451, #64144, #30541, #30175, #22893, #50988, #52706, #67984, #2112, #46810, #24986, #13531, #58232 ),
 .UNSPECIFIED., .F., .F.,
 ( 4, 2, 2, 2, 2, 2, 2, 2, 2, 2, 2, 2, 2, 2, 2, 2, 2, 2, 2, 2, 2, 2, 4 ),
 ( 0.01924954336552996831, 0.02045024950336954070, 0.02105060257228932863, 0.02165095564120911656, 0.02225130871012890449, 0.02285166177904869589, 0.02405236791688826481, 0.02525307405472783373, 0.02645378019256739918, 0.02705413326148718711, 0.02765448633040697157, 0.02825483939932675603, 0.02885519246824654049, 0.03005589860608610941, 0.03125660474392567834, 0.03245731088176524726, 0.03365801701960481618, 0.03485872315744438510, 0.03545907622636416956, 0.03605942929528395402, 0.03726013543312352294, 0.03786048850204330740, 0.03846084157096309186 ),
 .UNSPECIFIED. ) ;
#61571=LINE ( 'NONE', #68852, #36123 ) ;
#61572=CARTESIAN_POINT ( 'NONE',  ( 3.946875000614517681, -3.027376345333610441, -5.243569643749999898 ) ) ;
#61573=CARTESIAN_POINT ( 'NONE',  ( 23.27812500061451573, 6.421520780324663323E-16, -5.243569643749999010 ) ) ;
#61576=CARTESIAN_POINT ( 'NONE',  ( 9.309375000614517504, -4.541064518000417216, -2.621784821875001281 ) ) ;
#61577=CARTESIAN_POINT ( 'NONE',  ( 4.528125000614516615, 4.541064518000418104, 2.621784821874999949 ) ) ;
#61578=CARTESIAN_POINT ( 'NONE',  ( 29.35312500061451502, 0.000000000000000000, 5.243569643749999010 ) ) ;
#61579=CARTESIAN_POINT ( 'NONE',  ( 7.171875000614517326, 3.027376345333613106, -5.243569643749998122 ) ) ;
#61580=CARTESIAN_POINT ( 'NONE',  ( 29.52187500061451431, -6.054752690667223547, -1.112240025338166033E-15 ) ) ;
#61581=CARTESIAN_POINT ( 'NONE',  ( 30.00000000000000000, 0.000000000000000000, 0.000000000000000000 ) ) ;
#61582=CARTESIAN_POINT ( 'NONE',  ( 19.98749999999999716, 5.773502691896255534, 3.535250795749688894E-16 ) ) ;
#61583=ORIENTED_EDGE ( 'NONE', *, *, #15786, .T. ) ;
#61584=CARTESIAN_POINT ( 'NONE',  ( 26.55000000000000071, -4.330127018922190985, -2.500000000000001332 ) ) ;
#61585=( BOUNDED_CURVE ( )  B_SPLINE_CURVE ( 2, ( #34130, #17849, #11612, #5708, #23762, #1257, #56318 ),
 .UNSPECIFIED., .F., .F. ) 
 B_SPLINE_CURVE_WITH_KNOTS ( ( 3, 2, 2, 3 ),
 ( 0.04166666666666671293, 0.04444444444444448777, 0.04722222222222225568, 0.05000000000000003053 ),
 .UNSPECIFIED. ) 
 CURVE ( )  GEOMETRIC_REPRESENTATION_ITEM ( )  RATIONAL_B_SPLINE_CURVE ( ( 0.9999999999999976685, 0.8660254037844410391, 1.000000000000000000, 0.8660254037844387076, 1.000000000000000000, 0.8660254037844373753, 1.000000000000001332 ) ) 
 REPRESENTATION_ITEM ( '' )  );
#61586=CARTESIAN_POINT ( 'NONE',  ( 27.87187500061451573, 3.027376345333613106, -5.243569643749998122 ) ) ;
#61587=EDGE_CURVE ( 'NONE', #14259, #11117, #33949, .T. ) ;
#61588=ORIENTED_EDGE ( 'NONE', *, *, #22231, .T. ) ;
#61589=VECTOR ( 'NONE', #36794, 1000.000000000000000 ) ;
#61590=CARTESIAN_POINT ( 'NONE',  ( 17.05312500061451786, 4.541064518000418104, -2.621784821874998173 ) ) ;
#61591=CARTESIAN_POINT ( 'NONE',  ( 8.765625000614518214, -6.054752690667223547, -1.112240025338166033E-15 ) ) ;
#61593=CARTESIAN_POINT ( 'NONE',  ( 3.871875000614519280, -6.054752690667223547, -1.112240025338166033E-15 ) ) ;
#61594=CARTESIAN_POINT ( 'NONE',  ( 18.48750000122903359, -4.330127018922194537, 2.499999999999995559 ) ) ;
#61595=CARTESIAN_POINT ( 'NONE',  ( 24.22500000000000142, -4.330127018922194537, 2.499999999999995559 ) ) ;
#61596=CARTESIAN_POINT ( 'NONE',  ( 3.242103837493086330E-14, 11.00000000122903288, 26.00000000000000711 ) ) ;
#61597=CARTESIAN_POINT ( 'NONE',  ( 8.109375000614518214, 4.541064518000418104, -2.621784821874998173 ) ) ;
#61598=CARTESIAN_POINT ( 'NONE',  ( 11.70937500061451608, 4.541064518000418104, -2.621784821874998173 ) ) ;
#61599=CARTESIAN_POINT ( 'NONE',  ( 22.88437500061451857, 6.421520780324663323E-16, -5.243569643749999010 ) ) ;
#61600=CARTESIAN_POINT ( 'NONE',  ( -1.487416814333745711E-14, 15.72500000122903430, -26.00000000000000000 ) ) ;
#61601=ORIENTED_EDGE ( 'NONE', *, *, #38095, .T. ) ;
#61602=CARTESIAN_POINT ( 'NONE',  ( 3.646875000614520079, 6.054752690667223547, 3.707466751127219781E-16 ) ) ;
#61604=CARTESIAN_POINT ( 'NONE',  ( 7.846875000614518036, -3.027376345333614438, 5.243569643749998122 ) ) ;
#61606=CARTESIAN_POINT ( 'NONE',  ( 21.93750000000000000, -2.886751345948129988, 4.999999999999997335 ) ) ;
#61607=CARTESIAN_POINT ( 'NONE',  ( 16.00312500061451715, -4.541064518000417216, -2.621784821875001281 ) ) ;
#61609=CARTESIAN_POINT ( 'NONE',  ( 4.311958327294343363, 2.531208285321026263, 4.311958327294242999 ) ) ;
#61611=CARTESIAN_POINT ( 'NONE',  ( 10.82812500061451644, 4.541064518000418104, 2.621784821874999949 ) ) ;
#61612=CARTESIAN_POINT ( 'NONE',  ( 29.18437500061451573, 6.421520780324663323E-16, -5.243569643749999010 ) ) ;
#61613=CARTESIAN_POINT ( 'NONE',  ( 29.40937500061451715, 0.000000000000000000, 5.243569643749999010 ) ) ;
#61614=CARTESIAN_POINT ( 'NONE',  ( 10.76250000000000107, -5.773502691896255534, -1.060575238724906372E-15 ) ) ;
#61615=CARTESIAN_POINT ( 'NONE',  ( -1.999999999999997113, 14.78750000122903252, 33.46410161513775705 ) ) ;
#61616=CARTESIAN_POINT ( 'NONE',  ( 9.900000001229033231, -2.886751345948129988, 4.999999999999997335 ) ) ;
#61617=CARTESIAN_POINT ( 'NONE',  ( 20.37187500061451573, 3.027376345333611329, 5.243569643749999010 ) ) ;
#61618=CARTESIAN_POINT ( 'NONE',  ( 15.30937500061451750, 4.541064518000418104, -2.621784821874998173 ) ) ;
#61619=ORIENTED_EDGE ( 'NONE', *, *, #66024, .F. ) ;
#61620=CARTESIAN_POINT ( 'NONE',  ( 14.61562500061451608, -6.054752690667223547, -1.112240025338166033E-15 ) ) ;
#61621=CARTESIAN_POINT ( 'NONE',  ( 26.62500000122903288, -5.773502691896255534, -1.060575238724906372E-15 ) ) ;
#61622=CARTESIAN_POINT ( 'NONE',  ( 14.63437500061451679, -4.541064518000419881, 2.621784821874995952 ) ) ;
#61623=CARTESIAN_POINT ( 'NONE',  ( 5.989600911063007516, 8.007829439449656306, -29.59314995572118434 ) ) ;
#61624=CARTESIAN_POINT ( 'NONE',  ( 16.07812500061451289, 6.421520780324663323E-16, -5.243569643749999010 ) ) ;
#61625=CARTESIAN_POINT ( 'NONE',  ( -3.137519842735245283E-14, 14.37500000122903288, -26.00000000000000711 ) ) ;
#61626=CARTESIAN_POINT ( 'NONE',  ( 27.45937500061451786, 4.541064518000418104, -2.621784821874998173 ) ) ;
#61627=CARTESIAN_POINT ( 'NONE',  ( 2.121784821875001281, 10.50312500061451715, 33.67503911421598417 ) ) ;
#61628=CARTESIAN_POINT ( 'NONE',  ( 16.09687500061452070, -3.027376345333610441, -5.243569643749999898 ) ) ;
#61629=CARTESIAN_POINT ( 'NONE',  ( 14.88750000122903394, -4.330127018922194537, 2.499999999999995559 ) ) ;
#61630=FACE_OUTER_BOUND ( 'NONE', #18438, .T. ) ;
#61631=CARTESIAN_POINT ( 'NONE',  ( 2.121784821874999061, 18.80937500061451928, -33.67503911421598417 ) ) ;
#61632=CARTESIAN_POINT ( 'NONE',  ( 19.39687500061451786, 6.054752690667223547, 3.707466751127219781E-16 ) ) ;
#61633=CARTESIAN_POINT ( 'NONE',  ( 18.90000000122902790, -2.886751345948129988, 4.999999999999997335 ) ) ;
#61634=CARTESIAN_POINT ( 'NONE',  ( 17.25937500061451502, 0.000000000000000000, 5.243569643749999010 ) ) ;
#61635=CARTESIAN_POINT ( 'NONE',  ( 2.121784821875001281, 13.25937500061451857, 33.67503911421598417 ) ) ;
#61636=CARTESIAN_POINT ( 'NONE',  ( 16.94062500061451715, -3.027376345333610441, -5.243569643749999898 ) ) ;
#61637=ORIENTED_EDGE ( 'NONE', *, *, #53941, .T. ) ;
#61638=ORIENTED_EDGE ( 'NONE', *, *, #31768, .F. ) ;
#61639=CARTESIAN_POINT ( 'NONE',  ( 19.94999999999999929, 4.330127018922192761, -2.499999999999997780 ) ) ;
#61641=CARTESIAN_POINT ( 'NONE',  ( 23.35312500061451857, 4.541064518000418104, -2.621784821874998173 ) ) ;
#61642=CARTESIAN_POINT ( 'NONE',  ( 3.215625000614518836, 3.027376345333611329, 5.243569643749999010 ) ) ;
#61643=CARTESIAN_POINT ( 'NONE',  ( 17.36250000122903359, 4.330127018922192761, -2.499999999999997780 ) ) ;
#61644=CARTESIAN_POINT ( 'NONE',  ( 22.37812500061451360, 6.421520780324663323E-16, -5.243569643749999010 ) ) ;
#61645=CARTESIAN_POINT ( 'NONE',  ( 25.97812500061451502, 6.421520780324663323E-16, -5.243569643749999010 ) ) ;
#61646=CARTESIAN_POINT ( 'NONE',  ( 5.240625000614516971, -3.027376345333610441, -5.243569643749999898 ) ) ;
#61648=EDGE_CURVE ( 'NONE', #19531, #30832, #62034, .T. ) ;
#61651=CARTESIAN_POINT ( 'NONE',  ( 3.215625000614518836, 3.027376345333611329, 5.243569643749999010 ) ) ;
#61652=EDGE_CURVE ( 'NONE', #18641, #36195, #10203, .T. ) ;
#61655=CARTESIAN_POINT ( 'NONE',  ( -3.999999999999999112, 12.46250000122903323, -30.00000000000000000 ) ) ;
#61656=CARTESIAN_POINT ( 'NONE',  ( -4.243569643749999898, 18.95937500061451431, -30.00000000000000000 ) ) ;
#61657=CARTESIAN_POINT ( 'NONE',  ( 9.074999999999999289, 6.123233995736764310E-16, -4.999999999999998224 ) ) ;
#61658=ADVANCED_FACE ( 'NONE', ( #44698 ), #68238, .T. ) ;
#61659=CARTESIAN_POINT ( 'NONE',  ( 3.562500001229033764, 0.000000000000000000, 4.999999999999998224 ) ) ;
#61660=CARTESIAN_POINT ( 'NONE',  ( 11.93437500061451573, -4.541064518000419881, 2.621784821874995952 ) ) ;
#61661=CARTESIAN_POINT ( 'NONE',  ( 1.592000809091587073E-14, 16.85000000122903785, -34.00000000000000000 ) ) ;
#61662=CARTESIAN_POINT ( 'NONE',  ( 3.646875000614520079, 6.054752690667223547, 3.707466751127219781E-16 ) ) ;
#61663=DIRECTION ( 'NONE',  ( -1.000000000000000000, -0.000000000000000000, -0.000000000000000000 ) ) ;
#61666=CARTESIAN_POINT ( 'NONE',  ( 9.984375000614518214, 4.541064518000418104, 2.621784821874999949 ) ) ;
#61667=CARTESIAN_POINT ( 'NONE',  ( 3.562500000000000444, -5.773502691896255534, -1.060575238724906372E-15 ) ) ;
#61668=CARTESIAN_POINT ( 'NONE',  ( 19.52812500061451573, -4.541064518000419881, 2.621784821874995952 ) ) ;
#61670=CARTESIAN_POINT ( 'NONE',  ( -4.243569643749998122, 18.04062500061459673, 32.45002607614398471 ) ) ;
#61671=CARTESIAN_POINT ( 'NONE',  ( 23.55937500061451573, 0.000000000000000000, 5.243569643749999010 ) ) ;
#61672=CARTESIAN_POINT ( 'NONE',  ( 1.626862140677534273E-15, 15.27500000122903501, -26.00000000000000355 ) ) ;
#61673=CARTESIAN_POINT ( 'NONE',  ( 29.13750000122903216, 4.330127018922191873, 2.499999999999999556 ) ) ;
#61675=CARTESIAN_POINT ( 'NONE',  ( 24.02812500061451573, -4.541064518000419881, 2.621784821874995952 ) ) ;
#61676=CARTESIAN_POINT ( 'NONE',  ( 14.50312500061451537, 0.000000000000000000, 5.243569643749999010 ) ) ;
#61678=CARTESIAN_POINT ( 'NONE',  ( 12.94687500061451857, -3.027376345333610441, -5.243569643749999898 ) ) ;
#61679=CARTESIAN_POINT ( 'NONE',  ( 28.87499999999999645, 6.123233995736764310E-16, -4.999999999999998224 ) ) ;
#61680=CARTESIAN_POINT ( 'NONE',  ( 23.88750000122903216, -4.330127018922194537, 2.499999999999995559 ) ) ;
#61681=CARTESIAN_POINT ( 'NONE',  ( 4.246875000614519280, -3.027376345333614438, 5.243569643749998122 ) ) ;
#61682=CARTESIAN_POINT ( 'NONE',  ( 14.82187500061451679, 3.027376345333613106, -5.243569643749998122 ) ) ;
#61684=CARTESIAN_POINT ( 'NONE',  ( -1.999999999999997113, 11.52500000000000036, 33.46410161513775705 ) ) ;
#61686=CARTESIAN_POINT ( 'NONE',  ( 24.23437500061451644, 6.421520780324663323E-16, -5.243569643749999010 ) ) ;
#61687=CARTESIAN_POINT ( 'NONE',  ( 14.03437500061451715, 4.541064518000418104, 2.621784821874999949 ) ) ;
#61689=CARTESIAN_POINT ( 'NONE',  ( 27.97500000000000142, 6.123233995736764310E-16, -4.999999999999998224 ) ) ;
#61690=CARTESIAN_POINT ( 'NONE',  ( 3.562500001229033764, 0.000000000000000000, 4.999999999999998224 ) ) ;
#61691=CARTESIAN_POINT ( 'NONE',  ( 6.600000000000001421, 0.000000000000000000, 4.999999999999998224 ) ) ;
#61693=CARTESIAN_POINT ( 'NONE',  ( 19.11562500061451431, -6.054752690667223547, -1.112240025338166033E-15 ) ) ;
#61694=CARTESIAN_POINT ( 'NONE',  ( 8.512499999999999289, -5.773502691896255534, -1.060575238724906372E-15 ) ) ;
#61695=CARTESIAN_POINT ( 'NONE',  ( -3.999999999999999112, 14.15000000000000036, 30.00000000000000000 ) ) ;
#61696=CARTESIAN_POINT ( 'NONE',  ( 16.64999999999999858, -4.330127018922190985, -2.500000000000001332 ) ) ;
#61697=CARTESIAN_POINT ( 'NONE',  ( -2.121784821874996840, 12.67812500061451786, 33.67503911421598417 ) ) ;
#61699=CARTESIAN_POINT ( 'NONE',  ( 19.95000000122903572, -2.886751345948125991, -5.000000000000000000 ) ) ;
#61701=CARTESIAN_POINT ( 'NONE',  ( 27.12187500061451573, 3.027376345333611329, 5.243569643749999010 ) ) ;
#61703=CARTESIAN_POINT ( 'NONE',  ( 15.92812500061451608, -4.541064518000419881, 2.621784821874995952 ) ) ;
#61704=CARTESIAN_POINT ( 'NONE',  ( 22.00312500061451360, 4.541064518000418104, -2.621784821874998173 ) ) ;
#61705=CARTESIAN_POINT ( 'NONE',  ( 22.13437500061451502, 4.541064518000418104, 2.621784821874999949 ) ) ;
#61706=CARTESIAN_POINT ( 'NONE',  ( 6.600000000000001421, 0.000000000000000000, 4.999999999999998224 ) ) ;
#61707=CARTESIAN_POINT ( 'NONE',  ( 10.11562500061451608, -6.054752690667223547, -1.112240025338166033E-15 ) ) ;
#61708=CARTESIAN_POINT ( 'NONE',  ( 24.89062500061451644, -3.027376345333614438, 5.243569643749998122 ) ) ;
#61709=CARTESIAN_POINT ( 'NONE',  ( 15.12187500061451750, -6.054752690667223547, -1.112240025338166033E-15 ) ) ;
#61710=CARTESIAN_POINT ( 'NONE',  ( 18.42187500061451644, 3.027376345333613106, -5.243569643749998122 ) ) ;
#61711=CARTESIAN_POINT ( 'NONE',  ( 19.27500000000000213, -4.330127018922194537, 2.499999999999995559 ) ) ;
#61712=CARTESIAN_POINT ( 'NONE',  ( 4.243569643749999010, 17.81562500061451715, 27.54997392385601174 ) ) ;
#61713=CARTESIAN_POINT ( 'NONE',  ( 21.15000000122903145, -2.886751345948129988, 4.999999999999997335 ) ) ;
#61715=CARTESIAN_POINT ( 'NONE',  ( 12.32812500061451821, -4.541064518000419881, 2.621784821874995952 ) ) ;
#61716=CARTESIAN_POINT ( 'NONE',  ( 5.521875000614517859, 3.027376345333611329, 5.243569643749999010 ) ) ;
#61717=CARTESIAN_POINT ( 'NONE',  ( 4.321875000614517681, -6.054752690667223547, -1.112240025338166033E-15 ) ) ;
#61718=ORIENTED_EDGE ( 'NONE', *, *, #41944, .F. ) ;
#61719=CARTESIAN_POINT ( 'NONE',  ( 27.08437500061451786, 4.541064518000418104, 2.621784821874999949 ) ) ;
#61720=CARTESIAN_POINT ( 'NONE',  ( 18.21562500061451573, -6.054752690667223547, -1.112240025338166033E-15 ) ) ;
#61721=CARTESIAN_POINT ( 'NONE',  ( 27.90000000122903145, -2.886751345948129988, 4.999999999999997335 ) ) ;
#61722=CARTESIAN_POINT ( 'NONE',  ( 27.10312500061451502, 0.000000000000000000, 5.243569643749999010 ) ) ;
#61723=CARTESIAN_POINT ( 'NONE',  ( 25.24687500061451573, 6.054752690667223547, 3.707466751127219781E-16 ) ) ;
#61724=CARTESIAN_POINT ( 'NONE',  ( 20.31562500061451715, 3.027376345333611329, 5.243569643749999010 ) ) ;
#61725=CARTESIAN_POINT ( 'NONE',  ( 2.121784821874999061, 18.35937500061451644, 26.32496088578401583 ) ) ;
#61726=CARTESIAN_POINT ( 'NONE',  ( 25.11562500061451431, 3.027376345333613106, -5.243569643749998122 ) ) ;
#61727=CARTESIAN_POINT ( 'NONE',  ( 4.500000001229034652, -2.886751345948129988, 4.999999999999997335 ) ) ;
#61728=ORIENTED_EDGE ( 'NONE', *, *, #69660, .F. ) ;
#61729=CARTESIAN_POINT ( 'NONE',  ( 26.88749999999999574, -2.886751345948129988, 4.999999999999997335 ) ) ;
#61730=CARTESIAN_POINT ( 'NONE',  ( -1.999999999999997113, 14.67500000000000071, -26.53589838486224295 ) ) ;
#61732=CARTESIAN_POINT ( 'NONE',  ( 4.771875000614516971, -6.054752690667223547, -1.112240025338166033E-15 ) ) ;
#61733=CARTESIAN_POINT ( 'NONE',  ( 13.79062500061451502, -3.027376345333610441, -5.243569643749999898 ) ) ;
#61734=CARTESIAN_POINT ( 'NONE',  ( 6.721875000614518925, 3.027376345333613106, -5.243569643749998122 ) ) ;
#61735=CARTESIAN_POINT ( 'NONE',  ( 24.78750000122903074, -4.330127018922194537, 2.499999999999995559 ) ) ;
#61736=CARTESIAN_POINT ( 'NONE',  ( 15.12187500061451928, -6.054752690667223547, -1.112240025338166033E-15 ) ) ;
#61737=CARTESIAN_POINT ( 'NONE',  ( 3.421875000614516882, -6.054752690667223547, -1.112240025338166033E-15 ) ) ;
#61738=CARTESIAN_POINT ( 'NONE',  ( 27.93750000000000000, -2.886751345948125991, -5.000000000000000000 ) ) ;
#61739=CARTESIAN_POINT ( 'NONE',  ( 26.33437500061451431, -4.541064518000419881, 2.621784821874995952 ) ) ;
#61740=CARTESIAN_POINT ( 'NONE',  ( 3.140625000614516882, 6.054752690667223547, 3.707466751127219781E-16 ) ) ;
#61741=CARTESIAN_POINT ( 'NONE',  ( 13.90312500061451750, 4.541064518000418104, -2.621784821874998173 ) ) ;
#61743=CARTESIAN_POINT ( 'NONE',  ( 9.215625000614515727, -6.054752690667223547, -1.112240025338166033E-15 ) ) ;
#61744=CARTESIAN_POINT ( 'NONE',  ( 6.365625000614518747, 3.027376345333611329, 5.243569643749999010 ) ) ;
#61746=CARTESIAN_POINT ( 'NONE',  ( -0.7368805616696194605, 9.859898480082234684, 25.82089837893477480 ) ) ;
#61747=CARTESIAN_POINT ( 'NONE',  ( 15.03749999999999964, 5.773502691896255534, 3.535250795749688894E-16 ) ) ;
#61749=EDGE_CURVE ( 'NONE', #29431, #25241, #32415, .T. ) ;
#61750=CARTESIAN_POINT ( 'NONE',  ( 14.97187500061451892, 3.027376345333611329, 5.243569643749999010 ) ) ;
#61751=CARTESIAN_POINT ( 'NONE',  ( 12.56250000122903465, 0.000000000000000000, 4.999999999999998224 ) ) ;
#61753=CARTESIAN_POINT ( 'NONE',  ( 21.83437500061451786, -4.541064518000419881, 2.621784821874995952 ) ) ;
#61754=CARTESIAN_POINT ( 'NONE',  ( 4.243569643749999898, 13.27812500061451750, -30.00000000000000000 ) ) ;
#61755=CARTESIAN_POINT ( 'NONE',  ( 3.065815551951259543, -3.949781639713015657, 3.065815551951216467 ) ) ;
#61757=FACE_OUTER_BOUND ( 'NONE', #64025, .T. ) ;
#61758=CARTESIAN_POINT ( 'NONE',  ( 25.75312500061451715, 0.000000000000000000, 5.243569643749999010 ) ) ;
#61761=CARTESIAN_POINT ( 'NONE',  ( 25.53750000000000142, -2.886751345948129988, 4.999999999999997335 ) ) ;
#61762=CARTESIAN_POINT ( 'NONE',  ( 8.803125000614517859, -4.541064518000417216, -2.621784821875001281 ) ) ;
#61764=CARTESIAN_POINT ( 'NONE',  ( 20.52187500061451786, -6.054752690667223547, -1.112240025338166033E-15 ) ) ;
#61766=CARTESIAN_POINT ( 'NONE',  ( 5.653125000614517504, -4.541064518000417216, -2.621784821875001281 ) ) ;
#61767=CARTESIAN_POINT ( 'NONE',  ( 10.39687500061451786, 6.054752690667223547, 3.707466751127219781E-16 ) ) ;
#61768=ORIENTED_EDGE ( 'NONE', *, *, #53711, .T. ) ;
#61769=CARTESIAN_POINT ( 'NONE',  ( 20.59687500061451360, -3.027376345333610441, -5.243569643749999898 ) ) ;
#61770=CARTESIAN_POINT ( 'NONE',  ( 0.000000000000000000, 20.00000000000000000, 30.00000000000000000 ) ) ;
#61771=CARTESIAN_POINT ( 'NONE',  ( 29.43750000000000000, 5.773502691896255534, 3.535250795749688894E-16 ) ) ;
#61772=CARTESIAN_POINT ( 'NONE',  ( 6.075000000000000178, 4.330127018922191873, 2.499999999999999556 ) ) ;
#61773=ADVANCED_FACE ( 'NONE', ( #11250 ), #56316, .F. ) ;
#61774=CARTESIAN_POINT ( 'NONE',  ( 15.56250000122903465, 4.330127018922192761, -2.499999999999997780 ) ) ;
#61777=CARTESIAN_POINT ( 'NONE',  ( 12.33750000000000036, 5.773502691896255534, 3.535250795749688894E-16 ) ) ;
#61778=CARTESIAN_POINT ( 'NONE',  ( 25.94062500061451715, -3.027376345333610441, -5.243569643749999898 ) ) ;
#61779=CARTESIAN_POINT ( 'NONE',  ( 17.36249999999999716, 2.886751345948126879, 4.999999999999999112 ) ) ;
#61780=CARTESIAN_POINT ( 'NONE',  ( 11.62500000122903465, 2.886751345948126879, 4.999999999999999112 ) ) ;
#61781=CARTESIAN_POINT ( 'NONE',  ( 9.853125000614516793, 4.541064518000418104, -2.621784821874998173 ) ) ;
#61782=CARTESIAN_POINT ( 'NONE',  ( 7.912499999999999645, 2.886751345948126879, 4.999999999999999112 ) ) ;
#61783=DIRECTION ( 'NONE',  ( 0.000000000000000000, 0.000000000000000000, 1.000000000000000000 ) ) ;
#61784=CARTESIAN_POINT ( 'NONE',  ( -2.121784821874996840, 15.43437500061451928, -26.32496088578401583 ) ) ;
#61785=CARTESIAN_POINT ( 'NONE',  ( 27.60000000122903430, -2.886751345948125991, -5.000000000000000000 ) ) ;
#61787=CARTESIAN_POINT ( 'NONE',  ( 7.387500000000001066, 5.773502691896255534, 3.535250795749688894E-16 ) ) ;
#61788=CARTESIAN_POINT ( 'NONE',  ( -5.810221930991193690E-16, 12.68750000000000000, 26.00000000000000355 ) ) ;
#61789=VERTEX_POINT ( 'NONE', #45232 ) ;
#61790=CARTESIAN_POINT ( 'NONE',  ( 24.51562500061451289, -6.054752690667223547, -1.112240025338166033E-15 ) ) ;
#61791=CARTESIAN_POINT ( 'NONE',  ( 29.80312500061451431, 0.000000000000000000, 5.243569643749999010 ) ) ;
#61792=CARTESIAN_POINT ( 'NONE',  ( 28.77187500061451431, 3.027376345333613106, -5.243569643749998122 ) ) ;
#61793=CARTESIAN_POINT ( 'NONE',  ( 19.84687500061451360, 6.054752690667223547, 3.707466751127219781E-16 ) ) ;
#61794=CARTESIAN_POINT ( 'NONE',  ( 17.69062500061451715, -3.027376345333614438, 5.243569643749998122 ) ) ;
#61795=ADVANCED_FACE ( 'NONE', ( #67764 ), #6064, .F. ) ;
#61796=CARTESIAN_POINT ( 'NONE',  ( 4.243569643749999898, 11.44062500061459353, -27.54997392385601529 ) ) ;
#61797=CARTESIAN_POINT ( 'NONE',  ( 6.253125000614517148, 4.541064518000418104, -2.621784821874998173 ) ) ;
#61798=( BOUNDED_SURFACE ( )  B_SPLINE_SURFACE ( 1, 2, ( 
 ( #6719, #44808, #33699, #62142, #56246, #22254, #67341, #39259, #16701, #61413, #824, #5637, #29252, #72500, #33342, #61771, #57315, #51423, #22609, #11536, #6352, #16340, #28522, #28174, #23332, #11175, #22966, #44446, #38895, #27813, #50347, #45882, #34056, #45527, #21888, #68414, #72871, #10807, #50701, #55880, #56596, #17776, #103, #68057, #45161, #67692, #5992, #40335, #12251, #39985, #62497, #11895, #62857, #34420, #56948, #34782, #28883, #41070, #7438, #52144, #52867, #63584, #35866, #35150, #13327, #8529, #46603, #1547, #7802, #2266, #30339, #58389, #47684, #18136, #1184, #24781, #57673, #69146, #52505, #69505, #12616, #29608, #7079, #47325, #35509, #63942, #18865, #24420, #36241, #12971, #30694, #42150, #64677, #69858, #41426, #24057, #1916, #18505, #58755, #25143, #58028, #46969, #46240, #8165, #23692, #29964, #19225, #41779, #53225, #64308, #13698, #51784, #59122, #2622, #70220, #19594, #14062, #36601, #68780, #40703, #63221, #19963, #33516, #14795, #61962, #31058, #65040, #20328, #16887, #10996, #54338, #71322, #38062, #25518, #60218, #37338, #56066, #48431, #32164, #2990, #70588, #59488, #25891, #5458, #70956, #59861, #42882, #20697, #65405, #9265, #53972, #48063, #73055, #48793, #61595, #27998, #50527, #31800, #43255, #49166, #4101, #31432, #3732, #22437, #54697, #26257, #3370, #44985, #42516, #67522, #36966, #26629, #53595, #14431, #8900, #65776, #15158, #37695, #9630, #71697, #21069, #39441, #43620, #66142, #15520, #22793, #68969, #29795, #45346, #62688, #18326, #45712, #69332, #33883, #18690, #62328, #285, #28348, #56428, #46795, #67880, #17252, #39812, #5817, #17609, #12444, #57135, #35334, #1373, #68605, #11724, #50885, #34240, #56774, #6179, #28708, #40169, #51247, #1014, #23883, #650, #41254, #63043, #12084, #68246, #11365, #23158, #34605, #6544, #23520, #7266, #29078, #51613, #1733, #46070, #17966, #40899, #46430, #63412, #40527, #29437, #52331, #34975, #57504, #24247, #6906, #51974, #12798, #57857, #30158, #69687, #8718, #3187, #53423, #13890, #9088, #35696, #65227, #2097, #36430, #59307, #2813, #24608, #13154, #64129, #58216, #25714, #31250, #7621, #20151, #19791, #14616, #70775, #53792, #48252, #31625, #19052, #52691, #54159, #37155, #41610, #42705, #58583, #47515, #36063, #13515, #47155, #7990, #30526, #26077, #53053, #2447, #24970, #70044, #19417, #64865, #58944, #59681, #3555, #47887, #41977, #64498, #8352, #30881, #25341, #70415, #42342, #14253, #36792, #48616, #71141, #20514, #63766, #43808, #26818, #50448, #37524, #5375, #26446, #32720, #38997, #71516, #37888, #33436, #60407, #55257, #72610, #33079, #21992, #49352, #61155, #61512, #48986, #16083, #10910, #60045, #15347, #71882, #27547, #9456, #20891, #10550, #55617, #4653, #66333, #55981, #14986, #44550, #54520, #15711, #38631, #27182, #3923, #65598, #43445, #31986, #5013, #50079, #65967, #67081, #72244, #16440, #27913, #72973, #43072, #9816, #32348, #54886, #4293, #21255, #38249, #60778, #10185, #49716, #21621, #44179, #66709, #40441, #68520, #22711, #11644, #1285, #45984, #28627, #45264, #23795, #61877, #46346, #28272, #17881, #44907, #11284, #56348, #17170, #16806, #67796, #39730, #68164, #62957, #68880, #35250, #33805, #23438, #5738, #6820, #40810, #50803, #568, #29354, #56696, #7181, #67444, #29709, #51165, #62247, #18237, #206, #63326, #34159, #12352, #39362, #6096, #23074, #45631, #17527, #40089, #62603, #11999, #34887, #12714, #57771, #34522, #57416, #57052, #51887, #52247, #6458, #28993, #22355, #51530, #930, #8631, #46711, #7536, #47069, #64776, #31160, #7902, #36344, #31535, #9003, #69604, #35973, #19329, #58493, #24525, #18965, #41525, #64044, #63681, #3095, #30440, #1650, #24158, #35610, #13423, #59590, #53702, #24883, #41884, #25624, #69246, #30799, #52969, #48161, #2365, #2730, #18607, #41172, #30069, #47428, #70686, #69959, #64412, #13805, #58859, #8269, #53332, #25245, #13071, #42617, #47794, #20061, #65141, #14532, #52608, #2014, #37066, #70324, #19700, #58130, #42253, #14167, #36701, #59223, #10822, #15622, #27462, #9730, #27097, #26731, #43358, #3471, #21906, #66993, #3836, #21168, #37440, #44462, #42981, #49629, #16355, #38910, #65881, #32264, #54437, #55171, #15262, #38164, #59961, #60687, #54075, #48896, #26357, #10102, #4567, #32631, #72156, #49993, #20432, #25991, #71426, #72517, #20803, #60320, #37800, #43721, #54796, #4203, #49266, #48530, #61429, #71799, #10463, #61066, #71057, #9368, #31900, #4927, #21535, #44090, #65512, #32993, #66244, #14899, #66617, #15993, #38542, #55533, #62159, #6368, #6007, #22626, #55895, #1202, #46258, #56263, #474, #16720, #23707, #22270, #28900, #68797, #18153, #45177, #11556, #33718, #34436, #67708, #17442, #39275, #68073, #63237, #28189, #5654, #62513, #56964, #11911, #39999, #29269, #72889, #5284, #51439, #61787, #50718, #34072, #51077, #67357, #11191, #121, #841, #17080, #45544, #22982, #28542, #17793, #39641, #12268, #40720, #33357, #23350, #45899, #56612, #68430, #40353, #62872, #34798, #57331, #6735, #27830, #51799, #50362, #44822, #58046, #2640, #42167, #18879, #47341, #42530, #19977, #7454, #46985, #30354, #69521, #35525, #29981, #52522, #1931, #1564, #14077, #41442, #12631, #35166, #46619, #24436, #70604, #64693, #35881, #52883, #19610, #7095, #41795, #63960, #36617, #13344, #13716, #57690, #52161, #41087, #25159, #53242, #29624, #59138, #64323, #8547, #31074, #47700, #70237, #53614, #18522, #24074, #3005, #25534, #63599, #48076, #58406, #7819, #2281, #24798, #69875, #30709, #58772, #12989, #19240, #69163, #36257, #8181, #65421, #44002, #31447, #66524, #70971, #60601, #14447, #53988, #25907, #59876, #59503, #14810, #37354, #37712, #10010, #15904, #4839, #3386, #66159, #48447, #49544, #10377, #32545, #27012 ),
 ( #42897, #36981, #8916, #9281, #31815, #20346, #20713, #54354, #54714, #55083, #3748, #21813, #43635, #65793, #48809, #72429, #26272, #27373, #71339, #4117, #60978, #43272, #15174, #55446, #60233, #26645, #21446, #4483, #38451, #9647, #72066, #32909, #32181, #38079, #49905, #49182, #71712, #21084, #65056, #15535, #50277, #62430, #56879, #33990, #67625, #62790, #16271, #45812, #55810, #16991, #39916, #56527, #5197, #66903, #44738, #38827, #17359, #67272, #33628, #23262, #67985, #50632, #16631, #68348, #10738, #17709, #72801, #11828, #61342, #33271, #27738, #39186, #22184, #61701, #11100, #39549, #34346, #40269, #57240, #56172, #45453, #5566, #28813, #12183, #6283, #51351, #28103, #36, #29182, #22542, #51715, #45090, #62073, #11467, #5920, #6653, #28454, #50989, #387, #22894, #753, #34710, #1117, #44377, #13627, #7732, #1481, #46172, #18071, #69076, #18436, #29540, #52439, #41002, #13261, #36170, #68711, #53526, #2200, #24352, #7369, #30993, #40632, #59053, #7009, #35799, #19528, #52076, #63517, #13994, #12904, #58321, #53159, #58688, #2557, #29900, #41712, #42086, #23987, #69792, #64608, #63151, #35437, #1845, #8099, #12546, #46534, #64238, #30627, #30266, #46900, #36533, #35080, #25075, #57606, #69439, #19158, #52799, #57961, #18796, #41360, #63870, #47618, #70150, #24715, #8458, #47258, #23626, #9922, #66072, #15450, #43917, #8827, #64973, #66443, #26930, #31363, #37995, #70887, #59789, #48361, #54268, #65706, #20998, #25824, #48725, #43550, #4401, #15819, #42451, #4031, #14364, #60517, #21363, #32461, #54995, #36899, #59419, #60889, #25451, #10294, #53904, #3297, #19898, #47995, #38363, #20260, #42812, #65335, #70523, #9195, #26556, #71248, #49455, #71989, #60151, #14725, #37267, #31730, #3662, #26185, #20627, #43186, #15092, #37628, #32825, #9561, #2921, #54625, #32094, #49096, #71625, #49823, #17630, #38741, #45008, #51269, #10655, #50191, #45733, #72716, #67544, #11745, #45366, #34262, #39100, #305, #672, #61261, #28370, #23179, #72347, #27652, #61617, #39835, #21728, #33185, #22815, #67902, #16907, #5482, #68268, #27289, #56795, #66817, #28021, #50907, #39462, #16190, #4756, #55724, #44288, #17273, #62349, #5118, #6201, #11385, #28728, #40190, #62711, #12105, #55363, #22099, #44657, #67187, #16548, #11019, #33540, #56091, #50549, #73077, #22458, #61984, #33904, #56448, #5838, #23906, #14547, #58242, #40924, #34999, #37083, #1036, #59607, #40550, #31176, #57157, #23543, #68629, #29460, #29100, #57529, #13181, #18351, #46821, #1758, #7291, #20077, #68992, #9021, #26007, #48546, #35720, #24272, #6929, #57881, #63067, #53719, #17991, #25640, #29820, #51635, #42633, #6569, #12470, #51996, #48178, #65157, #63437, #69358, #65529, #42998, #1397, #12823, #52355, #35357, #46454, #18716, #41280, #63791, #46093, #31552, #8647, #34628, #3111, #70702, #54091, #20448, #3489, #71073, #55187, #21922, #9385, #44106, #21185, #38925, #32280, #16010, #59976, #54453, #43374, #9746, #61444, #54814, #43736, #4220, #4582, #26748, #71814, #37817, #31917, #55909, #32646, #44478, #67009, #10838, #20819, #65898, #33373, #49645, #66632, #72903, #16370, #15278, #3852, #60337, #44837, #72172, #5301, #66260, #61081, #60703, #49281, #37457, #27847, #50378, #15638, #27112, #71444, #22285, #26374, #10479, #14915, #48913, #38179, #10116, #21551, #38558, #33008, #55547, #4943, #27477, #50009, #72534, #67724, #23364, #68444, #45912, #857, #63251, #33734, #16735, #17806, #50734, #11573, #68090, #11926, #28205, #45192, #136, #39290, #29637, #22642, #17097, #56280, #61804, #490, #40367, #40015, #18166, #57343, #51454, #39657, #11207, #5669, #62176, #34088, #56629, #22999, #6023, #56979, #6749, #28558, #24086, #62885, #17457, #51093, #1577, #45559, #52175, #62529, #6383, #12643, #34451, #28916, #57703, #12280, #34813, #23721, #29282, #46271, #51812, #1215, #35179, #68810, #40735, #7108, #67372, #18892, #30369, #31089, #13001, #52534, #64707, #59153, #36273, #69889, #65072, #18536, #48094, #58058, #19254, #42182, #58787, #7467, #69175, #46998, #41100, #8561, #14091, #63610, #3020, #2656, #70618, #53628, #36631, #25551, #14463, #1943, #35538, #36996, #19992, #24449, #42545, #41454, #52898, #63972, #24811, #8197, #59519, #19626, #69533, #35896, #8932, #70253, #2296, #13355, #31462, #29993, #54005, #58420, #3401, #7832, #47357, #41809, #64339, #13731, #30726, #53258, #25174, #46633, #47715, #38842, #65436, #27028, #37369, #10392, #44393, #66539, #60993, #59892, #9297, #10754, #48462, #33285, #3763, #14827, #42913, #20729, #16287, #43288, #15550, #55462, #15919, #4854, #9663, #44017, #21828, #31830, #72080, #66918, #20362, #71355, #32196, #32924, #54368, #26287, #38467, #27388, #38093, #49196, #61357, #70986, #49920, #48824, #71729, #21463, #60616, #65808, #15190, #37728, #60248, #72444, #55824, #54729, #25922, #55099, #4132, #26662, #21099, #43650, #66174, #10025, #32561, #4499, #49559, #11115, #17722, #51, #62088, #50647, #56541, #67999, #23275, #51365, #5581, #67640, #57253, #28826, #11481, #28118, #6667, #44753, #29195, #33644, #767, #27753, #67287, #39202, #22556, #72816, #45104, #17006, #51003, #45825, #51729, #18084, #16646, #6297, #61716, #62803, #23639, #68361, #40282, #56188, #39563, #63164, #50293, #12559, #34004, #5934, #22199, #28468, #40645, #401, #22909, #45467, #17372, #39929, #12196, #62443, #1130, #34723, #11841, #34360, #56892, #46185, #68724, #35094, #5212, #69451, #57974, #7744, #13640, #7022, #8472, #47271, #41372, #24365, #59067, #52089, #14009, #69089, #30280, #19542, #41015, #36548, #69805, #52813, #35450, #63882, #63530, #64252, #18450, #36184, #13273, #29553, #30640, #1494, #12917, #7381, #58702, #53172, #46912, #2213, #57619, #24000, #18808, #35811, #24728, #58333 ) ),
 .UNSPECIFIED., .F., .F., .F. ) 
 B_SPLINE_SURFACE_WITH_KNOTS ( ( 2, 2 ),
 ( 3, 2, 2, 2, 2, 2, 2, 2, 2, 2, 2, 2, 2, 2, 2, 2, 2, 2, 2, 2, 2, 2, 2, 2, 2, 2, 2, 2, 2, 2, 2, 2, 2, 2, 2, 2, 2, 2, 2, 2, 2, 2, 2, 2, 2, 2, 2, 2, 2, 2, 2, 2, 2, 2, 2, 2, 2, 2, 2, 2, 2, 2, 2, 2, 2, 2, 2, 2, 2, 2, 2, 2, 2, 2, 2, 2, 2, 2, 2, 2, 2, 2, 2, 2, 2, 2, 2, 2, 2, 2, 2, 2, 2, 2, 2, 2, 2, 2, 2, 2, 2, 2, 2, 2, 2, 2, 2, 2, 2, 2, 2, 2, 2, 2, 2, 2, 2, 2, 2, 2, 2, 2, 2, 2, 2, 2, 2, 2, 2, 2, 2, 2, 2, 2, 2, 2, 2, 2, 2, 2, 2, 2, 2, 2, 2, 2, 2, 2, 2, 2, 2, 2, 2, 2, 2, 2, 2, 2, 2, 2, 2, 2, 2, 2, 2, 2, 2, 2, 2, 2, 2, 2, 2, 2, 2, 2, 2, 2, 2, 2, 2, 2, 2, 2, 2, 2, 2, 2, 2, 2, 2, 2, 2, 2, 2, 2, 2, 2, 2, 2, 2, 2, 2, 2, 2, 2, 2, 2, 2, 2, 2, 2, 2, 2, 2, 2, 2, 2, 2, 2, 2, 2, 2, 2, 2, 2, 2, 2, 2, 2, 2, 2, 2, 2, 2, 2, 2, 2, 2, 2, 2, 2, 2, 2, 2, 2, 2, 2, 2, 2, 2, 2, 2, 2, 2, 2, 2, 2, 2, 2, 2, 2, 2, 2, 2, 2, 2, 2, 2, 2, 2, 2, 2, 2, 2, 2, 2, 2, 2, 2, 2, 2, 2, 2, 2, 2, 2, 2, 2, 2, 2, 2, 2, 2, 2, 2, 2, 2, 2, 2, 2, 2, 2, 2, 2, 2, 2, 2, 2, 2, 2, 2, 2, 2, 2, 2, 2, 2, 2, 2, 2, 2, 2, 2, 2, 2, 2, 2, 2, 2, 2, 2, 2, 2, 2, 2, 2, 2, 2, 2, 2, 2, 2, 2, 2, 2, 2, 2, 2, 2, 2, 2, 2, 2, 2, 2, 2, 2, 2, 2, 3 ),
 ( 0.000000000000000000, 1.000000000000000000 ),
 ( 0.000000000000000000, 0.002777777777777777884, 0.005555555555555555768, 0.008333333333333333218, 0.01111111111111111154, 0.01388888888888888812, 0.01666666666666666644, 0.01944444444444444475, 0.02222222222222222307, 0.02500000000000000139, 0.02777777777777777624, 0.03055555555555555455, 0.03333333333333333287, 0.03611111111111110772, 0.03888888888888888951, 0.04166666666666666435, 0.04444444444444444614, 0.04722222222222222099, 0.05000000000000000278, 0.05277777777777777762, 0.05555555555555555247, 0.05833333333333333426, 0.06111111111111110911, 0.06388888888888888395, 0.06666666666666666574, 0.06944444444444444753, 0.07222222222222221544, 0.07499999999999999722, 0.07777777777777777901, 0.08055555555555556080, 0.08333333333333332871, 0.08611111111111111049, 0.08888888888888889228, 0.09166666666666666019, 0.09444444444444444198, 0.09722222222222222376, 0.1000000000000000056, 0.1027777777777777735, 0.1055555555555555552, 0.1083333333333333370, 0.1111111111111111049, 0.1138888888888888867, 0.1166666666666666685, 0.1194444444444444503, 0.1222222222222222182, 0.1250000000000000000, 0.1277777777777777679, 0.1305555555555555636, 0.1333333333333333315, 0.1361111111111110994, 0.1388888888888888951, 0.1416666666666666630, 0.1444444444444444309, 0.1472222222222222265, 0.1499999999999999944, 0.1527777777777777901, 0.1555555555555555580, 0.1583333333333333259, 0.1611111111111111216, 0.1638888888888888895, 0.1666666666666666574, 0.1694444444444444531, 0.1722222222222222210, 0.1749999999999999889, 0.1777777777777777846, 0.1805555555555555525, 0.1833333333333333204, 0.1861111111111111160, 0.1888888888888888840, 0.1916666666666666796, 0.1944444444444444475, 0.1972222222222222154, 0.2000000000000000111, 0.2027777777777777790, 0.2055555555555555469, 0.2083333333333333426, 0.2111111111111111105, 0.2138888888888888784, 0.2166666666666666741, 0.2194444444444444420, 0.2222222222222222099, 0.2250000000000000056, 0.2277777777777777735, 0.2305555555555555691, 0.2333333333333333370, 0.2361111111111111049, 0.2388888888888889006, 0.2416666666666666685, 0.2444444444444444364, 0.2472222222222222321, 0.2500000000000000000, 0.2527777777777777679, 0.2555555555555555358, 0.2583333333333333592, 0.2611111111111111271, 0.2638888888888888951, 0.2666666666666666630, 0.2694444444444444309, 0.2722222222222221988, 0.2750000000000000222, 0.2777777777777777901, 0.2805555555555555580, 0.2833333333333333259, 0.2861111111111110938, 0.2888888888888888618, 0.2916666666666666852, 0.2944444444444444531, 0.2972222222222222210, 0.2999999999999999889, 0.3027777777777777568, 0.3055555555555555802, 0.3083333333333333481, 0.3111111111111111160, 0.3138888888888888840, 0.3166666666666666519, 0.3194444444444444198, 0.3222222222222222432, 0.3250000000000000111, 0.3277777777777777790, 0.3305555555555555469, 0.3333333333333333148, 0.3361111111111111382, 0.3388888888888889062, 0.3416666666666666741, 0.3444444444444444420, 0.3472222222222222099, 0.3499999999999999778, 0.3527777777777778012, 0.3555555555555555691, 0.3583333333333333370, 0.3611111111111111049, 0.3638888888888888729, 0.3666666666666666408, 0.3694444444444444642, 0.3722222222222222321, 0.3750000000000000000, 0.3777777777777777679, 0.3805555555555555358, 0.3833333333333333592, 0.3861111111111111271, 0.3888888888888888951, 0.3916666666666666630, 0.3944444444444444309, 0.3972222222222221988, 0.4000000000000000222, 0.4027777777777777901, 0.4055555555555555580, 0.4083333333333333259, 0.4111111111111110938, 0.4138888888888888618, 0.4166666666666666852, 0.4194444444444444531, 0.4222222222222222210, 0.4249999999999999889, 0.4277777777777777568, 0.4305555555555555802, 0.4333333333333333481, 0.4361111111111111160, 0.4388888888888888840, 0.4416666666666666519, 0.4444444444444444198, 0.4472222222222222432, 0.4500000000000000111, 0.4527777777777777790, 0.4555555555555555469, 0.4583333333333333148, 0.4611111111111111382, 0.4638888888888889062, 0.4666666666666666741, 0.4694444444444444420, 0.4722222222222222099, 0.4749999999999999778, 0.4777777777777778012, 0.4805555555555555691, 0.4833333333333333370, 0.4861111111111111049, 0.4888888888888888729, 0.4916666666666666408, 0.4944444444444444642, 0.4972222222222222321, 0.5000000000000000000, 0.5027777777777777679, 0.5055555555555555358, 0.5083333333333333037, 0.5111111111111110716, 0.5138888888888888395, 0.5166666666666667185, 0.5194444444444444864, 0.5222222222222222543, 0.5250000000000000222, 0.5277777777777777901, 0.5305555555555555580, 0.5333333333333333259, 0.5361111111111110938, 0.5388888888888888618, 0.5416666666666666297, 0.5444444444444443976, 0.5472222222222222765, 0.5500000000000000444, 0.5527777777777778123, 0.5555555555555555802, 0.5583333333333333481, 0.5611111111111111160, 0.5638888888888888840, 0.5666666666666666519, 0.5694444444444444198, 0.5722222222222221877, 0.5749999999999999556, 0.5777777777777777235, 0.5805555555555556024, 0.5833333333333333703, 0.5861111111111111382, 0.5888888888888889062, 0.5916666666666666741, 0.5944444444444444420, 0.5972222222222222099, 0.5999999999999999778, 0.6027777777777777457, 0.6055555555555555136, 0.6083333333333332815, 0.6111111111111111605, 0.6138888888888889284, 0.6166666666666666963, 0.6194444444444444642, 0.6222222222222222321, 0.6250000000000000000, 0.6277777777777777679, 0.6305555555555555358, 0.6333333333333333037, 0.6361111111111110716, 0.6388888888888888395, 0.6416666666666667185, 0.6444444444444444864, 0.6472222222222222543, 0.6500000000000000222, 0.6527777777777777901, 0.6555555555555555580, 0.6583333333333333259, 0.6611111111111110938, 0.6638888888888888618, 0.6666666666666666297, 0.6694444444444443976, 0.6722222222222222765, 0.6750000000000000444, 0.6777777777777778123, 0.6805555555555555802, 0.6833333333333333481, 0.6861111111111111160, 0.6888888888888888840, 0.6916666666666666519, 0.6944444444444444198, 0.6972222222222221877, 0.6999999999999999556, 0.7027777777777777235, 0.7055555555555556024, 0.7083333333333333703, 0.7111111111111111382, 0.7138888888888889062, 0.7166666666666666741, 0.7194444444444444420, 0.7222222222222222099, 0.7249999999999999778, 0.7277777777777777457, 0.7305555555555555136, 0.7333333333333332815, 0.7361111111111111605, 0.7388888888888889284, 0.7416666666666666963, 0.7444444444444444642, 0.7472222222222222321, 0.7500000000000000000, 0.7527777777777777679, 0.7555555555555555358, 0.7583333333333333037, 0.7611111111111110716, 0.7638888888888888395, 0.7666666666666667185, 0.7694444444444444864, 0.7722222222222222543, 0.7750000000000000222, 0.7777777777777777901, 0.7805555555555555580, 0.7833333333333333259, 0.7861111111111110938, 0.7888888888888888618, 0.7916666666666666297, 0.7944444444444443976, 0.7972222222222222765, 0.8000000000000000444, 0.8027777777777778123, 0.8055555555555555802, 0.8083333333333333481, 0.8111111111111111160, 0.8138888888888888840, 0.8166666666666666519, 0.8194444444444444198, 0.8222222222222221877, 0.8249999999999999556, 0.8277777777777777235, 0.8305555555555556024, 0.8333333333333333703, 0.8361111111111111382, 0.8388888888888889062, 0.8416666666666666741, 0.8444444444444444420, 0.8472222222222222099, 0.8499999999999999778, 0.8527777777777777457, 0.8555555555555555136, 0.8583333333333332815, 0.8611111111111111605, 0.8638888888888889284, 0.8666666666666666963, 0.8694444444444444642, 0.8722222222222222321, 0.8750000000000000000, 0.8777777777777777679, 0.8805555555555555358, 0.8833333333333333037, 0.8861111111111110716, 0.8888888888888888395, 0.8916666666666667185, 0.8944444444444444864, 0.8972222222222222543, 0.9000000000000000222, 0.9027777777777777901, 0.9055555555555555580, 0.9083333333333333259, 0.9111111111111110938, 0.9138888888888888618, 0.9166666666666666297, 0.9194444444444443976, 0.9222222222222222765, 0.9250000000000000444, 0.9277777777777778123, 0.9305555555555555802, 0.9333333333333333481, 0.9361111111111111160, 0.9388888888888888840, 0.9416666666666666519, 0.9444444444444444198, 0.9472222222222221877, 0.9499999999999999556, 0.9527777777777777235, 0.9555555555555556024, 0.9583333333333333703, 0.9611111111111111382, 0.9638888888888889062, 0.9666666666666666741, 0.9694444444444444420, 0.9722222222222222099, 0.9749999999999999778, 0.9777777777777777457, 0.9805555555555555136, 0.9833333333333332815, 0.9861111111111111605, 0.9888888888888889284, 0.9916666666666666963, 0.9944444444444444642, 0.9972222222222222321, 1.000000000000000000 ),
 .UNSPECIFIED. ) 
 GEOMETRIC_REPRESENTATION_ITEM ( )  RATIONAL_B_SPLINE_SURFACE ( (
 ( 1.000000000000000000, 0.8660254037844387076, 1.000000000000000000, 0.8660254037844387076, 1.000000000000000000, 0.8660254037844387076, 1.000000000000000000, 0.8660254037844387076, 1.000000000000000000, 0.8660254037844387076, 1.000000000000000000, 0.8660254037844387076, 1.000000000000000000, 0.8660254037844387076, 1.000000000000000000, 0.8660254037844387076, 1.000000000000000000, 0.8660254037844387076, 1.000000000000000000, 0.8660254037844387076, 1.000000000000000000, 0.8660254037844387076, 1.000000000000000000, 0.8660254037844387076, 1.000000000000000000, 0.8660254037844387076, 1.000000000000000000, 0.8660254037844387076, 1.000000000000000000, 0.8660254037844387076, 1.000000000000000000, 0.8660254037844387076, 1.000000000000000000, 0.8660254037844387076, 1.000000000000000000, 0.8660254037844387076, 1.000000000000000000, 0.8660254037844387076, 1.000000000000000000, 0.8660254037844387076, 1.000000000000000000, 0.8660254037844387076, 1.000000000000000000, 0.8660254037844387076, 1.000000000000000000, 0.8660254037844387076, 1.000000000000000000, 0.8660254037844387076, 1.000000000000000000, 0.8660254037844387076, 1.000000000000000000, 0.8660254037844387076, 1.000000000000000000, 0.8660254037844387076, 1.000000000000000000, 0.8660254037844387076, 1.000000000000000000, 0.8660254037844387076, 1.000000000000000000, 0.8660254037844387076, 1.000000000000000000, 0.8660254037844387076, 1.000000000000000000, 0.8660254037844387076, 1.000000000000000000, 0.8660254037844387076, 1.000000000000000000, 0.8660254037844387076, 1.000000000000000000, 0.8660254037844387076, 1.000000000000000000, 0.8660254037844387076, 1.000000000000000000, 0.8660254037844387076, 1.000000000000000000, 0.8660254037844387076, 1.000000000000000000, 0.8660254037844387076, 1.000000000000000000, 0.8660254037844387076, 1.000000000000000000, 0.8660254037844387076, 1.000000000000000000, 0.8660254037844387076, 1.000000000000000000, 0.8660254037844387076, 1.000000000000000000, 0.8660254037844387076, 1.000000000000000000, 0.8660254037844387076, 1.000000000000000000, 0.8660254037844387076, 1.000000000000000000, 0.8660254037844387076, 1.000000000000000000, 0.8660254037844387076, 1.000000000000000000, 0.8660254037844387076, 1.000000000000000000, 0.8660254037844387076, 1.000000000000000000, 0.8660254037844387076, 1.000000000000000000, 0.8660254037844387076, 1.000000000000000000, 0.8660254037844387076, 1.000000000000000000, 0.8660254037844387076, 1.000000000000000000, 0.8660254037844387076, 1.000000000000000000, 0.8660254037844387076, 1.000000000000000000, 0.8660254037844387076, 1.000000000000000000, 0.8660254037844387076, 1.000000000000000000, 0.8660254037844387076, 1.000000000000000000, 0.8660254037844387076, 1.000000000000000000, 0.8660254037844387076, 1.000000000000000000, 0.8660254037844387076, 1.000000000000000000, 0.8660254037844387076, 1.000000000000000000, 0.8660254037844387076, 1.000000000000000000, 0.8660254037844387076, 1.000000000000000000, 0.8660254037844387076, 1.000000000000000000, 0.8660254037844387076, 1.000000000000000000, 0.8660254037844387076, 1.000000000000000000, 0.8660254037844387076, 1.000000000000000000, 0.8660254037844387076, 1.000000000000000000, 0.8660254037844387076, 1.000000000000000000, 0.8660254037844387076, 1.000000000000000000, 0.8660254037844387076, 1.000000000000000000, 0.8660254037844387076, 1.000000000000000000, 0.8660254037844387076, 1.000000000000000000, 0.8660254037844387076, 1.000000000000000000, 0.8660254037844387076, 1.000000000000000000, 0.8660254037844387076, 1.000000000000000000, 0.8660254037844387076, 1.000000000000000000, 0.8660254037844387076, 1.000000000000000000, 0.8660254037844387076, 1.000000000000000000, 0.8660254037844387076, 1.000000000000000000, 0.8660254037844387076, 1.000000000000000000, 0.8660254037844387076, 1.000000000000000000, 0.8660254037844387076, 1.000000000000000000, 0.8660254037844387076, 1.000000000000000000, 0.8660254037844387076, 1.000000000000000000, 0.8660254037844387076, 1.000000000000000000, 0.8660254037844387076, 1.000000000000000000, 0.8660254037844387076, 1.000000000000000000, 0.8660254037844387076, 1.000000000000000000, 0.8660254037844387076, 1.000000000000000000, 0.8660254037844387076, 1.000000000000000000, 0.8660254037844387076, 1.000000000000000000, 0.8660254037844387076, 1.000000000000000000, 0.8660254037844387076, 1.000000000000000000, 0.8660254037844387076, 1.000000000000000000, 0.8660254037844387076, 1.000000000000000000, 0.8660254037844387076, 1.000000000000000000, 0.8660254037844387076, 1.000000000000000000, 0.8660254037844387076, 1.000000000000000000, 0.8660254037844387076, 1.000000000000000000, 0.8660254037844387076, 1.000000000000000000, 0.8660254037844387076, 1.000000000000000000, 0.8660254037844387076, 1.000000000000000000, 0.8660254037844387076, 1.000000000000000000, 0.8660254037844387076, 1.000000000000000000, 0.8660254037844387076, 1.000000000000000000, 0.8660254037844387076, 1.000000000000000000, 0.8660254037844387076, 1.000000000000000000, 0.8660254037844387076, 1.000000000000000000, 0.8660254037844387076, 1.000000000000000000, 0.8660254037844387076, 1.000000000000000000, 0.8660254037844387076, 1.000000000000000000, 0.8660254037844387076, 1.000000000000000000, 0.8660254037844387076, 1.000000000000000000, 0.8660254037844387076, 1.000000000000000000, 0.8660254037844387076, 1.000000000000000000, 0.8660254037844387076, 1.000000000000000000, 0.8660254037844387076, 1.000000000000000000, 0.8660254037844387076, 1.000000000000000000, 0.8660254037844387076, 1.000000000000000000, 0.8660254037844387076, 1.000000000000000000, 0.8660254037844387076, 1.000000000000000000, 0.8660254037844387076, 1.000000000000000000, 0.8660254037844387076, 1.000000000000000000, 0.8660254037844387076, 1.000000000000000000, 0.8660254037844387076, 1.000000000000000000, 0.8660254037844387076, 1.000000000000000000, 0.8660254037844387076, 1.000000000000000000, 0.8660254037844387076, 1.000000000000000000, 0.8660254037844387076, 1.000000000000000000, 0.8660254037844387076, 1.000000000000000000, 0.8660254037844387076, 1.000000000000000000, 0.8660254037844387076, 1.000000000000000000, 0.8660254037844387076, 1.000000000000000000, 0.8660254037844387076, 1.000000000000000000, 0.8660254037844387076, 1.000000000000000000, 0.8660254037844387076, 1.000000000000000000, 0.8660254037844387076, 1.000000000000000000, 0.8660254037844387076, 1.000000000000000000, 0.8660254037844387076, 1.000000000000000000, 0.8660254037844387076, 1.000000000000000000, 0.8660254037844387076, 1.000000000000000000, 0.8660254037844387076, 1.000000000000000000, 0.8660254037844387076, 1.000000000000000000, 0.8660254037844387076, 1.000000000000000000, 0.8660254037844387076, 1.000000000000000000, 0.8660254037844387076, 1.000000000000000000, 0.8660254037844387076, 1.000000000000000000, 0.8660254037844387076, 1.000000000000000000, 0.8660254037844387076, 1.000000000000000000, 0.8660254037844387076, 1.000000000000000000, 0.8660254037844387076, 1.000000000000000000, 0.8660254037844387076, 1.000000000000000000, 0.8660254037844387076, 1.000000000000000000, 0.8660254037844387076, 1.000000000000000000, 0.8660254037844387076, 1.000000000000000000, 0.8660254037844387076, 1.000000000000000000, 0.8660254037844387076, 1.000000000000000000, 0.8660254037844387076, 1.000000000000000000, 0.8660254037844387076, 1.000000000000000000, 0.8660254037844387076, 1.000000000000000000, 0.8660254037844387076, 1.000000000000000000, 0.8660254037844387076, 1.000000000000000000, 0.8660254037844387076, 1.000000000000000000, 0.8660254037844387076, 1.000000000000000000, 0.8660254037844387076, 1.000000000000000000, 0.8660254037844387076, 1.000000000000000000, 0.8660254037844387076, 1.000000000000000000, 0.8660254037844387076, 1.000000000000000000, 0.8660254037844387076, 1.000000000000000000, 0.8660254037844387076, 1.000000000000000000, 0.8660254037844387076, 1.000000000000000000, 0.8660254037844387076, 1.000000000000000000, 0.8660254037844387076, 1.000000000000000000, 0.8660254037844387076, 1.000000000000000000, 0.8660254037844387076, 1.000000000000000000, 0.8660254037844387076, 1.000000000000000000, 0.8660254037844387076, 1.000000000000000000, 0.8660254037844387076, 1.000000000000000000, 0.8660254037844387076, 1.000000000000000000, 0.8660254037844387076, 1.000000000000000000, 0.8660254037844387076, 1.000000000000000000, 0.8660254037844387076, 1.000000000000000000, 0.8660254037844387076, 1.000000000000000000, 0.8660254037844387076, 1.000000000000000000, 0.8660254037844387076, 1.000000000000000000, 0.8660254037844387076, 1.000000000000000000, 0.8660254037844387076, 1.000000000000000000, 0.8660254037844387076, 1.000000000000000000, 0.8660254037844387076, 1.000000000000000000, 0.8660254037844387076, 1.000000000000000000, 0.8660254037844387076, 1.000000000000000000, 0.8660254037844387076, 1.000000000000000000, 0.8660254037844387076, 1.000000000000000000, 0.8660254037844387076, 1.000000000000000000, 0.8660254037844387076, 1.000000000000000000, 0.8660254037844387076, 1.000000000000000000, 0.8660254037844387076, 1.000000000000000000, 0.8660254037844387076, 1.000000000000000000, 0.8660254037844387076, 1.000000000000000000, 0.8660254037844387076, 1.000000000000000000, 0.8660254037844387076, 1.000000000000000000, 0.8660254037844387076, 1.000000000000000000, 0.8660254037844387076, 1.000000000000000000, 0.8660254037844387076, 1.000000000000000000, 0.8660254037844387076, 1.000000000000000000, 0.8660254037844387076, 1.000000000000000000, 0.8660254037844387076, 1.000000000000000000, 0.8660254037844387076, 1.000000000000000000, 0.8660254037844387076, 1.000000000000000000, 0.8660254037844387076, 1.000000000000000000, 0.8660254037844387076, 1.000000000000000000, 0.8660254037844387076, 1.000000000000000000, 0.8660254037844387076, 1.000000000000000000, 0.8660254037844387076, 1.000000000000000000, 0.8660254037844387076, 1.000000000000000000, 0.8660254037844387076, 1.000000000000000000, 0.8660254037844387076, 1.000000000000000000, 0.8660254037844387076, 1.000000000000000000, 0.8660254037844387076, 1.000000000000000000, 0.8660254037844387076, 1.000000000000000000, 0.8660254037844387076, 1.000000000000000000, 0.8660254037844387076, 1.000000000000000000, 0.8660254037844387076, 1.000000000000000000, 0.8660254037844387076, 1.000000000000000000, 0.8660254037844387076, 1.000000000000000000, 0.8660254037844387076, 1.000000000000000000, 0.8660254037844387076, 1.000000000000000000, 0.8660254037844387076, 1.000000000000000000, 0.8660254037844387076, 1.000000000000000000, 0.8660254037844387076, 1.000000000000000000, 0.8660254037844387076, 1.000000000000000000, 0.8660254037844387076, 1.000000000000000000, 0.8660254037844387076, 1.000000000000000000, 0.8660254037844387076, 1.000000000000000000, 0.8660254037844387076, 1.000000000000000000, 0.8660254037844387076, 1.000000000000000000, 0.8660254037844387076, 1.000000000000000000, 0.8660254037844387076, 1.000000000000000000, 0.8660254037844387076, 1.000000000000000000, 0.8660254037844387076, 1.000000000000000000, 0.8660254037844387076, 1.000000000000000000, 0.8660254037844387076, 1.000000000000000000, 0.8660254037844387076, 1.000000000000000000, 0.8660254037844387076, 1.000000000000000000, 0.8660254037844387076, 1.000000000000000000, 0.8660254037844387076, 1.000000000000000000, 0.8660254037844387076, 1.000000000000000000, 0.8660254037844387076, 1.000000000000000000, 0.8660254037844387076, 1.000000000000000000, 0.8660254037844387076, 1.000000000000000000, 0.8660254037844387076, 1.000000000000000000, 0.8660254037844387076, 1.000000000000000000, 0.8660254037844387076, 1.000000000000000000, 0.8660254037844387076, 1.000000000000000000, 0.8660254037844387076, 1.000000000000000000, 0.8660254037844387076, 1.000000000000000000, 0.8660254037844387076, 1.000000000000000000, 0.8660254037844387076, 1.000000000000000000, 0.8660254037844387076, 1.000000000000000000, 0.8660254037844387076, 1.000000000000000000, 0.8660254037844387076, 1.000000000000000000, 0.8660254037844387076, 1.000000000000000000, 0.8660254037844387076, 1.000000000000000000, 0.8660254037844387076, 1.000000000000000000, 0.8660254037844387076, 1.000000000000000000, 0.8660254037844387076, 1.000000000000000000, 0.8660254037844387076, 1.000000000000000000, 0.8660254037844387076, 1.000000000000000000, 0.8660254037844387076, 1.000000000000000000, 0.8660254037844387076, 1.000000000000000000, 0.8660254037844387076, 1.000000000000000000, 0.8660254037844387076, 1.000000000000000000, 0.8660254037844387076, 1.000000000000000000, 0.8660254037844387076, 1.000000000000000000, 0.8660254037844387076, 1.000000000000000000, 0.8660254037844387076, 1.000000000000000000, 0.8660254037844387076, 1.000000000000000000, 0.8660254037844387076, 1.000000000000000000, 0.8660254037844387076, 1.000000000000000000, 0.8660254037844387076, 1.000000000000000000, 0.8660254037844387076, 1.000000000000000000, 0.8660254037844387076, 1.000000000000000000, 0.8660254037844387076, 1.000000000000000000, 0.8660254037844387076, 1.000000000000000000, 0.8660254037844387076, 1.000000000000000000, 0.8660254037844387076, 1.000000000000000000, 0.8660254037844387076, 1.000000000000000000, 0.8660254037844387076, 1.000000000000000000, 0.8660254037844387076, 1.000000000000000000, 0.8660254037844387076, 1.000000000000000000, 0.8660254037844387076, 1.000000000000000000, 0.8660254037844387076, 1.000000000000000000, 0.8660254037844387076, 1.000000000000000000, 0.8660254037844387076, 1.000000000000000000, 0.8660254037844387076, 1.000000000000000000, 0.8660254037844387076, 1.000000000000000000, 0.8660254037844387076, 1.000000000000000000, 0.8660254037844387076, 1.000000000000000000, 0.8660254037844387076, 1.000000000000000000, 0.8660254037844387076, 1.000000000000000000, 0.8660254037844387076, 1.000000000000000000, 0.8660254037844387076, 1.000000000000000000, 0.8660254037844387076, 1.000000000000000000, 0.8660254037844387076, 1.000000000000000000, 0.8660254037844387076, 1.000000000000000000, 0.8660254037844387076, 1.000000000000000000, 0.8660254037844387076, 1.000000000000000000, 0.8660254037844387076, 1.000000000000000000, 0.8660254037844387076, 1.000000000000000000, 0.8660254037844387076, 1.000000000000000000, 0.8660254037844387076, 1.000000000000000000, 0.8660254037844387076, 1.000000000000000000, 0.8660254037844387076, 1.000000000000000000, 0.8660254037844387076, 1.000000000000000000, 0.8660254037844387076, 1.000000000000000000, 0.8660254037844387076, 1.000000000000000000, 0.8660254037844387076, 1.000000000000000000, 0.8660254037844387076, 1.000000000000000000, 0.8660254037844387076, 1.000000000000000000, 0.8660254037844387076, 1.000000000000000000, 0.8660254037844387076, 1.000000000000000000, 0.8660254037844387076, 1.000000000000000000, 0.8660254037844387076, 1.000000000000000000, 0.8660254037844387076, 1.000000000000000000, 0.8660254037844387076, 1.000000000000000000, 0.8660254037844387076, 1.000000000000000000, 0.8660254037844387076, 1.000000000000000000, 0.8660254037844387076, 1.000000000000000000, 0.8660254037844387076, 1.000000000000000000, 0.8660254037844387076, 1.000000000000000000, 0.8660254037844387076, 1.000000000000000000, 0.8660254037844387076, 1.000000000000000000, 0.8660254037844387076, 1.000000000000000000, 0.8660254037844387076, 1.000000000000000000, 0.8660254037844387076, 1.000000000000000000, 0.8660254037844387076, 1.000000000000000000, 0.8660254037844387076, 1.000000000000000000, 0.8660254037844387076, 1.000000000000000000, 0.8660254037844387076, 1.000000000000000000, 0.8660254037844387076, 1.000000000000000000, 0.8660254037844387076, 1.000000000000000000, 0.8660254037844387076, 1.000000000000000000, 0.8660254037844387076, 1.000000000000000000, 0.8660254037844387076, 1.000000000000000000, 0.8660254037844387076, 1.000000000000000000, 0.8660254037844387076, 1.000000000000000000, 0.8660254037844387076, 1.000000000000000000, 0.8660254037844387076, 1.000000000000000000, 0.8660254037844387076, 1.000000000000000000, 0.8660254037844387076, 1.000000000000000000, 0.8660254037844387076, 1.000000000000000000, 0.8660254037844387076, 1.000000000000000000, 0.8660254037844387076, 1.000000000000000000, 0.8660254037844387076, 1.000000000000000000, 0.8660254037844387076, 1.000000000000000000, 0.8660254037844387076, 1.000000000000000000, 0.8660254037844387076, 1.000000000000000000),
 ( 1.000000000000000000, 0.8660254037844387076, 1.000000000000000000, 0.8660254037844387076, 1.000000000000000000, 0.8660254037844387076, 1.000000000000000000, 0.8660254037844387076, 1.000000000000000000, 0.8660254037844387076, 1.000000000000000000, 0.8660254037844387076, 1.000000000000000000, 0.8660254037844387076, 1.000000000000000000, 0.8660254037844387076, 1.000000000000000000, 0.8660254037844387076, 1.000000000000000000, 0.8660254037844387076, 1.000000000000000000, 0.8660254037844387076, 1.000000000000000000, 0.8660254037844387076, 1.000000000000000000, 0.8660254037844387076, 1.000000000000000000, 0.8660254037844387076, 1.000000000000000000, 0.8660254037844387076, 1.000000000000000000, 0.8660254037844387076, 1.000000000000000000, 0.8660254037844387076, 1.000000000000000000, 0.8660254037844387076, 1.000000000000000000, 0.8660254037844387076, 1.000000000000000000, 0.8660254037844387076, 1.000000000000000000, 0.8660254037844387076, 1.000000000000000000, 0.8660254037844387076, 1.000000000000000000, 0.8660254037844387076, 1.000000000000000000, 0.8660254037844387076, 1.000000000000000000, 0.8660254037844387076, 1.000000000000000000, 0.8660254037844387076, 1.000000000000000000, 0.8660254037844387076, 1.000000000000000000, 0.8660254037844387076, 1.000000000000000000, 0.8660254037844387076, 1.000000000000000000, 0.8660254037844387076, 1.000000000000000000, 0.8660254037844387076, 1.000000000000000000, 0.8660254037844387076, 1.000000000000000000, 0.8660254037844387076, 1.000000000000000000, 0.8660254037844387076, 1.000000000000000000, 0.8660254037844387076, 1.000000000000000000, 0.8660254037844387076, 1.000000000000000000, 0.8660254037844387076, 1.000000000000000000, 0.8660254037844387076, 1.000000000000000000, 0.8660254037844387076, 1.000000000000000000, 0.8660254037844387076, 1.000000000000000000, 0.8660254037844387076, 1.000000000000000000, 0.8660254037844387076, 1.000000000000000000, 0.8660254037844387076, 1.000000000000000000, 0.8660254037844387076, 1.000000000000000000, 0.8660254037844387076, 1.000000000000000000, 0.8660254037844387076, 1.000000000000000000, 0.8660254037844387076, 1.000000000000000000, 0.8660254037844387076, 1.000000000000000000, 0.8660254037844387076, 1.000000000000000000, 0.8660254037844387076, 1.000000000000000000, 0.8660254037844387076, 1.000000000000000000, 0.8660254037844387076, 1.000000000000000000, 0.8660254037844387076, 1.000000000000000000, 0.8660254037844387076, 1.000000000000000000, 0.8660254037844387076, 1.000000000000000000, 0.8660254037844387076, 1.000000000000000000, 0.8660254037844387076, 1.000000000000000000, 0.8660254037844387076, 1.000000000000000000, 0.8660254037844387076, 1.000000000000000000, 0.8660254037844387076, 1.000000000000000000, 0.8660254037844387076, 1.000000000000000000, 0.8660254037844387076, 1.000000000000000000, 0.8660254037844387076, 1.000000000000000000, 0.8660254037844387076, 1.000000000000000000, 0.8660254037844387076, 1.000000000000000000, 0.8660254037844387076, 1.000000000000000000, 0.8660254037844387076, 1.000000000000000000, 0.8660254037844387076, 1.000000000000000000, 0.8660254037844387076, 1.000000000000000000, 0.8660254037844387076, 1.000000000000000000, 0.8660254037844387076, 1.000000000000000000, 0.8660254037844387076, 1.000000000000000000, 0.8660254037844387076, 1.000000000000000000, 0.8660254037844387076, 1.000000000000000000, 0.8660254037844387076, 1.000000000000000000, 0.8660254037844387076, 1.000000000000000000, 0.8660254037844387076, 1.000000000000000000, 0.8660254037844387076, 1.000000000000000000, 0.8660254037844387076, 1.000000000000000000, 0.8660254037844387076, 1.000000000000000000, 0.8660254037844387076, 1.000000000000000000, 0.8660254037844387076, 1.000000000000000000, 0.8660254037844387076, 1.000000000000000000, 0.8660254037844387076, 1.000000000000000000, 0.8660254037844387076, 1.000000000000000000, 0.8660254037844387076, 1.000000000000000000, 0.8660254037844387076, 1.000000000000000000, 0.8660254037844387076, 1.000000000000000000, 0.8660254037844387076, 1.000000000000000000, 0.8660254037844387076, 1.000000000000000000, 0.8660254037844387076, 1.000000000000000000, 0.8660254037844387076, 1.000000000000000000, 0.8660254037844387076, 1.000000000000000000, 0.8660254037844387076, 1.000000000000000000, 0.8660254037844387076, 1.000000000000000000, 0.8660254037844387076, 1.000000000000000000, 0.8660254037844387076, 1.000000000000000000, 0.8660254037844387076, 1.000000000000000000, 0.8660254037844387076, 1.000000000000000000, 0.8660254037844387076, 1.000000000000000000, 0.8660254037844387076, 1.000000000000000000, 0.8660254037844387076, 1.000000000000000000, 0.8660254037844387076, 1.000000000000000000, 0.8660254037844387076, 1.000000000000000000, 0.8660254037844387076, 1.000000000000000000, 0.8660254037844387076, 1.000000000000000000, 0.8660254037844387076, 1.000000000000000000, 0.8660254037844387076, 1.000000000000000000, 0.8660254037844387076, 1.000000000000000000, 0.8660254037844387076, 1.000000000000000000, 0.8660254037844387076, 1.000000000000000000, 0.8660254037844387076, 1.000000000000000000, 0.8660254037844387076, 1.000000000000000000, 0.8660254037844387076, 1.000000000000000000, 0.8660254037844387076, 1.000000000000000000, 0.8660254037844387076, 1.000000000000000000, 0.8660254037844387076, 1.000000000000000000, 0.8660254037844387076, 1.000000000000000000, 0.8660254037844387076, 1.000000000000000000, 0.8660254037844387076, 1.000000000000000000, 0.8660254037844387076, 1.000000000000000000, 0.8660254037844387076, 1.000000000000000000, 0.8660254037844387076, 1.000000000000000000, 0.8660254037844387076, 1.000000000000000000, 0.8660254037844387076, 1.000000000000000000, 0.8660254037844387076, 1.000000000000000000, 0.8660254037844387076, 1.000000000000000000, 0.8660254037844387076, 1.000000000000000000, 0.8660254037844387076, 1.000000000000000000, 0.8660254037844387076, 1.000000000000000000, 0.8660254037844387076, 1.000000000000000000, 0.8660254037844387076, 1.000000000000000000, 0.8660254037844387076, 1.000000000000000000, 0.8660254037844387076, 1.000000000000000000, 0.8660254037844387076, 1.000000000000000000, 0.8660254037844387076, 1.000000000000000000, 0.8660254037844387076, 1.000000000000000000, 0.8660254037844387076, 1.000000000000000000, 0.8660254037844387076, 1.000000000000000000, 0.8660254037844387076, 1.000000000000000000, 0.8660254037844387076, 1.000000000000000000, 0.8660254037844387076, 1.000000000000000000, 0.8660254037844387076, 1.000000000000000000, 0.8660254037844387076, 1.000000000000000000, 0.8660254037844387076, 1.000000000000000000, 0.8660254037844387076, 1.000000000000000000, 0.8660254037844387076, 1.000000000000000000, 0.8660254037844387076, 1.000000000000000000, 0.8660254037844387076, 1.000000000000000000, 0.8660254037844387076, 1.000000000000000000, 0.8660254037844387076, 1.000000000000000000, 0.8660254037844387076, 1.000000000000000000, 0.8660254037844387076, 1.000000000000000000, 0.8660254037844387076, 1.000000000000000000, 0.8660254037844387076, 1.000000000000000000, 0.8660254037844387076, 1.000000000000000000, 0.8660254037844387076, 1.000000000000000000, 0.8660254037844387076, 1.000000000000000000, 0.8660254037844387076, 1.000000000000000000, 0.8660254037844387076, 1.000000000000000000, 0.8660254037844387076, 1.000000000000000000, 0.8660254037844387076, 1.000000000000000000, 0.8660254037844387076, 1.000000000000000000, 0.8660254037844387076, 1.000000000000000000, 0.8660254037844387076, 1.000000000000000000, 0.8660254037844387076, 1.000000000000000000, 0.8660254037844387076, 1.000000000000000000, 0.8660254037844387076, 1.000000000000000000, 0.8660254037844387076, 1.000000000000000000, 0.8660254037844387076, 1.000000000000000000, 0.8660254037844387076, 1.000000000000000000, 0.8660254037844387076, 1.000000000000000000, 0.8660254037844387076, 1.000000000000000000, 0.8660254037844387076, 1.000000000000000000, 0.8660254037844387076, 1.000000000000000000, 0.8660254037844387076, 1.000000000000000000, 0.8660254037844387076, 1.000000000000000000, 0.8660254037844387076, 1.000000000000000000, 0.8660254037844387076, 1.000000000000000000, 0.8660254037844387076, 1.000000000000000000, 0.8660254037844387076, 1.000000000000000000, 0.8660254037844387076, 1.000000000000000000, 0.8660254037844387076, 1.000000000000000000, 0.8660254037844387076, 1.000000000000000000, 0.8660254037844387076, 1.000000000000000000, 0.8660254037844387076, 1.000000000000000000, 0.8660254037844387076, 1.000000000000000000, 0.8660254037844387076, 1.000000000000000000, 0.8660254037844387076, 1.000000000000000000, 0.8660254037844387076, 1.000000000000000000, 0.8660254037844387076, 1.000000000000000000, 0.8660254037844387076, 1.000000000000000000, 0.8660254037844387076, 1.000000000000000000, 0.8660254037844387076, 1.000000000000000000, 0.8660254037844387076, 1.000000000000000000, 0.8660254037844387076, 1.000000000000000000, 0.8660254037844387076, 1.000000000000000000, 0.8660254037844387076, 1.000000000000000000, 0.8660254037844387076, 1.000000000000000000, 0.8660254037844387076, 1.000000000000000000, 0.8660254037844387076, 1.000000000000000000, 0.8660254037844387076, 1.000000000000000000, 0.8660254037844387076, 1.000000000000000000, 0.8660254037844387076, 1.000000000000000000, 0.8660254037844387076, 1.000000000000000000, 0.8660254037844387076, 1.000000000000000000, 0.8660254037844387076, 1.000000000000000000, 0.8660254037844387076, 1.000000000000000000, 0.8660254037844387076, 1.000000000000000000, 0.8660254037844387076, 1.000000000000000000, 0.8660254037844387076, 1.000000000000000000, 0.8660254037844387076, 1.000000000000000000, 0.8660254037844387076, 1.000000000000000000, 0.8660254037844387076, 1.000000000000000000, 0.8660254037844387076, 1.000000000000000000, 0.8660254037844387076, 1.000000000000000000, 0.8660254037844387076, 1.000000000000000000, 0.8660254037844387076, 1.000000000000000000, 0.8660254037844387076, 1.000000000000000000, 0.8660254037844387076, 1.000000000000000000, 0.8660254037844387076, 1.000000000000000000, 0.8660254037844387076, 1.000000000000000000, 0.8660254037844387076, 1.000000000000000000, 0.8660254037844387076, 1.000000000000000000, 0.8660254037844387076, 1.000000000000000000, 0.8660254037844387076, 1.000000000000000000, 0.8660254037844387076, 1.000000000000000000, 0.8660254037844387076, 1.000000000000000000, 0.8660254037844387076, 1.000000000000000000, 0.8660254037844387076, 1.000000000000000000, 0.8660254037844387076, 1.000000000000000000, 0.8660254037844387076, 1.000000000000000000, 0.8660254037844387076, 1.000000000000000000, 0.8660254037844387076, 1.000000000000000000, 0.8660254037844387076, 1.000000000000000000, 0.8660254037844387076, 1.000000000000000000, 0.8660254037844387076, 1.000000000000000000, 0.8660254037844387076, 1.000000000000000000, 0.8660254037844387076, 1.000000000000000000, 0.8660254037844387076, 1.000000000000000000, 0.8660254037844387076, 1.000000000000000000, 0.8660254037844387076, 1.000000000000000000, 0.8660254037844387076, 1.000000000000000000, 0.8660254037844387076, 1.000000000000000000, 0.8660254037844387076, 1.000000000000000000, 0.8660254037844387076, 1.000000000000000000, 0.8660254037844387076, 1.000000000000000000, 0.8660254037844387076, 1.000000000000000000, 0.8660254037844387076, 1.000000000000000000, 0.8660254037844387076, 1.000000000000000000, 0.8660254037844387076, 1.000000000000000000, 0.8660254037844387076, 1.000000000000000000, 0.8660254037844387076, 1.000000000000000000, 0.8660254037844387076, 1.000000000000000000, 0.8660254037844387076, 1.000000000000000000, 0.8660254037844387076, 1.000000000000000000, 0.8660254037844387076, 1.000000000000000000, 0.8660254037844387076, 1.000000000000000000, 0.8660254037844387076, 1.000000000000000000, 0.8660254037844387076, 1.000000000000000000, 0.8660254037844387076, 1.000000000000000000, 0.8660254037844387076, 1.000000000000000000, 0.8660254037844387076, 1.000000000000000000, 0.8660254037844387076, 1.000000000000000000, 0.8660254037844387076, 1.000000000000000000, 0.8660254037844387076, 1.000000000000000000, 0.8660254037844387076, 1.000000000000000000, 0.8660254037844387076, 1.000000000000000000, 0.8660254037844387076, 1.000000000000000000, 0.8660254037844387076, 1.000000000000000000, 0.8660254037844387076, 1.000000000000000000, 0.8660254037844387076, 1.000000000000000000, 0.8660254037844387076, 1.000000000000000000, 0.8660254037844387076, 1.000000000000000000, 0.8660254037844387076, 1.000000000000000000, 0.8660254037844387076, 1.000000000000000000, 0.8660254037844387076, 1.000000000000000000, 0.8660254037844387076, 1.000000000000000000, 0.8660254037844387076, 1.000000000000000000, 0.8660254037844387076, 1.000000000000000000, 0.8660254037844387076, 1.000000000000000000, 0.8660254037844387076, 1.000000000000000000, 0.8660254037844387076, 1.000000000000000000, 0.8660254037844387076, 1.000000000000000000, 0.8660254037844387076, 1.000000000000000000, 0.8660254037844387076, 1.000000000000000000, 0.8660254037844387076, 1.000000000000000000, 0.8660254037844387076, 1.000000000000000000, 0.8660254037844387076, 1.000000000000000000, 0.8660254037844387076, 1.000000000000000000, 0.8660254037844387076, 1.000000000000000000, 0.8660254037844387076, 1.000000000000000000, 0.8660254037844387076, 1.000000000000000000, 0.8660254037844387076, 1.000000000000000000, 0.8660254037844387076, 1.000000000000000000, 0.8660254037844387076, 1.000000000000000000, 0.8660254037844387076, 1.000000000000000000, 0.8660254037844387076, 1.000000000000000000, 0.8660254037844387076, 1.000000000000000000, 0.8660254037844387076, 1.000000000000000000, 0.8660254037844387076, 1.000000000000000000, 0.8660254037844387076, 1.000000000000000000, 0.8660254037844387076, 1.000000000000000000, 0.8660254037844387076, 1.000000000000000000, 0.8660254037844387076, 1.000000000000000000, 0.8660254037844387076, 1.000000000000000000, 0.8660254037844387076, 1.000000000000000000, 0.8660254037844387076, 1.000000000000000000, 0.8660254037844387076, 1.000000000000000000, 0.8660254037844387076, 1.000000000000000000, 0.8660254037844387076, 1.000000000000000000, 0.8660254037844387076, 1.000000000000000000, 0.8660254037844387076, 1.000000000000000000, 0.8660254037844387076, 1.000000000000000000, 0.8660254037844387076, 1.000000000000000000, 0.8660254037844387076, 1.000000000000000000, 0.8660254037844387076, 1.000000000000000000, 0.8660254037844387076, 1.000000000000000000, 0.8660254037844387076, 1.000000000000000000, 0.8660254037844387076, 1.000000000000000000, 0.8660254037844387076, 1.000000000000000000, 0.8660254037844387076, 1.000000000000000000, 0.8660254037844387076, 1.000000000000000000, 0.8660254037844387076, 1.000000000000000000, 0.8660254037844387076, 1.000000000000000000, 0.8660254037844387076, 1.000000000000000000, 0.8660254037844387076, 1.000000000000000000, 0.8660254037844387076, 1.000000000000000000, 0.8660254037844387076, 1.000000000000000000, 0.8660254037844387076, 1.000000000000000000, 0.8660254037844387076, 1.000000000000000000, 0.8660254037844387076, 1.000000000000000000, 0.8660254037844387076, 1.000000000000000000, 0.8660254037844387076, 1.000000000000000000, 0.8660254037844387076, 1.000000000000000000, 0.8660254037844387076, 1.000000000000000000, 0.8660254037844387076, 1.000000000000000000, 0.8660254037844387076, 1.000000000000000000, 0.8660254037844387076, 1.000000000000000000, 0.8660254037844387076, 1.000000000000000000, 0.8660254037844387076, 1.000000000000000000, 0.8660254037844387076, 1.000000000000000000, 0.8660254037844387076, 1.000000000000000000, 0.8660254037844387076, 1.000000000000000000, 0.8660254037844387076, 1.000000000000000000, 0.8660254037844387076, 1.000000000000000000, 0.8660254037844387076, 1.000000000000000000, 0.8660254037844387076, 1.000000000000000000, 0.8660254037844387076, 1.000000000000000000, 0.8660254037844387076, 1.000000000000000000, 0.8660254037844387076, 1.000000000000000000, 0.8660254037844387076, 1.000000000000000000, 0.8660254037844387076, 1.000000000000000000, 0.8660254037844387076, 1.000000000000000000, 0.8660254037844387076, 1.000000000000000000, 0.8660254037844387076, 1.000000000000000000, 0.8660254037844387076, 1.000000000000000000, 0.8660254037844387076, 1.000000000000000000, 0.8660254037844387076, 1.000000000000000000, 0.8660254037844387076, 1.000000000000000000) ) ) 
 REPRESENTATION_ITEM ( '' )  SURFACE ( )  );
#61799=CARTESIAN_POINT ( 'NONE',  ( 27.90000000122903145, -2.886751345948129988, 4.999999999999997335 ) ) ;
#61801=CARTESIAN_POINT ( 'NONE',  ( 18.92812500061451431, 4.541064518000418104, 2.621784821874999949 ) ) ;
#61802=CARTESIAN_POINT ( 'NONE',  ( 1.626862140677534273E-15, 13.81250000000000000, 34.00000000000000000 ) ) ;
#61804=CARTESIAN_POINT ( 'NONE',  ( 13.17187500061451999, 3.027376345333611329, 5.243569643749999010 ) ) ;
#61805=CARTESIAN_POINT ( 'NONE',  ( 14.52187500061451608, 3.027376345333611329, 5.243569643749999010 ) ) ;
#61806=CARTESIAN_POINT ( 'NONE',  ( 22.95937500061451431, 4.541064518000418104, -2.621784821874998173 ) ) ;
#61807=ORIENTED_EDGE ( 'NONE', *, *, #15786, .F. ) ;
#61809=CARTESIAN_POINT ( 'NONE',  ( 25.97812500061451502, 6.421520780324663323E-16, -5.243569643749999010 ) ) ;
#61810=( BOUNDED_CURVE ( )  B_SPLINE_CURVE ( 2, ( #72785, #62415, #56864, #33973, #62058, #62777, #5184, #68335, #27722 ),
 .UNSPECIFIED., .F., .F. ) 
 B_SPLINE_CURVE_WITH_KNOTS ( ( 3, 2, 2, 2, 3 ),
 ( 0.7282608695652174058, 0.7318840579710145233, 0.7391304347826086474, 0.7463768115942028825, 0.7500000000000000000 ),
 .UNSPECIFIED. ) 
 CURVE ( )  GEOMETRIC_REPRESENTATION_ITEM ( )  RATIONAL_B_SPLINE_CURVE ( ( 0.9330127018922194093, 0.9330127018922194093, 1.000000000000000000, 0.8660254037844387076, 1.000000000000000000, 0.8660254037844387076, 1.000000000000000000, 0.9330127018922194093, 0.9330127018922194093 ) ) 
 REPRESENTATION_ITEM ( '' )  );
#61811=CARTESIAN_POINT ( 'NONE',  ( 26.76562500061451644, -6.054752690667223547, -1.112240025338166033E-15 ) ) ;
#61812=CYLINDRICAL_SURFACE ( 'NONE', #56839, 4.999999999999998224 ) ;
#61813=CARTESIAN_POINT ( 'NONE',  ( -3.999999999999997335, 16.88749999999999929, 32.30940107675850470 ) ) ;
#61814=CARTESIAN_POINT ( 'NONE',  ( 4.096875000614518925, 6.054752690667223547, 3.707466751127219781E-16 ) ) ;
#61815=CARTESIAN_POINT ( 'NONE',  ( 11.88750000122903216, 6.123233995736764310E-16, -4.999999999999998224 ) ) ;
#61816=CARTESIAN_POINT ( 'NONE',  ( 7.275000001229035007, -5.773502691896255534, -1.060575238724906372E-15 ) ) ;
#61817=CARTESIAN_POINT ( 'NONE',  ( 3.028125000614518392, 6.421520780324663323E-16, -5.243569643749999010 ) ) ;
#61820=CARTESIAN_POINT ( 'NONE',  ( 11.29687500061451644, 6.054752690667223547, 3.707466751127219781E-16 ) ) ;
#61821=CARTESIAN_POINT ( 'NONE',  ( 3.999999999999999112, 14.82500000000000107, -30.00000000000000000 ) ) ;
#61822=ORIENTED_EDGE ( 'NONE', *, *, #69469, .T. ) ;
#61823=CARTESIAN_POINT ( 'NONE',  ( 19.04062500061451146, -3.027376345333614438, 5.243569643749998122 ) ) ;
#61824=CARTESIAN_POINT ( 'NONE',  ( 14.22187500061451537, -6.054752690667223547, -1.112240025338166033E-15 ) ) ;
#61825=CARTESIAN_POINT ( 'NONE',  ( 4.790625000614518569, -3.027376345333610441, -5.243569643749999898 ) ) ;
#61826=CARTESIAN_POINT ( 'NONE',  ( 21.94687500061451502, -3.027376345333610441, -5.243569643749999898 ) ) ;
#61827=CARTESIAN_POINT ( 'NONE',  ( 9.121875000614517504, 3.027376345333611329, 5.243569643749999010 ) ) ;
#61828=CARTESIAN_POINT ( 'NONE',  ( 5.353125000614515905, 4.541064518000418104, -2.621784821874998173 ) ) ;
#61829=CARTESIAN_POINT ( 'NONE',  ( -1.999999999999997113, 17.82499999999999929, 33.46410161513775705 ) ) ;
#61830=CARTESIAN_POINT ( 'NONE',  ( 6.412500001229036073, -4.330127018922190985, -2.500000000000001332 ) ) ;
#61831=CARTESIAN_POINT ( 'NONE',  ( 18.92812500061451431, 4.541064518000418104, 2.621784821874999949 ) ) ;
#61832=( BOUNDED_CURVE ( )  B_SPLINE_CURVE ( 2, ( #42249, #35970, #7534, #14528, #70682, #59219, #7900, #41881, #64409 ),
 .UNSPECIFIED., .F., .F. ) 
 B_SPLINE_CURVE_WITH_KNOTS ( ( 3, 2, 2, 2, 3 ),
 ( 0.09782608695652174335, 0.1014492753623188470, 0.1086956521739130405, 0.1159420289855072478, 0.1195652173913043514 ),
 .UNSPECIFIED. ) 
 CURVE ( )  GEOMETRIC_REPRESENTATION_ITEM ( )  RATIONAL_B_SPLINE_CURVE ( ( 0.9330127018922194093, 0.9330127018922194093, 1.000000000000000000, 0.8660254037844387076, 1.000000000000000000, 0.8660254037844387076, 1.000000000000000000, 0.9330127018922194093, 0.9330127018922194093 ) ) 
 REPRESENTATION_ITEM ( '' )  );
#61833=CARTESIAN_POINT ( 'NONE',  ( 8.475000001229034297, 2.886751345948126879, 4.999999999999999112 ) ) ;
#61834=CARTESIAN_POINT ( 'NONE',  ( 17.20312500061451644, 0.000000000000000000, 5.243569643749999010 ) ) ;
#61835=CARTESIAN_POINT ( 'NONE',  ( 14.72812500061451679, 6.421520780324663323E-16, -5.243569643749999010 ) ) ;
#61837=CARTESIAN_POINT ( 'NONE',  ( 16.16250000000000142, -5.773502691896255534, -1.060575238724906372E-15 ) ) ;
#61838=CARTESIAN_POINT ( 'NONE',  ( 9.450000001229033941, -2.886751345948129988, 4.999999999999997335 ) ) ;
#61839=CARTESIAN_POINT ( 'NONE',  ( 5.465625000614517504, 3.027376345333611329, 5.243569643749999010 ) ) ;
#61841=CARTESIAN_POINT ( 'NONE',  ( 21.52500000122903145, 2.886751345948126879, 4.999999999999999112 ) ) ;
#61843=CARTESIAN_POINT ( 'NONE',  ( 4.243569643749999898, 10.63437500061451857, -30.00000000000000000 ) ) ;
#61844=CARTESIAN_POINT ( 'NONE',  ( 4.575021196052274419, -2.017510855256722468, 4.733783051837803235 ) ) ;
#61845=CARTESIAN_POINT ( 'NONE',  ( 23.92499999999999716, 6.123233995736764310E-16, -4.999999999999998224 ) ) ;
#61846=CARTESIAN_POINT ( 'NONE',  ( 4.434375000614519280, 6.421520780324663323E-16, -5.243569643749999010 ) ) ;
#61847=CARTESIAN_POINT ( 'NONE',  ( 21.87187500061451573, -6.054752690667223547, -1.112240025338166033E-15 ) ) ;
#61848=DIRECTION ( 'NONE',  ( -0.000000000000000000, -0.000000000000000000, -1.000000000000000000 ) ) ;
#61849=CARTESIAN_POINT ( 'NONE',  ( 17.27812500061451217, -4.541064518000419881, 2.621784821874995952 ) ) ;
#61851=CARTESIAN_POINT ( 'NONE',  ( 26.73749999999999716, 5.773502691896255534, 3.535250795749688401E-16 ) ) ;
#61852=CARTESIAN_POINT ( 'NONE',  ( 27.94687500061451502, 6.054752690667223547, 3.707466751127219781E-16 ) ) ;
#61855=CARTESIAN_POINT ( 'NONE',  ( 12.66562500061451502, 3.027376345333611329, 5.243569643749999010 ) ) ;
#61856=CARTESIAN_POINT ( 'NONE',  ( 10.17187500061451999, -6.054752690667223547, -1.112240025338166033E-15 ) ) ;
#61858=CARTESIAN_POINT ( 'NONE',  ( 2.817472997146174052, -4.130598735093008678, -2.817472997146206026 ) ) ;
#61859=CARTESIAN_POINT ( 'NONE',  ( 23.05312500061451431, 0.000000000000000000, 5.243569643749999010 ) ) ;
#61861=CARTESIAN_POINT ( 'NONE',  ( -5.810221930991193690E-16, 14.93750000000000000, 26.00000000000000355 ) ) ;
#61863=CARTESIAN_POINT ( 'NONE',  ( 13.04999999999999893, -4.330127018922190985, -2.500000000000001332 ) ) ;
#61864=CARTESIAN_POINT ( 'NONE',  ( 20.85000000122903430, -2.886751345948125991, -5.000000000000000000 ) ) ;
#61865=CARTESIAN_POINT ( 'NONE',  ( 16.45312500061451289, -4.541064518000417216, -2.621784821875001281 ) ) ;
#61867=EDGE_LOOP ( 'NONE', ( #15612, #56765, #25707, #72239 ) ) ;
#61868=CARTESIAN_POINT ( 'NONE',  ( 18.82500000000000284, -4.330127018922194537, 2.499999999999995559 ) ) ;
#61869=CARTESIAN_POINT ( 'NONE',  ( 24.89999999999999858, 4.330127018922192761, -2.499999999999997780 ) ) ;
#61870=CARTESIAN_POINT ( 'NONE',  ( 21.87187500061451573, -6.054752690667223547, -1.112240025338166033E-15 ) ) ;
#61871=CARTESIAN_POINT ( 'NONE',  ( 24.55312500061451786, -4.541064518000417216, -2.621784821875001281 ) ) ;
#61872=VECTOR ( 'NONE', #57770, 1000.000000000000000 ) ;
#61875=CARTESIAN_POINT ( 'NONE',  ( 8.053125000614516082, 4.541064518000418104, -2.621784821874998173 ) ) ;
#61876=CARTESIAN_POINT ( 'NONE',  ( 17.43750000122903288, 4.330127018922191873, 2.499999999999999556 ) ) ;
#61877=CARTESIAN_POINT ( 'NONE',  ( 15.52500000000000036, 4.330127018922191873, 2.499999999999999556 ) ) ;
#61878=CARTESIAN_POINT ( 'NONE',  ( 3.598985740823767987, -3.471053988920652422, -3.649034764177215173 ) ) ;
#61879=CARTESIAN_POINT ( 'NONE',  ( 4.884375000614518569, 6.421520780324663323E-16, -5.243569643749999010 ) ) ;
#61881=CARTESIAN_POINT ( 'NONE',  ( 28.47187500061451715, 3.027376345333611329, 5.243569643749999010 ) ) ;
#61882=ORIENTED_EDGE ( 'NONE', *, *, #45500, .T. ) ;
#61883=CARTESIAN_POINT ( 'NONE',  ( 24.92812500061451431, -4.541064518000419881, 2.621784821874995952 ) ) ;
#61884=CARTESIAN_POINT ( 'NONE',  ( 25.80937500061451928, 0.000000000000000000, 5.243569643749999010 ) ) ;
#61885=EDGE_CURVE ( 'NONE', #23724, #70091, #27683, .T. ) ;
#61886=CARTESIAN_POINT ( 'NONE',  ( 2.121784821875001281, 18.15312500061459389, -26.32496088578401938 ) ) ;
#61887=CARTESIAN_POINT ( 'NONE',  ( 11.17500000000000071, -4.330127018922194537, 2.499999999999995559 ) ) ;
#61888=CARTESIAN_POINT ( 'NONE',  ( 10.00312500061451715, 0.000000000000000000, 5.243569643749999010 ) ) ;
#61890=CARTESIAN_POINT ( 'NONE',  ( 1.510657702057710734E-15, 19.43750000000000000, -33.99999999999999289 ) ) ;
#61891=CARTESIAN_POINT ( 'NONE',  ( 26.72812500061451502, -4.541064518000419881, 2.621784821874995952 ) ) ;
#61894=CARTESIAN_POINT ( 'NONE',  ( 3.178125000614515638, 4.541064518000418104, 2.621784821874999949 ) ) ;
#61895=CARTESIAN_POINT ( 'NONE',  ( 19.35937500061451644, 4.541064518000418104, -2.621784821874998173 ) ) ;
#61896=CARTESIAN_POINT ( 'NONE',  ( 2.121784821874999061, 15.65937500061451892, 26.32496088578401583 ) ) ;
#61897=CARTESIAN_POINT ( 'NONE',  ( 20.93437500061451573, -4.541064518000419881, 2.621784821874995952 ) ) ;
#61898=CARTESIAN_POINT ( 'NONE',  ( 28.99687500061451573, -3.027376345333614438, 5.243569643749998122 ) ) ;
#61899=CARTESIAN_POINT ( 'NONE',  ( 4.243569643749999010, 18.77187500061451431, 27.54997392385601174 ) ) ;
#61900=CARTESIAN_POINT ( 'NONE',  ( 10.86562500061451431, 3.027376345333611329, 5.243569643749999010 ) ) ;
#61901=CARTESIAN_POINT ( 'NONE',  ( 2.700000001229035718, -2.886751345948129988, 4.999999999999997335 ) ) ;
#61902=CARTESIAN_POINT ( 'NONE',  ( 5.971875000614516260, 3.027376345333611329, 5.243569643749999010 ) ) ;
#61903=CARTESIAN_POINT ( 'NONE',  ( -1.071796769724488563, 16.15490381179669654, -26.00000000000000000 ) ) ;
#61904=CARTESIAN_POINT ( 'NONE',  ( 6.628125000614517148, 6.421520780324663323E-16, -5.243569643749999010 ) ) ;
#61905=CARTESIAN_POINT ( 'NONE',  ( 12.38437500061451857, -4.541064518000419881, 2.621784821874995952 ) ) ;
#61907=CARTESIAN_POINT ( 'NONE',  ( 19.68750000122903288, 4.330127018922191873, 2.499999999999999556 ) ) ;
#61908=CARTESIAN_POINT ( 'NONE',  ( 7.134375000614516793, 6.421520780324663323E-16, -5.243569643749999010 ) ) ;
#61909=CARTESIAN_POINT ( 'NONE',  ( 9.253125000614517148, -4.541064518000417216, -2.621784821875001281 ) ) ;
#61912=CARTESIAN_POINT ( 'NONE',  ( 18.08437500061451431, 4.541064518000418104, 2.621784821874999949 ) ) ;
#61913=CARTESIAN_POINT ( 'NONE',  ( 1.071796769724489895, 13.22990381179669939, 26.00000000000000355 ) ) ;
#61914=CARTESIAN_POINT ( 'NONE',  ( 27.62812500061451360, -4.541064518000419881, 2.621784821874995952 ) ) ;
#61915=CARTESIAN_POINT ( 'NONE',  ( 13.11562500061451786, 3.027376345333611329, 5.243569643749999010 ) ) ;
#61917=CARTESIAN_POINT ( 'NONE',  ( -4.243569643749998122, 11.79687500061451999, -27.54997392385601174 ) ) ;
#61918=CARTESIAN_POINT ( 'NONE',  ( 13.05000000122903536, -2.886751345948129988, 4.999999999999997335 ) ) ;
#61919=CARTESIAN_POINT ( 'NONE',  ( 28.45312500061451289, 0.000000000000000000, 5.243569643749999010 ) ) ;
#61920=CARTESIAN_POINT ( 'NONE',  ( 9.001249775931846008E-16, 16.31562500061451715, -25.09994784771203058 ) ) ;
#61921=CARTESIAN_POINT ( 'NONE',  ( 14.02500000122903323, -5.773502691896255534, -1.060575238724906372E-15 ) ) ;
#61922=AXIS2_PLACEMENT_3D ( 'NONE', #55587, #56315, #62215 ) ;
#61923=CARTESIAN_POINT ( 'NONE',  ( 12.90000000000000213, 0.000000000000000000, 4.999999999999998224 ) ) ;
#61924=CARTESIAN_POINT ( 'NONE',  ( 4.311958327294343363, 2.531208285321026263, 4.311958327294242999 ) ) ;
#61925=CARTESIAN_POINT ( 'NONE',  ( 21.89062500061451289, -3.027376345333610441, -5.243569643749999898 ) ) ;
#61926=CARTESIAN_POINT ( 'NONE',  ( 8.446875000614518569, -3.027376345333610441, -5.243569643749999898 ) ) ;
#61927=CARTESIAN_POINT ( 'NONE',  ( 8.512500001229033941, 0.000000000000000000, 4.999999999999998224 ) ) ;
#61929=CARTESIAN_POINT ( 'NONE',  ( 16.20000000122903216, -2.886751345948129988, 4.999999999999997335 ) ) ;
#61930=CARTESIAN_POINT ( 'NONE',  ( 12.89062500061451821, -3.027376345333610441, -5.243569643749999898 ) ) ;
#61931=CARTESIAN_POINT ( 'NONE',  ( 17.50312500061451715, 4.541064518000418104, -2.621784821874998173 ) ) ;
#61933=CIRCLE ( 'NONE', #5309, 9.999999999999998224 ) ;
#61934=CARTESIAN_POINT ( 'NONE',  ( 28.23750000122903359, 4.330127018922191873, 2.499999999999999556 ) ) ;
#61935=CARTESIAN_POINT ( 'NONE',  ( 23.09999999999999787, 4.330127018922192761, -2.499999999999997780 ) ) ;
#61937=CARTESIAN_POINT ( 'NONE',  ( 23.48437500061451644, 4.541064518000418104, 2.621784821874999949 ) ) ;
#61938=DIRECTION ( 'NONE',  ( -1.000000000000000000, -0.000000000000000000, -0.000000000000000000 ) ) ;
#61939=CARTESIAN_POINT ( 'NONE',  ( 9.750000001229032875, 5.773502691896255534, 3.535250795749688894E-16 ) ) ;
#61940=CARTESIAN_POINT ( 'NONE',  ( 28.20937500061451786, -4.541064518000417216, -2.621784821875001281 ) ) ;
#61941=CARTESIAN_POINT ( 'NONE',  ( 4.996875000614516615, 6.054752690667223547, 3.707466751127219781E-16 ) ) ;
#61942=CARTESIAN_POINT ( 'NONE',  ( 24.25312500061451715, 4.541064518000418104, -2.621784821874998173 ) ) ;
#61944=CARTESIAN_POINT ( 'NONE',  ( 9.384375000614518569, 6.421520780324663323E-16, -5.243569643749999010 ) ) ;
#61946=CARTESIAN_POINT ( 'NONE',  ( 29.12812500061451715, 6.421520780324663323E-16, -5.243569643749999010 ) ) ;
#61947=CARTESIAN_POINT ( 'NONE',  ( 6.159375000614517148, -4.541064518000417216, -2.621784821875001281 ) ) ;
#61948=CARTESIAN_POINT ( 'NONE',  ( 25.87500000000000000, 4.330127018922191873, 2.499999999999999556 ) ) ;
#61949=CARTESIAN_POINT ( 'NONE',  ( 27.90937500061451715, 4.541064518000418104, -2.621784821874998173 ) ) ;
#61951=CARTESIAN_POINT ( 'NONE',  ( 20.62499999999999645, -4.330127018922194537, 2.499999999999995559 ) ) ;
#61952=ORIENTED_EDGE ( 'NONE', *, *, #26233, .F. ) ;
#61953=CARTESIAN_POINT ( 'NONE',  ( 26.81250000000000000, 2.886751345948126879, 4.999999999999999112 ) ) ;
#61954=CARTESIAN_POINT ( 'NONE',  ( 29.48437500061451644, -4.541064518000419881, 2.621784821874995952 ) ) ;
#61956=CARTESIAN_POINT ( 'NONE',  ( 15.29062500061451679, 6.054752690667223547, 3.707466751127219781E-16 ) ) ;
#61957=CARTESIAN_POINT ( 'NONE',  ( 9.478125000614515017, 4.541064518000418104, 2.621784821874999949 ) ) ;
#61959=CARTESIAN_POINT ( 'NONE',  ( 4.021875000614516082, 3.027376345333613106, -5.243569643749998122 ) ) ;
#61960=CARTESIAN_POINT ( 'NONE',  ( 18.07500000122903216, -5.773502691896255534, -1.060575238724906372E-15 ) ) ;
#61962=CARTESIAN_POINT ( 'NONE',  ( 25.34999999999999787, 4.330127018922192761, -2.499999999999997780 ) ) ;
#61963=CARTESIAN_POINT ( 'NONE',  ( 23.88750000122903216, -4.330127018922194537, 2.499999999999995559 ) ) ;
#61964=CARTESIAN_POINT ( 'NONE',  ( 8.034375000614518925, 6.421520780324663323E-16, -5.243569643749999010 ) ) ;
#61965=CARTESIAN_POINT ( 'NONE',  ( 12.08437500061451608, 6.421520780324663323E-16, -5.243569643749999010 ) ) ;
#61966=CARTESIAN_POINT ( 'NONE',  ( 22.65937500061451715, 0.000000000000000000, 5.243569643749999010 ) ) ;
#61969=CARTESIAN_POINT ( 'NONE',  ( 4.171875000614517326, 3.027376345333611329, 5.243569643749999010 ) ) ;
#61970=CARTESIAN_POINT ( 'NONE',  ( 7.809375000614519280, 0.000000000000000000, 5.243569643749999010 ) ) ;
#61971=CARTESIAN_POINT ( 'NONE',  ( 19.72499999999999787, -4.330127018922194537, 2.499999999999995559 ) ) ;
#61972=CARTESIAN_POINT ( 'NONE',  ( 17.05312500061451786, 4.541064518000418104, -2.621784821874998173 ) ) ;
#61976=CARTESIAN_POINT ( 'NONE',  ( 9.103125000614515017, 0.000000000000000000, 5.243569643749999010 ) ) ;
#61977=CARTESIAN_POINT ( 'NONE',  ( 27.27187500061451431, -6.054752690667223547, -1.112240025338166033E-15 ) ) ;
#61979=CARTESIAN_POINT ( 'NONE',  ( 28.73437500061451644, 6.421520780324663323E-16, -5.243569643749999010 ) ) ;
#61980=CARTESIAN_POINT ( 'NONE',  ( 8.962500000000002132, -5.773502691896255534, -1.060575238724906372E-15 ) ) ;
#61981=CARTESIAN_POINT ( 'NONE',  ( 8.484601909799253346E-16, 15.27500000122903501, 34.61880215351700230 ) ) ;
#61982=CARTESIAN_POINT ( 'NONE',  ( 10.23750000122903359, 4.330127018922191873, 2.499999999999999556 ) ) ;
#61984=CARTESIAN_POINT ( 'NONE',  ( 18.90937500061451360, 4.541064518000418104, -2.621784821874998173 ) ) ;
#61985=CARTESIAN_POINT ( 'NONE',  ( 13.88437500061451679, 6.421520780324663323E-16, -5.243569643749999010 ) ) ;
#61986=CARTESIAN_POINT ( 'NONE',  ( -1.351880753582010319, 4.820610340066096455, -33.77395916724246661 ) ) ;
#61987=ORIENTED_EDGE ( 'NONE', *, *, #28959, .T. ) ;
#61988=CARTESIAN_POINT ( 'NONE',  ( 15.55312500061451608, -4.541064518000417216, -2.621784821875001281 ) ) ;
#61990=CARTESIAN_POINT ( 'NONE',  ( 26.36250000122903003, 4.330127018922192761, -2.499999999999997780 ) ) ;
#61991=CARTESIAN_POINT ( 'NONE',  ( 15.12187500061451750, -6.054752690667223547, -1.112240025338166033E-15 ) ) ;
#61992=CARTESIAN_POINT ( 'NONE',  ( 0.4052273161492611075, 10.00000000000000178, -23.99999999999999645 ) ) ;
#61993=CARTESIAN_POINT ( 'NONE',  ( 17.99062500061451786, 6.054752690667223547, 3.707466751127219781E-16 ) ) ;
#61995=CARTESIAN_POINT ( 'NONE',  ( 25.58437500061451431, 6.421520780324663323E-16, -5.243569643749999010 ) ) ;
#61996=CARTESIAN_POINT ( 'NONE',  ( -4.243569643749999898, 9.865625000614517859, 27.54997392385601529 ) ) ;
#61997=CARTESIAN_POINT ( 'NONE',  ( 15.00937500061451679, 0.000000000000000000, 5.243569643749999010 ) ) ;
#61998=CARTESIAN_POINT ( 'NONE',  ( 13.76250000122903394, 4.330127018922192761, -2.499999999999997780 ) ) ;
#62000=CARTESIAN_POINT ( 'NONE',  ( 2.121784821875001281, 19.10937500061451644, -26.32496088578401938 ) ) ;
#62001=CARTESIAN_POINT ( 'NONE',  ( 17.07187500061451502, 3.027376345333613106, -5.243569643749998122 ) ) ;
#62002=CARTESIAN_POINT ( 'NONE',  ( 19.72500000122903074, 2.886751345948126879, 4.999999999999999112 ) ) ;
#62003=CARTESIAN_POINT ( 'NONE',  ( 15.42187500061451821, 3.027376345333611329, 5.243569643749999010 ) ) ;
#62004=ADVANCED_FACE ( 'NONE', ( #30768 ), #13393, .F. ) ;
#62005=CARTESIAN_POINT ( 'NONE',  ( -2.121784821874996840, 12.73437500061451821, 33.67503911421598417 ) ) ;
#62006=CARTESIAN_POINT ( 'NONE',  ( 21.56250000122903288, 0.000000000000000000, 4.999999999999998224 ) ) ;
#62007=CARTESIAN_POINT ( 'NONE',  ( 15.14062500061451644, -3.027376345333610441, -5.243569643749999898 ) ) ;
#62008=VERTEX_POINT ( 'NONE', #18575 ) ;
#62009=ORIENTED_EDGE ( 'NONE', *, *, #11874, .F. ) ;
#62010=CARTESIAN_POINT ( 'NONE',  ( 20.06250000000000000, 2.886751345948126879, 4.999999999999999112 ) ) ;
#62012=CARTESIAN_POINT ( 'NONE',  ( 21.59062500061451928, 6.054752690667223547, 3.707466751127219781E-16 ) ) ;
#62013=CARTESIAN_POINT ( 'NONE',  ( 2.878125000614517592, -4.541064518000419881, 2.621784821874995952 ) ) ;
#62014=CARTESIAN_POINT ( 'NONE',  ( 13.83750000122903323, 4.330127018922191873, 2.499999999999999556 ) ) ;
#62015=CARTESIAN_POINT ( 'NONE',  ( 18.96562500061451573, 3.027376345333611329, 5.243569643749999010 ) ) ;
#62016=CARTESIAN_POINT ( 'NONE',  ( 24.29062500061451502, 6.054752690667223547, 3.707466751127219781E-16 ) ) ;
#62017=CARTESIAN_POINT ( 'NONE',  ( 5.540625000614515905, -3.027376345333614438, 5.243569643749998122 ) ) ;
#62019=EDGE_CURVE ( 'NONE', #14534, #15843, #37146, .T. ) ;
#62020=CARTESIAN_POINT ( 'NONE',  ( 1.071796769724491893, 14.28259618943233455, 33.99999999999999289 ) ) ;
#62021=CARTESIAN_POINT ( 'NONE',  ( 3.440625000614518036, -3.027376345333610441, -5.243569643749999898 ) ) ;
#62024=CARTESIAN_POINT ( 'NONE',  ( 3.999999999999998668, 13.06250000000000000, 27.69059892324149530 ) ) ;
#62025=CARTESIAN_POINT ( 'NONE',  ( 1.999999999999998668, 11.41250000122903430, -33.46410161513775705 ) ) ;
#62026=CARTESIAN_POINT ( 'NONE',  ( 2.121784821875001281, 17.30937500061451573, -26.32496088578401938 ) ) ;
#62027=CARTESIAN_POINT ( 'NONE',  ( 5.700000001229033941, 5.773502691896255534, 3.535250795749688894E-16 ) ) ;
#62029=CARTESIAN_POINT ( 'NONE',  ( 8.512499999999999289, -5.773502691896255534, -1.060575238724906372E-15 ) ) ;
#62030=( BOUNDED_CURVE ( )  B_SPLINE_CURVE ( 2, ( #91, #56583, #62130, #12238, #39245, #34769, #57302 ),
 .UNSPECIFIED., .F., .F. ) 
 B_SPLINE_CURVE_WITH_KNOTS ( ( 3, 2, 2, 3 ),
 ( 0.1833333333333333204, 0.1861111111111111160, 0.1888888888888888562, 0.1916666666666666519 ),
 .UNSPECIFIED. ) 
 CURVE ( )  GEOMETRIC_REPRESENTATION_ITEM ( )  RATIONAL_B_SPLINE_CURVE ( ( 1.000000000000000000, 0.8660254037844387076, 1.000000000000000000, 0.8660254037844387076, 1.000000000000000000, 0.8660254037844400399, 0.9999999999999986677 ) ) 
 REPRESENTATION_ITEM ( '' )  );
#62032=CARTESIAN_POINT ( 'NONE',  ( 3.187500001229033764, -4.330127018922194537, 2.499999999999995559 ) ) ;
#62033=CARTESIAN_POINT ( 'NONE',  ( 11.97187500061451892, -6.054752690667223547, -1.112240025338166033E-15 ) ) ;
#62034=LINE ( 'NONE', #51679, #543 ) ;
#62035=CARTESIAN_POINT ( 'NONE',  ( 3.651773823418189124, 3.415340091791402966, 3.978752903393068863 ) ) ;
#62036=CARTESIAN_POINT ( 'NONE',  ( 0.000000000000000000, 20.00000000000000000, -30.00000000000000000 ) ) ;
#62037=AXIS2_PLACEMENT_3D ( 'NONE', #53039, #24233, #52318 ) ;
#62038=B_SPLINE_CURVE_WITH_KNOTS ( 'NONE', 3,
 ( #54409, #19671, #69931, #42225 ),
 .UNSPECIFIED., .F., .F.,
 ( 4, 4 ),
 ( 2.168404344971008868E-19, 0.0006166911802265985596 ),
 .UNSPECIFIED. ) ;
#62039=CARTESIAN_POINT ( 'NONE',  ( 30.00000000000000000, 6.123233995736764310E-16, -4.999999999999998224 ) ) ;
#62040=CARTESIAN_POINT ( 'NONE',  ( 11.10937500061451644, -4.541064518000417216, -2.621784821875001281 ) ) ;
#62041=CARTESIAN_POINT ( 'NONE',  ( 20.43750000122903643, 6.123233995736764310E-16, -4.999999999999998224 ) ) ;
#62042=CARTESIAN_POINT ( 'NONE',  ( 3.999999999999999112, 14.37500000000000000, 30.00000000000000000 ) ) ;
#62043=CARTESIAN_POINT ( 'NONE',  ( 4.243569643749999898, 16.84062500061459389, 32.45002607614398471 ) ) ;
#62044=CARTESIAN_POINT ( 'NONE',  ( 22.02187500061452141, 3.027376345333613106, -5.243569643749998122 ) ) ;
#62046=CARTESIAN_POINT ( 'NONE',  ( 2.990625000614519191, -3.027376345333610441, -5.243569643749999898 ) ) ;
#62048=CARTESIAN_POINT ( 'NONE',  ( 22.56562500061451715, 3.027376345333611329, 5.243569643749999010 ) ) ;
#62049=CARTESIAN_POINT ( 'NONE',  ( 15.47812500061451679, -4.541064518000419881, 2.621784821874995952 ) ) ;
#62051=CARTESIAN_POINT ( 'NONE',  ( 11.29687500061451644, 6.054752690667223547, 3.707466751127219781E-16 ) ) ;
#62052=CARTESIAN_POINT ( 'NONE',  ( 28.76249999999999929, -5.773502691896255534, -1.060575238724906372E-15 ) ) ;
#62053=CARTESIAN_POINT ( 'NONE',  ( 26.10000000122903430, -2.886751345948129988, 4.999999999999997335 ) ) ;
#62054=CARTESIAN_POINT ( 'NONE',  ( 3.534375000614518036, 6.421520780324663323E-16, -5.243569643749999010 ) ) ;
#62055=CARTESIAN_POINT ( 'NONE',  ( 15.23437500061451644, 6.421520780324663323E-16, -5.243569643749999010 ) ) ;
#62056=CARTESIAN_POINT ( 'NONE',  ( 28.95937500061451431, 0.000000000000000000, 5.243569643749999010 ) ) ;
#62057=CARTESIAN_POINT ( 'NONE',  ( -1.071796769724475906, 11.35759618943233562, 25.99999999999999289 ) ) ;
#62058=CARTESIAN_POINT ( 'NONE',  ( -3.999999999999999112, 12.01250000122903394, 30.00000000000000000 ) ) ;
#62059=CARTESIAN_POINT ( 'NONE',  ( 22.35937500061451644, -4.541064518000417216, -2.621784821875001281 ) ) ;
#62060=CARTESIAN_POINT ( 'NONE',  ( 13.62187500061451750, 3.027376345333611329, 5.243569643749999010 ) ) ;
#62062=CARTESIAN_POINT ( 'NONE',  ( 27.26249999999999929, 2.886751345948126879, 4.999999999999999112 ) ) ;
#62063=CARTESIAN_POINT ( 'NONE',  ( 4.050000001229035362, -2.886751345948129988, 4.999999999999997335 ) ) ;
#62065=CARTESIAN_POINT ( 'NONE',  ( 18.44062500061451715, 6.054752690667223547, 3.707466751127219781E-16 ) ) ;
#62066=CARTESIAN_POINT ( 'NONE',  ( 7.050000000000000711, 0.000000000000000000, 4.999999999999998224 ) ) ;
#62067=CARTESIAN_POINT ( 'NONE',  ( 13.61250000122903359, -4.330127018922190985, -2.500000000000001332 ) ) ;
#62068=CARTESIAN_POINT ( 'NONE',  ( 16.38749999999999929, 5.773502691896255534, 3.535250795749688894E-16 ) ) ;
#62069=CARTESIAN_POINT ( 'NONE',  ( 2.121784821874999061, 13.80312500061451786, 26.32496088578401583 ) ) ;
#62071=CARTESIAN_POINT ( 'NONE',  ( 20.13750000122903216, 4.330127018922191873, 2.499999999999999556 ) ) ;
#62072=CARTESIAN_POINT ( 'NONE',  ( -2.000000000000000000, 13.28750000122903430, 26.53589838486224650 ) ) ;
#62073=CARTESIAN_POINT ( 'NONE',  ( 26.40937500061451715, -4.541064518000417216, -2.621784821875001281 ) ) ;
#62076=CARTESIAN_POINT ( 'NONE',  ( 22.71562500061451573, -6.054752690667223547, -1.112240025338166033E-15 ) ) ;
#62077=CARTESIAN_POINT ( 'NONE',  ( 21.79687500061451644, -3.027376345333614438, 5.243569643749998122 ) ) ;
#62078=CARTESIAN_POINT ( 'NONE',  ( 5.549999999999998934, 4.330127018922192761, -2.499999999999997780 ) ) ;
#62079=CARTESIAN_POINT ( 'NONE',  ( 9.178125000614517859, -4.541064518000419881, 2.621784821874995952 ) ) ;
#62080=CARTESIAN_POINT ( 'NONE',  ( 23.54062500061451146, -3.027376345333614438, 5.243569643749998122 ) ) ;
#62081=CARTESIAN_POINT ( 'NONE',  ( 13.54687500061451999, 6.054752690667223547, 3.707466751127219781E-16 ) ) ;
#62082=CARTESIAN_POINT ( 'NONE',  ( 17.40937500061451715, -4.541064518000417216, -2.621784821875001281 ) ) ;
#62083=CARTESIAN_POINT ( 'NONE',  ( 4.426899456784435749, 2.324341024790166799, -4.700261844762904317 ) ) ;
#62084=CARTESIAN_POINT ( 'NONE',  ( 2.121784821874999061, 18.30312500061451431, 26.32496088578401583 ) ) ;
#62085=CARTESIAN_POINT ( 'NONE',  ( 20.36250000122903359, -4.330127018922190985, -2.500000000000001332 ) ) ;
#62087=CARTESIAN_POINT ( 'NONE',  ( 11.95312500061451644, -4.541064518000417216, -2.621784821875001281 ) ) ;
#62088=CARTESIAN_POINT ( 'NONE',  ( 6.646875000614518747, -3.027376345333610441, -5.243569643749999898 ) ) ;
#62089=CARTESIAN_POINT ( 'NONE',  ( 4.771875000614516971, -6.054752690667223547, -1.112240025338166033E-15 ) ) ;
#62090=VERTEX_POINT ( 'NONE', #35578 ) ;
#62091=CARTESIAN_POINT ( 'NONE',  ( 28.69687500061451502, -3.027376345333610441, -5.243569643749999898 ) ) ;
#62092=CARTESIAN_POINT ( 'NONE',  ( 16.37812500061451715, -4.541064518000419881, 2.621784821874995952 ) ) ;
#62093=CARTESIAN_POINT ( 'NONE',  ( 28.12500000122902932, 2.886751345948129099, -4.999999999999998224 ) ) ;
#62094=CARTESIAN_POINT ( 'NONE',  ( 27.92812500061451431, 4.541064518000418104, 2.621784821874999949 ) ) ;
#62095=CARTESIAN_POINT ( 'NONE',  ( 20.85937500061451644, 0.000000000000000000, 5.243569643749999010 ) ) ;
#62096=CARTESIAN_POINT ( 'NONE',  ( 18.10312500061451502, 0.000000000000000000, 5.243569643749999010 ) ) ;
#62097=CARTESIAN_POINT ( 'NONE',  ( -0.6945855716117766976, 10.00052347946771825, 26.06076772914964934 ) ) ;
#62098=CARTESIAN_POINT ( 'NONE',  ( 23.72812500061451502, 6.421520780324663323E-16, -5.243569643749999010 ) ) ;
#62099=CARTESIAN_POINT ( 'NONE',  ( 4.800000001229032698, 5.773502691896255534, 3.535250795749688894E-16 ) ) ;
#62100=EDGE_LOOP ( 'NONE', ( #23302, #58773, #47934, #42024 ) ) ;
#62101=CARTESIAN_POINT ( 'NONE',  ( 27.56250000000000000, 2.886751345948129099, -4.999999999999998224 ) ) ;
#62102=CARTESIAN_POINT ( 'NONE',  ( 4.000000000000000000, 12.08750000000000036, -27.69059892324149530 ) ) ;
#62105=CARTESIAN_POINT ( 'NONE',  ( 3.946875000614517681, -3.027376345333610441, -5.243569643749999898 ) ) ;
#62106=CARTESIAN_POINT ( 'NONE',  ( 9.853125000614516793, 4.541064518000418104, -2.621784821874998173 ) ) ;
#62107=CARTESIAN_POINT ( 'NONE',  ( 24.86250000122903359, -4.330127018922190985, -2.500000000000001332 ) ) ;
#62108=CARTESIAN_POINT ( 'NONE',  ( 12.00937500061451857, -4.541064518000417216, -2.621784821875001281 ) ) ;
#62109=CARTESIAN_POINT ( 'NONE',  ( 29.61562500061451431, 3.027376345333613106, -5.243569643749998122 ) ) ;
#62110=CARTESIAN_POINT ( 'NONE',  ( 28.53749999999999787, 5.773502691896255534, 3.535250795749688894E-16 ) ) ;
#62111=DIRECTION ( 'NONE',  ( 0.000000000000000000, 0.000000000000000000, 1.000000000000000000 ) ) ;
#62112=CARTESIAN_POINT ( 'NONE',  ( 13.67812500061451786, -4.541064518000419881, 2.621784821874995952 ) ) ;
#62114=CARTESIAN_POINT ( 'NONE',  ( 10.00312500061451715, 0.000000000000000000, 5.243569643749999010 ) ) ;
#62115=CARTESIAN_POINT ( 'NONE',  ( 6.103125000614515905, -4.541064518000417216, -2.621784821875001281 ) ) ;
#62116=VECTOR ( 'NONE', #70518, 1000.000000000000000 ) ;
#62118=DIRECTION ( 'NONE',  ( -1.000000000000000000, -0.000000000000000000, -0.000000000000000000 ) ) ;
#62119=CARTESIAN_POINT ( 'NONE',  ( 16.27499999999999858, 6.123233995736764310E-16, -4.999999999999998224 ) ) ;
#62120=CARTESIAN_POINT ( 'NONE',  ( 16.05937500061451573, -4.541064518000417216, -2.621784821875001281 ) ) ;
#62121=CARTESIAN_POINT ( 'NONE',  ( 11.85000000122903430, -2.886751345948125991, -5.000000000000000000 ) ) ;
#62122=CARTESIAN_POINT ( 'NONE',  ( 19.69687500061451857, -3.027376345333610441, -5.243569643749999898 ) ) ;
#62124=CARTESIAN_POINT ( 'NONE',  ( 21.42187500061451644, -6.054752690667223547, -1.112240025338166033E-15 ) ) ;
#62125=CARTESIAN_POINT ( 'NONE',  ( -4.243569643749997233, 14.89062500061451644, -27.54997392385601174 ) ) ;
#62126=CARTESIAN_POINT ( 'NONE',  ( 7.312499999999998224, 2.886751345948062486, -5.000000000000113687 ) ) ;
#62128=CARTESIAN_POINT ( 'NONE',  ( 3.999999999999999112, 11.67500000000000071, -30.00000000000000000 ) ) ;
#62129=CARTESIAN_POINT ( 'NONE',  ( 27.92812500061451431, 4.541064518000418104, 2.621784821874999949 ) ) ;
#62130=CARTESIAN_POINT ( 'NONE',  ( 24.97499999999999787, 4.330127018922191873, 2.499999999999999556 ) ) ;
#62131=CARTESIAN_POINT ( 'NONE',  ( 28.95937500061451431, 0.000000000000000000, 5.243569643749999010 ) ) ;
#62132=CARTESIAN_POINT ( 'NONE',  ( 24.00000000000000000, 4.330127018922192761, -2.499999999999997780 ) ) ;
#62133=CARTESIAN_POINT ( 'NONE',  ( 8.915625000614515017, 3.027376345333613106, -5.243569643749998122 ) ) ;
#62135=CARTESIAN_POINT ( 'NONE',  ( 19.47187500061451360, 3.027376345333611329, 5.243569643749999010 ) ) ;
#62137=CARTESIAN_POINT ( 'NONE',  ( 6.253125000614517148, 4.541064518000418104, -2.621784821874998173 ) ) ;
#62138=CARTESIAN_POINT ( 'NONE',  ( 9.759375000614516793, -4.541064518000417216, -2.621784821875001281 ) ) ;
#62139=ORIENTED_EDGE ( 'NONE', *, *, #8132, .T. ) ;
#62140=CARTESIAN_POINT ( 'NONE',  ( 20.37187500061451573, 3.027376345333611329, 5.243569643749999010 ) ) ;
#62141=CARTESIAN_POINT ( 'NONE',  ( 28.87499999999999645, 6.123233995736764310E-16, -4.999999999999998224 ) ) ;
#62142=CARTESIAN_POINT ( 'NONE',  ( 29.88749999999999929, 5.773502691896255534, 3.535250795749688894E-16 ) ) ;
#62143=CARTESIAN_POINT ( 'NONE',  ( 4.987500000000002487, -2.886751345948125991, -5.000000000000000000 ) ) ;
#62144=CARTESIAN_POINT ( 'NONE',  ( 15.11250000122903359, 4.330127018922192761, -2.499999999999997780 ) ) ;
#62146=CARTESIAN_POINT ( 'NONE',  ( -5.810221930991193690E-16, 18.98750000000000071, -34.00000000000000000 ) ) ;
#62147=ORIENTED_EDGE ( 'NONE', *, *, #53394, .T. ) ;
#62148=CARTESIAN_POINT ( 'NONE',  ( 13.87500000000000178, -4.330127018922194537, 2.499999999999995559 ) ) ;
#62149=CARTESIAN_POINT ( 'NONE',  ( 24.59062500061451573, -3.027376345333610441, -5.243569643749999898 ) ) ;
#62150=CARTESIAN_POINT ( 'NONE',  ( 13.12500000000000178, 6.123233995736764310E-16, -4.999999999999998224 ) ) ;
#62151=CARTESIAN_POINT ( 'NONE',  ( 10.27500000122903323, 2.886751345948126879, 4.999999999999999112 ) ) ;
#62152=CARTESIAN_POINT ( 'NONE',  ( 8.465625000614515727, 3.027376345333613106, -5.243569643749998122 ) ) ;
#62153=ADVANCED_FACE ( 'NONE', ( #47037 ), #42223, .F. ) ;
#62154=CARTESIAN_POINT ( 'NONE',  ( 8.362500000000002487, 2.886751345948126879, 4.999999999999999112 ) ) ;
#62156=CARTESIAN_POINT ( 'NONE',  ( 4.243569643749999898, 13.78437500061451715, -30.00000000000000000 ) ) ;
#62157=CARTESIAN_POINT ( 'NONE',  ( 28.98750000122903359, 6.123233995736764310E-16, -4.999999999999998224 ) ) ;
#62159=CARTESIAN_POINT ( 'NONE',  ( 8.662499999999999645, 2.886751345948129099, -4.999999999999998224 ) ) ;
#62160=CARTESIAN_POINT ( 'NONE',  ( -3.999999999999999112, 12.76250000000000107, 27.69059892324149885 ) ) ;
#62161=ORIENTED_EDGE ( 'NONE', *, *, #36401, .F. ) ;
#62162=CARTESIAN_POINT ( 'NONE',  ( 22.11562500061451786, 3.027376345333611329, 5.243569643749999010 ) ) ;
#62163=CARTESIAN_POINT ( 'NONE',  ( 15.00000000122903465, -2.886751345948125991, -5.000000000000000000 ) ) ;
#62164=CARTESIAN_POINT ( 'NONE',  ( 28.56562500061451715, -6.054752690667223547, -1.112240025338166033E-15 ) ) ;
#62166=DIRECTION ( 'NONE',  ( -1.000000000000000000, -0.000000000000000000, -0.000000000000000000 ) ) ;
#62167=CARTESIAN_POINT ( 'NONE',  ( 18.38437500061451857, 6.421520780324663323E-16, -5.243569643749999010 ) ) ;
#62168=CARTESIAN_POINT ( 'NONE',  ( 16.22812500061451857, 4.541064518000418104, 2.621784821874999949 ) ) ;
#62169=CARTESIAN_POINT ( 'NONE',  ( -4.243569643749999898, 12.11562500061459247, -32.45002607614398471 ) ) ;
#62170=CARTESIAN_POINT ( 'NONE',  ( 6.890625000614516438, -3.027376345333614438, 5.243569643749998122 ) ) ;
#62171=CARTESIAN_POINT ( 'NONE',  ( 29.51250000122903216, 4.330127018922192761, -2.499999999999997780 ) ) ;
#62173=CARTESIAN_POINT ( 'NONE',  ( 18.96562500061451573, 3.027376345333611329, 5.243569643749999010 ) ) ;
#62174=CARTESIAN_POINT ( 'NONE',  ( 13.46249999999999858, -5.773502691896255534, -1.060575238724906372E-15 ) ) ;
#62175=CARTESIAN_POINT ( 'NONE',  ( 3.412500001229032964, 4.330127018922192761, -2.499999999999997780 ) ) ;
#62176=CARTESIAN_POINT ( 'NONE',  ( 12.79687500061451821, -3.027376345333614438, 5.243569643749998122 ) ) ;
#62177=CARTESIAN_POINT ( 'NONE',  ( 12.45937500061451786, -4.541064518000417216, -2.621784821875001281 ) ) ;
#62178=CARTESIAN_POINT ( 'NONE',  ( 20.18437500061451573, 6.421520780324663323E-16, -5.243569643749999010 ) ) ;
#62179=ORIENTED_EDGE ( 'NONE', *, *, #25113, .F. ) ;
#62180=CARTESIAN_POINT ( 'NONE',  ( 30.00000000000000000, 0.000000000000000000, 0.000000000000000000 ) ) ;
#62181=CARTESIAN_POINT ( 'NONE',  ( 24.10312500061451502, -4.541064518000417216, -2.621784821875001281 ) ) ;
#62182=CARTESIAN_POINT ( 'NONE',  ( 24.21562500061451573, 3.027376345333613106, -5.243569643749998122 ) ) ;
#62184=CARTESIAN_POINT ( 'NONE',  ( 1.999999999999998668, 17.15000000000000213, 26.53589838486224650 ) ) ;
#62185=CARTESIAN_POINT ( 'NONE',  ( 5.109375000614518214, 0.000000000000000000, 5.243569643749999010 ) ) ;
#62186=CARTESIAN_POINT ( 'NONE',  ( 12.26250000122903394, -4.330127018922190985, -2.500000000000001332 ) ) ;
#62187=B_SPLINE_CURVE_WITH_KNOTS ( 'NONE', 3,
 ( #45664, #27947, #963, #44939, #28304, #33114, #39032, #55652, #50839, #5048 ),
 .UNSPECIFIED., .F., .F.,
 ( 4, 3, 3, 4 ),
 ( 1.829295516389420302E-16, 0.0001572384447036336735, 0.0003144798658762968193, 0.0005339943342314175910 ),
 .UNSPECIFIED. ) ;
#62188=CARTESIAN_POINT ( 'NONE',  ( 7.837500001229035007, 6.123233995736764310E-16, -4.999999999999998224 ) ) ;
#62189=CARTESIAN_POINT ( 'NONE',  ( -0.1398361002794819008, 5.000000000000000888, 26.00000000000000000 ) ) ;
#62190=CARTESIAN_POINT ( 'NONE',  ( 27.45000000122903572, -2.886751345948129988, 4.999999999999997335 ) ) ;
#62193=CARTESIAN_POINT ( 'NONE',  ( 10.84687500061451892, 6.054752690667223547, 3.707466751127219781E-16 ) ) ;
#62194=CARTESIAN_POINT ( 'NONE',  ( 0.000000000000000000, 20.00000000000000000, 30.00000000000000000 ) ) ;
#62195=CARTESIAN_POINT ( 'NONE',  ( 17.57812500061451644, 4.541064518000418104, 2.621784821874999949 ) ) ;
#62196=CARTESIAN_POINT ( 'NONE',  ( 13.39687500061451608, -3.027376345333610441, -5.243569643749999898 ) ) ;
#62197=CARTESIAN_POINT ( 'NONE',  ( 4.115625000614516082, 3.027376345333611329, 5.243569643749999010 ) ) ;
#62198=CARTESIAN_POINT ( 'NONE',  ( 22.92187500061451644, 3.027376345333612662, -5.243569643749998122 ) ) ;
#62199=CARTESIAN_POINT ( 'NONE',  ( 9.159375000614515372, 0.000000000000000000, 5.243569643749999010 ) ) ;
#62200=CARTESIAN_POINT ( 'NONE',  ( 5.728125000614515905, 6.421520780324663323E-16, -5.243569643749999010 ) ) ;
#62201=( BOUNDED_CURVE ( )  B_SPLINE_CURVE ( 2, ( #25839, #37283, #7116, #63618, #64988, #59805, #66087 ),
 .UNSPECIFIED., .F., .F. ) 
 B_SPLINE_CURVE_WITH_KNOTS ( ( 3, 2, 2, 3 ),
 ( 0.7750000000000001332, 0.7777777777777779011, 0.7805555555555556690, 0.7833333333333334370 ),
 .UNSPECIFIED. ) 
 CURVE ( )  GEOMETRIC_REPRESENTATION_ITEM ( )  RATIONAL_B_SPLINE_CURVE ( ( 0.9999999999999946709, 0.8660254037844440367, 1.000000000000000000, 0.8660254037844387076, 1.000000000000000000, 0.8660254037844333785, 1.000000000000005329 ) ) 
 REPRESENTATION_ITEM ( '' )  );
#62202=CARTESIAN_POINT ( 'NONE',  ( 5.287500001229035185, 4.330127018922191873, 2.499999999999999556 ) ) ;
#62203=CARTESIAN_POINT ( 'NONE',  ( 20.35312500061451502, 0.000000000000000000, 5.243569643749999010 ) ) ;
#62204=CARTESIAN_POINT ( 'NONE',  ( 8.550000001229031810, -2.886751345948129988, 4.999999999999997335 ) ) ;
#62205=CARTESIAN_POINT ( 'NONE',  ( 17.12812500061451715, 4.541064518000418104, 2.621784821874999949 ) ) ;
#62206=CARTESIAN_POINT ( 'NONE',  ( 14.09062500061451750, -3.027376345333614438, 5.243569643749998122 ) ) ;
#62208=CARTESIAN_POINT ( 'NONE',  ( 14.32500000000000107, -4.330127018922194537, 2.499999999999995559 ) ) ;
#62209=CARTESIAN_POINT ( 'NONE',  ( 8.550000001229031810, -2.886751345948129988, 4.999999999999997335 ) ) ;
#62211=CARTESIAN_POINT ( 'NONE',  ( 6.440625000614517148, -3.027376345333614438, 5.243569643749998122 ) ) ;
#62212=CARTESIAN_POINT ( 'NONE',  ( 19.23750000122903714, 4.330127018922191873, 2.499999999999999556 ) ) ;
#62214=CARTESIAN_POINT ( 'NONE',  ( 4.243569643749999898, 10.14687500061451786, -27.54997392385601529 ) ) ;
#62215=DIRECTION ( 'NONE',  ( 0.000000000000000000, 0.000000000000000000, 1.000000000000000000 ) ) ;
#62216=CARTESIAN_POINT ( 'NONE',  ( 3.750000001229034652, -2.886751345948125991, -5.000000000000000000 ) ) ;
#62217=CARTESIAN_POINT ( 'NONE',  ( -3.999999999999997335, 11.48750000000000071, -27.69059892324149530 ) ) ;
#62218=CARTESIAN_POINT ( 'NONE',  ( 20.85937500061451644, 0.000000000000000000, 5.243569643749999010 ) ) ;
#62219=CARTESIAN_POINT ( 'NONE',  ( -1.999999999999997113, 16.58750000122903501, 33.46410161513775705 ) ) ;
#62220=CARTESIAN_POINT ( 'NONE',  ( 16.00312500061451715, -4.541064518000417216, -2.621784821875001281 ) ) ;
#62222=CARTESIAN_POINT ( 'NONE',  ( 11.02500000000000036, 4.330127018922191873, 2.499999999999999556 ) ) ;
#62223=CARTESIAN_POINT ( 'NONE',  ( 26.66250000000000142, 2.886751345948129099, -4.999999999999997335 ) ) ;
#62224=CARTESIAN_POINT ( 'NONE',  ( 25.35937500061451644, 0.000000000000000000, 5.243569643749999010 ) ) ;
#62226=CARTESIAN_POINT ( 'NONE',  ( 13.00312500061451537, 4.541064518000418104, -2.621784821874998173 ) ) ;
#62227=CARTESIAN_POINT ( 'NONE',  ( 9.684375000614517504, -4.541064518000419881, 2.621784821874995952 ) ) ;
#62229=CARTESIAN_POINT ( 'NONE',  ( 2.941572294020245337, -4.043263892169386864, -3.278731392431392333 ) ) ;
#62230=CARTESIAN_POINT ( 'NONE',  ( 20.57812500061451644, 6.421520780324663323E-16, -5.243569643749999010 ) ) ;
#62231=CARTESIAN_POINT ( 'NONE',  ( 4.000000000000000000, 11.18750000000000178, -27.69059892324149885 ) ) ;
#62232=CARTESIAN_POINT ( 'NONE',  ( -1.071796769724475906, 12.82009619066136707, 25.99999999999999289 ) ) ;
#62233=( BOUNDED_CURVE ( )  B_SPLINE_CURVE ( 2, ( #56228, #28157, #71767, #7420, #46224, #57298, #17410, #17759, #22950 ),
 .UNSPECIFIED., .F., .F. ) 
 B_SPLINE_CURVE_WITH_KNOTS ( ( 3, 2, 2, 2, 3 ),
 ( 0.2934782608695652439, 0.2971014492753623060, 0.3043478260869565410, 0.3115942028985507206, 0.3152173913043478382 ),
 .UNSPECIFIED. ) 
 CURVE ( )  GEOMETRIC_REPRESENTATION_ITEM ( )  RATIONAL_B_SPLINE_CURVE ( ( 0.9330127018922194093, 0.9330127018922198534, 1.000000000000000000, 0.8660254037844387076, 1.000000000000000000, 0.8660254037844387076, 1.000000000000000000, 0.9330127018922188542, 0.9330127018922194093 ) ) 
 REPRESENTATION_ITEM ( '' )  );
#62234=CARTESIAN_POINT ( 'NONE',  ( 11.25000000000000000, -4.330127018922190985, -2.500000000000001332 ) ) ;
#62235=CARTESIAN_POINT ( 'NONE',  ( 21.67500000122903359, -5.773502691896255534, -1.060575238724906372E-15 ) ) ;
#62236=CARTESIAN_POINT ( 'NONE',  ( 15.55312500061451608, -4.541064518000417216, -2.621784821875001281 ) ) ;
#62239=CARTESIAN_POINT ( 'NONE',  ( 20.21250000000000213, -5.773502691896255534, -1.060575238724906372E-15 ) ) ;
#62240=CARTESIAN_POINT ( 'NONE',  ( 23.62500000000000000, 4.330127018922191873, 2.499999999999999556 ) ) ;
#62241=( BOUNDED_CURVE ( )  B_SPLINE_CURVE ( 2, ( #33972, #56511, #45436, #11813, #49527, #40564, #52730 ),
 .UNSPECIFIED., .F., .F. ) 
 B_SPLINE_CURVE_WITH_KNOTS ( ( 3, 2, 2, 3 ),
 ( 0.7916666666666666297, 0.7944444444444443976, 0.7972222222222222765, 0.8000000000000000444 ),
 .UNSPECIFIED. ) 
 CURVE ( )  GEOMETRIC_REPRESENTATION_ITEM ( )  RATIONAL_B_SPLINE_CURVE ( ( 1.000000000000000000, 0.8660254037844387076, 1.000000000000000000, 0.8660254037844387076, 1.000000000000000000, 0.8660254037844387076, 1.000000000000000000 ) ) 
 REPRESENTATION_ITEM ( '' )  );
#62242=CARTESIAN_POINT ( 'NONE',  ( 22.58437500061451431, 4.541064518000418104, 2.621784821874999949 ) ) ;
#62243=CARTESIAN_POINT ( 'NONE',  ( 24.96562500061451573, -6.054752690667223547, -1.112240025338166033E-15 ) ) ;
#62244=ORIENTED_EDGE ( 'NONE', *, *, #8791, .F. ) ;
#62245=CARTESIAN_POINT ( 'NONE',  ( 7.640625000614517326, 6.054752690667223547, 3.707466751127219781E-16 ) ) ;
#62247=CARTESIAN_POINT ( 'NONE',  ( 14.47499999999999964, 6.123233995736764310E-16, -4.999999999999998224 ) ) ;
#62248=CARTESIAN_POINT ( 'NONE',  ( -3.000416591977282496E-16, 16.99062500061451786, 25.09994784771203058 ) ) ;
#62249=CARTESIAN_POINT ( 'NONE',  ( 4.696875000614518569, -3.027376345333614438, 5.243569643749998122 ) ) ;
#62250=CARTESIAN_POINT ( 'NONE',  ( 26.82187500061451857, -6.054752690667223547, -1.112240025338166033E-15 ) ) ;
#62251=ORIENTED_EDGE ( 'NONE', *, *, #73107, .F. ) ;
#62252=CARTESIAN_POINT ( 'NONE',  ( 23.16562500061451502, -6.054752690667223547, -1.112240025338166033E-15 ) ) ;
#62253=CARTESIAN_POINT ( 'NONE',  ( 26.03437500061451715, 6.421520780324663323E-16, -5.243569643749999010 ) ) ;
#62254=CARTESIAN_POINT ( 'NONE',  ( -4.243569643749998122, 18.49062500061459247, -27.54997392385601174 ) ) ;
#62255=CARTESIAN_POINT ( 'NONE',  ( 11.77500000000000036, 6.123233995736764310E-16, -4.999999999999998224 ) ) ;
#62256=CARTESIAN_POINT ( 'NONE',  ( 9.853125000614516793, 4.541064518000418104, -2.621784821874998173 ) ) ;
#62258=CARTESIAN_POINT ( 'NONE',  ( 27.89062500061451289, 6.054752690667223547, 3.707466751127219781E-16 ) ) ;
#62259=CARTESIAN_POINT ( 'NONE',  ( 25.86562500061451431, -6.054752690667223547, -1.112240025338166033E-15 ) ) ;
#62262=CARTESIAN_POINT ( 'NONE',  ( 2.915625000614516793, -6.054752690667223547, -1.112240025338166033E-15 ) ) ;
#62263=CARTESIAN_POINT ( 'NONE',  ( 18.57187500061451857, 3.027376345333611329, 5.243569643749999010 ) ) ;
#62264=CARTESIAN_POINT ( 'NONE',  ( -4.243569643749997233, 14.04687500061451999, 32.45002607614398471 ) ) ;
#62265=EDGE_CURVE ( 'NONE', #38080, #63662, #64989, .T. ) ;
#62266=CARTESIAN_POINT ( 'NONE',  ( 18.90937500061451360, 4.541064518000418104, -2.621784821874998173 ) ) ;
#62267=CARTESIAN_POINT ( 'NONE',  ( 29.74687500061451217, 6.054752690667223547, 3.707466751127219781E-16 ) ) ;
#62268=CARTESIAN_POINT ( 'NONE',  ( -4.243569643749998122, 17.19687500061451502, 32.45002607614398471 ) ) ;
#62269=CARTESIAN_POINT ( 'NONE',  ( 9.928125000614517859, 4.541064518000418104, 2.621784821874999949 ) ) ;
#62272=CARTESIAN_POINT ( 'NONE',  ( 6.721875000614518925, 3.027376345333613106, -5.243569643749998122 ) ) ;
#62273=DIRECTION ( 'NONE',  ( 0.000000000000000000, 0.000000000000000000, 1.000000000000000000 ) ) ;
#62274=CARTESIAN_POINT ( 'NONE',  ( 8.428125000614517859, 6.421520780324663323E-16, -5.243569643749999010 ) ) ;
#62275=CARTESIAN_POINT ( 'NONE',  ( 11.14687500061451608, -3.027376345333610441, -5.243569643749999898 ) ) ;
#62276=CARTESIAN_POINT ( 'NONE',  ( 20.02500000122903145, 2.886751345948129099, -4.999999999999998224 ) ) ;
#62277=CARTESIAN_POINT ( 'NONE',  ( 5.484375000614518214, 4.541064518000418104, 2.621784821874999949 ) ) ;
#62278=CARTESIAN_POINT ( 'NONE',  ( 8.690625000614515372, -3.027376345333614438, 5.243569643749998122 ) ) ;
#62281=CARTESIAN_POINT ( 'NONE',  ( 18.00937500061451502, 4.541064518000418104, -2.621784821874998173 ) ) ;
#62282=CARTESIAN_POINT ( 'NONE',  ( 3.999999999999998668, 13.17500000122903536, 27.69059892324149530 ) ) ;
#62283=ORIENTED_EDGE ( 'NONE', *, *, #13482, .F. ) ;
#62284=CARTESIAN_POINT ( 'NONE',  ( 27.10312500061451502, 0.000000000000000000, 5.243569643749999010 ) ) ;
#62285=CARTESIAN_POINT ( 'NONE',  ( 13.15312500061451750, 0.000000000000000000, 5.243569643749999010 ) ) ;
#62286=CARTESIAN_POINT ( 'NONE',  ( 29.78437500061451715, 4.541064518000418104, 2.621784821874999949 ) ) ;
#62287=CARTESIAN_POINT ( 'NONE',  ( 12.40312500061451573, -4.541064518000417216, -2.621784821875001281 ) ) ;
#62288=CARTESIAN_POINT ( 'NONE',  ( 2.121784821874999061, 10.70937500061451964, -33.67503911421598417 ) ) ;
#62289=CARTESIAN_POINT ( 'NONE',  ( 12.86250000122903359, 4.330127018922192761, -2.499999999999997780 ) ) ;
#62290=CARTESIAN_POINT ( 'NONE',  ( 26.57812500061451644, 4.541064518000418104, 2.621784821874999949 ) ) ;
#62291=CARTESIAN_POINT ( 'NONE',  ( -2.121784821874996840, 13.57812500061451644, -26.32496088578401583 ) ) ;
#62292=CARTESIAN_POINT ( 'NONE',  ( 15.26250000122903216, 0.000000000000000000, 4.999999999999998224 ) ) ;
#62293=CARTESIAN_POINT ( 'NONE',  ( 14.24999999999999822, 0.000000000000000000, 4.999999999999998224 ) ) ;
#62294=CARTESIAN_POINT ( 'NONE',  ( 21.32812500061451644, -4.541064518000419881, 2.621784821874995952 ) ) ;
#62295=CARTESIAN_POINT ( 'NONE',  ( 8.671875000614518214, 3.027376345333611329, 5.243569643749999010 ) ) ;
#62296=CARTESIAN_POINT ( 'NONE',  ( 8.400000001229035007, 5.773502691896255534, 3.535250795749688894E-16 ) ) ;
#62297=CARTESIAN_POINT ( 'NONE',  ( 15.45000000122903216, -2.886751345948125991, -5.000000000000000000 ) ) ;
#62298=CARTESIAN_POINT ( 'NONE',  ( 11.87812500061451537, -4.541064518000419881, 2.621784821874995952 ) ) ;
#62299=CARTESIAN_POINT ( 'NONE',  ( 16.90312500061451573, -4.541064518000417216, -2.621784821875001281 ) ) ;
#62300=CARTESIAN_POINT ( 'NONE',  ( 27.07500000122903216, -5.773502691896255534, -1.060575238724906372E-15 ) ) ;
#62301=CARTESIAN_POINT ( 'NONE',  ( 21.60000000000000142, -4.330127018922190985, -2.500000000000001332 ) ) ;
#62302=CARTESIAN_POINT ( 'NONE',  ( 24.27187500061452141, 3.027376345333613106, -5.243569643749998122 ) ) ;
#62304=ADVANCED_FACE ( 'NONE', ( #47397 ), #69929, .F. ) ;
#62305=CARTESIAN_POINT ( 'NONE',  ( 11.06250000122903288, 4.330127018922192761, -2.499999999999997780 ) ) ;
#62306=CARTESIAN_POINT ( 'NONE',  ( 28.17187500061451644, -6.054752690667223547, -1.112240025338166033E-15 ) ) ;
#62307=CARTESIAN_POINT ( 'NONE',  ( 4.509375000614518569, 4.541064518000418104, -2.621784821874998173 ) ) ;
#62308=CARTESIAN_POINT ( 'NONE',  ( 22.75312500061451360, -4.541064518000417216, -2.621784821875001281 ) ) ;
#62311=CARTESIAN_POINT ( 'NONE',  ( 10.80937500061451928, 4.541064518000418104, -2.621784821874998173 ) ) ;
#62312=CARTESIAN_POINT ( 'NONE',  ( 4.433683854237718158, 3.756322295769854325, -3.980998221622843669 ) ) ;
#62313=CARTESIAN_POINT ( 'NONE',  ( 29.16562500061451502, 3.027376345333613106, -5.243569643749998122 ) ) ;
#62314=CARTESIAN_POINT ( 'NONE',  ( 6.121875000614517504, -6.054752690667223547, -1.112240025338166033E-15 ) ) ;
#62316=CARTESIAN_POINT ( 'NONE',  ( 26.59687500061451360, 6.054752690667223547, 3.707466751127219781E-16 ) ) ;
#62317=CARTESIAN_POINT ( 'NONE',  ( -4.243569643749998122, 10.39062500061459637, 32.45002607614398471 ) ) ;
#62318=CARTESIAN_POINT ( 'NONE',  ( 18.33749999999999858, -2.886751345948129988, 4.999999999999997335 ) ) ;
#62319=VERTEX_POINT ( 'NONE', #10071 ) ;
#62320=CARTESIAN_POINT ( 'NONE',  ( 27.07499999999999929, 6.123233995736764310E-16, -4.999999999999998224 ) ) ;
#62321=CARTESIAN_POINT ( 'NONE',  ( 28.58437500061451786, -4.541064518000419881, 2.621784821874995952 ) ) ;
#62323=CARTESIAN_POINT ( 'NONE',  ( 16.52812500061451573, 6.421520780324663323E-16, -5.243569643749999010 ) ) ;
#62324=CARTESIAN_POINT ( 'NONE',  ( 8.990625000614516082, 6.054752690667223547, 3.707466751127219781E-16 ) ) ;
#62326=CARTESIAN_POINT ( 'NONE',  ( 5.071875000614519458, 3.027376345333611329, 5.243569643749999010 ) ) ;
#62327=CARTESIAN_POINT ( 'NONE',  ( 17.13750000122903216, -4.330127018922194537, 2.499999999999995559 ) ) ;
#62328=CARTESIAN_POINT ( 'NONE',  ( 22.68750000000000000, 5.773502691896255534, 3.535250795749688894E-16 ) ) ;
#62329=CARTESIAN_POINT ( 'NONE',  ( 27.97500000000000142, 6.123233995736764310E-16, -4.999999999999998224 ) ) ;
#62330=CARTESIAN_POINT ( 'NONE',  ( 3.646875000614520079, 6.054752690667223547, 3.707466751127219781E-16 ) ) ;
#62331=CARTESIAN_POINT ( 'NONE',  ( 11.22187500061451892, 3.027376345333613106, -5.243569643749998122 ) ) ;
#62332=CARTESIAN_POINT ( 'NONE',  ( 21.00937500061451857, -4.541064518000417216, -2.621784821875001281 ) ) ;
#62333=CARTESIAN_POINT ( 'NONE',  ( -1.071796769724483234, 15.07009619066136885, -34.00000000000000711 ) ) ;
#62334=EDGE_LOOP ( 'NONE', ( #50351, #53099, #16445, #71790, #36618, #20731, #40306, #70408, #10419, #45533, #11843, #19266, #60773, #42531, #9308, #25908, #21101, #39955, #5841, #57670, #67448, #20505, #58993, #4759, #70090, #15329, #51999, #56451, #65604, #4118, #56543, #48980, #33347, #42488, #57839, #63756, #62139, #1932, #3177, #46478, #63092, #70395, #72828 ) ) ;
#62335=CARTESIAN_POINT ( 'NONE',  ( 4.621875000614516615, 3.027376345333611329, 5.243569643749999010 ) ) ;
#62336=CARTESIAN_POINT ( 'NONE',  ( 7.734375000614517326, 4.541064518000418104, 2.621784821874999949 ) ) ;
#62337=CARTESIAN_POINT ( 'NONE',  ( 18.37500000000000355, -4.330127018922194537, 2.499999999999995559 ) ) ;
#62338=CARTESIAN_POINT ( 'NONE',  ( 15.74062500061451608, 6.054752690667223547, 3.707466751127219781E-16 ) ) ;
#62340=CARTESIAN_POINT ( 'NONE',  ( 24.78750000122903074, -4.330127018922194537, 2.499999999999995559 ) ) ;
#62341=EDGE_CURVE ( 'NONE', #13665, #40887, #37037, .T. ) ;
#62343=CARTESIAN_POINT ( 'NONE',  ( 9.965625000614517504, 3.027376345333611329, 5.243569643749999010 ) ) ;
#62344=CARTESIAN_POINT ( 'NONE',  ( 25.80937500061451928, 0.000000000000000000, 5.243569643749999010 ) ) ;
#62345=CARTESIAN_POINT ( 'NONE',  ( 27.53437500061451360, 4.541064518000418104, 2.621784821874999949 ) ) ;
#62346=CARTESIAN_POINT ( 'NONE',  ( 8.812500000000000000, 2.886751345948126879, 4.999999999999999112 ) ) ;
#62347=CARTESIAN_POINT ( 'NONE',  ( -1.999999999999997113, 16.58750000122903501, 33.46410161513775705 ) ) ;
#62348=CARTESIAN_POINT ( 'NONE',  ( 8.362500001229031810, 4.330127018922192761, -2.499999999999997780 ) ) ;
#62349=CARTESIAN_POINT ( 'NONE',  ( 19.62187500061451573, -6.054752690667223547, -1.112240025338166033E-15 ) ) ;
#62350=CARTESIAN_POINT ( 'NONE',  ( 15.12187500061451750, -6.054752690667223547, -1.112240025338166033E-15 ) ) ;
#62352=ORIENTED_EDGE ( 'NONE', *, *, #60856, .F. ) ;
#62353=CARTESIAN_POINT ( 'NONE',  ( 14.46562500061451750, 3.027376345333611329, 5.243569643749999010 ) ) ;
#62354=CARTESIAN_POINT ( 'NONE',  ( 26.21250000122903501, -4.330127018922190985, -2.500000000000001332 ) ) ;
#62355=CARTESIAN_POINT ( 'NONE',  ( 16.05937500061451573, -4.541064518000417216, -2.621784821875001281 ) ) ;
#62356=CARTESIAN_POINT ( 'NONE',  ( 4.150718249861528264, 3.881368968983215151, 3.764411030299838590 ) ) ;
#62357=CARTESIAN_POINT ( 'NONE',  ( 17.35312500061451502, -4.541064518000417216, -2.621784821875001281 ) ) ;
#62359=CARTESIAN_POINT ( 'NONE',  ( 25.43437500061451573, -4.541064518000419881, 2.621784821874995952 ) ) ;
#62360=CARTESIAN_POINT ( 'NONE',  ( 2.121784821875001281, 10.95312500061451821, 33.67503911421598417 ) ) ;
#62361=CARTESIAN_POINT ( 'NONE',  ( 14.48437500061451821, 4.541064518000418104, 2.621784821874999949 ) ) ;
#62362=CARTESIAN_POINT ( 'NONE',  ( 13.98750000122903359, -4.330127018922194537, 2.499999999999995559 ) ) ;
#62364=CARTESIAN_POINT ( 'NONE',  ( -2.121784821874999949, 17.08437500061451786, -33.67503911421598417 ) ) ;
#62365=CARTESIAN_POINT ( 'NONE',  ( 18.15937500061451715, 0.000000000000000000, 5.243569643749999010 ) ) ;
#62366=CARTESIAN_POINT ( 'NONE',  ( 20.28750000122903074, -4.330127018922194537, 2.499999999999995559 ) ) ;
#62367=CARTESIAN_POINT ( 'NONE',  ( 14.10937500061451644, 0.000000000000000000, 5.243569643749999010 ) ) ;
#62368=CARTESIAN_POINT ( 'NONE',  ( 2.121784821874999061, 11.15937500061451715, 26.32496088578401583 ) ) ;
#62369=CARTESIAN_POINT ( 'NONE',  ( 23.36250000122903359, 0.000000000000000000, 4.999999999999998224 ) ) ;
#62370=CARTESIAN_POINT ( 'NONE',  ( 15.36562500061451608, 3.027376345333611329, 5.243569643749999010 ) ) ;
#62371=CARTESIAN_POINT ( 'NONE',  ( 29.61562500061451431, 3.027376345333613106, -5.243569643749998122 ) ) ;
#62372=ORIENTED_EDGE ( 'NONE', *, *, #56499, .T. ) ;
#62373=ORIENTED_EDGE ( 'NONE', *, *, #61105, .F. ) ;
#62374=CARTESIAN_POINT ( 'NONE',  ( 20.21250000000000213, -5.773502691896255534, -1.060575238724906372E-15 ) ) ;
#62375=CARTESIAN_POINT ( 'NONE',  ( 17.55000000000000071, -4.330127018922190985, -2.500000000000001332 ) ) ;
#62376=CARTESIAN_POINT ( 'NONE',  ( 3.578402880298070077, 3.495305883107370448, 28.19419513515084219 ) ) ;
#62377=CARTESIAN_POINT ( 'NONE',  ( 15.03750000122903252, 6.123233995736764310E-16, -4.999999999999998224 ) ) ;
#62378=CARTESIAN_POINT ( 'NONE',  ( 20.95312500061451999, -4.541064518000417216, -2.621784821875001281 ) ) ;
#62379=CARTESIAN_POINT ( 'NONE',  ( 23.12812500061451360, -4.541064518000419881, 2.621784821874995952 ) ) ;
#62380=CARTESIAN_POINT ( 'NONE',  ( 5.503125000614516260, 0.000000000000000000, 5.243569643749999010 ) ) ;
#62381=CARTESIAN_POINT ( 'NONE',  ( 29.51249999999999929, 2.886751345948126879, 4.999999999999999112 ) ) ;
#62384=FACE_OUTER_BOUND ( 'NONE', #23909, .T. ) ;
#62385=CARTESIAN_POINT ( 'NONE',  ( -2.000000000000000000, 10.58750000122903323, -33.46410161513775705 ) ) ;
#62386=CARTESIAN_POINT ( 'NONE',  ( -4.243569643749997233, 18.09687500061452070, -27.54997392385601174 ) ) ;
#62387=CARTESIAN_POINT ( 'NONE',  ( 6.450000001229034829, -2.886751345948125991, -5.000000000000000000 ) ) ;
#62388=CARTESIAN_POINT ( 'NONE',  ( 9.150000000000002132, 4.330127018922192761, -2.499999999999997780 ) ) ;
#62390=CARTESIAN_POINT ( 'NONE',  ( 4.537500001229034297, -4.330127018922194537, 2.499999999999995559 ) ) ;
#62391=CARTESIAN_POINT ( 'NONE',  ( 12.23437500061451821, 4.541064518000418104, 2.621784821874999949 ) ) ;
#62392=FACE_OUTER_BOUND ( 'NONE', #40422, .T. ) ;
#62393=CARTESIAN_POINT ( 'NONE',  ( 4.546875000614517326, 6.054752690667223547, 3.707466751127219781E-16 ) ) ;
#62394=LINE ( 'NONE', #50239, #43251 ) ;
#62395=DIRECTION ( 'NONE',  ( -1.000000000000000000, -0.000000000000000000, -0.000000000000000000 ) ) ;
#62396=CARTESIAN_POINT ( 'NONE',  ( 9.196875000614518569, -3.027376345333614438, 5.243569643749998122 ) ) ;
#62397=CARTESIAN_POINT ( 'NONE',  ( 14.63437500061451679, -4.541064518000419881, 2.621784821874995952 ) ) ;
#62398=CARTESIAN_POINT ( 'NONE',  ( 2.000000000000001332, 17.11250000122903359, -26.53589838486224650 ) ) ;
#62399=CARTESIAN_POINT ( 'NONE',  ( 5.475000000000000533, 6.123233995736764310E-16, -4.999999999999998224 ) ) ;
#62400=CARTESIAN_POINT ( 'NONE',  ( -4.243569643749999898, 17.10312500061459318, 30.00000000000000000 ) ) ;
#62401=CARTESIAN_POINT ( 'NONE',  ( 21.45937500061451786, -4.541064518000417216, -2.621784821875001281 ) ) ;
#62402=CARTESIAN_POINT ( 'NONE',  ( -5.810221930991193690E-16, 12.68750000000000000, -34.00000000000000000 ) ) ;
#62403=CARTESIAN_POINT ( 'NONE',  ( 27.00000000122903288, -2.886751345948129988, 4.999999999999997335 ) ) ;
#62405=CARTESIAN_POINT ( 'NONE',  ( 23.69062500061451004, -3.027376345333610441, -5.243569643749999898 ) ) ;
#62406=CARTESIAN_POINT ( 'NONE',  ( 14.84062500061451750, 6.054752690667223547, 3.707466751127219781E-16 ) ) ;
#62408=CARTESIAN_POINT ( 'NONE',  ( 12.98437500061451821, 6.421520780324663323E-16, -5.243569643749999010 ) ) ;
#62409=CARTESIAN_POINT ( 'NONE',  ( 27.56250000000000000, 2.886751345948129099, -4.999999999999998224 ) ) ;
#62410=CARTESIAN_POINT ( 'NONE',  ( 24.18750000122903288, 4.330127018922191873, 2.499999999999999556 ) ) ;
#62411=CARTESIAN_POINT ( 'NONE',  ( 3.046875000614519990, -3.027376345333610441, -5.243569643749999898 ) ) ;
#62412=CARTESIAN_POINT ( 'NONE',  ( 13.50937500061451679, 4.541064518000418104, -2.621784821874998173 ) ) ;
#62413=CARTESIAN_POINT ( 'NONE',  ( 29.25937500061451502, 4.541064518000418104, -2.621784821874998173 ) ) ;
#62415=CARTESIAN_POINT ( 'NONE',  ( -1.071796769724488563, 12.10490381179670116, 34.00000000000000000 ) ) ;
#62416=CARTESIAN_POINT ( 'NONE',  ( 23.03437500061451715, 4.541064518000418104, 2.621784821874999949 ) ) ;
#62417=CARTESIAN_POINT ( 'NONE',  ( 13.43437500061451750, 6.421520780324663323E-16, -5.243569643749999010 ) ) ;
#62419=CARTESIAN_POINT ( 'NONE',  ( 26.28749999999999432, 5.773502691896255534, 3.535250795749688894E-16 ) ) ;
#62420=CARTESIAN_POINT ( 'NONE',  ( 3.187500001229033764, -4.330127018922194537, 2.499999999999995559 ) ) ;
#62422=CARTESIAN_POINT ( 'NONE',  ( 17.69062500061451715, -3.027376345333614438, 5.243569643749998122 ) ) ;
#62423=CARTESIAN_POINT ( 'NONE',  ( 6.712500000000000355, -5.773502691896255534, -1.060575238724906372E-15 ) ) ;
#62424=CARTESIAN_POINT ( 'NONE',  ( -2.000000000000000000, 14.07500000000000107, 26.53589838486224650 ) ) ;
#62425=CARTESIAN_POINT ( 'NONE',  ( 17.43750000000000355, -2.886751345948129988, 4.999999999999997335 ) ) ;
#62426=EDGE_CURVE ( 'NONE', #33889, #44184, #15592, .T. ) ;
#62427=CARTESIAN_POINT ( 'NONE',  ( 4.243569643749999010, 12.86562500061451608, 27.54997392385601174 ) ) ;
#62428=CARTESIAN_POINT ( 'NONE',  ( 3.242103837493086330E-14, 11.33750000000000213, -34.00000000000000000 ) ) ;
#62429=CARTESIAN_POINT ( 'NONE',  ( 20.62500000122903288, 2.886751345948126879, 4.999999999999999112 ) ) ;
#62430=CARTESIAN_POINT ( 'NONE',  ( 28.32187500061451502, 3.027376345333613106, -5.243569643749998122 ) ) ;
#62432=CARTESIAN_POINT ( 'NONE',  ( 20.99062500061451431, -3.027376345333610441, -5.243569643749999898 ) ) ;
#62433=CARTESIAN_POINT ( 'NONE',  ( 22.28437500061451715, -4.541064518000419881, 2.621784821874995952 ) ) ;
#62434=CARTESIAN_POINT ( 'NONE',  ( 4.200000000000001954, 4.330127018922192761, -2.499999999999997780 ) ) ;
#62435=CARTESIAN_POINT ( 'NONE',  ( 8.878125000614515372, 6.421520780324663323E-16, -5.243569643749999010 ) ) ;
#62436=CARTESIAN_POINT ( 'NONE',  ( 23.39062500061451289, 6.054752690667223547, 3.707466751127219781E-16 ) ) ;
#62437=CARTESIAN_POINT ( 'NONE',  ( 12.49687500061451573, -3.027376345333610441, -5.243569643749999898 ) ) ;
#62438=CARTESIAN_POINT ( 'NONE',  ( 15.90937500061451892, 0.000000000000000000, 5.243569643749999010 ) ) ;
#62439=CARTESIAN_POINT ( 'NONE',  ( -4.243569643749999898, 17.10312500061451502, 30.00000000000000000 ) ) ;
#62440=CARTESIAN_POINT ( 'NONE',  ( 20.43750000122903643, 6.123233995736764310E-16, -4.999999999999998224 ) ) ;
#62442=CARTESIAN_POINT ( 'NONE',  ( 11.24062500061451608, 6.054752690667223547, 3.707466751127219781E-16 ) ) ;
#62443=CARTESIAN_POINT ( 'NONE',  ( 4.734375000614518214, -4.541064518000419881, 2.621784821874995952 ) ) ;
#62444=CARTESIAN_POINT ( 'NONE',  ( 5.334375000614517859, 6.421520780324663323E-16, -5.243569643749999010 ) ) ;
#62446=CARTESIAN_POINT ( 'NONE',  ( 25.95937500061451431, -4.541064518000417216, -2.621784821875001281 ) ) ;
#62447=CARTESIAN_POINT ( 'NONE',  ( 16.04062500061451857, -3.027376345333610441, -5.243569643749999898 ) ) ;
#62448=CARTESIAN_POINT ( 'NONE',  ( 26.81250000122903288, 4.330127018922192761, -2.499999999999997780 ) ) ;
#62449=CARTESIAN_POINT ( 'NONE',  ( 27.47812500061451502, 4.541064518000418104, 2.621784821874999949 ) ) ;
#62450=CARTESIAN_POINT ( 'NONE',  ( 22.32187500061451502, -6.054752690667223547, -1.112240025338166033E-15 ) ) ;
#62451=CARTESIAN_POINT ( 'NONE',  ( 16.79062500061451857, -3.027376345333614438, 5.243569643749998122 ) ) ;
#62452=CARTESIAN_POINT ( 'NONE',  ( -4.243569643749999898, 19.37187500061451928, 27.54997392385601529 ) ) ;
#62453=CARTESIAN_POINT ( 'NONE',  ( 22.90312500061451573, 4.541064518000418104, -2.621784821874998173 ) ) ;
#62454=CARTESIAN_POINT ( 'NONE',  ( 3.487500001229035362, 4.330127018922191873, 2.499999999999999556 ) ) ;
#62456=CARTESIAN_POINT ( 'NONE',  ( 28.53749999999999787, 5.773502691896255534, 3.535250795749688894E-16 ) ) ;
#62457=CARTESIAN_POINT ( 'NONE',  ( -3.999999999999997335, 13.73749999999999893, -27.69059892324149175 ) ) ;
#62459=CARTESIAN_POINT ( 'NONE',  ( 29.01562500061451644, -6.054752690667223547, -1.112240025338166033E-15 ) ) ;
#62460=CARTESIAN_POINT ( 'NONE',  ( 10.79062500061451679, 6.054752690667223547, 3.707466751127219781E-16 ) ) ;
#62461=CARTESIAN_POINT ( 'NONE',  ( 22.27500000122903145, 2.886751345948129099, -4.999999999999998224 ) ) ;
#62462=CARTESIAN_POINT ( 'NONE',  ( 12.42187500061451821, -6.054752690667223547, -1.112240025338166033E-15 ) ) ;
#62463=CARTESIAN_POINT ( 'NONE',  ( 26.54062500061451146, 6.054752690667223547, 3.707466751127219781E-16 ) ) ;
#62464=CARTESIAN_POINT ( 'NONE',  ( 26.58750000000000213, -2.886751345948125991, -5.000000000000000000 ) ) ;
#62465=CARTESIAN_POINT ( 'NONE',  ( -3.999999999999999112, 17.86250000122903359, -30.00000000000000000 ) ) ;
#62466=DIRECTION ( 'NONE',  ( -1.000000000000000000, -0.000000000000000000, -0.000000000000000000 ) ) ;
#62467=CARTESIAN_POINT ( 'NONE',  ( 13.75312500061451715, -4.541064518000417216, -2.621784821875001281 ) ) ;
#62469=ORIENTED_EDGE ( 'NONE', *, *, #46996, .F. ) ;
#62470=CARTESIAN_POINT ( 'NONE',  ( 6.590625000614518392, -3.027376345333610441, -5.243569643749999898 ) ) ;
#62471=CARTESIAN_POINT ( 'NONE',  ( 5.728125000614515905, 6.421520780324663323E-16, -5.243569643749999010 ) ) ;
#62473=CARTESIAN_POINT ( 'NONE',  ( 2.812500001229033320, -4.330127018922190985, -2.500000000000001332 ) ) ;
#62474=CARTESIAN_POINT ( 'NONE',  ( 14.84999999999999964, -4.330127018922190985, -2.500000000000001332 ) ) ;
#62475=CARTESIAN_POINT ( 'NONE',  ( 16.28437500061452070, 4.541064518000418104, 2.621784821874999949 ) ) ;
#62476=CARTESIAN_POINT ( 'NONE',  ( 10.20000000122903572, 5.773502691896255534, 3.535250795749688894E-16 ) ) ;
#62477=CARTESIAN_POINT ( 'NONE',  ( 19.65937500061451360, -4.541064518000417216, -2.621784821875001281 ) ) ;
#62479=CARTESIAN_POINT ( 'NONE',  ( 20.93437500061451573, -4.541064518000419881, 2.621784821874995952 ) ) ;
#62480=CARTESIAN_POINT ( 'NONE',  ( -4.243569643749999898, 14.40312500061451750, -30.00000000000000000 ) ) ;
#62483=CARTESIAN_POINT ( 'NONE',  ( 3.999999999999998668, 11.71250000000000036, -32.30940107675850470 ) ) ;
#62484=CARTESIAN_POINT ( 'NONE',  ( 26.54062500061451146, 6.054752690667223547, 3.707466751127219781E-16 ) ) ;
#62485=CARTESIAN_POINT ( 'NONE',  ( -1.999999999999997113, 19.62500000000000000, -26.53589838486224295 ) ) ;
#62486=CARTESIAN_POINT ( 'NONE',  ( 29.63437500061451502, 6.421520780324663323E-16, -5.243569643749999010 ) ) ;
#62487=CARTESIAN_POINT ( 'NONE',  ( 24.03750000000000142, 5.773502691896255534, 3.535250795749688894E-16 ) ) ;
#62488=CARTESIAN_POINT ( 'NONE',  ( 6.065625000614516260, -6.054752690667223547, -1.112240025338166033E-15 ) ) ;
#62490=CARTESIAN_POINT ( 'NONE',  ( 18.45937500061451431, 4.541064518000418104, -2.621784821874998173 ) ) ;
#62492=CARTESIAN_POINT ( 'NONE',  ( 5.465625000614517504, 3.027376345333611329, 5.243569643749999010 ) ) ;
#62493=CARTESIAN_POINT ( 'NONE',  ( 11.55937500061451928, -4.541064518000417216, -2.621784821875001281 ) ) ;
#62494=ORIENTED_EDGE ( 'NONE', *, *, #54021, .T. ) ;
#62495=CARTESIAN_POINT ( 'NONE',  ( 20.44687500061451857, -3.027376345333614438, 5.243569643749998122 ) ) ;
#62497=CARTESIAN_POINT ( 'NONE',  ( 28.12499999999999645, 4.330127018922191873, 2.499999999999999556 ) ) ;
#62498=CARTESIAN_POINT ( 'NONE',  ( 28.92187500061451644, 3.027376345333611329, 5.243569643749999010 ) ) ;
#62500=CARTESIAN_POINT ( 'NONE',  ( 3.403125000614518836, -4.541064518000417216, -2.621784821875001281 ) ) ;
#62502=CARTESIAN_POINT ( 'NONE',  ( 9.525000000000002132, 6.123233995736764310E-16, -4.999999999999998224 ) ) ;
#62504=CARTESIAN_POINT ( 'NONE',  ( 23.35312500061451857, 4.541064518000418104, -2.621784821874998173 ) ) ;
#62505=CARTESIAN_POINT ( 'NONE',  ( 15.26249999999999929, -5.773502691896255534, -1.060575238724906372E-15 ) ) ;
#62506=CARTESIAN_POINT ( 'NONE',  ( 11.43750000122903465, 6.123233995736764310E-16, -4.999999999999998224 ) ) ;
#62507=CARTESIAN_POINT ( 'NONE',  ( 9.740625000614516082, -3.027376345333610441, -5.243569643749999898 ) ) ;
#62508=ADVANCED_FACE ( 'NONE', ( #38134 ), #72560, .T. ) ;
#62509=CARTESIAN_POINT ( 'NONE',  ( 8.737500000000002487, 5.773502691896255534, 3.535250795749688894E-16 ) ) ;
#62511=CARTESIAN_POINT ( 'NONE',  ( 28.23750000122903359, 4.330127018922191873, 2.499999999999999556 ) ) ;
#62513=CARTESIAN_POINT ( 'NONE',  ( 7.687500000000000000, -2.886751345948125991, -5.000000000000000000 ) ) ;
#62514=DIRECTION ( 'NONE',  ( 0.000000000000000000, 0.000000000000000000, 1.000000000000000000 ) ) ;
#62515=ORIENTED_EDGE ( 'NONE', *, *, #66601, .T. ) ;
#62516=CARTESIAN_POINT ( 'NONE',  ( 21.51562500061451644, 3.027376345333613106, -5.243569643749998122 ) ) ;
#62517=CARTESIAN_POINT ( 'NONE',  ( 28.22812500061451502, 6.421520780324663323E-16, -5.243569643749999010 ) ) ;
#62518=CARTESIAN_POINT ( 'NONE',  ( 29.18437500061451573, 6.421520780324663323E-16, -5.243569643749999010 ) ) ;
#62519=AXIS2_PLACEMENT_3D ( 'NONE', #17857, #23413, #57749 ) ;
#62520=CARTESIAN_POINT ( 'NONE',  ( 19.13437500061451857, -4.541064518000419881, 2.621784821874995952 ) ) ;
#62521=CARTESIAN_POINT ( 'NONE',  ( 16.11562500061451786, 3.027376345333613106, -5.243569643749998122 ) ) ;
#62522=CARTESIAN_POINT ( 'NONE',  ( -4.243569643749998122, 10.84062500061459211, -27.54997392385601174 ) ) ;
#62523=CARTESIAN_POINT ( 'NONE',  ( 5.315625000614516260, 3.027376345333613106, -5.243569643749998122 ) ) ;
#62524=CARTESIAN_POINT ( 'NONE',  ( 29.32500000122903216, -5.773502691896255534, -1.060575238724906372E-15 ) ) ;
#62526=CARTESIAN_POINT ( 'NONE',  ( 18.44062500061451715, 6.054752690667223547, 3.707466751127219781E-16 ) ) ;
#62528=CARTESIAN_POINT ( 'NONE',  ( 3.712500001229034563, -4.330127018922190985, -2.500000000000001332 ) ) ;
#62529=CARTESIAN_POINT ( 'NONE',  ( 12.23437500061451821, 4.541064518000418104, 2.621784821874999949 ) ) ;
#62530=CARTESIAN_POINT ( 'NONE',  ( 10.92187500061451644, 3.027376345333611329, 5.243569643749999010 ) ) ;
#62531=CARTESIAN_POINT ( 'NONE',  ( 20.10937500061451289, -4.541064518000417216, -2.621784821875001281 ) ) ;
#62532=ORIENTED_EDGE ( 'NONE', *, *, #16952, .F. ) ;
#62533=CARTESIAN_POINT ( 'NONE',  ( -2.698377630233220081, 9.636255672932170668, 24.62661337867154288 ) ) ;
#62534=CARTESIAN_POINT ( 'NONE',  ( 23.50312500061451360, 0.000000000000000000, 5.243569643749999010 ) ) ;
#62535=CARTESIAN_POINT ( 'NONE',  ( 18.83437500061451431, 6.421520780324663323E-16, -5.243569643749999010 ) ) ;
#62536=CARTESIAN_POINT ( 'NONE',  ( 24.62812500061451715, 6.421520780324663323E-16, -5.243569643749999010 ) ) ;
#62537=CARTESIAN_POINT ( 'NONE',  ( -5.810221930991193690E-16, 12.23750000000000071, -34.00000000000000000 ) ) ;
#62538=CARTESIAN_POINT ( 'NONE',  ( -3.999999999999999556, 16.81250000000000000, 27.69059892324149530 ) ) ;
#62539=CARTESIAN_POINT ( 'NONE',  ( 29.80312500061451431, 0.000000000000000000, 5.243569643749999010 ) ) ;
#62540=CARTESIAN_POINT ( 'NONE',  ( 11.17500000122903536, 2.886751345948126879, 4.999999999999999112 ) ) ;
#62541=CARTESIAN_POINT ( 'NONE',  ( 7.762500001229033053, -4.330127018922190985, -2.500000000000001332 ) ) ;
#62542=CARTESIAN_POINT ( 'NONE',  ( 28.83750000122903145, -4.330127018922194537, 2.499999999999995559 ) ) ;
#62543=CARTESIAN_POINT ( 'NONE',  ( 26.81250000122903288, 4.330127018922192761, -2.499999999999997780 ) ) ;
#62546=CARTESIAN_POINT ( 'NONE',  ( 8.896875000614517859, -3.027376345333610441, -5.243569643749999898 ) ) ;
#62549=CARTESIAN_POINT ( 'NONE',  ( 16.26562500061451289, 3.027376345333611329, 5.243569643749999010 ) ) ;
#62550=CARTESIAN_POINT ( 'NONE',  ( 12.38437500061451857, -4.541064518000419881, 2.621784821874995952 ) ) ;
#62551=CARTESIAN_POINT ( 'NONE',  ( 28.61250000122903359, 4.330127018922192761, -2.499999999999997780 ) ) ;
#62552=CARTESIAN_POINT ( 'NONE',  ( 20.10937500061451289, -4.541064518000417216, -2.621784821875001281 ) ) ;
#62553=CARTESIAN_POINT ( 'NONE',  ( 6.309375000614517504, 4.541064518000418104, -2.621784821874998173 ) ) ;
#62554=CARTESIAN_POINT ( 'NONE',  ( 3.253125000614518036, 0.000000000000000000, 5.243569643749999010 ) ) ;
#62555=CARTESIAN_POINT ( 'NONE',  ( 5.737499999999998934, -2.886751345948063374, 5.000000000000112799 ) ) ;
#62556=CARTESIAN_POINT ( 'NONE',  ( 9.178125000614517859, -4.541064518000419881, 2.621784821874995952 ) ) ;
#62557=CARTESIAN_POINT ( 'NONE',  ( 21.10312500061451502, 4.541064518000418104, -2.621784821874998173 ) ) ;
#62558=ORIENTED_EDGE ( 'NONE', *, *, #66024, .T. ) ;
#62559=CARTESIAN_POINT ( 'NONE',  ( 4.987500001229032698, -4.330127018922194537, 2.499999999999995559 ) ) ;
#62560=CARTESIAN_POINT ( 'NONE',  ( 17.95312500061451644, 4.541064518000418104, -2.621784821874998173 ) ) ;
#62561=CARTESIAN_POINT ( 'NONE',  ( 14.01562500061451644, 3.027376345333611329, 5.243569643749999010 ) ) ;
#62563=CARTESIAN_POINT ( 'NONE',  ( 12.82499999999999929, 4.330127018922191873, 2.499999999999999556 ) ) ;
#62564=CARTESIAN_POINT ( 'NONE',  ( 8.212500001229035007, -4.330127018922190985, -2.500000000000001332 ) ) ;
#62565=CARTESIAN_POINT ( 'NONE',  ( 5.315625000614516260, 3.027376345333613106, -5.243569643749998122 ) ) ;
#62566=EDGE_CURVE ( 'NONE', #23474, #26902, #41318, .T. ) ;
#62567=CARTESIAN_POINT ( 'NONE',  ( 18.86250000122903359, 0.000000000000000000, 4.999999999999998224 ) ) ;
#62569=EDGE_CURVE ( 'NONE', #964, #48607, #6959, .T. ) ;
#62570=CARTESIAN_POINT ( 'NONE',  ( -2.121784821874999949, 12.13437500061451857, -33.67503911421598417 ) ) ;
#62571=CARTESIAN_POINT ( 'NONE',  ( 1.626862140677534273E-15, 16.17500000122903359, 34.00000000000000000 ) ) ;
#62572=CARTESIAN_POINT ( 'NONE',  ( 2.700000001229035718, -2.886751345948129988, 4.999999999999997335 ) ) ;
#62574=CARTESIAN_POINT ( 'NONE',  ( 18.53437500061451715, 4.541064518000418104, 2.621784821874999949 ) ) ;
#62576=CARTESIAN_POINT ( 'NONE',  ( 16.67812500061451786, 4.541064518000418104, 2.621784821874999949 ) ) ;
#62579=CARTESIAN_POINT ( 'NONE',  ( 29.85937500061451644, 0.000000000000000000, 5.243569643749999010 ) ) ;
#62580=CARTESIAN_POINT ( 'NONE',  ( 26.82187500061451857, -6.054752690667223547, -1.112240025338166033E-15 ) ) ;
#62582=CARTESIAN_POINT ( 'NONE',  ( 12.81562500061451537, -6.054752690667223547, -1.112240025338166033E-15 ) ) ;
#62583=CARTESIAN_POINT ( 'NONE',  ( 11.37187500061451750, 3.027376345333611329, 5.243569643749999010 ) ) ;
#62584=ORIENTED_EDGE ( 'NONE', *, *, #30725, .T. ) ;
#62585=CARTESIAN_POINT ( 'NONE',  ( 28.94062500061452070, -3.027376345333614438, 5.243569643749998122 ) ) ;
#62586=CARTESIAN_POINT ( 'NONE',  ( 19.79062500061451502, 6.054752690667223547, 3.707466751127219781E-16 ) ) ;
#62587=FACE_OUTER_BOUND ( 'NONE', #45562, .T. ) ;
#62588=EDGE_CURVE ( 'NONE', #59726, #2356, #3299, .T. ) ;
#62590=CARTESIAN_POINT ( 'NONE',  ( 10.91250000000000320, 2.886751345948129099, -4.999999999999998224 ) ) ;
#62591=CARTESIAN_POINT ( 'NONE',  ( 21.33750000122903145, 6.123233995736764310E-16, -4.999999999999998224 ) ) ;
#62592=CARTESIAN_POINT ( 'NONE',  ( 15.32812500061451644, 4.541064518000418104, 2.621784821874999949 ) ) ;
#62595=CARTESIAN_POINT ( 'NONE',  ( 20.10000000000000142, 0.000000000000000000, 4.999999999999998224 ) ) ;
#62596=CARTESIAN_POINT ( 'NONE',  ( 21.18749999999999645, -2.886751345948125991, -5.000000000000000000 ) ) ;
#62597=CARTESIAN_POINT ( 'NONE',  ( 21.90937500061451715, -4.541064518000417216, -2.621784821875001281 ) ) ;
#62598=CARTESIAN_POINT ( 'NONE',  ( 25.64062500061451644, 6.054752690667223547, 3.707466751127219781E-16 ) ) ;
#62599=ORIENTED_EDGE ( 'NONE', *, *, #4648, .T. ) ;
#62601=CARTESIAN_POINT ( 'NONE',  ( 7.528125000614515727, 6.421520780324663323E-16, -5.243569643749999010 ) ) ;
#62602=CARTESIAN_POINT ( 'NONE',  ( 3.999999999999999112, 12.12500000000000000, 30.00000000000000000 ) ) ;
#62603=CARTESIAN_POINT ( 'NONE',  ( 14.02499999999999858, 6.123233995736764310E-16, -4.999999999999998224 ) ) ;
#62604=CARTESIAN_POINT ( 'NONE',  ( 4.243569643749999898, 16.84062500061451573, 32.45002607614398471 ) ) ;
#62605=CARTESIAN_POINT ( 'NONE',  ( 29.12812500061451715, 6.421520780324663323E-16, -5.243569643749999010 ) ) ;
#62606=CARTESIAN_POINT ( 'NONE',  ( 25.84687500061451360, -3.027376345333614438, 5.243569643749998122 ) ) ;
#62607=VERTEX_POINT ( 'NONE', #53528 ) ;
#62608=CARTESIAN_POINT ( 'NONE',  ( 23.50312500061451360, 0.000000000000000000, 5.243569643749999010 ) ) ;
#62609=CARTESIAN_POINT ( 'NONE',  ( 24.12187500061451217, -6.054752690667223547, -1.112240025338166033E-15 ) ) ;
#62610=CARTESIAN_POINT ( 'NONE',  ( 4.243569643749999010, 17.81562500061459176, -32.45002607614398471 ) ) ;
#62611=CARTESIAN_POINT ( 'NONE',  ( 10.98750000000000071, 5.773502691896255534, 3.535250795749688894E-16 ) ) ;
#62612=CARTESIAN_POINT ( 'NONE',  ( 9.403125000614517504, 4.541064518000418104, -2.621784821874998173 ) ) ;
#62613=CARTESIAN_POINT ( 'NONE',  ( 29.16562500061451502, 3.027376345333613106, -5.243569643749998122 ) ) ;
#62614=CARTESIAN_POINT ( 'NONE',  ( 26.80312500061451431, -4.541064518000417216, -2.621784821875001281 ) ) ;
#62617=CARTESIAN_POINT ( 'NONE',  ( 18.90937500061451360, 4.541064518000418104, -2.621784821874998173 ) ) ;
#62618=( BOUNDED_CURVE ( )  B_SPLINE_CURVE ( 2, ( #68636, #62356, #53727, #34269, #63075, #46461, #40557 ),
 .UNSPECIFIED., .F., .F. ) 
 B_SPLINE_CURVE_WITH_KNOTS ( ( 3, 2, 2, 3 ),
 ( 0.9514681797180121192, 0.9527777777777777235, 0.9555555555555556024, 0.9567451072665406064 ),
 .UNSPECIFIED. ) 
 CURVE ( )  GEOMETRIC_REPRESENTATION_ITEM ( )  RATIONAL_B_SPLINE_CURVE ( ( 0.9332310268437209455, 0.9368369663457591923, 1.000000000000000000, 0.8660254037844387076, 1.000000000000000000, 0.9426269043435712147, 0.9343925588410226801 ) ) 
 REPRESENTATION_ITEM ( '' )  );
#62619=CARTESIAN_POINT ( 'NONE',  ( -2.121784821874996840, 13.18437500061451750, 33.67503911421598417 ) ) ;
#62620=CARTESIAN_POINT ( 'NONE',  ( 20.40937500061451715, 0.000000000000000000, 5.243569643749999010 ) ) ;
#62621=CARTESIAN_POINT ( 'NONE',  ( 27.30937500061451573, -4.541064518000417216, -2.621784821875001281 ) ) ;
#62622=EDGE_CURVE ( 'NONE', #11718, #49995, #3664, .T. ) ;
#62623=CARTESIAN_POINT ( 'NONE',  ( -4.243569643749999898, 16.70937500061451786, 30.00000000000000000 ) ) ;
#62624=CARTESIAN_POINT ( 'NONE',  ( 7.115625000614516082, 3.027376345333613106, -5.243569643749998122 ) ) ;
#62625=CARTESIAN_POINT ( 'NONE',  ( -3.999999999999997335, 18.23750000000000071, -27.69059892324149530 ) ) ;
#62626=CARTESIAN_POINT ( 'NONE',  ( 5.184375000614516615, -4.541064518000419881, 2.621784821874995952 ) ) ;
#62627=CARTESIAN_POINT ( 'NONE',  ( -2.000000000000000000, 15.98750000122903181, -33.46410161513775705 ) ) ;
#62628=CARTESIAN_POINT ( 'NONE',  ( 6.703125000614516438, 4.541064518000418104, -2.621784821874998173 ) ) ;
#62629=CARTESIAN_POINT ( 'NONE',  ( 10.88437500061451679, 4.541064518000418104, 2.621784821874999949 ) ) ;
#62631=CARTESIAN_POINT ( 'NONE',  ( 18.48750000122903359, -4.330127018922194537, 2.499999999999995559 ) ) ;
#62632=CARTESIAN_POINT ( 'NONE',  ( 6.234375000614519102, 6.421520780324663323E-16, -5.243569643749999010 ) ) ;
#62633=CARTESIAN_POINT ( 'NONE',  ( 7.678125000614516082, 4.541064518000418104, 2.621784821874999949 ) ) ;
#62635=CARTESIAN_POINT ( 'NONE',  ( 15.83437500061451608, 4.541064518000418104, 2.621784821874999949 ) ) ;
#62636=DIRECTION ( 'NONE',  ( -1.000000000000000000, 0.000000000000000000, 0.000000000000000000 ) ) ;
#62637=ORIENTED_EDGE ( 'NONE', *, *, #4430, .F. ) ;
#62638=CARTESIAN_POINT ( 'NONE',  ( 25.67812500061451431, 4.541064518000418104, 2.621784821874999949 ) ) ;
#62639=CARTESIAN_POINT ( 'NONE',  ( 11.65312500061451573, 4.541064518000418104, -2.621784821874998173 ) ) ;
#62640=CARTESIAN_POINT ( 'NONE',  ( 27.15937500061451360, 0.000000000000000000, 5.243569643749999010 ) ) ;
#62641=CARTESIAN_POINT ( 'NONE',  ( 10.49062500061451431, -3.027376345333614438, 5.243569643749998122 ) ) ;
#62642=CARTESIAN_POINT ( 'NONE',  ( 1.592000809091587073E-14, 15.05000000122903714, -34.00000000000000000 ) ) ;
#62643=CARTESIAN_POINT ( 'NONE',  ( 12.60000000122903430, -2.886751345948129988, 4.999999999999997335 ) ) ;
#62644=CARTESIAN_POINT ( 'NONE',  ( 28.34062500061451928, 6.054752690667223547, 3.707466751127219781E-16 ) ) ;
#62645=CARTESIAN_POINT ( 'NONE',  ( 4.243569643749999898, 12.34062500061451750, -27.54997392385601529 ) ) ;
#62646=CARTESIAN_POINT ( 'NONE',  ( 12.93750000122903465, 4.330127018922191873, 2.499999999999999556 ) ) ;
#62647=CARTESIAN_POINT ( 'NONE',  ( 11.77500000000000036, 6.123233995736764310E-16, -4.999999999999998224 ) ) ;
#62648=CARTESIAN_POINT ( 'NONE',  ( 19.67812500061451786, 6.421520780324663323E-16, -5.243569643749999010 ) ) ;
#62649=CARTESIAN_POINT ( 'NONE',  ( 8.784375000614518925, -4.541064518000419881, 2.621784821874995952 ) ) ;
#62650=CARTESIAN_POINT ( 'NONE',  ( 20.40000000000000213, 4.330127018922192761, -2.499999999999997780 ) ) ;
#62651=CARTESIAN_POINT ( 'NONE',  ( 8.212500001229035007, -4.330127018922190985, -2.500000000000001332 ) ) ;
#62652=CARTESIAN_POINT ( 'NONE',  ( 16.87500000122903288, 2.886751345948129099, -4.999999999999998224 ) ) ;
#62653=CARTESIAN_POINT ( 'NONE',  ( 14.01562500061451644, 3.027376345333611329, 5.243569643749999010 ) ) ;
#62655=CARTESIAN_POINT ( 'NONE',  ( 16.41562500061451857, -6.054752690667223547, -1.112240025338166033E-15 ) ) ;
#62656=CARTESIAN_POINT ( 'NONE',  ( 24.52500000122903145, 2.886751345948129099, -4.999999999999998224 ) ) ;
#62657=CARTESIAN_POINT ( 'NONE',  ( 21.11249999999999716, -5.773502691896255534, -1.060575238724906372E-15 ) ) ;
#62658=CARTESIAN_POINT ( 'NONE',  ( 23.74687500061451573, -3.027376345333610441, -5.243569643749999898 ) ) ;
#62660=CARTESIAN_POINT ( 'NONE',  ( 9.150000001229033231, -2.886751345948125991, -5.000000000000000000 ) ) ;
#62661=CARTESIAN_POINT ( 'NONE',  ( 9.909375000614517148, 4.541064518000418104, -2.621784821874998173 ) ) ;
#62662=CARTESIAN_POINT ( 'NONE',  ( 28.62187500061451573, -6.054752690667223547, -1.112240025338166033E-15 ) ) ;
#62664=( BOUNDED_CURVE ( )  B_SPLINE_CURVE ( 2, ( #44177, #66707, #61876, #205, #50447, #16080, #10548 ),
 .UNSPECIFIED., .F., .F. ) 
 B_SPLINE_CURVE_WITH_KNOTS ( ( 3, 2, 2, 3 ),
 ( 0.4500000000000001221, 0.4527777777777778345, 0.4555555555555555469, 0.4583333333333332593 ),
 .UNSPECIFIED. ) 
 CURVE ( )  GEOMETRIC_REPRESENTATION_ITEM ( )  RATIONAL_B_SPLINE_CURVE ( ( 0.9999999999999946709, 0.8660254037844440367, 1.000000000000000000, 0.8660254037844387076, 1.000000000000000000, 0.8660254037844413721, 0.9999999999999973355 ) ) 
 REPRESENTATION_ITEM ( '' )  );
#62665=CARTESIAN_POINT ( 'NONE',  ( 4.226174930415019126, -2.672125389006213325, -4.285040371159579031 ) ) ;
#62666=CARTESIAN_POINT ( 'NONE',  ( 23.57812500061451289, -4.541064518000419881, 2.621784821874995952 ) ) ;
#62667=CARTESIAN_POINT ( 'NONE',  ( 25.65937500061451715, 4.541064518000418104, -2.621784821874998173 ) ) ;
#62670=CARTESIAN_POINT ( 'NONE',  ( 7.134375000614516793, 6.421520780324663323E-16, -5.243569643749999010 ) ) ;
#62671=CARTESIAN_POINT ( 'NONE',  ( 15.90000000000000036, 4.330127018922192761, -2.499999999999997780 ) ) ;
#62672=CARTESIAN_POINT ( 'NONE',  ( 26.35312500061451857, -4.541064518000417216, -2.621784821875001281 ) ) ;
#62673=CARTESIAN_POINT ( 'NONE',  ( 5.971875000614516260, 3.027376345333611329, 5.243569643749999010 ) ) ;
#62675=CARTESIAN_POINT ( 'NONE',  ( -2.000000000000000000, 16.43750000122903643, -33.46410161513775705 ) ) ;
#62676=CARTESIAN_POINT ( 'NONE',  ( 25.54687500061451644, -3.027376345333610441, -5.243569643749999898 ) ) ;
#62677=CARTESIAN_POINT ( 'NONE',  ( -4.243569643749999898, 10.76562500061459460, 27.54997392385601529 ) ) ;
#62678=CARTESIAN_POINT ( 'NONE',  ( 16.61250000000000426, -5.773502691896255534, -1.060575238724906372E-15 ) ) ;
#62679=ORIENTED_EDGE ( 'NONE', *, *, #45083, .F. ) ;
#62680=CARTESIAN_POINT ( 'NONE',  ( 26.32499999999999929, 4.330127018922191873, 2.499999999999999556 ) ) ;
#62681=CARTESIAN_POINT ( 'NONE',  ( 28.69687500061451502, -3.027376345333610441, -5.243569643749999898 ) ) ;
#62682=ORIENTED_EDGE ( 'NONE', *, *, #2964, .F. ) ;
#62683=CARTESIAN_POINT ( 'NONE',  ( 15.06562500061451537, -6.054752690667223547, -1.112240025338166033E-15 ) ) ;
#62684=CARTESIAN_POINT ( 'NONE',  ( 6.853125000614516793, 0.000000000000000000, 5.243569643749999010 ) ) ;
#62686=CARTESIAN_POINT ( 'NONE',  ( 5.184375000614516615, -4.541064518000419881, 2.621784821874995952 ) ) ;
#62687=CARTESIAN_POINT ( 'NONE',  ( 14.47500000122903430, -5.773502691896255534, -1.060575238724906372E-15 ) ) ;
#62688=CARTESIAN_POINT ( 'NONE',  ( 22.91249999999999432, -5.773502691896255534, -1.060575238724906372E-15 ) ) ;
#62690=CARTESIAN_POINT ( 'NONE',  ( 4.734375000614518214, -4.541064518000419881, 2.621784821874995952 ) ) ;
#62691=CARTESIAN_POINT ( 'NONE',  ( 8.296875000614516438, -3.027376345333614438, 5.243569643749998122 ) ) ;
#62692=CARTESIAN_POINT ( 'NONE',  ( 22.32187500061451502, -6.054752690667223547, -1.112240025338166033E-15 ) ) ;
#62693=CARTESIAN_POINT ( 'NONE',  ( -3.999999999999999112, 17.26249999999999929, -32.30940107675850470 ) ) ;
#62694=ORIENTED_EDGE ( 'NONE', *, *, #30819, .F. ) ;
#62695=CARTESIAN_POINT ( 'NONE',  ( 3.759375000614517681, 0.000000000000000000, 5.243569643749999010 ) ) ;
#62696=CARTESIAN_POINT ( 'NONE',  ( 6.796875000614516438, 6.054752690667223547, 3.707466751127219781E-16 ) ) ;
#62698=CARTESIAN_POINT ( 'NONE',  ( 17.96250000000000213, -5.773502691896255534, -1.060575238724906372E-15 ) ) ;
#62699=CARTESIAN_POINT ( 'NONE',  ( 16.19062500061451715, 6.054752690667223547, 3.707466751127219781E-16 ) ) ;
#62702=CARTESIAN_POINT ( 'NONE',  ( -3.999999999999999112, 20.00000000000000000, 30.00000000000000000 ) ) ;
#62704=CARTESIAN_POINT ( 'NONE',  ( 9.440625000614517148, 6.054752690667223547, 3.707466751127219781E-16 ) ) ;
#62705=CARTESIAN_POINT ( 'NONE',  ( 26.52187500061451431, 3.027376345333613106, -5.243569643749998122 ) ) ;
#62707=CARTESIAN_POINT ( 'NONE',  ( 25.35937500061451644, 0.000000000000000000, 5.243569643749999010 ) ) ;
#62708=CARTESIAN_POINT ( 'NONE',  ( 8.099999999999999645, -4.330127018922190985, -2.500000000000001332 ) ) ;
#62709=CARTESIAN_POINT ( 'NONE',  ( -2.828200636599751609E-16, 12.80000000122903181, 25.38119784648299770 ) ) ;
#62710=CARTESIAN_POINT ( 'NONE',  ( 7.762500001229033053, -4.330127018922190985, -2.500000000000001332 ) ) ;
#62711=CARTESIAN_POINT ( 'NONE',  ( 19.39687500061451786, 6.054752690667223547, 3.707466751127219781E-16 ) ) ;
#62712=CARTESIAN_POINT ( 'NONE',  ( 11.48437500061451644, -4.541064518000419881, 2.621784821874995952 ) ) ;
#62713=CARTESIAN_POINT ( 'NONE',  ( -4.000165449326166467, 2.999779401354842445, -30.13373215374999603 ) ) ;
#62714=ORIENTED_EDGE ( 'NONE', *, *, #34377, .F. ) ;
#62715=CARTESIAN_POINT ( 'NONE',  ( 14.80312500061451608, 4.541064518000418104, -2.621784821874998173 ) ) ;
#62716=CARTESIAN_POINT ( 'NONE',  ( 27.48750000122903359, -4.330127018922194537, 2.499999999999995559 ) ) ;
#62717=CARTESIAN_POINT ( 'NONE',  ( 13.24687500061451750, -3.027376345333614438, 5.243569643749998122 ) ) ;
#62718=CARTESIAN_POINT ( 'NONE',  ( 3.871875000614519280, -6.054752690667223547, -1.112240025338166033E-15 ) ) ;
#62719=CARTESIAN_POINT ( 'NONE',  ( 14.54062500061451679, -3.027376345333614438, 5.243569643749998122 ) ) ;
#62720=CARTESIAN_POINT ( 'NONE',  ( 26.43750000122903288, 4.330127018922191873, 2.499999999999999556 ) ) ;
#62722=CARTESIAN_POINT ( 'NONE',  ( 26.25937500061451857, 0.000000000000000000, 5.243569643749999010 ) ) ;
#62723=CARTESIAN_POINT ( 'NONE',  ( 2.226602359779148887, 9.751272476441998904, 25.29835638300850320 ) ) ;
#62724=CARTESIAN_POINT ( 'NONE',  ( 12.97500000122903252, 2.886751345948126879, 4.999999999999999112 ) ) ;
#62725=DIRECTION ( 'NONE',  ( -0.000000000000000000, -1.000000000000000000, -0.000000000000000000 ) ) ;
#62726=CARTESIAN_POINT ( 'NONE',  ( -4.243569643749999898, 17.15937500061451715, -30.00000000000000000 ) ) ;
#62727=CARTESIAN_POINT ( 'NONE',  ( 16.99687500061451573, -3.027376345333610441, -5.243569643749999898 ) ) ;
#62728=CARTESIAN_POINT ( 'NONE',  ( 19.23750000122903714, 4.330127018922191873, 2.499999999999999556 ) ) ;
#62729=CARTESIAN_POINT ( 'NONE',  ( 14.70937500061451786, -4.541064518000417216, -2.621784821875001281 ) ) ;
#62730=CARTESIAN_POINT ( 'NONE',  ( 4.243569643749999898, 10.63437500061451857, 30.00000000000000000 ) ) ;
#62731=CARTESIAN_POINT ( 'NONE',  ( 21.30000000122903359, -2.886751345948125991, -5.000000000000000000 ) ) ;
#62732=CARTESIAN_POINT ( 'NONE',  ( 16.04062500061451857, -3.027376345333610441, -5.243569643749999898 ) ) ;
#62733=CARTESIAN_POINT ( 'NONE',  ( 29.20312500061451644, 4.541064518000418104, -2.621784821874998173 ) ) ;
#62735=ORIENTED_EDGE ( 'NONE', *, *, #29767, .F. ) ;
#62736=CARTESIAN_POINT ( 'NONE',  ( 18.22499999999999787, 4.330127018922191873, 2.499999999999999556 ) ) ;
#62738=CARTESIAN_POINT ( 'NONE',  ( 3.403125000614518836, -4.541064518000417216, -2.621784821875001281 ) ) ;
#62739=CARTESIAN_POINT ( 'NONE',  ( 15.52500000122903323, 2.886751345948129099, -4.999999999999998224 ) ) ;
#62740=CARTESIAN_POINT ( 'NONE',  ( 20.99062500061451431, -3.027376345333610441, -5.243569643749999898 ) ) ;
#62741=ADVANCED_FACE ( 'NONE', ( #64975 ), #70152, .F. ) ;
#62742=CARTESIAN_POINT ( 'NONE',  ( 22.56562500061451715, 3.027376345333611329, 5.243569643749999010 ) ) ;
#62743=CARTESIAN_POINT ( 'NONE',  ( 3.815625000614518036, -6.054752690667223547, -1.112240025338166033E-15 ) ) ;
#62744=CARTESIAN_POINT ( 'NONE',  ( 27.63749999999999929, 5.773502691896255534, 3.535250795749688894E-16 ) ) ;
#62747=CARTESIAN_POINT ( 'NONE',  ( 29.44687500061451857, -3.027376345333614438, 5.243569643749998122 ) ) ;
#62748=CARTESIAN_POINT ( 'NONE',  ( 2.000000000000001332, 12.16250000122903430, -26.53589838486224650 ) ) ;
#62749=CARTESIAN_POINT ( 'NONE',  ( 2.121784821875001281, 16.40937500061452070, -26.32496088578401938 ) ) ;
#62750=CARTESIAN_POINT ( 'NONE',  ( 6.825000001229034829, -5.773502691896255534, -1.060575238724906372E-15 ) ) ;
#62751=CARTESIAN_POINT ( 'NONE',  ( 7.425000000000000711, 4.330127018922191873, 2.499999999999999556 ) ) ;
#62752=CARTESIAN_POINT ( 'NONE',  ( 4.312500001229034652, 4.330127018922192761, -2.499999999999997780 ) ) ;
#62753=CARTESIAN_POINT ( 'NONE',  ( 9.084375000614517859, 4.541064518000418104, 2.621784821874999949 ) ) ;
#62754=VECTOR ( 'NONE', #29034, 1000.000000000000000 ) ;
#62755=CARTESIAN_POINT ( 'NONE',  ( 3.590625000614518836, 6.054752690667223547, 3.707466751127219781E-16 ) ) ;
#62756=CARTESIAN_POINT ( 'NONE',  ( 28.12499999999999645, 4.330127018922191873, 2.499999999999999556 ) ) ;
#62758=CARTESIAN_POINT ( 'NONE',  ( 8.259375000614518569, 0.000000000000000000, 5.243569643749999010 ) ) ;
#62759=CARTESIAN_POINT ( 'NONE',  ( 12.68437500061451573, 4.541064518000418104, 2.621784821874999949 ) ) ;
#62760=CARTESIAN_POINT ( 'NONE',  ( 7.320879633048903241E-15, 18.53750000000000142, -34.00000000000000000 ) ) ;
#62761=CARTESIAN_POINT ( 'NONE',  ( 6.600000000000001421, 0.000000000000000000, 4.999999999999998224 ) ) ;
#62762=CARTESIAN_POINT ( 'NONE',  ( -4.243569643749998122, 17.14062500061459460, 32.45002607614398471 ) ) ;
#62763=CARTESIAN_POINT ( 'NONE',  ( 21.34687500061451715, -3.027376345333614438, 5.243569643749998122 ) ) ;
#62764=CARTESIAN_POINT ( 'NONE',  ( 26.40000000122902790, 5.773502691896255534, 3.535250795749688894E-16 ) ) ;
#62765=B_SPLINE_CURVE_WITH_KNOTS ( 'NONE', 3,
 ( #70018, #30499, #54134, #64470, #43044, #14960, #48224, #71116, #58918, #36405 ),
 .UNSPECIFIED., .F., .F.,
 ( 4, 3, 3, 4 ),
 ( 2.168404344971008868E-19, 0.0001572616466639377138, 0.0002553267708066046891, 0.0003534655997994981189 ),
 .UNSPECIFIED. ) ;
#62767=CARTESIAN_POINT ( 'NONE',  ( 23.65312500061451573, -4.541064518000417216, -2.621784821875001281 ) ) ;
#62768=CARTESIAN_POINT ( 'NONE',  ( 16.37812500061451715, -4.541064518000419881, 2.621784821874995952 ) ) ;
#62770=CARTESIAN_POINT ( 'NONE',  ( 12.68437500061451573, 4.541064518000418104, 2.621784821874999949 ) ) ;
#62771=CARTESIAN_POINT ( 'NONE',  ( 28.01249999999999574, 2.886751345948129099, -4.999999999999998224 ) ) ;
#62772=CARTESIAN_POINT ( 'NONE',  ( 25.72500000122903074, -5.773502691896255534, -1.060575238724906372E-15 ) ) ;
#62773=DIRECTION ( 'NONE',  ( -0.000000000000000000, -1.000000000000000000, -0.000000000000000000 ) ) ;
#62774=CARTESIAN_POINT ( 'NONE',  ( 12.64687500061451608, 6.054752690667223547, 3.707466751127219781E-16 ) ) ;
#62775=CARTESIAN_POINT ( 'NONE',  ( 27.90937500061451715, 4.541064518000418104, -2.621784821874998173 ) ) ;
#62776=DIRECTION ( 'NONE',  ( -0.000000000000000000, -1.000000000000000000, -0.000000000000000000 ) ) ;
#62777=CARTESIAN_POINT ( 'NONE',  ( -3.999999999999999112, 11.97500000122903430, 27.69059892324149885 ) ) ;
#62778=CARTESIAN_POINT ( 'NONE',  ( 22.09687500061451715, 6.054752690667223547, 3.707466751127219781E-16 ) ) ;
#62779=CARTESIAN_POINT ( 'NONE',  ( 13.47187500061451537, 3.027376345333613106, -5.243569643749998122 ) ) ;
#62781=CARTESIAN_POINT ( 'NONE',  ( 26.39999999999999858, 0.000000000000000000, 4.999999999999998224 ) ) ;
#62784=CARTESIAN_POINT ( 'NONE',  ( 17.80312500061451786, -4.541064518000417216, -2.621784821875001281 ) ) ;
#62785=CARTESIAN_POINT ( 'NONE',  ( 8.099999999999999645, -4.330127018922190985, -2.500000000000001332 ) ) ;
#62786=CARTESIAN_POINT ( 'NONE',  ( 2.000000000000001332, 13.51250000122903394, 33.46410161513774995 ) ) ;
#62787=CARTESIAN_POINT ( 'NONE',  ( 17.32499999999999929, 4.330127018922191873, 2.499999999999999556 ) ) ;
#62788=CARTESIAN_POINT ( 'NONE',  ( 4.243569643749999010, 11.06562500061451715, 27.54997392385601174 ) ) ;
#62790=CARTESIAN_POINT ( 'NONE',  ( 28.17187500061451644, -6.054752690667223547, -1.112240025338166033E-15 ) ) ;
#62791=EDGE_LOOP ( 'NONE', ( #51237, #19653, #28754, #39123 ) ) ;
#62792=CARTESIAN_POINT ( 'NONE',  ( 21.55312500061451431, 4.541064518000418104, -2.621784821874998173 ) ) ;
#62793=CARTESIAN_POINT ( 'NONE',  ( 19.80937500061451573, 4.541064518000418104, -2.621784821874998173 ) ) ;
#62794=CARTESIAN_POINT ( 'NONE',  ( 4.575000000000002842, 6.123233995736764310E-16, -4.999999999999998224 ) ) ;
#62795=CARTESIAN_POINT ( 'NONE',  ( 7.865625000614516971, -6.054752690667223547, -1.112240025338166033E-15 ) ) ;
#62796=CARTESIAN_POINT ( 'NONE',  ( 23.12812500061451360, -4.541064518000419881, 2.621784821874995952 ) ) ;
#62797=CARTESIAN_POINT ( 'NONE',  ( 12.68437500061451573, 4.541064518000418104, 2.621784821874999949 ) ) ;
#62798=CARTESIAN_POINT ( 'NONE',  ( 17.25937500061451502, 0.000000000000000000, 5.243569643749999010 ) ) ;
#62799=CARTESIAN_POINT ( 'NONE',  ( -2.121784821874999949, 18.37812500061451715, 26.32496088578401938 ) ) ;
#62800=CARTESIAN_POINT ( 'NONE',  ( 17.96250000122903501, 0.000000000000000000, 4.999999999999998224 ) ) ;
#62802=CARTESIAN_POINT ( 'NONE',  ( 9.178125000614517859, -4.541064518000419881, 2.621784821874995952 ) ) ;
#62803=CARTESIAN_POINT ( 'NONE',  ( 5.484375000614518214, 4.541064518000418104, 2.621784821874999949 ) ) ;
#62804=CARTESIAN_POINT ( 'NONE',  ( 4.584375000614516971, 4.541064518000418104, 2.621784821874999949 ) ) ;
#62805=ORIENTED_EDGE ( 'NONE', *, *, #38215, .F. ) ;
#62806=CARTESIAN_POINT ( 'NONE',  ( 26.22187500061451715, 3.027376345333611329, 5.243569643749999010 ) ) ;
#62807=CARTESIAN_POINT ( 'NONE',  ( 17.91562500061451502, 3.027376345333613106, -5.243569643749998122 ) ) ;
#62808=CARTESIAN_POINT ( 'NONE',  ( 28.20000000122903216, 5.773502691896255534, 3.535250795749688894E-16 ) ) ;
#62809=CARTESIAN_POINT ( 'NONE',  ( 27.36562500061451786, 3.027376345333613106, -5.243569643749998122 ) ) ;
#62810=VECTOR ( 'NONE', #11437, 1000.000000000000000 ) ;
#62811=CARTESIAN_POINT ( 'NONE',  ( 21.49687500061451573, -3.027376345333610441, -5.243569643749999898 ) ) ;
#62812=CARTESIAN_POINT ( 'NONE',  ( 17.35312500061451502, -4.541064518000417216, -2.621784821875001281 ) ) ;
#62813=CARTESIAN_POINT ( 'NONE',  ( 9.001249775931846008E-16, 16.82187500061451857, 34.90005215228797653 ) ) ;
#62814=CARTESIAN_POINT ( 'NONE',  ( 21.77812500061451928, -4.541064518000419881, 2.621784821874995952 ) ) ;
#62816=EDGE_LOOP ( 'NONE', ( #6952, #61638, #19423, #35701 ) ) ;
#62817=CARTESIAN_POINT ( 'NONE',  ( 28.64999999999999858, 0.000000000000000000, 4.999999999999998224 ) ) ;
#62818=CARTESIAN_POINT ( 'NONE',  ( -3.999999999999999112, 14.15000000000000036, -30.00000000000000000 ) ) ;
#62820=CARTESIAN_POINT ( 'NONE',  ( 29.50312500061451360, -4.541064518000417216, -2.621784821875001281 ) ) ;
#62821=CARTESIAN_POINT ( 'NONE',  ( 9.328125000614518214, 6.421520780324663323E-16, -5.243569643749999010 ) ) ;
#62822=CARTESIAN_POINT ( 'NONE',  ( 22.05000000122903714, -2.886751345948129988, 4.999999999999997335 ) ) ;
#62823=CARTESIAN_POINT ( 'NONE',  ( 28.34062500061451928, 6.054752690667223547, 3.707466751127219781E-16 ) ) ;
#62824=CARTESIAN_POINT ( 'NONE',  ( 28.35000000000000142, -4.330127018922190985, -2.500000000000001332 ) ) ;
#62825=CARTESIAN_POINT ( 'NONE',  ( -1.999999999999997113, 17.48750000122903359, -26.53589838486224295 ) ) ;
#62826=CARTESIAN_POINT ( 'NONE',  ( 1.592000809091587073E-14, 16.28750000000000142, 26.00000000000000000 ) ) ;
#62827=CARTESIAN_POINT ( 'NONE',  ( 11.65312500061451573, 4.541064518000418104, -2.621784821874998173 ) ) ;
#62829=CARTESIAN_POINT ( 'NONE',  ( 8.053125000614516082, 4.541064518000418104, -2.621784821874998173 ) ) ;
#62830=CARTESIAN_POINT ( 'NONE',  ( 5.690625000614516260, -3.027376345333610441, -5.243569643749999898 ) ) ;
#62834=CARTESIAN_POINT ( 'NONE',  ( 14.55000000000000071, 4.330127018922192761, -2.499999999999997780 ) ) ;
#62836=CARTESIAN_POINT ( 'NONE',  ( 16.88437500061451502, -4.541064518000419881, 2.621784821874995952 ) ) ;
#62837=CARTESIAN_POINT ( 'NONE',  ( 12.41250000122903430, 4.330127018922192761, -2.499999999999997780 ) ) ;
#62838=CARTESIAN_POINT ( 'NONE',  ( 18.94687500061451502, 6.054752690667223547, 3.707466751127219781E-16 ) ) ;
#62840=CARTESIAN_POINT ( 'NONE',  ( 21.64687500061451786, 6.054752690667223547, 3.707466751127219781E-16 ) ) ;
#62841=CARTESIAN_POINT ( 'NONE',  ( -3.000416591977282496E-16, 14.74062500061451786, -34.90005215228797653 ) ) ;
#62843=CARTESIAN_POINT ( 'NONE',  ( 4.140919957849956923, 2.802311140224996944, 4.431956019633390476 ) ) ;
#62844=CARTESIAN_POINT ( 'NONE',  ( 26.05312500061451431, 4.541064518000418104, -2.621784821874998173 ) ) ;
#62846=CARTESIAN_POINT ( 'NONE',  ( 28.92187500061451644, 3.027376345333611329, 5.243569643749999010 ) ) ;
#62847=CARTESIAN_POINT ( 'NONE',  ( 23.36250000000000071, -5.773502691896255534, -1.060575238724906372E-15 ) ) ;
#62848=CARTESIAN_POINT ( 'NONE',  ( 5.840625000614516615, 6.054752690667223547, 3.707466751127219781E-16 ) ) ;
#62850=CARTESIAN_POINT ( 'NONE',  ( 19.95937500061451786, 0.000000000000000000, 5.243569643749999010 ) ) ;
#62852=CARTESIAN_POINT ( 'NONE',  ( 4.940625000614515372, 6.054752690667223547, 3.707466751127219781E-16 ) ) ;
#62853=CARTESIAN_POINT ( 'NONE',  ( 8.371875000614515727, -6.054752690667223547, -1.112240025338166033E-15 ) ) ;
#62854=EDGE_LOOP ( 'NONE', ( #18107, #23708, #60618, #63238 ) ) ;
#62855=CARTESIAN_POINT ( 'NONE',  ( 18.19687500061451502, -3.027376345333614438, 5.243569643749998122 ) ) ;
#62856=CARTESIAN_POINT ( 'NONE',  ( -5.810221930991193690E-16, 11.90000000122903323, 26.00000000000000355 ) ) ;
#62857=CARTESIAN_POINT ( 'NONE',  ( 28.04999999999999716, 4.330127018922192761, -2.499999999999997780 ) ) ;
#62858=CARTESIAN_POINT ( 'NONE',  ( 3.337499999999999911, 5.773502691896255534, 3.535250795749688894E-16 ) ) ;
#62860=ORIENTED_EDGE ( 'NONE', *, *, #4790, .F. ) ;
#62861=CARTESIAN_POINT ( 'NONE',  ( 11.06250000000000000, 2.886751345948126879, 4.999999999999999112 ) ) ;
#62863=CARTESIAN_POINT ( 'NONE',  ( 24.44062500061451715, -3.027376345333614438, 5.243569643749998122 ) ) ;
#62864=CARTESIAN_POINT ( 'NONE',  ( 13.53749999999999964, -2.886751345948125991, -5.000000000000000000 ) ) ;
#62865=CARTESIAN_POINT ( 'NONE',  ( 9.975000001229034297, -5.773502691896255534, -1.060575238724906372E-15 ) ) ;
#62866=CARTESIAN_POINT ( 'NONE',  ( 10.07812500061451644, -4.541064518000419881, 2.621784821874995952 ) ) ;
#62867=CARTESIAN_POINT ( 'NONE',  ( 24.44999999999999929, 4.330127018922192761, -2.499999999999997780 ) ) ;
#62868=CARTESIAN_POINT ( 'NONE',  ( 21.29062500061451502, -3.027376345333614438, 5.243569643749998122 ) ) ;
#62870=CARTESIAN_POINT ( 'NONE',  ( 27.90000000122903145, -2.886751345948129988, 4.999999999999997335 ) ) ;
#62872=CARTESIAN_POINT ( 'NONE',  ( 6.562500000000001776, 2.886751345948126879, 4.999999999999999112 ) ) ;
#62874=CARTESIAN_POINT ( 'NONE',  ( 22.49062500061451431, 6.054752690667223547, 3.707466751127219781E-16 ) ) ;
#62875=CARTESIAN_POINT ( 'NONE',  ( 28.64062500061451289, -3.027376345333610441, -5.243569643749999898 ) ) ;
#62877=CARTESIAN_POINT ( 'NONE',  ( 19.35937500061451644, 4.541064518000418104, -2.621784821874998173 ) ) ;
#62878=CARTESIAN_POINT ( 'NONE',  ( 13.34062500061451750, -3.027376345333610441, -5.243569643749999898 ) ) ;
#62879=FACE_BOUND ( 'NONE', #70176, .T. ) ;
#62880=CARTESIAN_POINT ( 'NONE',  ( 26.47500000122903074, 2.886751345948126879, 4.999999999999999112 ) ) ;
#62882=CARTESIAN_POINT ( 'NONE',  ( 16.60312500061451857, 4.541064518000418104, -2.621784821874998173 ) ) ;
#62883=CARTESIAN_POINT ( 'NONE',  ( 30.00000000000000000, 0.000000000000000000, 0.000000000000000000 ) ) ;
#62884=CARTESIAN_POINT ( 'NONE',  ( 4.500000001229034652, -2.886751345948129988, 4.999999999999997335 ) ) ;
#62885=CARTESIAN_POINT ( 'NONE',  ( 12.45937500061451786, -4.541064518000417216, -2.621784821875001281 ) ) ;
#62886=CARTESIAN_POINT ( 'NONE',  ( 12.64687500061451608, 6.054752690667223547, 3.707466751127219781E-16 ) ) ;
#62887=CARTESIAN_POINT ( 'NONE',  ( 20.74687500061451573, 6.054752690667223547, 3.707466751127219781E-16 ) ) ;
#62888=ORIENTED_EDGE ( 'NONE', *, *, #9933, .F. ) ;
#62889=CARTESIAN_POINT ( 'NONE',  ( -5.959432963256015015, 8.030867404579451474, 30.80300165410438851 ) ) ;
#62890=CARTESIAN_POINT ( 'NONE',  ( 23.99062500061451786, -3.027376345333614438, 5.243569643749998122 ) ) ;
#62891=( BOUNDED_CURVE ( )  B_SPLINE_CURVE ( 2, ( #28203, #46269, #6021, #62174, #68808, #18164, #22283 ),
 .UNSPECIFIED., .F., .F. ) 
 B_SPLINE_CURVE_WITH_KNOTS ( ( 3, 2, 2, 3 ),
 ( 0.6083333333333332815, 0.6111111111111111605, 0.6138888888888889284, 0.6166666666666666963 ),
 .UNSPECIFIED. ) 
 CURVE ( )  GEOMETRIC_REPRESENTATION_ITEM ( )  RATIONAL_B_SPLINE_CURVE ( ( 1.000000000000000000, 0.8660254037844387076, 1.000000000000000000, 0.8660254037844387076, 1.000000000000000000, 0.8660254037844387076, 1.000000000000000000 ) ) 
 REPRESENTATION_ITEM ( '' )  );
#62892=CARTESIAN_POINT ( 'NONE',  ( 19.54687500061451644, -3.027376345333614438, 5.243569643749998122 ) ) ;
#62893=CARTESIAN_POINT ( 'NONE',  ( 24.02812500061451573, -4.541064518000419881, 2.621784821874995952 ) ) ;
#62895=CARTESIAN_POINT ( 'NONE',  ( 2.000000000000001332, 15.65000000000000036, 33.46410161513774995 ) ) ;
#62896=CARTESIAN_POINT ( 'NONE',  ( 28.86562500061451786, 3.027376345333611329, 5.243569643749999010 ) ) ;
#62897=CARTESIAN_POINT ( 'NONE',  ( 10.65000000122903323, 5.773502691896255534, 3.535250795749688894E-16 ) ) ;
#62898=CARTESIAN_POINT ( 'NONE',  ( 5.850000001229035185, -2.886751345948129988, 4.999999999999997335 ) ) ;
#62899=CARTESIAN_POINT ( 'NONE',  ( 30.00000000000000000, 0.000000000000000000, 4.999999999999998224 ) ) ;
#62900=CARTESIAN_POINT ( 'NONE',  ( 27.86250000122903359, 0.000000000000000000, 4.999999999999998224 ) ) ;
#62903=CARTESIAN_POINT ( 'NONE',  ( 9.421875000614519990, 3.027376345333613106, -5.243569643749998122 ) ) ;
#62905=CARTESIAN_POINT ( 'NONE',  ( 17.46562500061451217, 3.027376345333613106, -5.243569643749998122 ) ) ;
#62906=CARTESIAN_POINT ( 'NONE',  ( 10.54687500061451644, -3.027376345333614438, 5.243569643749998122 ) ) ;
#62907=CARTESIAN_POINT ( 'NONE',  ( 28.50000000122903288, -2.886751345948125991, -5.000000000000000000 ) ) ;
#62908=CARTESIAN_POINT ( 'NONE',  ( 19.99687500061451573, -3.027376345333614438, 5.243569643749998122 ) ) ;
#62909=CARTESIAN_POINT ( 'NONE',  ( 7.809375000614519280, 0.000000000000000000, 5.243569643749999010 ) ) ;
#62910=CARTESIAN_POINT ( 'NONE',  ( 2.803125000614518747, 0.000000000000000000, 5.243569643749999010 ) ) ;
#62911=CARTESIAN_POINT ( 'NONE',  ( 6.150000000000003020, 0.000000000000000000, 4.999999999999998224 ) ) ;
#62912=CARTESIAN_POINT ( 'NONE',  ( 8.990625000614516082, 6.054752690667223547, 3.707466751127219781E-16 ) ) ;
#62913=CARTESIAN_POINT ( 'NONE',  ( 19.15312500061451573, -4.541064518000417216, -2.621784821875001281 ) ) ;
#62914=EDGE_LOOP ( 'NONE', ( #24976, #71794, #72471 ) ) ;
#62915=CARTESIAN_POINT ( 'NONE',  ( 5.100000001229034297, -2.886751345948125991, -5.000000000000000000 ) ) ;
#62916=CARTESIAN_POINT ( 'NONE',  ( 14.24062500061451608, -3.027376345333610441, -5.243569643749999898 ) ) ;
#62917=CARTESIAN_POINT ( 'NONE',  ( 12.81562500061451537, -6.054752690667223547, -1.112240025338166033E-15 ) ) ;
#62919=CARTESIAN_POINT ( 'NONE',  ( 13.95000000000000107, -4.330127018922190985, -2.500000000000001332 ) ) ;
#62920=CARTESIAN_POINT ( 'NONE',  ( 7.912500001229033408, 4.330127018922192761, -2.499999999999997780 ) ) ;
#62921=CARTESIAN_POINT ( 'NONE',  ( 6.290625000614517681, 6.054752690667223547, 3.707466751127219781E-16 ) ) ;
#62922=EDGE_CURVE ( 'NONE', #16658, #60892, #29597, .T. ) ;
#62923=CARTESIAN_POINT ( 'NONE',  ( 19.12500000122903288, 2.886751345948129099, -4.999999999999998224 ) ) ;
#62925=CARTESIAN_POINT ( 'NONE',  ( 4.243569643749999898, 11.94687500061451857, -27.54997392385601529 ) ) ;
#62926=CARTESIAN_POINT ( 'NONE',  ( 8.512499999999999289, -5.773502691896255534, -1.060575238724906372E-15 ) ) ;
#62927=CARTESIAN_POINT ( 'NONE',  ( 3.337500001229034563, 6.123233995736764310E-16, -4.999999999999998224 ) ) ;
#62928=CARTESIAN_POINT ( 'NONE',  ( -3.999999999999999112, 11.41250000000000142, -32.30940107675850470 ) ) ;
#62930=CARTESIAN_POINT ( 'NONE',  ( 18.38437500061451857, 6.421520780324663323E-16, -5.243569643749999010 ) ) ;
#62931=CARTESIAN_POINT ( 'NONE',  ( 21.33750000122903145, 6.123233995736764310E-16, -4.999999999999998224 ) ) ;
#62932=CARTESIAN_POINT ( 'NONE',  ( 14.24062500061451608, -3.027376345333610441, -5.243569643749999898 ) ) ;
#62935=CARTESIAN_POINT ( 'NONE',  ( 26.63437500061451857, 4.541064518000418104, 2.621784821874999949 ) ) ;
#62937=CARTESIAN_POINT ( 'NONE',  ( 13.26562500061451644, -6.054752690667223547, -1.112240025338166033E-15 ) ) ;
#62938=CARTESIAN_POINT ( 'NONE',  ( 10.24687500061451750, -3.027376345333610441, -5.243569643749999898 ) ) ;
#62939=ORIENTED_EDGE ( 'NONE', *, *, #37818, .F. ) ;
#62940=CARTESIAN_POINT ( 'NONE',  ( 2.869618986945705608, -4.094575117703225686, -3.017297621565764310 ) ) ;
#62941=CARTESIAN_POINT ( 'NONE',  ( 20.20312500061451644, 4.541064518000418104, -2.621784821874998173 ) ) ;
#62942=LINE ( 'NONE', #35956, #30950 ) ;
#62944=CARTESIAN_POINT ( 'NONE',  ( 9.187500000000001776, 5.773502691896255534, 3.535250795749688894E-16 ) ) ;
#62945=CARTESIAN_POINT ( 'NONE',  ( 20.13750000122903216, 4.330127018922191873, 2.499999999999999556 ) ) ;
#62946=CARTESIAN_POINT ( 'NONE',  ( 3.999999999999998668, 10.36250000000000426, 27.69059892324149530 ) ) ;
#62948=VERTEX_POINT ( 'NONE', #52800 ) ;
#62949=CARTESIAN_POINT ( 'NONE',  ( 17.36249999999999716, 2.886751345948126879, 4.999999999999999112 ) ) ;
#62950=CARTESIAN_POINT ( 'NONE',  ( 20.51249999999999929, 2.886751345948126879, 4.999999999999999112 ) ) ;
#62951=CARTESIAN_POINT ( 'NONE',  ( 19.05937500061451928, 0.000000000000000000, 5.243569643749999010 ) ) ;
#62952=CARTESIAN_POINT ( 'NONE',  ( 24.36562500061451786, 3.027376345333611329, 5.243569643749999010 ) ) ;
#62953=ORIENTED_EDGE ( 'NONE', *, *, #53010, .T. ) ;
#62954=CARTESIAN_POINT ( 'NONE',  ( -3.999999999999999112, 16.92500000122903359, 27.69059892324149885 ) ) ;
#62955=CARTESIAN_POINT ( 'NONE',  ( 8.990625000614516082, 6.054752690667223547, 3.707466751127219781E-16 ) ) ;
#62956=LINE ( 'NONE', #1284, #61872 ) ;
#62957=CARTESIAN_POINT ( 'NONE',  ( 15.07499999999999929, 4.330127018922191873, 2.499999999999999556 ) ) ;
#62958=CARTESIAN_POINT ( 'NONE',  ( 2.121784821874999061, 18.75312500061451715, 26.32496088578401583 ) ) ;
#62959=CARTESIAN_POINT ( 'NONE',  ( 3.196875000614516793, 6.054752690667223547, 3.707466751127219781E-16 ) ) ;
#62962=CARTESIAN_POINT ( 'NONE',  ( 25.50937500061451502, -4.541064518000417216, -2.621784821875001281 ) ) ;
#62963=ORIENTED_EDGE ( 'NONE', *, *, #12710, .T. ) ;
#62964=CARTESIAN_POINT ( 'NONE',  ( 24.06562500061451715, -6.054752690667223547, -1.112240025338166033E-15 ) ) ;
#62965=CARTESIAN_POINT ( 'NONE',  ( 23.63437500061451502, -4.541064518000419881, 2.621784821874995952 ) ) ;
#62966=CARTESIAN_POINT ( 'NONE',  ( -4.243569643749999898, 17.06562500061459176, -32.45002607614398471 ) ) ;
#62967=CARTESIAN_POINT ( 'NONE',  ( 10.68750000000000000, -2.886751345948129988, 4.999999999999997335 ) ) ;
#62968=CARTESIAN_POINT ( 'NONE',  ( 8.015625000614518214, 3.027376345333613106, -5.243569643749998122 ) ) ;
#62969=CARTESIAN_POINT ( 'NONE',  ( 3.787500000000002753, 5.773502691896255534, 3.535250795749688401E-16 ) ) ;
#62970=CARTESIAN_POINT ( 'NONE',  ( 28.94062500061452070, -3.027376345333614438, 5.243569643749998122 ) ) ;
#62971=CARTESIAN_POINT ( 'NONE',  ( 27.29062500061451502, -3.027376345333610441, -5.243569643749999898 ) ) ;
#62974=CARTESIAN_POINT ( 'NONE',  ( 19.28437500061451360, 6.421520780324663323E-16, -5.243569643749999010 ) ) ;
#62975=CARTESIAN_POINT ( 'NONE',  ( -4.243569643749997233, 11.79687500061451999, 32.45002607614398471 ) ) ;
#62976=CARTESIAN_POINT ( 'NONE',  ( 18.34687500061451715, -3.027376345333610441, -5.243569643749999898 ) ) ;
#62977=CARTESIAN_POINT ( 'NONE',  ( 28.39687500061452141, 6.054752690667223547, 3.707466751127219781E-16 ) ) ;
#62978=CARTESIAN_POINT ( 'NONE',  ( 4.243569643749999898, 16.48437500061451644, 30.00000000000000000 ) ) ;
#62979=CARTESIAN_POINT ( 'NONE',  ( 8.203125000614518214, 0.000000000000000000, 5.243569643749999010 ) ) ;
#62980=CARTESIAN_POINT ( 'NONE',  ( -1.071796769724492338, 18.29240381056766651, -26.00000000000000711 ) ) ;
#62981=CARTESIAN_POINT ( 'NONE',  ( 3.534375000614518036, 6.421520780324663323E-16, -5.243569643749999010 ) ) ;
#62982=CARTESIAN_POINT ( 'NONE',  ( 0.000000000000000000, 20.00000000000000000, 26.00000000000000000 ) ) ;
#62983=CARTESIAN_POINT ( 'NONE',  ( 5.615625000614517859, -6.054752690667223547, -1.112240025338166033E-15 ) ) ;
#62984=CARTESIAN_POINT ( 'NONE',  ( 9.946875000614516793, 6.054752690667223547, 3.707466751127219781E-16 ) ) ;
#62986=CARTESIAN_POINT ( 'NONE',  ( 17.70000000122903216, -2.886751345948125991, -5.000000000000000000 ) ) ;
#62987=CARTESIAN_POINT ( 'NONE',  ( 5.446875000614518569, 6.054752690667223547, 3.707466751127219781E-16 ) ) ;
#62988=CARTESIAN_POINT ( 'NONE',  ( 6.890625000614516438, -3.027376345333614438, 5.243569643749998122 ) ) ;
#62991=CARTESIAN_POINT ( 'NONE',  ( 16.58437500061451786, 6.421520780324663323E-16, -5.243569643749999010 ) ) ;
#62993=ORIENTED_EDGE ( 'NONE', *, *, #33221, .T. ) ;
#62994=CARTESIAN_POINT ( 'NONE',  ( 23.61562500061451431, -6.054752690667223547, -1.112240025338166033E-15 ) ) ;
#62995=CARTESIAN_POINT ( 'NONE',  ( 9.103125000614515017, 0.000000000000000000, 5.243569643749999010 ) ) ;
#62996=CARTESIAN_POINT ( 'NONE',  ( 27.34687500061451360, -3.027376345333610441, -5.243569643749999898 ) ) ;
#62998=CARTESIAN_POINT ( 'NONE',  ( 10.79062500061451679, 6.054752690667223547, 3.707466751127219781E-16 ) ) ;
#62999=CARTESIAN_POINT ( 'NONE',  ( -2.121784821874996840, 10.03437500061451892, -26.32496088578401583 ) ) ;
#63000=CARTESIAN_POINT ( 'NONE',  ( 9.712500001229033231, 4.330127018922192761, -2.499999999999997780 ) ) ;
#63001=CARTESIAN_POINT ( 'NONE',  ( 26.99062500061451431, 6.054752690667223547, 3.707466751127219781E-16 ) ) ;
#63002=CARTESIAN_POINT ( 'NONE',  ( 2.121784821875001281, 11.85312500061451857, -26.32496088578401938 ) ) ;
#63003=CARTESIAN_POINT ( 'NONE',  ( 12.60000000122903430, -2.886751345948129988, 4.999999999999997335 ) ) ;
#63004=CARTESIAN_POINT ( 'NONE',  ( 10.46249999999999858, 2.886751345948129099, -4.999999999999998224 ) ) ;
#63005=CARTESIAN_POINT ( 'NONE',  ( 20.31562500061451715, 3.027376345333611329, 5.243569643749999010 ) ) ;
#63006=CARTESIAN_POINT ( 'NONE',  ( 30.00000000000000000, 0.000000000000000000, 4.999999999999998224 ) ) ;
#63007=EDGE_CURVE ( 'NONE', #72067, #9906, #26516, .T. ) ;
#63008=CARTESIAN_POINT ( 'NONE',  ( 20.77500000000000213, 6.123233995736764310E-16, -4.999999999999998224 ) ) ;
#63009=CARTESIAN_POINT ( 'NONE',  ( 7.162500001229032520, 0.000000000000000000, 4.999999999999998224 ) ) ;
#63010=CARTESIAN_POINT ( 'NONE',  ( 15.93750000122903110, 6.123233995736764310E-16, -4.999999999999998224 ) ) ;
#63011=CARTESIAN_POINT ( 'NONE',  ( 11.91562500061451857, -6.054752690667223547, -1.112240025338166033E-15 ) ) ;
#63012=CARTESIAN_POINT ( 'NONE',  ( 17.01562500061451644, 3.027376345333613106, -5.243569643749998122 ) ) ;
#63013=CARTESIAN_POINT ( 'NONE',  ( 26.66250000122903430, -4.330127018922190985, -2.500000000000001332 ) ) ;
#63014=CARTESIAN_POINT ( 'NONE',  ( 20.81250000000000000, 2.886751345948129099, -4.999999999999998224 ) ) ;
#63015=CARTESIAN_POINT ( 'NONE',  ( 24.42187500061451999, 3.027376345333611329, 5.243569643749999010 ) ) ;
#63017=CARTESIAN_POINT ( 'NONE',  ( 9.412500001229034297, 0.000000000000000000, 4.999999999999998224 ) ) ;
#63018=CARTESIAN_POINT ( 'NONE',  ( 9.346875000614517148, -3.027376345333610441, -5.243569643749999898 ) ) ;
#63019=CARTESIAN_POINT ( 'NONE',  ( 25.84687500061451360, -3.027376345333614438, 5.243569643749998122 ) ) ;
#63020=DIRECTION ( 'NONE',  ( -1.000000000000000000, -0.000000000000000000, -0.000000000000000000 ) ) ;
#63021=CARTESIAN_POINT ( 'NONE',  ( 20.99062500061451431, -3.027376345333610441, -5.243569643749999898 ) ) ;
#63022=CARTESIAN_POINT ( 'NONE',  ( 26.85937500061451644, -4.541064518000417216, -2.621784821875001281 ) ) ;
#63024=CARTESIAN_POINT ( 'NONE',  ( 18.56250000000000000, 2.886751345948129099, -4.999999999999997335 ) ) ;
#63025=CARTESIAN_POINT ( 'NONE',  ( 7.884375000614517681, -4.541064518000419881, 2.621784821874995952 ) ) ;
#63026=CARTESIAN_POINT ( 'NONE',  ( 19.19062500061452070, -3.027376345333610441, -5.243569643749999898 ) ) ;
#63028=CARTESIAN_POINT ( 'NONE',  ( 28.34062500061451928, 6.054752690667223547, 3.707466751127219781E-16 ) ) ;
#63029=CARTESIAN_POINT ( 'NONE',  ( 4.396875000614516971, -3.027376345333610441, -5.243569643749999898 ) ) ;
#63030=CARTESIAN_POINT ( 'NONE',  ( 4.898587196589411843E-16, 20.00000000000000000, -26.00000000000000000 ) ) ;
#63031=CARTESIAN_POINT ( 'NONE',  ( 4.040625000614517681, 6.054752690667223547, 3.707466751127219781E-16 ) ) ;
#63032=CARTESIAN_POINT ( 'NONE',  ( 18.22499999999999787, 4.330127018922191873, 2.499999999999999556 ) ) ;
#63033=ORIENTED_EDGE ( 'NONE', *, *, #31877, .F. ) ;
#63034=CARTESIAN_POINT ( 'NONE',  ( 25.08749999999999858, -2.886751345948129988, 4.999999999999997335 ) ) ;
#63035=( BOUNDED_CURVE ( )  B_SPLINE_CURVE ( 2, ( #55675, #4710, #72671, #5072, #33858, #27241, #50141 ),
 .UNSPECIFIED., .F., .F. ) 
 B_SPLINE_CURVE_WITH_KNOTS ( ( 3, 2, 2, 3 ),
 ( 0.4166666666666667407, 0.4194444444444445086, 0.4222222222222222210, 0.4249999999999999889 ),
 .UNSPECIFIED. ) 
 CURVE ( )  GEOMETRIC_REPRESENTATION_ITEM ( )  RATIONAL_B_SPLINE_CURVE ( ( 0.9999999999999973355, 0.8660254037844413721, 1.000000000000000000, 0.8660254037844387076, 1.000000000000000000, 0.8660254037844387076, 1.000000000000000000 ) ) 
 REPRESENTATION_ITEM ( '' )  );
#63036=CARTESIAN_POINT ( 'NONE',  ( 27.38437500061451857, 6.421520780324663323E-16, -5.243569643749999010 ) ) ;
#63038=CARTESIAN_POINT ( 'NONE',  ( 14.69062500061451537, -3.027376345333610441, -5.243569643749999898 ) ) ;
#63039=CARTESIAN_POINT ( 'NONE',  ( 6.365625000614518747, 3.027376345333611329, 5.243569643749999010 ) ) ;
#63041=CARTESIAN_POINT ( 'NONE',  ( 4.884375000614518569, 6.421520780324663323E-16, -5.243569643749999010 ) ) ;
#63042=CARTESIAN_POINT ( 'NONE',  ( 15.48750000122903359, 6.123233995736764310E-16, -4.999999999999998224 ) ) ;
#63043=CARTESIAN_POINT ( 'NONE',  ( 21.67500000000000071, 6.123233995736764310E-16, -4.999999999999998224 ) ) ;
#63044=CARTESIAN_POINT ( 'NONE',  ( 28.46249999999999858, 2.886751345948129099, -4.999999999999998224 ) ) ;
#63045=CARTESIAN_POINT ( 'NONE',  ( 4.134375000614517681, 4.541064518000418104, 2.621784821874999949 ) ) ;
#63046=CARTESIAN_POINT ( 'NONE',  ( 9.534375000614517148, 4.541064518000418104, 2.621784821874999949 ) ) ;
#63047=CARTESIAN_POINT ( 'NONE',  ( 20.78437500061451715, 4.541064518000418104, 2.621784821874999949 ) ) ;
#63049=ORIENTED_EDGE ( 'NONE', *, *, #70507, .F. ) ;
#63050=CARTESIAN_POINT ( 'NONE',  ( 4.209375000614516971, 0.000000000000000000, 5.243569643749999010 ) ) ;
#63051=CARTESIAN_POINT ( 'NONE',  ( 5.475000000000000533, 6.123233995736764310E-16, -4.999999999999998224 ) ) ;
#63052=CARTESIAN_POINT ( 'NONE',  ( 6.421875000614519102, 3.027376345333611329, 5.243569643749999010 ) ) ;
#63053=CARTESIAN_POINT ( 'NONE',  ( 18.75000000000000000, 0.000000000000000000, 4.999999999999998224 ) ) ;
#63054=CARTESIAN_POINT ( 'NONE',  ( 15.25312500061451715, 4.541064518000418104, -2.621784821874998173 ) ) ;
#63058=CARTESIAN_POINT ( 'NONE',  ( 9.253125000614517148, -4.541064518000417216, -2.621784821875001281 ) ) ;
#63059=CARTESIAN_POINT ( 'NONE',  ( 27.72187500061451715, -6.054752690667223547, -1.112240025338166033E-15 ) ) ;
#63060=CARTESIAN_POINT ( 'NONE',  ( -4.243569643749999898, 19.82187500061451857, 27.54997392385601529 ) ) ;
#63061=CARTESIAN_POINT ( 'NONE',  ( 25.84687500061451360, -3.027376345333614438, 5.243569643749998122 ) ) ;
#63062=CARTESIAN_POINT ( 'NONE',  ( 8.662499999999999645, 2.886751345948129099, -4.999999999999998224 ) ) ;
#63063=CARTESIAN_POINT ( 'NONE',  ( 3.999999999999999112, 12.68750000122903465, 30.00000000000000000 ) ) ;
#63064=CARTESIAN_POINT ( 'NONE',  ( 13.97812500061451679, 4.541064518000418104, 2.621784821874999949 ) ) ;
#63065=CARTESIAN_POINT ( 'NONE',  ( 7.200000001229035718, -2.886751345948129988, 4.999999999999997335 ) ) ;
#63066=ADVANCED_FACE ( 'NONE', ( #66074 ), #43919, .F. ) ;
#63067=CARTESIAN_POINT ( 'NONE',  ( 17.63437500061451502, 4.541064518000418104, 2.621784821874999949 ) ) ;
#63068=CARTESIAN_POINT ( 'NONE',  ( 11.63437500061451857, 6.421520780324663323E-16, -5.243569643749999010 ) ) ;
#63069=CARTESIAN_POINT ( 'NONE',  ( -3.963752180954430493, 3.047823949009541344, -29.44540563775499820 ) ) ;
#63071=VECTOR ( 'NONE', #39508, 1000.000000000000000 ) ;
#63072=CARTESIAN_POINT ( 'NONE',  ( 13.37812500061451715, 6.421520780324663323E-16, -5.243569643749999010 ) ) ;
#63073=CARTESIAN_POINT ( 'NONE',  ( 26.70000000122903572, -2.886751345948125991, -5.000000000000000000 ) ) ;
#63074=CARTESIAN_POINT ( 'NONE',  ( 12.79687500061451821, -3.027376345333614438, 5.243569643749998122 ) ) ;
#63075=CARTESIAN_POINT ( 'NONE',  ( 4.059375000614519280, 4.541064518000418104, -2.621784821874998173 ) ) ;
#63076=CARTESIAN_POINT ( 'NONE',  ( 13.67812500061451786, -4.541064518000419881, 2.621784821874995952 ) ) ;
#63078=CARTESIAN_POINT ( 'NONE',  ( 1.071796769724489895, 18.96740381056766722, -34.00000000000000000 ) ) ;
#63079=CARTESIAN_POINT ( 'NONE',  ( 22.84687500061451715, -3.027376345333610441, -5.243569643749999898 ) ) ;
#63080=CARTESIAN_POINT ( 'NONE',  ( -4.243569643749997233, 10.84062500061451395, 32.45002607614398471 ) ) ;
#63081=CARTESIAN_POINT ( 'NONE',  ( 10.61250000122903536, 4.330127018922192761, -2.499999999999997780 ) ) ;
#63083=CARTESIAN_POINT ( 'NONE',  ( 1.510657702057710734E-15, 19.43750000000000000, 26.00000000000000000 ) ) ;
#63084=CARTESIAN_POINT ( 'NONE',  ( 2.121784821874999061, 17.00937500061451857, -33.67503911421598417 ) ) ;
#63085=ADVANCED_FACE ( 'NONE', ( #5120 ), #55726, .F. ) ;
#63086=CARTESIAN_POINT ( 'NONE',  ( 18.72187500061451360, -6.054752690667223547, -1.112240025338166033E-15 ) ) ;
#63087=CARTESIAN_POINT ( 'NONE',  ( 20.02500000122903145, 2.886751345948129099, -4.999999999999998224 ) ) ;
#63088=CARTESIAN_POINT ( 'NONE',  ( 13.84687500061451537, -3.027376345333610441, -5.243569643749999898 ) ) ;
#63089=CARTESIAN_POINT ( 'NONE',  ( 4.243569643749999898, 19.54062500061451857, -27.54997392385601529 ) ) ;
#63090=CARTESIAN_POINT ( 'NONE',  ( 18.93750000122903288, -4.330127018922194537, 2.499999999999995559 ) ) ;
#63091=CARTESIAN_POINT ( 'NONE',  ( 14.80312500061451608, 4.541064518000418104, -2.621784821874998173 ) ) ;
#63092=ORIENTED_EDGE ( 'NONE', *, *, #32653, .T. ) ;
#63094=CARTESIAN_POINT ( 'NONE',  ( 17.69999999999999929, 4.330127018922192761, -2.499999999999997780 ) ) ;
#63095=CARTESIAN_POINT ( 'NONE',  ( 5.857864376269046325, 9.999999999999998224, -5.857864376269046325 ) ) ;
#63096=CARTESIAN_POINT ( 'NONE',  ( 3.992981257374419890, 3.009426956198104186, 30.27415453858231942 ) ) ;
#63097=CARTESIAN_POINT ( 'NONE',  ( 14.96250000122903323, -4.330127018922190985, -2.500000000000001332 ) ) ;
#63098=CARTESIAN_POINT ( 'NONE',  ( 27.38437500061451857, 6.421520780324663323E-16, -5.243569643749999010 ) ) ;
#63099=CARTESIAN_POINT ( 'NONE',  ( 19.41562500061451146, 3.027376345333611329, 5.243569643749999010 ) ) ;
#63100=CARTESIAN_POINT ( 'NONE',  ( 24.17812500061451786, 6.421520780324663323E-16, -5.243569643749999010 ) ) ;
#63101=CARTESIAN_POINT ( 'NONE',  ( 3.328125000614516438, -4.541064518000419881, 2.621784821874995952 ) ) ;
#63102=( BOUNDED_CURVE ( )  B_SPLINE_CURVE ( 2, ( #9472, #60061, #49368, #19806, #2829, #3939, #59322 ),
 .UNSPECIFIED., .F., .F. ) 
 B_SPLINE_CURVE_WITH_KNOTS ( ( 3, 2, 2, 3 ),
 ( 0.9600368262957028609, 0.9611111111111111382, 0.9638888888888889062, 0.9648669314804571018 ),
 .UNSPECIFIED. ) 
 CURVE ( )  GEOMETRIC_REPRESENTATION_ITEM ( )  RATIONAL_B_SPLINE_CURVE ( ( 0.9364497541642147205, 0.9481863252286599764, 1.000000000000000000, 0.8660254037844387076, 1.000000000000000000, 0.9528281699366905055, 0.9388743022987573461 ) ) 
 REPRESENTATION_ITEM ( '' )  );
#63103=CARTESIAN_POINT ( 'NONE',  ( 28.72500000000000142, -4.330127018922194537, 2.499999999999995559 ) ) ;
#63104=CARTESIAN_POINT ( 'NONE',  ( 4.633613603196540254, 1.878729617659674167, 4.895446622381335544 ) ) ;
#63107=CARTESIAN_POINT ( 'NONE',  ( 28.68749999999999289, -2.886751345948114000, 5.000000000000024869 ) ) ;
#63108=CARTESIAN_POINT ( 'NONE',  ( -2.121784821874996840, 16.78437500061452070, -26.32496088578401583 ) ) ;
#63110=CARTESIAN_POINT ( 'NONE',  ( 5.812500001229035540, 0.000000000000000000, 4.999999999999998224 ) ) ;
#63111=CARTESIAN_POINT ( 'NONE',  ( 5.437500000000001776, -2.886751345948125991, -5.000000000000000000 ) ) ;
#63112=CARTESIAN_POINT ( 'NONE',  ( 4.425000001229032698, 2.886751345948126879, 4.999999999999999112 ) ) ;
#63113=CARTESIAN_POINT ( 'NONE',  ( 9.346875000614517148, -3.027376345333610441, -5.243569643749999898 ) ) ;
#63114=CARTESIAN_POINT ( 'NONE',  ( 24.56250000122903288, 4.330127018922192761, -2.499999999999997780 ) ) ;
#63116=CARTESIAN_POINT ( 'NONE',  ( -6.000139530219994910, 7.999895352344700505, -29.59567021705531786 ) ) ;
#63117=VECTOR ( 'NONE', #70108, 1000.000000000000000 ) ;
#63119=CARTESIAN_POINT ( 'NONE',  ( 8.746875000614515727, -3.027376345333614438, 5.243569643749998122 ) ) ;
#63120=CARTESIAN_POINT ( 'NONE',  ( 14.18437500061451750, -4.541064518000419881, 2.621784821874995952 ) ) ;
#63121=CARTESIAN_POINT ( 'NONE',  ( 6.487499999999999822, 5.773502691896255534, 3.535250795749688894E-16 ) ) ;
#63122=CARTESIAN_POINT ( 'NONE',  ( 9.001249775931846008E-16, 16.31562500061459531, 34.90005215228797653 ) ) ;
#63123=CARTESIAN_POINT ( 'NONE',  ( 20.89687500061452141, -3.027376345333614438, 5.243569643749998122 ) ) ;
#63124=CARTESIAN_POINT ( 'NONE',  ( 9.600000000000001421, 4.330127018922192761, -2.499999999999997780 ) ) ;
#63125=CARTESIAN_POINT ( 'NONE',  ( 27.11250000122903359, -4.330127018922190985, -2.500000000000001332 ) ) ;
#63127=CARTESIAN_POINT ( 'NONE',  ( 21.70312500061451644, 0.000000000000000000, 5.243569643749999010 ) ) ;
#63128=CARTESIAN_POINT ( 'NONE',  ( 12.14062500061451821, 6.054752690667223547, 3.707466751127219781E-16 ) ) ;
#63130=CARTESIAN_POINT ( 'NONE',  ( 12.38437500061451857, -4.541064518000419881, 2.621784821874995952 ) ) ;
#63131=CARTESIAN_POINT ( 'NONE',  ( 29.43750000000000000, 5.773502691896255534, 3.535250795749688894E-16 ) ) ;
#63132=CARTESIAN_POINT ( 'NONE',  ( 23.32500000122903572, 2.886751345948126879, 4.999999999999999112 ) ) ;
#63133=FACE_OUTER_BOUND ( 'NONE', #62791, .T. ) ;
#63134=AXIS2_PLACEMENT_3D ( 'NONE', #36850, #64924, #42402 ) ;
#63135=CARTESIAN_POINT ( 'NONE',  ( 10.73437500061451644, 6.421520780324663323E-16, -5.243569643749999010 ) ) ;
#63136=CARTESIAN_POINT ( 'NONE',  ( 28.35937500061451289, 4.541064518000418104, -2.621784821874998173 ) ) ;
#63137=CARTESIAN_POINT ( 'NONE',  ( 3.534375000614518036, 6.421520780324663323E-16, -5.243569643749999010 ) ) ;
#63138=CARTESIAN_POINT ( 'NONE',  ( -1.071796769724488563, 13.00490381179669974, -26.00000000000000000 ) ) ;
#63139=CARTESIAN_POINT ( 'NONE',  ( 21.34687500061451715, -3.027376345333614438, 5.243569643749998122 ) ) ;
#63140=CARTESIAN_POINT ( 'NONE',  ( 13.69687500061451679, -3.027376345333614438, 5.243569643749998122 ) ) ;
#63142=CARTESIAN_POINT ( 'NONE',  ( 24.89999999999999858, 4.330127018922192761, -2.499999999999997780 ) ) ;
#63145=CARTESIAN_POINT ( 'NONE',  ( 16.64062500061451289, 6.054752690667223547, 3.707466751127219781E-16 ) ) ;
#63146=CARTESIAN_POINT ( 'NONE',  ( 7.350000000000002309, 4.330127018922192761, -2.499999999999997780 ) ) ;
#63148=CARTESIAN_POINT ( 'NONE',  ( 14.17500000000000071, 4.330127018922191873, 2.499999999999999556 ) ) ;
#63149=CARTESIAN_POINT ( 'NONE',  ( -4.243569643749999898, 10.35312500061451857, 30.00000000000000000 ) ) ;
#63151=CARTESIAN_POINT ( 'NONE',  ( 24.57187500061451502, -6.054752690667223547, -1.112240025338166033E-15 ) ) ;
#63152=ORIENTED_EDGE ( 'NONE', *, *, #19846, .F. ) ;
#63153=CARTESIAN_POINT ( 'NONE',  ( 23.01562500061451644, 3.027376345333611329, 5.243569643749999010 ) ) ;
#63154=CARTESIAN_POINT ( 'NONE',  ( 20.48437500061451289, -4.541064518000419881, 2.621784821874995952 ) ) ;
#63155=CARTESIAN_POINT ( 'NONE',  ( 4.537500000000000533, -2.886751345948125991, -5.000000000000000000 ) ) ;
#63156=CARTESIAN_POINT ( 'NONE',  ( 6.965625000614518392, -6.054752690667223547, -1.112240025338166033E-15 ) ) ;
#63157=CARTESIAN_POINT ( 'NONE',  ( 21.55312500061451431, 4.541064518000418104, -2.621784821874998173 ) ) ;
#63158=CARTESIAN_POINT ( 'NONE',  ( 12.98437500061451821, 6.421520780324663323E-16, -5.243569643749999010 ) ) ;
#63159=CARTESIAN_POINT ( 'NONE',  ( 17.97187500061451715, 3.027376345333613106, -5.243569643749998122 ) ) ;
#63160=CARTESIAN_POINT ( 'NONE',  ( -4.243569643749999898, 17.06562500061451360, 27.54997392385601529 ) ) ;
#63161=CARTESIAN_POINT ( 'NONE',  ( 19.27500000122903145, 2.886751345948126879, 4.999999999999999112 ) ) ;
#63163=CARTESIAN_POINT ( 'NONE',  ( 10.07812500061451644, -4.541064518000419881, 2.621784821874995952 ) ) ;
#63164=CARTESIAN_POINT ( 'NONE',  ( 5.259375000614518569, -4.541064518000417216, -2.621784821875001281 ) ) ;
#63165=CARTESIAN_POINT ( 'NONE',  ( 5.521875000614517859, 3.027376345333611329, 5.243569643749999010 ) ) ;
#63166=EDGE_CURVE ( 'NONE', #48969, #48104, #44731, .T. ) ;
#63167=CARTESIAN_POINT ( 'NONE',  ( 26.44687500061451502, -3.027376345333610441, -5.243569643749999898 ) ) ;
#63168=CARTESIAN_POINT ( 'NONE',  ( 17.84062500061451573, -3.027376345333610441, -5.243569643749999898 ) ) ;
#63169=CARTESIAN_POINT ( 'NONE',  ( 28.01250000122903216, -4.330127018922190985, -2.500000000000001332 ) ) ;
#63170=CARTESIAN_POINT ( 'NONE',  ( 26.42812500061451431, 6.421520780324663323E-16, -5.243569643749999010 ) ) ;
#63171=CARTESIAN_POINT ( 'NONE',  ( 22.95937500061451431, 4.541064518000418104, -2.621784821874998173 ) ) ;
#63172=CARTESIAN_POINT ( 'NONE',  ( 17.39062500061451644, -3.027376345333610441, -5.243569643749999898 ) ) ;
#63173=CARTESIAN_POINT ( 'NONE',  ( -2.121784821874999949, 17.53437500061451715, 26.32496088578401938 ) ) ;
#63174=AXIS2_PLACEMENT_3D ( 'NONE', #47459, #35642, #58891 ) ;
#63175=CARTESIAN_POINT ( 'NONE',  ( 21.21562500061451573, 3.027376345333611329, 5.243569643749999010 ) ) ;
#63176=CARTESIAN_POINT ( 'NONE',  ( 3.412500001229032964, 4.330127018922192761, -2.499999999999997780 ) ) ;
#63178=CARTESIAN_POINT ( 'NONE',  ( 26.32499999999999929, 4.330127018922191873, 2.499999999999999556 ) ) ;
#63179=CARTESIAN_POINT ( 'NONE',  ( -3.999999999999999556, 13.66250000000000142, -32.30940107675850470 ) ) ;
#63180=CARTESIAN_POINT ( 'NONE',  ( 28.15312500061451573, -4.541064518000417216, -2.621784821875001281 ) ) ;
#63181=CARTESIAN_POINT ( 'NONE',  ( 10.30312500061451431, 4.541064518000418104, -2.621784821874998173 ) ) ;
#63182=CARTESIAN_POINT ( 'NONE',  ( 23.02500000122903145, -5.773502691896255534, -1.060575238724906372E-15 ) ) ;
#63183=CARTESIAN_POINT ( 'NONE',  ( 26.87812500061451360, 6.421520780324663323E-16, -5.243569643749999010 ) ) ;
#63184=CARTESIAN_POINT ( 'NONE',  ( 28.49999999999999645, 4.330127018922192761, -2.499999999999997780 ) ) ;
#63185=CARTESIAN_POINT ( 'NONE',  ( 4.000000000000000000, 16.70000000122903572, -27.69059892324149530 ) ) ;
#63186=CARTESIAN_POINT ( 'NONE',  ( 29.46562500061451573, -6.054752690667223547, -1.112240025338166033E-15 ) ) ;
#63187=CARTESIAN_POINT ( 'NONE',  ( 10.86562500061451431, 3.027376345333611329, 5.243569643749999010 ) ) ;
#63190=CARTESIAN_POINT ( 'NONE',  ( 25.37812500061451715, -4.541064518000419881, 2.621784821874995952 ) ) ;
#63191=CARTESIAN_POINT ( 'NONE',  ( 7.003125000614518036, -4.541064518000417216, -2.621784821875001281 ) ) ;
#63192=AXIS2_PLACEMENT_3D ( 'NONE', #66722, #33449, #33090 ) ;
#63193=CARTESIAN_POINT ( 'NONE',  ( 5.953125000614519102, 0.000000000000000000, 5.243569643749999010 ) ) ;
#63195=CYLINDRICAL_SURFACE ( 'NONE', #68038, 4.999999999999998224 ) ;
#63196=CARTESIAN_POINT ( 'NONE',  ( 13.57500000000000107, 6.123233995736764310E-16, -4.999999999999998224 ) ) ;
#63197=CARTESIAN_POINT ( 'NONE',  ( 14.52187500061451608, 3.027376345333611329, 5.243569643749999010 ) ) ;
#63198=CARTESIAN_POINT ( 'NONE',  ( 11.55000000122903181, 5.773502691896255534, 3.535250795749688894E-16 ) ) ;
#63199=CARTESIAN_POINT ( 'NONE',  ( 18.04687500061451999, 6.054752690667223547, 3.707466751127219781E-16 ) ) ;
#63201=CARTESIAN_POINT ( 'NONE',  ( 20.18437500061451573, 6.421520780324663323E-16, -5.243569643749999010 ) ) ;
#63202=CARTESIAN_POINT ( 'NONE',  ( -4.243569643749999898, 11.21562500061451750, -32.45002607614398471 ) ) ;
#63205=CARTESIAN_POINT ( 'NONE',  ( 1.999999999999998668, 11.75000000000000178, -33.46410161513775705 ) ) ;
#63207=CARTESIAN_POINT ( 'NONE',  ( 24.51562500061451289, -6.054752690667223547, -1.112240025338166033E-15 ) ) ;
#63208=CARTESIAN_POINT ( 'NONE',  ( 17.10000000122903430, -2.886751345948096681, 5.000000000000054179 ) ) ;
#63209=CARTESIAN_POINT ( 'NONE',  ( 29.22187500061451715, 3.027376345333613106, -5.243569643749998122 ) ) ;
#63210=CARTESIAN_POINT ( 'NONE',  ( 25.19999999999999929, -4.330127018922190985, -2.500000000000001332 ) ) ;
#63211=CARTESIAN_POINT ( 'NONE',  ( 5.765625000614519102, 3.027376345333613106, -5.243569643749998122 ) ) ;
#63213=CARTESIAN_POINT ( 'NONE',  ( 18.27187500061451431, -6.054752690667223547, -1.112240025338166033E-15 ) ) ;
#63215=AXIS2_PLACEMENT_3D ( 'NONE', #43754, #66279, #38943 ) ;
#63216=CARTESIAN_POINT ( 'NONE',  ( 28.87500000122902932, -5.773502691896255534, -1.060575238724906372E-15 ) ) ;
#63217=CARTESIAN_POINT ( 'NONE',  ( 8.184375000614515727, 4.541064518000418104, 2.621784821874999949 ) ) ;
#63219=CARTESIAN_POINT ( 'NONE',  ( 18.53437500061451715, 4.541064518000418104, 2.621784821874999949 ) ) ;
#63220=CARTESIAN_POINT ( 'NONE',  ( 3.242103837493086330E-14, 12.80000000122903359, -34.00000000000000000 ) ) ;
#63221=CARTESIAN_POINT ( 'NONE',  ( 25.50000000000000000, 0.000000000000000000, 4.999999999999998224 ) ) ;
#63222=CARTESIAN_POINT ( 'NONE',  ( 29.33437500061451431, 4.541064518000418104, 2.621784821874999949 ) ) ;
#63224=CARTESIAN_POINT ( 'NONE',  ( 10.68749999999999645, -2.886751345948063374, 5.000000000000112799 ) ) ;
#63225=EDGE_LOOP ( 'NONE', ( #31832, #14981, #20372, #21900 ) ) ;
#63226=CARTESIAN_POINT ( 'NONE',  ( 9.600000000000001421, 4.330127018922192761, -2.499999999999997780 ) ) ;
#63228=CARTESIAN_POINT ( 'NONE',  ( 24.74062500061451786, 6.054752690667223547, 3.707466751127219781E-16 ) ) ;
#63229=CARTESIAN_POINT ( 'NONE',  ( 14.58750000000000036, 5.773502691896255534, 3.535250795749688894E-16 ) ) ;
#63230=CARTESIAN_POINT ( 'NONE',  ( 10.35000000122903074, -2.886751345948129988, 4.999999999999997335 ) ) ;
#63231=CARTESIAN_POINT ( 'NONE',  ( 8.390625000614518214, -3.027376345333610441, -5.243569643749999898 ) ) ;
#63232=CARTESIAN_POINT ( 'NONE',  ( 21.26249999999999574, 2.886751345948129099, -4.999999999999998224 ) ) ;
#63233=CARTESIAN_POINT ( 'NONE',  ( 21.96562500061451573, 3.027376345333613106, -5.243569643749998122 ) ) ;
#63234=DIRECTION ( 'NONE',  ( -1.000000000000000000, -0.000000000000000000, -0.000000000000000000 ) ) ;
#63235=CARTESIAN_POINT ( 'NONE',  ( 26.73750000122903003, 6.123233995736764310E-16, -4.999999999999998224 ) ) ;
#63237=CARTESIAN_POINT ( 'NONE',  ( 7.800000000000001599, 4.330127018922192761, -2.499999999999997780 ) ) ;
#63238=ORIENTED_EDGE ( 'NONE', *, *, #18393, .T. ) ;
#63239=CARTESIAN_POINT ( 'NONE',  ( 22.07812500061451644, 4.541064518000418104, 2.621784821874999949 ) ) ;
#63240=CARTESIAN_POINT ( 'NONE',  ( 29.61562500061451431, 3.027376345333613106, -5.243569643749998122 ) ) ;
#63241=CARTESIAN_POINT ( 'NONE',  ( 27.38437500061451857, 6.421520780324663323E-16, -5.243569643749999010 ) ) ;
#63242=CARTESIAN_POINT ( 'NONE',  ( 19.95937500061451786, 0.000000000000000000, 5.243569643749999010 ) ) ;
#63243=CARTESIAN_POINT ( 'NONE',  ( 15.32812500061451644, 4.541064518000418104, 2.621784821874999949 ) ) ;
#63245=CARTESIAN_POINT ( 'NONE',  ( 25.46250000122903501, 4.330127018922192761, -2.499999999999997780 ) ) ;
#63247=CARTESIAN_POINT ( 'NONE',  ( 17.39062500061451644, -3.027376345333610441, -5.243569643749999898 ) ) ;
#63248=FACE_OUTER_BOUND ( 'NONE', #15702, .T. ) ;
#63249=EDGE_CURVE ( 'NONE', #72719, #42898, #52263, .T. ) ;
#63251=CARTESIAN_POINT ( 'NONE',  ( 13.77187500061451786, -6.054752690667223547, -1.112240025338166033E-15 ) ) ;
#63252=CARTESIAN_POINT ( 'NONE',  ( 11.97187500061451892, -6.054752690667223547, -1.112240025338166033E-15 ) ) ;
#63253=CARTESIAN_POINT ( 'NONE',  ( 21.15937500061451715, 4.541064518000418104, -2.621784821874998173 ) ) ;
#63254=ORIENTED_EDGE ( 'NONE', *, *, #62341, .F. ) ;
#63255=LINE ( 'NONE', #23725, #14660 ) ;
#63256=CARTESIAN_POINT ( 'NONE',  ( 23.42812500061451786, 4.541064518000418104, 2.621784821874999949 ) ) ;
#63257=CARTESIAN_POINT ( 'NONE',  ( 19.32187500061451857, 3.027376345333613106, -5.243569643749998122 ) ) ;
#63258=CARTESIAN_POINT ( 'NONE',  ( 24.40312500061451573, 0.000000000000000000, 5.243569643749999010 ) ) ;
#63259=CARTESIAN_POINT ( 'NONE',  ( -3.999999999999999112, 9.725000001229036073, 27.69059892324149885 ) ) ;
#63260=CARTESIAN_POINT ( 'NONE',  ( -3.999999999999999556, 13.66250000000000142, 27.69059892324149530 ) ) ;
#63261=CARTESIAN_POINT ( 'NONE',  ( 3.309375000614518836, 0.000000000000000000, 5.243569643749999010 ) ) ;
#63262=CARTESIAN_POINT ( 'NONE',  ( 9.112500001229033586, -4.330127018922190985, -2.500000000000001332 ) ) ;
#63263=CARTESIAN_POINT ( 'NONE',  ( 4.912500001229034297, 0.000000000000000000, 4.999999999999998224 ) ) ;
#63264=DIRECTION ( 'NONE',  ( -1.000000000000000000, -0.000000000000000000, -0.000000000000000000 ) ) ;
#63265=CARTESIAN_POINT ( 'NONE',  ( 26.10000000122903430, -2.886751345948129988, 4.999999999999997335 ) ) ;
#63268=CARTESIAN_POINT ( 'NONE',  ( 9.796875000614519990, -3.027376345333610441, -5.243569643749999898 ) ) ;
#63269=CARTESIAN_POINT ( 'NONE',  ( 17.84999999999999787, 0.000000000000000000, 4.999999999999998224 ) ) ;
#63270=CARTESIAN_POINT ( 'NONE',  ( 16.94062500061451715, -3.027376345333610441, -5.243569643749999898 ) ) ;
#63271=CARTESIAN_POINT ( 'NONE',  ( 11.33437500061451608, 4.541064518000418104, 2.621784821874999949 ) ) ;
#63272=CARTESIAN_POINT ( 'NONE',  ( 3.253125000614518036, 0.000000000000000000, 5.243569643749999010 ) ) ;
#63273=CARTESIAN_POINT ( 'NONE',  ( 19.09687500061451360, -3.027376345333614438, 5.243569643749998122 ) ) ;
#63274=CARTESIAN_POINT ( 'NONE',  ( 7.846875000614518036, -3.027376345333614438, 5.243569643749998122 ) ) ;
#63275=CARTESIAN_POINT ( 'NONE',  ( 3.515625000614516882, 3.027376345333613106, -5.243569643749998122 ) ) ;
#63276=LINE ( 'NONE', #14485, #43891 ) ;
#63277=CARTESIAN_POINT ( 'NONE',  ( 7.115625000614516082, 3.027376345333613106, -5.243569643749998122 ) ) ;
#63278=CARTESIAN_POINT ( 'NONE',  ( 17.80312500061451786, -4.541064518000417216, -2.621784821875001281 ) ) ;
#63279=VERTEX_POINT ( 'NONE', #10296 ) ;
#63280=CARTESIAN_POINT ( 'NONE',  ( 6.375000001229031987, -5.773502691896255534, -1.060575238724906372E-15 ) ) ;
#63281=CARTESIAN_POINT ( 'NONE',  ( 14.01562500061451644, 3.027376345333611329, 5.243569643749999010 ) ) ;
#63282=CARTESIAN_POINT ( 'NONE',  ( 12.17812500061451608, 4.541064518000418104, 2.621784821874999949 ) ) ;
#63284=CARTESIAN_POINT ( 'NONE',  ( 12.67499999999999893, 6.123233995736764310E-16, -4.999999999999998224 ) ) ;
#63285=CARTESIAN_POINT ( 'NONE',  ( 5.625000001229036428, 2.886751345948129099, -4.999999999999998224 ) ) ;
#63287=CARTESIAN_POINT ( 'NONE',  ( 18.11250000122903359, -4.330127018922190985, -2.500000000000001332 ) ) ;
#63289=CARTESIAN_POINT ( 'NONE',  ( 4.243569643749999898, 11.53437500061451892, -30.00000000000000000 ) ) ;
#63292=( BOUNDED_CURVE ( )  B_SPLINE_CURVE ( 2, ( #27732, #1114, #749, #23621, #17704, #40265, #62786, #12178, #34706 ),
 .UNSPECIFIED., .F., .F. ) 
 B_SPLINE_CURVE_WITH_KNOTS ( ( 3, 2, 2, 2, 3 ),
 ( 0.5760869565217391353, 0.5797101449275362528, 0.5869565217391304879, 0.5942028985507246119, 0.5978260869565217295 ),
 .UNSPECIFIED. ) 
 CURVE ( )  GEOMETRIC_REPRESENTATION_ITEM ( )  RATIONAL_B_SPLINE_CURVE ( ( 0.9330127018922194093, 0.9330127018922194093, 1.000000000000000000, 0.8660254037844387076, 1.000000000000000000, 0.8660254037844387076, 1.000000000000000000, 0.9330127018922194093, 0.9330127018922194093 ) ) 
 REPRESENTATION_ITEM ( '' )  );
#63293=CARTESIAN_POINT ( 'NONE',  ( 6.562500000000002665, 2.886751345948126879, 4.999999999999998224 ) ) ;
#63295=CARTESIAN_POINT ( 'NONE',  ( 18.49687500061452283, 6.054752690667223547, 3.707466751127219781E-16 ) ) ;
#63296=CARTESIAN_POINT ( 'NONE',  ( -2.000000000000000000, 16.43750000122903643, 26.53589838486224650 ) ) ;
#63297=CARTESIAN_POINT ( 'NONE',  ( 14.20312500061451644, -4.541064518000417216, -2.621784821875001281 ) ) ;
#63299=DIRECTION ( 'NONE',  ( -0.000000000000000000, -1.000000000000000000, -0.000000000000000000 ) ) ;
#63300=CARTESIAN_POINT ( 'NONE',  ( 25.88437500061451502, -4.541064518000419881, 2.621784821874995952 ) ) ;
#63302=CARTESIAN_POINT ( 'NONE',  ( 13.04062500061451502, 6.054752690667223547, 3.707466751127219781E-16 ) ) ;
#63303=CARTESIAN_POINT ( 'NONE',  ( 15.27187500061451786, 3.027376345333613106, -5.243569643749998122 ) ) ;
#63304=ORIENTED_EDGE ( 'NONE', *, *, #34144, .F. ) ;
#63306=CARTESIAN_POINT ( 'NONE',  ( 26.80312500061451431, -4.541064518000417216, -2.621784821875001281 ) ) ;
#63307=CARTESIAN_POINT ( 'NONE',  ( 21.25312500061451715, 0.000000000000000000, 5.243569643749999010 ) ) ;
#63308=CARTESIAN_POINT ( 'NONE',  ( 29.12812500061451715, 6.421520780324663323E-16, -5.243569643749999010 ) ) ;
#63309=CARTESIAN_POINT ( 'NONE',  ( 4.000000000000000000, 12.65000000122903323, -27.69059892324149885 ) ) ;
#63310=CARTESIAN_POINT ( 'NONE',  ( 9.112500000000000711, 2.886751345948129099, -4.999999999999998224 ) ) ;
#63311=CARTESIAN_POINT ( 'NONE',  ( 18.93750000122903288, -4.330127018922194537, 2.499999999999995559 ) ) ;
#63314=EDGE_LOOP ( 'NONE', ( #12928, #51200, #59446, #67547 ) ) ;
#63315=CARTESIAN_POINT ( 'NONE',  ( 17.51249999999999929, -5.773502691896255534, -1.060575238724906372E-15 ) ) ;
#63316=CARTESIAN_POINT ( 'NONE',  ( 20.73750000000000071, -2.886751345948125991, -5.000000000000000000 ) ) ;
#63317=CARTESIAN_POINT ( 'NONE',  ( 18.34687500061451715, -3.027376345333610441, -5.243569643749999898 ) ) ;
#63318=CARTESIAN_POINT ( 'NONE',  ( 25.15312500061451217, 4.541064518000418104, -2.621784821874998173 ) ) ;
#63320=ORIENTED_EDGE ( 'NONE', *, *, #7307, .F. ) ;
#63321=EDGE_CURVE ( 'NONE', #12255, #18095, #32827, .T. ) ;
#63322=CARTESIAN_POINT ( 'NONE',  ( 27.90000000122903145, -2.886751345948137981, 4.999999999999982236 ) ) ;
#63323=CARTESIAN_POINT ( 'NONE',  ( 6.965625000614518392, -6.054752690667223547, -1.112240025338166033E-15 ) ) ;
#63324=CARTESIAN_POINT ( 'NONE',  ( 30.00000000000000000, 0.000000000000000000, 0.000000000000000000 ) ) ;
#63326=CARTESIAN_POINT ( 'NONE',  ( 14.36249999999999893, -5.773502691896255534, -1.060575238724906372E-15 ) ) ;
#63327=CARTESIAN_POINT ( 'NONE',  ( -2.121784821874999949, 17.92812500061451786, 26.32496088578401938 ) ) ;
#63328=CARTESIAN_POINT ( 'NONE',  ( 28.19062500061451715, -3.027376345333610441, -5.243569643749999898 ) ) ;
#63331=CARTESIAN_POINT ( 'NONE',  ( 25.39687500061451431, -3.027376345333614438, 5.243569643749998122 ) ) ;
#63332=EDGE_LOOP ( 'NONE', ( #11678, #13331, #21336, #5567 ) ) ;
#63333=CARTESIAN_POINT ( 'NONE',  ( 21.32812500061451644, -4.541064518000419881, 2.621784821874995952 ) ) ;
#63334=CARTESIAN_POINT ( 'NONE',  ( 22.50937500061451857, 4.541064518000418104, -2.621784821874998173 ) ) ;
#63335=CARTESIAN_POINT ( 'NONE',  ( 9.001249775931846008E-16, 15.86562500061459247, -25.09994784771203058 ) ) ;
#63336=CARTESIAN_POINT ( 'NONE',  ( 10.23750000000000071, -2.886751345948129988, 4.999999999999997335 ) ) ;
#63337=EDGE_CURVE ( 'NONE', #55474, #38159, #22911, .T. ) ;
#63338=CARTESIAN_POINT ( 'NONE',  ( 7.115625000614516082, 3.027376345333613106, -5.243569643749998122 ) ) ;
#63340=CARTESIAN_POINT ( 'NONE',  ( 22.90312500061451573, 4.541064518000418104, -2.621784821874998173 ) ) ;
#63343=CARTESIAN_POINT ( 'NONE',  ( 16.32187500061451502, 3.027376345333611329, 5.243569643749999010 ) ) ;
#63344=CARTESIAN_POINT ( 'NONE',  ( 20.33437500061451786, 4.541064518000418104, 2.621784821874999949 ) ) ;
#63345=CARTESIAN_POINT ( 'NONE',  ( 28.05937500061451573, 0.000000000000000000, 5.243569643749999010 ) ) ;
#63346=CARTESIAN_POINT ( 'NONE',  ( -3.000416591977282496E-16, 15.69687500061451857, 25.09994784771203058 ) ) ;
#63347=CARTESIAN_POINT ( 'NONE',  ( 8.653125000614515727, 0.000000000000000000, 5.243569643749999010 ) ) ;
#63348=CARTESIAN_POINT ( 'NONE',  ( 1.071796769724491893, 10.34509619066136921, -26.00000000000000355 ) ) ;
#63350=CARTESIAN_POINT ( 'NONE',  ( 3.984375000614517326, 6.421520780324663323E-16, -5.243569643749999010 ) ) ;
#63351=CARTESIAN_POINT ( 'NONE',  ( 30.00000000000000000, 0.000000000000000000, 0.000000000000000000 ) ) ;
#63353=CARTESIAN_POINT ( 'NONE',  ( 5.765625000614519102, 3.027376345333613106, -5.243569643749998122 ) ) ;
#63354=CARTESIAN_POINT ( 'NONE',  ( 10.02187500061451964, 3.027376345333611329, 5.243569643749999010 ) ) ;
#63356=CARTESIAN_POINT ( 'NONE',  ( 15.78750000122903430, -4.330127018922194537, 2.499999999999995559 ) ) ;
#63357=CARTESIAN_POINT ( 'NONE',  ( 5.034375000614519813, 4.541064518000418104, 2.621784821874999949 ) ) ;
#63358=CARTESIAN_POINT ( 'NONE',  ( 7.078125000614516438, 6.421520780324663323E-16, -5.243569643749999010 ) ) ;
#63361=CARTESIAN_POINT ( 'NONE',  ( 16.17187500061451644, 3.027376345333613106, -5.243569643749998122 ) ) ;
#63363=ORIENTED_EDGE ( 'NONE', *, *, #40617, .F. ) ;
#63364=CARTESIAN_POINT ( 'NONE',  ( 24.29062500061451502, 6.054752690667223547, 3.707466751127219781E-16 ) ) ;
#63365=CARTESIAN_POINT ( 'NONE',  ( 9.815625000614518925, 3.027376345333613106, -5.243569643749998122 ) ) ;
#63366=CARTESIAN_POINT ( 'NONE',  ( 27.19687500061451857, -3.027376345333614438, 5.243569643749998122 ) ) ;
#63367=CARTESIAN_POINT ( 'NONE',  ( 9.178125000614517859, -4.541064518000419881, 2.621784821874995952 ) ) ;
#63368=CARTESIAN_POINT ( 'NONE',  ( -2.121784821874999949, 10.33437500061451786, -33.67503911421598417 ) ) ;
#63369=EDGE_CURVE ( 'NONE', #25850, #68026, #30479, .T. ) ;
#63370=CARTESIAN_POINT ( 'NONE',  ( 11.58750000122903501, 4.330127018922191873, 2.499999999999999556 ) ) ;
#63371=CARTESIAN_POINT ( 'NONE',  ( 25.37812500061451715, -4.541064518000419881, 2.621784821874995952 ) ) ;
#63372=CARTESIAN_POINT ( 'NONE',  ( -4.243569643749997233, 13.54062500061451679, -27.54997392385601174 ) ) ;
#63373=CARTESIAN_POINT ( 'NONE',  ( 11.88750000122903216, 6.123233995736764310E-16, -4.999999999999998224 ) ) ;
#63374=CARTESIAN_POINT ( 'NONE',  ( 23.01562500061451644, 3.027376345333611329, 5.243569643749999010 ) ) ;
#63375=CARTESIAN_POINT ( 'NONE',  ( 11.62500000000000000, -4.330127018922194537, 2.499999999999995559 ) ) ;
#63376=CARTESIAN_POINT ( 'NONE',  ( 20.57812500061451644, 6.421520780324663323E-16, -5.243569643749999010 ) ) ;
#63377=CARTESIAN_POINT ( 'NONE',  ( 5.896875000614517859, 6.054752690667223547, 3.707466751127219781E-16 ) ) ;
#63378=CARTESIAN_POINT ( 'NONE',  ( 19.38749999999999929, -2.886751345948125991, -5.000000000000000000 ) ) ;
#63379=CARTESIAN_POINT ( 'NONE',  ( 15.07500000122903394, 2.886751345948129099, -4.999999999999998224 ) ) ;
#63380=CARTESIAN_POINT ( 'NONE',  ( 13.64062500061451644, -3.027376345333614438, 5.243569643749998122 ) ) ;
#63381=CARTESIAN_POINT ( 'NONE',  ( 16.94062500061451715, -3.027376345333610441, -5.243569643749999898 ) ) ;
#63382=CARTESIAN_POINT ( 'NONE',  ( 25.42500000122903359, 2.886751345948129099, -4.999999999999998224 ) ) ;
#63383=CARTESIAN_POINT ( 'NONE',  ( 19.46249999999999858, 2.886751345948129099, -4.999999999999998224 ) ) ;
#63384=CARTESIAN_POINT ( 'NONE',  ( 23.70937500061451786, -4.541064518000417216, -2.621784821875001281 ) ) ;
#63386=CARTESIAN_POINT ( 'NONE',  ( 11.17500000122903536, 2.886751345948126879, 4.999999999999999112 ) ) ;
#63387=CARTESIAN_POINT ( 'NONE',  ( 9.796875000614519990, -3.027376345333610441, -5.243569643749999898 ) ) ;
#63388=CARTESIAN_POINT ( 'NONE',  ( 24.53437500061451715, -4.541064518000419881, 2.621784821874995952 ) ) ;
#63389=CARTESIAN_POINT ( 'NONE',  ( 15.45000000122903216, -2.886751345948126435, -5.000000000000000000 ) ) ;
#63390=CARTESIAN_POINT ( 'NONE',  ( 20.50312500061451715, -4.541064518000417216, -2.621784821875001281 ) ) ;
#63391=CARTESIAN_POINT ( 'NONE',  ( 27.68437500061451573, -4.541064518000419881, 2.621784821874995952 ) ) ;
#63393=CARTESIAN_POINT ( 'NONE',  ( 6.684375000614518392, 6.421520780324663323E-16, -5.243569643749999010 ) ) ;
#63394=CARTESIAN_POINT ( 'NONE',  ( 19.11562500061451431, -6.054752690667223547, -1.112240025338166033E-15 ) ) ;
#63395=ORIENTED_EDGE ( 'NONE', *, *, #35455, .F. ) ;
#63396=CARTESIAN_POINT ( 'NONE',  ( 11.40000000000000036, 4.330127018922192761, -2.499999999999997780 ) ) ;
#63397=CARTESIAN_POINT ( 'NONE',  ( 27.14062500061451644, -3.027376345333614438, 5.243569643749998122 ) ) ;
#63398=CARTESIAN_POINT ( 'NONE',  ( 4.246875000614519280, -3.027376345333614438, 5.243569643749998122 ) ) ;
#63399=LINE ( 'NONE', #1360, #50190 ) ;
#63400=FACE_OUTER_BOUND ( 'NONE', #45879, .T. ) ;
#63401=CARTESIAN_POINT ( 'NONE',  ( 16.08749999999999503, -2.886751345948129988, 4.999999999999997335 ) ) ;
#63402=CARTESIAN_POINT ( 'NONE',  ( 21.74062500061451431, -3.027376345333614438, 5.243569643749998122 ) ) ;
#63403=ORIENTED_EDGE ( 'NONE', *, *, #7149, .T. ) ;
#63404=CARTESIAN_POINT ( 'NONE',  ( 24.18750000000000355, -2.886751345948129988, 4.999999999999997335 ) ) ;
#63405=CARTESIAN_POINT ( 'NONE',  ( 27.23437500061451644, -4.541064518000419881, 2.621784821874995952 ) ) ;
#63407=CARTESIAN_POINT ( 'NONE',  ( 14.57812500061451644, -4.541064518000419881, 2.621784821874995952 ) ) ;
#63408=CARTESIAN_POINT ( 'NONE',  ( 5.128125000614516260, -4.541064518000419881, 2.621784821874995952 ) ) ;
#63410=CARTESIAN_POINT ( 'NONE',  ( 29.61562500061451431, 3.027376345333613106, -5.243569643749998122 ) ) ;
#63411=CARTESIAN_POINT ( 'NONE',  ( 14.21250000122903323, 4.330127018922192761, -2.499999999999997780 ) ) ;
#63412=CARTESIAN_POINT ( 'NONE',  ( 21.07499999999999929, -4.330127018922194537, 2.499999999999995559 ) ) ;
#63413=CARTESIAN_POINT ( 'NONE',  ( 29.36250000000000071, 2.886751345948129099, -4.999999999999998224 ) ) ;
#63414=CARTESIAN_POINT ( 'NONE',  ( 4.434375000614519280, 6.421520780324663323E-16, -5.243569643749999010 ) ) ;
#63415=CARTESIAN_POINT ( 'NONE',  ( 10.28437500061451715, 6.421520780324663323E-16, -5.243569643749999010 ) ) ;
#63416=CARTESIAN_POINT ( 'NONE',  ( 19.99687500061451573, -3.027376345333614438, 5.243569643749998122 ) ) ;
#63417=CARTESIAN_POINT ( 'NONE',  ( 9.900000001229033231, -2.886751345948130876, 4.999999999999996447 ) ) ;
#63418=EDGE_LOOP ( 'NONE', ( #10813, #70972, #57549, #70153 ) ) ;
#63419=CARTESIAN_POINT ( 'NONE',  ( 29.76562500061451644, 3.027376345333611329, 5.243569643749999010 ) ) ;
#63420=CARTESIAN_POINT ( 'NONE',  ( 4.012500000000001954, -5.773502691896255534, -1.060575238724906372E-15 ) ) ;
#63421=CARTESIAN_POINT ( 'NONE',  ( 5.671875000614519102, -6.054752690667223547, -1.112240025338166033E-15 ) ) ;
#63422=CARTESIAN_POINT ( 'NONE',  ( 19.57500000000000284, 4.330127018922191873, 2.499999999999999556 ) ) ;
#63423=CARTESIAN_POINT ( 'NONE',  ( 13.07812500061451821, 4.541064518000418104, 2.621784821874999949 ) ) ;
#63428=CARTESIAN_POINT ( 'NONE',  ( 7.790625000614518569, -3.027376345333614438, 5.243569643749998122 ) ) ;
#63429=CARTESIAN_POINT ( 'NONE',  ( 23.97187500061451360, 3.027376345333611329, 5.243569643749999010 ) ) ;
#63430=CARTESIAN_POINT ( 'NONE',  ( -3.000416591977282496E-16, 18.39687500061451786, 25.09994784771203058 ) ) ;
#63431=CARTESIAN_POINT ( 'NONE',  ( 26.10937500061451644, 4.541064518000418104, -2.621784821874998173 ) ) ;
#63432=CARTESIAN_POINT ( 'NONE',  ( 6.600000000000001421, 0.000000000000000000, 4.999999999999998224 ) ) ;
#63433=CARTESIAN_POINT ( 'NONE',  ( 8.484601909799253346E-16, 13.92500000122903359, 34.61880215351700230 ) ) ;
#63434=CARTESIAN_POINT ( 'NONE',  ( 14.27812500061451573, 6.421520780324663323E-16, -5.243569643749999010 ) ) ;
#63435=CARTESIAN_POINT ( 'NONE',  ( 7.950000001229033053, 5.773502691896255534, 3.535250795749688894E-16 ) ) ;
#63436=EDGE_CURVE ( 'NONE', #70720, #32936, #6931, .T. ) ;
#63437=CARTESIAN_POINT ( 'NONE',  ( 17.18437500061451573, 4.541064518000418104, 2.621784821874999949 ) ) ;
#63438=CARTESIAN_POINT ( 'NONE',  ( 12.49687500061451573, -3.027376345333610441, -5.243569643749999898 ) ) ;
#63439=CARTESIAN_POINT ( 'NONE',  ( -3.942095835588579789, 3.076014195111399285, -29.30861973919568086 ) ) ;
#63440=ORIENTED_EDGE ( 'NONE', *, *, #65759, .F. ) ;
#63441=CARTESIAN_POINT ( 'NONE',  ( 11.99062500061451608, -3.027376345333610441, -5.243569643749999898 ) ) ;
#63443=CARTESIAN_POINT ( 'NONE',  ( 23.96250000122903145, -4.330127018922190985, -2.500000000000001332 ) ) ;
#63444=CARTESIAN_POINT ( 'NONE',  ( 13.47187500061451537, 3.027376345333613106, -5.243569643749998122 ) ) ;
#63445=CARTESIAN_POINT ( 'NONE',  ( 3.390184931900214860, 3.675138926287994767, 3.390184931900133147 ) ) ;
#63446=CARTESIAN_POINT ( 'NONE',  ( 14.99062500061451786, -3.027376345333614438, 5.243569643749998122 ) ) ;
#63447=FACE_OUTER_BOUND ( 'NONE', #12711, .T. ) ;
#63448=CARTESIAN_POINT ( 'NONE',  ( 24.27187500061452141, 3.027376345333613106, -5.243569643749998122 ) ) ;
#63449=DIRECTION ( 'NONE',  ( -0.000000000000000000, -1.000000000000000000, -0.000000000000000000 ) ) ;
#63450=CARTESIAN_POINT ( 'NONE',  ( 12.26250000122903394, -4.330127018922190985, -2.500000000000001332 ) ) ;
#63451=CARTESIAN_POINT ( 'NONE',  ( 23.88749999999999929, -2.886751345948159742, -4.999999999999942268 ) ) ;
#63453=CARTESIAN_POINT ( 'NONE',  ( 4.243569643749999898, 16.89687500061451786, -27.54997392385601529 ) ) ;
#63454=CARTESIAN_POINT ( 'NONE',  ( 18.94687500061451502, 6.054752690667223547, 3.707466751127219781E-16 ) ) ;
#63455=CARTESIAN_POINT ( 'NONE',  ( 18.75000000122903288, 5.773502691896255534, 3.535250795749688894E-16 ) ) ;
#63456=CARTESIAN_POINT ( 'NONE',  ( 15.04687500061451644, -3.027376345333614438, 5.243569643749998122 ) ) ;
#63458=CARTESIAN_POINT ( 'NONE',  ( 20.96250000122903145, 4.330127018922192761, -2.499999999999997780 ) ) ;
#63459=CARTESIAN_POINT ( 'NONE',  ( 15.55312500061451608, -4.541064518000417216, -2.621784821875001281 ) ) ;
#63460=ORIENTED_EDGE ( 'NONE', *, *, #39769, .T. ) ;
#63461=ORIENTED_EDGE ( 'NONE', *, *, #6614, .T. ) ;
#63462=CARTESIAN_POINT ( 'NONE',  ( 17.88749999999999929, -2.886751345948129988, 4.999999999999997335 ) ) ;
#63464=CARTESIAN_POINT ( 'NONE',  ( 24.82499999999999929, 6.123233995736764310E-16, -4.999999999999998224 ) ) ;
#63465=CARTESIAN_POINT ( 'NONE',  ( 14.88750000122903394, -4.330127018922194537, 2.499999999999995559 ) ) ;
#63466=CARTESIAN_POINT ( 'NONE',  ( 26.63437500061451857, 4.541064518000418104, 2.621784821874999949 ) ) ;
#63467=CARTESIAN_POINT ( 'NONE',  ( 19.30312500061451786, 4.541064518000418104, -2.621784821874998173 ) ) ;
#63468=CARTESIAN_POINT ( 'NONE',  ( 22.97812500061451857, 4.541064518000418104, 2.621784821874999949 ) ) ;
#63469=CARTESIAN_POINT ( 'NONE',  ( 3.853125000614517681, -4.541064518000417216, -2.621784821875001281 ) ) ;
#63470=CARTESIAN_POINT ( 'NONE',  ( 26.36249999999999716, 2.886751345948126879, 4.999999999999999112 ) ) ;
#63474=CARTESIAN_POINT ( 'NONE',  ( 3.965005778268202441, -3.046175387583509586, -4.212983158363885039 ) ) ;
#63475=CARTESIAN_POINT ( 'NONE',  ( -3.000416591977282496E-16, 16.14687500061451431, -34.90005215228797653 ) ) ;
#63476=CARTESIAN_POINT ( 'NONE',  ( 4.950000001229033941, -2.886751345948129988, 4.999999999999997335 ) ) ;
#63477=CARTESIAN_POINT ( 'NONE',  ( 7.087499999999999467, -2.886751345948129988, 4.999999999999997335 ) ) ;
#63478=( BOUNDED_CURVE ( )  B_SPLINE_CURVE ( 2, ( #37502, #31962, #70391, #42682, #3164, #49329, #9793, #48228, #14964 ),
 .UNSPECIFIED., .F., .F. ) 
 B_SPLINE_CURVE_WITH_KNOTS ( ( 3, 2, 2, 2, 3 ),
 ( 0.8152173913043478937, 0.8188405797101449002, 0.8260869565217391353, 0.8333333333333333703, 0.8369565217391304879 ),
 .UNSPECIFIED. ) 
 CURVE ( )  GEOMETRIC_REPRESENTATION_ITEM ( )  RATIONAL_B_SPLINE_CURVE ( ( 0.9330127018922192983, 0.9330127018922202975, 1.000000000000000000, 0.8660254037844387076, 1.000000000000000000, 0.8660254037844387076, 1.000000000000000000, 0.9330127018922182991, 0.9330127018922192983 ) ) 
 REPRESENTATION_ITEM ( '' )  );
#63480=CARTESIAN_POINT ( 'NONE',  ( 9.721875000614517148, -6.054752690667223547, -1.112240025338166033E-15 ) ) ;
#63481=CARTESIAN_POINT ( 'NONE',  ( 27.74062500061451431, -3.027376345333610441, -5.243569643749999898 ) ) ;
#63482=CARTESIAN_POINT ( 'NONE',  ( 27.48750000122903359, -4.330127018922194537, 2.499999999999995559 ) ) ;
#63484=CARTESIAN_POINT ( 'NONE',  ( 7.809375000614519280, 0.000000000000000000, 5.243569643749999010 ) ) ;
#63485=CARTESIAN_POINT ( 'NONE',  ( 11.93437500061451573, -4.541064518000419881, 2.621784821874995952 ) ) ;
#63486=CARTESIAN_POINT ( 'NONE',  ( 7.200000000000001954, -4.330127018922190985, -2.500000000000001332 ) ) ;
#63487=CARTESIAN_POINT ( 'NONE',  ( -4.243569643749999898, 15.30312500061459424, 30.00000000000000000 ) ) ;
#63489=CARTESIAN_POINT ( 'NONE',  ( 6.262500000000000178, -5.773502691896255534, -1.060575238724906372E-15 ) ) ;
#63490=CARTESIAN_POINT ( 'NONE',  ( 26.70000000122903572, -2.886751345948125991, -5.000000000000000000 ) ) ;
#63492=CARTESIAN_POINT ( 'NONE',  ( 22.41562500061451502, 3.027376345333613106, -5.243569643749998122 ) ) ;
#63493=CARTESIAN_POINT ( 'NONE',  ( 13.00312500061451537, 4.541064518000418104, -2.621784821874998173 ) ) ;
#63495=CARTESIAN_POINT ( 'NONE',  ( 8.746875000614515727, -3.027376345333614438, 5.243569643749998122 ) ) ;
#63496=CARTESIAN_POINT ( 'NONE',  ( 26.55000000000000071, -4.330127018922190985, -2.500000000000001332 ) ) ;
#63497=CARTESIAN_POINT ( 'NONE',  ( 21.45000000122903216, 5.773502691896255534, 3.535250795749688894E-16 ) ) ;
#63498=CARTESIAN_POINT ( 'NONE',  ( 1.626862140677534273E-15, 12.46250000000000213, -26.00000000000000355 ) ) ;
#63499=CARTESIAN_POINT ( 'NONE',  ( 11.89687500061451608, -3.027376345333614438, 5.243569643749998122 ) ) ;
#63500=CARTESIAN_POINT ( 'NONE',  ( 26.63437500061451857, 4.541064518000418104, 2.621784821874999949 ) ) ;
#63501=EDGE_CURVE ( 'NONE', #45031, #19466, #5840, .T. ) ;
#63502=CARTESIAN_POINT ( 'NONE',  ( 3.309375000614518836, 0.000000000000000000, 5.243569643749999010 ) ) ;
#63503=CARTESIAN_POINT ( 'NONE',  ( 1.626862140677534273E-15, 13.47500000122903252, -26.00000000000000355 ) ) ;
#63504=CARTESIAN_POINT ( 'NONE',  ( 23.10937500061451644, 0.000000000000000000, 5.243569643749999010 ) ) ;
#63505=CARTESIAN_POINT ( 'NONE',  ( 11.97187500061451892, -6.054752690667223547, -1.112240025338166033E-15 ) ) ;
#63507=CARTESIAN_POINT ( 'NONE',  ( 24.78750000000000497, -2.886751345948125991, -5.000000000000000000 ) ) ;
#63509=CARTESIAN_POINT ( 'NONE',  ( 9.001249775931846008E-16, 14.12187500061451750, -25.09994784771203058 ) ) ;
#63511=CARTESIAN_POINT ( 'NONE',  ( 17.05312500061451786, 4.541064518000418104, -2.621784821874998173 ) ) ;
#63512=CARTESIAN_POINT ( 'NONE',  ( 7.275000000000000355, 6.123233995736764310E-16, -4.999999999999998224 ) ) ;
#63514=CARTESIAN_POINT ( 'NONE',  ( 14.62500000000000000, 4.330127018922191873, 2.499999999999999556 ) ) ;
#63515=CARTESIAN_POINT ( 'NONE',  ( -3.000416591977282496E-16, 11.59062500061451750, 25.09994784771203058 ) ) ;
#63516=CARTESIAN_POINT ( 'NONE',  ( 13.72500000122903074, 2.886751345948129099, -4.999999999999998224 ) ) ;
#63517=CARTESIAN_POINT ( 'NONE',  ( 25.05937500061451573, -4.541064518000417216, -2.621784821875001281 ) ) ;
#63519=CARTESIAN_POINT ( 'NONE',  ( 20.46562500061451928, -6.054752690667223547, -1.112240025338166033E-15 ) ) ;
#63520=CARTESIAN_POINT ( 'NONE',  ( 20.67187500061451289, 3.027376345333613106, -5.243569643749998122 ) ) ;
#63521=CARTESIAN_POINT ( 'NONE',  ( 5.062500000000000888, 2.886751345948129099, -4.999999999999998224 ) ) ;
#63522=CARTESIAN_POINT ( 'NONE',  ( 8.165625000614516793, 3.027376345333611329, 5.243569643749999010 ) ) ;
#63523=CARTESIAN_POINT ( 'NONE',  ( 22.67812500061451431, -4.541064518000419881, 2.621784821874995952 ) ) ;
#63524=CARTESIAN_POINT ( 'NONE',  ( 12.12187500061451573, 3.027376345333613106, -5.243569643749998122 ) ) ;
#63525=CARTESIAN_POINT ( 'NONE',  ( 16.17187500061451644, 3.027376345333613106, -5.243569643749998122 ) ) ;
#63526=CARTESIAN_POINT ( 'NONE',  ( -4.243569643749999898, 15.75312500061451537, 30.00000000000000000 ) ) ;
#63527=CARTESIAN_POINT ( 'NONE',  ( 18.78750000122903430, 4.330127018922191873, 2.499999999999999556 ) ) ;
#63529=CARTESIAN_POINT ( 'NONE',  ( 8.578125000614518214, 4.541064518000418104, 2.621784821874999949 ) ) ;
#63530=CARTESIAN_POINT ( 'NONE',  ( 3.571875000614517237, 3.027376345333613106, -5.243569643749998122 ) ) ;
#63531=CARTESIAN_POINT ( 'NONE',  ( 29.12812500061451715, 6.421520780324663323E-16, -5.243569643749999010 ) ) ;
#63532=CARTESIAN_POINT ( 'NONE',  ( 25.13437500061451502, 6.421520780324663323E-16, -5.243569643749999010 ) ) ;
#63533=CARTESIAN_POINT ( 'NONE',  ( 17.99062500061451786, 6.054752690667223547, 3.707466751127219781E-16 ) ) ;
#63534=CARTESIAN_POINT ( 'NONE',  ( 24.82500000122902861, -5.773502691896255534, -1.060575238724906372E-15 ) ) ;
#63536=CARTESIAN_POINT ( 'NONE',  ( 25.26562500061451289, 3.027376345333611329, 5.243569643749999010 ) ) ;
#63537=CARTESIAN_POINT ( 'NONE',  ( 21.45937500061451786, -4.541064518000417216, -2.621784821875001281 ) ) ;
#63538=CARTESIAN_POINT ( 'NONE',  ( 16.41562500061451857, -6.054752690667223547, -1.112240025338166033E-15 ) ) ;
#63539=CARTESIAN_POINT ( 'NONE',  ( -4.243569643749997233, 17.19687500061451502, 32.45002607614398471 ) ) ;
#63540=CARTESIAN_POINT ( 'NONE',  ( 22.30312500061451431, -4.541064518000417216, -2.621784821875001281 ) ) ;
#63542=ORIENTED_EDGE ( 'NONE', *, *, #17977, .T. ) ;
#63543=CARTESIAN_POINT ( 'NONE',  ( 25.98750000000000071, -2.886751345948129988, 4.999999999999997335 ) ) ;
#63544=CARTESIAN_POINT ( 'NONE',  ( -2.828200636599751609E-16, 12.23750000000000249, -34.61880215351700230 ) ) ;
#63546=CARTESIAN_POINT ( 'NONE',  ( 29.27812500061451573, 4.541064518000418104, 2.621784821874999949 ) ) ;
#63547=CARTESIAN_POINT ( 'NONE',  ( 9.290625000614515017, -3.027376345333610441, -5.243569643749999898 ) ) ;
#63548=CARTESIAN_POINT ( 'NONE',  ( 21.52500000122903145, 2.886751345948126879, 4.999999999999999112 ) ) ;
#63549=CARTESIAN_POINT ( 'NONE',  ( 26.50312500061451360, 4.541064518000418104, -2.621784821874998173 ) ) ;
#63550=CARTESIAN_POINT ( 'NONE',  ( 25.27499999999999858, 6.123233995736764310E-16, -4.999999999999998224 ) ) ;
#63551=CARTESIAN_POINT ( 'NONE',  ( 8.484601909799253346E-16, 15.27500000122903501, -25.38119784648299770 ) ) ;
#63552=CARTESIAN_POINT ( 'NONE',  ( 25.35000000122903074, -2.886751345948159742, -4.999999999999942268 ) ) ;
#63553=CARTESIAN_POINT ( 'NONE',  ( 10.56562500061451715, -6.054752690667223547, -1.112240025338166033E-15 ) ) ;
#63555=CARTESIAN_POINT ( 'NONE',  ( 25.07812500061451644, 6.421520780324663323E-16, -5.243569643749999010 ) ) ;
#63556=CARTESIAN_POINT ( 'NONE',  ( 7.940625000614518036, -3.027376345333610441, -5.243569643749999898 ) ) ;
#63557=CARTESIAN_POINT ( 'NONE',  ( 2.840625000614518392, -3.027376345333614438, 5.243569643749998122 ) ) ;
#63559=CARTESIAN_POINT ( 'NONE',  ( 4.683223236373093457, -1.751405183929441556, 4.942428804804532838 ) ) ;
#63560=CARTESIAN_POINT ( 'NONE',  ( 13.64999999999999858, 4.330127018922192761, -2.499999999999997780 ) ) ;
#63561=CARTESIAN_POINT ( 'NONE',  ( 14.82187500061451679, 3.027376345333613106, -5.243569643749998122 ) ) ;
#63562=CARTESIAN_POINT ( 'NONE',  ( 12.03750000122903430, 4.330127018922191873, 2.499999999999999556 ) ) ;
#63563=CARTESIAN_POINT ( 'NONE',  ( 17.74687500061451928, -3.027376345333614438, 5.243569643749998122 ) ) ;
#63565=CARTESIAN_POINT ( 'NONE',  ( 7.509375000614517681, -4.541064518000417216, -2.621784821875001281 ) ) ;
#63566=CARTESIAN_POINT ( 'NONE',  ( -3.000416591977282496E-16, 10.69062500061451715, -34.90005215228797653 ) ) ;
#63569=ORIENTED_EDGE ( 'NONE', *, *, #16122, .T. ) ;
#63570=CARTESIAN_POINT ( 'NONE',  ( 23.95312500061451289, 0.000000000000000000, 5.243569643749999010 ) ) ;
#63571=CARTESIAN_POINT ( 'NONE',  ( 11.25000000000000000, -4.330127018922190985, -2.500000000000001332 ) ) ;
#63572=CARTESIAN_POINT ( 'NONE',  ( 27.53437500061451360, 4.541064518000418104, 2.621784821874999949 ) ) ;
#63574=CARTESIAN_POINT ( 'NONE',  ( 23.40000000000000213, -4.330127018922190985, -2.500000000000001332 ) ) ;
#63575=CARTESIAN_POINT ( 'NONE',  ( 7.828125000614517326, -4.541064518000419881, 2.621784821874995952 ) ) ;
#63577=CARTESIAN_POINT ( 'NONE',  ( 17.10937500061451999, 4.541064518000418104, -2.621784821874998173 ) ) ;
#63579=CARTESIAN_POINT ( 'NONE',  ( 29.58750000122903501, 4.330127018922191873, 2.499999999999999556 ) ) ;
#63580=CARTESIAN_POINT ( 'NONE',  ( 9.196875000614518569, -3.027376345333614438, 5.243569643749998122 ) ) ;
#63581=VERTEX_POINT ( 'NONE', #46456 ) ;
#63582=CARTESIAN_POINT ( 'NONE',  ( 19.80937500061451573, 4.541064518000418104, -2.621784821874998173 ) ) ;
#63583=DIRECTION ( 'NONE',  ( -0.000000000000000000, -1.000000000000000000, -0.000000000000000000 ) ) ;
#63584=CARTESIAN_POINT ( 'NONE',  ( 27.71250000000000568, 2.886751345948126879, 4.999999999999999112 ) ) ;
#63585=CARTESIAN_POINT ( 'NONE',  ( 28.50937500061451502, 0.000000000000000000, 5.243569643749999010 ) ) ;
#63587=CARTESIAN_POINT ( 'NONE',  ( 3.310802318797580579, -3.746810377620464205, 3.668301323911666412 ) ) ;
#63588=ORIENTED_EDGE ( 'NONE', *, *, #48710, .T. ) ;
#63589=CARTESIAN_POINT ( 'NONE',  ( 10.12500000000000178, 4.330127018922191873, 2.499999999999999556 ) ) ;
#63591=CARTESIAN_POINT ( 'NONE',  ( 23.46562500061451573, 3.027376345333611329, 5.243569643749999010 ) ) ;
#63592=CARTESIAN_POINT ( 'NONE',  ( 15.22500000000000142, -4.330127018922194537, 2.499999999999995559 ) ) ;
#63593=CARTESIAN_POINT ( 'NONE',  ( 8.775000001229033231, 2.886751345948129099, -4.999999999999998224 ) ) ;
#63594=CARTESIAN_POINT ( 'NONE',  ( 7.603125000614517681, 4.541064518000418104, -2.621784821874998173 ) ) ;
#63595=CARTESIAN_POINT ( 'NONE',  ( 22.34999999999999787, 0.000000000000000000, 4.999999999999998224 ) ) ;
#63596=CARTESIAN_POINT ( 'NONE',  ( 21.06562500061451715, 3.027376345333613106, -5.243569643749998122 ) ) ;
#63597=CARTESIAN_POINT ( 'NONE',  ( 24.82500000122902861, -5.773502691896255534, -1.060575238724906372E-15 ) ) ;
#63599=CARTESIAN_POINT ( 'NONE',  ( 4.387500000000002842, -2.886751345948129988, 4.999999999999997335 ) ) ;
#63600=ORIENTED_EDGE ( 'NONE', *, *, #19527, .T. ) ;
#63601=CARTESIAN_POINT ( 'NONE',  ( 22.34062500061451573, -3.027376345333610441, -5.243569643749999898 ) ) ;
#63602=CARTESIAN_POINT ( 'NONE',  ( 27.17812500061451786, -4.541064518000419881, 2.621784821874995952 ) ) ;
#63603=CARTESIAN_POINT ( 'NONE',  ( 28.17187500061451644, -6.054752690667223547, -1.112240025338166033E-15 ) ) ;
#63604=CARTESIAN_POINT ( 'NONE',  ( 15.02812500061451750, -4.541064518000419881, 2.621784821874995952 ) ) ;
#63605=CARTESIAN_POINT ( 'NONE',  ( 4.844509297411972781, 1.237226603047926421, -5.095516945469514170 ) ) ;
#63606=CARTESIAN_POINT ( 'NONE',  ( 26.70000000122903572, -2.886751345948125991, -5.000000000000000000 ) ) ;
#63608=CARTESIAN_POINT ( 'NONE',  ( 17.76562500061451644, -6.054752690667223547, -1.112240025338166033E-15 ) ) ;
#63609=CARTESIAN_POINT ( 'NONE',  ( 3.525000001229034119, 2.886751345948126879, 4.999999999999999112 ) ) ;
#63610=CARTESIAN_POINT ( 'NONE',  ( 10.73437500061451644, 6.421520780324663323E-16, -5.243569643749999010 ) ) ;
#63611=CARTESIAN_POINT ( 'NONE',  ( 10.62187500061451928, -6.054752690667223547, -1.112240025338166033E-15 ) ) ;
#63612=CARTESIAN_POINT ( 'NONE',  ( 18.90937500061451360, 4.541064518000418104, -2.621784821874998173 ) ) ;
#63614=DIRECTION ( 'NONE',  ( 0.000000000000000000, 0.000000000000000000, 1.000000000000000000 ) ) ;
#63615=CARTESIAN_POINT ( 'NONE',  ( 24.17812500061451786, 6.421520780324663323E-16, -5.243569643749999010 ) ) ;
#63616=CARTESIAN_POINT ( 'NONE',  ( 19.88437500061451857, 4.541064518000418104, 2.621784821874999949 ) ) ;
#63617=CARTESIAN_POINT ( 'NONE',  ( 23.57812500061451289, -4.541064518000419881, 2.621784821874995952 ) ) ;
#63618=CARTESIAN_POINT ( 'NONE',  ( 8.962500000000002132, -5.773502691896255534, -1.060575238724906372E-15 ) ) ;
#63619=CARTESIAN_POINT ( 'NONE',  ( -3.999999999999999556, 14.11249999999999893, 27.69059892324149530 ) ) ;
#63620=CARTESIAN_POINT ( 'NONE',  ( 29.09062500061451573, -3.027376345333610441, -5.243569643749999898 ) ) ;
#63621=CARTESIAN_POINT ( 'NONE',  ( 10.46250000122903323, -4.330127018922190985, -2.500000000000001332 ) ) ;
#63622=CARTESIAN_POINT ( 'NONE',  ( 4.500000001229034652, -2.886751345948129988, 4.999999999999997335 ) ) ;
#63623=CARTESIAN_POINT ( 'NONE',  ( 28.80000000122903359, -2.886751345948092240, 5.000000000000060396 ) ) ;
#63624=CARTESIAN_POINT ( 'NONE',  ( 26.92500000122903359, 2.886751345948126879, 4.999999999999999112 ) ) ;
#63626=CARTESIAN_POINT ( 'NONE',  ( 10.05937500061451750, 0.000000000000000000, 5.243569643749999010 ) ) ;
#63628=EDGE_CURVE ( 'NONE', #50439, #45851, #12472, .T. ) ;
#63629=CARTESIAN_POINT ( 'NONE',  ( 18.36562500061451431, 3.027376345333613106, -5.243569643749998122 ) ) ;
#63630=CARTESIAN_POINT ( 'NONE',  ( 11.29687500061451644, 6.054752690667223547, 3.707466751127219781E-16 ) ) ;
#63631=CARTESIAN_POINT ( 'NONE',  ( 2.840625000614518392, -3.027376345333614438, 5.243569643749998122 ) ) ;
#63633=CARTESIAN_POINT ( 'NONE',  ( 20.67187500061451289, 3.027376345333612662, -5.243569643749998122 ) ) ;
#63634=CARTESIAN_POINT ( 'NONE',  ( 8.446875000614518569, -3.027376345333610441, -5.243569643749999898 ) ) ;
#63635=CARTESIAN_POINT ( 'NONE',  ( 3.057638380960218338, -3.956115207028108038, -3.345374717763163641 ) ) ;
#63636=CARTESIAN_POINT ( 'NONE',  ( 6.853125000614516793, 0.000000000000000000, 5.243569643749999010 ) ) ;
#63637=CARTESIAN_POINT ( 'NONE',  ( 18.85312500061451502, 4.541064518000418104, -2.621784821874998173 ) ) ;
#63638=ORIENTED_EDGE ( 'NONE', *, *, #26043, .T. ) ;
#63639=CARTESIAN_POINT ( 'NONE',  ( 6.562500001229032875, 4.330127018922192761, -2.499999999999997780 ) ) ;
#63640=CARTESIAN_POINT ( 'NONE',  ( 15.89062500061451289, -3.027376345333614438, 5.243569643749998122 ) ) ;
#63641=CARTESIAN_POINT ( 'NONE',  ( 11.99062500061451608, -3.027376345333610441, -5.243569643749999898 ) ) ;
#63643=CARTESIAN_POINT ( 'NONE',  ( 14.51250000000000107, 2.886751345948129099, -4.999999999999998224 ) ) ;
#63644=CARTESIAN_POINT ( 'NONE',  ( 6.937500001229033764, 6.123233995736764310E-16, -4.999999999999998224 ) ) ;
#63645=CARTESIAN_POINT ( 'NONE',  ( 14.74687500061451573, -3.027376345333610441, -5.243569643749999898 ) ) ;
#63646=CARTESIAN_POINT ( 'NONE',  ( 18.67500000122903714, 2.886751345948129099, -4.999999999999998224 ) ) ;
#63648=CARTESIAN_POINT ( 'NONE',  ( -4.243569643749999898, 18.00312500061451715, -30.00000000000000000 ) ) ;
#63650=CARTESIAN_POINT ( 'NONE',  ( 4.378670304180260153, -3.762209243454259333, -3.970801729131952396 ) ) ;
#63651=CARTESIAN_POINT ( 'NONE',  ( 3.442799801882779231, -3.625940455515339167, 3.602703790535031203 ) ) ;
#63652=CARTESIAN_POINT ( 'NONE',  ( 22.57499999999999929, 6.123233995736764310E-16, -4.999999999999998224 ) ) ;
#63653=CARTESIAN_POINT ( 'NONE',  ( 17.44687500061451857, -3.027376345333610441, -5.243569643749999898 ) ) ;
#63655=CARTESIAN_POINT ( 'NONE',  ( 14.12812500061451715, -4.541064518000419881, 2.621784821874995952 ) ) ;
#63657=CARTESIAN_POINT ( 'NONE',  ( 15.90000000122903501, -2.886751345948193048, -4.999999999999883649 ) ) ;
#63658=CARTESIAN_POINT ( 'NONE',  ( 27.30937500061451573, -4.541064518000417216, -2.621784821875001281 ) ) ;
#63660=CARTESIAN_POINT ( 'NONE',  ( 10.60312500061451679, -4.541064518000417216, -2.621784821875001281 ) ) ;
#63661=CARTESIAN_POINT ( 'NONE',  ( 15.60937500061451644, -4.541064518000417216, -2.621784821875001281 ) ) ;
#63662=VERTEX_POINT ( 'NONE', #28372 ) ;
#63663=AXIS2_PLACEMENT_3D ( 'NONE', #51505, #30044, #11975 ) ;
#63664=CARTESIAN_POINT ( 'NONE',  ( 26.57812500061451644, 4.541064518000418104, 2.621784821874999949 ) ) ;
#63665=CARTESIAN_POINT ( 'NONE',  ( 19.97812500061451502, -4.541064518000419881, 2.621784821874995952 ) ) ;
#63666=CARTESIAN_POINT ( 'NONE',  ( 29.20312500061451644, 4.541064518000418104, -2.621784821874998173 ) ) ;
#63667=CARTESIAN_POINT ( 'NONE',  ( -5.810221930991193690E-16, 14.15000000122903145, -34.00000000000000000 ) ) ;
#63668=CARTESIAN_POINT ( 'NONE',  ( 9.562500000000001776, 2.886751345948129099, -4.999999999999998224 ) ) ;
#63669=CARTESIAN_POINT ( 'NONE',  ( 18.67500000122903714, 2.886751345948129099, -4.999999999999998224 ) ) ;
#63670=CARTESIAN_POINT ( 'NONE',  ( 23.21250000122903501, 4.330127018922192761, -2.499999999999997780 ) ) ;
#63672=EDGE_LOOP ( 'NONE', ( #54932, #56352, #18972, #27115 ) ) ;
#63673=CARTESIAN_POINT ( 'NONE',  ( 16.42500000000000071, 4.330127018922191873, 2.499999999999999556 ) ) ;
#63674=CARTESIAN_POINT ( 'NONE',  ( 20.43749999999999645, 5.773502691896255534, 3.535250795749688894E-16 ) ) ;
#63675=CARTESIAN_POINT ( 'NONE',  ( 18.12187500061451573, 3.027376345333611329, 5.243569643749999010 ) ) ;
#63676=CARTESIAN_POINT ( 'NONE',  ( 13.22812500061451502, -4.541064518000419881, 2.621784821874995952 ) ) ;
#63677=ORIENTED_EDGE ( 'NONE', *, *, #1559, .T. ) ;
#63678=CARTESIAN_POINT ( 'NONE',  ( 28.05000000122903003, -2.886751345948130432, -4.999999999999991118 ) ) ;
#63679=CARTESIAN_POINT ( 'NONE',  ( 4.865625000614517859, 3.027376345333613106, -5.243569643749998122 ) ) ;
#63680=CARTESIAN_POINT ( 'NONE',  ( 2.000000000000001332, 15.31250000122903465, 33.46410161513774995 ) ) ;
#63681=CARTESIAN_POINT ( 'NONE',  ( 12.78749999999999964, 5.773502691896255534, 3.535250795749688894E-16 ) ) ;
#63683=CARTESIAN_POINT ( 'NONE',  ( -2.121784821874999949, 17.47812500061451502, 26.32496088578401938 ) ) ;
#63684=CARTESIAN_POINT ( 'NONE',  ( 3.309375000614518836, 0.000000000000000000, 5.243569643749999010 ) ) ;
#63687=CARTESIAN_POINT ( 'NONE',  ( 26.93437500061451573, 6.421520780324663323E-16, -5.243569643749999010 ) ) ;
#63688=ORIENTED_EDGE ( 'NONE', *, *, #5826, .F. ) ;
#63689=CARTESIAN_POINT ( 'NONE',  ( 21.51562500061451644, 3.027376345333613106, -5.243569643749998122 ) ) ;
#63690=CARTESIAN_POINT ( 'NONE',  ( 24.04687500061451644, -3.027376345333614438, 5.243569643749998122 ) ) ;
#63691=CARTESIAN_POINT ( 'NONE',  ( 2.121784821874999061, 15.60312500061459495, -33.67503911421598417 ) ) ;
#63692=CARTESIAN_POINT ( 'NONE',  ( 6.515625000614516438, -6.054752690667223547, -1.112240025338166033E-15 ) ) ;
#63694=CARTESIAN_POINT ( 'NONE',  ( 23.31562500061451004, 3.027376345333612662, -5.243569643749998122 ) ) ;
#63697=CARTESIAN_POINT ( 'NONE',  ( 16.13437500061451502, 6.421520780324663323E-16, -5.243569643749999010 ) ) ;
#63698=CARTESIAN_POINT ( 'NONE',  ( 18.75937500061451857, -4.541064518000417216, -2.621784821875001281 ) ) ;
#63699=CARTESIAN_POINT ( 'NONE',  ( 28.09687500061451360, -3.027376345333614438, 5.243569643749998122 ) ) ;
#63700=CARTESIAN_POINT ( 'NONE',  ( 4.243569643749999898, 17.38437500061451502, 30.00000000000000000 ) ) ;
#63701=CARTESIAN_POINT ( 'NONE',  ( 7.190625000614518036, 6.054752690667223547, 3.707466751127219781E-16 ) ) ;
#63702=CARTESIAN_POINT ( 'NONE',  ( 4.000000000000000000, 16.13749999999999929, 32.30940107675849760 ) ) ;
#63703=CARTESIAN_POINT ( 'NONE',  ( 5.521875000614517859, 3.027376345333611329, 5.243569643749999010 ) ) ;
#63704=CARTESIAN_POINT ( 'NONE',  ( 6.328125000614515550, 4.541064518000418104, 2.621784821874999949 ) ) ;
#63705=CARTESIAN_POINT ( 'NONE',  ( 9.909375000614517148, 4.541064518000418104, -2.621784821874998173 ) ) ;
#63706=CARTESIAN_POINT ( 'NONE',  ( 16.53750000122903430, 4.330127018922191873, 2.499999999999999556 ) ) ;
#63707=CARTESIAN_POINT ( 'NONE',  ( 5.296875000614518214, -3.027376345333610441, -5.243569643749999898 ) ) ;
#63708=CARTESIAN_POINT ( 'NONE',  ( 7.265625000614516438, 3.027376345333611329, 5.243569643749999010 ) ) ;
#63711=CARTESIAN_POINT ( 'NONE',  ( 16.43437500061451573, -4.541064518000419881, 2.621784821874995952 ) ) ;
#63712=CARTESIAN_POINT ( 'NONE',  ( 27.59999999999999787, 4.330127018922192761, -2.499999999999997780 ) ) ;
#63713=ORIENTED_EDGE ( 'NONE', *, *, #66296, .F. ) ;
#63714=CARTESIAN_POINT ( 'NONE',  ( 24.51562500061451289, -6.054752690667223547, -1.112240025338166033E-15 ) ) ;
#63715=CARTESIAN_POINT ( 'NONE',  ( 8.540625000614518569, 6.054752690667223547, 3.707466751127219781E-16 ) ) ;
#63716=CARTESIAN_POINT ( 'NONE',  ( 27.60937500061451644, 0.000000000000000000, 5.243569643749999010 ) ) ;
#63717=CARTESIAN_POINT ( 'NONE',  ( 11.12812500061451715, 6.421520780324663323E-16, -5.243569643749999010 ) ) ;
#63718=CARTESIAN_POINT ( 'NONE',  ( -0.7368805616696195715, 9.859898480082234684, -34.17910162106521454 ) ) ;
#63719=CARTESIAN_POINT ( 'NONE',  ( 11.10000000122903252, 5.773502691896255534, 3.535250795749688894E-16 ) ) ;
#63720=CARTESIAN_POINT ( 'NONE',  ( 25.71562500061451573, 3.027376345333611329, 5.243569643749999010 ) ) ;
#63721=CARTESIAN_POINT ( 'NONE',  ( -3.000416591977282496E-16, 12.49062500061451608, -34.90005215228797653 ) ) ;
#63722=CARTESIAN_POINT ( 'NONE',  ( 12.22500000122903430, -5.773502691896255534, -1.060575238724906372E-15 ) ) ;
#63723=CARTESIAN_POINT ( 'NONE',  ( 21.44062500061452070, -3.027376345333610441, -5.243569643749999898 ) ) ;
#63724=CARTESIAN_POINT ( 'NONE',  ( 11.25000000000000000, -4.330127018922190985, -2.500000000000001332 ) ) ;
#63725=CARTESIAN_POINT ( 'NONE',  ( 19.52812500061451573, -4.541064518000419881, 2.621784821874995952 ) ) ;
#63726=CARTESIAN_POINT ( 'NONE',  ( 6.459375000614518747, 0.000000000000000000, 5.243569643749999010 ) ) ;
#63727=CARTESIAN_POINT ( 'NONE',  ( 20.21250000000000213, -5.773502691896255534, -1.060575238724906372E-15 ) ) ;
#63728=CARTESIAN_POINT ( 'NONE',  ( 13.83750000122903323, 4.330127018922191873, 2.499999999999999556 ) ) ;
#63729=( BOUNDED_CURVE ( )  B_SPLINE_CURVE ( 2, ( #11014, #53072, #35351, #8372, #52349, #35714, #40544 ),
 .UNSPECIFIED., .F., .T. ) 
 B_SPLINE_CURVE_WITH_KNOTS ( ( 3, 2, 2, 3 ),
 ( 0.3666666666666666408, 0.3694444444444444642, 0.3722222222222222321, 0.3750000000000000000 ),
 .UNSPECIFIED. ) 
 CURVE ( )  GEOMETRIC_REPRESENTATION_ITEM ( )  RATIONAL_B_SPLINE_CURVE ( ( 1.000000000000000000, 0.8660254037844387076, 1.000000000000000000, 0.8660254037844387076, 1.000000000000000000, 0.8660254037844387076, 1.000000000000000000 ) ) 
 REPRESENTATION_ITEM ( '' )  );
#63730=CARTESIAN_POINT ( 'NONE',  ( 10.86562500061451431, 3.027376345333611329, 5.243569643749999010 ) ) ;
#63731=CARTESIAN_POINT ( 'NONE',  ( 12.85312500061451502, -4.541064518000417216, -2.621784821875001281 ) ) ;
#63732=CARTESIAN_POINT ( 'NONE',  ( 24.60000000122903430, 5.773502691896255534, 3.535250795749688894E-16 ) ) ;
#63733=CARTESIAN_POINT ( 'NONE',  ( 20.25937500061451857, 4.541064518000418104, -2.621784821874998173 ) ) ;
#63735=EDGE_CURVE ( 'NONE', #47420, #33656, #30951, .T. ) ;
#63736=CARTESIAN_POINT ( 'NONE',  ( 7.275000001229035007, -5.773502691896255534, -1.060575238724906372E-15 ) ) ;
#63737=CARTESIAN_POINT ( 'NONE',  ( 9.196875000614518569, -3.027376345333614438, 5.243569643749998122 ) ) ;
#63738=CARTESIAN_POINT ( 'NONE',  ( 25.17187500061451644, 3.027376345333613106, -5.243569643749998122 ) ) ;
#63742=CARTESIAN_POINT ( 'NONE',  ( 20.95312500061451999, -4.541064518000417216, -2.621784821875001281 ) ) ;
#63743=CARTESIAN_POINT ( 'NONE',  ( 27.53437500061451360, 4.541064518000418104, 2.621784821874999949 ) ) ;
#63746=CARTESIAN_POINT ( 'NONE',  ( 8.971875000614515372, 3.027376345333613106, -5.243569643749998122 ) ) ;
#63747=CARTESIAN_POINT ( 'NONE',  ( 18.25312500061451715, -4.541064518000417216, -2.621784821875001281 ) ) ;
#63748=ORIENTED_EDGE ( 'NONE', *, *, #61508, .F. ) ;
#63749=CARTESIAN_POINT ( 'NONE',  ( -3.999999999999999112, 12.76250000000000107, -32.30940107675850470 ) ) ;
#63750=CARTESIAN_POINT ( 'NONE',  ( 26.76562500061451644, -6.054752690667223547, -1.112240025338166033E-15 ) ) ;
#63751=CARTESIAN_POINT ( 'NONE',  ( 4.809375000614516615, -4.541064518000417216, -2.621784821875001281 ) ) ;
#63752=CARTESIAN_POINT ( 'NONE',  ( 10.23750000122903359, 4.330127018922191873, 2.499999999999999556 ) ) ;
#63753=CARTESIAN_POINT ( 'NONE',  ( 3.727827348360245097, 3.332161949968362347, -3.727827348360304605 ) ) ;
#63754=CARTESIAN_POINT ( 'NONE',  ( 18.14999999999999858, 4.330127018922192761, -2.499999999999997780 ) ) ;
#63755=CARTESIAN_POINT ( 'NONE',  ( 21.89062500061451289, -3.027376345333610441, -5.243569643749999898 ) ) ;
#63756=ORIENTED_EDGE ( 'NONE', *, *, #1804, .T. ) ;
#63757=CARTESIAN_POINT ( 'NONE',  ( 24.63749999999999574, -2.886751345948129988, 4.999999999999997335 ) ) ;
#63758=CARTESIAN_POINT ( 'NONE',  ( 25.62187500061451573, 3.027376345333613106, -5.243569643749998122 ) ) ;
#63760=CARTESIAN_POINT ( 'NONE',  ( 14.27812500061451573, 6.421520780324663323E-16, -5.243569643749999010 ) ) ;
#63761=CARTESIAN_POINT ( 'NONE',  ( 5.278125000614516615, 6.421520780324663323E-16, -5.243569643749999010 ) ) ;
#63763=CARTESIAN_POINT ( 'NONE',  ( 29.24062500061451431, 6.054752690667223547, 3.707466751127219781E-16 ) ) ;
#63764=( BOUNDED_SURFACE ( )  B_SPLINE_SURFACE ( 1, 2, ( 
 ( #6688, #1153, #23662, #24020, #68747, #24387, #18830, #18105, #7046, #63186, #29575, #69828, #52112, #63908, #35832, #46569, #18473, #41037, #12938, #35475, #58355, #59455, #42849, #48032, #8136, #42119, #14029, #54661, #71659, #36569, #64645, #70924, #70185, #15126, #20294, #65741, #53938, #4065, #36206, #36935, #37303, #8862, #14397, #41746, #26590, #8494, #30662, #26222, #48762, #49131, #31769, #9232, #25859, #31398, #65371, #3335, #48398, #14759, #59826, #54305, #3697, #71285, #64275, #60186, #19564, #20664, #25110, #43222, #25485, #42486, #37663, #47653, #2957, #31026, #59089, #53195, #70557, #9595, #13663, #58724, #2591, #53561, #32127, #19933, #65009, #38773, #50939, #55754, #9958, #22490, #4787, #21032, #21759, #5148, #32495, #15851, #55029, #27684, #4433, #55393, #33573, #60922, #61645, #66850, #10324, #27321, #26961, #38397, #61293, #72379, #16579, #72019, #50221, #44320, #11047, #43585, #5870, #38029, #10685, #16222, #33215, #33935, #72747, #49488, #21395, #43951, #45039, #22132, #44688, #28402, #73108, #66474, #60551, #32858, #66106, #67218, #49853, #39131, #56121, #5513, #28052, #50580, #15485, #11418, #67574, #16939, #39494, #62016, #56478, #12135, #63100, #41310, #23210, #18024, #1429, #6602, #39867, #701, #45763, #13212, #30215, #68299, #17659, #29490, #28760, #46851, #52027, #24304, #12501, #35751, #67933, #68660, #69024, #40581, #46123, #335, #58272, #40220, #62379, #57911, #7320, #7679, #63468, #40953, #57557, #18386, #22845, #12855, #11778, #35388, #6960, #18746, #23936, #62742, #34294, #45397, #29851, #17307, #56826, #6232, #51665, #1069, #46485, #63820, #69391, #51300, #34660, #57189, #29132, #23578, #52387, #35029, #1794, #70471, #20207, #14669, #13574, #64186, #36847, #42033, #36119, #37212, #64921, #8407, #59734, #59363, #58639, #8047, #41664, #24663, #9142, #30581, #71196, #42761, #69741, #65281, #43127, #31308, #47209, #25027, #47569, #53107, #2504, #59001, #26131, #48308, #70832, #2869, #19475, #37576, #31679, #54213, #20570, #70099, #2152, #15039, #42398, #36483, #25399, #25770, #19109, #64557, #14311, #30936, #47942, #53477, #3610, #13946, #19848, #8774, #53848, #3242, #52748, #48671, #65650, #60100, #9509, #50133, #44605, #21675, #55310, #50497, #3978, #33486, #43496, #4704, #38689, #27601, #66764, #49771, #49404, #72665, #10964, #26501, #5427, #66022, #32041, #27234, #67493, #39048, #10603, #15766, #71571, #15401, #16137, #20945, #4348, #61208, #71935, #72296, #26874, #10240, #44232, #67135, #21311, #22044, #33131, #43865, #38306, #37943, #66389, #55668, #32773, #16492, #9871, #5065, #61562, #56035, #61931, #16856, #49043, #27966, #73024, #22408, #44955, #39412, #60462, #32404, #54943, #54574, #60835, #63012, #69298, #63381, #62299, #28320, #56745, #41222, #46038, #619, #29407, #23850, #11695, #34575, #68216, #11337, #1699, #62655, #40864, #35301, #23127, #50857, #45682, #982, #52298, #33854, #24211, #255, #57103, #6149, #68574, #28678, #6513, #51218, #12051, #23491, #51941, #46763, #6875, #22763, #1338, #17934, #29761, #12409, #17577, #45315, #56398, #46398, #5788, #67850, #17222, #29047, #51583, #57470, #18660, #57823, #39783, #40139, #34211, #40496, #34943, #68934, #18291, #12766, #7232, #31214, #25679, #24574, #2064, #47849, #53019, #47119, #48215, #2778, #19379, #70736, #70377, #69651, #19015, #52656, #35662, #20114, #41576, #9056, #53755, #7587, #3151, #54126, #42303, #58183, #36025, #58542, #64093, #13476, #70010, #37116, #59274, #8682, #13853, #30491, #7954, #30123, #41937, #25302, #20481, #71108, #2413, #24935, #19755, #47478, #64829, #8319, #63731, #14219, #64462, #65193, #36395, #13123, #58909, #36755, #30848, #53383, #42669, #14583, #59643, #31587, #3521, #26042, #48582, #71849, #15314, #32315, #3888, #43409, #43773, #4258, #27148, #48951, #60742, #26783, #72211, #67047, #21956, #37491, #66298, #49316, #21221, #50045, #15677, #31951, #26408, #71480, #10517, #38214, #32684, #44513, #61120, #20856, #60011, #65934, #43035, #10152, #60373, #21589, #66669, #37853, #55224, #54849, #65563, #72570, #4618, #33044, #4978, #9781, #54487, #49682, #44142, #14952, #16046, #38594, #55584, #27511, #9422, #36265, #8190, #48818, #65802, #30717, #58780, #65065, #64331, #9291, #14456, #59885, #48087, #71348, #30361, #31082, #31456, #53622, #8555, #35888, #20723, #2648, #24805, #20355, #42906, #43281, #25916, #3395, #19986, #3014, #59512, #25544, #70613, #42539, #58413, #54363, #13724, #53998, #19247, #48456, #19619, #36625, #8926, #41802, #70247, #25167, #42175, #7826, #59146, #36990, #47348, #53250, #69882, #70980, #47708, #64701, #65430, #14085, #14820, #37363, #31824, #3757, #26281, #52891, #2288, #11567, #22279, #56274, #27841, #16364, #33367, #38919, #39651, #66626, #60697, #50372, #16003, #67366, #38173, #10831, #22636, #4576, #44100, #5663, #50728, #72897, #61438, #56622, #10110, #62170, #49639, #55903, #44831, #33728, #16729, #5295, #55541, #28199, #17090, #32640, #34082, #72165, #55181, #39284, #483, #45186, #61797, #21916, #27106, #51087, #21545, #11201, #10473, #131, #4937, #67718, #33002, #6017, #28552, #22992, #45553, #68083, #38552, #61075, #27471, #50003, #72528, #44472, #67002, #48366, #59058, #62523, #51447, #17451, #69796, #19162, #64613, #36904, #42455, #28909, #13264, #34445, #6377, #30270, #13999, #69442, #2560, #36175, #8463, #53531, #850, #23358, #25080, #7735, #46903, #2927, #30631, #47262, #25456, #47623, #18799, #41363, #63873, #11920, #48000, #35802, #59424, #30998, #56973, #70528, #8832, #70156, #58324, #52803, #19903, #2204, #24719, #36538, #64978, #8103, #41716, #31368, #64243, #14369, #13631, #58692, #19533, #53909, #53163, #42091, #3302, #25829, #40009, #65340, #44294, #9200, #70892, #66077, #33190 ),
 ( #14730, #15455, #66448, #38000, #43555, #27657, #55729, #37633, #59794, #55368, #4761, #10660, #60894, #38369, #55000, #60522, #21368, #9928, #32467, #4406, #5123, #16195, #26190, #15825, #54273, #10299, #54630, #71630, #43922, #3667, #32098, #60156, #48730, #37272, #4037, #26935, #20265, #42817, #31735, #71253, #49460, #20633, #71994, #32830, #43191, #27294, #65711, #72352, #26561, #15097, #21003, #49828, #9566, #49101, #21733, #66822, #38746, #61266, #62716, #16912, #17635, #22820, #39467, #56453, #56096, #45013, #57534, #51640, #12110, #5843, #56800, #310, #40195, #6934, #35004, #67192, #17278, #50912, #28375, #63073, #45372, #61621, #68634, #67549, #72721, #12475, #39840, #33909, #61990, #23548, #34267, #68273, #62354, #67908, #11750, #6205, #1041, #5487, #22104, #28733, #28026, #51274, #50196, #678, #34633, #16553, #50554, #57162, #6575, #23184, #45738, #17996, #44662, #46098, #11024, #29105, #40555, #39105, #33546, #73082, #11390, #22463, #8383, #23911, #2844, #40929, #29465, #24639, #64897, #36461, #8021, #13187, #52001, #42375, #46459, #2128, #1765, #64159, #46827, #47185, #24279, #7653, #19085, #47545, #14287, #25003, #18358, #70074, #36094, #47918, #30557, #69364, #63443, #59339, #19449, #1402, #12829, #68997, #30192, #52721, #2478, #70447, #53454, #35363, #18722, #57887, #7296, #41286, #42009, #29826, #13547, #69717, #64529, #13923, #52361, #63797, #58614, #35726, #58248, #58976, #41640, #53083, #30913, #25373, #19823, #36824, #70808, #53825, #66366, #37188, #27212, #49382, #25747, #71913, #72275, #60439, #3218, #54190, #3587, #14647, #59712, #15016, #55288, #4325, #26850, #32016, #48648, #66741, #21287, #38281, #54552, #15742, #48284, #9119, #43840, #60809, #71548, #3954, #49747, #20183, #10217, #42738, #26477, #15379, #32750, #43474, #49017, #26109, #4682, #21652, #65257, #44209, #31656, #8750, #20922, #16111, #38663, #9849, #65629, #31283, #71173, #20545, #65998, #43103, #37921, #37554, #32378, #60076, #9487, #54918, #6123, #958, #56721, #50110, #28654, #67825, #6486, #62276, #27941, #72639, #17908, #51193, #33108, #22022, #61186, #39388, #61907, #34187, #29021, #12025, #44579, #56011, #5042, #67111, #73000, #596, #39026, #45291, #5767, #23101, #45658, #16467, #61540, #17198, #50474, #10942, #68191, #233, #16834, #17554, #39759, #33464, #5404, #22384, #55646, #40115, #44933, #51557, #62631, #27578, #34550, #23467, #11670, #67471, #11312, #33833, #56375, #28298, #50833, #57078, #46013, #68550, #22741, #10581, #25275, #58518, #69986, #58885, #57798, #62986, #2755, #30098, #24184, #7207, #13830, #24550, #7928, #52633, #18634, #35636, #41198, #41913, #68907, #12381, #2039, #18265, #69628, #40471, #30466, #30825, #18990, #34917, #12740, #35276, #46373, #40838, #46738, #36369, #35999, #52995, #63706, #29736, #47822, #2391, #19356, #8295, #52273, #57444, #70352, #47096, #69272, #1675, #53358, #41552, #24910, #64069, #13098, #58158, #7562, #64438, #63356, #6848, #13451, #47453, #29382, #51916, #1313, #23822, #59250, #25653, #37828, #32291, #9397, #43011, #38190, #64803, #21196, #31189, #65540, #26385, #15289, #54464, #37467, #37093, #60348, #71825, #14193, #66273, #53731, #19729, #14927, #55200, #26760, #71456, #3499, #42279, #32659, #36728, #59987, #65169, #3862, #59618, #31927, #14560, #71083, #48926, #9757, #4593, #54825, #8658, #4233, #20832, #60716, #43385, #9032, #3124, #49657, #49292, #48189, #70713, #20088, #20457, #65909, #43748, #10127, #15651, #42645, #31562, #54101, #26018, #48557, #27123, #50021, #56289, #16745, #39667, #34100, #33020, #10492, #5679, #61455, #55558, #56639, #11219, #27857, #6035, #28215, #4954, #27487, #61094, #44118, #28569, #72545, #17467, #62186, #16022, #38570, #44847, #44489, #33744, #16382, #67383, #67022, #50388, #61815, #17107, #11937, #67735, #21933, #11583, #50744, #40027, #147, #38937, #10849, #28928, #51105, #66645, #33383, #72185, #72913, #22295, #45202, #62540, #23011, #55919, #5314, #39301, #22653, #502, #45570, #68101, #34462, #56990, #6397, #21564, #12292, #62897, #35549, #40746, #34826, #35907, #63621, #7119, #13365, #58068, #57354, #6759, #40378, #23375, #58431, #29293, #69899, #18903, #68455, #41464, #41819, #30005, #45923, #23732, #46281, #51823, #1226, #57714, #24821, #47009, #69544, #1588, #18178, #36283, #63983, #7842, #19265, #68821, #868, #13741, #41111, #35189, #63262, #47368, #7478, #30379, #13011, #29648, #46645, #52186, #52908, #12654, #17817, #52547, #24098, #1954, #51465, #69186, #2306, #18546, #24461, #64350, #58797, #8207, #54015, #49205, #2666, #32205, #42193, #3411, #37378, #26297, #65446, #48471, #48103, #48834, #9672, #25183, #4141, #64717, #30736, #25931, #66184, #37738, #9307, #14472, #53268, #43662, #59529, #65818, #14837, #14101, #36641, #19636, #47726, #15200, #59163, #71739, #71365, #70265, #20739, #21109, #31841, #8571, #3031, #25562, #31099, #53639, #37006, #26672, #43297, #60258, #70995, #70626, #15562, #54739, #38105, #60627, #20001, #42554, #65081, #20371, #8941, #31472, #42922, #59902, #54377, #3772, #61368, #5223, #10765, #11493, #38480, #32572, #72827, #61004, #39215, #10038, #55836, #67651, #49570, #15931, #28130, #22568, #22210, #33298, #28479, #55110, #34015, #21476, #27765, #16657, #5593, #44764, #50305, #27401, #50658, #62099, #4510, #56552, #44029, #27039, #67299, #45479, #17017, #61727, #66930, #72092, #22921, #66551, #11128, #55473, #33655, #49931, #56200, #4865, #62, #45116, #39576, #68011, #5946, #10403, #51016, #412, #17383, #39941, #72456, #32935, #21841, #44404, #16299, #38853, #62454, #40655, #63176, #35462, #7755, #13284, #779, #57265, #6309, #51377, #1140, #57984, #40293, #46558, #7034, #29922, #24375, #23288, #45836, #69100, #51741, #68373, #46923 ) ),
 .UNSPECIFIED., .F., .F., .F. ) 
 B_SPLINE_SURFACE_WITH_KNOTS ( ( 2, 2 ),
 ( 3, 2, 2, 2, 2, 2, 2, 2, 2, 2, 2, 2, 2, 2, 2, 2, 2, 2, 2, 2, 2, 2, 2, 2, 2, 2, 2, 2, 2, 2, 2, 2, 2, 2, 2, 2, 2, 2, 2, 2, 2, 2, 2, 2, 2, 2, 2, 2, 2, 2, 2, 2, 2, 2, 2, 2, 2, 2, 2, 2, 2, 2, 2, 2, 2, 2, 2, 2, 2, 2, 2, 2, 2, 2, 2, 2, 2, 2, 2, 2, 2, 2, 2, 2, 2, 2, 2, 2, 2, 2, 2, 2, 2, 2, 2, 2, 2, 2, 2, 2, 2, 2, 2, 2, 2, 2, 2, 2, 2, 2, 2, 2, 2, 2, 2, 2, 2, 2, 2, 2, 2, 2, 2, 2, 2, 2, 2, 2, 2, 2, 2, 2, 2, 2, 2, 2, 2, 2, 2, 2, 2, 2, 2, 2, 2, 2, 2, 2, 2, 2, 2, 2, 2, 2, 2, 2, 2, 2, 2, 2, 2, 2, 2, 2, 2, 2, 2, 2, 2, 2, 2, 2, 2, 2, 2, 2, 2, 2, 2, 2, 2, 2, 2, 2, 2, 2, 2, 2, 2, 2, 2, 2, 2, 2, 2, 2, 2, 2, 2, 2, 2, 2, 2, 2, 2, 2, 2, 2, 2, 2, 2, 2, 2, 2, 2, 2, 2, 2, 2, 2, 2, 2, 2, 2, 2, 2, 2, 2, 2, 2, 2, 2, 2, 2, 2, 2, 2, 2, 2, 2, 2, 2, 2, 2, 2, 2, 2, 2, 2, 2, 2, 2, 2, 2, 2, 2, 2, 2, 2, 2, 2, 2, 2, 2, 2, 2, 2, 2, 2, 2, 2, 2, 2, 2, 2, 2, 2, 2, 2, 2, 2, 2, 2, 2, 2, 2, 2, 2, 2, 2, 2, 2, 2, 2, 2, 2, 2, 2, 2, 2, 2, 2, 2, 2, 2, 2, 2, 2, 2, 2, 2, 2, 2, 2, 2, 2, 2, 2, 2, 2, 2, 2, 2, 2, 2, 2, 2, 2, 2, 2, 2, 2, 2, 2, 2, 2, 2, 2, 2, 2, 2, 2, 2, 2, 2, 2, 2, 2, 2, 2, 2, 2, 2, 2, 2, 2, 2, 2, 2, 2, 3 ),
 ( 0.000000000000000000, 1.000000000000000000 ),
 ( 0.000000000000000000, 0.002777777777777777884, 0.005555555555555555768, 0.008333333333333333218, 0.01111111111111111154, 0.01388888888888888812, 0.01666666666666666644, 0.01944444444444444475, 0.02222222222222222307, 0.02500000000000000139, 0.02777777777777777624, 0.03055555555555555455, 0.03333333333333333287, 0.03611111111111110772, 0.03888888888888888951, 0.04166666666666666435, 0.04444444444444444614, 0.04722222222222222099, 0.05000000000000000278, 0.05277777777777777762, 0.05555555555555555247, 0.05833333333333333426, 0.06111111111111110911, 0.06388888888888888395, 0.06666666666666666574, 0.06944444444444444753, 0.07222222222222221544, 0.07499999999999999722, 0.07777777777777777901, 0.08055555555555556080, 0.08333333333333332871, 0.08611111111111111049, 0.08888888888888889228, 0.09166666666666666019, 0.09444444444444444198, 0.09722222222222222376, 0.1000000000000000056, 0.1027777777777777735, 0.1055555555555555552, 0.1083333333333333370, 0.1111111111111111049, 0.1138888888888888867, 0.1166666666666666685, 0.1194444444444444503, 0.1222222222222222182, 0.1250000000000000000, 0.1277777777777777679, 0.1305555555555555636, 0.1333333333333333315, 0.1361111111111110994, 0.1388888888888888951, 0.1416666666666666630, 0.1444444444444444309, 0.1472222222222222265, 0.1499999999999999944, 0.1527777777777777901, 0.1555555555555555580, 0.1583333333333333259, 0.1611111111111111216, 0.1638888888888888895, 0.1666666666666666574, 0.1694444444444444531, 0.1722222222222222210, 0.1749999999999999889, 0.1777777777777777846, 0.1805555555555555525, 0.1833333333333333204, 0.1861111111111111160, 0.1888888888888888840, 0.1916666666666666796, 0.1944444444444444475, 0.1972222222222222154, 0.2000000000000000111, 0.2027777777777777790, 0.2055555555555555469, 0.2083333333333333426, 0.2111111111111111105, 0.2138888888888888784, 0.2166666666666666741, 0.2194444444444444420, 0.2222222222222222099, 0.2250000000000000056, 0.2277777777777777735, 0.2305555555555555691, 0.2333333333333333370, 0.2361111111111111049, 0.2388888888888889006, 0.2416666666666666685, 0.2444444444444444364, 0.2472222222222222321, 0.2500000000000000000, 0.2527777777777777679, 0.2555555555555555358, 0.2583333333333333592, 0.2611111111111111271, 0.2638888888888888951, 0.2666666666666666630, 0.2694444444444444309, 0.2722222222222221988, 0.2750000000000000222, 0.2777777777777777901, 0.2805555555555555580, 0.2833333333333333259, 0.2861111111111110938, 0.2888888888888888618, 0.2916666666666666852, 0.2944444444444444531, 0.2972222222222222210, 0.2999999999999999889, 0.3027777777777777568, 0.3055555555555555802, 0.3083333333333333481, 0.3111111111111111160, 0.3138888888888888840, 0.3166666666666666519, 0.3194444444444444198, 0.3222222222222222432, 0.3250000000000000111, 0.3277777777777777790, 0.3305555555555555469, 0.3333333333333333148, 0.3361111111111111382, 0.3388888888888889062, 0.3416666666666666741, 0.3444444444444444420, 0.3472222222222222099, 0.3499999999999999778, 0.3527777777777778012, 0.3555555555555555691, 0.3583333333333333370, 0.3611111111111111049, 0.3638888888888888729, 0.3666666666666666408, 0.3694444444444444642, 0.3722222222222222321, 0.3750000000000000000, 0.3777777777777777679, 0.3805555555555555358, 0.3833333333333333592, 0.3861111111111111271, 0.3888888888888888951, 0.3916666666666666630, 0.3944444444444444309, 0.3972222222222221988, 0.4000000000000000222, 0.4027777777777777901, 0.4055555555555555580, 0.4083333333333333259, 0.4111111111111110938, 0.4138888888888888618, 0.4166666666666666852, 0.4194444444444444531, 0.4222222222222222210, 0.4249999999999999889, 0.4277777777777777568, 0.4305555555555555802, 0.4333333333333333481, 0.4361111111111111160, 0.4388888888888888840, 0.4416666666666666519, 0.4444444444444444198, 0.4472222222222222432, 0.4500000000000000111, 0.4527777777777777790, 0.4555555555555555469, 0.4583333333333333148, 0.4611111111111111382, 0.4638888888888889062, 0.4666666666666666741, 0.4694444444444444420, 0.4722222222222222099, 0.4749999999999999778, 0.4777777777777778012, 0.4805555555555555691, 0.4833333333333333370, 0.4861111111111111049, 0.4888888888888888729, 0.4916666666666666408, 0.4944444444444444642, 0.4972222222222222321, 0.5000000000000000000, 0.5027777777777777679, 0.5055555555555555358, 0.5083333333333333037, 0.5111111111111110716, 0.5138888888888888395, 0.5166666666666667185, 0.5194444444444444864, 0.5222222222222222543, 0.5250000000000000222, 0.5277777777777777901, 0.5305555555555555580, 0.5333333333333333259, 0.5361111111111110938, 0.5388888888888888618, 0.5416666666666666297, 0.5444444444444443976, 0.5472222222222222765, 0.5500000000000000444, 0.5527777777777778123, 0.5555555555555555802, 0.5583333333333333481, 0.5611111111111111160, 0.5638888888888888840, 0.5666666666666666519, 0.5694444444444444198, 0.5722222222222221877, 0.5749999999999999556, 0.5777777777777777235, 0.5805555555555556024, 0.5833333333333333703, 0.5861111111111111382, 0.5888888888888889062, 0.5916666666666666741, 0.5944444444444444420, 0.5972222222222222099, 0.5999999999999999778, 0.6027777777777777457, 0.6055555555555555136, 0.6083333333333332815, 0.6111111111111111605, 0.6138888888888889284, 0.6166666666666666963, 0.6194444444444444642, 0.6222222222222222321, 0.6250000000000000000, 0.6277777777777777679, 0.6305555555555555358, 0.6333333333333333037, 0.6361111111111110716, 0.6388888888888888395, 0.6416666666666667185, 0.6444444444444444864, 0.6472222222222222543, 0.6500000000000000222, 0.6527777777777777901, 0.6555555555555555580, 0.6583333333333333259, 0.6611111111111110938, 0.6638888888888888618, 0.6666666666666666297, 0.6694444444444443976, 0.6722222222222222765, 0.6750000000000000444, 0.6777777777777778123, 0.6805555555555555802, 0.6833333333333333481, 0.6861111111111111160, 0.6888888888888888840, 0.6916666666666666519, 0.6944444444444444198, 0.6972222222222221877, 0.6999999999999999556, 0.7027777777777777235, 0.7055555555555556024, 0.7083333333333333703, 0.7111111111111111382, 0.7138888888888889062, 0.7166666666666666741, 0.7194444444444444420, 0.7222222222222222099, 0.7249999999999999778, 0.7277777777777777457, 0.7305555555555555136, 0.7333333333333332815, 0.7361111111111111605, 0.7388888888888889284, 0.7416666666666666963, 0.7444444444444444642, 0.7472222222222222321, 0.7500000000000000000, 0.7527777777777777679, 0.7555555555555555358, 0.7583333333333333037, 0.7611111111111110716, 0.7638888888888888395, 0.7666666666666667185, 0.7694444444444444864, 0.7722222222222222543, 0.7750000000000000222, 0.7777777777777777901, 0.7805555555555555580, 0.7833333333333333259, 0.7861111111111110938, 0.7888888888888888618, 0.7916666666666666297, 0.7944444444444443976, 0.7972222222222222765, 0.8000000000000000444, 0.8027777777777778123, 0.8055555555555555802, 0.8083333333333333481, 0.8111111111111111160, 0.8138888888888888840, 0.8166666666666666519, 0.8194444444444444198, 0.8222222222222221877, 0.8249999999999999556, 0.8277777777777777235, 0.8305555555555556024, 0.8333333333333333703, 0.8361111111111111382, 0.8388888888888889062, 0.8416666666666666741, 0.8444444444444444420, 0.8472222222222222099, 0.8499999999999999778, 0.8527777777777777457, 0.8555555555555555136, 0.8583333333333332815, 0.8611111111111111605, 0.8638888888888889284, 0.8666666666666666963, 0.8694444444444444642, 0.8722222222222222321, 0.8750000000000000000, 0.8777777777777777679, 0.8805555555555555358, 0.8833333333333333037, 0.8861111111111110716, 0.8888888888888888395, 0.8916666666666667185, 0.8944444444444444864, 0.8972222222222222543, 0.9000000000000000222, 0.9027777777777777901, 0.9055555555555555580, 0.9083333333333333259, 0.9111111111111110938, 0.9138888888888888618, 0.9166666666666666297, 0.9194444444444443976, 0.9222222222222222765, 0.9250000000000000444, 0.9277777777777778123, 0.9305555555555555802, 0.9333333333333333481, 0.9361111111111111160, 0.9388888888888888840, 0.9416666666666666519, 0.9444444444444444198, 0.9472222222222221877, 0.9499999999999999556, 0.9527777777777777235, 0.9555555555555556024, 0.9583333333333333703, 0.9611111111111111382, 0.9638888888888889062, 0.9666666666666666741, 0.9694444444444444420, 0.9722222222222222099, 0.9749999999999999778, 0.9777777777777777457, 0.9805555555555555136, 0.9833333333333332815, 0.9861111111111111605, 0.9888888888888889284, 0.9916666666666666963, 0.9944444444444444642, 0.9972222222222222321, 1.000000000000000000 ),
 .UNSPECIFIED. ) 
 GEOMETRIC_REPRESENTATION_ITEM ( )  RATIONAL_B_SPLINE_SURFACE ( (
 ( 1.000000000000000000, 0.8660254037844387076, 1.000000000000000000, 0.8660254037844387076, 1.000000000000000000, 0.8660254037844387076, 1.000000000000000000, 0.8660254037844387076, 1.000000000000000000, 0.8660254037844387076, 1.000000000000000000, 0.8660254037844387076, 1.000000000000000000, 0.8660254037844387076, 1.000000000000000000, 0.8660254037844387076, 1.000000000000000000, 0.8660254037844387076, 1.000000000000000000, 0.8660254037844387076, 1.000000000000000000, 0.8660254037844387076, 1.000000000000000000, 0.8660254037844387076, 1.000000000000000000, 0.8660254037844387076, 1.000000000000000000, 0.8660254037844387076, 1.000000000000000000, 0.8660254037844387076, 1.000000000000000000, 0.8660254037844387076, 1.000000000000000000, 0.8660254037844387076, 1.000000000000000000, 0.8660254037844387076, 1.000000000000000000, 0.8660254037844387076, 1.000000000000000000, 0.8660254037844387076, 1.000000000000000000, 0.8660254037844387076, 1.000000000000000000, 0.8660254037844387076, 1.000000000000000000, 0.8660254037844387076, 1.000000000000000000, 0.8660254037844387076, 1.000000000000000000, 0.8660254037844387076, 1.000000000000000000, 0.8660254037844387076, 1.000000000000000000, 0.8660254037844387076, 1.000000000000000000, 0.8660254037844387076, 1.000000000000000000, 0.8660254037844387076, 1.000000000000000000, 0.8660254037844387076, 1.000000000000000000, 0.8660254037844387076, 1.000000000000000000, 0.8660254037844387076, 1.000000000000000000, 0.8660254037844387076, 1.000000000000000000, 0.8660254037844387076, 1.000000000000000000, 0.8660254037844387076, 1.000000000000000000, 0.8660254037844387076, 1.000000000000000000, 0.8660254037844387076, 1.000000000000000000, 0.8660254037844387076, 1.000000000000000000, 0.8660254037844387076, 1.000000000000000000, 0.8660254037844387076, 1.000000000000000000, 0.8660254037844387076, 1.000000000000000000, 0.8660254037844387076, 1.000000000000000000, 0.8660254037844387076, 1.000000000000000000, 0.8660254037844387076, 1.000000000000000000, 0.8660254037844387076, 1.000000000000000000, 0.8660254037844387076, 1.000000000000000000, 0.8660254037844387076, 1.000000000000000000, 0.8660254037844387076, 1.000000000000000000, 0.8660254037844387076, 1.000000000000000000, 0.8660254037844387076, 1.000000000000000000, 0.8660254037844387076, 1.000000000000000000, 0.8660254037844387076, 1.000000000000000000, 0.8660254037844387076, 1.000000000000000000, 0.8660254037844387076, 1.000000000000000000, 0.8660254037844387076, 1.000000000000000000, 0.8660254037844387076, 1.000000000000000000, 0.8660254037844387076, 1.000000000000000000, 0.8660254037844387076, 1.000000000000000000, 0.8660254037844387076, 1.000000000000000000, 0.8660254037844387076, 1.000000000000000000, 0.8660254037844387076, 1.000000000000000000, 0.8660254037844387076, 1.000000000000000000, 0.8660254037844387076, 1.000000000000000000, 0.8660254037844387076, 1.000000000000000000, 0.8660254037844387076, 1.000000000000000000, 0.8660254037844387076, 1.000000000000000000, 0.8660254037844387076, 1.000000000000000000, 0.8660254037844387076, 1.000000000000000000, 0.8660254037844387076, 1.000000000000000000, 0.8660254037844387076, 1.000000000000000000, 0.8660254037844387076, 1.000000000000000000, 0.8660254037844387076, 1.000000000000000000, 0.8660254037844387076, 1.000000000000000000, 0.8660254037844387076, 1.000000000000000000, 0.8660254037844387076, 1.000000000000000000, 0.8660254037844387076, 1.000000000000000000, 0.8660254037844387076, 1.000000000000000000, 0.8660254037844387076, 1.000000000000000000, 0.8660254037844387076, 1.000000000000000000, 0.8660254037844387076, 1.000000000000000000, 0.8660254037844387076, 1.000000000000000000, 0.8660254037844387076, 1.000000000000000000, 0.8660254037844387076, 1.000000000000000000, 0.8660254037844387076, 1.000000000000000000, 0.8660254037844387076, 1.000000000000000000, 0.8660254037844387076, 1.000000000000000000, 0.8660254037844387076, 1.000000000000000000, 0.8660254037844387076, 1.000000000000000000, 0.8660254037844387076, 1.000000000000000000, 0.8660254037844387076, 1.000000000000000000, 0.8660254037844387076, 1.000000000000000000, 0.8660254037844387076, 1.000000000000000000, 0.8660254037844387076, 1.000000000000000000, 0.8660254037844387076, 1.000000000000000000, 0.8660254037844387076, 1.000000000000000000, 0.8660254037844387076, 1.000000000000000000, 0.8660254037844387076, 1.000000000000000000, 0.8660254037844387076, 1.000000000000000000, 0.8660254037844387076, 1.000000000000000000, 0.8660254037844387076, 1.000000000000000000, 0.8660254037844387076, 1.000000000000000000, 0.8660254037844387076, 1.000000000000000000, 0.8660254037844387076, 1.000000000000000000, 0.8660254037844387076, 1.000000000000000000, 0.8660254037844387076, 1.000000000000000000, 0.8660254037844387076, 1.000000000000000000, 0.8660254037844387076, 1.000000000000000000, 0.8660254037844387076, 1.000000000000000000, 0.8660254037844387076, 1.000000000000000000, 0.8660254037844387076, 1.000000000000000000, 0.8660254037844387076, 1.000000000000000000, 0.8660254037844387076, 1.000000000000000000, 0.8660254037844387076, 1.000000000000000000, 0.8660254037844387076, 1.000000000000000000, 0.8660254037844387076, 1.000000000000000000, 0.8660254037844387076, 1.000000000000000000, 0.8660254037844387076, 1.000000000000000000, 0.8660254037844387076, 1.000000000000000000, 0.8660254037844387076, 1.000000000000000000, 0.8660254037844387076, 1.000000000000000000, 0.8660254037844387076, 1.000000000000000000, 0.8660254037844387076, 1.000000000000000000, 0.8660254037844387076, 1.000000000000000000, 0.8660254037844387076, 1.000000000000000000, 0.8660254037844387076, 1.000000000000000000, 0.8660254037844387076, 1.000000000000000000, 0.8660254037844387076, 1.000000000000000000, 0.8660254037844387076, 1.000000000000000000, 0.8660254037844387076, 1.000000000000000000, 0.8660254037844387076, 1.000000000000000000, 0.8660254037844387076, 1.000000000000000000, 0.8660254037844387076, 1.000000000000000000, 0.8660254037844387076, 1.000000000000000000, 0.8660254037844387076, 1.000000000000000000, 0.8660254037844387076, 1.000000000000000000, 0.8660254037844387076, 1.000000000000000000, 0.8660254037844387076, 1.000000000000000000, 0.8660254037844387076, 1.000000000000000000, 0.8660254037844387076, 1.000000000000000000, 0.8660254037844387076, 1.000000000000000000, 0.8660254037844387076, 1.000000000000000000, 0.8660254037844387076, 1.000000000000000000, 0.8660254037844387076, 1.000000000000000000, 0.8660254037844387076, 1.000000000000000000, 0.8660254037844387076, 1.000000000000000000, 0.8660254037844387076, 1.000000000000000000, 0.8660254037844387076, 1.000000000000000000, 0.8660254037844387076, 1.000000000000000000, 0.8660254037844387076, 1.000000000000000000, 0.8660254037844387076, 1.000000000000000000, 0.8660254037844387076, 1.000000000000000000, 0.8660254037844387076, 1.000000000000000000, 0.8660254037844387076, 1.000000000000000000, 0.8660254037844387076, 1.000000000000000000, 0.8660254037844387076, 1.000000000000000000, 0.8660254037844387076, 1.000000000000000000, 0.8660254037844387076, 1.000000000000000000, 0.8660254037844387076, 1.000000000000000000, 0.8660254037844387076, 1.000000000000000000, 0.8660254037844387076, 1.000000000000000000, 0.8660254037844387076, 1.000000000000000000, 0.8660254037844387076, 1.000000000000000000, 0.8660254037844387076, 1.000000000000000000, 0.8660254037844387076, 1.000000000000000000, 0.8660254037844387076, 1.000000000000000000, 0.8660254037844387076, 1.000000000000000000, 0.8660254037844387076, 1.000000000000000000, 0.8660254037844387076, 1.000000000000000000, 0.8660254037844387076, 1.000000000000000000, 0.8660254037844387076, 1.000000000000000000, 0.8660254037844387076, 1.000000000000000000, 0.8660254037844387076, 1.000000000000000000, 0.8660254037844387076, 1.000000000000000000, 0.8660254037844387076, 1.000000000000000000, 0.8660254037844387076, 1.000000000000000000, 0.8660254037844387076, 1.000000000000000000, 0.8660254037844387076, 1.000000000000000000, 0.8660254037844387076, 1.000000000000000000, 0.8660254037844387076, 1.000000000000000000, 0.8660254037844387076, 1.000000000000000000, 0.8660254037844387076, 1.000000000000000000, 0.8660254037844387076, 1.000000000000000000, 0.8660254037844387076, 1.000000000000000000, 0.8660254037844387076, 1.000000000000000000, 0.8660254037844387076, 1.000000000000000000, 0.8660254037844387076, 1.000000000000000000, 0.8660254037844387076, 1.000000000000000000, 0.8660254037844387076, 1.000000000000000000, 0.8660254037844387076, 1.000000000000000000, 0.8660254037844387076, 1.000000000000000000, 0.8660254037844387076, 1.000000000000000000, 0.8660254037844387076, 1.000000000000000000, 0.8660254037844387076, 1.000000000000000000, 0.8660254037844387076, 1.000000000000000000, 0.8660254037844387076, 1.000000000000000000, 0.8660254037844387076, 1.000000000000000000, 0.8660254037844387076, 1.000000000000000000, 0.8660254037844387076, 1.000000000000000000, 0.8660254037844387076, 1.000000000000000000, 0.8660254037844387076, 1.000000000000000000, 0.8660254037844387076, 1.000000000000000000, 0.8660254037844387076, 1.000000000000000000, 0.8660254037844387076, 1.000000000000000000, 0.8660254037844387076, 1.000000000000000000, 0.8660254037844387076, 1.000000000000000000, 0.8660254037844387076, 1.000000000000000000, 0.8660254037844387076, 1.000000000000000000, 0.8660254037844387076, 1.000000000000000000, 0.8660254037844387076, 1.000000000000000000, 0.8660254037844387076, 1.000000000000000000, 0.8660254037844387076, 1.000000000000000000, 0.8660254037844387076, 1.000000000000000000, 0.8660254037844387076, 1.000000000000000000, 0.8660254037844387076, 1.000000000000000000, 0.8660254037844387076, 1.000000000000000000, 0.8660254037844387076, 1.000000000000000000, 0.8660254037844387076, 1.000000000000000000, 0.8660254037844387076, 1.000000000000000000, 0.8660254037844387076, 1.000000000000000000, 0.8660254037844387076, 1.000000000000000000, 0.8660254037844387076, 1.000000000000000000, 0.8660254037844387076, 1.000000000000000000, 0.8660254037844387076, 1.000000000000000000, 0.8660254037844387076, 1.000000000000000000, 0.8660254037844387076, 1.000000000000000000, 0.8660254037844387076, 1.000000000000000000, 0.8660254037844387076, 1.000000000000000000, 0.8660254037844387076, 1.000000000000000000, 0.8660254037844387076, 1.000000000000000000, 0.8660254037844387076, 1.000000000000000000, 0.8660254037844387076, 1.000000000000000000, 0.8660254037844387076, 1.000000000000000000, 0.8660254037844387076, 1.000000000000000000, 0.8660254037844387076, 1.000000000000000000, 0.8660254037844387076, 1.000000000000000000, 0.8660254037844387076, 1.000000000000000000, 0.8660254037844387076, 1.000000000000000000, 0.8660254037844387076, 1.000000000000000000, 0.8660254037844387076, 1.000000000000000000, 0.8660254037844387076, 1.000000000000000000, 0.8660254037844387076, 1.000000000000000000, 0.8660254037844387076, 1.000000000000000000, 0.8660254037844387076, 1.000000000000000000, 0.8660254037844387076, 1.000000000000000000, 0.8660254037844387076, 1.000000000000000000, 0.8660254037844387076, 1.000000000000000000, 0.8660254037844387076, 1.000000000000000000, 0.8660254037844387076, 1.000000000000000000, 0.8660254037844387076, 1.000000000000000000, 0.8660254037844387076, 1.000000000000000000, 0.8660254037844387076, 1.000000000000000000, 0.8660254037844387076, 1.000000000000000000, 0.8660254037844387076, 1.000000000000000000, 0.8660254037844387076, 1.000000000000000000, 0.8660254037844387076, 1.000000000000000000, 0.8660254037844387076, 1.000000000000000000, 0.8660254037844387076, 1.000000000000000000, 0.8660254037844387076, 1.000000000000000000, 0.8660254037844387076, 1.000000000000000000, 0.8660254037844387076, 1.000000000000000000, 0.8660254037844387076, 1.000000000000000000, 0.8660254037844387076, 1.000000000000000000, 0.8660254037844387076, 1.000000000000000000, 0.8660254037844387076, 1.000000000000000000, 0.8660254037844387076, 1.000000000000000000, 0.8660254037844387076, 1.000000000000000000, 0.8660254037844387076, 1.000000000000000000, 0.8660254037844387076, 1.000000000000000000, 0.8660254037844387076, 1.000000000000000000, 0.8660254037844387076, 1.000000000000000000, 0.8660254037844387076, 1.000000000000000000, 0.8660254037844387076, 1.000000000000000000, 0.8660254037844387076, 1.000000000000000000, 0.8660254037844387076, 1.000000000000000000, 0.8660254037844387076, 1.000000000000000000, 0.8660254037844387076, 1.000000000000000000, 0.8660254037844387076, 1.000000000000000000, 0.8660254037844387076, 1.000000000000000000, 0.8660254037844387076, 1.000000000000000000, 0.8660254037844387076, 1.000000000000000000, 0.8660254037844387076, 1.000000000000000000, 0.8660254037844387076, 1.000000000000000000, 0.8660254037844387076, 1.000000000000000000, 0.8660254037844387076, 1.000000000000000000, 0.8660254037844387076, 1.000000000000000000, 0.8660254037844387076, 1.000000000000000000, 0.8660254037844387076, 1.000000000000000000, 0.8660254037844387076, 1.000000000000000000, 0.8660254037844387076, 1.000000000000000000, 0.8660254037844387076, 1.000000000000000000, 0.8660254037844387076, 1.000000000000000000, 0.8660254037844387076, 1.000000000000000000, 0.8660254037844387076, 1.000000000000000000, 0.8660254037844387076, 1.000000000000000000, 0.8660254037844387076, 1.000000000000000000, 0.8660254037844387076, 1.000000000000000000, 0.8660254037844387076, 1.000000000000000000, 0.8660254037844387076, 1.000000000000000000, 0.8660254037844387076, 1.000000000000000000, 0.8660254037844387076, 1.000000000000000000, 0.8660254037844387076, 1.000000000000000000, 0.8660254037844387076, 1.000000000000000000, 0.8660254037844387076, 1.000000000000000000, 0.8660254037844387076, 1.000000000000000000, 0.8660254037844387076, 1.000000000000000000, 0.8660254037844387076, 1.000000000000000000, 0.8660254037844387076, 1.000000000000000000, 0.8660254037844387076, 1.000000000000000000, 0.8660254037844387076, 1.000000000000000000, 0.8660254037844387076, 1.000000000000000000, 0.8660254037844387076, 1.000000000000000000, 0.8660254037844387076, 1.000000000000000000, 0.8660254037844387076, 1.000000000000000000, 0.8660254037844387076, 1.000000000000000000, 0.8660254037844387076, 1.000000000000000000, 0.8660254037844387076, 1.000000000000000000, 0.8660254037844387076, 1.000000000000000000, 0.8660254037844387076, 1.000000000000000000, 0.8660254037844387076, 1.000000000000000000, 0.8660254037844387076, 1.000000000000000000, 0.8660254037844387076, 1.000000000000000000, 0.8660254037844387076, 1.000000000000000000, 0.8660254037844387076, 1.000000000000000000, 0.8660254037844387076, 1.000000000000000000, 0.8660254037844387076, 1.000000000000000000, 0.8660254037844387076, 1.000000000000000000, 0.8660254037844387076, 1.000000000000000000, 0.8660254037844387076, 1.000000000000000000, 0.8660254037844387076, 1.000000000000000000, 0.8660254037844387076, 1.000000000000000000, 0.8660254037844387076, 1.000000000000000000, 0.8660254037844387076, 1.000000000000000000, 0.8660254037844387076, 1.000000000000000000, 0.8660254037844387076, 1.000000000000000000, 0.8660254037844387076, 1.000000000000000000, 0.8660254037844387076, 1.000000000000000000, 0.8660254037844387076, 1.000000000000000000, 0.8660254037844387076, 1.000000000000000000, 0.8660254037844387076, 1.000000000000000000, 0.8660254037844387076, 1.000000000000000000, 0.8660254037844387076, 1.000000000000000000, 0.8660254037844387076, 1.000000000000000000, 0.8660254037844387076, 1.000000000000000000, 0.8660254037844387076, 1.000000000000000000, 0.8660254037844387076, 1.000000000000000000, 0.8660254037844387076, 1.000000000000000000, 0.8660254037844387076, 1.000000000000000000, 0.8660254037844387076, 1.000000000000000000, 0.8660254037844387076, 1.000000000000000000, 0.8660254037844387076, 1.000000000000000000, 0.8660254037844387076, 1.000000000000000000, 0.8660254037844387076, 1.000000000000000000, 0.8660254037844387076, 1.000000000000000000, 0.8660254037844387076, 1.000000000000000000, 0.8660254037844387076, 1.000000000000000000, 0.8660254037844387076, 1.000000000000000000, 0.8660254037844387076, 1.000000000000000000, 0.8660254037844387076, 1.000000000000000000, 0.8660254037844387076, 1.000000000000000000, 0.8660254037844387076, 1.000000000000000000),
 ( 1.000000000000000000, 0.8660254037844387076, 1.000000000000000000, 0.8660254037844387076, 1.000000000000000000, 0.8660254037844387076, 1.000000000000000000, 0.8660254037844387076, 1.000000000000000000, 0.8660254037844387076, 1.000000000000000000, 0.8660254037844387076, 1.000000000000000000, 0.8660254037844387076, 1.000000000000000000, 0.8660254037844387076, 1.000000000000000000, 0.8660254037844387076, 1.000000000000000000, 0.8660254037844387076, 1.000000000000000000, 0.8660254037844387076, 1.000000000000000000, 0.8660254037844387076, 1.000000000000000000, 0.8660254037844387076, 1.000000000000000000, 0.8660254037844387076, 1.000000000000000000, 0.8660254037844387076, 1.000000000000000000, 0.8660254037844387076, 1.000000000000000000, 0.8660254037844387076, 1.000000000000000000, 0.8660254037844387076, 1.000000000000000000, 0.8660254037844387076, 1.000000000000000000, 0.8660254037844387076, 1.000000000000000000, 0.8660254037844387076, 1.000000000000000000, 0.8660254037844387076, 1.000000000000000000, 0.8660254037844387076, 1.000000000000000000, 0.8660254037844387076, 1.000000000000000000, 0.8660254037844387076, 1.000000000000000000, 0.8660254037844387076, 1.000000000000000000, 0.8660254037844387076, 1.000000000000000000, 0.8660254037844387076, 1.000000000000000000, 0.8660254037844387076, 1.000000000000000000, 0.8660254037844387076, 1.000000000000000000, 0.8660254037844387076, 1.000000000000000000, 0.8660254037844387076, 1.000000000000000000, 0.8660254037844387076, 1.000000000000000000, 0.8660254037844387076, 1.000000000000000000, 0.8660254037844387076, 1.000000000000000000, 0.8660254037844387076, 1.000000000000000000, 0.8660254037844387076, 1.000000000000000000, 0.8660254037844387076, 1.000000000000000000, 0.8660254037844387076, 1.000000000000000000, 0.8660254037844387076, 1.000000000000000000, 0.8660254037844387076, 1.000000000000000000, 0.8660254037844387076, 1.000000000000000000, 0.8660254037844387076, 1.000000000000000000, 0.8660254037844387076, 1.000000000000000000, 0.8660254037844387076, 1.000000000000000000, 0.8660254037844387076, 1.000000000000000000, 0.8660254037844387076, 1.000000000000000000, 0.8660254037844387076, 1.000000000000000000, 0.8660254037844387076, 1.000000000000000000, 0.8660254037844387076, 1.000000000000000000, 0.8660254037844387076, 1.000000000000000000, 0.8660254037844387076, 1.000000000000000000, 0.8660254037844387076, 1.000000000000000000, 0.8660254037844387076, 1.000000000000000000, 0.8660254037844387076, 1.000000000000000000, 0.8660254037844387076, 1.000000000000000000, 0.8660254037844387076, 1.000000000000000000, 0.8660254037844387076, 1.000000000000000000, 0.8660254037844387076, 1.000000000000000000, 0.8660254037844387076, 1.000000000000000000, 0.8660254037844387076, 1.000000000000000000, 0.8660254037844387076, 1.000000000000000000, 0.8660254037844387076, 1.000000000000000000, 0.8660254037844387076, 1.000000000000000000, 0.8660254037844387076, 1.000000000000000000, 0.8660254037844387076, 1.000000000000000000, 0.8660254037844387076, 1.000000000000000000, 0.8660254037844387076, 1.000000000000000000, 0.8660254037844387076, 1.000000000000000000, 0.8660254037844387076, 1.000000000000000000, 0.8660254037844387076, 1.000000000000000000, 0.8660254037844387076, 1.000000000000000000, 0.8660254037844387076, 1.000000000000000000, 0.8660254037844387076, 1.000000000000000000, 0.8660254037844387076, 1.000000000000000000, 0.8660254037844387076, 1.000000000000000000, 0.8660254037844387076, 1.000000000000000000, 0.8660254037844387076, 1.000000000000000000, 0.8660254037844387076, 1.000000000000000000, 0.8660254037844387076, 1.000000000000000000, 0.8660254037844387076, 1.000000000000000000, 0.8660254037844387076, 1.000000000000000000, 0.8660254037844387076, 1.000000000000000000, 0.8660254037844387076, 1.000000000000000000, 0.8660254037844387076, 1.000000000000000000, 0.8660254037844387076, 1.000000000000000000, 0.8660254037844387076, 1.000000000000000000, 0.8660254037844387076, 1.000000000000000000, 0.8660254037844387076, 1.000000000000000000, 0.8660254037844387076, 1.000000000000000000, 0.8660254037844387076, 1.000000000000000000, 0.8660254037844387076, 1.000000000000000000, 0.8660254037844387076, 1.000000000000000000, 0.8660254037844387076, 1.000000000000000000, 0.8660254037844387076, 1.000000000000000000, 0.8660254037844387076, 1.000000000000000000, 0.8660254037844387076, 1.000000000000000000, 0.8660254037844387076, 1.000000000000000000, 0.8660254037844387076, 1.000000000000000000, 0.8660254037844387076, 1.000000000000000000, 0.8660254037844387076, 1.000000000000000000, 0.8660254037844387076, 1.000000000000000000, 0.8660254037844387076, 1.000000000000000000, 0.8660254037844387076, 1.000000000000000000, 0.8660254037844387076, 1.000000000000000000, 0.8660254037844387076, 1.000000000000000000, 0.8660254037844387076, 1.000000000000000000, 0.8660254037844387076, 1.000000000000000000, 0.8660254037844387076, 1.000000000000000000, 0.8660254037844387076, 1.000000000000000000, 0.8660254037844387076, 1.000000000000000000, 0.8660254037844387076, 1.000000000000000000, 0.8660254037844387076, 1.000000000000000000, 0.8660254037844387076, 1.000000000000000000, 0.8660254037844387076, 1.000000000000000000, 0.8660254037844387076, 1.000000000000000000, 0.8660254037844387076, 1.000000000000000000, 0.8660254037844387076, 1.000000000000000000, 0.8660254037844387076, 1.000000000000000000, 0.8660254037844387076, 1.000000000000000000, 0.8660254037844387076, 1.000000000000000000, 0.8660254037844387076, 1.000000000000000000, 0.8660254037844387076, 1.000000000000000000, 0.8660254037844387076, 1.000000000000000000, 0.8660254037844387076, 1.000000000000000000, 0.8660254037844387076, 1.000000000000000000, 0.8660254037844387076, 1.000000000000000000, 0.8660254037844387076, 1.000000000000000000, 0.8660254037844387076, 1.000000000000000000, 0.8660254037844387076, 1.000000000000000000, 0.8660254037844387076, 1.000000000000000000, 0.8660254037844387076, 1.000000000000000000, 0.8660254037844387076, 1.000000000000000000, 0.8660254037844387076, 1.000000000000000000, 0.8660254037844387076, 1.000000000000000000, 0.8660254037844387076, 1.000000000000000000, 0.8660254037844387076, 1.000000000000000000, 0.8660254037844387076, 1.000000000000000000, 0.8660254037844387076, 1.000000000000000000, 0.8660254037844387076, 1.000000000000000000, 0.8660254037844387076, 1.000000000000000000, 0.8660254037844387076, 1.000000000000000000, 0.8660254037844387076, 1.000000000000000000, 0.8660254037844387076, 1.000000000000000000, 0.8660254037844387076, 1.000000000000000000, 0.8660254037844387076, 1.000000000000000000, 0.8660254037844387076, 1.000000000000000000, 0.8660254037844387076, 1.000000000000000000, 0.8660254037844387076, 1.000000000000000000, 0.8660254037844387076, 1.000000000000000000, 0.8660254037844387076, 1.000000000000000000, 0.8660254037844387076, 1.000000000000000000, 0.8660254037844387076, 1.000000000000000000, 0.8660254037844387076, 1.000000000000000000, 0.8660254037844387076, 1.000000000000000000, 0.8660254037844387076, 1.000000000000000000, 0.8660254037844387076, 1.000000000000000000, 0.8660254037844387076, 1.000000000000000000, 0.8660254037844387076, 1.000000000000000000, 0.8660254037844387076, 1.000000000000000000, 0.8660254037844387076, 1.000000000000000000, 0.8660254037844387076, 1.000000000000000000, 0.8660254037844387076, 1.000000000000000000, 0.8660254037844387076, 1.000000000000000000, 0.8660254037844387076, 1.000000000000000000, 0.8660254037844387076, 1.000000000000000000, 0.8660254037844387076, 1.000000000000000000, 0.8660254037844387076, 1.000000000000000000, 0.8660254037844387076, 1.000000000000000000, 0.8660254037844387076, 1.000000000000000000, 0.8660254037844387076, 1.000000000000000000, 0.8660254037844387076, 1.000000000000000000, 0.8660254037844387076, 1.000000000000000000, 0.8660254037844387076, 1.000000000000000000, 0.8660254037844387076, 1.000000000000000000, 0.8660254037844387076, 1.000000000000000000, 0.8660254037844387076, 1.000000000000000000, 0.8660254037844387076, 1.000000000000000000, 0.8660254037844387076, 1.000000000000000000, 0.8660254037844387076, 1.000000000000000000, 0.8660254037844387076, 1.000000000000000000, 0.8660254037844387076, 1.000000000000000000, 0.8660254037844387076, 1.000000000000000000, 0.8660254037844387076, 1.000000000000000000, 0.8660254037844387076, 1.000000000000000000, 0.8660254037844387076, 1.000000000000000000, 0.8660254037844387076, 1.000000000000000000, 0.8660254037844387076, 1.000000000000000000, 0.8660254037844387076, 1.000000000000000000, 0.8660254037844387076, 1.000000000000000000, 0.8660254037844387076, 1.000000000000000000, 0.8660254037844387076, 1.000000000000000000, 0.8660254037844387076, 1.000000000000000000, 0.8660254037844387076, 1.000000000000000000, 0.8660254037844387076, 1.000000000000000000, 0.8660254037844387076, 1.000000000000000000, 0.8660254037844387076, 1.000000000000000000, 0.8660254037844387076, 1.000000000000000000, 0.8660254037844387076, 1.000000000000000000, 0.8660254037844387076, 1.000000000000000000, 0.8660254037844387076, 1.000000000000000000, 0.8660254037844387076, 1.000000000000000000, 0.8660254037844387076, 1.000000000000000000, 0.8660254037844387076, 1.000000000000000000, 0.8660254037844387076, 1.000000000000000000, 0.8660254037844387076, 1.000000000000000000, 0.8660254037844387076, 1.000000000000000000, 0.8660254037844387076, 1.000000000000000000, 0.8660254037844387076, 1.000000000000000000, 0.8660254037844387076, 1.000000000000000000, 0.8660254037844387076, 1.000000000000000000, 0.8660254037844387076, 1.000000000000000000, 0.8660254037844387076, 1.000000000000000000, 0.8660254037844387076, 1.000000000000000000, 0.8660254037844387076, 1.000000000000000000, 0.8660254037844387076, 1.000000000000000000, 0.8660254037844387076, 1.000000000000000000, 0.8660254037844387076, 1.000000000000000000, 0.8660254037844387076, 1.000000000000000000, 0.8660254037844387076, 1.000000000000000000, 0.8660254037844387076, 1.000000000000000000, 0.8660254037844387076, 1.000000000000000000, 0.8660254037844387076, 1.000000000000000000, 0.8660254037844387076, 1.000000000000000000, 0.8660254037844387076, 1.000000000000000000, 0.8660254037844387076, 1.000000000000000000, 0.8660254037844387076, 1.000000000000000000, 0.8660254037844387076, 1.000000000000000000, 0.8660254037844387076, 1.000000000000000000, 0.8660254037844387076, 1.000000000000000000, 0.8660254037844387076, 1.000000000000000000, 0.8660254037844387076, 1.000000000000000000, 0.8660254037844387076, 1.000000000000000000, 0.8660254037844387076, 1.000000000000000000, 0.8660254037844387076, 1.000000000000000000, 0.8660254037844387076, 1.000000000000000000, 0.8660254037844387076, 1.000000000000000000, 0.8660254037844387076, 1.000000000000000000, 0.8660254037844387076, 1.000000000000000000, 0.8660254037844387076, 1.000000000000000000, 0.8660254037844387076, 1.000000000000000000, 0.8660254037844387076, 1.000000000000000000, 0.8660254037844387076, 1.000000000000000000, 0.8660254037844387076, 1.000000000000000000, 0.8660254037844387076, 1.000000000000000000, 0.8660254037844387076, 1.000000000000000000, 0.8660254037844387076, 1.000000000000000000, 0.8660254037844387076, 1.000000000000000000, 0.8660254037844387076, 1.000000000000000000, 0.8660254037844387076, 1.000000000000000000, 0.8660254037844387076, 1.000000000000000000, 0.8660254037844387076, 1.000000000000000000, 0.8660254037844387076, 1.000000000000000000, 0.8660254037844387076, 1.000000000000000000, 0.8660254037844387076, 1.000000000000000000, 0.8660254037844387076, 1.000000000000000000, 0.8660254037844387076, 1.000000000000000000, 0.8660254037844387076, 1.000000000000000000, 0.8660254037844387076, 1.000000000000000000, 0.8660254037844387076, 1.000000000000000000, 0.8660254037844387076, 1.000000000000000000, 0.8660254037844387076, 1.000000000000000000, 0.8660254037844387076, 1.000000000000000000, 0.8660254037844387076, 1.000000000000000000, 0.8660254037844387076, 1.000000000000000000, 0.8660254037844387076, 1.000000000000000000, 0.8660254037844387076, 1.000000000000000000, 0.8660254037844387076, 1.000000000000000000, 0.8660254037844387076, 1.000000000000000000, 0.8660254037844387076, 1.000000000000000000, 0.8660254037844387076, 1.000000000000000000, 0.8660254037844387076, 1.000000000000000000, 0.8660254037844387076, 1.000000000000000000, 0.8660254037844387076, 1.000000000000000000, 0.8660254037844387076, 1.000000000000000000, 0.8660254037844387076, 1.000000000000000000, 0.8660254037844387076, 1.000000000000000000, 0.8660254037844387076, 1.000000000000000000, 0.8660254037844387076, 1.000000000000000000, 0.8660254037844387076, 1.000000000000000000, 0.8660254037844387076, 1.000000000000000000, 0.8660254037844387076, 1.000000000000000000, 0.8660254037844387076, 1.000000000000000000, 0.8660254037844387076, 1.000000000000000000, 0.8660254037844387076, 1.000000000000000000, 0.8660254037844387076, 1.000000000000000000, 0.8660254037844387076, 1.000000000000000000, 0.8660254037844387076, 1.000000000000000000, 0.8660254037844387076, 1.000000000000000000, 0.8660254037844387076, 1.000000000000000000, 0.8660254037844387076, 1.000000000000000000, 0.8660254037844387076, 1.000000000000000000, 0.8660254037844387076, 1.000000000000000000, 0.8660254037844387076, 1.000000000000000000, 0.8660254037844387076, 1.000000000000000000, 0.8660254037844387076, 1.000000000000000000, 0.8660254037844387076, 1.000000000000000000, 0.8660254037844387076, 1.000000000000000000, 0.8660254037844387076, 1.000000000000000000, 0.8660254037844387076, 1.000000000000000000, 0.8660254037844387076, 1.000000000000000000, 0.8660254037844387076, 1.000000000000000000, 0.8660254037844387076, 1.000000000000000000, 0.8660254037844387076, 1.000000000000000000, 0.8660254037844387076, 1.000000000000000000, 0.8660254037844387076, 1.000000000000000000, 0.8660254037844387076, 1.000000000000000000, 0.8660254037844387076, 1.000000000000000000, 0.8660254037844387076, 1.000000000000000000, 0.8660254037844387076, 1.000000000000000000, 0.8660254037844387076, 1.000000000000000000, 0.8660254037844387076, 1.000000000000000000, 0.8660254037844387076, 1.000000000000000000, 0.8660254037844387076, 1.000000000000000000, 0.8660254037844387076, 1.000000000000000000, 0.8660254037844387076, 1.000000000000000000, 0.8660254037844387076, 1.000000000000000000, 0.8660254037844387076, 1.000000000000000000, 0.8660254037844387076, 1.000000000000000000, 0.8660254037844387076, 1.000000000000000000, 0.8660254037844387076, 1.000000000000000000, 0.8660254037844387076, 1.000000000000000000, 0.8660254037844387076, 1.000000000000000000, 0.8660254037844387076, 1.000000000000000000, 0.8660254037844387076, 1.000000000000000000, 0.8660254037844387076, 1.000000000000000000, 0.8660254037844387076, 1.000000000000000000, 0.8660254037844387076, 1.000000000000000000, 0.8660254037844387076, 1.000000000000000000, 0.8660254037844387076, 1.000000000000000000, 0.8660254037844387076, 1.000000000000000000, 0.8660254037844387076, 1.000000000000000000, 0.8660254037844387076, 1.000000000000000000, 0.8660254037844387076, 1.000000000000000000, 0.8660254037844387076, 1.000000000000000000, 0.8660254037844387076, 1.000000000000000000, 0.8660254037844387076, 1.000000000000000000, 0.8660254037844387076, 1.000000000000000000, 0.8660254037844387076, 1.000000000000000000, 0.8660254037844387076, 1.000000000000000000, 0.8660254037844387076, 1.000000000000000000, 0.8660254037844387076, 1.000000000000000000, 0.8660254037844387076, 1.000000000000000000, 0.8660254037844387076, 1.000000000000000000, 0.8660254037844387076, 1.000000000000000000, 0.8660254037844387076, 1.000000000000000000, 0.8660254037844387076, 1.000000000000000000, 0.8660254037844387076, 1.000000000000000000, 0.8660254037844387076, 1.000000000000000000, 0.8660254037844387076, 1.000000000000000000, 0.8660254037844387076, 1.000000000000000000, 0.8660254037844387076, 1.000000000000000000, 0.8660254037844387076, 1.000000000000000000, 0.8660254037844387076, 1.000000000000000000, 0.8660254037844387076, 1.000000000000000000, 0.8660254037844387076, 1.000000000000000000, 0.8660254037844387076, 1.000000000000000000, 0.8660254037844387076, 1.000000000000000000, 0.8660254037844387076, 1.000000000000000000, 0.8660254037844387076, 1.000000000000000000) ) ) 
 REPRESENTATION_ITEM ( '' )  SURFACE ( )  );
#63765=CARTESIAN_POINT ( 'NONE',  ( 15.18750000122903465, 4.330127018922191873, 2.499999999999999556 ) ) ;
#63766=CARTESIAN_POINT ( 'NONE',  ( 18.30000000000000071, 0.000000000000000000, 4.999999999999998224 ) ) ;
#63767=CARTESIAN_POINT ( 'NONE',  ( 28.12499999999999645, 4.330127018922191873, 2.499999999999999556 ) ) ;
#63768=CARTESIAN_POINT ( 'NONE',  ( 4.021875000614516082, 3.027376345333613106, -5.243569643749998122 ) ) ;
#63769=CARTESIAN_POINT ( 'NONE',  ( 8.896875000614517859, -3.027376345333610441, -5.243569643749999898 ) ) ;
#63770=CARTESIAN_POINT ( 'NONE',  ( 19.05937500061451928, 0.000000000000000000, 5.243569643749999010 ) ) ;
#63771=DIRECTION ( 'NONE',  ( 0.000000000000000000, 0.000000000000000000, 1.000000000000000000 ) ) ;
#63772=ORIENTED_EDGE ( 'NONE', *, *, #2473, .F. ) ;
#63773=CARTESIAN_POINT ( 'NONE',  ( 28.86562500061451786, 3.027376345333611329, 5.243569643749999010 ) ) ;
#63774=CARTESIAN_POINT ( 'NONE',  ( 3.412500000000002309, 2.886751345948126879, 4.999999999999999112 ) ) ;
#63775=CARTESIAN_POINT ( 'NONE',  ( 4.809375000614516615, -4.541064518000417216, -2.621784821875001281 ) ) ;
#63776=CARTESIAN_POINT ( 'NONE',  ( 16.12500000000000000, -4.330127018922194537, 2.499999999999995559 ) ) ;
#63777=CARTESIAN_POINT ( 'NONE',  ( 14.42812500061451786, 4.541064518000418104, 2.621784821874999949 ) ) ;
#63780=CARTESIAN_POINT ( 'NONE',  ( 17.55000000122903359, -2.886751345948129988, 4.999999999999997335 ) ) ;
#63781=CARTESIAN_POINT ( 'NONE',  ( 4.898587196589411843E-16, 20.00000000000000000, -26.00000000000000000 ) ) ;
#63783=CARTESIAN_POINT ( 'NONE',  ( 6.590625000614518392, -3.027376345333610441, -5.243569643749999898 ) ) ;
#63784=CARTESIAN_POINT ( 'NONE',  ( 24.90937500061451715, 0.000000000000000000, 5.243569643749999010 ) ) ;
#63785=CARTESIAN_POINT ( 'NONE',  ( 4.243569643749999898, 18.73437500061451644, 30.00000000000000000 ) ) ;
#63786=CARTESIAN_POINT ( 'NONE',  ( 27.60937500061451644, 0.000000000000000000, 5.243569643749999010 ) ) ;
#63787=CARTESIAN_POINT ( 'NONE',  ( 8.287499999999999645, 5.773502691896255534, 3.535250795749688894E-16 ) ) ;
#63788=CARTESIAN_POINT ( 'NONE',  ( 4.000000000000000000, 12.65000000122903501, 32.30940107675849049 ) ) ;
#63789=CARTESIAN_POINT ( 'NONE',  ( 14.76562500061451821, 3.027376345333613106, -5.243569643749998122 ) ) ;
#63790=CARTESIAN_POINT ( 'NONE',  ( 5.925000001229033586, -5.773502691896255534, -1.060575238724906372E-15 ) ) ;
#63791=CARTESIAN_POINT ( 'NONE',  ( 16.77187500061451786, 3.027376345333611329, 5.243569643749999010 ) ) ;
#63792=CARTESIAN_POINT ( 'NONE',  ( 12.00937500061451857, -4.541064518000417216, -2.621784821875001281 ) ) ;
#63794=ORIENTED_EDGE ( 'NONE', *, *, #55505, .F. ) ;
#63795=CARTESIAN_POINT ( 'NONE',  ( 11.42812500061451608, -4.541064518000419881, 2.621784821874995952 ) ) ;
#63797=CARTESIAN_POINT ( 'NONE',  ( 23.10000000122903074, -2.886751345948125991, -5.000000000000000000 ) ) ;
#63798=CARTESIAN_POINT ( 'NONE',  ( 12.23437500061451821, 4.541064518000418104, 2.621784821874999949 ) ) ;
#63799=CARTESIAN_POINT ( 'NONE',  ( 15.02812500061451750, -4.541064518000419881, 2.621784821874995952 ) ) ;
#63801=CARTESIAN_POINT ( 'NONE',  ( 23.40937500061451715, 4.541064518000418104, -2.621784821874998173 ) ) ;
#63802=DIRECTION ( 'NONE',  ( 0.000000000000000000, 0.000000000000000000, -1.000000000000000000 ) ) ;
#63804=CARTESIAN_POINT ( 'NONE',  ( -2.121784821874999949, 17.53437500061451715, -33.67503911421598417 ) ) ;
#63805=CARTESIAN_POINT ( 'NONE',  ( 14.70937500061451786, -4.541064518000417216, -2.621784821875001281 ) ) ;
#63806=CARTESIAN_POINT ( 'NONE',  ( 17.92500000122903359, 2.886751345948126879, 4.999999999999999112 ) ) ;
#63807=CARTESIAN_POINT ( 'NONE',  ( 12.42187500061451821, -6.054752690667223547, -1.112240025338166033E-15 ) ) ;
#63808=CARTESIAN_POINT ( 'NONE',  ( 9.001249775931846008E-16, 10.07187500061451857, 34.90005215228797653 ) ) ;
#63809=CARTESIAN_POINT ( 'NONE',  ( 18.90000000122902790, -2.886751345948129988, 4.999999999999997335 ) ) ;
#63810=CARTESIAN_POINT ( 'NONE',  ( 12.06562500061451537, 3.027376345333613106, -5.243569643749998122 ) ) ;
#63813=CARTESIAN_POINT ( 'NONE',  ( 18.71249999999999858, 2.886751345948126879, 4.999999999999999112 ) ) ;
#63814=CARTESIAN_POINT ( 'NONE',  ( -4.243569643749999898, 19.80312500061451786, 30.00000000000000000 ) ) ;
#63815=CARTESIAN_POINT ( 'NONE',  ( 12.08437500061451608, 6.421520780324663323E-16, -5.243569643749999010 ) ) ;
#63816=CARTESIAN_POINT ( 'NONE',  ( 4.077828214794575246, 2.893468368387148271, 4.305173067005224397 ) ) ;
#63817=CARTESIAN_POINT ( 'NONE',  ( 11.77500000122903501, -5.773502691896255534, -1.060575238724906372E-15 ) ) ;
#63818=CARTESIAN_POINT ( 'NONE',  ( 20.85000000122903430, -2.886751345948125991, -5.000000000000000000 ) ) ;
#63819=CARTESIAN_POINT ( 'NONE',  ( 17.05312500061451786, 4.541064518000418104, -2.621784821874998173 ) ) ;
#63820=CARTESIAN_POINT ( 'NONE',  ( 22.19062500061451715, -3.027376345333614438, 5.243569643749998122 ) ) ;
#63821=CARTESIAN_POINT ( 'NONE',  ( 29.21250000122903145, 0.000000000000000000, 4.999999999999998224 ) ) ;
#63822=CARTESIAN_POINT ( 'NONE',  ( 27.22499999999999787, 4.330127018922191873, 2.499999999999999556 ) ) ;
#63823=CARTESIAN_POINT ( 'NONE',  ( 4.615116929606795537, 1.923719243043608307, 4.877942894581709155 ) ) ;
#63826=CARTESIAN_POINT ( 'NONE',  ( 4.000000000000000000, 9.950000001229035718, -27.69059892324149530 ) ) ;
#63827=CARTESIAN_POINT ( 'NONE',  ( -4.243569643749999898, 15.32187500061451679, -32.45002607614398471 ) ) ;
#63828=CARTESIAN_POINT ( 'NONE',  ( 4.912500001229034297, 0.000000000000000000, 4.999999999999998224 ) ) ;
#63829=CARTESIAN_POINT ( 'NONE',  ( 6.675000000000000711, -4.330127018922194537, 2.499999999999995559 ) ) ;
#63831=CARTESIAN_POINT ( 'NONE',  ( 3.609375000614516882, 4.541064518000418104, -2.621784821874998173 ) ) ;
#63832=CARTESIAN_POINT ( 'NONE',  ( 10.28437500061451715, 6.421520780324663323E-16, -5.243569643749999010 ) ) ;
#63833=CARTESIAN_POINT ( 'NONE',  ( 29.57812500061451644, 6.421520780324663323E-16, -5.243569643749999010 ) ) ;
#63834=CARTESIAN_POINT ( 'NONE',  ( 1.071796769724489895, 10.86740381056766758, 26.00000000000000355 ) ) ;
#63835=CARTESIAN_POINT ( 'NONE',  ( -5.948681673321859265, 8.038272906428572284, -30.80841975699791746 ) ) ;
#63836=CARTESIAN_POINT ( 'NONE',  ( 29.83125000061451715, 0.000000000000000000, 4.999999999999998224 ) ) ;
#63837=CARTESIAN_POINT ( 'NONE',  ( 7.509375000614517681, -4.541064518000417216, -2.621784821875001281 ) ) ;
#63838=CARTESIAN_POINT ( 'NONE',  ( 12.00937500061451857, -4.541064518000417216, -2.621784821875001281 ) ) ;
#63839=CARTESIAN_POINT ( 'NONE',  ( 5.437500000000001776, -2.886751345948125991, -5.000000000000000000 ) ) ;
#63840=CARTESIAN_POINT ( 'NONE',  ( -2.121784821874996840, 14.92812500061459424, 33.67503911421598417 ) ) ;
#63841=MECHANICAL_DESIGN_GEOMETRIC_PRESENTATION_REPRESENTATION('',(#33226),#59152);
#63843=CARTESIAN_POINT ( 'NONE',  ( 6.487499999999999822, 5.773502691896255534, 3.535250795749688894E-16 ) ) ;
#63845=CARTESIAN_POINT ( 'NONE',  ( 19.49062500061451431, -3.027376345333614438, 5.243569643749998122 ) ) ;
#63846=CARTESIAN_POINT ( 'NONE',  ( 12.66562500061451502, 3.027376345333611329, 5.243569643749999010 ) ) ;
#63848=CARTESIAN_POINT ( 'NONE',  ( 8.334375000614516082, -4.541064518000419881, 2.621784821874995952 ) ) ;
#63849=CARTESIAN_POINT ( 'NONE',  ( 26.28749999999999432, 5.773502691896255534, 3.535250795749688894E-16 ) ) ;
#63850=CARTESIAN_POINT ( 'NONE',  ( 23.62500000122902932, 2.886751345948129099, -4.999999999999998224 ) ) ;
#63852=CARTESIAN_POINT ( 'NONE',  ( 12.34687500061452070, -3.027376345333614438, 5.243569643749998122 ) ) ;
#63853=CARTESIAN_POINT ( 'NONE',  ( 25.69687500061451502, 6.054752690667223547, 3.707466751127219781E-16 ) ) ;
#63856=CARTESIAN_POINT ( 'NONE',  ( 19.43437500061451928, 4.541064518000418104, 2.621784821874999949 ) ) ;
#63857=CARTESIAN_POINT ( 'NONE',  ( 12.64687500061451608, 6.054752690667223547, 3.707466751127219781E-16 ) ) ;
#63859=CARTESIAN_POINT ( 'NONE',  ( 26.66250000000000142, 2.886751345948129099, -4.999999999999998224 ) ) ;
#63861=CARTESIAN_POINT ( 'NONE',  ( -4.243569643749997233, 12.69687500061451857, -27.54997392385601174 ) ) ;
#63863=CARTESIAN_POINT ( 'NONE',  ( 14.50312500061451537, 0.000000000000000000, 5.243569643749999010 ) ) ;
#63864=CARTESIAN_POINT ( 'NONE',  ( 4.537500000000000533, -2.886751345948125991, -5.000000000000000000 ) ) ;
#63867=CARTESIAN_POINT ( 'NONE',  ( 13.76250000000000107, 2.886751345948126879, 4.999999999999999112 ) ) ;
#63868=CARTESIAN_POINT ( 'NONE',  ( -2.121784821874999949, 9.828125000614516438, 26.32496088578401938 ) ) ;
#63869=CARTESIAN_POINT ( 'NONE',  ( 14.02500000122903323, -5.773502691896255534, -1.060575238724906372E-15 ) ) ;
#63870=CARTESIAN_POINT ( 'NONE',  ( 23.82187500061451502, 3.027376345333613106, -5.243569643749998122 ) ) ;
#63872=CARTESIAN_POINT ( 'NONE',  ( 19.56562500061451715, -6.054752690667223547, -1.112240025338166033E-15 ) ) ;
#63873=CARTESIAN_POINT ( 'NONE',  ( 4.153125000614515727, 0.000000000000000000, 5.243569643749999010 ) ) ;
#63874=CARTESIAN_POINT ( 'NONE',  ( 19.35937500061451644, 4.541064518000418104, -2.621784821874998173 ) ) ;
#63875=CARTESIAN_POINT ( 'NONE',  ( 4.087500000000001243, -2.886751345948125991, -5.000000000000000000 ) ) ;
#63876=CARTESIAN_POINT ( 'NONE',  ( 7.828125000614517326, -4.541064518000419881, 2.621784821874995952 ) ) ;
#63877=CARTESIAN_POINT ( 'NONE',  ( 21.21562500061451573, 3.027376345333611329, 5.243569643749999010 ) ) ;
#63878=CARTESIAN_POINT ( 'NONE',  ( 2.121784821874999061, 14.25312500061451715, 26.32496088578401583 ) ) ;
#63879=CARTESIAN_POINT ( 'NONE',  ( 19.16250000122903430, 4.330127018922192761, -2.499999999999997780 ) ) ;
#63881=CARTESIAN_POINT ( 'NONE',  ( 9.590625000614517504, -3.027376345333614438, 5.243569643749998122 ) ) ;
#63882=CARTESIAN_POINT ( 'NONE',  ( 3.609375000614516882, 4.541064518000418104, -2.621784821874998173 ) ) ;
#63883=CARTESIAN_POINT ( 'NONE',  ( 3.009375000614516793, -4.541064518000417216, -2.621784821875001281 ) ) ;
#63884=CARTESIAN_POINT ( 'NONE',  ( 22.13437500061451502, 4.541064518000418104, 2.621784821874999949 ) ) ;
#63885=CARTESIAN_POINT ( 'NONE',  ( 13.56562500061451892, 3.027376345333611329, 5.243569643749999010 ) ) ;
#63886=CARTESIAN_POINT ( 'NONE',  ( 25.20000000122903216, -2.886751345948129988, 4.999999999999997335 ) ) ;
#63887=EDGE_CURVE ( 'NONE', #60322, #4907, #20343, .T. ) ;
#63888=CARTESIAN_POINT ( 'NONE',  ( 26.24062500061451431, -3.027376345333614438, 5.243569643749998122 ) ) ;
#63889=CARTESIAN_POINT ( 'NONE',  ( 19.65937500061451360, -4.541064518000417216, -2.621784821875001281 ) ) ;
#63890=CARTESIAN_POINT ( 'NONE',  ( 15.36562500061451608, 3.027376345333611329, 5.243569643749999010 ) ) ;
#63891=CARTESIAN_POINT ( 'NONE',  ( -4.243569643749999898, 16.25937500061451857, 30.00000000000000000 ) ) ;
#63893=CARTESIAN_POINT ( 'NONE',  ( 21.14062500061451289, 6.054752690667223547, 3.707466751127219781E-16 ) ) ;
#63896=CARTESIAN_POINT ( 'NONE',  ( 25.05000000000000071, 0.000000000000000000, 4.999999999999998224 ) ) ;
#63897=CARTESIAN_POINT ( 'NONE',  ( 1.999999999999998668, 10.85000000000000142, -33.46410161513775705 ) ) ;
#63899=CARTESIAN_POINT ( 'NONE',  ( 25.75312500061451715, 0.000000000000000000, 5.243569643749999010 ) ) ;
#63900=CARTESIAN_POINT ( 'NONE',  ( 6.740625000614516082, 6.054752690667223547, 3.707466751127219781E-16 ) ) ;
#63901=CARTESIAN_POINT ( 'NONE',  ( 22.83750000122903501, 4.330127018922191873, 2.499999999999999556 ) ) ;
#63902=CARTESIAN_POINT ( 'NONE',  ( 27.47812500061451502, 4.541064518000418104, 2.621784821874999949 ) ) ;
#63904=CARTESIAN_POINT ( 'NONE',  ( 24.29999999999999716, -4.330127018922190985, -2.500000000000001332 ) ) ;
#63905=CARTESIAN_POINT ( 'NONE',  ( -1.999999999999997113, 16.58750000122903501, -26.53589838486224295 ) ) ;
#63906=EDGE_CURVE ( 'NONE', #29785, #18820, #11276, .T. ) ;
#63907=( BOUNDED_CURVE ( )  B_SPLINE_CURVE ( 3, ( #22060, #67148, #23139, #55323 ),
 .UNSPECIFIED., .F., .F. ) 
 B_SPLINE_CURVE_WITH_KNOTS ( ( 4, 4 ),
 ( 5.853026561459537369, 5.913091855019096066 ),
 .UNSPECIFIED. ) 
 CURVE ( )  GEOMETRIC_REPRESENTATION_ITEM ( )  RATIONAL_B_SPLINE_CURVE ( ( 1.000000000000000000, 0.9996993693065544528, 0.9996993693065544528, 1.000000000000000000 ) ) 
 REPRESENTATION_ITEM ( '' )  );
#63908=CARTESIAN_POINT ( 'NONE',  ( 29.31562500061451715, 3.027376345333611329, 5.243569643749999010 ) ) ;
#63909=CARTESIAN_POINT ( 'NONE',  ( 11.69062500061451360, 6.054752690667223547, 3.707466751127219781E-16 ) ) ;
#63910=VERTEX_POINT ( 'NONE', #8379 ) ;
#63911=CARTESIAN_POINT ( 'NONE',  ( 24.85312500061451502, 0.000000000000000000, 5.243569643749999010 ) ) ;
#63912=CARTESIAN_POINT ( 'NONE',  ( 6.665625000614515905, 3.027376345333613106, -5.243569643749998122 ) ) ;
#63914=CARTESIAN_POINT ( 'NONE',  ( 3.778125000614519280, -4.541064518000419881, 2.621784821874995952 ) ) ;
#63918=CARTESIAN_POINT ( 'NONE',  ( 13.42499999999999893, -4.330127018922194537, 2.499999999999995559 ) ) ;
#63919=CARTESIAN_POINT ( 'NONE',  ( 12.57187500061451857, 3.027376345333613106, -5.243569643749998122 ) ) ;
#63920=CARTESIAN_POINT ( 'NONE',  ( 8.587500001229035007, -4.330127018922194537, 2.499999999999995559 ) ) ;
#63921=CARTESIAN_POINT ( 'NONE',  ( 17.29687500061451999, -3.027376345333614438, 5.243569643749998122 ) ) ;
#63923=CARTESIAN_POINT ( 'NONE',  ( 7.884375000614517681, -4.541064518000419881, 2.621784821874995952 ) ) ;
#63924=CARTESIAN_POINT ( 'NONE',  ( 2.121784821874999061, 10.65312500061451750, -33.67503911421598417 ) ) ;
#63925=FACE_OUTER_BOUND ( 'NONE', #22225, .T. ) ;
#63927=EDGE_LOOP ( 'NONE', ( #32847, #61601 ) ) ;
#63928=CARTESIAN_POINT ( 'NONE',  ( 23.84062500061451928, 6.054752690667223547, 3.707466751127219781E-16 ) ) ;
#63930=CARTESIAN_POINT ( 'NONE',  ( 26.89687500061451431, -3.027376345333610441, -5.243569643749999898 ) ) ;
#63931=CARTESIAN_POINT ( 'NONE',  ( 29.22187500061451715, 3.027376345333613106, -5.243569643749998122 ) ) ;
#63932=CARTESIAN_POINT ( 'NONE',  ( 22.23750000000000071, 5.773502691896255534, 3.535250795749688894E-16 ) ) ;
#63933=CARTESIAN_POINT ( 'NONE',  ( 7.753125000614518036, 0.000000000000000000, 5.243569643749999010 ) ) ;
#63935=CARTESIAN_POINT ( 'NONE',  ( 16.50937500061451502, -4.541064518000417216, -2.621784821875001281 ) ) ;
#63937=CARTESIAN_POINT ( 'NONE',  ( 3.103125000614517237, 4.541064518000418104, -2.621784821874998173 ) ) ;
#63938=CARTESIAN_POINT ( 'NONE',  ( 7.621875000614519280, 3.027376345333613106, -5.243569643749998122 ) ) ;
#63939=VERTEX_POINT ( 'NONE', #59708 ) ;
#63940=CARTESIAN_POINT ( 'NONE',  ( 19.88437500061451857, 4.541064518000418104, 2.621784821874999949 ) ) ;
#63942=CARTESIAN_POINT ( 'NONE',  ( 26.81250000000000000, 2.886751345948126879, 4.999999999999999112 ) ) ;
#63943=CARTESIAN_POINT ( 'NONE',  ( 26.48437500061451644, 6.421520780324663323E-16, -5.243569643749999010 ) ) ;
#63946=ORIENTED_EDGE ( 'NONE', *, *, #34637, .T. ) ;
#63947=CARTESIAN_POINT ( 'NONE',  ( 10.20000000000000107, 0.000000000000000000, 4.999999999999998224 ) ) ;
#63949=CARTESIAN_POINT ( 'NONE',  ( 21.44062500061452070, -3.027376345333610441, -5.243569643749999898 ) ) ;
#63950=CARTESIAN_POINT ( 'NONE',  ( 11.28749999999999787, -2.886751345948125991, -5.000000000000000000 ) ) ;
#63951=CARTESIAN_POINT ( 'NONE',  ( 8.662500001229034297, -4.330127018922190985, -2.500000000000001332 ) ) ;
#63952=CARTESIAN_POINT ( 'NONE',  ( 5.728125000614515905, 6.421520780324663323E-16, -5.243569643749999010 ) ) ;
#63954=CARTESIAN_POINT ( 'NONE',  ( 22.57499999999999929, 6.123233995736764310E-16, -4.999999999999998224 ) ) ;
#63955=CARTESIAN_POINT ( 'NONE',  ( 20.61562500061451431, 3.027376345333613106, -5.243569643749998122 ) ) ;
#63958=CARTESIAN_POINT ( 'NONE',  ( 25.50000000122903288, 5.773502691896255534, 3.535250795749688894E-16 ) ) ;
#63960=CARTESIAN_POINT ( 'NONE',  ( 5.175000000000002487, 4.330127018922191873, 2.499999999999999556 ) ) ;
#63961=VERTEX_POINT ( 'NONE', #9115 ) ;
#63962=CARTESIAN_POINT ( 'NONE',  ( 18.47812500061451857, 4.541064518000418104, 2.621784821874999949 ) ) ;
#63963=CARTESIAN_POINT ( 'NONE',  ( 27.29062500061451502, -3.027376345333610441, -5.243569643749999898 ) ) ;
#63964=CARTESIAN_POINT ( 'NONE',  ( 26.85937500061451644, -4.541064518000417216, -2.621784821875001281 ) ) ;
#63965=CARTESIAN_POINT ( 'NONE',  ( 14.27812500061451573, 6.421520780324663323E-16, -5.243569643749999010 ) ) ;
#63966=FACE_OUTER_BOUND ( 'NONE', #66108, .T. ) ;
#63967=CARTESIAN_POINT ( 'NONE',  ( 25.91250000122903074, 4.330127018922192761, -2.499999999999997780 ) ) ;
#63969=CARTESIAN_POINT ( 'NONE',  ( 17.31562500061451715, -6.054752690667223547, -1.112240025338166033E-15 ) ) ;
#63971=CARTESIAN_POINT ( 'NONE',  ( 28.54687500061451644, -3.027376345333614438, 5.243569643749998122 ) ) ;
#63972=CARTESIAN_POINT ( 'NONE',  ( 10.13437500061451679, -4.541064518000419881, 2.621784821874995952 ) ) ;
#63973=CARTESIAN_POINT ( 'NONE',  ( 9.759375000614516793, -4.541064518000417216, -2.621784821875001281 ) ) ;
#63974=CARTESIAN_POINT ( 'NONE',  ( 17.97187500061451715, 3.027376345333613106, -5.243569643749998122 ) ) ;
#63976=CARTESIAN_POINT ( 'NONE',  ( -5.918438294331348715, 8.060677219855273634, 28.99413606184803527 ) ) ;
#63977=CARTESIAN_POINT ( 'NONE',  ( 21.51562500061451644, 3.027376345333613106, -5.243569643749998122 ) ) ;
#63979=CARTESIAN_POINT ( 'NONE',  ( 18.57187500061451857, 3.027376345333611329, 5.243569643749999010 ) ) ;
#63980=CARTESIAN_POINT ( 'NONE',  ( 22.26562500061451644, -6.054752690667223547, -1.112240025338166033E-15 ) ) ;
#63981=CARTESIAN_POINT ( 'NONE',  ( -2.000000000000000000, 15.42500000000000071, 26.53589838486224650 ) ) ;
#63982=CARTESIAN_POINT ( 'NONE',  ( 29.65312500061451573, 4.541064518000418104, -2.621784821874998173 ) ) ;
#63983=CARTESIAN_POINT ( 'NONE',  ( 9.412500001229034297, 0.000000000000000000, 4.999999999999998224 ) ) ;
#63984=VERTEX_POINT ( 'NONE', #13183 ) ;
#63985=CARTESIAN_POINT ( 'NONE',  ( 3.937500001229034208, 4.330127018922191873, 2.499999999999999556 ) ) ;
#63986=CARTESIAN_POINT ( 'NONE',  ( -3.999999999999999556, 19.96250000000000213, -32.30940107675850470 ) ) ;
#63987=CARTESIAN_POINT ( 'NONE',  ( 25.08750000122903145, 4.330127018922191873, 2.499999999999999556 ) ) ;
#63990=CARTESIAN_POINT ( 'NONE',  ( 9.309375000614517504, -4.541064518000417216, -2.621784821875001281 ) ) ;
#63991=CARTESIAN_POINT ( 'NONE',  ( 30.00000000000000000, 0.000000000000000000, 0.000000000000000000 ) ) ;
#63992=CARTESIAN_POINT ( 'NONE',  ( 15.70312500061451644, 4.541064518000418104, -2.621784821874998173 ) ) ;
#63993=CARTESIAN_POINT ( 'NONE',  ( 9.834375000614517859, 6.421520780324663323E-16, -5.243569643749999010 ) ) ;
#63994=CARTESIAN_POINT ( 'NONE',  ( 28.72500000122903074, 2.886751345948126879, 4.999999999999999112 ) ) ;
#63995=CARTESIAN_POINT ( 'NONE',  ( 20.37187500061451573, 3.027376345333611329, 5.243569643749999010 ) ) ;
#63996=CARTESIAN_POINT ( 'NONE',  ( 6.684375000614518392, 6.421520780324663323E-16, -5.243569643749999010 ) ) ;
#63997=CARTESIAN_POINT ( 'NONE',  ( 4.818692141996693046, -1.334243621178544226, 4.818692141997074074 ) ) ;
#63998=ADVANCED_FACE ( 'NONE', ( #16107 ), #27937, .F. ) ;
#63999=CARTESIAN_POINT ( 'NONE',  ( 7.753125000614518036, 0.000000000000000000, 5.243569643749999010 ) ) ;
#64000=CARTESIAN_POINT ( 'NONE',  ( 17.27812500061451217, -4.541064518000419881, 2.621784821874995952 ) ) ;
#64002=CARTESIAN_POINT ( 'NONE',  ( 15.92812500061451608, -4.541064518000419881, 2.621784821874995952 ) ) ;
#64003=CARTESIAN_POINT ( 'NONE',  ( 9.928125000614517859, 4.541064518000418104, 2.621784821874999949 ) ) ;
#64005=CARTESIAN_POINT ( 'NONE',  ( 10.87500000000000000, 6.123233995736764310E-16, -4.999999999999998224 ) ) ;
#64006=CARTESIAN_POINT ( 'NONE',  ( 6.525000001229033231, 2.886751345948129099, -4.999999999999998224 ) ) ;
#64007=CARTESIAN_POINT ( 'NONE',  ( 15.34687500061451537, 6.054752690667223547, 3.707466751127219781E-16 ) ) ;
#64008=AXIS2_PLACEMENT_3D ( 'NONE', #25324, #47869, #70398 ) ;
#64009=CARTESIAN_POINT ( 'NONE',  ( 16.83750000122903145, 6.123233995736764310E-16, -4.999999999999998224 ) ) ;
#64011=CARTESIAN_POINT ( 'NONE',  ( -4.243569643749999898, 19.35312500061451857, -30.00000000000000000 ) ) ;
#64012=CARTESIAN_POINT ( 'NONE',  ( 16.35000000122903430, -2.886751345948126435, -5.000000000000000000 ) ) ;
#64013=CARTESIAN_POINT ( 'NONE',  ( 30.00000000000000000, 0.000000000000000000, 0.000000000000000000 ) ) ;
#64014=ADVANCED_FACE ( 'NONE', ( #55643 ), #72271, .F. ) ;
#64015=CARTESIAN_POINT ( 'NONE',  ( 1.626862140677534273E-15, 10.77500000122903323, -26.00000000000000355 ) ) ;
#64016=CYLINDRICAL_SURFACE ( 'NONE', #26699, 4.999999999999998224 ) ;
#64017=CARTESIAN_POINT ( 'NONE',  ( 17.78437500061451715, -4.541064518000419881, 2.621784821874995952 ) ) ;
#64018=FACE_OUTER_BOUND ( 'NONE', #71992, .T. ) ;
#64019=CARTESIAN_POINT ( 'NONE',  ( 13.79062500061451502, -3.027376345333610441, -5.243569643749999898 ) ) ;
#64021=CARTESIAN_POINT ( 'NONE',  ( 23.25937500061451857, -4.541064518000417216, -2.621784821875001281 ) ) ;
#64023=CARTESIAN_POINT ( 'NONE',  ( 10.56562500061451715, -6.054752690667223547, -1.112240025338166033E-15 ) ) ;
#64024=CARTESIAN_POINT ( 'NONE',  ( 15.68437500061451573, 6.421520780324663323E-16, -5.243569643749999010 ) ) ;
#64025=EDGE_LOOP ( 'NONE', ( #35822, #35981, #45091, #9732 ) ) ;
#64026=CARTESIAN_POINT ( 'NONE',  ( 26.07187500061451857, 3.027376345333613106, -5.243569643749998122 ) ) ;
#64027=CARTESIAN_POINT ( 'NONE',  ( 27.66562500061451146, -6.054752690667223547, -1.112240025338166033E-15 ) ) ;
#64028=CARTESIAN_POINT ( 'NONE',  ( 18.36562500061451431, 3.027376345333613106, -5.243569643749998122 ) ) ;
#64029=CARTESIAN_POINT ( 'NONE',  ( 18.97499999999999787, 6.123233995736764310E-16, -4.999999999999998224 ) ) ;
#64031=CARTESIAN_POINT ( 'NONE',  ( 8.737500000000002487, 5.773502691896255534, 3.535250795749688894E-16 ) ) ;
#64032=CARTESIAN_POINT ( 'NONE',  ( 19.08750000122903145, 6.123233995736764310E-16, -4.999999999999998224 ) ) ;
#64033=CARTESIAN_POINT ( 'NONE',  ( 1.626862140677534273E-15, 10.21250000000000036, 34.00000000000000000 ) ) ;
#64035=ORIENTED_EDGE ( 'NONE', *, *, #44978, .T. ) ;
#64036=CARTESIAN_POINT ( 'NONE',  ( 16.76249999999999929, 2.886751345948129099, -4.999999999999998224 ) ) ;
#64037=CARTESIAN_POINT ( 'NONE',  ( 22.12500000000000000, 6.123233995736764310E-16, -4.999999999999998224 ) ) ;
#64038=CARTESIAN_POINT ( 'NONE',  ( 18.83437500061451431, 6.421520780324663323E-16, -5.243569643749999010 ) ) ;
#64039=CARTESIAN_POINT ( 'NONE',  ( 14.24062500061451608, -3.027376345333610441, -5.243569643749999898 ) ) ;
#64041=CARTESIAN_POINT ( 'NONE',  ( 28.53749999999999787, 5.773502691896255534, 3.535250795749688401E-16 ) ) ;
#64042=CARTESIAN_POINT ( 'NONE',  ( 6.065625000614516260, -6.054752690667223547, -1.112240025338166033E-15 ) ) ;
#64044=CARTESIAN_POINT ( 'NONE',  ( 12.82499999999999929, 4.330127018922191873, 2.499999999999999556 ) ) ;
#64046=CARTESIAN_POINT ( 'NONE',  ( -3.000416591977282496E-16, 15.64062500061451644, 25.09994784771203058 ) ) ;
#64047=CARTESIAN_POINT ( 'NONE',  ( 28.64062500061451289, -3.027376345333610441, -5.243569643749999898 ) ) ;
#64050=CARTESIAN_POINT ( 'NONE',  ( 24.68437500061451573, 6.421520780324663323E-16, -5.243569643749999010 ) ) ;
#64052=CARTESIAN_POINT ( 'NONE',  ( 22.56562500061451715, 3.027376345333611329, 5.243569643749999010 ) ) ;
#64053=CARTESIAN_POINT ( 'NONE',  ( 24.00937500061451502, 0.000000000000000000, 5.243569643749999010 ) ) ;
#64054=CARTESIAN_POINT ( 'NONE',  ( 4.243569643749999010, 15.56562500061459531, -32.45002607614398471 ) ) ;
#64055=CARTESIAN_POINT ( 'NONE',  ( 6.440625000614517148, -3.027376345333614438, 5.243569643749998122 ) ) ;
#64057=CARTESIAN_POINT ( 'NONE',  ( 23.84062500061451573, 6.054752690667223547, 3.707466751127219781E-16 ) ) ;
#64060=CARTESIAN_POINT ( 'NONE',  ( 16.05937500061451573, -4.541064518000417216, -2.621784821875001281 ) ) ;
#64061=CARTESIAN_POINT ( 'NONE',  ( 27.04687500061451644, 6.054752690667223547, 3.707466751127219781E-16 ) ) ;
#64062=CARTESIAN_POINT ( 'NONE',  ( -3.000416591977282496E-16, 14.34687500061451715, 25.09994784771203058 ) ) ;
#64063=CARTESIAN_POINT ( 'NONE',  ( 6.328125000614515550, 4.541064518000418104, 2.621784821874999949 ) ) ;
#64064=DIRECTION ( 'NONE',  ( -1.000000000000000000, -0.000000000000000000, -0.000000000000000000 ) ) ;
#64065=CARTESIAN_POINT ( 'NONE',  ( 29.12812500061451715, 6.421520780324663323E-16, -5.243569643749999010 ) ) ;
#64067=CARTESIAN_POINT ( 'NONE',  ( 4.865625000614517859, 3.027376345333613106, -5.243569643749998122 ) ) ;
#64068=CARTESIAN_POINT ( 'NONE',  ( 8.634375000614518569, 4.541064518000418104, 2.621784821874999949 ) ) ;
#64069=CARTESIAN_POINT ( 'NONE',  ( 15.97500000122903430, 2.886751345948129099, -4.999999999999998224 ) ) ;
#64070=CARTESIAN_POINT ( 'NONE',  ( 4.171875000614517326, 3.027376345333611329, 5.243569643749999010 ) ) ;
#64071=CARTESIAN_POINT ( 'NONE',  ( 7.153125000614518392, 4.541064518000418104, -2.621784821874998173 ) ) ;
#64074=CARTESIAN_POINT ( 'NONE',  ( 17.52187500061451431, 3.027376345333613106, -5.243569643749998122 ) ) ;
#64076=ORIENTED_EDGE ( 'NONE', *, *, #57166, .F. ) ;
#64077=CARTESIAN_POINT ( 'NONE',  ( 25.64062500061451644, 6.054752690667223547, 3.707466751127219781E-16 ) ) ;
#64078=CARTESIAN_POINT ( 'NONE',  ( 9.928125000614517859, 4.541064518000418104, 2.621784821874999949 ) ) ;
#64079=CARTESIAN_POINT ( 'NONE',  ( 25.95937500061451431, -4.541064518000417216, -2.621784821875001281 ) ) ;
#64080=CARTESIAN_POINT ( 'NONE',  ( 10.86562500061451431, 3.027376345333611329, 5.243569643749999010 ) ) ;
#64082=CARTESIAN_POINT ( 'NONE',  ( 9.675000001229035362, 2.886751345948129099, -4.999999999999998224 ) ) ;
#64083=EDGE_CURVE ( 'NONE', #57497, #71040, #39542, .T. ) ;
#64084=CARTESIAN_POINT ( 'NONE',  ( 24.32812500061451289, 4.541064518000418104, 2.621784821874999949 ) ) ;
#64085=CARTESIAN_POINT ( 'NONE',  ( 4.243569643749999010, 10.16562500061451857, -32.45002607614398471 ) ) ;
#64086=CARTESIAN_POINT ( 'NONE',  ( 13.87500000122903465, 2.886751345948126879, 4.999999999999999112 ) ) ;
#64087=CARTESIAN_POINT ( 'NONE',  ( 21.25312500061451715, 0.000000000000000000, 5.243569643749999010 ) ) ;
#64088=CARTESIAN_POINT ( 'NONE',  ( 18.10312500061451502, 0.000000000000000000, 5.243569643749999010 ) ) ;
#64089=CARTESIAN_POINT ( 'NONE',  ( 5.034375000614519813, 4.541064518000418104, 2.621784821874999949 ) ) ;
#64090=CARTESIAN_POINT ( 'NONE',  ( 18.67500000000000071, 4.330127018922191873, 2.499999999999999556 ) ) ;
#64091=CARTESIAN_POINT ( 'NONE',  ( 13.57500000122903572, -5.773502691896255534, -1.060575238724906372E-15 ) ) ;
#64092=CARTESIAN_POINT ( 'NONE',  ( 10.79062500061451679, 6.054752690667223547, 3.707466751127219781E-16 ) ) ;
#64093=CARTESIAN_POINT ( 'NONE',  ( 13.60312500061451679, 0.000000000000000000, 5.243569643749999010 ) ) ;
#64094=CARTESIAN_POINT ( 'NONE',  ( 26.21250000122903501, -4.330127018922190985, -2.500000000000001332 ) ) ;
#64095=CARTESIAN_POINT ( 'NONE',  ( 20.97187500061451715, -6.054752690667223547, -1.112240025338166033E-15 ) ) ;
#64096=CARTESIAN_POINT ( 'NONE',  ( 22.09687500061451715, 6.054752690667223547, 3.707466751127219781E-16 ) ) ;
#64097=CARTESIAN_POINT ( 'NONE',  ( 4.809916128174254624, -1.365542690628744449, -5.062639209831853115 ) ) ;
#64098=CARTESIAN_POINT ( 'NONE',  ( 6.787500001229032520, -4.330127018922194537, 2.499999999999995559 ) ) ;
#64099=CARTESIAN_POINT ( 'NONE',  ( 6.646875000614518747, -3.027376345333610441, -5.243569643749999898 ) ) ;
#64100=CARTESIAN_POINT ( 'NONE',  ( 26.67187500061451644, 3.027376345333611329, 5.243569643749999010 ) ) ;
#64102=CARTESIAN_POINT ( 'NONE',  ( 3.684375000614518836, 4.541064518000418104, 2.621784821874999949 ) ) ;
#64103=CARTESIAN_POINT ( 'NONE',  ( 20.72812500061451502, 4.541064518000418104, 2.621784821874999949 ) ) ;
#64104=CARTESIAN_POINT ( 'NONE',  ( 26.37187500061451217, -6.054752690667223547, -1.112240025338166033E-15 ) ) ;
#64106=CARTESIAN_POINT ( 'NONE',  ( 3.282867099560692559, -3.771354186041921075, 3.570299421950303032 ) ) ;
#64107=FACE_OUTER_BOUND ( 'NONE', #40792, .T. ) ;
#64108=CARTESIAN_POINT ( 'NONE',  ( 7.209375000614519635, 4.541064518000418104, -2.621784821874998173 ) ) ;
#64109=CARTESIAN_POINT ( 'NONE',  ( 17.80312500061451786, -4.541064518000417216, -2.621784821875001281 ) ) ;
#64110=VERTEX_POINT ( 'NONE', #5038 ) ;
#64111=CARTESIAN_POINT ( 'NONE',  ( 23.02499999999999858, 6.123233995736764310E-16, -4.999999999999998224 ) ) ;
#64112=CARTESIAN_POINT ( 'NONE',  ( 26.50312500061451360, 4.541064518000418104, -2.621784821874998173 ) ) ;
#64113=CARTESIAN_POINT ( 'NONE',  ( 4.734375000614518214, -4.541064518000419881, 2.621784821874995952 ) ) ;
#64114=CARTESIAN_POINT ( 'NONE',  ( 4.652363956030752590, 1.832484597013495531, 4.879388851549410155 ) ) ;
#64117=CARTESIAN_POINT ( 'NONE',  ( 16.80000000000000071, 4.330127018922192761, -2.499999999999997780 ) ) ;
#64118=CARTESIAN_POINT ( 'NONE',  ( 22.00312500061451360, 4.541064518000418104, -2.621784821874998173 ) ) ;
#64119=EDGE_LOOP ( 'NONE', ( #63320, #49762, #28880, #54599 ) ) ;
#64120=CARTESIAN_POINT ( 'NONE',  ( 24.29999999999999716, -4.330127018922190985, -2.500000000000001332 ) ) ;
#64121=CARTESIAN_POINT ( 'NONE',  ( 25.32187500061451857, 3.027376345333611329, 5.243569643749999010 ) ) ;
#64122=ORIENTED_EDGE ( 'NONE', *, *, #57411, .T. ) ;
#64123=DIRECTION ( 'NONE',  ( 0.000000000000000000, 0.000000000000000000, 1.000000000000000000 ) ) ;
#64124=CARTESIAN_POINT ( 'NONE',  ( 13.94062500061451892, 6.054752690667223547, 3.707466751127219781E-16 ) ) ;
#64125=CARTESIAN_POINT ( 'NONE',  ( 4.790625000614518569, -3.027376345333610441, -5.243569643749999898 ) ) ;
#64127=CARTESIAN_POINT ( 'NONE',  ( 29.05312500061451431, -4.541064518000417216, -2.621784821875001281 ) ) ;
#64128=CARTESIAN_POINT ( 'NONE',  ( 15.11250000122903359, 4.330127018922192761, -2.499999999999997780 ) ) ;
#64129=CARTESIAN_POINT ( 'NONE',  ( 20.10000000000000142, 0.000000000000000000, 4.999999999999998224 ) ) ;
#64130=CARTESIAN_POINT ( 'NONE',  ( 25.53750000000000142, -2.886751345948129988, 4.999999999999997335 ) ) ;
#64132=CARTESIAN_POINT ( 'NONE',  ( 8.634375000614518569, 4.541064518000418104, 2.621784821874999949 ) ) ;
#64133=CARTESIAN_POINT ( 'NONE',  ( 19.54687500061451644, -3.027376345333614438, 5.243569643749998122 ) ) ;
#64134=CARTESIAN_POINT ( 'NONE',  ( 4.000000000000000000, 11.30000000122903536, 32.30940107675849760 ) ) ;
#64135=VERTEX_POINT ( 'NONE', #21648 ) ;
#64136=CARTESIAN_POINT ( 'NONE',  ( 28.00312500061451715, 0.000000000000000000, 5.243569643749999010 ) ) ;
#64137=CARTESIAN_POINT ( 'NONE',  ( 28.92187500061451644, 3.027376345333611329, 5.243569643749999010 ) ) ;
#64138=CARTESIAN_POINT ( 'NONE',  ( 5.221875000614519813, -6.054752690667223547, -1.112240025338166033E-15 ) ) ;
#64139=CARTESIAN_POINT ( 'NONE',  ( 16.83749999999999858, 5.773502691896255534, 3.535250795749688894E-16 ) ) ;
#64140=CARTESIAN_POINT ( 'NONE',  ( 13.19062500061451537, -3.027376345333614438, 5.243569643749998122 ) ) ;
#64143=CARTESIAN_POINT ( 'NONE',  ( 18.67500000122903714, 2.886751345948129099, -4.999999999999998224 ) ) ;
#64144=CARTESIAN_POINT ( 'NONE',  ( 3.680627977383748473, 9.304151242747314754, 25.24598017873988098 ) ) ;
#64146=CARTESIAN_POINT ( 'NONE',  ( 7.678125000614516082, 4.541064518000418104, 2.621784821874999949 ) ) ;
#64147=CARTESIAN_POINT ( 'NONE',  ( 24.04687500061451644, -3.027376345333614438, 5.243569643749998122 ) ) ;
#64148=CARTESIAN_POINT ( 'NONE',  ( 2.121784821874999061, 19.70937500061451786, 26.32496088578401583 ) ) ;
#64149=CARTESIAN_POINT ( 'NONE',  ( 23.78437500061451360, 6.421520780324663323E-16, -5.243569643749999010 ) ) ;
#64150=CARTESIAN_POINT ( 'NONE',  ( 6.750000000000002665, -4.330127018922190985, -2.500000000000001332 ) ) ;
#64151=CARTESIAN_POINT ( 'NONE',  ( 1.999999999999998668, 12.31250000122903465, 26.53589838486224650 ) ) ;
#64152=CARTESIAN_POINT ( 'NONE',  ( 15.81562500061451537, 3.027376345333611329, 5.243569643749999010 ) ) ;
#64153=CARTESIAN_POINT ( 'NONE',  ( 7.012500001229035718, 4.330127018922192761, -2.499999999999997780 ) ) ;
#64154=CARTESIAN_POINT ( 'NONE',  ( 12.60937500061451821, 4.541064518000418104, -2.621784821874998173 ) ) ;
#64155=CARTESIAN_POINT ( 'NONE',  ( 3.921850648269007422, -3.101535241682955579, 3.979058954293606565 ) ) ;
#64156=ORIENTED_EDGE ( 'NONE', *, *, #14379, .T. ) ;
#64157=CARTESIAN_POINT ( 'NONE',  ( 12.81562500061451537, -6.054752690667223547, -1.112240025338166033E-15 ) ) ;
#64158=DIRECTION ( 'NONE',  ( -1.000000000000000000, -0.000000000000000000, -0.000000000000000000 ) ) ;
#64159=CARTESIAN_POINT ( 'NONE',  ( 24.52500000122903145, 2.886751345948129099, -4.999999999999998224 ) ) ;
#64160=CARTESIAN_POINT ( 'NONE',  ( 11.70937500061451608, 4.541064518000418104, -2.621784821874998173 ) ) ;
#64161=CARTESIAN_POINT ( 'NONE',  ( 14.09062500061451750, -3.027376345333614438, 5.243569643749998122 ) ) ;
#64163=CARTESIAN_POINT ( 'NONE',  ( 23.03437500061451715, 4.541064518000418104, 2.621784821874999949 ) ) ;
#64164=CARTESIAN_POINT ( 'NONE',  ( 1.071796769724497445, 15.92990381179669868, 26.00000000000000355 ) ) ;
#64165=( BOUNDED_CURVE ( )  B_SPLINE_CURVE ( 2, ( #39796, #34960, #61577, #17950, #27982, #62312, #12066 ),
 .UNSPECIFIED., .F., .F. ) 
 B_SPLINE_CURVE_WITH_KNOTS ( ( 3, 2, 2, 3 ),
 ( 0.9343878867307400249, 0.9361111111111111160, 0.9388888888888888840, 0.9404282932007268503 ),
 .UNSPECIFIED. ) 
 CURVE ( )  GEOMETRIC_REPRESENTATION_ITEM ( )  RATIONAL_B_SPLINE_CURVE ( ( 0.9368944059126143031, 0.9168874154023497480, 1.000000000000000000, 0.8660254037844387076, 1.000000000000000000, 0.9257532144072448954, 0.9337994205692392580 ) ) 
 REPRESENTATION_ITEM ( '' )  );
#64167=CARTESIAN_POINT ( 'NONE',  ( -1.999999999999997113, 19.62500000000000000, 33.46410161513775705 ) ) ;
#64168=CARTESIAN_POINT ( 'NONE',  ( 4.243569643749999898, 15.09687500061451715, -27.54997392385601529 ) ) ;
#64169=CARTESIAN_POINT ( 'NONE',  ( 15.00937500061451679, 0.000000000000000000, 5.243569643749999010 ) ) ;
#64170=CARTESIAN_POINT ( 'NONE',  ( 17.55000000122903359, -2.886751345948129988, 4.999999999999997335 ) ) ;
#64172=CARTESIAN_POINT ( 'NONE',  ( 12.08437500061451608, 6.421520780324663323E-16, -5.243569643749999010 ) ) ;
#64173=CARTESIAN_POINT ( 'NONE',  ( 2.121784821874999061, 10.70937500061451964, 26.32496088578401583 ) ) ;
#64174=CARTESIAN_POINT ( 'NONE',  ( 19.08750000122903145, 6.123233995736764310E-16, -4.999999999999998224 ) ) ;
#64175=CARTESIAN_POINT ( 'NONE',  ( 13.07812500061451821, 4.541064518000418104, 2.621784821874999949 ) ) ;
#64178=ORIENTED_EDGE ( 'NONE', *, *, #67328, .T. ) ;
#64179=CARTESIAN_POINT ( 'NONE',  ( 17.06250000000000000, -5.773502691896255534, -1.060575238724906372E-15 ) ) ;
#64181=CARTESIAN_POINT ( 'NONE',  ( 11.67187500061451821, 3.027376345333612662, -5.243569643749998122 ) ) ;
#64182=CARTESIAN_POINT ( 'NONE',  ( 2.067223061484673163, 4.558648060312520123, 26.56624252461168822 ) ) ;
#64183=CARTESIAN_POINT ( 'NONE',  ( 12.67500000122903536, -5.773502691896255534, -1.060575238724906372E-15 ) ) ;
#64184=CARTESIAN_POINT ( 'NONE',  ( 20.62500000122903288, 2.886751345948126879, 4.999999999999999112 ) ) ;
#64185=CARTESIAN_POINT ( 'NONE',  ( 17.27812500061451217, -4.541064518000419881, 2.621784821874995952 ) ) ;
#64186=CARTESIAN_POINT ( 'NONE',  ( 21.66562500061451502, 3.027376345333611329, 5.243569643749999010 ) ) ;
#64187=CARTESIAN_POINT ( 'NONE',  ( 4.265625000614517326, -6.054752690667223547, -1.112240025338166033E-15 ) ) ;
#64188=( BOUNDED_CURVE ( )  B_SPLINE_CURVE ( 2, ( #3467, #25987, #48526, #37436, #30067, #43717, #50358 ),
 .UNSPECIFIED., .F., .F. ) 
 B_SPLINE_CURVE_WITH_KNOTS ( ( 3, 2, 2, 3 ),
 ( 0.9602520150385847053, 0.9611111111111111382, 0.9638888888888889062, 0.9646572887058436629 ),
 .UNSPECIFIED. ) 
 CURVE ( )  GEOMETRIC_REPRESENTATION_ITEM ( )  RATIONAL_B_SPLINE_CURVE ( ( 0.9427596708857610697, 0.9585650622062426018, 1.000000000000000000, 0.8660254037844387076, 1.000000000000000000, 0.9629394201248949736, 0.9463825270602228557 ) ) 
 REPRESENTATION_ITEM ( '' )  );
#64189=CARTESIAN_POINT ( 'NONE',  ( 26.77499999999999858, 4.330127018922191873, 2.499999999999999556 ) ) ;
#64190=CARTESIAN_POINT ( 'NONE',  ( 28.35000000000000142, -4.330127018922190985, -2.500000000000001332 ) ) ;
#64192=CARTESIAN_POINT ( 'NONE',  ( 29.18437500061451573, 6.421520780324663323E-16, -5.243569643749999010 ) ) ;
#64194=CARTESIAN_POINT ( 'NONE',  ( 2.121784821875001281, 15.50937500061451857, -26.32496088578401938 ) ) ;
#64195=CARTESIAN_POINT ( 'NONE',  ( 4.612500001229032698, -4.330127018922190985, -2.500000000000001332 ) ) ;
#64196=CARTESIAN_POINT ( 'NONE',  ( 5.924999999999999822, 6.123233995736764310E-16, -4.999999999999998224 ) ) ;
#64198=CARTESIAN_POINT ( 'NONE',  ( 9.571875000614518569, 3.027376345333611329, 5.243569643749999010 ) ) ;
#64199=CARTESIAN_POINT ( 'NONE',  ( 28.56562500061451715, -6.054752690667223547, -1.112240025338166033E-15 ) ) ;
#64202=CARTESIAN_POINT ( 'NONE',  ( 7.320879633048903241E-15, 17.75000000122903288, -34.00000000000000000 ) ) ;
#64203=CARTESIAN_POINT ( 'NONE',  ( 7.321875000614516793, 3.027376345333611329, 5.243569643749999010 ) ) ;
#64204=CARTESIAN_POINT ( 'NONE',  ( 12.30937500061451573, 0.000000000000000000, 5.243569643749999010 ) ) ;
#64205=CARTESIAN_POINT ( 'NONE',  ( 4.837500000000001243, -2.886751345948129988, 4.999999999999997335 ) ) ;
#64206=CARTESIAN_POINT ( 'NONE',  ( -2.121784821874999949, 14.77812500061459389, 26.32496088578401938 ) ) ;
#64208=CARTESIAN_POINT ( 'NONE',  ( 5.437500000000001776, -2.886751345948125991, -5.000000000000000000 ) ) ;
#64210=CARTESIAN_POINT ( 'NONE',  ( 19.82812500061451644, 4.541064518000418104, 2.621784821874999949 ) ) ;
#64211=CARTESIAN_POINT ( 'NONE',  ( 12.62812500061451537, 4.541064518000418104, 2.621784821874999949 ) ) ;
#64213=CARTESIAN_POINT ( 'NONE',  ( 8.859375000614518214, -4.541064518000417216, -2.621784821875001281 ) ) ;
#64214=CARTESIAN_POINT ( 'NONE',  ( 27.07499999999999929, 6.123233995736764310E-16, -4.999999999999998224 ) ) ;
#64215=CARTESIAN_POINT ( 'NONE',  ( 23.28750000122903430, 4.330127018922191873, 2.499999999999999556 ) ) ;
#64217=CARTESIAN_POINT ( 'NONE',  ( 17.02499999999999858, -4.330127018922194537, 2.499999999999995559 ) ) ;
#64218=CARTESIAN_POINT ( 'NONE',  ( 11.03437500061451715, -4.541064518000419881, 2.621784821874995952 ) ) ;
#64219=CARTESIAN_POINT ( 'NONE',  ( 25.50937500061451502, -4.541064518000417216, -2.621784821875001281 ) ) ;
#64220=CARTESIAN_POINT ( 'NONE',  ( 3.759375000614517681, 0.000000000000000000, 5.243569643749999010 ) ) ;
#64222=CARTESIAN_POINT ( 'NONE',  ( 19.62187500061451573, -6.054752690667223547, -1.112240025338166033E-15 ) ) ;
#64223=CARTESIAN_POINT ( 'NONE',  ( 11.07187500061451679, -6.054752690667223547, -1.112240025338166033E-15 ) ) ;
#64225=CARTESIAN_POINT ( 'NONE',  ( 22.83749999999999858, -2.886751345948129988, 4.999999999999997335 ) ) ;
#64227=CARTESIAN_POINT ( 'NONE',  ( -2.121784821874996840, 11.38437500061451679, -26.32496088578401583 ) ) ;
#64229=CARTESIAN_POINT ( 'NONE',  ( 14.05312500061451431, 0.000000000000000000, 5.243569643749999010 ) ) ;
#64230=CARTESIAN_POINT ( 'NONE',  ( 4.125000000000000000, 6.123233995736764310E-16, -4.999999999999998224 ) ) ;
#64231=CARTESIAN_POINT ( 'NONE',  ( 12.26250000122903394, -4.330127018922190985, -2.500000000000001332 ) ) ;
#64233=CARTESIAN_POINT ( 'NONE',  ( 13.72500000000000142, 4.330127018922191873, 2.499999999999999556 ) ) ;
#64234=CARTESIAN_POINT ( 'NONE',  ( -2.121784821874996840, 9.978125000614518569, 33.67503911421598417 ) ) ;
#64235=CARTESIAN_POINT ( 'NONE',  ( 15.07500000122903394, 2.886751345948129099, -4.999999999999998224 ) ) ;
#64238=CARTESIAN_POINT ( 'NONE',  ( 24.34687500061451715, 6.054752690667223547, 3.707466751127219781E-16 ) ) ;
#64241=CARTESIAN_POINT ( 'NONE',  ( 19.75312500061451360, 4.541064518000418104, -2.621784821874998173 ) ) ;
#64242=AXIS2_PLACEMENT_3D ( 'NONE', #29865, #52402, #30232 ) ;
#64243=CARTESIAN_POINT ( 'NONE',  ( 3.403125000614518836, -4.541064518000417216, -2.621784821875001281 ) ) ;
#64244=CARTESIAN_POINT ( 'NONE',  ( 18.90937500061451360, 4.541064518000418104, -2.621784821874998173 ) ) ;
#64245=CARTESIAN_POINT ( 'NONE',  ( 29.18437500061451573, 6.421520780324663323E-16, -5.243569643749999010 ) ) ;
#64246=CARTESIAN_POINT ( 'NONE',  ( 6.103125000614515905, -4.541064518000417216, -2.621784821875001281 ) ) ;
#64247=CARTESIAN_POINT ( 'NONE',  ( 22.37812500061451360, 6.421520780324663323E-16, -5.243569643749999010 ) ) ;
#64248=CARTESIAN_POINT ( 'NONE',  ( -2.121784821874999949, 16.12812500061451715, 26.32496088578401938 ) ) ;
#64249=CARTESIAN_POINT ( 'NONE',  ( 17.81250000122903288, 4.330127018922192761, -2.499999999999997780 ) ) ;
#64251=CARTESIAN_POINT ( 'NONE',  ( 8.728125000614518569, -4.541064518000419881, 2.621784821874995952 ) ) ;
#64252=CARTESIAN_POINT ( 'NONE',  ( 3.534375000614518036, 6.421520780324663323E-16, -5.243569643749999010 ) ) ;
#64253=CARTESIAN_POINT ( 'NONE',  ( 3.196875000614516793, 6.054752690667223547, 3.707466751127219781E-16 ) ) ;
#64254=CARTESIAN_POINT ( 'NONE',  ( 22.58437500061451431, 4.541064518000418104, 2.621784821874999949 ) ) ;
#64255=CARTESIAN_POINT ( 'NONE',  ( 14.84062500061451750, 6.054752690667223547, 3.707466751127219781E-16 ) ) ;
#64256=CARTESIAN_POINT ( 'NONE',  ( 24.71250000122903145, 0.000000000000000000, 4.999999999999998224 ) ) ;
#64257=EDGE_CURVE ( 'NONE', #9906, #64445, #30032, .T. ) ;
#64258=CARTESIAN_POINT ( 'NONE',  ( 25.49062500061451786, -3.027376345333610441, -5.243569643749999898 ) ) ;
#64259=CARTESIAN_POINT ( 'NONE',  ( 19.47187500061451360, 3.027376345333611329, 5.243569643749999010 ) ) ;
#64260=CARTESIAN_POINT ( 'NONE',  ( 14.57812500061451644, -4.541064518000419881, 2.621784821874995952 ) ) ;
#64261=CARTESIAN_POINT ( 'NONE',  ( 9.001249775931846008E-16, 17.72187500061451715, 34.90005215228797653 ) ) ;
#64262=CARTESIAN_POINT ( 'NONE',  ( 18.70312500061451644, -4.541064518000417216, -2.621784821875001281 ) ) ;
#64263=CARTESIAN_POINT ( 'NONE',  ( 29.16562500061451502, 3.027376345333613106, -5.243569643749998122 ) ) ;
#64264=VERTEX_POINT ( 'NONE', #37550 ) ;
#64265=CARTESIAN_POINT ( 'NONE',  ( 24.33749999999999858, -2.886751345948125991, -5.000000000000000000 ) ) ;
#64266=CARTESIAN_POINT ( 'NONE',  ( 3.999999999999999112, 11.22500000000000142, -30.00000000000000000 ) ) ;
#64268=CARTESIAN_POINT ( 'NONE',  ( 27.51562500061451644, 3.027376345333611329, 5.243569643749999010 ) ) ;
#64269=CARTESIAN_POINT ( 'NONE',  ( 7.340625000614518392, -3.027376345333614438, 5.243569643749998122 ) ) ;
#64270=CARTESIAN_POINT ( 'NONE',  ( 19.72500000122903074, 2.886751345948126879, 4.999999999999999112 ) ) ;
#64271=CARTESIAN_POINT ( 'NONE',  ( 25.71562500061451573, 3.027376345333611329, 5.243569643749999010 ) ) ;
#64272=CARTESIAN_POINT ( 'NONE',  ( 25.08749999999999858, -2.886751345948129988, 4.999999999999997335 ) ) ;
#64273=CARTESIAN_POINT ( 'NONE',  ( 3.999999999999999112, 14.93750000122903288, -30.00000000000000000 ) ) ;
#64275=CARTESIAN_POINT ( 'NONE',  ( 27.47812500061451502, 4.541064518000418104, 2.621784821874999949 ) ) ;
#64276=CARTESIAN_POINT ( 'NONE',  ( 9.365625000614519635, 3.027376345333613106, -5.243569643749998122 ) ) ;
#64278=CARTESIAN_POINT ( 'NONE',  ( 24.66562500061451502, 3.027376345333613106, -5.243569643749998122 ) ) ;
#64279=CARTESIAN_POINT ( 'NONE',  ( 5.090625000614516615, -3.027376345333614438, 5.243569643749998122 ) ) ;
#64280=AXIS2_PLACEMENT_3D ( 'NONE', #35996, #7925, #30821 ) ;
#64282=CYLINDRICAL_SURFACE ( 'NONE', #53855, 4.999999999999998224 ) ;
#64283=CARTESIAN_POINT ( 'NONE',  ( 12.67499999999999893, 6.123233995736764310E-16, -4.999999999999998224 ) ) ;
#64285=CARTESIAN_POINT ( 'NONE',  ( 14.03437500061451715, 4.541064518000418104, 2.621784821874999949 ) ) ;
#64286=CARTESIAN_POINT ( 'NONE',  ( 8.662500001229034297, -4.330127018922190985, -2.500000000000001332 ) ) ;
#64287=CARTESIAN_POINT ( 'NONE',  ( 17.97187500061451715, 3.027376345333613106, -5.243569643749998122 ) ) ;
#64289=CARTESIAN_POINT ( 'NONE',  ( 8.859375000614518214, -4.541064518000417216, -2.621784821875001281 ) ) ;
#64290=CARTESIAN_POINT ( 'NONE',  ( 2.121784821874999061, 12.00312500061451715, -33.67503911421598417 ) ) ;
#64292=CARTESIAN_POINT ( 'NONE',  ( -3.999999999999999112, 11.90000000000000036, -30.00000000000000000 ) ) ;
#64294=ORIENTED_EDGE ( 'NONE', *, *, #55830, .F. ) ;
#64295=CARTESIAN_POINT ( 'NONE',  ( 25.60312500061451502, 4.541064518000418104, -2.621784821874998173 ) ) ;
#64297=CARTESIAN_POINT ( 'NONE',  ( 25.32187500061451857, 3.027376345333611329, 5.243569643749999010 ) ) ;
#64298=CARTESIAN_POINT ( 'NONE',  ( 28.65937500061451715, -4.541064518000417216, -2.621784821875001281 ) ) ;
#64299=CARTESIAN_POINT ( 'NONE',  ( 22.53750000000000142, -2.886751345948125991, -5.000000000000000000 ) ) ;
#64300=CARTESIAN_POINT ( 'NONE',  ( 3.665625000614517681, 3.027376345333611329, 5.243569643749999010 ) ) ;
#64302=CARTESIAN_POINT ( 'NONE',  ( 17.22187500061451715, 3.027376345333611329, 5.243569643749999010 ) ) ;
#64304=CARTESIAN_POINT ( 'NONE',  ( 3.178125000614515638, 4.541064518000418104, 2.621784821874999949 ) ) ;
#64305=CARTESIAN_POINT ( 'NONE',  ( 8.971875000614515372, 3.027376345333613106, -5.243569643749998122 ) ) ;
#64306=CARTESIAN_POINT ( 'NONE',  ( 17.89687500061451431, -3.027376345333610441, -5.243569643749999898 ) ) ;
#64308=CARTESIAN_POINT ( 'NONE',  ( 25.91250000000000142, 2.886751345948126879, 4.999999999999999112 ) ) ;
#64309=CARTESIAN_POINT ( 'NONE',  ( 28.02187500061451431, 3.027376345333611329, 5.243569643749999010 ) ) ;
#64310=CYLINDRICAL_SURFACE ( 'NONE', #72656, 4.999999999999998224 ) ;
#64311=CARTESIAN_POINT ( 'NONE',  ( 14.28750000122903430, 4.330127018922191873, 2.499999999999999556 ) ) ;
#64312=ORIENTED_EDGE ( 'NONE', *, *, #58905, .T. ) ;
#64313=CARTESIAN_POINT ( 'NONE',  ( 8.775000000000002132, 4.330127018922191873, 2.499999999999999556 ) ) ;
#64315=CARTESIAN_POINT ( 'NONE',  ( 22.07812500061451644, 4.541064518000418104, 2.621784821874999949 ) ) ;
#64316=CARTESIAN_POINT ( 'NONE',  ( 11.17500000000000071, -4.330127018922194537, 2.499999999999995559 ) ) ;
#64317=CARTESIAN_POINT ( 'NONE',  ( 7.537500001229033408, 4.330127018922191873, 2.499999999999999556 ) ) ;
#64318=CARTESIAN_POINT ( 'NONE',  ( 6.553125000614518747, -4.541064518000417216, -2.621784821875001281 ) ) ;
#64319=CARTESIAN_POINT ( 'NONE',  ( 23.02499999999999858, 6.123233995736764310E-16, -4.999999999999998224 ) ) ;
#64320=CARTESIAN_POINT ( 'NONE',  ( 19.94062500061451715, -3.027376345333614438, 5.243569643749998122 ) ) ;
#64321=CARTESIAN_POINT ( 'NONE',  ( 25.65000000122903145, -2.886751345948129988, 4.999999999999997335 ) ) ;
#64323=CARTESIAN_POINT ( 'NONE',  ( 4.762499999999999289, 2.886751345948126879, 4.999999999999999112 ) ) ;
#64324=ORIENTED_EDGE ( 'NONE', *, *, #9299, .F. ) ;
#64325=CARTESIAN_POINT ( 'NONE',  ( 19.49062500061451431, -3.027376345333614438, 5.243569643749998122 ) ) ;
#64326=CARTESIAN_POINT ( 'NONE',  ( 25.75312500061451715, 0.000000000000000000, 5.243569643749999010 ) ) ;
#64327=CARTESIAN_POINT ( 'NONE',  ( 27.42187500061451644, 3.027376345333613106, -5.243569643749998122 ) ) ;
#64328=EDGE_CURVE ( 'NONE', #57266, #46535, #31551, .T. ) ;
#64329=CARTESIAN_POINT ( 'NONE',  ( 13.86562500061451431, 3.027376345333613106, -5.243569643749998122 ) ) ;
#64330=CARTESIAN_POINT ( 'NONE',  ( 28.97812500061451502, -4.541064518000419881, 2.621784821874995952 ) ) ;
#64331=CARTESIAN_POINT ( 'NONE',  ( 9.928125000614517859, 4.541064518000418104, 2.621784821874999949 ) ) ;
#64333=CARTESIAN_POINT ( 'NONE',  ( -4.243569643749997233, 13.14687500061451786, 32.45002607614398471 ) ) ;
#64334=AXIS2_PLACEMENT_3D ( 'NONE', #56877, #51714, #28100 ) ;
#64335=CARTESIAN_POINT ( 'NONE',  ( 25.83750000122903501, 6.123233995736764310E-16, -4.999999999999998224 ) ) ;
#64337=CARTESIAN_POINT ( 'NONE',  ( 16.90312500061451573, -4.541064518000417216, -2.621784821875001281 ) ) ;
#64339=CARTESIAN_POINT ( 'NONE',  ( 9.421875000614519990, 3.027376345333613106, -5.243569643749998122 ) ) ;
#64340=CARTESIAN_POINT ( 'NONE',  ( 8.634375000614518569, 4.541064518000418104, 2.621784821874999949 ) ) ;
#64341=CARTESIAN_POINT ( 'NONE',  ( 17.89687500061451431, -3.027376345333610441, -5.243569643749999898 ) ) ;
#64342=ORIENTED_EDGE ( 'NONE', *, *, #68280, .F. ) ;
#64343=CARTESIAN_POINT ( 'NONE',  ( 29.48437500061451644, -4.541064518000419881, 2.621784821874995952 ) ) ;
#64344=CARTESIAN_POINT ( 'NONE',  ( 22.11562500061451786, 3.027376345333611329, 5.243569643749999010 ) ) ;
#64346=CARTESIAN_POINT ( 'NONE',  ( 15.42187500061451821, 3.027376345333611329, 5.243569643749999010 ) ) ;
#64347=CARTESIAN_POINT ( 'NONE',  ( 22.67812500061451431, -4.541064518000419881, 2.621784821874995952 ) ) ;
#64348=CARTESIAN_POINT ( 'NONE',  ( -3.999999999999997335, 13.73749999999999893, 32.30940107675850470 ) ) ;
#64349=CARTESIAN_POINT ( 'NONE',  ( 26.95312500061451644, 4.541064518000418104, -2.621784821874998173 ) ) ;
#64350=CARTESIAN_POINT ( 'NONE',  ( 8.400000001229035007, 5.773502691896255534, 3.535250795749688894E-16 ) ) ;
#64351=VECTOR ( 'NONE', #31890, 1000.000000000000000 ) ;
#64353=CARTESIAN_POINT ( 'NONE',  ( 4.875000001229034652, 2.886751345948126879, 4.999999999999999112 ) ) ;
#64354=CARTESIAN_POINT ( 'NONE',  ( -2.000000000000000000, 16.77500000000000213, -33.46410161513775705 ) ) ;
#64355=CARTESIAN_POINT ( 'NONE',  ( 24.03750000122903430, 6.123233995736764310E-16, -4.999999999999998224 ) ) ;
#64357=CARTESIAN_POINT ( 'NONE',  ( 6.421875000614519102, 3.027376345333611329, 5.243569643749999010 ) ) ;
#64359=CARTESIAN_POINT ( 'NONE',  ( 14.50312500061451537, 0.000000000000000000, 5.243569643749999010 ) ) ;
#64360=CARTESIAN_POINT ( 'NONE',  ( 11.44687500061451857, -3.027376345333614438, 5.243569643749998122 ) ) ;
#64361=CARTESIAN_POINT ( 'NONE',  ( 27.60000000122903430, -2.886751345948125991, -5.000000000000000000 ) ) ;
#64362=CARTESIAN_POINT ( 'NONE',  ( 17.25937500061451502, 0.000000000000000000, 5.243569643749999010 ) ) ;
#64363=CARTESIAN_POINT ( 'NONE',  ( 4.996875000614516615, 6.054752690667223547, 3.707466751127219781E-16 ) ) ;
#64365=CARTESIAN_POINT ( 'NONE',  ( 7.865625000614516971, -6.054752690667223547, -1.112240025338166033E-15 ) ) ;
#64366=CARTESIAN_POINT ( 'NONE',  ( 17.09062500061451573, 6.054752690667223547, 3.707466751127219781E-16 ) ) ;
#64367=ORIENTED_EDGE ( 'NONE', *, *, #34144, .T. ) ;
#64368=CARTESIAN_POINT ( 'NONE',  ( 14.50312500061451537, 0.000000000000000000, 5.243569643749999010 ) ) ;
#64369=CARTESIAN_POINT ( 'NONE',  ( 8.775000001229033231, 2.886751345948129099, -4.999999999999998224 ) ) ;
#64370=CARTESIAN_POINT ( 'NONE',  ( 9.740625000614516082, -3.027376345333610441, -5.243569643749999898 ) ) ;
#64372=CARTESIAN_POINT ( 'NONE',  ( 10.38750000000000107, -2.886751345948125991, -5.000000000000000000 ) ) ;
#64373=CARTESIAN_POINT ( 'NONE',  ( 5.850000001229035185, -2.886751345948129988, 4.999999999999997335 ) ) ;
#64374=CARTESIAN_POINT ( 'NONE',  ( 15.12187500061451750, -6.054752690667223547, -1.112240025338166033E-15 ) ) ;
#64375=CARTESIAN_POINT ( 'NONE',  ( 16.38750000122903216, 6.123233995736764310E-16, -4.999999999999998224 ) ) ;
#64378=CARTESIAN_POINT ( 'NONE',  ( -4.243569643749999898, 19.31562500061451715, -32.45002607614398471 ) ) ;
#64382=CARTESIAN_POINT ( 'NONE',  ( 2.000000000000001332, 14.41250000122903430, 33.46410161513774995 ) ) ;
#64383=CARTESIAN_POINT ( 'NONE',  ( 15.23437500061451644, 6.421520780324663323E-16, -5.243569643749999010 ) ) ;
#64384=( BOUNDED_CURVE ( )  B_SPLINE_CURVE ( 2, ( #67059, #38607, #61490, #33055, #55955, #28604, #5351, #44526, #45238 ),
 .UNSPECIFIED., .F., .F. ) 
 B_SPLINE_CURVE_WITH_KNOTS ( ( 3, 2, 2, 2, 3 ),
 ( 0.4239130434782608647, 0.4275362318840579823, 0.4347826086956521618, 0.4420289855072463969, 0.4456521739130435145 ),
 .UNSPECIFIED. ) 
 CURVE ( )  GEOMETRIC_REPRESENTATION_ITEM ( )  RATIONAL_B_SPLINE_CURVE ( ( 0.9330127018922194093, 0.9330127018922194093, 1.000000000000000000, 0.8660254037844387076, 1.000000000000000000, 0.8660254037844387076, 1.000000000000000000, 0.9330127018922188542, 0.9330127018922194093 ) ) 
 REPRESENTATION_ITEM ( '' )  );
#64385=CARTESIAN_POINT ( 'NONE',  ( 29.69999999999999574, -4.330127018922190985, -2.500000000000001332 ) ) ;
#64387=CARTESIAN_POINT ( 'NONE',  ( 14.65312500061451573, -4.541064518000417216, -2.621784821875001281 ) ) ;
#64389=CARTESIAN_POINT ( 'NONE',  ( 22.84687500061451715, -3.027376345333610441, -5.243569643749999898 ) ) ;
#64391=CARTESIAN_POINT ( 'NONE',  ( 9.928125000614517859, 4.541064518000418104, 2.621784821874999949 ) ) ;
#64392=CARTESIAN_POINT ( 'NONE',  ( 14.52187500061451608, 3.027376345333611329, 5.243569643749999010 ) ) ;
#64393=ORIENTED_EDGE ( 'NONE', *, *, #7054, .T. ) ;
#64394=CARTESIAN_POINT ( 'NONE',  ( 26.48437500061451644, 6.421520780324663323E-16, -5.243569643749999010 ) ) ;
#64395=CARTESIAN_POINT ( 'NONE',  ( 28.37812500061451715, 4.541064518000418104, 2.621784821874999949 ) ) ;
#64396=CARTESIAN_POINT ( 'NONE',  ( 18.92812500061451431, 4.541064518000418104, 2.621784821874999949 ) ) ;
#64397=CARTESIAN_POINT ( 'NONE',  ( 29.61562500061451431, 3.027376345333613106, -5.243569643749998122 ) ) ;
#64398=CARTESIAN_POINT ( 'NONE',  ( 4.869452396223757695, 1.135286901598331566, -5.119236970012235766 ) ) ;
#64399=CARTESIAN_POINT ( 'NONE',  ( 7.987500000000000711, -2.886751345948129988, 4.999999999999997335 ) ) ;
#64400=CARTESIAN_POINT ( 'NONE',  ( 20.36250000122903359, -4.330127018922190985, -2.500000000000001332 ) ) ;
#64401=CARTESIAN_POINT ( 'NONE',  ( -5.810221930991193690E-16, 18.65000000122903501, -34.00000000000000000 ) ) ;
#64403=VERTEX_POINT ( 'NONE', #230 ) ;
#64404=CARTESIAN_POINT ( 'NONE',  ( 17.39999999999999858, 0.000000000000000000, 4.999999999999998224 ) ) ;
#64405=CARTESIAN_POINT ( 'NONE',  ( 19.20000000000000284, 0.000000000000000000, 4.999999999999998224 ) ) ;
#64406=CARTESIAN_POINT ( 'NONE',  ( 18.94687500061451502, 6.054752690667223547, 3.707466751127219781E-16 ) ) ;
#64407=CARTESIAN_POINT ( 'NONE',  ( 14.01562500061451644, 3.027376345333611329, 5.243569643749999010 ) ) ;
#64409=CARTESIAN_POINT ( 'NONE',  ( 1.626862140677534273E-15, 18.42500000122903359, -26.00000000000000355 ) ) ;
#64410=CARTESIAN_POINT ( 'NONE',  ( 5.240625000614516971, -3.027376345333610441, -5.243569643749999898 ) ) ;
#64412=CARTESIAN_POINT ( 'NONE',  ( 11.88749999999999751, 5.773502691896255534, 3.535250795749688894E-16 ) ) ;
#64414=CARTESIAN_POINT ( 'NONE',  ( 4.243569643749999010, 15.11562500061451608, 27.54997392385601174 ) ) ;
#64415=CARTESIAN_POINT ( 'NONE',  ( 26.84062500061451573, -3.027376345333610441, -5.243569643749999898 ) ) ;
#64418=CARTESIAN_POINT ( 'NONE',  ( 23.85937500061451644, 4.541064518000418104, -2.621784821874998173 ) ) ;
#64420=CARTESIAN_POINT ( 'NONE',  ( 22.45312500061451644, 4.541064518000418104, -2.621784821874998173 ) ) ;
#64421=CARTESIAN_POINT ( 'NONE',  ( 22.20937500061451431, 0.000000000000000000, 5.243569643749999010 ) ) ;
#64422=CARTESIAN_POINT ( 'NONE',  ( 9.001249775931846008E-16, 16.31562500061459176, -25.09994784771203058 ) ) ;
#64423=CARTESIAN_POINT ( 'NONE',  ( 7.678125000614516082, 4.541064518000418104, 2.621784821874999949 ) ) ;
#64425=CARTESIAN_POINT ( 'NONE',  ( 24.89062500061451644, -3.027376345333614438, 5.243569643749998122 ) ) ;
#64428=CARTESIAN_POINT ( 'NONE',  ( 16.84687500061451715, -3.027376345333614438, 5.243569643749998122 ) ) ;
#64429=CARTESIAN_POINT ( 'NONE',  ( 25.43437500061451573, -4.541064518000419881, 2.621784821874995952 ) ) ;
#64430=CARTESIAN_POINT ( 'NONE',  ( 4.243569643749999898, 13.78437500061451715, 30.00000000000000000 ) ) ;
#64431=CARTESIAN_POINT ( 'NONE',  ( 5.315625000614516260, 3.027376345333613106, -5.243569643749998122 ) ) ;
#64432=CARTESIAN_POINT ( 'NONE',  ( 29.42812500061451431, -4.541064518000419881, 2.621784821874995952 ) ) ;
#64433=CARTESIAN_POINT ( 'NONE',  ( 3.009375000614516793, -4.541064518000417216, -2.621784821875001281 ) ) ;
#64435=CARTESIAN_POINT ( 'NONE',  ( 4.228125000614517681, -4.541064518000419881, 2.621784821874995952 ) ) ;
#64436=CARTESIAN_POINT ( 'NONE',  ( 8.484375000614518214, 6.421520780324663323E-16, -5.243569643749999010 ) ) ;
#64438=CARTESIAN_POINT ( 'NONE',  ( 15.82500000122903216, -5.773502691896255534, -1.060575238724906372E-15 ) ) ;
#64439=CARTESIAN_POINT ( 'NONE',  ( 29.57812500061451644, 6.421520780324663323E-16, -5.243569643749999010 ) ) ;
#64440=CARTESIAN_POINT ( 'NONE',  ( 6.215625000614517504, 3.027376345333613106, -5.243569643749998122 ) ) ;
#64443=CARTESIAN_POINT ( 'NONE',  ( 14.03437500061451715, 4.541064518000418104, 2.621784821874999949 ) ) ;
#64444=CARTESIAN_POINT ( 'NONE',  ( 3.999999999999998668, 17.67500000122903359, 27.69059892324149530 ) ) ;
#64445=VERTEX_POINT ( 'NONE', #6483 ) ;
#64446=CARTESIAN_POINT ( 'NONE',  ( 21.06562500061451715, 3.027376345333613106, -5.243569643749998122 ) ) ;
#64447=CARTESIAN_POINT ( 'NONE',  ( 7.228125000614517681, 4.541064518000418104, 2.621784821874999949 ) ) ;
#64449=CARTESIAN_POINT ( 'NONE',  ( 24.53437500061451715, -4.541064518000419881, 2.621784821874995952 ) ) ;
#64450=CARTESIAN_POINT ( 'NONE',  ( 7.790625000614518569, -3.027376345333614438, 5.243569643749998122 ) ) ;
#64451=CARTESIAN_POINT ( 'NONE',  ( 18.97499999999999787, 6.123233995736764310E-16, -4.999999999999998224 ) ) ;
#64452=CARTESIAN_POINT ( 'NONE',  ( 10.87500000122903288, -5.773502691896255534, -1.060575238724906372E-15 ) ) ;
#64453=CARTESIAN_POINT ( 'NONE',  ( 25.19062500061451715, 6.054752690667223547, 3.707466751127219781E-16 ) ) ;
#64454=CARTESIAN_POINT ( 'NONE',  ( -0.7368814052146555049, 9.803648494990884643, -34.17910147232696261 ) ) ;
#64455=CARTESIAN_POINT ( 'NONE',  ( 10.05000000122903181, -2.886751345948125991, -5.000000000000000000 ) ) ;
#64456=CARTESIAN_POINT ( 'NONE',  ( 22.37812500061451360, 6.421520780324663323E-16, -5.243569643749999010 ) ) ;
#64457=CARTESIAN_POINT ( 'NONE',  ( 19.07812500061451644, -4.541064518000419881, 2.621784821874995952 ) ) ;
#64459=CARTESIAN_POINT ( 'NONE',  ( 18.52499999999999858, 6.123233995736764310E-16, -4.999999999999998224 ) ) ;
#64460=CARTESIAN_POINT ( 'NONE',  ( 13.76250000122903394, 4.330127018922192761, -2.499999999999997780 ) ) ;
#64461=CARTESIAN_POINT ( 'NONE',  ( 11.24062500061451608, 6.054752690667223547, 3.707466751127219781E-16 ) ) ;
#64462=CARTESIAN_POINT ( 'NONE',  ( 12.77812500061451750, -4.541064518000419881, 2.621784821874995952 ) ) ;
#64463=CARTESIAN_POINT ( 'NONE',  ( 22.72500000122903430, 2.886751345948129099, -4.999999999999998224 ) ) ;
#64464=CARTESIAN_POINT ( 'NONE',  ( 22.05937500061451573, 4.541064518000418104, -2.621784821874998173 ) ) ;
#64465=CARTESIAN_POINT ( 'NONE',  ( 21.98437500061451644, 6.421520780324663323E-16, -5.243569643749999010 ) ) ;
#64467=CARTESIAN_POINT ( 'NONE',  ( 7.875000001229034652, 2.886751345948129099, -4.999999999999998224 ) ) ;
#64468=CARTESIAN_POINT ( 'NONE',  ( 6.759375000614516793, 4.541064518000418104, -2.621784821874998173 ) ) ;
#64469=CARTESIAN_POINT ( 'NONE',  ( 24.30937500061451573, 4.541064518000418104, -2.621784821874998173 ) ) ;
#64470=CARTESIAN_POINT ( 'NONE',  ( 4.544030691951923551, 2.086093255490381715, -4.659623712765267989 ) ) ;
#64471=CARTESIAN_POINT ( 'NONE',  ( 22.04062500061451502, 6.054752690667223547, 3.707466751127219781E-16 ) ) ;
#64472=CARTESIAN_POINT ( 'NONE',  ( 23.07187500061451857, 3.027376345333611329, 5.243569643749999010 ) ) ;
#64476=CARTESIAN_POINT ( 'NONE',  ( 1.626862140677534273E-15, 15.61250000000000071, 34.00000000000000000 ) ) ;
#64477=CARTESIAN_POINT ( 'NONE',  ( 5.934375000614517504, 4.541064518000418104, 2.621784821874999949 ) ) ;
#64478=CARTESIAN_POINT ( 'NONE',  ( 17.01562500061451644, 3.027376345333613106, -5.243569643749998122 ) ) ;
#64479=EDGE_LOOP ( 'NONE', ( #33421, #13652, #66426, #7799 ) ) ;
#64480=FACE_OUTER_BOUND ( 'NONE', #54237, .T. ) ;
#64481=CARTESIAN_POINT ( 'NONE',  ( 25.60312500061451502, 4.541064518000418104, -2.621784821874998173 ) ) ;
#64482=CARTESIAN_POINT ( 'NONE',  ( 2.896875000614518747, -3.027376345333614438, 5.243569643749998122 ) ) ;
#64483=CARTESIAN_POINT ( 'NONE',  ( 4.720164951879130655, 1.649934272948560654, 4.824171440055819993 ) ) ;
#64484=CARTESIAN_POINT ( 'NONE',  ( 8.512500001229033941, 0.000000000000000000, 4.999999999999998224 ) ) ;
#64485=CARTESIAN_POINT ( 'NONE',  ( 13.61250000000000071, 2.886751345948129099, -4.999999999999998224 ) ) ;
#64486=CARTESIAN_POINT ( 'NONE',  ( 19.90312500061451573, 0.000000000000000000, 5.243569643749999010 ) ) ;
#64488=CARTESIAN_POINT ( 'NONE',  ( 24.22500000000000142, -4.330127018922194537, 2.499999999999995559 ) ) ;
#64489=EDGE_CURVE ( 'NONE', #44084, #41163, #46660, .T. ) ;
#64490=CARTESIAN_POINT ( 'NONE',  ( 25.92187500061451999, -6.054752690667223547, -1.112240025338166033E-15 ) ) ;
#64491=ORIENTED_EDGE ( 'NONE', *, *, #35816, .T. ) ;
#64492=CARTESIAN_POINT ( 'NONE',  ( 3.009043979185748174, -3.993209162649682842, -3.398434824636790363 ) ) ;
#64493=CARTESIAN_POINT ( 'NONE',  ( 13.15312500061451750, 0.000000000000000000, 5.243569643749999010 ) ) ;
#64494=CARTESIAN_POINT ( 'NONE',  ( 25.05000000122903359, 5.773502691896255534, 3.535250795749688401E-16 ) ) ;
#64496=CARTESIAN_POINT ( 'NONE',  ( 28.45312500061451289, 0.000000000000000000, 5.243569643749999010 ) ) ;
#64497=CARTESIAN_POINT ( 'NONE',  ( 13.57500000122903572, -5.773502691896255534, -1.060575238724906372E-15 ) ) ;
#64498=CARTESIAN_POINT ( 'NONE',  ( 18.71249999999999858, 2.886751345948126879, 4.999999999999999112 ) ) ;
#64499=CARTESIAN_POINT ( 'NONE',  ( 26.88749999999999574, -2.886751345948129988, 4.999999999999997335 ) ) ;
#64500=CARTESIAN_POINT ( 'NONE',  ( 3.182137239616405822, -4.123714228212172372, 2.857517440841834233 ) ) ;
#64501=CARTESIAN_POINT ( 'NONE',  ( 6.196875000614515905, -3.027376345333610441, -5.243569643749999898 ) ) ;
#64502=CARTESIAN_POINT ( 'NONE',  ( 18.90937500061451360, 4.541064518000418104, -2.621784821874998173 ) ) ;
#64504=ORIENTED_EDGE ( 'NONE', *, *, #21977, .F. ) ;
#64505=CARTESIAN_POINT ( 'NONE',  ( 2.859375000614519546, 0.000000000000000000, 5.243569643749999010 ) ) ;
#64506=CARTESIAN_POINT ( 'NONE',  ( 29.37187500061451928, 3.027376345333611329, 5.243569643749999010 ) ) ;
#64507=CARTESIAN_POINT ( 'NONE',  ( 4.996875000614516615, 6.054752690667223547, 3.707466751127219781E-16 ) ) ;
#64508=CARTESIAN_POINT ( 'NONE',  ( 17.36249999999999716, 2.886751345948126879, 4.999999999999999112 ) ) ;
#64509=CARTESIAN_POINT ( 'NONE',  ( 12.96562500061451750, 3.027376345333613106, -5.243569643749998122 ) ) ;
#64510=CARTESIAN_POINT ( 'NONE',  ( 3.586992791275801729, 3.483314903268937446, -3.919380039434936513 ) ) ;
#64512=CARTESIAN_POINT ( 'NONE',  ( 3.947751918878622757, -3.068428716296062841, 3.947751918878600108 ) ) ;
#64513=CARTESIAN_POINT ( 'NONE',  ( 17.81250000122903288, 4.330127018922192761, -2.499999999999997780 ) ) ;
#64516=CARTESIAN_POINT ( 'NONE',  ( 7.490625000614516082, -3.027376345333610441, -5.243569643749999898 ) ) ;
#64517=CARTESIAN_POINT ( 'NONE',  ( 24.72187500061451360, 3.027376345333613106, -5.243569643749998122 ) ) ;
#64518=CARTESIAN_POINT ( 'NONE',  ( 2.121784821875001281, 19.10937500061451644, 33.67503911421598417 ) ) ;
#64519=CARTESIAN_POINT ( 'NONE',  ( 23.52187500061451786, 3.027376345333611329, 5.243569643749999010 ) ) ;
#64520=CARTESIAN_POINT ( 'NONE',  ( 5.287500000000000533, -2.886751345948129988, 4.999999999999997335 ) ) ;
#64521=CARTESIAN_POINT ( 'NONE',  ( 2.000000000000001332, 11.71250000122903501, 33.46410161513774995 ) ) ;
#64522=CARTESIAN_POINT ( 'NONE',  ( 14.54062500061451679, -3.027376345333614438, 5.243569643749998122 ) ) ;
#64523=CARTESIAN_POINT ( 'NONE',  ( 4.650000001229035895, -2.886751345948125991, -5.000000000000000000 ) ) ;
#64524=CARTESIAN_POINT ( 'NONE',  ( 10.13437500061451679, -4.541064518000419881, 2.621784821874995952 ) ) ;
#64525=CARTESIAN_POINT ( 'NONE',  ( 4.000000000000000000, 14.90000000122903323, 32.30940107675849760 ) ) ;
#64527=CARTESIAN_POINT ( 'NONE',  ( 13.52812500061451750, 4.541064518000418104, 2.621784821874999949 ) ) ;
#64528=CARTESIAN_POINT ( 'NONE',  ( 3.422429900546629877, -3.645130117820770455, -3.769356580772429410 ) ) ;
#64529=CARTESIAN_POINT ( 'NONE',  ( 23.21250000122903501, 4.330127018922192761, -2.499999999999997780 ) ) ;
#64530=CARTESIAN_POINT ( 'NONE',  ( 11.29687500061451644, 6.054752690667223547, 3.707466751127219781E-16 ) ) ;
#64531=CARTESIAN_POINT ( 'NONE',  ( 11.57812500061451644, 6.421520780324663323E-16, -5.243569643749999010 ) ) ;
#64533=CARTESIAN_POINT ( 'NONE',  ( 24.00937500061451502, 0.000000000000000000, 5.243569643749999010 ) ) ;
#64534=CARTESIAN_POINT ( 'NONE',  ( 0.000000000000000000, 20.00000000000000000, -30.00000000000000000 ) ) ;
#64536=VECTOR ( 'NONE', #63020, 1000.000000000000000 ) ;
#64537=CARTESIAN_POINT ( 'NONE',  ( 20.47500000122903074, 2.886751345948162850, -4.999999999999940492 ) ) ;
#64538=CARTESIAN_POINT ( 'NONE',  ( -3.000416591977282496E-16, 13.89687500061451608, -34.90005215228797653 ) ) ;
#64539=CARTESIAN_POINT ( 'NONE',  ( 16.95937500061451786, -4.541064518000417216, -2.621784821875001281 ) ) ;
#64540=CARTESIAN_POINT ( 'NONE',  ( 16.80000000122903359, -2.886751345948125991, -5.000000000000000000 ) ) ;
#64541=CARTESIAN_POINT ( 'NONE',  ( 12.57187500061451857, 3.027376345333613106, -5.243569643749998122 ) ) ;
#64542=CARTESIAN_POINT ( 'NONE',  ( -4.243569643749997233, 16.69062500061451360, -27.54997392385601174 ) ) ;
#64543=CARTESIAN_POINT ( 'NONE',  ( 19.80000000122903359, -2.886751345948129988, 4.999999999999997335 ) ) ;
#64544=CARTESIAN_POINT ( 'NONE',  ( 12.66562500061451502, 3.027376345333611329, 5.243569643749999010 ) ) ;
#64547=CARTESIAN_POINT ( 'NONE',  ( 15.48749999999999893, 5.773502691896255534, 3.535250795749688894E-16 ) ) ;
#64549=CARTESIAN_POINT ( 'NONE',  ( 11.59687500061451892, -3.027376345333610441, -5.243569643749999898 ) ) ;
#64550=FACE_OUTER_BOUND ( 'NONE', #16802, .T. ) ;
#64551=EDGE_CURVE ( 'NONE', #72719, #46824, #28650, .T. ) ;
#64552=CARTESIAN_POINT ( 'NONE',  ( 12.41250000122903430, 4.330127018922192761, -2.499999999999997780 ) ) ;
#64553=CARTESIAN_POINT ( 'NONE',  ( 20.06250000122903643, 4.330127018922192761, -2.499999999999997780 ) ) ;
#64554=EDGE_CURVE ( 'NONE', #36412, #72350, #34183, .T. ) ;
#64555=CARTESIAN_POINT ( 'NONE',  ( 17.72812500061451502, -4.541064518000419881, 2.621784821874995952 ) ) ;
#64557=CARTESIAN_POINT ( 'NONE',  ( 20.01562500061451644, -6.054752690667223547, -1.112240025338166033E-15 ) ) ;
#64558=CARTESIAN_POINT ( 'NONE',  ( 27.97500000122903074, -5.773502691896255534, -1.060575238724906372E-15 ) ) ;
#64559=CARTESIAN_POINT ( 'NONE',  ( 25.46249999999999858, 2.886751345948126879, 4.999999999999999112 ) ) ;
#64560=CARTESIAN_POINT ( 'NONE',  ( 5.857864376269049878, -9.999999999999992895, 5.857864376269049878 ) ) ;
#64562=CARTESIAN_POINT ( 'NONE',  ( 28.92187500061451644, 3.027376345333611329, 5.243569643749999010 ) ) ;
#64563=LINE ( 'NONE', #13218, #22874 ) ;
#64564=CARTESIAN_POINT ( 'NONE',  ( -2.121784821874999949, 12.58437500061451786, -33.67503911421598417 ) ) ;
#64565=CARTESIAN_POINT ( 'NONE',  ( 4.462500001229035007, 0.000000000000000000, 4.999999999999998224 ) ) ;
#64566=CARTESIAN_POINT ( 'NONE',  ( 4.837500000000001243, -2.886751345948129988, 4.999999999999997335 ) ) ;
#64568=CARTESIAN_POINT ( 'NONE',  ( 7.996875000614519280, -3.027376345333610441, -5.243569643749999898 ) ) ;
#64569=CARTESIAN_POINT ( 'NONE',  ( 28.04062500061451502, -3.027376345333614438, 5.243569643749998122 ) ) ;
#64570=FACE_OUTER_BOUND ( 'NONE', #4929, .T. ) ;
#64571=CARTESIAN_POINT ( 'NONE',  ( -1.587936087009578445, 9.880963660774179758, -35.79978921151577964 ) ) ;
#64572=CARTESIAN_POINT ( 'NONE',  ( 16.83750000122903145, 6.123233995736764310E-16, -4.999999999999998224 ) ) ;
#64573=CARTESIAN_POINT ( 'NONE',  ( 5.596875000614516260, -3.027376345333614438, 5.243569643749998122 ) ) ;
#64574=CARTESIAN_POINT ( 'NONE',  ( 11.59687500061451892, -3.027376345333610441, -5.243569643749999898 ) ) ;
#64575=CARTESIAN_POINT ( 'NONE',  ( 4.612500000000002487, 2.886751345948129099, -4.999999999999998224 ) ) ;
#64576=CARTESIAN_POINT ( 'NONE',  ( 2.121784821875001281, 15.00312500061459353, 33.67503911421598417 ) ) ;
#64579=CARTESIAN_POINT ( 'NONE',  ( 6.862500000000002487, 2.886751345948129099, -4.999999999999998224 ) ) ;
#64581=CARTESIAN_POINT ( 'NONE',  ( 20.12812500061451715, 6.421520780324663323E-16, -5.243569643749999010 ) ) ;
#64582=CARTESIAN_POINT ( 'NONE',  ( 12.21562500061451573, 3.027376345333611329, 5.243569643749999010 ) ) ;
#64584=CARTESIAN_POINT ( 'NONE',  ( 10.58437500061451964, -4.541064518000419881, 2.621784821874995952 ) ) ;
#64585=CARTESIAN_POINT ( 'NONE',  ( 25.23749999999999716, -2.886751345948125991, -5.000000000000000000 ) ) ;
#64586=CARTESIAN_POINT ( 'NONE',  ( 22.23750000122903003, 6.123233995736764310E-16, -4.999999999999998224 ) ) ;
#64587=CARTESIAN_POINT ( 'NONE',  ( 1.999999999999998668, 10.96250000122903501, 26.53589838486224650 ) ) ;
#64588=CARTESIAN_POINT ( 'NONE',  ( 9.609375000614518214, 0.000000000000000000, 5.243569643749999010 ) ) ;
#64589=CARTESIAN_POINT ( 'NONE',  ( 27.57187500061451857, 3.027376345333611329, 5.243569643749999010 ) ) ;
#64591=LINE ( 'NONE', #36155, #39590 ) ;
#64592=CARTESIAN_POINT ( 'NONE',  ( 19.58437500061451786, -4.541064518000419881, 2.621784821874995952 ) ) ;
#64593=( BOUNDED_CURVE ( )  B_SPLINE_CURVE ( 2, ( #47958, #25787, #31324, #2167, #70115, #7336, #47586, #64936, #14327 ),
 .UNSPECIFIED., .F., .F. ) 
 B_SPLINE_CURVE_WITH_KNOTS ( ( 3, 2, 2, 2, 3 ),
 ( 0.03260869565217391908, 0.03623188405797101580, 0.04347826086956521618, 0.05072463768115942351, 0.05434782608695652717 ),
 .UNSPECIFIED. ) 
 CURVE ( )  GEOMETRIC_REPRESENTATION_ITEM ( )  RATIONAL_B_SPLINE_CURVE ( ( 0.9330127018922192983, 0.9330127018922194093, 1.000000000000000000, 0.8660254037844387076, 1.000000000000000000, 0.8660254037844387076, 1.000000000000000000, 0.9330127018922192983, 0.9330127018922194093 ) ) 
 REPRESENTATION_ITEM ( '' )  );
#64594=CARTESIAN_POINT ( 'NONE',  ( 12.94687500061451857, -3.027376345333610441, -5.243569643749999898 ) ) ;
#64596=CARTESIAN_POINT ( 'NONE',  ( 24.07499999999999929, 4.330127018922191873, 2.499999999999999556 ) ) ;
#64598=CARTESIAN_POINT ( 'NONE',  ( 4.243569643749999898, 12.88437500061451857, -30.00000000000000000 ) ) ;
#64600=CARTESIAN_POINT ( 'NONE',  ( 15.17812500061451608, 6.421520780324663323E-16, -5.243569643749999010 ) ) ;
#64601=CARTESIAN_POINT ( 'NONE',  ( 4.200000000000001954, 4.330127018922192761, -2.499999999999997780 ) ) ;
#64604=( BOUNDED_CURVE ( )  B_SPLINE_CURVE ( 2, ( #22081, #33888, #16172, #56071, #33168, #49806, #66425, #28353, #290 ),
 .UNSPECIFIED., .F., .F. ) 
 B_SPLINE_CURVE_WITH_KNOTS ( ( 3, 2, 2, 2, 3 ),
 ( 0.5108695652173913526, 0.5144927536231883591, 0.5217391304347825942, 0.5289855072463768293, 0.5326086956521739468 ),
 .UNSPECIFIED. ) 
 CURVE ( )  GEOMETRIC_REPRESENTATION_ITEM ( )  RATIONAL_B_SPLINE_CURVE ( ( 0.9330127018922192983, 0.9330127018922202975, 1.000000000000000000, 0.8660254037844387076, 1.000000000000000000, 0.8660254037844387076, 1.000000000000000000, 0.9330127018922194093, 0.9330127018922194093 ) ) 
 REPRESENTATION_ITEM ( '' )  );
#64605=CARTESIAN_POINT ( 'NONE',  ( 11.21250000000000036, -5.773502691896255534, -1.060575238724906372E-15 ) ) ;
#64606=CARTESIAN_POINT ( 'NONE',  ( 1.999999999999998668, 17.26250000122903572, 26.53589838486224650 ) ) ;
#64607=CARTESIAN_POINT ( 'NONE',  ( 13.83750000122903323, 4.330127018922191873, 2.499999999999999556 ) ) ;
#64608=CARTESIAN_POINT ( 'NONE',  ( 24.60937500061451644, -4.541064518000417216, -2.621784821875001281 ) ) ;
#64609=CARTESIAN_POINT ( 'NONE',  ( 16.95937500061451786, -4.541064518000417216, -2.621784821875001281 ) ) ;
#64610=DIRECTION ( 'NONE',  ( -1.000000000000000000, -0.000000000000000000, -0.000000000000000000 ) ) ;
#64612=CARTESIAN_POINT ( 'NONE',  ( 19.11562500061451431, -6.054752690667223547, -1.112240025338166033E-15 ) ) ;
#64613=CARTESIAN_POINT ( 'NONE',  ( 5.128125000614516260, -4.541064518000419881, 2.621784821874995952 ) ) ;
#64614=CARTESIAN_POINT ( 'NONE',  ( 18.49687500061452283, 6.054752690667223547, 3.707466751127219781E-16 ) ) ;
#64615=CARTESIAN_POINT ( 'NONE',  ( 28.69687500061451502, -3.027376345333610441, -5.243569643749999898 ) ) ;
#64616=CARTESIAN_POINT ( 'NONE',  ( 4.790625000614518569, -3.027376345333610441, -5.243569643749999898 ) ) ;
#64617=CARTESIAN_POINT ( 'NONE',  ( 22.41562500061451502, 3.027376345333613106, -5.243569643749998122 ) ) ;
#64618=CARTESIAN_POINT ( 'NONE',  ( 2.121784821875001281, 15.45312500061451644, 33.67503911421598417 ) ) ;
#64619=CARTESIAN_POINT ( 'NONE',  ( 16.16250000122903430, 0.000000000000000000, 4.999999999999998224 ) ) ;
#64621=CARTESIAN_POINT ( 'NONE',  ( 7.415625000614516793, -6.054752690667223547, -1.112240025338166033E-15 ) ) ;
#64622=CARTESIAN_POINT ( 'NONE',  ( 27.75000000000000000, 0.000000000000000000, 4.999999999999998224 ) ) ;
#64623=CARTESIAN_POINT ( 'NONE',  ( 29.76562500061451644, 3.027376345333611329, 5.243569643749999010 ) ) ;
#64624=CARTESIAN_POINT ( 'NONE',  ( 22.05937500061451573, 4.541064518000418104, -2.621784821874998173 ) ) ;
#64625=CARTESIAN_POINT ( 'NONE',  ( 14.69062500061451537, -3.027376345333610441, -5.243569643749999898 ) ) ;
#64626=CARTESIAN_POINT ( 'NONE',  ( 25.31250000122903288, -4.330127018922190985, -2.500000000000001332 ) ) ;
#64628=CARTESIAN_POINT ( 'NONE',  ( 25.34062500061451217, -3.027376345333614438, 5.243569643749998122 ) ) ;
#64629=CARTESIAN_POINT ( 'NONE',  ( 20.07187500061451857, -6.054752690667223547, -1.112240025338166033E-15 ) ) ;
#64630=CARTESIAN_POINT ( 'NONE',  ( 14.35312500061451679, 4.541064518000418104, -2.621784821874998173 ) ) ;
#64631=CARTESIAN_POINT ( 'NONE',  ( -3.000416591977282496E-16, 13.89687500061451786, 25.09994784771203058 ) ) ;
#64632=CARTESIAN_POINT ( 'NONE',  ( 20.69062500061451715, 6.054752690667223547, 3.707466751127219781E-16 ) ) ;
#64633=CARTESIAN_POINT ( 'NONE',  ( 28.56562500061451715, -6.054752690667223547, -1.112240025338166033E-15 ) ) ;
#64635=CARTESIAN_POINT ( 'NONE',  ( 26.09999999999999787, -4.330127018922190985, -2.500000000000001332 ) ) ;
#64636=CARTESIAN_POINT ( 'NONE',  ( 3.999999999999998668, 10.81250000000000178, -32.30940107675850470 ) ) ;
#64638=CARTESIAN_POINT ( 'NONE',  ( 26.69062500061451715, -3.027376345333614438, 5.243569643749998122 ) ) ;
#64639=CARTESIAN_POINT ( 'NONE',  ( 8.053125000614516082, 4.541064518000418104, -2.621784821874998173 ) ) ;
#64640=CARTESIAN_POINT ( 'NONE',  ( 19.87500000122903288, -5.773502691896255534, -1.060575238724906372E-15 ) ) ;
#64642=CARTESIAN_POINT ( 'NONE',  ( 25.67812500061451431, 4.541064518000418104, 2.621784821874999949 ) ) ;
#64643=CARTESIAN_POINT ( 'NONE',  ( 26.36249999999999716, 2.886751345948126879, 4.999999999999999112 ) ) ;
#64644=ADVANCED_FACE ( 'NONE', ( #57441 ), #39384, .F. ) ;
#64645=CARTESIAN_POINT ( 'NONE',  ( 28.67812500061451431, 6.421520780324663323E-16, -5.243569643749999010 ) ) ;
#64646=CARTESIAN_POINT ( 'NONE',  ( 9.178125000614517859, -4.541064518000419881, 2.621784821874995952 ) ) ;
#64648=CARTESIAN_POINT ( 'NONE',  ( 24.51562500061451289, -6.054752690667223547, -1.112240025338166033E-15 ) ) ;
#64649=CARTESIAN_POINT ( 'NONE',  ( 4.453125000614517326, 4.541064518000418104, -2.621784821874998173 ) ) ;
#64651=CARTESIAN_POINT ( 'NONE',  ( 3.478125000614517237, 6.421520780324663323E-16, -5.243569643749999010 ) ) ;
#64652=CYLINDRICAL_SURFACE ( 'NONE', #7861, 3.999999999999996447 ) ;
#64653=CARTESIAN_POINT ( 'NONE',  ( 13.79999999999999893, 0.000000000000000000, 4.999999999999998224 ) ) ;
#64654=CARTESIAN_POINT ( 'NONE',  ( 13.13437500061451857, 4.541064518000418104, 2.621784821874999949 ) ) ;
#64655=CARTESIAN_POINT ( 'NONE',  ( 8.812500001229034652, 4.330127018922192761, -2.499999999999997780 ) ) ;
#64656=CARTESIAN_POINT ( 'NONE',  ( 16.43437500061451573, -4.541064518000419881, 2.621784821874995952 ) ) ;
#64658=CARTESIAN_POINT ( 'NONE',  ( 7.696875000614516793, 6.054752690667223547, 3.707466751127219781E-16 ) ) ;
#64659=CARTESIAN_POINT ( 'NONE',  ( -4.243569643749997233, 11.29062500061451857, -27.54997392385601174 ) ) ;
#64660=CYLINDRICAL_SURFACE ( 'NONE', #6461, 4.999999999999998224 ) ;
#64663=CARTESIAN_POINT ( 'NONE',  ( 24.89062500061451644, -3.027376345333614438, 5.243569643749998122 ) ) ;
#64664=CARTESIAN_POINT ( 'NONE',  ( -1.473772837211104303, 9.872922166578582903, 25.95083099200021692 ) ) ;
#64665=CARTESIAN_POINT ( 'NONE',  ( 21.22500000122903074, -5.773502691896255534, -1.060575238724906372E-15 ) ) ;
#64666=CARTESIAN_POINT ( 'NONE',  ( 27.15937500061451360, 0.000000000000000000, 5.243569643749999010 ) ) ;
#64667=CARTESIAN_POINT ( 'NONE',  ( 27.90937500061451715, 4.541064518000418104, -2.621784821874998173 ) ) ;
#64668=ADVANCED_FACE ( 'NONE', ( #18261 ), #40834, .F. ) ;
#64669=CARTESIAN_POINT ( 'NONE',  ( 3.478125000614517237, 6.421520780324663323E-16, -5.243569643749999010 ) ) ;
#64671=CARTESIAN_POINT ( 'NONE',  ( 16.02187500061451786, -6.054752690667223547, -1.112240025338166033E-15 ) ) ;
#64673=CARTESIAN_POINT ( 'NONE',  ( 28.83750000122903145, -4.330127018922194537, 2.499999999999995559 ) ) ;
#64674=CARTESIAN_POINT ( 'NONE',  ( 6.571875000614517681, -6.054752690667223547, -1.112240025338166033E-15 ) ) ;
#64675=CARTESIAN_POINT ( 'NONE',  ( 15.75937500061451857, 4.541064518000418104, -2.621784821874998173 ) ) ;
#64677=CARTESIAN_POINT ( 'NONE',  ( 26.55000000000000071, -4.330127018922190985, -2.500000000000001332 ) ) ;
#64678=CARTESIAN_POINT ( 'NONE',  ( 26.70937500061451431, 0.000000000000000000, 5.243569643749999010 ) ) ;
#64680=CARTESIAN_POINT ( 'NONE',  ( 29.77499999999999858, 6.123233995736764310E-16, -4.999999999999998224 ) ) ;
#64681=VERTEX_POINT ( 'NONE', #35273 ) ;
#64682=CARTESIAN_POINT ( 'NONE',  ( 8.962500000000002132, -5.773502691896255534, -1.060575238724906372E-15 ) ) ;
#64684=CARTESIAN_POINT ( 'NONE',  ( 22.64062500061451644, -3.027376345333614438, 5.243569643749998122 ) ) ;
#64685=CARTESIAN_POINT ( 'NONE',  ( 12.93750000000000178, -2.886751345948129988, 4.999999999999997335 ) ) ;
#64686=CARTESIAN_POINT ( 'NONE',  ( 8.887500001229033941, 4.330127018922191873, 2.499999999999999556 ) ) ;
#64687=CARTESIAN_POINT ( 'NONE',  ( 7.640625000614517326, 6.054752690667223547, 3.707466751127219781E-16 ) ) ;
#64688=CARTESIAN_POINT ( 'NONE',  ( 22.27499999999999858, 4.330127018922191873, 2.499999999999999556 ) ) ;
#64689=CARTESIAN_POINT ( 'NONE',  ( 19.04062500061451146, -3.027376345333614438, 5.243569643749998122 ) ) ;
#64690=CARTESIAN_POINT ( 'NONE',  ( 4.837500001229035895, 4.330127018922191873, 2.499999999999999556 ) ) ;
#64691=CARTESIAN_POINT ( 'NONE',  ( 25.01250000122903216, 4.330127018922192761, -2.499999999999997780 ) ) ;
#64693=CARTESIAN_POINT ( 'NONE',  ( 5.400000000000002132, -4.330127018922190985, -2.500000000000001332 ) ) ;
#64694=EDGE_LOOP ( 'NONE', ( #8746, #65677, #68712, #34234 ) ) ;
#64695=CARTESIAN_POINT ( 'NONE',  ( 19.56562500061451715, -6.054752690667223547, -1.112240025338166033E-15 ) ) ;
#64696=CARTESIAN_POINT ( 'NONE',  ( 26.42812500061451431, 6.421520780324663323E-16, -5.243569643749999010 ) ) ;
#64697=CARTESIAN_POINT ( 'NONE',  ( 26.40937500061451715, -4.541064518000417216, -2.621784821875001281 ) ) ;
#64698=CARTESIAN_POINT ( 'NONE',  ( 9.000000000000001776, -4.330127018922190985, -2.500000000000001332 ) ) ;
#64699=CARTESIAN_POINT ( 'NONE',  ( 10.79062500061451679, 6.054752690667223547, 3.707466751127219781E-16 ) ) ;
#64700=CARTESIAN_POINT ( 'NONE',  ( 28.52812500061451573, -4.541064518000419881, 2.621784821874995952 ) ) ;
#64701=CARTESIAN_POINT ( 'NONE',  ( 8.165625000614516793, 3.027376345333611329, 5.243569643749999010 ) ) ;
#64703=CARTESIAN_POINT ( 'NONE',  ( -4.243569643749999898, 12.20937500061451608, 30.00000000000000000 ) ) ;
#64704=CARTESIAN_POINT ( 'NONE',  ( 24.56250000122903288, 4.330127018922192761, -2.499999999999997780 ) ) ;
#64706=CARTESIAN_POINT ( 'NONE',  ( 14.42812500061451786, 4.541064518000418104, 2.621784821874999949 ) ) ;
#64707=CARTESIAN_POINT ( 'NONE',  ( 11.37187500061451750, 3.027376345333611329, 5.243569643749999010 ) ) ;
#64708=CARTESIAN_POINT ( 'NONE',  ( 10.39687500061451786, 6.054752690667223547, 3.707466751127219781E-16 ) ) ;
#64709=CARTESIAN_POINT ( 'NONE',  ( 17.07187500061451502, 3.027376345333613106, -5.243569643749998122 ) ) ;
#64711=CARTESIAN_POINT ( 'NONE',  ( -2.699902572705014769, 9.635935948006316920, 35.37283348364390179 ) ) ;
#64712=CARTESIAN_POINT ( 'NONE',  ( 20.84062500061451573, -3.027376345333614438, 5.243569643749998122 ) ) ;
#64713=CARTESIAN_POINT ( 'NONE',  ( 16.24687500061451573, 6.054752690667223547, 3.707466751127219781E-16 ) ) ;
#64714=CARTESIAN_POINT ( 'NONE',  ( 22.97812500061451857, 4.541064518000418104, 2.621784821874999949 ) ) ;
#64715=CARTESIAN_POINT ( 'NONE',  ( -2.000000000000000000, 13.17500000000000071, 26.53589838486224650 ) ) ;
#64716=CARTESIAN_POINT ( 'NONE',  ( 27.81562500061452070, 3.027376345333613106, -5.243569643749998122 ) ) ;
#64717=CARTESIAN_POINT ( 'NONE',  ( 7.725000001229034297, -5.773502691896255534, -1.060575238724906372E-15 ) ) ;
#64718=ORIENTED_EDGE ( 'NONE', *, *, #58187, .F. ) ;
#64719=CARTESIAN_POINT ( 'NONE',  ( 5.625000001229036428, 2.886751345948129099, -4.999999999999998224 ) ) ;
#64720=CARTESIAN_POINT ( 'NONE',  ( -2.828200636599751609E-16, 17.18750000000000000, -34.61880215351700230 ) ) ;
#64721=CARTESIAN_POINT ( 'NONE',  ( 25.16250000122903074, 0.000000000000000000, 4.999999999999998224 ) ) ;
#64723=CARTESIAN_POINT ( 'NONE',  ( 7.696875000614516793, 6.054752690667223547, 3.707466751127219781E-16 ) ) ;
#64724=DIRECTION ( 'NONE',  ( -1.000000000000000000, -0.000000000000000000, -0.000000000000000000 ) ) ;
#64725=CARTESIAN_POINT ( 'NONE',  ( 15.06562500061451537, -6.054752690667223547, -1.112240025338166033E-15 ) ) ;
#64726=CARTESIAN_POINT ( 'NONE',  ( 9.009375000614518569, 4.541064518000418104, -2.621784821874998173 ) ) ;
#64727=CARTESIAN_POINT ( 'NONE',  ( 28.01250000122903216, -4.330127018922190985, -2.500000000000001332 ) ) ;
#64728=CARTESIAN_POINT ( 'NONE',  ( 17.37187500061451573, -6.054752690667223547, -1.112240025338166033E-15 ) ) ;
#64729=CARTESIAN_POINT ( 'NONE',  ( 4.134375000614517681, 4.541064518000418104, 2.621784821874999949 ) ) ;
#64731=CARTESIAN_POINT ( 'NONE',  ( 6.365625000614518747, 3.027376345333611329, 5.243569643749999010 ) ) ;
#64732=CARTESIAN_POINT ( 'NONE',  ( 15.59062500061451573, -3.027376345333610441, -5.243569643749999898 ) ) ;
#64734=CARTESIAN_POINT ( 'NONE',  ( 13.34062500061451750, -3.027376345333610441, -5.243569643749999898 ) ) ;
#64735=CARTESIAN_POINT ( 'NONE',  ( 5.175000001229033586, 2.886751345948129099, -4.999999999999998224 ) ) ;
#64736=CARTESIAN_POINT ( 'NONE',  ( 10.15312500061451750, -4.541064518000417216, -2.621784821875001281 ) ) ;
#64738=CARTESIAN_POINT ( 'NONE',  ( 9.975000000000001421, 6.123233995736764310E-16, -4.999999999999998224 ) ) ;
#64739=CARTESIAN_POINT ( 'NONE',  ( 5.737500001229033586, 4.330127018922191873, 2.499999999999999556 ) ) ;
#64740=CARTESIAN_POINT ( 'NONE',  ( 19.57500000000000284, 4.330127018922191873, 2.499999999999999556 ) ) ;
#64741=CARTESIAN_POINT ( 'NONE',  ( 13.92187500061451644, 3.027376345333613106, -5.243569643749998122 ) ) ;
#64742=CARTESIAN_POINT ( 'NONE',  ( 16.68750000122903288, -4.330127018922194537, 2.499999999999995559 ) ) ;
#64744=CARTESIAN_POINT ( 'NONE',  ( -2.121784821874999949, 9.884375000614518569, -33.67503911421598417 ) ) ;
#64745=CARTESIAN_POINT ( 'NONE',  ( 3.205315561573065963, 3.837448607643382026, 3.573382659177642751 ) ) ;
#64746=CARTESIAN_POINT ( 'NONE',  ( 30.00000000000000000, 0.000000000000000000, 0.000000000000000000 ) ) ;
#64747=CARTESIAN_POINT ( 'NONE',  ( 0.000000000000000000, 20.00000000000000000, -30.00000000000000000 ) ) ;
#64748=CARTESIAN_POINT ( 'NONE',  ( 0.000000000000000000, 20.00000000000000000, 30.00000000000000000 ) ) ;
#64750=CARTESIAN_POINT ( 'NONE',  ( 16.62187500061451573, 3.027376345333613106, -5.243569643749998122 ) ) ;
#64751=CARTESIAN_POINT ( 'NONE',  ( 28.19999999999999929, 0.000000000000000000, 4.999999999999998224 ) ) ;
#64752=EDGE_CURVE ( 'NONE', #3427, #65794, #34340, .T. ) ;
#64753=CARTESIAN_POINT ( 'NONE',  ( 10.79062500061451679, 6.054752690667223547, 3.707466751127219781E-16 ) ) ;
#64755=CARTESIAN_POINT ( 'NONE',  ( 22.77187500061451786, -6.054752690667223547, -1.112240025338166033E-15 ) ) ;
#64757=CARTESIAN_POINT ( 'NONE',  ( 10.64062500061451644, -3.027376345333610441, -5.243569643749999898 ) ) ;
#64758=CARTESIAN_POINT ( 'NONE',  ( 14.93437500061451750, 4.541064518000418104, 2.621784821874999949 ) ) ;
#64759=ORIENTED_EDGE ( 'NONE', *, *, #47041, .T. ) ;
#64760=CARTESIAN_POINT ( 'NONE',  ( 26.93437500061451573, 6.421520780324663323E-16, -5.243569643749999010 ) ) ;
#64761=CARTESIAN_POINT ( 'NONE',  ( 27.32812500061451644, 6.421520780324663323E-16, -5.243569643749999010 ) ) ;
#64762=CARTESIAN_POINT ( 'NONE',  ( 28.07812500061451289, -4.541064518000419881, 2.621784821874995952 ) ) ;
#64763=CARTESIAN_POINT ( 'NONE',  ( 4.874144969157243601, 1.114769402001472676, -5.123700985539431763 ) ) ;
#64764=CARTESIAN_POINT ( 'NONE',  ( 6.337499999999998579, -2.886751345948125991, -5.000000000000000000 ) ) ;
#64765=CARTESIAN_POINT ( 'NONE',  ( 16.68750000122903288, -4.330127018922194537, 2.499999999999995559 ) ) ;
#64768=ORIENTED_EDGE ( 'NONE', *, *, #57914, .F. ) ;
#64769=CARTESIAN_POINT ( 'NONE',  ( 14.21249999999999858, 2.886751345948126879, 4.999999999999999112 ) ) ;
#64770=CARTESIAN_POINT ( 'NONE',  ( 19.65000000000000213, 0.000000000000000000, 4.999999999999998224 ) ) ;
#64771=CARTESIAN_POINT ( 'NONE',  ( 14.05312500061451431, 0.000000000000000000, 5.243569643749999010 ) ) ;
#64773=CARTESIAN_POINT ( 'NONE',  ( 28.49999999999999645, 4.330127018922192761, -2.499999999999997780 ) ) ;
#64774=CARTESIAN_POINT ( 'NONE',  ( 2.121784821874999061, 16.55937500061451573, -33.67503911421598417 ) ) ;
#64775=CARTESIAN_POINT ( 'NONE',  ( 5.315625000614516260, 3.027376345333613106, -5.243569643749998122 ) ) ;
#64776=CARTESIAN_POINT ( 'NONE',  ( 13.31250000000000178, 2.886751345948126879, 4.999999999999999112 ) ) ;
#64778=ORIENTED_EDGE ( 'NONE', *, *, #45135, .F. ) ;
#64779=CARTESIAN_POINT ( 'NONE',  ( -3.000416591977282496E-16, 16.09062500061451573, 25.09994784771203058 ) ) ;
#64780=CARTESIAN_POINT ( 'NONE',  ( 25.56562500061452070, 3.027376345333613106, -5.243569643749998122 ) ) ;
#64783=CARTESIAN_POINT ( 'NONE',  ( 23.40937500061451715, 4.541064518000418104, -2.621784821874998173 ) ) ;
#64784=CARTESIAN_POINT ( 'NONE',  ( 22.15312500061451573, 0.000000000000000000, 5.243569643749999010 ) ) ;
#64785=CARTESIAN_POINT ( 'NONE',  ( -4.243569643749999898, 14.40312500061459389, -30.00000000000000000 ) ) ;
#64786=CARTESIAN_POINT ( 'NONE',  ( 24.15000000122903145, 5.773502691896255534, 3.535250795749688894E-16 ) ) ;
#64787=CARTESIAN_POINT ( 'NONE',  ( 5.840625000614516615, 6.054752690667223547, 3.707466751127219781E-16 ) ) ;
#64789=CARTESIAN_POINT ( 'NONE',  ( 25.11562500061451431, 3.027376345333612662, -5.243569643749998122 ) ) ;
#64792=CARTESIAN_POINT ( 'NONE',  ( 16.50937500061451502, -4.541064518000417216, -2.621784821875001281 ) ) ;
#64793=CARTESIAN_POINT ( 'NONE',  ( 25.02187500061451431, -6.054752690667223547, -1.112240025338166033E-15 ) ) ;
#64794=CARTESIAN_POINT ( 'NONE',  ( -2.121784821874999949, 13.48437500061451821, 26.32496088578401938 ) ) ;
#64795=CARTESIAN_POINT ( 'NONE',  ( 6.178125000614518747, 6.421520780324663323E-16, -5.243569643749999010 ) ) ;
#64796=CARTESIAN_POINT ( 'NONE',  ( 29.20312500061451644, 4.541064518000418104, -2.621784821874998173 ) ) ;
#64797=CARTESIAN_POINT ( 'NONE',  ( 29.20312500061451644, 4.541064518000418104, -2.621784821874998173 ) ) ;
#64799=CYLINDRICAL_SURFACE ( 'NONE', #4035, 3.999999999999996447 ) ;
#64800=CARTESIAN_POINT ( 'NONE',  ( 29.28750000122903074, -4.330127018922194537, 2.499999999999995559 ) ) ;
#64801=CARTESIAN_POINT ( 'NONE',  ( 8.034375000614518925, 6.421520780324663323E-16, -5.243569643749999010 ) ) ;
#64803=CARTESIAN_POINT ( 'NONE',  ( 15.22500000122903252, 2.886751345948126879, 4.999999999999999112 ) ) ;
#64804=CARTESIAN_POINT ( 'NONE',  ( 3.459375000614519635, -4.541064518000417216, -2.621784821875001281 ) ) ;
#64805=CARTESIAN_POINT ( 'NONE',  ( 11.10000000122903252, 5.773502691896255534, 3.535250795749688894E-16 ) ) ;
#64806=CARTESIAN_POINT ( 'NONE',  ( 4.040625000614517681, 6.054752690667223547, 3.707466751127219781E-16 ) ) ;
#64809=CARTESIAN_POINT ( 'NONE',  ( 13.80937500061451750, -4.541064518000417216, -2.621784821875001281 ) ) ;
#64810=CARTESIAN_POINT ( 'NONE',  ( 1.626862140677534273E-15, 17.52500000122903145, 34.00000000000000000 ) ) ;
#64812=CARTESIAN_POINT ( 'NONE',  ( 22.56562500061451715, 3.027376345333611329, 5.243569643749999010 ) ) ;
#64813=CARTESIAN_POINT ( 'NONE',  ( 7.828125000614517326, -4.541064518000419881, 2.621784821874995952 ) ) ;
#64814=CARTESIAN_POINT ( 'NONE',  ( 25.54687500061451644, -3.027376345333610441, -5.243569643749999898 ) ) ;
#64815=CARTESIAN_POINT ( 'NONE',  ( 6.590625000614518392, -3.027376345333610441, -5.243569643749999898 ) ) ;
#64817=CARTESIAN_POINT ( 'NONE',  ( 7.500000001229034652, 5.773502691896255534, 3.535250795749688894E-16 ) ) ;
#64819=CARTESIAN_POINT ( 'NONE',  ( 25.07812500061451644, 6.421520780324663323E-16, -5.243569643749999010 ) ) ;
#64820=CARTESIAN_POINT ( 'NONE',  ( -3.000416591977282496E-16, 11.59062500061451750, -34.90005215228797653 ) ) ;
#64821=CARTESIAN_POINT ( 'NONE',  ( 9.337500001229033231, 4.330127018922191873, 2.499999999999999556 ) ) ;
#64822=CARTESIAN_POINT ( 'NONE',  ( 20.31562500061451715, 3.027376345333611329, 5.243569643749999010 ) ) ;
#64824=CARTESIAN_POINT ( 'NONE',  ( 17.24062500061451786, -3.027376345333614438, 5.243569643749998122 ) ) ;
#64826=CARTESIAN_POINT ( 'NONE',  ( 19.31250000000000000, -5.773502691896255534, -1.060575238724906372E-15 ) ) ;
#64827=CARTESIAN_POINT ( 'NONE',  ( 13.53750000122903430, -4.330127018922194537, 2.499999999999995559 ) ) ;
#64828=CARTESIAN_POINT ( 'NONE',  ( 9.853125000614516793, 4.541064518000418104, -2.621784821874998173 ) ) ;
#64829=CARTESIAN_POINT ( 'NONE',  ( 12.92812500061451786, 6.421520780324663323E-16, -5.243569643749999010 ) ) ;
#64832=CARTESIAN_POINT ( 'NONE',  ( 23.40000000122903145, -2.886751345948129988, 4.999999999999997335 ) ) ;
#64833=CARTESIAN_POINT ( 'NONE',  ( 21.45937500061451786, -4.541064518000417216, -2.621784821875001281 ) ) ;
#64834=CARTESIAN_POINT ( 'NONE',  ( 21.68437500061451573, 4.541064518000418104, 2.621784821874999949 ) ) ;
#64836=EDGE_CURVE ( 'NONE', #10990, #11359, #33921, .T. ) ;
#64837=CARTESIAN_POINT ( 'NONE',  ( 7.950000001229033053, 5.773502691896255534, 3.535250795749688894E-16 ) ) ;
#64838=CARTESIAN_POINT ( 'NONE',  ( 5.671875000614519102, -6.054752690667223547, -1.112240025338166033E-15 ) ) ;
#64839=CARTESIAN_POINT ( 'NONE',  ( 23.25937500061451857, -4.541064518000417216, -2.621784821875001281 ) ) ;
#64841=CARTESIAN_POINT ( 'NONE',  ( 17.91562500061451502, 3.027376345333613106, -5.243569643749998122 ) ) ;
#64842=CARTESIAN_POINT ( 'NONE',  ( 24.60937500061451644, -4.541064518000417216, -2.621784821875001281 ) ) ;
#64845=CARTESIAN_POINT ( 'NONE',  ( 6.346875000614517148, 6.054752690667223547, 3.707466751127219781E-16 ) ) ;
#64846=CARTESIAN_POINT ( 'NONE',  ( 18.21562500061451573, -6.054752690667223547, -1.112240025338166033E-15 ) ) ;
#64848=CARTESIAN_POINT ( 'NONE',  ( 0.000000000000000000, 20.00000000000000000, 26.00000000000000000 ) ) ;
#64849=CARTESIAN_POINT ( 'NONE',  ( 24.66562500061451502, 3.027376345333613106, -5.243569643749998122 ) ) ;
#64850=CYLINDRICAL_SURFACE ( 'NONE', #66361, 4.999999999999998224 ) ;
#64852=CARTESIAN_POINT ( 'NONE',  ( 14.32500000000000107, -4.330127018922194537, 2.499999999999995559 ) ) ;
#64853=CARTESIAN_POINT ( 'NONE',  ( 25.42500000122903359, 2.886751345948129099, -4.999999999999998224 ) ) ;
#64854=CARTESIAN_POINT ( 'NONE',  ( 22.07812500061451644, 4.541064518000418104, 2.621784821874999949 ) ) ;
#64856=CARTESIAN_POINT ( 'NONE',  ( 23.40000000000000213, -4.330127018922190985, -2.500000000000001332 ) ) ;
#64857=CARTESIAN_POINT ( 'NONE',  ( 23.10937500061451644, 0.000000000000000000, 5.243569643749999010 ) ) ;
#64859=FACE_OUTER_BOUND ( 'NONE', #69203, .T. ) ;
#64860=CARTESIAN_POINT ( 'NONE',  ( 12.14062500061451821, 6.054752690667223547, 3.707466751127219781E-16 ) ) ;
#64861=CARTESIAN_POINT ( 'NONE',  ( 3.890625000614517326, -3.027376345333610441, -5.243569643749999898 ) ) ;
#64863=CARTESIAN_POINT ( 'NONE',  ( 25.75312500061451715, 0.000000000000000000, 5.243569643749999010 ) ) ;
#64864=CARTESIAN_POINT ( 'NONE',  ( 12.93750000122903465, 4.330127018922191873, 2.499999999999999556 ) ) ;
#64865=CARTESIAN_POINT ( 'NONE',  ( 18.93750000000000000, -2.886751345948125991, -5.000000000000000000 ) ) ;
#64866=CARTESIAN_POINT ( 'NONE',  ( 26.62500000000000000, 6.123233995736764310E-16, -4.999999999999998224 ) ) ;
#64867=CARTESIAN_POINT ( 'NONE',  ( 0.000000000000000000, 20.00000000000000000, -33.99999999999999289 ) ) ;
#64868=CARTESIAN_POINT ( 'NONE',  ( 6.234375000614519102, 6.421520780324663323E-16, -5.243569643749999010 ) ) ;
#64869=CARTESIAN_POINT ( 'NONE',  ( 20.03437500061451715, -4.541064518000419881, 2.621784821874995952 ) ) ;
#64870=CARTESIAN_POINT ( 'NONE',  ( 1.999999999999998668, 11.41250000122903430, 26.53589838486224650 ) ) ;
#64871=ORIENTED_EDGE ( 'NONE', *, *, #65098, .F. ) ;
#64872=CARTESIAN_POINT ( 'NONE',  ( 29.35312500061451502, 0.000000000000000000, 5.243569643749999010 ) ) ;
#64873=CARTESIAN_POINT ( 'NONE',  ( 3.075000000000001510, -4.330127018922194537, 2.499999999999995559 ) ) ;
#64874=CARTESIAN_POINT ( 'NONE',  ( 5.821875000614519458, 3.027376345333613106, -5.243569643749998122 ) ) ;
#64875=CARTESIAN_POINT ( 'NONE',  ( 15.26249999999999929, -5.773502691896255534, -1.060575238724906372E-15 ) ) ;
#64876=CARTESIAN_POINT ( 'NONE',  ( 13.79062500061451502, -3.027376345333610441, -5.243569643749999898 ) ) ;
#64880=CARTESIAN_POINT ( 'NONE',  ( 18.93750000122903288, -4.330127018922194537, 2.499999999999995559 ) ) ;
#64881=CARTESIAN_POINT ( 'NONE',  ( 0.000000000000000000, 20.00000000000000000, 26.00000000000000000 ) ) ;
#64883=CARTESIAN_POINT ( 'NONE',  ( 8.578125000614518214, 4.541064518000418104, 2.621784821874999949 ) ) ;
#64884=CARTESIAN_POINT ( 'NONE',  ( 23.40937500061451715, 4.541064518000418104, -2.621784821874998173 ) ) ;
#64885=CARTESIAN_POINT ( 'NONE',  ( 2.121784821874999061, 17.90937500061451715, 26.32496088578401583 ) ) ;
#64886=CARTESIAN_POINT ( 'NONE',  ( 25.20937500061451431, 4.541064518000418104, -2.621784821874998173 ) ) ;
#64887=CARTESIAN_POINT ( 'NONE',  ( 4.349999999999999645, 0.000000000000000000, 4.999999999999998224 ) ) ;
#64888=CARTESIAN_POINT ( 'NONE',  ( -1.389182545231912203, 9.676047173952133207, 26.18324276292616304 ) ) ;
#64889=CARTESIAN_POINT ( 'NONE',  ( 13.41562500061451502, 3.027376345333613106, -5.243569643749998122 ) ) ;
#64890=CARTESIAN_POINT ( 'NONE',  ( 3.600000001229033408, -2.886751345948129988, 4.999999999999997335 ) ) ;
#64891=CARTESIAN_POINT ( 'NONE',  ( 8.484375000614518214, 6.421520780324663323E-16, -5.243569643749999010 ) ) ;
#64892=CARTESIAN_POINT ( 'NONE',  ( 3.999999999999998668, 14.97500000122903252, 27.69059892324149530 ) ) ;
#64893=EDGE_LOOP ( 'NONE', ( #70037, #69313, #69817, #21188 ) ) ;
#64894=CARTESIAN_POINT ( 'NONE',  ( 10.37812500061451715, 4.541064518000418104, 2.621784821874999949 ) ) ;
#64895=CARTESIAN_POINT ( 'NONE',  ( 13.73437500061451821, -4.541064518000419881, 2.621784821874995952 ) ) ;
#64897=CARTESIAN_POINT ( 'NONE',  ( 24.86250000122903359, -4.330127018922190985, -2.500000000000001332 ) ) ;
#64898=CARTESIAN_POINT ( 'NONE',  ( 10.50937500061451679, 0.000000000000000000, 5.243569643749999010 ) ) ;
#64899=CARTESIAN_POINT ( 'NONE',  ( 12.55312500061451786, 4.541064518000418104, -2.621784821874998173 ) ) ;
#64901=CARTESIAN_POINT ( 'NONE',  ( 21.75937500061451502, 0.000000000000000000, 5.243569643749999010 ) ) ;
#64904=CARTESIAN_POINT ( 'NONE',  ( 4.898587196589411843E-16, 20.00000000000000000, -26.00000000000000000 ) ) ;
#64905=CARTESIAN_POINT ( 'NONE',  ( 4.243569643749999010, 13.82187500061451857, -32.45002607614398471 ) ) ;
#64906=CARTESIAN_POINT ( 'NONE',  ( 15.30937500061451750, 4.541064518000418104, -2.621784821874998173 ) ) ;
#64907=CARTESIAN_POINT ( 'NONE',  ( 17.85000000122903430, 5.773502691896255534, 3.535250795749688894E-16 ) ) ;
#64908=CARTESIAN_POINT ( 'NONE',  ( 11.18437500061451928, 6.421520780324663323E-16, -5.243569643749999010 ) ) ;
#64909=CARTESIAN_POINT ( 'NONE',  ( -4.243569643749999898, 17.51562500061451644, -32.45002607614398471 ) ) ;
#64910=CARTESIAN_POINT ( 'NONE',  ( 18.71250000122903145, 4.330127018922192761, -2.499999999999997780 ) ) ;
#64911=CARTESIAN_POINT ( 'NONE',  ( 11.65312500061451573, 4.541064518000418104, -2.621784821874998173 ) ) ;
#64913=CARTESIAN_POINT ( 'NONE',  ( 15.33750000000000036, -2.886751345948125991, -5.000000000000000000 ) ) ;
#64914=CARTESIAN_POINT ( 'NONE',  ( 19.23750000122903714, 4.330127018922191873, 2.499999999999999556 ) ) ;
#64915=CARTESIAN_POINT ( 'NONE',  ( 10.65937500061451715, -4.541064518000417216, -2.621784821875001281 ) ) ;
#64916=CARTESIAN_POINT ( 'NONE',  ( 30.00000000000000000, 0.000000000000000000, 0.000000000000000000 ) ) ;
#64917=CARTESIAN_POINT ( 'NONE',  ( 12.00000000122903465, 5.773502691896255534, 3.535250795749688894E-16 ) ) ;
#64918=CARTESIAN_POINT ( 'NONE',  ( 21.60000000122903430, -2.886751345948129988, 4.999999999999997335 ) ) ;
#64919=CARTESIAN_POINT ( 'NONE',  ( 18.44062500061451715, 6.054752690667223547, 3.707466751127219781E-16 ) ) ;
#64920=EDGE_CURVE ( 'NONE', #33359, #32339, #6088, .T. ) ;
#64921=CARTESIAN_POINT ( 'NONE',  ( 21.47812500061451502, 6.421520780324663323E-16, -5.243569643749999010 ) ) ;
#64922=CARTESIAN_POINT ( 'NONE',  ( 28.38750000122903216, -4.330127018922194537, 2.499999999999995559 ) ) ;
#64923=CARTESIAN_POINT ( 'NONE',  ( 25.27499999999999858, 6.123233995736764310E-16, -4.999999999999998224 ) ) ;
#64924=DIRECTION ( 'NONE',  ( 1.000000000000000000, 0.000000000000000000, 0.000000000000000000 ) ) ;
#64926=CARTESIAN_POINT ( 'NONE',  ( 29.07187500061451502, -6.054752690667223547, -1.112240025338166033E-15 ) ) ;
#64927=CARTESIAN_POINT ( 'NONE',  ( 11.62500000000000000, -4.330127018922194537, 2.499999999999995559 ) ) ;
#64928=CARTESIAN_POINT ( 'NONE',  ( 4.243569643749999898, 13.33437500061451786, -30.00000000000000000 ) ) ;
#64929=CARTESIAN_POINT ( 'NONE',  ( 3.675000001229035362, -5.773502691896255534, -1.060575238724906372E-15 ) ) ;
#64930=CARTESIAN_POINT ( 'NONE',  ( 4.425000000000001599, -4.330127018922194537, 2.499999999999995559 ) ) ;
#64932=CARTESIAN_POINT ( 'NONE',  ( 6.459375000614518747, 0.000000000000000000, 5.243569643749999010 ) ) ;
#64933=CARTESIAN_POINT ( 'NONE',  ( 28.71562500061451573, 3.027376345333613106, -5.243569643749998122 ) ) ;
#64934=CARTESIAN_POINT ( 'NONE',  ( 4.633613603196540254, 1.878729617659674167, 4.895446622381335544 ) ) ;
#64935=CARTESIAN_POINT ( 'NONE',  ( 5.475000000000000533, 6.123233995736764310E-16, -4.999999999999998224 ) ) ;
#64936=CARTESIAN_POINT ( 'NONE',  ( -1.071796769724490117, 19.12009619066136423, 26.00000000000000000 ) ) ;
#64937=CARTESIAN_POINT ( 'NONE',  ( 4.809375000614516615, -4.541064518000417216, -2.621784821875001281 ) ) ;
#64938=CARTESIAN_POINT ( 'NONE',  ( 12.08437500061451608, 6.421520780324663323E-16, -5.243569643749999010 ) ) ;
#64939=CARTESIAN_POINT ( 'NONE',  ( 4.987500000000002487, -2.886751345948125991, -5.000000000000000000 ) ) ;
#64941=CARTESIAN_POINT ( 'NONE',  ( -4.243569643749998122, 11.74062500061459424, 32.45002607614398471 ) ) ;
#64942=CARTESIAN_POINT ( 'NONE',  ( 2.000000000000001332, 17.89999999999999858, 33.46410161513774995 ) ) ;
#64943=CARTESIAN_POINT ( 'NONE',  ( 7.462500000000001243, 2.886751345948126879, 4.999999999999999112 ) ) ;
#64945=CARTESIAN_POINT ( 'NONE',  ( 20.76562500061451644, 3.027376345333611329, 5.243569643749999010 ) ) ;
#64946=CARTESIAN_POINT ( 'NONE',  ( 9.853125000614516793, 4.541064518000418104, -2.621784821874998173 ) ) ;
#64948=CARTESIAN_POINT ( 'NONE',  ( 9.984375000614518214, 4.541064518000418104, 2.621784821874999949 ) ) ;
#64949=CARTESIAN_POINT ( 'NONE',  ( 26.21249999999999858, 2.886751345948129099, -4.999999999999998224 ) ) ;
#64950=CARTESIAN_POINT ( 'NONE',  ( 21.22500000122903074, -5.773502691896255534, -1.060575238724906372E-15 ) ) ;
#64951=CARTESIAN_POINT ( 'NONE',  ( 27.51562500061451644, 3.027376345333611329, 5.243569643749999010 ) ) ;
#64953=CARTESIAN_POINT ( 'NONE',  ( 8.859375000614518214, -4.541064518000417216, -2.621784821875001281 ) ) ;
#64954=CARTESIAN_POINT ( 'NONE',  ( 14.85937500061451644, 4.541064518000418104, -2.621784821874998173 ) ) ;
#64955=CARTESIAN_POINT ( 'NONE',  ( 26.22187500061451715, 3.027376345333611329, 5.243569643749999010 ) ) ;
#64957=ADVANCED_FACE ( 'NONE', ( #31184 ), #13447, .F. ) ;
#64959=CARTESIAN_POINT ( 'NONE',  ( 19.95937500061451786, 0.000000000000000000, 5.243569643749999010 ) ) ;
#64960=CARTESIAN_POINT ( 'NONE',  ( 11.40937500061451892, 0.000000000000000000, 5.243569643749999010 ) ) ;
#64962=CARTESIAN_POINT ( 'NONE',  ( 22.61250000000000071, 2.886751345948129099, -4.999999999999998224 ) ) ;
#64964=CARTESIAN_POINT ( 'NONE',  ( -4.243569643749999898, 12.20937500061451608, -30.00000000000000000 ) ) ;
#64966=CARTESIAN_POINT ( 'NONE',  ( 15.81562500061451537, 3.027376345333611329, 5.243569643749999010 ) ) ;
#64967=CARTESIAN_POINT ( 'NONE',  ( 4.575000000000002842, 6.123233995736764310E-16, -4.999999999999998224 ) ) ;
#64970=CARTESIAN_POINT ( 'NONE',  ( 13.50000000000000178, -4.330127018922190985, -2.500000000000001332 ) ) ;
#64971=CARTESIAN_POINT ( 'NONE',  ( -2.000000000000000000, 18.68750000122903288, 26.53589838486224650 ) ) ;
#64972=CARTESIAN_POINT ( 'NONE',  ( 10.91250000122903252, -4.330127018922190985, -2.500000000000001332 ) ) ;
#64973=CARTESIAN_POINT ( 'NONE',  ( 23.37187500061451573, 3.027376345333613106, -5.243569643749998122 ) ) ;
#64974=CARTESIAN_POINT ( 'NONE',  ( 16.17187500061451644, 3.027376345333613106, -5.243569643749998122 ) ) ;
#64975=FACE_OUTER_BOUND ( 'NONE', #29103, .T. ) ;
#64976=ORIENTED_EDGE ( 'NONE', *, *, #12710, .F. ) ;
#64977=CARTESIAN_POINT ( 'NONE',  ( 20.09062500061451573, -3.027376345333610441, -5.243569643749999898 ) ) ;
#64978=CARTESIAN_POINT ( 'NONE',  ( 3.553125000614516082, 4.541064518000418104, -2.621784821874998173 ) ) ;
#64979=CARTESIAN_POINT ( 'NONE',  ( 16.50937500061451502, -4.541064518000417216, -2.621784821875001281 ) ) ;
#64980=CARTESIAN_POINT ( 'NONE',  ( 29.33437500061451431, 4.541064518000418104, 2.621784821874999949 ) ) ;
#64981=CARTESIAN_POINT ( 'NONE',  ( 3.853125000614517681, -4.541064518000417216, -2.621784821875001281 ) ) ;
#64982=CARTESIAN_POINT ( 'NONE',  ( 20.46562500061451928, -6.054752690667223547, -1.112240025338166033E-15 ) ) ;
#64983=CARTESIAN_POINT ( 'NONE',  ( 2.121784821875001281, 14.55312500061451786, 33.67503911421598417 ) ) ;
#64984=CARTESIAN_POINT ( 'NONE',  ( 15.97500000122903430, 2.886751345948129099, -4.999999999999998224 ) ) ;
#64986=CARTESIAN_POINT ( 'NONE',  ( 6.478125000614516793, -4.541064518000419881, 2.621784821874995952 ) ) ;
#64987=CARTESIAN_POINT ( 'NONE',  ( 3.609375000614516882, 4.541064518000418104, -2.621784821874998173 ) ) ;
#64988=CARTESIAN_POINT ( 'NONE',  ( 8.925000000000002487, -4.330127018922194537, 2.499999999999995559 ) ) ;
#64989=( BOUNDED_CURVE ( )  B_SPLINE_CURVE ( 2, ( #7148, #29679, #24127, #69572, #2334, #24852, #41852 ),
 .UNSPECIFIED., .F., .F. ) 
 B_SPLINE_CURVE_WITH_KNOTS ( ( 3, 2, 2, 3 ),
 ( 0.2250000000000000611, 0.2277777777777778290, 0.2305555555555555969, 0.2333333333333333648 ),
 .UNSPECIFIED. ) 
 CURVE ( )  GEOMETRIC_REPRESENTATION_ITEM ( )  RATIONAL_B_SPLINE_CURVE ( ( 0.9999999999999973355, 0.8660254037844413721, 1.000000000000000000, 0.8660254037844387076, 1.000000000000000000, 0.8660254037844373753, 1.000000000000001332 ) ) 
 REPRESENTATION_ITEM ( '' )  );
#64990=CARTESIAN_POINT ( 'NONE',  ( 22.80937500061451573, -4.541064518000417216, -2.621784821875001281 ) ) ;
#64991=CARTESIAN_POINT ( 'NONE',  ( 15.02812500061451750, -4.541064518000419881, 2.621784821874995952 ) ) ;
#64992=CARTESIAN_POINT ( 'NONE',  ( 24.41250000122903430, -4.330127018922190985, -2.500000000000001332 ) ) ;
#64993=CARTESIAN_POINT ( 'NONE',  ( 22.37812500061451360, 6.421520780324663323E-16, -5.243569643749999010 ) ) ;
#64994=CARTESIAN_POINT ( 'NONE',  ( 19.50937500061451857, 0.000000000000000000, 5.243569643749999010 ) ) ;
#64995=CARTESIAN_POINT ( 'NONE',  ( 13.75312500061451715, -4.541064518000417216, -2.621784821875001281 ) ) ;
#64996=CARTESIAN_POINT ( 'NONE',  ( 2.121784821875001281, 15.50937500061451857, 33.67503911421598417 ) ) ;
#64997=CARTESIAN_POINT ( 'NONE',  ( 19.45312500061451644, 0.000000000000000000, 5.243569643749999010 ) ) ;
#64998=CARTESIAN_POINT ( 'NONE',  ( 10.08749999999999858, 5.773502691896255534, 3.535250795749688401E-16 ) ) ;
#65000=ORIENTED_EDGE ( 'NONE', *, *, #66921, .F. ) ;
#65001=CARTESIAN_POINT ( 'NONE',  ( 23.02499999999999858, 6.123233995736764310E-16, -4.999999999999998224 ) ) ;
#65002=CARTESIAN_POINT ( 'NONE',  ( -2.000000000000000000, 10.92500000000000071, -33.46410161513775705 ) ) ;
#65003=CYLINDRICAL_SURFACE ( 'NONE', #4341, 9.999999999999998224 ) ;
#65004=CARTESIAN_POINT ( 'NONE',  ( 27.70312500061451289, -4.541064518000417216, -2.621784821875001281 ) ) ;
#65005=CARTESIAN_POINT ( 'NONE',  ( 8.015625000614518214, 3.027376345333613106, -5.243569643749998122 ) ) ;
#65006=CARTESIAN_POINT ( 'NONE',  ( 19.61250000122903359, 4.330127018922192761, -2.499999999999997780 ) ) ;
#65007=CARTESIAN_POINT ( 'NONE',  ( 25.41562500061451146, -6.054752690667223547, -1.112240025338166033E-15 ) ) ;
#65008=CARTESIAN_POINT ( 'NONE',  ( 25.64999999999999858, -4.330127018922190985, -2.500000000000001332 ) ) ;
#65009=CARTESIAN_POINT ( 'NONE',  ( 26.65312500061451573, 0.000000000000000000, 5.243569643749999010 ) ) ;
#65010=CARTESIAN_POINT ( 'NONE',  ( 8.803125000614517859, -4.541064518000417216, -2.621784821875001281 ) ) ;
#65011=ORIENTED_EDGE ( 'NONE', *, *, #27759, .F. ) ;
#65012=PRODUCT ( 'valve body', 'valve body', '', ( #4232 ) ) ;
#65013=CARTESIAN_POINT ( 'NONE',  ( 23.95312500061451289, 0.000000000000000000, 5.243569643749999010 ) ) ;
#65014=CARTESIAN_POINT ( 'NONE',  ( 4.190625000614518925, -3.027376345333614438, 5.243569643749998122 ) ) ;
#65016=CARTESIAN_POINT ( 'NONE',  ( 3.515625000614516882, 3.027376345333613106, -5.243569643749998122 ) ) ;
#65018=CARTESIAN_POINT ( 'NONE',  ( 9.899999999999998579, -4.330127018922190985, -2.500000000000001332 ) ) ;
#65019=CARTESIAN_POINT ( 'NONE',  ( 10.95937500061451964, 0.000000000000000000, 5.243569643749999010 ) ) ;
#65020=CARTESIAN_POINT ( 'NONE',  ( 9.675000001229035362, 2.886751345948129099, -4.999999999999998224 ) ) ;
#65021=CARTESIAN_POINT ( 'NONE',  ( 14.85937500061451644, 4.541064518000418104, -2.621784821874998173 ) ) ;
#65023=CARTESIAN_POINT ( 'NONE',  ( 5.671875000614519102, -6.054752690667223547, -1.112240025338166033E-15 ) ) ;
#65025=CARTESIAN_POINT ( 'NONE',  ( 13.54687500061451999, 6.054752690667223547, 3.707466751127219781E-16 ) ) ;
#65026=FACE_OUTER_BOUND ( 'NONE', #35851, .T. ) ;
#65027=CARTESIAN_POINT ( 'NONE',  ( 23.05312500061451431, 0.000000000000000000, 5.243569643749999010 ) ) ;
#65030=CARTESIAN_POINT ( 'NONE',  ( 25.39687500061451431, -3.027376345333614438, 5.243569643749998122 ) ) ;
#65031=( BOUNDED_CURVE ( )  B_SPLINE_CURVE ( 2, ( #51233, #73041, #67509, #68232, #17596, #40155, #62675, #12069, #34592 ),
 .UNSPECIFIED., .F., .F. ) 
 B_SPLINE_CURVE_WITH_KNOTS ( ( 3, 2, 2, 2, 3 ),
 ( 0.2934782608695652439, 0.2971014492753623060, 0.3043478260869565410, 0.3115942028985507206, 0.3152173913043478382 ),
 .UNSPECIFIED. ) 
 CURVE ( )  GEOMETRIC_REPRESENTATION_ITEM ( )  RATIONAL_B_SPLINE_CURVE ( ( 0.9330127018922194093, 0.9330127018922198534, 1.000000000000000000, 0.8660254037844387076, 1.000000000000000000, 0.8660254037844387076, 1.000000000000000000, 0.9330127018922188542, 0.9330127018922194093 ) ) 
 REPRESENTATION_ITEM ( '' )  );
#65032=CARTESIAN_POINT ( 'NONE',  ( 4.828125000614518214, 6.421520780324663323E-16, -5.243569643749999010 ) ) ;
#65034=CARTESIAN_POINT ( 'NONE',  ( 16.24687500061451573, 6.054752690667223547, 3.707466751127219781E-16 ) ) ;
#65036=CARTESIAN_POINT ( 'NONE',  ( 27.03750000122903430, -4.330127018922194537, 2.499999999999995559 ) ) ;
#65037=CARTESIAN_POINT ( 'NONE',  ( 6.834375000614518747, 4.541064518000418104, 2.621784821874999949 ) ) ;
#65038=CARTESIAN_POINT ( 'NONE',  ( 17.22187500061451715, 3.027376345333611329, 5.243569643749999010 ) ) ;
#65039=CARTESIAN_POINT ( 'NONE',  ( 21.60000000000000142, -4.330127018922190985, -2.500000000000001332 ) ) ;
#65040=CARTESIAN_POINT ( 'NONE',  ( 25.27499999999999858, 6.123233995736764310E-16, -4.999999999999998224 ) ) ;
#65042=CARTESIAN_POINT ( 'NONE',  ( 2.812500001229033320, -4.330127018922190985, -2.500000000000001332 ) ) ;
#65043=CARTESIAN_POINT ( 'NONE',  ( 27.72187500061451715, -6.054752690667223547, -1.112240025338166033E-15 ) ) ;
#65045=CARTESIAN_POINT ( 'NONE',  ( 21.86250000000000426, 2.886751345948126879, 4.999999999999998224 ) ) ;
#65046=CARTESIAN_POINT ( 'NONE',  ( 7.012500000000001066, 2.886751345948126879, 4.999999999999999112 ) ) ;
#65048=CARTESIAN_POINT ( 'NONE',  ( 23.05312500061451431, 0.000000000000000000, 5.243569643749999010 ) ) ;
#65049=CARTESIAN_POINT ( 'NONE',  ( 11.96250000000000213, 2.886751345948126879, 4.999999999999999112 ) ) ;
#65050=CARTESIAN_POINT ( 'NONE',  ( 5.765625000614519102, 3.027376345333613106, -5.243569643749998122 ) ) ;
#65051=CARTESIAN_POINT ( 'NONE',  ( 19.12500000000000000, 4.330127018922191873, 2.499999999999999556 ) ) ;
#65052=CARTESIAN_POINT ( 'NONE',  ( 18.32812500061451644, 6.421520780324663323E-16, -5.243569643749999010 ) ) ;
#65053=CYLINDRICAL_SURFACE ( 'NONE', #38407, 3.999999999999996447 ) ;
#65054=CARTESIAN_POINT ( 'NONE',  ( 24.00000000122902932, -2.886751345948125991, -5.000000000000000000 ) ) ;
#65056=CARTESIAN_POINT ( 'NONE',  ( 28.43437500061451573, 4.541064518000418104, 2.621784821874999949 ) ) ;
#65058=CARTESIAN_POINT ( 'NONE',  ( 19.04062500061451146, -3.027376345333614438, 5.243569643749998122 ) ) ;
#65059=CARTESIAN_POINT ( 'NONE',  ( 26.39062500061451644, -3.027376345333610441, -5.243569643749999898 ) ) ;
#65060=CARTESIAN_POINT ( 'NONE',  ( 23.97187500061451360, 3.027376345333611329, 5.243569643749999010 ) ) ;
#65061=CARTESIAN_POINT ( 'NONE',  ( 8.062500000000000000, -5.773502691896255534, -1.060575238724906372E-15 ) ) ;
#65062=CARTESIAN_POINT ( 'NONE',  ( 12.47812500061451502, 6.421520780324663323E-16, -5.243569643749999010 ) ) ;
#65063=CARTESIAN_POINT ( 'NONE',  ( 26.35312500061451857, -4.541064518000417216, -2.621784821875001281 ) ) ;
#65064=CARTESIAN_POINT ( 'NONE',  ( 18.27187500061451431, -6.054752690667223547, -1.112240025338166033E-15 ) ) ;
#65065=CARTESIAN_POINT ( 'NONE',  ( 9.965625000614517504, 3.027376345333611329, 5.243569643749999010 ) ) ;
#65066=CARTESIAN_POINT ( 'NONE',  ( 3.029947538045915323, -3.977363186420035834, 3.130101185692909294 ) ) ;
#65067=CARTESIAN_POINT ( 'NONE',  ( 2.121784821875001281, 13.25937500061451857, 33.67503911421598417 ) ) ;
#65068=CARTESIAN_POINT ( 'NONE',  ( 23.28750000122903430, 4.330127018922191873, 2.499999999999999556 ) ) ;
#65070=CARTESIAN_POINT ( 'NONE',  ( 13.15312500061451750, 0.000000000000000000, 5.243569643749999010 ) ) ;
#65072=CARTESIAN_POINT ( 'NONE',  ( 11.22187500061451892, 3.027376345333613106, -5.243569643749998122 ) ) ;
#65073=CARTESIAN_POINT ( 'NONE',  ( 8.896875000614517859, -3.027376345333610441, -5.243569643749999898 ) ) ;
#65074=VERTEX_POINT ( 'NONE', #25270 ) ;
#65075=CARTESIAN_POINT ( 'NONE',  ( -1.004196803065522836, 9.951383199219653974, 35.91870345184305080 ) ) ;
#65076=CARTESIAN_POINT ( 'NONE',  ( 21.77812500061451928, -4.541064518000419881, 2.621784821874995952 ) ) ;
#65077=CARTESIAN_POINT ( 'NONE',  ( 16.43437500061451573, -4.541064518000419881, 2.621784821874995952 ) ) ;
#65078=CARTESIAN_POINT ( 'NONE',  ( 21.85312500061451502, -4.541064518000417216, -2.621784821875001281 ) ) ;
#65079=CARTESIAN_POINT ( 'NONE',  ( -3.999999999999997335, 12.38750000000000107, 32.30940107675850470 ) ) ;
#65080=CARTESIAN_POINT ( 'NONE',  ( 26.42812500061451431, 6.421520780324663323E-16, -5.243569643749999010 ) ) ;
#65081=CARTESIAN_POINT ( 'NONE',  ( 6.187500001229032875, 4.330127018922191873, 2.499999999999999556 ) ) ;
#65082=ORIENTED_EDGE ( 'NONE', *, *, #14004, .T. ) ;
#65083=CARTESIAN_POINT ( 'NONE',  ( 29.62500000000000000, -4.330127018922194537, 2.499999999999995559 ) ) ;
#65084=CARTESIAN_POINT ( 'NONE',  ( -2.000000000000000000, 17.67500000000000071, -33.46410161513775705 ) ) ;
#65085=CARTESIAN_POINT ( 'NONE',  ( 25.57500000122903216, 2.886751345948126879, 4.999999999999999112 ) ) ;
#65087=CARTESIAN_POINT ( 'NONE',  ( 7.546875000614517326, -3.027376345333610441, -5.243569643749999898 ) ) ;
#65088=CARTESIAN_POINT ( 'NONE',  ( 23.40000000000000213, -4.330127018922190985, -2.500000000000001332 ) ) ;
#65089=CARTESIAN_POINT ( 'NONE',  ( 15.47812500061451679, -4.541064518000419881, 2.621784821874995952 ) ) ;
#65090=CARTESIAN_POINT ( 'NONE',  ( 7.921875000614517326, -6.054752690667223547, -1.112240025338166033E-15 ) ) ;
#65092=CARTESIAN_POINT ( 'NONE',  ( 28.16250000122903074, 4.330127018922192761, -2.499999999999997780 ) ) ;
#65093=CARTESIAN_POINT ( 'NONE',  ( 18.19687500061451502, -3.027376345333614438, 5.243569643749998122 ) ) ;
#65094=CARTESIAN_POINT ( 'NONE',  ( 5.934375000614517504, 4.541064518000418104, 2.621784821874999949 ) ) ;
#65095=CARTESIAN_POINT ( 'NONE',  ( 4.000000000000000000, 16.25000000122903643, 32.30940107675849760 ) ) ;
#65096=CARTESIAN_POINT ( 'NONE',  ( 4.640625000614518214, -3.027376345333614438, 5.243569643749998122 ) ) ;
#65097=CARTESIAN_POINT ( 'NONE',  ( 16.00312500061451715, -4.541064518000417216, -2.621784821875001281 ) ) ;
#65098=EDGE_CURVE ( 'NONE', #41592, #66380, #6522, .T. ) ;
#65099=VERTEX_POINT ( 'NONE', #49653 ) ;
#65100=CARTESIAN_POINT ( 'NONE',  ( 12.55312500061451786, 4.541064518000418104, -2.621784821874998173 ) ) ;
#65101=CARTESIAN_POINT ( 'NONE',  ( 6.337500001229033231, -4.330127018922194537, 2.499999999999995559 ) ) ;
#65102=CARTESIAN_POINT ( 'NONE',  ( 10.64062500061451644, -3.027376345333610441, -5.243569643749999898 ) ) ;
#65104=CARTESIAN_POINT ( 'NONE',  ( 11.66249999999999964, -5.773502691896255534, -1.060575238724906372E-15 ) ) ;
#65105=CARTESIAN_POINT ( 'NONE',  ( 3.675000001229035362, -5.773502691896255534, -1.060575238724906372E-15 ) ) ;
#65106=CARTESIAN_POINT ( 'NONE',  ( 20.32499999999999929, 6.123233995736764310E-16, -4.999999999999998224 ) ) ;
#65107=CARTESIAN_POINT ( 'NONE',  ( 15.68437500061451573, 6.421520780324663323E-16, -5.243569643749999010 ) ) ;
#65108=CARTESIAN_POINT ( 'NONE',  ( 17.06250000122903288, 0.000000000000000000, 4.999999999999998224 ) ) ;
#65110=CARTESIAN_POINT ( 'NONE',  ( -3.000416591977282496E-16, 17.89062500061451644, -34.90005215228797653 ) ) ;
#65111=CARTESIAN_POINT ( 'NONE',  ( 3.217156950473346377, 3.827526723824332677, 3.584008178510168730 ) ) ;
#65112=LINE ( 'NONE', #14502, #67799 ) ;
#65113=CARTESIAN_POINT ( 'NONE',  ( 28.94062500061452070, -3.027376345333614438, 5.243569643749998122 ) ) ;
#65114=CARTESIAN_POINT ( 'NONE',  ( 3.999999999999998668, 10.92500000122903536, -32.30940107675850470 ) ) ;
#65116=CARTESIAN_POINT ( 'NONE',  ( 16.13437500061451502, 6.421520780324663323E-16, -5.243569643749999010 ) ) ;
#65117=CARTESIAN_POINT ( 'NONE',  ( 29.43750000000000000, 5.773502691896255534, 3.535250795749688894E-16 ) ) ;
#65118=CARTESIAN_POINT ( 'NONE',  ( 12.62812500061451537, 4.541064518000418104, 2.621784821874999949 ) ) ;
#65119=VECTOR ( 'NONE', #31487, 1000.000000000000000 ) ;
#65121=CARTESIAN_POINT ( 'NONE',  ( 24.60937500061451644, -4.541064518000417216, -2.621784821875001281 ) ) ;
#65123=CARTESIAN_POINT ( 'NONE',  ( 10.82812500061451644, 4.541064518000418104, 2.621784821874999949 ) ) ;
#65124=CARTESIAN_POINT ( 'NONE',  ( 14.03437500061451715, 4.541064518000418104, 2.621784821874999949 ) ) ;
#65126=CARTESIAN_POINT ( 'NONE',  ( 23.85937500061451644, 4.541064518000418104, -2.621784821874998173 ) ) ;
#65127=CARTESIAN_POINT ( 'NONE',  ( 27.32812500061451644, 6.421520780324663323E-16, -5.243569643749999010 ) ) ;
#65129=CARTESIAN_POINT ( 'NONE',  ( 7.650000000000000355, -4.330127018922190985, -2.500000000000001332 ) ) ;
#65130=CARTESIAN_POINT ( 'NONE',  ( 16.01250000122903216, 4.330127018922192761, -2.499999999999997780 ) ) ;
#65131=CYLINDRICAL_SURFACE ( 'NONE', #45680, 3.999999999999996447 ) ;
#65133=CARTESIAN_POINT ( 'NONE',  ( 15.45000000000000107, 4.330127018922192761, -2.499999999999997780 ) ) ;
#65134=CARTESIAN_POINT ( 'NONE',  ( 18.48750000000000071, -2.886751345948125991, -5.000000000000000000 ) ) ;
#65135=CARTESIAN_POINT ( 'NONE',  ( 14.12812500061451715, -4.541064518000419881, 2.621784821874995952 ) ) ;
#65136=ORIENTED_EDGE ( 'NONE', *, *, #61648, .T. ) ;
#65138=CARTESIAN_POINT ( 'NONE',  ( -3.000416591977282496E-16, 17.94687500061451502, -34.90005215228797653 ) ) ;
#65139=CARTESIAN_POINT ( 'NONE',  ( 29.43750000122903288, 6.123233995736764310E-16, -4.999999999999998224 ) ) ;
#65141=CARTESIAN_POINT ( 'NONE',  ( 11.51250000000000107, 2.886751345948126879, 4.999999999999999112 ) ) ;
#65143=VERTEX_POINT ( 'NONE', #37825 ) ;
#65144=CARTESIAN_POINT ( 'NONE',  ( 2.121784821874999061, 15.15312500061451750, 26.32496088578401583 ) ) ;
#65145=CARTESIAN_POINT ( 'NONE',  ( 26.65312500061451573, 0.000000000000000000, 5.243569643749999010 ) ) ;
#65146=DIRECTION ( 'NONE',  ( 1.000000000000000000, 0.000000000000000000, 0.000000000000000000 ) ) ;
#65148=CARTESIAN_POINT ( 'NONE',  ( 22.73437500061451644, -4.541064518000419881, 2.621784821874995952 ) ) ;
#65149=CARTESIAN_POINT ( 'NONE',  ( 18.55312500061451431, 0.000000000000000000, 5.243569643749999010 ) ) ;
#65150=CARTESIAN_POINT ( 'NONE',  ( 2.121784821875001281, 14.55312500061459424, -26.32496088578401938 ) ) ;
#65151=CARTESIAN_POINT ( 'NONE',  ( 22.87500000122903288, 2.886751345948126879, 4.999999999999999112 ) ) ;
#65152=CARTESIAN_POINT ( 'NONE',  ( 4.003125000614518925, 4.541064518000418104, -2.621784821874998173 ) ) ;
#65154=CARTESIAN_POINT ( 'NONE',  ( 21.51562500061451644, 3.027376345333612662, -5.243569643749998122 ) ) ;
#65157=CARTESIAN_POINT ( 'NONE',  ( 17.22187500061451715, 3.027376345333611329, 5.243569643749999010 ) ) ;
#65158=CARTESIAN_POINT ( 'NONE',  ( 17.29687500061451999, -3.027376345333614438, 5.243569643749998122 ) ) ;
#65159=CARTESIAN_POINT ( 'NONE',  ( 24.68437500061451573, 6.421520780324663323E-16, -5.243569643749999010 ) ) ;
#65160=CARTESIAN_POINT ( 'NONE',  ( 2.121784821874999061, 13.40937500061451892, 26.32496088578401583 ) ) ;
#65161=CARTESIAN_POINT ( 'NONE',  ( 4.865625000614517859, 3.027376345333613106, -5.243569643749998122 ) ) ;
#65162=CARTESIAN_POINT ( 'NONE',  ( 28.52812500061451573, -4.541064518000419881, 2.621784821874995952 ) ) ;
#65163=CARTESIAN_POINT ( 'NONE',  ( 28.64062500061451289, -3.027376345333610441, -5.243569643749999898 ) ) ;
#65165=CARTESIAN_POINT ( 'NONE',  ( 3.999999999999999112, 19.77500000000000213, 30.00000000000000000 ) ) ;
#65166=CARTESIAN_POINT ( 'NONE',  ( 3.478125000614517237, 6.421520780324663323E-16, -5.243569643749999010 ) ) ;
#65167=CARTESIAN_POINT ( 'NONE',  ( 7.884375000614517681, -4.541064518000419881, 2.621784821874995952 ) ) ;
#65169=CARTESIAN_POINT ( 'NONE',  ( 14.32500000122903394, 2.886751345948126879, 4.999999999999999112 ) ) ;
#65170=CARTESIAN_POINT ( 'NONE',  ( 10.57500000122903572, 2.886751345948129099, -4.999999999999998224 ) ) ;
#65171=CARTESIAN_POINT ( 'NONE',  ( 5.240625000614516971, -3.027376345333610441, -5.243569643749999898 ) ) ;
#65174=CARTESIAN_POINT ( 'NONE',  ( 14.33437500061451786, 6.421520780324663323E-16, -5.243569643749999010 ) ) ;
#65177=CARTESIAN_POINT ( 'NONE',  ( 23.16562500061451502, -6.054752690667223547, -1.112240025338166033E-15 ) ) ;
#65178=CARTESIAN_POINT ( 'NONE',  ( 7.078125000614516438, 6.421520780324663323E-16, -5.243569643749999010 ) ) ;
#65179=CARTESIAN_POINT ( 'NONE',  ( 25.50937500061451502, -4.541064518000417216, -2.621784821875001281 ) ) ;
#65180=CARTESIAN_POINT ( 'NONE',  ( 8.653125000614515727, 0.000000000000000000, 5.243569643749999010 ) ) ;
#65181=CYLINDRICAL_SURFACE ( 'NONE', #8497, 4.999999999999998224 ) ;
#65182=CARTESIAN_POINT ( 'NONE',  ( 8.100000001229034297, -2.886751345948129988, 4.999999999999997335 ) ) ;
#65183=CARTESIAN_POINT ( 'NONE',  ( 23.27812500061451573, 6.421520780324663323E-16, -5.243569643749999010 ) ) ;
#65185=CARTESIAN_POINT ( 'NONE',  ( 9.001249775931846008E-16, 10.46562500061451928, -25.09994784771203058 ) ) ;
#65186=CARTESIAN_POINT ( 'NONE',  ( 10.76250000122903572, 0.000000000000000000, 4.999999999999998224 ) ) ;
#65187=CARTESIAN_POINT ( 'NONE',  ( 19.19062500061452070, -3.027376345333610441, -5.243569643749999898 ) ) ;
#65188=CARTESIAN_POINT ( 'NONE',  ( 18.85312500061451502, 4.541064518000418104, -2.621784821874998173 ) ) ;
#65190=CARTESIAN_POINT ( 'NONE',  ( 17.62500000000000000, 6.123233995736764310E-16, -4.999999999999998224 ) ) ;
#65191=CARTESIAN_POINT ( 'NONE',  ( 14.62500000122903288, 2.886751345948129099, -4.999999999999998224 ) ) ;
#65192=CARTESIAN_POINT ( 'NONE',  ( 11.57812500061451644, 6.421520780324663323E-16, -5.243569643749999010 ) ) ;
#65193=CARTESIAN_POINT ( 'NONE',  ( 12.74062500061451786, -3.027376345333614438, 5.243569643749998122 ) ) ;
#65194=CARTESIAN_POINT ( 'NONE',  ( 23.10000000122903074, -2.886751345948125991, -5.000000000000000000 ) ) ;
#65195=CARTESIAN_POINT ( 'NONE',  ( 22.28437500061451715, -4.541064518000419881, 2.621784821874995952 ) ) ;
#65196=CARTESIAN_POINT ( 'NONE',  ( 20.33437500061451786, 4.541064518000418104, 2.621784821874999949 ) ) ;
#65197=CARTESIAN_POINT ( 'NONE',  ( 3.531796677802674811, 3.539267187803308179, -3.868928841707397925 ) ) ;
#65198=CARTESIAN_POINT ( 'NONE',  ( 6.150000001229033231, 5.773502691896255534, 3.535250795749688894E-16 ) ) ;
#65199=CARTESIAN_POINT ( 'NONE',  ( 6.834375000614518747, 4.541064518000418104, 2.621784821874999949 ) ) ;
#65200=CARTESIAN_POINT ( 'NONE',  ( 22.47187500061451715, 3.027376345333613106, -5.243569643749998122 ) ) ;
#65201=CARTESIAN_POINT ( 'NONE',  ( 10.49999999999999822, 4.330127018922192761, -2.499999999999997780 ) ) ;
#65202=CARTESIAN_POINT ( 'NONE',  ( 19.56562500061451715, -6.054752690667223547, -1.112240025338166033E-15 ) ) ;
#65203=CARTESIAN_POINT ( 'NONE',  ( 23.63437500061451502, -4.541064518000419881, 2.621784821874995952 ) ) ;
#65205=DIRECTION ( 'NONE',  ( 0.000000000000000000, 0.000000000000000000, 1.000000000000000000 ) ) ;
#65206=CARTESIAN_POINT ( 'NONE',  ( 4.771875000614516971, -6.054752690667223547, -1.112240025338166033E-15 ) ) ;
#65207=CARTESIAN_POINT ( 'NONE',  ( 16.94062500061451715, -3.027376345333610441, -5.243569643749999898 ) ) ;
#65208=CARTESIAN_POINT ( 'NONE',  ( 13.92187500061451644, 3.027376345333613106, -5.243569643749998122 ) ) ;
#65211=CARTESIAN_POINT ( 'NONE',  ( 24.10312500061451502, -4.541064518000417216, -2.621784821875001281 ) ) ;
#65212=CARTESIAN_POINT ( 'NONE',  ( 1.999999999999998668, 13.10000000000000142, -33.46410161513775705 ) ) ;
#65213=DIRECTION ( 'NONE',  ( -0.000000000000000000, -1.000000000000000000, -0.000000000000000000 ) ) ;
#65214=CARTESIAN_POINT ( 'NONE',  ( 15.52500000000000036, 4.330127018922191873, 2.499999999999999556 ) ) ;
#65215=CARTESIAN_POINT ( 'NONE',  ( 24.86250000122903359, -4.330127018922190985, -2.500000000000001332 ) ) ;
#65216=CARTESIAN_POINT ( 'NONE',  ( 18.29062500061451502, -3.027376345333610441, -5.243569643749999898 ) ) ;
#65218=CARTESIAN_POINT ( 'NONE',  ( 22.01249999999999574, -5.773502691896255534, -1.060575238724906372E-15 ) ) ;
#65219=CARTESIAN_POINT ( 'NONE',  ( 24.49687500061451573, -3.027376345333614438, 5.243569643749998122 ) ) ;
#65220=ORIENTED_EDGE ( 'NONE', *, *, #27261, .F. ) ;
#65221=CARTESIAN_POINT ( 'NONE',  ( 19.98750000122903359, 6.123233995736764310E-16, -4.999999999999998224 ) ) ;
#65222=CARTESIAN_POINT ( 'NONE',  ( 12.06562500061451537, 3.027376345333613106, -5.243569643749998122 ) ) ;
#65223=CARTESIAN_POINT ( 'NONE',  ( 4.603125000614518569, 0.000000000000000000, 5.243569643749999010 ) ) ;
#65225=CARTESIAN_POINT ( 'NONE',  ( 26.16562500061451502, 3.027376345333611329, 5.243569643749999010 ) ) ;
#65226=CARTESIAN_POINT ( 'NONE',  ( 11.77500000122903501, -5.773502691896255534, -1.060575238724906372E-15 ) ) ;
#65227=CARTESIAN_POINT ( 'NONE',  ( 20.36249999999999716, 2.886751345948129099, -4.999999999999998224 ) ) ;
#65228=CARTESIAN_POINT ( 'NONE',  ( 25.61250000000000071, -5.773502691896255534, -1.060575238724906372E-15 ) ) ;
#65229=CARTESIAN_POINT ( 'NONE',  ( 6.346875000614517148, 6.054752690667223547, 3.707466751127219781E-16 ) ) ;
#65230=CARTESIAN_POINT ( 'NONE',  ( 17.78437500061451715, -4.541064518000419881, 2.621784821874995952 ) ) ;
#65231=FACE_OUTER_BOUND ( 'NONE', #24089, .T. ) ;
#65232=ORIENTED_EDGE ( 'NONE', *, *, #20108, .T. ) ;
#65233=CARTESIAN_POINT ( 'NONE',  ( 26.16562500061451502, 3.027376345333611329, 5.243569643749999010 ) ) ;
#65234=CARTESIAN_POINT ( 'NONE',  ( 28.13437500061451502, -4.541064518000419881, 2.621784821874995952 ) ) ;
#65235=CARTESIAN_POINT ( 'NONE',  ( 2.971875000614517592, -6.054752690667223547, -1.112240025338166033E-15 ) ) ;
#65236=CARTESIAN_POINT ( 'NONE',  ( 16.35000000000000142, 4.330127018922192761, -2.499999999999997780 ) ) ;
#65237=CARTESIAN_POINT ( 'NONE',  ( 10.97812500061451679, -4.541064518000419881, 2.621784821874995952 ) ) ;
#65240=CARTESIAN_POINT ( 'NONE',  ( 28.49062500061451431, -3.027376345333614438, 5.243569643749998122 ) ) ;
#65241=CARTESIAN_POINT ( 'NONE',  ( 19.50000000122903288, -2.886751345948125991, -5.000000000000000000 ) ) ;
#65242=CARTESIAN_POINT ( 'NONE',  ( 19.42499999999999716, 6.123233995736764310E-16, -4.999999999999998224 ) ) ;
#65244=CARTESIAN_POINT ( 'NONE',  ( 5.278125000614516615, 6.421520780324663323E-16, -5.243569643749999010 ) ) ;
#65245=CARTESIAN_POINT ( 'NONE',  ( 21.00937500061451857, -4.541064518000417216, -2.621784821875001281 ) ) ;
#65246=CARTESIAN_POINT ( 'NONE',  ( -2.121784821874999949, 16.18437500061451573, 26.32496088578401938 ) ) ;
#65247=CARTESIAN_POINT ( 'NONE',  ( 24.72187500061451360, 3.027376345333613106, -5.243569643749998122 ) ) ;
#65248=CARTESIAN_POINT ( 'NONE',  ( 4.762499999999999289, 2.886751345948126879, 4.999999999999999112 ) ) ;
#65249=CARTESIAN_POINT ( 'NONE',  ( 3.999999999999999112, 9.987500001229033586, 30.00000000000000000 ) ) ;
#65250=CARTESIAN_POINT ( 'NONE',  ( 11.42812500061451608, -4.541064518000419881, 2.621784821874995952 ) ) ;
#65251=CARTESIAN_POINT ( 'NONE',  ( 4.725000001229034297, 2.886751345948129099, -4.999999999999998224 ) ) ;
#65252=CARTESIAN_POINT ( 'NONE',  ( 10.02187500061451964, 3.027376345333611329, 5.243569643749999010 ) ) ;
#65254=CARTESIAN_POINT ( 'NONE',  ( 9.853125000614516793, 4.541064518000418104, -2.621784821874998173 ) ) ;
#65255=CARTESIAN_POINT ( 'NONE',  ( 13.24687500061451750, -3.027376345333614438, 5.243569643749998122 ) ) ;
#65256=DIRECTION ( 'NONE',  ( -1.000000000000000000, -0.000000000000000000, -0.000000000000000000 ) ) ;
#65257=CARTESIAN_POINT ( 'NONE',  ( 21.03750000122903074, 4.330127018922191873, 2.499999999999999556 ) ) ;
#65258=CARTESIAN_POINT ( 'NONE',  ( 11.25937500061451679, 4.541064518000418104, -2.621784821874998173 ) ) ;
#65259=CARTESIAN_POINT ( 'NONE',  ( 12.17812500061451608, 4.541064518000418104, 2.621784821874999949 ) ) ;
#65262=CARTESIAN_POINT ( 'NONE',  ( 20.97187500061451715, -6.054752690667223547, -1.112240025338166033E-15 ) ) ;
#65264=CARTESIAN_POINT ( 'NONE',  ( -1.999999999999997113, 12.08750000122903501, -26.53589838486224295 ) ) ;
#65265=CARTESIAN_POINT ( 'NONE',  ( 3.236638147732103565, 3.811095019601020262, -3.368060042915717034 ) ) ;
#65266=CARTESIAN_POINT ( 'NONE',  ( 4.243569643749999010, 14.72187500061451715, -32.45002607614398471 ) ) ;
#65267=CARTESIAN_POINT ( 'NONE',  ( 14.28750000122903430, 4.330127018922191873, 2.499999999999999556 ) ) ;
#65268=( BOUNDED_CURVE ( )  B_SPLINE_CURVE ( 2, ( #48959, #71489, #59282, #20866, #65201, #25311, #65941 ),
 .UNSPECIFIED., .F., .F. ) 
 B_SPLINE_CURVE_WITH_KNOTS ( ( 3, 2, 2, 3 ),
 ( 0.7166666666666667851, 0.7194444444444445530, 0.7222222222222222099, 0.7249999999999999778 ),
 .UNSPECIFIED. ) 
 CURVE ( )  GEOMETRIC_REPRESENTATION_ITEM ( )  RATIONAL_B_SPLINE_CURVE ( ( 0.9999999999999946709, 0.8660254037844440367, 1.000000000000000000, 0.8660254037844387076, 1.000000000000000000, 0.8660254037844387076, 1.000000000000000000 ) ) 
 REPRESENTATION_ITEM ( '' )  );
#65269=CARTESIAN_POINT ( 'NONE',  ( 13.39687500061451608, -3.027376345333610441, -5.243569643749999898 ) ) ;
#65270=CARTESIAN_POINT ( 'NONE',  ( -2.121784821874999949, 17.02812500061451573, -33.67503911421598417 ) ) ;
#65271=CARTESIAN_POINT ( 'NONE',  ( 18.37500000122903288, 2.886751345948126879, 4.999999999999999112 ) ) ;
#65272=CARTESIAN_POINT ( 'NONE',  ( 12.59062500061451573, 6.054752690667223547, 3.707466751127219781E-16 ) ) ;
#65274=CARTESIAN_POINT ( 'NONE',  ( 14.84999999999999964, -4.330127018922190985, -2.500000000000001332 ) ) ;
#65275=CARTESIAN_POINT ( 'NONE',  ( 19.20000000122903216, 5.773502691896255534, 3.535250795749688401E-16 ) ) ;
#65276=CARTESIAN_POINT ( 'NONE',  ( 9.684375000614517504, -4.541064518000419881, 2.621784821874995952 ) ) ;
#65277=CARTESIAN_POINT ( 'NONE',  ( 4.368064885651947726, -2.433106893405058813, -4.644891113268574401 ) ) ;
#65278=CARTESIAN_POINT ( 'NONE',  ( 11.55000000122903181, 5.773502691896255534, 3.535250795749688894E-16 ) ) ;
#65279=CARTESIAN_POINT ( 'NONE',  ( 22.01250000122903216, 0.000000000000000000, 4.999999999999998224 ) ) ;
#65280=CARTESIAN_POINT ( 'NONE',  ( 17.91562500061451502, 3.027376345333613106, -5.243569643749998122 ) ) ;
#65281=CARTESIAN_POINT ( 'NONE',  ( 20.99062500061451431, -3.027376345333610441, -5.243569643749999898 ) ) ;
#65282=CARTESIAN_POINT ( 'NONE',  ( 27.45000000122903572, -2.886751345948129988, 4.999999999999997335 ) ) ;
#65283=CARTESIAN_POINT ( 'NONE',  ( 4.265625000614517326, -6.054752690667223547, -1.112240025338166033E-15 ) ) ;
#65284=CARTESIAN_POINT ( 'NONE',  ( 24.89999999999999858, 4.330127018922192761, -2.499999999999997780 ) ) ;
#65285=CARTESIAN_POINT ( 'NONE',  ( 28.19999999999999929, 0.000000000000000000, 4.999999999999998224 ) ) ;
#65287=CARTESIAN_POINT ( 'NONE',  ( 29.03437500061451715, -4.541064518000419881, 2.621784821874995952 ) ) ;
#65288=CARTESIAN_POINT ( 'NONE',  ( 3.999999999999999112, 12.57500000000000107, -30.00000000000000000 ) ) ;
#65289=CARTESIAN_POINT ( 'NONE',  ( 2.925000001229034918, 2.886751345948129099, -4.999999999999998224 ) ) ;
#65290=CARTESIAN_POINT ( 'NONE',  ( 3.075000000000001510, -4.330127018922194537, 2.499999999999995559 ) ) ;
#65292=CARTESIAN_POINT ( 'NONE',  ( 7.659375000614518036, 4.541064518000418104, -2.621784821874998173 ) ) ;
#65293=CARTESIAN_POINT ( 'NONE',  ( 25.41562500061451146, -6.054752690667223547, -1.112240025338166033E-15 ) ) ;
#65296=FACE_OUTER_BOUND ( 'NONE', #28714, .T. ) ;
#65297=CARTESIAN_POINT ( 'NONE',  ( 6.271875000614517859, 3.027376345333613106, -5.243569643749998122 ) ) ;
#65298=CARTESIAN_POINT ( 'NONE',  ( 8.784375000614518925, -4.541064518000419881, 2.621784821874995952 ) ) ;
#65299=CARTESIAN_POINT ( 'NONE',  ( 3.675000000000001155, 6.123233995736764310E-16, -4.999999999999998224 ) ) ;
#65300=CARTESIAN_POINT ( 'NONE',  ( -3.000416591977282496E-16, 12.04062500061459495, 25.09994784771203058 ) ) ;
#65301=CARTESIAN_POINT ( 'NONE',  ( 29.25000000000000000, -4.330127018922190985, -2.500000000000001332 ) ) ;
#65302=CARTESIAN_POINT ( 'NONE',  ( 4.762499999999999289, 2.886751345948126879, 4.999999999999999112 ) ) ;
#65305=ORIENTED_EDGE ( 'NONE', *, *, #72200, .F. ) ;
#65306=CARTESIAN_POINT ( 'NONE',  ( 19.34062500061451573, 6.054752690667223547, 3.707466751127219781E-16 ) ) ;
#65307=CARTESIAN_POINT ( 'NONE',  ( 10.94062500061451537, -3.027376345333614438, 5.243569643749998122 ) ) ;
#65309=CARTESIAN_POINT ( 'NONE',  ( 7.659375000614518036, 4.541064518000418104, -2.621784821874998173 ) ) ;
#65310=CARTESIAN_POINT ( 'NONE',  ( 23.85000000000000142, -4.330127018922190985, -2.500000000000001332 ) ) ;
#65311=CARTESIAN_POINT ( 'NONE',  ( 20.36250000122903359, -4.330127018922190985, -2.500000000000001332 ) ) ;
#65312=CARTESIAN_POINT ( 'NONE',  ( 28.26562500061451289, 3.027376345333613106, -5.243569643749998122 ) ) ;
#65314=CARTESIAN_POINT ( 'NONE',  ( 10.62187500061451928, -6.054752690667223547, -1.112240025338166033E-15 ) ) ;
#65315=CARTESIAN_POINT ( 'NONE',  ( 13.47187500061451537, 3.027376345333613106, -5.243569643749998122 ) ) ;
#65316=CARTESIAN_POINT ( 'NONE',  ( 25.13437500061451502, 6.421520780324663323E-16, -5.243569643749999010 ) ) ;
#65320=CARTESIAN_POINT ( 'NONE',  ( 20.10937500061451289, -4.541064518000417216, -2.621784821875001281 ) ) ;
#65321=CARTESIAN_POINT ( 'NONE',  ( 10.47187500061451715, 3.027376345333611329, 5.243569643749999010 ) ) ;
#65323=CARTESIAN_POINT ( 'NONE',  ( 22.72499999999999787, 4.330127018922191873, 2.499999999999999556 ) ) ;
#65325=CARTESIAN_POINT ( 'NONE',  ( -4.243569643749999898, 10.85937500061451821, -30.00000000000000000 ) ) ;
#65327=CARTESIAN_POINT ( 'NONE',  ( 16.04062500061451857, -3.027376345333610441, -5.243569643749999898 ) ) ;
#65328=CARTESIAN_POINT ( 'NONE',  ( 3.750000000000000000, 4.330127018922192761, -2.499999999999997780 ) ) ;
#65329=EDGE_CURVE ( 'NONE', #23329, #3427, #16009, .T. ) ;
#65331=DIRECTION ( 'NONE',  ( -1.000000000000000000, -0.000000000000000000, -0.000000000000000000 ) ) ;
#65332=CARTESIAN_POINT ( 'NONE',  ( 13.23750000000000071, 5.773502691896255534, 3.535250795749688894E-16 ) ) ;
#65333=CARTESIAN_POINT ( 'NONE',  ( 3.999999999999998668, 18.12500000122903288, 27.69059892324149175 ) ) ;
#65334=CARTESIAN_POINT ( 'NONE',  ( 10.53750000122903252, 6.123233995736764310E-16, -4.999999999999998224 ) ) ;
#65335=CARTESIAN_POINT ( 'NONE',  ( 22.05937500061451573, 4.541064518000418104, -2.621784821874998173 ) ) ;
#65336=CARTESIAN_POINT ( 'NONE',  ( 16.13437500061451502, 6.421520780324663323E-16, -5.243569643749999010 ) ) ;
#65337=CARTESIAN_POINT ( 'NONE',  ( -3.999999999999999112, 19.83125000061451715, -30.00000000000000000 ) ) ;
#65339=CARTESIAN_POINT ( 'NONE',  ( 17.69062500061451715, -3.027376345333614438, 5.243569643749998122 ) ) ;
#65340=CARTESIAN_POINT ( 'NONE',  ( 2.990625000614519191, -3.027376345333610441, -5.243569643749999898 ) ) ;
#65341=CARTESIAN_POINT ( 'NONE',  ( 17.97187500061451715, 3.027376345333613106, -5.243569643749998122 ) ) ;
#65342=CARTESIAN_POINT ( 'NONE',  ( 28.02187500061451431, 3.027376345333611329, 5.243569643749999010 ) ) ;
#65343=CARTESIAN_POINT ( 'NONE',  ( 4.603125000614518569, 0.000000000000000000, 5.243569643749999010 ) ) ;
#65344=CARTESIAN_POINT ( 'NONE',  ( 20.65312500061451573, 4.541064518000418104, -2.621784821874998173 ) ) ;
#65345=CARTESIAN_POINT ( 'NONE',  ( 28.58437500061451786, -4.541064518000419881, 2.621784821874995952 ) ) ;
#65346=CARTESIAN_POINT ( 'NONE',  ( -3.000416591977282496E-16, 12.49062500061451608, 25.09994784771203058 ) ) ;
#65347=CARTESIAN_POINT ( 'NONE',  ( 16.61250000122903359, 0.000000000000000000, 4.999999999999998224 ) ) ;
#65349=CARTESIAN_POINT ( 'NONE',  ( 6.965625000614518392, -6.054752690667223547, -1.112240025338166033E-15 ) ) ;
#65350=CARTESIAN_POINT ( 'NONE',  ( 26.20312500061451644, 0.000000000000000000, 5.243569643749999010 ) ) ;
#65351=CYLINDRICAL_SURFACE ( 'NONE', #46255, 4.000000000000000000 ) ;
#65352=CARTESIAN_POINT ( 'NONE',  ( 23.44687500061451502, 6.054752690667223547, 3.707466751127219781E-16 ) ) ;
#65353=CARTESIAN_POINT ( 'NONE',  ( 13.60312500061451679, 0.000000000000000000, 5.243569643749999010 ) ) ;
#65354=CARTESIAN_POINT ( 'NONE',  ( 23.02500000122903145, -5.773502691896255534, -1.060575238724906372E-15 ) ) ;
#65355=CARTESIAN_POINT ( 'NONE',  ( 24.17812500061451786, 6.421520780324663323E-16, -5.243569643749999010 ) ) ;
#65356=CARTESIAN_POINT ( 'NONE',  ( 18.60937500061451644, 0.000000000000000000, 5.243569643749999010 ) ) ;
#65357=CARTESIAN_POINT ( 'NONE',  ( 11.54062500061451857, -3.027376345333610441, -5.243569643749999898 ) ) ;
#65358=CARTESIAN_POINT ( 'NONE',  ( 4.243569643749999010, 15.62187500061451928, 27.54997392385601174 ) ) ;
#65359=CARTESIAN_POINT ( 'NONE',  ( 20.05312500061451431, -4.541064518000417216, -2.621784821875001281 ) ) ;
#65360=CARTESIAN_POINT ( 'NONE',  ( 28.90312500061451217, 0.000000000000000000, 5.243569643749999010 ) ) ;
#65362=CARTESIAN_POINT ( 'NONE',  ( 22.27499999999999858, 4.330127018922191873, 2.499999999999999556 ) ) ;
#65363=CARTESIAN_POINT ( 'NONE',  ( 4.000000000000000000, 10.73750000000000071, -27.69059892324149530 ) ) ;
#65365=CARTESIAN_POINT ( 'NONE',  ( 27.06562500061451004, 3.027376345333611329, 5.243569643749999010 ) ) ;
#65366=CARTESIAN_POINT ( 'NONE',  ( 6.965625000614518392, -6.054752690667223547, -1.112240025338166033E-15 ) ) ;
#65367=CARTESIAN_POINT ( 'NONE',  ( 19.35000000122903430, -2.886751345948129988, 4.999999999999997335 ) ) ;
#65368=EDGE_CURVE ( 'NONE', #23474, #8958, #24409, .T. ) ;
#65369=CARTESIAN_POINT ( 'NONE',  ( 25.82812500061451644, -4.541064518000419881, 2.621784821874995952 ) ) ;
#65370=CARTESIAN_POINT ( 'NONE',  ( 22.12500000000000000, 6.123233995736764310E-16, -4.999999999999998224 ) ) ;
#65371=CARTESIAN_POINT ( 'NONE',  ( 27.77812500061451573, 6.421520780324663323E-16, -5.243569643749999010 ) ) ;
#65372=CARTESIAN_POINT ( 'NONE',  ( 7.453125000614516438, -4.541064518000417216, -2.621784821875001281 ) ) ;
#65374=CARTESIAN_POINT ( 'NONE',  ( 23.87812500061451715, 4.541064518000418104, 2.621784821874999949 ) ) ;
#65375=CARTESIAN_POINT ( 'NONE',  ( 5.428125000614517859, 4.541064518000418104, 2.621784821874999949 ) ) ;
#65377=CARTESIAN_POINT ( 'NONE',  ( 2.990625000614519191, -3.027376345333610441, -5.243569643749999898 ) ) ;
#65378=CARTESIAN_POINT ( 'NONE',  ( -1.999999999999997113, 13.43750000122903465, -26.53589838486224295 ) ) ;
#65380=CARTESIAN_POINT ( 'NONE',  ( 10.27499999999999858, -4.330127018922194537, 2.499999999999995559 ) ) ;
#65381=CARTESIAN_POINT ( 'NONE',  ( 11.63437500061451857, 6.421520780324663323E-16, -5.243569643749999010 ) ) ;
#65382=CARTESIAN_POINT ( 'NONE',  ( 7.800000001229035362, -2.886751345948125991, -5.000000000000000000 ) ) ;
#65383=CARTESIAN_POINT ( 'NONE',  ( 15.83437500061451608, 4.541064518000418104, 2.621784821874999949 ) ) ;
#65385=CARTESIAN_POINT ( 'NONE',  ( 6.084375000614518747, -4.541064518000419881, 2.621784821874995952 ) ) ;
#65386=CARTESIAN_POINT ( 'NONE',  ( 9.001249775931846008E-16, 10.01562500061451644, -25.09994784771203058 ) ) ;
#65388=CYLINDRICAL_SURFACE ( 'NONE', #53659, 4.999999999999998224 ) ;
#65389=CARTESIAN_POINT ( 'NONE',  ( 11.97187500061451892, -6.054752690667223547, -1.112240025338166033E-15 ) ) ;
#65391=CARTESIAN_POINT ( 'NONE',  ( 21.66562500061451502, 3.027376345333611329, 5.243569643749999010 ) ) ;
#65392=CARTESIAN_POINT ( 'NONE',  ( 4.243569643749999898, 10.14687500061451786, 32.45002607614398471 ) ) ;
#65393=CARTESIAN_POINT ( 'NONE',  ( 2.121784821874999061, 18.75312500061459531, 26.32496088578401583 ) ) ;
#65394=CARTESIAN_POINT ( 'NONE',  ( 25.35937500061451644, 0.000000000000000000, 5.243569643749999010 ) ) ;
#65395=CARTESIAN_POINT ( 'NONE',  ( 4.049280102667188963, 2.933370920535487425, -4.300716962760291473 ) ) ;
#65396=CARTESIAN_POINT ( 'NONE',  ( 3.853125000614517681, -4.541064518000417216, -2.621784821875001281 ) ) ;
#65397=AXIS2_PLACEMENT_3D ( 'NONE', #27545, #10909, #38996 ) ;
#65399=CARTESIAN_POINT ( 'NONE',  ( 13.17187500061451999, 3.027376345333611329, 5.243569643749999010 ) ) ;
#65401=CARTESIAN_POINT ( 'NONE',  ( 28.50000000122903288, -2.886751345948125991, -5.000000000000000000 ) ) ;
#65402=CARTESIAN_POINT ( 'NONE',  ( 5.146875000614517859, -3.027376345333614438, 5.243569643749998122 ) ) ;
#65403=CARTESIAN_POINT ( 'NONE',  ( 17.67187500061451644, 3.027376345333611329, 5.243569643749999010 ) ) ;
#65405=CARTESIAN_POINT ( 'NONE',  ( 24.44999999999999929, 4.330127018922192761, -2.499999999999997780 ) ) ;
#65406=CARTESIAN_POINT ( 'NONE',  ( 4.837500001229035895, 4.330127018922191873, 2.499999999999999556 ) ) ;
#65407=CARTESIAN_POINT ( 'NONE',  ( 26.14687500061451431, 6.054752690667223547, 3.707466751127219781E-16 ) ) ;
#65409=CARTESIAN_POINT ( 'NONE',  ( 29.73750000000000071, -2.886751345948125991, -5.000000000000000000 ) ) ;
#65410=CARTESIAN_POINT ( 'NONE',  ( 7.200000000000001954, -4.330127018922190985, -2.500000000000001332 ) ) ;
#65412=CARTESIAN_POINT ( 'NONE',  ( 21.40312500061451573, -4.541064518000417216, -2.621784821875001281 ) ) ;
#65413=CARTESIAN_POINT ( 'NONE',  ( 12.71250000000000036, 2.886751345948129099, -4.999999999999998224 ) ) ;
#65416=CARTESIAN_POINT ( 'NONE',  ( 5.053125000614517859, 0.000000000000000000, 5.243569643749999010 ) ) ;
#65417=CARTESIAN_POINT ( 'NONE',  ( 19.04999999999999716, 4.330127018922192761, -2.499999999999997780 ) ) ;
#65418=CARTESIAN_POINT ( 'NONE',  ( 19.52812500061451573, -4.541064518000419881, 2.621784821874995952 ) ) ;
#65419=CARTESIAN_POINT ( 'NONE',  ( 22.87500000122903288, 2.886751345948126879, 4.999999999999999112 ) ) ;
#65421=CARTESIAN_POINT ( 'NONE',  ( 3.862500000000001155, 2.886751345948126879, 4.999999999999999112 ) ) ;
#65423=CARTESIAN_POINT ( 'NONE',  ( 18.74062500061451431, -3.027376345333610441, -5.243569643749999898 ) ) ;
#65424=CARTESIAN_POINT ( 'NONE',  ( 24.32812500061451289, 4.541064518000418104, 2.621784821874999949 ) ) ;
#65425=CARTESIAN_POINT ( 'NONE',  ( 23.70937500061451786, -4.541064518000417216, -2.621784821875001281 ) ) ;
#65426=CARTESIAN_POINT ( 'NONE',  ( 9.412499999999999645, -5.773502691896255534, -1.060575238724906372E-15 ) ) ;
#65427=CARTESIAN_POINT ( 'NONE',  ( 11.35312500061451679, 0.000000000000000000, 5.243569643749999010 ) ) ;
#65428=CARTESIAN_POINT ( 'NONE',  ( 26.95312500061451644, 4.541064518000418104, -2.621784821874998173 ) ) ;
#65429=CARTESIAN_POINT ( 'NONE',  ( 18.23437500061451999, -4.541064518000419881, 2.621784821874995952 ) ) ;
#65430=CARTESIAN_POINT ( 'NONE',  ( 8.128125000614515372, 4.541064518000418104, 2.621784821874999949 ) ) ;
#65432=CARTESIAN_POINT ( 'NONE',  ( 4.243569643749999898, 10.59687500061451715, 32.45002607614398471 ) ) ;
#65433=CARTESIAN_POINT ( 'NONE',  ( 24.03750000122903430, 6.123233995736764310E-16, -4.999999999999998224 ) ) ;
#65435=CARTESIAN_POINT ( 'NONE',  ( 15.32812500061451644, 4.541064518000418104, 2.621784821874999949 ) ) ;
#65436=CARTESIAN_POINT ( 'NONE',  ( 9.121875000614517504, 3.027376345333611329, 5.243569643749999010 ) ) ;
#65437=CARTESIAN_POINT ( 'NONE',  ( 6.721875000614518925, 3.027376345333613106, -5.243569643749998122 ) ) ;
#65438=ORIENTED_EDGE ( 'NONE', *, *, #54421, .T. ) ;
#65439=CARTESIAN_POINT ( 'NONE',  ( 29.29687500061451644, 6.054752690667223547, 3.707466751127219781E-16 ) ) ;
#65440=CARTESIAN_POINT ( 'NONE',  ( 22.79062500061451502, -3.027376345333610441, -5.243569643749999898 ) ) ;
#65441=CARTESIAN_POINT ( 'NONE',  ( 16.95937500061451786, -4.541064518000417216, -2.621784821875001281 ) ) ;
#65442=CARTESIAN_POINT ( 'NONE',  ( 21.17812500061451431, 4.541064518000418104, 2.621784821874999949 ) ) ;
#65443=CARTESIAN_POINT ( 'NONE',  ( 3.999999999999999112, 10.77500000000000213, 30.00000000000000000 ) ) ;
#65445=CARTESIAN_POINT ( 'NONE',  ( 27.66562500061451146, -6.054752690667223547, -1.112240025338166033E-15 ) ) ;
#65446=CARTESIAN_POINT ( 'NONE',  ( 7.987500001229032698, 4.330127018922191873, 2.499999999999999556 ) ) ;
#65447=VERTEX_POINT ( 'NONE', #15285 ) ;
#65448=CARTESIAN_POINT ( 'NONE',  ( 29.28749999999999787, -2.886751345948125991, -5.000000000000000000 ) ) ;
#65449=CARTESIAN_POINT ( 'NONE',  ( 4.000000000000000000, 18.38749999999999929, -27.69059892324149530 ) ) ;
#65450=CARTESIAN_POINT ( 'NONE',  ( 24.63750000122903216, 4.330127018922191873, 2.499999999999999556 ) ) ;
#65452=CARTESIAN_POINT ( 'NONE',  ( 7.884375000614517681, -4.541064518000419881, 2.621784821874995952 ) ) ;
#65454=CARTESIAN_POINT ( 'NONE',  ( 14.12812500061451715, -4.541064518000419881, 2.621784821874995952 ) ) ;
#65455=CARTESIAN_POINT ( 'NONE',  ( 9.571875000614518569, 3.027376345333611329, 5.243569643749999010 ) ) ;
#65456=CARTESIAN_POINT ( 'NONE',  ( 27.41250000122903430, 0.000000000000000000, 4.999999999999998224 ) ) ;
#65457=CLOSED_SHELL ( 'NONE', ( #41666, #19708, #68201, #14121, #54911, #58593, #29653, #56735, #45259, #8386, #13765, #14129, #52831, #19028, #47994, #45841, #5966, #17309, #64957, #33767, #30642, #21800, #17132, #27070, #47350, #42352, #60819, #48169, #18756, #42083, #70101, #22596, #46252, #46043, #60662, #38659, #60169, #3139, #27990, #69969, #66109, #66251, #17388, #23787, #63066, #36658, #6338, #67131, #44776, #45948, #13297, #28585, #40854, #36547, #30311, #47929, #22954, #44228, #8593, #71206, #52581, #24043, #26572, #20548, #56825, #47580, #53597, #17669, #35201, #62304, #62153, #4799, #71669, #32797, #49020, #47721, #3812, #44864, #23406, #20387, #45415, #52323, #11268, #52661, #551, #63085, #61773, #57923, #14846, #71593, #49614, #6499, #67108, #56234, #40997, #36232, #62741, #52239, #113, #35482, #2159, #59378, #30029, #56419, #14459, #50043, #47487, #43593, #4227, #36882, #72771, #12578, #6639, #7981, #25535, #2294, #59653, #12462, #49128, #39569, #37666, #29501, #48586, #46311, #17842, #278, #49773, #31664, #22905, #13624, #60458, #18927, #44023, #6217, #52768, #11904, #4372, #43848, #9826, #70737, #6389, #64668, #13504, #72861, #52683, #38757, #39847, #6863, #50830, #18915, #61336, #28438, #1768, #66694, #66827, #23713, #36383, #50179, #48328, #314, #62004, #19547, #67105, #51206, #40006, #63998, #28988, #4328, #70009, #67944, #55039, #51361, #24686, #50827, #983, #64644, #55344, #50413, #20, #51047, #23932, #70599, #33895, #16942, #10696, #60400, #246, #57127, #39021, #61795, #13524, #29479, #43692, #5339, #71937, #53234, #11615, #45683, #23564, #71677, #34898, #52812, #6883, #22109, #11397, #39505, #46914, #20244, #2059, #59069, #6549, #51838, #2573, #23779, #37321, #16050, #65617, #64014, #66670, #42460, #52514, #21887, #9313, #71450, #23286, #49637, #70064, #34293, #21886, #10235, #44081, #45765, #58040, #68770, #12134, #51477, #53153, #7675, #58092, #51571, #70785, #55935, #42070, #24746, #801, #34627, #31107, #12435, #18534, #52015, #57496, #27394, #62508, #56867, #17066, #70671, #40161, #68286, #61658, #29148, #15873, #39419, #1303, #69565, #40074, #44067, #51161, #21132, #49227 ) ) ;
#65458=CARTESIAN_POINT ( 'NONE',  ( 17.78437500061451715, -4.541064518000419881, 2.621784821874995952 ) ) ;
#65459=CARTESIAN_POINT ( 'NONE',  ( 5.221875000614519813, -6.054752690667223547, -1.112240025338166033E-15 ) ) ;
#65460=DIRECTION ( 'NONE',  ( 0.000000000000000000, 0.000000000000000000, 1.000000000000000000 ) ) ;
#65461=CARTESIAN_POINT ( 'NONE',  ( 4.453125000614517326, 4.541064518000418104, -2.621784821874998173 ) ) ;
#65462=CARTESIAN_POINT ( 'NONE',  ( 16.45312500061451289, -4.541064518000417216, -2.621784821875001281 ) ) ;
#65463=ORIENTED_EDGE ( 'NONE', *, *, #71959, .F. ) ;
#65464=CARTESIAN_POINT ( 'NONE',  ( 12.74062500061451786, -3.027376345333614438, 5.243569643749998122 ) ) ;
#65465=CARTESIAN_POINT ( 'NONE',  ( 5.325000001229033941, 2.886751345948126879, 4.999999999999999112 ) ) ;
#65467=CARTESIAN_POINT ( 'NONE',  ( 11.76562500061451644, 3.027376345333611329, 5.243569643749999010 ) ) ;
#65469=CARTESIAN_POINT ( 'NONE',  ( 11.73750000000000249, -2.886751345948125991, -5.000000000000000000 ) ) ;
#65470=EDGE_CURVE ( 'NONE', #28698, #53581, #14922, .T. ) ;
#65471=CARTESIAN_POINT ( 'NONE',  ( 4.687500001229034652, 6.123233995736764310E-16, -4.999999999999998224 ) ) ;
#65472=CARTESIAN_POINT ( 'NONE',  ( 17.28750000000000142, 5.773502691896255534, 3.535250795749688894E-16 ) ) ;
#65474=CARTESIAN_POINT ( 'NONE',  ( 19.47187500061451360, 3.027376345333611329, 5.243569643749999010 ) ) ;
#65475=CARTESIAN_POINT ( 'NONE',  ( 16.50000000122903288, 5.773502691896255534, 3.535250795749688894E-16 ) ) ;
#65477=CARTESIAN_POINT ( 'NONE',  ( 4.243569643749999898, 15.97812500061451857, -30.00000000000000000 ) ) ;
#65479=CARTESIAN_POINT ( 'NONE',  ( 2.733878782416514941, -4.186395442746991158, 2.733878782416514941 ) ) ;
#65480=CARTESIAN_POINT ( 'NONE',  ( 30.00000000000000000, 0.000000000000000000, 4.999999999999998224 ) ) ;
#65481=CARTESIAN_POINT ( 'NONE',  ( 0.000000000000000000, 20.00000000000000000, -30.00000000000000000 ) ) ;
#65482=CARTESIAN_POINT ( 'NONE',  ( 30.00000000000000000, 0.000000000000000000, 0.000000000000000000 ) ) ;
#65483=CARTESIAN_POINT ( 'NONE',  ( 1.999999999999998668, 14.56250000122903288, 26.53589838486224650 ) ) ;
#65484=CARTESIAN_POINT ( 'NONE',  ( 16.50937500061451502, -4.541064518000417216, -2.621784821875001281 ) ) ;
#65485=CARTESIAN_POINT ( 'NONE',  ( 28.98750000000000071, 5.773502691896255534, 3.535250795749688894E-16 ) ) ;
#65486=CARTESIAN_POINT ( 'NONE',  ( 10.86562500061451431, 3.027376345333611329, 5.243569643749999010 ) ) ;
#65488=CARTESIAN_POINT ( 'NONE',  ( 24.27187500061452141, 3.027376345333613106, -5.243569643749998122 ) ) ;
#65490=CARTESIAN_POINT ( 'NONE',  ( 6.740625000614516082, 6.054752690667223547, 3.707466751127219781E-16 ) ) ;
#65491=CARTESIAN_POINT ( 'NONE',  ( 13.73437500061451821, -4.541064518000419881, 2.621784821874995952 ) ) ;
#65493=CARTESIAN_POINT ( 'NONE',  ( 24.64687500061451431, -3.027376345333610441, -5.243569643749999898 ) ) ;
#65494=CARTESIAN_POINT ( 'NONE',  ( 28.41562500061451502, 3.027376345333611329, 5.243569643749999010 ) ) ;
#65496=AXIS2_PLACEMENT_3D ( 'NONE', #22595, #45146, #3181 ) ;
#65497=CARTESIAN_POINT ( 'NONE',  ( 8.400000000000000355, 0.000000000000000000, 4.999999999999998224 ) ) ;
#65498=CARTESIAN_POINT ( 'NONE',  ( 15.86250000122903181, -4.330127018922190985, -2.500000000000001332 ) ) ;
#65500=DIRECTION ( 'NONE',  ( 0.000000000000000000, 0.000000000000000000, -1.000000000000000000 ) ) ;
#65501=ORIENTED_EDGE ( 'NONE', *, *, #28336, .F. ) ;
#65503=CARTESIAN_POINT ( 'NONE',  ( 16.35000000000000142, 4.330127018922192761, -2.499999999999997780 ) ) ;
#65504=CARTESIAN_POINT ( 'NONE',  ( 18.07499999999999929, 6.123233995736764310E-16, -4.999999999999998224 ) ) ;
#65505=CARTESIAN_POINT ( 'NONE',  ( 11.91562500061451857, -6.054752690667223547, -1.112240025338166033E-15 ) ) ;
#65509=CARTESIAN_POINT ( 'NONE',  ( 4.243569643749999010, 17.42187500061451999, -32.45002607614398471 ) ) ;
#65510=CARTESIAN_POINT ( 'NONE',  ( 4.565625000614516260, 3.027376345333611329, 5.243569643749999010 ) ) ;
#65512=CARTESIAN_POINT ( 'NONE',  ( 8.962500000000002132, -5.773502691896255534, -1.060575238724906372E-15 ) ) ;
#65513=CARTESIAN_POINT ( 'NONE',  ( 3.651773823418189124, 3.415340091791402966, 3.978752903393068863 ) ) ;
#65515=CARTESIAN_POINT ( 'NONE',  ( 4.243569643749999898, 16.39062500061451999, 32.45002607614398471 ) ) ;
#65516=CARTESIAN_POINT ( 'NONE',  ( 26.12812500061451360, 4.541064518000418104, 2.621784821874999949 ) ) ;
#65518=CIRCLE ( 'NONE', #623, 4.000000000000000000 ) ;
#65520=CARTESIAN_POINT ( 'NONE',  ( 22.65937500061451715, 0.000000000000000000, 5.243569643749999010 ) ) ;
#65521=CARTESIAN_POINT ( 'NONE',  ( 19.56562500061451715, -6.054752690667223547, -1.112240025338166033E-15 ) ) ;
#65522=CARTESIAN_POINT ( 'NONE',  ( -4.243569643749999898, 14.81562500061459353, -32.45002607614398471 ) ) ;
#65523=CARTESIAN_POINT ( 'NONE',  ( 22.72500000122903430, 2.886751345948129099, -4.999999999999998224 ) ) ;
#65524=CARTESIAN_POINT ( 'NONE',  ( 4.453125000614517326, 4.541064518000418104, -2.621784821874998173 ) ) ;
#65526=CARTESIAN_POINT ( 'NONE',  ( 20.87812500061451715, -4.541064518000419881, 2.621784821874995952 ) ) ;
#65529=CARTESIAN_POINT ( 'NONE',  ( 17.10937500061451999, 4.541064518000418104, -2.621784821874998173 ) ) ;
#65530=CARTESIAN_POINT ( 'NONE',  ( 17.03437500061451715, 6.421520780324663323E-16, -5.243569643749999010 ) ) ;
#65531=CARTESIAN_POINT ( 'NONE',  ( 25.88437500061451502, -4.541064518000419881, 2.621784821874995952 ) ) ;
#65532=CARTESIAN_POINT ( 'NONE',  ( 2.121784821874999061, 13.85937500061451821, 26.32496088578401583 ) ) ;
#65533=CARTESIAN_POINT ( 'NONE',  ( 4.453125000614517326, 4.541064518000418104, -2.621784821874998173 ) ) ;
#65534=CARTESIAN_POINT ( 'NONE',  ( 27.81562500061452070, 3.027376345333613106, -5.243569643749998122 ) ) ;
#65535=CARTESIAN_POINT ( 'NONE',  ( 3.309375000614518836, 0.000000000000000000, 5.243569643749999010 ) ) ;
#65537=CARTESIAN_POINT ( 'NONE',  ( 4.000000000000000000, 19.28750000000000142, 32.30940107675849049 ) ) ;
#65538=CARTESIAN_POINT ( 'NONE',  ( 8.071875000614518569, 3.027376345333613106, -5.243569643749998122 ) ) ;
#65540=CARTESIAN_POINT ( 'NONE',  ( 15.11250000122903359, 4.330127018922192761, -2.499999999999997780 ) ) ;
#65541=CARTESIAN_POINT ( 'NONE',  ( 9.150000001229033231, -2.886751345948125991, -5.000000000000000000 ) ) ;
#65542=CARTESIAN_POINT ( 'NONE',  ( 5.278125000614516615, 6.421520780324663323E-16, -5.243569643749999010 ) ) ;
#65545=CARTESIAN_POINT ( 'NONE',  ( 13.65937500061451715, 0.000000000000000000, 5.243569643749999010 ) ) ;
#65546=VERTEX_POINT ( 'NONE', #22292 ) ;
#65547=CARTESIAN_POINT ( 'NONE',  ( 21.55312500061451431, 4.541064518000418104, -2.621784821874998173 ) ) ;
#65548=CARTESIAN_POINT ( 'NONE',  ( 8.015625000614518214, 3.027376345333613106, -5.243569643749998122 ) ) ;
#65549=CARTESIAN_POINT ( 'NONE',  ( 24.45937500061451786, 0.000000000000000000, 5.243569643749999010 ) ) ;
#65550=CARTESIAN_POINT ( 'NONE',  ( 7.040625000614517681, -3.027376345333610441, -5.243569643749999898 ) ) ;
#65552=CARTESIAN_POINT ( 'NONE',  ( 8.025000001229035007, 2.886751345948126879, 4.999999999999999112 ) ) ;
#65553=CARTESIAN_POINT ( 'NONE',  ( 21.51562500061451644, 3.027376345333613106, -5.243569643749998122 ) ) ;
#65554=CARTESIAN_POINT ( 'NONE',  ( -4.243569643749997233, 9.940625000614515372, -27.54997392385601174 ) ) ;
#65555=CARTESIAN_POINT ( 'NONE',  ( 9.187500001229034652, 6.123233995736764310E-16, -4.999999999999998224 ) ) ;
#65556=CARTESIAN_POINT ( 'NONE',  ( 19.71562500061451928, 3.027376345333613106, -5.243569643749998122 ) ) ;
#65558=CARTESIAN_POINT ( 'NONE',  ( 17.39062500061451644, -3.027376345333610441, -5.243569643749999898 ) ) ;
#65560=CARTESIAN_POINT ( 'NONE',  ( 16.98750000000000426, -2.886751345948129988, 4.999999999999997335 ) ) ;
#65561=CARTESIAN_POINT ( 'NONE',  ( 11.81250000122903465, -4.330127018922190985, -2.500000000000001332 ) ) ;
#65562=CARTESIAN_POINT ( 'NONE',  ( 8.690625000614515372, -3.027376345333614438, 5.243569643749998122 ) ) ;
#65563=CARTESIAN_POINT ( 'NONE',  ( 10.75312500061451715, 4.541064518000418104, -2.621784821874998173 ) ) ;
#65564=CARTESIAN_POINT ( 'NONE',  ( 24.30000000122903359, -2.886751345948129988, 4.999999999999997335 ) ) ;
#65565=CARTESIAN_POINT ( 'NONE',  ( 22.35937500061451644, -4.541064518000417216, -2.621784821875001281 ) ) ;
#65566=CARTESIAN_POINT ( 'NONE',  ( 3.553828822764864448, 3.517143826812636931, -3.889051543804785016 ) ) ;
#65567=CARTESIAN_POINT ( 'NONE',  ( 5.850000001229035185, -2.886751345948129988, 4.999999999999997335 ) ) ;
#65568=CARTESIAN_POINT ( 'NONE',  ( 7.209375000614519635, 4.541064518000418104, -2.621784821874998173 ) ) ;
#65569=CARTESIAN_POINT ( 'NONE',  ( 23.14687500061451786, -3.027376345333614438, 5.243569643749998122 ) ) ;
#65571=CARTESIAN_POINT ( 'NONE',  ( 17.69062500061451715, -3.027376345333614438, 5.243569643749998122 ) ) ;
#65572=CARTESIAN_POINT ( 'NONE',  ( 23.40937500061451715, 4.541064518000418104, -2.621784821874998173 ) ) ;
#65575=CARTESIAN_POINT ( 'NONE',  ( 4.000000000000000000, 15.68750000000000000, 32.30940107675849760 ) ) ;
#65576=CARTESIAN_POINT ( 'NONE',  ( 4.846875000614519813, -3.027376345333610441, -5.243569643749999898 ) ) ;
#65577=CARTESIAN_POINT ( 'NONE',  ( 15.25312500061451715, 4.541064518000418104, -2.621784821874998173 ) ) ;
#65578=CARTESIAN_POINT ( 'NONE',  ( 14.10937500061451644, 0.000000000000000000, 5.243569643749999010 ) ) ;
#65580=CARTESIAN_POINT ( 'NONE',  ( 30.00000000000000000, 0.000000000000000000, 0.000000000000000000 ) ) ;
#65581=CARTESIAN_POINT ( 'NONE',  ( 23.99062500061451786, -3.027376345333614438, 5.243569643749998122 ) ) ;
#65582=CARTESIAN_POINT ( 'NONE',  ( -0.7368805616696194605, 9.859898480082234684, -34.17910162106521454 ) ) ;
#65584=CARTESIAN_POINT ( 'NONE',  ( 15.00000000000000000, 4.330127018922192761, -2.499999999999997780 ) ) ;
#65585=CARTESIAN_POINT ( 'NONE',  ( 24.82500000122902861, -5.773502691896255534, -1.060575238724906372E-15 ) ) ;
#65586=CARTESIAN_POINT ( 'NONE',  ( 19.52812500061451573, -4.541064518000419881, 2.621784821874995952 ) ) ;
#65587=ORIENTED_EDGE ( 'NONE', *, *, #27586, .F. ) ;
#65588=CARTESIAN_POINT ( 'NONE',  ( 21.52499999999999858, -4.330127018922194537, 2.499999999999995559 ) ) ;
#65589=CARTESIAN_POINT ( 'NONE',  ( 22.65937500061451715, 0.000000000000000000, 5.243569643749999010 ) ) ;
#65591=ORIENTED_EDGE ( 'NONE', *, *, #3605, .T. ) ;
#65593=CARTESIAN_POINT ( 'NONE',  ( 10.49062500061451431, -3.027376345333614438, 5.243569643749998122 ) ) ;
#65594=CARTESIAN_POINT ( 'NONE',  ( 2.990625000614519191, -3.027376345333610441, -5.243569643749999898 ) ) ;
#65596=CARTESIAN_POINT ( 'NONE',  ( 27.02812500061451573, 4.541064518000418104, 2.621784821874999949 ) ) ;
#65598=CARTESIAN_POINT ( 'NONE',  ( 16.76249999999999929, 2.886751345948129099, -4.999999999999998224 ) ) ;
#65599=CARTESIAN_POINT ( 'NONE',  ( 26.17500000000000071, 6.123233995736764310E-16, -4.999999999999998224 ) ) ;
#65600=CARTESIAN_POINT ( 'NONE',  ( 1.071796769724489895, 10.86740381056766758, -34.00000000000000000 ) ) ;
#65601=CARTESIAN_POINT ( 'NONE',  ( 7.059375000614518392, -4.541064518000417216, -2.621784821875001281 ) ) ;
#65602=CARTESIAN_POINT ( 'NONE',  ( 16.95937500061451786, -4.541064518000417216, -2.621784821875001281 ) ) ;
#65604=ORIENTED_EDGE ( 'NONE', *, *, #24878, .T. ) ;
#65605=CARTESIAN_POINT ( 'NONE',  ( 25.56562500061452070, 3.027376345333613106, -5.243569643749998122 ) ) ;
#65606=CARTESIAN_POINT ( 'NONE',  ( 28.65937500061451715, -4.541064518000417216, -2.621784821875001281 ) ) ;
#65608=CARTESIAN_POINT ( 'NONE',  ( 14.58750000000000036, 5.773502691896255534, 3.535250795749688894E-16 ) ) ;
#65609=CARTESIAN_POINT ( 'NONE',  ( 12.44062500061451537, -3.027376345333610441, -5.243569643749999898 ) ) ;
#65610=CARTESIAN_POINT ( 'NONE',  ( -1.071796769724491005, 14.95759618943233527, -34.00000000000000000 ) ) ;
#65612=CARTESIAN_POINT ( 'NONE',  ( 15.33750000122903323, -4.330127018922194537, 2.499999999999995559 ) ) ;
#65615=CARTESIAN_POINT ( 'NONE',  ( 5.915625000614515905, 3.027376345333611329, 5.243569643749999010 ) ) ;
#65616=CARTESIAN_POINT ( 'NONE',  ( 22.58437500061451431, 4.541064518000418104, 2.621784821874999949 ) ) ;
#65617=ADVANCED_FACE ( 'NONE', ( #28212 ), #61812, .F. ) ;
#65618=CARTESIAN_POINT ( 'NONE',  ( 4.243569643749999898, 16.89687500061451786, 32.45002607614398471 ) ) ;
#65619=CARTESIAN_POINT ( 'NONE',  ( 23.40937500061451715, 4.541064518000418104, -2.621784821874998173 ) ) ;
#65620=CARTESIAN_POINT ( 'NONE',  ( 4.612500000000002487, 2.886751345948129099, -4.999999999999998224 ) ) ;
#65621=CARTESIAN_POINT ( 'NONE',  ( -3.999999999999999112, 11.11250000122903536, 30.00000000000000000 ) ) ;
#65622=CARTESIAN_POINT ( 'NONE',  ( 12.55312500061451786, 4.541064518000418104, -2.621784821874998173 ) ) ;
#65623=CARTESIAN_POINT ( 'NONE',  ( 5.137500001229033941, 6.123233995736764310E-16, -4.999999999999998224 ) ) ;
#65624=CARTESIAN_POINT ( 'NONE',  ( 10.35937500061451644, 4.541064518000418104, -2.621784821874998173 ) ) ;
#65626=CARTESIAN_POINT ( 'NONE',  ( 9.403125000614517504, 4.541064518000418104, -2.621784821874998173 ) ) ;
#65627=CARTESIAN_POINT ( 'NONE',  ( 15.45937500061451608, 0.000000000000000000, 5.243569643749999010 ) ) ;
#65629=CARTESIAN_POINT ( 'NONE',  ( 20.73750000122903359, -4.330127018922194537, 2.499999999999995559 ) ) ;
#65630=CARTESIAN_POINT ( 'NONE',  ( 11.59687500061451892, -3.027376345333610441, -5.243569643749999898 ) ) ;
#65631=CARTESIAN_POINT ( 'NONE',  ( 13.00312500061451537, 4.541064518000418104, -2.621784821874998173 ) ) ;
#65633=CARTESIAN_POINT ( 'NONE',  ( 21.15937500061451715, 4.541064518000418104, -2.621784821874998173 ) ) ;
#65634=CARTESIAN_POINT ( 'NONE',  ( 1.626862140677534273E-15, 18.42500000122903359, 34.00000000000000000 ) ) ;
#65635=CARTESIAN_POINT ( 'NONE',  ( -0.2805529113108867767, 4.994030452822312505, 26.00745495759712611 ) ) ;
#65637=CARTESIAN_POINT ( 'NONE',  ( -4.243569643749998122, 14.94687500061451679, -27.54997392385601174 ) ) ;
#65638=CARTESIAN_POINT ( 'NONE',  ( 15.60000000122903607, 5.773502691896255534, 3.535250795749688894E-16 ) ) ;
#65639=CARTESIAN_POINT ( 'NONE',  ( 10.84687500061451892, 6.054752690667223547, 3.707466751127219781E-16 ) ) ;
#65640=CARTESIAN_POINT ( 'NONE',  ( 4.243569643749999898, 17.29062500061451502, -27.54997392385601529 ) ) ;
#65641=CARTESIAN_POINT ( 'NONE',  ( 16.87500000122903288, 2.886751345948129099, -4.999999999999998224 ) ) ;
#65642=CARTESIAN_POINT ( 'NONE',  ( 9.890625000614516438, 6.054752690667223547, 3.707466751127219781E-16 ) ) ;
#65643=VERTEX_POINT ( 'NONE', #34096 ) ;
#65644=CARTESIAN_POINT ( 'NONE',  ( 16.76249999999999929, 2.886751345948129099, -4.999999999999998224 ) ) ;
#65645=CARTESIAN_POINT ( 'NONE',  ( 10.46250000122903323, -4.330127018922190985, -2.500000000000001332 ) ) ;
#65646=CARTESIAN_POINT ( 'NONE',  ( 9.009375000614518569, 4.541064518000418104, -2.621784821874998173 ) ) ;
#65647=CARTESIAN_POINT ( 'NONE',  ( 9.412500001229034297, 0.000000000000000000, 4.999999999999998224 ) ) ;
#65648=CARTESIAN_POINT ( 'NONE',  ( 19.65000000122902790, 5.773502691896255534, 3.535250795749688894E-16 ) ) ;
#65649=CARTESIAN_POINT ( 'NONE',  ( 15.89062500061451289, -3.027376345333614438, 5.243569643749998122 ) ) ;
#65650=CARTESIAN_POINT ( 'NONE',  ( 19.52812500061451573, -4.541064518000419881, 2.621784821874995952 ) ) ;
#65651=CARTESIAN_POINT ( 'NONE',  ( 27.26250000122903216, 4.330127018922192761, -2.499999999999997780 ) ) ;
#65652=CARTESIAN_POINT ( 'NONE',  ( 3.028125000614518392, 6.421520780324663323E-16, -5.243569643749999010 ) ) ;
#65653=CARTESIAN_POINT ( 'NONE',  ( 24.29999999999999716, -4.330127018922190985, -2.500000000000001332 ) ) ;
#65654=CARTESIAN_POINT ( 'NONE',  ( 4.955394143245530181, -0.7664506687210094205, -5.056849431660869421 ) ) ;
#65655=AXIS2_PLACEMENT_3D ( 'NONE', #53301, #15235, #37772 ) ;
#65657=CARTESIAN_POINT ( 'NONE',  ( 27.57187500061451857, 3.027376345333611329, 5.243569643749999010 ) ) ;
#65659=CARTESIAN_POINT ( 'NONE',  ( 11.81250000122903465, -4.330127018922190985, -2.500000000000001332 ) ) ;
#65660=CARTESIAN_POINT ( 'NONE',  ( 29.78437500061451715, 4.541064518000418104, 2.621784821874999949 ) ) ;
#65661=CARTESIAN_POINT ( 'NONE',  ( 22.76249999999999929, 2.886751345948093572, 5.000000000000056843 ) ) ;
#65662=CARTESIAN_POINT ( 'NONE',  ( 7.246875000614518392, 6.054752690667223547, 3.707466751127219781E-16 ) ) ;
#65663=B_SPLINE_CURVE_WITH_KNOTS ( 'NONE', 3,
 ( #49124, #48025, #54655, #36928, #70918, #43579, #71653, #26955, #70179, #19926 ),
 .UNSPECIFIED., .F., .F.,
 ( 4, 3, 3, 4 ),
 ( 6.633699979077398476E-15, 0.0001572284277986207531, 0.0003144570899457547575, 0.0005090485883879889480 ),
 .UNSPECIFIED. ) ;
#65664=CARTESIAN_POINT ( 'NONE',  ( 25.75312500061451715, 0.000000000000000000, 5.243569643749999010 ) ) ;
#65665=DIRECTION ( 'NONE',  ( -0.000000000000000000, -1.000000000000000000, -0.000000000000000000 ) ) ;
#65666=CARTESIAN_POINT ( 'NONE',  ( 1.999999999999998668, 10.51250000122903572, 26.53589838486224650 ) ) ;
#65668=CARTESIAN_POINT ( 'NONE',  ( 5.934375000614517504, 4.541064518000418104, 2.621784821874999949 ) ) ;
#65669=CARTESIAN_POINT ( 'NONE',  ( 7.809375000614519280, 0.000000000000000000, 5.243569643749999010 ) ) ;
#65670=CARTESIAN_POINT ( 'NONE',  ( 4.275000000000001243, 4.330127018922191873, 2.499999999999999556 ) ) ;
#65671=( BOUNDED_CURVE ( )  B_SPLINE_CURVE ( 2, ( #56125, #73112, #22494, #45044, #16944, #23939, #29854, #23213, #1433 ),
 .UNSPECIFIED., .F., .F. ) 
 B_SPLINE_CURVE_WITH_KNOTS ( ( 3, 2, 2, 2, 3 ),
 ( 0.9021739130434782705, 0.9057971014492753881, 0.9130434782608695121, 0.9202898550724637472, 0.9239130434782608647 ),
 .UNSPECIFIED. ) 
 CURVE ( )  GEOMETRIC_REPRESENTATION_ITEM ( )  RATIONAL_B_SPLINE_CURVE ( ( 0.9330127018922194093, 0.9330127018922194093, 1.000000000000000000, 0.8660254037844387076, 1.000000000000000000, 0.8660254037844387076, 1.000000000000000000, 0.9330127018922194093, 0.9330127018922194093 ) ) 
 REPRESENTATION_ITEM ( '' )  );
#65672=CARTESIAN_POINT ( 'NONE',  ( -2.121784821874999949, 12.97812500061459318, 26.32496088578401938 ) ) ;
#65673=CARTESIAN_POINT ( 'NONE',  ( 21.63749999999999929, -2.886751345948125991, -5.000000000000000000 ) ) ;
#65674=CARTESIAN_POINT ( 'NONE',  ( 29.62500000000000000, -4.330127018922194537, 2.499999999999995559 ) ) ;
#65675=CARTESIAN_POINT ( 'NONE',  ( 3.225000000000002309, 6.123233995736764310E-16, -4.999999999999998224 ) ) ;
#65676=EDGE_CURVE ( 'NONE', #28753, #46571, #17814, .T. ) ;
#65677=ORIENTED_EDGE ( 'NONE', *, *, #9622, .T. ) ;
#65678=CARTESIAN_POINT ( 'NONE',  ( 17.72812500061451502, -4.541064518000419881, 2.621784821874995952 ) ) ;
#65679=CARTESIAN_POINT ( 'NONE',  ( 9.553125000614517859, 0.000000000000000000, 5.243569643749999010 ) ) ;
#65681=CARTESIAN_POINT ( 'NONE',  ( 6.234375000614519102, 6.421520780324663323E-16, -5.243569643749999010 ) ) ;
#65682=CARTESIAN_POINT ( 'NONE',  ( 22.87500000000000000, -4.330127018922194537, 2.499999999999995559 ) ) ;
#65683=CARTESIAN_POINT ( 'NONE',  ( 20.85000000122903430, -2.886751345948125991, -5.000000000000000000 ) ) ;
#65684=CARTESIAN_POINT ( 'NONE',  ( 0.000000000000000000, 20.00000000000000000, -30.00000000000000000 ) ) ;
#65685=CARTESIAN_POINT ( 'NONE',  ( 10.17187500061451999, -6.054752690667223547, -1.112240025338166033E-15 ) ) ;
#65686=CARTESIAN_POINT ( 'NONE',  ( 13.95937500061451786, 4.541064518000418104, -2.621784821874998173 ) ) ;
#65687=CARTESIAN_POINT ( 'NONE',  ( 23.67187500061451999, -6.054752690667223547, -1.112240025338166033E-15 ) ) ;
#65688=VECTOR ( 'NONE', #32399, 1000.000000000000000 ) ;
#65689=CARTESIAN_POINT ( 'NONE',  ( -6.275039685470489619E-15, 17.97500000122903074, -26.00000000000000355 ) ) ;
#65691=CARTESIAN_POINT ( 'NONE',  ( 17.63437500061451502, 4.541064518000418104, 2.621784821874999949 ) ) ;
#65692=CARTESIAN_POINT ( 'NONE',  ( 9.459375000614517859, 4.541064518000418104, -2.621784821874998173 ) ) ;
#65694=CARTESIAN_POINT ( 'NONE',  ( 22.68750000000000000, 5.773502691896255534, 3.535250795749688894E-16 ) ) ;
#65696=CARTESIAN_POINT ( 'NONE',  ( -1.473772837211104525, 9.872922166578584680, -34.04916900799978663 ) ) ;
#65698=CARTESIAN_POINT ( 'NONE',  ( 11.35312500061451679, 0.000000000000000000, 5.243569643749999010 ) ) ;
#65699=CARTESIAN_POINT ( 'NONE',  ( 28.73437500061451644, 6.421520780324663323E-16, -5.243569643749999010 ) ) ;
#65700=CARTESIAN_POINT ( 'NONE',  ( 30.00000000000000000, 0.000000000000000000, 4.999999999999998224 ) ) ;
#65701=CARTESIAN_POINT ( 'NONE',  ( 4.000000000000000000, 9.950000001229033941, -27.69059892324149885 ) ) ;
#65702=CARTESIAN_POINT ( 'NONE',  ( 12.90000000000000213, 0.000000000000000000, 4.999999999999998224 ) ) ;
#65703=CARTESIAN_POINT ( 'NONE',  ( 8.484601909799253346E-16, 18.42500000122903714, 34.61880215351700230 ) ) ;
#65704=CARTESIAN_POINT ( 'NONE',  ( 11.77500000122903501, -5.773502691896255534, -1.060575238724906372E-15 ) ) ;
#65706=CARTESIAN_POINT ( 'NONE',  ( 23.03437500061451715, 4.541064518000418104, 2.621784821874999949 ) ) ;
#65707=CARTESIAN_POINT ( 'NONE',  ( 16.92187500061451999, -6.054752690667223547, -1.112240025338166033E-15 ) ) ;
#65708=CARTESIAN_POINT ( 'NONE',  ( -3.999999999999999112, 16.36250000000000071, -32.30940107675850470 ) ) ;
#65709=ORIENTED_EDGE ( 'NONE', *, *, #35651, .T. ) ;
#65710=CARTESIAN_POINT ( 'NONE',  ( 17.16562500061451502, 3.027376345333611329, 5.243569643749999010 ) ) ;
#65711=CARTESIAN_POINT ( 'NONE',  ( 27.93750000122903288, -4.330127018922194537, 2.499999999999995559 ) ) ;
#65712=CARTESIAN_POINT ( 'NONE',  ( 17.89687500061451431, -3.027376345333610441, -5.243569643749999898 ) ) ;
#65713=CARTESIAN_POINT ( 'NONE',  ( 4.490625000614516971, 6.054752690667223547, 3.707466751127219781E-16 ) ) ;
#65714=CARTESIAN_POINT ( 'NONE',  ( 19.15312500061451573, -4.541064518000417216, -2.621784821875001281 ) ) ;
#65716=CARTESIAN_POINT ( 'NONE',  ( 29.70937500061451431, 4.541064518000418104, -2.621784821874998173 ) ) ;
#65717=CARTESIAN_POINT ( 'NONE',  ( -2.121784821874999949, 12.97812500061451679, 26.32496088578401938 ) ) ;
#65718=CARTESIAN_POINT ( 'NONE',  ( 17.70000000122903216, -2.886751345948125991, -5.000000000000000000 ) ) ;
#65720=CARTESIAN_POINT ( 'NONE',  ( 27.51562500061451644, 3.027376345333611329, 5.243569643749999010 ) ) ;
#65721=CARTESIAN_POINT ( 'NONE',  ( -2.000000000000000000, 9.687500001229034652, 26.53589838486224650 ) ) ;
#65722=CARTESIAN_POINT ( 'NONE',  ( 20.52187500061451786, -6.054752690667223547, -1.112240025338166033E-15 ) ) ;
#65723=CARTESIAN_POINT ( 'NONE',  ( 23.06250000122903288, -4.330127018922190985, -2.500000000000001332 ) ) ;
#65724=CARTESIAN_POINT ( 'NONE',  ( 22.45312500061451644, 4.541064518000418104, -2.621784821874998173 ) ) ;
#65725=CARTESIAN_POINT ( 'NONE',  ( 16.05937500061451573, -4.541064518000417216, -2.621784821875001281 ) ) ;
#65726=CARTESIAN_POINT ( 'NONE',  ( 12.77812500061451750, -4.541064518000419881, 2.621784821874995952 ) ) ;
#65727=CARTESIAN_POINT ( 'NONE',  ( 9.001249775931846008E-16, 15.02187500061451608, 34.90005215228797653 ) ) ;
#65728=( BOUNDED_CURVE ( )  B_SPLINE_CURVE ( 2, ( #10528, #50780, #28605, #72585, #55956, #60757, #66684, #10165, #5352 ),
 .UNSPECIFIED., .F., .F. ) 
 B_SPLINE_CURVE_WITH_KNOTS ( ( 3, 2, 2, 2, 3 ),
 ( 0.4239130434782608647, 0.4275362318840579823, 0.4347826086956521618, 0.4420289855072463969, 0.4456521739130435145 ),
 .UNSPECIFIED. ) 
 CURVE ( )  GEOMETRIC_REPRESENTATION_ITEM ( )  RATIONAL_B_SPLINE_CURVE ( ( 0.9330127018922194093, 0.9330127018922194093, 1.000000000000000000, 0.8660254037844387076, 1.000000000000000000, 0.8660254037844387076, 1.000000000000000000, 0.9330127018922188542, 0.9330127018922194093 ) ) 
 REPRESENTATION_ITEM ( '' )  );
#65729=CARTESIAN_POINT ( 'NONE',  ( 20.99062500061451431, -3.027376345333610441, -5.243569643749999898 ) ) ;
#65730=CARTESIAN_POINT ( 'NONE',  ( 29.27812500061451573, 4.541064518000418104, 2.621784821874999949 ) ) ;
#65731=ORIENTED_EDGE ( 'NONE', *, *, #33365, .F. ) ;
#65733=CARTESIAN_POINT ( 'NONE',  ( 22.94999999999999929, -4.330127018922190985, -2.500000000000001332 ) ) ;
#65734=CARTESIAN_POINT ( 'NONE',  ( 4.243569643749999898, 19.18437500061451928, -30.00000000000000000 ) ) ;
#65735=CARTESIAN_POINT ( 'NONE',  ( 12.44999999999999929, 0.000000000000000000, 4.999999999999998224 ) ) ;
#65736=CARTESIAN_POINT ( 'NONE',  ( 24.40312500061451573, 0.000000000000000000, 5.243569643749999010 ) ) ;
#65737=CARTESIAN_POINT ( 'NONE',  ( 4.228125000614517681, -4.541064518000419881, 2.621784821874995952 ) ) ;
#65738=CARTESIAN_POINT ( 'NONE',  ( 18.07500000122903216, -5.773502691896255534, -1.060575238724906372E-15 ) ) ;
#65739=CARTESIAN_POINT ( 'NONE',  ( 23.87812500061451715, 4.541064518000418104, 2.621784821874999949 ) ) ;
#65740=CARTESIAN_POINT ( 'NONE',  ( 23.51249999999999574, 2.886751345948129099, -4.999999999999998224 ) ) ;
#65741=CARTESIAN_POINT ( 'NONE',  ( 28.49062500061451431, -3.027376345333614438, 5.243569643749998122 ) ) ;
#65742=CARTESIAN_POINT ( 'NONE',  ( 8.428125000614517859, 6.421520780324663323E-16, -5.243569643749999010 ) ) ;
#65745=CARTESIAN_POINT ( 'NONE',  ( 23.69062500061451004, -3.027376345333610441, -5.243569643749999898 ) ) ;
#65746=CARTESIAN_POINT ( 'NONE',  ( 5.878125000614517148, 4.541064518000418104, 2.621784821874999949 ) ) ;
#65748=DIRECTION ( 'NONE',  ( -0.000000000000000000, -1.000000000000000000, -0.000000000000000000 ) ) ;
#65749=CARTESIAN_POINT ( 'NONE',  ( 3.999999999999999112, 12.68750000122903465, -30.00000000000000000 ) ) ;
#65750=CARTESIAN_POINT ( 'NONE',  ( -5.810221930991193690E-16, 13.58750000000000036, -34.00000000000000000 ) ) ;
#65751=CARTESIAN_POINT ( 'NONE',  ( 11.43750000000000000, 5.773502691896255534, 3.535250795749688894E-16 ) ) ;
#65752=CARTESIAN_POINT ( 'NONE',  ( 12.34687500061452070, -3.027376345333614438, 5.243569643749998122 ) ) ;
#65753=CARTESIAN_POINT ( 'NONE',  ( 6.525000001229033231, 2.886751345948129099, -4.999999999999998224 ) ) ;
#65754=CARTESIAN_POINT ( 'NONE',  ( 13.69687500061451679, -3.027376345333614438, 5.243569643749998122 ) ) ;
#65756=CARTESIAN_POINT ( 'NONE',  ( 5.596875000614516260, -3.027376345333614438, 5.243569643749998122 ) ) ;
#65757=CARTESIAN_POINT ( 'NONE',  ( 30.00000000000000000, 6.123233995736764310E-16, -4.999999999999998224 ) ) ;
#65758=CARTESIAN_POINT ( 'NONE',  ( 19.76249999999999929, -5.773502691896255534, -1.060575238724906372E-15 ) ) ;
#65759=EDGE_CURVE ( 'NONE', #29541, #58433, #31977, .T. ) ;
#65760=CARTESIAN_POINT ( 'NONE',  ( 11.48437500061451644, -4.541064518000419881, 2.621784821874995952 ) ) ;
#65761=CARTESIAN_POINT ( 'NONE',  ( 21.86250000122903003, 4.330127018922192761, -2.499999999999997780 ) ) ;
#65762=CARTESIAN_POINT ( 'NONE',  ( 22.19062500061451715, -3.027376345333614438, 5.243569643749998122 ) ) ;
#65763=CARTESIAN_POINT ( 'NONE',  ( 1.071796769724489895, 11.76740381056766616, 26.00000000000000355 ) ) ;
#65764=CARTESIAN_POINT ( 'NONE',  ( -2.121784821874996840, 18.52812500061459389, 33.67503911421598417 ) ) ;
#65765=CARTESIAN_POINT ( 'NONE',  ( 24.04687500061451644, -3.027376345333614438, 5.243569643749998122 ) ) ;
#65766=FACE_OUTER_BOUND ( 'NONE', #17887, .T. ) ;
#65767=CARTESIAN_POINT ( 'NONE',  ( 4.940625000614515372, 6.054752690667223547, 3.707466751127219781E-16 ) ) ;
#65769=CARTESIAN_POINT ( 'NONE',  ( 17.91562500061451502, 3.027376345333613106, -5.243569643749998122 ) ) ;
#65770=CARTESIAN_POINT ( 'NONE',  ( 15.12187500061451750, -6.054752690667223547, -1.112240025338166033E-15 ) ) ;
#65772=CARTESIAN_POINT ( 'NONE',  ( 28.53750000122903074, 6.123233995736764310E-16, -4.999999999999998224 ) ) ;
#65773=CARTESIAN_POINT ( 'NONE',  ( 5.634375000614519458, -4.541064518000419881, 2.621784821874995952 ) ) ;
#65774=CARTESIAN_POINT ( 'NONE',  ( 17.18437500061451573, 4.541064518000418104, 2.621784821874999949 ) ) ;
#65775=CYLINDRICAL_SURFACE ( 'NONE', #23119, 4.999999999999998224 ) ;
#65776=CARTESIAN_POINT ( 'NONE',  ( 23.43750000000000000, -2.886751345948125991, -5.000000000000000000 ) ) ;
#65777=CARTESIAN_POINT ( 'NONE',  ( 3.262500001229035718, -4.330127018922190985, -2.500000000000001332 ) ) ;
#65778=CARTESIAN_POINT ( 'NONE',  ( 23.70937500061451786, -4.541064518000417216, -2.621784821875001281 ) ) ;
#65779=CARTESIAN_POINT ( 'NONE',  ( 17.40937500061451715, -4.541064518000417216, -2.621784821875001281 ) ) ;
#65781=CARTESIAN_POINT ( 'NONE',  ( 29.43750000000000000, 5.773502691896255534, 3.535250795749688894E-16 ) ) ;
#65782=CARTESIAN_POINT ( 'NONE',  ( 7.724999999999999645, 6.123233995736764310E-16, -4.999999999999998224 ) ) ;
#65784=CARTESIAN_POINT ( 'NONE',  ( 19.15312500061451573, -4.541064518000417216, -2.621784821875001281 ) ) ;
#65785=CARTESIAN_POINT ( 'NONE',  ( 9.112500000000000711, 2.886751345948129099, -4.999999999999998224 ) ) ;
#65786=EDGE_CURVE ( 'NONE', #4423, #40887, #47085, .T. ) ;
#65787=CARTESIAN_POINT ( 'NONE',  ( 3.403125000614518836, -4.541064518000417216, -2.621784821875001281 ) ) ;
#65788=CARTESIAN_POINT ( 'NONE',  ( 18.86249999999999716, -5.773502691896255534, -1.060575238724906372E-15 ) ) ;
#65789=CARTESIAN_POINT ( 'NONE',  ( 17.42812500061451786, 6.421520780324663323E-16, -5.243569643749999010 ) ) ;
#65791=CARTESIAN_POINT ( 'NONE',  ( 22.65000000122903856, -2.886751345948125991, -5.000000000000000000 ) ) ;
#65792=LINE ( 'NONE', #16630, #4089 ) ;
#65793=CARTESIAN_POINT ( 'NONE',  ( 29.37187500061451928, 3.027376345333611329, 5.243569643749999010 ) ) ;
#65794=VERTEX_POINT ( 'NONE', #56987 ) ;
#65795=CARTESIAN_POINT ( 'NONE',  ( 17.91562500061451502, 3.027376345333613106, -5.243569643749998122 ) ) ;
#65796=CARTESIAN_POINT ( 'NONE',  ( 24.40312500061451573, 0.000000000000000000, 5.243569643749999010 ) ) ;
#65797=CARTESIAN_POINT ( 'NONE',  ( 25.69687500061451502, 6.054752690667223547, 3.707466751127219781E-16 ) ) ;
#65798=CARTESIAN_POINT ( 'NONE',  ( 8.662499999999999645, 2.886751345948129099, -4.999999999999998224 ) ) ;
#65799=CARTESIAN_POINT ( 'NONE',  ( 12.92812500061451786, 6.421520780324663323E-16, -5.243569643749999010 ) ) ;
#65800=CARTESIAN_POINT ( 'NONE',  ( 27.44062500061451715, 6.054752690667223547, 3.707466751127219781E-16 ) ) ;
#65801=CARTESIAN_POINT ( 'NONE',  ( 16.54687500061451644, -3.027376345333610441, -5.243569643749999898 ) ) ;
#65802=CARTESIAN_POINT ( 'NONE',  ( 10.07812500061451644, -4.541064518000419881, 2.621784821874995952 ) ) ;
#65803=CARTESIAN_POINT ( 'NONE',  ( 6.975000001229029856, 2.886751345948062486, -5.000000000000113687 ) ) ;
#65804=CARTESIAN_POINT ( 'NONE',  ( 4.243569643749999010, 19.16562500061451857, 27.54997392385601174 ) ) ;
#65805=CARTESIAN_POINT ( 'NONE',  ( 23.70000000122903216, 5.773502691896255534, 3.535250795749688894E-16 ) ) ;
#65807=CARTESIAN_POINT ( 'NONE',  ( 14.31562500061451892, 3.027376345333612662, -5.243569643749998122 ) ) ;
#65808=CARTESIAN_POINT ( 'NONE',  ( 7.434375000614519280, -4.541064518000419881, 2.621784821874995952 ) ) ;
#65809=CARTESIAN_POINT ( 'NONE',  ( 6.459375000614518747, 0.000000000000000000, 5.243569643749999010 ) ) ;
#65811=CARTESIAN_POINT ( 'NONE',  ( 29.22187500061451715, 3.027376345333613106, -5.243569643749998122 ) ) ;
#65812=CARTESIAN_POINT ( 'NONE',  ( 19.49062500061451431, -3.027376345333614438, 5.243569643749998122 ) ) ;
#65813=B_SPLINE_CURVE_WITH_KNOTS ( 'NONE', 1,
 ( #5976, #39605 ),
 .UNSPECIFIED., .F., .F.,
 ( 2, 2 ),
 ( 0.000000000000000000, 1.000000000000000000 ),
 .UNSPECIFIED. ) ;
#65814=CARTESIAN_POINT ( 'NONE',  ( 25.28437500061451715, 4.541064518000418104, 2.621784821874999949 ) ) ;
#65815=CARTESIAN_POINT ( 'NONE',  ( 19.00312500061451715, 0.000000000000000000, 5.243569643749999010 ) ) ;
#65816=CARTESIAN_POINT ( 'NONE',  ( -2.828200636599751609E-16, 13.13750000000000107, 25.38119784648299770 ) ) ;
#65817=CARTESIAN_POINT ( 'NONE',  ( 26.39062500061451644, -3.027376345333610441, -5.243569643749999898 ) ) ;
#65818=CARTESIAN_POINT ( 'NONE',  ( 7.350000001229033408, -2.886751345948125991, -5.000000000000000000 ) ) ;
#65820=CARTESIAN_POINT ( 'NONE',  ( 2.887500001229035274, 6.123233995736764310E-16, -4.999999999999998224 ) ) ;
#65821=CARTESIAN_POINT ( 'NONE',  ( 3.999999999999998668, 14.41250000000000142, -32.30940107675850470 ) ) ;
#65822=CARTESIAN_POINT ( 'NONE',  ( 22.68750000122903288, 6.123233995736764310E-16, -4.999999999999998224 ) ) ;
#65824=CARTESIAN_POINT ( 'NONE',  ( 6.196875000614515905, -3.027376345333610441, -5.243569643749999898 ) ) ;
#65826=CARTESIAN_POINT ( 'NONE',  ( 12.14062500061451821, 6.054752690667223547, 3.707466751127219781E-16 ) ) ;
#65827=CARTESIAN_POINT ( 'NONE',  ( 7.696875000614516793, 6.054752690667223547, 3.707466751127219781E-16 ) ) ;
#65828=CARTESIAN_POINT ( 'NONE',  ( 26.28750000122903430, 6.123233995736764310E-16, -4.999999999999998224 ) ) ;
#65829=CARTESIAN_POINT ( 'NONE',  ( 16.99687500061451573, -3.027376345333610441, -5.243569643749999898 ) ) ;
#65830=CARTESIAN_POINT ( 'NONE',  ( 4.059375000614519280, 4.541064518000418104, -2.621784821874998173 ) ) ;
#65831=CARTESIAN_POINT ( 'NONE',  ( 1.626862140677534273E-15, 11.11250000000000071, 34.00000000000000000 ) ) ;
#65832=CARTESIAN_POINT ( 'NONE',  ( 6.440625000614517148, -3.027376345333614438, 5.243569643749998122 ) ) ;
#65833=CARTESIAN_POINT ( 'NONE',  ( 14.69062500061451537, -3.027376345333610441, -5.243569643749999898 ) ) ;
#65834=ORIENTED_EDGE ( 'NONE', *, *, #66238, .F. ) ;
#65835=CARTESIAN_POINT ( 'NONE',  ( 11.99062500061451608, -3.027376345333610441, -5.243569643749999898 ) ) ;
#65836=CARTESIAN_POINT ( 'NONE',  ( 5.475000001229035185, -5.773502691896255534, -1.060575238724906372E-15 ) ) ;
#65837=CARTESIAN_POINT ( 'NONE',  ( 8.503125000614515372, 4.541064518000418104, -2.621784821874998173 ) ) ;
#65839=CARTESIAN_POINT ( 'NONE',  ( 9.375000000000001776, -4.330127018922194537, 2.499999999999995559 ) ) ;
#65840=CARTESIAN_POINT ( 'NONE',  ( 3.450000001229036162, 5.773502691896255534, 3.535250795749688894E-16 ) ) ;
#65841=CARTESIAN_POINT ( 'NONE',  ( 17.92500000000000071, -4.330127018922194537, 2.499999999999995559 ) ) ;
#65842=EDGE_CURVE ( 'NONE', #35743, #34653, #45199, .T. ) ;
#65843=CARTESIAN_POINT ( 'NONE',  ( 19.17187500061451999, -6.054752690667223547, -1.112240025338166033E-15 ) ) ;
#65844=CARTESIAN_POINT ( 'NONE',  ( 14.43750000122903288, -4.330127018922194537, 2.499999999999995559 ) ) ;
#65846=CARTESIAN_POINT ( 'NONE',  ( 9.001249775931846008E-16, 15.86562500061451608, -25.09994784771203058 ) ) ;
#65847=CARTESIAN_POINT ( 'NONE',  ( -3.999999999999999112, 16.06250000122903288, 30.00000000000000000 ) ) ;
#65848=DIRECTION ( 'NONE',  ( -0.000000000000000000, -1.000000000000000000, -0.000000000000000000 ) ) ;
#65852=CYLINDRICAL_SURFACE ( 'NONE', #65655, 4.999999999999998224 ) ;
#65853=CARTESIAN_POINT ( 'NONE',  ( 15.04687500061451644, -3.027376345333614438, 5.243569643749998122 ) ) ;
#65855=CARTESIAN_POINT ( 'NONE',  ( 27.37500000000000000, -4.330127018922194537, 2.499999999999995559 ) ) ;
#65856=CARTESIAN_POINT ( 'NONE',  ( 11.39062500061451644, -3.027376345333614438, 5.243569643749998122 ) ) ;
#65858=CARTESIAN_POINT ( 'NONE',  ( 21.04687500061451644, -3.027376345333610441, -5.243569643749999898 ) ) ;
#65860=CARTESIAN_POINT ( 'NONE',  ( 6.590625000614518392, -3.027376345333610441, -5.243569643749999898 ) ) ;
#65861=CARTESIAN_POINT ( 'NONE',  ( 11.97187500061451892, -6.054752690667223547, -1.112240025338166033E-15 ) ) ;
#65862=ORIENTED_EDGE ( 'NONE', *, *, #60328, .T. ) ;
#65863=CARTESIAN_POINT ( 'NONE',  ( 24.00937500061451502, 0.000000000000000000, 5.243569643749999010 ) ) ;
#65864=CARTESIAN_POINT ( 'NONE',  ( 3.942105046096217702, 3.076001935233272810, -30.69131329531799679 ) ) ;
#65865=CARTESIAN_POINT ( 'NONE',  ( 26.95312500061451644, 4.541064518000418104, -2.621784821874998173 ) ) ;
#65867=CARTESIAN_POINT ( 'NONE',  ( 7.837499999999999467, 5.773502691896255534, 3.535250795749688894E-16 ) ) ;
#65869=CARTESIAN_POINT ( 'NONE',  ( 17.88750000122903216, 4.330127018922191873, 2.499999999999999556 ) ) ;
#65870=CARTESIAN_POINT ( 'NONE',  ( 0.000000000000000000, 20.00000000000000000, 26.00000000000000000 ) ) ;
#65872=ORIENTED_EDGE ( 'NONE', *, *, #61587, .F. ) ;
#65873=CARTESIAN_POINT ( 'NONE',  ( 15.71250000000000213, -5.773502691896255534, -1.060575238724906372E-15 ) ) ;
#65874=CARTESIAN_POINT ( 'NONE',  ( 17.81250000000000355, 2.886751345948126879, 4.999999999999999112 ) ) ;
#65875=CARTESIAN_POINT ( 'NONE',  ( 11.50312500061451892, -4.541064518000417216, -2.621784821875001281 ) ) ;
#65876=EDGE_LOOP ( 'NONE', ( #68914, #18133, #53080, #14901 ) ) ;
#65878=CARTESIAN_POINT ( 'NONE',  ( -2.121784821874999949, 17.08437500061451786, -33.67503911421598417 ) ) ;
#65879=CARTESIAN_POINT ( 'NONE',  ( 2.915625000614516793, -6.054752690667223547, -1.112240025338166033E-15 ) ) ;
#65880=CARTESIAN_POINT ( 'NONE',  ( 2.000000000000001332, 12.05000000000000249, 33.46410161513774995 ) ) ;
#65881=CARTESIAN_POINT ( 'NONE',  ( 10.38750000000000107, -2.886751345948125991, -5.000000000000000000 ) ) ;
#65882=CARTESIAN_POINT ( 'NONE',  ( 3.193447721043152665, 3.847322660365763536, 3.562742055761627835 ) ) ;
#65883=ORIENTED_EDGE ( 'NONE', *, *, #52783, .T. ) ;
#65884=CARTESIAN_POINT ( 'NONE',  ( 2.121784821874999061, 12.90312500061451750, 26.32496088578401583 ) ) ;
#65885=CARTESIAN_POINT ( 'NONE',  ( 27.06562500061451004, 3.027376345333611329, 5.243569643749999010 ) ) ;
#65886=CARTESIAN_POINT ( 'NONE',  ( 3.563259964303803873, 3.507650584494903079, 3.697742481698767847 ) ) ;
#65888=CARTESIAN_POINT ( 'NONE',  ( 21.75937500061451502, 0.000000000000000000, 5.243569643749999010 ) ) ;
#65889=CARTESIAN_POINT ( 'NONE',  ( 19.49062500061451431, -3.027376345333614438, 5.243569643749998122 ) ) ;
#65891=CARTESIAN_POINT ( 'NONE',  ( 9.001249775931846008E-16, 14.51562500061459460, -25.09994784771203058 ) ) ;
#65892=CARTESIAN_POINT ( 'NONE',  ( 22.23750000122903003, 6.123233995736764310E-16, -4.999999999999998224 ) ) ;
#65893=CARTESIAN_POINT ( 'NONE',  ( 4.715625000614516615, -6.054752690667223547, -1.112240025338166033E-15 ) ) ;
#65895=CARTESIAN_POINT ( 'NONE',  ( 22.26562500061451644, -6.054752690667223547, -1.112240025338166033E-15 ) ) ;
#65898=CARTESIAN_POINT ( 'NONE',  ( 15.34687500061451537, 6.054752690667223547, 3.707466751127219781E-16 ) ) ;
#65899=CARTESIAN_POINT ( 'NONE',  ( 13.35937500061451821, -4.541064518000417216, -2.621784821875001281 ) ) ;
#65900=CARTESIAN_POINT ( 'NONE',  ( 21.23437500061451644, 4.541064518000418104, 2.621784821874999949 ) ) ;
#65901=CARTESIAN_POINT ( 'NONE',  ( 2.121784821874999061, 12.50937500061451857, 26.32496088578401583 ) ) ;
#65902=CARTESIAN_POINT ( 'NONE',  ( 4.153125000614515727, 0.000000000000000000, 5.243569643749999010 ) ) ;
#65903=CARTESIAN_POINT ( 'NONE',  ( 28.30312500061451431, 4.541064518000418104, -2.621784821874998173 ) ) ;
#65904=CARTESIAN_POINT ( 'NONE',  ( 27.29062500061451502, -3.027376345333610441, -5.243569643749999898 ) ) ;
#65907=CARTESIAN_POINT ( 'NONE',  ( 6.234375000614519102, 6.421520780324663323E-16, -5.243569643749999010 ) ) ;
#65909=CARTESIAN_POINT ( 'NONE',  ( 13.46250000122903323, 0.000000000000000000, 4.999999999999998224 ) ) ;
#65910=CARTESIAN_POINT ( 'NONE',  ( 8.925000001229033586, 2.886751345948126879, 4.999999999999999112 ) ) ;
#65911=CARTESIAN_POINT ( 'NONE',  ( 5.503125000614516260, 0.000000000000000000, 5.243569643749999010 ) ) ;
#65914=CARTESIAN_POINT ( 'NONE',  ( 13.95937500061451786, 4.541064518000418104, -2.621784821874998173 ) ) ;
#65915=VERTEX_POINT ( 'NONE', #24094 ) ;
#65916=CARTESIAN_POINT ( 'NONE',  ( 19.75312500061451360, 4.541064518000418104, -2.621784821874998173 ) ) ;
#65917=CARTESIAN_POINT ( 'NONE',  ( 6.778125000614518392, 4.541064518000418104, 2.621784821874999949 ) ) ;
#65918=CARTESIAN_POINT ( 'NONE',  ( 24.38437500061451502, 4.541064518000418104, 2.621784821874999949 ) ) ;
#65919=EDGE_CURVE ( 'NONE', #52475, #59726, #11702, .T. ) ;
#65920=CARTESIAN_POINT ( 'NONE',  ( 8.765625000614518214, -6.054752690667223547, -1.112240025338166033E-15 ) ) ;
#65922=CARTESIAN_POINT ( 'NONE',  ( 8.362500001229031810, 4.330127018922192761, -2.499999999999997780 ) ) ;
#65923=( BOUNDED_CURVE ( )  B_SPLINE_CURVE ( 2, ( #43086, #71898, #8732, #26462, #31266, #20167, #71532 ),
 .UNSPECIFIED., .F., .F. ) 
 B_SPLINE_CURVE_WITH_KNOTS ( ( 3, 2, 2, 3 ),
 ( 0.5333333333333334370, 0.5361111111111112049, 0.5388888888888888618, 0.5416666666666666297 ),
 .UNSPECIFIED. ) 
 CURVE ( )  GEOMETRIC_REPRESENTATION_ITEM ( )  RATIONAL_B_SPLINE_CURVE ( ( 0.9999999999999946709, 0.8660254037844440367, 1.000000000000000000, 0.8660254037844387076, 1.000000000000000000, 0.8660254037844387076, 1.000000000000000000 ) ) 
 REPRESENTATION_ITEM ( '' )  );
#65924=CARTESIAN_POINT ( 'NONE',  ( 22.49062500061451431, 6.054752690667223547, 3.707466751127219781E-16 ) ) ;
#65925=CARTESIAN_POINT ( 'NONE',  ( -2.000000000000000000, 17.33750000122903145, -33.46410161513775705 ) ) ;
#65926=CARTESIAN_POINT ( 'NONE',  ( 10.27500000122903323, 2.886751345948126879, 4.999999999999999112 ) ) ;
#65927=CARTESIAN_POINT ( 'NONE',  ( 20.09062500061451573, -3.027376345333610441, -5.243569643749999898 ) ) ;
#65928=CARTESIAN_POINT ( 'NONE',  ( 16.49062500061451786, -3.027376345333610441, -5.243569643749999898 ) ) ;
#65930=CARTESIAN_POINT ( 'NONE',  ( 14.69999999999999929, 0.000000000000000000, 4.999999999999998224 ) ) ;
#65931=CARTESIAN_POINT ( 'NONE',  ( 12.07500000122903216, 2.886751345948126879, 4.999999999999999112 ) ) ;
#65932=EDGE_CURVE ( 'NONE', #31631, #25241, #52183, .T. ) ;
#65933=CARTESIAN_POINT ( 'NONE',  ( 7.753125000614518036, 0.000000000000000000, 5.243569643749999010 ) ) ;
#65934=CARTESIAN_POINT ( 'NONE',  ( 11.09062500061451573, -3.027376345333610441, -5.243569643749999898 ) ) ;
#65935=CARTESIAN_POINT ( 'NONE',  ( 23.92500000122903359, -5.773502691896255534, -1.060575238724906372E-15 ) ) ;
#65936=CARTESIAN_POINT ( 'NONE',  ( 20.55937500061451573, -4.541064518000417216, -2.621784821875001281 ) ) ;
#65937=CARTESIAN_POINT ( 'NONE',  ( 4.678125000614516971, -4.541064518000419881, 2.621784821874995952 ) ) ;
#65938=CARTESIAN_POINT ( 'NONE',  ( 4.687500001229034652, 6.123233995736764310E-16, -4.999999999999998224 ) ) ;
#65939=CARTESIAN_POINT ( 'NONE',  ( 4.921875000614518214, 3.027376345333613106, -5.243569643749998122 ) ) ;
#65940=CARTESIAN_POINT ( 'NONE',  ( 23.63437500061451502, -4.541064518000419881, 2.621784821874995952 ) ) ;
#65941=CARTESIAN_POINT ( 'NONE',  ( 10.42500000000000071, 6.123233995736764310E-16, -4.999999999999998224 ) ) ;
#65942=CARTESIAN_POINT ( 'NONE',  ( 18.89062500061451644, 6.054752690667223547, 3.707466751127219781E-16 ) ) ;
#65943=CARTESIAN_POINT ( 'NONE',  ( 23.67187500061451999, -6.054752690667223547, -1.112240025338166033E-15 ) ) ;
#65946=CARTESIAN_POINT ( 'NONE',  ( 27.75937500061451502, -4.541064518000417216, -2.621784821875001281 ) ) ;
#65947=CARTESIAN_POINT ( 'NONE',  ( 5.559375000614517504, 0.000000000000000000, 5.243569643749999010 ) ) ;
#65948=CARTESIAN_POINT ( 'NONE',  ( 14.05312500061451431, 0.000000000000000000, 5.243569643749999010 ) ) ;
#65949=CARTESIAN_POINT ( 'NONE',  ( 14.22187500061451537, -6.054752690667223547, -1.112240025338166033E-15 ) ) ;
#65950=ORIENTED_EDGE ( 'NONE', *, *, #1615, .F. ) ;
#65951=DIRECTION ( 'NONE',  ( 0.000000000000000000, 0.000000000000000000, 1.000000000000000000 ) ) ;
#65952=CARTESIAN_POINT ( 'NONE',  ( 25.71562500061451573, 3.027376345333611329, 5.243569643749999010 ) ) ;
#65953=CARTESIAN_POINT ( 'NONE',  ( 1.071796769724505438, 13.11740381056766580, -33.99999999999999289 ) ) ;
#65955=CARTESIAN_POINT ( 'NONE',  ( 15.75000000000000000, -4.330127018922190985, -2.500000000000001332 ) ) ;
#65956=CARTESIAN_POINT ( 'NONE',  ( 24.75000000122902932, -2.886751345948129988, 4.999999999999997335 ) ) ;
#65957=CARTESIAN_POINT ( 'NONE',  ( 18.06562500061451715, 3.027376345333611329, 5.243569643749999010 ) ) ;
#65958=EDGE_LOOP ( 'NONE', ( #20415, #17615, #15296, #35182 ) ) ;
#65959=CARTESIAN_POINT ( 'NONE',  ( 22.94999999999999929, -4.330127018922190985, -2.500000000000001332 ) ) ;
#65960=CARTESIAN_POINT ( 'NONE',  ( 24.27187500061452141, 3.027376345333613106, -5.243569643749998122 ) ) ;
#65961=ORIENTED_EDGE ( 'NONE', *, *, #27532, .F. ) ;
#65962=CARTESIAN_POINT ( 'NONE',  ( 1.626862140677534273E-15, 17.86250000000000071, -26.00000000000000355 ) ) ;
#65963=CARTESIAN_POINT ( 'NONE',  ( 10.86562500061451431, 3.027376345333611329, 5.243569643749999010 ) ) ;
#65964=CARTESIAN_POINT ( 'NONE',  ( 3.028125000614518392, 6.421520780324663323E-16, -5.243569643749999010 ) ) ;
#65966=CARTESIAN_POINT ( 'NONE',  ( 26.12812500061451360, 4.541064518000418104, 2.621784821874999949 ) ) ;
#65967=CARTESIAN_POINT ( 'NONE',  ( 16.57499999999999929, -4.330127018922194537, 2.499999999999995559 ) ) ;
#65968=CARTESIAN_POINT ( 'NONE',  ( 24.29999999999999716, -4.330127018922190985, -2.500000000000001332 ) ) ;
#65969=CARTESIAN_POINT ( 'NONE',  ( -3.000416591977282496E-16, 19.24062500061451431, 25.09994784771203058 ) ) ;
#65970=CARTESIAN_POINT ( 'NONE',  ( 6.534375000614517148, -4.541064518000419881, 2.621784821874995952 ) ) ;
#65971=CARTESIAN_POINT ( 'NONE',  ( 16.58437500061451786, 6.421520780324663323E-16, -5.243569643749999010 ) ) ;
#65972=CARTESIAN_POINT ( 'NONE',  ( 28.62187500061451573, -6.054752690667223547, -1.112240025338166033E-15 ) ) ;
#65973=ORIENTED_EDGE ( 'NONE', *, *, #19460, .T. ) ;
#65974=CARTESIAN_POINT ( 'NONE',  ( 26.50312500061451360, 4.541064518000418104, -2.621784821874998173 ) ) ;
#65975=CARTESIAN_POINT ( 'NONE',  ( 26.70937500061451431, 0.000000000000000000, 5.243569643749999010 ) ) ;
#65976=LINE ( 'NONE', #66717, #12078 ) ;
#65977=CARTESIAN_POINT ( 'NONE',  ( 13.61250000000000071, 2.886751345948129099, -4.999999999999998224 ) ) ;
#65978=CARTESIAN_POINT ( 'NONE',  ( 10.22812500061451679, 6.421520780324663323E-16, -5.243569643749999010 ) ) ;
#65980=CARTESIAN_POINT ( 'NONE',  ( 5.250000000000000888, 0.000000000000000000, 4.999999999999998224 ) ) ;
#65981=CARTESIAN_POINT ( 'NONE',  ( 28.94062500061452070, -3.027376345333614438, 5.243569643749998122 ) ) ;
#65982=CARTESIAN_POINT ( 'NONE',  ( 17.06250000122903288, 0.000000000000000000, 4.999999999999998224 ) ) ;
#65985=CARTESIAN_POINT ( 'NONE',  ( 6.365625000614518747, 3.027376345333611329, 5.243569643749999010 ) ) ;
#65986=CARTESIAN_POINT ( 'NONE',  ( 22.88437500061451857, 6.421520780324663323E-16, -5.243569643749999010 ) ) ;
#65987=CARTESIAN_POINT ( 'NONE',  ( -2.121784821874996840, 16.33437500061451786, 33.67503911421598417 ) ) ;
#65988=CARTESIAN_POINT ( 'NONE',  ( 20.67187500061451289, 3.027376345333613106, -5.243569643749998122 ) ) ;
#65989=CARTESIAN_POINT ( 'NONE',  ( 4.912499999999999645, -5.773502691896255534, -1.060575238724906372E-15 ) ) ;
#65990=CARTESIAN_POINT ( 'NONE',  ( 2.000000000000001332, 9.912500001229034297, 33.46410161513774995 ) ) ;
#65991=CARTESIAN_POINT ( 'NONE',  ( 11.99062500061451608, -3.027376345333610441, -5.243569643749999898 ) ) ;
#65992=CARTESIAN_POINT ( 'NONE',  ( 4.162500001229033408, -4.330127018922190985, -2.500000000000001332 ) ) ;
#65993=CARTESIAN_POINT ( 'NONE',  ( 8.746875000614515727, -3.027376345333614438, 5.243569643749998122 ) ) ;
#65994=CARTESIAN_POINT ( 'NONE',  ( 3.928581913072007215, 3.092934553507882711, -4.135345885259243737 ) ) ;
#65995=CARTESIAN_POINT ( 'NONE',  ( 11.01562500061451821, -6.054752690667223547, -1.112240025338166033E-15 ) ) ;
#65996=CARTESIAN_POINT ( 'NONE',  ( 14.70937500061451786, -4.541064518000417216, -2.621784821875001281 ) ) ;
#65998=CARTESIAN_POINT ( 'NONE',  ( 20.58750000122903145, 4.330127018922191873, 2.499999999999999556 ) ) ;
#65999=CARTESIAN_POINT ( 'NONE',  ( 9.646875000614516082, -3.027376345333614438, 5.243569643749998122 ) ) ;
#66000=CARTESIAN_POINT ( 'NONE',  ( 12.32812500061451821, -4.541064518000419881, 2.621784821874995952 ) ) ;
#66002=EDGE_CURVE ( 'NONE', #10458, #403, #69832, .T. ) ;
#66003=CARTESIAN_POINT ( 'NONE',  ( 21.68437500061451573, 4.541064518000418104, 2.621784821874999949 ) ) ;
#66004=CARTESIAN_POINT ( 'NONE',  ( 14.10000000000000142, 4.330127018922192761, -2.499999999999997780 ) ) ;
#66005=CARTESIAN_POINT ( 'NONE',  ( -0.6909613911670718922, 4.953869264242466208, 26.05777829539367119 ) ) ;
#66006=CARTESIAN_POINT ( 'NONE',  ( 2.953125000614516438, -4.541064518000417216, -2.621784821875001281 ) ) ;
#66007=CARTESIAN_POINT ( 'NONE',  ( 2.121784821874999061, 12.50937500061451857, -33.67503911421598417 ) ) ;
#66008=CARTESIAN_POINT ( 'NONE',  ( 14.88750000122903394, -4.330127018922194537, 2.499999999999995559 ) ) ;
#66009=CARTESIAN_POINT ( 'NONE',  ( -2.121784821874996840, 16.72812500061451857, -26.32496088578401583 ) ) ;
#66010=CARTESIAN_POINT ( 'NONE',  ( 16.57500000122903216, 2.886751345948126879, 4.999999999999999112 ) ) ;
#66011=CARTESIAN_POINT ( 'NONE',  ( 9.065625000614517148, 3.027376345333611329, 5.243569643749999010 ) ) ;
#66013=CARTESIAN_POINT ( 'NONE',  ( 14.62500000000000000, 4.330127018922191873, 2.499999999999999556 ) ) ;
#66014=CARTESIAN_POINT ( 'NONE',  ( 4.957199372764754308, -3.163855285557799935, 4.520041897618551019 ) ) ;
#66015=CARTESIAN_POINT ( 'NONE',  ( 23.24062500061451786, -3.027376345333610441, -5.243569643749999898 ) ) ;
#66016=CARTESIAN_POINT ( 'NONE',  ( 11.22187500061451892, 3.027376345333612662, -5.243569643749998122 ) ) ;
#66017=CARTESIAN_POINT ( 'NONE',  ( 4.359768065504647794, -2.448001861170849836, -4.637088767021002589 ) ) ;
#66018=CARTESIAN_POINT ( 'NONE',  ( 9.975000001229034297, -5.773502691896255534, -1.060575238724906372E-15 ) ) ;
#66019=EDGE_CURVE ( 'NONE', #47866, #30305, #49471, .T. ) ;
#66020=CARTESIAN_POINT ( 'NONE',  ( 19.27500000122903145, 2.886751345948126879, 4.999999999999999112 ) ) ;
#66021=CARTESIAN_POINT ( 'NONE',  ( 16.41562500061451857, -6.054752690667223547, -1.112240025338166033E-15 ) ) ;
#66022=CARTESIAN_POINT ( 'NONE',  ( 18.74062500061451431, -3.027376345333610441, -5.243569643749999898 ) ) ;
#66023=CARTESIAN_POINT ( 'NONE',  ( 25.68750000122903288, -4.330127018922194537, 2.499999999999995559 ) ) ;
#66024=EDGE_CURVE ( 'NONE', #55912, #52358, #54642, .T. ) ;
#66025=CARTESIAN_POINT ( 'NONE',  ( 2.878125000614517592, -4.541064518000419881, 2.621784821874995952 ) ) ;
#66026=CARTESIAN_POINT ( 'NONE',  ( 24.52499999999999858, 4.330127018922191873, 2.499999999999999556 ) ) ;
#66028=CARTESIAN_POINT ( 'NONE',  ( 26.67187500061451644, 3.027376345333611329, 5.243569643749999010 ) ) ;
#66029=CARTESIAN_POINT ( 'NONE',  ( 1.071796769724495668, 17.43259618943233136, 34.00000000000000000 ) ) ;
#66030=CARTESIAN_POINT ( 'NONE',  ( 12.48750000122903359, 4.330127018922191873, 2.499999999999999556 ) ) ;
#66031=CARTESIAN_POINT ( 'NONE',  ( 3.112500000000000711, -5.773502691896255534, -1.060575238724906372E-15 ) ) ;
#66033=CARTESIAN_POINT ( 'NONE',  ( 6.646875000614518747, -3.027376345333610441, -5.243569643749999898 ) ) ;
#66034=CARTESIAN_POINT ( 'NONE',  ( 27.21562500061451928, -6.054752690667223547, -1.112240025338166033E-15 ) ) ;
#66036=CARTESIAN_POINT ( 'NONE',  ( 5.700000000000000178, 0.000000000000000000, 4.999999999999998224 ) ) ;
#66038=CARTESIAN_POINT ( 'NONE',  ( 5.671875000614519102, -6.054752690667223547, -1.112240025338166033E-15 ) ) ;
#66039=CARTESIAN_POINT ( 'NONE',  ( 9.159375000614515372, 0.000000000000000000, 5.243569643749999010 ) ) ;
#66040=CARTESIAN_POINT ( 'NONE',  ( 29.48437500061451644, -4.541064518000419881, 2.621784821874995952 ) ) ;
#66041=CARTESIAN_POINT ( 'NONE',  ( -4.243569643749998122, 12.64062500061459460, 32.45002607614398471 ) ) ;
#66042=CARTESIAN_POINT ( 'NONE',  ( 21.71249999999999858, 2.886751345948129099, -4.999999999999998224 ) ) ;
#66043=CARTESIAN_POINT ( 'NONE',  ( -3.999999999999997335, 17.78750000000000142, -27.69059892324149530 ) ) ;
#66044=CARTESIAN_POINT ( 'NONE',  ( 5.287500000000000533, -2.886751345948129988, 4.999999999999997335 ) ) ;
#66046=CARTESIAN_POINT ( 'NONE',  ( 18.89062500061451644, 6.054752690667223547, 3.707466751127219781E-16 ) ) ;
#66047=CARTESIAN_POINT ( 'NONE',  ( 11.46562500061451573, -6.054752690667223547, -1.112240025338166033E-15 ) ) ;
#66049=CARTESIAN_POINT ( 'NONE',  ( 7.884375000614517681, -4.541064518000419881, 2.621784821874995952 ) ) ;
#66050=CARTESIAN_POINT ( 'NONE',  ( 23.02499999999999858, 6.123233995736764310E-16, -4.999999999999998224 ) ) ;
#66051=CARTESIAN_POINT ( 'NONE',  ( 20.40000000122903145, -2.886751345948125991, -5.000000000000000000 ) ) ;
#66052=CARTESIAN_POINT ( 'NONE',  ( 10.32187500061451679, 3.027376345333613106, -5.243569643749998122 ) ) ;
#66053=CARTESIAN_POINT ( 'NONE',  ( 13.17187500061451999, 3.027376345333611329, 5.243569643749999010 ) ) ;
#66054=CARTESIAN_POINT ( 'NONE',  ( 23.52187500061451786, 3.027376345333611329, 5.243569643749999010 ) ) ;
#66055=CARTESIAN_POINT ( 'NONE',  ( 8.662500001229034297, -4.330127018922190985, -2.500000000000001332 ) ) ;
#66056=ORIENTED_EDGE ( 'NONE', *, *, #59373, .T. ) ;
#66058=CARTESIAN_POINT ( 'NONE',  ( 18.30937500061451928, -4.541064518000417216, -2.621784821875001281 ) ) ;
#66059=CARTESIAN_POINT ( 'NONE',  ( 8.596875000614518925, 6.054752690667223547, 3.707466751127219781E-16 ) ) ;
#66061=CARTESIAN_POINT ( 'NONE',  ( 20.13749999999999929, -2.886751345948129988, 4.999999999999997335 ) ) ;
#66063=CARTESIAN_POINT ( 'NONE',  ( 0.000000000000000000, 20.00000000000000000, -33.99999999999999289 ) ) ;
#66065=CARTESIAN_POINT ( 'NONE',  ( 12.14062500061451821, 6.054752690667223547, 3.707466751127219781E-16 ) ) ;
#66066=CARTESIAN_POINT ( 'NONE',  ( 28.17187500061451644, -6.054752690667223547, -1.112240025338166033E-15 ) ) ;
#66068=CARTESIAN_POINT ( 'NONE',  ( 1.071796769724489895, 10.07990381179669903, -34.00000000000000000 ) ) ;
#66069=CARTESIAN_POINT ( 'NONE',  ( 12.67499999999999893, 6.123233995736764310E-16, -4.999999999999998224 ) ) ;
#66070=CARTESIAN_POINT ( 'NONE',  ( 2.000000000000001332, 17.11250000122903359, 33.46410161513774995 ) ) ;
#66071=CARTESIAN_POINT ( 'NONE',  ( 12.48750000122903359, 4.330127018922191873, 2.499999999999999556 ) ) ;
#66072=CARTESIAN_POINT ( 'NONE',  ( 23.52187500061451786, 3.027376345333611329, 5.243569643749999010 ) ) ;
#66073=CARTESIAN_POINT ( 'NONE',  ( 15.98437500061451821, -4.541064518000419881, 2.621784821874995952 ) ) ;
#66074=FACE_OUTER_BOUND ( 'NONE', #12348, .T. ) ;
#66075=VERTEX_POINT ( 'NONE', #7475 ) ;
#66076=CARTESIAN_POINT ( 'NONE',  ( 16.19062500061451715, 6.054752690667223547, 3.707466751127219781E-16 ) ) ;
#66077=CARTESIAN_POINT ( 'NONE',  ( 2.840625000614518392, -3.027376345333614438, 5.243569643749998122 ) ) ;
#66078=CARTESIAN_POINT ( 'NONE',  ( 16.62187500061451573, 3.027376345333613106, -5.243569643749998122 ) ) ;
#66079=CARTESIAN_POINT ( 'NONE',  ( 5.278125000614516615, 6.421520780324663323E-16, -5.243569643749999010 ) ) ;
#66080=CARTESIAN_POINT ( 'NONE',  ( 19.41562500061451146, 3.027376345333611329, 5.243569643749999010 ) ) ;
#66082=CARTESIAN_POINT ( 'NONE',  ( 27.60937500061451644, 0.000000000000000000, 5.243569643749999010 ) ) ;
#66083=CARTESIAN_POINT ( 'NONE',  ( -2.121784821874999949, 12.07812500061451821, 26.32496088578401938 ) ) ;
#66084=CARTESIAN_POINT ( 'NONE',  ( 17.22187500061451715, 3.027376345333611329, 5.243569643749999010 ) ) ;
#66085=CARTESIAN_POINT ( 'NONE',  ( 15.82500000122903216, -5.773502691896255534, -1.060575238724906372E-15 ) ) ;
#66087=CARTESIAN_POINT ( 'NONE',  ( 8.849999999999999645, 0.000000000000000000, 4.999999999999998224 ) ) ;
#66088=CARTESIAN_POINT ( 'NONE',  ( 21.45937500061451786, -4.541064518000417216, -2.621784821875001281 ) ) ;
#66089=CARTESIAN_POINT ( 'NONE',  ( 21.82500000122903572, 2.886751345948129099, -4.999999999999998224 ) ) ;
#66090=CARTESIAN_POINT ( 'NONE',  ( 23.16562500061451502, -6.054752690667223547, -1.112240025338166033E-15 ) ) ;
#66091=CARTESIAN_POINT ( 'NONE',  ( 16.50937500061451502, -4.541064518000417216, -2.621784821875001281 ) ) ;
#66092=CARTESIAN_POINT ( 'NONE',  ( 11.27812500061451573, 4.541064518000418104, 2.621784821874999949 ) ) ;
#66093=CARTESIAN_POINT ( 'NONE',  ( -4.243569643749999898, 13.55937500061451750, 30.00000000000000000 ) ) ;
#66094=CARTESIAN_POINT ( 'NONE',  ( 17.61562500061451786, 3.027376345333611329, 5.243569643749999010 ) ) ;
#66095=CARTESIAN_POINT ( 'NONE',  ( 28.30312500061451431, 4.541064518000418104, -2.621784821874998173 ) ) ;
#66096=ORIENTED_EDGE ( 'NONE', *, *, #22499, .F. ) ;
#66097=ORIENTED_EDGE ( 'NONE', *, *, #70375, .T. ) ;
#66098=CARTESIAN_POINT ( 'NONE',  ( 22.12500000000000000, 6.123233995736764310E-16, -4.999999999999998224 ) ) ;
#66099=CARTESIAN_POINT ( 'NONE',  ( -4.243569643749999898, 19.37187500061451928, -32.45002607614398471 ) ) ;
#66101=CARTESIAN_POINT ( 'NONE',  ( 25.64062500061451644, 6.054752690667223547, 3.707466751127219781E-16 ) ) ;
#66102=CARTESIAN_POINT ( 'NONE',  ( 5.690625000614516260, -3.027376345333610441, -5.243569643749999898 ) ) ;
#66103=CARTESIAN_POINT ( 'NONE',  ( 16.80000000122903359, -2.886751345948125991, -5.000000000000000000 ) ) ;
#66104=CARTESIAN_POINT ( 'NONE',  ( 21.74062500061451431, -3.027376345333614438, 5.243569643749998122 ) ) ;
#66105=CARTESIAN_POINT ( 'NONE',  ( 23.36250000000000071, -5.773502691896255534, -1.060575238724906372E-15 ) ) ;
#66106=CARTESIAN_POINT ( 'NONE',  ( 24.77812500061451217, 4.541064518000418104, 2.621784821874999949 ) ) ;
#66107=CARTESIAN_POINT ( 'NONE',  ( 7.340625000614518392, -3.027376345333614438, 5.243569643749998122 ) ) ;
#66108=EDGE_LOOP ( 'NONE', ( #36284, #18072 ) ) ;
#66109=ADVANCED_FACE ( 'NONE', ( #15107 ), #65351, .F. ) ;
#66110=CARTESIAN_POINT ( 'NONE',  ( 23.35312500061451857, 4.541064518000418104, -2.621784821874998173 ) ) ;
#66111=CARTESIAN_POINT ( 'NONE',  ( 3.815625000614518036, -6.054752690667223547, -1.112240025338166033E-15 ) ) ;
#66113=CARTESIAN_POINT ( 'NONE',  ( 11.10000000122903252, 5.773502691896255534, 3.535250795749688401E-16 ) ) ;
#66114=CARTESIAN_POINT ( 'NONE',  ( -3.999999999999999112, 14.71250000122903501, -30.00000000000000000 ) ) ;
#66115=( BOUNDED_CURVE ( )  B_SPLINE_CURVE ( 2, ( #24871, #69948, #2718, #25234, #46699, #24514, #34875, #52597, #64401 ),
 .UNSPECIFIED., .F., .F. ) 
 B_SPLINE_CURVE_WITH_KNOTS ( ( 3, 2, 2, 2, 3 ),
 ( 0.07608695652173913526, 0.07971014492753622505, 0.08695652173913043237, 0.09420289855072463969, 0.09782608695652174335 ),
 .UNSPECIFIED. ) 
 CURVE ( )  GEOMETRIC_REPRESENTATION_ITEM ( )  RATIONAL_B_SPLINE_CURVE ( ( 0.9330127018922192983, 0.9330127018922194093, 1.000000000000000000, 0.8660254037844387076, 1.000000000000000000, 0.8660254037844387076, 1.000000000000000000, 0.9330127018922194093, 0.9330127018922194093 ) ) 
 REPRESENTATION_ITEM ( '' )  );
#66116=CARTESIAN_POINT ( 'NONE',  ( 10.65000000000000036, 0.000000000000000000, 4.999999999999998224 ) ) ;
#66117=CARTESIAN_POINT ( 'NONE',  ( 10.43437500061451750, 4.541064518000418104, 2.621784821874999949 ) ) ;
#66118=CARTESIAN_POINT ( 'NONE',  ( 5.325000001229033941, 2.886751345948126879, 4.999999999999999112 ) ) ;
#66119=CARTESIAN_POINT ( 'NONE',  ( 15.23437500061451644, 6.421520780324663323E-16, -5.243569643749999010 ) ) ;
#66120=CARTESIAN_POINT ( 'NONE',  ( 6.759375000614516793, 4.541064518000418104, -2.621784821874998173 ) ) ;
#66121=CARTESIAN_POINT ( 'NONE',  ( 30.00000000000000000, 6.123233995736764310E-16, -4.999999999999998224 ) ) ;
#66122=CARTESIAN_POINT ( 'NONE',  ( 0.000000000000000000, 20.00000000000000000, 30.00000000000000000 ) ) ;
#66123=CARTESIAN_POINT ( 'NONE',  ( 12.87187500061451750, -6.054752690667223547, -1.112240025338166033E-15 ) ) ;
#66124=CARTESIAN_POINT ( 'NONE',  ( 6.187500001229032875, 4.330127018922191873, 2.499999999999999556 ) ) ;
#66125=CARTESIAN_POINT ( 'NONE',  ( 21.62812500061451360, 4.541064518000418104, 2.621784821874999949 ) ) ;
#66126=CARTESIAN_POINT ( 'NONE',  ( -4.243569643749999898, 19.85937500061451644, 30.00000000000000000 ) ) ;
#66127=CYLINDRICAL_SURFACE ( 'NONE', #30190, 3.999999999999996447 ) ;
#66128=CARTESIAN_POINT ( 'NONE',  ( 22.73437500061451644, -4.541064518000419881, 2.621784821874995952 ) ) ;
#66129=CARTESIAN_POINT ( 'NONE',  ( 4.092234022020802442, 2.872911538668597053, -4.251154360391494080 ) ) ;
#66130=( BOUNDED_CURVE ( )  B_SPLINE_CURVE ( 2, ( #27218, #45204, #49753, #67737, #21659, #39669, #11585 ),
 .UNSPECIFIED., .F., .F. ) 
 B_SPLINE_CURVE_WITH_KNOTS ( ( 3, 2, 2, 3 ),
 ( 0.2916666666666667407, 0.2944444444444445086, 0.2972222222222222210, 0.2999999999999999889 ),
 .UNSPECIFIED. ) 
 CURVE ( )  GEOMETRIC_REPRESENTATION_ITEM ( )  RATIONAL_B_SPLINE_CURVE ( ( 0.9999999999999973355, 0.8660254037844413721, 1.000000000000000000, 0.8660254037844387076, 1.000000000000000000, 0.8660254037844387076, 1.000000000000000000 ) ) 
 REPRESENTATION_ITEM ( '' )  );
#66131=CARTESIAN_POINT ( 'NONE',  ( 27.86250000122903359, 0.000000000000000000, 4.999999999999998224 ) ) ;
#66133=CARTESIAN_POINT ( 'NONE',  ( 26.16562500061451502, 3.027376345333611329, 5.243569643749999010 ) ) ;
#66134=CARTESIAN_POINT ( 'NONE',  ( 17.61562500061451786, 3.027376345333611329, 5.243569643749999010 ) ) ;
#66136=CARTESIAN_POINT ( 'NONE',  ( 15.45937500061451608, 0.000000000000000000, 5.243569643749999010 ) ) ;
#66138=CARTESIAN_POINT ( 'NONE',  ( 28.46250000122903145, -4.330127018922190985, -2.500000000000001332 ) ) ;
#66139=CARTESIAN_POINT ( 'NONE',  ( 5.709375000614517859, -4.541064518000417216, -2.621784821875001281 ) ) ;
#66140=CARTESIAN_POINT ( 'NONE',  ( 16.05937500061451573, -4.541064518000417216, -2.621784821875001281 ) ) ;
#66141=DIRECTION ( 'NONE',  ( 0.000000000000000000, 0.000000000000000000, 1.000000000000000000 ) ) ;
#66142=CARTESIAN_POINT ( 'NONE',  ( 23.13749999999999929, 5.773502691896255534, 3.535250795749688894E-16 ) ) ;
#66143=CARTESIAN_POINT ( 'NONE',  ( 16.76250000122903216, -4.330127018922190985, -2.500000000000001332 ) ) ;
#66144=CARTESIAN_POINT ( 'NONE',  ( 25.17187500061451644, 3.027376345333613106, -5.243569643749998122 ) ) ;
#66145=CARTESIAN_POINT ( 'NONE',  ( 15.64687500061451608, -3.027376345333610441, -5.243569643749999898 ) ) ;
#66147=CARTESIAN_POINT ( 'NONE',  ( 28.80000000000000071, -4.330127018922190985, -2.500000000000001332 ) ) ;
#66148=CARTESIAN_POINT ( 'NONE',  ( 6.299999999999999822, -4.330127018922190985, -2.500000000000001332 ) ) ;
#66150=CARTESIAN_POINT ( 'NONE',  ( 20.61562500061451431, 3.027376345333613106, -5.243569643749998122 ) ) ;
#66151=CARTESIAN_POINT ( 'NONE',  ( 9.037499999999999645, -2.886751345948125991, -5.000000000000000000 ) ) ;
#66152=CARTESIAN_POINT ( 'NONE',  ( 4.078125000614517326, 4.541064518000418104, 2.621784821874999949 ) ) ;
#66153=CARTESIAN_POINT ( 'NONE',  ( 19.23749999999999716, -2.886751345948129988, 4.999999999999997335 ) ) ;
#66155=CARTESIAN_POINT ( 'NONE',  ( 15.52500000122903323, 2.886751345948129099, -4.999999999999997335 ) ) ;
#66156=CARTESIAN_POINT ( 'NONE',  ( 24.03750000122903430, 6.123233995736764310E-16, -4.999999999999998224 ) ) ;
#66157=CARTESIAN_POINT ( 'NONE',  ( 3.203040009831848334, 9.474684130322209796, 35.07722138099716602 ) ) ;
#66158=( BOUNDED_CURVE ( )  B_SPLINE_CURVE ( 1, ( #67477, #45297 ),
 .UNSPECIFIED., .F., .F. ) 
 B_SPLINE_CURVE_WITH_KNOTS ( ( 2, 2 ),
 ( 0.000000000000000000, 1.000000000000000000 ),
 .UNSPECIFIED. ) 
 CURVE ( )  GEOMETRIC_REPRESENTATION_ITEM ( )  RATIONAL_B_SPLINE_CURVE ( ( 0.9401542295229587953, 0.9401542295229587953 ) ) 
 REPRESENTATION_ITEM ( '' )  );
#66159=CARTESIAN_POINT ( 'NONE',  ( 3.187500000000002220, -2.886751345948125991, -5.000000000000000000 ) ) ;
#66160=ORIENTED_EDGE ( 'NONE', *, *, #14417, .T. ) ;
#66161=CARTESIAN_POINT ( 'NONE',  ( 17.99062500061451786, 6.054752690667223547, 3.707466751127219781E-16 ) ) ;
#66162=CARTESIAN_POINT ( 'NONE',  ( 23.42812500061451786, 4.541064518000418104, 2.621784821874999949 ) ) ;
#66163=CARTESIAN_POINT ( 'NONE',  ( 24.49687500061451573, -3.027376345333614438, 5.243569643749998122 ) ) ;
#66164=CARTESIAN_POINT ( 'NONE',  ( 9.262499999999999289, 2.886751345948126879, 4.999999999999999112 ) ) ;
#66165=CARTESIAN_POINT ( 'NONE',  ( 11.76562500061451644, 3.027376345333611329, 5.243569643749999010 ) ) ;
#66166=CARTESIAN_POINT ( 'NONE',  ( 26.65312500061451573, 0.000000000000000000, 5.243569643749999010 ) ) ;
#66167=CARTESIAN_POINT ( 'NONE',  ( 13.73437500061451821, -4.541064518000419881, 2.621784821874995952 ) ) ;
#66168=CARTESIAN_POINT ( 'NONE',  ( 19.24687500061452283, -3.027376345333610441, -5.243569643749999898 ) ) ;
#66169=CARTESIAN_POINT ( 'NONE',  ( 2.970509043979068231, -4.022057219312137555, 3.237209742923575106 ) ) ;
#66170=CARTESIAN_POINT ( 'NONE',  ( 5.190092854996874117, 9.755146338944483020, 24.77581305162949832 ) ) ;
#66171=CARTESIAN_POINT ( 'NONE',  ( 24.30000000122903359, -2.886751345948129988, 4.999999999999997335 ) ) ;
#66173=CARTESIAN_POINT ( 'NONE',  ( 14.05312500061451431, 0.000000000000000000, 5.243569643749999010 ) ) ;
#66174=CARTESIAN_POINT ( 'NONE',  ( 6.946875000614517681, -3.027376345333614438, 5.243569643749998122 ) ) ;
#66175=CARTESIAN_POINT ( 'NONE',  ( 8.146875000614516082, 6.054752690667223547, 3.707466751127219781E-16 ) ) ;
#66176=VERTEX_POINT ( 'NONE', #3312 ) ;
#66177=CARTESIAN_POINT ( 'NONE',  ( 26.59687500061451360, 6.054752690667223547, 3.707466751127219781E-16 ) ) ;
#66178=CARTESIAN_POINT ( 'NONE',  ( 20.50312500061451715, -4.541064518000417216, -2.621784821875001281 ) ) ;
#66179=CARTESIAN_POINT ( 'NONE',  ( 3.384375000614517237, -4.541064518000419881, 2.621784821874995952 ) ) ;
#66180=CARTESIAN_POINT ( 'NONE',  ( 24.87187500061451573, 3.027376345333611329, 5.243569643749999010 ) ) ;
#66181=CARTESIAN_POINT ( 'NONE',  ( 19.45312500061451644, 0.000000000000000000, 5.243569643749999010 ) ) ;
#66182=CARTESIAN_POINT ( 'NONE',  ( -3.999999999999997335, 11.48750000000000071, 32.30940107675850470 ) ) ;
#66183=CARTESIAN_POINT ( 'NONE',  ( 24.55312500061451786, -4.541064518000417216, -2.621784821875001281 ) ) ;
#66184=CARTESIAN_POINT ( 'NONE',  ( 7.612500001229035362, 0.000000000000000000, 4.999999999999998224 ) ) ;
#66186=CARTESIAN_POINT ( 'NONE',  ( 2.662500001229036073, 0.000000000000000000, 4.999999999999998224 ) ) ;
#66187=CARTESIAN_POINT ( 'NONE',  ( -3.999999999999997335, 15.98750000000000249, -27.69059892324149175 ) ) ;
#66188=CARTESIAN_POINT ( 'NONE',  ( 22.08750000122903501, -4.330127018922194537, 2.499999999999995559 ) ) ;
#66190=EDGE_CURVE ( 'NONE', #72082, #72537, #12651, .T. ) ;
#66191=CARTESIAN_POINT ( 'NONE',  ( 4.696875000614518569, -3.027376345333614438, 5.243569643749998122 ) ) ;
#66192=CARTESIAN_POINT ( 'NONE',  ( 29.31562500061451715, 3.027376345333611329, 5.243569643749999010 ) ) ;
#66193=CARTESIAN_POINT ( 'NONE',  ( 12.74062500061451786, -3.027376345333614438, 5.243569643749998122 ) ) ;
#66194=CARTESIAN_POINT ( 'NONE',  ( 5.896875000614518747, 6.054752690667223547, 3.707466751127219781E-16 ) ) ;
#66195=CARTESIAN_POINT ( 'NONE',  ( 23.55000000122903359, -2.886751345948125991, -5.000000000000000000 ) ) ;
#66196=CARTESIAN_POINT ( 'NONE',  ( 15.45937500061451608, 0.000000000000000000, 5.243569643749999010 ) ) ;
#66197=CARTESIAN_POINT ( 'NONE',  ( 28.79062500061451502, 6.054752690667223547, 3.707466751127219781E-16 ) ) ;
#66198=CARTESIAN_POINT ( 'NONE',  ( 29.32499999999999929, 6.123233995736764310E-16, -4.999999999999998224 ) ) ;
#66199=CARTESIAN_POINT ( 'NONE',  ( 5.540625000614515905, -3.027376345333614438, 5.243569643749998122 ) ) ;
#66200=CARTESIAN_POINT ( 'NONE',  ( 14.12812500061451715, -4.541064518000419881, 2.621784821874995952 ) ) ;
#66201=ORIENTED_EDGE ( 'NONE', *, *, #58318, .T. ) ;
#66202=CARTESIAN_POINT ( 'NONE',  ( 10.71562500061451928, 3.027376345333613106, -5.243569643749998122 ) ) ;
#66203=CARTESIAN_POINT ( 'NONE',  ( 8.053125000614516082, 4.541064518000418104, -2.621784821874998173 ) ) ;
#66205=CARTESIAN_POINT ( 'NONE',  ( 7.762500000000001954, 2.886751345948129099, -4.999999999999998224 ) ) ;
#66206=CARTESIAN_POINT ( 'NONE',  ( 4.500000001229034652, -2.886751345948129988, 4.999999999999997335 ) ) ;
#66207=CARTESIAN_POINT ( 'NONE',  ( 18.93750000000000000, -2.886751345948125991, -5.000000000000000000 ) ) ;
#66208=CARTESIAN_POINT ( 'NONE',  ( 18.23437500061451999, -4.541064518000419881, 2.621784821874995952 ) ) ;
#66209=CARTESIAN_POINT ( 'NONE',  ( 13.72500000122903074, 2.886751345948129099, -4.999999999999998224 ) ) ;
#66211=CARTESIAN_POINT ( 'NONE',  ( 4.243569643749999898, 17.32812500061451644, -30.00000000000000000 ) ) ;
#66212=B_SPLINE_CURVE_WITH_KNOTS ( 'NONE', 3,
 ( #4982, #16411, #39330, #11610, #61844, #56667, #27514, #28597, #51133, #45599 ),
 .UNSPECIFIED., .F., .F.,
 ( 4, 3, 3, 4 ),
 ( 1.879119738154566656E-16, 0.0001572461267887791201, 0.0003144877809832584913, 0.0005153498092345547071 ),
 .UNSPECIFIED. ) ;
#66214=CARTESIAN_POINT ( 'NONE',  ( 29.61562500061451431, 3.027376345333613106, -5.243569643749998122 ) ) ;
#66216=CARTESIAN_POINT ( 'NONE',  ( 24.26249999999999929, -5.773502691896255534, -1.060575238724906372E-15 ) ) ;
#66217=CARTESIAN_POINT ( 'NONE',  ( 13.80937500061451750, -4.541064518000417216, -2.621784821875001281 ) ) ;
#66218=CARTESIAN_POINT ( 'NONE',  ( 27.56250000000000000, 2.886751345948129099, -4.999999999999998224 ) ) ;
#66219=CARTESIAN_POINT ( 'NONE',  ( 11.76562500061451644, 3.027376345333611329, 5.243569643749999010 ) ) ;
#66221=CARTESIAN_POINT ( 'NONE',  ( 22.20937500061451431, 0.000000000000000000, 5.243569643749999010 ) ) ;
#66223=CARTESIAN_POINT ( 'NONE',  ( 8.315625000614515372, -6.054752690667223547, -1.112240025338166033E-15 ) ) ;
#66224=CARTESIAN_POINT ( 'NONE',  ( 13.95937500061451786, 4.541064518000418104, -2.621784821874998173 ) ) ;
#66225=EDGE_LOOP ( 'NONE', ( #69536, #61822, #49121, #11730 ) ) ;
#66226=CARTESIAN_POINT ( 'NONE',  ( 24.30937500061451573, 4.541064518000418104, -2.621784821874998173 ) ) ;
#66227=CARTESIAN_POINT ( 'NONE',  ( -3.305247878049081707E-15, 5.000000000000034639, -34.00000000000004263 ) ) ;
#66228=CARTESIAN_POINT ( 'NONE',  ( 24.82499999999999929, 6.123233995736764310E-16, -4.999999999999998224 ) ) ;
#66229=CARTESIAN_POINT ( 'NONE',  ( 4.612500000000002487, 2.886751345948129099, -4.999999999999998224 ) ) ;
#66230=CARTESIAN_POINT ( 'NONE',  ( 17.81250000122903288, 4.330127018922192761, -2.499999999999997780 ) ) ;
#66232=CARTESIAN_POINT ( 'NONE',  ( 3.752440054025286909, -3.304420318444254878, 4.071342403668507082 ) ) ;
#66235=CARTESIAN_POINT ( 'NONE',  ( 14.10000000000000142, 4.330127018922192761, -2.499999999999997780 ) ) ;
#66236=CARTESIAN_POINT ( 'NONE',  ( 17.73750000000000071, 5.773502691896255534, 3.535250795749688894E-16 ) ) ;
#66237=CARTESIAN_POINT ( 'NONE',  ( 11.24062500061451608, 6.054752690667223547, 3.707466751127219781E-16 ) ) ;
#66238=EDGE_CURVE ( 'NONE', #11468, #29843, #62201, .T. ) ;
#66239=ORIENTED_EDGE ( 'NONE', *, *, #30133, .F. ) ;
#66240=CARTESIAN_POINT ( 'NONE',  ( 26.25000000000000000, 4.330127018922192761, -2.499999999999997780 ) ) ;
#66241=CARTESIAN_POINT ( 'NONE',  ( -3.000416591977282496E-16, 17.49687500061451573, -34.90005215228797653 ) ) ;
#66242=CARTESIAN_POINT ( 'NONE',  ( 4.415625000614518569, 3.027376345333613106, -5.243569643749998122 ) ) ;
#66244=CARTESIAN_POINT ( 'NONE',  ( 8.887499999999999289, -2.886751345948129988, 4.999999999999997335 ) ) ;
#66245=CYLINDRICAL_SURFACE ( 'NONE', #57396, 4.999999999999998224 ) ;
#66246=ORIENTED_EDGE ( 'NONE', *, *, #27328, .F. ) ;
#66247=CARTESIAN_POINT ( 'NONE',  ( 23.27812500061451573, 6.421520780324663323E-16, -5.243569643749999010 ) ) ;
#66248=CARTESIAN_POINT ( 'NONE',  ( 4.192336996406676342, -2.724758798235080715, 4.480034832487019614 ) ) ;
#66250=CARTESIAN_POINT ( 'NONE',  ( 21.45937500061451786, -4.541064518000417216, -2.621784821875001281 ) ) ;
#66251=ADVANCED_FACE ( 'NONE', ( #67559 ), #56106, .F. ) ;
#66252=CARTESIAN_POINT ( 'NONE',  ( 18.96562500061451573, 3.027376345333611329, 5.243569643749999010 ) ) ;
#66253=CARTESIAN_POINT ( 'NONE',  ( -2.121784821874999949, 14.32812500061459282, -33.67503911421598417 ) ) ;
#66254=CARTESIAN_POINT ( 'NONE',  ( 23.96250000122903145, -4.330127018922190985, -2.500000000000001332 ) ) ;
#66255=CARTESIAN_POINT ( 'NONE',  ( 4.753125000614515372, -4.541064518000417216, -2.621784821875001281 ) ) ;
#66257=CARTESIAN_POINT ( 'NONE',  ( 22.64062500061451644, -3.027376345333614438, 5.243569643749998122 ) ) ;
#66260=CARTESIAN_POINT ( 'NONE',  ( 14.89687500061451786, 6.054752690667223547, 3.707466751127219781E-16 ) ) ;
#66261=EDGE_CURVE ( 'NONE', #11494, #29428, #38824, .T. ) ;
#66262=CARTESIAN_POINT ( 'NONE',  ( 13.73437500061451821, -4.541064518000419881, 2.621784821874995952 ) ) ;
#66263=CARTESIAN_POINT ( 'NONE',  ( 23.37187500061451573, 3.027376345333613106, -5.243569643749998122 ) ) ;
#66264=ORIENTED_EDGE ( 'NONE', *, *, #45500, .F. ) ;
#66265=CARTESIAN_POINT ( 'NONE',  ( 9.001249775931846008E-16, 11.42187500061451644, 34.90005215228797653 ) ) ;
#66266=CYLINDRICAL_SURFACE ( 'NONE', #58262, 4.999999999999998224 ) ;
#66267=CARTESIAN_POINT ( 'NONE',  ( 27.44062500061451715, 6.054752690667223547, 3.707466751127219781E-16 ) ) ;
#66268=CARTESIAN_POINT ( 'NONE',  ( 27.17812500061451786, -4.541064518000419881, 2.621784821874995952 ) ) ;
#66269=CARTESIAN_POINT ( 'NONE',  ( 3.999999999999999112, 19.43750000122903288, -30.00000000000000000 ) ) ;
#66270=DIRECTION ( 'NONE',  ( 0.000000000000000000, 0.000000000000000000, -1.000000000000000000 ) ) ;
#66271=CARTESIAN_POINT ( 'NONE',  ( 6.046875000614519102, -3.027376345333614438, 5.243569643749998122 ) ) ;
#66273=CARTESIAN_POINT ( 'NONE',  ( 14.77500000122903501, 2.886751345948126879, 4.999999999999999112 ) ) ;
#66274=CARTESIAN_POINT ( 'NONE',  ( 9.975000001229034297, -5.773502691896255534, -1.060575238724906372E-15 ) ) ;
#66275=CARTESIAN_POINT ( 'NONE',  ( 2.990625000614519191, -3.027376345333610441, -5.243569643749999898 ) ) ;
#66278=CARTESIAN_POINT ( 'NONE',  ( 12.68437500061451573, 4.541064518000418104, 2.621784821874999949 ) ) ;
#66279=DIRECTION ( 'NONE',  ( -0.000000000000000000, -1.000000000000000000, -0.000000000000000000 ) ) ;
#66281=CARTESIAN_POINT ( 'NONE',  ( 20.84062500061451573, -3.027376345333614438, 5.243569643749998122 ) ) ;
#66282=CARTESIAN_POINT ( 'NONE',  ( 15.08437500061451786, -4.541064518000419881, 2.621784821874995952 ) ) ;
#66283=CARTESIAN_POINT ( 'NONE',  ( 5.240625000614516971, -3.027376345333610441, -5.243569643749999898 ) ) ;
#66284=CARTESIAN_POINT ( 'NONE',  ( 21.00937500061451857, -4.541064518000417216, -2.621784821875001281 ) ) ;
#66285=CARTESIAN_POINT ( 'NONE',  ( 5.990625000614517859, -3.027376345333614438, 5.243569643749998122 ) ) ;
#66287=CARTESIAN_POINT ( 'NONE',  ( 6.937500001229033764, 6.123233995736764310E-16, -4.999999999999998224 ) ) ;
#66288=CARTESIAN_POINT ( 'NONE',  ( 23.50312500061451360, 0.000000000000000000, 5.243569643749999010 ) ) ;
#66289=CARTESIAN_POINT ( 'NONE',  ( -1.999999999999997113, 18.83750000122903501, -26.53589838486224295 ) ) ;
#66290=CARTESIAN_POINT ( 'NONE',  ( 7.612500001229035362, 0.000000000000000000, 4.999999999999998224 ) ) ;
#66291=CARTESIAN_POINT ( 'NONE',  ( 19.15312500061451573, -4.541064518000417216, -2.621784821875001281 ) ) ;
#66292=CARTESIAN_POINT ( 'NONE',  ( 14.65312500061451573, -4.541064518000417216, -2.621784821875001281 ) ) ;
#66294=CARTESIAN_POINT ( 'NONE',  ( 15.22500000000000142, -4.330127018922194537, 2.499999999999995559 ) ) ;
#66295=CARTESIAN_POINT ( 'NONE',  ( 11.32500000122903394, -5.773502691896255534, -1.060575238724906372E-15 ) ) ;
#66296=EDGE_CURVE ( 'NONE', #52378, #69635, #13620, .T. ) ;
#66297=CARTESIAN_POINT ( 'NONE',  ( 9.140625000614518214, -3.027376345333614438, 5.243569643749998122 ) ) ;
#66298=CARTESIAN_POINT ( 'NONE',  ( 11.65312500061451573, 4.541064518000418104, -2.621784821874998173 ) ) ;
#66299=( BOUNDED_SURFACE ( )  B_SPLINE_SURFACE ( 1, 2, ( 
 ( #36923, #70913, #48750, #3322, #59444, #59078, #71274, #20652, #36194, #15115, #25099, #41735, #8851, #4054, #65730, #20284, #25474, #64263, #26580, #58712, #53927, #14019, #25848, #53549, #65360, #2946, #42475, #14750, #37652, #49120, #32116, #42110, #8124, #64633, #70546, #23116, #61919, #33475, #51930, #62644, #66095, #56024, #21021, #245, #22754, #68207, #40486, #46028, #5415, #16846, #39038, #10954, #33845, #17568, #73013, #6138, #39774, #12040, #57092, #27955, #50487, #28668, #11324, #22397, #6501, #34202, #50846, #29037, #51209, #44945, #67483, #39402, #16480, #51572, #56389, #63001, #34564, #61552, #971, #12395, #609, #5779, #28310, #45305, #67840, #17212, #62290, #68564, #40130, #23481, #11686, #56736, #6864, #34932, #17922, #45671, #57458, #29396, #43574, #13112, #70000, #52288, #58532, #19004, #41927, #36384, #35291, #12755, #7943, #63720, #57812, #58898, #13466, #30112, #8309, #30481, #7222, #29750, #63371, #46387, #30839, #1689, #19745, #64453, #18278, #13844, #64819, #53009, #68922, #46752, #69286, #24199, #18650, #7577, #47838, #19370, #53372, #24564, #41212, #59264, #2769, #25292, #42294, #35652, #23838, #36744, #64084, #58172, #52647, #70367, #2404, #14208, #36014, #2053, #69642, #47110, #8673, #41565, #40853, #24925, #47467, #31204, #1327, #26399, #38205, #20104, #59633, #71840, #66288, #43399, #3877, #72201, #25668, #55214, #65183, #48941, #60363, #49306, #15304, #71470, #71098, #21211, #32674, #48205, #27139, #14574, #53745, #20846, #16037, #60733, #32306, #37481, #3142, #66660, #70727, #65924, #26032, #37842, #20471, #9772, #48571, #31942, #54840, #43764, #38585, #15667, #42659, #10142, #4247, #21579, #26774, #43025, #37107, #10507, #4609, #9046, #31577, #54115, #54478, #49673, #44133, #65553, #3512, #14943, #60002, #61110, #9411, #51121, #56304, #72929, #17833, #518, #62557, #51483, #50405, #55575, #68471, #22668, #16761, #22311, #6413, #17124, #23029, #45219, #11237, #28229, #33759, #34478, #61471, #4969, #67752, #10866, #62203, #33035, #5693, #17483, #72562, #38953, #45584, #68117, #39684, #50759, #884, #27503, #57007, #44505, #162, #11599, #28584, #34116, #56655, #44863, #40044, #11953, #50036, #28945, #67038, #21948, #6050, #40394, #23391, #45940, #39319, #16398, #62913, #33399, #55936, #5331, #27872, #67400, #61831, #57729, #63637, #1969, #30394, #25198, #7858, #1243, #52923, #18920, #30751, #13380, #52201, #23748, #42208, #2321, #57369, #46296, #12307, #13026, #35565, #58447, #53283, #36299, #68836, #7135, #29309, #18193, #24113, #24836, #63278, #69559, #30019, #47384, #69914, #40763, #12670, #41480, #1602, #35207, #19284, #24478, #41126, #41835, #64000, #29665, #46662, #69201, #6777, #64366, #18561, #2682, #13756, #51840, #58812, #47744, #35923, #58084, #7492, #8223, #52563, #70281, #34843, #19652, #47024, #31856, #65462, #42937, #4524, #59917, #3048, #70641, #42569, #15578, #26312, #43313, #49583, #43677, #65097, #8586, #37021, #21491, #48850, #54031, #9687, #4156, #14487, #14854, #48486, #64732, #55126, #37393, #21124, #38120, #3426, #31116, #25946, #54391, #32587, #59545, #9323, #31490, #32220, #53654, #8957, #71010, #27053, #14119, #20386, #3789, #20755, #20016, #60641, #65833, #10054, #71380, #72107, #59177, #15215, #60273, #37755, #54754, #36657, #25578, #26688, #48118, #49221, #71755, #66200, #34027, #11505, #28144, #39229, #67664, #61741, #33671, #11142, #51389, #62467, #72470, #62112, #27415, #56564, #27780, #44779, #17030, #49946, #5239, #10779, #21855, #10418, #50319, #5608, #791, #44044, #38495, #44418, #56215, #66945, #50672, #76, #66567, #22581, #32949, #45492, #72842, #15947, #67313, #45130, #55486, #38866, #4879, #39588, #16313, #22224, #5960, #33312, #28494, #16671, #55850, #51030, #61383, #426, #61020, #68025, #22934, #17397, #39954, #11865, #34386, #56918, #6322, #28851, #63909, #62827, #23663, #68748, #36207, #53196, #18106, #46208, #52474, #51754, #69829, #1881, #47294, #35476, #58725, #17746, #18474, #18831, #41038, #69114, #23301, #8137, #63187, #12220, #7768, #30304, #30663, #13295, #35833, #7406, #63553, #46937, #12939, #57997, #29934, #45850, #41747, #1154, #41394, #6689, #58356, #7047, #24021, #69474, #29217, #57640, #12583, #40668, #34748, #29576, #24388, #68385, #40305, #57280, #35117, #52837, #52113, #2236, #24751, #1517, #19194, #46570, #64276, #13664, #32496, #3336, #59827, #64646, #70558, #14030, #9233, #36570, #36936, #15127, #42487, #43223, #48399, #65010, #8863, #8495, #19934, #9959, #4066, #37664, #31399, #31770, #25860, #65742, #2592, #60552, #19565, #42850, #70925, #53939, #15486, #20295, #59090, #31027, #53562, #26591, #37304, #54306, #25111, #54662, #2958, #42120, #48033, #47654, #3698, #14398, #20665, #60187, #25486, #65372, #59456, #70186, #66107, #14760, #32128, #49132, #26223, #48763, #9596, #71286, #71660, #21033, #43586, #38030, #33216, #11419, #5871, #44321, #21396, #66851, #44689, #22846, #55394, #55755, #21760, #22491, #43952, #4788, #27322, #67934, #11779, #49854, #72380, #11048, #10325, #28403, #33574, #50940, #67219, #17308, #49489, #50222, #50581, #72748, #27685, #55030, #39868, #16223, #66475, #39495, #62017, #62380, #45041, #67575, #39132, #22133, #5514, #16580, #61646, #56122, #4434, #337, #32859, #73109, #38398, #16940, #38774, #5149, #28053, #60923, #61294, #10686, #33936, #15852, #56479, #45398, #26962, #72020, #28762, #40221, #46486, #17660, #18387, #52028, #64187, #69025, #23211, #35752, #18025, #34295, #35030, #40954, #45764, #29133, #68300, #63469, #62743, #68661, #46852, #1070, #1795, #6961, #23579, #40582, #12136, #51666, #41665, #58273, #69392, #63101, #12856, #57558, #24305, #56827, #19110, #51301, #1430, #29491, #12502, #47210, #23937, #34661, #57190, #6603 ),
 ( #7680, #46124, #6233, #35389, #69742, #41311, #57912, #7321, #702, #29852, #52388, #18747, #63821, #13213, #30216, #52749, #2153, #24664, #3243, #31680, #26502, #9143, #2505, #54214, #20208, #32042, #14670, #53478, #25028, #43497, #3611, #58640, #47570, #13575, #64922, #14312, #59735, #54575, #37577, #70100, #8408, #30582, #19476, #25400, #26132, #64558, #70833, #31309, #48672, #71197, #42034, #13947, #42762, #2870, #36484, #20571, #25771, #42399, #43128, #65282, #59002, #30937, #47943, #8048, #65651, #70472, #3979, #15040, #53108, #60101, #49044, #37213, #19849, #36848, #59364, #8775, #53849, #48309, #9510, #71572, #20946, #36120, #38307, #44956, #72666, #61563, #27967, #15767, #15402, #67494, #16138, #32774, #60836, #5428, #61209, #22045, #38690, #27235, #44233, #49772, #33487, #49405, #37944, #10604, #71936, #33132, #66023, #55669, #10965, #4349, #43866, #67136, #56036, #5066, #66765, #22409, #32405, #50498, #26875, #27602, #50134, #21312, #4705, #73025, #55311, #16493, #44606, #72297, #21676, #66390, #10241, #60463, #16857, #9872, #39049, #54944, #9014, #26367, #15632, #43730, #2739, #26001, #59601, #37077, #71808, #54085, #70334, #64786, #36711, #9740, #20442, #37451, #66254, #37811, #59233, #25257, #31170, #58868, #42992, #48172, #3846, #71438, #8641, #31545, #42627, #8278, #49275, #3483, #15272, #32274, #70696, #47805, #20071, #48540, #26742, #53713, #71067, #25634, #48906, #19711, #3105, #65151, #21178, #30808, #14541, #65523, #14909, #14177, #54807, #59970, #4213, #9378, #53341, #42263, #31911, #54447, #20813, #43368, #65892, #60331, #70469, #42759, #8044, #19845, #65279, #48305, #35749, #19107, #41308, #13210, #36117, #42396, #2150, #8405, #42031, #64918, #59360, #58270, #7677, #30934, #13572, #30213, #8772, #36480, #53105, #31306, #53475, #52745, #24661, #47207, #69389, #53846, #69738, #14667, #14309, #63818, #36845, #37210, #2867, #18744, #41662, #64184, #58637, #30579, #2502, #70830, #3240, #25768, #25025, #47567, #58999, #54210, #31677, #70097, #19473, #25397, #64553, #47940, #13944, #24301, #20204, #59732, #9140, #46849, #33483, #4346, #60832, #65648, #71569, #15037, #10238, #37574, #37941, #16134, #43494, #44230, #49402, #66020, #9869, #9507, #20943, #10962, #5063, #38686, #32401, #32771, #26871, #66762, #3607, #61560, #20567, #43862, #71933, #54941, #16489, #21309, #60098, #32037, #54572, #27599, #38303, #55308, #26129, #55666, #3975, #43125, #49040, #22042, #26498, #4702, #72294, #27232, #66387, #15399, #21672, #50131, #71194, #72663, #60460, #48668, #15764, #39046, #10601, #49769, #61206, #33129, #44602, #67133, #28676, #28317, #17575, #253, #51216, #50854, #34209, #45679, #979, #68931, #51580, #44953, #23489, #62652, #1336, #57101, #22761, #67491, #12763, #46036, #27964, #16854, #29045, #23848, #39781, #68572, #46396, #6873, #39410, #45313, #73021, #61929, #67848, #17931, #33852, #40137, #616, #40494, #63010, #11334, #56396, #12049, #17220, #5786, #12406, #68214, #11693, #23124, #18289, #34941, #34573, #62297, #56033, #40862, #22406, #6510, #56743, #57467, #6146, #29405, #51939, #63379, #5425, #50495, #48212, #30846, #24208, #53380, #41934, #53752, #36393, #2061, #46761, #65191, #2776, #7230, #69295, #8317, #3149, #19012, #25299, #25675, #59272, #18658, #30120, #52296, #41220, #47117, #47846, #13119, #19377, #53017, #70374, #19752, #63728, #35660, #64460, #24572, #58180, #42301, #47476, #64091, #64827, #13851, #7585, #52654, #69649, #29759, #14217, #41573, #70734, #36752, #1697, #8680, #20112, #58907, #13473, #36022, #58539, #7951, #30489, #2411, #31212, #42667, #35299, #24932, #70007, #57820, #32682, #44140, #33042, #31949, #37114, #50042, #4256, #71478, #54485, #61118, #71847, #55221, #26781, #65931, #9779, #15311, #16044, #43032, #59641, #49313, #65561, #43771, #14581, #60370, #72209, #54123, #20479, #4616, #27146, #21218, #37849, #55582, #9053, #66295, #4975, #14950, #15675, #10150, #38212, #32313, #3886, #49680, #66667, #31584, #10515, #26040, #3519, #54847, #60740, #21586, #21954, #27509, #37488, #38592, #71106, #72568, #20854, #44511, #48579, #60009, #48949, #26406, #9419, #43406, #170, #28591, #23755, #1250, #61477, #72935, #6057, #50411, #51128, #11605, #67045, #525, #55942, #68478, #50765, #16405, #67758, #23036, #5338, #61838, #27878, #45591, #22317, #28235, #6420, #33766, #34485, #39691, #56310, #22674, #44870, #11243, #38959, #17840, #28952, #45225, #68125, #17130, #57015, #10872, #51847, #33405, #34122, #62209, #56662, #6784, #17490, #67406, #16767, #39325, #40401, #40052, #62564, #5699, #45947, #11960, #51491, #891, #57377, #23398, #62920, #12315, #34850, #29316, #69566, #30027, #3055, #36665, #24486, #2689, #70288, #35572, #12678, #58091, #35931, #14127, #46669, #47030, #13033, #13764, #35214, #69210, #18568, #59184, #46304, #41135, #63644, #2327, #1609, #19660, #24844, #42215, #58453, #8594, #40771, #41486, #41844, #64006, #18926, #68843, #58820, #13386, #7865, #30401, #53291, #31123, #36306, #8231, #52930, #47390, #69920, #19290, #30759, #57736, #52208, #64373, #25205, #47753, #64739, #53663, #18200, #63285, #7142, #24120, #29672, #7499, #52570, #1977, #42944, #43683, #4531, #20023, #72114, #37029, #25586, #20763, #61027, #32594, #4164, #9330, #48125, #38501, #42577, #71389, #71017, #60280, #65471, #43320, #20395, #3797, #15223, #66206, #10424, #21130, #14494, #15584, #32226, #44050, #26694, #14861, #59553, #55492, #38126, #70648, #8964, #71761, #66574, #31863, #60647, #15953, #49589, #31498, #37400, #65105, #54038, #59924, #10062, #3434, #9693, #65840, #55132, #27059, #25953, #48493, #54760, #54398, #26319, #21497, #37762, #48858, #32956, #49228, #38872, #61390, #66951, #49952, #62473, #33317, #23307, #45501, #21863 ) ),
 .UNSPECIFIED., .F., .F., .F. ) 
 B_SPLINE_SURFACE_WITH_KNOTS ( ( 2, 2 ),
 ( 3, 2, 2, 2, 2, 2, 2, 2, 2, 2, 2, 2, 2, 2, 2, 2, 2, 2, 2, 2, 2, 2, 2, 2, 2, 2, 2, 2, 2, 2, 2, 2, 2, 2, 2, 2, 2, 2, 2, 2, 2, 2, 2, 2, 2, 2, 2, 2, 2, 2, 2, 2, 2, 2, 2, 2, 2, 2, 2, 2, 2, 2, 2, 2, 2, 2, 2, 2, 2, 2, 2, 2, 2, 2, 2, 2, 2, 2, 2, 2, 2, 2, 2, 2, 2, 2, 2, 2, 2, 2, 2, 2, 2, 2, 2, 2, 2, 2, 2, 2, 2, 2, 2, 2, 2, 2, 2, 2, 2, 2, 2, 2, 2, 2, 2, 2, 2, 2, 2, 2, 2, 2, 2, 2, 2, 2, 2, 2, 2, 2, 2, 2, 2, 2, 2, 2, 2, 2, 2, 2, 2, 2, 2, 2, 2, 2, 2, 2, 2, 2, 2, 2, 2, 2, 2, 2, 2, 2, 2, 2, 2, 2, 2, 2, 2, 2, 2, 2, 2, 2, 2, 2, 2, 2, 2, 2, 2, 2, 2, 2, 2, 2, 2, 2, 2, 2, 2, 2, 2, 2, 2, 2, 2, 2, 2, 2, 2, 2, 2, 2, 2, 2, 2, 2, 2, 2, 2, 2, 2, 2, 2, 2, 2, 2, 2, 2, 2, 2, 2, 2, 2, 2, 2, 2, 2, 2, 2, 2, 2, 2, 2, 2, 2, 2, 2, 2, 2, 2, 2, 2, 2, 2, 2, 2, 2, 2, 2, 2, 2, 2, 2, 2, 2, 2, 2, 2, 2, 2, 2, 2, 2, 2, 2, 2, 2, 2, 2, 2, 2, 2, 2, 2, 2, 2, 2, 2, 2, 2, 2, 2, 2, 2, 2, 2, 2, 2, 2, 2, 2, 2, 2, 2, 2, 2, 2, 2, 2, 2, 2, 2, 2, 2, 2, 2, 2, 2, 2, 2, 2, 2, 2, 2, 2, 2, 2, 2, 2, 2, 2, 2, 2, 2, 2, 2, 2, 2, 2, 2, 2, 2, 2, 2, 2, 2, 2, 2, 2, 2, 2, 2, 2, 2, 2, 2, 2, 2, 2, 2, 2, 2, 2, 2, 2, 2, 2, 2, 2, 2, 2, 2, 3 ),
 ( 0.000000000000000000, 1.000000000000000000 ),
 ( 0.000000000000000000, 0.002777777777777777884, 0.005555555555555555768, 0.008333333333333333218, 0.01111111111111111154, 0.01388888888888888812, 0.01666666666666666644, 0.01944444444444444475, 0.02222222222222222307, 0.02500000000000000139, 0.02777777777777777624, 0.03055555555555555455, 0.03333333333333333287, 0.03611111111111110772, 0.03888888888888888951, 0.04166666666666666435, 0.04444444444444444614, 0.04722222222222222099, 0.05000000000000000278, 0.05277777777777777762, 0.05555555555555555247, 0.05833333333333333426, 0.06111111111111110911, 0.06388888888888888395, 0.06666666666666666574, 0.06944444444444444753, 0.07222222222222221544, 0.07499999999999999722, 0.07777777777777777901, 0.08055555555555556080, 0.08333333333333332871, 0.08611111111111111049, 0.08888888888888889228, 0.09166666666666666019, 0.09444444444444444198, 0.09722222222222222376, 0.1000000000000000056, 0.1027777777777777735, 0.1055555555555555552, 0.1083333333333333370, 0.1111111111111111049, 0.1138888888888888867, 0.1166666666666666685, 0.1194444444444444503, 0.1222222222222222182, 0.1250000000000000000, 0.1277777777777777679, 0.1305555555555555636, 0.1333333333333333315, 0.1361111111111110994, 0.1388888888888888951, 0.1416666666666666630, 0.1444444444444444309, 0.1472222222222222265, 0.1499999999999999944, 0.1527777777777777901, 0.1555555555555555580, 0.1583333333333333259, 0.1611111111111111216, 0.1638888888888888895, 0.1666666666666666574, 0.1694444444444444531, 0.1722222222222222210, 0.1749999999999999889, 0.1777777777777777846, 0.1805555555555555525, 0.1833333333333333204, 0.1861111111111111160, 0.1888888888888888840, 0.1916666666666666796, 0.1944444444444444475, 0.1972222222222222154, 0.2000000000000000111, 0.2027777777777777790, 0.2055555555555555469, 0.2083333333333333426, 0.2111111111111111105, 0.2138888888888888784, 0.2166666666666666741, 0.2194444444444444420, 0.2222222222222222099, 0.2250000000000000056, 0.2277777777777777735, 0.2305555555555555691, 0.2333333333333333370, 0.2361111111111111049, 0.2388888888888889006, 0.2416666666666666685, 0.2444444444444444364, 0.2472222222222222321, 0.2500000000000000000, 0.2527777777777777679, 0.2555555555555555358, 0.2583333333333333592, 0.2611111111111111271, 0.2638888888888888951, 0.2666666666666666630, 0.2694444444444444309, 0.2722222222222221988, 0.2750000000000000222, 0.2777777777777777901, 0.2805555555555555580, 0.2833333333333333259, 0.2861111111111110938, 0.2888888888888888618, 0.2916666666666666852, 0.2944444444444444531, 0.2972222222222222210, 0.2999999999999999889, 0.3027777777777777568, 0.3055555555555555802, 0.3083333333333333481, 0.3111111111111111160, 0.3138888888888888840, 0.3166666666666666519, 0.3194444444444444198, 0.3222222222222222432, 0.3250000000000000111, 0.3277777777777777790, 0.3305555555555555469, 0.3333333333333333148, 0.3361111111111111382, 0.3388888888888889062, 0.3416666666666666741, 0.3444444444444444420, 0.3472222222222222099, 0.3499999999999999778, 0.3527777777777778012, 0.3555555555555555691, 0.3583333333333333370, 0.3611111111111111049, 0.3638888888888888729, 0.3666666666666666408, 0.3694444444444444642, 0.3722222222222222321, 0.3750000000000000000, 0.3777777777777777679, 0.3805555555555555358, 0.3833333333333333592, 0.3861111111111111271, 0.3888888888888888951, 0.3916666666666666630, 0.3944444444444444309, 0.3972222222222221988, 0.4000000000000000222, 0.4027777777777777901, 0.4055555555555555580, 0.4083333333333333259, 0.4111111111111110938, 0.4138888888888888618, 0.4166666666666666852, 0.4194444444444444531, 0.4222222222222222210, 0.4249999999999999889, 0.4277777777777777568, 0.4305555555555555802, 0.4333333333333333481, 0.4361111111111111160, 0.4388888888888888840, 0.4416666666666666519, 0.4444444444444444198, 0.4472222222222222432, 0.4500000000000000111, 0.4527777777777777790, 0.4555555555555555469, 0.4583333333333333148, 0.4611111111111111382, 0.4638888888888889062, 0.4666666666666666741, 0.4694444444444444420, 0.4722222222222222099, 0.4749999999999999778, 0.4777777777777778012, 0.4805555555555555691, 0.4833333333333333370, 0.4861111111111111049, 0.4888888888888888729, 0.4916666666666666408, 0.4944444444444444642, 0.4972222222222222321, 0.5000000000000000000, 0.5027777777777777679, 0.5055555555555555358, 0.5083333333333333037, 0.5111111111111110716, 0.5138888888888888395, 0.5166666666666667185, 0.5194444444444444864, 0.5222222222222222543, 0.5250000000000000222, 0.5277777777777777901, 0.5305555555555555580, 0.5333333333333333259, 0.5361111111111110938, 0.5388888888888888618, 0.5416666666666666297, 0.5444444444444443976, 0.5472222222222222765, 0.5500000000000000444, 0.5527777777777778123, 0.5555555555555555802, 0.5583333333333333481, 0.5611111111111111160, 0.5638888888888888840, 0.5666666666666666519, 0.5694444444444444198, 0.5722222222222221877, 0.5749999999999999556, 0.5777777777777777235, 0.5805555555555556024, 0.5833333333333333703, 0.5861111111111111382, 0.5888888888888889062, 0.5916666666666666741, 0.5944444444444444420, 0.5972222222222222099, 0.5999999999999999778, 0.6027777777777777457, 0.6055555555555555136, 0.6083333333333332815, 0.6111111111111111605, 0.6138888888888889284, 0.6166666666666666963, 0.6194444444444444642, 0.6222222222222222321, 0.6250000000000000000, 0.6277777777777777679, 0.6305555555555555358, 0.6333333333333333037, 0.6361111111111110716, 0.6388888888888888395, 0.6416666666666667185, 0.6444444444444444864, 0.6472222222222222543, 0.6500000000000000222, 0.6527777777777777901, 0.6555555555555555580, 0.6583333333333333259, 0.6611111111111110938, 0.6638888888888888618, 0.6666666666666666297, 0.6694444444444443976, 0.6722222222222222765, 0.6750000000000000444, 0.6777777777777778123, 0.6805555555555555802, 0.6833333333333333481, 0.6861111111111111160, 0.6888888888888888840, 0.6916666666666666519, 0.6944444444444444198, 0.6972222222222221877, 0.6999999999999999556, 0.7027777777777777235, 0.7055555555555556024, 0.7083333333333333703, 0.7111111111111111382, 0.7138888888888889062, 0.7166666666666666741, 0.7194444444444444420, 0.7222222222222222099, 0.7249999999999999778, 0.7277777777777777457, 0.7305555555555555136, 0.7333333333333332815, 0.7361111111111111605, 0.7388888888888889284, 0.7416666666666666963, 0.7444444444444444642, 0.7472222222222222321, 0.7500000000000000000, 0.7527777777777777679, 0.7555555555555555358, 0.7583333333333333037, 0.7611111111111110716, 0.7638888888888888395, 0.7666666666666667185, 0.7694444444444444864, 0.7722222222222222543, 0.7750000000000000222, 0.7777777777777777901, 0.7805555555555555580, 0.7833333333333333259, 0.7861111111111110938, 0.7888888888888888618, 0.7916666666666666297, 0.7944444444444443976, 0.7972222222222222765, 0.8000000000000000444, 0.8027777777777778123, 0.8055555555555555802, 0.8083333333333333481, 0.8111111111111111160, 0.8138888888888888840, 0.8166666666666666519, 0.8194444444444444198, 0.8222222222222221877, 0.8249999999999999556, 0.8277777777777777235, 0.8305555555555556024, 0.8333333333333333703, 0.8361111111111111382, 0.8388888888888889062, 0.8416666666666666741, 0.8444444444444444420, 0.8472222222222222099, 0.8499999999999999778, 0.8527777777777777457, 0.8555555555555555136, 0.8583333333333332815, 0.8611111111111111605, 0.8638888888888889284, 0.8666666666666666963, 0.8694444444444444642, 0.8722222222222222321, 0.8750000000000000000, 0.8777777777777777679, 0.8805555555555555358, 0.8833333333333333037, 0.8861111111111110716, 0.8888888888888888395, 0.8916666666666667185, 0.8944444444444444864, 0.8972222222222222543, 0.9000000000000000222, 0.9027777777777777901, 0.9055555555555555580, 0.9083333333333333259, 0.9111111111111110938, 0.9138888888888888618, 0.9166666666666666297, 0.9194444444444443976, 0.9222222222222222765, 0.9250000000000000444, 0.9277777777777778123, 0.9305555555555555802, 0.9333333333333333481, 0.9361111111111111160, 0.9388888888888888840, 0.9416666666666666519, 0.9444444444444444198, 0.9472222222222221877, 0.9499999999999999556, 0.9527777777777777235, 0.9555555555555556024, 0.9583333333333333703, 0.9611111111111111382, 0.9638888888888889062, 0.9666666666666666741, 0.9694444444444444420, 0.9722222222222222099, 0.9749999999999999778, 0.9777777777777777457, 0.9805555555555555136, 0.9833333333333332815, 0.9861111111111111605, 0.9888888888888889284, 0.9916666666666666963, 0.9944444444444444642, 0.9972222222222222321, 1.000000000000000000 ),
 .UNSPECIFIED. ) 
 GEOMETRIC_REPRESENTATION_ITEM ( )  RATIONAL_B_SPLINE_SURFACE ( (
 ( 1.000000000000000000, 0.8660254037844387076, 1.000000000000000000, 0.8660254037844387076, 1.000000000000000000, 0.8660254037844387076, 1.000000000000000000, 0.8660254037844387076, 1.000000000000000000, 0.8660254037844387076, 1.000000000000000000, 0.8660254037844387076, 1.000000000000000000, 0.8660254037844387076, 1.000000000000000000, 0.8660254037844387076, 1.000000000000000000, 0.8660254037844387076, 1.000000000000000000, 0.8660254037844387076, 1.000000000000000000, 0.8660254037844387076, 1.000000000000000000, 0.8660254037844387076, 1.000000000000000000, 0.8660254037844387076, 1.000000000000000000, 0.8660254037844387076, 1.000000000000000000, 0.8660254037844387076, 1.000000000000000000, 0.8660254037844387076, 1.000000000000000000, 0.8660254037844387076, 1.000000000000000000, 0.8660254037844387076, 1.000000000000000000, 0.8660254037844387076, 1.000000000000000000, 0.8660254037844387076, 1.000000000000000000, 0.8660254037844387076, 1.000000000000000000, 0.8660254037844387076, 1.000000000000000000, 0.8660254037844387076, 1.000000000000000000, 0.8660254037844387076, 1.000000000000000000, 0.8660254037844387076, 1.000000000000000000, 0.8660254037844387076, 1.000000000000000000, 0.8660254037844387076, 1.000000000000000000, 0.8660254037844387076, 1.000000000000000000, 0.8660254037844387076, 1.000000000000000000, 0.8660254037844387076, 1.000000000000000000, 0.8660254037844387076, 1.000000000000000000, 0.8660254037844387076, 1.000000000000000000, 0.8660254037844387076, 1.000000000000000000, 0.8660254037844387076, 1.000000000000000000, 0.8660254037844387076, 1.000000000000000000, 0.8660254037844387076, 1.000000000000000000, 0.8660254037844387076, 1.000000000000000000, 0.8660254037844387076, 1.000000000000000000, 0.8660254037844387076, 1.000000000000000000, 0.8660254037844387076, 1.000000000000000000, 0.8660254037844387076, 1.000000000000000000, 0.8660254037844387076, 1.000000000000000000, 0.8660254037844387076, 1.000000000000000000, 0.8660254037844387076, 1.000000000000000000, 0.8660254037844387076, 1.000000000000000000, 0.8660254037844387076, 1.000000000000000000, 0.8660254037844387076, 1.000000000000000000, 0.8660254037844387076, 1.000000000000000000, 0.8660254037844387076, 1.000000000000000000, 0.8660254037844387076, 1.000000000000000000, 0.8660254037844387076, 1.000000000000000000, 0.8660254037844387076, 1.000000000000000000, 0.8660254037844387076, 1.000000000000000000, 0.8660254037844387076, 1.000000000000000000, 0.8660254037844387076, 1.000000000000000000, 0.8660254037844387076, 1.000000000000000000, 0.8660254037844387076, 1.000000000000000000, 0.8660254037844387076, 1.000000000000000000, 0.8660254037844387076, 1.000000000000000000, 0.8660254037844387076, 1.000000000000000000, 0.8660254037844387076, 1.000000000000000000, 0.8660254037844387076, 1.000000000000000000, 0.8660254037844387076, 1.000000000000000000, 0.8660254037844387076, 1.000000000000000000, 0.8660254037844387076, 1.000000000000000000, 0.8660254037844387076, 1.000000000000000000, 0.8660254037844387076, 1.000000000000000000, 0.8660254037844387076, 1.000000000000000000, 0.8660254037844387076, 1.000000000000000000, 0.8660254037844387076, 1.000000000000000000, 0.8660254037844387076, 1.000000000000000000, 0.8660254037844387076, 1.000000000000000000, 0.8660254037844387076, 1.000000000000000000, 0.8660254037844387076, 1.000000000000000000, 0.8660254037844387076, 1.000000000000000000, 0.8660254037844387076, 1.000000000000000000, 0.8660254037844387076, 1.000000000000000000, 0.8660254037844387076, 1.000000000000000000, 0.8660254037844387076, 1.000000000000000000, 0.8660254037844387076, 1.000000000000000000, 0.8660254037844387076, 1.000000000000000000, 0.8660254037844387076, 1.000000000000000000, 0.8660254037844387076, 1.000000000000000000, 0.8660254037844387076, 1.000000000000000000, 0.8660254037844387076, 1.000000000000000000, 0.8660254037844387076, 1.000000000000000000, 0.8660254037844387076, 1.000000000000000000, 0.8660254037844387076, 1.000000000000000000, 0.8660254037844387076, 1.000000000000000000, 0.8660254037844387076, 1.000000000000000000, 0.8660254037844387076, 1.000000000000000000, 0.8660254037844387076, 1.000000000000000000, 0.8660254037844387076, 1.000000000000000000, 0.8660254037844387076, 1.000000000000000000, 0.8660254037844387076, 1.000000000000000000, 0.8660254037844387076, 1.000000000000000000, 0.8660254037844387076, 1.000000000000000000, 0.8660254037844387076, 1.000000000000000000, 0.8660254037844387076, 1.000000000000000000, 0.8660254037844387076, 1.000000000000000000, 0.8660254037844387076, 1.000000000000000000, 0.8660254037844387076, 1.000000000000000000, 0.8660254037844387076, 1.000000000000000000, 0.8660254037844387076, 1.000000000000000000, 0.8660254037844387076, 1.000000000000000000, 0.8660254037844387076, 1.000000000000000000, 0.8660254037844387076, 1.000000000000000000, 0.8660254037844387076, 1.000000000000000000, 0.8660254037844387076, 1.000000000000000000, 0.8660254037844387076, 1.000000000000000000, 0.8660254037844387076, 1.000000000000000000, 0.8660254037844387076, 1.000000000000000000, 0.8660254037844387076, 1.000000000000000000, 0.8660254037844387076, 1.000000000000000000, 0.8660254037844387076, 1.000000000000000000, 0.8660254037844387076, 1.000000000000000000, 0.8660254037844387076, 1.000000000000000000, 0.8660254037844387076, 1.000000000000000000, 0.8660254037844387076, 1.000000000000000000, 0.8660254037844387076, 1.000000000000000000, 0.8660254037844387076, 1.000000000000000000, 0.8660254037844387076, 1.000000000000000000, 0.8660254037844387076, 1.000000000000000000, 0.8660254037844387076, 1.000000000000000000, 0.8660254037844387076, 1.000000000000000000, 0.8660254037844387076, 1.000000000000000000, 0.8660254037844387076, 1.000000000000000000, 0.8660254037844387076, 1.000000000000000000, 0.8660254037844387076, 1.000000000000000000, 0.8660254037844387076, 1.000000000000000000, 0.8660254037844387076, 1.000000000000000000, 0.8660254037844387076, 1.000000000000000000, 0.8660254037844387076, 1.000000000000000000, 0.8660254037844387076, 1.000000000000000000, 0.8660254037844387076, 1.000000000000000000, 0.8660254037844387076, 1.000000000000000000, 0.8660254037844387076, 1.000000000000000000, 0.8660254037844387076, 1.000000000000000000, 0.8660254037844387076, 1.000000000000000000, 0.8660254037844387076, 1.000000000000000000, 0.8660254037844387076, 1.000000000000000000, 0.8660254037844387076, 1.000000000000000000, 0.8660254037844387076, 1.000000000000000000, 0.8660254037844387076, 1.000000000000000000, 0.8660254037844387076, 1.000000000000000000, 0.8660254037844387076, 1.000000000000000000, 0.8660254037844387076, 1.000000000000000000, 0.8660254037844387076, 1.000000000000000000, 0.8660254037844387076, 1.000000000000000000, 0.8660254037844387076, 1.000000000000000000, 0.8660254037844387076, 1.000000000000000000, 0.8660254037844387076, 1.000000000000000000, 0.8660254037844387076, 1.000000000000000000, 0.8660254037844387076, 1.000000000000000000, 0.8660254037844387076, 1.000000000000000000, 0.8660254037844387076, 1.000000000000000000, 0.8660254037844387076, 1.000000000000000000, 0.8660254037844387076, 1.000000000000000000, 0.8660254037844387076, 1.000000000000000000, 0.8660254037844387076, 1.000000000000000000, 0.8660254037844387076, 1.000000000000000000, 0.8660254037844387076, 1.000000000000000000, 0.8660254037844387076, 1.000000000000000000, 0.8660254037844387076, 1.000000000000000000, 0.8660254037844387076, 1.000000000000000000, 0.8660254037844387076, 1.000000000000000000, 0.8660254037844387076, 1.000000000000000000, 0.8660254037844387076, 1.000000000000000000, 0.8660254037844387076, 1.000000000000000000, 0.8660254037844387076, 1.000000000000000000, 0.8660254037844387076, 1.000000000000000000, 0.8660254037844387076, 1.000000000000000000, 0.8660254037844387076, 1.000000000000000000, 0.8660254037844387076, 1.000000000000000000, 0.8660254037844387076, 1.000000000000000000, 0.8660254037844387076, 1.000000000000000000, 0.8660254037844387076, 1.000000000000000000, 0.8660254037844387076, 1.000000000000000000, 0.8660254037844387076, 1.000000000000000000, 0.8660254037844387076, 1.000000000000000000, 0.8660254037844387076, 1.000000000000000000, 0.8660254037844387076, 1.000000000000000000, 0.8660254037844387076, 1.000000000000000000, 0.8660254037844387076, 1.000000000000000000, 0.8660254037844387076, 1.000000000000000000, 0.8660254037844387076, 1.000000000000000000, 0.8660254037844387076, 1.000000000000000000, 0.8660254037844387076, 1.000000000000000000, 0.8660254037844387076, 1.000000000000000000, 0.8660254037844387076, 1.000000000000000000, 0.8660254037844387076, 1.000000000000000000, 0.8660254037844387076, 1.000000000000000000, 0.8660254037844387076, 1.000000000000000000, 0.8660254037844387076, 1.000000000000000000, 0.8660254037844387076, 1.000000000000000000, 0.8660254037844387076, 1.000000000000000000, 0.8660254037844387076, 1.000000000000000000, 0.8660254037844387076, 1.000000000000000000, 0.8660254037844387076, 1.000000000000000000, 0.8660254037844387076, 1.000000000000000000, 0.8660254037844387076, 1.000000000000000000, 0.8660254037844387076, 1.000000000000000000, 0.8660254037844387076, 1.000000000000000000, 0.8660254037844387076, 1.000000000000000000, 0.8660254037844387076, 1.000000000000000000, 0.8660254037844387076, 1.000000000000000000, 0.8660254037844387076, 1.000000000000000000, 0.8660254037844387076, 1.000000000000000000, 0.8660254037844387076, 1.000000000000000000, 0.8660254037844387076, 1.000000000000000000, 0.8660254037844387076, 1.000000000000000000, 0.8660254037844387076, 1.000000000000000000, 0.8660254037844387076, 1.000000000000000000, 0.8660254037844387076, 1.000000000000000000, 0.8660254037844387076, 1.000000000000000000, 0.8660254037844387076, 1.000000000000000000, 0.8660254037844387076, 1.000000000000000000, 0.8660254037844387076, 1.000000000000000000, 0.8660254037844387076, 1.000000000000000000, 0.8660254037844387076, 1.000000000000000000, 0.8660254037844387076, 1.000000000000000000, 0.8660254037844387076, 1.000000000000000000, 0.8660254037844387076, 1.000000000000000000, 0.8660254037844387076, 1.000000000000000000, 0.8660254037844387076, 1.000000000000000000, 0.8660254037844387076, 1.000000000000000000, 0.8660254037844387076, 1.000000000000000000, 0.8660254037844387076, 1.000000000000000000, 0.8660254037844387076, 1.000000000000000000, 0.8660254037844387076, 1.000000000000000000, 0.8660254037844387076, 1.000000000000000000, 0.8660254037844387076, 1.000000000000000000, 0.8660254037844387076, 1.000000000000000000, 0.8660254037844387076, 1.000000000000000000, 0.8660254037844387076, 1.000000000000000000, 0.8660254037844387076, 1.000000000000000000, 0.8660254037844387076, 1.000000000000000000, 0.8660254037844387076, 1.000000000000000000, 0.8660254037844387076, 1.000000000000000000, 0.8660254037844387076, 1.000000000000000000, 0.8660254037844387076, 1.000000000000000000, 0.8660254037844387076, 1.000000000000000000, 0.8660254037844387076, 1.000000000000000000, 0.8660254037844387076, 1.000000000000000000, 0.8660254037844387076, 1.000000000000000000, 0.8660254037844387076, 1.000000000000000000, 0.8660254037844387076, 1.000000000000000000, 0.8660254037844387076, 1.000000000000000000, 0.8660254037844387076, 1.000000000000000000, 0.8660254037844387076, 1.000000000000000000, 0.8660254037844387076, 1.000000000000000000, 0.8660254037844387076, 1.000000000000000000, 0.8660254037844387076, 1.000000000000000000, 0.8660254037844387076, 1.000000000000000000, 0.8660254037844387076, 1.000000000000000000, 0.8660254037844387076, 1.000000000000000000, 0.8660254037844387076, 1.000000000000000000, 0.8660254037844387076, 1.000000000000000000, 0.8660254037844387076, 1.000000000000000000, 0.8660254037844387076, 1.000000000000000000, 0.8660254037844387076, 1.000000000000000000, 0.8660254037844387076, 1.000000000000000000, 0.8660254037844387076, 1.000000000000000000, 0.8660254037844387076, 1.000000000000000000, 0.8660254037844387076, 1.000000000000000000, 0.8660254037844387076, 1.000000000000000000, 0.8660254037844387076, 1.000000000000000000, 0.8660254037844387076, 1.000000000000000000, 0.8660254037844387076, 1.000000000000000000, 0.8660254037844387076, 1.000000000000000000, 0.8660254037844387076, 1.000000000000000000, 0.8660254037844387076, 1.000000000000000000, 0.8660254037844387076, 1.000000000000000000, 0.8660254037844387076, 1.000000000000000000, 0.8660254037844387076, 1.000000000000000000, 0.8660254037844387076, 1.000000000000000000, 0.8660254037844387076, 1.000000000000000000, 0.8660254037844387076, 1.000000000000000000, 0.8660254037844387076, 1.000000000000000000, 0.8660254037844387076, 1.000000000000000000, 0.8660254037844387076, 1.000000000000000000, 0.8660254037844387076, 1.000000000000000000, 0.8660254037844387076, 1.000000000000000000, 0.8660254037844387076, 1.000000000000000000, 0.8660254037844387076, 1.000000000000000000, 0.8660254037844387076, 1.000000000000000000, 0.8660254037844387076, 1.000000000000000000, 0.8660254037844387076, 1.000000000000000000, 0.8660254037844387076, 1.000000000000000000, 0.8660254037844387076, 1.000000000000000000, 0.8660254037844387076, 1.000000000000000000, 0.8660254037844387076, 1.000000000000000000, 0.8660254037844387076, 1.000000000000000000, 0.8660254037844387076, 1.000000000000000000, 0.8660254037844387076, 1.000000000000000000, 0.8660254037844387076, 1.000000000000000000, 0.8660254037844387076, 1.000000000000000000, 0.8660254037844387076, 1.000000000000000000, 0.8660254037844387076, 1.000000000000000000, 0.8660254037844387076, 1.000000000000000000, 0.8660254037844387076, 1.000000000000000000, 0.8660254037844387076, 1.000000000000000000, 0.8660254037844387076, 1.000000000000000000, 0.8660254037844387076, 1.000000000000000000, 0.8660254037844387076, 1.000000000000000000, 0.8660254037844387076, 1.000000000000000000, 0.8660254037844387076, 1.000000000000000000, 0.8660254037844387076, 1.000000000000000000, 0.8660254037844387076, 1.000000000000000000, 0.8660254037844387076, 1.000000000000000000, 0.8660254037844387076, 1.000000000000000000, 0.8660254037844387076, 1.000000000000000000, 0.8660254037844387076, 1.000000000000000000, 0.8660254037844387076, 1.000000000000000000, 0.8660254037844387076, 1.000000000000000000, 0.8660254037844387076, 1.000000000000000000, 0.8660254037844387076, 1.000000000000000000, 0.8660254037844387076, 1.000000000000000000, 0.8660254037844387076, 1.000000000000000000, 0.8660254037844387076, 1.000000000000000000, 0.8660254037844387076, 1.000000000000000000, 0.8660254037844387076, 1.000000000000000000, 0.8660254037844387076, 1.000000000000000000, 0.8660254037844387076, 1.000000000000000000, 0.8660254037844387076, 1.000000000000000000, 0.8660254037844387076, 1.000000000000000000, 0.8660254037844387076, 1.000000000000000000, 0.8660254037844387076, 1.000000000000000000, 0.8660254037844387076, 1.000000000000000000, 0.8660254037844387076, 1.000000000000000000, 0.8660254037844387076, 1.000000000000000000, 0.8660254037844387076, 1.000000000000000000, 0.8660254037844387076, 1.000000000000000000, 0.8660254037844387076, 1.000000000000000000, 0.8660254037844387076, 1.000000000000000000, 0.8660254037844387076, 1.000000000000000000, 0.8660254037844387076, 1.000000000000000000, 0.8660254037844387076, 1.000000000000000000, 0.8660254037844387076, 1.000000000000000000, 0.8660254037844387076, 1.000000000000000000, 0.8660254037844387076, 1.000000000000000000, 0.8660254037844387076, 1.000000000000000000, 0.8660254037844387076, 1.000000000000000000, 0.8660254037844387076, 1.000000000000000000, 0.8660254037844387076, 1.000000000000000000, 0.8660254037844387076, 1.000000000000000000, 0.8660254037844387076, 1.000000000000000000, 0.8660254037844387076, 1.000000000000000000, 0.8660254037844387076, 1.000000000000000000, 0.8660254037844387076, 1.000000000000000000, 0.8660254037844387076, 1.000000000000000000, 0.8660254037844387076, 1.000000000000000000, 0.8660254037844387076, 1.000000000000000000, 0.8660254037844387076, 1.000000000000000000, 0.8660254037844387076, 1.000000000000000000, 0.8660254037844387076, 1.000000000000000000, 0.8660254037844387076, 1.000000000000000000, 0.8660254037844387076, 1.000000000000000000, 0.8660254037844387076, 1.000000000000000000, 0.8660254037844387076, 1.000000000000000000),
 ( 1.000000000000000000, 0.8660254037844387076, 1.000000000000000000, 0.8660254037844387076, 1.000000000000000000, 0.8660254037844387076, 1.000000000000000000, 0.8660254037844387076, 1.000000000000000000, 0.8660254037844387076, 1.000000000000000000, 0.8660254037844387076, 1.000000000000000000, 0.8660254037844387076, 1.000000000000000000, 0.8660254037844387076, 1.000000000000000000, 0.8660254037844387076, 1.000000000000000000, 0.8660254037844387076, 1.000000000000000000, 0.8660254037844387076, 1.000000000000000000, 0.8660254037844387076, 1.000000000000000000, 0.8660254037844387076, 1.000000000000000000, 0.8660254037844387076, 1.000000000000000000, 0.8660254037844387076, 1.000000000000000000, 0.8660254037844387076, 1.000000000000000000, 0.8660254037844387076, 1.000000000000000000, 0.8660254037844387076, 1.000000000000000000, 0.8660254037844387076, 1.000000000000000000, 0.8660254037844387076, 1.000000000000000000, 0.8660254037844387076, 1.000000000000000000, 0.8660254037844387076, 1.000000000000000000, 0.8660254037844387076, 1.000000000000000000, 0.8660254037844387076, 1.000000000000000000, 0.8660254037844387076, 1.000000000000000000, 0.8660254037844387076, 1.000000000000000000, 0.8660254037844387076, 1.000000000000000000, 0.8660254037844387076, 1.000000000000000000, 0.8660254037844387076, 1.000000000000000000, 0.8660254037844387076, 1.000000000000000000, 0.8660254037844387076, 1.000000000000000000, 0.8660254037844387076, 1.000000000000000000, 0.8660254037844387076, 1.000000000000000000, 0.8660254037844387076, 1.000000000000000000, 0.8660254037844387076, 1.000000000000000000, 0.8660254037844387076, 1.000000000000000000, 0.8660254037844387076, 1.000000000000000000, 0.8660254037844387076, 1.000000000000000000, 0.8660254037844387076, 1.000000000000000000, 0.8660254037844387076, 1.000000000000000000, 0.8660254037844387076, 1.000000000000000000, 0.8660254037844387076, 1.000000000000000000, 0.8660254037844387076, 1.000000000000000000, 0.8660254037844387076, 1.000000000000000000, 0.8660254037844387076, 1.000000000000000000, 0.8660254037844387076, 1.000000000000000000, 0.8660254037844387076, 1.000000000000000000, 0.8660254037844387076, 1.000000000000000000, 0.8660254037844387076, 1.000000000000000000, 0.8660254037844387076, 1.000000000000000000, 0.8660254037844387076, 1.000000000000000000, 0.8660254037844387076, 1.000000000000000000, 0.8660254037844387076, 1.000000000000000000, 0.8660254037844387076, 1.000000000000000000, 0.8660254037844387076, 1.000000000000000000, 0.8660254037844387076, 1.000000000000000000, 0.8660254037844387076, 1.000000000000000000, 0.8660254037844387076, 1.000000000000000000, 0.8660254037844387076, 1.000000000000000000, 0.8660254037844387076, 1.000000000000000000, 0.8660254037844387076, 1.000000000000000000, 0.8660254037844387076, 1.000000000000000000, 0.8660254037844387076, 1.000000000000000000, 0.8660254037844387076, 1.000000000000000000, 0.8660254037844387076, 1.000000000000000000, 0.8660254037844387076, 1.000000000000000000, 0.8660254037844387076, 1.000000000000000000, 0.8660254037844387076, 1.000000000000000000, 0.8660254037844387076, 1.000000000000000000, 0.8660254037844387076, 1.000000000000000000, 0.8660254037844387076, 1.000000000000000000, 0.8660254037844387076, 1.000000000000000000, 0.8660254037844387076, 1.000000000000000000, 0.8660254037844387076, 1.000000000000000000, 0.8660254037844387076, 1.000000000000000000, 0.8660254037844387076, 1.000000000000000000, 0.8660254037844387076, 1.000000000000000000, 0.8660254037844387076, 1.000000000000000000, 0.8660254037844387076, 1.000000000000000000, 0.8660254037844387076, 1.000000000000000000, 0.8660254037844387076, 1.000000000000000000, 0.8660254037844387076, 1.000000000000000000, 0.8660254037844387076, 1.000000000000000000, 0.8660254037844387076, 1.000000000000000000, 0.8660254037844387076, 1.000000000000000000, 0.8660254037844387076, 1.000000000000000000, 0.8660254037844387076, 1.000000000000000000, 0.8660254037844387076, 1.000000000000000000, 0.8660254037844387076, 1.000000000000000000, 0.8660254037844387076, 1.000000000000000000, 0.8660254037844387076, 1.000000000000000000, 0.8660254037844387076, 1.000000000000000000, 0.8660254037844387076, 1.000000000000000000, 0.8660254037844387076, 1.000000000000000000, 0.8660254037844387076, 1.000000000000000000, 0.8660254037844387076, 1.000000000000000000, 0.8660254037844387076, 1.000000000000000000, 0.8660254037844387076, 1.000000000000000000, 0.8660254037844387076, 1.000000000000000000, 0.8660254037844387076, 1.000000000000000000, 0.8660254037844387076, 1.000000000000000000, 0.8660254037844387076, 1.000000000000000000, 0.8660254037844387076, 1.000000000000000000, 0.8660254037844387076, 1.000000000000000000, 0.8660254037844387076, 1.000000000000000000, 0.8660254037844387076, 1.000000000000000000, 0.8660254037844387076, 1.000000000000000000, 0.8660254037844387076, 1.000000000000000000, 0.8660254037844387076, 1.000000000000000000, 0.8660254037844387076, 1.000000000000000000, 0.8660254037844387076, 1.000000000000000000, 0.8660254037844387076, 1.000000000000000000, 0.8660254037844387076, 1.000000000000000000, 0.8660254037844387076, 1.000000000000000000, 0.8660254037844387076, 1.000000000000000000, 0.8660254037844387076, 1.000000000000000000, 0.8660254037844387076, 1.000000000000000000, 0.8660254037844387076, 1.000000000000000000, 0.8660254037844387076, 1.000000000000000000, 0.8660254037844387076, 1.000000000000000000, 0.8660254037844387076, 1.000000000000000000, 0.8660254037844387076, 1.000000000000000000, 0.8660254037844387076, 1.000000000000000000, 0.8660254037844387076, 1.000000000000000000, 0.8660254037844387076, 1.000000000000000000, 0.8660254037844387076, 1.000000000000000000, 0.8660254037844387076, 1.000000000000000000, 0.8660254037844387076, 1.000000000000000000, 0.8660254037844387076, 1.000000000000000000, 0.8660254037844387076, 1.000000000000000000, 0.8660254037844387076, 1.000000000000000000, 0.8660254037844387076, 1.000000000000000000, 0.8660254037844387076, 1.000000000000000000, 0.8660254037844387076, 1.000000000000000000, 0.8660254037844387076, 1.000000000000000000, 0.8660254037844387076, 1.000000000000000000, 0.8660254037844387076, 1.000000000000000000, 0.8660254037844387076, 1.000000000000000000, 0.8660254037844387076, 1.000000000000000000, 0.8660254037844387076, 1.000000000000000000, 0.8660254037844387076, 1.000000000000000000, 0.8660254037844387076, 1.000000000000000000, 0.8660254037844387076, 1.000000000000000000, 0.8660254037844387076, 1.000000000000000000, 0.8660254037844387076, 1.000000000000000000, 0.8660254037844387076, 1.000000000000000000, 0.8660254037844387076, 1.000000000000000000, 0.8660254037844387076, 1.000000000000000000, 0.8660254037844387076, 1.000000000000000000, 0.8660254037844387076, 1.000000000000000000, 0.8660254037844387076, 1.000000000000000000, 0.8660254037844387076, 1.000000000000000000, 0.8660254037844387076, 1.000000000000000000, 0.8660254037844387076, 1.000000000000000000, 0.8660254037844387076, 1.000000000000000000, 0.8660254037844387076, 1.000000000000000000, 0.8660254037844387076, 1.000000000000000000, 0.8660254037844387076, 1.000000000000000000, 0.8660254037844387076, 1.000000000000000000, 0.8660254037844387076, 1.000000000000000000, 0.8660254037844387076, 1.000000000000000000, 0.8660254037844387076, 1.000000000000000000, 0.8660254037844387076, 1.000000000000000000, 0.8660254037844387076, 1.000000000000000000, 0.8660254037844387076, 1.000000000000000000, 0.8660254037844387076, 1.000000000000000000, 0.8660254037844387076, 1.000000000000000000, 0.8660254037844387076, 1.000000000000000000, 0.8660254037844387076, 1.000000000000000000, 0.8660254037844387076, 1.000000000000000000, 0.8660254037844387076, 1.000000000000000000, 0.8660254037844387076, 1.000000000000000000, 0.8660254037844387076, 1.000000000000000000, 0.8660254037844387076, 1.000000000000000000, 0.8660254037844387076, 1.000000000000000000, 0.8660254037844387076, 1.000000000000000000, 0.8660254037844387076, 1.000000000000000000, 0.8660254037844387076, 1.000000000000000000, 0.8660254037844387076, 1.000000000000000000, 0.8660254037844387076, 1.000000000000000000, 0.8660254037844387076, 1.000000000000000000, 0.8660254037844387076, 1.000000000000000000, 0.8660254037844387076, 1.000000000000000000, 0.8660254037844387076, 1.000000000000000000, 0.8660254037844387076, 1.000000000000000000, 0.8660254037844387076, 1.000000000000000000, 0.8660254037844387076, 1.000000000000000000, 0.8660254037844387076, 1.000000000000000000, 0.8660254037844387076, 1.000000000000000000, 0.8660254037844387076, 1.000000000000000000, 0.8660254037844387076, 1.000000000000000000, 0.8660254037844387076, 1.000000000000000000, 0.8660254037844387076, 1.000000000000000000, 0.8660254037844387076, 1.000000000000000000, 0.8660254037844387076, 1.000000000000000000, 0.8660254037844387076, 1.000000000000000000, 0.8660254037844387076, 1.000000000000000000, 0.8660254037844387076, 1.000000000000000000, 0.8660254037844387076, 1.000000000000000000, 0.8660254037844387076, 1.000000000000000000, 0.8660254037844387076, 1.000000000000000000, 0.8660254037844387076, 1.000000000000000000, 0.8660254037844387076, 1.000000000000000000, 0.8660254037844387076, 1.000000000000000000, 0.8660254037844387076, 1.000000000000000000, 0.8660254037844387076, 1.000000000000000000, 0.8660254037844387076, 1.000000000000000000, 0.8660254037844387076, 1.000000000000000000, 0.8660254037844387076, 1.000000000000000000, 0.8660254037844387076, 1.000000000000000000, 0.8660254037844387076, 1.000000000000000000, 0.8660254037844387076, 1.000000000000000000, 0.8660254037844387076, 1.000000000000000000, 0.8660254037844387076, 1.000000000000000000, 0.8660254037844387076, 1.000000000000000000, 0.8660254037844387076, 1.000000000000000000, 0.8660254037844387076, 1.000000000000000000, 0.8660254037844387076, 1.000000000000000000, 0.8660254037844387076, 1.000000000000000000, 0.8660254037844387076, 1.000000000000000000, 0.8660254037844387076, 1.000000000000000000, 0.8660254037844387076, 1.000000000000000000, 0.8660254037844387076, 1.000000000000000000, 0.8660254037844387076, 1.000000000000000000, 0.8660254037844387076, 1.000000000000000000, 0.8660254037844387076, 1.000000000000000000, 0.8660254037844387076, 1.000000000000000000, 0.8660254037844387076, 1.000000000000000000, 0.8660254037844387076, 1.000000000000000000, 0.8660254037844387076, 1.000000000000000000, 0.8660254037844387076, 1.000000000000000000, 0.8660254037844387076, 1.000000000000000000, 0.8660254037844387076, 1.000000000000000000, 0.8660254037844387076, 1.000000000000000000, 0.8660254037844387076, 1.000000000000000000, 0.8660254037844387076, 1.000000000000000000, 0.8660254037844387076, 1.000000000000000000, 0.8660254037844387076, 1.000000000000000000, 0.8660254037844387076, 1.000000000000000000, 0.8660254037844387076, 1.000000000000000000, 0.8660254037844387076, 1.000000000000000000, 0.8660254037844387076, 1.000000000000000000, 0.8660254037844387076, 1.000000000000000000, 0.8660254037844387076, 1.000000000000000000, 0.8660254037844387076, 1.000000000000000000, 0.8660254037844387076, 1.000000000000000000, 0.8660254037844387076, 1.000000000000000000, 0.8660254037844387076, 1.000000000000000000, 0.8660254037844387076, 1.000000000000000000, 0.8660254037844387076, 1.000000000000000000, 0.8660254037844387076, 1.000000000000000000, 0.8660254037844387076, 1.000000000000000000, 0.8660254037844387076, 1.000000000000000000, 0.8660254037844387076, 1.000000000000000000, 0.8660254037844387076, 1.000000000000000000, 0.8660254037844387076, 1.000000000000000000, 0.8660254037844387076, 1.000000000000000000, 0.8660254037844387076, 1.000000000000000000, 0.8660254037844387076, 1.000000000000000000, 0.8660254037844387076, 1.000000000000000000, 0.8660254037844387076, 1.000000000000000000, 0.8660254037844387076, 1.000000000000000000, 0.8660254037844387076, 1.000000000000000000, 0.8660254037844387076, 1.000000000000000000, 0.8660254037844387076, 1.000000000000000000, 0.8660254037844387076, 1.000000000000000000, 0.8660254037844387076, 1.000000000000000000, 0.8660254037844387076, 1.000000000000000000, 0.8660254037844387076, 1.000000000000000000, 0.8660254037844387076, 1.000000000000000000, 0.8660254037844387076, 1.000000000000000000, 0.8660254037844387076, 1.000000000000000000, 0.8660254037844387076, 1.000000000000000000, 0.8660254037844387076, 1.000000000000000000, 0.8660254037844387076, 1.000000000000000000, 0.8660254037844387076, 1.000000000000000000, 0.8660254037844387076, 1.000000000000000000, 0.8660254037844387076, 1.000000000000000000, 0.8660254037844387076, 1.000000000000000000, 0.8660254037844387076, 1.000000000000000000, 0.8660254037844387076, 1.000000000000000000, 0.8660254037844387076, 1.000000000000000000, 0.8660254037844387076, 1.000000000000000000, 0.8660254037844387076, 1.000000000000000000, 0.8660254037844387076, 1.000000000000000000, 0.8660254037844387076, 1.000000000000000000, 0.8660254037844387076, 1.000000000000000000, 0.8660254037844387076, 1.000000000000000000, 0.8660254037844387076, 1.000000000000000000, 0.8660254037844387076, 1.000000000000000000, 0.8660254037844387076, 1.000000000000000000, 0.8660254037844387076, 1.000000000000000000, 0.8660254037844387076, 1.000000000000000000, 0.8660254037844387076, 1.000000000000000000, 0.8660254037844387076, 1.000000000000000000, 0.8660254037844387076, 1.000000000000000000, 0.8660254037844387076, 1.000000000000000000, 0.8660254037844387076, 1.000000000000000000, 0.8660254037844387076, 1.000000000000000000, 0.8660254037844387076, 1.000000000000000000, 0.8660254037844387076, 1.000000000000000000, 0.8660254037844387076, 1.000000000000000000, 0.8660254037844387076, 1.000000000000000000, 0.8660254037844387076, 1.000000000000000000, 0.8660254037844387076, 1.000000000000000000, 0.8660254037844387076, 1.000000000000000000, 0.8660254037844387076, 1.000000000000000000, 0.8660254037844387076, 1.000000000000000000, 0.8660254037844387076, 1.000000000000000000, 0.8660254037844387076, 1.000000000000000000, 0.8660254037844387076, 1.000000000000000000, 0.8660254037844387076, 1.000000000000000000, 0.8660254037844387076, 1.000000000000000000, 0.8660254037844387076, 1.000000000000000000, 0.8660254037844387076, 1.000000000000000000, 0.8660254037844387076, 1.000000000000000000, 0.8660254037844387076, 1.000000000000000000, 0.8660254037844387076, 1.000000000000000000, 0.8660254037844387076, 1.000000000000000000, 0.8660254037844387076, 1.000000000000000000, 0.8660254037844387076, 1.000000000000000000, 0.8660254037844387076, 1.000000000000000000, 0.8660254037844387076, 1.000000000000000000, 0.8660254037844387076, 1.000000000000000000, 0.8660254037844387076, 1.000000000000000000, 0.8660254037844387076, 1.000000000000000000, 0.8660254037844387076, 1.000000000000000000, 0.8660254037844387076, 1.000000000000000000, 0.8660254037844387076, 1.000000000000000000, 0.8660254037844387076, 1.000000000000000000, 0.8660254037844387076, 1.000000000000000000, 0.8660254037844387076, 1.000000000000000000, 0.8660254037844387076, 1.000000000000000000, 0.8660254037844387076, 1.000000000000000000, 0.8660254037844387076, 1.000000000000000000, 0.8660254037844387076, 1.000000000000000000, 0.8660254037844387076, 1.000000000000000000, 0.8660254037844387076, 1.000000000000000000, 0.8660254037844387076, 1.000000000000000000, 0.8660254037844387076, 1.000000000000000000, 0.8660254037844387076, 1.000000000000000000, 0.8660254037844387076, 1.000000000000000000, 0.8660254037844387076, 1.000000000000000000, 0.8660254037844387076, 1.000000000000000000, 0.8660254037844387076, 1.000000000000000000, 0.8660254037844387076, 1.000000000000000000, 0.8660254037844387076, 1.000000000000000000, 0.8660254037844387076, 1.000000000000000000, 0.8660254037844387076, 1.000000000000000000, 0.8660254037844387076, 1.000000000000000000, 0.8660254037844387076, 1.000000000000000000, 0.8660254037844387076, 1.000000000000000000, 0.8660254037844387076, 1.000000000000000000, 0.8660254037844387076, 1.000000000000000000, 0.8660254037844387076, 1.000000000000000000, 0.8660254037844387076, 1.000000000000000000, 0.8660254037844387076, 1.000000000000000000, 0.8660254037844387076, 1.000000000000000000, 0.8660254037844387076, 1.000000000000000000, 0.8660254037844387076, 1.000000000000000000) ) ) 
 REPRESENTATION_ITEM ( '' )  SURFACE ( )  );
#66301=CARTESIAN_POINT ( 'NONE',  ( 20.77500000122903145, -5.773502691896255534, -1.060575238724906372E-15 ) ) ;
#66302=CARTESIAN_POINT ( 'NONE',  ( 4.243569643749999898, 14.68437500061451750, -30.00000000000000000 ) ) ;
#66303=CARTESIAN_POINT ( 'NONE',  ( 20.63437500061451857, 6.421520780324663323E-16, -5.243569643749999010 ) ) ;
#66305=CARTESIAN_POINT ( 'NONE',  ( 5.100000001229034297, -2.886751345948125991, -5.000000000000000000 ) ) ;
#66306=CARTESIAN_POINT ( 'NONE',  ( 4.321875000614517681, -6.054752690667223547, -1.112240025338166033E-15 ) ) ;
#66307=CARTESIAN_POINT ( 'NONE',  ( 19.95937500061451786, 0.000000000000000000, 5.243569643749999010 ) ) ;
#66308=CARTESIAN_POINT ( 'NONE',  ( 5.250000000000000888, 0.000000000000000000, 4.999999999999998224 ) ) ;
#66309=CARTESIAN_POINT ( 'NONE',  ( 18.47812500061451857, 4.541064518000418104, 2.621784821874999949 ) ) ;
#66311=CARTESIAN_POINT ( 'NONE',  ( 0.000000000000000000, 20.00000000000000000, 26.00000000000000000 ) ) ;
#66313=CARTESIAN_POINT ( 'NONE',  ( 27.64687500061452141, -3.027376345333614438, 5.243569643749998122 ) ) ;
#66315=CARTESIAN_POINT ( 'NONE',  ( 15.14062500061451644, -3.027376345333610441, -5.243569643749999898 ) ) ;
#66316=CARTESIAN_POINT ( 'NONE',  ( 13.13437500061451857, 4.541064518000418104, 2.621784821874999949 ) ) ;
#66318=CARTESIAN_POINT ( 'NONE',  ( -1.487416814333745711E-14, 16.96250000000000213, -26.00000000000000000 ) ) ;
#66319=CARTESIAN_POINT ( 'NONE',  ( 23.39062500061451289, 6.054752690667223547, 3.707466751127219781E-16 ) ) ;
#66320=DIRECTION ( 'NONE',  ( 0.000000000000000000, 1.000000000000000000, 0.000000000000000000 ) ) ;
#66321=CARTESIAN_POINT ( 'NONE',  ( -1.071796769724488563, 18.40490381179670365, 34.00000000000000000 ) ) ;
#66322=CARTESIAN_POINT ( 'NONE',  ( 13.01249999999999929, -5.773502691896255534, -1.060575238724906372E-15 ) ) ;
#66323=CARTESIAN_POINT ( 'NONE',  ( 25.20000000122903216, -2.886751345948129988, 4.999999999999997335 ) ) ;
#66324=CARTESIAN_POINT ( 'NONE',  ( 17.72812500061451502, -4.541064518000419881, 2.621784821874995952 ) ) ;
#66326=CARTESIAN_POINT ( 'NONE',  ( 21.48750000000000071, -2.886751345948129988, 4.999999999999997335 ) ) ;
#66327=CARTESIAN_POINT ( 'NONE',  ( 22.80937500061451573, -4.541064518000417216, -2.621784821875001281 ) ) ;
#66328=ORIENTED_EDGE ( 'NONE', *, *, #72661, .T. ) ;
#66330=CARTESIAN_POINT ( 'NONE',  ( 10.07812500061451644, -4.541064518000419881, 2.621784821874995952 ) ) ;
#66331=CARTESIAN_POINT ( 'NONE',  ( 3.263151822586646933, 3.788417924198219655, 3.593707371173769261 ) ) ;
#66333=CARTESIAN_POINT ( 'NONE',  ( 17.10000000000000142, -4.330127018922190985, -2.500000000000001332 ) ) ;
#66334=CARTESIAN_POINT ( 'NONE',  ( 25.16249999999999432, -5.773502691896255534, -1.060575238724906372E-15 ) ) ;
#66335=CARTESIAN_POINT ( 'NONE',  ( 7.762500000000001066, 2.886751345948062486, -5.000000000000113687 ) ) ;
#66336=CARTESIAN_POINT ( 'NONE',  ( 4.321875000614517681, -6.054752690667223547, -1.112240025338166033E-15 ) ) ;
#66337=CARTESIAN_POINT ( 'NONE',  ( 16.39687500061451786, -3.027376345333614438, 5.243569643749998122 ) ) ;
#66338=CARTESIAN_POINT ( 'NONE',  ( 27.75937500061451502, -4.541064518000417216, -2.621784821875001281 ) ) ;
#66339=ORIENTED_EDGE ( 'NONE', *, *, #22055, .T. ) ;
#66340=CARTESIAN_POINT ( 'NONE',  ( 26.65312500061451573, 0.000000000000000000, 5.243569643749999010 ) ) ;
#66341=CARTESIAN_POINT ( 'NONE',  ( 28.88437500061451502, 4.541064518000418104, 2.621784821874999949 ) ) ;
#66343=CARTESIAN_POINT ( 'NONE',  ( 14.51250000000000107, 2.886751345948129099, -4.999999999999998224 ) ) ;
#66344=CARTESIAN_POINT ( 'NONE',  ( 10.49062500061451431, -3.027376345333614438, 5.243569643749998122 ) ) ;
#66345=CARTESIAN_POINT ( 'NONE',  ( 5.962500000000002132, 2.886751345948129099, -4.999999999999997335 ) ) ;
#66346=CARTESIAN_POINT ( 'NONE',  ( 7.275000000000000355, 6.123233995736764310E-16, -4.999999999999998224 ) ) ;
#66347=CARTESIAN_POINT ( 'NONE',  ( 28.64062500061451644, -3.027376345333610441, -5.243569643749999898 ) ) ;
#66348=CARTESIAN_POINT ( 'NONE',  ( 17.02500000122903145, 2.886751345948126879, 4.999999999999999112 ) ) ;
#66351=CARTESIAN_POINT ( 'NONE',  ( 4.565625000614516260, 3.027376345333611329, 5.243569643749999010 ) ) ;
#66352=CARTESIAN_POINT ( 'NONE',  ( 21.38437500061451502, -4.541064518000419881, 2.621784821874995952 ) ) ;
#66353=CARTESIAN_POINT ( 'NONE',  ( 9.001249775931846008E-16, 15.92187500061451821, 34.90005215228797653 ) ) ;
#66354=EDGE_CURVE ( 'NONE', #65915, #27313, #53305, .T. ) ;
#66355=CARTESIAN_POINT ( 'NONE',  ( 21.30937500061451573, 0.000000000000000000, 5.243569643749999010 ) ) ;
#66356=CARTESIAN_POINT ( 'NONE',  ( 28.62187500061451573, -6.054752690667223547, -1.112240025338166033E-15 ) ) ;
#66357=CARTESIAN_POINT ( 'NONE',  ( 9.001249775931846008E-16, 19.52187500061451786, 34.90005215228797653 ) ) ;
#66358=CARTESIAN_POINT ( 'NONE',  ( 11.35312500061451679, 0.000000000000000000, 5.243569643749999010 ) ) ;
#66359=CARTESIAN_POINT ( 'NONE',  ( -1.071796769724488563, 15.25490381179670152, 34.00000000000000000 ) ) ;
#66360=( BOUNDED_CURVE ( )  B_SPLINE_CURVE ( 2, ( #29331, #63657, #40064, #7157, #8891, #29686, #46322 ),
 .UNSPECIFIED., .F., .F. ) 
 B_SPLINE_CURVE_WITH_KNOTS ( ( 3, 2, 2, 3 ),
 ( 0.5083333333333334147, 0.5111111111111110716, 0.5138888888888888395, 0.5166666666666666075 ),
 .UNSPECIFIED. ) 
 CURVE ( )  GEOMETRIC_REPRESENTATION_ITEM ( )  RATIONAL_B_SPLINE_CURVE ( ( 0.9999999999999946709, 0.8660254037844440367, 1.000000000000000000, 0.8660254037844387076, 1.000000000000000000, 0.8660254037844440367, 0.9999999999999946709 ) ) 
 REPRESENTATION_ITEM ( '' )  );
#66361=AXIS2_PLACEMENT_3D ( 'NONE', #67781, #61499, #5360 ) ;
#66362=CARTESIAN_POINT ( 'NONE',  ( 7.059375000614518392, -4.541064518000417216, -2.621784821875001281 ) ) ;
#66363=CARTESIAN_POINT ( 'NONE',  ( 1.071796769724489895, 15.81740381056766509, -34.00000000000000000 ) ) ;
#66364=CARTESIAN_POINT ( 'NONE',  ( 10.75312500061451715, 4.541064518000418104, -2.621784821874998173 ) ) ;
#66365=CARTESIAN_POINT ( 'NONE',  ( 14.78437500061451715, 6.421520780324663323E-16, -5.243569643749999010 ) ) ;
#66366=CARTESIAN_POINT ( 'NONE',  ( 22.61250000122903003, -4.330127018922190985, -2.500000000000001332 ) ) ;
#66367=CARTESIAN_POINT ( 'NONE',  ( 8.334375000614516082, -4.541064518000419881, 2.621784821874995952 ) ) ;
#66368=B_SPLINE_CURVE_WITH_KNOTS ( 'NONE', 3,
 ( #63559, #6695, #29940, #7055, #58004, #24028, #47299, #23669, #29583, #52121 ),
 .UNSPECIFIED., .F., .F.,
 ( 4, 3, 3, 4 ),
 ( 2.168404344971008868E-19, 5.625121263557876196E-05, 0.0001067941766033528262, 0.0001573439915068947906 ),
 .UNSPECIFIED. ) ;
#66369=CARTESIAN_POINT ( 'NONE',  ( 9.028125000614517504, 4.541064518000418104, 2.621784821874999949 ) ) ;
#66371=CARTESIAN_POINT ( 'NONE',  ( 21.27187500061451786, 3.027376345333611329, 5.243569643749999010 ) ) ;
#66372=CARTESIAN_POINT ( 'NONE',  ( -5.810221930991193690E-16, 13.58750000000000036, 26.00000000000000355 ) ) ;
#66373=CARTESIAN_POINT ( 'NONE',  ( -1.349117715399773321, 4.821506530989291939, 33.77511393033235976 ) ) ;
#66374=CARTESIAN_POINT ( 'NONE',  ( 29.25937500061451502, 4.541064518000418104, -2.621784821874998173 ) ) ;
#66375=CARTESIAN_POINT ( 'NONE',  ( -4.243569643749999898, 11.75937500061451857, -30.00000000000000000 ) ) ;
#66376=CARTESIAN_POINT ( 'NONE',  ( 14.21250000122903323, 4.330127018922192761, -2.499999999999997780 ) ) ;
#66377=CARTESIAN_POINT ( 'NONE',  ( -2.121784821874999949, 16.57812500061451644, -33.67503911421598417 ) ) ;
#66378=CARTESIAN_POINT ( 'NONE',  ( 18.63750000122903216, 6.123233995736764310E-16, -4.999999999999998224 ) ) ;
#66379=CARTESIAN_POINT ( 'NONE',  ( 11.12812500061451715, 6.421520780324663323E-16, -5.243569643749999010 ) ) ;
#66380=VERTEX_POINT ( 'NONE', #46385 ) ;
#66381=CARTESIAN_POINT ( 'NONE',  ( 13.91249999999999964, -5.773502691896255534, -1.060575238724906372E-15 ) ) ;
#66383=CARTESIAN_POINT ( 'NONE',  ( 23.91562500061451502, 3.027376345333611329, 5.243569643749999010 ) ) ;
#66384=CARTESIAN_POINT ( 'NONE',  ( 10.50937500061451679, 0.000000000000000000, 5.243569643749999010 ) ) ;
#66385=CARTESIAN_POINT ( 'NONE',  ( -1.071796769724491005, 14.17009619066136672, 26.00000000000000355 ) ) ;
#66386=CARTESIAN_POINT ( 'NONE',  ( 10.50000000122903465, -2.886751345948125991, -5.000000000000000000 ) ) ;
#66387=CARTESIAN_POINT ( 'NONE',  ( 17.96250000122903501, 0.000000000000000000, 4.999999999999998224 ) ) ;
#66388=CARTESIAN_POINT ( 'NONE',  ( 15.51562500061451644, -6.054752690667223547, -1.112240025338166033E-15 ) ) ;
#66389=CARTESIAN_POINT ( 'NONE',  ( 17.80312500061451786, -4.541064518000417216, -2.621784821875001281 ) ) ;
#66390=CARTESIAN_POINT ( 'NONE',  ( 24.82500000122902861, -5.773502691896255534, -1.060575238724906372E-15 ) ) ;
#66391=CARTESIAN_POINT ( 'NONE',  ( 27.37500000122903288, 2.886751345948126879, 4.999999999999999112 ) ) ;
#66392=CARTESIAN_POINT ( 'NONE',  ( 23.13749999999999929, 5.773502691896255534, 3.535250795749688894E-16 ) ) ;
#66394=CARTESIAN_POINT ( 'NONE',  ( 25.02187500061451431, -6.054752690667223547, -1.112240025338166033E-15 ) ) ;
#66395=CARTESIAN_POINT ( 'NONE',  ( 3.999999999999998668, 12.61250000000000249, -32.30940107675850470 ) ) ;
#66396=EDGE_CURVE ( 'NONE', #14534, #54755, #14054, .T. ) ;
#66397=CARTESIAN_POINT ( 'NONE',  ( 12.03750000122903430, 4.330127018922191873, 2.499999999999999556 ) ) ;
#66398=CARTESIAN_POINT ( 'NONE',  ( 4.537500000000000533, -2.886751345948125991, -5.000000000000000000 ) ) ;
#66400=CARTESIAN_POINT ( 'NONE',  ( 5.821875000614519458, 3.027376345333613106, -5.243569643749998122 ) ) ;
#66402=CARTESIAN_POINT ( 'NONE',  ( 26.01562500061451289, 3.027376345333613106, -5.243569643749998122 ) ) ;
#66405=CARTESIAN_POINT ( 'NONE',  ( 11.40937500061451892, 0.000000000000000000, 5.243569643749999010 ) ) ;
#66406=CARTESIAN_POINT ( 'NONE',  ( 4.259027106289364539, -2.619388203951992455, 4.518412407730628466 ) ) ;
#66407=CARTESIAN_POINT ( 'NONE',  ( 3.346875000614518036, -3.027376345333614438, 5.243569643749998122 ) ) ;
#66408=CARTESIAN_POINT ( 'NONE',  ( 7.959375000614516971, -4.541064518000417216, -2.621784821875001281 ) ) ;
#66409=CARTESIAN_POINT ( 'NONE',  ( 28.35937500061451289, 4.541064518000418104, -2.621784821874998173 ) ) ;
#66410=CARTESIAN_POINT ( 'NONE',  ( 2.121784821874999061, 13.35312500061459318, 26.32496088578401583 ) ) ;
#66411=CARTESIAN_POINT ( 'NONE',  ( 22.61250000000000071, 2.886751345948129099, -4.999999999999998224 ) ) ;
#66413=CARTESIAN_POINT ( 'NONE',  ( 29.73750000000000071, -2.886751345948125991, -5.000000000000000000 ) ) ;
#66414=CARTESIAN_POINT ( 'NONE',  ( 3.337499999999999911, 5.773502691896255534, 3.535250795749688894E-16 ) ) ;
#66416=CARTESIAN_POINT ( 'NONE',  ( 17.57812500061451644, 4.541064518000418104, 2.621784821874999949 ) ) ;
#66417=CARTESIAN_POINT ( 'NONE',  ( 11.76562500061451644, 3.027376345333611329, 5.243569643749999010 ) ) ;
#66419=CARTESIAN_POINT ( 'NONE',  ( 6.459375000614518747, 0.000000000000000000, 5.243569643749999010 ) ) ;
#66420=CARTESIAN_POINT ( 'NONE',  ( 19.20000000122903572, 5.773502691896255534, 3.535250795749688894E-16 ) ) ;
#66421=DIRECTION ( 'NONE',  ( 1.000000000000000000, 0.000000000000000000, 0.000000000000000000 ) ) ;
#66422=CARTESIAN_POINT ( 'NONE',  ( 6.121875000614517504, -6.054752690667223547, -1.112240025338166033E-15 ) ) ;
#66423=CARTESIAN_POINT ( 'NONE',  ( 15.19687500061451857, -3.027376345333610441, -5.243569643749999898 ) ) ;
#66424=CARTESIAN_POINT ( 'NONE',  ( 24.38437500061451502, 4.541064518000418104, 2.621784821874999949 ) ) ;
#66425=CARTESIAN_POINT ( 'NONE',  ( -2.000000000000000000, 14.52500000000000036, -33.46410161513775705 ) ) ;
#66426=ORIENTED_EDGE ( 'NONE', *, *, #3972, .T. ) ;
#66428=CARTESIAN_POINT ( 'NONE',  ( 17.85937500061451999, -4.541064518000417216, -2.621784821875001281 ) ) ;
#66429=CARTESIAN_POINT ( 'NONE',  ( 10.43437500061451750, 4.541064518000418104, 2.621784821874999949 ) ) ;
#66431=CARTESIAN_POINT ( 'NONE',  ( 21.07499999999999929, -4.330127018922194537, 2.499999999999995559 ) ) ;
#66433=CARTESIAN_POINT ( 'NONE',  ( 4.243569643749999898, 10.63437500061451857, -30.00000000000000000 ) ) ;
#66435=CARTESIAN_POINT ( 'NONE',  ( 13.19062500061451537, -3.027376345333614438, 5.243569643749998122 ) ) ;
#66436=CARTESIAN_POINT ( 'NONE',  ( 28.47187500061451715, 3.027376345333611329, 5.243569643749999010 ) ) ;
#66437=CARTESIAN_POINT ( 'NONE',  ( 6.750000001229033764, -2.886751345948130876, 4.999999999999996447 ) ) ;
#66438=CARTESIAN_POINT ( 'NONE',  ( 27.64687500061452141, -3.027376345333614438, 5.243569643749998122 ) ) ;
#66439=CARTESIAN_POINT ( 'NONE',  ( 10.35000000000000142, -4.330127018922190985, -2.500000000000001332 ) ) ;
#66441=CARTESIAN_POINT ( 'NONE',  ( -2.828200636599751609E-16, 15.50000000122903465, 25.38119784648299770 ) ) ;
#66442=CARTESIAN_POINT ( 'NONE',  ( 11.55000000122903181, 5.773502691896255534, 3.535250795749688894E-16 ) ) ;
#66443=CARTESIAN_POINT ( 'NONE',  ( 23.33437500061451786, 6.421520780324663323E-16, -5.243569643749999010 ) ) ;
#66444=CARTESIAN_POINT ( 'NONE',  ( 13.84687500061451537, -3.027376345333610441, -5.243569643749999898 ) ) ;
#66445=CARTESIAN_POINT ( 'NONE',  ( 1.071796769724484344, 16.64509619066136992, 34.00000000000000000 ) ) ;
#66446=VERTEX_POINT ( 'NONE', #62642 ) ;
#66447=CARTESIAN_POINT ( 'NONE',  ( 16.41562500061451857, -6.054752690667223547, -1.112240025338166033E-15 ) ) ;
#66448=CARTESIAN_POINT ( 'NONE',  ( 29.58750000122903501, 4.330127018922191873, 2.499999999999999556 ) ) ;
#66449=CARTESIAN_POINT ( 'NONE',  ( 14.10937500061451644, 0.000000000000000000, 5.243569643749999010 ) ) ;
#66450=CARTESIAN_POINT ( 'NONE',  ( 4.765820465973555464, 8.794739343793304798, -26.33488593128669919 ) ) ;
#66451=CARTESIAN_POINT ( 'NONE',  ( 19.64062500061451644, -3.027376345333610441, -5.243569643749999898 ) ) ;
#66452=CARTESIAN_POINT ( 'NONE',  ( 1.999999999999998668, 16.69999999999999929, -33.46410161513775705 ) ) ;
#66453=CARTESIAN_POINT ( 'NONE',  ( 29.22187500061451715, 3.027376345333613106, -5.243569643749998122 ) ) ;
#66454=CARTESIAN_POINT ( 'NONE',  ( -2.121784821874996840, 13.12812500061451715, 33.67503911421598417 ) ) ;
#66455=CARTESIAN_POINT ( 'NONE',  ( 17.44687500061451857, -3.027376345333610441, -5.243569643749999898 ) ) ;
#66456=CARTESIAN_POINT ( 'NONE',  ( 14.36250000122903359, 0.000000000000000000, 4.999999999999998224 ) ) ;
#66458=CARTESIAN_POINT ( 'NONE',  ( 4.243569643749999010, 18.32187500061451502, -32.45002607614398471 ) ) ;
#66459=CARTESIAN_POINT ( 'NONE',  ( 21.12187500061451573, 3.027376345333613106, -5.243569643749998122 ) ) ;
#66460=CARTESIAN_POINT ( 'NONE',  ( 23.21250000122903501, 4.330127018922192761, -2.499999999999997780 ) ) ;
#66461=CARTESIAN_POINT ( 'NONE',  ( 16.09687500061452070, -3.027376345333610441, -5.243569643749999898 ) ) ;
#66462=CARTESIAN_POINT ( 'NONE',  ( 12.25312500061451537, 0.000000000000000000, 5.243569643749999010 ) ) ;
#66463=CARTESIAN_POINT ( 'NONE',  ( -4.243569643749999898, 11.30937500061451928, 30.00000000000000000 ) ) ;
#66464=CARTESIAN_POINT ( 'NONE',  ( 17.42812500061451786, 6.421520780324663323E-16, -5.243569643749999010 ) ) ;
#66465=ORIENTED_EDGE ( 'NONE', *, *, #13122, .T. ) ;
#66467=CARTESIAN_POINT ( 'NONE',  ( 19.76250000000000639, -5.773502691896255534, -1.060575238724906372E-15 ) ) ;
#66469=CARTESIAN_POINT ( 'NONE',  ( 23.87812500061451715, 4.541064518000418104, 2.621784821874999949 ) ) ;
#66470=CARTESIAN_POINT ( 'NONE',  ( 6.290625000614517681, 6.054752690667223547, 3.707466751127219781E-16 ) ) ;
#66471=CARTESIAN_POINT ( 'NONE',  ( 17.32500000122903216, 2.886751345948129099, -4.999999999999998224 ) ) ;
#66472=CARTESIAN_POINT ( 'NONE',  ( 22.60312500061451857, 0.000000000000000000, 5.243569643749999010 ) ) ;
#66473=CARTESIAN_POINT ( 'NONE',  ( 23.88749999999999929, -2.886751345948125991, -5.000000000000000000 ) ) ;
#66474=CARTESIAN_POINT ( 'NONE',  ( 24.89062500061451644, -3.027376345333614438, 5.243569643749998122 ) ) ;
#66475=CARTESIAN_POINT ( 'NONE',  ( 5.615625000614517859, -6.054752690667223547, -1.112240025338166033E-15 ) ) ;
#66477=CARTESIAN_POINT ( 'NONE',  ( 24.25312500061451715, 4.541064518000418104, -2.621784821874998173 ) ) ;
#66481=CARTESIAN_POINT ( 'NONE',  ( -3.999999999999997335, 13.40000000122903323, -27.69059892324149175 ) ) ;
#66482=CARTESIAN_POINT ( 'NONE',  ( -1.071796769724491005, 10.12009619066136956, 26.00000000000000355 ) ) ;
#66483=CARTESIAN_POINT ( 'NONE',  ( 10.76250000000000107, -5.773502691896255534, -1.060575238724906372E-15 ) ) ;
#66484=CARTESIAN_POINT ( 'NONE',  ( 11.03437500061451715, -4.541064518000419881, 2.621784821874995952 ) ) ;
#66485=CARTESIAN_POINT ( 'NONE',  ( 6.637500001229035718, 4.330127018922191873, 2.499999999999999556 ) ) ;
#66486=CARTESIAN_POINT ( 'NONE',  ( 15.15937500061451715, -4.541064518000417216, -2.621784821875001281 ) ) ;
#66487=CARTESIAN_POINT ( 'NONE',  ( 5.109375000614518214, 0.000000000000000000, 5.243569643749999010 ) ) ;
#66489=CARTESIAN_POINT ( 'NONE',  ( 12.75937500061451857, 0.000000000000000000, 5.243569643749999010 ) ) ;
#66490=CARTESIAN_POINT ( 'NONE',  ( 30.00000000000000000, 0.000000000000000000, 0.000000000000000000 ) ) ;
#66491=CARTESIAN_POINT ( 'NONE',  ( 19.79062500061451502, 6.054752690667223547, 3.707466751127219781E-16 ) ) ;
#66493=CARTESIAN_POINT ( 'NONE',  ( 24.42187500061451999, 3.027376345333611329, 5.243569643749999010 ) ) ;
#66494=( BOUNDED_CURVE ( )  B_SPLINE_CURVE ( 2, ( #10707, #33595, #28071, #26982, #4453, #72767, #55415 ),
 .UNSPECIFIED., .F., .F. ) 
 B_SPLINE_CURVE_WITH_KNOTS ( ( 3, 2, 2, 3 ),
 ( 0.4916666666666666408, 0.4944444444444444642, 0.4972222222222222321, 0.5000000000000000000 ),
 .UNSPECIFIED. ) 
 CURVE ( )  GEOMETRIC_REPRESENTATION_ITEM ( )  RATIONAL_B_SPLINE_CURVE ( ( 1.000000000000000000, 0.8660254037844387076, 1.000000000000000000, 0.8660254037844387076, 1.000000000000000000, 0.8660254037844387076, 1.000000000000000000 ) ) 
 REPRESENTATION_ITEM ( '' )  );
#66495=CARTESIAN_POINT ( 'NONE',  ( 1.071796769724490117, 19.23259618943233917, 33.99999999999999289 ) ) ;
#66496=CARTESIAN_POINT ( 'NONE',  ( 29.62500000122903288, 2.886751345948126879, 4.999999999999999112 ) ) ;
#66499=CARTESIAN_POINT ( 'NONE',  ( 25.49062500061451786, -3.027376345333610441, -5.243569643749999898 ) ) ;
#66500=CARTESIAN_POINT ( 'NONE',  ( 17.39062500061451644, -3.027376345333610441, -5.243569643749999898 ) ) ;
#66502=CARTESIAN_POINT ( 'NONE',  ( 13.84687500061451537, -3.027376345333610441, -5.243569643749999898 ) ) ;
#66503=CARTESIAN_POINT ( 'NONE',  ( 26.25000000122903288, -2.886751345948126435, -5.000000000000000000 ) ) ;
#66504=CARTESIAN_POINT ( 'NONE',  ( 27.33750000122903145, 4.330127018922191873, 2.499999999999999556 ) ) ;
#66505=CARTESIAN_POINT ( 'NONE',  ( 4.284375000614518925, -4.541064518000419881, 2.621784821874995952 ) ) ;
#66506=CARTESIAN_POINT ( 'NONE',  ( 14.18437500061451750, -4.541064518000419881, 2.621784821874995952 ) ) ;
#66507=CARTESIAN_POINT ( 'NONE',  ( 16.08750000000000213, -2.886751345948197045, 4.999999999999880096 ) ) ;
#66508=FACE_OUTER_BOUND ( 'NONE', #58245, .T. ) ;
#66509=CARTESIAN_POINT ( 'NONE',  ( 4.575000001229033941, -5.773502691896255534, -1.060575238724906372E-15 ) ) ;
#66510=CARTESIAN_POINT ( 'NONE',  ( 24.04687500061451644, -3.027376345333614438, 5.243569643749998122 ) ) ;
#66511=CARTESIAN_POINT ( 'NONE',  ( 16.69687500061451502, 6.054752690667223547, 3.707466751127219781E-16 ) ) ;
#66513=CARTESIAN_POINT ( 'NONE',  ( 27.89999999999999858, -4.330127018922190985, -2.500000000000001332 ) ) ;
#66514=FACE_OUTER_BOUND ( 'NONE', #33188, .T. ) ;
#66515=CARTESIAN_POINT ( 'NONE',  ( 5.775000000000002132, -4.330127018922194537, 2.499999999999995559 ) ) ;
#66517=CARTESIAN_POINT ( 'NONE',  ( 20.42812500061451431, -4.541064518000419881, 2.621784821874995952 ) ) ;
#66518=CARTESIAN_POINT ( 'NONE',  ( 9.750000000000001776, 0.000000000000000000, 4.999999999999998224 ) ) ;
#66519=CARTESIAN_POINT ( 'NONE',  ( 4.453125000614517326, 4.541064518000418104, -2.621784821874998173 ) ) ;
#66520=CARTESIAN_POINT ( 'NONE',  ( 20.17499999999999716, -4.330127018922194537, 2.499999999999995559 ) ) ;
#66521=EDGE_CURVE ( 'NONE', #63984, #59354, #29394, .T. ) ;
#66523=CARTESIAN_POINT ( 'NONE',  ( 23.66250000122903430, 4.330127018922192761, -2.499999999999997780 ) ) ;
#66524=CARTESIAN_POINT ( 'NONE',  ( 3.750000000000000000, 4.330127018922192761, -2.499999999999997780 ) ) ;
#66525=ORIENTED_EDGE ( 'NONE', *, *, #29318, .T. ) ;
#66526=CARTESIAN_POINT ( 'NONE',  ( 16.52812500061451573, 6.421520780324663323E-16, -5.243569643749999010 ) ) ;
#66527=CARTESIAN_POINT ( 'NONE',  ( 25.41562500061451146, -6.054752690667223547, -1.112240025338166033E-15 ) ) ;
#66528=CARTESIAN_POINT ( 'NONE',  ( 23.18437500061451573, -4.541064518000419881, 2.621784821874995952 ) ) ;
#66529=CARTESIAN_POINT ( 'NONE',  ( 6.750000000000002665, -4.330127018922190985, -2.500000000000001332 ) ) ;
#66530=CARTESIAN_POINT ( 'NONE',  ( 10.60312500061451679, -4.541064518000417216, -2.621784821875001281 ) ) ;
#66531=CARTESIAN_POINT ( 'NONE',  ( 25.52812500061451573, 6.421520780324663323E-16, -5.243569643749999010 ) ) ;
#66532=CARTESIAN_POINT ( 'NONE',  ( 14.52187500061451608, 3.027376345333611329, 5.243569643749999010 ) ) ;
#66533=CARTESIAN_POINT ( 'NONE',  ( 20.29687500061451644, 6.054752690667223547, 3.707466751127219781E-16 ) ) ;
#66535=CARTESIAN_POINT ( 'NONE',  ( -4.243569643749997233, 19.39062500061451999, 32.45002607614398471 ) ) ;
#66536=CARTESIAN_POINT ( 'NONE',  ( 21.22500000122903074, -5.773502691896255534, -1.060575238724906372E-15 ) ) ;
#66538=CARTESIAN_POINT ( 'NONE',  ( 11.20312500061451644, 4.541064518000418104, -2.621784821874998173 ) ) ;
#66539=CARTESIAN_POINT ( 'NONE',  ( 8.934375000614517504, 6.421520780324663323E-16, -5.243569643749999010 ) ) ;
#66540=CARTESIAN_POINT ( 'NONE',  ( 7.659375000614518036, 4.541064518000418104, -2.621784821874998173 ) ) ;
#66542=VERTEX_POINT ( 'NONE', #53370 ) ;
#66543=CARTESIAN_POINT ( 'NONE',  ( 26.63437500061451857, 4.541064518000418104, 2.621784821874999949 ) ) ;
#66544=CARTESIAN_POINT ( 'NONE',  ( 19.00312500061451715, 0.000000000000000000, 5.243569643749999010 ) ) ;
#66545=CARTESIAN_POINT ( 'NONE',  ( 28.65000000122903145, 5.773502691896255534, 3.535250795749688894E-16 ) ) ;
#66546=CARTESIAN_POINT ( 'NONE',  ( 29.16562500061451502, 3.027376345333613106, -5.243569643749998122 ) ) ;
#66547=CARTESIAN_POINT ( 'NONE',  ( 24.19687500061451857, -3.027376345333610441, -5.243569643749999898 ) ) ;
#66548=CARTESIAN_POINT ( 'NONE',  ( 20.16562500061451146, 3.027376345333613106, -5.243569643749998122 ) ) ;
#66549=CARTESIAN_POINT ( 'NONE',  ( -1.999999999999997113, 12.42500000000000249, 33.46410161513775705 ) ) ;
#66550=CARTESIAN_POINT ( 'NONE',  ( 24.25312500061451715, 4.541064518000418104, -2.621784821874998173 ) ) ;
#66551=CARTESIAN_POINT ( 'NONE',  ( 4.350000001229033408, 5.773502691896255534, 3.535250795749688894E-16 ) ) ;
#66553=CARTESIAN_POINT ( 'NONE',  ( 30.00000000000000000, 0.000000000000000000, 0.000000000000000000 ) ) ;
#66554=CARTESIAN_POINT ( 'NONE',  ( -3.999999999999999112, 16.40000000000000213, -30.00000000000000000 ) ) ;
#66556=CARTESIAN_POINT ( 'NONE',  ( 5.484375000614518214, 4.541064518000418104, 2.621784821874999949 ) ) ;
#66558=CARTESIAN_POINT ( 'NONE',  ( 12.59062500061451573, 6.054752690667223547, 3.707466751127219781E-16 ) ) ;
#66559=CARTESIAN_POINT ( 'NONE',  ( 5.559375000614517504, 0.000000000000000000, 5.243569643749999010 ) ) ;
#66560=CARTESIAN_POINT ( 'NONE',  ( 25.68750000122903288, -4.330127018922194537, 2.499999999999995559 ) ) ;
#66561=( BOUNDED_CURVE ( )  B_SPLINE_CURVE ( 2, ( #21239, #71499, #3907, #33062, #32705, #55242, #14600, #54144, #66318 ),
 .UNSPECIFIED., .F., .F. ) 
 B_SPLINE_CURVE_WITH_KNOTS ( ( 3, 2, 2, 2, 3 ),
 ( 0.2717391304347826497, 0.2753623188405797118, 0.2826086956521738913, 0.2898550724637681264, 0.2934782608695652439 ),
 .UNSPECIFIED. ) 
 CURVE ( )  GEOMETRIC_REPRESENTATION_ITEM ( )  RATIONAL_B_SPLINE_CURVE ( ( 0.9330127018922194093, 0.9330127018922198534, 1.000000000000000000, 0.8660254037844387076, 1.000000000000000000, 0.8660254037844387076, 1.000000000000000000, 0.9330127018922188542, 0.9330127018922194093 ) ) 
 REPRESENTATION_ITEM ( '' )  );
#66562=CARTESIAN_POINT ( 'NONE',  ( 15.34687500061451892, 6.054752690667223547, 3.707466751127219781E-16 ) ) ;
#66563=CARTESIAN_POINT ( 'NONE',  ( 28.60312500061451502, -4.541064518000417216, -2.621784821875001281 ) ) ;
#66564=CARTESIAN_POINT ( 'NONE',  ( -3.999999999999997335, 11.03749999999999964, 32.30940107675850470 ) ) ;
#66565=CARTESIAN_POINT ( 'NONE',  ( 27.12187500061451573, 3.027376345333611329, 5.243569643749999010 ) ) ;
#66566=CARTESIAN_POINT ( 'NONE',  ( 3.665625000614517681, 3.027376345333611329, 5.243569643749999010 ) ) ;
#66567=CARTESIAN_POINT ( 'NONE',  ( 12.89062500061451821, -3.027376345333610441, -5.243569643749999898 ) ) ;
#66568=ORIENTED_EDGE ( 'NONE', *, *, #58543, .F. ) ;
#66569=CARTESIAN_POINT ( 'NONE',  ( 9.440625000614517148, 6.054752690667223547, 3.707466751127219781E-16 ) ) ;
#66571=CARTESIAN_POINT ( 'NONE',  ( 8.728125000614518569, -4.541064518000419881, 2.621784821874995952 ) ) ;
#66573=CARTESIAN_POINT ( 'NONE',  ( 8.962500000000002132, -5.773502691896255534, -1.060575238724906372E-15 ) ) ;
#66574=CARTESIAN_POINT ( 'NONE',  ( 3.937500001229034208, 4.330127018922191873, 2.499999999999999556 ) ) ;
#66575=CARTESIAN_POINT ( 'NONE',  ( 17.81250000000000355, 2.886751345948126879, 4.999999999999999112 ) ) ;
#66576=EDGE_CURVE ( 'NONE', #35463, #40816, #3721, .T. ) ;
#66578=CARTESIAN_POINT ( 'NONE',  ( 19.39687500061451786, 6.054752690667223547, 3.707466751127219781E-16 ) ) ;
#66579=CARTESIAN_POINT ( 'NONE',  ( 13.31250000122903288, 4.330127018922192761, -2.499999999999997780 ) ) ;
#66581=CARTESIAN_POINT ( 'NONE',  ( 4.243569643749999898, 15.94062500061451537, -27.54997392385601529 ) ) ;
#66583=CARTESIAN_POINT ( 'NONE',  ( 3.507483327083503521, -3.563363679198468859, 3.507483327083555924 ) ) ;
#66584=CARTESIAN_POINT ( 'NONE',  ( 28.79062500061451502, 6.054752690667223547, 3.707466751127219781E-16 ) ) ;
#66585=LINE ( 'NONE', #38883, #51702 ) ;
#66587=CARTESIAN_POINT ( 'NONE',  ( 12.75937500061451857, 0.000000000000000000, 5.243569643749999010 ) ) ;
#66588=CARTESIAN_POINT ( 'NONE',  ( 27.67499999999999716, 4.330127018922191873, 2.499999999999999556 ) ) ;
#66589=CARTESIAN_POINT ( 'NONE',  ( 9.440625000614517148, 6.054752690667223547, 3.707466751127219781E-16 ) ) ;
#66590=B_SPLINE_CURVE_WITH_KNOTS ( 'NONE', 1,
 ( #44681, #28046 ),
 .UNSPECIFIED., .F., .F.,
 ( 2, 2 ),
 ( 0.000000000000000000, 1.000000000000000000 ),
 .UNSPECIFIED. ) ;
#66592=( BOUNDED_CURVE ( )  B_SPLINE_CURVE ( 3, ( #24496, #67144, #47039, #41494 ),
 .UNSPECIFIED., .F., .F. ) 
 B_SPLINE_CURVE_WITH_KNOTS ( ( 4, 4 ),
 ( 2.449615925479262657, 2.486570309407579948 ),
 .UNSPECIFIED. ) 
 CURVE ( )  GEOMETRIC_REPRESENTATION_ITEM ( )  RATIONAL_B_SPLINE_CURVE ( ( 1.000000000000000000, 0.9998862010300719749, 0.9998862010300719749, 1.000000000000000000 ) ) 
 REPRESENTATION_ITEM ( '' )  );
#66593=CARTESIAN_POINT ( 'NONE',  ( 21.75937500061451502, 0.000000000000000000, 5.243569643749999010 ) ) ;
#66595=CARTESIAN_POINT ( 'NONE',  ( 7.190625000614518036, 6.054752690667223547, 3.707466751127219781E-16 ) ) ;
#66596=CARTESIAN_POINT ( 'NONE',  ( 12.27187500061451786, 3.027376345333611329, 5.243569643749999010 ) ) ;
#66598=CARTESIAN_POINT ( 'NONE',  ( 24.94687500061451502, -3.027376345333614438, 5.243569643749998122 ) ) ;
#66599=DIRECTION ( 'NONE',  ( 0.000000000000000000, 0.000000000000000000, 1.000000000000000000 ) ) ;
#66601=EDGE_CURVE ( 'NONE', #14829, #39133, #20100, .T. ) ;
#66602=CARTESIAN_POINT ( 'NONE',  ( 8.662499999999999645, 2.886751345948129099, -4.999999999999997335 ) ) ;
#66603=CARTESIAN_POINT ( 'NONE',  ( 4.425000000000001599, -4.330127018922194537, 2.499999999999995559 ) ) ;
#66604=CARTESIAN_POINT ( 'NONE',  ( 14.21250000122903323, 4.330127018922192761, -2.499999999999997780 ) ) ;
#66605=CARTESIAN_POINT ( 'NONE',  ( 17.32499999999999929, 4.330127018922191873, 2.499999999999999556 ) ) ;
#66606=ORIENTED_EDGE ( 'NONE', *, *, #53813, .T. ) ;
#66607=CARTESIAN_POINT ( 'NONE',  ( 12.26249999999999929, 2.886751345948129099, -4.999999999999998224 ) ) ;
#66608=CARTESIAN_POINT ( 'NONE',  ( 17.32499999999999929, 4.330127018922191873, 2.499999999999999556 ) ) ;
#66609=CARTESIAN_POINT ( 'NONE',  ( 13.80000000122903181, 5.773502691896255534, 3.535250795749688894E-16 ) ) ;
#66610=CARTESIAN_POINT ( 'NONE',  ( 12.10312500061451857, 4.541064518000418104, -2.621784821874998173 ) ) ;
#66612=CARTESIAN_POINT ( 'NONE',  ( 9.637499999999999289, 5.773502691896255534, 3.535250795749688894E-16 ) ) ;
#66613=CARTESIAN_POINT ( 'NONE',  ( 16.83750000122903145, 6.123233995736764310E-16, -4.999999999999998224 ) ) ;
#66614=CARTESIAN_POINT ( 'NONE',  ( -2.121784821874996840, 14.08437500061451786, -26.32496088578401583 ) ) ;
#66615=CARTESIAN_POINT ( 'NONE',  ( 3.365625000614516082, -6.054752690667223547, -1.112240025338166033E-15 ) ) ;
#66617=CARTESIAN_POINT ( 'NONE',  ( 8.812500000000000000, 2.886751345948126879, 4.999999999999999112 ) ) ;
#66620=CARTESIAN_POINT ( 'NONE',  ( 24.29062500061451502, 6.054752690667223547, 3.707466751127219781E-16 ) ) ;
#66621=CARTESIAN_POINT ( 'NONE',  ( 29.40000000122903501, -2.886751345948115777, -5.000000000000017764 ) ) ;
#66623=CARTESIAN_POINT ( 'NONE',  ( 21.08437500061451786, 6.421520780324663323E-16, -5.243569643749999010 ) ) ;
#66624=CARTESIAN_POINT ( 'NONE',  ( 18.59062500061451573, -3.027376345333614438, 5.243569643749998122 ) ) ;
#66625=CARTESIAN_POINT ( 'NONE',  ( -2.121784821874996840, 12.67812500061459424, -26.32496088578401583 ) ) ;
#66626=CARTESIAN_POINT ( 'NONE',  ( 7.490625000614516082, -3.027376345333610441, -5.243569643749999898 ) ) ;
#66627=CARTESIAN_POINT ( 'NONE',  ( 3.815625000614518036, -6.054752690667223547, -1.112240025338166033E-15 ) ) ;
#66629=CARTESIAN_POINT ( 'NONE',  ( 18.70312500061451644, -4.541064518000417216, -2.621784821875001281 ) ) ;
#66630=FACE_OUTER_BOUND ( 'NONE', #37602, .T. ) ;
#66632=CARTESIAN_POINT ( 'NONE',  ( 15.23437500061451644, 6.421520780324663323E-16, -5.243569643749999010 ) ) ;
#66633=CARTESIAN_POINT ( 'NONE',  ( 15.45937500061451608, 0.000000000000000000, 5.243569643749999010 ) ) ;
#66634=CARTESIAN_POINT ( 'NONE',  ( 21.94687500061451857, -3.027376345333610441, -5.243569643749999898 ) ) ;
#66635=VERTEX_POINT ( 'NONE', #42657 ) ;
#66636=CARTESIAN_POINT ( 'NONE',  ( 9.001249775931846008E-16, 12.77187500061451786, 34.90005215228797653 ) ) ;
#66637=CARTESIAN_POINT ( 'NONE',  ( 3.665625000614517681, 3.027376345333611329, 5.243569643749999010 ) ) ;
#66638=CARTESIAN_POINT ( 'NONE',  ( 26.20312500061451644, 0.000000000000000000, 5.243569643749999010 ) ) ;
#66639=AXIS2_PLACEMENT_3D ( 'NONE', #32150, #44345, #4454 ) ;
#66640=CARTESIAN_POINT ( 'NONE',  ( 25.60312500061451502, 4.541064518000418104, -2.621784821874998173 ) ) ;
#66642=CARTESIAN_POINT ( 'NONE',  ( -2.828200636599751609E-16, 18.98749999999999716, 25.38119784648299770 ) ) ;
#66643=CARTESIAN_POINT ( 'NONE',  ( 5.184375000614516615, -4.541064518000419881, 2.621784821874995952 ) ) ;
#66645=CARTESIAN_POINT ( 'NONE',  ( 11.40000000122903501, -2.886751345948125991, -5.000000000000000000 ) ) ;
#66646=CARTESIAN_POINT ( 'NONE',  ( 9.300000001229035362, 5.773502691896255534, 3.535250795749688894E-16 ) ) ;
#66647=CARTESIAN_POINT ( 'NONE',  ( 3.178125000614515638, 4.541064518000418104, 2.621784821874999949 ) ) ;
#66650=CARTESIAN_POINT ( 'NONE',  ( 12.30937500061451573, 0.000000000000000000, 5.243569643749999010 ) ) ;
#66651=CARTESIAN_POINT ( 'NONE',  ( 4.000000000000000000, 14.78750000000000142, -27.69059892324149885 ) ) ;
#66652=EDGE_LOOP ( 'NONE', ( #58210, #44419, #64768, #48525 ) ) ;
#66653=CARTESIAN_POINT ( 'NONE',  ( 18.62812500061451715, -4.541064518000419881, 2.621784821874995952 ) ) ;
#66654=CARTESIAN_POINT ( 'NONE',  ( 12.42187500061451821, -6.054752690667223547, -1.112240025338166033E-15 ) ) ;
#66655=CARTESIAN_POINT ( 'NONE',  ( 5.540625000614515905, -3.027376345333614438, 5.243569643749998122 ) ) ;
#66656=CARTESIAN_POINT ( 'NONE',  ( 22.50937500061451857, 4.541064518000418104, -2.621784821874998173 ) ) ;
#66657=CARTESIAN_POINT ( 'NONE',  ( 5.765625000614519102, 3.027376345333613106, -5.243569643749998122 ) ) ;
#66658=CARTESIAN_POINT ( 'NONE',  ( 0.000000000000000000, 20.00000000000000000, -30.00000000000000000 ) ) ;
#66659=CARTESIAN_POINT ( 'NONE',  ( 6.487500001229034474, 6.123233995736764310E-16, -4.999999999999998224 ) ) ;
#66660=CARTESIAN_POINT ( 'NONE',  ( 22.56562500061451715, 3.027376345333611329, 5.243569643749999010 ) ) ;
#66661=CARTESIAN_POINT ( 'NONE',  ( 2.000000000000001332, 18.91250000122903430, -26.53589838486224650 ) ) ;
#66662=CARTESIAN_POINT ( 'NONE',  ( 8.887500001229033941, 4.330127018922191873, 2.499999999999999556 ) ) ;
#66663=CARTESIAN_POINT ( 'NONE',  ( 18.21562500061451573, -6.054752690667223547, -1.112240025338166033E-15 ) ) ;
#66664=CARTESIAN_POINT ( 'NONE',  ( 16.22812500061451857, 4.541064518000418104, 2.621784821874999949 ) ) ;
#66666=CARTESIAN_POINT ( 'NONE',  ( 14.92500000000000071, 6.123233995736764310E-16, -4.999999999999998224 ) ) ;
#66667=CARTESIAN_POINT ( 'NONE',  ( 10.98750000122903536, 6.123233995736764310E-16, -4.999999999999998224 ) ) ;
#66668=CARTESIAN_POINT ( 'NONE',  ( 7.265625000614516438, 3.027376345333611329, 5.243569643749999010 ) ) ;
#66669=CARTESIAN_POINT ( 'NONE',  ( 10.90312500061451928, 0.000000000000000000, 5.243569643749999010 ) ) ;
#66670=ADVANCED_FACE ( 'NONE', ( #19002 ), #25289, .F. ) ;
#66671=CARTESIAN_POINT ( 'NONE',  ( 19.68750000122903288, 4.330127018922191873, 2.499999999999999556 ) ) ;
#66673=CARTESIAN_POINT ( 'NONE',  ( -4.243569643749999898, 14.45937500061451964, -30.00000000000000000 ) ) ;
#66674=CARTESIAN_POINT ( 'NONE',  ( 20.18437500061451573, 6.421520780324663323E-16, -5.243569643749999010 ) ) ;
#66675=DIRECTION ( 'NONE',  ( -1.000000000000000000, -0.000000000000000000, -0.000000000000000000 ) ) ;
#66676=CARTESIAN_POINT ( 'NONE',  ( 6.375000001229031987, -5.773502691896255534, -1.060575238724906372E-15 ) ) ;
#66678=CARTESIAN_POINT ( 'NONE',  ( 3.009375000614516793, -4.541064518000417216, -2.621784821875001281 ) ) ;
#66679=CARTESIAN_POINT ( 'NONE',  ( 20.59687500061451360, -3.027376345333610441, -5.243569643749999898 ) ) ;
#66681=CARTESIAN_POINT ( 'NONE',  ( 17.42812500061451786, 6.421520780324663323E-16, -5.243569643749999010 ) ) ;
#66683=CARTESIAN_POINT ( 'NONE',  ( -3.999999999999999112, 14.71250000122903501, 30.00000000000000000 ) ) ;
#66684=CARTESIAN_POINT ( 'NONE',  ( -2.000000000000000000, 15.42500000000000071, 26.53589838486224650 ) ) ;
#66685=CARTESIAN_POINT ( 'NONE',  ( 28.92187500061451644, 3.027376345333611329, 5.243569643749999010 ) ) ;
#66687=CARTESIAN_POINT ( 'NONE',  ( 14.65312500061451573, -4.541064518000417216, -2.621784821875001281 ) ) ;
#66688=CIRCLE ( 'NONE', #63134, 9.999999999999998224 ) ;
#66689=CARTESIAN_POINT ( 'NONE',  ( 12.94687500061451857, -3.027376345333610441, -5.243569643749999898 ) ) ;
#66690=ORIENTED_EDGE ( 'NONE', *, *, #67682, .F. ) ;
#66691=CARTESIAN_POINT ( 'NONE',  ( 22.34999999999999787, 0.000000000000000000, 4.999999999999998224 ) ) ;
#66692=CARTESIAN_POINT ( 'NONE',  ( 22.97812500061451857, 4.541064518000418104, 2.621784821874999949 ) ) ;
#66693=CARTESIAN_POINT ( 'NONE',  ( 2.000000000000001332, 11.15000000000000213, -26.53589838486224650 ) ) ;
#66694=ADVANCED_FACE ( 'NONE', ( #19743 ), #65181, .F. ) ;
#66695=CARTESIAN_POINT ( 'NONE',  ( 1.626862140677534273E-15, 18.42500000122903359, 34.00000000000000000 ) ) ;
#66696=CARTESIAN_POINT ( 'NONE',  ( 13.38750000000000107, -2.886751345948129988, 4.999999999999997335 ) ) ;
#66697=CARTESIAN_POINT ( 'NONE',  ( 24.52500000122903145, 2.886751345948129099, -4.999999999999998224 ) ) ;
#66698=CARTESIAN_POINT ( 'NONE',  ( 19.22812500061451502, 6.421520780324663323E-16, -5.243569643749999010 ) ) ;
#66701=CARTESIAN_POINT ( 'NONE',  ( 21.15000000000000213, -4.330127018922190985, -2.500000000000001332 ) ) ;
#66702=CARTESIAN_POINT ( 'NONE',  ( 20.40937500061451715, 0.000000000000000000, 5.243569643749999010 ) ) ;
#66703=CARTESIAN_POINT ( 'NONE',  ( 27.96562500061451928, 3.027376345333611329, 5.243569643749999010 ) ) ;
#66704=VERTEX_POINT ( 'NONE', #35648 ) ;
#66705=CARTESIAN_POINT ( 'NONE',  ( 1.071796769724493892, 18.06740381056766864, -34.00000000000000000 ) ) ;
#66706=CARTESIAN_POINT ( 'NONE',  ( 11.80312500061451608, 0.000000000000000000, 5.243569643749999010 ) ) ;
#66707=CARTESIAN_POINT ( 'NONE',  ( 17.47500000122903430, 2.886751345948193936, 4.999999999999883649 ) ) ;
#66709=CARTESIAN_POINT ( 'NONE',  ( 15.90000000000000036, 4.330127018922192761, -2.499999999999997780 ) ) ;
#66710=CARTESIAN_POINT ( 'NONE',  ( 24.75000000000000000, -4.330127018922190985, -2.500000000000001332 ) ) ;
#66711=LINE ( 'NONE', #32350, #58043 ) ;
#66712=CARTESIAN_POINT ( 'NONE',  ( 5.371875000614516615, 3.027376345333613106, -5.243569643749998122 ) ) ;
#66713=CARTESIAN_POINT ( 'NONE',  ( 27.79687500061451999, -3.027376345333610441, -5.243569643749999898 ) ) ;
#66714=ORIENTED_EDGE ( 'NONE', *, *, #2252, .F. ) ;
#66715=CARTESIAN_POINT ( 'NONE',  ( 25.22812500061451502, 4.541064518000418104, 2.621784821874999949 ) ) ;
#66716=CARTESIAN_POINT ( 'NONE',  ( 27.53437500061451360, 4.541064518000418104, 2.621784821874999949 ) ) ;
#66717=CARTESIAN_POINT ( 'NONE',  ( 30.00000000000000000, 0.000000000000000000, 4.999999999999998224 ) ) ;
#66719=CARTESIAN_POINT ( 'NONE',  ( 12.71250000000000036, 2.886751345948129099, -4.999999999999998224 ) ) ;
#66720=CARTESIAN_POINT ( 'NONE',  ( 11.84062500061451750, -3.027376345333614438, 5.243569643749998122 ) ) ;
#66721=CARTESIAN_POINT ( 'NONE',  ( -5.810221930991193690E-16, 14.60000000122903252, -34.00000000000000000 ) ) ;
#66722=CARTESIAN_POINT ( 'NONE',  ( 0.000000000000000000, 20.00000000000000000, 30.00000000000000000 ) ) ;
#66723=CARTESIAN_POINT ( 'NONE',  ( 27.62812500061451360, -4.541064518000419881, 2.621784821874995952 ) ) ;
#66724=CARTESIAN_POINT ( 'NONE',  ( 16.57500000122903216, 2.886751345948126879, 4.999999999999999112 ) ) ;
#66727=CARTESIAN_POINT ( 'NONE',  ( 4.340625000614515727, -3.027376345333610441, -5.243569643749999898 ) ) ;
#66728=CARTESIAN_POINT ( 'NONE',  ( 22.24687500061451217, -3.027376345333614438, 5.243569643749998122 ) ) ;
#66729=CARTESIAN_POINT ( 'NONE',  ( 9.001249775931846008E-16, 14.12187500061451750, 34.90005215228797653 ) ) ;
#66730=CARTESIAN_POINT ( 'NONE',  ( 21.53437500061451715, 6.421520780324663323E-16, -5.243569643749999010 ) ) ;
#66731=CARTESIAN_POINT ( 'NONE',  ( 28.69687500061451502, -3.027376345333610441, -5.243569643749999898 ) ) ;
#66732=CARTESIAN_POINT ( 'NONE',  ( 2.121784821875001281, 19.10937500061451644, 33.67503911421598417 ) ) ;
#66733=CARTESIAN_POINT ( 'NONE',  ( 9.965625000614517504, 3.027376345333611329, 5.243569643749999010 ) ) ;
#66734=CARTESIAN_POINT ( 'NONE',  ( 2.887500001229035274, 6.123233995736764310E-16, -4.999999999999998224 ) ) ;
#66735=CARTESIAN_POINT ( 'NONE',  ( 6.459375000614518747, 0.000000000000000000, 5.243569643749999010 ) ) ;
#66738=CARTESIAN_POINT ( 'NONE',  ( 7.865625000614516971, -6.054752690667223547, -1.112240025338166033E-15 ) ) ;
#66739=CARTESIAN_POINT ( 'NONE',  ( 12.19687500061451679, 6.054752690667223547, 3.707466751127219781E-16 ) ) ;
#66740=FACE_OUTER_BOUND ( 'NONE', #14283, .T. ) ;
#66741=CARTESIAN_POINT ( 'NONE',  ( 21.90000000122903145, 5.773502691896255534, 3.535250795749688894E-16 ) ) ;
#66742=CARTESIAN_POINT ( 'NONE',  ( 7.434375000614519280, -4.541064518000419881, 2.621784821874995952 ) ) ;
#66743=CARTESIAN_POINT ( 'NONE',  ( 10.52812500061451750, -4.541064518000419881, 2.621784821874995952 ) ) ;
#66744=CARTESIAN_POINT ( 'NONE',  ( 7.378125000614518036, -4.541064518000419881, 2.621784821874995952 ) ) ;
#66746=CARTESIAN_POINT ( 'NONE',  ( 20.29687500061451644, 6.054752690667223547, 3.707466751127219781E-16 ) ) ;
#66747=CARTESIAN_POINT ( 'NONE',  ( 18.14999999999999858, 4.330127018922192761, -2.499999999999997780 ) ) ;
#66748=CARTESIAN_POINT ( 'NONE',  ( 11.91562500061451857, -6.054752690667223547, -1.112240025338166033E-15 ) ) ;
#66749=CARTESIAN_POINT ( 'NONE',  ( 28.69687500061451502, -3.027376345333610441, -5.243569643749999898 ) ) ;
#66750=CARTESIAN_POINT ( 'NONE',  ( 4.243569643749999898, 11.94687500061451857, -27.54997392385601529 ) ) ;
#66751=CARTESIAN_POINT ( 'NONE',  ( 15.15000000122903323, 5.773502691896255534, 3.535250795749688894E-16 ) ) ;
#66753=CARTESIAN_POINT ( 'NONE',  ( 2.121784821874999061, 16.05312500061451786, -33.67503911421598417 ) ) ;
#66754=CARTESIAN_POINT ( 'NONE',  ( 15.37500000122903465, -5.773502691896255534, -1.060575238724906372E-15 ) ) ;
#66755=CARTESIAN_POINT ( 'NONE',  ( 9.928125000614517859, 4.541064518000418104, 2.621784821874999949 ) ) ;
#66757=CARTESIAN_POINT ( 'NONE',  ( 13.31250000000000178, 2.886751345948126879, 4.999999999999999112 ) ) ;
#66759=CARTESIAN_POINT ( 'NONE',  ( 23.20312500061451644, -4.541064518000417216, -2.621784821875001281 ) ) ;
#66760=CARTESIAN_POINT ( 'NONE',  ( 8.109375000614518214, 4.541064518000418104, -2.621784821874998173 ) ) ;
#66761=CARTESIAN_POINT ( 'NONE',  ( 10.76250000122903572, 0.000000000000000000, 4.999999999999998224 ) ) ;
#66762=CARTESIAN_POINT ( 'NONE',  ( 18.90000000122902790, -2.886751345948129988, 4.999999999999997335 ) ) ;
#66763=CARTESIAN_POINT ( 'NONE',  ( 16.37812500061451715, -4.541064518000419881, 2.621784821874995952 ) ) ;
#66764=CARTESIAN_POINT ( 'NONE',  ( 19.00312500061451715, 0.000000000000000000, 5.243569643749999010 ) ) ;
#66765=CARTESIAN_POINT ( 'NONE',  ( 25.38750000122903216, 6.123233995736764310E-16, -4.999999999999998224 ) ) ;
#66766=CARTESIAN_POINT ( 'NONE',  ( 29.06250000122903288, 4.330127018922192761, -2.499999999999997780 ) ) ;
#66767=CARTESIAN_POINT ( 'NONE',  ( 23.47499999999999787, 6.123233995736764310E-16, -4.999999999999998224 ) ) ;
#66769=CARTESIAN_POINT ( 'NONE',  ( 26.48437500061451644, 6.421520780324663323E-16, -5.243569643749999010 ) ) ;
#66771=CARTESIAN_POINT ( 'NONE',  ( 13.38750000122903394, 4.330127018922191873, 2.499999999999999556 ) ) ;
#66772=CARTESIAN_POINT ( 'NONE',  ( 28.95937500061451431, 0.000000000000000000, 5.243569643749999010 ) ) ;
#66775=CARTESIAN_POINT ( 'NONE',  ( 4.321875000614517681, -6.054752690667223547, -1.112240025338166033E-15 ) ) ;
#66776=CARTESIAN_POINT ( 'NONE',  ( 25.22812500061451502, 4.541064518000418104, 2.621784821874999949 ) ) ;
#66779=CARTESIAN_POINT ( 'NONE',  ( 10.13437500061451679, -4.541064518000419881, 2.621784821874995952 ) ) ;
#66781=CARTESIAN_POINT ( 'NONE',  ( 3.909375000614518481, -4.541064518000417216, -2.621784821875001281 ) ) ;
#66782=CARTESIAN_POINT ( 'NONE',  ( 5.521875000614517859, 3.027376345333611329, 5.243569643749999010 ) ) ;
#66783=CARTESIAN_POINT ( 'NONE',  ( 27.79687500061451999, -3.027376345333610441, -5.243569643749999898 ) ) ;
#66784=CARTESIAN_POINT ( 'NONE',  ( -2.121784821874996840, 10.42812500061459424, 33.67503911421598417 ) ) ;
#66785=CARTESIAN_POINT ( 'NONE',  ( 19.20000000000000284, 0.000000000000000000, 4.999999999999998224 ) ) ;
#66787=VERTEX_POINT ( 'NONE', #36742 ) ;
#66788=CARTESIAN_POINT ( 'NONE',  ( 28.64999999999999858, 0.000000000000000000, 4.999999999999998224 ) ) ;
#66789=( BOUNDED_CURVE ( )  B_SPLINE_CURVE ( 2, ( #3631, #27260, #31699, #66043, #54234, #53872, #71958, #21334, #8796 ),
 .UNSPECIFIED., .F., .F. ) 
 B_SPLINE_CURVE_WITH_KNOTS ( ( 3, 2, 2, 2, 3 ),
 ( 0.2065217391304347838, 0.2101449275362318736, 0.2173913043478260809, 0.2246376811594202882, 0.2282608695652174058 ),
 .UNSPECIFIED. ) 
 CURVE ( )  GEOMETRIC_REPRESENTATION_ITEM ( )  RATIONAL_B_SPLINE_CURVE ( ( 0.9330127018922194093, 0.9330127018922194093, 1.000000000000000000, 0.8660254037844387076, 1.000000000000000000, 0.8660254037844387076, 1.000000000000000000, 0.9330127018922190762, 0.9330127018922194093 ) ) 
 REPRESENTATION_ITEM ( '' )  );
#66790=CARTESIAN_POINT ( 'NONE',  ( 28.95937500061451431, 0.000000000000000000, 5.243569643749999010 ) ) ;
#66791=VERTEX_POINT ( 'NONE', #24923 ) ;
#66792=CARTESIAN_POINT ( 'NONE',  ( 16.79062500061451857, -3.027376345333614438, 5.243569643749998122 ) ) ;
#66793=CARTESIAN_POINT ( 'NONE',  ( 7.753125000614518036, 0.000000000000000000, 5.243569643749999010 ) ) ;
#66795=CARTESIAN_POINT ( 'NONE',  ( 6.121875000614517504, -6.054752690667223547, -1.112240025338166033E-15 ) ) ;
#66796=CARTESIAN_POINT ( 'NONE',  ( 17.92500000122903359, 2.886751345948126879, 4.999999999999999112 ) ) ;
#66798=CARTESIAN_POINT ( 'NONE',  ( 5.934375000614517504, 4.541064518000418104, 2.621784821874999949 ) ) ;
#66799=CARTESIAN_POINT ( 'NONE',  ( 11.33437500061451608, 4.541064518000418104, 2.621784821874999949 ) ) ;
#66800=CARTESIAN_POINT ( 'NONE',  ( 23.03437500061451715, 4.541064518000418104, 2.621784821874999949 ) ) ;
#66801=CARTESIAN_POINT ( 'NONE',  ( 1.592000809091587073E-14, 15.95000000122903394, -34.00000000000000000 ) ) ;
#66804=CARTESIAN_POINT ( 'NONE',  ( 16.92187500061451999, -6.054752690667223547, -1.112240025338166033E-15 ) ) ;
#66805=CARTESIAN_POINT ( 'NONE',  ( 9.159375000614515372, 0.000000000000000000, 5.243569643749999010 ) ) ;
#66807=CARTESIAN_POINT ( 'NONE',  ( 20.36249999999999716, 2.886751345948129099, -4.999999999999998224 ) ) ;
#66809=CARTESIAN_POINT ( 'NONE',  ( -1.071796769724488563, 9.854903811796701163, -26.00000000000000000 ) ) ;
#66811=CARTESIAN_POINT ( 'NONE',  ( 12.36562500061451608, -6.054752690667223547, -1.112240025338166033E-15 ) ) ;
#66812=CARTESIAN_POINT ( 'NONE',  ( 28.05937500061451573, 0.000000000000000000, 5.243569643749999010 ) ) ;
#66813=CARTESIAN_POINT ( 'NONE',  ( 28.50937500061451502, 0.000000000000000000, 5.243569643749999010 ) ) ;
#66814=CARTESIAN_POINT ( 'NONE',  ( 10.16249999999999964, 2.886751345948126879, 4.999999999999999112 ) ) ;
#66815=CARTESIAN_POINT ( 'NONE',  ( 2.000000000000001332, 15.31250000122903465, 33.46410161513774995 ) ) ;
#66816=CARTESIAN_POINT ( 'NONE',  ( 9.750000001229032875, 5.773502691896255534, 3.535250795749688894E-16 ) ) ;
#66817=CARTESIAN_POINT ( 'NONE',  ( 19.95937500061451786, 0.000000000000000000, 5.243569643749999010 ) ) ;
#66818=CARTESIAN_POINT ( 'NONE',  ( 14.59687500061452070, -3.027376345333614438, 5.243569643749998122 ) ) ;
#66819=CARTESIAN_POINT ( 'NONE',  ( 4.008114575609427632, 2.989161209909902972, -4.308132060747937864 ) ) ;
#66821=CARTESIAN_POINT ( 'NONE',  ( 16.97812500061451502, 6.421520780324663323E-16, -5.243569643749999010 ) ) ;
#66822=CARTESIAN_POINT ( 'NONE',  ( 27.60000000122903430, -2.886751345948125991, -5.000000000000000000 ) ) ;
#66823=CARTESIAN_POINT ( 'NONE',  ( 15.64687500061451608, -3.027376345333610441, -5.243569643749999898 ) ) ;
#66824=CARTESIAN_POINT ( 'NONE',  ( 3.290625000614516793, -3.027376345333614438, 5.243569643749998122 ) ) ;
#66825=CARTESIAN_POINT ( 'NONE',  ( 17.01562500061451644, 3.027376345333613106, -5.243569643749998122 ) ) ;
#66827=ADVANCED_FACE ( 'NONE', ( #36012 ), #31202, .F. ) ;
#66828=CARTESIAN_POINT ( 'NONE',  ( 26.55937500061451573, 4.541064518000418104, -2.621784821874998173 ) ) ;
#66829=CARTESIAN_POINT ( 'NONE',  ( 9.001249775931846008E-16, 13.16562500061451857, 34.90005215228797653 ) ) ;
#66830=CARTESIAN_POINT ( 'NONE',  ( 14.85937500061451644, 4.541064518000418104, -2.621784821874998173 ) ) ;
#66831=CARTESIAN_POINT ( 'NONE',  ( 15.07500000122903394, 2.886751345948129099, -4.999999999999998224 ) ) ;
#66833=EDGE_CURVE ( 'NONE', #72537, #27078, #14051, .T. ) ;
#66834=CARTESIAN_POINT ( 'NONE',  ( -2.121784821874999949, 18.43437500061451928, -33.67503911421598417 ) ) ;
#66835=CARTESIAN_POINT ( 'NONE',  ( 21.49687500061451573, -3.027376345333610441, -5.243569643749999898 ) ) ;
#66836=CARTESIAN_POINT ( 'NONE',  ( 22.42500000122903359, 2.886751345948126879, 4.999999999999999112 ) ) ;
#66837=CARTESIAN_POINT ( 'NONE',  ( 16.47187500061452070, -6.054752690667223547, -1.112240025338166033E-15 ) ) ;
#66838=CARTESIAN_POINT ( 'NONE',  ( -4.243569643749999898, 11.72187500061451892, 27.54997392385601529 ) ) ;
#66839=AXIS2_PLACEMENT_3D ( 'NONE', #49964, #9702, #72488 ) ;
#66840=CARTESIAN_POINT ( 'NONE',  ( 17.20312500061451644, 0.000000000000000000, 5.243569643749999010 ) ) ;
#66841=VERTEX_POINT ( 'NONE', #64451 ) ;
#66843=CARTESIAN_POINT ( 'NONE',  ( 21.18749999999999645, -2.886751345948125991, -5.000000000000000000 ) ) ;
#66844=LINE ( 'NONE', #38391, #12588 ) ;
#66845=CARTESIAN_POINT ( 'NONE',  ( 24.89062500061451644, -3.027376345333614438, 5.243569643749998122 ) ) ;
#66846=CARTESIAN_POINT ( 'NONE',  ( 5.165625000614518569, -6.054752690667223547, -1.112240025338166033E-15 ) ) ;
#66847=CARTESIAN_POINT ( 'NONE',  ( 16.72500000122903430, -5.773502691896255534, -1.060575238724906372E-15 ) ) ;
#66848=CARTESIAN_POINT ( 'NONE',  ( 22.04062500061451502, 6.054752690667223547, 3.707466751127219781E-16 ) ) ;
#66849=CARTESIAN_POINT ( 'NONE',  ( 21.15000000000000213, -4.330127018922190985, -2.500000000000001332 ) ) ;
#66850=CARTESIAN_POINT ( 'NONE',  ( 25.94062500061451715, -3.027376345333610441, -5.243569643749999898 ) ) ;
#66851=CARTESIAN_POINT ( 'NONE',  ( 6.703125000614516438, 4.541064518000418104, -2.621784821874998173 ) ) ;
#66852=EDGE_LOOP ( 'NONE', ( #18539, #4600, #17863, #65463 ) ) ;
#66853=CARTESIAN_POINT ( 'NONE',  ( 3.390184931900214860, 3.675138926287994767, 3.390184931900133147 ) ) ;
#66856=CARTESIAN_POINT ( 'NONE',  ( 1.071796769724491893, 18.78259618943233278, 33.99999999999999289 ) ) ;
#66857=CARTESIAN_POINT ( 'NONE',  ( 4.000000000000000000, 12.20000000122903394, -27.69059892324149530 ) ) ;
#66858=CARTESIAN_POINT ( 'NONE',  ( -2.121784821874996840, 18.13437500061451502, -26.32496088578401583 ) ) ;
#66860=CARTESIAN_POINT ( 'NONE',  ( 8.437500000000000000, -2.886751345948129988, 4.999999999999997335 ) ) ;
#66861=CARTESIAN_POINT ( 'NONE',  ( 8.296875000614516438, -3.027376345333614438, 5.243569643749998122 ) ) ;
#66862=CARTESIAN_POINT ( 'NONE',  ( 6.600000001229032520, 5.773502691896255534, 3.535250795749688894E-16 ) ) ;
#66863=CARTESIAN_POINT ( 'NONE',  ( 12.00937500061451857, -4.541064518000417216, -2.621784821875001281 ) ) ;
#66864=CARTESIAN_POINT ( 'NONE',  ( 3.421875000614516882, -6.054752690667223547, -1.112240025338166033E-15 ) ) ;
#66865=CARTESIAN_POINT ( 'NONE',  ( 30.00000000000000000, 0.000000000000000000, 4.999999999999998224 ) ) ;
#66867=CARTESIAN_POINT ( 'NONE',  ( -0.6945831915928805111, 10.00052343484236950, 26.06076730949330411 ) ) ;
#66868=CARTESIAN_POINT ( 'NONE',  ( 10.24687500061451750, -3.027376345333610441, -5.243569643749999898 ) ) ;
#66869=DIRECTION ( 'NONE',  ( -0.000000000000000000, -1.000000000000000000, -0.000000000000000000 ) ) ;
#66870=CARTESIAN_POINT ( 'NONE',  ( 19.86562500061451786, 3.027376345333611329, 5.243569643749999010 ) ) ;
#66871=CARTESIAN_POINT ( 'NONE',  ( -3.137519842735245283E-14, 12.57500000122903572, -26.00000000000000711 ) ) ;
#66872=CARTESIAN_POINT ( 'NONE',  ( -4.243569643749999898, 19.80312500061451786, 30.00000000000000000 ) ) ;
#66873=CARTESIAN_POINT ( 'NONE',  ( 24.38437500061451502, 4.541064518000418104, 2.621784821874999949 ) ) ;
#66875=CARTESIAN_POINT ( 'NONE',  ( 28.57500000122903572, 2.886751345948129099, -4.999999999999998224 ) ) ;
#66877=CARTESIAN_POINT ( 'NONE',  ( 25.75312500061451715, 0.000000000000000000, 5.243569643749999010 ) ) ;
#66878=CARTESIAN_POINT ( 'NONE',  ( 14.99062500061451786, -3.027376345333614438, 5.243569643749998122 ) ) ;
#66880=CARTESIAN_POINT ( 'NONE',  ( 13.54687500061451999, 6.054752690667223547, 3.707466751127219781E-16 ) ) ;
#66882=VECTOR ( 'NONE', #60848, 1000.000000000000000 ) ;
#66883=CARTESIAN_POINT ( 'NONE',  ( 24.26250000122903216, 0.000000000000000000, 4.999999999999998224 ) ) ;
#66884=CARTESIAN_POINT ( 'NONE',  ( 4.471875000614518925, 3.027376345333613106, -5.243569643749998122 ) ) ;
#66885=CARTESIAN_POINT ( 'NONE',  ( 13.77187500061451786, -6.054752690667223547, -1.112240025338166033E-15 ) ) ;
#66886=CARTESIAN_POINT ( 'NONE',  ( 4.859524668404109349, -1.177064389673172728, -5.109794524303713281 ) ) ;
#66888=CARTESIAN_POINT ( 'NONE',  ( 16.68750000122903288, -4.330127018922194537, 2.499999999999995559 ) ) ;
#66889=CARTESIAN_POINT ( 'NONE',  ( 23.97187500061451360, 3.027376345333611329, 5.243569643749999010 ) ) ;
#66890=CARTESIAN_POINT ( 'NONE',  ( 15.94687500061451502, -3.027376345333614438, 5.243569643749998122 ) ) ;
#66892=CARTESIAN_POINT ( 'NONE',  ( 28.68749999999999645, -2.886751345948129988, 4.999999999999997335 ) ) ;
#66893=CARTESIAN_POINT ( 'NONE',  ( 2.662500001229036073, 0.000000000000000000, 4.999999999999998224 ) ) ;
#66894=CARTESIAN_POINT ( 'NONE',  ( 4.575000000000002842, 6.123233995736764310E-16, -4.999999999999998224 ) ) ;
#66896=CARTESIAN_POINT ( 'NONE',  ( 19.67812500061451786, 6.421520780324663323E-16, -5.243569643749999010 ) ) ;
#66897=CARTESIAN_POINT ( 'NONE',  ( 9.899999999999998579, -4.330127018922190985, -2.500000000000001332 ) ) ;
#66898=CARTESIAN_POINT ( 'NONE',  ( 4.340625000614515727, -3.027376345333610441, -5.243569643749999898 ) ) ;
#66899=CARTESIAN_POINT ( 'NONE',  ( 17.13749999999999929, -2.886751345948125991, -5.000000000000000000 ) ) ;
#66901=CARTESIAN_POINT ( 'NONE',  ( 20.96250000122903145, 4.330127018922192761, -2.499999999999997780 ) ) ;
#66902=CARTESIAN_POINT ( 'NONE',  ( 28.31250000122903288, 0.000000000000000000, 4.999999999999998224 ) ) ;
#66903=CARTESIAN_POINT ( 'NONE',  ( 27.87187500061451573, 3.027376345333613106, -5.243569643749998122 ) ) ;
#66904=VERTEX_POINT ( 'NONE', #3874 ) ;
#66905=CARTESIAN_POINT ( 'NONE',  ( 16.15312500061451573, 4.541064518000418104, -2.621784821874998173 ) ) ;
#66906=CARTESIAN_POINT ( 'NONE',  ( 25.11562500061451431, 3.027376345333613106, -5.243569643749998122 ) ) ;
#66907=CARTESIAN_POINT ( 'NONE',  ( 22.47187500061451715, 3.027376345333613106, -5.243569643749998122 ) ) ;
#66908=CARTESIAN_POINT ( 'NONE',  ( 6.975000000000002309, 4.330127018922191873, 2.499999999999999556 ) ) ;
#66909=CARTESIAN_POINT ( 'NONE',  ( 9.328125000614518214, 6.421520780324663323E-16, -5.243569643749999010 ) ) ;
#66910=CARTESIAN_POINT ( 'NONE',  ( 23.09062500061451573, -3.027376345333614438, 5.243569643749998122 ) ) ;
#66911=CARTESIAN_POINT ( 'NONE',  ( 15.79687500061451821, 6.054752690667223547, 3.707466751127219781E-16 ) ) ;
#66912=CARTESIAN_POINT ( 'NONE',  ( 18.72187500061451360, -6.054752690667223547, -1.112240025338166033E-15 ) ) ;
#66913=CARTESIAN_POINT ( 'NONE',  ( 4.432080220173729046, 2.314473833018743321, -4.705141300289269246 ) ) ;
#66914=CARTESIAN_POINT ( 'NONE',  ( -2.121784821874996840, 10.93437500061451928, 33.67503911421598417 ) ) ;
#66915=CARTESIAN_POINT ( 'NONE',  ( 21.33750000122903145, 6.123233995736764310E-16, -4.999999999999998224 ) ) ;
#66917=CARTESIAN_POINT ( 'NONE',  ( 12.29062500061451857, -3.027376345333614438, 5.243569643749998122 ) ) ;
#66918=CARTESIAN_POINT ( 'NONE',  ( 8.109375000614518214, 4.541064518000418104, -2.621784821874998173 ) ) ;
#66919=CARTESIAN_POINT ( 'NONE',  ( 6.684375000614518392, 6.421520780324663323E-16, -5.243569643749999010 ) ) ;
#66921=EDGE_CURVE ( 'NONE', #62090, #16892, #26373, .T. ) ;
#66922=CARTESIAN_POINT ( 'NONE',  ( 28.24687500061451573, -3.027376345333610441, -5.243569643749999898 ) ) ;
#66923=CARTESIAN_POINT ( 'NONE',  ( 19.04062500061451146, -3.027376345333614438, 5.243569643749998122 ) ) ;
#66924=CARTESIAN_POINT ( 'NONE',  ( 3.140625000614516882, 6.054752690667223547, 3.707466751127219781E-16 ) ) ;
#66925=CARTESIAN_POINT ( 'NONE',  ( 28.37812500061451715, 4.541064518000418104, 2.621784821874999949 ) ) ;
#66926=CARTESIAN_POINT ( 'NONE',  ( 23.89687500061451786, 6.054752690667223547, 3.707466751127219781E-16 ) ) ;
#66927=CARTESIAN_POINT ( 'NONE',  ( 19.86562500061451786, 3.027376345333611329, 5.243569643749999010 ) ) ;
#66928=CARTESIAN_POINT ( 'NONE',  ( -4.243569643749999898, 18.95937500061451431, 30.00000000000000000 ) ) ;
#66929=CARTESIAN_POINT ( 'NONE',  ( 24.85312500061451502, 0.000000000000000000, 5.243569643749999010 ) ) ;
#66930=CARTESIAN_POINT ( 'NONE',  ( 4.462500001229035007, 0.000000000000000000, 4.999999999999998224 ) ) ;
#66932=CARTESIAN_POINT ( 'NONE',  ( 27.59999999999999787, 4.330127018922192761, -2.499999999999997780 ) ) ;
#66933=CARTESIAN_POINT ( 'NONE',  ( -2.828200636599751609E-16, 15.38750000000000284, -34.61880215351700230 ) ) ;
#66935=CARTESIAN_POINT ( 'NONE',  ( 5.371875000614516615, 3.027376345333613106, -5.243569643749998122 ) ) ;
#66936=CARTESIAN_POINT ( 'NONE',  ( 13.52812500061451750, 4.541064518000418104, 2.621784821874999949 ) ) ;
#66937=CARTESIAN_POINT ( 'NONE',  ( 6.796875000614516438, 6.054752690667223547, 3.707466751127219781E-16 ) ) ;
#66938=CARTESIAN_POINT ( 'NONE',  ( 25.27500000122903145, -5.773502691896255534, -1.060575238724906372E-15 ) ) ;
#66940=CARTESIAN_POINT ( 'NONE',  ( 15.38437500061451679, 4.541064518000418104, 2.621784821874999949 ) ) ;
#66941=CARTESIAN_POINT ( 'NONE',  ( 29.20312500061451644, 4.541064518000418104, -2.621784821874998173 ) ) ;
#66942=CARTESIAN_POINT ( 'NONE',  ( 29.92500000000000071, 4.330127018922191873, 2.499999999999999556 ) ) ;
#66943=CARTESIAN_POINT ( 'NONE',  ( 27.04687500061451644, 6.054752690667223547, 3.707466751127219781E-16 ) ) ;
#66944=CARTESIAN_POINT ( 'NONE',  ( 3.965625000614515727, 3.027376345333613106, -5.243569643749998122 ) ) ;
#66945=CARTESIAN_POINT ( 'NONE',  ( 13.00312500061451537, 4.541064518000418104, -2.621784821874998173 ) ) ;
#66946=ORIENTED_EDGE ( 'NONE', *, *, #45929, .F. ) ;
#66947=CARTESIAN_POINT ( 'NONE',  ( 10.04062500061451502, -3.027376345333614438, 5.243569643749998122 ) ) ;
#66948=CARTESIAN_POINT ( 'NONE',  ( 7.378125000614518036, -4.541064518000419881, 2.621784821874995952 ) ) ;
#66950=CARTESIAN_POINT ( 'NONE',  ( 8.474999999999999645, -4.330127018922194537, 2.499999999999995559 ) ) ;
#66951=CARTESIAN_POINT ( 'NONE',  ( 2.887500001229035274, 6.123233995736764310E-16, -4.999999999999998224 ) ) ;
#66952=CARTESIAN_POINT ( 'NONE',  ( 18.78749999999999432, -2.886751345948129988, 4.999999999999997335 ) ) ;
#66955=CARTESIAN_POINT ( 'NONE',  ( 18.04687500061451999, 6.054752690667223547, 3.707466751127219781E-16 ) ) ;
#66956=CARTESIAN_POINT ( 'NONE',  ( 13.98750000122903359, -4.330127018922194537, 2.499999999999995559 ) ) ;
#66958=CARTESIAN_POINT ( 'NONE',  ( 9.001249775931846008E-16, 17.21562500061451928, -25.09994784771203058 ) ) ;
#66962=CARTESIAN_POINT ( 'NONE',  ( 27.44062500061451715, 6.054752690667223547, 3.707466751127219781E-16 ) ) ;
#66963=LINE ( 'NONE', #27798, #10425 ) ;
#66964=CARTESIAN_POINT ( 'NONE',  ( 24.33749999999999858, -2.886751345948092684, -5.000000000000057732 ) ) ;
#66965=CARTESIAN_POINT ( 'NONE',  ( 25.68750000000000000, -2.886751345948125991, -5.000000000000000000 ) ) ;
#66966=CARTESIAN_POINT ( 'NONE',  ( 8.690625000614515372, -3.027376345333614438, 5.243569643749998122 ) ) ;
#66968=CARTESIAN_POINT ( 'NONE',  ( 20.78437500061451715, 4.541064518000418104, 2.621784821874999949 ) ) ;
#66970=CARTESIAN_POINT ( 'NONE',  ( 7.415625000614516793, -6.054752690667223547, -1.112240025338166033E-15 ) ) ;
#66971=CARTESIAN_POINT ( 'NONE',  ( 10.62187500061451928, -6.054752690667223547, -1.112240025338166033E-15 ) ) ;
#66972=EDGE_LOOP ( 'NONE', ( #68556, #58892, #5366, #64778 ) ) ;
#66973=CARTESIAN_POINT ( 'NONE',  ( 20.82187500061451857, 3.027376345333611329, 5.243569643749999010 ) ) ;
#66974=CARTESIAN_POINT ( 'NONE',  ( 28.94999999999999929, 4.330127018922192761, -2.499999999999997780 ) ) ;
#66976=CARTESIAN_POINT ( 'NONE',  ( 4.012500000000001954, -5.773502691896255534, -1.060575238724906372E-15 ) ) ;
#66978=CARTESIAN_POINT ( 'NONE',  ( 14.47500000122903430, -5.773502691896255534, -1.060575238724906372E-15 ) ) ;
#66979=DIRECTION ( 'NONE',  ( -1.000000000000000000, -0.000000000000000000, -0.000000000000000000 ) ) ;
#66980=CARTESIAN_POINT ( 'NONE',  ( 3.781380313051493580, -3.271273037562549835, 4.098030693279675951 ) ) ;
#66981=VERTEX_POINT ( 'NONE', #16035 ) ;
#66982=CARTESIAN_POINT ( 'NONE',  ( 13.68750000000000178, 5.773502691896255534, 3.535250795749688894E-16 ) ) ;
#66983=CARTESIAN_POINT ( 'NONE',  ( 15.63749999999999751, -2.886751345948129988, 4.999999999999997335 ) ) ;
#66984=CARTESIAN_POINT ( 'NONE',  ( 13.91250000122903252, 0.000000000000000000, 4.999999999999998224 ) ) ;
#66985=CARTESIAN_POINT ( 'NONE',  ( 10.67812500061451608, 6.421520780324663323E-16, -5.243569643749999010 ) ) ;
#66986=CIRCLE ( 'NONE', #12688, 10.00000000000000000 ) ;
#66988=CARTESIAN_POINT ( 'NONE',  ( 9.787499999999999645, -2.886751345948129988, 4.999999999999997335 ) ) ;
#66989=CARTESIAN_POINT ( 'NONE',  ( -3.999999999999997335, 15.65000000122903501, 32.30940107675850470 ) ) ;
#66990=CARTESIAN_POINT ( 'NONE',  ( -4.243569643749997233, 14.94687500061451679, -27.54997392385601174 ) ) ;
#66991=CARTESIAN_POINT ( 'NONE',  ( 28.42500000122904069, -5.773502691896255534, -1.060575238724906372E-15 ) ) ;
#66993=CARTESIAN_POINT ( 'NONE',  ( 10.72500000000000142, -4.330127018922194537, 2.499999999999995559 ) ) ;
#66994=DIRECTION ( 'NONE',  ( 0.000000000000000000, 0.000000000000000000, 1.000000000000000000 ) ) ;
#66996=CARTESIAN_POINT ( 'NONE',  ( 25.30312500061451431, 0.000000000000000000, 5.243569643749999010 ) ) ;
#66997=CARTESIAN_POINT ( 'NONE',  ( 4.238135780288177834, -2.653016584470423656, 4.522920254035737386 ) ) ;
#66998=CARTESIAN_POINT ( 'NONE',  ( 30.00000000000000000, 0.000000000000000000, 0.000000000000000000 ) ) ;
#66999=CARTESIAN_POINT ( 'NONE',  ( 22.20937500061451431, 0.000000000000000000, 5.243569643749999010 ) ) ;
#67000=CARTESIAN_POINT ( 'NONE',  ( 17.80312500061451786, -4.541064518000417216, -2.621784821875001281 ) ) ;
#67001=CARTESIAN_POINT ( 'NONE',  ( -2.121784821874996840, 10.87812500061459353, -26.32496088578401583 ) ) ;
#67002=CARTESIAN_POINT ( 'NONE',  ( 5.428125000614517859, 4.541064518000418104, 2.621784821874999949 ) ) ;
#67003=( BOUNDED_CURVE ( )  B_SPLINE_CURVE ( 2, ( #4996, #26801, #48970, #43055, #72228, #15695, #9440 ),
 .UNSPECIFIED., .F., .F. ) 
 B_SPLINE_CURVE_WITH_KNOTS ( ( 3, 2, 2, 3 ),
 ( 0.2666666666666666075, 0.2694444444444444309, 0.2722222222222221988, 0.2750000000000000777 ),
 .UNSPECIFIED. ) 
 CURVE ( )  GEOMETRIC_REPRESENTATION_ITEM ( )  RATIONAL_B_SPLINE_CURVE ( ( 1.000000000000002665, 0.8660254037844360431, 1.000000000000000000, 0.8660254037844387076, 1.000000000000000000, 0.8660254037844360431, 1.000000000000002665 ) ) 
 REPRESENTATION_ITEM ( '' )  );
#67004=CARTESIAN_POINT ( 'NONE',  ( 29.55000000122903003, 5.773502691896255534, 3.535250795749688894E-16 ) ) ;
#67006=CARTESIAN_POINT ( 'NONE',  ( 19.56562500061451715, -6.054752690667223547, -1.112240025338166033E-15 ) ) ;
#67009=CARTESIAN_POINT ( 'NONE',  ( 15.45937500061451608, 0.000000000000000000, 5.243569643749999010 ) ) ;
#67010=CARTESIAN_POINT ( 'NONE',  ( 15.34687500061451537, 6.054752690667223547, 3.707466751127219781E-16 ) ) ;
#67011=CARTESIAN_POINT ( 'NONE',  ( 22.88437500061451857, 6.421520780324663323E-16, -5.243569643749999010 ) ) ;
#67012=ORIENTED_EDGE ( 'NONE', *, *, #20226, .F. ) ;
#67013=CARTESIAN_POINT ( 'NONE',  ( -2.121784821874996840, 11.83437500061451786, 33.67503911421598417 ) ) ;
#67014=CARTESIAN_POINT ( 'NONE',  ( 3.740625000614516527, -3.027376345333614438, 5.243569643749998122 ) ) ;
#67015=CARTESIAN_POINT ( 'NONE',  ( 27.02812500061451573, 4.541064518000418104, 2.621784821874999949 ) ) ;
#67017=CARTESIAN_POINT ( 'NONE',  ( 26.42812500061451431, 6.421520780324663323E-16, -5.243569643749999010 ) ) ;
#67019=CARTESIAN_POINT ( 'NONE',  ( 3.999999999999998668, 17.11250000000000071, 27.69059892324149175 ) ) ;
#67020=CARTESIAN_POINT ( 'NONE',  ( 4.134375000614517681, 4.541064518000418104, 2.621784821874999949 ) ) ;
#67022=CARTESIAN_POINT ( 'NONE',  ( 11.96250000122903501, 4.330127018922192761, -2.499999999999997780 ) ) ;
#67023=CARTESIAN_POINT ( 'NONE',  ( 7.875000001229034652, 2.886751345948129099, -4.999999999999998224 ) ) ;
#67024=CARTESIAN_POINT ( 'NONE',  ( 29.55000000122903003, 5.773502691896255534, 3.535250795749688894E-16 ) ) ;
#67027=CARTESIAN_POINT ( 'NONE',  ( 12.57187500061451857, 3.027376345333613106, -5.243569643749998122 ) ) ;
#67029=ORIENTED_EDGE ( 'NONE', *, *, #6241, .T. ) ;
#67030=CARTESIAN_POINT ( 'NONE',  ( 20.35312500061451502, 0.000000000000000000, 5.243569643749999010 ) ) ;
#67031=CARTESIAN_POINT ( 'NONE',  ( 14.14687500061451786, -3.027376345333614438, 5.243569643749998122 ) ) ;
#67032=CARTESIAN_POINT ( 'NONE',  ( 4.828125000614518214, 6.421520780324663323E-16, -5.243569643749999010 ) ) ;
#67033=CARTESIAN_POINT ( 'NONE',  ( 21.75937500061451502, 0.000000000000000000, 5.243569643749999010 ) ) ;
#67034=CARTESIAN_POINT ( 'NONE',  ( 9.721875000614517148, -6.054752690667223547, -1.112240025338166033E-15 ) ) ;
#67035=CARTESIAN_POINT ( 'NONE',  ( 4.603125000614518569, 0.000000000000000000, 5.243569643749999010 ) ) ;
#67036=CARTESIAN_POINT ( 'NONE',  ( 10.95000000122903216, -2.886751345948126435, -5.000000000000000000 ) ) ;
#67037=CARTESIAN_POINT ( 'NONE',  ( 5.362500001229033586, 0.000000000000000000, 4.999999999999998224 ) ) ;
#67038=CARTESIAN_POINT ( 'NONE',  ( 19.45312500061451644, 0.000000000000000000, 5.243569643749999010 ) ) ;
#67039=( BOUNDED_CURVE ( )  B_SPLINE_CURVE ( 2, ( #43440, #49347, #67442, #38245, #27543, #5009, #10907 ),
 .UNSPECIFIED., .F., .F. ) 
 B_SPLINE_CURVE_WITH_KNOTS ( ( 3, 2, 2, 3 ),
 ( 0.3666666666666666408, 0.3694444444444444642, 0.3722222222222222321, 0.3750000000000000000 ),
 .UNSPECIFIED. ) 
 CURVE ( )  GEOMETRIC_REPRESENTATION_ITEM ( )  RATIONAL_B_SPLINE_CURVE ( ( 1.000000000000000000, 0.8660254037844387076, 1.000000000000000000, 0.8660254037844387076, 1.000000000000000000, 0.8660254037844387076, 1.000000000000000000 ) ) 
 REPRESENTATION_ITEM ( '' )  );
#67040=CARTESIAN_POINT ( 'NONE',  ( 8.662500001229034297, -4.330127018922190985, -2.500000000000001332 ) ) ;
#67041=CARTESIAN_POINT ( 'NONE',  ( 17.61562500061451786, 3.027376345333611329, 5.243569643749999010 ) ) ;
#67042=CARTESIAN_POINT ( 'NONE',  ( 16.04062500061451857, -3.027376345333610441, -5.243569643749999898 ) ) ;
#67044=CARTESIAN_POINT ( 'NONE',  ( 16.57499999999999929, -4.330127018922194537, 2.499999999999995559 ) ) ;
#67045=CARTESIAN_POINT ( 'NONE',  ( 9.787500001229036073, 4.330127018922191873, 2.499999999999999556 ) ) ;
#67046=CARTESIAN_POINT ( 'NONE',  ( 8.503125000614515372, 4.541064518000418104, -2.621784821874998173 ) ) ;
#67047=CARTESIAN_POINT ( 'NONE',  ( 11.76562500061451644, 3.027376345333611329, 5.243569643749999010 ) ) ;
#67049=CARTESIAN_POINT ( 'NONE',  ( 20.70000000122903216, -2.886751345948129988, 4.999999999999997335 ) ) ;
#67051=CARTESIAN_POINT ( 'NONE',  ( -2.121784821874996840, 14.53437500061451715, -26.32496088578401583 ) ) ;
#67052=FACE_OUTER_BOUND ( 'NONE', #67666, .T. ) ;
#67053=CARTESIAN_POINT ( 'NONE',  ( 3.112500001229034918, 0.000000000000000000, 4.999999999999998224 ) ) ;
#67054=CARTESIAN_POINT ( 'NONE',  ( 3.309375000614518836, 0.000000000000000000, 5.243569643749999010 ) ) ;
#67055=CARTESIAN_POINT ( 'NONE',  ( 20.74687500061451573, 6.054752690667223547, 3.707466751127219781E-16 ) ) ;
#67057=CARTESIAN_POINT ( 'NONE',  ( 16.41562500061451857, -6.054752690667223547, -1.112240025338166033E-15 ) ) ;
#67059=CARTESIAN_POINT ( 'NONE',  ( 1.626862140677534273E-15, 15.61250000000000071, -26.00000000000000355 ) ) ;
#67060=CARTESIAN_POINT ( 'NONE',  ( 4.385796401931335353, -2.400997692794667682, 4.385796401931427724 ) ) ;
#67061=CARTESIAN_POINT ( 'NONE',  ( 29.40937500061451715, 0.000000000000000000, 5.243569643749999010 ) ) ;
#67063=CARTESIAN_POINT ( 'NONE',  ( 13.82812500061451466, 6.421520780324663323E-16, -5.243569643749999010 ) ) ;
#67064=CARTESIAN_POINT ( 'NONE',  ( 11.89687500061451608, -3.027376345333614438, 5.243569643749998122 ) ) ;
#67066=CARTESIAN_POINT ( 'NONE',  ( 29.05312500061451431, -4.541064518000417216, -2.621784821875001281 ) ) ;
#67067=CARTESIAN_POINT ( 'NONE',  ( 22.49062500061451431, 6.054752690667223547, 3.707466751127219781E-16 ) ) ;
#67068=CARTESIAN_POINT ( 'NONE',  ( 3.999999999999998668, 11.26250000000000107, -32.30940107675850470 ) ) ;
#67069=CARTESIAN_POINT ( 'NONE',  ( 13.35000000000000142, 0.000000000000000000, 4.999999999999998224 ) ) ;
#67070=CARTESIAN_POINT ( 'NONE',  ( 22.23750000122903003, 6.123233995736764310E-16, -4.999999999999998224 ) ) ;
#67071=CARTESIAN_POINT ( 'NONE',  ( 16.34062500061451573, -3.027376345333614438, 5.243569643749998122 ) ) ;
#67074=CARTESIAN_POINT ( 'NONE',  ( 20.73750000000000071, -2.886751345948125991, -5.000000000000000000 ) ) ;
#67075=CARTESIAN_POINT ( 'NONE',  ( 21.12187500061451573, 3.027376345333613106, -5.243569643749998122 ) ) ;
#67076=CARTESIAN_POINT ( 'NONE',  ( 26.80312500061451431, -4.541064518000417216, -2.621784821875001281 ) ) ;
#67077=ORIENTED_EDGE ( 'NONE', *, *, #12941, .F. ) ;
#67079=CARTESIAN_POINT ( 'NONE',  ( 11.31562500061451892, 3.027376345333611329, 5.243569643749999010 ) ) ;
#67080=CARTESIAN_POINT ( 'NONE',  ( 6.225000000000001421, -4.330127018922194537, 2.499999999999995559 ) ) ;
#67081=CARTESIAN_POINT ( 'NONE',  ( 16.53750000000000142, -2.886751345948129988, 4.999999999999997335 ) ) ;
#67082=CARTESIAN_POINT ( 'NONE',  ( 23.66250000000000142, 2.886751345948126879, 4.999999999999999112 ) ) ;
#67083=CARTESIAN_POINT ( 'NONE',  ( 7.800000000000001599, 4.330127018922192761, -2.499999999999997780 ) ) ;
#67084=CARTESIAN_POINT ( 'NONE',  ( 5.409375000614516260, 4.541064518000418104, -2.621784821874998173 ) ) ;
#67085=CARTESIAN_POINT ( 'NONE',  ( 29.37187500061451928, 3.027376345333611329, 5.243569643749999010 ) ) ;
#67087=CARTESIAN_POINT ( 'NONE',  ( 23.24062500061451786, -3.027376345333610441, -5.243569643749999898 ) ) ;
#67088=CARTESIAN_POINT ( 'NONE',  ( 25.58437500061451431, 6.421520780324663323E-16, -5.243569643749999010 ) ) ;
#67089=CARTESIAN_POINT ( 'NONE',  ( 4.243569643749999898, 19.54062500061459318, -27.54997392385601529 ) ) ;
#67090=CARTESIAN_POINT ( 'NONE',  ( 13.98750000000000249, -2.886751345948125991, -5.000000000000000000 ) ) ;
#67091=CARTESIAN_POINT ( 'NONE',  ( 7.828125000614517326, -4.541064518000419881, 2.621784821874995952 ) ) ;
#67093=CARTESIAN_POINT ( 'NONE',  ( 26.35312500061451857, -4.541064518000417216, -2.621784821875001281 ) ) ;
#67094=CARTESIAN_POINT ( 'NONE',  ( 15.63750000122903216, 4.330127018922191873, 2.499999999999999556 ) ) ;
#67095=CARTESIAN_POINT ( 'NONE',  ( -3.999999999999999112, 18.19999999999999929, 30.00000000000000000 ) ) ;
#67097=CARTESIAN_POINT ( 'NONE',  ( 3.890625000614517326, -3.027376345333610441, -5.243569643749999898 ) ) ;
#67098=CARTESIAN_POINT ( 'NONE',  ( 19.20937500061451786, -4.541064518000417216, -2.621784821875001281 ) ) ;
#67099=CARTESIAN_POINT ( 'NONE',  ( 2.121784821874999061, 13.85937500061451821, 26.32496088578401583 ) ) ;
#67100=CARTESIAN_POINT ( 'NONE',  ( 21.83437500061451786, -4.541064518000419881, 2.621784821874995952 ) ) ;
#67101=CARTESIAN_POINT ( 'NONE',  ( 28.47187500061451715, 3.027376345333611329, 5.243569643749999010 ) ) ;
#67103=CARTESIAN_POINT ( 'NONE',  ( 10.79062500061451679, 6.054752690667223547, 3.707466751127219781E-16 ) ) ;
#67104=CARTESIAN_POINT ( 'NONE',  ( -3.999999999999997335, 15.20000000122903572, 32.30940107675850470 ) ) ;
#67105=ADVANCED_FACE ( 'NONE', ( #49304 ), #9769, .F. ) ;
#67106=CARTESIAN_POINT ( 'NONE',  ( 6.271875000614517859, 3.027376345333613106, -5.243569643749998122 ) ) ;
#67107=DIRECTION ( 'NONE',  ( -0.000000000000000000, -1.000000000000000000, -0.000000000000000000 ) ) ;
#67108=ADVANCED_FACE ( 'NONE', ( #43761 ), #27137, .F. ) ;
#67109=CARTESIAN_POINT ( 'NONE',  ( 7.528125000614515727, 6.421520780324663323E-16, -5.243569643749999010 ) ) ;
#67110=CARTESIAN_POINT ( 'NONE',  ( 11.44687500061451857, -3.027376345333614438, 5.243569643749998122 ) ) ;
#67111=CARTESIAN_POINT ( 'NONE',  ( 19.42500000122903714, -5.773502691896255534, -1.060575238724906372E-15 ) ) ;
#67112=CARTESIAN_POINT ( 'NONE',  ( 8.034375000614518925, 6.421520780324663323E-16, -5.243569643749999010 ) ) ;
#67113=CARTESIAN_POINT ( 'NONE',  ( 10.71562500061451928, 3.027376345333613106, -5.243569643749998122 ) ) ;
#67114=CARTESIAN_POINT ( 'NONE',  ( 6.140625000614516438, -3.027376345333610441, -5.243569643749999898 ) ) ;
#67116=CARTESIAN_POINT ( 'NONE',  ( 18.45937500061451431, 4.541064518000418104, -2.621784821874998173 ) ) ;
#67117=CARTESIAN_POINT ( 'NONE',  ( 11.10000000000000142, 0.000000000000000000, 4.999999999999998224 ) ) ;
#67118=CARTESIAN_POINT ( 'NONE',  ( 27.81562500061452070, 3.027376345333613106, -5.243569643749998122 ) ) ;
#67119=CARTESIAN_POINT ( 'NONE',  ( 12.62812500061451537, 4.541064518000418104, 2.621784821874999949 ) ) ;
#67120=CARTESIAN_POINT ( 'NONE',  ( 28.84687500061452425, 6.054752690667223547, 3.707466751127219781E-16 ) ) ;
#67121=CARTESIAN_POINT ( 'NONE',  ( 9.001249775931846008E-16, 13.22187500061451892, -25.09994784771203058 ) ) ;
#67123=CARTESIAN_POINT ( 'NONE',  ( 14.06250000122903288, -4.330127018922190985, -2.500000000000001332 ) ) ;
#67124=CARTESIAN_POINT ( 'NONE',  ( 4.243569643749999010, 16.01562500061451644, -32.45002607614398471 ) ) ;
#67125=CARTESIAN_POINT ( 'NONE',  ( 14.10000000122903252, -2.886751345948125991, -5.000000000000000000 ) ) ;
#67126=CARTESIAN_POINT ( 'NONE',  ( 9.215625000614515727, -6.054752690667223547, -1.112240025338166033E-15 ) ) ;
#67127=CARTESIAN_POINT ( 'NONE',  ( 12.82499999999999929, 4.330127018922191873, 2.499999999999999556 ) ) ;
#67128=CARTESIAN_POINT ( 'NONE',  ( -5.810221930991193690E-16, 13.58750000000000036, -34.00000000000000000 ) ) ;
#67129=CARTESIAN_POINT ( 'NONE',  ( 23.50312500061451360, 0.000000000000000000, 5.243569643749999010 ) ) ;
#67130=CARTESIAN_POINT ( 'NONE',  ( 7.321875000614516793, 3.027376345333611329, 5.243569643749999010 ) ) ;
#67131=ADVANCED_FACE ( 'NONE', ( #55572 ), #50034, .F. ) ;
#67132=CARTESIAN_POINT ( 'NONE',  ( 9.900000001229033231, -2.886751345948129988, 4.999999999999997335 ) ) ;
#67133=CARTESIAN_POINT ( 'NONE',  ( 17.40000000122903145, 5.773502691896255534, 3.535250795749688894E-16 ) ) ;
#67134=CARTESIAN_POINT ( 'NONE',  ( 14.50312500061451537, 0.000000000000000000, 5.243569643749999010 ) ) ;
#67135=CARTESIAN_POINT ( 'NONE',  ( 18.06562500061451715, 3.027376345333611329, 5.243569643749999010 ) ) ;
#67136=CARTESIAN_POINT ( 'NONE',  ( 25.50000000122903288, 5.773502691896255534, 3.535250795749688894E-16 ) ) ;
#67137=CARTESIAN_POINT ( 'NONE',  ( 28.57500000122903572, 2.886751345948129099, -4.999999999999998224 ) ) ;
#67138=CARTESIAN_POINT ( 'NONE',  ( 22.68750000000000000, 5.773502691896255534, 3.535250795749688894E-16 ) ) ;
#67140=CARTESIAN_POINT ( 'NONE',  ( 25.95937500061451431, -4.541064518000417216, -2.621784821875001281 ) ) ;
#67142=CARTESIAN_POINT ( 'NONE',  ( 11.40000000122903501, -2.886751345948125991, -5.000000000000000000 ) ) ;
#67143=CARTESIAN_POINT ( 'NONE',  ( 27.75937500061451502, -4.541064518000417216, -2.621784821875001281 ) ) ;
#67144=CARTESIAN_POINT ( 'NONE',  ( 3.889232029978275662, 3.142875762045684418, 3.889232029978275662 ) ) ;
#67145=CARTESIAN_POINT ( 'NONE',  ( 4.134375000614517681, 4.541064518000418104, 2.621784821874999949 ) ) ;
#67146=CARTESIAN_POINT ( 'NONE',  ( 23.95312500061451289, 0.000000000000000000, 5.243569643749999010 ) ) ;
#67148=CARTESIAN_POINT ( 'NONE',  ( 4.586250975554630571, -1.994072912278271881, -4.586250975554630571 ) ) ;
#67149=CARTESIAN_POINT ( 'NONE',  ( 9.496875000614517504, 6.054752690667223547, 3.707466751127219781E-16 ) ) ;
#67151=CARTESIAN_POINT ( 'NONE',  ( 29.39062500061451289, -3.027376345333614438, 5.243569643749998122 ) ) ;
#67152=CARTESIAN_POINT ( 'NONE',  ( 7.396875000614519635, -3.027376345333614438, 5.243569643749998122 ) ) ;
#67153=CARTESIAN_POINT ( 'NONE',  ( 29.78437500061451715, 4.541064518000418104, 2.621784821874999949 ) ) ;
#67155=CARTESIAN_POINT ( 'NONE',  ( 20.21250000000000213, -5.773502691896255534, -1.060575238724906372E-15 ) ) ;
#67157=CARTESIAN_POINT ( 'NONE',  ( 27.03750000000000142, -2.886751345948125991, -5.000000000000000000 ) ) ;
#67158=CARTESIAN_POINT ( 'NONE',  ( 29.70937500061451431, 4.541064518000418104, -2.621784821874998173 ) ) ;
#67159=EDGE_LOOP ( 'NONE', ( #30343, #56692, #70072 ) ) ;
#67160=CARTESIAN_POINT ( 'NONE',  ( 17.50312500061451715, 4.541064518000418104, -2.621784821874998173 ) ) ;
#67161=CARTESIAN_POINT ( 'NONE',  ( 8.915625000614515017, 3.027376345333613106, -5.243569643749998122 ) ) ;
#67163=CARTESIAN_POINT ( 'NONE',  ( 4.059375000614519280, 4.541064518000418104, -2.621784821874998173 ) ) ;
#67164=CARTESIAN_POINT ( 'NONE',  ( 18.63750000122903216, 6.123233995736764310E-16, -4.999999999999998224 ) ) ;
#67165=CARTESIAN_POINT ( 'NONE',  ( 0.000000000000000000, 20.00000000000000000, -33.99999999999999289 ) ) ;
#67166=CARTESIAN_POINT ( 'NONE',  ( 7.809375000614519280, 0.000000000000000000, 5.243569643749999010 ) ) ;
#67167=CARTESIAN_POINT ( 'NONE',  ( 11.78437500061451892, 4.541064518000418104, 2.621784821874999949 ) ) ;
#67168=CARTESIAN_POINT ( 'NONE',  ( 21.75937500061451502, 0.000000000000000000, 5.243569643749999010 ) ) ;
#67169=CARTESIAN_POINT ( 'NONE',  ( 4.423774761630055785, -2.331624301134462396, 4.423774761630055785 ) ) ;
#67171=CARTESIAN_POINT ( 'NONE',  ( 4.884375000614518569, 6.421520780324663323E-16, -5.243569643749999010 ) ) ;
#67173=CARTESIAN_POINT ( 'NONE',  ( 7.471875000614519813, -6.054752690667223547, -1.112240025338166033E-15 ) ) ;
#67175=CARTESIAN_POINT ( 'NONE',  ( 21.63749999999999929, -2.886751345948125991, -5.000000000000000000 ) ) ;
#67176=CARTESIAN_POINT ( 'NONE',  ( 17.35312500061451502, -4.541064518000417216, -2.621784821875001281 ) ) ;
#67178=CARTESIAN_POINT ( 'NONE',  ( 4.182001429795429104, 2.740687966149290222, 4.445321778319560657 ) ) ;
#67180=CARTESIAN_POINT ( 'NONE',  ( 11.24062500061451608, 6.054752690667223547, 3.707466751127219781E-16 ) ) ;
#67181=CARTESIAN_POINT ( 'NONE',  ( 3.187500000000002220, -2.886751345948125991, -5.000000000000000000 ) ) ;
#67183=CARTESIAN_POINT ( 'NONE',  ( 29.70937500061451431, 4.541064518000418104, -2.621784821874998173 ) ) ;
#67184=CARTESIAN_POINT ( 'NONE',  ( 9.337500000000000355, -2.886751345948129988, 4.999999999999997335 ) ) ;
#67185=CARTESIAN_POINT ( 'NONE',  ( 8.484601909799253346E-16, 14.82500000122903216, 34.61880215351700230 ) ) ;
#67186=CARTESIAN_POINT ( 'NONE',  ( 10.01250000122903394, -4.330127018922190985, -2.500000000000001332 ) ) ;
#67187=CARTESIAN_POINT ( 'NONE',  ( 19.20937500061451786, -4.541064518000417216, -2.621784821875001281 ) ) ;
#67188=CARTESIAN_POINT ( 'NONE',  ( 14.37187500061451928, 3.027376345333613106, -5.243569643749998122 ) ) ;
#67189=CARTESIAN_POINT ( 'NONE',  ( -1.999999999999997113, 12.42500000000000249, 33.46410161513775705 ) ) ;
#67191=CARTESIAN_POINT ( 'NONE',  ( 14.76562500061451821, 3.027376345333613106, -5.243569643749998122 ) ) ;
#67192=CARTESIAN_POINT ( 'NONE',  ( 26.85000000122903430, 5.773502691896255534, 3.535250795749688894E-16 ) ) ;
#67193=CARTESIAN_POINT ( 'NONE',  ( 16.24687500061451573, 6.054752690667223547, 3.707466751127219781E-16 ) ) ;
#67194=CARTESIAN_POINT ( 'NONE',  ( 8.175000000000002487, 6.123233995736764310E-16, -4.999999999999998224 ) ) ;
#67195=CARTESIAN_POINT ( 'NONE',  ( 16.75312500061451715, 0.000000000000000000, 5.243569643749999010 ) ) ;
#67196=CARTESIAN_POINT ( 'NONE',  ( 17.96250000122903501, 0.000000000000000000, 4.999999999999998224 ) ) ;
#67197=CARTESIAN_POINT ( 'NONE',  ( 26.89687500061451431, -3.027376345333610441, -5.243569643749999898 ) ) ;
#67198=CARTESIAN_POINT ( 'NONE',  ( 4.243569643749999898, 11.47812500061451679, 30.00000000000000000 ) ) ;
#67199=CARTESIAN_POINT ( 'NONE',  ( 15.49687500061451750, -3.027376345333614438, 5.243569643749998122 ) ) ;
#67200=CARTESIAN_POINT ( 'NONE',  ( 15.30000000122903359, -2.886751345948129988, 4.999999999999997335 ) ) ;
#67202=CARTESIAN_POINT ( 'NONE',  ( 3.354550016499390441, -3.707702085728201702, 3.707832566801417595 ) ) ;
#67203=EDGE_CURVE ( 'NONE', #15264, #36412, #69740, .T. ) ;
#67204=CARTESIAN_POINT ( 'NONE',  ( 20.63437500061451857, 6.421520780324663323E-16, -5.243569643749999010 ) ) ;
#67205=CARTESIAN_POINT ( 'NONE',  ( 18.97500000122903074, -5.773502691896255534, -1.060575238724906372E-15 ) ) ;
#67206=CARTESIAN_POINT ( 'NONE',  ( 16.73437500061451644, 4.541064518000418104, 2.621784821874999949 ) ) ;
#67207=CARTESIAN_POINT ( 'NONE',  ( 2.121784821874999061, 12.95937500061451786, 26.32496088578401583 ) ) ;
#67208=CARTESIAN_POINT ( 'NONE',  ( 18.32812500061451644, 6.421520780324663323E-16, -5.243569643749999010 ) ) ;
#67210=ORIENTED_EDGE ( 'NONE', *, *, #39975, .T. ) ;
#67211=CARTESIAN_POINT ( 'NONE',  ( 20.92500000000000071, 4.330127018922191873, 2.499999999999999556 ) ) ;
#67212=FACE_OUTER_BOUND ( 'NONE', #3132, .T. ) ;
#67213=CARTESIAN_POINT ( 'NONE',  ( 23.42812500061451786, 4.541064518000418104, 2.621784821874999949 ) ) ;
#67214=CARTESIAN_POINT ( 'NONE',  ( 4.040625000614517681, 6.054752690667223547, 3.707466751127219781E-16 ) ) ;
#67215=CARTESIAN_POINT ( 'NONE',  ( 18.15000000122903501, -2.886751345948125991, -5.000000000000000000 ) ) ;
#67216=CARTESIAN_POINT ( 'NONE',  ( 22.34062500061451573, -3.027376345333610441, -5.243569643749999898 ) ) ;
#67217=CARTESIAN_POINT ( 'NONE',  ( 21.63749999999999929, -2.886751345948125991, -5.000000000000000000 ) ) ;
#67218=CARTESIAN_POINT ( 'NONE',  ( 24.74062500061451786, 6.054752690667223547, 3.707466751127219781E-16 ) ) ;
#67219=CARTESIAN_POINT ( 'NONE',  ( 5.990625000614517859, -3.027376345333614438, 5.243569643749998122 ) ) ;
#67220=ORIENTED_EDGE ( 'NONE', *, *, #64836, .F. ) ;
#67221=CARTESIAN_POINT ( 'NONE',  ( 29.73750000000000071, -2.886751345948125991, -5.000000000000000000 ) ) ;
#67222=CARTESIAN_POINT ( 'NONE',  ( 3.590625000614518836, 6.054752690667223547, 3.707466751127219781E-16 ) ) ;
#67224=CARTESIAN_POINT ( 'NONE',  ( -1.999999999999997113, 11.18750000122903288, 33.46410161513775705 ) ) ;
#67225=CARTESIAN_POINT ( 'NONE',  ( -3.999999999999999556, 12.42500000122903359, -32.30940107675850470 ) ) ;
#67226=CARTESIAN_POINT ( 'NONE',  ( 2.121784821875001281, 18.65937500061451715, -26.32496088578401938 ) ) ;
#67228=CARTESIAN_POINT ( 'NONE',  ( 9.262499999999999289, 2.886751345948126879, 4.999999999999999112 ) ) ;
#67229=( BOUNDED_CURVE ( )  B_SPLINE_CURVE ( 2, ( #53103, #2499, #36478, #52743, #19105, #2148, #18382 ),
 .UNSPECIFIED., .F., .F. ) 
 B_SPLINE_CURVE_WITH_KNOTS ( ( 3, 2, 2, 3 ),
 ( 0.2750000000000000777, 0.2777777777777778456, 0.2805555555555556135, 0.2833333333333333814 ),
 .UNSPECIFIED. ) 
 CURVE ( )  GEOMETRIC_REPRESENTATION_ITEM ( )  RATIONAL_B_SPLINE_CURVE ( ( 0.9999999999999973355, 0.8660254037844413721, 1.000000000000000000, 0.8660254037844387076, 1.000000000000000000, 0.8660254037844360431, 1.000000000000002665 ) ) 
 REPRESENTATION_ITEM ( '' )  );
#67230=CARTESIAN_POINT ( 'NONE',  ( 5.737500001229033586, 4.330127018922191873, 2.499999999999999556 ) ) ;
#67231=CARTESIAN_POINT ( 'NONE',  ( 13.13437500061451857, 4.541064518000418104, 2.621784821874999949 ) ) ;
#67232=CARTESIAN_POINT ( 'NONE',  ( 29.72812500061451502, 4.541064518000418104, 2.621784821874999949 ) ) ;
#67233=CARTESIAN_POINT ( 'NONE',  ( 4.134375000614517681, 4.541064518000418104, 2.621784821874999949 ) ) ;
#67234=CARTESIAN_POINT ( 'NONE',  ( 30.00000000000000000, 6.123233995736764310E-16, -4.999999999999998224 ) ) ;
#67235=CARTESIAN_POINT ( 'NONE',  ( 5.857864376269046325, -9.999999999999998224, -5.857864376269046325 ) ) ;
#67236=CARTESIAN_POINT ( 'NONE',  ( 9.609375000614518214, 0.000000000000000000, 5.243569643749999010 ) ) ;
#67239=CARTESIAN_POINT ( 'NONE',  ( 20.72812500061451502, 4.541064518000418104, 2.621784821874999949 ) ) ;
#67240=CARTESIAN_POINT ( 'NONE',  ( -3.999999999999999112, 12.42500000122903536, -32.30940107675850470 ) ) ;
#67241=CARTESIAN_POINT ( 'NONE',  ( 2.121784821875001281, 18.15312500061459389, 33.67503911421598417 ) ) ;
#67242=CARTESIAN_POINT ( 'NONE',  ( 23.07187500061451857, 3.027376345333611329, 5.243569643749999010 ) ) ;
#67244=CARTESIAN_POINT ( 'NONE',  ( 2.840625000614518392, -3.027376345333614438, 5.243569643749998122 ) ) ;
#67246=CARTESIAN_POINT ( 'NONE',  ( 24.14062500061451289, -3.027376345333610441, -5.243569643749999898 ) ) ;
#67247=CARTESIAN_POINT ( 'NONE',  ( 14.72812500061451679, 6.421520780324663323E-16, -5.243569643749999010 ) ) ;
#67249=CARTESIAN_POINT ( 'NONE',  ( 11.52187500061451608, -6.054752690667223547, -1.112240025338166033E-15 ) ) ;
#67251=CARTESIAN_POINT ( 'NONE',  ( 25.27500000122903145, -5.773502691896255534, -1.060575238724906372E-15 ) ) ;
#67252=CARTESIAN_POINT ( 'NONE',  ( 4.584375000614516971, 4.541064518000418104, 2.621784821874999949 ) ) ;
#67253=CARTESIAN_POINT ( 'NONE',  ( 14.78437500061451715, 6.421520780324663323E-16, -5.243569643749999010 ) ) ;
#67254=CARTESIAN_POINT ( 'NONE',  ( 27.79687500061451999, -3.027376345333610441, -5.243569643749999898 ) ) ;
#67257=CARTESIAN_POINT ( 'NONE',  ( 24.75937500061451502, 4.541064518000418104, -2.621784821874998173 ) ) ;
#67258=CARTESIAN_POINT ( 'NONE',  ( 16.58437500061451786, 6.421520780324663323E-16, -5.243569643749999010 ) ) ;
#67260=CARTESIAN_POINT ( 'NONE',  ( 28.38749999999999929, -2.886751345948125991, -5.000000000000000000 ) ) ;
#67261=CARTESIAN_POINT ( 'NONE',  ( 4.687500001229034652, 6.123233995736764310E-16, -4.999999999999998224 ) ) ;
#67262=CARTESIAN_POINT ( 'NONE',  ( 5.700000000000000178, 0.000000000000000000, 4.999999999999998224 ) ) ;
#67264=CARTESIAN_POINT ( 'NONE',  ( 19.41562500061451146, 3.027376345333611329, 5.243569643749999010 ) ) ;
#67265=CARTESIAN_POINT ( 'NONE',  ( 8.962500000000002132, -5.773502691896255534, -1.060575238724906372E-15 ) ) ;
#67266=CARTESIAN_POINT ( 'NONE',  ( 1.626862140677534273E-15, 14.26250000000000107, 34.00000000000000000 ) ) ;
#67267=CARTESIAN_POINT ( 'NONE',  ( 16.35000000000000142, 4.330127018922192761, -2.499999999999997780 ) ) ;
#67268=CARTESIAN_POINT ( 'NONE',  ( -4.243569643749999898, 11.66562500061451679, 27.54997392385601529 ) ) ;
#67270=CARTESIAN_POINT ( 'NONE',  ( 19.68750000122903288, 4.330127018922191873, 2.499999999999999556 ) ) ;
#67271=CARTESIAN_POINT ( 'NONE',  ( 7.285825576177820915E-16, 10.00000000000000000, 36.00000000000000000 ) ) ;
#67272=CARTESIAN_POINT ( 'NONE',  ( 27.72187500061451715, -6.054752690667223547, -1.112240025338166033E-15 ) ) ;
#67273=ORIENTED_EDGE ( 'NONE', *, *, #39819, .F. ) ;
#67274=CARTESIAN_POINT ( 'NONE',  ( 16.00312500061451715, -4.541064518000417216, -2.621784821875001281 ) ) ;
#67275=CARTESIAN_POINT ( 'NONE',  ( 23.12812500061451360, -4.541064518000419881, 2.621784821874995952 ) ) ;
#67276=CARTESIAN_POINT ( 'NONE',  ( 22.09687500061451715, 6.054752690667223547, 3.707466751127219781E-16 ) ) ;
#67277=CARTESIAN_POINT ( 'NONE',  ( 7.500000000000000000, 0.000000000000000000, 4.999999999999998224 ) ) ;
#67278=CARTESIAN_POINT ( 'NONE',  ( 9.140625000614518214, -3.027376345333614438, 5.243569643749998122 ) ) ;
#67279=CARTESIAN_POINT ( 'NONE',  ( 25.37812500061451715, -4.541064518000419881, 2.621784821874995952 ) ) ;
#67280=CARTESIAN_POINT ( 'NONE',  ( 13.80937500061451750, -4.541064518000417216, -2.621784821875001281 ) ) ;
#67281=CARTESIAN_POINT ( 'NONE',  ( 18.34687500061451715, -3.027376345333610441, -5.243569643749999898 ) ) ;
#67282=CARTESIAN_POINT ( 'NONE',  ( 4.027635003466097707, 2.962795348797195416, -4.326299380533228600 ) ) ;
#67283=CARTESIAN_POINT ( 'NONE',  ( -4.243569643749999898, 17.55312500061451786, 30.00000000000000000 ) ) ;
#67284=CARTESIAN_POINT ( 'NONE',  ( 22.46250000122903501, 0.000000000000000000, 4.999999999999998224 ) ) ;
#67286=CARTESIAN_POINT ( 'NONE',  ( 11.72812500061451857, 4.541064518000418104, 2.621784821874999949 ) ) ;
#67287=CARTESIAN_POINT ( 'NONE',  ( 5.971875000614516260, 3.027376345333611329, 5.243569643749999010 ) ) ;
#67288=CARTESIAN_POINT ( 'NONE',  ( 4.659375000614518925, 0.000000000000000000, 5.243569643749999010 ) ) ;
#67291=CARTESIAN_POINT ( 'NONE',  ( 28.88437500061451502, 4.541064518000418104, 2.621784821874999949 ) ) ;
#67292=CARTESIAN_POINT ( 'NONE',  ( 18.96562500061451573, 3.027376345333611329, 5.243569643749999010 ) ) ;
#67293=CARTESIAN_POINT ( 'NONE',  ( 3.890625000614517326, -3.027376345333610441, -5.243569643749999898 ) ) ;
#67294=CARTESIAN_POINT ( 'NONE',  ( 27.70312500061451289, -4.541064518000417216, -2.621784821875001281 ) ) ;
#67295=CARTESIAN_POINT ( 'NONE',  ( 23.14687500061451786, -3.027376345333614438, 5.243569643749998122 ) ) ;
#67296=CARTESIAN_POINT ( 'NONE',  ( 18.44062500061451715, 6.054752690667223547, 3.707466751127219781E-16 ) ) ;
#67297=CARTESIAN_POINT ( 'NONE',  ( -4.243569643749997233, 19.44687500061451502, 32.45002607614398471 ) ) ;
#67298=CARTESIAN_POINT ( 'NONE',  ( 25.15312500061451217, 4.541064518000418104, -2.621784821874998173 ) ) ;
#67299=CARTESIAN_POINT ( 'NONE',  ( 4.612500001229032698, -4.330127018922190985, -2.500000000000001332 ) ) ;
#67300=ORIENTED_EDGE ( 'NONE', *, *, #51252, .F. ) ;
#67301=CARTESIAN_POINT ( 'NONE',  ( 27.18750000000000000, 5.773502691896255534, 3.535250795749688894E-16 ) ) ;
#67302=CARTESIAN_POINT ( 'NONE',  ( 3.999999999999999112, 14.82500000000000107, -30.00000000000000000 ) ) ;
#67304=CARTESIAN_POINT ( 'NONE',  ( 5.559375000614517504, 0.000000000000000000, 5.243569643749999010 ) ) ;
#67305=CARTESIAN_POINT ( 'NONE',  ( 11.61562500061451608, 3.027376345333613106, -5.243569643749998122 ) ) ;
#67306=CARTESIAN_POINT ( 'NONE',  ( 7.134375000614516793, 6.421520780324663323E-16, -5.243569643749999010 ) ) ;
#67307=CARTESIAN_POINT ( 'NONE',  ( 24.63750000122903216, 4.330127018922191873, 2.499999999999999556 ) ) ;
#67308=CARTESIAN_POINT ( 'NONE',  ( 15.94687500061451502, -3.027376345333614438, 5.243569643749998122 ) ) ;
#67309=CARTESIAN_POINT ( 'NONE',  ( 3.459375000614519635, -4.541064518000417216, -2.621784821875001281 ) ) ;
#67310=CARTESIAN_POINT ( 'NONE',  ( 27.75000000000000000, 0.000000000000000000, 4.999999999999998224 ) ) ;
#67311=CARTESIAN_POINT ( 'NONE',  ( 26.67187500061451644, 3.027376345333611329, 5.243569643749999010 ) ) ;
#67312=CARTESIAN_POINT ( 'NONE',  ( 4.190625000614518925, -3.027376345333614438, 5.243569643749998122 ) ) ;
#67313=CARTESIAN_POINT ( 'NONE',  ( 12.66562500061451502, 3.027376345333611329, 5.243569643749999010 ) ) ;
#67314=ORIENTED_EDGE ( 'NONE', *, *, #46318, .F. ) ;
#67315=CARTESIAN_POINT ( 'NONE',  ( 9.590625000614517504, -3.027376345333614438, 5.243569643749998122 ) ) ;
#67316=CARTESIAN_POINT ( 'NONE',  ( 6.815625000614517148, 3.027376345333611329, 5.243569643749999010 ) ) ;
#67318=CARTESIAN_POINT ( 'NONE',  ( 0.000000000000000000, 20.00000000000000000, -30.00000000000000000 ) ) ;
#67319=CARTESIAN_POINT ( 'NONE',  ( 15.41250000000000142, 2.886751345948129099, -4.999999999999998224 ) ) ;
#67320=CARTESIAN_POINT ( 'NONE',  ( 15.83437500061451608, 4.541064518000418104, 2.621784821874999949 ) ) ;
#67321=CARTESIAN_POINT ( 'NONE',  ( 13.76250000122903394, 4.330127018922192761, -2.499999999999997780 ) ) ;
#67323=CARTESIAN_POINT ( 'NONE',  ( 19.95937500061451786, 0.000000000000000000, 5.243569643749999010 ) ) ;
#67324=CARTESIAN_POINT ( 'NONE',  ( -3.000416591977282496E-16, 13.84062500061451928, -34.90005215228797653 ) ) ;
#67327=CARTESIAN_POINT ( 'NONE',  ( 20.66250000000000142, -5.773502691896255534, -1.060575238724906372E-15 ) ) ;
#67328=EDGE_CURVE ( 'NONE', #60454, #20630, #1348, .T. ) ;
#67329=CARTESIAN_POINT ( 'NONE',  ( 26.39062500061451644, -3.027376345333610441, -5.243569643749999898 ) ) ;
#67330=CARTESIAN_POINT ( 'NONE',  ( 2.000000000000001332, 16.10000000000000142, -26.53589838486224650 ) ) ;
#67331=CARTESIAN_POINT ( 'NONE',  ( 25.61250000000000071, -5.773502691896255534, -1.060575238724906372E-15 ) ) ;
#67332=CARTESIAN_POINT ( 'NONE',  ( 10.26562500061451644, 3.027376345333613106, -5.243569643749998122 ) ) ;
#67334=CARTESIAN_POINT ( 'NONE',  ( 20.59687500061451360, -3.027376345333610441, -5.243569643749999898 ) ) ;
#67336=CARTESIAN_POINT ( 'NONE',  ( 4.453125000614517326, 4.541064518000418104, -2.621784821874998173 ) ) ;
#67337=CARTESIAN_POINT ( 'NONE',  ( 11.37187500061451750, 3.027376345333611329, 5.243569643749999010 ) ) ;
#67339=CARTESIAN_POINT ( 'NONE',  ( 20.70937500061451786, 4.541064518000418104, -2.621784821874998173 ) ) ;
#67340=FACE_OUTER_BOUND ( 'NONE', #2762, .T. ) ;
#67341=CARTESIAN_POINT ( 'NONE',  ( 29.77499999999999858, 6.123233995736764310E-16, -4.999999999999998224 ) ) ;
#67342=CARTESIAN_POINT ( 'NONE',  ( 4.387500000000002842, -2.886751345948129988, 4.999999999999997335 ) ) ;
#67343=CARTESIAN_POINT ( 'NONE',  ( 15.67500000122903181, 2.886751345948126879, 4.999999999999999112 ) ) ;
#67345=CARTESIAN_POINT ( 'NONE',  ( -1.999999999999997113, 19.17500000000000071, -26.53589838486224295 ) ) ;
#67346=VERTEX_POINT ( 'NONE', #62911 ) ;
#67347=CARTESIAN_POINT ( 'NONE',  ( 12.48750000000000249, -2.886751345948129988, 4.999999999999997335 ) ) ;
#67348=CARTESIAN_POINT ( 'NONE',  ( 27.55312500061451786, 0.000000000000000000, 5.243569643749999010 ) ) ;
#67349=CARTESIAN_POINT ( 'NONE',  ( 16.98750000000000426, -2.886751345948129988, 4.999999999999997335 ) ) ;
#67350=CARTESIAN_POINT ( 'NONE',  ( 9.562500001229032875, -4.330127018922190985, -2.500000000000001332 ) ) ;
#67351=CARTESIAN_POINT ( 'NONE',  ( 8.015625000614518214, 3.027376345333613106, -5.243569643749998122 ) ) ;
#67352=CARTESIAN_POINT ( 'NONE',  ( 8.587500000000002132, -2.886751345948125991, -5.000000000000000000 ) ) ;
#67353=CARTESIAN_POINT ( 'NONE',  ( 1.626862140677534273E-15, 11.11250000000000071, -26.00000000000000355 ) ) ;
#67354=CARTESIAN_POINT ( 'NONE',  ( 2.121784821874999061, 14.75937500061451679, -33.67503911421598417 ) ) ;
#67355=CARTESIAN_POINT ( 'NONE',  ( 27.45000000122903572, -2.886751345948129988, 4.999999999999997335 ) ) ;
#67357=CARTESIAN_POINT ( 'NONE',  ( 7.237500000000000711, -2.886751345948125991, -5.000000000000000000 ) ) ;
#67359=VERTEX_POINT ( 'NONE', #57727 ) ;
#67360=CARTESIAN_POINT ( 'NONE',  ( 24.10312500061451502, -4.541064518000417216, -2.621784821875001281 ) ) ;
#67361=CARTESIAN_POINT ( 'NONE',  ( 29.20312500061451644, 4.541064518000418104, -2.621784821874998173 ) ) ;
#67362=CARTESIAN_POINT ( 'NONE',  ( 29.25937500061451502, 4.541064518000418104, -2.621784821874998173 ) ) ;
#67363=CARTESIAN_POINT ( 'NONE',  ( 22.50937500061451857, 4.541064518000418104, -2.621784821874998173 ) ) ;
#67364=CARTESIAN_POINT ( 'NONE',  ( 15.59062500061451573, -3.027376345333610441, -5.243569643749999898 ) ) ;
#67365=CARTESIAN_POINT ( 'NONE',  ( -4.243569643749999898, 11.70312500061459282, -30.00000000000000000 ) ) ;
#67366=CARTESIAN_POINT ( 'NONE',  ( 7.340625000614518392, -3.027376345333614438, 5.243569643749998122 ) ) ;
#67367=CARTESIAN_POINT ( 'NONE',  ( 28.08750000122903145, 6.123233995736764310E-16, -4.999999999999998224 ) ) ;
#67369=CARTESIAN_POINT ( 'NONE',  ( 18.47812500061451857, 4.541064518000418104, 2.621784821874999949 ) ) ;
#67372=CARTESIAN_POINT ( 'NONE',  ( 11.59687500061451892, -3.027376345333610441, -5.243569643749999898 ) ) ;
#67373=CARTESIAN_POINT ( 'NONE',  ( 14.97187500061451892, 3.027376345333611329, 5.243569643749999010 ) ) ;
#67374=CARTESIAN_POINT ( 'NONE',  ( 22.58437500061451431, 4.541064518000418104, 2.621784821874999949 ) ) ;
#67377=CARTESIAN_POINT ( 'NONE',  ( 25.82812500061451644, -4.541064518000419881, 2.621784821874995952 ) ) ;
#67378=EDGE_CURVE ( 'NONE', #31619, #14728, #19214, .T. ) ;
#67379=CARTESIAN_POINT ( 'NONE',  ( 27.85312500061451502, 4.541064518000418104, -2.621784821874998173 ) ) ;
#67381=CARTESIAN_POINT ( 'NONE',  ( -2.000000000000000000, 15.87500000000000000, 26.53589838486224650 ) ) ;
#67382=CARTESIAN_POINT ( 'NONE',  ( 4.434375000614519280, 6.421520780324663323E-16, -5.243569643749999010 ) ) ;
#67383=CARTESIAN_POINT ( 'NONE',  ( 12.00000000122903465, 5.773502691896255534, 3.535250795749688894E-16 ) ) ;
#67384=CARTESIAN_POINT ( 'NONE',  ( 6.862500001229034474, -4.330127018922190985, -2.500000000000001332 ) ) ;
#67385=CARTESIAN_POINT ( 'NONE',  ( 29.58750000122903501, 4.330127018922191873, 2.499999999999999556 ) ) ;
#67388=CARTESIAN_POINT ( 'NONE',  ( 11.18437500061451928, 6.421520780324663323E-16, -5.243569643749999010 ) ) ;
#67391=CARTESIAN_POINT ( 'NONE',  ( 20.57812500061451644, 6.421520780324663323E-16, -5.243569643749999010 ) ) ;
#67392=CARTESIAN_POINT ( 'NONE',  ( 12.90937500061451537, -4.541064518000417216, -2.621784821875001281 ) ) ;
#67393=CARTESIAN_POINT ( 'NONE',  ( 4.303125000614516971, -4.541064518000417216, -2.621784821875001281 ) ) ;
#67394=CARTESIAN_POINT ( 'NONE',  ( 22.17187500061451644, 3.027376345333611329, 5.243569643749999010 ) ) ;
#67395=CARTESIAN_POINT ( 'NONE',  ( 9.684375000614517504, -4.541064518000419881, 2.621784821874995952 ) ) ;
#67396=CARTESIAN_POINT ( 'NONE',  ( 4.528125000614516615, 4.541064518000418104, 2.621784821874999949 ) ) ;
#67399=CARTESIAN_POINT ( 'NONE',  ( 6.037500001229035185, 6.123233995736764310E-16, -4.999999999999998224 ) ) ;
#67400=CARTESIAN_POINT ( 'NONE',  ( 18.96562500061451573, 3.027376345333611329, 5.243569643749999010 ) ) ;
#67401=CARTESIAN_POINT ( 'NONE',  ( 9.112500001229033586, -4.330127018922190985, -2.500000000000001332 ) ) ;
#67402=CARTESIAN_POINT ( 'NONE',  ( 18.10312500061451502, 0.000000000000000000, 5.243569643749999010 ) ) ;
#67403=CARTESIAN_POINT ( 'NONE',  ( 14.84062500061451750, 6.054752690667223547, 3.707466751127219781E-16 ) ) ;
#67405=CARTESIAN_POINT ( 'NONE',  ( 15.26249999999999929, -5.773502691896255534, -1.060575238724906372E-15 ) ) ;
#67406=CARTESIAN_POINT ( 'NONE',  ( 8.400000001229035007, 5.773502691896255534, 3.535250795749688894E-16 ) ) ;
#67407=CARTESIAN_POINT ( 'NONE',  ( 5.390625000614518214, 6.054752690667223547, 3.707466751127219781E-16 ) ) ;
#67408=CARTESIAN_POINT ( 'NONE',  ( 19.95000000122903572, -2.886751345948125991, -5.000000000000000000 ) ) ;
#67410=CARTESIAN_POINT ( 'NONE',  ( -2.121784821874996840, 10.03437500061451892, -26.32496088578401583 ) ) ;
#67411=LINE ( 'NONE', #11249, #27699 ) ;
#67412=CARTESIAN_POINT ( 'NONE',  ( 24.03750000000000142, 5.773502691896255534, 3.535250795749688401E-16 ) ) ;
#67413=CARTESIAN_POINT ( 'NONE',  ( 3.159375000614518036, 4.541064518000418104, -2.621784821874998173 ) ) ;
#67414=CARTESIAN_POINT ( 'NONE',  ( 21.72187500061451715, 3.027376345333611329, 5.243569643749999010 ) ) ;
#67416=CARTESIAN_POINT ( 'NONE',  ( 15.59062500061451573, -3.027376345333610441, -5.243569643749999898 ) ) ;
#67420=CARTESIAN_POINT ( 'NONE',  ( 28.43437500061451573, 4.541064518000418104, 2.621784821874999949 ) ) ;
#67422=CARTESIAN_POINT ( 'NONE',  ( 13.41562500061451502, 3.027376345333613106, -5.243569643749998122 ) ) ;
#67423=CARTESIAN_POINT ( 'NONE',  ( 10.62187500061451928, -6.054752690667223547, -1.112240025338166033E-15 ) ) ;
#67425=CARTESIAN_POINT ( 'NONE',  ( 29.69062500061451715, 6.054752690667223547, 3.707466751127219781E-16 ) ) ;
#67426=CARTESIAN_POINT ( 'NONE',  ( 23.87812500061451715, 4.541064518000418104, 2.621784821874999949 ) ) ;
#67427=CARTESIAN_POINT ( 'NONE',  ( 17.73750000122903359, 6.123233995736764310E-16, -4.999999999999998224 ) ) ;
#67428=CARTESIAN_POINT ( 'NONE',  ( -3.999999999999999112, 12.87500000122903465, 27.69059892324149885 ) ) ;
#67430=CARTESIAN_POINT ( 'NONE',  ( 12.56250000000000178, -5.773502691896255534, -1.060575238724906372E-15 ) ) ;
#67431=CARTESIAN_POINT ( 'NONE',  ( 22.16250000122903074, -4.330127018922190985, -2.500000000000001332 ) ) ;
#67432=CARTESIAN_POINT ( 'NONE',  ( 17.01562500061451644, 3.027376345333613106, -5.243569643749998122 ) ) ;
#67434=ORIENTED_EDGE ( 'NONE', *, *, #6454, .T. ) ;
#67435=CARTESIAN_POINT ( 'NONE',  ( 18.86249999999999716, -5.773502691896255534, -1.060575238724906372E-15 ) ) ;
#67436=CARTESIAN_POINT ( 'NONE',  ( 23.28750000000000142, -2.886751345948129988, 4.999999999999997335 ) ) ;
#67438=CARTESIAN_POINT ( 'NONE',  ( 20.85937500061451644, 0.000000000000000000, 5.243569643749999010 ) ) ;
#67439=CARTESIAN_POINT ( 'NONE',  ( 28.15312500061451573, -4.541064518000417216, -2.621784821875001281 ) ) ;
#67440=ORIENTED_EDGE ( 'NONE', *, *, #32319, .F. ) ;
#67442=CARTESIAN_POINT ( 'NONE',  ( 20.02500000000000213, 4.330127018922191873, 2.499999999999999556 ) ) ;
#67443=CARTESIAN_POINT ( 'NONE',  ( 8.315625000614515372, -6.054752690667223547, -1.112240025338166033E-15 ) ) ;
#67444=CARTESIAN_POINT ( 'NONE',  ( 14.58750000000000036, 5.773502691896255534, 3.535250795749688894E-16 ) ) ;
#67445=CARTESIAN_POINT ( 'NONE',  ( 4.243569643749999898, 19.54062500061451857, 32.45002607614398471 ) ) ;
#67446=CARTESIAN_POINT ( 'NONE',  ( 5.334375000614517859, 6.421520780324663323E-16, -5.243569643749999010 ) ) ;
#67447=CARTESIAN_POINT ( 'NONE',  ( 29.52187500061451431, -6.054752690667223547, -1.112240025338166033E-15 ) ) ;
#67448=ORIENTED_EDGE ( 'NONE', *, *, #24383, .T. ) ;
#67449=CARTESIAN_POINT ( 'NONE',  ( 25.11562500061451431, 3.027376345333613106, -5.243569643749998122 ) ) ;
#67450=CARTESIAN_POINT ( 'NONE',  ( 26.14687500061451431, 6.054752690667223547, 3.707466751127219781E-16 ) ) ;
#67451=CARTESIAN_POINT ( 'NONE',  ( 2.121784821874999061, 18.30312500061459247, -33.67503911421598417 ) ) ;
#67452=CARTESIAN_POINT ( 'NONE',  ( 12.11250000000000249, -5.773502691896255534, -1.060575238724906372E-15 ) ) ;
#67453=CARTESIAN_POINT ( 'NONE',  ( 9.928125000614517859, 4.541064518000418104, 2.621784821874999949 ) ) ;
#67455=CARTESIAN_POINT ( 'NONE',  ( 26.16562500061451502, 3.027376345333611329, 5.243569643749999010 ) ) ;
#67456=CARTESIAN_POINT ( 'NONE',  ( -1.999999999999997113, 18.27499999999999858, 33.46410161513775705 ) ) ;
#67458=CARTESIAN_POINT ( 'NONE',  ( 3.590625000614518836, 6.054752690667223547, 3.707466751127219781E-16 ) ) ;
#67459=CARTESIAN_POINT ( 'NONE',  ( 19.80937500061451573, 4.541064518000418104, -2.621784821874998173 ) ) ;
#67460=CARTESIAN_POINT ( 'NONE',  ( 2.121784821875001281, 15.50937500061451857, 33.67503911421598417 ) ) ;
#67461=CARTESIAN_POINT ( 'NONE',  ( 21.57187500061451502, 3.027376345333613106, -5.243569643749998122 ) ) ;
#67462=CARTESIAN_POINT ( 'NONE',  ( 29.29687500061451644, 6.054752690667223547, 3.707466751127219781E-16 ) ) ;
#67463=CARTESIAN_POINT ( 'NONE',  ( -4.243569643749998122, 18.99687500061451928, 32.45002607614398471 ) ) ;
#67464=CARTESIAN_POINT ( 'NONE',  ( 10.26562500061451644, 3.027376345333613106, -5.243569643749998122 ) ) ;
#67465=CARTESIAN_POINT ( 'NONE',  ( 3.037500001229032964, 4.330127018922191873, 2.499999999999999556 ) ) ;
#67466=EDGE_CURVE ( 'NONE', #68632, #8399, #29177, .T. ) ;
#67467=CARTESIAN_POINT ( 'NONE',  ( 6.234375000614519102, 6.421520780324663323E-16, -5.243569643749999010 ) ) ;
#67469=CARTESIAN_POINT ( 'NONE',  ( 6.740625000614516082, 6.054752690667223547, 3.707466751127219781E-16 ) ) ;
#67470=CARTESIAN_POINT ( 'NONE',  ( 13.09687500061451892, 6.054752690667223547, 3.707466751127219781E-16 ) ) ;
#67471=CARTESIAN_POINT ( 'NONE',  ( 18.30000000122903359, 5.773502691896255534, 3.535250795749688894E-16 ) ) ;
#67472=CARTESIAN_POINT ( 'NONE',  ( 7.284375000614518036, 4.541064518000418104, 2.621784821874999949 ) ) ;
#67473=CARTESIAN_POINT ( 'NONE',  ( 9.890625000614516438, 6.054752690667223547, 3.707466751127219781E-16 ) ) ;
#67474=CARTESIAN_POINT ( 'NONE',  ( 5.278125000614516615, 6.421520780324663323E-16, -5.243569643749999010 ) ) ;
#67476=CARTESIAN_POINT ( 'NONE',  ( 19.32187500061451857, 3.027376345333613106, -5.243569643749998122 ) ) ;
#67477=CARTESIAN_POINT ( 'NONE',  ( -0.7368881354385758975, 9.803648613939513368, -34.17910028561248481 ) ) ;
#67478=CARTESIAN_POINT ( 'NONE',  ( 27.29062500061451502, -3.027376345333610441, -5.243569643749999898 ) ) ;
#67479=CARTESIAN_POINT ( 'NONE',  ( 12.51562500061451821, 3.027376345333613106, -5.243569643749998122 ) ) ;
#67480=CARTESIAN_POINT ( 'NONE',  ( 28.24687500061451573, -3.027376345333610441, -5.243569643749999898 ) ) ;
#67481=CARTESIAN_POINT ( 'NONE',  ( -2.121784821874999949, 11.68437500061451750, -33.67503911421598417 ) ) ;
#67482=CARTESIAN_POINT ( 'NONE',  ( 12.03750000122903430, 4.330127018922191873, 2.499999999999999556 ) ) ;
#67483=CARTESIAN_POINT ( 'NONE',  ( 27.17812500061451786, -4.541064518000419881, 2.621784821874995952 ) ) ;
#67484=CARTESIAN_POINT ( 'NONE',  ( -3.000416591977282496E-16, 16.09062500061451573, -34.90005215228797653 ) ) ;
#67485=CARTESIAN_POINT ( 'NONE',  ( 14.96250000122903323, -4.330127018922190985, -2.500000000000001332 ) ) ;
#67486=CARTESIAN_POINT ( 'NONE',  ( 13.19999999999999929, 4.330127018922192761, -2.499999999999997780 ) ) ;
#67487=CARTESIAN_POINT ( 'NONE',  ( 10.35000000122903074, -2.886751345948063374, 5.000000000000112799 ) ) ;
#67488=CARTESIAN_POINT ( 'NONE',  ( 22.90312500061451573, 4.541064518000418104, -2.621784821874998173 ) ) ;
#67489=CARTESIAN_POINT ( 'NONE',  ( 8.596875000614518925, 6.054752690667223547, 3.707466751127219781E-16 ) ) ;
#67490=CARTESIAN_POINT ( 'NONE',  ( 8.887500001229033941, 4.330127018922191873, 2.499999999999999556 ) ) ;
#67491=CARTESIAN_POINT ( 'NONE',  ( 16.72500000122903430, -5.773502691896255534, -1.060575238724906372E-15 ) ) ;
#67492=CARTESIAN_POINT ( 'NONE',  ( 12.17812500061451608, 4.541064518000418104, 2.621784821874999949 ) ) ;
#67493=CARTESIAN_POINT ( 'NONE',  ( 18.62812500061451715, -4.541064518000419881, 2.621784821874995952 ) ) ;
#67494=CARTESIAN_POINT ( 'NONE',  ( 26.32500000122903216, 2.886751345948129099, -4.999999999999998224 ) ) ;
#67495=CARTESIAN_POINT ( 'NONE',  ( 28.95000000122903572, -2.886751345948125991, -5.000000000000000000 ) ) ;
#67496=CARTESIAN_POINT ( 'NONE',  ( 23.77499999999999858, -4.330127018922194537, 2.499999999999995559 ) ) ;
#67497=CARTESIAN_POINT ( 'NONE',  ( 26.89687500061451431, -3.027376345333610441, -5.243569643749999898 ) ) ;
#67499=CARTESIAN_POINT ( 'NONE',  ( 9.262500001229033941, 4.330127018922192761, -2.499999999999997780 ) ) ;
#67500=CARTESIAN_POINT ( 'NONE',  ( 28.73437500061451644, 6.421520780324663323E-16, -5.243569643749999010 ) ) ;
#67501=CARTESIAN_POINT ( 'NONE',  ( 5.259375000614518569, -4.541064518000417216, -2.621784821875001281 ) ) ;
#67502=CARTESIAN_POINT ( 'NONE',  ( 24.81562500061451715, 3.027376345333611329, 5.243569643749999010 ) ) ;
#67505=CARTESIAN_POINT ( 'NONE',  ( 9.459375000614517859, 4.541064518000418104, -2.621784821874998173 ) ) ;
#67506=CARTESIAN_POINT ( 'NONE',  ( 4.967063083088209652, -0.5913641066433281690, 5.048674133904348160 ) ) ;
#67507=CARTESIAN_POINT ( 'NONE',  ( 3.534375000614518036, 6.421520780324663323E-16, -5.243569643749999010 ) ) ;
#67508=CARTESIAN_POINT ( 'NONE',  ( 7.134375000614516793, 6.421520780324663323E-16, -5.243569643749999010 ) ) ;
#67509=CARTESIAN_POINT ( 'NONE',  ( -1.999999999999997113, 16.58750000122903501, -26.53589838486224295 ) ) ;
#67510=CARTESIAN_POINT ( 'NONE',  ( 28.69687500061451502, -3.027376345333610441, -5.243569643749999898 ) ) ;
#67511=CARTESIAN_POINT ( 'NONE',  ( 2.121784821874999061, 10.20312500061459637, 26.32496088578401583 ) ) ;
#67512=CARTESIAN_POINT ( 'NONE',  ( 18.86249999999999716, -5.773502691896255534, -1.060575238724906372E-15 ) ) ;
#67513=ORIENTED_EDGE ( 'NONE', *, *, #31048, .T. ) ;
#67514=CARTESIAN_POINT ( 'NONE',  ( 26.43750000000000000, -2.886751345948129988, 4.999999999999997335 ) ) ;
#67515=CARTESIAN_POINT ( 'NONE',  ( 29.18437500061451573, 6.421520780324663323E-16, -5.243569643749999010 ) ) ;
#67517=CARTESIAN_POINT ( 'NONE',  ( 15.89062500061451289, -3.027376345333614438, 5.243569643749998122 ) ) ;
#67518=CARTESIAN_POINT ( 'NONE',  ( 9.440625000614517148, 6.054752690667223547, 3.707466751127219781E-16 ) ) ;
#67520=CARTESIAN_POINT ( 'NONE',  ( 3.534375000614518036, 6.421520780324663323E-16, -5.243569643749999010 ) ) ;
#67521=CARTESIAN_POINT ( 'NONE',  ( 18.41250000122903430, 0.000000000000000000, 4.999999999999998224 ) ) ;
#67522=CARTESIAN_POINT ( 'NONE',  ( 23.66250000000000142, 2.886751345948126879, 4.999999999999999112 ) ) ;
#67523=DIRECTION ( 'NONE',  ( -0.000000000000000000, -1.000000000000000000, -0.000000000000000000 ) ) ;
#67524=CARTESIAN_POINT ( 'NONE',  ( 6.871875000614517504, 3.027376345333611329, 5.243569643749999010 ) ) ;
#67525=CARTESIAN_POINT ( 'NONE',  ( 11.74687500061451573, 6.054752690667223547, 3.707466751127219781E-16 ) ) ;
#67526=CARTESIAN_POINT ( 'NONE',  ( 21.87187500061451573, -6.054752690667223547, -1.112240025338166033E-15 ) ) ;
#67529=ORIENTED_EDGE ( 'NONE', *, *, #68939, .T. ) ;
#67530=CARTESIAN_POINT ( 'NONE',  ( 4.284375000614518925, -4.541064518000419881, 2.621784821874995952 ) ) ;
#67531=CARTESIAN_POINT ( 'NONE',  ( 6.909375000614518036, 0.000000000000000000, 5.243569643749999010 ) ) ;
#67532=CARTESIAN_POINT ( 'NONE',  ( 17.69999999999999929, 4.330127018922192761, -2.499999999999997780 ) ) ;
#67533=CARTESIAN_POINT ( 'NONE',  ( 16.94062500061451715, -3.027376345333610441, -5.243569643749999898 ) ) ;
#67535=DIRECTION ( 'NONE',  ( 0.000000000000000000, 0.000000000000000000, 1.000000000000000000 ) ) ;
#67537=CARTESIAN_POINT ( 'NONE',  ( 11.09062500061451573, -3.027376345333610441, -5.243569643749999898 ) ) ;
#67538=CARTESIAN_POINT ( 'NONE',  ( 25.88437500061451502, -4.541064518000419881, 2.621784821874995952 ) ) ;
#67540=CARTESIAN_POINT ( 'NONE',  ( 29.33437500061451431, 4.541064518000418104, 2.621784821874999949 ) ) ;
#67541=CARTESIAN_POINT ( 'NONE',  ( 10.65000000000000036, 0.000000000000000000, 4.999999999999998224 ) ) ;
#67542=CARTESIAN_POINT ( 'NONE',  ( -1.999999999999997113, 15.23750000122903536, 33.46410161513775705 ) ) ;
#67543=CARTESIAN_POINT ( 'NONE',  ( 10.16250000122903252, 4.330127018922192761, -2.499999999999997780 ) ) ;
#67544=CARTESIAN_POINT ( 'NONE',  ( 20.82187500061451857, 3.027376345333611329, 5.243569643749999010 ) ) ;
#67545=CARTESIAN_POINT ( 'NONE',  ( 14.40937500061451715, 4.541064518000418104, -2.621784821874998173 ) ) ;
#67547=ORIENTED_EDGE ( 'NONE', *, *, #1251, .F. ) ;
#67548=CARTESIAN_POINT ( 'NONE',  ( 14.57812500061451644, -4.541064518000419881, 2.621784821874995952 ) ) ;
#67549=CARTESIAN_POINT ( 'NONE',  ( 26.55000000122902648, -2.886751345948129988, 4.999999999999997335 ) ) ;
#67550=CARTESIAN_POINT ( 'NONE',  ( 16.20937500061451786, 4.541064518000418104, -2.621784821874998173 ) ) ;
#67551=CARTESIAN_POINT ( 'NONE',  ( 5.378878668797003826, 8.432125716319053055, -32.68706799072294444 ) ) ;
#67552=CARTESIAN_POINT ( 'NONE',  ( 15.96562500061451573, -6.054752690667223547, -1.112240025338166033E-15 ) ) ;
#67554=CARTESIAN_POINT ( 'NONE',  ( 25.77187500061451075, 3.027376345333611329, 5.243569643749999010 ) ) ;
#67555=CARTESIAN_POINT ( 'NONE',  ( 4.243569643749999898, 11.44062500061451715, 32.45002607614398471 ) ) ;
#67556=CARTESIAN_POINT ( 'NONE',  ( 16.13437500061451502, 6.421520780324663323E-16, -5.243569643749999010 ) ) ;
#67557=CARTESIAN_POINT ( 'NONE',  ( 13.91250000122903252, 0.000000000000000000, 4.999999999999998224 ) ) ;
#67558=DIRECTION ( 'NONE',  ( 0.000000000000000000, 0.000000000000000000, 1.000000000000000000 ) ) ;
#67559=FACE_OUTER_BOUND ( 'NONE', #2475, .T. ) ;
#67560=CARTESIAN_POINT ( 'NONE',  ( 18.23437500061451999, -4.541064518000419881, 2.621784821874995952 ) ) ;
#67561=CARTESIAN_POINT ( 'NONE',  ( 20.58750000122903145, 4.330127018922191873, 2.499999999999999556 ) ) ;
#67562=CARTESIAN_POINT ( 'NONE',  ( 13.69687500061451679, -3.027376345333614438, 5.243569643749998122 ) ) ;
#67563=CARTESIAN_POINT ( 'NONE',  ( -2.121784821874999949, 12.13437500061451857, 26.32496088578401938 ) ) ;
#67564=CARTESIAN_POINT ( 'NONE',  ( 22.72500000122903430, 2.886751345948129099, -4.999999999999998224 ) ) ;
#67565=CARTESIAN_POINT ( 'NONE',  ( 17.95312500061451644, 4.541064518000418104, -2.621784821874998173 ) ) ;
#67567=ORIENTED_EDGE ( 'NONE', *, *, #2964, .T. ) ;
#67568=CARTESIAN_POINT ( 'NONE',  ( 21.41250000000000497, 2.886751345948126879, 4.999999999999999112 ) ) ;
#67570=CARTESIAN_POINT ( 'NONE',  ( 22.64062500061451644, -3.027376345333614438, 5.243569643749998122 ) ) ;
#67571=CARTESIAN_POINT ( 'NONE',  ( 3.992467690304758232, 3.010110221998377078, 29.71877081132206655 ) ) ;
#67572=CARTESIAN_POINT ( 'NONE',  ( 14.17500000122903536, 2.886751345948129099, -4.999999999999998224 ) ) ;
#67573=CARTESIAN_POINT ( 'NONE',  ( 21.40312500061451573, -4.541064518000417216, -2.621784821875001281 ) ) ;
#67574=CARTESIAN_POINT ( 'NONE',  ( 24.40312500061451573, 0.000000000000000000, 5.243569643749999010 ) ) ;
#67575=CARTESIAN_POINT ( 'NONE',  ( 5.428125000614517859, 4.541064518000418104, 2.621784821874999949 ) ) ;
#67577=VECTOR ( 'NONE', #55265, 1000.000000000000000 ) ;
#67578=DIRECTION ( 'NONE',  ( -0.000000000000000000, -1.000000000000000000, -0.000000000000000000 ) ) ;
#67582=CARTESIAN_POINT ( 'NONE',  ( -3.999999999999999112, 11.11250000122903536, -30.00000000000000000 ) ) ;
#67583=CARTESIAN_POINT ( 'NONE',  ( -4.243569643749999898, 18.02187500061452141, -32.45002607614398471 ) ) ;
#67584=CARTESIAN_POINT ( 'NONE',  ( 5.625000001229036428, 2.886751345948129099, -4.999999999999998224 ) ) ;
#67585=CARTESIAN_POINT ( 'NONE',  ( 7.275000000000000355, 6.123233995736764310E-16, -4.999999999999998224 ) ) ;
#67587=CARTESIAN_POINT ( 'NONE',  ( 4.087500001229035007, -4.330127018922194537, 2.499999999999995559 ) ) ;
#67588=CARTESIAN_POINT ( 'NONE',  ( 12.79687500061451821, -3.027376345333614438, 5.243569643749998122 ) ) ;
#67589=CARTESIAN_POINT ( 'NONE',  ( 3.999999999999999112, 16.73750000122903359, -30.00000000000000000 ) ) ;
#67590=CARTESIAN_POINT ( 'NONE',  ( 2.971875000614517592, -6.054752690667223547, -1.112240025338166033E-15 ) ) ;
#67591=CARTESIAN_POINT ( 'NONE',  ( 12.93750000122903465, 4.330127018922191873, 2.499999999999999556 ) ) ;
#67593=CARTESIAN_POINT ( 'NONE',  ( 10.62187500061451928, -6.054752690667223547, -1.112240025338166033E-15 ) ) ;
#67594=CARTESIAN_POINT ( 'NONE',  ( 1.071796769724495668, 17.09509619066136921, -26.00000000000000711 ) ) ;
#67595=CARTESIAN_POINT ( 'NONE',  ( 4.494741915665276366, -2.190272839526016924, 4.494741915664858922 ) ) ;
#67596=CARTESIAN_POINT ( 'NONE',  ( -2.121784821874999949, 17.02812500061459744, 26.32496088578401938 ) ) ;
#67597=CARTESIAN_POINT ( 'NONE',  ( 20.67187500061451289, 3.027376345333613106, -5.243569643749998122 ) ) ;
#67599=CARTESIAN_POINT ( 'NONE',  ( 2.953125000614516438, -4.541064518000417216, -2.621784821875001281 ) ) ;
#67601=CARTESIAN_POINT ( 'NONE',  ( 25.15312500061451217, 4.541064518000418104, -2.621784821874998173 ) ) ;
#67602=CARTESIAN_POINT ( 'NONE',  ( 14.39062500061451821, 6.054752690667223547, 3.707466751127219781E-16 ) ) ;
#67604=CARTESIAN_POINT ( 'NONE',  ( 11.70937500061451608, 4.541064518000418104, -2.621784821874998173 ) ) ;
#67605=CARTESIAN_POINT ( 'NONE',  ( 29.51249999999999929, 2.886751345948126879, 4.999999999999999112 ) ) ;
#67606=CARTESIAN_POINT ( 'NONE',  ( 25.80000000122903714, -2.886751345948125991, -5.000000000000000000 ) ) ;
#67607=CARTESIAN_POINT ( 'NONE',  ( 3.159375000614518036, 4.541064518000418104, -2.621784821874998173 ) ) ;
#67608=CARTESIAN_POINT ( 'NONE',  ( 15.27187500061451786, 3.027376345333613106, -5.243569643749998122 ) ) ;
#67610=CARTESIAN_POINT ( 'NONE',  ( 30.00000000000000000, 6.123233995736764310E-16, -4.999999999999998224 ) ) ;
#67611=CARTESIAN_POINT ( 'NONE',  ( 21.83437500061451786, -4.541064518000419881, 2.621784821874995952 ) ) ;
#67612=CARTESIAN_POINT ( 'NONE',  ( 13.73437500061451821, -4.541064518000419881, 2.621784821874995952 ) ) ;
#67614=CARTESIAN_POINT ( 'NONE',  ( 27.82499999999999929, -4.330127018922194537, 2.499999999999995559 ) ) ;
#67615=CARTESIAN_POINT ( 'NONE',  ( 0.000000000000000000, 20.00000000000000000, 30.00000000000000000 ) ) ;
#67617=CARTESIAN_POINT ( 'NONE',  ( 17.31562500061451715, -6.054752690667223547, -1.112240025338166033E-15 ) ) ;
#67618=CARTESIAN_POINT ( 'NONE',  ( 7.650000000000000355, -4.330127018922190985, -2.500000000000001332 ) ) ;
#67619=CARTESIAN_POINT ( 'NONE',  ( 15.37500000000000000, 6.123233995736764310E-16, -4.999999999999998224 ) ) ;
#67620=CARTESIAN_POINT ( 'NONE',  ( 15.97499999999999964, 4.330127018922191873, 2.499999999999999556 ) ) ;
#67621=CARTESIAN_POINT ( 'NONE',  ( 2.121784821874999061, 13.35312500061451679, 26.32496088578401583 ) ) ;
#67623=CARTESIAN_POINT ( 'NONE',  ( 20.85000000122903430, -2.886751345948125991, -5.000000000000000000 ) ) ;
#67625=CARTESIAN_POINT ( 'NONE',  ( 28.20937500061451786, -4.541064518000417216, -2.621784821875001281 ) ) ;
#67627=CARTESIAN_POINT ( 'NONE',  ( 22.45312500061451644, 4.541064518000418104, -2.621784821874998173 ) ) ;
#67628=CARTESIAN_POINT ( 'NONE',  ( 22.39687500061451075, -3.027376345333610441, -5.243569643749999898 ) ) ;
#67629=CARTESIAN_POINT ( 'NONE',  ( 7.537500000000002309, -2.886751345948129988, 4.999999999999997335 ) ) ;
#67630=CARTESIAN_POINT ( 'NONE',  ( 10.00312500061451715, 0.000000000000000000, 5.243569643749999010 ) ) ;
#67631=CARTESIAN_POINT ( 'NONE',  ( 24.32812500061451289, 4.541064518000418104, 2.621784821874999949 ) ) ;
#67632=CARTESIAN_POINT ( 'NONE',  ( 15.53437500061451715, -4.541064518000419881, 2.621784821874995952 ) ) ;
#67633=CARTESIAN_POINT ( 'NONE',  ( 16.95937500061451786, -4.541064518000417216, -2.621784821875001281 ) ) ;
#67634=CARTESIAN_POINT ( 'NONE',  ( 19.31250000000000000, -5.773502691896255534, -1.060575238724906372E-15 ) ) ;
#67635=CARTESIAN_POINT ( 'NONE',  ( 4.243569643749999898, 18.67812500061451431, 30.00000000000000000 ) ) ;
#67637=CARTESIAN_POINT ( 'NONE',  ( 21.30000000122903359, -2.886751345948125991, -5.000000000000000000 ) ) ;
#67639=CARTESIAN_POINT ( 'NONE',  ( 12.21562500061451573, 3.027376345333611329, 5.243569643749999010 ) ) ;
#67640=CARTESIAN_POINT ( 'NONE',  ( 6.384375000614516793, 4.541064518000418104, 2.621784821874999949 ) ) ;
#67641=CARTESIAN_POINT ( 'NONE',  ( 3.834375000614519635, -4.541064518000419881, 2.621784821874995952 ) ) ;
#67642=ORIENTED_EDGE ( 'NONE', *, *, #67328, .F. ) ;
#67643=CARTESIAN_POINT ( 'NONE',  ( 27.23437500061451644, -4.541064518000419881, 2.621784821874995952 ) ) ;
#67644=CARTESIAN_POINT ( 'NONE',  ( 16.67812500061451786, 4.541064518000418104, 2.621784821874999949 ) ) ;
#67645=CARTESIAN_POINT ( 'NONE',  ( 27.07500000122903216, -5.773502691896255534, -1.060575238724906372E-15 ) ) ;
#67646=CARTESIAN_POINT ( 'NONE',  ( 26.61562500061451786, 3.027376345333611329, 5.243569643749999010 ) ) ;
#67647=CARTESIAN_POINT ( 'NONE',  ( 21.94687500061451857, -3.027376345333610441, -5.243569643749999898 ) ) ;
#67648=CARTESIAN_POINT ( 'NONE',  ( 17.65312500061451573, 0.000000000000000000, 5.243569643749999010 ) ) ;
#67649=CARTESIAN_POINT ( 'NONE',  ( 8.484601909799253346E-16, 10.66250000000000142, 34.61880215351700230 ) ) ;
#67650=CARTESIAN_POINT ( 'NONE',  ( 25.00312500061451715, -4.541064518000417216, -2.621784821875001281 ) ) ;
#67651=CARTESIAN_POINT ( 'NONE',  ( 5.475000001229035185, -5.773502691896255534, -1.060575238724906372E-15 ) ) ;
#67653=CARTESIAN_POINT ( 'NONE',  ( 28.08749999999999858, 5.773502691896255534, 3.535250795749688894E-16 ) ) ;
#67654=CARTESIAN_POINT ( 'NONE',  ( 8.484601909799253346E-16, 12.01250000000000107, -25.38119784648299770 ) ) ;
#67656=CARTESIAN_POINT ( 'NONE',  ( 4.209375000614516971, 0.000000000000000000, 5.243569643749999010 ) ) ;
#67657=CARTESIAN_POINT ( 'NONE',  ( 9.590625000614517504, -3.027376345333614438, 5.243569643749998122 ) ) ;
#67658=CARTESIAN_POINT ( 'NONE',  ( 6.234375000614519102, 6.421520780324663323E-16, -5.243569643749999010 ) ) ;
#67659=CARTESIAN_POINT ( 'NONE',  ( 24.11250000122903359, 4.330127018922192761, -2.499999999999997780 ) ) ;
#67660=CARTESIAN_POINT ( 'NONE',  ( 12.12187500061451573, 3.027376345333612662, -5.243569643749998122 ) ) ;
#67661=CARTESIAN_POINT ( 'NONE',  ( 28.64062500061451289, -3.027376345333610441, -5.243569643749999898 ) ) ;
#67662=CARTESIAN_POINT ( 'NONE',  ( 26.92499999999999716, -4.330127018922194537, 2.499999999999995559 ) ) ;
#67663=DIRECTION ( 'NONE',  ( -1.000000000000000000, -0.000000000000000000, -0.000000000000000000 ) ) ;
#67664=CARTESIAN_POINT ( 'NONE',  ( 13.94062500061451892, 6.054752690667223547, 3.707466751127219781E-16 ) ) ;
#67665=( BOUNDED_CURVE ( )  B_SPLINE_CURVE ( 2, ( #52147, #56951, #62500, #17429, #30342, #828, #63587 ),
 .UNSPECIFIED., .F., .F. ) 
 B_SPLINE_CURVE_WITH_KNOTS ( ( 3, 2, 2, 3 ),
 ( 0.9770271732711595103, 0.9777777777777777457, 0.9805555555555555136, 0.9812341018960827332 ),
 .UNSPECIFIED. ) 
 CURVE ( )  GEOMETRIC_REPRESENTATION_ITEM ( )  RATIONAL_B_SPLINE_CURVE ( ( 0.9471604034606007083, 0.9637977031509668002, 1.000000000000000000, 0.8660254037844387076, 1.000000000000000000, 0.9672731300851546976, 0.9505350825990019903 ) ) 
 REPRESENTATION_ITEM ( '' )  );
#67666=EDGE_LOOP ( 'NONE', ( #17773, #28121, #58726, #63946 ) ) ;
#67667=CARTESIAN_POINT ( 'NONE',  ( 10.79062500061451679, 6.054752690667223547, 3.707466751127219781E-16 ) ) ;
#67668=CARTESIAN_POINT ( 'NONE',  ( 6.065625000614516260, -6.054752690667223547, -1.112240025338166033E-15 ) ) ;
#67670=CARTESIAN_POINT ( 'NONE',  ( 25.38750000122903216, 6.123233995736764310E-16, -4.999999999999998224 ) ) ;
#67671=CARTESIAN_POINT ( 'NONE',  ( 16.12500000000000000, -4.330127018922194537, 2.499999999999995559 ) ) ;
#67672=CARTESIAN_POINT ( 'NONE',  ( 16.84687500061451715, -3.027376345333614438, 5.243569643749998122 ) ) ;
#67673=CARTESIAN_POINT ( 'NONE',  ( 11.88750000122903216, 6.123233995736764310E-16, -4.999999999999998224 ) ) ;
#67675=CARTESIAN_POINT ( 'NONE',  ( 20.14687500061451786, -3.027376345333610441, -5.243569643749999898 ) ) ;
#67676=CARTESIAN_POINT ( 'NONE',  ( 4.243569643749999898, 15.04062500061451679, -27.54997392385601529 ) ) ;
#67679=CARTESIAN_POINT ( 'NONE',  ( 2.000000000000001332, 11.60000000000000142, -26.53589838486224650 ) ) ;
#67680=CARTESIAN_POINT ( 'NONE',  ( 26.80312500061451431, -4.541064518000417216, -2.621784821875001281 ) ) ;
#67682=EDGE_CURVE ( 'NONE', #43575, #20886, #63276, .T. ) ;
#67683=CARTESIAN_POINT ( 'NONE',  ( 24.89999999999999858, 4.330127018922192761, -2.499999999999997780 ) ) ;
#67684=CARTESIAN_POINT ( 'NONE',  ( 10.15312500061451750, -4.541064518000417216, -2.621784821875001281 ) ) ;
#67686=CARTESIAN_POINT ( 'NONE',  ( 18.04687500061451999, 6.054752690667223547, 3.707466751127219781E-16 ) ) ;
#67688=CARTESIAN_POINT ( 'NONE',  ( 5.840625000614516615, 6.054752690667223547, 3.707466751127219781E-16 ) ) ;
#67689=CARTESIAN_POINT ( 'NONE',  ( 9.796875000614519990, -3.027376345333610441, -5.243569643749999898 ) ) ;
#67691=CARTESIAN_POINT ( 'NONE',  ( 20.55937500061451573, -4.541064518000417216, -2.621784821875001281 ) ) ;
#67692=CARTESIAN_POINT ( 'NONE',  ( 28.31250000000000000, -5.773502691896255534, -1.060575238724906372E-15 ) ) ;
#67693=CARTESIAN_POINT ( 'NONE',  ( 5.962500000000002132, 2.886751345948129099, -4.999999999999998224 ) ) ;
#67694=CARTESIAN_POINT ( 'NONE',  ( 14.28750000122903430, 4.330127018922191873, 2.499999999999999556 ) ) ;
#67695=CARTESIAN_POINT ( 'NONE',  ( 3.999999999999999112, 12.23750000122903359, 30.00000000000000000 ) ) ;
#67696=CARTESIAN_POINT ( 'NONE',  ( -1.071796769724490783, 19.19240381056767220, -26.00000000000000355 ) ) ;
#67698=CARTESIAN_POINT ( 'NONE',  ( 13.50000000000000178, -4.330127018922190985, -2.500000000000001332 ) ) ;
#67699=CARTESIAN_POINT ( 'NONE',  ( 24.06562500061451715, -6.054752690667223547, -1.112240025338166033E-15 ) ) ;
#67700=CARTESIAN_POINT ( 'NONE',  ( 16.12500000000000000, -4.330127018922194537, 2.499999999999995559 ) ) ;
#67701=CARTESIAN_POINT ( 'NONE',  ( 10.08750000122903323, 6.123233995736764310E-16, -4.999999999999998224 ) ) ;
#67702=CARTESIAN_POINT ( 'NONE',  ( 9.515625000614518214, 3.027376345333611329, 5.243569643749999010 ) ) ;
#67703=CARTESIAN_POINT ( 'NONE',  ( 9.074999999999999289, 6.123233995736764310E-16, -4.999999999999998224 ) ) ;
#67704=CARTESIAN_POINT ( 'NONE',  ( 18.86250000122903359, 0.000000000000000000, 4.999999999999998224 ) ) ;
#67705=CARTESIAN_POINT ( 'NONE',  ( -4.243569643749997233, 14.49687500061451928, -27.54997392385601174 ) ) ;
#67706=CARTESIAN_POINT ( 'NONE',  ( 26.96250000122903145, 0.000000000000000000, 4.999999999999998224 ) ) ;
#67708=CARTESIAN_POINT ( 'NONE',  ( 7.950000000000001954, 0.000000000000000000, 4.999999999999998224 ) ) ;
#67709=CARTESIAN_POINT ( 'NONE',  ( 4.898587196589411843E-16, 20.00000000000000000, 33.99999999999999289 ) ) ;
#67711=CARTESIAN_POINT ( 'NONE',  ( 23.54062500061451146, -3.027376345333614438, 5.243569643749998122 ) ) ;
#67712=CARTESIAN_POINT ( 'NONE',  ( 13.16250000122903430, -4.330127018922190985, -2.500000000000001332 ) ) ;
#67713=CARTESIAN_POINT ( 'NONE',  ( 29.31562500061451715, 3.027376345333611329, 5.243569643749999010 ) ) ;
#67714=CARTESIAN_POINT ( 'NONE',  ( 29.37187500061451928, 3.027376345333611329, 5.243569643749999010 ) ) ;
#67715=CARTESIAN_POINT ( 'NONE',  ( 18.64687500061451786, -3.027376345333614438, 5.243569643749998122 ) ) ;
#67716=CARTESIAN_POINT ( 'NONE',  ( 16.82812500061451644, -4.541064518000419881, 2.621784821874995952 ) ) ;
#67717=CARTESIAN_POINT ( 'NONE',  ( -4.243569643749998122, 12.19062500061459353, -27.54997392385601174 ) ) ;
#67718=CARTESIAN_POINT ( 'NONE',  ( 5.915625000614515905, 3.027376345333611329, 5.243569643749999010 ) ) ;
#67719=CARTESIAN_POINT ( 'NONE',  ( 28.35000000122903430, -2.886751345948129988, 4.999999999999997335 ) ) ;
#67721=CARTESIAN_POINT ( 'NONE',  ( 19.52812500061451573, -4.541064518000419881, 2.621784821874995952 ) ) ;
#67724=CARTESIAN_POINT ( 'NONE',  ( 13.95937500061451786, 4.541064518000418104, -2.621784821874998173 ) ) ;
#67725=CARTESIAN_POINT ( 'NONE',  ( 10.84687500061451892, 6.054752690667223547, 3.707466751127219781E-16 ) ) ;
#67726=CARTESIAN_POINT ( 'NONE',  ( 20.33437500061451786, 4.541064518000418104, 2.621784821874999949 ) ) ;
#67727=ORIENTED_EDGE ( 'NONE', *, *, #57642, .T. ) ;
#67728=CARTESIAN_POINT ( 'NONE',  ( 27.25312500061451360, -4.541064518000417216, -2.621784821875001281 ) ) ;
#67729=CARTESIAN_POINT ( 'NONE',  ( 25.11562500061451431, 3.027376345333613106, -5.243569643749998122 ) ) ;
#67731=CARTESIAN_POINT ( 'NONE',  ( 2.000000000000001332, 17.00000000000000000, 33.46410161513774995 ) ) ;
#67733=CARTESIAN_POINT ( 'NONE',  ( 4.396875000614516971, -3.027376345333610441, -5.243569643749999898 ) ) ;
#67735=CARTESIAN_POINT ( 'NONE',  ( 11.77500000122903501, -5.773502691896255534, -1.060575238724906372E-15 ) ) ;
#67736=CARTESIAN_POINT ( 'NONE',  ( 8.137500001229033941, -4.330127018922194537, 2.499999999999995559 ) ) ;
#67737=CARTESIAN_POINT ( 'NONE',  ( 21.67500000122902648, -5.773502691896255534, -1.060575238724906372E-15 ) ) ;
#67738=CARTESIAN_POINT ( 'NONE',  ( 28.65000000122903145, 5.773502691896255534, 3.535250795749688894E-16 ) ) ;
#67741=CARTESIAN_POINT ( 'NONE',  ( 10.99687500061451750, -3.027376345333614438, 5.243569643749998122 ) ) ;
#67743=EDGE_CURVE ( 'NONE', #60188, #29691, #18918, .T. ) ;
#67744=CARTESIAN_POINT ( 'NONE',  ( 16.52812500061451573, 6.421520780324663323E-16, -5.243569643749999010 ) ) ;
#67745=CARTESIAN_POINT ( 'NONE',  ( 13.32187500061451502, -6.054752690667223547, -1.112240025338166033E-15 ) ) ;
#67746=CARTESIAN_POINT ( 'NONE',  ( 4.715625000614516615, -6.054752690667223547, -1.112240025338166033E-15 ) ) ;
#67747=CARTESIAN_POINT ( 'NONE',  ( 22.09687500061451715, 6.054752690667223547, 3.707466751127219781E-16 ) ) ;
#67748=CARTESIAN_POINT ( 'NONE',  ( 10.50937500061451679, 0.000000000000000000, 5.243569643749999010 ) ) ;
#67749=CARTESIAN_POINT ( 'NONE',  ( 4.040625000614517681, 6.054752690667223547, 3.707466751127219781E-16 ) ) ;
#67751=CARTESIAN_POINT ( 'NONE',  ( 5.887500001229034829, -4.330127018922194537, 2.499999999999995559 ) ) ;
#67752=CARTESIAN_POINT ( 'NONE',  ( 20.42812500061451431, -4.541064518000419881, 2.621784821874995952 ) ) ;
#67753=CARTESIAN_POINT ( 'NONE',  ( 7.350000001229033408, -2.886751345948125991, -5.000000000000000000 ) ) ;
#67754=CARTESIAN_POINT ( 'NONE',  ( 18.44062500061451715, 6.054752690667223547, 3.707466751127219781E-16 ) ) ;
#67755=CARTESIAN_POINT ( 'NONE',  ( 12.77812500061451750, -4.541064518000419881, 2.621784821874995952 ) ) ;
#67757=CARTESIAN_POINT ( 'NONE',  ( 14.24999999999999822, 0.000000000000000000, 4.999999999999998224 ) ) ;
#67758=CARTESIAN_POINT ( 'NONE',  ( 9.562500001229032875, -4.330127018922190985, -2.500000000000001332 ) ) ;
#67759=CARTESIAN_POINT ( 'NONE',  ( 6.590625000614518392, -3.027376345333610441, -5.243569643749999898 ) ) ;
#67760=CARTESIAN_POINT ( 'NONE',  ( 21.93750000122903288, 4.330127018922191873, 2.499999999999999556 ) ) ;
#67762=CARTESIAN_POINT ( 'NONE',  ( -4.243569643749999898, 10.85937500061451821, -30.00000000000000000 ) ) ;
#67763=CARTESIAN_POINT ( 'NONE',  ( 1.626862140677534273E-15, 17.86250000000000071, 34.00000000000000000 ) ) ;
#67764=FACE_OUTER_BOUND ( 'NONE', #640, .T. ) ;
#67765=CARTESIAN_POINT ( 'NONE',  ( -3.999999999999999112, 11.45000000000000107, -30.00000000000000000 ) ) ;
#67766=CARTESIAN_POINT ( 'NONE',  ( 21.64687500061451786, 6.054752690667223547, 3.707466751127219781E-16 ) ) ;
#67768=CARTESIAN_POINT ( 'NONE',  ( 2.000000000000001332, 18.46250000122903501, 33.46410161513774995 ) ) ;
#67769=CARTESIAN_POINT ( 'NONE',  ( 16.86562500061451786, -6.054752690667223547, -1.112240025338166033E-15 ) ) ;
#67772=CARTESIAN_POINT ( 'NONE',  ( 4.385796401931335353, -2.400997692794667682, 4.385796401931427724 ) ) ;
#67773=CARTESIAN_POINT ( 'NONE',  ( 26.52187500061451431, 3.027376345333613106, -5.243569643749998122 ) ) ;
#67775=AXIS2_PLACEMENT_3D ( 'NONE', #58826, #31869, #8973 ) ;
#67776=CARTESIAN_POINT ( 'NONE',  ( 12.55312500061451786, 4.541064518000418104, -2.621784821874998173 ) ) ;
#67777=CARTESIAN_POINT ( 'NONE',  ( 9.796875000614519990, -3.027376345333610441, -5.243569643749999898 ) ) ;
#67778=ORIENTED_EDGE ( 'NONE', *, *, #24990, .F. ) ;
#67779=CARTESIAN_POINT ( 'NONE',  ( -5.810221930991193690E-16, 14.03750000000000142, -34.00000000000000000 ) ) ;
#67780=CARTESIAN_POINT ( 'NONE',  ( 23.76562500061451644, 3.027376345333613106, -5.243569643749998122 ) ) ;
#67781=CARTESIAN_POINT ( 'NONE',  ( 30.00000000000000000, 0.000000000000000000, 0.000000000000000000 ) ) ;
#67782=CARTESIAN_POINT ( 'NONE',  ( 26.62500000000000000, 6.123233995736764310E-16, -4.999999999999998224 ) ) ;
#67783=CARTESIAN_POINT ( 'NONE',  ( 11.92500000000000071, 4.330127018922191873, 2.499999999999999556 ) ) ;
#67784=CARTESIAN_POINT ( 'NONE',  ( 21.78750000122903074, 6.123233995736764310E-16, -4.999999999999998224 ) ) ;
#67785=CARTESIAN_POINT ( 'NONE',  ( 16.37812500061451715, -4.541064518000419881, 2.621784821874995952 ) ) ;
#67788=CARTESIAN_POINT ( 'NONE',  ( 20.47500000000000142, 4.330127018922191873, 2.499999999999999556 ) ) ;
#67789=CARTESIAN_POINT ( 'NONE',  ( 23.69999999999999929, 0.000000000000000000, 4.999999999999998224 ) ) ;
#67790=CARTESIAN_POINT ( 'NONE',  ( 22.09687500061451715, 6.054752690667223547, 3.707466751127219781E-16 ) ) ;
#67791=CARTESIAN_POINT ( 'NONE',  ( 25.22812500061451502, 4.541064518000418104, 2.621784821874999949 ) ) ;
#67794=CARTESIAN_POINT ( 'NONE',  ( 8.765625000614518214, -6.054752690667223547, -1.112240025338166033E-15 ) ) ;
#67795=CARTESIAN_POINT ( 'NONE',  ( 3.313217074437887266, 3.744712918542242974, 3.512650841967440041 ) ) ;
#67796=CARTESIAN_POINT ( 'NONE',  ( 15.18750000000000000, -2.886751345948129988, 4.999999999999997335 ) ) ;
#67797=CARTESIAN_POINT ( 'NONE',  ( 9.001249775931846008E-16, 18.11562500061451786, 34.90005215228797653 ) ) ;
#67798=CARTESIAN_POINT ( 'NONE',  ( 5.709375000614517859, -4.541064518000417216, -2.621784821875001281 ) ) ;
#67799=VECTOR ( 'NONE', #37036, 1000.000000000000000 ) ;
#67800=CARTESIAN_POINT ( 'NONE',  ( 26.37187500061451217, -6.054752690667223547, -1.112240025338166033E-15 ) ) ;
#67802=CARTESIAN_POINT ( 'NONE',  ( 23.42812500061451786, 4.541064518000418104, 2.621784821874999949 ) ) ;
#67803=CARTESIAN_POINT ( 'NONE',  ( 24.72187500061451360, 3.027376345333613106, -5.243569643749998122 ) ) ;
#67804=CARTESIAN_POINT ( 'NONE',  ( 2.121784821874999061, 19.20312500061459460, -33.67503911421598417 ) ) ;
#67805=CARTESIAN_POINT ( 'NONE',  ( 12.18750000000000000, -2.886751345948125991, -5.000000000000000000 ) ) ;
#67806=CARTESIAN_POINT ( 'NONE',  ( 8.390625000614518214, -3.027376345333610441, -5.243569643749999898 ) ) ;
#67807=DIRECTION ( 'NONE',  ( -0.000000000000000000, -1.000000000000000000, -0.000000000000000000 ) ) ;
#67808=CARTESIAN_POINT ( 'NONE',  ( 28.37812500061451715, 4.541064518000418104, 2.621784821874999949 ) ) ;
#67809=CARTESIAN_POINT ( 'NONE',  ( 27.14062500061451644, -3.027376345333614438, 5.243569643749998122 ) ) ;
#67812=CARTESIAN_POINT ( 'NONE',  ( 4.003125000614518925, 4.541064518000418104, -2.621784821874998173 ) ) ;
#67813=CARTESIAN_POINT ( 'NONE',  ( 19.73437500061451644, 6.421520780324663323E-16, -5.243569643749999010 ) ) ;
#67815=CARTESIAN_POINT ( 'NONE',  ( 4.243569643749999898, 14.68437500061451750, 30.00000000000000000 ) ) ;
#67816=CARTESIAN_POINT ( 'NONE',  ( 19.43437500061451928, 4.541064518000418104, 2.621784821874999949 ) ) ;
#67817=CARTESIAN_POINT ( 'NONE',  ( 3.262500000000001510, 2.886751345948129099, -4.999999999999998224 ) ) ;
#67818=CARTESIAN_POINT ( 'NONE',  ( 4.243569643749999898, 18.28437500061451715, 30.00000000000000000 ) ) ;
#67819=CARTESIAN_POINT ( 'NONE',  ( 10.56562500061451715, -6.054752690667223547, -1.112240025338166033E-15 ) ) ;
#67820=DIRECTION ( 'NONE',  ( -0.000000000000000000, -1.000000000000000000, -0.000000000000000000 ) ) ;
#67821=CARTESIAN_POINT ( 'NONE',  ( 7.546875000614517326, -3.027376345333610441, -5.243569643749999898 ) ) ;
#67822=CARTESIAN_POINT ( 'NONE',  ( 25.87500000122903643, 2.886751345948146419, -4.999999999999968914 ) ) ;
#67823=CARTESIAN_POINT ( 'NONE',  ( 7.415625000614516793, -6.054752690667223547, -1.112240025338166033E-15 ) ) ;
#67824=CARTESIAN_POINT ( 'NONE',  ( 12.87187500061451750, -6.054752690667223547, -1.112240025338166033E-15 ) ) ;
#67825=CARTESIAN_POINT ( 'NONE',  ( 20.10000000122903074, 5.773502691896255534, 3.535250795749688894E-16 ) ) ;
#67826=CARTESIAN_POINT ( 'NONE',  ( 6.009375000614519458, 0.000000000000000000, 5.243569643749999010 ) ) ;
#67827=CARTESIAN_POINT ( 'NONE',  ( 8.803125000614517859, -4.541064518000417216, -2.621784821875001281 ) ) ;
#67828=CARTESIAN_POINT ( 'NONE',  ( 5.840625000614517504, 6.054752690667223547, 3.707466751127219781E-16 ) ) ;
#67830=CARTESIAN_POINT ( 'NONE',  ( 19.35937500061451644, 4.541064518000418104, -2.621784821874998173 ) ) ;
#67831=CARTESIAN_POINT ( 'NONE',  ( -3.999999999999997335, 11.60000000122903430, 32.30940107675850470 ) ) ;
#67832=EDGE_LOOP ( 'NONE', ( #56417, #35908, #2806, #18880 ) ) ;
#67833=CARTESIAN_POINT ( 'NONE',  ( 26.05312500061451431, 4.541064518000418104, -2.621784821874998173 ) ) ;
#67834=CARTESIAN_POINT ( 'NONE',  ( 12.70312500061451821, 0.000000000000000000, 5.243569643749999010 ) ) ;
#67835=CARTESIAN_POINT ( 'NONE',  ( 28.62187500061451573, -6.054752690667223547, -1.112240025338166033E-15 ) ) ;
#67836=CARTESIAN_POINT ( 'NONE',  ( 13.04062500061451502, 6.054752690667223547, 3.707466751127219781E-16 ) ) ;
#67837=CARTESIAN_POINT ( 'NONE',  ( 4.456355333853387890, -2.267705344768013553, -4.623151165536616425 ) ) ;
#67838=CARTESIAN_POINT ( 'NONE',  ( 12.45000000122903394, 5.773502691896255534, 3.535250795749688894E-16 ) ) ;
#67839=EDGE_CURVE ( 'NONE', #69508, #43636, #4166, .T. ) ;
#67840=CARTESIAN_POINT ( 'NONE',  ( 26.65312500061451573, 0.000000000000000000, 5.243569643749999010 ) ) ;
#67841=CARTESIAN_POINT ( 'NONE',  ( -3.000416591977282496E-16, 14.74062500061451786, -34.90005215228797653 ) ) ;
#67842=CARTESIAN_POINT ( 'NONE',  ( 16.20000000122903216, -2.886751345948129988, 4.999999999999997335 ) ) ;
#67843=AXIS2_PLACEMENT_3D ( 'NONE', #47482, #29051, #41943 ) ;
#67844=CARTESIAN_POINT ( 'NONE',  ( 14.40000000000000036, -4.330127018922190985, -2.500000000000001332 ) ) ;
#67845=CARTESIAN_POINT ( 'NONE',  ( 20.39062500061451644, -3.027376345333614438, 5.243569643749998122 ) ) ;
#67846=CARTESIAN_POINT ( 'NONE',  ( 7.509375000614517681, -4.541064518000417216, -2.621784821875001281 ) ) ;
#67847=CARTESIAN_POINT ( 'NONE',  ( 7.650000001229034119, -2.886751345948129988, 4.999999999999997335 ) ) ;
#67848=CARTESIAN_POINT ( 'NONE',  ( 16.16250000122903430, 0.000000000000000000, 4.999999999999998224 ) ) ;
#67849=CARTESIAN_POINT ( 'NONE',  ( 13.19062500061451537, -3.027376345333614438, 5.243569643749998122 ) ) ;
#67850=CARTESIAN_POINT ( 'NONE',  ( 15.21562500061451750, 3.027376345333613106, -5.243569643749998122 ) ) ;
#67851=CARTESIAN_POINT ( 'NONE',  ( 28.68750000122903288, 4.330127018922191873, 2.499999999999999556 ) ) ;
#67852=CARTESIAN_POINT ( 'NONE',  ( 21.63749999999999929, -2.886751345948125991, -5.000000000000000000 ) ) ;
#67853=CARTESIAN_POINT ( 'NONE',  ( 23.33437500061451786, 6.421520780324663323E-16, -5.243569643749999010 ) ) ;
#67855=CARTESIAN_POINT ( 'NONE',  ( 9.525000001229033231, -5.773502691896255534, -1.060575238724906372E-15 ) ) ;
#67856=CARTESIAN_POINT ( 'NONE',  ( 28.05937500061451573, 0.000000000000000000, 5.243569643749999010 ) ) ;
#67858=EDGE_CURVE ( 'NONE', #4158, #41395, #36655, .T. ) ;
#67859=CARTESIAN_POINT ( 'NONE',  ( 5.034375000614519813, 4.541064518000418104, 2.621784821874999949 ) ) ;
#67860=CARTESIAN_POINT ( 'NONE',  ( 23.01562500061451644, 3.027376345333611329, 5.243569643749999010 ) ) ;
#67862=CARTESIAN_POINT ( 'NONE',  ( 6.862500000000002487, 2.886751345948129099, -4.999999999999997335 ) ) ;
#67863=CARTESIAN_POINT ( 'NONE',  ( 11.10937500061451644, -4.541064518000417216, -2.621784821875001281 ) ) ;
#67865=CARTESIAN_POINT ( 'NONE',  ( 2.896875000614518747, -3.027376345333614438, 5.243569643749998122 ) ) ;
#67866=CARTESIAN_POINT ( 'NONE',  ( 7.621875000614519280, 3.027376345333613106, -5.243569643749998122 ) ) ;
#67867=CARTESIAN_POINT ( 'NONE',  ( 6.750000000000002665, -4.330127018922190985, -2.500000000000001332 ) ) ;
#67868=CARTESIAN_POINT ( 'NONE',  ( 27.38437500061451857, 6.421520780324663323E-16, -5.243569643749999010 ) ) ;
#67869=CARTESIAN_POINT ( 'NONE',  ( 4.243569643749999010, 10.61562500061459602, 27.54997392385601174 ) ) ;
#67870=CARTESIAN_POINT ( 'NONE',  ( 18.45000000000000284, -4.330127018922190985, -2.500000000000001332 ) ) ;
#67872=CARTESIAN_POINT ( 'NONE',  ( 27.82499999999999929, -4.330127018922194537, 2.499999999999995559 ) ) ;
#67873=CARTESIAN_POINT ( 'NONE',  ( 29.63437500061451502, 6.421520780324663323E-16, -5.243569643749999010 ) ) ;
#67875=CARTESIAN_POINT ( 'NONE',  ( 14.80312500061451608, 4.541064518000418104, -2.621784821874998173 ) ) ;
#67876=CARTESIAN_POINT ( 'NONE',  ( 7.303125000614516082, 0.000000000000000000, 5.243569643749999010 ) ) ;
#67878=CARTESIAN_POINT ( 'NONE',  ( 4.734375000614518214, -4.541064518000419881, 2.621784821874995952 ) ) ;
#67879=CARTESIAN_POINT ( 'NONE',  ( 18.03750000122903430, -4.330127018922194537, 2.499999999999995559 ) ) ;
#67880=CARTESIAN_POINT ( 'NONE',  ( 22.50000000000000000, -4.330127018922190985, -2.500000000000001332 ) ) ;
#67881=CARTESIAN_POINT ( 'NONE',  ( 1.071796769724489895, 14.01740381056766793, -34.00000000000000000 ) ) ;
#67882=CARTESIAN_POINT ( 'NONE',  ( 6.909375000614518036, 0.000000000000000000, 5.243569643749999010 ) ) ;
#67883=CARTESIAN_POINT ( 'NONE',  ( 10.62187500061451928, -6.054752690667223547, -1.112240025338166033E-15 ) ) ;
#67884=CARTESIAN_POINT ( 'NONE',  ( 21.34687500061451715, -3.027376345333614438, 5.243569643749998122 ) ) ;
#67885=CARTESIAN_POINT ( 'NONE',  ( -2.000000000000000000, 16.32499999999999929, 26.53589838486224650 ) ) ;
#67887=CARTESIAN_POINT ( 'NONE',  ( 4.734375000614518214, -4.541064518000419881, 2.621784821874995952 ) ) ;
#67888=CARTESIAN_POINT ( 'NONE',  ( 6.234375000614519102, 6.421520780324663323E-16, -5.243569643749999010 ) ) ;
#67889=CARTESIAN_POINT ( 'NONE',  ( 18.82500000000000284, -4.330127018922194537, 2.499999999999995559 ) ) ;
#67890=CARTESIAN_POINT ( 'NONE',  ( 15.77812500061451573, 4.541064518000418104, 2.621784821874999949 ) ) ;
#67892=CARTESIAN_POINT ( 'NONE',  ( 24.86250000122903359, -4.330127018922190985, -2.500000000000001332 ) ) ;
#67894=CARTESIAN_POINT ( 'NONE',  ( 10.19062500061451892, -3.027376345333610441, -5.243569643749999898 ) ) ;
#67895=CARTESIAN_POINT ( 'NONE',  ( 27.68437500061451573, -4.541064518000419881, 2.621784821874995952 ) ) ;
#67897=CARTESIAN_POINT ( 'NONE',  ( 28.47187500061451715, 3.027376345333611329, 5.243569643749999010 ) ) ;
#67898=CARTESIAN_POINT ( 'NONE',  ( 9.262499999999999289, 2.886751345948126879, 4.999999999999999112 ) ) ;
#67899=CARTESIAN_POINT ( 'NONE',  ( 2.000000000000001332, 14.41250000122903430, 33.46410161513774995 ) ) ;
#67900=CARTESIAN_POINT ( 'NONE',  ( 9.562500001229032875, -4.330127018922190985, -2.500000000000001332 ) ) ;
#67901=CIRCLE ( 'NONE', #12469, 10.00000000000000000 ) ;
#67902=CARTESIAN_POINT ( 'NONE',  ( 20.18437500061451573, 6.421520780324663323E-16, -5.243569643749999010 ) ) ;
#67903=CARTESIAN_POINT ( 'NONE',  ( 14.48437500061451821, 4.541064518000418104, 2.621784821874999949 ) ) ;
#67906=CARTESIAN_POINT ( 'NONE',  ( 13.79062500061451502, -3.027376345333610441, -5.243569643749999898 ) ) ;
#67907=VECTOR ( 'NONE', #39987, 1000.000000000000000 ) ;
#67908=CARTESIAN_POINT ( 'NONE',  ( 26.17500000122903359, -5.773502691896255534, -1.060575238724906372E-15 ) ) ;
#67909=CARTESIAN_POINT ( 'NONE',  ( 15.68437500061451573, 6.421520780324663323E-16, -5.243569643749999010 ) ) ;
#67910=CARTESIAN_POINT ( 'NONE',  ( 3.403125000614518836, -4.541064518000417216, -2.621784821875001281 ) ) ;
#67911=CARTESIAN_POINT ( 'NONE',  ( 17.05312500061451786, 4.541064518000418104, -2.621784821874998173 ) ) ;
#67912=CARTESIAN_POINT ( 'NONE',  ( 20.88750000122903572, 6.123233995736764310E-16, -4.999999999999998224 ) ) ;
#67913=CARTESIAN_POINT ( 'NONE',  ( 25.50937500061451502, -4.541064518000417216, -2.621784821875001281 ) ) ;
#67914=CARTESIAN_POINT ( 'NONE',  ( -4.243569643749997233, 10.39062500061451644, 32.45002607614398471 ) ) ;
#67915=CARTESIAN_POINT ( 'NONE',  ( 15.45937500061451608, 0.000000000000000000, 5.243569643749999010 ) ) ;
#67916=CARTESIAN_POINT ( 'NONE',  ( 14.02500000122903323, -5.773502691896255534, -1.060575238724906372E-15 ) ) ;
#67918=CARTESIAN_POINT ( 'NONE',  ( 4.243569643749999898, 15.99687500061451573, -27.54997392385601529 ) ) ;
#67919=CARTESIAN_POINT ( 'NONE',  ( 18.49687500061452283, 6.054752690667223547, 3.707466751127219781E-16 ) ) ;
#67920=CARTESIAN_POINT ( 'NONE',  ( 20.51250000122903216, 4.330127018922192761, -2.499999999999997780 ) ) ;
#67921=CARTESIAN_POINT ( 'NONE',  ( 14.40937500061451715, 4.541064518000418104, -2.621784821874998173 ) ) ;
#67922=CARTESIAN_POINT ( 'NONE',  ( -2.121784821874999949, 13.48437500061451821, 26.32496088578401938 ) ) ;
#67923=CARTESIAN_POINT ( 'NONE',  ( 23.47500000122903430, -5.773502691896255534, -1.060575238724906372E-15 ) ) ;
#67924=CARTESIAN_POINT ( 'NONE',  ( 14.46562500061451750, 3.027376345333611329, 5.243569643749999010 ) ) ;
#67925=CARTESIAN_POINT ( 'NONE',  ( 29.39062500061451289, -3.027376345333614438, 5.243569643749998122 ) ) ;
#67926=VERTEX_POINT ( 'NONE', #35562 ) ;
#67928=CARTESIAN_POINT ( 'NONE',  ( 20.69999999999999929, -4.330127018922190985, -2.500000000000001332 ) ) ;
#67929=CARTESIAN_POINT ( 'NONE',  ( -3.999999999999999112, 17.82500000122903572, 27.69059892324149885 ) ) ;
#67930=CARTESIAN_POINT ( 'NONE',  ( 3.779877903161418473, 3.276378095916668620, 28.66642532236455665 ) ) ;
#67931=CARTESIAN_POINT ( 'NONE',  ( 16.08750000122903501, 4.330127018922191873, 2.499999999999999556 ) ) ;
#67932=CARTESIAN_POINT ( 'NONE',  ( 19.71562500061451928, 3.027376345333613106, -5.243569643749998122 ) ) ;
#67933=CARTESIAN_POINT ( 'NONE',  ( 23.42812500061451786, 4.541064518000418104, 2.621784821874999949 ) ) ;
#67934=CARTESIAN_POINT ( 'NONE',  ( 6.328125000614515550, 4.541064518000418104, 2.621784821874999949 ) ) ;
#67936=CARTESIAN_POINT ( 'NONE',  ( 4.589319506978690733, 1.984554166263133856, 4.853542117982821757 ) ) ;
#67939=CYLINDRICAL_SURFACE ( 'NONE', #18176, 4.000000000000000000 ) ;
#67940=CARTESIAN_POINT ( 'NONE',  ( 1.999999999999998668, 10.51250000122903572, -33.46410161513775705 ) ) ;
#67941=CARTESIAN_POINT ( 'NONE',  ( -4.243569643749997233, 19.44687500061451502, -27.54997392385601174 ) ) ;
#67942=CARTESIAN_POINT ( 'NONE',  ( 6.750000001229033764, -2.886751345948129988, 4.999999999999997335 ) ) ;
#67943=CARTESIAN_POINT ( 'NONE',  ( 7.312500000000000000, 2.886751345948129099, -4.999999999999998224 ) ) ;
#67944=ADVANCED_FACE ( 'NONE', ( #31113 ), #19280, .F. ) ;
#67945=CARTESIAN_POINT ( 'NONE',  ( 3.375000001229033320, 2.886751345948129099, -4.999999999999998224 ) ) ;
#67946=CARTESIAN_POINT ( 'NONE',  ( 12.83437500061451786, -4.541064518000419881, 2.621784821874995952 ) ) ;
#67947=CARTESIAN_POINT ( 'NONE',  ( 24.67500000122903359, 2.886751345948126879, 4.999999999999998224 ) ) ;
#67948=CARTESIAN_POINT ( 'NONE',  ( 3.271875000614519635, 3.027376345333611329, 5.243569643749999010 ) ) ;
#67949=CARTESIAN_POINT ( 'NONE',  ( -5.810221930991193690E-16, 15.83749999999999680, 26.00000000000000355 ) ) ;
#67952=CARTESIAN_POINT ( 'NONE',  ( 9.871875000614517504, 3.027376345333613106, -5.243569643749998122 ) ) ;
#67953=CARTESIAN_POINT ( 'NONE',  ( 12.98437500061451821, 6.421520780324663323E-16, -5.243569643749999010 ) ) ;
#67954=CARTESIAN_POINT ( 'NONE',  ( -1.071796769724488563, 18.74240381056766935, -26.00000000000000000 ) ) ;
#67955=CARTESIAN_POINT ( 'NONE',  ( 6.187500000000002665, -2.886751345948129988, 4.999999999999997335 ) ) ;
#67956=CARTESIAN_POINT ( 'NONE',  ( 4.243569643749999898, 16.39062500061459815, 32.45002607614398471 ) ) ;
#67957=CARTESIAN_POINT ( 'NONE',  ( 21.57187500061451502, 3.027376345333613106, -5.243569643749998122 ) ) ;
#67958=CARTESIAN_POINT ( 'NONE',  ( 27.48750000122903359, -4.330127018922194537, 2.499999999999995559 ) ) ;
#67960=CARTESIAN_POINT ( 'NONE',  ( 23.61562500061451431, -6.054752690667223547, -1.112240025338166033E-15 ) ) ;
#67961=CARTESIAN_POINT ( 'NONE',  ( 15.17812500061451608, 6.421520780324663323E-16, -5.243569643749999010 ) ) ;
#67963=CARTESIAN_POINT ( 'NONE',  ( 12.53437500061451537, 6.421520780324663323E-16, -5.243569643749999010 ) ) ;
#67964=CARTESIAN_POINT ( 'NONE',  ( 27.71250000000000568, 2.886751345948126879, 4.999999999999999112 ) ) ;
#67965=CARTESIAN_POINT ( 'NONE',  ( 24.78750000122903074, -4.330127018922194537, 2.499999999999995559 ) ) ;
#67966=CARTESIAN_POINT ( 'NONE',  ( 3.721875000614518036, 3.027376345333611329, 5.243569643749999010 ) ) ;
#67967=CARTESIAN_POINT ( 'NONE',  ( 13.62187500061451750, 3.027376345333611329, 5.243569643749999010 ) ) ;
#67968=CARTESIAN_POINT ( 'NONE',  ( 28.62187500061451573, -6.054752690667223547, -1.112240025338166033E-15 ) ) ;
#67969=CYLINDRICAL_SURFACE ( 'NONE', #54859, 4.999999999999998224 ) ;
#67970=CARTESIAN_POINT ( 'NONE',  ( 24.03750000122903430, 6.123233995736764310E-16, -4.999999999999998224 ) ) ;
#67971=CARTESIAN_POINT ( 'NONE',  ( 22.13437500061451502, 4.541064518000418104, 2.621784821874999949 ) ) ;
#67972=CARTESIAN_POINT ( 'NONE',  ( 14.07187500061451679, 3.027376345333611329, 5.243569643749999010 ) ) ;
#67974=CARTESIAN_POINT ( 'NONE',  ( 25.68750000000000000, -2.886751345948125991, -5.000000000000000000 ) ) ;
#67975=CARTESIAN_POINT ( 'NONE',  ( 4.087500001229035007, -4.330127018922194537, 2.499999999999995559 ) ) ;
#67977=CARTESIAN_POINT ( 'NONE',  ( 16.19062500061451715, 6.054752690667223547, 3.707466751127219781E-16 ) ) ;
#67978=CARTESIAN_POINT ( 'NONE',  ( 6.562500000000001776, 2.886751345948126879, 4.999999999999999112 ) ) ;
#67979=CARTESIAN_POINT ( 'NONE',  ( -5.810221930991193690E-16, 14.03750000000000142, 26.00000000000000355 ) ) ;
#67980=CARTESIAN_POINT ( 'NONE',  ( 16.46249999999999503, 2.886751345948126879, 4.999999999999999112 ) ) ;
#67981=CARTESIAN_POINT ( 'NONE',  ( 4.243569643749999898, 13.24062500061451786, 32.45002607614398471 ) ) ;
#67983=CARTESIAN_POINT ( 'NONE',  ( 21.86250000122903003, 4.330127018922192761, -2.499999999999997780 ) ) ;
#67984=CARTESIAN_POINT ( 'NONE',  ( 1.594043775273459307, 9.879932731042712746, 24.20196496940534914 ) ) ;
#67985=CARTESIAN_POINT ( 'NONE',  ( 27.60937500061451644, 0.000000000000000000, 5.243569643749999010 ) ) ;
#67987=CARTESIAN_POINT ( 'NONE',  ( 22.60312500061451857, 0.000000000000000000, 5.243569643749999010 ) ) ;
#67988=CARTESIAN_POINT ( 'NONE',  ( 23.29687500061451644, -3.027376345333610441, -5.243569643749999898 ) ) ;
#67989=CARTESIAN_POINT ( 'NONE',  ( 5.812500000000001776, -5.773502691896255534, -1.060575238724906372E-15 ) ) ;
#67990=CARTESIAN_POINT ( 'NONE',  ( 8.765625000614518214, -6.054752690667223547, -1.112240025338166033E-15 ) ) ;
#67991=CARTESIAN_POINT ( 'NONE',  ( 24.81562500061451715, 3.027376345333611329, 5.243569643749999010 ) ) ;
#67992=CARTESIAN_POINT ( 'NONE',  ( 13.35937500061451821, -4.541064518000417216, -2.621784821875001281 ) ) ;
#67993=CARTESIAN_POINT ( 'NONE',  ( 16.05937500061451573, -4.541064518000417216, -2.621784821875001281 ) ) ;
#67994=CARTESIAN_POINT ( 'NONE',  ( -0.6945831915928805111, 10.00052343484236950, 26.06076730949330411 ) ) ;
#67995=CARTESIAN_POINT ( 'NONE',  ( -2.121784821874999949, 17.92812500061451786, 26.32496088578401938 ) ) ;
#67996=CARTESIAN_POINT ( 'NONE',  ( 20.58750000122903145, 4.330127018922191873, 2.499999999999999556 ) ) ;
#67998=CARTESIAN_POINT ( 'NONE',  ( 12.77812500061451750, -4.541064518000419881, 2.621784821874995952 ) ) ;
#67999=CARTESIAN_POINT ( 'NONE',  ( 6.534375000614517148, -4.541064518000419881, 2.621784821874995952 ) ) ;
#68000=CARTESIAN_POINT ( 'NONE',  ( 3.796875000614517326, -3.027376345333614438, 5.243569643749998122 ) ) ;
#68001=ORIENTED_EDGE ( 'NONE', *, *, #29363, .F. ) ;
#68002=CARTESIAN_POINT ( 'NONE',  ( 26.52187500061451431, 3.027376345333613106, -5.243569643749998122 ) ) ;
#68003=CARTESIAN_POINT ( 'NONE',  ( 18.02812500061451573, 4.541064518000418104, 2.621784821874999949 ) ) ;
#68004=CARTESIAN_POINT ( 'NONE',  ( 26.85000000122903430, 5.773502691896255534, 3.535250795749688894E-16 ) ) ;
#68006=CARTESIAN_POINT ( 'NONE',  ( 28.30312500061451431, 4.541064518000418104, -2.621784821874998173 ) ) ;
#68007=CARTESIAN_POINT ( 'NONE',  ( 22.88437500061451857, 6.421520780324663323E-16, -5.243569643749999010 ) ) ;
#68008=CARTESIAN_POINT ( 'NONE',  ( 16.15312500061451573, 4.541064518000418104, -2.621784821874998173 ) ) ;
#68009=CARTESIAN_POINT ( 'NONE',  ( 2.121784821874999061, 19.70937500061451786, 26.32496088578401583 ) ) ;
#68010=CARTESIAN_POINT ( 'NONE',  ( 21.55312500061451431, 4.541064518000418104, -2.621784821874998173 ) ) ;
#68011=CARTESIAN_POINT ( 'NONE',  ( 3.975000001229033852, 2.886751345948126879, 4.999999999999999112 ) ) ;
#68013=CARTESIAN_POINT ( 'NONE',  ( 27.71250000000000568, 2.886751345948126879, 4.999999999999999112 ) ) ;
#68014=CARTESIAN_POINT ( 'NONE',  ( -3.999999999999999112, 11.90000000000000036, -30.00000000000000000 ) ) ;
#68016=CARTESIAN_POINT ( 'NONE',  ( 28.90312500061451217, 0.000000000000000000, 5.243569643749999010 ) ) ;
#68017=CARTESIAN_POINT ( 'NONE',  ( 10.97812500061451679, -4.541064518000419881, 2.621784821874995952 ) ) ;
#68018=CARTESIAN_POINT ( 'NONE',  ( 22.53750000122903430, -4.330127018922194537, 2.499999999999995559 ) ) ;
#68019=CARTESIAN_POINT ( 'NONE',  ( 12.87187500061451750, -6.054752690667223547, -1.112240025338166033E-15 ) ) ;
#68020=CARTESIAN_POINT ( 'NONE',  ( 26.24062500061451431, -3.027376345333614438, 5.243569643749998122 ) ) ;
#68021=CARTESIAN_POINT ( 'NONE',  ( 27.89999999999999858, -4.330127018922190985, -2.500000000000001332 ) ) ;
#68022=CARTESIAN_POINT ( 'NONE',  ( -2.000000000000000000, 18.23750000122903359, -33.46410161513775705 ) ) ;
#68024=CARTESIAN_POINT ( 'NONE',  ( 2.990625000614519191, -3.027376345333610441, -5.243569643749999898 ) ) ;
#68025=CARTESIAN_POINT ( 'NONE',  ( 12.02812500061451573, 6.421520780324663323E-16, -5.243569643749999010 ) ) ;
#68026=VERTEX_POINT ( 'NONE', #69557 ) ;
#68027=CARTESIAN_POINT ( 'NONE',  ( 7.528125000614515727, 6.421520780324663323E-16, -5.243569643749999010 ) ) ;
#68028=CARTESIAN_POINT ( 'NONE',  ( 4.865625000614517859, 3.027376345333613106, -5.243569643749998122 ) ) ;
#68031=EDGE_CURVE ( 'NONE', #71801, #16431, #36296, .T. ) ;
#68032=CARTESIAN_POINT ( 'NONE',  ( 14.13750000122903394, 6.123233995736764310E-16, -4.999999999999998224 ) ) ;
#68033=CARTESIAN_POINT ( 'NONE',  ( 15.93750000000000000, 5.773502691896255534, 3.535250795749688894E-16 ) ) ;
#68034=CARTESIAN_POINT ( 'NONE',  ( 15.75937500061451857, 4.541064518000418104, -2.621784821874998173 ) ) ;
#68035=CARTESIAN_POINT ( 'NONE',  ( 10.87500000122903288, -5.773502691896255534, -1.060575238724906372E-15 ) ) ;
#68036=CARTESIAN_POINT ( 'NONE',  ( 19.99687500061451573, -3.027376345333614438, 5.243569643749998122 ) ) ;
#68038=AXIS2_PLACEMENT_3D ( 'NONE', #35483, #69122, #1523 ) ;
#68039=CARTESIAN_POINT ( 'NONE',  ( 19.84687500061451360, 6.054752690667223547, 3.707466751127219781E-16 ) ) ;
#68040=CARTESIAN_POINT ( 'NONE',  ( -4.243569643749999898, 14.81562500061451715, -32.45002607614398471 ) ) ;
#68042=CARTESIAN_POINT ( 'NONE',  ( 3.144856541311010556, 3.887142566792906706, -3.519253510942787599 ) ) ;
#68043=CARTESIAN_POINT ( 'NONE',  ( 27.02812500061451573, 4.541064518000418104, 2.621784821874999949 ) ) ;
#68044=DIRECTION ( 'NONE',  ( 0.000000000000000000, 0.000000000000000000, 1.000000000000000000 ) ) ;
#68045=CARTESIAN_POINT ( 'NONE',  ( 28.62187500061451573, -6.054752690667223547, -1.112240025338166033E-15 ) ) ;
#68046=EDGE_CURVE ( 'NONE', #6716, #9071, #23982, .T. ) ;
#68047=CARTESIAN_POINT ( 'NONE',  ( 24.37500000000000000, 6.123233995736764310E-16, -4.999999999999998224 ) ) ;
#68048=CARTESIAN_POINT ( 'NONE',  ( 9.853125000614516793, 4.541064518000418104, -2.621784821874998173 ) ) ;
#68050=CARTESIAN_POINT ( 'NONE',  ( 19.77187500061451786, 3.027376345333613106, -5.243569643749998122 ) ) ;
#68052=CARTESIAN_POINT ( 'NONE',  ( 6.215625000614517504, 3.027376345333613106, -5.243569643749998122 ) ) ;
#68053=CARTESIAN_POINT ( 'NONE',  ( 10.47187500061451715, 3.027376345333611329, 5.243569643749999010 ) ) ;
#68055=CARTESIAN_POINT ( 'NONE',  ( 21.34687500061451715, -3.027376345333614438, 5.243569643749998122 ) ) ;
#68057=CARTESIAN_POINT ( 'NONE',  ( 28.38749999999999929, -2.886751345948125991, -5.000000000000000000 ) ) ;
#68059=CARTESIAN_POINT ( 'NONE',  ( 29.52187500061451431, -6.054752690667223547, -1.112240025338166033E-15 ) ) ;
#68060=CARTESIAN_POINT ( 'NONE',  ( 1.071796769724484344, 15.18259618943233669, -25.99999999999999645 ) ) ;
#68063=CARTESIAN_POINT ( 'NONE',  ( 12.93750000000000178, -2.886751345948129988, 4.999999999999997335 ) ) ;
#68065=CARTESIAN_POINT ( 'NONE',  ( 23.54062500061451146, -3.027376345333614438, 5.243569643749998122 ) ) ;
#68066=CARTESIAN_POINT ( 'NONE',  ( 15.11249999999999893, 2.886751345948126879, 4.999999999999999112 ) ) ;
#68067=CARTESIAN_POINT ( 'NONE',  ( 9.375000001229036428, 2.886751345948126879, 4.999999999999999112 ) ) ;
#68068=CARTESIAN_POINT ( 'NONE',  ( 8.278125000614515727, -4.541064518000419881, 2.621784821874995952 ) ) ;
#68069=CARTESIAN_POINT ( 'NONE',  ( 7.987500000000000711, -2.886751345948129988, 4.999999999999997335 ) ) ;
#68071=CARTESIAN_POINT ( 'NONE',  ( 28.72500000122903074, 2.886751345948126879, 4.999999999999999112 ) ) ;
#68073=CARTESIAN_POINT ( 'NONE',  ( 7.837499999999999467, 5.773502691896255534, 3.535250795749688894E-16 ) ) ;
#68075=ORIENTED_EDGE ( 'NONE', *, *, #26600, .T. ) ;
#68076=CARTESIAN_POINT ( 'NONE',  ( 21.47812500061451502, 6.421520780324663323E-16, -5.243569643749999010 ) ) ;
#68077=CARTESIAN_POINT ( 'NONE',  ( 28.30312500061451431, 4.541064518000418104, -2.621784821874998173 ) ) ;
#68078=CARTESIAN_POINT ( 'NONE',  ( 29.55937500061451573, -4.541064518000417216, -2.621784821875001281 ) ) ;
#68079=CARTESIAN_POINT ( 'NONE',  ( 19.92187500061451644, 3.027376345333611329, 5.243569643749999010 ) ) ;
#68080=CARTESIAN_POINT ( 'NONE',  ( 16.97812500061451502, 6.421520780324663323E-16, -5.243569643749999010 ) ) ;
#68081=AXIS2_PLACEMENT_3D ( 'NONE', #24676, #13587, #58653 ) ;
#68082=CARTESIAN_POINT ( 'NONE',  ( 9.001249775931846008E-16, 12.26562500061459637, -25.09994784771203058 ) ) ;
#68083=CARTESIAN_POINT ( 'NONE',  ( 5.690625000614516260, -3.027376345333610441, -5.243569643749999898 ) ) ;
#68085=CARTESIAN_POINT ( 'NONE',  ( 28.31250000122903288, 0.000000000000000000, 4.999999999999998224 ) ) ;
#68087=CARTESIAN_POINT ( 'NONE',  ( 19.37812500061451715, 4.541064518000418104, 2.621784821874999949 ) ) ;
#68088=CARTESIAN_POINT ( 'NONE',  ( 3.999999999999998668, 11.37500000122903643, -32.30940107675850470 ) ) ;
#68089=CARTESIAN_POINT ( 'NONE',  ( 4.462500001229035007, 0.000000000000000000, 4.999999999999998224 ) ) ;
#68090=CARTESIAN_POINT ( 'NONE',  ( 13.54687500061451999, 6.054752690667223547, 3.707466751127219781E-16 ) ) ;
#68091=CARTESIAN_POINT ( 'NONE',  ( 11.74687500061451573, 6.054752690667223547, 3.707466751127219781E-16 ) ) ;
#68092=CARTESIAN_POINT ( 'NONE',  ( 20.14687500061451786, -3.027376345333610441, -5.243569643749999898 ) ) ;
#68094=CARTESIAN_POINT ( 'NONE',  ( 29.51249999999999929, 2.886751345948106007, 5.000000000000033751 ) ) ;
#68095=CARTESIAN_POINT ( 'NONE',  ( 23.84062500061451928, 6.054752690667223547, 3.707466751127219781E-16 ) ) ;
#68096=( BOUNDED_CURVE ( )  B_SPLINE_CURVE ( 2, ( #18019, #2497, #64914, #65275, #2863, #9503, #25021 ),
 .UNSPECIFIED., .F., .F. ) 
 B_SPLINE_CURVE_WITH_KNOTS ( ( 3, 2, 2, 3 ),
 ( 0.3833333333333333037, 0.3861111111111111271, 0.3888888888888889506, 0.3916666666666667740 ),
 .UNSPECIFIED. ) 
 CURVE ( )  GEOMETRIC_REPRESENTATION_ITEM ( )  RATIONAL_B_SPLINE_CURVE ( ( 1.000000000000002665, 0.8660254037844360431, 1.000000000000000000, 0.8660254037844387076, 1.000000000000000000, 0.8660254037844333785, 1.000000000000005329 ) ) 
 REPRESENTATION_ITEM ( '' )  );
#68097=CARTESIAN_POINT ( 'NONE',  ( 18.30937500061451928, -4.541064518000417216, -2.621784821875001281 ) ) ;
#68098=CARTESIAN_POINT ( 'NONE',  ( 25.04062500061451502, -3.027376345333610441, -5.243569643749999898 ) ) ;
#68099=CARTESIAN_POINT ( 'NONE',  ( -3.999999999999999112, 17.75000000000000355, 30.00000000000000000 ) ) ;
#68100=CARTESIAN_POINT ( 'NONE',  ( 5.521875000614517859, 3.027376345333611329, 5.243569643749999010 ) ) ;
#68101=CARTESIAN_POINT ( 'NONE',  ( 10.87500000122903288, -5.773502691896255534, -1.060575238724906372E-15 ) ) ;
#68102=CARTESIAN_POINT ( 'NONE',  ( 7.350000001229033408, -2.886751345948125991, -5.000000000000000000 ) ) ;
#68103=CARTESIAN_POINT ( 'NONE',  ( 2.000000000000001332, 19.25000000000000000, -26.53589838486224650 ) ) ;
#68104=CARTESIAN_POINT ( 'NONE',  ( 27.63750000122903216, 6.123233995736764310E-16, -4.999999999999998224 ) ) ;
#68107=CARTESIAN_POINT ( 'NONE',  ( 10.24687500061451750, -3.027376345333610441, -5.243569643749999898 ) ) ;
#68108=DIRECTION ( 'NONE',  ( -0.000000000000000000, -1.000000000000000000, -0.000000000000000000 ) ) ;
#68109=CARTESIAN_POINT ( 'NONE',  ( 18.51562500061451289, 3.027376345333611329, 5.243569643749999010 ) ) ;
#68110=CARTESIAN_POINT ( 'NONE',  ( 14.33437500061451786, 6.421520780324663323E-16, -5.243569643749999010 ) ) ;
#68111=CARTESIAN_POINT ( 'NONE',  ( 29.28750000122903074, -4.330127018922194537, 2.499999999999995559 ) ) ;
#68112=CARTESIAN_POINT ( 'NONE',  ( 20.70937500061451786, 4.541064518000418104, -2.621784821874998173 ) ) ;
#68113=CARTESIAN_POINT ( 'NONE',  ( 8.109375000614518214, 4.541064518000418104, -2.621784821874998173 ) ) ;
#68114=CARTESIAN_POINT ( 'NONE',  ( 3.778125000614519280, -4.541064518000419881, 2.621784821874995952 ) ) ;
#68115=CARTESIAN_POINT ( 'NONE',  ( -3.999999999999999112, 17.75000000000000355, 30.00000000000000000 ) ) ;
#68117=CARTESIAN_POINT ( 'NONE',  ( 20.09062500061451573, -3.027376345333610441, -5.243569643749999898 ) ) ;
#68119=CARTESIAN_POINT ( 'NONE',  ( 6.225000001229036073, 2.886751345948126879, 4.999999999999999112 ) ) ;
#68120=( BOUNDED_CURVE ( )  B_SPLINE_CURVE ( 2, ( #50738, #11211, #43741, #61449, #5306, #10121, #61086, #32651, #50382 ),
 .UNSPECIFIED., .F., .F. ) 
 B_SPLINE_CURVE_WITH_KNOTS ( ( 3, 2, 2, 2, 3 ),
 ( 0.4673913043478261087, 0.4710144927536231707, 0.4782608695652174058, 0.4855072463768115854, 0.4891304347826087029 ),
 .UNSPECIFIED. ) 
 CURVE ( )  GEOMETRIC_REPRESENTATION_ITEM ( )  RATIONAL_B_SPLINE_CURVE ( ( 0.9330127018922194093, 0.9330127018922198534, 1.000000000000000000, 0.8660254037844387076, 1.000000000000000000, 0.8660254037844387076, 1.000000000000000000, 0.9330127018922194093, 0.9330127018922194093 ) ) 
 REPRESENTATION_ITEM ( '' )  );
#68121=CARTESIAN_POINT ( 'NONE',  ( 16.71562500061451573, 3.027376345333611329, 5.243569643749999010 ) ) ;
#68122=CARTESIAN_POINT ( 'NONE',  ( 12.29062500061451857, -3.027376345333614438, 5.243569643749998122 ) ) ;
#68124=CARTESIAN_POINT ( 'NONE',  ( 14.21249999999999858, 2.886751345948126879, 4.999999999999999112 ) ) ;
#68125=CARTESIAN_POINT ( 'NONE',  ( 8.812500001229034652, 4.330127018922192761, -2.499999999999997780 ) ) ;
#68126=CARTESIAN_POINT ( 'NONE',  ( 6.365625000614518747, 3.027376345333611329, 5.243569643749999010 ) ) ;
#68127=CARTESIAN_POINT ( 'NONE',  ( 18.75000000122903288, 5.773502691896255534, 3.535250795749688894E-16 ) ) ;
#68129=CARTESIAN_POINT ( 'NONE',  ( -2.121784821874999949, 11.23437500061451821, -33.67503911421598417 ) ) ;
#68130=CARTESIAN_POINT ( 'NONE',  ( 1.592000809091587073E-14, 16.28750000000000142, -34.00000000000000000 ) ) ;
#68131=CARTESIAN_POINT ( 'NONE',  ( 3.262500001229035718, -4.330127018922190985, -2.500000000000001332 ) ) ;
#68132=EDGE_CURVE ( 'NONE', #68526, #42547, #46659, .T. ) ;
#68134=CARTESIAN_POINT ( 'NONE',  ( -2.000000000000000000, 11.37500000000000178, -33.46410161513775705 ) ) ;
#68135=CARTESIAN_POINT ( 'NONE',  ( 18.27187500061451431, -6.054752690667223547, -1.112240025338166033E-15 ) ) ;
#68136=CARTESIAN_POINT ( 'NONE',  ( 6.487500001229034474, 6.123233995736764310E-16, -4.999999999999998224 ) ) ;
#68137=CARTESIAN_POINT ( 'NONE',  ( 15.66562500061451857, 3.027376345333613106, -5.243569643749998122 ) ) ;
#68139=CARTESIAN_POINT ( 'NONE',  ( 22.46250000122903501, 0.000000000000000000, 4.999999999999998224 ) ) ;
#68140=CARTESIAN_POINT ( 'NONE',  ( 29.70937500061451431, 4.541064518000418104, -2.621784821874998173 ) ) ;
#68141=CARTESIAN_POINT ( 'NONE',  ( 25.13437500061451502, 6.421520780324663323E-16, -5.243569643749999010 ) ) ;
#68143=CARTESIAN_POINT ( 'NONE',  ( 12.77812500061451750, -4.541064518000419881, 2.621784821874995952 ) ) ;
#68144=CARTESIAN_POINT ( 'NONE',  ( 11.74687500061451573, 6.054752690667223547, 3.707466751127219781E-16 ) ) ;
#68145=ORIENTED_EDGE ( 'NONE', *, *, #31407, .T. ) ;
#68146=CARTESIAN_POINT ( 'NONE',  ( 29.27812500061451573, 4.541064518000418104, 2.621784821874999949 ) ) ;
#68147=CARTESIAN_POINT ( 'NONE',  ( 20.31562500061451715, 3.027376345333611329, 5.243569643749999010 ) ) ;
#68149=CARTESIAN_POINT ( 'NONE',  ( 20.81249999999999645, 2.886751345948162850, -4.999999999999940492 ) ) ;
#68150=EDGE_CURVE ( 'NONE', #32497, #46707, #36717, .T. ) ;
#68151=CARTESIAN_POINT ( 'NONE',  ( 10.31250000000000355, -5.773502691896255534, -1.060575238724906372E-15 ) ) ;
#68152=CARTESIAN_POINT ( 'NONE',  ( 21.15000000122903145, -2.886751345948129988, 4.999999999999997335 ) ) ;
#68153=CARTESIAN_POINT ( 'NONE',  ( 16.41562500061451857, -6.054752690667223547, -1.112240025338166033E-15 ) ) ;
#68156=CARTESIAN_POINT ( 'NONE',  ( 20.69999999999999929, -4.330127018922190985, -2.500000000000001332 ) ) ;
#68157=CARTESIAN_POINT ( 'NONE',  ( 22.53750000000000142, -2.886751345948125991, -5.000000000000000000 ) ) ;
#68158=CARTESIAN_POINT ( 'NONE',  ( 22.54687500061451999, 6.054752690667223547, 3.707466751127219781E-16 ) ) ;
#68159=CARTESIAN_POINT ( 'NONE',  ( 24.59062500061451573, -3.027376345333610441, -5.243569643749999898 ) ) ;
#68161=CARTESIAN_POINT ( 'NONE',  ( 8.850000001229034297, 5.773502691896255534, 3.535250795749688401E-16 ) ) ;
#68162=CARTESIAN_POINT ( 'NONE',  ( 8.428125000614517859, 6.421520780324663323E-16, -5.243569643749999010 ) ) ;
#68163=CARTESIAN_POINT ( 'NONE',  ( 4.000000000000000000, 15.35000000122903252, 32.30940107675849760 ) ) ;
#68164=CARTESIAN_POINT ( 'NONE',  ( 15.11249999999999893, 2.886751345948126879, 4.999999999999999112 ) ) ;
#68165=CARTESIAN_POINT ( 'NONE',  ( -2.121784821874999949, 17.02812500061451573, 26.32496088578401938 ) ) ;
#68166=CARTESIAN_POINT ( 'NONE',  ( 2.971875000614517592, -6.054752690667223547, -1.112240025338166033E-15 ) ) ;
#68167=CARTESIAN_POINT ( 'NONE',  ( 26.67187500061451644, 3.027376345333611329, 5.243569643749999010 ) ) ;
#68168=ORIENTED_EDGE ( 'NONE', *, *, #3964, .F. ) ;
#68169=CARTESIAN_POINT ( 'NONE',  ( 24.32812500061451289, 4.541064518000418104, 2.621784821874999949 ) ) ;
#68170=CARTESIAN_POINT ( 'NONE',  ( 26.25937500061451857, 0.000000000000000000, 5.243569643749999010 ) ) ;
#68171=CARTESIAN_POINT ( 'NONE',  ( 4.243569643749999898, 18.19062500061459176, -27.54997392385601529 ) ) ;
#68172=CARTESIAN_POINT ( 'NONE',  ( 11.43750000000000000, 5.773502691896255534, 3.535250795749688894E-16 ) ) ;
#68173=CARTESIAN_POINT ( 'NONE',  ( 8.240625000614516082, -3.027376345333614438, 5.243569643749998122 ) ) ;
#68175=CARTESIAN_POINT ( 'NONE',  ( 29.35312500061451502, 0.000000000000000000, 5.243569643749999010 ) ) ;
#68176=CARTESIAN_POINT ( 'NONE',  ( 27.06562500061451715, 3.027376345333611329, 5.243569643749999010 ) ) ;
#68178=EDGE_CURVE ( 'NONE', #17518, #16738, #51837, .T. ) ;
#68180=CARTESIAN_POINT ( 'NONE',  ( 20.44687500061451857, -3.027376345333614438, 5.243569643749998122 ) ) ;
#68181=CARTESIAN_POINT ( 'NONE',  ( -2.121784821874999949, 15.73437500061451644, 26.32496088578401938 ) ) ;
#68182=CARTESIAN_POINT ( 'NONE',  ( 18.23437500061451999, -4.541064518000419881, 2.621784821874995952 ) ) ;
#68183=CARTESIAN_POINT ( 'NONE',  ( 27.42187500061451644, 3.027376345333613106, -5.243569643749998122 ) ) ;
#68184=CARTESIAN_POINT ( 'NONE',  ( 4.243569643749999010, 16.97187500061451715, 27.54997392385601174 ) ) ;
#68185=CARTESIAN_POINT ( 'NONE',  ( 10.49062500061451431, -3.027376345333614438, 5.243569643749998122 ) ) ;
#68186=CARTESIAN_POINT ( 'NONE',  ( 5.709375000614517859, -4.541064518000417216, -2.621784821875001281 ) ) ;
#68188=CARTESIAN_POINT ( 'NONE',  ( 8.653125000614515727, 0.000000000000000000, 5.243569643749999010 ) ) ;
#68189=CARTESIAN_POINT ( 'NONE',  ( 11.48437500061451644, -4.541064518000419881, 2.621784821874995952 ) ) ;
#68190=DIRECTION ( 'NONE',  ( 0.000000000000000000, 0.000000000000000000, 1.000000000000000000 ) ) ;
#68191=CARTESIAN_POINT ( 'NONE',  ( 18.93750000122903288, -4.330127018922194537, 2.499999999999995559 ) ) ;
#68192=CARTESIAN_POINT ( 'NONE',  ( 4.771875000614516971, -6.054752690667223547, -1.112240025338166033E-15 ) ) ;
#68193=CARTESIAN_POINT ( 'NONE',  ( 8.165625000614516793, 3.027376345333611329, 5.243569643749999010 ) ) ;
#68194=CARTESIAN_POINT ( 'NONE',  ( 5.465625000614517504, 3.027376345333611329, 5.243569643749999010 ) ) ;
#68196=CARTESIAN_POINT ( 'NONE',  ( 19.58437500061451786, -4.541064518000419881, 2.621784821874995952 ) ) ;
#68197=CARTESIAN_POINT ( 'NONE',  ( -1.071796769724491005, 11.47009619066136565, 26.00000000000000355 ) ) ;
#68199=CARTESIAN_POINT ( 'NONE',  ( 23.65312500061451573, -4.541064518000417216, -2.621784821875001281 ) ) ;
#68200=CARTESIAN_POINT ( 'NONE',  ( 11.69062500061451360, 6.054752690667223547, 3.707466751127219781E-16 ) ) ;
#68201=ADVANCED_FACE ( 'NONE', ( #32218 ), #42935, .T. ) ;
#68203=CARTESIAN_POINT ( 'NONE',  ( 27.90937500061451715, 4.541064518000418104, -2.621784821874998173 ) ) ;
#68204=CARTESIAN_POINT ( 'NONE',  ( 10.64062500061451644, -3.027376345333610441, -5.243569643749999898 ) ) ;
#68206=CARTESIAN_POINT ( 'NONE',  ( 12.30000000122903181, -2.886751345948125991, -5.000000000000000000 ) ) ;
#68207=CARTESIAN_POINT ( 'NONE',  ( 28.11562500061451431, -6.054752690667223547, -1.112240025338166033E-15 ) ) ;
#68208=CARTESIAN_POINT ( 'NONE',  ( -3.000416591977282496E-16, 13.39062500061451644, -34.90005215228797653 ) ) ;
#68209=CARTESIAN_POINT ( 'NONE',  ( 16.23750000122903359, -4.330127018922194537, 2.499999999999995559 ) ) ;
#68210=CARTESIAN_POINT ( 'NONE',  ( 12.15000000000000036, -4.330127018922190985, -2.500000000000001332 ) ) ;
#68211=CARTESIAN_POINT ( 'NONE',  ( 20.80312500061451431, 0.000000000000000000, 5.243569643749999010 ) ) ;
#68212=CARTESIAN_POINT ( 'NONE',  ( 7.471875000614519813, -6.054752690667223547, -1.112240025338166033E-15 ) ) ;
#68213=CARTESIAN_POINT ( 'NONE',  ( 8.700000001229032165, -2.886751345948125991, -5.000000000000000000 ) ) ;
#68214=CARTESIAN_POINT ( 'NONE',  ( 15.67500000122903181, 2.886751345948126879, 4.999999999999999112 ) ) ;
#68215=CARTESIAN_POINT ( 'NONE',  ( 13.71562500061451750, -6.054752690667223547, -1.112240025338166033E-15 ) ) ;
#68216=CARTESIAN_POINT ( 'NONE',  ( 16.52812500061451573, 6.421520780324663323E-16, -5.243569643749999010 ) ) ;
#68217=CARTESIAN_POINT ( 'NONE',  ( 25.50000000122903288, 5.773502691896255534, 3.535250795749688894E-16 ) ) ;
#68218=CARTESIAN_POINT ( 'NONE',  ( 21.37499999999999645, 4.330127018922191873, 2.499999999999999556 ) ) ;
#68219=CARTESIAN_POINT ( 'NONE',  ( 22.20937500061451431, 0.000000000000000000, 5.243569643749999010 ) ) ;
#68222=CARTESIAN_POINT ( 'NONE',  ( 10.95000000122903394, -2.886751345948125991, -5.000000000000000000 ) ) ;
#68223=CARTESIAN_POINT ( 'NONE',  ( 8.221875000614518925, 3.027376345333611329, 5.243569643749999010 ) ) ;
#68224=CARTESIAN_POINT ( 'NONE',  ( 27.30937500061451573, -4.541064518000417216, -2.621784821875001281 ) ) ;
#68225=CARTESIAN_POINT ( 'NONE',  ( 4.196151849995945149, -2.718880220196457476, -4.196151849995952254 ) ) ;
#68226=CARTESIAN_POINT ( 'NONE',  ( 24.51562500061451289, -6.054752690667223547, -1.112240025338166033E-15 ) ) ;
#68229=CARTESIAN_POINT ( 'NONE',  ( 7.921875000614517326, -6.054752690667223547, -1.112240025338166033E-15 ) ) ;
#68230=CARTESIAN_POINT ( 'NONE',  ( 28.07812500061451289, -4.541064518000419881, 2.621784821874995952 ) ) ;
#68231=CARTESIAN_POINT ( 'NONE',  ( 6.234375000614519102, 6.421520780324663323E-16, -5.243569643749999010 ) ) ;
#68232=CARTESIAN_POINT ( 'NONE',  ( -3.999999999999997335, 16.55000000122903359, -27.69059892324149530 ) ) ;
#68233=CARTESIAN_POINT ( 'NONE',  ( 25.95937500061451431, -4.541064518000417216, -2.621784821875001281 ) ) ;
#68234=CARTESIAN_POINT ( 'NONE',  ( -2.121784821874999949, 10.72812500061459318, 26.32496088578401938 ) ) ;
#68235=CARTESIAN_POINT ( 'NONE',  ( 20.36249999999999716, 2.886751345948129099, -4.999999999999998224 ) ) ;
#68236=ORIENTED_EDGE ( 'NONE', *, *, #34637, .F. ) ;
#68237=CARTESIAN_POINT ( 'NONE',  ( 26.69999999999999929, 4.330127018922192761, -2.499999999999997780 ) ) ;
#68238=( BOUNDED_SURFACE ( )  B_SPLINE_SURFACE ( 1, 2, ( 
 ( #28415, #39880, #67232, #16591, #57926, #30229, #63833, #36860, #70483, #35763, #2518, #35400, #2164, #1444, #13225, #14324, #52761, #52399, #25039, #13958, #36495, #23948, #47583, #58652, #46498, #6973, #1807, #7333, #36133, #64933, #8059, #24315, #53489, #64199, #70112, #41676, #47222, #29504, #52039, #8418, #29863, #69036, #69753, #46864, #30593, #18398, #24675, #64569, #40965, #12868, #19488, #42046, #19122, #13586, #25411, #63481, #19860, #2881, #69403, #53120, #59015, #30952, #47956, #18759, #42413, #41323, #58285, #7691, #9883, #66034, #10253, #43876, #43140, #43510, #48684, #37591, #15413, #59748, #21689, #37955, #31690, #71208, #3622, #54225, #60112, #49055, #4360, #3990, #60475, #20219, #38320, #26517, #70846, #32418, #4715, #59376, #54955, #48321, #42774, #32784, #16148, #66402, #3255, #71947, #55321, #21323, #26888, #44245, #65664, #71583, #60846, #49415, #37224, #15778, #20956, #27249, #49783, #65293, #14682, #72307, #20585, #9155, #66776, #8786, #15053, #31321, #53864, #25784, #9522, #26144, #32055, #54588, #55681, #67502, #28327, #5797, #50865, #993, #38700, #263, #45692, #68226, #17589, #44616, #44964, #12061, #34220, #56753, #61942, #5438, #23500, #22058, #51593, #27611, #27977, #50147, #67146, #72675, #39791, #16506, #39059, #34584, #68583, #23137, #5078, #51226, #62666, #630, #6158, #46048, #22417, #56406, #40148, #28687, #61573, #22772, #45324, #57112, #6524, #10976, #33497, #67860, #50508, #56046, #29056, #17231, #16866, #61220, #62308, #11704, #11346, #10614, #33143, #73034, #39421, #33863, #7596, #58193, #30135, #53395, #17944, #52666, #24945, #47489, #70019, #23859, #24222, #64471, #13488, #36036, #41230, #57833, #2788, #1350, #30857, #6884, #7242, #29417, #46407, #51950, #69661, #35311, #13865, #2073, #58556, #24582, #47130, #25313, #47859, #19390, #68944, #40506, #19026, #18302, #41585, #63021, #63742, #2422, #57480, #40873, #7964, #30500, #64103, #13131, #36406, #12420, #8327, #58919, #63390, #53028, #41951, #34952, #35670, #29771, #12775, #52307, #1709, #46771, #69307, #18668, #21230, #54860, #54135, #54497, #59655, #48592, #3898, #70749, #32696, #26419, #42679, #9064, #14591, #65202, #71117, #60019, #15322, #14961, #71490, #31224, #49326, #37499, #8692, #43420, #15686, #70388, #20867, #53766, #71858, #9431, #3161, #65942, #38224, #19764, #37863, #59283, #25690, #43782, #27158, #4268, #14228, #9790, #66309, #32323, #60382, #55233, #3530, #31959, #60754, #26792, #48225, #48960, #10162, #4628, #42315, #20124, #37126, #64841, #31598, #26052, #36766, #20489, #43045, #65571, #33778, #11256, #72947, #57024, #5710, #56321, #66681, #5349, #39336, #16778, #61849, #11973, #49692, #28246, #56671, #6069, #28602, #55592, #55953, #23048, #45236, #67769, #22329, #16416, #34496, #33053, #62576, #38604, #38972, #61130, #4987, #10525, #50777, #67057, #45604, #180, #17144, #22685, #39702, #6430, #72220, #51138, #27519, #21598, #62220, #50053, #11616, #44152, #44881, #34133, #16056, #72582, #537, #68137, #17501, #67416, #40062, #21966, #44524, #61488, #10885, #33414, #27888, #50421, #46683, #46320, #47043, #7879, #23411, #18939, #52582, #35585, #52943, #13397, #12689, #13046, #18212, #7154, #58104, #29329, #64387, #7511, #1261, #40784, #68855, #23768, #29684, #18582, #69577, #69221, #30042, #62932, #63297, #41147, #63655, #57388, #35226, #51859, #36319, #30415, #13777, #58834, #2340, #64019, #57747, #19304, #52221, #1988, #28965, #51503, #45958, #24499, #1625, #24133, #41857, #41498, #40415, #34861, #6795, #24857, #35945, #58466, #903, #47403, #69934, #12325, #68491, #17855, #59198, #70662, #26334, #20777, #8607, #31512, #65118, #38139, #71775, #37042, #3813, #36678, #3448, #2704, #14509, #15597, #54053, #53677, #48873, #15238, #37775, #25220, #71403, #59938, #47766, #8244, #3071, #31136, #37415, #66219, #14143, #20409, #25600, #48138, #70302, #20038, #30774, #42593, #43334, #65856, #4178, #59566, #60295, #19675, #9705, #42957, #71034, #25966, #8979, #32240, #48507, #53304, #42228, #65486, #14876, #64753, #26707, #9345, #54773, #31878, #49241, #54412, #21144, #43698, #44063, #21876, #27436, #38517, #27072, #67332, #27802, #33333, #67684, #10076, #50338, #4543, #56235, #49603, #5258, #45517, #68048, #72491, #22600, #50692, #60663, #61403, #44799, #72130, #55508, #21509, #448, #66589, #49967, #15967, #61040, #10438, #39249, #4901, #34047, #16692, #5628, #22245, #72862, #17417, #32607, #62133, #32968, #55145, #61762, #44437, #11166, #66966, #55871, #45152, #16331, #38886, #28165, #94, #33690, #10798, #5983, #17055, #51051, #56587, #39614, #11526, #28513, #22957, #57664, #57305, #58019, #18856, #34411, #29955, #63575, #46595, #63933, #24411, #23683, #24048, #29243, #18127, #69137, #40327, #2259, #18496, #12242, #51775, #6710, #34773, #40693, #29599, #7428, #7070, #41061, #815, #41417, #52135, #51413, #12962, #58380, #39976, #35499, #28874, #23323, #13318, #69850, #46960, #56938, #52496, #35857, #1906, #69496, #24773, #46231, #1538, #7792, #30329, #17767, #52859, #47317, #62488, #11886, #45872, #68405, #6343, #1175, #62848, #68771, #63211, #12607, #35141, #3362, #53964, #42508, #26618, #48423, #25883, #36233, #48055, #8892, #59480, #31424, #54687, #19217, #70949, #26249, #48786, #71311, #25135, #25510, #65767, #14788, #37329, #65032, #59114, #4088, #2614, #20320, #20688, #43247, #15149, #47676, #70580, #37686, #59853, #9257, #14423, #8521, #49155, #70212, #32154, #8157, #31050, #30686, #19586, #53217, #42874, #36593, #60209, #65396, #31792, #54330, #3724, #41771, #64300, #9621, #42142, #13689, #58747, #64669, #14053, #53587, #36958, #2982, #19956, #4457, #16602, #11072, #61315, #21783, #16964, #71686, #62046, #67599, #55056, #5173, #67244, #33244 ),
 ( #28426, #66496, #72041, #27708, #56500, #26987, #10712, #49516, #43976, #60576, #38424, #21058, #15879, #39158, #61673, #39519, #21419, #33599, #9982, #56144, #55782, #50249, #44350, #60947, #5538, #10350, #5893, #15509, #72772, #66875, #43609, #11441, #32880, #28076, #55420, #50604, #4813, #72402, #44708, #27346, #49877, #16243, #38799, #38050, #22156, #8, #22515, #45062, #66131, #33961, #32519, #46508, #17331, #68686, #36779, #59295, #57936, #7343, #67958, #69046, #29515, #39890, #8705, #45788, #51325, #6984, #50963, #56851, #63125, #6257, #23237, #62403, #17683, #359, #68323, #18409, #40975, #47874, #728, #63490, #11802, #35411, #12521, #40604, #23601, #40244, #12878, #62764, #22866, #34319, #35054, #46146, #45424, #70402, #28785, #29873, #12156, #53409, #34684, #51689, #23960, #57214, #6628, #29157, #1093, #18046, #57581, #52050, #1454, #2801, #25328, #19778, #42328, #64853, #14241, #48975, #16069, #38619, #43060, #66323, #21244, #31238, #31973, #15336, #20138, #26066, #42693, #37876, #65215, #65585, #71504, #65956, #59669, #14975, #54149, #61143, #10175, #66697, #53779, #32710, #15700, #60034, #21612, #31613, #60396, #3175, #25702, #48238, #20880, #54509, #9445, #44167, #26434, #14605, #37142, #9077, #55247, #9804, #32337, #70763, #4642, #3543, #48605, #27172, #71130, #20503, #37513, #49340, #43798, #3912, #43434, #54875, #4280, #26806, #71872, #38239, #60768, #49706, #72234, #16793, #17869, #56335, #55969, #6083, #45251, #194, #5725, #10898, #23063, #33426, #68506, #27535, #22699, #28260, #40428, #28980, #38986, #28615, #67070, #553, #67431, #11271, #56684, #16428, #44895, #50436, #61501, #50067, #17158, #50791, #67784, #17515, #39717, #62235, #5363, #11631, #34147, #51152, #45972, #10538, #45618, #40076, #62591, #11987, #27901, #39350, #57039, #68152, #34510, #33792, #72961, #33066, #22343, #23426, #72597, #61864, #21980, #6445, #44539, #51518, #917, #55605, #5001, #7892, #24513, #30058, #47779, #70314, #64400, #18224, #12339, #52596, #40798, #18953, #62945, #35598, #47417, #29342, #68868, #30428, #2353, #2003, #13059, #8257, #34874, #53318, #58847, #46334, #69591, #58481, #47057, #7525, #7169, #52956, #41871, #57403, #24870, #13411, #41513, #13793, #69947, #46698, #64032, #52235, #41160, #35960, #63311, #25233, #19317, #35239, #1639, #29697, #57760, #63669, #36333, #30787, #2717, #19688, #23782, #6808, #51874, #1273, #12702, #24145, #69234, #18596, #58117, #53689, #15609, #72141, #26719, #59211, #36689, #32251, #65869, #48884, #66230, #49253, #25979, #26345, #31524, #20420, #71414, #42604, #4554, #20790, #14520, #54063, #59578, #37053, #42968, #31889, #60307, #59949, #43347, #3083, #21156, #9356, #25612, #15250, #60674, #42241, #37787, #31148, #48149, #38151, #64765, #71787, #8619, #54784, #10088, #4190, #9718, #27083, #48518, #54424, #43709, #32618, #20049, #55158, #3824, #49615, #14155, #70674, #65130, #8991, #3459, #71045, #65498, #14887, #37427, #22611, #16704, #67343, #27815, #22968, #61774, #50349, #11177, #55519, #44810, #22256, #39261, #51063, #21520, #33701, #17067, #39626, #62144, #4913, #33345, #56598, #28176, #50703, #72874, #16342, #45530, #27448, #460, #10450, #38897, #32979, #49978, #72502, #56248, #66978, #5994, #5640, #106, #45163, #67694, #44075, #66604, #28524, #21891, #38528, #11539, #44448, #34058, #15978, #61051, #61416, #10809, #55882, #5270, #49051, #44241, #49779, #37586, #5073, #71578, #32050, #43505, #72303, #66771, #54582, #4356, #37951, #10970, #26882, #3986, #16144, #26511, #39055, #71204, #43872, #49411, #61568, #72672, #9518, #21684, #60108, #38696, #60469, #54950, #27242, #20952, #15408, #66030, #9878, #20580, #60842, #21319, #71942, #61215, #27608, #48680, #10610, #54221, #43135, #66397, #3618, #26139, #32413, #33139, #55676, #65659, #15773, #38315, #15048, #10247, #32780, #55317, #4711, #50143, #22052, #44612, #67142, #16501, #56403, #40869, #12416, #68940, #63386, #34948, #68579, #62305, #23855, #33860, #68222, #33493, #18298, #50503, #626, #34216, #11700, #46402, #28684, #44961, #39417, #11342, #57475, #17584, #260, #28324, #23496, #29052, #16862, #6880, #50862, #5793, #22769, #51588, #46044, #45321, #56750, #17228, #56042, #5434, #6154, #988, #61939, #51223, #27973, #39788, #73030, #23132, #67855, #17939, #40502, #63017, #22414, #29413, #12057, #67499, #45688, #40144, #62660, #34580, #57108, #6519, #51946, #1344, #58188, #1703, #52662, #42675, #30130, #53388, #2784, #8687, #35666, #25308, #24218, #70384, #47484, #2418, #70015, #30496, #47855, #19760, #46767, #69302, #19385, #2069, #18664, #42310, #24940, #41581, #64837, #41945, #64467, #36032, #20121, #13860, #58550, #36402, #41225, #58914, #53024, #8323, #48220, #12771, #30853, #14224, #36760, #59279, #63736, #19021, #31219, #53762, #3157, #7960, #24578, #70744, #13127, #25686, #7592, #47124, #69656, #64098, #13483, #35306, #57829, #7238, #29766, #52302, #26787, #32320, #50049, #72576, #66676, #20485, #14587, #54855, #43040, #21225, #65198, #37857, #49687, #31592, #71113, #10158, #9786, #54131, #65567, #44148, #37121, #55588, #61126, #48587, #71853, #60748, #49322, #4264, #9427, #32691, #16051, #59650, #55229, #15682, #43778, #38599, #72216, #48955, #66305, #54493, #43414, #38220, #14956, #27515, #4624, #37495, #3894, #31955, #60015, #65938, #27153, #21594, #10521, #33049, #26047, #4983, #21962, #3526, #9060, #26413, #71486, #20863, #15318, #60378, #17848, #1256, #28960, #61484, #57021, #68484, #6426, #11968, #29324, #28242, #62216, #45953, #40057, #22324, #11611, #45600, #5345, #23405, #34129, #55949, #17497, #62927, #44519, #68131, #33411, #27883, #40410, #67053, #51498, #10879, #898, #12321, #34856, #34492, #51853, #50773, #56669, #57383, #62572, #44877 ) ),
 .UNSPECIFIED., .F., .F., .F. ) 
 B_SPLINE_SURFACE_WITH_KNOTS ( ( 2, 2 ),
 ( 3, 2, 2, 2, 2, 2, 2, 2, 2, 2, 2, 2, 2, 2, 2, 2, 2, 2, 2, 2, 2, 2, 2, 2, 2, 2, 2, 2, 2, 2, 2, 2, 2, 2, 2, 2, 2, 2, 2, 2, 2, 2, 2, 2, 2, 2, 2, 2, 2, 2, 2, 2, 2, 2, 2, 2, 2, 2, 2, 2, 2, 2, 2, 2, 2, 2, 2, 2, 2, 2, 2, 2, 2, 2, 2, 2, 2, 2, 2, 2, 2, 2, 2, 2, 2, 2, 2, 2, 2, 2, 2, 2, 2, 2, 2, 2, 2, 2, 2, 2, 2, 2, 2, 2, 2, 2, 2, 2, 2, 2, 2, 2, 2, 2, 2, 2, 2, 2, 2, 2, 2, 2, 2, 2, 2, 2, 2, 2, 2, 2, 2, 2, 2, 2, 2, 2, 2, 2, 2, 2, 2, 2, 2, 2, 2, 2, 2, 2, 2, 2, 2, 2, 2, 2, 2, 2, 2, 2, 2, 2, 2, 2, 2, 2, 2, 2, 2, 2, 2, 2, 2, 2, 2, 2, 2, 2, 2, 2, 2, 2, 2, 2, 2, 2, 2, 2, 2, 2, 2, 2, 2, 2, 2, 2, 2, 2, 2, 2, 2, 2, 2, 2, 2, 2, 2, 2, 2, 2, 2, 2, 2, 2, 2, 2, 2, 2, 2, 2, 2, 2, 2, 2, 2, 2, 2, 2, 2, 2, 2, 2, 2, 2, 2, 2, 2, 2, 2, 2, 2, 2, 2, 2, 2, 2, 2, 2, 2, 2, 2, 2, 2, 2, 2, 2, 2, 2, 2, 2, 2, 2, 2, 2, 2, 2, 2, 2, 2, 2, 2, 2, 2, 2, 2, 2, 2, 2, 2, 2, 2, 2, 2, 2, 2, 2, 2, 2, 2, 2, 2, 2, 2, 2, 2, 2, 2, 2, 2, 2, 2, 2, 2, 2, 2, 2, 2, 2, 2, 2, 2, 2, 2, 2, 2, 2, 2, 2, 2, 2, 2, 2, 2, 2, 2, 2, 2, 2, 2, 2, 2, 2, 2, 2, 2, 2, 2, 2, 2, 2, 2, 2, 2, 2, 2, 2, 2, 2, 2, 2, 2, 2, 2, 2, 2, 2, 2, 2, 2, 2, 2, 2, 3 ),
 ( 0.000000000000000000, 1.000000000000000000 ),
 ( 0.000000000000000000, 0.002777777777777777884, 0.005555555555555555768, 0.008333333333333333218, 0.01111111111111111154, 0.01388888888888888812, 0.01666666666666666644, 0.01944444444444444475, 0.02222222222222222307, 0.02500000000000000139, 0.02777777777777777624, 0.03055555555555555455, 0.03333333333333333287, 0.03611111111111110772, 0.03888888888888888951, 0.04166666666666666435, 0.04444444444444444614, 0.04722222222222222099, 0.05000000000000000278, 0.05277777777777777762, 0.05555555555555555247, 0.05833333333333333426, 0.06111111111111110911, 0.06388888888888888395, 0.06666666666666666574, 0.06944444444444444753, 0.07222222222222221544, 0.07499999999999999722, 0.07777777777777777901, 0.08055555555555556080, 0.08333333333333332871, 0.08611111111111111049, 0.08888888888888889228, 0.09166666666666666019, 0.09444444444444444198, 0.09722222222222222376, 0.1000000000000000056, 0.1027777777777777735, 0.1055555555555555552, 0.1083333333333333370, 0.1111111111111111049, 0.1138888888888888867, 0.1166666666666666685, 0.1194444444444444503, 0.1222222222222222182, 0.1250000000000000000, 0.1277777777777777679, 0.1305555555555555636, 0.1333333333333333315, 0.1361111111111110994, 0.1388888888888888951, 0.1416666666666666630, 0.1444444444444444309, 0.1472222222222222265, 0.1499999999999999944, 0.1527777777777777901, 0.1555555555555555580, 0.1583333333333333259, 0.1611111111111111216, 0.1638888888888888895, 0.1666666666666666574, 0.1694444444444444531, 0.1722222222222222210, 0.1749999999999999889, 0.1777777777777777846, 0.1805555555555555525, 0.1833333333333333204, 0.1861111111111111160, 0.1888888888888888840, 0.1916666666666666796, 0.1944444444444444475, 0.1972222222222222154, 0.2000000000000000111, 0.2027777777777777790, 0.2055555555555555469, 0.2083333333333333426, 0.2111111111111111105, 0.2138888888888888784, 0.2166666666666666741, 0.2194444444444444420, 0.2222222222222222099, 0.2250000000000000056, 0.2277777777777777735, 0.2305555555555555691, 0.2333333333333333370, 0.2361111111111111049, 0.2388888888888889006, 0.2416666666666666685, 0.2444444444444444364, 0.2472222222222222321, 0.2500000000000000000, 0.2527777777777777679, 0.2555555555555555358, 0.2583333333333333592, 0.2611111111111111271, 0.2638888888888888951, 0.2666666666666666630, 0.2694444444444444309, 0.2722222222222221988, 0.2750000000000000222, 0.2777777777777777901, 0.2805555555555555580, 0.2833333333333333259, 0.2861111111111110938, 0.2888888888888888618, 0.2916666666666666852, 0.2944444444444444531, 0.2972222222222222210, 0.2999999999999999889, 0.3027777777777777568, 0.3055555555555555802, 0.3083333333333333481, 0.3111111111111111160, 0.3138888888888888840, 0.3166666666666666519, 0.3194444444444444198, 0.3222222222222222432, 0.3250000000000000111, 0.3277777777777777790, 0.3305555555555555469, 0.3333333333333333148, 0.3361111111111111382, 0.3388888888888889062, 0.3416666666666666741, 0.3444444444444444420, 0.3472222222222222099, 0.3499999999999999778, 0.3527777777777778012, 0.3555555555555555691, 0.3583333333333333370, 0.3611111111111111049, 0.3638888888888888729, 0.3666666666666666408, 0.3694444444444444642, 0.3722222222222222321, 0.3750000000000000000, 0.3777777777777777679, 0.3805555555555555358, 0.3833333333333333592, 0.3861111111111111271, 0.3888888888888888951, 0.3916666666666666630, 0.3944444444444444309, 0.3972222222222221988, 0.4000000000000000222, 0.4027777777777777901, 0.4055555555555555580, 0.4083333333333333259, 0.4111111111111110938, 0.4138888888888888618, 0.4166666666666666852, 0.4194444444444444531, 0.4222222222222222210, 0.4249999999999999889, 0.4277777777777777568, 0.4305555555555555802, 0.4333333333333333481, 0.4361111111111111160, 0.4388888888888888840, 0.4416666666666666519, 0.4444444444444444198, 0.4472222222222222432, 0.4500000000000000111, 0.4527777777777777790, 0.4555555555555555469, 0.4583333333333333148, 0.4611111111111111382, 0.4638888888888889062, 0.4666666666666666741, 0.4694444444444444420, 0.4722222222222222099, 0.4749999999999999778, 0.4777777777777778012, 0.4805555555555555691, 0.4833333333333333370, 0.4861111111111111049, 0.4888888888888888729, 0.4916666666666666408, 0.4944444444444444642, 0.4972222222222222321, 0.5000000000000000000, 0.5027777777777777679, 0.5055555555555555358, 0.5083333333333333037, 0.5111111111111110716, 0.5138888888888888395, 0.5166666666666667185, 0.5194444444444444864, 0.5222222222222222543, 0.5250000000000000222, 0.5277777777777777901, 0.5305555555555555580, 0.5333333333333333259, 0.5361111111111110938, 0.5388888888888888618, 0.5416666666666666297, 0.5444444444444443976, 0.5472222222222222765, 0.5500000000000000444, 0.5527777777777778123, 0.5555555555555555802, 0.5583333333333333481, 0.5611111111111111160, 0.5638888888888888840, 0.5666666666666666519, 0.5694444444444444198, 0.5722222222222221877, 0.5749999999999999556, 0.5777777777777777235, 0.5805555555555556024, 0.5833333333333333703, 0.5861111111111111382, 0.5888888888888889062, 0.5916666666666666741, 0.5944444444444444420, 0.5972222222222222099, 0.5999999999999999778, 0.6027777777777777457, 0.6055555555555555136, 0.6083333333333332815, 0.6111111111111111605, 0.6138888888888889284, 0.6166666666666666963, 0.6194444444444444642, 0.6222222222222222321, 0.6250000000000000000, 0.6277777777777777679, 0.6305555555555555358, 0.6333333333333333037, 0.6361111111111110716, 0.6388888888888888395, 0.6416666666666667185, 0.6444444444444444864, 0.6472222222222222543, 0.6500000000000000222, 0.6527777777777777901, 0.6555555555555555580, 0.6583333333333333259, 0.6611111111111110938, 0.6638888888888888618, 0.6666666666666666297, 0.6694444444444443976, 0.6722222222222222765, 0.6750000000000000444, 0.6777777777777778123, 0.6805555555555555802, 0.6833333333333333481, 0.6861111111111111160, 0.6888888888888888840, 0.6916666666666666519, 0.6944444444444444198, 0.6972222222222221877, 0.6999999999999999556, 0.7027777777777777235, 0.7055555555555556024, 0.7083333333333333703, 0.7111111111111111382, 0.7138888888888889062, 0.7166666666666666741, 0.7194444444444444420, 0.7222222222222222099, 0.7249999999999999778, 0.7277777777777777457, 0.7305555555555555136, 0.7333333333333332815, 0.7361111111111111605, 0.7388888888888889284, 0.7416666666666666963, 0.7444444444444444642, 0.7472222222222222321, 0.7500000000000000000, 0.7527777777777777679, 0.7555555555555555358, 0.7583333333333333037, 0.7611111111111110716, 0.7638888888888888395, 0.7666666666666667185, 0.7694444444444444864, 0.7722222222222222543, 0.7750000000000000222, 0.7777777777777777901, 0.7805555555555555580, 0.7833333333333333259, 0.7861111111111110938, 0.7888888888888888618, 0.7916666666666666297, 0.7944444444444443976, 0.7972222222222222765, 0.8000000000000000444, 0.8027777777777778123, 0.8055555555555555802, 0.8083333333333333481, 0.8111111111111111160, 0.8138888888888888840, 0.8166666666666666519, 0.8194444444444444198, 0.8222222222222221877, 0.8249999999999999556, 0.8277777777777777235, 0.8305555555555556024, 0.8333333333333333703, 0.8361111111111111382, 0.8388888888888889062, 0.8416666666666666741, 0.8444444444444444420, 0.8472222222222222099, 0.8499999999999999778, 0.8527777777777777457, 0.8555555555555555136, 0.8583333333333332815, 0.8611111111111111605, 0.8638888888888889284, 0.8666666666666666963, 0.8694444444444444642, 0.8722222222222222321, 0.8750000000000000000, 0.8777777777777777679, 0.8805555555555555358, 0.8833333333333333037, 0.8861111111111110716, 0.8888888888888888395, 0.8916666666666667185, 0.8944444444444444864, 0.8972222222222222543, 0.9000000000000000222, 0.9027777777777777901, 0.9055555555555555580, 0.9083333333333333259, 0.9111111111111110938, 0.9138888888888888618, 0.9166666666666666297, 0.9194444444444443976, 0.9222222222222222765, 0.9250000000000000444, 0.9277777777777778123, 0.9305555555555555802, 0.9333333333333333481, 0.9361111111111111160, 0.9388888888888888840, 0.9416666666666666519, 0.9444444444444444198, 0.9472222222222221877, 0.9499999999999999556, 0.9527777777777777235, 0.9555555555555556024, 0.9583333333333333703, 0.9611111111111111382, 0.9638888888888889062, 0.9666666666666666741, 0.9694444444444444420, 0.9722222222222222099, 0.9749999999999999778, 0.9777777777777777457, 0.9805555555555555136, 0.9833333333333332815, 0.9861111111111111605, 0.9888888888888889284, 0.9916666666666666963, 0.9944444444444444642, 0.9972222222222222321, 1.000000000000000000 ),
 .UNSPECIFIED. ) 
 GEOMETRIC_REPRESENTATION_ITEM ( )  RATIONAL_B_SPLINE_SURFACE ( (
 ( 1.000000000000000000, 0.8660254037844387076, 1.000000000000000000, 0.8660254037844387076, 1.000000000000000000, 0.8660254037844387076, 1.000000000000000000, 0.8660254037844387076, 1.000000000000000000, 0.8660254037844387076, 1.000000000000000000, 0.8660254037844387076, 1.000000000000000000, 0.8660254037844387076, 1.000000000000000000, 0.8660254037844387076, 1.000000000000000000, 0.8660254037844387076, 1.000000000000000000, 0.8660254037844387076, 1.000000000000000000, 0.8660254037844387076, 1.000000000000000000, 0.8660254037844387076, 1.000000000000000000, 0.8660254037844387076, 1.000000000000000000, 0.8660254037844387076, 1.000000000000000000, 0.8660254037844387076, 1.000000000000000000, 0.8660254037844387076, 1.000000000000000000, 0.8660254037844387076, 1.000000000000000000, 0.8660254037844387076, 1.000000000000000000, 0.8660254037844387076, 1.000000000000000000, 0.8660254037844387076, 1.000000000000000000, 0.8660254037844387076, 1.000000000000000000, 0.8660254037844387076, 1.000000000000000000, 0.8660254037844387076, 1.000000000000000000, 0.8660254037844387076, 1.000000000000000000, 0.8660254037844387076, 1.000000000000000000, 0.8660254037844387076, 1.000000000000000000, 0.8660254037844387076, 1.000000000000000000, 0.8660254037844387076, 1.000000000000000000, 0.8660254037844387076, 1.000000000000000000, 0.8660254037844387076, 1.000000000000000000, 0.8660254037844387076, 1.000000000000000000, 0.8660254037844387076, 1.000000000000000000, 0.8660254037844387076, 1.000000000000000000, 0.8660254037844387076, 1.000000000000000000, 0.8660254037844387076, 1.000000000000000000, 0.8660254037844387076, 1.000000000000000000, 0.8660254037844387076, 1.000000000000000000, 0.8660254037844387076, 1.000000000000000000, 0.8660254037844387076, 1.000000000000000000, 0.8660254037844387076, 1.000000000000000000, 0.8660254037844387076, 1.000000000000000000, 0.8660254037844387076, 1.000000000000000000, 0.8660254037844387076, 1.000000000000000000, 0.8660254037844387076, 1.000000000000000000, 0.8660254037844387076, 1.000000000000000000, 0.8660254037844387076, 1.000000000000000000, 0.8660254037844387076, 1.000000000000000000, 0.8660254037844387076, 1.000000000000000000, 0.8660254037844387076, 1.000000000000000000, 0.8660254037844387076, 1.000000000000000000, 0.8660254037844387076, 1.000000000000000000, 0.8660254037844387076, 1.000000000000000000, 0.8660254037844387076, 1.000000000000000000, 0.8660254037844387076, 1.000000000000000000, 0.8660254037844387076, 1.000000000000000000, 0.8660254037844387076, 1.000000000000000000, 0.8660254037844387076, 1.000000000000000000, 0.8660254037844387076, 1.000000000000000000, 0.8660254037844387076, 1.000000000000000000, 0.8660254037844387076, 1.000000000000000000, 0.8660254037844387076, 1.000000000000000000, 0.8660254037844387076, 1.000000000000000000, 0.8660254037844387076, 1.000000000000000000, 0.8660254037844387076, 1.000000000000000000, 0.8660254037844387076, 1.000000000000000000, 0.8660254037844387076, 1.000000000000000000, 0.8660254037844387076, 1.000000000000000000, 0.8660254037844387076, 1.000000000000000000, 0.8660254037844387076, 1.000000000000000000, 0.8660254037844387076, 1.000000000000000000, 0.8660254037844387076, 1.000000000000000000, 0.8660254037844387076, 1.000000000000000000, 0.8660254037844387076, 1.000000000000000000, 0.8660254037844387076, 1.000000000000000000, 0.8660254037844387076, 1.000000000000000000, 0.8660254037844387076, 1.000000000000000000, 0.8660254037844387076, 1.000000000000000000, 0.8660254037844387076, 1.000000000000000000, 0.8660254037844387076, 1.000000000000000000, 0.8660254037844387076, 1.000000000000000000, 0.8660254037844387076, 1.000000000000000000, 0.8660254037844387076, 1.000000000000000000, 0.8660254037844387076, 1.000000000000000000, 0.8660254037844387076, 1.000000000000000000, 0.8660254037844387076, 1.000000000000000000, 0.8660254037844387076, 1.000000000000000000, 0.8660254037844387076, 1.000000000000000000, 0.8660254037844387076, 1.000000000000000000, 0.8660254037844387076, 1.000000000000000000, 0.8660254037844387076, 1.000000000000000000, 0.8660254037844387076, 1.000000000000000000, 0.8660254037844387076, 1.000000000000000000, 0.8660254037844387076, 1.000000000000000000, 0.8660254037844387076, 1.000000000000000000, 0.8660254037844387076, 1.000000000000000000, 0.8660254037844387076, 1.000000000000000000, 0.8660254037844387076, 1.000000000000000000, 0.8660254037844387076, 1.000000000000000000, 0.8660254037844387076, 1.000000000000000000, 0.8660254037844387076, 1.000000000000000000, 0.8660254037844387076, 1.000000000000000000, 0.8660254037844387076, 1.000000000000000000, 0.8660254037844387076, 1.000000000000000000, 0.8660254037844387076, 1.000000000000000000, 0.8660254037844387076, 1.000000000000000000, 0.8660254037844387076, 1.000000000000000000, 0.8660254037844387076, 1.000000000000000000, 0.8660254037844387076, 1.000000000000000000, 0.8660254037844387076, 1.000000000000000000, 0.8660254037844387076, 1.000000000000000000, 0.8660254037844387076, 1.000000000000000000, 0.8660254037844387076, 1.000000000000000000, 0.8660254037844387076, 1.000000000000000000, 0.8660254037844387076, 1.000000000000000000, 0.8660254037844387076, 1.000000000000000000, 0.8660254037844387076, 1.000000000000000000, 0.8660254037844387076, 1.000000000000000000, 0.8660254037844387076, 1.000000000000000000, 0.8660254037844387076, 1.000000000000000000, 0.8660254037844387076, 1.000000000000000000, 0.8660254037844387076, 1.000000000000000000, 0.8660254037844387076, 1.000000000000000000, 0.8660254037844387076, 1.000000000000000000, 0.8660254037844387076, 1.000000000000000000, 0.8660254037844387076, 1.000000000000000000, 0.8660254037844387076, 1.000000000000000000, 0.8660254037844387076, 1.000000000000000000, 0.8660254037844387076, 1.000000000000000000, 0.8660254037844387076, 1.000000000000000000, 0.8660254037844387076, 1.000000000000000000, 0.8660254037844387076, 1.000000000000000000, 0.8660254037844387076, 1.000000000000000000, 0.8660254037844387076, 1.000000000000000000, 0.8660254037844387076, 1.000000000000000000, 0.8660254037844387076, 1.000000000000000000, 0.8660254037844387076, 1.000000000000000000, 0.8660254037844387076, 1.000000000000000000, 0.8660254037844387076, 1.000000000000000000, 0.8660254037844387076, 1.000000000000000000, 0.8660254037844387076, 1.000000000000000000, 0.8660254037844387076, 1.000000000000000000, 0.8660254037844387076, 1.000000000000000000, 0.8660254037844387076, 1.000000000000000000, 0.8660254037844387076, 1.000000000000000000, 0.8660254037844387076, 1.000000000000000000, 0.8660254037844387076, 1.000000000000000000, 0.8660254037844387076, 1.000000000000000000, 0.8660254037844387076, 1.000000000000000000, 0.8660254037844387076, 1.000000000000000000, 0.8660254037844387076, 1.000000000000000000, 0.8660254037844387076, 1.000000000000000000, 0.8660254037844387076, 1.000000000000000000, 0.8660254037844387076, 1.000000000000000000, 0.8660254037844387076, 1.000000000000000000, 0.8660254037844387076, 1.000000000000000000, 0.8660254037844387076, 1.000000000000000000, 0.8660254037844387076, 1.000000000000000000, 0.8660254037844387076, 1.000000000000000000, 0.8660254037844387076, 1.000000000000000000, 0.8660254037844387076, 1.000000000000000000, 0.8660254037844387076, 1.000000000000000000, 0.8660254037844387076, 1.000000000000000000, 0.8660254037844387076, 1.000000000000000000, 0.8660254037844387076, 1.000000000000000000, 0.8660254037844387076, 1.000000000000000000, 0.8660254037844387076, 1.000000000000000000, 0.8660254037844387076, 1.000000000000000000, 0.8660254037844387076, 1.000000000000000000, 0.8660254037844387076, 1.000000000000000000, 0.8660254037844387076, 1.000000000000000000, 0.8660254037844387076, 1.000000000000000000, 0.8660254037844387076, 1.000000000000000000, 0.8660254037844387076, 1.000000000000000000, 0.8660254037844387076, 1.000000000000000000, 0.8660254037844387076, 1.000000000000000000, 0.8660254037844387076, 1.000000000000000000, 0.8660254037844387076, 1.000000000000000000, 0.8660254037844387076, 1.000000000000000000, 0.8660254037844387076, 1.000000000000000000, 0.8660254037844387076, 1.000000000000000000, 0.8660254037844387076, 1.000000000000000000, 0.8660254037844387076, 1.000000000000000000, 0.8660254037844387076, 1.000000000000000000, 0.8660254037844387076, 1.000000000000000000, 0.8660254037844387076, 1.000000000000000000, 0.8660254037844387076, 1.000000000000000000, 0.8660254037844387076, 1.000000000000000000, 0.8660254037844387076, 1.000000000000000000, 0.8660254037844387076, 1.000000000000000000, 0.8660254037844387076, 1.000000000000000000, 0.8660254037844387076, 1.000000000000000000, 0.8660254037844387076, 1.000000000000000000, 0.8660254037844387076, 1.000000000000000000, 0.8660254037844387076, 1.000000000000000000, 0.8660254037844387076, 1.000000000000000000, 0.8660254037844387076, 1.000000000000000000, 0.8660254037844387076, 1.000000000000000000, 0.8660254037844387076, 1.000000000000000000, 0.8660254037844387076, 1.000000000000000000, 0.8660254037844387076, 1.000000000000000000, 0.8660254037844387076, 1.000000000000000000, 0.8660254037844387076, 1.000000000000000000, 0.8660254037844387076, 1.000000000000000000, 0.8660254037844387076, 1.000000000000000000, 0.8660254037844387076, 1.000000000000000000, 0.8660254037844387076, 1.000000000000000000, 0.8660254037844387076, 1.000000000000000000, 0.8660254037844387076, 1.000000000000000000, 0.8660254037844387076, 1.000000000000000000, 0.8660254037844387076, 1.000000000000000000, 0.8660254037844387076, 1.000000000000000000, 0.8660254037844387076, 1.000000000000000000, 0.8660254037844387076, 1.000000000000000000, 0.8660254037844387076, 1.000000000000000000, 0.8660254037844387076, 1.000000000000000000, 0.8660254037844387076, 1.000000000000000000, 0.8660254037844387076, 1.000000000000000000, 0.8660254037844387076, 1.000000000000000000, 0.8660254037844387076, 1.000000000000000000, 0.8660254037844387076, 1.000000000000000000, 0.8660254037844387076, 1.000000000000000000, 0.8660254037844387076, 1.000000000000000000, 0.8660254037844387076, 1.000000000000000000, 0.8660254037844387076, 1.000000000000000000, 0.8660254037844387076, 1.000000000000000000, 0.8660254037844387076, 1.000000000000000000, 0.8660254037844387076, 1.000000000000000000, 0.8660254037844387076, 1.000000000000000000, 0.8660254037844387076, 1.000000000000000000, 0.8660254037844387076, 1.000000000000000000, 0.8660254037844387076, 1.000000000000000000, 0.8660254037844387076, 1.000000000000000000, 0.8660254037844387076, 1.000000000000000000, 0.8660254037844387076, 1.000000000000000000, 0.8660254037844387076, 1.000000000000000000, 0.8660254037844387076, 1.000000000000000000, 0.8660254037844387076, 1.000000000000000000, 0.8660254037844387076, 1.000000000000000000, 0.8660254037844387076, 1.000000000000000000, 0.8660254037844387076, 1.000000000000000000, 0.8660254037844387076, 1.000000000000000000, 0.8660254037844387076, 1.000000000000000000, 0.8660254037844387076, 1.000000000000000000, 0.8660254037844387076, 1.000000000000000000, 0.8660254037844387076, 1.000000000000000000, 0.8660254037844387076, 1.000000000000000000, 0.8660254037844387076, 1.000000000000000000, 0.8660254037844387076, 1.000000000000000000, 0.8660254037844387076, 1.000000000000000000, 0.8660254037844387076, 1.000000000000000000, 0.8660254037844387076, 1.000000000000000000, 0.8660254037844387076, 1.000000000000000000, 0.8660254037844387076, 1.000000000000000000, 0.8660254037844387076, 1.000000000000000000, 0.8660254037844387076, 1.000000000000000000, 0.8660254037844387076, 1.000000000000000000, 0.8660254037844387076, 1.000000000000000000, 0.8660254037844387076, 1.000000000000000000, 0.8660254037844387076, 1.000000000000000000, 0.8660254037844387076, 1.000000000000000000, 0.8660254037844387076, 1.000000000000000000, 0.8660254037844387076, 1.000000000000000000, 0.8660254037844387076, 1.000000000000000000, 0.8660254037844387076, 1.000000000000000000, 0.8660254037844387076, 1.000000000000000000, 0.8660254037844387076, 1.000000000000000000, 0.8660254037844387076, 1.000000000000000000, 0.8660254037844387076, 1.000000000000000000, 0.8660254037844387076, 1.000000000000000000, 0.8660254037844387076, 1.000000000000000000, 0.8660254037844387076, 1.000000000000000000, 0.8660254037844387076, 1.000000000000000000, 0.8660254037844387076, 1.000000000000000000, 0.8660254037844387076, 1.000000000000000000, 0.8660254037844387076, 1.000000000000000000, 0.8660254037844387076, 1.000000000000000000, 0.8660254037844387076, 1.000000000000000000, 0.8660254037844387076, 1.000000000000000000, 0.8660254037844387076, 1.000000000000000000, 0.8660254037844387076, 1.000000000000000000, 0.8660254037844387076, 1.000000000000000000, 0.8660254037844387076, 1.000000000000000000, 0.8660254037844387076, 1.000000000000000000, 0.8660254037844387076, 1.000000000000000000, 0.8660254037844387076, 1.000000000000000000, 0.8660254037844387076, 1.000000000000000000, 0.8660254037844387076, 1.000000000000000000, 0.8660254037844387076, 1.000000000000000000, 0.8660254037844387076, 1.000000000000000000, 0.8660254037844387076, 1.000000000000000000, 0.8660254037844387076, 1.000000000000000000, 0.8660254037844387076, 1.000000000000000000, 0.8660254037844387076, 1.000000000000000000, 0.8660254037844387076, 1.000000000000000000, 0.8660254037844387076, 1.000000000000000000, 0.8660254037844387076, 1.000000000000000000, 0.8660254037844387076, 1.000000000000000000, 0.8660254037844387076, 1.000000000000000000, 0.8660254037844387076, 1.000000000000000000, 0.8660254037844387076, 1.000000000000000000, 0.8660254037844387076, 1.000000000000000000, 0.8660254037844387076, 1.000000000000000000, 0.8660254037844387076, 1.000000000000000000, 0.8660254037844387076, 1.000000000000000000, 0.8660254037844387076, 1.000000000000000000, 0.8660254037844387076, 1.000000000000000000, 0.8660254037844387076, 1.000000000000000000, 0.8660254037844387076, 1.000000000000000000, 0.8660254037844387076, 1.000000000000000000, 0.8660254037844387076, 1.000000000000000000, 0.8660254037844387076, 1.000000000000000000, 0.8660254037844387076, 1.000000000000000000, 0.8660254037844387076, 1.000000000000000000, 0.8660254037844387076, 1.000000000000000000, 0.8660254037844387076, 1.000000000000000000, 0.8660254037844387076, 1.000000000000000000, 0.8660254037844387076, 1.000000000000000000, 0.8660254037844387076, 1.000000000000000000, 0.8660254037844387076, 1.000000000000000000, 0.8660254037844387076, 1.000000000000000000, 0.8660254037844387076, 1.000000000000000000, 0.8660254037844387076, 1.000000000000000000, 0.8660254037844387076, 1.000000000000000000, 0.8660254037844387076, 1.000000000000000000, 0.8660254037844387076, 1.000000000000000000, 0.8660254037844387076, 1.000000000000000000, 0.8660254037844387076, 1.000000000000000000, 0.8660254037844387076, 1.000000000000000000, 0.8660254037844387076, 1.000000000000000000, 0.8660254037844387076, 1.000000000000000000, 0.8660254037844387076, 1.000000000000000000, 0.8660254037844387076, 1.000000000000000000, 0.8660254037844387076, 1.000000000000000000, 0.8660254037844387076, 1.000000000000000000, 0.8660254037844387076, 1.000000000000000000, 0.8660254037844387076, 1.000000000000000000, 0.8660254037844387076, 1.000000000000000000, 0.8660254037844387076, 1.000000000000000000, 0.8660254037844387076, 1.000000000000000000, 0.8660254037844387076, 1.000000000000000000, 0.8660254037844387076, 1.000000000000000000, 0.8660254037844387076, 1.000000000000000000, 0.8660254037844387076, 1.000000000000000000, 0.8660254037844387076, 1.000000000000000000, 0.8660254037844387076, 1.000000000000000000, 0.8660254037844387076, 1.000000000000000000, 0.8660254037844387076, 1.000000000000000000, 0.8660254037844387076, 1.000000000000000000, 0.8660254037844387076, 1.000000000000000000, 0.8660254037844387076, 1.000000000000000000, 0.8660254037844387076, 1.000000000000000000, 0.8660254037844387076, 1.000000000000000000, 0.8660254037844387076, 1.000000000000000000, 0.8660254037844387076, 1.000000000000000000, 0.8660254037844387076, 1.000000000000000000, 0.8660254037844387076, 1.000000000000000000, 0.8660254037844387076, 1.000000000000000000, 0.8660254037844387076, 1.000000000000000000, 0.8660254037844387076, 1.000000000000000000, 0.8660254037844387076, 1.000000000000000000),
 ( 1.000000000000000000, 0.8660254037844387076, 1.000000000000000000, 0.8660254037844387076, 1.000000000000000000, 0.8660254037844387076, 1.000000000000000000, 0.8660254037844387076, 1.000000000000000000, 0.8660254037844387076, 1.000000000000000000, 0.8660254037844387076, 1.000000000000000000, 0.8660254037844387076, 1.000000000000000000, 0.8660254037844387076, 1.000000000000000000, 0.8660254037844387076, 1.000000000000000000, 0.8660254037844387076, 1.000000000000000000, 0.8660254037844387076, 1.000000000000000000, 0.8660254037844387076, 1.000000000000000000, 0.8660254037844387076, 1.000000000000000000, 0.8660254037844387076, 1.000000000000000000, 0.8660254037844387076, 1.000000000000000000, 0.8660254037844387076, 1.000000000000000000, 0.8660254037844387076, 1.000000000000000000, 0.8660254037844387076, 1.000000000000000000, 0.8660254037844387076, 1.000000000000000000, 0.8660254037844387076, 1.000000000000000000, 0.8660254037844387076, 1.000000000000000000, 0.8660254037844387076, 1.000000000000000000, 0.8660254037844387076, 1.000000000000000000, 0.8660254037844387076, 1.000000000000000000, 0.8660254037844387076, 1.000000000000000000, 0.8660254037844387076, 1.000000000000000000, 0.8660254037844387076, 1.000000000000000000, 0.8660254037844387076, 1.000000000000000000, 0.8660254037844387076, 1.000000000000000000, 0.8660254037844387076, 1.000000000000000000, 0.8660254037844387076, 1.000000000000000000, 0.8660254037844387076, 1.000000000000000000, 0.8660254037844387076, 1.000000000000000000, 0.8660254037844387076, 1.000000000000000000, 0.8660254037844387076, 1.000000000000000000, 0.8660254037844387076, 1.000000000000000000, 0.8660254037844387076, 1.000000000000000000, 0.8660254037844387076, 1.000000000000000000, 0.8660254037844387076, 1.000000000000000000, 0.8660254037844387076, 1.000000000000000000, 0.8660254037844387076, 1.000000000000000000, 0.8660254037844387076, 1.000000000000000000, 0.8660254037844387076, 1.000000000000000000, 0.8660254037844387076, 1.000000000000000000, 0.8660254037844387076, 1.000000000000000000, 0.8660254037844387076, 1.000000000000000000, 0.8660254037844387076, 1.000000000000000000, 0.8660254037844387076, 1.000000000000000000, 0.8660254037844387076, 1.000000000000000000, 0.8660254037844387076, 1.000000000000000000, 0.8660254037844387076, 1.000000000000000000, 0.8660254037844387076, 1.000000000000000000, 0.8660254037844387076, 1.000000000000000000, 0.8660254037844387076, 1.000000000000000000, 0.8660254037844387076, 1.000000000000000000, 0.8660254037844387076, 1.000000000000000000, 0.8660254037844387076, 1.000000000000000000, 0.8660254037844387076, 1.000000000000000000, 0.8660254037844387076, 1.000000000000000000, 0.8660254037844387076, 1.000000000000000000, 0.8660254037844387076, 1.000000000000000000, 0.8660254037844387076, 1.000000000000000000, 0.8660254037844387076, 1.000000000000000000, 0.8660254037844387076, 1.000000000000000000, 0.8660254037844387076, 1.000000000000000000, 0.8660254037844387076, 1.000000000000000000, 0.8660254037844387076, 1.000000000000000000, 0.8660254037844387076, 1.000000000000000000, 0.8660254037844387076, 1.000000000000000000, 0.8660254037844387076, 1.000000000000000000, 0.8660254037844387076, 1.000000000000000000, 0.8660254037844387076, 1.000000000000000000, 0.8660254037844387076, 1.000000000000000000, 0.8660254037844387076, 1.000000000000000000, 0.8660254037844387076, 1.000000000000000000, 0.8660254037844387076, 1.000000000000000000, 0.8660254037844387076, 1.000000000000000000, 0.8660254037844387076, 1.000000000000000000, 0.8660254037844387076, 1.000000000000000000, 0.8660254037844387076, 1.000000000000000000, 0.8660254037844387076, 1.000000000000000000, 0.8660254037844387076, 1.000000000000000000, 0.8660254037844387076, 1.000000000000000000, 0.8660254037844387076, 1.000000000000000000, 0.8660254037844387076, 1.000000000000000000, 0.8660254037844387076, 1.000000000000000000, 0.8660254037844387076, 1.000000000000000000, 0.8660254037844387076, 1.000000000000000000, 0.8660254037844387076, 1.000000000000000000, 0.8660254037844387076, 1.000000000000000000, 0.8660254037844387076, 1.000000000000000000, 0.8660254037844387076, 1.000000000000000000, 0.8660254037844387076, 1.000000000000000000, 0.8660254037844387076, 1.000000000000000000, 0.8660254037844387076, 1.000000000000000000, 0.8660254037844387076, 1.000000000000000000, 0.8660254037844387076, 1.000000000000000000, 0.8660254037844387076, 1.000000000000000000, 0.8660254037844387076, 1.000000000000000000, 0.8660254037844387076, 1.000000000000000000, 0.8660254037844387076, 1.000000000000000000, 0.8660254037844387076, 1.000000000000000000, 0.8660254037844387076, 1.000000000000000000, 0.8660254037844387076, 1.000000000000000000, 0.8660254037844387076, 1.000000000000000000, 0.8660254037844387076, 1.000000000000000000, 0.8660254037844387076, 1.000000000000000000, 0.8660254037844387076, 1.000000000000000000, 0.8660254037844387076, 1.000000000000000000, 0.8660254037844387076, 1.000000000000000000, 0.8660254037844387076, 1.000000000000000000, 0.8660254037844387076, 1.000000000000000000, 0.8660254037844387076, 1.000000000000000000, 0.8660254037844387076, 1.000000000000000000, 0.8660254037844387076, 1.000000000000000000, 0.8660254037844387076, 1.000000000000000000, 0.8660254037844387076, 1.000000000000000000, 0.8660254037844387076, 1.000000000000000000, 0.8660254037844387076, 1.000000000000000000, 0.8660254037844387076, 1.000000000000000000, 0.8660254037844387076, 1.000000000000000000, 0.8660254037844387076, 1.000000000000000000, 0.8660254037844387076, 1.000000000000000000, 0.8660254037844387076, 1.000000000000000000, 0.8660254037844387076, 1.000000000000000000, 0.8660254037844387076, 1.000000000000000000, 0.8660254037844387076, 1.000000000000000000, 0.8660254037844387076, 1.000000000000000000, 0.8660254037844387076, 1.000000000000000000, 0.8660254037844387076, 1.000000000000000000, 0.8660254037844387076, 1.000000000000000000, 0.8660254037844387076, 1.000000000000000000, 0.8660254037844387076, 1.000000000000000000, 0.8660254037844387076, 1.000000000000000000, 0.8660254037844387076, 1.000000000000000000, 0.8660254037844387076, 1.000000000000000000, 0.8660254037844387076, 1.000000000000000000, 0.8660254037844387076, 1.000000000000000000, 0.8660254037844387076, 1.000000000000000000, 0.8660254037844387076, 1.000000000000000000, 0.8660254037844387076, 1.000000000000000000, 0.8660254037844387076, 1.000000000000000000, 0.8660254037844387076, 1.000000000000000000, 0.8660254037844387076, 1.000000000000000000, 0.8660254037844387076, 1.000000000000000000, 0.8660254037844387076, 1.000000000000000000, 0.8660254037844387076, 1.000000000000000000, 0.8660254037844387076, 1.000000000000000000, 0.8660254037844387076, 1.000000000000000000, 0.8660254037844387076, 1.000000000000000000, 0.8660254037844387076, 1.000000000000000000, 0.8660254037844387076, 1.000000000000000000, 0.8660254037844387076, 1.000000000000000000, 0.8660254037844387076, 1.000000000000000000, 0.8660254037844387076, 1.000000000000000000, 0.8660254037844387076, 1.000000000000000000, 0.8660254037844387076, 1.000000000000000000, 0.8660254037844387076, 1.000000000000000000, 0.8660254037844387076, 1.000000000000000000, 0.8660254037844387076, 1.000000000000000000, 0.8660254037844387076, 1.000000000000000000, 0.8660254037844387076, 1.000000000000000000, 0.8660254037844387076, 1.000000000000000000, 0.8660254037844387076, 1.000000000000000000, 0.8660254037844387076, 1.000000000000000000, 0.8660254037844387076, 1.000000000000000000, 0.8660254037844387076, 1.000000000000000000, 0.8660254037844387076, 1.000000000000000000, 0.8660254037844387076, 1.000000000000000000, 0.8660254037844387076, 1.000000000000000000, 0.8660254037844387076, 1.000000000000000000, 0.8660254037844387076, 1.000000000000000000, 0.8660254037844387076, 1.000000000000000000, 0.8660254037844387076, 1.000000000000000000, 0.8660254037844387076, 1.000000000000000000, 0.8660254037844387076, 1.000000000000000000, 0.8660254037844387076, 1.000000000000000000, 0.8660254037844387076, 1.000000000000000000, 0.8660254037844387076, 1.000000000000000000, 0.8660254037844387076, 1.000000000000000000, 0.8660254037844387076, 1.000000000000000000, 0.8660254037844387076, 1.000000000000000000, 0.8660254037844387076, 1.000000000000000000, 0.8660254037844387076, 1.000000000000000000, 0.8660254037844387076, 1.000000000000000000, 0.8660254037844387076, 1.000000000000000000, 0.8660254037844387076, 1.000000000000000000, 0.8660254037844387076, 1.000000000000000000, 0.8660254037844387076, 1.000000000000000000, 0.8660254037844387076, 1.000000000000000000, 0.8660254037844387076, 1.000000000000000000, 0.8660254037844387076, 1.000000000000000000, 0.8660254037844387076, 1.000000000000000000, 0.8660254037844387076, 1.000000000000000000, 0.8660254037844387076, 1.000000000000000000, 0.8660254037844387076, 1.000000000000000000, 0.8660254037844387076, 1.000000000000000000, 0.8660254037844387076, 1.000000000000000000, 0.8660254037844387076, 1.000000000000000000, 0.8660254037844387076, 1.000000000000000000, 0.8660254037844387076, 1.000000000000000000, 0.8660254037844387076, 1.000000000000000000, 0.8660254037844387076, 1.000000000000000000, 0.8660254037844387076, 1.000000000000000000, 0.8660254037844387076, 1.000000000000000000, 0.8660254037844387076, 1.000000000000000000, 0.8660254037844387076, 1.000000000000000000, 0.8660254037844387076, 1.000000000000000000, 0.8660254037844387076, 1.000000000000000000, 0.8660254037844387076, 1.000000000000000000, 0.8660254037844387076, 1.000000000000000000, 0.8660254037844387076, 1.000000000000000000, 0.8660254037844387076, 1.000000000000000000, 0.8660254037844387076, 1.000000000000000000, 0.8660254037844387076, 1.000000000000000000, 0.8660254037844387076, 1.000000000000000000, 0.8660254037844387076, 1.000000000000000000, 0.8660254037844387076, 1.000000000000000000, 0.8660254037844387076, 1.000000000000000000, 0.8660254037844387076, 1.000000000000000000, 0.8660254037844387076, 1.000000000000000000, 0.8660254037844387076, 1.000000000000000000, 0.8660254037844387076, 1.000000000000000000, 0.8660254037844387076, 1.000000000000000000, 0.8660254037844387076, 1.000000000000000000, 0.8660254037844387076, 1.000000000000000000, 0.8660254037844387076, 1.000000000000000000, 0.8660254037844387076, 1.000000000000000000, 0.8660254037844387076, 1.000000000000000000, 0.8660254037844387076, 1.000000000000000000, 0.8660254037844387076, 1.000000000000000000, 0.8660254037844387076, 1.000000000000000000, 0.8660254037844387076, 1.000000000000000000, 0.8660254037844387076, 1.000000000000000000, 0.8660254037844387076, 1.000000000000000000, 0.8660254037844387076, 1.000000000000000000, 0.8660254037844387076, 1.000000000000000000, 0.8660254037844387076, 1.000000000000000000, 0.8660254037844387076, 1.000000000000000000, 0.8660254037844387076, 1.000000000000000000, 0.8660254037844387076, 1.000000000000000000, 0.8660254037844387076, 1.000000000000000000, 0.8660254037844387076, 1.000000000000000000, 0.8660254037844387076, 1.000000000000000000, 0.8660254037844387076, 1.000000000000000000, 0.8660254037844387076, 1.000000000000000000, 0.8660254037844387076, 1.000000000000000000, 0.8660254037844387076, 1.000000000000000000, 0.8660254037844387076, 1.000000000000000000, 0.8660254037844387076, 1.000000000000000000, 0.8660254037844387076, 1.000000000000000000, 0.8660254037844387076, 1.000000000000000000, 0.8660254037844387076, 1.000000000000000000, 0.8660254037844387076, 1.000000000000000000, 0.8660254037844387076, 1.000000000000000000, 0.8660254037844387076, 1.000000000000000000, 0.8660254037844387076, 1.000000000000000000, 0.8660254037844387076, 1.000000000000000000, 0.8660254037844387076, 1.000000000000000000, 0.8660254037844387076, 1.000000000000000000, 0.8660254037844387076, 1.000000000000000000, 0.8660254037844387076, 1.000000000000000000, 0.8660254037844387076, 1.000000000000000000, 0.8660254037844387076, 1.000000000000000000, 0.8660254037844387076, 1.000000000000000000, 0.8660254037844387076, 1.000000000000000000, 0.8660254037844387076, 1.000000000000000000, 0.8660254037844387076, 1.000000000000000000, 0.8660254037844387076, 1.000000000000000000, 0.8660254037844387076, 1.000000000000000000, 0.8660254037844387076, 1.000000000000000000, 0.8660254037844387076, 1.000000000000000000, 0.8660254037844387076, 1.000000000000000000, 0.8660254037844387076, 1.000000000000000000, 0.8660254037844387076, 1.000000000000000000, 0.8660254037844387076, 1.000000000000000000, 0.8660254037844387076, 1.000000000000000000, 0.8660254037844387076, 1.000000000000000000, 0.8660254037844387076, 1.000000000000000000, 0.8660254037844387076, 1.000000000000000000, 0.8660254037844387076, 1.000000000000000000, 0.8660254037844387076, 1.000000000000000000, 0.8660254037844387076, 1.000000000000000000, 0.8660254037844387076, 1.000000000000000000, 0.8660254037844387076, 1.000000000000000000, 0.8660254037844387076, 1.000000000000000000, 0.8660254037844387076, 1.000000000000000000, 0.8660254037844387076, 1.000000000000000000, 0.8660254037844387076, 1.000000000000000000, 0.8660254037844387076, 1.000000000000000000, 0.8660254037844387076, 1.000000000000000000, 0.8660254037844387076, 1.000000000000000000, 0.8660254037844387076, 1.000000000000000000, 0.8660254037844387076, 1.000000000000000000, 0.8660254037844387076, 1.000000000000000000, 0.8660254037844387076, 1.000000000000000000, 0.8660254037844387076, 1.000000000000000000, 0.8660254037844387076, 1.000000000000000000, 0.8660254037844387076, 1.000000000000000000, 0.8660254037844387076, 1.000000000000000000, 0.8660254037844387076, 1.000000000000000000, 0.8660254037844387076, 1.000000000000000000, 0.8660254037844387076, 1.000000000000000000, 0.8660254037844387076, 1.000000000000000000, 0.8660254037844387076, 1.000000000000000000, 0.8660254037844387076, 1.000000000000000000, 0.8660254037844387076, 1.000000000000000000, 0.8660254037844387076, 1.000000000000000000, 0.8660254037844387076, 1.000000000000000000, 0.8660254037844387076, 1.000000000000000000, 0.8660254037844387076, 1.000000000000000000, 0.8660254037844387076, 1.000000000000000000, 0.8660254037844387076, 1.000000000000000000, 0.8660254037844387076, 1.000000000000000000, 0.8660254037844387076, 1.000000000000000000, 0.8660254037844387076, 1.000000000000000000, 0.8660254037844387076, 1.000000000000000000, 0.8660254037844387076, 1.000000000000000000, 0.8660254037844387076, 1.000000000000000000, 0.8660254037844387076, 1.000000000000000000, 0.8660254037844387076, 1.000000000000000000, 0.8660254037844387076, 1.000000000000000000, 0.8660254037844387076, 1.000000000000000000, 0.8660254037844387076, 1.000000000000000000, 0.8660254037844387076, 1.000000000000000000, 0.8660254037844387076, 1.000000000000000000, 0.8660254037844387076, 1.000000000000000000, 0.8660254037844387076, 1.000000000000000000, 0.8660254037844387076, 1.000000000000000000, 0.8660254037844387076, 1.000000000000000000, 0.8660254037844387076, 1.000000000000000000, 0.8660254037844387076, 1.000000000000000000, 0.8660254037844387076, 1.000000000000000000, 0.8660254037844387076, 1.000000000000000000, 0.8660254037844387076, 1.000000000000000000, 0.8660254037844387076, 1.000000000000000000, 0.8660254037844387076, 1.000000000000000000, 0.8660254037844387076, 1.000000000000000000, 0.8660254037844387076, 1.000000000000000000, 0.8660254037844387076, 1.000000000000000000, 0.8660254037844387076, 1.000000000000000000, 0.8660254037844387076, 1.000000000000000000, 0.8660254037844387076, 1.000000000000000000, 0.8660254037844387076, 1.000000000000000000, 0.8660254037844387076, 1.000000000000000000, 0.8660254037844387076, 1.000000000000000000, 0.8660254037844387076, 1.000000000000000000, 0.8660254037844387076, 1.000000000000000000, 0.8660254037844387076, 1.000000000000000000, 0.8660254037844387076, 1.000000000000000000, 0.8660254037844387076, 1.000000000000000000, 0.8660254037844387076, 1.000000000000000000, 0.8660254037844387076, 1.000000000000000000, 0.8660254037844387076, 1.000000000000000000, 0.8660254037844387076, 1.000000000000000000, 0.8660254037844387076, 1.000000000000000000, 0.8660254037844387076, 1.000000000000000000, 0.8660254037844387076, 1.000000000000000000, 0.8660254037844387076, 1.000000000000000000, 0.8660254037844387076, 1.000000000000000000) ) ) 
 REPRESENTATION_ITEM ( '' )  SURFACE ( )  );
#68239=CARTESIAN_POINT ( 'NONE',  ( 27.68437500061451573, -4.541064518000419881, 2.621784821874995952 ) ) ;
#68241=CARTESIAN_POINT ( 'NONE',  ( 14.87812500061451537, 4.541064518000418104, 2.621784821874999949 ) ) ;
#68242=CARTESIAN_POINT ( 'NONE',  ( 8.053125000614516082, 4.541064518000418104, -2.621784821874998173 ) ) ;
#68244=CARTESIAN_POINT ( 'NONE',  ( 4.209375000614516971, 0.000000000000000000, 5.243569643749999010 ) ) ;
#68245=CARTESIAN_POINT ( 'NONE',  ( 17.10000000122903430, -2.886751345948129988, 4.999999999999997335 ) ) ;
#68246=CARTESIAN_POINT ( 'NONE',  ( 21.60000000000000142, -4.330127018922190985, -2.500000000000001332 ) ) ;
#68247=CARTESIAN_POINT ( 'NONE',  ( 29.73750000000000071, -2.886751345948125991, -5.000000000000000000 ) ) ;
#68248=CARTESIAN_POINT ( 'NONE',  ( 3.534375000614518036, 6.421520780324663323E-16, -5.243569643749999010 ) ) ;
#68249=CARTESIAN_POINT ( 'NONE',  ( 12.00937500061451857, -4.541064518000417216, -2.621784821875001281 ) ) ;
#68250=CARTESIAN_POINT ( 'NONE',  ( 22.73437500061451644, -4.541064518000419881, 2.621784821874995952 ) ) ;
#68251=CARTESIAN_POINT ( 'NONE',  ( -3.999999999999999112, 15.12500000122903465, -32.30940107675850470 ) ) ;
#68252=VERTEX_POINT ( 'NONE', #27051 ) ;
#68254=CARTESIAN_POINT ( 'NONE',  ( 3.234375000614516438, 4.541064518000418104, 2.621784821874999949 ) ) ;
#68255=CARTESIAN_POINT ( 'NONE',  ( 7.434375000614519280, -4.541064518000419881, 2.621784821874995952 ) ) ;
#68256=CARTESIAN_POINT ( 'NONE',  ( 18.56250000000000000, 2.886751345948129099, -4.999999999999998224 ) ) ;
#68257=CARTESIAN_POINT ( 'NONE',  ( 16.64062500061451289, 6.054752690667223547, 3.707466751127219781E-16 ) ) ;
#68261=CARTESIAN_POINT ( 'NONE',  ( 9.628125000614517148, -4.541064518000419881, 2.621784821874995952 ) ) ;
#68262=CARTESIAN_POINT ( 'NONE',  ( 25.54687500061451644, -3.027376345333610441, -5.243569643749999898 ) ) ;
#68264=CARTESIAN_POINT ( 'NONE',  ( 25.39687500061451431, -3.027376345333614438, 5.243569643749998122 ) ) ;
#68265=CARTESIAN_POINT ( 'NONE',  ( 7.387500000000001066, 5.773502691896255534, 3.535250795749688894E-16 ) ) ;
#68266=CARTESIAN_POINT ( 'NONE',  ( -3.999999999999997335, 14.30000000122903359, 32.30940107675850470 ) ) ;
#68267=CARTESIAN_POINT ( 'NONE',  ( 8.625000001229034652, -5.773502691896255534, -1.060575238724906372E-15 ) ) ;
#68268=CARTESIAN_POINT ( 'NONE',  ( 20.07187500061451857, -6.054752690667223547, -1.112240025338166033E-15 ) ) ;
#68269=CARTESIAN_POINT ( 'NONE',  ( 12.19687500061451679, 6.054752690667223547, 3.707466751127219781E-16 ) ) ;
#68271=VERTEX_POINT ( 'NONE', #9321 ) ;
#68272=CARTESIAN_POINT ( 'NONE',  ( 14.99062500061451786, -3.027376345333614438, 5.243569643749998122 ) ) ;
#68273=CARTESIAN_POINT ( 'NONE',  ( 26.25000000122903288, -2.886751345948125991, -5.000000000000000000 ) ) ;
#68274=CARTESIAN_POINT ( 'NONE',  ( 11.63437500061451857, 6.421520780324663323E-16, -5.243569643749999010 ) ) ;
#68275=CARTESIAN_POINT ( 'NONE',  ( 4.000000000000000000, 12.65000000122903323, 32.30940107675849760 ) ) ;
#68276=CARTESIAN_POINT ( 'NONE',  ( 16.86562500061451786, -6.054752690667223547, -1.112240025338166033E-15 ) ) ;
#68277=CARTESIAN_POINT ( 'NONE',  ( 26.32500000122903216, 2.886751345948129099, -4.999999999999997335 ) ) ;
#68278=CARTESIAN_POINT ( 'NONE',  ( 26.85937500061451644, -4.541064518000417216, -2.621784821875001281 ) ) ;
#68279=CARTESIAN_POINT ( 'NONE',  ( -2.121784821874996840, 9.978125000614518569, 33.67503911421598417 ) ) ;
#68280=EDGE_CURVE ( 'NONE', #27910, #70559, #41901, .T. ) ;
#68281=CARTESIAN_POINT ( 'NONE',  ( 10.91250000122903252, -4.330127018922190985, -2.500000000000001332 ) ) ;
#68283=CARTESIAN_POINT ( 'NONE',  ( -4.243569643749999898, 17.12187500061451573, -32.45002607614398471 ) ) ;
#68284=CARTESIAN_POINT ( 'NONE',  ( 18.53437500061451715, 4.541064518000418104, 2.621784821874999949 ) ) ;
#68285=CARTESIAN_POINT ( 'NONE',  ( 19.98750000122903359, 6.123233995736764310E-16, -4.999999999999998224 ) ) ;
#68286=ADVANCED_FACE ( 'NONE', ( #31854 ), #18790, .T. ) ;
#68287=CARTESIAN_POINT ( 'NONE',  ( 15.38437500061451679, 4.541064518000418104, 2.621784821874999949 ) ) ;
#68288=CARTESIAN_POINT ( 'NONE',  ( -4.243569643749999898, 10.85937500061451821, 30.00000000000000000 ) ) ;
#68289=CARTESIAN_POINT ( 'NONE',  ( 21.93750000122903288, 4.330127018922191873, 2.499999999999999556 ) ) ;
#68290=CARTESIAN_POINT ( 'NONE',  ( 14.35312500061451679, 4.541064518000418104, -2.621784821874998173 ) ) ;
#68291=CARTESIAN_POINT ( 'NONE',  ( 28.90312500061451217, 0.000000000000000000, 5.243569643749999010 ) ) ;
#68292=VERTEX_POINT ( 'NONE', #20516 ) ;
#68293=VERTEX_POINT ( 'NONE', #2815 ) ;
#68294=CARTESIAN_POINT ( 'NONE',  ( 18.45000000000000284, -4.330127018922190985, -2.500000000000001332 ) ) ;
#68296=CARTESIAN_POINT ( 'NONE',  ( 0.6891293861215573857, 4.954145703890282526, 33.94256940425900382 ) ) ;
#68297=CARTESIAN_POINT ( 'NONE',  ( 14.66250000122903252, 4.330127018922192761, -2.499999999999997780 ) ) ;
#68298=CARTESIAN_POINT ( 'NONE',  ( 20.76562500061451644, 3.027376345333611329, 5.243569643749999010 ) ) ;
#68299=CARTESIAN_POINT ( 'NONE',  ( 23.76562500061451644, 3.027376345333613106, -5.243569643749998122 ) ) ;
#68300=CARTESIAN_POINT ( 'NONE',  ( 3.890625000614517326, -3.027376345333610441, -5.243569643749999898 ) ) ;
#68301=( BOUNDED_CURVE ( )  B_SPLINE_CURVE ( 3, ( #15727, #14631, #37905, #37171 ),
 .UNSPECIFIED., .F., .F. ) 
 B_SPLINE_CURVE_WITH_KNOTS ( ( 4, 4 ),
 ( 4.024033675728571069, 4.052330423520261959 ),
 .UNSPECIFIED. ) 
 CURVE ( )  GEOMETRIC_REPRESENTATION_ITEM ( )  RATIONAL_B_SPLINE_CURVE ( ( 1.000000000000000000, 0.9999332756184333704, 0.9999332756184333704, 1.000000000000000000 ) ) 
 REPRESENTATION_ITEM ( '' )  );
#68303=CARTESIAN_POINT ( 'NONE',  ( 5.812500001229035540, 0.000000000000000000, 4.999999999999998224 ) ) ;
#68305=CARTESIAN_POINT ( 'NONE',  ( 6.300000001229033586, -2.886751345948130876, 4.999999999999996447 ) ) ;
#68306=CARTESIAN_POINT ( 'NONE',  ( 8.484601909799253346E-16, 10.32500000122903572, -25.38119784648299770 ) ) ;
#68307=CARTESIAN_POINT ( 'NONE',  ( -2.121784821874999949, 15.73437500061451644, -33.67503911421598417 ) ) ;
#68308=CARTESIAN_POINT ( 'NONE',  ( 5.662500001229035185, 4.330127018922192761, -2.499999999999997780 ) ) ;
#68309=CARTESIAN_POINT ( 'NONE',  ( 8.662499999999999645, 2.886751345948129099, -4.999999999999998224 ) ) ;
#68310=CARTESIAN_POINT ( 'NONE',  ( 3.412500001229032964, 4.330127018922192761, -2.499999999999997780 ) ) ;
#68311=CARTESIAN_POINT ( 'NONE',  ( 11.70937500061451608, 4.541064518000418104, -2.621784821874998173 ) ) ;
#68312=DIRECTION ( 'NONE',  ( -1.000000000000000000, -0.000000000000000000, -0.000000000000000000 ) ) ;
#68313=CARTESIAN_POINT ( 'NONE',  ( 2.896875000614518747, -3.027376345333614438, 5.243569643749998122 ) ) ;
#68314=CARTESIAN_POINT ( 'NONE',  ( 4.000000000000000000, 18.95000000122903216, 32.30940107675849760 ) ) ;
#68315=CARTESIAN_POINT ( 'NONE',  ( 1.071796769724490339, 19.52990381179669654, 26.00000000000000355 ) ) ;
#68316=CARTESIAN_POINT ( 'NONE',  ( 7.884375000614517681, -4.541064518000419881, 2.621784821874995952 ) ) ;
#68317=CARTESIAN_POINT ( 'NONE',  ( 14.33437500061451786, 6.421520780324663323E-16, -5.243569643749999010 ) ) ;
#68318=CARTESIAN_POINT ( 'NONE',  ( -5.810221930991193690E-16, 14.15000000122903145, -34.00000000000000000 ) ) ;
#68319=CARTESIAN_POINT ( 'NONE',  ( 5.812500000000001776, -5.773502691896255534, -1.060575238724906372E-15 ) ) ;
#68320=CARTESIAN_POINT ( 'NONE',  ( -4.243569643749998122, 16.69062500061459531, 32.45002607614398471 ) ) ;
#68321=CARTESIAN_POINT ( 'NONE',  ( 20.59687500061451360, -3.027376345333610441, -5.243569643749999898 ) ) ;
#68323=CARTESIAN_POINT ( 'NONE',  ( 26.88750000122903216, 4.330127018922191873, 2.499999999999999556 ) ) ;
#68325=CARTESIAN_POINT ( 'NONE',  ( 22.64062500061451644, -3.027376345333614438, 5.243569643749998122 ) ) ;
#68326=CARTESIAN_POINT ( 'NONE',  ( 16.30312500061451786, 0.000000000000000000, 5.243569643749999010 ) ) ;
#68328=CARTESIAN_POINT ( 'NONE',  ( 12.83437500061451786, -4.541064518000419881, 2.621784821874995952 ) ) ;
#68329=CARTESIAN_POINT ( 'NONE',  ( 28.04999999999999716, 4.330127018922192761, -2.499999999999997780 ) ) ;
#68330=CARTESIAN_POINT ( 'NONE',  ( 23.92500000122903359, -5.773502691896255534, -1.060575238724906372E-15 ) ) ;
#68331=CYLINDRICAL_SURFACE ( 'NONE', #40241, 4.000000000000000000 ) ;
#68332=CARTESIAN_POINT ( 'NONE',  ( 10.80937500061451928, 4.541064518000418104, -2.621784821874998173 ) ) ;
#68333=CARTESIAN_POINT ( 'NONE',  ( 29.78437500061451715, 4.541064518000418104, 2.621784821874999949 ) ) ;
#68334=CARTESIAN_POINT ( 'NONE',  ( 3.084375000614519191, 6.421520780324663323E-16, -5.243569643749999010 ) ) ;
#68335=CARTESIAN_POINT ( 'NONE',  ( -1.071796769724491005, 11.92009619066136850, 26.00000000000000355 ) ) ;
#68336=CARTESIAN_POINT ( 'NONE',  ( 23.40937500061451715, 4.541064518000418104, -2.621784821874998173 ) ) ;
#68337=CARTESIAN_POINT ( 'NONE',  ( 14.40937500061451715, 4.541064518000418104, -2.621784821874998173 ) ) ;
#68339=CARTESIAN_POINT ( 'NONE',  ( 25.08749999999999858, -2.886751345948129988, 4.999999999999997335 ) ) ;
#68342=CARTESIAN_POINT ( 'NONE',  ( 18.02812500061451573, 4.541064518000418104, 2.621784821874999949 ) ) ;
#68343=CARTESIAN_POINT ( 'NONE',  ( 6.825000000000001066, 6.123233995736764310E-16, -4.999999999999998224 ) ) ;
#68344=DIRECTION ( 'NONE',  ( 0.1736464922939214561, 0.000000000000000000, 0.9848080501874549864 ) ) ;
#68345=CARTESIAN_POINT ( 'NONE',  ( 18.14999999999999858, 4.330127018922192761, -2.499999999999997780 ) ) ;
#68346=CARTESIAN_POINT ( 'NONE',  ( 4.243569643749999898, 12.79062500061451679, 32.45002607614398471 ) ) ;
#68347=DIRECTION ( 'NONE',  ( -1.000000000000000000, -0.000000000000000000, -0.000000000000000000 ) ) ;
#68348=CARTESIAN_POINT ( 'NONE',  ( 27.49687500061451217, 6.054752690667223547, 3.707466751127219781E-16 ) ) ;
#68349=EDGE_LOOP ( 'NONE', ( #32182, #25112, #1320, #21397 ) ) ;
#68350=CARTESIAN_POINT ( 'NONE',  ( 21.77812500061451928, -4.541064518000419881, 2.621784821874995952 ) ) ;
#68351=CARTESIAN_POINT ( 'NONE',  ( 20.29687500061451644, 6.054752690667223547, 3.707466751127219781E-16 ) ) ;
#68352=CARTESIAN_POINT ( 'NONE',  ( 3.337499999999999911, 5.773502691896255534, 3.535250795749688894E-16 ) ) ;
#68353=CARTESIAN_POINT ( 'NONE',  ( 6.290625000614517681, 6.054752690667223547, 3.707466751127219781E-16 ) ) ;
#68354=CARTESIAN_POINT ( 'NONE',  ( 24.14062500061451289, -3.027376345333610441, -5.243569643749999898 ) ) ;
#68355=CARTESIAN_POINT ( 'NONE',  ( 11.74687500061451573, 6.054752690667223547, 3.707466751127219781E-16 ) ) ;
#68356=CARTESIAN_POINT ( 'NONE',  ( 17.22187500061451715, 3.027376345333611329, 5.243569643749999010 ) ) ;
#68357=CARTESIAN_POINT ( 'NONE',  ( -3.000416591977282496E-16, 17.89062500061451644, 25.09994784771203058 ) ) ;
#68358=CARTESIAN_POINT ( 'NONE',  ( 19.20000000122903572, 5.773502691896255534, 3.535250795749688894E-16 ) ) ;
#68360=CARTESIAN_POINT ( 'NONE',  ( 9.403125000614517504, 4.541064518000418104, -2.621784821874998173 ) ) ;
#68361=CARTESIAN_POINT ( 'NONE',  ( 5.409375000614516260, 4.541064518000418104, -2.621784821874998173 ) ) ;
#68362=CARTESIAN_POINT ( 'NONE',  ( 4.021875000614516082, 3.027376345333613106, -5.243569643749998122 ) ) ;
#68364=CARTESIAN_POINT ( 'NONE',  ( 24.87187500061451573, 3.027376345333611329, 5.243569643749999010 ) ) ;
#68365=CARTESIAN_POINT ( 'NONE',  ( 17.01562500061451644, 3.027376345333613106, -5.243569643749998122 ) ) ;
#68366=CARTESIAN_POINT ( 'NONE',  ( 26.40000000122902790, 5.773502691896255534, 3.535250795749688894E-16 ) ) ;
#68368=CARTESIAN_POINT ( 'NONE',  ( 27.44062500061451715, 6.054752690667223547, 3.707466751127219781E-16 ) ) ;
#68369=CARTESIAN_POINT ( 'NONE',  ( 22.73437500061451644, -4.541064518000419881, 2.621784821874995952 ) ) ;
#68370=CARTESIAN_POINT ( 'NONE',  ( 16.90312500061451573, -4.541064518000417216, -2.621784821875001281 ) ) ;
#68371=CARTESIAN_POINT ( 'NONE',  ( 2.121784821874999061, 18.80937500061451928, 26.32496088578401583 ) ) ;
#68372=CARTESIAN_POINT ( 'NONE',  ( 23.09062500061451573, -3.027376345333614438, 5.243569643749998122 ) ) ;
#68373=CARTESIAN_POINT ( 'NONE',  ( 2.700000001229035718, -2.886751345948129988, 4.999999999999997335 ) ) ;
#68375=CARTESIAN_POINT ( 'NONE',  ( 26.77499999999999858, 4.330127018922191873, 2.499999999999999556 ) ) ;
#68376=CARTESIAN_POINT ( 'NONE',  ( 1.999999999999998668, 12.20000000000000107, -33.46410161513775705 ) ) ;
#68378=CARTESIAN_POINT ( 'NONE',  ( 3.496875000614518836, -3.027376345333610441, -5.243569643749999898 ) ) ;
#68379=CARTESIAN_POINT ( 'NONE',  ( 9.103125000614515017, 0.000000000000000000, 5.243569643749999010 ) ) ;
#68380=CARTESIAN_POINT ( 'NONE',  ( 21.93750000122903288, 4.330127018922191873, 2.499999999999999556 ) ) ;
#68381=CARTESIAN_POINT ( 'NONE',  ( 27.36562500061451786, 3.027376345333613106, -5.243569643749998122 ) ) ;
#68382=CARTESIAN_POINT ( 'NONE',  ( 27.63749999999999929, 5.773502691896255534, 3.535250795749688894E-16 ) ) ;
#68383=CARTESIAN_POINT ( 'NONE',  ( 3.999999999999998668, 18.12500000122903288, -32.30940107675850470 ) ) ;
#68384=DIRECTION ( 'NONE',  ( 0.1736464922939166267, 0.000000000000000000, 0.9848080501874559856 ) ) ;
#68385=CARTESIAN_POINT ( 'NONE',  ( 9.778125000614517504, 6.421520780324663323E-16, -5.243569643749999010 ) ) ;
#68386=ORIENTED_EDGE ( 'NONE', *, *, #31507, .T. ) ;
#68387=CARTESIAN_POINT ( 'NONE',  ( 8.728125000614518569, -4.541064518000419881, 2.621784821874995952 ) ) ;
#68388=CARTESIAN_POINT ( 'NONE',  ( 5.053125000614517859, 0.000000000000000000, 5.243569643749999010 ) ) ;
#68390=CARTESIAN_POINT ( 'NONE',  ( 13.95000000122903394, -2.886751345948063374, 5.000000000000112799 ) ) ;
#68391=CARTESIAN_POINT ( 'NONE',  ( 15.97499999999999964, 4.330127018922191873, 2.499999999999999556 ) ) ;
#68392=CARTESIAN_POINT ( 'NONE',  ( 16.50937500061451502, -4.541064518000417216, -2.621784821875001281 ) ) ;
#68393=CARTESIAN_POINT ( 'NONE',  ( 10.27500000122903323, 2.886751345948126879, 4.999999999999999112 ) ) ;
#68394=CARTESIAN_POINT ( 'NONE',  ( 19.47187500061451360, 3.027376345333611329, 5.243569643749999010 ) ) ;
#68396=CARTESIAN_POINT ( 'NONE',  ( 20.52187500061451786, -6.054752690667223547, -1.112240025338166033E-15 ) ) ;
#68397=CARTESIAN_POINT ( 'NONE',  ( -4.243569643749997233, 13.99062500061451786, -27.54997392385601174 ) ) ;
#68398=CYLINDRICAL_SURFACE ( 'NONE', #24162, 4.999999999999998224 ) ;
#68401=CARTESIAN_POINT ( 'NONE',  ( 26.12812500061451360, 4.541064518000418104, 2.621784821874999949 ) ) ;
#68403=CARTESIAN_POINT ( 'NONE',  ( 27.87187500061451573, 3.027376345333613106, -5.243569643749998122 ) ) ;
#68404=CARTESIAN_POINT ( 'NONE',  ( 23.21250000000000213, 2.886751345948126879, 4.999999999999999112 ) ) ;
#68405=CARTESIAN_POINT ( 'NONE',  ( 5.953125000614519102, 0.000000000000000000, 5.243569643749999010 ) ) ;
#68407=CARTESIAN_POINT ( 'NONE',  ( 18.49687500061452283, 6.054752690667223547, 3.707466751127219781E-16 ) ) ;
#68409=CARTESIAN_POINT ( 'NONE',  ( 5.278125000614516615, 6.421520780324663323E-16, -5.243569643749999010 ) ) ;
#68410=CARTESIAN_POINT ( 'NONE',  ( 11.63437500061451857, 6.421520780324663323E-16, -5.243569643749999010 ) ) ;
#68412=CARTESIAN_POINT ( 'NONE',  ( 19.62187500061451573, -6.054752690667223547, -1.112240025338166033E-15 ) ) ;
#68414=CARTESIAN_POINT ( 'NONE',  ( 28.68749999999999645, -2.886751345948129988, 4.999999999999997335 ) ) ;
#68415=CARTESIAN_POINT ( 'NONE',  ( 3.787500000000002753, 5.773502691896255534, 3.535250795749688894E-16 ) ) ;
#68416=DIRECTION ( 'NONE',  ( 0.000000000000000000, 0.000000000000000000, 1.000000000000000000 ) ) ;
#68417=CARTESIAN_POINT ( 'NONE',  ( 10.87500000000000000, 6.123233995736764310E-16, -4.999999999999998224 ) ) ;
#68418=VERTEX_POINT ( 'NONE', #24972 ) ;
#68419=CARTESIAN_POINT ( 'NONE',  ( 10.87500000000000000, 6.123233995736764310E-16, -4.999999999999998224 ) ) ;
#68421=CARTESIAN_POINT ( 'NONE',  ( 24.66562500061451502, 3.027376345333613106, -5.243569643749998122 ) ) ;
#68422=CARTESIAN_POINT ( 'NONE',  ( 15.29999999999999893, -4.330127018922190985, -2.500000000000001332 ) ) ;
#68423=CARTESIAN_POINT ( 'NONE',  ( 10.53750000122903252, 6.123233995736764310E-16, -4.999999999999998224 ) ) ;
#68424=CARTESIAN_POINT ( 'NONE',  ( 10.11562500061451608, -6.054752690667223547, -1.112240025338166033E-15 ) ) ;
#68425=CARTESIAN_POINT ( 'NONE',  ( 25.12499999999999645, -4.330127018922194537, 2.499999999999995559 ) ) ;
#68426=CARTESIAN_POINT ( 'NONE',  ( 20.12812500061451715, 6.421520780324663323E-16, -5.243569643749999010 ) ) ;
#68427=CARTESIAN_POINT ( 'NONE',  ( 18.67500000122903359, 2.886751345948095793, -5.000000000000055067 ) ) ;
#68428=CARTESIAN_POINT ( 'NONE',  ( 27.93750000122903288, -4.330127018922194537, 2.499999999999995559 ) ) ;
#68430=CARTESIAN_POINT ( 'NONE',  ( 6.637500000000001066, -2.886751345948129988, 4.999999999999997335 ) ) ;
#68432=CARTESIAN_POINT ( 'NONE',  ( 22.64062500061451644, -3.027376345333614438, 5.243569643749998122 ) ) ;
#68433=CARTESIAN_POINT ( 'NONE',  ( 28.52812500061451573, -4.541064518000419881, 2.621784821874995952 ) ) ;
#68434=DIRECTION ( 'NONE',  ( 0.000000000000000000, 0.000000000000000000, 1.000000000000000000 ) ) ;
#68435=CARTESIAN_POINT ( 'NONE',  ( 18.23437500061451999, -4.541064518000419881, 2.621784821874995952 ) ) ;
#68436=EDGE_CURVE ( 'NONE', #24236, #20715, #47517, .T. ) ;
#68437=CARTESIAN_POINT ( 'NONE',  ( 13.45312500061451466, 4.541064518000418104, -2.621784821874998173 ) ) ;
#68438=CARTESIAN_POINT ( 'NONE',  ( 28.91250000122903074, -4.330127018922190985, -2.500000000000001332 ) ) ;
#68440=CARTESIAN_POINT ( 'NONE',  ( 16.19062500061451715, 6.054752690667223547, 3.707466751127219781E-16 ) ) ;
#68441=CYLINDRICAL_SURFACE ( 'NONE', #6743, 4.999999999999998224 ) ;
#68442=CARTESIAN_POINT ( 'NONE',  ( 3.750000001229034652, -2.886751345948125991, -5.000000000000000000 ) ) ;
#68443=( BOUNDED_CURVE ( )  B_SPLINE_CURVE ( 2, ( #59666, #65953, #65212, #15332, #26803, #19774, #37874, #48972, #31970 ),
 .UNSPECIFIED., .F., .F. ) 
 B_SPLINE_CURVE_WITH_KNOTS ( ( 3, 2, 2, 2, 3 ),
 ( 0.6630434782608696231, 0.6666666666666666297, 0.6739130434782608647, 0.6811594202898550998, 0.6847826086956522174 ),
 .UNSPECIFIED. ) 
 CURVE ( )  GEOMETRIC_REPRESENTATION_ITEM ( )  RATIONAL_B_SPLINE_CURVE ( ( 0.9330127018922192983, 0.9330127018922202975, 1.000000000000000000, 0.8660254037844387076, 1.000000000000000000, 0.8660254037844387076, 1.000000000000000000, 0.9330127018922182991, 0.9330127018922192983 ) ) 
 REPRESENTATION_ITEM ( '' )  );
#68444=CARTESIAN_POINT ( 'NONE',  ( 13.88437500061451679, 6.421520780324663323E-16, -5.243569643749999010 ) ) ;
#68445=CARTESIAN_POINT ( 'NONE',  ( 12.94687500061451857, -3.027376345333610441, -5.243569643749999898 ) ) ;
#68446=CARTESIAN_POINT ( 'NONE',  ( 19.32187500061451857, 3.027376345333613106, -5.243569643749998122 ) ) ;
#68448=CARTESIAN_POINT ( 'NONE',  ( -5.790145606462770544, 8.153486631126844131, 31.58542748218363982 ) ) ;
#68449=CARTESIAN_POINT ( 'NONE',  ( 24.66562500061451502, 3.027376345333613106, -5.243569643749998122 ) ) ;
#68450=CARTESIAN_POINT ( 'NONE',  ( 17.78437500061451715, -4.541064518000419881, 2.621784821874995952 ) ) ;
#68451=CARTESIAN_POINT ( 'NONE',  ( 25.22812500061451502, 4.541064518000418104, 2.621784821874999949 ) ) ;
#68452=CARTESIAN_POINT ( 'NONE',  ( 1.626862140677534273E-15, 12.01250000000000284, -26.00000000000000355 ) ) ;
#68453=CARTESIAN_POINT ( 'NONE',  ( -1.999999999999997113, 17.82499999999999929, 33.46410161513775705 ) ) ;
#68454=CARTESIAN_POINT ( 'NONE',  ( 28.49062500061451431, -3.027376345333614438, 5.243569643749998122 ) ) ;
#68455=CARTESIAN_POINT ( 'NONE',  ( 10.01250000122903394, -4.330127018922190985, -2.500000000000001332 ) ) ;
#68456=CARTESIAN_POINT ( 'NONE',  ( 5.962500001229033231, -4.330127018922190985, -2.500000000000001332 ) ) ;
#68457=CARTESIAN_POINT ( 'NONE',  ( 28.76250000122903216, 0.000000000000000000, 4.999999999999998224 ) ) ;
#68458=CARTESIAN_POINT ( 'NONE',  ( 27.82500000122903572, 2.886751345948126879, 4.999999999999999112 ) ) ;
#68461=CARTESIAN_POINT ( 'NONE',  ( 8.671875000614518214, 3.027376345333611329, 5.243569643749999010 ) ) ;
#68463=CARTESIAN_POINT ( 'NONE',  ( 17.87812500061451715, 6.421520780324663323E-16, -5.243569643749999010 ) ) ;
#68464=CARTESIAN_POINT ( 'NONE',  ( 11.82187500061451679, 3.027376345333611329, 5.243569643749999010 ) ) ;
#68465=CARTESIAN_POINT ( 'NONE',  ( 3.703125000614516882, 0.000000000000000000, 5.243569643749999010 ) ) ;
#68466=CARTESIAN_POINT ( 'NONE',  ( 19.47187500061451360, 3.027376345333611329, 5.243569643749999010 ) ) ;
#68467=CARTESIAN_POINT ( 'NONE',  ( 6.384375000614516793, 4.541064518000418104, 2.621784821874999949 ) ) ;
#68470=CARTESIAN_POINT ( 'NONE',  ( 7.078125000614516438, 6.421520780324663323E-16, -5.243569643749999010 ) ) ;
#68471=CARTESIAN_POINT ( 'NONE',  ( 20.95312500061451999, -4.541064518000417216, -2.621784821875001281 ) ) ;
#68473=CARTESIAN_POINT ( 'NONE',  ( 5.662500001229035185, 4.330127018922192761, -2.499999999999997780 ) ) ;
#68474=CARTESIAN_POINT ( 'NONE',  ( 14.61562500061451608, -6.054752690667223547, -1.112240025338166033E-15 ) ) ;
#68475=CARTESIAN_POINT ( 'NONE',  ( 13.30312500061451786, -4.541064518000417216, -2.621784821875001281 ) ) ;
#68477=CARTESIAN_POINT ( 'NONE',  ( 13.61250000000000071, 2.886751345948129099, -4.999999999999998224 ) ) ;
#68478=CARTESIAN_POINT ( 'NONE',  ( 9.675000001229035362, 2.886751345948129099, -4.999999999999998224 ) ) ;
#68479=CARTESIAN_POINT ( 'NONE',  ( 5.953125000614519102, 0.000000000000000000, 5.243569643749999010 ) ) ;
#68480=CARTESIAN_POINT ( 'NONE',  ( 18.71250000122903145, 4.330127018922192761, -2.499999999999997780 ) ) ;
#68482=CARTESIAN_POINT ( 'NONE',  ( 9.001249775931846008E-16, 10.97187500061451715, -25.09994784771203058 ) ) ;
#68483=DIRECTION ( 'NONE',  ( 0.000000000000000000, 0.000000000000000000, -1.000000000000000000 ) ) ;
#68484=CARTESIAN_POINT ( 'NONE',  ( 3.937500001229034208, 4.330127018922191873, 2.499999999999999556 ) ) ;
#68487=CARTESIAN_POINT ( 'NONE',  ( -2.000000000000000000, 13.17500000000000071, 26.53589838486224650 ) ) ;
#68488=CARTESIAN_POINT ( 'NONE',  ( 17.85937500061451999, -4.541064518000417216, -2.621784821875001281 ) ) ;
#68489=CARTESIAN_POINT ( 'NONE',  ( -5.810221930991193690E-16, 13.70000000122903394, 26.00000000000000355 ) ) ;
#68490=EDGE_CURVE ( 'NONE', #5287, #13883, #1793, .T. ) ;
#68491=CARTESIAN_POINT ( 'NONE',  ( 12.92812500061451786, 6.421520780324663323E-16, -5.243569643749999010 ) ) ;
#68493=CARTESIAN_POINT ( 'NONE',  ( 22.61250000122903003, -4.330127018922190985, -2.500000000000001332 ) ) ;
#68494=CARTESIAN_POINT ( 'NONE',  ( 29.82187500061451502, 3.027376345333611329, 5.243569643749999010 ) ) ;
#68495=CARTESIAN_POINT ( 'NONE',  ( 26.85937500061451644, -4.541064518000417216, -2.621784821875001281 ) ) ;
#68497=CARTESIAN_POINT ( 'NONE',  ( 12.74062500061451786, -3.027376345333614438, 5.243569643749998122 ) ) ;
#68498=CARTESIAN_POINT ( 'NONE',  ( 9.871875000614517504, 3.027376345333613106, -5.243569643749998122 ) ) ;
#68499=ORIENTED_EDGE ( 'NONE', *, *, #57822, .F. ) ;
#68500=CARTESIAN_POINT ( 'NONE',  ( 29.46562500061451573, -6.054752690667223547, -1.112240025338166033E-15 ) ) ;
#68501=CARTESIAN_POINT ( 'NONE',  ( 20.87812500061451715, -4.541064518000419881, 2.621784821874995952 ) ) ;
#68502=FACE_OUTER_BOUND ( 'NONE', #46337, .T. ) ;
#68504=CARTESIAN_POINT ( 'NONE',  ( 1.071796769724491893, 15.29509619066137027, -26.00000000000000355 ) ) ;
#68505=CARTESIAN_POINT ( 'NONE',  ( 10.23750000000000071, -2.886751345948129988, 4.999999999999997335 ) ) ;
#68506=CARTESIAN_POINT ( 'NONE',  ( 22.53750000122903430, -4.330127018922194537, 2.499999999999995559 ) ) ;
#68507=CARTESIAN_POINT ( 'NONE',  ( 16.64062500061451289, 6.054752690667223547, 3.707466751127219781E-16 ) ) ;
#68509=ORIENTED_EDGE ( 'NONE', *, *, #39611, .T. ) ;
#68510=CARTESIAN_POINT ( 'NONE',  ( 18.56250000000000000, 2.886751345948129099, -4.999999999999998224 ) ) ;
#68512=CARTESIAN_POINT ( 'NONE',  ( 21.03750000000000142, -2.886751345948129988, 4.999999999999997335 ) ) ;
#68513=CARTESIAN_POINT ( 'NONE',  ( 19.43437500061451928, 4.541064518000418104, 2.621784821874999949 ) ) ;
#68514=CARTESIAN_POINT ( 'NONE',  ( 25.67812500061451431, 4.541064518000418104, 2.621784821874999949 ) ) ;
#68515=( BOUNDED_CURVE ( )  B_SPLINE_CURVE ( 2, ( #9589, #37657, #2951, #42843, #8856, #25479, #71279 ),
 .UNSPECIFIED., .F., .F. ) 
 B_SPLINE_CURVE_WITH_KNOTS ( ( 3, 2, 2, 3 ),
 ( 0.6083333333333332815, 0.6111111111111111605, 0.6138888888888889284, 0.6166666666666666963 ),
 .UNSPECIFIED. ) 
 CURVE ( )  GEOMETRIC_REPRESENTATION_ITEM ( )  RATIONAL_B_SPLINE_CURVE ( ( 1.000000000000000000, 0.8660254037844387076, 1.000000000000000000, 0.8660254037844387076, 1.000000000000000000, 0.8660254037844387076, 1.000000000000000000 ) ) 
 REPRESENTATION_ITEM ( '' )  );
#68517=CARTESIAN_POINT ( 'NONE',  ( 8.812500001229034652, 4.330127018922192761, -2.499999999999997780 ) ) ;
#68518=CARTESIAN_POINT ( 'NONE',  ( 9.253125000614517148, -4.541064518000417216, -2.621784821875001281 ) ) ;
#68520=CARTESIAN_POINT ( 'NONE',  ( 15.82499999999999929, 6.123233995736764310E-16, -4.999999999999998224 ) ) ;
#68521=CARTESIAN_POINT ( 'NONE',  ( 4.243569643749999010, 18.71562500061451217, 27.54997392385601174 ) ) ;
#68522=CARTESIAN_POINT ( 'NONE',  ( 27.96562500061451928, 3.027376345333611329, 5.243569643749999010 ) ) ;
#68525=CARTESIAN_POINT ( 'NONE',  ( 25.65937500061451715, 4.541064518000418104, -2.621784821874998173 ) ) ;
#68526=VERTEX_POINT ( 'NONE', #36432 ) ;
#68527=CARTESIAN_POINT ( 'NONE',  ( 24.85312500061451502, 0.000000000000000000, 5.243569643749999010 ) ) ;
#68528=CARTESIAN_POINT ( 'NONE',  ( 24.60937500061451644, -4.541064518000417216, -2.621784821875001281 ) ) ;
#68529=CARTESIAN_POINT ( 'NONE',  ( -2.121784821874996840, 18.07812500061459104, -26.32496088578401583 ) ) ;
#68530=CARTESIAN_POINT ( 'NONE',  ( 11.92500000000000071, 4.330127018922191873, 2.499999999999999556 ) ) ;
#68531=CARTESIAN_POINT ( 'NONE',  ( 8.915625000614515017, 3.027376345333613106, -5.243569643749998122 ) ) ;
#68533=CARTESIAN_POINT ( 'NONE',  ( 28.41562500061451502, 3.027376345333611329, 5.243569643749999010 ) ) ;
#68534=CARTESIAN_POINT ( 'NONE',  ( 27.47812500061451502, 4.541064518000418104, 2.621784821874999949 ) ) ;
#68537=CARTESIAN_POINT ( 'NONE',  ( 20.10937500061451289, -4.541064518000417216, -2.621784821875001281 ) ) ;
#68538=CARTESIAN_POINT ( 'NONE',  ( -2.121784821874996840, 12.73437500061451821, 33.67503911421598417 ) ) ;
#68539=CARTESIAN_POINT ( 'NONE',  ( 19.80937500061451573, 4.541064518000418104, -2.621784821874998173 ) ) ;
#68540=CARTESIAN_POINT ( 'NONE',  ( 27.68437500061451573, -4.541064518000419881, 2.621784821874995952 ) ) ;
#68541=CARTESIAN_POINT ( 'NONE',  ( 2.121784821874999061, 16.10937500061451644, 26.32496088578401583 ) ) ;
#68542=CARTESIAN_POINT ( 'NONE',  ( 8.465625000614515727, 3.027376345333613106, -5.243569643749998122 ) ) ;
#68543=CARTESIAN_POINT ( 'NONE',  ( 2.000000000000001332, 10.36250000122903359, -26.53589838486224650 ) ) ;
#68544=CARTESIAN_POINT ( 'NONE',  ( 5.484375000614518214, 4.541064518000418104, 2.621784821874999949 ) ) ;
#68547=CARTESIAN_POINT ( 'NONE',  ( 4.828125000614518214, 6.421520780324663323E-16, -5.243569643749999010 ) ) ;
#68548=CARTESIAN_POINT ( 'NONE',  ( 9.871875000614517504, 3.027376345333613106, -5.243569643749998122 ) ) ;
#68549=SURFACE_STYLE_FILL_AREA ( #34549 ) ;
#68550=CARTESIAN_POINT ( 'NONE',  ( 18.00000000122903288, -2.886751345948129988, 4.999999999999997335 ) ) ;
#68551=CARTESIAN_POINT ( 'NONE',  ( 5.709375000614517859, -4.541064518000417216, -2.621784821875001281 ) ) ;
#68552=CARTESIAN_POINT ( 'NONE',  ( 7.115625000614516082, 3.027376345333613106, -5.243569643749998122 ) ) ;
#68553=CARTESIAN_POINT ( 'NONE',  ( 4.196151849995945149, -2.718880220196457476, -4.196151849995952254 ) ) ;
#68555=CARTESIAN_POINT ( 'NONE',  ( 16.84687500061451715, -3.027376345333614438, 5.243569643749998122 ) ) ;
#68556=ORIENTED_EDGE ( 'NONE', *, *, #32955, .F. ) ;
#68557=CARTESIAN_POINT ( 'NONE',  ( 25.04062500061451502, -3.027376345333610441, -5.243569643749999898 ) ) ;
#68558=CARTESIAN_POINT ( 'NONE',  ( 9.215625000614515727, -6.054752690667223547, -1.112240025338166033E-15 ) ) ;
#68560=CARTESIAN_POINT ( 'NONE',  ( 27.68437500061451573, -4.541064518000419881, 2.621784821874995952 ) ) ;
#68561=CARTESIAN_POINT ( 'NONE',  ( 9.703125000614514661, -4.541064518000417216, -2.621784821875001281 ) ) ;
#68562=CARTESIAN_POINT ( 'NONE',  ( -4.243569643749999898, 10.85937500061451821, -30.00000000000000000 ) ) ;
#68563=CARTESIAN_POINT ( 'NONE',  ( 12.56250000122903465, 0.000000000000000000, 4.999999999999998224 ) ) ;
#68564=CARTESIAN_POINT ( 'NONE',  ( 26.54062500061451146, 6.054752690667223547, 3.707466751127219781E-16 ) ) ;
#68565=CARTESIAN_POINT ( 'NONE',  ( 2.121784821874999061, 13.35312500061451679, -33.67503911421598417 ) ) ;
#68566=CARTESIAN_POINT ( 'NONE',  ( 12.75000000122903643, -2.886751345948125991, -5.000000000000000000 ) ) ;
#68567=CARTESIAN_POINT ( 'NONE',  ( 10.95000000000000107, 4.330127018922192761, -2.499999999999997780 ) ) ;
#68568=CARTESIAN_POINT ( 'NONE',  ( 21.47812500061451502, 6.421520780324663323E-16, -5.243569643749999010 ) ) ;
#68569=CARTESIAN_POINT ( 'NONE',  ( 5.259375000614518569, -4.541064518000417216, -2.621784821875001281 ) ) ;
#68570=CARTESIAN_POINT ( 'NONE',  ( 20.47500000000000142, 4.330127018922191873, 2.499999999999999556 ) ) ;
#68571=CARTESIAN_POINT ( 'NONE',  ( 7.837500001229035007, 6.123233995736764310E-16, -4.999999999999998224 ) ) ;
#68572=CARTESIAN_POINT ( 'NONE',  ( 16.42500000122903359, 2.886751345948129099, -4.999999999999998224 ) ) ;
#68573=CARTESIAN_POINT ( 'NONE',  ( 12.70312500061451821, 0.000000000000000000, 5.243569643749999010 ) ) ;
#68574=CARTESIAN_POINT ( 'NONE',  ( 15.92812500061451608, -4.541064518000419881, 2.621784821874995952 ) ) ;
#68575=CARTESIAN_POINT ( 'NONE',  ( 25.95000000122903216, 5.773502691896255534, 3.535250795749688894E-16 ) ) ;
#68576=CARTESIAN_POINT ( 'NONE',  ( 21.22500000000000142, 6.123233995736764310E-16, -4.999999999999998224 ) ) ;
#68577=CARTESIAN_POINT ( 'NONE',  ( 24.30937500061451573, 4.541064518000418104, -2.621784821874998173 ) ) ;
#68579=CARTESIAN_POINT ( 'NONE',  ( 11.10000000122903252, 5.773502691896255534, 3.535250795749688894E-16 ) ) ;
#68580=CARTESIAN_POINT ( 'NONE',  ( 8.521875000614516082, 3.027376345333613106, -5.243569643749998122 ) ) ;
#68581=CARTESIAN_POINT ( 'NONE',  ( 26.55937500061451573, 4.541064518000418104, -2.621784821874998173 ) ) ;
#68582=CARTESIAN_POINT ( 'NONE',  ( 3.421875000614516882, -6.054752690667223547, -1.112240025338166033E-15 ) ) ;
#68583=CARTESIAN_POINT ( 'NONE',  ( 23.72812500061451502, 6.421520780324663323E-16, -5.243569643749999010 ) ) ;
#68584=CARTESIAN_POINT ( 'NONE',  ( 26.67187500061451644, 3.027376345333611329, 5.243569643749999010 ) ) ;
#68586=CARTESIAN_POINT ( 'NONE',  ( 7.396875000614519635, -3.027376345333614438, 5.243569643749998122 ) ) ;
#68587=CARTESIAN_POINT ( 'NONE',  ( 18.81562500061452070, 3.027376345333613106, -5.243569643749998122 ) ) ;
#68588=DIRECTION ( 'NONE',  ( 0.000000000000000000, 1.000000000000000000, 0.000000000000000000 ) ) ;
#68589=CARTESIAN_POINT ( 'NONE',  ( 28.15312500061451573, -4.541064518000417216, -2.621784821875001281 ) ) ;
#68590=CARTESIAN_POINT ( 'NONE',  ( 4.846875000614519813, -3.027376345333610441, -5.243569643749999898 ) ) ;
#68591=AXIS2_PLACEMENT_3D ( 'NONE', #68684, #1092, #23600 ) ;
#68593=CARTESIAN_POINT ( 'NONE',  ( 17.77499999999999858, 4.330127018922191873, 2.499999999999999556 ) ) ;
#68595=CARTESIAN_POINT ( 'NONE',  ( 24.71250000000000213, -5.773502691896255534, -1.060575238724906372E-15 ) ) ;
#68596=EDGE_CURVE ( 'NONE', #37144, #41179, #39116, .T. ) ;
#68597=EDGE_CURVE ( 'NONE', #39309, #26767, #39208, .T. ) ;
#68598=CARTESIAN_POINT ( 'NONE',  ( 27.04687500061451644, 6.054752690667223547, 3.707466751127219781E-16 ) ) ;
#68600=CARTESIAN_POINT ( 'NONE',  ( 14.95312500061451644, 0.000000000000000000, 5.243569643749999010 ) ) ;
#68601=CARTESIAN_POINT ( 'NONE',  ( 6.965625000614518392, -6.054752690667223547, -1.112240025338166033E-15 ) ) ;
#68603=CARTESIAN_POINT ( 'NONE',  ( 5.521875000614517859, 3.027376345333611329, 5.243569643749999010 ) ) ;
#68604=CARTESIAN_POINT ( 'NONE',  ( 14.40000000122903323, -2.886751345948129988, 4.999999999999997335 ) ) ;
#68605=CARTESIAN_POINT ( 'NONE',  ( 22.16250000000000142, 2.886751345948129099, -4.999999999999998224 ) ) ;
#68606=CARTESIAN_POINT ( 'NONE',  ( 29.28749999999999787, -2.886751345948125991, -5.000000000000000000 ) ) ;
#68607=CARTESIAN_POINT ( 'NONE',  ( 4.921875000614518214, 3.027376345333613106, -5.243569643749998122 ) ) ;
#68608=CARTESIAN_POINT ( 'NONE',  ( 8.334375000614516082, -4.541064518000419881, 2.621784821874995952 ) ) ;
#68609=CARTESIAN_POINT ( 'NONE',  ( 20.85937500061451644, 0.000000000000000000, 5.243569643749999010 ) ) ;
#68610=CYLINDRICAL_SURFACE ( 'NONE', #71382, 4.999999999999998224 ) ;
#68611=ORIENTED_EDGE ( 'NONE', *, *, #44097, .F. ) ;
#68612=CARTESIAN_POINT ( 'NONE',  ( 5.109375000614518214, 0.000000000000000000, 5.243569643749999010 ) ) ;
#68613=CARTESIAN_POINT ( 'NONE',  ( 5.250000000000000888, 0.000000000000000000, 4.999999999999998224 ) ) ;
#68614=CARTESIAN_POINT ( 'NONE',  ( 6.159375000614517148, -4.541064518000417216, -2.621784821875001281 ) ) ;
#68615=CARTESIAN_POINT ( 'NONE',  ( 19.50000000000000000, 4.330127018922192761, -2.499999999999997780 ) ) ;
#68616=CARTESIAN_POINT ( 'NONE',  ( 15.55312500061451608, -4.541064518000417216, -2.621784821875001281 ) ) ;
#68619=CARTESIAN_POINT ( 'NONE',  ( -1.071796769724490561, 19.90759618943233278, 26.00000000000000000 ) ) ;
#68621=CARTESIAN_POINT ( 'NONE',  ( 10.49062500061451431, -3.027376345333614438, 5.243569643749998122 ) ) ;
#68622=CARTESIAN_POINT ( 'NONE',  ( 27.34687500061451360, -3.027376345333610441, -5.243569643749999898 ) ) ;
#68623=CARTESIAN_POINT ( 'NONE',  ( 12.33750000122903145, 6.123233995736764310E-16, -4.999999999999998224 ) ) ;
#68624=CARTESIAN_POINT ( 'NONE',  ( 25.92187500061451999, -6.054752690667223547, -1.112240025338166033E-15 ) ) ;
#68625=CARTESIAN_POINT ( 'NONE',  ( 7.762500000000001954, 2.886751345948129099, -4.999999999999998224 ) ) ;
#68626=CARTESIAN_POINT ( 'NONE',  ( -2.828200636599751609E-16, 13.25000000122903288, 25.38119784648299770 ) ) ;
#68627=CARTESIAN_POINT ( 'NONE',  ( 15.14062500061451644, -3.027376345333610441, -5.243569643749999898 ) ) ;
#68628=CARTESIAN_POINT ( 'NONE',  ( 7.537500001229033408, 4.330127018922191873, 2.499999999999999556 ) ) ;
#68629=CARTESIAN_POINT ( 'NONE',  ( 18.30937500061451928, -4.541064518000417216, -2.621784821875001281 ) ) ;
#68630=CARTESIAN_POINT ( 'NONE',  ( 11.89687500061451608, -3.027376345333614438, 5.243569643749998122 ) ) ;
#68632=VERTEX_POINT ( 'NONE', #61514 ) ;
#68633=CARTESIAN_POINT ( 'NONE',  ( 11.65312500061451573, 4.541064518000418104, -2.621784821874998173 ) ) ;
#68634=CARTESIAN_POINT ( 'NONE',  ( 26.58750000122903145, -4.330127018922194537, 2.499999999999995559 ) ) ;
#68635=CARTESIAN_POINT ( 'NONE',  ( 12.38437500061451857, -4.541064518000419881, 2.621784821874995952 ) ) ;
#68636=CARTESIAN_POINT ( 'NONE',  ( 4.169580978743460342, 2.759455464706926708, 4.458747374224691029 ) ) ;
#68637=CARTESIAN_POINT ( 'NONE',  ( 13.94062500061451892, 6.054752690667223547, 3.707466751127219781E-16 ) ) ;
#68639=CARTESIAN_POINT ( 'NONE',  ( 23.22187500061451715, -6.054752690667223547, -1.112240025338166033E-15 ) ) ;
#68640=CARTESIAN_POINT ( 'NONE',  ( 2.867942972713479755, -4.095717654485441450, 3.274159358307527690 ) ) ;
#68641=CARTESIAN_POINT ( 'NONE',  ( 12.75000000122903643, -2.886751345948125991, -5.000000000000000000 ) ) ;
#68643=CARTESIAN_POINT ( 'NONE',  ( 3.193447721043152665, 3.847322660365763536, 3.562742055761627835 ) ) ;
#68644=CARTESIAN_POINT ( 'NONE',  ( 4.243569643749999010, 16.97187500061451715, -32.45002607614398471 ) ) ;
#68645=CARTESIAN_POINT ( 'NONE',  ( 17.93437500061451928, 6.421520780324663323E-16, -5.243569643749999010 ) ) ;
#68646=CARTESIAN_POINT ( 'NONE',  ( 19.12500000122903288, 2.886751345948129099, -4.999999999999998224 ) ) ;
#68647=CARTESIAN_POINT ( 'NONE',  ( 14.29687500061451821, -3.027376345333610441, -5.243569643749999898 ) ) ;
#68648=CARTESIAN_POINT ( 'NONE',  ( -2.121784821874996840, 10.03437500061451892, 33.67503911421598417 ) ) ;
#68649=CARTESIAN_POINT ( 'NONE',  ( 20.32500000122903572, -5.773502691896255534, -1.060575238724906372E-15 ) ) ;
#68650=CARTESIAN_POINT ( 'NONE',  ( 15.17812500061451608, 6.421520780324663323E-16, -5.243569643749999010 ) ) ;
#68651=FACE_OUTER_BOUND ( 'NONE', #19362, .T. ) ;
#68652=ORIENTED_EDGE ( 'NONE', *, *, #63249, .T. ) ;
#68654=CARTESIAN_POINT ( 'NONE',  ( 17.84999999999999787, 0.000000000000000000, 4.999999999999998224 ) ) ;
#68655=CARTESIAN_POINT ( 'NONE',  ( 4.115625000614516082, 3.027376345333611329, 5.243569643749999010 ) ) ;
#68656=EDGE_CURVE ( 'NONE', #45391, #6802, #66711, .T. ) ;
#68657=CARTESIAN_POINT ( 'NONE',  ( 15.33750000122903323, -4.330127018922194537, 2.499999999999995559 ) ) ;
#68658=CARTESIAN_POINT ( 'NONE',  ( 26.44687500061451502, -3.027376345333610441, -5.243569643749999898 ) ) ;
#68659=CARTESIAN_POINT ( 'NONE',  ( 20.27812500061451573, 4.541064518000418104, 2.621784821874999949 ) ) ;
#68660=CARTESIAN_POINT ( 'NONE',  ( 23.39062500061451289, 6.054752690667223547, 3.707466751127219781E-16 ) ) ;
#68661=CARTESIAN_POINT ( 'NONE',  ( 3.778125000614519280, -4.541064518000419881, 2.621784821874995952 ) ) ;
#68663=CARTESIAN_POINT ( 'NONE',  ( 28.12499999999999645, 4.330127018922191873, 2.499999999999999556 ) ) ;
#68664=CARTESIAN_POINT ( 'NONE',  ( 4.724999999999999645, 4.330127018922191873, 2.499999999999999556 ) ) ;
#68666=CARTESIAN_POINT ( 'NONE',  ( 6.337500001229033231, -4.330127018922194537, 2.499999999999995559 ) ) ;
#68667=CARTESIAN_POINT ( 'NONE',  ( 28.80000000000000071, -4.330127018922190985, -2.500000000000001332 ) ) ;
#68668=CARTESIAN_POINT ( 'NONE',  ( -4.243569643749999898, 17.12187500061451573, -32.45002607614398471 ) ) ;
#68669=CARTESIAN_POINT ( 'NONE',  ( 5.025000001229035895, -5.773502691896255534, -1.060575238724906372E-15 ) ) ;
#68670=CARTESIAN_POINT ( 'NONE',  ( 4.762499999999999289, 2.886751345948126879, 4.999999999999999112 ) ) ;
#68672=CARTESIAN_POINT ( 'NONE',  ( 3.225000001229033408, -5.773502691896255534, -1.060575238724906372E-15 ) ) ;
#68673=CARTESIAN_POINT ( 'NONE',  ( 9.946875000614516793, 6.054752690667223547, 3.707466751127219781E-16 ) ) ;
#68674=AXIS2_PLACEMENT_3D ( 'NONE', #21209, #44131, #50402 ) ;
#68675=CARTESIAN_POINT ( 'NONE',  ( 4.000000000000000000, 16.70000000122903216, -27.69059892324149885 ) ) ;
#68676=CYLINDRICAL_SURFACE ( 'NONE', #38967, 4.999999999999998224 ) ;
#68677=CARTESIAN_POINT ( 'NONE',  ( 5.512500001229033941, -4.330127018922190985, -2.500000000000001332 ) ) ;
#68678=CYLINDRICAL_SURFACE ( 'NONE', #47749, 4.999999999999998224 ) ;
#68679=CARTESIAN_POINT ( 'NONE',  ( 6.646875000614518747, -3.027376345333610441, -5.243569643749999898 ) ) ;
#68680=CARTESIAN_POINT ( 'NONE',  ( 13.20937500061451786, 0.000000000000000000, 5.243569643749999010 ) ) ;
#68681=CARTESIAN_POINT ( 'NONE',  ( 7.012500000000001066, 2.886751345948126879, 4.999999999999999112 ) ) ;
#68682=CARTESIAN_POINT ( 'NONE',  ( 4.243569643749999898, 17.32812500061459104, 30.00000000000000000 ) ) ;
#68683=CARTESIAN_POINT ( 'NONE',  ( 21.23437500061451644, 4.541064518000418104, 2.621784821874999949 ) ) ;
#68684=CARTESIAN_POINT ( 'NONE',  ( 0.000000000000000000, 20.00000000000000000, -30.00000000000000000 ) ) ;
#68686=CARTESIAN_POINT ( 'NONE',  ( 27.67500000122903359, 2.886751345948129099, -4.999999999999998224 ) ) ;
#68688=CARTESIAN_POINT ( 'NONE',  ( 21.66562500061451502, 3.027376345333611329, 5.243569643749999010 ) ) ;
#68689=CARTESIAN_POINT ( 'NONE',  ( 13.41562500061451502, 3.027376345333613106, -5.243569643749998122 ) ) ;
#68691=CARTESIAN_POINT ( 'NONE',  ( 11.07187500061451679, -6.054752690667223547, -1.112240025338166033E-15 ) ) ;
#68692=CARTESIAN_POINT ( 'NONE',  ( 29.06250000000000000, 2.886751345948126879, 4.999999999999999112 ) ) ;
#68693=CARTESIAN_POINT ( 'NONE',  ( 22.12500000122903288, -5.773502691896255534, -1.060575238724906372E-15 ) ) ;
#68695=CARTESIAN_POINT ( 'NONE',  ( 11.63437500061451857, 6.421520780324663323E-16, -5.243569643749999010 ) ) ;
#68696=CARTESIAN_POINT ( 'NONE',  ( 28.13437500061451502, -4.541064518000419881, 2.621784821874995952 ) ) ;
#68697=LINE ( 'NONE', #40255, #57215 ) ;
#68699=CARTESIAN_POINT ( 'NONE',  ( 21.87187500061451573, -6.054752690667223547, -1.112240025338166033E-15 ) ) ;
#68700=CARTESIAN_POINT ( 'NONE',  ( 14.70937500061451786, -4.541064518000417216, -2.621784821875001281 ) ) ;
#68702=CARTESIAN_POINT ( 'NONE',  ( 25.83749999999999858, 5.773502691896255534, 3.535250795749688894E-16 ) ) ;
#68705=CARTESIAN_POINT ( 'NONE',  ( 18.40312500061451573, 4.541064518000418104, -2.621784821874998173 ) ) ;
#68706=CARTESIAN_POINT ( 'NONE',  ( 6.787500000000001421, -2.886751345948125991, -5.000000000000000000 ) ) ;
#68707=CARTESIAN_POINT ( 'NONE',  ( -0.7368881354385758975, 9.803648613939515144, 25.82089971438751519 ) ) ;
#68708=CARTESIAN_POINT ( 'NONE',  ( 14.24999999999999822, 0.000000000000000000, 4.999999999999998224 ) ) ;
#68709=CARTESIAN_POINT ( 'NONE',  ( 4.243569643749999898, 10.57812500061451821, 30.00000000000000000 ) ) ;
#68711=CARTESIAN_POINT ( 'NONE',  ( 25.50937500061451502, -4.541064518000417216, -2.621784821875001281 ) ) ;
#68712=ORIENTED_EDGE ( 'NONE', *, *, #8736, .T. ) ;
#68713=CARTESIAN_POINT ( 'NONE',  ( 23.16562500061451502, -6.054752690667223547, -1.112240025338166033E-15 ) ) ;
#68714=CARTESIAN_POINT ( 'NONE',  ( 20.59687500061451360, -3.027376345333610441, -5.243569643749999898 ) ) ;
#68715=CARTESIAN_POINT ( 'NONE',  ( 3.787500000000002753, 5.773502691896255534, 3.535250795749688894E-16 ) ) ;
#68716=CARTESIAN_POINT ( 'NONE',  ( 7.903125000614515727, -4.541064518000417216, -2.621784821875001281 ) ) ;
#68717=CARTESIAN_POINT ( 'NONE',  ( 21.06562500061451715, 3.027376345333613106, -5.243569643749998122 ) ) ;
#68718=CARTESIAN_POINT ( 'NONE',  ( 13.20937500061451786, 0.000000000000000000, 5.243569643749999010 ) ) ;
#68719=CARTESIAN_POINT ( 'NONE',  ( 16.35937500061451644, 0.000000000000000000, 5.243569643749999010 ) ) ;
#68720=CARTESIAN_POINT ( 'NONE',  ( -4.243569643749997233, 18.49062500061451431, 32.45002607614398471 ) ) ;
#68721=CARTESIAN_POINT ( 'NONE',  ( 19.53750000122903430, 6.123233995736764310E-16, -4.999999999999998224 ) ) ;
#68723=CARTESIAN_POINT ( 'NONE',  ( 10.26562500061451644, 3.027376345333612662, -5.243569643749998122 ) ) ;
#68724=CARTESIAN_POINT ( 'NONE',  ( 4.471875000614518925, 3.027376345333613106, -5.243569643749998122 ) ) ;
#68725=CARTESIAN_POINT ( 'NONE',  ( 5.409375000614516260, 4.541064518000418104, -2.621784821874998173 ) ) ;
#68726=CARTESIAN_POINT ( 'NONE',  ( 26.33437500061451431, -4.541064518000419881, 2.621784821874995952 ) ) ;
#68727=CARTESIAN_POINT ( 'NONE',  ( 16.97812500061451502, 6.421520780324663323E-16, -5.243569643749999010 ) ) ;
#68728=CARTESIAN_POINT ( 'NONE',  ( 26.25000000122903288, -2.886751345948125991, -5.000000000000000000 ) ) ;
#68730=CARTESIAN_POINT ( 'NONE',  ( 26.12812500061451360, 4.541064518000418104, 2.621784821874999949 ) ) ;
#68732=CARTESIAN_POINT ( 'NONE',  ( 22.92187500061451644, 3.027376345333613106, -5.243569643749998122 ) ) ;
#68733=CARTESIAN_POINT ( 'NONE',  ( 17.50312500061451715, 4.541064518000418104, -2.621784821874998173 ) ) ;
#68734=CARTESIAN_POINT ( 'NONE',  ( 4.243569643749999010, 16.97187500061451360, 27.54997392385601174 ) ) ;
#68735=CARTESIAN_POINT ( 'NONE',  ( 21.29062500061451502, -3.027376345333614438, 5.243569643749998122 ) ) ;
#68737=ORIENTED_EDGE ( 'NONE', *, *, #47742, .F. ) ;
#68738=CARTESIAN_POINT ( 'NONE',  ( 26.47499999999999787, -4.330127018922194537, 2.499999999999995559 ) ) ;
#68739=CARTESIAN_POINT ( 'NONE',  ( -3.999999999999999112, 12.34999999999999964, -30.00000000000000000 ) ) ;
#68741=CARTESIAN_POINT ( 'NONE',  ( 29.46562500061451573, -6.054752690667223547, -1.112240025338166033E-15 ) ) ;
#68742=CARTESIAN_POINT ( 'NONE',  ( 10.75312500061451715, 4.541064518000418104, -2.621784821874998173 ) ) ;
#68743=CARTESIAN_POINT ( 'NONE',  ( 21.97500000122903074, 2.886751345948126879, 4.999999999999999112 ) ) ;
#68744=CARTESIAN_POINT ( 'NONE',  ( 26.84062500061451573, -3.027376345333610441, -5.243569643749999898 ) ) ;
#68745=CARTESIAN_POINT ( 'NONE',  ( 27.11249999999999716, 2.886751345948129099, -4.999999999999998224 ) ) ;
#68746=CARTESIAN_POINT ( 'NONE',  ( -3.999999999999999112, 15.61250000122903359, -30.00000000000000000 ) ) ;
#68747=CARTESIAN_POINT ( 'NONE',  ( 29.65312500061451573, 4.541064518000418104, -2.621784821874998173 ) ) ;
#68748=CARTESIAN_POINT ( 'NONE',  ( 11.57812500061451644, 6.421520780324663323E-16, -5.243569643749999010 ) ) ;
#68750=CARTESIAN_POINT ( 'NONE',  ( 26.65312500061451573, 0.000000000000000000, 5.243569643749999010 ) ) ;
#68751=CARTESIAN_POINT ( 'NONE',  ( 7.903125000614515727, -4.541064518000417216, -2.621784821875001281 ) ) ;
#68752=CARTESIAN_POINT ( 'NONE',  ( 4.828125000614518214, 6.421520780324663323E-16, -5.243569643749999010 ) ) ;
#68754=CARTESIAN_POINT ( 'NONE',  ( 13.04999999999999893, -4.330127018922190985, -2.500000000000001332 ) ) ;
#68755=CARTESIAN_POINT ( 'NONE',  ( 16.53750000000000142, -2.886751345948129988, 4.999999999999997335 ) ) ;
#68756=CARTESIAN_POINT ( 'NONE',  ( 15.04687500061451644, -3.027376345333614438, 5.243569643749998122 ) ) ;
#68757=CARTESIAN_POINT ( 'NONE',  ( 10.76250000122903572, 0.000000000000000000, 4.999999999999998224 ) ) ;
#68758=EDGE_CURVE ( 'NONE', #18233, #48333, #23561, .T. ) ;
#68759=CARTESIAN_POINT ( 'NONE',  ( 17.52187500061451431, 3.027376345333613106, -5.243569643749998122 ) ) ;
#68761=CARTESIAN_POINT ( 'NONE',  ( 21.98437500061451644, 6.421520780324663323E-16, -5.243569643749999010 ) ) ;
#68762=CARTESIAN_POINT ( 'NONE',  ( -2.121784821874996840, 13.12812500061451715, -26.32496088578401583 ) ) ;
#68766=CARTESIAN_POINT ( 'NONE',  ( 24.59062500061451573, -3.027376345333610441, -5.243569643749999898 ) ) ;
#68767=EDGE_CURVE ( 'NONE', #16738, #57497, #8890, .T. ) ;
#68768=CARTESIAN_POINT ( 'NONE',  ( 29.29687500061451644, 6.054752690667223547, 3.707466751127219781E-16 ) ) ;
#68769=CARTESIAN_POINT ( 'NONE',  ( 24.29999999999999716, -4.330127018922190985, -2.500000000000001332 ) ) ;
#68770=ADVANCED_FACE ( 'NONE', ( #27184 ), #54212, .T. ) ;
#68771=CARTESIAN_POINT ( 'NONE',  ( 5.803125000614517859, 4.541064518000418104, -2.621784821874998173 ) ) ;
#68773=CARTESIAN_POINT ( 'NONE',  ( 18.60937500061451644, 0.000000000000000000, 5.243569643749999010 ) ) ;
#68775=CARTESIAN_POINT ( 'NONE',  ( 3.478125000614517237, 6.421520780324663323E-16, -5.243569643749999010 ) ) ;
#68776=CARTESIAN_POINT ( 'NONE',  ( 7.771875000614516971, 3.027376345333611329, 5.243569643749999010 ) ) ;
#68778=CARTESIAN_POINT ( 'NONE',  ( 19.69687500061451857, -3.027376345333610441, -5.243569643749999898 ) ) ;
#68780=CARTESIAN_POINT ( 'NONE',  ( 25.57499999999999929, -4.330127018922194537, 2.499999999999995559 ) ) ;
#68781=CARTESIAN_POINT ( 'NONE',  ( 28.99687500061451573, -3.027376345333614438, 5.243569643749998122 ) ) ;
#68782=CARTESIAN_POINT ( 'NONE',  ( 3.999999999999999112, 10.32500000000000107, -30.00000000000000000 ) ) ;
#68785=CARTESIAN_POINT ( 'NONE',  ( 11.40000000000000036, 4.330127018922192761, -2.499999999999997780 ) ) ;
#68787=CARTESIAN_POINT ( 'NONE',  ( 24.77812500061451217, 4.541064518000418104, 2.621784821874999949 ) ) ;
#68788=CARTESIAN_POINT ( 'NONE',  ( 13.31250000000000178, 2.886751345948126879, 4.999999999999999112 ) ) ;
#68790=CARTESIAN_POINT ( 'NONE',  ( 9.900000001229033231, -2.886751345948129988, 4.999999999999997335 ) ) ;
#68791=CARTESIAN_POINT ( 'NONE',  ( 9.965625000614517504, 3.027376345333611329, 5.243569643749999010 ) ) ;
#68792=CARTESIAN_POINT ( 'NONE',  ( 22.42500000000000071, -4.330127018922194537, 2.499999999999995559 ) ) ;
#68793=CARTESIAN_POINT ( 'NONE',  ( 21.59062500061451928, 6.054752690667223547, 3.707466751127219781E-16 ) ) ;
#68794=CARTESIAN_POINT ( 'NONE',  ( 15.93750000122903110, 6.123233995736764310E-16, -4.999999999999998224 ) ) ;
#68795=CARTESIAN_POINT ( 'NONE',  ( 26.28750000122903430, 6.123233995736764310E-16, -4.999999999999998224 ) ) ;
#68797=CARTESIAN_POINT ( 'NONE',  ( 8.175000000000002487, 6.123233995736764310E-16, -4.999999999999998224 ) ) ;
#68799=CARTESIAN_POINT ( 'NONE',  ( 22.56562500061451715, 3.027376345333611329, 5.243569643749999010 ) ) ;
#68800=CARTESIAN_POINT ( 'NONE',  ( 29.65312500061451573, 4.541064518000418104, -2.621784821874998173 ) ) ;
#68801=CARTESIAN_POINT ( 'NONE',  ( 27.60937500061451644, 0.000000000000000000, 5.243569643749999010 ) ) ;
#68802=CARTESIAN_POINT ( 'NONE',  ( 19.58437500061451786, -4.541064518000419881, 2.621784821874995952 ) ) ;
#68803=CARTESIAN_POINT ( 'NONE',  ( 13.22812500061451502, -4.541064518000419881, 2.621784821874995952 ) ) ;
#68804=CARTESIAN_POINT ( 'NONE',  ( 2.121784821875001281, 10.05312500061459247, -26.32496088578401938 ) ) ;
#68805=CARTESIAN_POINT ( 'NONE',  ( 26.62500000122903288, -5.773502691896255534, -1.060575238724906372E-15 ) ) ;
#68807=CARTESIAN_POINT ( 'NONE',  ( 15.59062500061451573, -3.027376345333610441, -5.243569643749999898 ) ) ;
#68808=CARTESIAN_POINT ( 'NONE',  ( 13.42499999999999893, -4.330127018922194537, 2.499999999999995559 ) ) ;
#68809=CARTESIAN_POINT ( 'NONE',  ( 2.700000001229035718, -2.886751345948129988, 4.999999999999997335 ) ) ;
#68810=CARTESIAN_POINT ( 'NONE',  ( 11.70937500061451608, 4.541064518000418104, -2.621784821874998173 ) ) ;
#68811=CARTESIAN_POINT ( 'NONE',  ( 11.63437500061451857, 6.421520780324663323E-16, -5.243569643749999010 ) ) ;
#68812=CARTESIAN_POINT ( 'NONE',  ( 20.63437500061451857, 6.421520780324663323E-16, -5.243569643749999010 ) ) ;
#68813=ORIENTED_EDGE ( 'NONE', *, *, #62426, .F. ) ;
#68814=DIRECTION ( 'NONE',  ( -1.000000000000000000, -0.000000000000000000, -0.000000000000000000 ) ) ;
#68815=CARTESIAN_POINT ( 'NONE',  ( 23.87812500061451715, 4.541064518000418104, 2.621784821874999949 ) ) ;
#68816=CARTESIAN_POINT ( 'NONE',  ( 19.58437500061451786, -4.541064518000419881, 2.621784821874995952 ) ) ;
#68817=CARTESIAN_POINT ( 'NONE',  ( 24.44062500061451715, -3.027376345333614438, 5.243569643749998122 ) ) ;
#68818=CARTESIAN_POINT ( 'NONE',  ( 1.071796769724489895, 12.21740381056766900, -34.00000000000000000 ) ) ;
#68819=CARTESIAN_POINT ( 'NONE',  ( -1.999999999999997113, 14.22500000000000142, 33.46410161513775705 ) ) ;
#68820=CARTESIAN_POINT ( 'NONE',  ( 28.67812500061451431, 6.421520780324663323E-16, -5.243569643749999010 ) ) ;
#68821=CARTESIAN_POINT ( 'NONE',  ( 9.300000001229035362, 5.773502691896255534, 3.535250795749688894E-16 ) ) ;
#68822=CARTESIAN_POINT ( 'NONE',  ( 3.637500001229036162, -4.330127018922194537, 2.499999999999995559 ) ) ;
#68823=CARTESIAN_POINT ( 'NONE',  ( 28.87500000122902932, -5.773502691896255534, -1.060575238724906372E-15 ) ) ;
#68824=CARTESIAN_POINT ( 'NONE',  ( 26.21250000122903501, -4.330127018922190985, -2.500000000000001332 ) ) ;
#68827=CARTESIAN_POINT ( 'NONE',  ( 8.409375000614518925, -4.541064518000417216, -2.621784821875001281 ) ) ;
#68829=CARTESIAN_POINT ( 'NONE',  ( 17.27812500061451217, -4.541064518000419881, 2.621784821874995952 ) ) ;
#68830=CARTESIAN_POINT ( 'NONE',  ( 11.78437500061451892, 4.541064518000418104, 2.621784821874999949 ) ) ;
#68831=CARTESIAN_POINT ( 'NONE',  ( 3.478125000614517237, 6.421520780324663323E-16, -5.243569643749999010 ) ) ;
#68832=CARTESIAN_POINT ( 'NONE',  ( 19.20937500061451786, -4.541064518000417216, -2.621784821875001281 ) ) ;
#68833=CARTESIAN_POINT ( 'NONE',  ( 7.246875000614518392, 6.054752690667223547, 3.707466751127219781E-16 ) ) ;
#68834=CARTESIAN_POINT ( 'NONE',  ( 3.628125000614518036, 4.541064518000418104, 2.621784821874999949 ) ) ;
#68835=CARTESIAN_POINT ( 'NONE',  ( 8.765625000614518214, -6.054752690667223547, -1.112240025338166033E-15 ) ) ;
#68836=CARTESIAN_POINT ( 'NONE',  ( 18.02812500061451573, 4.541064518000418104, 2.621784821874999949 ) ) ;
#68838=CARTESIAN_POINT ( 'NONE',  ( 6.637500001229035718, 4.330127018922191873, 2.499999999999999556 ) ) ;
#68839=CARTESIAN_POINT ( 'NONE',  ( 15.40312500061451573, 0.000000000000000000, 5.243569643749999010 ) ) ;
#68840=CARTESIAN_POINT ( 'NONE',  ( 12.32812500061451821, -4.541064518000419881, 2.621784821874995952 ) ) ;
#68842=CARTESIAN_POINT ( 'NONE',  ( 13.42499999999999893, -4.330127018922194537, 2.499999999999995559 ) ) ;
#68843=CARTESIAN_POINT ( 'NONE',  ( 6.450000001229034829, -2.886751345948125991, -5.000000000000000000 ) ) ;
#68844=CARTESIAN_POINT ( 'NONE',  ( 4.528125000614516615, 4.541064518000418104, 2.621784821874999949 ) ) ;
#68845=CARTESIAN_POINT ( 'NONE',  ( 18.93750000122903288, -4.330127018922194537, 2.499999999999995559 ) ) ;
#68847=CARTESIAN_POINT ( 'NONE',  ( -4.243569643749997233, 10.44687500061451857, -27.54997392385601174 ) ) ;
#68848=CARTESIAN_POINT ( 'NONE',  ( 8.625000000000000000, 6.123233995736764310E-16, -4.999999999999998224 ) ) ;
#68849=EDGE_CURVE ( 'NONE', #69178, #52021, #59806, .T. ) ;
#68851=CARTESIAN_POINT ( 'NONE',  ( -3.137519842735245283E-14, 11.56250000000000178, -26.00000000000000711 ) ) ;
#68852=CARTESIAN_POINT ( 'NONE',  ( 30.00000000000000000, 0.000000000000000000, 4.999999999999998224 ) ) ;
#68853=CARTESIAN_POINT ( 'NONE',  ( 17.63437500061451502, 4.541064518000418104, 2.621784821874999949 ) ) ;
#68855=CARTESIAN_POINT ( 'NONE',  ( 14.50312500061451537, 0.000000000000000000, 5.243569643749999010 ) ) ;
#68858=CARTESIAN_POINT ( 'NONE',  ( 26.48437500061451644, 6.421520780324663323E-16, -5.243569643749999010 ) ) ;
#68860=CARTESIAN_POINT ( 'NONE',  ( 11.84062500061451750, -3.027376345333614438, 5.243569643749998122 ) ) ;
#68861=CARTESIAN_POINT ( 'NONE',  ( 16.43437500061451573, -4.541064518000419881, 2.621784821874995952 ) ) ;
#68863=CARTESIAN_POINT ( 'NONE',  ( 27.06562500061451004, 3.027376345333611329, 5.243569643749999010 ) ) ;
#68864=CARTESIAN_POINT ( 'NONE',  ( 20.24062500061451431, 6.054752690667223547, 3.707466751127219781E-16 ) ) ;
#68865=CARTESIAN_POINT ( 'NONE',  ( 3.089506346739232967, 3.931278485869285522, -3.469880700456108968 ) ) ;
#68866=DIRECTION ( 'NONE',  ( -1.000000000000000000, -0.000000000000000000, -0.000000000000000000 ) ) ;
#68867=CARTESIAN_POINT ( 'NONE',  ( 9.487500000000000711, -2.886751345948125991, -5.000000000000000000 ) ) ;
#68868=CARTESIAN_POINT ( 'NONE',  ( 19.98750000122903359, 6.123233995736764310E-16, -4.999999999999998224 ) ) ;
#68871=ORIENTED_EDGE ( 'NONE', *, *, #68849, .F. ) ;
#68872=CARTESIAN_POINT ( 'NONE',  ( 17.13749999999999929, -2.886751345948125991, -5.000000000000000000 ) ) ;
#68873=CARTESIAN_POINT ( 'NONE',  ( 20.96250000000000213, 2.886751345948126879, 4.999999999999999112 ) ) ;
#68874=CARTESIAN_POINT ( 'NONE',  ( 19.73437500061451644, 6.421520780324663323E-16, -5.243569643749999010 ) ) ;
#68875=CARTESIAN_POINT ( 'NONE',  ( 24.44062500061451715, -3.027376345333614438, 5.243569643749998122 ) ) ;
#68876=EDGE_LOOP ( 'NONE', ( #18921, #61882, #18868, #66690 ) ) ;
#68877=CARTESIAN_POINT ( 'NONE',  ( 27.86250000122903359, 0.000000000000000000, 4.999999999999998224 ) ) ;
#68878=CARTESIAN_POINT ( 'NONE',  ( 8.128125000614515372, 4.541064518000418104, 2.621784821874999949 ) ) ;
#68880=CARTESIAN_POINT ( 'NONE',  ( 15.03749999999999964, 5.773502691896255534, 3.535250795749688894E-16 ) ) ;
#68881=CARTESIAN_POINT ( 'NONE',  ( 2.121784821874999061, 18.30312500061451431, 26.32496088578401583 ) ) ;
#68882=CARTESIAN_POINT ( 'NONE',  ( 29.76562500061451644, 3.027376345333611329, 5.243569643749999010 ) ) ;
#68885=CARTESIAN_POINT ( 'NONE',  ( 27.00937500061451857, 4.541064518000418104, -2.621784821874998173 ) ) ;
#68887=CARTESIAN_POINT ( 'NONE',  ( 21.89062500061451289, -3.027376345333610441, -5.243569643749999898 ) ) ;
#68888=CARTESIAN_POINT ( 'NONE',  ( 23.78437500061451360, 6.421520780324663323E-16, -5.243569643749999010 ) ) ;
#68889=CARTESIAN_POINT ( 'NONE',  ( -4.243569643749999898, 16.16562500061459673, -32.45002607614398471 ) ) ;
#68890=CARTESIAN_POINT ( 'NONE',  ( 10.35000000000000142, -4.330127018922190985, -2.500000000000001332 ) ) ;
#68891=CARTESIAN_POINT ( 'NONE',  ( 5.315625000614516260, 3.027376345333613106, -5.243569643749998122 ) ) ;
#68893=CARTESIAN_POINT ( 'NONE',  ( 23.05312500061451431, 0.000000000000000000, 5.243569643749999010 ) ) ;
#68896=CARTESIAN_POINT ( 'NONE',  ( 17.97187500061451715, 3.027376345333613106, -5.243569643749998122 ) ) ;
#68897=CARTESIAN_POINT ( 'NONE',  ( 9.001249775931846008E-16, 13.22187500061451715, 34.90005215228797653 ) ) ;
#68898=CARTESIAN_POINT ( 'NONE',  ( 18.12187500061451573, 3.027376345333611329, 5.243569643749999010 ) ) ;
#68899=CARTESIAN_POINT ( 'NONE',  ( 26.33437500061451431, -4.541064518000419881, 2.621784821874995952 ) ) ;
#68900=CARTESIAN_POINT ( 'NONE',  ( -4.243569643749999898, 15.80937500061451573, 30.00000000000000000 ) ) ;
#68901=CARTESIAN_POINT ( 'NONE',  ( 7.528125000614515727, 6.421520780324663323E-16, -5.243569643749999010 ) ) ;
#68902=DIRECTION ( 'NONE',  ( -1.000000000000000000, -0.000000000000000000, -0.000000000000000000 ) ) ;
#68903=CARTESIAN_POINT ( 'NONE',  ( 3.796875000614517326, -3.027376345333614438, 5.243569643749998122 ) ) ;
#68904=DIRECTION ( 'NONE',  ( -1.000000000000000000, -0.000000000000000000, -0.000000000000000000 ) ) ;
#68905=CARTESIAN_POINT ( 'NONE',  ( 4.528125000614516615, 4.541064518000418104, 2.621784821874999949 ) ) ;
#68906=CARTESIAN_POINT ( 'NONE',  ( 9.271875000614516082, -6.054752690667223547, -1.112240025338166033E-15 ) ) ;
#68907=CARTESIAN_POINT ( 'NONE',  ( 17.21250000122903145, -4.330127018922190985, -2.500000000000001332 ) ) ;
#68908=CARTESIAN_POINT ( 'NONE',  ( 5.146875000614517859, -3.027376345333614438, 5.243569643749998122 ) ) ;
#68909=CARTESIAN_POINT ( 'NONE',  ( 6.403125000614517504, 0.000000000000000000, 5.243569643749999010 ) ) ;
#68912=CARTESIAN_POINT ( 'NONE',  ( 17.29687500061451999, -3.027376345333614438, 5.243569643749998122 ) ) ;
#68913=FACE_OUTER_BOUND ( 'NONE', #29084, .T. ) ;
#68914=ORIENTED_EDGE ( 'NONE', *, *, #42571, .F. ) ;
#68915=CARTESIAN_POINT ( 'NONE',  ( 25.34062500061451217, -3.027376345333614438, 5.243569643749998122 ) ) ;
#68916=CARTESIAN_POINT ( 'NONE',  ( 8.878125000614515372, 6.421520780324663323E-16, -5.243569643749999010 ) ) ;
#68917=CARTESIAN_POINT ( 'NONE',  ( 27.38437500061451857, 6.421520780324663323E-16, -5.243569643749999010 ) ) ;
#68918=CARTESIAN_POINT ( 'NONE',  ( 10.26562500061451644, 3.027376345333613106, -5.243569643749998122 ) ) ;
#68919=CARTESIAN_POINT ( 'NONE',  ( 4.413397852867026572, -2.350023558854721362, -4.663726614112597701 ) ) ;
#68920=CARTESIAN_POINT ( 'NONE',  ( 9.450000001229033941, -2.886751345948129988, 4.999999999999997335 ) ) ;
#68921=EDGE_CURVE ( 'NONE', #33991, #48298, #59475, .T. ) ;
#68922=CARTESIAN_POINT ( 'NONE',  ( 25.00312500061451715, -4.541064518000417216, -2.621784821875001281 ) ) ;
#68923=CARTESIAN_POINT ( 'NONE',  ( -3.000416591977282496E-16, 13.84062500061451928, -34.90005215228797653 ) ) ;
#68924=CARTESIAN_POINT ( 'NONE',  ( 12.26250000122903394, -4.330127018922190985, -2.500000000000001332 ) ) ;
#68925=CARTESIAN_POINT ( 'NONE',  ( 23.24062500061451786, -3.027376345333610441, -5.243569643749999898 ) ) ;
#68926=CARTESIAN_POINT ( 'NONE',  ( 11.43750000000000000, 5.773502691896255534, 3.535250795749688894E-16 ) ) ;
#68927=CARTESIAN_POINT ( 'NONE',  ( 19.49062500061451431, -3.027376345333614438, 5.243569643749998122 ) ) ;
#68928=CARTESIAN_POINT ( 'NONE',  ( 5.446875000614519458, 6.054752690667223547, 3.707466751127219781E-16 ) ) ;
#68929=CARTESIAN_POINT ( 'NONE',  ( 19.42499999999999716, 6.123233995736764310E-16, -4.999999999999998224 ) ) ;
#68930=CARTESIAN_POINT ( 'NONE',  ( 6.637500001229035718, 4.330127018922191873, 2.499999999999999556 ) ) ;
#68931=CARTESIAN_POINT ( 'NONE',  ( 17.02500000122903145, 2.886751345948126879, 4.999999999999999112 ) ) ;
#68933=CARTESIAN_POINT ( 'NONE',  ( 11.76562500061451644, 3.027376345333611329, 5.243569643749999010 ) ) ;
#68934=CARTESIAN_POINT ( 'NONE',  ( 14.76562500061451821, 3.027376345333613106, -5.243569643749998122 ) ) ;
#68935=CARTESIAN_POINT ( 'NONE',  ( 26.70000000122903572, -2.886751345948125991, -5.000000000000000000 ) ) ;
#68936=CARTESIAN_POINT ( 'NONE',  ( 21.52499999999999858, -4.330127018922194537, 2.499999999999995559 ) ) ;
#68937=CARTESIAN_POINT ( 'NONE',  ( 22.77187500061451786, -6.054752690667223547, -1.112240025338166033E-15 ) ) ;
#68939=EDGE_CURVE ( 'NONE', #17423, #51420, #36589, .T. ) ;
#68940=CARTESIAN_POINT ( 'NONE',  ( 11.21250000122903501, 0.000000000000000000, 4.999999999999998224 ) ) ;
#68941=CARTESIAN_POINT ( 'NONE',  ( 9.871875000614517504, 3.027376345333613106, -5.243569643749998122 ) ) ;
#68942=CARTESIAN_POINT ( 'NONE',  ( 24.64687500061451431, -3.027376345333610441, -5.243569643749999898 ) ) ;
#68943=( BOUNDED_CURVE ( )  B_SPLINE_CURVE ( 2, ( #20563, #43121, #65645, #15394, #22038, #67487, #33479 ),
 .UNSPECIFIED., .F., .F. ) 
 B_SPLINE_CURVE_WITH_KNOTS ( ( 3, 2, 2, 3 ),
 ( 0.7083333333333334814, 0.7111111111111112493, 0.7138888888888890172, 0.7166666666666667851 ),
 .UNSPECIFIED. ) 
 CURVE ( )  GEOMETRIC_REPRESENTATION_ITEM ( )  RATIONAL_B_SPLINE_CURVE ( ( 0.9999999999999946709, 0.8660254037844440367, 1.000000000000000000, 0.8660254037844387076, 1.000000000000000000, 0.8660254037844333785, 1.000000000000005329 ) ) 
 REPRESENTATION_ITEM ( '' )  );
#68944=CARTESIAN_POINT ( 'NONE',  ( 21.17812500061451431, 4.541064518000418104, 2.621784821874999949 ) ) ;
#68945=CARTESIAN_POINT ( 'NONE',  ( 27.45937500061451786, 4.541064518000418104, -2.621784821874998173 ) ) ;
#68948=CARTESIAN_POINT ( 'NONE',  ( 8.784375000614518925, -4.541064518000419881, 2.621784821874995952 ) ) ;
#68949=CARTESIAN_POINT ( 'NONE',  ( 20.01562500061451644, -6.054752690667223547, -1.112240025338166033E-15 ) ) ;
#68950=ORIENTED_EDGE ( 'NONE', *, *, #22648, .F. ) ;
#68951=CARTESIAN_POINT ( 'NONE',  ( 30.00000000000000000, 0.000000000000000000, 4.999999999999998224 ) ) ;
#68952=CARTESIAN_POINT ( 'NONE',  ( 27.70312500061451289, -4.541064518000417216, -2.621784821875001281 ) ) ;
#68953=CARTESIAN_POINT ( 'NONE',  ( 3.834375000614519635, -4.541064518000419881, 2.621784821874995952 ) ) ;
#68954=CARTESIAN_POINT ( 'NONE',  ( 22.76250000122903216, 4.330127018922192761, -2.499999999999997780 ) ) ;
#68955=EDGE_CURVE ( 'NONE', #5357, #69237, #28745, .T. ) ;
#68956=CARTESIAN_POINT ( 'NONE',  ( 3.586992791275801729, 3.483314903268937446, -3.919380039434936513 ) ) ;
#68957=CARTESIAN_POINT ( 'NONE',  ( 17.32499999999999929, 4.330127018922191873, 2.499999999999999556 ) ) ;
#68958=CARTESIAN_POINT ( 'NONE',  ( 20.42812500061451431, -4.541064518000419881, 2.621784821874995952 ) ) ;
#68960=CARTESIAN_POINT ( 'NONE',  ( 24.26249999999999929, -5.773502691896255534, -1.060575238724906372E-15 ) ) ;
#68961=CARTESIAN_POINT ( 'NONE',  ( 26.14687500061451431, 6.054752690667223547, 3.707466751127219781E-16 ) ) ;
#68963=CARTESIAN_POINT ( 'NONE',  ( 15.74062500061451608, 6.054752690667223547, 3.707466751127219781E-16 ) ) ;
#68964=CARTESIAN_POINT ( 'NONE',  ( 5.428125000614517859, 4.541064518000418104, 2.621784821874999949 ) ) ;
#68966=CARTESIAN_POINT ( 'NONE',  ( 2.859375000614519546, 0.000000000000000000, 5.243569643749999010 ) ) ;
#68968=CARTESIAN_POINT ( 'NONE',  ( 15.67500000122903181, 2.886751345948126879, 4.999999999999999112 ) ) ;
#68969=CARTESIAN_POINT ( 'NONE',  ( 23.02499999999999858, 6.123233995736764310E-16, -4.999999999999998224 ) ) ;
#68970=CARTESIAN_POINT ( 'NONE',  ( 29.25000000000000000, -4.330127018922190985, -2.500000000000001332 ) ) ;
#68971=CARTESIAN_POINT ( 'NONE',  ( 5.784375000614517148, 6.421520780324663323E-16, -5.243569643749999010 ) ) ;
#68972=CARTESIAN_POINT ( 'NONE',  ( 9.384375000614518569, 6.421520780324663323E-16, -5.243569643749999010 ) ) ;
#68973=CARTESIAN_POINT ( 'NONE',  ( 19.28437500061451360, 6.421520780324663323E-16, -5.243569643749999010 ) ) ;
#68974=CARTESIAN_POINT ( 'NONE',  ( 9.975000001229034297, -5.773502691896255534, -1.060575238724906372E-15 ) ) ;
#68976=CARTESIAN_POINT ( 'NONE',  ( 28.75312500061451715, 4.541064518000418104, -2.621784821874998173 ) ) ;
#68977=CARTESIAN_POINT ( 'NONE',  ( 4.050000000000001599, -4.330127018922190985, -2.500000000000001332 ) ) ;
#68978=CARTESIAN_POINT ( 'NONE',  ( 4.171875000614517326, 3.027376345333611329, 5.243569643749999010 ) ) ;
#68979=CARTESIAN_POINT ( 'NONE',  ( 19.20000000000000284, 0.000000000000000000, 4.999999999999998224 ) ) ;
#68980=CARTESIAN_POINT ( 'NONE',  ( 16.15312500061451573, 4.541064518000418104, -2.621784821874998173 ) ) ;
#68984=CARTESIAN_POINT ( 'NONE',  ( 7.415625000614516793, -6.054752690667223547, -1.112240025338166033E-15 ) ) ;
#68985=CARTESIAN_POINT ( 'NONE',  ( 26.40937500061451715, -4.541064518000417216, -2.621784821875001281 ) ) ;
#68986=CARTESIAN_POINT ( 'NONE',  ( 2.121784821874999061, 19.25937500061451857, 26.32496088578401583 ) ) ;
#68987=CARTESIAN_POINT ( 'NONE',  ( 26.40937500061451715, -4.541064518000417216, -2.621784821875001281 ) ) ;
#68988=CARTESIAN_POINT ( 'NONE',  ( 7.724999999999999645, 6.123233995736764310E-16, -4.999999999999998224 ) ) ;
#68989=CARTESIAN_POINT ( 'NONE',  ( 3.999999999999999112, 13.13750000122903394, 30.00000000000000000 ) ) ;
#68990=CARTESIAN_POINT ( 'NONE',  ( 14.50312500061451537, 0.000000000000000000, 5.243569643749999010 ) ) ;
#68991=CARTESIAN_POINT ( 'NONE',  ( 6.862500001229034474, -4.330127018922190985, -2.500000000000001332 ) ) ;
#68992=CARTESIAN_POINT ( 'NONE',  ( 17.93437500061451928, 6.421520780324663323E-16, -5.243569643749999010 ) ) ;
#68993=CARTESIAN_POINT ( 'NONE',  ( 12.27187500061451786, 3.027376345333611329, 5.243569643749999010 ) ) ;
#68994=CARTESIAN_POINT ( 'NONE',  ( -3.861264241427935673, 3.177798304702605492, -31.07837686909879693 ) ) ;
#68995=ORIENTED_EDGE ( 'NONE', *, *, #68656, .F. ) ;
#68996=CARTESIAN_POINT ( 'NONE',  ( 12.66562500061451502, 3.027376345333611329, 5.243569643749999010 ) ) ;
#68997=CARTESIAN_POINT ( 'NONE',  ( 23.77500000122903145, 2.886751345948126879, 4.999999999999999112 ) ) ;
#68998=CARTESIAN_POINT ( 'NONE',  ( 13.99687500061451928, 6.054752690667223547, 3.707466751127219781E-16 ) ) ;
#68999=CARTESIAN_POINT ( 'NONE',  ( 1.071796769724476572, 12.59509619066136921, 34.00000000000000000 ) ) ;
#69000=CARTESIAN_POINT ( 'NONE',  ( 15.51562500061451644, -6.054752690667223547, -1.112240025338166033E-15 ) ) ;
#69002=CARTESIAN_POINT ( 'NONE',  ( 24.53437500061451715, -4.541064518000419881, 2.621784821874995952 ) ) ;
#69004=CARTESIAN_POINT ( 'NONE',  ( 11.13750000122903216, 4.330127018922191873, 2.499999999999999556 ) ) ;
#69005=CARTESIAN_POINT ( 'NONE',  ( 30.00000000000000000, 0.000000000000000000, 0.000000000000000000 ) ) ;
#69006=CARTESIAN_POINT ( 'NONE',  ( 8.849999999999999645, 0.000000000000000000, 4.999999999999998224 ) ) ;
#69007=CARTESIAN_POINT ( 'NONE',  ( 9.001249775931846008E-16, 17.27187500061451786, -25.09994784771203058 ) ) ;
#69008=CARTESIAN_POINT ( 'NONE',  ( 17.10937500061451999, 4.541064518000418104, -2.621784821874998173 ) ) ;
#69009=CARTESIAN_POINT ( 'NONE',  ( 18.22500000122903430, 2.886751345948129099, -4.999999999999998224 ) ) ;
#69011=CARTESIAN_POINT ( 'NONE',  ( 15.64687500061451608, -3.027376345333610441, -5.243569643749999898 ) ) ;
#69013=CARTESIAN_POINT ( 'NONE',  ( 19.20000000122903572, 5.773502691896255534, 3.535250795749688894E-16 ) ) ;
#69014=CARTESIAN_POINT ( 'NONE',  ( 14.05312500061451431, 0.000000000000000000, 5.243569643749999010 ) ) ;
#69017=CARTESIAN_POINT ( 'NONE',  ( 18.93750000000000000, -2.886751345948125991, -5.000000000000000000 ) ) ;
#69019=CARTESIAN_POINT ( 'NONE',  ( 1.841668243974589059, 4.655663185590169562, 26.43913409586652818 ) ) ;
#69020=CARTESIAN_POINT ( 'NONE',  ( 14.02500000122903323, -5.773502691896255534, -1.060575238724906372E-15 ) ) ;
#69021=CARTESIAN_POINT ( 'NONE',  ( 27.79687500061451999, -3.027376345333610441, -5.243569643749999898 ) ) ;
#69022=CARTESIAN_POINT ( 'NONE',  ( 20.54062500061451502, -3.027376345333610441, -5.243569643749999898 ) ) ;
#69024=CARTESIAN_POINT ( 'NONE',  ( 23.35312500061451857, 4.541064518000418104, -2.621784821874998173 ) ) ;
#69025=CARTESIAN_POINT ( 'NONE',  ( 4.228125000614517681, -4.541064518000419881, 2.621784821874995952 ) ) ;
#69026=CARTESIAN_POINT ( 'NONE',  ( 26.66250000000000142, 2.886751345948129099, -4.999999999999998224 ) ) ;
#69027=CARTESIAN_POINT ( 'NONE',  ( 4.687500000000000000, 5.773502691896255534, 3.535250795749688401E-16 ) ) ;
#69029=CARTESIAN_POINT ( 'NONE',  ( 6.262500001229034829, 0.000000000000000000, 4.999999999999998224 ) ) ;
#69030=CARTESIAN_POINT ( 'NONE',  ( -3.999999999999997335, 9.800000001229033586, -27.69059892324149175 ) ) ;
#69031=CARTESIAN_POINT ( 'NONE',  ( -2.121784821874999949, 17.08437500061451786, -33.67503911421598417 ) ) ;
#69032=CARTESIAN_POINT ( 'NONE',  ( 6.262500001229034829, 0.000000000000000000, 4.999999999999998224 ) ) ;
#69033=CARTESIAN_POINT ( 'NONE',  ( 6.750000000000002665, -4.330127018922190985, -2.500000000000001332 ) ) ;
#69034=CARTESIAN_POINT ( 'NONE',  ( 4.762500001229033941, 4.330127018922192761, -2.499999999999997780 ) ) ;
#69035=CARTESIAN_POINT ( 'NONE',  ( 10.99687500061451750, -3.027376345333614438, 5.243569643749998122 ) ) ;
#69036=CARTESIAN_POINT ( 'NONE',  ( 28.26562500061451289, 3.027376345333613106, -5.243569643749998122 ) ) ;
#69038=CARTESIAN_POINT ( 'NONE',  ( 5.587500001229033231, 6.123233995736764310E-16, -4.999999999999998224 ) ) ;
#69039=CARTESIAN_POINT ( 'NONE',  ( 2.000000000000001332, 19.36250000122903359, 33.46410161513774995 ) ) ;
#69040=CARTESIAN_POINT ( 'NONE',  ( 7.846875000614518036, -3.027376345333614438, 5.243569643749998122 ) ) ;
#69041=CARTESIAN_POINT ( 'NONE',  ( 10.17187500061451999, -6.054752690667223547, -1.112240025338166033E-15 ) ) ;
#69042=CARTESIAN_POINT ( 'NONE',  ( 5.662500000000000533, 2.886751345948126879, 4.999999999999999112 ) ) ;
#69043=CARTESIAN_POINT ( 'NONE',  ( -4.243569643749998122, 14.89062500061459637, 32.45002607614398471 ) ) ;
#69044=CARTESIAN_POINT ( 'NONE',  ( 1.071796769724491893, 17.88259618943233065, 33.99999999999999289 ) ) ;
#69045=CARTESIAN_POINT ( 'NONE',  ( 6.825000000000001066, 6.123233995736764310E-16, -4.999999999999998224 ) ) ;
#69046=CARTESIAN_POINT ( 'NONE',  ( 27.45000000122903572, -2.886751345948129988, 4.999999999999997335 ) ) ;
#69049=CARTESIAN_POINT ( 'NONE',  ( 23.20312500061451644, -4.541064518000417216, -2.621784821875001281 ) ) ;
#69050=CARTESIAN_POINT ( 'NONE',  ( 14.20312500061451644, -4.541064518000417216, -2.621784821875001281 ) ) ;
#69052=CARTESIAN_POINT ( 'NONE',  ( 10.24687500061451750, -3.027376345333610441, -5.243569643749999898 ) ) ;
#69053=CARTESIAN_POINT ( 'NONE',  ( 29.13749999999999929, -2.886751345948129988, 4.999999999999997335 ) ) ;
#69054=CARTESIAN_POINT ( 'NONE',  ( 23.36250000122903359, 0.000000000000000000, 4.999999999999998224 ) ) ;
#69055=CARTESIAN_POINT ( 'NONE',  ( 11.32500000122903216, -5.773502691896255534, -1.060575238724906372E-15 ) ) ;
#69056=VECTOR ( 'NONE', #8335, 1000.000000000000000 ) ;
#69057=CARTESIAN_POINT ( 'NONE',  ( 12.94687500061451857, -3.027376345333610441, -5.243569643749999898 ) ) ;
#69058=CARTESIAN_POINT ( 'NONE',  ( 25.80937500061451928, 0.000000000000000000, 5.243569643749999010 ) ) ;
#69059=CARTESIAN_POINT ( 'NONE',  ( 3.946875000614517681, -3.027376345333610441, -5.243569643749999898 ) ) ;
#69061=CARTESIAN_POINT ( 'NONE',  ( 1.999999999999998668, 13.66250000122903607, -33.46410161513775705 ) ) ;
#69062=CARTESIAN_POINT ( 'NONE',  ( 22.43437500061451573, 6.421520780324663323E-16, -5.243569643749999010 ) ) ;
#69063=CARTESIAN_POINT ( 'NONE',  ( 12.38437500061451857, -4.541064518000419881, 2.621784821874995952 ) ) ;
#69064=EDGE_CURVE ( 'NONE', #23337, #16088, #36297, .T. ) ;
#69066=CARTESIAN_POINT ( 'NONE',  ( 25.53750000000000142, -2.886751345948129988, 4.999999999999997335 ) ) ;
#69068=CARTESIAN_POINT ( 'NONE',  ( -2.121784821874999949, 14.38437500061451679, -33.67503911421598417 ) ) ;
#69070=CARTESIAN_POINT ( 'NONE',  ( 17.27812500061451217, -4.541064518000419881, 2.621784821874995952 ) ) ;
#69071=CARTESIAN_POINT ( 'NONE',  ( 6.524999999999999467, 4.330127018922191873, 2.499999999999999556 ) ) ;
#69072=DIRECTION ( 'NONE',  ( -0.000000000000000000, -1.000000000000000000, -0.000000000000000000 ) ) ;
#69073=CARTESIAN_POINT ( 'NONE',  ( 15.15000000000000036, 0.000000000000000000, 4.999999999999998224 ) ) ;
#69074=CARTESIAN_POINT ( 'NONE',  ( 4.243569643749999010, 11.51562500061451644, 27.54997392385601174 ) ) ;
#69075=CARTESIAN_POINT ( 'NONE',  ( 13.98750000122903359, -4.330127018922194537, 2.499999999999995559 ) ) ;
#69076=CARTESIAN_POINT ( 'NONE',  ( 25.77187500061451075, 3.027376345333611329, 5.243569643749999010 ) ) ;
#69078=CARTESIAN_POINT ( 'NONE',  ( 18.96562500061451573, 3.027376345333611329, 5.243569643749999010 ) ) ;
#69079=CARTESIAN_POINT ( 'NONE',  ( 19.88437500061451857, 4.541064518000418104, 2.621784821874999949 ) ) ;
#69080=CARTESIAN_POINT ( 'NONE',  ( 4.125000000000000000, 6.123233995736764310E-16, -4.999999999999998224 ) ) ;
#69081=CARTESIAN_POINT ( 'NONE',  ( 7.378125000614518036, -4.541064518000419881, 2.621784821874995952 ) ) ;
#69082=CARTESIAN_POINT ( 'NONE',  ( 21.62812500061451360, 4.541064518000418104, 2.621784821874999949 ) ) ;
#69083=CARTESIAN_POINT ( 'NONE',  ( 12.83437500061451786, -4.541064518000419881, 2.621784821874995952 ) ) ;
#69084=CARTESIAN_POINT ( 'NONE',  ( 17.18437500061451573, 4.541064518000418104, 2.621784821874999949 ) ) ;
#69085=CARTESIAN_POINT ( 'NONE',  ( -4.243569643749999898, 14.36562500061451786, 27.54997392385601529 ) ) ;
#69086=CARTESIAN_POINT ( 'NONE',  ( 20.06250000122903643, 4.330127018922192761, -2.499999999999997780 ) ) ;
#69088=CARTESIAN_POINT ( 'NONE',  ( 10.41562500061451679, 3.027376345333611329, 5.243569643749999010 ) ) ;
#69089=CARTESIAN_POINT ( 'NONE',  ( 3.909375000614518481, -4.541064518000417216, -2.621784821875001281 ) ) ;
#69090=CARTESIAN_POINT ( 'NONE',  ( 3.121875000614518836, 3.027376345333613106, -5.243569643749998122 ) ) ;
#69091=CARTESIAN_POINT ( 'NONE',  ( 25.80937500061451928, 0.000000000000000000, 5.243569643749999010 ) ) ;
#69092=CARTESIAN_POINT ( 'NONE',  ( 17.69062500061451715, -3.027376345333614438, 5.243569643749998122 ) ) ;
#69093=CARTESIAN_POINT ( 'NONE',  ( 26.13750000122903216, -4.330127018922194537, 2.499999999999995559 ) ) ;
#69094=CARTESIAN_POINT ( 'NONE',  ( 25.00312500061451715, -4.541064518000417216, -2.621784821875001281 ) ) ;
#69095=CARTESIAN_POINT ( 'NONE',  ( 21.04687500061451644, -3.027376345333610441, -5.243569643749999898 ) ) ;
#69096=CARTESIAN_POINT ( 'NONE',  ( 16.86562500061451786, -6.054752690667223547, -1.112240025338166033E-15 ) ) ;
#69097=CARTESIAN_POINT ( 'NONE',  ( -3.000416591977282496E-16, 17.04687500061451644, 25.09994784771203058 ) ) ;
#69098=VECTOR ( 'NONE', #26180, 1000.000000000000000 ) ;
#69099=CARTESIAN_POINT ( 'NONE',  ( 23.24062500061451786, -3.027376345333610441, -5.243569643749999898 ) ) ;
#69100=CARTESIAN_POINT ( 'NONE',  ( 2.775000001229033675, -5.773502691896255534, -1.060575238724906372E-15 ) ) ;
#69102=CARTESIAN_POINT ( 'NONE',  ( 26.43750000000000000, -2.886751345948129988, 4.999999999999997335 ) ) ;
#69103=CARTESIAN_POINT ( 'NONE',  ( -2.000000000000000000, 12.72499999999999964, -33.46410161513775705 ) ) ;
#69105=CARTESIAN_POINT ( 'NONE',  ( 3.196875000614516793, 6.054752690667223547, 3.707466751127219781E-16 ) ) ;
#69106=CARTESIAN_POINT ( 'NONE',  ( 11.35312500061451679, 0.000000000000000000, 5.243569643749999010 ) ) ;
#69107=CARTESIAN_POINT ( 'NONE',  ( 21.75000000122903288, -2.886751345948125991, -5.000000000000000000 ) ) ;
#69109=EDGE_CURVE ( 'NONE', #26440, #18523, #66494, .T. ) ;
#69110=CARTESIAN_POINT ( 'NONE',  ( 26.46562500061451573, 3.027376345333613106, -5.243569643749998122 ) ) ;
#69111=CARTESIAN_POINT ( 'NONE',  ( 25.38749999999999929, 5.773502691896255534, 3.535250795749688894E-16 ) ) ;
#69112=CARTESIAN_POINT ( 'NONE',  ( 3.999999999999999112, 16.73750000122903359, -30.00000000000000000 ) ) ;
#69113=CARTESIAN_POINT ( 'NONE',  ( -3.999999999999999112, 15.61250000122903359, -30.00000000000000000 ) ) ;
#69114=CARTESIAN_POINT ( 'NONE',  ( 10.97812500061451679, -4.541064518000419881, 2.621784821874995952 ) ) ;
#69115=ORIENTED_EDGE ( 'NONE', *, *, #68939, .F. ) ;
#69116=CARTESIAN_POINT ( 'NONE',  ( 26.20312500061451644, 0.000000000000000000, 5.243569643749999010 ) ) ;
#69117=CARTESIAN_POINT ( 'NONE',  ( 6.703125000614516438, 4.541064518000418104, -2.621784821874998173 ) ) ;
#69120=CARTESIAN_POINT ( 'NONE',  ( 3.928125000614516527, 6.421520780324663323E-16, -5.243569643749999010 ) ) ;
#69122=DIRECTION ( 'NONE',  ( -1.000000000000000000, -0.000000000000000000, -0.000000000000000000 ) ) ;
#69123=CARTESIAN_POINT ( 'NONE',  ( 12.93750000000000178, -2.886751345948129988, 4.999999999999997335 ) ) ;
#69124=CARTESIAN_POINT ( 'NONE',  ( 13.47187500061451537, 3.027376345333613106, -5.243569643749998122 ) ) ;
#69125=CARTESIAN_POINT ( 'NONE',  ( 11.66250000122903430, 0.000000000000000000, 4.999999999999998224 ) ) ;
#69126=CARTESIAN_POINT ( 'NONE',  ( 16.54687500061451644, -3.027376345333610441, -5.243569643749999898 ) ) ;
#69128=CARTESIAN_POINT ( 'NONE',  ( 9.196875000614518569, -3.027376345333614438, 5.243569643749998122 ) ) ;
#69129=CARTESIAN_POINT ( 'NONE',  ( 9.001249775931846008E-16, 12.71562500061451750, -25.09994784771203058 ) ) ;
#69130=CARTESIAN_POINT ( 'NONE',  ( 7.275000000000000355, 6.123233995736764310E-16, -4.999999999999998224 ) ) ;
#69133=CARTESIAN_POINT ( 'NONE',  ( 24.40312500061451573, 0.000000000000000000, 5.243569643749999010 ) ) ;
#69135=CARTESIAN_POINT ( 'NONE',  ( 28.13437500061451502, -4.541064518000419881, 2.621784821874995952 ) ) ;
#69136=CARTESIAN_POINT ( 'NONE',  ( 23.66250000000000142, 2.886751345948126879, 4.999999999999999112 ) ) ;
#69137=CARTESIAN_POINT ( 'NONE',  ( 7.528125000614515727, 6.421520780324663323E-16, -5.243569643749999010 ) ) ;
#69139=CARTESIAN_POINT ( 'NONE',  ( 18.30937500061451928, -4.541064518000417216, -2.621784821875001281 ) ) ;
#69141=CARTESIAN_POINT ( 'NONE',  ( 29.47500000122903430, 2.886751345948129099, -4.999999999999998224 ) ) ;
#69142=CARTESIAN_POINT ( 'NONE',  ( 9.009375000614518569, 4.541064518000418104, -2.621784821874998173 ) ) ;
#69144=CARTESIAN_POINT ( 'NONE',  ( 18.04687500061451999, 6.054752690667223547, 3.707466751127219781E-16 ) ) ;
#69146=CARTESIAN_POINT ( 'NONE',  ( 27.11249999999999716, 2.886751345948129099, -4.999999999999998224 ) ) ;
#69147=CARTESIAN_POINT ( 'NONE',  ( 28.58437500061451786, -4.541064518000419881, 2.621784821874995952 ) ) ;
#69150=ORIENTED_EDGE ( 'NONE', *, *, #50466, .T. ) ;
#69151=CARTESIAN_POINT ( 'NONE',  ( 10.83750000000000036, -2.886751345948125991, -5.000000000000000000 ) ) ;
#69153=CARTESIAN_POINT ( 'NONE',  ( 23.87812500061451715, 4.541064518000418104, 2.621784821874999949 ) ) ;
#69154=CARTESIAN_POINT ( 'NONE',  ( 13.04999999999999893, -4.330127018922190985, -2.500000000000001332 ) ) ;
#69155=CARTESIAN_POINT ( 'NONE',  ( 8.437500001229034652, 4.330127018922191873, 2.499999999999999556 ) ) ;
#69156=CARTESIAN_POINT ( 'NONE',  ( 7.003125000614518036, -4.541064518000417216, -2.621784821875001281 ) ) ;
#69158=CARTESIAN_POINT ( 'NONE',  ( 20.99999999999999645, 0.000000000000000000, 4.999999999999998224 ) ) ;
#69159=CARTESIAN_POINT ( 'NONE',  ( 21.02812500061451573, 6.421520780324663323E-16, -5.243569643749999010 ) ) ;
#69160=CARTESIAN_POINT ( 'NONE',  ( 5.025000000000002132, 6.123233995736764310E-16, -4.999999999999998224 ) ) ;
#69161=CARTESIAN_POINT ( 'NONE',  ( 25.53750000122903074, 4.330127018922191873, 2.499999999999999556 ) ) ;
#69163=CARTESIAN_POINT ( 'NONE',  ( 3.975000000000002753, -4.330127018922194537, 2.499999999999995559 ) ) ;
#69165=CARTESIAN_POINT ( 'NONE',  ( 22.04062500061451502, 6.054752690667223547, 3.707466751127219781E-16 ) ) ;
#69166=CARTESIAN_POINT ( 'NONE',  ( 27.51562500061451644, 3.027376345333611329, 5.243569643749999010 ) ) ;
#69167=CARTESIAN_POINT ( 'NONE',  ( 27.49687500061451217, 6.054752690667223547, 3.707466751127219781E-16 ) ) ;
#69168=CARTESIAN_POINT ( 'NONE',  ( 13.79062500061451502, -3.027376345333610441, -5.243569643749999898 ) ) ;
#69169=CARTESIAN_POINT ( 'NONE',  ( -3.000416591977282496E-16, 10.24062500061459069, -34.90005215228797653 ) ) ;
#69170=CARTESIAN_POINT ( 'NONE',  ( 26.32500000122903216, 2.886751345948129099, -4.999999999999998224 ) ) ;
#69172=CARTESIAN_POINT ( 'NONE',  ( 17.87812500061451715, 6.421520780324663323E-16, -5.243569643749999010 ) ) ;
#69174=CARTESIAN_POINT ( 'NONE',  ( 5.962500001229033231, -4.330127018922190985, -2.500000000000001332 ) ) ;
#69175=CARTESIAN_POINT ( 'NONE',  ( 10.92187500061451644, 3.027376345333611329, 5.243569643749999010 ) ) ;
#69176=CARTESIAN_POINT ( 'NONE',  ( 11.70937500061451608, 4.541064518000418104, -2.621784821874998173 ) ) ;
#69177=CARTESIAN_POINT ( 'NONE',  ( 18.94687500061451502, 6.054752690667223547, 3.707466751127219781E-16 ) ) ;
#69178=VERTEX_POINT ( 'NONE', #66126 ) ;
#69179=CARTESIAN_POINT ( 'NONE',  ( 0.000000000000000000, 4.999999999999998224, 0.000000000000000000 ) ) ;
#69180=CARTESIAN_POINT ( 'NONE',  ( 24.89062500061451644, -3.027376345333614438, 5.243569643749998122 ) ) ;
#69181=CARTESIAN_POINT ( 'NONE',  ( 19.50937500061451857, 0.000000000000000000, 5.243569643749999010 ) ) ;
#69182=CARTESIAN_POINT ( 'NONE',  ( 23.80312500061451786, 4.541064518000418104, -2.621784821874998173 ) ) ;
#69183=DIRECTION ( 'NONE',  ( -1.000000000000000000, -0.000000000000000000, -0.000000000000000000 ) ) ;
#69184=CARTESIAN_POINT ( 'NONE',  ( 3.999999999999998668, 14.41250000000000142, 27.69059892324149175 ) ) ;
#69185=CARTESIAN_POINT ( 'NONE',  ( 3.609375000614516882, 4.541064518000418104, -2.621784821874998173 ) ) ;
#69186=CARTESIAN_POINT ( 'NONE',  ( 8.550000001229031810, -2.886751345948129988, 4.999999999999997335 ) ) ;
#69187=CARTESIAN_POINT ( 'NONE',  ( 5.062500001229035540, -4.330127018922190985, -2.500000000000001332 ) ) ;
#69188=CARTESIAN_POINT ( 'NONE',  ( 3.999999999999999112, 19.77500000000000213, -30.00000000000000000 ) ) ;
#69189=CARTESIAN_POINT ( 'NONE',  ( 28.16250000122903074, 4.330127018922192761, -2.499999999999997780 ) ) ;
#69191=CARTESIAN_POINT ( 'NONE',  ( 10.54687500061451644, -3.027376345333614438, 5.243569643749998122 ) ) ;
#69193=CARTESIAN_POINT ( 'NONE',  ( 16.67812500061451786, 4.541064518000418104, 2.621784821874999949 ) ) ;
#69194=CARTESIAN_POINT ( 'NONE',  ( 10.73437500061451644, 6.421520780324663323E-16, -5.243569643749999010 ) ) ;
#69195=CARTESIAN_POINT ( 'NONE',  ( 3.515625000614516882, 3.027376345333613106, -5.243569643749998122 ) ) ;
#69196=CARTESIAN_POINT ( 'NONE',  ( 18.60937500061451644, 0.000000000000000000, 5.243569643749999010 ) ) ;
#69197=CARTESIAN_POINT ( 'NONE',  ( 7.621875000614519280, 3.027376345333613106, -5.243569643749998122 ) ) ;
#69198=CARTESIAN_POINT ( 'NONE',  ( 3.045726060920115774, -3.965322109520783567, -3.366821969667765035 ) ) ;
#69199=CARTESIAN_POINT ( 'NONE',  ( 30.00000000000000000, 6.123233995736764310E-16, -4.999999999999998224 ) ) ;
#69200=CARTESIAN_POINT ( 'NONE',  ( 8.803125000614517859, -4.541064518000417216, -2.621784821875001281 ) ) ;
#69201=CARTESIAN_POINT ( 'NONE',  ( 17.16562500061451502, 3.027376345333611329, 5.243569643749999010 ) ) ;
#69202=EDGE_CURVE ( 'NONE', #38080, #64135, #15505, .T. ) ;
#69203=EDGE_LOOP ( 'NONE', ( #72332, #3462, #22428, #63304 ) ) ;
#69204=CARTESIAN_POINT ( 'NONE',  ( 5.737500001229033586, 4.330127018922191873, 2.499999999999999556 ) ) ;
#69205=CARTESIAN_POINT ( 'NONE',  ( 15.29062500061451679, 6.054752690667223547, 3.707466751127219781E-16 ) ) ;
#69206=AXIS2_PLACEMENT_3D ( 'NONE', #57648, #41754, #14036 ) ;
#69207=CARTESIAN_POINT ( 'NONE',  ( 12.02812500061451573, 6.421520780324663323E-16, -5.243569643749999010 ) ) ;
#69209=CARTESIAN_POINT ( 'NONE',  ( 13.08750000000000036, -2.886751345948125991, -5.000000000000000000 ) ) ;
#69210=CARTESIAN_POINT ( 'NONE',  ( 7.125000001229033764, 2.886751345948126879, 4.999999999999999112 ) ) ;
#69211=CARTESIAN_POINT ( 'NONE',  ( 25.16250000122903074, 0.000000000000000000, 4.999999999999998224 ) ) ;
#69212=CARTESIAN_POINT ( 'NONE',  ( 14.89687500061451786, 6.054752690667223547, 3.707466751127219781E-16 ) ) ;
#69213=CARTESIAN_POINT ( 'NONE',  ( 17.43750000122903288, 4.330127018922191873, 2.499999999999999556 ) ) ;
#69215=CARTESIAN_POINT ( 'NONE',  ( 4.243569643749999010, 18.71562500061451217, -32.45002607614398471 ) ) ;
#69218=FACE_OUTER_BOUND ( 'NONE', #31062, .T. ) ;
#69219=CARTESIAN_POINT ( 'NONE',  ( 17.70937500061451431, 0.000000000000000000, 5.243569643749999010 ) ) ;
#69220=CARTESIAN_POINT ( 'NONE',  ( 0.000000000000000000, 20.00000000000000000, -33.99999999999999289 ) ) ;
#69221=CARTESIAN_POINT ( 'NONE',  ( 14.31562500061451537, 3.027376345333613106, -5.243569643749998122 ) ) ;
#69224=CARTESIAN_POINT ( 'NONE',  ( 26.22187500061451715, 3.027376345333611329, 5.243569643749999010 ) ) ;
#69226=CARTESIAN_POINT ( 'NONE',  ( 11.24062500061451608, 6.054752690667223547, 3.707466751127219781E-16 ) ) ;
#69227=CARTESIAN_POINT ( 'NONE',  ( 16.20937500061451786, 4.541064518000418104, -2.621784821874998173 ) ) ;
#69228=ORIENTED_EDGE ( 'NONE', *, *, #19299, .T. ) ;
#69229=CARTESIAN_POINT ( 'NONE',  ( 27.51562500061451644, 3.027376345333611329, 5.243569643749999010 ) ) ;
#69230=CARTESIAN_POINT ( 'NONE',  ( 21.32812500061451644, -4.541064518000419881, 2.621784821874995952 ) ) ;
#69231=CARTESIAN_POINT ( 'NONE',  ( 29.39062500061451289, -3.027376345333614438, 5.243569643749998122 ) ) ;
#69232=CARTESIAN_POINT ( 'NONE',  ( -1.071796769724491005, 14.17009619066136672, -34.00000000000000000 ) ) ;
#69233=CARTESIAN_POINT ( 'NONE',  ( 9.937500000000001776, -2.886751345948125991, -5.000000000000000000 ) ) ;
#69234=CARTESIAN_POINT ( 'NONE',  ( 18.26250000122903216, 4.330127018922192761, -2.499999999999997780 ) ) ;
#69235=CARTESIAN_POINT ( 'NONE',  ( 3.752440054025286909, -3.304420318444254878, 4.071342403668507082 ) ) ;
#69237=VERTEX_POINT ( 'NONE', #16240 ) ;
#69238=CARTESIAN_POINT ( 'NONE',  ( 17.32499999999999929, 4.330127018922191873, 2.499999999999999556 ) ) ;
#69239=CARTESIAN_POINT ( 'NONE',  ( 20.81250000000000000, 2.886751345948129099, -4.999999999999998224 ) ) ;
#69240=CARTESIAN_POINT ( 'NONE',  ( 18.38437500061451857, 6.421520780324663323E-16, -5.243569643749999010 ) ) ;
#69241=CARTESIAN_POINT ( 'NONE',  ( 25.56562500061452070, 3.027376345333613106, -5.243569643749998122 ) ) ;
#69244=CARTESIAN_POINT ( 'NONE',  ( 5.840625000614516615, 6.054752690667223547, 3.707466751127219781E-16 ) ) ;
#69245=CARTESIAN_POINT ( 'NONE',  ( 3.250662400336420177, 3.799104362746421604, 3.614115195980558415 ) ) ;
#69246=CARTESIAN_POINT ( 'NONE',  ( 12.33750000000000036, 5.773502691896255534, 3.535250795749688894E-16 ) ) ;
#69247=CARTESIAN_POINT ( 'NONE',  ( 2.121784821874999061, 16.50312500061451715, 26.32496088578401583 ) ) ;
#69248=CARTESIAN_POINT ( 'NONE',  ( 28.37812500061451715, 4.541064518000418104, 2.621784821874999949 ) ) ;
#69251=CARTESIAN_POINT ( 'NONE',  ( 26.74687500061451573, -3.027376345333614438, 5.243569643749998122 ) ) ;
#69252=ORIENTED_EDGE ( 'NONE', *, *, #65786, .F. ) ;
#69253=CARTESIAN_POINT ( 'NONE',  ( 22.11562500061451786, 3.027376345333611329, 5.243569643749999010 ) ) ;
#69254=CARTESIAN_POINT ( 'NONE',  ( 22.77187500061451786, -6.054752690667223547, -1.112240025338166033E-15 ) ) ;
#69255=CARTESIAN_POINT ( 'NONE',  ( -2.121784821874999949, 16.12812500061459176, -33.67503911421598417 ) ) ;
#69256=CARTESIAN_POINT ( 'NONE',  ( 5.803125000614517859, 4.541064518000418104, -2.621784821874998173 ) ) ;
#69258=CARTESIAN_POINT ( 'NONE',  ( 23.99062500061451786, -3.027376345333614438, 5.243569643749998122 ) ) ;
#69261=CARTESIAN_POINT ( 'NONE',  ( 16.20937500061451786, 4.541064518000418104, -2.621784821874998173 ) ) ;
#69262=CARTESIAN_POINT ( 'NONE',  ( 18.98437500061451644, 4.541064518000418104, 2.621784821874999949 ) ) ;
#69263=CARTESIAN_POINT ( 'NONE',  ( 26.89687500061451431, -3.027376345333610441, -5.243569643749999898 ) ) ;
#69264=CARTESIAN_POINT ( 'NONE',  ( -4.243569643749999898, 17.57187500061451502, 27.54997392385601529 ) ) ;
#69265=CARTESIAN_POINT ( 'NONE',  ( 6.853125000614516793, 0.000000000000000000, 5.243569643749999010 ) ) ;
#69267=CARTESIAN_POINT ( 'NONE',  ( 5.146875000614517859, -3.027376345333614438, 5.243569643749998122 ) ) ;
#69268=CARTESIAN_POINT ( 'NONE',  ( 26.47499999999999787, -4.330127018922194537, 2.499999999999995559 ) ) ;
#69269=CARTESIAN_POINT ( 'NONE',  ( 5.990625000614517859, -3.027376345333614438, 5.243569643749998122 ) ) ;
#69270=CARTESIAN_POINT ( 'NONE',  ( 9.609375000614518214, 0.000000000000000000, 5.243569643749999010 ) ) ;
#69272=CARTESIAN_POINT ( 'NONE',  ( 16.16250000122903430, 0.000000000000000000, 4.999999999999998224 ) ) ;
#69273=CARTESIAN_POINT ( 'NONE',  ( 6.084375000614518747, -4.541064518000419881, 2.621784821874995952 ) ) ;
#69274=CARTESIAN_POINT ( 'NONE',  ( 8.090625000614515727, 6.054752690667223547, 3.707466751127219781E-16 ) ) ;
#69277=CARTESIAN_POINT ( 'NONE',  ( 17.85937500061451999, -4.541064518000417216, -2.621784821875001281 ) ) ;
#69280=CARTESIAN_POINT ( 'NONE',  ( 24.77812500061451217, 4.541064518000418104, 2.621784821874999949 ) ) ;
#69281=CARTESIAN_POINT ( 'NONE',  ( 9.778125000614517504, 6.421520780324663323E-16, -5.243569643749999010 ) ) ;
#69282=CARTESIAN_POINT ( 'NONE',  ( 26.22187500061451715, 3.027376345333611329, 5.243569643749999010 ) ) ;
#69283=CARTESIAN_POINT ( 'NONE',  ( 10.15312500061451750, -4.541064518000417216, -2.621784821875001281 ) ) ;
#69285=CARTESIAN_POINT ( 'NONE',  ( 10.91250000122903252, -4.330127018922190985, -2.500000000000001332 ) ) ;
#69286=CARTESIAN_POINT ( 'NONE',  ( 24.92812500061451431, -4.541064518000419881, 2.621784821874995952 ) ) ;
#69288=CARTESIAN_POINT ( 'NONE',  ( -4.243569643749999898, 13.50312500061451715, -30.00000000000000000 ) ) ;
#69289=CARTESIAN_POINT ( 'NONE',  ( 12.56250000122903465, 0.000000000000000000, 4.999999999999998224 ) ) ;
#69290=CARTESIAN_POINT ( 'NONE',  ( 21.70312500061451644, 0.000000000000000000, 5.243569643749999010 ) ) ;
#69291=CARTESIAN_POINT ( 'NONE',  ( 10.83750000000000036, -2.886751345948125991, -5.000000000000000000 ) ) ;
#69292=CARTESIAN_POINT ( 'NONE',  ( 20.99062500061451431, -3.027376345333610441, -5.243569643749999898 ) ) ;
#69293=CARTESIAN_POINT ( 'NONE',  ( 6.121875000614517504, -6.054752690667223547, -1.112240025338166033E-15 ) ) ;
#69294=CARTESIAN_POINT ( 'NONE',  ( 20.88749999999999929, 5.773502691896255534, 3.535250795749688894E-16 ) ) ;
#69295=CARTESIAN_POINT ( 'NONE',  ( 14.51250000122903394, -4.330127018922190985, -2.500000000000001332 ) ) ;
#69296=VECTOR ( 'NONE', #3736, 1000.000000000000000 ) ;
#69297=CARTESIAN_POINT ( 'NONE',  ( 10.22812500061451679, 6.421520780324663323E-16, -5.243569643749999010 ) ) ;
#69298=CARTESIAN_POINT ( 'NONE',  ( 16.97812500061451502, 6.421520780324663323E-16, -5.243569643749999010 ) ) ;
#69299=CARTESIAN_POINT ( 'NONE',  ( 24.75000000122902932, -2.886751345948129988, 4.999999999999997335 ) ) ;
#69300=CARTESIAN_POINT ( 'NONE',  ( 22.43437500061451573, 6.421520780324663323E-16, -5.243569643749999010 ) ) ;
#69301=DIRECTION ( 'NONE',  ( 0.000000000000000000, 0.000000000000000000, 1.000000000000000000 ) ) ;
#69302=CARTESIAN_POINT ( 'NONE',  ( 8.212500001229035007, -4.330127018922190985, -2.500000000000001332 ) ) ;
#69303=CARTESIAN_POINT ( 'NONE',  ( 9.159375000614515372, 0.000000000000000000, 5.243569643749999010 ) ) ;
#69304=CARTESIAN_POINT ( 'NONE',  ( 25.80937500061451928, 0.000000000000000000, 5.243569643749999010 ) ) ;
#69306=CARTESIAN_POINT ( 'NONE',  ( 3.309375000614518836, 0.000000000000000000, 5.243569643749999010 ) ) ;
#69307=CARTESIAN_POINT ( 'NONE',  ( 20.12812500061451715, 6.421520780324663323E-16, -5.243569643749999010 ) ) ;
#69308=CARTESIAN_POINT ( 'NONE',  ( 27.42187500061451644, 3.027376345333613106, -5.243569643749998122 ) ) ;
#69310=FACE_OUTER_BOUND ( 'NONE', #69584, .T. ) ;
#69311=CARTESIAN_POINT ( 'NONE',  ( 8.034375000614518925, 6.421520780324663323E-16, -5.243569643749999010 ) ) ;
#69312=CARTESIAN_POINT ( 'NONE',  ( 16.97812500061451502, 6.421520780324663323E-16, -5.243569643749999010 ) ) ;
#69313=ORIENTED_EDGE ( 'NONE', *, *, #33946, .F. ) ;
#69314=DIRECTION ( 'NONE',  ( 0.000000000000000000, 0.000000000000000000, -1.000000000000000000 ) ) ;
#69315=CARTESIAN_POINT ( 'NONE',  ( 28.60312500061451502, -4.541064518000417216, -2.621784821875001281 ) ) ;
#69316=CARTESIAN_POINT ( 'NONE',  ( 3.271875000614519635, 3.027376345333611329, 5.243569643749999010 ) ) ;
#69318=CARTESIAN_POINT ( 'NONE',  ( 3.714721736615232306, 3.346823739705472089, -3.745147025001839491 ) ) ;
#69319=CARTESIAN_POINT ( 'NONE',  ( 15.90000000000000036, 4.330127018922192761, -2.499999999999997780 ) ) ;
#69320=CARTESIAN_POINT ( 'NONE',  ( 20.24062500061451431, 6.054752690667223547, 3.707466751127219781E-16 ) ) ;
#69322=CARTESIAN_POINT ( 'NONE',  ( 24.67500000000000071, -4.330127018922194537, 2.499999999999995559 ) ) ;
#69323=CARTESIAN_POINT ( 'NONE',  ( 26.44687500061451502, -3.027376345333610441, -5.243569643749999898 ) ) ;
#69326=CARTESIAN_POINT ( 'NONE',  ( 12.32812500061451821, -4.541064518000419881, 2.621784821874995952 ) ) ;
#69327=CARTESIAN_POINT ( 'NONE',  ( 5.315625000614516260, 3.027376345333613106, -5.243569643749998122 ) ) ;
#69329=CARTESIAN_POINT ( 'NONE',  ( 29.42812500061451431, -4.541064518000419881, 2.621784821874995952 ) ) ;
#69330=EDGE_CURVE ( 'NONE', #48240, #66542, #72039, .T. ) ;
#69331=CARTESIAN_POINT ( 'NONE',  ( 15.63750000122903216, 4.330127018922191873, 2.499999999999999556 ) ) ;
#69332=CARTESIAN_POINT ( 'NONE',  ( 22.80000000000000071, 0.000000000000000000, 4.999999999999998224 ) ) ;
#69333=CARTESIAN_POINT ( 'NONE',  ( 29.58749999999999858, -2.886751345948129988, 4.999999999999997335 ) ) ;
#69334=CARTESIAN_POINT ( 'NONE',  ( 5.296875000614518214, -3.027376345333610441, -5.243569643749999898 ) ) ;
#69335=CARTESIAN_POINT ( 'NONE',  ( 10.02187500061451964, 3.027376345333611329, 5.243569643749999010 ) ) ;
#69336=CARTESIAN_POINT ( 'NONE',  ( 18.38437500061451857, 6.421520780324663323E-16, -5.243569643749999010 ) ) ;
#69338=CARTESIAN_POINT ( 'NONE',  ( 29.24062500061451431, 6.054752690667223547, 3.707466751127219781E-16 ) ) ;
#69339=CARTESIAN_POINT ( 'NONE',  ( 29.70937500061451431, 4.541064518000418104, -2.621784821874998173 ) ) ;
#69340=CARTESIAN_POINT ( 'NONE',  ( 3.984375000614517326, 6.421520780324663323E-16, -5.243569643749999010 ) ) ;
#69342=CARTESIAN_POINT ( 'NONE',  ( 16.01249999999999929, 2.886751345948126879, 4.999999999999999112 ) ) ;
#69343=CARTESIAN_POINT ( 'NONE',  ( 14.50312500061451537, 0.000000000000000000, 5.243569643749999010 ) ) ;
#69344=CARTESIAN_POINT ( 'NONE',  ( 3.999999999999998668, 14.07500000122903749, 27.69059892324149530 ) ) ;
#69345=CARTESIAN_POINT ( 'NONE',  ( 4.012500000000001954, -5.773502691896255534, -1.060575238724906372E-15 ) ) ;
#69346=CARTESIAN_POINT ( 'NONE',  ( 21.90000000122903145, 5.773502691896255534, 3.535250795749688894E-16 ) ) ;
#69347=CARTESIAN_POINT ( 'NONE',  ( -1.071796769724491005, 13.27009619066136636, 26.00000000000000355 ) ) ;
#69349=CARTESIAN_POINT ( 'NONE',  ( 8.728125000614518569, -4.541064518000419881, 2.621784821874995952 ) ) ;
#69350=CARTESIAN_POINT ( 'NONE',  ( 24.34687500061451715, 6.054752690667223547, 3.707466751127219781E-16 ) ) ;
#69351=EDGE_CURVE ( 'NONE', #60873, #62319, #60449, .T. ) ;
#69352=CARTESIAN_POINT ( 'NONE',  ( -3.000416591977282496E-16, 19.29687500061451644, 25.09994784771203058 ) ) ;
#69353=CARTESIAN_POINT ( 'NONE',  ( 26.33437500061451431, -4.541064518000419881, 2.621784821874995952 ) ) ;
#69354=CARTESIAN_POINT ( 'NONE',  ( 8.250000000000000000, 4.330127018922192761, -2.499999999999997780 ) ) ;
#69355=CARTESIAN_POINT ( 'NONE',  ( -3.999999999999999556, 13.77500000122903678, 27.69059892324149530 ) ) ;
#69356=CARTESIAN_POINT ( 'NONE',  ( 14.16562500061451679, -6.054752690667223547, -1.112240025338166033E-15 ) ) ;
#69357=CARTESIAN_POINT ( 'NONE',  ( 6.787500001229032520, -4.330127018922194537, 2.499999999999995559 ) ) ;
#69358=CARTESIAN_POINT ( 'NONE',  ( 17.14687500061451786, 6.054752690667223547, 3.707466751127219781E-16 ) ) ;
#69359=CARTESIAN_POINT ( 'NONE',  ( 11.10937500061451644, -4.541064518000417216, -2.621784821875001281 ) ) ;
#69362=CARTESIAN_POINT ( 'NONE',  ( 11.46562500061451573, -6.054752690667223547, -1.112240025338166033E-15 ) ) ;
#69364=CARTESIAN_POINT ( 'NONE',  ( 24.00000000122902932, -2.886751345948125991, -5.000000000000000000 ) ) ;
#69365=CARTESIAN_POINT ( 'NONE',  ( 12.64687500061451608, 6.054752690667223547, 3.707466751127219781E-16 ) ) ;
#69366=CARTESIAN_POINT ( 'NONE',  ( 13.79062500061451502, -3.027376345333610441, -5.243569643749999898 ) ) ;
#69369=CARTESIAN_POINT ( 'NONE',  ( 25.02187500061451431, -6.054752690667223547, -1.112240025338166033E-15 ) ) ;
#69371=( BOUNDED_CURVE ( )  B_SPLINE_CURVE ( 2, ( #64111, #30508, #2430, #47496, #70027, #14236, #8700 ),
 .UNSPECIFIED., .F., .F. ) 
 B_SPLINE_CURVE_WITH_KNOTS ( ( 3, 2, 2, 3 ),
 ( 0.2583333333333333037, 0.2611111111111110716, 0.2638888888888888395, 0.2666666666666666075 ),
 .UNSPECIFIED. ) 
 CURVE ( )  GEOMETRIC_REPRESENTATION_ITEM ( )  RATIONAL_B_SPLINE_CURVE ( ( 1.000000000000002665, 0.8660254037844360431, 1.000000000000000000, 0.8660254037844387076, 1.000000000000000000, 0.8660254037844413721, 0.9999999999999973355 ) ) 
 REPRESENTATION_ITEM ( '' )  );
#69372=CARTESIAN_POINT ( 'NONE',  ( 23.92499999999999716, 6.123233995736764310E-16, -4.999999999999998224 ) ) ;
#69374=CARTESIAN_POINT ( 'NONE',  ( 2.121784821875001281, 15.95937500061451608, -26.32496088578401938 ) ) ;
#69375=CARTESIAN_POINT ( 'NONE',  ( 15.12187500061451750, -6.054752690667223547, -1.112240025338166033E-15 ) ) ;
#69376=CARTESIAN_POINT ( 'NONE',  ( 18.00000000122903288, -2.886751345948129988, 4.999999999999997335 ) ) ;
#69377=( BOUNDED_CURVE ( )  B_SPLINE_CURVE ( 2, ( #30511, #47499, #63752, #7607, #13141, #8338, #7975 ),
 .UNSPECIFIED., .F., .F. ) 
 B_SPLINE_CURVE_WITH_KNOTS ( ( 3, 2, 2, 3 ),
 ( 0.7166666666666667851, 0.7194444444444445530, 0.7222222222222222099, 0.7249999999999999778 ),
 .UNSPECIFIED. ) 
 CURVE ( )  GEOMETRIC_REPRESENTATION_ITEM ( )  RATIONAL_B_SPLINE_CURVE ( ( 0.9999999999999946709, 0.8660254037844440367, 1.000000000000000000, 0.8660254037844387076, 1.000000000000000000, 0.8660254037844387076, 1.000000000000000000 ) ) 
 REPRESENTATION_ITEM ( '' )  );
#69378=CARTESIAN_POINT ( 'NONE',  ( 11.52187500061451608, -6.054752690667223547, -1.112240025338166033E-15 ) ) ;
#69379=CARTESIAN_POINT ( 'NONE',  ( 2.121784821875001281, 10.10937500061451821, 33.67503911421598417 ) ) ;
#69380=CARTESIAN_POINT ( 'NONE',  ( 19.31250000122903288, 0.000000000000000000, 4.999999999999998224 ) ) ;
#69381=CARTESIAN_POINT ( 'NONE',  ( 15.96562500061451573, -6.054752690667223547, -1.112240025338166033E-15 ) ) ;
#69384=CARTESIAN_POINT ( 'NONE',  ( 17.81250000000000355, 2.886751345948126879, 4.999999999999999112 ) ) ;
#69386=CARTESIAN_POINT ( 'NONE',  ( 12.45937500061451786, -4.541064518000417216, -2.621784821875001281 ) ) ;
#69387=CARTESIAN_POINT ( 'NONE',  ( 3.009823169949401578, 3.992613741101768365, -3.171945278996665785 ) ) ;
#69388=CARTESIAN_POINT ( 'NONE',  ( 13.38750000122903394, 4.330127018922191873, 2.499999999999999556 ) ) ;
#69389=CARTESIAN_POINT ( 'NONE',  ( 21.03750000122903074, 4.330127018922191873, 2.499999999999999556 ) ) ;
#69390=CARTESIAN_POINT ( 'NONE',  ( 18.74062500061451431, -3.027376345333610441, -5.243569643749999898 ) ) ;
#69391=CARTESIAN_POINT ( 'NONE',  ( 22.15312500061451573, 0.000000000000000000, 5.243569643749999010 ) ) ;
#69392=CARTESIAN_POINT ( 'NONE',  ( 3.365625000614516082, -6.054752690667223547, -1.112240025338166033E-15 ) ) ;
#69393=( BOUNDED_CURVE ( )  B_SPLINE_CURVE ( 2, ( #14595, #37130, #59659, #13492, #24949, #9067, #53399 ),
 .UNSPECIFIED., .F., .T. ) 
 B_SPLINE_CURVE_WITH_KNOTS ( ( 3, 2, 2, 3 ),
 ( 0.06666666666666665186, 0.06944444444444443365, 0.07222222222222218768, 0.07499999999999996947 ),
 .UNSPECIFIED. ) 
 CURVE ( )  GEOMETRIC_REPRESENTATION_ITEM ( )  RATIONAL_B_SPLINE_CURVE ( ( 1.000000000000000666, 0.8660254037844379305, 1.000000000000000000, 0.8660254037844387076, 1.000000000000000000, 0.8660254037844400399, 0.9999999999999986677 ) ) 
 REPRESENTATION_ITEM ( '' )  );
#69394=CARTESIAN_POINT ( 'NONE',  ( 27.48749999999999716, -2.886751345948125991, -5.000000000000000000 ) ) ;
#69395=LINE ( 'NONE', #5873, #14778 ) ;
#69398=CARTESIAN_POINT ( 'NONE',  ( 4.243569643749999898, 15.58437500061451786, -30.00000000000000000 ) ) ;
#69399=CARTESIAN_POINT ( 'NONE',  ( 2.700000001229035718, -2.886751345948129988, 4.999999999999997335 ) ) ;
#69400=CARTESIAN_POINT ( 'NONE',  ( 6.112499999999999822, 2.886751345948126879, 4.999999999999999112 ) ) ;
#69402=CARTESIAN_POINT ( 'NONE',  ( 10.73437500061451644, 6.421520780324663323E-16, -5.243569643749999010 ) ) ;
#69403=CARTESIAN_POINT ( 'NONE',  ( 27.62812500061451360, -4.541064518000419881, 2.621784821874995952 ) ) ;
#69404=CARTESIAN_POINT ( 'NONE',  ( 0.000000000000000000, 20.00000000000000000, 30.00000000000000000 ) ) ;
#69405=CARTESIAN_POINT ( 'NONE',  ( -5.376511845580211002, 8.433624770265602422, -32.69150760605022299 ) ) ;
#69407=CARTESIAN_POINT ( 'NONE',  ( 8.071875000614518569, 3.027376345333613106, -5.243569643749998122 ) ) ;
#69408=CARTESIAN_POINT ( 'NONE',  ( 10.54687500061451644, -3.027376345333614438, 5.243569643749998122 ) ) ;
#69409=CARTESIAN_POINT ( 'NONE',  ( 5.962500000000002132, 2.886751345948129099, -4.999999999999998224 ) ) ;
#69410=CARTESIAN_POINT ( 'NONE',  ( -3.000416591977282496E-16, 15.19062500061459353, 25.09994784771203058 ) ) ;
#69412=CARTESIAN_POINT ( 'NONE',  ( 6.000000000000001776, 4.330127018922192761, -2.499999999999997780 ) ) ;
#69414=CARTESIAN_POINT ( 'NONE',  ( 23.09062500061451573, -3.027376345333614438, 5.243569643749998122 ) ) ;
#69415=CARTESIAN_POINT ( 'NONE',  ( 13.75312500061451715, -4.541064518000417216, -2.621784821875001281 ) ) ;
#69417=CARTESIAN_POINT ( 'NONE',  ( 8.446875000614518569, -3.027376345333610441, -5.243569643749999898 ) ) ;
#69418=CARTESIAN_POINT ( 'NONE',  ( 26.47499999999999787, -4.330127018922194537, 2.499999999999995559 ) ) ;
#69419=CARTESIAN_POINT ( 'NONE',  ( 22.83750000122903501, 4.330127018922191873, 2.499999999999999556 ) ) ;
#69421=CARTESIAN_POINT ( 'NONE',  ( 12.49687500061451573, -3.027376345333610441, -5.243569643749999898 ) ) ;
#69422=CARTESIAN_POINT ( 'NONE',  ( 27.15937500061451360, 0.000000000000000000, 5.243569643749999010 ) ) ;
#69423=CARTESIAN_POINT ( 'NONE',  ( 0.000000000000000000, 20.00000000000000000, -33.99999999999999289 ) ) ;
#69424=CARTESIAN_POINT ( 'NONE',  ( 18.98437500061451644, 4.541064518000418104, 2.621784821874999949 ) ) ;
#69425=CARTESIAN_POINT ( 'NONE',  ( 12.60937500061451821, 4.541064518000418104, -2.621784821874998173 ) ) ;
#69427=CARTESIAN_POINT ( 'NONE',  ( 24.60000000000000142, 0.000000000000000000, 4.999999999999998224 ) ) ;
#69429=CARTESIAN_POINT ( 'NONE',  ( 4.243569643749999898, 11.08437500061451786, -30.00000000000000000 ) ) ;
#69431=CARTESIAN_POINT ( 'NONE',  ( 15.02812500061451750, -4.541064518000419881, 2.621784821874995952 ) ) ;
#69432=CARTESIAN_POINT ( 'NONE',  ( 5.400000000000002132, -4.330127018922190985, -2.500000000000001332 ) ) ;
#69433=EDGE_CURVE ( 'NONE', #47010, #65143, #31114, .T. ) ;
#69434=CARTESIAN_POINT ( 'NONE',  ( 12.33750000122903145, 6.123233995736764310E-16, -4.999999999999998224 ) ) ;
#69436=CARTESIAN_POINT ( 'NONE',  ( 13.79999999999999893, 0.000000000000000000, 4.999999999999998224 ) ) ;
#69437=CARTESIAN_POINT ( 'NONE',  ( -4.243569643749999898, 9.865625000614517859, 27.54997392385601529 ) ) ;
#69438=CARTESIAN_POINT ( 'NONE',  ( 13.91250000122903252, 0.000000000000000000, 4.999999999999998224 ) ) ;
#69439=CARTESIAN_POINT ( 'NONE',  ( 24.04687500061451644, -3.027376345333614438, 5.243569643749998122 ) ) ;
#69440=ORIENTED_EDGE ( 'NONE', *, *, #23832, .T. ) ;
#69441=CARTESIAN_POINT ( 'NONE',  ( 18.77812500061451573, 6.421520780324663323E-16, -5.243569643749999010 ) ) ;
#69442=CARTESIAN_POINT ( 'NONE',  ( 4.790625000614518569, -3.027376345333610441, -5.243569643749999898 ) ) ;
#69443=CARTESIAN_POINT ( 'NONE',  ( 19.47187500061451360, 3.027376345333611329, 5.243569643749999010 ) ) ;
#69444=CARTESIAN_POINT ( 'NONE',  ( 4.237500000000001599, 5.773502691896255534, 3.535250795749688894E-16 ) ) ;
#69445=CARTESIAN_POINT ( 'NONE',  ( 6.815625000614517148, 3.027376345333611329, 5.243569643749999010 ) ) ;
#69446=CARTESIAN_POINT ( 'NONE',  ( 22.82812500061451644, 6.421520780324663323E-16, -5.243569643749999010 ) ) ;
#69447=CARTESIAN_POINT ( 'NONE',  ( -3.000416591977282496E-16, 14.29062500061451679, 25.09994784771203058 ) ) ;
#69448=CARTESIAN_POINT ( 'NONE',  ( 20.13750000122903216, 4.330127018922191873, 2.499999999999999556 ) ) ;
#69450=CARTESIAN_POINT ( 'NONE',  ( 9.553125000614517859, 0.000000000000000000, 5.243569643749999010 ) ) ;
#69451=CARTESIAN_POINT ( 'NONE',  ( 4.359375000614517326, -4.541064518000417216, -2.621784821875001281 ) ) ;
#69452=CARTESIAN_POINT ( 'NONE',  ( 28.22812500061451502, 6.421520780324663323E-16, -5.243569643749999010 ) ) ;
#69453=CARTESIAN_POINT ( 'NONE',  ( 24.38437500061451502, 4.541064518000418104, 2.621784821874999949 ) ) ;
#69454=CARTESIAN_POINT ( 'NONE',  ( 13.64062500061451644, -3.027376345333614438, 5.243569643749998122 ) ) ;
#69455=CARTESIAN_POINT ( 'NONE',  ( 25.05000000122903714, 5.773502691896255534, 3.535250795749688894E-16 ) ) ;
#69456=CARTESIAN_POINT ( 'NONE',  ( 25.52812500061451573, 6.421520780324663323E-16, -5.243569643749999010 ) ) ;
#69457=CARTESIAN_POINT ( 'NONE',  ( 18.45937500061451431, 4.541064518000418104, -2.621784821874998173 ) ) ;
#69458=CARTESIAN_POINT ( 'NONE',  ( 14.42812500061451786, 4.541064518000418104, 2.621784821874999949 ) ) ;
#69459=CARTESIAN_POINT ( 'NONE',  ( -2.121784821874996840, 16.33437500061451786, 33.67503911421598417 ) ) ;
#69460=CARTESIAN_POINT ( 'NONE',  ( 22.71562500061451573, -6.054752690667223547, -1.112240025338166033E-15 ) ) ;
#69463=CARTESIAN_POINT ( 'NONE',  ( 26.36249999999999716, 2.886751345948126879, 4.999999999999999112 ) ) ;
#69464=CARTESIAN_POINT ( 'NONE',  ( -1.999999999999997113, 11.52500000000000036, -26.53589838486224295 ) ) ;
#69466=CARTESIAN_POINT ( 'NONE',  ( 3.234375000614516438, 4.541064518000418104, 2.621784821874999949 ) ) ;
#69467=CARTESIAN_POINT ( 'NONE',  ( 7.378125000614518036, -4.541064518000419881, 2.621784821874995952 ) ) ;
#69468=CARTESIAN_POINT ( 'NONE',  ( 23.21250000122903501, 4.330127018922192761, -2.499999999999997780 ) ) ;
#69469=EDGE_CURVE ( 'NONE', #27313, #30796, #45043, .T. ) ;
#69470=CARTESIAN_POINT ( 'NONE',  ( 28.26562500061451289, 3.027376345333613106, -5.243569643749998122 ) ) ;
#69471=CARTESIAN_POINT ( 'NONE',  ( 25.16249999999999432, -5.773502691896255534, -1.060575238724906372E-15 ) ) ;
#69472=CARTESIAN_POINT ( 'NONE',  ( -3.999999999999999556, 16.47500000122903430, -32.30940107675850470 ) ) ;
#69473=CARTESIAN_POINT ( 'NONE',  ( -5.810221930991193690E-16, 12.35000000122903430, 26.00000000000000355 ) ) ;
#69474=CARTESIAN_POINT ( 'NONE',  ( 10.07812500061451644, -4.541064518000419881, 2.621784821874995952 ) ) ;
#69476=CARTESIAN_POINT ( 'NONE',  ( 26.80312500061451431, -4.541064518000417216, -2.621784821875001281 ) ) ;
#69477=CARTESIAN_POINT ( 'NONE',  ( 6.778125000614518392, 4.541064518000418104, 2.621784821874999949 ) ) ;
#69478=CARTESIAN_POINT ( 'NONE',  ( 3.065625000614517592, 3.027376345333613106, -5.243569643749998122 ) ) ;
#69481=CARTESIAN_POINT ( 'NONE',  ( 12.93750000000000178, -2.886751345948130876, 4.999999999999996447 ) ) ;
#69482=CARTESIAN_POINT ( 'NONE',  ( 12.59999999999999964, -4.330127018922190985, -2.500000000000001332 ) ) ;
#69483=CARTESIAN_POINT ( 'NONE',  ( 12.72187500061451537, 3.027376345333611329, 5.243569643749999010 ) ) ;
#69484=CARTESIAN_POINT ( 'NONE',  ( 8.625000001229034652, -5.773502691896255534, -1.060575238724906372E-15 ) ) ;
#69485=CARTESIAN_POINT ( 'NONE',  ( 16.50937500061451502, -4.541064518000417216, -2.621784821875001281 ) ) ;
#69487=CARTESIAN_POINT ( 'NONE',  ( 9.084375000614517859, 4.541064518000418104, 2.621784821874999949 ) ) ;
#69488=CARTESIAN_POINT ( 'NONE',  ( -4.243569643749997233, 11.74062500061451786, -27.54997392385601174 ) ) ;
#69489=CARTESIAN_POINT ( 'NONE',  ( -1.071796769724488563, 11.99240381056766758, -26.00000000000000000 ) ) ;
#69491=VERTEX_POINT ( 'NONE', #11050 ) ;
#69492=CARTESIAN_POINT ( 'NONE',  ( 24.32812500061451289, 4.541064518000418104, 2.621784821874999949 ) ) ;
#69493=CARTESIAN_POINT ( 'NONE',  ( 11.13750000000000107, -2.886751345948130876, 4.999999999999996447 ) ) ;
#69494=CARTESIAN_POINT ( 'NONE',  ( 27.30937500061451573, -4.541064518000417216, -2.621784821875001281 ) ) ;
#69495=CARTESIAN_POINT ( 'NONE',  ( 22.08749999999999858, -2.886751345948125991, -5.000000000000000000 ) ) ;
#69496=CARTESIAN_POINT ( 'NONE',  ( 6.403125000614517504, 0.000000000000000000, 5.243569643749999010 ) ) ;
#69498=CARTESIAN_POINT ( 'NONE',  ( 15.75937500061451857, 4.541064518000418104, -2.621784821874998173 ) ) ;
#69500=CARTESIAN_POINT ( 'NONE',  ( 28.95000000122903572, -2.886751345948125991, -5.000000000000000000 ) ) ;
#69501=CARTESIAN_POINT ( 'NONE',  ( 9.046875000614518214, 6.054752690667223547, 3.707466751127219781E-16 ) ) ;
#69502=VERTEX_POINT ( 'NONE', #66853 ) ;
#69503=CARTESIAN_POINT ( 'NONE',  ( 20.10937500061451289, -4.541064518000417216, -2.621784821875001281 ) ) ;
#69505=CARTESIAN_POINT ( 'NONE',  ( 27.03750000000000142, -2.886751345948125991, -5.000000000000000000 ) ) ;
#69506=CARTESIAN_POINT ( 'NONE',  ( 29.14687500061451075, -3.027376345333610441, -5.243569643749999898 ) ) ;
#69507=CARTESIAN_POINT ( 'NONE',  ( 1.999999999999998668, 10.40000000000000213, -33.46410161513775705 ) ) ;
#69508=VERTEX_POINT ( 'NONE', #45766 ) ;
#69509=CARTESIAN_POINT ( 'NONE',  ( 11.25000000000000000, -4.330127018922190985, -2.500000000000001332 ) ) ;
#69511=CARTESIAN_POINT ( 'NONE',  ( 21.21562500061451573, 3.027376345333611329, 5.243569643749999010 ) ) ;
#69512=CARTESIAN_POINT ( 'NONE',  ( 14.21249999999999858, 2.886751345948126879, 4.999999999999999112 ) ) ;
#69513=EDGE_CURVE ( 'NONE', #69611, #860, #55718, .T. ) ;
#69514=CARTESIAN_POINT ( 'NONE',  ( 8.700000001229032165, -2.886751345948125991, -5.000000000000000000 ) ) ;
#69515=CARTESIAN_POINT ( 'NONE',  ( 5.953125000614519102, 0.000000000000000000, 5.243569643749999010 ) ) ;
#69516=CARTESIAN_POINT ( 'NONE',  ( 20.73750000000000071, -2.886751345948125991, -5.000000000000000000 ) ) ;
#69517=CARTESIAN_POINT ( 'NONE',  ( 21.66562500061451502, 3.027376345333611329, 5.243569643749999010 ) ) ;
#69518=CARTESIAN_POINT ( 'NONE',  ( 23.69999999999999929, 0.000000000000000000, 4.999999999999998224 ) ) ;
#69519=CARTESIAN_POINT ( 'NONE',  ( 24.56250000122903288, 4.330127018922192761, -2.499999999999997780 ) ) ;
#69521=CARTESIAN_POINT ( 'NONE',  ( 5.887500000000000178, -2.886751345948125991, -5.000000000000000000 ) ) ;
#69522=ORIENTED_EDGE ( 'NONE', *, *, #69109, .T. ) ;
#69523=CARTESIAN_POINT ( 'NONE',  ( 20.84062500061451573, -3.027376345333614438, 5.243569643749998122 ) ) ;
#69524=CARTESIAN_POINT ( 'NONE',  ( 26.35312500061451857, -4.541064518000417216, -2.621784821875001281 ) ) ;
#69525=CARTESIAN_POINT ( 'NONE',  ( 27.15937500061451360, 0.000000000000000000, 5.243569643749999010 ) ) ;
#69526=CARTESIAN_POINT ( 'NONE',  ( 15.14062500061451644, -3.027376345333610441, -5.243569643749999898 ) ) ;
#69527=CARTESIAN_POINT ( 'NONE',  ( -4.243569643749998122, 9.940625000614591755, -27.54997392385601174 ) ) ;
#69528=CARTESIAN_POINT ( 'NONE',  ( 26.51250000122903216, 0.000000000000000000, 4.999999999999998224 ) ) ;
#69530=CARTESIAN_POINT ( 'NONE',  ( 15.96562500061451573, -6.054752690667223547, -1.112240025338166033E-15 ) ) ;
#69531=CARTESIAN_POINT ( 'NONE',  ( 2.000000000000001332, 14.41250000122903430, -26.53589838486224650 ) ) ;
#69532=CARTESIAN_POINT ( 'NONE',  ( 3.937500001229034208, 4.330127018922191873, 2.499999999999999556 ) ) ;
#69533=CARTESIAN_POINT ( 'NONE',  ( 9.946875000614516793, 6.054752690667223547, 3.707466751127219781E-16 ) ) ;
#69534=CARTESIAN_POINT ( 'NONE',  ( 9.121875000614517504, 3.027376345333611329, 5.243569643749999010 ) ) ;
#69535=CARTESIAN_POINT ( 'NONE',  ( 18.00937500061451502, 4.541064518000418104, -2.621784821874998173 ) ) ;
#69536=ORIENTED_EDGE ( 'NONE', *, *, #41902, .F. ) ;
#69537=CARTESIAN_POINT ( 'NONE',  ( -5.193763058582910652, 8.549021686977596346, 26.97145083886558581 ) ) ;
#69538=CARTESIAN_POINT ( 'NONE',  ( 24.55312500061451786, -4.541064518000417216, -2.621784821875001281 ) ) ;
#69539=CARTESIAN_POINT ( 'NONE',  ( 20.03437500061451715, -4.541064518000419881, 2.621784821874995952 ) ) ;
#69540=CARTESIAN_POINT ( 'NONE',  ( 23.01562500061451644, 3.027376345333611329, 5.243569643749999010 ) ) ;
#69541=CARTESIAN_POINT ( 'NONE',  ( 1.626862140677534273E-15, 9.875000001229034652, 34.00000000000000000 ) ) ;
#69542=CARTESIAN_POINT ( 'NONE',  ( 1.999999999999998668, 13.55000000000000071, 26.53589838486224650 ) ) ;
#69543=CARTESIAN_POINT ( 'NONE',  ( 29.39062500061451289, -3.027376345333614438, 5.243569643749998122 ) ) ;
#69544=CARTESIAN_POINT ( 'NONE',  ( 9.562500001229032875, -4.330127018922190985, -2.500000000000001332 ) ) ;
#69545=EDGE_LOOP ( 'NONE', ( #56123, #24837, #36559, #52680 ) ) ;
#69546=CARTESIAN_POINT ( 'NONE',  ( 5.137500001229033941, 6.123233995736764310E-16, -4.999999999999998224 ) ) ;
#69547=CARTESIAN_POINT ( 'NONE',  ( 1.999999999999998668, 19.40000000000000213, -33.46410161513775705 ) ) ;
#69548=CARTESIAN_POINT ( 'NONE',  ( 27.41250000122903430, 0.000000000000000000, 4.999999999999998224 ) ) ;
#69550=CARTESIAN_POINT ( 'NONE',  ( 9.384375000614518569, 6.421520780324663323E-16, -5.243569643749999010 ) ) ;
#69551=CARTESIAN_POINT ( 'NONE',  ( 17.77499999999999858, 4.330127018922191873, 2.499999999999999556 ) ) ;
#69552=CARTESIAN_POINT ( 'NONE',  ( 14.01562500061451644, 3.027376345333611329, 5.243569643749999010 ) ) ;
#69553=CARTESIAN_POINT ( 'NONE',  ( 12.15937500061451892, 4.541064518000418104, -2.621784821874998173 ) ) ;
#69554=CARTESIAN_POINT ( 'NONE',  ( 3.590625000614518836, 6.054752690667223547, 3.707466751127219781E-16 ) ) ;
#69555=CARTESIAN_POINT ( 'NONE',  ( 20.82187500061451857, 3.027376345333611329, 5.243569643749999010 ) ) ;
#69556=CARTESIAN_POINT ( 'NONE',  ( 6.759375000614516793, 4.541064518000418104, -2.621784821874998173 ) ) ;
#69557=CARTESIAN_POINT ( 'NONE',  ( 10.00000000000000000, 1.224646799147353256E-15, 10.00000000000000178 ) ) ;
#69558=CARTESIAN_POINT ( 'NONE',  ( 8.728125000614518569, -4.541064518000419881, 2.621784821874995952 ) ) ;
#69559=CARTESIAN_POINT ( 'NONE',  ( 17.76562500061451644, -6.054752690667223547, -1.112240025338166033E-15 ) ) ;
#69560=VERTEX_POINT ( 'NONE', #27687 ) ;
#69561=CARTESIAN_POINT ( 'NONE',  ( 15.47812500061451679, -4.541064518000419881, 2.621784821874995952 ) ) ;
#69562=CARTESIAN_POINT ( 'NONE',  ( 10.37812500061451715, 4.541064518000418104, 2.621784821874999949 ) ) ;
#69564=CARTESIAN_POINT ( 'NONE',  ( 11.51250000000000107, 2.886751345948126879, 4.999999999999999112 ) ) ;
#69565=ADVANCED_FACE ( 'NONE', ( #55758 ), #43417, .T. ) ;
#69566=CARTESIAN_POINT ( 'NONE',  ( 7.762500001229033053, -4.330127018922190985, -2.500000000000001332 ) ) ;
#69567=CARTESIAN_POINT ( 'NONE',  ( 14.18437500061451750, -4.541064518000419881, 2.621784821874995952 ) ) ;
#69568=CARTESIAN_POINT ( 'NONE',  ( 16.72500000122903430, -5.773502691896255534, -1.060575238724906372E-15 ) ) ;
#69570=CARTESIAN_POINT ( 'NONE',  ( -2.121784821874999949, 19.27812500061451573, -33.67503911421598417 ) ) ;
#69572=CARTESIAN_POINT ( 'NONE',  ( 23.47500000122903430, -5.773502691896255534, -1.060575238724906372E-15 ) ) ;
#69573=CARTESIAN_POINT ( 'NONE',  ( 3.408588963864223054, -3.658193339867878535, 3.653826635041531379 ) ) ;
#69574=CARTESIAN_POINT ( 'NONE',  ( 4.489140539347876491, 3.724300126011093504, -4.036462246613610638 ) ) ;
#69575=CARTESIAN_POINT ( 'NONE',  ( 17.93437500061451928, 6.421520780324663323E-16, -5.243569643749999010 ) ) ;
#69576=( BOUNDED_CURVE ( )  B_SPLINE_CURVE ( 2, ( #52492, #25508, #36228, #64665, #35853, #24769, #30325 ),
 .UNSPECIFIED., .F., .F. ) 
 B_SPLINE_CURVE_WITH_KNOTS ( ( 3, 2, 2, 3 ),
 ( 0.3083333333333333481, 0.3111111111111111160, 0.3138888888888888840, 0.3166666666666666519 ),
 .UNSPECIFIED. ) 
 CURVE ( )  GEOMETRIC_REPRESENTATION_ITEM ( )  RATIONAL_B_SPLINE_CURVE ( ( 1.000000000000000000, 0.8660254037844387076, 1.000000000000000000, 0.8660254037844387076, 1.000000000000000000, 0.8660254037844387076, 1.000000000000000000 ) ) 
 REPRESENTATION_ITEM ( '' )  );
#69577=CARTESIAN_POINT ( 'NONE',  ( 14.35312500061451679, 4.541064518000418104, -2.621784821874998173 ) ) ;
#69580=CARTESIAN_POINT ( 'NONE',  ( 24.34687500061451715, 6.054752690667223547, 3.707466751127219781E-16 ) ) ;
#69582=CARTESIAN_POINT ( 'NONE',  ( 10.00312500061451715, 0.000000000000000000, 5.243569643749999010 ) ) ;
#69583=CARTESIAN_POINT ( 'NONE',  ( 16.17187500061451644, 3.027376345333613106, -5.243569643749998122 ) ) ;
#69584=EDGE_LOOP ( 'NONE', ( #55101, #51272, #24240, #52884 ) ) ;
#69585=CARTESIAN_POINT ( 'NONE',  ( 27.00937500061451857, 4.541064518000418104, -2.621784821874998173 ) ) ;
#69586=CARTESIAN_POINT ( 'NONE',  ( 27.89062500061451289, 6.054752690667223547, 3.707466751127219781E-16 ) ) ;
#69587=CARTESIAN_POINT ( 'NONE',  ( 17.99062500061451786, 6.054752690667223547, 3.707466751127219781E-16 ) ) ;
#69589=CYLINDRICAL_SURFACE ( 'NONE', #46682, 4.999999999999998224 ) ;
#69590=CARTESIAN_POINT ( 'NONE',  ( 8.812500000000000000, 2.886751345948126879, 4.999999999999999112 ) ) ;
#69591=CARTESIAN_POINT ( 'NONE',  ( 19.61250000122903359, 4.330127018922192761, -2.499999999999997780 ) ) ;
#69595=CARTESIAN_POINT ( 'NONE',  ( 17.10000000000000142, -4.330127018922190985, -2.500000000000001332 ) ) ;
#69596=CARTESIAN_POINT ( 'NONE',  ( 21.67500000000000071, 6.123233995736764310E-16, -4.999999999999998224 ) ) ;
#69597=CARTESIAN_POINT ( 'NONE',  ( 18.27187500061451431, -6.054752690667223547, -1.112240025338166033E-15 ) ) ;
#69598=CARTESIAN_POINT ( 'NONE',  ( 14.54062500061451679, -3.027376345333614438, 5.243569643749998122 ) ) ;
#69599=EDGE_CURVE ( 'NONE', #57032, #40816, #32130, .T. ) ;
#69602=CARTESIAN_POINT ( 'NONE',  ( 6.028125000614517504, -4.541064518000419881, 2.621784821874995952 ) ) ;
#69603=DIRECTION ( 'NONE',  ( 0.000000000000000000, 0.000000000000000000, 1.000000000000000000 ) ) ;
#69604=CARTESIAN_POINT ( 'NONE',  ( 13.08750000000000036, -2.886751345948125991, -5.000000000000000000 ) ) ;
#69606=CARTESIAN_POINT ( 'NONE',  ( 4.243569643749999010, 15.56562500061451715, 27.54997392385601174 ) ) ;
#69607=CARTESIAN_POINT ( 'NONE',  ( 28.86562500061451786, 3.027376345333611329, 5.243569643749999010 ) ) ;
#69610=CARTESIAN_POINT ( 'NONE',  ( 24.15937500061451715, -4.541064518000417216, -2.621784821875001281 ) ) ;
#69611=VERTEX_POINT ( 'NONE', #20500 ) ;
#69612=CARTESIAN_POINT ( 'NONE',  ( 21.66562500061451502, 3.027376345333611329, 5.243569643749999010 ) ) ;
#69613=CARTESIAN_POINT ( 'NONE',  ( 23.25937500061451857, -4.541064518000417216, -2.621784821875001281 ) ) ;
#69614=CARTESIAN_POINT ( 'NONE',  ( 4.243569643749999898, 15.94062500061459176, -27.54997392385601529 ) ) ;
#69615=CARTESIAN_POINT ( 'NONE',  ( 7.265625000614516438, 3.027376345333611329, 5.243569643749999010 ) ) ;
#69616=CARTESIAN_POINT ( 'NONE',  ( 23.95312500061451289, 0.000000000000000000, 5.243569643749999010 ) ) ;
#69619=CARTESIAN_POINT ( 'NONE',  ( 17.33437500061451431, -4.541064518000419881, 2.621784821874995952 ) ) ;
#69620=CARTESIAN_POINT ( 'NONE',  ( 27.34687500061451360, -3.027376345333610441, -5.243569643749999898 ) ) ;
#69621=CARTESIAN_POINT ( 'NONE',  ( -4.243569643749998122, 17.64687500061451786, 32.45002607614398471 ) ) ;
#69622=CARTESIAN_POINT ( 'NONE',  ( 6.403125000614517504, 0.000000000000000000, 5.243569643749999010 ) ) ;
#69623=CARTESIAN_POINT ( 'NONE',  ( 2.000000000000001332, 16.10000000000000142, 33.46410161513774995 ) ) ;
#69624=CARTESIAN_POINT ( 'NONE',  ( 4.209375000614516971, 0.000000000000000000, 5.243569643749999010 ) ) ;
#69625=CARTESIAN_POINT ( 'NONE',  ( 26.62500000000000000, 6.123233995736764310E-16, -4.999999999999998224 ) ) ;
#69626=CARTESIAN_POINT ( 'NONE',  ( 6.365625000614518747, 3.027376345333611329, 5.243569643749999010 ) ) ;
#69627=CARTESIAN_POINT ( 'NONE',  ( 9.496875000614517504, 6.054752690667223547, 3.707466751127219781E-16 ) ) ;
#69628=CARTESIAN_POINT ( 'NONE',  ( 17.06250000122903288, 0.000000000000000000, 4.999999999999998224 ) ) ;
#69629=CARTESIAN_POINT ( 'NONE',  ( 29.80312500061451431, 0.000000000000000000, 5.243569643749999010 ) ) ;
#69630=CARTESIAN_POINT ( 'NONE',  ( 7.303125000614516082, 0.000000000000000000, 5.243569643749999010 ) ) ;
#69633=CARTESIAN_POINT ( 'NONE',  ( 15.64687500061451608, -3.027376345333610441, -5.243569643749999898 ) ) ;
#69635=VERTEX_POINT ( 'NONE', #65582 ) ;
#69636=CARTESIAN_POINT ( 'NONE',  ( 25.19062500061451715, 6.054752690667223547, 3.707466751127219781E-16 ) ) ;
#69637=CARTESIAN_POINT ( 'NONE',  ( 10.49062500061451431, -3.027376345333614438, 5.243569643749998122 ) ) ;
#69638=CARTESIAN_POINT ( 'NONE',  ( 26.63437500061451857, 4.541064518000418104, 2.621784821874999949 ) ) ;
#69639=CARTESIAN_POINT ( 'NONE',  ( 9.365625000614519635, 3.027376345333613106, -5.243569643749998122 ) ) ;
#69640=CARTESIAN_POINT ( 'NONE',  ( 3.412500001229032964, 4.330127018922192761, -2.499999999999997780 ) ) ;
#69641=CARTESIAN_POINT ( 'NONE',  ( 10.95000000122903394, -2.886751345948125991, -5.000000000000000000 ) ) ;
#69642=CARTESIAN_POINT ( 'NONE',  ( 24.02812500061451573, -4.541064518000419881, 2.621784821874995952 ) ) ;
#69643=CARTESIAN_POINT ( 'NONE',  ( -4.243569643749999898, 13.91562500061451679, -32.45002607614398471 ) ) ;
#69644=CARTESIAN_POINT ( 'NONE',  ( 12.86250000122903359, 4.330127018922192761, -2.499999999999997780 ) ) ;
#69645=CARTESIAN_POINT ( 'NONE',  ( 21.89062500061451289, -3.027376345333610441, -5.243569643749999898 ) ) ;
#69646=CARTESIAN_POINT ( 'NONE',  ( 18.77812500061451573, 6.421520780324663323E-16, -5.243569643749999010 ) ) ;
#69647=CARTESIAN_POINT ( 'NONE',  ( 6.496875000614518392, -3.027376345333614438, 5.243569643749998122 ) ) ;
#69648=CARTESIAN_POINT ( 'NONE',  ( 18.56250000000000000, 2.886751345948129099, -4.999999999999998224 ) ) ;
#69649=CARTESIAN_POINT ( 'NONE',  ( 13.38750000122903394, 4.330127018922191873, 2.499999999999999556 ) ) ;
#69650=CARTESIAN_POINT ( 'NONE',  ( 9.740625000614516082, -3.027376345333610441, -5.243569643749999898 ) ) ;
#69651=CARTESIAN_POINT ( 'NONE',  ( 14.16562500061451679, -6.054752690667223547, -1.112240025338166033E-15 ) ) ;
#69652=CARTESIAN_POINT ( 'NONE',  ( 25.68750000122903288, -4.330127018922194537, 2.499999999999995559 ) ) ;
#69653=CARTESIAN_POINT ( 'NONE',  ( 21.75937500061451502, 0.000000000000000000, 5.243569643749999010 ) ) ;
#69654=CARTESIAN_POINT ( 'NONE',  ( 20.18437500061451573, 6.421520780324663323E-16, -5.243569643749999010 ) ) ;
#69655=CARTESIAN_POINT ( 'NONE',  ( 13.79999999999999893, 0.000000000000000000, 4.999999999999998224 ) ) ;
#69656=CARTESIAN_POINT ( 'NONE',  ( 6.825000001229034829, -5.773502691896255534, -1.060575238724906372E-15 ) ) ;
#69657=CARTESIAN_POINT ( 'NONE',  ( 5.709375000614517859, -4.541064518000417216, -2.621784821875001281 ) ) ;
#69658=CARTESIAN_POINT ( 'NONE',  ( 26.25937500061451857, 0.000000000000000000, 5.243569643749999010 ) ) ;
#69660=EDGE_CURVE ( 'NONE', #18895, #71251, #68443, .T. ) ;
#69661=CARTESIAN_POINT ( 'NONE',  ( 21.55312500061451431, 4.541064518000418104, -2.621784821874998173 ) ) ;
#69662=CARTESIAN_POINT ( 'NONE',  ( 27.75937500061451502, -4.541064518000417216, -2.621784821875001281 ) ) ;
#69665=CARTESIAN_POINT ( 'NONE',  ( 2.000000000000001332, 13.96250000122903323, -26.53589838486224650 ) ) ;
#69666=CARTESIAN_POINT ( 'NONE',  ( 7.959375000614516971, -4.541064518000417216, -2.621784821875001281 ) ) ;
#69667=CARTESIAN_POINT ( 'NONE',  ( 17.50312500061451715, 4.541064518000418104, -2.621784821874998173 ) ) ;
#69669=DIRECTION ( 'NONE',  ( -1.000000000000000000, -0.000000000000000000, -0.000000000000000000 ) ) ;
#69670=CARTESIAN_POINT ( 'NONE',  ( 26.61562500061451786, 3.027376345333611329, 5.243569643749999010 ) ) ;
#69671=CARTESIAN_POINT ( 'NONE',  ( 4.096875000614518925, 6.054752690667223547, 3.707466751127219781E-16 ) ) ;
#69672=CARTESIAN_POINT ( 'NONE',  ( -1.999999999999997113, 16.02500000000000213, -26.53589838486224295 ) ) ;
#69674=CARTESIAN_POINT ( 'NONE',  ( 17.55000000000000071, -4.330127018922190985, -2.500000000000001332 ) ) ;
#69675=CARTESIAN_POINT ( 'NONE',  ( 20.95312500061451999, -4.541064518000417216, -2.621784821875001281 ) ) ;
#69676=ORIENTED_EDGE ( 'NONE', *, *, #58649, .F. ) ;
#69677=CARTESIAN_POINT ( 'NONE',  ( 25.05000000000000071, 0.000000000000000000, 4.999999999999998224 ) ) ;
#69678=CARTESIAN_POINT ( 'NONE',  ( 25.39687500061451431, -3.027376345333614438, 5.243569643749998122 ) ) ;
#69679=EDGE_CURVE ( 'NONE', #7528, #69491, #20305, .T. ) ;
#69680=ORIENTED_EDGE ( 'NONE', *, *, #63249, .F. ) ;
#69681=CARTESIAN_POINT ( 'NONE',  ( 3.021917804904423743, -3.983467431823952687, -3.409840147052992432 ) ) ;
#69682=CARTESIAN_POINT ( 'NONE',  ( 12.85312500061451502, -4.541064518000417216, -2.621784821875001281 ) ) ;
#69683=CARTESIAN_POINT ( 'NONE',  ( 6.928125000614516082, -4.541064518000419881, 2.621784821874995952 ) ) ;
#69685=CARTESIAN_POINT ( 'NONE',  ( 3.159375000614518036, 4.541064518000418104, -2.621784821874998173 ) ) ;
#69686=CARTESIAN_POINT ( 'NONE',  ( 16.46250000122903501, 4.330127018922192761, -2.499999999999997780 ) ) ;
#69687=CARTESIAN_POINT ( 'NONE',  ( 20.62499999999999645, -4.330127018922194537, 2.499999999999995559 ) ) ;
#69688=CARTESIAN_POINT ( 'NONE',  ( 29.51249999999999929, 2.886751345948126879, 4.999999999999999112 ) ) ;
#69689=CARTESIAN_POINT ( 'NONE',  ( 2.971875000614517592, -6.054752690667223547, -1.112240025338166033E-15 ) ) ;
#69690=CARTESIAN_POINT ( 'NONE',  ( 9.159375000614515372, 0.000000000000000000, 5.243569643749999010 ) ) ;
#69691=CARTESIAN_POINT ( 'NONE',  ( 19.02187500061451786, 3.027376345333611329, 5.243569643749999010 ) ) ;
#69694=CARTESIAN_POINT ( 'NONE',  ( 27.77812500061451573, 6.421520780324663323E-16, -5.243569643749999010 ) ) ;
#69695=CARTESIAN_POINT ( 'NONE',  ( 29.10937500061451644, -4.541064518000417216, -2.621784821875001281 ) ) ;
#69696=CARTESIAN_POINT ( 'NONE',  ( 4.096875000614518925, 6.054752690667223547, 3.707466751127219781E-16 ) ) ;
#69697=CARTESIAN_POINT ( 'NONE',  ( 16.72500000000000142, 6.123233995736764310E-16, -4.999999999999998224 ) ) ;
#69698=CARTESIAN_POINT ( 'NONE',  ( 14.16562500061451679, -6.054752690667223547, -1.112240025338166033E-15 ) ) ;
#69701=CARTESIAN_POINT ( 'NONE',  ( 19.46250000122903145, -4.330127018922190985, -2.500000000000001332 ) ) ;
#69702=CARTESIAN_POINT ( 'NONE',  ( -3.999999999999997335, 13.40000000122903323, 32.30940107675850470 ) ) ;
#69704=CARTESIAN_POINT ( 'NONE',  ( 6.665625000614515905, 3.027376345333613106, -5.243569643749998122 ) ) ;
#69705=CARTESIAN_POINT ( 'NONE',  ( 25.35937500061451644, 0.000000000000000000, 5.243569643749999010 ) ) ;
#69706=CARTESIAN_POINT ( 'NONE',  ( -3.000416591977282496E-16, 19.74687500061451928, 25.09994784771203058 ) ) ;
#69707=CARTESIAN_POINT ( 'NONE',  ( 26.82187500061451857, -6.054752690667223547, -1.112240025338166033E-15 ) ) ;
#69708=CARTESIAN_POINT ( 'NONE',  ( 7.275000000000000355, 6.123233995736764310E-16, -4.999999999999998224 ) ) ;
#69709=CARTESIAN_POINT ( 'NONE',  ( -3.999999999999999112, 13.81250000122903465, 30.00000000000000000 ) ) ;
#69710=CARTESIAN_POINT ( 'NONE',  ( 15.85312500061451857, 0.000000000000000000, 5.243569643749999010 ) ) ;
#69711=CARTESIAN_POINT ( 'NONE',  ( 6.825000001229034829, -5.773502691896255534, -1.060575238724906372E-15 ) ) ;
#69712=CARTESIAN_POINT ( 'NONE',  ( 11.18437500061451928, 6.421520780324663323E-16, -5.243569643749999010 ) ) ;
#69715=CARTESIAN_POINT ( 'NONE',  ( 11.20312500061451644, 4.541064518000418104, -2.621784821874998173 ) ) ;
#69717=CARTESIAN_POINT ( 'NONE',  ( 23.25000000122903288, 5.773502691896255534, 3.535250795749688894E-16 ) ) ;
#69718=CARTESIAN_POINT ( 'NONE',  ( 11.78437500061451892, 4.541064518000418104, 2.621784821874999949 ) ) ;
#69719=CARTESIAN_POINT ( 'NONE',  ( 15.62812500061451537, 6.421520780324663323E-16, -5.243569643749999010 ) ) ;
#69720=CARTESIAN_POINT ( 'NONE',  ( 23.74687500061451573, -3.027376345333610441, -5.243569643749999898 ) ) ;
#69723=CARTESIAN_POINT ( 'NONE',  ( -4.243569643749999898, 14.42187500061451999, -32.45002607614398471 ) ) ;
#69724=VECTOR ( 'NONE', #23245, 1000.000000000000000 ) ;
#69725=CARTESIAN_POINT ( 'NONE',  ( 15.34687500061451537, 6.054752690667223547, 3.707466751127219781E-16 ) ) ;
#69726=CARTESIAN_POINT ( 'NONE',  ( 18.56250000122903288, -4.330127018922190985, -2.500000000000001332 ) ) ;
#69727=CARTESIAN_POINT ( 'NONE',  ( 11.82187500061451679, 3.027376345333611329, 5.243569643749999010 ) ) ;
#69728=CARTESIAN_POINT ( 'NONE',  ( 2.121784821875001281, 19.05312500061451431, -26.32496088578401938 ) ) ;
#69729=CARTESIAN_POINT ( 'NONE',  ( 19.16250000122903430, 4.330127018922192761, -2.499999999999997780 ) ) ;
#69730=CARTESIAN_POINT ( 'NONE',  ( 13.37812500061451715, 6.421520780324663323E-16, -5.243569643749999010 ) ) ;
#69731=VERTEX_POINT ( 'NONE', #32334 ) ;
#69732=ORIENTED_EDGE ( 'NONE', *, *, #4648, .F. ) ;
#69733=CARTESIAN_POINT ( 'NONE',  ( 18.41250000000000142, -5.773502691896255534, -1.060575238724906372E-15 ) ) ;
#69734=CARTESIAN_POINT ( 'NONE',  ( 27.52500000000000213, 6.123233995736764310E-16, -4.999999999999998224 ) ) ;
#69735=CARTESIAN_POINT ( 'NONE',  ( 13.28437500061451715, -4.541064518000419881, 2.621784821874995952 ) ) ;
#69736=CARTESIAN_POINT ( 'NONE',  ( 2.483674929639041906, 4.345807424128183882, 26.85429492329592804 ) ) ;
#69737=CARTESIAN_POINT ( 'NONE',  ( 13.01250000122903394, 0.000000000000000000, 4.999999999999998224 ) ) ;
#69738=CARTESIAN_POINT ( 'NONE',  ( 20.96250000122903145, 4.330127018922192761, -2.499999999999997780 ) ) ;
#69739=CARTESIAN_POINT ( 'NONE',  ( 18.21562500061451573, -6.054752690667223547, -1.112240025338166033E-15 ) ) ;
#69740=( BOUNDED_CURVE ( )  B_SPLINE_CURVE ( 2, ( #44503, #67036, #16396, #38951, #61469, #10864, #33397 ),
 .UNSPECIFIED., .F., .F. ) 
 B_SPLINE_CURVE_WITH_KNOTS ( ( 3, 2, 2, 3 ),
 ( 0.6916666666666666519, 0.6944444444444444198, 0.6972222222222221877, 0.6999999999999999556 ),
 .UNSPECIFIED. ) 
 CURVE ( )  GEOMETRIC_REPRESENTATION_ITEM ( )  RATIONAL_B_SPLINE_CURVE ( ( 1.000000000000000000, 0.8660254037844387076, 1.000000000000000000, 0.8660254037844387076, 1.000000000000000000, 0.8660254037844387076, 1.000000000000000000 ) ) 
 REPRESENTATION_ITEM ( '' )  );
#69741=CARTESIAN_POINT ( 'NONE',  ( 21.02812500061451573, 6.421520780324663323E-16, -5.243569643749999010 ) ) ;
#69742=CARTESIAN_POINT ( 'NONE',  ( 29.51250000122903216, 4.330127018922192761, -2.499999999999997780 ) ) ;
#69743=CARTESIAN_POINT ( 'NONE',  ( 27.07499999999999929, 6.123233995736764310E-16, -4.999999999999998224 ) ) ;
#69744=CARTESIAN_POINT ( 'NONE',  ( 5.000000000000000000, 6.176262757673013563E-16, -5.043301270189223473 ) ) ;
#69746=CARTESIAN_POINT ( 'NONE',  ( 28.69687500061451502, -3.027376345333610441, -5.243569643749999898 ) ) ;
#69747=CARTESIAN_POINT ( 'NONE',  ( 1.999999999999998668, 14.45000000000000107, -33.46410161513775705 ) ) ;
#69748=CARTESIAN_POINT ( 'NONE',  ( -3.000416591977282496E-16, 14.79687500061451821, -34.90005215228797653 ) ) ;
#69749=CARTESIAN_POINT ( 'NONE',  ( 4.537500001229034297, -4.330127018922194537, 2.499999999999995559 ) ) ;
#69750=CARTESIAN_POINT ( 'NONE',  ( 6.075000000000000178, 4.330127018922191873, 2.499999999999999556 ) ) ;
#69752=CARTESIAN_POINT ( 'NONE',  ( 9.684375000614517504, -4.541064518000419881, 2.621784821874995952 ) ) ;
#69753=CARTESIAN_POINT ( 'NONE',  ( 28.22812500061451502, 6.421520780324663323E-16, -5.243569643749999010 ) ) ;
#69755=CARTESIAN_POINT ( 'NONE',  ( 5.550000001229033586, -2.886751345948126435, -5.000000000000000000 ) ) ;
#69756=CARTESIAN_POINT ( 'NONE',  ( 15.26250000122903216, 0.000000000000000000, 4.999999999999998224 ) ) ;
#69758=CARTESIAN_POINT ( 'NONE',  ( 8.671875000614518214, 3.027376345333611329, 5.243569643749999010 ) ) ;
#69759=CARTESIAN_POINT ( 'NONE',  ( 10.65937500061451715, -4.541064518000417216, -2.621784821875001281 ) ) ;
#69760=CARTESIAN_POINT ( 'NONE',  ( 4.650000000000001243, 4.330127018922192761, -2.499999999999997780 ) ) ;
#69761=CARTESIAN_POINT ( 'NONE',  ( 2.121784821875001281, 14.55312500061459602, 33.67503911421598417 ) ) ;
#69762=CARTESIAN_POINT ( 'NONE',  ( 2.733878782416514941, -4.186395442746991158, 2.733878782416514941 ) ) ;
#69763=CARTESIAN_POINT ( 'NONE',  ( 5.662500000000000533, 2.886751345948126879, 4.999999999999999112 ) ) ;
#69765=CARTESIAN_POINT ( 'NONE',  ( 20.35312500061451502, 0.000000000000000000, 5.243569643749999010 ) ) ;
#69766=CARTESIAN_POINT ( 'NONE',  ( 12.29062500061451857, -3.027376345333614438, 5.243569643749998122 ) ) ;
#69768=CARTESIAN_POINT ( 'NONE',  ( 9.234375000614518214, -4.541064518000419881, 2.621784821874995952 ) ) ;
#69769=CARTESIAN_POINT ( 'NONE',  ( 25.72499999999999787, 6.123233995736764310E-16, -4.999999999999998224 ) ) ;
#69770=CARTESIAN_POINT ( 'NONE',  ( 22.35000000122903074, 5.773502691896255534, 3.535250795749688894E-16 ) ) ;
#69771=CARTESIAN_POINT ( 'NONE',  ( -2.000000000000000000, 18.23750000122903359, -33.46410161513775705 ) ) ;
#69772=CARTESIAN_POINT ( 'NONE',  ( 11.18437500061451928, 6.421520780324663323E-16, -5.243569643749999010 ) ) ;
#69773=CARTESIAN_POINT ( 'NONE',  ( 25.65937500061451715, 4.541064518000418104, -2.621784821874998173 ) ) ;
#69774=CARTESIAN_POINT ( 'NONE',  ( 4.059375000614519280, 4.541064518000418104, -2.621784821874998173 ) ) ;
#69775=CARTESIAN_POINT ( 'NONE',  ( 24.30000000122903359, -2.886751345948163738, 4.999999999999939604 ) ) ;
#69776=CARTESIAN_POINT ( 'NONE',  ( 19.99687500061451573, -3.027376345333614438, 5.243569643749998122 ) ) ;
#69778=CARTESIAN_POINT ( 'NONE',  ( 11.85937500061451644, 0.000000000000000000, 5.243569643749999010 ) ) ;
#69780=CARTESIAN_POINT ( 'NONE',  ( 23.36250000000000071, -5.773502691896255534, -1.060575238724906372E-15 ) ) ;
#69782=CARTESIAN_POINT ( 'NONE',  ( 4.243569643749999898, 11.98437500061451821, -30.00000000000000000 ) ) ;
#69784=CARTESIAN_POINT ( 'NONE',  ( 13.86562500061451431, 3.027376345333613106, -5.243569643749998122 ) ) ;
#69785=CARTESIAN_POINT ( 'NONE',  ( 5.700000000000000178, 0.000000000000000000, 4.999999999999998224 ) ) ;
#69787=CARTESIAN_POINT ( 'NONE',  ( -1.071796769724504328, 12.89240381056766616, 33.99999999999999289 ) ) ;
#69788=( BOUNDED_CURVE ( )  B_SPLINE_CURVE ( 2, ( #35783, #7717, #52062, #30251, #47243, #69775, #13610 ),
 .UNSPECIFIED., .F., .F. ) 
 B_SPLINE_CURVE_WITH_KNOTS ( ( 3, 2, 2, 3 ),
 ( 0.1916666666666666519, 0.1944444444444444198, 0.1972222222222221599, 0.1999999999999999556 ),
 .UNSPECIFIED. ) 
 CURVE ( )  GEOMETRIC_REPRESENTATION_ITEM ( )  RATIONAL_B_SPLINE_CURVE ( ( 1.000000000000001332, 0.8660254037844373753, 1.000000000000000000, 0.8660254037844387076, 1.000000000000000000, 0.8660254037844413721, 0.9999999999999973355 ) ) 
 REPRESENTATION_ITEM ( '' )  );
#69789=CARTESIAN_POINT ( 'NONE',  ( 14.06250000000000000, 2.886751345948129099, -4.999999999999998224 ) ) ;
#69790=CARTESIAN_POINT ( 'NONE',  ( 2.121784821875001281, 10.95312500061451821, 33.67503911421598417 ) ) ;
#69791=CARTESIAN_POINT ( 'NONE',  ( 13.08750000122903323, -4.330127018922194537, 2.499999999999995559 ) ) ;
#69792=CARTESIAN_POINT ( 'NONE',  ( 24.64687500061451431, -3.027376345333610441, -5.243569643749999898 ) ) ;
#69793=CARTESIAN_POINT ( 'NONE',  ( 20.43750000122903643, 6.123233995736764310E-16, -4.999999999999998224 ) ) ;
#69794=VERTEX_POINT ( 'NONE', #53776 ) ;
#69795=CARTESIAN_POINT ( 'NONE',  ( 19.94062500061451715, -3.027376345333614438, 5.243569643749998122 ) ) ;
#69796=CARTESIAN_POINT ( 'NONE',  ( 5.203125000614518214, -4.541064518000417216, -2.621784821875001281 ) ) ;
#69797=CARTESIAN_POINT ( 'NONE',  ( 19.02187500061451786, 3.027376345333611329, 5.243569643749999010 ) ) ;
#69798=CARTESIAN_POINT ( 'NONE',  ( 29.82187500061451502, 3.027376345333611329, 5.243569643749999010 ) ) ;
#69799=CARTESIAN_POINT ( 'NONE',  ( 6.890625000614516438, -3.027376345333614438, 5.243569643749998122 ) ) ;
#69800=CARTESIAN_POINT ( 'NONE',  ( 22.75312500061451360, -4.541064518000417216, -2.621784821875001281 ) ) ;
#69801=CARTESIAN_POINT ( 'NONE',  ( -2.121784821874996840, 14.02812500061451750, 33.67503911421598417 ) ) ;
#69802=CARTESIAN_POINT ( 'NONE',  ( 17.85000000122903430, 5.773502691896255534, 3.535250795749688894E-16 ) ) ;
#69804=CARTESIAN_POINT ( 'NONE',  ( 10.64062500061451466, -3.027376345333610441, -5.243569643749999898 ) ) ;
#69805=CARTESIAN_POINT ( 'NONE',  ( 3.721875000614518036, 3.027376345333611329, 5.243569643749999010 ) ) ;
#69806=CARTESIAN_POINT ( 'NONE',  ( 28.86562500061451786, 3.027376345333611329, 5.243569643749999010 ) ) ;
#69807=CARTESIAN_POINT ( 'NONE',  ( 22.20937500061451431, 0.000000000000000000, 5.243569643749999010 ) ) ;
#69808=CARTESIAN_POINT ( 'NONE',  ( 15.10312500061451502, -4.541064518000417216, -2.621784821875001281 ) ) ;
#69809=CARTESIAN_POINT ( 'NONE',  ( 23.92500000122903359, -5.773502691896255534, -1.060575238724906372E-15 ) ) ;
#69811=CARTESIAN_POINT ( 'NONE',  ( 26.39062500061451644, -3.027376345333610441, -5.243569643749999898 ) ) ;
#69812=CARTESIAN_POINT ( 'NONE',  ( 20.52187500061451786, -6.054752690667223547, -1.112240025338166033E-15 ) ) ;
#69813=CARTESIAN_POINT ( 'NONE',  ( 14.27812500061451573, 6.421520780324663323E-16, -5.243569643749999010 ) ) ;
#69814=CARTESIAN_POINT ( 'NONE',  ( 4.243569643749999898, 15.99687500061451573, 32.45002607614398471 ) ) ;
#69815=CARTESIAN_POINT ( 'NONE',  ( 20.01562500061451644, -6.054752690667223547, -1.112240025338166033E-15 ) ) ;
#69816=CARTESIAN_POINT ( 'NONE',  ( 30.00000000000000000, 0.000000000000000000, 0.000000000000000000 ) ) ;
#69817=ORIENTED_EDGE ( 'NONE', *, *, #68436, .T. ) ;
#69818=CARTESIAN_POINT ( 'NONE',  ( 26.02499999999999858, -4.330127018922194537, 2.499999999999995559 ) ) ;
#69819=CARTESIAN_POINT ( 'NONE',  ( 3.999999999999998668, 11.71250000000000036, -32.30940107675850470 ) ) ;
#69821=CARTESIAN_POINT ( 'NONE',  ( 27.36562500061451786, 3.027376345333613106, -5.243569643749998122 ) ) ;
#69822=CARTESIAN_POINT ( 'NONE',  ( 8.915625000614515017, 3.027376345333613106, -5.243569643749998122 ) ) ;
#69823=CARTESIAN_POINT ( 'NONE',  ( 20.36250000122903359, -4.330127018922190985, -2.500000000000001332 ) ) ;
#69824=CARTESIAN_POINT ( 'NONE',  ( 25.26562500061451289, 3.027376345333611329, 5.243569643749999010 ) ) ;
#69826=CARTESIAN_POINT ( 'NONE',  ( 25.01249999999999929, 2.886751345948126879, 4.999999999999999112 ) ) ;
#69827=CARTESIAN_POINT ( 'NONE',  ( -2.828200636599751609E-16, 15.95000000122903216, -34.61880215351700230 ) ) ;
#69828=CARTESIAN_POINT ( 'NONE',  ( 29.39062500061451289, -3.027376345333614438, 5.243569643749998122 ) ) ;
#69829=CARTESIAN_POINT ( 'NONE',  ( 11.31562500061451892, 3.027376345333611329, 5.243569643749999010 ) ) ;
#69831=EDGE_CURVE ( 'NONE', #26824, #65546, #33052, .T. ) ;
#69832=CIRCLE ( 'NONE', #59199, 5.000000000000000000 ) ;
#69833=CARTESIAN_POINT ( 'NONE',  ( 25.34062500061451217, -3.027376345333614438, 5.243569643749998122 ) ) ;
#69834=CARTESIAN_POINT ( 'NONE',  ( 6.140625000614516438, -3.027376345333610441, -5.243569643749999898 ) ) ;
#69836=CARTESIAN_POINT ( 'NONE',  ( 14.24999999999999822, 0.000000000000000000, 4.999999999999998224 ) ) ;
#69837=CARTESIAN_POINT ( 'NONE',  ( 14.10937500061451644, 0.000000000000000000, 5.243569643749999010 ) ) ;
#69838=CARTESIAN_POINT ( 'NONE',  ( 8.100000001229034297, -2.886751345948129988, 4.999999999999997335 ) ) ;
#69839=CARTESIAN_POINT ( 'NONE',  ( 18.23437500061451999, -4.541064518000419881, 2.621784821874995952 ) ) ;
#69841=CARTESIAN_POINT ( 'NONE',  ( 7.359375000614516438, 0.000000000000000000, 5.243569643749999010 ) ) ;
#69842=CARTESIAN_POINT ( 'NONE',  ( 2.121784821875001281, 12.30312500061451608, -26.32496088578401938 ) ) ;
#69844=FACE_OUTER_BOUND ( 'NONE', #41836, .T. ) ;
#69845=CARTESIAN_POINT ( 'NONE',  ( 24.77812500061451217, 4.541064518000418104, 2.621784821874999949 ) ) ;
#69846=CARTESIAN_POINT ( 'NONE',  ( -2.000000000000000000, 17.33750000122903145, 26.53589838486224650 ) ) ;
#69847=CARTESIAN_POINT ( 'NONE',  ( 26.40937500061451715, -4.541064518000417216, -2.621784821875001281 ) ) ;
#69848=CARTESIAN_POINT ( 'NONE',  ( 28.88437500061451502, 4.541064518000418104, 2.621784821874999949 ) ) ;
#69849=CARTESIAN_POINT ( 'NONE',  ( 20.88749999999999929, 5.773502691896255534, 3.535250795749688894E-16 ) ) ;
#69850=CARTESIAN_POINT ( 'NONE',  ( 6.628125000614517148, 6.421520780324663323E-16, -5.243569643749999010 ) ) ;
#69852=CARTESIAN_POINT ( 'NONE',  ( 16.84687500061451715, -3.027376345333614438, 5.243569643749998122 ) ) ;
#69854=CARTESIAN_POINT ( 'NONE',  ( 3.440625000614518036, -3.027376345333610441, -5.243569643749999898 ) ) ;
#69855=CARTESIAN_POINT ( 'NONE',  ( 7.846875000614518036, -3.027376345333614438, 5.243569643749998122 ) ) ;
#69856=CARTESIAN_POINT ( 'NONE',  ( 18.94687500061451502, 6.054752690667223547, 3.707466751127219781E-16 ) ) ;
#69858=CARTESIAN_POINT ( 'NONE',  ( 26.51249999999999929, -5.773502691896255534, -1.060575238724906372E-15 ) ) ;
#69859=CARTESIAN_POINT ( 'NONE',  ( 27.83437500061451786, 6.421520780324663323E-16, -5.243569643749999010 ) ) ;
#69860=EDGE_CURVE ( 'NONE', #22838, #24963, #55244, .T. ) ;
#69862=ORIENTED_EDGE ( 'NONE', *, *, #53711, .F. ) ;
#69863=CARTESIAN_POINT ( 'NONE',  ( 8.512499999999999289, -5.773502691896255534, -1.060575238724906372E-15 ) ) ;
#69865=CARTESIAN_POINT ( 'NONE',  ( 23.16562500061451502, -6.054752690667223547, -1.112240025338166033E-15 ) ) ;
#69866=CARTESIAN_POINT ( 'NONE',  ( 11.92500000000000071, 4.330127018922191873, 2.499999999999999556 ) ) ;
#69867=CARTESIAN_POINT ( 'NONE',  ( 8.400000001229035007, 5.773502691896255534, 3.535250795749688894E-16 ) ) ;
#69868=CARTESIAN_POINT ( 'NONE',  ( 5.428125000614517859, 4.541064518000418104, 2.621784821874999949 ) ) ;
#69869=CARTESIAN_POINT ( 'NONE',  ( 23.09999999999999787, 4.330127018922192761, -2.499999999999997780 ) ) ;
#69870=CARTESIAN_POINT ( 'NONE',  ( 19.97812500061451502, -4.541064518000419881, 2.621784821874995952 ) ) ;
#69871=FACE_OUTER_BOUND ( 'NONE', #2143, .T. ) ;
#69873=CARTESIAN_POINT ( 'NONE',  ( 26.02500000122903145, 2.886751345948126879, 4.999999999999999112 ) ) ;
#69875=CARTESIAN_POINT ( 'NONE',  ( 4.162499999999999645, 2.886751345948129099, -4.999999999999998224 ) ) ;
#69876=ORIENTED_EDGE ( 'NONE', *, *, #57675, .T. ) ;
#69877=CARTESIAN_POINT ( 'NONE',  ( 18.40312500061451573, 4.541064518000418104, -2.621784821874998173 ) ) ;
#69878=CARTESIAN_POINT ( 'NONE',  ( 26.16562500061451502, 3.027376345333611329, 5.243569643749999010 ) ) ;
#69879=CARTESIAN_POINT ( 'NONE',  ( 26.25937500061451857, 0.000000000000000000, 5.243569643749999010 ) ) ;
#69880=CARTESIAN_POINT ( 'NONE',  ( 14.31562500061451537, 3.027376345333613106, -5.243569643749998122 ) ) ;
#69881=CARTESIAN_POINT ( 'NONE',  ( 28.07812500061451289, -4.541064518000419881, 2.621784821874995952 ) ) ;
#69882=CARTESIAN_POINT ( 'NONE',  ( 8.278125000614515727, -4.541064518000419881, 2.621784821874995952 ) ) ;
#69883=FACE_OUTER_BOUND ( 'NONE', #34526, .T. ) ;
#69884=CARTESIAN_POINT ( 'NONE',  ( 27.37500000122903288, 2.886751345948126879, 4.999999999999999112 ) ) ;
#69886=CARTESIAN_POINT ( 'NONE',  ( 16.94062500061451715, -3.027376345333610441, -5.243569643749999898 ) ) ;
#69887=CARTESIAN_POINT ( 'NONE',  ( -6.275039685470489619E-15, 18.31250000000000000, -26.00000000000000355 ) ) ;
#69888=CARTESIAN_POINT ( 'NONE',  ( 28.84687500061452070, 6.054752690667223547, 3.707466751127219781E-16 ) ) ;
#69889=CARTESIAN_POINT ( 'NONE',  ( 11.25937500061451679, 4.541064518000418104, -2.621784821874998173 ) ) ;
#69890=CARTESIAN_POINT ( 'NONE',  ( 9.984375000614518214, 4.541064518000418104, 2.621784821874999949 ) ) ;
#69891=CARTESIAN_POINT ( 'NONE',  ( 18.79687500061451644, -3.027376345333610441, -5.243569643749999898 ) ) ;
#69892=ORIENTED_EDGE ( 'NONE', *, *, #64489, .F. ) ;
#69893=CARTESIAN_POINT ( 'NONE',  ( 29.03437500061451715, -4.541064518000419881, 2.621784821874995952 ) ) ;
#69894=CARTESIAN_POINT ( 'NONE',  ( 21.59062500061451928, 6.054752690667223547, 3.707466751127219781E-16 ) ) ;
#69895=CARTESIAN_POINT ( 'NONE',  ( 17.22187500061451715, 3.027376345333611329, 5.243569643749999010 ) ) ;
#69896=CARTESIAN_POINT ( 'NONE',  ( 22.19062500061451715, -3.027376345333614438, 5.243569643749998122 ) ) ;
#69897=CARTESIAN_POINT ( 'NONE',  ( 3.999999999999999112, 14.37500000000000000, 30.00000000000000000 ) ) ;
#69898=CARTESIAN_POINT ( 'NONE',  ( 28.07812500061451289, -4.541064518000419881, 2.621784821874995952 ) ) ;
#69899=CARTESIAN_POINT ( 'NONE',  ( 10.08750000122903323, 6.123233995736764310E-16, -4.999999999999998224 ) ) ;
#69901=CARTESIAN_POINT ( 'NONE',  ( 4.650000001229035895, -2.886751345948125991, -5.000000000000000000 ) ) ;
#69902=CARTESIAN_POINT ( 'NONE',  ( -2.000000000000000000, 18.12500000000000355, -33.46410161513775705 ) ) ;
#69903=CARTESIAN_POINT ( 'NONE',  ( 23.88750000122903216, -4.330127018922194537, 2.499999999999995559 ) ) ;
#69905=CARTESIAN_POINT ( 'NONE',  ( 6.234375000614519102, 6.421520780324663323E-16, -5.243569643749999010 ) ) ;
#69907=CARTESIAN_POINT ( 'NONE',  ( 15.59062500061451573, -3.027376345333610441, -5.243569643749999898 ) ) ;
#69908=CARTESIAN_POINT ( 'NONE',  ( 11.48437500061451644, -4.541064518000419881, 2.621784821874995952 ) ) ;
#69909=CARTESIAN_POINT ( 'NONE',  ( 26.47500000122903074, 2.886751345948126879, 4.999999999999999112 ) ) ;
#69910=CARTESIAN_POINT ( 'NONE',  ( 18.49687500061452283, 6.054752690667223547, 3.707466751127219781E-16 ) ) ;
#69911=CARTESIAN_POINT ( 'NONE',  ( 5.746875000614517504, -3.027376345333610441, -5.243569643749999898 ) ) ;
#69912=CARTESIAN_POINT ( 'NONE',  ( 3.999999999999999112, 17.52499999999999858, -30.00000000000000000 ) ) ;
#69913=CARTESIAN_POINT ( 'NONE',  ( 7.678125000614516082, 4.541064518000418104, 2.621784821874999949 ) ) ;
#69914=CARTESIAN_POINT ( 'NONE',  ( 17.65312500061451573, 0.000000000000000000, 5.243569643749999010 ) ) ;
#69916=CARTESIAN_POINT ( 'NONE',  ( 14.54062500061451679, -3.027376345333614438, 5.243569643749998122 ) ) ;
#69917=CARTESIAN_POINT ( 'NONE',  ( 10.49062500061451431, -3.027376345333614438, 5.243569643749998122 ) ) ;
#69919=CARTESIAN_POINT ( 'NONE',  ( 10.65000000000000036, 0.000000000000000000, 4.999999999999998224 ) ) ;
#69920=CARTESIAN_POINT ( 'NONE',  ( 6.037500001229035185, 6.123233995736764310E-16, -4.999999999999998224 ) ) ;
#69921=EDGE_CURVE ( 'NONE', #37790, #37474, #71127, .T. ) ;
#69922=CARTESIAN_POINT ( 'NONE',  ( 15.75937500061451857, 4.541064518000418104, -2.621784821874998173 ) ) ;
#69924=CARTESIAN_POINT ( 'NONE',  ( 16.42500000122903359, 2.886751345948129099, -4.999999999999998224 ) ) ;
#69926=CARTESIAN_POINT ( 'NONE',  ( -4.243569643749999898, 18.86562500061451431, -32.45002607614398471 ) ) ;
#69927=CARTESIAN_POINT ( 'NONE',  ( 12.00000000122903465, 5.773502691896255534, 3.535250795749688401E-16 ) ) ;
#69928=CARTESIAN_POINT ( 'NONE',  ( -1.071796769724488563, 18.74240381056766935, 34.00000000000000000 ) ) ;
#69929=CYLINDRICAL_SURFACE ( 'NONE', #7650, 3.999999999999996447 ) ;
#69931=CARTESIAN_POINT ( 'NONE',  ( 4.764378199515531875, -1.525943107988289249, -4.942298803467851442 ) ) ;
#69932=CARTESIAN_POINT ( 'NONE',  ( 16.54687500061451644, -3.027376345333610441, -5.243569643749999898 ) ) ;
#69934=CARTESIAN_POINT ( 'NONE',  ( 13.00312500061451537, 4.541064518000418104, -2.621784821874998173 ) ) ;
#69936=CARTESIAN_POINT ( 'NONE',  ( 23.10937500061451644, 0.000000000000000000, 5.243569643749999010 ) ) ;
#69938=CARTESIAN_POINT ( 'NONE',  ( 9.815625000614518925, 3.027376345333613106, -5.243569643749998122 ) ) ;
#69939=CARTESIAN_POINT ( 'NONE',  ( 14.78437500061451715, 6.421520780324663323E-16, -5.243569643749999010 ) ) ;
#69941=CARTESIAN_POINT ( 'NONE',  ( 26.55937500061451573, 4.541064518000418104, -2.621784821874998173 ) ) ;
#69942=CARTESIAN_POINT ( 'NONE',  ( 28.15312500061451573, -4.541064518000417216, -2.621784821875001281 ) ) ;
#69943=CARTESIAN_POINT ( 'NONE',  ( 16.75312500061451715, 0.000000000000000000, 5.243569643749999010 ) ) ;
#69944=CARTESIAN_POINT ( 'NONE',  ( 3.126873471466460330, 3.901623033231208737, -3.503192874424200465 ) ) ;
#69945=CARTESIAN_POINT ( 'NONE',  ( 4.890128389269437825, 1.043072884460970684, -5.138907771842282202 ) ) ;
#69946=CARTESIAN_POINT ( 'NONE',  ( 8.662499999999999645, 2.886751345948129099, -4.999999999999998224 ) ) ;
#69947=CARTESIAN_POINT ( 'NONE',  ( 19.16250000122903430, 4.330127018922192761, -2.499999999999997780 ) ) ;
#69948=CARTESIAN_POINT ( 'NONE',  ( -1.071796769724490783, 18.85490381179670649, -26.00000000000000355 ) ) ;
#69950=EDGE_LOOP ( 'NONE', ( #59091, #20875, #63588, #49648 ) ) ;
#69951=CARTESIAN_POINT ( 'NONE',  ( 16.50000000000000000, 0.000000000000000000, 4.999999999999998224 ) ) ;
#69952=CARTESIAN_POINT ( 'NONE',  ( 18.71249999999999858, 2.886751345948126879, 4.999999999999999112 ) ) ;
#69953=CARTESIAN_POINT ( 'NONE',  ( 19.95937500061451786, 0.000000000000000000, 5.243569643749999010 ) ) ;
#69954=CARTESIAN_POINT ( 'NONE',  ( 14.72812500061451679, 6.421520780324663323E-16, -5.243569643749999010 ) ) ;
#69956=CARTESIAN_POINT ( 'NONE',  ( 28.46249999999999503, 2.886751345948125103, -5.000000000000004441 ) ) ;
#69957=CARTESIAN_POINT ( 'NONE',  ( 5.428125000614517859, 4.541064518000418104, 2.621784821874999949 ) ) ;
#69959=CARTESIAN_POINT ( 'NONE',  ( 11.92500000000000071, 4.330127018922191873, 2.499999999999999556 ) ) ;
#69961=CARTESIAN_POINT ( 'NONE',  ( 4.243569643749999898, 15.04062500061451679, 32.45002607614398471 ) ) ;
#69962=CARTESIAN_POINT ( 'NONE',  ( 25.82812500061451644, -4.541064518000419881, 2.621784821874995952 ) ) ;
#69965=CARTESIAN_POINT ( 'NONE',  ( 24.94687500061451502, -3.027376345333614438, 5.243569643749998122 ) ) ;
#69967=CARTESIAN_POINT ( 'NONE',  ( 20.80312500061451431, 0.000000000000000000, 5.243569643749999010 ) ) ;
#69968=CARTESIAN_POINT ( 'NONE',  ( 23.03437500061451715, 4.541064518000418104, 2.621784821874999949 ) ) ;
#69969=ADVANCED_FACE ( 'NONE', ( #21241 ), #43793, .F. ) ;
#69970=CARTESIAN_POINT ( 'NONE',  ( 2.121784821874999061, 16.50312500061459176, -33.67503911421598417 ) ) ;
#69971=CARTESIAN_POINT ( 'NONE',  ( 6.290625000614517681, 6.054752690667223547, 3.707466751127219781E-16 ) ) ;
#69973=CARTESIAN_POINT ( 'NONE',  ( 24.55312500061451786, -4.541064518000417216, -2.621784821875001281 ) ) ;
#69976=CARTESIAN_POINT ( 'NONE',  ( 17.59687500061451715, 6.054752690667223547, 3.707466751127219781E-16 ) ) ;
#69977=CARTESIAN_POINT ( 'NONE',  ( 24.08437500061451786, -4.541064518000419881, 2.621784821874995952 ) ) ;
#69978=CARTESIAN_POINT ( 'NONE',  ( 4.243569643749999010, 14.72187500061451715, 27.54997392385601174 ) ) ;
#69979=CARTESIAN_POINT ( 'NONE',  ( 7.490625000614516082, -3.027376345333610441, -5.243569643749999898 ) ) ;
#69980=CARTESIAN_POINT ( 'NONE',  ( 27.89062500061451289, 6.054752690667223547, 3.707466751127219781E-16 ) ) ;
#69981=CARTESIAN_POINT ( 'NONE',  ( 3.271875000614519635, 3.027376345333611329, 5.243569643749999010 ) ) ;
#69982=CARTESIAN_POINT ( 'NONE',  ( 4.200000000000001954, 4.330127018922192761, -2.499999999999997780 ) ) ;
#69983=CARTESIAN_POINT ( 'NONE',  ( 4.603125000614518569, 0.000000000000000000, 5.243569643749999010 ) ) ;
#69984=CARTESIAN_POINT ( 'NONE',  ( 8.896875000614517859, -3.027376345333610441, -5.243569643749999898 ) ) ;
#69986=CARTESIAN_POINT ( 'NONE',  ( 17.81250000122903288, 4.330127018922192761, -2.499999999999997780 ) ) ;
#69987=CARTESIAN_POINT ( 'NONE',  ( 29.01562500061451644, -6.054752690667223547, -1.112240025338166033E-15 ) ) ;
#69988=CARTESIAN_POINT ( 'NONE',  ( 5.128125000614516260, -4.541064518000419881, 2.621784821874995952 ) ) ;
#69991=CARTESIAN_POINT ( 'NONE',  ( 15.87187500061451573, 3.027376345333611329, 5.243569643749999010 ) ) ;
#69992=CARTESIAN_POINT ( 'NONE',  ( -1.999999999999997113, 10.62500000000000000, 33.46410161513775705 ) ) ;
#69994=CARTESIAN_POINT ( 'NONE',  ( 22.49062500061451431, 6.054752690667223547, 3.707466751127219781E-16 ) ) ;
#69995=CARTESIAN_POINT ( 'NONE',  ( 9.440625000614517148, 6.054752690667223547, 3.707466751127219781E-16 ) ) ;
#69996=CARTESIAN_POINT ( 'NONE',  ( 24.42187500061451644, 3.027376345333611329, 5.243569643749999010 ) ) ;
#69997=CARTESIAN_POINT ( 'NONE',  ( 7.115625000614516082, 3.027376345333613106, -5.243569643749998122 ) ) ;
#69999=CARTESIAN_POINT ( 'NONE',  ( 10.20000000122903572, 5.773502691896255534, 3.535250795749688894E-16 ) ) ;
#70000=CARTESIAN_POINT ( 'NONE',  ( 26.05312500061451431, 4.541064518000418104, -2.621784821874998173 ) ) ;
#70001=CARTESIAN_POINT ( 'NONE',  ( 4.243569643749999898, 10.54062500061451679, -27.54997392385601529 ) ) ;
#70002=CARTESIAN_POINT ( 'NONE',  ( 13.38750000122903394, 4.330127018922191873, 2.499999999999999556 ) ) ;
#70003=CARTESIAN_POINT ( 'NONE',  ( 22.34062500061451573, -3.027376345333610441, -5.243569643749999898 ) ) ;
#70004=CARTESIAN_POINT ( 'NONE',  ( 18.29062500061451502, -3.027376345333610441, -5.243569643749999898 ) ) ;
#70006=CARTESIAN_POINT ( 'NONE',  ( 19.16250000000000142, 2.886751345948126879, 4.999999999999999112 ) ) ;
#70007=CARTESIAN_POINT ( 'NONE',  ( 12.63750000122903394, -4.330127018922194537, 2.499999999999995559 ) ) ;
#70008=CARTESIAN_POINT ( 'NONE',  ( 11.35312500061451679, 0.000000000000000000, 5.243569643749999010 ) ) ;
#70009=ADVANCED_FACE ( 'NONE', ( #42325 ), #64850, .F. ) ;
#70010=CARTESIAN_POINT ( 'NONE',  ( 13.52812500061451750, 4.541064518000418104, 2.621784821874999949 ) ) ;
#70012=CARTESIAN_POINT ( 'NONE',  ( 23.58750000122903145, 6.123233995736764310E-16, -4.999999999999998224 ) ) ;
#70013=CARTESIAN_POINT ( 'NONE',  ( 22.84687500061451715, -3.027376345333610441, -5.243569643749999898 ) ) ;
#70014=CARTESIAN_POINT ( 'NONE',  ( 21.75937500061451502, 0.000000000000000000, 5.243569643749999010 ) ) ;
#70015=CARTESIAN_POINT ( 'NONE',  ( 8.400000001229035007, 5.773502691896255534, 3.535250795749688894E-16 ) ) ;
#70016=CARTESIAN_POINT ( 'NONE',  ( 5.896875000614518747, 6.054752690667223547, 3.707466751127219781E-16 ) ) ;
#70017=CARTESIAN_POINT ( 'NONE',  ( 24.49687500061451573, -3.027376345333614438, 5.243569643749998122 ) ) ;
#70018=CARTESIAN_POINT ( 'NONE',  ( 4.603329117574985752, 1.951758446961684434, -4.603329117574985752 ) ) ;
#70019=CARTESIAN_POINT ( 'NONE',  ( 22.15312500061451573, 0.000000000000000000, 5.243569643749999010 ) ) ;
#70020=CARTESIAN_POINT ( 'NONE',  ( 26.97187500061451360, 3.027376345333613106, -5.243569643749998122 ) ) ;
#70024=CARTESIAN_POINT ( 'NONE',  ( 5.521875000614517859, 3.027376345333611329, 5.243569643749999010 ) ) ;
#70025=CARTESIAN_POINT ( 'NONE',  ( 16.52812500061451573, 6.421520780324663323E-16, -5.243569643749999010 ) ) ;
#70026=EDGE_LOOP ( 'NONE', ( #4961, #15617, #13358, #62694 ) ) ;
#70027=CARTESIAN_POINT ( 'NONE',  ( 22.87500000000000000, -4.330127018922194537, 2.499999999999995559 ) ) ;
#70028=CARTESIAN_POINT ( 'NONE',  ( 25.11562500061451431, 3.027376345333613106, -5.243569643749998122 ) ) ;
#70029=CARTESIAN_POINT ( 'NONE',  ( 3.009375000614516793, -4.541064518000417216, -2.621784821875001281 ) ) ;
#70030=CARTESIAN_POINT ( 'NONE',  ( -3.999999999999999112, 15.91249999999999964, -32.30940107675850470 ) ) ;
#70032=CARTESIAN_POINT ( 'NONE',  ( 16.16250000000000142, -5.773502691896255534, -1.060575238724906372E-15 ) ) ;
#70033=CARTESIAN_POINT ( 'NONE',  ( 22.15312500061451573, 0.000000000000000000, 5.243569643749999010 ) ) ;
#70035=CARTESIAN_POINT ( 'NONE',  ( 25.50000000000000000, 0.000000000000000000, 4.999999999999998224 ) ) ;
#70036=CARTESIAN_POINT ( 'NONE',  ( 26.82187500061451857, -6.054752690667223547, -1.112240025338166033E-15 ) ) ;
#70037=ORIENTED_EDGE ( 'NONE', *, *, #5968, .F. ) ;
#70039=CARTESIAN_POINT ( 'NONE',  ( 14.05312500061451431, 0.000000000000000000, 5.243569643749999010 ) ) ;
#70040=CARTESIAN_POINT ( 'NONE',  ( 6.815625000614517148, 3.027376345333611329, 5.243569643749999010 ) ) ;
#70042=CARTESIAN_POINT ( 'NONE',  ( 29.57812500061451644, 6.421520780324663323E-16, -5.243569643749999010 ) ) ;
#70043=CARTESIAN_POINT ( 'NONE',  ( 13.98750000122903359, -4.330127018922194537, 2.499999999999995559 ) ) ;
#70044=CARTESIAN_POINT ( 'NONE',  ( 19.01249999999999929, 2.886751345948129099, -4.999999999999998224 ) ) ;
#70045=CARTESIAN_POINT ( 'NONE',  ( 27.59999999999999787, 4.330127018922192761, -2.499999999999997780 ) ) ;
#70047=CARTESIAN_POINT ( 'NONE',  ( 7.621875000614519280, 3.027376345333613106, -5.243569643749998122 ) ) ;
#70048=CARTESIAN_POINT ( 'NONE',  ( 18.49687500061452283, 6.054752690667223547, 3.707466751127219781E-16 ) ) ;
#70049=CARTESIAN_POINT ( 'NONE',  ( -5.810221930991193690E-16, 11.45000000122903216, 26.00000000000000355 ) ) ;
#70051=CARTESIAN_POINT ( 'NONE',  ( 27.74062500061451431, -3.027376345333610441, -5.243569643749999898 ) ) ;
#70052=CARTESIAN_POINT ( 'NONE',  ( 3.300000000000000711, 4.330127018922192761, -2.499999999999997780 ) ) ;
#70053=CARTESIAN_POINT ( 'NONE',  ( 3.646875000614520079, 6.054752690667223547, 3.707466751127219781E-16 ) ) ;
#70054=CARTESIAN_POINT ( 'NONE',  ( 16.42500000000000071, 4.330127018922191873, 2.499999999999999556 ) ) ;
#70055=CARTESIAN_POINT ( 'NONE',  ( 13.60312500061451679, 0.000000000000000000, 5.243569643749999010 ) ) ;
#70058=CARTESIAN_POINT ( 'NONE',  ( 18.18750000122903288, 6.123233995736764310E-16, -4.999999999999998224 ) ) ;
#70059=CARTESIAN_POINT ( 'NONE',  ( 5.191822204397939622, 8.550203871005528811, 26.96813994412839222 ) ) ;
#70061=CARTESIAN_POINT ( 'NONE',  ( 7.828125000614517326, -4.541064518000419881, 2.621784821874995952 ) ) ;
#70062=CARTESIAN_POINT ( 'NONE',  ( 23.29687500061451644, -3.027376345333610441, -5.243569643749999898 ) ) ;
#70063=CARTESIAN_POINT ( 'NONE',  ( 4.243569643749999898, 19.59687500061452070, 32.45002607614398471 ) ) ;
#70064=ADVANCED_FACE ( 'NONE', ( #62587 ), #27898, .T. ) ;
#70065=CARTESIAN_POINT ( 'NONE',  ( 22.88437500061451857, 6.421520780324663323E-16, -5.243569643749999010 ) ) ;
#70066=CARTESIAN_POINT ( 'NONE',  ( 6.037500000000001421, 5.773502691896255534, 3.535250795749688894E-16 ) ) ;
#70067=CARTESIAN_POINT ( 'NONE',  ( 3.999999999999999112, 10.43750000122903465, 30.00000000000000000 ) ) ;
#70068=CARTESIAN_POINT ( 'NONE',  ( 14.61562500061451608, -6.054752690667223547, -1.112240025338166033E-15 ) ) ;
#70069=CARTESIAN_POINT ( 'NONE',  ( 5.962500001229033231, -4.330127018922190985, -2.500000000000001332 ) ) ;
#70070=CARTESIAN_POINT ( 'NONE',  ( 9.759375000614516793, -4.541064518000417216, -2.621784821875001281 ) ) ;
#70071=CARTESIAN_POINT ( 'NONE',  ( -0.5524690355592173363, 4.971316854763022874, -26.03590284058948612 ) ) ;
#70072=ORIENTED_EDGE ( 'NONE', *, *, #7700, .T. ) ;
#70073=CARTESIAN_POINT ( 'NONE',  ( 12.92812500061451786, 6.421520780324663323E-16, -5.243569643749999010 ) ) ;
#70074=CARTESIAN_POINT ( 'NONE',  ( 24.15000000122903145, 5.773502691896255534, 3.535250795749688894E-16 ) ) ;
#70075=CARTESIAN_POINT ( 'NONE',  ( 10.62187500061451928, -6.054752690667223547, -1.112240025338166033E-15 ) ) ;
#70076=CARTESIAN_POINT ( 'NONE',  ( 11.99062500061451608, -3.027376345333610441, -5.243569643749999898 ) ) ;
#70078=CARTESIAN_POINT ( 'NONE',  ( 22.77187500061451786, -6.054752690667223547, -1.112240025338166033E-15 ) ) ;
#70080=FACE_OUTER_BOUND ( 'NONE', #59079, .T. ) ;
#70082=CARTESIAN_POINT ( 'NONE',  ( -2.121784821874999949, 13.93437500061451750, -33.67503911421598417 ) ) ;
#70083=CARTESIAN_POINT ( 'NONE',  ( 15.79687500061451821, 6.054752690667223547, 3.707466751127219781E-16 ) ) ;
#70084=CARTESIAN_POINT ( 'NONE',  ( 16.98750000122903359, 4.330127018922191873, 2.499999999999999556 ) ) ;
#70085=CARTESIAN_POINT ( 'NONE',  ( 12.00937500061451857, -4.541064518000417216, -2.621784821875001281 ) ) ;
#70086=CARTESIAN_POINT ( 'NONE',  ( 4.243569643749999010, 17.81562500061451715, -32.45002607614398471 ) ) ;
#70087=CARTESIAN_POINT ( 'NONE',  ( 20.55000000122903359, 5.773502691896255534, 3.535250795749688894E-16 ) ) ;
#70088=CARTESIAN_POINT ( 'NONE',  ( 13.56562500061451892, 3.027376345333611329, 5.243569643749999010 ) ) ;
#70090=ORIENTED_EDGE ( 'NONE', *, *, #2540, .T. ) ;
#70091=VERTEX_POINT ( 'NONE', #11627 ) ;
#70092=CARTESIAN_POINT ( 'NONE',  ( 15.59999999999999964, 0.000000000000000000, 4.999999999999998224 ) ) ;
#70093=CARTESIAN_POINT ( 'NONE',  ( -3.999999999999997335, 17.45000000122903572, -27.69059892324149530 ) ) ;
#70094=CARTESIAN_POINT ( 'NONE',  ( 12.23437500061451821, 4.541064518000418104, 2.621784821874999949 ) ) ;
#70095=CARTESIAN_POINT ( 'NONE',  ( 2.675063744352810247, 4.229653939133389606, 27.01553149349311767 ) ) ;
#70096=CARTESIAN_POINT ( 'NONE',  ( 13.27500000122903323, 2.886751345948129099, -4.999999999999998224 ) ) ;
#70097=CARTESIAN_POINT ( 'NONE',  ( 20.17500000122903359, 2.886751345948126879, 4.999999999999999112 ) ) ;
#70098=CARTESIAN_POINT ( 'NONE',  ( 17.69062500061451715, -3.027376345333614438, 5.243569643749998122 ) ) ;
#70099=CARTESIAN_POINT ( 'NONE',  ( 20.31562500061451715, 3.027376345333611329, 5.243569643749999010 ) ) ;
#70100=CARTESIAN_POINT ( 'NONE',  ( 28.20000000122903216, 5.773502691896255534, 3.535250795749688894E-16 ) ) ;
#70101=ADVANCED_FACE ( 'NONE', ( #44164 ), #44536, .F. ) ;
#70102=CARTESIAN_POINT ( 'NONE',  ( 27.82499999999999929, -4.330127018922194537, 2.499999999999995559 ) ) ;
#70105=CARTESIAN_POINT ( 'NONE',  ( 26.97187500061451360, 3.027376345333613106, -5.243569643749998122 ) ) ;
#70107=CARTESIAN_POINT ( 'NONE',  ( 2.121784821874999061, 12.95937500061451786, -33.67503911421598417 ) ) ;
#70108=DIRECTION ( 'NONE',  ( -1.000000000000000000, -0.000000000000000000, -0.000000000000000000 ) ) ;
#70109=CARTESIAN_POINT ( 'NONE',  ( 5.137500000000000178, 5.773502691896255534, 3.535250795749688894E-16 ) ) ;
#70111=CARTESIAN_POINT ( 'NONE',  ( 7.621875000614519280, 3.027376345333613106, -5.243569643749998122 ) ) ;
#70112=CARTESIAN_POINT ( 'NONE',  ( 28.52812500061451573, -4.541064518000419881, 2.621784821874995952 ) ) ;
#70114=CARTESIAN_POINT ( 'NONE',  ( -3.968938398713114601, 9.180052406904112061, -25.49615315276739480 ) ) ;
#70115=CARTESIAN_POINT ( 'NONE',  ( -3.999999999999999112, 19.21250000122903501, 30.00000000000000000 ) ) ;
#70116=CARTESIAN_POINT ( 'NONE',  ( 6.234375000614519102, 6.421520780324663323E-16, -5.243569643749999010 ) ) ;
#70117=CARTESIAN_POINT ( 'NONE',  ( 10.77187500061451786, 3.027376345333613106, -5.243569643749998122 ) ) ;
#70118=CARTESIAN_POINT ( 'NONE',  ( 3.712499999999999911, 2.886751345948129099, -4.999999999999998224 ) ) ;
#70119=CARTESIAN_POINT ( 'NONE',  ( 4.243569643749999898, 14.59062500061459744, 32.45002607614398471 ) ) ;
#70121=CARTESIAN_POINT ( 'NONE',  ( 7.275000000000000355, 6.123233995736764310E-16, -4.999999999999998224 ) ) ;
#70123=CARTESIAN_POINT ( 'NONE',  ( 19.30312500061451786, 4.541064518000418104, -2.621784821874998173 ) ) ;
#70124=CARTESIAN_POINT ( 'NONE',  ( 12.47812500061451502, 6.421520780324663323E-16, -5.243569643749999010 ) ) ;
#70126=CARTESIAN_POINT ( 'NONE',  ( 9.084375000614517859, 4.541064518000418104, 2.621784821874999949 ) ) ;
#70127=CARTESIAN_POINT ( 'NONE',  ( 25.46249999999999858, 2.886751345948126879, 4.999999999999999112 ) ) ;
#70128=CARTESIAN_POINT ( 'NONE',  ( 21.75000000122903288, -2.886751345948125991, -5.000000000000000000 ) ) ;
#70130=CARTESIAN_POINT ( 'NONE',  ( 2.000000000000001332, 10.81250000122903465, 33.46410161513774995 ) ) ;
#70131=CARTESIAN_POINT ( 'NONE',  ( 9.646875000614516082, -3.027376345333614438, 5.243569643749998122 ) ) ;
#70132=CARTESIAN_POINT ( 'NONE',  ( 26.55937500061451573, 4.541064518000418104, -2.621784821874998173 ) ) ;
#70133=CARTESIAN_POINT ( 'NONE',  ( 4.211513410512504940, -3.870537385557588195, 3.783171883119448076 ) ) ;
#70135=CARTESIAN_POINT ( 'NONE',  ( 19.05937500061451928, 0.000000000000000000, 5.243569643749999010 ) ) ;
#70136=CARTESIAN_POINT ( 'NONE',  ( 11.22187500061451892, 3.027376345333613106, -5.243569643749998122 ) ) ;
#70138=CARTESIAN_POINT ( 'NONE',  ( 24.14999999999999858, 0.000000000000000000, 4.999999999999998224 ) ) ;
#70140=CARTESIAN_POINT ( 'NONE',  ( -2.121784821874996840, 13.18437500061451750, -26.32496088578401583 ) ) ;
#70142=CARTESIAN_POINT ( 'NONE',  ( 15.10312500061451502, -4.541064518000417216, -2.621784821875001281 ) ) ;
#70143=CARTESIAN_POINT ( 'NONE',  ( 3.825000000000001954, 4.330127018922191873, 2.499999999999999556 ) ) ;
#70146=CARTESIAN_POINT ( 'NONE',  ( 15.29999999999999893, -4.330127018922190985, -2.500000000000001332 ) ) ;
#70147=CARTESIAN_POINT ( 'NONE',  ( 4.243569643749999010, 10.61562500061451786, 27.54997392385601174 ) ) ;
#70148=CARTESIAN_POINT ( 'NONE',  ( 12.97500000122903252, 2.886751345948126879, 4.999999999999999112 ) ) ;
#70150=CARTESIAN_POINT ( 'NONE',  ( 23.74687500061451573, -3.027376345333610441, -5.243569643749999898 ) ) ;
#70151=CARTESIAN_POINT ( 'NONE',  ( 18.45937500061451431, 4.541064518000418104, -2.621784821874998173 ) ) ;
#70152=CYLINDRICAL_SURFACE ( 'NONE', #7694, 4.999999999999998224 ) ;
#70153=ORIENTED_EDGE ( 'NONE', *, *, #4728, .T. ) ;
#70154=CARTESIAN_POINT ( 'NONE',  ( 20.31562500061451715, 3.027376345333611329, 5.243569643749999010 ) ) ;
#70156=CARTESIAN_POINT ( 'NONE',  ( 3.815625000614518036, -6.054752690667223547, -1.112240025338166033E-15 ) ) ;
#70157=CARTESIAN_POINT ( 'NONE',  ( 17.18437500061451573, 4.541064518000418104, 2.621784821874999949 ) ) ;
#70158=CARTESIAN_POINT ( 'NONE',  ( 27.87187500061451573, 3.027376345333613106, -5.243569643749998122 ) ) ;
#70159=CARTESIAN_POINT ( 'NONE',  ( 5.578125000614518214, -4.541064518000419881, 2.621784821874995952 ) ) ;
#70160=CARTESIAN_POINT ( 'NONE',  ( 22.90312500061451573, 4.541064518000418104, -2.621784821874998173 ) ) ;
#70161=CARTESIAN_POINT ( 'NONE',  ( -4.243569643749997233, 15.79062500061451857, 32.45002607614398471 ) ) ;
#70162=CARTESIAN_POINT ( 'NONE',  ( 16.98750000122903359, 4.330127018922191873, 2.499999999999999556 ) ) ;
#70164=CARTESIAN_POINT ( 'NONE',  ( 6.740625000614515194, 6.054752690667223547, 3.707466751127219781E-16 ) ) ;
#70165=CARTESIAN_POINT ( 'NONE',  ( 0.000000000000000000, 20.00000000000000000, -33.99999999999999289 ) ) ;
#70166=CARTESIAN_POINT ( 'NONE',  ( 28.79062500061451502, 6.054752690667223547, 3.707466751127219781E-16 ) ) ;
#70167=( BOUNDED_CURVE ( )  B_SPLINE_CURVE ( 2, ( #15047, #20579, #32779, #43871, #53858, #43504, #8780, #15407, #9150 ),
 .UNSPECIFIED., .F., .F. ) 
 B_SPLINE_CURVE_WITH_KNOTS ( ( 3, 2, 2, 2, 3 ),
 ( 0.3804347826086956763, 0.3840579710144927383, 0.3913043478260869734, 0.3985507246376811530, 0.4021739130434782705 ),
 .UNSPECIFIED. ) 
 CURVE ( )  GEOMETRIC_REPRESENTATION_ITEM ( )  RATIONAL_B_SPLINE_CURVE ( ( 0.9330127018922194093, 0.9330127018922198534, 1.000000000000000000, 0.8660254037844387076, 1.000000000000000000, 0.8660254037844387076, 1.000000000000000000, 0.9330127018922194093, 0.9330127018922194093 ) ) 
 REPRESENTATION_ITEM ( '' )  );
#70168=CARTESIAN_POINT ( 'NONE',  ( 22.65937500061451715, 0.000000000000000000, 5.243569643749999010 ) ) ;
#70169=CARTESIAN_POINT ( 'NONE',  ( 14.05312500061451431, 0.000000000000000000, 5.243569643749999010 ) ) ;
#70170=CARTESIAN_POINT ( 'NONE',  ( 23.77500000122903145, 2.886751345948126879, 4.999999999999999112 ) ) ;
#70171=CARTESIAN_POINT ( 'NONE',  ( 24.96562500061451573, -6.054752690667223547, -1.112240025338166033E-15 ) ) ;
#70172=CARTESIAN_POINT ( 'NONE',  ( 20.55937500061451573, -4.541064518000417216, -2.621784821875001281 ) ) ;
#70173=CARTESIAN_POINT ( 'NONE',  ( 14.84062500061451750, 6.054752690667223547, 3.707466751127219781E-16 ) ) ;
#70174=CARTESIAN_POINT ( 'NONE',  ( -2.121784821874996840, 18.13437500061451502, 33.67503911421598417 ) ) ;
#70175=CARTESIAN_POINT ( 'NONE',  ( 19.97812500061451502, -4.541064518000419881, 2.621784821874995952 ) ) ;
#70176=EDGE_LOOP ( 'NONE', ( #73046, #40521 ) ) ;
#70177=CARTESIAN_POINT ( 'NONE',  ( 26.13749999999999929, -2.886751345948125991, -5.000000000000000000 ) ) ;
#70178=CARTESIAN_POINT ( 'NONE',  ( 3.999999999999998668, 11.26250000000000107, -32.30940107675850470 ) ) ;
#70179=CARTESIAN_POINT ( 'NONE',  ( 3.862478830110306571, -3.175243778317320409, -4.133272023037573462 ) ) ;
#70180=CARTESIAN_POINT ( 'NONE',  ( 27.74062500061451431, -3.027376345333610441, -5.243569643749999898 ) ) ;
#70181=CARTESIAN_POINT ( 'NONE',  ( 8.465625000614515727, 3.027376345333613106, -5.243569643749998122 ) ) ;
#70182=CARTESIAN_POINT ( 'NONE',  ( 20.92500000122903714, 2.886751345948129099, -4.999999999999998224 ) ) ;
#70183=CARTESIAN_POINT ( 'NONE',  ( 23.91562500061451502, 3.027376345333611329, 5.243569643749999010 ) ) ;
#70184=CARTESIAN_POINT ( 'NONE',  ( 26.47499999999999787, -4.330127018922194537, 2.499999999999995559 ) ) ;
#70185=CARTESIAN_POINT ( 'NONE',  ( 28.60312500061451502, -4.541064518000417216, -2.621784821875001281 ) ) ;
#70186=CARTESIAN_POINT ( 'NONE',  ( 7.378125000614518036, -4.541064518000419881, 2.621784821874995952 ) ) ;
#70187=ORIENTED_EDGE ( 'NONE', *, *, #16958, .T. ) ;
#70189=CARTESIAN_POINT ( 'NONE',  ( 26.09062500061451573, 6.054752690667223547, 3.707466751127219781E-16 ) ) ;
#70190=CARTESIAN_POINT ( 'NONE',  ( 5.540625000614515905, -3.027376345333614438, 5.243569643749998122 ) ) ;
#70192=CARTESIAN_POINT ( 'NONE',  ( 13.01249999999999929, -5.773502691896255534, -1.060575238724906372E-15 ) ) ;
#70193=VECTOR ( 'NONE', #26813, 1000.000000000000000 ) ;
#70194=CARTESIAN_POINT ( 'NONE',  ( 12.11250000000000249, -5.773502691896255534, -1.060575238724906372E-15 ) ) ;
#70195=AXIS2_PLACEMENT_3D ( 'NONE', #10723, #50615, #33255 ) ;
#70196=CARTESIAN_POINT ( 'NONE',  ( 13.02187500061451608, 3.027376345333613106, -5.243569643749998122 ) ) ;
#70197=CARTESIAN_POINT ( 'NONE',  ( 9.862500001229033586, 0.000000000000000000, 4.999999999999998224 ) ) ;
#70198=CARTESIAN_POINT ( 'NONE',  ( 17.03437500061451715, 6.421520780324663323E-16, -5.243569643749999010 ) ) ;
#70200=CARTESIAN_POINT ( 'NONE',  ( 8.709375000614517859, 0.000000000000000000, 5.243569643749999010 ) ) ;
#70201=CARTESIAN_POINT ( 'NONE',  ( 2.121784821874999061, 12.45312500061451821, -33.67503911421598417 ) ) ;
#70203=CARTESIAN_POINT ( 'NONE',  ( 30.00000000000000000, 6.123233995736764310E-16, -4.999999999999998224 ) ) ;
#70205=DIRECTION ( 'NONE',  ( 0.000000000000000000, 0.000000000000000000, 1.000000000000000000 ) ) ;
#70206=CARTESIAN_POINT ( 'NONE',  ( 24.10312500061451502, -4.541064518000417216, -2.621784821875001281 ) ) ;
#70207=CARTESIAN_POINT ( 'NONE',  ( -4.243569643749999898, 11.27187500061451786, 27.54997392385601529 ) ) ;
#70208=CARTESIAN_POINT ( 'NONE',  ( 1.626862140677534273E-15, 17.52500000122903145, 34.00000000000000000 ) ) ;
#70209=CARTESIAN_POINT ( 'NONE',  ( 25.73437500061451644, 4.541064518000418104, 2.621784821874999949 ) ) ;
#70210=CARTESIAN_POINT ( 'NONE',  ( 29.14687500061451075, -3.027376345333610441, -5.243569643749999898 ) ) ;
#70212=CARTESIAN_POINT ( 'NONE',  ( 4.228125000614517681, -4.541064518000419881, 2.621784821874995952 ) ) ;
#70214=CARTESIAN_POINT ( 'NONE',  ( 16.69687500061451502, 6.054752690667223547, 3.707466751127219781E-16 ) ) ;
#70216=CARTESIAN_POINT ( 'NONE',  ( 28.98750000122903359, 6.123233995736764310E-16, -4.999999999999998224 ) ) ;
#70217=CARTESIAN_POINT ( 'NONE',  ( 9.421875000614519990, 3.027376345333613106, -5.243569643749998122 ) ) ;
#70218=CARTESIAN_POINT ( 'NONE',  ( 15.72187500061451892, 3.027376345333613106, -5.243569643749998122 ) ) ;
#70220=CARTESIAN_POINT ( 'NONE',  ( 25.72499999999999787, 6.123233995736764310E-16, -4.999999999999998224 ) ) ;
#70221=CARTESIAN_POINT ( 'NONE',  ( 27.64687500061452141, -3.027376345333614438, 5.243569643749998122 ) ) ;
#70223=CARTESIAN_POINT ( 'NONE',  ( -2.556497649636125342E-15, 19.21250000000000213, -26.00000000000000355 ) ) ;
#70224=ORIENTED_EDGE ( 'NONE', *, *, #34645, .T. ) ;
#70225=CARTESIAN_POINT ( 'NONE',  ( 8.287499999999999645, 5.773502691896255534, 3.535250795749688894E-16 ) ) ;
#70227=CARTESIAN_POINT ( 'NONE',  ( 22.71562500061451573, -6.054752690667223547, -1.112240025338166033E-15 ) ) ;
#70228=CARTESIAN_POINT ( 'NONE',  ( 12.37500000000000000, 4.330127018922191873, 2.499999999999999556 ) ) ;
#70229=CARTESIAN_POINT ( 'NONE',  ( 7.875000001229034652, 2.886751345948129099, -4.999999999999998224 ) ) ;
#70230=CARTESIAN_POINT ( 'NONE',  ( 7.678125000614516082, 4.541064518000418104, 2.621784821874999949 ) ) ;
#70231=CARTESIAN_POINT ( 'NONE',  ( 21.48750000000000071, -2.886751345948129988, 4.999999999999997335 ) ) ;
#70232=EDGE_CURVE ( 'NONE', #5506, #20508, #30670, .T. ) ;
#70233=CARTESIAN_POINT ( 'NONE',  ( 18.44062500061451715, 6.054752690667223547, 3.707466751127219781E-16 ) ) ;
#70234=CARTESIAN_POINT ( 'NONE',  ( 4.148274082013050368, -2.791383553096713044, 4.344604658505033079 ) ) ;
#70235=CARTESIAN_POINT ( 'NONE',  ( 26.66250000122903430, -4.330127018922190985, -2.500000000000001332 ) ) ;
#70237=CARTESIAN_POINT ( 'NONE',  ( 4.612500000000002487, 2.886751345948129099, -4.999999999999998224 ) ) ;
#70240=ORIENTED_EDGE ( 'NONE', *, *, #35309, .F. ) ;
#70241=CARTESIAN_POINT ( 'NONE',  ( 19.34062500061451573, 6.054752690667223547, 3.707466751127219781E-16 ) ) ;
#70242=CARTESIAN_POINT ( 'NONE',  ( 25.64062500061451644, 6.054752690667223547, 3.707466751127219781E-16 ) ) ;
#70243=CARTESIAN_POINT ( 'NONE',  ( 26.89687500061451431, -3.027376345333610441, -5.243569643749999898 ) ) ;
#70244=CARTESIAN_POINT ( 'NONE',  ( 9.937500000000001776, -2.886751345948125991, -5.000000000000000000 ) ) ;
#70245=CARTESIAN_POINT ( 'NONE',  ( 12.10312500061451857, 4.541064518000418104, -2.621784821874998173 ) ) ;
#70246=CARTESIAN_POINT ( 'NONE',  ( 29.05312500061451431, -4.541064518000417216, -2.621784821875001281 ) ) ;
#70247=CARTESIAN_POINT ( 'NONE',  ( 8.578125000614518214, 4.541064518000418104, 2.621784821874999949 ) ) ;
#70249=CARTESIAN_POINT ( 'NONE',  ( -4.243569643749999898, 13.10937500061451821, 30.00000000000000000 ) ) ;
#70250=CARTESIAN_POINT ( 'NONE',  ( 26.96250000122903145, 0.000000000000000000, 4.999999999999998224 ) ) ;
#70252=CARTESIAN_POINT ( 'NONE',  ( 13.60312500061451679, 0.000000000000000000, 5.243569643749999010 ) ) ;
#70253=CARTESIAN_POINT ( 'NONE',  ( 9.834375000614517859, 6.421520780324663323E-16, -5.243569643749999010 ) ) ;
#70254=CARTESIAN_POINT ( 'NONE',  ( 10.09687500061451715, -3.027376345333614438, 5.243569643749998122 ) ) ;
#70255=CARTESIAN_POINT ( 'NONE',  ( 17.74687500061451928, -3.027376345333614438, 5.243569643749998122 ) ) ;
#70256=EDGE_CURVE ( 'NONE', #72227, #755, #10837, .T. ) ;
#70257=ORIENTED_EDGE ( 'NONE', *, *, #35738, .F. ) ;
#70258=CARTESIAN_POINT ( 'NONE',  ( 29.33437500061451431, 4.541064518000418104, 2.621784821874999949 ) ) ;
#70259=CARTESIAN_POINT ( 'NONE',  ( 22.37812500061451360, 6.421520780324663323E-16, -5.243569643749999010 ) ) ;
#70260=AXIS2_PLACEMENT_3D ( 'NONE', #20066, #42622, #65146 ) ;
#70261=CARTESIAN_POINT ( 'NONE',  ( 16.69687500061451502, 6.054752690667223547, 3.707466751127219781E-16 ) ) ;
#70262=CARTESIAN_POINT ( 'NONE',  ( 21.25312500061451715, 0.000000000000000000, 5.243569643749999010 ) ) ;
#70263=CARTESIAN_POINT ( 'NONE',  ( -1.999999999999997113, 13.77500000000000036, 33.46410161513775705 ) ) ;
#70264=CARTESIAN_POINT ( 'NONE',  ( 27.06562500061451004, 3.027376345333611329, 5.243569643749999010 ) ) ;
#70265=CARTESIAN_POINT ( 'NONE',  ( 6.975000001229032520, 2.886751345948129099, -4.999999999999998224 ) ) ;
#70266=ORIENTED_EDGE ( 'NONE', *, *, #29620, .T. ) ;
#70267=CARTESIAN_POINT ( 'NONE',  ( 3.525000001229034119, 2.886751345948126879, 4.999999999999999112 ) ) ;
#70268=CARTESIAN_POINT ( 'NONE',  ( 4.000000000000000000, 17.93750000000000355, -27.69059892324149530 ) ) ;
#70269=CARTESIAN_POINT ( 'NONE',  ( 24.75000000122902932, -2.886751345948129988, 4.999999999999997335 ) ) ;
#70272=CARTESIAN_POINT ( 'NONE',  ( 7.959375000614516971, -4.541064518000417216, -2.621784821875001281 ) ) ;
#70273=CARTESIAN_POINT ( 'NONE',  ( 23.28750000000000142, -2.886751345948130876, 4.999999999999996447 ) ) ;
#70274=CARTESIAN_POINT ( 'NONE',  ( 15.14062500061451644, -3.027376345333610441, -5.243569643749999898 ) ) ;
#70275=CARTESIAN_POINT ( 'NONE',  ( 8.184375000614515727, 4.541064518000418104, 2.621784821874999949 ) ) ;
#70276=CARTESIAN_POINT ( 'NONE',  ( 27.52500000122903145, -5.773502691896255534, -1.060575238724906372E-15 ) ) ;
#70277=CARTESIAN_POINT ( 'NONE',  ( 16.77187500061451786, 3.027376345333611329, 5.243569643749999010 ) ) ;
#70278=CARTESIAN_POINT ( 'NONE',  ( 5.146875000614517859, -3.027376345333614438, 5.243569643749998122 ) ) ;
#70280=CARTESIAN_POINT ( 'NONE',  ( 4.528125000614516615, 4.541064518000418104, 2.621784821874999949 ) ) ;
#70281=CARTESIAN_POINT ( 'NONE',  ( 16.64062500061451289, 6.054752690667223547, 3.707466751127219781E-16 ) ) ;
#70283=CARTESIAN_POINT ( 'NONE',  ( 13.67812500061451786, -4.541064518000419881, 2.621784821874995952 ) ) ;
#70284=CARTESIAN_POINT ( 'NONE',  ( 4.950000001229033941, -2.886751345948129988, 4.999999999999997335 ) ) ;
#70285=CARTESIAN_POINT ( 'NONE',  ( 11.31562500061451892, 3.027376345333611329, 5.243569643749999010 ) ) ;
#70287=CARTESIAN_POINT ( 'NONE',  ( 10.12500000000000178, 4.330127018922191873, 2.499999999999999556 ) ) ;
#70288=CARTESIAN_POINT ( 'NONE',  ( 7.537500001229033408, 4.330127018922191873, 2.499999999999999556 ) ) ;
#70289=CARTESIAN_POINT ( 'NONE',  ( 21.26249999999999574, 2.886751345948129099, -4.999999999999998224 ) ) ;
#70291=CARTESIAN_POINT ( 'NONE',  ( 16.05937500061451573, -4.541064518000417216, -2.621784821875001281 ) ) ;
#70292=CARTESIAN_POINT ( 'NONE',  ( 15.71250000122903501, 0.000000000000000000, 4.999999999999998224 ) ) ;
#70295=CARTESIAN_POINT ( 'NONE',  ( 4.243569643749999898, 19.54062500061451857, -27.54997392385601529 ) ) ;
#70298=CARTESIAN_POINT ( 'NONE',  ( 3.486133158594716510E-16, 19.88749999999999929, 26.00000000000000355 ) ) ;
#70299=CARTESIAN_POINT ( 'NONE',  ( 1.626862140677534273E-15, 10.32500000122903572, -26.00000000000000355 ) ) ;
#70300=CARTESIAN_POINT ( 'NONE',  ( 16.88437500061451502, -4.541064518000419881, 2.621784821874995952 ) ) ;
#70301=CARTESIAN_POINT ( 'NONE',  ( 28.12499999999999645, 4.330127018922191873, 2.499999999999999556 ) ) ;
#70302=CARTESIAN_POINT ( 'NONE',  ( 11.57812500061451644, 6.421520780324663323E-16, -5.243569643749999010 ) ) ;
#70304=CARTESIAN_POINT ( 'NONE',  ( 23.48437500061451644, 4.541064518000418104, 2.621784821874999949 ) ) ;
#70306=CARTESIAN_POINT ( 'NONE',  ( 9.290625000614515017, -3.027376345333610441, -5.243569643749999898 ) ) ;
#70307=CARTESIAN_POINT ( 'NONE',  ( 15.45937500061451608, 0.000000000000000000, 5.243569643749999010 ) ) ;
#70308=VERTEX_POINT ( 'NONE', #28612 ) ;
#70309=CARTESIAN_POINT ( 'NONE',  ( 27.04687500061451644, 6.054752690667223547, 3.707466751127219781E-16 ) ) ;
#70310=CARTESIAN_POINT ( 'NONE',  ( 27.10312500061451502, 0.000000000000000000, 5.243569643749999010 ) ) ;
#70311=CARTESIAN_POINT ( 'NONE',  ( 28.82812500061451644, 4.541064518000418104, 2.621784821874999949 ) ) ;
#70312=CARTESIAN_POINT ( 'NONE',  ( 1.999999999999998668, 12.76250000122903394, -33.46410161513775705 ) ) ;
#70313=CARTESIAN_POINT ( 'NONE',  ( 6.562500000000001776, 2.886751345948126879, 4.999999999999999112 ) ) ;
#70314=CARTESIAN_POINT ( 'NONE',  ( 20.40000000122903145, -2.886751345948125991, -5.000000000000000000 ) ) ;
#70316=ORIENTED_EDGE ( 'NONE', *, *, #68178, .T. ) ;
#70317=CARTESIAN_POINT ( 'NONE',  ( 16.31250000000000000, 2.886751345948129099, -4.999999999999998224 ) ) ;
#70318=CARTESIAN_POINT ( 'NONE',  ( 19.50000000000000000, 4.330127018922192761, -2.499999999999997780 ) ) ;
#70319=CARTESIAN_POINT ( 'NONE',  ( 14.42812500061451786, 4.541064518000418104, 2.621784821874999949 ) ) ;
#70320=ORIENTED_EDGE ( 'NONE', *, *, #72450, .T. ) ;
#70321=CARTESIAN_POINT ( 'NONE',  ( 2.121784821875001281, 15.95937500061451608, -26.32496088578401938 ) ) ;
#70322=CARTESIAN_POINT ( 'NONE',  ( 6.365625000614518747, 3.027376345333611329, 5.243569643749999010 ) ) ;
#70324=CARTESIAN_POINT ( 'NONE',  ( 11.32500000000000107, 6.123233995736764310E-16, -4.999999999999998224 ) ) ;
#70326=EDGE_LOOP ( 'NONE', ( #68995, #39942, #51005, #39734 ) ) ;
#70327=CARTESIAN_POINT ( 'NONE',  ( -4.243569643749997233, 16.24062500061451431, 32.45002607614398471 ) ) ;
#70328=CARTESIAN_POINT ( 'NONE',  ( 25.71562500061451573, 3.027376345333611329, 5.243569643749999010 ) ) ;
#70331=CARTESIAN_POINT ( 'NONE',  ( 24.49687500061451573, -3.027376345333614438, 5.243569643749998122 ) ) ;
#70332=CARTESIAN_POINT ( 'NONE',  ( 21.36562500061451431, -6.054752690667223547, -1.112240025338166033E-15 ) ) ;
#70333=CARTESIAN_POINT ( 'NONE',  ( 4.243569643749999898, 15.04062500061459495, -27.54997392385601529 ) ) ;
#70334=CARTESIAN_POINT ( 'NONE',  ( 24.18750000122903288, 4.330127018922191873, 2.499999999999999556 ) ) ;
#70335=CARTESIAN_POINT ( 'NONE',  ( 6.103125000614515905, -4.541064518000417216, -2.621784821875001281 ) ) ;
#70337=CARTESIAN_POINT ( 'NONE',  ( 24.36562500061451786, 3.027376345333611329, 5.243569643749999010 ) ) ;
#70341=CARTESIAN_POINT ( 'NONE',  ( 16.99687500061451573, -3.027376345333610441, -5.243569643749999898 ) ) ;
#70342=CARTESIAN_POINT ( 'NONE',  ( 25.84687500061451360, -3.027376345333614438, 5.243569643749998122 ) ) ;
#70343=CARTESIAN_POINT ( 'NONE',  ( 4.243569643749999898, 14.23437500061451821, 30.00000000000000000 ) ) ;
#70344=CARTESIAN_POINT ( 'NONE',  ( 5.915625000614515905, 3.027376345333611329, 5.243569643749999010 ) ) ;
#70345=CARTESIAN_POINT ( 'NONE',  ( 29.69062500061451715, 6.054752690667223547, 3.707466751127219781E-16 ) ) ;
#70346=CARTESIAN_POINT ( 'NONE',  ( 29.39062500061451289, -3.027376345333614438, 5.243569643749998122 ) ) ;
#70348=CARTESIAN_POINT ( 'NONE',  ( 3.203127373816005541, 9.474626018533117033, -35.07709628816699166 ) ) ;
#70349=AXIS2_PLACEMENT_3D ( 'NONE', #69816, #1505, #34735 ) ;
#70350=CARTESIAN_POINT ( 'NONE',  ( 29.47500000122903430, 2.886751345948129099, -4.999999999999998224 ) ) ;
#70351=CARTESIAN_POINT ( 'NONE',  ( 8.371875000614515727, -6.054752690667223547, -1.112240025338166033E-15 ) ) ;
#70352=CARTESIAN_POINT ( 'NONE',  ( 16.23750000122903359, -4.330127018922194537, 2.499999999999995559 ) ) ;
#70353=CARTESIAN_POINT ( 'NONE',  ( 3.346875000614518036, -3.027376345333614438, 5.243569643749998122 ) ) ;
#70354=CARTESIAN_POINT ( 'NONE',  ( 11.47500000122903252, 2.886751345948129099, -4.999999999999998224 ) ) ;
#70355=CARTESIAN_POINT ( 'NONE',  ( 4.153125000614515727, 0.000000000000000000, 5.243569643749999010 ) ) ;
#70358=CARTESIAN_POINT ( 'NONE',  ( 14.29687500061451821, -3.027376345333610441, -5.243569643749999898 ) ) ;
#70359=CARTESIAN_POINT ( 'NONE',  ( 11.84999999999999964, 4.330127018922192761, -2.499999999999997780 ) ) ;
#70361=CARTESIAN_POINT ( 'NONE',  ( 22.97812500061451857, 4.541064518000418104, 2.621784821874999949 ) ) ;
#70362=CARTESIAN_POINT ( 'NONE',  ( 7.640625000614517326, 6.054752690667223547, 3.707466751127219781E-16 ) ) ;
#70363=CARTESIAN_POINT ( 'NONE',  ( 24.90937500061451715, 0.000000000000000000, 5.243569643749999010 ) ) ;
#70364=CARTESIAN_POINT ( 'NONE',  ( 6.965625000614518392, -6.054752690667223547, -1.112240025338166033E-15 ) ) ;
#70365=CARTESIAN_POINT ( 'NONE',  ( 3.405214727565324839, 4.049716704864715133, -2.985684910913894097 ) ) ;
#70366=CARTESIAN_POINT ( 'NONE',  ( 11.32500000122903394, -5.773502691896255534, -1.060575238724906372E-15 ) ) ;
#70367=CARTESIAN_POINT ( 'NONE',  ( 24.21562500061451573, 3.027376345333613106, -5.243569643749998122 ) ) ;
#70368=CARTESIAN_POINT ( 'NONE',  ( -4.243569643749997233, 11.74062500061451786, -27.54997392385601174 ) ) ;
#70369=CARTESIAN_POINT ( 'NONE',  ( 10.53750000122903252, 6.123233995736764310E-16, -4.999999999999998224 ) ) ;
#70370=CARTESIAN_POINT ( 'NONE',  ( 19.97812500061451502, -4.541064518000419881, 2.621784821874995952 ) ) ;
#70371=CARTESIAN_POINT ( 'NONE',  ( 17.69062500061451715, -3.027376345333614438, 5.243569643749998122 ) ) ;
#70373=CARTESIAN_POINT ( 'NONE',  ( 17.81250000000000355, 2.886751345948126879, 4.999999999999999112 ) ) ;
#70374=CARTESIAN_POINT ( 'NONE',  ( 13.91250000122903252, 0.000000000000000000, 4.999999999999998224 ) ) ;
#70375=EDGE_CURVE ( 'NONE', #3193, #1870, #10415, .T. ) ;
#70376=CARTESIAN_POINT ( 'NONE',  ( 10.82812500061451644, 4.541064518000418104, 2.621784821874999949 ) ) ;
#70377=CARTESIAN_POINT ( 'NONE',  ( 14.20312500061451644, -4.541064518000417216, -2.621784821875001281 ) ) ;
#70378=CARTESIAN_POINT ( 'NONE',  ( 24.07500000122903216, 2.886751345948129099, -4.999999999999998224 ) ) ;
#70379=CARTESIAN_POINT ( 'NONE',  ( 21.34687500061451715, -3.027376345333614438, 5.243569643749998122 ) ) ;
#70380=CARTESIAN_POINT ( 'NONE',  ( 21.19687500061451502, 6.054752690667223547, 3.707466751127219781E-16 ) ) ;
#70382=AXIS2_PLACEMENT_3D ( 'NONE', #10823, #15623, #38165 ) ;
#70384=CARTESIAN_POINT ( 'NONE',  ( 8.512500001229033941, 0.000000000000000000, 4.999999999999998224 ) ) ;
#70385=CARTESIAN_POINT ( 'NONE',  ( 5.371875000614516615, 3.027376345333613106, -5.243569643749998122 ) ) ;
#70386=CARTESIAN_POINT ( 'NONE',  ( 24.08437500061451786, -4.541064518000419881, 2.621784821874995952 ) ) ;
#70387=CARTESIAN_POINT ( 'NONE',  ( 26.55000000122903359, -2.886751345948121994, 5.000000000000011546 ) ) ;
#70388=CARTESIAN_POINT ( 'NONE',  ( 19.11562500061451431, -6.054752690667223547, -1.112240025338166033E-15 ) ) ;
#70389=CARTESIAN_POINT ( 'NONE',  ( 25.09687500061451715, -3.027376345333610441, -5.243569643749999898 ) ) ;
#70391=CARTESIAN_POINT ( 'NONE',  ( -1.999999999999997113, 11.18750000122903288, -26.53589838486224295 ) ) ;
#70393=CARTESIAN_POINT ( 'NONE',  ( 4.734375000614518214, -4.541064518000419881, 2.621784821874995952 ) ) ;
#70394=CARTESIAN_POINT ( 'NONE',  ( 16.37812500061451715, -4.541064518000419881, 2.621784821874995952 ) ) ;
#70395=ORIENTED_EDGE ( 'NONE', *, *, #21542, .T. ) ;
#70396=CARTESIAN_POINT ( 'NONE',  ( -1.071796769724491005, 12.70759618943233349, -34.00000000000000000 ) ) ;
#70397=CARTESIAN_POINT ( 'NONE',  ( 24.77812500061451217, 4.541064518000418104, 2.621784821874999949 ) ) ;
#70398=DIRECTION ( 'NONE',  ( 0.000000000000000000, 0.000000000000000000, -1.000000000000000000 ) ) ;
#70400=DIRECTION ( 'NONE',  ( -1.000000000000000000, -0.000000000000000000, -0.000000000000000000 ) ) ;
#70401=CARTESIAN_POINT ( 'NONE',  ( 14.40000000000000036, -4.330127018922190985, -2.500000000000001332 ) ) ;
#70402=CARTESIAN_POINT ( 'NONE',  ( 26.17500000122903359, -5.773502691896255534, -1.060575238724906372E-15 ) ) ;
#70403=CARTESIAN_POINT ( 'NONE',  ( 20.72812500061451502, 4.541064518000418104, 2.621784821874999949 ) ) ;
#70404=EDGE_CURVE ( 'NONE', #66841, #53581, #52897, .T. ) ;
#70405=ORIENTED_EDGE ( 'NONE', *, *, #54179, .T. ) ;
#70406=CARTESIAN_POINT ( 'NONE',  ( 23.32499999999999929, -4.330127018922194537, 2.499999999999995559 ) ) ;
#70407=CARTESIAN_POINT ( 'NONE',  ( 23.29687500061451644, -3.027376345333610441, -5.243569643749999898 ) ) ;
#70408=ORIENTED_EDGE ( 'NONE', *, *, #71580, .T. ) ;
#70410=CARTESIAN_POINT ( 'NONE',  ( 12.47812500061451502, 6.421520780324663323E-16, -5.243569643749999010 ) ) ;
#70411=CARTESIAN_POINT ( 'NONE',  ( 3.703125000614516882, 0.000000000000000000, 5.243569643749999010 ) ) ;
#70413=CARTESIAN_POINT ( 'NONE',  ( 28.22812500061451502, 6.421520780324663323E-16, -5.243569643749999010 ) ) ;
#70414=CARTESIAN_POINT ( 'NONE',  ( 13.16250000122903430, -4.330127018922190985, -2.500000000000001332 ) ) ;
#70415=CARTESIAN_POINT ( 'NONE',  ( 18.56250000000000000, 2.886751345948129099, -4.999999999999998224 ) ) ;
#70416=CARTESIAN_POINT ( 'NONE',  ( 27.18750000000000000, 5.773502691896255534, 3.535250795749688894E-16 ) ) ;
#70418=CARTESIAN_POINT ( 'NONE',  ( 6.834375000614518747, 4.541064518000418104, 2.621784821874999949 ) ) ;
#70419=CARTESIAN_POINT ( 'NONE',  ( 20.40937500061451715, 0.000000000000000000, 5.243569643749999010 ) ) ;
#70422=CARTESIAN_POINT ( 'NONE',  ( 27.59062500061451573, -3.027376345333614438, 5.243569643749998122 ) ) ;
#70423=CARTESIAN_POINT ( 'NONE',  ( 28.99687500061451573, -3.027376345333614438, 5.243569643749998122 ) ) ;
#70424=CARTESIAN_POINT ( 'NONE',  ( 4.959375000614516971, 4.541064518000418104, -2.621784821874998173 ) ) ;
#70425=CARTESIAN_POINT ( 'NONE',  ( 16.16250000000000142, -5.773502691896255534, -1.060575238724906372E-15 ) ) ;
#70426=CARTESIAN_POINT ( 'NONE',  ( 13.26562500061451644, -6.054752690667223547, -1.112240025338166033E-15 ) ) ;
#70429=CARTESIAN_POINT ( 'NONE',  ( 0.000000000000000000, 20.00000000000000000, -30.00000000000000000 ) ) ;
#70430=CARTESIAN_POINT ( 'NONE',  ( 17.36250000122903359, 4.330127018922192761, -2.499999999999997780 ) ) ;
#70431=CARTESIAN_POINT ( 'NONE',  ( -5.810221930991193690E-16, 10.55000000122903359, 26.00000000000000355 ) ) ;
#70433=CARTESIAN_POINT ( 'NONE',  ( 8.128125000614515372, 4.541064518000418104, 2.621784821874999949 ) ) ;
#70434=CARTESIAN_POINT ( 'NONE',  ( 23.25937500061451857, -4.541064518000417216, -2.621784821875001281 ) ) ;
#70435=CARTESIAN_POINT ( 'NONE',  ( 4.243569643749999898, 16.44687500061451857, 32.45002607614398471 ) ) ;
#70436=CARTESIAN_POINT ( 'NONE',  ( 23.33437500061451786, 6.421520780324663323E-16, -5.243569643749999010 ) ) ;
#70437=CARTESIAN_POINT ( 'NONE',  ( 6.075000000000000178, 4.330127018922191873, 2.499999999999999556 ) ) ;
#70438=CARTESIAN_POINT ( 'NONE',  ( 1.999999999999998668, 10.06250000122903465, 26.53589838486224650 ) ) ;
#70439=CARTESIAN_POINT ( 'NONE',  ( 12.70312500061451821, 0.000000000000000000, 5.243569643749999010 ) ) ;
#70440=CARTESIAN_POINT ( 'NONE',  ( 3.675000001229035362, -5.773502691896255534, -1.060575238724906372E-15 ) ) ;
#70441=CARTESIAN_POINT ( 'NONE',  ( 8.559375000614515727, 4.541064518000418104, -2.621784821874998173 ) ) ;
#70442=CARTESIAN_POINT ( 'NONE',  ( 3.895888853841904531, -3.134084140313734501, 4.010892849215046851 ) ) ;
#70444=CARTESIAN_POINT ( 'NONE',  ( 10.52812500061451750, -4.541064518000419881, 2.621784821874995952 ) ) ;
#70445=CARTESIAN_POINT ( 'NONE',  ( 14.18437500061451750, -4.541064518000419881, 2.621784821874995952 ) ) ;
#70446=CARTESIAN_POINT ( 'NONE',  ( 29.17500000122903359, 2.886751345948106007, 5.000000000000033751 ) ) ;
#70447=CARTESIAN_POINT ( 'NONE',  ( 23.62500000122902932, 2.886751345948129099, -4.999999999999998224 ) ) ;
#70448=CARTESIAN_POINT ( 'NONE',  ( 9.834375000614517859, 6.421520780324663323E-16, -5.243569643749999010 ) ) ;
#70449=CARTESIAN_POINT ( 'NONE',  ( 12.51562500061451821, 3.027376345333613106, -5.243569643749998122 ) ) ;
#70451=CARTESIAN_POINT ( 'NONE',  ( 22.24687500061451217, -3.027376345333614438, 5.243569643749998122 ) ) ;
#70452=CYLINDRICAL_SURFACE ( 'NONE', #14811, 3.999999999999996447 ) ;
#70453=CARTESIAN_POINT ( 'NONE',  ( 5.362500000000002487, -5.773502691896255534, -1.060575238724906372E-15 ) ) ;
#70455=CARTESIAN_POINT ( 'NONE',  ( -4.243569643749999898, 14.45937500061451964, -30.00000000000000000 ) ) ;
#70456=CARTESIAN_POINT ( 'NONE',  ( 16.50937500061451502, -4.541064518000417216, -2.621784821875001281 ) ) ;
#70457=CARTESIAN_POINT ( 'NONE',  ( 16.65000000122903501, -2.886751345948129988, 4.999999999999997335 ) ) ;
#70459=CARTESIAN_POINT ( 'NONE',  ( 11.29687500061451644, 6.054752690667223547, 3.707466751127219781E-16 ) ) ;
#70460=CARTESIAN_POINT ( 'NONE',  ( -4.243569643749999898, 18.00312500061451715, -30.00000000000000000 ) ) ;
#70461=CARTESIAN_POINT ( 'NONE',  ( 16.80000000122903359, -2.886751345948125991, -5.000000000000000000 ) ) ;
#70462=CARTESIAN_POINT ( 'NONE',  ( 13.26562500061451644, -6.054752690667223547, -1.112240025338166033E-15 ) ) ;
#70464=CARTESIAN_POINT ( 'NONE',  ( 15.56250000000000000, 2.886751345948126879, 4.999999999999999112 ) ) ;
#70466=CARTESIAN_POINT ( 'NONE',  ( 9.721875000614517148, -6.054752690667223547, -1.112240025338166033E-15 ) ) ;
#70467=CARTESIAN_POINT ( 'NONE',  ( 3.458282317606259149, 3.615826433065254530, 27.97484066355150034 ) ) ;
#70468=CARTESIAN_POINT ( 'NONE',  ( 11.88750000122903216, 6.123233995736764310E-16, -4.999999999999998224 ) ) ;
#70469=CARTESIAN_POINT ( 'NONE',  ( 22.16250000122903074, -4.330127018922190985, -2.500000000000001332 ) ) ;
#70470=CARTESIAN_POINT ( 'NONE',  ( 17.16562500061451502, 3.027376345333611329, 5.243569643749999010 ) ) ;
#70471=CARTESIAN_POINT ( 'NONE',  ( 21.81562500061451004, -6.054752690667223547, -1.112240025338166033E-15 ) ) ;
#70472=CARTESIAN_POINT ( 'NONE',  ( 27.22500000122903430, 2.886751345948129099, -4.999999999999998224 ) ) ;
#70473=CARTESIAN_POINT ( 'NONE',  ( 24.93750000000000355, 5.773502691896255534, 3.535250795749688894E-16 ) ) ;
#70476=CARTESIAN_POINT ( 'NONE',  ( 27.53437500061451360, 4.541064518000418104, 2.621784821874999949 ) ) ;
#70478=CARTESIAN_POINT ( 'NONE',  ( 4.243569643749999898, 13.29687500061451644, -27.54997392385601529 ) ) ;
#70479=CARTESIAN_POINT ( 'NONE',  ( 3.487500001229035362, 4.330127018922191873, 2.499999999999999556 ) ) ;
#70480=CARTESIAN_POINT ( 'NONE',  ( 29.37187500061451928, 3.027376345333611329, 5.243569643749999010 ) ) ;
#70482=CARTESIAN_POINT ( 'NONE',  ( 7.396875000614519635, -3.027376345333614438, 5.243569643749998122 ) ) ;
#70483=CARTESIAN_POINT ( 'NONE',  ( 29.50312500061451360, -4.541064518000417216, -2.621784821875001281 ) ) ;
#70484=CARTESIAN_POINT ( 'NONE',  ( 4.837952263367122363, -3.387542794378833211, -4.619743054822007089 ) ) ;
#70485=CARTESIAN_POINT ( 'NONE',  ( 11.43750000122903465, 6.123233995736764310E-16, -4.999999999999998224 ) ) ;
#70486=CARTESIAN_POINT ( 'NONE',  ( -3.999999999999999112, 20.00000000000000000, 30.00000000000000000 ) ) ;
#70487=CARTESIAN_POINT ( 'NONE',  ( 6.046875000614519102, -3.027376345333614438, 5.243569643749998122 ) ) ;
#70488=CARTESIAN_POINT ( 'NONE',  ( 10.50937500061451679, 0.000000000000000000, 5.243569643749999010 ) ) ;
#70489=CARTESIAN_POINT ( 'NONE',  ( 4.012500000000001954, -5.773502691896255534, -1.060575238724906372E-15 ) ) ;
#70490=CARTESIAN_POINT ( 'NONE',  ( 4.243569643749999898, 13.69062500061459176, 32.45002607614398471 ) ) ;
#70491=CARTESIAN_POINT ( 'NONE',  ( 5.850000000000001421, -4.330127018922190985, -2.500000000000001332 ) ) ;
#70494=CARTESIAN_POINT ( 'NONE',  ( 21.21562500061451573, 3.027376345333611329, 5.243569643749999010 ) ) ;
#70495=CARTESIAN_POINT ( 'NONE',  ( 11.87812500061451537, -4.541064518000419881, 2.621784821874995952 ) ) ;
#70497=CARTESIAN_POINT ( 'NONE',  ( 8.971875000614515372, 3.027376345333613106, -5.243569643749998122 ) ) ;
#70498=CARTESIAN_POINT ( 'NONE',  ( 25.05000000000000071, 0.000000000000000000, 4.999999999999998224 ) ) ;
#70499=CARTESIAN_POINT ( 'NONE',  ( 19.61250000122903359, 4.330127018922192761, -2.499999999999997780 ) ) ;
#70500=CARTESIAN_POINT ( 'NONE',  ( 28.45312500061451289, 0.000000000000000000, 5.243569643749999010 ) ) ;
#70502=CARTESIAN_POINT ( 'NONE',  ( 8.971875000614515372, 3.027376345333613106, -5.243569643749998122 ) ) ;
#70503=CARTESIAN_POINT ( 'NONE',  ( 13.58437500061451786, 4.541064518000418104, 2.621784821874999949 ) ) ;
#70504=CARTESIAN_POINT ( 'NONE',  ( 26.40937500061451715, -4.541064518000417216, -2.621784821875001281 ) ) ;
#70505=CARTESIAN_POINT ( 'NONE',  ( 8.700000001229032165, -2.886751345948193048, -4.999999999999883649 ) ) ;
#70507=EDGE_CURVE ( 'NONE', #1970, #68292, #50712, .T. ) ;
#70508=CARTESIAN_POINT ( 'NONE',  ( 20.52187500061451786, -6.054752690667223547, -1.112240025338166033E-15 ) ) ;
#70509=CARTESIAN_POINT ( 'NONE',  ( 12.23437500061451821, 4.541064518000418104, 2.621784821874999949 ) ) ;
#70511=CARTESIAN_POINT ( 'NONE',  ( 24.22500000000000142, -4.330127018922194537, 2.499999999999995559 ) ) ;
#70513=CARTESIAN_POINT ( 'NONE',  ( 9.001249775931846008E-16, 11.87187500061451750, -25.09994784771203058 ) ) ;
#70515=CARTESIAN_POINT ( 'NONE',  ( 15.59062500061451573, -3.027376345333610441, -5.243569643749999898 ) ) ;
#70516=CARTESIAN_POINT ( 'NONE',  ( 5.250000000000000888, 0.000000000000000000, 4.999999999999998224 ) ) ;
#70518=DIRECTION ( 'NONE',  ( -0.000000000000000000, -1.000000000000000000, -0.000000000000000000 ) ) ;
#70519=CARTESIAN_POINT ( 'NONE',  ( 13.46249999999999858, -5.773502691896255534, -1.060575238724906372E-15 ) ) ;
#70520=EDGE_CURVE ( 'NONE', #43636, #27655, #62942, .T. ) ;
#70521=CARTESIAN_POINT ( 'NONE',  ( -2.828200636599751609E-16, 17.30000000122903359, 25.38119784648299770 ) ) ;
#70522=CARTESIAN_POINT ( 'NONE',  ( 11.10000000122903252, 5.773502691896255534, 3.535250795749688894E-16 ) ) ;
#70523=CARTESIAN_POINT ( 'NONE',  ( 22.02187500061452141, 3.027376345333613106, -5.243569643749998122 ) ) ;
#70524=CARTESIAN_POINT ( 'NONE',  ( 16.65937500061452070, 4.541064518000418104, -2.621784821874998173 ) ) ;
#70526=VERTEX_POINT ( 'NONE', #19314 ) ;
#70527=CARTESIAN_POINT ( 'NONE',  ( 18.51562500061451289, 3.027376345333611329, 5.243569643749999010 ) ) ;
#70528=CARTESIAN_POINT ( 'NONE',  ( 3.890625000614517326, -3.027376345333610441, -5.243569643749999898 ) ) ;
#70529=CARTESIAN_POINT ( 'NONE',  ( 18.75937500061451857, -4.541064518000417216, -2.621784821875001281 ) ) ;
#70530=CARTESIAN_POINT ( 'NONE',  ( 28.17187500061451644, -6.054752690667223547, -1.112240025338166033E-15 ) ) ;
#70531=CARTESIAN_POINT ( 'NONE',  ( 4.153125000614515727, 0.000000000000000000, 5.243569643749999010 ) ) ;
#70532=CARTESIAN_POINT ( 'NONE',  ( 19.67812500061451786, 6.421520780324663323E-16, -5.243569643749999010 ) ) ;
#70533=CARTESIAN_POINT ( 'NONE',  ( -3.000416591977282496E-16, 14.74062500061451786, 25.09994784771203058 ) ) ;
#70534=CARTESIAN_POINT ( 'NONE',  ( 16.23750000122903359, -4.330127018922194537, 2.499999999999995559 ) ) ;
#70536=CARTESIAN_POINT ( 'NONE',  ( 7.340625000614518392, -3.027376345333614438, 5.243569643749998122 ) ) ;
#70537=CARTESIAN_POINT ( 'NONE',  ( 29.09062500061451573, -3.027376345333610441, -5.243569643749999898 ) ) ;
#70538=CARTESIAN_POINT ( 'NONE',  ( 23.10937500061451644, 0.000000000000000000, 5.243569643749999010 ) ) ;
#70539=CARTESIAN_POINT ( 'NONE',  ( 14.99062500061451786, -3.027376345333614438, 5.243569643749998122 ) ) ;
#70540=CARTESIAN_POINT ( 'NONE',  ( 25.68750000122903288, -4.330127018922194537, 2.499999999999995559 ) ) ;
#70541=CARTESIAN_POINT ( 'NONE',  ( 23.61562500061451431, -6.054752690667223547, -1.112240025338166033E-15 ) ) ;
#70542=CARTESIAN_POINT ( 'NONE',  ( 18.75937500061451857, -4.541064518000417216, -2.621784821875001281 ) ) ;
#70543=CARTESIAN_POINT ( 'NONE',  ( 15.70312500061451644, 4.541064518000418104, -2.621784821874998173 ) ) ;
#70544=CARTESIAN_POINT ( 'NONE',  ( -4.243569643749999898, 14.87187500061451928, 27.54997392385601529 ) ) ;
#70545=CARTESIAN_POINT ( 'NONE',  ( 20.72812500061451502, 4.541064518000418104, 2.621784821874999949 ) ) ;
#70546=CARTESIAN_POINT ( 'NONE',  ( 28.52812500061451573, -4.541064518000419881, 2.621784821874995952 ) ) ;
#70547=ORIENTED_EDGE ( 'NONE', *, *, #65932, .T. ) ;
#70549=CARTESIAN_POINT ( 'NONE',  ( 23.21250000000000213, 2.886751345948126879, 4.999999999999999112 ) ) ;
#70550=CARTESIAN_POINT ( 'NONE',  ( -3.000416591977282496E-16, 19.74687500061451928, -34.90005215228797653 ) ) ;
#70552=CARTESIAN_POINT ( 'NONE',  ( 27.55312500061451786, 0.000000000000000000, 5.243569643749999010 ) ) ;
#70553=CARTESIAN_POINT ( 'NONE',  ( 8.278125000614515727, -4.541064518000419881, 2.621784821874995952 ) ) ;
#70554=CARTESIAN_POINT ( 'NONE',  ( 20.10000000122903074, 5.773502691896255534, 3.535250795749688894E-16 ) ) ;
#70555=CARTESIAN_POINT ( 'NONE',  ( 25.97812500061451502, 6.421520780324663323E-16, -5.243569643749999010 ) ) ;
#70556=CARTESIAN_POINT ( 'NONE',  ( 24.41250000000000142, 2.886751345948129099, -4.999999999999998224 ) ) ;
#70557=CARTESIAN_POINT ( 'NONE',  ( 26.95312500061451644, 4.541064518000418104, -2.621784821874998173 ) ) ;
#70558=CARTESIAN_POINT ( 'NONE',  ( 9.140625000614518214, -3.027376345333614438, 5.243569643749998122 ) ) ;
#70559=VERTEX_POINT ( 'NONE', #1635 ) ;
#70560=CARTESIAN_POINT ( 'NONE',  ( 22.56562500061451715, 3.027376345333611329, 5.243569643749999010 ) ) ;
#70561=CARTESIAN_POINT ( 'NONE',  ( 4.940625000614515372, 6.054752690667223547, 3.707466751127219781E-16 ) ) ;
#70562=UNCERTAINTY_MEASURE_WITH_UNIT (LENGTH_MEASURE( 1.000000000000000082E-05 ), #54189, 'distance_accuracy_value', 'NONE');
#70564=CARTESIAN_POINT ( 'NONE',  ( 3.290625000614516793, -3.027376345333614438, 5.243569643749998122 ) ) ;
#70565=CARTESIAN_POINT ( 'NONE',  ( 2.121784821874999061, 19.70937500061451786, -33.67503911421598417 ) ) ;
#70566=CARTESIAN_POINT ( 'NONE',  ( 13.95000000000000107, -4.330127018922190985, -2.500000000000001332 ) ) ;
#70567=CARTESIAN_POINT ( 'NONE',  ( 14.33437500061451786, 6.421520780324663323E-16, -5.243569643749999010 ) ) ;
#70568=CARTESIAN_POINT ( 'NONE',  ( 8.212500001229035007, -4.330127018922190985, -2.500000000000001332 ) ) ;
#70569=CARTESIAN_POINT ( 'NONE',  ( 15.49687500061451750, -3.027376345333614438, 5.243569643749998122 ) ) ;
#70571=CARTESIAN_POINT ( 'NONE',  ( 8.896875000614517859, -3.027376345333610441, -5.243569643749999898 ) ) ;
#70574=CARTESIAN_POINT ( 'NONE',  ( 12.57187500061451857, 3.027376345333613106, -5.243569643749998122 ) ) ;
#70576=CARTESIAN_POINT ( 'NONE',  ( 23.16562500061451502, -6.054752690667223547, -1.112240025338166033E-15 ) ) ;
#70577=DIRECTION ( 'NONE',  ( -1.000000000000000000, -0.000000000000000000, -0.000000000000000000 ) ) ;
#70579=CARTESIAN_POINT ( 'NONE',  ( 26.25937500061451857, 0.000000000000000000, 5.243569643749999010 ) ) ;
#70580=CARTESIAN_POINT ( 'NONE',  ( 4.490625000614516971, 6.054752690667223547, 3.707466751127219781E-16 ) ) ;
#70582=CARTESIAN_POINT ( 'NONE',  ( 16.99687500061451573, -3.027376345333610441, -5.243569643749999898 ) ) ;
#70584=CARTESIAN_POINT ( 'NONE',  ( 26.55000000122902648, -2.886751345948129988, 4.999999999999997335 ) ) ;
#70585=CARTESIAN_POINT ( 'NONE',  ( 6.159375000614517148, -4.541064518000417216, -2.621784821875001281 ) ) ;
#70586=CARTESIAN_POINT ( 'NONE',  ( 15.60937500061451644, -4.541064518000417216, -2.621784821875001281 ) ) ;
#70587=CARTESIAN_POINT ( 'NONE',  ( 6.600000000000001421, 0.000000000000000000, 4.999999999999998224 ) ) ;
#70588=CARTESIAN_POINT ( 'NONE',  ( 24.75000000000000000, -4.330127018922190985, -2.500000000000001332 ) ) ;
#70589=CARTESIAN_POINT ( 'NONE',  ( 27.60937500061451644, 0.000000000000000000, 5.243569643749999010 ) ) ;
#70592=CARTESIAN_POINT ( 'NONE',  ( 7.237500000000000711, -2.886751345948125991, -5.000000000000000000 ) ) ;
#70594=CARTESIAN_POINT ( 'NONE',  ( 22.97812500061451857, 4.541064518000418104, 2.621784821874999949 ) ) ;
#70595=CARTESIAN_POINT ( 'NONE',  ( 12.78749999999999964, 5.773502691896255534, 3.535250795749688894E-16 ) ) ;
#70596=( BOUNDED_CURVE ( )  B_SPLINE_CURVE ( 2, ( #53632, #54371, #30730, #2300, #59522, #53262, #8935 ),
 .UNSPECIFIED., .F., .F. ) 
 B_SPLINE_CURVE_WITH_KNOTS ( ( 3, 2, 2, 3 ),
 ( 0.5416666666666666297, 0.5444444444444443976, 0.5472222222222222765, 0.5500000000000000444 ),
 .UNSPECIFIED. ) 
 CURVE ( )  GEOMETRIC_REPRESENTATION_ITEM ( )  RATIONAL_B_SPLINE_CURVE ( ( 1.000000000000000000, 0.8660254037844387076, 1.000000000000000000, 0.8660254037844387076, 1.000000000000000000, 0.8660254037844387076, 1.000000000000000000 ) ) 
 REPRESENTATION_ITEM ( '' )  );
#70597=CARTESIAN_POINT ( 'NONE',  ( 6.028125000614517504, -4.541064518000419881, 2.621784821874995952 ) ) ;
#70598=CARTESIAN_POINT ( 'NONE',  ( 18.59999999999999787, 4.330127018922192761, -2.499999999999997780 ) ) ;
#70599=ADVANCED_FACE ( 'NONE', ( #68502 ), #40425, .F. ) ;
#70600=CARTESIAN_POINT ( 'NONE',  ( 19.34062500061451573, 6.054752690667223547, 3.707466751127219781E-16 ) ) ;
#70601=CARTESIAN_POINT ( 'NONE',  ( 14.88749999999999929, -2.886751345948126435, -5.000000000000000000 ) ) ;
#70602=CARTESIAN_POINT ( 'NONE',  ( 24.26250000122903216, 0.000000000000000000, 4.999999999999998224 ) ) ;
#70604=CARTESIAN_POINT ( 'NONE',  ( 5.437500000000001776, -2.886751345948125991, -5.000000000000000000 ) ) ;
#70606=CARTESIAN_POINT ( 'NONE',  ( 19.52812500061451573, -4.541064518000419881, 2.621784821874995952 ) ) ;
#70607=CARTESIAN_POINT ( 'NONE',  ( 27.66562500061451146, -6.054752690667223547, -1.112240025338166033E-15 ) ) ;
#70608=CARTESIAN_POINT ( 'NONE',  ( 24.15937500061451715, -4.541064518000417216, -2.621784821875001281 ) ) ;
#70609=CARTESIAN_POINT ( 'NONE',  ( 7.912499999999999645, 2.886751345948126879, 4.999999999999999112 ) ) ;
#70610=CARTESIAN_POINT ( 'NONE',  ( 11.84062500061451750, -3.027376345333614438, 5.243569643749998122 ) ) ;
#70611=CARTESIAN_POINT ( 'NONE',  ( 26.76562500061451644, -6.054752690667223547, -1.112240025338166033E-15 ) ) ;
#70612=CARTESIAN_POINT ( 'NONE',  ( 15.94687500061451502, -3.027376345333614438, 5.243569643749998122 ) ) ;
#70613=CARTESIAN_POINT ( 'NONE',  ( 9.028125000614517504, 4.541064518000418104, 2.621784821874999949 ) ) ;
#70614=CARTESIAN_POINT ( 'NONE',  ( 4.243569643749999898, 11.49687500061451928, 32.45002607614398471 ) ) ;
#70615=CARTESIAN_POINT ( 'NONE',  ( 23.81250000122903288, 0.000000000000000000, 4.999999999999998224 ) ) ;
#70617=CARTESIAN_POINT ( 'NONE',  ( 13.19062500061451537, -3.027376345333614438, 5.243569643749998122 ) ) ;
#70618=CARTESIAN_POINT ( 'NONE',  ( 10.62187500061451928, -6.054752690667223547, -1.112240025338166033E-15 ) ) ;
#70619=CARTESIAN_POINT ( 'NONE',  ( 9.834375000614517859, 6.421520780324663323E-16, -5.243569643749999010 ) ) ;
#70621=CARTESIAN_POINT ( 'NONE',  ( 21.70312500061451644, 0.000000000000000000, 5.243569643749999010 ) ) ;
#70622=CARTESIAN_POINT ( 'NONE',  ( 16.65937500061452070, 4.541064518000418104, -2.621784821874998173 ) ) ;
#70623=CARTESIAN_POINT ( 'NONE',  ( 22.75312500061451360, -4.541064518000417216, -2.621784821875001281 ) ) ;
#70624=CARTESIAN_POINT ( 'NONE',  ( -3.999999999999999556, 12.31250000000000000, 27.69059892324149530 ) ) ;
#70625=CARTESIAN_POINT ( 'NONE',  ( 28.00312500061451715, 0.000000000000000000, 5.243569643749999010 ) ) ;
#70626=CARTESIAN_POINT ( 'NONE',  ( 6.450000001229034829, -2.886751345948125991, -5.000000000000000000 ) ) ;
#70628=CARTESIAN_POINT ( 'NONE',  ( 29.58749999999999858, -2.886751345948129988, 4.999999999999997335 ) ) ;
#70629=CARTESIAN_POINT ( 'NONE',  ( -3.999999999999999556, 17.71249999999999858, -32.30940107675850470 ) ) ;
#70630=CARTESIAN_POINT ( 'NONE',  ( 23.62500000122902932, 2.886751345948129099, -4.999999999999998224 ) ) ;
#70632=CARTESIAN_POINT ( 'NONE',  ( 6.384375000614516793, 4.541064518000418104, 2.621784821874999949 ) ) ;
#70633=CARTESIAN_POINT ( 'NONE',  ( 4.396896640047911475, 2.380805009064795197, -4.642950682235516879 ) ) ;
#70634=CARTESIAN_POINT ( 'NONE',  ( 15.40312500061451573, 0.000000000000000000, 5.243569643749999010 ) ) ;
#70635=CARTESIAN_POINT ( 'NONE',  ( 7.996875000614519280, -3.027376345333610441, -5.243569643749999898 ) ) ;
#70636=CARTESIAN_POINT ( 'NONE',  ( 26.10000000122903430, -2.886751345948129988, 4.999999999999997335 ) ) ;
#70637=CARTESIAN_POINT ( 'NONE',  ( 16.95937500061451786, -4.541064518000417216, -2.621784821875001281 ) ) ;
#70638=CARTESIAN_POINT ( 'NONE',  ( 6.121875000614517504, -6.054752690667223547, -1.112240025338166033E-15 ) ) ;
#70640=CARTESIAN_POINT ( 'NONE',  ( 5.503125000614516260, 0.000000000000000000, 5.243569643749999010 ) ) ;
#70641=CARTESIAN_POINT ( 'NONE',  ( 16.26562500061451289, 3.027376345333611329, 5.243569643749999010 ) ) ;
#70642=EDGE_LOOP ( 'NONE', ( #5452, #42815, #60176, #59164 ) ) ;
#70643=CARTESIAN_POINT ( 'NONE',  ( 11.72812500061451857, 4.541064518000418104, 2.621784821874999949 ) ) ;
#70644=CARTESIAN_POINT ( 'NONE',  ( 4.687500001229034652, 6.123233995736764310E-16, -4.999999999999998224 ) ) ;
#70645=CARTESIAN_POINT ( 'NONE',  ( 10.34062500061451750, 6.054752690667223547, 3.707466751127219781E-16 ) ) ;
#70647=CARTESIAN_POINT ( 'NONE',  ( 11.32500000000000107, 6.123233995736764310E-16, -4.999999999999998224 ) ) ;
#70648=CARTESIAN_POINT ( 'NONE',  ( 4.050000001229035362, -2.886751345948129988, 4.999999999999997335 ) ) ;
#70649=CARTESIAN_POINT ( 'NONE',  ( 19.34999999999999787, -4.330127018922190985, -2.500000000000001332 ) ) ;
#70651=CARTESIAN_POINT ( 'NONE',  ( 15.87187500061451573, 3.027376345333611329, 5.243569643749999010 ) ) ;
#70652=CARTESIAN_POINT ( 'NONE',  ( 16.01250000122903216, 4.330127018922192761, -2.499999999999997780 ) ) ;
#70654=CARTESIAN_POINT ( 'NONE',  ( -2.121784821874999949, 17.92812500061451786, -33.67503911421598417 ) ) ;
#70655=CARTESIAN_POINT ( 'NONE',  ( -3.999999999999997335, 16.10000000122903430, 32.30940107675850470 ) ) ;
#70657=CARTESIAN_POINT ( 'NONE',  ( 28.41562500061451502, 3.027376345333611329, 5.243569643749999010 ) ) ;
#70660=CARTESIAN_POINT ( 'NONE',  ( 15.83437500061451608, 4.541064518000418104, 2.621784821874999949 ) ) ;
#70661=CARTESIAN_POINT ( 'NONE',  ( 29.28749999999999787, -2.886751345948125991, -5.000000000000000000 ) ) ;
#70662=CARTESIAN_POINT ( 'NONE',  ( 12.81562500061451537, -6.054752690667223547, -1.112240025338166033E-15 ) ) ;
#70664=CARTESIAN_POINT ( 'NONE',  ( 24.79687500061451999, 6.054752690667223547, 3.707466751127219781E-16 ) ) ;
#70666=CARTESIAN_POINT ( 'NONE',  ( 10.26562500061451644, 3.027376345333613106, -5.243569643749998122 ) ) ;
#70667=CARTESIAN_POINT ( 'NONE',  ( 13.50937500061451679, 4.541064518000418104, -2.621784821874998173 ) ) ;
#70669=CARTESIAN_POINT ( 'NONE',  ( 23.74687500061451573, -3.027376345333610441, -5.243569643749999898 ) ) ;
#70670=CARTESIAN_POINT ( 'NONE',  ( 27.62812500061451360, -4.541064518000419881, 2.621784821874995952 ) ) ;
#70671=ADVANCED_FACE ( 'NONE', ( #52231 ), #48590, .T. ) ;
#70672=DIRECTION ( 'NONE',  ( -0.000000000000000000, -1.000000000000000000, -0.000000000000000000 ) ) ;
#70673=CARTESIAN_POINT ( 'NONE',  ( 6.675000000000000711, -4.330127018922194537, 2.499999999999995559 ) ) ;
#70674=CARTESIAN_POINT ( 'NONE',  ( 16.05000000122903359, 5.773502691896255534, 3.535250795749688894E-16 ) ) ;
#70675=CARTESIAN_POINT ( 'NONE',  ( -1.999999999999997113, 17.93750000122903288, -26.53589838486224295 ) ) ;
#70676=FACE_OUTER_BOUND ( 'NONE', #64893, .T. ) ;
#70678=CARTESIAN_POINT ( 'NONE',  ( 14.28750000000000142, -2.886751345948129988, 4.999999999999997335 ) ) ;
#70679=CARTESIAN_POINT ( 'NONE',  ( 19.01249999999999929, 2.886751345948129099, -4.999999999999998224 ) ) ;
#70680=CARTESIAN_POINT ( 'NONE',  ( 14.35312500061451679, 4.541064518000418104, -2.621784821874998173 ) ) ;
#70682=CARTESIAN_POINT ( 'NONE',  ( 3.999999999999999112, 18.53750000122903430, -30.00000000000000000 ) ) ;
#70683=CARTESIAN_POINT ( 'NONE',  ( -3.000416591977282496E-16, 17.04687500061451644, -34.90005215228797653 ) ) ;
#70684=CARTESIAN_POINT ( 'NONE',  ( 6.928125000614516082, -4.541064518000419881, 2.621784821874995952 ) ) ;
#70686=CARTESIAN_POINT ( 'NONE',  ( 11.96250000000000213, 2.886751345948126879, 4.999999999999999112 ) ) ;
#70688=ORIENTED_EDGE ( 'NONE', *, *, #40125, .F. ) ;
#70689=CARTESIAN_POINT ( 'NONE',  ( 4.243569643749999898, 15.49062500061451786, 32.45002607614398471 ) ) ;
#70690=CARTESIAN_POINT ( 'NONE',  ( 27.47812500061451502, 4.541064518000418104, 2.621784821874999949 ) ) ;
#70691=DIRECTION ( 'NONE',  ( -0.000000000000000000, -1.000000000000000000, -0.000000000000000000 ) ) ;
#70693=CARTESIAN_POINT ( 'NONE',  ( 22.88437500061451857, 6.421520780324663323E-16, -5.243569643749999010 ) ) ;
#70694=CARTESIAN_POINT ( 'NONE',  ( 19.82812500061451644, 4.541064518000418104, 2.621784821874999949 ) ) ;
#70695=CARTESIAN_POINT ( 'NONE',  ( 4.243569643749999010, 13.31562500061459531, -32.45002607614398471 ) ) ;
#70696=CARTESIAN_POINT ( 'NONE',  ( 23.28750000122903430, 4.330127018922191873, 2.499999999999999556 ) ) ;
#70697=CARTESIAN_POINT ( 'NONE',  ( 4.490625000614516971, 6.054752690667223547, 3.707466751127219781E-16 ) ) ;
#70699=CARTESIAN_POINT ( 'NONE',  ( 20.46562500061451573, -6.054752690667223547, -1.112240025338166033E-15 ) ) ;
#70702=CARTESIAN_POINT ( 'NONE',  ( 16.54687500061451644, -3.027376345333610441, -5.243569643749999898 ) ) ;
#70703=CARTESIAN_POINT ( 'NONE',  ( 17.74687500061451928, -3.027376345333614438, 5.243569643749998122 ) ) ;
#70704=CARTESIAN_POINT ( 'NONE',  ( 23.70937500061451786, -4.541064518000417216, -2.621784821875001281 ) ) ;
#70705=CARTESIAN_POINT ( 'NONE',  ( -4.243569643749999898, 14.87187500061451928, 27.54997392385601529 ) ) ;
#70706=CARTESIAN_POINT ( 'NONE',  ( 4.265625000614517326, -6.054752690667223547, -1.112240025338166033E-15 ) ) ;
#70707=CARTESIAN_POINT ( 'NONE',  ( 28.64062500061451289, -3.027376345333610441, -5.243569643749999898 ) ) ;
#70708=CARTESIAN_POINT ( 'NONE',  ( 28.45312500061451289, 0.000000000000000000, 5.243569643749999010 ) ) ;
#70710=CARTESIAN_POINT ( 'NONE',  ( 3.999999999999999112, 19.32500000000000284, 30.00000000000000000 ) ) ;
#70711=CARTESIAN_POINT ( 'NONE',  ( 2.953125000614516438, -4.541064518000417216, -2.621784821875001281 ) ) ;
#70712=CARTESIAN_POINT ( 'NONE',  ( 6.534375000614517148, -4.541064518000419881, 2.621784821874995952 ) ) ;
#70713=CARTESIAN_POINT ( 'NONE',  ( 13.57500000122903572, -5.773502691896255534, -1.060575238724906372E-15 ) ) ;
#70714=CARTESIAN_POINT ( 'NONE',  ( 12.03750000122903430, 4.330127018922191873, 2.499999999999999556 ) ) ;
#70715=CARTESIAN_POINT ( 'NONE',  ( 4.678125000614516971, -4.541064518000419881, 2.621784821874995952 ) ) ;
#70718=CARTESIAN_POINT ( 'NONE',  ( 14.70937500061451786, -4.541064518000417216, -2.621784821875001281 ) ) ;
#70719=CARTESIAN_POINT ( 'NONE',  ( 21.22500000000000142, 6.123233995736764310E-16, -4.999999999999998224 ) ) ;
#70720=VERTEX_POINT ( 'NONE', #26675 ) ;
#70721=CARTESIAN_POINT ( 'NONE',  ( 22.45312500061451644, 4.541064518000418104, -2.621784821874998173 ) ) ;
#70722=CARTESIAN_POINT ( 'NONE',  ( 8.053125000614516082, 4.541064518000418104, -2.621784821874998173 ) ) ;
#70723=CARTESIAN_POINT ( 'NONE',  ( 24.60937500061451644, -4.541064518000417216, -2.621784821875001281 ) ) ;
#70724=CARTESIAN_POINT ( 'NONE',  ( 7.265625000614516438, 3.027376345333611329, 5.243569643749999010 ) ) ;
#70726=CARTESIAN_POINT ( 'NONE',  ( 7.875000001229034652, 2.886751345948129099, -4.999999999999998224 ) ) ;
#70727=CARTESIAN_POINT ( 'NONE',  ( 22.52812500061451573, 4.541064518000418104, 2.621784821874999949 ) ) ;
#70728=CARTESIAN_POINT ( 'NONE',  ( 4.243569643749999010, 11.51562500061451644, -32.45002607614398471 ) ) ;
#70729=CARTESIAN_POINT ( 'NONE',  ( 10.72500000122903252, 2.886751345948126879, 4.999999999999999112 ) ) ;
#70730=CARTESIAN_POINT ( 'NONE',  ( 19.86562500061451786, 3.027376345333611329, 5.243569643749999010 ) ) ;
#70731=CARTESIAN_POINT ( 'NONE',  ( 18.70312500061451644, -4.541064518000417216, -2.621784821875001281 ) ) ;
#70733=CARTESIAN_POINT ( 'NONE',  ( 17.21249999999999858, 2.886751345948129099, -4.999999999999998224 ) ) ;
#70734=CARTESIAN_POINT ( 'NONE',  ( 13.23750000122903359, 6.123233995736764310E-16, -4.999999999999998224 ) ) ;
#70735=CARTESIAN_POINT ( 'NONE',  ( 9.290625000614515017, -3.027376345333610441, -5.243569643749999898 ) ) ;
#70736=CARTESIAN_POINT ( 'NONE',  ( 14.24062500061451608, -3.027376345333610441, -5.243569643749999898 ) ) ;
#70737=ADVANCED_FACE ( 'NONE', ( #48836 ), #31843, .F. ) ;
#70738=CARTESIAN_POINT ( 'NONE',  ( 22.38750000122903216, 4.330127018922191873, 2.499999999999999556 ) ) ;
#70739=CARTESIAN_POINT ( 'NONE',  ( 22.73437500061451644, -4.541064518000419881, 2.621784821874995952 ) ) ;
#70740=CARTESIAN_POINT ( 'NONE',  ( 20.44687500061451857, -3.027376345333614438, 5.243569643749998122 ) ) ;
#70741=CARTESIAN_POINT ( 'NONE',  ( 3.581485683406023135, 3.488985925492861906, -3.914339967783176721 ) ) ;
#70743=EDGE_CURVE ( 'NONE', #5008, #68026, #49572, .T. ) ;
#70744=CARTESIAN_POINT ( 'NONE',  ( 7.012500001229035718, 4.330127018922192761, -2.499999999999997780 ) ) ;
#70745=CARTESIAN_POINT ( 'NONE',  ( 7.434375000614519280, -4.541064518000419881, 2.621784821874995952 ) ) ;
#70746=CARTESIAN_POINT ( 'NONE',  ( 22.62187500061451573, 3.027376345333611329, 5.243569643749999010 ) ) ;
#70749=CARTESIAN_POINT ( 'NONE',  ( 19.79062500061451502, 6.054752690667223547, 3.707466751127219781E-16 ) ) ;
#70750=CARTESIAN_POINT ( 'NONE',  ( 24.57187500061451502, -6.054752690667223547, -1.112240025338166033E-15 ) ) ;
#70752=LINE ( 'NONE', #36769, #10245 ) ;
#70754=CARTESIAN_POINT ( 'NONE',  ( 5.409375000614516260, 4.541064518000418104, -2.621784821874998173 ) ) ;
#70755=CARTESIAN_POINT ( 'NONE',  ( 16.34062500061451573, -3.027376345333614438, 5.243569643749998122 ) ) ;
#70756=CARTESIAN_POINT ( 'NONE',  ( 13.65937500061451715, 0.000000000000000000, 5.243569643749999010 ) ) ;
#70757=EDGE_LOOP ( 'NONE', ( #3097, #50429, #24557, #54296 ) ) ;
#70759=CARTESIAN_POINT ( 'NONE',  ( 24.17812500061451786, 6.421520780324663323E-16, -5.243569643749999010 ) ) ;
#70760=CARTESIAN_POINT ( 'NONE',  ( 3.517413553188016628, 3.553619953230496176, -3.820619027221005659 ) ) ;
#70762=CARTESIAN_POINT ( 'NONE',  ( 15.41250000000000142, 2.886751345948129099, -4.999999999999998224 ) ) ;
#70763=CARTESIAN_POINT ( 'NONE',  ( 23.70000000122903216, 5.773502691896255534, 3.535250795749688894E-16 ) ) ;
#70764=CARTESIAN_POINT ( 'NONE',  ( 18.17812500061451786, -4.541064518000419881, 2.621784821874995952 ) ) ;
#70765=VERTEX_POINT ( 'NONE', #32937 ) ;
#70766=CARTESIAN_POINT ( 'NONE',  ( 22.38749999999999929, -2.886751345948129988, 4.999999999999997335 ) ) ;
#70767=CARTESIAN_POINT ( 'NONE',  ( 24.04687500061451644, -3.027376345333614438, 5.243569643749998122 ) ) ;
#70768=ORIENTED_EDGE ( 'NONE', *, *, #19616, .T. ) ;
#70769=CARTESIAN_POINT ( 'NONE',  ( 13.31250000122903288, 4.330127018922192761, -2.499999999999997780 ) ) ;
#70770=CARTESIAN_POINT ( 'NONE',  ( 12.10312500061451857, 4.541064518000418104, -2.621784821874998173 ) ) ;
#70771=CARTESIAN_POINT ( 'NONE',  ( 4.228125000614517681, -4.541064518000419881, 2.621784821874995952 ) ) ;
#70773=CARTESIAN_POINT ( 'NONE',  ( 27.81562500061452070, 3.027376345333613106, -5.243569643749998122 ) ) ;
#70774=CARTESIAN_POINT ( 'NONE',  ( 12.90000000122903145, 5.773502691896255534, 3.535250795749688894E-16 ) ) ;
#70775=CARTESIAN_POINT ( 'NONE',  ( 19.79999999999999716, -4.330127018922190985, -2.500000000000001332 ) ) ;
#70776=CARTESIAN_POINT ( 'NONE',  ( 26.69999999999999929, 4.330127018922192761, -2.499999999999997780 ) ) ;
#70778=CARTESIAN_POINT ( 'NONE',  ( 6.309375000614517504, 4.541064518000418104, -2.621784821874998173 ) ) ;
#70779=CARTESIAN_POINT ( 'NONE',  ( 16.80937500061451573, 0.000000000000000000, 5.243569643749999010 ) ) ;
#70780=DIRECTION ( 'NONE',  ( 0.000000000000000000, 0.000000000000000000, 1.000000000000000000 ) ) ;
#70781=ORIENTED_EDGE ( 'NONE', *, *, #9299, .T. ) ;
#70782=CARTESIAN_POINT ( 'NONE',  ( 26.27812500061451573, -4.541064518000419881, 2.621784821874995952 ) ) ;
#70783=CARTESIAN_POINT ( 'NONE',  ( 26.67187500061451644, 3.027376345333611329, 5.243569643749999010 ) ) ;
#70785=ADVANCED_FACE ( 'NONE', ( #38107 ), #35408, .T. ) ;
#70786=CARTESIAN_POINT ( 'NONE',  ( 16.57499999999999929, -4.330127018922194537, 2.499999999999995559 ) ) ;
#70787=CARTESIAN_POINT ( 'NONE',  ( 14.27812500061451573, 6.421520780324663323E-16, -5.243569643749999010 ) ) ;
#70788=CARTESIAN_POINT ( 'NONE',  ( -3.999999999999999112, 15.01250000000000107, -32.30940107675850470 ) ) ;
#70790=CARTESIAN_POINT ( 'NONE',  ( 29.24062500061451431, 6.054752690667223547, 3.707466751127219781E-16 ) ) ;
#70791=CARTESIAN_POINT ( 'NONE',  ( 18.03750000122903430, -4.330127018922194537, 2.499999999999995559 ) ) ;
#70794=CARTESIAN_POINT ( 'NONE',  ( 4.078125000614517326, 4.541064518000418104, 2.621784821874999949 ) ) ;
#70795=CARTESIAN_POINT ( 'NONE',  ( 25.13437500061451502, 6.421520780324663323E-16, -5.243569643749999010 ) ) ;
#70796=CARTESIAN_POINT ( 'NONE',  ( -4.243569643749997233, 18.09687500061452070, 32.45002607614398471 ) ) ;
#70797=CARTESIAN_POINT ( 'NONE',  ( 24.83437500061451431, 4.541064518000418104, 2.621784821874999949 ) ) ;
#70798=CARTESIAN_POINT ( 'NONE',  ( 5.737499999999998934, -2.886751345948129988, 4.999999999999997335 ) ) ;
#70799=CARTESIAN_POINT ( 'NONE',  ( 8.484601909799253346E-16, 10.77500000122903501, 34.61880215351700230 ) ) ;
#70800=CARTESIAN_POINT ( 'NONE',  ( 12.14062500061451821, 6.054752690667223547, 3.707466751127219781E-16 ) ) ;
#70801=CARTESIAN_POINT ( 'NONE',  ( 3.562500001229033764, 0.000000000000000000, 4.999999999999998224 ) ) ;
#70802=CARTESIAN_POINT ( 'NONE',  ( 8.334375000614516082, -4.541064518000419881, 2.621784821874995952 ) ) ;
#70805=CARTESIAN_POINT ( 'NONE',  ( 11.09062500061451573, -3.027376345333610441, -5.243569643749999898 ) ) ;
#70806=CARTESIAN_POINT ( 'NONE',  ( 13.47187500061451537, 3.027376345333613106, -5.243569643749998122 ) ) ;
#70808=CARTESIAN_POINT ( 'NONE',  ( 22.68750000122903288, 6.123233995736764310E-16, -4.999999999999998224 ) ) ;
#70809=CARTESIAN_POINT ( 'NONE',  ( 10.02187500061451964, 3.027376345333611329, 5.243569643749999010 ) ) ;
#70810=CARTESIAN_POINT ( 'NONE',  ( 13.19062500061451537, -3.027376345333614438, 5.243569643749998122 ) ) ;
#70812=CARTESIAN_POINT ( 'NONE',  ( 20.55937500061451573, -4.541064518000417216, -2.621784821875001281 ) ) ;
#70814=CARTESIAN_POINT ( 'NONE',  ( -3.992479141629563077, 3.010095094815110617, 30.28109884793043705 ) ) ;
#70815=FACE_OUTER_BOUND ( 'NONE', #16224, .T. ) ;
#70816=CARTESIAN_POINT ( 'NONE',  ( -2.121784821874996840, 14.53437500061451715, -26.32496088578401583 ) ) ;
#70817=( BOUNDED_CURVE ( )  B_SPLINE_CURVE ( 2, ( #10387, #55093, #15914, #4493, #60988, #32919, #72439, #16281, #61352 ),
 .UNSPECIFIED., .F., .F. ) 
 B_SPLINE_CURVE_WITH_KNOTS ( ( 3, 2, 2, 2, 3 ),
 ( 0.7500000000000000000, 0.7536231884057971175, 0.7608695652173913526, 0.7681159420289854767, 0.7717391304347825942 ),
 .UNSPECIFIED. ) 
 CURVE ( )  GEOMETRIC_REPRESENTATION_ITEM ( )  RATIONAL_B_SPLINE_CURVE ( ( 0.9330127018922194093, 0.9330127018922194093, 1.000000000000000000, 0.8660254037844387076, 1.000000000000000000, 0.8660254037844387076, 1.000000000000000000, 0.9330127018922194093, 0.9330127018922194093 ) ) 
 REPRESENTATION_ITEM ( '' )  );
#70818=CARTESIAN_POINT ( 'NONE',  ( 15.98437500061451821, -4.541064518000419881, 2.621784821874995952 ) ) ;
#70819=CARTESIAN_POINT ( 'NONE',  ( 15.41250000122903252, -4.330127018922190985, -2.500000000000001332 ) ) ;
#70820=CARTESIAN_POINT ( 'NONE',  ( 12.15937500061451892, 4.541064518000418104, -2.621784821874998173 ) ) ;
#70821=CARTESIAN_POINT ( 'NONE',  ( 2.121784821874999061, 16.95312500061451999, -33.67503911421598417 ) ) ;
#70822=CARTESIAN_POINT ( 'NONE',  ( 17.13750000122903216, -4.330127018922194537, 2.499999999999995559 ) ) ;
#70823=CARTESIAN_POINT ( 'NONE',  ( 13.19062500061451537, -3.027376345333614438, 5.243569643749998122 ) ) ;
#70825=CARTESIAN_POINT ( 'NONE',  ( 16.57499999999999929, -4.330127018922194537, 2.499999999999995559 ) ) ;
#70826=CARTESIAN_POINT ( 'NONE',  ( 30.00000000000000000, 0.000000000000000000, 0.000000000000000000 ) ) ;
#70827=CARTESIAN_POINT ( 'NONE',  ( 9.759375000614516793, -4.541064518000417216, -2.621784821875001281 ) ) ;
#70828=CARTESIAN_POINT ( 'NONE',  ( 30.00000000000000000, 0.000000000000000000, 4.999999999999998224 ) ) ;
#70829=CARTESIAN_POINT ( 'NONE',  ( 11.70000000122903216, -2.886751345948129988, 4.999999999999997335 ) ) ;
#70830=CARTESIAN_POINT ( 'NONE',  ( 20.47500000122903074, 2.886751345948129099, -4.999999999999998224 ) ) ;
#70831=CARTESIAN_POINT ( 'NONE',  ( 17.65312500061451573, 0.000000000000000000, 5.243569643749999010 ) ) ;
#70832=CARTESIAN_POINT ( 'NONE',  ( 20.57812500061451644, 6.421520780324663323E-16, -5.243569643749999010 ) ) ;
#70833=CARTESIAN_POINT ( 'NONE',  ( 27.93750000122903288, -4.330127018922194537, 2.499999999999995559 ) ) ;
#70834=CARTESIAN_POINT ( 'NONE',  ( 3.628125000614518036, 4.541064518000418104, 2.621784821874999949 ) ) ;
#70835=CARTESIAN_POINT ( 'NONE',  ( 25.34999999999999787, 4.330127018922192761, -2.499999999999997780 ) ) ;
#70837=CARTESIAN_POINT ( 'NONE',  ( 28.54687500061451644, -3.027376345333614438, 5.243569643749998122 ) ) ;
#70838=CARTESIAN_POINT ( 'NONE',  ( 1.071796769724493892, 17.61740381056766580, 26.00000000000000711 ) ) ;
#70839=CARTESIAN_POINT ( 'NONE',  ( -3.000416591977282496E-16, 13.44687500061451857, -34.90005215228797653 ) ) ;
#70840=CARTESIAN_POINT ( 'NONE',  ( 3.075000001229035718, 2.886751345948126879, 4.999999999999999112 ) ) ;
#70841=CARTESIAN_POINT ( 'NONE',  ( 4.275000000000001243, 4.330127018922191873, 2.499999999999999556 ) ) ;
#70843=B_SPLINE_CURVE_WITH_KNOTS ( 'NONE', 3,
 ( #22903, #5929, #44012, #39558, #21457, #66913, #62083, #27383, #11476, #28463 ),
 .UNSPECIFIED., .F., .F.,
 ( 4, 3, 3, 4 ),
 ( 2.022162326929778336E-16, 5.625099572120405517E-05, 9.274853646366114607E-05, 0.0001292481992272784394 ),
 .UNSPECIFIED. ) ;
#70844=DIRECTION ( 'NONE',  ( 0.000000000000000000, 0.000000000000000000, -1.000000000000000000 ) ) ;
#70845=CARTESIAN_POINT ( 'NONE',  ( 7.584375000614516082, 6.421520780324663323E-16, -5.243569643749999010 ) ) ;
#70846=CARTESIAN_POINT ( 'NONE',  ( 26.35312500061451857, -4.541064518000417216, -2.621784821875001281 ) ) ;
#70848=CARTESIAN_POINT ( 'NONE',  ( 5.512499999999997513, 2.886751345948062486, -5.000000000000113687 ) ) ;
#70849=CARTESIAN_POINT ( 'NONE',  ( 8.175000000000002487, 6.123233995736764310E-16, -4.999999999999998224 ) ) ;
#70850=CARTESIAN_POINT ( 'NONE',  ( 5.071875000614519458, 3.027376345333611329, 5.243569643749999010 ) ) ;
#70851=CARTESIAN_POINT ( 'NONE',  ( 9.759375000614516793, -4.541064518000417216, -2.621784821875001281 ) ) ;
#70852=CARTESIAN_POINT ( 'NONE',  ( 3.149999999999999911, -4.330127018922190985, -2.500000000000001332 ) ) ;
#70853=( BOUNDED_CURVE ( )  B_SPLINE_CURVE ( 2, ( #38263, #60791, #30716, #52889, #28638, #51176, #56706, #39741, #943 ),
 .UNSPECIFIED., .F., .F. ) 
 B_SPLINE_CURVE_WITH_KNOTS ( ( 3, 2, 2, 2, 3 ),
 ( 0.8369565217391304879, 0.8405797101449274944, 0.8478260869565217295, 0.8550724637681159646, 0.8586956521739130821 ),
 .UNSPECIFIED. ) 
 CURVE ( )  GEOMETRIC_REPRESENTATION_ITEM ( )  RATIONAL_B_SPLINE_CURVE ( ( 0.9330127018922192983, 0.9330127018922202975, 1.000000000000000000, 0.8660254037844387076, 1.000000000000000000, 0.8660254037844387076, 1.000000000000000000, 0.9330127018922194093, 0.9330127018922194093 ) ) 
 REPRESENTATION_ITEM ( '' )  );
#70854=CARTESIAN_POINT ( 'NONE',  ( -4.243569643749999898, 12.60312500061459495, 30.00000000000000000 ) ) ;
#70855=CARTESIAN_POINT ( 'NONE',  ( 28.49999999999999645, 4.330127018922192761, -2.499999999999997780 ) ) ;
#70856=CARTESIAN_POINT ( 'NONE',  ( 4.237500000000001599, 5.773502691896255534, 3.535250795749688894E-16 ) ) ;
#70859=CARTESIAN_POINT ( 'NONE',  ( 20.01562500061451644, -6.054752690667223547, -1.112240025338166033E-15 ) ) ;
#70860=CARTESIAN_POINT ( 'NONE',  ( 10.15312500061451750, -4.541064518000417216, -2.621784821875001281 ) ) ;
#70862=CARTESIAN_POINT ( 'NONE',  ( 7.359375000614516438, 0.000000000000000000, 5.243569643749999010 ) ) ;
#70863=CARTESIAN_POINT ( 'NONE',  ( 23.17500000000000071, 4.330127018922191873, 2.499999999999999556 ) ) ;
#70864=CARTESIAN_POINT ( 'NONE',  ( 20.02500000122903145, 2.886751345948129099, -4.999999999999998224 ) ) ;
#70865=CARTESIAN_POINT ( 'NONE',  ( 27.14062500061451644, -3.027376345333614438, 5.243569643749998122 ) ) ;
#70866=CARTESIAN_POINT ( 'NONE',  ( 0.000000000000000000, 20.00000000000000000, -33.99999999999999289 ) ) ;
#70867=CARTESIAN_POINT ( 'NONE',  ( 8.746875000614515727, -3.027376345333614438, 5.243569643749998122 ) ) ;
#70868=CARTESIAN_POINT ( 'NONE',  ( 13.54687500061451999, 6.054752690667223547, 3.707466751127219781E-16 ) ) ;
#70869=CARTESIAN_POINT ( 'NONE',  ( 24.45937500061451786, 0.000000000000000000, 5.243569643749999010 ) ) ;
#70872=CARTESIAN_POINT ( 'NONE',  ( 20.25937500061451857, 4.541064518000418104, -2.621784821874998173 ) ) ;
#70873=CARTESIAN_POINT ( 'NONE',  ( 8.821875000614518569, -6.054752690667223547, -1.112240025338166033E-15 ) ) ;
#70875=CARTESIAN_POINT ( 'NONE',  ( 22.91249999999999432, -5.773502691896255534, -1.060575238724906372E-15 ) ) ;
#70877=CARTESIAN_POINT ( 'NONE',  ( 4.243569643749999898, 11.94687500061451857, -27.54997392385601529 ) ) ;
#70879=CARTESIAN_POINT ( 'NONE',  ( 13.79062500061451502, -3.027376345333610441, -5.243569643749999898 ) ) ;
#70880=CARTESIAN_POINT ( 'NONE',  ( 5.775000000000002132, -4.330127018922194537, 2.499999999999995559 ) ) ;
#70881=LINE ( 'NONE', #54990, #69098 ) ;
#70882=DIRECTION ( 'NONE',  ( 0.000000000000000000, 0.000000000000000000, 1.000000000000000000 ) ) ;
#70883=CARTESIAN_POINT ( 'NONE',  ( 12.63749999999999929, -2.886751345948125991, -5.000000000000000000 ) ) ;
#70884=CARTESIAN_POINT ( 'NONE',  ( 8.484601909799253346E-16, 18.87500000122903643, 34.61880215351700230 ) ) ;
#70885=CARTESIAN_POINT ( 'NONE',  ( 11.02500000122903501, 2.886751345948129099, -4.999999999999998224 ) ) ;
#70886=( BOUNDED_CURVE ( )  B_SPLINE_CURVE ( 2, ( #58956, #60057, #14265, #37167, #31262, #70788, #19429, #65610, #19802 ),
 .UNSPECIFIED., .F., .F. ) 
 B_SPLINE_CURVE_WITH_KNOTS ( ( 3, 2, 2, 2, 3 ),
 ( 0.4673913043478261087, 0.4710144927536231707, 0.4782608695652174058, 0.4855072463768115854, 0.4891304347826087029 ),
 .UNSPECIFIED. ) 
 CURVE ( )  GEOMETRIC_REPRESENTATION_ITEM ( )  RATIONAL_B_SPLINE_CURVE ( ( 0.9330127018922194093, 0.9330127018922198534, 1.000000000000000000, 0.8660254037844387076, 1.000000000000000000, 0.8660254037844387076, 1.000000000000000000, 0.9330127018922194093, 0.9330127018922194093 ) ) 
 REPRESENTATION_ITEM ( '' )  );
#70887=CARTESIAN_POINT ( 'NONE',  ( 23.18437500061451573, -4.541064518000419881, 2.621784821874995952 ) ) ;
#70888=CARTESIAN_POINT ( 'NONE',  ( 15.75937500061451857, 4.541064518000418104, -2.621784821874998173 ) ) ;
#70889=DIRECTION ( 'NONE',  ( 0.000000000000000000, 1.000000000000000000, 0.000000000000000000 ) ) ;
#70890=ORIENTED_EDGE ( 'NONE', *, *, #17622, .F. ) ;
#70891=CARTESIAN_POINT ( 'NONE',  ( 18.21562500061451573, -6.054752690667223547, -1.112240025338166033E-15 ) ) ;
#70892=CARTESIAN_POINT ( 'NONE',  ( 2.878125000614517592, -4.541064518000419881, 2.621784821874995952 ) ) ;
#70893=CARTESIAN_POINT ( 'NONE',  ( 18.53437500061451715, 4.541064518000418104, 2.621784821874999949 ) ) ;
#70894=CARTESIAN_POINT ( 'NONE',  ( 28.62187500061451573, -6.054752690667223547, -1.112240025338166033E-15 ) ) ;
#70895=CARTESIAN_POINT ( 'NONE',  ( 5.203125000614518214, -4.541064518000417216, -2.621784821875001281 ) ) ;
#70896=CARTESIAN_POINT ( 'NONE',  ( 19.82812500061451644, 4.541064518000418104, 2.621784821874999949 ) ) ;
#70898=CARTESIAN_POINT ( 'NONE',  ( -2.121784821874996840, 13.57812500061451644, 33.67503911421598417 ) ) ;
#70899=CARTESIAN_POINT ( 'NONE',  ( 17.32500000122903216, 2.886751345948129099, -4.999999999999998224 ) ) ;
#70901=CARTESIAN_POINT ( 'NONE',  ( 7.453125000614516438, -4.541064518000417216, -2.621784821875001281 ) ) ;
#70902=CARTESIAN_POINT ( 'NONE',  ( 27.89062500061451289, 6.054752690667223547, 3.707466751127219781E-16 ) ) ;
#70903=CARTESIAN_POINT ( 'NONE',  ( 9.637500001229033941, 6.123233995736764310E-16, -4.999999999999998224 ) ) ;
#70904=CARTESIAN_POINT ( 'NONE',  ( 23.63437500061451502, -4.541064518000419881, 2.621784821874995952 ) ) ;
#70905=CARTESIAN_POINT ( 'NONE',  ( 13.79062500061451502, -3.027376345333610441, -5.243569643749999898 ) ) ;
#70906=CARTESIAN_POINT ( 'NONE',  ( 21.67500000122903359, -5.773502691896255534, -1.060575238724906372E-15 ) ) ;
#70907=CARTESIAN_POINT ( 'NONE',  ( 23.76562500061451644, 3.027376345333613106, -5.243569643749998122 ) ) ;
#70908=CARTESIAN_POINT ( 'NONE',  ( 18.79687500061451644, -3.027376345333610441, -5.243569643749999898 ) ) ;
#70909=CARTESIAN_POINT ( 'NONE',  ( 15.47812500061451679, -4.541064518000419881, 2.621784821874995952 ) ) ;
#70910=CARTESIAN_POINT ( 'NONE',  ( 2.121784821874999061, 13.85937500061451821, 26.32496088578401583 ) ) ;
#70911=( BOUNDED_CURVE ( )  B_SPLINE_CURVE ( 2, ( #31688, #65661, #43138, #33141, #71581, #55679, #63652 ),
 .UNSPECIFIED., .F., .F. ) 
 B_SPLINE_CURVE_WITH_KNOTS ( ( 3, 2, 2, 3 ),
 ( 0.2666666666666666075, 0.2694444444444444309, 0.2722222222222221988, 0.2750000000000000777 ),
 .UNSPECIFIED. ) 
 CURVE ( )  GEOMETRIC_REPRESENTATION_ITEM ( )  RATIONAL_B_SPLINE_CURVE ( ( 1.000000000000002665, 0.8660254037844360431, 1.000000000000000000, 0.8660254037844387076, 1.000000000000000000, 0.8660254037844360431, 1.000000000000002665 ) ) 
 REPRESENTATION_ITEM ( '' )  );
#70912=CARTESIAN_POINT ( 'NONE',  ( 18.85312500061451502, 4.541064518000418104, -2.621784821874998173 ) ) ;
#70913=CARTESIAN_POINT ( 'NONE',  ( 29.76562500061451644, 3.027376345333611329, 5.243569643749999010 ) ) ;
#70916=CARTESIAN_POINT ( 'NONE',  ( 23.58749999999999858, 5.773502691896255534, 3.535250795749688894E-16 ) ) ;
#70917=CARTESIAN_POINT ( 'NONE',  ( -2.000000000000000000, 10.02500000000000036, -33.46410161513775705 ) ) ;
#70918=CARTESIAN_POINT ( 'NONE',  ( 3.794436392317134921, -3.256190485932382472, -3.923912810455655542 ) ) ;
#70919=CARTESIAN_POINT ( 'NONE',  ( 25.86562500061451431, -6.054752690667223547, -1.112240025338166033E-15 ) ) ;
#70920=CARTESIAN_POINT ( 'NONE',  ( 7.003125000614518036, -4.541064518000417216, -2.621784821875001281 ) ) ;
#70921=CARTESIAN_POINT ( 'NONE',  ( 19.01250000122903216, -4.330127018922190985, -2.500000000000001332 ) ) ;
#70922=CARTESIAN_POINT ( 'NONE',  ( 24.36562500061451786, 3.027376345333611329, 5.243569643749999010 ) ) ;
#70923=CARTESIAN_POINT ( 'NONE',  ( 24.14999999999999858, 0.000000000000000000, 4.999999999999998224 ) ) ;
#70924=CARTESIAN_POINT ( 'NONE',  ( 28.64062500061451289, -3.027376345333610441, -5.243569643749999898 ) ) ;
#70925=CARTESIAN_POINT ( 'NONE',  ( 8.240625000614516082, -3.027376345333614438, 5.243569643749998122 ) ) ;
#70927=CARTESIAN_POINT ( 'NONE',  ( 22.37812500061451360, 6.421520780324663323E-16, -5.243569643749999010 ) ) ;
#70928=CARTESIAN_POINT ( 'NONE',  ( 5.390625000614518214, 6.054752690667223547, 3.707466751127219781E-16 ) ) ;
#70930=CARTESIAN_POINT ( 'NONE',  ( 3.440625000614518036, -3.027376345333610441, -5.243569643749999898 ) ) ;
#70931=CARTESIAN_POINT ( 'NONE',  ( -3.999999999999999112, 13.36250000122903359, -30.00000000000000000 ) ) ;
#70934=CARTESIAN_POINT ( 'NONE',  ( 11.62500000000000000, -4.330127018922194537, 2.499999999999995559 ) ) ;
#70935=CARTESIAN_POINT ( 'NONE',  ( 11.44687500061451857, -3.027376345333614438, 5.243569643749998122 ) ) ;
#70936=CARTESIAN_POINT ( 'NONE',  ( 7.950000001229033053, 5.773502691896255534, 3.535250795749688894E-16 ) ) ;
#70937=CARTESIAN_POINT ( 'NONE',  ( 14.37187500061451928, 3.027376345333613106, -5.243569643749998122 ) ) ;
#70939=CARTESIAN_POINT ( 'NONE',  ( 7.134375000614516793, 6.421520780324663323E-16, -5.243569643749999010 ) ) ;
#70940=DIRECTION ( 'NONE',  ( -1.000000000000000000, -0.000000000000000000, -0.000000000000000000 ) ) ;
#70941=DIRECTION ( 'NONE',  ( -1.000000000000000000, -0.000000000000000000, -0.000000000000000000 ) ) ;
#70942=CARTESIAN_POINT ( 'NONE',  ( 12.12187500061451573, 3.027376345333613106, -5.243569643749998122 ) ) ;
#70943=CARTESIAN_POINT ( 'NONE',  ( 3.651773823418189124, 3.415340091791402966, 3.978752903393068863 ) ) ;
#70944=CARTESIAN_POINT ( 'NONE',  ( 22.82812500061451644, 6.421520780324663323E-16, -5.243569643749999010 ) ) ;
#70945=CARTESIAN_POINT ( 'NONE',  ( 4.243569643749999898, 11.08437500061451786, 30.00000000000000000 ) ) ;
#70946=CARTESIAN_POINT ( 'NONE',  ( -4.243569643749998122, 19.39062500061459104, 32.45002607614398471 ) ) ;
#70947=CARTESIAN_POINT ( 'NONE',  ( 27.00937500061451857, 4.541064518000418104, -2.621784821874998173 ) ) ;
#70948=CARTESIAN_POINT ( 'NONE',  ( 29.62500000000000000, -4.330127018922194537, 2.499999999999995559 ) ) ;
#70949=CARTESIAN_POINT ( 'NONE',  ( 5.165625000614518569, -6.054752690667223547, -1.112240025338166033E-15 ) ) ;
#70951=CARTESIAN_POINT ( 'NONE',  ( 17.44687500061451857, -3.027376345333610441, -5.243569643749999898 ) ) ;
#70953=CARTESIAN_POINT ( 'NONE',  ( 26.32500000122903216, 2.886751345948129099, -4.999999999999998224 ) ) ;
#70954=CARTESIAN_POINT ( 'NONE',  ( 5.296875000614518214, -3.027376345333610441, -5.243569643749999898 ) ) ;
#70955=CARTESIAN_POINT ( 'NONE',  ( 16.02187500061451786, -6.054752690667223547, -1.112240025338166033E-15 ) ) ;
#70956=CARTESIAN_POINT ( 'NONE',  ( 24.60000000000000142, 0.000000000000000000, 4.999999999999998224 ) ) ;
#70957=CARTESIAN_POINT ( 'NONE',  ( 4.387500001229033053, 4.330127018922191873, 2.499999999999999556 ) ) ;
#70958=CARTESIAN_POINT ( 'NONE',  ( 27.23437500061451644, -4.541064518000419881, 2.621784821874995952 ) ) ;
#70960=CARTESIAN_POINT ( 'NONE',  ( 5.662500001229035185, 4.330127018922192761, -2.499999999999997780 ) ) ;
#70961=CARTESIAN_POINT ( 'NONE',  ( 7.312500000000000000, 2.886751345948129099, -4.999999999999998224 ) ) ;
#70963=CARTESIAN_POINT ( 'NONE',  ( 22.22812500061451502, -4.541064518000419881, 2.621784821874995952 ) ) ;
#70964=CARTESIAN_POINT ( 'NONE',  ( 11.47499999999999964, 4.330127018922191873, 2.499999999999999556 ) ) ;
#70965=CARTESIAN_POINT ( 'NONE',  ( 4.678125000614516971, -4.541064518000419881, 2.621784821874995952 ) ) ;
#70966=CARTESIAN_POINT ( 'NONE',  ( 19.68750000000000355, -2.886751345948129988, 4.999999999999997335 ) ) ;
#70967=CARTESIAN_POINT ( 'NONE',  ( 19.19062500061452070, -3.027376345333610441, -5.243569643749999898 ) ) ;
#70968=CARTESIAN_POINT ( 'NONE',  ( -2.556497649636125342E-15, 18.87500000122903288, 34.00000000000000000 ) ) ;
#70969=CARTESIAN_POINT ( 'NONE',  ( 23.10000000122903074, -2.886751345948125991, -5.000000000000000000 ) ) ;
#70971=CARTESIAN_POINT ( 'NONE',  ( 3.712499999999999911, 2.886751345948129099, -4.999999999999998224 ) ) ;
#70972=ORIENTED_EDGE ( 'NONE', *, *, #61389, .F. ) ;
#70973=CARTESIAN_POINT ( 'NONE',  ( 20.05312500061451431, -4.541064518000417216, -2.621784821875001281 ) ) ;
#70974=CARTESIAN_POINT ( 'NONE',  ( 25.37812500061451715, -4.541064518000419881, 2.621784821874995952 ) ) ;
#70975=CARTESIAN_POINT ( 'NONE',  ( 23.93437500061451573, 4.541064518000418104, 2.621784821874999949 ) ) ;
#70976=CARTESIAN_POINT ( 'NONE',  ( 9.600000000000001421, 4.330127018922192761, -2.499999999999997780 ) ) ;
#70977=CARTESIAN_POINT ( 'NONE',  ( 12.89062500061451821, -3.027376345333610441, -5.243569643749999898 ) ) ;
#70978=CARTESIAN_POINT ( 'NONE',  ( 25.82812500061451644, -4.541064518000419881, 2.621784821874995952 ) ) ;
#70979=CARTESIAN_POINT ( 'NONE',  ( 16.39687500061451786, -3.027376345333614438, 5.243569643749998122 ) ) ;
#70980=CARTESIAN_POINT ( 'NONE',  ( 8.240625000614516082, -3.027376345333614438, 5.243569643749998122 ) ) ;
#70982=CARTESIAN_POINT ( 'NONE',  ( 4.243569643749999010, 11.57187500061451679, 27.54997392385601174 ) ) ;
#70983=CARTESIAN_POINT ( 'NONE',  ( 24.67500000122903359, 2.886751345948126879, 4.999999999999999112 ) ) ;
#70985=CARTESIAN_POINT ( 'NONE',  ( 15.40312500061451573, 0.000000000000000000, 5.243569643749999010 ) ) ;
#70986=CARTESIAN_POINT ( 'NONE',  ( 7.659375000614518036, 4.541064518000418104, -2.621784821874998173 ) ) ;
#70987=CARTESIAN_POINT ( 'NONE',  ( 10.69687500061451679, -3.027376345333610441, -5.243569643749999898 ) ) ;
#70988=ORIENTED_EDGE ( 'NONE', *, *, #39769, .F. ) ;
#70989=CARTESIAN_POINT ( 'NONE',  ( 29.52187500061451431, -6.054752690667223547, -1.112240025338166033E-15 ) ) ;
#70990=CARTESIAN_POINT ( 'NONE',  ( 20.72812500061451502, 4.541064518000418104, 2.621784821874999949 ) ) ;
#70991=CARTESIAN_POINT ( 'NONE',  ( 17.63437500061451502, 4.541064518000418104, 2.621784821874999949 ) ) ;
#70992=CARTESIAN_POINT ( 'NONE',  ( 21.96562500061451573, 3.027376345333613106, -5.243569643749998122 ) ) ;
#70993=CARTESIAN_POINT ( 'NONE',  ( -2.000000000000000000, 12.27500000000000036, 26.53589838486224650 ) ) ;
#70994=CARTESIAN_POINT ( 'NONE',  ( 26.87812500061451360, 6.421520780324663323E-16, -5.243569643749999010 ) ) ;
#70995=CARTESIAN_POINT ( 'NONE',  ( 6.487500001229034474, 6.123233995736764310E-16, -4.999999999999998224 ) ) ;
#70998=CARTESIAN_POINT ( 'NONE',  ( -3.999999999999999112, 17.30000000000000071, -30.00000000000000000 ) ) ;
#70999=CARTESIAN_POINT ( 'NONE',  ( 25.76250000122903216, -4.330127018922190985, -2.500000000000001332 ) ) ;
#71001=CARTESIAN_POINT ( 'NONE',  ( 7.846875000614518036, -3.027376345333614438, 5.243569643749998122 ) ) ;
#71002=CARTESIAN_POINT ( 'NONE',  ( 4.352828865414680948, 2.460460882526558812, -4.510749027574212811 ) ) ;
#71003=CARTESIAN_POINT ( 'NONE',  ( 14.57812500061451644, -4.541064518000419881, 2.621784821874995952 ) ) ;
#71004=CARTESIAN_POINT ( 'NONE',  ( 8.446875000614518569, -3.027376345333610441, -5.243569643749999898 ) ) ;
#71005=CARTESIAN_POINT ( 'NONE',  ( 27.67500000122903359, 2.886751345948129099, -4.999999999999998224 ) ) ;
#71006=CARTESIAN_POINT ( 'NONE',  ( 17.18437500061451573, 4.541064518000418104, 2.621784821874999949 ) ) ;
#71007=CARTESIAN_POINT ( 'NONE',  ( 5.184375000614516615, -4.541064518000419881, 2.621784821874995952 ) ) ;
#71008=CARTESIAN_POINT ( 'NONE',  ( -1.999999999999997113, 11.07500000000000107, 33.46410161513775705 ) ) ;
#71009=CARTESIAN_POINT ( 'NONE',  ( 5.053125000614517859, 0.000000000000000000, 5.243569643749999010 ) ) ;
#71010=CARTESIAN_POINT ( 'NONE',  ( 14.99062500061451786, -3.027376345333614438, 5.243569643749998122 ) ) ;
#71012=CARTESIAN_POINT ( 'NONE',  ( 13.37812500061451715, 6.421520780324663323E-16, -5.243569643749999010 ) ) ;
#71013=CARTESIAN_POINT ( 'NONE',  ( 6.075000001229034829, 2.886751345948129099, -4.999999999999998224 ) ) ;
#71014=CARTESIAN_POINT ( 'NONE',  ( 9.815625000614518925, 3.027376345333613106, -5.243569643749998122 ) ) ;
#71016=CARTESIAN_POINT ( 'NONE',  ( 10.80000000000000071, -4.330127018922190985, -2.500000000000001332 ) ) ;
#71017=CARTESIAN_POINT ( 'NONE',  ( 4.762500001229033941, 4.330127018922192761, -2.499999999999997780 ) ) ;
#71018=CARTESIAN_POINT ( 'NONE',  ( 17.73750000000000071, 5.773502691896255534, 3.535250795749688894E-16 ) ) ;
#71020=CARTESIAN_POINT ( 'NONE',  ( 17.67187500061451644, 3.027376345333611329, 5.243569643749999010 ) ) ;
#71021=CARTESIAN_POINT ( 'NONE',  ( 17.21250000122903145, -4.330127018922190985, -2.500000000000001332 ) ) ;
#71023=CARTESIAN_POINT ( 'NONE',  ( -2.121784821874996840, 17.62812500061451715, -26.32496088578401583 ) ) ;
#71025=CARTESIAN_POINT ( 'NONE',  ( 2.737500001229034474, -4.330127018922194537, 2.499999999999995559 ) ) ;
#71026=LINE ( 'NONE', #65480, #58364 ) ;
#71027=CARTESIAN_POINT ( 'NONE',  ( 28.71562500061451573, 3.027376345333613106, -5.243569643749998122 ) ) ;
#71028=CARTESIAN_POINT ( 'NONE',  ( 3.507483327083503521, -3.563363679198468859, 3.507483327083555924 ) ) ;
#71029=CARTESIAN_POINT ( 'NONE',  ( 3.939080010846523372, -3.079553322829319928, -4.243980907203444453 ) ) ;
#71030=CARTESIAN_POINT ( 'NONE',  ( 17.18437500061451573, 4.541064518000418104, 2.621784821874999949 ) ) ;
#71031=EDGE_CURVE ( 'NONE', #4525, #66981, #60787, .T. ) ;
#71032=( BOUNDED_SURFACE ( )  B_SPLINE_SURFACE ( 1, 2, ( 
 ( #62579, #68494, #23414, #57027, #68140, #19215, #52857, #7789, #25134, #51506, #6433, #23051, #17504, #40065, #30327, #53586, #31049, #63931, #45961, #70210, #2981, #35855, #47315, #11976, #906, #34499, #69848, #28968, #17858, #41769, #36592, #58746, #64298, #41415, #51141, #19585, #540, #45606, #13316, #58378, #14052, #2256, #8519, #24771, #13686, #36230, #2613, #8156, #30685, #53216, #47675, #42141, #64667, #59113, #21853, #69021, #5606, #23576, #29849, #23934, #44416, #27413, #46121, #61381, #18384, #28142, #63098, #33669, #22222, #39227, #44777, #46483, #72468, #66565, #56213, #66943, #1066, #44042, #16669, #29488, #10416, #49944, #12499, #57555, #50670, #67311, #63466, #15945, #35386, #40951, #16311, #68658, #40578, #18022, #61739, #10777, #35027, #12853, #38493, #6957, #52025, #1427, #57909, #7318, #27778, #52385, #33310, #61018, #1791, #32947, #11140, #38865, #55485, #55848, #4877, #5237, #50317, #72840, #50654, #71735, #4861, #21105, #65814, #61723, #11124, #33651, #56196, #43658, #28126, #58, #21472, #10761, #27397, #66180, #49927, #55469, #38476, #15558, #72452, #61000, #16295, #10399, #21836, #32931, #22564, #5589, #38101, #33294, #49201, #55832, #49566, #66547, #38849, #60623, #27035, #32568, #10033, #32201, #44400, #66926, #61364, #72823, #55106, #4506, #60254, #54735, #4137, #5219, #15196, #37734, #44025, #72088, #44760, #9668, #15926, #27761, #26668, #50301, #22206, #67295, #16653, #39211, #46191, #12923, #63171, #68732, #68007, #52458, #24006, #12566, #68369, #11848, #29918, #51736, #45474, #17379, #39937, #56548, #28475, #5942, #23646, #62450, #18457, #29201, #35100, #34731, #23283, #40289, #45832, #46554, #408, #67647, #57260, #22917, #1136, #45112, #17730, #29559, #11489, #51012, #57625, #7029, #6673, #62811, #63537, #17013, #35457, #41021, #34367, #18090, #40651, #52096, #12203, #56900, #1501, #69095, #39571, #57980, #7390, #1865, #62095, #34011, #28833, #6305, #51372, #775, #37288, #41378, #70172, #69812, #59074, #41731, #19549, #19178, #2576, #14015, #42471, #42106, #25470, #58340, #3318, #64629, #8478, #59440, #14746, #36190, #58708, #2941, #53179, #8119, #30647, #31383, #63889, #36919, #48381, #8847, #64994, #64259, #13279, #35818, #25095, #19917, #2221, #31012, #36554, #14384, #53923, #7750, #30287, #53545, #13646, #52819, #25844, #48016, #47639, #70908, #70542, #20280, #42834, #31753, #65356, #24371, #59811, #9216, #69457, #54290, #46919, #18815, #24734, #47278, #5136, #32843, #27671, #9580, #9943, #50209, #72366, #10311, #37648, #38014, #4774, #44675, #21746, #27308, #26576, #11036, #55742, #39119, #33561, #72733, #38761, #32481, #55380, #26948, #44308, #3683, #61634, #20648, #43937, #4419, #55014, #16567, #72006, #15111, #32112, #54646, #22120, #38384, #49841, #26207, #67206, #4050, #60171, #48746, #71644, #49116, #66091, #66837, #16208, #21017, #49474, #60536, #71270, #43205, #21381, #61280, #43570, #66461, #65725, #15838, #15470, #60907, #10673, #33203, #22833, #23565, #22477, #56466, #28389, #69011, #12843, #50927, #5857, #12122, #40942, #62003, #68287, #11405, #56110, #52016, #1417, #23923, #46473, #33924, #18374, #63456, #11765, #1054, #17647, #324, #40207, #45750, #28748, #45385, #62729, #51288, #6590, #689, #34648, #23197, #5500, #28039, #67921, #46110, #39481, #68647, #39855, #56813, #29119, #17292, #62367, #34281, #6220, #45027, #57176, #51653, #18011, #63088, #40568, #12489, #50568, #67562, #16927, #35016, #73095, #57545, #6947, #29478, #14298, #65269, #36105, #19462, #24290, #30203, #46838, #30568, #29838, #41651, #42748, #8033, #35739, #58626, #2139, #2856, #1779, #58258, #7664, #48294, #35376, #52734, #24650, #64541, #20194, #41297, #47556, #63807, #57899, #31295, #53836, #3231, #25758, #13199, #70820, #7308, #64172, #53465, #70085, #47196, #42020, #25014, #53094, #69727, #13934, #2490, #58989, #36471, #8395, #30924, #52373, #69378, #19096, #25386, #18733, #47930, #13560, #70459, #19834, #42386, #64908, #36836, #59350, #8761, #22307, #55931, #61467, #22664, #9497, #65639, #9130, #54200, #3597, #33395, #514, #23025, #44501, #26487, #67748, #45581, #16394, #72925, #26119, #32026, #48658, #44859, #71183, #49029, #16757, #56651, #33755, #39315, #37564, #14656, #17120, #51117, #37199, #39679, #50755, #67034, #67395, #38949, #56300, #59722, #31667, #20556, #5327, #10862, #27868, #28580, #50400, #43114, #15027, #60088, #62199, #61827, #11232, #54562, #11595, #3965, #71558, #34112, #20933, #5690, #28225, #158, #45214, #6046, #18189, #51835, #24833, #58444, #23744, #63634, #23387, #18557, #1598, #18917, #52560, #1239, #52197, #57365, #68113, #7855, #11949, #40759, #40390, #29660, #12303, #63274, #62909, #46292, #57725, #13022, #12666, #69197, #28941, #47021, #35203, #24109, #30017, #30391, #6773, #29305, #46657, #68833, #7130, #41122, #1966, #34474, #7488, #41476, #24475, #35560, #34839, #57002, #6409, #58080, #69556, #45936, #63996, #13377, #35920, #52920, #51479, #880, #2318, #17479, #68467, #40039, #62553, #17829, #9320, #31486, #8953, #70638, #54751, #3423, #47381, #71377, #65094, #19279, #14484, #59542, #9684, #69911, #31853, #37390, #41832, #48115, #54028, #36295, #42205, #58809, #25943, #8220, #8583, #48483, #15212, #65459, #71007, #70278, #4153, #26309, #32217, #64363, #48847, #54389, #3044, #20383, #20013, #14851, #13753, #30748, #53280, #37018, #42566, #25575, #60270, #42934, #2679, #25195, #47740, #20752, #59914, #3785, #19649, #43310, #64729, #14115, #65830, #36654, #59175, #31112, #37752, #53651, #4521, #49942, #10413, #56561, #17027, #55483, #22220, #27050, #10775, #44414, #67309, #61737, #60638, #38117, #33308, #15943, #10051, #11138, #38863, #4875, #33667, #55846, #61379, #72466, #34024, #5234, #26685 ),
 ( #44774, #50315, #49581, #49218, #5604, #62109, #71752, #28140, #56211, #27411, #27776, #21851, #16667, #21121, #11502, #43674, #66941, #16309, #72838, #39585, #39225, #32584, #55123, #72103, #50668, #72, #22578, #66197, #45127, #21488, #44040, #67661, #66563, #38491, #61016, #15575, #32945, #56913, #29213, #62823, #35829, #69470, #34744, #1513, #34381, #1150, #422, #12215, #13292, #51749, #6318, #6685, #45846, #46566, #45489, #28847, #51385, #18827, #5956, #787, #23296, #35113, #63902, #11861, #18102, #68381, #28488, #1878, #24384, #46932, #41390, #17742, #51026, #22930, #57276, #24017, #40664, #40301, #63183, #68744, #23659, #46203, #12579, #57636, #29572, #7042, #52108, #62463, #63549, #69110, #18470, #41034, #12935, #35471, #57992, #68020, #7402, #17393, #29930, #52470, #39950, #25483, #70555, #20662, #58352, #48029, #65369, #14757, #37301, #64271, #64642, #31766, #53936, #3332, #8492, #25107, #43219, #65007, #58720, #30659, #8133, #69824, #41743, #19190, #36933, #2588, #54303, #42484, #25857, #19930, #36567, #53558, #59087, #59824, #13660, #7763, #14395, #36202, #59453, #30300, #31024, #42847, #24747, #53192, #48394, #70922, #8860, #2955, #3695, #52833, #48759, #26220, #47651, #31396, #20292, #9230, #71283, #70183, #65739, #15124, #2233, #47290, #19561, #42117, #14027, #22130, #21393, #21757, #26959, #37661, #50579, #54659, #10322, #9956, #72377, #55027, #32855, #32492, #15849, #27319, #55752, #55391, #38771, #71657, #16577, #4785, #44318, #72745, #28051, #49486, #72017, #16218, #66472, #43949, #38395, #44685, #4062, #50219, #61644, #67216, #5146, #4431, #26588, #49129, #60919, #33213, #15483, #66848, #49851, #27681, #39129, #21030, #43583, #61291, #10683, #66104, #11046, #33572, #56120, #5512, #73106, #22488, #45038, #32125, #67573, #60184, #9593, #38026, #60549, #700, #1068, #6231, #16938, #29850, #33934, #62740, #62378, #51664, #34292, #12132, #11777, #68298, #6601, #35028, #34659, #18023, #50938, #69022, #57188, #23577, #52026, #7319, #28759, #51299, #68659, #45762, #23209, #17658, #23935, #56477, #29489, #40952, #1428, #57556, #56824, #5868, #28400, #40219, #12500, #67932, #46122, #29131, #6958, #46484, #334, #22844, #40579, #63099, #45396, #18385, #63467, #12854, #35387, #57910, #52386, #1792, #24302, #46850, #39493, #62015, #11417, #17305, #39866, #8406, #31678, #69390, #36481, #3241, #25769, #48307, #2151, #2503, #42760, #64919, #14310, #19474, #36118, #54211, #2868, #69739, #41663, #19108, #7678, #52746, #30214, #47941, #13573, #65280, #53476, #36846, #59000, #47568, #64555, #70098, #70831, #24662, #18745, #30935, #47208, #25398, #41309, #42032, #53847, #35750, #64185, #59361, #8773, #70470, #13945, #14668, #63819, #59733, #37211, #58638, #31307, #20205, #19847, #42397, #9141, #13211, #3609, #26130, #8045, #58271, #30580, #53106, #25026, #66021, #66763, #27600, #43126, #38687, #72295, #55309, #72664, #33130, #32402, #32772, #37942, #48669, #61561, #65649, #21310, #20944, #10239, #15400, #43863, #43495, #26873, #38305, #16135, #66388, #49770, #9508, #50132, #15765, #4703, #10602, #39047, #60461, #9870, #27233, #4347, #54942, #49403, #55667, #15038, #61207, #22043, #5064, #44603, #71934, #37575, #60099, #60833, #44231, #26500, #21674, #67134, #16491, #10963, #32040, #54573, #33484, #56034, #3976, #5426, #71195, #20569, #49041, #71570, #62653, #51217, #35300, #57102, #27965, #51940, #45681, #73022, #68215, #40138, #63380, #50496, #17576, #34942, #57469, #6874, #33853, #34210, #1337, #23490, #46037, #618, #67849, #12764, #34574, #28318, #254, #50855, #39411, #11336, #61930, #6512, #45314, #23849, #12050, #68573, #29046, #6148, #23125, #28677, #29406, #56397, #22407, #51582, #5787, #981, #44954, #17932, #12408, #67492, #57821, #22762, #17221, #40495, #16855, #39782, #63011, #62298, #11694, #46397, #68933, #18290, #40863, #56744, #42668, #65192, #36024, #25300, #19378, #35661, #41936, #70008, #53018, #7586, #64461, #2412, #30847, #24933, #13852, #47477, #14582, #25678, #58182, #47848, #63730, #70376, #64092, #7953, #53382, #13120, #41574, #47118, #30122, #46762, #36394, #58908, #8318, #14218, #2063, #52655, #1698, #69297, #18659, #2777, #37115, #7231, #19013, #42302, #19754, #29760, #30490, #64828, #41221, #24573, #69650, #36753, #13475, #58541, #59273, #48214, #8681, #31213, #53754, #52297, #3150, #24210, #70735, #20113, #21588, #15312, #66297, #9780, #27147, #16406, #44512, #3520, #26782, #60371, #37852, #72569, #54848, #71107, #65562, #37490, #10516, #21220, #38213, #67046, #38593, #60010, #43034, #33043, #54486, #9421, #48950, #4617, #72210, #31950, #32314, #43408, #59642, #50044, #4257, #55223, #14951, #49315, #54125, #65933, #9055, #71848, #3887, #43772, #26407, #49681, #26041, #71479, #20855, #21955, #55583, #44141, #66668, #15676, #48580, #20480, #60741, #16045, #10151, #32683, #61119, #4976, #27510, #31586, #50412, #23037, #28236, #22318, #23399, #51129, #67759, #892, #45593, #526, #62211, #46305, #68126, #38960, #62921, #56663, #10873, #6058, #17492, #1252, #61478, #28592, #45949, #68479, #17841, #44871, #45226, #12316, #34486, #57016, #11606, #5700, #23756, #40053, #39326, #11244, #61839, #72937, #67407, #16768, #62565, #56311, #34851, #11962, #6421, #28953, #17131, #34123, #39692, #40402, #33768, #33406, #51492, #50766, #57378, #55943, #6785, #29317, #5340, #171, #51848, #68844, #27879, #22675, #37670, #18201, #9602, #15132, #1610, #25865, #14766, #53945, #36941, #36576, #37310, #71291, #12679, #9239, #42855, #48404, #43228, #3703, #2963, #3342, #8502, #40772, #32134, #35215, #65016, #64651, #70930, #59096, #14404, #14035, #70564, #8869, #59832, #59461, #20301, #52209, #20670, #31405, #65377, #54312, #54667, #31032, #53568, #31775 ) ),
 .UNSPECIFIED., .F., .F., .F. ) 
 B_SPLINE_SURFACE_WITH_KNOTS ( ( 2, 2 ),
 ( 3, 2, 2, 2, 2, 2, 2, 2, 2, 2, 2, 2, 2, 2, 2, 2, 2, 2, 2, 2, 2, 2, 2, 2, 2, 2, 2, 2, 2, 2, 2, 2, 2, 2, 2, 2, 2, 2, 2, 2, 2, 2, 2, 2, 2, 2, 2, 2, 2, 2, 2, 2, 2, 2, 2, 2, 2, 2, 2, 2, 2, 2, 2, 2, 2, 2, 2, 2, 2, 2, 2, 2, 2, 2, 2, 2, 2, 2, 2, 2, 2, 2, 2, 2, 2, 2, 2, 2, 2, 2, 2, 2, 2, 2, 2, 2, 2, 2, 2, 2, 2, 2, 2, 2, 2, 2, 2, 2, 2, 2, 2, 2, 2, 2, 2, 2, 2, 2, 2, 2, 2, 2, 2, 2, 2, 2, 2, 2, 2, 2, 2, 2, 2, 2, 2, 2, 2, 2, 2, 2, 2, 2, 2, 2, 2, 2, 2, 2, 2, 2, 2, 2, 2, 2, 2, 2, 2, 2, 2, 2, 2, 2, 2, 2, 2, 2, 2, 2, 2, 2, 2, 2, 2, 2, 2, 2, 2, 2, 2, 2, 2, 2, 2, 2, 2, 2, 2, 2, 2, 2, 2, 2, 2, 2, 2, 2, 2, 2, 2, 2, 2, 2, 2, 2, 2, 2, 2, 2, 2, 2, 2, 2, 2, 2, 2, 2, 2, 2, 2, 2, 2, 2, 2, 2, 2, 2, 2, 2, 2, 2, 2, 2, 2, 2, 2, 2, 2, 2, 2, 2, 2, 2, 2, 2, 2, 2, 2, 2, 2, 2, 2, 2, 2, 2, 2, 2, 2, 2, 2, 2, 2, 2, 2, 2, 2, 2, 2, 2, 2, 2, 2, 2, 2, 2, 2, 2, 2, 2, 2, 2, 2, 2, 2, 2, 2, 2, 2, 2, 2, 2, 2, 2, 2, 2, 2, 2, 2, 2, 2, 2, 2, 2, 2, 2, 2, 2, 2, 2, 2, 2, 2, 2, 2, 2, 2, 2, 2, 2, 2, 2, 2, 2, 2, 2, 2, 2, 2, 2, 2, 2, 2, 2, 2, 2, 2, 2, 2, 2, 2, 2, 2, 2, 2, 2, 2, 2, 2, 2, 2, 2, 2, 2, 2, 2, 2, 2, 2, 2, 2, 2, 3 ),
 ( 0.000000000000000000, 1.000000000000000000 ),
 ( 0.000000000000000000, 0.002777777777777777884, 0.005555555555555555768, 0.008333333333333333218, 0.01111111111111111154, 0.01388888888888888812, 0.01666666666666666644, 0.01944444444444444475, 0.02222222222222222307, 0.02500000000000000139, 0.02777777777777777624, 0.03055555555555555455, 0.03333333333333333287, 0.03611111111111110772, 0.03888888888888888951, 0.04166666666666666435, 0.04444444444444444614, 0.04722222222222222099, 0.05000000000000000278, 0.05277777777777777762, 0.05555555555555555247, 0.05833333333333333426, 0.06111111111111110911, 0.06388888888888888395, 0.06666666666666666574, 0.06944444444444444753, 0.07222222222222221544, 0.07499999999999999722, 0.07777777777777777901, 0.08055555555555556080, 0.08333333333333332871, 0.08611111111111111049, 0.08888888888888889228, 0.09166666666666666019, 0.09444444444444444198, 0.09722222222222222376, 0.1000000000000000056, 0.1027777777777777735, 0.1055555555555555552, 0.1083333333333333370, 0.1111111111111111049, 0.1138888888888888867, 0.1166666666666666685, 0.1194444444444444503, 0.1222222222222222182, 0.1250000000000000000, 0.1277777777777777679, 0.1305555555555555636, 0.1333333333333333315, 0.1361111111111110994, 0.1388888888888888951, 0.1416666666666666630, 0.1444444444444444309, 0.1472222222222222265, 0.1499999999999999944, 0.1527777777777777901, 0.1555555555555555580, 0.1583333333333333259, 0.1611111111111111216, 0.1638888888888888895, 0.1666666666666666574, 0.1694444444444444531, 0.1722222222222222210, 0.1749999999999999889, 0.1777777777777777846, 0.1805555555555555525, 0.1833333333333333204, 0.1861111111111111160, 0.1888888888888888840, 0.1916666666666666796, 0.1944444444444444475, 0.1972222222222222154, 0.2000000000000000111, 0.2027777777777777790, 0.2055555555555555469, 0.2083333333333333426, 0.2111111111111111105, 0.2138888888888888784, 0.2166666666666666741, 0.2194444444444444420, 0.2222222222222222099, 0.2250000000000000056, 0.2277777777777777735, 0.2305555555555555691, 0.2333333333333333370, 0.2361111111111111049, 0.2388888888888889006, 0.2416666666666666685, 0.2444444444444444364, 0.2472222222222222321, 0.2500000000000000000, 0.2527777777777777679, 0.2555555555555555358, 0.2583333333333333592, 0.2611111111111111271, 0.2638888888888888951, 0.2666666666666666630, 0.2694444444444444309, 0.2722222222222221988, 0.2750000000000000222, 0.2777777777777777901, 0.2805555555555555580, 0.2833333333333333259, 0.2861111111111110938, 0.2888888888888888618, 0.2916666666666666852, 0.2944444444444444531, 0.2972222222222222210, 0.2999999999999999889, 0.3027777777777777568, 0.3055555555555555802, 0.3083333333333333481, 0.3111111111111111160, 0.3138888888888888840, 0.3166666666666666519, 0.3194444444444444198, 0.3222222222222222432, 0.3250000000000000111, 0.3277777777777777790, 0.3305555555555555469, 0.3333333333333333148, 0.3361111111111111382, 0.3388888888888889062, 0.3416666666666666741, 0.3444444444444444420, 0.3472222222222222099, 0.3499999999999999778, 0.3527777777777778012, 0.3555555555555555691, 0.3583333333333333370, 0.3611111111111111049, 0.3638888888888888729, 0.3666666666666666408, 0.3694444444444444642, 0.3722222222222222321, 0.3750000000000000000, 0.3777777777777777679, 0.3805555555555555358, 0.3833333333333333592, 0.3861111111111111271, 0.3888888888888888951, 0.3916666666666666630, 0.3944444444444444309, 0.3972222222222221988, 0.4000000000000000222, 0.4027777777777777901, 0.4055555555555555580, 0.4083333333333333259, 0.4111111111111110938, 0.4138888888888888618, 0.4166666666666666852, 0.4194444444444444531, 0.4222222222222222210, 0.4249999999999999889, 0.4277777777777777568, 0.4305555555555555802, 0.4333333333333333481, 0.4361111111111111160, 0.4388888888888888840, 0.4416666666666666519, 0.4444444444444444198, 0.4472222222222222432, 0.4500000000000000111, 0.4527777777777777790, 0.4555555555555555469, 0.4583333333333333148, 0.4611111111111111382, 0.4638888888888889062, 0.4666666666666666741, 0.4694444444444444420, 0.4722222222222222099, 0.4749999999999999778, 0.4777777777777778012, 0.4805555555555555691, 0.4833333333333333370, 0.4861111111111111049, 0.4888888888888888729, 0.4916666666666666408, 0.4944444444444444642, 0.4972222222222222321, 0.5000000000000000000, 0.5027777777777777679, 0.5055555555555555358, 0.5083333333333333037, 0.5111111111111110716, 0.5138888888888888395, 0.5166666666666667185, 0.5194444444444444864, 0.5222222222222222543, 0.5250000000000000222, 0.5277777777777777901, 0.5305555555555555580, 0.5333333333333333259, 0.5361111111111110938, 0.5388888888888888618, 0.5416666666666666297, 0.5444444444444443976, 0.5472222222222222765, 0.5500000000000000444, 0.5527777777777778123, 0.5555555555555555802, 0.5583333333333333481, 0.5611111111111111160, 0.5638888888888888840, 0.5666666666666666519, 0.5694444444444444198, 0.5722222222222221877, 0.5749999999999999556, 0.5777777777777777235, 0.5805555555555556024, 0.5833333333333333703, 0.5861111111111111382, 0.5888888888888889062, 0.5916666666666666741, 0.5944444444444444420, 0.5972222222222222099, 0.5999999999999999778, 0.6027777777777777457, 0.6055555555555555136, 0.6083333333333332815, 0.6111111111111111605, 0.6138888888888889284, 0.6166666666666666963, 0.6194444444444444642, 0.6222222222222222321, 0.6250000000000000000, 0.6277777777777777679, 0.6305555555555555358, 0.6333333333333333037, 0.6361111111111110716, 0.6388888888888888395, 0.6416666666666667185, 0.6444444444444444864, 0.6472222222222222543, 0.6500000000000000222, 0.6527777777777777901, 0.6555555555555555580, 0.6583333333333333259, 0.6611111111111110938, 0.6638888888888888618, 0.6666666666666666297, 0.6694444444444443976, 0.6722222222222222765, 0.6750000000000000444, 0.6777777777777778123, 0.6805555555555555802, 0.6833333333333333481, 0.6861111111111111160, 0.6888888888888888840, 0.6916666666666666519, 0.6944444444444444198, 0.6972222222222221877, 0.6999999999999999556, 0.7027777777777777235, 0.7055555555555556024, 0.7083333333333333703, 0.7111111111111111382, 0.7138888888888889062, 0.7166666666666666741, 0.7194444444444444420, 0.7222222222222222099, 0.7249999999999999778, 0.7277777777777777457, 0.7305555555555555136, 0.7333333333333332815, 0.7361111111111111605, 0.7388888888888889284, 0.7416666666666666963, 0.7444444444444444642, 0.7472222222222222321, 0.7500000000000000000, 0.7527777777777777679, 0.7555555555555555358, 0.7583333333333333037, 0.7611111111111110716, 0.7638888888888888395, 0.7666666666666667185, 0.7694444444444444864, 0.7722222222222222543, 0.7750000000000000222, 0.7777777777777777901, 0.7805555555555555580, 0.7833333333333333259, 0.7861111111111110938, 0.7888888888888888618, 0.7916666666666666297, 0.7944444444444443976, 0.7972222222222222765, 0.8000000000000000444, 0.8027777777777778123, 0.8055555555555555802, 0.8083333333333333481, 0.8111111111111111160, 0.8138888888888888840, 0.8166666666666666519, 0.8194444444444444198, 0.8222222222222221877, 0.8249999999999999556, 0.8277777777777777235, 0.8305555555555556024, 0.8333333333333333703, 0.8361111111111111382, 0.8388888888888889062, 0.8416666666666666741, 0.8444444444444444420, 0.8472222222222222099, 0.8499999999999999778, 0.8527777777777777457, 0.8555555555555555136, 0.8583333333333332815, 0.8611111111111111605, 0.8638888888888889284, 0.8666666666666666963, 0.8694444444444444642, 0.8722222222222222321, 0.8750000000000000000, 0.8777777777777777679, 0.8805555555555555358, 0.8833333333333333037, 0.8861111111111110716, 0.8888888888888888395, 0.8916666666666667185, 0.8944444444444444864, 0.8972222222222222543, 0.9000000000000000222, 0.9027777777777777901, 0.9055555555555555580, 0.9083333333333333259, 0.9111111111111110938, 0.9138888888888888618, 0.9166666666666666297, 0.9194444444444443976, 0.9222222222222222765, 0.9250000000000000444, 0.9277777777777778123, 0.9305555555555555802, 0.9333333333333333481, 0.9361111111111111160, 0.9388888888888888840, 0.9416666666666666519, 0.9444444444444444198, 0.9472222222222221877, 0.9499999999999999556, 0.9527777777777777235, 0.9555555555555556024, 0.9583333333333333703, 0.9611111111111111382, 0.9638888888888889062, 0.9666666666666666741, 0.9694444444444444420, 0.9722222222222222099, 0.9749999999999999778, 0.9777777777777777457, 0.9805555555555555136, 0.9833333333333332815, 0.9861111111111111605, 0.9888888888888889284, 0.9916666666666666963, 0.9944444444444444642, 0.9972222222222222321, 1.000000000000000000 ),
 .UNSPECIFIED. ) 
 GEOMETRIC_REPRESENTATION_ITEM ( )  RATIONAL_B_SPLINE_SURFACE ( (
 ( 1.000000000000000000, 0.8660254037844387076, 1.000000000000000000, 0.8660254037844387076, 1.000000000000000000, 0.8660254037844387076, 1.000000000000000000, 0.8660254037844387076, 1.000000000000000000, 0.8660254037844387076, 1.000000000000000000, 0.8660254037844387076, 1.000000000000000000, 0.8660254037844387076, 1.000000000000000000, 0.8660254037844387076, 1.000000000000000000, 0.8660254037844387076, 1.000000000000000000, 0.8660254037844387076, 1.000000000000000000, 0.8660254037844387076, 1.000000000000000000, 0.8660254037844387076, 1.000000000000000000, 0.8660254037844387076, 1.000000000000000000, 0.8660254037844387076, 1.000000000000000000, 0.8660254037844387076, 1.000000000000000000, 0.8660254037844387076, 1.000000000000000000, 0.8660254037844387076, 1.000000000000000000, 0.8660254037844387076, 1.000000000000000000, 0.8660254037844387076, 1.000000000000000000, 0.8660254037844387076, 1.000000000000000000, 0.8660254037844387076, 1.000000000000000000, 0.8660254037844387076, 1.000000000000000000, 0.8660254037844387076, 1.000000000000000000, 0.8660254037844387076, 1.000000000000000000, 0.8660254037844387076, 1.000000000000000000, 0.8660254037844387076, 1.000000000000000000, 0.8660254037844387076, 1.000000000000000000, 0.8660254037844387076, 1.000000000000000000, 0.8660254037844387076, 1.000000000000000000, 0.8660254037844387076, 1.000000000000000000, 0.8660254037844387076, 1.000000000000000000, 0.8660254037844387076, 1.000000000000000000, 0.8660254037844387076, 1.000000000000000000, 0.8660254037844387076, 1.000000000000000000, 0.8660254037844387076, 1.000000000000000000, 0.8660254037844387076, 1.000000000000000000, 0.8660254037844387076, 1.000000000000000000, 0.8660254037844387076, 1.000000000000000000, 0.8660254037844387076, 1.000000000000000000, 0.8660254037844387076, 1.000000000000000000, 0.8660254037844387076, 1.000000000000000000, 0.8660254037844387076, 1.000000000000000000, 0.8660254037844387076, 1.000000000000000000, 0.8660254037844387076, 1.000000000000000000, 0.8660254037844387076, 1.000000000000000000, 0.8660254037844387076, 1.000000000000000000, 0.8660254037844387076, 1.000000000000000000, 0.8660254037844387076, 1.000000000000000000, 0.8660254037844387076, 1.000000000000000000, 0.8660254037844387076, 1.000000000000000000, 0.8660254037844387076, 1.000000000000000000, 0.8660254037844387076, 1.000000000000000000, 0.8660254037844387076, 1.000000000000000000, 0.8660254037844387076, 1.000000000000000000, 0.8660254037844387076, 1.000000000000000000, 0.8660254037844387076, 1.000000000000000000, 0.8660254037844387076, 1.000000000000000000, 0.8660254037844387076, 1.000000000000000000, 0.8660254037844387076, 1.000000000000000000, 0.8660254037844387076, 1.000000000000000000, 0.8660254037844387076, 1.000000000000000000, 0.8660254037844387076, 1.000000000000000000, 0.8660254037844387076, 1.000000000000000000, 0.8660254037844387076, 1.000000000000000000, 0.8660254037844387076, 1.000000000000000000, 0.8660254037844387076, 1.000000000000000000, 0.8660254037844387076, 1.000000000000000000, 0.8660254037844387076, 1.000000000000000000, 0.8660254037844387076, 1.000000000000000000, 0.8660254037844387076, 1.000000000000000000, 0.8660254037844387076, 1.000000000000000000, 0.8660254037844387076, 1.000000000000000000, 0.8660254037844387076, 1.000000000000000000, 0.8660254037844387076, 1.000000000000000000, 0.8660254037844387076, 1.000000000000000000, 0.8660254037844387076, 1.000000000000000000, 0.8660254037844387076, 1.000000000000000000, 0.8660254037844387076, 1.000000000000000000, 0.8660254037844387076, 1.000000000000000000, 0.8660254037844387076, 1.000000000000000000, 0.8660254037844387076, 1.000000000000000000, 0.8660254037844387076, 1.000000000000000000, 0.8660254037844387076, 1.000000000000000000, 0.8660254037844387076, 1.000000000000000000, 0.8660254037844387076, 1.000000000000000000, 0.8660254037844387076, 1.000000000000000000, 0.8660254037844387076, 1.000000000000000000, 0.8660254037844387076, 1.000000000000000000, 0.8660254037844387076, 1.000000000000000000, 0.8660254037844387076, 1.000000000000000000, 0.8660254037844387076, 1.000000000000000000, 0.8660254037844387076, 1.000000000000000000, 0.8660254037844387076, 1.000000000000000000, 0.8660254037844387076, 1.000000000000000000, 0.8660254037844387076, 1.000000000000000000, 0.8660254037844387076, 1.000000000000000000, 0.8660254037844387076, 1.000000000000000000, 0.8660254037844387076, 1.000000000000000000, 0.8660254037844387076, 1.000000000000000000, 0.8660254037844387076, 1.000000000000000000, 0.8660254037844387076, 1.000000000000000000, 0.8660254037844387076, 1.000000000000000000, 0.8660254037844387076, 1.000000000000000000, 0.8660254037844387076, 1.000000000000000000, 0.8660254037844387076, 1.000000000000000000, 0.8660254037844387076, 1.000000000000000000, 0.8660254037844387076, 1.000000000000000000, 0.8660254037844387076, 1.000000000000000000, 0.8660254037844387076, 1.000000000000000000, 0.8660254037844387076, 1.000000000000000000, 0.8660254037844387076, 1.000000000000000000, 0.8660254037844387076, 1.000000000000000000, 0.8660254037844387076, 1.000000000000000000, 0.8660254037844387076, 1.000000000000000000, 0.8660254037844387076, 1.000000000000000000, 0.8660254037844387076, 1.000000000000000000, 0.8660254037844387076, 1.000000000000000000, 0.8660254037844387076, 1.000000000000000000, 0.8660254037844387076, 1.000000000000000000, 0.8660254037844387076, 1.000000000000000000, 0.8660254037844387076, 1.000000000000000000, 0.8660254037844387076, 1.000000000000000000, 0.8660254037844387076, 1.000000000000000000, 0.8660254037844387076, 1.000000000000000000, 0.8660254037844387076, 1.000000000000000000, 0.8660254037844387076, 1.000000000000000000, 0.8660254037844387076, 1.000000000000000000, 0.8660254037844387076, 1.000000000000000000, 0.8660254037844387076, 1.000000000000000000, 0.8660254037844387076, 1.000000000000000000, 0.8660254037844387076, 1.000000000000000000, 0.8660254037844387076, 1.000000000000000000, 0.8660254037844387076, 1.000000000000000000, 0.8660254037844387076, 1.000000000000000000, 0.8660254037844387076, 1.000000000000000000, 0.8660254037844387076, 1.000000000000000000, 0.8660254037844387076, 1.000000000000000000, 0.8660254037844387076, 1.000000000000000000, 0.8660254037844387076, 1.000000000000000000, 0.8660254037844387076, 1.000000000000000000, 0.8660254037844387076, 1.000000000000000000, 0.8660254037844387076, 1.000000000000000000, 0.8660254037844387076, 1.000000000000000000, 0.8660254037844387076, 1.000000000000000000, 0.8660254037844387076, 1.000000000000000000, 0.8660254037844387076, 1.000000000000000000, 0.8660254037844387076, 1.000000000000000000, 0.8660254037844387076, 1.000000000000000000, 0.8660254037844387076, 1.000000000000000000, 0.8660254037844387076, 1.000000000000000000, 0.8660254037844387076, 1.000000000000000000, 0.8660254037844387076, 1.000000000000000000, 0.8660254037844387076, 1.000000000000000000, 0.8660254037844387076, 1.000000000000000000, 0.8660254037844387076, 1.000000000000000000, 0.8660254037844387076, 1.000000000000000000, 0.8660254037844387076, 1.000000000000000000, 0.8660254037844387076, 1.000000000000000000, 0.8660254037844387076, 1.000000000000000000, 0.8660254037844387076, 1.000000000000000000, 0.8660254037844387076, 1.000000000000000000, 0.8660254037844387076, 1.000000000000000000, 0.8660254037844387076, 1.000000000000000000, 0.8660254037844387076, 1.000000000000000000, 0.8660254037844387076, 1.000000000000000000, 0.8660254037844387076, 1.000000000000000000, 0.8660254037844387076, 1.000000000000000000, 0.8660254037844387076, 1.000000000000000000, 0.8660254037844387076, 1.000000000000000000, 0.8660254037844387076, 1.000000000000000000, 0.8660254037844387076, 1.000000000000000000, 0.8660254037844387076, 1.000000000000000000, 0.8660254037844387076, 1.000000000000000000, 0.8660254037844387076, 1.000000000000000000, 0.8660254037844387076, 1.000000000000000000, 0.8660254037844387076, 1.000000000000000000, 0.8660254037844387076, 1.000000000000000000, 0.8660254037844387076, 1.000000000000000000, 0.8660254037844387076, 1.000000000000000000, 0.8660254037844387076, 1.000000000000000000, 0.8660254037844387076, 1.000000000000000000, 0.8660254037844387076, 1.000000000000000000, 0.8660254037844387076, 1.000000000000000000, 0.8660254037844387076, 1.000000000000000000, 0.8660254037844387076, 1.000000000000000000, 0.8660254037844387076, 1.000000000000000000, 0.8660254037844387076, 1.000000000000000000, 0.8660254037844387076, 1.000000000000000000, 0.8660254037844387076, 1.000000000000000000, 0.8660254037844387076, 1.000000000000000000, 0.8660254037844387076, 1.000000000000000000, 0.8660254037844387076, 1.000000000000000000, 0.8660254037844387076, 1.000000000000000000, 0.8660254037844387076, 1.000000000000000000, 0.8660254037844387076, 1.000000000000000000, 0.8660254037844387076, 1.000000000000000000, 0.8660254037844387076, 1.000000000000000000, 0.8660254037844387076, 1.000000000000000000, 0.8660254037844387076, 1.000000000000000000, 0.8660254037844387076, 1.000000000000000000, 0.8660254037844387076, 1.000000000000000000, 0.8660254037844387076, 1.000000000000000000, 0.8660254037844387076, 1.000000000000000000, 0.8660254037844387076, 1.000000000000000000, 0.8660254037844387076, 1.000000000000000000, 0.8660254037844387076, 1.000000000000000000, 0.8660254037844387076, 1.000000000000000000, 0.8660254037844387076, 1.000000000000000000, 0.8660254037844387076, 1.000000000000000000, 0.8660254037844387076, 1.000000000000000000, 0.8660254037844387076, 1.000000000000000000, 0.8660254037844387076, 1.000000000000000000, 0.8660254037844387076, 1.000000000000000000, 0.8660254037844387076, 1.000000000000000000, 0.8660254037844387076, 1.000000000000000000, 0.8660254037844387076, 1.000000000000000000, 0.8660254037844387076, 1.000000000000000000, 0.8660254037844387076, 1.000000000000000000, 0.8660254037844387076, 1.000000000000000000, 0.8660254037844387076, 1.000000000000000000, 0.8660254037844387076, 1.000000000000000000, 0.8660254037844387076, 1.000000000000000000, 0.8660254037844387076, 1.000000000000000000, 0.8660254037844387076, 1.000000000000000000, 0.8660254037844387076, 1.000000000000000000, 0.8660254037844387076, 1.000000000000000000, 0.8660254037844387076, 1.000000000000000000, 0.8660254037844387076, 1.000000000000000000, 0.8660254037844387076, 1.000000000000000000, 0.8660254037844387076, 1.000000000000000000, 0.8660254037844387076, 1.000000000000000000, 0.8660254037844387076, 1.000000000000000000, 0.8660254037844387076, 1.000000000000000000, 0.8660254037844387076, 1.000000000000000000, 0.8660254037844387076, 1.000000000000000000, 0.8660254037844387076, 1.000000000000000000, 0.8660254037844387076, 1.000000000000000000, 0.8660254037844387076, 1.000000000000000000, 0.8660254037844387076, 1.000000000000000000, 0.8660254037844387076, 1.000000000000000000, 0.8660254037844387076, 1.000000000000000000, 0.8660254037844387076, 1.000000000000000000, 0.8660254037844387076, 1.000000000000000000, 0.8660254037844387076, 1.000000000000000000, 0.8660254037844387076, 1.000000000000000000, 0.8660254037844387076, 1.000000000000000000, 0.8660254037844387076, 1.000000000000000000, 0.8660254037844387076, 1.000000000000000000, 0.8660254037844387076, 1.000000000000000000, 0.8660254037844387076, 1.000000000000000000, 0.8660254037844387076, 1.000000000000000000, 0.8660254037844387076, 1.000000000000000000, 0.8660254037844387076, 1.000000000000000000, 0.8660254037844387076, 1.000000000000000000, 0.8660254037844387076, 1.000000000000000000, 0.8660254037844387076, 1.000000000000000000, 0.8660254037844387076, 1.000000000000000000, 0.8660254037844387076, 1.000000000000000000, 0.8660254037844387076, 1.000000000000000000, 0.8660254037844387076, 1.000000000000000000, 0.8660254037844387076, 1.000000000000000000, 0.8660254037844387076, 1.000000000000000000, 0.8660254037844387076, 1.000000000000000000, 0.8660254037844387076, 1.000000000000000000, 0.8660254037844387076, 1.000000000000000000, 0.8660254037844387076, 1.000000000000000000, 0.8660254037844387076, 1.000000000000000000, 0.8660254037844387076, 1.000000000000000000, 0.8660254037844387076, 1.000000000000000000, 0.8660254037844387076, 1.000000000000000000, 0.8660254037844387076, 1.000000000000000000, 0.8660254037844387076, 1.000000000000000000, 0.8660254037844387076, 1.000000000000000000, 0.8660254037844387076, 1.000000000000000000, 0.8660254037844387076, 1.000000000000000000, 0.8660254037844387076, 1.000000000000000000, 0.8660254037844387076, 1.000000000000000000, 0.8660254037844387076, 1.000000000000000000, 0.8660254037844387076, 1.000000000000000000, 0.8660254037844387076, 1.000000000000000000, 0.8660254037844387076, 1.000000000000000000, 0.8660254037844387076, 1.000000000000000000, 0.8660254037844387076, 1.000000000000000000, 0.8660254037844387076, 1.000000000000000000, 0.8660254037844387076, 1.000000000000000000, 0.8660254037844387076, 1.000000000000000000, 0.8660254037844387076, 1.000000000000000000, 0.8660254037844387076, 1.000000000000000000, 0.8660254037844387076, 1.000000000000000000, 0.8660254037844387076, 1.000000000000000000, 0.8660254037844387076, 1.000000000000000000, 0.8660254037844387076, 1.000000000000000000, 0.8660254037844387076, 1.000000000000000000, 0.8660254037844387076, 1.000000000000000000, 0.8660254037844387076, 1.000000000000000000, 0.8660254037844387076, 1.000000000000000000, 0.8660254037844387076, 1.000000000000000000, 0.8660254037844387076, 1.000000000000000000, 0.8660254037844387076, 1.000000000000000000, 0.8660254037844387076, 1.000000000000000000, 0.8660254037844387076, 1.000000000000000000, 0.8660254037844387076, 1.000000000000000000, 0.8660254037844387076, 1.000000000000000000, 0.8660254037844387076, 1.000000000000000000, 0.8660254037844387076, 1.000000000000000000, 0.8660254037844387076, 1.000000000000000000, 0.8660254037844387076, 1.000000000000000000, 0.8660254037844387076, 1.000000000000000000, 0.8660254037844387076, 1.000000000000000000, 0.8660254037844387076, 1.000000000000000000, 0.8660254037844387076, 1.000000000000000000, 0.8660254037844387076, 1.000000000000000000, 0.8660254037844387076, 1.000000000000000000, 0.8660254037844387076, 1.000000000000000000, 0.8660254037844387076, 1.000000000000000000, 0.8660254037844387076, 1.000000000000000000, 0.8660254037844387076, 1.000000000000000000, 0.8660254037844387076, 1.000000000000000000, 0.8660254037844387076, 1.000000000000000000, 0.8660254037844387076, 1.000000000000000000, 0.8660254037844387076, 1.000000000000000000, 0.8660254037844387076, 1.000000000000000000, 0.8660254037844387076, 1.000000000000000000, 0.8660254037844387076, 1.000000000000000000, 0.8660254037844387076, 1.000000000000000000, 0.8660254037844387076, 1.000000000000000000, 0.8660254037844387076, 1.000000000000000000, 0.8660254037844387076, 1.000000000000000000, 0.8660254037844387076, 1.000000000000000000, 0.8660254037844387076, 1.000000000000000000, 0.8660254037844387076, 1.000000000000000000, 0.8660254037844387076, 1.000000000000000000, 0.8660254037844387076, 1.000000000000000000, 0.8660254037844387076, 1.000000000000000000, 0.8660254037844387076, 1.000000000000000000, 0.8660254037844387076, 1.000000000000000000, 0.8660254037844387076, 1.000000000000000000, 0.8660254037844387076, 1.000000000000000000, 0.8660254037844387076, 1.000000000000000000, 0.8660254037844387076, 1.000000000000000000, 0.8660254037844387076, 1.000000000000000000, 0.8660254037844387076, 1.000000000000000000, 0.8660254037844387076, 1.000000000000000000, 0.8660254037844387076, 1.000000000000000000, 0.8660254037844387076, 1.000000000000000000, 0.8660254037844387076, 1.000000000000000000, 0.8660254037844387076, 1.000000000000000000, 0.8660254037844387076, 1.000000000000000000, 0.8660254037844387076, 1.000000000000000000, 0.8660254037844387076, 1.000000000000000000, 0.8660254037844387076, 1.000000000000000000, 0.8660254037844387076, 1.000000000000000000, 0.8660254037844387076, 1.000000000000000000, 0.8660254037844387076, 1.000000000000000000, 0.8660254037844387076, 1.000000000000000000, 0.8660254037844387076, 1.000000000000000000, 0.8660254037844387076, 1.000000000000000000, 0.8660254037844387076, 1.000000000000000000, 0.8660254037844387076, 1.000000000000000000, 0.8660254037844387076, 1.000000000000000000),
 ( 1.000000000000000000, 0.8660254037844387076, 1.000000000000000000, 0.8660254037844387076, 1.000000000000000000, 0.8660254037844387076, 1.000000000000000000, 0.8660254037844387076, 1.000000000000000000, 0.8660254037844387076, 1.000000000000000000, 0.8660254037844387076, 1.000000000000000000, 0.8660254037844387076, 1.000000000000000000, 0.8660254037844387076, 1.000000000000000000, 0.8660254037844387076, 1.000000000000000000, 0.8660254037844387076, 1.000000000000000000, 0.8660254037844387076, 1.000000000000000000, 0.8660254037844387076, 1.000000000000000000, 0.8660254037844387076, 1.000000000000000000, 0.8660254037844387076, 1.000000000000000000, 0.8660254037844387076, 1.000000000000000000, 0.8660254037844387076, 1.000000000000000000, 0.8660254037844387076, 1.000000000000000000, 0.8660254037844387076, 1.000000000000000000, 0.8660254037844387076, 1.000000000000000000, 0.8660254037844387076, 1.000000000000000000, 0.8660254037844387076, 1.000000000000000000, 0.8660254037844387076, 1.000000000000000000, 0.8660254037844387076, 1.000000000000000000, 0.8660254037844387076, 1.000000000000000000, 0.8660254037844387076, 1.000000000000000000, 0.8660254037844387076, 1.000000000000000000, 0.8660254037844387076, 1.000000000000000000, 0.8660254037844387076, 1.000000000000000000, 0.8660254037844387076, 1.000000000000000000, 0.8660254037844387076, 1.000000000000000000, 0.8660254037844387076, 1.000000000000000000, 0.8660254037844387076, 1.000000000000000000, 0.8660254037844387076, 1.000000000000000000, 0.8660254037844387076, 1.000000000000000000, 0.8660254037844387076, 1.000000000000000000, 0.8660254037844387076, 1.000000000000000000, 0.8660254037844387076, 1.000000000000000000, 0.8660254037844387076, 1.000000000000000000, 0.8660254037844387076, 1.000000000000000000, 0.8660254037844387076, 1.000000000000000000, 0.8660254037844387076, 1.000000000000000000, 0.8660254037844387076, 1.000000000000000000, 0.8660254037844387076, 1.000000000000000000, 0.8660254037844387076, 1.000000000000000000, 0.8660254037844387076, 1.000000000000000000, 0.8660254037844387076, 1.000000000000000000, 0.8660254037844387076, 1.000000000000000000, 0.8660254037844387076, 1.000000000000000000, 0.8660254037844387076, 1.000000000000000000, 0.8660254037844387076, 1.000000000000000000, 0.8660254037844387076, 1.000000000000000000, 0.8660254037844387076, 1.000000000000000000, 0.8660254037844387076, 1.000000000000000000, 0.8660254037844387076, 1.000000000000000000, 0.8660254037844387076, 1.000000000000000000, 0.8660254037844387076, 1.000000000000000000, 0.8660254037844387076, 1.000000000000000000, 0.8660254037844387076, 1.000000000000000000, 0.8660254037844387076, 1.000000000000000000, 0.8660254037844387076, 1.000000000000000000, 0.8660254037844387076, 1.000000000000000000, 0.8660254037844387076, 1.000000000000000000, 0.8660254037844387076, 1.000000000000000000, 0.8660254037844387076, 1.000000000000000000, 0.8660254037844387076, 1.000000000000000000, 0.8660254037844387076, 1.000000000000000000, 0.8660254037844387076, 1.000000000000000000, 0.8660254037844387076, 1.000000000000000000, 0.8660254037844387076, 1.000000000000000000, 0.8660254037844387076, 1.000000000000000000, 0.8660254037844387076, 1.000000000000000000, 0.8660254037844387076, 1.000000000000000000, 0.8660254037844387076, 1.000000000000000000, 0.8660254037844387076, 1.000000000000000000, 0.8660254037844387076, 1.000000000000000000, 0.8660254037844387076, 1.000000000000000000, 0.8660254037844387076, 1.000000000000000000, 0.8660254037844387076, 1.000000000000000000, 0.8660254037844387076, 1.000000000000000000, 0.8660254037844387076, 1.000000000000000000, 0.8660254037844387076, 1.000000000000000000, 0.8660254037844387076, 1.000000000000000000, 0.8660254037844387076, 1.000000000000000000, 0.8660254037844387076, 1.000000000000000000, 0.8660254037844387076, 1.000000000000000000, 0.8660254037844387076, 1.000000000000000000, 0.8660254037844387076, 1.000000000000000000, 0.8660254037844387076, 1.000000000000000000, 0.8660254037844387076, 1.000000000000000000, 0.8660254037844387076, 1.000000000000000000, 0.8660254037844387076, 1.000000000000000000, 0.8660254037844387076, 1.000000000000000000, 0.8660254037844387076, 1.000000000000000000, 0.8660254037844387076, 1.000000000000000000, 0.8660254037844387076, 1.000000000000000000, 0.8660254037844387076, 1.000000000000000000, 0.8660254037844387076, 1.000000000000000000, 0.8660254037844387076, 1.000000000000000000, 0.8660254037844387076, 1.000000000000000000, 0.8660254037844387076, 1.000000000000000000, 0.8660254037844387076, 1.000000000000000000, 0.8660254037844387076, 1.000000000000000000, 0.8660254037844387076, 1.000000000000000000, 0.8660254037844387076, 1.000000000000000000, 0.8660254037844387076, 1.000000000000000000, 0.8660254037844387076, 1.000000000000000000, 0.8660254037844387076, 1.000000000000000000, 0.8660254037844387076, 1.000000000000000000, 0.8660254037844387076, 1.000000000000000000, 0.8660254037844387076, 1.000000000000000000, 0.8660254037844387076, 1.000000000000000000, 0.8660254037844387076, 1.000000000000000000, 0.8660254037844387076, 1.000000000000000000, 0.8660254037844387076, 1.000000000000000000, 0.8660254037844387076, 1.000000000000000000, 0.8660254037844387076, 1.000000000000000000, 0.8660254037844387076, 1.000000000000000000, 0.8660254037844387076, 1.000000000000000000, 0.8660254037844387076, 1.000000000000000000, 0.8660254037844387076, 1.000000000000000000, 0.8660254037844387076, 1.000000000000000000, 0.8660254037844387076, 1.000000000000000000, 0.8660254037844387076, 1.000000000000000000, 0.8660254037844387076, 1.000000000000000000, 0.8660254037844387076, 1.000000000000000000, 0.8660254037844387076, 1.000000000000000000, 0.8660254037844387076, 1.000000000000000000, 0.8660254037844387076, 1.000000000000000000, 0.8660254037844387076, 1.000000000000000000, 0.8660254037844387076, 1.000000000000000000, 0.8660254037844387076, 1.000000000000000000, 0.8660254037844387076, 1.000000000000000000, 0.8660254037844387076, 1.000000000000000000, 0.8660254037844387076, 1.000000000000000000, 0.8660254037844387076, 1.000000000000000000, 0.8660254037844387076, 1.000000000000000000, 0.8660254037844387076, 1.000000000000000000, 0.8660254037844387076, 1.000000000000000000, 0.8660254037844387076, 1.000000000000000000, 0.8660254037844387076, 1.000000000000000000, 0.8660254037844387076, 1.000000000000000000, 0.8660254037844387076, 1.000000000000000000, 0.8660254037844387076, 1.000000000000000000, 0.8660254037844387076, 1.000000000000000000, 0.8660254037844387076, 1.000000000000000000, 0.8660254037844387076, 1.000000000000000000, 0.8660254037844387076, 1.000000000000000000, 0.8660254037844387076, 1.000000000000000000, 0.8660254037844387076, 1.000000000000000000, 0.8660254037844387076, 1.000000000000000000, 0.8660254037844387076, 1.000000000000000000, 0.8660254037844387076, 1.000000000000000000, 0.8660254037844387076, 1.000000000000000000, 0.8660254037844387076, 1.000000000000000000, 0.8660254037844387076, 1.000000000000000000, 0.8660254037844387076, 1.000000000000000000, 0.8660254037844387076, 1.000000000000000000, 0.8660254037844387076, 1.000000000000000000, 0.8660254037844387076, 1.000000000000000000, 0.8660254037844387076, 1.000000000000000000, 0.8660254037844387076, 1.000000000000000000, 0.8660254037844387076, 1.000000000000000000, 0.8660254037844387076, 1.000000000000000000, 0.8660254037844387076, 1.000000000000000000, 0.8660254037844387076, 1.000000000000000000, 0.8660254037844387076, 1.000000000000000000, 0.8660254037844387076, 1.000000000000000000, 0.8660254037844387076, 1.000000000000000000, 0.8660254037844387076, 1.000000000000000000, 0.8660254037844387076, 1.000000000000000000, 0.8660254037844387076, 1.000000000000000000, 0.8660254037844387076, 1.000000000000000000, 0.8660254037844387076, 1.000000000000000000, 0.8660254037844387076, 1.000000000000000000, 0.8660254037844387076, 1.000000000000000000, 0.8660254037844387076, 1.000000000000000000, 0.8660254037844387076, 1.000000000000000000, 0.8660254037844387076, 1.000000000000000000, 0.8660254037844387076, 1.000000000000000000, 0.8660254037844387076, 1.000000000000000000, 0.8660254037844387076, 1.000000000000000000, 0.8660254037844387076, 1.000000000000000000, 0.8660254037844387076, 1.000000000000000000, 0.8660254037844387076, 1.000000000000000000, 0.8660254037844387076, 1.000000000000000000, 0.8660254037844387076, 1.000000000000000000, 0.8660254037844387076, 1.000000000000000000, 0.8660254037844387076, 1.000000000000000000, 0.8660254037844387076, 1.000000000000000000, 0.8660254037844387076, 1.000000000000000000, 0.8660254037844387076, 1.000000000000000000, 0.8660254037844387076, 1.000000000000000000, 0.8660254037844387076, 1.000000000000000000, 0.8660254037844387076, 1.000000000000000000, 0.8660254037844387076, 1.000000000000000000, 0.8660254037844387076, 1.000000000000000000, 0.8660254037844387076, 1.000000000000000000, 0.8660254037844387076, 1.000000000000000000, 0.8660254037844387076, 1.000000000000000000, 0.8660254037844387076, 1.000000000000000000, 0.8660254037844387076, 1.000000000000000000, 0.8660254037844387076, 1.000000000000000000, 0.8660254037844387076, 1.000000000000000000, 0.8660254037844387076, 1.000000000000000000, 0.8660254037844387076, 1.000000000000000000, 0.8660254037844387076, 1.000000000000000000, 0.8660254037844387076, 1.000000000000000000, 0.8660254037844387076, 1.000000000000000000, 0.8660254037844387076, 1.000000000000000000, 0.8660254037844387076, 1.000000000000000000, 0.8660254037844387076, 1.000000000000000000, 0.8660254037844387076, 1.000000000000000000, 0.8660254037844387076, 1.000000000000000000, 0.8660254037844387076, 1.000000000000000000, 0.8660254037844387076, 1.000000000000000000, 0.8660254037844387076, 1.000000000000000000, 0.8660254037844387076, 1.000000000000000000, 0.8660254037844387076, 1.000000000000000000, 0.8660254037844387076, 1.000000000000000000, 0.8660254037844387076, 1.000000000000000000, 0.8660254037844387076, 1.000000000000000000, 0.8660254037844387076, 1.000000000000000000, 0.8660254037844387076, 1.000000000000000000, 0.8660254037844387076, 1.000000000000000000, 0.8660254037844387076, 1.000000000000000000, 0.8660254037844387076, 1.000000000000000000, 0.8660254037844387076, 1.000000000000000000, 0.8660254037844387076, 1.000000000000000000, 0.8660254037844387076, 1.000000000000000000, 0.8660254037844387076, 1.000000000000000000, 0.8660254037844387076, 1.000000000000000000, 0.8660254037844387076, 1.000000000000000000, 0.8660254037844387076, 1.000000000000000000, 0.8660254037844387076, 1.000000000000000000, 0.8660254037844387076, 1.000000000000000000, 0.8660254037844387076, 1.000000000000000000, 0.8660254037844387076, 1.000000000000000000, 0.8660254037844387076, 1.000000000000000000, 0.8660254037844387076, 1.000000000000000000, 0.8660254037844387076, 1.000000000000000000, 0.8660254037844387076, 1.000000000000000000, 0.8660254037844387076, 1.000000000000000000, 0.8660254037844387076, 1.000000000000000000, 0.8660254037844387076, 1.000000000000000000, 0.8660254037844387076, 1.000000000000000000, 0.8660254037844387076, 1.000000000000000000, 0.8660254037844387076, 1.000000000000000000, 0.8660254037844387076, 1.000000000000000000, 0.8660254037844387076, 1.000000000000000000, 0.8660254037844387076, 1.000000000000000000, 0.8660254037844387076, 1.000000000000000000, 0.8660254037844387076, 1.000000000000000000, 0.8660254037844387076, 1.000000000000000000, 0.8660254037844387076, 1.000000000000000000, 0.8660254037844387076, 1.000000000000000000, 0.8660254037844387076, 1.000000000000000000, 0.8660254037844387076, 1.000000000000000000, 0.8660254037844387076, 1.000000000000000000, 0.8660254037844387076, 1.000000000000000000, 0.8660254037844387076, 1.000000000000000000, 0.8660254037844387076, 1.000000000000000000, 0.8660254037844387076, 1.000000000000000000, 0.8660254037844387076, 1.000000000000000000, 0.8660254037844387076, 1.000000000000000000, 0.8660254037844387076, 1.000000000000000000, 0.8660254037844387076, 1.000000000000000000, 0.8660254037844387076, 1.000000000000000000, 0.8660254037844387076, 1.000000000000000000, 0.8660254037844387076, 1.000000000000000000, 0.8660254037844387076, 1.000000000000000000, 0.8660254037844387076, 1.000000000000000000, 0.8660254037844387076, 1.000000000000000000, 0.8660254037844387076, 1.000000000000000000, 0.8660254037844387076, 1.000000000000000000, 0.8660254037844387076, 1.000000000000000000, 0.8660254037844387076, 1.000000000000000000, 0.8660254037844387076, 1.000000000000000000, 0.8660254037844387076, 1.000000000000000000, 0.8660254037844387076, 1.000000000000000000, 0.8660254037844387076, 1.000000000000000000, 0.8660254037844387076, 1.000000000000000000, 0.8660254037844387076, 1.000000000000000000, 0.8660254037844387076, 1.000000000000000000, 0.8660254037844387076, 1.000000000000000000, 0.8660254037844387076, 1.000000000000000000, 0.8660254037844387076, 1.000000000000000000, 0.8660254037844387076, 1.000000000000000000, 0.8660254037844387076, 1.000000000000000000, 0.8660254037844387076, 1.000000000000000000, 0.8660254037844387076, 1.000000000000000000, 0.8660254037844387076, 1.000000000000000000, 0.8660254037844387076, 1.000000000000000000, 0.8660254037844387076, 1.000000000000000000, 0.8660254037844387076, 1.000000000000000000, 0.8660254037844387076, 1.000000000000000000, 0.8660254037844387076, 1.000000000000000000, 0.8660254037844387076, 1.000000000000000000, 0.8660254037844387076, 1.000000000000000000, 0.8660254037844387076, 1.000000000000000000, 0.8660254037844387076, 1.000000000000000000, 0.8660254037844387076, 1.000000000000000000, 0.8660254037844387076, 1.000000000000000000, 0.8660254037844387076, 1.000000000000000000, 0.8660254037844387076, 1.000000000000000000, 0.8660254037844387076, 1.000000000000000000, 0.8660254037844387076, 1.000000000000000000, 0.8660254037844387076, 1.000000000000000000, 0.8660254037844387076, 1.000000000000000000, 0.8660254037844387076, 1.000000000000000000, 0.8660254037844387076, 1.000000000000000000, 0.8660254037844387076, 1.000000000000000000, 0.8660254037844387076, 1.000000000000000000, 0.8660254037844387076, 1.000000000000000000, 0.8660254037844387076, 1.000000000000000000, 0.8660254037844387076, 1.000000000000000000, 0.8660254037844387076, 1.000000000000000000, 0.8660254037844387076, 1.000000000000000000, 0.8660254037844387076, 1.000000000000000000, 0.8660254037844387076, 1.000000000000000000, 0.8660254037844387076, 1.000000000000000000, 0.8660254037844387076, 1.000000000000000000, 0.8660254037844387076, 1.000000000000000000, 0.8660254037844387076, 1.000000000000000000, 0.8660254037844387076, 1.000000000000000000, 0.8660254037844387076, 1.000000000000000000, 0.8660254037844387076, 1.000000000000000000, 0.8660254037844387076, 1.000000000000000000, 0.8660254037844387076, 1.000000000000000000, 0.8660254037844387076, 1.000000000000000000, 0.8660254037844387076, 1.000000000000000000, 0.8660254037844387076, 1.000000000000000000, 0.8660254037844387076, 1.000000000000000000, 0.8660254037844387076, 1.000000000000000000, 0.8660254037844387076, 1.000000000000000000, 0.8660254037844387076, 1.000000000000000000, 0.8660254037844387076, 1.000000000000000000, 0.8660254037844387076, 1.000000000000000000, 0.8660254037844387076, 1.000000000000000000, 0.8660254037844387076, 1.000000000000000000, 0.8660254037844387076, 1.000000000000000000, 0.8660254037844387076, 1.000000000000000000, 0.8660254037844387076, 1.000000000000000000, 0.8660254037844387076, 1.000000000000000000, 0.8660254037844387076, 1.000000000000000000, 0.8660254037844387076, 1.000000000000000000, 0.8660254037844387076, 1.000000000000000000, 0.8660254037844387076, 1.000000000000000000, 0.8660254037844387076, 1.000000000000000000, 0.8660254037844387076, 1.000000000000000000, 0.8660254037844387076, 1.000000000000000000, 0.8660254037844387076, 1.000000000000000000, 0.8660254037844387076, 1.000000000000000000, 0.8660254037844387076, 1.000000000000000000, 0.8660254037844387076, 1.000000000000000000, 0.8660254037844387076, 1.000000000000000000, 0.8660254037844387076, 1.000000000000000000, 0.8660254037844387076, 1.000000000000000000, 0.8660254037844387076, 1.000000000000000000, 0.8660254037844387076, 1.000000000000000000, 0.8660254037844387076, 1.000000000000000000) ) ) 
 REPRESENTATION_ITEM ( '' )  SURFACE ( )  );
#71033=CARTESIAN_POINT ( 'NONE',  ( 28.61249999999999716, 2.886751345948126879, 4.999999999999999112 ) ) ;
#71034=CARTESIAN_POINT ( 'NONE',  ( 11.12812500061451715, 6.421520780324663323E-16, -5.243569643749999010 ) ) ;
#71036=CARTESIAN_POINT ( 'NONE',  ( 24.68437500061451573, 6.421520780324663323E-16, -5.243569643749999010 ) ) ;
#71038=CARTESIAN_POINT ( 'NONE',  ( 7.828125000614517326, -4.541064518000419881, 2.621784821874995952 ) ) ;
#71039=CARTESIAN_POINT ( 'NONE',  ( 12.42187500061451821, -6.054752690667223547, -1.112240025338166033E-15 ) ) ;
#71040=VERTEX_POINT ( 'NONE', #31634 ) ;
#71041=CARTESIAN_POINT ( 'NONE',  ( 23.10937500061451644, 0.000000000000000000, 5.243569643749999010 ) ) ;
#71042=CARTESIAN_POINT ( 'NONE',  ( 27.36562500061451786, 3.027376345333613106, -5.243569643749998122 ) ) ;
#71043=PLANE ( 'NONE',  #14832 ) ;
#71044=CARTESIAN_POINT ( 'NONE',  ( 7.124999999999999112, -4.330127018922194537, 2.499999999999995559 ) ) ;
#71045=CARTESIAN_POINT ( 'NONE',  ( 15.90000000122903501, -2.886751345948125991, -5.000000000000000000 ) ) ;
#71046=CARTESIAN_POINT ( 'NONE',  ( -2.000000000000000000, 17.78750000122903430, -33.46410161513775705 ) ) ;
#71048=EDGE_LOOP ( 'NONE', ( #54295, #52949, #67727, #1632 ) ) ;
#71049=CARTESIAN_POINT ( 'NONE',  ( 15.26249999999999929, -5.773502691896255534, -1.060575238724906372E-15 ) ) ;
#71050=CARTESIAN_POINT ( 'NONE',  ( 18.18750000000000000, 5.773502691896255534, 3.535250795749688894E-16 ) ) ;
#71051=CARTESIAN_POINT ( 'NONE',  ( 11.05312500061451608, -4.541064518000417216, -2.621784821875001281 ) ) ;
#71052=ORIENTED_EDGE ( 'NONE', *, *, #37057, .F. ) ;
#71054=CARTESIAN_POINT ( 'NONE',  ( 2.121784821874999061, 17.90937500061451715, -33.67503911421598417 ) ) ;
#71055=CARTESIAN_POINT ( 'NONE',  ( 3.290625000614516793, -3.027376345333614438, 5.243569643749998122 ) ) ;
#71056=CARTESIAN_POINT ( 'NONE',  ( 10.42500000000000071, 6.123233995736764310E-16, -4.999999999999998224 ) ) ;
#71057=CARTESIAN_POINT ( 'NONE',  ( 9.187500000000001776, 5.773502691896255534, 3.535250795749688894E-16 ) ) ;
#71058=CARTESIAN_POINT ( 'NONE',  ( 3.850967645426020436, 3.886246437104829088, -3.268823720200904503 ) ) ;
#71059=ORIENTED_EDGE ( 'NONE', *, *, #18452, .F. ) ;
#71060=CARTESIAN_POINT ( 'NONE',  ( -4.243569643749999898, 15.71562500061451573, 27.54997392385601529 ) ) ;
#71061=CARTESIAN_POINT ( 'NONE',  ( 26.01562500061451289, 3.027376345333613106, -5.243569643749998122 ) ) ;
#71064=CARTESIAN_POINT ( 'NONE',  ( 23.70937500061451786, -4.541064518000417216, -2.621784821875001281 ) ) ;
#71065=CARTESIAN_POINT ( 'NONE',  ( 17.95312500061451644, 4.541064518000418104, -2.621784821874998173 ) ) ;
#71066=CARTESIAN_POINT ( 'NONE',  ( -3.000416591977282496E-16, 12.94062500061459176, -34.90005215228797653 ) ) ;
#71067=CARTESIAN_POINT ( 'NONE',  ( 23.06250000122903288, -4.330127018922190985, -2.500000000000001332 ) ) ;
#71068=CARTESIAN_POINT ( 'NONE',  ( 3.665625000614517681, 3.027376345333611329, 5.243569643749999010 ) ) ;
#71070=CARTESIAN_POINT ( 'NONE',  ( 22.00312500061451360, 4.541064518000418104, -2.621784821874998173 ) ) ;
#71073=CARTESIAN_POINT ( 'NONE',  ( 16.39687500061451786, -3.027376345333614438, 5.243569643749998122 ) ) ;
#71074=CARTESIAN_POINT ( 'NONE',  ( 16.47187500061452070, -6.054752690667223547, -1.112240025338166033E-15 ) ) ;
#71075=CARTESIAN_POINT ( 'NONE',  ( 25.50937500061451502, -4.541064518000417216, -2.621784821875001281 ) ) ;
#71076=CARTESIAN_POINT ( 'NONE',  ( 4.243569643749999010, 15.17187500061451644, 27.54997392385601174 ) ) ;
#71077=CARTESIAN_POINT ( 'NONE',  ( 4.678125000614516971, -4.541064518000419881, 2.621784821874995952 ) ) ;
#71078=CARTESIAN_POINT ( 'NONE',  ( 29.12812500061451715, 6.421520780324663323E-16, -5.243569643749999010 ) ) ;
#71079=CARTESIAN_POINT ( 'NONE',  ( 28.86562500061451786, 3.027376345333611329, 5.243569643749999010 ) ) ;
#71080=CARTESIAN_POINT ( 'NONE',  ( 1.999999999999998668, 16.36250000122903359, -33.46410161513775705 ) ) ;
#71081=CARTESIAN_POINT ( 'NONE',  ( -1.999999999999997113, 19.62500000000000000, 33.46410161513775705 ) ) ;
#71082=CARTESIAN_POINT ( 'NONE',  ( 8.184375000614515727, 4.541064518000418104, 2.621784821874999949 ) ) ;
#71083=CARTESIAN_POINT ( 'NONE',  ( 14.13750000122903394, 6.123233995736764310E-16, -4.999999999999998224 ) ) ;
#71084=CARTESIAN_POINT ( 'NONE',  ( 8.737500001229033586, 6.123233995736764310E-16, -4.999999999999998224 ) ) ;
#71085=CARTESIAN_POINT ( 'NONE',  ( 6.178125000614518747, 6.421520780324663323E-16, -5.243569643749999010 ) ) ;
#71088=CARTESIAN_POINT ( 'NONE',  ( 15.38437500061451679, 4.541064518000418104, 2.621784821874999949 ) ) ;
#71089=CARTESIAN_POINT ( 'NONE',  ( 7.724999999999999645, 6.123233995736764310E-16, -4.999999999999998224 ) ) ;
#71091=CARTESIAN_POINT ( 'NONE',  ( 21.85312500061451502, -4.541064518000417216, -2.621784821875001281 ) ) ;
#71092=CARTESIAN_POINT ( 'NONE',  ( 7.865625000614516971, -6.054752690667223547, -1.112240025338166033E-15 ) ) ;
#71093=CARTESIAN_POINT ( 'NONE',  ( 24.64687500061451431, -3.027376345333610441, -5.243569643749999898 ) ) ;
#71094=CARTESIAN_POINT ( 'NONE',  ( 8.390625000614518214, -3.027376345333610441, -5.243569643749999898 ) ) ;
#71096=CARTESIAN_POINT ( 'NONE',  ( 7.650000001229034119, -2.886751345948129988, 4.999999999999997335 ) ) ;
#71097=( BOUNDED_CURVE ( )  B_SPLINE_CURVE ( 2, ( #12250, #34781, #57314, #29251, #40702, #47683, #2621 ),
 .UNSPECIFIED., .F., .F. ) 
 B_SPLINE_CURVE_WITH_KNOTS ( ( 3, 2, 2, 3 ),
 ( 0.5833333333333334814, 0.5861111111111112493, 0.5888888888888890172, 0.5916666666666667851 ),
 .UNSPECIFIED. ) 
 CURVE ( )  GEOMETRIC_REPRESENTATION_ITEM ( )  RATIONAL_B_SPLINE_CURVE ( ( 0.9999999999999946709, 0.8660254037844440367, 1.000000000000000000, 0.8660254037844387076, 1.000000000000000000, 0.8660254037844333785, 1.000000000000005329 ) ) 
 REPRESENTATION_ITEM ( '' )  );
#71098=CARTESIAN_POINT ( 'NONE',  ( 23.05312500061451431, 0.000000000000000000, 5.243569643749999010 ) ) ;
#71100=CARTESIAN_POINT ( 'NONE',  ( 2.121784821874999061, 11.10312500061451679, -33.67503911421598417 ) ) ;
#71101=CARTESIAN_POINT ( 'NONE',  ( 9.412500001229034297, 0.000000000000000000, 4.999999999999998224 ) ) ;
#71102=CARTESIAN_POINT ( 'NONE',  ( 19.11562500061451431, -6.054752690667223547, -1.112240025338166033E-15 ) ) ;
#71103=CARTESIAN_POINT ( 'NONE',  ( 16.97812500061451502, 6.421520780324663323E-16, -5.243569643749999010 ) ) ;
#71105=CARTESIAN_POINT ( 'NONE',  ( 18.07499999999999929, 6.123233995736764310E-16, -4.999999999999998224 ) ) ;
#71106=CARTESIAN_POINT ( 'NONE',  ( 10.53750000122903252, 6.123233995736764310E-16, -4.999999999999998224 ) ) ;
#71107=CARTESIAN_POINT ( 'NONE',  ( 8.728125000614518569, -4.541064518000419881, 2.621784821874995952 ) ) ;
#71108=CARTESIAN_POINT ( 'NONE',  ( 13.11562500061451786, 3.027376345333611329, 5.243569643749999010 ) ) ;
#71110=CARTESIAN_POINT ( 'NONE',  ( 23.73750000122903359, 4.330127018922191873, 2.499999999999999556 ) ) ;
#71111=CARTESIAN_POINT ( 'NONE',  ( 22.77187500061451786, -6.054752690667223547, -1.112240025338166033E-15 ) ) ;
#71113=CARTESIAN_POINT ( 'NONE',  ( 6.000000001229033764, -2.886751345948125991, -5.000000000000000000 ) ) ;
#71114=CARTESIAN_POINT ( 'NONE',  ( 6.046875000614519102, -3.027376345333614438, 5.243569643749998122 ) ) ;
#71115=CARTESIAN_POINT ( 'NONE',  ( 22.69687500061451857, -3.027376345333614438, 5.243569643749998122 ) ) ;
#71116=CARTESIAN_POINT ( 'NONE',  ( 4.492467025342753217, 2.195141042190226877, -4.710191972078852984 ) ) ;
#71117=CARTESIAN_POINT ( 'NONE',  ( 19.52812500061451573, -4.541064518000419881, 2.621784821874995952 ) ) ;
#71118=CARTESIAN_POINT ( 'NONE',  ( 25.13437500061451502, 6.421520780324663323E-16, -5.243569643749999010 ) ) ;
#71120=CARTESIAN_POINT ( 'NONE',  ( 30.00000000000000000, 0.000000000000000000, 0.000000000000000000 ) ) ;
#71122=CARTESIAN_POINT ( 'NONE',  ( 5.784375000614517148, 6.421520780324663323E-16, -5.243569643749999010 ) ) ;
#71123=CARTESIAN_POINT ( 'NONE',  ( 14.99062500061451786, -3.027376345333614438, 5.243569643749998122 ) ) ;
#71124=CARTESIAN_POINT ( 'NONE',  ( 14.18437500061451750, -4.541064518000419881, 2.621784821874995952 ) ) ;
#71125=ORIENTED_EDGE ( 'NONE', *, *, #36482, .F. ) ;
#71126=CARTESIAN_POINT ( 'NONE',  ( 24.51562500061451289, -6.054752690667223547, -1.112240025338166033E-15 ) ) ;
#71127=LINE ( 'NONE', #71869, #3878 ) ;
#71129=CARTESIAN_POINT ( 'NONE',  ( 15.82499999999999929, 6.123233995736764310E-16, -4.999999999999998224 ) ) ;
#71130=CARTESIAN_POINT ( 'NONE',  ( 23.51250000122903216, -4.330127018922190985, -2.500000000000001332 ) ) ;
#71131=CARTESIAN_POINT ( 'NONE',  ( 17.39062500061451644, -3.027376345333610441, -5.243569643749999898 ) ) ;
#71133=CARTESIAN_POINT ( 'NONE',  ( 22.87500000000000000, -4.330127018922194537, 2.499999999999995559 ) ) ;
#71134=CARTESIAN_POINT ( 'NONE',  ( 24.08437500061451786, -4.541064518000419881, 2.621784821874995952 ) ) ;
#71136=CARTESIAN_POINT ( 'NONE',  ( 13.23750000122903359, 6.123233995736764310E-16, -4.999999999999998224 ) ) ;
#71137=CARTESIAN_POINT ( 'NONE',  ( 11.09062500061451573, -3.027376345333610441, -5.243569643749999898 ) ) ;
#71138=CARTESIAN_POINT ( 'NONE',  ( 4.378125000614518925, 6.421520780324663323E-16, -5.243569643749999010 ) ) ;
#71140=CARTESIAN_POINT ( 'NONE',  ( 27.77812500061451573, 6.421520780324663323E-16, -5.243569643749999010 ) ) ;
#71141=CARTESIAN_POINT ( 'NONE',  ( 18.37500000000000355, -4.330127018922194537, 2.499999999999995559 ) ) ;
#71142=CARTESIAN_POINT ( 'NONE',  ( 27.41250000000000142, -5.773502691896255534, -1.060575238724906372E-15 ) ) ;
#71144=CARTESIAN_POINT ( 'NONE',  ( 6.871875000614517504, 3.027376345333611329, 5.243569643749999010 ) ) ;
#71145=CARTESIAN_POINT ( 'NONE',  ( 17.44687500061451857, -3.027376345333610441, -5.243569643749999898 ) ) ;
#71146=CYLINDRICAL_SURFACE ( 'NONE', #25385, 4.999999999999998224 ) ;
#71148=CARTESIAN_POINT ( 'NONE',  ( 26.31562500061451715, -6.054752690667223547, -1.112240025338166033E-15 ) ) ;
#71149=CARTESIAN_POINT ( 'NONE',  ( 27.04687500061451644, 6.054752690667223547, 3.707466751127219781E-16 ) ) ;
#71151=CARTESIAN_POINT ( 'NONE',  ( 12.93750000000000178, -2.886751345948129988, 4.999999999999997335 ) ) ;
#71152=CARTESIAN_POINT ( 'NONE',  ( 11.39062500061451644, -3.027376345333614438, 5.243569643749998122 ) ) ;
#71155=CARTESIAN_POINT ( 'NONE',  ( 29.80312500061451431, 0.000000000000000000, 5.243569643749999010 ) ) ;
#71156=CARTESIAN_POINT ( 'NONE',  ( 18.63750000122903216, 6.123233995736764310E-16, -4.999999999999998224 ) ) ;
#71159=CARTESIAN_POINT ( 'NONE',  ( 4.865625000614517859, 3.027376345333613106, -5.243569643749998122 ) ) ;
#71160=CARTESIAN_POINT ( 'NONE',  ( 21.30937500061451573, 0.000000000000000000, 5.243569643749999010 ) ) ;
#71161=CARTESIAN_POINT ( 'NONE',  ( -4.243569643749999898, 17.60937500061451999, 30.00000000000000000 ) ) ;
#71162=CARTESIAN_POINT ( 'NONE',  ( 23.44687500061451502, 6.054752690667223547, 3.707466751127219781E-16 ) ) ;
#71163=CARTESIAN_POINT ( 'NONE',  ( 4.425000000000001599, -4.330127018922194537, 2.499999999999995559 ) ) ;
#71164=CARTESIAN_POINT ( 'NONE',  ( -3.999999999999999556, 11.07500000122903394, 27.69059892324149530 ) ) ;
#71165=CARTESIAN_POINT ( 'NONE',  ( 11.57812500061451644, 6.421520780324663323E-16, -5.243569643749999010 ) ) ;
#71166=CARTESIAN_POINT ( 'NONE',  ( 3.525000001229034119, 2.886751345948126879, 4.999999999999999112 ) ) ;
#71167=EDGE_CURVE ( 'NONE', #15981, #16013, #65976, .T. ) ;
#71168=CARTESIAN_POINT ( 'NONE',  ( 10.39687500061451786, 6.054752690667223547, 3.707466751127219781E-16 ) ) ;
#71169=CARTESIAN_POINT ( 'NONE',  ( 1.592000809091587073E-14, 15.05000000122903714, 26.00000000000000000 ) ) ;
#71170=CARTESIAN_POINT ( 'NONE',  ( 9.515625000614518214, 3.027376345333611329, 5.243569643749999010 ) ) ;
#71171=CARTESIAN_POINT ( 'NONE',  ( 13.77187500061451786, -6.054752690667223547, -1.112240025338166033E-15 ) ) ;
#71173=CARTESIAN_POINT ( 'NONE',  ( 20.66250000122903074, 0.000000000000000000, 4.999999999999998224 ) ) ;
#71174=CARTESIAN_POINT ( 'NONE',  ( 10.20937500061451786, -4.541064518000417216, -2.621784821875001281 ) ) ;
#71175=CARTESIAN_POINT ( 'NONE',  ( 12.47812500061451502, 6.421520780324663323E-16, -5.243569643749999010 ) ) ;
#71177=CARTESIAN_POINT ( 'NONE',  ( 20.40937500061451715, 0.000000000000000000, 5.243569643749999010 ) ) ;
#71179=CARTESIAN_POINT ( 'NONE',  ( -2.506492529888153964, 4.347006505069262339, 26.84353589692258879 ) ) ;
#71180=CARTESIAN_POINT ( 'NONE',  ( 2.964777361493091679, -4.026176250088806086, -3.359304602455296607 ) ) ;
#71181=CARTESIAN_POINT ( 'NONE',  ( -4.243569643749999898, 14.90937500061451715, -30.00000000000000000 ) ) ;
#71182=CARTESIAN_POINT ( 'NONE',  ( 15.56250000122903465, 4.330127018922192761, -2.499999999999997780 ) ) ;
#71183=CARTESIAN_POINT ( 'NONE',  ( 10.20937500061451786, -4.541064518000417216, -2.621784821875001281 ) ) ;
#71184=CARTESIAN_POINT ( 'NONE',  ( -4.243569643749999898, 17.96562500061451573, -32.45002607614398471 ) ) ;
#71185=CARTESIAN_POINT ( 'NONE',  ( 18.41250000122903430, 0.000000000000000000, 4.999999999999998224 ) ) ;
#71186=CARTESIAN_POINT ( 'NONE',  ( 9.440625000614517148, 6.054752690667223547, 3.707466751127219781E-16 ) ) ;
#71188=CARTESIAN_POINT ( 'NONE',  ( 15.97499999999999964, 4.330127018922191873, 2.499999999999999556 ) ) ;
#71189=CARTESIAN_POINT ( 'NONE',  ( 4.987500001229032698, -4.330127018922194537, 2.499999999999995559 ) ) ;
#71190=CARTESIAN_POINT ( 'NONE',  ( 9.309375000614517504, -4.541064518000417216, -2.621784821875001281 ) ) ;
#71192=CARTESIAN_POINT ( 'NONE',  ( 5.137500001229033941, 6.123233995736764310E-16, -4.999999999999998224 ) ) ;
#71193=CARTESIAN_POINT ( 'NONE',  ( 10.95000000122903394, -2.886751345948125991, -5.000000000000000000 ) ) ;
#71194=CARTESIAN_POINT ( 'NONE',  ( 17.81250000122903288, 4.330127018922192761, -2.499999999999997780 ) ) ;
#71195=CARTESIAN_POINT ( 'NONE',  ( 14.16562500061451679, -6.054752690667223547, -1.112240025338166033E-15 ) ) ;
#71196=CARTESIAN_POINT ( 'NONE',  ( 21.10312500061451502, 4.541064518000418104, -2.621784821874998173 ) ) ;
#71197=CARTESIAN_POINT ( 'NONE',  ( 27.82500000122903572, 2.886751345948126879, 4.999999999999999112 ) ) ;
#71198=CARTESIAN_POINT ( 'NONE',  ( 3.253125000614518036, 0.000000000000000000, 5.243569643749999010 ) ) ;
#71199=CARTESIAN_POINT ( 'NONE',  ( 24.44999999999999929, 4.330127018922192761, -2.499999999999997780 ) ) ;
#71200=CARTESIAN_POINT ( 'NONE',  ( 4.898587196589411843E-16, 20.00000000000000000, 33.99999999999999289 ) ) ;
#71202=CARTESIAN_POINT ( 'NONE',  ( 29.25937500061451502, 4.541064518000418104, -2.621784821874998173 ) ) ;
#71204=CARTESIAN_POINT ( 'NONE',  ( 13.01250000122903394, 0.000000000000000000, 4.999999999999998224 ) ) ;
#71205=CARTESIAN_POINT ( 'NONE',  ( 29.25937500061451502, 4.541064518000418104, -2.621784821874998173 ) ) ;
#71206=ADVANCED_FACE ( 'NONE', ( #71525 ), #15720, .F. ) ;
#71207=CARTESIAN_POINT ( 'NONE',  ( 8.109375000614518214, 4.541064518000418104, -2.621784821874998173 ) ) ;
#71208=CARTESIAN_POINT ( 'NONE',  ( 26.76562500061451644, -6.054752690667223547, -1.112240025338166033E-15 ) ) ;
#71210=CARTESIAN_POINT ( 'NONE',  ( 11.58750000122903501, 4.330127018922191873, 2.499999999999999556 ) ) ;
#71211=CARTESIAN_POINT ( 'NONE',  ( 3.752440054025286909, -3.304420318444254878, 4.071342403668507082 ) ) ;
#71212=CARTESIAN_POINT ( 'NONE',  ( 6.534375000614517148, -4.541064518000419881, 2.621784821874995952 ) ) ;
#71213=CARTESIAN_POINT ( 'NONE',  ( 8.371875000614515727, -6.054752690667223547, -1.112240025338166033E-15 ) ) ;
#71214=CARTESIAN_POINT ( 'NONE',  ( 3.000000000000002665, 0.000000000000000000, 4.999999999999998224 ) ) ;
#71215=CARTESIAN_POINT ( 'NONE',  ( 4.243569643749999010, 13.31562500061459353, 27.54997392385601174 ) ) ;
#71216=CARTESIAN_POINT ( 'NONE',  ( 22.94999999999999929, -4.330127018922190985, -2.500000000000001332 ) ) ;
#71217=CARTESIAN_POINT ( 'NONE',  ( 29.69999999999999574, -4.330127018922190985, -2.500000000000001332 ) ) ;
#71218=CARTESIAN_POINT ( 'NONE',  ( 4.500000000000000888, -4.330127018922190985, -2.500000000000001332 ) ) ;
#71221=CARTESIAN_POINT ( 'NONE',  ( 18.70312500061451644, -4.541064518000417216, -2.621784821875001281 ) ) ;
#71222=CARTESIAN_POINT ( 'NONE',  ( 11.50312500061451892, -4.541064518000417216, -2.621784821875001281 ) ) ;
#71224=CARTESIAN_POINT ( 'NONE',  ( 6.084375000614518747, -4.541064518000419881, 2.621784821874995952 ) ) ;
#71225=CARTESIAN_POINT ( 'NONE',  ( 23.88749999999999929, -2.886751345948125991, -5.000000000000000000 ) ) ;
#71226=CARTESIAN_POINT ( 'NONE',  ( 19.80000000122903359, -2.886751345948129988, 4.999999999999997335 ) ) ;
#71227=CARTESIAN_POINT ( 'NONE',  ( 27.02812500061451573, 4.541064518000418104, 2.621784821874999949 ) ) ;
#71228=FACE_OUTER_BOUND ( 'NONE', #66972, .T. ) ;
#71229=CARTESIAN_POINT ( 'NONE',  ( 8.896875000614517859, -3.027376345333610441, -5.243569643749999898 ) ) ;
#71230=CARTESIAN_POINT ( 'NONE',  ( 14.52187500061451608, 3.027376345333611329, 5.243569643749999010 ) ) ;
#71231=CARTESIAN_POINT ( 'NONE',  ( 23.74687500061451573, -3.027376345333610441, -5.243569643749999898 ) ) ;
#71234=CARTESIAN_POINT ( 'NONE',  ( 18.72187500061451360, -6.054752690667223547, -1.112240025338166033E-15 ) ) ;
#71235=CARTESIAN_POINT ( 'NONE',  ( 9.721875000614517148, -6.054752690667223547, -1.112240025338166033E-15 ) ) ;
#71237=CARTESIAN_POINT ( 'NONE',  ( 23.47499999999999787, 6.123233995736764310E-16, -4.999999999999998224 ) ) ;
#71239=CARTESIAN_POINT ( 'NONE',  ( -1.389182545231912203, 9.676047173952133207, -33.81675723707382275 ) ) ;
#71241=CARTESIAN_POINT ( 'NONE',  ( 12.06562500061451537, 3.027376345333613106, -5.243569643749998122 ) ) ;
#71242=CARTESIAN_POINT ( 'NONE',  ( 29.78437500061451715, 4.541064518000418104, 2.621784821874999949 ) ) ;
#71244=CARTESIAN_POINT ( 'NONE',  ( 1.999999999999998668, 10.06250000122903465, -33.46410161513775705 ) ) ;
#71245=CARTESIAN_POINT ( 'NONE',  ( 12.37500000000000000, 4.330127018922191873, 2.499999999999999556 ) ) ;
#71246=CARTESIAN_POINT ( 'NONE',  ( -3.999999999999999556, 18.72500000122903074, 27.69059892324149530 ) ) ;
#71247=CARTESIAN_POINT ( 'NONE',  ( 12.00000000122903465, 5.773502691896255534, 3.535250795749688894E-16 ) ) ;
#71248=CARTESIAN_POINT ( 'NONE',  ( 21.90937500061451715, -4.541064518000417216, -2.621784821875001281 ) ) ;
#71249=CARTESIAN_POINT ( 'NONE',  ( 17.18437500061451573, 4.541064518000418104, 2.621784821874999949 ) ) ;
#71250=CARTESIAN_POINT ( 'NONE',  ( -3.999999999999999112, 16.40000000000000213, -30.00000000000000000 ) ) ;
#71251=VERTEX_POINT ( 'NONE', #39005 ) ;
#71252=CARTESIAN_POINT ( 'NONE',  ( 18.10312500061451502, 0.000000000000000000, 5.243569643749999010 ) ) ;
#71253=CARTESIAN_POINT ( 'NONE',  ( 28.20000000122903216, 5.773502691896255534, 3.535250795749688894E-16 ) ) ;
#71254=CARTESIAN_POINT ( 'NONE',  ( 18.57187500061451857, 3.027376345333611329, 5.243569643749999010 ) ) ;
#71255=CARTESIAN_POINT ( 'NONE',  ( 29.52187500061451431, -6.054752690667223547, -1.112240025338166033E-15 ) ) ;
#71256=CARTESIAN_POINT ( 'NONE',  ( 5.353125000614515905, 4.541064518000418104, -2.621784821874998173 ) ) ;
#71257=CARTESIAN_POINT ( 'NONE',  ( 19.94062500061451715, -3.027376345333614438, 5.243569643749998122 ) ) ;
#71258=CARTESIAN_POINT ( 'NONE',  ( 27.98437500061451289, 4.541064518000418104, 2.621784821874999949 ) ) ;
#71259=CARTESIAN_POINT ( 'NONE',  ( -2.121784821874999949, 12.52812500061451573, 26.32496088578401938 ) ) ;
#71260=CARTESIAN_POINT ( 'NONE',  ( 17.77500000122903145, 2.886751345948129099, -4.999999999999998224 ) ) ;
#71262=CARTESIAN_POINT ( 'NONE',  ( 7.153125000614518392, 4.541064518000418104, -2.621784821874998173 ) ) ;
#71263=CARTESIAN_POINT ( 'NONE',  ( 27.59062500061451573, -3.027376345333614438, 5.243569643749998122 ) ) ;
#71264=DIRECTION ( 'NONE',  ( -0.000000000000000000, -1.000000000000000000, -0.000000000000000000 ) ) ;
#71265=EDGE_CURVE ( 'NONE', #23627, #8722, #2853, .T. ) ;
#71266=CARTESIAN_POINT ( 'NONE',  ( 22.73437500061451644, -4.541064518000419881, 2.621784821874995952 ) ) ;
#71267=CARTESIAN_POINT ( 'NONE',  ( 12.14062500061451821, 6.054752690667223547, 3.707466751127219781E-16 ) ) ;
#71268=CARTESIAN_POINT ( 'NONE',  ( 23.58750000122903145, 6.123233995736764310E-16, -4.999999999999998224 ) ) ;
#71269=CARTESIAN_POINT ( 'NONE',  ( 22.97812500061451857, 4.541064518000418104, 2.621784821874999949 ) ) ;
#71270=CARTESIAN_POINT ( 'NONE',  ( 16.28437500061452070, 4.541064518000418104, 2.621784821874999949 ) ) ;
#71271=CARTESIAN_POINT ( 'NONE',  ( 13.41562500061451502, 3.027376345333613106, -5.243569643749998122 ) ) ;
#71272=CARTESIAN_POINT ( 'NONE',  ( -2.121784821874999949, 14.38437500061451679, 26.32496088578401938 ) ) ;
#71273=CARTESIAN_POINT ( 'NONE',  ( 19.71562500061451928, 3.027376345333613106, -5.243569643749998122 ) ) ;
#71274=CARTESIAN_POINT ( 'NONE',  ( 29.57812500061451644, 6.421520780324663323E-16, -5.243569643749999010 ) ) ;
#71275=EDGE_LOOP ( 'NONE', ( #1061, #64504, #21894, #33313 ) ) ;
#71277=CARTESIAN_POINT ( 'NONE',  ( 22.83749999999999858, -2.886751345948129988, 4.999999999999997335 ) ) ;
#71278=CARTESIAN_POINT ( 'NONE',  ( -4.243569643749999898, 18.50937500061451857, -30.00000000000000000 ) ) ;
#71279=CARTESIAN_POINT ( 'NONE',  ( 13.01250000122903394, 0.000000000000000000, 4.999999999999998224 ) ) ;
#71280=CARTESIAN_POINT ( 'NONE',  ( 25.79062500061451502, -3.027376345333614438, 5.243569643749998122 ) ) ;
#71281=CARTESIAN_POINT ( 'NONE',  ( 5.615625000614517859, -6.054752690667223547, -1.112240025338166033E-15 ) ) ;
#71282=CARTESIAN_POINT ( 'NONE',  ( 20.47500000122903074, 2.886751345948129099, -4.999999999999998224 ) ) ;
#71283=CARTESIAN_POINT ( 'NONE',  ( 23.95312500061451289, 0.000000000000000000, 5.243569643749999010 ) ) ;
#71284=CARTESIAN_POINT ( 'NONE',  ( 23.62500000000000000, 4.330127018922191873, 2.499999999999999556 ) ) ;
#71285=CARTESIAN_POINT ( 'NONE',  ( 27.51562500061451644, 3.027376345333611329, 5.243569643749999010 ) ) ;
#71286=CARTESIAN_POINT ( 'NONE',  ( 7.078125000614516438, 6.421520780324663323E-16, -5.243569643749999010 ) ) ;
#71288=CARTESIAN_POINT ( 'NONE',  ( 24.44062500061451715, -3.027376345333614438, 5.243569643749998122 ) ) ;
#71289=CARTESIAN_POINT ( 'NONE',  ( 5.840625000614516615, 6.054752690667223547, 3.707466751127219781E-16 ) ) ;
#71291=CARTESIAN_POINT ( 'NONE',  ( 4.003125000614518925, 4.541064518000418104, -2.621784821874998173 ) ) ;
#71292=CARTESIAN_POINT ( 'NONE',  ( -2.000000000000000000, 13.28750000122903430, -33.46410161513775705 ) ) ;
#71293=DIRECTION ( 'NONE',  ( 0.000000000000000000, 0.000000000000000000, -1.000000000000000000 ) ) ;
#71294=( BOUNDED_CURVE ( )  B_SPLINE_CURVE ( 2, ( #2116, #24265, #24991, #17985, #41628, #41998, #30179 ),
 .UNSPECIFIED., .F., .F. ) 
 B_SPLINE_CURVE_WITH_KNOTS ( ( 3, 2, 2, 3 ),
 ( 0.09166666666666660468, 0.09444444444444442810, 0.09722222222222223764, 0.1000000000000000611 ),
 .UNSPECIFIED. ) 
 CURVE ( )  GEOMETRIC_REPRESENTATION_ITEM ( )  RATIONAL_B_SPLINE_CURVE ( ( 1.000000000000002665, 0.8660254037844360431, 1.000000000000000000, 0.8660254037844387076, 1.000000000000000000, 0.8660254037844360431, 1.000000000000002665 ) ) 
 REPRESENTATION_ITEM ( '' )  );
#71295=CARTESIAN_POINT ( 'NONE',  ( 9.937500000000001776, -2.886751345948125991, -5.000000000000000000 ) ) ;
#71296=CARTESIAN_POINT ( 'NONE',  ( 11.97187500061451892, -6.054752690667223547, -1.112240025338166033E-15 ) ) ;
#71297=CARTESIAN_POINT ( 'NONE',  ( 7.462500001229035007, 4.330127018922192761, -2.499999999999997780 ) ) ;
#71298=CARTESIAN_POINT ( 'NONE',  ( 13.58437500061451786, 4.541064518000418104, 2.621784821874999949 ) ) ;
#71300=CARTESIAN_POINT ( 'NONE',  ( 6.684375000614518392, 6.421520780324663323E-16, -5.243569643749999010 ) ) ;
#71301=CARTESIAN_POINT ( 'NONE',  ( 4.243569643749999898, 10.12812500061451715, -30.00000000000000000 ) ) ;
#71302=DIRECTION ( 'NONE',  ( -0.000000000000000000, -1.000000000000000000, -0.000000000000000000 ) ) ;
#71303=CARTESIAN_POINT ( 'NONE',  ( 12.04687500061451821, -3.027376345333610441, -5.243569643749999898 ) ) ;
#71304=CARTESIAN_POINT ( 'NONE',  ( 22.01250000122903216, 0.000000000000000000, 4.999999999999998224 ) ) ;
#71306=CARTESIAN_POINT ( 'NONE',  ( 21.17812500061451431, 4.541064518000418104, 2.621784821874999949 ) ) ;
#71307=CARTESIAN_POINT ( 'NONE',  ( 4.898587196589411843E-16, 20.00000000000000000, -26.00000000000000000 ) ) ;
#71308=CARTESIAN_POINT ( 'NONE',  ( -2.121784821874996840, 19.42812500061459602, 33.67503911421598417 ) ) ;
#71309=CARTESIAN_POINT ( 'NONE',  ( 24.87187500061451573, 3.027376345333611329, 5.243569643749999010 ) ) ;
#71310=( BOUNDED_CURVE ( )  B_SPLINE_CURVE ( 2, ( #10464, #43359, #71800, #32994, #38543, #71058, #44091 ),
 .UNSPECIFIED., .F., .F. ) 
 B_SPLINE_CURVE_WITH_KNOTS ( ( 3, 2, 2, 3 ),
 ( 0.9517299907128293768, 0.9527777777777777235, 0.9555555555555556024, 0.9564971600366024562 ),
 .UNSPECIFIED. ) 
 CURVE ( )  GEOMETRIC_REPRESENTATION_ITEM ( )  RATIONAL_B_SPLINE_CURVE ( ( 0.9370531128228860585, 0.9494643343793163215, 1.000000000000000000, 0.8660254037844387076, 1.000000000000000000, 0.9545856111485142570, 0.9399601445705541014 ) ) 
 REPRESENTATION_ITEM ( '' )  );
#71311=CARTESIAN_POINT ( 'NONE',  ( 5.053125000614517859, 0.000000000000000000, 5.243569643749999010 ) ) ;
#71314=CARTESIAN_POINT ( 'NONE',  ( 17.95312500061451644, 4.541064518000418104, -2.621784821874998173 ) ) ;
#71315=CARTESIAN_POINT ( 'NONE',  ( 15.34687500061451537, 6.054752690667223547, 3.707466751127219781E-16 ) ) ;
#71316=CARTESIAN_POINT ( 'NONE',  ( 29.84999999999999787, 4.330127018922192761, -2.499999999999997780 ) ) ;
#71317=CARTESIAN_POINT ( 'NONE',  ( 26.25000000122903288, -2.886751345948125991, -5.000000000000000000 ) ) ;
#71318=CARTESIAN_POINT ( 'NONE',  ( 6.984375000614516438, -4.541064518000419881, 2.621784821874995952 ) ) ;
#71320=CARTESIAN_POINT ( 'NONE',  ( 17.03437500061451715, 6.421520780324663323E-16, -5.243569643749999010 ) ) ;
#71321=DIRECTION ( 'NONE',  ( -1.000000000000000000, -0.000000000000000000, -0.000000000000000000 ) ) ;
#71322=CARTESIAN_POINT ( 'NONE',  ( 25.08749999999999858, -2.886751345948129988, 4.999999999999997335 ) ) ;
#71323=CARTESIAN_POINT ( 'NONE',  ( 3.750000001229034652, -2.886751345948125991, -5.000000000000000000 ) ) ;
#71324=CARTESIAN_POINT ( 'NONE',  ( 28.24687500061451573, -3.027376345333610441, -5.243569643749999898 ) ) ;
#71325=CARTESIAN_POINT ( 'NONE',  ( 15.57187500061451679, -6.054752690667223547, -1.112240025338166033E-15 ) ) ;
#71327=LINE ( 'NONE', #2993, #69296 ) ;
#71328=CARTESIAN_POINT ( 'NONE',  ( 9.150000000000002132, 4.330127018922192761, -2.499999999999997780 ) ) ;
#71330=CARTESIAN_POINT ( 'NONE',  ( 20.31562500061451715, 3.027376345333611329, 5.243569643749999010 ) ) ;
#71331=CARTESIAN_POINT ( 'NONE',  ( 12.44999999999999929, 0.000000000000000000, 4.999999999999998224 ) ) ;
#71332=CARTESIAN_POINT ( 'NONE',  ( 3.515625000614516882, 3.027376345333613106, -5.243569643749998122 ) ) ;
#71333=CARTESIAN_POINT ( 'NONE',  ( 18.67500000000000071, 4.330127018922191873, 2.499999999999999556 ) ) ;
#71334=CARTESIAN_POINT ( 'NONE',  ( 18.74062500061451431, -3.027376345333610441, -5.243569643749999898 ) ) ;
#71336=CARTESIAN_POINT ( 'NONE',  ( 22.53750000122903430, -4.330127018922194537, 2.499999999999995559 ) ) ;
#71339=CARTESIAN_POINT ( 'NONE',  ( 29.18437500061451573, 6.421520780324663323E-16, -5.243569643749999010 ) ) ;
#71340=ORIENTED_EDGE ( 'NONE', *, *, #56383, .F. ) ;
#71341=CARTESIAN_POINT ( 'NONE',  ( 17.57812500061451644, 4.541064518000418104, 2.621784821874999949 ) ) ;
#71342=CARTESIAN_POINT ( 'NONE',  ( 25.07812500061451644, 6.421520780324663323E-16, -5.243569643749999010 ) ) ;
#71343=CARTESIAN_POINT ( 'NONE',  ( 25.54687500061451644, -3.027376345333610441, -5.243569643749999898 ) ) ;
#71344=CARTESIAN_POINT ( 'NONE',  ( 8.699999999999999289, 4.330127018922192761, -2.499999999999997780 ) ) ;
#71345=CARTESIAN_POINT ( 'NONE',  ( 11.09062500061451573, -3.027376345333610441, -5.243569643749999898 ) ) ;
#71346=CARTESIAN_POINT ( 'NONE',  ( 26.24062500061451431, -3.027376345333614438, 5.243569643749998122 ) ) ;
#71347=CARTESIAN_POINT ( 'NONE',  ( 17.82187500061451502, -6.054752690667223547, -1.112240025338166033E-15 ) ) ;
#71348=CARTESIAN_POINT ( 'NONE',  ( 9.740625000614516082, -3.027376345333610441, -5.243569643749999898 ) ) ;
#71349=CARTESIAN_POINT ( 'NONE',  ( 7.162500001229032520, 0.000000000000000000, 4.999999999999998224 ) ) ;
#71350=CARTESIAN_POINT ( 'NONE',  ( 2.121784821875001281, 19.50312500061451360, 33.67503911421598417 ) ) ;
#71352=CARTESIAN_POINT ( 'NONE',  ( 24.18750000122903288, 4.330127018922191873, 2.499999999999999556 ) ) ;
#71354=CARTESIAN_POINT ( 'NONE',  ( 14.50312500061451537, 0.000000000000000000, 5.243569643749999010 ) ) ;
#71355=CARTESIAN_POINT ( 'NONE',  ( 8.034375000614518925, 6.421520780324663323E-16, -5.243569643749999010 ) ) ;
#71356=CARTESIAN_POINT ( 'NONE',  ( 6.084375000614518747, -4.541064518000419881, 2.621784821874995952 ) ) ;
#71358=CARTESIAN_POINT ( 'NONE',  ( 3.999999999999998668, 13.51250000000000107, 27.69059892324149530 ) ) ;
#71359=CARTESIAN_POINT ( 'NONE',  ( 22.49062500061451431, 6.054752690667223547, 3.707466751127219781E-16 ) ) ;
#71360=CARTESIAN_POINT ( 'NONE',  ( 15.64687500061451608, -3.027376345333610441, -5.243569643749999898 ) ) ;
#71361=CARTESIAN_POINT ( 'NONE',  ( 19.52812500061451573, -4.541064518000419881, 2.621784821874995952 ) ) ;
#71362=CARTESIAN_POINT ( 'NONE',  ( 3.999999999999999112, 13.02500000000000213, 30.00000000000000000 ) ) ;
#71363=AXIS2_PLACEMENT_3D ( 'NONE', #64747, #36673, #58099 ) ;
#71364=CARTESIAN_POINT ( 'NONE',  ( 26.12812500061451360, 4.541064518000418104, 2.621784821874999949 ) ) ;
#71365=CARTESIAN_POINT ( 'NONE',  ( 7.012500001229035718, 4.330127018922192761, -2.499999999999997780 ) ) ;
#71367=CARTESIAN_POINT ( 'NONE',  ( 2.850000001229036073, -2.886751345948125991, -5.000000000000000000 ) ) ;
#71368=CARTESIAN_POINT ( 'NONE',  ( -2.828200636599751609E-16, 18.53750000000000142, -34.61880215351700230 ) ) ;
#71369=CARTESIAN_POINT ( 'NONE',  ( 21.86250000122903003, 4.330127018922192761, -2.499999999999997780 ) ) ;
#71371=CARTESIAN_POINT ( 'NONE',  ( 6.534375000614517148, -4.541064518000419881, 2.621784821874995952 ) ) ;
#71372=LINE ( 'NONE', #19644, #59680 ) ;
#71373=CARTESIAN_POINT ( 'NONE',  ( 13.22812500061451502, -4.541064518000419881, 2.621784821874995952 ) ) ;
#71374=CARTESIAN_POINT ( 'NONE',  ( 8.784375000614518925, -4.541064518000419881, 2.621784821874995952 ) ) ;
#71375=CARTESIAN_POINT ( 'NONE',  ( 26.40000000122902790, 5.773502691896255534, 3.535250795749688894E-16 ) ) ;
#71376=CARTESIAN_POINT ( 'NONE',  ( 16.50937500061451502, -4.541064518000417216, -2.621784821875001281 ) ) ;
#71377=CARTESIAN_POINT ( 'NONE',  ( 5.971875000614516260, 3.027376345333611329, 5.243569643749999010 ) ) ;
#71378=CARTESIAN_POINT ( 'NONE',  ( 29.62500000000000000, -4.330127018922194537, 2.499999999999995559 ) ) ;
#71379=CARTESIAN_POINT ( 'NONE',  ( 5.278125000614516615, 6.421520780324663323E-16, -5.243569643749999010 ) ) ;
#71380=CARTESIAN_POINT ( 'NONE',  ( 14.61562500061451608, -6.054752690667223547, -1.112240025338166033E-15 ) ) ;
#71381=EDGE_LOOP ( 'NONE', ( #26452, #32987, #43290, #65973 ) ) ;
#71382=AXIS2_PLACEMENT_3D ( 'NONE', #40904, #12449, #63771 ) ;
#71383=CARTESIAN_POINT ( 'NONE',  ( 11.42812500061451608, -4.541064518000419881, 2.621784821874995952 ) ) ;
#71384=CARTESIAN_POINT ( 'NONE',  ( 6.487500001229034474, 6.123233995736764310E-16, -4.999999999999998224 ) ) ;
#71386=CARTESIAN_POINT ( 'NONE',  ( 8.803125000614517859, -4.541064518000417216, -2.621784821875001281 ) ) ;
#71388=CARTESIAN_POINT ( 'NONE',  ( 9.187500000000001776, 5.773502691896255534, 3.535250795749688894E-16 ) ) ;
#71389=CARTESIAN_POINT ( 'NONE',  ( 4.800000001229032698, 5.773502691896255534, 3.535250795749688894E-16 ) ) ;
#71390=CARTESIAN_POINT ( 'NONE',  ( 16.98750000000000426, -2.886751345948129988, 4.999999999999997335 ) ) ;
#71391=CARTESIAN_POINT ( 'NONE',  ( 17.40937500061451715, -4.541064518000417216, -2.621784821875001281 ) ) ;
#71392=CARTESIAN_POINT ( 'NONE',  ( 13.68750000122903288, 6.123233995736764310E-16, -4.999999999999998224 ) ) ;
#71395=CARTESIAN_POINT ( 'NONE',  ( -2.121784821874996840, 16.27812500061451573, -26.32496088578401583 ) ) ;
#71397=CARTESIAN_POINT ( 'NONE',  ( 3.544807824988736478, -3.526624500747946200, 3.544807824988736478 ) ) ;
#71398=CARTESIAN_POINT ( 'NONE',  ( 28.07812500061451289, -4.541064518000419881, 2.621784821874995952 ) ) ;
#71399=CARTESIAN_POINT ( 'NONE',  ( 1.626862140677534273E-15, 12.12500000122903465, 34.00000000000000000 ) ) ;
#71400=DIRECTION ( 'NONE',  ( -1.000000000000000000, -0.000000000000000000, -0.000000000000000000 ) ) ;
#71401=CARTESIAN_POINT ( 'NONE',  ( 14.97187500061451892, 3.027376345333611329, 5.243569643749999010 ) ) ;
#71402=CARTESIAN_POINT ( 'NONE',  ( 27.11249999999999716, 2.886751345948129099, -4.999999999999998224 ) ) ;
#71403=CARTESIAN_POINT ( 'NONE',  ( 12.02812500061451573, 6.421520780324663323E-16, -5.243569643749999010 ) ) ;
#71405=CARTESIAN_POINT ( 'NONE',  ( 21.15937500061451715, 4.541064518000418104, -2.621784821874998173 ) ) ;
#71407=CARTESIAN_POINT ( 'NONE',  ( 6.665625000614515905, 3.027376345333613106, -5.243569643749998122 ) ) ;
#71408=CARTESIAN_POINT ( 'NONE',  ( 12.04687500061451821, -3.027376345333610441, -5.243569643749999898 ) ) ;
#71409=VERTEX_POINT ( 'NONE', #23357 ) ;
#71410=CARTESIAN_POINT ( 'NONE',  ( 24.98437500061451644, -4.541064518000419881, 2.621784821874995952 ) ) ;
#71411=CARTESIAN_POINT ( 'NONE',  ( 28.22812500061451502, 6.421520780324663323E-16, -5.243569643749999010 ) ) ;
#71412=DIRECTION ( 'NONE',  ( 0.000000000000000000, -0.000000000000000000, 1.000000000000000000 ) ) ;
#71413=CARTESIAN_POINT ( 'NONE',  ( 8.250000000000000000, 4.330127018922192761, -2.499999999999997780 ) ) ;
#71414=CARTESIAN_POINT ( 'NONE',  ( 17.58750000122903145, -4.330127018922194537, 2.499999999999995559 ) ) ;
#71415=CARTESIAN_POINT ( 'NONE',  ( -1.071796769724492338, 17.95490381179670081, -26.00000000000000711 ) ) ;
#71417=VERTEX_POINT ( 'NONE', #57338 ) ;
#71418=CARTESIAN_POINT ( 'NONE',  ( 15.93750000000000000, 5.773502691896255534, 3.535250795749688894E-16 ) ) ;
#71419=CARTESIAN_POINT ( 'NONE',  ( 17.96250000000000213, -5.773502691896255534, -1.060575238724906372E-15 ) ) ;
#71420=CARTESIAN_POINT ( 'NONE',  ( 10.56562500061451715, -6.054752690667223547, -1.112240025338166033E-15 ) ) ;
#71422=CARTESIAN_POINT ( 'NONE',  ( -5.810221930991193690E-16, 10.88749999999999929, -34.00000000000000000 ) ) ;
#71423=CARTESIAN_POINT ( 'NONE',  ( 4.243569643749999010, 16.97187500061451360, -32.45002607614398471 ) ) ;
#71424=CARTESIAN_POINT ( 'NONE',  ( 4.528125000614516615, 4.541064518000418104, 2.621784821874999949 ) ) ;
#71426=CARTESIAN_POINT ( 'NONE',  ( 9.712500000000002132, 2.886751345948126879, 4.999999999999999112 ) ) ;
#71427=DIRECTION ( 'NONE',  ( -1.000000000000000000, -0.000000000000000000, -0.000000000000000000 ) ) ;
#71428=ORIENTED_EDGE ( 'NONE', *, *, #45249, .F. ) ;
#71429=CARTESIAN_POINT ( 'NONE',  ( -3.000416591977282496E-16, 13.39062500061451644, 25.09994784771203058 ) ) ;
#71430=CARTESIAN_POINT ( 'NONE',  ( 25.79062500061451502, -3.027376345333614438, 5.243569643749998122 ) ) ;
#71433=CYLINDRICAL_SURFACE ( 'NONE', #52548, 4.999999999999998224 ) ;
#71434=CARTESIAN_POINT ( 'NONE',  ( 20.33437500061451786, 4.541064518000418104, 2.621784821874999949 ) ) ;
#71435=CARTESIAN_POINT ( 'NONE',  ( 19.45312500061451644, 0.000000000000000000, 5.243569643749999010 ) ) ;
#71437=CARTESIAN_POINT ( 'NONE',  ( 9.001249775931846008E-16, 14.96562500061459744, -25.09994784771203058 ) ) ;
#71438=CARTESIAN_POINT ( 'NONE',  ( 23.62500000122902932, 2.886751345948129099, -4.999999999999998224 ) ) ;
#71439=CARTESIAN_POINT ( 'NONE',  ( 3.065625000614517592, 3.027376345333613106, -5.243569643749998122 ) ) ;
#71441=CARTESIAN_POINT ( 'NONE',  ( 21.21562500061451573, 3.027376345333611329, 5.243569643749999010 ) ) ;
#71444=CARTESIAN_POINT ( 'NONE',  ( 14.55937500061451573, 0.000000000000000000, 5.243569643749999010 ) ) ;
#71445=CARTESIAN_POINT ( 'NONE',  ( 15.00937500061451679, 0.000000000000000000, 5.243569643749999010 ) ) ;
#71446=CARTESIAN_POINT ( 'NONE',  ( 24.49687500061451573, -3.027376345333614438, 5.243569643749998122 ) ) ;
#71447=CARTESIAN_POINT ( 'NONE',  ( -2.121784821874996840, 14.98437500061451644, 33.67503911421598417 ) ) ;
#71448=CARTESIAN_POINT ( 'NONE',  ( 4.190625000614518925, -3.027376345333614438, 5.243569643749998122 ) ) ;
#71449=CARTESIAN_POINT ( 'NONE',  ( 28.79062500061451502, 6.054752690667223547, 3.707466751127219781E-16 ) ) ;
#71450=ADVANCED_FACE ( 'NONE', ( #62879, #63966 ), #1571, .T. ) ;
#71452=CARTESIAN_POINT ( 'NONE',  ( 28.00312500061451715, 0.000000000000000000, 5.243569643749999010 ) ) ;
#71453=CARTESIAN_POINT ( 'NONE',  ( 4.000000000000000000, 16.25000000122903643, -27.69059892324149885 ) ) ;
#71454=CARTESIAN_POINT ( 'NONE',  ( -3.999999999999997335, 19.58749999999999858, 32.30940107675850470 ) ) ;
#71455=CARTESIAN_POINT ( 'NONE',  ( 6.271875000614517859, 3.027376345333613106, -5.243569643749998122 ) ) ;
#71456=CARTESIAN_POINT ( 'NONE',  ( 14.55000000122903181, -2.886751345948125991, -5.000000000000000000 ) ) ;
#71457=CARTESIAN_POINT ( 'NONE',  ( 9.525000001229033231, -5.773502691896255534, -1.060575238724906372E-15 ) ) ;
#71458=CARTESIAN_POINT ( 'NONE',  ( 4.415625000614518569, 3.027376345333613106, -5.243569643749998122 ) ) ;
#71461=CARTESIAN_POINT ( 'NONE',  ( 13.54687500061451999, 6.054752690667223547, 3.707466751127219781E-16 ) ) ;
#71462=CARTESIAN_POINT ( 'NONE',  ( 1.071796769724491893, 17.54509619066136850, 33.99999999999999289 ) ) ;
#71463=ORIENTED_EDGE ( 'NONE', *, *, #6663, .F. ) ;
#71464=CARTESIAN_POINT ( 'NONE',  ( 21.36562500061451431, -6.054752690667223547, -1.112240025338166033E-15 ) ) ;
#71465=CARTESIAN_POINT ( 'NONE',  ( 6.290625000614517681, 6.054752690667223547, 3.707466751127219781E-16 ) ) ;
#71466=CARTESIAN_POINT ( 'NONE',  ( 25.62187500061451928, 3.027376345333612662, -5.243569643749998122 ) ) ;
#71467=CARTESIAN_POINT ( 'NONE',  ( 6.665625000614515905, 3.027376345333613106, -5.243569643749998122 ) ) ;
#71469=CARTESIAN_POINT ( 'NONE',  ( 8.550000001229031810, -2.886751345948129988, 4.999999999999997335 ) ) ;
#71470=CARTESIAN_POINT ( 'NONE',  ( 23.09062500061451573, -3.027376345333614438, 5.243569643749998122 ) ) ;
#71471=CARTESIAN_POINT ( 'NONE',  ( 2.121784821874999061, 10.20312500061451821, -33.67503911421598417 ) ) ;
#71472=CARTESIAN_POINT ( 'NONE',  ( 11.06250000122903288, 4.330127018922192761, -2.499999999999997780 ) ) ;
#71473=CARTESIAN_POINT ( 'NONE',  ( 18.55312500061451431, 0.000000000000000000, 5.243569643749999010 ) ) ;
#71474=AXIS2_PLACEMENT_3D ( 'NONE', #2849, #58252, #42014 ) ;
#71475=CARTESIAN_POINT ( 'NONE',  ( 14.54062500061451679, -3.027376345333614438, 5.243569643749998122 ) ) ;
#71477=CARTESIAN_POINT ( 'NONE',  ( 14.81250000000000000, -5.773502691896255534, -1.060575238724906372E-15 ) ) ;
#71478=CARTESIAN_POINT ( 'NONE',  ( 12.30000000122903181, -2.886751345948125991, -5.000000000000000000 ) ) ;
#71479=CARTESIAN_POINT ( 'NONE',  ( 7.453125000614516438, -4.541064518000417216, -2.621784821875001281 ) ) ;
#71480=CARTESIAN_POINT ( 'NONE',  ( 11.39062500061451644, -3.027376345333614438, 5.243569643749998122 ) ) ;
#71481=( BOUNDED_CURVE ( )  B_SPLINE_CURVE ( 3, ( #69179, #52179, #40019, #30373 ),
 .UNSPECIFIED., .F., .F. ) 
 B_SPLINE_CURVE_WITH_KNOTS ( ( 4, 4 ),
 ( 1.570796326794896558, 2.225934242759671111 ),
 .UNSPECIFIED. ) 
 CURVE ( )  GEOMETRIC_REPRESENTATION_ITEM ( )  RATIONAL_B_SPLINE_CURVE ( ( 1.000000000000000000, 0.9645515396217719806, 0.9645515396217719806, 1.000000000000000000 ) ) 
 REPRESENTATION_ITEM ( '' )  );
#71483=CARTESIAN_POINT ( 'NONE',  ( 24.26250000122903216, 0.000000000000000000, 4.999999999999998224 ) ) ;
#71484=CARTESIAN_POINT ( 'NONE',  ( 18.75937500061451857, -4.541064518000417216, -2.621784821875001281 ) ) ;
#71486=CARTESIAN_POINT ( 'NONE',  ( 4.275000001229035895, 2.886751345948129099, -4.999999999999998224 ) ) ;
#71487=CARTESIAN_POINT ( 'NONE',  ( 4.959375000614516971, 4.541064518000418104, -2.621784821874998173 ) ) ;
#71488=CARTESIAN_POINT ( 'NONE',  ( 22.28437500061451715, -4.541064518000419881, 2.621784821874995952 ) ) ;
#71489=CARTESIAN_POINT ( 'NONE',  ( 10.61249999999999893, 2.886751345948193936, 4.999999999999883649 ) ) ;
#71490=CARTESIAN_POINT ( 'NONE',  ( 19.37812500061451715, 4.541064518000418104, 2.621784821874999949 ) ) ;
#71491=CARTESIAN_POINT ( 'NONE',  ( 24.27187500061452141, 3.027376345333613106, -5.243569643749998122 ) ) ;
#71493=CARTESIAN_POINT ( 'NONE',  ( 12.41250000122903430, 4.330127018922192761, -2.499999999999997780 ) ) ;
#71494=DIRECTION ( 'NONE',  ( -0.000000000000000000, -1.000000000000000000, -0.000000000000000000 ) ) ;
#71495=CARTESIAN_POINT ( 'NONE',  ( 4.434375000614519280, 6.421520780324663323E-16, -5.243569643749999010 ) ) ;
#71496=CARTESIAN_POINT ( 'NONE',  ( 14.16562500061451679, -6.054752690667223547, -1.112240025338166033E-15 ) ) ;
#71497=CARTESIAN_POINT ( 'NONE',  ( 13.09687500061451892, 6.054752690667223547, 3.707466751127219781E-16 ) ) ;
#71499=CARTESIAN_POINT ( 'NONE',  ( 1.071796769724497445, 17.16740381056766651, -33.99999999999998579 ) ) ;
#71500=CARTESIAN_POINT ( 'NONE',  ( 26.01562500061451289, 3.027376345333613106, -5.243569643749998122 ) ) ;
#71501=CARTESIAN_POINT ( 'NONE',  ( -2.000000000000000000, 10.58750000122903323, -33.46410161513775705 ) ) ;
#71502=DIRECTION ( 'NONE',  ( -1.000000000000000000, -0.000000000000000000, -0.000000000000000000 ) ) ;
#71503=CARTESIAN_POINT ( 'NONE',  ( 14.21249999999999858, 2.886751345948126879, 4.999999999999999112 ) ) ;
#71504=CARTESIAN_POINT ( 'NONE',  ( 24.78750000122903074, -4.330127018922194537, 2.499999999999995559 ) ) ;
#71505=CARTESIAN_POINT ( 'NONE',  ( 19.07812500061451644, -4.541064518000419881, 2.621784821874995952 ) ) ;
#71506=ORIENTED_EDGE ( 'NONE', *, *, #58401, .F. ) ;
#71507=CARTESIAN_POINT ( 'NONE',  ( 22.80000000000000071, 0.000000000000000000, 4.999999999999998224 ) ) ;
#71508=CARTESIAN_POINT ( 'NONE',  ( 24.38437500061451502, 4.541064518000418104, 2.621784821874999949 ) ) ;
#71511=CARTESIAN_POINT ( 'NONE',  ( 11.50312500061451892, -4.541064518000417216, -2.621784821875001281 ) ) ;
#71512=CARTESIAN_POINT ( 'NONE',  ( 4.490625000614516971, 6.054752690667223547, 3.707466751127219781E-16 ) ) ;
#71514=CARTESIAN_POINT ( 'NONE',  ( 26.69062500061451715, -3.027376345333614438, 5.243569643749998122 ) ) ;
#71515=AXIS2_PLACEMENT_3D ( 'NONE', #55117, #11769, #4516 ) ;
#71516=CARTESIAN_POINT ( 'NONE',  ( 17.96250000000000213, -5.773502691896255534, -1.060575238724906372E-15 ) ) ;
#71517=CARTESIAN_POINT ( 'NONE',  ( 25.87500000000000000, 4.330127018922191873, 2.499999999999999556 ) ) ;
#71518=CARTESIAN_POINT ( 'NONE',  ( 7.837500001229035007, 6.123233995736764310E-16, -4.999999999999998224 ) ) ;
#71519=CARTESIAN_POINT ( 'NONE',  ( 6.271875000614517859, 3.027376345333613106, -5.243569643749998122 ) ) ;
#71520=CARTESIAN_POINT ( 'NONE',  ( 17.03437500061451715, 6.421520780324663323E-16, -5.243569643749999010 ) ) ;
#71521=CARTESIAN_POINT ( 'NONE',  ( 28.05937500061451573, 0.000000000000000000, 5.243569643749999010 ) ) ;
#71522=ORIENTED_EDGE ( 'NONE', *, *, #13592, .T. ) ;
#71523=CARTESIAN_POINT ( 'NONE',  ( 26.46562500061451573, 3.027376345333613106, -5.243569643749998122 ) ) ;
#71524=CARTESIAN_POINT ( 'NONE',  ( 26.85937500061451644, -4.541064518000417216, -2.621784821875001281 ) ) ;
#71525=FACE_OUTER_BOUND ( 'NONE', #18154, .T. ) ;
#71526=CARTESIAN_POINT ( 'NONE',  ( 14.40000000000000036, -4.330127018922190985, -2.500000000000001332 ) ) ;
#71527=CARTESIAN_POINT ( 'NONE',  ( 10.30312500061451431, 4.541064518000418104, -2.621784821874998173 ) ) ;
#71530=CARTESIAN_POINT ( 'NONE',  ( 29.35312500061451502, 0.000000000000000000, 5.243569643749999010 ) ) ;
#71531=CARTESIAN_POINT ( 'NONE',  ( 16.01250000122903216, 4.330127018922192761, -2.499999999999997780 ) ) ;
#71532=CARTESIAN_POINT ( 'NONE',  ( 15.03750000122903252, 6.123233995736764310E-16, -4.999999999999998224 ) ) ;
#71534=CARTESIAN_POINT ( 'NONE',  ( 5.390625000614518214, 6.054752690667223547, 3.707466751127219781E-16 ) ) ;
#71535=CARTESIAN_POINT ( 'NONE',  ( 21.72187500061451715, 3.027376345333611329, 5.243569643749999010 ) ) ;
#71536=CARTESIAN_POINT ( 'NONE',  ( -2.121784821874999949, 17.98437500061451999, 26.32496088578401938 ) ) ;
#71537=CARTESIAN_POINT ( 'NONE',  ( 22.95937500061451431, 4.541064518000418104, -2.621784821874998173 ) ) ;
#71538=CARTESIAN_POINT ( 'NONE',  ( 5.062500000000000888, 2.886751345948129099, -4.999999999999998224 ) ) ;
#71539=CARTESIAN_POINT ( 'NONE',  ( 2.000000000000001332, 10.36250000122903359, 33.46410161513774995 ) ) ;
#71540=CARTESIAN_POINT ( 'NONE',  ( 12.62812500061451537, 4.541064518000418104, 2.621784821874999949 ) ) ;
#71541=CARTESIAN_POINT ( 'NONE',  ( 5.325000001229033941, 2.886751345948126879, 4.999999999999999112 ) ) ;
#71542=( BOUNDED_SURFACE ( )  B_SPLINE_SURFACE ( 1, 2, ( 
 ( #57136, #6180, #12085, #34606, #34976, #1374, #46071, #68247, #46796, #57505, #6545, #69333, #30159, #69688, #28709, #23521, #51248, #63413, #29796, #68606, #68970, #651, #23159, #45713, #24609, #17610, #52332, #35697, #18327, #40170, #29079, #51614, #47156, #1015, #1734, #58217, #12445, #12799, #41255, #17967, #19053, #63044, #40900, #6907, #24248, #29438, #23884, #46431, #35335, #57858, #63767, #13155, #7622, #52692, #62329, #2098, #42343, #25342, #48987, #36064, #3924, #24971, #31251, #37525, #70045, #42706, #47516, #8353, #59682, #71142, #31626, #20515, #47888, #43073, #54521, #70416, #19418, #9089, #14617, #48253, #41978, #26078, #7991, #64499, #54160, #37156, #53424, #19792, #70776, #53054, #64866, #13891, #14254, #36431, #36793, #58945, #30527, #30882, #58584, #3556, #48617, #13516, #65599, #20152, #14987, #2448, #59308, #2814, #26447, #8719, #71517, #60046, #53793, #9457, #3188, #25715, #41611, #65228, #31987, #64130, #61513, #20892, #38632, #4654, #49353, #44551, #27183, #21256, #836, #66334, #68425, #33437, #29264, #43446, #60408, #54887, #15712, #15348, #43809, #38250, #66710, #33080, #49717, #26819, #5376, #16084, #60779, #28895, #62867, #51794, #37889, #55258, #65968, #21993, #10911, #72245, #55982, #61156, #21622, #40347, #23345, #44180, #10551, #51434, #9817, #50080, #55618, #45893, #10186, #67082, #32349, #4294, #71883, #5014, #32721, #27548, #72611, #16441, #38998, #17787, #12263, #34793, #57326, #6730, #69869, #18148, #64319, #2276, #7090, #52155, #25155, #35876, #13709, #35520, #24431, #29975, #19605, #42161, #63954, #1196, #47695, #24793, #68792, #12626, #63595, #23703, #64688, #14073, #24069, #41437, #57685, #36612, #13338, #58039, #35161, #47336, #46251, #7814, #59133, #52878, #7449, #8541, #58400, #58767, #52517, #19235, #41789, #70231, #29619, #1558, #36252, #8176, #40715, #63232, #30704, #46614, #53237, #2634, #18875, #31069, #69158, #18516, #41082, #1926, #30350, #12984, #46980, #69516, #3380, #19972, #4479, #4113, #27008, #37349, #10006, #37706, #31810, #43998, #26641, #49178, #32541, #49539, #66520, #71708, #59498, #25901, #43631, #55079, #9641, #48442, #31442, #32175, #53608, #59871, #53982, #70966, #43267, #3000, #38447, #42892, #42525, #72062, #9275, #10373, #21441, #20339, #15900, #66153, #60973, #25528, #65051, #14441, #65417, #48071, #14805, #54348, #26267, #65788, #3742, #8911, #38074, #48804, #71333, #60597, #70598, #36976, #20709, #15169, #60228, #54708, #21081, #15531, #39544, #21808, #49901, #4835, #68345, #61338, #50984, #6279, #56167, #33983, #39912, #55443, #40266, #39180, #11462, #33267, #45447, #27369, #5194, #27734, #38822, #55805, #10734, #62425, #72425, #44372, #62787, #56522, #33623, #16626, #32905, #66899, #17705, #16267, #22537, #28808, #50271, #5915, #72796, #22179, #382, #11824, #22889, #34342, #61696, #56875, #45809, #11095, #44733, #67980, #28449, #62068, #67267, #17355, #5561, #28098, #51347, #750, #50626, #31, #23259, #45085, #67620, #16986, #57958, #35077, #40999, #12543, #1115, #57603, #6650, #24712, #52796, #57237, #41709, #41357, #13623, #51712, #7366, #7007, #70146, #29537, #47615, #30263, #69073, #58317, #29179, #1842, #19524, #52072, #36167, #23622, #2197, #12180, #29896, #18432, #40629, #35795, #63514, #1477, #42082, #46168, #46531, #34707, #13257, #47255, #12901, #18793, #68708, #18068, #63148, #23984, #35434, #69789, #58685, #52435, #7729, #19155, #24349, #46897, #69436, #63867, #64233, #8095, #30624, #53156, #2554, #25072, #64970, #70519, #20995, #59050, #13991, #21360, #43183, #65332, #48358, #71986, #8455, #26927, #47991, #54264, #60513, #19895, #65702, #42448, #31360, #9557, #43547, #54622, #66069, #70883, #15447, #4398, #20257, #14361, #32091, #37625, #71245, #36896, #49093, #30990, #59416, #4028, #60148, #3293, #42809, #20624, #2917, #14721, #8823, #37264, #53901, #59786, #25820, #53523, #9192, #25448, #26553, #71622, #36530, #37991, #15089, #9919, #31727, #3659, #26182, #49452, #48722, #64605, #32457, #54992, #16904, #38359, #33537, #6197, #10652, #45363, #32821, #11382, #43914, #61614, #27649, #72344, #67541, #50185, #44284, #22812, #16187, #17270, #56445, #51266, #66439, #10291, #4753, #38738, #60886, #66814, #61258, #16545, #56087, #72713, #49820, #28367, #39097, #33182, #50903, #11742, #302, #15816, #668, #22096, #22455, #55721, #5835, #55359, #5115, #44654, #21725, #67184, #11016, #67898, #27286, #5479, #28018, #45004, #50546, #73074, #39459, #61980, #28725, #33901, #39831, #62346, #34259, #56792, #6565, #63062, #41276, #52712, #13177, #2118, #6925, #24630, #36085, #51992, #29097, #63787, #69354, #29816, #51632, #7643, #62708, #1033, #35716, #18711, #34995, #29455, #52351, #34623, #23902, #68625, #68988, #46089, #1393, #23539, #12102, #17987, #17627, #58238, #30181, #68265, #47175, #1754, #69708, #57154, #18345, #40546, #8012, #12465, #58605, #19074, #46450, #41631, #40187, #12819, #30547, #57524, #64150, #40920, #13537, #23176, #63432, #35353, #57877, #46816, #7287, #24267, #53074, #45730, #49007, #15008, #9840, #24993, #42000, #36452, #70437, #70066, #2835, #25364, #48274, #14637, #59328, #8374, #60067, #70798, #19812, #9479, #43465, #32369, #19439, #36813, #47537, #3577, #43092, #8739, #9110, #64520, #13913, #58966, #37912, #30903, #20536, #71538, #25737, #26100, #31648, #65989, #54181, #31272, #2469, #65248, #32008, #53815, #48638, #65620, #26468, #53445, #47908, #37545, #71163, #42365, #64887, #54543, #14275, #3945, #20913, #20173, #15370, #3208, #42727, #60429, #37178, #59703, #22015, #27569, #39379, #4673, #21277, #5757, #5395, #28291, #38652, #11303, #39017, #33099, #45283, #27932, #50465, #33824, #50822, #67817, #72993, #60800, #27203, #44926, #56367, #10930, #49738 ),
 ( #33457, #55638, #61176, #62267, #49374, #17190, #38272, #44571, #225, #10206, #56001, #32741, #21643, #22374, #22730, #67462, #39750, #10571, #11662, #54907, #5032, #55278, #16825, #61898, #61532, #72265, #4315, #43831, #44200, #26840, #71904, #66731, #50101, #66356, #15733, #72631, #16102, #67101, #16459, #62977, #34540, #23092, #57070, #28645, #46728, #1667, #6114, #63699, #63345, #35628, #587, #29374, #6477, #18982, #29012, #2031, #41543, #51183, #68540, #56713, #35267, #24176, #40461, #40829, #45649, #68183, #17546, #69620, #62621, #52265, #7554, #57436, #57789, #41190, #40107, #64061, #12373, #12731, #51549, #69263, #12017, #950, #23458, #46004, #17901, #34908, #13090, #6839, #51906, #34177, #7198, #1305, #23814, #46365, #68899, #18256, #29727, #18625, #30088, #58149, #52626, #24542, #47087, #31554, #43000, #3491, #65531, #70342, #14917, #26376, #42270, #19347, #54094, #59609, #20079, #41904, #71075, #52986, #64429, #26009, #9023, #25265, #19718, #42635, #24900, #14184, #58875, #59240, #36361, #64793, #13821, #2382, #8285, #7920, #48548, #20450, #58509, #37459, #65159, #59978, #47445, #8649, #30815, #71446, #53348, #48915, #9388, #36719, #31919, #30457, #3113, #20821, #2746, #54455, #69977, #3854, #13442, #31178, #53721, #47812, #37085, #25643, #48180, #43376, #70704, #35991, #14549, #138, #15280, #32282, #26750, #60705, #60339, #66263, #15640, #38560, #4945, #49647, #71816, #50380, #61083, #10118, #72905, #55549, #61806, #21187, #67011, #49283, #32648, #10840, #22287, #55911, #44839, #72174, #67374, #5671, #21554, #43738, #33375, #38927, #72536, #38181, #16737, #54816, #55189, #5304, #61446, #4584, #44108, #21924, #4222, #66634, #27114, #10481, #16012, #33010, #27479, #50012, #44480, #9748, #27849, #39292, #37820, #11209, #16372, #33736, #56282, #28207, #50736, #22644, #65900, #7469, #63253, #28918, #18168, #39659, #34815, #29995, #11928, #46635, #34090, #12645, #45194, #62887, #51456, #492, #68812, #859, #45561, #24088, #17459, #18538, #57705, #52536, #67726, #11575, #6026, #40017, #62178, #68092, #62531, #17808, #57345, #23366, #51095, #29639, #40369, #34453, #52177, #13003, #1945, #56631, #6385, #17099, #46273, #35181, #45914, #51814, #28560, #23001, #56981, #68446, #12282, #7110, #41102, #6751, #40737, #1579, #29284, #1217, #23723, #69177, #63612, #35540, #58060, #69891, #19256, #30371, #24813, #52900, #55007, #18894, #47000, #55374, #3022, #25176, #8199, #32837, #41456, #60901, #7834, #4413, #41811, #72000, #38007, #24451, #69535, #63974, #58422, #64341, #13357, #47359, #13733, #70255, #36633, #30728, #2298, #9936, #19628, #36275, #32474, #66455, #35898, #58789, #53260, #2658, #25553, #66084, #47717, #31091, #42184, #64709, #14093, #10304, #59155, #43562, #21375, #8563, #49108, #26942, #53630, #71637, #21010, #15462, #60529, #49467, #43929, #15832, #38377, #38753, #10667, #61274, #318, #49835, #27301, #28741, #67556, #61628, #44669, #6213, #72359, #34275, #16202, #28033, #39848, #33197, #16919, #55736, #50203, #11398, #22827, #33917, #45379, #67199, #67915, #56807, #16561, #5130, #56460, #39474, #22470, #27664, #28382, #21740, #72728, #5851, #61997, #22112, #39112, #45021, #66830, #11030, #33553, #56103, #5494, #50562, #73089, #44301, #50920, #17286, #62361, #11757, #4768, #27165, #26799, #72226, #37134, #65949, #71124, #55599, #65578, #33060, #15693, #54503, #43789, #65208, #60389, #4994, #37506, #21605, #59662, #38232, #70756, #15328, #3905, #26059, #21237, #26427, #20496, #44160, #9070, #60762, #20131, #37870, #48968, #48599, #66316, #71497, #43053, #49699, #14968, #66689, #10169, #27526, #42686, #31605, #54142, #60026, #14598, #9438, #31966, #43427, #9797, #20874, #3536, #55240, #32330, #54868, #4635, #38612, #4275, #49333, #71865, #32703, #16063, #61135, #10532, #56678, #38979, #67064, #21972, #12332, #5356, #68144, #23418, #187, #51145, #57031, #72590, #57394, #56328, #28609, #50428, #62583, #44531, #22336, #44888, #55961, #72954, #27894, #6438, #16421, #61495, #6801, #545, #50784, #33785, #50060, #10892, #34867, #33420, #39709, #45965, #67423, #23056, #16785, #39343, #17508, #28973, #40069, #51510, #5717, #910, #62938, #28253, #61856, #11980, #45610, #6076, #11263, #34503, #22692, #45243, #68498, #17862, #67777, #17151, #40421, #62227, #11623, #34139, #42132, #53207, #2973, #8510, #1897, #35130, #53575, #25501, #35490, #52849, #69128, #48046, #2247, #69487, #24036, #36221, #57655, #19206, #70571, #64289, #46950, #19947, #24763, #70200, #41407, #41760, #14043, #52127, #7782, #12953, #42500, #7418, #12598, #30675, #18846, #58737, #7061, #47306, #29589, #52486, #36583, #1529, #2603, #46586, #30319, #63923, #41052, #8148, #13308, #58010, #64658, #29946, #59103, #25124, #18486, #63565, #24401, #35846, #58371, #69841, #13677, #47666, #19576, #31039, #48776, #70939, #49504, #37677, #9247, #72033, #32871, #72392, #8879, #26239, #14412, #66120, #32509, #71300, #71673, #53954, #31414, #36949, #27336, #20310, #9972, #38414, #15139, #15499, #21409, #59469, #21772, #20679, #43599, #65385, #4447, #3351, #37318, #59842, #42863, #14776, #31782, #43966, #25873, #48413, #65023, #38041, #65756, #43236, #54321, #3712, #49868, #60199, #54675, #60935, #9611, #60565, #32142, #4078, #55044, #66487, #26975, #15866, #26606, #10339, #4803, #49144, #21047, #55408, #17321, #50953, #50238, #28774, #10700, #72760, #62393, #39881, #56133, #28065, #351, #55771, #45054, #16592, #16956, #11062, #12147, #67233, #22858, #44699, #38788, #56841, #11791, #16235, #718, #56491, #50595, #22146, #51314, #39509, #61662, #23225, #34674, #51680, #61305, #5527, #66864, #45412, #34308, #28527, #67948, #33233, #5163, #27697, #6618, #39145, #6247, #17673, #67590, #45778, #68313, #33588 ) ),
 .UNSPECIFIED., .F., .F., .F. ) 
 B_SPLINE_SURFACE_WITH_KNOTS ( ( 2, 2 ),
 ( 3, 2, 2, 2, 2, 2, 2, 2, 2, 2, 2, 2, 2, 2, 2, 2, 2, 2, 2, 2, 2, 2, 2, 2, 2, 2, 2, 2, 2, 2, 2, 2, 2, 2, 2, 2, 2, 2, 2, 2, 2, 2, 2, 2, 2, 2, 2, 2, 2, 2, 2, 2, 2, 2, 2, 2, 2, 2, 2, 2, 2, 2, 2, 2, 2, 2, 2, 2, 2, 2, 2, 2, 2, 2, 2, 2, 2, 2, 2, 2, 2, 2, 2, 2, 2, 2, 2, 2, 2, 2, 2, 2, 2, 2, 2, 2, 2, 2, 2, 2, 2, 2, 2, 2, 2, 2, 2, 2, 2, 2, 2, 2, 2, 2, 2, 2, 2, 2, 2, 2, 2, 2, 2, 2, 2, 2, 2, 2, 2, 2, 2, 2, 2, 2, 2, 2, 2, 2, 2, 2, 2, 2, 2, 2, 2, 2, 2, 2, 2, 2, 2, 2, 2, 2, 2, 2, 2, 2, 2, 2, 2, 2, 2, 2, 2, 2, 2, 2, 2, 2, 2, 2, 2, 2, 2, 2, 2, 2, 2, 2, 2, 2, 2, 2, 2, 2, 2, 2, 2, 2, 2, 2, 2, 2, 2, 2, 2, 2, 2, 2, 2, 2, 2, 2, 2, 2, 2, 2, 2, 2, 2, 2, 2, 2, 2, 2, 2, 2, 2, 2, 2, 2, 2, 2, 2, 2, 2, 2, 2, 2, 2, 2, 2, 2, 2, 2, 2, 2, 2, 2, 2, 2, 2, 2, 2, 2, 2, 2, 2, 2, 2, 2, 2, 2, 2, 2, 2, 2, 2, 2, 2, 2, 2, 2, 2, 2, 2, 2, 2, 2, 2, 2, 2, 2, 2, 2, 2, 2, 2, 2, 2, 2, 2, 2, 2, 2, 2, 2, 2, 2, 2, 2, 2, 2, 2, 2, 2, 2, 2, 2, 2, 2, 2, 2, 2, 2, 2, 2, 2, 2, 2, 2, 2, 2, 2, 2, 2, 2, 2, 2, 2, 2, 2, 2, 2, 2, 2, 2, 2, 2, 2, 2, 2, 2, 2, 2, 2, 2, 2, 2, 2, 2, 2, 2, 2, 2, 2, 2, 2, 2, 2, 2, 2, 2, 2, 2, 2, 2, 2, 2, 3 ),
 ( 0.000000000000000000, 1.000000000000000000 ),
 ( 0.000000000000000000, 0.002777777777777777884, 0.005555555555555555768, 0.008333333333333333218, 0.01111111111111111154, 0.01388888888888888812, 0.01666666666666666644, 0.01944444444444444475, 0.02222222222222222307, 0.02500000000000000139, 0.02777777777777777624, 0.03055555555555555455, 0.03333333333333333287, 0.03611111111111110772, 0.03888888888888888951, 0.04166666666666666435, 0.04444444444444444614, 0.04722222222222222099, 0.05000000000000000278, 0.05277777777777777762, 0.05555555555555555247, 0.05833333333333333426, 0.06111111111111110911, 0.06388888888888888395, 0.06666666666666666574, 0.06944444444444444753, 0.07222222222222221544, 0.07499999999999999722, 0.07777777777777777901, 0.08055555555555556080, 0.08333333333333332871, 0.08611111111111111049, 0.08888888888888889228, 0.09166666666666666019, 0.09444444444444444198, 0.09722222222222222376, 0.1000000000000000056, 0.1027777777777777735, 0.1055555555555555552, 0.1083333333333333370, 0.1111111111111111049, 0.1138888888888888867, 0.1166666666666666685, 0.1194444444444444503, 0.1222222222222222182, 0.1250000000000000000, 0.1277777777777777679, 0.1305555555555555636, 0.1333333333333333315, 0.1361111111111110994, 0.1388888888888888951, 0.1416666666666666630, 0.1444444444444444309, 0.1472222222222222265, 0.1499999999999999944, 0.1527777777777777901, 0.1555555555555555580, 0.1583333333333333259, 0.1611111111111111216, 0.1638888888888888895, 0.1666666666666666574, 0.1694444444444444531, 0.1722222222222222210, 0.1749999999999999889, 0.1777777777777777846, 0.1805555555555555525, 0.1833333333333333204, 0.1861111111111111160, 0.1888888888888888840, 0.1916666666666666796, 0.1944444444444444475, 0.1972222222222222154, 0.2000000000000000111, 0.2027777777777777790, 0.2055555555555555469, 0.2083333333333333426, 0.2111111111111111105, 0.2138888888888888784, 0.2166666666666666741, 0.2194444444444444420, 0.2222222222222222099, 0.2250000000000000056, 0.2277777777777777735, 0.2305555555555555691, 0.2333333333333333370, 0.2361111111111111049, 0.2388888888888889006, 0.2416666666666666685, 0.2444444444444444364, 0.2472222222222222321, 0.2500000000000000000, 0.2527777777777777679, 0.2555555555555555358, 0.2583333333333333592, 0.2611111111111111271, 0.2638888888888888951, 0.2666666666666666630, 0.2694444444444444309, 0.2722222222222221988, 0.2750000000000000222, 0.2777777777777777901, 0.2805555555555555580, 0.2833333333333333259, 0.2861111111111110938, 0.2888888888888888618, 0.2916666666666666852, 0.2944444444444444531, 0.2972222222222222210, 0.2999999999999999889, 0.3027777777777777568, 0.3055555555555555802, 0.3083333333333333481, 0.3111111111111111160, 0.3138888888888888840, 0.3166666666666666519, 0.3194444444444444198, 0.3222222222222222432, 0.3250000000000000111, 0.3277777777777777790, 0.3305555555555555469, 0.3333333333333333148, 0.3361111111111111382, 0.3388888888888889062, 0.3416666666666666741, 0.3444444444444444420, 0.3472222222222222099, 0.3499999999999999778, 0.3527777777777778012, 0.3555555555555555691, 0.3583333333333333370, 0.3611111111111111049, 0.3638888888888888729, 0.3666666666666666408, 0.3694444444444444642, 0.3722222222222222321, 0.3750000000000000000, 0.3777777777777777679, 0.3805555555555555358, 0.3833333333333333592, 0.3861111111111111271, 0.3888888888888888951, 0.3916666666666666630, 0.3944444444444444309, 0.3972222222222221988, 0.4000000000000000222, 0.4027777777777777901, 0.4055555555555555580, 0.4083333333333333259, 0.4111111111111110938, 0.4138888888888888618, 0.4166666666666666852, 0.4194444444444444531, 0.4222222222222222210, 0.4249999999999999889, 0.4277777777777777568, 0.4305555555555555802, 0.4333333333333333481, 0.4361111111111111160, 0.4388888888888888840, 0.4416666666666666519, 0.4444444444444444198, 0.4472222222222222432, 0.4500000000000000111, 0.4527777777777777790, 0.4555555555555555469, 0.4583333333333333148, 0.4611111111111111382, 0.4638888888888889062, 0.4666666666666666741, 0.4694444444444444420, 0.4722222222222222099, 0.4749999999999999778, 0.4777777777777778012, 0.4805555555555555691, 0.4833333333333333370, 0.4861111111111111049, 0.4888888888888888729, 0.4916666666666666408, 0.4944444444444444642, 0.4972222222222222321, 0.5000000000000000000, 0.5027777777777777679, 0.5055555555555555358, 0.5083333333333333037, 0.5111111111111110716, 0.5138888888888888395, 0.5166666666666667185, 0.5194444444444444864, 0.5222222222222222543, 0.5250000000000000222, 0.5277777777777777901, 0.5305555555555555580, 0.5333333333333333259, 0.5361111111111110938, 0.5388888888888888618, 0.5416666666666666297, 0.5444444444444443976, 0.5472222222222222765, 0.5500000000000000444, 0.5527777777777778123, 0.5555555555555555802, 0.5583333333333333481, 0.5611111111111111160, 0.5638888888888888840, 0.5666666666666666519, 0.5694444444444444198, 0.5722222222222221877, 0.5749999999999999556, 0.5777777777777777235, 0.5805555555555556024, 0.5833333333333333703, 0.5861111111111111382, 0.5888888888888889062, 0.5916666666666666741, 0.5944444444444444420, 0.5972222222222222099, 0.5999999999999999778, 0.6027777777777777457, 0.6055555555555555136, 0.6083333333333332815, 0.6111111111111111605, 0.6138888888888889284, 0.6166666666666666963, 0.6194444444444444642, 0.6222222222222222321, 0.6250000000000000000, 0.6277777777777777679, 0.6305555555555555358, 0.6333333333333333037, 0.6361111111111110716, 0.6388888888888888395, 0.6416666666666667185, 0.6444444444444444864, 0.6472222222222222543, 0.6500000000000000222, 0.6527777777777777901, 0.6555555555555555580, 0.6583333333333333259, 0.6611111111111110938, 0.6638888888888888618, 0.6666666666666666297, 0.6694444444444443976, 0.6722222222222222765, 0.6750000000000000444, 0.6777777777777778123, 0.6805555555555555802, 0.6833333333333333481, 0.6861111111111111160, 0.6888888888888888840, 0.6916666666666666519, 0.6944444444444444198, 0.6972222222222221877, 0.6999999999999999556, 0.7027777777777777235, 0.7055555555555556024, 0.7083333333333333703, 0.7111111111111111382, 0.7138888888888889062, 0.7166666666666666741, 0.7194444444444444420, 0.7222222222222222099, 0.7249999999999999778, 0.7277777777777777457, 0.7305555555555555136, 0.7333333333333332815, 0.7361111111111111605, 0.7388888888888889284, 0.7416666666666666963, 0.7444444444444444642, 0.7472222222222222321, 0.7500000000000000000, 0.7527777777777777679, 0.7555555555555555358, 0.7583333333333333037, 0.7611111111111110716, 0.7638888888888888395, 0.7666666666666667185, 0.7694444444444444864, 0.7722222222222222543, 0.7750000000000000222, 0.7777777777777777901, 0.7805555555555555580, 0.7833333333333333259, 0.7861111111111110938, 0.7888888888888888618, 0.7916666666666666297, 0.7944444444444443976, 0.7972222222222222765, 0.8000000000000000444, 0.8027777777777778123, 0.8055555555555555802, 0.8083333333333333481, 0.8111111111111111160, 0.8138888888888888840, 0.8166666666666666519, 0.8194444444444444198, 0.8222222222222221877, 0.8249999999999999556, 0.8277777777777777235, 0.8305555555555556024, 0.8333333333333333703, 0.8361111111111111382, 0.8388888888888889062, 0.8416666666666666741, 0.8444444444444444420, 0.8472222222222222099, 0.8499999999999999778, 0.8527777777777777457, 0.8555555555555555136, 0.8583333333333332815, 0.8611111111111111605, 0.8638888888888889284, 0.8666666666666666963, 0.8694444444444444642, 0.8722222222222222321, 0.8750000000000000000, 0.8777777777777777679, 0.8805555555555555358, 0.8833333333333333037, 0.8861111111111110716, 0.8888888888888888395, 0.8916666666666667185, 0.8944444444444444864, 0.8972222222222222543, 0.9000000000000000222, 0.9027777777777777901, 0.9055555555555555580, 0.9083333333333333259, 0.9111111111111110938, 0.9138888888888888618, 0.9166666666666666297, 0.9194444444444443976, 0.9222222222222222765, 0.9250000000000000444, 0.9277777777777778123, 0.9305555555555555802, 0.9333333333333333481, 0.9361111111111111160, 0.9388888888888888840, 0.9416666666666666519, 0.9444444444444444198, 0.9472222222222221877, 0.9499999999999999556, 0.9527777777777777235, 0.9555555555555556024, 0.9583333333333333703, 0.9611111111111111382, 0.9638888888888889062, 0.9666666666666666741, 0.9694444444444444420, 0.9722222222222222099, 0.9749999999999999778, 0.9777777777777777457, 0.9805555555555555136, 0.9833333333333332815, 0.9861111111111111605, 0.9888888888888889284, 0.9916666666666666963, 0.9944444444444444642, 0.9972222222222222321, 1.000000000000000000 ),
 .UNSPECIFIED. ) 
 GEOMETRIC_REPRESENTATION_ITEM ( )  RATIONAL_B_SPLINE_SURFACE ( (
 ( 1.000000000000000000, 0.8660254037844387076, 1.000000000000000000, 0.8660254037844387076, 1.000000000000000000, 0.8660254037844387076, 1.000000000000000000, 0.8660254037844387076, 1.000000000000000000, 0.8660254037844387076, 1.000000000000000000, 0.8660254037844387076, 1.000000000000000000, 0.8660254037844387076, 1.000000000000000000, 0.8660254037844387076, 1.000000000000000000, 0.8660254037844387076, 1.000000000000000000, 0.8660254037844387076, 1.000000000000000000, 0.8660254037844387076, 1.000000000000000000, 0.8660254037844387076, 1.000000000000000000, 0.8660254037844387076, 1.000000000000000000, 0.8660254037844387076, 1.000000000000000000, 0.8660254037844387076, 1.000000000000000000, 0.8660254037844387076, 1.000000000000000000, 0.8660254037844387076, 1.000000000000000000, 0.8660254037844387076, 1.000000000000000000, 0.8660254037844387076, 1.000000000000000000, 0.8660254037844387076, 1.000000000000000000, 0.8660254037844387076, 1.000000000000000000, 0.8660254037844387076, 1.000000000000000000, 0.8660254037844387076, 1.000000000000000000, 0.8660254037844387076, 1.000000000000000000, 0.8660254037844387076, 1.000000000000000000, 0.8660254037844387076, 1.000000000000000000, 0.8660254037844387076, 1.000000000000000000, 0.8660254037844387076, 1.000000000000000000, 0.8660254037844387076, 1.000000000000000000, 0.8660254037844387076, 1.000000000000000000, 0.8660254037844387076, 1.000000000000000000, 0.8660254037844387076, 1.000000000000000000, 0.8660254037844387076, 1.000000000000000000, 0.8660254037844387076, 1.000000000000000000, 0.8660254037844387076, 1.000000000000000000, 0.8660254037844387076, 1.000000000000000000, 0.8660254037844387076, 1.000000000000000000, 0.8660254037844387076, 1.000000000000000000, 0.8660254037844387076, 1.000000000000000000, 0.8660254037844387076, 1.000000000000000000, 0.8660254037844387076, 1.000000000000000000, 0.8660254037844387076, 1.000000000000000000, 0.8660254037844387076, 1.000000000000000000, 0.8660254037844387076, 1.000000000000000000, 0.8660254037844387076, 1.000000000000000000, 0.8660254037844387076, 1.000000000000000000, 0.8660254037844387076, 1.000000000000000000, 0.8660254037844387076, 1.000000000000000000, 0.8660254037844387076, 1.000000000000000000, 0.8660254037844387076, 1.000000000000000000, 0.8660254037844387076, 1.000000000000000000, 0.8660254037844387076, 1.000000000000000000, 0.8660254037844387076, 1.000000000000000000, 0.8660254037844387076, 1.000000000000000000, 0.8660254037844387076, 1.000000000000000000, 0.8660254037844387076, 1.000000000000000000, 0.8660254037844387076, 1.000000000000000000, 0.8660254037844387076, 1.000000000000000000, 0.8660254037844387076, 1.000000000000000000, 0.8660254037844387076, 1.000000000000000000, 0.8660254037844387076, 1.000000000000000000, 0.8660254037844387076, 1.000000000000000000, 0.8660254037844387076, 1.000000000000000000, 0.8660254037844387076, 1.000000000000000000, 0.8660254037844387076, 1.000000000000000000, 0.8660254037844387076, 1.000000000000000000, 0.8660254037844387076, 1.000000000000000000, 0.8660254037844387076, 1.000000000000000000, 0.8660254037844387076, 1.000000000000000000, 0.8660254037844387076, 1.000000000000000000, 0.8660254037844387076, 1.000000000000000000, 0.8660254037844387076, 1.000000000000000000, 0.8660254037844387076, 1.000000000000000000, 0.8660254037844387076, 1.000000000000000000, 0.8660254037844387076, 1.000000000000000000, 0.8660254037844387076, 1.000000000000000000, 0.8660254037844387076, 1.000000000000000000, 0.8660254037844387076, 1.000000000000000000, 0.8660254037844387076, 1.000000000000000000, 0.8660254037844387076, 1.000000000000000000, 0.8660254037844387076, 1.000000000000000000, 0.8660254037844387076, 1.000000000000000000, 0.8660254037844387076, 1.000000000000000000, 0.8660254037844387076, 1.000000000000000000, 0.8660254037844387076, 1.000000000000000000, 0.8660254037844387076, 1.000000000000000000, 0.8660254037844387076, 1.000000000000000000, 0.8660254037844387076, 1.000000000000000000, 0.8660254037844387076, 1.000000000000000000, 0.8660254037844387076, 1.000000000000000000, 0.8660254037844387076, 1.000000000000000000, 0.8660254037844387076, 1.000000000000000000, 0.8660254037844387076, 1.000000000000000000, 0.8660254037844387076, 1.000000000000000000, 0.8660254037844387076, 1.000000000000000000, 0.8660254037844387076, 1.000000000000000000, 0.8660254037844387076, 1.000000000000000000, 0.8660254037844387076, 1.000000000000000000, 0.8660254037844387076, 1.000000000000000000, 0.8660254037844387076, 1.000000000000000000, 0.8660254037844387076, 1.000000000000000000, 0.8660254037844387076, 1.000000000000000000, 0.8660254037844387076, 1.000000000000000000, 0.8660254037844387076, 1.000000000000000000, 0.8660254037844387076, 1.000000000000000000, 0.8660254037844387076, 1.000000000000000000, 0.8660254037844387076, 1.000000000000000000, 0.8660254037844387076, 1.000000000000000000, 0.8660254037844387076, 1.000000000000000000, 0.8660254037844387076, 1.000000000000000000, 0.8660254037844387076, 1.000000000000000000, 0.8660254037844387076, 1.000000000000000000, 0.8660254037844387076, 1.000000000000000000, 0.8660254037844387076, 1.000000000000000000, 0.8660254037844387076, 1.000000000000000000, 0.8660254037844387076, 1.000000000000000000, 0.8660254037844387076, 1.000000000000000000, 0.8660254037844387076, 1.000000000000000000, 0.8660254037844387076, 1.000000000000000000, 0.8660254037844387076, 1.000000000000000000, 0.8660254037844387076, 1.000000000000000000, 0.8660254037844387076, 1.000000000000000000, 0.8660254037844387076, 1.000000000000000000, 0.8660254037844387076, 1.000000000000000000, 0.8660254037844387076, 1.000000000000000000, 0.8660254037844387076, 1.000000000000000000, 0.8660254037844387076, 1.000000000000000000, 0.8660254037844387076, 1.000000000000000000, 0.8660254037844387076, 1.000000000000000000, 0.8660254037844387076, 1.000000000000000000, 0.8660254037844387076, 1.000000000000000000, 0.8660254037844387076, 1.000000000000000000, 0.8660254037844387076, 1.000000000000000000, 0.8660254037844387076, 1.000000000000000000, 0.8660254037844387076, 1.000000000000000000, 0.8660254037844387076, 1.000000000000000000, 0.8660254037844387076, 1.000000000000000000, 0.8660254037844387076, 1.000000000000000000, 0.8660254037844387076, 1.000000000000000000, 0.8660254037844387076, 1.000000000000000000, 0.8660254037844387076, 1.000000000000000000, 0.8660254037844387076, 1.000000000000000000, 0.8660254037844387076, 1.000000000000000000, 0.8660254037844387076, 1.000000000000000000, 0.8660254037844387076, 1.000000000000000000, 0.8660254037844387076, 1.000000000000000000, 0.8660254037844387076, 1.000000000000000000, 0.8660254037844387076, 1.000000000000000000, 0.8660254037844387076, 1.000000000000000000, 0.8660254037844387076, 1.000000000000000000, 0.8660254037844387076, 1.000000000000000000, 0.8660254037844387076, 1.000000000000000000, 0.8660254037844387076, 1.000000000000000000, 0.8660254037844387076, 1.000000000000000000, 0.8660254037844387076, 1.000000000000000000, 0.8660254037844387076, 1.000000000000000000, 0.8660254037844387076, 1.000000000000000000, 0.8660254037844387076, 1.000000000000000000, 0.8660254037844387076, 1.000000000000000000, 0.8660254037844387076, 1.000000000000000000, 0.8660254037844387076, 1.000000000000000000, 0.8660254037844387076, 1.000000000000000000, 0.8660254037844387076, 1.000000000000000000, 0.8660254037844387076, 1.000000000000000000, 0.8660254037844387076, 1.000000000000000000, 0.8660254037844387076, 1.000000000000000000, 0.8660254037844387076, 1.000000000000000000, 0.8660254037844387076, 1.000000000000000000, 0.8660254037844387076, 1.000000000000000000, 0.8660254037844387076, 1.000000000000000000, 0.8660254037844387076, 1.000000000000000000, 0.8660254037844387076, 1.000000000000000000, 0.8660254037844387076, 1.000000000000000000, 0.8660254037844387076, 1.000000000000000000, 0.8660254037844387076, 1.000000000000000000, 0.8660254037844387076, 1.000000000000000000, 0.8660254037844387076, 1.000000000000000000, 0.8660254037844387076, 1.000000000000000000, 0.8660254037844387076, 1.000000000000000000, 0.8660254037844387076, 1.000000000000000000, 0.8660254037844387076, 1.000000000000000000, 0.8660254037844387076, 1.000000000000000000, 0.8660254037844387076, 1.000000000000000000, 0.8660254037844387076, 1.000000000000000000, 0.8660254037844387076, 1.000000000000000000, 0.8660254037844387076, 1.000000000000000000, 0.8660254037844387076, 1.000000000000000000, 0.8660254037844387076, 1.000000000000000000, 0.8660254037844387076, 1.000000000000000000, 0.8660254037844387076, 1.000000000000000000, 0.8660254037844387076, 1.000000000000000000, 0.8660254037844387076, 1.000000000000000000, 0.8660254037844387076, 1.000000000000000000, 0.8660254037844387076, 1.000000000000000000, 0.8660254037844387076, 1.000000000000000000, 0.8660254037844387076, 1.000000000000000000, 0.8660254037844387076, 1.000000000000000000, 0.8660254037844387076, 1.000000000000000000, 0.8660254037844387076, 1.000000000000000000, 0.8660254037844387076, 1.000000000000000000, 0.8660254037844387076, 1.000000000000000000, 0.8660254037844387076, 1.000000000000000000, 0.8660254037844387076, 1.000000000000000000, 0.8660254037844387076, 1.000000000000000000, 0.8660254037844387076, 1.000000000000000000, 0.8660254037844387076, 1.000000000000000000, 0.8660254037844387076, 1.000000000000000000, 0.8660254037844387076, 1.000000000000000000, 0.8660254037844387076, 1.000000000000000000, 0.8660254037844387076, 1.000000000000000000, 0.8660254037844387076, 1.000000000000000000, 0.8660254037844387076, 1.000000000000000000, 0.8660254037844387076, 1.000000000000000000, 0.8660254037844387076, 1.000000000000000000, 0.8660254037844387076, 1.000000000000000000, 0.8660254037844387076, 1.000000000000000000, 0.8660254037844387076, 1.000000000000000000, 0.8660254037844387076, 1.000000000000000000, 0.8660254037844387076, 1.000000000000000000, 0.8660254037844387076, 1.000000000000000000, 0.8660254037844387076, 1.000000000000000000, 0.8660254037844387076, 1.000000000000000000, 0.8660254037844387076, 1.000000000000000000, 0.8660254037844387076, 1.000000000000000000, 0.8660254037844387076, 1.000000000000000000, 0.8660254037844387076, 1.000000000000000000, 0.8660254037844387076, 1.000000000000000000, 0.8660254037844387076, 1.000000000000000000, 0.8660254037844387076, 1.000000000000000000, 0.8660254037844387076, 1.000000000000000000, 0.8660254037844387076, 1.000000000000000000, 0.8660254037844387076, 1.000000000000000000, 0.8660254037844387076, 1.000000000000000000, 0.8660254037844387076, 1.000000000000000000, 0.8660254037844387076, 1.000000000000000000, 0.8660254037844387076, 1.000000000000000000, 0.8660254037844387076, 1.000000000000000000, 0.8660254037844387076, 1.000000000000000000, 0.8660254037844387076, 1.000000000000000000, 0.8660254037844387076, 1.000000000000000000, 0.8660254037844387076, 1.000000000000000000, 0.8660254037844387076, 1.000000000000000000, 0.8660254037844387076, 1.000000000000000000, 0.8660254037844387076, 1.000000000000000000, 0.8660254037844387076, 1.000000000000000000, 0.8660254037844387076, 1.000000000000000000, 0.8660254037844387076, 1.000000000000000000, 0.8660254037844387076, 1.000000000000000000, 0.8660254037844387076, 1.000000000000000000, 0.8660254037844387076, 1.000000000000000000, 0.8660254037844387076, 1.000000000000000000, 0.8660254037844387076, 1.000000000000000000, 0.8660254037844387076, 1.000000000000000000, 0.8660254037844387076, 1.000000000000000000, 0.8660254037844387076, 1.000000000000000000, 0.8660254037844387076, 1.000000000000000000, 0.8660254037844387076, 1.000000000000000000, 0.8660254037844387076, 1.000000000000000000, 0.8660254037844387076, 1.000000000000000000, 0.8660254037844387076, 1.000000000000000000, 0.8660254037844387076, 1.000000000000000000, 0.8660254037844387076, 1.000000000000000000, 0.8660254037844387076, 1.000000000000000000, 0.8660254037844387076, 1.000000000000000000, 0.8660254037844387076, 1.000000000000000000, 0.8660254037844387076, 1.000000000000000000, 0.8660254037844387076, 1.000000000000000000, 0.8660254037844387076, 1.000000000000000000, 0.8660254037844387076, 1.000000000000000000, 0.8660254037844387076, 1.000000000000000000, 0.8660254037844387076, 1.000000000000000000, 0.8660254037844387076, 1.000000000000000000, 0.8660254037844387076, 1.000000000000000000, 0.8660254037844387076, 1.000000000000000000, 0.8660254037844387076, 1.000000000000000000, 0.8660254037844387076, 1.000000000000000000, 0.8660254037844387076, 1.000000000000000000, 0.8660254037844387076, 1.000000000000000000, 0.8660254037844387076, 1.000000000000000000, 0.8660254037844387076, 1.000000000000000000, 0.8660254037844387076, 1.000000000000000000, 0.8660254037844387076, 1.000000000000000000, 0.8660254037844387076, 1.000000000000000000, 0.8660254037844387076, 1.000000000000000000, 0.8660254037844387076, 1.000000000000000000, 0.8660254037844387076, 1.000000000000000000, 0.8660254037844387076, 1.000000000000000000, 0.8660254037844387076, 1.000000000000000000, 0.8660254037844387076, 1.000000000000000000, 0.8660254037844387076, 1.000000000000000000, 0.8660254037844387076, 1.000000000000000000, 0.8660254037844387076, 1.000000000000000000, 0.8660254037844387076, 1.000000000000000000, 0.8660254037844387076, 1.000000000000000000, 0.8660254037844387076, 1.000000000000000000, 0.8660254037844387076, 1.000000000000000000, 0.8660254037844387076, 1.000000000000000000, 0.8660254037844387076, 1.000000000000000000, 0.8660254037844387076, 1.000000000000000000, 0.8660254037844387076, 1.000000000000000000, 0.8660254037844387076, 1.000000000000000000, 0.8660254037844387076, 1.000000000000000000, 0.8660254037844387076, 1.000000000000000000, 0.8660254037844387076, 1.000000000000000000, 0.8660254037844387076, 1.000000000000000000, 0.8660254037844387076, 1.000000000000000000, 0.8660254037844387076, 1.000000000000000000, 0.8660254037844387076, 1.000000000000000000, 0.8660254037844387076, 1.000000000000000000, 0.8660254037844387076, 1.000000000000000000, 0.8660254037844387076, 1.000000000000000000, 0.8660254037844387076, 1.000000000000000000, 0.8660254037844387076, 1.000000000000000000, 0.8660254037844387076, 1.000000000000000000, 0.8660254037844387076, 1.000000000000000000, 0.8660254037844387076, 1.000000000000000000, 0.8660254037844387076, 1.000000000000000000, 0.8660254037844387076, 1.000000000000000000, 0.8660254037844387076, 1.000000000000000000, 0.8660254037844387076, 1.000000000000000000, 0.8660254037844387076, 1.000000000000000000, 0.8660254037844387076, 1.000000000000000000, 0.8660254037844387076, 1.000000000000000000, 0.8660254037844387076, 1.000000000000000000, 0.8660254037844387076, 1.000000000000000000, 0.8660254037844387076, 1.000000000000000000, 0.8660254037844387076, 1.000000000000000000, 0.8660254037844387076, 1.000000000000000000, 0.8660254037844387076, 1.000000000000000000, 0.8660254037844387076, 1.000000000000000000, 0.8660254037844387076, 1.000000000000000000, 0.8660254037844387076, 1.000000000000000000, 0.8660254037844387076, 1.000000000000000000, 0.8660254037844387076, 1.000000000000000000, 0.8660254037844387076, 1.000000000000000000, 0.8660254037844387076, 1.000000000000000000, 0.8660254037844387076, 1.000000000000000000, 0.8660254037844387076, 1.000000000000000000, 0.8660254037844387076, 1.000000000000000000, 0.8660254037844387076, 1.000000000000000000, 0.8660254037844387076, 1.000000000000000000, 0.8660254037844387076, 1.000000000000000000, 0.8660254037844387076, 1.000000000000000000, 0.8660254037844387076, 1.000000000000000000, 0.8660254037844387076, 1.000000000000000000, 0.8660254037844387076, 1.000000000000000000, 0.8660254037844387076, 1.000000000000000000, 0.8660254037844387076, 1.000000000000000000, 0.8660254037844387076, 1.000000000000000000, 0.8660254037844387076, 1.000000000000000000, 0.8660254037844387076, 1.000000000000000000, 0.8660254037844387076, 1.000000000000000000, 0.8660254037844387076, 1.000000000000000000, 0.8660254037844387076, 1.000000000000000000, 0.8660254037844387076, 1.000000000000000000, 0.8660254037844387076, 1.000000000000000000, 0.8660254037844387076, 1.000000000000000000, 0.8660254037844387076, 1.000000000000000000, 0.8660254037844387076, 1.000000000000000000, 0.8660254037844387076, 1.000000000000000000),
 ( 1.000000000000000000, 0.8660254037844387076, 1.000000000000000000, 0.8660254037844387076, 1.000000000000000000, 0.8660254037844387076, 1.000000000000000000, 0.8660254037844387076, 1.000000000000000000, 0.8660254037844387076, 1.000000000000000000, 0.8660254037844387076, 1.000000000000000000, 0.8660254037844387076, 1.000000000000000000, 0.8660254037844387076, 1.000000000000000000, 0.8660254037844387076, 1.000000000000000000, 0.8660254037844387076, 1.000000000000000000, 0.8660254037844387076, 1.000000000000000000, 0.8660254037844387076, 1.000000000000000000, 0.8660254037844387076, 1.000000000000000000, 0.8660254037844387076, 1.000000000000000000, 0.8660254037844387076, 1.000000000000000000, 0.8660254037844387076, 1.000000000000000000, 0.8660254037844387076, 1.000000000000000000, 0.8660254037844387076, 1.000000000000000000, 0.8660254037844387076, 1.000000000000000000, 0.8660254037844387076, 1.000000000000000000, 0.8660254037844387076, 1.000000000000000000, 0.8660254037844387076, 1.000000000000000000, 0.8660254037844387076, 1.000000000000000000, 0.8660254037844387076, 1.000000000000000000, 0.8660254037844387076, 1.000000000000000000, 0.8660254037844387076, 1.000000000000000000, 0.8660254037844387076, 1.000000000000000000, 0.8660254037844387076, 1.000000000000000000, 0.8660254037844387076, 1.000000000000000000, 0.8660254037844387076, 1.000000000000000000, 0.8660254037844387076, 1.000000000000000000, 0.8660254037844387076, 1.000000000000000000, 0.8660254037844387076, 1.000000000000000000, 0.8660254037844387076, 1.000000000000000000, 0.8660254037844387076, 1.000000000000000000, 0.8660254037844387076, 1.000000000000000000, 0.8660254037844387076, 1.000000000000000000, 0.8660254037844387076, 1.000000000000000000, 0.8660254037844387076, 1.000000000000000000, 0.8660254037844387076, 1.000000000000000000, 0.8660254037844387076, 1.000000000000000000, 0.8660254037844387076, 1.000000000000000000, 0.8660254037844387076, 1.000000000000000000, 0.8660254037844387076, 1.000000000000000000, 0.8660254037844387076, 1.000000000000000000, 0.8660254037844387076, 1.000000000000000000, 0.8660254037844387076, 1.000000000000000000, 0.8660254037844387076, 1.000000000000000000, 0.8660254037844387076, 1.000000000000000000, 0.8660254037844387076, 1.000000000000000000, 0.8660254037844387076, 1.000000000000000000, 0.8660254037844387076, 1.000000000000000000, 0.8660254037844387076, 1.000000000000000000, 0.8660254037844387076, 1.000000000000000000, 0.8660254037844387076, 1.000000000000000000, 0.8660254037844387076, 1.000000000000000000, 0.8660254037844387076, 1.000000000000000000, 0.8660254037844387076, 1.000000000000000000, 0.8660254037844387076, 1.000000000000000000, 0.8660254037844387076, 1.000000000000000000, 0.8660254037844387076, 1.000000000000000000, 0.8660254037844387076, 1.000000000000000000, 0.8660254037844387076, 1.000000000000000000, 0.8660254037844387076, 1.000000000000000000, 0.8660254037844387076, 1.000000000000000000, 0.8660254037844387076, 1.000000000000000000, 0.8660254037844387076, 1.000000000000000000, 0.8660254037844387076, 1.000000000000000000, 0.8660254037844387076, 1.000000000000000000, 0.8660254037844387076, 1.000000000000000000, 0.8660254037844387076, 1.000000000000000000, 0.8660254037844387076, 1.000000000000000000, 0.8660254037844387076, 1.000000000000000000, 0.8660254037844387076, 1.000000000000000000, 0.8660254037844387076, 1.000000000000000000, 0.8660254037844387076, 1.000000000000000000, 0.8660254037844387076, 1.000000000000000000, 0.8660254037844387076, 1.000000000000000000, 0.8660254037844387076, 1.000000000000000000, 0.8660254037844387076, 1.000000000000000000, 0.8660254037844387076, 1.000000000000000000, 0.8660254037844387076, 1.000000000000000000, 0.8660254037844387076, 1.000000000000000000, 0.8660254037844387076, 1.000000000000000000, 0.8660254037844387076, 1.000000000000000000, 0.8660254037844387076, 1.000000000000000000, 0.8660254037844387076, 1.000000000000000000, 0.8660254037844387076, 1.000000000000000000, 0.8660254037844387076, 1.000000000000000000, 0.8660254037844387076, 1.000000000000000000, 0.8660254037844387076, 1.000000000000000000, 0.8660254037844387076, 1.000000000000000000, 0.8660254037844387076, 1.000000000000000000, 0.8660254037844387076, 1.000000000000000000, 0.8660254037844387076, 1.000000000000000000, 0.8660254037844387076, 1.000000000000000000, 0.8660254037844387076, 1.000000000000000000, 0.8660254037844387076, 1.000000000000000000, 0.8660254037844387076, 1.000000000000000000, 0.8660254037844387076, 1.000000000000000000, 0.8660254037844387076, 1.000000000000000000, 0.8660254037844387076, 1.000000000000000000, 0.8660254037844387076, 1.000000000000000000, 0.8660254037844387076, 1.000000000000000000, 0.8660254037844387076, 1.000000000000000000, 0.8660254037844387076, 1.000000000000000000, 0.8660254037844387076, 1.000000000000000000, 0.8660254037844387076, 1.000000000000000000, 0.8660254037844387076, 1.000000000000000000, 0.8660254037844387076, 1.000000000000000000, 0.8660254037844387076, 1.000000000000000000, 0.8660254037844387076, 1.000000000000000000, 0.8660254037844387076, 1.000000000000000000, 0.8660254037844387076, 1.000000000000000000, 0.8660254037844387076, 1.000000000000000000, 0.8660254037844387076, 1.000000000000000000, 0.8660254037844387076, 1.000000000000000000, 0.8660254037844387076, 1.000000000000000000, 0.8660254037844387076, 1.000000000000000000, 0.8660254037844387076, 1.000000000000000000, 0.8660254037844387076, 1.000000000000000000, 0.8660254037844387076, 1.000000000000000000, 0.8660254037844387076, 1.000000000000000000, 0.8660254037844387076, 1.000000000000000000, 0.8660254037844387076, 1.000000000000000000, 0.8660254037844387076, 1.000000000000000000, 0.8660254037844387076, 1.000000000000000000, 0.8660254037844387076, 1.000000000000000000, 0.8660254037844387076, 1.000000000000000000, 0.8660254037844387076, 1.000000000000000000, 0.8660254037844387076, 1.000000000000000000, 0.8660254037844387076, 1.000000000000000000, 0.8660254037844387076, 1.000000000000000000, 0.8660254037844387076, 1.000000000000000000, 0.8660254037844387076, 1.000000000000000000, 0.8660254037844387076, 1.000000000000000000, 0.8660254037844387076, 1.000000000000000000, 0.8660254037844387076, 1.000000000000000000, 0.8660254037844387076, 1.000000000000000000, 0.8660254037844387076, 1.000000000000000000, 0.8660254037844387076, 1.000000000000000000, 0.8660254037844387076, 1.000000000000000000, 0.8660254037844387076, 1.000000000000000000, 0.8660254037844387076, 1.000000000000000000, 0.8660254037844387076, 1.000000000000000000, 0.8660254037844387076, 1.000000000000000000, 0.8660254037844387076, 1.000000000000000000, 0.8660254037844387076, 1.000000000000000000, 0.8660254037844387076, 1.000000000000000000, 0.8660254037844387076, 1.000000000000000000, 0.8660254037844387076, 1.000000000000000000, 0.8660254037844387076, 1.000000000000000000, 0.8660254037844387076, 1.000000000000000000, 0.8660254037844387076, 1.000000000000000000, 0.8660254037844387076, 1.000000000000000000, 0.8660254037844387076, 1.000000000000000000, 0.8660254037844387076, 1.000000000000000000, 0.8660254037844387076, 1.000000000000000000, 0.8660254037844387076, 1.000000000000000000, 0.8660254037844387076, 1.000000000000000000, 0.8660254037844387076, 1.000000000000000000, 0.8660254037844387076, 1.000000000000000000, 0.8660254037844387076, 1.000000000000000000, 0.8660254037844387076, 1.000000000000000000, 0.8660254037844387076, 1.000000000000000000, 0.8660254037844387076, 1.000000000000000000, 0.8660254037844387076, 1.000000000000000000, 0.8660254037844387076, 1.000000000000000000, 0.8660254037844387076, 1.000000000000000000, 0.8660254037844387076, 1.000000000000000000, 0.8660254037844387076, 1.000000000000000000, 0.8660254037844387076, 1.000000000000000000, 0.8660254037844387076, 1.000000000000000000, 0.8660254037844387076, 1.000000000000000000, 0.8660254037844387076, 1.000000000000000000, 0.8660254037844387076, 1.000000000000000000, 0.8660254037844387076, 1.000000000000000000, 0.8660254037844387076, 1.000000000000000000, 0.8660254037844387076, 1.000000000000000000, 0.8660254037844387076, 1.000000000000000000, 0.8660254037844387076, 1.000000000000000000, 0.8660254037844387076, 1.000000000000000000, 0.8660254037844387076, 1.000000000000000000, 0.8660254037844387076, 1.000000000000000000, 0.8660254037844387076, 1.000000000000000000, 0.8660254037844387076, 1.000000000000000000, 0.8660254037844387076, 1.000000000000000000, 0.8660254037844387076, 1.000000000000000000, 0.8660254037844387076, 1.000000000000000000, 0.8660254037844387076, 1.000000000000000000, 0.8660254037844387076, 1.000000000000000000, 0.8660254037844387076, 1.000000000000000000, 0.8660254037844387076, 1.000000000000000000, 0.8660254037844387076, 1.000000000000000000, 0.8660254037844387076, 1.000000000000000000, 0.8660254037844387076, 1.000000000000000000, 0.8660254037844387076, 1.000000000000000000, 0.8660254037844387076, 1.000000000000000000, 0.8660254037844387076, 1.000000000000000000, 0.8660254037844387076, 1.000000000000000000, 0.8660254037844387076, 1.000000000000000000, 0.8660254037844387076, 1.000000000000000000, 0.8660254037844387076, 1.000000000000000000, 0.8660254037844387076, 1.000000000000000000, 0.8660254037844387076, 1.000000000000000000, 0.8660254037844387076, 1.000000000000000000, 0.8660254037844387076, 1.000000000000000000, 0.8660254037844387076, 1.000000000000000000, 0.8660254037844387076, 1.000000000000000000, 0.8660254037844387076, 1.000000000000000000, 0.8660254037844387076, 1.000000000000000000, 0.8660254037844387076, 1.000000000000000000, 0.8660254037844387076, 1.000000000000000000, 0.8660254037844387076, 1.000000000000000000, 0.8660254037844387076, 1.000000000000000000, 0.8660254037844387076, 1.000000000000000000, 0.8660254037844387076, 1.000000000000000000, 0.8660254037844387076, 1.000000000000000000, 0.8660254037844387076, 1.000000000000000000, 0.8660254037844387076, 1.000000000000000000, 0.8660254037844387076, 1.000000000000000000, 0.8660254037844387076, 1.000000000000000000, 0.8660254037844387076, 1.000000000000000000, 0.8660254037844387076, 1.000000000000000000, 0.8660254037844387076, 1.000000000000000000, 0.8660254037844387076, 1.000000000000000000, 0.8660254037844387076, 1.000000000000000000, 0.8660254037844387076, 1.000000000000000000, 0.8660254037844387076, 1.000000000000000000, 0.8660254037844387076, 1.000000000000000000, 0.8660254037844387076, 1.000000000000000000, 0.8660254037844387076, 1.000000000000000000, 0.8660254037844387076, 1.000000000000000000, 0.8660254037844387076, 1.000000000000000000, 0.8660254037844387076, 1.000000000000000000, 0.8660254037844387076, 1.000000000000000000, 0.8660254037844387076, 1.000000000000000000, 0.8660254037844387076, 1.000000000000000000, 0.8660254037844387076, 1.000000000000000000, 0.8660254037844387076, 1.000000000000000000, 0.8660254037844387076, 1.000000000000000000, 0.8660254037844387076, 1.000000000000000000, 0.8660254037844387076, 1.000000000000000000, 0.8660254037844387076, 1.000000000000000000, 0.8660254037844387076, 1.000000000000000000, 0.8660254037844387076, 1.000000000000000000, 0.8660254037844387076, 1.000000000000000000, 0.8660254037844387076, 1.000000000000000000, 0.8660254037844387076, 1.000000000000000000, 0.8660254037844387076, 1.000000000000000000, 0.8660254037844387076, 1.000000000000000000, 0.8660254037844387076, 1.000000000000000000, 0.8660254037844387076, 1.000000000000000000, 0.8660254037844387076, 1.000000000000000000, 0.8660254037844387076, 1.000000000000000000, 0.8660254037844387076, 1.000000000000000000, 0.8660254037844387076, 1.000000000000000000, 0.8660254037844387076, 1.000000000000000000, 0.8660254037844387076, 1.000000000000000000, 0.8660254037844387076, 1.000000000000000000, 0.8660254037844387076, 1.000000000000000000, 0.8660254037844387076, 1.000000000000000000, 0.8660254037844387076, 1.000000000000000000, 0.8660254037844387076, 1.000000000000000000, 0.8660254037844387076, 1.000000000000000000, 0.8660254037844387076, 1.000000000000000000, 0.8660254037844387076, 1.000000000000000000, 0.8660254037844387076, 1.000000000000000000, 0.8660254037844387076, 1.000000000000000000, 0.8660254037844387076, 1.000000000000000000, 0.8660254037844387076, 1.000000000000000000, 0.8660254037844387076, 1.000000000000000000, 0.8660254037844387076, 1.000000000000000000, 0.8660254037844387076, 1.000000000000000000, 0.8660254037844387076, 1.000000000000000000, 0.8660254037844387076, 1.000000000000000000, 0.8660254037844387076, 1.000000000000000000, 0.8660254037844387076, 1.000000000000000000, 0.8660254037844387076, 1.000000000000000000, 0.8660254037844387076, 1.000000000000000000, 0.8660254037844387076, 1.000000000000000000, 0.8660254037844387076, 1.000000000000000000, 0.8660254037844387076, 1.000000000000000000, 0.8660254037844387076, 1.000000000000000000, 0.8660254037844387076, 1.000000000000000000, 0.8660254037844387076, 1.000000000000000000, 0.8660254037844387076, 1.000000000000000000, 0.8660254037844387076, 1.000000000000000000, 0.8660254037844387076, 1.000000000000000000, 0.8660254037844387076, 1.000000000000000000, 0.8660254037844387076, 1.000000000000000000, 0.8660254037844387076, 1.000000000000000000, 0.8660254037844387076, 1.000000000000000000, 0.8660254037844387076, 1.000000000000000000, 0.8660254037844387076, 1.000000000000000000, 0.8660254037844387076, 1.000000000000000000, 0.8660254037844387076, 1.000000000000000000, 0.8660254037844387076, 1.000000000000000000, 0.8660254037844387076, 1.000000000000000000, 0.8660254037844387076, 1.000000000000000000, 0.8660254037844387076, 1.000000000000000000, 0.8660254037844387076, 1.000000000000000000, 0.8660254037844387076, 1.000000000000000000, 0.8660254037844387076, 1.000000000000000000, 0.8660254037844387076, 1.000000000000000000, 0.8660254037844387076, 1.000000000000000000, 0.8660254037844387076, 1.000000000000000000, 0.8660254037844387076, 1.000000000000000000, 0.8660254037844387076, 1.000000000000000000, 0.8660254037844387076, 1.000000000000000000, 0.8660254037844387076, 1.000000000000000000, 0.8660254037844387076, 1.000000000000000000, 0.8660254037844387076, 1.000000000000000000, 0.8660254037844387076, 1.000000000000000000, 0.8660254037844387076, 1.000000000000000000, 0.8660254037844387076, 1.000000000000000000, 0.8660254037844387076, 1.000000000000000000, 0.8660254037844387076, 1.000000000000000000, 0.8660254037844387076, 1.000000000000000000, 0.8660254037844387076, 1.000000000000000000, 0.8660254037844387076, 1.000000000000000000, 0.8660254037844387076, 1.000000000000000000, 0.8660254037844387076, 1.000000000000000000, 0.8660254037844387076, 1.000000000000000000, 0.8660254037844387076, 1.000000000000000000, 0.8660254037844387076, 1.000000000000000000, 0.8660254037844387076, 1.000000000000000000, 0.8660254037844387076, 1.000000000000000000, 0.8660254037844387076, 1.000000000000000000, 0.8660254037844387076, 1.000000000000000000, 0.8660254037844387076, 1.000000000000000000, 0.8660254037844387076, 1.000000000000000000, 0.8660254037844387076, 1.000000000000000000, 0.8660254037844387076, 1.000000000000000000, 0.8660254037844387076, 1.000000000000000000, 0.8660254037844387076, 1.000000000000000000, 0.8660254037844387076, 1.000000000000000000, 0.8660254037844387076, 1.000000000000000000, 0.8660254037844387076, 1.000000000000000000, 0.8660254037844387076, 1.000000000000000000, 0.8660254037844387076, 1.000000000000000000, 0.8660254037844387076, 1.000000000000000000, 0.8660254037844387076, 1.000000000000000000, 0.8660254037844387076, 1.000000000000000000, 0.8660254037844387076, 1.000000000000000000, 0.8660254037844387076, 1.000000000000000000, 0.8660254037844387076, 1.000000000000000000, 0.8660254037844387076, 1.000000000000000000, 0.8660254037844387076, 1.000000000000000000, 0.8660254037844387076, 1.000000000000000000, 0.8660254037844387076, 1.000000000000000000, 0.8660254037844387076, 1.000000000000000000, 0.8660254037844387076, 1.000000000000000000, 0.8660254037844387076, 1.000000000000000000, 0.8660254037844387076, 1.000000000000000000, 0.8660254037844387076, 1.000000000000000000, 0.8660254037844387076, 1.000000000000000000, 0.8660254037844387076, 1.000000000000000000, 0.8660254037844387076, 1.000000000000000000, 0.8660254037844387076, 1.000000000000000000) ) ) 
 REPRESENTATION_ITEM ( '' )  SURFACE ( )  );
#71544=CARTESIAN_POINT ( 'NONE',  ( 10.24687500061451750, -3.027376345333610441, -5.243569643749999898 ) ) ;
#71545=CARTESIAN_POINT ( 'NONE',  ( 7.387500001229032165, 6.123233995736764310E-16, -4.999999999999998224 ) ) ;
#71546=CARTESIAN_POINT ( 'NONE',  ( 10.07812500061451644, -4.541064518000419881, 2.621784821874995952 ) ) ;
#71547=CARTESIAN_POINT ( 'NONE',  ( 14.97187500061451892, 3.027376345333611329, 5.243569643749999010 ) ) ;
#71548=CARTESIAN_POINT ( 'NONE',  ( 21.56250000122903288, 0.000000000000000000, 4.999999999999998224 ) ) ;
#71549=CARTESIAN_POINT ( 'NONE',  ( 9.909375000614517148, 4.541064518000418104, -2.621784821874998173 ) ) ;
#71550=CARTESIAN_POINT ( 'NONE',  ( 11.50312500061451892, -4.541064518000417216, -2.621784821875001281 ) ) ;
#71552=CARTESIAN_POINT ( 'NONE',  ( 22.17187500061451644, 3.027376345333611329, 5.243569643749999010 ) ) ;
#71553=CARTESIAN_POINT ( 'NONE',  ( 14.17500000000000071, 4.330127018922191873, 2.499999999999999556 ) ) ;
#71554=CARTESIAN_POINT ( 'NONE',  ( -3.942095835588578900, 3.076014195111398397, 30.69138026080431203 ) ) ;
#71556=CARTESIAN_POINT ( 'NONE',  ( 2.121784821875001281, 13.25937500061451857, -26.32496088578401938 ) ) ;
#71557=CARTESIAN_POINT ( 'NONE',  ( 16.42500000122903359, 2.886751345948129099, -4.999999999999998224 ) ) ;
#71558=CARTESIAN_POINT ( 'NONE',  ( 8.934375000614517504, 6.421520780324663323E-16, -5.243569643749999010 ) ) ;
#71559=CARTESIAN_POINT ( 'NONE',  ( 4.243569643749999010, 17.36562500061451786, -32.45002607614398471 ) ) ;
#71560=CARTESIAN_POINT ( 'NONE',  ( 17.21250000122903145, -4.330127018922190985, -2.500000000000001332 ) ) ;
#71561=CARTESIAN_POINT ( 'NONE',  ( 9.628125000614517148, -4.541064518000419881, 2.621784821874995952 ) ) ;
#71563=CARTESIAN_POINT ( 'NONE',  ( 14.81250000000000000, -5.773502691896255534, -1.060575238724906372E-15 ) ) ;
#71564=CARTESIAN_POINT ( 'NONE',  ( 17.96249999999999858, -5.773502691896255534, -1.060575238724906372E-15 ) ) ;
#71565=VECTOR ( 'NONE', #8094, 1000.000000000000000 ) ;
#71566=CARTESIAN_POINT ( 'NONE',  ( 9.496875000614517504, 6.054752690667223547, 3.707466751127219781E-16 ) ) ;
#71567=CARTESIAN_POINT ( 'NONE',  ( 2.955228467731844333, 4.033190387708875946, -2.955228467731844333 ) ) ;
#71568=CARTESIAN_POINT ( 'NONE',  ( 10.20000000122903572, 5.773502691896255534, 3.535250795749688894E-16 ) ) ;
#71569=CARTESIAN_POINT ( 'NONE',  ( 19.61250000122903359, 4.330127018922192761, -2.499999999999997780 ) ) ;
#71570=CARTESIAN_POINT ( 'NONE',  ( 14.05312500061451431, 0.000000000000000000, 5.243569643749999010 ) ) ;
#71571=CARTESIAN_POINT ( 'NONE',  ( 18.47812500061451857, 4.541064518000418104, 2.621784821874999949 ) ) ;
#71572=CARTESIAN_POINT ( 'NONE',  ( 26.70000000122903572, -2.886751345948125991, -5.000000000000000000 ) ) ;
#71573=CARTESIAN_POINT ( 'NONE',  ( 2.803125000614518747, 0.000000000000000000, 5.243569643749999010 ) ) ;
#71574=CARTESIAN_POINT ( 'NONE',  ( 25.53750000000000142, -2.886751345948129988, 4.999999999999997335 ) ) ;
#71576=CARTESIAN_POINT ( 'NONE',  ( 24.83437500061451431, 4.541064518000418104, 2.621784821874999949 ) ) ;
#71577=CARTESIAN_POINT ( 'NONE',  ( 0.000000000000000000, 20.00000000000000000, 30.00000000000000000 ) ) ;
#71578=CARTESIAN_POINT ( 'NONE',  ( 13.53750000122903430, -4.330127018922194537, 2.499999999999995559 ) ) ;
#71579=CARTESIAN_POINT ( 'NONE',  ( 4.724999999999999645, 4.330127018922191873, 2.499999999999999556 ) ) ;
#71580=EDGE_CURVE ( 'NONE', #53469, #47796, #19816, .T. ) ;
#71581=CARTESIAN_POINT ( 'NONE',  ( 22.64999999999999858, 4.330127018922192761, -2.499999999999997780 ) ) ;
#71582=CARTESIAN_POINT ( 'NONE',  ( 8.409375000614518925, -4.541064518000417216, -2.621784821875001281 ) ) ;
#71583=CARTESIAN_POINT ( 'NONE',  ( 25.71562500061451573, 3.027376345333611329, 5.243569643749999010 ) ) ;
#71585=CARTESIAN_POINT ( 'NONE',  ( 11.47500000122903252, 2.886751345948129099, -4.999999999999997335 ) ) ;
#71586=DIRECTION ( 'NONE',  ( -1.000000000000000000, -0.000000000000000000, -0.000000000000000000 ) ) ;
#71587=CARTESIAN_POINT ( 'NONE',  ( 5.484375000614518214, 4.541064518000418104, 2.621784821874999949 ) ) ;
#71588=CARTESIAN_POINT ( 'NONE',  ( 9.046875000614518214, 6.054752690667223547, 3.707466751127219781E-16 ) ) ;
#71589=CARTESIAN_POINT ( 'NONE',  ( 28.50937500061451502, 0.000000000000000000, 5.243569643749999010 ) ) ;
#71590=CARTESIAN_POINT ( 'NONE',  ( -4.243569643749999898, 11.70312500061459460, 30.00000000000000000 ) ) ;
#71591=CARTESIAN_POINT ( 'NONE',  ( 21.82499999999999574, 4.330127018922191873, 2.499999999999999556 ) ) ;
#71592=CARTESIAN_POINT ( 'NONE',  ( 29.77499999999999858, 6.123233995736764310E-16, -4.999999999999998224 ) ) ;
#71593=ADVANCED_FACE ( 'NONE', ( #69883 ), #41093, .F. ) ;
#71594=CARTESIAN_POINT ( 'NONE',  ( 5.175000000000002487, 4.330127018922191873, 2.499999999999999556 ) ) ;
#71596=CARTESIAN_POINT ( 'NONE',  ( 17.01562500061451644, 3.027376345333613106, -5.243569643749998122 ) ) ;
#71597=CARTESIAN_POINT ( 'NONE',  ( 11.01562500061451821, -6.054752690667223547, -1.112240025338166033E-15 ) ) ;
#71599=CARTESIAN_POINT ( 'NONE',  ( 8.259375000614518569, 0.000000000000000000, 5.243569643749999010 ) ) ;
#71600=CARTESIAN_POINT ( 'NONE',  ( 22.80000000000000071, 0.000000000000000000, 4.999999999999998224 ) ) ;
#71601=CARTESIAN_POINT ( 'NONE',  ( 19.83750000122903145, -4.330127018922194537, 2.499999999999995559 ) ) ;
#71603=CARTESIAN_POINT ( 'NONE',  ( 9.759375000614516793, -4.541064518000417216, -2.621784821875001281 ) ) ;
#71604=CARTESIAN_POINT ( 'NONE',  ( 13.84687500061451537, -3.027376345333610441, -5.243569643749999898 ) ) ;
#71605=CARTESIAN_POINT ( 'NONE',  ( 24.90937500061451715, 0.000000000000000000, 5.243569643749999010 ) ) ;
#71607=CARTESIAN_POINT ( 'NONE',  ( 4.321628989681628674, -3.794150667385939979, -3.915477560016185965 ) ) ;
#71608=ORIENTED_EDGE ( 'NONE', *, *, #16221, .T. ) ;
#71611=CARTESIAN_POINT ( 'NONE',  ( 17.07187500061451502, 3.027376345333613106, -5.243569643749998122 ) ) ;
#71612=CARTESIAN_POINT ( 'NONE',  ( 9.871875000614517504, 3.027376345333613106, -5.243569643749998122 ) ) ;
#71614=CARTESIAN_POINT ( 'NONE',  ( 19.94999999999999929, 4.330127018922192761, -2.499999999999997780 ) ) ;
#71616=CARTESIAN_POINT ( 'NONE',  ( 4.243569643749999010, 10.22187500061451892, -32.45002607614398471 ) ) ;
#71618=CARTESIAN_POINT ( 'NONE',  ( 12.55312500061451786, 4.541064518000418104, -2.621784821874998173 ) ) ;
#71619=CARTESIAN_POINT ( 'NONE',  ( 28.50937500061451502, 0.000000000000000000, 5.243569643749999010 ) ) ;
#71620=CARTESIAN_POINT ( 'NONE',  ( 0.000000000000000000, 20.00000000000000000, -33.99999999999999289 ) ) ;
#71622=CARTESIAN_POINT ( 'NONE',  ( 11.58750000000000036, -2.886751345948129988, 4.999999999999997335 ) ) ;
#71623=CARTESIAN_POINT ( 'NONE',  ( -3.999999999999999556, 17.37500000122903288, 27.69059892324149530 ) ) ;
#71624=CARTESIAN_POINT ( 'NONE',  ( 12.26250000122903394, -4.330127018922190985, -2.500000000000001332 ) ) ;
#71625=CARTESIAN_POINT ( 'NONE',  ( 21.19687500061451502, 6.054752690667223547, 3.707466751127219781E-16 ) ) ;
#71626=CARTESIAN_POINT ( 'NONE',  ( 16.09687500061452070, -3.027376345333610441, -5.243569643749999898 ) ) ;
#71627=CARTESIAN_POINT ( 'NONE',  ( -3.999999999999997335, 12.38750000000000107, 32.30940107675850470 ) ) ;
#71629=CARTESIAN_POINT ( 'NONE',  ( 16.56562500061451715, 3.027376345333613106, -5.243569643749998122 ) ) ;
#71630=CARTESIAN_POINT ( 'NONE',  ( 28.65000000122903145, 5.773502691896255534, 3.535250795749688894E-16 ) ) ;
#71631=CARTESIAN_POINT ( 'NONE',  ( 18.64687500061451786, -3.027376345333614438, 5.243569643749998122 ) ) ;
#71632=CARTESIAN_POINT ( 'NONE',  ( 5.090625000614516615, -3.027376345333614438, 5.243569643749998122 ) ) ;
#71633=CARTESIAN_POINT ( 'NONE',  ( 20.09062500061451573, -3.027376345333610441, -5.243569643749999898 ) ) ;
#71634=CARTESIAN_POINT ( 'NONE',  ( 1.999999999999998668, 18.50000000000000000, -33.46410161513775705 ) ) ;
#71635=CARTESIAN_POINT ( 'NONE',  ( 27.72187500061451715, -6.054752690667223547, -1.112240025338166033E-15 ) ) ;
#71636=CARTESIAN_POINT ( 'NONE',  ( -4.243569643749999898, 13.46562500061451928, 27.54997392385601529 ) ) ;
#71637=CARTESIAN_POINT ( 'NONE',  ( 16.69687500061451502, 6.054752690667223547, 3.707466751127219781E-16 ) ) ;
#71638=CARTESIAN_POINT ( 'NONE',  ( 16.50000000122903288, 5.773502691896255534, 3.535250795749688894E-16 ) ) ;
#71640=CARTESIAN_POINT ( 'NONE',  ( 1.071796769724490117, 18.89509619066136992, -26.00000000000000000 ) ) ;
#71641=CARTESIAN_POINT ( 'NONE',  ( 20.40937500061451715, 0.000000000000000000, 5.243569643749999010 ) ) ;
#71642=CARTESIAN_POINT ( 'NONE',  ( 21.63750000122903572, -4.330127018922194537, 2.499999999999995559 ) ) ;
#71643=CARTESIAN_POINT ( 'NONE',  ( 23.42812500061451786, 4.541064518000418104, 2.621784821874999949 ) ) ;
#71644=CARTESIAN_POINT ( 'NONE',  ( 16.58437500061451786, 6.421520780324663323E-16, -5.243569643749999010 ) ) ;
#71645=CARTESIAN_POINT ( 'NONE',  ( 11.69062500061451360, 6.054752690667223547, 3.707466751127219781E-16 ) ) ;
#71646=CARTESIAN_POINT ( 'NONE',  ( 4.243569643749999010, 13.82187500061451857, 27.54997392385601174 ) ) ;
#71647=CARTESIAN_POINT ( 'NONE',  ( 16.97812500061451502, 6.421520780324663323E-16, -5.243569643749999010 ) ) ;
#71651=CARTESIAN_POINT ( 'NONE',  ( 23.43750000000000000, -2.886751345948125991, -5.000000000000000000 ) ) ;
#71652=CARTESIAN_POINT ( 'NONE',  ( -2.121784821874996840, 18.58437500061451786, -26.32496088578401583 ) ) ;
#71653=CARTESIAN_POINT ( 'NONE',  ( 3.824725165337683030, -3.220477823186019606, -4.017693170146901416 ) ) ;
#71654=CARTESIAN_POINT ( 'NONE',  ( 24.47812500061451502, -4.541064518000419881, 2.621784821874995952 ) ) ;
#71655=CARTESIAN_POINT ( 'NONE',  ( 6.103125000614515905, -4.541064518000417216, -2.621784821875001281 ) ) ;
#71656=CARTESIAN_POINT ( 'NONE',  ( 17.47500000122903430, 2.886751345948126879, 4.999999999999999112 ) ) ;
#71657=CARTESIAN_POINT ( 'NONE',  ( 22.94062500061451715, 6.054752690667223547, 3.707466751127219781E-16 ) ) ;
#71658=CARTESIAN_POINT ( 'NONE',  ( 23.58749999999999858, 5.773502691896255534, 3.535250795749688894E-16 ) ) ;
#71659=CARTESIAN_POINT ( 'NONE',  ( 28.75312500061451715, 4.541064518000418104, -2.621784821874998173 ) ) ;
#71660=CARTESIAN_POINT ( 'NONE',  ( 7.040625000614517681, -3.027376345333610441, -5.243569643749999898 ) ) ;
#71662=CARTESIAN_POINT ( 'NONE',  ( 23.91562500061451502, 3.027376345333611329, 5.243569643749999010 ) ) ;
#71663=CARTESIAN_POINT ( 'NONE',  ( 3.403125000614518836, -4.541064518000417216, -2.621784821875001281 ) ) ;
#71666=CARTESIAN_POINT ( 'NONE',  ( 3.999999999999999112, 13.58750000122903323, -30.00000000000000000 ) ) ;
#71668=CARTESIAN_POINT ( 'NONE',  ( 11.77500000000000036, 6.123233995736764310E-16, -4.999999999999998224 ) ) ;
#71669=ADVANCED_FACE ( 'NONE', ( #48457 ), #15545, .F. ) ;
#71670=CARTESIAN_POINT ( 'NONE',  ( 11.40937500061451892, 0.000000000000000000, 5.243569643749999010 ) ) ;
#71671=CARTESIAN_POINT ( 'NONE',  ( 5.400000001229032343, -2.886751345948129988, 4.999999999999997335 ) ) ;
#71672=CARTESIAN_POINT ( 'NONE',  ( 15.00937500061451679, 0.000000000000000000, 5.243569643749999010 ) ) ;
#71673=CARTESIAN_POINT ( 'NONE',  ( 6.646875000614518747, -3.027376345333610441, -5.243569643749999898 ) ) ;
#71674=LINE ( 'NONE', #66121, #38507 ) ;
#71675=CARTESIAN_POINT ( 'NONE',  ( 10.76250000122903572, 0.000000000000000000, 4.999999999999998224 ) ) ;
#71676=CARTESIAN_POINT ( 'NONE',  ( 11.67187500061451821, 3.027376345333613106, -5.243569643749998122 ) ) ;
#71677=ADVANCED_FACE ( 'NONE', ( #8556 ), #21094, .F. ) ;
#71678=CARTESIAN_POINT ( 'NONE',  ( 21.97500000122902364, 2.886751345948161074, 4.999999999999941380 ) ) ;
#71679=CARTESIAN_POINT ( 'NONE',  ( 22.22812500061451502, -4.541064518000419881, 2.621784821874995952 ) ) ;
#71680=CARTESIAN_POINT ( 'NONE',  ( -4.243569643749998122, 10.89687500061451786, 32.45002607614398471 ) ) ;
#71682=CARTESIAN_POINT ( 'NONE',  ( 23.97187500061451360, 3.027376345333611329, 5.243569643749999010 ) ) ;
#71685=CARTESIAN_POINT ( 'NONE',  ( 4.104815315424666267, 2.854990486726923571, -4.236757528529293992 ) ) ;
#71686=CARTESIAN_POINT ( 'NONE',  ( 3.028125000614518392, 6.421520780324663323E-16, -5.243569643749999010 ) ) ;
#71688=CARTESIAN_POINT ( 'NONE',  ( 25.26562500061451289, 3.027376345333611329, 5.243569643749999010 ) ) ;
#71689=CARTESIAN_POINT ( 'NONE',  ( 18.17812500061451786, -4.541064518000419881, 2.621784821874995952 ) ) ;
#71691=CARTESIAN_POINT ( 'NONE',  ( 14.85937500061451644, 4.541064518000418104, -2.621784821874998173 ) ) ;
#71693=CARTESIAN_POINT ( 'NONE',  ( 28.31250000122903288, 0.000000000000000000, 4.999999999999998224 ) ) ;
#71694=CARTESIAN_POINT ( 'NONE',  ( 5.971875000614516260, 3.027376345333611329, 5.243569643749999010 ) ) ;
#71695=CARTESIAN_POINT ( 'NONE',  ( 16.95937500061451786, -4.541064518000417216, -2.621784821875001281 ) ) ;
#71696=CARTESIAN_POINT ( 'NONE',  ( 25.27499999999999858, 6.123233995736764310E-16, -4.999999999999998224 ) ) ;
#71697=CARTESIAN_POINT ( 'NONE',  ( 23.28750000000000142, -2.886751345948129988, 4.999999999999997335 ) ) ;
#71698=CARTESIAN_POINT ( 'NONE',  ( 2.850000001229036073, -2.886751345948125991, -5.000000000000000000 ) ) ;
#71699=CARTESIAN_POINT ( 'NONE',  ( 25.54687500061451644, -3.027376345333610441, -5.243569643749999898 ) ) ;
#71700=CARTESIAN_POINT ( 'NONE',  ( 15.72187500061451892, 3.027376345333613106, -5.243569643749998122 ) ) ;
#71702=CARTESIAN_POINT ( 'NONE',  ( 29.32499999999999929, 6.123233995736764310E-16, -4.999999999999998224 ) ) ;
#71703=CARTESIAN_POINT ( 'NONE',  ( 6.262500000000000178, -5.773502691896255534, -1.060575238724906372E-15 ) ) ;
#71705=CARTESIAN_POINT ( 'NONE',  ( 18.51562500061451289, 3.027376345333611329, 5.243569643749999010 ) ) ;
#71706=CARTESIAN_POINT ( 'NONE',  ( 9.975000000000001421, 6.123233995736764310E-16, -4.999999999999998224 ) ) ;
#71707=CARTESIAN_POINT ( 'NONE',  ( 3.365625000614516082, -6.054752690667223547, -1.112240025338166033E-15 ) ) ;
#71708=CARTESIAN_POINT ( 'NONE',  ( 20.13749999999999929, -2.886751345948129988, 4.999999999999997335 ) ) ;
#71710=CARTESIAN_POINT ( 'NONE',  ( 24.07500000122903216, 2.886751345948129099, -4.999999999999998224 ) ) ;
#71712=CARTESIAN_POINT ( 'NONE',  ( 28.50937500061451502, 0.000000000000000000, 5.243569643749999010 ) ) ;
#71714=CARTESIAN_POINT ( 'NONE',  ( 17.95312500061451644, 4.541064518000418104, -2.621784821874998173 ) ) ;
#71715=CARTESIAN_POINT ( 'NONE',  ( 23.91562500061451502, 3.027376345333611329, 5.243569643749999010 ) ) ;
#71716=CARTESIAN_POINT ( 'NONE',  ( 23.74687500061451573, -3.027376345333610441, -5.243569643749999898 ) ) ;
#71717=CARTESIAN_POINT ( 'NONE',  ( 9.787499999999999645, -2.886751345948129988, 4.999999999999997335 ) ) ;
#71718=CARTESIAN_POINT ( 'NONE',  ( 11.87812500061451537, -4.541064518000419881, 2.621784821874995952 ) ) ;
#71719=CARTESIAN_POINT ( 'NONE',  ( 27.25312500061451360, -4.541064518000417216, -2.621784821875001281 ) ) ;
#71720=CARTESIAN_POINT ( 'NONE',  ( 13.99687500061451928, 6.054752690667223547, 3.707466751127219781E-16 ) ) ;
#71721=CARTESIAN_POINT ( 'NONE',  ( 19.47187500061451360, 3.027376345333611329, 5.243569643749999010 ) ) ;
#71723=CARTESIAN_POINT ( 'NONE',  ( -2.121784821874999949, 19.27812500061451573, 26.32496088578401938 ) ) ;
#71724=EDGE_CURVE ( 'NONE', #10011, #42322, #38688, .T. ) ;
#71725=AXIS2_PLACEMENT_3D ( 'NONE', #27193, #67807, #17181 ) ;
#71726=CARTESIAN_POINT ( 'NONE',  ( 23.47500000122903430, -5.773502691896255534, -1.060575238724906372E-15 ) ) ;
#71728=CARTESIAN_POINT ( 'NONE',  ( 13.75312500061451715, -4.541064518000417216, -2.621784821875001281 ) ) ;
#71729=CARTESIAN_POINT ( 'NONE',  ( 7.546875000614517326, -3.027376345333610441, -5.243569643749999898 ) ) ;
#71730=CARTESIAN_POINT ( 'NONE',  ( 7.059375000614518392, -4.541064518000417216, -2.621784821875001281 ) ) ;
#71731=EDGE_LOOP ( 'NONE', ( #5947, #28661, #1761, #22211 ) ) ;
#71732=CARTESIAN_POINT ( 'NONE',  ( 27.42187500061451644, 3.027376345333613106, -5.243569643749998122 ) ) ;
#71733=CARTESIAN_POINT ( 'NONE',  ( 19.60312500061451502, -4.541064518000417216, -2.621784821875001281 ) ) ;
#71734=CARTESIAN_POINT ( 'NONE',  ( 29.27812500061451573, 4.541064518000418104, 2.621784821874999949 ) ) ;
#71735=CARTESIAN_POINT ( 'NONE',  ( 25.39687500061451431, -3.027376345333614438, 5.243569643749998122 ) ) ;
#71736=CARTESIAN_POINT ( 'NONE',  ( 20.61562500061451431, 3.027376345333613106, -5.243569643749998122 ) ) ;
#71737=CARTESIAN_POINT ( 'NONE',  ( -2.000000000000000000, 11.37500000000000178, 26.53589838486224650 ) ) ;
#71738=CARTESIAN_POINT ( 'NONE',  ( 25.49062500061451786, -3.027376345333610441, -5.243569643749999898 ) ) ;
#71739=CARTESIAN_POINT ( 'NONE',  ( 7.050000001229036251, 5.773502691896255534, 3.535250795749688894E-16 ) ) ;
#71740=ORIENTED_EDGE ( 'NONE', *, *, #15748, .T. ) ;
#71741=CARTESIAN_POINT ( 'NONE',  ( 2.812500001229033320, -4.330127018922190985, -2.500000000000001332 ) ) ;
#71742=CARTESIAN_POINT ( 'NONE',  ( 2.000000000000001332, 14.30000000000000071, -26.53589838486224650 ) ) ;
#71743=CARTESIAN_POINT ( 'NONE',  ( 21.78750000122903074, 6.123233995736764310E-16, -4.999999999999998224 ) ) ;
#71745=CARTESIAN_POINT ( 'NONE',  ( 4.996875000614516615, 6.054752690667223547, 3.707466751127219781E-16 ) ) ;
#71747=CARTESIAN_POINT ( 'NONE',  ( 13.56562500061451892, 3.027376345333611329, 5.243569643749999010 ) ) ;
#71748=CARTESIAN_POINT ( 'NONE',  ( 9.346875000614517148, -3.027376345333610441, -5.243569643749999898 ) ) ;
#71749=CARTESIAN_POINT ( 'NONE',  ( 23.88750000122903216, -4.330127018922194537, 2.499999999999995559 ) ) ;
#71750=( BOUNDED_CURVE ( )  B_SPLINE_CURVE ( 2, ( #23461, #51909, #12734, #18628, #24179, #51552, #40464, #30091, #1670 ),
 .UNSPECIFIED., .F., .F. ) 
 B_SPLINE_CURVE_WITH_KNOTS ( ( 3, 2, 2, 2, 3 ),
 ( 0.07608695652173913526, 0.07971014492753622505, 0.08695652173913043237, 0.09420289855072463969, 0.09782608695652174335 ),
 .UNSPECIFIED. ) 
 CURVE ( )  GEOMETRIC_REPRESENTATION_ITEM ( )  RATIONAL_B_SPLINE_CURVE ( ( 0.9330127018922192983, 0.9330127018922194093, 1.000000000000000000, 0.8660254037844387076, 1.000000000000000000, 0.8660254037844387076, 1.000000000000000000, 0.9330127018922194093, 0.9330127018922194093 ) ) 
 REPRESENTATION_ITEM ( '' )  );
#71751=CARTESIAN_POINT ( 'NONE',  ( 15.42187500061451821, 3.027376345333611329, 5.243569643749999010 ) ) ;
#71752=CARTESIAN_POINT ( 'NONE',  ( 29.57812500061451644, 6.421520780324663323E-16, -5.243569643749999010 ) ) ;
#71754=CARTESIAN_POINT ( 'NONE',  ( 4.265625000614517326, -6.054752690667223547, -1.112240025338166033E-15 ) ) ;
#71755=CARTESIAN_POINT ( 'NONE',  ( 14.16562500061451679, -6.054752690667223547, -1.112240025338166033E-15 ) ) ;
#71757=CARTESIAN_POINT ( 'NONE',  ( 12.25312500061451537, 0.000000000000000000, 5.243569643749999010 ) ) ;
#71758=CARTESIAN_POINT ( 'NONE',  ( 8.240625000614516082, -3.027376345333614438, 5.243569643749998122 ) ) ;
#71760=CARTESIAN_POINT ( 'NONE',  ( 7.912499999999999645, 2.886751345948126879, 4.999999999999999112 ) ) ;
#71761=CARTESIAN_POINT ( 'NONE',  ( 3.975000001229033852, 2.886751345948126879, 4.999999999999999112 ) ) ;
#71762=CARTESIAN_POINT ( 'NONE',  ( 17.77499999999999858, 4.330127018922191873, 2.499999999999999556 ) ) ;
#71763=CARTESIAN_POINT ( 'NONE',  ( 18.49687500061452283, 6.054752690667223547, 3.707466751127219781E-16 ) ) ;
#71764=CARTESIAN_POINT ( 'NONE',  ( 13.08750000122903323, -4.330127018922194537, 2.499999999999995559 ) ) ;
#71766=CARTESIAN_POINT ( 'NONE',  ( -3.000416591977282496E-16, 17.44062500061451360, -34.90005215228797653 ) ) ;
#71767=CARTESIAN_POINT ( 'NONE',  ( -1.999999999999997113, 16.92500000000000426, 33.46410161513775705 ) ) ;
#71769=CARTESIAN_POINT ( 'NONE',  ( 28.64062500061451289, -3.027376345333610441, -5.243569643749999898 ) ) ;
#71770=FACE_OUTER_BOUND ( 'NONE', #55346, .T. ) ;
#71771=CARTESIAN_POINT ( 'NONE',  ( 24.22500000000000142, -4.330127018922194537, 2.499999999999995559 ) ) ;
#71772=CARTESIAN_POINT ( 'NONE',  ( 14.07187500061451679, 3.027376345333611329, 5.243569643749999010 ) ) ;
#71773=EDGE_CURVE ( 'NONE', #35438, #26212, #47031, .T. ) ;
#71774=CARTESIAN_POINT ( 'NONE',  ( 27.63749999999999929, 5.773502691896255534, 3.535250795749688894E-16 ) ) ;
#71775=CARTESIAN_POINT ( 'NONE',  ( 12.55312500061451786, 4.541064518000418104, -2.621784821874998173 ) ) ;
#71777=( BOUNDED_SURFACE ( )  B_SPLINE_SURFACE ( 1, 2, ( 
 ( #50690, #92, #22598, #45149, #17053, #32236, #62486, #34408, #40324, #51773, #7068, #1904, #57662, #51049, #29596, #68768, #7425, #63209, #28871, #445, #18852, #52133, #34045, #22953, #62131, #62846, #12239, #35137, #29953, #12960, #45515, #56936, #5981, #68045, #813, #1536, #39972, #46229, #6707, #24044, #46593, #17415, #11883, #18125, #51410, #6341, #69135, #1173, #17764, #18494, #40691, #23320, #45870, #68403, #56584, #34770, #12604, #57303, #35497, #28511, #41059, #52493, #63572, #29240, #23681, #58017, #24408, #46958, #69494, #11523, #36956, #59477, #64666, #8155, #26247, #8889, #70947, #59850, #58745, #63930, #3720, #31047, #25133, #14050, #14422, #35854, #7788, #53585, #19584, #36591, #42140, #42872, #69847, #13315, #2980, #19213, #70579, #41414, #59112, #25881, #30326, #47313, #31422, #53962, #25509, #8518, #9255, #58377, #48420, #48054, #70209, #3359, #19954, #2255, #24770, #52856, #41768, #47674, #42507, #65030, #65394, #64297, #20318, #31790, #14785, #13685, #36229, #30684, #53215, #2611, #37327, #54328, #48784, #71309, #43974, #60573, #5536, #38797, #50247, #39154, #38048, #43244, #56142, #10348, #4455, #66493, #66873, #15147, #60207, #32878, #72040, #15876, #21417, #22154, #49153, #65765, #55417, #71682, #49875, #20686, #38422, #5171, #9619, #26616, #61313, #33242, #4812, #60944, #61671, #37684, #44707, #32151, #27344, #72400, #16242, #21781, #44346, #9980, #10709, #72769, #54684, #67242, #4086, #21056, #55779, #28073, #27706, #16600, #26984, #43607, #66128, #11070, #15507, #32517, #33597, #55054, #49513, #50601, #34316, #23235, #6626, #6981, #57212, #39517, #29155, #17681, #35050, #12155, #45421, #62044, #23956, #51687, #22513, #11439, #6, #6255, #28783, #1091, #29512, #57578, #33958, #67957, #56497, #5892, #62401, #23599, #50960, #62763, #45786, #46144, #68683, #28423, #358, #40240, #39888, #22865, #45060, #52047, #51323, #63123, #1451, #11799, #17329, #56849, #34682, #67597, #727, #68321, #18044, #40601, #12519, #16963, #32555, #60987, #60610, #66533, #4848, #33280, #28112, #10747, #4126, #55819, #21822, #33638, #16280, #55092, #26655, #45098, #5206, #60242, #49191, #15183, #15913, #38461, #61351, #56182, #39195, #71721, #10019, #32190, #21093, #27021, #27747, #66168, #72438, #32918, #50286, #72810, #43644, #15544, #44387, #4492, #38088, #22193, #27382, #44011, #44747, #66912, #49553, #72075, #21456, #9656, #10386, #38836, #55455, #61710, #54723, #67281, #5575, #16640, #49914, #11109, #50641, #45, #22550, #37722, #41010, #63159, #12554, #17717, #34354, #52447, #35088, #23995, #12912, #11836, #17000, #29907, #57248, #51359, #40277, #40640, #62082, #33998, #6661, #45820, #62798, #68356, #69084, #22902, #39557, #29190, #45461, #23634, #67633, #12191, #52084, #56535, #395, #57614, #7017, #51724, #34718, #35445, #11475, #18445, #5928, #1125, #46180, #29548, #68719, #18079, #56887, #1489, #46543, #63525, #762, #28462, #67993, #39924, #7376, #24360, #62438, #17367, #57969, #6292, #1853, #50997, #28821, #23270, #10215, #42373, #43101, #43472, #65627, #20543, #4680, #32748, #14645, #36822, #32376, #54916, #60807, #37919, #15377, #32015, #15014, #71547, #37552, #60074, #9486, #55286, #66365, #3216, #65996, #31281, #60437, #31655, #48646, #20920, #53823, #9117, #37186, #25745, #14285, #54188, #54550, #47916, #70445, #20181, #3585, #3952, #26107, #26475, #49015, #19821, #9847, #59337, #49381, #71171, #64895, #4323, #26848, #8748, #42736, #48282, #71911, #70806, #21285, #43838, #59710, #15740, #38279, #65255, #33463, #33106, #22021, #67470, #5403, #22739, #5040, #33831, #50472, #67824, #57077, #12024, #44207, #16833, #27939, #72999, #40114, #22383, #38661, #55645, #27576, #51191, #61905, #5766, #34548, #6122, #50108, #66739, #72637, #27210, #11310, #16466, #45290, #39757, #44577, #44932, #10940, #49745, #17553, #39386, #56720, #595, #39025, #16110, #61539, #56374, #68189, #67110, #28297, #50832, #28652, #56009, #72273, #232, #17197, #62275, #21650, #11669, #34185, #61184, #23099, #45657, #62629, #10579, #29734, #24908, #51555, #7927, #17907, #52272, #13097, #2038, #41197, #24183, #23821, #24549, #58517, #957, #52994, #40469, #6485, #1674, #41911, #13449, #58157, #63354, #46011, #62984, #63705, #68548, #51914, #35635, #46372, #46736, #1312, #57796, #69270, #47094, #19354, #69627, #12379, #18989, #7561, #47452, #30096, #68906, #34916, #36368, #41551, #23465, #57443, #29020, #7205, #18632, #52632, #69984, #30464, #6846, #18263, #29381, #40837, #12738, #64068, #35275, #35998, #2390, #64436, #13828, #19727, #70351, #43009, #48188, #42278, #43383, #71082, #14558, #20830, #65538, #64801, #14192, #47820, #30824, #65167, #59985, #31561, #9755, #2754, #48924, #49290, #37466, #53356, #31187, #53729, #36727, #59249, #37092, #32289, #54462, #3860, #9031, #25651, #43746, #26383, #15287, #4231, #3122, #8293, #21195, #48555, #42643, #54100, #31926, #25273, #8657, #20456, #59616, #15649, #14925, #70712, #60346, #3498, #58883, #26016, #9396, #20086, #71455, #65907, #37827, #54823, #26758, #71823, #66271, #5678, #10848, #4953, #44488, #44116, #33018, #5313, #16381, #33743, #16020, #44846, #61454, #28214, #68100, #23010, #55198, #27855, #38936, #33382, #51104, #55918, #49655, #66643, #38568, #62185, #72912, #16744, #45569, #17106, #61092, #4592, #10491, #38189, #22294, #27486, #56288, #50743, #55557, #50387, #21932, #60714, #28568, #67382, #67733, #11582, #50020, #27121, #72544, #39299, #6034, #67020, #61814, #11217, #146, #72183, #22652, #45201, #500, #10126, #39666, #34098, #56638, #32658, #21562, #69185, #41463, #29647, #52907, #11936, #12653, #13010, #35188, #63261, #47367, #2305, #57353, #6396, #1953, #24460, #30378, #7477, #58067, #1587, #57713, #41110 ),
 ( #62539, #23731, #18545, #7118, #63982, #34461, #35548, #52185, #24097, #34825, #30004, #69543, #56989, #13364, #28927, #17466, #46644, #24820, #47008, #63620, #1225, #51464, #867, #52546, #23374, #62896, #18902, #6758, #35906, #12291, #68820, #58430, #7841, #40025, #45922, #68454, #17816, #40377, #29292, #51822, #46280, #18177, #40745, #37377, #41818, #30735, #69898, #48102, #70625, #42921, #15199, #20738, #8206, #64716, #13740, #58796, #8570, #65445, #47725, #54014, #14471, #59901, #31840, #53267, #2665, #3410, #59162, #25182, #54376, #8940, #25561, #3771, #25930, #70264, #19635, #42192, #64349, #3030, #70994, #42553, #43296, #36282, #9306, #60257, #48470, #14100, #36640, #31098, #53638, #20000, #65080, #65817, #14836, #26296, #37005, #59528, #54738, #48833, #71364, #37737, #31471, #19264, #32204, #20370, #9671, #4140, #26671, #43661, #15561, #38852, #27400, #44403, #49930, #50657, #4509, #71738, #61367, #27038, #5222, #49204, #21840, #33654, #38104, #55109, #67298, #61726, #10764, #72455, #67650, #21108, #61, #60626, #66929, #55835, #49569, #16656, #11127, #33297, #16298, #17016, #66183, #22567, #10037, #27764, #50304, #44763, #72826, #22209, #66550, #39214, #28129, #32571, #45115, #72091, #21475, #56199, #11492, #5592, #39575, #32934, #44028, #15930, #62098, #38479, #61003, #34014, #10402, #56551, #55472, #5945, #4864, #46557, #41381, #24009, #17382, #69099, #35103, #46922, #29562, #68372, #39940, #58343, #18461, #411, #62453, #28478, #6676, #29204, #1504, #69460, #52461, #11851, #23287, #45478, #34370, #40292, #41024, #6308, #12569, #46194, #63540, #12926, #56903, #28837, #57628, #17733, #51376, #35461, #40654, #57264, #57983, #7033, #778, #45835, #62814, #22920, #34734, #52099, #1139, #1868, #68010, #7393, #18818, #29921, #12206, #51740, #23650, #68735, #18093, #63175, #24374, #63893, #13283, #35821, #51015, #65729, #25847, #37291, #26210, #25098, #30290, #43209, #70545, #64632, #53548, #53926, #2224, #47281, #19920, #59077, #2945, #8481, #9219, #36193, #52822, #42474, #58711, #36922, #7754, #25473, #65359, #69815, #70175, #48384, #20283, #8123, #31015, #14018, #37651, #71273, #48019, #59814, #31756, #19552, #19181, #42109, #64997, #48749, #30650, #14387, #8850, #36557, #41734, #53182, #2579, #20651, #24737, #47642, #59443, #31387, #3321, #54293, #70912, #3686, #42837, #15114, #64262, #14749, #13650, #55383, #32846, #16930, #22480, #26951, #49119, #44677, #67208, #73098, #50211, #27673, #44310, #4777, #10675, #27311, #49844, #72369, #67565, #5504, #15473, #5138, #43573, #72736, #43940, #60911, #33205, #66094, #21384, #49477, #38017, #26579, #66464, #21749, #60174, #9583, #32484, #15841, #66840, #38387, #16210, #38763, #32115, #61282, #71647, #61636, #10314, #54649, #55744, #22122, #21020, #55018, #60540, #16569, #9946, #39121, #11038, #72009, #33563, #56112, #28042, #50571, #4422, #45030, #4053, #17650, #35020, #17297, #46113, #62732, #6950, #69381, #24293, #56469, #6593, #40210, #12124, #52376, #34651, #50930, #45388, #39858, #63459, #1058, #18014, #46841, #18377, #62370, #5860, #11768, #39484, #23568, #68650, #62007, #11409, #34284, #692, #57179, #23201, #40571, #29123, #33927, #63091, #28392, #40945, #45754, #327, #51656, #12492, #22836, #56816, #67924, #57548, #6223, #68290, #52019, #28751, #29482, #1420, #51291, #23926, #46476, #69014, #12846, #35379, #57902, #7311, #29841, #1782, #59353, #48661, #3600, #35742, #58992, #19465, #70088, #31670, #13937, #30206, #24653, #69730, #42751, #53468, #70462, #26122, #70823, #19099, #58261, #64175, #18736, #2859, #8036, #36839, #31298, #41654, #42023, #2493, #41300, #9133, #64544, #48297, #65272, #30571, #7667, #53097, #8398, #59725, #13563, #36474, #19837, #25017, #52737, #36108, #58629, #54203, #63810, #47559, #30927, #47933, #47199, #14659, #42389, #37202, #25389, #13202, #2142, #64911, #14301, #8764, #53839, #3234, #25761, #20197, #60091, #55659, #5055, #11952, #61199, #38678, #55300, #66379, #21665, #15755, #60823, #38294, #6412, #17482, #26490, #16125, #54565, #10594, #54931, #71925, #44222, #3968, #32391, #37933, #49032, #37567, #4338, #21300, #60453, #57006, #33122, #27592, #40042, #15391, #20559, #34477, #10229, #26863, #43854, #66755, #65642, #9500, #32763, #49394, #4694, #27224, #72655, #71561, #43117, #49761, #20936, #72287, #71186, #50124, #22036, #32029, #43487, #44595, #67126, #62556, #28944, #15030, #66011, #9861, #62912, #1601, #58083, #47023, #13025, #69200, #68835, #69558, #30393, #45939, #24835, #12306, #51482, #46661, #13755, #58446, #30018, #35206, #17832, #34841, #35564, #40393, #23747, #7491, #18192, #24112, #46295, #29663, #41125, #18919, #64365, #41479, #57368, #63999, #52562, #69913, #1968, #40762, #6776, #8222, #13379, #23390, #29308, #883, #52200, #18560, #24476, #19282, #2320, #51839, #63277, #68470, #1242, #12669, #35922, #57728, #7857, #63636, #52922, #47383, #7134, #41834, #36298, #58811, #14117, #15214, #42936, #59544, #65832, #14853, #64731, #36656, #19651, #2681, #37020, #31855, #3425, #54753, #47743, #20754, #21123, #9322, #25197, #3047, #25577, #59176, #8585, #8955, #4155, #26311, #48849, #60640, #66199, #70640, #42207, #37754, #60272, #43676, #43312, #71379, #37392, #25945, #54390, #48485, #20385, #71009, #38119, #49220, #31115, #9686, #53653, #32219, #14486, #31489, #3787, #48117, #65096, #20015, #42568, #70280, #54030, #65461, #30750, #53282, #59916, #26687, #71754, #15577, #67312, #27779, #39953, #44778, #72106, #11504, #66944, #10053, #10778, #16670, #21490, #4878, #44043, #39228, #66566, #44417, #22580, #49945, #50671, #55849, #72469, #16312, #15946, #27414, #50318, #61382, #5607, #61019, #61740, #33311, #75, #32586, #68024, #27052, #72841, #5238, #22223, #22933 ) ),
 .UNSPECIFIED., .F., .F., .F. ) 
 B_SPLINE_SURFACE_WITH_KNOTS ( ( 2, 2 ),
 ( 3, 2, 2, 2, 2, 2, 2, 2, 2, 2, 2, 2, 2, 2, 2, 2, 2, 2, 2, 2, 2, 2, 2, 2, 2, 2, 2, 2, 2, 2, 2, 2, 2, 2, 2, 2, 2, 2, 2, 2, 2, 2, 2, 2, 2, 2, 2, 2, 2, 2, 2, 2, 2, 2, 2, 2, 2, 2, 2, 2, 2, 2, 2, 2, 2, 2, 2, 2, 2, 2, 2, 2, 2, 2, 2, 2, 2, 2, 2, 2, 2, 2, 2, 2, 2, 2, 2, 2, 2, 2, 2, 2, 2, 2, 2, 2, 2, 2, 2, 2, 2, 2, 2, 2, 2, 2, 2, 2, 2, 2, 2, 2, 2, 2, 2, 2, 2, 2, 2, 2, 2, 2, 2, 2, 2, 2, 2, 2, 2, 2, 2, 2, 2, 2, 2, 2, 2, 2, 2, 2, 2, 2, 2, 2, 2, 2, 2, 2, 2, 2, 2, 2, 2, 2, 2, 2, 2, 2, 2, 2, 2, 2, 2, 2, 2, 2, 2, 2, 2, 2, 2, 2, 2, 2, 2, 2, 2, 2, 2, 2, 2, 2, 2, 2, 2, 2, 2, 2, 2, 2, 2, 2, 2, 2, 2, 2, 2, 2, 2, 2, 2, 2, 2, 2, 2, 2, 2, 2, 2, 2, 2, 2, 2, 2, 2, 2, 2, 2, 2, 2, 2, 2, 2, 2, 2, 2, 2, 2, 2, 2, 2, 2, 2, 2, 2, 2, 2, 2, 2, 2, 2, 2, 2, 2, 2, 2, 2, 2, 2, 2, 2, 2, 2, 2, 2, 2, 2, 2, 2, 2, 2, 2, 2, 2, 2, 2, 2, 2, 2, 2, 2, 2, 2, 2, 2, 2, 2, 2, 2, 2, 2, 2, 2, 2, 2, 2, 2, 2, 2, 2, 2, 2, 2, 2, 2, 2, 2, 2, 2, 2, 2, 2, 2, 2, 2, 2, 2, 2, 2, 2, 2, 2, 2, 2, 2, 2, 2, 2, 2, 2, 2, 2, 2, 2, 2, 2, 2, 2, 2, 2, 2, 2, 2, 2, 2, 2, 2, 2, 2, 2, 2, 2, 2, 2, 2, 2, 2, 2, 2, 2, 2, 2, 2, 2, 2, 2, 2, 2, 2, 2, 3 ),
 ( 0.000000000000000000, 1.000000000000000000 ),
 ( 0.000000000000000000, 0.002777777777777777884, 0.005555555555555555768, 0.008333333333333333218, 0.01111111111111111154, 0.01388888888888888812, 0.01666666666666666644, 0.01944444444444444475, 0.02222222222222222307, 0.02500000000000000139, 0.02777777777777777624, 0.03055555555555555455, 0.03333333333333333287, 0.03611111111111110772, 0.03888888888888888951, 0.04166666666666666435, 0.04444444444444444614, 0.04722222222222222099, 0.05000000000000000278, 0.05277777777777777762, 0.05555555555555555247, 0.05833333333333333426, 0.06111111111111110911, 0.06388888888888888395, 0.06666666666666666574, 0.06944444444444444753, 0.07222222222222221544, 0.07499999999999999722, 0.07777777777777777901, 0.08055555555555556080, 0.08333333333333332871, 0.08611111111111111049, 0.08888888888888889228, 0.09166666666666666019, 0.09444444444444444198, 0.09722222222222222376, 0.1000000000000000056, 0.1027777777777777735, 0.1055555555555555552, 0.1083333333333333370, 0.1111111111111111049, 0.1138888888888888867, 0.1166666666666666685, 0.1194444444444444503, 0.1222222222222222182, 0.1250000000000000000, 0.1277777777777777679, 0.1305555555555555636, 0.1333333333333333315, 0.1361111111111110994, 0.1388888888888888951, 0.1416666666666666630, 0.1444444444444444309, 0.1472222222222222265, 0.1499999999999999944, 0.1527777777777777901, 0.1555555555555555580, 0.1583333333333333259, 0.1611111111111111216, 0.1638888888888888895, 0.1666666666666666574, 0.1694444444444444531, 0.1722222222222222210, 0.1749999999999999889, 0.1777777777777777846, 0.1805555555555555525, 0.1833333333333333204, 0.1861111111111111160, 0.1888888888888888840, 0.1916666666666666796, 0.1944444444444444475, 0.1972222222222222154, 0.2000000000000000111, 0.2027777777777777790, 0.2055555555555555469, 0.2083333333333333426, 0.2111111111111111105, 0.2138888888888888784, 0.2166666666666666741, 0.2194444444444444420, 0.2222222222222222099, 0.2250000000000000056, 0.2277777777777777735, 0.2305555555555555691, 0.2333333333333333370, 0.2361111111111111049, 0.2388888888888889006, 0.2416666666666666685, 0.2444444444444444364, 0.2472222222222222321, 0.2500000000000000000, 0.2527777777777777679, 0.2555555555555555358, 0.2583333333333333592, 0.2611111111111111271, 0.2638888888888888951, 0.2666666666666666630, 0.2694444444444444309, 0.2722222222222221988, 0.2750000000000000222, 0.2777777777777777901, 0.2805555555555555580, 0.2833333333333333259, 0.2861111111111110938, 0.2888888888888888618, 0.2916666666666666852, 0.2944444444444444531, 0.2972222222222222210, 0.2999999999999999889, 0.3027777777777777568, 0.3055555555555555802, 0.3083333333333333481, 0.3111111111111111160, 0.3138888888888888840, 0.3166666666666666519, 0.3194444444444444198, 0.3222222222222222432, 0.3250000000000000111, 0.3277777777777777790, 0.3305555555555555469, 0.3333333333333333148, 0.3361111111111111382, 0.3388888888888889062, 0.3416666666666666741, 0.3444444444444444420, 0.3472222222222222099, 0.3499999999999999778, 0.3527777777777778012, 0.3555555555555555691, 0.3583333333333333370, 0.3611111111111111049, 0.3638888888888888729, 0.3666666666666666408, 0.3694444444444444642, 0.3722222222222222321, 0.3750000000000000000, 0.3777777777777777679, 0.3805555555555555358, 0.3833333333333333592, 0.3861111111111111271, 0.3888888888888888951, 0.3916666666666666630, 0.3944444444444444309, 0.3972222222222221988, 0.4000000000000000222, 0.4027777777777777901, 0.4055555555555555580, 0.4083333333333333259, 0.4111111111111110938, 0.4138888888888888618, 0.4166666666666666852, 0.4194444444444444531, 0.4222222222222222210, 0.4249999999999999889, 0.4277777777777777568, 0.4305555555555555802, 0.4333333333333333481, 0.4361111111111111160, 0.4388888888888888840, 0.4416666666666666519, 0.4444444444444444198, 0.4472222222222222432, 0.4500000000000000111, 0.4527777777777777790, 0.4555555555555555469, 0.4583333333333333148, 0.4611111111111111382, 0.4638888888888889062, 0.4666666666666666741, 0.4694444444444444420, 0.4722222222222222099, 0.4749999999999999778, 0.4777777777777778012, 0.4805555555555555691, 0.4833333333333333370, 0.4861111111111111049, 0.4888888888888888729, 0.4916666666666666408, 0.4944444444444444642, 0.4972222222222222321, 0.5000000000000000000, 0.5027777777777777679, 0.5055555555555555358, 0.5083333333333333037, 0.5111111111111110716, 0.5138888888888888395, 0.5166666666666667185, 0.5194444444444444864, 0.5222222222222222543, 0.5250000000000000222, 0.5277777777777777901, 0.5305555555555555580, 0.5333333333333333259, 0.5361111111111110938, 0.5388888888888888618, 0.5416666666666666297, 0.5444444444444443976, 0.5472222222222222765, 0.5500000000000000444, 0.5527777777777778123, 0.5555555555555555802, 0.5583333333333333481, 0.5611111111111111160, 0.5638888888888888840, 0.5666666666666666519, 0.5694444444444444198, 0.5722222222222221877, 0.5749999999999999556, 0.5777777777777777235, 0.5805555555555556024, 0.5833333333333333703, 0.5861111111111111382, 0.5888888888888889062, 0.5916666666666666741, 0.5944444444444444420, 0.5972222222222222099, 0.5999999999999999778, 0.6027777777777777457, 0.6055555555555555136, 0.6083333333333332815, 0.6111111111111111605, 0.6138888888888889284, 0.6166666666666666963, 0.6194444444444444642, 0.6222222222222222321, 0.6250000000000000000, 0.6277777777777777679, 0.6305555555555555358, 0.6333333333333333037, 0.6361111111111110716, 0.6388888888888888395, 0.6416666666666667185, 0.6444444444444444864, 0.6472222222222222543, 0.6500000000000000222, 0.6527777777777777901, 0.6555555555555555580, 0.6583333333333333259, 0.6611111111111110938, 0.6638888888888888618, 0.6666666666666666297, 0.6694444444444443976, 0.6722222222222222765, 0.6750000000000000444, 0.6777777777777778123, 0.6805555555555555802, 0.6833333333333333481, 0.6861111111111111160, 0.6888888888888888840, 0.6916666666666666519, 0.6944444444444444198, 0.6972222222222221877, 0.6999999999999999556, 0.7027777777777777235, 0.7055555555555556024, 0.7083333333333333703, 0.7111111111111111382, 0.7138888888888889062, 0.7166666666666666741, 0.7194444444444444420, 0.7222222222222222099, 0.7249999999999999778, 0.7277777777777777457, 0.7305555555555555136, 0.7333333333333332815, 0.7361111111111111605, 0.7388888888888889284, 0.7416666666666666963, 0.7444444444444444642, 0.7472222222222222321, 0.7500000000000000000, 0.7527777777777777679, 0.7555555555555555358, 0.7583333333333333037, 0.7611111111111110716, 0.7638888888888888395, 0.7666666666666667185, 0.7694444444444444864, 0.7722222222222222543, 0.7750000000000000222, 0.7777777777777777901, 0.7805555555555555580, 0.7833333333333333259, 0.7861111111111110938, 0.7888888888888888618, 0.7916666666666666297, 0.7944444444444443976, 0.7972222222222222765, 0.8000000000000000444, 0.8027777777777778123, 0.8055555555555555802, 0.8083333333333333481, 0.8111111111111111160, 0.8138888888888888840, 0.8166666666666666519, 0.8194444444444444198, 0.8222222222222221877, 0.8249999999999999556, 0.8277777777777777235, 0.8305555555555556024, 0.8333333333333333703, 0.8361111111111111382, 0.8388888888888889062, 0.8416666666666666741, 0.8444444444444444420, 0.8472222222222222099, 0.8499999999999999778, 0.8527777777777777457, 0.8555555555555555136, 0.8583333333333332815, 0.8611111111111111605, 0.8638888888888889284, 0.8666666666666666963, 0.8694444444444444642, 0.8722222222222222321, 0.8750000000000000000, 0.8777777777777777679, 0.8805555555555555358, 0.8833333333333333037, 0.8861111111111110716, 0.8888888888888888395, 0.8916666666666667185, 0.8944444444444444864, 0.8972222222222222543, 0.9000000000000000222, 0.9027777777777777901, 0.9055555555555555580, 0.9083333333333333259, 0.9111111111111110938, 0.9138888888888888618, 0.9166666666666666297, 0.9194444444444443976, 0.9222222222222222765, 0.9250000000000000444, 0.9277777777777778123, 0.9305555555555555802, 0.9333333333333333481, 0.9361111111111111160, 0.9388888888888888840, 0.9416666666666666519, 0.9444444444444444198, 0.9472222222222221877, 0.9499999999999999556, 0.9527777777777777235, 0.9555555555555556024, 0.9583333333333333703, 0.9611111111111111382, 0.9638888888888889062, 0.9666666666666666741, 0.9694444444444444420, 0.9722222222222222099, 0.9749999999999999778, 0.9777777777777777457, 0.9805555555555555136, 0.9833333333333332815, 0.9861111111111111605, 0.9888888888888889284, 0.9916666666666666963, 0.9944444444444444642, 0.9972222222222222321, 1.000000000000000000 ),
 .UNSPECIFIED. ) 
 GEOMETRIC_REPRESENTATION_ITEM ( )  RATIONAL_B_SPLINE_SURFACE ( (
 ( 1.000000000000000000, 0.8660254037844387076, 1.000000000000000000, 0.8660254037844387076, 1.000000000000000000, 0.8660254037844387076, 1.000000000000000000, 0.8660254037844387076, 1.000000000000000000, 0.8660254037844387076, 1.000000000000000000, 0.8660254037844387076, 1.000000000000000000, 0.8660254037844387076, 1.000000000000000000, 0.8660254037844387076, 1.000000000000000000, 0.8660254037844387076, 1.000000000000000000, 0.8660254037844387076, 1.000000000000000000, 0.8660254037844387076, 1.000000000000000000, 0.8660254037844387076, 1.000000000000000000, 0.8660254037844387076, 1.000000000000000000, 0.8660254037844387076, 1.000000000000000000, 0.8660254037844387076, 1.000000000000000000, 0.8660254037844387076, 1.000000000000000000, 0.8660254037844387076, 1.000000000000000000, 0.8660254037844387076, 1.000000000000000000, 0.8660254037844387076, 1.000000000000000000, 0.8660254037844387076, 1.000000000000000000, 0.8660254037844387076, 1.000000000000000000, 0.8660254037844387076, 1.000000000000000000, 0.8660254037844387076, 1.000000000000000000, 0.8660254037844387076, 1.000000000000000000, 0.8660254037844387076, 1.000000000000000000, 0.8660254037844387076, 1.000000000000000000, 0.8660254037844387076, 1.000000000000000000, 0.8660254037844387076, 1.000000000000000000, 0.8660254037844387076, 1.000000000000000000, 0.8660254037844387076, 1.000000000000000000, 0.8660254037844387076, 1.000000000000000000, 0.8660254037844387076, 1.000000000000000000, 0.8660254037844387076, 1.000000000000000000, 0.8660254037844387076, 1.000000000000000000, 0.8660254037844387076, 1.000000000000000000, 0.8660254037844387076, 1.000000000000000000, 0.8660254037844387076, 1.000000000000000000, 0.8660254037844387076, 1.000000000000000000, 0.8660254037844387076, 1.000000000000000000, 0.8660254037844387076, 1.000000000000000000, 0.8660254037844387076, 1.000000000000000000, 0.8660254037844387076, 1.000000000000000000, 0.8660254037844387076, 1.000000000000000000, 0.8660254037844387076, 1.000000000000000000, 0.8660254037844387076, 1.000000000000000000, 0.8660254037844387076, 1.000000000000000000, 0.8660254037844387076, 1.000000000000000000, 0.8660254037844387076, 1.000000000000000000, 0.8660254037844387076, 1.000000000000000000, 0.8660254037844387076, 1.000000000000000000, 0.8660254037844387076, 1.000000000000000000, 0.8660254037844387076, 1.000000000000000000, 0.8660254037844387076, 1.000000000000000000, 0.8660254037844387076, 1.000000000000000000, 0.8660254037844387076, 1.000000000000000000, 0.8660254037844387076, 1.000000000000000000, 0.8660254037844387076, 1.000000000000000000, 0.8660254037844387076, 1.000000000000000000, 0.8660254037844387076, 1.000000000000000000, 0.8660254037844387076, 1.000000000000000000, 0.8660254037844387076, 1.000000000000000000, 0.8660254037844387076, 1.000000000000000000, 0.8660254037844387076, 1.000000000000000000, 0.8660254037844387076, 1.000000000000000000, 0.8660254037844387076, 1.000000000000000000, 0.8660254037844387076, 1.000000000000000000, 0.8660254037844387076, 1.000000000000000000, 0.8660254037844387076, 1.000000000000000000, 0.8660254037844387076, 1.000000000000000000, 0.8660254037844387076, 1.000000000000000000, 0.8660254037844387076, 1.000000000000000000, 0.8660254037844387076, 1.000000000000000000, 0.8660254037844387076, 1.000000000000000000, 0.8660254037844387076, 1.000000000000000000, 0.8660254037844387076, 1.000000000000000000, 0.8660254037844387076, 1.000000000000000000, 0.8660254037844387076, 1.000000000000000000, 0.8660254037844387076, 1.000000000000000000, 0.8660254037844387076, 1.000000000000000000, 0.8660254037844387076, 1.000000000000000000, 0.8660254037844387076, 1.000000000000000000, 0.8660254037844387076, 1.000000000000000000, 0.8660254037844387076, 1.000000000000000000, 0.8660254037844387076, 1.000000000000000000, 0.8660254037844387076, 1.000000000000000000, 0.8660254037844387076, 1.000000000000000000, 0.8660254037844387076, 1.000000000000000000, 0.8660254037844387076, 1.000000000000000000, 0.8660254037844387076, 1.000000000000000000, 0.8660254037844387076, 1.000000000000000000, 0.8660254037844387076, 1.000000000000000000, 0.8660254037844387076, 1.000000000000000000, 0.8660254037844387076, 1.000000000000000000, 0.8660254037844387076, 1.000000000000000000, 0.8660254037844387076, 1.000000000000000000, 0.8660254037844387076, 1.000000000000000000, 0.8660254037844387076, 1.000000000000000000, 0.8660254037844387076, 1.000000000000000000, 0.8660254037844387076, 1.000000000000000000, 0.8660254037844387076, 1.000000000000000000, 0.8660254037844387076, 1.000000000000000000, 0.8660254037844387076, 1.000000000000000000, 0.8660254037844387076, 1.000000000000000000, 0.8660254037844387076, 1.000000000000000000, 0.8660254037844387076, 1.000000000000000000, 0.8660254037844387076, 1.000000000000000000, 0.8660254037844387076, 1.000000000000000000, 0.8660254037844387076, 1.000000000000000000, 0.8660254037844387076, 1.000000000000000000, 0.8660254037844387076, 1.000000000000000000, 0.8660254037844387076, 1.000000000000000000, 0.8660254037844387076, 1.000000000000000000, 0.8660254037844387076, 1.000000000000000000, 0.8660254037844387076, 1.000000000000000000, 0.8660254037844387076, 1.000000000000000000, 0.8660254037844387076, 1.000000000000000000, 0.8660254037844387076, 1.000000000000000000, 0.8660254037844387076, 1.000000000000000000, 0.8660254037844387076, 1.000000000000000000, 0.8660254037844387076, 1.000000000000000000, 0.8660254037844387076, 1.000000000000000000, 0.8660254037844387076, 1.000000000000000000, 0.8660254037844387076, 1.000000000000000000, 0.8660254037844387076, 1.000000000000000000, 0.8660254037844387076, 1.000000000000000000, 0.8660254037844387076, 1.000000000000000000, 0.8660254037844387076, 1.000000000000000000, 0.8660254037844387076, 1.000000000000000000, 0.8660254037844387076, 1.000000000000000000, 0.8660254037844387076, 1.000000000000000000, 0.8660254037844387076, 1.000000000000000000, 0.8660254037844387076, 1.000000000000000000, 0.8660254037844387076, 1.000000000000000000, 0.8660254037844387076, 1.000000000000000000, 0.8660254037844387076, 1.000000000000000000, 0.8660254037844387076, 1.000000000000000000, 0.8660254037844387076, 1.000000000000000000, 0.8660254037844387076, 1.000000000000000000, 0.8660254037844387076, 1.000000000000000000, 0.8660254037844387076, 1.000000000000000000, 0.8660254037844387076, 1.000000000000000000, 0.8660254037844387076, 1.000000000000000000, 0.8660254037844387076, 1.000000000000000000, 0.8660254037844387076, 1.000000000000000000, 0.8660254037844387076, 1.000000000000000000, 0.8660254037844387076, 1.000000000000000000, 0.8660254037844387076, 1.000000000000000000, 0.8660254037844387076, 1.000000000000000000, 0.8660254037844387076, 1.000000000000000000, 0.8660254037844387076, 1.000000000000000000, 0.8660254037844387076, 1.000000000000000000, 0.8660254037844387076, 1.000000000000000000, 0.8660254037844387076, 1.000000000000000000, 0.8660254037844387076, 1.000000000000000000, 0.8660254037844387076, 1.000000000000000000, 0.8660254037844387076, 1.000000000000000000, 0.8660254037844387076, 1.000000000000000000, 0.8660254037844387076, 1.000000000000000000, 0.8660254037844387076, 1.000000000000000000, 0.8660254037844387076, 1.000000000000000000, 0.8660254037844387076, 1.000000000000000000, 0.8660254037844387076, 1.000000000000000000, 0.8660254037844387076, 1.000000000000000000, 0.8660254037844387076, 1.000000000000000000, 0.8660254037844387076, 1.000000000000000000, 0.8660254037844387076, 1.000000000000000000, 0.8660254037844387076, 1.000000000000000000, 0.8660254037844387076, 1.000000000000000000, 0.8660254037844387076, 1.000000000000000000, 0.8660254037844387076, 1.000000000000000000, 0.8660254037844387076, 1.000000000000000000, 0.8660254037844387076, 1.000000000000000000, 0.8660254037844387076, 1.000000000000000000, 0.8660254037844387076, 1.000000000000000000, 0.8660254037844387076, 1.000000000000000000, 0.8660254037844387076, 1.000000000000000000, 0.8660254037844387076, 1.000000000000000000, 0.8660254037844387076, 1.000000000000000000, 0.8660254037844387076, 1.000000000000000000, 0.8660254037844387076, 1.000000000000000000, 0.8660254037844387076, 1.000000000000000000, 0.8660254037844387076, 1.000000000000000000, 0.8660254037844387076, 1.000000000000000000, 0.8660254037844387076, 1.000000000000000000, 0.8660254037844387076, 1.000000000000000000, 0.8660254037844387076, 1.000000000000000000, 0.8660254037844387076, 1.000000000000000000, 0.8660254037844387076, 1.000000000000000000, 0.8660254037844387076, 1.000000000000000000, 0.8660254037844387076, 1.000000000000000000, 0.8660254037844387076, 1.000000000000000000, 0.8660254037844387076, 1.000000000000000000, 0.8660254037844387076, 1.000000000000000000, 0.8660254037844387076, 1.000000000000000000, 0.8660254037844387076, 1.000000000000000000, 0.8660254037844387076, 1.000000000000000000, 0.8660254037844387076, 1.000000000000000000, 0.8660254037844387076, 1.000000000000000000, 0.8660254037844387076, 1.000000000000000000, 0.8660254037844387076, 1.000000000000000000, 0.8660254037844387076, 1.000000000000000000, 0.8660254037844387076, 1.000000000000000000, 0.8660254037844387076, 1.000000000000000000, 0.8660254037844387076, 1.000000000000000000, 0.8660254037844387076, 1.000000000000000000, 0.8660254037844387076, 1.000000000000000000, 0.8660254037844387076, 1.000000000000000000, 0.8660254037844387076, 1.000000000000000000, 0.8660254037844387076, 1.000000000000000000, 0.8660254037844387076, 1.000000000000000000, 0.8660254037844387076, 1.000000000000000000, 0.8660254037844387076, 1.000000000000000000, 0.8660254037844387076, 1.000000000000000000, 0.8660254037844387076, 1.000000000000000000, 0.8660254037844387076, 1.000000000000000000, 0.8660254037844387076, 1.000000000000000000, 0.8660254037844387076, 1.000000000000000000, 0.8660254037844387076, 1.000000000000000000, 0.8660254037844387076, 1.000000000000000000, 0.8660254037844387076, 1.000000000000000000, 0.8660254037844387076, 1.000000000000000000, 0.8660254037844387076, 1.000000000000000000, 0.8660254037844387076, 1.000000000000000000, 0.8660254037844387076, 1.000000000000000000, 0.8660254037844387076, 1.000000000000000000, 0.8660254037844387076, 1.000000000000000000, 0.8660254037844387076, 1.000000000000000000, 0.8660254037844387076, 1.000000000000000000, 0.8660254037844387076, 1.000000000000000000, 0.8660254037844387076, 1.000000000000000000, 0.8660254037844387076, 1.000000000000000000, 0.8660254037844387076, 1.000000000000000000, 0.8660254037844387076, 1.000000000000000000, 0.8660254037844387076, 1.000000000000000000, 0.8660254037844387076, 1.000000000000000000, 0.8660254037844387076, 1.000000000000000000, 0.8660254037844387076, 1.000000000000000000, 0.8660254037844387076, 1.000000000000000000, 0.8660254037844387076, 1.000000000000000000, 0.8660254037844387076, 1.000000000000000000, 0.8660254037844387076, 1.000000000000000000, 0.8660254037844387076, 1.000000000000000000, 0.8660254037844387076, 1.000000000000000000, 0.8660254037844387076, 1.000000000000000000, 0.8660254037844387076, 1.000000000000000000, 0.8660254037844387076, 1.000000000000000000, 0.8660254037844387076, 1.000000000000000000, 0.8660254037844387076, 1.000000000000000000, 0.8660254037844387076, 1.000000000000000000, 0.8660254037844387076, 1.000000000000000000, 0.8660254037844387076, 1.000000000000000000, 0.8660254037844387076, 1.000000000000000000, 0.8660254037844387076, 1.000000000000000000, 0.8660254037844387076, 1.000000000000000000, 0.8660254037844387076, 1.000000000000000000, 0.8660254037844387076, 1.000000000000000000, 0.8660254037844387076, 1.000000000000000000, 0.8660254037844387076, 1.000000000000000000, 0.8660254037844387076, 1.000000000000000000, 0.8660254037844387076, 1.000000000000000000, 0.8660254037844387076, 1.000000000000000000, 0.8660254037844387076, 1.000000000000000000, 0.8660254037844387076, 1.000000000000000000, 0.8660254037844387076, 1.000000000000000000, 0.8660254037844387076, 1.000000000000000000, 0.8660254037844387076, 1.000000000000000000, 0.8660254037844387076, 1.000000000000000000, 0.8660254037844387076, 1.000000000000000000, 0.8660254037844387076, 1.000000000000000000, 0.8660254037844387076, 1.000000000000000000, 0.8660254037844387076, 1.000000000000000000, 0.8660254037844387076, 1.000000000000000000, 0.8660254037844387076, 1.000000000000000000, 0.8660254037844387076, 1.000000000000000000, 0.8660254037844387076, 1.000000000000000000, 0.8660254037844387076, 1.000000000000000000, 0.8660254037844387076, 1.000000000000000000, 0.8660254037844387076, 1.000000000000000000, 0.8660254037844387076, 1.000000000000000000, 0.8660254037844387076, 1.000000000000000000, 0.8660254037844387076, 1.000000000000000000, 0.8660254037844387076, 1.000000000000000000, 0.8660254037844387076, 1.000000000000000000, 0.8660254037844387076, 1.000000000000000000, 0.8660254037844387076, 1.000000000000000000, 0.8660254037844387076, 1.000000000000000000, 0.8660254037844387076, 1.000000000000000000, 0.8660254037844387076, 1.000000000000000000, 0.8660254037844387076, 1.000000000000000000, 0.8660254037844387076, 1.000000000000000000, 0.8660254037844387076, 1.000000000000000000, 0.8660254037844387076, 1.000000000000000000, 0.8660254037844387076, 1.000000000000000000, 0.8660254037844387076, 1.000000000000000000, 0.8660254037844387076, 1.000000000000000000, 0.8660254037844387076, 1.000000000000000000, 0.8660254037844387076, 1.000000000000000000, 0.8660254037844387076, 1.000000000000000000, 0.8660254037844387076, 1.000000000000000000, 0.8660254037844387076, 1.000000000000000000, 0.8660254037844387076, 1.000000000000000000, 0.8660254037844387076, 1.000000000000000000, 0.8660254037844387076, 1.000000000000000000, 0.8660254037844387076, 1.000000000000000000, 0.8660254037844387076, 1.000000000000000000, 0.8660254037844387076, 1.000000000000000000, 0.8660254037844387076, 1.000000000000000000, 0.8660254037844387076, 1.000000000000000000, 0.8660254037844387076, 1.000000000000000000, 0.8660254037844387076, 1.000000000000000000, 0.8660254037844387076, 1.000000000000000000, 0.8660254037844387076, 1.000000000000000000, 0.8660254037844387076, 1.000000000000000000, 0.8660254037844387076, 1.000000000000000000, 0.8660254037844387076, 1.000000000000000000, 0.8660254037844387076, 1.000000000000000000, 0.8660254037844387076, 1.000000000000000000, 0.8660254037844387076, 1.000000000000000000, 0.8660254037844387076, 1.000000000000000000, 0.8660254037844387076, 1.000000000000000000, 0.8660254037844387076, 1.000000000000000000, 0.8660254037844387076, 1.000000000000000000, 0.8660254037844387076, 1.000000000000000000, 0.8660254037844387076, 1.000000000000000000, 0.8660254037844387076, 1.000000000000000000, 0.8660254037844387076, 1.000000000000000000, 0.8660254037844387076, 1.000000000000000000, 0.8660254037844387076, 1.000000000000000000, 0.8660254037844387076, 1.000000000000000000, 0.8660254037844387076, 1.000000000000000000, 0.8660254037844387076, 1.000000000000000000, 0.8660254037844387076, 1.000000000000000000, 0.8660254037844387076, 1.000000000000000000, 0.8660254037844387076, 1.000000000000000000, 0.8660254037844387076, 1.000000000000000000, 0.8660254037844387076, 1.000000000000000000, 0.8660254037844387076, 1.000000000000000000, 0.8660254037844387076, 1.000000000000000000, 0.8660254037844387076, 1.000000000000000000, 0.8660254037844387076, 1.000000000000000000, 0.8660254037844387076, 1.000000000000000000, 0.8660254037844387076, 1.000000000000000000, 0.8660254037844387076, 1.000000000000000000, 0.8660254037844387076, 1.000000000000000000, 0.8660254037844387076, 1.000000000000000000, 0.8660254037844387076, 1.000000000000000000, 0.8660254037844387076, 1.000000000000000000, 0.8660254037844387076, 1.000000000000000000, 0.8660254037844387076, 1.000000000000000000, 0.8660254037844387076, 1.000000000000000000, 0.8660254037844387076, 1.000000000000000000, 0.8660254037844387076, 1.000000000000000000, 0.8660254037844387076, 1.000000000000000000, 0.8660254037844387076, 1.000000000000000000, 0.8660254037844387076, 1.000000000000000000, 0.8660254037844387076, 1.000000000000000000, 0.8660254037844387076, 1.000000000000000000, 0.8660254037844387076, 1.000000000000000000, 0.8660254037844387076, 1.000000000000000000, 0.8660254037844387076, 1.000000000000000000),
 ( 1.000000000000000000, 0.8660254037844387076, 1.000000000000000000, 0.8660254037844387076, 1.000000000000000000, 0.8660254037844387076, 1.000000000000000000, 0.8660254037844387076, 1.000000000000000000, 0.8660254037844387076, 1.000000000000000000, 0.8660254037844387076, 1.000000000000000000, 0.8660254037844387076, 1.000000000000000000, 0.8660254037844387076, 1.000000000000000000, 0.8660254037844387076, 1.000000000000000000, 0.8660254037844387076, 1.000000000000000000, 0.8660254037844387076, 1.000000000000000000, 0.8660254037844387076, 1.000000000000000000, 0.8660254037844387076, 1.000000000000000000, 0.8660254037844387076, 1.000000000000000000, 0.8660254037844387076, 1.000000000000000000, 0.8660254037844387076, 1.000000000000000000, 0.8660254037844387076, 1.000000000000000000, 0.8660254037844387076, 1.000000000000000000, 0.8660254037844387076, 1.000000000000000000, 0.8660254037844387076, 1.000000000000000000, 0.8660254037844387076, 1.000000000000000000, 0.8660254037844387076, 1.000000000000000000, 0.8660254037844387076, 1.000000000000000000, 0.8660254037844387076, 1.000000000000000000, 0.8660254037844387076, 1.000000000000000000, 0.8660254037844387076, 1.000000000000000000, 0.8660254037844387076, 1.000000000000000000, 0.8660254037844387076, 1.000000000000000000, 0.8660254037844387076, 1.000000000000000000, 0.8660254037844387076, 1.000000000000000000, 0.8660254037844387076, 1.000000000000000000, 0.8660254037844387076, 1.000000000000000000, 0.8660254037844387076, 1.000000000000000000, 0.8660254037844387076, 1.000000000000000000, 0.8660254037844387076, 1.000000000000000000, 0.8660254037844387076, 1.000000000000000000, 0.8660254037844387076, 1.000000000000000000, 0.8660254037844387076, 1.000000000000000000, 0.8660254037844387076, 1.000000000000000000, 0.8660254037844387076, 1.000000000000000000, 0.8660254037844387076, 1.000000000000000000, 0.8660254037844387076, 1.000000000000000000, 0.8660254037844387076, 1.000000000000000000, 0.8660254037844387076, 1.000000000000000000, 0.8660254037844387076, 1.000000000000000000, 0.8660254037844387076, 1.000000000000000000, 0.8660254037844387076, 1.000000000000000000, 0.8660254037844387076, 1.000000000000000000, 0.8660254037844387076, 1.000000000000000000, 0.8660254037844387076, 1.000000000000000000, 0.8660254037844387076, 1.000000000000000000, 0.8660254037844387076, 1.000000000000000000, 0.8660254037844387076, 1.000000000000000000, 0.8660254037844387076, 1.000000000000000000, 0.8660254037844387076, 1.000000000000000000, 0.8660254037844387076, 1.000000000000000000, 0.8660254037844387076, 1.000000000000000000, 0.8660254037844387076, 1.000000000000000000, 0.8660254037844387076, 1.000000000000000000, 0.8660254037844387076, 1.000000000000000000, 0.8660254037844387076, 1.000000000000000000, 0.8660254037844387076, 1.000000000000000000, 0.8660254037844387076, 1.000000000000000000, 0.8660254037844387076, 1.000000000000000000, 0.8660254037844387076, 1.000000000000000000, 0.8660254037844387076, 1.000000000000000000, 0.8660254037844387076, 1.000000000000000000, 0.8660254037844387076, 1.000000000000000000, 0.8660254037844387076, 1.000000000000000000, 0.8660254037844387076, 1.000000000000000000, 0.8660254037844387076, 1.000000000000000000, 0.8660254037844387076, 1.000000000000000000, 0.8660254037844387076, 1.000000000000000000, 0.8660254037844387076, 1.000000000000000000, 0.8660254037844387076, 1.000000000000000000, 0.8660254037844387076, 1.000000000000000000, 0.8660254037844387076, 1.000000000000000000, 0.8660254037844387076, 1.000000000000000000, 0.8660254037844387076, 1.000000000000000000, 0.8660254037844387076, 1.000000000000000000, 0.8660254037844387076, 1.000000000000000000, 0.8660254037844387076, 1.000000000000000000, 0.8660254037844387076, 1.000000000000000000, 0.8660254037844387076, 1.000000000000000000, 0.8660254037844387076, 1.000000000000000000, 0.8660254037844387076, 1.000000000000000000, 0.8660254037844387076, 1.000000000000000000, 0.8660254037844387076, 1.000000000000000000, 0.8660254037844387076, 1.000000000000000000, 0.8660254037844387076, 1.000000000000000000, 0.8660254037844387076, 1.000000000000000000, 0.8660254037844387076, 1.000000000000000000, 0.8660254037844387076, 1.000000000000000000, 0.8660254037844387076, 1.000000000000000000, 0.8660254037844387076, 1.000000000000000000, 0.8660254037844387076, 1.000000000000000000, 0.8660254037844387076, 1.000000000000000000, 0.8660254037844387076, 1.000000000000000000, 0.8660254037844387076, 1.000000000000000000, 0.8660254037844387076, 1.000000000000000000, 0.8660254037844387076, 1.000000000000000000, 0.8660254037844387076, 1.000000000000000000, 0.8660254037844387076, 1.000000000000000000, 0.8660254037844387076, 1.000000000000000000, 0.8660254037844387076, 1.000000000000000000, 0.8660254037844387076, 1.000000000000000000, 0.8660254037844387076, 1.000000000000000000, 0.8660254037844387076, 1.000000000000000000, 0.8660254037844387076, 1.000000000000000000, 0.8660254037844387076, 1.000000000000000000, 0.8660254037844387076, 1.000000000000000000, 0.8660254037844387076, 1.000000000000000000, 0.8660254037844387076, 1.000000000000000000, 0.8660254037844387076, 1.000000000000000000, 0.8660254037844387076, 1.000000000000000000, 0.8660254037844387076, 1.000000000000000000, 0.8660254037844387076, 1.000000000000000000, 0.8660254037844387076, 1.000000000000000000, 0.8660254037844387076, 1.000000000000000000, 0.8660254037844387076, 1.000000000000000000, 0.8660254037844387076, 1.000000000000000000, 0.8660254037844387076, 1.000000000000000000, 0.8660254037844387076, 1.000000000000000000, 0.8660254037844387076, 1.000000000000000000, 0.8660254037844387076, 1.000000000000000000, 0.8660254037844387076, 1.000000000000000000, 0.8660254037844387076, 1.000000000000000000, 0.8660254037844387076, 1.000000000000000000, 0.8660254037844387076, 1.000000000000000000, 0.8660254037844387076, 1.000000000000000000, 0.8660254037844387076, 1.000000000000000000, 0.8660254037844387076, 1.000000000000000000, 0.8660254037844387076, 1.000000000000000000, 0.8660254037844387076, 1.000000000000000000, 0.8660254037844387076, 1.000000000000000000, 0.8660254037844387076, 1.000000000000000000, 0.8660254037844387076, 1.000000000000000000, 0.8660254037844387076, 1.000000000000000000, 0.8660254037844387076, 1.000000000000000000, 0.8660254037844387076, 1.000000000000000000, 0.8660254037844387076, 1.000000000000000000, 0.8660254037844387076, 1.000000000000000000, 0.8660254037844387076, 1.000000000000000000, 0.8660254037844387076, 1.000000000000000000, 0.8660254037844387076, 1.000000000000000000, 0.8660254037844387076, 1.000000000000000000, 0.8660254037844387076, 1.000000000000000000, 0.8660254037844387076, 1.000000000000000000, 0.8660254037844387076, 1.000000000000000000, 0.8660254037844387076, 1.000000000000000000, 0.8660254037844387076, 1.000000000000000000, 0.8660254037844387076, 1.000000000000000000, 0.8660254037844387076, 1.000000000000000000, 0.8660254037844387076, 1.000000000000000000, 0.8660254037844387076, 1.000000000000000000, 0.8660254037844387076, 1.000000000000000000, 0.8660254037844387076, 1.000000000000000000, 0.8660254037844387076, 1.000000000000000000, 0.8660254037844387076, 1.000000000000000000, 0.8660254037844387076, 1.000000000000000000, 0.8660254037844387076, 1.000000000000000000, 0.8660254037844387076, 1.000000000000000000, 0.8660254037844387076, 1.000000000000000000, 0.8660254037844387076, 1.000000000000000000, 0.8660254037844387076, 1.000000000000000000, 0.8660254037844387076, 1.000000000000000000, 0.8660254037844387076, 1.000000000000000000, 0.8660254037844387076, 1.000000000000000000, 0.8660254037844387076, 1.000000000000000000, 0.8660254037844387076, 1.000000000000000000, 0.8660254037844387076, 1.000000000000000000, 0.8660254037844387076, 1.000000000000000000, 0.8660254037844387076, 1.000000000000000000, 0.8660254037844387076, 1.000000000000000000, 0.8660254037844387076, 1.000000000000000000, 0.8660254037844387076, 1.000000000000000000, 0.8660254037844387076, 1.000000000000000000, 0.8660254037844387076, 1.000000000000000000, 0.8660254037844387076, 1.000000000000000000, 0.8660254037844387076, 1.000000000000000000, 0.8660254037844387076, 1.000000000000000000, 0.8660254037844387076, 1.000000000000000000, 0.8660254037844387076, 1.000000000000000000, 0.8660254037844387076, 1.000000000000000000, 0.8660254037844387076, 1.000000000000000000, 0.8660254037844387076, 1.000000000000000000, 0.8660254037844387076, 1.000000000000000000, 0.8660254037844387076, 1.000000000000000000, 0.8660254037844387076, 1.000000000000000000, 0.8660254037844387076, 1.000000000000000000, 0.8660254037844387076, 1.000000000000000000, 0.8660254037844387076, 1.000000000000000000, 0.8660254037844387076, 1.000000000000000000, 0.8660254037844387076, 1.000000000000000000, 0.8660254037844387076, 1.000000000000000000, 0.8660254037844387076, 1.000000000000000000, 0.8660254037844387076, 1.000000000000000000, 0.8660254037844387076, 1.000000000000000000, 0.8660254037844387076, 1.000000000000000000, 0.8660254037844387076, 1.000000000000000000, 0.8660254037844387076, 1.000000000000000000, 0.8660254037844387076, 1.000000000000000000, 0.8660254037844387076, 1.000000000000000000, 0.8660254037844387076, 1.000000000000000000, 0.8660254037844387076, 1.000000000000000000, 0.8660254037844387076, 1.000000000000000000, 0.8660254037844387076, 1.000000000000000000, 0.8660254037844387076, 1.000000000000000000, 0.8660254037844387076, 1.000000000000000000, 0.8660254037844387076, 1.000000000000000000, 0.8660254037844387076, 1.000000000000000000, 0.8660254037844387076, 1.000000000000000000, 0.8660254037844387076, 1.000000000000000000, 0.8660254037844387076, 1.000000000000000000, 0.8660254037844387076, 1.000000000000000000, 0.8660254037844387076, 1.000000000000000000, 0.8660254037844387076, 1.000000000000000000, 0.8660254037844387076, 1.000000000000000000, 0.8660254037844387076, 1.000000000000000000, 0.8660254037844387076, 1.000000000000000000, 0.8660254037844387076, 1.000000000000000000, 0.8660254037844387076, 1.000000000000000000, 0.8660254037844387076, 1.000000000000000000, 0.8660254037844387076, 1.000000000000000000, 0.8660254037844387076, 1.000000000000000000, 0.8660254037844387076, 1.000000000000000000, 0.8660254037844387076, 1.000000000000000000, 0.8660254037844387076, 1.000000000000000000, 0.8660254037844387076, 1.000000000000000000, 0.8660254037844387076, 1.000000000000000000, 0.8660254037844387076, 1.000000000000000000, 0.8660254037844387076, 1.000000000000000000, 0.8660254037844387076, 1.000000000000000000, 0.8660254037844387076, 1.000000000000000000, 0.8660254037844387076, 1.000000000000000000, 0.8660254037844387076, 1.000000000000000000, 0.8660254037844387076, 1.000000000000000000, 0.8660254037844387076, 1.000000000000000000, 0.8660254037844387076, 1.000000000000000000, 0.8660254037844387076, 1.000000000000000000, 0.8660254037844387076, 1.000000000000000000, 0.8660254037844387076, 1.000000000000000000, 0.8660254037844387076, 1.000000000000000000, 0.8660254037844387076, 1.000000000000000000, 0.8660254037844387076, 1.000000000000000000, 0.8660254037844387076, 1.000000000000000000, 0.8660254037844387076, 1.000000000000000000, 0.8660254037844387076, 1.000000000000000000, 0.8660254037844387076, 1.000000000000000000, 0.8660254037844387076, 1.000000000000000000, 0.8660254037844387076, 1.000000000000000000, 0.8660254037844387076, 1.000000000000000000, 0.8660254037844387076, 1.000000000000000000, 0.8660254037844387076, 1.000000000000000000, 0.8660254037844387076, 1.000000000000000000, 0.8660254037844387076, 1.000000000000000000, 0.8660254037844387076, 1.000000000000000000, 0.8660254037844387076, 1.000000000000000000, 0.8660254037844387076, 1.000000000000000000, 0.8660254037844387076, 1.000000000000000000, 0.8660254037844387076, 1.000000000000000000, 0.8660254037844387076, 1.000000000000000000, 0.8660254037844387076, 1.000000000000000000, 0.8660254037844387076, 1.000000000000000000, 0.8660254037844387076, 1.000000000000000000, 0.8660254037844387076, 1.000000000000000000, 0.8660254037844387076, 1.000000000000000000, 0.8660254037844387076, 1.000000000000000000, 0.8660254037844387076, 1.000000000000000000, 0.8660254037844387076, 1.000000000000000000, 0.8660254037844387076, 1.000000000000000000, 0.8660254037844387076, 1.000000000000000000, 0.8660254037844387076, 1.000000000000000000, 0.8660254037844387076, 1.000000000000000000, 0.8660254037844387076, 1.000000000000000000, 0.8660254037844387076, 1.000000000000000000, 0.8660254037844387076, 1.000000000000000000, 0.8660254037844387076, 1.000000000000000000, 0.8660254037844387076, 1.000000000000000000, 0.8660254037844387076, 1.000000000000000000, 0.8660254037844387076, 1.000000000000000000, 0.8660254037844387076, 1.000000000000000000, 0.8660254037844387076, 1.000000000000000000, 0.8660254037844387076, 1.000000000000000000, 0.8660254037844387076, 1.000000000000000000, 0.8660254037844387076, 1.000000000000000000, 0.8660254037844387076, 1.000000000000000000, 0.8660254037844387076, 1.000000000000000000, 0.8660254037844387076, 1.000000000000000000, 0.8660254037844387076, 1.000000000000000000, 0.8660254037844387076, 1.000000000000000000, 0.8660254037844387076, 1.000000000000000000, 0.8660254037844387076, 1.000000000000000000, 0.8660254037844387076, 1.000000000000000000, 0.8660254037844387076, 1.000000000000000000, 0.8660254037844387076, 1.000000000000000000, 0.8660254037844387076, 1.000000000000000000, 0.8660254037844387076, 1.000000000000000000, 0.8660254037844387076, 1.000000000000000000, 0.8660254037844387076, 1.000000000000000000, 0.8660254037844387076, 1.000000000000000000, 0.8660254037844387076, 1.000000000000000000, 0.8660254037844387076, 1.000000000000000000, 0.8660254037844387076, 1.000000000000000000, 0.8660254037844387076, 1.000000000000000000, 0.8660254037844387076, 1.000000000000000000, 0.8660254037844387076, 1.000000000000000000, 0.8660254037844387076, 1.000000000000000000, 0.8660254037844387076, 1.000000000000000000, 0.8660254037844387076, 1.000000000000000000, 0.8660254037844387076, 1.000000000000000000, 0.8660254037844387076, 1.000000000000000000, 0.8660254037844387076, 1.000000000000000000, 0.8660254037844387076, 1.000000000000000000, 0.8660254037844387076, 1.000000000000000000, 0.8660254037844387076, 1.000000000000000000, 0.8660254037844387076, 1.000000000000000000, 0.8660254037844387076, 1.000000000000000000, 0.8660254037844387076, 1.000000000000000000, 0.8660254037844387076, 1.000000000000000000, 0.8660254037844387076, 1.000000000000000000, 0.8660254037844387076, 1.000000000000000000, 0.8660254037844387076, 1.000000000000000000, 0.8660254037844387076, 1.000000000000000000, 0.8660254037844387076, 1.000000000000000000, 0.8660254037844387076, 1.000000000000000000, 0.8660254037844387076, 1.000000000000000000, 0.8660254037844387076, 1.000000000000000000, 0.8660254037844387076, 1.000000000000000000, 0.8660254037844387076, 1.000000000000000000, 0.8660254037844387076, 1.000000000000000000, 0.8660254037844387076, 1.000000000000000000, 0.8660254037844387076, 1.000000000000000000, 0.8660254037844387076, 1.000000000000000000, 0.8660254037844387076, 1.000000000000000000, 0.8660254037844387076, 1.000000000000000000, 0.8660254037844387076, 1.000000000000000000, 0.8660254037844387076, 1.000000000000000000, 0.8660254037844387076, 1.000000000000000000, 0.8660254037844387076, 1.000000000000000000, 0.8660254037844387076, 1.000000000000000000, 0.8660254037844387076, 1.000000000000000000, 0.8660254037844387076, 1.000000000000000000, 0.8660254037844387076, 1.000000000000000000, 0.8660254037844387076, 1.000000000000000000, 0.8660254037844387076, 1.000000000000000000, 0.8660254037844387076, 1.000000000000000000, 0.8660254037844387076, 1.000000000000000000, 0.8660254037844387076, 1.000000000000000000, 0.8660254037844387076, 1.000000000000000000, 0.8660254037844387076, 1.000000000000000000, 0.8660254037844387076, 1.000000000000000000, 0.8660254037844387076, 1.000000000000000000, 0.8660254037844387076, 1.000000000000000000, 0.8660254037844387076, 1.000000000000000000, 0.8660254037844387076, 1.000000000000000000, 0.8660254037844387076, 1.000000000000000000, 0.8660254037844387076, 1.000000000000000000, 0.8660254037844387076, 1.000000000000000000, 0.8660254037844387076, 1.000000000000000000) ) ) 
 REPRESENTATION_ITEM ( '' )  SURFACE ( )  );
#71778=CARTESIAN_POINT ( 'NONE',  ( 21.60937500061451644, 4.541064518000418104, -2.621784821874998173 ) ) ;
#71780=CARTESIAN_POINT ( 'NONE',  ( 7.078125000614516438, 6.421520780324663323E-16, -5.243569643749999010 ) ) ;
#71781=CARTESIAN_POINT ( 'NONE',  ( 14.22187500061451537, -6.054752690667223547, -1.112240025338166033E-15 ) ) ;
#71783=CARTESIAN_POINT ( 'NONE',  ( 22.88437500061451857, 6.421520780324663323E-16, -5.243569643749999010 ) ) ;
#71784=CARTESIAN_POINT ( 'NONE',  ( 3.780892357739494170, 3.275126314170736741, -28.66976688362063186 ) ) ;
#71785=CARTESIAN_POINT ( 'NONE',  ( 8.699999999999999289, 4.330127018922192761, -2.499999999999997780 ) ) ;
#71786=CARTESIAN_POINT ( 'NONE',  ( 6.262500000000000178, -5.773502691896255534, -1.060575238724906372E-15 ) ) ;
#71787=CARTESIAN_POINT ( 'NONE',  ( 16.65000000122903501, -2.886751345948129988, 4.999999999999997335 ) ) ;
#71788=LINE ( 'NONE', #53690, #67907 ) ;
#71790=ORIENTED_EDGE ( 'NONE', *, *, #18349, .F. ) ;
#71791=CARTESIAN_POINT ( 'NONE',  ( 14.13750000000000107, 5.773502691896255534, 3.535250795749688894E-16 ) ) ;
#71792=CARTESIAN_POINT ( 'NONE',  ( 15.93750000000000000, 5.773502691896255534, 3.535250795749688894E-16 ) ) ;
#71793=CARTESIAN_POINT ( 'NONE',  ( 11.09062500061451573, -3.027376345333610441, -5.243569643749999898 ) ) ;
#71794=ORIENTED_EDGE ( 'NONE', *, *, #51099, .F. ) ;
#71795=CARTESIAN_POINT ( 'NONE',  ( -3.999999999999999112, 16.92500000122903359, -32.30940107675850470 ) ) ;
#71796=CARTESIAN_POINT ( 'NONE',  ( -2.121784821874999949, 16.18437500061451573, -33.67503911421598417 ) ) ;
#71797=CARTESIAN_POINT ( 'NONE',  ( 29.21250000122903145, 0.000000000000000000, 4.999999999999998224 ) ) ;
#71799=CARTESIAN_POINT ( 'NONE',  ( 9.299999999999998934, 0.000000000000000000, 4.999999999999998224 ) ) ;
#71800=CARTESIAN_POINT ( 'NONE',  ( 3.937500001229034208, 4.330127018922191873, 2.499999999999999556 ) ) ;
#71801=VERTEX_POINT ( 'NONE', #53999 ) ;
#71802=CARTESIAN_POINT ( 'NONE',  ( 23.46562500061451573, 3.027376345333611329, 5.243569643749999010 ) ) ;
#71805=CARTESIAN_POINT ( 'NONE',  ( 20.40937500061451715, 0.000000000000000000, 5.243569643749999010 ) ) ;
#71806=CARTESIAN_POINT ( 'NONE',  ( 19.86562500061451786, 3.027376345333611329, 5.243569643749999010 ) ) ;
#71807=CARTESIAN_POINT ( 'NONE',  ( -2.121784821874996840, 14.02812500061459389, -26.32496088578401583 ) ) ;
#71808=CARTESIAN_POINT ( 'NONE',  ( 24.26250000122903216, 0.000000000000000000, 4.999999999999998224 ) ) ;
#71809=CARTESIAN_POINT ( 'NONE',  ( 4.978125000614518569, 4.541064518000418104, 2.621784821874999949 ) ) ;
#71811=CARTESIAN_POINT ( 'NONE',  ( 20.80312500061451431, 0.000000000000000000, 5.243569643749999010 ) ) ;
#71814=CARTESIAN_POINT ( 'NONE',  ( 15.68437500061451573, 6.421520780324663323E-16, -5.243569643749999010 ) ) ;
#71815=CARTESIAN_POINT ( 'NONE',  ( 13.80937500061451750, -4.541064518000417216, -2.621784821875001281 ) ) ;
#71816=CARTESIAN_POINT ( 'NONE',  ( 23.18437500061451573, -4.541064518000419881, 2.621784821874995952 ) ) ;
#71817=CARTESIAN_POINT ( 'NONE',  ( 4.243569643749999898, 12.84687500061451715, 32.45002607614398471 ) ) ;
#71818=CARTESIAN_POINT ( 'NONE',  ( 5.090625000614516615, -3.027376345333614438, 5.243569643749998122 ) ) ;
#71819=CARTESIAN_POINT ( 'NONE',  ( 27.62812500061451360, -4.541064518000419881, 2.621784821874995952 ) ) ;
#71820=CARTESIAN_POINT ( 'NONE',  ( 26.80312500061451431, -4.541064518000417216, -2.621784821875001281 ) ) ;
#71821=CARTESIAN_POINT ( 'NONE',  ( -1.394453263437886604E-15, 19.32500000122903216, -26.00000000000000000 ) ) ;
#71822=CARTESIAN_POINT ( 'NONE',  ( 1.999999999999998668, 18.05000000000000071, 26.53589838486224650 ) ) ;
#71823=CARTESIAN_POINT ( 'NONE',  ( 6.084375000614518747, -4.541064518000419881, 2.621784821874995952 ) ) ;
#71825=CARTESIAN_POINT ( 'NONE',  ( 14.85000000122903252, -2.886751345948129988, 4.999999999999997335 ) ) ;
#71826=CARTESIAN_POINT ( 'NONE',  ( 10.08750000122903323, 6.123233995736764310E-16, -4.999999999999998224 ) ) ;
#71827=CARTESIAN_POINT ( 'NONE',  ( 28.38750000122903216, -4.330127018922194537, 2.499999999999995559 ) ) ;
#71830=CARTESIAN_POINT ( 'NONE',  ( 15.49687500061451750, -3.027376345333614438, 5.243569643749998122 ) ) ;
#71831=CYLINDRICAL_SURFACE ( 'NONE', #63215, 4.000000000000000000 ) ;
#71834=CARTESIAN_POINT ( 'NONE',  ( 18.70312500061451644, -4.541064518000417216, -2.621784821875001281 ) ) ;
#71835=CARTESIAN_POINT ( 'NONE',  ( 8.428125000614517859, 6.421520780324663323E-16, -5.243569643749999010 ) ) ;
#71836=CARTESIAN_POINT ( 'NONE',  ( 23.18437500061451573, -4.541064518000419881, 2.621784821874995952 ) ) ;
#71837=CARTESIAN_POINT ( 'NONE',  ( 5.540625000614515905, -3.027376345333614438, 5.243569643749998122 ) ) ;
#71839=CARTESIAN_POINT ( 'NONE',  ( 7.012500001229035718, 4.330127018922192761, -2.499999999999997780 ) ) ;
#71840=CARTESIAN_POINT ( 'NONE',  ( 23.54062500061451146, -3.027376345333614438, 5.243569643749998122 ) ) ;
#71841=CARTESIAN_POINT ( 'NONE',  ( 3.999999999999999112, 17.63750000122903572, -30.00000000000000000 ) ) ;
#71842=CARTESIAN_POINT ( 'NONE',  ( 9.637500001229033941, 6.123233995736764310E-16, -4.999999999999998224 ) ) ;
#71843=CARTESIAN_POINT ( 'NONE',  ( 18.85312500061451502, 4.541064518000418104, -2.621784821874998173 ) ) ;
#71844=CARTESIAN_POINT ( 'NONE',  ( 16.30312500061451786, 0.000000000000000000, 5.243569643749999010 ) ) ;
#71846=CARTESIAN_POINT ( 'NONE',  ( 15.45000000000000107, 4.330127018922192761, -2.499999999999997780 ) ) ;
#71847=CARTESIAN_POINT ( 'NONE',  ( 12.18750000122903465, -4.330127018922194537, 2.499999999999995559 ) ) ;
#71848=CARTESIAN_POINT ( 'NONE',  ( 7.678125000614516082, 4.541064518000418104, 2.621784821874999949 ) ) ;
#71849=CARTESIAN_POINT ( 'NONE',  ( 12.21562500061451573, 3.027376345333611329, 5.243569643749999010 ) ) ;
#71850=CARTESIAN_POINT ( 'NONE',  ( 21.26250000122903572, -4.330127018922190985, -2.500000000000001332 ) ) ;
#71851=CARTESIAN_POINT ( 'NONE',  ( 19.05937500061451928, 0.000000000000000000, 5.243569643749999010 ) ) ;
#71853=CARTESIAN_POINT ( 'NONE',  ( 5.625000001229036428, 2.886751345948129099, -4.999999999999998224 ) ) ;
#71854=CARTESIAN_POINT ( 'NONE',  ( 4.021875000614516082, 3.027376345333613106, -5.243569643749998122 ) ) ;
#71855=CARTESIAN_POINT ( 'NONE',  ( 24.15937500061451715, -4.541064518000417216, -2.621784821875001281 ) ) ;
#71857=CARTESIAN_POINT ( 'NONE',  ( 1.626862140677534273E-15, 18.42500000122903359, 34.00000000000000000 ) ) ;
#71858=CARTESIAN_POINT ( 'NONE',  ( 19.00312500061451715, 0.000000000000000000, 5.243569643749999010 ) ) ;
#71859=CARTESIAN_POINT ( 'NONE',  ( 23.14687500061451786, -3.027376345333614438, 5.243569643749998122 ) ) ;
#71862=CARTESIAN_POINT ( 'NONE',  ( 28.32187500061451502, 3.027376345333613106, -5.243569643749998122 ) ) ;
#71864=CARTESIAN_POINT ( 'NONE',  ( 15.32812500061451644, 4.541064518000418104, 2.621784821874999949 ) ) ;
#71865=CARTESIAN_POINT ( 'NONE',  ( 12.15937500061451892, 4.541064518000418104, -2.621784821874998173 ) ) ;
#71866=VERTEX_POINT ( 'NONE', #50642 ) ;
#71868=CARTESIAN_POINT ( 'NONE',  ( 21.77812500061451928, -4.541064518000419881, 2.621784821874995952 ) ) ;
#71869=CARTESIAN_POINT ( 'NONE',  ( -3.999999999999999112, 19.83125000061451715, 30.00000000000000000 ) ) ;
#71871=CARTESIAN_POINT ( 'NONE',  ( 15.48749999999999893, 5.773502691896255534, 3.535250795749688894E-16 ) ) ;
#71872=CARTESIAN_POINT ( 'NONE',  ( 23.13750000122903216, 6.123233995736764310E-16, -4.999999999999998224 ) ) ;
#71873=CARTESIAN_POINT ( 'NONE',  ( 19.00312500061451715, 0.000000000000000000, 5.243569643749999010 ) ) ;
#71874=ORIENTED_EDGE ( 'NONE', *, *, #11525, .F. ) ;
#71875=CARTESIAN_POINT ( 'NONE',  ( 22.72499999999999787, 4.330127018922191873, 2.499999999999999556 ) ) ;
#71876=CARTESIAN_POINT ( 'NONE',  ( 24.53437500061451715, -4.541064518000419881, 2.621784821874995952 ) ) ;
#71879=CARTESIAN_POINT ( 'NONE',  ( 11.87812500061451537, -4.541064518000419881, 2.621784821874995952 ) ) ;
#71880=DIRECTION ( 'NONE',  ( -1.000000000000000000, -0.000000000000000000, -0.000000000000000000 ) ) ;
#71882=CARTESIAN_POINT ( 'NONE',  ( 17.36249999999999716, 2.886751345948126879, 4.999999999999999112 ) ) ;
#71883=CARTESIAN_POINT ( 'NONE',  ( 23.55000000000000071, 4.330127018922192761, -2.499999999999997780 ) ) ;
#71884=CARTESIAN_POINT ( 'NONE',  ( 9.001249775931846008E-16, 19.01562500061451644, 34.90005215228797653 ) ) ;
#71885=CARTESIAN_POINT ( 'NONE',  ( 5.109375000614518214, 0.000000000000000000, 5.243569643749999010 ) ) ;
#71886=CARTESIAN_POINT ( 'NONE',  ( 17.40937500061451715, -4.541064518000417216, -2.621784821875001281 ) ) ;
#71887=CARTESIAN_POINT ( 'NONE',  ( 28.65937500061451715, -4.541064518000417216, -2.621784821875001281 ) ) ;
#71889=CARTESIAN_POINT ( 'NONE',  ( 25.64062500061451644, 6.054752690667223547, 3.707466751127219781E-16 ) ) ;
#71890=CARTESIAN_POINT ( 'NONE',  ( 27.45937500061451786, 4.541064518000418104, -2.621784821874998173 ) ) ;
#71891=DIRECTION ( 'NONE',  ( -1.000000000000000000, -0.000000000000000000, -0.000000000000000000 ) ) ;
#71892=CARTESIAN_POINT ( 'NONE',  ( 14.66249999999999964, 2.886751345948126879, 4.999999999999999112 ) ) ;
#71893=CARTESIAN_POINT ( 'NONE',  ( 11.91562500061451857, -6.054752690667223547, -1.112240025338166033E-15 ) ) ;
#71894=CARTESIAN_POINT ( 'NONE',  ( 30.00000000000000000, 0.000000000000000000, 0.000000000000000000 ) ) ;
#71895=CARTESIAN_POINT ( 'NONE',  ( 1.071796769724490783, 19.41740381056767006, -34.00000000000000000 ) ) ;
#71896=CARTESIAN_POINT ( 'NONE',  ( 29.05312500061451431, -4.541064518000417216, -2.621784821875001281 ) ) ;
#71897=CARTESIAN_POINT ( 'NONE',  ( 16.23750000122903359, -4.330127018922194537, 2.499999999999995559 ) ) ;
#71898=CARTESIAN_POINT ( 'NONE',  ( 15.22500000122903074, 2.886751345948193936, 4.999999999999883649 ) ) ;
#71900=CARTESIAN_POINT ( 'NONE',  ( 4.828125000614518214, 6.421520780324663323E-16, -5.243569643749999010 ) ) ;
#71901=CARTESIAN_POINT ( 'NONE',  ( 22.28437500061451715, -4.541064518000419881, 2.621784821874995952 ) ) ;
#71902=CARTESIAN_POINT ( 'NONE',  ( 9.001249775931846008E-16, 17.72187500061451715, 34.90005215228797653 ) ) ;
#71903=CARTESIAN_POINT ( 'NONE',  ( 22.32187500061451502, -6.054752690667223547, -1.112240025338166033E-15 ) ) ;
#71904=CARTESIAN_POINT ( 'NONE',  ( 28.73437500061451644, 6.421520780324663323E-16, -5.243569643749999010 ) ) ;
#71905=CARTESIAN_POINT ( 'NONE',  ( -2.121784821874999949, 19.78437500061451715, 26.32496088578401938 ) ) ;
#71906=CARTESIAN_POINT ( 'NONE',  ( 11.54062500061451857, -3.027376345333610441, -5.243569643749999898 ) ) ;
#71907=CARTESIAN_POINT ( 'NONE',  ( 2.000000000000001332, 17.11250000122903359, 33.46410161513774995 ) ) ;
#71908=CARTESIAN_POINT ( 'NONE',  ( 8.146875000614516082, 6.054752690667223547, 3.707466751127219781E-16 ) ) ;
#71909=CARTESIAN_POINT ( 'NONE',  ( 3.867736846495323011, 3.168783417359460231, -3.937610184585229156 ) ) ;
#71910=CARTESIAN_POINT ( 'NONE',  ( 10.00312500061451715, 0.000000000000000000, 5.243569643749999010 ) ) ;
#71911=CARTESIAN_POINT ( 'NONE',  ( 13.50937500061451679, 4.541064518000418104, -2.621784821874998173 ) ) ;
#71912=CARTESIAN_POINT ( 'NONE',  ( 6.037500001229035185, 6.123233995736764310E-16, -4.999999999999998224 ) ) ;
#71913=CARTESIAN_POINT ( 'NONE',  ( 22.42500000122903359, 2.886751345948126879, 4.999999999999999112 ) ) ;
#71914=CARTESIAN_POINT ( 'NONE',  ( 9.159375000614515372, 0.000000000000000000, 5.243569643749999010 ) ) ;
#71915=CARTESIAN_POINT ( 'NONE',  ( 10.34062500061451750, 6.054752690667223547, 3.707466751127219781E-16 ) ) ;
#71917=CARTESIAN_POINT ( 'NONE',  ( 21.38437500061451502, -4.541064518000419881, 2.621784821874995952 ) ) ;
#71918=CARTESIAN_POINT ( 'NONE',  ( 25.42500000122902648, 2.886751345948095793, -5.000000000000055067 ) ) ;
#71919=CARTESIAN_POINT ( 'NONE',  ( -3.182292052831501739, 3.860956188314066395, 32.43599349108946939 ) ) ;
#71920=LINE ( 'NONE', #2851, #57283 ) ;
#71921=CARTESIAN_POINT ( 'NONE',  ( 4.243569643749999010, 11.12187500061451928, -32.45002607614398471 ) ) ;
#71922=CARTESIAN_POINT ( 'NONE',  ( 15.93750000122903110, 6.123233995736764310E-16, -4.999999999999998224 ) ) ;
#71923=CARTESIAN_POINT ( 'NONE',  ( 4.243569643749999010, 15.11562500061451608, -32.45002607614398471 ) ) ;
#71924=CARTESIAN_POINT ( 'NONE',  ( 16.42500000122903359, 2.886751345948129099, -4.999999999999998224 ) ) ;
#71925=CARTESIAN_POINT ( 'NONE',  ( 10.67812500061451608, 6.421520780324663323E-16, -5.243569643749999010 ) ) ;
#71926=ORIENTED_EDGE ( 'NONE', *, *, #47179, .F. ) ;
#71927=CARTESIAN_POINT ( 'NONE',  ( 13.61250000000000071, 2.886751345948129099, -4.999999999999998224 ) ) ;
#71929=CARTESIAN_POINT ( 'NONE',  ( 22.60312500061451857, 0.000000000000000000, 5.243569643749999010 ) ) ;
#71930=CARTESIAN_POINT ( 'NONE',  ( 10.88437500061451679, 4.541064518000418104, 2.621784821874999949 ) ) ;
#71932=CARTESIAN_POINT ( 'NONE',  ( 9.187500001229034652, 6.123233995736764310E-16, -4.999999999999998224 ) ) ;
#71933=CARTESIAN_POINT ( 'NONE',  ( 18.71250000122903145, 4.330127018922192761, -2.499999999999997780 ) ) ;
#71934=CARTESIAN_POINT ( 'NONE',  ( 14.76562500061451821, 3.027376345333613106, -5.243569643749998122 ) ) ;
#71935=CARTESIAN_POINT ( 'NONE',  ( 18.25312500061451715, -4.541064518000417216, -2.621784821875001281 ) ) ;
#71936=CARTESIAN_POINT ( 'NONE',  ( 25.76250000122903216, -4.330127018922190985, -2.500000000000001332 ) ) ;
#71937=ADVANCED_FACE ( 'NONE', ( #45462 ), #4849, .F. ) ;
#71938=CARTESIAN_POINT ( 'NONE',  ( 28.91250000122903074, -4.330127018922190985, -2.500000000000001332 ) ) ;
#71939=CARTESIAN_POINT ( 'NONE',  ( 22.53750000000000142, -2.886751345948125991, -5.000000000000000000 ) ) ;
#71941=CARTESIAN_POINT ( 'NONE',  ( 25.35937500061451644, 0.000000000000000000, 5.243569643749999010 ) ) ;
#71942=CARTESIAN_POINT ( 'NONE',  ( 12.30000000122903181, -2.886751345948125991, -5.000000000000000000 ) ) ;
#71943=CARTESIAN_POINT ( 'NONE',  ( 29.67187500061451644, 3.027376345333613106, -5.243569643749998122 ) ) ;
#71944=EDGE_CURVE ( 'NONE', #2861, #37056, #22551, .T. ) ;
#71945=FACE_OUTER_BOUND ( 'NONE', #58935, .T. ) ;
#71946=CARTESIAN_POINT ( 'NONE',  ( 6.046875000614519102, -3.027376345333614438, 5.243569643749998122 ) ) ;
#71947=CARTESIAN_POINT ( 'NONE',  ( 25.94062500061451715, -3.027376345333610441, -5.243569643749999898 ) ) ;
#71949=CARTESIAN_POINT ( 'NONE',  ( 16.27499999999999858, 6.123233995736764310E-16, -4.999999999999998224 ) ) ;
#71950=CARTESIAN_POINT ( 'NONE',  ( 10.84687500061451892, 6.054752690667223547, 3.707466751127219781E-16 ) ) ;
#71951=CARTESIAN_POINT ( 'NONE',  ( 4.317513935836856831, -2.521720328239906550, 4.456045716080967445 ) ) ;
#71952=CARTESIAN_POINT ( 'NONE',  ( 28.90312500061451217, 0.000000000000000000, 5.243569643749999010 ) ) ;
#71953=CARTESIAN_POINT ( 'NONE',  ( 8.296875000614516438, -3.027376345333614438, 5.243569643749998122 ) ) ;
#71954=CARTESIAN_POINT ( 'NONE',  ( 29.22187500061451715, 3.027376345333613106, -5.243569643749998122 ) ) ;
#71955=CARTESIAN_POINT ( 'NONE',  ( 2.121784821875001281, 11.40312500061459566, 33.67503911421598417 ) ) ;
#71956=CARTESIAN_POINT ( 'NONE',  ( 23.06250000000000355, 2.886751345948129099, -4.999999999999998224 ) ) ;
#71958=CARTESIAN_POINT ( 'NONE',  ( -2.000000000000000000, 17.67500000000000071, -33.46410161513775705 ) ) ;
#71959=EDGE_CURVE ( 'NONE', #45966, #29431, #55456, .T. ) ;
#71961=CARTESIAN_POINT ( 'NONE',  ( 3.487500000000000711, -2.886751345948129988, 4.999999999999997335 ) ) ;
#71962=ORIENTED_EDGE ( 'NONE', *, *, #37402, .T. ) ;
#71963=CARTESIAN_POINT ( 'NONE',  ( 17.80312500061451786, -4.541064518000417216, -2.621784821875001281 ) ) ;
#71964=CARTESIAN_POINT ( 'NONE',  ( 11.91562500061451857, -6.054752690667223547, -1.112240025338166033E-15 ) ) ;
#71966=CARTESIAN_POINT ( 'NONE',  ( 6.909375000614518036, 0.000000000000000000, 5.243569643749999010 ) ) ;
#71967=CARTESIAN_POINT ( 'NONE',  ( 19.35000000122903430, -2.886751345948129988, 4.999999999999997335 ) ) ;
#71969=CARTESIAN_POINT ( 'NONE',  ( 7.321875000614516793, 3.027376345333611329, 5.243569643749999010 ) ) ;
#71970=CARTESIAN_POINT ( 'NONE',  ( 14.29687500061451821, -3.027376345333610441, -5.243569643749999898 ) ) ;
#71971=CARTESIAN_POINT ( 'NONE',  ( 23.93437500061451573, 4.541064518000418104, 2.621784821874999949 ) ) ;
#71972=VECTOR ( 'NONE', #3256, 1000.000000000000000 ) ;
#71975=CARTESIAN_POINT ( 'NONE',  ( 17.25937500061451502, 0.000000000000000000, 5.243569643749999010 ) ) ;
#71976=CARTESIAN_POINT ( 'NONE',  ( 10.02187500061451964, 3.027376345333611329, 5.243569643749999010 ) ) ;
#71978=CARTESIAN_POINT ( 'NONE',  ( 21.89999999999999858, 0.000000000000000000, 4.999999999999998224 ) ) ;
#71980=CARTESIAN_POINT ( 'NONE',  ( -2.121784821874999949, 10.33437500061451786, -33.67503911421598417 ) ) ;
#71982=CARTESIAN_POINT ( 'NONE',  ( 12.02812500061451573, 6.421520780324663323E-16, -5.243569643749999010 ) ) ;
#71983=CARTESIAN_POINT ( 'NONE',  ( 28.13437500061451502, -4.541064518000419881, 2.621784821874995952 ) ) ;
#71985=CARTESIAN_POINT ( 'NONE',  ( 27.87187500061451573, 3.027376345333613106, -5.243569643749998122 ) ) ;
#71986=CARTESIAN_POINT ( 'NONE',  ( 13.16249999999999964, 2.886751345948129099, -4.999999999999998224 ) ) ;
#71987=CARTESIAN_POINT ( 'NONE',  ( 3.999999999999999112, 16.73750000122903359, 30.00000000000000000 ) ) ;
#71988=CARTESIAN_POINT ( 'NONE',  ( 11.21250000122903501, 0.000000000000000000, 4.999999999999998224 ) ) ;
#71989=CARTESIAN_POINT ( 'NONE',  ( 21.83437500061451786, -4.541064518000419881, 2.621784821874995952 ) ) ;
#71990=CARTESIAN_POINT ( 'NONE',  ( 16.32187500061451502, 3.027376345333611329, 5.243569643749999010 ) ) ;
#71991=CARTESIAN_POINT ( 'NONE',  ( 4.017893810940423194, 2.976003446579597256, -4.317231760934856943 ) ) ;
#71992=EDGE_LOOP ( 'NONE', ( #59581, #17603, #9712, #64718 ) ) ;
#71993=CARTESIAN_POINT ( 'NONE',  ( 16.37812500061451715, -4.541064518000419881, 2.621784821874995952 ) ) ;
#71994=CARTESIAN_POINT ( 'NONE',  ( 28.08750000122903145, 6.123233995736764310E-16, -4.999999999999998224 ) ) ;
#71995=CARTESIAN_POINT ( 'NONE',  ( 14.55937500061451573, 0.000000000000000000, 5.243569643749999010 ) ) ;
#71997=CARTESIAN_POINT ( 'NONE',  ( 20.01562500061451644, -6.054752690667223547, -1.112240025338166033E-15 ) ) ;
#71998=CARTESIAN_POINT ( 'NONE',  ( 28.35937500061451289, 4.541064518000418104, -2.621784821874998173 ) ) ;
#71999=CARTESIAN_POINT ( 'NONE',  ( -4.243569643749999898, 13.50312500061451715, 30.00000000000000000 ) ) ;
#72000=CARTESIAN_POINT ( 'NONE',  ( 18.12187500061451573, 3.027376345333611329, 5.243569643749999010 ) ) ;
#72001=CARTESIAN_POINT ( 'NONE',  ( 13.65000000122903323, -2.886751345948125991, -5.000000000000000000 ) ) ;
#72003=CARTESIAN_POINT ( 'NONE',  ( 4.243569643749999898, 18.73437500061451644, -30.00000000000000000 ) ) ;
#72004=CARTESIAN_POINT ( 'NONE',  ( 21.19687500061451502, 6.054752690667223547, 3.707466751127219781E-16 ) ) ;
#72005=CARTESIAN_POINT ( 'NONE',  ( 22.72500000122903430, 2.886751345948129099, -4.999999999999998224 ) ) ;
#72006=CARTESIAN_POINT ( 'NONE',  ( 17.03437500061451715, 6.421520780324663323E-16, -5.243569643749999010 ) ) ;
#72007=CARTESIAN_POINT ( 'NONE',  ( 13.45312500061451466, 4.541064518000418104, -2.621784821874998173 ) ) ;
#72008=CARTESIAN_POINT ( 'NONE',  ( 4.243569643749999898, 11.98437500061451821, 30.00000000000000000 ) ) ;
#72009=CARTESIAN_POINT ( 'NONE',  ( 16.49062500061451786, -3.027376345333610441, -5.243569643749999898 ) ) ;
#72012=CARTESIAN_POINT ( 'NONE',  ( 24.00000000000000000, 4.330127018922192761, -2.499999999999997780 ) ) ;
#72013=CARTESIAN_POINT ( 'NONE',  ( 4.243569643749999010, 18.32187500061451502, -32.45002607614398471 ) ) ;
#72014=CARTESIAN_POINT ( 'NONE',  ( 24.25312500061451715, 4.541064518000418104, -2.621784821874998173 ) ) ;
#72015=CARTESIAN_POINT ( 'NONE',  ( 5.578125000614518214, -4.541064518000419881, 2.621784821874995952 ) ) ;
#72016=CARTESIAN_POINT ( 'NONE',  ( 18.11250000122903359, -4.330127018922190985, -2.500000000000001332 ) ) ;
#72017=CARTESIAN_POINT ( 'NONE',  ( 22.67812500061451431, -4.541064518000419881, 2.621784821874995952 ) ) ;
#72018=CARTESIAN_POINT ( 'NONE',  ( 23.66250000000000142, 2.886751345948126879, 4.999999999999999112 ) ) ;
#72019=CARTESIAN_POINT ( 'NONE',  ( 25.64062500061451644, 6.054752690667223547, 3.707466751127219781E-16 ) ) ;
#72020=CARTESIAN_POINT ( 'NONE',  ( 4.528125000614516615, 4.541064518000418104, 2.621784821874999949 ) ) ;
#72021=ORIENTED_EDGE ( 'NONE', *, *, #28241, .T. ) ;
#72022=CARTESIAN_POINT ( 'NONE',  ( 22.19062500061451715, -3.027376345333614438, 5.243569643749998122 ) ) ;
#72025=CARTESIAN_POINT ( 'NONE',  ( 4.000000000000000000, 18.83749999999999858, 32.30940107675849760 ) ) ;
#72026=CARTESIAN_POINT ( 'NONE',  ( 8.484601909799253346E-16, 13.92500000122903359, -25.38119784648299770 ) ) ;
#72028=CARTESIAN_POINT ( 'NONE',  ( -2.000000000000000000, 10.13750000122903572, 26.53589838486224650 ) ) ;
#72029=CARTESIAN_POINT ( 'NONE',  ( 10.72500000000000142, -4.330127018922194537, 2.499999999999995559 ) ) ;
#72030=CARTESIAN_POINT ( 'NONE',  ( 12.23437500061451821, 4.541064518000418104, 2.621784821874999949 ) ) ;
#72031=CARTESIAN_POINT ( 'NONE',  ( 7.050000001229036251, 5.773502691896255534, 3.535250795749688894E-16 ) ) ;
#72032=CARTESIAN_POINT ( 'NONE',  ( 13.80937500061451750, -4.541064518000417216, -2.621784821875001281 ) ) ;
#72033=CARTESIAN_POINT ( 'NONE',  ( 6.984375000614516438, -4.541064518000419881, 2.621784821874995952 ) ) ;
#72035=CARTESIAN_POINT ( 'NONE',  ( -0.7368805616696195715, 9.859898480082234684, 25.82089837893477480 ) ) ;
#72036=CARTESIAN_POINT ( 'NONE',  ( 13.58437500061451786, 4.541064518000418104, 2.621784821874999949 ) ) ;
#72037=CARTESIAN_POINT ( 'NONE',  ( 3.684201729119676916, 3.380333950832448142, 4.008536514702806919 ) ) ;
#72038=CARTESIAN_POINT ( 'NONE',  ( 21.96562500061451573, 3.027376345333613106, -5.243569643749998122 ) ) ;
#72039=LINE ( 'NONE', #45058, #62810 ) ;
#72040=CARTESIAN_POINT ( 'NONE',  ( 24.23437500061451644, 6.421520780324663323E-16, -5.243569643749999010 ) ) ;
#72041=CARTESIAN_POINT ( 'NONE',  ( 29.58750000122903501, 4.330127018922191873, 2.499999999999999556 ) ) ;
#72043=CARTESIAN_POINT ( 'NONE',  ( 24.25312500061451715, 4.541064518000418104, -2.621784821874998173 ) ) ;
#72044=CARTESIAN_POINT ( 'NONE',  ( 18.77812500061451573, 6.421520780324663323E-16, -5.243569643749999010 ) ) ;
#72046=CARTESIAN_POINT ( 'NONE',  ( 14.07187500061451679, 3.027376345333611329, 5.243569643749999010 ) ) ;
#72047=CARTESIAN_POINT ( 'NONE',  ( 30.00000000000000000, 0.000000000000000000, 4.999999999999998224 ) ) ;
#72048=CARTESIAN_POINT ( 'NONE',  ( 28.23750000122903359, 4.330127018922191873, 2.499999999999999556 ) ) ;
#72049=CARTESIAN_POINT ( 'NONE',  ( 4.021875000614516082, 3.027376345333613106, -5.243569643749998122 ) ) ;
#72050=CARTESIAN_POINT ( 'NONE',  ( 13.39687500061451608, -3.027376345333610441, -5.243569643749999898 ) ) ;
#72052=CARTESIAN_POINT ( 'NONE',  ( 4.537500001229034297, -4.330127018922194537, 2.499999999999995559 ) ) ;
#72053=CARTESIAN_POINT ( 'NONE',  ( 25.13437500061451502, 6.421520780324663323E-16, -5.243569643749999010 ) ) ;
#72054=CARTESIAN_POINT ( 'NONE',  ( 17.25937500061451502, 0.000000000000000000, 5.243569643749999010 ) ) ;
#72056=CARTESIAN_POINT ( 'NONE',  ( 29.25000000000000000, -4.330127018922190985, -2.500000000000001332 ) ) ;
#72057=CARTESIAN_POINT ( 'NONE',  ( 6.412500000000001421, 2.886751345948129099, -4.999999999999998224 ) ) ;
#72059=CARTESIAN_POINT ( 'NONE',  ( 19.90312500061451573, 0.000000000000000000, 5.243569643749999010 ) ) ;
#72060=CARTESIAN_POINT ( 'NONE',  ( 8.587500000000002132, -2.886751345948125991, -5.000000000000000000 ) ) ;
#72061=CARTESIAN_POINT ( 'NONE',  ( 5.015625000614518214, 3.027376345333611329, 5.243569643749999010 ) ) ;
#72062=CARTESIAN_POINT ( 'NONE',  ( 19.46249999999999858, 2.886751345948129099, -4.999999999999998224 ) ) ;
#72064=CARTESIAN_POINT ( 'NONE',  ( 22.08750000122903501, -4.330127018922194537, 2.499999999999995559 ) ) ;
#72065=CARTESIAN_POINT ( 'NONE',  ( 5.959992197959415705, 8.030459126529553515, 29.19994738672135526 ) ) ;
#72066=CARTESIAN_POINT ( 'NONE',  ( 28.73437500061451644, 6.421520780324663323E-16, -5.243569643749999010 ) ) ;
#72067=VERTEX_POINT ( 'NONE', #67282 ) ;
#72068=CARTESIAN_POINT ( 'NONE',  ( 17.54062500061451502, 6.054752690667223547, 3.707466751127219781E-16 ) ) ;
#72069=CARTESIAN_POINT ( 'NONE',  ( 24.62812500061451715, 6.421520780324663323E-16, -5.243569643749999010 ) ) ;
#72070=CARTESIAN_POINT ( 'NONE',  ( 25.77187500061451075, 3.027376345333611329, 5.243569643749999010 ) ) ;
#72071=CARTESIAN_POINT ( 'NONE',  ( 6.000000000000001776, 4.330127018922192761, -2.499999999999997780 ) ) ;
#72072=CARTESIAN_POINT ( 'NONE',  ( 9.590625000614517504, -3.027376345333614438, 5.243569643749998122 ) ) ;
#72073=CARTESIAN_POINT ( 'NONE',  ( 25.60312500061451502, 4.541064518000418104, -2.621784821874998173 ) ) ;
#72074=CARTESIAN_POINT ( 'NONE',  ( 14.74687500061451573, -3.027376345333610441, -5.243569643749999898 ) ) ;
#72075=CARTESIAN_POINT ( 'NONE',  ( 18.64687500061451786, -3.027376345333614438, 5.243569643749998122 ) ) ;
#72076=CARTESIAN_POINT ( 'NONE',  ( 9.001249775931846008E-16, 19.46562500061451573, 34.90005215228797653 ) ) ;
#72077=CARTESIAN_POINT ( 'NONE',  ( 24.97500000122903430, 2.886751345948129099, -4.999999999999998224 ) ) ;
#72079=CARTESIAN_POINT ( 'NONE',  ( 11.35312500061451679, 0.000000000000000000, 5.243569643749999010 ) ) ;
#72080=CARTESIAN_POINT ( 'NONE',  ( 8.146875000614516082, 6.054752690667223547, 3.707466751127219781E-16 ) ) ;
#72081=CARTESIAN_POINT ( 'NONE',  ( 7.771875000614516971, 3.027376345333611329, 5.243569643749999010 ) ) ;
#72082=VERTEX_POINT ( 'NONE', #50998 ) ;
#72083=CARTESIAN_POINT ( 'NONE',  ( 26.78437500061451360, -4.541064518000419881, 2.621784821874995952 ) ) ;
#72084=CARTESIAN_POINT ( 'NONE',  ( 18.70312500061451644, -4.541064518000417216, -2.621784821875001281 ) ) ;
#72085=CARTESIAN_POINT ( 'NONE',  ( 29.36250000122903003, -4.330127018922190985, -2.500000000000001332 ) ) ;
#72086=EDGE_CURVE ( 'NONE', #23724, #40333, #28113, .T. ) ;
#72087=CARTESIAN_POINT ( 'NONE',  ( 3.946875000614517681, -3.027376345333610441, -5.243569643749999898 ) ) ;
#72088=CARTESIAN_POINT ( 'NONE',  ( 23.44687500061451502, 6.054752690667223547, 3.707466751127219781E-16 ) ) ;
#72089=CARTESIAN_POINT ( 'NONE',  ( 18.81562500061452070, 3.027376345333613106, -5.243569643749998122 ) ) ;
#72090=CARTESIAN_POINT ( 'NONE',  ( 2.000000000000001332, 11.15000000000000213, 33.46410161513774995 ) ) ;
#72091=CARTESIAN_POINT ( 'NONE',  ( 24.06562500061451715, -6.054752690667223547, -1.112240025338166033E-15 ) ) ;
#72092=CARTESIAN_POINT ( 'NONE',  ( 4.425000001229032698, 2.886751345948126879, 4.999999999999999112 ) ) ;
#72094=CARTESIAN_POINT ( 'NONE',  ( 29.39999999999999858, 4.330127018922192761, -2.499999999999997780 ) ) ;
#72095=CARTESIAN_POINT ( 'NONE',  ( 4.000000000000000000, 15.68750000000000000, -27.69059892324149530 ) ) ;
#72097=CARTESIAN_POINT ( 'NONE',  ( 4.471875000614518925, 3.027376345333613106, -5.243569643749998122 ) ) ;
#72098=FACE_OUTER_BOUND ( 'NONE', #32910, .T. ) ;
#72099=CARTESIAN_POINT ( 'NONE',  ( 13.41562500061451502, 3.027376345333613106, -5.243569643749998122 ) ) ;
#72100=CARTESIAN_POINT ( 'NONE',  ( 6.871875000614517504, 3.027376345333611329, 5.243569643749999010 ) ) ;
#72101=CARTESIAN_POINT ( 'NONE',  ( 25.31250000122903288, -4.330127018922190985, -2.500000000000001332 ) ) ;
#72102=CARTESIAN_POINT ( 'NONE',  ( 16.05937500061451573, -4.541064518000417216, -2.621784821875001281 ) ) ;
#72103=CARTESIAN_POINT ( 'NONE',  ( 28.94062500061452070, -3.027376345333614438, 5.243569643749998122 ) ) ;
#72104=CARTESIAN_POINT ( 'NONE',  ( 30.00000000000000000, 0.000000000000000000, 0.000000000000000000 ) ) ;
#72106=CARTESIAN_POINT ( 'NONE',  ( 4.040625000614517681, 6.054752690667223547, 3.707466751127219781E-16 ) ) ;
#72107=CARTESIAN_POINT ( 'NONE',  ( 14.57812500061451644, -4.541064518000419881, 2.621784821874995952 ) ) ;
#72109=CARTESIAN_POINT ( 'NONE',  ( 10.11562500061451608, -6.054752690667223547, -1.112240025338166033E-15 ) ) ;
#72110=CARTESIAN_POINT ( 'NONE',  ( 8.390625000614518214, -3.027376345333610441, -5.243569643749999898 ) ) ;
#72112=CARTESIAN_POINT ( 'NONE',  ( 8.062500000000000000, -5.773502691896255534, -1.060575238724906372E-15 ) ) ;
#72113=EDGE_CURVE ( 'NONE', #26808, #6811, #48153, .T. ) ;
#72114=CARTESIAN_POINT ( 'NONE',  ( 5.212500001229032343, 4.330127018922192761, -2.499999999999997780 ) ) ;
#72115=CARTESIAN_POINT ( 'NONE',  ( 19.04999999999999716, 4.330127018922192761, -2.499999999999997780 ) ) ;
#72117=CARTESIAN_POINT ( 'NONE',  ( 17.89687500061451431, -3.027376345333610441, -5.243569643749999898 ) ) ;
#72118=CARTESIAN_POINT ( 'NONE',  ( 13.95000000122903572, -2.886751345948129988, 4.999999999999997335 ) ) ;
#72120=CARTESIAN_POINT ( 'NONE',  ( 2.121784821874999061, 16.05312500061451786, -33.67503911421598417 ) ) ;
#72122=AXIS2_PLACEMENT_3D ( 'NONE', #37328, #10349, #21057 ) ;
#72124=CARTESIAN_POINT ( 'NONE',  ( 28.75312500061451715, 4.541064518000418104, -2.621784821874998173 ) ) ;
#72127=CARTESIAN_POINT ( 'NONE',  ( 1.071796769724484344, 16.08259618943233704, -25.99999999999999645 ) ) ;
#72128=CARTESIAN_POINT ( 'NONE',  ( 13.92187500061451644, 3.027376345333613106, -5.243569643749998122 ) ) ;
#72129=CARTESIAN_POINT ( 'NONE',  ( 26.06250000000000000, -5.773502691896255534, -1.060575238724906372E-15 ) ) ;
#72130=CARTESIAN_POINT ( 'NONE',  ( 9.590625000614517504, -3.027376345333614438, 5.243569643749998122 ) ) ;
#72132=CARTESIAN_POINT ( 'NONE',  ( 22.62187500061451573, 3.027376345333611329, 5.243569643749999010 ) ) ;
#72134=CARTESIAN_POINT ( 'NONE',  ( 7.228125000614517681, 4.541064518000418104, 2.621784821874999949 ) ) ;
#72135=CARTESIAN_POINT ( 'NONE',  ( 12.94687500061451857, -3.027376345333610441, -5.243569643749999898 ) ) ;
#72136=EDGE_LOOP ( 'NONE', ( #40284, #21516, #13505, #32764 ) ) ;
#72137=CARTESIAN_POINT ( 'NONE',  ( 23.22187500061451715, -6.054752690667223547, -1.112240025338166033E-15 ) ) ;
#72138=CARTESIAN_POINT ( 'NONE',  ( 2.067223061484678048, 4.558648060312520123, -33.43375747538831888 ) ) ;
#72140=CARTESIAN_POINT ( 'NONE',  ( 4.762499999999999289, 2.886751345948126879, 4.999999999999999112 ) ) ;
#72141=CARTESIAN_POINT ( 'NONE',  ( 18.07500000122903216, -5.773502691896255534, -1.060575238724906372E-15 ) ) ;
#72143=CARTESIAN_POINT ( 'NONE',  ( 19.16250000000000142, 2.886751345948060266, 5.000000000000114575 ) ) ;
#72145=VERTEX_POINT ( 'NONE', #67994 ) ;
#72146=CARTESIAN_POINT ( 'NONE',  ( 12.44999999999999929, 0.000000000000000000, 4.999999999999998224 ) ) ;
#72147=CARTESIAN_POINT ( 'NONE',  ( 16.53750000000000142, -2.886751345948129988, 4.999999999999997335 ) ) ;
#72148=CARTESIAN_POINT ( 'NONE',  ( 13.08750000122903323, -4.330127018922194537, 2.499999999999995559 ) ) ;
#72149=CARTESIAN_POINT ( 'NONE',  ( 11.84062500061451750, -3.027376345333614438, 5.243569643749998122 ) ) ;
#72151=CARTESIAN_POINT ( 'NONE',  ( 10.08749999999999858, 5.773502691896255534, 3.535250795749688894E-16 ) ) ;
#72152=CARTESIAN_POINT ( 'NONE',  ( 18.60000000122903430, -2.886751345948159742, -4.999999999999942268 ) ) ;
#72153=CARTESIAN_POINT ( 'NONE',  ( -2.121784821874996840, 14.53437500061451715, -26.32496088578401583 ) ) ;
#72154=CARTESIAN_POINT ( 'NONE',  ( 4.303125000614516971, -4.541064518000417216, -2.621784821875001281 ) ) ;
#72156=CARTESIAN_POINT ( 'NONE',  ( 9.862500000000000711, -5.773502691896255534, -1.060575238724906372E-15 ) ) ;
#72158=VERTEX_POINT ( 'NONE', #32556 ) ;
#72159=CARTESIAN_POINT ( 'NONE',  ( 24.85312500061451502, 0.000000000000000000, 5.243569643749999010 ) ) ;
#72160=CARTESIAN_POINT ( 'NONE',  ( 4.219924060640600771, -2.681835364526683474, 4.505860815252779261 ) ) ;
#72162=CARTESIAN_POINT ( 'NONE',  ( 22.24687500061451217, -3.027376345333614438, 5.243569643749998122 ) ) ;
#72163=CARTESIAN_POINT ( 'NONE',  ( 19.07812500061451644, -4.541064518000419881, 2.621784821874995952 ) ) ;
#72164=CARTESIAN_POINT ( 'NONE',  ( -4.243569643749998122, 11.74062500061459424, -27.54997392385601174 ) ) ;
#72165=CARTESIAN_POINT ( 'NONE',  ( 6.440625000614517148, -3.027376345333614438, 5.243569643749998122 ) ) ;
#72167=CARTESIAN_POINT ( 'NONE',  ( 3.440625000614518036, -3.027376345333610441, -5.243569643749999898 ) ) ;
#72169=CARTESIAN_POINT ( 'NONE',  ( 21.96562500061451928, 3.027376345333612662, -5.243569643749998122 ) ) ;
#72172=CARTESIAN_POINT ( 'NONE',  ( 14.97187500061451892, 3.027376345333611329, 5.243569643749999010 ) ) ;
#72173=CARTESIAN_POINT ( 'NONE',  ( 14.40937500061451715, 4.541064518000418104, -2.621784821874998173 ) ) ;
#72174=CARTESIAN_POINT ( 'NONE',  ( 22.62187500061451573, 3.027376345333611329, 5.243569643749999010 ) ) ;
#72176=CARTESIAN_POINT ( 'NONE',  ( 4.243569643749999898, 12.39687500061451786, 32.45002607614398471 ) ) ;
#72178=CARTESIAN_POINT ( 'NONE',  ( 27.55312500061451786, 0.000000000000000000, 5.243569643749999010 ) ) ;
#72179=( BOUNDED_CURVE ( )  B_SPLINE_CURVE ( 3, ( #72699, #44640, #67169, #16530 ),
 .UNSPECIFIED., .F., .F. ) 
 B_SPLINE_CURVE_WITH_KNOTS ( ( 4, 4 ),
 ( 3.595026063070182243, 3.642474834530476269 ),
 .UNSPECIFIED. ) 
 CURVE ( )  GEOMETRIC_REPRESENTATION_ITEM ( )  RATIONAL_B_SPLINE_CURVE ( ( 1.000000000000000000, 0.9998123933069705815, 0.9998123933069705815, 1.000000000000000000 ) ) 
 REPRESENTATION_ITEM ( '' )  );
#72180=CARTESIAN_POINT ( 'NONE',  ( 27.44062500061451715, 6.054752690667223547, 3.707466751127219781E-16 ) ) ;
#72182=CARTESIAN_POINT ( 'NONE',  ( 1.999999999999998668, 18.50000000000000000, 26.53589838486224650 ) ) ;
#72183=CARTESIAN_POINT ( 'NONE',  ( 3.984375000614517326, 6.421520780324663323E-16, -5.243569643749999010 ) ) ;
#72184=SHAPE_DEFINITION_REPRESENTATION ( #8981, #13196 ) ;
#72185=CARTESIAN_POINT ( 'NONE',  ( 11.32500000122903394, -5.773502691896255534, -1.060575238724906372E-15 ) ) ;
#72186=CARTESIAN_POINT ( 'NONE',  ( 10.16250000122903252, 4.330127018922192761, -2.499999999999997780 ) ) ;
#72187=CARTESIAN_POINT ( 'NONE',  ( 28.98750000122903359, 6.123233995736764310E-16, -4.999999999999998224 ) ) ;
#72190=CARTESIAN_POINT ( 'NONE',  ( 12.98437500061451821, 6.421520780324663323E-16, -5.243569643749999010 ) ) ;
#72192=ORIENTED_EDGE ( 'NONE', *, *, #23389, .F. ) ;
#72193=CARTESIAN_POINT ( 'NONE',  ( 19.00312500061451715, 0.000000000000000000, 5.243569643749999010 ) ) ;
#72194=CARTESIAN_POINT ( 'NONE',  ( 14.29687500061451821, -3.027376345333610441, -5.243569643749999898 ) ) ;
#72195=CARTESIAN_POINT ( 'NONE',  ( 4.640625000614518214, -3.027376345333614438, 5.243569643749998122 ) ) ;
#72196=CARTESIAN_POINT ( 'NONE',  ( 22.77187500061451786, -6.054752690667223547, -1.112240025338166033E-15 ) ) ;
#72197=CARTESIAN_POINT ( 'NONE',  ( 6.103125000614515905, -4.541064518000417216, -2.621784821875001281 ) ) ;
#72198=CARTESIAN_POINT ( 'NONE',  ( 6.487500001229034474, 6.123233995736764310E-16, -4.999999999999998224 ) ) ;
#72199=CARTESIAN_POINT ( 'NONE',  ( 4.987500001229032698, -4.330127018922194537, 2.499999999999995559 ) ) ;
#72200=EDGE_CURVE ( 'NONE', #70765, #54526, #70843, .T. ) ;
#72201=CARTESIAN_POINT ( 'NONE',  ( 23.39062500061451289, 6.054752690667223547, 3.707466751127219781E-16 ) ) ;
#72202=( BOUNDED_CURVE ( )  B_SPLINE_CURVE ( 2, ( #39969, #34766, #63205, #62483, #62128, #12236, #67679, #7065, #45866 ),
 .UNSPECIFIED., .F., .F. ) 
 B_SPLINE_CURVE_WITH_KNOTS ( ( 3, 2, 2, 2, 3 ),
 ( 0.7934782608695651884, 0.7971014492753623060, 0.8043478260869565410, 0.8115942028985507761, 0.8152173913043478937 ),
 .UNSPECIFIED. ) 
 CURVE ( )  GEOMETRIC_REPRESENTATION_ITEM ( )  RATIONAL_B_SPLINE_CURVE ( ( 0.9330127018922194093, 0.9330127018922194093, 1.000000000000000000, 0.8660254037844387076, 1.000000000000000000, 0.8660254037844387076, 1.000000000000000000, 0.9330127018922182991, 0.9330127018922192983 ) ) 
 REPRESENTATION_ITEM ( '' )  );
#72203=CARTESIAN_POINT ( 'NONE',  ( -2.000000000000000000, 18.68750000122903288, -33.46410161513775705 ) ) ;
#72204=CARTESIAN_POINT ( 'NONE',  ( 8.400000001229035007, 5.773502691896255534, 3.535250795749688894E-16 ) ) ;
#72205=CARTESIAN_POINT ( 'NONE',  ( 16.56562500061451715, 3.027376345333613106, -5.243569643749998122 ) ) ;
#72206=CARTESIAN_POINT ( 'NONE',  ( 14.39062500061451821, 6.054752690667223547, 3.707466751127219781E-16 ) ) ;
#72208=CARTESIAN_POINT ( 'NONE',  ( 16.23750000000000071, -2.886751345948125991, -5.000000000000000000 ) ) ;
#72209=CARTESIAN_POINT ( 'NONE',  ( 11.66250000122903430, 0.000000000000000000, 4.999999999999998224 ) ) ;
#72210=CARTESIAN_POINT ( 'NONE',  ( 8.165625000614516793, 3.027376345333611329, 5.243569643749999010 ) ) ;
#72211=CARTESIAN_POINT ( 'NONE',  ( 11.80312500061451608, 0.000000000000000000, 5.243569643749999010 ) ) ;
#72212=CARTESIAN_POINT ( 'NONE',  ( 19.76250000122903216, 0.000000000000000000, 4.999999999999998224 ) ) ;
#72213=CARTESIAN_POINT ( 'NONE',  ( 4.243569643749999010, 14.72187500061451715, -32.45002607614398471 ) ) ;
#72214=CARTESIAN_POINT ( 'NONE',  ( 19.58437500061451786, -4.541064518000419881, 2.621784821874995952 ) ) ;
#72216=CARTESIAN_POINT ( 'NONE',  ( 5.175000001229033586, 2.886751345948129099, -4.999999999999998224 ) ) ;
#72217=CARTESIAN_POINT ( 'NONE',  ( 3.271875000614519635, 3.027376345333611329, 5.243569643749999010 ) ) ;
#72218=CARTESIAN_POINT ( 'NONE',  ( 20.93437500061451573, -4.541064518000419881, 2.621784821874995952 ) ) ;
#72220=CARTESIAN_POINT ( 'NONE',  ( 16.15312500061451573, 4.541064518000418104, -2.621784821874998173 ) ) ;
#72223=CARTESIAN_POINT ( 'NONE',  ( 27.49687500061451217, 6.054752690667223547, 3.707466751127219781E-16 ) ) ;
#72225=CARTESIAN_POINT ( 'NONE',  ( 14.46562500061451750, 3.027376345333611329, 5.243569643749999010 ) ) ;
#72226=CARTESIAN_POINT ( 'NONE',  ( 14.29687500061451821, -3.027376345333610441, -5.243569643749999898 ) ) ;
#72227=VERTEX_POINT ( 'NONE', #49915 ) ;
#72228=CARTESIAN_POINT ( 'NONE',  ( 22.31250000122903288, 4.330127018922192761, -2.499999999999997780 ) ) ;
#72229=CARTESIAN_POINT ( 'NONE',  ( 22.15312500061451573, 0.000000000000000000, 5.243569643749999010 ) ) ;
#72230=DIRECTION ( 'NONE',  ( 0.000000000000000000, 0.000000000000000000, -1.000000000000000000 ) ) ;
#72231=CARTESIAN_POINT ( 'NONE',  ( 14.62500000000000000, 4.330127018922191873, 2.499999999999999556 ) ) ;
#72232=EDGE_CURVE ( 'NONE', #14992, #61789, #70817, .T. ) ;
#72233=CARTESIAN_POINT ( 'NONE',  ( 11.66249999999999964, -5.773502691896255534, -1.060575238724906372E-15 ) ) ;
#72234=CARTESIAN_POINT ( 'NONE',  ( 22.98750000122903003, -4.330127018922194537, 2.499999999999995559 ) ) ;
#72235=CARTESIAN_POINT ( 'NONE',  ( 17.54062500061451502, 6.054752690667223547, 3.707466751127219781E-16 ) ) ;
#72236=ORIENTED_EDGE ( 'NONE', *, *, #17352, .T. ) ;
#72237=CARTESIAN_POINT ( 'NONE',  ( 20.43749999999999645, 5.773502691896255534, 3.535250795749688894E-16 ) ) ;
#72238=CARTESIAN_POINT ( 'NONE',  ( 20.55937500061451573, -4.541064518000417216, -2.621784821875001281 ) ) ;
#72239=ORIENTED_EDGE ( 'NONE', *, *, #25043, .F. ) ;
#72240=DIRECTION ( 'NONE',  ( -1.000000000000000000, -0.000000000000000000, -0.000000000000000000 ) ) ;
#72241=CARTESIAN_POINT ( 'NONE',  ( 10.45312500061451644, 0.000000000000000000, 5.243569643749999010 ) ) ;
#72244=CARTESIAN_POINT ( 'NONE',  ( 16.50000000000000000, 0.000000000000000000, 4.999999999999998224 ) ) ;
#72245=CARTESIAN_POINT ( 'NONE',  ( 24.18750000000000355, -2.886751345948129988, 4.999999999999997335 ) ) ;
#72247=CARTESIAN_POINT ( 'NONE',  ( 3.459375000614519635, -4.541064518000417216, -2.621784821875001281 ) ) ;
#72248=CARTESIAN_POINT ( 'NONE',  ( 27.49687500061451217, 6.054752690667223547, 3.707466751127219781E-16 ) ) ;
#72250=CARTESIAN_POINT ( 'NONE',  ( 26.12812500061451360, 4.541064518000418104, 2.621784821874999949 ) ) ;
#72251=CARTESIAN_POINT ( 'NONE',  ( 27.79687500061451999, -3.027376345333610441, -5.243569643749999898 ) ) ;
#72253=CARTESIAN_POINT ( 'NONE',  ( 14.73749999999999893, -2.886751345948129988, 4.999999999999997335 ) ) ;
#72254=CARTESIAN_POINT ( 'NONE',  ( 10.64062500061451644, -3.027376345333610441, -5.243569643749999898 ) ) ;
#72255=DIRECTION ( 'NONE',  ( 0.000000000000000000, 0.000000000000000000, -1.000000000000000000 ) ) ;
#72256=CARTESIAN_POINT ( 'NONE',  ( 0.000000000000000000, 20.00000000000000000, -30.00000000000000000 ) ) ;
#72257=CARTESIAN_POINT ( 'NONE',  ( 27.70312500061451289, -4.541064518000417216, -2.621784821875001281 ) ) ;
#72258=CARTESIAN_POINT ( 'NONE',  ( 16.95000000122903216, 5.773502691896255534, 3.535250795749688894E-16 ) ) ;
#72261=CARTESIAN_POINT ( 'NONE',  ( 6.065625000614516260, -6.054752690667223547, -1.112240025338166033E-15 ) ) ;
#72262=CARTESIAN_POINT ( 'NONE',  ( 22.32187500061451502, -6.054752690667223547, -1.112240025338166033E-15 ) ) ;
#72263=CARTESIAN_POINT ( 'NONE',  ( -4.243569643749997233, 15.84687500061451715, 32.45002607614398471 ) ) ;
#72264=CARTESIAN_POINT ( 'NONE',  ( 20.97187500061451715, -6.054752690667223547, -1.112240025338166033E-15 ) ) ;
#72265=CARTESIAN_POINT ( 'NONE',  ( 28.92187500061451644, 3.027376345333611329, 5.243569643749999010 ) ) ;
#72266=CARTESIAN_POINT ( 'NONE',  ( -4.243569643749999898, 18.02187500061451786, 27.54997392385601529 ) ) ;
#72267=CARTESIAN_POINT ( 'NONE',  ( 9.478125000614515017, 4.541064518000418104, 2.621784821874999949 ) ) ;
#72270=CARTESIAN_POINT ( 'NONE',  ( 6.871875000614517504, 3.027376345333611329, 5.243569643749999010 ) ) ;
#72271=CYLINDRICAL_SURFACE ( 'NONE', #13544, 3.999999999999996447 ) ;
#72272=CARTESIAN_POINT ( 'NONE',  ( 6.928125000614516082, -4.541064518000419881, 2.621784821874995952 ) ) ;
#72273=CARTESIAN_POINT ( 'NONE',  ( 11.25937500061451679, 4.541064518000418104, -2.621784821874998173 ) ) ;
#72274=CARTESIAN_POINT ( 'NONE',  ( 3.450849747961474367, -3.618245071504076371, -3.795178659245230790 ) ) ;
#72275=CARTESIAN_POINT ( 'NONE',  ( 22.38750000122903216, 4.330127018922191873, 2.499999999999999556 ) ) ;
#72276=CARTESIAN_POINT ( 'NONE',  ( 7.321875000614516793, 3.027376345333611329, 5.243569643749999010 ) ) ;
#72277=CARTESIAN_POINT ( 'NONE',  ( 10.64062500061451644, -3.027376345333610441, -5.243569643749999898 ) ) ;
#72279=CARTESIAN_POINT ( 'NONE',  ( 19.20937500061451786, -4.541064518000417216, -2.621784821875001281 ) ) ;
#72280=CARTESIAN_POINT ( 'NONE',  ( -2.482458701038963156, 4.346511033910187116, 33.14667641405304011 ) ) ;
#72281=CARTESIAN_POINT ( 'NONE',  ( 29.03437500061451715, -4.541064518000419881, 2.621784821874995952 ) ) ;
#72282=EDGE_CURVE ( 'NONE', #62319, #13801, #58486, .T. ) ;
#72283=CARTESIAN_POINT ( 'NONE',  ( -4.243569643749999898, 12.65937500061451715, -30.00000000000000000 ) ) ;
#72284=CARTESIAN_POINT ( 'NONE',  ( 14.55000000122903181, -2.886751345948125991, -5.000000000000000000 ) ) ;
#72285=CARTESIAN_POINT ( 'NONE',  ( 4.243569643749999898, 15.97812500061451857, -30.00000000000000000 ) ) ;
#72286=CARTESIAN_POINT ( 'NONE',  ( 14.36250000122903359, 0.000000000000000000, 4.999999999999998224 ) ) ;
#72287=CARTESIAN_POINT ( 'NONE',  ( 9.478125000614515017, 4.541064518000418104, 2.621784821874999949 ) ) ;
#72288=ORIENTED_EDGE ( 'NONE', *, *, #17583, .T. ) ;
#72289=CARTESIAN_POINT ( 'NONE',  ( 13.79999999999999893, 0.000000000000000000, 4.999999999999998224 ) ) ;
#72291=CARTESIAN_POINT ( 'NONE',  ( 21.81562500061451004, -6.054752690667223547, -1.112240025338166033E-15 ) ) ;
#72292=CARTESIAN_POINT ( 'NONE',  ( 6.984375000614516438, -4.541064518000419881, 2.621784821874995952 ) ) ;
#72293=CARTESIAN_POINT ( 'NONE',  ( 11.25000000122903288, -2.886751345948129988, 4.999999999999997335 ) ) ;
#72294=CARTESIAN_POINT ( 'NONE',  ( 18.03750000122903430, -4.330127018922194537, 2.499999999999995559 ) ) ;
#72295=CARTESIAN_POINT ( 'NONE',  ( 16.22812500061451857, 4.541064518000418104, 2.621784821874999949 ) ) ;
#72296=CARTESIAN_POINT ( 'NONE',  ( 18.21562500061451573, -6.054752690667223547, -1.112240025338166033E-15 ) ) ;
#72297=CARTESIAN_POINT ( 'NONE',  ( 24.90000000122903145, -2.886751345948125991, -5.000000000000000000 ) ) ;
#72298=CARTESIAN_POINT ( 'NONE',  ( 27.78750000122903074, 4.330127018922191873, 2.499999999999999556 ) ) ;
#72299=CARTESIAN_POINT ( 'NONE',  ( 23.43750000000000000, -2.886751345948125991, -5.000000000000000000 ) ) ;
#72301=CARTESIAN_POINT ( 'NONE',  ( 26.40937500061451715, -4.541064518000417216, -2.621784821875001281 ) ) ;
#72303=CARTESIAN_POINT ( 'NONE',  ( 13.42500000122903536, 2.886751345948126879, 4.999999999999999112 ) ) ;
#72304=CARTESIAN_POINT ( 'NONE',  ( 27.79687500061451999, -3.027376345333610441, -5.243569643749999898 ) ) ;
#72305=DIRECTION ( 'NONE',  ( 0.000000000000000000, -0.000000000000000000, -1.000000000000000000 ) ) ;
#72306=CARTESIAN_POINT ( 'NONE',  ( 4.809375000614516615, -4.541064518000417216, -2.621784821875001281 ) ) ;
#72307=CARTESIAN_POINT ( 'NONE',  ( 25.34062500061451217, -3.027376345333614438, 5.243569643749998122 ) ) ;
#72310=CARTESIAN_POINT ( 'NONE',  ( 10.28437500061451715, 6.421520780324663323E-16, -5.243569643749999010 ) ) ;
#72311=CARTESIAN_POINT ( 'NONE',  ( 4.270834433354036008, -2.600094210001211437, 4.505651273120875544 ) ) ;
#72312=CARTESIAN_POINT ( 'NONE',  ( 3.009375000614516793, -4.541064518000417216, -2.621784821875001281 ) ) ;
#72313=CARTESIAN_POINT ( 'NONE',  ( 9.609375000614518214, 0.000000000000000000, 5.243569643749999010 ) ) ;
#72314=CARTESIAN_POINT ( 'NONE',  ( 28.54687500061451644, -3.027376345333614438, 5.243569643749998122 ) ) ;
#72315=CARTESIAN_POINT ( 'NONE',  ( 2.121784821874999061, 12.90312500061459566, 26.32496088578401583 ) ) ;
#72316=CARTESIAN_POINT ( 'NONE',  ( 20.28750000000000142, -2.886751345948125991, -5.000000000000000000 ) ) ;
#72317=ORIENTED_EDGE ( 'NONE', *, *, #53813, .F. ) ;
#72318=CARTESIAN_POINT ( 'NONE',  ( 28.91250000000000497, 2.886751345948129099, -4.999999999999998224 ) ) ;
#72320=CARTESIAN_POINT ( 'NONE',  ( 5.025000000000002132, 6.123233995736764310E-16, -4.999999999999998224 ) ) ;
#72322=CARTESIAN_POINT ( 'NONE',  ( 16.90312500061451573, -4.541064518000417216, -2.621784821875001281 ) ) ;
#72323=CARTESIAN_POINT ( 'NONE',  ( 8.165625000614516793, 3.027376345333611329, 5.243569643749999010 ) ) ;
#72325=CARTESIAN_POINT ( 'NONE',  ( 7.771875000614516971, 3.027376345333611329, 5.243569643749999010 ) ) ;
#72326=CARTESIAN_POINT ( 'NONE',  ( 18.90000000122902790, -2.886751345948129988, 4.999999999999997335 ) ) ;
#72327=CARTESIAN_POINT ( 'NONE',  ( 3.199564126591990743, -3.842561905972809555, -3.199564126591990743 ) ) ;
#72328=CARTESIAN_POINT ( 'NONE',  ( 6.984375000614516438, -4.541064518000419881, 2.621784821874995952 ) ) ;
#72329=CARTESIAN_POINT ( 'NONE',  ( 12.34687500061452070, -3.027376345333614438, 5.243569643749998122 ) ) ;
#72330=CARTESIAN_POINT ( 'NONE',  ( 24.04687500061451644, -3.027376345333614438, 5.243569643749998122 ) ) ;
#72332=ORIENTED_EDGE ( 'NONE', *, *, #45751, .F. ) ;
#72334=CARTESIAN_POINT ( 'NONE',  ( 17.14687500061451786, 6.054752690667223547, 3.707466751127219781E-16 ) ) ;
#72335=CARTESIAN_POINT ( 'NONE',  ( 8.746875000614515727, -3.027376345333614438, 5.243569643749998122 ) ) ;
#72337=CARTESIAN_POINT ( 'NONE',  ( 21.82499999999999574, 4.330127018922191873, 2.499999999999999556 ) ) ;
#72340=CARTESIAN_POINT ( 'NONE',  ( 12.47812500061451502, 6.421520780324663323E-16, -5.243569643749999010 ) ) ;
#72341=CARTESIAN_POINT ( 'NONE',  ( 28.95937500061451431, 0.000000000000000000, 5.243569643749999010 ) ) ;
#72343=CARTESIAN_POINT ( 'NONE',  ( 29.44687500061451857, -3.027376345333614438, 5.243569643749998122 ) ) ;
#72344=CARTESIAN_POINT ( 'NONE',  ( 10.68750000000000000, -2.886751345948129988, 4.999999999999997335 ) ) ;
#72345=CARTESIAN_POINT ( 'NONE',  ( 1.999999999999998668, 15.91250000122903430, 26.53589838486224650 ) ) ;
#72346=CARTESIAN_POINT ( 'NONE',  ( 7.987500001229032698, 4.330127018922191873, 2.499999999999999556 ) ) ;
#72347=CARTESIAN_POINT ( 'NONE',  ( 20.44687500061451857, -3.027376345333614438, 5.243569643749998122 ) ) ;
#72348=CARTESIAN_POINT ( 'NONE',  ( 14.89687500061451786, 6.054752690667223547, 3.707466751127219781E-16 ) ) ;
#72349=CARTESIAN_POINT ( 'NONE',  ( -2.000000000000000000, 12.27500000000000036, 26.53589838486224650 ) ) ;
#72350=VERTEX_POINT ( 'NONE', #46826 ) ;
#72351=CARTESIAN_POINT ( 'NONE',  ( 17.80312500061451786, -4.541064518000417216, -2.621784821875001281 ) ) ;
#72352=CARTESIAN_POINT ( 'NONE',  ( 27.90000000122903145, -2.886751345948129988, 4.999999999999997335 ) ) ;
#72353=CARTESIAN_POINT ( 'NONE',  ( 16.28437500061452070, 4.541064518000418104, 2.621784821874999949 ) ) ;
#72354=CARTESIAN_POINT ( 'NONE',  ( 5.800002967315412761, 8.146762937617081590, -31.58794104515360601 ) ) ;
#72355=CARTESIAN_POINT ( 'NONE',  ( 17.54062500061451502, 6.054752690667223547, 3.707466751127219781E-16 ) ) ;
#72356=CARTESIAN_POINT ( 'NONE',  ( 1.071796769724476572, 14.39509619066136636, -25.99999999999999289 ) ) ;
#72357=CARTESIAN_POINT ( 'NONE',  ( 25.35937500061451644, 0.000000000000000000, 5.243569643749999010 ) ) ;
#72358=CARTESIAN_POINT ( 'NONE',  ( 4.243569643749999898, 12.79062500061451679, 32.45002607614398471 ) ) ;
#72359=CARTESIAN_POINT ( 'NONE',  ( 15.98437500061451821, -4.541064518000419881, 2.621784821874995952 ) ) ;
#72360=CARTESIAN_POINT ( 'NONE',  ( 14.77500000122903501, 2.886751345948126879, 4.999999999999999112 ) ) ;
#72362=CARTESIAN_POINT ( 'NONE',  ( -2.121784821874996840, 19.48437500061451644, -26.32496088578401583 ) ) ;
#72363=CARTESIAN_POINT ( 'NONE',  ( 21.15937500061451715, 4.541064518000418104, -2.621784821874998173 ) ) ;
#72364=CARTESIAN_POINT ( 'NONE',  ( 23.36250000122903359, 0.000000000000000000, 4.999999999999998224 ) ) ;
#72366=CARTESIAN_POINT ( 'NONE',  ( 18.00937500061451502, 4.541064518000418104, -2.621784821874998173 ) ) ;
#72367=CARTESIAN_POINT ( 'NONE',  ( 12.66562500061451502, 3.027376345333611329, 5.243569643749999010 ) ) ;
#72368=CARTESIAN_POINT ( 'NONE',  ( -2.121784821874996840, 13.18437500061451750, 33.67503911421598417 ) ) ;
#72369=CARTESIAN_POINT ( 'NONE',  ( 17.99062500061451786, 6.054752690667223547, 3.707466751127219781E-16 ) ) ;
#72370=ORIENTED_EDGE ( 'NONE', *, *, #11236, .F. ) ;
#72372=CARTESIAN_POINT ( 'NONE',  ( 20.58750000000000213, -2.886751345948129988, 4.999999999999997335 ) ) ;
#72373=CARTESIAN_POINT ( 'NONE',  ( 28.31250000122903288, 0.000000000000000000, 4.999999999999998224 ) ) ;
#72374=CARTESIAN_POINT ( 'NONE',  ( 25.22812500061451502, 4.541064518000418104, 2.621784821874999949 ) ) ;
#72375=CARTESIAN_POINT ( 'NONE',  ( 5.053125000614517859, 0.000000000000000000, 5.243569643749999010 ) ) ;
#72376=CARTESIAN_POINT ( 'NONE',  ( 17.85000000122903430, 5.773502691896255534, 3.535250795749688894E-16 ) ) ;
#72377=CARTESIAN_POINT ( 'NONE',  ( 23.27812500061451573, 6.421520780324663323E-16, -5.243569643749999010 ) ) ;
#72378=CARTESIAN_POINT ( 'NONE',  ( 22.16250000000000142, 2.886751345948129099, -4.999999999999998224 ) ) ;
#72379=CARTESIAN_POINT ( 'NONE',  ( 25.71562500061451573, 3.027376345333611329, 5.243569643749999010 ) ) ;
#72380=CARTESIAN_POINT ( 'NONE',  ( 6.215625000614517504, 3.027376345333613106, -5.243569643749998122 ) ) ;
#72381=ORIENTED_EDGE ( 'NONE', *, *, #36827, .T. ) ;
#72382=CARTESIAN_POINT ( 'NONE',  ( 29.32499999999999929, 6.123233995736764310E-16, -4.999999999999998224 ) ) ;
#72383=CARTESIAN_POINT ( 'NONE',  ( 2.915625000614516793, -6.054752690667223547, -1.112240025338166033E-15 ) ) ;
#72385=CARTESIAN_POINT ( 'NONE',  ( 3.999999999999999112, 14.48750000122903536, -30.00000000000000000 ) ) ;
#72386=CARTESIAN_POINT ( 'NONE',  ( 2.121784821875001281, 18.20937500061451786, -26.32496088578401938 ) ) ;
#72387=CARTESIAN_POINT ( 'NONE',  ( 11.88749999999999751, 5.773502691896255534, 3.535250795749688894E-16 ) ) ;
#72388=( BOUNDED_CURVE ( )  B_SPLINE_CURVE ( 2, ( #57167, #18000, #62720, #45742, #6579, #68277, #7656 ),
 .UNSPECIFIED., .F., .F. ) 
 B_SPLINE_CURVE_WITH_KNOTS ( ( 3, 2, 2, 3 ),
 ( 0.1166666666666666824, 0.1194444444444444642, 0.1222222222222222182, 0.1250000000000000000 ),
 .UNSPECIFIED. ) 
 CURVE ( )  GEOMETRIC_REPRESENTATION_ITEM ( )  RATIONAL_B_SPLINE_CURVE ( ( 0.9999999999999993339, 0.8660254037844393737, 1.000000000000000000, 0.8660254037844387076, 1.000000000000000000, 0.8660254037844387076, 1.000000000000000000 ) ) 
 REPRESENTATION_ITEM ( '' )  );
#72389=CARTESIAN_POINT ( 'NONE',  ( 9.309375000614517504, -4.541064518000417216, -2.621784821875001281 ) ) ;
#72390=CARTESIAN_POINT ( 'NONE',  ( 6.450000001229034829, -2.886751345948125991, -5.000000000000000000 ) ) ;
#72391=CARTESIAN_POINT ( 'NONE',  ( 12.19687500061451679, 6.054752690667223547, 3.707466751127219781E-16 ) ) ;
#72392=CARTESIAN_POINT ( 'NONE',  ( 6.909375000614518036, 0.000000000000000000, 5.243569643749999010 ) ) ;
#72393=CARTESIAN_POINT ( 'NONE',  ( 27.97500000000000142, 6.123233995736764310E-16, -4.999999999999998224 ) ) ;
#72394=LINE ( 'NONE', #26609, #571 ) ;
#72395=CARTESIAN_POINT ( 'NONE',  ( 11.33437500061451608, 4.541064518000418104, 2.621784821874999949 ) ) ;
#72396=FACE_OUTER_BOUND ( 'NONE', #19337, .T. ) ;
#72397=CARTESIAN_POINT ( 'NONE',  ( 20.65312500061451573, 4.541064518000418104, -2.621784821874998173 ) ) ;
#72399=CARTESIAN_POINT ( 'NONE',  ( 0.000000000000000000, 20.00000000000000000, -30.00000000000000000 ) ) ;
#72400=CARTESIAN_POINT ( 'NONE',  ( 23.37187500061451573, 3.027376345333613106, -5.243569643749998122 ) ) ;
#72401=CARTESIAN_POINT ( 'NONE',  ( 4.428044609675158227, 2.322158679919935409, 4.428044609675073850 ) ) ;
#72402=CARTESIAN_POINT ( 'NONE',  ( 28.27500000122903145, 2.886751345948126879, 4.999999999999999112 ) ) ;
#72404=CARTESIAN_POINT ( 'NONE',  ( 24.29062500061451502, 6.054752690667223547, 3.707466751127219781E-16 ) ) ;
#72405=CARTESIAN_POINT ( 'NONE',  ( 15.89062500061451289, -3.027376345333614438, 5.243569643749998122 ) ) ;
#72407=CARTESIAN_POINT ( 'NONE',  ( 14.44687500061451679, 6.054752690667223547, 3.707466751127219781E-16 ) ) ;
#72408=CARTESIAN_POINT ( 'NONE',  ( 7.275000001229035007, -5.773502691896255534, -1.060575238724906372E-15 ) ) ;
#72409=CARTESIAN_POINT ( 'NONE',  ( 24.52500000122903145, 2.886751345948129099, -4.999999999999998224 ) ) ;
#72410=CARTESIAN_POINT ( 'NONE',  ( 4.546875000614517326, 6.054752690667223547, 3.707466751127219781E-16 ) ) ;
#72411=CARTESIAN_POINT ( 'NONE',  ( 14.44687500061451679, 6.054752690667223547, 3.707466751127219781E-16 ) ) ;
#72412=CARTESIAN_POINT ( 'NONE',  ( 16.19999999999999929, -4.330127018922190985, -2.500000000000001332 ) ) ;
#72414=CARTESIAN_POINT ( 'NONE',  ( 3.187500001229033764, -4.330127018922194537, 2.499999999999995559 ) ) ;
#72415=CARTESIAN_POINT ( 'NONE',  ( 25.35937500061451644, 0.000000000000000000, 5.243569643749999010 ) ) ;
#72416=CARTESIAN_POINT ( 'NONE',  ( 16.17187500061451644, 3.027376345333613106, -5.243569643749998122 ) ) ;
#72418=CARTESIAN_POINT ( 'NONE',  ( 27.44999999999999929, -4.330127018922190985, -2.500000000000001332 ) ) ;
#72419=CARTESIAN_POINT ( 'NONE',  ( 3.300000001229034918, -2.886751345948125991, -5.000000000000000000 ) ) ;
#72420=CARTESIAN_POINT ( 'NONE',  ( 4.875000000000000888, -4.330127018922194537, 2.499999999999995559 ) ) ;
#72422=CARTESIAN_POINT ( 'NONE',  ( 20.27812500061451573, 4.541064518000418104, 2.621784821874999949 ) ) ;
#72423=CARTESIAN_POINT ( 'NONE',  ( 10.38750000000000107, -2.886751345948125991, -5.000000000000000000 ) ) ;
#72424=CARTESIAN_POINT ( 'NONE',  ( 3.290625000614516793, -3.027376345333614438, 5.243569643749998122 ) ) ;
#72425=CARTESIAN_POINT ( 'NONE',  ( 17.39999999999999858, 0.000000000000000000, 4.999999999999998224 ) ) ;
#72427=CARTESIAN_POINT ( 'NONE',  ( 20.17500000122903359, 2.886751345948126879, 4.999999999999999112 ) ) ;
#72429=CARTESIAN_POINT ( 'NONE',  ( 29.29687500061451644, 6.054752690667223547, 3.707466751127219781E-16 ) ) ;
#72430=ORIENTED_EDGE ( 'NONE', *, *, #29578, .F. ) ;
#72431=CARTESIAN_POINT ( 'NONE',  ( 17.24062500061451786, -3.027376345333614438, 5.243569643749998122 ) ) ;
#72432=CARTESIAN_POINT ( 'NONE',  ( 25.04062500061451502, -3.027376345333610441, -5.243569643749999898 ) ) ;
#72433=CARTESIAN_POINT ( 'NONE',  ( 21.98437500061451644, 6.421520780324663323E-16, -5.243569643749999010 ) ) ;
#72434=CARTESIAN_POINT ( 'NONE',  ( 6.150000000000003020, 0.000000000000000000, 4.999999999999998224 ) ) ;
#72435=CARTESIAN_POINT ( 'NONE',  ( 9.403125000614517504, 4.541064518000418104, -2.621784821874998173 ) ) ;
#72436=CARTESIAN_POINT ( 'NONE',  ( 23.16562500061451502, -6.054752690667223547, -1.112240025338166033E-15 ) ) ;
#72437=CARTESIAN_POINT ( 'NONE',  ( 15.19687500061451857, -3.027376345333610441, -5.243569643749999898 ) ) ;
#72438=CARTESIAN_POINT ( 'NONE',  ( 19.20937500061451786, -4.541064518000417216, -2.621784821875001281 ) ) ;
#72439=CARTESIAN_POINT ( 'NONE',  ( 2.000000000000001332, 11.71250000122903501, -26.53589838486224650 ) ) ;
#72440=CARTESIAN_POINT ( 'NONE',  ( 9.001249775931846008E-16, 10.97187500061451715, 34.90005215228797653 ) ) ;
#72441=CARTESIAN_POINT ( 'NONE',  ( 20.85000000122903430, -2.886751345948125991, -5.000000000000000000 ) ) ;
#72443=CARTESIAN_POINT ( 'NONE',  ( 10.79062500061451679, 6.054752690667223547, 3.707466751127219781E-16 ) ) ;
#72444=CARTESIAN_POINT ( 'NONE',  ( 7.284375000614518036, 4.541064518000418104, 2.621784821874999949 ) ) ;
#72445=CARTESIAN_POINT ( 'NONE',  ( 6.834375000614518747, 4.541064518000418104, 2.621784821874999949 ) ) ;
#72446=ORIENTED_EDGE ( 'NONE', *, *, #57275, .T. ) ;
#72447=CARTESIAN_POINT ( 'NONE',  ( 28.58437500061451786, -4.541064518000419881, 2.621784821874995952 ) ) ;
#72448=CARTESIAN_POINT ( 'NONE',  ( 18.25312500061451715, -4.541064518000417216, -2.621784821875001281 ) ) ;
#72449=CARTESIAN_POINT ( 'NONE',  ( 29.17500000122903714, 2.886751345948126879, 4.999999999999999112 ) ) ;
#72450=EDGE_CURVE ( 'NONE', #47076, #29843, #25372, .T. ) ;
#72451=CARTESIAN_POINT ( 'NONE',  ( 28.11562500061451431, -6.054752690667223547, -1.112240025338166033E-15 ) ) ;
#72452=CARTESIAN_POINT ( 'NONE',  ( 24.68437500061451573, 6.421520780324663323E-16, -5.243569643749999010 ) ) ;
#72453=CARTESIAN_POINT ( 'NONE',  ( 19.94062500061451715, -3.027376345333614438, 5.243569643749998122 ) ) ;
#72454=CARTESIAN_POINT ( 'NONE',  ( -4.243569643749999898, 19.82187500061451857, 27.54997392385601529 ) ) ;
#72455=CARTESIAN_POINT ( 'NONE',  ( 25.04062500061451502, -3.027376345333610441, -5.243569643749999898 ) ) ;
#72456=CARTESIAN_POINT ( 'NONE',  ( 3.712500001229034563, -4.330127018922190985, -2.500000000000001332 ) ) ;
#72458=CARTESIAN_POINT ( 'NONE',  ( 28.46249999999999858, 2.886751345948129099, -4.999999999999998224 ) ) ;
#72459=CARTESIAN_POINT ( 'NONE',  ( 3.999999999999998668, 15.76249999999999751, -32.30940107675850470 ) ) ;
#72461=CARTESIAN_POINT ( 'NONE',  ( 3.871875000614519280, -6.054752690667223547, -1.112240025338166033E-15 ) ) ;
#72462=CARTESIAN_POINT ( 'NONE',  ( 12.44062500061451537, -3.027376345333610441, -5.243569643749999898 ) ) ;
#72463=CARTESIAN_POINT ( 'NONE',  ( 6.271875000614517859, 3.027376345333613106, -5.243569643749998122 ) ) ;
#72464=CARTESIAN_POINT ( 'NONE',  ( 23.62500000122902932, 2.886751345948129099, -4.999999999999998224 ) ) ;
#72465=CARTESIAN_POINT ( 'NONE',  ( 14.82187500061451502, 3.027376345333612662, -5.243569643749998122 ) ) ;
#72466=CARTESIAN_POINT ( 'NONE',  ( 2.971875000614517592, -6.054752690667223547, -1.112240025338166033E-15 ) ) ;
#72467=CARTESIAN_POINT ( 'NONE',  ( -1.071796769724491005, 10.90759618943233455, 26.00000000000000355 ) ) ;
#72468=CARTESIAN_POINT ( 'NONE',  ( 27.15937500061451360, 0.000000000000000000, 5.243569643749999010 ) ) ;
#72469=CARTESIAN_POINT ( 'NONE',  ( 3.440625000614518036, -3.027376345333610441, -5.243569643749999898 ) ) ;
#72470=CARTESIAN_POINT ( 'NONE',  ( 13.71562500061451750, -6.054752690667223547, -1.112240025338166033E-15 ) ) ;
#72471=ORIENTED_EDGE ( 'NONE', *, *, #48761, .F. ) ;
#72472=CARTESIAN_POINT ( 'NONE',  ( 11.27812500061451573, 4.541064518000418104, 2.621784821874999949 ) ) ;
#72474=CARTESIAN_POINT ( 'NONE',  ( 9.365625000614519635, 3.027376345333613106, -5.243569643749998122 ) ) ;
#72476=CARTESIAN_POINT ( 'NONE',  ( 9.112500000000000711, 2.886751345948129099, -4.999999999999998224 ) ) ;
#72477=CARTESIAN_POINT ( 'NONE',  ( 1.510657702057710734E-15, 19.43750000000000000, 26.00000000000000000 ) ) ;
#72478=CARTESIAN_POINT ( 'NONE',  ( 16.80000000000000071, 4.330127018922192761, -2.499999999999997780 ) ) ;
#72479=CARTESIAN_POINT ( 'NONE',  ( 18.90937500061451360, 4.541064518000418104, -2.621784821874998173 ) ) ;
#72480=CARTESIAN_POINT ( 'NONE',  ( 12.75000000122903643, -2.886751345948125991, -5.000000000000000000 ) ) ;
#72482=CARTESIAN_POINT ( 'NONE',  ( 4.243569643749999898, 16.42812500061451786, -30.00000000000000000 ) ) ;
#72483=FACE_OUTER_BOUND ( 'NONE', #64479, .T. ) ;
#72486=CARTESIAN_POINT ( 'NONE',  ( 27.06562500061451004, 3.027376345333611329, 5.243569643749999010 ) ) ;
#72487=CARTESIAN_POINT ( 'NONE',  ( 2.000000000000001332, 19.69999999999999929, 33.46410161513774995 ) ) ;
#72488=DIRECTION ( 'NONE',  ( 0.000000000000000000, 0.000000000000000000, 1.000000000000000000 ) ) ;
#72489=CARTESIAN_POINT ( 'NONE',  ( 25.91250000000000142, 2.886751345948126879, 4.999999999999999112 ) ) ;
#72491=CARTESIAN_POINT ( 'NONE',  ( 9.815625000614518925, 3.027376345333613106, -5.243569643749998122 ) ) ;
#72493=CARTESIAN_POINT ( 'NONE',  ( 21.42187500061451644, -6.054752690667223547, -1.112240025338166033E-15 ) ) ;
#72496=CARTESIAN_POINT ( 'NONE',  ( 8.240625000614516082, -3.027376345333614438, 5.243569643749998122 ) ) ;
#72497=CARTESIAN_POINT ( 'NONE',  ( 9.646875000614516082, -3.027376345333614438, 5.243569643749998122 ) ) ;
#72498=ORIENTED_EDGE ( 'NONE', *, *, #826, .T. ) ;
#72499=CARTESIAN_POINT ( 'NONE',  ( 22.47187500061451715, 3.027376345333613106, -5.243569643749998122 ) ) ;
#72500=CARTESIAN_POINT ( 'NONE',  ( 29.51249999999999929, 2.886751345948126879, 4.999999999999999112 ) ) ;
#72501=CARTESIAN_POINT ( 'NONE',  ( 4.087500000000001243, -2.886751345948125991, -5.000000000000000000 ) ) ;
#72502=CARTESIAN_POINT ( 'NONE',  ( 14.55000000122903181, -2.886751345948125991, -5.000000000000000000 ) ) ;
#72504=CARTESIAN_POINT ( 'NONE',  ( 14.40000000122902790, -2.886751345948063374, 5.000000000000112799 ) ) ;
#72506=CARTESIAN_POINT ( 'NONE',  ( 13.76250000000000107, 2.886751345948126879, 4.999999999999999112 ) ) ;
#72507=CARTESIAN_POINT ( 'NONE',  ( 17.69999999999999929, 4.330127018922192761, -2.499999999999997780 ) ) ;
#72509=CARTESIAN_POINT ( 'NONE',  ( 13.61250000122903359, -4.330127018922190985, -2.500000000000001332 ) ) ;
#72510=CARTESIAN_POINT ( 'NONE',  ( 12.14062500061451821, 6.054752690667223547, 3.707466751127219781E-16 ) ) ;
#72511=ORIENTED_EDGE ( 'NONE', *, *, #10210, .T. ) ;
#72512=CARTESIAN_POINT ( 'NONE',  ( 8.550000000000002487, -4.330127018922190985, -2.500000000000001332 ) ) ;
#72513=CARTESIAN_POINT ( 'NONE',  ( 26.39999999999999858, 0.000000000000000000, 4.999999999999998224 ) ) ;
#72514=CARTESIAN_POINT ( 'NONE',  ( 4.243569643749999010, 14.27187500061451964, -32.45002607614398471 ) ) ;
#72515=CARTESIAN_POINT ( 'NONE',  ( 27.33750000122903145, 4.330127018922191873, 2.499999999999999556 ) ) ;
#72517=CARTESIAN_POINT ( 'NONE',  ( 9.674999999999998934, 4.330127018922191873, 2.499999999999999556 ) ) ;
#72521=CARTESIAN_POINT ( 'NONE',  ( 23.80312500061451786, 4.541064518000418104, -2.621784821874998173 ) ) ;
#72522=CARTESIAN_POINT ( 'NONE',  ( 3.999999999999999112, 13.47500000000000142, -30.00000000000000000 ) ) ;
#72524=CARTESIAN_POINT ( 'NONE',  ( 20.74687500061451573, 6.054752690667223547, 3.707466751127219781E-16 ) ) ;
#72525=EDGE_CURVE ( 'NONE', #14829, #43953, #5236, .T. ) ;
#72526=CARTESIAN_POINT ( 'NONE',  ( 17.24062500061451786, -3.027376345333614438, 5.243569643749998122 ) ) ;
#72527=CARTESIAN_POINT ( 'NONE',  ( -3.000416591977282496E-16, 11.59062500061459389, -34.90005215228797653 ) ) ;
#72528=CARTESIAN_POINT ( 'NONE',  ( 5.503125000614516260, 0.000000000000000000, 5.243569643749999010 ) ) ;
#72529=CARTESIAN_POINT ( 'NONE',  ( 29.58750000122903501, 4.330127018922191873, 2.499999999999999556 ) ) ;
#72531=CARTESIAN_POINT ( 'NONE',  ( 18.10312500061451502, 0.000000000000000000, 5.243569643749999010 ) ) ;
#72534=CARTESIAN_POINT ( 'NONE',  ( 13.99687500061451928, 6.054752690667223547, 3.707466751127219781E-16 ) ) ;
#72535=CARTESIAN_POINT ( 'NONE',  ( 14.78437500061451715, 6.421520780324663323E-16, -5.243569643749999010 ) ) ;
#72536=CARTESIAN_POINT ( 'NONE',  ( 22.35937500061451644, -4.541064518000417216, -2.621784821875001281 ) ) ;
#72537=VERTEX_POINT ( 'NONE', #19822 ) ;
#72538=CARTESIAN_POINT ( 'NONE',  ( -2.121784821874996840, 12.28437500061451892, 33.67503911421598417 ) ) ;
#72539=CARTESIAN_POINT ( 'NONE',  ( 3.515625000614516882, 3.027376345333613106, -5.243569643749998122 ) ) ;
#72540=CARTESIAN_POINT ( 'NONE',  ( 27.14062500061451644, -3.027376345333614438, 5.243569643749998122 ) ) ;
#72541=CARTESIAN_POINT ( 'NONE',  ( 26.46562500061451573, 3.027376345333613106, -5.243569643749998122 ) ) ;
#72543=CARTESIAN_POINT ( 'NONE',  ( -2.828200636599751609E-16, 17.18750000000000000, 25.38119784648299770 ) ) ;
#72544=CARTESIAN_POINT ( 'NONE',  ( 4.246875000614519280, -3.027376345333614438, 5.243569643749998122 ) ) ;
#72545=CARTESIAN_POINT ( 'NONE',  ( 12.33750000122903145, 6.123233995736764310E-16, -4.999999999999998224 ) ) ;
#72546=AXIS2_PLACEMENT_3D ( 'NONE', #38509, #43689, #33325 ) ;
#72547=CARTESIAN_POINT ( 'NONE',  ( 9.450000001229033941, -2.886751345948129988, 4.999999999999997335 ) ) ;
#72548=CARTESIAN_POINT ( 'NONE',  ( 3.740625000614516527, -3.027376345333614438, 5.243569643749998122 ) ) ;
#72551=CARTESIAN_POINT ( 'NONE',  ( 12.19687500061451679, 6.054752690667223547, 3.707466751127219781E-16 ) ) ;
#72552=CARTESIAN_POINT ( 'NONE',  ( 26.51250000122903216, 0.000000000000000000, 4.999999999999998224 ) ) ;
#72553=ORIENTED_EDGE ( 'NONE', *, *, #41935, .F. ) ;
#72554=CARTESIAN_POINT ( 'NONE',  ( 20.69062500061451715, 6.054752690667223547, 3.707466751127219781E-16 ) ) ;
#72555=CARTESIAN_POINT ( 'NONE',  ( 14.10937500061451644, 0.000000000000000000, 5.243569643749999010 ) ) ;
#72556=CARTESIAN_POINT ( 'NONE',  ( 5.578125000614518214, -4.541064518000419881, 2.621784821874995952 ) ) ;
#72557=CARTESIAN_POINT ( 'NONE',  ( 21.19687500061451502, 6.054752690667223547, 3.707466751127219781E-16 ) ) ;
#72558=CARTESIAN_POINT ( 'NONE',  ( 4.678125000614516971, -4.541064518000419881, 2.621784821874995952 ) ) ;
#72559=DIRECTION ( 'NONE',  ( -0.000000000000000000, -1.000000000000000000, -0.000000000000000000 ) ) ;
#72560=( BOUNDED_SURFACE ( )  B_SPLINE_SURFACE ( 1, 2, ( 
 ( #14503, #54768, #20405, #49598, #9701, #66214, #37771, #43329, #10433, #32963, #4539, #31506, #25595, #15233, #54046, #32234, #3064, #48867, #32602, #42587, #8974, #55140, #4173, #65113, #25961, #27066, #48133, #66584, #72124, #71027, #26703, #71769, #49236, #21505, #14871, #44058, #15961, #70657, #38511, #20031, #37410, #59932, #9340, #31872, #3807, #26329, #71398, #39608, #55866, #17762, #62129, #27797, #44795, #72858, #50334, #33686, #45147, #443, #90, #56582, #16328, #34406, #22597, #66962, #28509, #811, #55500, #5979, #44434, #38882, #28869, #12237, #39970, #72486, #68043, #6339, #17413, #22952, #40322, #39244, #67680, #56934, #51048, #33328, #11521, #17051, #45513, #62484, #61399, #10793, #34043, #67329, #5255, #11882, #51408, #11161, #23318, #45868, #68401, #5624, #62844, #4896, #28160, #27430, #22241, #49962, #21872, #16688, #61758, #56230, #50688, #41766, #64295, #13682, #40689, #41057, #8153, #30324, #52854, #58015, #1534, #19581, #18124, #47671, #23680, #24041, #46227, #19211, #42137, #1171, #52491, #64663, #34768, #46591, #69845, #24768, #57301, #35495, #18851, #68766, #29594, #63207, #41412, #12602, #69133, #1902, #69492, #35135, #18492, #57660, #6706, #36226, #70206, #29239, #58742, #30680, #63570, #25130, #7066, #63928, #51772, #52131, #12958, #24406, #7423, #29951, #46956, #13313, #35852, #58375, #7787, #53212, #2253, #47311, #2608, #4083, #9616, #70576, #38045, #8886, #65027, #3356, #32147, #26613, #14418, #37324, #70944, #43971, #4452, #42869, #54680, #42504, #9252, #8515, #20315, #21414, #59847, #59474, #49150, #21053, #43604, #31044, #71679, #65762, #53582, #14048, #31419, #36953, #43242, #72038, #19951, #26244, #53959, #25878, #2978, #48417, #36588, #65391, #66125, #15504, #9977, #14782, #60570, #25506, #32514, #48781, #3717, #31787, #54326, #55051, #71306, #59109, #48051, #20683, #15144, #37681, #26981, #60204, #49510, #49872, #57485, #50244, #67239, #40511, #72397, #27703, #33239, #44342, #32875, #3, #33594, #39150, #1355, #18307, #60941, #72766, #16239, #1714, #46412, #29776, #24227, #68949, #29421, #22151, #57838, #66870, #28070, #66491, #52312, #10345, #56139, #16597, #44704, #7247, #61668, #4809, #21778, #38794, #40879, #50599, #55776, #61311, #6889, #63026, #10706, #63394, #5168, #11067, #5533, #12425, #51955, #22510, #46053, #68587, #15872, #38419, #17949, #34958, #23864, #12779, #55414, #35316, #27341, #19396, #19033, #42321, #53772, #3168, #63747, #64846, #25319, #13136, #3535, #41591, #47136, #2793, #31604, #52671, #58925, #2079, #64109, #35675, #13494, #46777, #36042, #14234, #36772, #42685, #69667, #59289, #58198, #31230, #8333, #36411, #41957, #58563, #8698, #7970, #54141, #7601, #30863, #64478, #69312, #65207, #24588, #25695, #30140, #48231, #30506, #47494, #19770, #53033, #2428, #24951, #70025, #13871, #53401, #47865, #70394, #70755, #20130, #41235, #14597, #18673, #37132, #59661, #9069, #10891, #37869, #61134, #16062, #26058, #26798, #10168, #14967, #20873, #37505, #32702, #60025, #60388, #43788, #60760, #54502, #3904, #55239, #48598, #71864, #10531, #65577, #31965, #44159, #66315, #9437, #26426, #4993, #71123, #16420, #21971, #48966, #4634, #21604, #27164, #15692, #43426, #66687, #27525, #20495, #38611, #49698, #72225, #50059, #33059, #9796, #55598, #15327, #4274, #72588, #71496, #61494, #44530, #65948, #32329, #54866, #49332, #21236, #38231, #67063, #38978, #33419, #55960, #43051, #45609, #16784, #51509, #23773, #5355, #6437, #67422, #39342, #51864, #35231, #62937, #22335, #17861, #29334, #40420, #45964, #63302, #62226, #23054, #6800, #909, #56327, #62582, #68143, #68497, #12331, #61855, #11262, #11979, #67776, #33784, #34866, #17507, #34138, #57393, #34502, #40068, #28608, #12694, #57030, #51144, #28971, #5716, #23417, #1266, #46325, #40789, #27893, #68860, #18216, #50427, #72953, #28252, #11622, #44887, #50783, #186, #544, #45242, #22691, #17150, #39708, #56677, #6075, #69226, #41152, #18587, #36323, #1993, #31140, #41861, #2708, #19308, #24861, #42597, #65123, #59203, #13051, #7160, #47408, #64757, #63660, #64023, #53681, #53309, #25224, #7883, #24504, #14513, #35590, #70666, #46688, #47048, #58109, #7516, #30047, #58838, #69582, #3076, #64391, #47770, #13781, #69938, #57752, #29689, #8611, #52587, #52226, #8248, #18944, #30778, #1630, #30419, #42232, #24137, #41503, #70306, #2344, #13402, #35950, #36682, #58470, #48142, #25604, #52947, #19679, #14147, #20042, #54777, #54416, #55149, #15971, #31516, #27076, #60667, #43702, #61044, #21514, #20782, #21148, #26338, #15242, #66223, #37419, #72496, #15602, #9349, #48877, #3817, #31882, #37779, #26711, #4547, #4183, #38143, #71038, #38521, #49245, #48511, #10081, #55512, #37046, #32611, #25970, #20413, #10442, #66970, #44068, #54057, #49607, #32972, #72134, #66595, #21881, #43338, #71780, #4905, #27441, #14880, #49971, #44441, #59571, #8984, #42961, #65490, #3452, #71407, #59942, #65860, #60299, #9710, #32244, #452, #51057, #39619, #23687, #45522, #62137, #68052, #22249, #5987, #56591, #28517, #51779, #16335, #22961, #23327, #45877, #67688, #17421, #16696, #1179, #39980, #61766, #5632, #33694, #11170, #17059, #62492, #34415, #34051, #11890, #50342, #68409, #56943, #27808, #6347, #34777, #38890, #28878, #5262, #72866, #62852, #46235, #819, #33337, #51418, #40331, #17771, #12246, #61408, #98, #57310, #6714, #29247, #67336, #10802, #55875, #44803, #39254, #56241, #28169, #50696, #22604, #45156, #11531, #7797, #24415, #30690, #52863, #30335, #18860, #2986, #24777, #41421, #47321, #1542, #58384, #35861, #2263, #31054, #68775, #69854, #2618, #25139, #47680, #24052, #1911, #42146, #64304, #13694, #63937, #35504, #53591, #52139, #8525, #57668, #58023, #7074, #46599 ),
 ( #19221, #7433, #63579, #58751, #36237, #69141, #19590, #12966, #18500, #29959, #8161, #53221, #41065, #13322, #52500, #25514, #59118, #46964, #70216, #69500, #41775, #63216, #64673, #18131, #14058, #36597, #40698, #12611, #35145, #29603, #65772, #65401, #66138, #26994, #42512, #38058, #71693, #54693, #72048, #32526, #31796, #32160, #37334, #26253, #4096, #48427, #10357, #26625, #20324, #59857, #14792, #42878, #48790, #37691, #15516, #15154, #49162, #8896, #49523, #60214, #59484, #21065, #66504, #48059, #43616, #36962, #31428, #21426, #4819, #55063, #65036, #60583, #43983, #9991, #4464, #32887, #54334, #9627, #15886, #38431, #25887, #60955, #55427, #70584, #19960, #53968, #3366, #14427, #9261, #70953, #3728, #71317, #20693, #43252, #11448, #62053, #50611, #34691, #56507, #15, #5900, #33251, #16971, #67606, #39527, #62772, #27353, #33968, #34326, #56858, #6264, #55789, #33607, #735, #22873, #45431, #22522, #67251, #12163, #10719, #40251, #16250, #16609, #38806, #5179, #61321, #28433, #44715, #23244, #50970, #67965, #366, #17338, #57222, #49884, #28792, #27716, #72409, #39897, #39165, #21791, #45795, #11079, #11809, #66883, #50256, #62410, #45069, #72780, #22163, #51333, #44357, #17690, #68330, #61680, #56151, #5545, #28083, #8077, #2180, #57588, #63850, #24331, #47237, #41692, #40611, #18053, #13241, #69054, #63132, #64215, #18774, #35418, #13604, #35779, #41340, #29880, #13974, #58302, #52416, #7711, #12528, #69419, #46880, #30245, #42063, #6635, #52778, #36150, #58669, #30609, #35061, #12885, #53137, #24693, #69770, #1824, #46515, #64586, #6991, #19506, #68693, #18416, #29522, #52057, #1461, #19138, #23967, #2536, #25056, #47599, #70128, #36512, #29164, #51696, #1100, #40982, #23608, #46153, #63497, #57943, #7350, #42790, #43529, #25428, #64950, #4010, #3640, #47971, #14342, #37973, #59032, #49433, #54972, #42429, #65683, #54605, #20604, #26164, #3273, #26533, #60494, #53505, #49073, #9539, #15071, #9900, #66051, #65311, #43163, #48339, #37245, #37608, #59394, #21341, #60130, #31340, #70864, #25801, #53881, #59766, #48703, #71601, #71226, #32073, #19876, #32436, #20976, #70499, #15429, #4378, #8434, #26907, #36876, #8804, #71967, #15798, #43896, #2897, #66420, #30970, #20238, #14701, #9173, #31708, #54243, #284, #72326, #49801, #22436, #27631, #21706, #22792, #50526, #67164, #45345, #44984, #73054, #61594, #45711, #67521, #10995, #16886, #44263, #27997, #5457, #39440, #649, #38338, #61960, #67879, #17251, #39811, #66796, #44635, #11723, #33882, #56427, #33515, #5095, #23157, #16167, #51246, #27268, #50164, #38719, #61239, #10633, #11364, #55701, #34239, #5816, #28347, #50884, #62327, #68245, #60867, #56773, #33163, #10270, #6178, #72694, #32803, #28707, #22076, #55339, #4734, #16525, #39077, #56064, #57134, #46069, #69686, #17608, #7989, #13514, #1013, #24245, #13153, #52330, #35333, #34974, #35695, #19051, #12083, #7620, #41253, #46794, #41609, #2096, #1372, #1732, #6905, #68968, #69331, #17965, #53052, #18689, #63042, #29436, #57503, #12442, #18324, #7265, #58215, #57856, #63765, #51612, #64128, #29794, #29077, #30156, #36061, #40168, #52690, #6543, #23519, #58582, #47514, #24607, #34604, #47154, #30525, #2446, #24969, #62687, #23882, #68604, #40526, #46429, #51973, #40898, #63411, #12797, #15615, #36429, #25340, #49984, #70043, #61422, #66984, #53422, #4561, #66609, #32624, #38157, #14252, #15984, #72509, #64497, #61057, #21526, #27089, #21897, #55525, #53790, #55164, #59306, #48251, #49621, #70414, #33350, #72148, #42341, #8717, #36791, #64864, #70774, #60680, #38534, #10094, #44082, #30880, #44454, #10456, #8351, #32985, #16348, #19416, #4919, #58943, #2812, #38903, #27822, #27454, #13889, #10816, #55888, #5276, #41976, #47885, #3186, #19790, #31249, #25713, #20150, #42704, #65226, #17785, #12261, #11184, #61780, #34429, #39633, #33709, #34791, #62506, #6001, #57324, #56958, #11905, #468, #57683, #6361, #22976, #28893, #56256, #39993, #17435, #51432, #12624, #50354, #834, #6728, #29262, #51792, #5646, #56605, #23701, #45891, #68423, #45538, #17073, #35159, #28182, #63230, #39268, #62151, #50710, #114, #22619, #23343, #67701, #46249, #40345, #62865, #1193, #68790, #7088, #72881, #18146, #45170, #22263, #40713, #11548, #44816, #67350, #16712, #34064, #28534, #51070, #68067, #2632, #24791, #52876, #35874, #58037, #8174, #7447, #8539, #46612, #2274, #58398, #31067, #64686, #12982, #36250, #63593, #30702, #69514, #63951, #13707, #41080, #46978, #1924, #35518, #69155, #69867, #30348, #7812, #25153, #19603, #24067, #53235, #53605, #18514, #47334, #29617, #52153, #18873, #47693, #70229, #1556, #58764, #42159, #41435, #19233, #13336, #14071, #41787, #64317, #36610, #59131, #29973, #52515, #24429, #29859, #1438, #57921, #52395, #23944, #57565, #51308, #12864, #22852, #57197, #22500, #7328, #39503, #62750, #23219, #67942, #16950, #50948, #39875, #28411, #346, #46493, #6612, #62387, #17315, #12509, #18033, #5879, #69032, #11786, #45407, #34303, #40589, #35037, #56834, #45772, #6242, #45049, #35395, #712, #63110, #28769, #17667, #62027, #68308, #67584, #40228, #12143, #6968, #29499, #52035, #11426, #18394, #1078, #33943, #56486, #34669, #29140, #51673, #23586, #46131, #68669, #40961, #63476, #63828, #41672, #31686, #19117, #42407, #37221, #8414, #47217, #64195, #13582, #69749, #53115, #64565, #19856, #19484, #2877, #35759, #53860, #42042, #13220, #47951, #20215, #1802, #25408, #58280, #7687, #48317, #24312, #59371, #18754, #14320, #25779, #36855, #64929, #59743, #58647, #13953, #3251, #70479, #52757, #59011, #36491, #8782, #31316, #30224, #2160, #30944, #36128, #24671, #70840, #53485, #30590, #42769, #65289, #14677, #25035, #9151, #46860, #47578, #69399, #8055 ) ),
 .UNSPECIFIED., .F., .F., .F. ) 
 B_SPLINE_SURFACE_WITH_KNOTS ( ( 2, 2 ),
 ( 3, 2, 2, 2, 2, 2, 2, 2, 2, 2, 2, 2, 2, 2, 2, 2, 2, 2, 2, 2, 2, 2, 2, 2, 2, 2, 2, 2, 2, 2, 2, 2, 2, 2, 2, 2, 2, 2, 2, 2, 2, 2, 2, 2, 2, 2, 2, 2, 2, 2, 2, 2, 2, 2, 2, 2, 2, 2, 2, 2, 2, 2, 2, 2, 2, 2, 2, 2, 2, 2, 2, 2, 2, 2, 2, 2, 2, 2, 2, 2, 2, 2, 2, 2, 2, 2, 2, 2, 2, 2, 2, 2, 2, 2, 2, 2, 2, 2, 2, 2, 2, 2, 2, 2, 2, 2, 2, 2, 2, 2, 2, 2, 2, 2, 2, 2, 2, 2, 2, 2, 2, 2, 2, 2, 2, 2, 2, 2, 2, 2, 2, 2, 2, 2, 2, 2, 2, 2, 2, 2, 2, 2, 2, 2, 2, 2, 2, 2, 2, 2, 2, 2, 2, 2, 2, 2, 2, 2, 2, 2, 2, 2, 2, 2, 2, 2, 2, 2, 2, 2, 2, 2, 2, 2, 2, 2, 2, 2, 2, 2, 2, 2, 2, 2, 2, 2, 2, 2, 2, 2, 2, 2, 2, 2, 2, 2, 2, 2, 2, 2, 2, 2, 2, 2, 2, 2, 2, 2, 2, 2, 2, 2, 2, 2, 2, 2, 2, 2, 2, 2, 2, 2, 2, 2, 2, 2, 2, 2, 2, 2, 2, 2, 2, 2, 2, 2, 2, 2, 2, 2, 2, 2, 2, 2, 2, 2, 2, 2, 2, 2, 2, 2, 2, 2, 2, 2, 2, 2, 2, 2, 2, 2, 2, 2, 2, 2, 2, 2, 2, 2, 2, 2, 2, 2, 2, 2, 2, 2, 2, 2, 2, 2, 2, 2, 2, 2, 2, 2, 2, 2, 2, 2, 2, 2, 2, 2, 2, 2, 2, 2, 2, 2, 2, 2, 2, 2, 2, 2, 2, 2, 2, 2, 2, 2, 2, 2, 2, 2, 2, 2, 2, 2, 2, 2, 2, 2, 2, 2, 2, 2, 2, 2, 2, 2, 2, 2, 2, 2, 2, 2, 2, 2, 2, 2, 2, 2, 2, 2, 2, 2, 2, 2, 2, 2, 2, 2, 2, 2, 2, 2, 3 ),
 ( 0.000000000000000000, 1.000000000000000000 ),
 ( 0.000000000000000000, 0.002777777777777777884, 0.005555555555555555768, 0.008333333333333333218, 0.01111111111111111154, 0.01388888888888888812, 0.01666666666666666644, 0.01944444444444444475, 0.02222222222222222307, 0.02500000000000000139, 0.02777777777777777624, 0.03055555555555555455, 0.03333333333333333287, 0.03611111111111110772, 0.03888888888888888951, 0.04166666666666666435, 0.04444444444444444614, 0.04722222222222222099, 0.05000000000000000278, 0.05277777777777777762, 0.05555555555555555247, 0.05833333333333333426, 0.06111111111111110911, 0.06388888888888888395, 0.06666666666666666574, 0.06944444444444444753, 0.07222222222222221544, 0.07499999999999999722, 0.07777777777777777901, 0.08055555555555556080, 0.08333333333333332871, 0.08611111111111111049, 0.08888888888888889228, 0.09166666666666666019, 0.09444444444444444198, 0.09722222222222222376, 0.1000000000000000056, 0.1027777777777777735, 0.1055555555555555552, 0.1083333333333333370, 0.1111111111111111049, 0.1138888888888888867, 0.1166666666666666685, 0.1194444444444444503, 0.1222222222222222182, 0.1250000000000000000, 0.1277777777777777679, 0.1305555555555555636, 0.1333333333333333315, 0.1361111111111110994, 0.1388888888888888951, 0.1416666666666666630, 0.1444444444444444309, 0.1472222222222222265, 0.1499999999999999944, 0.1527777777777777901, 0.1555555555555555580, 0.1583333333333333259, 0.1611111111111111216, 0.1638888888888888895, 0.1666666666666666574, 0.1694444444444444531, 0.1722222222222222210, 0.1749999999999999889, 0.1777777777777777846, 0.1805555555555555525, 0.1833333333333333204, 0.1861111111111111160, 0.1888888888888888840, 0.1916666666666666796, 0.1944444444444444475, 0.1972222222222222154, 0.2000000000000000111, 0.2027777777777777790, 0.2055555555555555469, 0.2083333333333333426, 0.2111111111111111105, 0.2138888888888888784, 0.2166666666666666741, 0.2194444444444444420, 0.2222222222222222099, 0.2250000000000000056, 0.2277777777777777735, 0.2305555555555555691, 0.2333333333333333370, 0.2361111111111111049, 0.2388888888888889006, 0.2416666666666666685, 0.2444444444444444364, 0.2472222222222222321, 0.2500000000000000000, 0.2527777777777777679, 0.2555555555555555358, 0.2583333333333333592, 0.2611111111111111271, 0.2638888888888888951, 0.2666666666666666630, 0.2694444444444444309, 0.2722222222222221988, 0.2750000000000000222, 0.2777777777777777901, 0.2805555555555555580, 0.2833333333333333259, 0.2861111111111110938, 0.2888888888888888618, 0.2916666666666666852, 0.2944444444444444531, 0.2972222222222222210, 0.2999999999999999889, 0.3027777777777777568, 0.3055555555555555802, 0.3083333333333333481, 0.3111111111111111160, 0.3138888888888888840, 0.3166666666666666519, 0.3194444444444444198, 0.3222222222222222432, 0.3250000000000000111, 0.3277777777777777790, 0.3305555555555555469, 0.3333333333333333148, 0.3361111111111111382, 0.3388888888888889062, 0.3416666666666666741, 0.3444444444444444420, 0.3472222222222222099, 0.3499999999999999778, 0.3527777777777778012, 0.3555555555555555691, 0.3583333333333333370, 0.3611111111111111049, 0.3638888888888888729, 0.3666666666666666408, 0.3694444444444444642, 0.3722222222222222321, 0.3750000000000000000, 0.3777777777777777679, 0.3805555555555555358, 0.3833333333333333592, 0.3861111111111111271, 0.3888888888888888951, 0.3916666666666666630, 0.3944444444444444309, 0.3972222222222221988, 0.4000000000000000222, 0.4027777777777777901, 0.4055555555555555580, 0.4083333333333333259, 0.4111111111111110938, 0.4138888888888888618, 0.4166666666666666852, 0.4194444444444444531, 0.4222222222222222210, 0.4249999999999999889, 0.4277777777777777568, 0.4305555555555555802, 0.4333333333333333481, 0.4361111111111111160, 0.4388888888888888840, 0.4416666666666666519, 0.4444444444444444198, 0.4472222222222222432, 0.4500000000000000111, 0.4527777777777777790, 0.4555555555555555469, 0.4583333333333333148, 0.4611111111111111382, 0.4638888888888889062, 0.4666666666666666741, 0.4694444444444444420, 0.4722222222222222099, 0.4749999999999999778, 0.4777777777777778012, 0.4805555555555555691, 0.4833333333333333370, 0.4861111111111111049, 0.4888888888888888729, 0.4916666666666666408, 0.4944444444444444642, 0.4972222222222222321, 0.5000000000000000000, 0.5027777777777777679, 0.5055555555555555358, 0.5083333333333333037, 0.5111111111111110716, 0.5138888888888888395, 0.5166666666666667185, 0.5194444444444444864, 0.5222222222222222543, 0.5250000000000000222, 0.5277777777777777901, 0.5305555555555555580, 0.5333333333333333259, 0.5361111111111110938, 0.5388888888888888618, 0.5416666666666666297, 0.5444444444444443976, 0.5472222222222222765, 0.5500000000000000444, 0.5527777777777778123, 0.5555555555555555802, 0.5583333333333333481, 0.5611111111111111160, 0.5638888888888888840, 0.5666666666666666519, 0.5694444444444444198, 0.5722222222222221877, 0.5749999999999999556, 0.5777777777777777235, 0.5805555555555556024, 0.5833333333333333703, 0.5861111111111111382, 0.5888888888888889062, 0.5916666666666666741, 0.5944444444444444420, 0.5972222222222222099, 0.5999999999999999778, 0.6027777777777777457, 0.6055555555555555136, 0.6083333333333332815, 0.6111111111111111605, 0.6138888888888889284, 0.6166666666666666963, 0.6194444444444444642, 0.6222222222222222321, 0.6250000000000000000, 0.6277777777777777679, 0.6305555555555555358, 0.6333333333333333037, 0.6361111111111110716, 0.6388888888888888395, 0.6416666666666667185, 0.6444444444444444864, 0.6472222222222222543, 0.6500000000000000222, 0.6527777777777777901, 0.6555555555555555580, 0.6583333333333333259, 0.6611111111111110938, 0.6638888888888888618, 0.6666666666666666297, 0.6694444444444443976, 0.6722222222222222765, 0.6750000000000000444, 0.6777777777777778123, 0.6805555555555555802, 0.6833333333333333481, 0.6861111111111111160, 0.6888888888888888840, 0.6916666666666666519, 0.6944444444444444198, 0.6972222222222221877, 0.6999999999999999556, 0.7027777777777777235, 0.7055555555555556024, 0.7083333333333333703, 0.7111111111111111382, 0.7138888888888889062, 0.7166666666666666741, 0.7194444444444444420, 0.7222222222222222099, 0.7249999999999999778, 0.7277777777777777457, 0.7305555555555555136, 0.7333333333333332815, 0.7361111111111111605, 0.7388888888888889284, 0.7416666666666666963, 0.7444444444444444642, 0.7472222222222222321, 0.7500000000000000000, 0.7527777777777777679, 0.7555555555555555358, 0.7583333333333333037, 0.7611111111111110716, 0.7638888888888888395, 0.7666666666666667185, 0.7694444444444444864, 0.7722222222222222543, 0.7750000000000000222, 0.7777777777777777901, 0.7805555555555555580, 0.7833333333333333259, 0.7861111111111110938, 0.7888888888888888618, 0.7916666666666666297, 0.7944444444444443976, 0.7972222222222222765, 0.8000000000000000444, 0.8027777777777778123, 0.8055555555555555802, 0.8083333333333333481, 0.8111111111111111160, 0.8138888888888888840, 0.8166666666666666519, 0.8194444444444444198, 0.8222222222222221877, 0.8249999999999999556, 0.8277777777777777235, 0.8305555555555556024, 0.8333333333333333703, 0.8361111111111111382, 0.8388888888888889062, 0.8416666666666666741, 0.8444444444444444420, 0.8472222222222222099, 0.8499999999999999778, 0.8527777777777777457, 0.8555555555555555136, 0.8583333333333332815, 0.8611111111111111605, 0.8638888888888889284, 0.8666666666666666963, 0.8694444444444444642, 0.8722222222222222321, 0.8750000000000000000, 0.8777777777777777679, 0.8805555555555555358, 0.8833333333333333037, 0.8861111111111110716, 0.8888888888888888395, 0.8916666666666667185, 0.8944444444444444864, 0.8972222222222222543, 0.9000000000000000222, 0.9027777777777777901, 0.9055555555555555580, 0.9083333333333333259, 0.9111111111111110938, 0.9138888888888888618, 0.9166666666666666297, 0.9194444444444443976, 0.9222222222222222765, 0.9250000000000000444, 0.9277777777777778123, 0.9305555555555555802, 0.9333333333333333481, 0.9361111111111111160, 0.9388888888888888840, 0.9416666666666666519, 0.9444444444444444198, 0.9472222222222221877, 0.9499999999999999556, 0.9527777777777777235, 0.9555555555555556024, 0.9583333333333333703, 0.9611111111111111382, 0.9638888888888889062, 0.9666666666666666741, 0.9694444444444444420, 0.9722222222222222099, 0.9749999999999999778, 0.9777777777777777457, 0.9805555555555555136, 0.9833333333333332815, 0.9861111111111111605, 0.9888888888888889284, 0.9916666666666666963, 0.9944444444444444642, 0.9972222222222222321, 1.000000000000000000 ),
 .UNSPECIFIED. ) 
 GEOMETRIC_REPRESENTATION_ITEM ( )  RATIONAL_B_SPLINE_SURFACE ( (
 ( 1.000000000000000000, 0.8660254037844387076, 1.000000000000000000, 0.8660254037844387076, 1.000000000000000000, 0.8660254037844387076, 1.000000000000000000, 0.8660254037844387076, 1.000000000000000000, 0.8660254037844387076, 1.000000000000000000, 0.8660254037844387076, 1.000000000000000000, 0.8660254037844387076, 1.000000000000000000, 0.8660254037844387076, 1.000000000000000000, 0.8660254037844387076, 1.000000000000000000, 0.8660254037844387076, 1.000000000000000000, 0.8660254037844387076, 1.000000000000000000, 0.8660254037844387076, 1.000000000000000000, 0.8660254037844387076, 1.000000000000000000, 0.8660254037844387076, 1.000000000000000000, 0.8660254037844387076, 1.000000000000000000, 0.8660254037844387076, 1.000000000000000000, 0.8660254037844387076, 1.000000000000000000, 0.8660254037844387076, 1.000000000000000000, 0.8660254037844387076, 1.000000000000000000, 0.8660254037844387076, 1.000000000000000000, 0.8660254037844387076, 1.000000000000000000, 0.8660254037844387076, 1.000000000000000000, 0.8660254037844387076, 1.000000000000000000, 0.8660254037844387076, 1.000000000000000000, 0.8660254037844387076, 1.000000000000000000, 0.8660254037844387076, 1.000000000000000000, 0.8660254037844387076, 1.000000000000000000, 0.8660254037844387076, 1.000000000000000000, 0.8660254037844387076, 1.000000000000000000, 0.8660254037844387076, 1.000000000000000000, 0.8660254037844387076, 1.000000000000000000, 0.8660254037844387076, 1.000000000000000000, 0.8660254037844387076, 1.000000000000000000, 0.8660254037844387076, 1.000000000000000000, 0.8660254037844387076, 1.000000000000000000, 0.8660254037844387076, 1.000000000000000000, 0.8660254037844387076, 1.000000000000000000, 0.8660254037844387076, 1.000000000000000000, 0.8660254037844387076, 1.000000000000000000, 0.8660254037844387076, 1.000000000000000000, 0.8660254037844387076, 1.000000000000000000, 0.8660254037844387076, 1.000000000000000000, 0.8660254037844387076, 1.000000000000000000, 0.8660254037844387076, 1.000000000000000000, 0.8660254037844387076, 1.000000000000000000, 0.8660254037844387076, 1.000000000000000000, 0.8660254037844387076, 1.000000000000000000, 0.8660254037844387076, 1.000000000000000000, 0.8660254037844387076, 1.000000000000000000, 0.8660254037844387076, 1.000000000000000000, 0.8660254037844387076, 1.000000000000000000, 0.8660254037844387076, 1.000000000000000000, 0.8660254037844387076, 1.000000000000000000, 0.8660254037844387076, 1.000000000000000000, 0.8660254037844387076, 1.000000000000000000, 0.8660254037844387076, 1.000000000000000000, 0.8660254037844387076, 1.000000000000000000, 0.8660254037844387076, 1.000000000000000000, 0.8660254037844387076, 1.000000000000000000, 0.8660254037844387076, 1.000000000000000000, 0.8660254037844387076, 1.000000000000000000, 0.8660254037844387076, 1.000000000000000000, 0.8660254037844387076, 1.000000000000000000, 0.8660254037844387076, 1.000000000000000000, 0.8660254037844387076, 1.000000000000000000, 0.8660254037844387076, 1.000000000000000000, 0.8660254037844387076, 1.000000000000000000, 0.8660254037844387076, 1.000000000000000000, 0.8660254037844387076, 1.000000000000000000, 0.8660254037844387076, 1.000000000000000000, 0.8660254037844387076, 1.000000000000000000, 0.8660254037844387076, 1.000000000000000000, 0.8660254037844387076, 1.000000000000000000, 0.8660254037844387076, 1.000000000000000000, 0.8660254037844387076, 1.000000000000000000, 0.8660254037844387076, 1.000000000000000000, 0.8660254037844387076, 1.000000000000000000, 0.8660254037844387076, 1.000000000000000000, 0.8660254037844387076, 1.000000000000000000, 0.8660254037844387076, 1.000000000000000000, 0.8660254037844387076, 1.000000000000000000, 0.8660254037844387076, 1.000000000000000000, 0.8660254037844387076, 1.000000000000000000, 0.8660254037844387076, 1.000000000000000000, 0.8660254037844387076, 1.000000000000000000, 0.8660254037844387076, 1.000000000000000000, 0.8660254037844387076, 1.000000000000000000, 0.8660254037844387076, 1.000000000000000000, 0.8660254037844387076, 1.000000000000000000, 0.8660254037844387076, 1.000000000000000000, 0.8660254037844387076, 1.000000000000000000, 0.8660254037844387076, 1.000000000000000000, 0.8660254037844387076, 1.000000000000000000, 0.8660254037844387076, 1.000000000000000000, 0.8660254037844387076, 1.000000000000000000, 0.8660254037844387076, 1.000000000000000000, 0.8660254037844387076, 1.000000000000000000, 0.8660254037844387076, 1.000000000000000000, 0.8660254037844387076, 1.000000000000000000, 0.8660254037844387076, 1.000000000000000000, 0.8660254037844387076, 1.000000000000000000, 0.8660254037844387076, 1.000000000000000000, 0.8660254037844387076, 1.000000000000000000, 0.8660254037844387076, 1.000000000000000000, 0.8660254037844387076, 1.000000000000000000, 0.8660254037844387076, 1.000000000000000000, 0.8660254037844387076, 1.000000000000000000, 0.8660254037844387076, 1.000000000000000000, 0.8660254037844387076, 1.000000000000000000, 0.8660254037844387076, 1.000000000000000000, 0.8660254037844387076, 1.000000000000000000, 0.8660254037844387076, 1.000000000000000000, 0.8660254037844387076, 1.000000000000000000, 0.8660254037844387076, 1.000000000000000000, 0.8660254037844387076, 1.000000000000000000, 0.8660254037844387076, 1.000000000000000000, 0.8660254037844387076, 1.000000000000000000, 0.8660254037844387076, 1.000000000000000000, 0.8660254037844387076, 1.000000000000000000, 0.8660254037844387076, 1.000000000000000000, 0.8660254037844387076, 1.000000000000000000, 0.8660254037844387076, 1.000000000000000000, 0.8660254037844387076, 1.000000000000000000, 0.8660254037844387076, 1.000000000000000000, 0.8660254037844387076, 1.000000000000000000, 0.8660254037844387076, 1.000000000000000000, 0.8660254037844387076, 1.000000000000000000, 0.8660254037844387076, 1.000000000000000000, 0.8660254037844387076, 1.000000000000000000, 0.8660254037844387076, 1.000000000000000000, 0.8660254037844387076, 1.000000000000000000, 0.8660254037844387076, 1.000000000000000000, 0.8660254037844387076, 1.000000000000000000, 0.8660254037844387076, 1.000000000000000000, 0.8660254037844387076, 1.000000000000000000, 0.8660254037844387076, 1.000000000000000000, 0.8660254037844387076, 1.000000000000000000, 0.8660254037844387076, 1.000000000000000000, 0.8660254037844387076, 1.000000000000000000, 0.8660254037844387076, 1.000000000000000000, 0.8660254037844387076, 1.000000000000000000, 0.8660254037844387076, 1.000000000000000000, 0.8660254037844387076, 1.000000000000000000, 0.8660254037844387076, 1.000000000000000000, 0.8660254037844387076, 1.000000000000000000, 0.8660254037844387076, 1.000000000000000000, 0.8660254037844387076, 1.000000000000000000, 0.8660254037844387076, 1.000000000000000000, 0.8660254037844387076, 1.000000000000000000, 0.8660254037844387076, 1.000000000000000000, 0.8660254037844387076, 1.000000000000000000, 0.8660254037844387076, 1.000000000000000000, 0.8660254037844387076, 1.000000000000000000, 0.8660254037844387076, 1.000000000000000000, 0.8660254037844387076, 1.000000000000000000, 0.8660254037844387076, 1.000000000000000000, 0.8660254037844387076, 1.000000000000000000, 0.8660254037844387076, 1.000000000000000000, 0.8660254037844387076, 1.000000000000000000, 0.8660254037844387076, 1.000000000000000000, 0.8660254037844387076, 1.000000000000000000, 0.8660254037844387076, 1.000000000000000000, 0.8660254037844387076, 1.000000000000000000, 0.8660254037844387076, 1.000000000000000000, 0.8660254037844387076, 1.000000000000000000, 0.8660254037844387076, 1.000000000000000000, 0.8660254037844387076, 1.000000000000000000, 0.8660254037844387076, 1.000000000000000000, 0.8660254037844387076, 1.000000000000000000, 0.8660254037844387076, 1.000000000000000000, 0.8660254037844387076, 1.000000000000000000, 0.8660254037844387076, 1.000000000000000000, 0.8660254037844387076, 1.000000000000000000, 0.8660254037844387076, 1.000000000000000000, 0.8660254037844387076, 1.000000000000000000, 0.8660254037844387076, 1.000000000000000000, 0.8660254037844387076, 1.000000000000000000, 0.8660254037844387076, 1.000000000000000000, 0.8660254037844387076, 1.000000000000000000, 0.8660254037844387076, 1.000000000000000000, 0.8660254037844387076, 1.000000000000000000, 0.8660254037844387076, 1.000000000000000000, 0.8660254037844387076, 1.000000000000000000, 0.8660254037844387076, 1.000000000000000000, 0.8660254037844387076, 1.000000000000000000, 0.8660254037844387076, 1.000000000000000000, 0.8660254037844387076, 1.000000000000000000, 0.8660254037844387076, 1.000000000000000000, 0.8660254037844387076, 1.000000000000000000, 0.8660254037844387076, 1.000000000000000000, 0.8660254037844387076, 1.000000000000000000, 0.8660254037844387076, 1.000000000000000000, 0.8660254037844387076, 1.000000000000000000, 0.8660254037844387076, 1.000000000000000000, 0.8660254037844387076, 1.000000000000000000, 0.8660254037844387076, 1.000000000000000000, 0.8660254037844387076, 1.000000000000000000, 0.8660254037844387076, 1.000000000000000000, 0.8660254037844387076, 1.000000000000000000, 0.8660254037844387076, 1.000000000000000000, 0.8660254037844387076, 1.000000000000000000, 0.8660254037844387076, 1.000000000000000000, 0.8660254037844387076, 1.000000000000000000, 0.8660254037844387076, 1.000000000000000000, 0.8660254037844387076, 1.000000000000000000, 0.8660254037844387076, 1.000000000000000000, 0.8660254037844387076, 1.000000000000000000, 0.8660254037844387076, 1.000000000000000000, 0.8660254037844387076, 1.000000000000000000, 0.8660254037844387076, 1.000000000000000000, 0.8660254037844387076, 1.000000000000000000, 0.8660254037844387076, 1.000000000000000000, 0.8660254037844387076, 1.000000000000000000, 0.8660254037844387076, 1.000000000000000000, 0.8660254037844387076, 1.000000000000000000, 0.8660254037844387076, 1.000000000000000000, 0.8660254037844387076, 1.000000000000000000, 0.8660254037844387076, 1.000000000000000000, 0.8660254037844387076, 1.000000000000000000, 0.8660254037844387076, 1.000000000000000000, 0.8660254037844387076, 1.000000000000000000, 0.8660254037844387076, 1.000000000000000000, 0.8660254037844387076, 1.000000000000000000, 0.8660254037844387076, 1.000000000000000000, 0.8660254037844387076, 1.000000000000000000, 0.8660254037844387076, 1.000000000000000000, 0.8660254037844387076, 1.000000000000000000, 0.8660254037844387076, 1.000000000000000000, 0.8660254037844387076, 1.000000000000000000, 0.8660254037844387076, 1.000000000000000000, 0.8660254037844387076, 1.000000000000000000, 0.8660254037844387076, 1.000000000000000000, 0.8660254037844387076, 1.000000000000000000, 0.8660254037844387076, 1.000000000000000000, 0.8660254037844387076, 1.000000000000000000, 0.8660254037844387076, 1.000000000000000000, 0.8660254037844387076, 1.000000000000000000, 0.8660254037844387076, 1.000000000000000000, 0.8660254037844387076, 1.000000000000000000, 0.8660254037844387076, 1.000000000000000000, 0.8660254037844387076, 1.000000000000000000, 0.8660254037844387076, 1.000000000000000000, 0.8660254037844387076, 1.000000000000000000, 0.8660254037844387076, 1.000000000000000000, 0.8660254037844387076, 1.000000000000000000, 0.8660254037844387076, 1.000000000000000000, 0.8660254037844387076, 1.000000000000000000, 0.8660254037844387076, 1.000000000000000000, 0.8660254037844387076, 1.000000000000000000, 0.8660254037844387076, 1.000000000000000000, 0.8660254037844387076, 1.000000000000000000, 0.8660254037844387076, 1.000000000000000000, 0.8660254037844387076, 1.000000000000000000, 0.8660254037844387076, 1.000000000000000000, 0.8660254037844387076, 1.000000000000000000, 0.8660254037844387076, 1.000000000000000000, 0.8660254037844387076, 1.000000000000000000, 0.8660254037844387076, 1.000000000000000000, 0.8660254037844387076, 1.000000000000000000, 0.8660254037844387076, 1.000000000000000000, 0.8660254037844387076, 1.000000000000000000, 0.8660254037844387076, 1.000000000000000000, 0.8660254037844387076, 1.000000000000000000, 0.8660254037844387076, 1.000000000000000000, 0.8660254037844387076, 1.000000000000000000, 0.8660254037844387076, 1.000000000000000000, 0.8660254037844387076, 1.000000000000000000, 0.8660254037844387076, 1.000000000000000000, 0.8660254037844387076, 1.000000000000000000, 0.8660254037844387076, 1.000000000000000000, 0.8660254037844387076, 1.000000000000000000, 0.8660254037844387076, 1.000000000000000000, 0.8660254037844387076, 1.000000000000000000, 0.8660254037844387076, 1.000000000000000000, 0.8660254037844387076, 1.000000000000000000, 0.8660254037844387076, 1.000000000000000000, 0.8660254037844387076, 1.000000000000000000, 0.8660254037844387076, 1.000000000000000000, 0.8660254037844387076, 1.000000000000000000, 0.8660254037844387076, 1.000000000000000000, 0.8660254037844387076, 1.000000000000000000, 0.8660254037844387076, 1.000000000000000000, 0.8660254037844387076, 1.000000000000000000, 0.8660254037844387076, 1.000000000000000000, 0.8660254037844387076, 1.000000000000000000, 0.8660254037844387076, 1.000000000000000000, 0.8660254037844387076, 1.000000000000000000, 0.8660254037844387076, 1.000000000000000000, 0.8660254037844387076, 1.000000000000000000, 0.8660254037844387076, 1.000000000000000000, 0.8660254037844387076, 1.000000000000000000, 0.8660254037844387076, 1.000000000000000000, 0.8660254037844387076, 1.000000000000000000, 0.8660254037844387076, 1.000000000000000000, 0.8660254037844387076, 1.000000000000000000, 0.8660254037844387076, 1.000000000000000000, 0.8660254037844387076, 1.000000000000000000, 0.8660254037844387076, 1.000000000000000000, 0.8660254037844387076, 1.000000000000000000, 0.8660254037844387076, 1.000000000000000000, 0.8660254037844387076, 1.000000000000000000, 0.8660254037844387076, 1.000000000000000000, 0.8660254037844387076, 1.000000000000000000, 0.8660254037844387076, 1.000000000000000000, 0.8660254037844387076, 1.000000000000000000, 0.8660254037844387076, 1.000000000000000000, 0.8660254037844387076, 1.000000000000000000, 0.8660254037844387076, 1.000000000000000000, 0.8660254037844387076, 1.000000000000000000, 0.8660254037844387076, 1.000000000000000000, 0.8660254037844387076, 1.000000000000000000, 0.8660254037844387076, 1.000000000000000000, 0.8660254037844387076, 1.000000000000000000, 0.8660254037844387076, 1.000000000000000000, 0.8660254037844387076, 1.000000000000000000, 0.8660254037844387076, 1.000000000000000000, 0.8660254037844387076, 1.000000000000000000, 0.8660254037844387076, 1.000000000000000000, 0.8660254037844387076, 1.000000000000000000, 0.8660254037844387076, 1.000000000000000000, 0.8660254037844387076, 1.000000000000000000, 0.8660254037844387076, 1.000000000000000000, 0.8660254037844387076, 1.000000000000000000, 0.8660254037844387076, 1.000000000000000000, 0.8660254037844387076, 1.000000000000000000, 0.8660254037844387076, 1.000000000000000000, 0.8660254037844387076, 1.000000000000000000, 0.8660254037844387076, 1.000000000000000000, 0.8660254037844387076, 1.000000000000000000, 0.8660254037844387076, 1.000000000000000000, 0.8660254037844387076, 1.000000000000000000, 0.8660254037844387076, 1.000000000000000000, 0.8660254037844387076, 1.000000000000000000, 0.8660254037844387076, 1.000000000000000000, 0.8660254037844387076, 1.000000000000000000, 0.8660254037844387076, 1.000000000000000000, 0.8660254037844387076, 1.000000000000000000, 0.8660254037844387076, 1.000000000000000000, 0.8660254037844387076, 1.000000000000000000, 0.8660254037844387076, 1.000000000000000000, 0.8660254037844387076, 1.000000000000000000, 0.8660254037844387076, 1.000000000000000000, 0.8660254037844387076, 1.000000000000000000, 0.8660254037844387076, 1.000000000000000000, 0.8660254037844387076, 1.000000000000000000, 0.8660254037844387076, 1.000000000000000000, 0.8660254037844387076, 1.000000000000000000, 0.8660254037844387076, 1.000000000000000000, 0.8660254037844387076, 1.000000000000000000, 0.8660254037844387076, 1.000000000000000000, 0.8660254037844387076, 1.000000000000000000, 0.8660254037844387076, 1.000000000000000000, 0.8660254037844387076, 1.000000000000000000, 0.8660254037844387076, 1.000000000000000000, 0.8660254037844387076, 1.000000000000000000, 0.8660254037844387076, 1.000000000000000000, 0.8660254037844387076, 1.000000000000000000, 0.8660254037844387076, 1.000000000000000000, 0.8660254037844387076, 1.000000000000000000, 0.8660254037844387076, 1.000000000000000000),
 ( 1.000000000000000000, 0.8660254037844387076, 1.000000000000000000, 0.8660254037844387076, 1.000000000000000000, 0.8660254037844387076, 1.000000000000000000, 0.8660254037844387076, 1.000000000000000000, 0.8660254037844387076, 1.000000000000000000, 0.8660254037844387076, 1.000000000000000000, 0.8660254037844387076, 1.000000000000000000, 0.8660254037844387076, 1.000000000000000000, 0.8660254037844387076, 1.000000000000000000, 0.8660254037844387076, 1.000000000000000000, 0.8660254037844387076, 1.000000000000000000, 0.8660254037844387076, 1.000000000000000000, 0.8660254037844387076, 1.000000000000000000, 0.8660254037844387076, 1.000000000000000000, 0.8660254037844387076, 1.000000000000000000, 0.8660254037844387076, 1.000000000000000000, 0.8660254037844387076, 1.000000000000000000, 0.8660254037844387076, 1.000000000000000000, 0.8660254037844387076, 1.000000000000000000, 0.8660254037844387076, 1.000000000000000000, 0.8660254037844387076, 1.000000000000000000, 0.8660254037844387076, 1.000000000000000000, 0.8660254037844387076, 1.000000000000000000, 0.8660254037844387076, 1.000000000000000000, 0.8660254037844387076, 1.000000000000000000, 0.8660254037844387076, 1.000000000000000000, 0.8660254037844387076, 1.000000000000000000, 0.8660254037844387076, 1.000000000000000000, 0.8660254037844387076, 1.000000000000000000, 0.8660254037844387076, 1.000000000000000000, 0.8660254037844387076, 1.000000000000000000, 0.8660254037844387076, 1.000000000000000000, 0.8660254037844387076, 1.000000000000000000, 0.8660254037844387076, 1.000000000000000000, 0.8660254037844387076, 1.000000000000000000, 0.8660254037844387076, 1.000000000000000000, 0.8660254037844387076, 1.000000000000000000, 0.8660254037844387076, 1.000000000000000000, 0.8660254037844387076, 1.000000000000000000, 0.8660254037844387076, 1.000000000000000000, 0.8660254037844387076, 1.000000000000000000, 0.8660254037844387076, 1.000000000000000000, 0.8660254037844387076, 1.000000000000000000, 0.8660254037844387076, 1.000000000000000000, 0.8660254037844387076, 1.000000000000000000, 0.8660254037844387076, 1.000000000000000000, 0.8660254037844387076, 1.000000000000000000, 0.8660254037844387076, 1.000000000000000000, 0.8660254037844387076, 1.000000000000000000, 0.8660254037844387076, 1.000000000000000000, 0.8660254037844387076, 1.000000000000000000, 0.8660254037844387076, 1.000000000000000000, 0.8660254037844387076, 1.000000000000000000, 0.8660254037844387076, 1.000000000000000000, 0.8660254037844387076, 1.000000000000000000, 0.8660254037844387076, 1.000000000000000000, 0.8660254037844387076, 1.000000000000000000, 0.8660254037844387076, 1.000000000000000000, 0.8660254037844387076, 1.000000000000000000, 0.8660254037844387076, 1.000000000000000000, 0.8660254037844387076, 1.000000000000000000, 0.8660254037844387076, 1.000000000000000000, 0.8660254037844387076, 1.000000000000000000, 0.8660254037844387076, 1.000000000000000000, 0.8660254037844387076, 1.000000000000000000, 0.8660254037844387076, 1.000000000000000000, 0.8660254037844387076, 1.000000000000000000, 0.8660254037844387076, 1.000000000000000000, 0.8660254037844387076, 1.000000000000000000, 0.8660254037844387076, 1.000000000000000000, 0.8660254037844387076, 1.000000000000000000, 0.8660254037844387076, 1.000000000000000000, 0.8660254037844387076, 1.000000000000000000, 0.8660254037844387076, 1.000000000000000000, 0.8660254037844387076, 1.000000000000000000, 0.8660254037844387076, 1.000000000000000000, 0.8660254037844387076, 1.000000000000000000, 0.8660254037844387076, 1.000000000000000000, 0.8660254037844387076, 1.000000000000000000, 0.8660254037844387076, 1.000000000000000000, 0.8660254037844387076, 1.000000000000000000, 0.8660254037844387076, 1.000000000000000000, 0.8660254037844387076, 1.000000000000000000, 0.8660254037844387076, 1.000000000000000000, 0.8660254037844387076, 1.000000000000000000, 0.8660254037844387076, 1.000000000000000000, 0.8660254037844387076, 1.000000000000000000, 0.8660254037844387076, 1.000000000000000000, 0.8660254037844387076, 1.000000000000000000, 0.8660254037844387076, 1.000000000000000000, 0.8660254037844387076, 1.000000000000000000, 0.8660254037844387076, 1.000000000000000000, 0.8660254037844387076, 1.000000000000000000, 0.8660254037844387076, 1.000000000000000000, 0.8660254037844387076, 1.000000000000000000, 0.8660254037844387076, 1.000000000000000000, 0.8660254037844387076, 1.000000000000000000, 0.8660254037844387076, 1.000000000000000000, 0.8660254037844387076, 1.000000000000000000, 0.8660254037844387076, 1.000000000000000000, 0.8660254037844387076, 1.000000000000000000, 0.8660254037844387076, 1.000000000000000000, 0.8660254037844387076, 1.000000000000000000, 0.8660254037844387076, 1.000000000000000000, 0.8660254037844387076, 1.000000000000000000, 0.8660254037844387076, 1.000000000000000000, 0.8660254037844387076, 1.000000000000000000, 0.8660254037844387076, 1.000000000000000000, 0.8660254037844387076, 1.000000000000000000, 0.8660254037844387076, 1.000000000000000000, 0.8660254037844387076, 1.000000000000000000, 0.8660254037844387076, 1.000000000000000000, 0.8660254037844387076, 1.000000000000000000, 0.8660254037844387076, 1.000000000000000000, 0.8660254037844387076, 1.000000000000000000, 0.8660254037844387076, 1.000000000000000000, 0.8660254037844387076, 1.000000000000000000, 0.8660254037844387076, 1.000000000000000000, 0.8660254037844387076, 1.000000000000000000, 0.8660254037844387076, 1.000000000000000000, 0.8660254037844387076, 1.000000000000000000, 0.8660254037844387076, 1.000000000000000000, 0.8660254037844387076, 1.000000000000000000, 0.8660254037844387076, 1.000000000000000000, 0.8660254037844387076, 1.000000000000000000, 0.8660254037844387076, 1.000000000000000000, 0.8660254037844387076, 1.000000000000000000, 0.8660254037844387076, 1.000000000000000000, 0.8660254037844387076, 1.000000000000000000, 0.8660254037844387076, 1.000000000000000000, 0.8660254037844387076, 1.000000000000000000, 0.8660254037844387076, 1.000000000000000000, 0.8660254037844387076, 1.000000000000000000, 0.8660254037844387076, 1.000000000000000000, 0.8660254037844387076, 1.000000000000000000, 0.8660254037844387076, 1.000000000000000000, 0.8660254037844387076, 1.000000000000000000, 0.8660254037844387076, 1.000000000000000000, 0.8660254037844387076, 1.000000000000000000, 0.8660254037844387076, 1.000000000000000000, 0.8660254037844387076, 1.000000000000000000, 0.8660254037844387076, 1.000000000000000000, 0.8660254037844387076, 1.000000000000000000, 0.8660254037844387076, 1.000000000000000000, 0.8660254037844387076, 1.000000000000000000, 0.8660254037844387076, 1.000000000000000000, 0.8660254037844387076, 1.000000000000000000, 0.8660254037844387076, 1.000000000000000000, 0.8660254037844387076, 1.000000000000000000, 0.8660254037844387076, 1.000000000000000000, 0.8660254037844387076, 1.000000000000000000, 0.8660254037844387076, 1.000000000000000000, 0.8660254037844387076, 1.000000000000000000, 0.8660254037844387076, 1.000000000000000000, 0.8660254037844387076, 1.000000000000000000, 0.8660254037844387076, 1.000000000000000000, 0.8660254037844387076, 1.000000000000000000, 0.8660254037844387076, 1.000000000000000000, 0.8660254037844387076, 1.000000000000000000, 0.8660254037844387076, 1.000000000000000000, 0.8660254037844387076, 1.000000000000000000, 0.8660254037844387076, 1.000000000000000000, 0.8660254037844387076, 1.000000000000000000, 0.8660254037844387076, 1.000000000000000000, 0.8660254037844387076, 1.000000000000000000, 0.8660254037844387076, 1.000000000000000000, 0.8660254037844387076, 1.000000000000000000, 0.8660254037844387076, 1.000000000000000000, 0.8660254037844387076, 1.000000000000000000, 0.8660254037844387076, 1.000000000000000000, 0.8660254037844387076, 1.000000000000000000, 0.8660254037844387076, 1.000000000000000000, 0.8660254037844387076, 1.000000000000000000, 0.8660254037844387076, 1.000000000000000000, 0.8660254037844387076, 1.000000000000000000, 0.8660254037844387076, 1.000000000000000000, 0.8660254037844387076, 1.000000000000000000, 0.8660254037844387076, 1.000000000000000000, 0.8660254037844387076, 1.000000000000000000, 0.8660254037844387076, 1.000000000000000000, 0.8660254037844387076, 1.000000000000000000, 0.8660254037844387076, 1.000000000000000000, 0.8660254037844387076, 1.000000000000000000, 0.8660254037844387076, 1.000000000000000000, 0.8660254037844387076, 1.000000000000000000, 0.8660254037844387076, 1.000000000000000000, 0.8660254037844387076, 1.000000000000000000, 0.8660254037844387076, 1.000000000000000000, 0.8660254037844387076, 1.000000000000000000, 0.8660254037844387076, 1.000000000000000000, 0.8660254037844387076, 1.000000000000000000, 0.8660254037844387076, 1.000000000000000000, 0.8660254037844387076, 1.000000000000000000, 0.8660254037844387076, 1.000000000000000000, 0.8660254037844387076, 1.000000000000000000, 0.8660254037844387076, 1.000000000000000000, 0.8660254037844387076, 1.000000000000000000, 0.8660254037844387076, 1.000000000000000000, 0.8660254037844387076, 1.000000000000000000, 0.8660254037844387076, 1.000000000000000000, 0.8660254037844387076, 1.000000000000000000, 0.8660254037844387076, 1.000000000000000000, 0.8660254037844387076, 1.000000000000000000, 0.8660254037844387076, 1.000000000000000000, 0.8660254037844387076, 1.000000000000000000, 0.8660254037844387076, 1.000000000000000000, 0.8660254037844387076, 1.000000000000000000, 0.8660254037844387076, 1.000000000000000000, 0.8660254037844387076, 1.000000000000000000, 0.8660254037844387076, 1.000000000000000000, 0.8660254037844387076, 1.000000000000000000, 0.8660254037844387076, 1.000000000000000000, 0.8660254037844387076, 1.000000000000000000, 0.8660254037844387076, 1.000000000000000000, 0.8660254037844387076, 1.000000000000000000, 0.8660254037844387076, 1.000000000000000000, 0.8660254037844387076, 1.000000000000000000, 0.8660254037844387076, 1.000000000000000000, 0.8660254037844387076, 1.000000000000000000, 0.8660254037844387076, 1.000000000000000000, 0.8660254037844387076, 1.000000000000000000, 0.8660254037844387076, 1.000000000000000000, 0.8660254037844387076, 1.000000000000000000, 0.8660254037844387076, 1.000000000000000000, 0.8660254037844387076, 1.000000000000000000, 0.8660254037844387076, 1.000000000000000000, 0.8660254037844387076, 1.000000000000000000, 0.8660254037844387076, 1.000000000000000000, 0.8660254037844387076, 1.000000000000000000, 0.8660254037844387076, 1.000000000000000000, 0.8660254037844387076, 1.000000000000000000, 0.8660254037844387076, 1.000000000000000000, 0.8660254037844387076, 1.000000000000000000, 0.8660254037844387076, 1.000000000000000000, 0.8660254037844387076, 1.000000000000000000, 0.8660254037844387076, 1.000000000000000000, 0.8660254037844387076, 1.000000000000000000, 0.8660254037844387076, 1.000000000000000000, 0.8660254037844387076, 1.000000000000000000, 0.8660254037844387076, 1.000000000000000000, 0.8660254037844387076, 1.000000000000000000, 0.8660254037844387076, 1.000000000000000000, 0.8660254037844387076, 1.000000000000000000, 0.8660254037844387076, 1.000000000000000000, 0.8660254037844387076, 1.000000000000000000, 0.8660254037844387076, 1.000000000000000000, 0.8660254037844387076, 1.000000000000000000, 0.8660254037844387076, 1.000000000000000000, 0.8660254037844387076, 1.000000000000000000, 0.8660254037844387076, 1.000000000000000000, 0.8660254037844387076, 1.000000000000000000, 0.8660254037844387076, 1.000000000000000000, 0.8660254037844387076, 1.000000000000000000, 0.8660254037844387076, 1.000000000000000000, 0.8660254037844387076, 1.000000000000000000, 0.8660254037844387076, 1.000000000000000000, 0.8660254037844387076, 1.000000000000000000, 0.8660254037844387076, 1.000000000000000000, 0.8660254037844387076, 1.000000000000000000, 0.8660254037844387076, 1.000000000000000000, 0.8660254037844387076, 1.000000000000000000, 0.8660254037844387076, 1.000000000000000000, 0.8660254037844387076, 1.000000000000000000, 0.8660254037844387076, 1.000000000000000000, 0.8660254037844387076, 1.000000000000000000, 0.8660254037844387076, 1.000000000000000000, 0.8660254037844387076, 1.000000000000000000, 0.8660254037844387076, 1.000000000000000000, 0.8660254037844387076, 1.000000000000000000, 0.8660254037844387076, 1.000000000000000000, 0.8660254037844387076, 1.000000000000000000, 0.8660254037844387076, 1.000000000000000000, 0.8660254037844387076, 1.000000000000000000, 0.8660254037844387076, 1.000000000000000000, 0.8660254037844387076, 1.000000000000000000, 0.8660254037844387076, 1.000000000000000000, 0.8660254037844387076, 1.000000000000000000, 0.8660254037844387076, 1.000000000000000000, 0.8660254037844387076, 1.000000000000000000, 0.8660254037844387076, 1.000000000000000000, 0.8660254037844387076, 1.000000000000000000, 0.8660254037844387076, 1.000000000000000000, 0.8660254037844387076, 1.000000000000000000, 0.8660254037844387076, 1.000000000000000000, 0.8660254037844387076, 1.000000000000000000, 0.8660254037844387076, 1.000000000000000000, 0.8660254037844387076, 1.000000000000000000, 0.8660254037844387076, 1.000000000000000000, 0.8660254037844387076, 1.000000000000000000, 0.8660254037844387076, 1.000000000000000000, 0.8660254037844387076, 1.000000000000000000, 0.8660254037844387076, 1.000000000000000000, 0.8660254037844387076, 1.000000000000000000, 0.8660254037844387076, 1.000000000000000000, 0.8660254037844387076, 1.000000000000000000, 0.8660254037844387076, 1.000000000000000000, 0.8660254037844387076, 1.000000000000000000, 0.8660254037844387076, 1.000000000000000000, 0.8660254037844387076, 1.000000000000000000, 0.8660254037844387076, 1.000000000000000000, 0.8660254037844387076, 1.000000000000000000, 0.8660254037844387076, 1.000000000000000000, 0.8660254037844387076, 1.000000000000000000, 0.8660254037844387076, 1.000000000000000000, 0.8660254037844387076, 1.000000000000000000, 0.8660254037844387076, 1.000000000000000000, 0.8660254037844387076, 1.000000000000000000, 0.8660254037844387076, 1.000000000000000000, 0.8660254037844387076, 1.000000000000000000, 0.8660254037844387076, 1.000000000000000000, 0.8660254037844387076, 1.000000000000000000, 0.8660254037844387076, 1.000000000000000000, 0.8660254037844387076, 1.000000000000000000, 0.8660254037844387076, 1.000000000000000000, 0.8660254037844387076, 1.000000000000000000, 0.8660254037844387076, 1.000000000000000000, 0.8660254037844387076, 1.000000000000000000, 0.8660254037844387076, 1.000000000000000000, 0.8660254037844387076, 1.000000000000000000, 0.8660254037844387076, 1.000000000000000000, 0.8660254037844387076, 1.000000000000000000, 0.8660254037844387076, 1.000000000000000000, 0.8660254037844387076, 1.000000000000000000, 0.8660254037844387076, 1.000000000000000000, 0.8660254037844387076, 1.000000000000000000, 0.8660254037844387076, 1.000000000000000000, 0.8660254037844387076, 1.000000000000000000, 0.8660254037844387076, 1.000000000000000000, 0.8660254037844387076, 1.000000000000000000, 0.8660254037844387076, 1.000000000000000000, 0.8660254037844387076, 1.000000000000000000, 0.8660254037844387076, 1.000000000000000000, 0.8660254037844387076, 1.000000000000000000, 0.8660254037844387076, 1.000000000000000000, 0.8660254037844387076, 1.000000000000000000, 0.8660254037844387076, 1.000000000000000000, 0.8660254037844387076, 1.000000000000000000, 0.8660254037844387076, 1.000000000000000000, 0.8660254037844387076, 1.000000000000000000, 0.8660254037844387076, 1.000000000000000000, 0.8660254037844387076, 1.000000000000000000, 0.8660254037844387076, 1.000000000000000000, 0.8660254037844387076, 1.000000000000000000, 0.8660254037844387076, 1.000000000000000000, 0.8660254037844387076, 1.000000000000000000, 0.8660254037844387076, 1.000000000000000000, 0.8660254037844387076, 1.000000000000000000, 0.8660254037844387076, 1.000000000000000000, 0.8660254037844387076, 1.000000000000000000, 0.8660254037844387076, 1.000000000000000000, 0.8660254037844387076, 1.000000000000000000, 0.8660254037844387076, 1.000000000000000000, 0.8660254037844387076, 1.000000000000000000, 0.8660254037844387076, 1.000000000000000000, 0.8660254037844387076, 1.000000000000000000, 0.8660254037844387076, 1.000000000000000000, 0.8660254037844387076, 1.000000000000000000, 0.8660254037844387076, 1.000000000000000000, 0.8660254037844387076, 1.000000000000000000, 0.8660254037844387076, 1.000000000000000000) ) ) 
 REPRESENTATION_ITEM ( '' )  SURFACE ( )  );
#72561=CARTESIAN_POINT ( 'NONE',  ( 6.750000001229033764, -2.886751345948129988, 4.999999999999997335 ) ) ;
#72562=CARTESIAN_POINT ( 'NONE',  ( 20.20312500061451644, 4.541064518000418104, -2.621784821874998173 ) ) ;
#72563=CARTESIAN_POINT ( 'NONE',  ( 7.800000001229035362, -2.886751345948125991, -5.000000000000000000 ) ) ;
#72564=CARTESIAN_POINT ( 'NONE',  ( 17.24062500061451786, -3.027376345333614438, 5.243569643749998122 ) ) ;
#72565=CARTESIAN_POINT ( 'NONE',  ( 16.11562500061451786, 3.027376345333613106, -5.243569643749998122 ) ) ;
#72567=CARTESIAN_POINT ( 'NONE',  ( 15.37500000000000000, 6.123233995736764310E-16, -4.999999999999998224 ) ) ;
#72568=CARTESIAN_POINT ( 'NONE',  ( 10.50000000122903465, -2.886751345948125991, -5.000000000000000000 ) ) ;
#72569=CARTESIAN_POINT ( 'NONE',  ( 8.803125000614517859, -4.541064518000417216, -2.621784821875001281 ) ) ;
#72570=CARTESIAN_POINT ( 'NONE',  ( 10.71562500061451928, 3.027376345333613106, -5.243569643749998122 ) ) ;
#72571=CARTESIAN_POINT ( 'NONE',  ( 21.48750000122903003, 4.330127018922191873, 2.499999999999999556 ) ) ;
#72574=CARTESIAN_POINT ( 'NONE',  ( 2.121784821875001281, 12.80937500061451928, -26.32496088578401938 ) ) ;
#72576=CARTESIAN_POINT ( 'NONE',  ( 6.412500001229036073, -4.330127018922190985, -2.500000000000001332 ) ) ;
#72577=VECTOR ( 'NONE', #58856, 1000.000000000000000 ) ;
#72578=CARTESIAN_POINT ( 'NONE',  ( 4.096875000614518925, 6.054752690667223547, 3.707466751127219781E-16 ) ) ;
#72579=CARTESIAN_POINT ( 'NONE',  ( 19.77187500061451786, 3.027376345333613106, -5.243569643749998122 ) ) ;
#72582=CARTESIAN_POINT ( 'NONE',  ( 15.74062500061451608, 6.054752690667223547, 3.707466751127219781E-16 ) ) ;
#72585=CARTESIAN_POINT ( 'NONE',  ( -3.999999999999997335, 15.53750000000000142, 32.30940107675850470 ) ) ;
#72586=CARTESIAN_POINT ( 'NONE',  ( 29.18437500061451573, 6.421520780324663323E-16, -5.243569643749999010 ) ) ;
#72588=CARTESIAN_POINT ( 'NONE',  ( 14.20312500061451644, -4.541064518000417216, -2.621784821875001281 ) ) ;
#72589=VECTOR ( 'NONE', #22421, 1000.000000000000000 ) ;
#72590=CARTESIAN_POINT ( 'NONE',  ( 11.55937500061451928, -4.541064518000417216, -2.621784821875001281 ) ) ;
#72591=ORIENTED_EDGE ( 'NONE', *, *, #48506, .T. ) ;
#72592=CARTESIAN_POINT ( 'NONE',  ( 9.449999999999999289, -4.330127018922190985, -2.500000000000001332 ) ) ;
#72593=CARTESIAN_POINT ( 'NONE',  ( 21.59062500061451928, 6.054752690667223547, 3.707466751127219781E-16 ) ) ;
#72594=CARTESIAN_POINT ( 'NONE',  ( 17.55000000122903003, -2.886751345948063374, 5.000000000000112799 ) ) ;
#72595=CARTESIAN_POINT ( 'NONE',  ( 28.61250000122903359, 4.330127018922192761, -2.499999999999997780 ) ) ;
#72596=CARTESIAN_POINT ( 'NONE',  ( 12.07499999999999929, -4.330127018922194537, 2.499999999999995559 ) ) ;
#72597=CARTESIAN_POINT ( 'NONE',  ( 20.88750000122903572, 6.123233995736764310E-16, -4.999999999999998224 ) ) ;
#72598=CARTESIAN_POINT ( 'NONE',  ( 16.26562500061451289, 3.027376345333611329, 5.243569643749999010 ) ) ;
#72601=CARTESIAN_POINT ( 'NONE',  ( 20.81250000000000000, 2.886751345948129099, -4.999999999999998224 ) ) ;
#72604=CARTESIAN_POINT ( 'NONE',  ( 20.78437500061451715, 4.541064518000418104, 2.621784821874999949 ) ) ;
#72605=CARTESIAN_POINT ( 'NONE',  ( 27.36562500061451786, 3.027376345333613106, -5.243569643749998122 ) ) ;
#72607=CARTESIAN_POINT ( 'NONE',  ( 14.36250000122903359, 0.000000000000000000, 4.999999999999998224 ) ) ;
#72608=CARTESIAN_POINT ( 'NONE',  ( 10.79062500061451679, 6.054752690667223547, 3.707466751127219781E-16 ) ) ;
#72609=CARTESIAN_POINT ( 'NONE',  ( 30.00000000000000000, 0.000000000000000000, 4.999999999999998224 ) ) ;
#72610=CARTESIAN_POINT ( 'NONE',  ( 17.77499999999999858, 4.330127018922191873, 2.499999999999999556 ) ) ;
#72611=CARTESIAN_POINT ( 'NONE',  ( 23.40000000000000213, -4.330127018922190985, -2.500000000000001332 ) ) ;
#72613=CARTESIAN_POINT ( 'NONE',  ( 4.809375000614516615, -4.541064518000417216, -2.621784821875001281 ) ) ;
#72614=CARTESIAN_POINT ( 'NONE',  ( 28.13437500061451502, -4.541064518000419881, 2.621784821874995952 ) ) ;
#72615=ORIENTED_EDGE ( 'NONE', *, *, #32398, .T. ) ;
#72616=CARTESIAN_POINT ( 'NONE',  ( 24.66562500061451502, 3.027376345333613106, -5.243569643749998122 ) ) ;
#72617=CARTESIAN_POINT ( 'NONE',  ( 24.45937500061451786, 0.000000000000000000, 5.243569643749999010 ) ) ;
#72618=CARTESIAN_POINT ( 'NONE',  ( -3.000416591977282496E-16, 19.69062500061459176, -34.90005215228797653 ) ) ;
#72619=CARTESIAN_POINT ( 'NONE',  ( 14.24999999999999822, 0.000000000000000000, 4.999999999999998224 ) ) ;
#72620=CARTESIAN_POINT ( 'NONE',  ( 8.090625000614515727, 6.054752690667223547, 3.707466751127219781E-16 ) ) ;
#72621=CARTESIAN_POINT ( 'NONE',  ( 3.761592534273730415, 3.294057342109477649, 3.962396521687911566 ) ) ;
#72622=CARTESIAN_POINT ( 'NONE',  ( 19.65000000000000213, 0.000000000000000000, 4.999999999999998224 ) ) ;
#72623=CARTESIAN_POINT ( 'NONE',  ( 26.24062500061451431, -3.027376345333614438, 5.243569643749998122 ) ) ;
#72624=CARTESIAN_POINT ( 'NONE',  ( 17.17500000122903359, -5.773502691896255534, -1.060575238724906372E-15 ) ) ;
#72625=CYLINDRICAL_SURFACE ( 'NONE', #14724, 4.000000000000000000 ) ;
#72627=CARTESIAN_POINT ( 'NONE',  ( 3.703125000614516882, 0.000000000000000000, 5.243569643749999010 ) ) ;
#72628=CARTESIAN_POINT ( 'NONE',  ( 21.08437500061451786, 6.421520780324663323E-16, -5.243569643749999010 ) ) ;
#72629=CARTESIAN_POINT ( 'NONE',  ( -2.121784821874996840, 15.88437500061451857, 33.67503911421598417 ) ) ;
#72630=CARTESIAN_POINT ( 'NONE',  ( 21.15937500061451715, 4.541064518000418104, -2.621784821874998173 ) ) ;
#72631=CARTESIAN_POINT ( 'NONE',  ( 28.54687500061451644, -3.027376345333614438, 5.243569643749998122 ) ) ;
#72633=CARTESIAN_POINT ( 'NONE',  ( 10.00312500061451715, 0.000000000000000000, 5.243569643749999010 ) ) ;
#72634=CARTESIAN_POINT ( 'NONE',  ( 1.071796769724495668, 17.09509619066136921, 34.00000000000000000 ) ) ;
#72635=CARTESIAN_POINT ( 'NONE',  ( 6.346875000614517148, 6.054752690667223547, 3.707466751127219781E-16 ) ) ;
#72636=CARTESIAN_POINT ( 'NONE',  ( 8.315625000614515372, -6.054752690667223547, -1.112240025338166033E-15 ) ) ;
#72637=CARTESIAN_POINT ( 'NONE',  ( 12.15937500061451892, 4.541064518000418104, -2.621784821874998173 ) ) ;
#72638=PRESENTATION_STYLE_ASSIGNMENT (( #56010 ) ) ;
#72639=CARTESIAN_POINT ( 'NONE',  ( 19.95000000122903572, -2.886751345948125991, -5.000000000000000000 ) ) ;
#72640=CARTESIAN_POINT ( 'NONE',  ( 7.921875000614517326, -6.054752690667223547, -1.112240025338166033E-15 ) ) ;
#72641=CARTESIAN_POINT ( 'NONE',  ( 9.703125000614514661, -4.541064518000417216, -2.621784821875001281 ) ) ;
#72642=CARTESIAN_POINT ( 'NONE',  ( 8.128125000614515372, 4.541064518000418104, 2.621784821874999949 ) ) ;
#72644=CARTESIAN_POINT ( 'NONE',  ( 18.30937500061451928, -4.541064518000417216, -2.621784821875001281 ) ) ;
#72645=CARTESIAN_POINT ( 'NONE',  ( -5.810221930991193690E-16, 11.45000000122903216, 26.00000000000000355 ) ) ;
#72646=CARTESIAN_POINT ( 'NONE',  ( 26.50312500061451360, 4.541064518000418104, -2.621784821874998173 ) ) ;
#72647=VECTOR ( 'NONE', #19237, 1000.000000000000000 ) ;
#72648=CARTESIAN_POINT ( 'NONE',  ( 11.87812500061451537, -4.541064518000419881, 2.621784821874995952 ) ) ;
#72650=CARTESIAN_POINT ( 'NONE',  ( 28.54687500061451644, -3.027376345333614438, 5.243569643749998122 ) ) ;
#72651=CARTESIAN_POINT ( 'NONE',  ( 2.121784821874999061, 12.05937500061451750, -33.67503911421598417 ) ) ;
#72652=CARTESIAN_POINT ( 'NONE',  ( 11.77500000122903501, -5.773502691896255534, -1.060575238724906372E-15 ) ) ;
#72653=CARTESIAN_POINT ( 'NONE',  ( 4.243569643749999010, 15.56562500061451715, -32.45002607614398471 ) ) ;
#72654=CARTESIAN_POINT ( 'NONE',  ( 14.58750000122903323, 6.123233995736764310E-16, -4.999999999999998224 ) ) ;
#72655=CARTESIAN_POINT ( 'NONE',  ( 9.665625000614515017, -6.054752690667223547, -1.112240025338166033E-15 ) ) ;
#72656=AXIS2_PLACEMENT_3D ( 'NONE', #29966, #52507, #13700 ) ;
#72657=CARTESIAN_POINT ( 'NONE',  ( 12.59999999999999964, -4.330127018922190985, -2.500000000000001332 ) ) ;
#72659=CARTESIAN_POINT ( 'NONE',  ( 23.57812500061451289, -4.541064518000419881, 2.621784821874995952 ) ) ;
#72660=CARTESIAN_POINT ( 'NONE',  ( 7.584375000614516082, 6.421520780324663323E-16, -5.243569643749999010 ) ) ;
#72661=EDGE_CURVE ( 'NONE', #62948, #39309, #55032, .T. ) ;
#72662=CARTESIAN_POINT ( 'NONE',  ( 10.08750000122903323, 6.123233995736764310E-16, -4.999999999999998224 ) ) ;
#72663=CARTESIAN_POINT ( 'NONE',  ( 17.77500000122903145, 2.886751345948129099, -4.999999999999998224 ) ) ;
#72664=CARTESIAN_POINT ( 'NONE',  ( 16.15312500061451573, 4.541064518000418104, -2.621784821874998173 ) ) ;
#72665=CARTESIAN_POINT ( 'NONE',  ( 18.89062500061451644, 6.054752690667223547, 3.707466751127219781E-16 ) ) ;
#72666=CARTESIAN_POINT ( 'NONE',  ( 26.51250000122903216, 0.000000000000000000, 4.999999999999998224 ) ) ;
#72667=CARTESIAN_POINT ( 'NONE',  ( 27.60000000122903430, -2.886751345948125991, -5.000000000000000000 ) ) ;
#72668=CARTESIAN_POINT ( 'NONE',  ( 22.12500000000000000, 6.123233995736764310E-16, -4.999999999999998224 ) ) ;
#72670=CARTESIAN_POINT ( 'NONE',  ( 25.32187500061451857, 3.027376345333611329, 5.243569643749999010 ) ) ;
#72671=CARTESIAN_POINT ( 'NONE',  ( 18.33750000122903501, 4.330127018922191873, 2.499999999999999556 ) ) ;
#72672=CARTESIAN_POINT ( 'NONE',  ( 12.86250000122903359, 4.330127018922192761, -2.499999999999997780 ) ) ;
#72673=CARTESIAN_POINT ( 'NONE',  ( 27.68437500061451573, -4.541064518000419881, 2.621784821874995952 ) ) ;
#72674=CARTESIAN_POINT ( 'NONE',  ( 4.284375000614518925, -4.541064518000419881, 2.621784821874995952 ) ) ;
#72675=CARTESIAN_POINT ( 'NONE',  ( 23.91562500061451502, 3.027376345333611329, 5.243569643749999010 ) ) ;
#72679=CARTESIAN_POINT ( 'NONE',  ( 10.54687500061451644, -3.027376345333614438, 5.243569643749998122 ) ) ;
#72680=CARTESIAN_POINT ( 'NONE',  ( 30.00000000000000000, 6.123233995736764310E-16, -4.999999999999998224 ) ) ;
#72681=CARTESIAN_POINT ( 'NONE',  ( 2.971875000614517592, -6.054752690667223547, -1.112240025338166033E-15 ) ) ;
#72682=CARTESIAN_POINT ( 'NONE',  ( 6.796875000614516438, 6.054752690667223547, 3.707466751127219781E-16 ) ) ;
#72683=CARTESIAN_POINT ( 'NONE',  ( 29.14687500061451075, -3.027376345333610441, -5.243569643749999898 ) ) ;
#72684=CARTESIAN_POINT ( 'NONE',  ( -4.243569643749999898, 10.31562500061459531, 27.54997392385601529 ) ) ;
#72685=CARTESIAN_POINT ( 'NONE',  ( 20.32499999999999929, 6.123233995736764310E-16, -4.999999999999998224 ) ) ;
#72686=ORIENTED_EDGE ( 'NONE', *, *, #40409, .F. ) ;
#72687=CARTESIAN_POINT ( 'NONE',  ( 28.16249999999999787, 2.886751345948126879, 4.999999999999999112 ) ) ;
#72688=CARTESIAN_POINT ( 'NONE',  ( 29.10937500061451644, -4.541064518000417216, -2.621784821875001281 ) ) ;
#72689=VERTEX_POINT ( 'NONE', #71912 ) ;
#72690=CARTESIAN_POINT ( 'NONE',  ( 18.81562500061452070, 3.027376345333613106, -5.243569643749998122 ) ) ;
#72691=CARTESIAN_POINT ( 'NONE',  ( 7.228125000614517681, 4.541064518000418104, 2.621784821874999949 ) ) ;
#72693=CARTESIAN_POINT ( 'NONE',  ( 5.221875000614519813, -6.054752690667223547, -1.112240025338166033E-15 ) ) ;
#72694=CARTESIAN_POINT ( 'NONE',  ( 16.87500000122903288, 2.886751345948129099, -4.999999999999998224 ) ) ;
#72695=CARTESIAN_POINT ( 'NONE',  ( 1.071796769724491893, 13.83259618943233527, -26.00000000000000355 ) ) ;
#72696=CARTESIAN_POINT ( 'NONE',  ( 6.009375000614519458, 0.000000000000000000, 5.243569643749999010 ) ) ;
#72697=CARTESIAN_POINT ( 'NONE',  ( 12.23437500061451821, 4.541064518000418104, 2.621784821874999949 ) ) ;
#72698=CARTESIAN_POINT ( 'NONE',  ( 20.63437500061451857, 6.421520780324663323E-16, -5.243569643749999010 ) ) ;
#72699=CARTESIAN_POINT ( 'NONE',  ( 4.494741915665277254, -2.190272839526016924, 4.494741915664858922 ) ) ;
#72702=CARTESIAN_POINT ( 'NONE',  ( 6.084375000614518747, -4.541064518000419881, 2.621784821874995952 ) ) ;
#72704=CARTESIAN_POINT ( 'NONE',  ( 22.12500000000000000, 6.123233995736764310E-16, -4.999999999999998224 ) ) ;
#72705=CARTESIAN_POINT ( 'NONE',  ( 17.76562500061451644, -6.054752690667223547, -1.112240025338166033E-15 ) ) ;
#72707=CARTESIAN_POINT ( 'NONE',  ( -2.121784821874996840, 10.93437500061451928, -26.32496088578401583 ) ) ;
#72709=CARTESIAN_POINT ( 'NONE',  ( 11.50312500061451892, -4.541064518000417216, -2.621784821875001281 ) ) ;
#72710=CARTESIAN_POINT ( 'NONE',  ( 29.48437500061451644, -4.541064518000419881, 2.621784821874995952 ) ) ;
#72712=CARTESIAN_POINT ( 'NONE',  ( 29.63437500061451502, 6.421520780324663323E-16, -5.243569643749999010 ) ) ;
#72713=CARTESIAN_POINT ( 'NONE',  ( 10.01250000000000107, 2.886751345948129099, -4.999999999999998224 ) ) ;
#72714=CARTESIAN_POINT ( 'NONE',  ( -1.999999999999997113, 15.68750000122903465, 33.46410161513775705 ) ) ;
#72715=CARTESIAN_POINT ( 'NONE',  ( 8.587500001229035007, -4.330127018922194537, 2.499999999999995559 ) ) ;
#72716=CARTESIAN_POINT ( 'NONE',  ( 20.85937500061451644, 0.000000000000000000, 5.243569643749999010 ) ) ;
#72717=CARTESIAN_POINT ( 'NONE',  ( 13.24687500061451750, -3.027376345333614438, 5.243569643749998122 ) ) ;
#72718=CARTESIAN_POINT ( 'NONE',  ( 1.592000809091587073E-14, 16.85000000122903785, 26.00000000000000000 ) ) ;
#72719=VERTEX_POINT ( 'NONE', #10580 ) ;
#72720=CARTESIAN_POINT ( 'NONE',  ( 14.09062500061451750, -3.027376345333614438, 5.243569643749998122 ) ) ;
#72721=CARTESIAN_POINT ( 'NONE',  ( 26.51250000122903216, 0.000000000000000000, 4.999999999999998224 ) ) ;
#72722=CARTESIAN_POINT ( 'NONE',  ( 14.89687500061451786, 6.054752690667223547, 3.707466751127219781E-16 ) ) ;
#72723=CARTESIAN_POINT ( 'NONE',  ( 3.979525575715637586, 9.178911176227741109, -25.49336387293115180 ) ) ;
#72724=CARTESIAN_POINT ( 'NONE',  ( 16.15312500061451573, 4.541064518000418104, -2.621784821874998173 ) ) ;
#72725=CARTESIAN_POINT ( 'NONE',  ( 0.000000000000000000, 0.000000000000000000, 50.00000000000000000 ) ) ;
#72726=CARTESIAN_POINT ( 'NONE',  ( 26.29687500061451644, -3.027376345333614438, 5.243569643749998122 ) ) ;
#72727=CARTESIAN_POINT ( 'NONE',  ( 2.121784821874999061, 10.20312500061451821, 26.32496088578401583 ) ) ;
#72728=CARTESIAN_POINT ( 'NONE',  ( 15.08437500061451786, -4.541064518000419881, 2.621784821874995952 ) ) ;
#72729=CARTESIAN_POINT ( 'NONE',  ( 14.28750000122903430, 4.330127018922191873, 2.499999999999999556 ) ) ;
#72731=CARTESIAN_POINT ( 'NONE',  ( 19.43437500061451928, 4.541064518000418104, 2.621784821874999949 ) ) ;
#72732=CARTESIAN_POINT ( 'NONE',  ( 20.70000000122903216, -2.886751345948129988, 4.999999999999997335 ) ) ;
#72733=CARTESIAN_POINT ( 'NONE',  ( 17.52187500061451431, 3.027376345333613106, -5.243569643749998122 ) ) ;
#72734=CARTESIAN_POINT ( 'NONE',  ( -4.243569643749999898, 12.65937500061451715, 30.00000000000000000 ) ) ;
#72736=CARTESIAN_POINT ( 'NONE',  ( 17.76562500061451644, -6.054752690667223547, -1.112240025338166033E-15 ) ) ;
#72739=CARTESIAN_POINT ( 'NONE',  ( 19.53749999999999432, 5.773502691896255534, 3.535250795749688894E-16 ) ) ;
#72741=CARTESIAN_POINT ( 'NONE',  ( 23.61562500061451431, -6.054752690667223547, -1.112240025338166033E-15 ) ) ;
#72742=CARTESIAN_POINT ( 'NONE',  ( 4.490625000614516971, 6.054752690667223547, 3.707466751127219781E-16 ) ) ;
#72744=CARTESIAN_POINT ( 'NONE',  ( 16.27500000122903501, -5.773502691896255534, -1.060575238724906372E-15 ) ) ;
#72745=CARTESIAN_POINT ( 'NONE',  ( 22.79062500061451502, -3.027376345333610441, -5.243569643749999898 ) ) ;
#72746=CARTESIAN_POINT ( 'NONE',  ( 21.56250000000000000, -5.773502691896255534, -1.060575238724906372E-15 ) ) ;
#72747=CARTESIAN_POINT ( 'NONE',  ( 25.22812500061451502, 4.541064518000418104, 2.621784821874999949 ) ) ;
#72748=CARTESIAN_POINT ( 'NONE',  ( 5.803125000614517859, 4.541064518000418104, -2.621784821874998173 ) ) ;
#72749=ORIENTED_EDGE ( 'NONE', *, *, #23832, .F. ) ;
#72750=CARTESIAN_POINT ( 'NONE',  ( 29.28749999999999787, -2.886751345948125991, -5.000000000000000000 ) ) ;
#72753=CARTESIAN_POINT ( 'NONE',  ( 23.25000000000000000, 0.000000000000000000, 4.999999999999998224 ) ) ;
#72754=CARTESIAN_POINT ( 'NONE',  ( 1.999999999999998668, 12.31250000122903465, -33.46410161513775705 ) ) ;
#72755=CARTESIAN_POINT ( 'NONE',  ( -2.121784821874999949, 17.53437500061451715, -33.67503911421598417 ) ) ;
#72756=CARTESIAN_POINT ( 'NONE',  ( 8.362500000000002487, 2.886751345948126879, 4.999999999999999112 ) ) ;
#72757=CARTESIAN_POINT ( 'NONE',  ( 5.962500001229033231, -4.330127018922190985, -2.500000000000001332 ) ) ;
#72758=CARTESIAN_POINT ( 'NONE',  ( 11.89687500061451608, -3.027376345333614438, 5.243569643749998122 ) ) ;
#72759=CARTESIAN_POINT ( 'NONE',  ( 24.60000000122903430, 5.773502691896255534, 3.535250795749688401E-16 ) ) ;
#72760=CARTESIAN_POINT ( 'NONE',  ( 4.584375000614516971, 4.541064518000418104, 2.621784821874999949 ) ) ;
#72761=CARTESIAN_POINT ( 'NONE',  ( 13.01250000122903394, 0.000000000000000000, 4.999999999999998224 ) ) ;
#72762=VECTOR ( 'NONE', #5058, 1000.000000000000000 ) ;
#72763=CYLINDRICAL_SURFACE ( 'NONE', #54826, 4.000000000000000000 ) ;
#72764=CARTESIAN_POINT ( 'NONE',  ( 10.28437500061451715, 6.421520780324663323E-16, -5.243569643749999010 ) ) ;
#72765=CARTESIAN_POINT ( 'NONE',  ( 4.000000000000000000, 14.00000000122903465, -27.69059892324149885 ) ) ;
#72766=CARTESIAN_POINT ( 'NONE',  ( 20.24062500061451431, 6.054752690667223547, 3.707466751127219781E-16 ) ) ;
#72767=CARTESIAN_POINT ( 'NONE',  ( 16.53750000000000142, -2.886751345948130876, 4.999999999999996447 ) ) ;
#72768=CARTESIAN_POINT ( 'NONE',  ( -4.243569643749999898, 18.41562500061459318, 27.54997392385601529 ) ) ;
#72769=CARTESIAN_POINT ( 'NONE',  ( 23.14687500061451786, -3.027376345333614438, 5.243569643749998122 ) ) ;
#72770=CARTESIAN_POINT ( 'NONE',  ( 7.320879633048903241E-15, 17.63749999999999574, 26.00000000000000355 ) ) ;
#72771=ADVANCED_FACE ( 'NONE', ( #20182 ), #27577, .F. ) ;
#72772=CARTESIAN_POINT ( 'NONE',  ( 28.61250000122903359, 4.330127018922192761, -2.499999999999997780 ) ) ;
#72774=CARTESIAN_POINT ( 'NONE',  ( 24.66562500061451502, 3.027376345333613106, -5.243569643749998122 ) ) ;
#72775=CARTESIAN_POINT ( 'NONE',  ( 16.71562500061451573, 3.027376345333611329, 5.243569643749999010 ) ) ;
#72777=CARTESIAN_POINT ( 'NONE',  ( 13.20937500061451786, 0.000000000000000000, 5.243569643749999010 ) ) ;
#72779=AXIS2_PLACEMENT_3D ( 'NONE', #7245, #7599, #2076 ) ;
#72780=CARTESIAN_POINT ( 'NONE',  ( 24.11250000122903359, 4.330127018922192761, -2.499999999999997780 ) ) ;
#72781=DIRECTION ( 'NONE',  ( -0.000000000000000000, -1.000000000000000000, -0.000000000000000000 ) ) ;
#72782=CARTESIAN_POINT ( 'NONE',  ( 13.09687500061451892, 6.054752690667223547, 3.707466751127219781E-16 ) ) ;
#72784=CARTESIAN_POINT ( 'NONE',  ( 3.112500000000000711, -5.773502691896255534, -1.060575238724906372E-15 ) ) ;
#72785=CARTESIAN_POINT ( 'NONE',  ( 1.626862140677534273E-15, 12.12500000122903465, 34.00000000000000000 ) ) ;
#72786=CARTESIAN_POINT ( 'NONE',  ( 24.83437500061451431, 4.541064518000418104, 2.621784821874999949 ) ) ;
#72787=CARTESIAN_POINT ( 'NONE',  ( 17.70937500061451431, 0.000000000000000000, 5.243569643749999010 ) ) ;
#72789=CARTESIAN_POINT ( 'NONE',  ( 28.94999999999999929, 4.330127018922192761, -2.499999999999997780 ) ) ;
#72790=CARTESIAN_POINT ( 'NONE',  ( 3.600000001229033408, -2.886751345948129988, 4.999999999999997335 ) ) ;
#72791=CARTESIAN_POINT ( 'NONE',  ( 5.812500000000001776, -5.773502691896255534, -1.060575238724906372E-15 ) ) ;
#72793=CARTESIAN_POINT ( 'NONE',  ( 20.01562500061451644, -6.054752690667223547, -1.112240025338166033E-15 ) ) ;
#72794=CARTESIAN_POINT ( 'NONE',  ( 9.637499999999999289, 5.773502691896255534, 3.535250795749688894E-16 ) ) ;
#72795=PLANE ( 'NONE',  #5419 ) ;
#72796=CARTESIAN_POINT ( 'NONE',  ( 16.87500000000000000, 4.330127018922191873, 2.499999999999999556 ) ) ;
#72797=CARTESIAN_POINT ( 'NONE',  ( -2.121784821874996840, 11.77812500061451750, 33.67503911421598417 ) ) ;
#72799=CARTESIAN_POINT ( 'NONE',  ( 19.76250000122903216, 0.000000000000000000, 4.999999999999998224 ) ) ;
#72801=CARTESIAN_POINT ( 'NONE',  ( 27.38437500061451857, 6.421520780324663323E-16, -5.243569643749999010 ) ) ;
#72802=ORIENTED_EDGE ( 'NONE', *, *, #36502, .F. ) ;
#72803=CARTESIAN_POINT ( 'NONE',  ( 16.90312500061451573, -4.541064518000417216, -2.621784821875001281 ) ) ;
#72804=CARTESIAN_POINT ( 'NONE',  ( 21.92812500061451431, 6.421520780324663323E-16, -5.243569643749999010 ) ) ;
#72805=CARTESIAN_POINT ( 'NONE',  ( 23.25937500061451857, -4.541064518000417216, -2.621784821875001281 ) ) ;
#72806=CARTESIAN_POINT ( 'NONE',  ( 7.087499999999999467, -2.886751345948129988, 4.999999999999997335 ) ) ;
#72807=CARTESIAN_POINT ( 'NONE',  ( 10.67812500061451608, 6.421520780324663323E-16, -5.243569643749999010 ) ) ;
#72808=CARTESIAN_POINT ( 'NONE',  ( 25.41562500061451146, -6.054752690667223547, -1.112240025338166033E-15 ) ) ;
#72809=CARTESIAN_POINT ( 'NONE',  ( 13.92187500061451644, 3.027376345333613106, -5.243569643749998122 ) ) ;
#72810=CARTESIAN_POINT ( 'NONE',  ( 19.09687500061451360, -3.027376345333614438, 5.243569643749998122 ) ) ;
#72811=CARTESIAN_POINT ( 'NONE',  ( 1.999999999999998668, 12.31250000122903465, -33.46410161513775705 ) ) ;
#72812=CARTESIAN_POINT ( 'NONE',  ( 4.243569643749999898, 11.08437500061451786, 30.00000000000000000 ) ) ;
#72813=CARTESIAN_POINT ( 'NONE',  ( 20.96250000122903145, 4.330127018922192761, -2.499999999999997780 ) ) ;
#72815=CARTESIAN_POINT ( 'NONE',  ( 12.47812500061451502, 6.421520780324663323E-16, -5.243569643749999010 ) ) ;
#72816=CARTESIAN_POINT ( 'NONE',  ( 5.859375000614519102, 4.541064518000418104, -2.621784821874998173 ) ) ;
#72817=CARTESIAN_POINT ( 'NONE',  ( 6.234375000614519102, 6.421520780324663323E-16, -5.243569643749999010 ) ) ;
#72819=CARTESIAN_POINT ( 'NONE',  ( 28.73437500061451644, 6.421520780324663323E-16, -5.243569643749999010 ) ) ;
#72820=CARTESIAN_POINT ( 'NONE',  ( 18.51562500061451289, 3.027376345333611329, 5.243569643749999010 ) ) ;
#72821=CARTESIAN_POINT ( 'NONE',  ( 28.72500000122903074, 2.886751345948126879, 4.999999999999999112 ) ) ;
#72822=CARTESIAN_POINT ( 'NONE',  ( 27.06562500061451004, 3.027376345333611329, 5.243569643749999010 ) ) ;
#72823=CARTESIAN_POINT ( 'NONE',  ( 23.82187500061451502, 3.027376345333613106, -5.243569643749998122 ) ) ;
#72824=CARTESIAN_POINT ( 'NONE',  ( 18.85312500061451502, 4.541064518000418104, -2.621784821874998173 ) ) ;
#72825=CARTESIAN_POINT ( 'NONE',  ( 8.484601909799253346E-16, 10.21250000000000213, 34.61880215351700230 ) ) ;
#72826=CARTESIAN_POINT ( 'NONE',  ( 24.32812500061451289, 4.541064518000418104, 2.621784821874999949 ) ) ;
#72827=CARTESIAN_POINT ( 'NONE',  ( 5.662500001229035185, 4.330127018922192761, -2.499999999999997780 ) ) ;
#72828=ORIENTED_EDGE ( 'NONE', *, *, #60362, .T. ) ;
#72829=CARTESIAN_POINT ( 'NONE',  ( 27.82499999999999929, -4.330127018922194537, 2.499999999999995559 ) ) ;
#72830=CARTESIAN_POINT ( 'NONE',  ( -3.999999999999999556, 16.36250000000000071, -32.30940107675850470 ) ) ;
#72832=CARTESIAN_POINT ( 'NONE',  ( 4.659375000614518925, 0.000000000000000000, 5.243569643749999010 ) ) ;
#72833=CARTESIAN_POINT ( 'NONE',  ( 12.25312500061451537, 0.000000000000000000, 5.243569643749999010 ) ) ;
#72834=CARTESIAN_POINT ( 'NONE',  ( 6.909375000614518036, 0.000000000000000000, 5.243569643749999010 ) ) ;
#72835=CARTESIAN_POINT ( 'NONE',  ( 25.08750000122903145, 4.330127018922191873, 2.499999999999999556 ) ) ;
#72837=CARTESIAN_POINT ( 'NONE',  ( 15.19687500061451679, -3.027376345333610441, -5.243569643749999898 ) ) ;
#72838=CARTESIAN_POINT ( 'NONE',  ( 29.12812500061451715, 6.421520780324663323E-16, -5.243569643749999010 ) ) ;
#72839=CARTESIAN_POINT ( 'NONE',  ( 28.94999999999999929, 4.330127018922192761, -2.499999999999997780 ) ) ;
#72840=CARTESIAN_POINT ( 'NONE',  ( 25.47187500061451715, -6.054752690667223547, -1.112240025338166033E-15 ) ) ;
#72841=CARTESIAN_POINT ( 'NONE',  ( 2.915625000614516793, -6.054752690667223547, -1.112240025338166033E-15 ) ) ;
#72842=CARTESIAN_POINT ( 'NONE',  ( 12.74062500061451786, -3.027376345333614438, 5.243569643749998122 ) ) ;
#72843=( BOUNDED_CURVE ( )  B_SPLINE_CURVE ( 2, ( #66308, #38223, #11254, #21965, #50420, #21597, #10524 ),
 .UNSPECIFIED., .F., .F. ) 
 B_SPLINE_CURVE_WITH_KNOTS ( ( 3, 2, 2, 3 ),
 ( 0.9166666666666666297, 0.9194444444444443976, 0.9222222222222221655, 0.9249999999999999334 ),
 .UNSPECIFIED. ) 
 CURVE ( )  GEOMETRIC_REPRESENTATION_ITEM ( )  RATIONAL_B_SPLINE_CURVE ( ( 1.000000000000000000, 0.8660254037844387076, 1.000000000000000000, 0.8660254037844387076, 1.000000000000000000, 0.8660254037844440367, 0.9999999999999946709 ) ) 
 REPRESENTATION_ITEM ( '' )  );
#72845=CARTESIAN_POINT ( 'NONE',  ( 10.49062500061451431, -3.027376345333614438, 5.243569643749998122 ) ) ;
#72846=CARTESIAN_POINT ( 'NONE',  ( 7.790625000614518569, -3.027376345333614438, 5.243569643749998122 ) ) ;
#72848=DIRECTION ( 'NONE',  ( -0.000000000000000000, -1.000000000000000000, -0.000000000000000000 ) ) ;
#72849=CARTESIAN_POINT ( 'NONE',  ( 16.19999999999999929, -4.330127018922190985, -2.500000000000001332 ) ) ;
#72850=CARTESIAN_POINT ( 'NONE',  ( 15.68437500061451573, 6.421520780324663323E-16, -5.243569643749999010 ) ) ;
#72851=CARTESIAN_POINT ( 'NONE',  ( 14.47500000122903430, -5.773502691896255534, -1.060575238724906372E-15 ) ) ;
#72853=CARTESIAN_POINT ( 'NONE',  ( 21.15937500061451715, 4.541064518000418104, -2.621784821874998173 ) ) ;
#72854=CARTESIAN_POINT ( 'NONE',  ( -2.121784821874999949, 13.87812500061451715, -33.67503911421598417 ) ) ;
#72857=CARTESIAN_POINT ( 'NONE',  ( 20.69999999999999929, -4.330127018922190985, -2.500000000000001332 ) ) ;
#72858=CARTESIAN_POINT ( 'NONE',  ( 27.81562500061452070, 3.027376345333613106, -5.243569643749998122 ) ) ;
#72859=CARTESIAN_POINT ( 'NONE',  ( -1.487416814333745711E-14, 16.06250000000000000, -26.00000000000000000 ) ) ;
#72860=CARTESIAN_POINT ( 'NONE',  ( 27.75000000000000000, 0.000000000000000000, 4.999999999999998224 ) ) ;
#72861=ADVANCED_FACE ( 'NONE', ( #66740 ), #42737, .F. ) ;
#72862=CARTESIAN_POINT ( 'NONE',  ( 9.028125000614517504, 4.541064518000418104, 2.621784821874999949 ) ) ;
#72864=CARTESIAN_POINT ( 'NONE',  ( 20.55937500061451573, -4.541064518000417216, -2.621784821875001281 ) ) ;
#72866=CARTESIAN_POINT ( 'NONE',  ( 4.978125000614518569, 4.541064518000418104, 2.621784821874999949 ) ) ;
#72867=CARTESIAN_POINT ( 'NONE',  ( 10.50937500061451679, 0.000000000000000000, 5.243569643749999010 ) ) ;
#72868=ORIENTED_EDGE ( 'NONE', *, *, #66396, .T. ) ;
#72869=CARTESIAN_POINT ( 'NONE',  ( 21.60937500061451644, 4.541064518000418104, -2.621784821874998173 ) ) ;
#72870=CARTESIAN_POINT ( 'NONE',  ( 1.347985686992486443, 4.821799686897913162, -26.22451506405455390 ) ) ;
#72871=CARTESIAN_POINT ( 'NONE',  ( 28.64999999999999858, 0.000000000000000000, 4.999999999999998224 ) ) ;
#72872=CARTESIAN_POINT ( 'NONE',  ( 4.500000000000000888, -4.330127018922190985, -2.500000000000001332 ) ) ;
#72874=CARTESIAN_POINT ( 'NONE',  ( 14.88750000122903394, -4.330127018922194537, 2.499999999999995559 ) ) ;
#72876=CARTESIAN_POINT ( 'NONE',  ( 19.20000000000000284, 0.000000000000000000, 4.999999999999998224 ) ) ;
#72877=ORIENTED_EDGE ( 'NONE', *, *, #9144, .T. ) ;
#72878=CARTESIAN_POINT ( 'NONE',  ( 13.83749999999999858, -2.886751345948129988, 4.999999999999997335 ) ) ;
#72879=CARTESIAN_POINT ( 'NONE',  ( 26.35312500061451857, -4.541064518000417216, -2.621784821875001281 ) ) ;
#72880=CARTESIAN_POINT ( 'NONE',  ( 17.39999999999999858, 0.000000000000000000, 4.999999999999998224 ) ) ;
#72881=CARTESIAN_POINT ( 'NONE',  ( 9.825000001229033941, 2.886751345948126879, 4.999999999999999112 ) ) ;
#72882=CARTESIAN_POINT ( 'NONE',  ( 9.665625000614515017, -6.054752690667223547, -1.112240025338166033E-15 ) ) ;
#72883=AXIS2_PLACEMENT_3D ( 'NONE', #65482, #44059, #32964 ) ;
#72884=CARTESIAN_POINT ( 'NONE',  ( 9.562500000000001776, 2.886751345948129099, -4.999999999999998224 ) ) ;
#72885=CARTESIAN_POINT ( 'NONE',  ( 18.41250000122903430, 0.000000000000000000, 4.999999999999998224 ) ) ;
#72886=CARTESIAN_POINT ( 'NONE',  ( -4.243569643749999898, 15.35937500061451644, -30.00000000000000000 ) ) ;
#72887=CARTESIAN_POINT ( 'NONE',  ( 27.63750000122903216, 6.123233995736764310E-16, -4.999999999999998224 ) ) ;
#72889=CARTESIAN_POINT ( 'NONE',  ( 7.500000000000000000, 0.000000000000000000, 4.999999999999998224 ) ) ;
#72890=CARTESIAN_POINT ( 'NONE',  ( -3.999999999999997335, 12.83750000000000213, 32.30940107675850470 ) ) ;
#72891=EDGE_LOOP ( 'NONE', ( #63403, #46209 ) ) ;
#72892=CARTESIAN_POINT ( 'NONE',  ( 24.02812500061451573, -4.541064518000419881, 2.621784821874995952 ) ) ;
#72893=CARTESIAN_POINT ( 'NONE',  ( 4.080569135018654592, -2.889455923578380769, -4.080569135022440896 ) ) ;
#72894=CARTESIAN_POINT ( 'NONE',  ( 21.19687500061451502, 6.054752690667223547, 3.707466751127219781E-16 ) ) ;
#72895=CARTESIAN_POINT ( 'NONE',  ( 15.74062500061451608, 6.054752690667223547, 3.707466751127219781E-16 ) ) ;
#72896=CARTESIAN_POINT ( 'NONE',  ( 2.121784821875001281, 11.40312500061459389, -26.32496088578401938 ) ) ;
#72897=CARTESIAN_POINT ( 'NONE',  ( 7.040625000614517681, -3.027376345333610441, -5.243569643749999898 ) ) ;
#72898=CARTESIAN_POINT ( 'NONE',  ( 28.61250000122903359, 4.330127018922192761, -2.499999999999997780 ) ) ;
#72900=CARTESIAN_POINT ( 'NONE',  ( 19.49062500061451786, -3.027376345333614438, 5.243569643749998122 ) ) ;
#72901=CARTESIAN_POINT ( 'NONE',  ( 3.999999999999999112, 11.33750000122903501, -30.00000000000000000 ) ) ;
#72903=CARTESIAN_POINT ( 'NONE',  ( 15.19687500061451857, -3.027376345333610441, -5.243569643749999898 ) ) ;
#72904=CARTESIAN_POINT ( 'NONE',  ( 14.10937500061451644, 0.000000000000000000, 5.243569643749999010 ) ) ;
#72905=CARTESIAN_POINT ( 'NONE',  ( 23.03437500061451715, 4.541064518000418104, 2.621784821874999949 ) ) ;
#72907=CARTESIAN_POINT ( 'NONE',  ( 3.028125000614518392, 6.421520780324663323E-16, -5.243569643749999010 ) ) ;
#72908=CARTESIAN_POINT ( 'NONE',  ( 26.24062500061451431, -3.027376345333614438, 5.243569643749998122 ) ) ;
#72909=CARTESIAN_POINT ( 'NONE',  ( 25.71562500061451573, 3.027376345333611329, 5.243569643749999010 ) ) ;
#72911=CARTESIAN_POINT ( 'NONE',  ( -3.999999999999999556, 16.36250000000000071, 27.69059892324149530 ) ) ;
#72912=CARTESIAN_POINT ( 'NONE',  ( 5.071875000614519458, 3.027376345333611329, 5.243569643749999010 ) ) ;
#72913=CARTESIAN_POINT ( 'NONE',  ( 11.28750000122903252, -4.330127018922194537, 2.499999999999995559 ) ) ;
#72914=CARTESIAN_POINT ( 'NONE',  ( 7.912500001229033408, 4.330127018922192761, -2.499999999999997780 ) ) ;
#72915=CARTESIAN_POINT ( 'NONE',  ( 29.21250000122903145, 0.000000000000000000, 4.999999999999998224 ) ) ;
#72918=CARTESIAN_POINT ( 'NONE',  ( 11.10937500061451644, -4.541064518000417216, -2.621784821875001281 ) ) ;
#72921=CARTESIAN_POINT ( 'NONE',  ( 19.11562500061451431, -6.054752690667223547, -1.112240025338166033E-15 ) ) ;
#72922=CARTESIAN_POINT ( 'NONE',  ( 13.92187500061451644, 3.027376345333613106, -5.243569643749998122 ) ) ;
#72923=CARTESIAN_POINT ( 'NONE',  ( 4.415625000614518569, 3.027376345333613106, -5.243569643749998122 ) ) ;
#72924=CARTESIAN_POINT ( 'NONE',  ( 22.58437500061451431, 4.541064518000418104, 2.621784821874999949 ) ) ;
#72925=CARTESIAN_POINT ( 'NONE',  ( 10.39687500061451786, 6.054752690667223547, 3.707466751127219781E-16 ) ) ;
#72926=CARTESIAN_POINT ( 'NONE',  ( 4.228125000614517681, -4.541064518000419881, 2.621784821874995952 ) ) ;
#72928=CARTESIAN_POINT ( 'NONE',  ( 4.950000001229033941, -2.886751345948129988, 4.999999999999997335 ) ) ;
#72929=CARTESIAN_POINT ( 'NONE',  ( 21.21562500061451573, 3.027376345333611329, 5.243569643749999010 ) ) ;
#72930=CARTESIAN_POINT ( 'NONE',  ( 7.125000001229033764, 2.886751345948126879, 4.999999999999999112 ) ) ;
#72931=CARTESIAN_POINT ( 'NONE',  ( 16.86562500061451786, -6.054752690667223547, -1.112240025338166033E-15 ) ) ;
#72932=CARTESIAN_POINT ( 'NONE',  ( 14.87812500061451537, 4.541064518000418104, 2.621784821874999949 ) ) ;
#72934=CARTESIAN_POINT ( 'NONE',  ( 15.41250000000000142, 2.886751345948129099, -4.999999999999998224 ) ) ;
#72935=CARTESIAN_POINT ( 'NONE',  ( 9.975000001229034297, -5.773502691896255534, -1.060575238724906372E-15 ) ) ;
#72937=CARTESIAN_POINT ( 'NONE',  ( 5.428125000614517859, 4.541064518000418104, 2.621784821874999949 ) ) ;
#72938=CARTESIAN_POINT ( 'NONE',  ( 19.98750000122903359, 6.123233995736764310E-16, -4.999999999999998224 ) ) ;
#72940=CARTESIAN_POINT ( 'NONE',  ( 4.243569643749999898, 10.18437500061451750, -30.00000000000000000 ) ) ;
#72941=CARTESIAN_POINT ( 'NONE',  ( 4.999999999999050537, 0.1750410927365727287, 5.155377002944480758 ) ) ;
#72943=CARTESIAN_POINT ( 'NONE',  ( 24.11249999999999716, 2.886751345948161074, 4.999999999999941380 ) ) ;
#72944=CARTESIAN_POINT ( 'NONE',  ( 3.196875000614516793, 6.054752690667223547, 3.707466751127219781E-16 ) ) ;
#72945=CARTESIAN_POINT ( 'NONE',  ( 21.08437500061451786, 6.421520780324663323E-16, -5.243569643749999010 ) ) ;
#72946=CARTESIAN_POINT ( 'NONE',  ( 12.26249999999999929, 2.886751345948062486, -5.000000000000113687 ) ) ;
#72947=CARTESIAN_POINT ( 'NONE',  ( 17.57812500061451644, 4.541064518000418104, 2.621784821874999949 ) ) ;
#72949=CARTESIAN_POINT ( 'NONE',  ( 23.06250000000000355, 2.886751345948162850, -4.999999999999940492 ) ) ;
#72951=CARTESIAN_POINT ( 'NONE',  ( 28.77187500061451431, 3.027376345333613106, -5.243569643749998122 ) ) ;
#72953=CARTESIAN_POINT ( 'NONE',  ( 11.72812500061451857, 4.541064518000418104, 2.621784821874999949 ) ) ;
#72954=CARTESIAN_POINT ( 'NONE',  ( 11.18437500061451928, 6.421520780324663323E-16, -5.243569643749999010 ) ) ;
#72955=EDGE_LOOP ( 'NONE', ( #11194, #16551 ) ) ;
#72956=CARTESIAN_POINT ( 'NONE',  ( 28.71562500061451573, 3.027376345333613106, -5.243569643749998122 ) ) ;
#72957=CARTESIAN_POINT ( 'NONE',  ( 22.07812500061451644, 4.541064518000418104, 2.621784821874999949 ) ) ;
#72958=CARTESIAN_POINT ( 'NONE',  ( 1.626862140677534273E-15, 11.11250000000000071, -26.00000000000000355 ) ) ;
#72959=CARTESIAN_POINT ( 'NONE',  ( 19.08750000122903145, 6.123233995736764310E-16, -4.999999999999998224 ) ) ;
#72960=CARTESIAN_POINT ( 'NONE',  ( 11.43750000000000000, 5.773502691896255534, 3.535250795749688894E-16 ) ) ;
#72961=CARTESIAN_POINT ( 'NONE',  ( 21.03750000122903074, 4.330127018922191873, 2.499999999999999556 ) ) ;
#72962=CARTESIAN_POINT ( 'NONE',  ( 16.82812500061451644, -4.541064518000419881, 2.621784821874995952 ) ) ;
#72965=CARTESIAN_POINT ( 'NONE',  ( 20.77500000000000213, 6.123233995736764310E-16, -4.999999999999998224 ) ) ;
#72966=CARTESIAN_POINT ( 'NONE',  ( 23.36250000000000071, -5.773502691896255534, -1.060575238724906372E-15 ) ) ;
#72967=CARTESIAN_POINT ( 'NONE',  ( 20.37187500061451573, 3.027376345333611329, 5.243569643749999010 ) ) ;
#72968=CARTESIAN_POINT ( 'NONE',  ( 26.46562500061451573, 3.027376345333613106, -5.243569643749998122 ) ) ;
#72969=VERTEX_POINT ( 'NONE', #37553 ) ;
#72971=CARTESIAN_POINT ( 'NONE',  ( 7.828125000614517326, -4.541064518000419881, 2.621784821874995952 ) ) ;
#72972=CARTESIAN_POINT ( 'NONE',  ( 3.347192403100067715, 3.714448376624780224, 3.458182559776492138 ) ) ;
#72973=CARTESIAN_POINT ( 'NONE',  ( 16.38749999999999929, 5.773502691896255534, 3.535250795749688894E-16 ) ) ;
#72974=CARTESIAN_POINT ( 'NONE',  ( 4.243569643749999010, 19.61562500061451431, 27.54997392385601174 ) ) ;
#72975=CARTESIAN_POINT ( 'NONE',  ( 4.246875000614519280, -3.027376345333614438, 5.243569643749998122 ) ) ;
#72976=CARTESIAN_POINT ( 'NONE',  ( 28.92187500061451644, 3.027376345333611329, 5.243569643749999010 ) ) ;
#72977=ORIENTED_EDGE ( 'NONE', *, *, #38408, .F. ) ;
#72978=CARTESIAN_POINT ( 'NONE',  ( 24.17812500061451786, 6.421520780324663323E-16, -5.243569643749999010 ) ) ;
#72979=CARTESIAN_POINT ( 'NONE',  ( 25.50937500061451502, -4.541064518000417216, -2.621784821875001281 ) ) ;
#72980=CARTESIAN_POINT ( 'NONE',  ( 2.121784821874999061, 19.65312500061459389, -33.67503911421598417 ) ) ;
#72981=CARTESIAN_POINT ( 'NONE',  ( 12.44999999999999929, 0.000000000000000000, 4.999999999999998224 ) ) ;
#72982=CARTESIAN_POINT ( 'NONE',  ( 8.653125000614515727, 0.000000000000000000, 5.243569643749999010 ) ) ;
#72983=CARTESIAN_POINT ( 'NONE',  ( 4.898587196589411843E-16, 20.00000000000000000, -26.00000000000000000 ) ) ;
#72985=CARTESIAN_POINT ( 'NONE',  ( 27.02812500061451573, 4.541064518000418104, 2.621784821874999949 ) ) ;
#72986=CARTESIAN_POINT ( 'NONE',  ( 12.75000000122903465, -2.886751345948126435, -5.000000000000000000 ) ) ;
#72988=CARTESIAN_POINT ( 'NONE',  ( 3.290625000614516793, -3.027376345333614438, 5.243569643749998122 ) ) ;
#72989=CARTESIAN_POINT ( 'NONE',  ( 19.13437500061451857, -4.541064518000419881, 2.621784821874995952 ) ) ;
#72990=( BOUNDED_CURVE ( )  B_SPLINE_CURVE ( 2, ( #18170, #68094, #6753, #7836, #46275, #861, #1219 ),
 .UNSPECIFIED., .F., .F. ) 
 B_SPLINE_CURVE_WITH_KNOTS ( ( 3, 2, 2, 3 ),
 ( 0.01666666666666663174, 0.01944444444444440312, 0.02222222222222217797, 0.02499999999999994935 ),
 .UNSPECIFIED. ) 
 CURVE ( )  GEOMETRIC_REPRESENTATION_ITEM ( )  RATIONAL_B_SPLINE_CURVE ( ( 1.000000000000001554, 0.8660254037844370423, 1.000000000000000000, 0.8660254037844387076, 1.000000000000000000, 0.8660254037844412611, 0.9999999999999974465 ) ) 
 REPRESENTATION_ITEM ( '' )  );
#72991=CARTESIAN_POINT ( 'NONE',  ( -4.243569643749999898, 14.90937500061451715, 30.00000000000000000 ) ) ;
#72992=CARTESIAN_POINT ( 'NONE',  ( 21.72187500061451715, 3.027376345333611329, 5.243569643749999010 ) ) ;
#72993=CARTESIAN_POINT ( 'NONE',  ( 3.225000000000002309, 6.123233995736764310E-16, -4.999999999999998224 ) ) ;
#72995=CARTESIAN_POINT ( 'NONE',  ( 9.440625000614517148, 6.054752690667223547, 3.707466751127219781E-16 ) ) ;
#72996=CARTESIAN_POINT ( 'NONE',  ( 1.071796769724493892, 17.27990381179670010, 26.00000000000000711 ) ) ;
#72997=CARTESIAN_POINT ( 'NONE',  ( 6.046875000614519102, -3.027376345333614438, 5.243569643749998122 ) ) ;
#72998=CARTESIAN_POINT ( 'NONE',  ( 7.453125000614516438, -4.541064518000417216, -2.621784821875001281 ) ) ;
#72999=CARTESIAN_POINT ( 'NONE',  ( 12.64687500061451608, 6.054752690667223547, 3.707466751127219781E-16 ) ) ;
#73000=CARTESIAN_POINT ( 'NONE',  ( 19.38750000122903216, -4.330127018922194537, 2.499999999999995559 ) ) ;
#73001=CARTESIAN_POINT ( 'NONE',  ( 8.221875000614518925, 3.027376345333611329, 5.243569643749999010 ) ) ;
#73002=CARTESIAN_POINT ( 'NONE',  ( 9.215625000614515727, -6.054752690667223547, -1.112240025338166033E-15 ) ) ;
#73005=CARTESIAN_POINT ( 'NONE',  ( 18.12187500061451573, 3.027376345333611329, 5.243569643749999010 ) ) ;
#73006=CARTESIAN_POINT ( 'NONE',  ( 18.26249999999999929, 2.886751345948126879, 4.999999999999998224 ) ) ;
#73007=CARTESIAN_POINT ( 'NONE',  ( 28.19062500061451715, -3.027376345333610441, -5.243569643749999898 ) ) ;
#73008=CARTESIAN_POINT ( 'NONE',  ( 11.05312500061451608, -4.541064518000417216, -2.621784821875001281 ) ) ;
#73009=CARTESIAN_POINT ( 'NONE',  ( 28.20937500061451786, -4.541064518000417216, -2.621784821875001281 ) ) ;
#73010=CARTESIAN_POINT ( 'NONE',  ( -3.000416591977282496E-16, 12.09687500061451892, -34.90005215228797653 ) ) ;
#73011=CARTESIAN_POINT ( 'NONE',  ( 12.22500000122903430, -5.773502691896255534, -1.060575238724906372E-15 ) ) ;
#73013=CARTESIAN_POINT ( 'NONE',  ( 27.77812500061451573, 6.421520780324663323E-16, -5.243569643749999010 ) ) ;
#73014=CARTESIAN_POINT ( 'NONE',  ( -4.243569643749997233, 16.24062500061451431, -27.54997392385601174 ) ) ;
#73015=CARTESIAN_POINT ( 'NONE',  ( 15.97500000122903430, 2.886751345948129099, -4.999999999999998224 ) ) ;
#73016=CARTESIAN_POINT ( 'NONE',  ( 12.41249999999999964, 2.886751345948126879, 4.999999999999999112 ) ) ;
#73017=CARTESIAN_POINT ( 'NONE',  ( -3.999999999999999112, 13.70000000000000107, 30.00000000000000000 ) ) ;
#73018=CARTESIAN_POINT ( 'NONE',  ( 22.64062500061451644, -3.027376345333614438, 5.243569643749998122 ) ) ;
#73019=CARTESIAN_POINT ( 'NONE',  ( 7.546875000614515550, -3.027376345333610441, -5.243569643749999898 ) ) ;
#73020=CARTESIAN_POINT ( 'NONE',  ( 8.100000001229034297, -2.886751345948129988, 4.999999999999997335 ) ) ;
#73021=CARTESIAN_POINT ( 'NONE',  ( 16.23750000122903359, -4.330127018922194537, 2.499999999999995559 ) ) ;
#73022=CARTESIAN_POINT ( 'NONE',  ( 13.75312500061451715, -4.541064518000417216, -2.621784821875001281 ) ) ;
#73023=EDGE_CURVE ( 'NONE', #54151, #55851, #5041, .T. ) ;
#73024=CARTESIAN_POINT ( 'NONE',  ( 17.35312500061451502, -4.541064518000417216, -2.621784821875001281 ) ) ;
#73025=CARTESIAN_POINT ( 'NONE',  ( 25.05000000122903714, 5.773502691896255534, 3.535250795749688894E-16 ) ) ;
#73026=CARTESIAN_POINT ( 'NONE',  ( 28.72500000122903074, 2.886751345948126879, 4.999999999999999112 ) ) ;
#73027=CARTESIAN_POINT ( 'NONE',  ( 22.57499999999999929, 6.123233995736764310E-16, -4.999999999999998224 ) ) ;
#73028=CARTESIAN_POINT ( 'NONE',  ( 25.62187500061451573, 3.027376345333613106, -5.243569643749998122 ) ) ;
#73030=CARTESIAN_POINT ( 'NONE',  ( 9.600000001229034297, -2.886751345948125991, -5.000000000000000000 ) ) ;
#73031=CARTESIAN_POINT ( 'NONE',  ( 28.69687500061451502, -3.027376345333610441, -5.243569643749999898 ) ) ;
#73032=( BOUNDED_CURVE ( )  B_SPLINE_CURVE ( 2, ( #36616, #28102, #10376, #5196, #39185, #22183, #55445, #49904, #21812 ),
 .UNSPECIFIED., .F., .F. ) 
 B_SPLINE_CURVE_WITH_KNOTS ( ( 3, 2, 2, 2, 3 ),
 ( 0.9456521739130434590, 0.9492753623188405765, 0.9565217391304348116, 0.9637681159420289356, 0.9662083058201528241 ),
 .UNSPECIFIED. ) 
 CURVE ( )  GEOMETRIC_REPRESENTATION_ITEM ( )  RATIONAL_B_SPLINE_CURVE ( ( 0.9330127018922194093, 0.9330127018922194093, 1.000000000000000000, 0.8660254037844387076, 1.000000000000000000, 0.8660254037844387076, 1.000000000000000000, 0.9548845634016894790, 0.9401540307620559478 ) ) 
 REPRESENTATION_ITEM ( '' )  );
#73033=CARTESIAN_POINT ( 'NONE',  ( 6.084375000614518747, -4.541064518000419881, 2.621784821874995952 ) ) ;
#73034=CARTESIAN_POINT ( 'NONE',  ( 22.56562500061451715, 3.027376345333611329, 5.243569643749999010 ) ) ;
#73037=CARTESIAN_POINT ( 'NONE',  ( 9.571875000614518569, 3.027376345333611329, 5.243569643749999010 ) ) ;
#73038=CARTESIAN_POINT ( 'NONE',  ( 10.53750000122903252, 6.123233995736764310E-16, -4.999999999999998224 ) ) ;
#73039=CARTESIAN_POINT ( 'NONE',  ( 3.496875000614518836, -3.027376345333610441, -5.243569643749999898 ) ) ;
#73040=CARTESIAN_POINT ( 'NONE',  ( 5.334375000614517859, 6.421520780324663323E-16, -5.243569643749999010 ) ) ;
#73041=CARTESIAN_POINT ( 'NONE',  ( -1.071796769724496556, 16.60490381179669939, -26.00000000000000355 ) ) ;
#73042=CARTESIAN_POINT ( 'NONE',  ( 27.53437500061451360, 4.541064518000418104, 2.621784821874999949 ) ) ;
#73044=CARTESIAN_POINT ( 'NONE',  ( -2.121784821874999949, 9.828125000614594597, 26.32496088578401938 ) ) ;
#73045=CARTESIAN_POINT ( 'NONE',  ( 20.43749999999999645, 5.773502691896255534, 3.535250795749688894E-16 ) ) ;
#73046=ORIENTED_EDGE ( 'NONE', *, *, #60961, .F. ) ;
#73047=CARTESIAN_POINT ( 'NONE',  ( 26.92499999999999716, -4.330127018922194537, 2.499999999999995559 ) ) ;
#73048=CARTESIAN_POINT ( 'NONE',  ( 28.05937500061451573, 0.000000000000000000, 5.243569643749999010 ) ) ;
#73050=CARTESIAN_POINT ( 'NONE',  ( 14.84062500061451750, 6.054752690667223547, 3.707466751127219781E-16 ) ) ;
#73051=CARTESIAN_POINT ( 'NONE',  ( 9.253125000614517148, -4.541064518000417216, -2.621784821875001281 ) ) ;
#73053=CARTESIAN_POINT ( 'NONE',  ( 5.859375000614519102, 4.541064518000418104, -2.621784821874998173 ) ) ;
#73054=CARTESIAN_POINT ( 'NONE',  ( 18.52500000122903145, -5.773502691896255534, -1.060575238724906372E-15 ) ) ;
#73055=CARTESIAN_POINT ( 'NONE',  ( 24.29999999999999716, -4.330127018922190985, -2.500000000000001332 ) ) ;
#73057=CARTESIAN_POINT ( 'NONE',  ( 6.796875000614516438, 6.054752690667223547, 3.707466751127219781E-16 ) ) ;
#73058=CARTESIAN_POINT ( 'NONE',  ( 11.18437500061451928, 6.421520780324663323E-16, -5.243569643749999010 ) ) ;
#73059=CARTESIAN_POINT ( 'NONE',  ( 21.38437500061451502, -4.541064518000419881, 2.621784821874995952 ) ) ;
#73060=CARTESIAN_POINT ( 'NONE',  ( 1.626862140677534273E-15, 16.51249999999999929, 34.00000000000000000 ) ) ;
#73062=CARTESIAN_POINT ( 'NONE',  ( 4.546875000614517326, 6.054752690667223547, 3.707466751127219781E-16 ) ) ;
#73064=CARTESIAN_POINT ( 'NONE',  ( 7.621875000614519280, 3.027376345333613106, -5.243569643749998122 ) ) ;
#73065=CARTESIAN_POINT ( 'NONE',  ( 20.73750000000000071, -2.886751345948125991, -5.000000000000000000 ) ) ;
#73066=CARTESIAN_POINT ( 'NONE',  ( 16.45312500061451289, -4.541064518000417216, -2.621784821875001281 ) ) ;
#73068=CARTESIAN_POINT ( 'NONE',  ( 4.243387908797823016, 2.644552713687023271, 4.380842878058396117 ) ) ;
#73070=CARTESIAN_POINT ( 'NONE',  ( 10.75312500061451715, 4.541064518000418104, -2.621784821874998173 ) ) ;
#73071=CARTESIAN_POINT ( 'NONE',  ( 26.10937500061451644, 4.541064518000418104, -2.621784821874998173 ) ) ;
#73072=DIRECTION ( 'NONE',  ( -0.000000000000000000, -1.000000000000000000, -0.000000000000000000 ) ) ;
#73073=CARTESIAN_POINT ( 'NONE',  ( 28.32187500061451502, 3.027376345333613106, -5.243569643749998122 ) ) ;
#73074=CARTESIAN_POINT ( 'NONE',  ( 9.037499999999999645, -2.886751345948125991, -5.000000000000000000 ) ) ;
#73075=CARTESIAN_POINT ( 'NONE',  ( 3.999999999999999112, 14.93750000122903288, 30.00000000000000000 ) ) ;
#73076=CARTESIAN_POINT ( 'NONE',  ( 8.737500001229033586, 6.123233995736764310E-16, -4.999999999999998224 ) ) ;
#73077=CARTESIAN_POINT ( 'NONE',  ( 18.98437500061451644, 4.541064518000418104, 2.621784821874999949 ) ) ;
#73078=CARTESIAN_POINT ( 'NONE',  ( 14.78437500061451715, 6.421520780324663323E-16, -5.243569643749999010 ) ) ;
#73079=CARTESIAN_POINT ( 'NONE',  ( 9.187500001229034652, 6.123233995736764310E-16, -4.999999999999998224 ) ) ;
#73080=ORIENTED_EDGE ( 'NONE', *, *, #27328, .T. ) ;
#73081=CARTESIAN_POINT ( 'NONE',  ( 14.65312500061451573, -4.541064518000417216, -2.621784821875001281 ) ) ;
#73082=CARTESIAN_POINT ( 'NONE',  ( 25.20000000122903216, -2.886751345948129988, 4.999999999999997335 ) ) ;
#73083=CARTESIAN_POINT ( 'NONE',  ( 14.67187500061451821, -6.054752690667223547, -1.112240025338166033E-15 ) ) ;
#73084=CARTESIAN_POINT ( 'NONE',  ( 3.328125000614516438, -4.541064518000419881, 2.621784821874995952 ) ) ;
#73085=CARTESIAN_POINT ( 'NONE',  ( 16.79062500061451857, -3.027376345333614438, 5.243569643749998122 ) ) ;
#73087=CARTESIAN_POINT ( 'NONE',  ( 25.84687500061451360, -3.027376345333614438, 5.243569643749998122 ) ) ;
#73088=CARTESIAN_POINT ( 'NONE',  ( 9.001249775931846008E-16, 11.36562500061451786, 34.90005215228797653 ) ) ;
#73089=CARTESIAN_POINT ( 'NONE',  ( 14.63437500061451679, -4.541064518000419881, 2.621784821874995952 ) ) ;
#73090=CARTESIAN_POINT ( 'NONE',  ( 14.58750000122903323, 6.123233995736764310E-16, -4.999999999999998224 ) ) ;
#73092=CARTESIAN_POINT ( 'NONE',  ( -4.243569643749998122, 18.99687500061451928, -27.54997392385601174 ) ) ;
#73093=CARTESIAN_POINT ( 'NONE',  ( 21.30937500061451573, 0.000000000000000000, 5.243569643749999010 ) ) ;
#73094=CARTESIAN_POINT ( 'NONE',  ( 20.96250000122903145, 4.330127018922192761, -2.499999999999997780 ) ) ;
#73095=CARTESIAN_POINT ( 'NONE',  ( 13.58437500061451786, 4.541064518000418104, 2.621784821874999949 ) ) ;
#73096=CARTESIAN_POINT ( 'NONE',  ( 2.121784821874999061, 11.60937500061451821, 26.32496088578401583 ) ) ;
#73097=CARTESIAN_POINT ( 'NONE',  ( 21.75000000122903288, -2.886751345948125991, -5.000000000000000000 ) ) ;
#73098=CARTESIAN_POINT ( 'NONE',  ( 18.29062500061451502, -3.027376345333610441, -5.243569643749999898 ) ) ;
#73100=ORIENTED_EDGE ( 'NONE', *, *, #48794, .T. ) ;
#73101=CARTESIAN_POINT ( 'NONE',  ( 21.48750000000000071, -2.886751345948129988, 4.999999999999997335 ) ) ;
#73102=CARTESIAN_POINT ( 'NONE',  ( 30.00000000000000000, 0.000000000000000000, 0.000000000000000000 ) ) ;
#73103=CARTESIAN_POINT ( 'NONE',  ( 25.04062500061451502, -3.027376345333610441, -5.243569643749999898 ) ) ;
#73104=CARTESIAN_POINT ( 'NONE',  ( 3.943546631589880391, 3.074146327801218437, 30.68299680867395907 ) ) ;
#73105=CARTESIAN_POINT ( 'NONE',  ( 18.52500000122903145, -5.773502691896255534, -1.060575238724906372E-15 ) ) ;
#73106=CARTESIAN_POINT ( 'NONE',  ( 21.55312500061451431, 4.541064518000418104, -2.621784821874998173 ) ) ;
#73107=EDGE_CURVE ( 'NONE', #37048, #48891, #47355, .T. ) ;
#73108=CARTESIAN_POINT ( 'NONE',  ( 24.92812500061451431, -4.541064518000419881, 2.621784821874995952 ) ) ;
#73109=CARTESIAN_POINT ( 'NONE',  ( 5.053125000614517859, 0.000000000000000000, 5.243569643749999010 ) ) ;
#73110=EDGE_LOOP ( 'NONE', ( #47495, #330, #25184, #41516 ) ) ;
#73111=CARTESIAN_POINT ( 'NONE',  ( 26.88750000122903216, 4.330127018922191873, 2.499999999999999556 ) ) ;
#73112=CARTESIAN_POINT ( 'NONE',  ( -1.071796769724488563, 10.30490381179670045, -26.00000000000000000 ) ) ;
#73115=CARTESIAN_POINT ( 'NONE',  ( 3.999999999999998668, 10.92500000122903536, -32.30940107675850470 ) ) ;
#73116=CARTESIAN_POINT ( 'NONE',  ( -2.121784821874999949, 19.33437500061451786, -33.67503911421598417 ) ) ;
#73117=CARTESIAN_POINT ( 'NONE',  ( 7.387500000000001066, 5.773502691896255534, 3.535250795749688894E-16 ) ) ;
#73118=CARTESIAN_POINT ( 'NONE',  ( 29.55000000122903003, 5.773502691896255534, 3.535250795749688401E-16 ) ) ;
#73124=COLOUR_RGB('Dark Blue',0.08,0.2,0.34);
#73125=FILL_AREA_STYLE_COLOUR('',#73124);
#73126=FILL_AREA_STYLE('',(#73125));
#73127=SURFACE_STYLE_FILL_AREA(#73126);
#73128=SURFACE_SIDE_STYLE('',(#73127));
#73129=SURFACE_STYLE_USAGE(.BOTH.,#73128);
#73130=PRESENTATION_STYLE_ASSIGNMENT((#73129));
ENDSEC;
END-ISO-10303-21;
